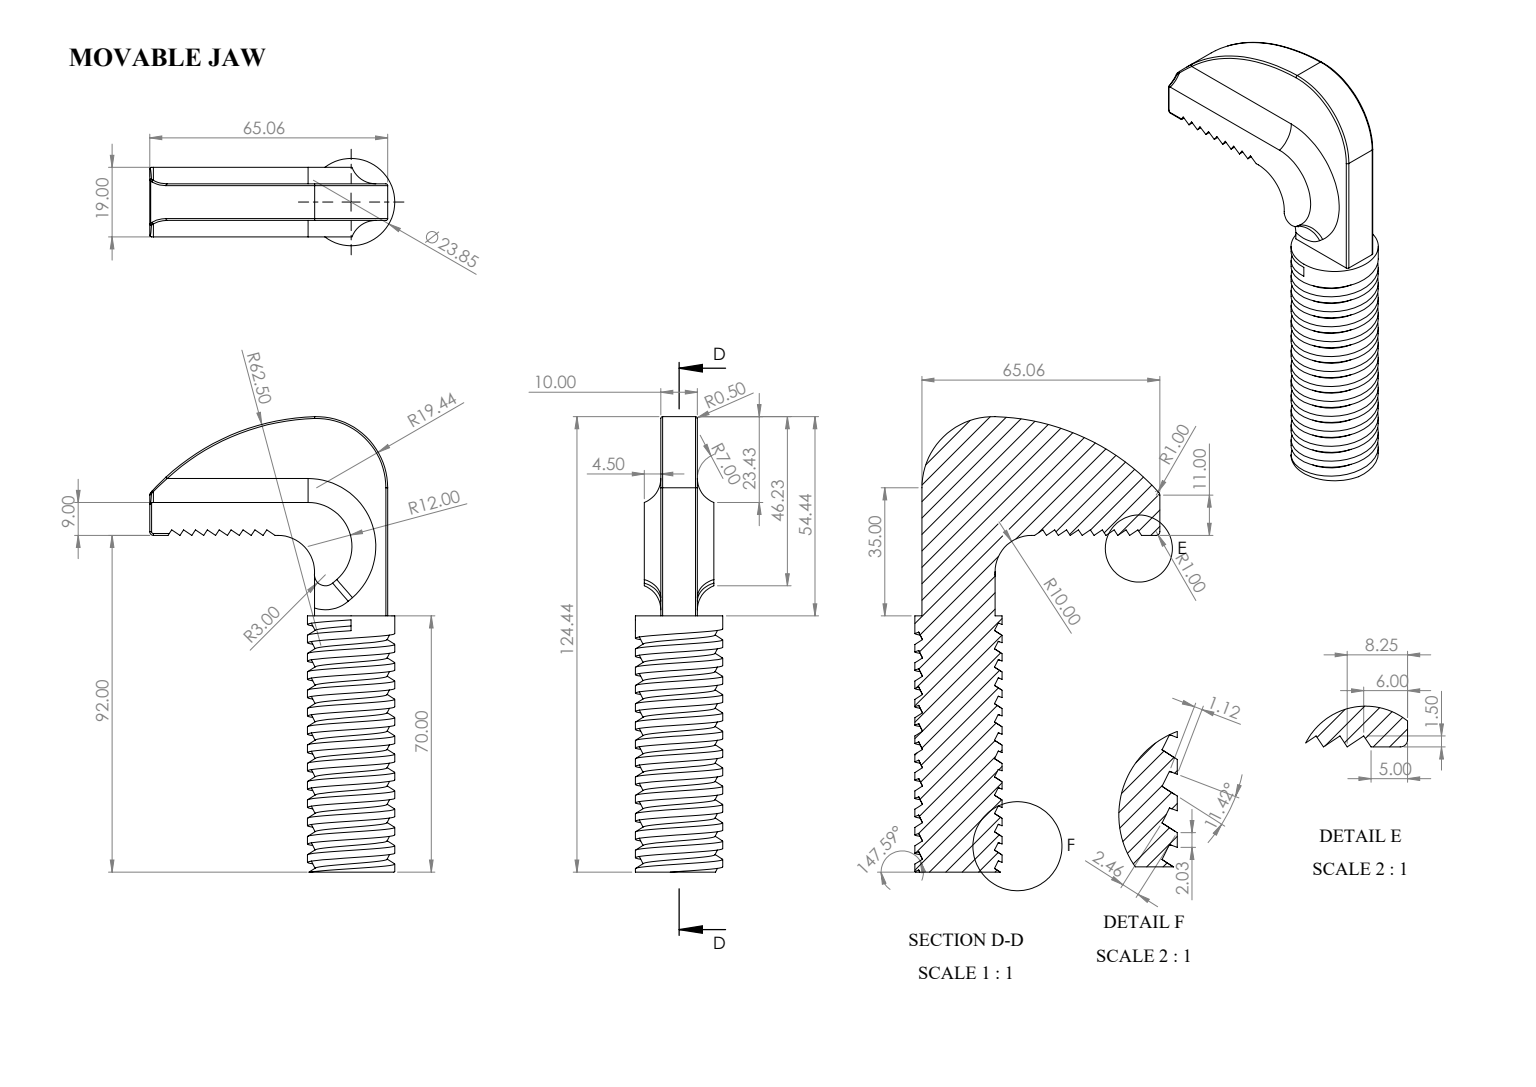
ISO-10303-21;
HEADER;
FILE_DESCRIPTION (('STEP AP214'),
    '1' );
FILE_NAME ('1.2 Movable Jaw.step',
    '2026-10-07T05:30:18',
    ( '' ),
    ( '' ),
    'SwSTEP 2.0',
    'SolidWorks 2021',
    '' );
FILE_SCHEMA (( 'AUTOMOTIVE_DESIGN' ));
ENDSEC;

DATA;
#1=CARTESIAN_POINT ( 'NONE',  ( 7.084665262690076126, 22.02201867748817321, -10.88017736071110164 ) ) ;
#3=CARTESIAN_POINT ( 'NONE',  ( 10.00000000000000000, 59.75893115100078745, -9.846743663894594434 ) ) ;
#5=CARTESIAN_POINT ( 'NONE',  ( 14.92337183194729988, 29.34226448433411960, -8.527530157486177487 ) ) ;
#6=CARTESIAN_POINT ( 'NONE',  ( -1.099225684535947600, 54.54030133659708923, 6.408140936763237150 ) ) ;
#9=CARTESIAN_POINT ( 'NONE',  ( 4.559911319644449179, 47.23035201082150536, -9.422509992056141925 ) ) ;
#10=CARTESIAN_POINT ( 'NONE',  ( 10.00000000000000000, 49.75893115100078745, -9.846743663894594434 ) ) ;
#11=CARTESIAN_POINT ( 'NONE',  ( 6.204703633549690345, 40.76208216824731778, -14.16423886937410259 ) ) ;
#13=CARTESIAN_POINT ( 'NONE',  ( 17.08211943468705840, 5.137082168247300906, -12.26659068614894466 ) ) ;
#14=CARTESIAN_POINT ( 'NONE',  ( 0.5774900079438590739, 67.64701867748817676, -5.440088680355550821 ) ) ;
#16=CARTESIAN_POINT ( 'NONE',  ( 24.16423886937410614, 59.51208216824728936, -3.795296366450302550 ) ) ;
#17=CARTESIAN_POINT ( 'NONE',  ( 13.43411237798106583, 7.665301336597086568, -12.81628187352647252 ) ) ;
#18=CARTESIAN_POINT ( 'NONE',  ( 18.95386800104995473, 43.23810908735726599, -6.499999999999990230 ) ) ;
#19=CARTESIAN_POINT ( 'NONE',  ( 0.5774900079438607392, 58.48035201082151247, 5.440088680355550821 ) ) ;
#21=CARTESIAN_POINT ( 'NONE',  ( -46.94000000000001194, 100.5254250115999923, -8.865097534344174690 ) ) ;
#22=CARTESIAN_POINT ( 'NONE',  ( 0.6178305044545818747, 33.49863466993042493, -9.382169495545419124 ) ) ;
#23=CARTESIAN_POINT ( 'NONE',  ( -2.266590686148945544, 67.22041550158063217, 7.082119434687048631 ) ) ;
#25=CARTESIAN_POINT ( 'NONE',  ( 20.88017736071110875, 15.77201867748817143, -2.915334737309920765 ) ) ;
#26=CARTESIAN_POINT ( 'NONE',  ( 19.42250999205614193, 30.14701867748817321, 5.440088680355555262 ) ) ;
#27=CARTESIAN_POINT ( 'NONE',  ( 7.361572987183169658, 49.96726448433410894, -9.846743663894592657 ) ) ;
#28=CARTESIAN_POINT ( 'NONE',  ( 19.84674366389459266, 58.71726448433411605, -2.638427012816827677 ) ) ;
#29=CARTESIAN_POINT ( 'NONE',  ( -2.816281873526473856, 49.12363466993042493, 9.499525473075851096E-16 ) ) ;
#34=CARTESIAN_POINT ( 'NONE',  ( 20.88017736071110875, 20.77201867748816611, -2.915334737309920765 ) ) ;
#35=CARTESIAN_POINT ( 'NONE',  ( 6.565887622018943937, 23.08196800326375708, -12.81628187352647608 ) ) ;
#37=CARTESIAN_POINT ( 'NONE',  ( 10.00000000000000000, 54.75893115100078745, -9.846743663894594434 ) ) ;
#38=CARTESIAN_POINT ( 'NONE',  ( 12.91533473730992121, 29.52201867748817321, 10.88017736071110164 ) ) ;
#39=CARTESIAN_POINT ( 'NONE',  ( 3.591859063236763294, 18.29030133659708568, -11.09922568453595026 ) ) ;
#40=CARTESIAN_POINT ( 'NONE',  ( -0.8801773607111008646, 43.27201867748817676, 2.915334737309923430 ) ) ;
#42=DIRECTION ( 'NONE',  ( -1.000000000000000000, 0.000000000000000000, 0.000000000000000000 ) ) ;
#43=CARTESIAN_POINT ( 'NONE',  ( 21.09922568453594849, 56.20696800326375353, 6.408140936763242479 ) ) ;
#45=CARTESIAN_POINT ( 'NONE',  ( 12.63842701281683034, 62.46726448433410894, 9.846743663894596210 ) ) ;
#46=CARTESIAN_POINT ( 'NONE',  ( -0.8801773607110991993, 42.85535201082150536, -2.915334737309923874 ) ) ;
#47=CARTESIAN_POINT ( 'NONE',  ( 13.43411237798106583, 32.66530133659708213, -12.81628187352647252 ) ) ;
#48=CARTESIAN_POINT ( 'NONE',  ( -4.164238869374099039, 6.803748834913967869, 8.674139862899312516E-16 ) ) ;
#49=CARTESIAN_POINT ( 'NONE',  ( 10.00000000000000000, 9.758931151000785675, -9.846743663894594434 ) ) ;
#50=CARTESIAN_POINT ( 'NONE',  ( 2.035157376598824452, 58.68868534415482685, 7.964842623401179544 ) ) ;
#51=CARTESIAN_POINT ( 'NONE',  ( -4.164238869374099039, 46.80374883491397497, 8.674139862899312516E-16 ) ) ;
#53=CARTESIAN_POINT ( 'NONE',  ( 0.1532563361054083140, 11.00893115100078568, 1.131784320476157264E-15 ) ) ;
#54=CARTESIAN_POINT ( 'NONE',  ( 0.1532563361054082862, 6.217264484334118713, 2.638427012816831674 ) ) ;
#56=CARTESIAN_POINT ( 'NONE',  ( 2.917880565312950480, 45.97041550158063927, -12.26659068614894821 ) ) ;
#58=CARTESIAN_POINT ( 'NONE',  ( 0.5774900079438590739, 12.64701867748817143, -5.440088680355550821 ) ) ;
#60=ORIENTED_EDGE ( 'NONE', *, *, #26638, .T. ) ;
#62=CARTESIAN_POINT ( 'NONE',  ( 15.44008868035555793, 11.39701867748817143, -9.422509992056140149 ) ) ;
#63=CARTESIAN_POINT ( 'NONE',  ( 22.26659068614895176, 59.72041550158063927, -7.082119434687042414 ) ) ;
#65=CARTESIAN_POINT ( 'NONE',  ( 17.20831665107776587, 42.88393115100077324, 7.208316651077764980 ) ) ;
#66=CARTESIAN_POINT ( 'NONE',  ( -2.816281873526473856, 34.33196800326376064, 3.434112377981055619 ) ) ;
#69=CARTESIAN_POINT ( 'NONE',  ( -2.266590686148945544, 11.38708216824730179, -7.082119434687050408 ) ) ;
#70=CARTESIAN_POINT ( 'NONE',  ( 12.91533473730992121, 29.52201867748817321, 10.88017736071110164 ) ) ;
#71=CARTESIAN_POINT ( 'NONE',  ( -0.8801773607111009756, 8.063685344154837509, 1.068504757029289695E-15 ) ) ;
#72=CARTESIAN_POINT ( 'NONE',  ( 19.84674366389459266, 48.71726448433413026, -2.638427012816827677 ) ) ;
#75=CARTESIAN_POINT ( 'NONE',  ( 17.20831665107776587, 17.88393115100078745, 7.208316651077764980 ) ) ;
#76=CARTESIAN_POINT ( 'NONE',  ( 1.274849032794231007, 33.57228050351031357, 6.499999999999895195 ) ) ;
#78=EDGE_LOOP ( 'NONE', ( #8782, #50817, #67592, #16515 ) ) ;
#81=CARTESIAN_POINT ( 'NONE',  ( 12.63842701281683922, 59.55059781766744464, -9.846743663894590881 ) ) ;
#82=CARTESIAN_POINT ( 'NONE',  ( 20.88017736071110519, 30.56368534415484106, 2.639326808657452039E-16 ) ) ;
#83=CARTESIAN_POINT ( 'NONE',  ( 2.035157376598824452, 33.68868534415484106, 7.964842623401179544 ) ) ;
#84=CARTESIAN_POINT ( 'NONE',  ( 2.791683348922240793, 56.63393115100078035, 7.208316651077764092 ) ) ;
#85=CARTESIAN_POINT ( 'NONE',  ( 16.40814093676323893, 25.79030133659708923, 11.09922568453595026 ) ) ;
#86=CARTESIAN_POINT ( 'NONE',  ( -2.266590686148945544, 21.38708216824730357, -7.082119434687050408 ) ) ;
#89=CARTESIAN_POINT ( 'NONE',  ( 19.38216949554541202, 40.99863466993042493, 9.382169495545424454 ) ) ;
#91=CARTESIAN_POINT ( 'NONE',  ( 0.1532563361054083140, 51.00893115100078745, 1.131784320476157264E-15 ) ) ;
#92=CARTESIAN_POINT ( 'NONE',  ( -0.8801773607110991993, 2.855352010821504471, -2.915334737309923874 ) ) ;
#94=CARTESIAN_POINT ( 'NONE',  ( 17.96484262340118221, 11.18868534415484106, -7.964842623401177768 ) ) ;
#95=ORIENTED_EDGE ( 'NONE', *, *, #4795, .T. ) ;
#96=CARTESIAN_POINT ( 'NONE',  ( 20.88017736071110164, 60.35535201082151957, 2.915334737309930979 ) ) ;
#97=CARTESIAN_POINT ( 'NONE',  ( 15.44008868035555793, 61.39701867748817676, -9.422509992056140149 ) ) ;
#98=CARTESIAN_POINT ( 'NONE',  ( 10.00000000000000178, 59.31368534415484106, 10.88017736071110342 ) ) ;
#100=CARTESIAN_POINT ( 'NONE',  ( 0.5774900079438590739, 52.64701867748817676, -5.440088680355550821 ) ) ;
#103=CARTESIAN_POINT ( 'NONE',  ( -46.78604402846880106, 100.7423487049318140, 9.213902555517821114 ) ) ;
#106=CARTESIAN_POINT ( 'NONE',  ( 7.361572987183170547, 42.05059781766745886, 9.846743663894590881 ) ) ;
#107=VERTEX_POINT ( 'NONE', #70238 ) ;
#108=CARTESIAN_POINT ( 'NONE',  ( 1.472469842513823179, 65.59226448433412315, -4.923371831947296329 ) ) ;
#110=CARTESIAN_POINT ( 'NONE',  ( -4.164238869374098151, 16.59541550158063927, -3.795296366450310543 ) ) ;
#113=CARTESIAN_POINT ( 'NONE',  ( 10.00000000000000178, 64.31368534415483396, 10.88017736071110342 ) ) ;
#114=CARTESIAN_POINT ( 'NONE',  ( 7.084665262690076126, 12.02201867748817321, -10.88017736071110164 ) ) ;
#115=CARTESIAN_POINT ( 'NONE',  ( 0.6081133539230425544, 48.33703382326399378, 6.499999999999948486 ) ) ;
#116=CARTESIAN_POINT ( 'NONE',  ( 6.565887622018943937, 45.16530133659708923, 12.81628187352647430 ) ) ;
#118=CARTESIAN_POINT ( 'NONE',  ( 5.076628168052703671, 46.84226448433412315, 8.527530157486179263 ) ) ;
#119=CARTESIAN_POINT ( 'NONE',  ( 12.63842701281683034, 2.467264484334118269, 9.846743663894596210 ) ) ;
#120=CARTESIAN_POINT ( 'NONE',  ( 16.40814093676324603, 17.45696800326375353, -11.09922568453594671 ) ) ;
#121=CARTESIAN_POINT ( 'NONE',  ( 14.92337183194729988, 19.34226448433411960, -8.527530157486177487 ) ) ;
#122=CARTESIAN_POINT ( 'NONE',  ( 0.6178305044545818747, 13.49863466993041783, -9.382169495545419124 ) ) ;
#125=CARTESIAN_POINT ( 'NONE',  ( 12.63842701281683034, 12.46726448433411782, 9.846743663894596210 ) ) ;
#126=EDGE_LOOP ( 'NONE', ( #78693, #55595, #4509, #60539 ) ) ;
#128=CARTESIAN_POINT ( 'NONE',  ( -0.8801773607110991993, 22.85535201082150181, -2.915334737309923874 ) ) ;
#129=CARTESIAN_POINT ( 'NONE',  ( 24.16423886937410614, 19.30374883491397142, 8.672049930838204340E-16 ) ) ;
#130=CARTESIAN_POINT ( 'NONE',  ( 0.1532563361054082862, 46.21726448433411605, 2.638427012816831674 ) ) ;
#131=CARTESIAN_POINT ( 'NONE',  ( 1.472469842513823179, 5.592264484334118713, -4.923371831947296329 ) ) ;
#132=CARTESIAN_POINT ( 'NONE',  ( -2.816281873526473856, 44.33196800326375353, 3.434112377981055619 ) ) ;
#134=CARTESIAN_POINT ( 'NONE',  ( -0.8801773607111008646, 18.27201867748817321, 2.915334737309923430 ) ) ;
#136=CARTESIAN_POINT ( 'NONE',  ( 6.565887622018943937, 13.08196800326374998, -12.81628187352647608 ) ) ;
#137=CARTESIAN_POINT ( 'NONE',  ( 3.591859063236761518, 4.956968003263753531, 11.09922568453594849 ) ) ;
#138=CARTESIAN_POINT ( 'NONE',  ( 19.84674366389459266, 33.30059781766744464, 2.638427012816836559 ) ) ;
#140=CARTESIAN_POINT ( 'NONE',  ( 19.38216949554541202, 30.99863466993042138, 9.382169495545424454 ) ) ;
#142=CARTESIAN_POINT ( 'NONE',  ( 2.035157376598822676, 42.43868534415483396, -7.964842623401177768 ) ) ;
#144=ADVANCED_FACE ( 'NONE', ( #16249 ), #24174, .T. ) ;
#146=CARTESIAN_POINT ( 'NONE',  ( 2.035157376598824452, 68.68868534415484817, 7.964842623401179544 ) ) ;
#147=CARTESIAN_POINT ( 'NONE',  ( 2.035157376598822676, 42.43868534415483396, -7.964842623401177768 ) ) ;
#149=CARTESIAN_POINT ( 'NONE',  ( 2.035157376598824452, 48.68868534415483396, 7.964842623401179544 ) ) ;
#150=CARTESIAN_POINT ( 'NONE',  ( 5.076628168052703671, 61.84226448433412315, 8.527530157486179263 ) ) ;
#151=CARTESIAN_POINT ( 'NONE',  ( 19.42250999205614548, 65.98035201082151957, -5.440088680355545492 ) ) ;
#152=CARTESIAN_POINT ( 'NONE',  ( 1.472469842513823179, 50.59226448433411605, -4.923371831947296329 ) ) ;
#153=CARTESIAN_POINT ( 'NONE',  ( 15.44008868035555793, 6.397018677488170546, -9.422509992056140149 ) ) ;
#155=CARTESIAN_POINT ( 'NONE',  ( 3.591859063236763294, 8.290301336597087456, -11.09922568453595026 ) ) ;
#156=VERTEX_POINT ( 'NONE', #67375 ) ;
#157=CARTESIAN_POINT ( 'NONE',  ( -0.8801773607111009756, 38.06368534415484106, 1.068504757029289695E-15 ) ) ;
#158=CARTESIAN_POINT ( 'NONE',  ( 19.84674366389459266, 63.71726448433412315, -2.638427012816827677 ) ) ;
#159=CARTESIAN_POINT ( 'NONE',  ( 0.9413316022086131163, 23.45508385108959004, 6.499999999999978684 ) ) ;
#160=CARTESIAN_POINT ( 'NONE',  ( 20.88017736071110164, 20.35535201082150891, 2.915334737309930979 ) ) ;
#161=CARTESIAN_POINT ( 'NONE',  ( 4.559911319644449179, 23.89701867748817321, 9.422509992056141925 ) ) ;
#162=CARTESIAN_POINT ( 'NONE',  ( 20.36894250292379738, 39.92874883491396787, -10.36894250292379027 ) ) ;
#163=CARTESIAN_POINT ( 'NONE',  ( 18.52753015748618282, 23.92559781766745530, -4.923371831947291888 ) ) ;
#164=CARTESIAN_POINT ( 'NONE',  ( 0.5774900079438590739, 42.64701867748816966, -5.440088680355550821 ) ) ;
#165=CARTESIAN_POINT ( 'NONE',  ( 24.16423886937410614, 4.512082168247300906, -3.795296366450302550 ) ) ;
#167=CARTESIAN_POINT ( 'NONE',  ( 7.361572987183170547, 57.05059781766744464, 9.846743663894590881 ) ) ;
#170=CARTESIAN_POINT ( 'NONE',  ( -2.266590686148945544, 32.22041550158063927, 7.082119434687048631 ) ) ;
#171=CARTESIAN_POINT ( 'NONE',  ( 13.79529636645030344, 23.26208216824730002, 14.16423886937410614 ) ) ;
#173=CARTESIAN_POINT ( 'NONE',  ( 0.1532563361054100626, 0.8005978176674514168, -2.638427012816831230 ) ) ;
#174=CARTESIAN_POINT ( 'NONE',  ( 17.20831665107776587, 47.88393115100078745, 7.208316651077764980 ) ) ;
#176=CARTESIAN_POINT ( 'NONE',  ( 4.559911319644449179, 52.23035201082151247, -9.422509992056141925 ) ) ;
#177=CARTESIAN_POINT ( 'NONE',  ( 16.40814093676324603, 22.45696800326375353, -11.09922568453594671 ) ) ;
#178=CARTESIAN_POINT ( 'NONE',  ( 6.204703633549690345, 30.76208216824730357, -14.16423886937410259 ) ) ;
#179=CARTESIAN_POINT ( 'NONE',  ( 0.5774900079438590739, 7.647018677488171434, -5.440088680355550821 ) ) ;
#180=CARTESIAN_POINT ( 'NONE',  ( 20.88017736071110519, 25.56368534415483751, 2.639326808657452039E-16 ) ) ;
#182=CARTESIAN_POINT ( 'NONE',  ( -0.8801773607110991993, 62.85535201082150536, -2.915334737309923874 ) ) ;
#183=CARTESIAN_POINT ( 'NONE',  ( -1.099225684535947600, 44.54030133659708923, 6.408140936763237150 ) ) ;
#191=CARTESIAN_POINT ( 'NONE',  ( -0.3689425029237881626, 62.42874883491396787, 10.36894250292379027 ) ) ;
#192=CARTESIAN_POINT ( 'NONE',  ( 17.08211943468705840, 60.13708216824729647, -12.26659068614894466 ) ) ;
#193=CARTESIAN_POINT ( 'NONE',  ( 19.84674366389459621, 18.50893115100078745, 7.409399052514197653E-17 ) ) ;
#194=CARTESIAN_POINT ( 'NONE',  ( 2.791683348922237240, 60.38393115100078745, -7.208316651077763204 ) ) ;
#197=CARTESIAN_POINT ( 'NONE',  ( 21.09922568453595559, 2.040301336597086568, -6.408140936763230044 ) ) ;
#200=CARTESIAN_POINT ( 'NONE',  ( 24.16423886937409904, 34.09541550158064638, 3.795296366450317205 ) ) ;
#202=CARTESIAN_POINT ( 'NONE',  ( 22.26659068614895176, 49.72041550158063927, -7.082119434687042414 ) ) ;
#204=CARTESIAN_POINT ( 'NONE',  ( 13.43411237798106583, 52.66530133659708213, -12.81628187352647252 ) ) ;
#206=CARTESIAN_POINT ( 'NONE',  ( -0.8801773607111008646, 28.27201867748817321, 2.915334737309923430 ) ) ;
#207=CARTESIAN_POINT ( 'NONE',  ( 1.472469842513823179, 50.59226448433411605, -4.923371831947296329 ) ) ;
#208=CARTESIAN_POINT ( 'NONE',  ( 19.42250999205614548, 25.98035201082150891, -5.440088680355545492 ) ) ;
#209=CARTESIAN_POINT ( 'NONE',  ( 22.81628187352647785, 61.41530133659709634, 3.434112377981063169 ) ) ;
#211=CARTESIAN_POINT ( 'NONE',  ( 0.1532563361054083140, 51.00893115100078745, 1.131784320476157264E-15 ) ) ;
#212=CARTESIAN_POINT ( 'NONE',  ( 7.361572987183169658, 54.96726448433413026, -9.846743663894592657 ) ) ;
#214=CARTESIAN_POINT ( 'NONE',  ( -46.30928139467842897, 104.0823827281712255, -5.529860068218142466 ) ) ;
#216=ORIENTED_EDGE ( 'NONE', *, *, #69949, .F. ) ;
#218=CARTESIAN_POINT ( 'NONE',  ( 18.52753015748617571, 3.092264484334118269, 4.923371831947298993 ) ) ;
#221=CARTESIAN_POINT ( 'NONE',  ( 0.9408516040111366552, 57.46693863883976405, -6.499999999999915623 ) ) ;
#222=CARTESIAN_POINT ( 'NONE',  ( 12.63842701281683034, 37.46726448433411605, 9.846743663894596210 ) ) ;
#224=CARTESIAN_POINT ( 'NONE',  ( 16.40814093676324603, 32.45696800326375353, -11.09922568453594671 ) ) ;
#229=CARTESIAN_POINT ( 'NONE',  ( 18.52753015748618282, 63.92559781766745886, -4.923371831947291888 ) ) ;
#231=CARTESIAN_POINT ( 'NONE',  ( 17.20831665107776587, 57.88393115100078745, 7.208316651077764980 ) ) ;
#232=CARTESIAN_POINT ( 'NONE',  ( 2.917880565312948704, 37.63708216824731068, 12.26659068614894643 ) ) ;
#233=CARTESIAN_POINT ( 'NONE',  ( 14.92337183194729633, 62.67559781766745886, 8.527530157486181039 ) ) ;
#235=CARTESIAN_POINT ( 'NONE',  ( 14.92337183194729988, 9.342264484334119601, -8.527530157486177487 ) ) ;
#236=CARTESIAN_POINT ( 'NONE',  ( 20.15039907845753220, 46.74884699246888431, 6.262539305110077947 ) ) ;
#237=CARTESIAN_POINT ( 'NONE',  ( 10.00000000000000000, 44.75893115100078745, -9.846743663894594434 ) ) ;
#238=CARTESIAN_POINT ( 'NONE',  ( 15.44008868035555260, 54.73035201082150536, 9.422509992056143702 ) ) ;
#239=CARTESIAN_POINT ( 'NONE',  ( 10.00000000000000178, 47.25893115100078745, 9.846743663894594434 ) ) ;
#242=CARTESIAN_POINT ( 'NONE',  ( 17.96484262340118221, 49.93868534415484106, 7.964842623401181321 ) ) ;
#245=CARTESIAN_POINT ( 'NONE',  ( 7.084665262690076126, 27.02201867748817676, -10.88017736071110164 ) ) ;
#246=CARTESIAN_POINT ( 'NONE',  ( -2.816281873526473856, -0.6680319967362464695, 3.434112377981055619 ) ) ;
#247=CARTESIAN_POINT ( 'NONE',  ( 19.42250999205614193, 60.14701867748817676, 5.440088680355555262 ) ) ;
#249=LINE ( 'NONE', #54676, #20391 ) ;
#251=CARTESIAN_POINT ( 'NONE',  ( 19.42250999205614193, 45.14701867748817676, 5.440088680355555262 ) ) ;
#252=CARTESIAN_POINT ( 'NONE',  ( -35.44000000000001194, 93.50000000000000000, 9.500000000000000000 ) ) ;
#253=CARTESIAN_POINT ( 'NONE',  ( 19.84674366389459266, 8.300597817667451750, 2.638427012816836559 ) ) ;
#254=CARTESIAN_POINT ( 'NONE',  ( 14.92337183194729633, 42.67559781766745886, 8.527530157486181039 ) ) ;
#256=CARTESIAN_POINT ( 'NONE',  ( 19.38216949554541202, 0.9986346699304200492, 9.382169495545424454 ) ) ;
#257=CARTESIAN_POINT ( 'NONE',  ( -4.164238869374098151, 61.59541550158063217, -3.795296366450310543 ) ) ;
#261=CARTESIAN_POINT ( 'NONE',  ( 24.16423886937410614, 24.30374883491396787, 8.672049930838204340E-16 ) ) ;
#262=EDGE_CURVE ( 'NONE', #31207, #19224, #78615, .T. ) ;
#263=CARTESIAN_POINT ( 'NONE',  ( -4.164238869374098151, 56.59541550158063927, -3.795296366450310543 ) ) ;
#265=( BOUNDED_CURVE ( )  B_SPLINE_CURVE ( 2, ( #5381, #12855, #20864, #27367, #66849, #65855, #27855, #66344, #19866 ),
 .UNSPECIFIED., .F., .F. ) 
 B_SPLINE_CURVE_WITH_KNOTS ( ( 3, 2, 2, 2, 3 ),
 ( 0.7962860886497512558, 0.7976190476190476719, 0.8035714285714286031, 0.8095238095238095344, 0.8108567684931060615 ),
 .UNSPECIFIED. ) 
 CURVE ( )  GEOMETRIC_REPRESENTATION_ITEM ( )  RATIONAL_B_SPLINE_CURVE ( ( 0.9881565478350734510, 0.9923695281211492025, 1.000000000000000000, 0.9659258262890683122, 1.000000000000000000, 0.9659258262890683122, 1.000000000000000000, 0.9923695281211484254, 0.9881565478350726739 ) ) 
 REPRESENTATION_ITEM ( '' )  );
#266=CARTESIAN_POINT ( 'NONE',  ( 17.20831665107776587, 14.13393115100078568, -7.208316651077762316 ) ) ;
#267=CARTESIAN_POINT ( 'NONE',  ( 19.88565890683626947, 32.71691075486303646, -6.480892540919838574 ) ) ;
#270=CARTESIAN_POINT ( 'NONE',  ( 14.92337183194729633, 22.67559781766745175, 8.527530157486181039 ) ) ;
#271=CARTESIAN_POINT ( 'NONE',  ( 7.084665262690076126, 24.10535201082150181, 10.88017736071109987 ) ) ;
#272=CARTESIAN_POINT ( 'NONE',  ( -1.099225684535947600, -1.293031996736246469, -6.408140936763238038 ) ) ;
#273=CARTESIAN_POINT ( 'NONE',  ( 6.204703633549690345, 12.84541550158063572, 14.16423886937410082 ) ) ;
#276=CARTESIAN_POINT ( 'NONE',  ( 14.92337183194729633, 12.67559781766745353, 8.527530157486181039 ) ) ;
#277=CARTESIAN_POINT ( 'NONE',  ( 13.43411237798105340, 40.58196800326375353, 12.81628187352647963 ) ) ;
#278=CARTESIAN_POINT ( 'NONE',  ( 0.1532563361054083140, 46.00893115100079456, 1.131784320476157264E-15 ) ) ;
#280=CARTESIAN_POINT ( 'NONE',  ( 1.472469842513823179, 16.42559781766745175, 4.923371831947296329 ) ) ;
#283=CARTESIAN_POINT ( 'NONE',  ( 24.16423886937410614, 59.30374883491397497, 8.672049930838204340E-16 ) ) ;
#284=CARTESIAN_POINT ( 'NONE',  ( 2.035157376598822676, 57.43868534415484106, -7.964842623401177768 ) ) ;
#287=CARTESIAN_POINT ( 'NONE',  ( 10.00000000000000000, 34.75893115100078745, -9.846743663894594434 ) ) ;
#288=CARTESIAN_POINT ( 'NONE',  ( -0.8801773607111008646, 3.272018677488171434, 2.915334737309923430 ) ) ;
#289=CARTESIAN_POINT ( 'NONE',  ( 10.00000000000000178, 42.25893115100078745, 9.846743663894594434 ) ) ;
#291=CARTESIAN_POINT ( 'NONE',  ( 17.20831665107776587, 52.88393115100078035, 7.208316651077764980 ) ) ;
#292=CARTESIAN_POINT ( 'NONE',  ( 7.084665262690076126, 49.10535201082149825, 10.88017736071109987 ) ) ;
#299=ADVANCED_FACE ( 'NONE', ( #45868 ), #51618, .T. ) ;
#300=CARTESIAN_POINT ( 'NONE',  ( 19.84674366389459621, 8.508931151000785675, 7.409399052514197653E-17 ) ) ;
#301=CARTESIAN_POINT ( 'NONE',  ( 22.81628187352647785, 56.41530133659708213, 3.434112377981063169 ) ) ;
#302=CARTESIAN_POINT ( 'NONE',  ( 7.084665262690076126, 2.022018677488171434, -10.88017736071110164 ) ) ;
#303=CARTESIAN_POINT ( 'NONE',  ( 2.791683348922237240, 55.38393115100078745, -7.208316651077763204 ) ) ;
#304=CARTESIAN_POINT ( 'NONE',  ( 20.00000000000000711, 81.00839193781131087, 4.500000000000000888 ) ) ;
#305=CARTESIAN_POINT ( 'NONE',  ( 6.204703633549690345, 30.76208216824730357, -14.16423886937410259 ) ) ;
#306=CARTESIAN_POINT ( 'NONE',  ( 2.917880565312948704, 52.63708216824730357, 12.26659068614894643 ) ) ;
#307=CARTESIAN_POINT ( 'NONE',  ( 18.52753015748617571, 58.09226448433411605, 4.923371831947298993 ) ) ;
#310=CARTESIAN_POINT ( 'NONE',  ( 17.96484262340118221, 56.18868534415484817, -7.964842623401177768 ) ) ;
#312=CARTESIAN_POINT ( 'NONE',  ( 1.472469842513823179, 0.5922644843341181575, -4.923371831947296329 ) ) ;
#314=CARTESIAN_POINT ( 'NONE',  ( 13.43411237798106583, 62.66530133659708923, -12.81628187352647252 ) ) ;
#317=CARTESIAN_POINT ( 'NONE',  ( 10.00000000000000178, 7.258931151000785675, 9.846743663894594434 ) ) ;
#319=CARTESIAN_POINT ( 'NONE',  ( 10.00000000000000178, 23.05374883491397142, 14.16423886937410082 ) ) ;
#320=CARTESIAN_POINT ( 'NONE',  ( 17.20831665107776587, 19.13393115100078035, -7.208316651077762316 ) ) ;
#321=CARTESIAN_POINT ( 'NONE',  ( 15.44008868035555260, 34.73035201082151247, 9.422509992056143702 ) ) ;
#322=CARTESIAN_POINT ( 'NONE',  ( 0.5600000000000076028, 107.5383484153110203, -5.000000000000000000 ) ) ;
#324=CARTESIAN_POINT ( 'NONE',  ( 12.91533473730993009, 21.60535201082150536, -10.88017736071109987 ) ) ;
#326=CARTESIAN_POINT ( 'NONE',  ( 17.96484262340118221, 34.93868534415482685, 7.964842623401181321 ) ) ;
#327=PRESENTATION_STYLE_ASSIGNMENT (( #76290 ) ) ;
#331=CARTESIAN_POINT ( 'NONE',  ( 16.40814093676324603, 22.45696800326375353, -11.09922568453594671 ) ) ;
#332=CARTESIAN_POINT ( 'NONE',  ( 2.603489959281199972, 21.58210964143324873, 6.499999999999559464 ) ) ;
#333=CARTESIAN_POINT ( 'NONE',  ( 0.1532563361054082862, 6.217264484334118713, 2.638427012816831674 ) ) ;
#335=CARTESIAN_POINT ( 'NONE',  ( -0.03932841506541424198, 58.12161441960502373, 6.397827110479012092 ) ) ;
#336=CARTESIAN_POINT ( 'NONE',  ( 2.791683348922240793, 21.63393115100078745, 7.208316651077764092 ) ) ;
#337=CARTESIAN_POINT ( 'NONE',  ( 7.084665262690076126, 29.10535201082150181, 10.88017736071109987 ) ) ;
#342=CARTESIAN_POINT ( 'NONE',  ( -0.1503990784575247319, 52.22266099184918176, -6.262539305110083276 ) ) ;
#343=CARTESIAN_POINT ( 'NONE',  ( 10.00000000000000000, 56.81368534415484106, -10.88017736071110342 ) ) ;
#345=CARTESIAN_POINT ( 'NONE',  ( 21.09922568453594849, 61.20696800326376064, 6.408140936763242479 ) ) ;
#346=CARTESIAN_POINT ( 'NONE',  ( 15.44008868035555260, 64.73035201082151957, 9.422509992056143702 ) ) ;
#347=CARTESIAN_POINT ( 'NONE',  ( 7.361572987183170547, 67.05059781766746596, 9.846743663894590881 ) ) ;
#349=CARTESIAN_POINT ( 'NONE',  ( 5.076628168052704559, 30.17559781766745175, -8.527530157486179263 ) ) ;
#350=CARTESIAN_POINT ( 'NONE',  ( 3.591859063236761518, 49.95696800326375353, 11.09922568453594849 ) ) ;
#352=CARTESIAN_POINT ( 'NONE',  ( 19.84674366389459266, 13.30059781766745353, 2.638427012816836559 ) ) ;
#353=CARTESIAN_POINT ( 'NONE',  ( 0.6178305044545838731, 14.74863466993041783, 9.382169495545420901 ) ) ;
#355=CARTESIAN_POINT ( 'NONE',  ( 19.42250999205614548, 30.98035201082150536, -5.440088680355545492 ) ) ;
#356=CARTESIAN_POINT ( 'NONE',  ( 10.00000000000000000, 64.75893115100078035, -9.846743663894594434 ) ) ;
#358=CARTESIAN_POINT ( 'NONE',  ( 5.076628168052704559, 20.17559781766745175, -8.527530157486179263 ) ) ;
#359=CARTESIAN_POINT ( 'NONE',  ( 5.076628168052703671, 1.842264484334118047, 8.527530157486179263 ) ) ;
#360=CARTESIAN_POINT ( 'NONE',  ( 0.5774900079438607392, 13.48035201082150358, 5.440088680355550821 ) ) ;
#361=CARTESIAN_POINT ( 'NONE',  ( 0.6178305044545838731, 19.74863466993042138, 9.382169495545420901 ) ) ;
#366=CARTESIAN_POINT ( 'NONE',  ( -2.266590686148945544, 67.22041550158063217, 7.082119434687048631 ) ) ;
#367=CARTESIAN_POINT ( 'NONE',  ( 7.361572987183169658, 49.96726448433410894, -9.846743663894592657 ) ) ;
#371=CARTESIAN_POINT ( 'NONE',  ( 2.035157376598824452, 23.68868534415484461, 7.964842623401179544 ) ) ;
#372=CARTESIAN_POINT ( 'NONE',  ( -0.8801773607111009756, 13.27201867748817321, 2.915334737309923874 ) ) ;
#374=CARTESIAN_POINT ( 'NONE',  ( 7.084665262690076126, 29.10535201082150181, 10.88017736071109987 ) ) ;
#375=CARTESIAN_POINT ( 'NONE',  ( 17.08211943468705840, 65.13708216824730357, -12.26659068614894466 ) ) ;
#377=( LENGTH_UNIT ( ) NAMED_UNIT ( * ) SI_UNIT ( .MILLI., .METRE. ) );
#378=CARTESIAN_POINT ( 'NONE',  ( 10.00000000000000000, 24.75893115100078745, -9.846743663894594434 ) ) ;
#379=CARTESIAN_POINT ( 'NONE',  ( 0.6178305044545818747, 8.498634669930421381, -9.382169495545419124 ) ) ;
#381=CARTESIAN_POINT ( 'NONE',  ( -2.816281873526473856, -0.8763653300695799508, 9.499525473075851096E-16 ) ) ;
#383=ADVANCED_FACE ( 'NONE', ( #38841 ), #20965, .T. ) ;
#385=CARTESIAN_POINT ( 'NONE',  ( -0.3689425029237898834, 11.17874883491396787, -10.36894250292378850 ) ) ;
#386=CARTESIAN_POINT ( 'NONE',  ( 5.076628168052703671, 31.84226448433412315, 8.527530157486179263 ) ) ;
#387=EDGE_LOOP ( 'NONE', ( #36571, #85483, #95211, #2832, #77271 ) ) ;
#388=CARTESIAN_POINT ( 'NONE',  ( 6.204703633549690345, 57.84541550158063927, 14.16423886937410082 ) ) ;
#390=CARTESIAN_POINT ( 'NONE',  ( 14.92337183194729633, 12.67559781766745353, 8.527530157486181039 ) ) ;
#393=CARTESIAN_POINT ( 'NONE',  ( 10.00000000000000178, 44.31368534415484106, 10.88017736071110342 ) ) ;
#394=CARTESIAN_POINT ( 'NONE',  ( 22.81628187352647785, 46.41530133659708213, 3.434112377981063169 ) ) ;
#395=CARTESIAN_POINT ( 'NONE',  ( 10.00000000000000000, 16.81368534415483751, -10.88017736071110342 ) ) ;
#396=CARTESIAN_POINT ( 'NONE',  ( 19.38216949554541557, 47.24863466993041783, -9.382169495545420901 ) ) ;
#397=CARTESIAN_POINT ( 'NONE',  ( 1.472469842513823179, 65.59226448433412315, -4.923371831947296329 ) ) ;
#401=CARTESIAN_POINT ( 'NONE',  ( -4.164238869374098151, 36.59541550158063217, -3.795296366450310543 ) ) ;
#402=CARTESIAN_POINT ( 'NONE',  ( 13.79529636645030344, 13.26208216824729824, 14.16423886937410614 ) ) ;
#403=CARTESIAN_POINT ( 'NONE',  ( 19.42250999205614193, 15.14701867748817143, 5.440088680355555262 ) ) ;
#404=CARTESIAN_POINT ( 'NONE',  ( 15.44008868035555260, 34.73035201082151247, 9.422509992056143702 ) ) ;
#407=CARTESIAN_POINT ( 'NONE',  ( 19.84674366389459621, 3.508931151000785231, 7.409399052514197653E-17 ) ) ;
#408=CARTESIAN_POINT ( 'NONE',  ( 0.5774900079438607392, 58.48035201082151247, 5.440088680355550821 ) ) ;
#409=CARTESIAN_POINT ( 'NONE',  ( -2.816281873526473856, 24.33196800326375353, 3.434112377981055619 ) ) ;
#410=DIRECTION ( 'NONE',  ( 1.000000000000000000, 0.000000000000000000, 0.000000000000000000 ) ) ;
#412=CARTESIAN_POINT ( 'NONE',  ( 7.361572987183170547, 37.05059781766744464, 9.846743663894590881 ) ) ;
#413=CARTESIAN_POINT ( 'NONE',  ( 19.42250999205614193, 20.14701867748817321, 5.440088680355555262 ) ) ;
#415=CARTESIAN_POINT ( 'NONE',  ( 6.565887622018943937, 18.08196800326375708, -12.81628187352647608 ) ) ;
#417=CARTESIAN_POINT ( 'NONE',  ( 10.00000000000000178, 12.25893115100078568, 9.846743663894594434 ) ) ;
#418=CARTESIAN_POINT ( 'NONE',  ( 15.44008868035555260, 14.73035201082150536, 9.422509992056143702 ) ) ;
#419=CARTESIAN_POINT ( 'NONE',  ( 5.076628168052704559, 35.17559781766745175, -8.527530157486179263 ) ) ;
#420=CARTESIAN_POINT ( 'NONE',  ( -2.816281873526473856, 59.33196800326374643, 3.434112377981055619 ) ) ;
#421=CARTESIAN_POINT ( 'NONE',  ( 17.20831665107776587, 37.88393115100078745, 7.208316651077764980 ) ) ;
#422=CARTESIAN_POINT ( 'NONE',  ( 17.08211943468705130, 3.470415501580634388, 12.26659068614894998 ) ) ;
#423=CARTESIAN_POINT ( 'NONE',  ( 22.26659068614894466, 13.88708216824730179, 7.082119434687054849 ) ) ;
#424=CARTESIAN_POINT ( 'NONE',  ( 0.5774900079438607392, 33.48035201082150536, 5.440088680355550821 ) ) ;
#425=CARTESIAN_POINT ( 'NONE',  ( -0.8801773607111008646, 13.27201867748817143, 2.915334737309923430 ) ) ;
#426=CARTESIAN_POINT ( 'NONE',  ( 20.36894250292379382, 43.67874883491397497, 10.36894250292379205 ) ) ;
#428=CARTESIAN_POINT ( 'NONE',  ( 2.035157376598822676, 37.43868534415484106, -7.964842623401177768 ) ) ;
#429=CARTESIAN_POINT ( 'NONE',  ( 15.44008868035555260, 14.73035201082150536, 9.422509992056143702 ) ) ;
#430=ORIENTED_EDGE ( 'NONE', *, *, #84794, .F. ) ;
#431=CARTESIAN_POINT ( 'NONE',  ( 10.00000000000000000, 36.81368534415484106, -10.88017736071110342 ) ) ;
#432=CARTESIAN_POINT ( 'NONE',  ( 16.40814093676324603, 57.45696800326375353, -11.09922568453594671 ) ) ;
#433=CARTESIAN_POINT ( 'NONE',  ( 7.084665262690076126, 44.10535201082151247, 10.88017736071109987 ) ) ;
#434=CARTESIAN_POINT ( 'NONE',  ( 15.44008868035555260, 44.73035201082151247, 9.422509992056143702 ) ) ;
#437=CARTESIAN_POINT ( 'NONE',  ( 12.91533473730993009, 46.60535201082150536, -10.88017736071109987 ) ) ;
#439=CARTESIAN_POINT ( 'NONE',  ( 20.36894250292379382, 48.67874883491396076, 10.36894250292379205 ) ) ;
#440=CARTESIAN_POINT ( 'NONE',  ( 20.88017736071110875, 65.77201867748817676, -2.915334737309920765 ) ) ;
#444=CARTESIAN_POINT ( 'NONE',  ( 19.84674366389459621, 38.50893115100078745, 7.409399052514197653E-17 ) ) ;
#447=CARTESIAN_POINT ( 'NONE',  ( 2.791683348922237240, 40.38393115100078035, -7.208316651077763204 ) ) ;
#448=CARTESIAN_POINT ( 'NONE',  ( 17.96484262340118221, 39.93868534415484106, 7.964842623401181321 ) ) ;
#449=CARTESIAN_POINT ( 'NONE',  ( 7.361572987183169658, 34.96726448433411605, -9.846743663894592657 ) ) ;
#450=CARTESIAN_POINT ( 'NONE',  ( 6.565887622018943937, 20.16530133659708213, 12.81628187352647430 ) ) ;
#452=CARTESIAN_POINT ( 'NONE',  ( 19.42250999205614548, 55.98035201082150536, -5.440088680355545492 ) ) ;
#453=CARTESIAN_POINT ( 'NONE',  ( 19.42250999205614193, 40.14701867748817676, 5.440088680355555262 ) ) ;
#454=CARTESIAN_POINT ( 'NONE',  ( 0.5774900079438607392, 3.480352010821504027, 5.440088680355550821 ) ) ;
#455=CARTESIAN_POINT ( 'NONE',  ( -4.164238869374099927, 52.01208216824729647, 3.795296366450308767 ) ) ;
#456=EDGE_CURVE ( 'NONE', #94075, #88696, #79322, .T. ) ;
#457=( GEOMETRIC_REPRESENTATION_CONTEXT ( 3 ) GLOBAL_UNCERTAINTY_ASSIGNED_CONTEXT ( ( #37162 ) ) GLOBAL_UNIT_ASSIGNED_CONTEXT ( ( #27747, #58230, #95771 ) ) REPRESENTATION_CONTEXT ( 'NONE', 'WORKASPACE' ) );
#458=CARTESIAN_POINT ( 'NONE',  ( 10.00000000000000000, 22.87363466993042138, -12.81628187352647608 ) ) ;
#459=CARTESIAN_POINT ( 'NONE',  ( 2.603489959281613420, 50.43575266056826933, -6.500000000000031086 ) ) ;
#461=CARTESIAN_POINT ( 'NONE',  ( 22.81628187352647785, 21.62363466993041783, 6.195893100308588602E-16 ) ) ;
#462=CARTESIAN_POINT ( 'NONE',  ( 4.559911319644449179, 22.23035201082150536, -9.422509992056141925 ) ) ;
#463=CARTESIAN_POINT ( 'NONE',  ( 17.96484262340118221, 59.93868534415484106, 7.964842623401181321 ) ) ;
#465=ORIENTED_EDGE ( 'NONE', *, *, #55676, .T. ) ;
#466=CARTESIAN_POINT ( 'NONE',  ( 7.361572987183170547, 2.050597817667451750, 9.846743663894590881 ) ) ;
#467=CARTESIAN_POINT ( 'NONE',  ( 18.52753015748618282, 48.92559781766745886, -4.923371831947291888 ) ) ;
#468=CARTESIAN_POINT ( 'NONE',  ( 1.472469842513823179, 40.59226448433411605, -4.923371831947296329 ) ) ;
#469=CARTESIAN_POINT ( 'NONE',  ( 7.361572987183170547, 32.05059781766745175, 9.846743663894590881 ) ) ;
#470=CARTESIAN_POINT ( 'NONE',  ( 0.2751277870542967463, 70.00000000000000000, 6.000000000000000000 ) ) ;
#472=CARTESIAN_POINT ( 'NONE',  ( -2.816281873526473856, 39.12363466993041783, 9.499525473075851096E-16 ) ) ;
#473=CARTESIAN_POINT ( 'NONE',  ( 19.84674366389459621, 13.50893115100078568, 7.409399052514197653E-17 ) ) ;
#474=CARTESIAN_POINT ( 'NONE',  ( 19.89103541497710737, 50.66234555792570404, -6.479102184480820981 ) ) ;
#476=CARTESIAN_POINT ( 'NONE',  ( 1.472469842513823179, 40.59226448433411605, -4.923371831947296329 ) ) ;
#479=CARTESIAN_POINT ( 'NONE',  ( 0.000000000000000000, 70.00000000000000000, 6.000000000000000000 ) ) ;
#480=CARTESIAN_POINT ( 'NONE',  ( 0.6178305044545838731, 9.748634669930416052, 9.382169495545420901 ) ) ;
#481=CARTESIAN_POINT ( 'NONE',  ( 4.559911319644449179, 48.89701867748817676, 9.422509992056141925 ) ) ;
#482=CARTESIAN_POINT ( 'NONE',  ( -2.266590686148945544, 37.22041550158063217, 7.082119434687048631 ) ) ;
#484=CARTESIAN_POINT ( 'NONE',  ( 20.00000000000000711, 93.00652443313256867, 4.825407043044950051 ) ) ;
#485=CARTESIAN_POINT ( 'NONE',  ( 24.16423886937409904, 29.09541550158063572, 3.795296366450317205 ) ) ;
#486=CARTESIAN_POINT ( 'NONE',  ( 17.08211943468705840, 65.13708216824730357, -12.26659068614894466 ) ) ;
#487=CARTESIAN_POINT ( 'NONE',  ( 24.16423886937410614, 14.30374883491396787, 8.672049930838204340E-16 ) ) ;
#488=CARTESIAN_POINT ( 'NONE',  ( -4.164238869374098151, 31.59541550158063927, -3.795296366450310543 ) ) ;
#490=CARTESIAN_POINT ( 'NONE',  ( 7.084665262690076126, 59.10535201082150536, 10.88017736071109987 ) ) ;
#491=CARTESIAN_POINT ( 'NONE',  ( 1.274849032794231007, 38.57228050351032067, 6.499999999999895195 ) ) ;
#494=CARTESIAN_POINT ( 'NONE',  ( 10.00000000000000000, 39.75893115100078745, -9.846743663894594434 ) ) ;
#495=CARTESIAN_POINT ( 'NONE',  ( 0.5774900079438607392, 23.48035201082150536, 5.440088680355550821 ) ) ;
#496=CARTESIAN_POINT ( 'NONE',  ( 20.24186590665278018, 55.59014588040356841, -6.114288769123040090 ) ) ;
#497=CARTESIAN_POINT ( 'NONE',  ( 1.472469842513823179, 66.42559781766745175, 4.923371831947296329 ) ) ;
#498=CARTESIAN_POINT ( 'NONE',  ( 20.00000000000000711, 85.79222437201093499, -4.885465336748874066 ) ) ;
#499=CARTESIAN_POINT ( 'NONE',  ( 7.361572987183169658, 34.96726448433411605, -9.846743663894592657 ) ) ;
#500=CARTESIAN_POINT ( 'NONE',  ( 22.81628187352647785, 51.62363466993042493, 6.195893100308588602E-16 ) ) ;
#503=CARTESIAN_POINT ( 'NONE',  ( 0.1532563361054083140, 36.00893115100078745, 1.131784320476157264E-15 ) ) ;
#504=CARTESIAN_POINT ( 'NONE',  ( 10.00000000000000000, 54.75893115100078745, -9.846743663894594434 ) ) ;
#506=CARTESIAN_POINT ( 'NONE',  ( -4.164238869374099927, 42.01208216824728936, 3.795296366450308767 ) ) ;
#507=VERTEX_POINT ( 'NONE', #94282 ) ;
#508=CARTESIAN_POINT ( 'NONE',  ( -2.266590686148945544, 7.220415501580634832, 7.082119434687048631 ) ) ;
#510=EDGE_CURVE ( 'NONE', #54365, #74552, #66998, .T. ) ;
#511=CARTESIAN_POINT ( 'NONE',  ( 19.42250999205614193, 60.14701867748817676, 5.440088680355555262 ) ) ;
#513=CARTESIAN_POINT ( 'NONE',  ( 22.26659068614894466, 53.88708216824731068, 7.082119434687054849 ) ) ;
#514=CARTESIAN_POINT ( 'NONE',  ( 16.40814093676323893, 10.79030133659708923, 11.09922568453595026 ) ) ;
#516=CARTESIAN_POINT ( 'NONE',  ( 19.84674366389459621, 3.508931151000785231, 7.409399052514197653E-17 ) ) ;
#517=AXIS2_PLACEMENT_3D ( 'NONE', #48549, #24101, #1611 ) ;
#519=CARTESIAN_POINT ( 'NONE',  ( 2.603489959281582777, 31.58210964143329136, 6.499999999999995559 ) ) ;
#520=CARTESIAN_POINT ( 'NONE',  ( 2.917880565312948704, 57.63708216824731068, 12.26659068614894643 ) ) ;
#521=LINE ( 'NONE', #78442, #17689 ) ;
#522=CARTESIAN_POINT ( 'NONE',  ( 4.559911319644449179, 28.89701867748817321, 9.422509992056141925 ) ) ;
#523=CARTESIAN_POINT ( 'NONE',  ( 20.88017736071110519, 30.56368534415484106, 2.639326808657452039E-16 ) ) ;
#524=VECTOR ( 'NONE', #59815, 1000.000000000000000 ) ;
#525=CARTESIAN_POINT ( 'NONE',  ( 10.00000000000000000, 54.75893115100078745, -9.846743663894594434 ) ) ;
#526=CARTESIAN_POINT ( 'NONE',  ( 22.81628187352647785, 51.62363466993042493, 6.195893100308588602E-16 ) ) ;
#529=CARTESIAN_POINT ( 'NONE',  ( 7.084665262690076126, 17.02201867748817676, -10.88017736071110164 ) ) ;
#530=CARTESIAN_POINT ( 'NONE',  ( -2.816281873526473856, 14.33196800326375531, 3.434112377981055619 ) ) ;
#531=CARTESIAN_POINT ( 'NONE',  ( -10.00000000000000000, 82.00000000000000000, 5.000000000000000000 ) ) ;
#532=CARTESIAN_POINT ( 'NONE',  ( 17.20831665107776587, 42.88393115100077324, 7.208316651077764980 ) ) ;
#533=CARTESIAN_POINT ( 'NONE',  ( -0.8801773607111009756, 48.06368534415484817, 1.068504757029289695E-15 ) ) ;
#534=CARTESIAN_POINT ( 'NONE',  ( 10.00000000000000000, 27.87363466993042138, -12.81628187352647608 ) ) ;
#535=CARTESIAN_POINT ( 'NONE',  ( 0.5774900079438590739, 52.64701867748817676, -5.440088680355550821 ) ) ;
#537=CARTESIAN_POINT ( 'NONE',  ( 19.50000000000000000, 3.304235192336776005E-17, -4.500000000000001776 ) ) ;
#541=CARTESIAN_POINT ( 'NONE',  ( 20.88017736071110164, 50.35535201082151247, 2.915334737309930979 ) ) ;
#542=CARTESIAN_POINT ( 'NONE',  ( 22.81628187352647785, 41.62363466993042493, 6.195893100308588602E-16 ) ) ;
#545=CARTESIAN_POINT ( 'NONE',  ( 18.52753015748618282, 63.92559781766745886, -4.923371831947291888 ) ) ;
#546=CARTESIAN_POINT ( 'NONE',  ( 14.92337183194729633, 32.67559781766745175, 8.527530157486181039 ) ) ;
#547=CARTESIAN_POINT ( 'NONE',  ( 1.472469842513823179, 10.59226448433411782, -4.923371831947296329 ) ) ;
#549=CARTESIAN_POINT ( 'NONE',  ( 10.00000000000000178, 48.05374883491396787, 14.16423886937410082 ) ) ;
#550=( BOUNDED_CURVE ( )  B_SPLINE_CURVE ( 2, ( #98605, #14593, #6092, #22091, #15581, #28586, #76549, #67588, #76059 ),
 .UNSPECIFIED., .F., .T. ) 
 B_SPLINE_CURVE_WITH_KNOTS ( ( 3, 2, 2, 2, 3 ),
 ( 0.5115695083688026612, 0.5119047619047618625, 0.5178571428571427937, 0.5238095238095238360, 0.5241447773454830372 ),
 .UNSPECIFIED. ) 
 CURVE ( )  GEOMETRIC_REPRESENTATION_ITEM ( )  RATIONAL_B_SPLINE_CURVE ( ( 0.9963778908391753841, 0.9980808541467917072, 1.000000000000000000, 0.9659258262890683122, 1.000000000000000000, 0.9659258262890683122, 1.000000000000000000, 0.9980808541467917072, 0.9963778908391753841 ) ) 
 REPRESENTATION_ITEM ( '' )  );
#551=CARTESIAN_POINT ( 'NONE',  ( 0.5774900079438607392, 3.480352010821504027, 5.440088680355550821 ) ) ;
#552=CARTESIAN_POINT ( 'NONE',  ( -0.8801773607111008646, 3.272018677488171434, 2.915334737309923430 ) ) ;
#555=ORIENTED_EDGE ( 'NONE', *, *, #26429, .F. ) ;
#557=VECTOR ( 'NONE', #45943, 1000.000000000000000 ) ;
#558=CARTESIAN_POINT ( 'NONE',  ( 2.035157376598824452, 3.688685344154837953, 7.964842623401179544 ) ) ;
#559=CARTESIAN_POINT ( 'NONE',  ( -0.8801773607110991993, 12.85535201082150358, -2.915334737309923874 ) ) ;
#560=CARTESIAN_POINT ( 'NONE',  ( 19.84674366389459266, 43.30059781766744464, 2.638427012816836559 ) ) ;
#561=CARTESIAN_POINT ( 'NONE',  ( 10.00000000000000178, 35.37363466993042493, 12.81628187352647608 ) ) ;
#562=CARTESIAN_POINT ( 'NONE',  ( -13.69000000000001549, 92.00000000000000000, -10.09898361729590199 ) ) ;
#564=CARTESIAN_POINT ( 'NONE',  ( 2.917880565312948704, 12.63708216824730179, 12.26659068614894643 ) ) ;
#565=CARTESIAN_POINT ( 'NONE',  ( 15.44008868035555793, 26.39701867748817321, -9.422509992056140149 ) ) ;
#566=CARTESIAN_POINT ( 'NONE',  ( 10.00000000000000178, 68.05374883491397497, 14.16423886937410082 ) ) ;
#567=CARTESIAN_POINT ( 'NONE',  ( 19.84674366389459266, 38.30059781766745175, 2.638427012816836559 ) ) ;
#569=CARTESIAN_POINT ( 'NONE',  ( 2.791683348922240793, 21.63393115100078745, 7.208316651077764092 ) ) ;
#570=SURFACE_SIDE_STYLE ('',( #91028 ) ) ;
#573=CARTESIAN_POINT ( 'NONE',  ( 2.035157376598822676, 2.438685344154837953, -7.964842623401177768 ) ) ;
#575=CARTESIAN_POINT ( 'NONE',  ( 0.1532563361054082862, 56.21726448433411605, 2.638427012816831674 ) ) ;
#576=CARTESIAN_POINT ( 'NONE',  ( 20.88017736071110875, 35.77201867748816966, -2.915334737309920765 ) ) ;
#577=CARTESIAN_POINT ( 'NONE',  ( 20.88017736071110875, 40.77201867748818387, -2.915334737309920765 ) ) ;
#578=CARTESIAN_POINT ( 'NONE',  ( 12.91533473730993009, 6.605352010821504471, -10.88017736071109987 ) ) ;
#579=CARTESIAN_POINT ( 'NONE',  ( 16.40814093676324603, 32.45696800326375353, -11.09922568453594671 ) ) ;
#580=CARTESIAN_POINT ( 'NONE',  ( 13.79529636645031943, 15.34541550158063750, -14.16423886937409904 ) ) ;
#582=CARTESIAN_POINT ( 'NONE',  ( 22.81628187352648496, 51.83196800326376064, -3.434112377981050290 ) ) ;
#583=ORIENTED_EDGE ( 'NONE', *, *, #80611, .T. ) ;
#585=CARTESIAN_POINT ( 'NONE',  ( 5.076628168052704559, 40.17559781766745175, -8.527530157486179263 ) ) ;
#586=CARTESIAN_POINT ( 'NONE',  ( 2.035157376598824452, 23.68868534415484461, 7.964842623401179544 ) ) ;
#588=AXIS2_PLACEMENT_3D ( 'NONE', #25960, #34918, #10951 ) ;
#589=CARTESIAN_POINT ( 'NONE',  ( 20.88017736071110875, 15.77201867748817143, -2.915334737309920765 ) ) ;
#591=CARTESIAN_POINT ( 'NONE',  ( 17.96484262340118221, 54.93868534415484106, 7.964842623401181321 ) ) ;
#592=CARTESIAN_POINT ( 'NONE',  ( -0.8801773607111008646, 68.27201867748817676, 2.915334737309923430 ) ) ;
#593=CARTESIAN_POINT ( 'NONE',  ( 20.88017736071110164, 60.35535201082151957, 2.915334737309930979 ) ) ;
#596=CARTESIAN_POINT ( 'NONE',  ( 2.791683348922237240, 15.38393115100078212, -7.208316651077763204 ) ) ;
#597=CARTESIAN_POINT ( 'NONE',  ( 7.084665262690076126, 49.10535201082149825, 10.88017736071109987 ) ) ;
#600=CARTESIAN_POINT ( 'NONE',  ( -46.94000000000001194, 100.9546402834806713, 8.718409068399685324 ) ) ;
#603=CARTESIAN_POINT ( 'NONE',  ( 5.076628168052704559, 40.17559781766745175, -8.527530157486179263 ) ) ;
#608=CARTESIAN_POINT ( 'NONE',  ( -0.3689425029237881626, 22.42874883491397142, 10.36894250292379027 ) ) ;
#609=CARTESIAN_POINT ( 'NONE',  ( 20.15039907845753220, 29.72266099184918531, 6.262539305110077947 ) ) ;
#610=CARTESIAN_POINT ( 'NONE',  ( 19.39188664607694079, 10.83703382326400266, -6.499999999999999112 ) ) ;
#611=CARTESIAN_POINT ( 'NONE',  ( 2.035157376598822676, 57.43868534415484106, -7.964842623401177768 ) ) ;
#612=CARTESIAN_POINT ( 'NONE',  ( -0.8801773607111008646, 3.272018677488171434, 2.915334737309923430 ) ) ;
#613=CARTESIAN_POINT ( 'NONE',  ( 1.472469842513823179, 65.59226448433412315, -4.923371831947296329 ) ) ;
#614=CARTESIAN_POINT ( 'NONE',  ( 5.076628168052703671, 1.842264484334118047, 8.527530157486179263 ) ) ;
#615=CARTESIAN_POINT ( 'NONE',  ( 7.361572987183169658, 4.967264484334119601, -9.846743663894592657 ) ) ;
#616=CARTESIAN_POINT ( 'NONE',  ( 10.00000000000000000, 37.87363466993041783, -12.81628187352647608 ) ) ;
#617=CARTESIAN_POINT ( 'NONE',  ( 5.076628168052704559, 25.17559781766745175, -8.527530157486179263 ) ) ;
#619=CARTESIAN_POINT ( 'NONE',  ( 22.81628187352647785, 21.41530133659708923, 3.434112377981063169 ) ) ;
#621=CARTESIAN_POINT ( 'NONE',  ( 7.361572987183169658, -0.03273551566588185635, -9.846743663894592657 ) ) ;
#625=CARTESIAN_POINT ( 'NONE',  ( 15.44008868035555260, 19.73035201082150536, 9.422509992056143702 ) ) ;
#626=CARTESIAN_POINT ( 'NONE',  ( 20.36894250292379382, 18.67874883491397142, 10.36894250292379205 ) ) ;
#627=CARTESIAN_POINT ( 'NONE',  ( 14.92337183194729633, 42.67559781766745886, 8.527530157486181039 ) ) ;
#628=CARTESIAN_POINT ( 'NONE',  ( 12.91533473730993009, 66.60535201082150536, -10.88017736071109987 ) ) ;
#629=CARTESIAN_POINT ( 'NONE',  ( 22.81628187352648496, 46.83196800326376064, -3.434112377981050290 ) ) ;
#631=CARTESIAN_POINT ( 'NONE',  ( 7.084665262690076126, 22.02201867748817321, -10.88017736071110164 ) ) ;
#633=CARTESIAN_POINT ( 'NONE',  ( 16.40814093676323893, 10.79030133659708923, 11.09922568453595026 ) ) ;
#634=CARTESIAN_POINT ( 'NONE',  ( 3.591859063236763294, 3.290301336597087012, -11.09922568453595026 ) ) ;
#635=CARTESIAN_POINT ( 'NONE',  ( 1.472469842513823179, 31.42559781766745530, 4.923371831947296329 ) ) ;
#637=CARTESIAN_POINT ( 'NONE',  ( 22.81628187352648496, 46.83196800326376064, -3.434112377981050290 ) ) ;
#638=CARTESIAN_POINT ( 'NONE',  ( 0.5774900079438607392, 48.48035201082150536, 5.440088680355550821 ) ) ;
#641=CARTESIAN_POINT ( 'NONE',  ( 20.10421743870887212, 20.60736173766201773, -6.337391062633416894 ) ) ;
#642=CARTESIAN_POINT ( 'NONE',  ( 19.42250999205614193, 45.14701867748817676, 5.440088680355555262 ) ) ;
#643=CARTESIAN_POINT ( 'NONE',  ( 19.42250999205614193, 50.14701867748817676, 5.440088680355555262 ) ) ;
#644=CARTESIAN_POINT ( 'NONE',  ( 18.52753015748618282, 63.92559781766745886, -4.923371831947291888 ) ) ;
#645=CARTESIAN_POINT ( 'NONE',  ( 7.084665262690076126, 62.02201867748816966, -10.88017736071110164 ) ) ;
#647=CARTESIAN_POINT ( 'NONE',  ( 10.00000000000000178, 52.25893115100078745, 9.846743663894594434 ) ) ;
#648=CARTESIAN_POINT ( 'NONE',  ( 4.559911319644449179, 13.89701867748817143, 9.422509992056141925 ) ) ;
#650=CARTESIAN_POINT ( 'NONE',  ( -2.816281873526471635, 13.91530133659708746, -3.434112377981056508 ) ) ;
#651=VERTEX_POINT ( 'NONE', #85315 ) ;
#652=CARTESIAN_POINT ( 'NONE',  ( -0.8801773607110991993, 37.85535201082151247, -2.915334737309923874 ) ) ;
#653=CARTESIAN_POINT ( 'NONE',  ( 3.591859063236763294, 3.290301336597087012, -11.09922568453595026 ) ) ;
#656=CARTESIAN_POINT ( 'NONE',  ( 17.96484262340118221, 16.18868534415483396, -7.964842623401177768 ) ) ;
#657=CARTESIAN_POINT ( 'NONE',  ( 0.5774900079438590739, 27.64701867748817676, -5.440088680355550821 ) ) ;
#658=CARTESIAN_POINT ( 'NONE',  ( 24.16423886937410614, 34.51208216824731068, -3.795296366450302550 ) ) ;
#659=CARTESIAN_POINT ( 'NONE',  ( 17.20831665107776587, 24.13393115100078035, -7.208316651077762316 ) ) ;
#660=CARTESIAN_POINT ( 'NONE',  ( 2.035157376598822676, 57.43868534415484106, -7.964842623401177768 ) ) ;
#662=CARTESIAN_POINT ( 'NONE',  ( 19.84674366389459621, 63.50893115100078745, 7.409399052514197653E-17 ) ) ;
#663=VERTEX_POINT ( 'NONE', #55810 ) ;
#665=CARTESIAN_POINT ( 'NONE',  ( 6.204703633549690345, 32.84541550158063927, 14.16423886937410082 ) ) ;
#666=CARTESIAN_POINT ( 'NONE',  ( 24.16423886937410614, 39.51208216824731068, -3.795296366450302550 ) ) ;
#667=CARTESIAN_POINT ( 'NONE',  ( 0.1532563361054082862, 1.217264484334117824, 2.638427012816831674 ) ) ;
#668=CARTESIAN_POINT ( 'NONE',  ( 19.84674366389459266, 58.30059781766745886, 2.638427012816836559 ) ) ;
#670=CARTESIAN_POINT ( 'NONE',  ( 19.42250999205614193, 60.14701867748817676, 5.440088680355555262 ) ) ;
#671=CARTESIAN_POINT ( 'NONE',  ( 22.81628187352648496, 21.83196800326374643, -3.434112377981050290 ) ) ;
#672=CARTESIAN_POINT ( 'NONE',  ( 17.08211943468705840, 25.13708216824730357, -12.26659068614894466 ) ) ;
#673=CARTESIAN_POINT ( 'NONE',  ( 10.00000000000000178, 19.31368534415484106, 10.88017736071110342 ) ) ;
#674=CARTESIAN_POINT ( 'NONE',  ( 12.91533473730993009, 26.60535201082150536, -10.88017736071109987 ) ) ;
#676=CARTESIAN_POINT ( 'NONE',  ( 2.035157376598822676, 57.43868534415484106, -7.964842623401177768 ) ) ;
#677=CARTESIAN_POINT ( 'NONE',  ( 10.00000000000000000, 52.87363466993041783, -12.81628187352647608 ) ) ;
#680=SURFACE_SIDE_STYLE ('',( #69155 ) ) ;
#681=ORIENTED_EDGE ( 'NONE', *, *, #51264, .T. ) ;
#682=CARTESIAN_POINT ( 'NONE',  ( -0.1503990784575277295, 54.24884699246889852, -6.262539305110077947 ) ) ;
#684=CARTESIAN_POINT ( 'NONE',  ( -4.164238869374099039, 56.80374883491397497, 8.674139862899312516E-16 ) ) ;
#685=CARTESIAN_POINT ( 'NONE',  ( -0.8801773607111008646, 3.272018677488171434, 2.915334737309923430 ) ) ;
#686=CARTESIAN_POINT ( 'NONE',  ( 12.63842701281683922, 34.55059781766745886, -9.846743663894590881 ) ) ;
#687=CARTESIAN_POINT ( 'NONE',  ( 1.472469842513823179, 56.42559781766745886, 4.923371831947296329 ) ) ;
#689=CARTESIAN_POINT ( 'NONE',  ( 0.1532563361054100626, 10.80059781766745175, -2.638427012816831230 ) ) ;
#690=CARTESIAN_POINT ( 'NONE',  ( 19.38216949554541557, 2.248634669930420049, -9.382169495545420901 ) ) ;
#693=CARTESIAN_POINT ( 'NONE',  ( 24.16423886937410614, 49.30374883491396787, 8.672049930838204340E-16 ) ) ;
#695=CARTESIAN_POINT ( 'NONE',  ( -0.3689425029237881626, 37.42874883491396787, 10.36894250292379027 ) ) ;
#697=CARTESIAN_POINT ( 'NONE',  ( 6.565887622018943937, 58.08196800326376064, -12.81628187352647608 ) ) ;
#698=CARTESIAN_POINT ( 'NONE',  ( 19.42250999205614193, 30.14701867748817321, 5.440088680355555262 ) ) ;
#699=CARTESIAN_POINT ( 'NONE',  ( 18.52753015748618282, 43.92559781766745175, -4.923371831947291888 ) ) ;
#700=CARTESIAN_POINT ( 'NONE',  ( 7.084665262690076126, 24.10535201082150181, 10.88017736071109987 ) ) ;
#701=CARTESIAN_POINT ( 'NONE',  ( -1.926860441876563801, 64.89664270246085209, 3.195792623639529761 ) ) ;
#702=CARTESIAN_POINT ( 'NONE',  ( 19.84674366389459266, 53.71726448433411605, -2.638427012816827677 ) ) ;
#703=CARTESIAN_POINT ( 'NONE',  ( 19.84674366389459266, 48.30059781766745175, 2.638427012816836559 ) ) ;
#708=CARTESIAN_POINT ( 'NONE',  ( 17.85158348494335812, 19.73726573380441351, -6.499999999999992895 ) ) ;
#709=EDGE_LOOP ( 'NONE', ( #92265, #29499, #42364, #81425, #71041, #49947 ) ) ;
#711=CARTESIAN_POINT ( 'NONE',  ( 2.791683348922237240, 35.38393115100079456, -7.208316651077763204 ) ) ;
#713=CARTESIAN_POINT ( 'NONE',  ( 13.43411237798106583, 32.66530133659708213, -12.81628187352647252 ) ) ;
#716=DIRECTION ( 'NONE',  ( 0.000000000000000000, 0.000000000000000000, 1.000000000000000000 ) ) ;
#718=CARTESIAN_POINT ( 'NONE',  ( 10.00000000000000000, 64.75893115100078035, -9.846743663894594434 ) ) ;
#720=CARTESIAN_POINT ( 'NONE',  ( 10.00000000000000178, 57.25893115100078745, 9.846743663894594434 ) ) ;
#721=CARTESIAN_POINT ( 'NONE',  ( 24.16423886937410614, 39.30374883491396787, 8.672049930838204340E-16 ) ) ;
#722=CARTESIAN_POINT ( 'NONE',  ( 2.791683348922237240, 60.38393115100078745, -7.208316651077763204 ) ) ;
#724=CARTESIAN_POINT ( 'NONE',  ( 2.791683348922237240, 15.38393115100078212, -7.208316651077763204 ) ) ;
#725=CARTESIAN_POINT ( 'NONE',  ( -2.816281873526471635, 53.91530133659709634, -3.434112377981056508 ) ) ;
#726=CARTESIAN_POINT ( 'NONE',  ( 5.076628168052703671, 61.84226448433412315, 8.527530157486179263 ) ) ;
#727=CARTESIAN_POINT ( 'NONE',  ( 7.084665262690076126, 49.10535201082149825, 10.88017736071109987 ) ) ;
#728=CARTESIAN_POINT ( 'NONE',  ( 7.361572987183170547, 47.05059781766745175, 9.846743663894590881 ) ) ;
#731=EDGE_CURVE ( 'NONE', #11978, #70278, #61820, .T. ) ;
#732=CARTESIAN_POINT ( 'NONE',  ( 0.5774900079438607392, 53.48035201082151247, 5.440088680355550821 ) ) ;
#733=ORIENTED_EDGE ( 'NONE', *, *, #34970, .T. ) ;
#736=CARTESIAN_POINT ( 'NONE',  ( 4.559911319644449179, 32.23035201082150536, -9.422509992056141925 ) ) ;
#737=CARTESIAN_POINT ( 'NONE',  ( 10.00000000000000000, 2.873634669930420049, -12.81628187352647608 ) ) ;
#738=CARTESIAN_POINT ( 'NONE',  ( 4.559911319644449179, 58.89701867748817676, 9.422509992056141925 ) ) ;
#740=CARTESIAN_POINT ( 'NONE',  ( 20.10421743870887568, 10.60736173766201773, -6.337391062633407124 ) ) ;
#742=CARTESIAN_POINT ( 'NONE',  ( 19.42250999205614548, 45.98035201082150536, -5.440088680355545492 ) ) ;
#744=CARTESIAN_POINT ( 'NONE',  ( 7.361572987183169658, 34.96726448433411605, -9.846743663894592657 ) ) ;
#745=DIRECTION ( 'NONE',  ( -0.8320502943378437211, 0.5547001962252290364, 0.000000000000000000 ) ) ;
#747=CARTESIAN_POINT ( 'NONE',  ( 7.361572987183170547, 62.05059781766745886, 9.846743663894590881 ) ) ;
#748=CARTESIAN_POINT ( 'NONE',  ( -0.8801773607110991993, 7.855352010821506248, -2.915334737309923874 ) ) ;
#751=CARTESIAN_POINT ( 'NONE',  ( 2.917880565312948704, 27.63708216824730357, 12.26659068614894643 ) ) ;
#752=CARTESIAN_POINT ( 'NONE',  ( 10.00000000000000178, 58.05374883491397497, 14.16423886937410082 ) ) ;
#753=CARTESIAN_POINT ( 'NONE',  ( 12.63842701281683922, 34.55059781766745886, -9.846743663894590881 ) ) ;
#754=CARTESIAN_POINT ( 'NONE',  ( 0.1532563361054082862, 21.21726448433412315, 2.638427012816831674 ) ) ;
#757=CARTESIAN_POINT ( 'NONE',  ( 18.52753015748618282, 28.92559781766745175, -4.923371831947291888 ) ) ;
#758=CARTESIAN_POINT ( 'NONE',  ( 0.5774900079438590739, 27.64701867748817676, -5.440088680355550821 ) ) ;
#759=CARTESIAN_POINT ( 'NONE',  ( 0.1532563361054100626, 55.80059781766745175, -2.638427012816831230 ) ) ;
#760=CARTESIAN_POINT ( 'NONE',  ( 22.26659068614894466, 3.887082168247300906, 7.082119434687054849 ) ) ;
#762=CARTESIAN_POINT ( 'NONE',  ( 0.1532563361054082862, 11.21726448433411605, 2.638427012816831674 ) ) ;
#763=CARTESIAN_POINT ( 'NONE',  ( 21.09922568453595559, 32.04030133659708923, -6.408140936763230044 ) ) ;
#764=CARTESIAN_POINT ( 'NONE',  ( 17.20831665107776587, 37.88393115100078745, 7.208316651077764980 ) ) ;
#766=CARTESIAN_POINT ( 'NONE',  ( 0.1532563361054082862, 21.21726448433412315, 2.638427012816831674 ) ) ;
#768=CARTESIAN_POINT ( 'NONE',  ( -46.58960623550384383, 101.6399765164375850, -8.033401704989589831 ) ) ;
#769=CARTESIAN_POINT ( 'NONE',  ( -4.164238869374099039, 51.80374883491396787, 8.674139862899312516E-16 ) ) ;
#770=CARTESIAN_POINT ( 'NONE',  ( 10.00000000000000178, 54.31368534415484106, 10.88017736071110342 ) ) ;
#771=CARTESIAN_POINT ( 'NONE',  ( 2.035157376598822676, 52.43868534415483396, -7.964842623401177768 ) ) ;
#772=CARTESIAN_POINT ( 'NONE',  ( 2.791683348922240793, 31.63393115100078745, 7.208316651077764092 ) ) ;
#773=CARTESIAN_POINT ( 'NONE',  ( 7.084665262690076126, 2.022018677488170990, -10.88017736071110164 ) ) ;
#775=CARTESIAN_POINT ( 'NONE',  ( 12.63842701281683922, 44.55059781766745175, -9.846743663894590881 ) ) ;
#777=CARTESIAN_POINT ( 'NONE',  ( 4.559911319644449179, 53.89701867748817676, 9.422509992056141925 ) ) ;
#778=CARTESIAN_POINT ( 'NONE',  ( 17.20831665107776587, 4.133931151000785675, -7.208316651077762316 ) ) ;
#783=CARTESIAN_POINT ( 'NONE',  ( 5.076628168052704559, 20.17559781766745175, -8.527530157486179263 ) ) ;
#784=CARTESIAN_POINT ( 'NONE',  ( 10.00000000000000178, 55.37363466993042493, 12.81628187352647608 ) ) ;
#785=CARTESIAN_POINT ( 'NONE',  ( 4.559911319644449179, 13.89701867748817321, 9.422509992056141925 ) ) ;
#786=CARTESIAN_POINT ( 'NONE',  ( 2.791683348922240793, 46.63393115100077324, 7.208316651077764092 ) ) ;
#788=CARTESIAN_POINT ( 'NONE',  ( 10.00000000000000178, 28.05374883491396787, 14.16423886937410082 ) ) ;
#789=CARTESIAN_POINT ( 'NONE',  ( 20.36894250292379738, 59.92874883491397497, -10.36894250292379027 ) ) ;
#790=CARTESIAN_POINT ( 'NONE',  ( 12.63842701281683922, 54.55059781766745175, -9.846743663894590881 ) ) ;
#791=CARTESIAN_POINT ( 'NONE',  ( 15.44008868035555260, 49.73035201082150536, 9.422509992056143702 ) ) ;
#793=CARTESIAN_POINT ( 'NONE',  ( 1.472469842513823179, 15.59226448433411960, -4.923371831947296329 ) ) ;
#795=EDGE_LOOP ( 'NONE', ( #13304, #46664, #87844, #53045 ) ) ;
#796=B_SPLINE_CURVE_WITH_KNOTS ( 'NONE', 3,
 ( #44696, #708, #68688, #75192 ),
 .UNSPECIFIED., .F., .F.,
 ( 4, 4 ),
 ( 0.000000000000000000, 0.002392975128318422604 ),
 .UNSPECIFIED. ) ;
#799=CARTESIAN_POINT ( 'NONE',  ( 19.84674366389459621, 8.508931151000785675, 7.409399052514197653E-17 ) ) ;
#800=VERTEX_POINT ( 'NONE', #21761 ) ;
#801=CARTESIAN_POINT ( 'NONE',  ( -4.164238869374098151, 21.59541550158063217, -3.795296366450310543 ) ) ;
#802=CARTESIAN_POINT ( 'NONE',  ( 19.84674366389459266, 18.71726448433411960, -2.638427012816827677 ) ) ;
#803=CARTESIAN_POINT ( 'NONE',  ( 15.44008868035555793, 41.39701867748817676, -9.422509992056140149 ) ) ;
#806=CARTESIAN_POINT ( 'NONE',  ( 2.035157376598824452, 23.68868534415484461, 7.964842623401179544 ) ) ;
#810=CARTESIAN_POINT ( 'NONE',  ( 2.035157376598822676, 32.43868534415483396, -7.964842623401177768 ) ) ;
#812=EDGE_LOOP ( 'NONE', ( #36804, #71222, #33329, #97808 ) ) ;
#813=CARTESIAN_POINT ( 'NONE',  ( 13.43411237798106583, 22.66530133659708923, -12.81628187352647252 ) ) ;
#815=CARTESIAN_POINT ( 'NONE',  ( 5.076628168052704559, 5.175597817667451750, -8.527530157486179263 ) ) ;
#816=CARTESIAN_POINT ( 'NONE',  ( 19.84674366389459621, 18.50893115100078745, 7.409399052514197653E-17 ) ) ;
#817=CARTESIAN_POINT ( 'NONE',  ( 2.035157376598824452, 33.68868534415484106, 7.964842623401179544 ) ) ;
#820=ORIENTED_EDGE ( 'NONE', *, *, #72852, .F. ) ;
#822=CARTESIAN_POINT ( 'NONE',  ( 0.5774900079438607392, 63.48035201082149825, 5.440088680355550821 ) ) ;
#824=CARTESIAN_POINT ( 'NONE',  ( 10.00000000000000000, 66.81368534415484817, -10.88017736071110342 ) ) ;
#825=CARTESIAN_POINT ( 'NONE',  ( 13.43411237798105340, 5.581968003263753531, 12.81628187352647963 ) ) ;
#827=CARTESIAN_POINT ( 'NONE',  ( 12.63842701281683034, 32.46726448433412315, 9.846743663894596210 ) ) ;
#828=CARTESIAN_POINT ( 'NONE',  ( -1.099225684535947600, 49.54030133659708923, 6.408140936763237150 ) ) ;
#829=CARTESIAN_POINT ( 'NONE',  ( 2.153642693323476909, 36.13791097397317742, -6.500000000000079936 ) ) ;
#830=CARTESIAN_POINT ( 'NONE',  ( 17.20831665107776587, 14.13393115100078568, -7.208316651077762316 ) ) ;
#831=CARTESIAN_POINT ( 'NONE',  ( -2.816281873526471635, 13.91530133659708746, -3.434112377981056508 ) ) ;
#833=CARTESIAN_POINT ( 'NONE',  ( 20.88017736071110164, 35.35535201082150536, 2.915334737309930979 ) ) ;
#834=CARTESIAN_POINT ( 'NONE',  ( 0.1532563361054083140, 61.00893115100078745, 1.131784320476157264E-15 ) ) ;
#836=CARTESIAN_POINT ( 'NONE',  ( 2.791683348922237240, 20.38393115100078745, -7.208316651077763204 ) ) ;
#837=CARTESIAN_POINT ( 'NONE',  ( 18.52753015748618282, 3.925597817667451306, -4.923371831947291888 ) ) ;
#838=CARTESIAN_POINT ( 'NONE',  ( 19.42250999205614548, 10.98035201082150358, -5.440088680355545492 ) ) ;
#839=CARTESIAN_POINT ( 'NONE',  ( 19.38216949554541557, 12.24863466993041961, -9.382169495545420901 ) ) ;
#840=CARTESIAN_POINT ( 'NONE',  ( 14.92337183194729988, 64.34226448433412315, -8.527530157486177487 ) ) ;
#841=EDGE_CURVE ( 'NONE', #25175, #32896, #62196, .T. ) ;
#844=CARTESIAN_POINT ( 'NONE',  ( 10.00000000000000178, 24.31368534415484106, 10.88017736071110342 ) ) ;
#845=CARTESIAN_POINT ( 'NONE',  ( 1.472469842513823179, 46.42559781766745175, 4.923371831947296329 ) ) ;
#848=ADVANCED_FACE ( 'NONE', ( #33166 ), #69709, .F. ) ;
#849=CARTESIAN_POINT ( 'NONE',  ( -0.8801773607111008646, 18.27201867748817321, 2.915334737309923430 ) ) ;
#851=CARTESIAN_POINT ( 'NONE',  ( -0.8801773607111009756, 28.06368534415484106, 1.068504757029289695E-15 ) ) ;
#852=CARTESIAN_POINT ( 'NONE',  ( -4.164238869374099039, 66.80374883491396076, 8.674139862899312516E-16 ) ) ;
#854=CARTESIAN_POINT ( 'NONE',  ( 1.472469842513823179, 0.5922644843341181575, -4.923371831947296329 ) ) ;
#855=CARTESIAN_POINT ( 'NONE',  ( 18.52753015748617571, 23.09226448433411960, 4.923371831947298993 ) ) ;
#856=CARTESIAN_POINT ( 'NONE',  ( 0.6178305044545838731, 9.748634669930416052, 9.382169495545420901 ) ) ;
#859=CARTESIAN_POINT ( 'NONE',  ( 14.92337183194729988, 64.34226448433412315, -8.527530157486177487 ) ) ;
#862=CARTESIAN_POINT ( 'NONE',  ( 2.917880565312950480, 10.97041550158063572, -12.26659068614894821 ) ) ;
#863=CARTESIAN_POINT ( 'NONE',  ( 1.472469842513823179, 35.59226448433412315, -4.923371831947296329 ) ) ;
#866=CARTESIAN_POINT ( 'NONE',  ( 22.26659068614894466, 53.88708216824731068, 7.082119434687054849 ) ) ;
#867=CARTESIAN_POINT ( 'NONE',  ( 2.791683348922240793, 16.63393115100078745, 7.208316651077764092 ) ) ;
#870=CARTESIAN_POINT ( 'NONE',  ( 4.559911319644449179, 43.89701867748816966, 9.422509992056141925 ) ) ;
#871=CARTESIAN_POINT ( 'NONE',  ( 21.09922568453594849, 56.20696800326375353, 6.408140936763242479 ) ) ;
#872=CARTESIAN_POINT ( 'NONE',  ( 4.559911319644449179, 23.89701867748817321, 9.422509992056141925 ) ) ;
#873=CARTESIAN_POINT ( 'NONE',  ( 21.09922568453594849, 46.20696800326376064, 6.408140936763242479 ) ) ;
#874=CARTESIAN_POINT ( 'NONE',  ( -1.099225684535947600, 3.706968003263753531, -6.408140936763238038 ) ) ;
#878=CARTESIAN_POINT ( 'NONE',  ( 20.36894250292379382, 53.67874883491397497, 10.36894250292379205 ) ) ;
#879=CARTESIAN_POINT ( 'NONE',  ( -0.3689425029237881626, 17.42874883491397142, 10.36894250292379027 ) ) ;
#880=CARTESIAN_POINT ( 'NONE',  ( 10.00000000000000178, 14.31368534415483751, 10.88017736071110342 ) ) ;
#881=CARTESIAN_POINT ( 'NONE',  ( 0.5774900079438607392, 33.48035201082150536, 5.440088680355550821 ) ) ;
#883=CARTESIAN_POINT ( 'NONE',  ( -46.76873188434316830, 100.6386073946591466, -9.384976975161267276 ) ) ;
#884=CARTESIAN_POINT ( 'NONE',  ( 7.084665262690076126, 64.10535201082150536, 10.88017736071109987 ) ) ;
#885=CARTESIAN_POINT ( 'NONE',  ( 17.96484262340118221, 66.18868534415483396, -7.964842623401177768 ) ) ;
#886=CARTESIAN_POINT ( 'NONE',  ( -2.816281873526473856, 29.33196800326376064, 3.434112377981055619 ) ) ;
#888=CARTESIAN_POINT ( 'NONE',  ( 17.20831665107776587, 14.13393115100078568, -7.208316651077762316 ) ) ;
#889=CARTESIAN_POINT ( 'NONE',  ( 18.52753015748617571, 43.09226448433412315, 4.923371831947298993 ) ) ;
#890=STYLED_ITEM ( 'NONE', ( #61535 ), #52669 ) ;
#891=EDGE_CURVE ( 'NONE', #46987, #90157, #82265, .T. ) ;
#892=CARTESIAN_POINT ( 'NONE',  ( 10.00000000000000178, 14.31368534415483751, 10.88017736071110342 ) ) ;
#893=CARTESIAN_POINT ( 'NONE',  ( 16.40814093676323893, 35.79030133659708923, 11.09922568453595026 ) ) ;
#895=CARTESIAN_POINT ( 'NONE',  ( 0.1532563361054100626, 10.80059781766745175, -2.638427012816831230 ) ) ;
#897=CARTESIAN_POINT ( 'NONE',  ( 19.84674366389459621, 53.50893115100078745, 7.409399052514197653E-17 ) ) ;
#898=CARTESIAN_POINT ( 'NONE',  ( 19.84674366389459266, 28.30059781766745886, 2.638427012816836559 ) ) ;
#899=CARTESIAN_POINT ( 'NONE',  ( 2.917880565312948704, 17.63708216824730357, 12.26659068614894643 ) ) ;
#900=CARTESIAN_POINT ( 'NONE',  ( 10.00000000000000000, 36.81368534415484106, -10.88017736071110342 ) ) ;
#901=CARTESIAN_POINT ( 'NONE',  ( 19.42250999205614193, 5.147018677488171434, 5.440088680355555262 ) ) ;
#902=EDGE_CURVE ( 'NONE', #80852, #61558, #58673, .T. ) ;
#903=CARTESIAN_POINT ( 'NONE',  ( 20.88017736071110519, 35.56368534415484106, 2.639326808657452039E-16 ) ) ;
#904=CARTESIAN_POINT ( 'NONE',  ( -0.8801773607111009756, 28.06368534415484106, 1.068504757029289695E-15 ) ) ;
#906=CARTESIAN_POINT ( 'NONE',  ( 20.88017736071110164, 35.35535201082150536, 2.915334737309930979 ) ) ;
#908=CARTESIAN_POINT ( 'NONE',  ( 0.6178305044545818747, 63.49863466993043204, -9.382169495545419124 ) ) ;
#909=CARTESIAN_POINT ( 'NONE',  ( 7.084665262690076126, 54.10535201082151247, 10.88017736071109987 ) ) ;
#911=ORIENTED_EDGE ( 'NONE', *, *, #98370, .F. ) ;
#912=CARTESIAN_POINT ( 'NONE',  ( 17.96484262340118221, 44.93868534415483396, 7.964842623401181321 ) ) ;
#914=CARTESIAN_POINT ( 'NONE',  ( -0.1503990784575247319, 37.22266099184918176, -6.262539305110083276 ) ) ;
#915=CARTESIAN_POINT ( 'NONE',  ( -0.3689425029237881626, 62.42874883491396787, 10.36894250292379027 ) ) ;
#916=CARTESIAN_POINT ( 'NONE',  ( 7.084665262690076126, 64.10535201082150536, 10.88017736071109987 ) ) ;
#919=CARTESIAN_POINT ( 'NONE',  ( 2.035157376598822676, 2.438685344154837953, -7.964842623401177768 ) ) ;
#920=CARTESIAN_POINT ( 'NONE',  ( 14.92337183194729988, 29.34226448433411960, -8.527530157486177487 ) ) ;
#922=CARTESIAN_POINT ( 'NONE',  ( 5.076628168052704559, 35.17559781766745175, -8.527530157486179263 ) ) ;
#923=CARTESIAN_POINT ( 'NONE',  ( 2.035157376598822676, 37.43868534415484106, -7.964842623401177768 ) ) ;
#924=CARTESIAN_POINT ( 'NONE',  ( 19.84674366389459266, 43.71726448433410894, -2.638427012816827677 ) ) ;
#925=CARTESIAN_POINT ( 'NONE',  ( 10.00000000000000000, 17.87363466993041783, -12.81628187352647608 ) ) ;
#926=CARTESIAN_POINT ( 'NONE',  ( -0.8801773607110991993, 67.85535201082151957, -2.915334737309923874 ) ) ;
#927=CARTESIAN_POINT ( 'NONE',  ( 0.5774900079438607392, 68.48035201082150536, 5.440088680355550821 ) ) ;
#928=CARTESIAN_POINT ( 'NONE',  ( 10.00000000000000000, 51.81368534415484106, -10.88017736071110342 ) ) ;
#929=CARTESIAN_POINT ( 'NONE',  ( -0.3689425029237898834, 56.17874883491396076, -10.36894250292378850 ) ) ;
#932=CARTESIAN_POINT ( 'NONE',  ( 3.591859063236761518, 19.95696800326375353, 11.09922568453594849 ) ) ;
#936=CARTESIAN_POINT ( 'NONE',  ( 22.81628187352648496, 21.83196800326374643, -3.434112377981050290 ) ) ;
#937=CARTESIAN_POINT ( 'NONE',  ( 2.035157376598824452, 23.68868534415484461, 7.964842623401179544 ) ) ;
#938=CARTESIAN_POINT ( 'NONE',  ( 4.559911319644449179, 62.23035201082150536, -9.422509992056141925 ) ) ;
#939=EDGE_LOOP ( 'NONE', ( #2928, #68689, #25232, #41405 ) ) ;
#940=CARTESIAN_POINT ( 'NONE',  ( 1.472469842513823179, 5.592264484334118713, -4.923371831947296329 ) ) ;
#941=CARTESIAN_POINT ( 'NONE',  ( 2.791683348922237240, 50.38393115100078035, -7.208316651077763204 ) ) ;
#943=CARTESIAN_POINT ( 'NONE',  ( 17.20831665107776587, 37.88393115100078745, 7.208316651077764980 ) ) ;
#945=CARTESIAN_POINT ( 'NONE',  ( 17.20831665107776587, 22.88393115100078745, 7.208316651077764980 ) ) ;
#948=CARTESIAN_POINT ( 'NONE',  ( 1.472469842513823179, 15.59226448433411960, -4.923371831947296329 ) ) ;
#951=CARTESIAN_POINT ( 'NONE',  ( 10.00000000000000178, 47.25893115100078745, 9.846743663894594434 ) ) ;
#954=CARTESIAN_POINT ( 'NONE',  ( 0.6178305044545838731, 14.74863466993041783, 9.382169495545420901 ) ) ;
#956=CARTESIAN_POINT ( 'NONE',  ( -0.8801773607110991993, 47.85535201082150536, -2.915334737309923874 ) ) ;
#957=CARTESIAN_POINT ( 'NONE',  ( 17.08211943468705130, 43.47041550158063927, 12.26659068614894998 ) ) ;
#958=CARTESIAN_POINT ( 'NONE',  ( 10.00000000000000178, 2.258931151000784787, 9.846743663894594434 ) ) ;
#959=CARTESIAN_POINT ( 'NONE',  ( -46.94000000000001194, 100.4376529975699981, 9.000000000001183054 ) ) ;
#961=CARTESIAN_POINT ( 'NONE',  ( 13.79529636645031943, 50.34541550158064638, -14.16423886937409904 ) ) ;
#962=CARTESIAN_POINT ( 'NONE',  ( 10.00000000000000000, 65.55374883491396076, -14.16423886937410082 ) ) ;
#963=CARTESIAN_POINT ( 'NONE',  ( 10.00000000000000000, 20.55374883491396787, -14.16423886937410082 ) ) ;
#964=CARTESIAN_POINT ( 'NONE',  ( 24.16423886937410614, 29.51208216824729647, -3.795296366450302550 ) ) ;
#968=CARTESIAN_POINT ( 'NONE',  ( 5.076628168052704559, 40.17559781766745175, -8.527530157486179263 ) ) ;
#969=CARTESIAN_POINT ( 'NONE',  ( 15.44008868035555793, 26.39701867748817321, -9.422509992056140149 ) ) ;
#971=CARTESIAN_POINT ( 'NONE',  ( 1.472469842513823179, 65.59226448433412315, -4.923371831947296329 ) ) ;
#972=CARTESIAN_POINT ( 'NONE',  ( 20.00000000000000711, 88.18949240714360371, -4.994480956907769276 ) ) ;
#973=CARTESIAN_POINT ( 'NONE',  ( 17.20831665107776587, 42.88393115100077324, 7.208316651077764980 ) ) ;
#974=CARTESIAN_POINT ( 'NONE',  ( 0.6178305044545838731, 59.74863466993041783, 9.382169495545420901 ) ) ;
#977=CARTESIAN_POINT ( 'NONE',  ( 1.472469842513823179, 36.42559781766745175, 4.923371831947296329 ) ) ;
#978=CARTESIAN_POINT ( 'NONE',  ( 17.20831665107776587, 57.88393115100078745, 7.208316651077764980 ) ) ;
#979=VECTOR ( 'NONE', #94838, 1000.000000000000000 ) ;
#980=CARTESIAN_POINT ( 'NONE',  ( 20.36894250292379382, 33.67874883491396076, 10.36894250292379205 ) ) ;
#982=CARTESIAN_POINT ( 'NONE',  ( 13.79529636645030344, 13.26208216824729824, 14.16423886937410614 ) ) ;
#987=CARTESIAN_POINT ( 'NONE',  ( 2.035157376598824452, 8.688685344154839285, 7.964842623401179544 ) ) ;
#988=CARTESIAN_POINT ( 'NONE',  ( 21.09922568453594849, 6.206968003263753531, 6.408140936763242479 ) ) ;
#990=CARTESIAN_POINT ( 'NONE',  ( 14.92337183194729988, 4.342264484334117824, -8.527530157486177487 ) ) ;
#992=CARTESIAN_POINT ( 'NONE',  ( -46.52365679472261206, 102.3054413859459828, -7.234551493516248932 ) ) ;
#993=CARTESIAN_POINT ( 'NONE',  ( 2.917880565312950480, 65.97041550158063217, -12.26659068614894821 ) ) ;
#995=CARTESIAN_POINT ( 'NONE',  ( 12.91533473730992121, 29.52201867748817321, 10.88017736071110164 ) ) ;
#996=CARTESIAN_POINT ( 'NONE',  ( -0.8801773607111009756, 18.06368534415484106, 1.068504757029289695E-15 ) ) ;
#997=CARTESIAN_POINT ( 'NONE',  ( 2.791683348922237240, 60.38393115100078745, -7.208316651077763204 ) ) ;
#998=CARTESIAN_POINT ( 'NONE',  ( 0.1532563361054082862, 51.21726448433412315, 2.638427012816831674 ) ) ;
#999=CARTESIAN_POINT ( 'NONE',  ( -44.79861740791880464, 105.6822567946284153, -4.824280223375575716 ) ) ;
#1001=ORIENTED_EDGE ( 'NONE', *, *, #82418, .F. ) ;
#1002=CARTESIAN_POINT ( 'NONE',  ( 4.559911319644449179, 33.89701867748817676, 9.422509992056141925 ) ) ;
#1004=CARTESIAN_POINT ( 'NONE',  ( 13.43411237798105340, 20.58196800326374643, 12.81628187352647963 ) ) ;
#1005=CARTESIAN_POINT ( 'NONE',  ( 19.39235739573469530, 34.87576471608600315, 6.499999999999993783 ) ) ;
#1006=CARTESIAN_POINT ( 'NONE',  ( 10.00000000000000178, 67.25893115100079456, 9.846743663894594434 ) ) ;
#1007=CARTESIAN_POINT ( 'NONE',  ( 0.5774900079438590739, 52.64701867748817676, -5.440088680355550821 ) ) ;
#1008=CARTESIAN_POINT ( 'NONE',  ( 0.6178305044545838731, 24.74863466993042493, 9.382169495545420901 ) ) ;
#1009=CARTESIAN_POINT ( 'NONE',  ( -0.8801773607110991993, 67.85535201082151957, -2.915334737309923874 ) ) ;
#1012=CARTESIAN_POINT ( 'NONE',  ( -1.099225684535947600, 64.54030133659709634, 6.408140936763237150 ) ) ;
#1014=CARTESIAN_POINT ( 'NONE',  ( -0.8801773607110990882, 47.85535201082150536, -2.915334737309924318 ) ) ;
#1015=CARTESIAN_POINT ( 'NONE',  ( -46.94000000000001194, 103.0000000000000000, 5.997726559847112782 ) ) ;
#1016=CARTESIAN_POINT ( 'NONE',  ( 12.91533473730992121, 49.52201867748817676, 10.88017736071110164 ) ) ;
#1017=CARTESIAN_POINT ( 'NONE',  ( 3.591859063236763294, 53.29030133659708923, -11.09922568453595026 ) ) ;
#1018=CARTESIAN_POINT ( 'NONE',  ( 10.00000000000000178, 13.05374883491396787, 14.16423886937410082 ) ) ;
#1020=CARTESIAN_POINT ( 'NONE',  ( 10.00000000000000000, 24.75893115100078745, -9.846743663894594434 ) ) ;
#1022=CARTESIAN_POINT ( 'NONE',  ( 13.79529636645031943, 55.34541550158062506, -14.16423886937409904 ) ) ;
#1025=CARTESIAN_POINT ( 'NONE',  ( 4.559911319644449179, 3.897018677488170990, 9.422509992056141925 ) ) ;
#1026=CARTESIAN_POINT ( 'NONE',  ( 0.5774900079438607392, 3.480352010821504027, 5.440088680355550821 ) ) ;
#1029=CARTESIAN_POINT ( 'NONE',  ( 20.88017736071110875, 5.772018677488170546, -2.915334737309920765 ) ) ;
#1030=CARTESIAN_POINT ( 'NONE',  ( 10.00000000000000000, 6.813685344154838397, -10.88017736071110342 ) ) ;
#1031=CARTESIAN_POINT ( 'NONE',  ( 1.472469842513823179, 45.59226448433412315, -4.923371831947296329 ) ) ;
#1032=CARTESIAN_POINT ( 'NONE',  ( 6.565887622018943937, 35.16530133659708923, 12.81628187352647430 ) ) ;
#1033=CARTESIAN_POINT ( 'NONE',  ( 19.80832241502127999, 64.75868815902069286, 6.499999999999992006 ) ) ;
#1034=CARTESIAN_POINT ( 'NONE',  ( 18.72515096720570327, 11.07228050351031712, -6.499999999999992006 ) ) ;
#1035=CARTESIAN_POINT ( 'NONE',  ( -4.164238869374099927, 22.01208216824730357, 3.795296366450308767 ) ) ;
#1036=CARTESIAN_POINT ( 'NONE',  ( 12.91533473730993009, 21.60535201082150536, -10.88017736071109987 ) ) ;
#1037=CARTESIAN_POINT ( 'NONE',  ( 24.16423886937410614, 64.30374883491396076, 8.672049930838204340E-16 ) ) ;
#1038=CARTESIAN_POINT ( 'NONE',  ( 5.076628168052704559, 45.17559781766745175, -8.527530157486179263 ) ) ;
#1039=CARTESIAN_POINT ( 'NONE',  ( -45.94000000000000483, 92.50000000000000000, -9.000000000000000000 ) ) ;
#1040=CARTESIAN_POINT ( 'NONE',  ( 10.00000000000000178, 22.25893115100078745, 9.846743663894594434 ) ) ;
#1041=DIRECTION ( 'NONE',  ( 0.000000000000000000, -1.000000000000000000, 0.000000000000000000 ) ) ;
#1045=CARTESIAN_POINT ( 'NONE',  ( 18.52753015748617571, 63.09226448433412315, 4.923371831947298993 ) ) ;
#1046=CARTESIAN_POINT ( 'NONE',  ( 10.00000000000000000, 36.81368534415484106, -10.88017736071110342 ) ) ;
#1047=CARTESIAN_POINT ( 'NONE',  ( 17.96484262340118221, 36.18868534415484106, -7.964842623401177768 ) ) ;
#1048=CARTESIAN_POINT ( 'NONE',  ( 21.09922568453594849, 31.20696800326375353, 6.408140936763242479 ) ) ;
#1049=CARTESIAN_POINT ( 'NONE',  ( -4.164238869374099927, 17.01208216824730357, 3.795296366450308767 ) ) ;
#1055=CARTESIAN_POINT ( 'NONE',  ( -1.099225684535947600, 38.70696800326375353, -6.408140936763238038 ) ) ;
#1058=CARTESIAN_POINT ( 'NONE',  ( 0.1532563361054082862, 46.21726448433411605, 2.638427012816831674 ) ) ;
#1059=CARTESIAN_POINT ( 'NONE',  ( -0.8801773607110991993, 17.85535201082150536, -2.915334737309923874 ) ) ;
#1061=CARTESIAN_POINT ( 'NONE',  ( 0.5774900079438590739, 12.64701867748817321, -5.440088680355550821 ) ) ;
#1063=ORIENTED_EDGE ( 'NONE', *, *, #45515, .F. ) ;
#1064=CARTESIAN_POINT ( 'NONE',  ( 15.44008868035555260, 59.73035201082151247, 9.422509992056143702 ) ) ;
#1065=CARTESIAN_POINT ( 'NONE',  ( 2.035157376598822676, 67.43868534415484817, -7.964842623401177768 ) ) ;
#1067=CARTESIAN_POINT ( 'NONE',  ( 5.076628168052704559, 5.175597817667451750, -8.527530157486179263 ) ) ;
#1068=CARTESIAN_POINT ( 'NONE',  ( 4.559911319644449179, 63.89701867748817676, 9.422509992056141925 ) ) ;
#1070=( GEOMETRIC_REPRESENTATION_CONTEXT ( 3 ) GLOBAL_UNCERTAINTY_ASSIGNED_CONTEXT ( ( #63324 ) ) GLOBAL_UNIT_ASSIGNED_CONTEXT ( ( #52443, #14458, #5965 ) ) REPRESENTATION_CONTEXT ( 'NONE', 'WORKASPACE' ) );
#1071=CARTESIAN_POINT ( 'NONE',  ( -46.67091953292581508, 101.1773697441846736, 8.660634561519810148 ) ) ;
#1072=CARTESIAN_POINT ( 'NONE',  ( 10.00000000000000000, 4.758931151000784787, -9.846743663894594434 ) ) ;
#1076=CARTESIAN_POINT ( 'NONE',  ( 7.361572987183170547, 47.05059781766745175, 9.846743663894590881 ) ) ;
#1078=VERTEX_POINT ( 'NONE', #64147 ) ;
#1079=CARTESIAN_POINT ( 'NONE',  ( 5.500000000000000000, 11.50000000000000000, -6.000000000000000000 ) ) ;
#1081=LINE ( 'NONE', #65482, #88658 ) ;
#1083=CARTESIAN_POINT ( 'NONE',  ( 13.79529636645030344, 8.262082168247300018, 14.16423886937410614 ) ) ;
#1084=CARTESIAN_POINT ( 'NONE',  ( -2.266590686148945544, 21.38708216824730357, -7.082119434687050408 ) ) ;
#1086=DIRECTION ( 'NONE',  ( 1.000000000000000000, 0.000000000000000000, 0.000000000000000000 ) ) ;
#1087=CARTESIAN_POINT ( 'NONE',  ( -0.8801773607110991993, 27.85535201082150181, -2.915334737309923874 ) ) ;
#1090=CARTESIAN_POINT ( 'NONE',  ( 1.472469842513823179, 6.425597817667451750, 4.923371831947296329 ) ) ;
#1091=STYLED_ITEM ( 'NONE', ( #64075 ), #55484 ) ;
#1092=CARTESIAN_POINT ( 'NONE',  ( 3.591859063236763294, 28.29030133659708568, -11.09922568453595026 ) ) ;
#1093=CARTESIAN_POINT ( 'NONE',  ( 19.84674366389459266, 23.71726448433412315, -2.638427012816827677 ) ) ;
#1095=CARTESIAN_POINT ( 'NONE',  ( 6.565887622018943937, 10.16530133659708746, 12.81628187352647430 ) ) ;
#1097=CARTESIAN_POINT ( 'NONE',  ( 14.92337183194729633, 2.675597817667451750, 8.527530157486181039 ) ) ;
#1098=ORIENTED_EDGE ( 'NONE', *, *, #58474, .T. ) ;
#1100=CARTESIAN_POINT ( 'NONE',  ( 7.084665262690076126, 17.02201867748817676, -10.88017736071110164 ) ) ;
#1101=CARTESIAN_POINT ( 'NONE',  ( -0.3689425029237898834, 36.17874883491396787, -10.36894250292378850 ) ) ;
#1102=CARTESIAN_POINT ( 'NONE',  ( 17.20831665107776587, 37.88393115100078745, 7.208316651077764980 ) ) ;
#1103=CARTESIAN_POINT ( 'NONE',  ( 0.1532563361054082862, 1.217264484334117824, 2.638427012816831674 ) ) ;
#1104=CARTESIAN_POINT ( 'NONE',  ( 10.00000000000000178, 50.37363466993042493, 12.81628187352647608 ) ) ;
#1106=CARTESIAN_POINT ( 'NONE',  ( -0.8801773607111008646, 23.27201867748817676, 2.915334737309923430 ) ) ;
#1108=CARTESIAN_POINT ( 'NONE',  ( -1.099225684535947600, 18.70696800326375353, -6.408140936763238038 ) ) ;
#1109=CARTESIAN_POINT ( 'NONE',  ( 22.81628187352648496, 6.831968003263753531, -3.434112377981050290 ) ) ;
#1110=CARTESIAN_POINT ( 'NONE',  ( 19.84674366389459266, 38.30059781766745175, 2.638427012816836559 ) ) ;
#1112=CARTESIAN_POINT ( 'NONE',  ( -1.099225684535947600, 44.54030133659708923, 6.408140936763237150 ) ) ;
#1115=CARTESIAN_POINT ( 'NONE',  ( 10.00000000000000178, 59.31368534415484106, 10.88017736071110342 ) ) ;
#1120=CARTESIAN_POINT ( 'NONE',  ( 19.42250999205614193, 60.14701867748817676, 5.440088680355555262 ) ) ;
#1121=CARTESIAN_POINT ( 'NONE',  ( 15.44008868035555260, 59.73035201082151247, 9.422509992056143702 ) ) ;
#1124=CARTESIAN_POINT ( 'NONE',  ( 20.88017736071110875, 5.772018677488170546, -2.915334737309920765 ) ) ;
#1125=CARTESIAN_POINT ( 'NONE',  ( 19.84674366389459266, 53.30059781766744464, 2.638427012816836559 ) ) ;
#1126=CARTESIAN_POINT ( 'NONE',  ( 10.00000000000000000, 21.81368534415484106, -10.88017736071110342 ) ) ;
#1128=CARTESIAN_POINT ( 'NONE',  ( 10.00000000000000178, 30.37363466993042138, 12.81628187352647608 ) ) ;
#1130=CARTESIAN_POINT ( 'NONE',  ( -0.8801773607111009756, 43.06368534415484106, 1.068504757029289695E-15 ) ) ;
#1131=CARTESIAN_POINT ( 'NONE',  ( 10.00000000000000178, 5.373634669930420493, 12.81628187352647608 ) ) ;
#1133=CARTESIAN_POINT ( 'NONE',  ( 10.00000000000000178, 9.313685344154839285, 10.88017736071110342 ) ) ;
#1134=CARTESIAN_POINT ( 'NONE',  ( -0.8801773607110991993, 42.85535201082150536, -2.915334737309923874 ) ) ;
#1135=CARTESIAN_POINT ( 'NONE',  ( -0.3689425029237898834, 41.17874883491397497, -10.36894250292378850 ) ) ;
#1136=CARTESIAN_POINT ( 'NONE',  ( 10.00000000000000178, 22.25893115100078745, 9.846743663894594434 ) ) ;
#1137=CARTESIAN_POINT ( 'NONE',  ( 10.00000000000000178, 64.31368534415483396, 10.88017736071110342 ) ) ;
#1139=CARTESIAN_POINT ( 'NONE',  ( 24.16423886937409904, 9.095415501580633943, 3.795296366450317205 ) ) ;
#1144=CARTESIAN_POINT ( 'NONE',  ( 1.472469842513823179, 55.59226448433412315, -4.923371831947296329 ) ) ;
#1147=CARTESIAN_POINT ( 'NONE',  ( -0.3689425029237898834, 36.17874883491396787, -10.36894250292378850 ) ) ;
#1148=CARTESIAN_POINT ( 'NONE',  ( 20.36894250292379738, 34.92874883491396076, -10.36894250292379027 ) ) ;
#1149=AXIS2_PLACEMENT_3D ( 'NONE', #2580, #34009, #40556 ) ;
#1150=CARTESIAN_POINT ( 'NONE',  ( 19.84674366389459266, 3.300597817667451750, 2.638427012816836559 ) ) ;
#1151=CARTESIAN_POINT ( 'NONE',  ( 19.38216949554541557, 7.248634669930421381, -9.382169495545420901 ) ) ;
#1152=CARTESIAN_POINT ( 'NONE',  ( 10.00000000000000178, 57.25893115100078745, 9.846743663894594434 ) ) ;
#1154=CARTESIAN_POINT ( 'NONE',  ( 19.42250999205614548, 65.98035201082151957, -5.440088680355545492 ) ) ;
#1155=CARTESIAN_POINT ( 'NONE',  ( 22.81628187352648496, 16.83196800326374998, -3.434112377981050290 ) ) ;
#1156=CARTESIAN_POINT ( 'NONE',  ( -4.164238869374099039, 31.80374883491396432, 8.674139862899312516E-16 ) ) ;
#1157=CARTESIAN_POINT ( 'NONE',  ( -0.8801773607110991993, 32.85535201082151247, -2.915334737309923874 ) ) ;
#1158=CARTESIAN_POINT ( 'NONE',  ( 15.44008868035555793, 26.39701867748817321, -9.422509992056140149 ) ) ;
#1160=CARTESIAN_POINT ( 'NONE',  ( 20.88017736071110519, 55.56368534415484817, 2.639326808657452039E-16 ) ) ;
#1169=CARTESIAN_POINT ( 'NONE',  ( 13.79529636645031943, 60.34541550158063927, -14.16423886937409904 ) ) ;
#1170=CARTESIAN_POINT ( 'NONE',  ( 2.035157376598824452, 3.688685344154837953, 7.964842623401179544 ) ) ;
#1171=CARTESIAN_POINT ( 'NONE',  ( 14.92337183194729988, 39.34226448433412315, -8.527530157486177487 ) ) ;
#1172=CARTESIAN_POINT ( 'NONE',  ( 1.472469842513823179, 66.42559781766745175, 4.923371831947296329 ) ) ;
#1174=CARTESIAN_POINT ( 'NONE',  ( 20.10493008474205823, 49.71697413083879269, 6.336235997365754713 ) ) ;
#1175=ADVANCED_FACE ( 'NONE', ( #75612 ), #52125, .F. ) ;
#1176=B_SPLINE_CURVE_WITH_KNOTS ( 'NONE', 3,
 ( #51662, #22649, #81158, #20665, #74645, #43162 ),
 .UNSPECIFIED., .F., .F.,
 ( 4, 2, 4 ),
 ( 7.822990134193277425E-18, 0.0002626113303185972870, 0.0005252226606371867678 ),
 .UNSPECIFIED. ) ;
#1177=CARTESIAN_POINT ( 'NONE',  ( 3.591859063236761518, 9.956968003263753531, 11.09922568453594849 ) ) ;
#1180=CARTESIAN_POINT ( 'NONE',  ( 2.917880565312948704, 42.63708216824729647, 12.26659068614894643 ) ) ;
#1181=CARTESIAN_POINT ( 'NONE',  ( 13.79529636645031943, 45.34541550158062506, -14.16423886937409904 ) ) ;
#1183=CARTESIAN_POINT ( 'NONE',  ( 7.084665262690076126, 22.02201867748817321, -10.88017736071110164 ) ) ;
#1184=CARTESIAN_POINT ( 'NONE',  ( 19.38216949554541202, 55.99863466993041072, 9.382169495545424454 ) ) ;
#1185=CARTESIAN_POINT ( 'NONE',  ( 15.44008868035555793, 26.39701867748817321, -9.422509992056140149 ) ) ;
#1186=CARTESIAN_POINT ( 'NONE',  ( 19.84674366389459621, 53.50893115100078745, 7.409399052514197653E-17 ) ) ;
#1187=CARTESIAN_POINT ( 'NONE',  ( 4.559911319644449179, 38.89701867748817676, 9.422509992056141925 ) ) ;
#1188=CARTESIAN_POINT ( 'NONE',  ( -0.3289641300568005855, 65.10497603579418069, 5.963430220938281678 ) ) ;
#1189=CARTESIAN_POINT ( 'NONE',  ( 19.84674366389459266, 58.71726448433411605, -2.638427012816827677 ) ) ;
#1191=CARTESIAN_POINT ( 'NONE',  ( 2.035157376598822676, 27.43868534415483396, -7.964842623401177768 ) ) ;
#1193=VECTOR ( 'NONE', #97289, 1000.000000000000000 ) ;
#1196=CARTESIAN_POINT ( 'NONE',  ( 5.076628168052704559, 0.1755978176674514724, -8.527530157486179263 ) ) ;
#1200=CIRCLE ( 'NONE', #26713, 0.5000000000000004441 ) ;
#1202=CARTESIAN_POINT ( 'NONE',  ( 0.1532563361054100626, 25.80059781766744820, -2.638427012816831230 ) ) ;
#1203=CARTESIAN_POINT ( 'NONE',  ( 20.15039907845753575, 47.62777174578613426, -6.262539305110073506 ) ) ;
#1204=CARTESIAN_POINT ( 'NONE',  ( -2.816281873526473856, 49.33196800326374643, 3.434112377981055619 ) ) ;
#1211=CARTESIAN_POINT ( 'NONE',  ( 7.361572987183170547, 57.05059781766744464, 9.846743663894590881 ) ) ;
#1212=CARTESIAN_POINT ( 'NONE',  ( -0.3689425029237881626, 52.42874883491396076, 10.36894250292379027 ) ) ;
#1213=CARTESIAN_POINT ( 'NONE',  ( 12.63842701281683922, 64.55059781766745175, -9.846743663894590881 ) ) ;
#1214=CARTESIAN_POINT ( 'NONE',  ( 19.80448550324509682, 41.82703681773342907, 6.500000000002703615 ) ) ;
#1215=CARTESIAN_POINT ( 'NONE',  ( 0.1532563361054082862, 16.21726448433411960, 2.638427012816831674 ) ) ;
#1216=CARTESIAN_POINT ( 'NONE',  ( -1.099225684535947600, 48.70696800326375353, -6.408140936763238038 ) ) ;
#1217=CARTESIAN_POINT ( 'NONE',  ( 1.472469842513823179, 55.59226448433412315, -4.923371831947296329 ) ) ;
#1218=CARTESIAN_POINT ( 'NONE',  ( 2.035157376598822676, 57.43868534415484106, -7.964842623401177768 ) ) ;
#1220=CARTESIAN_POINT ( 'NONE',  ( 10.00000000000000000, 49.75893115100078745, -9.846743663894594434 ) ) ;
#1223=CARTESIAN_POINT ( 'NONE',  ( 7.084665262690076126, 54.10535201082151247, 10.88017736071109987 ) ) ;
#1226=CARTESIAN_POINT ( 'NONE',  ( 20.88017736071110164, 35.35535201082150536, 2.915334737309930979 ) ) ;
#1227=CARTESIAN_POINT ( 'NONE',  ( 0.6178305044545838731, 9.748634669930416052, 9.382169495545420901 ) ) ;
#1228=CARTESIAN_POINT ( 'NONE',  ( 19.42250999205614548, 60.98035201082151247, -5.440088680355545492 ) ) ;
#1232=CARTESIAN_POINT ( 'NONE',  ( 2.035157376598822676, 42.43868534415483396, -7.964842623401177768 ) ) ;
#1233=CARTESIAN_POINT ( 'NONE',  ( -0.1503990784575277295, 54.24884699246889852, -6.262539305110077947 ) ) ;
#1234=CARTESIAN_POINT ( 'NONE',  ( 7.361572987183170547, 42.05059781766745886, 9.846743663894590881 ) ) ;
#1235=CARTESIAN_POINT ( 'NONE',  ( 7.361572987183169658, 4.967264484334119601, -9.846743663894592657 ) ) ;
#1237=CARTESIAN_POINT ( 'NONE',  ( 3.591859063236763294, 13.29030133659708746, -11.09922568453595026 ) ) ;
#1238=CARTESIAN_POINT ( 'NONE',  ( 0.5774900079438590739, 7.647018677488171434, -5.440088680355550821 ) ) ;
#1240=CARTESIAN_POINT ( 'NONE',  ( -4.164238869374098151, 26.59541550158063217, -3.795296366450310543 ) ) ;
#1241=CARTESIAN_POINT ( 'NONE',  ( -2.266590686148945544, 66.38708216824730357, -7.082119434687050408 ) ) ;
#1242=CARTESIAN_POINT ( 'NONE',  ( 2.791683348922237240, 35.38393115100079456, -7.208316651077763204 ) ) ;
#1243=CARTESIAN_POINT ( 'NONE',  ( 10.00000000000000000, 19.75893115100078390, -9.846743663894594434 ) ) ;
#1244=CARTESIAN_POINT ( 'NONE',  ( 0.5774900079438607392, 18.48035201082150536, 5.440088680355550821 ) ) ;
#1246=CARTESIAN_POINT ( 'NONE',  ( 14.92337183194729633, 42.67559781766745886, 8.527530157486181039 ) ) ;
#1247=CARTESIAN_POINT ( 'NONE',  ( 19.42250999205614548, 30.98035201082150536, -5.440088680355545492 ) ) ;
#1248=CARTESIAN_POINT ( 'NONE',  ( 5.076628168052703671, 66.84226448433412315, 8.527530157486179263 ) ) ;
#1249=CARTESIAN_POINT ( 'NONE',  ( 17.08211943468705130, 13.47041550158063572, 12.26659068614894998 ) ) ;
#1252=UNCERTAINTY_MEASURE_WITH_UNIT (LENGTH_MEASURE( 1.000000000000000082E-05 ), #79189, 'distance_accuracy_value', 'NONE');
#1253=CARTESIAN_POINT ( 'NONE',  ( 2.791683348922237240, 5.383931151000785675, -7.208316651077763204 ) ) ;
#1254=CARTESIAN_POINT ( 'NONE',  ( 3.591859063236763294, 38.29030133659708923, -11.09922568453595026 ) ) ;
#1255=CARTESIAN_POINT ( 'NONE',  ( 0.1532563361054100626, 60.80059781766744464, -2.638427012816831230 ) ) ;
#1257=CARTESIAN_POINT ( 'NONE',  ( 19.84674366389459266, 18.71726448433411960, -2.638427012816827677 ) ) ;
#1258=FACE_OUTER_BOUND ( 'NONE', #92860, .T. ) ;
#1259=CARTESIAN_POINT ( 'NONE',  ( 17.08211943468705840, 50.13708216824730357, -12.26659068614894466 ) ) ;
#1260=CARTESIAN_POINT ( 'NONE',  ( 12.91533473730992121, 49.52201867748817676, 10.88017736071110164 ) ) ;
#1261=CARTESIAN_POINT ( 'NONE',  ( 2.917880565312948704, 2.637082168247300906, 12.26659068614894643 ) ) ;
#1263=CARTESIAN_POINT ( 'NONE',  ( 19.42250999205614548, 60.98035201082151247, -5.440088680355545492 ) ) ;
#1264=CARTESIAN_POINT ( 'NONE',  ( 10.00000000000000000, 39.75893115100078745, -9.846743663894594434 ) ) ;
#1265=CARTESIAN_POINT ( 'NONE',  ( 10.00000000000000178, 19.31368534415484106, 10.88017736071110342 ) ) ;
#1266=CARTESIAN_POINT ( 'NONE',  ( 17.39651004071841101, 37.93575266056827644, 6.500000000000005329 ) ) ;
#1267=CARTESIAN_POINT ( 'NONE',  ( 1.472469842513823179, 45.59226448433412315, -4.923371831947296329 ) ) ;
#1269=CARTESIAN_POINT ( 'NONE',  ( 7.084665262690076126, 54.10535201082151247, 10.88017736071109987 ) ) ;
#1270=ORIENTED_EDGE ( 'NONE', *, *, #68403, .F. ) ;
#1277=CARTESIAN_POINT ( 'NONE',  ( 13.79529636645030344, 3.262082168247301350, 14.16423886937410614 ) ) ;
#1278=CARTESIAN_POINT ( 'NONE',  ( 12.63842701281683922, 44.55059781766745175, -9.846743663894590881 ) ) ;
#1279=CARTESIAN_POINT ( 'NONE',  ( 10.00000000000000178, 22.25893115100078745, 9.846743663894594434 ) ) ;
#1280=CARTESIAN_POINT ( 'NONE',  ( -1.099225684535947600, 53.70696800326376064, -6.408140936763238038 ) ) ;
#1281=CARTESIAN_POINT ( 'NONE',  ( 15.44008868035555793, 16.39701867748817321, -9.422509992056140149 ) ) ;
#1282=CARTESIAN_POINT ( 'NONE',  ( 10.00000000000000000, 54.75893115100078745, -9.846743663894594434 ) ) ;
#1284=CARTESIAN_POINT ( 'NONE',  ( 20.36894250292379738, 44.92874883491396787, -10.36894250292379027 ) ) ;
#1285=CARTESIAN_POINT ( 'NONE',  ( 17.08211943468705130, 53.47041550158063217, 12.26659068614894998 ) ) ;
#1286=CARTESIAN_POINT ( 'NONE',  ( 14.92337183194729633, 57.67559781766745886, 8.527530157486181039 ) ) ;
#1288=CARTESIAN_POINT ( 'NONE',  ( 0.5774900079438607392, 53.48035201082151247, 5.440088680355550821 ) ) ;
#1289=CARTESIAN_POINT ( 'NONE',  ( 7.361572987183169658, 19.96726448433411960, -9.846743663894592657 ) ) ;
#1296=CARTESIAN_POINT ( 'NONE',  ( 2.791683348922237240, 10.38393115100078390, -7.208316651077763204 ) ) ;
#1298=CARTESIAN_POINT ( 'NONE',  ( -0.3689425029237898834, 16.17874883491396076, -10.36894250292378850 ) ) ;
#1299=CARTESIAN_POINT ( 'NONE',  ( 2.791683348922237240, 15.38393115100078212, -7.208316651077763204 ) ) ;
#1300=CARTESIAN_POINT ( 'NONE',  ( 2.035157376598824452, 43.68868534415484106, 7.964842623401179544 ) ) ;
#1303=VECTOR ( 'NONE', #84637, 1000.000000000000114 ) ;
#1304=CARTESIAN_POINT ( 'NONE',  ( 17.96484262340118221, 39.93868534415484106, 7.964842623401181321 ) ) ;
#1306=CARTESIAN_POINT ( 'NONE',  ( -0.1042174387088607435, 43.10736173766202484, 6.337391062633419558 ) ) ;
#1308=ORIENTED_EDGE ( 'NONE', *, *, #88059, .T. ) ;
#1309=CARTESIAN_POINT ( 'NONE',  ( 10.00000000000000178, 3.053748834913967425, 14.16423886937410082 ) ) ;
#1312=CARTESIAN_POINT ( 'NONE',  ( 3.591859063236763294, 23.29030133659708568, -11.09922568453595026 ) ) ;
#1313=CARTESIAN_POINT ( 'NONE',  ( 2.791683348922240793, 16.63393115100078745, 7.208316651077764092 ) ) ;
#1315=CARTESIAN_POINT ( 'NONE',  ( 19.10478245763051319, 10.10160829253885950, 5.990408912944328534 ) ) ;
#1316=CARTESIAN_POINT ( 'NONE',  ( 18.52753015748618282, 13.92559781766745175, -4.923371831947291888 ) ) ;
#1317=CARTESIAN_POINT ( 'NONE',  ( 10.00000000000000000, 36.81368534415484106, -10.88017736071110342 ) ) ;
#1319=ORIENTED_EDGE ( 'NONE', *, *, #41541, .F. ) ;
#1321=CARTESIAN_POINT ( 'NONE',  ( -0.8801773607110991993, 57.85535201082149825, -2.915334737309923874 ) ) ;
#1323=CARTESIAN_POINT ( 'NONE',  ( 20.88017736071110519, 60.56368534415484106, 2.639326808657452039E-16 ) ) ;
#1325=CARTESIAN_POINT ( 'NONE',  ( 14.92337183194729633, 32.67559781766745175, 8.527530157486181039 ) ) ;
#1326=CARTESIAN_POINT ( 'NONE',  ( 10.00000000000000000, 57.87363466993042493, -12.81628187352647608 ) ) ;
#1328=CARTESIAN_POINT ( 'NONE',  ( 2.791683348922237240, 20.38393115100078745, -7.208316651077763204 ) ) ;
#1329=CARTESIAN_POINT ( 'NONE',  ( 0.6178305044545818747, 18.49863466993041428, -9.382169495545419124 ) ) ;
#1332=CARTESIAN_POINT ( 'NONE',  ( 17.96484262340118221, 46.18868534415484106, -7.964842623401177768 ) ) ;
#1333=CARTESIAN_POINT ( 'NONE',  ( 10.00000000000000178, 57.25893115100078745, 9.846743663894594434 ) ) ;
#1335=CARTESIAN_POINT ( 'NONE',  ( 19.84674366389459621, 33.50893115100078745, 7.409399052514197653E-17 ) ) ;
#1336=CARTESIAN_POINT ( 'NONE',  ( 0.1532563361054100626, 20.80059781766744464, -2.638427012816831230 ) ) ;
#1337=CARTESIAN_POINT ( 'NONE',  ( 17.96484262340118221, 14.93868534415483751, 7.964842623401181321 ) ) ;
#1338=CARTESIAN_POINT ( 'NONE',  ( 22.81628187352647785, 11.41530133659708390, 3.434112377981063169 ) ) ;
#1340=PRESENTATION_STYLE_ASSIGNMENT (( #34861 ) ) ;
#1342=CARTESIAN_POINT ( 'NONE',  ( 17.96484262340118221, 19.93868534415484106, 7.964842623401181321 ) ) ;
#1344=CARTESIAN_POINT ( 'NONE',  ( 18.52753015748617571, 33.09226448433411605, 4.923371831947298993 ) ) ;
#1345=CARTESIAN_POINT ( 'NONE',  ( 0.5774900079438607392, 13.48035201082150358, 5.440088680355550821 ) ) ;
#1347=CARTESIAN_POINT ( 'NONE',  ( 2.035157376598824452, 33.68868534415484106, 7.964842623401179544 ) ) ;
#1349=CARTESIAN_POINT ( 'NONE',  ( 22.26659068614894466, 63.88708216824730357, 7.082119434687054849 ) ) ;
#1351=CARTESIAN_POINT ( 'NONE',  ( 19.84674366389459266, 18.71726448433411960, -2.638427012816827677 ) ) ;
#1352=CARTESIAN_POINT ( 'NONE',  ( 0.1532563361054100626, 40.80059781766745886, -2.638427012816831230 ) ) ;
#1354=CARTESIAN_POINT ( 'NONE',  ( 19.84674366389459621, 63.50893115100078745, 7.409399052514197653E-17 ) ) ;
#1359=CARTESIAN_POINT ( 'NONE',  ( -4.164238869374098151, 21.59541550158063217, -3.795296366450310543 ) ) ;
#1360=CARTESIAN_POINT ( 'NONE',  ( 17.20831665107776587, 34.13393115100078745, -7.208316651077762316 ) ) ;
#1363=CARTESIAN_POINT ( 'NONE',  ( 2.917880565312950480, 50.97041550158064638, -12.26659068614894821 ) ) ;
#1364=CARTESIAN_POINT ( 'NONE',  ( 1.472469842513823179, 25.59226448433412315, -4.923371831947296329 ) ) ;
#1367=CARTESIAN_POINT ( 'NONE',  ( 12.91533473730993009, 51.60535201082149825, -10.88017736071109987 ) ) ;
#1368=CARTESIAN_POINT ( 'NONE',  ( 19.38216949554541557, 52.24863466993041072, -9.382169495545420901 ) ) ;
#1369=CARTESIAN_POINT ( 'NONE',  ( 20.88017736071110164, 20.35535201082150891, 2.915334737309930979 ) ) ;
#1370=CARTESIAN_POINT ( 'NONE',  ( 0.6178305044545818747, 43.49863466993042493, -9.382169495545419124 ) ) ;
#1371=CARTESIAN_POINT ( 'NONE',  ( 0.6178305044545838731, -0.2513653300695798953, 9.382169495545420901 ) ) ;
#1375=CARTESIAN_POINT ( 'NONE',  ( 24.16423886937410614, 59.51208216824728936, -3.795296366450302550 ) ) ;
#1376=CARTESIAN_POINT ( 'NONE',  ( 24.16423886937410614, 19.51208216824729647, -3.795296366450302550 ) ) ;
#1377=CARTESIAN_POINT ( 'NONE',  ( 7.084665262690076126, 19.10535201082150181, 10.88017736071109987 ) ) ;
#1378=CARTESIAN_POINT ( 'NONE',  ( 2.035157376598824452, 38.68868534415483396, 7.964842623401179544 ) ) ;
#1379=CARTESIAN_POINT ( 'NONE',  ( 20.15039907845753930, 70.00000000000000000, -6.262539305110068177 ) ) ;
#1380=CARTESIAN_POINT ( 'NONE',  ( 2.791683348922237240, 0.3839311510007847872, -7.208316651077763204 ) ) ;
#1382=CARTESIAN_POINT ( 'NONE',  ( 2.791683348922237240, 15.38393115100078212, -7.208316651077763204 ) ) ;
#1383=CARTESIAN_POINT ( 'NONE',  ( 2.603489959281614308, 61.58210964143329846, 6.500000000000031086 ) ) ;
#1385=CARTESIAN_POINT ( 'NONE',  ( 19.84674366389459266, 13.71726448433411782, -2.638427012816827677 ) ) ;
#1386=CARTESIAN_POINT ( 'NONE',  ( 1.472469842513823179, 35.59226448433412315, -4.923371831947296329 ) ) ;
#1388=CARTESIAN_POINT ( 'NONE',  ( 15.44008868035555793, 16.39701867748817321, -9.422509992056140149 ) ) ;
#1389=CARTESIAN_POINT ( 'NONE',  ( -1.099225684535947600, 34.54030133659708923, 6.408140936763237150 ) ) ;
#1390=CARTESIAN_POINT ( 'NONE',  ( 18.52753015748618282, 3.925597817667451306, -4.923371831947291888 ) ) ;
#1392=CARTESIAN_POINT ( 'NONE',  ( 1.472469842513823179, 46.42559781766745175, 4.923371831947296329 ) ) ;
#1393=CARTESIAN_POINT ( 'NONE',  ( 12.63842701281683922, 29.55059781766745175, -9.846743663894590881 ) ) ;
#1394=CARTESIAN_POINT ( 'NONE',  ( 22.26659068614894466, 3.887082168247300906, 7.082119434687054849 ) ) ;
#1395=CARTESIAN_POINT ( 'NONE',  ( -2.266590686148945544, 21.38708216824730357, -7.082119434687050408 ) ) ;
#1396=CARTESIAN_POINT ( 'NONE',  ( 2.035157376598822676, 52.43868534415483396, -7.964842623401177768 ) ) ;
#1397=CARTESIAN_POINT ( 'NONE',  ( 20.88017736071110164, 10.35535201082150714, 2.915334737309930979 ) ) ;
#1398=CARTESIAN_POINT ( 'NONE',  ( 17.96484262340118221, 44.93868534415483396, 7.964842623401181321 ) ) ;
#1399=CARTESIAN_POINT ( 'NONE',  ( 20.88017736071110519, 30.56368534415484106, 2.639326808657452039E-16 ) ) ;
#1401=CARTESIAN_POINT ( 'NONE',  ( 10.00000000000000178, 30.37363466993042138, 12.81628187352647608 ) ) ;
#1402=CARTESIAN_POINT ( 'NONE',  ( 7.084665262690076126, 42.02201867748816966, -10.88017736071110164 ) ) ;
#1403=ORIENTED_EDGE ( 'NONE', *, *, #70327, .T. ) ;
#1404=CARTESIAN_POINT ( 'NONE',  ( 21.09922568453594849, 56.20696800326375353, 6.408140936763242479 ) ) ;
#1405=CARTESIAN_POINT ( 'NONE',  ( 0.5774900079438607392, 53.48035201082151247, 5.440088680355550821 ) ) ;
#1408=CARTESIAN_POINT ( 'NONE',  ( 2.035157376598824452, 53.68868534415484817, 7.964842623401179544 ) ) ;
#1411=CARTESIAN_POINT ( 'NONE',  ( 10.00000000000000178, 70.00000000000000000, 0.000000000000000000 ) ) ;
#1412=CARTESIAN_POINT ( 'NONE',  ( 24.16423886937410614, 59.30374883491397497, 8.672049930838204340E-16 ) ) ;
#1413=CARTESIAN_POINT ( 'NONE',  ( 10.00000000000000178, 64.31368534415483396, 10.88017736071110342 ) ) ;
#1414=CARTESIAN_POINT ( 'NONE',  ( 2.917880565312950480, 10.97041550158063572, -12.26659068614894821 ) ) ;
#1415=SURFACE_STYLE_USAGE ( .BOTH. , #69895 ) ;
#1416=CARTESIAN_POINT ( 'NONE',  ( 4.559911319644449179, 12.23035201082150536, -9.422509992056141925 ) ) ;
#1417=CARTESIAN_POINT ( 'NONE',  ( 0.1532563361054083140, 41.00893115100078745, 1.131784320476157264E-15 ) ) ;
#1418=VERTEX_POINT ( 'NONE', #21138 ) ;
#1419=CARTESIAN_POINT ( 'NONE',  ( 12.63842701281683922, 34.55059781766745886, -9.846743663894590881 ) ) ;
#1421=CARTESIAN_POINT ( 'NONE',  ( 7.084665262690076126, 39.10535201082150536, 10.88017736071109987 ) ) ;
#1422=CARTESIAN_POINT ( 'NONE',  ( 17.20831665107776587, 44.13393115100078745, -7.208316651077762316 ) ) ;
#1423=CARTESIAN_POINT ( 'NONE',  ( 16.40814093676323893, 20.79030133659708923, 11.09922568453595026 ) ) ;
#1424=SURFACE_STYLE_USAGE ( .BOTH. , #10872 ) ;
#1426=CARTESIAN_POINT ( 'NONE',  ( 4.559911319644449179, 47.23035201082150536, -9.422509992056141925 ) ) ;
#1427=CARTESIAN_POINT ( 'NONE',  ( 10.00000000000000178, 53.05374883491396787, 14.16423886937410082 ) ) ;
#1430=CARTESIAN_POINT ( 'NONE',  ( -1.099225684535947600, 19.54030133659708568, 6.408140936763237150 ) ) ;
#1433=CARTESIAN_POINT ( 'NONE',  ( 0.6178305044545818747, 23.49863466993041783, -9.382169495545419124 ) ) ;
#1434=CARTESIAN_POINT ( 'NONE',  ( 20.88017736071110164, 15.35535201082150358, 2.915334737309930979 ) ) ;
#1438=CARTESIAN_POINT ( 'NONE',  ( 19.42250999205614193, 65.14701867748817676, 5.440088680355555262 ) ) ;
#1439=CARTESIAN_POINT ( 'NONE',  ( 19.84674366389459621, 48.50893115100078745, 7.409399052514197653E-17 ) ) ;
#1440=CARTESIAN_POINT ( 'NONE',  ( 19.84674366389459266, 33.71726448433410894, -2.638427012816827677 ) ) ;
#1442=CARTESIAN_POINT ( 'NONE',  ( -1.099225684535947600, 64.54030133659709634, 6.408140936763237150 ) ) ;
#1443=CARTESIAN_POINT ( 'NONE',  ( 0.1532563361054083140, 31.00893115100078390, 1.131784320476157264E-15 ) ) ;
#1447=CARTESIAN_POINT ( 'NONE',  ( 5.076628168052704559, 10.17559781766745175, -8.527530157486179263 ) ) ;
#1448=CARTESIAN_POINT ( 'NONE',  ( 10.00000000000000178, 2.258931151000784787, 9.846743663894594434 ) ) ;
#1449=CARTESIAN_POINT ( 'NONE',  ( 0.1532563361054082862, 46.21726448433411605, 2.638427012816831674 ) ) ;
#1451=CARTESIAN_POINT ( 'NONE',  ( 20.32896413005680003, 16.77164270246083788, 5.963430220938287007 ) ) ;
#1452=CARTESIAN_POINT ( 'NONE',  ( 13.43411237798106583, 27.66530133659708568, -12.81628187352647252 ) ) ;
#1453=CARTESIAN_POINT ( 'NONE',  ( 10.00000000000000000, 46.81368534415484106, -10.88017736071110342 ) ) ;
#1454=CARTESIAN_POINT ( 'NONE',  ( 22.26659068614895176, 39.72041550158063217, -7.082119434687042414 ) ) ;
#1455=CARTESIAN_POINT ( 'NONE',  ( 0.1532563361054100626, 0.8005978176674514168, -2.638427012816831230 ) ) ;
#1457=CARTESIAN_POINT ( 'NONE',  ( 24.16423886937410614, 39.30374883491396787, 8.672049930838204340E-16 ) ) ;
#1459=CARTESIAN_POINT ( 'NONE',  ( 20.36894250292379738, 54.92874883491396076, -10.36894250292379027 ) ) ;
#1460=CARTESIAN_POINT ( 'NONE',  ( 24.16423886937410614, 24.51208216824730002, -3.795296366450302550 ) ) ;
#1461=CARTESIAN_POINT ( 'NONE',  ( -4.164238869374099039, 31.80374883491396432, 8.674139862899312516E-16 ) ) ;
#1465=CARTESIAN_POINT ( 'NONE',  ( 5.076628168052703671, 46.84226448433412315, 8.527530157486179263 ) ) ;
#1466=CARTESIAN_POINT ( 'NONE',  ( -0.8801773607111008646, 43.27201867748817676, 2.915334737309923430 ) ) ;
#1467=CARTESIAN_POINT ( 'NONE',  ( 10.00000000000000178, 70.00000000000000000, 0.000000000000000000 ) ) ;
#1468=CARTESIAN_POINT ( 'NONE',  ( 20.00000000000000711, 92.21878522475820716, -5.248003389973252553 ) ) ;
#1469=CARTESIAN_POINT ( 'NONE',  ( 12.63842701281683922, 39.55059781766744464, -9.846743663894590881 ) ) ;
#1470=CARTESIAN_POINT ( 'NONE',  ( 10.00000000000000178, 50.37363466993042493, 12.81628187352647608 ) ) ;
#1472=CARTESIAN_POINT ( 'NONE',  ( 17.20831665107776587, 39.13393115100079456, -7.208316651077762316 ) ) ;
#1473=CARTESIAN_POINT ( 'NONE',  ( 1.472469842513823179, 66.42559781766745175, 4.923371831947296329 ) ) ;
#1474=CARTESIAN_POINT ( 'NONE',  ( 10.00000000000000178, 38.05374883491396787, 14.16423886937410082 ) ) ;
#1476=CARTESIAN_POINT ( 'NONE',  ( -2.266590686148945544, 16.38708216824730357, -7.082119434687050408 ) ) ;
#1480=CARTESIAN_POINT ( 'NONE',  ( 0.5774900079438590739, 2.647018677488171434, -5.440088680355550821 ) ) ;
#1481=CARTESIAN_POINT ( 'NONE',  ( 6.565887622018943937, 8.081968003263751754, -12.81628187352647608 ) ) ;
#1483=CARTESIAN_POINT ( 'NONE',  ( 10.00000000000000000, -0.2410688489992152128, -9.846743663894594434 ) ) ;
#1485=CARTESIAN_POINT ( 'NONE',  ( -0.03743638938523759230, 14.25197528031018557, -6.399506433553937335 ) ) ;
#1487=CARTESIAN_POINT ( 'NONE',  ( -2.266590686148945544, 62.22041550158063927, 7.082119434687048631 ) ) ;
#1489=CARTESIAN_POINT ( 'NONE',  ( 10.00000000000000178, 24.31368534415484106, 10.88017736071110342 ) ) ;
#1490=CARTESIAN_POINT ( 'NONE',  ( 15.44008868035555260, 19.73035201082150536, 9.422509992056143702 ) ) ;
#1491=CARTESIAN_POINT ( 'NONE',  ( 7.361572987183170547, 67.05059781766746596, 9.846743663894590881 ) ) ;
#1492=CARTESIAN_POINT ( 'NONE',  ( 12.63842701281683922, 54.55059781766745175, -9.846743663894590881 ) ) ;
#1493=CARTESIAN_POINT ( 'NONE',  ( 6.565887622018943937, 60.16530133659707502, 12.81628187352647430 ) ) ;
#1494=B_SPLINE_CURVE_WITH_KNOTS ( 'NONE', 3,
 ( #6532, #84018, #74530, #29510 ),
 .UNSPECIFIED., .F., .F.,
 ( 4, 4 ),
 ( 5.421010862427522170E-20, 0.002657014572711347174 ),
 .UNSPECIFIED. ) ;
#1498=CARTESIAN_POINT ( 'NONE',  ( 0.5774900079438590739, 32.64701867748816966, -5.440088680355550821 ) ) ;
#1500=CARTESIAN_POINT ( 'NONE',  ( 3.591859063236761518, 34.95696800326375353, 11.09922568453594849 ) ) ;
#1504=CARTESIAN_POINT ( 'NONE',  ( 1.472469842513823179, 55.59226448433412315, -4.923371831947296329 ) ) ;
#1506=CARTESIAN_POINT ( 'NONE',  ( 7.084665262690076126, 52.02201867748816255, -10.88017736071110164 ) ) ;
#1508=CARTESIAN_POINT ( 'NONE',  ( 2.791683348922240793, 11.63393115100078568, 7.208316651077764092 ) ) ;
#1509=CARTESIAN_POINT ( 'NONE',  ( 6.565887622018943937, 25.16530133659708213, 12.81628187352647430 ) ) ;
#1510=CARTESIAN_POINT ( 'NONE',  ( 10.00000000000000178, 64.31368534415483396, 10.88017736071110342 ) ) ;
#1511=CARTESIAN_POINT ( 'NONE',  ( 19.72487221294571569, 17.80223176428831522, -6.499999999999990230 ) ) ;
#1512=( BOUNDED_SURFACE ( )  B_SPLINE_SURFACE ( 3, 2, ( 
 ( #55462, #86934, #71457 ),
 ( #47941, #9463, #86457 ),
 ( #32453, #78447, #23989 ),
 ( #40469, #69481, #999 ),
 ( #17955, #31461, #48442 ),
 ( #78941, #10452, #2971 ),
 ( #33421, #94431, #18447 ),
 ( #54460, #16485, #57418 ) ),
 .UNSPECIFIED., .F., .F., .T. ) 
 B_SPLINE_SURFACE_WITH_KNOTS ( ( 4, 2, 2, 4 ),
 ( 3, 3 ),
 ( 8.673617379884035472E-19, 0.002726357873101972664, 0.004089536809652958779, 0.005452715746203944461 ),
 ( 0.000000000000000000, 1.000000000000000000 ),
 .UNSPECIFIED. ) 
 GEOMETRIC_REPRESENTATION_ITEM ( )  RATIONAL_B_SPLINE_SURFACE ( (
 ( 1.000000000000000000, 0.7071067811865475727, 1.000000000000000000),
 ( 1.000000000000000000, 0.7287458841150015187, 1.000000000000000000),
 ( 1.000000000000000000, 0.7487351283423555603, 1.000000000000000000),
 ( 1.000000000000000000, 0.7766004504404603326, 1.000000000000000000),
 ( 1.000000000000000000, 0.7855344611292480739, 1.000000000000000000),
 ( 1.000000000000000000, 0.8027290847944021923, 1.000000000000000000),
 ( 1.000000000000000000, 0.8110176777142721338, 1.000000000000000000),
 ( 1.000000000000000000, 0.8188293140827601624, 1.000000000000000000) ) ) 
 REPRESENTATION_ITEM ( '' )  SURFACE ( )  );
#1513=CARTESIAN_POINT ( 'NONE',  ( 18.28836319691949797, 54.34492782695772917, 6.499999999999920952 ) ) ;
#1514=CARTESIAN_POINT ( 'NONE',  ( 3.591859063236763294, 63.29030133659708923, -11.09922568453595026 ) ) ;
#1517=CARTESIAN_POINT ( 'NONE',  ( 19.05914839598885280, 24.96693863883976050, 6.499999999999962697 ) ) ;
#1518=CARTESIAN_POINT ( 'NONE',  ( 15.44008868035555260, 49.73035201082150536, 9.422509992056143702 ) ) ;
#1519=CARTESIAN_POINT ( 'NONE',  ( 22.81628187352648496, 41.83196800326375353, -3.434112377981050290 ) ) ;
#1520=CARTESIAN_POINT ( 'NONE',  ( 19.84674366389459266, 23.71726448433412315, -2.638427012816827677 ) ) ;
#1521=CARTESIAN_POINT ( 'NONE',  ( 0.5774900079438590739, 2.647018677488170990, -5.440088680355550821 ) ) ;
#1522=CARTESIAN_POINT ( 'NONE',  ( 0.1532563361054100626, 25.80059781766744820, -2.638427012816831230 ) ) ;
#1524=CARTESIAN_POINT ( 'NONE',  ( 20.36894250292379738, 59.92874883491397497, -10.36894250292379027 ) ) ;
#1527=CARTESIAN_POINT ( 'NONE',  ( 12.91533473730993009, 11.60535201082150536, -10.88017736071109987 ) ) ;
#1528=DIRECTION ( 'NONE',  ( 0.000000000000000000, -0.000000000000000000, 1.000000000000000000 ) ) ;
#1529=VERTEX_POINT ( 'NONE', #54573 ) ;
#1531=CARTESIAN_POINT ( 'NONE',  ( -0.8801773607110991993, 7.855352010821506248, -2.915334737309923874 ) ) ;
#1532=CARTESIAN_POINT ( 'NONE',  ( 20.88017736071110875, 15.77201867748817143, -2.915334737309920765 ) ) ;
#1533=CARTESIAN_POINT ( 'NONE',  ( 10.00000000000000000, 44.75893115100078745, -9.846743663894594434 ) ) ;
#1535=CARTESIAN_POINT ( 'NONE',  ( 22.81628187352648496, 51.83196800326376064, -3.434112377981050290 ) ) ;
#1537=CARTESIAN_POINT ( 'NONE',  ( 19.84674366389459266, 63.71726448433412315, -2.638427012816827677 ) ) ;
#1538=CARTESIAN_POINT ( 'NONE',  ( -4.164238869374099039, 26.80374883491397142, 8.674139862899312516E-16 ) ) ;
#1539=CARTESIAN_POINT ( 'NONE',  ( 20.88017736071110519, 25.56368534415483751, 2.639326808657452039E-16 ) ) ;
#1540=CARTESIAN_POINT ( 'NONE',  ( 4.559911319644449179, 2.230352010821504916, -9.422509992056141925 ) ) ;
#1541=CARTESIAN_POINT ( 'NONE',  ( 0.1532563361054082862, 36.21726448433410894, 2.638427012816831674 ) ) ;
#1543=CARTESIAN_POINT ( 'NONE',  ( 19.84674366389459266, 33.30059781766744464, 2.638427012816836559 ) ) ;
#1546=EDGE_LOOP ( 'NONE', ( #6604, #81096, #63230, #9148 ) ) ;
#1547=CARTESIAN_POINT ( 'NONE',  ( 20.88017736071110875, 5.772018677488170546, -2.915334737309920765 ) ) ;
#1548=CARTESIAN_POINT ( 'NONE',  ( 20.88017736071110519, 65.56368534415483396, 2.639326808657452039E-16 ) ) ;
#1549=CARTESIAN_POINT ( 'NONE',  ( 17.20831665107776587, 59.13393115100078745, -7.208316651077762316 ) ) ;
#1550=CARTESIAN_POINT ( 'NONE',  ( 17.96484262340118221, 41.18868534415484106, -7.964842623401177768 ) ) ;
#1551=CARTESIAN_POINT ( 'NONE',  ( 0.5774900079438590739, 7.647018677488171434, -5.440088680355550821 ) ) ;
#1552=CARTESIAN_POINT ( 'NONE',  ( 0.6178305044545838731, 34.74863466993042493, 9.382169495545420901 ) ) ;
#1553=CARTESIAN_POINT ( 'NONE',  ( 24.16423886937410614, 24.30374883491396787, 8.672049930838204340E-16 ) ) ;
#1555=CARTESIAN_POINT ( 'NONE',  ( 16.40814093676323893, 45.79030133659708923, 11.09922568453595026 ) ) ;
#1557=CARTESIAN_POINT ( 'NONE',  ( 18.52753015748617571, 53.09226448433412315, 4.923371831947298993 ) ) ;
#1558=CARTESIAN_POINT ( 'NONE',  ( 10.00000000000000000, 16.81368534415483751, -10.88017736071110342 ) ) ;
#1560=CARTESIAN_POINT ( 'NONE',  ( 4.559911319644449179, 23.89701867748817321, 9.422509992056141925 ) ) ;
#1562=CARTESIAN_POINT ( 'NONE',  ( 20.88017736071110164, 65.35535201082150536, 2.915334737309930979 ) ) ;
#1563=CARTESIAN_POINT ( 'NONE',  ( 20.15039907845753220, 31.74884699246888786, 6.262539305110077059 ) ) ;
#1564=CARTESIAN_POINT ( 'NONE',  ( 18.52753015748617571, 3.092264484334118269, 4.923371831947298993 ) ) ;
#1565=CARTESIAN_POINT ( 'NONE',  ( 10.00000000000000000, -0.2410688489992152128, -9.846743663894594434 ) ) ;
#1568=CARTESIAN_POINT ( 'NONE',  ( -46.58521628013341598, 101.6760492933278215, 7.987317478326372289 ) ) ;
#1569=CARTESIAN_POINT ( 'NONE',  ( 14.92337183194729633, 12.67559781766745353, 8.527530157486181039 ) ) ;
#1571=CARTESIAN_POINT ( 'NONE',  ( 14.92337183194729988, 44.34226448433412315, -8.527530157486177487 ) ) ;
#1572=VERTEX_POINT ( 'NONE', #23124 ) ;
#1575=CARTESIAN_POINT ( 'NONE',  ( -0.3689425029237881626, 12.42874883491396609, 10.36894250292379027 ) ) ;
#1576=CARTESIAN_POINT ( 'NONE',  ( 6.565887622018943937, 63.08196800326376064, -12.81628187352647608 ) ) ;
#1578=CARTESIAN_POINT ( 'NONE',  ( 24.16423886937410614, 14.51208216824730179, -3.795296366450302550 ) ) ;
#1581=CARTESIAN_POINT ( 'NONE',  ( -0.8801773607111008646, 63.27201867748817676, 2.915334737309923430 ) ) ;
#1582=CARTESIAN_POINT ( 'NONE',  ( 7.084665262690076126, 17.02201867748817676, -10.88017736071110164 ) ) ;
#1585=( LENGTH_UNIT ( ) NAMED_UNIT ( * ) SI_UNIT ( .MILLI., .METRE. ) );
#1586=CARTESIAN_POINT ( 'NONE',  ( 18.52753015748618282, 8.925597817667451750, -4.923371831947291888 ) ) ;
#1588=CARTESIAN_POINT ( 'NONE',  ( 22.81628187352648496, 36.83196800326376064, -3.434112377981050290 ) ) ;
#1589=CARTESIAN_POINT ( 'NONE',  ( 18.52753015748617571, 28.09226448433411960, 4.923371831947298993 ) ) ;
#1591=CARTESIAN_POINT ( 'NONE',  ( -2.816281873526473856, 19.12363466993042138, 9.499525473075851096E-16 ) ) ;
#1593=CARTESIAN_POINT ( 'NONE',  ( 1.472469842513823179, 11.42559781766745175, 4.923371831947296329 ) ) ;
#1595=ORIENTED_EDGE ( 'NONE', *, *, #22327, .T. ) ;
#1596=CARTESIAN_POINT ( 'NONE',  ( -0.8801773607111009756, 43.06368534415484106, 1.068504757029289695E-15 ) ) ;
#1597=CARTESIAN_POINT ( 'NONE',  ( 24.16423886937409904, 29.09541550158063572, 3.795296366450317205 ) ) ;
#1598=CARTESIAN_POINT ( 'NONE',  ( 19.84674366389459266, 43.30059781766744464, 2.638427012816836559 ) ) ;
#1600=CARTESIAN_POINT ( 'NONE',  ( 10.00000000000000178, 2.258931151000784787, 9.846743663894594434 ) ) ;
#1601=B_SPLINE_CURVE_WITH_KNOTS ( 'NONE', 3,
 ( #20973, #97472, #89943, #21460 ),
 .UNSPECIFIED., .F., .F.,
 ( 4, 4 ),
 ( 3.469446951953614189E-18, 0.002392975128318428242 ),
 .UNSPECIFIED. ) ;
#1602=CARTESIAN_POINT ( 'NONE',  ( 6.565887622018943937, 60.16530133659707502, 12.81628187352647430 ) ) ;
#1603=CARTESIAN_POINT ( 'NONE',  ( 13.99999999999999822, 61.50000000000000711, -6.000000000000000000 ) ) ;
#1604=CARTESIAN_POINT ( 'NONE',  ( 15.44008868035555260, 29.73035201082150891, 9.422509992056143702 ) ) ;
#1607=CARTESIAN_POINT ( 'NONE',  ( 19.38216949554541202, 25.99863466993042138, 9.382169495545424454 ) ) ;
#1608=CARTESIAN_POINT ( 'NONE',  ( 0.1532563361054083140, 36.00893115100078745, 1.131784320476157264E-15 ) ) ;
#1610=CARTESIAN_POINT ( 'NONE',  ( 0.6178305044545838731, 49.74863466993041072, 9.382169495545420901 ) ) ;
#1611=DIRECTION ( 'NONE',  ( -0.8320502943378437211, 0.5547001962252290364, 0.000000000000000000 ) ) ;
#1612=CARTESIAN_POINT ( 'NONE',  ( 4.559911319644449179, 47.23035201082150536, -9.422509992056141925 ) ) ;
#1616=CARTESIAN_POINT ( 'NONE',  ( 1.042145700049407653, 14.74216108172003104, -6.499999999999879208 ) ) ;
#1617=CARTESIAN_POINT ( 'NONE',  ( 0.5774900079438590739, 57.64701867748817676, -5.440088680355550821 ) ) ;
#1618=CARTESIAN_POINT ( 'NONE',  ( 19.42250999205614548, 55.98035201082150536, -5.440088680355545492 ) ) ;
#1621=EDGE_CURVE ( 'NONE', #64078, #31259, #50151, .T. ) ;
#1623=CARTESIAN_POINT ( 'NONE',  ( 17.96484262340118221, 11.18868534415484106, -7.964842623401177768 ) ) ;
#1624=CARTESIAN_POINT ( 'NONE',  ( 0.1532563361054083140, 51.00893115100078745, 1.131784320476157264E-15 ) ) ;
#1625=CARTESIAN_POINT ( 'NONE',  ( 2.035157376598822676, 17.43868534415483751, -7.964842623401177768 ) ) ;
#1627=CARTESIAN_POINT ( 'NONE',  ( 22.81628187352648496, 31.83196800326375353, -3.434112377981050290 ) ) ;
#1629=CARTESIAN_POINT ( 'NONE',  ( 2.035157376598824452, 43.68868534415484106, 7.964842623401179544 ) ) ;
#1630=CARTESIAN_POINT ( 'NONE',  ( 13.43411237798105340, 0.5819680032637533085, 12.81628187352647963 ) ) ;
#1632=CARTESIAN_POINT ( 'NONE',  ( -0.8801773607111008646, 18.27201867748817321, 2.915334737309923430 ) ) ;
#1633=CARTESIAN_POINT ( 'NONE',  ( 10.00000000000000178, 44.31368534415484106, 10.88017736071110342 ) ) ;
#1634=CARTESIAN_POINT ( 'NONE',  ( 2.917880565312948704, 57.63708216824731068, 12.26659068614894643 ) ) ;
#1635=CARTESIAN_POINT ( 'NONE',  ( 12.63842701281683922, 29.55059781766745175, -9.846743663894590881 ) ) ;
#1636=CARTESIAN_POINT ( 'NONE',  ( 19.42250999205614193, 65.14701867748817676, 5.440088680355555262 ) ) ;
#1638=CARTESIAN_POINT ( 'NONE',  ( 24.16423886937410614, 19.51208216824729647, -3.795296366450302550 ) ) ;
#1642=CARTESIAN_POINT ( 'NONE',  ( 2.917880565312950480, 40.97041550158063217, -12.26659068614894821 ) ) ;
#1643=CARTESIAN_POINT ( 'NONE',  ( 13.79529636645031943, 30.34541550158063927, -14.16423886937409904 ) ) ;
#1644=CARTESIAN_POINT ( 'NONE',  ( 19.84674366389459621, 3.508931151000785231, 7.409399052514197653E-17 ) ) ;
#1645=CARTESIAN_POINT ( 'NONE',  ( 12.63842701281683034, 62.46726448433410894, 9.846743663894596210 ) ) ;
#1646=CARTESIAN_POINT ( 'NONE',  ( 0.000000000000000000, 69.50000000000000000, -6.000000000000000000 ) ) ;
#1647=CARTESIAN_POINT ( 'NONE',  ( 17.96484262340118221, 61.18868534415482685, -7.964842623401177768 ) ) ;
#1648=CARTESIAN_POINT ( 'NONE',  ( 19.38216949554541557, 37.24863466993041783, -9.382169495545420901 ) ) ;
#1649=CARTESIAN_POINT ( 'NONE',  ( 13.79529636645031943, 30.34541550158063927, -14.16423886937409904 ) ) ;
#1651=CARTESIAN_POINT ( 'NONE',  ( 4.559911319644449179, 28.89701867748817321, 9.422509992056141925 ) ) ;
#1652=CARTESIAN_POINT ( 'NONE',  ( 10.00000000000000178, 29.31368534415483751, 10.88017736071110342 ) ) ;
#1654=CARTESIAN_POINT ( 'NONE',  ( 1.472469842513823179, 0.5922644843341181575, -4.923371831947296329 ) ) ;
#1663=CARTESIAN_POINT ( 'NONE',  ( 24.16423886937409904, 4.095415501580634832, 3.795296366450317205 ) ) ;
#1664=CARTESIAN_POINT ( 'NONE',  ( 17.08211943468705130, 63.47041550158063927, 12.26659068614894998 ) ) ;
#1665=CARTESIAN_POINT ( 'NONE',  ( 20.88017736071110519, 15.56368534415483751, 2.639326808657452039E-16 ) ) ;
#1666=CARTESIAN_POINT ( 'NONE',  ( 0.1532563361054100626, 30.80059781766744820, -2.638427012816831230 ) ) ;
#1667=CARTESIAN_POINT ( 'NONE',  ( 17.20831665107776587, 54.13393115100079456, -7.208316651077762316 ) ) ;
#1669=CARTESIAN_POINT ( 'NONE',  ( -1.099225684535947600, -0.4596986634029132657, 6.408140936763237150 ) ) ;
#1671=CARTESIAN_POINT ( 'NONE',  ( -0.3689425029237898834, 51.17874883491397497, -10.36894250292378850 ) ) ;
#1673=CARTESIAN_POINT ( 'NONE',  ( 13.79529636645030344, 43.26208216824730357, 14.16423886937410614 ) ) ;
#1674=ORIENTED_EDGE ( 'NONE', *, *, #63110, .F. ) ;
#1675=CARTESIAN_POINT ( 'NONE',  ( 20.88017736071110164, 25.35535201082150891, 2.915334737309930979 ) ) ;
#1677=CARTESIAN_POINT ( 'NONE',  ( 12.91533473730992121, 44.52201867748816966, 10.88017736071110164 ) ) ;
#1678=CARTESIAN_POINT ( 'NONE',  ( 2.791683348922237240, 45.38393115100079456, -7.208316651077763204 ) ) ;
#1679=CARTESIAN_POINT ( 'NONE',  ( 12.91533473730992121, 39.52201867748817676, 10.88017736071110164 ) ) ;
#1681=CARTESIAN_POINT ( 'NONE',  ( 17.96484262340118221, 61.18868534415482685, -7.964842623401177768 ) ) ;
#1682=CARTESIAN_POINT ( 'NONE',  ( 0.5774900079438607392, 33.48035201082150536, 5.440088680355550821 ) ) ;
#1685=CARTESIAN_POINT ( 'NONE',  ( 1.472469842513823179, 6.425597817667451750, 4.923371831947296329 ) ) ;
#1688=CARTESIAN_POINT ( 'NONE',  ( 18.52753015748617571, 43.09226448433412315, 4.923371831947298993 ) ) ;
#1689=CARTESIAN_POINT ( 'NONE',  ( 18.29284471827482150, 10.40189080397285437, -6.499999999999984901 ) ) ;
#1693=CARTESIAN_POINT ( 'NONE',  ( 0.8952175423695086787, 53.52576239577083328, 5.990408912944362285 ) ) ;
#1694=CARTESIAN_POINT ( 'NONE',  ( 19.84674366389459266, 53.30059781766744464, 2.638427012816836559 ) ) ;
#1695=CARTESIAN_POINT ( 'NONE',  ( 13.79529636645030344, 53.26208216824730357, 14.16423886937410614 ) ) ;
#1696=CARTESIAN_POINT ( 'NONE',  ( 1.472469842513823179, 61.42559781766745175, 4.923371831947296329 ) ) ;
#1699=CARTESIAN_POINT ( 'NONE',  ( 14.92337183194729633, 22.67559781766745175, 8.527530157486181039 ) ) ;
#1700=CARTESIAN_POINT ( 'NONE',  ( 13.43411237798105340, 55.58196800326374643, 12.81628187352647963 ) ) ;
#1701=EDGE_CURVE ( 'NONE', #97107, #26202, #14406, .T. ) ;
#1702=CARTESIAN_POINT ( 'NONE',  ( 14.92337183194729988, 64.34226448433412315, -8.527530157486177487 ) ) ;
#1703=CARTESIAN_POINT ( 'NONE',  ( 20.88017736071110164, 55.35535201082149825, 2.915334737309930979 ) ) ;
#1706=CARTESIAN_POINT ( 'NONE',  ( 10.00000000000000178, 63.05374883491396076, 14.16423886937410082 ) ) ;
#1708=CARTESIAN_POINT ( 'NONE',  ( 2.035157376598822676, 32.43868534415483396, -7.964842623401177768 ) ) ;
#1709=VECTOR ( 'NONE', #83376, 1000.000000000000114 ) ;
#1710=CARTESIAN_POINT ( 'NONE',  ( 6.565887622018943937, 10.16530133659708746, 12.81628187352647430 ) ) ;
#1711=CARTESIAN_POINT ( 'NONE',  ( 10.00000000000000000, 61.81368534415484106, -10.88017736071110342 ) ) ;
#1712=CARTESIAN_POINT ( 'NONE',  ( 18.72515096720583827, 65.05509018479936856, 6.499999999999810818 ) ) ;
#1716=CARTESIAN_POINT ( 'NONE',  ( 2.035157376598824452, 53.68868534415484817, 7.964842623401179544 ) ) ;
#1718=CARTESIAN_POINT ( 'NONE',  ( 2.791683348922240793, 41.63393115100078745, 7.208316651077764092 ) ) ;
#1719=CARTESIAN_POINT ( 'NONE',  ( 19.84674366389459266, 3.717264484334118713, -2.638427012816827677 ) ) ;
#1721=CARTESIAN_POINT ( 'NONE',  ( 0.6178305044545838731, 14.74863466993041783, 9.382169495545420901 ) ) ;
#1724=CARTESIAN_POINT ( 'NONE',  ( -0.8801773607111008646, 18.27201867748817321, 2.915334737309923430 ) ) ;
#1725=CARTESIAN_POINT ( 'NONE',  ( 1.274849032794292736, 67.55509018479936856, -6.499999999999977796 ) ) ;
#1726=CARTESIAN_POINT ( 'NONE',  ( 6.204703633549690345, 40.76208216824731778, -14.16423886937410259 ) ) ;
#1727=CARTESIAN_POINT ( 'NONE',  ( -2.266590686148945544, 26.38708216824730357, -7.082119434687050408 ) ) ;
#1728=CARTESIAN_POINT ( 'NONE',  ( -0.3689425029237881626, 62.42874883491396787, 10.36894250292379027 ) ) ;
#1729=CARTESIAN_POINT ( 'NONE',  ( 12.63842701281683922, 29.55059781766745175, -9.846743663894590881 ) ) ;
#1730=CARTESIAN_POINT ( 'NONE',  ( 12.63842701281683922, 24.55059781766745175, -9.846743663894590881 ) ) ;
#1731=CARTESIAN_POINT ( 'NONE',  ( 15.44008868035555793, 16.39701867748817321, -9.422509992056140149 ) ) ;
#1734=CARTESIAN_POINT ( 'NONE',  ( 10.00000000000000178, 42.25893115100078745, 9.846743663894594434 ) ) ;
#1735=CARTESIAN_POINT ( 'NONE',  ( 20.88017736071110519, 30.56368534415484106, 2.639326808657452039E-16 ) ) ;
#1736=CARTESIAN_POINT ( 'NONE',  ( 10.00000000000000000, 59.75893115100078745, -9.846743663894594434 ) ) ;
#1737=CARTESIAN_POINT ( 'NONE',  ( 13.79529636645030344, 18.26208216824730002, 14.16423886937410614 ) ) ;
#1738=CARTESIAN_POINT ( 'NONE',  ( 1.959929470562282283, 61.50257860105349295, 5.767676674365853629 ) ) ;
#1741=CARTESIAN_POINT ( 'NONE',  ( 12.63842701281683922, 9.550597817667449974, -9.846743663894590881 ) ) ;
#1742=CARTESIAN_POINT ( 'NONE',  ( 16.40814093676323893, 45.79030133659708923, 11.09922568453595026 ) ) ;
#1743=CARTESIAN_POINT ( 'NONE',  ( 5.076628168052704559, 55.17559781766745175, -8.527530157486179263 ) ) ;
#1747=CARTESIAN_POINT ( 'NONE',  ( 17.96484262340118221, 6.188685344154837509, -7.964842623401177768 ) ) ;
#1748=CARTESIAN_POINT ( 'NONE',  ( 7.084665262690076126, 52.02201867748816255, -10.88017736071110164 ) ) ;
#1749=CARTESIAN_POINT ( 'NONE',  ( 22.26659068614895176, 4.720415501580633943, -7.082119434687042414 ) ) ;
#1750=CARTESIAN_POINT ( 'NONE',  ( 4.559911319644449179, 53.89701867748817676, 9.422509992056141925 ) ) ;
#1751=CARTESIAN_POINT ( 'NONE',  ( 19.84674366389459266, 38.30059781766745175, 2.638427012816836559 ) ) ;
#1752=CARTESIAN_POINT ( 'NONE',  ( -0.8801773607111009756, 23.06368534415484106, 1.068504757029289695E-15 ) ) ;
#1754=CARTESIAN_POINT ( 'NONE',  ( 1.472469842513823179, 65.59226448433412315, -4.923371831947296329 ) ) ;
#1762=CARTESIAN_POINT ( 'NONE',  ( 0.1532563361054100626, 40.80059781766745886, -2.638427012816831230 ) ) ;
#1763=CARTESIAN_POINT ( 'NONE',  ( 1.472469842513823179, 16.42559781766745175, 4.923371831947296329 ) ) ;
#1764=CARTESIAN_POINT ( 'NONE',  ( 0.6178305044545818747, 63.49863466993043204, -9.382169495545419124 ) ) ;
#1765=CARTESIAN_POINT ( 'NONE',  ( 15.44008868035555260, 24.73035201082150891, 9.422509992056143702 ) ) ;
#1766=CARTESIAN_POINT ( 'NONE',  ( 5.076628168052703671, 46.84226448433412315, 8.527530157486179263 ) ) ;
#1768=CARTESIAN_POINT ( 'NONE',  ( 2.917880565312948704, 37.63708216824731068, 12.26659068614894643 ) ) ;
#1769=CARTESIAN_POINT ( 'NONE',  ( 22.26659068614894466, 53.88708216824731068, 7.082119434687054849 ) ) ;
#1772=CARTESIAN_POINT ( 'NONE',  ( 10.00000000000000000, 46.81368534415484106, -10.88017736071110342 ) ) ;
#1774=CARTESIAN_POINT ( 'NONE',  ( 1.472469842513823179, 20.59226448433411960, -4.923371831947296329 ) ) ;
#1779=CARTESIAN_POINT ( 'NONE',  ( 7.361572987183170547, 7.050597817667451750, 9.846743663894590881 ) ) ;
#1781=CARTESIAN_POINT ( 'NONE',  ( 13.79529636645030344, 23.26208216824730002, 14.16423886937410614 ) ) ;
#1782=CARTESIAN_POINT ( 'NONE',  ( 1.472469842513823179, 26.42559781766745175, 4.923371831947296329 ) ) ;
#1783=CARTESIAN_POINT ( 'NONE',  ( 19.42250999205614548, 45.98035201082150536, -5.440088680355545492 ) ) ;
#1786=STYLED_ITEM ( 'NONE', ( #71662 ), #61780 ) ;
#1787=CARTESIAN_POINT ( 'NONE',  ( -0.8801773607110991993, 42.85535201082150536, -2.915334737309923874 ) ) ;
#1791=CARTESIAN_POINT ( 'NONE',  ( 15.44008868035555793, 46.39701867748817676, -9.422509992056140149 ) ) ;
#1793=CARTESIAN_POINT ( 'NONE',  ( 10.00000000000000000, 10.55374883491396787, -14.16423886937410082 ) ) ;
#1794=MECHANICAL_DESIGN_GEOMETRIC_PRESENTATION_REPRESENTATION('',(#87976),#62411);
#1795=VERTEX_POINT ( 'NONE', #12892 ) ;
#1796=CARTESIAN_POINT ( 'NONE',  ( -1.099225684535947600, 28.70696800326375353, -6.408140936763238038 ) ) ;
#1797=CARTESIAN_POINT ( 'NONE',  ( 10.00000000000000000, 4.758931151000784787, -9.846743663894594434 ) ) ;
#1798=CARTESIAN_POINT ( 'NONE',  ( 19.42250999205614548, 5.980352010821504471, -5.440088680355545492 ) ) ;
#1800=CARTESIAN_POINT ( 'NONE',  ( 14.92337183194729988, 14.34226448433411782, -8.527530157486177487 ) ) ;
#1801=CARTESIAN_POINT ( 'NONE',  ( 20.88017736071110164, 50.35535201082151247, 2.915334737309930979 ) ) ;
#1803=CARTESIAN_POINT ( 'NONE',  ( 10.00000000000000000, 62.87363466993042493, -12.81628187352647608 ) ) ;
#1804=CARTESIAN_POINT ( 'NONE',  ( 19.42250999205614193, 55.14701867748817676, 5.440088680355555262 ) ) ;
#1807=CARTESIAN_POINT ( 'NONE',  ( 10.00000000000000178, 59.31368534415484106, 10.88017736071110342 ) ) ;
#1808=CARTESIAN_POINT ( 'NONE',  ( 0.6178305044545818747, 8.498634669930421381, -9.382169495545419124 ) ) ;
#1809=DIRECTION ( 'NONE',  ( 0.000000000000000000, -1.000000000000000000, 0.000000000000000000 ) ) ;
#1811=CARTESIAN_POINT ( 'NONE',  ( 5.076628168052704559, 25.17559781766745175, -8.527530157486179263 ) ) ;
#1812=CARTESIAN_POINT ( 'NONE',  ( 18.72515096720568906, 36.07228050351032778, -6.500000000000007105 ) ) ;
#1813=CARTESIAN_POINT ( 'NONE',  ( 6.204703633549690345, 5.762082168247301794, -14.16423886937410259 ) ) ;
#1814=CARTESIAN_POINT ( 'NONE',  ( 2.791683348922240793, 16.63393115100078745, 7.208316651077764092 ) ) ;
#1815=CARTESIAN_POINT ( 'NONE',  ( 19.38216949554541202, 20.99863466993042138, 9.382169495545424454 ) ) ;
#1816=CARTESIAN_POINT ( 'NONE',  ( 10.00000000000000178, 70.00000000000000000, 0.000000000000000000 ) ) ;
#1817=CARTESIAN_POINT ( 'NONE',  ( 20.88017736071110519, 55.56368534415484817, 2.639326808657452039E-16 ) ) ;
#1818=CARTESIAN_POINT ( 'NONE',  ( 5.076628168052704559, 65.17559781766745175, -8.527530157486179263 ) ) ;
#1823=CARTESIAN_POINT ( 'NONE',  ( 10.00000000000000000, 34.75893115100078745, -9.846743663894594434 ) ) ;
#1824=CARTESIAN_POINT ( 'NONE',  ( 19.84674366389459266, 28.30059781766745886, 2.638427012816836559 ) ) ;
#1825=CARTESIAN_POINT ( 'NONE',  ( 12.91533473730992121, 14.52201867748817143, 10.88017736071110164 ) ) ;
#1826=CARTESIAN_POINT ( 'NONE',  ( 16.40814093676323893, 15.79030133659708746, 11.09922568453595026 ) ) ;
#1827=CARTESIAN_POINT ( 'NONE',  ( 18.52753015748618282, 18.92559781766745175, -4.923371831947291888 ) ) ;
#1828=SHAPE_REPRESENTATION_RELATIONSHIP ( 'NONE' , 'NONE' ,  #19841, #54890 ) ;
#1831=CARTESIAN_POINT ( 'NONE',  ( 19.42250999205614548, 20.98035201082150891, -5.440088680355545492 ) ) ;
#1833=CARTESIAN_POINT ( 'NONE',  ( 0.1532563361054083140, 46.00893115100079456, 1.131784320476157264E-15 ) ) ;
#1834=CARTESIAN_POINT ( 'NONE',  ( 20.88017736071110875, 15.77201867748817143, -2.915334737309920765 ) ) ;
#1835=CARTESIAN_POINT ( 'NONE',  ( 20.88017736071110875, 40.77201867748818387, -2.915334737309920765 ) ) ;
#1836=CARTESIAN_POINT ( 'NONE',  ( 0.5774900079438607392, 13.48035201082150358, 5.440088680355550821 ) ) ;
#1837=CARTESIAN_POINT ( 'NONE',  ( -0.2418659066527494572, 19.26028685723174405, -6.114288769123083611 ) ) ;
#1838=CARTESIAN_POINT ( 'NONE',  ( 0.1532563361054100626, 20.80059781766744464, -2.638427012816831230 ) ) ;
#1839=CARTESIAN_POINT ( 'NONE',  ( 1.472469842513823179, 35.59226448433412315, -4.923371831947296329 ) ) ;
#1841=CARTESIAN_POINT ( 'NONE',  ( 19.72487221294571569, 30.71833443783938122, -6.499999999999989342 ) ) ;
#1842=CARTESIAN_POINT ( 'NONE',  ( 1.472469842513823179, 65.59226448433412315, -4.923371831947296329 ) ) ;
#1843=CARTESIAN_POINT ( 'NONE',  ( 10.00000000000000000, 0.5537488349139675359, -14.16423886937410082 ) ) ;
#1844=CARTESIAN_POINT ( 'NONE',  ( 13.79529636645031943, 30.34541550158063927, -14.16423886937409904 ) ) ;
#1846=CARTESIAN_POINT ( 'NONE',  ( 19.84674366389459266, 33.30059781766744464, 2.638427012816836559 ) ) ;
#1849=CARTESIAN_POINT ( 'NONE',  ( 10.00000000000000178, 58.05374883491397497, 14.16423886937410082 ) ) ;
#1850=CARTESIAN_POINT ( 'NONE',  ( 18.52753015748618282, 18.92559781766745175, -4.923371831947291888 ) ) ;
#1853=CARTESIAN_POINT ( 'NONE',  ( 20.88017736071110164, 45.35535201082149115, 2.915334737309930979 ) ) ;
#1856=CARTESIAN_POINT ( 'NONE',  ( 20.88017736071110519, 20.56368534415484106, 2.639326808657452039E-16 ) ) ;
#1857=VECTOR ( 'NONE', #90994, 1000.000000000000000 ) ;
#1858=CARTESIAN_POINT ( 'NONE',  ( 13.43411237798105340, 50.58196800326375353, 12.81628187352647963 ) ) ;
#1859=CARTESIAN_POINT ( 'NONE',  ( 19.38216949554541202, 15.99863466993042138, 9.382169495545424454 ) ) ;
#1860=CARTESIAN_POINT ( 'NONE',  ( 1.472469842513823179, 20.59226448433411960, -4.923371831947296329 ) ) ;
#1862=DIRECTION ( 'NONE',  ( -0.000000000000000000, -0.000000000000000000, -1.000000000000000000 ) ) ;
#1864=CARTESIAN_POINT ( 'NONE',  ( 13.79529636645031943, 50.34541550158064638, -14.16423886937409904 ) ) ;
#1865=CARTESIAN_POINT ( 'NONE',  ( -2.266590686148945544, 21.38708216824730357, -7.082119434687050408 ) ) ;
#1866=CARTESIAN_POINT ( 'NONE',  ( 19.42250999205614193, 20.14701867748817321, 5.440088680355555262 ) ) ;
#1867=CARTESIAN_POINT ( 'NONE',  ( 12.91533473730993009, 31.60535201082150891, -10.88017736071109987 ) ) ;
#1870=CARTESIAN_POINT ( 'NONE',  ( 2.791683348922240793, 1.633931151000784565, 7.208316651077764092 ) ) ;
#1871=CARTESIAN_POINT ( 'NONE',  ( 1.274849032794231007, 33.57228050351031357, 6.499999999999895195 ) ) ;
#1872=CARTESIAN_POINT ( 'NONE',  ( 14.92337183194729988, 19.34226448433411960, -8.527530157486177487 ) ) ;
#1875=CARTESIAN_POINT ( 'NONE',  ( 19.84674366389459621, 18.50893115100078745, 7.409399052514197653E-17 ) ) ;
#1876=CARTESIAN_POINT ( 'NONE',  ( 7.361572987183169658, 34.96726448433411605, -9.846743663894592657 ) ) ;
#1877=CARTESIAN_POINT ( 'NONE',  ( 2.035157376598824452, 8.688685344154839285, 7.964842623401179544 ) ) ;
#1878=B_SPLINE_CURVE_WITH_KNOTS ( 'NONE', 3,
 ( #8995, #40988, #86487, #77985, #32481, #31974 ),
 .UNSPECIFIED., .F., .F.,
 ( 4, 2, 4 ),
 ( 0.000000000000000000, 0.0002626113303184896258, 0.0005252226606369792515 ),
 .UNSPECIFIED. ) ;
#1879=CARTESIAN_POINT ( 'NONE',  ( 6.565887622018943937, 30.16530133659708568, 12.81628187352647430 ) ) ;
#1880=CARTESIAN_POINT ( 'NONE',  ( 10.00000000000000178, 59.31368534415484106, 10.88017736071110342 ) ) ;
#1881=CARTESIAN_POINT ( 'NONE',  ( -0.3689425029237881626, 52.42874883491396076, 10.36894250292379027 ) ) ;
#1882=CARTESIAN_POINT ( 'NONE',  ( 7.361572987183169658, 9.967264484334119601, -9.846743663894592657 ) ) ;
#1885=CARTESIAN_POINT ( 'NONE',  ( 5.076628168052704559, 50.17559781766745886, -8.527530157486179263 ) ) ;
#1886=CARTESIAN_POINT ( 'NONE',  ( 12.63842701281683034, 37.46726448433411605, 9.846743663894596210 ) ) ;
#1887=CARTESIAN_POINT ( 'NONE',  ( 24.16423886937410614, 14.51208216824730179, -3.795296366450302550 ) ) ;
#1888=CARTESIAN_POINT ( 'NONE',  ( 20.36894250292379382, 13.67874883491396965, 10.36894250292379205 ) ) ;
#1889=CARTESIAN_POINT ( 'NONE',  ( 7.084665262690076126, 44.10535201082151247, 10.88017736071109987 ) ) ;
#1890=CARTESIAN_POINT ( 'NONE',  ( 20.88017736071110519, 15.56368534415483751, 2.639326808657452039E-16 ) ) ;
#1892=CARTESIAN_POINT ( 'NONE',  ( 17.96484262340118221, 46.18868534415484106, -7.964842623401177768 ) ) ;
#1893=CARTESIAN_POINT ( 'NONE',  ( 12.91533473730993009, 26.60535201082150536, -10.88017736071109987 ) ) ;
#1895=CARTESIAN_POINT ( 'NONE',  ( 13.43411237798105340, 35.58196800326375353, 12.81628187352647963 ) ) ;
#1896=CARTESIAN_POINT ( 'NONE',  ( 20.88017736071110875, 40.77201867748818387, -2.915334737309920765 ) ) ;
#1898=VERTEX_POINT ( 'NONE', #63551 ) ;
#1899=CARTESIAN_POINT ( 'NONE',  ( -2.816281873526473856, 64.33196800326376774, 3.434112377981055619 ) ) ;
#1900=CARTESIAN_POINT ( 'NONE',  ( 12.91533473730992121, 54.52201867748816255, 10.88017736071110164 ) ) ;
#1902=CARTESIAN_POINT ( 'NONE',  ( 17.96484262340118221, 54.93868534415484106, 7.964842623401181321 ) ) ;
#1903=( NAMED_UNIT ( * ) SI_UNIT ( $, .STERADIAN. ) SOLID_ANGLE_UNIT ( ) );
#1904=CARTESIAN_POINT ( 'NONE',  ( 19.84674366389459266, 8.300597817667453526, 2.638427012816836559 ) ) ;
#1906=CARTESIAN_POINT ( 'NONE',  ( 20.36894250292379382, 58.67874883491396076, 10.36894250292379205 ) ) ;
#1907=CARTESIAN_POINT ( 'NONE',  ( 19.42250999205614193, 60.14701867748817676, 5.440088680355555262 ) ) ;
#1908=CARTESIAN_POINT ( 'NONE',  ( 0.1532563361054100626, 10.80059781766745175, -2.638427012816831230 ) ) ;
#1909=CARTESIAN_POINT ( 'NONE',  ( 15.44008868035555793, 16.39701867748817321, -9.422509992056140149 ) ) ;
#1910=CARTESIAN_POINT ( 'NONE',  ( 19.84674366389459621, 48.50893115100078745, 7.409399052514197653E-17 ) ) ;
#1911=VERTEX_POINT ( 'NONE', #18561 ) ;
#1912=CARTESIAN_POINT ( 'NONE',  ( 18.52753015748618282, 43.92559781766745175, -4.923371831947291888 ) ) ;
#1913=CARTESIAN_POINT ( 'NONE',  ( 17.96484262340118221, 41.18868534415484106, -7.964842623401177768 ) ) ;
#1914=CARTESIAN_POINT ( 'NONE',  ( 14.92337183194729633, 52.67559781766745175, 8.527530157486181039 ) ) ;
#1915=CARTESIAN_POINT ( 'NONE',  ( 13.43411237798106583, 27.66530133659708568, -12.81628187352647252 ) ) ;
#1916=SURFACE_SIDE_STYLE ('',( #70397 ) ) ;
#1917=CARTESIAN_POINT ( 'NONE',  ( 17.96484262340118221, 64.93868534415483396, 7.964842623401181321 ) ) ;
#1918=CARTESIAN_POINT ( 'NONE',  ( 20.88017736071110164, 50.35535201082151247, 2.915334737309930979 ) ) ;
#1919=CARTESIAN_POINT ( 'NONE',  ( 17.08211943468705840, 55.13708216824731068, -12.26659068614894466 ) ) ;
#1920=COLOUR_RGB ( '', 0.72549020, 0.75294118, 0.79215686) ;
#1921=MECHANICAL_DESIGN_GEOMETRIC_PRESENTATION_REPRESENTATION('',(#25810),#22686);
#1922=CARTESIAN_POINT ( 'NONE',  ( 10.00000000000000000, 27.87363466993042138, -12.81628187352647608 ) ) ;
#1925=CARTESIAN_POINT ( 'NONE',  ( 13.43411237798106583, 32.66530133659708213, -12.81628187352647252 ) ) ;
#1926=CARTESIAN_POINT ( 'NONE',  ( 2.035157376598822676, 27.43868534415483396, -7.964842623401177768 ) ) ;
#1928=ORIENTED_EDGE ( 'NONE', *, *, #82443, .T. ) ;
#1929=CARTESIAN_POINT ( 'NONE',  ( 12.91533473730993009, 66.60535201082150536, -10.88017736071109987 ) ) ;
#1930=COLOUR_RGB ( '', 0.31764706, 0.68627451, 0.89019608) ;
#1931=CARTESIAN_POINT ( 'NONE',  ( 10.00000000000000000, 44.75893115100078745, -9.846743663894594434 ) ) ;
#1932=CARTESIAN_POINT ( 'NONE',  ( 14.92337183194729988, 9.342264484334119601, -8.527530157486177487 ) ) ;
#1933=CARTESIAN_POINT ( 'NONE',  ( 0.1532563361054100626, 35.80059781766745175, -2.638427012816831230 ) ) ;
#1937=LINE ( 'NONE', #47399, #8515 ) ;
#1938=EDGE_CURVE ( 'NONE', #89108, #507, #93384, .T. ) ;
#1939=CARTESIAN_POINT ( 'NONE',  ( 14.92337183194729633, 27.67559781766745530, 8.527530157486181039 ) ) ;
#1941=CARTESIAN_POINT ( 'NONE',  ( 1.472469842513823179, 45.59226448433412315, -4.923371831947296329 ) ) ;
#1942=EDGE_LOOP ( 'NONE', ( #82166, #11641, #33187, #89350, #49488, #32510 ) ) ;
#1944=CARTESIAN_POINT ( 'NONE',  ( 22.81628187352648496, 26.83196800326374998, -3.434112377981050290 ) ) ;
#1946=CARTESIAN_POINT ( 'NONE',  ( 2.917880565312950480, 50.97041550158064638, -12.26659068614894821 ) ) ;
#1947=CARTESIAN_POINT ( 'NONE',  ( 7.361572987183169658, 24.96726448433412315, -9.846743663894592657 ) ) ;
#1949=CARTESIAN_POINT ( 'NONE',  ( 20.36894250292379382, 38.67874883491396076, 10.36894250292379205 ) ) ;
#1950=CARTESIAN_POINT ( 'NONE',  ( 2.791683348922237240, 65.38393115100078035, -7.208316651077763204 ) ) ;
#1951=CARTESIAN_POINT ( 'NONE',  ( 10.00000000000000000, 55.55374883491396787, -14.16423886937410082 ) ) ;
#1952=CARTESIAN_POINT ( 'NONE',  ( 2.917880565312948704, 27.63708216824730357, 12.26659068614894643 ) ) ;
#1953=CARTESIAN_POINT ( 'NONE',  ( -2.266590686148945544, 36.38708216824730357, -7.082119434687050408 ) ) ;
#1954=CARTESIAN_POINT ( 'NONE',  ( -45.72064753280899652, 104.7206091210568957, -5.189487810365704057 ) ) ;
#1957=CARTESIAN_POINT ( 'NONE',  ( 7.361572987183170547, 62.05059781766745886, 9.846743663894590881 ) ) ;
#1958=CARTESIAN_POINT ( 'NONE',  ( -0.8801773607110991993, 42.85535201082150536, -2.915334737309923874 ) ) ;
#1959=CARTESIAN_POINT ( 'NONE',  ( 0.2751277870542909176, 64.36607318730132477, -6.499999999999992006 ) ) ;
#1960=CARTESIAN_POINT ( 'NONE',  ( 10.00000000000000000, 34.75893115100078745, -9.846743663894594434 ) ) ;
#1961=CARTESIAN_POINT ( 'NONE',  ( 19.38216949554541557, 57.24863466993042493, -9.382169495545420901 ) ) ;
#1963=CARTESIAN_POINT ( 'NONE',  ( 19.84674366389459266, 48.71726448433413026, -2.638427012816827677 ) ) ;
#1968=CARTESIAN_POINT ( 'NONE',  ( -0.3689425029237881626, 17.42874883491397142, 10.36894250292379027 ) ) ;
#1972=CARTESIAN_POINT ( 'NONE',  ( 12.91533473730993009, 11.60535201082150714, -10.88017736071109987 ) ) ;
#1973=CARTESIAN_POINT ( 'NONE',  ( 22.81628187352647785, 11.41530133659708390, 3.434112377981063169 ) ) ;
#1975=CARTESIAN_POINT ( 'NONE',  ( 0.1957200283969096621, 55.25733960839544068, 6.499999999999992006 ) ) ;
#1976=CARTESIAN_POINT ( 'NONE',  ( 7.084665262690076126, 69.10535201082151957, 10.88017736071109987 ) ) ;
#1977=CARTESIAN_POINT ( 'NONE',  ( 20.15039907845753220, 26.74884699246889141, 6.262539305110078836 ) ) ;
#1980=CARTESIAN_POINT ( 'NONE',  ( 24.16423886937409904, 59.09541550158063217, 3.795296366450317205 ) ) ;
#1981=CARTESIAN_POINT ( 'NONE',  ( 17.39651004071838969, 44.08210964143329846, -6.500000000000027534 ) ) ;
#1983=CARTESIAN_POINT ( 'NONE',  ( 7.084665262690076126, 24.10535201082150181, 10.88017736071109987 ) ) ;
#1984=CARTESIAN_POINT ( 'NONE',  ( 7.084665262690076126, 39.10535201082150536, 10.88017736071109987 ) ) ;
#1985=CARTESIAN_POINT ( 'NONE',  ( -1.099225684535947600, 3.706968003263753531, -6.408140936763238038 ) ) ;
#1986=CARTESIAN_POINT ( 'NONE',  ( 10.00000000000000178, 52.25893115100078745, 9.846743663894594434 ) ) ;
#1987=CARTESIAN_POINT ( 'NONE',  ( 0.6178305044545838731, 59.74863466993041783, 9.382169495545420901 ) ) ;
#1988=ORIENTED_EDGE ( 'NONE', *, *, #46418, .F. ) ;
#1990=CARTESIAN_POINT ( 'NONE',  ( 20.88017736071110875, 25.77201867748816966, -2.915334737309920765 ) ) ;
#1991=CARTESIAN_POINT ( 'NONE',  ( 13.43411237798105340, 35.58196800326375353, 12.81628187352647963 ) ) ;
#1992=CARTESIAN_POINT ( 'NONE',  ( -1.319618665598680717E-31, 72.38931350946023713, 5.123507015312970481 ) ) ;
#1994=CARTESIAN_POINT ( 'NONE',  ( 1.472469842513823179, 66.42559781766745175, 4.923371831947296329 ) ) ;
#1995=CARTESIAN_POINT ( 'NONE',  ( 0.5774900079438607392, 48.48035201082150536, 5.440088680355550821 ) ) ;
#1996=CARTESIAN_POINT ( 'NONE',  ( 7.361572987183170547, 12.05059781766744997, 9.846743663894590881 ) ) ;
#1997=CARTESIAN_POINT ( 'NONE',  ( 0.6178305044545818747, 33.49863466993042493, -9.382169495545419124 ) ) ;
#1999=CARTESIAN_POINT ( 'NONE',  ( 4.559911319644449179, 57.23035201082150536, -9.422509992056141925 ) ) ;
#2001=PRESENTATION_STYLE_ASSIGNMENT (( #23520 ) ) ;
#2002=CARTESIAN_POINT ( 'NONE',  ( -2.816281873526473856, 59.33196800326374643, 3.434112377981055619 ) ) ;
#2005=CARTESIAN_POINT ( 'NONE',  ( 1.602071938427501063, 17.02224192338641373, -6.499999999999984901 ) ) ;
#2006=CARTESIAN_POINT ( 'NONE',  ( 7.084665262690076126, 7.022018677488169658, -10.88017736071110164 ) ) ;
#2007=CARTESIAN_POINT ( 'NONE',  ( 10.00000000000000000, 42.87363466993042493, -12.81628187352647608 ) ) ;
#2008=CARTESIAN_POINT ( 'NONE',  ( -4.164238869374099039, 16.80374883491396787, 8.674139862899312516E-16 ) ) ;
#2009=CARTESIAN_POINT ( 'NONE',  ( 0.1532563361054082862, 16.21726448433411960, 2.638427012816831674 ) ) ;
#2010=CARTESIAN_POINT ( 'NONE',  ( 12.91533473730992121, 4.522018677488169658, 10.88017736071110164 ) ) ;
#2011=CARTESIAN_POINT ( 'NONE',  ( 17.20831665107776587, 22.88393115100078745, 7.208316651077764980 ) ) ;
#2012=CARTESIAN_POINT ( 'NONE',  ( 10.00000000000000178, 53.05374883491396787, 14.16423886937410082 ) ) ;
#2017=CARTESIAN_POINT ( 'NONE',  ( 4.559911319644449179, 22.23035201082150536, -9.422509992056141925 ) ) ;
#2018=CARTESIAN_POINT ( 'NONE',  ( 1.492507162822237499, 32.19955587570479594, -6.499999999999986677 ) ) ;
#2022=CARTESIAN_POINT ( 'NONE',  ( 0.5774900079438590739, 17.64701867748817321, -5.440088680355550821 ) ) ;
#2023=CARTESIAN_POINT ( 'NONE',  ( 19.42250999205614193, 15.14701867748817143, 5.440088680355555262 ) ) ;
#2024=CARTESIAN_POINT ( 'NONE',  ( 1.472469842513823179, 51.42559781766745886, 4.923371831947296329 ) ) ;
#2025=CARTESIAN_POINT ( 'NONE',  ( -2.816281873526473856, 54.33196800326376064, 3.434112377981055619 ) ) ;
#2026=CARTESIAN_POINT ( 'NONE',  ( 20.10493008474205823, 64.71697413083879269, 6.336235997365761818 ) ) ;
#2028=CARTESIAN_POINT ( 'NONE',  ( 22.26659068614894466, 13.88708216824730179, 7.082119434687054849 ) ) ;
#2029=CARTESIAN_POINT ( 'NONE',  ( 4.559911319644449179, 22.23035201082150536, -9.422509992056141925 ) ) ;
#2030=CARTESIAN_POINT ( 'NONE',  ( 12.91533473730992121, 4.522018677488170546, 10.88017736071110164 ) ) ;
#2031=CARTESIAN_POINT ( 'NONE',  ( 5.076628168052703671, 56.84226448433412315, 8.527530157486179263 ) ) ;
#2033=CARTESIAN_POINT ( 'NONE',  ( 17.20831665107776587, 37.88393115100078745, 7.208316651077764980 ) ) ;
#2035=CARTESIAN_POINT ( 'NONE',  ( 19.84674366389459621, 3.508931151000785231, 7.409399052514197653E-17 ) ) ;
#2038=CARTESIAN_POINT ( 'NONE',  ( 17.96484262340118221, 6.188685344154836621, -7.964842623401177768 ) ) ;
#2039=CARTESIAN_POINT ( 'NONE',  ( 10.00000000000000178, 2.258931151000784787, 9.846743663894594434 ) ) ;
#2040=CARTESIAN_POINT ( 'NONE',  ( 3.591859063236763294, 3.290301336597087012, -11.09922568453595026 ) ) ;
#2041=CARTESIAN_POINT ( 'NONE',  ( 19.42250999205614193, 40.14701867748817676, 5.440088680355555262 ) ) ;
#2042=CARTESIAN_POINT ( 'NONE',  ( 7.084665262690076126, 47.02201867748818387, -10.88017736071110164 ) ) ;
#2043=CARTESIAN_POINT ( 'NONE',  ( -0.8801773607110991993, 12.85535201082150358, -2.915334737309923874 ) ) ;
#2044=CARTESIAN_POINT ( 'NONE',  ( 3.591859063236761518, 44.95696800326376064, 11.09922568453594849 ) ) ;
#2045=CARTESIAN_POINT ( 'NONE',  ( 24.16423886937409904, 19.09541550158063927, 3.795296366450317205 ) ) ;
#2047=CARTESIAN_POINT ( 'NONE',  ( 22.81628187352647785, 46.41530133659708213, 3.434112377981063169 ) ) ;
#2049=CARTESIAN_POINT ( 'NONE',  ( 0.1532563361054100626, 55.80059781766745175, -2.638427012816831230 ) ) ;
#2050=CARTESIAN_POINT ( 'NONE',  ( 19.42250999205614548, 20.98035201082150891, -5.440088680355545492 ) ) ;
#2051=CARTESIAN_POINT ( 'NONE',  ( 17.96484262340118221, 26.18868534415483396, -7.964842623401177768 ) ) ;
#2053=CARTESIAN_POINT ( 'NONE',  ( -0.8801773607111008646, 68.27201867748817676, 2.915334737309923430 ) ) ;
#2054=( NAMED_UNIT ( * ) PLANE_ANGLE_UNIT ( ) SI_UNIT ( $, .RADIAN. ) );
#2055=CARTESIAN_POINT ( 'NONE',  ( 20.15039907845753930, 70.00000000000000000, 6.262539305110068177 ) ) ;
#2056=CARTESIAN_POINT ( 'NONE',  ( 2.791683348922237240, 10.38393115100078390, -7.208316651077763204 ) ) ;
#2057=CARTESIAN_POINT ( 'NONE',  ( 2.791683348922237240, 0.3839311510007847872, -7.208316651077763204 ) ) ;
#2059=CARTESIAN_POINT ( 'NONE',  ( 10.00000000000000178, 54.31368534415484106, 10.88017736071110342 ) ) ;
#2061=CARTESIAN_POINT ( 'NONE',  ( 7.084665262690076126, 69.10535201082151957, 10.88017736071109987 ) ) ;
#2062=CARTESIAN_POINT ( 'NONE',  ( 7.361572987183170547, 7.050597817667451750, 9.846743663894590881 ) ) ;
#2064=ORIENTED_EDGE ( 'NONE', *, *, #89439, .F. ) ;
#2066=CARTESIAN_POINT ( 'NONE',  ( 2.791683348922240793, 61.63393115100079456, 7.208316651077764092 ) ) ;
#2070=CARTESIAN_POINT ( 'NONE',  ( 10.00000000000000000, 10.55374883491396787, -14.16423886937410082 ) ) ;
#2072=CARTESIAN_POINT ( 'NONE',  ( 13.43411237798106583, 57.66530133659708923, -12.81628187352647252 ) ) ;
#2073=( GEOMETRIC_REPRESENTATION_CONTEXT ( 3 ) GLOBAL_UNCERTAINTY_ASSIGNED_CONTEXT ( ( #64491 ) ) GLOBAL_UNIT_ASSIGNED_CONTEXT ( ( #85888, #78872, #74305 ) ) REPRESENTATION_CONTEXT ( 'NONE', 'WORKASPACE' ) );
#2074=CARTESIAN_POINT ( 'NONE',  ( 20.36894250292379382, 3.678748834913967869, 10.36894250292379205 ) ) ;
#2075=CARTESIAN_POINT ( 'NONE',  ( 17.08211943468705840, 20.13708216824730357, -12.26659068614894466 ) ) ;
#2076=CARTESIAN_POINT ( 'NONE',  ( 19.72487221294570858, 56.86607318730075633, 6.500000000000000888 ) ) ;
#2078=CARTESIAN_POINT ( 'NONE',  ( -0.8801773607111009756, 23.06368534415484106, 1.068504757029289695E-15 ) ) ;
#2080=CARTESIAN_POINT ( 'NONE',  ( 0.1532563361054083140, 1.008931151000784787, 1.131784320476157264E-15 ) ) ;
#2082=CARTESIAN_POINT ( 'NONE',  ( 22.81628187352647785, 26.62363466993042138, 6.195893100308588602E-16 ) ) ;
#2083=CARTESIAN_POINT ( 'NONE',  ( 10.00000000000000000, 34.75893115100078745, -9.846743663894594434 ) ) ;
#2085=CARTESIAN_POINT ( 'NONE',  ( 10.00000000000000000, 12.87363466993042138, -12.81628187352647608 ) ) ;
#2087=CARTESIAN_POINT ( 'NONE',  ( 19.84674366389459621, 23.50893115100078390, 7.409399052514197653E-17 ) ) ;
#2088=CARTESIAN_POINT ( 'NONE',  ( 10.00000000000000178, 12.25893115100078568, 9.846743663894594434 ) ) ;
#2092=CARTESIAN_POINT ( 'NONE',  ( 0.5774900079438607392, 38.48035201082150536, 5.440088680355550821 ) ) ;
#2093=CARTESIAN_POINT ( 'NONE',  ( -4.164238869374099039, 26.80374883491397142, 8.674139862899312516E-16 ) ) ;
#2094=CARTESIAN_POINT ( 'NONE',  ( 7.361572987183169658, 34.96726448433411605, -9.846743663894592657 ) ) ;
#2095=CARTESIAN_POINT ( 'NONE',  ( 1.472469842513823179, 15.59226448433411960, -4.923371831947296329 ) ) ;
#2096=CARTESIAN_POINT ( 'NONE',  ( -1.099225684535947600, 53.70696800326376064, -6.408140936763238038 ) ) ;
#2098=CARTESIAN_POINT ( 'NONE',  ( 2.035157376598824452, 33.68868534415484106, 7.964842623401179544 ) ) ;
#2100=CARTESIAN_POINT ( 'NONE',  ( -0.1503990784575328643, 70.00000000000000000, 6.262539305110068177 ) ) ;
#2101=CARTESIAN_POINT ( 'NONE',  ( 16.40814093676323893, 20.79030133659708923, 11.09922568453595026 ) ) ;
#2102=CARTESIAN_POINT ( 'NONE',  ( 22.81628187352647785, 16.41530133659708923, 3.434112377981063169 ) ) ;
#2103=CARTESIAN_POINT ( 'NONE',  ( 12.63842701281683922, 34.55059781766745886, -9.846743663894590881 ) ) ;
#2105=CARTESIAN_POINT ( 'NONE',  ( 10.00000000000000178, 45.37363466993041783, 12.81628187352647608 ) ) ;
#2106=FILL_AREA_STYLE ('',( #17588 ) ) ;
#2107=CARTESIAN_POINT ( 'NONE',  ( 10.00000000000000000, 56.81368534415484106, -10.88017736071110342 ) ) ;
#2111=CARTESIAN_POINT ( 'NONE',  ( 15.44008868035555793, 51.39701867748816966, -9.422509992056140149 ) ) ;
#2113=CARTESIAN_POINT ( 'NONE',  ( 20.88017736071110875, 55.77201867748816966, -2.915334737309920765 ) ) ;
#2116=CARTESIAN_POINT ( 'NONE',  ( 7.084665262690076126, 14.10535201082150358, 10.88017736071109987 ) ) ;
#2117=CARTESIAN_POINT ( 'NONE',  ( 5.076628168052704559, 60.17559781766745175, -8.527530157486179263 ) ) ;
#2118=CARTESIAN_POINT ( 'NONE',  ( 4.559911319644449179, 18.89701867748817321, 9.422509992056141925 ) ) ;
#2121=CARTESIAN_POINT ( 'NONE',  ( 22.81628187352648496, 21.83196800326374643, -3.434112377981050290 ) ) ;
#2123=CARTESIAN_POINT ( 'NONE',  ( 17.96484262340118221, 54.93868534415484106, 7.964842623401181321 ) ) ;
#2124=CARTESIAN_POINT ( 'NONE',  ( 5.076628168052704559, 40.17559781766745175, -8.527530157486179263 ) ) ;
#2125=CARTESIAN_POINT ( 'NONE',  ( 22.81628187352648496, 1.831968003263753753, -3.434112377981050290 ) ) ;
#2126=CARTESIAN_POINT ( 'NONE',  ( 19.80427997160309062, 47.75733960839543357, -6.499999999999980460 ) ) ;
#2127=CARTESIAN_POINT ( 'NONE',  ( 19.42250999205614548, 15.98035201082150714, -5.440088680355545492 ) ) ;
#2128=CARTESIAN_POINT ( 'NONE',  ( 19.42250999205614548, 40.98035201082150536, -5.440088680355545492 ) ) ;
#2129=CARTESIAN_POINT ( 'NONE',  ( 17.08211943468705840, 55.13708216824731068, -12.26659068614894466 ) ) ;
#2130=CARTESIAN_POINT ( 'NONE',  ( 10.00000000000000178, 37.25893115100078745, 9.846743663894594434 ) ) ;
#2131=CARTESIAN_POINT ( 'NONE',  ( 15.44008868035555793, 56.39701867748817676, -9.422509992056140149 ) ) ;
#2132=DIRECTION ( 'NONE',  ( 0.000000000000000000, -1.000000000000000000, 0.000000000000000000 ) ) ;
#2133=CARTESIAN_POINT ( 'NONE',  ( -4.164238869374098151, 11.59541550158063217, -3.795296366450310543 ) ) ;
#2139=CARTESIAN_POINT ( 'NONE',  ( -2.266590686148945544, 31.38708216824730002, -7.082119434687050408 ) ) ;
#2140=CARTESIAN_POINT ( 'NONE',  ( -0.3689425029237881626, 37.42874883491396787, 10.36894250292379027 ) ) ;
#2141=CARTESIAN_POINT ( 'NONE',  ( 1.472469842513823179, 5.592264484334118713, -4.923371831947296329 ) ) ;
#2142=CARTESIAN_POINT ( 'NONE',  ( 5.076628168052703671, 66.84226448433412315, 8.527530157486179263 ) ) ;
#2143=CARTESIAN_POINT ( 'NONE',  ( 19.72487221294570858, 70.00000000000000000, -6.000000000000000000 ) ) ;
#2144=CARTESIAN_POINT ( 'NONE',  ( 0.5774900079438590739, 62.64701867748817676, -5.440088680355550821 ) ) ;
#2145=CARTESIAN_POINT ( 'NONE',  ( -2.816281873526471635, 38.91530133659708213, -3.434112377981056508 ) ) ;
#2146=CARTESIAN_POINT ( 'NONE',  ( 20.36894250292379382, 28.67874883491396787, 10.36894250292379205 ) ) ;
#2147=CARTESIAN_POINT ( 'NONE',  ( -0.8801773607111009756, 28.06368534415484106, 1.068504757029289695E-15 ) ) ;
#2150=CARTESIAN_POINT ( 'NONE',  ( 10.00000000000000178, 2.258931151000784787, 9.846743663894594434 ) ) ;
#2152=EDGE_CURVE ( 'NONE', #46415, #92145, #11040, .T. ) ;
#2154=CARTESIAN_POINT ( 'NONE',  ( 19.84674366389459266, 8.300597817667451750, 2.638427012816836559 ) ) ;
#2161=CARTESIAN_POINT ( 'NONE',  ( 10.00000000000000178, 68.05374883491397497, 14.16423886937410082 ) ) ;
#2162=CARTESIAN_POINT ( 'NONE',  ( 7.084665262690076126, 17.02201867748817676, -10.88017736071110164 ) ) ;
#2163=CARTESIAN_POINT ( 'NONE',  ( 14.92337183194729633, 42.67559781766745886, 8.527530157486181039 ) ) ;
#2164=CARTESIAN_POINT ( 'NONE',  ( -1.099225684535947600, 9.540301336597087456, 6.408140936763237150 ) ) ;
#2167=CARTESIAN_POINT ( 'NONE',  ( 22.81628187352647785, 1.415301336597087012, 3.434112377981063169 ) ) ;
#2169=CARTESIAN_POINT ( 'NONE',  ( 10.00000000000000000, 45.55374883491397497, -14.16423886937410082 ) ) ;
#2171=CARTESIAN_POINT ( 'NONE',  ( 13.79529636645030344, 58.26208216824728936, 14.16423886937410614 ) ) ;
#2173=CARTESIAN_POINT ( 'NONE',  ( 19.42250999205614548, 30.98035201082150536, -5.440088680355545492 ) ) ;
#2174=CARTESIAN_POINT ( 'NONE',  ( 12.91533473730993009, 41.60535201082149825, -10.88017736071109987 ) ) ;
#2175=CARTESIAN_POINT ( 'NONE',  ( 10.00000000000000000, 64.75893115100078035, -9.846743663894594434 ) ) ;
#2176=CARTESIAN_POINT ( 'NONE',  ( 0.5774900079438607392, 38.48035201082150536, 5.440088680355550821 ) ) ;
#2177=CARTESIAN_POINT ( 'NONE',  ( 10.00000000000000000, 61.81368534415484106, -10.88017736071110342 ) ) ;
#2178=CARTESIAN_POINT ( 'NONE',  ( -0.8801773607111009756, 23.06368534415484106, 1.068504757029289695E-15 ) ) ;
#2179=EDGE_CURVE ( 'NONE', #80524, #56195, #29858, .T. ) ;
#2181=CARTESIAN_POINT ( 'NONE',  ( 0.1532563361054082862, 16.21726448433411960, 2.638427012816831674 ) ) ;
#2185=CARTESIAN_POINT ( 'NONE',  ( 5.076628168052704559, 40.17559781766745175, -8.527530157486179263 ) ) ;
#2186=ADVANCED_FACE ( 'NONE', ( #16355 ), #98403, .T. ) ;
#2187=FACE_OUTER_BOUND ( 'NONE', #9592, .T. ) ;
#2190=CARTESIAN_POINT ( 'NONE',  ( 0.2751277870542913062, 49.36607318730131055, -6.499999999999992006 ) ) ;
#2191=CARTESIAN_POINT ( 'NONE',  ( 18.52753015748618282, 48.92559781766745886, -4.923371831947291888 ) ) ;
#2192=CARTESIAN_POINT ( 'NONE',  ( 17.08211943468705840, 45.13708216824730357, -12.26659068614894466 ) ) ;
#2193=CARTESIAN_POINT ( 'NONE',  ( 2.791683348922240793, 61.63393115100079456, 7.208316651077764092 ) ) ;
#2194=ORIENTED_EDGE ( 'NONE', *, *, #27099, .F. ) ;
#2196=CARTESIAN_POINT ( 'NONE',  ( 19.84674366389459621, 23.50893115100078390, 7.409399052514197653E-17 ) ) ;
#2197=EDGE_CURVE ( 'NONE', #39981, #14329, #74238, .T. ) ;
#2198=CARTESIAN_POINT ( 'NONE',  ( 6.565887622018943937, 50.16530133659708213, 12.81628187352647430 ) ) ;
#2199=CARTESIAN_POINT ( 'NONE',  ( 7.361572987183170547, 67.05059781766746596, 9.846743663894590881 ) ) ;
#2200=CARTESIAN_POINT ( 'NONE',  ( 7.084665262690076126, 69.10535201082151957, 10.88017736071109987 ) ) ;
#2204=CARTESIAN_POINT ( 'NONE',  ( 13.79529636645031943, 60.34541550158063927, -14.16423886937409904 ) ) ;
#2205=CARTESIAN_POINT ( 'NONE',  ( 4.559911319644449179, 38.89701867748817676, 9.422509992056141925 ) ) ;
#2206=CARTESIAN_POINT ( 'NONE',  ( -2.816281873526473856, 9.331968003263753531, 3.434112377981055619 ) ) ;
#2207=CARTESIAN_POINT ( 'NONE',  ( 19.42250999205614548, 55.98035201082150536, -5.440088680355545492 ) ) ;
#2213=CARTESIAN_POINT ( 'NONE',  ( 18.52753015748618282, 53.92559781766745175, -4.923371831947291888 ) ) ;
#2214=CARTESIAN_POINT ( 'NONE',  ( 18.52753015748617571, 3.092264484334118269, 4.923371831947298993 ) ) ;
#2216=CARTESIAN_POINT ( 'NONE',  ( 10.00000000000000000, 2.873634669930420049, -12.81628187352647608 ) ) ;
#2218=CARTESIAN_POINT ( 'NONE',  ( 12.91533473730992121, 9.522018677488171434, 10.88017736071110164 ) ) ;
#2220=CARTESIAN_POINT ( 'NONE',  ( 10.00000000000000000, 30.55374883491397142, -14.16423886937410082 ) ) ;
#2221=CARTESIAN_POINT ( 'NONE',  ( 6.204703633549690345, 32.84541550158063927, 14.16423886937410082 ) ) ;
#2222=CARTESIAN_POINT ( 'NONE',  ( 13.79529636645031943, 65.34541550158063217, -14.16423886937409904 ) ) ;
#2223=CARTESIAN_POINT ( 'NONE',  ( 1.472469842513823179, 20.59226448433411960, -4.923371831947296329 ) ) ;
#2224=CARTESIAN_POINT ( 'NONE',  ( 12.91533473730992121, 9.522018677488171434, 10.88017736071110164 ) ) ;
#2225=B_SPLINE_CURVE_WITH_KNOTS ( 'NONE', 3,
 ( #42817, #4825, #20312, #72310 ),
 .UNSPECIFIED., .F., .F.,
 ( 4, 4 ),
 ( 5.421010862427522170E-20, 0.0003153491572467390460 ),
 .UNSPECIFIED. ) ;
#2226=ORIENTED_EDGE ( 'NONE', *, *, #49530, .F. ) ;
#2227=CARTESIAN_POINT ( 'NONE',  ( 14.92337183194729633, 32.67559781766745175, 8.527530157486181039 ) ) ;
#2228=CARTESIAN_POINT ( 'NONE',  ( 12.91533473730992121, 34.52201867748817676, 10.88017736071110164 ) ) ;
#2229=CARTESIAN_POINT ( 'NONE',  ( 10.00000000000000178, 62.25893115100078745, 9.846743663894594434 ) ) ;
#2230=CARTESIAN_POINT ( 'NONE',  ( -4.164238869374098151, 21.59541550158063217, -3.795296366450310543 ) ) ;
#2231=CARTESIAN_POINT ( 'NONE',  ( -0.1503990784575407469, 17.22266099184918531, -6.262539305110056631 ) ) ;
#2233=UNCERTAINTY_MEASURE_WITH_UNIT (LENGTH_MEASURE( 1.000000000000000082E-05 ), #61801, 'distance_accuracy_value', 'NONE');
#2234=CARTESIAN_POINT ( 'NONE',  ( 0.1532563361054083140, 31.00893115100078390, 1.131784320476157264E-15 ) ) ;
#2235=CARTESIAN_POINT ( 'NONE',  ( 19.38216949554541557, 47.24863466993041783, -9.382169495545420901 ) ) ;
#2236=CARTESIAN_POINT ( 'NONE',  ( 19.84674366389459266, 53.30059781766744464, 2.638427012816836559 ) ) ;
#2239=FACE_OUTER_BOUND ( 'NONE', #44031, .T. ) ;
#2240=CARTESIAN_POINT ( 'NONE',  ( 2.917880565312950480, 60.97041550158063927, -12.26659068614894821 ) ) ;
#2241=CARTESIAN_POINT ( 'NONE',  ( 4.559911319644449179, 57.23035201082150536, -9.422509992056141925 ) ) ;
#2242=CARTESIAN_POINT ( 'NONE',  ( 6.204703633549690345, 10.76208216824729824, -14.16423886937410259 ) ) ;
#2243=CARTESIAN_POINT ( 'NONE',  ( 18.52753015748617571, 3.092264484334118269, 4.923371831947298993 ) ) ;
#2244=CARTESIAN_POINT ( 'NONE',  ( 0.1532563361054100626, 55.80059781766745175, -2.638427012816831230 ) ) ;
#2245=CARTESIAN_POINT ( 'NONE',  ( 20.88017736071110875, 20.77201867748816611, -2.915334737309920765 ) ) ;
#2246=CARTESIAN_POINT ( 'NONE',  ( 18.28836319691944112, 39.34492782695771496, 6.500000000000040856 ) ) ;
#2247=CARTESIAN_POINT ( 'NONE',  ( 19.84674366389459266, 63.30059781766745886, 2.638427012816836559 ) ) ;
#2251=DIRECTION ( 'NONE',  ( -0.000000000000000000, -0.000000000000000000, 1.000000000000000000 ) ) ;
#2252=ORIENTED_EDGE ( 'NONE', *, *, #16102, .F. ) ;
#2253=ORIENTED_EDGE ( 'NONE', *, *, #72228, .F. ) ;
#2254=LINE ( 'NONE', #32711, #64468 ) ;
#2257=CARTESIAN_POINT ( 'NONE',  ( 13.79529636645031943, 45.34541550158062506, -14.16423886937409904 ) ) ;
#2258=CARTESIAN_POINT ( 'NONE',  ( 14.92337183194729633, 62.67559781766745886, 8.527530157486181039 ) ) ;
#2259=CARTESIAN_POINT ( 'NONE',  ( 17.20831665107776587, 24.13393115100078035, -7.208316651077762316 ) ) ;
#2260=CARTESIAN_POINT ( 'NONE',  ( 17.39651004071838614, 52.93575266056826933, 6.500000000000032863 ) ) ;
#2261=CARTESIAN_POINT ( 'NONE',  ( -0.8801773607111009756, 13.06368534415483929, 1.068504757029289695E-15 ) ) ;
#2262=CARTESIAN_POINT ( 'NONE',  ( 10.00000000000000000, -2.126365330069579951, -12.81628187352647608 ) ) ;
#2263=CARTESIAN_POINT ( 'NONE',  ( -0.1503990784575242878, 34.24884699246889141, -6.262539305110083276 ) ) ;
#2264=CARTESIAN_POINT ( 'NONE',  ( 17.08211943468705840, 40.13708216824731068, -12.26659068614894466 ) ) ;
#2265=CARTESIAN_POINT ( 'NONE',  ( -4.164238869374099039, 61.80374883491397497, 8.674139862899312516E-16 ) ) ;
#2266=CARTESIAN_POINT ( 'NONE',  ( 6.000000000000000000, 11.50000000000000000, 6.500000000000000888 ) ) ;
#2267=CARTESIAN_POINT ( 'NONE',  ( 2.603489959281590771, 66.58210964143327715, 6.500000000000003553 ) ) ;
#2268=CARTESIAN_POINT ( 'NONE',  ( 2.035157376598824452, 68.68868534415484817, 7.964842623401179544 ) ) ;
#2269=CARTESIAN_POINT ( 'NONE',  ( 18.52753015748618282, 13.92559781766745175, -4.923371831947291888 ) ) ;
#2272=CARTESIAN_POINT ( 'NONE',  ( 20.15039907845753220, 29.72266099184918531, 6.262539305110077947 ) ) ;
#2273=ORIENTED_EDGE ( 'NONE', *, *, #21380, .F. ) ;
#2274=CARTESIAN_POINT ( 'NONE',  ( 10.00000000000000000, 24.75893115100078745, -9.846743663894594434 ) ) ;
#2276=CARTESIAN_POINT ( 'NONE',  ( 24.16423886937409904, 34.09541550158064638, 3.795296366450317205 ) ) ;
#2277=CARTESIAN_POINT ( 'NONE',  ( 7.361572987183169658, 39.96726448433411605, -9.846743663894592657 ) ) ;
#2278=CARTESIAN_POINT ( 'NONE',  ( 2.035157376598824452, 48.68868534415483396, 7.964842623401179544 ) ) ;
#2281=CARTESIAN_POINT ( 'NONE',  ( 7.084665262690076126, 42.02201867748816966, -10.88017736071110164 ) ) ;
#2286=CARTESIAN_POINT ( 'NONE',  ( 20.36894250292379738, 9.928748834913966093, -10.36894250292379027 ) ) ;
#2289=( LENGTH_UNIT ( ) NAMED_UNIT ( * ) SI_UNIT ( .MILLI., .METRE. ) );
#2290=CARTESIAN_POINT ( 'NONE',  ( 3.591859063236763294, 28.29030133659708568, -11.09922568453595026 ) ) ;
#2292=CARTESIAN_POINT ( 'NONE',  ( 10.00000000000000000, 19.75893115100078390, -9.846743663894594434 ) ) ;
#2293=CARTESIAN_POINT ( 'NONE',  ( 7.084665262690076126, 2.022018677488170990, -10.88017736071110164 ) ) ;
#2295=CARTESIAN_POINT ( 'NONE',  ( 14.92337183194729633, 27.67559781766745530, 8.527530157486181039 ) ) ;
#2299=CARTESIAN_POINT ( 'NONE',  ( 10.00000000000000000, 51.81368534415484106, -10.88017736071110342 ) ) ;
#2302=CARTESIAN_POINT ( 'NONE',  ( 3.591859063236763294, 63.29030133659708923, -11.09922568453595026 ) ) ;
#2303=CARTESIAN_POINT ( 'NONE',  ( 5.076628168052704559, 10.17559781766745175, -8.527530157486179263 ) ) ;
#2305=CARTESIAN_POINT ( 'NONE',  ( 22.81628187352647785, 11.41530133659708390, 3.434112377981063169 ) ) ;
#2306=CARTESIAN_POINT ( 'NONE',  ( 4.999999999999999112, 60.50000000000000711, 6.000000000000000000 ) ) ;
#2307=B_SPLINE_CURVE_WITH_KNOTS ( 'NONE', 3,
 ( #22595, #53072, #115, #77058 ),
 .UNSPECIFIED., .F., .F.,
 ( 4, 4 ),
 ( 2.168404344971008868E-18, 0.001060528352561995475 ),
 .UNSPECIFIED. ) ;
#2308=CARTESIAN_POINT ( 'NONE',  ( 0.1532563361054100626, 25.80059781766744820, -2.638427012816831230 ) ) ;
#2309=DIRECTION ( 'NONE',  ( 1.000000000000000000, -0.000000000000000000, 0.000000000000000000 ) ) ;
#2310=CARTESIAN_POINT ( 'NONE',  ( 6.204703633549690345, 7.845415501580634832, 14.16423886937410082 ) ) ;
#2311=CARTESIAN_POINT ( 'NONE',  ( 14.92337183194729633, 22.67559781766745175, 8.527530157486181039 ) ) ;
#2312=CARTESIAN_POINT ( 'NONE',  ( 3.591859063236763294, 33.29030133659708213, -11.09922568453595026 ) ) ;
#2315=CARTESIAN_POINT ( 'NONE',  ( -0.8801773607110991993, 52.85535201082151247, -2.915334737309923874 ) ) ;
#2316=CARTESIAN_POINT ( 'NONE',  ( 19.38216949554541202, 5.998634669930420493, 9.382169495545424454 ) ) ;
#2319=CARTESIAN_POINT ( 'NONE',  ( 2.791683348922237240, 30.38393115100078390, -7.208316651077763204 ) ) ;
#2320=CARTESIAN_POINT ( 'NONE',  ( 14.92337183194729988, 24.34226448433411960, -8.527530157486177487 ) ) ;
#2321=CARTESIAN_POINT ( 'NONE',  ( 7.084665262690076126, 32.02201867748816966, -10.88017736071110164 ) ) ;
#2322=CARTESIAN_POINT ( 'NONE',  ( 6.565887622018943937, 23.08196800326375708, -12.81628187352647608 ) ) ;
#2323=CARTESIAN_POINT ( 'NONE',  ( 1.472469842513823179, 25.59226448433412315, -4.923371831947296329 ) ) ;
#2325=CARTESIAN_POINT ( 'NONE',  ( -0.8801773607111008646, 13.27201867748817321, 2.915334737309923430 ) ) ;
#2326=CARTESIAN_POINT ( 'NONE',  ( 0.5774900079438590739, 62.64701867748817676, -5.440088680355550821 ) ) ;
#2328=CARTESIAN_POINT ( 'NONE',  ( 19.84674366389459621, 48.50893115100078745, 7.409399052514197653E-17 ) ) ;
#2329=CARTESIAN_POINT ( 'NONE',  ( 7.084665262690076126, 22.02201867748817321, -10.88017736071110164 ) ) ;
#2331=ADVANCED_FACE ( 'NONE', ( #94301 ), #32810, .F. ) ;
#2332=CARTESIAN_POINT ( 'NONE',  ( 20.88017736071110519, 45.56368534415484106, 2.639326808657452039E-16 ) ) ;
#2333=CARTESIAN_POINT ( 'NONE',  ( 0.5774900079438590739, 7.647018677488171434, -5.440088680355550821 ) ) ;
#2334=CARTESIAN_POINT ( 'NONE',  ( 17.20831665107776587, 14.13393115100078568, -7.208316651077762316 ) ) ;
#2335=CARTESIAN_POINT ( 'NONE',  ( 18.52753015748618282, 33.92559781766745886, -4.923371831947291888 ) ) ;
#2338=CARTESIAN_POINT ( 'NONE',  ( -4.164238869374098151, 1.595415501580634388, -3.795296366450310543 ) ) ;
#2339=CARTESIAN_POINT ( 'NONE',  ( 17.08211943468705130, 23.47041550158063572, 12.26659068614894998 ) ) ;
#2340=CARTESIAN_POINT ( 'NONE',  ( 17.20831665107776587, 32.88393115100078745, 7.208316651077764980 ) ) ;
#2342=VERTEX_POINT ( 'NONE', #87294 ) ;
#2343=CARTESIAN_POINT ( 'NONE',  ( 12.91533473730993009, 6.605352010821504471, -10.88017736071109987 ) ) ;
#2344=CARTESIAN_POINT ( 'NONE',  ( 2.791683348922237240, 20.38393115100078745, -7.208316651077763204 ) ) ;
#2346=CARTESIAN_POINT ( 'NONE',  ( 4.559911319644449179, 47.23035201082150536, -9.422509992056141925 ) ) ;
#2349=CARTESIAN_POINT ( 'NONE',  ( 15.44008868035555793, 21.39701867748817321, -9.422509992056140149 ) ) ;
#2350=CARTESIAN_POINT ( 'NONE',  ( 10.00000000000000000, 47.87363466993042493, -12.81628187352647608 ) ) ;
#2351=CARTESIAN_POINT ( 'NONE',  ( -2.816281873526473856, 14.12363466993041961, 9.499525473075851096E-16 ) ) ;
#2352=CARTESIAN_POINT ( 'NONE',  ( 19.84674366389459266, 18.71726448433411960, -2.638427012816827677 ) ) ;
#2356=CARTESIAN_POINT ( 'NONE',  ( 22.26659068614895176, 54.72041550158063217, -7.082119434687042414 ) ) ;
#2357=CARTESIAN_POINT ( 'NONE',  ( 24.16423886937410614, 24.51208216824730002, -3.795296366450302550 ) ) ;
#2358=CARTESIAN_POINT ( 'NONE',  ( 17.96484262340118221, 19.93868534415484106, 7.964842623401181321 ) ) ;
#2359=CARTESIAN_POINT ( 'NONE',  ( -0.8801773607111009756, 53.06368534415484106, 1.068504757029289695E-15 ) ) ;
#2362=CARTESIAN_POINT ( 'NONE',  ( 7.084665262690076126, 67.02201867748817676, -10.88017736071110164 ) ) ;
#2363=DIRECTION ( 'NONE',  ( -0.8320502943378437211, 0.5547001962252290364, 0.000000000000000000 ) ) ;
#2364=CARTESIAN_POINT ( 'NONE',  ( 12.63842701281683922, 19.55059781766745175, -9.846743663894590881 ) ) ;
#2365=CARTESIAN_POINT ( 'NONE',  ( 17.20831665107776587, 17.88393115100078745, 7.208316651077764980 ) ) ;
#2366=CARTESIAN_POINT ( 'NONE',  ( 2.791683348922240793, 56.63393115100078035, 7.208316651077764092 ) ) ;
#2367=CARTESIAN_POINT ( 'NONE',  ( 4.559911319644449179, 8.897018677488171434, 9.422509992056141925 ) ) ;
#2368=UNCERTAINTY_MEASURE_WITH_UNIT (LENGTH_MEASURE( 1.000000000000000082E-05 ), #13505, 'distance_accuracy_value', 'NONE');
#2369=( BOUNDED_CURVE ( )  B_SPLINE_CURVE ( 2, ( #47773, #71759, #57235, #63747, #71279, #78271, #40779, #87733, #1812 ),
 .UNSPECIFIED., .F., .F. ) 
 B_SPLINE_CURVE_WITH_KNOTS ( ( 3, 2, 2, 2, 3 ),
 ( 0.4748575172211798034, 0.4761904761904761640, 0.4821428571428571508, 0.4880952380952380820, 0.4894281970645347202 ),
 .UNSPECIFIED. ) 
 CURVE ( )  GEOMETRIC_REPRESENTATION_ITEM ( )  RATIONAL_B_SPLINE_CURVE ( ( 0.9881565478350737841, 0.9923695281211494246, 1.000000000000000000, 0.9659258262890683122, 1.000000000000000000, 0.9659258262890683122, 1.000000000000000000, 0.9923695281211478703, 0.9881565478350720078 ) ) 
 REPRESENTATION_ITEM ( '' )  );
#2370=CARTESIAN_POINT ( 'NONE',  ( 13.43411237798105340, 25.58196800326374998, 12.81628187352647963 ) ) ;
#2372=CARTESIAN_POINT ( 'NONE',  ( -0.8801773607110991993, 52.85535201082151247, -2.915334737309923874 ) ) ;
#2373=CARTESIAN_POINT ( 'NONE',  ( 12.63842701281683922, 34.55059781766745886, -9.846743663894590881 ) ) ;
#2374=CARTESIAN_POINT ( 'NONE',  ( 24.16423886937410614, 44.51208216824730357, -3.795296366450302550 ) ) ;
#2375=CARTESIAN_POINT ( 'NONE',  ( 14.92337183194729633, 27.67559781766745530, 8.527530157486181039 ) ) ;
#2377=CARTESIAN_POINT ( 'NONE',  ( 0.1532563361054100626, 55.80059781766745175, -2.638427012816831230 ) ) ;
#2378=CARTESIAN_POINT ( 'NONE',  ( 1.472469842513823179, 35.59226448433412315, -4.923371831947296329 ) ) ;
#2379=CARTESIAN_POINT ( 'NONE',  ( 17.08211943468705840, 15.13708216824730179, -12.26659068614894466 ) ) ;
#2380=( BOUNDED_SURFACE ( )  B_SPLINE_SURFACE ( 1, 2, ( 
 ( #32034, #18046, #25556, #70552, #77060, #63039, #2080, #92066, #62538, #9550, #614, #56048, #16074, #31059, #8085, #71052, #48524, #38581, #78542, #61559, #23595, #16572, #85556, #10052, #62048, #2575, #86052, #17563, #40552, #54059, #78048, #77543, #8572, #84573, #46561, #33031, #9061, #39076, #69570, #17068, #92548, #24077, #54544, #85060, #47551, #39574, #70063, #32540, #93537, #57989, #42035, #57503, #65988, #49021, #20502, #87513, #71546, #79025, #49503, #11028, #19998, #33510, #56530, #72994, #42510, #96515, #18531, #64007, #64500, #35493, #94520, #64986, #72500, #4524, #4032, #87019, #27006, #27987, #34987, #11512, #34495, #95513, #50007, #65491, #41547, #72011, #73482, #87999, #42999, #3056, #80512, #19512, #95006, #12011, #27496, #79528, #96011, #80008, #26514, #88495, #26038, #50500, #57010, #3542, #58483, #80997, #34002, #12500, #5009, #19026, #88996, #10538, #41048, #44472, #31796, #8815, #14490, #20997, #6981, #44962, #35984, #74972, #52468, #12986, #39327, #58984, #43482, #50988, #14987, #81482, #28491, #21992, #59963, #67975, #89487, #13491, #43970, #6477, #52955, #69822, #36491, #21490, #36981, #67480, #75465, #62294, #98001, #29455, #51485, #13995, #92802, #73983, #81979, #74472, #5996, #66983, #83466, #82971, #97504, #90455, #1344, #98500, #5508, #29955, #37486, #51987, #66485, #97013, #28969, #77300, #59472, #60461, #90950, #22480, #46808, #89972, #82475, #9304, #33271, #79279, #11268, #79769, #72260, #24329, #25316, #39813, #10789, #55803, #86296, #32784, #56770, #47792, #63281, #70316, #94272, #3789, #18787, #85308, #25795, #93787, #16816, #78793, #41788, #34244, #24818, #85805, #56294, #17803, #87266, #71300, #55294, #86789, #18290, #41306, #64744, #10301, #62794, #33753, #40799, #93294, #48281, #54792, #1833, #78290, #2821, #63765, #48773, #71779, #3288, #64255, #94770, #32289, #9806, #77794, #2328, #47293, #17317, #26269, #49269, #40307, #70813, #27247, #74726, #36241, #21243, #27741, #28731, #95763, #19265, #66737, #89240, #35240, #36742, #81241, #35742, #13239, #57745, #4768, #58223, #50241, #97262, #51741, #65238, #11763, #88744, #87751, #26762, #50755, #65738, #28240, #12740, #88248, #19756, #59222, #43733, #74219, #89726, #57254, #66230, #96267, #80756, #49749, #13739, #5752, #20254, #4275, #42271, #43239, #95256, #12251, #42758, #82225, #73734, #44222, #73240, #80259, #6240, #72742, #5264, #96765, #34749, #58735, #20748, #51239, #81725, #67233, #37737, #98253, #8218, #21748, #44721, #61204, #30694, #84701, #6730, #52229, #52715, #23725, #82721, #53214, #60706, #91710, #30203, #75218, #15236 ),
 ( #37246, #22238, #91203, #22731, #38228, #23229, #68715, #246, #46211, #14240, #83222, #67735, #45219, #90215, #29711, #76698, #75716, #60219, #90713, #14745, #46689, #38712, #92201, #98753, #737, #7230, #68236, #69211, #53701, #83716, #8694, #45717, #7732, #84222, #76219, #15731, #31190, #61684, #54188, #16206, #77186, #97756, #29222, #59721, #69697, #93668, #78174, #71178, #25202, #9190, #33155, #18665, #55680, #32667, #39704, #2206, #49153, #1227, #70191, #1710, #62669, #16699, #71664, #40678, #47172, #63160, #10184, #63649, #2704, #94157, #18173, #54673, #93170, #92681, #17203, #62172, #77677, #48655, #47680, #24206, #85192, #32168, #79654, #79155, #64135, #70688, #3174, #24695, #55167, #10669, #25683, #9685, #39210, #86179, #78675, #56176, #85682, #40181, #17690, #48161, #41183, #94653, #86669, #33639, #26161, #31680, #56656, #87142, #50133, #43126, #65619, #80137, #5138, #89616, #96144, #4658, #11647, #73117, #21128, #72141, #42160, #72625, #34625, #87636, #43617, #12624, #19150, #27627, #59106, #58620, #51627, #89121, #58112, #12136, #41673, #3668, #34131, #36115, #49628, #88621, #50632, #73615, #81123, #35629, #57140, #95132, #20128, #66114, #97148, #66621, #11152, #64623, #42639, #26644, #96643, #35119, #28120, #19640, #74104, #65124, #80640, #4158, #20632, #95643, #5637, #27129, #51121, #81613, #57632, #13121, #28619, #88128, #82606, #44608, #83605, #52599, #46097, #30087, #14124, #15119, #76093, #38115, #92084, #37617, #21629, #91596, #68111, #52114, #14630, #13618, #59605, #37123, #45095, #75103, #97638, #75601, #74610, #44099, #98636, #22119, #45595, #60594, #6610, #7623, #61573, #91089, #7113, #67619, #22617, #23610, #6123, #98127, #29588, #60090, #90101, #15613, #68604, #90592, #53093, #31075, #30582, #82107, #61086, #132, #83102, #36629, #67113, #29103, #8101, #23112, #53584, #84098, #76581, #38597, #69095, #629, #39093, #63056, #10069, #41065, #10554, #3074, #54075, #55054, #69584, #40568, #85573, #17087, #62554, #86559, #77560, #93058, #1104, #25086, #33530, #48542, #16090, #55569, #24591, #46577, #9568, #71562, #64025, #54561, #16586, #86068, #47567, #18063, #2096, #85077, #17579, #48045, #71066, #94538, #40070, #92566, #63541, #70571, #24092, #78065, #84590, #31567, #9076, #32555, #93553, #78559, #2591, #33046, #94051, #25572, #62063, #39589, #8587, #32051, #77075, #47062, #56064, #79041, #70080, #1602, #57029, #5526, #66005, #51006, #57523, #58504, #26533, #49042, #96533, #20018, #65007, #66509, #12029, #65509, #43019, #87530, #34514, #88019, #80029, #28008, #81501, #19532, #26056, #19044, #49520 ) ),
 .UNSPECIFIED., .F., .F., .F. ) 
 B_SPLINE_SURFACE_WITH_KNOTS ( ( 2, 2 ),
 ( 3, 2, 2, 2, 2, 2, 2, 2, 2, 2, 2, 2, 2, 2, 2, 2, 2, 2, 2, 2, 2, 2, 2, 2, 2, 2, 2, 2, 2, 2, 2, 2, 2, 2, 2, 2, 2, 2, 2, 2, 2, 2, 2, 2, 2, 2, 2, 2, 2, 2, 2, 2, 2, 2, 2, 2, 2, 2, 2, 2, 2, 2, 2, 2, 2, 2, 2, 2, 2, 2, 2, 2, 2, 2, 2, 2, 2, 2, 2, 2, 2, 2, 2, 2, 2, 2, 2, 2, 2, 2, 2, 2, 2, 2, 2, 2, 2, 2, 2, 2, 2, 2, 2, 2, 2, 2, 2, 2, 2, 2, 2, 2, 2, 2, 2, 2, 2, 2, 2, 2, 2, 2, 2, 2, 2, 2, 2, 2, 2, 2, 2, 2, 2, 2, 2, 2, 2, 2, 2, 2, 2, 2, 2, 2, 2, 2, 2, 2, 2, 2, 2, 2, 2, 2, 2, 2, 2, 2, 2, 2, 2, 2, 3 ),
 ( 0.000000000000000000, 1.000000000000000000 ),
 ( 0.000000000000000000, 0.005952380952380952051, 0.01190476190476190410, 0.01785714285714285615, 0.02380952380952380820, 0.02976190476190476025, 0.03571428571428571230, 0.04166666666666666435, 0.04761904761904761640, 0.05357142857142856845, 0.05952380952380952051, 0.06547619047619047949, 0.07142857142857142461, 0.07738095238095238360, 0.08333333333333332871, 0.08928571428571428770, 0.09523809523809523281, 0.1011904761904761918, 0.1071428571428571369, 0.1130952380952380959, 0.1190476190476190410, 0.1250000000000000000, 0.1309523809523809590, 0.1369047619047619180, 0.1428571428571428492, 0.1488095238095238082, 0.1547619047619047672, 0.1607142857142857262, 0.1666666666666666574, 0.1726190476190476164, 0.1785714285714285754, 0.1845238095238095344, 0.1904761904761904656, 0.1964285714285714246, 0.2023809523809523836, 0.2083333333333333426, 0.2142857142857142738, 0.2202380952380952328, 0.2261904761904761918, 0.2321428571428571508, 0.2380952380952380820, 0.2440476190476190410, 0.2500000000000000000, 0.2559523809523809312, 0.2619047619047619180, 0.2678571428571428492, 0.2738095238095238360, 0.2797619047619047672, 0.2857142857142856984, 0.2916666666666666852, 0.2976190476190476164, 0.3035714285714285476, 0.3095238095238095344, 0.3154761904761904656, 0.3214285714285714524, 0.3273809523809523836, 0.3333333333333333148, 0.3392857142857143016, 0.3452380952380952328, 0.3511904761904761640, 0.3571428571428571508, 0.3630952380952380820, 0.3690476190476190688, 0.3750000000000000000, 0.3809523809523809312, 0.3869047619047619180, 0.3928571428571428492, 0.3988095238095238360, 0.4047619047619047672, 0.4107142857142856984, 0.4166666666666666852, 0.4226190476190476164, 0.4285714285714285476, 0.4345238095238095344, 0.4404761904761904656, 0.4464285714285714524, 0.4523809523809523836, 0.4583333333333333148, 0.4642857142857143016, 0.4702380952380952328, 0.4761904761904761640, 0.4821428571428571508, 0.4880952380952380820, 0.4940476190476190688, 0.5000000000000000000, 0.5059523809523809312, 0.5119047619047618625, 0.5178571428571429047, 0.5238095238095238360, 0.5297619047619047672, 0.5357142857142856984, 0.5416666666666666297, 0.5476190476190476719, 0.5535714285714286031, 0.5595238095238095344, 0.5654761904761904656, 0.5714285714285713969, 0.5773809523809523281, 0.5833333333333333703, 0.5892857142857143016, 0.5952380952380952328, 0.6011904761904761640, 0.6071428571428570953, 0.6130952380952381375, 0.6190476190476190688, 0.6250000000000000000, 0.6309523809523809312, 0.6369047619047618625, 0.6428571428571429047, 0.6488095238095238360, 0.6547619047619047672, 0.6607142857142856984, 0.6666666666666666297, 0.6726190476190476719, 0.6785714285714286031, 0.6845238095238095344, 0.6904761904761904656, 0.6964285714285713969, 0.7023809523809523281, 0.7083333333333333703, 0.7142857142857143016, 0.7202380952380952328, 0.7261904761904761640, 0.7321428571428570953, 0.7380952380952381375, 0.7440476190476190688, 0.7500000000000000000, 0.7559523809523809312, 0.7619047619047618625, 0.7678571428571429047, 0.7738095238095238360, 0.7797619047619047672, 0.7857142857142856984, 0.7916666666666666297, 0.7976190476190476719, 0.8035714285714286031, 0.8095238095238095344, 0.8154761904761904656, 0.8214285714285713969, 0.8273809523809523281, 0.8333333333333333703, 0.8392857142857143016, 0.8452380952380952328, 0.8511904761904761640, 0.8571428571428570953, 0.8630952380952381375, 0.8690476190476190688, 0.8750000000000000000, 0.8809523809523809312, 0.8869047619047618625, 0.8928571428571429047, 0.8988095238095238360, 0.9047619047619047672, 0.9107142857142856984, 0.9166666666666666297, 0.9226190476190476719, 0.9285714285714286031, 0.9345238095238095344, 0.9404761904761904656, 0.9464285714285713969, 0.9523809523809523281, 0.9583333333333333703, 0.9642857142857143016 ),
 .UNSPECIFIED. ) 
 GEOMETRIC_REPRESENTATION_ITEM ( )  RATIONAL_B_SPLINE_SURFACE ( (
 ( 1.000000000000000000, 0.9659258262890683122, 1.000000000000000000, 0.9659258262890683122, 1.000000000000000000, 0.9659258262890683122, 1.000000000000000000, 0.9659258262890683122, 1.000000000000000000, 0.9659258262890683122, 1.000000000000000000, 0.9659258262890683122, 1.000000000000000000, 0.9659258262890683122, 1.000000000000000000, 0.9659258262890683122, 1.000000000000000000, 0.9659258262890683122, 1.000000000000000000, 0.9659258262890683122, 1.000000000000000000, 0.9659258262890683122, 1.000000000000000000, 0.9659258262890683122, 1.000000000000000000, 0.9659258262890683122, 1.000000000000000000, 0.9659258262890683122, 1.000000000000000000, 0.9659258262890683122, 1.000000000000000000, 0.9659258262890683122, 1.000000000000000000, 0.9659258262890683122, 1.000000000000000000, 0.9659258262890683122, 1.000000000000000000, 0.9659258262890683122, 1.000000000000000000, 0.9659258262890683122, 1.000000000000000000, 0.9659258262890683122, 1.000000000000000000, 0.9659258262890683122, 1.000000000000000000, 0.9659258262890683122, 1.000000000000000000, 0.9659258262890683122, 1.000000000000000000, 0.9659258262890683122, 1.000000000000000000, 0.9659258262890683122, 1.000000000000000000, 0.9659258262890683122, 1.000000000000000000, 0.9659258262890683122, 1.000000000000000000, 0.9659258262890683122, 1.000000000000000000, 0.9659258262890683122, 1.000000000000000000, 0.9659258262890683122, 1.000000000000000000, 0.9659258262890683122, 1.000000000000000000, 0.9659258262890683122, 1.000000000000000000, 0.9659258262890683122, 1.000000000000000000, 0.9659258262890683122, 1.000000000000000000, 0.9659258262890683122, 1.000000000000000000, 0.9659258262890683122, 1.000000000000000000, 0.9659258262890683122, 1.000000000000000000, 0.9659258262890683122, 1.000000000000000000, 0.9659258262890683122, 1.000000000000000000, 0.9659258262890683122, 1.000000000000000000, 0.9659258262890683122, 1.000000000000000000, 0.9659258262890683122, 1.000000000000000000, 0.9659258262890683122, 1.000000000000000000, 0.9659258262890683122, 1.000000000000000000, 0.9659258262890683122, 1.000000000000000000, 0.9659258262890683122, 1.000000000000000000, 0.9659258262890683122, 1.000000000000000000, 0.9659258262890683122, 1.000000000000000000, 0.9659258262890683122, 1.000000000000000000, 0.9659258262890683122, 1.000000000000000000, 0.9659258262890683122, 1.000000000000000000, 0.9659258262890683122, 1.000000000000000000, 0.9659258262890683122, 1.000000000000000000, 0.9659258262890683122, 1.000000000000000000, 0.9659258262890683122, 1.000000000000000000, 0.9659258262890683122, 1.000000000000000000, 0.9659258262890683122, 1.000000000000000000, 0.9659258262890683122, 1.000000000000000000, 0.9659258262890683122, 1.000000000000000000, 0.9659258262890683122, 1.000000000000000000, 0.9659258262890683122, 1.000000000000000000, 0.9659258262890683122, 1.000000000000000000, 0.9659258262890683122, 1.000000000000000000, 0.9659258262890683122, 1.000000000000000000, 0.9659258262890683122, 1.000000000000000000, 0.9659258262890683122, 1.000000000000000000, 0.9659258262890683122, 1.000000000000000000, 0.9659258262890683122, 1.000000000000000000, 0.9659258262890683122, 1.000000000000000000, 0.9659258262890683122, 1.000000000000000000, 0.9659258262890683122, 1.000000000000000000, 0.9659258262890683122, 1.000000000000000000, 0.9659258262890683122, 1.000000000000000000, 0.9659258262890683122, 1.000000000000000000, 0.9659258262890683122, 1.000000000000000000, 0.9659258262890683122, 1.000000000000000000, 0.9659258262890683122, 1.000000000000000000, 0.9659258262890683122, 1.000000000000000000, 0.9659258262890683122, 1.000000000000000000, 0.9659258262890683122, 1.000000000000000000, 0.9659258262890683122, 1.000000000000000000, 0.9659258262890683122, 1.000000000000000000, 0.9659258262890683122, 1.000000000000000000, 0.9659258262890683122, 1.000000000000000000, 0.9659258262890683122, 1.000000000000000000, 0.9659258262890683122, 1.000000000000000000, 0.9659258262890683122, 1.000000000000000000, 0.9659258262890683122, 1.000000000000000000, 0.9659258262890683122, 1.000000000000000000, 0.9659258262890683122, 1.000000000000000000, 0.9659258262890683122, 1.000000000000000000, 0.9659258262890683122, 1.000000000000000000, 0.9659258262890683122, 1.000000000000000000, 0.9659258262890683122, 1.000000000000000000, 0.9659258262890683122, 1.000000000000000000, 0.9659258262890683122, 1.000000000000000000, 0.9659258262890683122, 1.000000000000000000, 0.9659258262890683122, 1.000000000000000000, 0.9659258262890683122, 1.000000000000000000, 0.9659258262890683122, 1.000000000000000000, 0.9659258262890683122, 1.000000000000000000, 0.9659258262890683122, 1.000000000000000000, 0.9659258262890683122, 1.000000000000000000, 0.9659258262890683122, 1.000000000000000000, 0.9659258262890683122, 1.000000000000000000, 0.9659258262890683122, 1.000000000000000000, 0.9659258262890683122, 1.000000000000000000, 0.9659258262890683122, 1.000000000000000000, 0.9659258262890683122, 1.000000000000000000, 0.9659258262890683122, 1.000000000000000000, 0.9659258262890683122, 1.000000000000000000, 0.9659258262890683122, 1.000000000000000000, 0.9659258262890683122, 1.000000000000000000, 0.9659258262890683122, 1.000000000000000000, 0.9659258262890683122, 1.000000000000000000, 0.9659258262890683122, 1.000000000000000000, 0.9659258262890683122, 1.000000000000000000, 0.9659258262890683122, 1.000000000000000000, 0.9659258262890683122, 1.000000000000000000, 0.9659258262890683122, 1.000000000000000000, 0.9659258262890683122, 1.000000000000000000, 0.9659258262890683122, 1.000000000000000000, 0.9659258262890683122, 1.000000000000000000, 0.9659258262890683122, 1.000000000000000000, 0.9659258262890683122, 1.000000000000000000, 0.9659258262890683122, 1.000000000000000000, 0.9659258262890683122, 1.000000000000000000, 0.9659258262890683122, 1.000000000000000000, 0.9659258262890683122, 1.000000000000000000, 0.9659258262890683122, 1.000000000000000000, 0.9659258262890683122, 1.000000000000000000, 0.9659258262890683122, 1.000000000000000000, 0.9659258262890683122, 1.000000000000000000, 0.9659258262890683122, 1.000000000000000000, 0.9659258262890683122, 1.000000000000000000, 0.9659258262890683122, 1.000000000000000000, 0.9659258262890683122, 1.000000000000000000, 0.9659258262890683122, 1.000000000000000000, 0.9659258262890683122, 1.000000000000000000, 0.9659258262890683122, 1.000000000000000000, 0.9659258262890683122, 1.000000000000000000, 0.9659258262890683122, 1.000000000000000000, 0.9659258262890683122, 1.000000000000000000, 0.9659258262890683122, 1.000000000000000000, 0.9659258262890683122, 1.000000000000000000, 0.9659258262890683122, 1.000000000000000000, 0.9659258262890683122, 1.000000000000000000, 0.9659258262890683122, 1.000000000000000000, 0.9659258262890683122, 1.000000000000000000, 0.9659258262890683122, 1.000000000000000000, 0.9659258262890683122, 1.000000000000000000, 0.9659258262890683122, 1.000000000000000000, 0.9659258262890683122, 1.000000000000000000, 0.9659258262890683122, 1.000000000000000000, 0.9659258262890683122, 1.000000000000000000, 0.9659258262890683122, 1.000000000000000000, 0.9659258262890683122, 1.000000000000000000, 0.9659258262890683122, 1.000000000000000000, 0.9659258262890683122, 1.000000000000000000, 0.9659258262890683122, 1.000000000000000000, 0.9659258262890683122, 1.000000000000000000),
 ( 1.000000000000000000, 0.9659258262890683122, 1.000000000000000000, 0.9659258262890683122, 1.000000000000000000, 0.9659258262890683122, 1.000000000000000000, 0.9659258262890683122, 1.000000000000000000, 0.9659258262890683122, 1.000000000000000000, 0.9659258262890683122, 1.000000000000000000, 0.9659258262890683122, 1.000000000000000000, 0.9659258262890683122, 1.000000000000000000, 0.9659258262890683122, 1.000000000000000000, 0.9659258262890683122, 1.000000000000000000, 0.9659258262890683122, 1.000000000000000000, 0.9659258262890683122, 1.000000000000000000, 0.9659258262890683122, 1.000000000000000000, 0.9659258262890683122, 1.000000000000000000, 0.9659258262890683122, 1.000000000000000000, 0.9659258262890683122, 1.000000000000000000, 0.9659258262890683122, 1.000000000000000000, 0.9659258262890683122, 1.000000000000000000, 0.9659258262890683122, 1.000000000000000000, 0.9659258262890683122, 1.000000000000000000, 0.9659258262890683122, 1.000000000000000000, 0.9659258262890683122, 1.000000000000000000, 0.9659258262890683122, 1.000000000000000000, 0.9659258262890683122, 1.000000000000000000, 0.9659258262890683122, 1.000000000000000000, 0.9659258262890683122, 1.000000000000000000, 0.9659258262890683122, 1.000000000000000000, 0.9659258262890683122, 1.000000000000000000, 0.9659258262890683122, 1.000000000000000000, 0.9659258262890683122, 1.000000000000000000, 0.9659258262890683122, 1.000000000000000000, 0.9659258262890683122, 1.000000000000000000, 0.9659258262890683122, 1.000000000000000000, 0.9659258262890683122, 1.000000000000000000, 0.9659258262890683122, 1.000000000000000000, 0.9659258262890683122, 1.000000000000000000, 0.9659258262890683122, 1.000000000000000000, 0.9659258262890683122, 1.000000000000000000, 0.9659258262890683122, 1.000000000000000000, 0.9659258262890683122, 1.000000000000000000, 0.9659258262890683122, 1.000000000000000000, 0.9659258262890683122, 1.000000000000000000, 0.9659258262890683122, 1.000000000000000000, 0.9659258262890683122, 1.000000000000000000, 0.9659258262890683122, 1.000000000000000000, 0.9659258262890683122, 1.000000000000000000, 0.9659258262890683122, 1.000000000000000000, 0.9659258262890683122, 1.000000000000000000, 0.9659258262890683122, 1.000000000000000000, 0.9659258262890683122, 1.000000000000000000, 0.9659258262890683122, 1.000000000000000000, 0.9659258262890683122, 1.000000000000000000, 0.9659258262890683122, 1.000000000000000000, 0.9659258262890683122, 1.000000000000000000, 0.9659258262890683122, 1.000000000000000000, 0.9659258262890683122, 1.000000000000000000, 0.9659258262890683122, 1.000000000000000000, 0.9659258262890683122, 1.000000000000000000, 0.9659258262890683122, 1.000000000000000000, 0.9659258262890683122, 1.000000000000000000, 0.9659258262890683122, 1.000000000000000000, 0.9659258262890683122, 1.000000000000000000, 0.9659258262890683122, 1.000000000000000000, 0.9659258262890683122, 1.000000000000000000, 0.9659258262890683122, 1.000000000000000000, 0.9659258262890683122, 1.000000000000000000, 0.9659258262890683122, 1.000000000000000000, 0.9659258262890683122, 1.000000000000000000, 0.9659258262890683122, 1.000000000000000000, 0.9659258262890683122, 1.000000000000000000, 0.9659258262890683122, 1.000000000000000000, 0.9659258262890683122, 1.000000000000000000, 0.9659258262890683122, 1.000000000000000000, 0.9659258262890683122, 1.000000000000000000, 0.9659258262890683122, 1.000000000000000000, 0.9659258262890683122, 1.000000000000000000, 0.9659258262890683122, 1.000000000000000000, 0.9659258262890683122, 1.000000000000000000, 0.9659258262890683122, 1.000000000000000000, 0.9659258262890683122, 1.000000000000000000, 0.9659258262890683122, 1.000000000000000000, 0.9659258262890683122, 1.000000000000000000, 0.9659258262890683122, 1.000000000000000000, 0.9659258262890683122, 1.000000000000000000, 0.9659258262890683122, 1.000000000000000000, 0.9659258262890683122, 1.000000000000000000, 0.9659258262890683122, 1.000000000000000000, 0.9659258262890683122, 1.000000000000000000, 0.9659258262890683122, 1.000000000000000000, 0.9659258262890683122, 1.000000000000000000, 0.9659258262890683122, 1.000000000000000000, 0.9659258262890683122, 1.000000000000000000, 0.9659258262890683122, 1.000000000000000000, 0.9659258262890683122, 1.000000000000000000, 0.9659258262890683122, 1.000000000000000000, 0.9659258262890683122, 1.000000000000000000, 0.9659258262890683122, 1.000000000000000000, 0.9659258262890683122, 1.000000000000000000, 0.9659258262890683122, 1.000000000000000000, 0.9659258262890683122, 1.000000000000000000, 0.9659258262890683122, 1.000000000000000000, 0.9659258262890683122, 1.000000000000000000, 0.9659258262890683122, 1.000000000000000000, 0.9659258262890683122, 1.000000000000000000, 0.9659258262890683122, 1.000000000000000000, 0.9659258262890683122, 1.000000000000000000, 0.9659258262890683122, 1.000000000000000000, 0.9659258262890683122, 1.000000000000000000, 0.9659258262890683122, 1.000000000000000000, 0.9659258262890683122, 1.000000000000000000, 0.9659258262890683122, 1.000000000000000000, 0.9659258262890683122, 1.000000000000000000, 0.9659258262890683122, 1.000000000000000000, 0.9659258262890683122, 1.000000000000000000, 0.9659258262890683122, 1.000000000000000000, 0.9659258262890683122, 1.000000000000000000, 0.9659258262890683122, 1.000000000000000000, 0.9659258262890683122, 1.000000000000000000, 0.9659258262890683122, 1.000000000000000000, 0.9659258262890683122, 1.000000000000000000, 0.9659258262890683122, 1.000000000000000000, 0.9659258262890683122, 1.000000000000000000, 0.9659258262890683122, 1.000000000000000000, 0.9659258262890683122, 1.000000000000000000, 0.9659258262890683122, 1.000000000000000000, 0.9659258262890683122, 1.000000000000000000, 0.9659258262890683122, 1.000000000000000000, 0.9659258262890683122, 1.000000000000000000, 0.9659258262890683122, 1.000000000000000000, 0.9659258262890683122, 1.000000000000000000, 0.9659258262890683122, 1.000000000000000000, 0.9659258262890683122, 1.000000000000000000, 0.9659258262890683122, 1.000000000000000000, 0.9659258262890683122, 1.000000000000000000, 0.9659258262890683122, 1.000000000000000000, 0.9659258262890683122, 1.000000000000000000, 0.9659258262890683122, 1.000000000000000000, 0.9659258262890683122, 1.000000000000000000, 0.9659258262890683122, 1.000000000000000000, 0.9659258262890683122, 1.000000000000000000, 0.9659258262890683122, 1.000000000000000000, 0.9659258262890683122, 1.000000000000000000, 0.9659258262890683122, 1.000000000000000000, 0.9659258262890683122, 1.000000000000000000, 0.9659258262890683122, 1.000000000000000000, 0.9659258262890683122, 1.000000000000000000, 0.9659258262890683122, 1.000000000000000000, 0.9659258262890683122, 1.000000000000000000, 0.9659258262890683122, 1.000000000000000000, 0.9659258262890683122, 1.000000000000000000, 0.9659258262890683122, 1.000000000000000000, 0.9659258262890683122, 1.000000000000000000, 0.9659258262890683122, 1.000000000000000000, 0.9659258262890683122, 1.000000000000000000, 0.9659258262890683122, 1.000000000000000000, 0.9659258262890683122, 1.000000000000000000, 0.9659258262890683122, 1.000000000000000000, 0.9659258262890683122, 1.000000000000000000, 0.9659258262890683122, 1.000000000000000000, 0.9659258262890683122, 1.000000000000000000, 0.9659258262890683122, 1.000000000000000000, 0.9659258262890683122, 1.000000000000000000) ) ) 
 REPRESENTATION_ITEM ( '' )  SURFACE ( )  );
#2381=CARTESIAN_POINT ( 'NONE',  ( 17.08211943468705840, 15.13708216824730179, -12.26659068614894466 ) ) ;
#2382=CARTESIAN_POINT ( 'NONE',  ( 5.076628168052703671, 26.84226448433411960, 8.527530157486179263 ) ) ;
#2383=CARTESIAN_POINT ( 'NONE',  ( 12.91533473730993009, 41.60535201082149825, -10.88017736071109987 ) ) ;
#2384=CARTESIAN_POINT ( 'NONE',  ( 2.035157376598824452, 18.68868534415484106, 7.964842623401179544 ) ) ;
#2385=CARTESIAN_POINT ( 'NONE',  ( 10.00000000000000178, 44.31368534415484106, 10.88017736071110342 ) ) ;
#2387=CARTESIAN_POINT ( 'NONE',  ( 17.96484262340118221, 29.93868534415484106, 7.964842623401181321 ) ) ;
#2388=VERTEX_POINT ( 'NONE', #48309 ) ;
#2389=CARTESIAN_POINT ( 'NONE',  ( 10.00000000000000000, 37.87363466993041783, -12.81628187352647608 ) ) ;
#2390=CARTESIAN_POINT ( 'NONE',  ( 7.084665262690076126, 44.10535201082151247, 10.88017736071109987 ) ) ;
#2393=CARTESIAN_POINT ( 'NONE',  ( -2.816281873526473856, 59.33196800326374643, 3.434112377981055619 ) ) ;
#2394=CARTESIAN_POINT ( 'NONE',  ( 2.035157376598824452, 63.68868534415484106, 7.964842623401179544 ) ) ;
#2396=CARTESIAN_POINT ( 'NONE',  ( 20.88017736071110164, 65.35535201082150536, 2.915334737309930979 ) ) ;
#2397=CARTESIAN_POINT ( 'NONE',  ( 2.603489959281614308, 61.58210964143329846, 6.500000000000031086 ) ) ;
#2399=CARTESIAN_POINT ( 'NONE',  ( -2.266590686148945544, 56.38708216824731068, -7.082119434687050408 ) ) ;
#2400=CARTESIAN_POINT ( 'NONE',  ( 7.361572987183169658, 9.967264484334119601, -9.846743663894592657 ) ) ;
#2402=( NAMED_UNIT ( * ) PLANE_ANGLE_UNIT ( ) SI_UNIT ( $, .RADIAN. ) );
#2403=CARTESIAN_POINT ( 'NONE',  ( 0.1532563361054083140, 6.008931151000784787, 1.131784320476157264E-15 ) ) ;
#2404=CARTESIAN_POINT ( 'NONE',  ( 12.91533473730992121, 4.522018677488169658, 10.88017736071110164 ) ) ;
#2405=CARTESIAN_POINT ( 'NONE',  ( 10.00000000000000000, 39.75893115100078745, -9.846743663894594434 ) ) ;
#2407=CARTESIAN_POINT ( 'NONE',  ( 17.20831665107776587, 49.13393115100078745, -7.208316651077762316 ) ) ;
#2408=CARTESIAN_POINT ( 'NONE',  ( 17.96484262340118221, 46.18868534415484106, -7.964842623401177768 ) ) ;
#2409=CARTESIAN_POINT ( 'NONE',  ( 18.52753015748617571, 48.09226448433412315, 4.923371831947298993 ) ) ;
#2412=CARTESIAN_POINT ( 'NONE',  ( 10.00000000000000178, 54.31368534415484106, 10.88017736071110342 ) ) ;
#2413=CARTESIAN_POINT ( 'NONE',  ( 19.42250999205614193, 10.14701867748816966, 5.440088680355555262 ) ) ;
#2414=EDGE_CURVE ( 'NONE', #37014, #48374, #2847, .T. ) ;
#2415=B_SPLINE_CURVE_WITH_KNOTS ( 'NONE', 3,
 ( #47096, #84620, #16124, #31600 ),
 .UNSPECIFIED., .F., .F.,
 ( 4, 4 ),
 ( 0.000000000000000000, 0.001036303429213394781 ),
 .UNSPECIFIED. ) ;
#2417=CARTESIAN_POINT ( 'NONE',  ( 13.43411237798105340, 40.58196800326375353, 12.81628187352647963 ) ) ;
#2420=CARTESIAN_POINT ( 'NONE',  ( -2.816281873526473856, 34.12363466993042493, 9.499525473075851096E-16 ) ) ;
#2421=CARTESIAN_POINT ( 'NONE',  ( -0.8801773607111009756, 28.06368534415484106, 1.068504757029289695E-15 ) ) ;
#2422=EDGE_CURVE ( 'NONE', #19080, #91846, #96963, .T. ) ;
#2425=CARTESIAN_POINT ( 'NONE',  ( 10.00000000000000000, -0.2410688489992152128, -9.846743663894594434 ) ) ;
#2426=CARTESIAN_POINT ( 'NONE',  ( 12.63842701281683922, 44.55059781766745175, -9.846743663894590881 ) ) ;
#2427=CARTESIAN_POINT ( 'NONE',  ( 18.52753015748618282, 13.92559781766745175, -4.923371831947291888 ) ) ;
#2428=CARTESIAN_POINT ( 'NONE',  ( 12.63842701281683034, 42.46726448433412315, 9.846743663894596210 ) ) ;
#2431=CARTESIAN_POINT ( 'NONE',  ( 7.361572987183169658, 29.96726448433411960, -9.846743663894592657 ) ) ;
#2433=CARTESIAN_POINT ( 'NONE',  ( 2.603489959281614308, 61.58210964143329846, 6.500000000000031086 ) ) ;
#2434=CARTESIAN_POINT ( 'NONE',  ( 14.92337183194729633, 32.67559781766745175, 8.527530157486181039 ) ) ;
#2435=CARTESIAN_POINT ( 'NONE',  ( 0.2751277870542967463, 70.00000000000000000, -6.000000000000000000 ) ) ;
#2437=CARTESIAN_POINT ( 'NONE',  ( 10.00000000000000000, 39.75893115100078745, -9.846743663894594434 ) ) ;
#2440=CARTESIAN_POINT ( 'NONE',  ( 6.565887622018943937, 23.08196800326375708, -12.81628187352647608 ) ) ;
#2444=CARTESIAN_POINT ( 'NONE',  ( -0.3689425029237881626, 42.42874883491396787, 10.36894250292379027 ) ) ;
#2445=CARTESIAN_POINT ( 'NONE',  ( 5.076628168052703671, 21.84226448433411960, 8.527530157486179263 ) ) ;
#2446=CARTESIAN_POINT ( 'NONE',  ( 14.92337183194729633, 2.675597817667451750, 8.527530157486181039 ) ) ;
#2448=CARTESIAN_POINT ( 'NONE',  ( -0.3689425029237898834, 46.17874883491397497, -10.36894250292378850 ) ) ;
#2449=CARTESIAN_POINT ( 'NONE',  ( 19.84674366389459266, 58.30059781766745886, 2.638427012816836559 ) ) ;
#2450=EDGE_CURVE ( 'NONE', #84403, #23604, #32460, .T. ) ;
#2451=CARTESIAN_POINT ( 'NONE',  ( 0.5774900079438607392, 8.480352010821505360, 5.440088680355550821 ) ) ;
#2452=CARTESIAN_POINT ( 'NONE',  ( 20.36894250292379382, 23.67874883491397142, 10.36894250292379205 ) ) ;
#2453=CARTESIAN_POINT ( 'NONE',  ( 10.00000000000000000, 35.55374883491396787, -14.16423886937410082 ) ) ;
#2456=CARTESIAN_POINT ( 'NONE',  ( 0.1532563361054100626, 50.80059781766745175, -2.638427012816831230 ) ) ;
#2458=CARTESIAN_POINT ( 'NONE',  ( 7.084665262690076126, 32.02201867748816966, -10.88017736071110164 ) ) ;
#2460=COLOUR_RGB ( '', 0.66274510, 0.83137255, 0.94901961) ;
#2462=CARTESIAN_POINT ( 'NONE',  ( 14.92337183194729988, 39.34226448433412315, -8.527530157486177487 ) ) ;
#2465=CARTESIAN_POINT ( 'NONE',  ( 0.1532563361054100626, 55.80059781766745175, -2.638427012816831230 ) ) ;
#2466=CARTESIAN_POINT ( 'NONE',  ( 12.63842701281683922, 64.55059781766745175, -9.846743663894590881 ) ) ;
#2469=CARTESIAN_POINT ( 'NONE',  ( 17.08211943468705130, 18.47041550158063572, 12.26659068614894998 ) ) ;
#2473=CARTESIAN_POINT ( 'NONE',  ( 0.5774900079438590739, 7.647018677488171434, -5.440088680355550821 ) ) ;
#2474=CARTESIAN_POINT ( 'NONE',  ( 13.43411237798106583, 22.66530133659708923, -12.81628187352647252 ) ) ;
#2475=CARTESIAN_POINT ( 'NONE',  ( -0.1503990784575328643, 55.12777174578612716, 6.262539305110068177 ) ) ;
#2476=CARTESIAN_POINT ( 'NONE',  ( 7.084665262690076126, 64.10535201082150536, 10.88017736071109987 ) ) ;
#2477=CARTESIAN_POINT ( 'NONE',  ( 21.92686044187656691, 42.18830936912751639, 4.562052436263911564E-16 ) ) ;
#2479=CARTESIAN_POINT ( 'NONE',  ( 7.084665262690076126, 14.10535201082150358, 10.88017736071109987 ) ) ;
#2481=CARTESIAN_POINT ( 'NONE',  ( 0.9413316022086114510, 3.455083851089586489, 6.499999999999963585 ) ) ;
#2482=CARTESIAN_POINT ( 'NONE',  ( 17.96484262340118221, 29.93868534415484106, 7.964842623401181321 ) ) ;
#2483=CARTESIAN_POINT ( 'NONE',  ( 20.88017736071110519, 40.56368534415484106, 2.639326808657452039E-16 ) ) ;
#2485=CARTESIAN_POINT ( 'NONE',  ( 3.591859063236763294, -1.709698663402913210, -11.09922568453595026 ) ) ;
#2486=DIRECTION ( 'NONE',  ( 0.000000000000000000, -1.000000000000000000, -0.000000000000000000 ) ) ;
#2487=CARTESIAN_POINT ( 'NONE',  ( 0.6178305044545838731, 64.74863466993043914, 9.382169495545420901 ) ) ;
#2488=CARTESIAN_POINT ( 'NONE',  ( 18.52753015748618282, 13.92559781766745175, -4.923371831947291888 ) ) ;
#2490=CARTESIAN_POINT ( 'NONE',  ( 12.91533473730992121, 24.52201867748816966, 10.88017736071110164 ) ) ;
#2491=CARTESIAN_POINT ( 'NONE',  ( 22.81628187352648496, 26.83196800326374998, -3.434112377981050290 ) ) ;
#2493=CARTESIAN_POINT ( 'NONE',  ( 19.84674366389459266, 63.71726448433412315, -2.638427012816827677 ) ) ;
#2494=CARTESIAN_POINT ( 'NONE',  ( 17.96484262340118221, 46.18868534415484106, -7.964842623401177768 ) ) ;
#2496=CARTESIAN_POINT ( 'NONE',  ( 2.791683348922237240, 15.38393115100078212, -7.208316651077763204 ) ) ;
#2497=CARTESIAN_POINT ( 'NONE',  ( 22.81628187352647785, 41.62363466993042493, 6.195893100308588602E-16 ) ) ;
#2498=CARTESIAN_POINT ( 'NONE',  ( -0.8801773607111008646, 68.27201867748817676, 2.915334737309923430 ) ) ;
#2501=CARTESIAN_POINT ( 'NONE',  ( -2.816281873526473856, 64.12363466993042493, 9.499525473075851096E-16 ) ) ;
#2505=( NAMED_UNIT ( * ) SI_UNIT ( $, .STERADIAN. ) SOLID_ANGLE_UNIT ( ) );
#2506=CARTESIAN_POINT ( 'NONE',  ( 13.43411237798106583, 52.66530133659708213, -12.81628187352647252 ) ) ;
#2507=CARTESIAN_POINT ( 'NONE',  ( -0.3689425029237881626, 17.42874883491397142, 10.36894250292379027 ) ) ;
#2508=CARTESIAN_POINT ( 'NONE',  ( 0.1532563361054100626, 10.80059781766745175, -2.638427012816831230 ) ) ;
#2509=CARTESIAN_POINT ( 'NONE',  ( 2.035157376598822676, 7.438685344154837509, -7.964842623401177768 ) ) ;
#2510=CARTESIAN_POINT ( 'NONE',  ( 19.84674366389459621, 13.50893115100078568, 7.409399052514197653E-17 ) ) ;
#2511=CARTESIAN_POINT ( 'NONE',  ( 13.79529636645031943, 60.34541550158063927, -14.16423886937409904 ) ) ;
#2513=CARTESIAN_POINT ( 'NONE',  ( 20.88017736071110875, 5.772018677488170546, -2.915334737309920765 ) ) ;
#2515=CARTESIAN_POINT ( 'NONE',  ( 7.084665262690076126, 24.10535201082150181, 10.88017736071109987 ) ) ;
#2517=ORIENTED_EDGE ( 'NONE', *, *, #4236, .T. ) ;
#2518=CARTESIAN_POINT ( 'NONE',  ( 4.559911319644449179, 13.89701867748817321, 9.422509992056141925 ) ) ;
#2519=CARTESIAN_POINT ( 'NONE',  ( 7.361572987183170547, 57.05059781766744464, 9.846743663894590881 ) ) ;
#2521=CARTESIAN_POINT ( 'NONE',  ( 21.09922568453594849, 56.20696800326375353, 6.408140936763242479 ) ) ;
#2524=CARTESIAN_POINT ( 'NONE',  ( -4.164238869374098151, 21.59541550158063217, -3.795296366450310543 ) ) ;
#2525=CARTESIAN_POINT ( 'NONE',  ( 2.035157376598822676, 42.43868534415483396, -7.964842623401177768 ) ) ;
#2526=CARTESIAN_POINT ( 'NONE',  ( -0.8801773607111009756, 23.06368534415484106, 1.068504757029289695E-15 ) ) ;
#2527=CARTESIAN_POINT ( 'NONE',  ( 1.472469842513823179, 56.42559781766745886, 4.923371831947296329 ) ) ;
#2529=CARTESIAN_POINT ( 'NONE',  ( 19.72487221294570858, 31.86607318730074567, 6.500000000000000888 ) ) ;
#2530=CARTESIAN_POINT ( 'NONE',  ( 14.92337183194729988, 34.34226448433411605, -8.527530157486177487 ) ) ;
#2531=CARTESIAN_POINT ( 'NONE',  ( 2.791683348922237240, 5.383931151000785675, -7.208316651077763204 ) ) ;
#2533=ORIENTED_EDGE ( 'NONE', *, *, #11199, .F. ) ;
#2534=CARTESIAN_POINT ( 'NONE',  ( 17.96484262340118221, 4.938685344154837509, 7.964842623401181321 ) ) ;
#2535=CARTESIAN_POINT ( 'NONE',  ( 14.92337183194729633, 17.67559781766745175, 8.527530157486181039 ) ) ;
#2536=CARTESIAN_POINT ( 'NONE',  ( 13.43411237798105340, 5.581968003263753531, 12.81628187352647963 ) ) ;
#2537=CARTESIAN_POINT ( 'NONE',  ( 2.035157376598824452, 43.68868534415484106, 7.964842623401179544 ) ) ;
#2538=CARTESIAN_POINT ( 'NONE',  ( 15.44008868035555793, 6.397018677488170546, -9.422509992056140149 ) ) ;
#2539=CARTESIAN_POINT ( 'NONE',  ( 6.565887622018943937, 43.08196800326374643, -12.81628187352647608 ) ) ;
#2540=CARTESIAN_POINT ( 'NONE',  ( 6.204703633549690345, 25.76208216824730712, -14.16423886937410259 ) ) ;
#2544=CARTESIAN_POINT ( 'NONE',  ( 3.591859063236763294, 63.29030133659708923, -11.09922568453595026 ) ) ;
#2545=ORIENTED_EDGE ( 'NONE', *, *, #97325, .F. ) ;
#2546=CARTESIAN_POINT ( 'NONE',  ( 19.84674366389459266, 58.71726448433411605, -2.638427012816827677 ) ) ;
#2548=CARTESIAN_POINT ( 'NONE',  ( 12.91533473730992121, 24.52201867748816966, 10.88017736071110164 ) ) ;
#2549=ORIENTED_EDGE ( 'NONE', *, *, #98491, .T. ) ;
#2550=CARTESIAN_POINT ( 'NONE',  ( 12.63842701281683034, 2.467264484334118269, 9.846743663894596210 ) ) ;
#2552=CARTESIAN_POINT ( 'NONE',  ( 5.076628168052703671, 11.84226448433411960, 8.527530157486179263 ) ) ;
#2553=CARTESIAN_POINT ( 'NONE',  ( 14.92337183194729633, 2.675597817667451750, 8.527530157486181039 ) ) ;
#2554=CARTESIAN_POINT ( 'NONE',  ( 20.88017736071110164, 60.35535201082151957, 2.915334737309930979 ) ) ;
#2556=CARTESIAN_POINT ( 'NONE',  ( -0.8801773607111008646, 68.27201867748817676, 2.915334737309923430 ) ) ;
#2558=CARTESIAN_POINT ( 'NONE',  ( 19.84674366389459266, 3.300597817667451750, 2.638427012816836559 ) ) ;
#2562=CARTESIAN_POINT ( 'NONE',  ( 0.1532563361054100626, 50.80059781766745175, -2.638427012816831230 ) ) ;
#2565=FACE_OUTER_BOUND ( 'NONE', #78621, .T. ) ;
#2567=CARTESIAN_POINT ( 'NONE',  ( -0.3689425029237898834, 6.178748834913968757, -10.36894250292378850 ) ) ;
#2568=CARTESIAN_POINT ( 'NONE',  ( -2.816281873526473856, 59.12363466993042493, 9.499525473075851096E-16 ) ) ;
#2569=CARTESIAN_POINT ( 'NONE',  ( -0.3689425029237898834, 6.178748834913968757, -10.36894250292378850 ) ) ;
#2570=CARTESIAN_POINT ( 'NONE',  ( 22.26659068614895176, 29.72041550158063572, -7.082119434687042414 ) ) ;
#2571=CARTESIAN_POINT ( 'NONE',  ( 0.1957200283969079413, 45.25733960839543357, 6.499999999999982236 ) ) ;
#2572=CARTESIAN_POINT ( 'NONE',  ( 19.42250999205614548, 25.98035201082150891, -5.440088680355545492 ) ) ;
#2574=ORIENTED_EDGE ( 'NONE', *, *, #72852, .T. ) ;
#2575=CARTESIAN_POINT ( 'NONE',  ( 7.361572987183169658, 4.967264484334119601, -9.846743663894592657 ) ) ;
#2576=CARTESIAN_POINT ( 'NONE',  ( 19.84674366389459266, 13.30059781766745353, 2.638427012816836559 ) ) ;
#2577=CARTESIAN_POINT ( 'NONE',  ( -1.099225684535947600, 28.70696800326375353, -6.408140936763238038 ) ) ;
#2578=CARTESIAN_POINT ( 'NONE',  ( 18.52753015748618282, 43.92559781766745175, -4.923371831947291888 ) ) ;
#2579=EDGE_CURVE ( 'NONE', #91901, #78236, #2756, .T. ) ;
#2580=CARTESIAN_POINT ( 'NONE',  ( 5.500000000000000000, 11.00000000000000000, -6.500000000000000888 ) ) ;
#2581=CARTESIAN_POINT ( 'NONE',  ( 16.40814093676324603, 32.45696800326375353, -11.09922568453594671 ) ) ;
#2582=CARTESIAN_POINT ( 'NONE',  ( 19.72487221294571569, 40.71833443783938122, -6.499999999999989342 ) ) ;
#2583=CARTESIAN_POINT ( 'NONE',  ( 12.63842701281683034, 32.46726448433412315, 9.846743663894596210 ) ) ;
#2584=AXIS2_PLACEMENT_3D ( 'NONE', #55942, #40945, #72394 ) ;
#2585=CARTESIAN_POINT ( 'NONE',  ( -2.266590686148945544, 12.22041550158063394, 7.082119434687048631 ) ) ;
#2586=ORIENTED_EDGE ( 'NONE', *, *, #2422, .T. ) ;
#2587=CARTESIAN_POINT ( 'NONE',  ( 20.88017736071110519, 30.56368534415484106, 2.639326808657452039E-16 ) ) ;
#2588=CARTESIAN_POINT ( 'NONE',  ( -4.164238869374098151, 31.59541550158063927, -3.795296366450310543 ) ) ;
#2589=CARTESIAN_POINT ( 'NONE',  ( 14.92337183194729988, 54.34226448433412315, -8.527530157486177487 ) ) ;
#2590=CARTESIAN_POINT ( 'NONE',  ( 0.1532563361054082862, 11.21726448433411605, 2.638427012816831674 ) ) ;
#2591=CARTESIAN_POINT ( 'NONE',  ( 16.40814093676324603, 57.45696800326375353, -11.09922568453594671 ) ) ;
#2593=CARTESIAN_POINT ( 'NONE',  ( 10.00000000000000178, 34.31368534415484106, 10.88017736071110342 ) ) ;
#2595=CARTESIAN_POINT ( 'NONE',  ( 16.40814093676324603, 17.45696800326375353, -11.09922568453594671 ) ) ;
#2596=CARTESIAN_POINT ( 'NONE',  ( 22.81628187352647785, 21.62363466993041783, 6.195893100308588602E-16 ) ) ;
#2597=CARTESIAN_POINT ( 'NONE',  ( 2.791683348922237240, 45.38393115100079456, -7.208316651077763204 ) ) ;
#2599=CARTESIAN_POINT ( 'NONE',  ( -2.816281873526471635, 43.91530133659708923, -3.434112377981056508 ) ) ;
#2600=CARTESIAN_POINT ( 'NONE',  ( 7.084665262690076126, 57.02201867748817676, -10.88017736071110164 ) ) ;
#2606=CARTESIAN_POINT ( 'NONE',  ( -0.8801773607111008646, 48.27201867748816966, 2.915334737309923430 ) ) ;
#2607=CARTESIAN_POINT ( 'NONE',  ( 10.00000000000000178, 54.31368534415484106, 10.88017736071110342 ) ) ;
#2608=LINE ( 'NONE', #24109, #48873 ) ;
#2610=CARTESIAN_POINT ( 'NONE',  ( -0.8801773607110991993, 2.855352010821504471, -2.915334737309923874 ) ) ;
#2611=CARTESIAN_POINT ( 'NONE',  ( 17.20831665107776587, 59.13393115100078745, -7.208316651077762316 ) ) ;
#2612=CARTESIAN_POINT ( 'NONE',  ( -0.8801773607110991993, 22.85535201082150181, -2.915334737309923874 ) ) ;
#2614=CARTESIAN_POINT ( 'NONE',  ( 20.32896413005680003, 51.77164270246084499, 5.963430220938287007 ) ) ;
#2615=CARTESIAN_POINT ( 'NONE',  ( -2.816281873526471635, 23.91530133659708568, -3.434112377981056508 ) ) ;
#2616=ORIENTED_EDGE ( 'NONE', *, *, #83073, .F. ) ;
#2617=CARTESIAN_POINT ( 'NONE',  ( 17.96484262340118221, 46.18868534415484106, -7.964842623401177768 ) ) ;
#2618=CARTESIAN_POINT ( 'NONE',  ( 17.20831665107776587, 39.13393115100079456, -7.208316651077762316 ) ) ;
#2619=CARTESIAN_POINT ( 'NONE',  ( -2.816281873526471635, 8.915301336597083903, -3.434112377981056508 ) ) ;
#2621=CARTESIAN_POINT ( 'NONE',  ( 12.91533473730993009, 31.60535201082150891, -10.88017736071109987 ) ) ;
#2622=CARTESIAN_POINT ( 'NONE',  ( 15.44008868035555260, 34.73035201082151247, 9.422509992056143702 ) ) ;
#2623=CARTESIAN_POINT ( 'NONE',  ( 13.79529636645030344, 48.26208216824728936, 14.16423886937410614 ) ) ;
#2624=CARTESIAN_POINT ( 'NONE',  ( 0.1532563361054083140, 41.00893115100078745, 1.131784320476157264E-15 ) ) ;
#2625=CARTESIAN_POINT ( 'NONE',  ( 15.44008868035555260, 59.73035201082151247, 9.422509992056143702 ) ) ;
#2627=CARTESIAN_POINT ( 'NONE',  ( 10.00000000000000178, 18.05374883491396787, 14.16423886937410082 ) ) ;
#2635=CARTESIAN_POINT ( 'NONE',  ( 20.36894250292379382, 43.67874883491397497, 10.36894250292379205 ) ) ;
#2636=CARTESIAN_POINT ( 'NONE',  ( -0.3689425029237881626, 42.42874883491396787, 10.36894250292379027 ) ) ;
#2637=CARTESIAN_POINT ( 'NONE',  ( 19.84674366389459621, 23.50893115100078390, 7.409399052514197653E-17 ) ) ;
#2638=CARTESIAN_POINT ( 'NONE',  ( 19.38216949554541202, 20.99863466993042138, 9.382169495545424454 ) ) ;
#2639=CARTESIAN_POINT ( 'NONE',  ( 5.076628168052703671, 61.84226448433412315, 8.527530157486179263 ) ) ;
#2640=CARTESIAN_POINT ( 'NONE',  ( 18.72515096720568906, 36.07228050351032778, -6.500000000000007105 ) ) ;
#2641=CARTESIAN_POINT ( 'NONE',  ( 4.559911319644449179, 53.89701867748817676, 9.422509992056141925 ) ) ;
#2642=CARTESIAN_POINT ( 'NONE',  ( 21.09922568453594849, 31.20696800326375353, 6.408140936763242479 ) ) ;
#2643=CARTESIAN_POINT ( 'NONE',  ( 17.08211943468705840, 40.13708216824731068, -12.26659068614894466 ) ) ;
#2644=VECTOR ( 'NONE', #2309, 1000.000000000000000 ) ;
#2646=CARTESIAN_POINT ( 'NONE',  ( 10.00000000000000000, 66.81368534415484817, -10.88017736071110342 ) ) ;
#2649=CARTESIAN_POINT ( 'NONE',  ( -0.1503990784575403861, 9.248846992468887862, -6.262539305110056631 ) ) ;
#2653=CARTESIAN_POINT ( 'NONE',  ( 10.00000000000000178, 3.053748834913967425, 14.16423886937410082 ) ) ;
#2654=CARTESIAN_POINT ( 'NONE',  ( 20.88017736071110519, 10.56368534415483929, 2.639326808657452039E-16 ) ) ;
#2655=CARTESIAN_POINT ( 'NONE',  ( 15.44008868035555793, 6.397018677488171434, -9.422509992056140149 ) ) ;
#2656=CARTESIAN_POINT ( 'NONE',  ( 14.92337183194729633, 32.67559781766745175, 8.527530157486181039 ) ) ;
#2657=CARTESIAN_POINT ( 'NONE',  ( -2.816281873526471635, 8.915301336597083903, -3.434112377981056508 ) ) ;
#2659=STYLED_ITEM ( 'NONE', ( #90423 ), #60882 ) ;
#2660=VECTOR ( 'NONE', #61914, 1000.000000000000000 ) ;
#2662=CARTESIAN_POINT ( 'NONE',  ( 21.09922568453595559, 17.04030133659708923, -6.408140936763230044 ) ) ;
#2663=ORIENTED_EDGE ( 'NONE', *, *, #69776, .T. ) ;
#2664=CARTESIAN_POINT ( 'NONE',  ( -2.266590686148945544, 47.22041550158063927, 7.082119434687048631 ) ) ;
#2665=ORIENTED_EDGE ( 'NONE', *, *, #18588, .T. ) ;
#2666=CARTESIAN_POINT ( 'NONE',  ( -4.164238869374099039, 56.80374883491397497, 8.674139862899312516E-16 ) ) ;
#2668=CARTESIAN_POINT ( 'NONE',  ( 12.91533473730993009, 36.60535201082151247, -10.88017736071109987 ) ) ;
#2669=CARTESIAN_POINT ( 'NONE',  ( 15.44008868035555260, 34.73035201082151247, 9.422509992056143702 ) ) ;
#2670=CARTESIAN_POINT ( 'NONE',  ( 19.42250999205614193, 40.14701867748817676, 5.440088680355555262 ) ) ;
#2671=CARTESIAN_POINT ( 'NONE',  ( 20.88017736071110164, 60.35535201082151957, 2.915334737309930979 ) ) ;
#2672=CARTESIAN_POINT ( 'NONE',  ( 19.42250999205614548, 30.98035201082150536, -5.440088680355545492 ) ) ;
#2676=CARTESIAN_POINT ( 'NONE',  ( 12.63842701281683922, 14.55059781766744997, -9.846743663894590881 ) ) ;
#2679=CARTESIAN_POINT ( 'NONE',  ( 14.92337183194729988, 39.34226448433412315, -8.527530157486177487 ) ) ;
#2680=CARTESIAN_POINT ( 'NONE',  ( 18.95386800104995828, 53.23810908735728020, -6.499999999999990230 ) ) ;
#2685=CARTESIAN_POINT ( 'NONE',  ( 1.472469842513823179, 61.42559781766745175, 4.923371831947296329 ) ) ;
#2686=CARTESIAN_POINT ( 'NONE',  ( 13.79529636645031943, 50.34541550158064638, -14.16423886937409904 ) ) ;
#2688=ORIENTED_EDGE ( 'NONE', *, *, #38184, .T. ) ;
#2690=CARTESIAN_POINT ( 'NONE',  ( 10.00000000000000000, 24.75893115100078745, -9.846743663894594434 ) ) ;
#2692=CARTESIAN_POINT ( 'NONE',  ( 14.92337183194729988, 59.34226448433412315, -8.527530157486177487 ) ) ;
#2693=CARTESIAN_POINT ( 'NONE',  ( 2.791683348922240793, 1.633931151000784565, 7.208316651077764092 ) ) ;
#2696=CARTESIAN_POINT ( 'NONE',  ( 7.361572987183170547, 57.05059781766744464, 9.846743663894590881 ) ) ;
#2699=ORIENTED_EDGE ( 'NONE', *, *, #38085, .F. ) ;
#2700=( BOUNDED_CURVE ( )  B_SPLINE_CURVE ( 2, ( #6769, #35777, #13774, #66266, #58264, #81279, #28277, #82759, #88780 ),
 .UNSPECIFIED., .F., .F. ) 
 B_SPLINE_CURVE_WITH_KNOTS ( ( 3, 2, 2, 2, 3 ),
 ( 0.4044266512259456214, 0.4047619047619047672, 0.4107142857142856984, 0.4166666666666666297, 0.4170019202026257754 ),
 .UNSPECIFIED. ) 
 CURVE ( )  GEOMETRIC_REPRESENTATION_ITEM ( )  RATIONAL_B_SPLINE_CURVE ( ( 0.9963778908391760503, 0.9980808541467920403, 1.000000000000000000, 0.9659258262890682012, 1.000000000000000000, 0.9659258262890682012, 1.000000000000000000, 0.9980808541467920403, 0.9963778908391760503 ) ) 
 REPRESENTATION_ITEM ( '' )  );
#2701=CARTESIAN_POINT ( 'NONE',  ( 22.26659068614894466, 63.88708216824730357, 7.082119434687054849 ) ) ;
#2703=CARTESIAN_POINT ( 'NONE',  ( -0.8801773607111008646, 38.27201867748816255, 2.915334737309923430 ) ) ;
#2704=CARTESIAN_POINT ( 'NONE',  ( 21.09922568453595559, 12.04030133659708746, -6.408140936763230044 ) ) ;
#2705=CARTESIAN_POINT ( 'NONE',  ( 19.42250999205614548, 65.98035201082151957, -5.440088680355545492 ) ) ;
#2707=CARTESIAN_POINT ( 'NONE',  ( 20.03932841506541962, 45.62161441960500241, -6.397827110479002322 ) ) ;
#2709=CARTESIAN_POINT ( 'NONE',  ( 17.20831665107776587, 47.88393115100078745, 7.208316651077764980 ) ) ;
#2710=CARTESIAN_POINT ( 'NONE',  ( 5.076628168052703671, 6.842264484334118713, 8.527530157486179263 ) ) ;
#2712=CARTESIAN_POINT ( 'NONE',  ( -2.816281873526471635, 3.915301336597087456, -3.434112377981056508 ) ) ;
#2713=CARTESIAN_POINT ( 'NONE',  ( -0.8801773607111008646, 13.27201867748817321, 2.915334737309923430 ) ) ;
#2714=CARTESIAN_POINT ( 'NONE',  ( 17.08211943468705130, 33.47041550158063927, 12.26659068614894998 ) ) ;
#2716=CARTESIAN_POINT ( 'NONE',  ( 17.08211943468705130, 33.47041550158063927, 12.26659068614894998 ) ) ;
#2717=CARTESIAN_POINT ( 'NONE',  ( -4.164238869374099927, 62.01208216824728936, 3.795296366450308767 ) ) ;
#2718=CARTESIAN_POINT ( 'NONE',  ( 0.1532563361054082862, 31.21726448433412315, 2.638427012816831674 ) ) ;
#2720=CARTESIAN_POINT ( 'NONE',  ( 22.81628187352647785, 36.41530133659707502, 3.434112377981063169 ) ) ;
#2721=CARTESIAN_POINT ( 'NONE',  ( 7.084665262690076126, 12.02201867748817143, -10.88017736071110164 ) ) ;
#2723=CARTESIAN_POINT ( 'NONE',  ( 7.361572987183170547, 32.05059781766745175, 9.846743663894590881 ) ) ;
#2724=CARTESIAN_POINT ( 'NONE',  ( 20.88017736071110875, 40.77201867748818387, -2.915334737309920765 ) ) ;
#2725=CARTESIAN_POINT ( 'NONE',  ( 0.6178305044545818747, 3.498634669930420049, -9.382169495545419124 ) ) ;
#2726=CARTESIAN_POINT ( 'NONE',  ( 6.204703633549690345, 27.84541550158063217, 14.16423886937410082 ) ) ;
#2727=CARTESIAN_POINT ( 'NONE',  ( 1.042145700049402990, 44.74216108172000617, -6.499999999999941380 ) ) ;
#2729=CARTESIAN_POINT ( 'NONE',  ( 12.63842701281683034, 22.46726448433411605, 9.846743663894596210 ) ) ;
#2730=CARTESIAN_POINT ( 'NONE',  ( 21.09922568453595559, 52.04030133659708923, -6.408140936763230044 ) ) ;
#2731=CARTESIAN_POINT ( 'NONE',  ( 7.361572987183170547, 52.05059781766745175, 9.846743663894590881 ) ) ;
#2734=CARTESIAN_POINT ( 'NONE',  ( 17.08211943468705130, 63.47041550158063927, 12.26659068614894998 ) ) ;
#2735=CARTESIAN_POINT ( 'NONE',  ( 24.16423886937409904, 9.095415501580633943, 3.795296366450317205 ) ) ;
#2736=CARTESIAN_POINT ( 'NONE',  ( 18.52753015748618282, 3.925597817667451306, -4.923371831947291888 ) ) ;
#2737=CARTESIAN_POINT ( 'NONE',  ( 10.00000000000000000, 54.75893115100078745, -9.846743663894594434 ) ) ;
#2738=CARTESIAN_POINT ( 'NONE',  ( 0.5774900079438590739, 17.64701867748817321, -5.440088680355550821 ) ) ;
#2743=B_SPLINE_CURVE_WITH_KNOTS ( 'NONE', 3,
 ( #67360, #29348, #73371, #12384 ),
 .UNSPECIFIED., .F., .F.,
 ( 4, 4 ),
 ( 4.336808689942017736E-19, 0.002562518741975335079 ),
 .UNSPECIFIED. ) ;
#2745=EDGE_LOOP ( 'NONE', ( #38210, #90387, #43418, #77232 ) ) ;
#2748=CARTESIAN_POINT ( 'NONE',  ( 22.26659068614895176, 14.72041550158063572, -7.082119434687042414 ) ) ;
#2749=CARTESIAN_POINT ( 'NONE',  ( 6.204703633549690345, 0.7620821682473009062, -14.16423886937410259 ) ) ;
#2750=CARTESIAN_POINT ( 'NONE',  ( 0.1532563361054082862, 51.21726448433412315, 2.638427012816831674 ) ) ;
#2751=CARTESIAN_POINT ( 'NONE',  ( 7.361572987183170547, 27.05059781766745175, 9.846743663894590881 ) ) ;
#2752=CARTESIAN_POINT ( 'NONE',  ( -2.816281873526471635, 63.91530133659708923, -3.434112377981056508 ) ) ;
#2753=CARTESIAN_POINT ( 'NONE',  ( 17.96484262340118221, 14.93868534415484106, 7.964842623401181321 ) ) ;
#2754=CARTESIAN_POINT ( 'NONE',  ( 10.00000000000000178, 62.25893115100078745, 9.846743663894594434 ) ) ;
#2756=B_SPLINE_CURVE_WITH_KNOTS ( 'NONE', 3,
 ( #65267, #72769, #81756, #43760, #19297, #4796, #88280, #59254, #49295, #87781 ),
 .UNSPECIFIED., .F., .F.,
 ( 4, 3, 3, 4 ),
 ( 1.474514954580286030E-17, 0.0006253016069560837905, 0.001250604074564929313, 0.002501455912506545670 ),
 .UNSPECIFIED. ) ;
#2758=CARTESIAN_POINT ( 'NONE',  ( 6.204703633549690345, 40.76208216824731778, -14.16423886937410259 ) ) ;
#2759=CARTESIAN_POINT ( 'NONE',  ( 12.91533473730992121, 9.522018677488171434, 10.88017736071110164 ) ) ;
#2761=CARTESIAN_POINT ( 'NONE',  ( 4.999999999999999112, 60.50000000000000000, -6.000000000000000000 ) ) ;
#2762=CARTESIAN_POINT ( 'NONE',  ( 17.96484262340118221, 61.18868534415482685, -7.964842623401177768 ) ) ;
#2763=CARTESIAN_POINT ( 'NONE',  ( 2.791683348922240793, 16.63393115100078745, 7.208316651077764092 ) ) ;
#2766=CYLINDRICAL_SURFACE ( 'NONE', #37890, 0.5000000000000004441 ) ;
#2768=CARTESIAN_POINT ( 'NONE',  ( 10.00000000000000178, 27.25893115100078390, 9.846743663894594434 ) ) ;
#2769=ORIENTED_EDGE ( 'NONE', *, *, #81676, .T. ) ;
#2770=CARTESIAN_POINT ( 'NONE',  ( 10.00000000000000000, 35.55374883491396787, -14.16423886937410082 ) ) ;
#2771=CARTESIAN_POINT ( 'NONE',  ( 19.84674366389459621, 28.50893115100078745, 7.409399052514197653E-17 ) ) ;
#2772=CARTESIAN_POINT ( 'NONE',  ( 2.035157376598822676, 47.43868534415484817, -7.964842623401177768 ) ) ;
#2775=CARTESIAN_POINT ( 'NONE',  ( 0.5774900079438590739, 42.64701867748816966, -5.440088680355550821 ) ) ;
#2777=AXIS2_PLACEMENT_3D ( 'NONE', #29083, #61553, #15591 ) ;
#2780=CARTESIAN_POINT ( 'NONE',  ( -4.164238869374098151, 1.595415501580634388, -3.795296366450310543 ) ) ;
#2783=ORIENTED_EDGE ( 'NONE', *, *, #80156, .F. ) ;
#2784=CARTESIAN_POINT ( 'NONE',  ( 13.43411237798106583, 27.66530133659708568, -12.81628187352647252 ) ) ;
#2786=CARTESIAN_POINT ( 'NONE',  ( 17.20831665107776587, 22.88393115100078745, 7.208316651077764980 ) ) ;
#2787=CARTESIAN_POINT ( 'NONE',  ( 0.5774900079438607392, 3.480352010821504027, 5.440088680355550821 ) ) ;
#2789=CARTESIAN_POINT ( 'NONE',  ( 12.63842701281683922, 34.55059781766745886, -9.846743663894590881 ) ) ;
#2790=STYLED_ITEM ( 'NONE', ( #32997 ), #31045 ) ;
#2791=VECTOR ( 'NONE', #20359, 1000.000000000000000 ) ;
#2793=CARTESIAN_POINT ( 'NONE',  ( 20.88017736071110164, 55.35535201082149825, 2.915334737309930979 ) ) ;
#2795=CARTESIAN_POINT ( 'NONE',  ( 19.42250999205614193, 65.14701867748817676, 5.440088680355555262 ) ) ;
#2797=CARTESIAN_POINT ( 'NONE',  ( 17.20831665107776587, 9.133931151000787452, -7.208316651077762316 ) ) ;
#2798=CARTESIAN_POINT ( 'NONE',  ( 6.565887622018943937, 13.08196800326374998, -12.81628187352647608 ) ) ;
#2800=CARTESIAN_POINT ( 'NONE',  ( 0.1532563361054082862, 41.21726448433411605, 2.638427012816831674 ) ) ;
#2801=CARTESIAN_POINT ( 'NONE',  ( -1.099225684535947600, 64.54030133659709634, 6.408140936763237150 ) ) ;
#2802=CARTESIAN_POINT ( 'NONE',  ( 2.917880565312950480, 10.97041550158063572, -12.26659068614894821 ) ) ;
#2803=CARTESIAN_POINT ( 'NONE',  ( 10.00000000000000178, 32.25893115100078745, 9.846743663894594434 ) ) ;
#2804=CARTESIAN_POINT ( 'NONE',  ( 0.6178305044545818747, 28.49863466993041783, -9.382169495545419124 ) ) ;
#2805=CARTESIAN_POINT ( 'NONE',  ( 2.603489959281115151, 16.58210964143323807, 6.499999999999462652 ) ) ;
#2807=CARTESIAN_POINT ( 'NONE',  ( 17.96484262340118221, 44.93868534415483396, 7.964842623401181321 ) ) ;
#2808=CARTESIAN_POINT ( 'NONE',  ( 10.00000000000000178, 5.373634669930420493, 12.81628187352647608 ) ) ;
#2811=CARTESIAN_POINT ( 'NONE',  ( 14.92337183194729633, 27.67559781766745530, 8.527530157486181039 ) ) ;
#2812=CARTESIAN_POINT ( 'NONE',  ( 4.559911319644449179, 23.89701867748817321, 9.422509992056141925 ) ) ;
#2813=EDGE_CURVE ( 'NONE', #50944, #76767, #55120, .T. ) ;
#2814=CARTESIAN_POINT ( 'NONE',  ( 3.591859063236761518, 29.95696800326375708, 11.09922568453594849 ) ) ;
#2816=CARTESIAN_POINT ( 'NONE',  ( 4.559911319644449179, 17.23035201082150536, -9.422509992056141925 ) ) ;
#2819=CARTESIAN_POINT ( 'NONE',  ( 20.88017736071110164, 55.35535201082149825, 2.915334737309930979 ) ) ;
#2820=CARTESIAN_POINT ( 'NONE',  ( 0.5774900079438590739, 2.647018677488170990, -5.440088680355550821 ) ) ;
#2821=CARTESIAN_POINT ( 'NONE',  ( 1.472469842513823179, 46.42559781766745175, 4.923371831947296329 ) ) ;
#2822=CARTESIAN_POINT ( 'NONE',  ( 20.88017736071110875, 30.77201867748816966, -2.915334737309920765 ) ) ;
#2823=CARTESIAN_POINT ( 'NONE',  ( 17.96484262340118221, 41.18868534415484106, -7.964842623401177768 ) ) ;
#2824=CARTESIAN_POINT ( 'NONE',  ( 2.035157376598824452, 13.68868534415483751, 7.964842623401179544 ) ) ;
#2826=CARTESIAN_POINT ( 'NONE',  ( 14.92337183194729988, 34.34226448433411605, -8.527530157486177487 ) ) ;
#2827=CARTESIAN_POINT ( 'NONE',  ( 1.274849032794280523, 48.57228050351032067, 6.499999999999960032 ) ) ;
#2828=CARTESIAN_POINT ( 'NONE',  ( 19.50000000000000711, 79.40087001978915282, -4.500000000000000888 ) ) ;
#2830=CARTESIAN_POINT ( 'NONE',  ( 13.79529636645030344, 23.26208216824730002, 14.16423886937410614 ) ) ;
#2832=ORIENTED_EDGE ( 'NONE', *, *, #61604, .F. ) ;
#2833=CARTESIAN_POINT ( 'NONE',  ( -4.164238869374098151, 61.59541550158063217, -3.795296366450310543 ) ) ;
#2834=CARTESIAN_POINT ( 'NONE',  ( 19.84674366389459621, 28.50893115100078745, 7.409399052514197653E-17 ) ) ;
#2837=CARTESIAN_POINT ( 'NONE',  ( 7.084665262690076126, 54.10535201082151247, 10.88017736071109987 ) ) ;
#2838=CARTESIAN_POINT ( 'NONE',  ( 19.38216949554541557, 62.24863466993041072, -9.382169495545420901 ) ) ;
#2840=CARTESIAN_POINT ( 'NONE',  ( 7.084665262690076126, 37.02201867748817676, -10.88017736071110164 ) ) ;
#2842=CARTESIAN_POINT ( 'NONE',  ( -1.099225684535947600, 8.706968003263753531, -6.408140936763238038 ) ) ;
#2844=CARTESIAN_POINT ( 'NONE',  ( 0.1532563361054083140, 11.00893115100078568, 1.131784320476157264E-15 ) ) ;
#2846=CARTESIAN_POINT ( 'NONE',  ( 5.076628168052704559, 0.1755978176674514724, -8.527530157486179263 ) ) ;
#2847=LINE ( 'NONE', #10328, #31688 ) ;
#2848=CARTESIAN_POINT ( 'NONE',  ( 10.00000000000000178, 53.05374883491396787, 14.16423886937410082 ) ) ;
#2849=CARTESIAN_POINT ( 'NONE',  ( -0.3689425029237881626, 22.42874883491397142, 10.36894250292379027 ) ) ;
#2850=AXIS2_PLACEMENT_3D ( 'NONE', #93611, #55110, #25148 ) ;
#2851=CARTESIAN_POINT ( 'NONE',  ( 19.42250999205614548, 45.98035201082150536, -5.440088680355545492 ) ) ;
#2854=CARTESIAN_POINT ( 'NONE',  ( 0.1532563361054083140, 6.008931151000784787, 1.131784320476157264E-15 ) ) ;
#2856=CARTESIAN_POINT ( 'NONE',  ( 0.1532563361054083140, 21.00893115100078745, 1.131784320476157264E-15 ) ) ;
#2857=CARTESIAN_POINT ( 'NONE',  ( 10.00000000000000178, 22.25893115100078745, 9.846743663894594434 ) ) ;
#2858=CARTESIAN_POINT ( 'NONE',  ( 0.1532563361054082862, 46.21726448433411605, 2.638427012816831674 ) ) ;
#2860=CARTESIAN_POINT ( 'NONE',  ( 2.035157376598824452, 28.68868534415484106, 7.964842623401179544 ) ) ;
#2862=VECTOR ( 'NONE', #79215, 1000.000000000000000 ) ;
#2863=CARTESIAN_POINT ( 'NONE',  ( 10.00000000000000178, 35.37363466993042493, 12.81628187352647608 ) ) ;
#2864=CARTESIAN_POINT ( 'NONE',  ( 4.559911319644449179, 53.89701867748817676, 9.422509992056141925 ) ) ;
#2865=CARTESIAN_POINT ( 'NONE',  ( 14.92337183194729633, 22.67559781766745175, 8.527530157486181039 ) ) ;
#2866=CARTESIAN_POINT ( 'NONE',  ( 24.16423886937409904, 44.09541550158063927, 3.795296366450317205 ) ) ;
#2867=CARTESIAN_POINT ( 'NONE',  ( 17.20831665107776587, 17.88393115100078745, 7.208316651077764980 ) ) ;
#2871=CARTESIAN_POINT ( 'NONE',  ( 17.20831665107776587, 52.88393115100078035, 7.208316651077764980 ) ) ;
#2872=CARTESIAN_POINT ( 'NONE',  ( 18.52753015748618282, 48.92559781766745886, -4.923371831947291888 ) ) ;
#2873=CARTESIAN_POINT ( 'NONE',  ( -4.164238869374099927, 7.012082168247302683, 3.795296366450308767 ) ) ;
#2874=CARTESIAN_POINT ( 'NONE',  ( 10.00000000000000178, 38.05374883491396787, 14.16423886937410082 ) ) ;
#2875=CARTESIAN_POINT ( 'NONE',  ( 0.1532563361054082862, 26.21726448433411605, 2.638427012816831674 ) ) ;
#2876=CARTESIAN_POINT ( 'NONE',  ( 20.88017736071110164, 25.35535201082150891, 2.915334737309930979 ) ) ;
#2877=CARTESIAN_POINT ( 'NONE',  ( 20.88017736071110164, 45.35535201082149115, 2.915334737309930979 ) ) ;
#2878=CARTESIAN_POINT ( 'NONE',  ( 12.91533473730993009, 31.60535201082150891, -10.88017736071109987 ) ) ;
#2880=CARTESIAN_POINT ( 'NONE',  ( 21.09922568453595559, 32.04030133659708923, -6.408140936763230044 ) ) ;
#2881=CARTESIAN_POINT ( 'NONE',  ( 20.88017736071110875, 55.77201867748816966, -2.915334737309920765 ) ) ;
#2882=ORIENTED_EDGE ( 'NONE', *, *, #91334, .T. ) ;
#2883=CARTESIAN_POINT ( 'NONE',  ( -0.8801773607110991993, 62.85535201082150536, -2.915334737309923874 ) ) ;
#2885=CARTESIAN_POINT ( 'NONE',  ( 15.44008868035555260, 59.73035201082151247, 9.422509992056143702 ) ) ;
#2886=CARTESIAN_POINT ( 'NONE',  ( 0.5774900079438590739, 2.647018677488170990, -5.440088680355550821 ) ) ;
#2889=CARTESIAN_POINT ( 'NONE',  ( 10.00000000000000000, 65.55374883491396076, -14.16423886937410082 ) ) ;
#2890=CARTESIAN_POINT ( 'NONE',  ( 1.472469842513823179, 15.59226448433411960, -4.923371831947296329 ) ) ;
#2892=CARTESIAN_POINT ( 'NONE',  ( 20.36894250292379382, 3.678748834913967869, 10.36894250292379205 ) ) ;
#2893=CARTESIAN_POINT ( 'NONE',  ( 1.472469842513823179, 0.5922644843341181575, -4.923371831947296329 ) ) ;
#2894=CARTESIAN_POINT ( 'NONE',  ( 10.00000000000000000, 6.813685344154838397, -10.88017736071110342 ) ) ;
#2895=CARTESIAN_POINT ( 'NONE',  ( 18.52753015748617571, 48.09226448433412315, 4.923371831947298993 ) ) ;
#2896=ORIENTED_EDGE ( 'NONE', *, *, #42226, .T. ) ;
#2897=ADVANCED_FACE ( 'NONE', ( #61715 ), #32200, .T. ) ;
#2898=CARTESIAN_POINT ( 'NONE',  ( 19.84674366389459266, 53.30059781766744464, 2.638427012816836559 ) ) ;
#2900=CARTESIAN_POINT ( 'NONE',  ( 12.91533473730992121, 59.52201867748816966, 10.88017736071110164 ) ) ;
#2901=CARTESIAN_POINT ( 'NONE',  ( 12.63842701281683034, 57.46726448433411605, 9.846743663894596210 ) ) ;
#2903=CARTESIAN_POINT ( 'NONE',  ( -0.8801773607111008646, 53.27201867748816966, 2.915334737309923430 ) ) ;
#2904=CARTESIAN_POINT ( 'NONE',  ( 17.96484262340118221, 9.938685344154839285, 7.964842623401181321 ) ) ;
#2906=CARTESIAN_POINT ( 'NONE',  ( 13.43411237798106583, 42.66530133659707502, -12.81628187352647252 ) ) ;
#2908=EDGE_LOOP ( 'NONE', ( #82923, #13926, #7024, #19525 ) ) ;
#2909=CARTESIAN_POINT ( 'NONE',  ( 3.591859063236761518, 34.95696800326375353, 11.09922568453594849 ) ) ;
#2910=CARTESIAN_POINT ( 'NONE',  ( -0.8801773607111008646, 33.27201867748817676, 2.915334737309923430 ) ) ;
#2914=CARTESIAN_POINT ( 'NONE',  ( 2.791683348922237240, 10.38393115100078390, -7.208316651077763204 ) ) ;
#2915=CARTESIAN_POINT ( 'NONE',  ( -1.099225684535947600, -0.4596986634029132657, 6.408140936763237150 ) ) ;
#2916=CARTESIAN_POINT ( 'NONE',  ( 10.00000000000000000, 9.758931151000785675, -9.846743663894594434 ) ) ;
#2917=CARTESIAN_POINT ( 'NONE',  ( 19.84674366389459266, 48.30059781766745175, 2.638427012816836559 ) ) ;
#2920=CARTESIAN_POINT ( 'NONE',  ( 19.84674366389459266, 43.30059781766744464, 2.638427012816836559 ) ) ;
#2923=CARTESIAN_POINT ( 'NONE',  ( 5.076628168052704559, 25.17559781766745175, -8.527530157486179263 ) ) ;
#2927=CARTESIAN_POINT ( 'NONE',  ( 10.00000000000000000, 64.75893115100078035, -9.846743663894594434 ) ) ;
#2928=ORIENTED_EDGE ( 'NONE', *, *, #29948, .T. ) ;
#2930=CARTESIAN_POINT ( 'NONE',  ( 0.8952175423694859191, 7.601608292538859502, -5.990408912944324094 ) ) ;
#2931=CARTESIAN_POINT ( 'NONE',  ( 13.43411237798106583, 22.66530133659708923, -12.81628187352647252 ) ) ;
#2932=CARTESIAN_POINT ( 'NONE',  ( 18.52753015748617571, 38.09226448433412315, 4.923371831947298993 ) ) ;
#2933=CARTESIAN_POINT ( 'NONE',  ( 13.99999999999999822, 61.50000000000000711, -6.500000000000000888 ) ) ;
#2934=CARTESIAN_POINT ( 'NONE',  ( -4.164238869374098151, 41.59541550158061796, -3.795296366450310543 ) ) ;
#2935=CARTESIAN_POINT ( 'NONE',  ( 19.84674366389459621, 18.50893115100078745, 7.409399052514197653E-17 ) ) ;
#2936=CARTESIAN_POINT ( 'NONE',  ( -0.1503990784575328643, 40.12777174578613426, 6.262539305110068177 ) ) ;
#2937=CARTESIAN_POINT ( 'NONE',  ( 6.204703633549690345, 45.76208216824729647, -14.16423886937410259 ) ) ;
#2938=CARTESIAN_POINT ( 'NONE',  ( 1.472469842513823179, 60.59226448433412315, -4.923371831947296329 ) ) ;
#2939=CARTESIAN_POINT ( 'NONE',  ( 10.00000000000000178, 68.05374883491397497, 14.16423886937410082 ) ) ;
#2940=CARTESIAN_POINT ( 'NONE',  ( 17.08211943468705840, 20.13708216824730357, -12.26659068614894466 ) ) ;
#2941=CARTESIAN_POINT ( 'NONE',  ( 13.79529636645031943, 40.34541550158063217, -14.16423886937409904 ) ) ;
#2942=FILL_AREA_STYLE ('',( #40929 ) ) ;
#2943=CARTESIAN_POINT ( 'NONE',  ( 1.274849032794317383, 27.55509018479935790, -6.500000000000010658 ) ) ;
#2944=CARTESIAN_POINT ( 'NONE',  ( 19.84674366389459266, 53.71726448433411605, -2.638427012816827677 ) ) ;
#2945=CARTESIAN_POINT ( 'NONE',  ( 20.88017736071110519, 30.56368534415484106, 2.639326808657452039E-16 ) ) ;
#2949=CARTESIAN_POINT ( 'NONE',  ( 16.40814093676324603, 62.45696800326376064, -11.09922568453594671 ) ) ;
#2951=CARTESIAN_POINT ( 'NONE',  ( 7.361572987183169658, 54.96726448433413026, -9.846743663894592657 ) ) ;
#2952=CARTESIAN_POINT ( 'NONE',  ( 5.076628168052703671, 61.84226448433412315, 8.527530157486179263 ) ) ;
#2953=VERTEX_POINT ( 'NONE', #77220 ) ;
#2954=CARTESIAN_POINT ( 'NONE',  ( -2.266590686148945544, 21.38708216824730357, -7.082119434687050408 ) ) ;
#2955=LINE ( 'NONE', #77940, #13527 ) ;
#2958=CARTESIAN_POINT ( 'NONE',  ( 12.91533473730992121, 9.522018677488171434, 10.88017736071110164 ) ) ;
#2959=CARTESIAN_POINT ( 'NONE',  ( 22.81628187352647785, 31.41530133659709279, 3.434112377981063169 ) ) ;
#2961=CARTESIAN_POINT ( 'NONE',  ( 10.00000000000000178, 17.25893115100078745, 9.846743663894594434 ) ) ;
#2963=CARTESIAN_POINT ( 'NONE',  ( -0.1503990784575403861, 9.248846992468887862, -6.262539305110056631 ) ) ;
#2965=CARTESIAN_POINT ( 'NONE',  ( 19.42250999205614548, 15.98035201082150714, -5.440088680355545492 ) ) ;
#2967=CARTESIAN_POINT ( 'NONE',  ( 2.035157376598822676, 42.43868534415483396, -7.964842623401177768 ) ) ;
#2968=CARTESIAN_POINT ( 'NONE',  ( 0.5774900079438590739, 32.64701867748816966, -5.440088680355550821 ) ) ;
#2969=CARTESIAN_POINT ( 'NONE',  ( 6.565887622018943937, 5.165301336597086568, 12.81628187352647430 ) ) ;
#2970=CARTESIAN_POINT ( 'NONE',  ( 18.52753015748618282, 63.92559781766745886, -4.923371831947291888 ) ) ;
#2971=CARTESIAN_POINT ( 'NONE',  ( -45.72097266785441150, 104.7202616008577678, -5.189651444387643586 ) ) ;
#2972=CARTESIAN_POINT ( 'NONE',  ( 7.361572987183169658, 9.967264484334119601, -9.846743663894592657 ) ) ;
#2973=EDGE_CURVE ( 'NONE', #97455, #75793, #44509, .T. ) ;
#2975=CARTESIAN_POINT ( 'NONE',  ( -0.8801773607111009756, 28.06368534415484106, 1.068504757029289695E-15 ) ) ;
#2976=CARTESIAN_POINT ( 'NONE',  ( 22.81628187352647785, 26.62363466993042138, 6.195893100308588602E-16 ) ) ;
#2977=CARTESIAN_POINT ( 'NONE',  ( 19.72487221294570858, 36.86607318730075633, 6.500000000000000888 ) ) ;
#2978=ADVANCED_FACE ( 'NONE', ( #1258 ), #62208, .T. ) ;
#2979=CARTESIAN_POINT ( 'NONE',  ( 14.92337183194729988, 64.34226448433412315, -8.527530157486177487 ) ) ;
#2980=CARTESIAN_POINT ( 'NONE',  ( -0.8801773607111009756, 68.06368534415484817, 1.068504757029289695E-15 ) ) ;
#2982=CARTESIAN_POINT ( 'NONE',  ( 12.63842701281683922, 9.550597817667449974, -9.846743663894590881 ) ) ;
#2983=CARTESIAN_POINT ( 'NONE',  ( 6.565887622018943937, 30.16530133659708568, 12.81628187352647430 ) ) ;
#2984=CARTESIAN_POINT ( 'NONE',  ( 12.91533473730993009, 56.60535201082151247, -10.88017736071109987 ) ) ;
#2988=CARTESIAN_POINT ( 'NONE',  ( 17.96484262340118221, 9.938685344154837509, 7.964842623401181321 ) ) ;
#2990=CARTESIAN_POINT ( 'NONE',  ( -1.099225684535947600, 58.70696800326375353, -6.408140936763238038 ) ) ;
#2991=CARTESIAN_POINT ( 'NONE',  ( 5.076628168052704559, 20.17559781766745175, -8.527530157486179263 ) ) ;
#2993=CARTESIAN_POINT ( 'NONE',  ( -0.8801773607110991993, 7.855352010821504471, -2.915334737309923874 ) ) ;
#2994=CARTESIAN_POINT ( 'NONE',  ( 14.92337183194729988, 24.34226448433411960, -8.527530157486177487 ) ) ;
#2995=CARTESIAN_POINT ( 'NONE',  ( -4.164238869374099039, 51.80374883491396787, 8.674139862899312516E-16 ) ) ;
#2996=ORIENTED_EDGE ( 'NONE', *, *, #76081, .F. ) ;
#2997=CARTESIAN_POINT ( 'NONE',  ( 7.084665262690076126, 12.02201867748817143, -10.88017736071110164 ) ) ;
#2999=CARTESIAN_POINT ( 'NONE',  ( 12.91533473730993009, 16.60535201082150891, -10.88017736071109987 ) ) ;
#3003=LINE ( 'NONE', #65925, #79619 ) ;
#3004=CARTESIAN_POINT ( 'NONE',  ( -0.8801773607111008646, 28.27201867748817321, 2.915334737309923430 ) ) ;
#3005=CARTESIAN_POINT ( 'NONE',  ( 0.1532563361054100626, 60.80059781766744464, -2.638427012816831230 ) ) ;
#3006=CARTESIAN_POINT ( 'NONE',  ( 6.565887622018943937, 48.08196800326375353, -12.81628187352647608 ) ) ;
#3008=CARTESIAN_POINT ( 'NONE',  ( -2.266590686148945544, 21.38708216824730357, -7.082119434687050408 ) ) ;
#3009=CARTESIAN_POINT ( 'NONE',  ( 15.44008868035555793, 36.39701867748816966, -9.422509992056140149 ) ) ;
#3010=CARTESIAN_POINT ( 'NONE',  ( 7.084665262690076126, 22.02201867748817321, -10.88017736071110164 ) ) ;
#3011=CARTESIAN_POINT ( 'NONE',  ( 12.63842701281683922, 49.55059781766744464, -9.846743663894590881 ) ) ;
#3013=CARTESIAN_POINT ( 'NONE',  ( 19.84674366389459266, 33.71726448433410894, -2.638427012816827677 ) ) ;
#3014=EDGE_CURVE ( 'NONE', #74488, #1418, #76428, .T. ) ;
#3015=CARTESIAN_POINT ( 'NONE',  ( 7.361572987183170547, 12.05059781766744997, 9.846743663894590881 ) ) ;
#3017=ORIENTED_EDGE ( 'NONE', *, *, #18470, .F. ) ;
#3019=CARTESIAN_POINT ( 'NONE',  ( 20.88017736071110519, 15.56368534415483751, 2.639326808657452039E-16 ) ) ;
#3020=CARTESIAN_POINT ( 'NONE',  ( 0.1532563361054100626, 5.800597817667452638, -2.638427012816831230 ) ) ;
#3021=CARTESIAN_POINT ( 'NONE',  ( 5.076628168052703671, 66.84226448433412315, 8.527530157486179263 ) ) ;
#3022=CARTESIAN_POINT ( 'NONE',  ( 10.00000000000000000, 41.81368534415484106, -10.88017736071110342 ) ) ;
#3023=CARTESIAN_POINT ( 'NONE',  ( 2.035157376598824452, 48.68868534415483396, 7.964842623401179544 ) ) ;
#3024=CARTESIAN_POINT ( 'NONE',  ( 2.035157376598824452, 23.68868534415484461, 7.964842623401179544 ) ) ;
#3025=CARTESIAN_POINT ( 'NONE',  ( 22.81628187352647785, 46.62363466993041783, 6.195893100308588602E-16 ) ) ;
#3026=CARTESIAN_POINT ( 'NONE',  ( 10.00000000000000178, 28.05374883491396787, 14.16423886937410082 ) ) ;
#3027=LINE ( 'NONE', #49469, #4344 ) ;
#3028=CARTESIAN_POINT ( 'NONE',  ( 13.43411237798106583, 57.66530133659708923, -12.81628187352647252 ) ) ;
#3029=ORIENTED_EDGE ( 'NONE', *, *, #67068, .F. ) ;
#3030=CARTESIAN_POINT ( 'NONE',  ( 10.00000000000000178, 52.25893115100078745, 9.846743663894594434 ) ) ;
#3031=CARTESIAN_POINT ( 'NONE',  ( 4.559911319644449179, 32.23035201082150536, -9.422509992056141925 ) ) ;
#3032=ORIENTED_EDGE ( 'NONE', *, *, #52405, .T. ) ;
#3033=CARTESIAN_POINT ( 'NONE',  ( 14.92337183194729633, 2.675597817667451750, 8.527530157486181039 ) ) ;
#3035=VECTOR ( 'NONE', #87176, 1000.000000000000000 ) ;
#3036=CARTESIAN_POINT ( 'NONE',  ( 12.63842701281683034, 22.46726448433411605, 9.846743663894596210 ) ) ;
#3037=CARTESIAN_POINT ( 'NONE',  ( 1.472469842513823179, 1.425597817667451528, 4.923371831947296329 ) ) ;
#3038=CARTESIAN_POINT ( 'NONE',  ( 18.52753015748618282, 3.925597817667451306, -4.923371831947291888 ) ) ;
#3039=CARTESIAN_POINT ( 'NONE',  ( 2.035157376598824452, 58.68868534415482685, 7.964842623401179544 ) ) ;
#3040=CARTESIAN_POINT ( 'NONE',  ( 15.44008868035555793, 66.39701867748817676, -9.422509992056140149 ) ) ;
#3041=ORIENTED_EDGE ( 'NONE', *, *, #39008, .T. ) ;
#3043=CARTESIAN_POINT ( 'NONE',  ( 17.20831665107776587, 52.88393115100078035, 7.208316651077764980 ) ) ;
#3044=VERTEX_POINT ( 'NONE', #33669 ) ;
#3046=CARTESIAN_POINT ( 'NONE',  ( -4.164238869374099927, 7.012082168247302683, 3.795296366450308767 ) ) ;
#3047=CARTESIAN_POINT ( 'NONE',  ( 3.059999999999993392, 76.92054879330447648, -9.500000000000000000 ) ) ;
#3048=CARTESIAN_POINT ( 'NONE',  ( 6.204703633549690345, 7.845415501580634832, 14.16423886937410082 ) ) ;
#3049=CARTESIAN_POINT ( 'NONE',  ( 6.204703633549690345, 32.84541550158063927, 14.16423886937410082 ) ) ;
#3051=DIRECTION ( 'NONE',  ( 0.000000000000000000, -1.000000000000000000, 0.000000000000000000 ) ) ;
#3052=CARTESIAN_POINT ( 'NONE',  ( 17.08211943468705840, 5.137082168247300906, -12.26659068614894466 ) ) ;
#3053=CARTESIAN_POINT ( 'NONE',  ( 10.00000000000000000, 26.81368534415484106, -10.88017736071110342 ) ) ;
#3054=FILL_AREA_STYLE_COLOUR ( '', #32366 ) ;
#3056=CARTESIAN_POINT ( 'NONE',  ( 19.84674366389459266, 18.30059781766745175, 2.638427012816836559 ) ) ;
#3057=CARTESIAN_POINT ( 'NONE',  ( 17.96484262340118221, 56.18868534415484817, -7.964842623401177768 ) ) ;
#3058=CARTESIAN_POINT ( 'NONE',  ( 5.076628168052704559, 20.17559781766745175, -8.527530157486179263 ) ) ;
#3059=CARTESIAN_POINT ( 'NONE',  ( 22.81628187352647785, 46.62363466993041783, 6.195893100308588602E-16 ) ) ;
#3060=CARTESIAN_POINT ( 'NONE',  ( 7.361572987183169658, 39.96726448433411605, -9.846743663894592657 ) ) ;
#3061=EDGE_CURVE ( 'NONE', #29028, #87186, #28152, .T. ) ;
#3062=MECHANICAL_DESIGN_GEOMETRIC_PRESENTATION_REPRESENTATION('',(#65331),#34994);
#3063=CARTESIAN_POINT ( 'NONE',  ( 0.1957200283969089960, 25.25733960839544423, 6.499999999999985789 ) ) ;
#3064=CARTESIAN_POINT ( 'NONE',  ( -0.8801773607111008646, 53.27201867748816966, 2.915334737309923430 ) ) ;
#3065=CARTESIAN_POINT ( 'NONE',  ( 3.591859063236761518, 29.95696800326375708, 11.09922568453594849 ) ) ;
#3066=COLOUR_RGB ( '', 0.31764706, 0.68627451, 0.89019608) ;
#3068=CARTESIAN_POINT ( 'NONE',  ( 17.20831665107776587, 27.88393115100078390, 7.208316651077764980 ) ) ;
#3069=CARTESIAN_POINT ( 'NONE',  ( 6.204703633549690345, 15.76208216824730179, -14.16423886937410259 ) ) ;
#3070=CARTESIAN_POINT ( 'NONE',  ( 15.44008868035555793, 36.39701867748816966, -9.422509992056140149 ) ) ;
#3071=CARTESIAN_POINT ( 'NONE',  ( 2.917880565312950480, 35.97041550158063217, -12.26659068614894821 ) ) ;
#3072=CARTESIAN_POINT ( 'NONE',  ( 5.076628168052703671, 51.84226448433412315, 8.527530157486179263 ) ) ;
#3073=CARTESIAN_POINT ( 'NONE',  ( 10.00000000000000178, 12.25893115100078568, 9.846743663894594434 ) ) ;
#3074=CARTESIAN_POINT ( 'NONE',  ( 6.565887622018943937, 48.08196800326375353, -12.81628187352647608 ) ) ;
#3076=CARTESIAN_POINT ( 'NONE',  ( 15.44008868035555793, 41.39701867748817676, -9.422509992056140149 ) ) ;
#3077=CARTESIAN_POINT ( 'NONE',  ( 3.591859063236763294, 18.29030133659708568, -11.09922568453595026 ) ) ;
#3078=CARTESIAN_POINT ( 'NONE',  ( 0.1532563361054082862, 46.21726448433411605, 2.638427012816831674 ) ) ;
#3081=CARTESIAN_POINT ( 'NONE',  ( 7.084665262690076126, 64.10535201082150536, 10.88017736071109987 ) ) ;
#3086=CARTESIAN_POINT ( 'NONE',  ( 10.00000000000000178, 59.31368534415484106, 10.88017736071110342 ) ) ;
#3087=CARTESIAN_POINT ( 'NONE',  ( 7.084665262690076126, 62.02201867748816966, -10.88017736071110164 ) ) ;
#3091=CARTESIAN_POINT ( 'NONE',  ( 17.20831665107776587, 22.88393115100078745, 7.208316651077764980 ) ) ;
#3092=CARTESIAN_POINT ( 'NONE',  ( 10.00000000000000000, 16.81368534415483751, -10.88017736071110342 ) ) ;
#3093=ADVANCED_FACE ( 'NONE', ( #27655 ), #42188, .T. ) ;
#3094=CARTESIAN_POINT ( 'NONE',  ( 22.81628187352647785, 1.415301336597087012, 3.434112377981063169 ) ) ;
#3095=CARTESIAN_POINT ( 'NONE',  ( -0.8801773607111008646, 23.27201867748817676, 2.915334737309923430 ) ) ;
#3098=CARTESIAN_POINT ( 'NONE',  ( 13.43411237798105340, 20.58196800326374643, 12.81628187352647963 ) ) ;
#3100=CARTESIAN_POINT ( 'NONE',  ( 4.559911319644449179, 52.23035201082151247, -9.422509992056141925 ) ) ;
#3101=CARTESIAN_POINT ( 'NONE',  ( 10.00000000000000178, 47.25893115100078745, 9.846743663894594434 ) ) ;
#3102=CARTESIAN_POINT ( 'NONE',  ( 13.43411237798105340, 25.58196800326374998, 12.81628187352647963 ) ) ;
#3103=CARTESIAN_POINT ( 'NONE',  ( 20.88017736071110164, 25.35535201082150891, 2.915334737309930979 ) ) ;
#3104=CARTESIAN_POINT ( 'NONE',  ( 2.035157376598824452, 38.68868534415483396, 7.964842623401179544 ) ) ;
#3105=CARTESIAN_POINT ( 'NONE',  ( 10.00000000000000178, 53.05374883491396787, 14.16423886937410082 ) ) ;
#3106=CARTESIAN_POINT ( 'NONE',  ( 0.1532563361054082862, 41.21726448433411605, 2.638427012816831674 ) ) ;
#3108=CARTESIAN_POINT ( 'NONE',  ( 10.00000000000000000, 9.758931151000785675, -9.846743663894594434 ) ) ;
#3109=CARTESIAN_POINT ( 'NONE',  ( 20.88017736071110519, 45.56368534415484106, 2.639326808657452039E-16 ) ) ;
#3111=CARTESIAN_POINT ( 'NONE',  ( -2.266590686148945544, 16.38708216824730357, -7.082119434687050408 ) ) ;
#3113=CARTESIAN_POINT ( 'NONE',  ( 1.472469842513823179, 66.42559781766745175, 4.923371831947296329 ) ) ;
#3115=CARTESIAN_POINT ( 'NONE',  ( 24.16423886937409904, 44.09541550158063927, 3.795296366450317205 ) ) ;
#3116=CARTESIAN_POINT ( 'NONE',  ( 20.36894250292379738, 44.92874883491396787, -10.36894250292379027 ) ) ;
#3117=CARTESIAN_POINT ( 'NONE',  ( 0.1532563361054100626, 15.80059781766745353, -2.638427012816831230 ) ) ;
#3120=CARTESIAN_POINT ( 'NONE',  ( -1.099225684535947600, 34.54030133659708923, 6.408140936763237150 ) ) ;
#3121=CARTESIAN_POINT ( 'NONE',  ( -4.164238869374099927, 42.01208216824728936, 3.795296366450308767 ) ) ;
#3122=EDGE_CURVE ( 'NONE', #26466, #76186, #72652, .T. ) ;
#3123=SURFACE_SIDE_STYLE ('',( #64567 ) ) ;
#3126=CARTESIAN_POINT ( 'NONE',  ( 14.92337183194729633, 17.67559781766745175, 8.527530157486181039 ) ) ;
#3127=LINE ( 'NONE', #32614, #20601 ) ;
#3129=CARTESIAN_POINT ( 'NONE',  ( 2.035157376598822676, 12.43868534415483751, -7.964842623401177768 ) ) ;
#3130=CARTESIAN_POINT ( 'NONE',  ( -0.8801773607110991993, 7.855352010821506248, -2.915334737309923874 ) ) ;
#3131=CARTESIAN_POINT ( 'NONE',  ( 0.1532563361054083140, 56.00893115100078745, 1.131784320476157264E-15 ) ) ;
#3132=CARTESIAN_POINT ( 'NONE',  ( 21.09922568453595559, 7.040301336597086568, -6.408140936763230044 ) ) ;
#3134=CARTESIAN_POINT ( 'NONE',  ( -2.816281873526473856, 14.12363466993041961, 9.499525473075851096E-16 ) ) ;
#3136=CARTESIAN_POINT ( 'NONE',  ( -2.266590686148945544, 57.22041550158063217, 7.082119434687048631 ) ) ;
#3138=CARTESIAN_POINT ( 'NONE',  ( -4.164238869374099039, 51.80374883491396787, 8.674139862899312516E-16 ) ) ;
#3139=ORIENTED_EDGE ( 'NONE', *, *, #48244, .T. ) ;
#3140=CARTESIAN_POINT ( 'NONE',  ( 2.035157376598824452, 33.68868534415484106, 7.964842623401179544 ) ) ;
#3142=CARTESIAN_POINT ( 'NONE',  ( 12.91533473730992121, 39.52201867748817676, 10.88017736071110164 ) ) ;
#3143=CARTESIAN_POINT ( 'NONE',  ( -0.8801773607111008646, 63.27201867748817676, 2.915334737309923430 ) ) ;
#3144=CARTESIAN_POINT ( 'NONE',  ( 7.084665262690076126, 32.02201867748816966, -10.88017736071110164 ) ) ;
#3146=CARTESIAN_POINT ( 'NONE',  ( 0.2751277870542911952, 33.21833443783938122, 6.499999999999992006 ) ) ;
#3147=CARTESIAN_POINT ( 'NONE',  ( 14.92337183194729633, 12.67559781766745353, 8.527530157486181039 ) ) ;
#3148=ORIENTED_EDGE ( 'NONE', *, *, #73132, .F. ) ;
#3150=CARTESIAN_POINT ( 'NONE',  ( 18.52753015748618282, 43.92559781766745175, -4.923371831947291888 ) ) ;
#3152=CARTESIAN_POINT ( 'NONE',  ( -1.099225684535947600, 48.70696800326375353, -6.408140936763238038 ) ) ;
#3153=( LENGTH_UNIT ( ) NAMED_UNIT ( * ) SI_UNIT ( .MILLI., .METRE. ) );
#3156=CARTESIAN_POINT ( 'NONE',  ( -44.76764016918902200, 105.1727941590568349, 5.383302543209945945 ) ) ;
#3158=CARTESIAN_POINT ( 'NONE',  ( -4.164238869374099039, 51.80374883491396787, 8.674139862899312516E-16 ) ) ;
#3159=CARTESIAN_POINT ( 'NONE',  ( 19.05866839779138999, 5.955083851089585600, -6.499999999999964473 ) ) ;
#3162=CARTESIAN_POINT ( 'NONE',  ( 14.92337183194729633, 27.67559781766745530, 8.527530157486181039 ) ) ;
#3164=CARTESIAN_POINT ( 'NONE',  ( 6.565887622018943937, 3.081968003263753531, -12.81628187352647608 ) ) ;
#3165=CARTESIAN_POINT ( 'NONE',  ( -0.8801773607111009756, 68.06368534415484817, 1.068504757029289695E-15 ) ) ;
#3166=EDGE_CURVE ( 'NONE', #66548, #85989, #98203, .T. ) ;
#3167=CARTESIAN_POINT ( 'NONE',  ( 0.1532563361054082862, 56.21726448433411605, 2.638427012816831674 ) ) ;
#3168=CARTESIAN_POINT ( 'NONE',  ( -0.1491070598754174470, 61.94583914210339515, 5.000000000000000000 ) ) ;
#3171=CARTESIAN_POINT ( 'NONE',  ( 10.00000000000000000, 1.813685344154838175, -10.88017736071110342 ) ) ;
#3173=CARTESIAN_POINT ( 'NONE',  ( 0.5774900079438590739, 42.64701867748816966, -5.440088680355550821 ) ) ;
#3174=CARTESIAN_POINT ( 'NONE',  ( 16.40814093676323893, 15.79030133659708746, 11.09922568453595026 ) ) ;
#3178=CARTESIAN_POINT ( 'NONE',  ( -0.1503990784575247319, 67.22266099184919597, -6.262539305110083276 ) ) ;
#3179=CARTESIAN_POINT ( 'NONE',  ( 2.791683348922237240, 45.38393115100079456, -7.208316651077763204 ) ) ;
#3180=CARTESIAN_POINT ( 'NONE',  ( 0.1532563361054100626, 0.8005978176674514168, -2.638427012816831230 ) ) ;
#3182=CARTESIAN_POINT ( 'NONE',  ( 19.38216949554541202, 10.99863466993042138, 9.382169495545424454 ) ) ;
#3184=CARTESIAN_POINT ( 'NONE',  ( 12.91533473730992121, 29.52201867748817321, 10.88017736071110164 ) ) ;
#3187=CARTESIAN_POINT ( 'NONE',  ( -4.164238869374098151, 36.59541550158063217, -3.795296366450310543 ) ) ;
#3188=CARTESIAN_POINT ( 'NONE',  ( 2.917880565312950480, 30.97041550158063572, -12.26659068614894821 ) ) ;
#3189=CARTESIAN_POINT ( 'NONE',  ( 10.00000000000000000, 6.813685344154838397, -10.88017736071110342 ) ) ;
#3190=CARTESIAN_POINT ( 'NONE',  ( 17.20831665107776587, 37.88393115100078745, 7.208316651077764980 ) ) ;
#3191=CARTESIAN_POINT ( 'NONE',  ( -1.099225684535947600, 39.54030133659708923, 6.408140936763237150 ) ) ;
#3192=CARTESIAN_POINT ( 'NONE',  ( 4.559911319644449179, 12.23035201082150536, -9.422509992056141925 ) ) ;
#3194=CARTESIAN_POINT ( 'NONE',  ( 10.00000000000000178, 32.25893115100078745, 9.846743663894594434 ) ) ;
#3196=CARTESIAN_POINT ( 'NONE',  ( 2.035157376598822676, 37.43868534415484106, -7.964842623401177768 ) ) ;
#3197=CARTESIAN_POINT ( 'NONE',  ( 10.00000000000000000, 2.873634669930420049, -12.81628187352647608 ) ) ;
#3198=CARTESIAN_POINT ( 'NONE',  ( 13.79529636645031943, 20.34541550158063572, -14.16423886937409904 ) ) ;
#3202=CARTESIAN_POINT ( 'NONE',  ( 12.63842701281683922, 24.55059781766745175, -9.846743663894590881 ) ) ;
#3203=CARTESIAN_POINT ( 'NONE',  ( 10.00000000000000178, 50.37363466993042493, 12.81628187352647608 ) ) ;
#3204=CARTESIAN_POINT ( 'NONE',  ( 5.076628168052704559, 60.17559781766745175, -8.527530157486179263 ) ) ;
#3209=CARTESIAN_POINT ( 'NONE',  ( 20.88017736071110875, 5.772018677488170546, -2.915334737309920765 ) ) ;
#3210=CARTESIAN_POINT ( 'NONE',  ( 24.16423886937410614, 9.512082168247301794, -3.795296366450302550 ) ) ;
#3211=CARTESIAN_POINT ( 'NONE',  ( 0.1532563361054082862, 1.217264484334117824, 2.638427012816831674 ) ) ;
#3212=CARTESIAN_POINT ( 'NONE',  ( 19.84674366389459266, 48.71726448433413026, -2.638427012816827677 ) ) ;
#3213=CARTESIAN_POINT ( 'NONE',  ( 10.00000000000000000, 26.81368534415484106, -10.88017736071110342 ) ) ;
#3215=CARTESIAN_POINT ( 'NONE',  ( 19.84674366389459266, 58.30059781766745886, 2.638427012816836559 ) ) ;
#3221=CARTESIAN_POINT ( 'NONE',  ( 2.917880565312950480, 5.970415501580634832, -12.26659068614894821 ) ) ;
#3222=CARTESIAN_POINT ( 'NONE',  ( 2.917880565312948704, 42.63708216824729647, 12.26659068614894643 ) ) ;
#3223=CARTESIAN_POINT ( 'NONE',  ( 17.20831665107776587, 54.13393115100079456, -7.208316651077762316 ) ) ;
#3224=CARTESIAN_POINT ( 'NONE',  ( 10.00000000000000000, 39.75893115100078745, -9.846743663894594434 ) ) ;
#3226=CARTESIAN_POINT ( 'NONE',  ( 12.91533473730993009, 26.60535201082150536, -10.88017736071109987 ) ) ;
#3227=CARTESIAN_POINT ( 'NONE',  ( 0.1532563361054082862, 66.21726448433413736, 2.638427012816831674 ) ) ;
#3228=CARTESIAN_POINT ( 'NONE',  ( 6.204703633549690345, 37.84541550158063927, 14.16423886937410082 ) ) ;
#3229=CARTESIAN_POINT ( 'NONE',  ( 19.42250999205614548, 10.98035201082150536, -5.440088680355545492 ) ) ;
#3230=CARTESIAN_POINT ( 'NONE',  ( 1.472469842513823179, 65.59226448433412315, -4.923371831947296329 ) ) ;
#3231=CARTESIAN_POINT ( 'NONE',  ( -0.8801773607111008646, 58.27201867748816966, 2.915334737309923430 ) ) ;
#3232=CARTESIAN_POINT ( 'NONE',  ( 12.63842701281683922, 24.55059781766745175, -9.846743663894590881 ) ) ;
#3234=EDGE_CURVE ( 'NONE', #1418, #39614, #35148, .T. ) ;
#3238=CARTESIAN_POINT ( 'NONE',  ( 1.472469842513823179, 21.42559781766745175, 4.923371831947296329 ) ) ;
#3240=CARTESIAN_POINT ( 'NONE',  ( 24.16423886937409904, 29.09541550158063572, 3.795296366450317205 ) ) ;
#3241=CARTESIAN_POINT ( 'NONE',  ( 12.63842701281683922, 29.55059781766745175, -9.846743663894590881 ) ) ;
#3242=CARTESIAN_POINT ( 'NONE',  ( 4.559911319644449179, 53.89701867748817676, 9.422509992056141925 ) ) ;
#3244=CARTESIAN_POINT ( 'NONE',  ( 15.44008868035555793, 41.39701867748817676, -9.422509992056140149 ) ) ;
#3245=CARTESIAN_POINT ( 'NONE',  ( 1.472469842513823179, 50.59226448433411605, -4.923371831947296329 ) ) ;
#3248=CARTESIAN_POINT ( 'NONE',  ( 7.084665262690076126, 42.02201867748816966, -10.88017736071110164 ) ) ;
#3249=CARTESIAN_POINT ( 'NONE',  ( -4.164238869374099927, 7.012082168247302683, 3.795296366450308767 ) ) ;
#3251=CARTESIAN_POINT ( 'NONE',  ( 22.81628187352647785, 31.62363466993042138, 6.195893100308588602E-16 ) ) ;
#3252=CARTESIAN_POINT ( 'NONE',  ( 1.472469842513823179, 26.42559781766745175, 4.923371831947296329 ) ) ;
#3254=CARTESIAN_POINT ( 'NONE',  ( 3.591859063236763294, 43.29030133659708923, -11.09922568453595026 ) ) ;
#3256=CARTESIAN_POINT ( 'NONE',  ( 19.84674366389459266, 28.71726448433411960, -2.638427012816827677 ) ) ;
#3257=CARTESIAN_POINT ( 'NONE',  ( 7.084665262690076126, 64.10535201082150536, 10.88017736071109987 ) ) ;
#3259=B_SPLINE_CURVE_WITH_KNOTS ( 'NONE', 3,
 ( #18118, #59547, #98575, #43068 ),
 .UNSPECIFIED., .F., .F.,
 ( 4, 4 ),
 ( 0.0004294207726287377542, 0.0005403323854458763099 ),
 .UNSPECIFIED. ) ;
#3263=CARTESIAN_POINT ( 'NONE',  ( 5.076628168052703671, 6.842264484334118713, 8.527530157486179263 ) ) ;
#3264=CARTESIAN_POINT ( 'NONE',  ( -2.816281873526473856, 14.33196800326375531, 3.434112377981055619 ) ) ;
#3268=CARTESIAN_POINT ( 'NONE',  ( 7.361572987183169658, 49.96726448433410894, -9.846743663894592657 ) ) ;
#3270=CARTESIAN_POINT ( 'NONE',  ( 24.16423886937409904, 9.095415501580633943, 3.795296366450317205 ) ) ;
#3271=CARTESIAN_POINT ( 'NONE',  ( 5.076628168052704559, 35.17559781766745175, -8.527530157486179263 ) ) ;
#3272=CARTESIAN_POINT ( 'NONE',  ( 10.00000000000000000, 32.87363466993042493, -12.81628187352647608 ) ) ;
#3275=CARTESIAN_POINT ( 'NONE',  ( 7.084665262690076126, 54.10535201082151247, 10.88017736071109987 ) ) ;
#3276=CARTESIAN_POINT ( 'NONE',  ( 21.09922568453595559, 7.040301336597086568, -6.408140936763230044 ) ) ;
#3278=CARTESIAN_POINT ( 'NONE',  ( 0.1532563361054082862, 21.21726448433412315, 2.638427012816831674 ) ) ;
#3279=CARTESIAN_POINT ( 'NONE',  ( -0.8801773607110991993, 22.85535201082150181, -2.915334737309923874 ) ) ;
#3281=CARTESIAN_POINT ( 'NONE',  ( 21.09922568453594849, 36.20696800326375353, 6.408140936763242479 ) ) ;
#3282=CARTESIAN_POINT ( 'NONE',  ( 19.84674366389459266, 23.30059781766745530, 2.638427012816836559 ) ) ;
#3285=CARTESIAN_POINT ( 'NONE',  ( 20.88017736071110164, 35.35535201082150536, 2.915334737309930979 ) ) ;
#3286=CARTESIAN_POINT ( 'NONE',  ( 2.035157376598822676, 62.43868534415483396, -7.964842623401177768 ) ) ;
#3287=CARTESIAN_POINT ( 'NONE',  ( -0.8801773607110991993, 2.855352010821504471, -2.915334737309923874 ) ) ;
#3288=CARTESIAN_POINT ( 'NONE',  ( 10.00000000000000178, 47.25893115100078745, 9.846743663894594434 ) ) ;
#3289=CARTESIAN_POINT ( 'NONE',  ( 17.96484262340118221, 24.93868534415484461, 7.964842623401181321 ) ) ;
#3290=PRESENTATION_STYLE_ASSIGNMENT (( #70815 ) ) ;
#3291=CARTESIAN_POINT ( 'NONE',  ( 2.035157376598824452, 43.68868534415484106, 7.964842623401179544 ) ) ;
#3292=CARTESIAN_POINT ( 'NONE',  ( 2.035157376598824452, 8.688685344154839285, 7.964842623401179544 ) ) ;
#3295=CARTESIAN_POINT ( 'NONE',  ( 12.63842701281683034, 42.46726448433412315, 9.846743663894596210 ) ) ;
#3296=CARTESIAN_POINT ( 'NONE',  ( 2.917880565312950480, 50.97041550158064638, -12.26659068614894821 ) ) ;
#3298=CARTESIAN_POINT ( 'NONE',  ( 24.16423886937410614, 19.51208216824729647, -3.795296366450302550 ) ) ;
#3303=CARTESIAN_POINT ( 'NONE',  ( 24.16423886937410614, 64.51208216824728936, -3.795296366450302550 ) ) ;
#3304=CARTESIAN_POINT ( 'NONE',  ( 17.20831665107776587, 34.13393115100078745, -7.208316651077762316 ) ) ;
#3306=CARTESIAN_POINT ( 'NONE',  ( 0.5774900079438590739, 57.64701867748817676, -5.440088680355550821 ) ) ;
#3307=CARTESIAN_POINT ( 'NONE',  ( -2.816281873526473856, 59.33196800326374643, 3.434112377981055619 ) ) ;
#3308=CARTESIAN_POINT ( 'NONE',  ( 15.44008868035555260, 24.73035201082150891, 9.422509992056143702 ) ) ;
#3309=CARTESIAN_POINT ( 'NONE',  ( 10.00000000000000178, 65.37363466993042493, 12.81628187352647608 ) ) ;
#3310=CARTESIAN_POINT ( 'NONE',  ( 13.43411237798105340, 15.58196800326374998, 12.81628187352647963 ) ) ;
#3311=CARTESIAN_POINT ( 'NONE',  ( 18.52753015748617571, 13.09226448433411960, 4.923371831947298993 ) ) ;
#3313=ORIENTED_EDGE ( 'NONE', *, *, #81525, .T. ) ;
#3315=CARTESIAN_POINT ( 'NONE',  ( 22.26659068614895176, 64.72041550158064638, -7.082119434687042414 ) ) ;
#3316=CARTESIAN_POINT ( 'NONE',  ( -4.164238869374098151, 21.59541550158063217, -3.795296366450310543 ) ) ;
#3317=CARTESIAN_POINT ( 'NONE',  ( 20.88017736071110164, 30.35535201082151247, 2.915334737309930979 ) ) ;
#3318=CARTESIAN_POINT ( 'NONE',  ( 17.96484262340118221, 44.93868534415483396, 7.964842623401181321 ) ) ;
#3321=CARTESIAN_POINT ( 'NONE',  ( 19.84674366389459621, 13.50893115100078568, 7.409399052514197653E-17 ) ) ;
#3322=FILL_AREA_STYLE ('',( #11307 ) ) ;
#3323=CARTESIAN_POINT ( 'NONE',  ( 5.076628168052703671, 21.84226448433411960, 8.527530157486179263 ) ) ;
#3326=CARTESIAN_POINT ( 'NONE',  ( 10.00000000000000000, 19.75893115100078390, -9.846743663894594434 ) ) ;
#3327=CARTESIAN_POINT ( 'NONE',  ( 19.84674366389459621, 53.50893115100078745, 7.409399052514197653E-17 ) ) ;
#3328=AXIS2_PLACEMENT_3D ( 'NONE', #4753, #95750, #57240 ) ;
#3329=CARTESIAN_POINT ( 'NONE',  ( 19.42250999205614548, 25.98035201082150891, -5.440088680355545492 ) ) ;
#3330=B_SPLINE_CURVE_WITH_KNOTS ( 'NONE', 3,
 ( #81763, #82258, #72294, #50278, #5302, #43767 ),
 .UNSPECIFIED., .F., .F.,
 ( 4, 2, 4 ),
 ( 0.000000000000000000, 0.0002626113303185885592, 0.0005252226606371771184 ),
 .UNSPECIFIED. ) ;
#3332=CARTESIAN_POINT ( 'NONE',  ( 10.00000000000000000, 47.87363466993042493, -12.81628187352647608 ) ) ;
#3333=CARTESIAN_POINT ( 'NONE',  ( -0.8801773607111008646, 48.27201867748816966, 2.915334737309923430 ) ) ;
#3334=CARTESIAN_POINT ( 'NONE',  ( 19.84674366389459266, 28.71726448433411960, -2.638427012816827677 ) ) ;
#3335=CARTESIAN_POINT ( 'NONE',  ( -4.164238869374098151, 41.59541550158061796, -3.795296366450310543 ) ) ;
#3336=CARTESIAN_POINT ( 'NONE',  ( 17.20831665107776587, 24.13393115100078035, -7.208316651077762316 ) ) ;
#3338=CARTESIAN_POINT ( 'NONE',  ( 12.63842701281683922, 64.55059781766745175, -9.846743663894590881 ) ) ;
#3339=CARTESIAN_POINT ( 'NONE',  ( 22.26659068614895176, 9.720415501580633943, -7.082119434687042414 ) ) ;
#3340=CARTESIAN_POINT ( 'NONE',  ( 13.79529636645031943, 25.34541550158063572, -14.16423886937409904 ) ) ;
#3341=CARTESIAN_POINT ( 'NONE',  ( 10.00000000000000178, 32.25893115100078745, 9.846743663894594434 ) ) ;
#3343=CARTESIAN_POINT ( 'NONE',  ( 20.88017736071110875, 20.77201867748816611, -2.915334737309920765 ) ) ;
#3344=CARTESIAN_POINT ( 'NONE',  ( 2.035157376598824452, 48.68868534415483396, 7.964842623401179544 ) ) ;
#3345=CARTESIAN_POINT ( 'NONE',  ( 7.084665262690076126, 44.10535201082151247, 10.88017736071109987 ) ) ;
#3347=CARTESIAN_POINT ( 'NONE',  ( 6.565887622018943937, 45.16530133659708923, 12.81628187352647430 ) ) ;
#3348=CARTESIAN_POINT ( 'NONE',  ( 20.88017736071110519, 50.56368534415484106, 2.639326808657452039E-16 ) ) ;
#3351=EDGE_CURVE ( 'NONE', #107, #61640, #69627, .T. ) ;
#3352=CARTESIAN_POINT ( 'NONE',  ( 20.88017736071110164, 65.35535201082150536, 2.915334737309930979 ) ) ;
#3353=ORIENTED_EDGE ( 'NONE', *, *, #39054, .T. ) ;
#3354=CARTESIAN_POINT ( 'NONE',  ( 2.035157376598824452, 63.68868534415484106, 7.964842623401179544 ) ) ;
#3355=CARTESIAN_POINT ( 'NONE',  ( 0.5774900079438607392, 3.480352010821504027, 5.440088680355550821 ) ) ;
#3356=CARTESIAN_POINT ( 'NONE',  ( 19.10478245763052740, 40.10160829253885595, 5.990408912944308994 ) ) ;
#3358=CARTESIAN_POINT ( 'NONE',  ( 19.42250999205614548, 5.980352010821504471, -5.440088680355545492 ) ) ;
#3359=CARTESIAN_POINT ( 'NONE',  ( 12.63842701281683034, 7.467264484334118713, 9.846743663894596210 ) ) ;
#3360=CARTESIAN_POINT ( 'NONE',  ( 13.79529636645031943, 10.34541550158063394, -14.16423886937409904 ) ) ;
#3361=CARTESIAN_POINT ( 'NONE',  ( 1.472469842513823179, 10.59226448433411782, -4.923371831947296329 ) ) ;
#3362=CARTESIAN_POINT ( 'NONE',  ( 7.084665262690076126, 12.02201867748817143, -10.88017736071110164 ) ) ;
#3363=CARTESIAN_POINT ( 'NONE',  ( 1.472469842513823179, 50.59226448433411605, -4.923371831947296329 ) ) ;
#3364=B_SPLINE_CURVE_WITH_KNOTS ( 'NONE', 3,
 ( #26424, #35900, #18945, #49421, #79924, #11432, #41952, #87914, #15801, #44427 ),
 .UNSPECIFIED., .F., .F.,
 ( 4, 3, 3, 4 ),
 ( 0.000000000000000000, 0.0006253016069560996199, 0.001250604074564917820, 0.002501455912506563017 ),
 .UNSPECIFIED. ) ;
#3367=CARTESIAN_POINT ( 'NONE',  ( 1.472469842513823179, 46.42559781766745175, 4.923371831947296329 ) ) ;
#3368=EDGE_LOOP ( 'NONE', ( #67416, #80626, #82600, #56636 ) ) ;
#3369=CARTESIAN_POINT ( 'NONE',  ( 18.29284471827483571, 30.40189080397291832, -6.500000000000035527 ) ) ;
#3370=CARTESIAN_POINT ( 'NONE',  ( 0.5774900079438607392, 53.48035201082151247, 5.440088680355550821 ) ) ;
#3371=CARTESIAN_POINT ( 'NONE',  ( 1.472469842513823179, 50.59226448433411605, -4.923371831947296329 ) ) ;
#3372=CARTESIAN_POINT ( 'NONE',  ( 22.81628187352647785, 31.62363466993042138, 6.195893100308588602E-16 ) ) ;
#3373=FILL_AREA_STYLE_COLOUR ( '', #62700 ) ;
#3374=CARTESIAN_POINT ( 'NONE',  ( 2.035157376598824452, 58.68868534415482685, 7.964842623401179544 ) ) ;
#3375=CARTESIAN_POINT ( 'NONE',  ( 4.559911319644449179, 2.230352010821504916, -9.422509992056141925 ) ) ;
#3376=CIRCLE ( 'NONE', #83233, 1.000000000000000888 ) ;
#3377=CARTESIAN_POINT ( 'NONE',  ( 22.81628187352647785, 41.62363466993042493, 6.195893100308588602E-16 ) ) ;
#3380=CARTESIAN_POINT ( 'NONE',  ( 16.40814093676324603, 22.45696800326375353, -11.09922568453594671 ) ) ;
#3381=CARTESIAN_POINT ( 'NONE',  ( 7.084665262690076126, 39.10535201082150536, 10.88017736071109987 ) ) ;
#3383=CARTESIAN_POINT ( 'NONE',  ( 12.63842701281683034, 7.467264484334118713, 9.846743663894596210 ) ) ;
#3384=CARTESIAN_POINT ( 'NONE',  ( -2.816281873526473856, -0.6680319967362464695, 3.434112377981055619 ) ) ;
#3385=CARTESIAN_POINT ( 'NONE',  ( 17.20831665107776587, 17.88393115100078745, 7.208316651077764980 ) ) ;
#3386=CARTESIAN_POINT ( 'NONE',  ( 14.92337183194729633, 52.67559781766745175, 8.527530157486181039 ) ) ;
#3388=SURFACE_SIDE_STYLE ('',( #25896 ) ) ;
#3390=CARTESIAN_POINT ( 'NONE',  ( 2.791683348922240793, 41.63393115100078745, 7.208316651077764092 ) ) ;
#3392=CARTESIAN_POINT ( 'NONE',  ( -29.94000000000000838, 92.00000000000000000, -10.09898361729590199 ) ) ;
#3393=CARTESIAN_POINT ( 'NONE',  ( 12.63842701281683922, 24.55059781766745175, -9.846743663894590881 ) ) ;
#3394=CARTESIAN_POINT ( 'NONE',  ( 7.361572987183169658, -0.03273551566588185635, -9.846743663894592657 ) ) ;
#3397=CARTESIAN_POINT ( 'NONE',  ( 19.84674366389459266, 63.71726448433412315, -2.638427012816827677 ) ) ;
#3400=CARTESIAN_POINT ( 'NONE',  ( 3.591859063236763294, 63.29030133659708923, -11.09922568453595026 ) ) ;
#3402=CARTESIAN_POINT ( 'NONE',  ( 22.81628187352648496, 21.83196800326374643, -3.434112377981050290 ) ) ;
#3403=CARTESIAN_POINT ( 'NONE',  ( 5.076628168052703671, 41.84226448433411605, 8.527530157486179263 ) ) ;
#3406=CARTESIAN_POINT ( 'NONE',  ( -4.164238869374098151, 61.59541550158063217, -3.795296366450310543 ) ) ;
#3408=CARTESIAN_POINT ( 'NONE',  ( 18.52753015748618282, 13.92559781766745175, -4.923371831947291888 ) ) ;
#3412=CARTESIAN_POINT ( 'NONE',  ( 13.79529636645030344, 63.26208216824730357, 14.16423886937410614 ) ) ;
#3413=CARTESIAN_POINT ( 'NONE',  ( 18.52753015748617571, 58.09226448433411605, 4.923371831947298993 ) ) ;
#3414=CARTESIAN_POINT ( 'NONE',  ( 17.96484262340118221, 9.938685344154839285, 7.964842623401181321 ) ) ;
#3415=CARTESIAN_POINT ( 'NONE',  ( -0.3689425029237881626, 37.42874883491396787, 10.36894250292379027 ) ) ;
#3416=CARTESIAN_POINT ( 'NONE',  ( 13.79529636645031943, 45.34541550158062506, -14.16423886937409904 ) ) ;
#3420=CARTESIAN_POINT ( 'NONE',  ( 19.84674366389459266, 53.30059781766744464, 2.638427012816836559 ) ) ;
#3421=B_SPLINE_CURVE_WITH_KNOTS ( 'NONE', 3,
 ( #98692, #60649, #91148, #22674, #13678, #53153 ),
 .UNSPECIFIED., .F., .F.,
 ( 4, 2, 4 ),
 ( 0.000000000000000000, 0.0002565770811490986373, 0.0005131541622981972747 ),
 .UNSPECIFIED. ) ;
#3423=CARTESIAN_POINT ( 'NONE',  ( 17.96484262340118221, 31.18868534415483751, -7.964842623401177768 ) ) ;
#3425=CARTESIAN_POINT ( 'NONE',  ( 19.84674366389459621, 48.50893115100078745, 7.409399052514197653E-17 ) ) ;
#3428=CARTESIAN_POINT ( 'NONE',  ( 0.1532563361054083140, 56.00893115100078745, 1.131784320476157264E-15 ) ) ;
#3429=CARTESIAN_POINT ( 'NONE',  ( 0.1532563361054082862, 66.21726448433413736, 2.638427012816831674 ) ) ;
#3432=CARTESIAN_POINT ( 'NONE',  ( 22.26659068614894466, 28.88708216824730357, 7.082119434687054849 ) ) ;
#3433=( NAMED_UNIT ( * ) PLANE_ANGLE_UNIT ( ) SI_UNIT ( $, .RADIAN. ) );
#3435=CARTESIAN_POINT ( 'NONE',  ( 18.72515096720571037, 45.05509018479935435, 6.499999999999982236 ) ) ;
#3436=CARTESIAN_POINT ( 'NONE',  ( -0.8801773607111009756, 23.06368534415484106, 1.068504757029289695E-15 ) ) ;
#3437=CARTESIAN_POINT ( 'NONE',  ( -1.099225684535947600, 29.54030133659708923, 6.408140936763237150 ) ) ;
#3438=DIRECTION ( 'NONE',  ( 0.000000000000000000, -1.000000000000000000, 0.000000000000000000 ) ) ;
#3439=CARTESIAN_POINT ( 'NONE',  ( 1.472469842513823179, 5.592264484334118713, -4.923371831947296329 ) ) ;
#3442=CARTESIAN_POINT ( 'NONE',  ( 22.26659068614894466, 28.88708216824730357, 7.082119434687054849 ) ) ;
#3445=CARTESIAN_POINT ( 'NONE',  ( 10.00000000000000000, 6.813685344154838397, -10.88017736071110342 ) ) ;
#3446=CYLINDRICAL_SURFACE ( 'NONE', #79772, 0.5000000000000004441 ) ;
#3448=CARTESIAN_POINT ( 'NONE',  ( 2.035157376598824452, 33.68868534415484106, 7.964842623401179544 ) ) ;
#3449=CARTESIAN_POINT ( 'NONE',  ( 4.559911319644449179, 42.23035201082151247, -9.422509992056141925 ) ) ;
#3450=CARTESIAN_POINT ( 'NONE',  ( -2.816281873526473856, -0.6680319967362464695, 3.434112377981055619 ) ) ;
#3451=CARTESIAN_POINT ( 'NONE',  ( 18.52753015748617571, 63.09226448433412315, 4.923371831947298993 ) ) ;
#3452=LINE ( 'NONE', #71931, #75477 ) ;
#3453=CARTESIAN_POINT ( 'NONE',  ( 19.84674366389459621, 3.508931151000785231, 7.409399052514197653E-17 ) ) ;
#3455=B_SPLINE_CURVE_WITH_KNOTS ( 'NONE', 3,
 ( #53189, #83196, #82201, #37705, #68690, #98728, #30670, #30178 ),
 .UNSPECIFIED., .F., .F.,
 ( 4, 2, 2, 4 ),
 ( 0.000000000000000000, 0.004806130321901048823, 0.007209195482851595352, 0.009612260643802141014 ),
 .UNSPECIFIED. ) ;
#3457=CARTESIAN_POINT ( 'NONE',  ( 0.5774900079438590739, 47.64701867748817676, -5.440088680355550821 ) ) ;
#3459=COLOUR_RGB ( '', 0.40784314, 0.44705882, 0.49803922) ;
#3460=CARTESIAN_POINT ( 'NONE',  ( 21.09922568453594849, 11.20696800326375531, 6.408140936763242479 ) ) ;
#3461=CARTESIAN_POINT ( 'NONE',  ( 12.91533473730992121, 59.52201867748816966, 10.88017736071110164 ) ) ;
#3462=CARTESIAN_POINT ( 'NONE',  ( 0.1532563361054082862, 26.21726448433411605, 2.638427012816831674 ) ) ;
#3463=CARTESIAN_POINT ( 'NONE',  ( 22.81628187352648496, 31.83196800326375353, -3.434112377981050290 ) ) ;
#3464=CARTESIAN_POINT ( 'NONE',  ( 14.92337183194729633, 7.675597817667451750, 8.527530157486181039 ) ) ;
#3467=CARTESIAN_POINT ( 'NONE',  ( 0.8952175423695025724, 48.52576239577081907, 5.990408912944351627 ) ) ;
#3469=CARTESIAN_POINT ( 'NONE',  ( 0.5774900079438607392, 8.480352010821505360, 5.440088680355550821 ) ) ;
#3470=CARTESIAN_POINT ( 'NONE',  ( -1.099225684535947600, 63.70696800326376774, -6.408140936763238038 ) ) ;
#3471=CARTESIAN_POINT ( 'NONE',  ( 18.52753015748617571, 13.09226448433411960, 4.923371831947298993 ) ) ;
#3472=PRESENTATION_STYLE_ASSIGNMENT (( #40980 ) ) ;
#3473=CARTESIAN_POINT ( 'NONE',  ( -0.8801773607110991993, 7.855352010821506248, -2.915334737309923874 ) ) ;
#3474=EDGE_LOOP ( 'NONE', ( #29821, #1595, #46121, #23054 ) ) ;
#3475=CARTESIAN_POINT ( 'NONE',  ( 7.084665262690076126, 17.02201867748817676, -10.88017736071110164 ) ) ;
#3477=CARTESIAN_POINT ( 'NONE',  ( -0.8801773607111008646, 18.27201867748817321, 2.915334737309923430 ) ) ;
#3478=CARTESIAN_POINT ( 'NONE',  ( 2.603489959281581889, 30.43575266056827999, -6.499999999999995559 ) ) ;
#3481=CARTESIAN_POINT ( 'NONE',  ( 10.00000000000000178, 62.25893115100078745, 9.846743663894594434 ) ) ;
#3482=CARTESIAN_POINT ( 'NONE',  ( 20.88017736071110519, 20.56368534415484106, 2.639326808657452039E-16 ) ) ;
#3483=CARTESIAN_POINT ( 'NONE',  ( 0.1532563361054100626, 50.80059781766745175, -2.638427012816831230 ) ) ;
#3484=STYLED_ITEM ( 'NONE', ( #72806 ), #32638 ) ;
#3486=CARTESIAN_POINT ( 'NONE',  ( -1.926860441876562025, 4.479976035794175360, -3.195792623639529761 ) ) ;
#3487=CARTESIAN_POINT ( 'NONE',  ( 24.16423886937410614, 29.30374883491396787, 8.672049930838204340E-16 ) ) ;
#3488=CARTESIAN_POINT ( 'NONE',  ( 2.035157376598824452, 38.68868534415483396, 7.964842623401179544 ) ) ;
#3489=CARTESIAN_POINT ( 'NONE',  ( 10.00000000000000000, 11.81368534415483751, -10.88017736071110342 ) ) ;
#3490=CARTESIAN_POINT ( 'NONE',  ( 2.791683348922237240, 60.38393115100078745, -7.208316651077763204 ) ) ;
#3492=CARTESIAN_POINT ( 'NONE',  ( 12.63842701281683034, 42.46726448433412315, 9.846743663894596210 ) ) ;
#3494=CARTESIAN_POINT ( 'NONE',  ( 17.20831665107776587, 12.88393115100078390, 7.208316651077764980 ) ) ;
#3498=CARTESIAN_POINT ( 'NONE',  ( 12.91533473730993009, 11.60535201082150536, -10.88017736071109987 ) ) ;
#3499=CARTESIAN_POINT ( 'NONE',  ( 12.63842701281683034, 12.46726448433411782, 9.846743663894596210 ) ) ;
#3500=CARTESIAN_POINT ( 'NONE',  ( 14.92337183194729988, 64.34226448433412315, -8.527530157486177487 ) ) ;
#3501=CARTESIAN_POINT ( 'NONE',  ( 19.42250999205614193, 45.14701867748817676, 5.440088680355555262 ) ) ;
#3502=CARTESIAN_POINT ( 'NONE',  ( 4.559911319644449179, 23.89701867748817321, 9.422509992056141925 ) ) ;
#3503=CARTESIAN_POINT ( 'NONE',  ( 10.00000000000000000, 42.87363466993042493, -12.81628187352647608 ) ) ;
#3504=CARTESIAN_POINT ( 'NONE',  ( 2.917880565312948704, 37.63708216824731068, 12.26659068614894643 ) ) ;
#3506=CARTESIAN_POINT ( 'NONE',  ( -1.099225684535947600, 64.54030133659709634, 6.408140936763237150 ) ) ;
#3508=CARTESIAN_POINT ( 'NONE',  ( 12.63842701281683034, 52.46726448433413026, 9.846743663894596210 ) ) ;
#3510=CARTESIAN_POINT ( 'NONE',  ( 2.035157376598824452, 33.68868534415484106, 7.964842623401179544 ) ) ;
#3512=CARTESIAN_POINT ( 'NONE',  ( 17.20831665107776587, 4.133931151000785675, -7.208316651077762316 ) ) ;
#3514=CARTESIAN_POINT ( 'NONE',  ( 18.52753015748617571, 8.092264484334117824, 4.923371831947298993 ) ) ;
#3515=CARTESIAN_POINT ( 'NONE',  ( 10.00000000000000000, 24.75893115100078745, -9.846743663894594434 ) ) ;
#3517=CARTESIAN_POINT ( 'NONE',  ( 7.361572987183169658, 4.967264484334119601, -9.846743663894592657 ) ) ;
#3518=CARTESIAN_POINT ( 'NONE',  ( 10.00000000000000000, -0.2410688489992152128, -9.846743663894594434 ) ) ;
#3519=CARTESIAN_POINT ( 'NONE',  ( 12.91533473730993009, 61.60535201082150536, -10.88017736071109987 ) ) ;
#3521=CARTESIAN_POINT ( 'NONE',  ( 20.88017736071110164, 60.35535201082151957, 2.915334737309930979 ) ) ;
#3522=CARTESIAN_POINT ( 'NONE',  ( 2.791683348922240793, 16.63393115100078745, 7.208316651077764092 ) ) ;
#3524=EDGE_CURVE ( 'NONE', #29181, #68203, #24300, .T. ) ;
#3527=CARTESIAN_POINT ( 'NONE',  ( 7.361572987183169658, 49.96726448433410894, -9.846743663894592657 ) ) ;
#3530=CARTESIAN_POINT ( 'NONE',  ( 13.79529636645030344, 3.262082168247301350, 14.16423886937410614 ) ) ;
#3531=EDGE_CURVE ( 'NONE', #34568, #83562, #70881, .T. ) ;
#3532=( BOUNDED_SURFACE ( )  B_SPLINE_SURFACE ( 1, 2, ( 
 ( #81264, #58756, #97280, #12763, #21263, #31705, #75737, #22263, #38250, #98276, #37270, #61227, #45743, #38735, #91732, #7256, #760, #85219, #23254, #31211, #47198, #46236, #8717, #67757, #37760, #68256, #30224, #83244, #39235, #8241, #14767, #53729, #54697, #54209, #16723, #84726, #84246, #7756, #29733, #60241, #90736, #62198, #45240, #69236, #91228, #98776, #69723, #61707, #52737, #60729, #15750, #92221, #92706, #24231, #6753, #22752, #68741, #53235, #23749, #273, #30718, #15262, #1249, #83740, #76239, #76722, #16231, #46711, #77211, #39725, #48677, #86201, #70218, #33180, #95157, #64646, #78195, #40206, #79180, #48185, #41694, #25708, #47703, #93193, #10207, #1737, #9212, #63673, #17713, #10695, #94177, #9708, #71687, #57160, #56200, #3198, #19171, #18197, #79677, #32191, #70712, #2230, #32689, #55193, #11174, #41207, #85710, #86692, #26666, #26185, #87658, #56677, #33662, #78697, #62693, #24720, #17224, #3691, #63184, #64158, #93691, #25225, #72164, #94676, #55705, #40700, #87166, #18692, #77701, #34152, #71203, #2726, #49175, #34650, #89141, #27646, #58132, #35140, #5659, #80662, #65640, #65146, #35646, #89634, #66644, #11669, #66133, #96164, #42182, #50654, #21146, #59125, #57653, #19662, #96664, #88642, #36137, #43143, #88150, #28144, #58642, #20651, #51646, #81142, #27151, #13138, #12645, #97168, #50152, #73634, #4179, #12157, #20149, #5160, #51142, #81631, #43636, #74122, #28636, #42662, #82126, #49651, #80159, #95666, #73138, #72646, #4678, #41357, #86343, #54840, #48331, #24864, #24375, #63328, #71348, #85854, #17366, #3335, #79328, #17846, #91510, #78835, #10346, #7537, #47835, #25362, #83518, #10838, #30498, #2866, #78338, #2374, #71826, #85353, #64304, #32340, #15037, #22533, #93342, #16867, #63812, #76009, #51, #40846, #33317, #33797, #61000, #38028, #9353, #53004, #68520, #9859, #40358, #94322, #70859, #47341, #32829, #45509, #25843, #55347, #93836, #55848, #56341, #86835, #18339, #48819, #77844, #39858, #70364, #1881, #62842, #57795, #80309, #73294, #43289, #57305, #34293, #81293, #35792, #19801, #87314, #96318, #42317, #3834, #13290, #58278, #26811, #20304, #95816, #95307, #35292, #73784, #88303, #50292, #74269, #51290, #88796, #64790, #50804, #12789, #79814, #80805, #27793, #56816, #81775, #87797, #18832, #94815, #58785, #26318, #72304, #65785, #4818, #5314, #19315, #49801, #11809, #12302, #96815, #72790, #4327, #34799, #66280, #42810, #43778, #49312, #28291, #5800, #36290, #65289, #89291, #20801, #27296, #11318, #41837, #45772, #68770, #28779, #37786, #75272, #67285, #21293, #84275, #37296, #8265 ),
 ( #59277, #302, #51786, #52276, #23281, #82272, #52764, #60267, #60756, #29759, #44274, #14796, #15774, #91256, #98305, #90766, #22291, #68283, #30746, #83272, #83767, #13787, #45269, #61253, #89776, #98804, #75764, #82775, #7285, #15290, #29274, #6288, #53261, #7782, #30252, #74779, #22782, #14295, #36791, #46263, #76265, #97813, #38277, #67783, #59770, #91758, #53757, #76748, #66788, #97307, #90263, #21796, #44767, #6782, #2261, #23776, #32221, #40237, #785, #94206, #46741, #31238, #38765, #2753, #69265, #16259, #9737, #47728, #55737, #77239, #1281, #31734, #93222, #40728, #92737, #62230, #24261, #78725, #55225, #25736, #61733, #10235, #56228, #79209, #47226, #24746, #71230, #54725, #33209, #86228, #17739, #63703, #92251, #70745, #77729, #39264, #54241, #86722, #9241, #84754, #8743, #69753, #62722, #85245, #16751, #39752, #48215, #17252, #18226, #70249, #1765, #48706, #85739, #78225, #32716, #63214, #93718, #25252, #19200, #3226, #10719, #80187, #41723, #50686, #64188, #87197, #4710, #73171, #28176, #49202, #43177, #34183, #49683, #56706, #80690, #58670, #5192, #71714, #12186, #11700, #33690, #65176, #89172, #96697, #11204, #72193, #42692, #42209, #73665, #57683, #3722, #35172, #65673, #96194, #20683, #95697, #79706, #20183, #27181, #35680, #64675, #88179, #94708, #95185, #72676, #4211, #27679, #58164, #88675, #81178, #12678, #26693, #51177, #41236, #66164, #26213, #57189, #18720, #34681, #87686, #19693, #50180, #61131, #22665, #7669, #14172, #15165, #82156, #5687, #53141, #75648, #21677, #23159, #67670, #22166, #98683, #44152, #90147, #44656, #36675, #83650, #38160, #51677, #97198, #75151, #74154, #13170, #37177, #52163, #14676, #98180, #13668, #7160, #91641, #29636, #37663, #81660, #52648, #45646, #43667, #74660, #6171, #67163, #59158, #76143, #83151, #89664, #60144, #30624, #30132, #36173, #60638, #90641, #82656, #66673, #28666, #21175, #68646, #97687, #45142, #29149, #59656, #176, #68163, #6661, #91139, #62598, #9617, #40615, #10117, #2641, #53634, #54606, #69142, #40118, #85122, #16633, #62105, #84633, #33095, #93602, #78608, #47108, #86114, #54120, #76629, #25139, #47616, #92615, #94097, #39636, #93103, #70619, #16135, #24139, #77608, #8631, #55617, #71114, #23658, #670, #9121, #46143, #84154, #70125, #1647, #85620, #32099, #46621, #78111, #63588, #24633, #2144, #15660, #55100, #17625, #8148, #77119, #39140, #69630, #31120, #48095, #17137, #61615, #32604, #38641, #63100, #92133, #1154, #31614, #26576, #56111, #86605, #48589, #50565, #64071, #57565, #11095, #94586, #27560, #19575, #71608, #10604, #34558, #80576 ) ),
 .UNSPECIFIED., .F., .F., .F. ) 
 B_SPLINE_SURFACE_WITH_KNOTS ( ( 2, 2 ),
 ( 3, 2, 2, 2, 2, 2, 2, 2, 2, 2, 2, 2, 2, 2, 2, 2, 2, 2, 2, 2, 2, 2, 2, 2, 2, 2, 2, 2, 2, 2, 2, 2, 2, 2, 2, 2, 2, 2, 2, 2, 2, 2, 2, 2, 2, 2, 2, 2, 2, 2, 2, 2, 2, 2, 2, 2, 2, 2, 2, 2, 2, 2, 2, 2, 2, 2, 2, 2, 2, 2, 2, 2, 2, 2, 2, 2, 2, 2, 2, 2, 2, 2, 2, 2, 2, 2, 2, 2, 2, 2, 2, 2, 2, 2, 2, 2, 2, 2, 2, 2, 2, 2, 2, 2, 2, 2, 2, 2, 2, 2, 2, 2, 2, 2, 2, 2, 2, 2, 2, 2, 2, 2, 2, 2, 2, 2, 2, 2, 2, 2, 2, 2, 2, 2, 2, 2, 2, 2, 2, 2, 2, 2, 2, 2, 2, 2, 2, 2, 2, 2, 2, 2, 2, 2, 2, 2, 2, 2, 2, 2, 2, 2, 3 ),
 ( 0.000000000000000000, 1.000000000000000000 ),
 ( 0.000000000000000000, 0.005952380952380952051, 0.01190476190476190410, 0.01785714285714285615, 0.02380952380952380820, 0.02976190476190476025, 0.03571428571428571230, 0.04166666666666666435, 0.04761904761904761640, 0.05357142857142856845, 0.05952380952380952051, 0.06547619047619047949, 0.07142857142857142461, 0.07738095238095238360, 0.08333333333333332871, 0.08928571428571428770, 0.09523809523809523281, 0.1011904761904761918, 0.1071428571428571369, 0.1130952380952380959, 0.1190476190476190410, 0.1250000000000000000, 0.1309523809523809590, 0.1369047619047619180, 0.1428571428571428492, 0.1488095238095238082, 0.1547619047619047672, 0.1607142857142857262, 0.1666666666666666574, 0.1726190476190476164, 0.1785714285714285754, 0.1845238095238095344, 0.1904761904761904656, 0.1964285714285714246, 0.2023809523809523836, 0.2083333333333333426, 0.2142857142857142738, 0.2202380952380952328, 0.2261904761904761918, 0.2321428571428571508, 0.2380952380952380820, 0.2440476190476190410, 0.2500000000000000000, 0.2559523809523809312, 0.2619047619047619180, 0.2678571428571428492, 0.2738095238095238360, 0.2797619047619047672, 0.2857142857142856984, 0.2916666666666666852, 0.2976190476190476164, 0.3035714285714285476, 0.3095238095238095344, 0.3154761904761904656, 0.3214285714285714524, 0.3273809523809523836, 0.3333333333333333148, 0.3392857142857143016, 0.3452380952380952328, 0.3511904761904761640, 0.3571428571428571508, 0.3630952380952380820, 0.3690476190476190688, 0.3750000000000000000, 0.3809523809523809312, 0.3869047619047619180, 0.3928571428571428492, 0.3988095238095238360, 0.4047619047619047672, 0.4107142857142856984, 0.4166666666666666852, 0.4226190476190476164, 0.4285714285714285476, 0.4345238095238095344, 0.4404761904761904656, 0.4464285714285714524, 0.4523809523809523836, 0.4583333333333333148, 0.4642857142857143016, 0.4702380952380952328, 0.4761904761904761640, 0.4821428571428571508, 0.4880952380952380820, 0.4940476190476190688, 0.5000000000000000000, 0.5059523809523809312, 0.5119047619047618625, 0.5178571428571429047, 0.5238095238095238360, 0.5297619047619047672, 0.5357142857142856984, 0.5416666666666666297, 0.5476190476190476719, 0.5535714285714286031, 0.5595238095238095344, 0.5654761904761904656, 0.5714285714285713969, 0.5773809523809523281, 0.5833333333333333703, 0.5892857142857143016, 0.5952380952380952328, 0.6011904761904761640, 0.6071428571428570953, 0.6130952380952381375, 0.6190476190476190688, 0.6250000000000000000, 0.6309523809523809312, 0.6369047619047618625, 0.6428571428571429047, 0.6488095238095238360, 0.6547619047619047672, 0.6607142857142856984, 0.6666666666666666297, 0.6726190476190476719, 0.6785714285714286031, 0.6845238095238095344, 0.6904761904761904656, 0.6964285714285713969, 0.7023809523809523281, 0.7083333333333333703, 0.7142857142857143016, 0.7202380952380952328, 0.7261904761904761640, 0.7321428571428570953, 0.7380952380952381375, 0.7440476190476190688, 0.7500000000000000000, 0.7559523809523809312, 0.7619047619047618625, 0.7678571428571429047, 0.7738095238095238360, 0.7797619047619047672, 0.7857142857142856984, 0.7916666666666666297, 0.7976190476190476719, 0.8035714285714286031, 0.8095238095238095344, 0.8154761904761904656, 0.8214285714285713969, 0.8273809523809523281, 0.8333333333333333703, 0.8392857142857143016, 0.8452380952380952328, 0.8511904761904761640, 0.8571428571428570953, 0.8630952380952381375, 0.8690476190476190688, 0.8750000000000000000, 0.8809523809523809312, 0.8869047619047618625, 0.8928571428571429047, 0.8988095238095238360, 0.9047619047619047672, 0.9107142857142856984, 0.9166666666666666297, 0.9226190476190476719, 0.9285714285714286031, 0.9345238095238095344, 0.9404761904761904656, 0.9464285714285713969, 0.9523809523809523281, 0.9583333333333333703, 0.9642857142857143016 ),
 .UNSPECIFIED. ) 
 GEOMETRIC_REPRESENTATION_ITEM ( )  RATIONAL_B_SPLINE_SURFACE ( (
 ( 1.000000000000000000, 0.9659258262890683122, 1.000000000000000000, 0.9659258262890683122, 1.000000000000000000, 0.9659258262890683122, 1.000000000000000000, 0.9659258262890683122, 1.000000000000000000, 0.9659258262890683122, 1.000000000000000000, 0.9659258262890683122, 1.000000000000000000, 0.9659258262890683122, 1.000000000000000000, 0.9659258262890683122, 1.000000000000000000, 0.9659258262890683122, 1.000000000000000000, 0.9659258262890683122, 1.000000000000000000, 0.9659258262890683122, 1.000000000000000000, 0.9659258262890683122, 1.000000000000000000, 0.9659258262890683122, 1.000000000000000000, 0.9659258262890683122, 1.000000000000000000, 0.9659258262890683122, 1.000000000000000000, 0.9659258262890683122, 1.000000000000000000, 0.9659258262890683122, 1.000000000000000000, 0.9659258262890683122, 1.000000000000000000, 0.9659258262890683122, 1.000000000000000000, 0.9659258262890683122, 1.000000000000000000, 0.9659258262890683122, 1.000000000000000000, 0.9659258262890683122, 1.000000000000000000, 0.9659258262890683122, 1.000000000000000000, 0.9659258262890683122, 1.000000000000000000, 0.9659258262890683122, 1.000000000000000000, 0.9659258262890683122, 1.000000000000000000, 0.9659258262890683122, 1.000000000000000000, 0.9659258262890683122, 1.000000000000000000, 0.9659258262890683122, 1.000000000000000000, 0.9659258262890683122, 1.000000000000000000, 0.9659258262890683122, 1.000000000000000000, 0.9659258262890683122, 1.000000000000000000, 0.9659258262890683122, 1.000000000000000000, 0.9659258262890683122, 1.000000000000000000, 0.9659258262890683122, 1.000000000000000000, 0.9659258262890683122, 1.000000000000000000, 0.9659258262890683122, 1.000000000000000000, 0.9659258262890683122, 1.000000000000000000, 0.9659258262890683122, 1.000000000000000000, 0.9659258262890683122, 1.000000000000000000, 0.9659258262890683122, 1.000000000000000000, 0.9659258262890683122, 1.000000000000000000, 0.9659258262890683122, 1.000000000000000000, 0.9659258262890683122, 1.000000000000000000, 0.9659258262890683122, 1.000000000000000000, 0.9659258262890683122, 1.000000000000000000, 0.9659258262890683122, 1.000000000000000000, 0.9659258262890683122, 1.000000000000000000, 0.9659258262890683122, 1.000000000000000000, 0.9659258262890683122, 1.000000000000000000, 0.9659258262890683122, 1.000000000000000000, 0.9659258262890683122, 1.000000000000000000, 0.9659258262890683122, 1.000000000000000000, 0.9659258262890683122, 1.000000000000000000, 0.9659258262890683122, 1.000000000000000000, 0.9659258262890683122, 1.000000000000000000, 0.9659258262890683122, 1.000000000000000000, 0.9659258262890683122, 1.000000000000000000, 0.9659258262890683122, 1.000000000000000000, 0.9659258262890683122, 1.000000000000000000, 0.9659258262890683122, 1.000000000000000000, 0.9659258262890683122, 1.000000000000000000, 0.9659258262890683122, 1.000000000000000000, 0.9659258262890683122, 1.000000000000000000, 0.9659258262890683122, 1.000000000000000000, 0.9659258262890683122, 1.000000000000000000, 0.9659258262890683122, 1.000000000000000000, 0.9659258262890683122, 1.000000000000000000, 0.9659258262890683122, 1.000000000000000000, 0.9659258262890683122, 1.000000000000000000, 0.9659258262890683122, 1.000000000000000000, 0.9659258262890683122, 1.000000000000000000, 0.9659258262890683122, 1.000000000000000000, 0.9659258262890683122, 1.000000000000000000, 0.9659258262890683122, 1.000000000000000000, 0.9659258262890683122, 1.000000000000000000, 0.9659258262890683122, 1.000000000000000000, 0.9659258262890683122, 1.000000000000000000, 0.9659258262890683122, 1.000000000000000000, 0.9659258262890683122, 1.000000000000000000, 0.9659258262890683122, 1.000000000000000000, 0.9659258262890683122, 1.000000000000000000, 0.9659258262890683122, 1.000000000000000000, 0.9659258262890683122, 1.000000000000000000, 0.9659258262890683122, 1.000000000000000000, 0.9659258262890683122, 1.000000000000000000, 0.9659258262890683122, 1.000000000000000000, 0.9659258262890683122, 1.000000000000000000, 0.9659258262890683122, 1.000000000000000000, 0.9659258262890683122, 1.000000000000000000, 0.9659258262890683122, 1.000000000000000000, 0.9659258262890683122, 1.000000000000000000, 0.9659258262890683122, 1.000000000000000000, 0.9659258262890683122, 1.000000000000000000, 0.9659258262890683122, 1.000000000000000000, 0.9659258262890683122, 1.000000000000000000, 0.9659258262890683122, 1.000000000000000000, 0.9659258262890683122, 1.000000000000000000, 0.9659258262890683122, 1.000000000000000000, 0.9659258262890683122, 1.000000000000000000, 0.9659258262890683122, 1.000000000000000000, 0.9659258262890683122, 1.000000000000000000, 0.9659258262890683122, 1.000000000000000000, 0.9659258262890683122, 1.000000000000000000, 0.9659258262890683122, 1.000000000000000000, 0.9659258262890683122, 1.000000000000000000, 0.9659258262890683122, 1.000000000000000000, 0.9659258262890683122, 1.000000000000000000, 0.9659258262890683122, 1.000000000000000000, 0.9659258262890683122, 1.000000000000000000, 0.9659258262890683122, 1.000000000000000000, 0.9659258262890683122, 1.000000000000000000, 0.9659258262890683122, 1.000000000000000000, 0.9659258262890683122, 1.000000000000000000, 0.9659258262890683122, 1.000000000000000000, 0.9659258262890683122, 1.000000000000000000, 0.9659258262890683122, 1.000000000000000000, 0.9659258262890683122, 1.000000000000000000, 0.9659258262890683122, 1.000000000000000000, 0.9659258262890683122, 1.000000000000000000, 0.9659258262890683122, 1.000000000000000000, 0.9659258262890683122, 1.000000000000000000, 0.9659258262890683122, 1.000000000000000000, 0.9659258262890683122, 1.000000000000000000, 0.9659258262890683122, 1.000000000000000000, 0.9659258262890683122, 1.000000000000000000, 0.9659258262890683122, 1.000000000000000000, 0.9659258262890683122, 1.000000000000000000, 0.9659258262890683122, 1.000000000000000000, 0.9659258262890683122, 1.000000000000000000, 0.9659258262890683122, 1.000000000000000000, 0.9659258262890683122, 1.000000000000000000, 0.9659258262890683122, 1.000000000000000000, 0.9659258262890683122, 1.000000000000000000, 0.9659258262890683122, 1.000000000000000000, 0.9659258262890683122, 1.000000000000000000, 0.9659258262890683122, 1.000000000000000000, 0.9659258262890683122, 1.000000000000000000, 0.9659258262890683122, 1.000000000000000000, 0.9659258262890683122, 1.000000000000000000, 0.9659258262890683122, 1.000000000000000000, 0.9659258262890683122, 1.000000000000000000, 0.9659258262890683122, 1.000000000000000000, 0.9659258262890683122, 1.000000000000000000, 0.9659258262890683122, 1.000000000000000000, 0.9659258262890683122, 1.000000000000000000, 0.9659258262890683122, 1.000000000000000000, 0.9659258262890683122, 1.000000000000000000, 0.9659258262890683122, 1.000000000000000000, 0.9659258262890683122, 1.000000000000000000, 0.9659258262890683122, 1.000000000000000000, 0.9659258262890683122, 1.000000000000000000, 0.9659258262890683122, 1.000000000000000000, 0.9659258262890683122, 1.000000000000000000, 0.9659258262890683122, 1.000000000000000000, 0.9659258262890683122, 1.000000000000000000, 0.9659258262890683122, 1.000000000000000000, 0.9659258262890683122, 1.000000000000000000, 0.9659258262890683122, 1.000000000000000000, 0.9659258262890683122, 1.000000000000000000, 0.9659258262890683122, 1.000000000000000000, 0.9659258262890683122, 1.000000000000000000),
 ( 1.000000000000000000, 0.9659258262890683122, 1.000000000000000000, 0.9659258262890683122, 1.000000000000000000, 0.9659258262890683122, 1.000000000000000000, 0.9659258262890683122, 1.000000000000000000, 0.9659258262890683122, 1.000000000000000000, 0.9659258262890683122, 1.000000000000000000, 0.9659258262890683122, 1.000000000000000000, 0.9659258262890683122, 1.000000000000000000, 0.9659258262890683122, 1.000000000000000000, 0.9659258262890683122, 1.000000000000000000, 0.9659258262890683122, 1.000000000000000000, 0.9659258262890683122, 1.000000000000000000, 0.9659258262890683122, 1.000000000000000000, 0.9659258262890683122, 1.000000000000000000, 0.9659258262890683122, 1.000000000000000000, 0.9659258262890683122, 1.000000000000000000, 0.9659258262890683122, 1.000000000000000000, 0.9659258262890683122, 1.000000000000000000, 0.9659258262890683122, 1.000000000000000000, 0.9659258262890683122, 1.000000000000000000, 0.9659258262890683122, 1.000000000000000000, 0.9659258262890683122, 1.000000000000000000, 0.9659258262890683122, 1.000000000000000000, 0.9659258262890683122, 1.000000000000000000, 0.9659258262890683122, 1.000000000000000000, 0.9659258262890683122, 1.000000000000000000, 0.9659258262890683122, 1.000000000000000000, 0.9659258262890683122, 1.000000000000000000, 0.9659258262890683122, 1.000000000000000000, 0.9659258262890683122, 1.000000000000000000, 0.9659258262890683122, 1.000000000000000000, 0.9659258262890683122, 1.000000000000000000, 0.9659258262890683122, 1.000000000000000000, 0.9659258262890683122, 1.000000000000000000, 0.9659258262890683122, 1.000000000000000000, 0.9659258262890683122, 1.000000000000000000, 0.9659258262890683122, 1.000000000000000000, 0.9659258262890683122, 1.000000000000000000, 0.9659258262890683122, 1.000000000000000000, 0.9659258262890683122, 1.000000000000000000, 0.9659258262890683122, 1.000000000000000000, 0.9659258262890683122, 1.000000000000000000, 0.9659258262890683122, 1.000000000000000000, 0.9659258262890683122, 1.000000000000000000, 0.9659258262890683122, 1.000000000000000000, 0.9659258262890683122, 1.000000000000000000, 0.9659258262890683122, 1.000000000000000000, 0.9659258262890683122, 1.000000000000000000, 0.9659258262890683122, 1.000000000000000000, 0.9659258262890683122, 1.000000000000000000, 0.9659258262890683122, 1.000000000000000000, 0.9659258262890683122, 1.000000000000000000, 0.9659258262890683122, 1.000000000000000000, 0.9659258262890683122, 1.000000000000000000, 0.9659258262890683122, 1.000000000000000000, 0.9659258262890683122, 1.000000000000000000, 0.9659258262890683122, 1.000000000000000000, 0.9659258262890683122, 1.000000000000000000, 0.9659258262890683122, 1.000000000000000000, 0.9659258262890683122, 1.000000000000000000, 0.9659258262890683122, 1.000000000000000000, 0.9659258262890683122, 1.000000000000000000, 0.9659258262890683122, 1.000000000000000000, 0.9659258262890683122, 1.000000000000000000, 0.9659258262890683122, 1.000000000000000000, 0.9659258262890683122, 1.000000000000000000, 0.9659258262890683122, 1.000000000000000000, 0.9659258262890683122, 1.000000000000000000, 0.9659258262890683122, 1.000000000000000000, 0.9659258262890683122, 1.000000000000000000, 0.9659258262890683122, 1.000000000000000000, 0.9659258262890683122, 1.000000000000000000, 0.9659258262890683122, 1.000000000000000000, 0.9659258262890683122, 1.000000000000000000, 0.9659258262890683122, 1.000000000000000000, 0.9659258262890683122, 1.000000000000000000, 0.9659258262890683122, 1.000000000000000000, 0.9659258262890683122, 1.000000000000000000, 0.9659258262890683122, 1.000000000000000000, 0.9659258262890683122, 1.000000000000000000, 0.9659258262890683122, 1.000000000000000000, 0.9659258262890683122, 1.000000000000000000, 0.9659258262890683122, 1.000000000000000000, 0.9659258262890683122, 1.000000000000000000, 0.9659258262890683122, 1.000000000000000000, 0.9659258262890683122, 1.000000000000000000, 0.9659258262890683122, 1.000000000000000000, 0.9659258262890683122, 1.000000000000000000, 0.9659258262890683122, 1.000000000000000000, 0.9659258262890683122, 1.000000000000000000, 0.9659258262890683122, 1.000000000000000000, 0.9659258262890683122, 1.000000000000000000, 0.9659258262890683122, 1.000000000000000000, 0.9659258262890683122, 1.000000000000000000, 0.9659258262890683122, 1.000000000000000000, 0.9659258262890683122, 1.000000000000000000, 0.9659258262890683122, 1.000000000000000000, 0.9659258262890683122, 1.000000000000000000, 0.9659258262890683122, 1.000000000000000000, 0.9659258262890683122, 1.000000000000000000, 0.9659258262890683122, 1.000000000000000000, 0.9659258262890683122, 1.000000000000000000, 0.9659258262890683122, 1.000000000000000000, 0.9659258262890683122, 1.000000000000000000, 0.9659258262890683122, 1.000000000000000000, 0.9659258262890683122, 1.000000000000000000, 0.9659258262890683122, 1.000000000000000000, 0.9659258262890683122, 1.000000000000000000, 0.9659258262890683122, 1.000000000000000000, 0.9659258262890683122, 1.000000000000000000, 0.9659258262890683122, 1.000000000000000000, 0.9659258262890683122, 1.000000000000000000, 0.9659258262890683122, 1.000000000000000000, 0.9659258262890683122, 1.000000000000000000, 0.9659258262890683122, 1.000000000000000000, 0.9659258262890683122, 1.000000000000000000, 0.9659258262890683122, 1.000000000000000000, 0.9659258262890683122, 1.000000000000000000, 0.9659258262890683122, 1.000000000000000000, 0.9659258262890683122, 1.000000000000000000, 0.9659258262890683122, 1.000000000000000000, 0.9659258262890683122, 1.000000000000000000, 0.9659258262890683122, 1.000000000000000000, 0.9659258262890683122, 1.000000000000000000, 0.9659258262890683122, 1.000000000000000000, 0.9659258262890683122, 1.000000000000000000, 0.9659258262890683122, 1.000000000000000000, 0.9659258262890683122, 1.000000000000000000, 0.9659258262890683122, 1.000000000000000000, 0.9659258262890683122, 1.000000000000000000, 0.9659258262890683122, 1.000000000000000000, 0.9659258262890683122, 1.000000000000000000, 0.9659258262890683122, 1.000000000000000000, 0.9659258262890683122, 1.000000000000000000, 0.9659258262890683122, 1.000000000000000000, 0.9659258262890683122, 1.000000000000000000, 0.9659258262890683122, 1.000000000000000000, 0.9659258262890683122, 1.000000000000000000, 0.9659258262890683122, 1.000000000000000000, 0.9659258262890683122, 1.000000000000000000, 0.9659258262890683122, 1.000000000000000000, 0.9659258262890683122, 1.000000000000000000, 0.9659258262890683122, 1.000000000000000000, 0.9659258262890683122, 1.000000000000000000, 0.9659258262890683122, 1.000000000000000000, 0.9659258262890683122, 1.000000000000000000, 0.9659258262890683122, 1.000000000000000000, 0.9659258262890683122, 1.000000000000000000, 0.9659258262890683122, 1.000000000000000000, 0.9659258262890683122, 1.000000000000000000, 0.9659258262890683122, 1.000000000000000000, 0.9659258262890683122, 1.000000000000000000, 0.9659258262890683122, 1.000000000000000000, 0.9659258262890683122, 1.000000000000000000, 0.9659258262890683122, 1.000000000000000000, 0.9659258262890683122, 1.000000000000000000, 0.9659258262890683122, 1.000000000000000000, 0.9659258262890683122, 1.000000000000000000, 0.9659258262890683122, 1.000000000000000000, 0.9659258262890683122, 1.000000000000000000, 0.9659258262890683122, 1.000000000000000000, 0.9659258262890683122, 1.000000000000000000) ) ) 
 REPRESENTATION_ITEM ( '' )  SURFACE ( )  );
#3533=UNCERTAINTY_MEASURE_WITH_UNIT (LENGTH_MEASURE( 1.000000000000000082E-05 ), #4520, 'distance_accuracy_value', 'NONE');
#3535=CARTESIAN_POINT ( 'NONE',  ( 13.79529636645030344, 23.26208216824730002, 14.16423886937410614 ) ) ;
#3536=CARTESIAN_POINT ( 'NONE',  ( 10.00000000000000178, 28.05374883491396787, 14.16423886937410082 ) ) ;
#3537=CARTESIAN_POINT ( 'NONE',  ( 2.917880565312948704, 2.637082168247300906, 12.26659068614894643 ) ) ;
#3538=CARTESIAN_POINT ( 'NONE',  ( 4.555630843329476320, 77.03495325336415078, 9.500000000000000000 ) ) ;
#3539=CARTESIAN_POINT ( 'NONE',  ( 0.5774900079438590739, 32.64701867748816966, -5.440088680355550821 ) ) ;
#3542=CARTESIAN_POINT ( 'NONE',  ( 0.1532563361054082862, 21.21726448433412315, 2.638427012816831674 ) ) ;
#3543=CARTESIAN_POINT ( 'NONE',  ( 7.084665262690076126, 52.02201867748816255, -10.88017736071110164 ) ) ;
#3544=CARTESIAN_POINT ( 'NONE',  ( 14.92337183194729988, 19.34226448433411960, -8.527530157486177487 ) ) ;
#3547=CARTESIAN_POINT ( 'NONE',  ( 19.38216949554541202, 45.99863466993041072, 9.382169495545424454 ) ) ;
#3548=CARTESIAN_POINT ( 'NONE',  ( 18.52753015748618282, 38.92559781766745175, -4.923371831947291888 ) ) ;
#3550=CARTESIAN_POINT ( 'NONE',  ( 19.38216949554541202, 30.99863466993042138, 9.382169495545424454 ) ) ;
#3552=COLOUR_RGB ( '', 0.40784314, 0.44705882, 0.49803922) ;
#3553=CARTESIAN_POINT ( 'NONE',  ( 5.076628168052704559, 25.17559781766745175, -8.527530157486179263 ) ) ;
#3554=CARTESIAN_POINT ( 'NONE',  ( 20.36894250292379382, 13.67874883491396965, 10.36894250292379205 ) ) ;
#3556=CARTESIAN_POINT ( 'NONE',  ( 19.42250999205614548, 40.98035201082150536, -5.440088680355545492 ) ) ;
#3557=CARTESIAN_POINT ( 'NONE',  ( 12.91533473730992121, 49.52201867748817676, 10.88017736071110164 ) ) ;
#3558=CARTESIAN_POINT ( 'NONE',  ( 13.79529636645031943, 40.34541550158063217, -14.16423886937409904 ) ) ;
#3559=CARTESIAN_POINT ( 'NONE',  ( 7.361572987183170547, 57.05059781766744464, 9.846743663894590881 ) ) ;
#3560=CARTESIAN_POINT ( 'NONE',  ( 17.20831665107776587, 14.13393115100078568, -7.208316651077762316 ) ) ;
#3564=CARTESIAN_POINT ( 'NONE',  ( -0.8801773607111008646, 43.27201867748817676, 2.915334737309923430 ) ) ;
#3565=EDGE_CURVE ( 'NONE', #78790, #60237, #48075, .T. ) ;
#3568=CARTESIAN_POINT ( 'NONE',  ( 21.09922568453594849, 16.20696800326375353, 6.408140936763242479 ) ) ;
#3569=CARTESIAN_POINT ( 'NONE',  ( 0.1532563361054083140, 51.00893115100078745, 1.131784320476157264E-15 ) ) ;
#3571=SURFACE_SIDE_STYLE ('',( #26063 ) ) ;
#3573=CARTESIAN_POINT ( 'NONE',  ( 12.91533473730992121, 64.52201867748817676, 10.88017736071110164 ) ) ;
#3577=CARTESIAN_POINT ( 'NONE',  ( 0.1532563361054083140, 1.008931151000784787, 1.131784320476157264E-15 ) ) ;
#3578=CARTESIAN_POINT ( 'NONE',  ( 7.361572987183169658, -0.03273551566588185635, -9.846743663894592657 ) ) ;
#3580=CARTESIAN_POINT ( 'NONE',  ( 0.1532563361054100626, 25.80059781766744820, -2.638427012816831230 ) ) ;
#3581=CARTESIAN_POINT ( 'NONE',  ( -0.8801773607110991993, 17.85535201082150536, -2.915334737309923874 ) ) ;
#3582=CARTESIAN_POINT ( 'NONE',  ( 7.361572987183170547, 62.05059781766745886, 9.846743663894590881 ) ) ;
#3583=CARTESIAN_POINT ( 'NONE',  ( 19.42250999205614548, 40.98035201082150536, -5.440088680355545492 ) ) ;
#3584=CARTESIAN_POINT ( 'NONE',  ( 19.39188664607695145, 55.83703382326400799, -6.499999999999960920 ) ) ;
#3585=CARTESIAN_POINT ( 'NONE',  ( -2.816281873526473856, 44.33196800326375353, 3.434112377981055619 ) ) ;
#3586=VERTEX_POINT ( 'NONE', #85602 ) ;
#3587=CARTESIAN_POINT ( 'NONE',  ( 20.88017736071110875, 50.77201867748817676, -2.915334737309920765 ) ) ;
#3588=CARTESIAN_POINT ( 'NONE',  ( -1.099225684535947600, 23.70696800326375708, -6.408140936763238038 ) ) ;
#3589=SURFACE_SIDE_STYLE ('',( #48571 ) ) ;
#3590=CARTESIAN_POINT ( 'NONE',  ( 17.08211943468705130, 48.47041550158063927, 12.26659068614894998 ) ) ;
#3591=CARTESIAN_POINT ( 'NONE',  ( 0.1532563361054082862, 46.21726448433411605, 2.638427012816831674 ) ) ;
#3592=CARTESIAN_POINT ( 'NONE',  ( 1.472469842513823179, 1.425597817667451528, 4.923371831947296329 ) ) ;
#3593=CARTESIAN_POINT ( 'NONE',  ( 7.084665262690076126, 69.10535201082151957, 10.88017736071109987 ) ) ;
#3595=CARTESIAN_POINT ( 'NONE',  ( 22.26659068614895176, 29.72041550158063572, -7.082119434687042414 ) ) ;
#3596=CARTESIAN_POINT ( 'NONE',  ( -45.94000000000001194, 107.5383484153110061, -12.00000000000000000 ) ) ;
#3601=CARTESIAN_POINT ( 'NONE',  ( 20.36894250292379382, 48.67874883491396076, 10.36894250292379205 ) ) ;
#3602=CARTESIAN_POINT ( 'NONE',  ( -4.164238869374099927, 52.01208216824729647, 3.795296366450308767 ) ) ;
#3603=CARTESIAN_POINT ( 'NONE',  ( 1.472469842513823179, 11.42559781766745175, 4.923371831947296329 ) ) ;
#3605=DIRECTION ( 'NONE',  ( 0.000000000000000000, 0.000000000000000000, -1.000000000000000000 ) ) ;
#3606=CARTESIAN_POINT ( 'NONE',  ( 19.42250999205614548, 5.980352010821504471, -5.440088680355545492 ) ) ;
#3607=CARTESIAN_POINT ( 'NONE',  ( 13.43411237798106583, 32.66530133659708213, -12.81628187352647252 ) ) ;
#3608=CARTESIAN_POINT ( 'NONE',  ( 20.36894250292379382, 48.67874883491396076, 10.36894250292379205 ) ) ;
#3611=VERTEX_POINT ( 'NONE', #54590 ) ;
#3612=CARTESIAN_POINT ( 'NONE',  ( 10.00000000000000000, 24.75893115100078745, -9.846743663894594434 ) ) ;
#3614=CARTESIAN_POINT ( 'NONE',  ( 10.00000000000000178, 9.313685344154839285, 10.88017736071110342 ) ) ;
#3615=CARTESIAN_POINT ( 'NONE',  ( 10.00000000000000178, 9.313685344154839285, 10.88017736071110342 ) ) ;
#3616=CARTESIAN_POINT ( 'NONE',  ( 7.361572987183169658, 44.96726448433412315, -9.846743663894592657 ) ) ;
#3617=CARTESIAN_POINT ( 'NONE',  ( -1.099225684535947600, 8.706968003263753531, -6.408140936763238038 ) ) ;
#3620=LINE ( 'NONE', #54624, #14493 ) ;
#3622=CARTESIAN_POINT ( 'NONE',  ( 19.38216949554541202, 20.99863466993042138, 9.382169495545424454 ) ) ;
#3624=VECTOR ( 'NONE', #76938, 1000.000000000000000 ) ;
#3625=CARTESIAN_POINT ( 'NONE',  ( 24.16423886937410614, 54.51208216824730357, -3.795296366450302550 ) ) ;
#3628=CARTESIAN_POINT ( 'NONE',  ( -4.164238869374098151, 56.59541550158063927, -3.795296366450310543 ) ) ;
#3630=CARTESIAN_POINT ( 'NONE',  ( 2.035157376598824452, 38.68868534415483396, 7.964842623401179544 ) ) ;
#3631=CARTESIAN_POINT ( 'NONE',  ( 4.559911319644449179, 47.23035201082150536, -9.422509992056141925 ) ) ;
#3632=CARTESIAN_POINT ( 'NONE',  ( 17.96484262340118221, 34.93868534415482685, 7.964842623401181321 ) ) ;
#3635=CARTESIAN_POINT ( 'NONE',  ( 10.00000000000000000, 46.81368534415484106, -10.88017736071110342 ) ) ;
#3637=EDGE_CURVE ( 'NONE', #55747, #22305, #17116, .T. ) ;
#3638=CARTESIAN_POINT ( 'NONE',  ( 1.472469842513823179, 15.59226448433411960, -4.923371831947296329 ) ) ;
#3641=CARTESIAN_POINT ( 'NONE',  ( 0.1532563361054100626, 40.80059781766745886, -2.638427012816831230 ) ) ;
#3642=DIRECTION ( 'NONE',  ( 0.000000000000000000, -1.000000000000000000, -0.000000000000000000 ) ) ;
#3643=EDGE_CURVE ( 'NONE', #45856, #25477, #79177, .T. ) ;
#3644=CARTESIAN_POINT ( 'NONE',  ( 13.43411237798105340, 60.58196800326376064, 12.81628187352647963 ) ) ;
#3647=LINE ( 'NONE', #34112, #18881 ) ;
#3648=CARTESIAN_POINT ( 'NONE',  ( -43.79988333157628233, 106.6859424350824668, 5.014248105693637214 ) ) ;
#3650=CARTESIAN_POINT ( 'NONE',  ( -0.3689425029237898834, 61.17874883491396076, -10.36894250292378850 ) ) ;
#3651=CARTESIAN_POINT ( 'NONE',  ( 1.274849032794278747, 57.55509018479938277, -6.499999999999960032 ) ) ;
#3652=ORIENTED_EDGE ( 'NONE', *, *, #46207, .T. ) ;
#3654=CARTESIAN_POINT ( 'NONE',  ( 10.00000000000000178, 32.25893115100078745, 9.846743663894594434 ) ) ;
#3656=CARTESIAN_POINT ( 'NONE',  ( 13.43411237798105340, 10.58196800326375353, 12.81628187352647963 ) ) ;
#3657=CARTESIAN_POINT ( 'NONE',  ( 20.88017736071110519, 60.56368534415484106, 2.639326808657452039E-16 ) ) ;
#3659=CARTESIAN_POINT ( 'NONE',  ( 5.076628168052704559, 15.17559781766745175, -8.527530157486179263 ) ) ;
#3660=CARTESIAN_POINT ( 'NONE',  ( 10.00000000000000000, 54.75893115100078745, -9.846743663894594434 ) ) ;
#3665=CARTESIAN_POINT ( 'NONE',  ( 24.16423886937410614, 64.51208216824728936, -3.795296366450302550 ) ) ;
#3667=CARTESIAN_POINT ( 'NONE',  ( 19.42250999205614193, 40.14701867748817676, 5.440088680355555262 ) ) ;
#3668=CARTESIAN_POINT ( 'NONE',  ( 19.38216949554541202, 25.99863466993042138, 9.382169495545424454 ) ) ;
#3674=CARTESIAN_POINT ( 'NONE',  ( 0.1532563361054100626, 50.80059781766745175, -2.638427012816831230 ) ) ;
#3675=CARTESIAN_POINT ( 'NONE',  ( 5.076628168052704559, 10.17559781766745175, -8.527530157486179263 ) ) ;
#3677=CARTESIAN_POINT ( 'NONE',  ( 0.6178305044545838731, 19.74863466993042138, 9.382169495545420901 ) ) ;
#3679=CARTESIAN_POINT ( 'NONE',  ( 7.084665262690076126, 24.10535201082150181, 10.88017736071109987 ) ) ;
#3682=CARTESIAN_POINT ( 'NONE',  ( 2.917880565312950480, 40.97041550158063217, -12.26659068614894821 ) ) ;
#3683=CARTESIAN_POINT ( 'NONE',  ( 13.79529636645031943, 35.34541550158063927, -14.16423886937409904 ) ) ;
#3685=CARTESIAN_POINT ( 'NONE',  ( 7.361572987183169658, 39.96726448433411605, -9.846743663894592657 ) ) ;
#3686=CARTESIAN_POINT ( 'NONE',  ( -2.816281873526473856, 34.12363466993042493, 9.499525473075851096E-16 ) ) ;
#3687=CARTESIAN_POINT ( 'NONE',  ( 7.084665262690076126, 27.02201867748817676, -10.88017736071110164 ) ) ;
#3688=CARTESIAN_POINT ( 'NONE',  ( 14.92337183194729988, 54.34226448433412315, -8.527530157486177487 ) ) ;
#3689=CARTESIAN_POINT ( 'NONE',  ( 4.559911319644449179, 42.23035201082151247, -9.422509992056141925 ) ) ;
#3690=CARTESIAN_POINT ( 'NONE',  ( 16.40814093676323893, 5.790301336597087456, 11.09922568453595026 ) ) ;
#3691=CARTESIAN_POINT ( 'NONE',  ( 20.36894250292379738, 24.92874883491396787, -10.36894250292379027 ) ) ;
#3692=CARTESIAN_POINT ( 'NONE',  ( -0.1503990784575359729, 13.10158574516642105, 6.262539305110062848 ) ) ;
#3693=VECTOR ( 'NONE', #41023, 1000.000000000000000 ) ;
#3695=CARTESIAN_POINT ( 'NONE',  ( 19.84674366389459266, 28.71726448433411960, -2.638427012816827677 ) ) ;
#3696=CARTESIAN_POINT ( 'NONE',  ( 21.09922568453594849, 51.20696800326375353, 6.408140936763242479 ) ) ;
#3697=CARTESIAN_POINT ( 'NONE',  ( -2.816281873526473856, 4.123634669930420493, 9.499525473075851096E-16 ) ) ;
#3700=CARTESIAN_POINT ( 'NONE',  ( 20.00000000000000355, 70.00000000000000000, 4.500000000000000888 ) ) ;
#3702=CARTESIAN_POINT ( 'NONE',  ( 10.00000000000000178, 68.05374883491397497, 14.16423886937410082 ) ) ;
#3703=CARTESIAN_POINT ( 'NONE',  ( 4.559911319644449179, 62.23035201082150536, -9.422509992056141925 ) ) ;
#3704=CARTESIAN_POINT ( 'NONE',  ( -4.164238869374099927, 17.01208216824730357, 3.795296366450308767 ) ) ;
#3705=CARTESIAN_POINT ( 'NONE',  ( 2.791683348922240793, 1.633931151000784565, 7.208316651077764092 ) ) ;
#3706=CARTESIAN_POINT ( 'NONE',  ( 19.84674366389459266, 48.30059781766745175, 2.638427012816836559 ) ) ;
#3707=CARTESIAN_POINT ( 'NONE',  ( 2.035157376598824452, 28.68868534415484106, 7.964842623401179544 ) ) ;
#3710=CARTESIAN_POINT ( 'NONE',  ( 7.361572987183169658, 64.96726448433412315, -9.846743663894592657 ) ) ;
#3716=CARTESIAN_POINT ( 'NONE',  ( -4.164238869374098151, 6.595415501580634832, -3.795296366450310543 ) ) ;
#3717=CARTESIAN_POINT ( 'NONE',  ( 20.36894250292379738, 4.928748834913967869, -10.36894250292379027 ) ) ;
#3718=CARTESIAN_POINT ( 'NONE',  ( -2.266590686148945544, 57.22041550158063217, 7.082119434687048631 ) ) ;
#3719=CARTESIAN_POINT ( 'NONE',  ( 18.52753015748617571, 63.09226448433412315, 4.923371831947298993 ) ) ;
#3720=CARTESIAN_POINT ( 'NONE',  ( 1.472469842513823179, 40.59226448433411605, -4.923371831947296329 ) ) ;
#3722=CARTESIAN_POINT ( 'NONE',  ( -0.8801773607111009756, 33.06368534415484106, 1.068504757029289695E-15 ) ) ;
#3723=CARTESIAN_POINT ( 'NONE',  ( 2.791683348922240793, 56.63393115100078035, 7.208316651077764092 ) ) ;
#3724=( NAMED_UNIT ( * ) PLANE_ANGLE_UNIT ( ) SI_UNIT ( $, .RADIAN. ) );
#3725=CARTESIAN_POINT ( 'NONE',  ( 22.26659068614894466, 53.88708216824731068, 7.082119434687054849 ) ) ;
#3726=CARTESIAN_POINT ( 'NONE',  ( 20.88017736071110519, 5.563685344154838397, 2.639326808657452039E-16 ) ) ;
#3729=CARTESIAN_POINT ( 'NONE',  ( 7.084665262690076126, 67.02201867748817676, -10.88017736071110164 ) ) ;
#3730=CARTESIAN_POINT ( 'NONE',  ( 17.20831665107776587, 34.13393115100078745, -7.208316651077762316 ) ) ;
#3733=CYLINDRICAL_SURFACE ( 'NONE', #61901, 0.5000000000000004441 ) ;
#3734=( BOUNDED_SURFACE ( )  B_SPLINE_SURFACE ( 1, 2, ( 
 ( #38910, #97953, #69397, #919, #92385, #21944, #82921, #6930, #37438, #60411, #67929, #22434, #33344, #2404, #40876, #39403, #86373, #24896, #87345, #79357, #71382, #62368, #70886, #78864, #2894, #55874, #56846, #48848, #18860, #94352, #70390, #10864, #63838, #17875, #56369, #16896, #41385, #40389, #32862, #86861, #69896, #77374, #47862, #18367, #63360, #62872, #64333, #93863, #71852, #3362, #1416, #26345, #32367, #9381, #33826, #94844, #25391, #8887, #55381, #93369, #31869, #92872, #77871, #24404, #78368, #54872, #85382, #47373, #39886, #85881, #1909, #17394, #9887, #57822, #80831, #73319, #66306, #27818, #34825, #19344, #49341, #19828, #74295, #4842, #88331, #81321, #35318, #43314, #96345, #28802, #41865, #50316, #89318, #95841, #12331, #42344, #5822, #20332, #42835, #3861, #49827, #80339, #36315, #34322, #65813, #66809, #96843, #57330, #26836, #58303, #88820, #28317, #87826, #50828, #12815, #73808, #65315, #11837, #51315, #5341, #81798, #97331, #59302, #35819, #58809, #89799, #20825, #72821, #13315, #4359, #64820, #95337, #27326, #43802, #79840, #11345, #72328, #60781, #91784, #75295, #60297, #37319, #46285, #52304, #90789, #21822, #52788, #810, #90284, #45295, #22316, #61275, #74801, #67811, #15314, #59792, #91283, #51809, #45798, #326, #15799, #82797, #98327, #76773, #23307, #6807, #22805, #75789, #29297, #29786, #38787, #31264, #37811, #53284, #84300, #8289, #83793, #30770, #13817, #44299, #76289, #69288, #7803, #61762, #21318, #38302, #82296, #6309, #36814, #67307, #97833, #24775, #9765, #3248, #70274, #71739, #55760, #40753, #24284, #18251, #55251, #17277, #33235, #46765, #39288, #62749, #63728, #85766, #77753, #79234, #48730, #10747, #41265, #69779, #1791, #32246, #93251, #81202, #12703, #80713, #81681, #11720, #19225, #72218, #64699, #80214, #73197, #65198, #4234, #96220, #50710, #73685, #5221, #85032, #84545, #87969, #95731, #20218, #44933, #74946, #44444, #30422, #75441, #43944, #59935, #22955, #66453, #83928, #6448, #14961, #90425, #67454, #15457, #7456, #96989, #6953, #81950, #52445, #21966, #36958, #97975, #74442, #60432, #22454, #5969, #82945, #28466, #52928, #53421, #37461, #90925, #58963, #67948, #13462, #29431, #82445, #14460, #36463, #59444, #37954, #66958, #97476, #45430, #83440, #13969, #98472, #28941, #45938, #29926, #75933, #5487, #68447, #89459, #98968, #51960, #60922, #35957, #91428, #89945, #20977, #21463, #51460, #8424, #32387, #1438, #39907, #38439, #85404, #23933, #17896, #78387, #1929, #61412, #31890, #77892, #62892, #54889, #55897, #47885, #76427, #93391, #69419, #9908, #47391, #9405 ),
 ( #2425, #24916, #15930, #62387, #93885, #68936, #7943, #77393, #85902, #92894, #39423, #466, #70905, #30914, #55401, #53923, #24426, #17416, #8907, #32882, #46421, #63381, #25413, #76913, #91921, #23446, #84433, #38931, #940, #31402, #61903, #92409, #54402, #84913, #16425, #46901, #41406, #3383, #73340, #64356, #94865, #88353, #50342, #56865, #41889, #4867, #27840, #35344, #58328, #88845, #48379, #2914, #78882, #10393, #33364, #68325, #97852, #89338, #29808, #43824, #20848, #51339, #75316, #44322, #82817, #81342, #29316, #66831, #30299, #22336, #14337, #5363, #13840, #21843, #44810, #59812, #98845, #90808, #60801, #37342, #13340, #52810, #90307, #52324, #67832, #58831, #83317, #82320, #74823, #6828, #12838, #20353, #89824, #98350, #6327, #5846, #7333, #36839, #60317, #14842, #43338, #50849, #74319, #81823, #45314, #75811, #67327, #37834, #97353, #36337, #73834, #35842, #28822, #66329, #21342, #96865, #28341, #59322, #51833, #53304, #70791, #92295, #1811, #46788, #54282, #2308, #93274, #83812, #62272, #68816, #39309, #77281, #23819, #84797, #61296, #47273, #9287, #30796, #8792, #15338, #39796, #40283, #24309, #77774, #45821, #54774, #349, #16306, #69305, #69802, #91805, #46307, #24797, #23327, #53808, #32266, #70296, #827, #1325, #84318, #32763, #31777, #85290, #91301, #92778, #76308, #16797, #38812, #47772, #22828, #62775, #15819, #55274, #76793, #8309, #31287, #85785, #17297, #78270, #7826, #9784, #61785, #38322, #65217, #26739, #48259, #56749, #64721, #57234, #41766, #42738, #34726, #4747, #80235, #56273, #95744, #34224, #72237, #11743, #2800, #27228, #26253, #87242, #87732, #25293, #73219, #33732, #3770, #18768, #48750, #50220, #49250, #42251, #57723, #55780, #12229, #18271, #94251, #72721, #4255, #79750, #80734, #10769, #79258, #88226, #19735, #63746, #11248, #64233, #63258, #93767, #33255, #86275, #78772, #86768, #25779, #41284, #17784, #95231, #19244, #94750, #3268, #10278, #49728, #71758, #40778, #71278, #89221, #35723, #66211, #90197, #59204, #97739, #96243, #44201, #81705, #45201, #37228, #29201, #20231, #28713, #36725, #59700, #13717, #14725, #6710, #75700, #52209, #28218, #67715, #6221, #74711, #82703, #73712, #98228, #97244, #89707, #21727, #27723, #35217, #5733, #67216, #21221, #20730, #22222, #51725, #44701, #29689, #58203, #83203, #51221, #13219, #75200, #60198, #82207, #52698, #43715, #74199, #90693, #88720, #36219, #81224, #66719, #12723, #43218, #5245, #85173, #91187, #229, #38212, #45696, #70176, #718, #46672, #76679, #46196, #32148, #77170, #76196, #61663, #24678, #68214, #85663, #8199, #16683 ) ),
 .UNSPECIFIED., .F., .F., .T. ) 
 B_SPLINE_SURFACE_WITH_KNOTS ( ( 2, 2 ),
 ( 3, 2, 2, 2, 2, 2, 2, 2, 2, 2, 2, 2, 2, 2, 2, 2, 2, 2, 2, 2, 2, 2, 2, 2, 2, 2, 2, 2, 2, 2, 2, 2, 2, 2, 2, 2, 2, 2, 2, 2, 2, 2, 2, 2, 2, 2, 2, 2, 2, 2, 2, 2, 2, 2, 2, 2, 2, 2, 2, 2, 2, 2, 2, 2, 2, 2, 2, 2, 2, 2, 2, 2, 2, 2, 2, 2, 2, 2, 2, 2, 2, 2, 2, 2, 2, 2, 2, 2, 2, 2, 2, 2, 2, 2, 2, 2, 2, 2, 2, 2, 2, 2, 2, 2, 2, 2, 2, 2, 2, 2, 2, 2, 2, 2, 2, 2, 2, 2, 2, 2, 2, 2, 2, 2, 2, 2, 2, 2, 2, 2, 2, 2, 2, 2, 2, 2, 2, 2, 2, 2, 2, 2, 2, 2, 2, 2, 2, 2, 2, 2, 2, 2, 2, 2, 2, 2, 2, 2, 2, 2, 2, 2, 3 ),
 ( 0.000000000000000000, 1.000000000000000000 ),
 ( 0.000000000000000000, 0.005952380952380952051, 0.01190476190476190410, 0.01785714285714285615, 0.02380952380952380820, 0.02976190476190476025, 0.03571428571428571230, 0.04166666666666666435, 0.04761904761904761640, 0.05357142857142856845, 0.05952380952380952051, 0.06547619047619047949, 0.07142857142857142461, 0.07738095238095238360, 0.08333333333333332871, 0.08928571428571428770, 0.09523809523809523281, 0.1011904761904761918, 0.1071428571428571369, 0.1130952380952380959, 0.1190476190476190410, 0.1250000000000000000, 0.1309523809523809590, 0.1369047619047619180, 0.1428571428571428492, 0.1488095238095238082, 0.1547619047619047672, 0.1607142857142857262, 0.1666666666666666574, 0.1726190476190476164, 0.1785714285714285754, 0.1845238095238095344, 0.1904761904761904656, 0.1964285714285714246, 0.2023809523809523836, 0.2083333333333333426, 0.2142857142857142738, 0.2202380952380952328, 0.2261904761904761918, 0.2321428571428571508, 0.2380952380952380820, 0.2440476190476190410, 0.2500000000000000000, 0.2559523809523809312, 0.2619047619047619180, 0.2678571428571428492, 0.2738095238095238360, 0.2797619047619047672, 0.2857142857142856984, 0.2916666666666666852, 0.2976190476190476164, 0.3035714285714285476, 0.3095238095238095344, 0.3154761904761904656, 0.3214285714285714524, 0.3273809523809523836, 0.3333333333333333148, 0.3392857142857143016, 0.3452380952380952328, 0.3511904761904761640, 0.3571428571428571508, 0.3630952380952380820, 0.3690476190476190688, 0.3750000000000000000, 0.3809523809523809312, 0.3869047619047619180, 0.3928571428571428492, 0.3988095238095238360, 0.4047619047619047672, 0.4107142857142856984, 0.4166666666666666852, 0.4226190476190476164, 0.4285714285714285476, 0.4345238095238095344, 0.4404761904761904656, 0.4464285714285714524, 0.4523809523809523836, 0.4583333333333333148, 0.4642857142857143016, 0.4702380952380952328, 0.4761904761904761640, 0.4821428571428571508, 0.4880952380952380820, 0.4940476190476190688, 0.5000000000000000000, 0.5059523809523809312, 0.5119047619047618625, 0.5178571428571429047, 0.5238095238095238360, 0.5297619047619047672, 0.5357142857142856984, 0.5416666666666666297, 0.5476190476190476719, 0.5535714285714286031, 0.5595238095238095344, 0.5654761904761904656, 0.5714285714285713969, 0.5773809523809523281, 0.5833333333333333703, 0.5892857142857143016, 0.5952380952380952328, 0.6011904761904761640, 0.6071428571428570953, 0.6130952380952381375, 0.6190476190476190688, 0.6250000000000000000, 0.6309523809523809312, 0.6369047619047618625, 0.6428571428571429047, 0.6488095238095238360, 0.6547619047619047672, 0.6607142857142856984, 0.6666666666666666297, 0.6726190476190476719, 0.6785714285714286031, 0.6845238095238095344, 0.6904761904761904656, 0.6964285714285713969, 0.7023809523809523281, 0.7083333333333333703, 0.7142857142857143016, 0.7202380952380952328, 0.7261904761904761640, 0.7321428571428570953, 0.7380952380952381375, 0.7440476190476190688, 0.7500000000000000000, 0.7559523809523809312, 0.7619047619047618625, 0.7678571428571429047, 0.7738095238095238360, 0.7797619047619047672, 0.7857142857142856984, 0.7916666666666666297, 0.7976190476190476719, 0.8035714285714286031, 0.8095238095238095344, 0.8154761904761904656, 0.8214285714285713969, 0.8273809523809523281, 0.8333333333333333703, 0.8392857142857143016, 0.8452380952380952328, 0.8511904761904761640, 0.8571428571428570953, 0.8630952380952381375, 0.8690476190476190688, 0.8750000000000000000, 0.8809523809523809312, 0.8869047619047618625, 0.8928571428571429047, 0.8988095238095238360, 0.9047619047619047672, 0.9107142857142856984, 0.9166666666666666297, 0.9226190476190476719, 0.9285714285714286031, 0.9345238095238095344, 0.9404761904761904656, 0.9464285714285713969, 0.9523809523809523281, 0.9583333333333333703, 0.9642857142857143016 ),
 .UNSPECIFIED. ) 
 GEOMETRIC_REPRESENTATION_ITEM ( )  RATIONAL_B_SPLINE_SURFACE ( (
 ( 1.000000000000000000, 0.9659258262890683122, 1.000000000000000000, 0.9659258262890683122, 1.000000000000000000, 0.9659258262890683122, 1.000000000000000000, 0.9659258262890683122, 1.000000000000000000, 0.9659258262890683122, 1.000000000000000000, 0.9659258262890683122, 1.000000000000000000, 0.9659258262890683122, 1.000000000000000000, 0.9659258262890683122, 1.000000000000000000, 0.9659258262890683122, 1.000000000000000000, 0.9659258262890683122, 1.000000000000000000, 0.9659258262890683122, 1.000000000000000000, 0.9659258262890683122, 1.000000000000000000, 0.9659258262890683122, 1.000000000000000000, 0.9659258262890683122, 1.000000000000000000, 0.9659258262890683122, 1.000000000000000000, 0.9659258262890683122, 1.000000000000000000, 0.9659258262890683122, 1.000000000000000000, 0.9659258262890683122, 1.000000000000000000, 0.9659258262890683122, 1.000000000000000000, 0.9659258262890683122, 1.000000000000000000, 0.9659258262890683122, 1.000000000000000000, 0.9659258262890683122, 1.000000000000000000, 0.9659258262890683122, 1.000000000000000000, 0.9659258262890683122, 1.000000000000000000, 0.9659258262890683122, 1.000000000000000000, 0.9659258262890683122, 1.000000000000000000, 0.9659258262890683122, 1.000000000000000000, 0.9659258262890683122, 1.000000000000000000, 0.9659258262890683122, 1.000000000000000000, 0.9659258262890683122, 1.000000000000000000, 0.9659258262890683122, 1.000000000000000000, 0.9659258262890683122, 1.000000000000000000, 0.9659258262890683122, 1.000000000000000000, 0.9659258262890683122, 1.000000000000000000, 0.9659258262890683122, 1.000000000000000000, 0.9659258262890683122, 1.000000000000000000, 0.9659258262890683122, 1.000000000000000000, 0.9659258262890683122, 1.000000000000000000, 0.9659258262890683122, 1.000000000000000000, 0.9659258262890683122, 1.000000000000000000, 0.9659258262890683122, 1.000000000000000000, 0.9659258262890683122, 1.000000000000000000, 0.9659258262890683122, 1.000000000000000000, 0.9659258262890683122, 1.000000000000000000, 0.9659258262890683122, 1.000000000000000000, 0.9659258262890683122, 1.000000000000000000, 0.9659258262890683122, 1.000000000000000000, 0.9659258262890683122, 1.000000000000000000, 0.9659258262890683122, 1.000000000000000000, 0.9659258262890683122, 1.000000000000000000, 0.9659258262890683122, 1.000000000000000000, 0.9659258262890683122, 1.000000000000000000, 0.9659258262890683122, 1.000000000000000000, 0.9659258262890683122, 1.000000000000000000, 0.9659258262890683122, 1.000000000000000000, 0.9659258262890683122, 1.000000000000000000, 0.9659258262890683122, 1.000000000000000000, 0.9659258262890683122, 1.000000000000000000, 0.9659258262890683122, 1.000000000000000000, 0.9659258262890683122, 1.000000000000000000, 0.9659258262890683122, 1.000000000000000000, 0.9659258262890683122, 1.000000000000000000, 0.9659258262890683122, 1.000000000000000000, 0.9659258262890683122, 1.000000000000000000, 0.9659258262890683122, 1.000000000000000000, 0.9659258262890683122, 1.000000000000000000, 0.9659258262890683122, 1.000000000000000000, 0.9659258262890683122, 1.000000000000000000, 0.9659258262890683122, 1.000000000000000000, 0.9659258262890683122, 1.000000000000000000, 0.9659258262890683122, 1.000000000000000000, 0.9659258262890683122, 1.000000000000000000, 0.9659258262890683122, 1.000000000000000000, 0.9659258262890683122, 1.000000000000000000, 0.9659258262890683122, 1.000000000000000000, 0.9659258262890683122, 1.000000000000000000, 0.9659258262890683122, 1.000000000000000000, 0.9659258262890683122, 1.000000000000000000, 0.9659258262890683122, 1.000000000000000000, 0.9659258262890683122, 1.000000000000000000, 0.9659258262890683122, 1.000000000000000000, 0.9659258262890683122, 1.000000000000000000, 0.9659258262890683122, 1.000000000000000000, 0.9659258262890683122, 1.000000000000000000, 0.9659258262890683122, 1.000000000000000000, 0.9659258262890683122, 1.000000000000000000, 0.9659258262890683122, 1.000000000000000000, 0.9659258262890683122, 1.000000000000000000, 0.9659258262890683122, 1.000000000000000000, 0.9659258262890683122, 1.000000000000000000, 0.9659258262890683122, 1.000000000000000000, 0.9659258262890683122, 1.000000000000000000, 0.9659258262890683122, 1.000000000000000000, 0.9659258262890683122, 1.000000000000000000, 0.9659258262890683122, 1.000000000000000000, 0.9659258262890683122, 1.000000000000000000, 0.9659258262890683122, 1.000000000000000000, 0.9659258262890683122, 1.000000000000000000, 0.9659258262890683122, 1.000000000000000000, 0.9659258262890683122, 1.000000000000000000, 0.9659258262890683122, 1.000000000000000000, 0.9659258262890683122, 1.000000000000000000, 0.9659258262890683122, 1.000000000000000000, 0.9659258262890683122, 1.000000000000000000, 0.9659258262890683122, 1.000000000000000000, 0.9659258262890683122, 1.000000000000000000, 0.9659258262890683122, 1.000000000000000000, 0.9659258262890683122, 1.000000000000000000, 0.9659258262890683122, 1.000000000000000000, 0.9659258262890683122, 1.000000000000000000, 0.9659258262890683122, 1.000000000000000000, 0.9659258262890683122, 1.000000000000000000, 0.9659258262890683122, 1.000000000000000000, 0.9659258262890683122, 1.000000000000000000, 0.9659258262890683122, 1.000000000000000000, 0.9659258262890683122, 1.000000000000000000, 0.9659258262890683122, 1.000000000000000000, 0.9659258262890683122, 1.000000000000000000, 0.9659258262890683122, 1.000000000000000000, 0.9659258262890683122, 1.000000000000000000, 0.9659258262890683122, 1.000000000000000000, 0.9659258262890683122, 1.000000000000000000, 0.9659258262890683122, 1.000000000000000000, 0.9659258262890683122, 1.000000000000000000, 0.9659258262890683122, 1.000000000000000000, 0.9659258262890683122, 1.000000000000000000, 0.9659258262890683122, 1.000000000000000000, 0.9659258262890683122, 1.000000000000000000, 0.9659258262890683122, 1.000000000000000000, 0.9659258262890683122, 1.000000000000000000, 0.9659258262890683122, 1.000000000000000000, 0.9659258262890683122, 1.000000000000000000, 0.9659258262890683122, 1.000000000000000000, 0.9659258262890683122, 1.000000000000000000, 0.9659258262890683122, 1.000000000000000000, 0.9659258262890683122, 1.000000000000000000, 0.9659258262890683122, 1.000000000000000000, 0.9659258262890683122, 1.000000000000000000, 0.9659258262890683122, 1.000000000000000000, 0.9659258262890683122, 1.000000000000000000, 0.9659258262890683122, 1.000000000000000000, 0.9659258262890683122, 1.000000000000000000, 0.9659258262890683122, 1.000000000000000000, 0.9659258262890683122, 1.000000000000000000, 0.9659258262890683122, 1.000000000000000000, 0.9659258262890683122, 1.000000000000000000, 0.9659258262890683122, 1.000000000000000000, 0.9659258262890683122, 1.000000000000000000, 0.9659258262890683122, 1.000000000000000000, 0.9659258262890683122, 1.000000000000000000, 0.9659258262890683122, 1.000000000000000000, 0.9659258262890683122, 1.000000000000000000, 0.9659258262890683122, 1.000000000000000000, 0.9659258262890683122, 1.000000000000000000, 0.9659258262890683122, 1.000000000000000000, 0.9659258262890683122, 1.000000000000000000, 0.9659258262890683122, 1.000000000000000000, 0.9659258262890683122, 1.000000000000000000, 0.9659258262890683122, 1.000000000000000000, 0.9659258262890683122, 1.000000000000000000, 0.9659258262890683122, 1.000000000000000000, 0.9659258262890683122, 1.000000000000000000),
 ( 1.000000000000000000, 0.9659258262890683122, 1.000000000000000000, 0.9659258262890683122, 1.000000000000000000, 0.9659258262890683122, 1.000000000000000000, 0.9659258262890683122, 1.000000000000000000, 0.9659258262890683122, 1.000000000000000000, 0.9659258262890683122, 1.000000000000000000, 0.9659258262890683122, 1.000000000000000000, 0.9659258262890683122, 1.000000000000000000, 0.9659258262890683122, 1.000000000000000000, 0.9659258262890683122, 1.000000000000000000, 0.9659258262890683122, 1.000000000000000000, 0.9659258262890683122, 1.000000000000000000, 0.9659258262890683122, 1.000000000000000000, 0.9659258262890683122, 1.000000000000000000, 0.9659258262890683122, 1.000000000000000000, 0.9659258262890683122, 1.000000000000000000, 0.9659258262890683122, 1.000000000000000000, 0.9659258262890683122, 1.000000000000000000, 0.9659258262890683122, 1.000000000000000000, 0.9659258262890683122, 1.000000000000000000, 0.9659258262890683122, 1.000000000000000000, 0.9659258262890683122, 1.000000000000000000, 0.9659258262890683122, 1.000000000000000000, 0.9659258262890683122, 1.000000000000000000, 0.9659258262890683122, 1.000000000000000000, 0.9659258262890683122, 1.000000000000000000, 0.9659258262890683122, 1.000000000000000000, 0.9659258262890683122, 1.000000000000000000, 0.9659258262890683122, 1.000000000000000000, 0.9659258262890683122, 1.000000000000000000, 0.9659258262890683122, 1.000000000000000000, 0.9659258262890683122, 1.000000000000000000, 0.9659258262890683122, 1.000000000000000000, 0.9659258262890683122, 1.000000000000000000, 0.9659258262890683122, 1.000000000000000000, 0.9659258262890683122, 1.000000000000000000, 0.9659258262890683122, 1.000000000000000000, 0.9659258262890683122, 1.000000000000000000, 0.9659258262890683122, 1.000000000000000000, 0.9659258262890683122, 1.000000000000000000, 0.9659258262890683122, 1.000000000000000000, 0.9659258262890683122, 1.000000000000000000, 0.9659258262890683122, 1.000000000000000000, 0.9659258262890683122, 1.000000000000000000, 0.9659258262890683122, 1.000000000000000000, 0.9659258262890683122, 1.000000000000000000, 0.9659258262890683122, 1.000000000000000000, 0.9659258262890683122, 1.000000000000000000, 0.9659258262890683122, 1.000000000000000000, 0.9659258262890683122, 1.000000000000000000, 0.9659258262890683122, 1.000000000000000000, 0.9659258262890683122, 1.000000000000000000, 0.9659258262890683122, 1.000000000000000000, 0.9659258262890683122, 1.000000000000000000, 0.9659258262890683122, 1.000000000000000000, 0.9659258262890683122, 1.000000000000000000, 0.9659258262890683122, 1.000000000000000000, 0.9659258262890683122, 1.000000000000000000, 0.9659258262890683122, 1.000000000000000000, 0.9659258262890683122, 1.000000000000000000, 0.9659258262890683122, 1.000000000000000000, 0.9659258262890683122, 1.000000000000000000, 0.9659258262890683122, 1.000000000000000000, 0.9659258262890683122, 1.000000000000000000, 0.9659258262890683122, 1.000000000000000000, 0.9659258262890683122, 1.000000000000000000, 0.9659258262890683122, 1.000000000000000000, 0.9659258262890683122, 1.000000000000000000, 0.9659258262890683122, 1.000000000000000000, 0.9659258262890683122, 1.000000000000000000, 0.9659258262890683122, 1.000000000000000000, 0.9659258262890683122, 1.000000000000000000, 0.9659258262890683122, 1.000000000000000000, 0.9659258262890683122, 1.000000000000000000, 0.9659258262890683122, 1.000000000000000000, 0.9659258262890683122, 1.000000000000000000, 0.9659258262890683122, 1.000000000000000000, 0.9659258262890683122, 1.000000000000000000, 0.9659258262890683122, 1.000000000000000000, 0.9659258262890683122, 1.000000000000000000, 0.9659258262890683122, 1.000000000000000000, 0.9659258262890683122, 1.000000000000000000, 0.9659258262890683122, 1.000000000000000000, 0.9659258262890683122, 1.000000000000000000, 0.9659258262890683122, 1.000000000000000000, 0.9659258262890683122, 1.000000000000000000, 0.9659258262890683122, 1.000000000000000000, 0.9659258262890683122, 1.000000000000000000, 0.9659258262890683122, 1.000000000000000000, 0.9659258262890683122, 1.000000000000000000, 0.9659258262890683122, 1.000000000000000000, 0.9659258262890683122, 1.000000000000000000, 0.9659258262890683122, 1.000000000000000000, 0.9659258262890683122, 1.000000000000000000, 0.9659258262890683122, 1.000000000000000000, 0.9659258262890683122, 1.000000000000000000, 0.9659258262890683122, 1.000000000000000000, 0.9659258262890683122, 1.000000000000000000, 0.9659258262890683122, 1.000000000000000000, 0.9659258262890683122, 1.000000000000000000, 0.9659258262890683122, 1.000000000000000000, 0.9659258262890683122, 1.000000000000000000, 0.9659258262890683122, 1.000000000000000000, 0.9659258262890683122, 1.000000000000000000, 0.9659258262890683122, 1.000000000000000000, 0.9659258262890683122, 1.000000000000000000, 0.9659258262890683122, 1.000000000000000000, 0.9659258262890683122, 1.000000000000000000, 0.9659258262890683122, 1.000000000000000000, 0.9659258262890683122, 1.000000000000000000, 0.9659258262890683122, 1.000000000000000000, 0.9659258262890683122, 1.000000000000000000, 0.9659258262890683122, 1.000000000000000000, 0.9659258262890683122, 1.000000000000000000, 0.9659258262890683122, 1.000000000000000000, 0.9659258262890683122, 1.000000000000000000, 0.9659258262890683122, 1.000000000000000000, 0.9659258262890683122, 1.000000000000000000, 0.9659258262890683122, 1.000000000000000000, 0.9659258262890683122, 1.000000000000000000, 0.9659258262890683122, 1.000000000000000000, 0.9659258262890683122, 1.000000000000000000, 0.9659258262890683122, 1.000000000000000000, 0.9659258262890683122, 1.000000000000000000, 0.9659258262890683122, 1.000000000000000000, 0.9659258262890683122, 1.000000000000000000, 0.9659258262890683122, 1.000000000000000000, 0.9659258262890683122, 1.000000000000000000, 0.9659258262890683122, 1.000000000000000000, 0.9659258262890683122, 1.000000000000000000, 0.9659258262890683122, 1.000000000000000000, 0.9659258262890683122, 1.000000000000000000, 0.9659258262890683122, 1.000000000000000000, 0.9659258262890683122, 1.000000000000000000, 0.9659258262890683122, 1.000000000000000000, 0.9659258262890683122, 1.000000000000000000, 0.9659258262890683122, 1.000000000000000000, 0.9659258262890683122, 1.000000000000000000, 0.9659258262890683122, 1.000000000000000000, 0.9659258262890683122, 1.000000000000000000, 0.9659258262890683122, 1.000000000000000000, 0.9659258262890683122, 1.000000000000000000, 0.9659258262890683122, 1.000000000000000000, 0.9659258262890683122, 1.000000000000000000, 0.9659258262890683122, 1.000000000000000000, 0.9659258262890683122, 1.000000000000000000, 0.9659258262890683122, 1.000000000000000000, 0.9659258262890683122, 1.000000000000000000, 0.9659258262890683122, 1.000000000000000000, 0.9659258262890683122, 1.000000000000000000, 0.9659258262890683122, 1.000000000000000000, 0.9659258262890683122, 1.000000000000000000, 0.9659258262890683122, 1.000000000000000000, 0.9659258262890683122, 1.000000000000000000, 0.9659258262890683122, 1.000000000000000000, 0.9659258262890683122, 1.000000000000000000, 0.9659258262890683122, 1.000000000000000000, 0.9659258262890683122, 1.000000000000000000, 0.9659258262890683122, 1.000000000000000000, 0.9659258262890683122, 1.000000000000000000, 0.9659258262890683122, 1.000000000000000000, 0.9659258262890683122, 1.000000000000000000) ) ) 
 REPRESENTATION_ITEM ( '' )  SURFACE ( )  );
#3736=CARTESIAN_POINT ( 'NONE',  ( 12.63842701281683034, 17.46726448433411250, 9.846743663894596210 ) ) ;
#3738=CARTESIAN_POINT ( 'NONE',  ( -2.266590686148945544, 37.22041550158063217, 7.082119434687048631 ) ) ;
#3739=CARTESIAN_POINT ( 'NONE',  ( 10.00000000000000178, 37.25893115100078745, 9.846743663894594434 ) ) ;
#3740=CARTESIAN_POINT ( 'NONE',  ( 10.00000000000000178, 54.31368534415484106, 10.88017736071110342 ) ) ;
#3742=FILL_AREA_STYLE ('',( #86247 ) ) ;
#3744=CARTESIAN_POINT ( 'NONE',  ( 10.00000000000000178, 54.31368534415484106, 10.88017736071110342 ) ) ;
#3746=CARTESIAN_POINT ( 'NONE',  ( 0.1532563361054082862, 46.21726448433411605, 2.638427012816831674 ) ) ;
#3749=CARTESIAN_POINT ( 'NONE',  ( -2.266590686148945544, 26.38708216824730357, -7.082119434687050408 ) ) ;
#3752=CARTESIAN_POINT ( 'NONE',  ( 0.6178305044545838731, 29.74863466993042138, 9.382169495545420901 ) ) ;
#3753=CARTESIAN_POINT ( 'NONE',  ( 19.84674366389459266, 18.71726448433411960, -2.638427012816827677 ) ) ;
#3754=SURFACE_SIDE_STYLE ('',( #78759 ) ) ;
#3755=CARTESIAN_POINT ( 'NONE',  ( -1.099225684535947600, 53.70696800326376064, -6.408140936763238038 ) ) ;
#3756=FACE_OUTER_BOUND ( 'NONE', #55982, .T. ) ;
#3757=CARTESIAN_POINT ( 'NONE',  ( 19.84674366389459266, 33.30059781766744464, 2.638427012816836559 ) ) ;
#3759=EDGE_CURVE ( 'NONE', #72785, #16271, #76612, .T. ) ;
#3761=CARTESIAN_POINT ( 'NONE',  ( -0.8801773607111009756, 68.06368534415484817, 1.068504757029289695E-15 ) ) ;
#3762=CARTESIAN_POINT ( 'NONE',  ( 17.39651004071838969, 39.08210964143329846, -6.500000000000027534 ) ) ;
#3764=CARTESIAN_POINT ( 'NONE',  ( 19.84674366389459621, 3.508931151000785231, 7.409399052514197653E-17 ) ) ;
#3767=CARTESIAN_POINT ( 'NONE',  ( 3.591859063236763294, 18.29030133659708568, -11.09922568453595026 ) ) ;
#3768=COLOUR_RGB ( '', 0.66274510, 0.83137255, 0.94901961) ;
#3770=CARTESIAN_POINT ( 'NONE',  ( 17.20831665107776587, 42.88393115100077324, 7.208316651077764980 ) ) ;
#3772=CARTESIAN_POINT ( 'NONE',  ( 24.16423886937410614, 9.512082168247301794, -3.795296366450302550 ) ) ;
#3773=CARTESIAN_POINT ( 'NONE',  ( 14.92337183194729988, 34.34226448433411605, -8.527530157486177487 ) ) ;
#3775=CARTESIAN_POINT ( 'NONE',  ( 3.591859063236761518, 29.95696800326375708, 11.09922568453594849 ) ) ;
#3776=CARTESIAN_POINT ( 'NONE',  ( 17.39651004071841456, 14.08210964143329669, -6.500000000000003553 ) ) ;
#3777=FACE_OUTER_BOUND ( 'NONE', #50735, .T. ) ;
#3778=CARTESIAN_POINT ( 'NONE',  ( 19.42250999205614548, 55.98035201082150536, -5.440088680355545492 ) ) ;
#3779=CARTESIAN_POINT ( 'NONE',  ( 0.6178305044545818747, 8.498634669930421381, -9.382169495545419124 ) ) ;
#3781=CARTESIAN_POINT ( 'NONE',  ( 0.1532563361054083140, 41.00893115100078745, 1.131784320476157264E-15 ) ) ;
#3782=CARTESIAN_POINT ( 'NONE',  ( 2.035157376598822676, 22.43868534415483396, -7.964842623401177768 ) ) ;
#3783=CARTESIAN_POINT ( 'NONE',  ( -1.099225684535947600, 28.70696800326375353, -6.408140936763238038 ) ) ;
#3784=CARTESIAN_POINT ( 'NONE',  ( 7.361572987183170547, 17.05059781766745530, 9.846743663894590881 ) ) ;
#3786=CARTESIAN_POINT ( 'NONE',  ( -0.8801773607111009756, 33.06368534415484106, 1.068504757029289695E-15 ) ) ;
#3787=CARTESIAN_POINT ( 'NONE',  ( 20.88017736071110875, 65.77201867748817676, -2.915334737309920765 ) ) ;
#3788=CARTESIAN_POINT ( 'NONE',  ( 12.91533473730993009, 6.605352010821504471, -10.88017736071109987 ) ) ;
#3789=CARTESIAN_POINT ( 'NONE',  ( 2.791683348922237240, 40.38393115100078035, -7.208316651077763204 ) ) ;
#3790=CARTESIAN_POINT ( 'NONE',  ( 0.5774900079438607392, 28.48035201082150891, 5.440088680355550821 ) ) ;
#3791=CARTESIAN_POINT ( 'NONE',  ( 5.500000000000000000, 11.00000000000000000, -6.500000000000000888 ) ) ;
#3792=CARTESIAN_POINT ( 'NONE',  ( 19.42250999205614548, 40.98035201082150536, -5.440088680355545492 ) ) ;
#3793=CARTESIAN_POINT ( 'NONE',  ( 10.00000000000000000, 6.813685344154838397, -10.88017736071110342 ) ) ;
#3794=FACE_OUTER_BOUND ( 'NONE', #19494, .T. ) ;
#3796=CARTESIAN_POINT ( 'NONE',  ( 18.52753015748617571, 58.09226448433411605, 4.923371831947298993 ) ) ;
#3797=CARTESIAN_POINT ( 'NONE',  ( 20.36894250292379382, 48.67874883491396076, 10.36894250292379205 ) ) ;
#3801=CARTESIAN_POINT ( 'NONE',  ( 20.36894250292379738, 39.92874883491396787, -10.36894250292379027 ) ) ;
#3804=CARTESIAN_POINT ( 'NONE',  ( 24.16423886937409904, 64.09541550158064638, 3.795296366450317205 ) ) ;
#3805=CARTESIAN_POINT ( 'NONE',  ( 0.1532563361054083140, 36.00893115100078745, 1.131784320476157264E-15 ) ) ;
#3808=CARTESIAN_POINT ( 'NONE',  ( 2.035157376598824452, 63.68868534415484106, 7.964842623401179544 ) ) ;
#3809=CARTESIAN_POINT ( 'NONE',  ( 16.40814093676324603, 62.45696800326376064, -11.09922568453594671 ) ) ;
#3810=CARTESIAN_POINT ( 'NONE',  ( 15.44008868035555260, 34.73035201082151247, 9.422509992056143702 ) ) ;
#3811=CARTESIAN_POINT ( 'NONE',  ( 21.09922568453594849, 56.20696800326375353, 6.408140936763242479 ) ) ;
#3812=CARTESIAN_POINT ( 'NONE',  ( 21.09922568453595559, 17.04030133659708923, -6.408140936763230044 ) ) ;
#3813=CARTESIAN_POINT ( 'NONE',  ( 19.84674366389459266, 13.30059781766745353, 2.638427012816836559 ) ) ;
#3815=( NAMED_UNIT ( * ) SI_UNIT ( $, .STERADIAN. ) SOLID_ANGLE_UNIT ( ) );
#3817=CARTESIAN_POINT ( 'NONE',  ( -0.8801773607111008646, 3.272018677488171434, 2.915334737309923430 ) ) ;
#3818=CARTESIAN_POINT ( 'NONE',  ( -0.3689425029237881626, 32.42874883491395366, 10.36894250292379027 ) ) ;
#3819=CARTESIAN_POINT ( 'NONE',  ( 4.559911319644449179, 38.89701867748817676, 9.422509992056141925 ) ) ;
#3820=CARTESIAN_POINT ( 'NONE',  ( 12.91533473730993009, 46.60535201082150536, -10.88017736071109987 ) ) ;
#3823=CARTESIAN_POINT ( 'NONE',  ( 17.20831665107776587, 4.133931151000785675, -7.208316651077762316 ) ) ;
#3826=CARTESIAN_POINT ( 'NONE',  ( -46.52481518344757205, 102.2792363782860576, 7.261093659072778372 ) ) ;
#3827=CARTESIAN_POINT ( 'NONE',  ( 10.00000000000000000, 24.75893115100078745, -9.846743663894594434 ) ) ;
#3828=CARTESIAN_POINT ( 'NONE',  ( 0.1532563361054082862, 56.21726448433411605, 2.638427012816831674 ) ) ;
#3829=CARTESIAN_POINT ( 'NONE',  ( 0.5774900079438590739, 22.64701867748817321, -5.440088680355550821 ) ) ;
#3830=CARTESIAN_POINT ( 'NONE',  ( 22.81628187352648496, 41.83196800326375353, -3.434112377981050290 ) ) ;
#3832=CARTESIAN_POINT ( 'NONE',  ( 20.88017736071110875, 60.77201867748817676, -2.915334737309920765 ) ) ;
#3833=CARTESIAN_POINT ( 'NONE',  ( 5.076628168052703671, 26.84226448433411960, 8.527530157486179263 ) ) ;
#3834=CARTESIAN_POINT ( 'NONE',  ( 13.79529636645031943, 55.34541550158062506, -14.16423886937409904 ) ) ;
#3835=CARTESIAN_POINT ( 'NONE',  ( 12.63842701281683034, 27.46726448433411250, 9.846743663894596210 ) ) ;
#3836=CARTESIAN_POINT ( 'NONE',  ( 0.1129803114748860748, 44.29427333184091964, -6.480634945678686698 ) ) ;
#3837=CARTESIAN_POINT ( 'NONE',  ( -42.60666666666667624, 92.50000000000000000, -9.500000000000000000 ) ) ;
#3838=CARTESIAN_POINT ( 'NONE',  ( 2.917880565312950480, 5.970415501580634832, -12.26659068614894821 ) ) ;
#3839=CARTESIAN_POINT ( 'NONE',  ( 2.917880565312948704, 37.63708216824731068, 12.26659068614894643 ) ) ;
#3840=CARTESIAN_POINT ( 'NONE',  ( 2.791683348922240793, 31.63393115100078745, 7.208316651077764092 ) ) ;
#3842=CARTESIAN_POINT ( 'NONE',  ( 19.42250999205614193, 20.14701867748817321, 5.440088680355555262 ) ) ;
#3844=CARTESIAN_POINT ( 'NONE',  ( 0.5774900079438607392, 53.48035201082151247, 5.440088680355550821 ) ) ;
#3846=EDGE_LOOP ( 'NONE', ( #4746, #67108, #37781, #17654 ) ) ;
#3847=CARTESIAN_POINT ( 'NONE',  ( -1.099225684535947600, 38.70696800326375353, -6.408140936763238038 ) ) ;
#3848=CARTESIAN_POINT ( 'NONE',  ( 0.5774900079438607392, 48.48035201082150536, 5.440088680355550821 ) ) ;
#3850=FACE_OUTER_BOUND ( 'NONE', #26365, .T. ) ;
#3852=CARTESIAN_POINT ( 'NONE',  ( 12.91533473730993009, 61.60535201082150536, -10.88017736071109987 ) ) ;
#3854=CARTESIAN_POINT ( 'NONE',  ( 4.559911319644449179, 62.23035201082150536, -9.422509992056141925 ) ) ;
#3857=CARTESIAN_POINT ( 'NONE',  ( 2.035157376598822676, 7.438685344154837509, -7.964842623401177768 ) ) ;
#3858=CARTESIAN_POINT ( 'NONE',  ( 5.076628168052703671, 6.842264484334118713, 8.527530157486179263 ) ) ;
#3859=CARTESIAN_POINT ( 'NONE',  ( -0.3689425029237881626, 12.42874883491396609, 10.36894250292379027 ) ) ;
#3860=CARTESIAN_POINT ( 'NONE',  ( 18.52753015748618282, 8.925597817667451750, -4.923371831947291888 ) ) ;
#3861=CARTESIAN_POINT ( 'NONE',  ( 2.035157376598822676, 22.43868534415483396, -7.964842623401177768 ) ) ;
#3862=CARTESIAN_POINT ( 'NONE',  ( 10.00000000000000000, 59.75893115100078745, -9.846743663894594434 ) ) ;
#3863=VERTEX_POINT ( 'NONE', #72062 ) ;
#3864=CARTESIAN_POINT ( 'NONE',  ( 5.076628168052703671, 46.84226448433412315, 8.527530157486179263 ) ) ;
#3865=EDGE_LOOP ( 'NONE', ( #8215, #61037, #25643, #64355, #6806, #79339, #24164, #19615 ) ) ;
#3866=CARTESIAN_POINT ( 'NONE',  ( 19.72487221294570858, 70.00000000000000000, 6.000000000000000000 ) ) ;
#3867=CARTESIAN_POINT ( 'NONE',  ( 15.44008868035555793, 56.39701867748817676, -9.422509992056140149 ) ) ;
#3868=CARTESIAN_POINT ( 'NONE',  ( 17.20831665107776587, 52.88393115100078035, 7.208316651077764980 ) ) ;
#3869=CARTESIAN_POINT ( 'NONE',  ( 2.035157376598822676, 12.43868534415483751, -7.964842623401177768 ) ) ;
#3871=CARTESIAN_POINT ( 'NONE',  ( 7.084665262690076126, 64.10535201082150536, 10.88017736071109987 ) ) ;
#3872=CARTESIAN_POINT ( 'NONE',  ( 6.204703633549690345, 65.76208216824731778, -14.16423886937410259 ) ) ;
#3875=CARTESIAN_POINT ( 'NONE',  ( 0.6178305044545838731, 44.74863466993042493, 9.382169495545420901 ) ) ;
#3876=CARTESIAN_POINT ( 'NONE',  ( -0.8801773607111009756, 33.06368534415484106, 1.068504757029289695E-15 ) ) ;
#3879=CARTESIAN_POINT ( 'NONE',  ( 16.40814093676324603, 42.45696800326375353, -11.09922568453594671 ) ) ;
#3880=CARTESIAN_POINT ( 'NONE',  ( 10.00000000000000000, 36.81368534415484106, -10.88017736071110342 ) ) ;
#3881=EDGE_CURVE ( 'NONE', #85215, #57334, #12414, .T. ) ;
#3883=CARTESIAN_POINT ( 'NONE',  ( 0.1532563361054100626, 65.80059781766745175, -2.638427012816831230 ) ) ;
#3884=CARTESIAN_POINT ( 'NONE',  ( 12.63842701281683922, 14.55059781766744997, -9.846743663894590881 ) ) ;
#3885=CARTESIAN_POINT ( 'NONE',  ( 0.1532563361054100626, 45.80059781766745886, -2.638427012816831230 ) ) ;
#3886=CARTESIAN_POINT ( 'NONE',  ( 10.00000000000000000, 16.81368534415483751, -10.88017736071110342 ) ) ;
#3888=CARTESIAN_POINT ( 'NONE',  ( 2.791683348922237240, 40.38393115100078035, -7.208316651077763204 ) ) ;
#3891=CARTESIAN_POINT ( 'NONE',  ( 14.92337183194729988, 24.34226448433411960, -8.527530157486177487 ) ) ;
#3892=CARTESIAN_POINT ( 'NONE',  ( 17.20831665107776587, 14.13393115100078568, -7.208316651077762316 ) ) ;
#3894=CARTESIAN_POINT ( 'NONE',  ( 10.00000000000000178, 62.25893115100078745, 9.846743663894594434 ) ) ;
#3896=CARTESIAN_POINT ( 'NONE',  ( 20.10239578412225470, 7.633775574782964313, -6.340343622311918281 ) ) ;
#3897=CARTESIAN_POINT ( 'NONE',  ( -2.816281873526471635, 43.91530133659708923, -3.434112377981056508 ) ) ;
#3898=CARTESIAN_POINT ( 'NONE',  ( 2.791683348922240793, 46.63393115100077324, 7.208316651077764092 ) ) ;
#3900=CARTESIAN_POINT ( 'NONE',  ( 0.1916775849787255848, 12.25868815902069642, -6.500000000000001776 ) ) ;
#3901=CARTESIAN_POINT ( 'NONE',  ( 17.08211943468705130, 63.47041550158063927, 12.26659068614894998 ) ) ;
#3902=CARTESIAN_POINT ( 'NONE',  ( 12.63842701281683922, 24.55059781766745175, -9.846743663894590881 ) ) ;
#3905=CARTESIAN_POINT ( 'NONE',  ( 17.08211943468705130, 53.47041550158063217, 12.26659068614894998 ) ) ;
#3906=CARTESIAN_POINT ( 'NONE',  ( 19.84674366389459266, 63.71726448433412315, -2.638427012816827677 ) ) ;
#3907=CARTESIAN_POINT ( 'NONE',  ( 17.96484262340118221, 4.938685344154837509, 7.964842623401181321 ) ) ;
#3908=CARTESIAN_POINT ( 'NONE',  ( -2.266590686148945544, 31.38708216824730002, -7.082119434687050408 ) ) ;
#3909=CARTESIAN_POINT ( 'NONE',  ( 22.26659068614895176, 34.72041550158063927, -7.082119434687042414 ) ) ;
#3912=CARTESIAN_POINT ( 'NONE',  ( 0.1532563361054100626, 60.80059781766744464, -2.638427012816831230 ) ) ;
#3913=CARTESIAN_POINT ( 'NONE',  ( 19.42250999205614548, 45.98035201082150536, -5.440088680355545492 ) ) ;
#3917=CARTESIAN_POINT ( 'NONE',  ( 18.52753015748617571, 58.09226448433411605, 4.923371831947298993 ) ) ;
#3918=CARTESIAN_POINT ( 'NONE',  ( 2.917880565312950480, 0.9704155015806342766, -12.26659068614894821 ) ) ;
#3920=CARTESIAN_POINT ( 'NONE',  ( 24.16423886937410614, 24.30374883491396787, 8.672049930838204340E-16 ) ) ;
#3924=CARTESIAN_POINT ( 'NONE',  ( 2.035157376598822676, 17.43868534415483751, -7.964842623401177768 ) ) ;
#3925=CARTESIAN_POINT ( 'NONE',  ( 22.81628187352648496, 26.83196800326374998, -3.434112377981050290 ) ) ;
#3927=CARTESIAN_POINT ( 'NONE',  ( 7.361572987183170547, 12.05059781766744997, 9.846743663894590881 ) ) ;
#3933=CARTESIAN_POINT ( 'NONE',  ( 7.084665262690076126, 7.022018677488170546, -10.88017736071110164 ) ) ;
#3935=CARTESIAN_POINT ( 'NONE',  ( 20.88017736071110164, 35.35535201082150536, 2.915334737309930979 ) ) ;
#3936=CARTESIAN_POINT ( 'NONE',  ( -0.8801773607111008646, 43.27201867748817676, 2.915334737309923430 ) ) ;
#3937=CARTESIAN_POINT ( 'NONE',  ( 22.81628187352647785, 11.62363466993042138, 6.195893100308588602E-16 ) ) ;
#3938=CARTESIAN_POINT ( 'NONE',  ( 1.472469842513823179, 61.42559781766745175, 4.923371831947296329 ) ) ;
#3940=CARTESIAN_POINT ( 'NONE',  ( 19.84674366389459266, 13.71726448433411782, -2.638427012816827677 ) ) ;
#3943=CARTESIAN_POINT ( 'NONE',  ( 19.42250999205614548, 45.98035201082150536, -5.440088680355545492 ) ) ;
#3944=CARTESIAN_POINT ( 'NONE',  ( 13.43411237798105340, 0.5819680032637533085, 12.81628187352647963 ) ) ;
#3945=CARTESIAN_POINT ( 'NONE',  ( 19.42250999205614193, 60.14701867748817676, 5.440088680355555262 ) ) ;
#3946=CARTESIAN_POINT ( 'NONE',  ( 12.63842701281683922, 24.55059781766745175, -9.846743663894590881 ) ) ;
#3947=CARTESIAN_POINT ( 'NONE',  ( 13.43411237798105340, 45.58196800326374643, 12.81628187352647963 ) ) ;
#3948=CARTESIAN_POINT ( 'NONE',  ( 10.00000000000000000, -0.2410688489992152128, -9.846743663894594434 ) ) ;
#3949=CARTESIAN_POINT ( 'NONE',  ( 5.500000000000000000, 10.49999999999999822, 6.500000000000000888 ) ) ;
#3953=CARTESIAN_POINT ( 'NONE',  ( 19.42250999205614548, 5.980352010821504471, -5.440088680355545492 ) ) ;
#3954=CARTESIAN_POINT ( 'NONE',  ( 6.565887622018943937, 60.16530133659707502, 12.81628187352647430 ) ) ;
#3955=CARTESIAN_POINT ( 'NONE',  ( 17.08211943468705130, 23.47041550158063572, 12.26659068614894998 ) ) ;
#3956=CARTESIAN_POINT ( 'NONE',  ( 2.791683348922237240, 25.38393115100078390, -7.208316651077763204 ) ) ;
#3957=CARTESIAN_POINT ( 'NONE',  ( 20.88017736071110875, 20.77201867748816611, -2.915334737309920765 ) ) ;
#3958=CARTESIAN_POINT ( 'NONE',  ( 2.917880565312948704, 67.63708216824730357, 12.26659068614894643 ) ) ;
#3961=CARTESIAN_POINT ( 'NONE',  ( 20.88017736071110164, 15.35535201082150358, 2.915334737309930979 ) ) ;
#3962=EDGE_CURVE ( 'NONE', #97016, #51739, #66195, .T. ) ;
#3963=CARTESIAN_POINT ( 'NONE',  ( 4.559911319644449179, 27.23035201082150536, -9.422509992056141925 ) ) ;
#3965=CARTESIAN_POINT ( 'NONE',  ( 12.91533473730993009, 31.60535201082150891, -10.88017736071109987 ) ) ;
#3967=CARTESIAN_POINT ( 'NONE',  ( 18.52753015748617571, 63.09226448433412315, 4.923371831947298993 ) ) ;
#3968=CARTESIAN_POINT ( 'NONE',  ( 15.44008868035555260, 24.73035201082150891, 9.422509992056143702 ) ) ;
#3969=CARTESIAN_POINT ( 'NONE',  ( 18.52753015748617571, 63.09226448433412315, 4.923371831947298993 ) ) ;
#3971=CARTESIAN_POINT ( 'NONE',  ( 10.00000000000000000, 57.87363466993042493, -12.81628187352647608 ) ) ;
#3972=CARTESIAN_POINT ( 'NONE',  ( 0.8952175423694801459, 67.60160829253887016, -5.990408912944315212 ) ) ;
#3974=CARTESIAN_POINT ( 'NONE',  ( 20.36894250292379738, 34.92874883491396076, -10.36894250292379027 ) ) ;
#3975=CARTESIAN_POINT ( 'NONE',  ( 20.88017736071110875, 45.77201867748816966, -2.915334737309920765 ) ) ;
#3976=CARTESIAN_POINT ( 'NONE',  ( 4.559911319644449179, 12.23035201082150714, -9.422509992056141925 ) ) ;
#3977=ADVANCED_FACE ( 'NONE', ( #73527 ), #10732, .T. ) ;
#3978=CARTESIAN_POINT ( 'NONE',  ( 19.84674366389459266, 53.71726448433411605, -2.638427012816827677 ) ) ;
#3980=CARTESIAN_POINT ( 'NONE',  ( 0.1532563361054100626, 45.80059781766745886, -2.638427012816831230 ) ) ;
#3982=CARTESIAN_POINT ( 'NONE',  ( 20.15039907845753930, 70.00000000000000000, -6.262539305110068177 ) ) ;
#3983=CARTESIAN_POINT ( 'NONE',  ( 0.1532563361054083140, 11.00893115100078568, 1.131784320476157264E-15 ) ) ;
#3985=ORIENTED_EDGE ( 'NONE', *, *, #43233, .F. ) ;
#3987=CARTESIAN_POINT ( 'NONE',  ( 2.035157376598824452, 13.68868534415483751, 7.964842623401179544 ) ) ;
#3988=CARTESIAN_POINT ( 'NONE',  ( 12.63842701281683034, 7.467264484334118713, 9.846743663894596210 ) ) ;
#3990=CARTESIAN_POINT ( 'NONE',  ( 10.00000000000000000, 64.75893115100078035, -9.846743663894594434 ) ) ;
#3991=CARTESIAN_POINT ( 'NONE',  ( 20.88017736071110164, 65.35535201082150536, 2.915334737309930979 ) ) ;
#3992=CARTESIAN_POINT ( 'NONE',  ( 15.44008868035555260, 49.73035201082150536, 9.422509992056143702 ) ) ;
#3993=CARTESIAN_POINT ( 'NONE',  ( -0.8801773607110991993, 22.85535201082150181, -2.915334737309923874 ) ) ;
#3994=CARTESIAN_POINT ( 'NONE',  ( 10.00000000000000000, 62.87363466993042493, -12.81628187352647608 ) ) ;
#3995=CARTESIAN_POINT ( 'NONE',  ( 13.79529636645031943, 30.34541550158063927, -14.16423886937409904 ) ) ;
#3996=CARTESIAN_POINT ( 'NONE',  ( 2.791683348922240793, 11.63393115100078568, 7.208316651077764092 ) ) ;
#3999=CARTESIAN_POINT ( 'NONE',  ( 3.591859063236763294, 53.29030133659708923, -11.09922568453595026 ) ) ;
#4001=CARTESIAN_POINT ( 'NONE',  ( 10.00000000000000178, 5.373634669930420493, 12.81628187352647608 ) ) ;
#4003=CARTESIAN_POINT ( 'NONE',  ( 0.5774900079438607392, 28.48035201082150891, 5.440088680355550821 ) ) ;
#4007=CARTESIAN_POINT ( 'NONE',  ( 17.20831665107776587, 9.133931151000787452, -7.208316651077762316 ) ) ;
#4009=CARTESIAN_POINT ( 'NONE',  ( 19.84674366389459621, 8.508931151000785675, 7.409399052514197653E-17 ) ) ;
#4010=CARTESIAN_POINT ( 'NONE',  ( 1.472469842513823179, 25.59226448433412315, -4.923371831947296329 ) ) ;
#4011=CARTESIAN_POINT ( 'NONE',  ( 0.1532563361054082862, 11.21726448433411605, 2.638427012816831674 ) ) ;
#4012=CARTESIAN_POINT ( 'NONE',  ( 14.92337183194729633, 2.675597817667451750, 8.527530157486181039 ) ) ;
#4014=CARTESIAN_POINT ( 'NONE',  ( 0.5774900079438607392, 53.48035201082151247, 5.440088680355550821 ) ) ;
#4016=CARTESIAN_POINT ( 'NONE',  ( 19.42250999205614548, 60.98035201082151247, -5.440088680355545492 ) ) ;
#4017=CARTESIAN_POINT ( 'NONE',  ( 2.791683348922240793, 21.63393115100078745, 7.208316651077764092 ) ) ;
#4020=CARTESIAN_POINT ( 'NONE',  ( 12.63842701281683922, 54.55059781766745175, -9.846743663894590881 ) ) ;
#4022=CARTESIAN_POINT ( 'NONE',  ( 19.42250999205614193, 5.147018677488171434, 5.440088680355555262 ) ) ;
#4023=CARTESIAN_POINT ( 'NONE',  ( 22.26659068614895176, 24.72041550158063572, -7.082119434687042414 ) ) ;
#4026=CARTESIAN_POINT ( 'NONE',  ( 20.36894250292379738, 14.92874883491396432, -10.36894250292379027 ) ) ;
#4027=CARTESIAN_POINT ( 'NONE',  ( 13.79529636645031943, 30.34541550158063927, -14.16423886937409904 ) ) ;
#4029=( NAMED_UNIT ( * ) PLANE_ANGLE_UNIT ( ) SI_UNIT ( $, .RADIAN. ) );
#4030=CARTESIAN_POINT ( 'NONE',  ( 17.96484262340118221, 39.93868534415484106, 7.964842623401181321 ) ) ;
#4032=CARTESIAN_POINT ( 'NONE',  ( 5.076628168052704559, 15.17559781766745175, -8.527530157486179263 ) ) ;
#4033=CARTESIAN_POINT ( 'NONE',  ( 0.5774900079438607392, 58.48035201082151247, 5.440088680355550821 ) ) ;
#4034=CARTESIAN_POINT ( 'NONE',  ( 2.791683348922237240, 20.38393115100078745, -7.208316651077763204 ) ) ;
#4035=CARTESIAN_POINT ( 'NONE',  ( 17.96484262340118221, 9.938685344154839285, 7.964842623401181321 ) ) ;
#4036=CARTESIAN_POINT ( 'NONE',  ( 10.00000000000000000, 42.87363466993042493, -12.81628187352647608 ) ) ;
#4037=CARTESIAN_POINT ( 'NONE',  ( 7.361572987183169658, 44.96726448433412315, -9.846743663894592657 ) ) ;
#4038=CARTESIAN_POINT ( 'NONE',  ( 18.04007052943772749, 58.01528370094807485, 5.767676674365840306 ) ) ;
#4040=CARTESIAN_POINT ( 'NONE',  ( 13.43411237798106583, 32.66530133659708213, -12.81628187352647252 ) ) ;
#4042=CARTESIAN_POINT ( 'NONE',  ( 19.84674366389459621, 28.50893115100078745, 7.409399052514197653E-17 ) ) ;
#4043=CARTESIAN_POINT ( 'NONE',  ( 10.00000000000000000, 10.55374883491396787, -14.16423886937410082 ) ) ;
#4047=CARTESIAN_POINT ( 'NONE',  ( 19.42250999205614193, 45.14701867748817676, 5.440088680355555262 ) ) ;
#4048=CARTESIAN_POINT ( 'NONE',  ( 12.91533473730993009, 46.60535201082150536, -10.88017736071109987 ) ) ;
#4049=CARTESIAN_POINT ( 'NONE',  ( 20.36894250292379382, 48.67874883491396076, 10.36894250292379205 ) ) ;
#4050=CARTESIAN_POINT ( 'NONE',  ( 18.52753015748618282, 53.92559781766745175, -4.923371831947291888 ) ) ;
#4051=CARTESIAN_POINT ( 'NONE',  ( 19.84674366389459621, 8.508931151000785675, 7.409399052514197653E-17 ) ) ;
#4053=CARTESIAN_POINT ( 'NONE',  ( 2.035157376598822676, 47.43868534415484817, -7.964842623401177768 ) ) ;
#4054=FACE_OUTER_BOUND ( 'NONE', #51584, .T. ) ;
#4055=CARTESIAN_POINT ( 'NONE',  ( 16.40814093676324603, 27.45696800326375708, -11.09922568453594671 ) ) ;
#4056=CARTESIAN_POINT ( 'NONE',  ( 17.20831665107776587, 57.88393115100078745, 7.208316651077764980 ) ) ;
#4058=CARTESIAN_POINT ( 'NONE',  ( 10.00000000000000000, 66.81368534415484817, -10.88017736071110342 ) ) ;
#4059=( LENGTH_UNIT ( ) NAMED_UNIT ( * ) SI_UNIT ( .MILLI., .METRE. ) );
#4060=CARTESIAN_POINT ( 'NONE',  ( 10.00000000000000178, 2.258931151000784787, 9.846743663894594434 ) ) ;
#4061=CARTESIAN_POINT ( 'NONE',  ( 0.5774900079438607392, 68.48035201082150536, 5.440088680355550821 ) ) ;
#4063=AXIS2_PLACEMENT_3D ( 'NONE', #64970, #11991, #27478 ) ;
#4064=CARTESIAN_POINT ( 'NONE',  ( 18.52753015748617571, 33.09226448433411605, 4.923371831947298993 ) ) ;
#4065=CARTESIAN_POINT ( 'NONE',  ( 10.00000000000000000, 21.81368534415484106, -10.88017736071110342 ) ) ;
#4066=CARTESIAN_POINT ( 'NONE',  ( 0.1532563361054100626, 60.80059781766744464, -2.638427012816831230 ) ) ;
#4067=CARTESIAN_POINT ( 'NONE',  ( 2.035157376598824452, 33.68868534415484106, 7.964842623401179544 ) ) ;
#4070=CARTESIAN_POINT ( 'NONE',  ( 3.591859063236761518, 39.95696800326375353, 11.09922568453594849 ) ) ;
#4072=CARTESIAN_POINT ( 'NONE',  ( 19.42250999205614193, 55.14701867748817676, 5.440088680355555262 ) ) ;
#4073=CARTESIAN_POINT ( 'NONE',  ( 16.40814093676324603, 17.45696800326375353, -11.09922568453594671 ) ) ;
#4075=CARTESIAN_POINT ( 'NONE',  ( 12.63842701281683034, 2.467264484334118269, 9.846743663894596210 ) ) ;
#4076=CARTESIAN_POINT ( 'NONE',  ( 17.96484262340118221, 29.93868534415484106, 7.964842623401181321 ) ) ;
#4077=CARTESIAN_POINT ( 'NONE',  ( 22.26659068614895176, 59.72041550158063927, -7.082119434687042414 ) ) ;
#4078=CARTESIAN_POINT ( 'NONE',  ( 10.00000000000000000, 49.75893115100078745, -9.846743663894594434 ) ) ;
#4079=CARTESIAN_POINT ( 'NONE',  ( 17.20831665107776587, 7.883931151000784787, 7.208316651077764980 ) ) ;
#4080=CARTESIAN_POINT ( 'NONE',  ( 4.559911319644449179, 62.23035201082150536, -9.422509992056141925 ) ) ;
#4082=CARTESIAN_POINT ( 'NONE',  ( 24.16423886937409904, 29.09541550158063572, 3.795296366450317205 ) ) ;
#4088=CARTESIAN_POINT ( 'NONE',  ( 2.917880565312948704, 52.63708216824730357, 12.26659068614894643 ) ) ;
#4089=CARTESIAN_POINT ( 'NONE',  ( 2.917880565312948704, 47.63708216824730357, 12.26659068614894643 ) ) ;
#4090=CARTESIAN_POINT ( 'NONE',  ( 10.00000000000000178, 22.25893115100078745, 9.846743663894594434 ) ) ;
#4092=CARTESIAN_POINT ( 'NONE',  ( -1.099225684535947600, 14.54030133659708568, 6.408140936763237150 ) ) ;
#4095=SURFACE_SIDE_STYLE ('',( #12072 ) ) ;
#4096=CARTESIAN_POINT ( 'NONE',  ( 22.81628187352647785, 51.41530133659708923, 3.434112377981063169 ) ) ;
#4097=CARTESIAN_POINT ( 'NONE',  ( 22.26659068614894466, 48.88708216824730357, 7.082119434687054849 ) ) ;
#4101=CARTESIAN_POINT ( 'NONE',  ( 19.84674366389459266, 8.717264484334116048, -2.638427012816827677 ) ) ;
#4104=CARTESIAN_POINT ( 'NONE',  ( 18.52753015748618282, 13.92559781766745175, -4.923371831947291888 ) ) ;
#4106=CARTESIAN_POINT ( 'NONE',  ( 20.88017736071110164, 5.355352010821503583, 2.915334737309930979 ) ) ;
#4107=CARTESIAN_POINT ( 'NONE',  ( 19.42250999205614548, 30.98035201082150536, -5.440088680355545492 ) ) ;
#4108=CARTESIAN_POINT ( 'NONE',  ( 17.20831665107776587, 49.13393115100078745, -7.208316651077762316 ) ) ;
#4109=CARTESIAN_POINT ( 'NONE',  ( 21.09922568453594849, 6.206968003263753531, 6.408140936763242479 ) ) ;
#4113=CARTESIAN_POINT ( 'NONE',  ( 0.6178305044545818747, 18.49863466993041428, -9.382169495545419124 ) ) ;
#4114=ORIENTED_EDGE ( 'NONE', *, *, #3061, .T. ) ;
#4115=( BOUNDED_CURVE ( )  B_SPLINE_CURVE ( 2, ( #19207, #21682, #28182, #21182, #51682, #45149, #6666, #60643, #82161 ),
 .UNSPECIFIED., .F., .T. ) 
 B_SPLINE_CURVE_WITH_KNOTS ( ( 3, 2, 2, 2, 3 ),
 ( 0.9401409369402312644, 0.9404761904761904656, 0.9464285714285713969, 0.9523809523809524391, 0.9527162059169116404 ),
 .UNSPECIFIED. ) 
 CURVE ( )  GEOMETRIC_REPRESENTATION_ITEM ( )  RATIONAL_B_SPLINE_CURVE ( ( 0.9963778908391753841, 0.9980808541467917072, 1.000000000000000000, 0.9659258262890682012, 1.000000000000000000, 0.9659258262890682012, 1.000000000000000000, 0.9980808541467917072, 0.9963778908391753841 ) ) 
 REPRESENTATION_ITEM ( '' )  );
#4116=CARTESIAN_POINT ( 'NONE',  ( 1.472469842513823179, 35.59226448433412315, -4.923371831947296329 ) ) ;
#4117=CARTESIAN_POINT ( 'NONE',  ( -0.3689425029237881626, 57.42874883491397497, 10.36894250292379027 ) ) ;
#4120=CARTESIAN_POINT ( 'NONE',  ( 20.36894250292379382, 58.67874883491396076, 10.36894250292379205 ) ) ;
#4121=ORIENTED_EDGE ( 'NONE', *, *, #50935, .F. ) ;
#4122=CARTESIAN_POINT ( 'NONE',  ( 0.5774900079438607392, 28.48035201082150891, 5.440088680355550821 ) ) ;
#4123=CARTESIAN_POINT ( 'NONE',  ( 15.44008868035555793, 41.39701867748817676, -9.422509992056140149 ) ) ;
#4124=CARTESIAN_POINT ( 'NONE',  ( 2.035157376598822676, 52.43868534415483396, -7.964842623401177768 ) ) ;
#4126=CARTESIAN_POINT ( 'NONE',  ( 4.559911319644449179, 43.89701867748816966, 9.422509992056141925 ) ) ;
#4132=CARTESIAN_POINT ( 'NONE',  ( 19.84674366389459266, 18.30059781766745175, 2.638427012816836559 ) ) ;
#4135=CARTESIAN_POINT ( 'NONE',  ( 1.472469842513823179, 61.42559781766745175, 4.923371831947296329 ) ) ;
#4137=CARTESIAN_POINT ( 'NONE',  ( 22.81628187352647785, 61.41530133659709634, 3.434112377981063169 ) ) ;
#4142=CARTESIAN_POINT ( 'NONE',  ( 17.08211943468705130, 63.47041550158063927, 12.26659068614894998 ) ) ;
#4146=CARTESIAN_POINT ( 'NONE',  ( 19.84674366389459266, 33.30059781766744464, 2.638427012816836559 ) ) ;
#4147=CARTESIAN_POINT ( 'NONE',  ( 19.38216949554541557, 62.24863466993041072, -9.382169495545420901 ) ) ;
#4148=CARTESIAN_POINT ( 'NONE',  ( -1.099225684535947600, -0.4596986634029132657, 6.408140936763237150 ) ) ;
#4149=CARTESIAN_POINT ( 'NONE',  ( 17.96484262340118221, 61.18868534415482685, -7.964842623401177768 ) ) ;
#4151=CARTESIAN_POINT ( 'NONE',  ( 1.472469842513823179, 15.59226448433411960, -4.923371831947296329 ) ) ;
#4152=CARTESIAN_POINT ( 'NONE',  ( 0.1532563361054083140, 61.00893115100078745, 1.131784320476157264E-15 ) ) ;
#4155=CARTESIAN_POINT ( 'NONE',  ( 12.91533473730993009, 16.60535201082150891, -10.88017736071109987 ) ) ;
#4156=CARTESIAN_POINT ( 'NONE',  ( 0.1532563361054082862, 11.21726448433411605, 2.638427012816831674 ) ) ;
#4157=CARTESIAN_POINT ( 'NONE',  ( 10.00000000000000000, 36.81368534415484106, -10.88017736071110342 ) ) ;
#4158=CARTESIAN_POINT ( 'NONE',  ( 22.81628187352647785, 31.41530133659709279, 3.434112377981063169 ) ) ;
#4160=( NAMED_UNIT ( * ) PLANE_ANGLE_UNIT ( ) SI_UNIT ( $, .RADIAN. ) );
#4161=CARTESIAN_POINT ( 'NONE',  ( -0.2418659066527703572, 58.09014588040358262, 6.114288769123046308 ) ) ;
#4162=CARTESIAN_POINT ( 'NONE',  ( 1.472469842513823179, 50.59226448433411605, -4.923371831947296329 ) ) ;
#4163=CARTESIAN_POINT ( 'NONE',  ( 7.361572987183170547, 17.05059781766745530, 9.846743663894590881 ) ) ;
#4165=CARTESIAN_POINT ( 'NONE',  ( 6.565887622018943937, 20.16530133659708213, 12.81628187352647430 ) ) ;
#4166=FACE_OUTER_BOUND ( 'NONE', #50419, .T. ) ;
#4167=CARTESIAN_POINT ( 'NONE',  ( 17.96484262340118221, 26.18868534415483396, -7.964842623401177768 ) ) ;
#4171=CARTESIAN_POINT ( 'NONE',  ( 13.79529636645030344, 48.26208216824728936, 14.16423886937410614 ) ) ;
#4173=CARTESIAN_POINT ( 'NONE',  ( 12.63842701281683922, 39.55059781766744464, -9.846743663894590881 ) ) ;
#4174=CARTESIAN_POINT ( 'NONE',  ( 21.09922568453595559, 32.04030133659708923, -6.408140936763230044 ) ) ;
#4175=CARTESIAN_POINT ( 'NONE',  ( 17.96484262340118221, 31.18868534415483751, -7.964842623401177768 ) ) ;
#4176=CARTESIAN_POINT ( 'NONE',  ( 2.791683348922237240, 50.38393115100078035, -7.208316651077763204 ) ) ;
#4177=CARTESIAN_POINT ( 'NONE',  ( -0.8801773607111009756, 43.06368534415484106, 1.068504757029289695E-15 ) ) ;
#4178=CARTESIAN_POINT ( 'NONE',  ( 22.81628187352647785, 11.62363466993042138, 6.195893100308588602E-16 ) ) ;
#4179=CARTESIAN_POINT ( 'NONE',  ( 2.917880565312950480, 35.97041550158063217, -12.26659068614894821 ) ) ;
#4183=CARTESIAN_POINT ( 'NONE',  ( 5.076628168052704559, 25.17559781766745175, -8.527530157486179263 ) ) ;
#4184=CARTESIAN_POINT ( 'NONE',  ( 6.565887622018943937, 58.08196800326376064, -12.81628187352647608 ) ) ;
#4185=CARTESIAN_POINT ( 'NONE',  ( 5.076628168052703671, 61.84226448433412315, 8.527530157486179263 ) ) ;
#4186=ORIENTED_EDGE ( 'NONE', *, *, #89747, .T. ) ;
#4187=CARTESIAN_POINT ( 'NONE',  ( 20.15039907845753575, 7.627771745786129820, -6.262539305110077059 ) ) ;
#4189=CARTESIAN_POINT ( 'NONE',  ( -0.8801773607111008646, 8.272018677488171434, 2.915334737309923430 ) ) ;
#4190=CARTESIAN_POINT ( 'NONE',  ( 20.88017736071110519, 60.56368534415484106, 2.639326808657452039E-16 ) ) ;
#4191=CARTESIAN_POINT ( 'NONE',  ( 2.917880565312950480, 30.97041550158063572, -12.26659068614894821 ) ) ;
#4192=CARTESIAN_POINT ( 'NONE',  ( 0.1532563361054082862, 6.217264484334118713, 2.638427012816831674 ) ) ;
#4193=CARTESIAN_POINT ( 'NONE',  ( 18.52753015748618282, 53.92559781766745175, -4.923371831947291888 ) ) ;
#4194=CARTESIAN_POINT ( 'NONE',  ( 0.5774900079438607392, 38.48035201082150536, 5.440088680355550821 ) ) ;
#4196=CARTESIAN_POINT ( 'NONE',  ( -43.49126349454923712, 106.3716649516064479, -5.070890430955789618 ) ) ;
#4200=ADVANCED_FACE ( 'NONE', ( #30938 ), #97316, .T. ) ;
#4202=ORIENTED_EDGE ( 'NONE', *, *, #72345, .T. ) ;
#4204=CARTESIAN_POINT ( 'NONE',  ( 13.79529636645030344, 3.262082168247301350, 14.16423886937410614 ) ) ;
#4205=CARTESIAN_POINT ( 'NONE',  ( 13.79529636645031943, 15.34541550158063750, -14.16423886937409904 ) ) ;
#4206=CARTESIAN_POINT ( 'NONE',  ( 4.559911319644449179, 47.23035201082150536, -9.422509992056141925 ) ) ;
#4207=CARTESIAN_POINT ( 'NONE',  ( 6.204703633549690345, 60.76208216824730357, -14.16423886937410259 ) ) ;
#4208=CARTESIAN_POINT ( 'NONE',  ( 7.361572987183169658, 59.96726448433410894, -9.846743663894592657 ) ) ;
#4209=CARTESIAN_POINT ( 'NONE',  ( 18.52753015748618282, 33.92559781766745886, -4.923371831947291888 ) ) ;
#4211=CARTESIAN_POINT ( 'NONE',  ( 17.96484262340118221, 36.18868534415484106, -7.964842623401177768 ) ) ;
#4212=CARTESIAN_POINT ( 'NONE',  ( 5.076628168052703671, 56.84226448433412315, 8.527530157486179263 ) ) ;
#4213=( NAMED_UNIT ( * ) SI_UNIT ( $, .STERADIAN. ) SOLID_ANGLE_UNIT ( ) );
#4214=CARTESIAN_POINT ( 'NONE',  ( 2.917880565312948704, 47.63708216824730357, 12.26659068614894643 ) ) ;
#4215=EDGE_CURVE ( 'NONE', #90918, #14329, #66068, .T. ) ;
#4216=CARTESIAN_POINT ( 'NONE',  ( 10.00000000000000178, 4.313685344154837509, 10.88017736071110342 ) ) ;
#4217=CARTESIAN_POINT ( 'NONE',  ( 17.39651004071838969, 39.08210964143329846, -6.500000000000027534 ) ) ;
#4220=ORIENTED_EDGE ( 'NONE', *, *, #79658, .F. ) ;
#4223=CARTESIAN_POINT ( 'NONE',  ( 17.20831665107776587, 24.13393115100078035, -7.208316651077762316 ) ) ;
#4226=CARTESIAN_POINT ( 'NONE',  ( 24.16423886937410614, 39.51208216824731068, -3.795296366450302550 ) ) ;
#4227=CARTESIAN_POINT ( 'NONE',  ( 0.1532563361054082862, 31.21726448433412315, 2.638427012816831674 ) ) ;
#4228=CARTESIAN_POINT ( 'NONE',  ( 12.91533473730993009, 61.60535201082150536, -10.88017736071109987 ) ) ;
#4229=CARTESIAN_POINT ( 'NONE',  ( 19.88701968852527102, 36.79427333184084858, 6.480634945678612091 ) ) ;
#4230=CARTESIAN_POINT ( 'NONE',  ( 15.44008868035555793, 56.39701867748817676, -9.422509992056140149 ) ) ;
#4231=EDGE_CURVE ( 'NONE', #90354, #87694, #86076, .T. ) ;
#4233=ORIENTED_EDGE ( 'NONE', *, *, #87033, .T. ) ;
#4234=CARTESIAN_POINT ( 'NONE',  ( 10.00000000000000178, 49.31368534415484106, 10.88017736071110342 ) ) ;
#4235=CARTESIAN_POINT ( 'NONE',  ( -2.266590686148945544, 17.22041550158063572, 7.082119434687048631 ) ) ;
#4236=EDGE_CURVE ( 'NONE', #98371, #507, #24760, .T. ) ;
#4238=CARTESIAN_POINT ( 'NONE',  ( -2.816281873526471635, 48.91530133659708213, -3.434112377981056508 ) ) ;
#4239=CARTESIAN_POINT ( 'NONE',  ( 19.42250999205614193, 20.14701867748817321, 5.440088680355555262 ) ) ;
#4240=CARTESIAN_POINT ( 'NONE',  ( 7.361572987183170547, 22.05059781766745530, 9.846743663894590881 ) ) ;
#4241=CARTESIAN_POINT ( 'NONE',  ( 7.084665262690076126, 19.10535201082150181, 10.88017736071109987 ) ) ;
#4242=CARTESIAN_POINT ( 'NONE',  ( 0.6178305044545818747, 48.49863466993042493, -9.382169495545419124 ) ) ;
#4244=CARTESIAN_POINT ( 'NONE',  ( 0.1532563361054100626, 35.80059781766745175, -2.638427012816831230 ) ) ;
#4247=DIRECTION ( 'NONE',  ( 1.000000000000000000, 0.000000000000000000, 0.000000000000000000 ) ) ;
#4250=AXIS2_PLACEMENT_3D ( 'NONE', #22093, #75074, #61052 ) ;
#4251=CARTESIAN_POINT ( 'NONE',  ( -0.3289641300568005855, 44.27164270246084499, -5.963430220938281678 ) ) ;
#4252=CARTESIAN_POINT ( 'NONE',  ( 10.00000000000000000, -0.2410688489992152128, -9.846743663894594434 ) ) ;
#4253=CARTESIAN_POINT ( 'NONE',  ( 16.40814093676324603, 27.45696800326375708, -11.09922568453594671 ) ) ;
#4255=CARTESIAN_POINT ( 'NONE',  ( 2.791683348922237240, 45.38393115100079456, -7.208316651077763204 ) ) ;
#4257=CARTESIAN_POINT ( 'NONE',  ( 13.79529636645030344, 18.26208216824730002, 14.16423886937410614 ) ) ;
#4258=CARTESIAN_POINT ( 'NONE',  ( 2.791683348922240793, 26.63393115100078745, 7.208316651077764092 ) ) ;
#4259=CARTESIAN_POINT ( 'NONE',  ( -1.099225684535947600, 38.70696800326375353, -6.408140936763238038 ) ) ;
#4261=CARTESIAN_POINT ( 'NONE',  ( 19.72487221294570858, 70.00000000000000000, 6.000000000000000000 ) ) ;
#4262=CARTESIAN_POINT ( 'NONE',  ( 7.084665262690076126, 69.10535201082151957, 10.88017736071109987 ) ) ;
#4263=CARTESIAN_POINT ( 'NONE',  ( -2.816281873526471635, 3.915301336597087456, -3.434112377981056508 ) ) ;
#4264=CARTESIAN_POINT ( 'NONE',  ( 2.791683348922237240, 30.38393115100078390, -7.208316651077763204 ) ) ;
#4265=CARTESIAN_POINT ( 'NONE',  ( 12.91533473730993009, 21.60535201082150536, -10.88017736071109987 ) ) ;
#4266=CARTESIAN_POINT ( 'NONE',  ( 21.09922568453595559, 32.04030133659708923, -6.408140936763230044 ) ) ;
#4268=COLOUR_RGB ( '', 0.66274510, 0.83137255, 0.94901961) ;
#4271=CARTESIAN_POINT ( 'NONE',  ( 7.084665262690076126, 34.10535201082151247, 10.88017736071109987 ) ) ;
#4275=CARTESIAN_POINT ( 'NONE',  ( 17.20831665107776587, 59.13393115100078745, -7.208316651077762316 ) ) ;
#4276=CARTESIAN_POINT ( 'NONE',  ( 19.42250999205614193, 35.14701867748816966, 5.440088680355555262 ) ) ;
#4278=CARTESIAN_POINT ( 'NONE',  ( 0.5774900079438590739, 62.64701867748817676, -5.440088680355550821 ) ) ;
#4279=CARTESIAN_POINT ( 'NONE',  ( 7.084665262690076126, 27.02201867748817676, -10.88017736071110164 ) ) ;
#4281=CARTESIAN_POINT ( 'NONE',  ( 12.63842701281683034, 2.467264484334118269, 9.846743663894596210 ) ) ;
#4283=CARTESIAN_POINT ( 'NONE',  ( 19.84674366389459266, 53.30059781766744464, 2.638427012816836559 ) ) ;
#4284=CARTESIAN_POINT ( 'NONE',  ( 24.16423886937410614, 49.30374883491396787, 8.672049930838204340E-16 ) ) ;
#4287=EDGE_CURVE ( 'NONE', #94783, #87107, #77936, .T. ) ;
#4288=CARTESIAN_POINT ( 'NONE',  ( 24.16423886937410614, 14.51208216824730179, -3.795296366450302550 ) ) ;
#4289=CARTESIAN_POINT ( 'NONE',  ( 22.26659068614894466, 38.88708216824731068, 7.082119434687054849 ) ) ;
#4291=CARTESIAN_POINT ( 'NONE',  ( 19.38216949554541202, 10.99863466993042138, 9.382169495545424454 ) ) ;
#4294=CARTESIAN_POINT ( 'NONE',  ( -4.164238869374099927, 67.01208216824728936, 3.795296366450308767 ) ) ;
#4295=CARTESIAN_POINT ( 'NONE',  ( 12.63842701281683034, 37.46726448433411605, 9.846743663894596210 ) ) ;
#4298=CARTESIAN_POINT ( 'NONE',  ( 10.00000000000000178, 59.31368534415484106, 10.88017736071110342 ) ) ;
#4300=STYLED_ITEM ( 'NONE', ( #86456 ), #29558 ) ;
#4301=CARTESIAN_POINT ( 'NONE',  ( -2.816281873526471635, 63.91530133659708923, -3.434112377981056508 ) ) ;
#4302=CARTESIAN_POINT ( 'NONE',  ( 6.565887622018943937, 30.16530133659708568, 12.81628187352647430 ) ) ;
#4303=CARTESIAN_POINT ( 'NONE',  ( 0.1532563361054082862, 26.21726448433411605, 2.638427012816831674 ) ) ;
#4307=CARTESIAN_POINT ( 'NONE',  ( 10.00000000000000000, 1.813685344154838175, -10.88017736071110342 ) ) ;
#4308=CARTESIAN_POINT ( 'NONE',  ( 24.16423886937410614, 34.51208216824731068, -3.795296366450302550 ) ) ;
#4309=CARTESIAN_POINT ( 'NONE',  ( 0.5774900079438590739, 27.64701867748817676, -5.440088680355550821 ) ) ;
#4310=CARTESIAN_POINT ( 'NONE',  ( 10.00000000000000178, 49.31368534415484106, 10.88017736071110342 ) ) ;
#4313=CARTESIAN_POINT ( 'NONE',  ( 14.92337183194729988, 14.34226448433411782, -8.527530157486177487 ) ) ;
#4316=CARTESIAN_POINT ( 'NONE',  ( 2.791683348922237240, 40.38393115100078035, -7.208316651077763204 ) ) ;
#4317=CARTESIAN_POINT ( 'NONE',  ( 0.1532563361054100626, 50.80059781766745175, -2.638427012816831230 ) ) ;
#4318=CARTESIAN_POINT ( 'NONE',  ( 2.035157376598824452, 23.68868534415484461, 7.964842623401179544 ) ) ;
#4319=UNCERTAINTY_MEASURE_WITH_UNIT (LENGTH_MEASURE( 1.000000000000000082E-05 ), #64257, 'distance_accuracy_value', 'NONE');
#4320=( BOUNDED_CURVE ( )  B_SPLINE_CURVE ( 2, ( #86993, #57474, #27466, #49974, #42481, #26482, #34960, #18500, #65458 ),
 .UNSPECIFIED., .F., .T. ) 
 B_SPLINE_CURVE_WITH_KNOTS ( ( 3, 2, 2, 2, 3 ),
 ( 0.7258552226545170738, 0.7261904761904762751, 0.7321428571428572063, 0.7380952380952381375, 0.7384304916311973388 ),
 .UNSPECIFIED. ) 
 CURVE ( )  GEOMETRIC_REPRESENTATION_ITEM ( )  RATIONAL_B_SPLINE_CURVE ( ( 0.9963778908391753841, 0.9980808541467917072, 1.000000000000000000, 0.9659258262890683122, 1.000000000000000000, 0.9659258262890683122, 1.000000000000000000, 0.9980808541467917072, 0.9963778908391753841 ) ) 
 REPRESENTATION_ITEM ( '' )  );
#4321=ADVANCED_FACE ( 'NONE', ( #44348 ), #65368, .T. ) ;
#4323=CARTESIAN_POINT ( 'NONE',  ( 22.81628187352648496, 51.83196800326376064, -3.434112377981050290 ) ) ;
#4325=CARTESIAN_POINT ( 'NONE',  ( 4.559911319644449179, 68.89701867748817676, 9.422509992056141925 ) ) ;
#4326=CARTESIAN_POINT ( 'NONE',  ( 1.472469842513823179, 25.59226448433412315, -4.923371831947296329 ) ) ;
#4327=CARTESIAN_POINT ( 'NONE',  ( 10.00000000000000178, 63.05374883491396076, 14.16423886937410082 ) ) ;
#4328=CARTESIAN_POINT ( 'NONE',  ( 14.92337183194729633, 17.67559781766745175, 8.527530157486181039 ) ) ;
#4332=CARTESIAN_POINT ( 'NONE',  ( 20.36894250292379382, 23.67874883491397142, 10.36894250292379205 ) ) ;
#4334=CARTESIAN_POINT ( 'NONE',  ( 17.08211943468705130, 33.47041550158063927, 12.26659068614894998 ) ) ;
#4335=CARTESIAN_POINT ( 'NONE',  ( 19.84674366389459266, 43.71726448433410894, -2.638427012816827677 ) ) ;
#4337=CARTESIAN_POINT ( 'NONE',  ( 15.44008868035555260, 29.73035201082150891, 9.422509992056143702 ) ) ;
#4338=CARTESIAN_POINT ( 'NONE',  ( 12.91533473730993009, 56.60535201082151247, -10.88017736071109987 ) ) ;
#4341=CARTESIAN_POINT ( 'NONE',  ( 22.81628187352647785, 51.62363466993042493, 6.195893100308588602E-16 ) ) ;
#4344=VECTOR ( 'NONE', #48493, 1000.000000000000000 ) ;
#4345=CARTESIAN_POINT ( 'NONE',  ( 2.035157376598822676, 47.43868534415484817, -7.964842623401177768 ) ) ;
#4349=CARTESIAN_POINT ( 'NONE',  ( 2.347401019785370746, 0.3355287360789229734, -6.482960602445015041 ) ) ;
#4352=CARTESIAN_POINT ( 'NONE',  ( 4.559911319644449179, 67.23035201082150536, -9.422509992056141925 ) ) ;
#4353=CARTESIAN_POINT ( 'NONE',  ( 12.91533473730992121, 9.522018677488171434, 10.88017736071110164 ) ) ;
#4356=CARTESIAN_POINT ( 'NONE',  ( 20.88017736071110164, 5.355352010821503583, 2.915334737309930979 ) ) ;
#4357=CARTESIAN_POINT ( 'NONE',  ( 2.791683348922240793, 6.633931151000785675, 7.208316651077764092 ) ) ;
#4358=CARTESIAN_POINT ( 'NONE',  ( 17.08211943468705840, 15.13708216824730179, -12.26659068614894466 ) ) ;
#4359=CARTESIAN_POINT ( 'NONE',  ( 2.035157376598824452, 28.68868534415484106, 7.964842623401179544 ) ) ;
#4360=CARTESIAN_POINT ( 'NONE',  ( 2.791683348922237240, 60.38393115100078745, -7.208316651077763204 ) ) ;
#4361=ORIENTED_EDGE ( 'NONE', *, *, #26104, .T. ) ;
#4362=CARTESIAN_POINT ( 'NONE',  ( 12.63842701281683034, 62.46726448433410894, 9.846743663894596210 ) ) ;
#4365=CARTESIAN_POINT ( 'NONE',  ( -0.8801773607111008646, 53.27201867748816966, 2.915334737309923430 ) ) ;
#4366=CARTESIAN_POINT ( 'NONE',  ( 2.791683348922237240, 60.38393115100078745, -7.208316651077763204 ) ) ;
#4367=CARTESIAN_POINT ( 'NONE',  ( 19.38216949554541557, 42.24863466993041783, -9.382169495545420901 ) ) ;
#4368=CARTESIAN_POINT ( 'NONE',  ( 10.00000000000000000, 6.813685344154838397, -10.88017736071110342 ) ) ;
#4370=CARTESIAN_POINT ( 'NONE',  ( 12.91533473730993009, 56.60535201082151247, -10.88017736071109987 ) ) ;
#4371=CARTESIAN_POINT ( 'NONE',  ( 17.96484262340118221, 6.188685344154837509, -7.964842623401177768 ) ) ;
#4372=CARTESIAN_POINT ( 'NONE',  ( 21.09922568453595559, 47.04030133659708923, -6.408140936763230044 ) ) ;
#4373=CARTESIAN_POINT ( 'NONE',  ( 19.42250999205614193, 25.14701867748817321, 5.440088680355555262 ) ) ;
#4374=CARTESIAN_POINT ( 'NONE',  ( -46.94000000000002615, 100.7935499705929203, -8.437539667946047928 ) ) ;
#4376=CARTESIAN_POINT ( 'NONE',  ( 13.43411237798105340, 35.58196800326375353, 12.81628187352647963 ) ) ;
#4377=CARTESIAN_POINT ( 'NONE',  ( 19.42250999205614548, 40.98035201082150536, -5.440088680355545492 ) ) ;
#4378=CARTESIAN_POINT ( 'NONE',  ( 1.472469842513823179, 51.42559781766745886, 4.923371831947296329 ) ) ;
#4379=VERTEX_POINT ( 'NONE', #49878 ) ;
#4380=CARTESIAN_POINT ( 'NONE',  ( 10.00000000000000000, 59.75893115100078745, -9.846743663894594434 ) ) ;
#4382=CARTESIAN_POINT ( 'NONE',  ( 1.472469842513823179, 50.59226448433411605, -4.923371831947296329 ) ) ;
#4383=CARTESIAN_POINT ( 'NONE',  ( -0.8801773607111008646, 23.27201867748817676, 2.915334737309923430 ) ) ;
#4385=CARTESIAN_POINT ( 'NONE',  ( 19.84674366389459621, 33.50893115100078745, 7.409399052514197653E-17 ) ) ;
#4388=CARTESIAN_POINT ( 'NONE',  ( 7.361572987183170547, 47.05059781766745175, 9.846743663894590881 ) ) ;
#4389=( LENGTH_UNIT ( ) NAMED_UNIT ( * ) SI_UNIT ( .MILLI., .METRE. ) );
#4390=CARTESIAN_POINT ( 'NONE',  ( 17.20831665107776587, 52.88393115100078035, 7.208316651077764980 ) ) ;
#4392=( BOUNDED_SURFACE ( )  B_SPLINE_SURFACE ( 1, 2, ( 
 ( #71327, #56320, #2846, #63792, #42788, #94300, #25823, #65265, #27275, #88279, #58763, #51269, #44254, #66258, #29739, #21270, #5780, #68263, #89267, #43759, #20778, #50779, #36270, #6266, #60735, #66764, #21777, #90742, #13267, #83252, #37276, #75250, #59749, #12771, #81753, #74248, #14274, #35770, #98783, #60249, #90246, #28761, #97287, #37766, #59253, #97790, #30231, #67765, #29253, #52744, #89753, #43267, #22270, #98284, #82251, #14774, #51767, #13766, #74758, #36771, #73762, #20282, #67263, #7265, #52256, #6762, #82752, #44747, #45247, #75743, #81271, #5293, #96793, #28268, #85227, #77219, #84733, #16730, #54216, #16239, #280, #46719, #62207, #23756, #8724, #39242, #92713, #69730, #91740, #47207, #38744, #1257, #77708, #24239, #92230, #8247, #31712, #94556, #54706, #61234, #9220, #61714, #69245, #766, #41082, #31219, #26074, #72051, #15757, #71580, #30727, #3091, #33547, #23261, #64043, #56565, #87059, #18568, #49061, #46242, #79566, #53736, #11064, #84255, #41584, #3580, #34037, #91237, #22760, #53242, #76728, #83747, #15270, #45751, #76247, #7763, #38256, #68748, #65021, #58520, #12042, #50534, #89028, #66022, #65524, #80545, #43036, #66523, #73517, #34525, #81029, #35023, #42541, #73025, #5045, #4560, #97050, #44008, #88033, #96047, #4064, #20538, #27531, #95549, #35528, #13022, #58023, #88531, #74510, #20033, #96548, #28524, #51522, #28023, #49536, #12535, #51022, #26549, #21032, #72530, #57044, #64533, #59016, #95040, #42069, #81516, #43519, #74014, #27037, #57536, #5543, #11549, #36020, #89522, #50041, #13525, #19546, #82014, #6031, #87547, #19058, #80044, #76978, #52502, #38014, #8005, #29490, #532, #53485, #91496, #75996, #29002, #6513, #75008, #30485, #52021, #84493, #46002, #7524, #44998, #98036, #53985, #83010, #15023, #46482, #83996, #45494, #68999, #60000, #59513, #38503, #15520, #98540, #30979, #37021, #7015, #90493, #75503, #90007, #36531, #37522, #23513, #83506, #23017, #90988, #22029, #14528, #61477, #76492, #15994, #91983, #67020, #97541, #68013, #82512, #21527, #29992, #14030, #44508, #67518, #60499, #22519, #52991, #68507, #37, #60984, #24491, #69981, #1504, #77462, #48937, #54955, #86941, #32949, #54469, #10459, #77964, #71466, #55469, #8974, #55965, #62455, #63449, #32459, #62955, #46968, #17963, #93460, #17482, #47948, #38995, #40476, #92470, #85473, #93956, #48450, #78948, #86466, #85972, #25481, #23996, #92957, #61970, #16984, #84974, #31468, #40969, #2493, #39490, #47462, #2979, #25952, #33428, #63925, #39972, #94440, #31953, #16492, #56455, #18453, #1994, #9470, #8491, #69488, #1006 ),
 ( #70474, #78457, #9971, #24986, #70973, #11435, #4447, #26430, #88915, #80432, #64907, #28409, #18947, #3944, #79927, #10945, #95432, #65409, #20917, #26926, #80922, #50909, #72418, #43404, #96433, #35410, #19920, #71937, #49424, #41954, #73402, #94929, #58903, #20423, #50412, #87917, #34416, #96933, #57423, #95934, #19433, #4930, #49921, #27416, #65902, #12415, #11930, #42434, #57908, #81405, #88419, #72917, #42922, #34912, #27905, #58396, #12907, #73901, #5434, #89401, #35904, #66401, #79445, #41469, #3460, #33915, #64422, #56930, #87431, #44877, #30866, #90374, #60376, #83878, #38385, #14905, #36405, #75379, #52877, #13404, #7891, #59389, #43889, #51406, #15405, #81893, #28884, #22402, #90873, #68391, #89890, #82387, #6896, #97418, #60870, #52389, #36903, #415, #21408, #74889, #51903, #74387, #67395, #37408, #91873, #97921, #83387, #22897, #44391, #45888, #98912, #7404, #45377, #5913, #13911, #6388, #75883, #66899, #61364, #91371, #37902, #59883, #29381, #68886, #21913, #29874, #82889, #30365, #53369, #76376, #14405, #67896, #98419, #2370, #85351, #93833, #92360, #92847, #77347, #31844, #15886, #23395, #24374, #10342, #70362, #9856, #77842, #8858, #9351, #39374, #39856, #61856, #93340, #16373, #17363, #1879, #16863, #47832, #47339, #32338, #31355, #62839, #24861, #54838, #55345, #85852, #78335, #71345, #46852, #62340, #69372, #40355, #70855, #53880, #69869, #84864, #1389, #23886, #63809, #32825, #2863, #63325, #893, #25359, #55845, #86340, #17843, #54352, #48328, #78832, #40842, #33314, #84387, #46371, #76860, #8373, #38880, #34796, #25840, #27292, #79325, #72301, #50287, #35288, #65781, #42807, #42312, #19796, #10835, #49309, #48815, #3830, #41354, #18335, #80801, #88298, #94811, #79810, #12298, #12786, #96314, #20300, #26807, #27787, #26314, #71823, #58273, #73290, #87793, #34287, #81290, #73780, #4814, #56813, #64786, #57302, #11314, #88792, #50800, #64301, #3332, #19311, #86831, #56338, #49796, #95303, #57791, #80305, #87311, #43286, #33794, #18830, #95812, #5310, #35787, #94319, #41833, #11804, #72786, #4323, #65285, #98800, #30248, #14792, #52272, #15286, #45265, #45768, #51287, #36787, #22778, #51782, #60263, #58782, #36286, #97303, #6779, #22286, #29270, #67778, #75759, #7280, #89772, #91252, #52760, #53257, #83763, #76261, #66275, #67281, #81772, #83268, #44269, #13286, #28287, #37782, #28775, #74775, #97809, #21289, #68279, #7778, #66784, #43774, #59764, #89287, #96811, #21792, #6284, #98300, #82770, #59273, #20798, #74266, #82267, #29755, #60751, #5795, #90762, #13783, #90258, #44763, #14291, #75268, #37292 ) ),
 .UNSPECIFIED., .F., .F., .F. ) 
 B_SPLINE_SURFACE_WITH_KNOTS ( ( 2, 2 ),
 ( 3, 2, 2, 2, 2, 2, 2, 2, 2, 2, 2, 2, 2, 2, 2, 2, 2, 2, 2, 2, 2, 2, 2, 2, 2, 2, 2, 2, 2, 2, 2, 2, 2, 2, 2, 2, 2, 2, 2, 2, 2, 2, 2, 2, 2, 2, 2, 2, 2, 2, 2, 2, 2, 2, 2, 2, 2, 2, 2, 2, 2, 2, 2, 2, 2, 2, 2, 2, 2, 2, 2, 2, 2, 2, 2, 2, 2, 2, 2, 2, 2, 2, 2, 2, 2, 2, 2, 2, 2, 2, 2, 2, 2, 2, 2, 2, 2, 2, 2, 2, 2, 2, 2, 2, 2, 2, 2, 2, 2, 2, 2, 2, 2, 2, 2, 2, 2, 2, 2, 2, 2, 2, 2, 2, 2, 2, 2, 2, 2, 2, 2, 2, 2, 2, 2, 2, 2, 2, 2, 2, 2, 2, 2, 2, 2, 2, 2, 2, 2, 2, 2, 2, 2, 2, 2, 2, 2, 2, 2, 2, 2, 2, 3 ),
 ( 0.000000000000000000, 1.000000000000000000 ),
 ( 0.000000000000000000, 0.005952380952380952051, 0.01190476190476190410, 0.01785714285714285615, 0.02380952380952380820, 0.02976190476190476025, 0.03571428571428571230, 0.04166666666666666435, 0.04761904761904761640, 0.05357142857142856845, 0.05952380952380952051, 0.06547619047619047949, 0.07142857142857142461, 0.07738095238095238360, 0.08333333333333332871, 0.08928571428571428770, 0.09523809523809523281, 0.1011904761904761918, 0.1071428571428571369, 0.1130952380952380959, 0.1190476190476190410, 0.1250000000000000000, 0.1309523809523809590, 0.1369047619047619180, 0.1428571428571428492, 0.1488095238095238082, 0.1547619047619047672, 0.1607142857142857262, 0.1666666666666666574, 0.1726190476190476164, 0.1785714285714285754, 0.1845238095238095344, 0.1904761904761904656, 0.1964285714285714246, 0.2023809523809523836, 0.2083333333333333426, 0.2142857142857142738, 0.2202380952380952328, 0.2261904761904761918, 0.2321428571428571508, 0.2380952380952380820, 0.2440476190476190410, 0.2500000000000000000, 0.2559523809523809312, 0.2619047619047619180, 0.2678571428571428492, 0.2738095238095238360, 0.2797619047619047672, 0.2857142857142856984, 0.2916666666666666852, 0.2976190476190476164, 0.3035714285714285476, 0.3095238095238095344, 0.3154761904761904656, 0.3214285714285714524, 0.3273809523809523836, 0.3333333333333333148, 0.3392857142857143016, 0.3452380952380952328, 0.3511904761904761640, 0.3571428571428571508, 0.3630952380952380820, 0.3690476190476190688, 0.3750000000000000000, 0.3809523809523809312, 0.3869047619047619180, 0.3928571428571428492, 0.3988095238095238360, 0.4047619047619047672, 0.4107142857142856984, 0.4166666666666666852, 0.4226190476190476164, 0.4285714285714285476, 0.4345238095238095344, 0.4404761904761904656, 0.4464285714285714524, 0.4523809523809523836, 0.4583333333333333148, 0.4642857142857143016, 0.4702380952380952328, 0.4761904761904761640, 0.4821428571428571508, 0.4880952380952380820, 0.4940476190476190688, 0.5000000000000000000, 0.5059523809523809312, 0.5119047619047618625, 0.5178571428571429047, 0.5238095238095238360, 0.5297619047619047672, 0.5357142857142856984, 0.5416666666666666297, 0.5476190476190476719, 0.5535714285714286031, 0.5595238095238095344, 0.5654761904761904656, 0.5714285714285713969, 0.5773809523809523281, 0.5833333333333333703, 0.5892857142857143016, 0.5952380952380952328, 0.6011904761904761640, 0.6071428571428570953, 0.6130952380952381375, 0.6190476190476190688, 0.6250000000000000000, 0.6309523809523809312, 0.6369047619047618625, 0.6428571428571429047, 0.6488095238095238360, 0.6547619047619047672, 0.6607142857142856984, 0.6666666666666666297, 0.6726190476190476719, 0.6785714285714286031, 0.6845238095238095344, 0.6904761904761904656, 0.6964285714285713969, 0.7023809523809523281, 0.7083333333333333703, 0.7142857142857143016, 0.7202380952380952328, 0.7261904761904761640, 0.7321428571428570953, 0.7380952380952381375, 0.7440476190476190688, 0.7500000000000000000, 0.7559523809523809312, 0.7619047619047618625, 0.7678571428571429047, 0.7738095238095238360, 0.7797619047619047672, 0.7857142857142856984, 0.7916666666666666297, 0.7976190476190476719, 0.8035714285714286031, 0.8095238095238095344, 0.8154761904761904656, 0.8214285714285713969, 0.8273809523809523281, 0.8333333333333333703, 0.8392857142857143016, 0.8452380952380952328, 0.8511904761904761640, 0.8571428571428570953, 0.8630952380952381375, 0.8690476190476190688, 0.8750000000000000000, 0.8809523809523809312, 0.8869047619047618625, 0.8928571428571429047, 0.8988095238095238360, 0.9047619047619047672, 0.9107142857142856984, 0.9166666666666666297, 0.9226190476190476719, 0.9285714285714286031, 0.9345238095238095344, 0.9404761904761904656, 0.9464285714285713969, 0.9523809523809523281, 0.9583333333333333703, 0.9642857142857143016 ),
 .UNSPECIFIED. ) 
 GEOMETRIC_REPRESENTATION_ITEM ( )  RATIONAL_B_SPLINE_SURFACE ( (
 ( 1.000000000000000000, 0.9659258262890683122, 1.000000000000000000, 0.9659258262890683122, 1.000000000000000000, 0.9659258262890683122, 1.000000000000000000, 0.9659258262890683122, 1.000000000000000000, 0.9659258262890683122, 1.000000000000000000, 0.9659258262890683122, 1.000000000000000000, 0.9659258262890683122, 1.000000000000000000, 0.9659258262890683122, 1.000000000000000000, 0.9659258262890683122, 1.000000000000000000, 0.9659258262890683122, 1.000000000000000000, 0.9659258262890683122, 1.000000000000000000, 0.9659258262890683122, 1.000000000000000000, 0.9659258262890683122, 1.000000000000000000, 0.9659258262890683122, 1.000000000000000000, 0.9659258262890683122, 1.000000000000000000, 0.9659258262890683122, 1.000000000000000000, 0.9659258262890683122, 1.000000000000000000, 0.9659258262890683122, 1.000000000000000000, 0.9659258262890683122, 1.000000000000000000, 0.9659258262890683122, 1.000000000000000000, 0.9659258262890683122, 1.000000000000000000, 0.9659258262890683122, 1.000000000000000000, 0.9659258262890683122, 1.000000000000000000, 0.9659258262890683122, 1.000000000000000000, 0.9659258262890683122, 1.000000000000000000, 0.9659258262890683122, 1.000000000000000000, 0.9659258262890683122, 1.000000000000000000, 0.9659258262890683122, 1.000000000000000000, 0.9659258262890683122, 1.000000000000000000, 0.9659258262890683122, 1.000000000000000000, 0.9659258262890683122, 1.000000000000000000, 0.9659258262890683122, 1.000000000000000000, 0.9659258262890683122, 1.000000000000000000, 0.9659258262890683122, 1.000000000000000000, 0.9659258262890683122, 1.000000000000000000, 0.9659258262890683122, 1.000000000000000000, 0.9659258262890683122, 1.000000000000000000, 0.9659258262890683122, 1.000000000000000000, 0.9659258262890683122, 1.000000000000000000, 0.9659258262890683122, 1.000000000000000000, 0.9659258262890683122, 1.000000000000000000, 0.9659258262890683122, 1.000000000000000000, 0.9659258262890683122, 1.000000000000000000, 0.9659258262890683122, 1.000000000000000000, 0.9659258262890683122, 1.000000000000000000, 0.9659258262890683122, 1.000000000000000000, 0.9659258262890683122, 1.000000000000000000, 0.9659258262890683122, 1.000000000000000000, 0.9659258262890683122, 1.000000000000000000, 0.9659258262890683122, 1.000000000000000000, 0.9659258262890683122, 1.000000000000000000, 0.9659258262890683122, 1.000000000000000000, 0.9659258262890683122, 1.000000000000000000, 0.9659258262890683122, 1.000000000000000000, 0.9659258262890683122, 1.000000000000000000, 0.9659258262890683122, 1.000000000000000000, 0.9659258262890683122, 1.000000000000000000, 0.9659258262890683122, 1.000000000000000000, 0.9659258262890683122, 1.000000000000000000, 0.9659258262890683122, 1.000000000000000000, 0.9659258262890683122, 1.000000000000000000, 0.9659258262890683122, 1.000000000000000000, 0.9659258262890683122, 1.000000000000000000, 0.9659258262890683122, 1.000000000000000000, 0.9659258262890683122, 1.000000000000000000, 0.9659258262890683122, 1.000000000000000000, 0.9659258262890683122, 1.000000000000000000, 0.9659258262890683122, 1.000000000000000000, 0.9659258262890683122, 1.000000000000000000, 0.9659258262890683122, 1.000000000000000000, 0.9659258262890683122, 1.000000000000000000, 0.9659258262890683122, 1.000000000000000000, 0.9659258262890683122, 1.000000000000000000, 0.9659258262890683122, 1.000000000000000000, 0.9659258262890683122, 1.000000000000000000, 0.9659258262890683122, 1.000000000000000000, 0.9659258262890683122, 1.000000000000000000, 0.9659258262890683122, 1.000000000000000000, 0.9659258262890683122, 1.000000000000000000, 0.9659258262890683122, 1.000000000000000000, 0.9659258262890683122, 1.000000000000000000, 0.9659258262890683122, 1.000000000000000000, 0.9659258262890683122, 1.000000000000000000, 0.9659258262890683122, 1.000000000000000000, 0.9659258262890683122, 1.000000000000000000, 0.9659258262890683122, 1.000000000000000000, 0.9659258262890683122, 1.000000000000000000, 0.9659258262890683122, 1.000000000000000000, 0.9659258262890683122, 1.000000000000000000, 0.9659258262890683122, 1.000000000000000000, 0.9659258262890683122, 1.000000000000000000, 0.9659258262890683122, 1.000000000000000000, 0.9659258262890683122, 1.000000000000000000, 0.9659258262890683122, 1.000000000000000000, 0.9659258262890683122, 1.000000000000000000, 0.9659258262890683122, 1.000000000000000000, 0.9659258262890683122, 1.000000000000000000, 0.9659258262890683122, 1.000000000000000000, 0.9659258262890683122, 1.000000000000000000, 0.9659258262890683122, 1.000000000000000000, 0.9659258262890683122, 1.000000000000000000, 0.9659258262890683122, 1.000000000000000000, 0.9659258262890683122, 1.000000000000000000, 0.9659258262890683122, 1.000000000000000000, 0.9659258262890683122, 1.000000000000000000, 0.9659258262890683122, 1.000000000000000000, 0.9659258262890683122, 1.000000000000000000, 0.9659258262890683122, 1.000000000000000000, 0.9659258262890683122, 1.000000000000000000, 0.9659258262890683122, 1.000000000000000000, 0.9659258262890683122, 1.000000000000000000, 0.9659258262890683122, 1.000000000000000000, 0.9659258262890683122, 1.000000000000000000, 0.9659258262890683122, 1.000000000000000000, 0.9659258262890683122, 1.000000000000000000, 0.9659258262890683122, 1.000000000000000000, 0.9659258262890683122, 1.000000000000000000, 0.9659258262890683122, 1.000000000000000000, 0.9659258262890683122, 1.000000000000000000, 0.9659258262890683122, 1.000000000000000000, 0.9659258262890683122, 1.000000000000000000, 0.9659258262890683122, 1.000000000000000000, 0.9659258262890683122, 1.000000000000000000, 0.9659258262890683122, 1.000000000000000000, 0.9659258262890683122, 1.000000000000000000, 0.9659258262890683122, 1.000000000000000000, 0.9659258262890683122, 1.000000000000000000, 0.9659258262890683122, 1.000000000000000000, 0.9659258262890683122, 1.000000000000000000, 0.9659258262890683122, 1.000000000000000000, 0.9659258262890683122, 1.000000000000000000, 0.9659258262890683122, 1.000000000000000000, 0.9659258262890683122, 1.000000000000000000, 0.9659258262890683122, 1.000000000000000000, 0.9659258262890683122, 1.000000000000000000, 0.9659258262890683122, 1.000000000000000000, 0.9659258262890683122, 1.000000000000000000, 0.9659258262890683122, 1.000000000000000000, 0.9659258262890683122, 1.000000000000000000, 0.9659258262890683122, 1.000000000000000000, 0.9659258262890683122, 1.000000000000000000, 0.9659258262890683122, 1.000000000000000000, 0.9659258262890683122, 1.000000000000000000, 0.9659258262890683122, 1.000000000000000000, 0.9659258262890683122, 1.000000000000000000, 0.9659258262890683122, 1.000000000000000000, 0.9659258262890683122, 1.000000000000000000, 0.9659258262890683122, 1.000000000000000000, 0.9659258262890683122, 1.000000000000000000, 0.9659258262890683122, 1.000000000000000000, 0.9659258262890683122, 1.000000000000000000, 0.9659258262890683122, 1.000000000000000000, 0.9659258262890683122, 1.000000000000000000, 0.9659258262890683122, 1.000000000000000000, 0.9659258262890683122, 1.000000000000000000, 0.9659258262890683122, 1.000000000000000000, 0.9659258262890683122, 1.000000000000000000, 0.9659258262890683122, 1.000000000000000000, 0.9659258262890683122, 1.000000000000000000, 0.9659258262890683122, 1.000000000000000000, 0.9659258262890683122, 1.000000000000000000, 0.9659258262890683122, 1.000000000000000000),
 ( 1.000000000000000000, 0.9659258262890683122, 1.000000000000000000, 0.9659258262890683122, 1.000000000000000000, 0.9659258262890683122, 1.000000000000000000, 0.9659258262890683122, 1.000000000000000000, 0.9659258262890683122, 1.000000000000000000, 0.9659258262890683122, 1.000000000000000000, 0.9659258262890683122, 1.000000000000000000, 0.9659258262890683122, 1.000000000000000000, 0.9659258262890683122, 1.000000000000000000, 0.9659258262890683122, 1.000000000000000000, 0.9659258262890683122, 1.000000000000000000, 0.9659258262890683122, 1.000000000000000000, 0.9659258262890683122, 1.000000000000000000, 0.9659258262890683122, 1.000000000000000000, 0.9659258262890683122, 1.000000000000000000, 0.9659258262890683122, 1.000000000000000000, 0.9659258262890683122, 1.000000000000000000, 0.9659258262890683122, 1.000000000000000000, 0.9659258262890683122, 1.000000000000000000, 0.9659258262890683122, 1.000000000000000000, 0.9659258262890683122, 1.000000000000000000, 0.9659258262890683122, 1.000000000000000000, 0.9659258262890683122, 1.000000000000000000, 0.9659258262890683122, 1.000000000000000000, 0.9659258262890683122, 1.000000000000000000, 0.9659258262890683122, 1.000000000000000000, 0.9659258262890683122, 1.000000000000000000, 0.9659258262890683122, 1.000000000000000000, 0.9659258262890683122, 1.000000000000000000, 0.9659258262890683122, 1.000000000000000000, 0.9659258262890683122, 1.000000000000000000, 0.9659258262890683122, 1.000000000000000000, 0.9659258262890683122, 1.000000000000000000, 0.9659258262890683122, 1.000000000000000000, 0.9659258262890683122, 1.000000000000000000, 0.9659258262890683122, 1.000000000000000000, 0.9659258262890683122, 1.000000000000000000, 0.9659258262890683122, 1.000000000000000000, 0.9659258262890683122, 1.000000000000000000, 0.9659258262890683122, 1.000000000000000000, 0.9659258262890683122, 1.000000000000000000, 0.9659258262890683122, 1.000000000000000000, 0.9659258262890683122, 1.000000000000000000, 0.9659258262890683122, 1.000000000000000000, 0.9659258262890683122, 1.000000000000000000, 0.9659258262890683122, 1.000000000000000000, 0.9659258262890683122, 1.000000000000000000, 0.9659258262890683122, 1.000000000000000000, 0.9659258262890683122, 1.000000000000000000, 0.9659258262890683122, 1.000000000000000000, 0.9659258262890683122, 1.000000000000000000, 0.9659258262890683122, 1.000000000000000000, 0.9659258262890683122, 1.000000000000000000, 0.9659258262890683122, 1.000000000000000000, 0.9659258262890683122, 1.000000000000000000, 0.9659258262890683122, 1.000000000000000000, 0.9659258262890683122, 1.000000000000000000, 0.9659258262890683122, 1.000000000000000000, 0.9659258262890683122, 1.000000000000000000, 0.9659258262890683122, 1.000000000000000000, 0.9659258262890683122, 1.000000000000000000, 0.9659258262890683122, 1.000000000000000000, 0.9659258262890683122, 1.000000000000000000, 0.9659258262890683122, 1.000000000000000000, 0.9659258262890683122, 1.000000000000000000, 0.9659258262890683122, 1.000000000000000000, 0.9659258262890683122, 1.000000000000000000, 0.9659258262890683122, 1.000000000000000000, 0.9659258262890683122, 1.000000000000000000, 0.9659258262890683122, 1.000000000000000000, 0.9659258262890683122, 1.000000000000000000, 0.9659258262890683122, 1.000000000000000000, 0.9659258262890683122, 1.000000000000000000, 0.9659258262890683122, 1.000000000000000000, 0.9659258262890683122, 1.000000000000000000, 0.9659258262890683122, 1.000000000000000000, 0.9659258262890683122, 1.000000000000000000, 0.9659258262890683122, 1.000000000000000000, 0.9659258262890683122, 1.000000000000000000, 0.9659258262890683122, 1.000000000000000000, 0.9659258262890683122, 1.000000000000000000, 0.9659258262890683122, 1.000000000000000000, 0.9659258262890683122, 1.000000000000000000, 0.9659258262890683122, 1.000000000000000000, 0.9659258262890683122, 1.000000000000000000, 0.9659258262890683122, 1.000000000000000000, 0.9659258262890683122, 1.000000000000000000, 0.9659258262890683122, 1.000000000000000000, 0.9659258262890683122, 1.000000000000000000, 0.9659258262890683122, 1.000000000000000000, 0.9659258262890683122, 1.000000000000000000, 0.9659258262890683122, 1.000000000000000000, 0.9659258262890683122, 1.000000000000000000, 0.9659258262890683122, 1.000000000000000000, 0.9659258262890683122, 1.000000000000000000, 0.9659258262890683122, 1.000000000000000000, 0.9659258262890683122, 1.000000000000000000, 0.9659258262890683122, 1.000000000000000000, 0.9659258262890683122, 1.000000000000000000, 0.9659258262890683122, 1.000000000000000000, 0.9659258262890683122, 1.000000000000000000, 0.9659258262890683122, 1.000000000000000000, 0.9659258262890683122, 1.000000000000000000, 0.9659258262890683122, 1.000000000000000000, 0.9659258262890683122, 1.000000000000000000, 0.9659258262890683122, 1.000000000000000000, 0.9659258262890683122, 1.000000000000000000, 0.9659258262890683122, 1.000000000000000000, 0.9659258262890683122, 1.000000000000000000, 0.9659258262890683122, 1.000000000000000000, 0.9659258262890683122, 1.000000000000000000, 0.9659258262890683122, 1.000000000000000000, 0.9659258262890683122, 1.000000000000000000, 0.9659258262890683122, 1.000000000000000000, 0.9659258262890683122, 1.000000000000000000, 0.9659258262890683122, 1.000000000000000000, 0.9659258262890683122, 1.000000000000000000, 0.9659258262890683122, 1.000000000000000000, 0.9659258262890683122, 1.000000000000000000, 0.9659258262890683122, 1.000000000000000000, 0.9659258262890683122, 1.000000000000000000, 0.9659258262890683122, 1.000000000000000000, 0.9659258262890683122, 1.000000000000000000, 0.9659258262890683122, 1.000000000000000000, 0.9659258262890683122, 1.000000000000000000, 0.9659258262890683122, 1.000000000000000000, 0.9659258262890683122, 1.000000000000000000, 0.9659258262890683122, 1.000000000000000000, 0.9659258262890683122, 1.000000000000000000, 0.9659258262890683122, 1.000000000000000000, 0.9659258262890683122, 1.000000000000000000, 0.9659258262890683122, 1.000000000000000000, 0.9659258262890683122, 1.000000000000000000, 0.9659258262890683122, 1.000000000000000000, 0.9659258262890683122, 1.000000000000000000, 0.9659258262890683122, 1.000000000000000000, 0.9659258262890683122, 1.000000000000000000, 0.9659258262890683122, 1.000000000000000000, 0.9659258262890683122, 1.000000000000000000, 0.9659258262890683122, 1.000000000000000000, 0.9659258262890683122, 1.000000000000000000, 0.9659258262890683122, 1.000000000000000000, 0.9659258262890683122, 1.000000000000000000, 0.9659258262890683122, 1.000000000000000000, 0.9659258262890683122, 1.000000000000000000, 0.9659258262890683122, 1.000000000000000000, 0.9659258262890683122, 1.000000000000000000, 0.9659258262890683122, 1.000000000000000000, 0.9659258262890683122, 1.000000000000000000, 0.9659258262890683122, 1.000000000000000000, 0.9659258262890683122, 1.000000000000000000, 0.9659258262890683122, 1.000000000000000000, 0.9659258262890683122, 1.000000000000000000, 0.9659258262890683122, 1.000000000000000000, 0.9659258262890683122, 1.000000000000000000, 0.9659258262890683122, 1.000000000000000000, 0.9659258262890683122, 1.000000000000000000, 0.9659258262890683122, 1.000000000000000000, 0.9659258262890683122, 1.000000000000000000, 0.9659258262890683122, 1.000000000000000000, 0.9659258262890683122, 1.000000000000000000, 0.9659258262890683122, 1.000000000000000000) ) ) 
 REPRESENTATION_ITEM ( '' )  SURFACE ( )  );
#4394=CARTESIAN_POINT ( 'NONE',  ( 6.565887622018943937, 40.16530133659708923, 12.81628187352647430 ) ) ;
#4395=CARTESIAN_POINT ( 'NONE',  ( 5.076628168052704559, 45.17559781766745175, -8.527530157486179263 ) ) ;
#4397=CARTESIAN_POINT ( 'NONE',  ( -0.3689425029237881626, 57.42874883491397497, 10.36894250292379027 ) ) ;
#4398=CARTESIAN_POINT ( 'NONE',  ( 18.52753015748617571, 38.09226448433412315, 4.923371831947298993 ) ) ;
#4399=ORIENTED_EDGE ( 'NONE', *, *, #72108, .F. ) ;
#4401=CARTESIAN_POINT ( 'NONE',  ( 24.16423886937409904, 54.09541550158063217, 3.795296366450317205 ) ) ;
#4403=CARTESIAN_POINT ( 'NONE',  ( -0.3689425029237881626, 67.42874883491396076, 10.36894250292379027 ) ) ;
#4404=CARTESIAN_POINT ( 'NONE',  ( 24.16423886937409904, 39.09541550158062506, 3.795296366450317205 ) ) ;
#4406=CARTESIAN_POINT ( 'NONE',  ( 13.79529636645030344, 58.26208216824728936, 14.16423886937410614 ) ) ;
#4408=CARTESIAN_POINT ( 'NONE',  ( 19.42250999205614193, 5.147018677488171434, 5.440088680355555262 ) ) ;
#4409=CARTESIAN_POINT ( 'NONE',  ( 2.791683348922240793, 6.633931151000785675, 7.208316651077764092 ) ) ;
#4411=CARTESIAN_POINT ( 'NONE',  ( 21.09922568453594849, 1.206968003263753531, 6.408140936763242479 ) ) ;
#4413=CARTESIAN_POINT ( 'NONE',  ( 20.88017736071110519, 50.56368534415484106, 2.639326808657452039E-16 ) ) ;
#4414=CARTESIAN_POINT ( 'NONE',  ( -0.8801773607111009756, 18.06368534415484106, 1.068504757029289695E-15 ) ) ;
#4416=CARTESIAN_POINT ( 'NONE',  ( 18.52753015748617571, 48.09226448433412315, 4.923371831947298993 ) ) ;
#4419=CARTESIAN_POINT ( 'NONE',  ( 18.52753015748618282, 53.92559781766745175, -4.923371831947291888 ) ) ;
#4420=( NAMED_UNIT ( * ) SI_UNIT ( $, .STERADIAN. ) SOLID_ANGLE_UNIT ( ) );
#4421=CARTESIAN_POINT ( 'NONE',  ( 13.79529636645030344, 23.26208216824730002, 14.16423886937410614 ) ) ;
#4422=FILL_AREA_STYLE ('',( #88396 ) ) ;
#4424=FILL_AREA_STYLE ('',( #5889 ) ) ;
#4425=CARTESIAN_POINT ( 'NONE',  ( 20.88017736071110875, 25.77201867748816966, -2.915334737309920765 ) ) ;
#4426=CARTESIAN_POINT ( 'NONE',  ( -2.816281873526471635, 43.91530133659708923, -3.434112377981056508 ) ) ;
#4428=CARTESIAN_POINT ( 'NONE',  ( 18.52753015748617571, 8.092264484334117824, 4.923371831947298993 ) ) ;
#4429=CARTESIAN_POINT ( 'NONE',  ( 3.591859063236763294, 63.29030133659708923, -11.09922568453595026 ) ) ;
#4430=ORIENTED_EDGE ( 'NONE', *, *, #52943, .T. ) ;
#4432=CARTESIAN_POINT ( 'NONE',  ( 13.79529636645030344, 33.26208216824730357, 14.16423886937410614 ) ) ;
#4433=CARTESIAN_POINT ( 'NONE',  ( 0.1532563361054083140, 21.00893115100078745, 1.131784320476157264E-15 ) ) ;
#4434=CYLINDRICAL_SURFACE ( 'NONE', #75816, 11.92686044187656513 ) ;
#4435=CARTESIAN_POINT ( 'NONE',  ( 12.91533473730993009, 11.60535201082150714, -10.88017736071109987 ) ) ;
#4438=CARTESIAN_POINT ( 'NONE',  ( 2.035157376598824452, 43.68868534415484106, 7.964842623401179544 ) ) ;
#4439=CARTESIAN_POINT ( 'NONE',  ( -0.8801773607111009756, 48.06368534415484817, 1.068504757029289695E-15 ) ) ;
#4440=CARTESIAN_POINT ( 'NONE',  ( 13.43411237798105340, 15.58196800326374998, 12.81628187352647963 ) ) ;
#4441=CARTESIAN_POINT ( 'NONE',  ( 12.63842701281683034, 62.46726448433410894, 9.846743663894596210 ) ) ;
#4443=CARTESIAN_POINT ( 'NONE',  ( 18.52753015748618282, 3.925597817667451306, -4.923371831947291888 ) ) ;
#4445=CARTESIAN_POINT ( 'NONE',  ( 15.44008868035555793, 46.39701867748817676, -9.422509992056140149 ) ) ;
#4447=CARTESIAN_POINT ( 'NONE',  ( -2.816281873526473856, -0.8763653300695799508, 9.499525473075851096E-16 ) ) ;
#4448=CARTESIAN_POINT ( 'NONE',  ( 2.035157376598824452, 58.68868534415482685, 7.964842623401179544 ) ) ;
#4449=CARTESIAN_POINT ( 'NONE',  ( 0.1532563361054082862, 31.21726448433412315, 2.638427012816831674 ) ) ;
#4450=CARTESIAN_POINT ( 'NONE',  ( 0.6178305044545838731, 44.74863466993042493, 9.382169495545420901 ) ) ;
#4451=CARTESIAN_POINT ( 'NONE',  ( 18.52753015748617571, 8.092264484334117824, 4.923371831947298993 ) ) ;
#4455=CARTESIAN_POINT ( 'NONE',  ( 7.084665262690076126, 17.02201867748817676, -10.88017736071110164 ) ) ;
#4457=CARTESIAN_POINT ( 'NONE',  ( 5.076628168052703671, 26.84226448433411960, 8.527530157486179263 ) ) ;
#4458=CARTESIAN_POINT ( 'NONE',  ( 17.96484262340118221, 14.93868534415483751, 7.964842623401181321 ) ) ;
#4459=CARTESIAN_POINT ( 'NONE',  ( 15.44008868035555260, 4.730352010821505360, 9.422509992056143702 ) ) ;
#4461=CARTESIAN_POINT ( 'NONE',  ( 12.91533473730992121, 14.52201867748817143, 10.88017736071110164 ) ) ;
#4462=CARTESIAN_POINT ( 'NONE',  ( 12.91533473730992121, 29.52201867748817321, 10.88017736071110164 ) ) ;
#4464=CARTESIAN_POINT ( 'NONE',  ( 17.96484262340118221, 26.18868534415483396, -7.964842623401177768 ) ) ;
#4466=VERTEX_POINT ( 'NONE', #11893 ) ;
#4467=CARTESIAN_POINT ( 'NONE',  ( 20.24186590665277663, 26.76028685723174760, 6.114288769123037426 ) ) ;
#4468=CARTESIAN_POINT ( 'NONE',  ( -0.8801773607111008646, 18.27201867748817321, 2.915334737309923430 ) ) ;
#4471=CARTESIAN_POINT ( 'NONE',  ( 16.40814093676323893, 60.79030133659709634, 11.09922568453595026 ) ) ;
#4472=CARTESIAN_POINT ( 'NONE',  ( -0.8801773607110990882, 67.85535201082149115, -2.915334737309924318 ) ) ;
#4473=CARTESIAN_POINT ( 'NONE',  ( -4.164238869374098151, 36.59541550158063217, -3.795296366450310543 ) ) ;
#4474=CARTESIAN_POINT ( 'NONE',  ( 7.084665262690076126, 39.10535201082150536, 10.88017736071109987 ) ) ;
#4475=CARTESIAN_POINT ( 'NONE',  ( 10.00000000000000178, 14.31368534415483929, 10.88017736071110342 ) ) ;
#4476=CARTESIAN_POINT ( 'NONE',  ( 19.84674366389459266, 63.30059781766745886, 2.638427012816836559 ) ) ;
#4477=CARTESIAN_POINT ( 'NONE',  ( 10.00000000000000000, 54.75893115100078745, -9.846743663894594434 ) ) ;
#4478=CARTESIAN_POINT ( 'NONE',  ( 10.00000000000000000, 24.75893115100078745, -9.846743663894594434 ) ) ;
#4482=CARTESIAN_POINT ( 'NONE',  ( -0.8801773607110991993, 7.855352010821504471, -2.915334737309923874 ) ) ;
#4483=CARTESIAN_POINT ( 'NONE',  ( 10.00000000000000178, 7.258931151000785675, 9.846743663894594434 ) ) ;
#4484=CARTESIAN_POINT ( 'NONE',  ( 10.00000000000000000, 56.81368534415484106, -10.88017736071110342 ) ) ;
#4485=CARTESIAN_POINT ( 'NONE',  ( 12.91533473730992121, 24.52201867748816966, 10.88017736071110164 ) ) ;
#4486=CARTESIAN_POINT ( 'NONE',  ( 22.81628187352648496, 61.83196800326376774, -3.434112377981050290 ) ) ;
#4487=CARTESIAN_POINT ( 'NONE',  ( 17.08211943468705130, 33.47041550158063927, 12.26659068614894998 ) ) ;
#4490=CARTESIAN_POINT ( 'NONE',  ( 20.32896413005680714, 12.60497603579417536, -5.963430220938276349 ) ) ;
#4492=CARTESIAN_POINT ( 'NONE',  ( 13.43411237798106583, 52.66530133659708213, -12.81628187352647252 ) ) ;
#4493=ORIENTED_EDGE ( 'NONE', *, *, #93755, .F. ) ;
#4494=CARTESIAN_POINT ( 'NONE',  ( 2.791683348922237240, 65.38393115100078035, -7.208316651077763204 ) ) ;
#4496=CARTESIAN_POINT ( 'NONE',  ( 20.88017736071110875, 30.77201867748816966, -2.915334737309920765 ) ) ;
#4499=CARTESIAN_POINT ( 'NONE',  ( 2.791683348922240793, 11.63393115100078568, 7.208316651077764092 ) ) ;
#4501=B_SPLINE_CURVE_WITH_KNOTS ( 'NONE', 3,
 ( #26248, #33728, #64716, #40770 ),
 .UNSPECIFIED., .F., .F.,
 ( 4, 4 ),
 ( 0.000000000000000000, 0.001036303429213241041 ),
 .UNSPECIFIED. ) ;
#4502=CARTESIAN_POINT ( 'NONE',  ( 5.076628168052703671, 21.84226448433411960, 8.527530157486179263 ) ) ;
#4503=CARTESIAN_POINT ( 'NONE',  ( 10.00000000000000000, 9.758931151000785675, -9.846743663894594434 ) ) ;
#4504=CARTESIAN_POINT ( 'NONE',  ( 2.791683348922240793, 1.633931151000784565, 7.208316651077764092 ) ) ;
#4505=CARTESIAN_POINT ( 'NONE',  ( 10.00000000000000000, 66.81368534415484817, -10.88017736071110342 ) ) ;
#4507=CARTESIAN_POINT ( 'NONE',  ( 1.472469842513823179, 5.592264484334118713, -4.923371831947296329 ) ) ;
#4508=CARTESIAN_POINT ( 'NONE',  ( 5.076628168052704559, 15.17559781766745175, -8.527530157486179263 ) ) ;
#4509=ORIENTED_EDGE ( 'NONE', *, *, #3234, .F. ) ;
#4511=CARTESIAN_POINT ( 'NONE',  ( -1.099225684535947600, 4.540301336597087456, 6.408140936763237150 ) ) ;
#4512=ORIENTED_EDGE ( 'NONE', *, *, #83547, .F. ) ;
#4513=EDGE_LOOP ( 'NONE', ( #31366, #36200, #2533, #9399, #53295, #97738 ) ) ;
#4514=SURFACE_STYLE_FILL_AREA ( #72985 ) ;
#4515=CARTESIAN_POINT ( 'NONE',  ( 17.08211943468705130, 13.47041550158063572, 12.26659068614894998 ) ) ;
#4518=CARTESIAN_POINT ( 'NONE',  ( 24.16423886937410614, 14.30374883491396787, 8.672049930838204340E-16 ) ) ;
#4519=CARTESIAN_POINT ( 'NONE',  ( 17.08211943468705130, 33.47041550158063927, 12.26659068614894998 ) ) ;
#4520=( LENGTH_UNIT ( ) NAMED_UNIT ( * ) SI_UNIT ( .MILLI., .METRE. ) );
#4521=CARTESIAN_POINT ( 'NONE',  ( 17.08211943468705130, 3.470415501580634388, 12.26659068614894998 ) ) ;
#4522=CARTESIAN_POINT ( 'NONE',  ( 0.5774900079438607392, 38.48035201082150536, 5.440088680355550821 ) ) ;
#4524=CARTESIAN_POINT ( 'NONE',  ( 7.361572987183169658, 14.96726448433411960, -9.846743663894592657 ) ) ;
#4525=CARTESIAN_POINT ( 'NONE',  ( 15.44008868035555793, 51.39701867748816966, -9.422509992056140149 ) ) ;
#4526=CARTESIAN_POINT ( 'NONE',  ( 5.076628168052703671, 26.84226448433411960, 8.527530157486179263 ) ) ;
#4527=CARTESIAN_POINT ( 'NONE',  ( 19.42250999205614548, 10.98035201082150536, -5.440088680355545492 ) ) ;
#4528=CARTESIAN_POINT ( 'NONE',  ( 0.6178305044545818747, 48.49863466993042493, -9.382169495545419124 ) ) ;
#4529=CARTESIAN_POINT ( 'NONE',  ( 0.1532563361054083140, 46.00893115100079456, 1.131784320476157264E-15 ) ) ;
#4532=CARTESIAN_POINT ( 'NONE',  ( 19.38216949554541557, 27.24863466993041783, -9.382169495545420901 ) ) ;
#4535=CARTESIAN_POINT ( 'NONE',  ( 10.00000000000000000, 39.75893115100078745, -9.846743663894594434 ) ) ;
#4536=CARTESIAN_POINT ( 'NONE',  ( 6.204703633549690345, 7.845415501580634832, 14.16423886937410082 ) ) ;
#4537=EDGE_LOOP ( 'NONE', ( #85668, #68586, #87009, #52697 ) ) ;
#4540=CARTESIAN_POINT ( 'NONE',  ( 4.559911319644449179, 53.89701867748817676, 9.422509992056141925 ) ) ;
#4541=CARTESIAN_POINT ( 'NONE',  ( -0.8801773607110991993, 47.85535201082150536, -2.915334737309923874 ) ) ;
#4542=CARTESIAN_POINT ( 'NONE',  ( 2.917880565312950480, 45.97041550158063927, -12.26659068614894821 ) ) ;
#4543=CARTESIAN_POINT ( 'NONE',  ( 0.1532563361054082862, 51.21726448433412315, 2.638427012816831674 ) ) ;
#4545=CARTESIAN_POINT ( 'NONE',  ( 19.42250999205614193, 35.14701867748816966, 5.440088680355555262 ) ) ;
#4548=CARTESIAN_POINT ( 'NONE',  ( 14.92337183194729633, 57.67559781766745886, 8.527530157486181039 ) ) ;
#4550=CARTESIAN_POINT ( 'NONE',  ( 0.2751277870542983006, 13.21833443783938122, 6.500000000000002665 ) ) ;
#4552=CARTESIAN_POINT ( 'NONE',  ( 12.91533473730992121, 4.522018677488169658, 10.88017736071110164 ) ) ;
#4555=CARTESIAN_POINT ( 'NONE',  ( 15.44008868035555793, 61.39701867748817676, -9.422509992056140149 ) ) ;
#4556=B_SPLINE_CURVE_WITH_KNOTS ( 'NONE', 3,
 ( #9266, #39773, #40749, #25758, #93245, #18246 ),
 .UNSPECIFIED., .F., .F.,
 ( 4, 2, 4 ),
 ( 0.000000000000000000, 0.0002701661927229329508, 0.0005403323854458659016 ),
 .UNSPECIFIED. ) ;
#4557=CARTESIAN_POINT ( 'NONE',  ( 5.076628168052704559, 0.1755978176674514724, -8.527530157486179263 ) ) ;
#4560=CARTESIAN_POINT ( 'NONE',  ( 7.361572987183170547, 32.05059781766745175, 9.846743663894590881 ) ) ;
#4561=CARTESIAN_POINT ( 'NONE',  ( 17.96484262340118221, 16.18868534415483396, -7.964842623401177768 ) ) ;
#4562=CARTESIAN_POINT ( 'NONE',  ( 3.591859063236761518, 4.956968003263753531, 11.09922568453594849 ) ) ;
#4563=CARTESIAN_POINT ( 'NONE',  ( -0.8801773607110991993, 32.85535201082151247, -2.915334737309923874 ) ) ;
#4566=CARTESIAN_POINT ( 'NONE',  ( 13.43411237798106583, 37.66530133659708923, -12.81628187352647252 ) ) ;
#4568=CARTESIAN_POINT ( 'NONE',  ( -0.8801773607111008646, 63.27201867748817676, 2.915334737309923430 ) ) ;
#4570=CARTESIAN_POINT ( 'NONE',  ( 19.38216949554541557, 17.24863466993041783, -9.382169495545420901 ) ) ;
#4571=CARTESIAN_POINT ( 'NONE',  ( 19.84674366389459266, 18.30059781766745175, 2.638427012816836559 ) ) ;
#4572=( NAMED_UNIT ( * ) PLANE_ANGLE_UNIT ( ) SI_UNIT ( $, .RADIAN. ) );
#4573=CARTESIAN_POINT ( 'NONE',  ( 10.00000000000000178, 29.31368534415483751, 10.88017736071110342 ) ) ;
#4574=CARTESIAN_POINT ( 'NONE',  ( 10.00000000000000178, 63.05374883491396076, 14.16423886937410082 ) ) ;
#4575=CARTESIAN_POINT ( 'NONE',  ( 14.92337183194729988, 54.34226448433412315, -8.527530157486177487 ) ) ;
#4576=CARTESIAN_POINT ( 'NONE',  ( 2.791683348922240793, 1.633931151000784565, 7.208316651077764092 ) ) ;
#4577=CARTESIAN_POINT ( 'NONE',  ( 0.5774900079438607392, 58.48035201082151247, 5.440088680355550821 ) ) ;
#4578=CARTESIAN_POINT ( 'NONE',  ( 0.2751277870542914172, 43.21833443783938122, 6.499999999999992006 ) ) ;
#4579=CARTESIAN_POINT ( 'NONE',  ( 2.917880565312948704, 32.63708216824730357, 12.26659068614894643 ) ) ;
#4580=B_SPLINE_CURVE_WITH_KNOTS ( 'NONE', 3,
 ( #19206, #58677, #12190, #20689 ),
 .UNSPECIFIED., .F., .F.,
 ( 4, 4 ),
 ( 6.046421166978534523E-20, 0.0003153927346769890092 ),
 .UNSPECIFIED. ) ;
#4585=CARTESIAN_POINT ( 'NONE',  ( -4.164238869374098151, 46.59541550158063927, -3.795296366450310543 ) ) ;
#4586=CARTESIAN_POINT ( 'NONE',  ( 22.26659068614894466, 48.88708216824730357, 7.082119434687054849 ) ) ;
#4587=CARTESIAN_POINT ( 'NONE',  ( 18.52753015748617571, 23.09226448433411960, 4.923371831947298993 ) ) ;
#4588=CARTESIAN_POINT ( 'NONE',  ( 19.38216949554541557, 32.24863466993041783, -9.382169495545420901 ) ) ;
#4591=( LENGTH_UNIT ( ) NAMED_UNIT ( * ) SI_UNIT ( .MILLI., .METRE. ) );
#4592=CARTESIAN_POINT ( 'NONE',  ( 20.36894250292379738, 39.92874883491396787, -10.36894250292379027 ) ) ;
#4594=CARTESIAN_POINT ( 'NONE',  ( 5.076628168052704559, 10.17559781766745175, -8.527530157486179263 ) ) ;
#4597=ORIENTED_EDGE ( 'NONE', *, *, #73216, .F. ) ;
#4599=( BOUNDED_CURVE ( )  B_SPLINE_CURVE ( 2, ( #81791, #73801, #13308, #5331, #35812, #67301, #43794, #66804, #44294 ),
 .UNSPECIFIED., .F., .T. ) 
 B_SPLINE_CURVE_WITH_KNOTS ( ( 3, 2, 2, 2, 3 ),
 ( 0.08299807979737425234, 0.08333333333333337034, 0.08928571428571430157, 0.09523809523809523281, 0.09557334877405435081 ),
 .UNSPECIFIED. ) 
 CURVE ( )  GEOMETRIC_REPRESENTATION_ITEM ( )  RATIONAL_B_SPLINE_CURVE ( ( 0.9963778908391762723, 0.9980808541467921513, 1.000000000000000000, 0.9659258262890683122, 1.000000000000000000, 0.9659258262890683122, 1.000000000000000000, 0.9980808541467921513, 0.9963778908391762723 ) ) 
 REPRESENTATION_ITEM ( '' )  );
#4603=CARTESIAN_POINT ( 'NONE',  ( 6.204703633549690345, 12.84541550158063572, 14.16423886937410082 ) ) ;
#4604=CARTESIAN_POINT ( 'NONE',  ( 20.88017736071110519, 15.56368534415483751, 2.639326808657452039E-16 ) ) ;
#4605=CARTESIAN_POINT ( 'NONE',  ( 20.88017736071110519, 20.56368534415484106, 2.639326808657452039E-16 ) ) ;
#4606=CARTESIAN_POINT ( 'NONE',  ( 7.361572987183170547, 52.05059781766745175, 9.846743663894590881 ) ) ;
#4607=CARTESIAN_POINT ( 'NONE',  ( 13.43411237798106583, 17.66530133659708923, -12.81628187352647252 ) ) ;
#4610=CARTESIAN_POINT ( 'NONE',  ( 19.38216949554541557, 17.24863466993041783, -9.382169495545420901 ) ) ;
#4612=CARTESIAN_POINT ( 'NONE',  ( 19.84674366389459621, 33.50893115100078745, 7.409399052514197653E-17 ) ) ;
#4613=CARTESIAN_POINT ( 'NONE',  ( 10.00000000000000178, 63.05374883491396076, 14.16423886937410082 ) ) ;
#4615=CARTESIAN_POINT ( 'NONE',  ( 20.88017736071110519, 5.563685344154838397, 2.639326808657452039E-16 ) ) ;
#4617=CARTESIAN_POINT ( 'NONE',  ( 4.559911319644449179, 47.23035201082150536, -9.422509992056141925 ) ) ;
#4618=CARTESIAN_POINT ( 'NONE',  ( 17.96484262340118221, 49.93868534415484106, 7.964842623401181321 ) ) ;
#4620=CARTESIAN_POINT ( 'NONE',  ( 15.44008868035555260, 54.73035201082150536, 9.422509992056143702 ) ) ;
#4621=CARTESIAN_POINT ( 'NONE',  ( 0.5774900079438590739, 37.64701867748817676, -5.440088680355550821 ) ) ;
#4623=VECTOR ( 'NONE', #31133, 1000.000000000000000 ) ;
#4627=CARTESIAN_POINT ( 'NONE',  ( 1.472469842513823179, 26.42559781766745175, 4.923371831947296329 ) ) ;
#4628=ORIENTED_EDGE ( 'NONE', *, *, #66191, .F. ) ;
#4629=CARTESIAN_POINT ( 'NONE',  ( 14.92337183194729988, 54.34226448433412315, -8.527530157486177487 ) ) ;
#4635=CARTESIAN_POINT ( 'NONE',  ( 0.1532563361054083140, 66.00893115100079456, 1.131784320476157264E-15 ) ) ;
#4636=CARTESIAN_POINT ( 'NONE',  ( 1.472469842513823179, 30.59226448433411960, -4.923371831947296329 ) ) ;
#4637=CARTESIAN_POINT ( 'NONE',  ( 24.16423886937410614, 59.30374883491397497, 8.672049930838204340E-16 ) ) ;
#4641=CARTESIAN_POINT ( 'NONE',  ( 17.20831665107776587, 32.88393115100078745, 7.208316651077764980 ) ) ;
#4642=CARTESIAN_POINT ( 'NONE',  ( -2.816281873526473856, 59.33196800326374643, 3.434112377981055619 ) ) ;
#4643=CARTESIAN_POINT ( 'NONE',  ( 0.6178305044545838731, -0.2513653300695798953, 9.382169495545420901 ) ) ;
#4644=CARTESIAN_POINT ( 'NONE',  ( 17.20831665107776587, 14.13393115100078568, -7.208316651077762316 ) ) ;
#4648=CARTESIAN_POINT ( 'NONE',  ( 17.20831665107776587, 7.883931151000784787, 7.208316651077764980 ) ) ;
#4649=CARTESIAN_POINT ( 'NONE',  ( 5.076628168052704559, 65.17559781766745175, -8.527530157486179263 ) ) ;
#4651=ADVANCED_FACE ( 'NONE', ( #91330 ), #60829, .T. ) ;
#4653=EDGE_LOOP ( 'NONE', ( #16581, #78021, #48136, #88770 ) ) ;
#4654=CARTESIAN_POINT ( 'NONE',  ( -0.8801773607111009756, 8.063685344154837509, 1.068504757029289695E-15 ) ) ;
#4655=CARTESIAN_POINT ( 'NONE',  ( 10.00000000000000000, 10.55374883491396787, -14.16423886937410082 ) ) ;
#4656=CARTESIAN_POINT ( 'NONE',  ( 12.63842701281683922, 9.550597817667449974, -9.846743663894590881 ) ) ;
#4657=CARTESIAN_POINT ( 'NONE',  ( 4.559911319644449179, 53.89701867748817676, 9.422509992056141925 ) ) ;
#4658=CARTESIAN_POINT ( 'NONE',  ( 22.81628187352648496, 21.83196800326374643, -3.434112377981050290 ) ) ;
#4659=CARTESIAN_POINT ( 'NONE',  ( 15.44008868035555260, 64.73035201082151957, 9.422509992056143702 ) ) ;
#4663=CARTESIAN_POINT ( 'NONE',  ( 19.38216949554541557, 7.248634669930421381, -9.382169495545420901 ) ) ;
#4664=CARTESIAN_POINT ( 'NONE',  ( 6.565887622018943937, 0.1653013365970866511, 12.81628187352647430 ) ) ;
#4665=CARTESIAN_POINT ( 'NONE',  ( 12.63842701281683922, 9.550597817667449974, -9.846743663894590881 ) ) ;
#4667=CARTESIAN_POINT ( 'NONE',  ( 6.565887622018943937, 25.16530133659708213, 12.81628187352647430 ) ) ;
#4670=CARTESIAN_POINT ( 'NONE',  ( 0.5774900079438607392, 33.48035201082150536, 5.440088680355550821 ) ) ;
#4672=CARTESIAN_POINT ( 'NONE',  ( 20.36894250292379382, 48.67874883491396076, 10.36894250292379205 ) ) ;
#4674=CARTESIAN_POINT ( 'NONE',  ( 6.565887622018943937, 38.08196800326376064, -12.81628187352647608 ) ) ;
#4675=CARTESIAN_POINT ( 'NONE',  ( -0.8801773607111009756, 33.06368534415484106, 1.068504757029289695E-15 ) ) ;
#4676=CARTESIAN_POINT ( 'NONE',  ( 0.1532563361054082862, 46.21726448433411605, 2.638427012816831674 ) ) ;
#4677=CARTESIAN_POINT ( 'NONE',  ( 4.559911319644449179, 48.89701867748817676, 9.422509992056141925 ) ) ;
#4678=CARTESIAN_POINT ( 'NONE',  ( 24.16423886937410614, 39.30374883491396787, 8.672049930838204340E-16 ) ) ;
#4680=CARTESIAN_POINT ( 'NONE',  ( 10.00000000000000178, 32.25893115100078745, 9.846743663894594434 ) ) ;
#4681=CARTESIAN_POINT ( 'NONE',  ( 0.6178305044545838731, 64.74863466993043914, 9.382169495545420901 ) ) ;
#4682=CARTESIAN_POINT ( 'NONE',  ( 10.00000000000000000, 64.75893115100078035, -9.846743663894594434 ) ) ;
#4687=CARTESIAN_POINT ( 'NONE',  ( 19.42250999205614548, 15.98035201082150714, -5.440088680355545492 ) ) ;
#4688=CARTESIAN_POINT ( 'NONE',  ( 20.88017736071110164, 60.35535201082151957, 2.915334737309930979 ) ) ;
#4690=CARTESIAN_POINT ( 'NONE',  ( 20.36894250292379738, 24.92874883491396787, -10.36894250292379027 ) ) ;
#4691=CARTESIAN_POINT ( 'NONE',  ( 2.791683348922240793, 16.63393115100078745, 7.208316651077764092 ) ) ;
#4692=CARTESIAN_POINT ( 'NONE',  ( 7.361572987183170547, 67.05059781766746596, 9.846743663894590881 ) ) ;
#4693=CARTESIAN_POINT ( 'NONE',  ( 7.084665262690076126, 32.02201867748816966, -10.88017736071110164 ) ) ;
#4699=CARTESIAN_POINT ( 'NONE',  ( 0.1532563361054100626, 45.80059781766745886, -2.638427012816831230 ) ) ;
#4701=VERTEX_POINT ( 'NONE', #67859 ) ;
#4702=DIRECTION ( 'NONE',  ( -0.000000000000000000, 1.000000000000000000, 0.000000000000000000 ) ) ;
#4703=CARTESIAN_POINT ( 'NONE',  ( -4.164238869374099039, 11.80374883491396965, 8.674139862899312516E-16 ) ) ;
#4704=CARTESIAN_POINT ( 'NONE',  ( 24.16423886937409904, 9.095415501580633943, 3.795296366450317205 ) ) ;
#4705=CARTESIAN_POINT ( 'NONE',  ( 19.42250999205614548, 50.98035201082151247, -5.440088680355545492 ) ) ;
#4706=CARTESIAN_POINT ( 'NONE',  ( 22.26659068614894466, 48.88708216824730357, 7.082119434687054849 ) ) ;
#4707=CARTESIAN_POINT ( 'NONE',  ( 0.6178305044545838731, -0.2513653300695798953, 9.382169495545420901 ) ) ;
#4708=CARTESIAN_POINT ( 'NONE',  ( 17.20831665107776587, 34.13393115100078745, -7.208316651077762316 ) ) ;
#4710=CARTESIAN_POINT ( 'NONE',  ( -0.8801773607111009756, 28.06368534415484106, 1.068504757029289695E-15 ) ) ;
#4711=CARTESIAN_POINT ( 'NONE',  ( 0.6178305044545838731, 9.748634669930416052, 9.382169495545420901 ) ) ;
#4712=CARTESIAN_POINT ( 'NONE',  ( 24.16423886937409904, 4.095415501580634832, 3.795296366450317205 ) ) ;
#4713=CARTESIAN_POINT ( 'NONE',  ( -4.164238869374099039, 46.80374883491397497, 8.674139862899312516E-16 ) ) ;
#4714=CARTESIAN_POINT ( 'NONE',  ( -4.164238869374099039, 66.80374883491396076, 8.674139862899312516E-16 ) ) ;
#4715=CARTESIAN_POINT ( 'NONE',  ( -1.926860441876564023, 67.87045670184116375, 3.195792623639529761 ) ) ;
#4720=ORIENTED_EDGE ( 'NONE', *, *, #82743, .F. ) ;
#4721=CARTESIAN_POINT ( 'NONE',  ( -4.164238869374099039, 51.80374883491396787, 8.674139862899312516E-16 ) ) ;
#4722=CARTESIAN_POINT ( 'NONE',  ( 5.076628168052703671, 51.84226448433412315, 8.527530157486179263 ) ) ;
#4723=CARTESIAN_POINT ( 'NONE',  ( -0.8801773607111009756, 58.06368534415484106, 1.068504757029289695E-15 ) ) ;
#4726=CARTESIAN_POINT ( 'NONE',  ( 17.96484262340118221, 54.93868534415484106, 7.964842623401181321 ) ) ;
#4729=CARTESIAN_POINT ( 'NONE',  ( 10.00000000000000178, 23.05374883491397142, 14.16423886937410082 ) ) ;
#4730=CARTESIAN_POINT ( 'NONE',  ( 6.565887622018943937, 30.16530133659708568, 12.81628187352647430 ) ) ;
#4732=CARTESIAN_POINT ( 'NONE',  ( 13.43411237798105340, 50.58196800326375353, 12.81628187352647963 ) ) ;
#4734=CARTESIAN_POINT ( 'NONE',  ( 15.44008868035555260, 19.73035201082150536, 9.422509992056143702 ) ) ;
#4735=CARTESIAN_POINT ( 'NONE',  ( 5.076628168052703671, 41.84226448433411605, 8.527530157486179263 ) ) ;
#4736=CARTESIAN_POINT ( 'NONE',  ( 0.5774900079438607392, 13.48035201082150358, 5.440088680355550821 ) ) ;
#4737=CARTESIAN_POINT ( 'NONE',  ( 0.1532563361054082862, 41.21726448433411605, 2.638427012816831674 ) ) ;
#4741=CARTESIAN_POINT ( 'NONE',  ( 15.44008868035555793, 66.39701867748817676, -9.422509992056140149 ) ) ;
#4742=CARTESIAN_POINT ( 'NONE',  ( 19.72487221294570858, 69.50000000000000000, 6.500000000000000888 ) ) ;
#4744=CARTESIAN_POINT ( 'NONE',  ( 19.84674366389459266, 23.30059781766745530, 2.638427012816836559 ) ) ;
#4745=CARTESIAN_POINT ( 'NONE',  ( 3.591859063236763294, 23.29030133659708568, -11.09922568453595026 ) ) ;
#4746=ORIENTED_EDGE ( 'NONE', *, *, #35243, .T. ) ;
#4747=CARTESIAN_POINT ( 'NONE',  ( 10.00000000000000000, 39.75893115100078745, -9.846743663894594434 ) ) ;
#4749=CARTESIAN_POINT ( 'NONE',  ( 17.08211943468705840, 25.13708216824730357, -12.26659068614894466 ) ) ;
#4750=CARTESIAN_POINT ( 'NONE',  ( 19.84674366389459266, 33.71726448433410894, -2.638427012816827677 ) ) ;
#4751=CARTESIAN_POINT ( 'NONE',  ( 10.00000000000000178, 45.37363466993041783, 12.81628187352647608 ) ) ;
#4753=CARTESIAN_POINT ( 'NONE',  ( 19.50000000000000000, 3.304235192336776005E-17, -4.500000000000001776 ) ) ;
#4754=CARTESIAN_POINT ( 'NONE',  ( 17.96484262340118221, 61.18868534415482685, -7.964842623401177768 ) ) ;
#4756=CARTESIAN_POINT ( 'NONE',  ( -2.816281873526473856, 14.33196800326375531, 3.434112377981055619 ) ) ;
#4757=CARTESIAN_POINT ( 'NONE',  ( 4.999999999999999112, 60.50000000000000000, -6.500000000000000888 ) ) ;
#4758=CARTESIAN_POINT ( 'NONE',  ( 10.00000000000000000, 39.75893115100078745, -9.846743663894594434 ) ) ;
#4759=CARTESIAN_POINT ( 'NONE',  ( 4.559911319644449179, 37.23035201082150536, -9.422509992056141925 ) ) ;
#4760=CARTESIAN_POINT ( 'NONE',  ( 10.00000000000000178, 25.37363466993041783, 12.81628187352647608 ) ) ;
#4761=CARTESIAN_POINT ( 'NONE',  ( 5.076628168052703671, 31.84226448433412315, 8.527530157486179263 ) ) ;
#4765=CARTESIAN_POINT ( 'NONE',  ( 10.00000000000000000, 26.81368534415484106, -10.88017736071110342 ) ) ;
#4768=CARTESIAN_POINT ( 'NONE',  ( 19.84674366389459266, 53.30059781766744464, 2.638427012816836559 ) ) ;
#4769=CARTESIAN_POINT ( 'NONE',  ( 12.91533473730992121, 29.52201867748817321, 10.88017736071110164 ) ) ;
#4770=CARTESIAN_POINT ( 'NONE',  ( 2.035157376598822676, 62.43868534415483396, -7.964842623401177768 ) ) ;
#4772=CARTESIAN_POINT ( 'NONE',  ( 10.00000000000000178, 29.31368534415483751, 10.88017736071110342 ) ) ;
#4773=CARTESIAN_POINT ( 'NONE',  ( 3.640395162852212874, 107.5383484153110203, -12.00000000000000000 ) ) ;
#4774=PRESENTATION_STYLE_ASSIGNMENT (( #88750 ) ) ;
#4775=CARTESIAN_POINT ( 'NONE',  ( 2.791683348922237240, 30.38393115100078390, -7.208316651077763204 ) ) ;
#4776=CARTESIAN_POINT ( 'NONE',  ( 5.076628168052704559, 45.17559781766745175, -8.527530157486179263 ) ) ;
#4778=CARTESIAN_POINT ( 'NONE',  ( 22.26659068614895176, 54.72041550158063217, -7.082119434687042414 ) ) ;
#4781=CARTESIAN_POINT ( 'NONE',  ( -2.266590686148945544, 12.22041550158063394, 7.082119434687048631 ) ) ;
#4782=CARTESIAN_POINT ( 'NONE',  ( -0.3689425029237898834, 41.17874883491397497, -10.36894250292378850 ) ) ;
#4783=CARTESIAN_POINT ( 'NONE',  ( 21.09922568453594849, 11.20696800326375531, 6.408140936763242479 ) ) ;
#4784=LINE ( 'NONE', #12267, #31352 ) ;
#4785=CARTESIAN_POINT ( 'NONE',  ( -0.8801773607111009756, 18.06368534415484106, 1.068504757029289695E-15 ) ) ;
#4786=CARTESIAN_POINT ( 'NONE',  ( 17.20831665107776587, 37.88393115100078745, 7.208316651077764980 ) ) ;
#4788=CARTESIAN_POINT ( 'NONE',  ( 10.00000000000000178, 64.31368534415483396, 10.88017736071110342 ) ) ;
#4790=CARTESIAN_POINT ( 'NONE',  ( 13.43411237798105340, 60.58196800326376064, 12.81628187352647963 ) ) ;
#4791=CARTESIAN_POINT ( 'NONE',  ( -1.099225684535947600, 24.54030133659708923, 6.408140936763237150 ) ) ;
#4792=CARTESIAN_POINT ( 'NONE',  ( 14.92337183194729988, 34.34226448433411605, -8.527530157486177487 ) ) ;
#4795=EDGE_CURVE ( 'NONE', #96981, #27072, #60342, .T. ) ;
#4796=CARTESIAN_POINT ( 'NONE',  ( 18.17829156368507526, 4.167925641218962696, 6.500000000000000888 ) ) ;
#4797=CARTESIAN_POINT ( 'NONE',  ( 20.88017736071110164, 5.355352010821503583, 2.915334737309930979 ) ) ;
#4798=CARTESIAN_POINT ( 'NONE',  ( 4.559911319644449179, 12.23035201082150536, -9.422509992056141925 ) ) ;
#4799=CARTESIAN_POINT ( 'NONE',  ( 17.08211943468705840, 45.13708216824730357, -12.26659068614894466 ) ) ;
#4800=CARTESIAN_POINT ( 'NONE',  ( 12.91533473730992121, 34.52201867748817676, 10.88017736071110164 ) ) ;
#4801=CARTESIAN_POINT ( 'NONE',  ( -0.8801773607111009756, 63.06368534415484106, 1.068504757029289695E-15 ) ) ;
#4805=CARTESIAN_POINT ( 'NONE',  ( 10.00000000000000000, 14.75893115100078568, -9.846743663894594434 ) ) ;
#4806=( LENGTH_UNIT ( ) NAMED_UNIT ( * ) SI_UNIT ( .MILLI., .METRE. ) );
#4807=CARTESIAN_POINT ( 'NONE',  ( 12.63842701281683034, 7.467264484334118713, 9.846743663894596210 ) ) ;
#4808=DIRECTION ( 'NONE',  ( -0.000000000000000000, -1.000000000000000000, 0.000000000000000000 ) ) ;
#4809=CARTESIAN_POINT ( 'NONE',  ( 14.92337183194729988, 34.34226448433411605, -8.527530157486177487 ) ) ;
#4810=CARTESIAN_POINT ( 'NONE',  ( -2.816281873526473856, -0.8763653300695799508, 9.499525473075851096E-16 ) ) ;
#4811=CARTESIAN_POINT ( 'NONE',  ( 10.00000000000000178, 24.31368534415484106, 10.88017736071110342 ) ) ;
#4814=CARTESIAN_POINT ( 'NONE',  ( 21.09922568453594849, 46.20696800326376064, 6.408140936763242479 ) ) ;
#4815=CARTESIAN_POINT ( 'NONE',  ( -46.70923076923077133, 98.84615384615385381, -9.500000000000000000 ) ) ;
#4816=CARTESIAN_POINT ( 'NONE',  ( 10.00000000000000000, -0.2410688489992152128, -9.846743663894594434 ) ) ;
#4817=CARTESIAN_POINT ( 'NONE',  ( 22.81628187352647785, 41.62363466993042493, 6.195893100308588602E-16 ) ) ;
#4818=CARTESIAN_POINT ( 'NONE',  ( -2.266590686148945544, 61.38708216824730357, -7.082119434687050408 ) ) ;
#4819=CARTESIAN_POINT ( 'NONE',  ( 10.00000000000000000, 29.75893115100078745, -9.846743663894594434 ) ) ;
#4821=CARTESIAN_POINT ( 'NONE',  ( 19.84674366389459266, 58.71726448433411605, -2.638427012816827677 ) ) ;
#4822=CARTESIAN_POINT ( 'NONE',  ( -0.3689425029237881626, 17.42874883491397142, 10.36894250292379027 ) ) ;
#4823=CARTESIAN_POINT ( 'NONE',  ( 24.16423886937409904, 34.09541550158064638, 3.795296366450317205 ) ) ;
#4824=CARTESIAN_POINT ( 'NONE',  ( 10.00000000000000000, 49.75893115100078745, -9.846743663894594434 ) ) ;
#4825=CARTESIAN_POINT ( 'NONE',  ( -0.2002492713866858565, 69.97537705844109723, 6.181741512438951425 ) ) ;
#4826=CARTESIAN_POINT ( 'NONE',  ( 7.084665262690076126, 42.02201867748816966, -10.88017736071110164 ) ) ;
#4827=CARTESIAN_POINT ( 'NONE',  ( 4.559911319644449179, 52.23035201082151247, -9.422509992056141925 ) ) ;
#4830=CARTESIAN_POINT ( 'NONE',  ( 22.81628187352647785, 41.41530133659708923, 3.434112377981063169 ) ) ;
#4831=CARTESIAN_POINT ( 'NONE',  ( 12.63842701281683034, 2.467264484334118269, 9.846743663894596210 ) ) ;
#4835=DIRECTION ( 'NONE',  ( -0.000000000000000000, -1.000000000000000000, -0.000000000000000000 ) ) ;
#4839=CARTESIAN_POINT ( 'NONE',  ( 19.42250999205614548, 15.98035201082150714, -5.440088680355545492 ) ) ;
#4841=CARTESIAN_POINT ( 'NONE',  ( -0.3689425029237898834, 21.17874883491396432, -10.36894250292378850 ) ) ;
#4842=CARTESIAN_POINT ( 'NONE',  ( 7.084665262690076126, 19.10535201082150181, 10.88017736071109987 ) ) ;
#4843=CARTESIAN_POINT ( 'NONE',  ( 14.92337183194729633, 57.67559781766745886, 8.527530157486181039 ) ) ;
#4844=ORIENTED_EDGE ( 'NONE', *, *, #25859, .F. ) ;
#4845=AXIS2_PLACEMENT_3D ( 'NONE', #76117, #69606, #55077 ) ;
#4846=CARTESIAN_POINT ( 'NONE',  ( 17.20831665107776587, 62.88393115100078745, 7.208316651077764980 ) ) ;
#4849=CARTESIAN_POINT ( 'NONE',  ( -0.8801773607110991993, 52.85535201082151247, -2.915334737309923874 ) ) ;
#4850=CARTESIAN_POINT ( 'NONE',  ( 0.1532563361054082862, 61.21726448433412315, 2.638427012816831674 ) ) ;
#4851=CARTESIAN_POINT ( 'NONE',  ( -2.816281873526473856, 34.12363466993042493, 9.499525473075851096E-16 ) ) ;
#4852=CARTESIAN_POINT ( 'NONE',  ( 12.91533473730992121, 9.522018677488171434, 10.88017736071110164 ) ) ;
#4854=CARTESIAN_POINT ( 'NONE',  ( 2.791683348922237240, 5.383931151000785675, -7.208316651077763204 ) ) ;
#4855=VECTOR ( 'NONE', #70283, 1000.000000000000000 ) ;
#4856=CARTESIAN_POINT ( 'NONE',  ( -0.8801773607111009756, 23.06368534415484106, 1.068504757029289695E-15 ) ) ;
#4859=CARTESIAN_POINT ( 'NONE',  ( -2.816281873526473856, 59.12363466993042493, 9.499525473075851096E-16 ) ) ;
#4860=CARTESIAN_POINT ( 'NONE',  ( 12.91533473730992121, 29.52201867748817321, 10.88017736071110164 ) ) ;
#4861=CARTESIAN_POINT ( 'NONE',  ( 19.65595853167378948, 92.20263838533996648, 5.361990343729008401 ) ) ;
#4862=CARTESIAN_POINT ( 'NONE',  ( 10.00000000000000178, 40.37363466993042493, 12.81628187352647608 ) ) ;
#4863=CARTESIAN_POINT ( 'NONE',  ( 7.084665262690076126, 52.02201867748816255, -10.88017736071110164 ) ) ;
#4864=CARTESIAN_POINT ( 'NONE',  ( 19.84674366389459621, 53.50893115100078745, 7.409399052514197653E-17 ) ) ;
#4866=CARTESIAN_POINT ( 'NONE',  ( -0.03743638938522138304, 49.25197528031019090, -6.399506433553975526 ) ) ;
#4867=CARTESIAN_POINT ( 'NONE',  ( 17.20831665107776587, 9.133931151000787452, -7.208316651077762316 ) ) ;
#4868=CARTESIAN_POINT ( 'NONE',  ( 7.361572987183170547, 67.05059781766746596, 9.846743663894590881 ) ) ;
#4869=CARTESIAN_POINT ( 'NONE',  ( 17.39651004071841811, 4.082109641433293135, -6.499999999999999112 ) ) ;
#4870=CARTESIAN_POINT ( 'NONE',  ( 14.92337183194729988, 49.34226448433411605, -8.527530157486177487 ) ) ;
#4871=CARTESIAN_POINT ( 'NONE',  ( 19.42250999205614548, 15.98035201082150714, -5.440088680355545492 ) ) ;
#4872=CARTESIAN_POINT ( 'NONE',  ( 5.076628168052703671, 36.84226448433412315, 8.527530157486179263 ) ) ;
#4874=SURFACE_STYLE_FILL_AREA ( #50350 ) ;
#4875=CARTESIAN_POINT ( 'NONE',  ( 0.1532563361054082862, 41.21726448433411605, 2.638427012816831674 ) ) ;
#4876=CARTESIAN_POINT ( 'NONE',  ( 18.52753015748617571, 8.092264484334117824, 4.923371831947298993 ) ) ;
#4877=CARTESIAN_POINT ( 'NONE',  ( 19.84674366389459266, 53.30059781766744464, 2.638427012816836559 ) ) ;
#4881=VECTOR ( 'NONE', #65106, 1000.000000000000000 ) ;
#4882=CARTESIAN_POINT ( 'NONE',  ( -1.099225684535947600, 38.70696800326375353, -6.408140936763238038 ) ) ;
#4883=CARTESIAN_POINT ( 'NONE',  ( 1.472469842513823179, 46.42559781766745175, 4.923371831947296329 ) ) ;
#4885=CARTESIAN_POINT ( 'NONE',  ( 22.26659068614895176, 59.72041550158063927, -7.082119434687042414 ) ) ;
#4886=CARTESIAN_POINT ( 'NONE',  ( 5.076628168052703671, 31.84226448433412315, 8.527530157486179263 ) ) ;
#4887=EDGE_CURVE ( 'NONE', #4978, #24202, #32405, .T. ) ;
#4888=CARTESIAN_POINT ( 'NONE',  ( 20.00000000000000000, 88.20477317201525125, 5.338983947147861286 ) ) ;
#4889=CARTESIAN_POINT ( 'NONE',  ( 2.917880565312948704, 52.63708216824730357, 12.26659068614894643 ) ) ;
#4891=CARTESIAN_POINT ( 'NONE',  ( 20.88017736071110519, 20.56368534415484106, 2.639326808657452039E-16 ) ) ;
#4892=CARTESIAN_POINT ( 'NONE',  ( -4.164238869374099927, 42.01208216824728936, 3.795296366450308767 ) ) ;
#4893=CARTESIAN_POINT ( 'NONE',  ( 13.79529636645030344, 53.26208216824730357, 14.16423886937410614 ) ) ;
#4894=CARTESIAN_POINT ( 'NONE',  ( 20.88017736071110519, 5.563685344154838397, 2.639326808657452039E-16 ) ) ;
#4895=CARTESIAN_POINT ( 'NONE',  ( 19.84674366389459266, 18.30059781766745175, 2.638427012816836559 ) ) ;
#4896=CARTESIAN_POINT ( 'NONE',  ( 6.565887622018943937, 0.1653013365970866511, 12.81628187352647430 ) ) ;
#4897=CARTESIAN_POINT ( 'NONE',  ( 4.559911319644449179, 43.89701867748816966, 9.422509992056141925 ) ) ;
#4898=CARTESIAN_POINT ( 'NONE',  ( 1.274849032794305170, 17.55509018479936145, -6.499999999999995559 ) ) ;
#4900=( BOUNDED_SURFACE ( )  B_SPLINE_SURFACE ( 1, 2, ( 
 ( #35972, #66472, #88485, #28478, #20988, #51473, #81964, #87988, #5986, #36478, #66972, #42024, #19500, #97491, #19987, #72489, #4022, #34979, #50487, #64979, #80987, #4999, #11999, #35480, #42501, #65976, #84811, #69316, #70804, #16317, #69814, #47284, #91818, #38825, #61798, #54296, #77786, #8805, #15831, #45833, #92306, #21477, #59460, #46800, #838, #62287, #77293, #24320, #39318, #9797, #51976, #76804, #16809, #23833, #82462, #89961, #360, #61307, #23339, #32278, #31298, #1825, #85302, #1337, #15349, #31788, #92791, #85795, #54786, #9298, #39808, #38336, #17308, #53819, #70309, #76319, #62786, #47785, #28957, #84331, #24809, #7837, #30809, #93285, #68829, #46318, #8321, #55286, #78282, #40296, #49740, #95755, #33265, #79269, #57734, #4265, #63757, #72248, #34738, #3782, #41778, #3279, #26751, #34236, #64732, #80247, #2812, #50231, #80745, #72732, #25305, #40789, #11754, #10779, #19746, #27239, #41295, #71769, #55792, #18283, #64244, #17795, #49261, #42263, #79761, #56760, #33743, #42750, #87254, #95244, #19255, #94263, #94762, #26262, #18779, #65229, #11260, #86780, #48270, #57246, #93778, #32774, #87743, #88238, #12240, #2321, #63269, #86287, #78784, #10291, #48762, #71288, #25789, #56284, #35230, #43230, #5255, #96752, #50746, #6721, #74720, #81234, #98241, #82714, #43725, #44212, #97253, #74211, #83214, #28227, #4759, #96254, #29700, #12733, #6232, #58726, #73724, #75210, #89230, #35733, #14232, #51735, #29213, #60209, #90704, #22232, #5741, #97749, #36735, #67226, #52220, #66222, #52707, #14735, #44711, #27733, #20739, #37237, #81716, #73231, #65728, #51232, #36230, #58215, #13228, #66729, #88731, #21232, #67727, #82217, #28723, #59213, #20243, #89718, #13727, #90208, #59712, #21738, #76688, #69203, #62165, #23719, #30686, #60696, #8209, #37722, #75709, #727, #84214, #77179, #31183, #39200, #92193, #24688, #68226, #91702, #31673, #38704, #98746, #7223, #15227, #76207, #68706, #22721, #77667, #46682, #53204, #70186, #54665, #15720, #16200, #61673, #46205, #55160, #238, #30195, #91195, #1703, #83709, #8686, #61194, #45706, #47162, #23220, #7724, #85181, #54178, #1218, #32159, #62661, #93163, #38221, #9181, #53693, #16692, #92670, #84690, #69687, #24198, #39698, #85674, #45211, #3657, #10659, #25192, #4149, #10173, #25674, #78168, #71656, #34614, #17193, #48154, #11633, #47673, #86171, #56647, #9677, #70679, #55671, #94643, #40175, #11143, #64614, #42149, #78667, #94147, #72614, #19139, #40671, #87132, #49616, #18655, #49143, #57128, #65109, #57619, #56168, #3165, #79644, #33627, #86660, #41662, #2200, #87625 ),
 ( #80126, #71169, #17680, #95632, #26153, #72130, #27120, #32661, #63154, #2693, #93657, #18165, #33145, #34122, #48643, #63639, #64126, #95123, #79147, #26630, #41173, #81598, #96134, #75092, #81112, #96631, #50120, #43606, #6598, #88118, #20118, #82595, #19628, #58101, #28607, #80630, #42627, #27615, #66609, #12126, #82097, #36617, #14110, #50621, #66102, #44594, #90090, #12613, #59096, #21617, #89605, #21114, #89110, #13608, #51614, #44089, #67104, #88608, #37111, #67608, #59592, #73105, #43114, #97628, #28108, #98114, #29576, #58608, #20621, #4644, #5128, #51111, #35108, #36103, #29092, #97137, #74092, #13110, #65607, #5626, #74598, #6112, #73603, #52103, #35617, #84084, #77064, #38584, #45584, #75590, #91584, #52587, #90581, #15599, #121, #92070, #46082, #54062, #8088, #39577, #83090, #7608, #46563, #23100, #14619, #22107, #30075, #91076, #53080, #76079, #61562, #83592, #69082, #77546, #22603, #1093, #62050, #15107, #53571, #76570, #16077, #98626, #617, #45085, #60584, #84576, #23598, #9065, #38103, #8575, #68591, #30568, #70066, #31063, #16575, #39079, #1589, #69573, #60080, #31554, #92552, #7102, #24080, #37604, #54547, #61072, #85064, #68099, #47050, #32038, #34008, #33034, #87023, #94038, #17567, #10541, #79532, #93540, #70555, #18535, #72018, #56052, #24580, #33515, #78545, #87517, #80014, #41051, #2083, #19030, #86055, #63530, #32543, #25559, #18050, #64012, #86543, #49507, #94524, #63043, #49026, #26043, #17071, #48527, #56534, #11032, #71550, #11517, #3548, #62541, #95010, #93047, #9554, #3060, #41552, #64504, #25071, #26518, #79029, #57015, #42041, #48032, #71055, #72505, #55554, #55041, #85559, #47554, #78051, #40056, #10056, #40555, #2578, #5513, #20507, #12505, #73988, #4037, #43975, #35990, #96018, #43004, #4529, #57509, #21495, #73488, #44478, #34500, #42515, #89001, #5015, #74477, #27011, #21002, #81488, #36496, #72999, #43487, #95518, #88006, #34993, #12991, #64991, #97019, #51490, #97510, #65498, #81003, #59477, #6002, #27501, #66492, #66988, #28496, #58989, #35498, #89493, #81985, #13496, #28974, #57996, #51992, #82481, #89978, #19517, #88502, #14000, #65993, #50014, #80518, #96520, #27993, #12016, #20005, #58489, #50505, #50993, #84461, #53451, #30451, #14992, #16454, #60951, #15486, #91950, #37491, #83471, #7490, #3, #23482, #83960, #60466, #90461, #37986, #67485, #6483, #91460, #45463, #7974, #22986, #68965, #45969, #54434, #98007, #22487, #61444, #68477, #29460, #36988, #44968, #6987, #98506, #52472, #8453, #76459, #82977, #971, #15959, #75962, #38473, #497, #30946, #84943, #29960, #59968 ) ),
 .UNSPECIFIED., .F., .F., .F. ) 
 B_SPLINE_SURFACE_WITH_KNOTS ( ( 2, 2 ),
 ( 3, 2, 2, 2, 2, 2, 2, 2, 2, 2, 2, 2, 2, 2, 2, 2, 2, 2, 2, 2, 2, 2, 2, 2, 2, 2, 2, 2, 2, 2, 2, 2, 2, 2, 2, 2, 2, 2, 2, 2, 2, 2, 2, 2, 2, 2, 2, 2, 2, 2, 2, 2, 2, 2, 2, 2, 2, 2, 2, 2, 2, 2, 2, 2, 2, 2, 2, 2, 2, 2, 2, 2, 2, 2, 2, 2, 2, 2, 2, 2, 2, 2, 2, 2, 2, 2, 2, 2, 2, 2, 2, 2, 2, 2, 2, 2, 2, 2, 2, 2, 2, 2, 2, 2, 2, 2, 2, 2, 2, 2, 2, 2, 2, 2, 2, 2, 2, 2, 2, 2, 2, 2, 2, 2, 2, 2, 2, 2, 2, 2, 2, 2, 2, 2, 2, 2, 2, 2, 2, 2, 2, 2, 2, 2, 2, 2, 2, 2, 2, 2, 2, 2, 2, 2, 2, 2, 2, 2, 2, 2, 2, 2, 3 ),
 ( 0.000000000000000000, 1.000000000000000000 ),
 ( 0.000000000000000000, 0.005952380952380952051, 0.01190476190476190410, 0.01785714285714285615, 0.02380952380952380820, 0.02976190476190476025, 0.03571428571428571230, 0.04166666666666666435, 0.04761904761904761640, 0.05357142857142856845, 0.05952380952380952051, 0.06547619047619047949, 0.07142857142857142461, 0.07738095238095238360, 0.08333333333333332871, 0.08928571428571428770, 0.09523809523809523281, 0.1011904761904761918, 0.1071428571428571369, 0.1130952380952380959, 0.1190476190476190410, 0.1250000000000000000, 0.1309523809523809590, 0.1369047619047619180, 0.1428571428571428492, 0.1488095238095238082, 0.1547619047619047672, 0.1607142857142857262, 0.1666666666666666574, 0.1726190476190476164, 0.1785714285714285754, 0.1845238095238095344, 0.1904761904761904656, 0.1964285714285714246, 0.2023809523809523836, 0.2083333333333333426, 0.2142857142857142738, 0.2202380952380952328, 0.2261904761904761918, 0.2321428571428571508, 0.2380952380952380820, 0.2440476190476190410, 0.2500000000000000000, 0.2559523809523809312, 0.2619047619047619180, 0.2678571428571428492, 0.2738095238095238360, 0.2797619047619047672, 0.2857142857142856984, 0.2916666666666666852, 0.2976190476190476164, 0.3035714285714285476, 0.3095238095238095344, 0.3154761904761904656, 0.3214285714285714524, 0.3273809523809523836, 0.3333333333333333148, 0.3392857142857143016, 0.3452380952380952328, 0.3511904761904761640, 0.3571428571428571508, 0.3630952380952380820, 0.3690476190476190688, 0.3750000000000000000, 0.3809523809523809312, 0.3869047619047619180, 0.3928571428571428492, 0.3988095238095238360, 0.4047619047619047672, 0.4107142857142856984, 0.4166666666666666852, 0.4226190476190476164, 0.4285714285714285476, 0.4345238095238095344, 0.4404761904761904656, 0.4464285714285714524, 0.4523809523809523836, 0.4583333333333333148, 0.4642857142857143016, 0.4702380952380952328, 0.4761904761904761640, 0.4821428571428571508, 0.4880952380952380820, 0.4940476190476190688, 0.5000000000000000000, 0.5059523809523809312, 0.5119047619047618625, 0.5178571428571429047, 0.5238095238095238360, 0.5297619047619047672, 0.5357142857142856984, 0.5416666666666666297, 0.5476190476190476719, 0.5535714285714286031, 0.5595238095238095344, 0.5654761904761904656, 0.5714285714285713969, 0.5773809523809523281, 0.5833333333333333703, 0.5892857142857143016, 0.5952380952380952328, 0.6011904761904761640, 0.6071428571428570953, 0.6130952380952381375, 0.6190476190476190688, 0.6250000000000000000, 0.6309523809523809312, 0.6369047619047618625, 0.6428571428571429047, 0.6488095238095238360, 0.6547619047619047672, 0.6607142857142856984, 0.6666666666666666297, 0.6726190476190476719, 0.6785714285714286031, 0.6845238095238095344, 0.6904761904761904656, 0.6964285714285713969, 0.7023809523809523281, 0.7083333333333333703, 0.7142857142857143016, 0.7202380952380952328, 0.7261904761904761640, 0.7321428571428570953, 0.7380952380952381375, 0.7440476190476190688, 0.7500000000000000000, 0.7559523809523809312, 0.7619047619047618625, 0.7678571428571429047, 0.7738095238095238360, 0.7797619047619047672, 0.7857142857142856984, 0.7916666666666666297, 0.7976190476190476719, 0.8035714285714286031, 0.8095238095238095344, 0.8154761904761904656, 0.8214285714285713969, 0.8273809523809523281, 0.8333333333333333703, 0.8392857142857143016, 0.8452380952380952328, 0.8511904761904761640, 0.8571428571428570953, 0.8630952380952381375, 0.8690476190476190688, 0.8750000000000000000, 0.8809523809523809312, 0.8869047619047618625, 0.8928571428571429047, 0.8988095238095238360, 0.9047619047619047672, 0.9107142857142856984, 0.9166666666666666297, 0.9226190476190476719, 0.9285714285714286031, 0.9345238095238095344, 0.9404761904761904656, 0.9464285714285713969, 0.9523809523809523281, 0.9583333333333333703, 0.9642857142857143016 ),
 .UNSPECIFIED. ) 
 GEOMETRIC_REPRESENTATION_ITEM ( )  RATIONAL_B_SPLINE_SURFACE ( (
 ( 1.000000000000000000, 0.9659258262890683122, 1.000000000000000000, 0.9659258262890683122, 1.000000000000000000, 0.9659258262890683122, 1.000000000000000000, 0.9659258262890683122, 1.000000000000000000, 0.9659258262890683122, 1.000000000000000000, 0.9659258262890683122, 1.000000000000000000, 0.9659258262890683122, 1.000000000000000000, 0.9659258262890683122, 1.000000000000000000, 0.9659258262890683122, 1.000000000000000000, 0.9659258262890683122, 1.000000000000000000, 0.9659258262890683122, 1.000000000000000000, 0.9659258262890683122, 1.000000000000000000, 0.9659258262890683122, 1.000000000000000000, 0.9659258262890683122, 1.000000000000000000, 0.9659258262890683122, 1.000000000000000000, 0.9659258262890683122, 1.000000000000000000, 0.9659258262890683122, 1.000000000000000000, 0.9659258262890683122, 1.000000000000000000, 0.9659258262890683122, 1.000000000000000000, 0.9659258262890683122, 1.000000000000000000, 0.9659258262890683122, 1.000000000000000000, 0.9659258262890683122, 1.000000000000000000, 0.9659258262890683122, 1.000000000000000000, 0.9659258262890683122, 1.000000000000000000, 0.9659258262890683122, 1.000000000000000000, 0.9659258262890683122, 1.000000000000000000, 0.9659258262890683122, 1.000000000000000000, 0.9659258262890683122, 1.000000000000000000, 0.9659258262890683122, 1.000000000000000000, 0.9659258262890683122, 1.000000000000000000, 0.9659258262890683122, 1.000000000000000000, 0.9659258262890683122, 1.000000000000000000, 0.9659258262890683122, 1.000000000000000000, 0.9659258262890683122, 1.000000000000000000, 0.9659258262890683122, 1.000000000000000000, 0.9659258262890683122, 1.000000000000000000, 0.9659258262890683122, 1.000000000000000000, 0.9659258262890683122, 1.000000000000000000, 0.9659258262890683122, 1.000000000000000000, 0.9659258262890683122, 1.000000000000000000, 0.9659258262890683122, 1.000000000000000000, 0.9659258262890683122, 1.000000000000000000, 0.9659258262890683122, 1.000000000000000000, 0.9659258262890683122, 1.000000000000000000, 0.9659258262890683122, 1.000000000000000000, 0.9659258262890683122, 1.000000000000000000, 0.9659258262890683122, 1.000000000000000000, 0.9659258262890683122, 1.000000000000000000, 0.9659258262890683122, 1.000000000000000000, 0.9659258262890683122, 1.000000000000000000, 0.9659258262890683122, 1.000000000000000000, 0.9659258262890683122, 1.000000000000000000, 0.9659258262890683122, 1.000000000000000000, 0.9659258262890683122, 1.000000000000000000, 0.9659258262890683122, 1.000000000000000000, 0.9659258262890683122, 1.000000000000000000, 0.9659258262890683122, 1.000000000000000000, 0.9659258262890683122, 1.000000000000000000, 0.9659258262890683122, 1.000000000000000000, 0.9659258262890683122, 1.000000000000000000, 0.9659258262890683122, 1.000000000000000000, 0.9659258262890683122, 1.000000000000000000, 0.9659258262890683122, 1.000000000000000000, 0.9659258262890683122, 1.000000000000000000, 0.9659258262890683122, 1.000000000000000000, 0.9659258262890683122, 1.000000000000000000, 0.9659258262890683122, 1.000000000000000000, 0.9659258262890683122, 1.000000000000000000, 0.9659258262890683122, 1.000000000000000000, 0.9659258262890683122, 1.000000000000000000, 0.9659258262890683122, 1.000000000000000000, 0.9659258262890683122, 1.000000000000000000, 0.9659258262890683122, 1.000000000000000000, 0.9659258262890683122, 1.000000000000000000, 0.9659258262890683122, 1.000000000000000000, 0.9659258262890683122, 1.000000000000000000, 0.9659258262890683122, 1.000000000000000000, 0.9659258262890683122, 1.000000000000000000, 0.9659258262890683122, 1.000000000000000000, 0.9659258262890683122, 1.000000000000000000, 0.9659258262890683122, 1.000000000000000000, 0.9659258262890683122, 1.000000000000000000, 0.9659258262890683122, 1.000000000000000000, 0.9659258262890683122, 1.000000000000000000, 0.9659258262890683122, 1.000000000000000000, 0.9659258262890683122, 1.000000000000000000, 0.9659258262890683122, 1.000000000000000000, 0.9659258262890683122, 1.000000000000000000, 0.9659258262890683122, 1.000000000000000000, 0.9659258262890683122, 1.000000000000000000, 0.9659258262890683122, 1.000000000000000000, 0.9659258262890683122, 1.000000000000000000, 0.9659258262890683122, 1.000000000000000000, 0.9659258262890683122, 1.000000000000000000, 0.9659258262890683122, 1.000000000000000000, 0.9659258262890683122, 1.000000000000000000, 0.9659258262890683122, 1.000000000000000000, 0.9659258262890683122, 1.000000000000000000, 0.9659258262890683122, 1.000000000000000000, 0.9659258262890683122, 1.000000000000000000, 0.9659258262890683122, 1.000000000000000000, 0.9659258262890683122, 1.000000000000000000, 0.9659258262890683122, 1.000000000000000000, 0.9659258262890683122, 1.000000000000000000, 0.9659258262890683122, 1.000000000000000000, 0.9659258262890683122, 1.000000000000000000, 0.9659258262890683122, 1.000000000000000000, 0.9659258262890683122, 1.000000000000000000, 0.9659258262890683122, 1.000000000000000000, 0.9659258262890683122, 1.000000000000000000, 0.9659258262890683122, 1.000000000000000000, 0.9659258262890683122, 1.000000000000000000, 0.9659258262890683122, 1.000000000000000000, 0.9659258262890683122, 1.000000000000000000, 0.9659258262890683122, 1.000000000000000000, 0.9659258262890683122, 1.000000000000000000, 0.9659258262890683122, 1.000000000000000000, 0.9659258262890683122, 1.000000000000000000, 0.9659258262890683122, 1.000000000000000000, 0.9659258262890683122, 1.000000000000000000, 0.9659258262890683122, 1.000000000000000000, 0.9659258262890683122, 1.000000000000000000, 0.9659258262890683122, 1.000000000000000000, 0.9659258262890683122, 1.000000000000000000, 0.9659258262890683122, 1.000000000000000000, 0.9659258262890683122, 1.000000000000000000, 0.9659258262890683122, 1.000000000000000000, 0.9659258262890683122, 1.000000000000000000, 0.9659258262890683122, 1.000000000000000000, 0.9659258262890683122, 1.000000000000000000, 0.9659258262890683122, 1.000000000000000000, 0.9659258262890683122, 1.000000000000000000, 0.9659258262890683122, 1.000000000000000000, 0.9659258262890683122, 1.000000000000000000, 0.9659258262890683122, 1.000000000000000000, 0.9659258262890683122, 1.000000000000000000, 0.9659258262890683122, 1.000000000000000000, 0.9659258262890683122, 1.000000000000000000, 0.9659258262890683122, 1.000000000000000000, 0.9659258262890683122, 1.000000000000000000, 0.9659258262890683122, 1.000000000000000000, 0.9659258262890683122, 1.000000000000000000, 0.9659258262890683122, 1.000000000000000000, 0.9659258262890683122, 1.000000000000000000, 0.9659258262890683122, 1.000000000000000000, 0.9659258262890683122, 1.000000000000000000, 0.9659258262890683122, 1.000000000000000000, 0.9659258262890683122, 1.000000000000000000, 0.9659258262890683122, 1.000000000000000000, 0.9659258262890683122, 1.000000000000000000, 0.9659258262890683122, 1.000000000000000000, 0.9659258262890683122, 1.000000000000000000, 0.9659258262890683122, 1.000000000000000000, 0.9659258262890683122, 1.000000000000000000, 0.9659258262890683122, 1.000000000000000000, 0.9659258262890683122, 1.000000000000000000, 0.9659258262890683122, 1.000000000000000000, 0.9659258262890683122, 1.000000000000000000, 0.9659258262890683122, 1.000000000000000000, 0.9659258262890683122, 1.000000000000000000, 0.9659258262890683122, 1.000000000000000000, 0.9659258262890683122, 1.000000000000000000),
 ( 1.000000000000000000, 0.9659258262890683122, 1.000000000000000000, 0.9659258262890683122, 1.000000000000000000, 0.9659258262890683122, 1.000000000000000000, 0.9659258262890683122, 1.000000000000000000, 0.9659258262890683122, 1.000000000000000000, 0.9659258262890683122, 1.000000000000000000, 0.9659258262890683122, 1.000000000000000000, 0.9659258262890683122, 1.000000000000000000, 0.9659258262890683122, 1.000000000000000000, 0.9659258262890683122, 1.000000000000000000, 0.9659258262890683122, 1.000000000000000000, 0.9659258262890683122, 1.000000000000000000, 0.9659258262890683122, 1.000000000000000000, 0.9659258262890683122, 1.000000000000000000, 0.9659258262890683122, 1.000000000000000000, 0.9659258262890683122, 1.000000000000000000, 0.9659258262890683122, 1.000000000000000000, 0.9659258262890683122, 1.000000000000000000, 0.9659258262890683122, 1.000000000000000000, 0.9659258262890683122, 1.000000000000000000, 0.9659258262890683122, 1.000000000000000000, 0.9659258262890683122, 1.000000000000000000, 0.9659258262890683122, 1.000000000000000000, 0.9659258262890683122, 1.000000000000000000, 0.9659258262890683122, 1.000000000000000000, 0.9659258262890683122, 1.000000000000000000, 0.9659258262890683122, 1.000000000000000000, 0.9659258262890683122, 1.000000000000000000, 0.9659258262890683122, 1.000000000000000000, 0.9659258262890683122, 1.000000000000000000, 0.9659258262890683122, 1.000000000000000000, 0.9659258262890683122, 1.000000000000000000, 0.9659258262890683122, 1.000000000000000000, 0.9659258262890683122, 1.000000000000000000, 0.9659258262890683122, 1.000000000000000000, 0.9659258262890683122, 1.000000000000000000, 0.9659258262890683122, 1.000000000000000000, 0.9659258262890683122, 1.000000000000000000, 0.9659258262890683122, 1.000000000000000000, 0.9659258262890683122, 1.000000000000000000, 0.9659258262890683122, 1.000000000000000000, 0.9659258262890683122, 1.000000000000000000, 0.9659258262890683122, 1.000000000000000000, 0.9659258262890683122, 1.000000000000000000, 0.9659258262890683122, 1.000000000000000000, 0.9659258262890683122, 1.000000000000000000, 0.9659258262890683122, 1.000000000000000000, 0.9659258262890683122, 1.000000000000000000, 0.9659258262890683122, 1.000000000000000000, 0.9659258262890683122, 1.000000000000000000, 0.9659258262890683122, 1.000000000000000000, 0.9659258262890683122, 1.000000000000000000, 0.9659258262890683122, 1.000000000000000000, 0.9659258262890683122, 1.000000000000000000, 0.9659258262890683122, 1.000000000000000000, 0.9659258262890683122, 1.000000000000000000, 0.9659258262890683122, 1.000000000000000000, 0.9659258262890683122, 1.000000000000000000, 0.9659258262890683122, 1.000000000000000000, 0.9659258262890683122, 1.000000000000000000, 0.9659258262890683122, 1.000000000000000000, 0.9659258262890683122, 1.000000000000000000, 0.9659258262890683122, 1.000000000000000000, 0.9659258262890683122, 1.000000000000000000, 0.9659258262890683122, 1.000000000000000000, 0.9659258262890683122, 1.000000000000000000, 0.9659258262890683122, 1.000000000000000000, 0.9659258262890683122, 1.000000000000000000, 0.9659258262890683122, 1.000000000000000000, 0.9659258262890683122, 1.000000000000000000, 0.9659258262890683122, 1.000000000000000000, 0.9659258262890683122, 1.000000000000000000, 0.9659258262890683122, 1.000000000000000000, 0.9659258262890683122, 1.000000000000000000, 0.9659258262890683122, 1.000000000000000000, 0.9659258262890683122, 1.000000000000000000, 0.9659258262890683122, 1.000000000000000000, 0.9659258262890683122, 1.000000000000000000, 0.9659258262890683122, 1.000000000000000000, 0.9659258262890683122, 1.000000000000000000, 0.9659258262890683122, 1.000000000000000000, 0.9659258262890683122, 1.000000000000000000, 0.9659258262890683122, 1.000000000000000000, 0.9659258262890683122, 1.000000000000000000, 0.9659258262890683122, 1.000000000000000000, 0.9659258262890683122, 1.000000000000000000, 0.9659258262890683122, 1.000000000000000000, 0.9659258262890683122, 1.000000000000000000, 0.9659258262890683122, 1.000000000000000000, 0.9659258262890683122, 1.000000000000000000, 0.9659258262890683122, 1.000000000000000000, 0.9659258262890683122, 1.000000000000000000, 0.9659258262890683122, 1.000000000000000000, 0.9659258262890683122, 1.000000000000000000, 0.9659258262890683122, 1.000000000000000000, 0.9659258262890683122, 1.000000000000000000, 0.9659258262890683122, 1.000000000000000000, 0.9659258262890683122, 1.000000000000000000, 0.9659258262890683122, 1.000000000000000000, 0.9659258262890683122, 1.000000000000000000, 0.9659258262890683122, 1.000000000000000000, 0.9659258262890683122, 1.000000000000000000, 0.9659258262890683122, 1.000000000000000000, 0.9659258262890683122, 1.000000000000000000, 0.9659258262890683122, 1.000000000000000000, 0.9659258262890683122, 1.000000000000000000, 0.9659258262890683122, 1.000000000000000000, 0.9659258262890683122, 1.000000000000000000, 0.9659258262890683122, 1.000000000000000000, 0.9659258262890683122, 1.000000000000000000, 0.9659258262890683122, 1.000000000000000000, 0.9659258262890683122, 1.000000000000000000, 0.9659258262890683122, 1.000000000000000000, 0.9659258262890683122, 1.000000000000000000, 0.9659258262890683122, 1.000000000000000000, 0.9659258262890683122, 1.000000000000000000, 0.9659258262890683122, 1.000000000000000000, 0.9659258262890683122, 1.000000000000000000, 0.9659258262890683122, 1.000000000000000000, 0.9659258262890683122, 1.000000000000000000, 0.9659258262890683122, 1.000000000000000000, 0.9659258262890683122, 1.000000000000000000, 0.9659258262890683122, 1.000000000000000000, 0.9659258262890683122, 1.000000000000000000, 0.9659258262890683122, 1.000000000000000000, 0.9659258262890683122, 1.000000000000000000, 0.9659258262890683122, 1.000000000000000000, 0.9659258262890683122, 1.000000000000000000, 0.9659258262890683122, 1.000000000000000000, 0.9659258262890683122, 1.000000000000000000, 0.9659258262890683122, 1.000000000000000000, 0.9659258262890683122, 1.000000000000000000, 0.9659258262890683122, 1.000000000000000000, 0.9659258262890683122, 1.000000000000000000, 0.9659258262890683122, 1.000000000000000000, 0.9659258262890683122, 1.000000000000000000, 0.9659258262890683122, 1.000000000000000000, 0.9659258262890683122, 1.000000000000000000, 0.9659258262890683122, 1.000000000000000000, 0.9659258262890683122, 1.000000000000000000, 0.9659258262890683122, 1.000000000000000000, 0.9659258262890683122, 1.000000000000000000, 0.9659258262890683122, 1.000000000000000000, 0.9659258262890683122, 1.000000000000000000, 0.9659258262890683122, 1.000000000000000000, 0.9659258262890683122, 1.000000000000000000, 0.9659258262890683122, 1.000000000000000000, 0.9659258262890683122, 1.000000000000000000, 0.9659258262890683122, 1.000000000000000000, 0.9659258262890683122, 1.000000000000000000, 0.9659258262890683122, 1.000000000000000000, 0.9659258262890683122, 1.000000000000000000, 0.9659258262890683122, 1.000000000000000000, 0.9659258262890683122, 1.000000000000000000, 0.9659258262890683122, 1.000000000000000000, 0.9659258262890683122, 1.000000000000000000, 0.9659258262890683122, 1.000000000000000000, 0.9659258262890683122, 1.000000000000000000, 0.9659258262890683122, 1.000000000000000000, 0.9659258262890683122, 1.000000000000000000, 0.9659258262890683122, 1.000000000000000000, 0.9659258262890683122, 1.000000000000000000) ) ) 
 REPRESENTATION_ITEM ( '' )  SURFACE ( )  );
#4902=CARTESIAN_POINT ( 'NONE',  ( -0.1503990784575328643, 60.12777174578613426, 6.262539305110068177 ) ) ;
#4905=CARTESIAN_POINT ( 'NONE',  ( -0.3689425029237898834, 41.17874883491397497, -10.36894250292378850 ) ) ;
#4906=( LENGTH_UNIT ( ) NAMED_UNIT ( * ) SI_UNIT ( .MILLI., .METRE. ) );
#4908=CARTESIAN_POINT ( 'NONE',  ( 17.96484262340118221, 19.93868534415484106, 7.964842623401181321 ) ) ;
#4909=CARTESIAN_POINT ( 'NONE',  ( -2.816281873526471635, 33.91530133659708213, -3.434112377981056508 ) ) ;
#4912=CARTESIAN_POINT ( 'NONE',  ( -2.816281873526473856, 59.12363466993042493, 9.499525473075851096E-16 ) ) ;
#4917=CARTESIAN_POINT ( 'NONE',  ( 17.08211943468705840, 25.13708216824730357, -12.26659068614894466 ) ) ;
#4918=CARTESIAN_POINT ( 'NONE',  ( 2.917880565312950480, 5.970415501580634832, -12.26659068614894821 ) ) ;
#4919=CARTESIAN_POINT ( 'NONE',  ( 20.03743638938529159, 61.75197528031018379, 6.399506433553906248 ) ) ;
#4920=CARTESIAN_POINT ( 'NONE',  ( 12.91533473730993009, 21.60535201082150536, -10.88017736071109987 ) ) ;
#4922=CARTESIAN_POINT ( 'NONE',  ( 20.88017736071110875, 40.77201867748818387, -2.915334737309920765 ) ) ;
#4923=CARTESIAN_POINT ( 'NONE',  ( 0.5774900079438590739, 57.64701867748817676, -5.440088680355550821 ) ) ;
#4924=CARTESIAN_POINT ( 'NONE',  ( 19.38216949554541557, 12.24863466993041961, -9.382169495545420901 ) ) ;
#4926=CYLINDRICAL_SURFACE ( 'NONE', #54689, 0.5000000000000004441 ) ;
#4927=CARTESIAN_POINT ( 'NONE',  ( 17.20831665107776587, 29.13393115100078390, -7.208316651077762316 ) ) ;
#4929=CARTESIAN_POINT ( 'NONE',  ( 10.00000000000000178, 39.31368534415484106, 10.88017736071110342 ) ) ;
#4930=CARTESIAN_POINT ( 'NONE',  ( 22.81628187352647785, 6.415301336597088344, 3.434112377981063169 ) ) ;
#4931=CARTESIAN_POINT ( 'NONE',  ( 12.91533473730993009, 56.60535201082151247, -10.88017736071109987 ) ) ;
#4932=CARTESIAN_POINT ( 'NONE',  ( 17.20831665107776587, 22.88393115100078745, 7.208316651077764980 ) ) ;
#4933=CARTESIAN_POINT ( 'NONE',  ( -1.099225684535947600, 53.70696800326376064, -6.408140936763238038 ) ) ;
#4934=CARTESIAN_POINT ( 'NONE',  ( 0.1532563361054083140, 11.00893115100078568, 1.131784320476157264E-15 ) ) ;
#4937=DIRECTION ( 'NONE',  ( 0.000000000000000000, -1.000000000000000000, 0.000000000000000000 ) ) ;
#4938=CARTESIAN_POINT ( 'NONE',  ( 20.88017736071110164, 15.35535201082150358, 2.915334737309930979 ) ) ;
#4939=CARTESIAN_POINT ( 'NONE',  ( 22.81628187352647785, 56.41530133659708213, 3.434112377981063169 ) ) ;
#4940=CARTESIAN_POINT ( 'NONE',  ( 6.204703633549690345, 22.84541550158062861, 14.16423886937410082 ) ) ;
#4941=CARTESIAN_POINT ( 'NONE',  ( 2.791683348922240793, 31.63393115100078745, 7.208316651077764092 ) ) ;
#4942=CARTESIAN_POINT ( 'NONE',  ( 10.00000000000000178, 19.31368534415484106, 10.88017736071110342 ) ) ;
#4943=CARTESIAN_POINT ( 'NONE',  ( -2.266590686148945544, 67.22041550158063217, 7.082119434687048631 ) ) ;
#4945=CARTESIAN_POINT ( 'NONE',  ( 4.559911319644449179, 17.23035201082150536, -9.422509992056141925 ) ) ;
#4946=CARTESIAN_POINT ( 'NONE',  ( 4.559911319644449179, 32.23035201082150536, -9.422509992056141925 ) ) ;
#4948=CARTESIAN_POINT ( 'NONE',  ( 4.559911319644449179, 43.89701867748816966, 9.422509992056141925 ) ) ;
#4949=ORIENTED_EDGE ( 'NONE', *, *, #43822, .T. ) ;
#4950=CARTESIAN_POINT ( 'NONE',  ( 0.1532563361054082862, 66.21726448433413736, 2.638427012816831674 ) ) ;
#4951=CARTESIAN_POINT ( 'NONE',  ( 4.559911319644449179, 18.89701867748817321, 9.422509992056141925 ) ) ;
#4953=COLOUR_RGB ( '', 0.08235294, 0.09019608, 0.10196078) ;
#4955=CARTESIAN_POINT ( 'NONE',  ( -2.816281873526473856, 64.12363466993042493, 9.499525473075851096E-16 ) ) ;
#4956=CARTESIAN_POINT ( 'NONE',  ( 20.15039907845753220, 30.60158574516642815, -6.262539305110077947 ) ) ;
#4957=CARTESIAN_POINT ( 'NONE',  ( -2.266590686148945544, 27.22041550158063572, 7.082119434687048631 ) ) ;
#4958=CARTESIAN_POINT ( 'NONE',  ( -0.8801773607111008646, 53.27201867748816966, 2.915334737309923430 ) ) ;
#4959=CARTESIAN_POINT ( 'NONE',  ( 19.42250999205614193, 35.14701867748816966, 5.440088680355555262 ) ) ;
#4962=CARTESIAN_POINT ( 'NONE',  ( 17.20831665107776587, 52.88393115100078035, 7.208316651077764980 ) ) ;
#4963=ORIENTED_EDGE ( 'NONE', *, *, #8053, .F. ) ;
#4964=CARTESIAN_POINT ( 'NONE',  ( 0.1077916266722469679, 22.24062864464239553, -6.478736007405950126 ) ) ;
#4965=CARTESIAN_POINT ( 'NONE',  ( 7.361572987183170547, 22.05059781766745530, 9.846743663894590881 ) ) ;
#4967=CARTESIAN_POINT ( 'NONE',  ( 4.559911319644449179, 17.23035201082150536, -9.422509992056141925 ) ) ;
#4968=CARTESIAN_POINT ( 'NONE',  ( 2.791683348922237240, 30.38393115100078390, -7.208316651077763204 ) ) ;
#4970=CARTESIAN_POINT ( 'NONE',  ( 3.591859063236761518, 14.95696800326375531, 11.09922568453594849 ) ) ;
#4971=CARTESIAN_POINT ( 'NONE',  ( 2.035157376598824452, 58.68868534415482685, 7.964842623401179544 ) ) ;
#4972=CARTESIAN_POINT ( 'NONE',  ( 12.91533473730993009, 16.60535201082150891, -10.88017736071109987 ) ) ;
#4973=CARTESIAN_POINT ( 'NONE',  ( 6.565887622018943937, 55.16530133659709634, 12.81628187352647430 ) ) ;
#4974=CARTESIAN_POINT ( 'NONE',  ( 24.16423886937410614, 49.30374883491396787, 8.672049930838204340E-16 ) ) ;
#4975=EDGE_CURVE ( 'NONE', #65472, #96338, #92100, .T. ) ;
#4977=CARTESIAN_POINT ( 'NONE',  ( -42.83369174045569849, 106.9566484930309684, 5.017862233661315230 ) ) ;
#4978=VERTEX_POINT ( 'NONE', #79774 ) ;
#4979=CARTESIAN_POINT ( 'NONE',  ( -2.816281873526473856, -0.8763653300695799508, 9.499525473075851096E-16 ) ) ;
#4980=CARTESIAN_POINT ( 'NONE',  ( 19.05866839779139355, 20.95508385108958649, -6.499999999999974243 ) ) ;
#4981=CARTESIAN_POINT ( 'NONE',  ( 10.00000000000000178, 29.31368534415483751, 10.88017736071110342 ) ) ;
#4982=CARTESIAN_POINT ( 'NONE',  ( 19.84674366389459266, 63.30059781766745886, 2.638427012816836559 ) ) ;
#4984=CARTESIAN_POINT ( 'NONE',  ( 19.84674366389459621, 13.50893115100078568, 7.409399052514197653E-17 ) ) ;
#4985=CARTESIAN_POINT ( 'NONE',  ( 10.00000000000000000, 14.75893115100078568, -9.846743663894594434 ) ) ;
#4986=CARTESIAN_POINT ( 'NONE',  ( 19.84674366389459266, 28.30059781766745886, 2.638427012816836559 ) ) ;
#4987=CARTESIAN_POINT ( 'NONE',  ( 5.076628168052704559, 5.175597817667451750, -8.527530157486179263 ) ) ;
#4988=CARTESIAN_POINT ( 'NONE',  ( 19.84674366389459266, 3.717264484334118713, -2.638427012816827677 ) ) ;
#4990=CARTESIAN_POINT ( 'NONE',  ( 17.20831665107776587, 4.133931151000785675, -7.208316651077762316 ) ) ;
#4992=CARTESIAN_POINT ( 'NONE',  ( 18.52753015748617571, 8.092264484334117824, 4.923371831947298993 ) ) ;
#4993=CARTESIAN_POINT ( 'NONE',  ( 19.84674366389459266, 23.71726448433412315, -2.638427012816827677 ) ) ;
#4996=EDGE_CURVE ( 'NONE', #91846, #36347, #58603, .T. ) ;
#4997=CARTESIAN_POINT ( 'NONE',  ( 10.00000000000000178, 62.25893115100078745, 9.846743663894594434 ) ) ;
#4999=CARTESIAN_POINT ( 'NONE',  ( 17.96484262340118221, 6.188685344154836621, -7.964842623401177768 ) ) ;
#5000=CARTESIAN_POINT ( 'NONE',  ( 2.917880565312948704, 22.63708216824730002, 12.26659068614894643 ) ) ;
#5003=CARTESIAN_POINT ( 'NONE',  ( 13.79529636645031943, 15.34541550158063750, -14.16423886937409904 ) ) ;
#5004=CARTESIAN_POINT ( 'NONE',  ( 2.917880565312950480, 45.97041550158063927, -12.26659068614894821 ) ) ;
#5005=FILL_AREA_STYLE_COLOUR ( '', #71005 ) ;
#5006=CARTESIAN_POINT ( 'NONE',  ( 22.26659068614894466, 18.88708216824730002, 7.082119434687054849 ) ) ;
#5007=CARTESIAN_POINT ( 'NONE',  ( -0.8801773607111009756, 33.06368534415484106, 1.068504757029289695E-15 ) ) ;
#5009=CARTESIAN_POINT ( 'NONE',  ( 10.00000000000000178, 22.25893115100078745, 9.846743663894594434 ) ) ;
#5010=CARTESIAN_POINT ( 'NONE',  ( 0.5774900079438590739, 52.64701867748817676, -5.440088680355550821 ) ) ;
#5011=CARTESIAN_POINT ( 'NONE',  ( 18.52753015748617571, 23.09226448433411960, 4.923371831947298993 ) ) ;
#5013=CARTESIAN_POINT ( 'NONE',  ( -0.8801773607110991993, 12.85535201082150358, -2.915334737309923874 ) ) ;
#5014=CARTESIAN_POINT ( 'NONE',  ( 3.591859063236763294, 48.29030133659708923, -11.09922568453595026 ) ) ;
#5015=CARTESIAN_POINT ( 'NONE',  ( 14.92337183194729633, 47.67559781766745175, 8.527530157486181039 ) ) ;
#5017=CARTESIAN_POINT ( 'NONE',  ( -2.816281873526471635, 48.91530133659708213, -3.434112377981056508 ) ) ;
#5019=CARTESIAN_POINT ( 'NONE',  ( 10.00000000000000000, 34.75893115100078745, -9.846743663894594434 ) ) ;
#5020=CARTESIAN_POINT ( 'NONE',  ( 24.16423886937410614, 24.30374883491396787, 8.672049930838204340E-16 ) ) ;
#5023=CARTESIAN_POINT ( 'NONE',  ( 20.88017736071110875, 55.77201867748816966, -2.915334737309920765 ) ) ;
#5024=CARTESIAN_POINT ( 'NONE',  ( 0.5774900079438590739, 62.64701867748817676, -5.440088680355550821 ) ) ;
#5025=CARTESIAN_POINT ( 'NONE',  ( -4.164238869374099039, 41.80374883491397497, 8.674139862899312516E-16 ) ) ;
#5026=CARTESIAN_POINT ( 'NONE',  ( 2.791683348922240793, 66.63393115100079456, 7.208316651077764092 ) ) ;
#5027=CARTESIAN_POINT ( 'NONE',  ( -0.04068437667222699061, 57.21974360917722180, -6.396802510829763477 ) ) ;
#5028=CARTESIAN_POINT ( 'NONE',  ( 20.88017736071110519, 35.56368534415484106, 2.639326808657452039E-16 ) ) ;
#5030=CARTESIAN_POINT ( 'NONE',  ( 13.43411237798106583, 27.66530133659708568, -12.81628187352647252 ) ) ;
#5031=CARTESIAN_POINT ( 'NONE',  ( 2.791683348922237240, 55.38393115100078745, -7.208316651077763204 ) ) ;
#5034=CARTESIAN_POINT ( 'NONE',  ( 4.559911319644449179, 13.89701867748817321, 9.422509992056141925 ) ) ;
#5039=CARTESIAN_POINT ( 'NONE',  ( 10.00000000000000000, 6.813685344154838397, -10.88017736071110342 ) ) ;
#5040=PLANE ( 'NONE',  #44846 ) ;
#5041=CARTESIAN_POINT ( 'NONE',  ( 12.91533473730993009, 66.60535201082150536, -10.88017736071109987 ) ) ;
#5043=CARTESIAN_POINT ( 'NONE',  ( 20.88017736071110519, 65.56368534415483396, 2.639326808657452039E-16 ) ) ;
#5045=CARTESIAN_POINT ( 'NONE',  ( 5.076628168052703671, 31.84226448433412315, 8.527530157486179263 ) ) ;
#5046=CARTESIAN_POINT ( 'NONE',  ( 20.88017736071110519, 25.56368534415483751, 2.639326808657452039E-16 ) ) ;
#5047=CARTESIAN_POINT ( 'NONE',  ( 13.43411237798106583, 12.66530133659708746, -12.81628187352647252 ) ) ;
#5048=CARTESIAN_POINT ( 'NONE',  ( 12.91533473730992121, 29.52201867748817321, 10.88017736071110164 ) ) ;
#5051=CARTESIAN_POINT ( 'NONE',  ( -2.816281873526471635, 33.91530133659708213, -3.434112377981056508 ) ) ;
#5053=CARTESIAN_POINT ( 'NONE',  ( 2.035157376598824452, 63.68868534415484106, 7.964842623401179544 ) ) ;
#5054=CARTESIAN_POINT ( 'NONE',  ( -1.099225684535947600, 24.54030133659708923, 6.408140936763237150 ) ) ;
#5055=FILL_AREA_STYLE ('',( #42553 ) ) ;
#5056=CARTESIAN_POINT ( 'NONE',  ( 7.084665262690076126, 44.10535201082151247, 10.88017736071109987 ) ) ;
#5057=CARTESIAN_POINT ( 'NONE',  ( 0.1957200283969144639, 15.25733960839543890, 6.500000000000003553 ) ) ;
#5058=CARTESIAN_POINT ( 'NONE',  ( -4.164238869374098151, 66.59541550158060375, -3.795296366450310543 ) ) ;
#5059=CARTESIAN_POINT ( 'NONE',  ( 17.20831665107776587, 54.13393115100079456, -7.208316651077762316 ) ) ;
#5060=CARTESIAN_POINT ( 'NONE',  ( 7.084665262690076126, 67.02201867748817676, -10.88017736071110164 ) ) ;
#5061=CARTESIAN_POINT ( 'NONE',  ( 2.035157376598822676, 67.43868534415484817, -7.964842623401177768 ) ) ;
#5063=CARTESIAN_POINT ( 'NONE',  ( 20.36894250292379738, 24.92874883491396787, -10.36894250292379027 ) ) ;
#5068=CARTESIAN_POINT ( 'NONE',  ( 22.26659068614894466, 63.88708216824730357, 7.082119434687054849 ) ) ;
#5069=CARTESIAN_POINT ( 'NONE',  ( 10.00000000000000000, 55.55374883491396787, -14.16423886937410082 ) ) ;
#5070=CARTESIAN_POINT ( 'NONE',  ( 7.361572987183169658, 24.96726448433412315, -9.846743663894592657 ) ) ;
#5071=CARTESIAN_POINT ( 'NONE',  ( 10.00000000000000000, 22.87363466993042138, -12.81628187352647608 ) ) ;
#5074=CARTESIAN_POINT ( 'NONE',  ( 0.5774900079438607392, 3.480352010821504027, 5.440088680355550821 ) ) ;
#5075=CARTESIAN_POINT ( 'NONE',  ( -4.164238869374099039, 61.80374883491397497, 8.674139862899312516E-16 ) ) ;
#5077=CARTESIAN_POINT ( 'NONE',  ( 0.1532563361054083140, 6.008931151000784787, 1.131784320476157264E-15 ) ) ;
#5084=CARTESIAN_POINT ( 'NONE',  ( 22.26659068614894466, 13.88708216824730179, 7.082119434687054849 ) ) ;
#5085=CARTESIAN_POINT ( 'NONE',  ( -0.8801773607111009756, 23.06368534415484106, 1.068504757029289695E-15 ) ) ;
#5086=CARTESIAN_POINT ( 'NONE',  ( 0.5774900079438590739, 22.64701867748817321, -5.440088680355550821 ) ) ;
#5087=CARTESIAN_POINT ( 'NONE',  ( 7.361572987183169658, 49.96726448433410894, -9.846743663894592657 ) ) ;
#5088=CARTESIAN_POINT ( 'NONE',  ( -1.099225684535947600, 19.54030133659708568, 6.408140936763237150 ) ) ;
#5090=MECHANICAL_DESIGN_GEOMETRIC_PRESENTATION_REPRESENTATION('',(#9945),#64154);
#5091=CARTESIAN_POINT ( 'NONE',  ( -2.816281873526473856, 34.12363466993042493, 9.499525473075851096E-16 ) ) ;
#5093=CARTESIAN_POINT ( 'NONE',  ( 19.84674366389459266, 33.30059781766744464, 2.638427012816836559 ) ) ;
#5094=CARTESIAN_POINT ( 'NONE',  ( 20.36894250292379382, 58.67874883491396076, 10.36894250292379205 ) ) ;
#5096=CARTESIAN_POINT ( 'NONE',  ( 7.084665262690076126, 7.022018677488170546, -10.88017736071110164 ) ) ;
#5097=ORIENTED_EDGE ( 'NONE', *, *, #26477, .F. ) ;
#5098=CARTESIAN_POINT ( 'NONE',  ( -0.8801773607110991993, 42.85535201082150536, -2.915334737309923874 ) ) ;
#5099=CARTESIAN_POINT ( 'NONE',  ( 19.42250999205614193, 45.14701867748817676, 5.440088680355555262 ) ) ;
#5100=CARTESIAN_POINT ( 'NONE',  ( 0.5774900079438590739, 52.64701867748817676, -5.440088680355550821 ) ) ;
#5101=CARTESIAN_POINT ( 'NONE',  ( 20.88017736071110164, 40.35535201082150536, 2.915334737309930979 ) ) ;
#5102=CARTESIAN_POINT ( 'NONE',  ( 20.15039907845753220, 64.72266099184918176, 6.262539305110077947 ) ) ;
#5104=AXIS2_PLACEMENT_3D ( 'NONE', #58198, #88713, #20223 ) ;
#5105=VERTEX_POINT ( 'NONE', #73740 ) ;
#5107=EDGE_CURVE ( 'NONE', #27101, #17129, #42763, .T. ) ;
#5108=CARTESIAN_POINT ( 'NONE',  ( 1.472469842513823179, 25.59226448433412315, -4.923371831947296329 ) ) ;
#5110=CARTESIAN_POINT ( 'NONE',  ( 7.361572987183170547, 62.05059781766745886, 9.846743663894590881 ) ) ;
#5111=FACE_OUTER_BOUND ( 'NONE', #56104, .T. ) ;
#5112=AXIS2_PLACEMENT_3D ( 'NONE', #92284, #31765, #46290 ) ;
#5113=EDGE_CURVE ( 'NONE', #46963, #88123, #79864, .T. ) ;
#5118=DIRECTION ( 'NONE',  ( -0.000000000000000000, -0.000000000000000000, 1.000000000000000000 ) ) ;
#5119=CARTESIAN_POINT ( 'NONE',  ( 18.72515096720571037, 45.05509018479935435, 6.499999999999982236 ) ) ;
#5121=CARTESIAN_POINT ( 'NONE',  ( 22.26659068614895176, 54.72041550158063217, -7.082119434687042414 ) ) ;
#5122=CARTESIAN_POINT ( 'NONE',  ( 18.61655166652077398, 64.87718327197430312, 6.499999999999981348 ) ) ;
#5125=CARTESIAN_POINT ( 'NONE',  ( 0.1532563361054100626, 35.80059781766745175, -2.638427012816831230 ) ) ;
#5126=DIRECTION ( 'NONE',  ( 0.000000000000000000, 0.000000000000000000, -1.000000000000000000 ) ) ;
#5127=CARTESIAN_POINT ( 'NONE',  ( 6.565887622018943937, 8.081968003263751754, -12.81628187352647608 ) ) ;
#5128=CARTESIAN_POINT ( 'NONE',  ( 14.92337183194729988, 14.34226448433411782, -8.527530157486177487 ) ) ;
#5130=CARTESIAN_POINT ( 'NONE',  ( 5.076628168052704559, 5.175597817667451750, -8.527530157486179263 ) ) ;
#5131=CARTESIAN_POINT ( 'NONE',  ( -2.816281873526471635, -1.084698663402913210, -3.434112377981056508 ) ) ;
#5132=DIRECTION ( 'NONE',  ( -1.000000000000000000, 0.000000000000000000, 0.000000000000000000 ) ) ;
#5134=CARTESIAN_POINT ( 'NONE',  ( 2.035157376598824452, 3.688685344154837953, 7.964842623401179544 ) ) ;
#5135=CARTESIAN_POINT ( 'NONE',  ( 24.16423886937409904, 4.095415501580634832, 3.795296366450317205 ) ) ;
#5136=CARTESIAN_POINT ( 'NONE',  ( 5.076628168052704559, 25.17559781766745175, -8.527530157486179263 ) ) ;
#5137=CARTESIAN_POINT ( 'NONE',  ( 7.084665262690076126, 49.10535201082149825, 10.88017736071109987 ) ) ;
#5138=CARTESIAN_POINT ( 'NONE',  ( 21.09922568453594849, 21.20696800326375353, 6.408140936763242479 ) ) ;
#5140=CARTESIAN_POINT ( 'NONE',  ( 0.5774900079438590739, 2.647018677488170990, -5.440088680355550821 ) ) ;
#5143=CARTESIAN_POINT ( 'NONE',  ( 3.591859063236763294, 3.290301336597087012, -11.09922568453595026 ) ) ;
#5144=CARTESIAN_POINT ( 'NONE',  ( 16.40814093676323893, 0.7903013365970867898, 11.09922568453595026 ) ) ;
#5145=CARTESIAN_POINT ( 'NONE',  ( 19.84674366389459266, 13.71726448433411782, -2.638427012816827677 ) ) ;
#5147=CARTESIAN_POINT ( 'NONE',  ( 22.81628187352648496, 21.83196800326374643, -3.434112377981050290 ) ) ;
#5149=CARTESIAN_POINT ( 'NONE',  ( 4.559911319644449179, 23.89701867748817321, 9.422509992056141925 ) ) ;
#5153=CARTESIAN_POINT ( 'NONE',  ( 20.36894250292379738, 49.92874883491396787, -10.36894250292379027 ) ) ;
#5155=DIRECTION ( 'NONE',  ( 0.000000000000000000, -1.000000000000000000, 0.000000000000000000 ) ) ;
#5156=CARTESIAN_POINT ( 'NONE',  ( 19.42250999205614548, 30.98035201082150536, -5.440088680355545492 ) ) ;
#5157=AXIS2_PLACEMENT_3D ( 'NONE', #29918, #67941, #91914 ) ;
#5158=CARTESIAN_POINT ( 'NONE',  ( 2.791683348922240793, 46.63393115100077324, 7.208316651077764092 ) ) ;
#5159=CARTESIAN_POINT ( 'NONE',  ( 20.88017736071110875, 50.77201867748817676, -2.915334737309920765 ) ) ;
#5160=CARTESIAN_POINT ( 'NONE',  ( -4.164238869374098151, 36.59541550158063217, -3.795296366450310543 ) ) ;
#5162=UNCERTAINTY_MEASURE_WITH_UNIT (LENGTH_MEASURE( 1.000000000000000082E-05 ), #13393, 'distance_accuracy_value', 'NONE');
#5163=CARTESIAN_POINT ( 'NONE',  ( 1.472469842513823179, 41.42559781766745886, 4.923371831947296329 ) ) ;
#5164=CARTESIAN_POINT ( 'NONE',  ( 3.591859063236763294, 63.29030133659708923, -11.09922568453595026 ) ) ;
#5165=CARTESIAN_POINT ( 'NONE',  ( -1.099225684535947600, -0.4596986634029132657, 6.408140936763237150 ) ) ;
#5167=CARTESIAN_POINT ( 'NONE',  ( 7.084665262690076126, 19.10535201082150181, 10.88017736071109987 ) ) ;
#5169=CARTESIAN_POINT ( 'NONE',  ( 20.15039907845753930, 70.00000000000000000, 6.262539305110068177 ) ) ;
#5170=CARTESIAN_POINT ( 'NONE',  ( -0.8801773607111009756, 3.063685344154837509, 1.068504757029289695E-15 ) ) ;
#5171=CARTESIAN_POINT ( 'NONE',  ( -0.8801773607111009756, 13.06368534415483929, 1.068504757029289695E-15 ) ) ;
#5172=CARTESIAN_POINT ( 'NONE',  ( 0.1532563361054100626, 5.800597817667452638, -2.638427012816831230 ) ) ;
#5173=CARTESIAN_POINT ( 'NONE',  ( 10.00000000000000178, 18.05374883491396787, 14.16423886937410082 ) ) ;
#5174=CARTESIAN_POINT ( 'NONE',  ( 14.92337183194729988, 19.34226448433411960, -8.527530157486177487 ) ) ;
#5175=CARTESIAN_POINT ( 'NONE',  ( 14.92337183194729633, 62.67559781766745886, 8.527530157486181039 ) ) ;
#5176=CARTESIAN_POINT ( 'NONE',  ( 19.42250999205614548, 35.98035201082151247, -5.440088680355545492 ) ) ;
#5177=( BOUNDED_SURFACE ( )  B_SPLINE_SURFACE ( 1, 2, ( 
 ( #33333, #63827, #94341, #56833, #75781, #37803, #5814, #66803, #29776, #60286, #51308, #67802, #50819, #81312, #96832, #37313, #97324, #7304, #83290, #36307, #28794, #51804, #88811, #52295, #6799, #52781, #89309, #59296, #14815, #90783, #20817, #29289, #82288, #66298, #89793, #68300, #98819, #21311, #13808, #22309, #45286, #81790, #98322, #12807, #43307, #28309, #58295, #44292, #20323, #73800, #74796, #6304, #36806, #67300, #5330, #82791, #97827, #14313, #35811, #75289, #58801, #59786, #90279, #21811, #13307, #43793, #44783, #74287, #54258, #47245, #8764, #15791, #32240, #55243, #22798, #1299, #84769, #69280, #62247, #16278, #24278, #77255, #9754, #53276, #76764, #16770, #61751, #83783, #23298, #85757, #31752, #802, #15306, #320, #30762, #17268, #45791, #91276, #62739, #47743, #38293, #7797, #92269, #46760, #77746, #68788, #39281, #23793, #92753, #46279, #61268, #93239, #54742, #24765, #78240, #40256, #69769, #9259, #70763, #70266, #91776, #85263, #53776, #76282, #84292, #8284, #39766, #38781, #1782, #30272, #60774, #31255, #71731, #33225, #32733, #93736, #63720, #41256, #2771, #33707, #80704, #71248, #26229, #3241, #65190, #94223, #56722, #34697, #40744, #79721, #95203, #4227, #19706, #50193, #64207, #87700, #12199, #42224, #25753, #11221, #56247, #55753, #48234, #86740, #19216, #86244, #94722, #41740, #72211, #72690, #87214, #18242, #63233, #25270, #48723, #18737, #79227, #49217, #42708, #10737, #3739, #34199, #95712, #64692, #26708, #27195, #57203, #49697, #17757, #80206, #11712, #57697, #88197, #2277, #78743, #10251, #35694, #44170, #97212, #81193, #81673, #90660, #52667, #20699, #13188, #44674, #75168, #66178, #82674, #65687, #96211, #12694, #52180, #43680, #22186, #98198, #51191, #74167, #66687, #51692, #21694, #97705, #5701, #29171, #60164, #90164, #83169, #82171, #36187, #89679, #14190, #96712, #28680, #59174, #21192, #6678, #13684, #58685, #37198, #29655, #27693, #74678, #6190, #36694, #67182, #59672, #67689, #14694, #73186, #58177, #4722, #35185, #88689, #20197, #28190, #50699, #43190, #73678, #5210, #89186, #45665, #1667, #98700, #7179, #47123, #32116, #53162, #22681, #8167, #69163, #62123, #83667, #687, #38658, #77139, #30641, #15185, #77623, #62614, #31138, #24154, #39654, #37682, #93121, #9138, #53654, #61631, #46163, #92150, #24648, #91659, #194, #70146, #55117, #76162, #23675, #15678, #85635, #45164, #7684, #54622, #30149, #38177, #68667, #61150, #75668, #54137, #84650, #76646, #84173, #68181, #16153, #23177, #46637, #60658, #91157, #8648, #39158, #85143, #69648, #1172, #31632, #92631, #16651, #87100 ),
 ( #41133, #49580, #55631, #94602, #47632, #11109, #64577, #11595, #48112, #94109, #72576, #19099, #78626, #18614, #71621, #25154, #25637, #34573, #95595, #63604, #56127, #87587, #80090, #10137, #26591, #9638, #40136, #86131, #95086, #86622, #65069, #42114, #18133, #48605, #10621, #26119, #57093, #41628, #79109, #72093, #4109, #34086, #27080, #56611, #3132, #33592, #57581, #40632, #64087, #49103, #79606, #17153, #3617, #2657, #78128, #70636, #2164, #32619, #63117, #93619, #17644, #71130, #33109, #36069, #67570, #80591, #35575, #74560, #20585, #42591, #81077, #13069, #6076, #27575, #43561, #51070, #21076, #73564, #58070, #90055, #82060, #21578, #6562, #37072, #81562, #36577, #98082, #29051, #20077, #66570, #50582, #73071, #35068, #12580, #67065, #4607, #74059, #97099, #28570, #59558, #58566, #43078, #19589, #12086, #5088, #28069, #88573, #5592, #29541, #66066, #59063, #89071, #52066, #96594, #89567, #82561, #51574, #13568, #50087, #44055, #97591, #14077, #44557, #75053, #88077, #65567, #96093, #31024, #84044, #68059, #68553, #77505, #39536, #7575, #85, #31516, #62015, #53037, #69535, #52551, #83055, #98589, #39041, #30532, #9019, #85025, #38061, #61033, #53531, #38550, #8540, #84540, #91545, #16037, #47015, #77026, #70028, #69045, #23062, #76535, #1048, #22568, #15565, #46049, #8050, #92515, #579, #45545, #24040, #16538, #14576, #61520, #92030, #23560, #54028, #46526, #54512, #1552, #60046, #45043, #90544, #22076, #75552, #7068, #83553, #37568, #30038, #60546, #91039, #15076, #76042, #87475, #85520, #93007, #33960, #18990, #40017, #9517, #93999, #49467, #79973, #63497, #18494, #11479, #71978, #63003, #10498, #93505, #17030, #78010, #25030, #48982, #47509, #25523, #41011, #71511, #3503, #2539, #55517, #62504, #24541, #86016, #71017, #32505, #56009, #41996, #2044, #86513, #32994, #94972, #17529, #18010, #64465, #70521, #3025, #55002, #26000, #79491, #26474, #47996, #10019, #72460, #56972, #78506, #33473, #48490, #40520, #78993, #31998, #63970, #94482, #56495, #86985, #10991, #41512, #13446, #95478, #26966, #42473, #81936, #12461, #21451, #28928, #80961, #73447, #96476, #81448, #51450, #28450, #42966, #58947, #89934, #20962, #82433, #12949, #4973, #20464, #43933, #65451, #35453, #65949, #27949, #74430, #43444, #88459, #5958, #59432, #57467, #73945, #58441, #88955, #35946, #50953, #96976, #5474, #13958, #87960, #50455, #89449, #66442, #19476, #95976, #51948, #36451, #66943, #49966, #72957, #4486, #44432, #80472, #64950, #97463, #3994, #11970, #34953, #34459, #27459, #57952, #19960, #75921, #83429, #22942, #67939, #82932, #30904 ) ),
 .UNSPECIFIED., .F., .F., .F. ) 
 B_SPLINE_SURFACE_WITH_KNOTS ( ( 2, 2 ),
 ( 3, 2, 2, 2, 2, 2, 2, 2, 2, 2, 2, 2, 2, 2, 2, 2, 2, 2, 2, 2, 2, 2, 2, 2, 2, 2, 2, 2, 2, 2, 2, 2, 2, 2, 2, 2, 2, 2, 2, 2, 2, 2, 2, 2, 2, 2, 2, 2, 2, 2, 2, 2, 2, 2, 2, 2, 2, 2, 2, 2, 2, 2, 2, 2, 2, 2, 2, 2, 2, 2, 2, 2, 2, 2, 2, 2, 2, 2, 2, 2, 2, 2, 2, 2, 2, 2, 2, 2, 2, 2, 2, 2, 2, 2, 2, 2, 2, 2, 2, 2, 2, 2, 2, 2, 2, 2, 2, 2, 2, 2, 2, 2, 2, 2, 2, 2, 2, 2, 2, 2, 2, 2, 2, 2, 2, 2, 2, 2, 2, 2, 2, 2, 2, 2, 2, 2, 2, 2, 2, 2, 2, 2, 2, 2, 2, 2, 2, 2, 2, 2, 2, 2, 2, 2, 2, 2, 2, 2, 2, 2, 2, 2, 3 ),
 ( 0.000000000000000000, 1.000000000000000000 ),
 ( 0.000000000000000000, 0.005952380952380952051, 0.01190476190476190410, 0.01785714285714285615, 0.02380952380952380820, 0.02976190476190476025, 0.03571428571428571230, 0.04166666666666666435, 0.04761904761904761640, 0.05357142857142856845, 0.05952380952380952051, 0.06547619047619047949, 0.07142857142857142461, 0.07738095238095238360, 0.08333333333333332871, 0.08928571428571428770, 0.09523809523809523281, 0.1011904761904761918, 0.1071428571428571369, 0.1130952380952380959, 0.1190476190476190410, 0.1250000000000000000, 0.1309523809523809590, 0.1369047619047619180, 0.1428571428571428492, 0.1488095238095238082, 0.1547619047619047672, 0.1607142857142857262, 0.1666666666666666574, 0.1726190476190476164, 0.1785714285714285754, 0.1845238095238095344, 0.1904761904761904656, 0.1964285714285714246, 0.2023809523809523836, 0.2083333333333333426, 0.2142857142857142738, 0.2202380952380952328, 0.2261904761904761918, 0.2321428571428571508, 0.2380952380952380820, 0.2440476190476190410, 0.2500000000000000000, 0.2559523809523809312, 0.2619047619047619180, 0.2678571428571428492, 0.2738095238095238360, 0.2797619047619047672, 0.2857142857142856984, 0.2916666666666666852, 0.2976190476190476164, 0.3035714285714285476, 0.3095238095238095344, 0.3154761904761904656, 0.3214285714285714524, 0.3273809523809523836, 0.3333333333333333148, 0.3392857142857143016, 0.3452380952380952328, 0.3511904761904761640, 0.3571428571428571508, 0.3630952380952380820, 0.3690476190476190688, 0.3750000000000000000, 0.3809523809523809312, 0.3869047619047619180, 0.3928571428571428492, 0.3988095238095238360, 0.4047619047619047672, 0.4107142857142856984, 0.4166666666666666852, 0.4226190476190476164, 0.4285714285714285476, 0.4345238095238095344, 0.4404761904761904656, 0.4464285714285714524, 0.4523809523809523836, 0.4583333333333333148, 0.4642857142857143016, 0.4702380952380952328, 0.4761904761904761640, 0.4821428571428571508, 0.4880952380952380820, 0.4940476190476190688, 0.5000000000000000000, 0.5059523809523809312, 0.5119047619047618625, 0.5178571428571429047, 0.5238095238095238360, 0.5297619047619047672, 0.5357142857142856984, 0.5416666666666666297, 0.5476190476190476719, 0.5535714285714286031, 0.5595238095238095344, 0.5654761904761904656, 0.5714285714285713969, 0.5773809523809523281, 0.5833333333333333703, 0.5892857142857143016, 0.5952380952380952328, 0.6011904761904761640, 0.6071428571428570953, 0.6130952380952381375, 0.6190476190476190688, 0.6250000000000000000, 0.6309523809523809312, 0.6369047619047618625, 0.6428571428571429047, 0.6488095238095238360, 0.6547619047619047672, 0.6607142857142856984, 0.6666666666666666297, 0.6726190476190476719, 0.6785714285714286031, 0.6845238095238095344, 0.6904761904761904656, 0.6964285714285713969, 0.7023809523809523281, 0.7083333333333333703, 0.7142857142857143016, 0.7202380952380952328, 0.7261904761904761640, 0.7321428571428570953, 0.7380952380952381375, 0.7440476190476190688, 0.7500000000000000000, 0.7559523809523809312, 0.7619047619047618625, 0.7678571428571429047, 0.7738095238095238360, 0.7797619047619047672, 0.7857142857142856984, 0.7916666666666666297, 0.7976190476190476719, 0.8035714285714286031, 0.8095238095238095344, 0.8154761904761904656, 0.8214285714285713969, 0.8273809523809523281, 0.8333333333333333703, 0.8392857142857143016, 0.8452380952380952328, 0.8511904761904761640, 0.8571428571428570953, 0.8630952380952381375, 0.8690476190476190688, 0.8750000000000000000, 0.8809523809523809312, 0.8869047619047618625, 0.8928571428571429047, 0.8988095238095238360, 0.9047619047619047672, 0.9107142857142856984, 0.9166666666666666297, 0.9226190476190476719, 0.9285714285714286031, 0.9345238095238095344, 0.9404761904761904656, 0.9464285714285713969, 0.9523809523809523281, 0.9583333333333333703, 0.9642857142857143016 ),
 .UNSPECIFIED. ) 
 GEOMETRIC_REPRESENTATION_ITEM ( )  RATIONAL_B_SPLINE_SURFACE ( (
 ( 1.000000000000000000, 0.9659258262890683122, 1.000000000000000000, 0.9659258262890683122, 1.000000000000000000, 0.9659258262890683122, 1.000000000000000000, 0.9659258262890683122, 1.000000000000000000, 0.9659258262890683122, 1.000000000000000000, 0.9659258262890683122, 1.000000000000000000, 0.9659258262890683122, 1.000000000000000000, 0.9659258262890683122, 1.000000000000000000, 0.9659258262890683122, 1.000000000000000000, 0.9659258262890683122, 1.000000000000000000, 0.9659258262890683122, 1.000000000000000000, 0.9659258262890683122, 1.000000000000000000, 0.9659258262890683122, 1.000000000000000000, 0.9659258262890683122, 1.000000000000000000, 0.9659258262890683122, 1.000000000000000000, 0.9659258262890683122, 1.000000000000000000, 0.9659258262890683122, 1.000000000000000000, 0.9659258262890683122, 1.000000000000000000, 0.9659258262890683122, 1.000000000000000000, 0.9659258262890683122, 1.000000000000000000, 0.9659258262890683122, 1.000000000000000000, 0.9659258262890683122, 1.000000000000000000, 0.9659258262890683122, 1.000000000000000000, 0.9659258262890683122, 1.000000000000000000, 0.9659258262890683122, 1.000000000000000000, 0.9659258262890683122, 1.000000000000000000, 0.9659258262890683122, 1.000000000000000000, 0.9659258262890683122, 1.000000000000000000, 0.9659258262890683122, 1.000000000000000000, 0.9659258262890683122, 1.000000000000000000, 0.9659258262890683122, 1.000000000000000000, 0.9659258262890683122, 1.000000000000000000, 0.9659258262890683122, 1.000000000000000000, 0.9659258262890683122, 1.000000000000000000, 0.9659258262890683122, 1.000000000000000000, 0.9659258262890683122, 1.000000000000000000, 0.9659258262890683122, 1.000000000000000000, 0.9659258262890683122, 1.000000000000000000, 0.9659258262890683122, 1.000000000000000000, 0.9659258262890683122, 1.000000000000000000, 0.9659258262890683122, 1.000000000000000000, 0.9659258262890683122, 1.000000000000000000, 0.9659258262890683122, 1.000000000000000000, 0.9659258262890683122, 1.000000000000000000, 0.9659258262890683122, 1.000000000000000000, 0.9659258262890683122, 1.000000000000000000, 0.9659258262890683122, 1.000000000000000000, 0.9659258262890683122, 1.000000000000000000, 0.9659258262890683122, 1.000000000000000000, 0.9659258262890683122, 1.000000000000000000, 0.9659258262890683122, 1.000000000000000000, 0.9659258262890683122, 1.000000000000000000, 0.9659258262890683122, 1.000000000000000000, 0.9659258262890683122, 1.000000000000000000, 0.9659258262890683122, 1.000000000000000000, 0.9659258262890683122, 1.000000000000000000, 0.9659258262890683122, 1.000000000000000000, 0.9659258262890683122, 1.000000000000000000, 0.9659258262890683122, 1.000000000000000000, 0.9659258262890683122, 1.000000000000000000, 0.9659258262890683122, 1.000000000000000000, 0.9659258262890683122, 1.000000000000000000, 0.9659258262890683122, 1.000000000000000000, 0.9659258262890683122, 1.000000000000000000, 0.9659258262890683122, 1.000000000000000000, 0.9659258262890683122, 1.000000000000000000, 0.9659258262890683122, 1.000000000000000000, 0.9659258262890683122, 1.000000000000000000, 0.9659258262890683122, 1.000000000000000000, 0.9659258262890683122, 1.000000000000000000, 0.9659258262890683122, 1.000000000000000000, 0.9659258262890683122, 1.000000000000000000, 0.9659258262890683122, 1.000000000000000000, 0.9659258262890683122, 1.000000000000000000, 0.9659258262890683122, 1.000000000000000000, 0.9659258262890683122, 1.000000000000000000, 0.9659258262890683122, 1.000000000000000000, 0.9659258262890683122, 1.000000000000000000, 0.9659258262890683122, 1.000000000000000000, 0.9659258262890683122, 1.000000000000000000, 0.9659258262890683122, 1.000000000000000000, 0.9659258262890683122, 1.000000000000000000, 0.9659258262890683122, 1.000000000000000000, 0.9659258262890683122, 1.000000000000000000, 0.9659258262890683122, 1.000000000000000000, 0.9659258262890683122, 1.000000000000000000, 0.9659258262890683122, 1.000000000000000000, 0.9659258262890683122, 1.000000000000000000, 0.9659258262890683122, 1.000000000000000000, 0.9659258262890683122, 1.000000000000000000, 0.9659258262890683122, 1.000000000000000000, 0.9659258262890683122, 1.000000000000000000, 0.9659258262890683122, 1.000000000000000000, 0.9659258262890683122, 1.000000000000000000, 0.9659258262890683122, 1.000000000000000000, 0.9659258262890683122, 1.000000000000000000, 0.9659258262890683122, 1.000000000000000000, 0.9659258262890683122, 1.000000000000000000, 0.9659258262890683122, 1.000000000000000000, 0.9659258262890683122, 1.000000000000000000, 0.9659258262890683122, 1.000000000000000000, 0.9659258262890683122, 1.000000000000000000, 0.9659258262890683122, 1.000000000000000000, 0.9659258262890683122, 1.000000000000000000, 0.9659258262890683122, 1.000000000000000000, 0.9659258262890683122, 1.000000000000000000, 0.9659258262890683122, 1.000000000000000000, 0.9659258262890683122, 1.000000000000000000, 0.9659258262890683122, 1.000000000000000000, 0.9659258262890683122, 1.000000000000000000, 0.9659258262890683122, 1.000000000000000000, 0.9659258262890683122, 1.000000000000000000, 0.9659258262890683122, 1.000000000000000000, 0.9659258262890683122, 1.000000000000000000, 0.9659258262890683122, 1.000000000000000000, 0.9659258262890683122, 1.000000000000000000, 0.9659258262890683122, 1.000000000000000000, 0.9659258262890683122, 1.000000000000000000, 0.9659258262890683122, 1.000000000000000000, 0.9659258262890683122, 1.000000000000000000, 0.9659258262890683122, 1.000000000000000000, 0.9659258262890683122, 1.000000000000000000, 0.9659258262890683122, 1.000000000000000000, 0.9659258262890683122, 1.000000000000000000, 0.9659258262890683122, 1.000000000000000000, 0.9659258262890683122, 1.000000000000000000, 0.9659258262890683122, 1.000000000000000000, 0.9659258262890683122, 1.000000000000000000, 0.9659258262890683122, 1.000000000000000000, 0.9659258262890683122, 1.000000000000000000, 0.9659258262890683122, 1.000000000000000000, 0.9659258262890683122, 1.000000000000000000, 0.9659258262890683122, 1.000000000000000000, 0.9659258262890683122, 1.000000000000000000, 0.9659258262890683122, 1.000000000000000000, 0.9659258262890683122, 1.000000000000000000, 0.9659258262890683122, 1.000000000000000000, 0.9659258262890683122, 1.000000000000000000, 0.9659258262890683122, 1.000000000000000000, 0.9659258262890683122, 1.000000000000000000, 0.9659258262890683122, 1.000000000000000000, 0.9659258262890683122, 1.000000000000000000, 0.9659258262890683122, 1.000000000000000000, 0.9659258262890683122, 1.000000000000000000, 0.9659258262890683122, 1.000000000000000000, 0.9659258262890683122, 1.000000000000000000, 0.9659258262890683122, 1.000000000000000000, 0.9659258262890683122, 1.000000000000000000, 0.9659258262890683122, 1.000000000000000000, 0.9659258262890683122, 1.000000000000000000, 0.9659258262890683122, 1.000000000000000000, 0.9659258262890683122, 1.000000000000000000, 0.9659258262890683122, 1.000000000000000000, 0.9659258262890683122, 1.000000000000000000, 0.9659258262890683122, 1.000000000000000000, 0.9659258262890683122, 1.000000000000000000, 0.9659258262890683122, 1.000000000000000000, 0.9659258262890683122, 1.000000000000000000, 0.9659258262890683122, 1.000000000000000000, 0.9659258262890683122, 1.000000000000000000, 0.9659258262890683122, 1.000000000000000000, 0.9659258262890683122, 1.000000000000000000),
 ( 1.000000000000000000, 0.9659258262890683122, 1.000000000000000000, 0.9659258262890683122, 1.000000000000000000, 0.9659258262890683122, 1.000000000000000000, 0.9659258262890683122, 1.000000000000000000, 0.9659258262890683122, 1.000000000000000000, 0.9659258262890683122, 1.000000000000000000, 0.9659258262890683122, 1.000000000000000000, 0.9659258262890683122, 1.000000000000000000, 0.9659258262890683122, 1.000000000000000000, 0.9659258262890683122, 1.000000000000000000, 0.9659258262890683122, 1.000000000000000000, 0.9659258262890683122, 1.000000000000000000, 0.9659258262890683122, 1.000000000000000000, 0.9659258262890683122, 1.000000000000000000, 0.9659258262890683122, 1.000000000000000000, 0.9659258262890683122, 1.000000000000000000, 0.9659258262890683122, 1.000000000000000000, 0.9659258262890683122, 1.000000000000000000, 0.9659258262890683122, 1.000000000000000000, 0.9659258262890683122, 1.000000000000000000, 0.9659258262890683122, 1.000000000000000000, 0.9659258262890683122, 1.000000000000000000, 0.9659258262890683122, 1.000000000000000000, 0.9659258262890683122, 1.000000000000000000, 0.9659258262890683122, 1.000000000000000000, 0.9659258262890683122, 1.000000000000000000, 0.9659258262890683122, 1.000000000000000000, 0.9659258262890683122, 1.000000000000000000, 0.9659258262890683122, 1.000000000000000000, 0.9659258262890683122, 1.000000000000000000, 0.9659258262890683122, 1.000000000000000000, 0.9659258262890683122, 1.000000000000000000, 0.9659258262890683122, 1.000000000000000000, 0.9659258262890683122, 1.000000000000000000, 0.9659258262890683122, 1.000000000000000000, 0.9659258262890683122, 1.000000000000000000, 0.9659258262890683122, 1.000000000000000000, 0.9659258262890683122, 1.000000000000000000, 0.9659258262890683122, 1.000000000000000000, 0.9659258262890683122, 1.000000000000000000, 0.9659258262890683122, 1.000000000000000000, 0.9659258262890683122, 1.000000000000000000, 0.9659258262890683122, 1.000000000000000000, 0.9659258262890683122, 1.000000000000000000, 0.9659258262890683122, 1.000000000000000000, 0.9659258262890683122, 1.000000000000000000, 0.9659258262890683122, 1.000000000000000000, 0.9659258262890683122, 1.000000000000000000, 0.9659258262890683122, 1.000000000000000000, 0.9659258262890683122, 1.000000000000000000, 0.9659258262890683122, 1.000000000000000000, 0.9659258262890683122, 1.000000000000000000, 0.9659258262890683122, 1.000000000000000000, 0.9659258262890683122, 1.000000000000000000, 0.9659258262890683122, 1.000000000000000000, 0.9659258262890683122, 1.000000000000000000, 0.9659258262890683122, 1.000000000000000000, 0.9659258262890683122, 1.000000000000000000, 0.9659258262890683122, 1.000000000000000000, 0.9659258262890683122, 1.000000000000000000, 0.9659258262890683122, 1.000000000000000000, 0.9659258262890683122, 1.000000000000000000, 0.9659258262890683122, 1.000000000000000000, 0.9659258262890683122, 1.000000000000000000, 0.9659258262890683122, 1.000000000000000000, 0.9659258262890683122, 1.000000000000000000, 0.9659258262890683122, 1.000000000000000000, 0.9659258262890683122, 1.000000000000000000, 0.9659258262890683122, 1.000000000000000000, 0.9659258262890683122, 1.000000000000000000, 0.9659258262890683122, 1.000000000000000000, 0.9659258262890683122, 1.000000000000000000, 0.9659258262890683122, 1.000000000000000000, 0.9659258262890683122, 1.000000000000000000, 0.9659258262890683122, 1.000000000000000000, 0.9659258262890683122, 1.000000000000000000, 0.9659258262890683122, 1.000000000000000000, 0.9659258262890683122, 1.000000000000000000, 0.9659258262890683122, 1.000000000000000000, 0.9659258262890683122, 1.000000000000000000, 0.9659258262890683122, 1.000000000000000000, 0.9659258262890683122, 1.000000000000000000, 0.9659258262890683122, 1.000000000000000000, 0.9659258262890683122, 1.000000000000000000, 0.9659258262890683122, 1.000000000000000000, 0.9659258262890683122, 1.000000000000000000, 0.9659258262890683122, 1.000000000000000000, 0.9659258262890683122, 1.000000000000000000, 0.9659258262890683122, 1.000000000000000000, 0.9659258262890683122, 1.000000000000000000, 0.9659258262890683122, 1.000000000000000000, 0.9659258262890683122, 1.000000000000000000, 0.9659258262890683122, 1.000000000000000000, 0.9659258262890683122, 1.000000000000000000, 0.9659258262890683122, 1.000000000000000000, 0.9659258262890683122, 1.000000000000000000, 0.9659258262890683122, 1.000000000000000000, 0.9659258262890683122, 1.000000000000000000, 0.9659258262890683122, 1.000000000000000000, 0.9659258262890683122, 1.000000000000000000, 0.9659258262890683122, 1.000000000000000000, 0.9659258262890683122, 1.000000000000000000, 0.9659258262890683122, 1.000000000000000000, 0.9659258262890683122, 1.000000000000000000, 0.9659258262890683122, 1.000000000000000000, 0.9659258262890683122, 1.000000000000000000, 0.9659258262890683122, 1.000000000000000000, 0.9659258262890683122, 1.000000000000000000, 0.9659258262890683122, 1.000000000000000000, 0.9659258262890683122, 1.000000000000000000, 0.9659258262890683122, 1.000000000000000000, 0.9659258262890683122, 1.000000000000000000, 0.9659258262890683122, 1.000000000000000000, 0.9659258262890683122, 1.000000000000000000, 0.9659258262890683122, 1.000000000000000000, 0.9659258262890683122, 1.000000000000000000, 0.9659258262890683122, 1.000000000000000000, 0.9659258262890683122, 1.000000000000000000, 0.9659258262890683122, 1.000000000000000000, 0.9659258262890683122, 1.000000000000000000, 0.9659258262890683122, 1.000000000000000000, 0.9659258262890683122, 1.000000000000000000, 0.9659258262890683122, 1.000000000000000000, 0.9659258262890683122, 1.000000000000000000, 0.9659258262890683122, 1.000000000000000000, 0.9659258262890683122, 1.000000000000000000, 0.9659258262890683122, 1.000000000000000000, 0.9659258262890683122, 1.000000000000000000, 0.9659258262890683122, 1.000000000000000000, 0.9659258262890683122, 1.000000000000000000, 0.9659258262890683122, 1.000000000000000000, 0.9659258262890683122, 1.000000000000000000, 0.9659258262890683122, 1.000000000000000000, 0.9659258262890683122, 1.000000000000000000, 0.9659258262890683122, 1.000000000000000000, 0.9659258262890683122, 1.000000000000000000, 0.9659258262890683122, 1.000000000000000000, 0.9659258262890683122, 1.000000000000000000, 0.9659258262890683122, 1.000000000000000000, 0.9659258262890683122, 1.000000000000000000, 0.9659258262890683122, 1.000000000000000000, 0.9659258262890683122, 1.000000000000000000, 0.9659258262890683122, 1.000000000000000000, 0.9659258262890683122, 1.000000000000000000, 0.9659258262890683122, 1.000000000000000000, 0.9659258262890683122, 1.000000000000000000, 0.9659258262890683122, 1.000000000000000000, 0.9659258262890683122, 1.000000000000000000, 0.9659258262890683122, 1.000000000000000000, 0.9659258262890683122, 1.000000000000000000, 0.9659258262890683122, 1.000000000000000000, 0.9659258262890683122, 1.000000000000000000, 0.9659258262890683122, 1.000000000000000000, 0.9659258262890683122, 1.000000000000000000, 0.9659258262890683122, 1.000000000000000000, 0.9659258262890683122, 1.000000000000000000, 0.9659258262890683122, 1.000000000000000000, 0.9659258262890683122, 1.000000000000000000, 0.9659258262890683122, 1.000000000000000000, 0.9659258262890683122, 1.000000000000000000, 0.9659258262890683122, 1.000000000000000000, 0.9659258262890683122, 1.000000000000000000) ) ) 
 REPRESENTATION_ITEM ( '' )  SURFACE ( )  );
#5179=ORIENTED_EDGE ( 'NONE', *, *, #70842, .T. ) ;
#5182=CARTESIAN_POINT ( 'NONE',  ( 18.52753015748617571, 43.09226448433412315, 4.923371831947298993 ) ) ;
#5183=ORIENTED_EDGE ( 'NONE', *, *, #2414, .T. ) ;
#5186=CARTESIAN_POINT ( 'NONE',  ( 6.204703633549690345, 15.76208216824730179, -14.16423886937410259 ) ) ;
#5187=CARTESIAN_POINT ( 'NONE',  ( 6.204703633549690345, 12.84541550158063572, 14.16423886937410082 ) ) ;
#5188=CARTESIAN_POINT ( 'NONE',  ( 19.42250999205614193, 55.14701867748817676, 5.440088680355555262 ) ) ;
#5189=CARTESIAN_POINT ( 'NONE',  ( 20.36894250292379382, 53.67874883491397497, 10.36894250292379205 ) ) ;
#5190=CARTESIAN_POINT ( 'NONE',  ( 19.84674366389459621, 38.50893115100078745, 7.409399052514197653E-17 ) ) ;
#5192=CARTESIAN_POINT ( 'NONE',  ( 19.42250999205614193, 30.14701867748817321, 5.440088680355555262 ) ) ;
#5193=CARTESIAN_POINT ( 'NONE',  ( 22.81628187352647785, 1.623634669930420271, 6.195893100308588602E-16 ) ) ;
#5194=CARTESIAN_POINT ( 'NONE',  ( 24.16423886937409904, 9.095415501580633943, 3.795296366450317205 ) ) ;
#5195=CARTESIAN_POINT ( 'NONE',  ( 6.204703633549690345, 55.76208216824730357, -14.16423886937410259 ) ) ;
#5197=CARTESIAN_POINT ( 'NONE',  ( 12.91533473730993009, 21.60535201082150536, -10.88017736071109987 ) ) ;
#5198=CARTESIAN_POINT ( 'NONE',  ( 18.52753015748617571, 38.09226448433412315, 4.923371831947298993 ) ) ;
#5201=CARTESIAN_POINT ( 'NONE',  ( 19.42250999205614193, 50.14701867748817676, 5.440088680355555262 ) ) ;
#5204=ORIENTED_EDGE ( 'NONE', *, *, #10522, .T. ) ;
#5208=ORIENTED_EDGE ( 'NONE', *, *, #82294, .F. ) ;
#5209=CARTESIAN_POINT ( 'NONE',  ( 24.16423886937409904, 44.09541550158063927, 3.795296366450317205 ) ) ;
#5210=CARTESIAN_POINT ( 'NONE',  ( 19.84674366389459621, 53.50893115100078745, 7.409399052514197653E-17 ) ) ;
#5211=CARTESIAN_POINT ( 'NONE',  ( 0.5774900079438590739, 62.64701867748817676, -5.440088680355550821 ) ) ;
#5213=EDGE_CURVE ( 'NONE', #72980, #65756, #51552, .T. ) ;
#5215=CARTESIAN_POINT ( 'NONE',  ( 2.035157376598822676, 52.43868534415483396, -7.964842623401177768 ) ) ;
#5217=EDGE_CURVE ( 'NONE', #34081, #74857, #90844, .T. ) ;
#5218=CARTESIAN_POINT ( 'NONE',  ( 10.00000000000000178, 60.37363466993041783, 12.81628187352647608 ) ) ;
#5221=CARTESIAN_POINT ( 'NONE',  ( 19.42250999205614193, 50.14701867748817676, 5.440088680355555262 ) ) ;
#5222=CARTESIAN_POINT ( 'NONE',  ( 6.204703633549690345, 15.76208216824730179, -14.16423886937410259 ) ) ;
#5223=CARTESIAN_POINT ( 'NONE',  ( 22.81628187352647785, 21.41530133659708923, 3.434112377981063169 ) ) ;
#5226=CARTESIAN_POINT ( 'NONE',  ( 19.38216949554541202, 40.99863466993042493, 9.382169495545424454 ) ) ;
#5227=CARTESIAN_POINT ( 'NONE',  ( 2.035157376598824452, 18.68868534415484106, 7.964842623401179544 ) ) ;
#5228=CARTESIAN_POINT ( 'NONE',  ( 10.00000000000000000, 39.75893115100078745, -9.846743663894594434 ) ) ;
#5229=CARTESIAN_POINT ( 'NONE',  ( 10.00000000000000000, 6.813685344154838397, -10.88017736071110342 ) ) ;
#5231=DIRECTION ( 'NONE',  ( 0.000000000000000000, 0.000000000000000000, -1.000000000000000000 ) ) ;
#5232=CARTESIAN_POINT ( 'NONE',  ( 18.52753015748618282, 48.92559781766745886, -4.923371831947291888 ) ) ;
#5233=CARTESIAN_POINT ( 'NONE',  ( 20.15039907845753220, 21.74884699246888786, 6.262539305110078836 ) ) ;
#5235=VECTOR ( 'NONE', #31884, 1000.000000000000000 ) ;
#5236=CARTESIAN_POINT ( 'NONE',  ( -0.1503990784575328088, 3.101585745166421493, 6.262539305110068177 ) ) ;
#5239=CARTESIAN_POINT ( 'NONE',  ( -0.1503990784575242878, 44.24884699246889852, -6.262539305110083276 ) ) ;
#5240=CARTESIAN_POINT ( 'NONE',  ( 12.63842701281683922, 24.55059781766745175, -9.846743663894590881 ) ) ;
#5241=CARTESIAN_POINT ( 'NONE',  ( 13.43411237798105340, 20.58196800326374643, 12.81628187352647963 ) ) ;
#5245=CARTESIAN_POINT ( 'NONE',  ( 19.84674366389459266, 63.30059781766745886, 2.638427012816836559 ) ) ;
#5247=CARTESIAN_POINT ( 'NONE',  ( -4.164238869374098151, 26.59541550158063217, -3.795296366450310543 ) ) ;
#5248=CARTESIAN_POINT ( 'NONE',  ( 2.791683348922237240, 45.38393115100079456, -7.208316651077763204 ) ) ;
#5249=CARTESIAN_POINT ( 'NONE',  ( 19.38216949554541202, 40.99863466993042493, 9.382169495545424454 ) ) ;
#5252=CARTESIAN_POINT ( 'NONE',  ( 19.42250999205614193, 60.14701867748817676, 5.440088680355555262 ) ) ;
#5254=CARTESIAN_POINT ( 'NONE',  ( 5.076628168052704559, 30.17559781766745175, -8.527530157486179263 ) ) ;
#5255=CARTESIAN_POINT ( 'NONE',  ( 10.00000000000000178, 34.31368534415484106, 10.88017736071110342 ) ) ;
#5256=CARTESIAN_POINT ( 'NONE',  ( 19.38216949554541202, 40.99863466993042493, 9.382169495545424454 ) ) ;
#5257=( GEOMETRIC_REPRESENTATION_CONTEXT ( 3 ) GLOBAL_UNCERTAINTY_ASSIGNED_CONTEXT ( ( #75265 ) ) GLOBAL_UNIT_ASSIGNED_CONTEXT ( ( #40154, #55139, #53674 ) ) REPRESENTATION_CONTEXT ( 'NONE', 'WORKASPACE' ) );
#5258=CARTESIAN_POINT ( 'NONE',  ( -45.94000000000000483, 92.00000000000000000, 9.500000000000000000 ) ) ;
#5259=CARTESIAN_POINT ( 'NONE',  ( 4.559911319644449179, 28.89701867748817321, 9.422509992056141925 ) ) ;
#5262=CARTESIAN_POINT ( 'NONE',  ( -45.94000000000001194, 107.5383484153110061, 12.00000000000000000 ) ) ;
#5263=CARTESIAN_POINT ( 'NONE',  ( 15.44008868035555793, 21.39701867748817321, -9.422509992056140149 ) ) ;
#5264=CARTESIAN_POINT ( 'NONE',  ( 5.076628168052703671, 61.84226448433412315, 8.527530157486179263 ) ) ;
#5265=CARTESIAN_POINT ( 'NONE',  ( 10.00000000000000178, 39.31368534415484106, 10.88017736071110342 ) ) ;
#5267=STYLED_ITEM ( 'NONE', ( #27313 ), #91888 ) ;
#5268=CARTESIAN_POINT ( 'NONE',  ( 19.42250999205614193, 55.14701867748817676, 5.440088680355555262 ) ) ;
#5269=CARTESIAN_POINT ( 'NONE',  ( 10.00000000000000000, 31.81368534415483751, -10.88017736071110342 ) ) ;
#5270=DIRECTION ( 'NONE',  ( -1.000000000000000000, -2.653152395358074805E-16, 0.000000000000000000 ) ) ;
#5271=CARTESIAN_POINT ( 'NONE',  ( 17.20831665107776587, 2.883931151000785231, 7.208316651077764980 ) ) ;
#5272=CARTESIAN_POINT ( 'NONE',  ( 19.84674366389459621, 28.50893115100078745, 7.409399052514197653E-17 ) ) ;
#5275=CARTESIAN_POINT ( 'NONE',  ( 5.076628168052704559, 55.17559781766745175, -8.527530157486179263 ) ) ;
#5276=CARTESIAN_POINT ( 'NONE',  ( 24.16423886937409904, 49.09541550158063217, 3.795296366450317205 ) ) ;
#5278=CARTESIAN_POINT ( 'NONE',  ( 6.000000000000000000, 11.50000000000000000, -6.500000000000000888 ) ) ;
#5279=CARTESIAN_POINT ( 'NONE',  ( -0.3689425029237898834, 11.17874883491396787, -10.36894250292378850 ) ) ;
#5281=CARTESIAN_POINT ( 'NONE',  ( 24.16423886937410614, 34.51208216824731068, -3.795296366450302550 ) ) ;
#5282=CARTESIAN_POINT ( 'NONE',  ( 21.09922568453595559, 7.040301336597086568, -6.408140936763230044 ) ) ;
#5284=CARTESIAN_POINT ( 'NONE',  ( 4.559911319644449179, 12.23035201082150714, -9.422509992056141925 ) ) ;
#5285=CARTESIAN_POINT ( 'NONE',  ( 2.791683348922237240, 30.38393115100078390, -7.208316651077763204 ) ) ;
#5289=CARTESIAN_POINT ( 'NONE',  ( 18.52753015748617571, 3.092264484334118269, 4.923371831947298993 ) ) ;
#5290=CARTESIAN_POINT ( 'NONE',  ( 0.6178305044545818747, 23.49863466993041783, -9.382169495545419124 ) ) ;
#5291=CARTESIAN_POINT ( 'NONE',  ( 19.84674366389459266, 23.30059781766745530, 2.638427012816836559 ) ) ;
#5293=CARTESIAN_POINT ( 'NONE',  ( 12.63842701281683922, 14.55059781766744997, -9.846743663894590881 ) ) ;
#5294=CARTESIAN_POINT ( 'NONE',  ( 0.5774900079438590739, 2.647018677488171434, -5.440088680355550821 ) ) ;
#5295=CARTESIAN_POINT ( 'NONE',  ( 20.88017736071110875, 10.77201867748817143, -2.915334737309920765 ) ) ;
#5297=CARTESIAN_POINT ( 'NONE',  ( -2.266590686148945544, 36.38708216824730357, -7.082119434687050408 ) ) ;
#5298=CARTESIAN_POINT ( 'NONE',  ( 20.88017736071110875, 60.77201867748817676, -2.915334737309920765 ) ) ;
#5299=DIRECTION ( 'NONE',  ( 0.000000000000000000, -1.000000000000000000, 0.000000000000000000 ) ) ;
#5300=CARTESIAN_POINT ( 'NONE',  ( 17.39651004071843232, 17.93575266056828355, 6.499999999999984013 ) ) ;
#5301=CARTESIAN_POINT ( 'NONE',  ( 2.791683348922240793, 21.63393115100078745, 7.208316651077764092 ) ) ;
#5302=CARTESIAN_POINT ( 'NONE',  ( 19.80448550324510038, 21.82703681773340421, 6.500000000002801315 ) ) ;
#5303=CARTESIAN_POINT ( 'NONE',  ( 1.472469842513823179, 1.425597817667451528, 4.923371831947296329 ) ) ;
#5304=LINE ( 'NONE', #19791, #19655 ) ;
#5305=CARTESIAN_POINT ( 'NONE',  ( 14.92337183194729633, 32.67559781766745175, 8.527530157486181039 ) ) ;
#5306=CARTESIAN_POINT ( 'NONE',  ( 2.791683348922237240, 60.38393115100078745, -7.208316651077763204 ) ) ;
#5308=CARTESIAN_POINT ( 'NONE',  ( 10.00000000000000178, 34.31368534415484106, 10.88017736071110342 ) ) ;
#5310=CARTESIAN_POINT ( 'NONE',  ( 13.43411237798105340, 50.58196800326375353, 12.81628187352647963 ) ) ;
#5312=CARTESIAN_POINT ( 'NONE',  ( 12.91533473730992121, 64.52201867748817676, 10.88017736071110164 ) ) ;
#5313=CARTESIAN_POINT ( 'NONE',  ( -2.816281873526473856, 44.12363466993042493, 9.499525473075851096E-16 ) ) ;
#5314=CARTESIAN_POINT ( 'NONE',  ( -4.164238869374098151, 61.59541550158063217, -3.795296366450310543 ) ) ;
#5315=CARTESIAN_POINT ( 'NONE',  ( 14.92337183194729633, 32.67559781766745175, 8.527530157486181039 ) ) ;
#5318=CARTESIAN_POINT ( 'NONE',  ( 17.08211943468705840, 20.13708216824730357, -12.26659068614894466 ) ) ;
#5319=CARTESIAN_POINT ( 'NONE',  ( 10.00000000000000000, 45.55374883491397497, -14.16423886937410082 ) ) ;
#5320=CARTESIAN_POINT ( 'NONE',  ( 7.361572987183169658, 49.96726448433410894, -9.846743663894592657 ) ) ;
#5321=CARTESIAN_POINT ( 'NONE',  ( 20.10239578412225825, 12.63377557478296609, -6.340343622311917393 ) ) ;
#5322=CARTESIAN_POINT ( 'NONE',  ( -0.8801773607111009756, 38.06368534415484106, 1.068504757029289695E-15 ) ) ;
#5323=CARTESIAN_POINT ( 'NONE',  ( 17.96484262340118221, 56.18868534415484817, -7.964842623401177768 ) ) ;
#5324=ORIENTED_EDGE ( 'NONE', *, *, #51919, .T. ) ;
#5325=CARTESIAN_POINT ( 'NONE',  ( 13.43411237798105340, 40.58196800326375353, 12.81628187352647963 ) ) ;
#5327=CARTESIAN_POINT ( 'NONE',  ( 20.88017736071110519, 65.56368534415483396, 2.639326808657452039E-16 ) ) ;
#5329=CARTESIAN_POINT ( 'NONE',  ( -4.164238869374099039, 1.803748834913967647, 8.674139862899312516E-16 ) ) ;
#5330=CARTESIAN_POINT ( 'NONE',  ( 0.1532563361054083140, 11.00893115100078568, 1.131784320476157264E-15 ) ) ;
#5331=CARTESIAN_POINT ( 'NONE',  ( -1.926860441876563801, 59.89664270246083788, 3.195792623639529761 ) ) ;
#5335=CARTESIAN_POINT ( 'NONE',  ( 2.035157376598824452, 13.68868534415483751, 7.964842623401179544 ) ) ;
#5337=CARTESIAN_POINT ( 'NONE',  ( -4.164238869374099039, 21.80374883491396787, 8.674139862899312516E-16 ) ) ;
#5339=EDGE_CURVE ( 'NONE', #41390, #43512, #29659, .T. ) ;
#5341=CARTESIAN_POINT ( 'NONE',  ( 12.91533473730993009, 26.60535201082150536, -10.88017736071109987 ) ) ;
#5342=CARTESIAN_POINT ( 'NONE',  ( 0.1532563361054082862, 66.21726448433413736, 2.638427012816831674 ) ) ;
#5343=ORIENTED_EDGE ( 'NONE', *, *, #15317, .T. ) ;
#5345=CARTESIAN_POINT ( 'NONE',  ( 10.00000000000000000, 59.75893115100078745, -9.846743663894594434 ) ) ;
#5347=CARTESIAN_POINT ( 'NONE',  ( 14.92337183194729633, 2.675597817667451750, 8.527530157486181039 ) ) ;
#5348=CARTESIAN_POINT ( 'NONE',  ( 2.791683348922240793, 66.63393115100079456, 7.208316651077764092 ) ) ;
#5349=CARTESIAN_POINT ( 'NONE',  ( 6.565887622018943937, 38.08196800326376064, -12.81628187352647608 ) ) ;
#5350=CARTESIAN_POINT ( 'NONE',  ( 10.00000000000000000, 11.81368534415483751, -10.88017736071110342 ) ) ;
#5352=CARTESIAN_POINT ( 'NONE',  ( 2.035157376598824452, 68.68868534415484817, 7.964842623401179544 ) ) ;
#5353=CARTESIAN_POINT ( 'NONE',  ( -0.8801773607111009756, 13.06368534415483929, 1.068504757029289695E-15 ) ) ;
#5355=CARTESIAN_POINT ( 'NONE',  ( 13.43411237798105340, 55.58196800326374643, 12.81628187352647963 ) ) ;
#5356=CARTESIAN_POINT ( 'NONE',  ( 17.96484262340118221, 41.18868534415484106, -7.964842623401177768 ) ) ;
#5357=CARTESIAN_POINT ( 'NONE',  ( 19.67858290521088449, 89.80181819993967451, 5.461713021790604472 ) ) ;
#5358=CARTESIAN_POINT ( 'NONE',  ( 21.09922568453595559, 42.04030133659708213, -6.408140936763230044 ) ) ;
#5359=CARTESIAN_POINT ( 'NONE',  ( 17.96484262340118221, 49.93868534415484106, 7.964842623401181321 ) ) ;
#5360=CARTESIAN_POINT ( 'NONE',  ( 18.52753015748617571, 53.09226448433412315, 4.923371831947298993 ) ) ;
#5362=VERTEX_POINT ( 'NONE', #98759 ) ;
#5363=CARTESIAN_POINT ( 'NONE',  ( 12.63842701281683922, 14.55059781766744997, -9.846743663894590881 ) ) ;
#5364=CARTESIAN_POINT ( 'NONE',  ( 10.00000000000000000, 2.873634669930420049, -12.81628187352647608 ) ) ;
#5366=CARTESIAN_POINT ( 'NONE',  ( 19.84674366389459266, 58.30059781766745886, 2.638427012816836559 ) ) ;
#5367=CARTESIAN_POINT ( 'NONE',  ( 2.035157376598822676, 17.43868534415483751, -7.964842623401177768 ) ) ;
#5368=CARTESIAN_POINT ( 'NONE',  ( 2.791683348922237240, 55.38393115100078745, -7.208316651077763204 ) ) ;
#5369=CARTESIAN_POINT ( 'NONE',  ( 5.500000000000000000, 11.00000000000000000, -6.000000000000000000 ) ) ;
#5370=( NAMED_UNIT ( * ) PLANE_ANGLE_UNIT ( ) SI_UNIT ( $, .RADIAN. ) );
#5372=CARTESIAN_POINT ( 'NONE',  ( 1.472469842513823179, 11.42559781766745175, 4.923371831947296329 ) ) ;
#5373=FILL_AREA_STYLE_COLOUR ( '', #4268 ) ;
#5374=CARTESIAN_POINT ( 'NONE',  ( -2.816281873526473856, -0.8763653300695799508, 9.499525473075851096E-16 ) ) ;
#5377=CARTESIAN_POINT ( 'NONE',  ( 1.274849032794294290, 63.57228050351031357, 6.499999999999979572 ) ) ;
#5379=CARTESIAN_POINT ( 'NONE',  ( 6.565887622018943937, 43.08196800326374643, -12.81628187352647608 ) ) ;
#5380=CARTESIAN_POINT ( 'NONE',  ( 7.361572987183169658, 29.96726448433411960, -9.846743663894592657 ) ) ;
#5381=CARTESIAN_POINT ( 'NONE',  ( 1.274849032794278747, 57.55509018479938277, -6.499999999999960032 ) ) ;
#5382=CARTESIAN_POINT ( 'NONE',  ( 17.08211943468705130, 58.47041550158063927, 12.26659068614894998 ) ) ;
#5383=CARTESIAN_POINT ( 'NONE',  ( 1.472469842513823179, 31.42559781766745530, 4.923371831947296329 ) ) ;
#5386=CARTESIAN_POINT ( 'NONE',  ( 10.00000000000000000, 50.55374883491396787, -14.16423886937410082 ) ) ;
#5388=CARTESIAN_POINT ( 'NONE',  ( 12.91533473730992121, 14.52201867748817143, 10.88017736071110164 ) ) ;
#5389=CARTESIAN_POINT ( 'NONE',  ( 6.204703633549690345, 35.76208216824729647, -14.16423886937410259 ) ) ;
#5390=CARTESIAN_POINT ( 'NONE',  ( 24.16423886937410614, 59.51208216824728936, -3.795296366450302550 ) ) ;
#5391=CARTESIAN_POINT ( 'NONE',  ( 0.2751277870542967463, 70.00000000000000000, -6.000000000000000000 ) ) ;
#5393=CARTESIAN_POINT ( 'NONE',  ( 2.791683348922240793, 11.63393115100078568, 7.208316651077764092 ) ) ;
#5394=CARTESIAN_POINT ( 'NONE',  ( 13.43411237798105340, 5.581968003263753531, 12.81628187352647963 ) ) ;
#5395=CARTESIAN_POINT ( 'NONE',  ( 18.28836319691945889, 14.34492782695770785, 6.500000000000000888 ) ) ;
#5396=ORIENTED_EDGE ( 'NONE', *, *, #9194, .T. ) ;
#5397=CARTESIAN_POINT ( 'NONE',  ( 10.00000000000000000, 51.81368534415484106, -10.88017736071110342 ) ) ;
#5398=FACE_OUTER_BOUND ( 'NONE', #18255, .T. ) ;
#5401=CARTESIAN_POINT ( 'NONE',  ( 20.00000000000000711, 79.40087001978915282, -4.500000000000000000 ) ) ;
#5404=CARTESIAN_POINT ( 'NONE',  ( -0.3689425029237881626, 37.42874883491396787, 10.36894250292379027 ) ) ;
#5405=EDGE_LOOP ( 'NONE', ( #34767, #10259, #30265, #6912, #72865, #6651 ) ) ;
#5406=CARTESIAN_POINT ( 'NONE',  ( 5.076628168052704559, 0.1755978176674514724, -8.527530157486179263 ) ) ;
#5409=CARTESIAN_POINT ( 'NONE',  ( 20.88017736071110519, 20.56368534415484106, 2.639326808657452039E-16 ) ) ;
#5410=CARTESIAN_POINT ( 'NONE',  ( 13.43411237798106583, 42.66530133659707502, -12.81628187352647252 ) ) ;
#5411=CARTESIAN_POINT ( 'NONE',  ( 10.00000000000000000, 6.813685344154838397, -10.88017736071110342 ) ) ;
#5412=CARTESIAN_POINT ( 'NONE',  ( -1.099225684535947600, 28.70696800326375353, -6.408140936763238038 ) ) ;
#5413=CARTESIAN_POINT ( 'NONE',  ( 16.40814093676324603, 57.45696800326375353, -11.09922568453594671 ) ) ;
#5415=AXIS2_PLACEMENT_3D ( 'NONE', #52469, #75958, #14491 ) ;
#5418=CARTESIAN_POINT ( 'NONE',  ( 24.16423886937410614, 24.30374883491396787, 8.672049930838204340E-16 ) ) ;
#5419=CARTESIAN_POINT ( 'NONE',  ( -2.266590686148945544, 6.387082168247300906, -7.082119434687050408 ) ) ;
#5421=CARTESIAN_POINT ( 'NONE',  ( 0.5774900079438607392, 28.48035201082150891, 5.440088680355550821 ) ) ;
#5424=CARTESIAN_POINT ( 'NONE',  ( -0.8801773607111009756, 58.06368534415484106, 1.068504757029289695E-15 ) ) ;
#5425=CARTESIAN_POINT ( 'NONE',  ( 17.96484262340118221, 49.93868534415484106, 7.964842623401181321 ) ) ;
#5426=CARTESIAN_POINT ( 'NONE',  ( 19.38216949554541202, 15.99863466993042138, 9.382169495545424454 ) ) ;
#5427=CARTESIAN_POINT ( 'NONE',  ( 0.1089645850228985746, 48.16234555792571115, 6.479102184480827198 ) ) ;
#5429=CARTESIAN_POINT ( 'NONE',  ( 7.361572987183169658, 24.96726448433412315, -9.846743663894592657 ) ) ;
#5432=CARTESIAN_POINT ( 'NONE',  ( -0.8801773607111008646, 38.27201867748816255, 2.915334737309923430 ) ) ;
#5434=CARTESIAN_POINT ( 'NONE',  ( 3.591859063236761518, 9.956968003263753531, 11.09922568453594849 ) ) ;
#5435=CARTESIAN_POINT ( 'NONE',  ( 1.472469842513823179, 26.42559781766745175, 4.923371831947296329 ) ) ;
#5436=CARTESIAN_POINT ( 'NONE',  ( 0.6178305044545838731, 54.74863466993042493, 9.382169495545420901 ) ) ;
#5437=CARTESIAN_POINT ( 'NONE',  ( 0.1532563361054100626, 10.80059781766745175, -2.638427012816831230 ) ) ;
#5438=ORIENTED_EDGE ( 'NONE', *, *, #12359, .T. ) ;
#5439=CARTESIAN_POINT ( 'NONE',  ( 20.15039907845753220, 41.74884699246887720, 6.262539305110078836 ) ) ;
#5440=CARTESIAN_POINT ( 'NONE',  ( 18.95785429995060767, 27.24216108172003104, 6.499999999999853451 ) ) ;
#5441=CARTESIAN_POINT ( 'NONE',  ( 0.5774900079438607392, 13.48035201082150358, 5.440088680355550821 ) ) ;
#5442=( NAMED_UNIT ( * ) PLANE_ANGLE_UNIT ( ) SI_UNIT ( $, .RADIAN. ) );
#5443=CARTESIAN_POINT ( 'NONE',  ( 17.08211943468705840, 30.13708216824730357, -12.26659068614894466 ) ) ;
#5444=CARTESIAN_POINT ( 'NONE',  ( 1.472469842513823179, 30.59226448433411960, -4.923371831947296329 ) ) ;
#5445=CARTESIAN_POINT ( 'NONE',  ( 19.42250999205614548, 15.98035201082150714, -5.440088680355545492 ) ) ;
#5446=CARTESIAN_POINT ( 'NONE',  ( 0.5774900079438607392, 3.480352010821504916, 5.440088680355550821 ) ) ;
#5448=CARTESIAN_POINT ( 'NONE',  ( 19.42250999205614548, 30.98035201082150536, -5.440088680355545492 ) ) ;
#5449=CARTESIAN_POINT ( 'NONE',  ( -0.8801773607111009756, 38.06368534415484106, 1.068504757029289695E-15 ) ) ;
#5451=ORIENTED_EDGE ( 'NONE', *, *, #51194, .F. ) ;
#5452=CARTESIAN_POINT ( 'NONE',  ( 0.1532563361054082862, 51.21726448433412315, 2.638427012816831674 ) ) ;
#5453=CARTESIAN_POINT ( 'NONE',  ( -0.8801773607110991993, 37.85535201082151247, -2.915334737309923874 ) ) ;
#5457=CARTESIAN_POINT ( 'NONE',  ( 10.00000000000000178, 65.37363466993042493, 12.81628187352647608 ) ) ;
#5459=CARTESIAN_POINT ( 'NONE',  ( 6.204703633549690345, 37.84541550158063927, 14.16423886937410082 ) ) ;
#5460=CARTESIAN_POINT ( 'NONE',  ( 19.42250999205614193, 55.14701867748817676, 5.440088680355555262 ) ) ;
#5464=CARTESIAN_POINT ( 'NONE',  ( 12.63842701281683922, 44.55059781766745175, -9.846743663894590881 ) ) ;
#5467=CARTESIAN_POINT ( 'NONE',  ( 0.1532563361054083140, 16.00893115100078390, 1.131784320476157264E-15 ) ) ;
#5469=CARTESIAN_POINT ( 'NONE',  ( 2.035157376598822676, 27.43868534415483396, -7.964842623401177768 ) ) ;
#5470=CARTESIAN_POINT ( 'NONE',  ( 12.63842701281683034, 27.46726448433411250, 9.846743663894596210 ) ) ;
#5471=CARTESIAN_POINT ( 'NONE',  ( 21.09922568453594849, 6.206968003263753531, 6.408140936763242479 ) ) ;
#5472=CARTESIAN_POINT ( 'NONE',  ( 0.5774900079438607392, 53.48035201082151247, 5.440088680355550821 ) ) ;
#5473=CARTESIAN_POINT ( 'NONE',  ( 4.559911319644449179, 32.23035201082150536, -9.422509992056141925 ) ) ;
#5474=CARTESIAN_POINT ( 'NONE',  ( -2.816281873526473856, 59.12363466993042493, 9.499525473075851096E-16 ) ) ;
#5475=CARTESIAN_POINT ( 'NONE',  ( 20.36894250292379382, 43.67874883491397497, 10.36894250292379205 ) ) ;
#5476=CARTESIAN_POINT ( 'NONE',  ( 21.92686044187657046, 35.16212336850780673, 4.562052436263912550E-16 ) ) ;
#5477=ORIENTED_EDGE ( 'NONE', *, *, #33964, .F. ) ;
#5478=CARTESIAN_POINT ( 'NONE',  ( 1.472469842513823179, 66.42559781766745175, 4.923371831947296329 ) ) ;
#5479=CARTESIAN_POINT ( 'NONE',  ( 0.5774900079438590739, 12.64701867748817143, -5.440088680355550821 ) ) ;
#5480=CARTESIAN_POINT ( 'NONE',  ( 19.42250999205614548, 50.98035201082151247, -5.440088680355545492 ) ) ;
#5481=CARTESIAN_POINT ( 'NONE',  ( 1.472469842513823179, 61.42559781766745175, 4.923371831947296329 ) ) ;
#5483=EDGE_CURVE ( 'NONE', #35669, #12094, #7472, .T. ) ;
#5485=CARTESIAN_POINT ( 'NONE',  ( 19.84674366389459621, 18.50893115100078745, 7.409399052514197653E-17 ) ) ;
#5487=CARTESIAN_POINT ( 'NONE',  ( 4.559911319644449179, 62.23035201082150536, -9.422509992056141925 ) ) ;
#5488=CARTESIAN_POINT ( 'NONE',  ( 14.92337183194729633, 42.67559781766745886, 8.527530157486181039 ) ) ;
#5489=CARTESIAN_POINT ( 'NONE',  ( 5.076628168052704559, 15.17559781766745175, -8.527530157486179263 ) ) ;
#5490=CARTESIAN_POINT ( 'NONE',  ( 5.076628168052704559, 15.17559781766745175, -8.527530157486179263 ) ) ;
#5491=CARTESIAN_POINT ( 'NONE',  ( 19.50000000000000711, 79.40087001978915282, 4.500000000000000888 ) ) ;
#5492=CARTESIAN_POINT ( 'NONE',  ( 4.559911319644449179, 67.23035201082150536, -9.422509992056141925 ) ) ;
#5494=CARTESIAN_POINT ( 'NONE',  ( 10.00000000000000178, 7.258931151000785675, 9.846743663894594434 ) ) ;
#5495=CARTESIAN_POINT ( 'NONE',  ( 0.1532563361054100626, 30.80059781766744820, -2.638427012816831230 ) ) ;
#5496=VERTEX_POINT ( 'NONE', #252 ) ;
#5498=CARTESIAN_POINT ( 'NONE',  ( 3.591859063236763294, 3.290301336597087012, -11.09922568453595026 ) ) ;
#5499=CARTESIAN_POINT ( 'NONE',  ( -4.164238869374099039, 21.80374883491396787, 8.674139862899312516E-16 ) ) ;
#5502=CARTESIAN_POINT ( 'NONE',  ( 20.36894250292379738, 19.92874883491396787, -10.36894250292379027 ) ) ;
#5503=CARTESIAN_POINT ( 'NONE',  ( -0.3689425029237898834, 41.17874883491397497, -10.36894250292378850 ) ) ;
#5504=CARTESIAN_POINT ( 'NONE',  ( 24.16423886937410614, 19.51208216824729647, -3.795296366450302550 ) ) ;
#5505=CARTESIAN_POINT ( 'NONE',  ( -0.8801773607111008646, 68.27201867748817676, 2.915334737309923430 ) ) ;
#5506=CARTESIAN_POINT ( 'NONE',  ( 15.44008868035555793, 36.39701867748816966, -9.422509992056140149 ) ) ;
#5508=CARTESIAN_POINT ( 'NONE',  ( 19.84674366389459621, 33.50893115100078745, 7.409399052514197653E-17 ) ) ;
#5509=CARTESIAN_POINT ( 'NONE',  ( 0.2751277870542967463, 70.00000000000000000, -6.500000000000000888 ) ) ;
#5510=CARTESIAN_POINT ( 'NONE',  ( 17.20831665107776587, 22.88393115100078745, 7.208316651077764980 ) ) ;
#5511=CARTESIAN_POINT ( 'NONE',  ( 15.44008868035555793, 11.39701867748817143, -9.422509992056140149 ) ) ;
#5512=CARTESIAN_POINT ( 'NONE',  ( 19.38216949554541557, 57.24863466993042493, -9.382169495545420901 ) ) ;
#5513=CARTESIAN_POINT ( 'NONE',  ( 17.20831665107776587, 44.13393115100078745, -7.208316651077762316 ) ) ;
#5516=CARTESIAN_POINT ( 'NONE',  ( -1.099225684535947600, 44.54030133659708923, 6.408140936763237150 ) ) ;
#5518=CARTESIAN_POINT ( 'NONE',  ( 10.00000000000000178, 49.31368534415484106, 10.88017736071110342 ) ) ;
#5519=CARTESIAN_POINT ( 'NONE',  ( 0.1532563361054100626, 45.80059781766745886, -2.638427012816831230 ) ) ;
#5520=CARTESIAN_POINT ( 'NONE',  ( 17.08211943468705840, 20.13708216824730357, -12.26659068614894466 ) ) ;
#5521=ORIENTED_EDGE ( 'NONE', *, *, #52221, .F. ) ;
#5522=CARTESIAN_POINT ( 'NONE',  ( 17.96484262340118221, 54.93868534415484106, 7.964842623401181321 ) ) ;
#5524=CARTESIAN_POINT ( 'NONE',  ( -2.266590686148945544, 52.22041550158064638, 7.082119434687048631 ) ) ;
#5525=CARTESIAN_POINT ( 'NONE',  ( 16.40814093676324603, 2.456968003263753531, -11.09922568453594671 ) ) ;
#5526=CARTESIAN_POINT ( 'NONE',  ( 13.43411237798105340, 60.58196800326376064, 12.81628187352647963 ) ) ;
#5527=CARTESIAN_POINT ( 'NONE',  ( 20.88017736071110164, 60.35535201082151957, 2.915334737309930979 ) ) ;
#5529=CARTESIAN_POINT ( 'NONE',  ( 10.00000000000000000, 27.87363466993042138, -12.81628187352647608 ) ) ;
#5530=CARTESIAN_POINT ( 'NONE',  ( 22.81628187352647785, 1.623634669930420271, 6.195893100308588602E-16 ) ) ;
#5532=CARTESIAN_POINT ( 'NONE',  ( -0.8801773607110991993, 17.85535201082150536, -2.915334737309923874 ) ) ;
#5533=CARTESIAN_POINT ( 'NONE',  ( 10.00000000000000178, 9.313685344154839285, 10.88017736071110342 ) ) ;
#5537=EDGE_CURVE ( 'NONE', #26466, #93630, #20565, .T. ) ;
#5538=CARTESIAN_POINT ( 'NONE',  ( 19.42250999205614193, 10.14701867748816966, 5.440088680355555262 ) ) ;
#5540=CARTESIAN_POINT ( 'NONE',  ( 10.00000000000000178, 69.31368534415484817, 10.88017736071110342 ) ) ;
#5541=CARTESIAN_POINT ( 'NONE',  ( 2.791683348922240793, 1.633931151000784565, 7.208316651077764092 ) ) ;
#5542=STYLED_ITEM ( 'NONE', ( #14352 ), #54890 ) ;
#5543=CARTESIAN_POINT ( 'NONE',  ( 14.92337183194729988, 39.34226448433412315, -8.527530157486177487 ) ) ;
#5544=CARTESIAN_POINT ( 'NONE',  ( 15.44008868035555793, 31.39701867748817676, -9.422509992056140149 ) ) ;
#5546=CARTESIAN_POINT ( 'NONE',  ( 22.81628187352647785, 6.415301336597088344, 3.434112377981063169 ) ) ;
#5547=CARTESIAN_POINT ( 'NONE',  ( 12.91533473730993009, 41.60535201082149825, -10.88017736071109987 ) ) ;
#5549=CARTESIAN_POINT ( 'NONE',  ( 0.6178305044545818747, 38.49863466993042493, -9.382169495545419124 ) ) ;
#5550=ORIENTED_EDGE ( 'NONE', *, *, #43101, .T. ) ;
#5551=CARTESIAN_POINT ( 'NONE',  ( 17.96484262340118221, 61.18868534415482685, -7.964842623401177768 ) ) ;
#5553=CARTESIAN_POINT ( 'NONE',  ( 0.6178305044545838731, 34.74863466993042493, 9.382169495545420901 ) ) ;
#5554=CARTESIAN_POINT ( 'NONE',  ( -2.266590686148945544, 7.220415501580634832, 7.082119434687048631 ) ) ;
#5555=CARTESIAN_POINT ( 'NONE',  ( 1.472469842513823179, 0.5922644843341181575, -4.923371831947296329 ) ) ;
#5556=CARTESIAN_POINT ( 'NONE',  ( 10.00000000000000000, 41.81368534415484106, -10.88017736071110342 ) ) ;
#5558=CARTESIAN_POINT ( 'NONE',  ( 17.08211943468705840, 60.13708216824729647, -12.26659068614894466 ) ) ;
#5559=CARTESIAN_POINT ( 'NONE',  ( 14.92337183194729633, 47.67559781766745175, 8.527530157486181039 ) ) ;
#5560=CARTESIAN_POINT ( 'NONE',  ( 19.84674366389459266, 13.71726448433411782, -2.638427012816827677 ) ) ;
#5561=CARTESIAN_POINT ( 'NONE',  ( 4.559911319644449179, 67.23035201082150536, -9.422509992056141925 ) ) ;
#5563=CARTESIAN_POINT ( 'NONE',  ( 2.917880565312948704, 27.63708216824730357, 12.26659068614894643 ) ) ;
#5566=( BOUNDED_SURFACE ( )  B_SPLINE_SURFACE ( 1, 2, ( 
 ( #7722, #83707, #53691, #38219, #90702, #68704, #84688, #84211, #30684, #61192, #15718, #46203, #8207, #44709, #38702, #37235, #69201, #46680, #92191, #6719, #23716, #60694, #67724, #60207, #83212, #14733, #7219, #37720, #68224, #30193, #11524, #80021, #86552, #71556, #42046, #4536, #27016, #12021, #18542, #19524, #18056, #10062, #57515, #72510, #26050, #27506, #72026, #26524, #4043, #48534, #94531, #49034, #41058, #88012, #42521, #56058, #2585, #79539, #78551, #17572, #41560, #56540, #19037, #3554, #79034, #34505, #65502, #34014, #11038, #10548, #64511, #96025, #48039, #3069, #33523, #64019, #63536, #50020, #87522, #94044, #95015, #34999, #64997, #86061, #87030, #57020, #80523, #49513, #95524, #40560, #73004, #71060, #33039, #25566, #5520, #29468, #58997, #12998, #90469, #35998, #14006, #44975, #14504, #6994, #58001, #89499, #73493, #44485, #21010, #51497, #66501, #22004, #81494, #97026, #5020, #28981, #37498, #52479, #20010, #59485, #28503, #50512, #13503, #75480, #43494, #67988, #74486, #81992, #81009, #89985, #43984, #12510, #6009, #98514, #73994, #88508, #36503, #66995, #97518, #82985, #21502, #58497, #51999, #82489, #74986, #43011, #6489, #96526, #67493, #36997, #89007, #98014, #35504, #65998, #59976, #27999, #50999, #20514, #54441, #980, #31442, #8948, #45470, #83969, #83479, #7981, #75972, #52967, #84951, #23967, #30459, #15494, #16461, #48781, #69955, #56304, #61452, #63771, #60959, #15000, #1474, #46941, #68974, #71787, #15966, #69460, #77435, #91468, #38480, #91960, #45976, #31928, #86797, #11, #7499, #23489, #22495, #60473, #84468, #506, #61943, #46458, #22993, #39465, #10797, #76952, #53961, #53459, #8462, #41315, #90962, #76466, #30953, #38968, #37992, #94281, #92444, #68484, #25802, #79288, #18298, #29967, #80271, #11771, #73745, #12260, #96277, #94776, #72269, #34252, #56778, #3797, #49759, #5276, #4284, #57265, #35753, #42280, #58235, #89250, #58746, #51250, #3296, #34758, #18794, #88755, #65248, #95775, #72751, #66240, #26770, #27255, #49277, #73251, #81736, #96775, #20265, #65747, #87273, #57755, #4778, #64264, #20760, #11276, #26276, #33760, #28252, #79777, #41796, #35251, #42769, #50764, #64753, #95265, #87760, #88258, #13252, #43743, #19275, #19764, #50249, #80765, #27751, #81253, #43250, #12752, #15741, #82734, #29724, #45730, #67245, #38239, #91215, #257, #68730, #5763, #76231, #13751, #68247, #89736, #23242, #59733, #44235, #14252, #59234, #91721, #44734, #7745, #21254, #22743, #52727, #30706, #97770, #66748, #61218, #53226, #37260, #83232, #53714, #74738, #74230, #75230, #97272, #36252, #6743 ),
 ( #84234, #90725, #67748, #98267, #28744, #22250, #6251, #7244, #98765, #30215, #51752, #60230, #36755, #83729, #14757, #29235, #15252, #82236, #90229, #37749, #21760, #52241, #45230, #60719, #75728, #47690, #25212, #61694, #1238, #748, #24218, #92210, #69223, #70698, #40191, #46701, #31693, #2218, #63659, #86190, #71188, #77687, #78684, #77200, #31201, #17701, #32676, #85206, #86678, #17213, #63170, #46224, #55692, #76710, #55178, #2713, #32178, #33165, #9202, #62184, #24707, #93677, #16216, #62681, #16710, #92694, #54684, #85693, #47183, #48171, #25695, #69708, #39714, #84715, #10194, #70203, #8705, #78183, #40687, #1724, #93181, #56185, #94165, #9696, #39223, #8229, #38723, #23737, #54199, #19651, #79165, #73626, #26172, #10678, #18184, #81133, #48663, #94663, #88138, #27139, #35131, #56664, #79666, #11162, #72635, #20140, #5149, #3679, #87646, #42172, #34636, #35639, #41194, #58123, #66125, #58633, #26653, #4167, #88631, #41682, #12636, #65630, #43134, #96654, #71674, #50644, #87152, #12146, #33650, #28133, #34141, #18677, #57149, #3184, #64146, #19160, #49163, #72151, #96155, #95655, #64633, #95143, #49639, #80147, #27638, #11658, #57643, #65134, #50143, #80652, #42651, #73128, #4670, #59616, #21137, #30097, #43628, #66633, #83112, #52611, #7634, #28629, #60604, #6622, #44109, #51132, #75115, #82618, #14642, #52124, #97161, #37135, #38125, #45104, #21638, #14134, #44619, #51638, #91099, #74114, #59116, #75611, #7122, #68613, #89626, #22627, #67630, #74621, #81623, #98140, #29601, #37626, #60102, #82118, #90603, #142, #68122, #22129, #98648, #53105, #83615, #15130, #30591, #45606, #20643, #76104, #89133, #13131, #5648, #36124, #6135, #13628, #36640, #67123, #97650, #90113, #29113, #39104, #1612, #8596, #63063, #40579, #84601, #77085, #638, #85582, #62071, #61582, #32061, #9579, #24102, #54572, #71075, #17589, #24599, #31087, #17096, #55064, #46109, #85087, #62565, #23123, #48054, #69105, #53594, #61096, #25096, #91606, #38606, #93068, #70088, #78074, #92093, #23621, #54086, #16595, #93562, #78569, #46588, #31577, #47073, #77570, #10078, #84108, #2107, #2600, #15624, #69594, #9086, #32565, #16100, #55579, #40079, #86077, #76593, #8111, #1115, #92579, #47578, #39600, #70581, #18560, #71569, #72043, #18070, #50526, #41575, #65516, #48550, #50034, #11542, #96038, #26064, #25581, #35015, #12035, #95032, #42061, #20025, #3081, #73510, #3573, #56073, #33054, #34030, #63550, #72524, #88523, #19051, #58013, #26541, #49052, #4058, #80537, #33539, #49529, #64526, #79555, #11055, #34519, #57037, #27522, #12525, #56555, #87539 ) ),
 .UNSPECIFIED., .F., .F., .F. ) 
 B_SPLINE_SURFACE_WITH_KNOTS ( ( 2, 2 ),
 ( 3, 2, 2, 2, 2, 2, 2, 2, 2, 2, 2, 2, 2, 2, 2, 2, 2, 2, 2, 2, 2, 2, 2, 2, 2, 2, 2, 2, 2, 2, 2, 2, 2, 2, 2, 2, 2, 2, 2, 2, 2, 2, 2, 2, 2, 2, 2, 2, 2, 2, 2, 2, 2, 2, 2, 2, 2, 2, 2, 2, 2, 2, 2, 2, 2, 2, 2, 2, 2, 2, 2, 2, 2, 2, 2, 2, 2, 2, 2, 2, 2, 2, 2, 2, 2, 2, 2, 2, 2, 2, 2, 2, 2, 2, 2, 2, 2, 2, 2, 2, 2, 2, 2, 2, 2, 2, 2, 2, 2, 2, 2, 2, 2, 2, 2, 2, 2, 2, 2, 2, 2, 2, 2, 2, 2, 2, 2, 2, 2, 2, 2, 2, 2, 2, 2, 2, 2, 2, 2, 2, 2, 2, 2, 2, 2, 2, 2, 2, 2, 2, 2, 2, 2, 2, 2, 2, 2, 2, 2, 2, 2, 2, 3 ),
 ( 0.000000000000000000, 1.000000000000000000 ),
 ( 0.000000000000000000, 0.005952380952380952051, 0.01190476190476190410, 0.01785714285714285615, 0.02380952380952380820, 0.02976190476190476025, 0.03571428571428571230, 0.04166666666666666435, 0.04761904761904761640, 0.05357142857142856845, 0.05952380952380952051, 0.06547619047619047949, 0.07142857142857142461, 0.07738095238095238360, 0.08333333333333332871, 0.08928571428571428770, 0.09523809523809523281, 0.1011904761904761918, 0.1071428571428571369, 0.1130952380952380959, 0.1190476190476190410, 0.1250000000000000000, 0.1309523809523809590, 0.1369047619047619180, 0.1428571428571428492, 0.1488095238095238082, 0.1547619047619047672, 0.1607142857142857262, 0.1666666666666666574, 0.1726190476190476164, 0.1785714285714285754, 0.1845238095238095344, 0.1904761904761904656, 0.1964285714285714246, 0.2023809523809523836, 0.2083333333333333426, 0.2142857142857142738, 0.2202380952380952328, 0.2261904761904761918, 0.2321428571428571508, 0.2380952380952380820, 0.2440476190476190410, 0.2500000000000000000, 0.2559523809523809312, 0.2619047619047619180, 0.2678571428571428492, 0.2738095238095238360, 0.2797619047619047672, 0.2857142857142856984, 0.2916666666666666852, 0.2976190476190476164, 0.3035714285714285476, 0.3095238095238095344, 0.3154761904761904656, 0.3214285714285714524, 0.3273809523809523836, 0.3333333333333333148, 0.3392857142857143016, 0.3452380952380952328, 0.3511904761904761640, 0.3571428571428571508, 0.3630952380952380820, 0.3690476190476190688, 0.3750000000000000000, 0.3809523809523809312, 0.3869047619047619180, 0.3928571428571428492, 0.3988095238095238360, 0.4047619047619047672, 0.4107142857142856984, 0.4166666666666666852, 0.4226190476190476164, 0.4285714285714285476, 0.4345238095238095344, 0.4404761904761904656, 0.4464285714285714524, 0.4523809523809523836, 0.4583333333333333148, 0.4642857142857143016, 0.4702380952380952328, 0.4761904761904761640, 0.4821428571428571508, 0.4880952380952380820, 0.4940476190476190688, 0.5000000000000000000, 0.5059523809523809312, 0.5119047619047618625, 0.5178571428571429047, 0.5238095238095238360, 0.5297619047619047672, 0.5357142857142856984, 0.5416666666666666297, 0.5476190476190476719, 0.5535714285714286031, 0.5595238095238095344, 0.5654761904761904656, 0.5714285714285713969, 0.5773809523809523281, 0.5833333333333333703, 0.5892857142857143016, 0.5952380952380952328, 0.6011904761904761640, 0.6071428571428570953, 0.6130952380952381375, 0.6190476190476190688, 0.6250000000000000000, 0.6309523809523809312, 0.6369047619047618625, 0.6428571428571429047, 0.6488095238095238360, 0.6547619047619047672, 0.6607142857142856984, 0.6666666666666666297, 0.6726190476190476719, 0.6785714285714286031, 0.6845238095238095344, 0.6904761904761904656, 0.6964285714285713969, 0.7023809523809523281, 0.7083333333333333703, 0.7142857142857143016, 0.7202380952380952328, 0.7261904761904761640, 0.7321428571428570953, 0.7380952380952381375, 0.7440476190476190688, 0.7500000000000000000, 0.7559523809523809312, 0.7619047619047618625, 0.7678571428571429047, 0.7738095238095238360, 0.7797619047619047672, 0.7857142857142856984, 0.7916666666666666297, 0.7976190476190476719, 0.8035714285714286031, 0.8095238095238095344, 0.8154761904761904656, 0.8214285714285713969, 0.8273809523809523281, 0.8333333333333333703, 0.8392857142857143016, 0.8452380952380952328, 0.8511904761904761640, 0.8571428571428570953, 0.8630952380952381375, 0.8690476190476190688, 0.8750000000000000000, 0.8809523809523809312, 0.8869047619047618625, 0.8928571428571429047, 0.8988095238095238360, 0.9047619047619047672, 0.9107142857142856984, 0.9166666666666666297, 0.9226190476190476719, 0.9285714285714286031, 0.9345238095238095344, 0.9404761904761904656, 0.9464285714285713969, 0.9523809523809523281, 0.9583333333333333703, 0.9642857142857143016 ),
 .UNSPECIFIED. ) 
 GEOMETRIC_REPRESENTATION_ITEM ( )  RATIONAL_B_SPLINE_SURFACE ( (
 ( 1.000000000000000000, 0.9659258262890683122, 1.000000000000000000, 0.9659258262890683122, 1.000000000000000000, 0.9659258262890683122, 1.000000000000000000, 0.9659258262890683122, 1.000000000000000000, 0.9659258262890683122, 1.000000000000000000, 0.9659258262890683122, 1.000000000000000000, 0.9659258262890683122, 1.000000000000000000, 0.9659258262890683122, 1.000000000000000000, 0.9659258262890683122, 1.000000000000000000, 0.9659258262890683122, 1.000000000000000000, 0.9659258262890683122, 1.000000000000000000, 0.9659258262890683122, 1.000000000000000000, 0.9659258262890683122, 1.000000000000000000, 0.9659258262890683122, 1.000000000000000000, 0.9659258262890683122, 1.000000000000000000, 0.9659258262890683122, 1.000000000000000000, 0.9659258262890683122, 1.000000000000000000, 0.9659258262890683122, 1.000000000000000000, 0.9659258262890683122, 1.000000000000000000, 0.9659258262890683122, 1.000000000000000000, 0.9659258262890683122, 1.000000000000000000, 0.9659258262890683122, 1.000000000000000000, 0.9659258262890683122, 1.000000000000000000, 0.9659258262890683122, 1.000000000000000000, 0.9659258262890683122, 1.000000000000000000, 0.9659258262890683122, 1.000000000000000000, 0.9659258262890683122, 1.000000000000000000, 0.9659258262890683122, 1.000000000000000000, 0.9659258262890683122, 1.000000000000000000, 0.9659258262890683122, 1.000000000000000000, 0.9659258262890683122, 1.000000000000000000, 0.9659258262890683122, 1.000000000000000000, 0.9659258262890683122, 1.000000000000000000, 0.9659258262890683122, 1.000000000000000000, 0.9659258262890683122, 1.000000000000000000, 0.9659258262890683122, 1.000000000000000000, 0.9659258262890683122, 1.000000000000000000, 0.9659258262890683122, 1.000000000000000000, 0.9659258262890683122, 1.000000000000000000, 0.9659258262890683122, 1.000000000000000000, 0.9659258262890683122, 1.000000000000000000, 0.9659258262890683122, 1.000000000000000000, 0.9659258262890683122, 1.000000000000000000, 0.9659258262890683122, 1.000000000000000000, 0.9659258262890683122, 1.000000000000000000, 0.9659258262890683122, 1.000000000000000000, 0.9659258262890683122, 1.000000000000000000, 0.9659258262890683122, 1.000000000000000000, 0.9659258262890683122, 1.000000000000000000, 0.9659258262890683122, 1.000000000000000000, 0.9659258262890683122, 1.000000000000000000, 0.9659258262890683122, 1.000000000000000000, 0.9659258262890683122, 1.000000000000000000, 0.9659258262890683122, 1.000000000000000000, 0.9659258262890683122, 1.000000000000000000, 0.9659258262890683122, 1.000000000000000000, 0.9659258262890683122, 1.000000000000000000, 0.9659258262890683122, 1.000000000000000000, 0.9659258262890683122, 1.000000000000000000, 0.9659258262890683122, 1.000000000000000000, 0.9659258262890683122, 1.000000000000000000, 0.9659258262890683122, 1.000000000000000000, 0.9659258262890683122, 1.000000000000000000, 0.9659258262890683122, 1.000000000000000000, 0.9659258262890683122, 1.000000000000000000, 0.9659258262890683122, 1.000000000000000000, 0.9659258262890683122, 1.000000000000000000, 0.9659258262890683122, 1.000000000000000000, 0.9659258262890683122, 1.000000000000000000, 0.9659258262890683122, 1.000000000000000000, 0.9659258262890683122, 1.000000000000000000, 0.9659258262890683122, 1.000000000000000000, 0.9659258262890683122, 1.000000000000000000, 0.9659258262890683122, 1.000000000000000000, 0.9659258262890683122, 1.000000000000000000, 0.9659258262890683122, 1.000000000000000000, 0.9659258262890683122, 1.000000000000000000, 0.9659258262890683122, 1.000000000000000000, 0.9659258262890683122, 1.000000000000000000, 0.9659258262890683122, 1.000000000000000000, 0.9659258262890683122, 1.000000000000000000, 0.9659258262890683122, 1.000000000000000000, 0.9659258262890683122, 1.000000000000000000, 0.9659258262890683122, 1.000000000000000000, 0.9659258262890683122, 1.000000000000000000, 0.9659258262890683122, 1.000000000000000000, 0.9659258262890683122, 1.000000000000000000, 0.9659258262890683122, 1.000000000000000000, 0.9659258262890683122, 1.000000000000000000, 0.9659258262890683122, 1.000000000000000000, 0.9659258262890683122, 1.000000000000000000, 0.9659258262890683122, 1.000000000000000000, 0.9659258262890683122, 1.000000000000000000, 0.9659258262890683122, 1.000000000000000000, 0.9659258262890683122, 1.000000000000000000, 0.9659258262890683122, 1.000000000000000000, 0.9659258262890683122, 1.000000000000000000, 0.9659258262890683122, 1.000000000000000000, 0.9659258262890683122, 1.000000000000000000, 0.9659258262890683122, 1.000000000000000000, 0.9659258262890683122, 1.000000000000000000, 0.9659258262890683122, 1.000000000000000000, 0.9659258262890683122, 1.000000000000000000, 0.9659258262890683122, 1.000000000000000000, 0.9659258262890683122, 1.000000000000000000, 0.9659258262890683122, 1.000000000000000000, 0.9659258262890683122, 1.000000000000000000, 0.9659258262890683122, 1.000000000000000000, 0.9659258262890683122, 1.000000000000000000, 0.9659258262890683122, 1.000000000000000000, 0.9659258262890683122, 1.000000000000000000, 0.9659258262890683122, 1.000000000000000000, 0.9659258262890683122, 1.000000000000000000, 0.9659258262890683122, 1.000000000000000000, 0.9659258262890683122, 1.000000000000000000, 0.9659258262890683122, 1.000000000000000000, 0.9659258262890683122, 1.000000000000000000, 0.9659258262890683122, 1.000000000000000000, 0.9659258262890683122, 1.000000000000000000, 0.9659258262890683122, 1.000000000000000000, 0.9659258262890683122, 1.000000000000000000, 0.9659258262890683122, 1.000000000000000000, 0.9659258262890683122, 1.000000000000000000, 0.9659258262890683122, 1.000000000000000000, 0.9659258262890683122, 1.000000000000000000, 0.9659258262890683122, 1.000000000000000000, 0.9659258262890683122, 1.000000000000000000, 0.9659258262890683122, 1.000000000000000000, 0.9659258262890683122, 1.000000000000000000, 0.9659258262890683122, 1.000000000000000000, 0.9659258262890683122, 1.000000000000000000, 0.9659258262890683122, 1.000000000000000000, 0.9659258262890683122, 1.000000000000000000, 0.9659258262890683122, 1.000000000000000000, 0.9659258262890683122, 1.000000000000000000, 0.9659258262890683122, 1.000000000000000000, 0.9659258262890683122, 1.000000000000000000, 0.9659258262890683122, 1.000000000000000000, 0.9659258262890683122, 1.000000000000000000, 0.9659258262890683122, 1.000000000000000000, 0.9659258262890683122, 1.000000000000000000, 0.9659258262890683122, 1.000000000000000000, 0.9659258262890683122, 1.000000000000000000, 0.9659258262890683122, 1.000000000000000000, 0.9659258262890683122, 1.000000000000000000, 0.9659258262890683122, 1.000000000000000000, 0.9659258262890683122, 1.000000000000000000, 0.9659258262890683122, 1.000000000000000000, 0.9659258262890683122, 1.000000000000000000, 0.9659258262890683122, 1.000000000000000000, 0.9659258262890683122, 1.000000000000000000, 0.9659258262890683122, 1.000000000000000000, 0.9659258262890683122, 1.000000000000000000, 0.9659258262890683122, 1.000000000000000000, 0.9659258262890683122, 1.000000000000000000, 0.9659258262890683122, 1.000000000000000000, 0.9659258262890683122, 1.000000000000000000, 0.9659258262890683122, 1.000000000000000000, 0.9659258262890683122, 1.000000000000000000, 0.9659258262890683122, 1.000000000000000000, 0.9659258262890683122, 1.000000000000000000, 0.9659258262890683122, 1.000000000000000000),
 ( 1.000000000000000000, 0.9659258262890683122, 1.000000000000000000, 0.9659258262890683122, 1.000000000000000000, 0.9659258262890683122, 1.000000000000000000, 0.9659258262890683122, 1.000000000000000000, 0.9659258262890683122, 1.000000000000000000, 0.9659258262890683122, 1.000000000000000000, 0.9659258262890683122, 1.000000000000000000, 0.9659258262890683122, 1.000000000000000000, 0.9659258262890683122, 1.000000000000000000, 0.9659258262890683122, 1.000000000000000000, 0.9659258262890683122, 1.000000000000000000, 0.9659258262890683122, 1.000000000000000000, 0.9659258262890683122, 1.000000000000000000, 0.9659258262890683122, 1.000000000000000000, 0.9659258262890683122, 1.000000000000000000, 0.9659258262890683122, 1.000000000000000000, 0.9659258262890683122, 1.000000000000000000, 0.9659258262890683122, 1.000000000000000000, 0.9659258262890683122, 1.000000000000000000, 0.9659258262890683122, 1.000000000000000000, 0.9659258262890683122, 1.000000000000000000, 0.9659258262890683122, 1.000000000000000000, 0.9659258262890683122, 1.000000000000000000, 0.9659258262890683122, 1.000000000000000000, 0.9659258262890683122, 1.000000000000000000, 0.9659258262890683122, 1.000000000000000000, 0.9659258262890683122, 1.000000000000000000, 0.9659258262890683122, 1.000000000000000000, 0.9659258262890683122, 1.000000000000000000, 0.9659258262890683122, 1.000000000000000000, 0.9659258262890683122, 1.000000000000000000, 0.9659258262890683122, 1.000000000000000000, 0.9659258262890683122, 1.000000000000000000, 0.9659258262890683122, 1.000000000000000000, 0.9659258262890683122, 1.000000000000000000, 0.9659258262890683122, 1.000000000000000000, 0.9659258262890683122, 1.000000000000000000, 0.9659258262890683122, 1.000000000000000000, 0.9659258262890683122, 1.000000000000000000, 0.9659258262890683122, 1.000000000000000000, 0.9659258262890683122, 1.000000000000000000, 0.9659258262890683122, 1.000000000000000000, 0.9659258262890683122, 1.000000000000000000, 0.9659258262890683122, 1.000000000000000000, 0.9659258262890683122, 1.000000000000000000, 0.9659258262890683122, 1.000000000000000000, 0.9659258262890683122, 1.000000000000000000, 0.9659258262890683122, 1.000000000000000000, 0.9659258262890683122, 1.000000000000000000, 0.9659258262890683122, 1.000000000000000000, 0.9659258262890683122, 1.000000000000000000, 0.9659258262890683122, 1.000000000000000000, 0.9659258262890683122, 1.000000000000000000, 0.9659258262890683122, 1.000000000000000000, 0.9659258262890683122, 1.000000000000000000, 0.9659258262890683122, 1.000000000000000000, 0.9659258262890683122, 1.000000000000000000, 0.9659258262890683122, 1.000000000000000000, 0.9659258262890683122, 1.000000000000000000, 0.9659258262890683122, 1.000000000000000000, 0.9659258262890683122, 1.000000000000000000, 0.9659258262890683122, 1.000000000000000000, 0.9659258262890683122, 1.000000000000000000, 0.9659258262890683122, 1.000000000000000000, 0.9659258262890683122, 1.000000000000000000, 0.9659258262890683122, 1.000000000000000000, 0.9659258262890683122, 1.000000000000000000, 0.9659258262890683122, 1.000000000000000000, 0.9659258262890683122, 1.000000000000000000, 0.9659258262890683122, 1.000000000000000000, 0.9659258262890683122, 1.000000000000000000, 0.9659258262890683122, 1.000000000000000000, 0.9659258262890683122, 1.000000000000000000, 0.9659258262890683122, 1.000000000000000000, 0.9659258262890683122, 1.000000000000000000, 0.9659258262890683122, 1.000000000000000000, 0.9659258262890683122, 1.000000000000000000, 0.9659258262890683122, 1.000000000000000000, 0.9659258262890683122, 1.000000000000000000, 0.9659258262890683122, 1.000000000000000000, 0.9659258262890683122, 1.000000000000000000, 0.9659258262890683122, 1.000000000000000000, 0.9659258262890683122, 1.000000000000000000, 0.9659258262890683122, 1.000000000000000000, 0.9659258262890683122, 1.000000000000000000, 0.9659258262890683122, 1.000000000000000000, 0.9659258262890683122, 1.000000000000000000, 0.9659258262890683122, 1.000000000000000000, 0.9659258262890683122, 1.000000000000000000, 0.9659258262890683122, 1.000000000000000000, 0.9659258262890683122, 1.000000000000000000, 0.9659258262890683122, 1.000000000000000000, 0.9659258262890683122, 1.000000000000000000, 0.9659258262890683122, 1.000000000000000000, 0.9659258262890683122, 1.000000000000000000, 0.9659258262890683122, 1.000000000000000000, 0.9659258262890683122, 1.000000000000000000, 0.9659258262890683122, 1.000000000000000000, 0.9659258262890683122, 1.000000000000000000, 0.9659258262890683122, 1.000000000000000000, 0.9659258262890683122, 1.000000000000000000, 0.9659258262890683122, 1.000000000000000000, 0.9659258262890683122, 1.000000000000000000, 0.9659258262890683122, 1.000000000000000000, 0.9659258262890683122, 1.000000000000000000, 0.9659258262890683122, 1.000000000000000000, 0.9659258262890683122, 1.000000000000000000, 0.9659258262890683122, 1.000000000000000000, 0.9659258262890683122, 1.000000000000000000, 0.9659258262890683122, 1.000000000000000000, 0.9659258262890683122, 1.000000000000000000, 0.9659258262890683122, 1.000000000000000000, 0.9659258262890683122, 1.000000000000000000, 0.9659258262890683122, 1.000000000000000000, 0.9659258262890683122, 1.000000000000000000, 0.9659258262890683122, 1.000000000000000000, 0.9659258262890683122, 1.000000000000000000, 0.9659258262890683122, 1.000000000000000000, 0.9659258262890683122, 1.000000000000000000, 0.9659258262890683122, 1.000000000000000000, 0.9659258262890683122, 1.000000000000000000, 0.9659258262890683122, 1.000000000000000000, 0.9659258262890683122, 1.000000000000000000, 0.9659258262890683122, 1.000000000000000000, 0.9659258262890683122, 1.000000000000000000, 0.9659258262890683122, 1.000000000000000000, 0.9659258262890683122, 1.000000000000000000, 0.9659258262890683122, 1.000000000000000000, 0.9659258262890683122, 1.000000000000000000, 0.9659258262890683122, 1.000000000000000000, 0.9659258262890683122, 1.000000000000000000, 0.9659258262890683122, 1.000000000000000000, 0.9659258262890683122, 1.000000000000000000, 0.9659258262890683122, 1.000000000000000000, 0.9659258262890683122, 1.000000000000000000, 0.9659258262890683122, 1.000000000000000000, 0.9659258262890683122, 1.000000000000000000, 0.9659258262890683122, 1.000000000000000000, 0.9659258262890683122, 1.000000000000000000, 0.9659258262890683122, 1.000000000000000000, 0.9659258262890683122, 1.000000000000000000, 0.9659258262890683122, 1.000000000000000000, 0.9659258262890683122, 1.000000000000000000, 0.9659258262890683122, 1.000000000000000000, 0.9659258262890683122, 1.000000000000000000, 0.9659258262890683122, 1.000000000000000000, 0.9659258262890683122, 1.000000000000000000, 0.9659258262890683122, 1.000000000000000000, 0.9659258262890683122, 1.000000000000000000, 0.9659258262890683122, 1.000000000000000000, 0.9659258262890683122, 1.000000000000000000, 0.9659258262890683122, 1.000000000000000000, 0.9659258262890683122, 1.000000000000000000, 0.9659258262890683122, 1.000000000000000000, 0.9659258262890683122, 1.000000000000000000, 0.9659258262890683122, 1.000000000000000000, 0.9659258262890683122, 1.000000000000000000, 0.9659258262890683122, 1.000000000000000000, 0.9659258262890683122, 1.000000000000000000, 0.9659258262890683122, 1.000000000000000000, 0.9659258262890683122, 1.000000000000000000, 0.9659258262890683122, 1.000000000000000000) ) ) 
 REPRESENTATION_ITEM ( '' )  SURFACE ( )  );
#5568=ORIENTED_EDGE ( 'NONE', *, *, #25107, .T. ) ;
#5569=CARTESIAN_POINT ( 'NONE',  ( -4.164238869374099039, 56.80374883491397497, 8.674139862899312516E-16 ) ) ;
#5570=CARTESIAN_POINT ( 'NONE',  ( -0.8801773607111009756, 3.063685344154838397, 1.068504757029289695E-15 ) ) ;
#5572=CARTESIAN_POINT ( 'NONE',  ( 14.92337183194729988, 29.34226448433411960, -8.527530157486177487 ) ) ;
#5574=CARTESIAN_POINT ( 'NONE',  ( -2.816281873526473856, 29.12363466993041783, 9.499525473075851096E-16 ) ) ;
#5577=CARTESIAN_POINT ( 'NONE',  ( 20.88017736071110519, 15.56368534415483751, 2.639326808657452039E-16 ) ) ;
#5578=CARTESIAN_POINT ( 'NONE',  ( -4.164238869374099927, 62.01208216824728936, 3.795296366450308767 ) ) ;
#5579=CARTESIAN_POINT ( 'NONE',  ( 17.20831665107776587, 22.88393115100078745, 7.208316651077764980 ) ) ;
#5582=CARTESIAN_POINT ( 'NONE',  ( 0.1532563361054083140, 11.00893115100078568, 1.131784320476157264E-15 ) ) ;
#5583=CARTESIAN_POINT ( 'NONE',  ( 18.61655166652078108, 59.87718327197428181, 6.499999999999962697 ) ) ;
#5589=CARTESIAN_POINT ( 'NONE',  ( 10.00000000000000178, 14.31368534415483929, 10.88017736071110342 ) ) ;
#5590=CARTESIAN_POINT ( 'NONE',  ( 4.559911319644449179, 18.89701867748817321, 9.422509992056141925 ) ) ;
#5591=CARTESIAN_POINT ( 'NONE',  ( 19.84674366389459266, 58.30059781766745886, 2.638427012816836559 ) ) ;
#5592=CARTESIAN_POINT ( 'NONE',  ( 6.565887622018943937, 20.16530133659708213, 12.81628187352647430 ) ) ;
#5593=CARTESIAN_POINT ( 'NONE',  ( -2.266590686148945544, 11.38708216824730179, -7.082119434687050408 ) ) ;
#5594=CARTESIAN_POINT ( 'NONE',  ( 22.81628187352647785, 36.41530133659707502, 3.434112377981063169 ) ) ;
#5596=CARTESIAN_POINT ( 'NONE',  ( 12.63842701281683922, 29.55059781766745175, -9.846743663894590881 ) ) ;
#5597=CARTESIAN_POINT ( 'NONE',  ( 12.91533473730992121, 4.522018677488170546, 10.88017736071110164 ) ) ;
#5599=CARTESIAN_POINT ( 'NONE',  ( 2.035157376598822676, 7.438685344154837509, -7.964842623401177768 ) ) ;
#5600=VERTEX_POINT ( 'NONE', #3178 ) ;
#5601=CARTESIAN_POINT ( 'NONE',  ( 15.44008868035555260, 49.73035201082150536, 9.422509992056143702 ) ) ;
#5602=CARTESIAN_POINT ( 'NONE',  ( 17.96484262340118221, 61.18868534415482685, -7.964842623401177768 ) ) ;
#5603=CARTESIAN_POINT ( 'NONE',  ( 2.035157376598822676, 47.43868534415484817, -7.964842623401177768 ) ) ;
#5606=CARTESIAN_POINT ( 'NONE',  ( 19.42250999205614548, 40.98035201082150536, -5.440088680355545492 ) ) ;
#5607=CARTESIAN_POINT ( 'NONE',  ( 1.492507162822263256, 47.19955587570481725, -6.500000000000077272 ) ) ;
#5609=CARTESIAN_POINT ( 'NONE',  ( 10.00000000000000000, 34.75893115100078745, -9.846743663894594434 ) ) ;
#5610=ORIENTED_EDGE ( 'NONE', *, *, #17730, .F. ) ;
#5611=CARTESIAN_POINT ( 'NONE',  ( 0.1532563361054100626, 55.80059781766745175, -2.638427012816831230 ) ) ;
#5614=CARTESIAN_POINT ( 'NONE',  ( 24.16423886937410614, 4.512082168247300906, -3.795296366450302550 ) ) ;
#5615=ORIENTED_EDGE ( 'NONE', *, *, #37205, .F. ) ;
#5619=CARTESIAN_POINT ( 'NONE',  ( 17.08211943468705840, 55.13708216824731068, -12.26659068614894466 ) ) ;
#5621=ORIENTED_EDGE ( 'NONE', *, *, #24086, .F. ) ;
#5623=CARTESIAN_POINT ( 'NONE',  ( 0.1532563361054100626, 45.80059781766745886, -2.638427012816831230 ) ) ;
#5624=DIRECTION ( 'NONE',  ( -0.000000000000000000, -1.000000000000000000, 0.000000000000000000 ) ) ;
#5625=CARTESIAN_POINT ( 'NONE',  ( 6.565887622018943937, 23.08196800326375708, -12.81628187352647608 ) ) ;
#5626=CARTESIAN_POINT ( 'NONE',  ( 0.1532563361054082862, 16.21726448433411960, 2.638427012816831674 ) ) ;
#5628=CARTESIAN_POINT ( 'NONE',  ( 18.52753015748618282, 3.925597817667451306, -4.923371831947291888 ) ) ;
#5629=CARTESIAN_POINT ( 'NONE',  ( 0.6178305044545838731, -0.2513653300695798953, 9.382169495545420901 ) ) ;
#5633=CARTESIAN_POINT ( 'NONE',  ( 17.96484262340118221, 16.18868534415483396, -7.964842623401177768 ) ) ;
#5634=CARTESIAN_POINT ( 'NONE',  ( 6.204703633549690345, 7.845415501580634832, 14.16423886937410082 ) ) ;
#5635=CARTESIAN_POINT ( 'NONE',  ( 10.00000000000000178, 22.25893115100078745, 9.846743663894594434 ) ) ;
#5636=CARTESIAN_POINT ( 'NONE',  ( 20.88017736071110875, 50.77201867748817676, -2.915334737309920765 ) ) ;
#5637=CARTESIAN_POINT ( 'NONE',  ( 21.09922568453595559, 32.04030133659708923, -6.408140936763230044 ) ) ;
#5639=CARTESIAN_POINT ( 'NONE',  ( 7.084665262690076126, 7.022018677488169658, -10.88017736071110164 ) ) ;
#5642=CARTESIAN_POINT ( 'NONE',  ( -2.816281873526473856, 4.123634669930420493, 9.499525473075851096E-16 ) ) ;
#5643=CARTESIAN_POINT ( 'NONE',  ( 19.84674366389459266, 63.30059781766745886, 2.638427012816836559 ) ) ;
#5644=CARTESIAN_POINT ( 'NONE',  ( 18.52753015748618282, 18.92559781766745175, -4.923371831947291888 ) ) ;
#5646=CARTESIAN_POINT ( 'NONE',  ( 13.43411237798106583, 22.66530133659708923, -12.81628187352647252 ) ) ;
#5647=CARTESIAN_POINT ( 'NONE',  ( 2.603489959281613420, 50.43575266056826933, -6.500000000000031086 ) ) ;
#5648=CARTESIAN_POINT ( 'NONE',  ( 19.42250999205614193, 45.14701867748817676, 5.440088680355555262 ) ) ;
#5652=EDGE_CURVE ( 'NONE', #97107, #57318, #38453, .T. ) ;
#5654=CARTESIAN_POINT ( 'NONE',  ( 0.5774900079438607392, 33.48035201082150536, 5.440088680355550821 ) ) ;
#5655=CARTESIAN_POINT ( 'NONE',  ( 12.91533473730993009, 26.60535201082150536, -10.88017736071109987 ) ) ;
#5656=CARTESIAN_POINT ( 'NONE',  ( 0.1532563361054100626, 50.80059781766745175, -2.638427012816831230 ) ) ;
#5657=CARTESIAN_POINT ( 'NONE',  ( 19.42250999205614548, 50.98035201082151247, -5.440088680355545492 ) ) ;
#5659=CARTESIAN_POINT ( 'NONE',  ( 24.16423886937410614, 29.30374883491396787, 8.672049930838204340E-16 ) ) ;
#5660=CARTESIAN_POINT ( 'NONE',  ( 0.1532563361054083140, 36.00893115100078745, 1.131784320476157264E-15 ) ) ;
#5661=CARTESIAN_POINT ( 'NONE',  ( 19.38216949554541202, 60.99863466993042493, 9.382169495545424454 ) ) ;
#5662=CARTESIAN_POINT ( 'NONE',  ( 22.81628187352648496, 1.831968003263753753, -3.434112377981050290 ) ) ;
#5664=CARTESIAN_POINT ( 'NONE',  ( 17.96484262340118221, 19.93868534415484106, 7.964842623401181321 ) ) ;
#5665=CARTESIAN_POINT ( 'NONE',  ( 10.00000000000000000, 6.813685344154838397, -10.88017736071110342 ) ) ;
#5666=CARTESIAN_POINT ( 'NONE',  ( 19.42250999205614193, 10.14701867748816966, 5.440088680355555262 ) ) ;
#5667=CARTESIAN_POINT ( 'NONE',  ( 12.91533473730993009, 66.60535201082150536, -10.88017736071109987 ) ) ;
#5668=CARTESIAN_POINT ( 'NONE',  ( -2.266590686148945544, 27.22041550158063572, 7.082119434687048631 ) ) ;
#5669=CARTESIAN_POINT ( 'NONE',  ( 1.472469842513823179, 20.59226448433411960, -4.923371831947296329 ) ) ;
#5670=CARTESIAN_POINT ( 'NONE',  ( 19.84674366389459266, 63.30059781766745886, 2.638427012816836559 ) ) ;
#5671=CARTESIAN_POINT ( 'NONE',  ( 7.084665262690076126, 29.10535201082150181, 10.88017736071109987 ) ) ;
#5675=CARTESIAN_POINT ( 'NONE',  ( 3.558677480090427281, 70.40124509038875544, 5.000000000000000000 ) ) ;
#5676=CARTESIAN_POINT ( 'NONE',  ( 19.84674366389459621, 43.50893115100078745, 7.409399052514197653E-17 ) ) ;
#5680=CARTESIAN_POINT ( 'NONE',  ( -4.164238869374099927, 27.01208216824730357, 3.795296366450308767 ) ) ;
#5681=CARTESIAN_POINT ( 'NONE',  ( 13.79529636645030344, 13.26208216824729824, 14.16423886937410614 ) ) ;
#5682=EDGE_CURVE ( 'NONE', #507, #90918, #33633, .T. ) ;
#5683=CARTESIAN_POINT ( 'NONE',  ( 20.88017736071110519, 60.56368534415484106, 2.639326808657452039E-16 ) ) ;
#5684=CARTESIAN_POINT ( 'NONE',  ( 6.204703633549690345, 57.84541550158063927, 14.16423886937410082 ) ) ;
#5685=CARTESIAN_POINT ( 'NONE',  ( 0.6178305044545818747, -1.501365330069579951, -9.382169495545419124 ) ) ;
#5686=CARTESIAN_POINT ( 'NONE',  ( 19.84674366389459621, 48.50893115100078745, 7.409399052514197653E-17 ) ) ;
#5687=CARTESIAN_POINT ( 'NONE',  ( 19.42250999205614548, 40.98035201082150536, -5.440088680355545492 ) ) ;
#5688=CARTESIAN_POINT ( 'NONE',  ( 0.6178305044545838731, -0.2513653300695798953, 9.382169495545420901 ) ) ;
#5689=CARTESIAN_POINT ( 'NONE',  ( 10.00000000000000000, 15.55374883491396787, -14.16423886937410082 ) ) ;
#5691=CARTESIAN_POINT ( 'NONE',  ( 20.88017736071110519, 15.56368534415483751, 2.639326808657452039E-16 ) ) ;
#5692=CARTESIAN_POINT ( 'NONE',  ( 20.04068437667225666, 14.71974360917720226, 6.396802510829714628 ) ) ;
#5694=CARTESIAN_POINT ( 'NONE',  ( -0.8801773607110991993, 47.85535201082150536, -2.915334737309923874 ) ) ;
#5696=EDGE_LOOP ( 'NONE', ( #72256, #44786, #30246, #34006 ) ) ;
#5699=ORIENTED_EDGE ( 'NONE', *, *, #5339, .T. ) ;
#5700=CARTESIAN_POINT ( 'NONE',  ( 17.08211943468705130, 43.47041550158063927, 12.26659068614894998 ) ) ;
#5701=CARTESIAN_POINT ( 'NONE',  ( 0.1532563361054083140, 46.00893115100079456, 1.131784320476157264E-15 ) ) ;
#5702=CARTESIAN_POINT ( 'NONE',  ( 12.91533473730992121, 64.52201867748817676, 10.88017736071110164 ) ) ;
#5704=CARTESIAN_POINT ( 'NONE',  ( 19.42250999205614193, 60.14701867748817676, 5.440088680355555262 ) ) ;
#5706=CARTESIAN_POINT ( 'NONE',  ( -1.099225684535947600, 54.54030133659708923, 6.408140936763237150 ) ) ;
#5709=CARTESIAN_POINT ( 'NONE',  ( 2.917880565312948704, 22.63708216824730002, 12.26659068614894643 ) ) ;
#5710=CARTESIAN_POINT ( 'NONE',  ( 3.591859063236763294, 18.29030133659708568, -11.09922568453595026 ) ) ;
#5712=CARTESIAN_POINT ( 'NONE',  ( 6.565887622018943937, 45.16530133659708923, 12.81628187352647430 ) ) ;
#5714=CARTESIAN_POINT ( 'NONE',  ( 2.791683348922240793, 31.63393115100078745, 7.208316651077764092 ) ) ;
#5715=CARTESIAN_POINT ( 'NONE',  ( 7.084665262690076126, 9.105352010821503583, 10.88017736071109987 ) ) ;
#5716=CARTESIAN_POINT ( 'NONE',  ( 0.6178305044545818747, 53.49863466993041072, -9.382169495545419124 ) ) ;
#5718=CARTESIAN_POINT ( 'NONE',  ( 18.52753015748617571, 48.09226448433412315, 4.923371831947298993 ) ) ;
#5720=EDGE_CURVE ( 'NONE', #4379, #97455, #15796, .T. ) ;
#5721=CARTESIAN_POINT ( 'NONE',  ( 18.72515096720568550, 20.05509018479935790, 6.500000000000015099 ) ) ;
#5725=CARTESIAN_POINT ( 'NONE',  ( 14.49999999999999822, 60.50000000000000000, 6.000000000000000000 ) ) ;
#5728=CARTESIAN_POINT ( 'NONE',  ( 19.84674366389459266, 13.71726448433411782, -2.638427012816827677 ) ) ;
#5729=CARTESIAN_POINT ( 'NONE',  ( -2.816281873526473856, 19.33196800326375708, 3.434112377981055619 ) ) ;
#5732=ORIENTED_EDGE ( 'NONE', *, *, #57354, .F. ) ;
#5733=CARTESIAN_POINT ( 'NONE',  ( 18.52753015748617571, 58.09226448433411605, 4.923371831947298993 ) ) ;
#5734=CARTESIAN_POINT ( 'NONE',  ( 18.72515096720570327, 6.072280503510315341, -6.499999999999985789 ) ) ;
#5735=CARTESIAN_POINT ( 'NONE',  ( 20.36894250292379738, 24.92874883491396787, -10.36894250292379027 ) ) ;
#5736=CARTESIAN_POINT ( 'NONE',  ( 17.20831665107776587, 47.88393115100078745, 7.208316651077764980 ) ) ;
#5737=CARTESIAN_POINT ( 'NONE',  ( 16.40814093676324603, 42.45696800326375353, -11.09922568453594671 ) ) ;
#5739=CARTESIAN_POINT ( 'NONE',  ( 7.361572987183169658, 9.967264484334119601, -9.846743663894592657 ) ) ;
#5740=CARTESIAN_POINT ( 'NONE',  ( 14.92337183194729633, 37.67559781766745175, 8.527530157486181039 ) ) ;
#5741=CARTESIAN_POINT ( 'NONE',  ( 20.88017736071110519, 40.56368534415484106, 2.639326808657452039E-16 ) ) ;
#5743=CARTESIAN_POINT ( 'NONE',  ( 14.92337183194729988, 34.34226448433411605, -8.527530157486177487 ) ) ;
#5747=CARTESIAN_POINT ( 'NONE',  ( 7.084665262690076126, 52.02201867748816255, -10.88017736071110164 ) ) ;
#5748=STYLED_ITEM ( 'NONE', ( #82397 ), #86608 ) ;
#5751=CARTESIAN_POINT ( 'NONE',  ( 19.42250999205614548, 10.98035201082150358, -5.440088680355545492 ) ) ;
#5752=CARTESIAN_POINT ( 'NONE',  ( 19.84674366389459266, 58.71726448433411605, -2.638427012816827677 ) ) ;
#5753=CARTESIAN_POINT ( 'NONE',  ( 17.96484262340118221, 44.93868534415483396, 7.964842623401181321 ) ) ;
#5755=CARTESIAN_POINT ( 'NONE',  ( 15.44008868035555793, 56.39701867748817676, -9.422509992056140149 ) ) ;
#5756=CARTESIAN_POINT ( 'NONE',  ( 20.88017736071110519, 20.56368534415484106, 2.639326808657452039E-16 ) ) ;
#5758=CARTESIAN_POINT ( 'NONE',  ( 18.72515096720571037, 50.05509018479936856, 6.499999999999982236 ) ) ;
#5759=CARTESIAN_POINT ( 'NONE',  ( 18.52753015748618282, 18.92559781766745175, -4.923371831947291888 ) ) ;
#5760=CARTESIAN_POINT ( 'NONE',  ( -46.68456736488007408, 103.6675473310227034, 5.000000000000000000 ) ) ;
#5762=CARTESIAN_POINT ( 'NONE',  ( 17.20831665107776587, 49.13393115100078745, -7.208316651077762316 ) ) ;
#5763=CARTESIAN_POINT ( 'NONE',  ( -4.164238869374099927, 62.01208216824728936, 3.795296366450308767 ) ) ;
#5764=CARTESIAN_POINT ( 'NONE',  ( 2.153642693323417845, 61.13791097397316321, -6.499999999999922728 ) ) ;
#5765=CARTESIAN_POINT ( 'NONE',  ( 20.36894250292379382, 13.67874883491396965, 10.36894250292379205 ) ) ;
#5767=CARTESIAN_POINT ( 'NONE',  ( 22.26659068614894466, 33.88708216824730357, 7.082119434687054849 ) ) ;
#5768=CARTESIAN_POINT ( 'NONE',  ( 0.6178305044545838731, 9.748634669930416052, 9.382169495545420901 ) ) ;
#5770=CARTESIAN_POINT ( 'NONE',  ( 20.88017736071110875, 15.77201867748817143, -2.915334737309920765 ) ) ;
#5771=EDGE_CURVE ( 'NONE', #59748, #53014, #17034, .T. ) ;
#5772=CARTESIAN_POINT ( 'NONE',  ( 10.00000000000000178, 52.25893115100078745, 9.846743663894594434 ) ) ;
#5776=CARTESIAN_POINT ( 'NONE',  ( 14.92337183194729988, 4.342264484334117824, -8.527530157486177487 ) ) ;
#5777=CARTESIAN_POINT ( 'NONE',  ( 0.6178305044545838731, 29.74863466993042138, 9.382169495545420901 ) ) ;
#5778=CARTESIAN_POINT ( 'NONE',  ( 5.076628168052703671, 26.84226448433411960, 8.527530157486179263 ) ) ;
#5779=EDGE_LOOP ( 'NONE', ( #78866, #86254, #22881, #76246 ) ) ;
#5780=CARTESIAN_POINT ( 'NONE',  ( 18.52753015748617571, 3.092264484334118269, 4.923371831947298993 ) ) ;
#5783=CARTESIAN_POINT ( 'NONE',  ( 7.084665262690076126, 17.02201867748817676, -10.88017736071110164 ) ) ;
#5784=CARTESIAN_POINT ( 'NONE',  ( -2.266590686148945544, 42.22041550158063217, 7.082119434687048631 ) ) ;
#5785=CARTESIAN_POINT ( 'NONE',  ( 10.00000000000000178, 59.31368534415484106, 10.88017736071110342 ) ) ;
#5786=CARTESIAN_POINT ( 'NONE',  ( 14.92337183194729988, 19.34226448433411960, -8.527530157486177487 ) ) ;
#5787=CARTESIAN_POINT ( 'NONE',  ( 17.20831665107776587, 9.133931151000787452, -7.208316651077762316 ) ) ;
#5788=CARTESIAN_POINT ( 'NONE',  ( -1.468748247964608566, 5.397528278722328812E-15, 2.247705202101426103 ) ) ;
#5789=CARTESIAN_POINT ( 'NONE',  ( 7.361572987183169658, 34.96726448433411605, -9.846743663894592657 ) ) ;
#5790=CARTESIAN_POINT ( 'NONE',  ( 12.63842701281683034, 57.46726448433411605, 9.846743663894596210 ) ) ;
#5793=CARTESIAN_POINT ( 'NONE',  ( 12.91533473730993009, 36.60535201082151247, -10.88017736071109987 ) ) ;
#5794=ORIENTED_EDGE ( 'NONE', *, *, #82294, .T. ) ;
#5795=CARTESIAN_POINT ( 'NONE',  ( -2.816281873526471635, 63.91530133659708923, -3.434112377981056508 ) ) ;
#5798=CARTESIAN_POINT ( 'NONE',  ( 17.96484262340118221, 66.18868534415483396, -7.964842623401177768 ) ) ;
#5799=CARTESIAN_POINT ( 'NONE',  ( 21.09922568453594849, 46.20696800326376064, 6.408140936763242479 ) ) ;
#5800=CARTESIAN_POINT ( 'NONE',  ( 24.16423886937410614, 64.51208216824728936, -3.795296366450302550 ) ) ;
#5801=CARTESIAN_POINT ( 'NONE',  ( 2.791683348922240793, 36.63393115100078035, 7.208316651077764092 ) ) ;
#5802=CARTESIAN_POINT ( 'NONE',  ( 2.917880565312948704, 42.63708216824729647, 12.26659068614894643 ) ) ;
#5803=CARTESIAN_POINT ( 'NONE',  ( 18.52753015748617571, 48.09226448433412315, 4.923371831947298993 ) ) ;
#5805=CARTESIAN_POINT ( 'NONE',  ( -0.8801773607111008646, 43.27201867748817676, 2.915334737309923430 ) ) ;
#5807=CARTESIAN_POINT ( 'NONE',  ( 2.791683348922237240, 0.3839311510007847872, -7.208316651077763204 ) ) ;
#5808=CARTESIAN_POINT ( 'NONE',  ( 1.959929470562272291, 55.51528370094808906, -5.767676674365837641 ) ) ;
#5810=CARTESIAN_POINT ( 'NONE',  ( 19.38216949554541202, 60.99863466993042493, 9.382169495545424454 ) ) ;
#5812=CARTESIAN_POINT ( 'NONE',  ( 19.84674366389459621, 3.508931151000785231, 7.409399052514197653E-17 ) ) ;
#5814=CARTESIAN_POINT ( 'NONE',  ( 0.1532563361054083140, 1.008931151000784787, 1.131784320476157264E-15 ) ) ;
#5815=CARTESIAN_POINT ( 'NONE',  ( 1.361758211743682168, 0.02824709245459683729, -6.170260303628292142 ) ) ;
#5816=COLOUR_RGB ( '', 0.08235294, 0.09019608, 0.10196078) ;
#5819=CARTESIAN_POINT ( 'NONE',  ( 7.084665262690076126, 14.10535201082150358, 10.88017736071109987 ) ) ;
#5822=CARTESIAN_POINT ( 'NONE',  ( 10.00000000000000000, 21.81368534415484106, -10.88017736071110342 ) ) ;
#5823=CARTESIAN_POINT ( 'NONE',  ( 7.361572987183170547, 62.05059781766745886, 9.846743663894590881 ) ) ;
#5825=CARTESIAN_POINT ( 'NONE',  ( 1.472469842513823179, 65.59226448433412315, -4.923371831947296329 ) ) ;
#5827=CARTESIAN_POINT ( 'NONE',  ( 20.88017736071110519, 60.56368534415484106, 2.639326808657452039E-16 ) ) ;
#5828=CARTESIAN_POINT ( 'NONE',  ( 5.076628168052704559, 65.17559781766745175, -8.527530157486179263 ) ) ;
#5829=CARTESIAN_POINT ( 'NONE',  ( 3.591859063236761518, 39.95696800326375353, 11.09922568453594849 ) ) ;
#5830=CARTESIAN_POINT ( 'NONE',  ( 20.88017736071110164, 5.355352010821502695, 2.915334737309930979 ) ) ;
#5832=CARTESIAN_POINT ( 'NONE',  ( 0.1532563361054083140, 1.008931151000784787, 1.131784320476157264E-15 ) ) ;
#5833=CARTESIAN_POINT ( 'NONE',  ( 15.44008868035555260, 24.73035201082150891, 9.422509992056143702 ) ) ;
#5836=ORIENTED_EDGE ( 'NONE', *, *, #96583, .F. ) ;
#5838=CARTESIAN_POINT ( 'NONE',  ( -2.816281873526471635, 53.91530133659709634, -3.434112377981056508 ) ) ;
#5839=CARTESIAN_POINT ( 'NONE',  ( -0.8801773607111008646, 43.27201867748817676, 2.915334737309923430 ) ) ;
#5841=CARTESIAN_POINT ( 'NONE',  ( 10.00000000000000178, 60.37363466993041783, 12.81628187352647608 ) ) ;
#5842=CARTESIAN_POINT ( 'NONE',  ( 19.42250999205614193, 50.14701867748817676, 5.440088680355555262 ) ) ;
#5843=CARTESIAN_POINT ( 'NONE',  ( 1.472469842513823179, 60.59226448433412315, -4.923371831947296329 ) ) ;
#5844=CARTESIAN_POINT ( 'NONE',  ( 0.1129803114748853671, 49.29427333184091964, -6.480634945678684922 ) ) ;
#5845=B_SPLINE_CURVE_WITH_KNOTS ( 'NONE', 3,
 ( #87370, #63385, #86398, #63862, #9409, #55405 ),
 .UNSPECIFIED., .F., .F.,
 ( 4, 2, 4 ),
 ( 0.000000000000000000, 0.0002605067024380848333, 0.0005210134048761696666 ),
 .UNSPECIFIED. ) ;
#5846=CARTESIAN_POINT ( 'NONE',  ( 12.63842701281683922, 19.55059781766745175, -9.846743663894590881 ) ) ;
#5847=CARTESIAN_POINT ( 'NONE',  ( 6.565887622018943937, 3.081968003263753531, -12.81628187352647608 ) ) ;
#5848=FACE_OUTER_BOUND ( 'NONE', #62243, .T. ) ;
#5849=CARTESIAN_POINT ( 'NONE',  ( 19.50000000000000711, 105.0000000000000000, 4.500000000000000888 ) ) ;
#5850=CARTESIAN_POINT ( 'NONE',  ( 20.88017736071110519, 25.56368534415483751, 2.639326808657452039E-16 ) ) ;
#5851=CARTESIAN_POINT ( 'NONE',  ( 0.1532563361054083140, 56.00893115100078745, 1.131784320476157264E-15 ) ) ;
#5852=CARTESIAN_POINT ( 'NONE',  ( 17.20831665107776587, 4.133931151000785675, -7.208316651077762316 ) ) ;
#5854=CARTESIAN_POINT ( 'NONE',  ( 3.591859063236763294, 3.290301336597087012, -11.09922568453595026 ) ) ;
#5855=ORIENTED_EDGE ( 'NONE', *, *, #56361, .T. ) ;
#5858=CARTESIAN_POINT ( 'NONE',  ( -2.816281873526473856, 44.33196800326375353, 3.434112377981055619 ) ) ;
#5859=CARTESIAN_POINT ( 'NONE',  ( 7.361572987183170547, 32.05059781766745175, 9.846743663894590881 ) ) ;
#5861=CARTESIAN_POINT ( 'NONE',  ( 4.559911319644449179, 12.23035201082150714, -9.422509992056141925 ) ) ;
#5862=CARTESIAN_POINT ( 'NONE',  ( 5.076628168052703671, 36.84226448433412315, 8.527530157486179263 ) ) ;
#5863=VECTOR ( 'NONE', #21053, 1000.000000000000000 ) ;
#5867=CARTESIAN_POINT ( 'NONE',  ( 22.26659068614894466, 63.88708216824730357, 7.082119434687054849 ) ) ;
#5869=CARTESIAN_POINT ( 'NONE',  ( 4.559911319644449179, 13.89701867748817321, 9.422509992056141925 ) ) ;
#5870=CARTESIAN_POINT ( 'NONE',  ( 13.79529636645030344, 43.26208216824730357, 14.16423886937410614 ) ) ;
#5871=CARTESIAN_POINT ( 'NONE',  ( 6.204703633549690345, 50.76208216824730357, -14.16423886937410259 ) ) ;
#5873=CARTESIAN_POINT ( 'NONE',  ( 18.52753015748618282, 13.92559781766745175, -4.923371831947291888 ) ) ;
#5874=CARTESIAN_POINT ( 'NONE',  ( 6.565887622018943937, -1.918031996736246692, -12.81628187352647608 ) ) ;
#5875=CARTESIAN_POINT ( 'NONE',  ( 19.42250999205614193, 45.14701867748817676, 5.440088680355555262 ) ) ;
#5878=CARTESIAN_POINT ( 'NONE',  ( 1.472469842513823179, 66.42559781766745175, 4.923371831947296329 ) ) ;
#5879=CARTESIAN_POINT ( 'NONE',  ( -4.164238869374099039, 1.803748834913967647, 8.674139862899312516E-16 ) ) ;
#5881=CARTESIAN_POINT ( 'NONE',  ( 10.00000000000000000, 29.75893115100078745, -9.846743663894594434 ) ) ;
#5884=CARTESIAN_POINT ( 'NONE',  ( 22.26659068614894466, 43.88708216824729647, 7.082119434687054849 ) ) ;
#5887=EDGE_CURVE ( 'NONE', #31069, #43200, #20133, .T. ) ;
#5888=CARTESIAN_POINT ( 'NONE',  ( 7.361572987183169658, 14.96726448433411960, -9.846743663894592657 ) ) ;
#5889=FILL_AREA_STYLE_COLOUR ( '', #83789 ) ;
#5890=CARTESIAN_POINT ( 'NONE',  ( 10.00000000000000178, 34.31368534415484106, 10.88017736071110342 ) ) ;
#5891=CARTESIAN_POINT ( 'NONE',  ( 16.40814093676323893, 35.79030133659708923, 11.09922568453595026 ) ) ;
#5892=( BOUNDED_CURVE ( )  B_SPLINE_CURVE ( 2, ( #7354, #20868, #54304, #15842, #46807, #91828, #54791, #93293, #45842 ),
 .UNSPECIFIED., .F., .F. ) 
 B_SPLINE_CURVE_WITH_KNOTS ( ( 3, 2, 2, 2, 3 ),
 ( 0.2258552226545170460, 0.2261904761904761640, 0.2321428571428572063, 0.2380952380952381375, 0.2384304916311972555 ),
 .UNSPECIFIED. ) 
 CURVE ( )  GEOMETRIC_REPRESENTATION_ITEM ( )  RATIONAL_B_SPLINE_CURVE ( ( 0.9963778908391762723, 0.9980808541467921513, 1.000000000000000000, 0.9659258262890683122, 1.000000000000000000, 0.9659258262890683122, 1.000000000000000000, 0.9980808541467921513, 0.9963778908391762723 ) ) 
 REPRESENTATION_ITEM ( '' )  );
#5893=CARTESIAN_POINT ( 'NONE',  ( -0.8801773607111009756, 3.063685344154837509, 1.068504757029289695E-15 ) ) ;
#5894=CARTESIAN_POINT ( 'NONE',  ( 6.565887622018943937, 35.16530133659708923, 12.81628187352647430 ) ) ;
#5895=CARTESIAN_POINT ( 'NONE',  ( 10.00000000000000000, 57.87363466993042493, -12.81628187352647608 ) ) ;
#5897=CARTESIAN_POINT ( 'NONE',  ( -4.164238869374099039, 46.80374883491397497, 8.674139862899312516E-16 ) ) ;
#5899=CARTESIAN_POINT ( 'NONE',  ( 17.96484262340118221, 9.938685344154837509, 7.964842623401181321 ) ) ;
#5900=CARTESIAN_POINT ( 'NONE',  ( -0.8801773607111008646, 18.27201867748817321, 2.915334737309923430 ) ) ;
#5903=CARTESIAN_POINT ( 'NONE',  ( 12.91533473730992121, 54.52201867748816255, 10.88017736071110164 ) ) ;
#5904=CARTESIAN_POINT ( 'NONE',  ( 15.44008868035555260, 49.73035201082150536, 9.422509992056143702 ) ) ;
#5905=CARTESIAN_POINT ( 'NONE',  ( 16.40814093676324603, 17.45696800326375353, -11.09922568453594671 ) ) ;
#5906=FACE_OUTER_BOUND ( 'NONE', #48931, .T. ) ;
#5908=CARTESIAN_POINT ( 'NONE',  ( 1.472469842513823179, 25.59226448433412315, -4.923371831947296329 ) ) ;
#5909=CARTESIAN_POINT ( 'NONE',  ( -0.8801773607111009756, 58.06368534415484106, 1.068504757029289695E-15 ) ) ;
#5910=STYLED_ITEM ( 'NONE', ( #81472 ), #56452 ) ;
#5911=AXIS2_PLACEMENT_3D ( 'NONE', #24622, #2132, #91629 ) ;
#5913=CARTESIAN_POINT ( 'NONE',  ( 22.81628187352647785, 21.41530133659708923, 3.434112377981063169 ) ) ;
#5914=CARTESIAN_POINT ( 'NONE',  ( 0.1532563361054083140, 1.008931151000784787, 1.131784320476157264E-15 ) ) ;
#5915=CARTESIAN_POINT ( 'NONE',  ( 14.92337183194729988, 44.34226448433412315, -8.527530157486177487 ) ) ;
#5916=CARTESIAN_POINT ( 'NONE',  ( -2.816281873526471635, 43.91530133659708923, -3.434112377981056508 ) ) ;
#5917=CARTESIAN_POINT ( 'NONE',  ( 10.00000000000000000, 24.75893115100078745, -9.846743663894594434 ) ) ;
#5918=CARTESIAN_POINT ( 'NONE',  ( 6.204703633549690345, 0.7620821682473009062, -14.16423886937410259 ) ) ;
#5920=CARTESIAN_POINT ( 'NONE',  ( 12.91533473730993009, 16.60535201082150891, -10.88017736071109987 ) ) ;
#5922=CARTESIAN_POINT ( 'NONE',  ( 22.26659068614895176, 29.72041550158063572, -7.082119434687042414 ) ) ;
#5924=CARTESIAN_POINT ( 'NONE',  ( 7.361572987183170547, 32.05059781766745175, 9.846743663894590881 ) ) ;
#5925=CARTESIAN_POINT ( 'NONE',  ( 15.44008868035555260, 19.73035201082150536, 9.422509992056143702 ) ) ;
#5927=CARTESIAN_POINT ( 'NONE',  ( -0.8801773607111008646, 23.27201867748817676, 2.915334737309923430 ) ) ;
#5930=CARTESIAN_POINT ( 'NONE',  ( 17.96484262340118221, 26.18868534415483396, -7.964842623401177768 ) ) ;
#5931=CARTESIAN_POINT ( 'NONE',  ( -1.099225684535947600, 43.70696800326375353, -6.408140936763238038 ) ) ;
#5932=CARTESIAN_POINT ( 'NONE',  ( 4.559911319644449179, 38.89701867748817676, 9.422509992056141925 ) ) ;
#5934=CARTESIAN_POINT ( 'NONE',  ( 0.5774900079438607392, 38.48035201082150536, 5.440088680355550821 ) ) ;
#5937=CARTESIAN_POINT ( 'NONE',  ( 18.52753015748618282, 58.92559781766745886, -4.923371831947291888 ) ) ;
#5938=CARTESIAN_POINT ( 'NONE',  ( 20.88017736071110519, 35.56368534415484106, 2.639326808657452039E-16 ) ) ;
#5941=CARTESIAN_POINT ( 'NONE',  ( -2.816281873526473856, 59.33196800326374643, 3.434112377981055619 ) ) ;
#5943=CARTESIAN_POINT ( 'NONE',  ( -2.266590686148945544, 52.22041550158064638, 7.082119434687048631 ) ) ;
#5944=CARTESIAN_POINT ( 'NONE',  ( 4.559911319644449179, 53.89701867748817676, 9.422509992056141925 ) ) ;
#5945=CARTESIAN_POINT ( 'NONE',  ( 1.472469842513823179, 66.42559781766745175, 4.923371831947296329 ) ) ;
#5948=CARTESIAN_POINT ( 'NONE',  ( 18.52753015748618282, 53.92559781766745175, -4.923371831947291888 ) ) ;
#5949=CARTESIAN_POINT ( 'NONE',  ( 7.361572987183169658, 14.96726448433411960, -9.846743663894592657 ) ) ;
#5951=CARTESIAN_POINT ( 'NONE',  ( 0.1532563361054082862, 26.21726448433411605, 2.638427012816831674 ) ) ;
#5953=CARTESIAN_POINT ( 'NONE',  ( 2.035157376598824452, 28.68868534415484106, 7.964842623401179544 ) ) ;
#5954=CARTESIAN_POINT ( 'NONE',  ( 5.076628168052703671, 26.84226448433411960, 8.527530157486179263 ) ) ;
#5955=CARTESIAN_POINT ( 'NONE',  ( 12.91533473730992121, 64.52201867748817676, 10.88017736071110164 ) ) ;
#5956=CARTESIAN_POINT ( 'NONE',  ( 2.035157376598822676, 52.43868534415483396, -7.964842623401177768 ) ) ;
#5957=CARTESIAN_POINT ( 'NONE',  ( -0.8801773607110991993, 37.85535201082151247, -2.915334737309923874 ) ) ;
#5958=CARTESIAN_POINT ( 'NONE',  ( 19.38216949554541557, 57.24863466993042493, -9.382169495545420901 ) ) ;
#5959=CARTESIAN_POINT ( 'NONE',  ( 13.79529636645031943, 50.34541550158064638, -14.16423886937409904 ) ) ;
#5962=CARTESIAN_POINT ( 'NONE',  ( 3.591859063236761518, 4.956968003263753531, 11.09922568453594849 ) ) ;
#5963=CARTESIAN_POINT ( 'NONE',  ( 0.5774900079438590739, 2.647018677488170990, -5.440088680355550821 ) ) ;
#5964=CARTESIAN_POINT ( 'NONE',  ( 7.084665262690076126, 52.02201867748816255, -10.88017736071110164 ) ) ;
#5965=( NAMED_UNIT ( * ) SI_UNIT ( $, .STERADIAN. ) SOLID_ANGLE_UNIT ( ) );
#5966=ORIENTED_EDGE ( 'NONE', *, *, #11212, .T. ) ;
#5967=CARTESIAN_POINT ( 'NONE',  ( 1.472469842513823179, 16.42559781766745175, 4.923371831947296329 ) ) ;
#5969=CARTESIAN_POINT ( 'NONE',  ( 10.00000000000000000, 56.81368534415484106, -10.88017736071110342 ) ) ;
#5970=CARTESIAN_POINT ( 'NONE',  ( 19.84674366389459266, 33.30059781766744464, 2.638427012816836559 ) ) ;
#5971=CARTESIAN_POINT ( 'NONE',  ( 17.20831665107776587, 27.88393115100078390, 7.208316651077764980 ) ) ;
#5972=CARTESIAN_POINT ( 'NONE',  ( 1.472469842513823179, 16.42559781766745175, 4.923371831947296329 ) ) ;
#5975=CARTESIAN_POINT ( 'NONE',  ( 22.81628187352647785, 36.62363466993041783, 6.195893100308588602E-16 ) ) ;
#5976=CARTESIAN_POINT ( 'NONE',  ( 12.91533473730992121, 64.52201867748817676, 10.88017736071110164 ) ) ;
#5980=CARTESIAN_POINT ( 'NONE',  ( 17.20831665107776587, 37.88393115100078745, 7.208316651077764980 ) ) ;
#5981=ORIENTED_EDGE ( 'NONE', *, *, #47684, .F. ) ;
#5983=CARTESIAN_POINT ( 'NONE',  ( 16.40814093676323893, 55.79030133659708923, 11.09922568453595026 ) ) ;
#5984=CARTESIAN_POINT ( 'NONE',  ( 17.39651004071838969, 54.08210964143329846, -6.500000000000027534 ) ) ;
#5985=CARTESIAN_POINT ( 'NONE',  ( 17.20831665107776587, 64.13393115100079456, -7.208316651077762316 ) ) ;
#5986=CARTESIAN_POINT ( 'NONE',  ( 0.5774900079438607392, 3.480352010821504027, 5.440088680355550821 ) ) ;
#5987=CARTESIAN_POINT ( 'NONE',  ( 22.26659068614894466, 13.88708216824730179, 7.082119434687054849 ) ) ;
#5989=CARTESIAN_POINT ( 'NONE',  ( 2.917880565312950480, 30.97041550158063572, -12.26659068614894821 ) ) ;
#5990=CARTESIAN_POINT ( 'NONE',  ( 6.204703633549690345, 42.84541550158063217, 14.16423886937410082 ) ) ;
#5991=CARTESIAN_POINT ( 'NONE',  ( 6.204703633549690345, 15.76208216824730179, -14.16423886937410259 ) ) ;
#5992=CARTESIAN_POINT ( 'NONE',  ( -2.266590686148945544, 16.38708216824730357, -7.082119434687050408 ) ) ;
#5993=CARTESIAN_POINT ( 'NONE',  ( 19.42250999205614548, 65.98035201082151957, -5.440088680355545492 ) ) ;
#5994=CARTESIAN_POINT ( 'NONE',  ( 20.88017736071110519, 50.56368534415484106, 2.639326808657452039E-16 ) ) ;
#5996=CARTESIAN_POINT ( 'NONE',  ( 5.076628168052703671, 31.84226448433412315, 8.527530157486179263 ) ) ;
#5998=CARTESIAN_POINT ( 'NONE',  ( 17.96484262340118221, 64.93868534415483396, 7.964842623401181321 ) ) ;
#5999=CARTESIAN_POINT ( 'NONE',  ( 0.1532563361054100626, 25.80059781766744820, -2.638427012816831230 ) ) ;
#6000=CARTESIAN_POINT ( 'NONE',  ( -0.8801773607110991993, 7.855352010821506248, -2.915334737309923874 ) ) ;
#6001=CARTESIAN_POINT ( 'NONE',  ( -2.816281873526473856, 64.33196800326376774, 3.434112377981055619 ) ) ;
#6002=CARTESIAN_POINT ( 'NONE',  ( 2.791683348922240793, 51.63393115100078745, 7.208316651077764092 ) ) ;
#6003=CARTESIAN_POINT ( 'NONE',  ( 0.1532563361054082862, 26.21726448433411605, 2.638427012816831674 ) ) ;
#6004=CARTESIAN_POINT ( 'NONE',  ( -2.816281873526473856, 44.12363466993042493, 9.499525473075851096E-16 ) ) ;
#6006=CARTESIAN_POINT ( 'NONE',  ( 15.44008868035555260, 39.73035201082150536, 9.422509992056143702 ) ) ;
#6007=CARTESIAN_POINT ( 'NONE',  ( 12.63842701281683034, 42.46726448433412315, 9.846743663894596210 ) ) ;
#6008=EDGE_CURVE ( 'NONE', #65472, #14954, #19310, .T. ) ;
#6009=CARTESIAN_POINT ( 'NONE',  ( 10.00000000000000178, 28.05374883491396787, 14.16423886937410082 ) ) ;
#6011=CARTESIAN_POINT ( 'NONE',  ( 22.26659068614894466, 3.887082168247300906, 7.082119434687054849 ) ) ;
#6012=EDGE_CURVE ( 'NONE', #55863, #70171, #56003, .T. ) ;
#6014=CARTESIAN_POINT ( 'NONE',  ( 20.88017736071110519, 50.56368534415484106, 2.639326808657452039E-16 ) ) ;
#6015=CARTESIAN_POINT ( 'NONE',  ( 19.42250999205614193, 60.14701867748817676, 5.440088680355555262 ) ) ;
#6016=CARTESIAN_POINT ( 'NONE',  ( 6.204703633549690345, 60.76208216824730357, -14.16423886937410259 ) ) ;
#6017=CARTESIAN_POINT ( 'NONE',  ( 6.565887622018943937, 3.081968003263753531, -12.81628187352647608 ) ) ;
#6018=CARTESIAN_POINT ( 'NONE',  ( -0.1042174387088606741, 53.10736173766203905, 6.337391062633418670 ) ) ;
#6019=CARTESIAN_POINT ( 'NONE',  ( 19.42250999205614548, 60.98035201082151247, -5.440088680355545492 ) ) ;
#6020=CARTESIAN_POINT ( 'NONE',  ( 21.09922568453594849, 1.206968003263753531, 6.408140936763242479 ) ) ;
#6022=CARTESIAN_POINT ( 'NONE',  ( 17.96484262340118221, 9.938685344154837509, 7.964842623401181321 ) ) ;
#6023=CARTESIAN_POINT ( 'NONE',  ( 19.42250999205614193, 10.14701867748816966, 5.440088680355555262 ) ) ;
#6024=CARTESIAN_POINT ( 'NONE',  ( 12.63842701281683034, 47.46726448433412315, 9.846743663894596210 ) ) ;
#6025=LINE ( 'NONE', #59992, #61549 ) ;
#6027=SURFACE_SIDE_STYLE ('',( #49531 ) ) ;
#6028=CARTESIAN_POINT ( 'NONE',  ( 21.09922568453595559, 7.040301336597086568, -6.408140936763230044 ) ) ;
#6029=CARTESIAN_POINT ( 'NONE',  ( 0.5600000000000083800, 105.0000000000000000, 5.000000000000000000 ) ) ;
#6030=CARTESIAN_POINT ( 'NONE',  ( 5.076628168052704559, 5.175597817667451750, -8.527530157486179263 ) ) ;
#6031=CARTESIAN_POINT ( 'NONE',  ( 0.1532563361054083140, 41.00893115100078745, 1.131784320476157264E-15 ) ) ;
#6032=CARTESIAN_POINT ( 'NONE',  ( 20.88017736071110519, 40.56368534415484106, 2.639326808657452039E-16 ) ) ;
#6033=B_SPLINE_CURVE_WITH_KNOTS ( 'NONE', 3,
 ( #39635, #18113, #34066, #71607 ),
 .UNSPECIFIED., .F., .F.,
 ( 4, 4 ),
 ( 2.168404344971008868E-18, 0.001060528352562004149 ),
 .UNSPECIFIED. ) ;
#6034=CARTESIAN_POINT ( 'NONE',  ( 3.591859063236763294, 3.290301336597087012, -11.09922568453595026 ) ) ;
#6035=CARTESIAN_POINT ( 'NONE',  ( 19.42250999205614193, 50.14701867748817676, 5.440088680355555262 ) ) ;
#6037=CARTESIAN_POINT ( 'NONE',  ( 19.38216949554541557, 47.24863466993041783, -9.382169495545420901 ) ) ;
#6039=CARTESIAN_POINT ( 'NONE',  ( 7.084665262690076126, 69.10535201082151957, 10.88017736071109987 ) ) ;
#6040=CARTESIAN_POINT ( 'NONE',  ( 16.40814093676324603, 37.45696800326376064, -11.09922568453594671 ) ) ;
#6042=CARTESIAN_POINT ( 'NONE',  ( 7.361572987183170547, 2.050597817667451750, 9.846743663894590881 ) ) ;
#6043=CARTESIAN_POINT ( 'NONE',  ( 7.084665262690076126, 39.10535201082150536, 10.88017736071109987 ) ) ;
#6044=CARTESIAN_POINT ( 'NONE',  ( 7.361572987183169658, 64.96726448433412315, -9.846743663894592657 ) ) ;
#6046=CARTESIAN_POINT ( 'NONE',  ( 18.52753015748618282, 58.92559781766745886, -4.923371831947291888 ) ) ;
#6047=CARTESIAN_POINT ( 'NONE',  ( 1.472469842513823179, 21.42559781766745175, 4.923371831947296329 ) ) ;
#6048=CARTESIAN_POINT ( 'NONE',  ( 1.472469842513823179, 1.425597817667451528, 4.923371831947296329 ) ) ;
#6050=CARTESIAN_POINT ( 'NONE',  ( 13.79529636645030344, 48.26208216824728936, 14.16423886937410614 ) ) ;
#6054=ORIENTED_EDGE ( 'NONE', *, *, #17895, .T. ) ;
#6055=CARTESIAN_POINT ( 'NONE',  ( 6.204703633549690345, 55.76208216824730357, -14.16423886937410259 ) ) ;
#6056=CARTESIAN_POINT ( 'NONE',  ( 2.917880565312950480, 65.97041550158063217, -12.26659068614894821 ) ) ;
#6057=CARTESIAN_POINT ( 'NONE',  ( 7.361572987183170547, 32.05059781766745175, 9.846743663894590881 ) ) ;
#6059=( NAMED_UNIT ( * ) PLANE_ANGLE_UNIT ( ) SI_UNIT ( $, .RADIAN. ) );
#6060=CARTESIAN_POINT ( 'NONE',  ( -4.164238869374098151, 11.59541550158063217, -3.795296366450310543 ) ) ;
#6061=CARTESIAN_POINT ( 'NONE',  ( 12.91533473730992121, 9.522018677488171434, 10.88017736071110164 ) ) ;
#6062=CARTESIAN_POINT ( 'NONE',  ( 22.26659068614895176, 54.72041550158063217, -7.082119434687042414 ) ) ;
#6063=CARTESIAN_POINT ( 'NONE',  ( 1.472469842513823179, 30.59226448433411960, -4.923371831947296329 ) ) ;
#6065=CARTESIAN_POINT ( 'NONE',  ( 18.52753015748618282, 8.925597817667451750, -4.923371831947291888 ) ) ;
#6066=CARTESIAN_POINT ( 'NONE',  ( 18.72515096720571037, 55.05509018479936145, 6.499999999999982236 ) ) ;
#6068=VERTEX_POINT ( 'NONE', #72145 ) ;
#6069=EDGE_LOOP ( 'NONE', ( #37105, #93758, #9070, #87712 ) ) ;
#6071=EDGE_LOOP ( 'NONE', ( #98466, #96969, #7617, #47754 ) ) ;
#6072=CARTESIAN_POINT ( 'NONE',  ( 17.20831665107776587, 42.88393115100077324, 7.208316651077764980 ) ) ;
#6073=CARTESIAN_POINT ( 'NONE',  ( 4.559911319644449179, 23.89701867748817321, 9.422509992056141925 ) ) ;
#6074=CARTESIAN_POINT ( 'NONE',  ( 17.96484262340118221, 24.93868534415484461, 7.964842623401181321 ) ) ;
#6075=CARTESIAN_POINT ( 'NONE',  ( 0.1532563361054100626, 60.80059781766744464, -2.638427012816831230 ) ) ;
#6076=CARTESIAN_POINT ( 'NONE',  ( 10.00000000000000000, 12.87363466993042138, -12.81628187352647608 ) ) ;
#6077=CARTESIAN_POINT ( 'NONE',  ( -2.266590686148945544, 6.387082168247300906, -7.082119434687050408 ) ) ;
#6079=CARTESIAN_POINT ( 'NONE',  ( 3.591859063236761518, 29.95696800326375708, 11.09922568453594849 ) ) ;
#6081=CARTESIAN_POINT ( 'NONE',  ( 17.20831665107776587, 34.13393115100078745, -7.208316651077762316 ) ) ;
#6082=CARTESIAN_POINT ( 'NONE',  ( 20.88017736071110519, 10.56368534415483929, 2.639326808657452039E-16 ) ) ;
#6083=ORIENTED_EDGE ( 'NONE', *, *, #26901, .T. ) ;
#6084=CARTESIAN_POINT ( 'NONE',  ( 20.88017736071110164, 5.355352010821503583, 2.915334737309930979 ) ) ;
#6086=CARTESIAN_POINT ( 'NONE',  ( -0.8801773607110991993, 47.85535201082150536, -2.915334737309923874 ) ) ;
#6087=CARTESIAN_POINT ( 'NONE',  ( 4.559911319644449179, 62.23035201082150536, -9.422509992056141925 ) ) ;
#6088=CARTESIAN_POINT ( 'NONE',  ( -0.8801773607111009756, 48.06368534415484817, 1.068504757029289695E-15 ) ) ;
#6091=CARTESIAN_POINT ( 'NONE',  ( 4.559911319644449179, 58.89701867748817676, 9.422509992056141925 ) ) ;
#6092=CARTESIAN_POINT ( 'NONE',  ( -0.3289641300568005855, 30.10497603579417714, 5.963430220938281678 ) ) ;
#6095=CARTESIAN_POINT ( 'NONE',  ( 1.472469842513823179, 31.42559781766745530, 4.923371831947296329 ) ) ;
#6097=CARTESIAN_POINT ( 'NONE',  ( 10.00000000000000000, 59.75893115100078745, -9.846743663894594434 ) ) ;
#6099=CARTESIAN_POINT ( 'NONE',  ( 2.917880565312948704, 12.63708216824730179, 12.26659068614894643 ) ) ;
#6101=VERTEX_POINT ( 'NONE', #23973 ) ;
#6105=CARTESIAN_POINT ( 'NONE',  ( 4.559911319644449179, 2.230352010821504916, -9.422509992056141925 ) ) ;
#6109=CARTESIAN_POINT ( 'NONE',  ( 7.361572987183169658, 39.96726448433411605, -9.846743663894592657 ) ) ;
#6111=CARTESIAN_POINT ( 'NONE',  ( 21.09922568453594849, 16.20696800326375353, 6.408140936763242479 ) ) ;
#6112=CARTESIAN_POINT ( 'NONE',  ( 2.791683348922240793, 16.63393115100078745, 7.208316651077764092 ) ) ;
#6114=DIRECTION ( 'NONE',  ( 0.000000000000000000, 0.000000000000000000, -1.000000000000000000 ) ) ;
#6115=CARTESIAN_POINT ( 'NONE',  ( -2.816281873526473856, 4.123634669930420493, 9.499525473075851096E-16 ) ) ;
#6117=ORIENTED_EDGE ( 'NONE', *, *, #3759, .F. ) ;
#6119=CARTESIAN_POINT ( 'NONE',  ( 0.5774900079438590739, 12.64701867748817321, -5.440088680355550821 ) ) ;
#6120=CARTESIAN_POINT ( 'NONE',  ( -0.3689425029237898834, 6.178748834913968757, -10.36894250292378850 ) ) ;
#6121=CARTESIAN_POINT ( 'NONE',  ( 1.472469842513823179, 21.42559781766745175, 4.923371831947296329 ) ) ;
#6122=CARTESIAN_POINT ( 'NONE',  ( 19.42250999205614193, 55.14701867748817676, 5.440088680355555262 ) ) ;
#6123=CARTESIAN_POINT ( 'NONE',  ( 22.81628187352647785, 41.62363466993042493, 6.195893100308588602E-16 ) ) ;
#6125=CARTESIAN_POINT ( 'NONE',  ( 7.084665262690076126, 9.105352010821503583, 10.88017736071109987 ) ) ;
#6129=CARTESIAN_POINT ( 'NONE',  ( 0.6178305044545818747, 3.498634669930420049, -9.382169495545419124 ) ) ;
#6130=CARTESIAN_POINT ( 'NONE',  ( 5.076628168052704559, 65.17559781766745175, -8.527530157486179263 ) ) ;
#6131=CARTESIAN_POINT ( 'NONE',  ( 12.63842701281683034, 27.46726448433411250, 9.846743663894596210 ) ) ;
#6133=CARTESIAN_POINT ( 'NONE',  ( 16.40814093676323893, 30.79030133659708923, 11.09922568453595026 ) ) ;
#6135=CARTESIAN_POINT ( 'NONE',  ( 20.88017736071110519, 45.56368534415484106, 2.639326808657452039E-16 ) ) ;
#6138=( BOUNDED_CURVE ( )  B_SPLINE_CURVE ( 2, ( #34182, #57188, #80186, #42208, #89171 ),
 .UNSPECIFIED., .F., .F. ) 
 B_SPLINE_CURVE_WITH_KNOTS ( ( 3, 2, 3 ),
 ( 0.9401409369402312644, 0.9404761904761904656, 0.9419949716883659896 ),
 .UNSPECIFIED. ) 
 CURVE ( )  GEOMETRIC_REPRESENTATION_ITEM ( )  RATIONAL_B_SPLINE_CURVE ( ( 0.9963778908391753841, 0.9980808541467917072, 1.000000000000000000, 0.9913057959047685275, 0.9870483353379817526 ) ) 
 REPRESENTATION_ITEM ( '' )  );
#6139=CARTESIAN_POINT ( 'NONE',  ( 20.88017736071110519, 45.56368534415484106, 2.639326808657452039E-16 ) ) ;
#6140=CARTESIAN_POINT ( 'NONE',  ( 2.035157376598822676, 32.43868534415483396, -7.964842623401177768 ) ) ;
#6141=CARTESIAN_POINT ( 'NONE',  ( 1.472469842513823179, 61.42559781766745175, 4.923371831947296329 ) ) ;
#6142=CARTESIAN_POINT ( 'NONE',  ( 17.96484262340118221, 59.93868534415484106, 7.964842623401181321 ) ) ;
#6144=CARTESIAN_POINT ( 'NONE',  ( 19.84674366389459266, 33.30059781766744464, 2.638427012816836559 ) ) ;
#6145=CARTESIAN_POINT ( 'NONE',  ( -40.17076923076924544, 96.15384615384614619, -9.500000000000000000 ) ) ;
#6146=CARTESIAN_POINT ( 'NONE',  ( 22.81628187352647785, 16.41530133659708923, 3.434112377981063169 ) ) ;
#6148=CARTESIAN_POINT ( 'NONE',  ( 20.88017736071110519, 20.56368534415484106, 2.639326808657452039E-16 ) ) ;
#6149=CARTESIAN_POINT ( 'NONE',  ( 4.559911319644449179, 12.23035201082150714, -9.422509992056141925 ) ) ;
#6150=CARTESIAN_POINT ( 'NONE',  ( 14.92337183194729988, 4.342264484334117824, -8.527530157486177487 ) ) ;
#6151=CARTESIAN_POINT ( 'NONE',  ( -4.164238869374098151, 26.59541550158063217, -3.795296366450310543 ) ) ;
#6152=CARTESIAN_POINT ( 'NONE',  ( 7.361572987183170547, 12.05059781766744997, 9.846743663894590881 ) ) ;
#6153=CARTESIAN_POINT ( 'NONE',  ( 17.20831665107776587, 62.88393115100078745, 7.208316651077764980 ) ) ;
#6154=CARTESIAN_POINT ( 'NONE',  ( 2.035157376598822676, 47.43868534415484817, -7.964842623401177768 ) ) ;
#6156=FACE_OUTER_BOUND ( 'NONE', #93578, .T. ) ;
#6160=CARTESIAN_POINT ( 'NONE',  ( 19.84674366389459266, 48.30059781766745175, 2.638427012816836559 ) ) ;
#6164=CARTESIAN_POINT ( 'NONE',  ( 6.204703633549690345, 20.76208216824730357, -14.16423886937410259 ) ) ;
#6165=CARTESIAN_POINT ( 'NONE',  ( -4.164238869374099039, 21.80374883491396787, 8.674139862899312516E-16 ) ) ;
#6166=CARTESIAN_POINT ( 'NONE',  ( 7.084665262690076126, 59.10535201082150536, 10.88017736071109987 ) ) ;
#6167=CARTESIAN_POINT ( 'NONE',  ( -0.8801773607111009756, 3.063685344154838397, 1.068504757029289695E-15 ) ) ;
#6168=CARTESIAN_POINT ( 'NONE',  ( -2.816281873526473856, 4.331968003263754419, 3.434112377981055619 ) ) ;
#6169=CARTESIAN_POINT ( 'NONE',  ( 7.361572987183169658, 49.96726448433410894, -9.846743663894592657 ) ) ;
#6171=CARTESIAN_POINT ( 'NONE',  ( -0.8801773607110991993, 47.85535201082150536, -2.915334737309923874 ) ) ;
#6172=CARTESIAN_POINT ( 'NONE',  ( 21.09922568453595559, 2.040301336597086568, -6.408140936763230044 ) ) ;
#6173=CARTESIAN_POINT ( 'NONE',  ( -4.164238869374099039, 16.80374883491396787, 8.674139862899312516E-16 ) ) ;
#6174=CARTESIAN_POINT ( 'NONE',  ( 17.96484262340118221, 19.93868534415484106, 7.964842623401181321 ) ) ;
#6175=CARTESIAN_POINT ( 'NONE',  ( 2.035157376598822676, 12.43868534415483751, -7.964842623401177768 ) ) ;
#6177=CARTESIAN_POINT ( 'NONE',  ( 2.035157376598824452, 43.68868534415484106, 7.964842623401179544 ) ) ;
#6178=( GEOMETRIC_REPRESENTATION_CONTEXT ( 3 ) GLOBAL_UNCERTAINTY_ASSIGNED_CONTEXT ( ( #39237 ) ) GLOBAL_UNIT_ASSIGNED_CONTEXT ( ( #47414, #69936, #55418 ) ) REPRESENTATION_CONTEXT ( 'NONE', 'WORKASPACE' ) );
#6179=CARTESIAN_POINT ( 'NONE',  ( 13.43411237798105340, 45.58196800326374643, 12.81628187352647963 ) ) ;
#6182=CARTESIAN_POINT ( 'NONE',  ( 20.10493008474208665, 4.716974130838791801, 6.336235997365754713 ) ) ;
#6184=CARTESIAN_POINT ( 'NONE',  ( 1.472469842513823179, 30.59226448433411960, -4.923371831947296329 ) ) ;
#6186=DIRECTION ( 'NONE',  ( 0.000000000000000000, 0.000000000000000000, 1.000000000000000000 ) ) ;
#6187=CARTESIAN_POINT ( 'NONE',  ( -2.266590686148945544, 47.22041550158063927, 7.082119434687048631 ) ) ;
#6188=CARTESIAN_POINT ( 'NONE',  ( 10.00000000000000178, 4.313685344154837509, 10.88017736071110342 ) ) ;
#6189=CARTESIAN_POINT ( 'NONE',  ( 17.20831665107776587, 27.88393115100078390, 7.208316651077764980 ) ) ;
#6190=CARTESIAN_POINT ( 'NONE',  ( 5.076628168052704559, 50.17559781766745886, -8.527530157486179263 ) ) ;
#6195=CARTESIAN_POINT ( 'NONE',  ( 1.472469842513823179, 0.5922644843341181575, -4.923371831947296329 ) ) ;
#6198=CARTESIAN_POINT ( 'NONE',  ( -0.3689425029237881626, 32.42874883491395366, 10.36894250292379027 ) ) ;
#6199=CARTESIAN_POINT ( 'NONE',  ( 6.565887622018943937, 28.08196800326375353, -12.81628187352647608 ) ) ;
#6201=CARTESIAN_POINT ( 'NONE',  ( 10.00000000000000000, 47.87363466993042493, -12.81628187352647608 ) ) ;
#6202=CARTESIAN_POINT ( 'NONE',  ( 17.96484262340118221, 14.93868534415484106, 7.964842623401181321 ) ) ;
#6203=CARTESIAN_POINT ( 'NONE',  ( 7.361572987183170547, 32.05059781766745175, 9.846743663894590881 ) ) ;
#6204=CARTESIAN_POINT ( 'NONE',  ( -0.8801773607110991993, 17.85535201082150536, -2.915334737309923874 ) ) ;
#6207=CARTESIAN_POINT ( 'NONE',  ( 5.076628168052703671, 46.84226448433412315, 8.527530157486179263 ) ) ;
#6208=CARTESIAN_POINT ( 'NONE',  ( 1.472469842513823179, 50.59226448433411605, -4.923371831947296329 ) ) ;
#6216=CARTESIAN_POINT ( 'NONE',  ( 14.92337183194729988, 19.34226448433411960, -8.527530157486177487 ) ) ;
#6217=CARTESIAN_POINT ( 'NONE',  ( 13.43411237798105340, 40.58196800326375353, 12.81628187352647963 ) ) ;
#6221=CARTESIAN_POINT ( 'NONE',  ( 0.1532563361054083140, 56.00893115100078745, 1.131784320476157264E-15 ) ) ;
#6222=CARTESIAN_POINT ( 'NONE',  ( 17.39651004071841811, 4.082109641433293135, -6.499999999999999112 ) ) ;
#6223=CARTESIAN_POINT ( 'NONE',  ( 22.26659068614895176, 29.72041550158063572, -7.082119434687042414 ) ) ;
#6224=CARTESIAN_POINT ( 'NONE',  ( 2.791683348922240793, 41.63393115100078745, 7.208316651077764092 ) ) ;
#6225=CARTESIAN_POINT ( 'NONE',  ( 22.81628187352647785, 46.41530133659708213, 3.434112377981063169 ) ) ;
#6229=CARTESIAN_POINT ( 'NONE',  ( 17.20831665107776587, 2.883931151000785231, 7.208316651077764980 ) ) ;
#6231=CARTESIAN_POINT ( 'NONE',  ( 12.63842701281683034, 47.46726448433412315, 9.846743663894596210 ) ) ;
#6232=CARTESIAN_POINT ( 'NONE',  ( -0.8801773607111009756, 38.06368534415484106, 1.068504757029289695E-15 ) ) ;
#6233=CARTESIAN_POINT ( 'NONE',  ( 19.50000000000000711, 105.0000000000000000, 5.000000000000000000 ) ) ;
#6235=CARTESIAN_POINT ( 'NONE',  ( 2.035157376598824452, 43.68868534415484106, 7.964842623401179544 ) ) ;
#6238=DIRECTION ( 'NONE',  ( -1.000000000000000000, -2.799047438454523236E-16, 0.000000000000000000 ) ) ;
#6239=CARTESIAN_POINT ( 'NONE',  ( 20.88017736071110164, 10.35535201082150714, 2.915334737309930979 ) ) ;
#6240=CARTESIAN_POINT ( 'NONE',  ( 1.472469842513823179, 61.42559781766745175, 4.923371831947296329 ) ) ;
#6241=CARTESIAN_POINT ( 'NONE',  ( 10.00000000000000178, 44.31368534415484106, 10.88017736071110342 ) ) ;
#6242=CARTESIAN_POINT ( 'NONE',  ( 4.559911319644449179, 63.89701867748817676, 9.422509992056141925 ) ) ;
#6244=CARTESIAN_POINT ( 'NONE',  ( 4.559911319644449179, 22.23035201082150536, -9.422509992056141925 ) ) ;
#6246=CARTESIAN_POINT ( 'NONE',  ( 19.84674366389459621, 13.50893115100078568, 7.409399052514197653E-17 ) ) ;
#6247=CARTESIAN_POINT ( 'NONE',  ( 17.20831665107776587, 19.13393115100078035, -7.208316651077762316 ) ) ;
#6250=CARTESIAN_POINT ( 'NONE',  ( 2.791683348922237240, 65.38393115100078035, -7.208316651077763204 ) ) ;
#6251=CARTESIAN_POINT ( 'NONE',  ( -0.8801773607111009756, 3.063685344154838397, 1.068504757029289695E-15 ) ) ;
#6253=CARTESIAN_POINT ( 'NONE',  ( 24.16423886937410614, 9.512082168247301794, -3.795296366450302550 ) ) ;
#6255=CARTESIAN_POINT ( 'NONE',  ( -2.266590686148945544, 51.38708216824730357, -7.082119434687050408 ) ) ;
#6256=CARTESIAN_POINT ( 'NONE',  ( 13.43411237798106583, 7.665301336597086568, -12.81628187352647252 ) ) ;
#6257=ORIENTED_EDGE ( 'NONE', *, *, #4996, .T. ) ;
#6258=CARTESIAN_POINT ( 'NONE',  ( 19.84674366389459266, 8.717264484334116048, -2.638427012816827677 ) ) ;
#6259=CARTESIAN_POINT ( 'NONE',  ( 10.00000000000000000, 11.81368534415483751, -10.88017736071110342 ) ) ;
#6260=CARTESIAN_POINT ( 'NONE',  ( 14.92337183194729633, 42.67559781766745886, 8.527530157486181039 ) ) ;
#6261=DIRECTION ( 'NONE',  ( -0.000000000000000000, -0.000000000000000000, 1.000000000000000000 ) ) ;
#6263=CARTESIAN_POINT ( 'NONE',  ( 22.81628187352647785, 21.62363466993041783, 6.195893100308588602E-16 ) ) ;
#6264=CARTESIAN_POINT ( 'NONE',  ( 19.84674366389459621, 23.50893115100078390, 7.409399052514197653E-17 ) ) ;
#6265=VERTEX_POINT ( 'NONE', #16962 ) ;
#6266=CARTESIAN_POINT ( 'NONE',  ( 12.63842701281683922, 4.550597817667451750, -9.846743663894590881 ) ) ;
#6268=CARTESIAN_POINT ( 'NONE',  ( -46.70132286185116044, 101.0484326958216599, -8.835676566301254198 ) ) ;
#6269=CARTESIAN_POINT ( 'NONE',  ( 7.084665262690076126, 14.10535201082150358, 10.88017736071109987 ) ) ;
#6270=CARTESIAN_POINT ( 'NONE',  ( -2.266590686148945544, 46.38708216824730357, -7.082119434687050408 ) ) ;
#6271=CARTESIAN_POINT ( 'NONE',  ( 7.084665262690076126, 57.02201867748817676, -10.88017736071110164 ) ) ;
#6274=CARTESIAN_POINT ( 'NONE',  ( 10.00000000000000000, 24.75893115100078745, -9.846743663894594434 ) ) ;
#6275=CARTESIAN_POINT ( 'NONE',  ( 17.96484262340118221, 6.188685344154836621, -7.964842623401177768 ) ) ;
#6276=CARTESIAN_POINT ( 'NONE',  ( 2.791683348922240793, 11.63393115100078568, 7.208316651077764092 ) ) ;
#6278=CARTESIAN_POINT ( 'NONE',  ( 18.52753015748617571, 38.09226448433412315, 4.923371831947298993 ) ) ;
#6280=STYLED_ITEM ( 'NONE', ( #76066 ), #26594 ) ;
#6281=CARTESIAN_POINT ( 'NONE',  ( 2.035157376598822676, 37.43868534415484106, -7.964842623401177768 ) ) ;
#6282=UNCERTAINTY_MEASURE_WITH_UNIT (LENGTH_MEASURE( 1.000000000000000082E-05 ), #74854, 'distance_accuracy_value', 'NONE');
#6284=CARTESIAN_POINT ( 'NONE',  ( 21.09922568453595559, 62.04030133659709634, -6.408140936763230044 ) ) ;
#6286=CARTESIAN_POINT ( 'NONE',  ( 19.84674366389459266, 8.300597817667451750, 2.638427012816836559 ) ) ;
#6287=CARTESIAN_POINT ( 'NONE',  ( -2.816281873526473856, 39.33196800326374643, 3.434112377981055619 ) ) ;
#6288=CARTESIAN_POINT ( 'NONE',  ( -0.8801773607111008646, 8.272018677488171434, 2.915334737309923430 ) ) ;
#6289=CARTESIAN_POINT ( 'NONE',  ( 0.1532563361054083140, 31.00893115100078390, 1.131784320476157264E-15 ) ) ;
#6291=SURFACE_SIDE_STYLE ('',( #59773 ) ) ;
#6292=CARTESIAN_POINT ( 'NONE',  ( 6.204703633549690345, 22.84541550158062861, 14.16423886937410082 ) ) ;
#6293=CARTESIAN_POINT ( 'NONE',  ( -2.266590686148945544, 47.22041550158063927, 7.082119434687048631 ) ) ;
#6294=CARTESIAN_POINT ( 'NONE',  ( 10.00000000000000178, 47.25893115100078745, 9.846743663894594434 ) ) ;
#6296=CARTESIAN_POINT ( 'NONE',  ( 0.5774900079438590739, 32.64701867748816966, -5.440088680355550821 ) ) ;
#6297=CARTESIAN_POINT ( 'NONE',  ( 20.88017736071110519, 65.56368534415483396, 2.639326808657452039E-16 ) ) ;
#6299=VERTEX_POINT ( 'NONE', #21632 ) ;
#6300=CARTESIAN_POINT ( 'NONE',  ( 19.38216949554541557, 57.24863466993042493, -9.382169495545420901 ) ) ;
#6301=CARTESIAN_POINT ( 'NONE',  ( 4.559911319644449179, 68.89701867748817676, 9.422509992056141925 ) ) ;
#6303=CARTESIAN_POINT ( 'NONE',  ( -4.164238869374099927, 7.012082168247302683, 3.795296366450308767 ) ) ;
#6304=CARTESIAN_POINT ( 'NONE',  ( 2.791683348922237240, 10.38393115100078390, -7.208316651077763204 ) ) ;
#6307=CARTESIAN_POINT ( 'NONE',  ( 17.96484262340118221, 16.18868534415483396, -7.964842623401177768 ) ) ;
#6309=CARTESIAN_POINT ( 'NONE',  ( 20.88017736071110875, 40.77201867748818387, -2.915334737309920765 ) ) ;
#6311=CARTESIAN_POINT ( 'NONE',  ( 22.81628187352647785, 11.62363466993042138, 6.195893100308588602E-16 ) ) ;
#6312=ORIENTED_EDGE ( 'NONE', *, *, #62855, .F. ) ;
#6313=CARTESIAN_POINT ( 'NONE',  ( 2.791683348922237240, 0.3839311510007847872, -7.208316651077763204 ) ) ;
#6314=CARTESIAN_POINT ( 'NONE',  ( 19.84674366389459266, 58.30059781766745886, 2.638427012816836559 ) ) ;
#6315=CARTESIAN_POINT ( 'NONE',  ( 2.035157376598824452, 18.68868534415484106, 7.964842623401179544 ) ) ;
#6317=CARTESIAN_POINT ( 'NONE',  ( 0.1532563361054083140, 6.008931151000784787, 1.131784320476157264E-15 ) ) ;
#6318=CARTESIAN_POINT ( 'NONE',  ( 15.44008868035555260, 14.73035201082150536, 9.422509992056143702 ) ) ;
#6320=CARTESIAN_POINT ( 'NONE',  ( -2.816281873526471635, 58.91530133659707502, -3.434112377981056508 ) ) ;
#6321=CARTESIAN_POINT ( 'NONE',  ( 0.5774900079438590739, 42.64701867748816966, -5.440088680355550821 ) ) ;
#6322=CARTESIAN_POINT ( 'NONE',  ( 0.2751277870542909731, 47.28217586085238366, -6.499999999999992006 ) ) ;
#6323=CARTESIAN_POINT ( 'NONE',  ( 22.81628187352647785, 51.62363466993042493, 6.195893100308588602E-16 ) ) ;
#6324=CARTESIAN_POINT ( 'NONE',  ( 17.96484262340118221, 41.18868534415484106, -7.964842623401177768 ) ) ;
#6326=VECTOR ( 'NONE', #51893, 1000.000000000000000 ) ;
#6327=CARTESIAN_POINT ( 'NONE',  ( 14.92337183194729988, 19.34226448433411960, -8.527530157486177487 ) ) ;
#6328=CARTESIAN_POINT ( 'NONE',  ( 21.09922568453595559, 7.040301336597086568, -6.408140936763230044 ) ) ;
#6330=CARTESIAN_POINT ( 'NONE',  ( 5.076628168052704559, 65.17559781766745175, -8.527530157486179263 ) ) ;
#6331=CARTESIAN_POINT ( 'NONE',  ( 20.88017736071110875, 40.77201867748818387, -2.915334737309920765 ) ) ;
#6333=CARTESIAN_POINT ( 'NONE',  ( 14.92337183194729988, 44.34226448433412315, -8.527530157486177487 ) ) ;
#6335=CARTESIAN_POINT ( 'NONE',  ( 0.1532563361054083140, 21.00893115100078745, 1.131784320476157264E-15 ) ) ;
#6336=CARTESIAN_POINT ( 'NONE',  ( 7.361572987183170547, 12.05059781766744997, 9.846743663894590881 ) ) ;
#6337=CARTESIAN_POINT ( 'NONE',  ( 10.00000000000000178, 5.373634669930420493, 12.81628187352647608 ) ) ;
#6339=CARTESIAN_POINT ( 'NONE',  ( 0.1532563361054082862, 66.21726448433413736, 2.638427012816831674 ) ) ;
#6340=CARTESIAN_POINT ( 'NONE',  ( 10.00000000000000178, 50.37363466993042493, 12.81628187352647608 ) ) ;
#6342=CARTESIAN_POINT ( 'NONE',  ( 14.92337183194729988, 29.34226448433411960, -8.527530157486177487 ) ) ;
#6344=CARTESIAN_POINT ( 'NONE',  ( 2.035157376598822676, 2.438685344154838397, -7.964842623401177768 ) ) ;
#6345=CARTESIAN_POINT ( 'NONE',  ( 2.791683348922237240, 30.38393115100078390, -7.208316651077763204 ) ) ;
#6349=CARTESIAN_POINT ( 'NONE',  ( 12.91533473730993009, 6.605352010821504471, -10.88017736071109987 ) ) ;
#6351=CARTESIAN_POINT ( 'NONE',  ( 7.084665262690076126, 24.10535201082150181, 10.88017736071109987 ) ) ;
#6352=CARTESIAN_POINT ( 'NONE',  ( 10.00000000000000000, 50.55374883491396787, -14.16423886937410082 ) ) ;
#6353=CARTESIAN_POINT ( 'NONE',  ( 17.08211943468705840, 55.13708216824731068, -12.26659068614894466 ) ) ;
#6354=DIRECTION ( 'NONE',  ( 0.000000000000000000, 0.000000000000000000, -1.000000000000000000 ) ) ;
#6356=CARTESIAN_POINT ( 'NONE',  ( 2.791683348922237240, 15.38393115100078212, -7.208316651077763204 ) ) ;
#6357=CARTESIAN_POINT ( 'NONE',  ( -1.099225684535947600, -0.4596986634029132657, 6.408140936763237150 ) ) ;
#6360=CARTESIAN_POINT ( 'NONE',  ( 0.5600000000000083800, 105.0000000000000000, -4.500000000000001776 ) ) ;
#6361=CARTESIAN_POINT ( 'NONE',  ( -0.3689425029237881626, 12.42874883491396609, 10.36894250292379027 ) ) ;
#6362=CARTESIAN_POINT ( 'NONE',  ( 1.472469842513823179, 26.42559781766745175, 4.923371831947296329 ) ) ;
#6363=DIRECTION ( 'NONE',  ( -0.000000000000000000, -0.000000000000000000, 1.000000000000000000 ) ) ;
#6364=CARTESIAN_POINT ( 'NONE',  ( -2.266590686148945544, 46.38708216824730357, -7.082119434687050408 ) ) ;
#6365=CARTESIAN_POINT ( 'NONE',  ( 19.84674366389459266, 3.300597817667451750, 2.638427012816836559 ) ) ;
#6366=CARTESIAN_POINT ( 'NONE',  ( 1.274849032794131976, 13.57228050351029403, 6.499999999999760192 ) ) ;
#6368=CARTESIAN_POINT ( 'NONE',  ( -0.8801773607111008646, 28.27201867748817321, 2.915334737309923430 ) ) ;
#6369=CARTESIAN_POINT ( 'NONE',  ( 16.40814093676324603, 32.45696800326375353, -11.09922568453594671 ) ) ;
#6370=( NAMED_UNIT ( * ) SI_UNIT ( $, .STERADIAN. ) SOLID_ANGLE_UNIT ( ) );
#6371=CARTESIAN_POINT ( 'NONE',  ( 10.00000000000000178, 30.37363466993042138, 12.81628187352647608 ) ) ;
#6372=CARTESIAN_POINT ( 'NONE',  ( 6.565887622018943937, 63.08196800326376064, -12.81628187352647608 ) ) ;
#6374=CARTESIAN_POINT ( 'NONE',  ( 2.603489959281591659, 10.43575266056827644, -6.500000000000006217 ) ) ;
#6375=DIRECTION ( 'NONE',  ( 0.000000000000000000, 0.000000000000000000, -1.000000000000000000 ) ) ;
#6376=CARTESIAN_POINT ( 'NONE',  ( 17.08211943468705840, 35.13708216824730357, -12.26659068614894466 ) ) ;
#6377=CARTESIAN_POINT ( 'NONE',  ( 10.00000000000000000, 0.5537488349139675359, -14.16423886937410082 ) ) ;
#6378=CARTESIAN_POINT ( 'NONE',  ( 12.91533473730992121, 9.522018677488171434, 10.88017736071110164 ) ) ;
#6379=CARTESIAN_POINT ( 'NONE',  ( 0.5774900079438590739, 27.64701867748817676, -5.440088680355550821 ) ) ;
#6381=CARTESIAN_POINT ( 'NONE',  ( 20.88017736071110875, 50.77201867748817676, -2.915334737309920765 ) ) ;
#6382=CARTESIAN_POINT ( 'NONE',  ( 19.42250999205614548, 45.98035201082150536, -5.440088680355545492 ) ) ;
#6383=CARTESIAN_POINT ( 'NONE',  ( 10.00000000000000000, 22.87363466993042138, -12.81628187352647608 ) ) ;
#6384=CARTESIAN_POINT ( 'NONE',  ( 20.15039907845753220, 26.74884699246889141, 6.262539305110078836 ) ) ;
#6385=CARTESIAN_POINT ( 'NONE',  ( 1.472469842513823179, 21.42559781766745175, 4.923371831947296329 ) ) ;
#6386=CARTESIAN_POINT ( 'NONE',  ( 7.084665262690076126, 52.02201867748816255, -10.88017736071110164 ) ) ;
#6388=CARTESIAN_POINT ( 'NONE',  ( 22.81628187352648496, 21.83196800326374643, -3.434112377981050290 ) ) ;
#6389=FILL_AREA_STYLE ('',( #97419 ) ) ;
#6390=CARTESIAN_POINT ( 'NONE',  ( 10.00000000000000000, 6.813685344154838397, -10.88017736071110342 ) ) ;
#6391=CARTESIAN_POINT ( 'NONE',  ( 19.84674366389459621, 33.50893115100078745, 7.409399052514197653E-17 ) ) ;
#6392=CARTESIAN_POINT ( 'NONE',  ( -2.816281873526471635, 63.91530133659708923, -3.434112377981056508 ) ) ;
#6393=CARTESIAN_POINT ( 'NONE',  ( 12.63842701281683922, 14.55059781766744997, -9.846743663894590881 ) ) ;
#6394=CARTESIAN_POINT ( 'NONE',  ( 10.00000000000000178, 8.053748834913967869, 14.16423886937410082 ) ) ;
#6396=CARTESIAN_POINT ( 'NONE',  ( -0.8801773607111008646, 38.27201867748816255, 2.915334737309923430 ) ) ;
#6397=CARTESIAN_POINT ( 'NONE',  ( 0.5774900079438590739, 2.647018677488170990, -5.440088680355550821 ) ) ;
#6398=CARTESIAN_POINT ( 'NONE',  ( 24.16423886937410614, 29.51208216824729647, -3.795296366450302550 ) ) ;
#6399=CARTESIAN_POINT ( 'NONE',  ( 10.00000000000000178, 42.25893115100078745, 9.846743663894594434 ) ) ;
#6402=B_SPLINE_CURVE_WITH_KNOTS ( 'NONE', 3,
 ( #57336, #17880, #3369, #64338 ),
 .UNSPECIFIED., .F., .F.,
 ( 4, 4 ),
 ( 2.146014906638809613E-16, 0.002392975128318425206 ),
 .UNSPECIFIED. ) ;
#6403=CARTESIAN_POINT ( 'NONE',  ( -0.8801773607111009756, 38.06368534415484106, 1.068504757029289695E-15 ) ) ;
#6404=CARTESIAN_POINT ( 'NONE',  ( 10.00000000000000178, 14.31368534415483929, 10.88017736071110342 ) ) ;
#6407=CARTESIAN_POINT ( 'NONE',  ( 12.91533473730992121, 29.52201867748817321, 10.88017736071110164 ) ) ;
#6409=CARTESIAN_POINT ( 'NONE',  ( -1.099225684535947600, 39.54030133659708923, 6.408140936763237150 ) ) ;
#6410=CARTESIAN_POINT ( 'NONE',  ( 7.084665262690076126, 37.02201867748817676, -10.88017736071110164 ) ) ;
#6411=CARTESIAN_POINT ( 'NONE',  ( 0.1532563361054082862, 46.21726448433411605, 2.638427012816831674 ) ) ;
#6412=CARTESIAN_POINT ( 'NONE',  ( 15.44008868035555260, 34.73035201082151247, 9.422509992056143702 ) ) ;
#6413=ORIENTED_EDGE ( 'NONE', *, *, #44925, .F. ) ;
#6414=CARTESIAN_POINT ( 'NONE',  ( 17.20831665107776587, 59.13393115100078745, -7.208316651077762316 ) ) ;
#6415=CARTESIAN_POINT ( 'NONE',  ( 7.084665262690076126, 34.10535201082151247, 10.88017736071109987 ) ) ;
#6418=CARTESIAN_POINT ( 'NONE',  ( -2.266590686148945544, 46.38708216824730357, -7.082119434687050408 ) ) ;
#6419=CARTESIAN_POINT ( 'NONE',  ( -0.8801773607111009756, 48.06368534415484817, 1.068504757029289695E-15 ) ) ;
#6420=CARTESIAN_POINT ( 'NONE',  ( 17.20831665107776587, 62.88393115100078745, 7.208316651077764980 ) ) ;
#6422=CARTESIAN_POINT ( 'NONE',  ( 14.92337183194729633, 62.67559781766745886, 8.527530157486181039 ) ) ;
#6423=SURFACE_STYLE_USAGE ( .BOTH. , #45916 ) ;
#6424=CARTESIAN_POINT ( 'NONE',  ( 14.92337183194729633, 2.675597817667451750, 8.527530157486181039 ) ) ;
#6425=CARTESIAN_POINT ( 'NONE',  ( 5.076628168052704559, 20.17559781766745175, -8.527530157486179263 ) ) ;
#6426=ORIENTED_EDGE ( 'NONE', *, *, #39741, .T. ) ;
#6427=CARTESIAN_POINT ( 'NONE',  ( 12.63842701281683034, 27.46726448433411250, 9.846743663894596210 ) ) ;
#6429=CARTESIAN_POINT ( 'NONE',  ( 4.559911319644449179, 23.89701867748817321, 9.422509992056141925 ) ) ;
#6430=CARTESIAN_POINT ( 'NONE',  ( 12.63842701281683034, 22.46726448433411605, 9.846743663894596210 ) ) ;
#6432=CARTESIAN_POINT ( 'NONE',  ( 0.6178305044545818747, 13.49863466993041783, -9.382169495545419124 ) ) ;
#6433=CARTESIAN_POINT ( 'NONE',  ( 18.72515096720568195, 26.07228050351032778, -6.500000000000018652 ) ) ;
#6434=CARTESIAN_POINT ( 'NONE',  ( 10.00000000000000000, 56.81368534415484106, -10.88017736071110342 ) ) ;
#6435=CARTESIAN_POINT ( 'NONE',  ( 12.91533473730992121, 34.52201867748817676, 10.88017736071110164 ) ) ;
#6436=CARTESIAN_POINT ( 'NONE',  ( 7.084665262690076126, 4.105352010821503583, 10.88017736071109987 ) ) ;
#6437=CARTESIAN_POINT ( 'NONE',  ( 22.26659068614894466, 48.88708216824730357, 7.082119434687054849 ) ) ;
#6439=B_SPLINE_CURVE_WITH_KNOTS ( 'NONE', 3,
 ( #36105, #36619, #75591, #20119, #60081, #98115 ),
 .UNSPECIFIED., .F., .F.,
 ( 4, 2, 4 ),
 ( 0.000000000000000000, 0.0004042018129159926330, 0.0008084036258319852661 ),
 .UNSPECIFIED. ) ;
#6442=EDGE_CURVE ( 'NONE', #89305, #57072, #69420, .T. ) ;
#6444=CARTESIAN_POINT ( 'NONE',  ( -1.099225684535947600, 18.70696800326375353, -6.408140936763238038 ) ) ;
#6445=CARTESIAN_POINT ( 'NONE',  ( 12.91533473730992121, 49.52201867748817676, 10.88017736071110164 ) ) ;
#6446=FILL_AREA_STYLE ('',( #67946 ) ) ;
#6447=ORIENTED_EDGE ( 'NONE', *, *, #70155, .F. ) ;
#6448=CARTESIAN_POINT ( 'NONE',  ( 0.5774900079438607392, 53.48035201082151247, 5.440088680355550821 ) ) ;
#6449=CARTESIAN_POINT ( 'NONE',  ( 19.84674366389459621, 38.50893115100078745, 7.409399052514197653E-17 ) ) ;
#6451=CARTESIAN_POINT ( 'NONE',  ( 7.361572987183169658, 19.96726448433411960, -9.846743663894592657 ) ) ;
#6452=CARTESIAN_POINT ( 'NONE',  ( 17.20831665107776587, 12.88393115100078390, 7.208316651077764980 ) ) ;
#6453=DIRECTION ( 'NONE',  ( 0.000000000000000000, -1.000000000000000000, 0.000000000000000000 ) ) ;
#6454=CARTESIAN_POINT ( 'NONE',  ( -1.099225684535947600, 39.54030133659708923, 6.408140936763237150 ) ) ;
#6455=CARTESIAN_POINT ( 'NONE',  ( -0.8801773607111009756, 68.06368534415484817, 1.068504757029289695E-15 ) ) ;
#6458=CARTESIAN_POINT ( 'NONE',  ( 0.1532563361054083140, 31.00893115100078390, 1.131784320476157264E-15 ) ) ;
#6459=VERTEX_POINT ( 'NONE', #94908 ) ;
#6461=CARTESIAN_POINT ( 'NONE',  ( 10.00000000000000178, 55.37363466993042493, 12.81628187352647608 ) ) ;
#6463=CARTESIAN_POINT ( 'NONE',  ( 14.92337183194729633, 62.67559781766745886, 8.527530157486181039 ) ) ;
#6464=EDGE_CURVE ( 'NONE', #73005, #90157, #41933, .T. ) ;
#6465=CARTESIAN_POINT ( 'NONE',  ( 13.79529636645031943, 30.34541550158063927, -14.16423886937409904 ) ) ;
#6469=ADVANCED_FACE ( 'NONE', ( #87890 ), #11412, .T. ) ;
#6470=CARTESIAN_POINT ( 'NONE',  ( 13.79529636645031943, 30.34541550158063927, -14.16423886937409904 ) ) ;
#6471=CARTESIAN_POINT ( 'NONE',  ( 17.08211943468705130, 48.47041550158063927, 12.26659068614894998 ) ) ;
#6472=CARTESIAN_POINT ( 'NONE',  ( 2.917880565312948704, 12.63708216824730179, 12.26659068614894643 ) ) ;
#6473=CARTESIAN_POINT ( 'NONE',  ( 17.08211943468705130, 18.47041550158063572, 12.26659068614894998 ) ) ;
#6475=CARTESIAN_POINT ( 'NONE',  ( 15.44008868035555260, 44.73035201082151247, 9.422509992056143702 ) ) ;
#6477=CARTESIAN_POINT ( 'NONE',  ( 19.84674366389459266, 28.30059781766745886, 2.638427012816836559 ) ) ;
#6478=CARTESIAN_POINT ( 'NONE',  ( 12.91533473730993009, 66.60535201082150536, -10.88017736071109987 ) ) ;
#6479=CARTESIAN_POINT ( 'NONE',  ( 17.20831665107776587, 29.13393115100078390, -7.208316651077762316 ) ) ;
#6481=CARTESIAN_POINT ( 'NONE',  ( 12.91533473730992121, 19.52201867748816611, 10.88017736071110164 ) ) ;
#6482=CARTESIAN_POINT ( 'NONE',  ( 0.6178305044545818747, 53.49863466993041072, -9.382169495545419124 ) ) ;
#6483=CARTESIAN_POINT ( 'NONE',  ( 0.1532563361054082862, 61.21726448433412315, 2.638427012816831674 ) ) ;
#6484=CARTESIAN_POINT ( 'NONE',  ( 2.791683348922237240, 30.38393115100078390, -7.208316651077763204 ) ) ;
#6485=CARTESIAN_POINT ( 'NONE',  ( 22.81628187352648496, 36.83196800326376064, -3.434112377981050290 ) ) ;
#6487=CARTESIAN_POINT ( 'NONE',  ( 2.035157376598824452, 38.68868534415483396, 7.964842623401179544 ) ) ;
#6488=CARTESIAN_POINT ( 'NONE',  ( 1.472469842513823179, 45.59226448433412315, -4.923371831947296329 ) ) ;
#6489=CARTESIAN_POINT ( 'NONE',  ( 2.917880565312950480, 30.97041550158063572, -12.26659068614894821 ) ) ;
#6490=EDGE_LOOP ( 'NONE', ( #733, #24227, #78705, #12836, #93610, #35062, #85868, #41735 ) ) ;
#6491=SURFACE_STYLE_USAGE ( .BOTH. , #98016 ) ;
#6492=CARTESIAN_POINT ( 'NONE',  ( 10.00000000000000178, 69.31368534415484817, 10.88017736071110342 ) ) ;
#6493=CARTESIAN_POINT ( 'NONE',  ( 12.91533473730993009, 61.60535201082150536, -10.88017736071109987 ) ) ;
#6494=CARTESIAN_POINT ( 'NONE',  ( 6.204703633549690345, 57.84541550158063927, 14.16423886937410082 ) ) ;
#6495=CARTESIAN_POINT ( 'NONE',  ( 19.84674366389459266, 63.30059781766745886, 2.638427012816836559 ) ) ;
#6497=CARTESIAN_POINT ( 'NONE',  ( 12.91533473730992121, 54.52201867748816255, 10.88017736071110164 ) ) ;
#6501=CARTESIAN_POINT ( 'NONE',  ( 17.96484262340118221, 11.18868534415483929, -7.964842623401177768 ) ) ;
#6502=CARTESIAN_POINT ( 'NONE',  ( 4.559911319644449179, 17.23035201082150536, -9.422509992056141925 ) ) ;
#6503=CARTESIAN_POINT ( 'NONE',  ( 12.63842701281683034, 37.46726448433411605, 9.846743663894596210 ) ) ;
#6504=CARTESIAN_POINT ( 'NONE',  ( 13.43411237798105340, 45.58196800326374643, 12.81628187352647963 ) ) ;
#6508=CARTESIAN_POINT ( 'NONE',  ( -0.8801773607111008646, 23.27201867748817676, 2.915334737309923430 ) ) ;
#6510=CARTESIAN_POINT ( 'NONE',  ( 13.43411237798105340, 25.58196800326374998, 12.81628187352647963 ) ) ;
#6511=CARTESIAN_POINT ( 'NONE',  ( 19.89220837332773684, 39.74062864464239908, 6.478736007406005193 ) ) ;
#6512=CARTESIAN_POINT ( 'NONE',  ( 1.472469842513823179, 5.592264484334118713, -4.923371831947296329 ) ) ;
#6513=CARTESIAN_POINT ( 'NONE',  ( 18.52753015748618282, 43.92559781766745175, -4.923371831947291888 ) ) ;
#6514=CARTESIAN_POINT ( 'NONE',  ( 17.96484262340118221, 36.18868534415484106, -7.964842623401177768 ) ) ;
#6515=CARTESIAN_POINT ( 'NONE',  ( -1.099225684535947600, 14.54030133659708568, 6.408140936763237150 ) ) ;
#6516=CARTESIAN_POINT ( 'NONE',  ( 17.96484262340118221, 54.93868534415484106, 7.964842623401181321 ) ) ;
#6518=DIRECTION ( 'NONE',  ( 0.000000000000000000, 0.000000000000000000, 1.000000000000000000 ) ) ;
#6519=CARTESIAN_POINT ( 'NONE',  ( 21.09922568453594849, 51.20696800326375353, 6.408140936763242479 ) ) ;
#6521=CARTESIAN_POINT ( 'NONE',  ( 20.88017736071110875, 65.77201867748817676, -2.915334737309920765 ) ) ;
#6522=CARTESIAN_POINT ( 'NONE',  ( 13.43411237798105340, 30.58196800326374998, 12.81628187352647963 ) ) ;
#6523=CARTESIAN_POINT ( 'NONE',  ( 24.16423886937410614, 4.512082168247300906, -3.795296366450302550 ) ) ;
#6524=CARTESIAN_POINT ( 'NONE',  ( 18.52753015748618282, 3.925597817667451306, -4.923371831947291888 ) ) ;
#6525=CARTESIAN_POINT ( 'NONE',  ( 20.88017736071110164, 35.35535201082150536, 2.915334737309930979 ) ) ;
#6527=CARTESIAN_POINT ( 'NONE',  ( 0.1532563361054100626, 65.80059781766745175, -2.638427012816831230 ) ) ;
#6528=CARTESIAN_POINT ( 'NONE',  ( 18.52753015748617571, 18.09226448433411960, 4.923371831947298993 ) ) ;
#6529=CARTESIAN_POINT ( 'NONE',  ( 12.63842701281683034, 7.467264484334118713, 9.846743663894596210 ) ) ;
#6531=CARTESIAN_POINT ( 'NONE',  ( 22.26659068614895176, 44.72041550158063927, -7.082119434687042414 ) ) ;
#6532=CARTESIAN_POINT ( 'NONE',  ( 0.2751277870542911397, 55.30223176428831522, 6.499999999999992006 ) ) ;
#6534=CARTESIAN_POINT ( 'NONE',  ( 0.1077916266722467875, 7.240628644642391087, -6.478736007405949238 ) ) ;
#6538=CARTESIAN_POINT ( 'NONE',  ( 22.26659068614895176, 64.72041550158064638, -7.082119434687042414 ) ) ;
#6539=CARTESIAN_POINT ( 'NONE',  ( 20.36894250292379382, 63.67874883491396787, 10.36894250292379205 ) ) ;
#6540=CARTESIAN_POINT ( 'NONE',  ( 1.472469842513823179, 26.42559781766745175, 4.923371831947296329 ) ) ;
#6541=CARTESIAN_POINT ( 'NONE',  ( 0.6178305044545838731, 24.74863466993042493, 9.382169495545420901 ) ) ;
#6543=CARTESIAN_POINT ( 'NONE',  ( 10.00000000000000000, 5.553748834913967869, -14.16423886937410082 ) ) ;
#6544=CARTESIAN_POINT ( 'NONE',  ( 10.00000000000000000, 16.81368534415483751, -10.88017736071110342 ) ) ;
#6545=CARTESIAN_POINT ( 'NONE',  ( 24.16423886937410614, 59.30374883491397497, 8.672049930838204340E-16 ) ) ;
#6546=CARTESIAN_POINT ( 'NONE',  ( 17.20831665107776587, 27.88393115100078390, 7.208316651077764980 ) ) ;
#6548=CARTESIAN_POINT ( 'NONE',  ( 14.92337183194729988, 24.34226448433411960, -8.527530157486177487 ) ) ;
#6550=CARTESIAN_POINT ( 'NONE',  ( 19.84674366389459266, 3.300597817667451750, 2.638427012816836559 ) ) ;
#6557=CARTESIAN_POINT ( 'NONE',  ( 17.20831665107776587, 49.13393115100078745, -7.208316651077762316 ) ) ;
#6558=CARTESIAN_POINT ( 'NONE',  ( 13.79529636645031943, 20.34541550158063572, -14.16423886937409904 ) ) ;
#6559=CARTESIAN_POINT ( 'NONE',  ( 7.084665262690076126, 24.10535201082150181, 10.88017736071109987 ) ) ;
#6560=CARTESIAN_POINT ( 'NONE',  ( 12.91533473730992121, 44.52201867748816966, 10.88017736071110164 ) ) ;
#6561=CARTESIAN_POINT ( 'NONE',  ( 5.076628168052703671, 66.84226448433412315, 8.527530157486179263 ) ) ;
#6562=CARTESIAN_POINT ( 'NONE',  ( 3.591859063236761518, 14.95696800326375531, 11.09922568453594849 ) ) ;
#6563=ADVANCED_FACE ( 'NONE', ( #24963 ), #55448, .T. ) ;
#6564=CARTESIAN_POINT ( 'NONE',  ( 19.38216949554541202, 25.99863466993042138, 9.382169495545424454 ) ) ;
#6567=CARTESIAN_POINT ( 'NONE',  ( 0.1532563361054083140, 46.00893115100079456, 1.131784320476157264E-15 ) ) ;
#6568=CARTESIAN_POINT ( 'NONE',  ( 4.559911319644449179, 2.230352010821504916, -9.422509992056141925 ) ) ;
#6570=CARTESIAN_POINT ( 'NONE',  ( -0.8801773607110991993, 2.855352010821504471, -2.915334737309923874 ) ) ;
#6572=CARTESIAN_POINT ( 'NONE',  ( 15.44008868035555793, 46.39701867748817676, -9.422509992056140149 ) ) ;
#6573=CARTESIAN_POINT ( 'NONE',  ( -0.8801773607110991993, 62.85535201082150536, -2.915334737309923874 ) ) ;
#6574=FILL_AREA_STYLE ('',( #44068 ) ) ;
#6575=CARTESIAN_POINT ( 'NONE',  ( -0.8801773607110991993, 57.85535201082149825, -2.915334737309923874 ) ) ;
#6576=AXIS2_PLACEMENT_3D ( 'NONE', #39343, #77314, #8828 ) ;
#6582=CARTESIAN_POINT ( 'NONE',  ( 19.84674366389459266, 33.30059781766744464, 2.638427012816836559 ) ) ;
#6585=CARTESIAN_POINT ( 'NONE',  ( 20.30776406404415724, 70.00000000000000000, -6.000000000000001776 ) ) ;
#6587=CARTESIAN_POINT ( 'NONE',  ( 13.79529636645030344, 3.262082168247301350, 14.16423886937410614 ) ) ;
#6591=CARTESIAN_POINT ( 'NONE',  ( 0.5774900079438590739, 12.64701867748817321, -5.440088680355550821 ) ) ;
#6592=CARTESIAN_POINT ( 'NONE',  ( 18.39792806157253224, 64.52224192338641728, 6.499999999999917399 ) ) ;
#6594=SURFACE_STYLE_FILL_AREA ( #14106 ) ;
#6595=CARTESIAN_POINT ( 'NONE',  ( 17.20831665107776587, 44.13393115100078745, -7.208316651077762316 ) ) ;
#6597=CARTESIAN_POINT ( 'NONE',  ( 21.09922568453595559, 22.04030133659708923, -6.408140936763230044 ) ) ;
#6598=CARTESIAN_POINT ( 'NONE',  ( 1.472469842513823179, 5.592264484334118713, -4.923371831947296329 ) ) ;
#6600=CARTESIAN_POINT ( 'NONE',  ( 7.361572987183169658, 19.96726448433411960, -9.846743663894592657 ) ) ;
#6601=CARTESIAN_POINT ( 'NONE',  ( 6.565887622018943937, 8.081968003263751754, -12.81628187352647608 ) ) ;
#6602=CARTESIAN_POINT ( 'NONE',  ( 0.1532563361054100626, 25.80059781766744820, -2.638427012816831230 ) ) ;
#6604=ORIENTED_EDGE ( 'NONE', *, *, #19988, .F. ) ;
#6605=ORIENTED_EDGE ( 'NONE', *, *, #39008, .F. ) ;
#6606=CARTESIAN_POINT ( 'NONE',  ( -0.8801773607111008646, 18.27201867748817321, 2.915334737309923430 ) ) ;
#6607=CARTESIAN_POINT ( 'NONE',  ( -2.266590686148945544, 17.22041550158063572, 7.082119434687048631 ) ) ;
#6608=CARTESIAN_POINT ( 'NONE',  ( 19.84674366389459621, 33.50893115100078745, 7.409399052514197653E-17 ) ) ;
#6609=CARTESIAN_POINT ( 'NONE',  ( 4.559911319644449179, 58.89701867748817676, 9.422509992056141925 ) ) ;
#6610=CARTESIAN_POINT ( 'NONE',  ( 3.591859063236761518, 39.95696800326375353, 11.09922568453594849 ) ) ;
#6612=CARTESIAN_POINT ( 'NONE',  ( 4.559911319644449179, 12.23035201082150536, -9.422509992056141925 ) ) ;
#6615=CARTESIAN_POINT ( 'NONE',  ( 0.6178305044545838731, 9.748634669930416052, 9.382169495545420901 ) ) ;
#6616=CARTESIAN_POINT ( 'NONE',  ( 0.1532563361054100626, 65.80059781766745175, -2.638427012816831230 ) ) ;
#6617=CARTESIAN_POINT ( 'NONE',  ( 5.076628168052704559, 30.17559781766745175, -8.527530157486179263 ) ) ;
#6619=CARTESIAN_POINT ( 'NONE',  ( 21.09922568453595559, 42.04030133659708213, -6.408140936763230044 ) ) ;
#6621=( GEOMETRIC_REPRESENTATION_CONTEXT ( 3 ) GLOBAL_UNCERTAINTY_ASSIGNED_CONTEXT ( ( #69131 ) ) GLOBAL_UNIT_ASSIGNED_CONTEXT ( ( #47099, #83640, #40107 ) ) REPRESENTATION_CONTEXT ( 'NONE', 'WORKASPACE' ) );
#6622=CARTESIAN_POINT ( 'NONE',  ( 20.88017736071110875, 35.77201867748816966, -2.915334737309920765 ) ) ;
#6625=CARTESIAN_POINT ( 'NONE',  ( 0.5774900079438590739, 67.64701867748817676, -5.440088680355550821 ) ) ;
#6626=CARTESIAN_POINT ( 'NONE',  ( 12.91533473730993009, 46.60535201082150536, -10.88017736071109987 ) ) ;
#6628=CARTESIAN_POINT ( 'NONE',  ( -0.8801773607111009756, 43.06368534415484106, 1.068504757029289695E-15 ) ) ;
#6629=CARTESIAN_POINT ( 'NONE',  ( 19.84674366389459266, 63.71726448433412315, -2.638427012816827677 ) ) ;
#6630=CARTESIAN_POINT ( 'NONE',  ( 7.084665262690076126, 67.02201867748817676, -10.88017736071110164 ) ) ;
#6631=CARTESIAN_POINT ( 'NONE',  ( 10.00000000000000178, 37.25893115100078745, 9.846743663894594434 ) ) ;
#6632=CARTESIAN_POINT ( 'NONE',  ( 4.559911319644449179, 2.230352010821504471, -9.422509992056141925 ) ) ;
#6633=CARTESIAN_POINT ( 'NONE',  ( 21.09922568453594849, 6.206968003263753531, 6.408140936763242479 ) ) ;
#6635=CARTESIAN_POINT ( 'NONE',  ( 7.084665262690076126, 29.10535201082150181, 10.88017736071109987 ) ) ;
#6636=CARTESIAN_POINT ( 'NONE',  ( 2.035157376598824452, 33.68868534415484106, 7.964842623401179544 ) ) ;
#6637=CARTESIAN_POINT ( 'NONE',  ( 7.084665262690076126, 69.10535201082151957, 10.88017736071109987 ) ) ;
#6638=CARTESIAN_POINT ( 'NONE',  ( 13.79529636645030344, 43.26208216824730357, 14.16423886937410614 ) ) ;
#6640=CARTESIAN_POINT ( 'NONE',  ( 2.791683348922240793, 11.63393115100078568, 7.208316651077764092 ) ) ;
#6641=CARTESIAN_POINT ( 'NONE',  ( -0.8801773607111008646, 53.27201867748816966, 2.915334737309923430 ) ) ;
#6643=CARTESIAN_POINT ( 'NONE',  ( 22.26659068614895176, 4.720415501580633943, -7.082119434687042414 ) ) ;
#6645=ADVANCED_FACE ( 'NONE', ( #28862 ), #65385, .F. ) ;
#6648=CARTESIAN_POINT ( 'NONE',  ( 5.076628168052704559, 65.17559781766745175, -8.527530157486179263 ) ) ;
#6649=( BOUNDED_SURFACE ( )  B_SPLINE_SURFACE ( 1, 2, ( 
 ( #97964, #59925, #75428, #76416, #29420, #52917, #68433, #30411, #454, #14948, #44920, #6436, #67445, #6942, #37943, #98460, #91416, #8413, #83917, #15446, #45927, #23434, #68925, #84422, #15919, #52434, #74935, #90413, #59256, #13770, #59753, #96297, #43271, #21780, #67266, #27774, #36272, #89270, #73276, #73766, #82754, #44750, #12774, #5295, #36774, #97794, #58259, #74761, #57776, #88282, #4798, #44257, #35773, #14277, #90248, #66261, #96796, #58766, #43762, #6269, #89757, #28271, #21274, #52259, #82254, #75253, #74251, #20781, #81758, #29256, #88774, #51272, #13270, #5783, #6766, #66767, #50783, #65269, #95797, #19782, #97290, #28764, #51770, #27278, #50270, #80787, #12284, #42791, #35274, #65769, #20285, #81274, #93636, #33606, #77154, #18147, #56143, #71633, #69665, #26133, #41148, #85649, #2178, #78144, #70656, #94620, #63134, #48130, #54643, #25170, #55646, #9654, #40151, #47142, #33123, #32636, #87113, #86146, #39175, #25650, #56624, #10151, #63617, #1191, #40646, #85160, #17659, #55135, #78645, #16668, #32134, #10636, #77639, #9156, #48619, #94124, #17169, #71144, #39674, #18628, #2672, #86638, #8663, #79123, #31650, #3144, #24665, #64102, #62140, #92648, #70165, #24172, #1682, #62634, #93138, #47649, #87601, #11610, #58584, #58083, #95606, #59075, #51087, #12592, #34101, #42607, #50599, #43091, #27594, #28585, #20600, #49120, #4621, #42126, #81091, #20095, #88587, #66081, #19112, #81578, #12104, #73085, #73577, #65084, #88093, #5101, #49592, #65582, #5606, #79622, #89086, #28086, #43582, #41642, #97114, #13084, #57596, #35083, #50101, #96109, #66587, #27093, #4126, #74073, #36084, #80104, #35594, #19606, #89580, #11123, #72592, #72106, #64592, #34590, #80607, #96609, #3635, #95100, #26607, #57105, #60061, #46062, #91054, #59576, #75569, #38563, #82075, #597, #22090, #30546, #7081, #90562, #22581, #37583, #31039, #67587, #29556, #91562, #23079, #14090, #61048, #13586, #44069, #90069, #100, #52566, #69059, #76548, #98096, #83071, #14590, #98604, #68569, #45562, #45059, #76058, #8067, #38080, #61539, #30054, #68076, #60563, #53548, #82576, #53054, #83571, #15090, #84061, #7588, #6575, #15580, #21091, #74575, #51591, #6091, #36594, #67080, #97607, #29068, #21593, #52083, #44573, #75071, #37088, #24558, #46542, #54044, #62028, #24056, #16554, #77043, #92528, #54525, #48503, #8556, #84554, #94011, #79006, #1068, #69552, #55017, #17047, #10031, #31532, #47527, #85534, #25045, #77520, #85041, #25534, #86028, #56025, #10509, #41025, #78029, #78517, #71527, #33010, #47028, #70535, #9037, #39057, #39554, #70043, #40532 ),
 ( #1565, #40033, #9531, #2057, #32519, #32014, #48009, #63017, #3037, #93518, #16054, #71030, #33487, #55531, #2553, #62517, #17542, #93022, #63509, #86523, #18021, #92047, #23575, #96491, #33975, #3517, #4987, #49482, #64478, #65964, #57967, #27962, #81460, #12963, #95492, #50471, #43458, #35468, #94985, #42490, #26491, #18507, #11008, #56985, #80976, #48997, #26985, #72972, #4503, #58456, #34473, #87492, #94496, #56510, #19006, #4011, #79990, #57483, #73960, #11492, #87978, #64966, #88971, #42013, #19489, #20480, #72478, #34968, #26015, #88471, #12475, #50966, #49982, #80490, #5489, #63986, #11987, #65465, #95992, #71992, #27474, #87001, #79506, #19974, #42979, #41524, #73459, #28944, #45433, #28468, #58965, #74444, #14963, #44446, #53423, #60925, #13971, #6451, #29433, #14462, #83442, #60434, #74948, #90927, #22958, #52931, #15459, #44937, #36961, #52447, #75935, #97478, #67456, #97977, #59937, #7458, #75443, #21465, #37956, #91430, #89461, #6955, #90427, #21968, #67950, #82947, #29928, #37463, #45940, #20979, #82447, #22456, #98474, #51462, #96991, #5971, #66960, #59446, #81952, #36465, #89947, #83930, #13465, #43946, #68449, #76430, #51963, #98970, #30424, #35960, #66455, #46423, #62390, #69919, #39910, #8426, #63384, #61416, #68938, #9911, #93888, #15932, #84435, #1440, #31892, #24919, #76916, #92898, #24429, #70413, #92411, #38933, #40413, #1933, #70908, #25416, #55900, #39426, #93394, #86397, #47888, #69422, #85408, #943, #91923, #53925, #31404, #55404, #23448, #54893, #16918, #47394, #78390, #77396, #61905, #38441, #468, #23935, #46903, #54404, #77896, #17900, #84916, #9408, #8909, #2428, #16427, #32390, #32885, #62895, #85905, #30916, #17419, #48383, #7945, #10886, #56868, #35347, #80856, #41410, #49856, #3885, #86880, #87369, #96370, #58331, #26369, #18884, #50345, #12353, #71874, #88356, #71401, #2917, #18390, #57846, #49365, #27843, #4870, #79867, #11371, #72353, #57359, #27353, #4382, #41893, #34847, #65841, #95871, #88848, #87853, #34352, #95362, #19852, #3386, #64843, #26862, #19371, #42860, #80365, #64359, #73343, #20356, #33367, #11865, #42372, #72846, #65343, #78885, #10396, #40900, #63861, #94375, #25894, #56393, #48869, #79381, #33851, #94868, #81827, #74323, #5366, #20851, #97356, #59325, #22342, #52815, #43827, #60323, #43341, #73838, #89341, #29814, #89828, #68331, #75818, #28825, #21345, #44325, #29319, #98356, #75320, #51836, #6833, #37840, #67838, #30305, #59816, #82323, #67330, #90813, #13343, #13843, #74826, #6330, #83323, #90311, #36340, #14849, #7339, #35845, #21847, #36842, #97856, #82821 ) ),
 .UNSPECIFIED., .F., .F., .T. ) 
 B_SPLINE_SURFACE_WITH_KNOTS ( ( 2, 2 ),
 ( 3, 2, 2, 2, 2, 2, 2, 2, 2, 2, 2, 2, 2, 2, 2, 2, 2, 2, 2, 2, 2, 2, 2, 2, 2, 2, 2, 2, 2, 2, 2, 2, 2, 2, 2, 2, 2, 2, 2, 2, 2, 2, 2, 2, 2, 2, 2, 2, 2, 2, 2, 2, 2, 2, 2, 2, 2, 2, 2, 2, 2, 2, 2, 2, 2, 2, 2, 2, 2, 2, 2, 2, 2, 2, 2, 2, 2, 2, 2, 2, 2, 2, 2, 2, 2, 2, 2, 2, 2, 2, 2, 2, 2, 2, 2, 2, 2, 2, 2, 2, 2, 2, 2, 2, 2, 2, 2, 2, 2, 2, 2, 2, 2, 2, 2, 2, 2, 2, 2, 2, 2, 2, 2, 2, 2, 2, 2, 2, 2, 2, 2, 2, 2, 2, 2, 2, 2, 2, 2, 2, 2, 2, 2, 2, 2, 2, 2, 2, 2, 2, 2, 2, 2, 2, 2, 2, 2, 2, 2, 2, 2, 2, 3 ),
 ( 0.000000000000000000, 1.000000000000000000 ),
 ( 0.000000000000000000, 0.005952380952380952051, 0.01190476190476190410, 0.01785714285714285615, 0.02380952380952380820, 0.02976190476190476025, 0.03571428571428571230, 0.04166666666666666435, 0.04761904761904761640, 0.05357142857142856845, 0.05952380952380952051, 0.06547619047619047949, 0.07142857142857142461, 0.07738095238095238360, 0.08333333333333332871, 0.08928571428571428770, 0.09523809523809523281, 0.1011904761904761918, 0.1071428571428571369, 0.1130952380952380959, 0.1190476190476190410, 0.1250000000000000000, 0.1309523809523809590, 0.1369047619047619180, 0.1428571428571428492, 0.1488095238095238082, 0.1547619047619047672, 0.1607142857142857262, 0.1666666666666666574, 0.1726190476190476164, 0.1785714285714285754, 0.1845238095238095344, 0.1904761904761904656, 0.1964285714285714246, 0.2023809523809523836, 0.2083333333333333426, 0.2142857142857142738, 0.2202380952380952328, 0.2261904761904761918, 0.2321428571428571508, 0.2380952380952380820, 0.2440476190476190410, 0.2500000000000000000, 0.2559523809523809312, 0.2619047619047619180, 0.2678571428571428492, 0.2738095238095238360, 0.2797619047619047672, 0.2857142857142856984, 0.2916666666666666852, 0.2976190476190476164, 0.3035714285714285476, 0.3095238095238095344, 0.3154761904761904656, 0.3214285714285714524, 0.3273809523809523836, 0.3333333333333333148, 0.3392857142857143016, 0.3452380952380952328, 0.3511904761904761640, 0.3571428571428571508, 0.3630952380952380820, 0.3690476190476190688, 0.3750000000000000000, 0.3809523809523809312, 0.3869047619047619180, 0.3928571428571428492, 0.3988095238095238360, 0.4047619047619047672, 0.4107142857142856984, 0.4166666666666666852, 0.4226190476190476164, 0.4285714285714285476, 0.4345238095238095344, 0.4404761904761904656, 0.4464285714285714524, 0.4523809523809523836, 0.4583333333333333148, 0.4642857142857143016, 0.4702380952380952328, 0.4761904761904761640, 0.4821428571428571508, 0.4880952380952380820, 0.4940476190476190688, 0.5000000000000000000, 0.5059523809523809312, 0.5119047619047618625, 0.5178571428571429047, 0.5238095238095238360, 0.5297619047619047672, 0.5357142857142856984, 0.5416666666666666297, 0.5476190476190476719, 0.5535714285714286031, 0.5595238095238095344, 0.5654761904761904656, 0.5714285714285713969, 0.5773809523809523281, 0.5833333333333333703, 0.5892857142857143016, 0.5952380952380952328, 0.6011904761904761640, 0.6071428571428570953, 0.6130952380952381375, 0.6190476190476190688, 0.6250000000000000000, 0.6309523809523809312, 0.6369047619047618625, 0.6428571428571429047, 0.6488095238095238360, 0.6547619047619047672, 0.6607142857142856984, 0.6666666666666666297, 0.6726190476190476719, 0.6785714285714286031, 0.6845238095238095344, 0.6904761904761904656, 0.6964285714285713969, 0.7023809523809523281, 0.7083333333333333703, 0.7142857142857143016, 0.7202380952380952328, 0.7261904761904761640, 0.7321428571428570953, 0.7380952380952381375, 0.7440476190476190688, 0.7500000000000000000, 0.7559523809523809312, 0.7619047619047618625, 0.7678571428571429047, 0.7738095238095238360, 0.7797619047619047672, 0.7857142857142856984, 0.7916666666666666297, 0.7976190476190476719, 0.8035714285714286031, 0.8095238095238095344, 0.8154761904761904656, 0.8214285714285713969, 0.8273809523809523281, 0.8333333333333333703, 0.8392857142857143016, 0.8452380952380952328, 0.8511904761904761640, 0.8571428571428570953, 0.8630952380952381375, 0.8690476190476190688, 0.8750000000000000000, 0.8809523809523809312, 0.8869047619047618625, 0.8928571428571429047, 0.8988095238095238360, 0.9047619047619047672, 0.9107142857142856984, 0.9166666666666666297, 0.9226190476190476719, 0.9285714285714286031, 0.9345238095238095344, 0.9404761904761904656, 0.9464285714285713969, 0.9523809523809523281, 0.9583333333333333703, 0.9642857142857143016 ),
 .UNSPECIFIED. ) 
 GEOMETRIC_REPRESENTATION_ITEM ( )  RATIONAL_B_SPLINE_SURFACE ( (
 ( 1.000000000000000000, 0.9659258262890683122, 1.000000000000000000, 0.9659258262890683122, 1.000000000000000000, 0.9659258262890683122, 1.000000000000000000, 0.9659258262890683122, 1.000000000000000000, 0.9659258262890683122, 1.000000000000000000, 0.9659258262890683122, 1.000000000000000000, 0.9659258262890683122, 1.000000000000000000, 0.9659258262890683122, 1.000000000000000000, 0.9659258262890683122, 1.000000000000000000, 0.9659258262890683122, 1.000000000000000000, 0.9659258262890683122, 1.000000000000000000, 0.9659258262890683122, 1.000000000000000000, 0.9659258262890683122, 1.000000000000000000, 0.9659258262890683122, 1.000000000000000000, 0.9659258262890683122, 1.000000000000000000, 0.9659258262890683122, 1.000000000000000000, 0.9659258262890683122, 1.000000000000000000, 0.9659258262890683122, 1.000000000000000000, 0.9659258262890683122, 1.000000000000000000, 0.9659258262890683122, 1.000000000000000000, 0.9659258262890683122, 1.000000000000000000, 0.9659258262890683122, 1.000000000000000000, 0.9659258262890683122, 1.000000000000000000, 0.9659258262890683122, 1.000000000000000000, 0.9659258262890683122, 1.000000000000000000, 0.9659258262890683122, 1.000000000000000000, 0.9659258262890683122, 1.000000000000000000, 0.9659258262890683122, 1.000000000000000000, 0.9659258262890683122, 1.000000000000000000, 0.9659258262890683122, 1.000000000000000000, 0.9659258262890683122, 1.000000000000000000, 0.9659258262890683122, 1.000000000000000000, 0.9659258262890683122, 1.000000000000000000, 0.9659258262890683122, 1.000000000000000000, 0.9659258262890683122, 1.000000000000000000, 0.9659258262890683122, 1.000000000000000000, 0.9659258262890683122, 1.000000000000000000, 0.9659258262890683122, 1.000000000000000000, 0.9659258262890683122, 1.000000000000000000, 0.9659258262890683122, 1.000000000000000000, 0.9659258262890683122, 1.000000000000000000, 0.9659258262890683122, 1.000000000000000000, 0.9659258262890683122, 1.000000000000000000, 0.9659258262890683122, 1.000000000000000000, 0.9659258262890683122, 1.000000000000000000, 0.9659258262890683122, 1.000000000000000000, 0.9659258262890683122, 1.000000000000000000, 0.9659258262890683122, 1.000000000000000000, 0.9659258262890683122, 1.000000000000000000, 0.9659258262890683122, 1.000000000000000000, 0.9659258262890683122, 1.000000000000000000, 0.9659258262890683122, 1.000000000000000000, 0.9659258262890683122, 1.000000000000000000, 0.9659258262890683122, 1.000000000000000000, 0.9659258262890683122, 1.000000000000000000, 0.9659258262890683122, 1.000000000000000000, 0.9659258262890683122, 1.000000000000000000, 0.9659258262890683122, 1.000000000000000000, 0.9659258262890683122, 1.000000000000000000, 0.9659258262890683122, 1.000000000000000000, 0.9659258262890683122, 1.000000000000000000, 0.9659258262890683122, 1.000000000000000000, 0.9659258262890683122, 1.000000000000000000, 0.9659258262890683122, 1.000000000000000000, 0.9659258262890683122, 1.000000000000000000, 0.9659258262890683122, 1.000000000000000000, 0.9659258262890683122, 1.000000000000000000, 0.9659258262890683122, 1.000000000000000000, 0.9659258262890683122, 1.000000000000000000, 0.9659258262890683122, 1.000000000000000000, 0.9659258262890683122, 1.000000000000000000, 0.9659258262890683122, 1.000000000000000000, 0.9659258262890683122, 1.000000000000000000, 0.9659258262890683122, 1.000000000000000000, 0.9659258262890683122, 1.000000000000000000, 0.9659258262890683122, 1.000000000000000000, 0.9659258262890683122, 1.000000000000000000, 0.9659258262890683122, 1.000000000000000000, 0.9659258262890683122, 1.000000000000000000, 0.9659258262890683122, 1.000000000000000000, 0.9659258262890683122, 1.000000000000000000, 0.9659258262890683122, 1.000000000000000000, 0.9659258262890683122, 1.000000000000000000, 0.9659258262890683122, 1.000000000000000000, 0.9659258262890683122, 1.000000000000000000, 0.9659258262890683122, 1.000000000000000000, 0.9659258262890683122, 1.000000000000000000, 0.9659258262890683122, 1.000000000000000000, 0.9659258262890683122, 1.000000000000000000, 0.9659258262890683122, 1.000000000000000000, 0.9659258262890683122, 1.000000000000000000, 0.9659258262890683122, 1.000000000000000000, 0.9659258262890683122, 1.000000000000000000, 0.9659258262890683122, 1.000000000000000000, 0.9659258262890683122, 1.000000000000000000, 0.9659258262890683122, 1.000000000000000000, 0.9659258262890683122, 1.000000000000000000, 0.9659258262890683122, 1.000000000000000000, 0.9659258262890683122, 1.000000000000000000, 0.9659258262890683122, 1.000000000000000000, 0.9659258262890683122, 1.000000000000000000, 0.9659258262890683122, 1.000000000000000000, 0.9659258262890683122, 1.000000000000000000, 0.9659258262890683122, 1.000000000000000000, 0.9659258262890683122, 1.000000000000000000, 0.9659258262890683122, 1.000000000000000000, 0.9659258262890683122, 1.000000000000000000, 0.9659258262890683122, 1.000000000000000000, 0.9659258262890683122, 1.000000000000000000, 0.9659258262890683122, 1.000000000000000000, 0.9659258262890683122, 1.000000000000000000, 0.9659258262890683122, 1.000000000000000000, 0.9659258262890683122, 1.000000000000000000, 0.9659258262890683122, 1.000000000000000000, 0.9659258262890683122, 1.000000000000000000, 0.9659258262890683122, 1.000000000000000000, 0.9659258262890683122, 1.000000000000000000, 0.9659258262890683122, 1.000000000000000000, 0.9659258262890683122, 1.000000000000000000, 0.9659258262890683122, 1.000000000000000000, 0.9659258262890683122, 1.000000000000000000, 0.9659258262890683122, 1.000000000000000000, 0.9659258262890683122, 1.000000000000000000, 0.9659258262890683122, 1.000000000000000000, 0.9659258262890683122, 1.000000000000000000, 0.9659258262890683122, 1.000000000000000000, 0.9659258262890683122, 1.000000000000000000, 0.9659258262890683122, 1.000000000000000000, 0.9659258262890683122, 1.000000000000000000, 0.9659258262890683122, 1.000000000000000000, 0.9659258262890683122, 1.000000000000000000, 0.9659258262890683122, 1.000000000000000000, 0.9659258262890683122, 1.000000000000000000, 0.9659258262890683122, 1.000000000000000000, 0.9659258262890683122, 1.000000000000000000, 0.9659258262890683122, 1.000000000000000000, 0.9659258262890683122, 1.000000000000000000, 0.9659258262890683122, 1.000000000000000000, 0.9659258262890683122, 1.000000000000000000, 0.9659258262890683122, 1.000000000000000000, 0.9659258262890683122, 1.000000000000000000, 0.9659258262890683122, 1.000000000000000000, 0.9659258262890683122, 1.000000000000000000, 0.9659258262890683122, 1.000000000000000000, 0.9659258262890683122, 1.000000000000000000, 0.9659258262890683122, 1.000000000000000000, 0.9659258262890683122, 1.000000000000000000, 0.9659258262890683122, 1.000000000000000000, 0.9659258262890683122, 1.000000000000000000, 0.9659258262890683122, 1.000000000000000000, 0.9659258262890683122, 1.000000000000000000, 0.9659258262890683122, 1.000000000000000000, 0.9659258262890683122, 1.000000000000000000, 0.9659258262890683122, 1.000000000000000000, 0.9659258262890683122, 1.000000000000000000, 0.9659258262890683122, 1.000000000000000000, 0.9659258262890683122, 1.000000000000000000, 0.9659258262890683122, 1.000000000000000000, 0.9659258262890683122, 1.000000000000000000, 0.9659258262890683122, 1.000000000000000000, 0.9659258262890683122, 1.000000000000000000, 0.9659258262890683122, 1.000000000000000000),
 ( 1.000000000000000000, 0.9659258262890683122, 1.000000000000000000, 0.9659258262890683122, 1.000000000000000000, 0.9659258262890683122, 1.000000000000000000, 0.9659258262890683122, 1.000000000000000000, 0.9659258262890683122, 1.000000000000000000, 0.9659258262890683122, 1.000000000000000000, 0.9659258262890683122, 1.000000000000000000, 0.9659258262890683122, 1.000000000000000000, 0.9659258262890683122, 1.000000000000000000, 0.9659258262890683122, 1.000000000000000000, 0.9659258262890683122, 1.000000000000000000, 0.9659258262890683122, 1.000000000000000000, 0.9659258262890683122, 1.000000000000000000, 0.9659258262890683122, 1.000000000000000000, 0.9659258262890683122, 1.000000000000000000, 0.9659258262890683122, 1.000000000000000000, 0.9659258262890683122, 1.000000000000000000, 0.9659258262890683122, 1.000000000000000000, 0.9659258262890683122, 1.000000000000000000, 0.9659258262890683122, 1.000000000000000000, 0.9659258262890683122, 1.000000000000000000, 0.9659258262890683122, 1.000000000000000000, 0.9659258262890683122, 1.000000000000000000, 0.9659258262890683122, 1.000000000000000000, 0.9659258262890683122, 1.000000000000000000, 0.9659258262890683122, 1.000000000000000000, 0.9659258262890683122, 1.000000000000000000, 0.9659258262890683122, 1.000000000000000000, 0.9659258262890683122, 1.000000000000000000, 0.9659258262890683122, 1.000000000000000000, 0.9659258262890683122, 1.000000000000000000, 0.9659258262890683122, 1.000000000000000000, 0.9659258262890683122, 1.000000000000000000, 0.9659258262890683122, 1.000000000000000000, 0.9659258262890683122, 1.000000000000000000, 0.9659258262890683122, 1.000000000000000000, 0.9659258262890683122, 1.000000000000000000, 0.9659258262890683122, 1.000000000000000000, 0.9659258262890683122, 1.000000000000000000, 0.9659258262890683122, 1.000000000000000000, 0.9659258262890683122, 1.000000000000000000, 0.9659258262890683122, 1.000000000000000000, 0.9659258262890683122, 1.000000000000000000, 0.9659258262890683122, 1.000000000000000000, 0.9659258262890683122, 1.000000000000000000, 0.9659258262890683122, 1.000000000000000000, 0.9659258262890683122, 1.000000000000000000, 0.9659258262890683122, 1.000000000000000000, 0.9659258262890683122, 1.000000000000000000, 0.9659258262890683122, 1.000000000000000000, 0.9659258262890683122, 1.000000000000000000, 0.9659258262890683122, 1.000000000000000000, 0.9659258262890683122, 1.000000000000000000, 0.9659258262890683122, 1.000000000000000000, 0.9659258262890683122, 1.000000000000000000, 0.9659258262890683122, 1.000000000000000000, 0.9659258262890683122, 1.000000000000000000, 0.9659258262890683122, 1.000000000000000000, 0.9659258262890683122, 1.000000000000000000, 0.9659258262890683122, 1.000000000000000000, 0.9659258262890683122, 1.000000000000000000, 0.9659258262890683122, 1.000000000000000000, 0.9659258262890683122, 1.000000000000000000, 0.9659258262890683122, 1.000000000000000000, 0.9659258262890683122, 1.000000000000000000, 0.9659258262890683122, 1.000000000000000000, 0.9659258262890683122, 1.000000000000000000, 0.9659258262890683122, 1.000000000000000000, 0.9659258262890683122, 1.000000000000000000, 0.9659258262890683122, 1.000000000000000000, 0.9659258262890683122, 1.000000000000000000, 0.9659258262890683122, 1.000000000000000000, 0.9659258262890683122, 1.000000000000000000, 0.9659258262890683122, 1.000000000000000000, 0.9659258262890683122, 1.000000000000000000, 0.9659258262890683122, 1.000000000000000000, 0.9659258262890683122, 1.000000000000000000, 0.9659258262890683122, 1.000000000000000000, 0.9659258262890683122, 1.000000000000000000, 0.9659258262890683122, 1.000000000000000000, 0.9659258262890683122, 1.000000000000000000, 0.9659258262890683122, 1.000000000000000000, 0.9659258262890683122, 1.000000000000000000, 0.9659258262890683122, 1.000000000000000000, 0.9659258262890683122, 1.000000000000000000, 0.9659258262890683122, 1.000000000000000000, 0.9659258262890683122, 1.000000000000000000, 0.9659258262890683122, 1.000000000000000000, 0.9659258262890683122, 1.000000000000000000, 0.9659258262890683122, 1.000000000000000000, 0.9659258262890683122, 1.000000000000000000, 0.9659258262890683122, 1.000000000000000000, 0.9659258262890683122, 1.000000000000000000, 0.9659258262890683122, 1.000000000000000000, 0.9659258262890683122, 1.000000000000000000, 0.9659258262890683122, 1.000000000000000000, 0.9659258262890683122, 1.000000000000000000, 0.9659258262890683122, 1.000000000000000000, 0.9659258262890683122, 1.000000000000000000, 0.9659258262890683122, 1.000000000000000000, 0.9659258262890683122, 1.000000000000000000, 0.9659258262890683122, 1.000000000000000000, 0.9659258262890683122, 1.000000000000000000, 0.9659258262890683122, 1.000000000000000000, 0.9659258262890683122, 1.000000000000000000, 0.9659258262890683122, 1.000000000000000000, 0.9659258262890683122, 1.000000000000000000, 0.9659258262890683122, 1.000000000000000000, 0.9659258262890683122, 1.000000000000000000, 0.9659258262890683122, 1.000000000000000000, 0.9659258262890683122, 1.000000000000000000, 0.9659258262890683122, 1.000000000000000000, 0.9659258262890683122, 1.000000000000000000, 0.9659258262890683122, 1.000000000000000000, 0.9659258262890683122, 1.000000000000000000, 0.9659258262890683122, 1.000000000000000000, 0.9659258262890683122, 1.000000000000000000, 0.9659258262890683122, 1.000000000000000000, 0.9659258262890683122, 1.000000000000000000, 0.9659258262890683122, 1.000000000000000000, 0.9659258262890683122, 1.000000000000000000, 0.9659258262890683122, 1.000000000000000000, 0.9659258262890683122, 1.000000000000000000, 0.9659258262890683122, 1.000000000000000000, 0.9659258262890683122, 1.000000000000000000, 0.9659258262890683122, 1.000000000000000000, 0.9659258262890683122, 1.000000000000000000, 0.9659258262890683122, 1.000000000000000000, 0.9659258262890683122, 1.000000000000000000, 0.9659258262890683122, 1.000000000000000000, 0.9659258262890683122, 1.000000000000000000, 0.9659258262890683122, 1.000000000000000000, 0.9659258262890683122, 1.000000000000000000, 0.9659258262890683122, 1.000000000000000000, 0.9659258262890683122, 1.000000000000000000, 0.9659258262890683122, 1.000000000000000000, 0.9659258262890683122, 1.000000000000000000, 0.9659258262890683122, 1.000000000000000000, 0.9659258262890683122, 1.000000000000000000, 0.9659258262890683122, 1.000000000000000000, 0.9659258262890683122, 1.000000000000000000, 0.9659258262890683122, 1.000000000000000000, 0.9659258262890683122, 1.000000000000000000, 0.9659258262890683122, 1.000000000000000000, 0.9659258262890683122, 1.000000000000000000, 0.9659258262890683122, 1.000000000000000000, 0.9659258262890683122, 1.000000000000000000, 0.9659258262890683122, 1.000000000000000000, 0.9659258262890683122, 1.000000000000000000, 0.9659258262890683122, 1.000000000000000000, 0.9659258262890683122, 1.000000000000000000, 0.9659258262890683122, 1.000000000000000000, 0.9659258262890683122, 1.000000000000000000, 0.9659258262890683122, 1.000000000000000000, 0.9659258262890683122, 1.000000000000000000, 0.9659258262890683122, 1.000000000000000000, 0.9659258262890683122, 1.000000000000000000, 0.9659258262890683122, 1.000000000000000000, 0.9659258262890683122, 1.000000000000000000, 0.9659258262890683122, 1.000000000000000000, 0.9659258262890683122, 1.000000000000000000, 0.9659258262890683122, 1.000000000000000000) ) ) 
 REPRESENTATION_ITEM ( '' )  SURFACE ( )  );
#6650=EDGE_LOOP ( 'NONE', ( #51499, #60296, #62086, #64666 ) ) ;
#6651=ORIENTED_EDGE ( 'NONE', *, *, #48371, .F. ) ;
#6654=CARTESIAN_POINT ( 'NONE',  ( 10.00000000000000178, 18.05374883491396787, 14.16423886937410082 ) ) ;
#6655=CARTESIAN_POINT ( 'NONE',  ( 24.16423886937409904, 19.09541550158063927, 3.795296366450317205 ) ) ;
#6656=CARTESIAN_POINT ( 'NONE',  ( 17.96484262340118221, 59.93868534415484106, 7.964842623401181321 ) ) ;
#6657=CARTESIAN_POINT ( 'NONE',  ( 10.00000000000000000, 1.813685344154838175, -10.88017736071110342 ) ) ;
#6658=CARTESIAN_POINT ( 'NONE',  ( -1.099225684535947600, -0.4596986634029132657, 6.408140936763237150 ) ) ;
#6659=CARTESIAN_POINT ( 'NONE',  ( 17.20831665107776587, 42.88393115100077324, 7.208316651077764980 ) ) ;
#6661=CARTESIAN_POINT ( 'NONE',  ( 0.5774900079438590739, 52.64701867748817676, -5.440088680355550821 ) ) ;
#6662=CARTESIAN_POINT ( 'NONE',  ( 21.09922568453594849, 1.206968003263753531, 6.408140936763242479 ) ) ;
#6663=CARTESIAN_POINT ( 'NONE',  ( 24.16423886937409904, 14.09541550158063217, 3.795296366450317205 ) ) ;
#6664=CARTESIAN_POINT ( 'NONE',  ( -0.8801773607110991993, 12.85535201082150358, -2.915334737309923874 ) ) ;
#6665=CARTESIAN_POINT ( 'NONE',  ( 7.084665262690076126, 12.02201867748817321, -10.88017736071110164 ) ) ;
#6666=CARTESIAN_POINT ( 'NONE',  ( -0.3289641300568009741, 2.245456701841137548, -5.963430220938281678 ) ) ;
#6667=CARTESIAN_POINT ( 'NONE',  ( 10.00000000000000178, 54.31368534415484106, 10.88017736071110342 ) ) ;
#6668=CARTESIAN_POINT ( 'NONE',  ( 19.38216949554541557, 47.24863466993041783, -9.382169495545420901 ) ) ;
#6670=ORIENTED_EDGE ( 'NONE', *, *, #86362, .F. ) ;
#6671=CARTESIAN_POINT ( 'NONE',  ( -46.20903833114419967, 103.7402771300235855, -6.114030023718171059 ) ) ;
#6672=ORIENTED_EDGE ( 'NONE', *, *, #25922, .T. ) ;
#6674=CARTESIAN_POINT ( 'NONE',  ( -0.1503990784575242878, 19.24884699246888786, -6.262539305110083276 ) ) ;
#6675=CARTESIAN_POINT ( 'NONE',  ( 20.36894250292379738, 49.92874883491396787, -10.36894250292379027 ) ) ;
#6676=CARTESIAN_POINT ( 'NONE',  ( 24.16423886937410614, 64.51208216824728936, -3.795296366450302550 ) ) ;
#6677=CARTESIAN_POINT ( 'NONE',  ( 14.92337183194729988, 29.34226448433411960, -8.527530157486177487 ) ) ;
#6678=CARTESIAN_POINT ( 'NONE',  ( 19.84674366389459266, 48.71726448433413026, -2.638427012816827677 ) ) ;
#6681=CARTESIAN_POINT ( 'NONE',  ( 19.84674366389459266, 3.300597817667451750, 2.638427012816836559 ) ) ;
#6682=EDGE_CURVE ( 'NONE', #66913, #69767, #42313, .T. ) ;
#6687=CARTESIAN_POINT ( 'NONE',  ( 6.204703633549690345, 32.84541550158063927, 14.16423886937410082 ) ) ;
#6688=CARTESIAN_POINT ( 'NONE',  ( -1.099225684535947600, 29.54030133659708923, 6.408140936763237150 ) ) ;
#6690=CARTESIAN_POINT ( 'NONE',  ( -2.816281873526473856, 64.12363466993042493, 9.499525473075851096E-16 ) ) ;
#6691=CARTESIAN_POINT ( 'NONE',  ( 7.084665262690076126, 29.10535201082150181, 10.88017736071109987 ) ) ;
#6692=CARTESIAN_POINT ( 'NONE',  ( 19.84674366389459266, 33.71726448433410894, -2.638427012816827677 ) ) ;
#6693=CARTESIAN_POINT ( 'NONE',  ( -0.8801773607111009756, 33.06368534415484106, 1.068504757029289695E-15 ) ) ;
#6695=CARTESIAN_POINT ( 'NONE',  ( 19.38216949554541557, 62.24863466993041072, -9.382169495545420901 ) ) ;
#6697=CARTESIAN_POINT ( 'NONE',  ( 10.00000000000000000, 44.75893115100078745, -9.846743663894594434 ) ) ;
#6698=CARTESIAN_POINT ( 'NONE',  ( 0.1532563361054082862, 56.21726448433411605, 2.638427012816831674 ) ) ;
#6705=CARTESIAN_POINT ( 'NONE',  ( 18.52753015748618282, 13.92559781766745175, -4.923371831947291888 ) ) ;
#6706=CARTESIAN_POINT ( 'NONE',  ( 0.6178305044545838731, 34.74863466993042493, 9.382169495545420901 ) ) ;
#6708=EDGE_CURVE ( 'NONE', #22423, #28167, #51881, .T. ) ;
#6710=CARTESIAN_POINT ( 'NONE',  ( 7.361572987183169658, 54.96726448433413026, -9.846743663894592657 ) ) ;
#6712=CARTESIAN_POINT ( 'NONE',  ( 19.84674366389459266, 43.71726448433410894, -2.638427012816827677 ) ) ;
#6713=CARTESIAN_POINT ( 'NONE',  ( 24.16423886937409904, 29.09541550158063572, 3.795296366450317205 ) ) ;
#6714=CARTESIAN_POINT ( 'NONE',  ( 14.92337183194729988, 49.34226448433411605, -8.527530157486177487 ) ) ;
#6715=CARTESIAN_POINT ( 'NONE',  ( 22.81628187352648496, 46.83196800326376064, -3.434112377981050290 ) ) ;
#6717=CARTESIAN_POINT ( 'NONE',  ( 1.816707512666851709, 10.10290668512023338, -6.499999999999988454 ) ) ;
#6718=CARTESIAN_POINT ( 'NONE',  ( 18.52753015748617571, 3.092264484334118269, 4.923371831947298993 ) ) ;
#6719=CARTESIAN_POINT ( 'NONE',  ( 24.16423886937410614, 4.512082168247300906, -3.795296366450302550 ) ) ;
#6720=CARTESIAN_POINT ( 'NONE',  ( 10.00000000000000000, 54.75893115100078745, -9.846743663894594434 ) ) ;
#6721=CARTESIAN_POINT ( 'NONE',  ( 17.96484262340118221, 34.93868534415482685, 7.964842623401181321 ) ) ;
#6722=CARTESIAN_POINT ( 'NONE',  ( 1.472469842513823179, 45.59226448433412315, -4.923371831947296329 ) ) ;
#6726=CARTESIAN_POINT ( 'NONE',  ( 20.88017736071110519, 50.56368534415484106, 2.639326808657452039E-16 ) ) ;
#6727=ORIENTED_EDGE ( 'NONE', *, *, #91334, .F. ) ;
#6729=CARTESIAN_POINT ( 'NONE',  ( 12.91533473730993009, 21.60535201082150536, -10.88017736071109987 ) ) ;
#6730=CARTESIAN_POINT ( 'NONE',  ( 5.076628168052704559, 65.17559781766745175, -8.527530157486179263 ) ) ;
#6731=CARTESIAN_POINT ( 'NONE',  ( 2.035157376598824452, 38.68868534415483396, 7.964842623401179544 ) ) ;
#6735=CARTESIAN_POINT ( 'NONE',  ( 20.88017736071110875, 35.77201867748816966, -2.915334737309920765 ) ) ;
#6736=CARTESIAN_POINT ( 'NONE',  ( 20.00000000000000711, 92.18909449965150316, -4.886738312308601451 ) ) ;
#6737=CARTESIAN_POINT ( 'NONE',  ( 17.20831665107776587, 14.13393115100078568, -7.208316651077762316 ) ) ;
#6739=CARTESIAN_POINT ( 'NONE',  ( 7.361572987183170547, 27.05059781766745175, 9.846743663894590881 ) ) ;
#6740=FACE_OUTER_BOUND ( 'NONE', #43969, .T. ) ;
#6742=CARTESIAN_POINT ( 'NONE',  ( 6.565887622018943937, 0.1653013365970866511, 12.81628187352647430 ) ) ;
#6743=CARTESIAN_POINT ( 'NONE',  ( 10.00000000000000178, 68.05374883491397497, 14.16423886937410082 ) ) ;
#6745=CARTESIAN_POINT ( 'NONE',  ( 10.00000000000000178, 23.05374883491397142, 14.16423886937410082 ) ) ;
#6746=CARTESIAN_POINT ( 'NONE',  ( -4.164238869374099927, 57.01208216824731068, 3.795296366450308767 ) ) ;
#6748=DIRECTION ( 'NONE',  ( 0.000000000000000000, 0.000000000000000000, 1.000000000000000000 ) ) ;
#6749=VERTEX_POINT ( 'NONE', #57884 ) ;
#6750=CARTESIAN_POINT ( 'NONE',  ( 19.84674366389459266, 28.30059781766745886, 2.638427012816836559 ) ) ;
#6751=CARTESIAN_POINT ( 'NONE',  ( 12.91533473730992121, 14.52201867748817143, 10.88017736071110164 ) ) ;
#6752=CARTESIAN_POINT ( 'NONE',  ( 19.84674366389459621, 53.50893115100078745, 7.409399052514197653E-17 ) ) ;
#6753=CARTESIAN_POINT ( 'NONE',  ( -4.164238869374099039, 11.80374883491396965, 8.674139862899312516E-16 ) ) ;
#6755=CARTESIAN_POINT ( 'NONE',  ( 14.49999999999999822, 60.50000000000000000, 5.000000000000000000 ) ) ;
#6758=CARTESIAN_POINT ( 'NONE',  ( 2.791683348922237240, 0.3839311510007847872, -7.208316651077763204 ) ) ;
#6759=CARTESIAN_POINT ( 'NONE',  ( 22.81628187352647785, 36.41530133659707502, 3.434112377981063169 ) ) ;
#6760=CARTESIAN_POINT ( 'NONE',  ( 19.84674366389459266, 38.71726448433412315, -2.638427012816827677 ) ) ;
#6762=CARTESIAN_POINT ( 'NONE',  ( 19.84674366389459266, 13.30059781766745353, 2.638427012816836559 ) ) ;
#6765=CARTESIAN_POINT ( 'NONE',  ( 20.15039907845753575, 16.74884699246888431, 6.262539305110077059 ) ) ;
#6766=CARTESIAN_POINT ( 'NONE',  ( 4.559911319644449179, 17.23035201082150536, -9.422509992056141925 ) ) ;
#6767=CARTESIAN_POINT ( 'NONE',  ( 10.00000000000000000, 60.55374883491397497, -14.16423886937410082 ) ) ;
#6768=CARTESIAN_POINT ( 'NONE',  ( 4.559911319644449179, 68.89701867748817676, 9.422509992056141925 ) ) ;
#6769=CARTESIAN_POINT ( 'NONE',  ( 20.15039907845753220, 40.60158574516643171, -6.262539305110077947 ) ) ;
#6770=CARTESIAN_POINT ( 'NONE',  ( 18.52753015748617571, 18.09226448433411960, 4.923371831947298993 ) ) ;
#6771=CARTESIAN_POINT ( 'NONE',  ( 19.42250999205614193, 10.14701867748816966, 5.440088680355555262 ) ) ;
#6772=CARTESIAN_POINT ( 'NONE',  ( 2.791683348922237240, 0.3839311510007847872, -7.208316651077763204 ) ) ;
#6775=CARTESIAN_POINT ( 'NONE',  ( 7.361572987183169658, 44.96726448433412315, -9.846743663894592657 ) ) ;
#6777=CARTESIAN_POINT ( 'NONE',  ( 15.44008868035555260, 39.73035201082150536, 9.422509992056143702 ) ) ;
#6779=CARTESIAN_POINT ( 'NONE',  ( 10.00000000000000178, 55.37363466993042493, 12.81628187352647608 ) ) ;
#6780=CARTESIAN_POINT ( 'NONE',  ( 2.791683348922240793, 6.633931151000785675, 7.208316651077764092 ) ) ;
#6781=CARTESIAN_POINT ( 'NONE',  ( 16.40814093676323893, 40.79030133659708923, 11.09922568453595026 ) ) ;
#6782=CARTESIAN_POINT ( 'NONE',  ( -0.8801773607110991993, 12.85535201082150358, -2.915334737309923874 ) ) ;
#6783=CARTESIAN_POINT ( 'NONE',  ( 17.20831665107776587, 37.88393115100078745, 7.208316651077764980 ) ) ;
#6784=( LENGTH_UNIT ( ) NAMED_UNIT ( * ) SI_UNIT ( .MILLI., .METRE. ) );
#6785=FILL_AREA_STYLE ('',( #98807 ) ) ;
#6786=CARTESIAN_POINT ( 'NONE',  ( 24.16423886937410614, 34.51208216824731068, -3.795296366450302550 ) ) ;
#6787=CARTESIAN_POINT ( 'NONE',  ( 13.79529636645031943, 45.34541550158062506, -14.16423886937409904 ) ) ;
#6788=CARTESIAN_POINT ( 'NONE',  ( 5.076628168052704559, 55.17559781766745175, -8.527530157486179263 ) ) ;
#6790=CARTESIAN_POINT ( 'NONE',  ( 2.035157376598822676, 42.43868534415483396, -7.964842623401177768 ) ) ;
#6791=CARTESIAN_POINT ( 'NONE',  ( 7.361572987183169658, 4.967264484334119601, -9.846743663894592657 ) ) ;
#6795=CARTESIAN_POINT ( 'NONE',  ( 3.591859063236761518, 64.95696800326376774, 11.09922568453594849 ) ) ;
#6796=CARTESIAN_POINT ( 'NONE',  ( 20.88017736071110519, 60.56368534415484106, 2.639326808657452039E-16 ) ) ;
#6797=ORIENTED_EDGE ( 'NONE', *, *, #50588, .T. ) ;
#6798=CARTESIAN_POINT ( 'NONE',  ( -4.164238869374099927, 12.01208216824730357, 3.795296366450308767 ) ) ;
#6799=CARTESIAN_POINT ( 'NONE',  ( 10.00000000000000000, 4.758931151000784787, -9.846743663894594434 ) ) ;
#6800=CARTESIAN_POINT ( 'NONE',  ( 20.88017736071110164, 25.35535201082150891, 2.915334737309930979 ) ) ;
#6802=CARTESIAN_POINT ( 'NONE',  ( 7.084665262690076126, 24.10535201082150181, 10.88017736071109987 ) ) ;
#6806=ORIENTED_EDGE ( 'NONE', *, *, #49225, .F. ) ;
#6807=CARTESIAN_POINT ( 'NONE',  ( 17.96484262340118221, 36.18868534415484106, -7.964842623401177768 ) ) ;
#6810=ORIENTED_EDGE ( 'NONE', *, *, #86183, .T. ) ;
#6811=CARTESIAN_POINT ( 'NONE',  ( 2.035157376598822676, 62.43868534415483396, -7.964842623401177768 ) ) ;
#6813=CARTESIAN_POINT ( 'NONE',  ( 0.5774900079438607392, 18.48035201082150536, 5.440088680355550821 ) ) ;
#6815=CARTESIAN_POINT ( 'NONE',  ( 0.1532563361054082862, 1.217264484334117824, 2.638427012816831674 ) ) ;
#6816=CARTESIAN_POINT ( 'NONE',  ( 12.91533473730992121, 14.52201867748817143, 10.88017736071110164 ) ) ;
#6817=COLOUR_RGB ( '', 0.40784314, 0.44705882, 0.49803922) ;
#6819=CARTESIAN_POINT ( 'NONE',  ( 19.38216949554541557, 57.24863466993042493, -9.382169495545420901 ) ) ;
#6820=CARTESIAN_POINT ( 'NONE',  ( 0.5774900079438607392, 38.48035201082150536, 5.440088680355550821 ) ) ;
#6821=CARTESIAN_POINT ( 'NONE',  ( -0.3289641300568009741, 22.24545670184114243, -5.963430220938281678 ) ) ;
#6822=CARTESIAN_POINT ( 'NONE',  ( 22.81628187352647785, 56.41530133659708213, 3.434112377981063169 ) ) ;
#6823=CARTESIAN_POINT ( 'NONE',  ( 12.91533473730993009, 41.60535201082149825, -10.88017736071109987 ) ) ;
#6826=CARTESIAN_POINT ( 'NONE',  ( 1.472469842513823179, 65.59226448433412315, -4.923371831947296329 ) ) ;
#6828=CARTESIAN_POINT ( 'NONE',  ( 19.84674366389459266, 18.30059781766745175, 2.638427012816836559 ) ) ;
#6829=CARTESIAN_POINT ( 'NONE',  ( -2.816281873526473856, 59.12363466993042493, 9.499525473075851096E-16 ) ) ;
#6830=CARTESIAN_POINT ( 'NONE',  ( 1.383448333479235348, 37.37718327197428181, -6.499999999999977796 ) ) ;
#6831=CARTESIAN_POINT ( 'NONE',  ( 13.43411237798105340, 5.581968003263753531, 12.81628187352647963 ) ) ;
#6833=CARTESIAN_POINT ( 'NONE',  ( 17.20831665107776587, 62.88393115100078745, 7.208316651077764980 ) ) ;
#6834=CARTESIAN_POINT ( 'NONE',  ( -0.8801773607111009756, 33.06368534415484106, 1.068504757029289695E-15 ) ) ;
#6835=CARTESIAN_POINT ( 'NONE',  ( 0.1532563361054083140, 51.00893115100078745, 1.131784320476157264E-15 ) ) ;
#6838=CARTESIAN_POINT ( 'NONE',  ( 1.472469842513823179, 10.59226448433411782, -4.923371831947296329 ) ) ;
#6839=CARTESIAN_POINT ( 'NONE',  ( -2.816281873526471635, -1.084698663402913210, -3.434112377981056508 ) ) ;
#6841=CARTESIAN_POINT ( 'NONE',  ( 20.88017736071110519, 5.563685344154837509, 2.639326808657452039E-16 ) ) ;
#6843=CARTESIAN_POINT ( 'NONE',  ( 19.84674366389459266, 63.30059781766745886, 2.638427012816836559 ) ) ;
#6845=CARTESIAN_POINT ( 'NONE',  ( 7.084665262690076126, 7.022018677488170546, -10.88017736071110164 ) ) ;
#6846=CARTESIAN_POINT ( 'NONE',  ( 12.63842701281683922, 39.55059781766744464, -9.846743663894590881 ) ) ;
#6848=LINE ( 'NONE', #66348, #15402 ) ;
#6849=CARTESIAN_POINT ( 'NONE',  ( 0.5774900079438607392, 3.480352010821504916, 5.440088680355550821 ) ) ;
#6850=CARTESIAN_POINT ( 'NONE',  ( 0.1532563361054082862, 6.217264484334118713, 2.638427012816831674 ) ) ;
#6851=CARTESIAN_POINT ( 'NONE',  ( 12.91533473730993009, 21.60535201082150536, -10.88017736071109987 ) ) ;
#6853=CARTESIAN_POINT ( 'NONE',  ( -0.3689425029237898834, 51.17874883491397497, -10.36894250292378850 ) ) ;
#6854=CARTESIAN_POINT ( 'NONE',  ( 2.917880565312948704, 67.63708216824730357, 12.26659068614894643 ) ) ;
#6856=CARTESIAN_POINT ( 'NONE',  ( 0.1532563361054100626, 5.800597817667452638, -2.638427012816831230 ) ) ;
#6857=CARTESIAN_POINT ( 'NONE',  ( 2.791683348922240793, 21.63393115100078745, 7.208316651077764092 ) ) ;
#6858=CARTESIAN_POINT ( 'NONE',  ( 3.591859063236763294, 13.29030133659708746, -11.09922568453595026 ) ) ;
#6861=TOROIDAL_SURFACE ( 'NONE', #91518, 1.000000000000000000, 0.5000000000000000000 ) ;
#6864=CARTESIAN_POINT ( 'NONE',  ( 5.076628168052704559, 65.17559781766745175, -8.527530157486179263 ) ) ;
#6865=CARTESIAN_POINT ( 'NONE',  ( 20.36894250292379738, 4.928748834913967869, -10.36894250292379027 ) ) ;
#6867=CARTESIAN_POINT ( 'NONE',  ( 12.63842701281683922, 29.55059781766745175, -9.846743663894590881 ) ) ;
#6870=CARTESIAN_POINT ( 'NONE',  ( 20.36894250292379738, 34.92874883491396076, -10.36894250292379027 ) ) ;
#6871=CARTESIAN_POINT ( 'NONE',  ( 19.84674366389459621, 13.50893115100078568, 7.409399052514197653E-17 ) ) ;
#6874=CARTESIAN_POINT ( 'NONE',  ( 20.88017736071110164, 35.35535201082150536, 2.915334737309930979 ) ) ;
#6875=CARTESIAN_POINT ( 'NONE',  ( -2.816281873526471635, 53.91530133659709634, -3.434112377981056508 ) ) ;
#6876=CARTESIAN_POINT ( 'NONE',  ( 2.035157376598824452, 3.688685344154837953, 7.964842623401179544 ) ) ;
#6877=CARTESIAN_POINT ( 'NONE',  ( 0.6178305044545838731, 39.74863466993041072, 9.382169495545420901 ) ) ;
#6878=CARTESIAN_POINT ( 'NONE',  ( 5.076628168052703671, 1.842264484334118047, 8.527530157486179263 ) ) ;
#6881=CARTESIAN_POINT ( 'NONE',  ( 1.274849032793998305, 2.555090184799397424, -6.499999999999581668 ) ) ;
#6882=CARTESIAN_POINT ( 'NONE',  ( 13.79529636645031943, 40.34541550158063217, -14.16423886937409904 ) ) ;
#6883=CARTESIAN_POINT ( 'NONE',  ( 2.035157376598824452, 8.688685344154839285, 7.964842623401179544 ) ) ;
#6884=CARTESIAN_POINT ( 'NONE',  ( 19.42250999205614548, 20.98035201082150891, -5.440088680355545492 ) ) ;
#6887=CARTESIAN_POINT ( 'NONE',  ( 4.559911319644449179, 58.89701867748817676, 9.422509992056141925 ) ) ;
#6888=CARTESIAN_POINT ( 'NONE',  ( 4.559911319644449179, 67.23035201082150536, -9.422509992056141925 ) ) ;
#6889=CARTESIAN_POINT ( 'NONE',  ( 6.565887622018943937, 20.16530133659708213, 12.81628187352647430 ) ) ;
#6890=CARTESIAN_POINT ( 'NONE',  ( 0.2751277870542876980, 48.21833443783936701, 6.499999999999984901 ) ) ;
#6892=CARTESIAN_POINT ( 'NONE',  ( 5.076628168052704559, 20.17559781766745175, -8.527530157486179263 ) ) ;
#6893=CARTESIAN_POINT ( 'NONE',  ( 10.00000000000000000, 56.81368534415484106, -10.88017736071110342 ) ) ;
#6896=CARTESIAN_POINT ( 'NONE',  ( 21.09922568453595559, 17.04030133659708923, -6.408140936763230044 ) ) ;
#6897=CARTESIAN_POINT ( 'NONE',  ( 2.035157376598824452, 8.688685344154839285, 7.964842623401179544 ) ) ;
#6898=CARTESIAN_POINT ( 'NONE',  ( 12.63842701281683034, 42.46726448433412315, 9.846743663894596210 ) ) ;
#6899=CARTESIAN_POINT ( 'NONE',  ( 22.81628187352647785, 61.41530133659709634, 3.434112377981063169 ) ) ;
#6901=CARTESIAN_POINT ( 'NONE',  ( 12.63842701281683034, 17.46726448433411250, 9.846743663894596210 ) ) ;
#6902=VECTOR ( 'NONE', #42884, 1000.000000000000000 ) ;
#6903=CARTESIAN_POINT ( 'NONE',  ( -4.164238869374098151, 1.595415501580634388, -3.795296366450310543 ) ) ;
#6905=CARTESIAN_POINT ( 'NONE',  ( 20.88017736071110875, 30.77201867748816966, -2.915334737309920765 ) ) ;
#6906=CARTESIAN_POINT ( 'NONE',  ( 4.559911319644449179, 3.897018677488170990, 9.422509992056141925 ) ) ;
#6907=CARTESIAN_POINT ( 'NONE',  ( 10.00000000000000000, 35.55374883491396787, -14.16423886937410082 ) ) ;
#6908=CARTESIAN_POINT ( 'NONE',  ( 19.84674366389459266, 48.71726448433413026, -2.638427012816827677 ) ) ;
#6910=CARTESIAN_POINT ( 'NONE',  ( 4.559911319644449179, 27.23035201082150536, -9.422509992056141925 ) ) ;
#6911=CARTESIAN_POINT ( 'NONE',  ( -0.8801773607111008646, 13.27201867748817321, 2.915334737309923430 ) ) ;
#6912=ORIENTED_EDGE ( 'NONE', *, *, #88945, .F. ) ;
#6914=CARTESIAN_POINT ( 'NONE',  ( 2.035157376598822676, 22.43868534415483396, -7.964842623401177768 ) ) ;
#6915=CARTESIAN_POINT ( 'NONE',  ( 21.09922568453594849, 51.20696800326375353, 6.408140936763242479 ) ) ;
#6916=CARTESIAN_POINT ( 'NONE',  ( 2.035157376598824452, 48.68868534415483396, 7.964842623401179544 ) ) ;
#6918=CARTESIAN_POINT ( 'NONE',  ( 20.88017736071110519, 40.56368534415484106, 2.639326808657452039E-16 ) ) ;
#6920=CARTESIAN_POINT ( 'NONE',  ( 12.63842701281683034, 57.46726448433411605, 9.846743663894596210 ) ) ;
#6921=CARTESIAN_POINT ( 'NONE',  ( -0.8801773607111008646, 43.27201867748817676, 2.915334737309923430 ) ) ;
#6924=ADVANCED_FACE ( 'NONE', ( #8348 ), #7128, .T. ) ;
#6925=CYLINDRICAL_SURFACE ( 'NONE', #61969, 0.5000000000000004441 ) ;
#6926=CARTESIAN_POINT ( 'NONE',  ( 2.917880565312948704, 42.63708216824729647, 12.26659068614894643 ) ) ;
#6927=CARTESIAN_POINT ( 'NONE',  ( 2.035157376598822676, 52.43868534415483396, -7.964842623401177768 ) ) ;
#6929=CARTESIAN_POINT ( 'NONE',  ( 10.00000000000000000, 64.75893115100078035, -9.846743663894594434 ) ) ;
#6930=CARTESIAN_POINT ( 'NONE',  ( -0.8801773607111008646, 3.272018677488171434, 2.915334737309923430 ) ) ;
#6931=CARTESIAN_POINT ( 'NONE',  ( 0.1532563361054083140, 36.00893115100078745, 1.131784320476157264E-15 ) ) ;
#6934=CARTESIAN_POINT ( 'NONE',  ( 19.84674366389459621, 28.50893115100078745, 7.409399052514197653E-17 ) ) ;
#6936=CARTESIAN_POINT ( 'NONE',  ( 15.44008868035555260, 24.73035201082150891, 9.422509992056143702 ) ) ;
#6937=CARTESIAN_POINT ( 'NONE',  ( 19.84674366389459621, 28.50893115100078745, 7.409399052514197653E-17 ) ) ;
#6938=CARTESIAN_POINT ( 'NONE',  ( -2.816281873526471635, 18.91530133659708213, -3.434112377981056508 ) ) ;
#6939=CARTESIAN_POINT ( 'NONE',  ( 2.148416515056620124, 37.23726573380441351, 6.499999999999959144 ) ) ;
#6940=CARTESIAN_POINT ( 'NONE',  ( -0.8801773607111008646, 58.27201867748816966, 2.915334737309923430 ) ) ;
#6941=CARTESIAN_POINT ( 'NONE',  ( 0.5774900079438590739, 37.64701867748817676, -5.440088680355550821 ) ) ;
#6942=CARTESIAN_POINT ( 'NONE',  ( 12.91533473730992121, 4.522018677488169658, 10.88017736071110164 ) ) ;
#6943=CARTESIAN_POINT ( 'NONE',  ( 24.16423886937409904, 44.09541550158063927, 3.795296366450317205 ) ) ;
#6948=CARTESIAN_POINT ( 'NONE',  ( 0.6178305044545818747, 13.49863466993041783, -9.382169495545419124 ) ) ;
#6949=CARTESIAN_POINT ( 'NONE',  ( 15.44008868035555260, 4.730352010821504471, 9.422509992056143702 ) ) ;
#6950=CARTESIAN_POINT ( 'NONE',  ( 12.91533473730993009, 46.60535201082150536, -10.88017736071109987 ) ) ;
#6951=VERTEX_POINT ( 'NONE', #92336 ) ;
#6953=CARTESIAN_POINT ( 'NONE',  ( 17.96484262340118221, 54.93868534415484106, 7.964842623401181321 ) ) ;
#6954=CARTESIAN_POINT ( 'NONE',  ( 12.63842701281683922, 39.55059781766744464, -9.846743663894590881 ) ) ;
#6955=CARTESIAN_POINT ( 'NONE',  ( 7.361572987183169658, 24.96726448433412315, -9.846743663894592657 ) ) ;
#6956=CARTESIAN_POINT ( 'NONE',  ( 12.63842701281683922, 9.550597817667449974, -9.846743663894590881 ) ) ;
#6959=CARTESIAN_POINT ( 'NONE',  ( 7.361572987183170547, 17.05059781766745530, 9.846743663894590881 ) ) ;
#6962=CARTESIAN_POINT ( 'NONE',  ( 2.791683348922240793, 36.63393115100078035, 7.208316651077764092 ) ) ;
#6963=VERTEX_POINT ( 'NONE', #83362 ) ;
#6964=CARTESIAN_POINT ( 'NONE',  ( 19.38216949554541202, 55.99863466993041072, 9.382169495545424454 ) ) ;
#6965=CARTESIAN_POINT ( 'NONE',  ( 19.72487221294570858, 5.718334437839381224, -6.500000000000000888 ) ) ;
#6966=CARTESIAN_POINT ( 'NONE',  ( 3.591859063236763294, 8.290301336597087456, -11.09922568453595026 ) ) ;
#6968=CARTESIAN_POINT ( 'NONE',  ( 2.035157376598824452, 58.68868534415482685, 7.964842623401179544 ) ) ;
#6969=CARTESIAN_POINT ( 'NONE',  ( 24.16423886937410614, 34.30374883491396787, 8.672049930838204340E-16 ) ) ;
#6972=VECTOR ( 'NONE', #59473, 1000.000000000000000 ) ;
#6973=CARTESIAN_POINT ( 'NONE',  ( 22.26659068614895176, 24.72041550158063572, -7.082119434687042414 ) ) ;
#6975=CARTESIAN_POINT ( 'NONE',  ( 2.917880565312950480, 50.97041550158064638, -12.26659068614894821 ) ) ;
#6976=CARTESIAN_POINT ( 'NONE',  ( 24.16423886937410614, 9.512082168247301794, -3.795296366450302550 ) ) ;
#6977=CARTESIAN_POINT ( 'NONE',  ( 22.26659068614895176, 9.720415501580633943, -7.082119434687042414 ) ) ;
#6978=CARTESIAN_POINT ( 'NONE',  ( -1.926860441876562247, 37.45379003517448524, -3.195792623639530650 ) ) ;
#6979=CARTESIAN_POINT ( 'NONE',  ( 2.035157376598824452, 43.68868534415484106, 7.964842623401179544 ) ) ;
#6981=CARTESIAN_POINT ( 'NONE',  ( 14.92337183194729988, 24.34226448433411960, -8.527530157486177487 ) ) ;
#6982=LINE ( 'NONE', #29956, #62853 ) ;
#6983=CARTESIAN_POINT ( 'NONE',  ( 1.472469842513823179, 41.42559781766745886, 4.923371831947296329 ) ) ;
#6985=CARTESIAN_POINT ( 'NONE',  ( 20.88017736071110519, 25.56368534415483751, 2.639326808657452039E-16 ) ) ;
#6986=CARTESIAN_POINT ( 'NONE',  ( 21.09922568453595559, 62.04030133659709634, -6.408140936763230044 ) ) ;
#6987=CARTESIAN_POINT ( 'NONE',  ( 14.92337183194729988, 64.34226448433412315, -8.527530157486177487 ) ) ;
#6989=CARTESIAN_POINT ( 'NONE',  ( 1.472469842513823179, 30.59226448433411960, -4.923371831947296329 ) ) ;
#6990=CARTESIAN_POINT ( 'NONE',  ( -2.816281873526471635, 38.91530133659708213, -3.434112377981056508 ) ) ;
#6992=CARTESIAN_POINT ( 'NONE',  ( 2.035157376598824452, 43.68868534415484106, 7.964842623401179544 ) ) ;
#6993=CARTESIAN_POINT ( 'NONE',  ( 14.92337183194729988, 49.34226448433411605, -8.527530157486177487 ) ) ;
#6994=CARTESIAN_POINT ( 'NONE',  ( -4.164238869374099927, 22.01208216824730357, 3.795296366450308767 ) ) ;
#6995=ORIENTED_EDGE ( 'NONE', *, *, #64077, .F. ) ;
#6996=CARTESIAN_POINT ( 'NONE',  ( -0.8801773607111008646, 58.27201867748816966, 2.915334737309923430 ) ) ;
#6997=CARTESIAN_POINT ( 'NONE',  ( 17.96484262340118221, 64.93868534415483396, 7.964842623401181321 ) ) ;
#6998=CARTESIAN_POINT ( 'NONE',  ( 20.36894250292379738, 64.92874883491397497, -10.36894250292379027 ) ) ;
#6999=CARTESIAN_POINT ( 'NONE',  ( 2.791683348922240793, 61.63393115100079456, 7.208316651077764092 ) ) ;
#7001=CARTESIAN_POINT ( 'NONE',  ( 2.035157376598824452, 53.68868534415484817, 7.964842623401179544 ) ) ;
#7003=CARTESIAN_POINT ( 'NONE',  ( -0.3689425029237898834, 46.17874883491397497, -10.36894250292378850 ) ) ;
#7005=CARTESIAN_POINT ( 'NONE',  ( 12.91533473730992121, 9.522018677488171434, 10.88017736071110164 ) ) ;
#7006=CARTESIAN_POINT ( 'NONE',  ( 10.00000000000000178, 24.31368534415484106, 10.88017736071110342 ) ) ;
#7007=CARTESIAN_POINT ( 'NONE',  ( 7.361572987183170547, 52.05059781766745175, 9.846743663894590881 ) ) ;
#7008=CARTESIAN_POINT ( 'NONE',  ( 16.40814093676324603, 57.45696800326375353, -11.09922568453594671 ) ) ;
#7011=CARTESIAN_POINT ( 'NONE',  ( 12.91533473730993009, 11.60535201082150536, -10.88017736071109987 ) ) ;
#7013=CARTESIAN_POINT ( 'NONE',  ( -2.816281873526471635, 18.91530133659708213, -3.434112377981056508 ) ) ;
#7015=CARTESIAN_POINT ( 'NONE',  ( 19.84674366389459266, 48.71726448433413026, -2.638427012816827677 ) ) ;
#7016=B_SPLINE_CURVE_WITH_KNOTS ( 'NONE', 3,
 ( #85392, #38918, #56380, #93873, #23919, #25399 ),
 .UNSPECIFIED., .F., .F.,
 ( 4, 2, 4 ),
 ( 0.000000000000000000, 0.0002626113303184793800, 0.0005252226606369587601 ),
 .UNSPECIFIED. ) ;
#7018=CARTESIAN_POINT ( 'NONE',  ( 2.035157376598824452, 33.68868534415484106, 7.964842623401179544 ) ) ;
#7019=CARTESIAN_POINT ( 'NONE',  ( 16.40814093676324603, 27.45696800326375708, -11.09922568453594671 ) ) ;
#7020=CARTESIAN_POINT ( 'NONE',  ( -0.8801773607110991993, 47.85535201082150536, -2.915334737309923874 ) ) ;
#7023=CARTESIAN_POINT ( 'NONE',  ( -2.816281873526473856, 49.12363466993042493, 9.499525473075851096E-16 ) ) ;
#7024=ORIENTED_EDGE ( 'NONE', *, *, #64473, .F. ) ;
#7026=CARTESIAN_POINT ( 'NONE',  ( 4.559911319644449179, 53.89701867748817676, 9.422509992056141925 ) ) ;
#7027=CARTESIAN_POINT ( 'NONE',  ( 6.565887622018943937, 40.16530133659708923, 12.81628187352647430 ) ) ;
#7028=CARTESIAN_POINT ( 'NONE',  ( 5.076628168052703671, 6.842264484334118713, 8.527530157486179263 ) ) ;
#7029=CARTESIAN_POINT ( 'NONE',  ( 19.42250999205614548, 45.98035201082150536, -5.440088680355545492 ) ) ;
#7030=CARTESIAN_POINT ( 'NONE',  ( -0.03447792253739143109, 15.15514106990689847, 6.401564815979740253 ) ) ;
#7031=SURFACE_STYLE_FILL_AREA ( #69503 ) ;
#7032=CARTESIAN_POINT ( 'NONE',  ( 0.1532563361054083140, 21.00893115100078745, 1.131784320476157264E-15 ) ) ;
#7033=CARTESIAN_POINT ( 'NONE',  ( 1.472469842513823179, 0.5922644843341181575, -4.923371831947296329 ) ) ;
#7034=CARTESIAN_POINT ( 'NONE',  ( -0.03447792253739536544, 5.155141069906901130, 6.401564815979722489 ) ) ;
#7035=CARTESIAN_POINT ( 'NONE',  ( 6.204703633549690345, 37.84541550158063927, 14.16423886937410082 ) ) ;
#7036=ADVANCED_FACE ( 'NONE', ( #30341 ), #38856, .T. ) ;
#7038=CARTESIAN_POINT ( 'NONE',  ( 2.035157376598822676, 12.43868534415483751, -7.964842623401177768 ) ) ;
#7041=CARTESIAN_POINT ( 'NONE',  ( 17.08211943468705840, 60.13708216824729647, -12.26659068614894466 ) ) ;
#7042=CARTESIAN_POINT ( 'NONE',  ( 6.204703633549690345, 62.84541550158063927, 14.16423886937410082 ) ) ;
#7043=CARTESIAN_POINT ( 'NONE',  ( 2.791683348922240793, 36.63393115100078035, 7.208316651077764092 ) ) ;
#7045=CARTESIAN_POINT ( 'NONE',  ( -1.099225684535947600, 39.54030133659708923, 6.408140936763237150 ) ) ;
#7049=CARTESIAN_POINT ( 'NONE',  ( -0.3689425029237898834, 1.178748834913967869, -10.36894250292378850 ) ) ;
#7050=CARTESIAN_POINT ( 'NONE',  ( 12.91533473730992121, 19.52201867748816611, 10.88017736071110164 ) ) ;
#7051=CARTESIAN_POINT ( 'NONE',  ( 10.00000000000000178, 63.05374883491396076, 14.16423886937410082 ) ) ;
#7052=CARTESIAN_POINT ( 'NONE',  ( 12.63842701281683034, 37.46726448433411605, 9.846743663894596210 ) ) ;
#7054=CARTESIAN_POINT ( 'NONE',  ( 19.84674366389459266, 28.30059781766745886, 2.638427012816836559 ) ) ;
#7063=CARTESIAN_POINT ( 'NONE',  ( 17.20831665107776587, 57.88393115100078745, 7.208316651077764980 ) ) ;
#7064=CARTESIAN_POINT ( 'NONE',  ( -4.164238869374098151, 21.59541550158063217, -3.795296366450310543 ) ) ;
#7065=CARTESIAN_POINT ( 'NONE',  ( 17.96484262340118221, 31.18868534415483751, -7.964842623401177768 ) ) ;
#7066=CARTESIAN_POINT ( 'NONE',  ( 4.559911319644449179, 33.89701867748817676, 9.422509992056141925 ) ) ;
#7067=CARTESIAN_POINT ( 'NONE',  ( 5.076628168052703671, 56.84226448433412315, 8.527530157486179263 ) ) ;
#7068=CARTESIAN_POINT ( 'NONE',  ( 19.38216949554541202, 35.99863466993041072, 9.382169495545424454 ) ) ;
#7069=CARTESIAN_POINT ( 'NONE',  ( 10.00000000000000000, 5.553748834913967869, -14.16423886937410082 ) ) ;
#7070=CARTESIAN_POINT ( 'NONE',  ( 4.559911319644449179, 68.89701867748817676, 9.422509992056141925 ) ) ;
#7071=CARTESIAN_POINT ( 'NONE',  ( 10.00000000000000178, 25.37363466993041783, 12.81628187352647608 ) ) ;
#7073=CARTESIAN_POINT ( 'NONE',  ( 18.52753015748617571, 43.09226448433412315, 4.923371831947298993 ) ) ;
#7074=CARTESIAN_POINT ( 'NONE',  ( -0.8801773607111009756, 3.063685344154838397, 1.068504757029289695E-15 ) ) ;
#7075=ORIENTED_EDGE ( 'NONE', *, *, #77438, .T. ) ;
#7076=CARTESIAN_POINT ( 'NONE',  ( 20.88017736071110519, 15.56368534415483751, 2.639326808657452039E-16 ) ) ;
#7078=CARTESIAN_POINT ( 'NONE',  ( 17.96484262340118221, 66.18868534415483396, -7.964842623401177768 ) ) ;
#7079=CARTESIAN_POINT ( 'NONE',  ( 2.035157376598822676, 52.43868534415483396, -7.964842623401177768 ) ) ;
#7080=CARTESIAN_POINT ( 'NONE',  ( 12.91533473730992121, 64.52201867748817676, 10.88017736071110164 ) ) ;
#7081=CARTESIAN_POINT ( 'NONE',  ( 15.44008868035555260, 49.73035201082150536, 9.422509992056143702 ) ) ;
#7084=CARTESIAN_POINT ( 'NONE',  ( 20.15039907845753930, 70.00000000000000000, -6.262539305110068177 ) ) ;
#7087=CARTESIAN_POINT ( 'NONE',  ( 12.63842701281683034, 47.46726448433412315, 9.846743663894596210 ) ) ;
#7089=DIRECTION ( 'NONE',  ( 0.000000000000000000, -1.000000000000000000, 0.000000000000000000 ) ) ;
#7090=CARTESIAN_POINT ( 'NONE',  ( 20.36894250292379382, 8.678748834913967869, 10.36894250292379205 ) ) ;
#7093=CARTESIAN_POINT ( 'NONE',  ( 17.39651004071838614, 42.93575266056826933, 6.500000000000032863 ) ) ;
#7094=CARTESIAN_POINT ( 'NONE',  ( 0.5774900079438607392, 8.480352010821505360, 5.440088680355550821 ) ) ;
#7096=CARTESIAN_POINT ( 'NONE',  ( 16.40814093676324603, 37.45696800326376064, -11.09922568453594671 ) ) ;
#7099=CARTESIAN_POINT ( 'NONE',  ( 0.1532563361054083140, 41.00893115100078745, 1.131784320476157264E-15 ) ) ;
#7101=CARTESIAN_POINT ( 'NONE',  ( -2.816281873526471635, 13.91530133659708746, -3.434112377981056508 ) ) ;
#7102=CARTESIAN_POINT ( 'NONE',  ( 17.20831665107776587, 29.13393115100078390, -7.208316651077762316 ) ) ;
#7103=CARTESIAN_POINT ( 'NONE',  ( 17.20831665107776587, 17.88393115100078745, 7.208316651077764980 ) ) ;
#7104=CARTESIAN_POINT ( 'NONE',  ( 13.43411237798106583, 2.665301336597086568, -12.81628187352647252 ) ) ;
#7107=ORIENTED_EDGE ( 'NONE', *, *, #16746, .F. ) ;
#7109=CARTESIAN_POINT ( 'NONE',  ( 17.96484262340118221, 24.93868534415484461, 7.964842623401181321 ) ) ;
#7110=CARTESIAN_POINT ( 'NONE',  ( 24.16423886937410614, 14.51208216824730179, -3.795296366450302550 ) ) ;
#7111=CARTESIAN_POINT ( 'NONE',  ( 7.361572987183170547, 32.05059781766745175, 9.846743663894590881 ) ) ;
#7112=CARTESIAN_POINT ( 'NONE',  ( 7.084665262690076126, 69.10535201082151957, 10.88017736071109987 ) ) ;
#7113=CARTESIAN_POINT ( 'NONE',  ( 16.40814093676323893, 40.79030133659708923, 11.09922568453595026 ) ) ;
#7114=CARTESIAN_POINT ( 'NONE',  ( -0.8801773607110991993, 12.85535201082150358, -2.915334737309923874 ) ) ;
#7116=CARTESIAN_POINT ( 'NONE',  ( -0.1503990784575328643, 70.00000000000000000, 6.262539305110068177 ) ) ;
#7117=CARTESIAN_POINT ( 'NONE',  ( 0.6178305044545818747, 3.498634669930420049, -9.382169495545419124 ) ) ;
#7118=CARTESIAN_POINT ( 'NONE',  ( 18.52753015748618282, 28.92559781766745175, -4.923371831947291888 ) ) ;
#7120=CARTESIAN_POINT ( 'NONE',  ( 3.591859063236763294, 38.29030133659708923, -11.09922568453595026 ) ) ;
#7122=CARTESIAN_POINT ( 'NONE',  ( 15.44008868035555260, 39.73035201082150536, 9.422509992056143702 ) ) ;
#7125=CARTESIAN_POINT ( 'NONE',  ( 15.44008868035555793, 41.39701867748817676, -9.422509992056140149 ) ) ;
#7126=CARTESIAN_POINT ( 'NONE',  ( -0.8801773607110991993, 47.85535201082150536, -2.915334737309923874 ) ) ;
#7127=DIRECTION ( 'NONE',  ( 1.000000000000000000, 1.790682297782510536E-15, 0.000000000000000000 ) ) ;
#7128=TOROIDAL_SURFACE ( 'NONE', #96574, 62.00000000000000000, 0.5000000000000000000 ) ;
#7129=CARTESIAN_POINT ( 'NONE',  ( 0.5774900079438590739, 62.64701867748817676, -5.440088680355550821 ) ) ;
#7130=ADVANCED_FACE ( 'NONE', ( #90849 ), #72277, .F. ) ;
#7133=CARTESIAN_POINT ( 'NONE',  ( 10.00000000000000000, 54.75893115100078745, -9.846743663894594434 ) ) ;
#7134=CARTESIAN_POINT ( 'NONE',  ( 2.035157376598822676, 7.438685344154837509, -7.964842623401177768 ) ) ;
#7136=CARTESIAN_POINT ( 'NONE',  ( 13.43411237798105340, 10.58196800326375353, 12.81628187352647963 ) ) ;
#7138=CARTESIAN_POINT ( 'NONE',  ( 17.96484262340118221, 36.18868534415484106, -7.964842623401177768 ) ) ;
#7140=CARTESIAN_POINT ( 'NONE',  ( 10.00000000000000178, 24.31368534415484106, 10.88017736071110342 ) ) ;
#7141=CARTESIAN_POINT ( 'NONE',  ( 14.92337183194729633, 2.675597817667451750, 8.527530157486181039 ) ) ;
#7142=CARTESIAN_POINT ( 'NONE',  ( 13.79529636645031943, 40.34541550158063217, -14.16423886937409904 ) ) ;
#7143=CARTESIAN_POINT ( 'NONE',  ( 1.472469842513823179, 31.42559781766745530, 4.923371831947296329 ) ) ;
#7144=CARTESIAN_POINT ( 'NONE',  ( -0.8801773607111008646, 48.27201867748816966, 2.915334737309923430 ) ) ;
#7146=SURFACE_STYLE_FILL_AREA ( #75634 ) ;
#7150=CARTESIAN_POINT ( 'NONE',  ( 12.63842701281683034, 57.46726448433411605, 9.846743663894596210 ) ) ;
#7151=ORIENTED_EDGE ( 'NONE', *, *, #42484, .T. ) ;
#7153=CARTESIAN_POINT ( 'NONE',  ( -4.164238869374099039, 16.80374883491396787, 8.674139862899312516E-16 ) ) ;
#7154=CARTESIAN_POINT ( 'NONE',  ( 6.204703633549690345, 25.76208216824730712, -14.16423886937410259 ) ) ;
#7155=CARTESIAN_POINT ( 'NONE',  ( -0.8801773607111008646, 63.27201867748817676, 2.915334737309923430 ) ) ;
#7156=CARTESIAN_POINT ( 'NONE',  ( -4.164238869374099927, 67.01208216824728936, 3.795296366450308767 ) ) ;
#7157=CARTESIAN_POINT ( 'NONE',  ( 13.43411237798106583, 7.665301336597086568, -12.81628187352647252 ) ) ;
#7158=CARTESIAN_POINT ( 'NONE',  ( 2.791683348922240793, 46.63393115100077324, 7.208316651077764092 ) ) ;
#7160=CARTESIAN_POINT ( 'NONE',  ( 19.42250999205614548, 45.98035201082150536, -5.440088680355545492 ) ) ;
#7161=CARTESIAN_POINT ( 'NONE',  ( 22.81628187352647785, 16.62363466993042138, 6.195893100308588602E-16 ) ) ;
#7162=CARTESIAN_POINT ( 'NONE',  ( 10.00000000000000178, 18.05374883491396787, 14.16423886937410082 ) ) ;
#7163=CARTESIAN_POINT ( 'NONE',  ( 2.035157376598824452, 8.688685344154839285, 7.964842623401179544 ) ) ;
#7164=CARTESIAN_POINT ( 'NONE',  ( 7.084665262690076126, 24.10535201082150181, 10.88017736071109987 ) ) ;
#7166=CARTESIAN_POINT ( 'NONE',  ( 2.035157376598824452, 53.68868534415484817, 7.964842623401179544 ) ) ;
#7171=STYLED_ITEM ( 'NONE', ( #11421 ), #10384 ) ;
#7172=ORIENTED_EDGE ( 'NONE', *, *, #91952, .T. ) ;
#7173=PLANE ( 'NONE',  #27096 ) ;
#7175=CARTESIAN_POINT ( 'NONE',  ( -0.1491070598754174470, 61.94583914210339515, 5.000000000000000000 ) ) ;
#7176=CARTESIAN_POINT ( 'NONE',  ( 10.00000000000000000, 65.55374883491396076, -14.16423886937410082 ) ) ;
#7177=CARTESIAN_POINT ( 'NONE',  ( -4.164238869374098151, 66.59541550158060375, -3.795296366450310543 ) ) ;
#7178=CARTESIAN_POINT ( 'NONE',  ( 12.63842701281683922, 29.55059781766745175, -9.846743663894590881 ) ) ;
#7179=CARTESIAN_POINT ( 'NONE',  ( 12.63842701281683922, 54.55059781766745175, -9.846743663894590881 ) ) ;
#7180=CARTESIAN_POINT ( 'NONE',  ( 7.084665262690076126, 67.02201867748817676, -10.88017736071110164 ) ) ;
#7181=CARTESIAN_POINT ( 'NONE',  ( 17.96484262340118221, 64.93868534415483396, 7.964842623401181321 ) ) ;
#7186=CARTESIAN_POINT ( 'NONE',  ( 20.36894250292379738, 39.92874883491396787, -10.36894250292379027 ) ) ;
#7188=CARTESIAN_POINT ( 'NONE',  ( -4.164238869374098151, 41.59541550158061796, -3.795296366450310543 ) ) ;
#7190=CARTESIAN_POINT ( 'NONE',  ( -2.816281873526471635, 53.91530133659709634, -3.434112377981056508 ) ) ;
#7191=CARTESIAN_POINT ( 'NONE',  ( 0.5774900079438590739, 22.64701867748817321, -5.440088680355550821 ) ) ;
#7192=CARTESIAN_POINT ( 'NONE',  ( 10.00000000000000000, 49.75893115100078745, -9.846743663894594434 ) ) ;
#7193=CARTESIAN_POINT ( 'NONE',  ( 7.084665262690076126, 22.02201867748817321, -10.88017736071110164 ) ) ;
#7196=CARTESIAN_POINT ( 'NONE',  ( 2.791683348922237240, 55.38393115100078745, -7.208316651077763204 ) ) ;
#7197=CARTESIAN_POINT ( 'NONE',  ( 19.84674366389459621, 53.50893115100078745, 7.409399052514197653E-17 ) ) ;
#7202=FACE_OUTER_BOUND ( 'NONE', #83288, .T. ) ;
#7204=CARTESIAN_POINT ( 'NONE',  ( 0.6076426042653103599, 67.37576471608602446, -6.499999999999992006 ) ) ;
#7205=CARTESIAN_POINT ( 'NONE',  ( 7.361572987183169658, 24.96726448433412315, -9.846743663894592657 ) ) ;
#7206=CYLINDRICAL_SURFACE ( 'NONE', #61199, 0.5000000000000004441 ) ;
#7207=CARTESIAN_POINT ( 'NONE',  ( 21.09922568453595559, 32.04030133659708923, -6.408140936763230044 ) ) ;
#7212=CARTESIAN_POINT ( 'NONE',  ( 0.1143410931637171279, 65.21691075486303646, 6.480892540919849232 ) ) ;
#7213=CARTESIAN_POINT ( 'NONE',  ( 18.52753015748618282, 38.92559781766745175, -4.923371831947291888 ) ) ;
#7214=CARTESIAN_POINT ( 'NONE',  ( 2.917880565312948704, 32.63708216824730357, 12.26659068614894643 ) ) ;
#7215=CARTESIAN_POINT ( 'NONE',  ( 0.1532563361054100626, 50.80059781766745175, -2.638427012816831230 ) ) ;
#7218=CARTESIAN_POINT ( 'NONE',  ( 0.1532563361054083140, 1.008931151000784787, 1.131784320476157264E-15 ) ) ;
#7219=CARTESIAN_POINT ( 'NONE',  ( 2.917880565312950480, 5.970415501580634832, -12.26659068614894821 ) ) ;
#7222=CARTESIAN_POINT ( 'NONE',  ( 5.076628168052703671, 46.84226448433412315, 8.527530157486179263 ) ) ;
#7223=CARTESIAN_POINT ( 'NONE',  ( 12.91533473730993009, 51.60535201082149825, -10.88017736071109987 ) ) ;
#7224=CARTESIAN_POINT ( 'NONE',  ( 0.1532563361054100626, 45.80059781766745886, -2.638427012816831230 ) ) ;
#7226=CARTESIAN_POINT ( 'NONE',  ( 17.96484262340118221, 44.93868534415483396, 7.964842623401181321 ) ) ;
#7229=CARTESIAN_POINT ( 'NONE',  ( 4.559911319644449179, 18.89701867748817321, 9.422509992056141925 ) ) ;
#7230=CARTESIAN_POINT ( 'NONE',  ( 6.565887622018943937, 3.081968003263753531, -12.81628187352647608 ) ) ;
#7231=CARTESIAN_POINT ( 'NONE',  ( 10.00000000000000178, 49.31368534415484106, 10.88017736071110342 ) ) ;
#7232=CARTESIAN_POINT ( 'NONE',  ( -1.926860441876563801, 47.66212336850780673, 1.004413902775740978E-15 ) ) ;
#7233=CARTESIAN_POINT ( 'NONE',  ( 20.15039907845753575, 10.60158574516642460, -6.262539305110077059 ) ) ;
#7235=CARTESIAN_POINT ( 'NONE',  ( 20.88017736071110519, 45.56368534415484106, 2.639326808657452039E-16 ) ) ;
#7237=CARTESIAN_POINT ( 'NONE',  ( 18.52753015748618282, 13.92559781766745175, -4.923371831947291888 ) ) ;
#7239=CARTESIAN_POINT ( 'NONE',  ( 5.076628168052703671, 36.84226448433412315, 8.527530157486179263 ) ) ;
#7242=CARTESIAN_POINT ( 'NONE',  ( 7.361572987183170547, 67.05059781766746596, 9.846743663894590881 ) ) ;
#7244=CARTESIAN_POINT ( 'NONE',  ( -0.8801773607111008646, 3.272018677488171434, 2.915334737309923430 ) ) ;
#7246=CARTESIAN_POINT ( 'NONE',  ( 13.79529636645031943, 25.34541550158063572, -14.16423886937409904 ) ) ;
#7247=B_SPLINE_CURVE_WITH_KNOTS ( 'NONE', 3,
 ( #80036, #64033, #73018, #65014, #94547, #4550 ),
 .UNSPECIFIED., .F., .F.,
 ( 4, 2, 4 ),
 ( 0.000000000000000000, 0.0002605067024380935069, 0.0005210134048761870139 ),
 .UNSPECIFIED. ) ;
#7248=CARTESIAN_POINT ( 'NONE',  ( 13.79529636645030344, 48.26208216824728936, 14.16423886937410614 ) ) ;
#7249=FILL_AREA_STYLE ('',( #45234 ) ) ;
#7252=CARTESIAN_POINT ( 'NONE',  ( 18.52753015748617571, 23.09226448433411960, 4.923371831947298993 ) ) ;
#7254=CARTESIAN_POINT ( 'NONE',  ( -0.8801773607111008646, 33.27201867748817676, 2.915334737309923430 ) ) ;
#7255=CARTESIAN_POINT ( 'NONE',  ( 0.1532563361054100626, 50.80059781766745175, -2.638427012816831230 ) ) ;
#7256=CARTESIAN_POINT ( 'NONE',  ( 20.36894250292379382, 3.678748834913967869, 10.36894250292379205 ) ) ;
#7261=CARTESIAN_POINT ( 'NONE',  ( 19.38216949554541202, 40.99863466993042493, 9.382169495545424454 ) ) ;
#7263=CARTESIAN_POINT ( 'NONE',  ( 18.52753015748618282, 38.92559781766745175, -4.923371831947291888 ) ) ;
#7264=ORIENTED_EDGE ( 'NONE', *, *, #86712, .T. ) ;
#7265=CARTESIAN_POINT ( 'NONE',  ( 17.20831665107776587, 12.88393115100078390, 7.208316651077764980 ) ) ;
#7267=CARTESIAN_POINT ( 'NONE',  ( 20.10384461210892226, 16.74302437010793199, 6.337995344473751125 ) ) ;
#7268=CARTESIAN_POINT ( 'NONE',  ( 4.559911319644449179, 8.897018677488173211, 9.422509992056141925 ) ) ;
#7269=CARTESIAN_POINT ( 'NONE',  ( 22.26659068614894466, 48.88708216824730357, 7.082119434687054849 ) ) ;
#7270=CARTESIAN_POINT ( 'NONE',  ( 4.559911319644449179, 43.89701867748816966, 9.422509992056141925 ) ) ;
#7271=CARTESIAN_POINT ( 'NONE',  ( 0.2751277870542908621, 32.28217586085237656, -6.499999999999992006 ) ) ;
#7272=LINE ( 'NONE', #47593, #83200 ) ;
#7273=CARTESIAN_POINT ( 'NONE',  ( 17.20831665107776587, 32.88393115100078745, 7.208316651077764980 ) ) ;
#7274=CARTESIAN_POINT ( 'NONE',  ( 19.42250999205614548, 5.980352010821504471, -5.440088680355545492 ) ) ;
#7275=CARTESIAN_POINT ( 'NONE',  ( 5.076628168052704559, 45.17559781766745175, -8.527530157486179263 ) ) ;
#7276=CARTESIAN_POINT ( 'NONE',  ( 17.20831665107776587, 54.13393115100079456, -7.208316651077762316 ) ) ;
#7277=CARTESIAN_POINT ( 'NONE',  ( 17.96484262340118221, 29.93868534415484106, 7.964842623401181321 ) ) ;
#7280=CARTESIAN_POINT ( 'NONE',  ( 22.81628187352647785, 56.41530133659708213, 3.434112377981063169 ) ) ;
#7281=VECTOR ( 'NONE', #85220, 1000.000000000000000 ) ;
#7282=CARTESIAN_POINT ( 'NONE',  ( 6.000000000000000000, 61.00000000000000711, -6.500000000000000888 ) ) ;
#7283=CARTESIAN_POINT ( 'NONE',  ( 10.00000000000000000, 9.758931151000785675, -9.846743663894594434 ) ) ;
#7284=CARTESIAN_POINT ( 'NONE',  ( 21.09922568453595559, 52.04030133659708923, -6.408140936763230044 ) ) ;
#7285=CARTESIAN_POINT ( 'NONE',  ( 0.5774900079438590739, 7.647018677488171434, -5.440088680355550821 ) ) ;
#7286=CARTESIAN_POINT ( 'NONE',  ( 10.00000000000000178, 52.25893115100078745, 9.846743663894594434 ) ) ;
#7287=FILL_AREA_STYLE_COLOUR ( '', #48816 ) ;
#7288=B_SPLINE_CURVE_WITH_KNOTS ( 'NONE', 3,
 ( #67598, #8078, #97620, #69073, #29566, #609 ),
 .UNSPECIFIED., .F., .F.,
 ( 4, 2, 4 ),
 ( 0.000000000000000000, 0.0002565770811490998300, 0.0005131541622981996599 ),
 .UNSPECIFIED. ) ;
#7289=CARTESIAN_POINT ( 'NONE',  ( 17.08211943468705840, 25.13708216824730357, -12.26659068614894466 ) ) ;
#7290=CARTESIAN_POINT ( 'NONE',  ( -4.164238869374098151, 51.59541550158063217, -3.795296366450310543 ) ) ;
#7291=CARTESIAN_POINT ( 'NONE',  ( 7.361572987183169658, 59.96726448433410894, -9.846743663894592657 ) ) ;
#7293=CARTESIAN_POINT ( 'NONE',  ( 15.44008868035555260, 54.73035201082150536, 9.422509992056143702 ) ) ;
#7295=CARTESIAN_POINT ( 'NONE',  ( 2.791683348922237240, 5.383931151000785675, -7.208316651077763204 ) ) ;
#7298=CARTESIAN_POINT ( 'NONE',  ( 0.6178305044545838731, 54.74863466993042493, 9.382169495545420901 ) ) ;
#7300=CARTESIAN_POINT ( 'NONE',  ( 5.076628168052704559, 10.17559781766745175, -8.527530157486179263 ) ) ;
#7303=CARTESIAN_POINT ( 'NONE',  ( 6.204703633549690345, 25.76208216824730712, -14.16423886937410259 ) ) ;
#7304=CARTESIAN_POINT ( 'NONE',  ( 19.84674366389459266, 3.300597817667451750, 2.638427012816836559 ) ) ;
#7305=CARTESIAN_POINT ( 'NONE',  ( 0.5774900079438607392, 28.48035201082150891, 5.440088680355550821 ) ) ;
#7306=DIRECTION ( 'NONE',  ( 0.7353630527936689809, 0.6776733583268385042, 0.000000000000000000 ) ) ;
#7307=ORIENTED_EDGE ( 'NONE', *, *, #48449, .T. ) ;
#7308=CARTESIAN_POINT ( 'NONE',  ( 7.084665262690076126, 32.02201867748816966, -10.88017736071110164 ) ) ;
#7313=CARTESIAN_POINT ( 'NONE',  ( 13.43411237798106583, 12.66530133659708746, -12.81628187352647252 ) ) ;
#7314=CARTESIAN_POINT ( 'NONE',  ( 19.42250999205614548, 60.98035201082151247, -5.440088680355545492 ) ) ;
#7317=CARTESIAN_POINT ( 'NONE',  ( 1.472469842513823179, 11.42559781766745175, 4.923371831947296329 ) ) ;
#7318=CARTESIAN_POINT ( 'NONE',  ( -0.8801773607111008646, 38.27201867748816255, 2.915334737309923430 ) ) ;
#7319=COLOUR_RGB ( '', 0.08235294, 0.09019608, 0.10196078) ;
#7323=ORIENTED_EDGE ( 'NONE', *, *, #9855, .F. ) ;
#7325=CARTESIAN_POINT ( 'NONE',  ( 15.44008868035555260, 44.73035201082151247, 9.422509992056143702 ) ) ;
#7326=CARTESIAN_POINT ( 'NONE',  ( -1.926860441876563801, 22.66212336850780673, 1.004413902775740978E-15 ) ) ;
#7329=CARTESIAN_POINT ( 'NONE',  ( 13.43411237798106583, 52.66530133659708213, -12.81628187352647252 ) ) ;
#7330=CARTESIAN_POINT ( 'NONE',  ( 12.91533473730993009, 56.60535201082151247, -10.88017736071109987 ) ) ;
#7331=CARTESIAN_POINT ( 'NONE',  ( -2.816281873526471635, -1.084698663402913210, -3.434112377981056508 ) ) ;
#7333=CARTESIAN_POINT ( 'NONE',  ( 10.00000000000000000, 19.75893115100078390, -9.846743663894594434 ) ) ;
#7334=CARTESIAN_POINT ( 'NONE',  ( 21.09922568453595559, 57.04030133659708923, -6.408140936763230044 ) ) ;
#7336=CARTESIAN_POINT ( 'NONE',  ( 10.00000000000000178, 2.258931151000784787, 9.846743663894594434 ) ) ;
#7337=CARTESIAN_POINT ( 'NONE',  ( 6.565887622018943937, 8.081968003263751754, -12.81628187352647608 ) ) ;
#7339=CARTESIAN_POINT ( 'NONE',  ( 0.1532563361054082862, 66.21726448433413736, 2.638427012816831674 ) ) ;
#7340=CARTESIAN_POINT ( 'NONE',  ( 4.559911319644449179, 33.89701867748817676, 9.422509992056141925 ) ) ;
#7341=CARTESIAN_POINT ( 'NONE',  ( 10.00000000000000000, 44.75893115100078745, -9.846743663894594434 ) ) ;
#7342=CARTESIAN_POINT ( 'NONE',  ( -1.926860441876563801, 32.66212336850780673, 1.004413902775740978E-15 ) ) ;
#7344=CARTESIAN_POINT ( 'NONE',  ( 2.791683348922237240, 15.38393115100078212, -7.208316651077763204 ) ) ;
#7345=CARTESIAN_POINT ( 'NONE',  ( 12.63842701281683034, 7.467264484334118713, 9.846743663894596210 ) ) ;
#7346=CARTESIAN_POINT ( 'NONE',  ( 3.591859063236761518, -0.04303199673624671928, 11.09922568453594849 ) ) ;
#7348=CARTESIAN_POINT ( 'NONE',  ( 2.035157376598824452, 3.688685344154837953, 7.964842623401179544 ) ) ;
#7349=CARTESIAN_POINT ( 'NONE',  ( 19.84674366389459266, 63.71726448433412315, -2.638427012816827677 ) ) ;
#7352=CARTESIAN_POINT ( 'NONE',  ( 0.5774900079438590739, 7.647018677488171434, -5.440088680355550821 ) ) ;
#7353=CARTESIAN_POINT ( 'NONE',  ( 7.361572987183169658, 39.96726448433411605, -9.846743663894592657 ) ) ;
#7354=CARTESIAN_POINT ( 'NONE',  ( -0.1503990784575328643, 50.12777174578613426, 6.262539305110068177 ) ) ;
#7355=CARTESIAN_POINT ( 'NONE',  ( -0.8801773607111008646, 8.272018677488171434, 2.915334737309923430 ) ) ;
#7357=CARTESIAN_POINT ( 'NONE',  ( 10.00000000000000178, 39.31368534415484106, 10.88017736071110342 ) ) ;
#7358=CARTESIAN_POINT ( 'NONE',  ( 13.79529636645031943, 45.34541550158062506, -14.16423886937409904 ) ) ;
#7359=CARTESIAN_POINT ( 'NONE',  ( 6.204703633549690345, 62.84541550158063927, 14.16423886937410082 ) ) ;
#7361=CARTESIAN_POINT ( 'NONE',  ( 5.076628168052703671, 6.842264484334118713, 8.527530157486179263 ) ) ;
#7362=CARTESIAN_POINT ( 'NONE',  ( 1.472469842513823179, 31.42559781766745530, 4.923371831947296329 ) ) ;
#7363=CARTESIAN_POINT ( 'NONE',  ( 19.38216949554541202, 15.99863466993042138, 9.382169495545424454 ) ) ;
#7368=CARTESIAN_POINT ( 'NONE',  ( 12.63842701281683034, 57.46726448433411605, 9.846743663894596210 ) ) ;
#7371=CARTESIAN_POINT ( 'NONE',  ( -4.164238869374098151, 6.595415501580634832, -3.795296366450310543 ) ) ;
#7372=CARTESIAN_POINT ( 'NONE',  ( 14.92337183194729633, 22.67559781766745175, 8.527530157486181039 ) ) ;
#7376=CARTESIAN_POINT ( 'NONE',  ( -2.266590686148945544, 52.22041550158064638, 7.082119434687048631 ) ) ;
#7377=CARTESIAN_POINT ( 'NONE',  ( 1.472469842513823179, 11.42559781766745175, 4.923371831947296329 ) ) ;
#7380=CARTESIAN_POINT ( 'NONE',  ( 15.44008868035555260, 34.73035201082151247, 9.422509992056143702 ) ) ;
#7381=CARTESIAN_POINT ( 'NONE',  ( 10.00000000000000000, 47.87363466993042493, -12.81628187352647608 ) ) ;
#7383=CARTESIAN_POINT ( 'NONE',  ( 19.42250999205614193, 10.14701867748816966, 5.440088680355555262 ) ) ;
#7384=CARTESIAN_POINT ( 'NONE',  ( 3.591859063236761518, 34.95696800326375353, 11.09922568453594849 ) ) ;
#7386=CARTESIAN_POINT ( 'NONE',  ( 2.791683348922237240, 5.383931151000785675, -7.208316651077763204 ) ) ;
#7389=CARTESIAN_POINT ( 'NONE',  ( -0.3689425029237881626, 42.42874883491396787, 10.36894250292379027 ) ) ;
#7390=CARTESIAN_POINT ( 'NONE',  ( 6.204703633549690345, 12.84541550158063572, 14.16423886937410082 ) ) ;
#7391=CARTESIAN_POINT ( 'NONE',  ( 15.44008868035555260, 4.730352010821504471, 9.422509992056143702 ) ) ;
#7392=CARTESIAN_POINT ( 'NONE',  ( 19.42250999205614548, 40.98035201082150536, -5.440088680355545492 ) ) ;
#7395=CARTESIAN_POINT ( 'NONE',  ( 12.91533473730992121, 59.52201867748816966, 10.88017736071110164 ) ) ;
#7396=CARTESIAN_POINT ( 'NONE',  ( 19.42250999205614193, 65.14701867748817676, 5.440088680355555262 ) ) ;
#7397=CARTESIAN_POINT ( 'NONE',  ( 19.38216949554541202, 25.99863466993042138, 9.382169495545424454 ) ) ;
#7400=CARTESIAN_POINT ( 'NONE',  ( 0.1532563361054100626, 30.80059781766744820, -2.638427012816831230 ) ) ;
#7404=CARTESIAN_POINT ( 'NONE',  ( 19.38216949554541202, 20.99863466993042138, 9.382169495545424454 ) ) ;
#7405=EDGE_CURVE ( 'NONE', #53047, #62035, #19287, .T. ) ;
#7406=CARTESIAN_POINT ( 'NONE',  ( 7.361572987183169658, -0.03273551566588185635, -9.846743663894592657 ) ) ;
#7407=CARTESIAN_POINT ( 'NONE',  ( 4.559911319644449179, 8.897018677488171434, 9.422509992056141925 ) ) ;
#7409=CARTESIAN_POINT ( 'NONE',  ( 19.84674366389459266, 38.71726448433412315, -2.638427012816827677 ) ) ;
#7410=CARTESIAN_POINT ( 'NONE',  ( -23.44000000000000838, 92.00000000000000000, -10.09898361729590199 ) ) ;
#7411=CARTESIAN_POINT ( 'NONE',  ( 10.00000000000000178, 17.25893115100078745, 9.846743663894594434 ) ) ;
#7412=CARTESIAN_POINT ( 'NONE',  ( 6.204703633549690345, 2.845415501580634388, 14.16423886937410082 ) ) ;
#7413=CARTESIAN_POINT ( 'NONE',  ( 2.917880565312950480, 0.9704155015806342766, -12.26659068614894821 ) ) ;
#7415=CARTESIAN_POINT ( 'NONE',  ( 4.559911319644449179, 38.89701867748817676, 9.422509992056141925 ) ) ;
#7417=CARTESIAN_POINT ( 'NONE',  ( 20.36894250292379738, 44.92874883491396787, -10.36894250292379027 ) ) ;
#7418=CARTESIAN_POINT ( 'NONE',  ( 20.88017736071110519, 25.56368534415483751, 2.639326808657452039E-16 ) ) ;
#7419=CARTESIAN_POINT ( 'NONE',  ( 4.559911319644449179, 13.89701867748817321, 9.422509992056141925 ) ) ;
#7420=ORIENTED_EDGE ( 'NONE', *, *, #36870, .F. ) ;
#7421=CARTESIAN_POINT ( 'NONE',  ( 12.91533473730992121, 24.52201867748816966, 10.88017736071110164 ) ) ;
#7422=CARTESIAN_POINT ( 'NONE',  ( 22.81628187352647785, 46.41530133659708213, 3.434112377981063169 ) ) ;
#7423=CARTESIAN_POINT ( 'NONE',  ( 20.88017736071110875, 45.77201867748816966, -2.915334737309920765 ) ) ;
#7425=CARTESIAN_POINT ( 'NONE',  ( 0.5774900079438590739, 57.64701867748817676, -5.440088680355550821 ) ) ;
#7427=MECHANICAL_DESIGN_GEOMETRIC_PRESENTATION_REPRESENTATION('',(#95248),#79273);
#7428=CARTESIAN_POINT ( 'NONE',  ( -0.8801773607111009756, 38.06368534415484106, 1.068504757029289695E-15 ) ) ;
#7431=CARTESIAN_POINT ( 'NONE',  ( -4.164238869374099039, 41.80374883491397497, 8.674139862899312516E-16 ) ) ;
#7432=CARTESIAN_POINT ( 'NONE',  ( 2.035157376598822676, 67.43868534415484817, -7.964842623401177768 ) ) ;
#7433=CARTESIAN_POINT ( 'NONE',  ( 19.80777595082616216, 25.68878173731741299, -6.499999999999960920 ) ) ;
#7434=CARTESIAN_POINT ( 'NONE',  ( 10.00000000000000000, -0.2410688489992152128, -9.846743663894594434 ) ) ;
#7435=CARTESIAN_POINT ( 'NONE',  ( 0.1532563361054100626, 60.80059781766744464, -2.638427012816831230 ) ) ;
#7437=CARTESIAN_POINT ( 'NONE',  ( 12.63842701281683034, 27.46726448433411250, 9.846743663894596210 ) ) ;
#7438=CARTESIAN_POINT ( 'NONE',  ( 17.20831665107776587, 39.13393115100079456, -7.208316651077762316 ) ) ;
#7440=CARTESIAN_POINT ( 'NONE',  ( 4.559911319644449179, 27.23035201082150536, -9.422509992056141925 ) ) ;
#7441=CARTESIAN_POINT ( 'NONE',  ( 17.20831665107776587, 42.88393115100077324, 7.208316651077764980 ) ) ;
#7442=CARTESIAN_POINT ( 'NONE',  ( 19.39188664607695500, 25.83703382326400089, -6.499999999999964473 ) ) ;
#7443=CARTESIAN_POINT ( 'NONE',  ( 17.96484262340118221, 56.18868534415484817, -7.964842623401177768 ) ) ;
#7444=CARTESIAN_POINT ( 'NONE',  ( 2.035157376598822676, 37.43868534415484106, -7.964842623401177768 ) ) ;
#7445=PRESENTATION_STYLE_ASSIGNMENT (( #98955 ) ) ;
#7446=CARTESIAN_POINT ( 'NONE',  ( 20.36894250292379382, 53.67874883491397497, 10.36894250292379205 ) ) ;
#7447=MECHANICAL_DESIGN_GEOMETRIC_PRESENTATION_REPRESENTATION('',(#1091),#26608);
#7449=CARTESIAN_POINT ( 'NONE',  ( -1.099225684535947600, 23.70696800326375708, -6.408140936763238038 ) ) ;
#7450=DIRECTION ( 'NONE',  ( -0.000000000000000000, -1.000000000000000000, 0.000000000000000000 ) ) ;
#7452=CARTESIAN_POINT ( 'NONE',  ( -2.816281873526473856, 14.33196800326375531, 3.434112377981055619 ) ) ;
#7453=CARTESIAN_POINT ( 'NONE',  ( 0.5774900079438607392, 13.48035201082150358, 5.440088680355550821 ) ) ;
#7454=CARTESIAN_POINT ( 'NONE',  ( 7.084665262690076126, 47.02201867748818387, -10.88017736071110164 ) ) ;
#7456=CARTESIAN_POINT ( 'NONE',  ( 12.91533473730992121, 54.52201867748816255, 10.88017736071110164 ) ) ;
#7457=CARTESIAN_POINT ( 'NONE',  ( 14.92337183194729988, 39.34226448433412315, -8.527530157486177487 ) ) ;
#7458=CARTESIAN_POINT ( 'NONE',  ( 19.84674366389459266, 23.71726448433412315, -2.638427012816827677 ) ) ;
#7460=CARTESIAN_POINT ( 'NONE',  ( 19.84674366389459266, 18.71726448433411960, -2.638427012816827677 ) ) ;
#7463=CARTESIAN_POINT ( 'NONE',  ( 19.38216949554541202, 35.99863466993041072, 9.382169495545424454 ) ) ;
#7465=CARTESIAN_POINT ( 'NONE',  ( 0.1532563361054082862, 16.21726448433411960, 2.638427012816831674 ) ) ;
#7469=CARTESIAN_POINT ( 'NONE',  ( 18.52753015748618282, 28.92559781766745175, -4.923371831947291888 ) ) ;
#7472=B_SPLINE_CURVE_WITH_KNOTS ( 'NONE', 3,
 ( #54194, #97762, #91715, #29718, #29227, #68723 ),
 .UNSPECIFIED., .F., .F.,
 ( 4, 2, 4 ),
 ( 2.221529986854170345E-17, 0.0002504968758227833921, 0.0005009937516455445581 ),
 .UNSPECIFIED. ) ;
#7473=CARTESIAN_POINT ( 'NONE',  ( 10.00000000000000178, 15.37363466993042138, 12.81628187352647608 ) ) ;
#7474=CARTESIAN_POINT ( 'NONE',  ( 4.559911319644449179, 58.89701867748817676, 9.422509992056141925 ) ) ;
#7475=CIRCLE ( 'NONE', #44120, 0.5000000000000004441 ) ;
#7476=CARTESIAN_POINT ( 'NONE',  ( 24.16423886937410614, 34.51208216824731068, -3.795296366450302550 ) ) ;
#7479=CARTESIAN_POINT ( 'NONE',  ( 13.79529636645030344, 33.26208216824730357, 14.16423886937410614 ) ) ;
#7480=CARTESIAN_POINT ( 'NONE',  ( -0.3689425029237898834, 56.17874883491396076, -10.36894250292378850 ) ) ;
#7481=CARTESIAN_POINT ( 'NONE',  ( 22.26659068614894466, 8.887082168247300018, 7.082119434687054849 ) ) ;
#7482=CARTESIAN_POINT ( 'NONE',  ( 13.79529636645031943, 20.34541550158063572, -14.16423886937409904 ) ) ;
#7483=CARTESIAN_POINT ( 'NONE',  ( -0.3289641300567998083, 38.07879003517447103, 5.963430220938281678 ) ) ;
#7484=CARTESIAN_POINT ( 'NONE',  ( 10.00000000000000178, 49.31368534415484106, 10.88017736071110342 ) ) ;
#7486=DIRECTION ( 'NONE',  ( -1.000000000000000000, 0.000000000000000000, -0.000000000000000000 ) ) ;
#7487=CARTESIAN_POINT ( 'NONE',  ( 17.20831665107776587, 47.88393115100078745, 7.208316651077764980 ) ) ;
#7488=CARTESIAN_POINT ( 'NONE',  ( 2.035157376598824452, 18.68868534415484106, 7.964842623401179544 ) ) ;
#7489=CARTESIAN_POINT ( 'NONE',  ( 13.43411237798106583, 57.66530133659708923, -12.81628187352647252 ) ) ;
#7490=CARTESIAN_POINT ( 'NONE',  ( 12.63842701281683922, 59.55059781766744464, -9.846743663894590881 ) ) ;
#7491=CARTESIAN_POINT ( 'NONE',  ( 20.00000000000000711, 79.40087001978915282, -4.500000000000000888 ) ) ;
#7492=CARTESIAN_POINT ( 'NONE',  ( 7.361572987183169658, 29.96726448433411960, -9.846743663894592657 ) ) ;
#7494=CARTESIAN_POINT ( 'NONE',  ( 0.6178305044545818747, 58.49863466993042493, -9.382169495545419124 ) ) ;
#7497=CARTESIAN_POINT ( 'NONE',  ( 7.084665262690076126, 47.02201867748818387, -10.88017736071110164 ) ) ;
#7498=CARTESIAN_POINT ( 'NONE',  ( 1.472469842513823179, 50.59226448433411605, -4.923371831947296329 ) ) ;
#7499=CARTESIAN_POINT ( 'NONE',  ( 2.917880565312950480, 40.97041550158063217, -12.26659068614894821 ) ) ;
#7503=CARTESIAN_POINT ( 'NONE',  ( 24.16423886937410614, 4.512082168247300906, -3.795296366450302550 ) ) ;
#7504=CARTESIAN_POINT ( 'NONE',  ( 12.91533473730992121, 64.52201867748817676, 10.88017736071110164 ) ) ;
#7506=CARTESIAN_POINT ( 'NONE',  ( 24.16423886937409904, 59.09541550158063217, 3.795296366450317205 ) ) ;
#7507=CARTESIAN_POINT ( 'NONE',  ( 19.38216949554541202, 15.99863466993042138, 9.382169495545424454 ) ) ;
#7509=CARTESIAN_POINT ( 'NONE',  ( 4.559911319644449179, 57.23035201082150536, -9.422509992056141925 ) ) ;
#7511=CARTESIAN_POINT ( 'NONE',  ( -46.69421152571126044, 101.0768001808267229, -8.798454068542781670 ) ) ;
#7512=CARTESIAN_POINT ( 'NONE',  ( 7.084665262690076126, 2.022018677488171434, -10.88017736071110164 ) ) ;
#7514=CARTESIAN_POINT ( 'NONE',  ( 10.00000000000000000, 11.81368534415483751, -10.88017736071110342 ) ) ;
#7515=CARTESIAN_POINT ( 'NONE',  ( 15.44008868035555793, 21.39701867748817321, -9.422509992056140149 ) ) ;
#7516=CARTESIAN_POINT ( 'NONE',  ( 14.92337183194729988, 59.34226448433412315, -8.527530157486177487 ) ) ;
#7517=CARTESIAN_POINT ( 'NONE',  ( 19.38216949554541557, 52.24863466993041072, -9.382169495545420901 ) ) ;
#7518=FACE_OUTER_BOUND ( 'NONE', #65659, .T. ) ;
#7520=CARTESIAN_POINT ( 'NONE',  ( 2.035157376598824452, 13.68868534415483751, 7.964842623401179544 ) ) ;
#7521=CARTESIAN_POINT ( 'NONE',  ( 21.09922568453594849, 21.20696800326375353, 6.408140936763242479 ) ) ;
#7524=CARTESIAN_POINT ( 'NONE',  ( 5.076628168052704559, 45.17559781766745175, -8.527530157486179263 ) ) ;
#7525=CARTESIAN_POINT ( 'NONE',  ( 2.035157376598822676, 32.43868534415483396, -7.964842623401177768 ) ) ;
#7526=CARTESIAN_POINT ( 'NONE',  ( 0.6178305044545818747, 28.49863466993041783, -9.382169495545419124 ) ) ;
#7527=CARTESIAN_POINT ( 'NONE',  ( 4.559911319644449179, 43.89701867748816966, 9.422509992056141925 ) ) ;
#7528=CARTESIAN_POINT ( 'NONE',  ( 19.10478245763048477, 16.02576239577082262, -5.990408912944377384 ) ) ;
#7530=CARTESIAN_POINT ( 'NONE',  ( 10.00000000000000000, 52.87363466993041783, -12.81628187352647608 ) ) ;
#7532=CARTESIAN_POINT ( 'NONE',  ( 20.88017736071110519, 55.56368534415484817, 2.639326808657452039E-16 ) ) ;
#7533=CARTESIAN_POINT ( 'NONE',  ( 10.00000000000000000, 27.87363466993042138, -12.81628187352647608 ) ) ;
#7534=CARTESIAN_POINT ( 'NONE',  ( 2.917880565312948704, 7.637082168247301794, 12.26659068614894643 ) ) ;
#7535=CARTESIAN_POINT ( 'NONE',  ( 2.791683348922237240, 5.383931151000785675, -7.208316651077763204 ) ) ;
#7536=CARTESIAN_POINT ( 'NONE',  ( -0.8801773607111008646, 58.27201867748816966, 2.915334737309923430 ) ) ;
#7537=CARTESIAN_POINT ( 'NONE',  ( 6.204703633549690345, 42.84541550158063217, 14.16423886937410082 ) ) ;
#7538=CARTESIAN_POINT ( 'NONE',  ( 12.63842701281683034, 62.46726448433410894, 9.846743663894596210 ) ) ;
#7539=CARTESIAN_POINT ( 'NONE',  ( 17.20831665107776587, 12.88393115100078390, 7.208316651077764980 ) ) ;
#7541=CARTESIAN_POINT ( 'NONE',  ( 2.791683348922237240, 5.383931151000785675, -7.208316651077763204 ) ) ;
#7543=CARTESIAN_POINT ( 'NONE',  ( -2.266590686148945544, 42.22041550158063217, 7.082119434687048631 ) ) ;
#7544=( BOUNDED_CURVE ( )  B_SPLINE_CURVE ( 2, ( #57325, #87819, #13311, #11339, #95836, #74291, #73806, #64813, #34315 ),
 .UNSPECIFIED., .F., .T. ) 
 B_SPLINE_CURVE_WITH_KNOTS ( ( 3, 2, 2, 2, 3 ),
 ( 0.009663273234349279567, 0.01190476190476190410, 0.01785714285714285615, 0.02380952380952380820, 0.02605726409658919510 ),
 .UNSPECIFIED. ) 
 CURVE ( )  GEOMETRIC_REPRESENTATION_ITEM ( )  RATIONAL_B_SPLINE_CURVE ( ( 0.9840011491998950088, 0.9871686851131101781, 1.000000000000000000, 0.9659258262890683122, 1.000000000000000000, 0.9659258262890683122, 1.000000000000000000, 0.9871328979762477029, 0.9839835555609426354 ) ) 
 REPRESENTATION_ITEM ( '' )  );
#7547=CARTESIAN_POINT ( 'NONE',  ( 20.88017736071110164, 10.35535201082150714, 2.915334737309930979 ) ) ;
#7549=COLOUR_RGB ( '', 0.40784314, 0.44705882, 0.49803922) ;
#7550=VERTEX_POINT ( 'NONE', #14266 ) ;
#7551=CARTESIAN_POINT ( 'NONE',  ( 15.44008868035555260, 4.730352010821505360, 9.422509992056143702 ) ) ;
#7552=CARTESIAN_POINT ( 'NONE',  ( 0.5774900079438590739, 2.647018677488171434, -5.440088680355550821 ) ) ;
#7553=CARTESIAN_POINT ( 'NONE',  ( 12.63842701281683922, 49.55059781766744464, -9.846743663894590881 ) ) ;
#7554=CARTESIAN_POINT ( 'NONE',  ( 22.81628187352648496, 41.83196800326375353, -3.434112377981050290 ) ) ;
#7557=CARTESIAN_POINT ( 'NONE',  ( 13.79529636645030344, 3.262082168247301350, 14.16423886937410614 ) ) ;
#7558=CARTESIAN_POINT ( 'NONE',  ( -0.8801773607110991993, 12.85535201082150358, -2.915334737309923874 ) ) ;
#7559=CARTESIAN_POINT ( 'NONE',  ( 2.917880565312948704, 67.63708216824730357, 12.26659068614894643 ) ) ;
#7562=CARTESIAN_POINT ( 'NONE',  ( 14.92337183194729633, 47.67559781766745175, 8.527530157486181039 ) ) ;
#7563=CARTESIAN_POINT ( 'NONE',  ( 18.06765999051787119, 43.99127512925446126, 6.499999999999926281 ) ) ;
#7564=CARTESIAN_POINT ( 'NONE',  ( 1.472469842513823179, 26.42559781766745175, 4.923371831947296329 ) ) ;
#7565=CARTESIAN_POINT ( 'NONE',  ( 0.8952175423694952450, 33.52576239577081907, 5.990408912944338304 ) ) ;
#7567=ORIENTED_EDGE ( 'NONE', *, *, #23183, .F. ) ;
#7568=ORIENTED_EDGE ( 'NONE', *, *, #83927, .F. ) ;
#7569=CARTESIAN_POINT ( 'NONE',  ( -22.44000000000001194, 93.50000000000000000, -10.09898361729590199 ) ) ;
#7570=EDGE_LOOP ( 'NONE', ( #82632, #60248, #32625, #25427, #36388, #54669 ) ) ;
#7571=CARTESIAN_POINT ( 'NONE',  ( 14.92337183194729633, 52.67559781766745175, 8.527530157486181039 ) ) ;
#7572=CARTESIAN_POINT ( 'NONE',  ( 4.559911319644449179, 28.89701867748817321, 9.422509992056141925 ) ) ;
#7573=CARTESIAN_POINT ( 'NONE',  ( 20.88017736071110519, 35.56368534415484106, 2.639326808657452039E-16 ) ) ;
#7574=CARTESIAN_POINT ( 'NONE',  ( 14.92337183194729988, 59.34226448433412315, -8.527530157486177487 ) ) ;
#7575=CARTESIAN_POINT ( 'NONE',  ( 13.43411237798105340, 25.58196800326374998, 12.81628187352647963 ) ) ;
#7578=CARTESIAN_POINT ( 'NONE',  ( 21.09922568453595559, 42.04030133659708213, -6.408140936763230044 ) ) ;
#7580=CARTESIAN_POINT ( 'NONE',  ( 17.20831665107776587, 49.13393115100078745, -7.208316651077762316 ) ) ;
#7581=CARTESIAN_POINT ( 'NONE',  ( 20.88017736071110519, 5.563685344154838397, 2.639326808657452039E-16 ) ) ;
#7583=CARTESIAN_POINT ( 'NONE',  ( 12.91533473730993009, 21.60535201082150536, -10.88017736071109987 ) ) ;
#7585=CARTESIAN_POINT ( 'NONE',  ( 2.035157376598824452, 63.68868534415484106, 7.964842623401179544 ) ) ;
#7586=CARTESIAN_POINT ( 'NONE',  ( 20.88017736071110164, 60.35535201082151957, 2.915334737309930979 ) ) ;
#7588=CARTESIAN_POINT ( 'NONE',  ( 0.5774900079438590739, 57.64701867748817676, -5.440088680355550821 ) ) ;
#7589=EDGE_CURVE ( 'NONE', #35045, #55728, #38736, .T. ) ;
#7590=CARTESIAN_POINT ( 'NONE',  ( -46.94000000000240647, 102.7387969410439723, 6.737038697110675045 ) ) ;
#7591=ORIENTED_EDGE ( 'NONE', *, *, #42129, .T. ) ;
#7592=CARTESIAN_POINT ( 'NONE',  ( 12.63842701281683034, 42.46726448433412315, 9.846743663894596210 ) ) ;
#7599=CARTESIAN_POINT ( 'NONE',  ( 2.035157376598824452, 58.68868534415482685, 7.964842623401179544 ) ) ;
#7600=CARTESIAN_POINT ( 'NONE',  ( 10.00000000000000178, 9.313685344154839285, 10.88017736071110342 ) ) ;
#7601=CARTESIAN_POINT ( 'NONE',  ( -0.03743638938522109161, 59.25197528031019090, -6.399506433553975526 ) ) ;
#7602=CARTESIAN_POINT ( 'NONE',  ( 21.09922568453594849, 41.20696800326375353, 6.408140936763242479 ) ) ;
#7605=CARTESIAN_POINT ( 'NONE',  ( 18.52753015748617571, 43.09226448433412315, 4.923371831947298993 ) ) ;
#7606=CARTESIAN_POINT ( 'NONE',  ( 12.63842701281683922, 4.550597817667451750, -9.846743663894590881 ) ) ;
#7607=CARTESIAN_POINT ( 'NONE',  ( 0.6178305044545838731, 24.74863466993042493, 9.382169495545420901 ) ) ;
#7608=CARTESIAN_POINT ( 'NONE',  ( 0.1532563361054100626, 20.80059781766744464, -2.638427012816831230 ) ) ;
#7610=CARTESIAN_POINT ( 'NONE',  ( 0.1532563361054100626, 20.80059781766744464, -2.638427012816831230 ) ) ;
#7611=CARTESIAN_POINT ( 'NONE',  ( -1.099225684535947600, 14.54030133659708568, 6.408140936763237150 ) ) ;
#7612=( BOUNDED_CURVE ( )  B_SPLINE_CURVE ( 2, ( #90633, #22157, #73658, #96689, #58662, #48510, #33495, #63994, #56517 ),
 .UNSPECIFIED., .F., .F. ) 
 B_SPLINE_CURVE_WITH_KNOTS ( ( 3, 2, 2, 2, 3 ),
 ( 0.8677146600783226527, 0.8690476190476190688, 0.8750000000000000000, 0.8809523809523809312, 0.8822853399216774584 ),
 .UNSPECIFIED. ) 
 CURVE ( )  GEOMETRIC_REPRESENTATION_ITEM ( )  RATIONAL_B_SPLINE_CURVE ( ( 0.9881565478350733400, 0.9923695281211490915, 1.000000000000000000, 0.9659258262890683122, 1.000000000000000000, 0.9659258262890683122, 1.000000000000000000, 0.9923695281211484254, 0.9881565478350726739 ) ) 
 REPRESENTATION_ITEM ( '' )  );
#7615=CARTESIAN_POINT ( 'NONE',  ( 5.076628168052704559, 5.175597817667451750, -8.527530157486179263 ) ) ;
#7616=EDGE_CURVE ( 'NONE', #45856, #9878, #63951, .T. ) ;
#7617=ORIENTED_EDGE ( 'NONE', *, *, #48609, .T. ) ;
#7619=CARTESIAN_POINT ( 'NONE',  ( 4.559911319644449179, 23.89701867748817321, 9.422509992056141925 ) ) ;
#7620=CARTESIAN_POINT ( 'NONE',  ( -4.164238869374099039, 21.80374883491396787, 8.674139862899312516E-16 ) ) ;
#7621=CARTESIAN_POINT ( 'NONE',  ( 0.1532563361054100626, 45.80059781766745886, -2.638427012816831230 ) ) ;
#7622=CARTESIAN_POINT ( 'NONE',  ( 10.00000000000000178, 64.31368534415483396, 10.88017736071110342 ) ) ;
#7623=CARTESIAN_POINT ( 'NONE',  ( 6.565887622018943937, 40.16530133659708923, 12.81628187352647430 ) ) ;
#7625=CARTESIAN_POINT ( 'NONE',  ( 20.88017736071110519, 15.56368534415483751, 2.639326808657452039E-16 ) ) ;
#7629=CARTESIAN_POINT ( 'NONE',  ( -2.816281873526473856, 9.123634669930421381, 9.499525473075851096E-16 ) ) ;
#7630=CARTESIAN_POINT ( 'NONE',  ( 5.076628168052703671, 21.84226448433411960, 8.527530157486179263 ) ) ;
#7632=CARTESIAN_POINT ( 'NONE',  ( 3.591859063236761518, 34.95696800326375353, 11.09922568453594849 ) ) ;
#7634=CARTESIAN_POINT ( 'NONE',  ( 19.42250999205614193, 35.14701867748816966, 5.440088680355555262 ) ) ;
#7638=CARTESIAN_POINT ( 'NONE',  ( 20.03932841506543383, 20.62161441960503083, -6.397827110478934820 ) ) ;
#7640=CARTESIAN_POINT ( 'NONE',  ( 10.00000000000000000, 41.81368534415484106, -10.88017736071110342 ) ) ;
#7641=CARTESIAN_POINT ( 'NONE',  ( 10.00000000000000178, 39.31368534415484106, 10.88017736071110342 ) ) ;
#7642=CARTESIAN_POINT ( 'NONE',  ( 0.1532563361054100626, 60.80059781766744464, -2.638427012816831230 ) ) ;
#7643=CARTESIAN_POINT ( 'NONE',  ( 2.035157376598822676, 67.43868534415484817, -7.964842623401177768 ) ) ;
#7644=CARTESIAN_POINT ( 'NONE',  ( 7.361572987183169658, 49.96726448433410894, -9.846743663894592657 ) ) ;
#7645=CARTESIAN_POINT ( 'NONE',  ( -0.8801773607110991993, 12.85535201082150358, -2.915334737309923874 ) ) ;
#7647=CARTESIAN_POINT ( 'NONE',  ( -1.099225684535947600, 14.54030133659708568, 6.408140936763237150 ) ) ;
#7649=CARTESIAN_POINT ( 'NONE',  ( -0.8801773607110991993, 32.85535201082151247, -2.915334737309923874 ) ) ;
#7650=CARTESIAN_POINT ( 'NONE',  ( 3.591859063236761518, -0.04303199673624671928, 11.09922568453594849 ) ) ;
#7651=CARTESIAN_POINT ( 'NONE',  ( 7.084665262690076126, 19.10535201082150181, 10.88017736071109987 ) ) ;
#7652=CARTESIAN_POINT ( 'NONE',  ( 17.96484262340118221, 31.18868534415483751, -7.964842623401177768 ) ) ;
#7653=CARTESIAN_POINT ( 'NONE',  ( 24.16423886937410614, 39.51208216824731068, -3.795296366450302550 ) ) ;
#7654=CARTESIAN_POINT ( 'NONE',  ( 1.472469842513823179, 25.59226448433412315, -4.923371831947296329 ) ) ;
#7655=CARTESIAN_POINT ( 'NONE',  ( 7.084665262690076126, 49.10535201082149825, 10.88017736071109987 ) ) ;
#7657=CARTESIAN_POINT ( 'NONE',  ( 6.204703633549690345, 0.7620821682473009062, -14.16423886937410259 ) ) ;
#7659=FILL_AREA_STYLE ('',( #70116 ) ) ;
#7660=CARTESIAN_POINT ( 'NONE',  ( 14.92337183194729988, 59.34226448433412315, -8.527530157486177487 ) ) ;
#7663=CARTESIAN_POINT ( 'NONE',  ( 13.79529636645030344, 38.26208216824729647, 14.16423886937410614 ) ) ;
#7664=CARTESIAN_POINT ( 'NONE',  ( 2.917880565312948704, 17.63708216824730357, 12.26659068614894643 ) ) ;
#7665=CARTESIAN_POINT ( 'NONE',  ( 18.52753015748618282, 8.925597817667451750, -4.923371831947291888 ) ) ;
#7666=CARTESIAN_POINT ( 'NONE',  ( 3.591859063236761518, 9.956968003263753531, 11.09922568453594849 ) ) ;
#7667=CARTESIAN_POINT ( 'NONE',  ( 19.84674366389459621, 53.50893115100078745, 7.409399052514197653E-17 ) ) ;
#7669=CARTESIAN_POINT ( 'NONE',  ( 19.42250999205614193, 40.14701867748817676, 5.440088680355555262 ) ) ;
#7670=CARTESIAN_POINT ( 'NONE',  ( 22.81628187352647785, 16.41530133659708923, 3.434112377981063169 ) ) ;
#7671=CARTESIAN_POINT ( 'NONE',  ( 13.79529636645031943, 20.34541550158063572, -14.16423886937409904 ) ) ;
#7672=CARTESIAN_POINT ( 'NONE',  ( -0.8801773607111008646, 18.27201867748817321, 2.915334737309923430 ) ) ;
#7673=CARTESIAN_POINT ( 'NONE',  ( 7.084665262690076126, 29.10535201082150181, 10.88017736071109987 ) ) ;
#7674=CARTESIAN_POINT ( 'NONE',  ( 17.96484262340118221, 59.93868534415484106, 7.964842623401181321 ) ) ;
#7676=ORIENTED_EDGE ( 'NONE', *, *, #49106, .T. ) ;
#7681=CARTESIAN_POINT ( 'NONE',  ( 17.08211943468705840, 55.13708216824731068, -12.26659068614894466 ) ) ;
#7682=CARTESIAN_POINT ( 'NONE',  ( -2.266590686148945544, 62.22041550158063927, 7.082119434687048631 ) ) ;
#7683=CARTESIAN_POINT ( 'NONE',  ( 14.92337183194729633, 17.67559781766745175, 8.527530157486181039 ) ) ;
#7684=CARTESIAN_POINT ( 'NONE',  ( 7.361572987183170547, 62.05059781766745886, 9.846743663894590881 ) ) ;
#7685=CARTESIAN_POINT ( 'NONE',  ( 2.035157376598822676, 67.43868534415484817, -7.964842623401177768 ) ) ;
#7686=CARTESIAN_POINT ( 'NONE',  ( 0.1532563361054082862, 11.21726448433411605, 2.638427012816831674 ) ) ;
#7688=ORIENTED_EDGE ( 'NONE', *, *, #14714, .F. ) ;
#7690=CARTESIAN_POINT ( 'NONE',  ( -4.164238869374099927, 32.01208216824730357, 3.795296366450308767 ) ) ;
#7691=CARTESIAN_POINT ( 'NONE',  ( 20.36894250292379382, 48.67874883491396076, 10.36894250292379205 ) ) ;
#7693=CARTESIAN_POINT ( 'NONE',  ( 3.591859063236761518, 54.95696800326376064, 11.09922568453594849 ) ) ;
#7695=CARTESIAN_POINT ( 'NONE',  ( 15.44008868035555260, 24.73035201082150891, 9.422509992056143702 ) ) ;
#7696=CARTESIAN_POINT ( 'NONE',  ( 19.84674366389459621, 43.50893115100078745, 7.409399052514197653E-17 ) ) ;
#7697=CARTESIAN_POINT ( 'NONE',  ( 19.42250999205614193, 20.14701867748817321, 5.440088680355555262 ) ) ;
#7699=CARTESIAN_POINT ( 'NONE',  ( 1.472469842513823179, 60.59226448433412315, -4.923371831947296329 ) ) ;
#7700=CARTESIAN_POINT ( 'NONE',  ( 18.52753015748618282, 53.92559781766745175, -4.923371831947291888 ) ) ;
#7702=EDGE_CURVE ( 'NONE', #42198, #39274, #22192, .T. ) ;
#7704=CARTESIAN_POINT ( 'NONE',  ( 19.50000000000000355, 98.59912998021083297, -5.000000000000000000 ) ) ;
#7708=CARTESIAN_POINT ( 'NONE',  ( 0.9408516040111539747, 7.466938638839759612, -6.499999999999972466 ) ) ;
#7709=CARTESIAN_POINT ( 'NONE',  ( 5.076628168052704559, 35.17559781766745175, -8.527530157486179263 ) ) ;
#7712=CARTESIAN_POINT ( 'NONE',  ( 22.81628187352647785, 31.41530133659709279, 3.434112377981063169 ) ) ;
#7713=CARTESIAN_POINT ( 'NONE',  ( 1.274849032794231007, 38.57228050351032067, 6.499999999999895195 ) ) ;
#7717=CARTESIAN_POINT ( 'NONE',  ( 12.63842701281683922, 39.55059781766744464, -9.846743663894590881 ) ) ;
#7718=CARTESIAN_POINT ( 'NONE',  ( 2.917880565312950480, 30.97041550158063572, -12.26659068614894821 ) ) ;
#7719=CARTESIAN_POINT ( 'NONE',  ( 18.52753015748618282, 58.92559781766745886, -4.923371831947291888 ) ) ;
#7721=CARTESIAN_POINT ( 'NONE',  ( 10.00000000000000178, 69.31368534415484817, 10.88017736071110342 ) ) ;
#7722=CARTESIAN_POINT ( 'NONE',  ( 10.00000000000000000, 0.5537488349139675359, -14.16423886937410082 ) ) ;
#7723=CARTESIAN_POINT ( 'NONE',  ( 17.20831665107776587, 47.88393115100078745, 7.208316651077764980 ) ) ;
#7724=CARTESIAN_POINT ( 'NONE',  ( 10.00000000000000000, 56.81368534415484106, -10.88017736071110342 ) ) ;
#7725=CARTESIAN_POINT ( 'NONE',  ( 5.076628168052703671, 46.84226448433412315, 8.527530157486179263 ) ) ;
#7728=CARTESIAN_POINT ( 'NONE',  ( 12.91533473730992121, 49.52201867748817676, 10.88017736071110164 ) ) ;
#7730=CARTESIAN_POINT ( 'NONE',  ( 0.8719017118913385822, 123.9374316453451144, -4.500000000000000888 ) ) ;
#7731=CARTESIAN_POINT ( 'NONE',  ( 20.88017736071110519, 25.56368534415483751, 2.639326808657452039E-16 ) ) ;
#7732=CARTESIAN_POINT ( 'NONE',  ( -1.099225684535947600, 4.540301336597087456, 6.408140936763237150 ) ) ;
#7733=CARTESIAN_POINT ( 'NONE',  ( -0.8801773607110991993, 57.85535201082149825, -2.915334737309923874 ) ) ;
#7736=CARTESIAN_POINT ( 'NONE',  ( 2.035157376598824452, 68.68868534415484817, 7.964842623401179544 ) ) ;
#7737=CARTESIAN_POINT ( 'NONE',  ( -46.48928645636213730, 103.2957187381727238, -6.397878122524045530 ) ) ;
#7738=CARTESIAN_POINT ( 'NONE',  ( 0.5774900079438590739, 42.64701867748816966, -5.440088680355550821 ) ) ;
#7739=CARTESIAN_POINT ( 'NONE',  ( 10.00000000000000000, 14.75893115100078568, -9.846743663894594434 ) ) ;
#7740=AXIS2_PLACEMENT_3D ( 'NONE', #9337, #56798, #55830 ) ;
#7741=CARTESIAN_POINT ( 'NONE',  ( 18.52753015748618282, 33.92559781766745886, -4.923371831947291888 ) ) ;
#7744=CARTESIAN_POINT ( 'NONE',  ( 1.472469842513823179, 61.42559781766745175, 4.923371831947296329 ) ) ;
#7745=CARTESIAN_POINT ( 'NONE',  ( 24.16423886937410614, 64.51208216824728936, -3.795296366450302550 ) ) ;
#7747=CARTESIAN_POINT ( 'NONE',  ( -2.266590686148945544, 26.38708216824730357, -7.082119434687050408 ) ) ;
#7748=CARTESIAN_POINT ( 'NONE',  ( 17.08211943468705840, 55.13708216824731068, -12.26659068614894466 ) ) ;
#7750=CARTESIAN_POINT ( 'NONE',  ( 12.63842701281683922, 19.55059781766745175, -9.846743663894590881 ) ) ;
#7751=CARTESIAN_POINT ( 'NONE',  ( -0.8801773607110991993, 2.855352010821504471, -2.915334737309923874 ) ) ;
#7753=CARTESIAN_POINT ( 'NONE',  ( 17.20831665107776587, 27.88393115100078390, 7.208316651077764980 ) ) ;
#7754=CARTESIAN_POINT ( 'NONE',  ( 7.084665262690076126, 22.02201867748817321, -10.88017736071110164 ) ) ;
#7755=CARTESIAN_POINT ( 'NONE',  ( 7.361572987183169658, 49.96726448433410894, -9.846743663894592657 ) ) ;
#7756=CARTESIAN_POINT ( 'NONE',  ( 13.79529636645030344, 8.262082168247300018, 14.16423886937410614 ) ) ;
#7759=CARTESIAN_POINT ( 'NONE',  ( 5.076628168052704559, 5.175597817667451750, -8.527530157486179263 ) ) ;
#7760=CARTESIAN_POINT ( 'NONE',  ( 16.40814093676324603, 37.45696800326376064, -11.09922568453594671 ) ) ;
#7761=CARTESIAN_POINT ( 'NONE',  ( 12.63842701281683922, 44.55059781766745175, -9.846743663894590881 ) ) ;
#7762=EDGE_LOOP ( 'NONE', ( #4949, #82036, #54167, #23373, #61872, #75045 ) ) ;
#7763=CARTESIAN_POINT ( 'NONE',  ( 17.20831665107776587, 27.88393115100078390, 7.208316651077764980 ) ) ;
#7765=CARTESIAN_POINT ( 'NONE',  ( -0.3689425029237898834, 56.17874883491396076, -10.36894250292378850 ) ) ;
#7766=CARTESIAN_POINT ( 'NONE',  ( 17.96484262340118221, 51.18868534415483396, -7.964842623401177768 ) ) ;
#7769=CARTESIAN_POINT ( 'NONE',  ( 0.1532563361054083140, 36.00893115100078745, 1.131784320476157264E-15 ) ) ;
#7770=CARTESIAN_POINT ( 'NONE',  ( 2.035157376598822676, 7.438685344154837509, -7.964842623401177768 ) ) ;
#7771=CARTESIAN_POINT ( 'NONE',  ( 7.361572987183170547, 37.05059781766744464, 9.846743663894590881 ) ) ;
#7773=CARTESIAN_POINT ( 'NONE',  ( 5.076628168052703671, 51.84226448433412315, 8.527530157486179263 ) ) ;
#7774=CARTESIAN_POINT ( 'NONE',  ( 20.88017736071110164, 45.35535201082149115, 2.915334737309930979 ) ) ;
#7777=ORIENTED_EDGE ( 'NONE', *, *, #25585, .F. ) ;
#7778=CARTESIAN_POINT ( 'NONE',  ( 13.43411237798105340, 60.58196800326376064, 12.81628187352647963 ) ) ;
#7779=DIRECTION ( 'NONE',  ( 0.000000000000000000, -0.000000000000000000, -1.000000000000000000 ) ) ;
#7780=CARTESIAN_POINT ( 'NONE',  ( 18.52753015748618282, 13.92559781766745175, -4.923371831947291888 ) ) ;
#7781=CARTESIAN_POINT ( 'NONE',  ( 13.43411237798105340, 55.58196800326374643, 12.81628187352647963 ) ) ;
#7782=CARTESIAN_POINT ( 'NONE',  ( 2.035157376598824452, 8.688685344154839285, 7.964842623401179544 ) ) ;
#7783=CARTESIAN_POINT ( 'NONE',  ( 19.84674366389459266, 53.71726448433411605, -2.638427012816827677 ) ) ;
#7785=CARTESIAN_POINT ( 'NONE',  ( 6.204703633549690345, 25.76208216824730712, -14.16423886937410259 ) ) ;
#7786=CARTESIAN_POINT ( 'NONE',  ( 17.08211943468705130, 58.47041550158063927, 12.26659068614894998 ) ) ;
#7787=CARTESIAN_POINT ( 'NONE',  ( 1.472469842513823179, 61.42559781766745175, 4.923371831947296329 ) ) ;
#7789=CARTESIAN_POINT ( 'NONE',  ( 12.91533473730992121, 54.52201867748816255, 10.88017736071110164 ) ) ;
#7790=CARTESIAN_POINT ( 'NONE',  ( 10.00000000000000178, 69.31368534415484817, 10.88017736071110342 ) ) ;
#7791=ORIENTED_EDGE ( 'NONE', *, *, #81606, .F. ) ;
#7792=CARTESIAN_POINT ( 'NONE',  ( 13.43411237798106583, 52.66530133659708213, -12.81628187352647252 ) ) ;
#7794=CARTESIAN_POINT ( 'NONE',  ( 18.52753015748618282, 3.925597817667451306, -4.923371831947291888 ) ) ;
#7796=CARTESIAN_POINT ( 'NONE',  ( -2.266590686148945544, 16.38708216824730357, -7.082119434687050408 ) ) ;
#7797=CARTESIAN_POINT ( 'NONE',  ( 0.1532563361054100626, 20.80059781766744464, -2.638427012816831230 ) ) ;
#7798=CARTESIAN_POINT ( 'NONE',  ( 7.084665262690076126, 27.02201867748817676, -10.88017736071110164 ) ) ;
#7801=CARTESIAN_POINT ( 'NONE',  ( 12.91533473730992121, 29.52201867748817321, 10.88017736071110164 ) ) ;
#7803=CARTESIAN_POINT ( 'NONE',  ( 15.44008868035555260, 39.73035201082150536, 9.422509992056143702 ) ) ;
#7807=CARTESIAN_POINT ( 'NONE',  ( 13.43411237798105340, 20.58196800326374643, 12.81628187352647963 ) ) ;
#7809=( BOUNDED_SURFACE ( )  B_SPLINE_SURFACE ( 3, 2, ( 
 ( #35201, #49714, #57221 ),
 ( #58194, #56262, #65208 ),
 ( #42241, #80224, #26726 ),
 ( #56737, #50210, #42725 ) ),
 .UNSPECIFIED., .F., .F., .F. ) 
 B_SPLINE_SURFACE_WITH_KNOTS ( ( 4, 4 ),
 ( 3, 3 ),
 ( 2.168404344971008868E-19, 0.0006068291151710755033 ),
 ( 0.000000000000000000, 1.000000000000000000 ),
 .UNSPECIFIED. ) 
 GEOMETRIC_REPRESENTATION_ITEM ( )  RATIONAL_B_SPLINE_SURFACE ( (
 ( 1.000000000000000000, 0.8188293140827536121, 1.000000000000000000),
 ( 1.000000000000000000, 0.8260591074388915489, 1.000000000000000000),
 ( 1.000000000000000000, 0.8336435218269933056, 1.000000000000000000),
 ( 1.000000000000000000, 0.8414823709351006986, 1.000000000000000000) ) ) 
 REPRESENTATION_ITEM ( '' )  SURFACE ( )  );
#7810=CARTESIAN_POINT ( 'NONE',  ( 5.076628168052704559, 10.17559781766745175, -8.527530157486179263 ) ) ;
#7812=EDGE_CURVE ( 'NONE', #25175, #10365, #82848, .T. ) ;
#7814=CARTESIAN_POINT ( 'NONE',  ( 14.92337183194729988, 19.34226448433411960, -8.527530157486177487 ) ) ;
#7815=CARTESIAN_POINT ( 'NONE',  ( 20.88017736071110875, 35.77201867748816966, -2.915334737309920765 ) ) ;
#7819=CARTESIAN_POINT ( 'NONE',  ( 19.42250999205614548, 50.98035201082151247, -5.440088680355545492 ) ) ;
#7821=CARTESIAN_POINT ( 'NONE',  ( -2.816281873526473856, 59.33196800326374643, 3.434112377981055619 ) ) ;
#7822=CARTESIAN_POINT ( 'NONE',  ( 17.96484262340118221, 56.18868534415484817, -7.964842623401177768 ) ) ;
#7824=CARTESIAN_POINT ( 'NONE',  ( 19.38216949554541557, 2.248634669930420049, -9.382169495545420901 ) ) ;
#7826=CARTESIAN_POINT ( 'NONE',  ( 7.361572987183170547, 37.05059781766744464, 9.846743663894590881 ) ) ;
#7827=CARTESIAN_POINT ( 'NONE',  ( -1.099225684535947600, 53.70696800326376064, -6.408140936763238038 ) ) ;
#7828=CARTESIAN_POINT ( 'NONE',  ( 20.15039907845753220, 37.62777174578614847, -6.262539305110077947 ) ) ;
#7829=CARTESIAN_POINT ( 'NONE',  ( 19.84674366389459266, 3.300597817667451750, 2.638427012816836559 ) ) ;
#7830=CARTESIAN_POINT ( 'NONE',  ( 3.591859063236763294, 18.29030133659708568, -11.09922568453595026 ) ) ;
#7833=CARTESIAN_POINT ( 'NONE',  ( 10.00000000000000000, 31.81368534415483751, -10.88017736071110342 ) ) ;
#7834=CARTESIAN_POINT ( 'NONE',  ( 14.92337183194729633, 57.67559781766745886, 8.527530157486181039 ) ) ;
#7836=CARTESIAN_POINT ( 'NONE',  ( 5.076628168052703671, 6.842264484334118713, 8.527530157486179263 ) ) ;
#7837=CARTESIAN_POINT ( 'NONE',  ( 2.035157376598824452, 18.68868534415484106, 7.964842623401179544 ) ) ;
#7838=CARTESIAN_POINT ( 'NONE',  ( 0.6178305044545838731, 14.74863466993041783, 9.382169495545420901 ) ) ;
#7839=STYLED_ITEM ( 'NONE', ( #31868 ), #71516 ) ;
#7840=( NAMED_UNIT ( * ) SI_UNIT ( $, .STERADIAN. ) SOLID_ANGLE_UNIT ( ) );
#7843=CARTESIAN_POINT ( 'NONE',  ( 20.88017736071110519, 10.56368534415483929, 2.639326808657452039E-16 ) ) ;
#7844=CARTESIAN_POINT ( 'NONE',  ( 12.63842701281683922, 44.55059781766745175, -9.846743663894590881 ) ) ;
#7846=CARTESIAN_POINT ( 'NONE',  ( 15.44008868035555260, 4.730352010821505360, 9.422509992056143702 ) ) ;
#7848=CARTESIAN_POINT ( 'NONE',  ( 7.084665262690076126, 34.10535201082151247, 10.88017736071109987 ) ) ;
#7849=CARTESIAN_POINT ( 'NONE',  ( 13.79529636645030344, 63.26208216824730357, 14.16423886937410614 ) ) ;
#7851=CARTESIAN_POINT ( 'NONE',  ( 5.076628168052703671, 21.84226448433411960, 8.527530157486179263 ) ) ;
#7852=CARTESIAN_POINT ( 'NONE',  ( 13.43411237798105340, 10.58196800326375353, 12.81628187352647963 ) ) ;
#7855=CARTESIAN_POINT ( 'NONE',  ( 17.20831665107776587, 64.13393115100079456, -7.208316651077762316 ) ) ;
#7858=EDGE_CURVE ( 'NONE', #16435, #9403, #52194, .T. ) ;
#7860=CARTESIAN_POINT ( 'NONE',  ( -2.266590686148945544, 16.38708216824730357, -7.082119434687050408 ) ) ;
#7861=CARTESIAN_POINT ( 'NONE',  ( 0.1532563361054083140, 21.00893115100078745, 1.131784320476157264E-15 ) ) ;
#7862=LINE ( 'NONE', #44848, #80011 ) ;
#7864=CARTESIAN_POINT ( 'NONE',  ( 22.26659068614895176, 49.72041550158063927, -7.082119434687042414 ) ) ;
#7865=CARTESIAN_POINT ( 'NONE',  ( 17.20831665107776587, 7.883931151000784787, 7.208316651077764980 ) ) ;
#7868=CARTESIAN_POINT ( 'NONE',  ( 7.084665262690076126, 39.10535201082150536, 10.88017736071109987 ) ) ;
#7869=CARTESIAN_POINT ( 'NONE',  ( 21.09922568453594849, 46.20696800326376064, 6.408140936763242479 ) ) ;
#7870=CARTESIAN_POINT ( 'NONE',  ( -0.8801773607111008646, 13.27201867748817143, 2.915334737309923430 ) ) ;
#7871=CARTESIAN_POINT ( 'NONE',  ( 6.565887622018943937, 45.16530133659708923, 12.81628187352647430 ) ) ;
#7872=CARTESIAN_POINT ( 'NONE',  ( 2.791683348922237240, 65.38393115100078035, -7.208316651077763204 ) ) ;
#7873=CARTESIAN_POINT ( 'NONE',  ( 0.1532563361054082862, 1.217264484334117824, 2.638427012816831674 ) ) ;
#7877=CARTESIAN_POINT ( 'NONE',  ( 24.16423886937410614, 44.51208216824730357, -3.795296366450302550 ) ) ;
#7878=CARTESIAN_POINT ( 'NONE',  ( -2.266590686148945544, 11.38708216824730179, -7.082119434687050408 ) ) ;
#7879=CARTESIAN_POINT ( 'NONE',  ( 0.5774900079438590739, 7.647018677488171434, -5.440088680355550821 ) ) ;
#7880=CARTESIAN_POINT ( 'NONE',  ( 0.5774900079438607392, 38.48035201082150536, 5.440088680355550821 ) ) ;
#7884=CARTESIAN_POINT ( 'NONE',  ( -0.8801773607111008646, 63.27201867748817676, 2.915334737309923430 ) ) ;
#7886=CARTESIAN_POINT ( 'NONE',  ( 16.40814093676323893, 30.79030133659708923, 11.09922568453595026 ) ) ;
#7889=CARTESIAN_POINT ( 'NONE',  ( 19.84674366389459266, 38.71726448433412315, -2.638427012816827677 ) ) ;
#7890=CARTESIAN_POINT ( 'NONE',  ( 10.00000000000000000, 16.81368534415483751, -10.88017736071110342 ) ) ;
#7891=CARTESIAN_POINT ( 'NONE',  ( -1.099225684535947600, 14.54030133659708568, 6.408140936763237150 ) ) ;
#7892=CARTESIAN_POINT ( 'NONE',  ( 10.00000000000000000, 4.758931151000784787, -9.846743663894594434 ) ) ;
#7893=CARTESIAN_POINT ( 'NONE',  ( -0.8801773607110991993, 12.85535201082150358, -2.915334737309923874 ) ) ;
#7894=CARTESIAN_POINT ( 'NONE',  ( 7.361572987183169658, 34.96726448433411605, -9.846743663894592657 ) ) ;
#7895=CARTESIAN_POINT ( 'NONE',  ( 16.40814093676324603, 62.45696800326376064, -11.09922568453594671 ) ) ;
#7896=CARTESIAN_POINT ( 'NONE',  ( 19.84674366389459621, 23.50893115100078390, 7.409399052514197653E-17 ) ) ;
#7897=CARTESIAN_POINT ( 'NONE',  ( 13.79529636645030344, 8.262082168247300018, 14.16423886937410614 ) ) ;
#7899=CARTESIAN_POINT ( 'NONE',  ( 0.5774900079438607392, 28.48035201082150891, 5.440088680355550821 ) ) ;
#7900=CARTESIAN_POINT ( 'NONE',  ( 19.42250999205614548, 5.980352010821504471, -5.440088680355545492 ) ) ;
#7901=CARTESIAN_POINT ( 'NONE',  ( 24.16423886937410614, 39.51208216824731068, -3.795296366450302550 ) ) ;
#7902=CARTESIAN_POINT ( 'NONE',  ( 4.559911319644449179, 33.89701867748817676, 9.422509992056141925 ) ) ;
#7904=CARTESIAN_POINT ( 'NONE',  ( 20.88017736071110875, 10.77201867748817143, -2.915334737309920765 ) ) ;
#7905=ORIENTED_EDGE ( 'NONE', *, *, #68674, .T. ) ;
#7906=CARTESIAN_POINT ( 'NONE',  ( 20.88017736071110875, 45.77201867748816966, -2.915334737309920765 ) ) ;
#7907=EDGE_CURVE ( 'NONE', #13653, #26237, #78196, .T. ) ;
#7908=CARTESIAN_POINT ( 'NONE',  ( 0.6178305044545818747, 53.49863466993041072, -9.382169495545419124 ) ) ;
#7909=CARTESIAN_POINT ( 'NONE',  ( 12.91533473730993009, 46.60535201082150536, -10.88017736071109987 ) ) ;
#7910=CARTESIAN_POINT ( 'NONE',  ( 19.42250999205614548, 55.98035201082150536, -5.440088680355545492 ) ) ;
#7912=CARTESIAN_POINT ( 'NONE',  ( 19.42250999205614193, 50.14701867748817676, 5.440088680355555262 ) ) ;
#7914=CARTESIAN_POINT ( 'NONE',  ( -0.1503990784575260087, 24.24884699246888786, -6.262539305110081500 ) ) ;
#7915=CARTESIAN_POINT ( 'NONE',  ( 17.08211943468705840, 50.13708216824730357, -12.26659068614894466 ) ) ;
#7916=CARTESIAN_POINT ( 'NONE',  ( 0.1532563361054082862, 1.217264484334117824, 2.638427012816831674 ) ) ;
#7919=CARTESIAN_POINT ( 'NONE',  ( 12.63842701281683922, 59.55059781766744464, -9.846743663894590881 ) ) ;
#7920=( LENGTH_UNIT ( ) NAMED_UNIT ( * ) SI_UNIT ( .MILLI., .METRE. ) );
#7921=CARTESIAN_POINT ( 'NONE',  ( 19.84674366389459266, 33.71726448433410894, -2.638427012816827677 ) ) ;
#7922=ORIENTED_EDGE ( 'NONE', *, *, #2450, .T. ) ;
#7923=CARTESIAN_POINT ( 'NONE',  ( 2.791683348922237240, 35.38393115100079456, -7.208316651077763204 ) ) ;
#7925=CARTESIAN_POINT ( 'NONE',  ( -0.8801773607111009756, 43.06368534415484106, 1.068504757029289695E-15 ) ) ;
#7926=CARTESIAN_POINT ( 'NONE',  ( 2.791683348922240793, 31.63393115100078745, 7.208316651077764092 ) ) ;
#7927=CARTESIAN_POINT ( 'NONE',  ( 3.591859063236761518, 24.95696800326375353, 11.09922568453594849 ) ) ;
#7928=CARTESIAN_POINT ( 'NONE',  ( 10.00000000000000178, 70.00000000000000000, 0.000000000000000000 ) ) ;
#7929=CARTESIAN_POINT ( 'NONE',  ( 19.42250999205614193, 55.14701867748817676, 5.440088680355555262 ) ) ;
#7930=CARTESIAN_POINT ( 'NONE',  ( 17.96484262340118221, 44.93868534415483396, 7.964842623401181321 ) ) ;
#7931=( LENGTH_UNIT ( ) NAMED_UNIT ( * ) SI_UNIT ( .MILLI., .METRE. ) );
#7932=CARTESIAN_POINT ( 'NONE',  ( 20.36894250292379382, 58.67874883491396076, 10.36894250292379205 ) ) ;
#7933=EDGE_CURVE ( 'NONE', #87224, #2388, #51928, .T. ) ;
#7934=CARTESIAN_POINT ( 'NONE',  ( 16.40814093676324603, 17.45696800326375353, -11.09922568453594671 ) ) ;
#7935=LINE ( 'NONE', #8417, #91441 ) ;
#7937=CARTESIAN_POINT ( 'NONE',  ( 19.38216949554541557, 12.24863466993041961, -9.382169495545420901 ) ) ;
#7938=CARTESIAN_POINT ( 'NONE',  ( 19.42250999205614193, 15.14701867748817143, 5.440088680355555262 ) ) ;
#7940=CARTESIAN_POINT ( 'NONE',  ( 7.084665262690076126, 54.10535201082151247, 10.88017736071109987 ) ) ;
#7941=ORIENTED_EDGE ( 'NONE', *, *, #92769, .T. ) ;
#7943=CARTESIAN_POINT ( 'NONE',  ( 0.1532563361054083140, 1.008931151000784787, 1.131784320476157264E-15 ) ) ;
#7944=CARTESIAN_POINT ( 'NONE',  ( 1.472469842513823179, 55.59226448433412315, -4.923371831947296329 ) ) ;
#7945=CARTESIAN_POINT ( 'NONE',  ( 14.92337183194729988, 44.34226448433412315, -8.527530157486177487 ) ) ;
#7946=CARTESIAN_POINT ( 'NONE',  ( 0.1532563361054082862, 31.21726448433412315, 2.638427012816831674 ) ) ;
#7950=CARTESIAN_POINT ( 'NONE',  ( -1.099225684535947600, 34.54030133659708923, 6.408140936763237150 ) ) ;
#7951=CARTESIAN_POINT ( 'NONE',  ( 2.791683348922237240, 20.38393115100078745, -7.208316651077763204 ) ) ;
#7953=CARTESIAN_POINT ( 'NONE',  ( 21.92686044187657046, 45.16212336850780673, 4.562052436263912550E-16 ) ) ;
#7954=CARTESIAN_POINT ( 'NONE',  ( 14.92337183194729988, 44.34226448433412315, -8.527530157486177487 ) ) ;
#7955=ORIENTED_EDGE ( 'NONE', *, *, #51347, .F. ) ;
#7957=CARTESIAN_POINT ( 'NONE',  ( 16.40814093676323893, 15.79030133659708746, 11.09922568453595026 ) ) ;
#7959=CARTESIAN_POINT ( 'NONE',  ( 10.00000000000000000, 51.81368534415484106, -10.88017736071110342 ) ) ;
#7960=CARTESIAN_POINT ( 'NONE',  ( -4.164238869374099927, 27.01208216824730357, 3.795296366450308767 ) ) ;
#7961=CARTESIAN_POINT ( 'NONE',  ( 1.602071938427519049, 42.02224192338641018, -6.500000000000035527 ) ) ;
#7962=CARTESIAN_POINT ( 'NONE',  ( 17.08211943468705840, 30.13708216824730357, -12.26659068614894466 ) ) ;
#7963=ADVANCED_FACE ( 'NONE', ( #16556 ), #86656, .T. ) ;
#7964=CARTESIAN_POINT ( 'NONE',  ( 6.204703633549690345, 55.76208216824730357, -14.16423886937410259 ) ) ;
#7965=CARTESIAN_POINT ( 'NONE',  ( 13.79529636645030344, 8.262082168247300018, 14.16423886937410614 ) ) ;
#7966=CARTESIAN_POINT ( 'NONE',  ( 10.00000000000000000, 30.55374883491397142, -14.16423886937410082 ) ) ;
#7968=CARTESIAN_POINT ( 'NONE',  ( 15.44008868035555793, 56.39701867748817676, -9.422509992056140149 ) ) ;
#7969=CARTESIAN_POINT ( 'NONE',  ( 19.89220837332776526, 24.74062864464239553, 6.478736007405958119 ) ) ;
#7971=CARTESIAN_POINT ( 'NONE',  ( 17.20831665107776587, 49.13393115100078745, -7.208316651077762316 ) ) ;
#7972=CARTESIAN_POINT ( 'NONE',  ( 15.44008868035555793, 21.39701867748817321, -9.422509992056140149 ) ) ;
#7974=CARTESIAN_POINT ( 'NONE',  ( 5.076628168052703671, 61.84226448433412315, 8.527530157486179263 ) ) ;
#7976=CARTESIAN_POINT ( 'NONE',  ( 0.1532563361054083140, 31.00893115100078390, 1.131784320476157264E-15 ) ) ;
#7977=CARTESIAN_POINT ( 'NONE',  ( 13.43411237798105340, 50.58196800326375353, 12.81628187352647963 ) ) ;
#7979=CARTESIAN_POINT ( 'NONE',  ( 14.92337183194729988, 44.34226448433412315, -8.527530157486177487 ) ) ;
#7980=CARTESIAN_POINT ( 'NONE',  ( 0.1532563361054083140, 56.00893115100078745, 1.131784320476157264E-15 ) ) ;
#7981=CARTESIAN_POINT ( 'NONE',  ( 20.36894250292379738, 34.92874883491396076, -10.36894250292379027 ) ) ;
#7983=CARTESIAN_POINT ( 'NONE',  ( 17.08211943468705130, 8.470415501580635720, 12.26659068614894998 ) ) ;
#7984=CARTESIAN_POINT ( 'NONE',  ( 7.084665262690076126, 64.10535201082150536, 10.88017736071109987 ) ) ;
#7986=CARTESIAN_POINT ( 'NONE',  ( -4.164238869374099039, 56.80374883491397497, 8.674139862899312516E-16 ) ) ;
#7987=CARTESIAN_POINT ( 'NONE',  ( 16.40814093676324603, 17.45696800326375353, -11.09922568453594671 ) ) ;
#7989=CARTESIAN_POINT ( 'NONE',  ( 17.20831665107776587, 2.883931151000785231, 7.208316651077764980 ) ) ;
#7992=CARTESIAN_POINT ( 'NONE',  ( 13.79529636645031943, 60.34541550158063927, -14.16423886937409904 ) ) ;
#7994=CARTESIAN_POINT ( 'NONE',  ( 20.88017736071110875, 25.77201867748816966, -2.915334737309920765 ) ) ;
#7995=CARTESIAN_POINT ( 'NONE',  ( -0.8801773607111008646, 28.27201867748817321, 2.915334737309923430 ) ) ;
#7996=CARTESIAN_POINT ( 'NONE',  ( 10.00000000000000178, 57.25893115100078745, 9.846743663894594434 ) ) ;
#7997=CARTESIAN_POINT ( 'NONE',  ( 10.00000000000000000, 59.75893115100078745, -9.846743663894594434 ) ) ;
#7998=CARTESIAN_POINT ( 'NONE',  ( 21.09922568453594849, 51.20696800326375353, 6.408140936763242479 ) ) ;
#7999=VECTOR ( 'NONE', #78259, 1000.000000000000000 ) ;
#8002=CARTESIAN_POINT ( 'NONE',  ( -0.8801773607111008646, 18.27201867748817321, 2.915334737309923430 ) ) ;
#8003=CARTESIAN_POINT ( 'NONE',  ( 16.40814093676323893, 25.79030133659708923, 11.09922568453595026 ) ) ;
#8005=CARTESIAN_POINT ( 'NONE',  ( 12.63842701281683034, 42.46726448433412315, 9.846743663894596210 ) ) ;
#8006=CARTESIAN_POINT ( 'NONE',  ( -0.8801773607110991993, 47.85535201082150536, -2.915334737309923874 ) ) ;
#8007=CARTESIAN_POINT ( 'NONE',  ( 10.00000000000000178, 20.37363466993042138, 12.81628187352647608 ) ) ;
#8008=CARTESIAN_POINT ( 'NONE',  ( 10.00000000000000000, 51.81368534415484106, -10.88017736071110342 ) ) ;
#8010=DIRECTION ( 'NONE',  ( 0.000000000000000000, -1.000000000000000000, 0.000000000000000000 ) ) ;
#8011=CARTESIAN_POINT ( 'NONE',  ( 10.00000000000000178, 45.37363466993041783, 12.81628187352647608 ) ) ;
#8013=CARTESIAN_POINT ( 'NONE',  ( 7.361572987183170547, 57.05059781766744464, 9.846743663894590881 ) ) ;
#8015=CARTESIAN_POINT ( 'NONE',  ( 10.00000000000000178, 54.31368534415484106, 10.88017736071110342 ) ) ;
#8016=CARTESIAN_POINT ( 'NONE',  ( 10.00000000000000178, 45.37363466993041783, 12.81628187352647608 ) ) ;
#8017=CARTESIAN_POINT ( 'NONE',  ( 24.16423886937410614, 19.51208216824729647, -3.795296366450302550 ) ) ;
#8018=CARTESIAN_POINT ( 'NONE',  ( 1.472469842513823179, 10.59226448433411782, -4.923371831947296329 ) ) ;
#8019=DIRECTION ( 'NONE',  ( 0.000000000000000000, -1.000000000000000000, 0.000000000000000000 ) ) ;
#8020=CARTESIAN_POINT ( 'NONE',  ( 19.84674366389459621, 28.50893115100078745, 7.409399052514197653E-17 ) ) ;
#8021=CARTESIAN_POINT ( 'NONE',  ( 14.92337183194729988, 9.342264484334119601, -8.527530157486177487 ) ) ;
#8022=CARTESIAN_POINT ( 'NONE',  ( -42.16485527613927076, 107.5383484153110061, 5.000000000000000000 ) ) ;
#8023=CARTESIAN_POINT ( 'NONE',  ( -2.266590686148945544, 46.38708216824730357, -7.082119434687050408 ) ) ;
#8026=CARTESIAN_POINT ( 'NONE',  ( 20.88017736071110875, 10.77201867748817143, -2.915334737309920765 ) ) ;
#8029=CARTESIAN_POINT ( 'NONE',  ( 19.42250999205614193, 15.14701867748817143, 5.440088680355555262 ) ) ;
#8030=CARTESIAN_POINT ( 'NONE',  ( 2.035157376598822676, 7.438685344154837509, -7.964842623401177768 ) ) ;
#8031=CARTESIAN_POINT ( 'NONE',  ( 7.361572987183169658, 39.96726448433411605, -9.846743663894592657 ) ) ;
#8032=CARTESIAN_POINT ( 'NONE',  ( 10.00000000000000000, 37.87363466993041783, -12.81628187352647608 ) ) ;
#8034=CARTESIAN_POINT ( 'NONE',  ( 1.274849032794199255, 23.57228050351030646, 6.499999999999850786 ) ) ;
#8035=CARTESIAN_POINT ( 'NONE',  ( 13.79529636645031943, 5.345415501580634832, -14.16423886937409904 ) ) ;
#8036=CARTESIAN_POINT ( 'NONE',  ( 17.96484262340118221, 29.93868534415484106, 7.964842623401181321 ) ) ;
#8037=CARTESIAN_POINT ( 'NONE',  ( -0.3689425029237898834, 66.17874883491396076, -10.36894250292378850 ) ) ;
#8038=CARTESIAN_POINT ( 'NONE',  ( 19.84674366389459266, 43.71726448433410894, -2.638427012816827677 ) ) ;
#8039=DIRECTION ( 'NONE',  ( 1.000000000000000000, -0.000000000000000000, -0.000000000000000000 ) ) ;
#8040=CARTESIAN_POINT ( 'NONE',  ( 2.791683348922240793, 26.63393115100078745, 7.208316651077764092 ) ) ;
#8041=FILL_AREA_STYLE_COLOUR ( '', #84950 ) ;
#8047=CARTESIAN_POINT ( 'NONE',  ( 10.00000000000000178, 34.31368534415484106, 10.88017736071110342 ) ) ;
#8048=CARTESIAN_POINT ( 'NONE',  ( 20.88017736071110519, 40.56368534415484106, 2.639326808657452039E-16 ) ) ;
#8049=CARTESIAN_POINT ( 'NONE',  ( 7.084665262690076126, 2.022018677488170990, -10.88017736071110164 ) ) ;
#8050=CARTESIAN_POINT ( 'NONE',  ( 21.09922568453595559, 32.04030133659708923, -6.408140936763230044 ) ) ;
#8051=CARTESIAN_POINT ( 'NONE',  ( 24.16423886937410614, 19.51208216824729647, -3.795296366450302550 ) ) ;
#8053=EDGE_CURVE ( 'NONE', #68797, #97455, #34947, .T. ) ;
#8054=CARTESIAN_POINT ( 'NONE',  ( 19.38216949554541557, 42.24863466993041783, -9.382169495545420901 ) ) ;
#8056=CARTESIAN_POINT ( 'NONE',  ( 0.1532563361054100626, 50.80059781766745175, -2.638427012816831230 ) ) ;
#8057=EDGE_CURVE ( 'NONE', #25434, #98109, #45062, .T. ) ;
#8058=CARTESIAN_POINT ( 'NONE',  ( 17.96484262340118221, 24.93868534415484461, 7.964842623401181321 ) ) ;
#8061=CARTESIAN_POINT ( 'NONE',  ( 2.035157376598822676, 22.43868534415483396, -7.964842623401177768 ) ) ;
#8063=CARTESIAN_POINT ( 'NONE',  ( 10.00000000000000000, 56.81368534415484106, -10.88017736071110342 ) ) ;
#8065=CARTESIAN_POINT ( 'NONE',  ( 12.91533473730993009, 61.60535201082150536, -10.88017736071109987 ) ) ;
#8066=CARTESIAN_POINT ( 'NONE',  ( 1.472469842513823179, 0.5922644843341181575, -4.923371831947296329 ) ) ;
#8067=CARTESIAN_POINT ( 'NONE',  ( 19.42250999205614193, 55.14701867748817676, 5.440088680355555262 ) ) ;
#8068=CARTESIAN_POINT ( 'NONE',  ( -46.94000000000000483, 101.1610691152320953, 7.882642855612810528 ) ) ;
#8069=CARTESIAN_POINT ( 'NONE',  ( 1.472469842513823179, 10.59226448433411782, -4.923371831947296329 ) ) ;
#8070=FACE_OUTER_BOUND ( 'NONE', #91251, .T. ) ;
#8071=ORIENTED_EDGE ( 'NONE', *, *, #891, .T. ) ;
#8072=CARTESIAN_POINT ( 'NONE',  ( 19.84674366389459621, 43.50893115100078745, 7.409399052514197653E-17 ) ) ;
#8074=CARTESIAN_POINT ( 'NONE',  ( 5.076628168052703671, 66.84226448433412315, 8.527530157486179263 ) ) ;
#8075=CARTESIAN_POINT ( 'NONE',  ( 17.08211943468705840, 15.13708216824730179, -12.26659068614894466 ) ) ;
#8076=VERTEX_POINT ( 'NONE', #63989 ) ;
#8078=CARTESIAN_POINT ( 'NONE',  ( 19.80832241502127289, 29.75868815902069997, 6.499999999999991118 ) ) ;
#8079=CARTESIAN_POINT ( 'NONE',  ( 19.72487221294570858, 9.782175860852373006, 6.500000000000000000 ) ) ;
#8080=CARTESIAN_POINT ( 'NONE',  ( 7.084665262690076126, 59.10535201082150536, 10.88017736071109987 ) ) ;
#8081=CARTESIAN_POINT ( 'NONE',  ( -0.8801773607110991993, 7.855352010821506248, -2.915334737309923874 ) ) ;
#8083=CARTESIAN_POINT ( 'NONE',  ( 6.565887622018943937, 40.16530133659708923, 12.81628187352647430 ) ) ;
#8085=CARTESIAN_POINT ( 'NONE',  ( 14.92337183194729633, 2.675597817667451750, 8.527530157486181039 ) ) ;
#8086=( NAMED_UNIT ( * ) PLANE_ANGLE_UNIT ( ) SI_UNIT ( $, .RADIAN. ) );
#8087=CARTESIAN_POINT ( 'NONE',  ( 3.591859063236763294, 33.29030133659708213, -11.09922568453595026 ) ) ;
#8088=CARTESIAN_POINT ( 'NONE',  ( 5.076628168052704559, 20.17559781766745175, -8.527530157486179263 ) ) ;
#8091=CARTESIAN_POINT ( 'NONE',  ( -2.816281873526473856, 19.33196800326375708, 3.434112377981055619 ) ) ;
#8094=CARTESIAN_POINT ( 'NONE',  ( 1.472469842513823179, 6.425597817667451750, 4.923371831947296329 ) ) ;
#8097=CARTESIAN_POINT ( 'NONE',  ( 10.00000000000000000, 16.81368534415483751, -10.88017736071110342 ) ) ;
#8098=CARTESIAN_POINT ( 'NONE',  ( 10.00000000000000178, 13.05374883491396787, 14.16423886937410082 ) ) ;
#8099=CARTESIAN_POINT ( 'NONE',  ( 2.791683348922237240, 35.38393115100079456, -7.208316651077763204 ) ) ;
#8100=CARTESIAN_POINT ( 'NONE',  ( 2.035157376598824452, 68.68868534415484817, 7.964842623401179544 ) ) ;
#8101=CARTESIAN_POINT ( 'NONE',  ( 10.00000000000000178, 45.37363466993041783, 12.81628187352647608 ) ) ;
#8103=CARTESIAN_POINT ( 'NONE',  ( 2.035157376598822676, 12.43868534415483751, -7.964842623401177768 ) ) ;
#8105=CARTESIAN_POINT ( 'NONE',  ( -2.816281873526473856, 14.33196800326375531, 3.434112377981055619 ) ) ;
#8106=CARTESIAN_POINT ( 'NONE',  ( 13.43411237798106583, 7.665301336597086568, -12.81628187352647252 ) ) ;
#8107=CARTESIAN_POINT ( 'NONE',  ( 14.92337183194729633, 22.67559781766745175, 8.527530157486181039 ) ) ;
#8109=CARTESIAN_POINT ( 'NONE',  ( -2.816281873526473856, 29.33196800326376064, 3.434112377981055619 ) ) ;
#8111=CARTESIAN_POINT ( 'NONE',  ( 7.084665262690076126, 59.10535201082150536, 10.88017736071109987 ) ) ;
#8114=CARTESIAN_POINT ( 'NONE',  ( 7.084665262690076126, 69.10535201082151957, 10.88017736071109987 ) ) ;
#8115=CARTESIAN_POINT ( 'NONE',  ( 4.559911319644449179, 43.89701867748816966, 9.422509992056141925 ) ) ;
#8117=CARTESIAN_POINT ( 'NONE',  ( 20.88017736071110164, 40.35535201082150536, 2.915334737309930979 ) ) ;
#8118=CARTESIAN_POINT ( 'NONE',  ( 20.15039907845753220, 56.74884699246889141, 6.262539305110074395 ) ) ;
#8120=CARTESIAN_POINT ( 'NONE',  ( 2.791683348922237240, 50.38393115100078035, -7.208316651077763204 ) ) ;
#8121=CARTESIAN_POINT ( 'NONE',  ( 7.084665262690076126, 7.022018677488169658, -10.88017736071110164 ) ) ;
#8124=CARTESIAN_POINT ( 'NONE',  ( 16.40814093676324603, 7.456968003263754419, -11.09922568453594671 ) ) ;
#8126=CARTESIAN_POINT ( 'NONE',  ( 20.88017736071110164, 35.35535201082150536, 2.915334737309930979 ) ) ;
#8127=CARTESIAN_POINT ( 'NONE',  ( 0.6178305044545818747, 3.498634669930420049, -9.382169495545419124 ) ) ;
#8128=CARTESIAN_POINT ( 'NONE',  ( -20.19000000000001194, 92.00000000000000000, -10.09898361729590199 ) ) ;
#8129=CARTESIAN_POINT ( 'NONE',  ( -0.8801773607110991993, 12.85535201082150358, -2.915334737309923874 ) ) ;
#8131=CARTESIAN_POINT ( 'NONE',  ( 19.42250999205614548, 30.98035201082150536, -5.440088680355545492 ) ) ;
#8132=CARTESIAN_POINT ( 'NONE',  ( 17.08211943468705840, 35.13708216824730357, -12.26659068614894466 ) ) ;
#8133=CARTESIAN_POINT ( 'NONE',  ( 19.84674366389459621, 33.50893115100078745, 7.409399052514197653E-17 ) ) ;
#8134=CARTESIAN_POINT ( 'NONE',  ( 20.88017736071110164, 45.35535201082149115, 2.915334737309930979 ) ) ;
#8136=CARTESIAN_POINT ( 'NONE',  ( 2.917880565312950480, 5.970415501580634832, -12.26659068614894821 ) ) ;
#8140=CARTESIAN_POINT ( 'NONE',  ( 19.84674366389459266, 63.71726448433412315, -2.638427012816827677 ) ) ;
#8142=ORIENTED_EDGE ( 'NONE', *, *, #52894, .T. ) ;
#8143=CARTESIAN_POINT ( 'NONE',  ( 10.00000000000000178, 33.05374883491396787, 14.16423886937410082 ) ) ;
#8144=CARTESIAN_POINT ( 'NONE',  ( 10.00000000000000178, 18.05374883491396787, 14.16423886937410082 ) ) ;
#8145=CARTESIAN_POINT ( 'NONE',  ( 18.52753015748617571, 3.092264484334118269, 4.923371831947298993 ) ) ;
#8146=CARTESIAN_POINT ( 'NONE',  ( 17.20831665107776587, 62.88393115100078745, 7.208316651077764980 ) ) ;
#8148=CARTESIAN_POINT ( 'NONE',  ( 0.5774900079438607392, 63.48035201082149825, 5.440088680355550821 ) ) ;
#8149=CARTESIAN_POINT ( 'NONE',  ( 13.43411237798105340, 15.58196800326374998, 12.81628187352647963 ) ) ;
#8150=CARTESIAN_POINT ( 'NONE',  ( -2.266590686148945544, 27.22041550158063572, 7.082119434687048631 ) ) ;
#8151=CARTESIAN_POINT ( 'NONE',  ( 2.035157376598822676, 17.43868534415483751, -7.964842623401177768 ) ) ;
#8152=CARTESIAN_POINT ( 'NONE',  ( 20.88017736071110164, 35.35535201082150536, 2.915334737309930979 ) ) ;
#8153=LINE ( 'NONE', #15665, #1303 ) ;
#8154=CARTESIAN_POINT ( 'NONE',  ( 17.96484262340118221, 56.18868534415484817, -7.964842623401177768 ) ) ;
#8155=CARTESIAN_POINT ( 'NONE',  ( 13.43411237798106583, 52.66530133659708213, -12.81628187352647252 ) ) ;
#8157=EDGE_LOOP ( 'NONE', ( #43861, #13677, #27585, #4220, #97678, #42682 ) ) ;
#8158=FILL_AREA_STYLE_COLOUR ( '', #93820 ) ;
#8164=CARTESIAN_POINT ( 'NONE',  ( 13.79529636645031943, 55.34541550158062506, -14.16423886937409904 ) ) ;
#8165=CARTESIAN_POINT ( 'NONE',  ( 10.00000000000000000, 65.55374883491396076, -14.16423886937410082 ) ) ;
#8166=CARTESIAN_POINT ( 'NONE',  ( 19.84674366389459266, 18.30059781766745175, 2.638427012816836559 ) ) ;
#8167=CARTESIAN_POINT ( 'NONE',  ( 1.472469842513823179, 55.59226448433412315, -4.923371831947296329 ) ) ;
#8169=STYLED_ITEM ( 'NONE', ( #35882 ), #80046 ) ;
#8171=CARTESIAN_POINT ( 'NONE',  ( -2.816281873526473856, -0.8763653300695799508, 9.499525473075851096E-16 ) ) ;
#8173=ORIENTED_EDGE ( 'NONE', *, *, #29529, .F. ) ;
#8174=CARTESIAN_POINT ( 'NONE',  ( 17.08211943468705130, 28.47041550158063572, 12.26659068614894998 ) ) ;
#8176=CARTESIAN_POINT ( 'NONE',  ( 22.26659068614895176, 39.72041550158063217, -7.082119434687042414 ) ) ;
#8177=ORIENTED_EDGE ( 'NONE', *, *, #62796, .F. ) ;
#8178=CARTESIAN_POINT ( 'NONE',  ( -1.099225684535947600, 54.54030133659708923, 6.408140936763237150 ) ) ;
#8179=CARTESIAN_POINT ( 'NONE',  ( 19.84674366389459266, 48.30059781766745175, 2.638427012816836559 ) ) ;
#8180=CARTESIAN_POINT ( 'NONE',  ( 2.035157376598822676, 22.43868534415483396, -7.964842623401177768 ) ) ;
#8182=CARTESIAN_POINT ( 'NONE',  ( 12.63842701281683034, 52.46726448433413026, 9.846743663894596210 ) ) ;
#8183=CARTESIAN_POINT ( 'NONE',  ( 7.361572987183170547, 47.05059781766745175, 9.846743663894590881 ) ) ;
#8184=STYLED_ITEM ( 'NONE', ( #77535 ), #33405 ) ;
#8188=CARTESIAN_POINT ( 'NONE',  ( 12.63842701281683922, 4.550597817667451750, -9.846743663894590881 ) ) ;
#8189=DIRECTION ( 'NONE',  ( -0.000000000000000000, -0.000000000000000000, 1.000000000000000000 ) ) ;
#8192=CARTESIAN_POINT ( 'NONE',  ( 19.84674366389459621, 33.50893115100078745, 7.409399052514197653E-17 ) ) ;
#8194=CARTESIAN_POINT ( 'NONE',  ( 3.591859063236763294, 38.29030133659708923, -11.09922568453595026 ) ) ;
#8197=DIRECTION ( 'NONE',  ( -0.8320502943378436100, 0.5547001962252291474, -0.000000000000000000 ) ) ;
#8199=CARTESIAN_POINT ( 'NONE',  ( 7.361572987183170547, 67.05059781766746596, 9.846743663894590881 ) ) ;
#8201=CARTESIAN_POINT ( 'NONE',  ( 17.20831665107776587, 59.13393115100078745, -7.208316651077762316 ) ) ;
#8202=CARTESIAN_POINT ( 'NONE',  ( 13.79529636645030344, 28.26208216824729647, 14.16423886937410614 ) ) ;
#8203=CARTESIAN_POINT ( 'NONE',  ( 0.1532563361054083140, 56.00893115100078745, 1.131784320476157264E-15 ) ) ;
#8205=CARTESIAN_POINT ( 'NONE',  ( 14.92337183194729988, 24.34226448433411960, -8.527530157486177487 ) ) ;
#8206=CARTESIAN_POINT ( 'NONE',  ( 3.591859063236763294, 48.29030133659708923, -11.09922568453595026 ) ) ;
#8207=CARTESIAN_POINT ( 'NONE',  ( 10.00000000000000178, 3.053748834913967425, 14.16423886937410082 ) ) ;
#8208=CARTESIAN_POINT ( 'NONE',  ( 7.361572987183170547, 52.05059781766745175, 9.846743663894590881 ) ) ;
#8209=CARTESIAN_POINT ( 'NONE',  ( 0.5774900079438607392, 48.48035201082150536, 5.440088680355550821 ) ) ;
#8211=CARTESIAN_POINT ( 'NONE',  ( 10.00000000000000000, 39.75893115100078745, -9.846743663894594434 ) ) ;
#8213=ORIENTED_EDGE ( 'NONE', *, *, #11124, .F. ) ;
#8214=CARTESIAN_POINT ( 'NONE',  ( 19.42250999205614548, 60.98035201082151247, -5.440088680355545492 ) ) ;
#8215=ORIENTED_EDGE ( 'NONE', *, *, #47389, .F. ) ;
#8217=CARTESIAN_POINT ( 'NONE',  ( 19.42250999205614548, 25.98035201082150891, -5.440088680355545492 ) ) ;
#8218=CARTESIAN_POINT ( 'NONE',  ( 18.52753015748618282, 63.92559781766745886, -4.923371831947291888 ) ) ;
#8219=CARTESIAN_POINT ( 'NONE',  ( 4.559911319644449179, 57.23035201082150536, -9.422509992056141925 ) ) ;
#8220=CARTESIAN_POINT ( 'NONE',  ( 7.084665262690076126, 69.10535201082151957, 10.88017736071109987 ) ) ;
#8222=CARTESIAN_POINT ( 'NONE',  ( -0.8801773607111008646, 43.27201867748817676, 2.915334737309923430 ) ) ;
#8225=CARTESIAN_POINT ( 'NONE',  ( 19.84674366389459621, 43.50893115100078745, 7.409399052514197653E-17 ) ) ;
#8228=CARTESIAN_POINT ( 'NONE',  ( 0.1532563361054082862, 61.21726448433412315, 2.638427012816831674 ) ) ;
#8229=CARTESIAN_POINT ( 'NONE',  ( 12.91533473730992121, 19.52201867748816611, 10.88017736071110164 ) ) ;
#8232=CARTESIAN_POINT ( 'NONE',  ( 24.16423886937409904, 19.09541550158063927, 3.795296366450317205 ) ) ;
#8233=CARTESIAN_POINT ( 'NONE',  ( 2.917880565312950480, 55.97041550158063217, -12.26659068614894821 ) ) ;
#8234=CARTESIAN_POINT ( 'NONE',  ( 19.84674366389459621, 18.50893115100078745, 7.409399052514197653E-17 ) ) ;
#8235=CARTESIAN_POINT ( 'NONE',  ( 20.15039907845753575, 32.62777174578613426, -6.262539305110076171 ) ) ;
#8238=CARTESIAN_POINT ( 'NONE',  ( 5.076628168052704559, 20.17559781766745175, -8.527530157486179263 ) ) ;
#8239=CARTESIAN_POINT ( 'NONE',  ( -0.8801773607110991993, 22.85535201082150181, -2.915334737309923874 ) ) ;
#8240=CARTESIAN_POINT ( 'NONE',  ( 19.84674366389459266, 63.71726448433412315, -2.638427012816827677 ) ) ;
#8241=CARTESIAN_POINT ( 'NONE',  ( -4.164238869374098151, 6.595415501580634832, -3.795296366450310543 ) ) ;
#8243=CARTESIAN_POINT ( 'NONE',  ( 0.1532563361054100626, 15.80059781766745353, -2.638427012816831230 ) ) ;
#8244=CARTESIAN_POINT ( 'NONE',  ( -2.816281873526473856, 44.12363466993042493, 9.499525473075851096E-16 ) ) ;
#8245=CARTESIAN_POINT ( 'NONE',  ( 1.472469842513823179, 40.59226448433411605, -4.923371831947296329 ) ) ;
#8247=CARTESIAN_POINT ( 'NONE',  ( 12.63842701281683922, 19.55059781766745175, -9.846743663894590881 ) ) ;
#8249=CARTESIAN_POINT ( 'NONE',  ( -4.164238869374099927, 57.01208216824731068, 3.795296366450308767 ) ) ;
#8251=CARTESIAN_POINT ( 'NONE',  ( 2.791683348922237240, 35.38393115100079456, -7.208316651077763204 ) ) ;
#8252=CARTESIAN_POINT ( 'NONE',  ( 20.88017736071110164, 5.355352010821502695, 2.915334737309930979 ) ) ;
#8253=CARTESIAN_POINT ( 'NONE',  ( 14.92337183194729633, 52.67559781766745175, 8.527530157486181039 ) ) ;
#8254=CARTESIAN_POINT ( 'NONE',  ( 20.88017736071110164, 55.35535201082149825, 2.915334737309930979 ) ) ;
#8256=CARTESIAN_POINT ( 'NONE',  ( 10.00000000000000178, 2.258931151000784787, 9.846743663894594434 ) ) ;
#8260=ORIENTED_EDGE ( 'NONE', *, *, #60753, .F. ) ;
#8263=CARTESIAN_POINT ( 'NONE',  ( 2.791683348922237240, 25.38393115100078390, -7.208316651077763204 ) ) ;
#8264=CARTESIAN_POINT ( 'NONE',  ( 6.565887622018943937, 63.08196800326376064, -12.81628187352647608 ) ) ;
#8265=CARTESIAN_POINT ( 'NONE',  ( 10.00000000000000178, 68.05374883491397497, 14.16423886937410082 ) ) ;
#8266=CARTESIAN_POINT ( 'NONE',  ( 17.20831665107776587, 42.88393115100077324, 7.208316651077764980 ) ) ;
#8268=EDGE_CURVE ( 'NONE', #50375, #49115, #21547, .T. ) ;
#8269=CARTESIAN_POINT ( 'NONE',  ( 24.16423886937410614, 24.30374883491396787, 8.672049930838204340E-16 ) ) ;
#8270=CARTESIAN_POINT ( 'NONE',  ( 24.16423886937409904, 54.09541550158063217, 3.795296366450317205 ) ) ;
#8271=CARTESIAN_POINT ( 'NONE',  ( 14.92337183194729633, 62.67559781766745886, 8.527530157486181039 ) ) ;
#8272=CARTESIAN_POINT ( 'NONE',  ( 1.707155281725165397, 67.90189080397283306, 6.499999999999919176 ) ) ;
#8273=CARTESIAN_POINT ( 'NONE',  ( 19.42250999205614548, 50.98035201082151247, -5.440088680355545492 ) ) ;
#8274=CARTESIAN_POINT ( 'NONE',  ( 12.63842701281683922, 9.550597817667449974, -9.846743663894590881 ) ) ;
#8278=CIRCLE ( 'NONE', #35448, 9.538348415311009632 ) ;
#8281=CARTESIAN_POINT ( 'NONE',  ( 1.472469842513823179, 5.592264484334118713, -4.923371831947296329 ) ) ;
#8283=CARTESIAN_POINT ( 'NONE',  ( -0.3689425029237881626, 22.42874883491397142, 10.36894250292379027 ) ) ;
#8284=CARTESIAN_POINT ( 'NONE',  ( 0.1532563361054100626, 25.80059781766744820, -2.638427012816831230 ) ) ;
#8285=CARTESIAN_POINT ( 'NONE',  ( -0.8801773607110991993, 32.85535201082151247, -2.915334737309923874 ) ) ;
#8287=CARTESIAN_POINT ( 'NONE',  ( 10.00000000000000178, 24.31368534415484106, 10.88017736071110342 ) ) ;
#8289=CARTESIAN_POINT ( 'NONE',  ( -0.8801773607111008646, 38.27201867748816255, 2.915334737309923430 ) ) ;
#8290=( LENGTH_UNIT ( ) NAMED_UNIT ( * ) SI_UNIT ( .MILLI., .METRE. ) );
#8293=ORIENTED_EDGE ( 'NONE', *, *, #60962, .T. ) ;
#8294=CARTESIAN_POINT ( 'NONE',  ( 16.40814093676323893, 20.79030133659708923, 11.09922568453595026 ) ) ;
#8295=CARTESIAN_POINT ( 'NONE',  ( 1.472469842513823179, 10.59226448433411782, -4.923371831947296329 ) ) ;
#8297=CARTESIAN_POINT ( 'NONE',  ( 1.472469842513823179, 15.59226448433411960, -4.923371831947296329 ) ) ;
#8298=CARTESIAN_POINT ( 'NONE',  ( 0.5774900079438590739, 27.64701867748817676, -5.440088680355550821 ) ) ;
#8299=VERTEX_POINT ( 'NONE', #95995 ) ;
#8302=CARTESIAN_POINT ( 'NONE',  ( 19.38216949554541557, 62.24863466993041072, -9.382169495545420901 ) ) ;
#8303=CARTESIAN_POINT ( 'NONE',  ( 20.88017736071110519, 60.56368534415484106, 2.639326808657452039E-16 ) ) ;
#8306=CARTESIAN_POINT ( 'NONE',  ( 20.88017736071110519, 55.56368534415484817, 2.639326808657452039E-16 ) ) ;
#8307=CARTESIAN_POINT ( 'NONE',  ( 3.591859063236761518, 4.956968003263753531, 11.09922568453594849 ) ) ;
#8309=CARTESIAN_POINT ( 'NONE',  ( 0.1532563361054083140, 36.00893115100078745, 1.131784320476157264E-15 ) ) ;
#8310=CARTESIAN_POINT ( 'NONE',  ( 21.09922568453595559, 52.04030133659708923, -6.408140936763230044 ) ) ;
#8312=CARTESIAN_POINT ( 'NONE',  ( 18.52753015748617571, 18.09226448433411960, 4.923371831947298993 ) ) ;
#8313=CARTESIAN_POINT ( 'NONE',  ( 21.09922568453594849, 21.20696800326375353, 6.408140936763242479 ) ) ;
#8315=CARTESIAN_POINT ( 'NONE',  ( 14.49999999999999822, 11.00000000000000000, 5.000000000000000000 ) ) ;
#8316=CARTESIAN_POINT ( 'NONE',  ( 20.88017736071110875, 30.77201867748816966, -2.915334737309920765 ) ) ;
#8317=CARTESIAN_POINT ( 'NONE',  ( 10.00000000000000178, 67.25893115100079456, 9.846743663894594434 ) ) ;
#8319=CARTESIAN_POINT ( 'NONE',  ( 0.1532563361054100626, 25.80059781766744820, -2.638427012816831230 ) ) ;
#8320=CARTESIAN_POINT ( 'NONE',  ( 19.84674366389459266, 3.717264484334118713, -2.638427012816827677 ) ) ;
#8321=CARTESIAN_POINT ( 'NONE',  ( 15.44008868035555260, 19.73035201082150536, 9.422509992056143702 ) ) ;
#8322=EDGE_CURVE ( 'NONE', #8299, #93646, #58274, .T. ) ;
#8323=CARTESIAN_POINT ( 'NONE',  ( 6.565887622018943937, 20.16530133659708213, 12.81628187352647430 ) ) ;
#8324=CARTESIAN_POINT ( 'NONE',  ( 10.00000000000000178, 67.25893115100079456, 9.846743663894594434 ) ) ;
#8326=CARTESIAN_POINT ( 'NONE',  ( 20.88017736071110519, 20.56368534415484106, 2.639326808657452039E-16 ) ) ;
#8327=CARTESIAN_POINT ( 'NONE',  ( 10.00000000000000000, 49.75893115100078745, -9.846743663894594434 ) ) ;
#8328=MECHANICAL_DESIGN_GEOMETRIC_PRESENTATION_REPRESENTATION('',(#19531),#29079);
#8329=CARTESIAN_POINT ( 'NONE',  ( 15.44008868035555793, 21.39701867748817321, -9.422509992056140149 ) ) ;
#8330=CARTESIAN_POINT ( 'NONE',  ( 0.1532563361054100626, 5.800597817667451750, -2.638427012816831230 ) ) ;
#8332=CARTESIAN_POINT ( 'NONE',  ( 10.00000000000000000, 31.81368534415483751, -10.88017736071110342 ) ) ;
#8333=CARTESIAN_POINT ( 'NONE',  ( 19.42250999205614193, 5.147018677488171434, 5.440088680355555262 ) ) ;
#8335=( NAMED_UNIT ( * ) SI_UNIT ( $, .STERADIAN. ) SOLID_ANGLE_UNIT ( ) );
#8336=CARTESIAN_POINT ( 'NONE',  ( 19.84674366389459266, 28.71726448433411960, -2.638427012816827677 ) ) ;
#8337=CARTESIAN_POINT ( 'NONE',  ( 16.40814093676323893, 10.79030133659708923, 11.09922568453595026 ) ) ;
#8341=CARTESIAN_POINT ( 'NONE',  ( 6.204703633549690345, 12.84541550158063572, 14.16423886937410082 ) ) ;
#8342=CARTESIAN_POINT ( 'NONE',  ( 18.52753015748618282, 33.92559781766745886, -4.923371831947291888 ) ) ;
#8345=CARTESIAN_POINT ( 'NONE',  ( 10.00000000000000178, 48.05374883491396787, 14.16423886937410082 ) ) ;
#8346=CARTESIAN_POINT ( 'NONE',  ( 12.63842701281683034, 22.46726448433411605, 9.846743663894596210 ) ) ;
#8348=FACE_OUTER_BOUND ( 'NONE', #30508, .T. ) ;
#8349=CARTESIAN_POINT ( 'NONE',  ( -0.8801773607110991993, 47.85535201082150536, -2.915334737309923874 ) ) ;
#8350=CARTESIAN_POINT ( 'NONE',  ( 0.6178305044545818747, 48.49863466993042493, -9.382169495545419124 ) ) ;
#8351=CARTESIAN_POINT ( 'NONE',  ( -0.8801773607111009756, 18.06368534415484106, 1.068504757029289695E-15 ) ) ;
#8352=CARTESIAN_POINT ( 'NONE',  ( 10.00000000000000178, 50.37363466993042493, 12.81628187352647608 ) ) ;
#8353=CARTESIAN_POINT ( 'NONE',  ( -2.816281873526471635, -1.084698663402913210, -3.434112377981056508 ) ) ;
#8354=CARTESIAN_POINT ( 'NONE',  ( 0.1532563361054100626, 5.800597817667452638, -2.638427012816831230 ) ) ;
#8355=ORIENTED_EDGE ( 'NONE', *, *, #29891, .T. ) ;
#8357=CARTESIAN_POINT ( 'NONE',  ( 0.000000000000000000, 10.49999999999999822, -6.500000000000000888 ) ) ;
#8358=CARTESIAN_POINT ( 'NONE',  ( 20.36894250292379738, 59.92874883491397497, -10.36894250292379027 ) ) ;
#8359=CARTESIAN_POINT ( 'NONE',  ( 24.16423886937410614, 14.51208216824730179, -3.795296366450302550 ) ) ;
#8360=CARTESIAN_POINT ( 'NONE',  ( 10.00000000000000178, 24.31368534415484106, 10.88017736071110342 ) ) ;
#8361=CARTESIAN_POINT ( 'NONE',  ( 4.559911319644449179, 38.89701867748817676, 9.422509992056141925 ) ) ;
#8364=CARTESIAN_POINT ( 'NONE',  ( 20.88017736071110875, 65.77201867748817676, -2.915334737309920765 ) ) ;
#8365=CARTESIAN_POINT ( 'NONE',  ( 20.88017736071110875, 60.77201867748817676, -2.915334737309920765 ) ) ;
#8366=CARTESIAN_POINT ( 'NONE',  ( 6.565887622018943937, 25.16530133659708213, 12.81628187352647430 ) ) ;
#8367=CYLINDRICAL_SURFACE ( 'NONE', #74584, 0.5000000000000004441 ) ;
#8369=CARTESIAN_POINT ( 'NONE',  ( 14.92337183194729633, 7.675597817667451750, 8.527530157486181039 ) ) ;
#8370=CARTESIAN_POINT ( 'NONE',  ( 14.92337183194729633, 42.67559781766745886, 8.527530157486181039 ) ) ;
#8371=CARTESIAN_POINT ( 'NONE',  ( 19.42250999205614548, 10.98035201082150358, -5.440088680355545492 ) ) ;
#8373=CARTESIAN_POINT ( 'NONE',  ( 0.6178305044545818747, 38.49863466993042493, -9.382169495545419124 ) ) ;
#8374=CARTESIAN_POINT ( 'NONE',  ( 19.84674366389459621, 13.50893115100078568, 7.409399052514197653E-17 ) ) ;
#8378=CARTESIAN_POINT ( 'NONE',  ( 17.20831665107776587, 57.88393115100078745, 7.208316651077764980 ) ) ;
#8379=CARTESIAN_POINT ( 'NONE',  ( 0.1532563361054100626, 25.80059781766744820, -2.638427012816831230 ) ) ;
#8380=CARTESIAN_POINT ( 'NONE',  ( 20.36894250292379382, 3.678748834913967869, 10.36894250292379205 ) ) ;
#8381=CARTESIAN_POINT ( 'NONE',  ( -2.266590686148945544, 12.22041550158063394, 7.082119434687048631 ) ) ;
#8382=CARTESIAN_POINT ( 'NONE',  ( 0.5774900079438590739, 32.64701867748816966, -5.440088680355550821 ) ) ;
#8383=CARTESIAN_POINT ( 'NONE',  ( 15.44008868035555793, 6.397018677488170546, -9.422509992056140149 ) ) ;
#8384=CARTESIAN_POINT ( 'NONE',  ( -0.8801773607111008646, 28.27201867748817321, 2.915334737309923430 ) ) ;
#8385=CARTESIAN_POINT ( 'NONE',  ( 19.42250999205614193, 35.14701867748816966, 5.440088680355555262 ) ) ;
#8387=( BOUNDED_SURFACE ( )  B_SPLINE_SURFACE ( 1, 2, ( 
 ( #38391, #54846, #22904, #15412, #46860, #69874, #14912, #68894, #45895, #14412, #67902, #7412, #54357, #37908, #422, #8380, #1394, #49316, #78840, #25848, #55853, #25368, #11322, #56345, #24871, #71354, #3838, #47346, #64794, #86348, #94819, #2873, #48336, #95313, #87319, #77849, #86839, #62848, #33322, #63817, #17851, #10351, #55353, #41363, #3339, #47840, #94327, #9358, #33801, #34297, #18344, #71830, #79333, #18836, #26815, #85360, #10842, #64308, #16872, #26322, #78343, #79820, #9864, #39863, #32345, #40363, #41841, #1887, #72307, #70864, #2379, #32834, #63336, #93841, #73298, #82276, #88307, #96323, #19805, #20309, #36794, #4822, #12793, #43293, #97310, #11813, #35296, #81779, #65789, #35797, #19321, #13294, #28783, #51789, #5318, #66284, #13793, #59280, #96819, #89295, #20805, #74273, #89780, #74783, #67288, #21297, #44279, #6292, #49805, #80313, #72794, #4332, #34803, #67787, #8269, #37789, #46745, #54244, #7289, #98808, #22786, #7785, #69268, #53760, #68287, #15777, #16262, #46266, #8747, #38280, #60760, #45775, #788, #52768, #91260, #53264, #83770, #31241, #68775, #14801, #98309, #90266, #15293, #84756, #76268, #305, #61256, #30749, #23284, #91761, #39267, #21799, #61736, #92254, #69755, #52281, #83276, #82779, #14299, #44770, #75275, #29763, #60271, #6786, #37299, #45273, #71233, #10238, #9244, #77732, #63218, #25255, #18228, #70252, #55740, #93721, #63706, #85742, #1768, #3228, #70750, #56709, #86231, #40240, #94209, #17742, #25739, #78728, #11207, #92740, #2264, #41240, #40730, #2758, #93225, #87200, #56231, #86725, #54728, #32224, #62725, #18723, #48709, #79212, #10722, #71717, #24750, #55228, #33693, #64191, #94710, #17255, #41726, #1284, #31737, #62233, #24264, #85249, #16754, #47229, #89667, #21178, #4713, #58674, #51680, #13173, #4214, #81180, #34684, #26696, #19204, #65178, #20686, #57191, #35175, #12681, #43180, #43670, #27184, #12188, #88182, #97201, #95701, #42695, #72678, #65676, #82159, #42212, #96198, #73174, #36176, #87689, #19696, #66167, #57687, #73668, #3725, #96700, #51180, #66676, #50183, #80693, #28669, #59161, #27682, #5195, #58167, #80190, #88678, #13671, #72196, #20186, #35683, #34186, #64678, #28179, #95188, #49686, #29653, #45162, #84648, #15183, #24152, #31630, #83665, #76160, #192, #84171, #54135, #31136, #45663, #61629, #92629, #23673, #85141, #15676, #7682, #23175, #16151, #68179, #38175, #68665, #30639, #46635, #46161, #91155, #75666, #6676, #38656, #47121, #61148, #98196, #8165, #53160, #62121, #54620, #76644, #7177, #77137, #30147, #37680, #98698, #16649, #60656, #22679 ),
 ( #69161, #37196, #8646, #67687, #39156, #91657, #69646, #685, #92148, #1170, #53652, #60162, #90658, #22184, #52665, #83167, #14692, #48110, #56125, #71128, #63115, #64575, #2655, #56609, #72091, #70144, #26589, #17642, #63602, #3130, #33107, #94107, #95084, #25152, #32617, #11107, #3615, #78126, #25635, #78624, #19097, #77621, #17151, #87098, #62612, #70634, #9636, #47630, #41626, #86620, #18131, #10135, #40630, #34084, #48603, #40134, #79107, #57091, #39652, #87585, #10619, #18612, #41131, #71619, #9136, #79604, #1665, #33590, #55115, #64085, #94600, #26117, #49101, #2162, #32114, #93119, #93617, #24646, #85633, #55629, #86129, #81560, #5590, #11593, #13067, #27078, #43076, #27573, #12578, #57579, #4605, #82058, #19587, #88075, #89566, #66568, #58068, #73562, #12084, #29049, #5086, #96091, #43559, #50085, #28067, #80088, #74057, #97097, #44053, #80589, #88571, #6074, #51572, #42589, #20583, #35573, #73069, #20075, #67063, #90053, #50580, #81075, #21074, #13566, #35066, #59061, #42112, #72574, #65565, #28568, #66064, #97589, #74558, #96592, #58564, #89069, #51068, #36575, #36067, #49578, #4107, #34571, #65067, #95593, #30530, #98587, #38059, #38548, #83054, #30036, #53035, #45543, #69043, #83, #7066, #90542, #21576, #91037, #46524, #76040, #60544, #53529, #7573, #15563, #68552, #1047, #14075, #22566, #61518, #68057, #83551, #14574, #77024, #91543, #15074, #75051, #22074, #52549, #8538, #61031, #76533, #23060, #84042, #29539, #98080, #46048, #8048, #577, #60044, #31022, #92028, #23558, #37566, #45041, #54027, #84538, #16035, #39039, #69533, #31514, #62013, #52064, #82559, #75550, #44555, #6560, #37070, #67568, #55000, #41009, #9017, #25029, #32992, #25521, #63968, #70519, #32503, #2042, #41510, #85518, #63001, #47994, #18008, #92513, #78991, #3023, #86983, #31996, #18988, #19958, #3992, #27947, #50453, #51448, #13444, #58439, #34457, #89447, #80470, #64948, #12459, #43931, #20462, #5956, #94970, #26472, #82930, #46408, #38426, #98953, #21449, #29914, #37941, #30409, #14946, #15917, #7929, #76896, #53408, #29418, #452, #7443, #45415, #45925, #6434, #30902, #98458, #60419, #91414, #97461, #36449, #6940, #75919, #22443, #21953, #23432, #52915, #76414, #91907, #28926, #84420, #75426, #83427, #22940, #68431, #53911, #66941, #14448, #90411, #59430, #51946, #67443, #82431, #37447, #13956, #44430, #97962, #59923, #52432, #44918, #39410, #46890, #71389, #1917, #47870, #77879, #47380, #33352, #78375, #77381, #62881, #25879, #69406, #86869, #9391, #17884, #93378, #70398, #18378, #10381, #927, #9896, #84900, #55388, #24905 ) ),
 .UNSPECIFIED., .F., .F., .F. ) 
 B_SPLINE_SURFACE_WITH_KNOTS ( ( 2, 2 ),
 ( 3, 2, 2, 2, 2, 2, 2, 2, 2, 2, 2, 2, 2, 2, 2, 2, 2, 2, 2, 2, 2, 2, 2, 2, 2, 2, 2, 2, 2, 2, 2, 2, 2, 2, 2, 2, 2, 2, 2, 2, 2, 2, 2, 2, 2, 2, 2, 2, 2, 2, 2, 2, 2, 2, 2, 2, 2, 2, 2, 2, 2, 2, 2, 2, 2, 2, 2, 2, 2, 2, 2, 2, 2, 2, 2, 2, 2, 2, 2, 2, 2, 2, 2, 2, 2, 2, 2, 2, 2, 2, 2, 2, 2, 2, 2, 2, 2, 2, 2, 2, 2, 2, 2, 2, 2, 2, 2, 2, 2, 2, 2, 2, 2, 2, 2, 2, 2, 2, 2, 2, 2, 2, 2, 2, 2, 2, 2, 2, 2, 2, 2, 2, 2, 2, 2, 2, 2, 2, 2, 2, 2, 2, 2, 2, 2, 2, 2, 2, 2, 2, 2, 2, 2, 2, 2, 2, 2, 2, 2, 2, 2, 2, 3 ),
 ( 0.000000000000000000, 1.000000000000000000 ),
 ( 0.000000000000000000, 0.005952380952380952051, 0.01190476190476190410, 0.01785714285714285615, 0.02380952380952380820, 0.02976190476190476025, 0.03571428571428571230, 0.04166666666666666435, 0.04761904761904761640, 0.05357142857142856845, 0.05952380952380952051, 0.06547619047619047949, 0.07142857142857142461, 0.07738095238095238360, 0.08333333333333332871, 0.08928571428571428770, 0.09523809523809523281, 0.1011904761904761918, 0.1071428571428571369, 0.1130952380952380959, 0.1190476190476190410, 0.1250000000000000000, 0.1309523809523809590, 0.1369047619047619180, 0.1428571428571428492, 0.1488095238095238082, 0.1547619047619047672, 0.1607142857142857262, 0.1666666666666666574, 0.1726190476190476164, 0.1785714285714285754, 0.1845238095238095344, 0.1904761904761904656, 0.1964285714285714246, 0.2023809523809523836, 0.2083333333333333426, 0.2142857142857142738, 0.2202380952380952328, 0.2261904761904761918, 0.2321428571428571508, 0.2380952380952380820, 0.2440476190476190410, 0.2500000000000000000, 0.2559523809523809312, 0.2619047619047619180, 0.2678571428571428492, 0.2738095238095238360, 0.2797619047619047672, 0.2857142857142856984, 0.2916666666666666852, 0.2976190476190476164, 0.3035714285714285476, 0.3095238095238095344, 0.3154761904761904656, 0.3214285714285714524, 0.3273809523809523836, 0.3333333333333333148, 0.3392857142857143016, 0.3452380952380952328, 0.3511904761904761640, 0.3571428571428571508, 0.3630952380952380820, 0.3690476190476190688, 0.3750000000000000000, 0.3809523809523809312, 0.3869047619047619180, 0.3928571428571428492, 0.3988095238095238360, 0.4047619047619047672, 0.4107142857142856984, 0.4166666666666666852, 0.4226190476190476164, 0.4285714285714285476, 0.4345238095238095344, 0.4404761904761904656, 0.4464285714285714524, 0.4523809523809523836, 0.4583333333333333148, 0.4642857142857143016, 0.4702380952380952328, 0.4761904761904761640, 0.4821428571428571508, 0.4880952380952380820, 0.4940476190476190688, 0.5000000000000000000, 0.5059523809523809312, 0.5119047619047618625, 0.5178571428571429047, 0.5238095238095238360, 0.5297619047619047672, 0.5357142857142856984, 0.5416666666666666297, 0.5476190476190476719, 0.5535714285714286031, 0.5595238095238095344, 0.5654761904761904656, 0.5714285714285713969, 0.5773809523809523281, 0.5833333333333333703, 0.5892857142857143016, 0.5952380952380952328, 0.6011904761904761640, 0.6071428571428570953, 0.6130952380952381375, 0.6190476190476190688, 0.6250000000000000000, 0.6309523809523809312, 0.6369047619047618625, 0.6428571428571429047, 0.6488095238095238360, 0.6547619047619047672, 0.6607142857142856984, 0.6666666666666666297, 0.6726190476190476719, 0.6785714285714286031, 0.6845238095238095344, 0.6904761904761904656, 0.6964285714285713969, 0.7023809523809523281, 0.7083333333333333703, 0.7142857142857143016, 0.7202380952380952328, 0.7261904761904761640, 0.7321428571428570953, 0.7380952380952381375, 0.7440476190476190688, 0.7500000000000000000, 0.7559523809523809312, 0.7619047619047618625, 0.7678571428571429047, 0.7738095238095238360, 0.7797619047619047672, 0.7857142857142856984, 0.7916666666666666297, 0.7976190476190476719, 0.8035714285714286031, 0.8095238095238095344, 0.8154761904761904656, 0.8214285714285713969, 0.8273809523809523281, 0.8333333333333333703, 0.8392857142857143016, 0.8452380952380952328, 0.8511904761904761640, 0.8571428571428570953, 0.8630952380952381375, 0.8690476190476190688, 0.8750000000000000000, 0.8809523809523809312, 0.8869047619047618625, 0.8928571428571429047, 0.8988095238095238360, 0.9047619047619047672, 0.9107142857142856984, 0.9166666666666666297, 0.9226190476190476719, 0.9285714285714286031, 0.9345238095238095344, 0.9404761904761904656, 0.9464285714285713969, 0.9523809523809523281, 0.9583333333333333703, 0.9642857142857143016 ),
 .UNSPECIFIED. ) 
 GEOMETRIC_REPRESENTATION_ITEM ( )  RATIONAL_B_SPLINE_SURFACE ( (
 ( 1.000000000000000000, 0.9659258262890683122, 1.000000000000000000, 0.9659258262890683122, 1.000000000000000000, 0.9659258262890683122, 1.000000000000000000, 0.9659258262890683122, 1.000000000000000000, 0.9659258262890683122, 1.000000000000000000, 0.9659258262890683122, 1.000000000000000000, 0.9659258262890683122, 1.000000000000000000, 0.9659258262890683122, 1.000000000000000000, 0.9659258262890683122, 1.000000000000000000, 0.9659258262890683122, 1.000000000000000000, 0.9659258262890683122, 1.000000000000000000, 0.9659258262890683122, 1.000000000000000000, 0.9659258262890683122, 1.000000000000000000, 0.9659258262890683122, 1.000000000000000000, 0.9659258262890683122, 1.000000000000000000, 0.9659258262890683122, 1.000000000000000000, 0.9659258262890683122, 1.000000000000000000, 0.9659258262890683122, 1.000000000000000000, 0.9659258262890683122, 1.000000000000000000, 0.9659258262890683122, 1.000000000000000000, 0.9659258262890683122, 1.000000000000000000, 0.9659258262890683122, 1.000000000000000000, 0.9659258262890683122, 1.000000000000000000, 0.9659258262890683122, 1.000000000000000000, 0.9659258262890683122, 1.000000000000000000, 0.9659258262890683122, 1.000000000000000000, 0.9659258262890683122, 1.000000000000000000, 0.9659258262890683122, 1.000000000000000000, 0.9659258262890683122, 1.000000000000000000, 0.9659258262890683122, 1.000000000000000000, 0.9659258262890683122, 1.000000000000000000, 0.9659258262890683122, 1.000000000000000000, 0.9659258262890683122, 1.000000000000000000, 0.9659258262890683122, 1.000000000000000000, 0.9659258262890683122, 1.000000000000000000, 0.9659258262890683122, 1.000000000000000000, 0.9659258262890683122, 1.000000000000000000, 0.9659258262890683122, 1.000000000000000000, 0.9659258262890683122, 1.000000000000000000, 0.9659258262890683122, 1.000000000000000000, 0.9659258262890683122, 1.000000000000000000, 0.9659258262890683122, 1.000000000000000000, 0.9659258262890683122, 1.000000000000000000, 0.9659258262890683122, 1.000000000000000000, 0.9659258262890683122, 1.000000000000000000, 0.9659258262890683122, 1.000000000000000000, 0.9659258262890683122, 1.000000000000000000, 0.9659258262890683122, 1.000000000000000000, 0.9659258262890683122, 1.000000000000000000, 0.9659258262890683122, 1.000000000000000000, 0.9659258262890683122, 1.000000000000000000, 0.9659258262890683122, 1.000000000000000000, 0.9659258262890683122, 1.000000000000000000, 0.9659258262890683122, 1.000000000000000000, 0.9659258262890683122, 1.000000000000000000, 0.9659258262890683122, 1.000000000000000000, 0.9659258262890683122, 1.000000000000000000, 0.9659258262890683122, 1.000000000000000000, 0.9659258262890683122, 1.000000000000000000, 0.9659258262890683122, 1.000000000000000000, 0.9659258262890683122, 1.000000000000000000, 0.9659258262890683122, 1.000000000000000000, 0.9659258262890683122, 1.000000000000000000, 0.9659258262890683122, 1.000000000000000000, 0.9659258262890683122, 1.000000000000000000, 0.9659258262890683122, 1.000000000000000000, 0.9659258262890683122, 1.000000000000000000, 0.9659258262890683122, 1.000000000000000000, 0.9659258262890683122, 1.000000000000000000, 0.9659258262890683122, 1.000000000000000000, 0.9659258262890683122, 1.000000000000000000, 0.9659258262890683122, 1.000000000000000000, 0.9659258262890683122, 1.000000000000000000, 0.9659258262890683122, 1.000000000000000000, 0.9659258262890683122, 1.000000000000000000, 0.9659258262890683122, 1.000000000000000000, 0.9659258262890683122, 1.000000000000000000, 0.9659258262890683122, 1.000000000000000000, 0.9659258262890683122, 1.000000000000000000, 0.9659258262890683122, 1.000000000000000000, 0.9659258262890683122, 1.000000000000000000, 0.9659258262890683122, 1.000000000000000000, 0.9659258262890683122, 1.000000000000000000, 0.9659258262890683122, 1.000000000000000000, 0.9659258262890683122, 1.000000000000000000, 0.9659258262890683122, 1.000000000000000000, 0.9659258262890683122, 1.000000000000000000, 0.9659258262890683122, 1.000000000000000000, 0.9659258262890683122, 1.000000000000000000, 0.9659258262890683122, 1.000000000000000000, 0.9659258262890683122, 1.000000000000000000, 0.9659258262890683122, 1.000000000000000000, 0.9659258262890683122, 1.000000000000000000, 0.9659258262890683122, 1.000000000000000000, 0.9659258262890683122, 1.000000000000000000, 0.9659258262890683122, 1.000000000000000000, 0.9659258262890683122, 1.000000000000000000, 0.9659258262890683122, 1.000000000000000000, 0.9659258262890683122, 1.000000000000000000, 0.9659258262890683122, 1.000000000000000000, 0.9659258262890683122, 1.000000000000000000, 0.9659258262890683122, 1.000000000000000000, 0.9659258262890683122, 1.000000000000000000, 0.9659258262890683122, 1.000000000000000000, 0.9659258262890683122, 1.000000000000000000, 0.9659258262890683122, 1.000000000000000000, 0.9659258262890683122, 1.000000000000000000, 0.9659258262890683122, 1.000000000000000000, 0.9659258262890683122, 1.000000000000000000, 0.9659258262890683122, 1.000000000000000000, 0.9659258262890683122, 1.000000000000000000, 0.9659258262890683122, 1.000000000000000000, 0.9659258262890683122, 1.000000000000000000, 0.9659258262890683122, 1.000000000000000000, 0.9659258262890683122, 1.000000000000000000, 0.9659258262890683122, 1.000000000000000000, 0.9659258262890683122, 1.000000000000000000, 0.9659258262890683122, 1.000000000000000000, 0.9659258262890683122, 1.000000000000000000, 0.9659258262890683122, 1.000000000000000000, 0.9659258262890683122, 1.000000000000000000, 0.9659258262890683122, 1.000000000000000000, 0.9659258262890683122, 1.000000000000000000, 0.9659258262890683122, 1.000000000000000000, 0.9659258262890683122, 1.000000000000000000, 0.9659258262890683122, 1.000000000000000000, 0.9659258262890683122, 1.000000000000000000, 0.9659258262890683122, 1.000000000000000000, 0.9659258262890683122, 1.000000000000000000, 0.9659258262890683122, 1.000000000000000000, 0.9659258262890683122, 1.000000000000000000, 0.9659258262890683122, 1.000000000000000000, 0.9659258262890683122, 1.000000000000000000, 0.9659258262890683122, 1.000000000000000000, 0.9659258262890683122, 1.000000000000000000, 0.9659258262890683122, 1.000000000000000000, 0.9659258262890683122, 1.000000000000000000, 0.9659258262890683122, 1.000000000000000000, 0.9659258262890683122, 1.000000000000000000, 0.9659258262890683122, 1.000000000000000000, 0.9659258262890683122, 1.000000000000000000, 0.9659258262890683122, 1.000000000000000000, 0.9659258262890683122, 1.000000000000000000, 0.9659258262890683122, 1.000000000000000000, 0.9659258262890683122, 1.000000000000000000, 0.9659258262890683122, 1.000000000000000000, 0.9659258262890683122, 1.000000000000000000, 0.9659258262890683122, 1.000000000000000000, 0.9659258262890683122, 1.000000000000000000, 0.9659258262890683122, 1.000000000000000000, 0.9659258262890683122, 1.000000000000000000, 0.9659258262890683122, 1.000000000000000000, 0.9659258262890683122, 1.000000000000000000, 0.9659258262890683122, 1.000000000000000000, 0.9659258262890683122, 1.000000000000000000, 0.9659258262890683122, 1.000000000000000000, 0.9659258262890683122, 1.000000000000000000, 0.9659258262890683122, 1.000000000000000000, 0.9659258262890683122, 1.000000000000000000, 0.9659258262890683122, 1.000000000000000000, 0.9659258262890683122, 1.000000000000000000, 0.9659258262890683122, 1.000000000000000000),
 ( 1.000000000000000000, 0.9659258262890683122, 1.000000000000000000, 0.9659258262890683122, 1.000000000000000000, 0.9659258262890683122, 1.000000000000000000, 0.9659258262890683122, 1.000000000000000000, 0.9659258262890683122, 1.000000000000000000, 0.9659258262890683122, 1.000000000000000000, 0.9659258262890683122, 1.000000000000000000, 0.9659258262890683122, 1.000000000000000000, 0.9659258262890683122, 1.000000000000000000, 0.9659258262890683122, 1.000000000000000000, 0.9659258262890683122, 1.000000000000000000, 0.9659258262890683122, 1.000000000000000000, 0.9659258262890683122, 1.000000000000000000, 0.9659258262890683122, 1.000000000000000000, 0.9659258262890683122, 1.000000000000000000, 0.9659258262890683122, 1.000000000000000000, 0.9659258262890683122, 1.000000000000000000, 0.9659258262890683122, 1.000000000000000000, 0.9659258262890683122, 1.000000000000000000, 0.9659258262890683122, 1.000000000000000000, 0.9659258262890683122, 1.000000000000000000, 0.9659258262890683122, 1.000000000000000000, 0.9659258262890683122, 1.000000000000000000, 0.9659258262890683122, 1.000000000000000000, 0.9659258262890683122, 1.000000000000000000, 0.9659258262890683122, 1.000000000000000000, 0.9659258262890683122, 1.000000000000000000, 0.9659258262890683122, 1.000000000000000000, 0.9659258262890683122, 1.000000000000000000, 0.9659258262890683122, 1.000000000000000000, 0.9659258262890683122, 1.000000000000000000, 0.9659258262890683122, 1.000000000000000000, 0.9659258262890683122, 1.000000000000000000, 0.9659258262890683122, 1.000000000000000000, 0.9659258262890683122, 1.000000000000000000, 0.9659258262890683122, 1.000000000000000000, 0.9659258262890683122, 1.000000000000000000, 0.9659258262890683122, 1.000000000000000000, 0.9659258262890683122, 1.000000000000000000, 0.9659258262890683122, 1.000000000000000000, 0.9659258262890683122, 1.000000000000000000, 0.9659258262890683122, 1.000000000000000000, 0.9659258262890683122, 1.000000000000000000, 0.9659258262890683122, 1.000000000000000000, 0.9659258262890683122, 1.000000000000000000, 0.9659258262890683122, 1.000000000000000000, 0.9659258262890683122, 1.000000000000000000, 0.9659258262890683122, 1.000000000000000000, 0.9659258262890683122, 1.000000000000000000, 0.9659258262890683122, 1.000000000000000000, 0.9659258262890683122, 1.000000000000000000, 0.9659258262890683122, 1.000000000000000000, 0.9659258262890683122, 1.000000000000000000, 0.9659258262890683122, 1.000000000000000000, 0.9659258262890683122, 1.000000000000000000, 0.9659258262890683122, 1.000000000000000000, 0.9659258262890683122, 1.000000000000000000, 0.9659258262890683122, 1.000000000000000000, 0.9659258262890683122, 1.000000000000000000, 0.9659258262890683122, 1.000000000000000000, 0.9659258262890683122, 1.000000000000000000, 0.9659258262890683122, 1.000000000000000000, 0.9659258262890683122, 1.000000000000000000, 0.9659258262890683122, 1.000000000000000000, 0.9659258262890683122, 1.000000000000000000, 0.9659258262890683122, 1.000000000000000000, 0.9659258262890683122, 1.000000000000000000, 0.9659258262890683122, 1.000000000000000000, 0.9659258262890683122, 1.000000000000000000, 0.9659258262890683122, 1.000000000000000000, 0.9659258262890683122, 1.000000000000000000, 0.9659258262890683122, 1.000000000000000000, 0.9659258262890683122, 1.000000000000000000, 0.9659258262890683122, 1.000000000000000000, 0.9659258262890683122, 1.000000000000000000, 0.9659258262890683122, 1.000000000000000000, 0.9659258262890683122, 1.000000000000000000, 0.9659258262890683122, 1.000000000000000000, 0.9659258262890683122, 1.000000000000000000, 0.9659258262890683122, 1.000000000000000000, 0.9659258262890683122, 1.000000000000000000, 0.9659258262890683122, 1.000000000000000000, 0.9659258262890683122, 1.000000000000000000, 0.9659258262890683122, 1.000000000000000000, 0.9659258262890683122, 1.000000000000000000, 0.9659258262890683122, 1.000000000000000000, 0.9659258262890683122, 1.000000000000000000, 0.9659258262890683122, 1.000000000000000000, 0.9659258262890683122, 1.000000000000000000, 0.9659258262890683122, 1.000000000000000000, 0.9659258262890683122, 1.000000000000000000, 0.9659258262890683122, 1.000000000000000000, 0.9659258262890683122, 1.000000000000000000, 0.9659258262890683122, 1.000000000000000000, 0.9659258262890683122, 1.000000000000000000, 0.9659258262890683122, 1.000000000000000000, 0.9659258262890683122, 1.000000000000000000, 0.9659258262890683122, 1.000000000000000000, 0.9659258262890683122, 1.000000000000000000, 0.9659258262890683122, 1.000000000000000000, 0.9659258262890683122, 1.000000000000000000, 0.9659258262890683122, 1.000000000000000000, 0.9659258262890683122, 1.000000000000000000, 0.9659258262890683122, 1.000000000000000000, 0.9659258262890683122, 1.000000000000000000, 0.9659258262890683122, 1.000000000000000000, 0.9659258262890683122, 1.000000000000000000, 0.9659258262890683122, 1.000000000000000000, 0.9659258262890683122, 1.000000000000000000, 0.9659258262890683122, 1.000000000000000000, 0.9659258262890683122, 1.000000000000000000, 0.9659258262890683122, 1.000000000000000000, 0.9659258262890683122, 1.000000000000000000, 0.9659258262890683122, 1.000000000000000000, 0.9659258262890683122, 1.000000000000000000, 0.9659258262890683122, 1.000000000000000000, 0.9659258262890683122, 1.000000000000000000, 0.9659258262890683122, 1.000000000000000000, 0.9659258262890683122, 1.000000000000000000, 0.9659258262890683122, 1.000000000000000000, 0.9659258262890683122, 1.000000000000000000, 0.9659258262890683122, 1.000000000000000000, 0.9659258262890683122, 1.000000000000000000, 0.9659258262890683122, 1.000000000000000000, 0.9659258262890683122, 1.000000000000000000, 0.9659258262890683122, 1.000000000000000000, 0.9659258262890683122, 1.000000000000000000, 0.9659258262890683122, 1.000000000000000000, 0.9659258262890683122, 1.000000000000000000, 0.9659258262890683122, 1.000000000000000000, 0.9659258262890683122, 1.000000000000000000, 0.9659258262890683122, 1.000000000000000000, 0.9659258262890683122, 1.000000000000000000, 0.9659258262890683122, 1.000000000000000000, 0.9659258262890683122, 1.000000000000000000, 0.9659258262890683122, 1.000000000000000000, 0.9659258262890683122, 1.000000000000000000, 0.9659258262890683122, 1.000000000000000000, 0.9659258262890683122, 1.000000000000000000, 0.9659258262890683122, 1.000000000000000000, 0.9659258262890683122, 1.000000000000000000, 0.9659258262890683122, 1.000000000000000000, 0.9659258262890683122, 1.000000000000000000, 0.9659258262890683122, 1.000000000000000000, 0.9659258262890683122, 1.000000000000000000, 0.9659258262890683122, 1.000000000000000000, 0.9659258262890683122, 1.000000000000000000, 0.9659258262890683122, 1.000000000000000000, 0.9659258262890683122, 1.000000000000000000, 0.9659258262890683122, 1.000000000000000000, 0.9659258262890683122, 1.000000000000000000, 0.9659258262890683122, 1.000000000000000000, 0.9659258262890683122, 1.000000000000000000, 0.9659258262890683122, 1.000000000000000000, 0.9659258262890683122, 1.000000000000000000, 0.9659258262890683122, 1.000000000000000000, 0.9659258262890683122, 1.000000000000000000, 0.9659258262890683122, 1.000000000000000000, 0.9659258262890683122, 1.000000000000000000, 0.9659258262890683122, 1.000000000000000000, 0.9659258262890683122, 1.000000000000000000, 0.9659258262890683122, 1.000000000000000000) ) ) 
 REPRESENTATION_ITEM ( '' )  SURFACE ( )  );
#8388=CARTESIAN_POINT ( 'NONE',  ( 19.42250999205614193, 35.14701867748816966, 5.440088680355555262 ) ) ;
#8389=EDGE_LOOP ( 'NONE', ( #87511, #90186, #92006, #53340 ) ) ;
#8390=CARTESIAN_POINT ( 'NONE',  ( 13.43411237798106583, 57.66530133659708923, -12.81628187352647252 ) ) ;
#8391=CARTESIAN_POINT ( 'NONE',  ( -0.8801773607111008646, 48.27201867748816966, 2.915334737309923430 ) ) ;
#8392=AXIS2_PLACEMENT_3D ( 'NONE', #51612, #73601, #5126 ) ;
#8394=CARTESIAN_POINT ( 'NONE',  ( 15.44008868035555793, 51.39701867748816966, -9.422509992056140149 ) ) ;
#8397=CARTESIAN_POINT ( 'NONE',  ( -0.3689425029237881626, 57.42874883491397497, 10.36894250292379027 ) ) ;
#8398=CARTESIAN_POINT ( 'NONE',  ( -0.8801773607111008646, 63.27201867748817676, 2.915334737309923430 ) ) ;
#8402=CARTESIAN_POINT ( 'NONE',  ( 19.84674366389459266, 33.30059781766744464, 2.638427012816836559 ) ) ;
#8403=ORIENTED_EDGE ( 'NONE', *, *, #62283, .T. ) ;
#8406=CARTESIAN_POINT ( 'NONE',  ( 10.00000000000000178, 37.25893115100078745, 9.846743663894594434 ) ) ;
#8407=CARTESIAN_POINT ( 'NONE',  ( 20.88017736071110875, 35.77201867748816966, -2.915334737309920765 ) ) ;
#8408=CARTESIAN_POINT ( 'NONE',  ( 14.92337183194729633, 42.67559781766745886, 8.527530157486181039 ) ) ;
#8409=CARTESIAN_POINT ( 'NONE',  ( -2.816281873526473856, 19.33196800326375708, 3.434112377981055619 ) ) ;
#8410=CARTESIAN_POINT ( 'NONE',  ( 19.88565890683628723, 2.716910754863021804, -6.480892540919843903 ) ) ;
#8412=CARTESIAN_POINT ( 'NONE',  ( 12.91533473730993009, 51.60535201082149825, -10.88017736071109987 ) ) ;
#8413=CARTESIAN_POINT ( 'NONE',  ( 20.88017736071110164, 5.355352010821502695, 2.915334737309930979 ) ) ;
#8414=CARTESIAN_POINT ( 'NONE',  ( 10.00000000000000178, 58.05374883491397497, 14.16423886937410082 ) ) ;
#8415=MECHANICAL_DESIGN_GEOMETRIC_PRESENTATION_REPRESENTATION('',(#54644),#457);
#8416=CARTESIAN_POINT ( 'NONE',  ( 3.591859063236761518, 24.95696800326375353, 11.09922568453594849 ) ) ;
#8417=CARTESIAN_POINT ( 'NONE',  ( 19.72487221294570858, 70.00000000000000000, 6.500000000000000888 ) ) ;
#8418=ORIENTED_EDGE ( 'NONE', *, *, #70327, .F. ) ;
#8419=CARTESIAN_POINT ( 'NONE',  ( 6.565887622018943937, 15.16530133659708568, 12.81628187352647430 ) ) ;
#8420=CARTESIAN_POINT ( 'NONE',  ( 20.88017736071110875, 25.77201867748816966, -2.915334737309920765 ) ) ;
#8421=CARTESIAN_POINT ( 'NONE',  ( 12.91533473730993009, 66.60535201082150536, -10.88017736071109987 ) ) ;
#8424=CARTESIAN_POINT ( 'NONE',  ( 15.44008868035555260, 64.73035201082151957, 9.422509992056143702 ) ) ;
#8425=CARTESIAN_POINT ( 'NONE',  ( 7.361572987183170547, 47.05059781766745175, 9.846743663894590881 ) ) ;
#8426=CARTESIAN_POINT ( 'NONE',  ( 7.361572987183170547, 32.05059781766745175, 9.846743663894590881 ) ) ;
#8428=CARTESIAN_POINT ( 'NONE',  ( 5.076628168052704559, 30.17559781766745175, -8.527530157486179263 ) ) ;
#8429=CYLINDRICAL_SURFACE ( 'NONE', #60422, 0.5000000000000004441 ) ;
#8431=CARTESIAN_POINT ( 'NONE',  ( 2.791683348922237240, 15.38393115100078212, -7.208316651077763204 ) ) ;
#8434=CARTESIAN_POINT ( 'NONE',  ( 2.791683348922237240, 45.38393115100079456, -7.208316651077763204 ) ) ;
#8438=CARTESIAN_POINT ( 'NONE',  ( 0.6178305044545818747, 18.49863466993041428, -9.382169495545419124 ) ) ;
#8439=CARTESIAN_POINT ( 'NONE',  ( 17.96484262340118221, 54.93868534415484106, 7.964842623401181321 ) ) ;
#8440=CARTESIAN_POINT ( 'NONE',  ( -4.164238869374099039, 36.80374883491396787, 8.674139862899312516E-16 ) ) ;
#8442=CARTESIAN_POINT ( 'NONE',  ( 20.36894250292379738, 39.92874883491396787, -10.36894250292379027 ) ) ;
#8443=CARTESIAN_POINT ( 'NONE',  ( 17.08211943468705840, 55.13708216824731068, -12.26659068614894466 ) ) ;
#8444=CARTESIAN_POINT ( 'NONE',  ( 24.16423886937410614, 24.30374883491396787, 8.672049930838204340E-16 ) ) ;
#8445=CARTESIAN_POINT ( 'NONE',  ( 24.16423886937409904, 24.09541550158063927, 3.795296366450317205 ) ) ;
#8446=CARTESIAN_POINT ( 'NONE',  ( -0.1503990784575280903, 38.10158574516643171, 6.262539305110076171 ) ) ;
#8449=CARTESIAN_POINT ( 'NONE',  ( 7.361572987183169658, 39.96726448433411605, -9.846743663894592657 ) ) ;
#8451=CARTESIAN_POINT ( 'NONE',  ( -0.8801773607111008646, 23.27201867748817676, 2.915334737309923430 ) ) ;
#8453=CARTESIAN_POINT ( 'NONE',  ( 7.361572987183169658, 64.96726448433412315, -9.846743663894592657 ) ) ;
#8455=CARTESIAN_POINT ( 'NONE',  ( 19.67853978997394293, 88.18036594423148244, -5.461515559775651063 ) ) ;
#8456=CARTESIAN_POINT ( 'NONE',  ( 0.1532563361054100626, 45.80059781766745886, -2.638427012816831230 ) ) ;
#8457=CARTESIAN_POINT ( 'NONE',  ( -1.099225684535947600, 49.54030133659708923, 6.408140936763237150 ) ) ;
#8460=CARTESIAN_POINT ( 'NONE',  ( 5.076628168052703671, 36.84226448433412315, 8.527530157486179263 ) ) ;
#8461=CARTESIAN_POINT ( 'NONE',  ( 18.52753015748618282, 48.92559781766745886, -4.923371831947291888 ) ) ;
#8462=CARTESIAN_POINT ( 'NONE',  ( 22.26659068614894466, 43.88708216824729647, 7.082119434687054849 ) ) ;
#8463=ORIENTED_EDGE ( 'NONE', *, *, #88174, .T. ) ;
#8464=CARTESIAN_POINT ( 'NONE',  ( -4.164238869374099927, 17.01208216824730357, 3.795296366450308767 ) ) ;
#8465=CARTESIAN_POINT ( 'NONE',  ( 15.44008868035555260, 64.73035201082151957, 9.422509992056143702 ) ) ;
#8467=CARTESIAN_POINT ( 'NONE',  ( -0.8801773607111008646, 3.272018677488171434, 2.915334737309923430 ) ) ;
#8468=CARTESIAN_POINT ( 'NONE',  ( -1.099225684535947600, 14.54030133659708568, 6.408140936763237150 ) ) ;
#8469=AXIS2_PLACEMENT_3D ( 'NONE', #97882, #44349, #6354 ) ;
#8470=CARTESIAN_POINT ( 'NONE',  ( 20.24186590665274821, 1.760286857231739610, 6.114288769123088052 ) ) ;
#8471=CARTESIAN_POINT ( 'NONE',  ( 18.52753015748618282, 3.925597817667451306, -4.923371831947291888 ) ) ;
#8472=( GEOMETRIC_REPRESENTATION_CONTEXT ( 3 ) GLOBAL_UNCERTAINTY_ASSIGNED_CONTEXT ( ( #95505 ) ) GLOBAL_UNIT_ASSIGNED_CONTEXT ( ( #47072, #92092, #9085 ) ) REPRESENTATION_CONTEXT ( 'NONE', 'WORKASPACE' ) );
#8476=CARTESIAN_POINT ( 'NONE',  ( 13.79529636645031943, 65.34541550158063217, -14.16423886937409904 ) ) ;
#8478=CARTESIAN_POINT ( 'NONE',  ( 15.44008868035555260, 24.73035201082150891, 9.422509992056143702 ) ) ;
#8479=CARTESIAN_POINT ( 'NONE',  ( 17.96484262340118221, 26.18868534415483396, -7.964842623401177768 ) ) ;
#8481=CARTESIAN_POINT ( 'NONE',  ( 0.1532563361054082862, 56.21726448433411605, 2.638427012816831674 ) ) ;
#8482=CARTESIAN_POINT ( 'NONE',  ( 14.92337183194729633, 52.67559781766745175, 8.527530157486181039 ) ) ;
#8483=CARTESIAN_POINT ( 'NONE',  ( -2.816281873526473856, 59.33196800326374643, 3.434112377981055619 ) ) ;
#8484=CARTESIAN_POINT ( 'NONE',  ( 17.20831665107776587, 2.883931151000785231, 7.208316651077764980 ) ) ;
#8486=ORIENTED_EDGE ( 'NONE', *, *, #70639, .F. ) ;
#8487=CARTESIAN_POINT ( 'NONE',  ( 7.084665262690076126, 22.02201867748817321, -10.88017736071110164 ) ) ;
#8488=CARTESIAN_POINT ( 'NONE',  ( -2.816281873526473856, 19.33196800326375708, 3.434112377981055619 ) ) ;
#8491=CARTESIAN_POINT ( 'NONE',  ( 5.076628168052703671, 66.84226448433412315, 8.527530157486179263 ) ) ;
#8492=CARTESIAN_POINT ( 'NONE',  ( 17.96484262340118221, 51.18868534415483396, -7.964842623401177768 ) ) ;
#8494=CARTESIAN_POINT ( 'NONE',  ( -2.816281873526473856, 24.33196800326375353, 3.434112377981055619 ) ) ;
#8495=CARTESIAN_POINT ( 'NONE',  ( 0.5774900079438607392, 58.48035201082151247, 5.440088680355550821 ) ) ;
#8502=CARTESIAN_POINT ( 'NONE',  ( 10.00000000000000178, 49.31368534415484106, 10.88017736071110342 ) ) ;
#8503=CARTESIAN_POINT ( 'NONE',  ( 22.81628187352648496, 51.83196800326376064, -3.434112377981050290 ) ) ;
#8504=CARTESIAN_POINT ( 'NONE',  ( 6.204703633549690345, 17.84541550158063217, 14.16423886937410082 ) ) ;
#8505=CARTESIAN_POINT ( 'NONE',  ( 19.84674366389459266, 3.717264484334118713, -2.638427012816827677 ) ) ;
#8507=CARTESIAN_POINT ( 'NONE',  ( 19.84674366389459621, 23.50893115100078390, 7.409399052514197653E-17 ) ) ;
#8509=CARTESIAN_POINT ( 'NONE',  ( 2.917880565312950480, 55.97041550158063217, -12.26659068614894821 ) ) ;
#8510=FILL_AREA_STYLE_COLOUR ( '', #9071 ) ;
#8511=CARTESIAN_POINT ( 'NONE',  ( 7.084665262690076126, 7.022018677488169658, -10.88017736071110164 ) ) ;
#8514=ORIENTED_EDGE ( 'NONE', *, *, #46418, .T. ) ;
#8515=VECTOR ( 'NONE', #32395, 1000.000000000000000 ) ;
#8516=CARTESIAN_POINT ( 'NONE',  ( 19.42250999205614548, 10.98035201082150536, -5.440088680355545492 ) ) ;
#8517=CARTESIAN_POINT ( 'NONE',  ( 10.00000000000000178, 14.31368534415483929, 10.88017736071110342 ) ) ;
#8518=CARTESIAN_POINT ( 'NONE',  ( 7.361572987183170547, 37.05059781766744464, 9.846743663894590881 ) ) ;
#8519=CARTESIAN_POINT ( 'NONE',  ( -1.099225684535947600, 34.54030133659708923, 6.408140936763237150 ) ) ;
#8522=CARTESIAN_POINT ( 'NONE',  ( -0.3689425029237898834, 16.17874883491396076, -10.36894250292378850 ) ) ;
#8523=CARTESIAN_POINT ( 'NONE',  ( 0.5774900079438590739, 22.64701867748817321, -5.440088680355550821 ) ) ;
#8524=EDGE_CURVE ( 'NONE', #38545, #83562, #30665, .T. ) ;
#8525=CARTESIAN_POINT ( 'NONE',  ( -4.164238869374098151, 66.59541550158060375, -3.795296366450310543 ) ) ;
#8527=CARTESIAN_POINT ( 'NONE',  ( 5.076628168052703671, 41.84226448433411605, 8.527530157486179263 ) ) ;
#8529=CARTESIAN_POINT ( 'NONE',  ( 19.84674366389459266, 23.71726448433412315, -2.638427012816827677 ) ) ;
#8531=CARTESIAN_POINT ( 'NONE',  ( 0.1532563361054083140, 1.008931151000784787, 1.131784320476157264E-15 ) ) ;
#8534=SURFACE_STYLE_USAGE ( .BOTH. , #47503 ) ;
#8536=CARTESIAN_POINT ( 'NONE',  ( 17.20831665107776587, 62.88393115100078745, 7.208316651077764980 ) ) ;
#8537=CARTESIAN_POINT ( 'NONE',  ( 0.5774900079438590739, 27.64701867748817676, -5.440088680355550821 ) ) ;
#8538=CARTESIAN_POINT ( 'NONE',  ( 4.559911319644449179, 38.89701867748817676, 9.422509992056141925 ) ) ;
#8539=( LENGTH_UNIT ( ) NAMED_UNIT ( * ) SI_UNIT ( .MILLI., .METRE. ) );
#8540=CARTESIAN_POINT ( 'NONE',  ( -2.816281873526473856, 29.12363466993041783, 9.499525473075851096E-16 ) ) ;
#8541=CARTESIAN_POINT ( 'NONE',  ( 22.26659068614894466, 23.88708216824730357, 7.082119434687054849 ) ) ;
#8542=EDGE_CURVE ( 'NONE', #76182, #68558, #89953, .T. ) ;
#8544=CARTESIAN_POINT ( 'NONE',  ( 10.00000000000000000, 42.87363466993042493, -12.81628187352647608 ) ) ;
#8545=ORIENTED_EDGE ( 'NONE', *, *, #58920, .T. ) ;
#8547=CARTESIAN_POINT ( 'NONE',  ( 19.84674366389459266, 48.30059781766745175, 2.638427012816836559 ) ) ;
#8548=CARTESIAN_POINT ( 'NONE',  ( 12.91533473730993009, 26.60535201082150536, -10.88017736071109987 ) ) ;
#8550=CARTESIAN_POINT ( 'NONE',  ( 0.5774900079438607392, 23.48035201082150536, 5.440088680355550821 ) ) ;
#8551=ORIENTED_EDGE ( 'NONE', *, *, #76610, .T. ) ;
#8552=CARTESIAN_POINT ( 'NONE',  ( 15.44008868035555793, 56.39701867748817676, -9.422509992056140149 ) ) ;
#8553=CARTESIAN_POINT ( 'NONE',  ( 10.00000000000000178, 70.00000000000000000, 0.000000000000000000 ) ) ;
#8554=CARTESIAN_POINT ( 'NONE',  ( 2.035157376598824452, 68.68868534415484817, 7.964842623401179544 ) ) ;
#8555=CARTESIAN_POINT ( 'NONE',  ( 18.52753015748618282, 3.925597817667451306, -4.923371831947291888 ) ) ;
#8556=CARTESIAN_POINT ( 'NONE',  ( -0.8801773607111009756, 63.06368534415484106, 1.068504757029289695E-15 ) ) ;
#8558=CARTESIAN_POINT ( 'NONE',  ( -46.94000000000001194, 101.5930487410390270, 7.918115197747519929 ) ) ;
#8559=CARTESIAN_POINT ( 'NONE',  ( 10.00000000000000178, 12.25893115100078568, 9.846743663894594434 ) ) ;
#8561=CARTESIAN_POINT ( 'NONE',  ( 12.63842701281683922, 39.55059781766744464, -9.846743663894590881 ) ) ;
#8562=VERTEX_POINT ( 'NONE', #74953 ) ;
#8563=CARTESIAN_POINT ( 'NONE',  ( 19.72487221294571569, 19.78217586085237301, 6.499999999999990230 ) ) ;
#8564=CARTESIAN_POINT ( 'NONE',  ( 20.25387647958519821, 70.00000000000000000, -6.092576751097364074 ) ) ;
#8566=CARTESIAN_POINT ( 'NONE',  ( 6.204703633549690345, 15.76208216824730179, -14.16423886937410259 ) ) ;
#8569=CARTESIAN_POINT ( 'NONE',  ( 4.559911319644449179, 27.23035201082150536, -9.422509992056141925 ) ) ;
#8572=CARTESIAN_POINT ( 'NONE',  ( 1.472469842513823179, 6.425597817667451750, 4.923371831947296329 ) ) ;
#8573=CARTESIAN_POINT ( 'NONE',  ( 7.361572987183169658, -0.03273551566588185635, -9.846743663894592657 ) ) ;
#8574=CARTESIAN_POINT ( 'NONE',  ( 10.00000000000000178, 35.37363466993042493, 12.81628187352647608 ) ) ;
#8575=CARTESIAN_POINT ( 'NONE',  ( 2.791683348922240793, 26.63393115100078745, 7.208316651077764092 ) ) ;
#8578=CARTESIAN_POINT ( 'NONE',  ( 13.43411237798105340, 15.58196800326374998, 12.81628187352647963 ) ) ;
#8580=CARTESIAN_POINT ( 'NONE',  ( 7.361572987183169658, 4.967264484334119601, -9.846743663894592657 ) ) ;
#8583=CARTESIAN_POINT ( 'NONE',  ( 2.035157376598822676, 17.43868534415483751, -7.964842623401177768 ) ) ;
#8584=CARTESIAN_POINT ( 'NONE',  ( 17.08211943468705130, 13.47041550158063572, 12.26659068614894998 ) ) ;
#8585=CARTESIAN_POINT ( 'NONE',  ( 17.20831665107776587, 42.88393115100077324, 7.208316651077764980 ) ) ;
#8586=CARTESIAN_POINT ( 'NONE',  ( 20.88017736071110875, 65.77201867748817676, -2.915334737309920765 ) ) ;
#8587=CARTESIAN_POINT ( 'NONE',  ( -1.099225684535947600, 58.70696800326375353, -6.408140936763238038 ) ) ;
#8589=CARTESIAN_POINT ( 'NONE',  ( 4.559911319644449179, 22.23035201082150536, -9.422509992056141925 ) ) ;
#8591=CARTESIAN_POINT ( 'NONE',  ( 0.6178305044545838731, 14.74863466993041783, 9.382169495545420901 ) ) ;
#8592=CARTESIAN_POINT ( 'NONE',  ( 10.00000000000000178, 47.25893115100078745, 9.846743663894594434 ) ) ;
#8594=CARTESIAN_POINT ( 'NONE',  ( 16.40814093676324603, 42.45696800326375353, -11.09922568453594671 ) ) ;
#8596=CARTESIAN_POINT ( 'NONE',  ( 2.035157376598822676, 47.43868534415484817, -7.964842623401177768 ) ) ;
#8599=CARTESIAN_POINT ( 'NONE',  ( 10.00000000000000000, 56.81368534415484106, -10.88017736071110342 ) ) ;
#8600=CARTESIAN_POINT ( 'NONE',  ( 10.00000000000000000, 46.81368534415484106, -10.88017736071110342 ) ) ;
#8603=CARTESIAN_POINT ( 'NONE',  ( 4.559911319644449179, 67.23035201082150536, -9.422509992056141925 ) ) ;
#8606=CARTESIAN_POINT ( 'NONE',  ( 0.1532563361054083140, 56.00893115100078745, 1.131784320476157264E-15 ) ) ;
#8607=CARTESIAN_POINT ( 'NONE',  ( 0.5774900079438607392, 28.48035201082150891, 5.440088680355550821 ) ) ;
#8609=CARTESIAN_POINT ( 'NONE',  ( 0.6178305044545838731, 19.74863466993042138, 9.382169495545420901 ) ) ;
#8611=CARTESIAN_POINT ( 'NONE',  ( -0.8801773607110991993, 42.85535201082150536, -2.915334737309923874 ) ) ;
#8613=CARTESIAN_POINT ( 'NONE',  ( 6.565887622018943937, 10.16530133659708746, 12.81628187352647430 ) ) ;
#8614=CARTESIAN_POINT ( 'NONE',  ( 0.2751277870542914172, 23.21833443783937767, 6.499999999999992006 ) ) ;
#8615=CARTESIAN_POINT ( 'NONE',  ( 7.084665262690076126, 12.02201867748817143, -10.88017736071110164 ) ) ;
#8616=CARTESIAN_POINT ( 'NONE',  ( 20.88017736071110519, 30.56368534415484106, 2.639326808657452039E-16 ) ) ;
#8617=CARTESIAN_POINT ( 'NONE',  ( 17.08211943468705130, 38.47041550158063217, 12.26659068614894998 ) ) ;
#8618=CARTESIAN_POINT ( 'NONE',  ( 19.84674366389459621, 28.50893115100078745, 7.409399052514197653E-17 ) ) ;
#8619=CARTESIAN_POINT ( 'NONE',  ( 7.084665262690076126, 57.02201867748817676, -10.88017736071110164 ) ) ;
#8621=CARTESIAN_POINT ( 'NONE',  ( -4.164238869374099039, 6.803748834913967869, 8.674139862899312516E-16 ) ) ;
#8623=CARTESIAN_POINT ( 'NONE',  ( 10.00000000000000000, 54.75893115100078745, -9.846743663894594434 ) ) ;
#8626=CARTESIAN_POINT ( 'NONE',  ( 10.00000000000000000, 30.55374883491397142, -14.16423886937410082 ) ) ;
#8627=CARTESIAN_POINT ( 'NONE',  ( -2.266590686148945544, 36.38708216824730357, -7.082119434687050408 ) ) ;
#8628=CARTESIAN_POINT ( 'NONE',  ( 18.52753015748618282, 3.925597817667451306, -4.923371831947291888 ) ) ;
#8629=CARTESIAN_POINT ( 'NONE',  ( 7.361572987183169658, 59.96726448433410894, -9.846743663894592657 ) ) ;
#8631=CARTESIAN_POINT ( 'NONE',  ( 10.00000000000000178, 59.31368534415484106, 10.88017736071110342 ) ) ;
#8632=CARTESIAN_POINT ( 'NONE',  ( -2.816281873526473856, 24.12363466993042138, 9.499525473075851096E-16 ) ) ;
#8633=CARTESIAN_POINT ( 'NONE',  ( -0.3689425029237898834, 36.17874883491396787, -10.36894250292378850 ) ) ;
#8634=CARTESIAN_POINT ( 'NONE',  ( -0.8801773607111009756, 23.06368534415484106, 1.068504757029289695E-15 ) ) ;
#8635=CARTESIAN_POINT ( 'NONE',  ( 19.42250999205614193, 35.14701867748816966, 5.440088680355555262 ) ) ;
#8637=CARTESIAN_POINT ( 'NONE',  ( 4.559911319644449179, 52.23035201082151247, -9.422509992056141925 ) ) ;
#8641=ORIENTED_EDGE ( 'NONE', *, *, #95637, .T. ) ;
#8644=CARTESIAN_POINT ( 'NONE',  ( -0.3689425029237898834, 1.178748834913967869, -10.36894250292378850 ) ) ;
#8645=CARTESIAN_POINT ( 'NONE',  ( 22.26659068614895176, 54.72041550158063217, -7.082119434687042414 ) ) ;
#8646=CARTESIAN_POINT ( 'NONE',  ( 4.559911319644449179, 2.230352010821504916, -9.422509992056141925 ) ) ;
#8647=CARTESIAN_POINT ( 'NONE',  ( 10.00000000000000000, 39.75893115100078745, -9.846743663894594434 ) ) ;
#8648=CARTESIAN_POINT ( 'NONE',  ( 1.472469842513823179, 65.59226448433412315, -4.923371831947296329 ) ) ;
#8650=CARTESIAN_POINT ( 'NONE',  ( -2.816281873526473856, 9.331968003263753531, 3.434112377981055619 ) ) ;
#8652=CARTESIAN_POINT ( 'NONE',  ( 6.204703633549690345, 45.76208216824729647, -14.16423886937410259 ) ) ;
#8653=CARTESIAN_POINT ( 'NONE',  ( -2.266590686148945544, 42.22041550158063217, 7.082119434687048631 ) ) ;
#8654=ORIENTED_EDGE ( 'NONE', *, *, #42653, .T. ) ;
#8655=CARTESIAN_POINT ( 'NONE',  ( 2.035157376598822676, 17.43868534415483751, -7.964842623401177768 ) ) ;
#8656=CARTESIAN_POINT ( 'NONE',  ( 16.40814093676324603, 57.45696800326375353, -11.09922568453594671 ) ) ;
#8657=CARTESIAN_POINT ( 'NONE',  ( 17.96484262340118221, 26.18868534415483396, -7.964842623401177768 ) ) ;
#8658=CARTESIAN_POINT ( 'NONE',  ( 18.52753015748617571, 48.09226448433412315, 4.923371831947298993 ) ) ;
#8659=CARTESIAN_POINT ( 'NONE',  ( 12.91533473730993009, 21.60535201082150536, -10.88017736071109987 ) ) ;
#8661=CARTESIAN_POINT ( 'NONE',  ( 7.361572987183170547, 57.05059781766744464, 9.846743663894590881 ) ) ;
#8663=CARTESIAN_POINT ( 'NONE',  ( 15.44008868035555793, 31.39701867748817676, -9.422509992056140149 ) ) ;
#8668=SURFACE_STYLE_USAGE ( .BOTH. , #16179 ) ;
#8672=CARTESIAN_POINT ( 'NONE',  ( 19.84674366389459266, 33.30059781766744464, 2.638427012816836559 ) ) ;
#8674=CARTESIAN_POINT ( 'NONE',  ( -2.816281873526471635, 48.91530133659708213, -3.434112377981056508 ) ) ;
#8675=DIRECTION ( 'NONE',  ( 0.000000000000000000, 0.000000000000000000, -1.000000000000000000 ) ) ;
#8680=CARTESIAN_POINT ( 'NONE',  ( 2.791683348922237240, 60.38393115100078745, -7.208316651077763204 ) ) ;
#8681=CARTESIAN_POINT ( 'NONE',  ( -2.266590686148945544, 52.22041550158064638, 7.082119434687048631 ) ) ;
#8682=CARTESIAN_POINT ( 'NONE',  ( 17.20831665107776587, 57.88393115100078745, 7.208316651077764980 ) ) ;
#8683=CARTESIAN_POINT ( 'NONE',  ( 12.63842701281683922, 19.55059781766745175, -9.846743663894590881 ) ) ;
#8684=CARTESIAN_POINT ( 'NONE',  ( 16.40814093676323893, 55.79030133659708923, 11.09922568453595026 ) ) ;
#8685=CARTESIAN_POINT ( 'NONE',  ( 7.361572987183170547, 62.05059781766745886, 9.846743663894590881 ) ) ;
#8686=CARTESIAN_POINT ( 'NONE',  ( 20.88017736071110875, 55.77201867748816966, -2.915334737309920765 ) ) ;
#8688=CARTESIAN_POINT ( 'NONE',  ( 12.63842701281683922, 44.55059781766745175, -9.846743663894590881 ) ) ;
#8690=CARTESIAN_POINT ( 'NONE',  ( 2.035157376598824452, 53.68868534415484817, 7.964842623401179544 ) ) ;
#8693=CARTESIAN_POINT ( 'NONE',  ( 20.88017736071110519, 30.56368534415484106, 2.639326808657452039E-16 ) ) ;
#8694=CARTESIAN_POINT ( 'NONE',  ( -2.816281873526473856, 4.123634669930420493, 9.499525473075851096E-16 ) ) ;
#8695=CARTESIAN_POINT ( 'NONE',  ( 12.91533473730993009, 51.60535201082149825, -10.88017736071109987 ) ) ;
#8697=CARTESIAN_POINT ( 'NONE',  ( 7.084665262690076126, 67.02201867748817676, -10.88017736071110164 ) ) ;
#8699=CARTESIAN_POINT ( 'NONE',  ( 7.084665262690076126, 37.02201867748817676, -10.88017736071110164 ) ) ;
#8700=CARTESIAN_POINT ( 'NONE',  ( -0.1503990784575247319, 62.22266099184918176, -6.262539305110083276 ) ) ;
#8701=CARTESIAN_POINT ( 'NONE',  ( 19.84674366389459266, 38.30059781766745175, 2.638427012816836559 ) ) ;
#8702=CARTESIAN_POINT ( 'NONE',  ( 19.84674366389459266, 3.300597817667451750, 2.638427012816836559 ) ) ;
#8704=CARTESIAN_POINT ( 'NONE',  ( -2.816281873526471635, 13.91530133659708746, -3.434112377981056508 ) ) ;
#8705=CARTESIAN_POINT ( 'NONE',  ( 0.5774900079438590739, 17.64701867748817321, -5.440088680355550821 ) ) ;
#8706=( NAMED_UNIT ( * ) SI_UNIT ( $, .STERADIAN. ) SOLID_ANGLE_UNIT ( ) );
#8708=CARTESIAN_POINT ( 'NONE',  ( -0.3689425029237898834, 21.17874883491396432, -10.36894250292378850 ) ) ;
#8709=CARTESIAN_POINT ( 'NONE',  ( 10.00000000000000178, 63.05374883491396076, 14.16423886937410082 ) ) ;
#8710=CARTESIAN_POINT ( 'NONE',  ( 14.92337183194729988, 14.34226448433411782, -8.527530157486177487 ) ) ;
#8711=SURFACE_STYLE_USAGE ( .BOTH. , #77206 ) ;
#8713=CARTESIAN_POINT ( 'NONE',  ( 0.1532563361054082862, 21.21726448433412315, 2.638427012816831674 ) ) ;
#8714=EDGE_CURVE ( 'NONE', #93646, #32106, #89848, .T. ) ;
#8715=CARTESIAN_POINT ( 'NONE',  ( 20.88017736071110875, 20.77201867748816611, -2.915334737309920765 ) ) ;
#8716=CARTESIAN_POINT ( 'NONE',  ( 0.1532563361054100626, 60.80059781766744464, -2.638427012816831230 ) ) ;
#8717=CARTESIAN_POINT ( 'NONE',  ( 17.08211943468705840, 5.137082168247300906, -12.26659068614894466 ) ) ;
#8720=CARTESIAN_POINT ( 'NONE',  ( 18.52753015748618282, 13.92559781766745175, -4.923371831947291888 ) ) ;
#8721=CARTESIAN_POINT ( 'NONE',  ( 19.38216949554541557, 37.24863466993041783, -9.382169495545420901 ) ) ;
#8722=CARTESIAN_POINT ( 'NONE',  ( 19.84674366389459266, 43.30059781766744464, 2.638427012816836559 ) ) ;
#8724=CARTESIAN_POINT ( 'NONE',  ( 10.00000000000000178, 17.25893115100078745, 9.846743663894594434 ) ) ;
#8725=CARTESIAN_POINT ( 'NONE',  ( 2.603489959281592991, 11.58210964143329313, 6.500000000000006217 ) ) ;
#8726=CARTESIAN_POINT ( 'NONE',  ( 2.917880565312948704, 47.63708216824730357, 12.26659068614894643 ) ) ;
#8727=CARTESIAN_POINT ( 'NONE',  ( 15.44008868035555260, 49.73035201082150536, 9.422509992056143702 ) ) ;
#8728=CARTESIAN_POINT ( 'NONE',  ( -0.04068437667224335946, 32.21974360917720759, -6.396802510829702193 ) ) ;
#8729=CARTESIAN_POINT ( 'NONE',  ( 12.91533473730993009, 56.60535201082151247, -10.88017736071109987 ) ) ;
#8730=CARTESIAN_POINT ( 'NONE',  ( 5.076628168052703671, 31.84226448433412315, 8.527530157486179263 ) ) ;
#8731=CARTESIAN_POINT ( 'NONE',  ( 12.91533473730992121, 14.52201867748817143, 10.88017736071110164 ) ) ;
#8733=CARTESIAN_POINT ( 'NONE',  ( 1.472469842513823179, 55.59226448433412315, -4.923371831947296329 ) ) ;
#8734=CARTESIAN_POINT ( 'NONE',  ( 7.084665262690076126, 47.02201867748818387, -10.88017736071110164 ) ) ;
#8735=CARTESIAN_POINT ( 'NONE',  ( 5.076628168052704559, 0.1755978176674514724, -8.527530157486179263 ) ) ;
#8740=CARTESIAN_POINT ( 'NONE',  ( 18.52753015748618282, 43.92559781766745175, -4.923371831947291888 ) ) ;
#8741=CARTESIAN_POINT ( 'NONE',  ( 1.472469842513823179, 21.42559781766745175, 4.923371831947296329 ) ) ;
#8742=CARTESIAN_POINT ( 'NONE',  ( 13.43411237798106583, 57.66530133659708923, -12.81628187352647252 ) ) ;
#8743=CARTESIAN_POINT ( 'NONE',  ( 0.5774900079438590739, 22.64701867748817321, -5.440088680355550821 ) ) ;
#8744=CARTESIAN_POINT ( 'NONE',  ( 18.52753015748617571, 53.09226448433412315, 4.923371831947298993 ) ) ;
#8747=CARTESIAN_POINT ( 'NONE',  ( -2.266590686148945544, 27.22041550158063572, 7.082119434687048631 ) ) ;
#8749=CARTESIAN_POINT ( 'NONE',  ( 22.26659068614895176, 54.72041550158063217, -7.082119434687042414 ) ) ;
#8750=CARTESIAN_POINT ( 'NONE',  ( 19.84674366389459266, 63.30059781766745886, 2.638427012816836559 ) ) ;
#8752=CARTESIAN_POINT ( 'NONE',  ( 20.88017736071110519, 50.56368534415484106, 2.639326808657452039E-16 ) ) ;
#8754=CARTESIAN_POINT ( 'NONE',  ( 17.20831665107776587, 9.133931151000787452, -7.208316651077762316 ) ) ;
#8756=EDGE_CURVE ( 'NONE', #80446, #51688, #61650, .T. ) ;
#8758=DIRECTION ( 'NONE',  ( 0.000000000000000000, 0.000000000000000000, -1.000000000000000000 ) ) ;
#8761=CARTESIAN_POINT ( 'NONE',  ( 7.361572987183169658, 14.96726448433411960, -9.846743663894592657 ) ) ;
#8763=CARTESIAN_POINT ( 'NONE',  ( 24.16423886937410614, 14.30374883491396787, 8.672049930838204340E-16 ) ) ;
#8764=CARTESIAN_POINT ( 'NONE',  ( 14.92337183194729988, 14.34226448433411782, -8.527530157486177487 ) ) ;
#8765=CARTESIAN_POINT ( 'NONE',  ( 2.035157376598822676, 42.43868534415483396, -7.964842623401177768 ) ) ;
#8769=CARTESIAN_POINT ( 'NONE',  ( 20.88017736071110519, 25.56368534415483751, 2.639326808657452039E-16 ) ) ;
#8773=CARTESIAN_POINT ( 'NONE',  ( 6.204703633549690345, 7.845415501580634832, 14.16423886937410082 ) ) ;
#8775=CARTESIAN_POINT ( 'NONE',  ( -2.816281873526473856, 24.33196800326375353, 3.434112377981055619 ) ) ;
#8776=CARTESIAN_POINT ( 'NONE',  ( 14.92337183194729633, 12.67559781766745353, 8.527530157486181039 ) ) ;
#8779=CARTESIAN_POINT ( 'NONE',  ( 12.63842701281683922, 19.55059781766745175, -9.846743663894590881 ) ) ;
#8780=CARTESIAN_POINT ( 'NONE',  ( -0.8801773607111009756, 28.06368534415484106, 1.068504757029289695E-15 ) ) ;
#8782=ORIENTED_EDGE ( 'NONE', *, *, #22584, .F. ) ;
#8784=CARTESIAN_POINT ( 'NONE',  ( 19.42250999205614548, 55.98035201082150536, -5.440088680355545492 ) ) ;
#8787=CARTESIAN_POINT ( 'NONE',  ( 7.084665262690076126, 67.02201867748817676, -10.88017736071110164 ) ) ;
#8788=CARTESIAN_POINT ( 'NONE',  ( 21.09922568453595559, 17.04030133659708923, -6.408140936763230044 ) ) ;
#8789=B_SPLINE_CURVE_WITH_KNOTS ( 'NONE', 3,
 ( #9844, #69362, #32326, #46842, #883, #85341 ),
 .UNSPECIFIED., .F., .F.,
 ( 4, 2, 4 ),
 ( 0.000000000000000000, 0.0002496607219482335272, 0.0004993214438964670545 ),
 .UNSPECIFIED. ) ;
#8791=DIRECTION ( 'NONE',  ( -0.000000000000000000, -1.000000000000000000, -0.000000000000000000 ) ) ;
#8792=CARTESIAN_POINT ( 'NONE',  ( 19.84674366389459621, 28.50893115100078745, 7.409399052514197653E-17 ) ) ;
#8793=CARTESIAN_POINT ( 'NONE',  ( 21.09922568453594849, 56.20696800326375353, 6.408140936763242479 ) ) ;
#8794=CARTESIAN_POINT ( 'NONE',  ( 1.821708436314968482, 36.66792564121895026, -6.500000000000079936 ) ) ;
#8795=CARTESIAN_POINT ( 'NONE',  ( 19.84674366389459621, 18.50893115100078745, 7.409399052514197653E-17 ) ) ;
#8796=CARTESIAN_POINT ( 'NONE',  ( 0.6178305044545818747, 23.49863466993041783, -9.382169495545419124 ) ) ;
#8800=CARTESIAN_POINT ( 'NONE',  ( 20.88017736071110164, 55.35535201082149825, 2.915334737309930979 ) ) ;
#8801=CARTESIAN_POINT ( 'NONE',  ( 2.791683348922240793, 56.63393115100078035, 7.208316651077764092 ) ) ;
#8803=CARTESIAN_POINT ( 'NONE',  ( 12.63842701281683922, 29.55059781766745175, -9.846743663894590881 ) ) ;
#8804=CARTESIAN_POINT ( 'NONE',  ( 14.92337183194729633, 17.67559781766745175, 8.527530157486181039 ) ) ;
#8805=CARTESIAN_POINT ( 'NONE',  ( 12.91533473730992121, 9.522018677488171434, 10.88017736071110164 ) ) ;
#8806=EDGE_CURVE ( 'NONE', #31975, #10378, #36715, .T. ) ;
#8807=CARTESIAN_POINT ( 'NONE',  ( -1.099225684535947600, 14.54030133659708568, 6.408140936763237150 ) ) ;
#8808=CARTESIAN_POINT ( 'NONE',  ( -0.8801773607111008646, 3.272018677488171434, 2.915334737309923430 ) ) ;
#8809=CARTESIAN_POINT ( 'NONE',  ( 0.000000000000000000, 81.99999999999992895, 5.000000000000000000 ) ) ;
#8811=CARTESIAN_POINT ( 'NONE',  ( 2.035157376598824452, 18.68868534415484106, 7.964842623401179544 ) ) ;
#8815=CARTESIAN_POINT ( 'NONE',  ( 19.84674366389459266, 23.71726448433412315, -2.638427012816827677 ) ) ;
#8816=CARTESIAN_POINT ( 'NONE',  ( 17.96484262340118221, 11.18868534415484106, -7.964842623401177768 ) ) ;
#8817=CARTESIAN_POINT ( 'NONE',  ( 7.084665262690076126, 37.02201867748817676, -10.88017736071110164 ) ) ;
#8818=CARTESIAN_POINT ( 'NONE',  ( -0.3689425029237881626, 67.42874883491396076, 10.36894250292379027 ) ) ;
#8819=CARTESIAN_POINT ( 'NONE',  ( 1.046131998950050601, 40.73810908735726599, 6.499999999999992006 ) ) ;
#8820=CARTESIAN_POINT ( 'NONE',  ( 1.472469842513823179, 1.425597817667451528, 4.923371831947296329 ) ) ;
#8821=CARTESIAN_POINT ( 'NONE',  ( 0.1532563361054100626, 35.80059781766745175, -2.638427012816831230 ) ) ;
#8822=DIRECTION ( 'NONE',  ( 2.478176394252579169E-16, -1.000000000000000000, 0.000000000000000000 ) ) ;
#8826=CARTESIAN_POINT ( 'NONE',  ( 24.16423886937410614, 24.30374883491396787, 8.672049930838204340E-16 ) ) ;
#8827=CARTESIAN_POINT ( 'NONE',  ( 7.361572987183169658, 39.96726448433411605, -9.846743663894592657 ) ) ;
#8828=DIRECTION ( 'NONE',  ( 0.000000000000000000, 0.000000000000000000, -1.000000000000000000 ) ) ;
#8831=CARTESIAN_POINT ( 'NONE',  ( 22.26659068614894466, 48.88708216824730357, 7.082119434687054849 ) ) ;
#8832=CARTESIAN_POINT ( 'NONE',  ( 10.00000000000000000, 24.75893115100078745, -9.846743663894594434 ) ) ;
#8835=CARTESIAN_POINT ( 'NONE',  ( -0.8801773607110991993, 42.85535201082150536, -2.915334737309923874 ) ) ;
#8836=CARTESIAN_POINT ( 'NONE',  ( 13.43411237798106583, 57.66530133659708923, -12.81628187352647252 ) ) ;
#8837=CARTESIAN_POINT ( 'NONE',  ( 17.96484262340118221, 19.93868534415484106, 7.964842623401181321 ) ) ;
#8838=CARTESIAN_POINT ( 'NONE',  ( 6.565887622018943937, 53.08196800326374643, -12.81628187352647608 ) ) ;
#8839=CARTESIAN_POINT ( 'NONE',  ( 18.52753015748617571, 63.09226448433412315, 4.923371831947298993 ) ) ;
#8843=CARTESIAN_POINT ( 'NONE',  ( -0.1503990784575328643, 20.12777174578613071, 6.262539305110068177 ) ) ;
#8844=CARTESIAN_POINT ( 'NONE',  ( 10.00000000000000178, 48.05374883491396787, 14.16423886937410082 ) ) ;
#8845=CARTESIAN_POINT ( 'NONE',  ( 20.36894250292379382, 8.678748834913967869, 10.36894250292379205 ) ) ;
#8846=CARTESIAN_POINT ( 'NONE',  ( 15.44008868035555260, 24.73035201082150891, 9.422509992056143702 ) ) ;
#8847=CARTESIAN_POINT ( 'NONE',  ( 0.5774900079438590739, 42.64701867748816966, -5.440088680355550821 ) ) ;
#8850=CARTESIAN_POINT ( 'NONE',  ( 10.00000000000000178, 69.31368534415484817, 10.88017736071110342 ) ) ;
#8851=CARTESIAN_POINT ( 'NONE',  ( 19.42250999205614193, 60.14701867748817676, 5.440088680355555262 ) ) ;
#8852=CARTESIAN_POINT ( 'NONE',  ( 1.472469842513823179, 26.42559781766745175, 4.923371831947296329 ) ) ;
#8854=CARTESIAN_POINT ( 'NONE',  ( 17.20831665107776587, 12.88393115100078390, 7.208316651077764980 ) ) ;
#8855=CARTESIAN_POINT ( 'NONE',  ( 10.00000000000000000, 34.75893115100078745, -9.846743663894594434 ) ) ;
#8857=CARTESIAN_POINT ( 'NONE',  ( -0.8801773607111008646, 8.272018677488171434, 2.915334737309923430 ) ) ;
#8858=CARTESIAN_POINT ( 'NONE',  ( 0.6178305044545818747, 28.49863466993041783, -9.382169495545419124 ) ) ;
#8860=CARTESIAN_POINT ( 'NONE',  ( 1.472469842513823179, 6.425597817667451750, 4.923371831947296329 ) ) ;
#8862=CARTESIAN_POINT ( 'NONE',  ( 17.20831665107776587, 47.88393115100078745, 7.208316651077764980 ) ) ;
#8863=CARTESIAN_POINT ( 'NONE',  ( 14.92337183194729633, 32.67559781766745175, 8.527530157486181039 ) ) ;
#8864=CARTESIAN_POINT ( 'NONE',  ( -4.164238869374098151, 16.59541550158063927, -3.795296366450310543 ) ) ;
#8865=CARTESIAN_POINT ( 'NONE',  ( 7.084665262690076126, 52.02201867748816255, -10.88017736071110164 ) ) ;
#8866=CARTESIAN_POINT ( 'NONE',  ( 7.084665262690076126, 9.105352010821503583, 10.88017736071109987 ) ) ;
#8867=CARTESIAN_POINT ( 'NONE',  ( 12.91533473730993009, 51.60535201082149825, -10.88017736071109987 ) ) ;
#8868=CARTESIAN_POINT ( 'NONE',  ( 15.44008868035555793, 36.39701867748816966, -9.422509992056140149 ) ) ;
#8870=CARTESIAN_POINT ( 'NONE',  ( 12.91533473730993009, 41.60535201082149825, -10.88017736071109987 ) ) ;
#8872=CARTESIAN_POINT ( 'NONE',  ( 0.6178305044545838731, 54.74863466993042493, 9.382169495545420901 ) ) ;
#8874=CARTESIAN_POINT ( 'NONE',  ( 20.88017736071110164, 50.35535201082151247, 2.915334737309930979 ) ) ;
#8876=ORIENTED_EDGE ( 'NONE', *, *, #68114, .T. ) ;
#8877=CARTESIAN_POINT ( 'NONE',  ( 15.44008868035555260, 49.73035201082150536, 9.422509992056143702 ) ) ;
#8878=FILL_AREA_STYLE ('',( #91394 ) ) ;
#8879=CARTESIAN_POINT ( 'NONE',  ( 1.383448333479224024, 27.37718327197428891, -6.499999999999968026 ) ) ;
#8881=CARTESIAN_POINT ( 'NONE',  ( 2.917880565312950480, 60.97041550158063927, -12.26659068614894821 ) ) ;
#8882=CARTESIAN_POINT ( 'NONE',  ( 10.00000000000000000, 61.81368534415484106, -10.88017736071110342 ) ) ;
#8884=CARTESIAN_POINT ( 'NONE',  ( 13.79529636645031943, 5.345415501580634832, -14.16423886937409904 ) ) ;
#8886=FILL_AREA_STYLE_COLOUR ( '', #3066 ) ;
#8887=CARTESIAN_POINT ( 'NONE',  ( 2.035157376598824452, 13.68868534415483751, 7.964842623401179544 ) ) ;
#8888=CARTESIAN_POINT ( 'NONE',  ( 18.52753015748618282, 33.92559781766745886, -4.923371831947291888 ) ) ;
#8889=ORIENTED_EDGE ( 'NONE', *, *, #86910, .F. ) ;
#8890=CARTESIAN_POINT ( 'NONE',  ( 7.361572987183170547, 32.05059781766745175, 9.846743663894590881 ) ) ;
#8891=CARTESIAN_POINT ( 'NONE',  ( 20.88017736071110164, 35.35535201082150536, 2.915334737309930979 ) ) ;
#8892=CARTESIAN_POINT ( 'NONE',  ( 1.472469842513823179, 41.42559781766745886, 4.923371831947296329 ) ) ;
#8893=CARTESIAN_POINT ( 'NONE',  ( 21.09922568453595559, 17.04030133659708923, -6.408140936763230044 ) ) ;
#8895=CARTESIAN_POINT ( 'NONE',  ( -0.8801773607110991993, 52.85535201082151247, -2.915334737309923874 ) ) ;
#8896=CARTESIAN_POINT ( 'NONE',  ( 2.917880565312948704, 57.63708216824731068, 12.26659068614894643 ) ) ;
#8898=CARTESIAN_POINT ( 'NONE',  ( 16.40814093676323893, 15.79030133659708746, 11.09922568453595026 ) ) ;
#8901=CARTESIAN_POINT ( 'NONE',  ( 3.591859063236761518, 29.95696800326375708, 11.09922568453594849 ) ) ;
#8902=CARTESIAN_POINT ( 'NONE',  ( -0.8801773607111009756, 23.06368534415484106, 1.068504757029289695E-15 ) ) ;
#8904=ORIENTED_EDGE ( 'NONE', *, *, #91447, .T. ) ;
#8907=CARTESIAN_POINT ( 'NONE',  ( 19.84674366389459621, 3.508931151000785231, 7.409399052514197653E-17 ) ) ;
#8908=CARTESIAN_POINT ( 'NONE',  ( 19.84674366389459266, 43.71726448433410894, -2.638427012816827677 ) ) ;
#8909=CARTESIAN_POINT ( 'NONE',  ( 10.00000000000000178, 42.25893115100078745, 9.846743663894594434 ) ) ;
#8911=CARTESIAN_POINT ( 'NONE',  ( 19.39235739573469530, 14.87576471608601203, 6.499999999999995559 ) ) ;
#8912=CARTESIAN_POINT ( 'NONE',  ( 10.00000000000000178, 27.25893115100078390, 9.846743663894594434 ) ) ;
#8916=CARTESIAN_POINT ( 'NONE',  ( 19.84674366389459621, 8.508931151000785675, 7.409399052514197653E-17 ) ) ;
#8920=CARTESIAN_POINT ( 'NONE',  ( 7.361572987183169658, 39.96726448433411605, -9.846743663894592657 ) ) ;
#8922=DIRECTION ( 'NONE',  ( 1.000000000000000000, -0.000000000000000000, -0.000000000000000000 ) ) ;
#8923=CARTESIAN_POINT ( 'NONE',  ( 21.09922568453594849, 6.206968003263753531, 6.408140936763242479 ) ) ;
#8925=CARTESIAN_POINT ( 'NONE',  ( 20.88017736071110164, 50.35535201082151247, 2.915334737309930979 ) ) ;
#8926=CARTESIAN_POINT ( 'NONE',  ( 2.917880565312948704, 52.63708216824730357, 12.26659068614894643 ) ) ;
#8930=CARTESIAN_POINT ( 'NONE',  ( -4.164238869374098151, 46.59541550158063927, -3.795296366450310543 ) ) ;
#8931=CARTESIAN_POINT ( 'NONE',  ( 24.16423886937409904, 59.09541550158063217, 3.795296366450317205 ) ) ;
#8932=CARTESIAN_POINT ( 'NONE',  ( -0.3689425029237898834, 26.17874883491396432, -10.36894250292378850 ) ) ;
#8933=CARTESIAN_POINT ( 'NONE',  ( -4.164238869374099927, 22.01208216824730357, 3.795296366450308767 ) ) ;
#8936=CARTESIAN_POINT ( 'NONE',  ( 1.472469842513823179, 36.42559781766745175, 4.923371831947296329 ) ) ;
#8938=CARTESIAN_POINT ( 'NONE',  ( -0.8801773607111009756, 43.06368534415484106, 1.068504757029289695E-15 ) ) ;
#8939=CARTESIAN_POINT ( 'NONE',  ( 20.10239578412225470, 22.63377557478296964, -6.340343622311920058 ) ) ;
#8941=CARTESIAN_POINT ( 'NONE',  ( 1.472469842513823179, 40.59226448433411605, -4.923371831947296329 ) ) ;
#8942=CARTESIAN_POINT ( 'NONE',  ( -2.816281873526471635, 58.91530133659707502, -3.434112377981056508 ) ) ;
#8945=CARTESIAN_POINT ( 'NONE',  ( 0.1532563361054100626, 35.80059781766745175, -2.638427012816831230 ) ) ;
#8946=CARTESIAN_POINT ( 'NONE',  ( 19.84674366389459621, 63.50893115100078745, 7.409399052514197653E-17 ) ) ;
#8947=COLOUR_RGB ( '', 0.66274510, 0.83137255, 0.94901961) ;
#8948=CARTESIAN_POINT ( 'NONE',  ( 24.16423886937409904, 34.09541550158064638, 3.795296366450317205 ) ) ;
#8950=CARTESIAN_POINT ( 'NONE',  ( -2.266590686148945544, 11.38708216824730179, -7.082119434687050408 ) ) ;
#8951=VECTOR ( 'NONE', #28893, 1000.000000000000000 ) ;
#8952=CARTESIAN_POINT ( 'NONE',  ( 0.1922240491738397838, 68.18878173731741299, 6.499999999999944933 ) ) ;
#8954=CARTESIAN_POINT ( 'NONE',  ( 19.42250999205614193, 10.14701867748816966, 5.440088680355555262 ) ) ;
#8955=CARTESIAN_POINT ( 'NONE',  ( 3.591859063236763294, 13.29030133659708746, -11.09922568453595026 ) ) ;
#8957=CARTESIAN_POINT ( 'NONE',  ( 0.1532563361054100626, 0.8005978176674514168, -2.638427012816831230 ) ) ;
#8958=ADVANCED_FACE ( 'NONE', ( #86405 ), #92905, .T. ) ;
#8959=CARTESIAN_POINT ( 'NONE',  ( 0.2751277870542980231, 14.36607318730130878, -6.500000000000002665 ) ) ;
#8960=DIRECTION ( 'NONE',  ( 0.000000000000000000, 0.000000000000000000, 1.000000000000000000 ) ) ;
#8961=CARTESIAN_POINT ( 'NONE',  ( 22.26659068614895176, 64.72041550158064638, -7.082119434687042414 ) ) ;
#8963=( BOUNDED_SURFACE ( )  B_SPLINE_SURFACE ( 1, 2, ( 
 ( #23671, #9134, #93615, #8644, #47628, #92146, #86127, #17640, #63600, #31628, #70142, #25633, #2653, #62119, #40132, #24644, #77135, #1663, #86618, #48601, #32112, #62610, #33105, #94105, #92627, #78622, #54133, #84646, #39154, #10133, #55113, #18129, #56123, #85631, #78124, #9634, #70632, #79105, #10617, #69159, #16149, #46633, #69644, #24150, #54618, #85139, #80587, #58066, #34082, #42110, #72572, #65065, #50578, #12082, #87583, #11105, #41129, #73067, #28065, #4603, #65563, #96089, #81073, #12576, #5084, #20581, #64083, #35571, #58562, #89067, #51066, #64573, #91035, #98078, #29047, #97095, #21072, #51570, #15072, #97587, #83052, #29537, #37068, #82056, #28566, #52062, #82557, #14572, #90051, #21574, #74556, #45541, #75049, #90540, #13065, #6558, #36573, #45039, #67566, #74055, #75548, #7064, #68055, #30034, #26912, #34400, #64888, #51392, #41941, #57408, #43390, #12400, #49907, #13391, #5418, #96417, #87415, #95920, #4917, #58380, #80906, #81879, #73887, #43874, #20409, #87900, #35888, #73389, #42906, #50895, #72404, #66384, #65394, #27400, #88900, #64408, #3442, #72898, #81390, #57892, #19415, #89389, #88407, #96918, #28394, #94914, #33900, #42418, #19905, #58888, #50396, #20903, #26413, #80418, #11916, #56914, #18932, #4432, #49410, #34898, #79911, #11419, #13894, #53356, #59374, #67379, #6376, #44378, #38370, #67882, #14894, #44864, #14393, #401, #45364, #74877, #29859, #91859, #36392, #53861, #75367, #83863, #60362, #37394, #84372, #76363, #66886, #75868, #51889, #22389, #90858, #6882, #98404, #36891, #30351, #91358, #97908, #52865, #97404, #22884, #23377, #7389, #60858, #28872, #37887, #82371, #83371, #52372, #68380, #29368, #59870, #7877, #90357, #21895, #15387, #45872, #98899, #68871, #30853, #61350, #15871, #74370, #5897, #89879, #21395, #82878, #62825, #63307, #8844, #54824, #77823, #70346, #93817, #24846, #31829, #16356, #46356, #16849, #71329, #1864, #85336, #78319, #32322, #40340, #93325, #25825, #38866, #47324, #86325, #92833, #9338, #39358, #2848, #17349, #39840, #878, #46837, #77332, #33302, #24361, #2356, #47819, #55328, #54335, #23871, #85835, #9839, #25348, #84849, #70843, #32811, #55831, #62325, #69852, #48310, #17829, #78819, #63794, #94302, #10329, #40828, #56322, #86818, #1375, #76844, #8358, #31338, #92345, #69357, #61838, #71809, #49784, #95796, #57775, #88773, #72285, #57288, #34272, #43270, #49296, #87782, #18814, #80291, #96795, #87295, #42298, #19298, #58258, #3315, #64773, #12283, #56799, #27277, #48802, #42790, #65768, #12773, #79798, #95289, #73765, #20284, #11300, #88281, #72770, #26299 ),
 ( #4307, #10818, #19781, #26791, #5294, #66260, #50269, #3817, #27773, #11790, #34781, #73275, #65268, #28270, #41338, #80786, #50782, #4797, #35273, #96296, #35772, #81273, #58765, #33778, #18321, #79311, #64284, #94797, #179, #15168, #53144, #52166, #82659, #7163, #68166, #61134, #14175, #98686, #37666, #76147, #29639, #44659, #46146, #38163, #76632, #61618, #92136, #75651, #30627, #23661, #84157, #75154, #22668, #6664, #97690, #90150, #37180, #91644, #29152, #30135, #83653, #45649, #15663, #98183, #83154, #60147, #69145, #67673, #14679, #90644, #60641, #54123, #22169, #91142, #45145, #8151, #59659, #52651, #68649, #7672, #23162, #74663, #53637, #38644, #673, #31123, #44155, #6174, #36678, #67166, #86117, #40121, #54609, #24636, #34932, #95953, #62601, #55103, #87936, #19452, #9124, #26945, #8634, #39143, #85125, #95454, #85623, #65429, #42453, #93106, #17140, #9621, #93605, #64926, #40618, #47619, #71117, #4464, #34433, #27434, #25143, #78114, #32607, #57446, #77611, #70622, #2147, #63103, #49946, #55620, #1651, #16636, #16138, #17628, #72935, #48099, #78611, #10120, #39639, #47111, #70130, #57929, #32102, #3965, #80451, #11949, #46624, #77122, #69633, #1157, #31617, #62108, #92618, #51923, #66919, #67916, #59901, #29894, #6412, #81424, #52409, #89912, #97440, #36924, #27924, #82910, #51424, #13424, #82407, #50431, #98438, #58923, #28904, #81914, #73924, #75399, #5934, #67414, #14428, #80940, #88438, #28425, #36426, #13933, #21426, #44409, #6918, #35923, #43422, #44897, #19938, #88931, #74912, #89423, #12433, #42941, #58416, #97942, #73424, #12927, #20441, #50929, #4948, #29400, #96452, #20936, #434, #85372, #31373, #98933, #15900, #77861, #22422, #39874, #61381, #69886, #46391, #23412, #70381, #62358, #52896, #61871, #37922, #8391, #76877, #91890, #53895, #30388, #16389, #77364, #60891, #38901, #83406, #8874, #9372, #92376, #46874, #14928, #23902, #68411, #84401, #38405, #69388, #91390, #15428, #92862, #22919, #53388, #1405, #39392, #68906, #909, #83896, #1900, #54371, #84882, #60397, #31859, #45394, #24392, #7910, #16883, #90894, #54860, #45907, #47361, #76394, #75900, #7425, #30885, #49818, #80327, #63829, #18849, #11827, #72318, #63348, #10854, #93853, #85871, #78357, #25381, #49329, #17383, #94342, #41375, #71842, #3852, #86363, #71369, #48347, #57321, #55865, #2883, #32847, #25860, #42335, #2394, #56356, #33334, #34310, #47852, #78853, #26336, #70877, #3352, #62863, #56834, #79831, #26827, #17862, #10364, #87814, #64807, #40863, #33814, #86852, #40376, #18358, #72807, #32356, #48834, #79346, #95327, #19335 ) ),
 .UNSPECIFIED., .F., .F., .F. ) 
 B_SPLINE_SURFACE_WITH_KNOTS ( ( 2, 2 ),
 ( 3, 2, 2, 2, 2, 2, 2, 2, 2, 2, 2, 2, 2, 2, 2, 2, 2, 2, 2, 2, 2, 2, 2, 2, 2, 2, 2, 2, 2, 2, 2, 2, 2, 2, 2, 2, 2, 2, 2, 2, 2, 2, 2, 2, 2, 2, 2, 2, 2, 2, 2, 2, 2, 2, 2, 2, 2, 2, 2, 2, 2, 2, 2, 2, 2, 2, 2, 2, 2, 2, 2, 2, 2, 2, 2, 2, 2, 2, 2, 2, 2, 2, 2, 2, 2, 2, 2, 2, 2, 2, 2, 2, 2, 2, 2, 2, 2, 2, 2, 2, 2, 2, 2, 2, 2, 2, 2, 2, 2, 2, 2, 2, 2, 2, 2, 2, 2, 2, 2, 2, 2, 2, 2, 2, 2, 2, 2, 2, 2, 2, 2, 2, 2, 2, 2, 2, 2, 2, 2, 2, 2, 2, 2, 2, 2, 2, 2, 2, 2, 2, 2, 2, 2, 2, 2, 2, 2, 2, 2, 2, 2, 2, 3 ),
 ( 0.000000000000000000, 1.000000000000000000 ),
 ( 0.000000000000000000, 0.005952380952380952051, 0.01190476190476190410, 0.01785714285714285615, 0.02380952380952380820, 0.02976190476190476025, 0.03571428571428571230, 0.04166666666666666435, 0.04761904761904761640, 0.05357142857142856845, 0.05952380952380952051, 0.06547619047619047949, 0.07142857142857142461, 0.07738095238095238360, 0.08333333333333332871, 0.08928571428571428770, 0.09523809523809523281, 0.1011904761904761918, 0.1071428571428571369, 0.1130952380952380959, 0.1190476190476190410, 0.1250000000000000000, 0.1309523809523809590, 0.1369047619047619180, 0.1428571428571428492, 0.1488095238095238082, 0.1547619047619047672, 0.1607142857142857262, 0.1666666666666666574, 0.1726190476190476164, 0.1785714285714285754, 0.1845238095238095344, 0.1904761904761904656, 0.1964285714285714246, 0.2023809523809523836, 0.2083333333333333426, 0.2142857142857142738, 0.2202380952380952328, 0.2261904761904761918, 0.2321428571428571508, 0.2380952380952380820, 0.2440476190476190410, 0.2500000000000000000, 0.2559523809523809312, 0.2619047619047619180, 0.2678571428571428492, 0.2738095238095238360, 0.2797619047619047672, 0.2857142857142856984, 0.2916666666666666852, 0.2976190476190476164, 0.3035714285714285476, 0.3095238095238095344, 0.3154761904761904656, 0.3214285714285714524, 0.3273809523809523836, 0.3333333333333333148, 0.3392857142857143016, 0.3452380952380952328, 0.3511904761904761640, 0.3571428571428571508, 0.3630952380952380820, 0.3690476190476190688, 0.3750000000000000000, 0.3809523809523809312, 0.3869047619047619180, 0.3928571428571428492, 0.3988095238095238360, 0.4047619047619047672, 0.4107142857142856984, 0.4166666666666666852, 0.4226190476190476164, 0.4285714285714285476, 0.4345238095238095344, 0.4404761904761904656, 0.4464285714285714524, 0.4523809523809523836, 0.4583333333333333148, 0.4642857142857143016, 0.4702380952380952328, 0.4761904761904761640, 0.4821428571428571508, 0.4880952380952380820, 0.4940476190476190688, 0.5000000000000000000, 0.5059523809523809312, 0.5119047619047618625, 0.5178571428571429047, 0.5238095238095238360, 0.5297619047619047672, 0.5357142857142856984, 0.5416666666666666297, 0.5476190476190476719, 0.5535714285714286031, 0.5595238095238095344, 0.5654761904761904656, 0.5714285714285713969, 0.5773809523809523281, 0.5833333333333333703, 0.5892857142857143016, 0.5952380952380952328, 0.6011904761904761640, 0.6071428571428570953, 0.6130952380952381375, 0.6190476190476190688, 0.6250000000000000000, 0.6309523809523809312, 0.6369047619047618625, 0.6428571428571429047, 0.6488095238095238360, 0.6547619047619047672, 0.6607142857142856984, 0.6666666666666666297, 0.6726190476190476719, 0.6785714285714286031, 0.6845238095238095344, 0.6904761904761904656, 0.6964285714285713969, 0.7023809523809523281, 0.7083333333333333703, 0.7142857142857143016, 0.7202380952380952328, 0.7261904761904761640, 0.7321428571428570953, 0.7380952380952381375, 0.7440476190476190688, 0.7500000000000000000, 0.7559523809523809312, 0.7619047619047618625, 0.7678571428571429047, 0.7738095238095238360, 0.7797619047619047672, 0.7857142857142856984, 0.7916666666666666297, 0.7976190476190476719, 0.8035714285714286031, 0.8095238095238095344, 0.8154761904761904656, 0.8214285714285713969, 0.8273809523809523281, 0.8333333333333333703, 0.8392857142857143016, 0.8452380952380952328, 0.8511904761904761640, 0.8571428571428570953, 0.8630952380952381375, 0.8690476190476190688, 0.8750000000000000000, 0.8809523809523809312, 0.8869047619047618625, 0.8928571428571429047, 0.8988095238095238360, 0.9047619047619047672, 0.9107142857142856984, 0.9166666666666666297, 0.9226190476190476719, 0.9285714285714286031, 0.9345238095238095344, 0.9404761904761904656, 0.9464285714285713969, 0.9523809523809523281, 0.9583333333333333703, 0.9642857142857143016 ),
 .UNSPECIFIED. ) 
 GEOMETRIC_REPRESENTATION_ITEM ( )  RATIONAL_B_SPLINE_SURFACE ( (
 ( 1.000000000000000000, 0.9659258262890683122, 1.000000000000000000, 0.9659258262890683122, 1.000000000000000000, 0.9659258262890683122, 1.000000000000000000, 0.9659258262890683122, 1.000000000000000000, 0.9659258262890683122, 1.000000000000000000, 0.9659258262890683122, 1.000000000000000000, 0.9659258262890683122, 1.000000000000000000, 0.9659258262890683122, 1.000000000000000000, 0.9659258262890683122, 1.000000000000000000, 0.9659258262890683122, 1.000000000000000000, 0.9659258262890683122, 1.000000000000000000, 0.9659258262890683122, 1.000000000000000000, 0.9659258262890683122, 1.000000000000000000, 0.9659258262890683122, 1.000000000000000000, 0.9659258262890683122, 1.000000000000000000, 0.9659258262890683122, 1.000000000000000000, 0.9659258262890683122, 1.000000000000000000, 0.9659258262890683122, 1.000000000000000000, 0.9659258262890683122, 1.000000000000000000, 0.9659258262890683122, 1.000000000000000000, 0.9659258262890683122, 1.000000000000000000, 0.9659258262890683122, 1.000000000000000000, 0.9659258262890683122, 1.000000000000000000, 0.9659258262890683122, 1.000000000000000000, 0.9659258262890683122, 1.000000000000000000, 0.9659258262890683122, 1.000000000000000000, 0.9659258262890683122, 1.000000000000000000, 0.9659258262890683122, 1.000000000000000000, 0.9659258262890683122, 1.000000000000000000, 0.9659258262890683122, 1.000000000000000000, 0.9659258262890683122, 1.000000000000000000, 0.9659258262890683122, 1.000000000000000000, 0.9659258262890683122, 1.000000000000000000, 0.9659258262890683122, 1.000000000000000000, 0.9659258262890683122, 1.000000000000000000, 0.9659258262890683122, 1.000000000000000000, 0.9659258262890683122, 1.000000000000000000, 0.9659258262890683122, 1.000000000000000000, 0.9659258262890683122, 1.000000000000000000, 0.9659258262890683122, 1.000000000000000000, 0.9659258262890683122, 1.000000000000000000, 0.9659258262890683122, 1.000000000000000000, 0.9659258262890683122, 1.000000000000000000, 0.9659258262890683122, 1.000000000000000000, 0.9659258262890683122, 1.000000000000000000, 0.9659258262890683122, 1.000000000000000000, 0.9659258262890683122, 1.000000000000000000, 0.9659258262890683122, 1.000000000000000000, 0.9659258262890683122, 1.000000000000000000, 0.9659258262890683122, 1.000000000000000000, 0.9659258262890683122, 1.000000000000000000, 0.9659258262890683122, 1.000000000000000000, 0.9659258262890683122, 1.000000000000000000, 0.9659258262890683122, 1.000000000000000000, 0.9659258262890683122, 1.000000000000000000, 0.9659258262890683122, 1.000000000000000000, 0.9659258262890683122, 1.000000000000000000, 0.9659258262890683122, 1.000000000000000000, 0.9659258262890683122, 1.000000000000000000, 0.9659258262890683122, 1.000000000000000000, 0.9659258262890683122, 1.000000000000000000, 0.9659258262890683122, 1.000000000000000000, 0.9659258262890683122, 1.000000000000000000, 0.9659258262890683122, 1.000000000000000000, 0.9659258262890683122, 1.000000000000000000, 0.9659258262890683122, 1.000000000000000000, 0.9659258262890683122, 1.000000000000000000, 0.9659258262890683122, 1.000000000000000000, 0.9659258262890683122, 1.000000000000000000, 0.9659258262890683122, 1.000000000000000000, 0.9659258262890683122, 1.000000000000000000, 0.9659258262890683122, 1.000000000000000000, 0.9659258262890683122, 1.000000000000000000, 0.9659258262890683122, 1.000000000000000000, 0.9659258262890683122, 1.000000000000000000, 0.9659258262890683122, 1.000000000000000000, 0.9659258262890683122, 1.000000000000000000, 0.9659258262890683122, 1.000000000000000000, 0.9659258262890683122, 1.000000000000000000, 0.9659258262890683122, 1.000000000000000000, 0.9659258262890683122, 1.000000000000000000, 0.9659258262890683122, 1.000000000000000000, 0.9659258262890683122, 1.000000000000000000, 0.9659258262890683122, 1.000000000000000000, 0.9659258262890683122, 1.000000000000000000, 0.9659258262890683122, 1.000000000000000000, 0.9659258262890683122, 1.000000000000000000, 0.9659258262890683122, 1.000000000000000000, 0.9659258262890683122, 1.000000000000000000, 0.9659258262890683122, 1.000000000000000000, 0.9659258262890683122, 1.000000000000000000, 0.9659258262890683122, 1.000000000000000000, 0.9659258262890683122, 1.000000000000000000, 0.9659258262890683122, 1.000000000000000000, 0.9659258262890683122, 1.000000000000000000, 0.9659258262890683122, 1.000000000000000000, 0.9659258262890683122, 1.000000000000000000, 0.9659258262890683122, 1.000000000000000000, 0.9659258262890683122, 1.000000000000000000, 0.9659258262890683122, 1.000000000000000000, 0.9659258262890683122, 1.000000000000000000, 0.9659258262890683122, 1.000000000000000000, 0.9659258262890683122, 1.000000000000000000, 0.9659258262890683122, 1.000000000000000000, 0.9659258262890683122, 1.000000000000000000, 0.9659258262890683122, 1.000000000000000000, 0.9659258262890683122, 1.000000000000000000, 0.9659258262890683122, 1.000000000000000000, 0.9659258262890683122, 1.000000000000000000, 0.9659258262890683122, 1.000000000000000000, 0.9659258262890683122, 1.000000000000000000, 0.9659258262890683122, 1.000000000000000000, 0.9659258262890683122, 1.000000000000000000, 0.9659258262890683122, 1.000000000000000000, 0.9659258262890683122, 1.000000000000000000, 0.9659258262890683122, 1.000000000000000000, 0.9659258262890683122, 1.000000000000000000, 0.9659258262890683122, 1.000000000000000000, 0.9659258262890683122, 1.000000000000000000, 0.9659258262890683122, 1.000000000000000000, 0.9659258262890683122, 1.000000000000000000, 0.9659258262890683122, 1.000000000000000000, 0.9659258262890683122, 1.000000000000000000, 0.9659258262890683122, 1.000000000000000000, 0.9659258262890683122, 1.000000000000000000, 0.9659258262890683122, 1.000000000000000000, 0.9659258262890683122, 1.000000000000000000, 0.9659258262890683122, 1.000000000000000000, 0.9659258262890683122, 1.000000000000000000, 0.9659258262890683122, 1.000000000000000000, 0.9659258262890683122, 1.000000000000000000, 0.9659258262890683122, 1.000000000000000000, 0.9659258262890683122, 1.000000000000000000, 0.9659258262890683122, 1.000000000000000000, 0.9659258262890683122, 1.000000000000000000, 0.9659258262890683122, 1.000000000000000000, 0.9659258262890683122, 1.000000000000000000, 0.9659258262890683122, 1.000000000000000000, 0.9659258262890683122, 1.000000000000000000, 0.9659258262890683122, 1.000000000000000000, 0.9659258262890683122, 1.000000000000000000, 0.9659258262890683122, 1.000000000000000000, 0.9659258262890683122, 1.000000000000000000, 0.9659258262890683122, 1.000000000000000000, 0.9659258262890683122, 1.000000000000000000, 0.9659258262890683122, 1.000000000000000000, 0.9659258262890683122, 1.000000000000000000, 0.9659258262890683122, 1.000000000000000000, 0.9659258262890683122, 1.000000000000000000, 0.9659258262890683122, 1.000000000000000000, 0.9659258262890683122, 1.000000000000000000, 0.9659258262890683122, 1.000000000000000000, 0.9659258262890683122, 1.000000000000000000, 0.9659258262890683122, 1.000000000000000000, 0.9659258262890683122, 1.000000000000000000, 0.9659258262890683122, 1.000000000000000000, 0.9659258262890683122, 1.000000000000000000, 0.9659258262890683122, 1.000000000000000000, 0.9659258262890683122, 1.000000000000000000, 0.9659258262890683122, 1.000000000000000000, 0.9659258262890683122, 1.000000000000000000, 0.9659258262890683122, 1.000000000000000000),
 ( 1.000000000000000000, 0.9659258262890683122, 1.000000000000000000, 0.9659258262890683122, 1.000000000000000000, 0.9659258262890683122, 1.000000000000000000, 0.9659258262890683122, 1.000000000000000000, 0.9659258262890683122, 1.000000000000000000, 0.9659258262890683122, 1.000000000000000000, 0.9659258262890683122, 1.000000000000000000, 0.9659258262890683122, 1.000000000000000000, 0.9659258262890683122, 1.000000000000000000, 0.9659258262890683122, 1.000000000000000000, 0.9659258262890683122, 1.000000000000000000, 0.9659258262890683122, 1.000000000000000000, 0.9659258262890683122, 1.000000000000000000, 0.9659258262890683122, 1.000000000000000000, 0.9659258262890683122, 1.000000000000000000, 0.9659258262890683122, 1.000000000000000000, 0.9659258262890683122, 1.000000000000000000, 0.9659258262890683122, 1.000000000000000000, 0.9659258262890683122, 1.000000000000000000, 0.9659258262890683122, 1.000000000000000000, 0.9659258262890683122, 1.000000000000000000, 0.9659258262890683122, 1.000000000000000000, 0.9659258262890683122, 1.000000000000000000, 0.9659258262890683122, 1.000000000000000000, 0.9659258262890683122, 1.000000000000000000, 0.9659258262890683122, 1.000000000000000000, 0.9659258262890683122, 1.000000000000000000, 0.9659258262890683122, 1.000000000000000000, 0.9659258262890683122, 1.000000000000000000, 0.9659258262890683122, 1.000000000000000000, 0.9659258262890683122, 1.000000000000000000, 0.9659258262890683122, 1.000000000000000000, 0.9659258262890683122, 1.000000000000000000, 0.9659258262890683122, 1.000000000000000000, 0.9659258262890683122, 1.000000000000000000, 0.9659258262890683122, 1.000000000000000000, 0.9659258262890683122, 1.000000000000000000, 0.9659258262890683122, 1.000000000000000000, 0.9659258262890683122, 1.000000000000000000, 0.9659258262890683122, 1.000000000000000000, 0.9659258262890683122, 1.000000000000000000, 0.9659258262890683122, 1.000000000000000000, 0.9659258262890683122, 1.000000000000000000, 0.9659258262890683122, 1.000000000000000000, 0.9659258262890683122, 1.000000000000000000, 0.9659258262890683122, 1.000000000000000000, 0.9659258262890683122, 1.000000000000000000, 0.9659258262890683122, 1.000000000000000000, 0.9659258262890683122, 1.000000000000000000, 0.9659258262890683122, 1.000000000000000000, 0.9659258262890683122, 1.000000000000000000, 0.9659258262890683122, 1.000000000000000000, 0.9659258262890683122, 1.000000000000000000, 0.9659258262890683122, 1.000000000000000000, 0.9659258262890683122, 1.000000000000000000, 0.9659258262890683122, 1.000000000000000000, 0.9659258262890683122, 1.000000000000000000, 0.9659258262890683122, 1.000000000000000000, 0.9659258262890683122, 1.000000000000000000, 0.9659258262890683122, 1.000000000000000000, 0.9659258262890683122, 1.000000000000000000, 0.9659258262890683122, 1.000000000000000000, 0.9659258262890683122, 1.000000000000000000, 0.9659258262890683122, 1.000000000000000000, 0.9659258262890683122, 1.000000000000000000, 0.9659258262890683122, 1.000000000000000000, 0.9659258262890683122, 1.000000000000000000, 0.9659258262890683122, 1.000000000000000000, 0.9659258262890683122, 1.000000000000000000, 0.9659258262890683122, 1.000000000000000000, 0.9659258262890683122, 1.000000000000000000, 0.9659258262890683122, 1.000000000000000000, 0.9659258262890683122, 1.000000000000000000, 0.9659258262890683122, 1.000000000000000000, 0.9659258262890683122, 1.000000000000000000, 0.9659258262890683122, 1.000000000000000000, 0.9659258262890683122, 1.000000000000000000, 0.9659258262890683122, 1.000000000000000000, 0.9659258262890683122, 1.000000000000000000, 0.9659258262890683122, 1.000000000000000000, 0.9659258262890683122, 1.000000000000000000, 0.9659258262890683122, 1.000000000000000000, 0.9659258262890683122, 1.000000000000000000, 0.9659258262890683122, 1.000000000000000000, 0.9659258262890683122, 1.000000000000000000, 0.9659258262890683122, 1.000000000000000000, 0.9659258262890683122, 1.000000000000000000, 0.9659258262890683122, 1.000000000000000000, 0.9659258262890683122, 1.000000000000000000, 0.9659258262890683122, 1.000000000000000000, 0.9659258262890683122, 1.000000000000000000, 0.9659258262890683122, 1.000000000000000000, 0.9659258262890683122, 1.000000000000000000, 0.9659258262890683122, 1.000000000000000000, 0.9659258262890683122, 1.000000000000000000, 0.9659258262890683122, 1.000000000000000000, 0.9659258262890683122, 1.000000000000000000, 0.9659258262890683122, 1.000000000000000000, 0.9659258262890683122, 1.000000000000000000, 0.9659258262890683122, 1.000000000000000000, 0.9659258262890683122, 1.000000000000000000, 0.9659258262890683122, 1.000000000000000000, 0.9659258262890683122, 1.000000000000000000, 0.9659258262890683122, 1.000000000000000000, 0.9659258262890683122, 1.000000000000000000, 0.9659258262890683122, 1.000000000000000000, 0.9659258262890683122, 1.000000000000000000, 0.9659258262890683122, 1.000000000000000000, 0.9659258262890683122, 1.000000000000000000, 0.9659258262890683122, 1.000000000000000000, 0.9659258262890683122, 1.000000000000000000, 0.9659258262890683122, 1.000000000000000000, 0.9659258262890683122, 1.000000000000000000, 0.9659258262890683122, 1.000000000000000000, 0.9659258262890683122, 1.000000000000000000, 0.9659258262890683122, 1.000000000000000000, 0.9659258262890683122, 1.000000000000000000, 0.9659258262890683122, 1.000000000000000000, 0.9659258262890683122, 1.000000000000000000, 0.9659258262890683122, 1.000000000000000000, 0.9659258262890683122, 1.000000000000000000, 0.9659258262890683122, 1.000000000000000000, 0.9659258262890683122, 1.000000000000000000, 0.9659258262890683122, 1.000000000000000000, 0.9659258262890683122, 1.000000000000000000, 0.9659258262890683122, 1.000000000000000000, 0.9659258262890683122, 1.000000000000000000, 0.9659258262890683122, 1.000000000000000000, 0.9659258262890683122, 1.000000000000000000, 0.9659258262890683122, 1.000000000000000000, 0.9659258262890683122, 1.000000000000000000, 0.9659258262890683122, 1.000000000000000000, 0.9659258262890683122, 1.000000000000000000, 0.9659258262890683122, 1.000000000000000000, 0.9659258262890683122, 1.000000000000000000, 0.9659258262890683122, 1.000000000000000000, 0.9659258262890683122, 1.000000000000000000, 0.9659258262890683122, 1.000000000000000000, 0.9659258262890683122, 1.000000000000000000, 0.9659258262890683122, 1.000000000000000000, 0.9659258262890683122, 1.000000000000000000, 0.9659258262890683122, 1.000000000000000000, 0.9659258262890683122, 1.000000000000000000, 0.9659258262890683122, 1.000000000000000000, 0.9659258262890683122, 1.000000000000000000, 0.9659258262890683122, 1.000000000000000000, 0.9659258262890683122, 1.000000000000000000, 0.9659258262890683122, 1.000000000000000000, 0.9659258262890683122, 1.000000000000000000, 0.9659258262890683122, 1.000000000000000000, 0.9659258262890683122, 1.000000000000000000, 0.9659258262890683122, 1.000000000000000000, 0.9659258262890683122, 1.000000000000000000, 0.9659258262890683122, 1.000000000000000000, 0.9659258262890683122, 1.000000000000000000, 0.9659258262890683122, 1.000000000000000000, 0.9659258262890683122, 1.000000000000000000, 0.9659258262890683122, 1.000000000000000000, 0.9659258262890683122, 1.000000000000000000, 0.9659258262890683122, 1.000000000000000000, 0.9659258262890683122, 1.000000000000000000, 0.9659258262890683122, 1.000000000000000000) ) ) 
 REPRESENTATION_ITEM ( '' )  SURFACE ( )  );
#8964=CARTESIAN_POINT ( 'NONE',  ( 20.88017736071110875, 30.77201867748816966, -2.915334737309920765 ) ) ;
#8965=CARTESIAN_POINT ( 'NONE',  ( 2.035157376598824452, 28.68868534415484106, 7.964842623401179544 ) ) ;
#8966=CARTESIAN_POINT ( 'NONE',  ( 13.43411237798106583, 2.665301336597086568, -12.81628187352647252 ) ) ;
#8967=CARTESIAN_POINT ( 'NONE',  ( 2.791683348922237240, 55.38393115100078745, -7.208316651077763204 ) ) ;
#8968=CARTESIAN_POINT ( 'NONE',  ( 3.591859063236763294, 58.29030133659708923, -11.09922568453595026 ) ) ;
#8971=CARTESIAN_POINT ( 'NONE',  ( 15.44008868035555260, 24.73035201082150891, 9.422509992056143702 ) ) ;
#8972=CARTESIAN_POINT ( 'NONE',  ( 19.38216949554541202, 30.99863466993042138, 9.382169495545424454 ) ) ;
#8973=CARTESIAN_POINT ( 'NONE',  ( 19.05914839598885635, 34.96693863883976405, 6.499999999999962697 ) ) ;
#8974=CARTESIAN_POINT ( 'NONE',  ( 17.20831665107776587, 57.88393115100078745, 7.208316651077764980 ) ) ;
#8975=CARTESIAN_POINT ( 'NONE',  ( 10.00000000000000178, 44.31368534415484106, 10.88017736071110342 ) ) ;
#8976=CARTESIAN_POINT ( 'NONE',  ( 17.20831665107776587, 17.88393115100078745, 7.208316651077764980 ) ) ;
#8977=CARTESIAN_POINT ( 'NONE',  ( 16.40814093676324603, 17.45696800326375353, -11.09922568453594671 ) ) ;
#8978=CARTESIAN_POINT ( 'NONE',  ( 7.084665262690076126, 62.02201867748816966, -10.88017736071110164 ) ) ;
#8979=CARTESIAN_POINT ( 'NONE',  ( 19.42250999205614548, 15.98035201082150714, -5.440088680355545492 ) ) ;
#8980=FILL_AREA_STYLE_COLOUR ( '', #13029 ) ;
#8982=CARTESIAN_POINT ( 'NONE',  ( 0.5774900079438607392, 48.48035201082150536, 5.440088680355550821 ) ) ;
#8983=CARTESIAN_POINT ( 'NONE',  ( 19.39235739573469175, 24.87576471608601381, 6.499999999999993783 ) ) ;
#8984=CARTESIAN_POINT ( 'NONE',  ( -0.8801773607111009756, 43.06368534415484106, 1.068504757029289695E-15 ) ) ;
#8985=CARTESIAN_POINT ( 'NONE',  ( 16.40814093676324603, 47.45696800326375353, -11.09922568453594671 ) ) ;
#8986=CARTESIAN_POINT ( 'NONE',  ( 24.16423886937410614, 9.512082168247301794, -3.795296366450302550 ) ) ;
#8987=CARTESIAN_POINT ( 'NONE',  ( 18.52753015748617571, 23.09226448433411960, 4.923371831947298993 ) ) ;
#8988=CARTESIAN_POINT ( 'NONE',  ( 20.88017736071110164, 10.35535201082150714, 2.915334737309930979 ) ) ;
#8989=CARTESIAN_POINT ( 'NONE',  ( 7.361572987183170547, 17.05059781766745530, 9.846743663894590881 ) ) ;
#8991=CARTESIAN_POINT ( 'NONE',  ( 24.16423886937410614, 59.30374883491397497, 8.672049930838204340E-16 ) ) ;
#8995=CARTESIAN_POINT ( 'NONE',  ( 20.15039907845753220, 46.74884699246888431, 6.262539305110077947 ) ) ;
#8998=CARTESIAN_POINT ( 'NONE',  ( 17.96484262340118221, 11.18868534415484106, -7.964842623401177768 ) ) ;
#8999=CARTESIAN_POINT ( 'NONE',  ( 19.42250999205614193, 5.147018677488171434, 5.440088680355555262 ) ) ;
#9000=CARTESIAN_POINT ( 'NONE',  ( 14.92337183194729633, 42.67559781766745886, 8.527530157486181039 ) ) ;
#9001=CARTESIAN_POINT ( 'NONE',  ( 16.40814093676324603, 42.45696800326375353, -11.09922568453594671 ) ) ;
#9002=CARTESIAN_POINT ( 'NONE',  ( 20.04068437667222469, 64.71974360917720048, 6.396802510829778576 ) ) ;
#9004=CARTESIAN_POINT ( 'NONE',  ( 24.16423886937409904, 14.09541550158063217, 3.795296366450317205 ) ) ;
#9005=CARTESIAN_POINT ( 'NONE',  ( 19.42250999205614548, 30.98035201082150536, -5.440088680355545492 ) ) ;
#9006=CARTESIAN_POINT ( 'NONE',  ( 6.204703633549690345, 65.76208216824731778, -14.16423886937410259 ) ) ;
#9007=CARTESIAN_POINT ( 'NONE',  ( 12.63842701281683034, 42.46726448433412315, 9.846743663894596210 ) ) ;
#9008=LINE ( 'NONE', #91534, #34860 ) ;
#9009=CARTESIAN_POINT ( 'NONE',  ( 0.1532563361054082862, 41.21726448433411605, 2.638427012816831674 ) ) ;
#9010=CARTESIAN_POINT ( 'NONE',  ( 2.791683348922237240, 0.3839311510007847872, -7.208316651077763204 ) ) ;
#9012=VERTEX_POINT ( 'NONE', #10893 ) ;
#9013=CARTESIAN_POINT ( 'NONE',  ( 20.88017736071110164, 5.355352010821502695, 2.915334737309930979 ) ) ;
#9014=CARTESIAN_POINT ( 'NONE',  ( 15.44008868035555260, 64.73035201082151957, 9.422509992056143702 ) ) ;
#9015=CARTESIAN_POINT ( 'NONE',  ( 2.791683348922240793, 56.63393115100078035, 7.208316651077764092 ) ) ;
#9016=CARTESIAN_POINT ( 'NONE',  ( 7.084665262690076126, 47.02201867748818387, -10.88017736071110164 ) ) ;
#9017=CARTESIAN_POINT ( 'NONE',  ( 20.88017736071110519, 45.56368534415484106, 2.639326808657452039E-16 ) ) ;
#9018=CARTESIAN_POINT ( 'NONE',  ( 19.42250999205614548, 10.98035201082150358, -5.440088680355545492 ) ) ;
#9019=CARTESIAN_POINT ( 'NONE',  ( 10.00000000000000000, 27.87363466993042138, -12.81628187352647608 ) ) ;
#9020=CARTESIAN_POINT ( 'NONE',  ( -0.3689425029237881626, 22.42874883491397142, 10.36894250292379027 ) ) ;
#9021=EDGE_CURVE ( 'NONE', #97143, #17007, #48391, .T. ) ;
#9023=CIRCLE ( 'NONE', #80892, 0.5000000000000004441 ) ;
#9026=CARTESIAN_POINT ( 'NONE',  ( -2.816281873526473856, 49.33196800326374643, 3.434112377981055619 ) ) ;
#9028=CARTESIAN_POINT ( 'NONE',  ( 12.63842701281683034, 57.46726448433411605, 9.846743663894596210 ) ) ;
#9029=CARTESIAN_POINT ( 'NONE',  ( 20.88017736071110164, 15.35535201082150358, 2.915334737309930979 ) ) ;
#9031=CARTESIAN_POINT ( 'NONE',  ( 19.42250999205614193, 20.14701867748817321, 5.440088680355555262 ) ) ;
#9032=ORIENTED_EDGE ( 'NONE', *, *, #77438, .F. ) ;
#9033=CARTESIAN_POINT ( 'NONE',  ( 17.96484262340118221, 64.93868534415483396, 7.964842623401181321 ) ) ;
#9034=FILL_AREA_STYLE ('',( #69547 ) ) ;
#9035=CARTESIAN_POINT ( 'NONE',  ( 10.00000000000000000, 9.758931151000785675, -9.846743663894594434 ) ) ;
#9037=CARTESIAN_POINT ( 'NONE',  ( 0.5774900079438607392, 68.48035201082150536, 5.440088680355550821 ) ) ;
#9038=COLOUR_RGB ( '', 0.66274510, 0.83137255, 0.94901961) ;
#9041=CARTESIAN_POINT ( 'NONE',  ( -46.94000000000001194, 100.3306229069515325, 9.153711987617667134 ) ) ;
#9042=CARTESIAN_POINT ( 'NONE',  ( 1.472469842513823179, 11.42559781766745175, 4.923371831947296329 ) ) ;
#9043=VERTEX_POINT ( 'NONE', #63391 ) ;
#9047=CARTESIAN_POINT ( 'NONE',  ( 10.00000000000000000, 44.75893115100078745, -9.846743663894594434 ) ) ;
#9050=CARTESIAN_POINT ( 'NONE',  ( 2.917880565312948704, 7.637082168247301794, 12.26659068614894643 ) ) ;
#9051=ADVANCED_FACE ( 'NONE', ( #39433 ), #31747, .T. ) ;
#9052=CARTESIAN_POINT ( 'NONE',  ( 13.43411237798106583, 62.66530133659708923, -12.81628187352647252 ) ) ;
#9053=CARTESIAN_POINT ( 'NONE',  ( -2.266590686148945544, 1.387082168247301128, -7.082119434687050408 ) ) ;
#9054=CARTESIAN_POINT ( 'NONE',  ( 24.16423886937409904, 14.09541550158063217, 3.795296366450317205 ) ) ;
#9057=CARTESIAN_POINT ( 'NONE',  ( 2.035157376598822676, 62.43868534415483396, -7.964842623401177768 ) ) ;
#9058=CARTESIAN_POINT ( 'NONE',  ( 17.96484262340118221, 14.93868534415484106, 7.964842623401181321 ) ) ;
#9059=CARTESIAN_POINT ( 'NONE',  ( 1.472469842513823179, 66.42559781766745175, 4.923371831947296329 ) ) ;
#9060=ORIENTED_EDGE ( 'NONE', *, *, #95734, .T. ) ;
#9061=CARTESIAN_POINT ( 'NONE',  ( 10.00000000000000178, 7.258931151000785675, 9.846743663894594434 ) ) ;
#9062=CARTESIAN_POINT ( 'NONE',  ( 18.52753015748617571, 8.092264484334117824, 4.923371831947298993 ) ) ;
#9063=COLOUR_RGB ( '', 0.09019608, 0.27058824, 0.51372549) ;
#9064=CARTESIAN_POINT ( 'NONE',  ( 13.43411237798105340, 30.58196800326374998, 12.81628187352647963 ) ) ;
#9065=CARTESIAN_POINT ( 'NONE',  ( 0.1532563361054082862, 26.21726448433411605, 2.638427012816831674 ) ) ;
#9067=CARTESIAN_POINT ( 'NONE',  ( 22.81628187352648496, 16.83196800326374998, -3.434112377981050290 ) ) ;
#9069=CARTESIAN_POINT ( 'NONE',  ( 7.361572987183170547, 2.050597817667451750, 9.846743663894590881 ) ) ;
#9070=ORIENTED_EDGE ( 'NONE', *, *, #41733, .T. ) ;
#9071=COLOUR_RGB ( '', 0.66274510, 0.83137255, 0.94901961) ;
#9072=CARTESIAN_POINT ( 'NONE',  ( 4.559911319644449179, 42.23035201082151247, -9.422509992056141925 ) ) ;
#9073=CARTESIAN_POINT ( 'NONE',  ( -2.266590686148945544, 31.38708216824730002, -7.082119434687050408 ) ) ;
#9074=CARTESIAN_POINT ( 'NONE',  ( 14.92337183194729633, 37.67559781766745175, 8.527530157486181039 ) ) ;
#9075=CARTESIAN_POINT ( 'NONE',  ( 19.84674366389459621, 3.508931151000785231, 7.409399052514197653E-17 ) ) ;
#9076=CARTESIAN_POINT ( 'NONE',  ( 22.81628187352647785, 56.62363466993042493, 6.195893100308588602E-16 ) ) ;
#9078=CARTESIAN_POINT ( 'NONE',  ( 7.084665262690076126, 24.10535201082150181, 10.88017736071109987 ) ) ;
#9081=CARTESIAN_POINT ( 'NONE',  ( 0.6178305044545818747, 8.498634669930421381, -9.382169495545419124 ) ) ;
#9082=CARTESIAN_POINT ( 'NONE',  ( 5.076628168052703671, 41.84226448433411605, 8.527530157486179263 ) ) ;
#9084=CARTESIAN_POINT ( 'NONE',  ( 3.591859063236761518, 54.95696800326376064, 11.09922568453594849 ) ) ;
#9085=( NAMED_UNIT ( * ) SI_UNIT ( $, .STERADIAN. ) SOLID_ANGLE_UNIT ( ) );
#9086=CARTESIAN_POINT ( 'NONE',  ( 0.5774900079438590739, 57.64701867748817676, -5.440088680355550821 ) ) ;
#9090=CARTESIAN_POINT ( 'NONE',  ( 4.559911319644449179, 53.89701867748817676, 9.422509992056141925 ) ) ;
#9091=CARTESIAN_POINT ( 'NONE',  ( 15.44008868035555260, 54.73035201082150536, 9.422509992056143702 ) ) ;
#9095=CARTESIAN_POINT ( 'NONE',  ( 10.00000000000000178, 9.313685344154839285, 10.88017736071110342 ) ) ;
#9096=CARTESIAN_POINT ( 'NONE',  ( 0.1532563361054100626, 50.80059781766745175, -2.638427012816831230 ) ) ;
#9097=CARTESIAN_POINT ( 'NONE',  ( 19.42250999205614193, 20.14701867748817321, 5.440088680355555262 ) ) ;
#9099=CARTESIAN_POINT ( 'NONE',  ( -2.816281873526471635, 28.91530133659708213, -3.434112377981056508 ) ) ;
#9101=CARTESIAN_POINT ( 'NONE',  ( 15.44008868035555793, 36.39701867748816966, -9.422509992056140149 ) ) ;
#9102=CARTESIAN_POINT ( 'NONE',  ( 21.09922568453595559, 12.04030133659708746, -6.408140936763230044 ) ) ;
#9104=CARTESIAN_POINT ( 'NONE',  ( 20.88017736071110164, 10.35535201082150714, 2.915334737309930979 ) ) ;
#9105=CARTESIAN_POINT ( 'NONE',  ( 4.559911319644449179, 42.23035201082151247, -9.422509992056141925 ) ) ;
#9106=CARTESIAN_POINT ( 'NONE',  ( -0.3689425029237881626, 47.42874883491396787, 10.36894250292379027 ) ) ;
#9107=CARTESIAN_POINT ( 'NONE',  ( 17.20831665107776587, 29.13393115100078390, -7.208316651077762316 ) ) ;
#9108=CARTESIAN_POINT ( 'NONE',  ( 7.084665262690076126, 62.02201867748816966, -10.88017736071110164 ) ) ;
#9109=LINE ( 'NONE', #39623, #87335 ) ;
#9110=CARTESIAN_POINT ( 'NONE',  ( 13.79529636645030344, 23.26208216824730002, 14.16423886937410614 ) ) ;
#9112=SURFACE_SIDE_STYLE ('',( #54110 ) ) ;
#9113=CARTESIAN_POINT ( 'NONE',  ( 1.932340009482153231, 21.49127512925448613, -6.500000000000008882 ) ) ;
#9116=CARTESIAN_POINT ( 'NONE',  ( 13.79529636645031943, 40.34541550158063217, -14.16423886937409904 ) ) ;
#9117=CARTESIAN_POINT ( 'NONE',  ( -2.266590686148945544, 31.38708216824730002, -7.082119434687050408 ) ) ;
#9118=CARTESIAN_POINT ( 'NONE',  ( 5.076628168052704559, 0.1755978176674514724, -8.527530157486179263 ) ) ;
#9119=CARTESIAN_POINT ( 'NONE',  ( 18.52753015748618282, 63.92559781766745886, -4.923371831947291888 ) ) ;
#9121=CARTESIAN_POINT ( 'NONE',  ( 20.88017736071110164, 60.35535201082151957, 2.915334737309930979 ) ) ;
#9122=CARTESIAN_POINT ( 'NONE',  ( 10.00000000000000000, 22.87363466993042138, -12.81628187352647608 ) ) ;
#9123=CARTESIAN_POINT ( 'NONE',  ( -2.266590686148945544, 36.38708216824730357, -7.082119434687050408 ) ) ;
#9124=CARTESIAN_POINT ( 'NONE',  ( 0.5774900079438590739, 22.64701867748817321, -5.440088680355550821 ) ) ;
#9125=CARTESIAN_POINT ( 'NONE',  ( 10.00000000000000000, 26.81368534415484106, -10.88017736071110342 ) ) ;
#9126=DIRECTION ( 'NONE',  ( 0.000000000000000000, -1.000000000000000000, 0.000000000000000000 ) ) ;
#9130=CARTESIAN_POINT ( 'NONE',  ( 19.72487221294570858, 0.5000000000000000000, 6.500000000000000888 ) ) ;
#9131=VERTEX_POINT ( 'NONE', #23193 ) ;
#9133=ORIENTED_EDGE ( 'NONE', *, *, #86940, .F. ) ;
#9134=CARTESIAN_POINT ( 'NONE',  ( 6.204703633549690345, 0.7620821682473009062, -14.16423886937410259 ) ) ;
#9135=CARTESIAN_POINT ( 'NONE',  ( 24.16423886937410614, 54.30374883491396787, 8.672049930838204340E-16 ) ) ;
#9136=CARTESIAN_POINT ( 'NONE',  ( 19.42250999205614193, 15.14701867748817143, 5.440088680355555262 ) ) ;
#9137=CARTESIAN_POINT ( 'NONE',  ( 7.361572987183170547, 37.05059781766744464, 9.846743663894590881 ) ) ;
#9138=CARTESIAN_POINT ( 'NONE',  ( 18.52753015748618282, 58.92559781766745886, -4.923371831947291888 ) ) ;
#9142=CARTESIAN_POINT ( 'NONE',  ( 6.565887622018943937, 3.081968003263753531, -12.81628187352647608 ) ) ;
#9143=AXIS2_PLACEMENT_3D ( 'NONE', #60867, #91367, #22893 ) ;
#9144=ORIENTED_EDGE ( 'NONE', *, *, #98768, .T. ) ;
#9145=CARTESIAN_POINT ( 'NONE',  ( -4.164238869374099927, 47.01208216824729647, 3.795296366450308767 ) ) ;
#9147=CARTESIAN_POINT ( 'NONE',  ( 6.204703633549690345, 37.84541550158063927, 14.16423886937410082 ) ) ;
#9148=ORIENTED_EDGE ( 'NONE', *, *, #12731, .T. ) ;
#9149=CARTESIAN_POINT ( 'NONE',  ( 10.00000000000000178, 24.31368534415484106, 10.88017736071110342 ) ) ;
#9151=CARTESIAN_POINT ( 'NONE',  ( 4.559911319644449179, 33.89701867748817676, 9.422509992056141925 ) ) ;
#9152=CARTESIAN_POINT ( 'NONE',  ( 19.84674366389459266, 53.30059781766744464, 2.638427012816836559 ) ) ;
#9153=CARTESIAN_POINT ( 'NONE',  ( 12.91533473730992121, 34.52201867748817676, 10.88017736071110164 ) ) ;
#9155=CARTESIAN_POINT ( 'NONE',  ( -0.8801773607111008646, 68.27201867748817676, 2.915334737309923430 ) ) ;
#9156=CARTESIAN_POINT ( 'NONE',  ( 12.91533473730992121, 29.52201867748817321, 10.88017736071110164 ) ) ;
#9160=CARTESIAN_POINT ( 'NONE',  ( 17.20831665107776587, 4.133931151000785675, -7.208316651077762316 ) ) ;
#9164=CARTESIAN_POINT ( 'NONE',  ( 17.20831665107776587, 29.13393115100078390, -7.208316651077762316 ) ) ;
#9172=CARTESIAN_POINT ( 'NONE',  ( 14.92337183194729633, 52.67559781766745175, 8.527530157486181039 ) ) ;
#9173=CARTESIAN_POINT ( 'NONE',  ( 22.26659068614894466, 48.88708216824730357, 7.082119434687054849 ) ) ;
#9174=CARTESIAN_POINT ( 'NONE',  ( 2.791683348922237240, 65.38393115100078035, -7.208316651077763204 ) ) ;
#9177=CARTESIAN_POINT ( 'NONE',  ( 19.84674366389459266, 18.30059781766745175, 2.638427012816836559 ) ) ;
#9179=CARTESIAN_POINT ( 'NONE',  ( 16.40814093676323893, 45.79030133659708923, 11.09922568453595026 ) ) ;
#9180=CARTESIAN_POINT ( 'NONE',  ( 1.472469842513823179, 60.59226448433412315, -4.923371831947296329 ) ) ;
#9181=CARTESIAN_POINT ( 'NONE',  ( 0.5774900079438607392, 58.48035201082151247, 5.440088680355550821 ) ) ;
#9183=CARTESIAN_POINT ( 'NONE',  ( 17.20831665107776587, 49.13393115100078745, -7.208316651077762316 ) ) ;
#9187=CARTESIAN_POINT ( 'NONE',  ( 6.204703633549690345, 50.76208216824730357, -14.16423886937410259 ) ) ;
#9188=SURFACE_STYLE_FILL_AREA ( #17201 ) ;
#9189=CARTESIAN_POINT ( 'NONE',  ( 4.559911319644449179, 23.89701867748817321, 9.422509992056141925 ) ) ;
#9190=CARTESIAN_POINT ( 'NONE',  ( 6.565887622018943937, 8.081968003263751754, -12.81628187352647608 ) ) ;
#9191=CARTESIAN_POINT ( 'NONE',  ( -0.8801773607110991993, 62.85535201082150536, -2.915334737309923874 ) ) ;
#9194=EDGE_CURVE ( 'NONE', #36460, #52625, #45181, .T. ) ;
#9195=CARTESIAN_POINT ( 'NONE',  ( 20.10421743870887568, 45.60736173766201063, -6.337391062633419558 ) ) ;
#9196=CARTESIAN_POINT ( 'NONE',  ( -0.8801773607111009756, 58.06368534415484106, 1.068504757029289695E-15 ) ) ;
#9197=CARTESIAN_POINT ( 'NONE',  ( 0.1955144967549070634, 54.32703681773340065, -6.500000000002873257 ) ) ;
#9198=CARTESIAN_POINT ( 'NONE',  ( 7.361572987183170547, 37.05059781766744464, 9.846743663894590881 ) ) ;
#9199=FILL_AREA_STYLE_COLOUR ( '', #12218 ) ;
#9201=CARTESIAN_POINT ( 'NONE',  ( 3.591859063236763294, 3.290301336597087012, -11.09922568453595026 ) ) ;
#9202=CARTESIAN_POINT ( 'NONE',  ( 4.559911319644449179, 13.89701867748817321, 9.422509992056141925 ) ) ;
#9204=CARTESIAN_POINT ( 'NONE',  ( -2.266590686148945544, 42.22041550158063217, 7.082119434687048631 ) ) ;
#9205=CARTESIAN_POINT ( 'NONE',  ( 24.16423886937410614, 59.51208216824728936, -3.795296366450302550 ) ) ;
#9206=CARTESIAN_POINT ( 'NONE',  ( 1.472469842513823179, 15.59226448433411960, -4.923371831947296329 ) ) ;
#9207=CARTESIAN_POINT ( 'NONE',  ( 19.42250999205614193, 10.14701867748816966, 5.440088680355555262 ) ) ;
#9209=CARTESIAN_POINT ( 'NONE',  ( 17.20831665107776587, 37.88393115100078745, 7.208316651077764980 ) ) ;
#9210=CARTESIAN_POINT ( 'NONE',  ( -0.8801773607111009756, 28.06368534415484106, 1.068504757029289695E-15 ) ) ;
#9211=CARTESIAN_POINT ( 'NONE',  ( 6.565887622018943937, -1.918031996736246692, -12.81628187352647608 ) ) ;
#9212=CARTESIAN_POINT ( 'NONE',  ( 17.08211943468705130, 18.47041550158063572, 12.26659068614894998 ) ) ;
#9213=CARTESIAN_POINT ( 'NONE',  ( 0.1532563361054100626, 60.80059781766744464, -2.638427012816831230 ) ) ;
#9216=CARTESIAN_POINT ( 'NONE',  ( 2.791683348922237240, 10.38393115100078390, -7.208316651077763204 ) ) ;
#9217=CARTESIAN_POINT ( 'NONE',  ( 13.43411237798106583, 57.66530133659708923, -12.81628187352647252 ) ) ;
#9218=CARTESIAN_POINT ( 'NONE',  ( 14.92337183194729633, 57.67559781766745886, 8.527530157486181039 ) ) ;
#9220=CARTESIAN_POINT ( 'NONE',  ( 1.472469842513823179, 20.59226448433411960, -4.923371831947296329 ) ) ;
#9223=CARTESIAN_POINT ( 'NONE',  ( 10.00000000000000000, 1.813685344154838175, -10.88017736071110342 ) ) ;
#9224=CARTESIAN_POINT ( 'NONE',  ( 19.42250999205614548, 55.98035201082150536, -5.440088680355545492 ) ) ;
#9225=CARTESIAN_POINT ( 'NONE',  ( 13.79529636645031943, 10.34541550158063394, -14.16423886937409904 ) ) ;
#9227=CARTESIAN_POINT ( 'NONE',  ( 20.88017736071110519, 50.56368534415484106, 2.639326808657452039E-16 ) ) ;
#9228=CARTESIAN_POINT ( 'NONE',  ( 5.076628168052704559, 35.17559781766745175, -8.527530157486179263 ) ) ;
#9229=CARTESIAN_POINT ( 'NONE',  ( 7.084665262690076126, 22.02201867748817321, -10.88017736071110164 ) ) ;
#9231=CARTESIAN_POINT ( 'NONE',  ( 17.20831665107776587, 57.88393115100078745, 7.208316651077764980 ) ) ;
#9237=CARTESIAN_POINT ( 'NONE',  ( 0.2751277870542908621, 32.28217586085237656, -6.499999999999992006 ) ) ;
#9238=CARTESIAN_POINT ( 'NONE',  ( 0.1532563361054082862, 46.21726448433411605, 2.638427012816831674 ) ) ;
#9239=CARTESIAN_POINT ( 'NONE',  ( 0.1532563361054082862, 26.21726448433411605, 2.638427012816831674 ) ) ;
#9240=CARTESIAN_POINT ( 'NONE',  ( 3.591859063236763294, 63.29030133659708923, -11.09922568453595026 ) ) ;
#9241=CARTESIAN_POINT ( 'NONE',  ( 4.559911319644449179, 22.23035201082150536, -9.422509992056141925 ) ) ;
#9242=CARTESIAN_POINT ( 'NONE',  ( 14.92337183194729633, 47.67559781766745175, 8.527530157486181039 ) ) ;
#9243=CARTESIAN_POINT ( 'NONE',  ( -0.2418659066527639179, 34.26028685723174050, -6.114288769123057854 ) ) ;
#9244=CARTESIAN_POINT ( 'NONE',  ( 10.00000000000000000, 35.55374883491396787, -14.16423886937410082 ) ) ;
#9245=CARTESIAN_POINT ( 'NONE',  ( 24.16423886937410614, 54.30374883491396787, 8.672049930838204340E-16 ) ) ;
#9248=CARTESIAN_POINT ( 'NONE',  ( 7.084665262690076126, 54.10535201082151247, 10.88017736071109987 ) ) ;
#9249=CARTESIAN_POINT ( 'NONE',  ( 14.92337183194729633, 17.67559781766745175, 8.527530157486181039 ) ) ;
#9253=CARTESIAN_POINT ( 'NONE',  ( 0.8719017118913385822, 123.9374316453451144, 4.500000000000000888 ) ) ;
#9256=CARTESIAN_POINT ( 'NONE',  ( 2.791683348922240793, 11.63393115100078568, 7.208316651077764092 ) ) ;
#9258=CARTESIAN_POINT ( 'NONE',  ( 17.08211943468705130, 18.47041550158063572, 12.26659068614894998 ) ) ;
#9259=CARTESIAN_POINT ( 'NONE',  ( 17.20831665107776587, 24.13393115100078035, -7.208316651077762316 ) ) ;
#9260=CARTESIAN_POINT ( 'NONE',  ( -0.8801773607111008646, 38.27201867748816255, 2.915334737309923430 ) ) ;
#9262=MECHANICAL_DESIGN_GEOMETRIC_PRESENTATION_REPRESENTATION('',(#47580),#14047);
#9265=CARTESIAN_POINT ( 'NONE',  ( 17.96484262340118221, 41.18868534415484106, -7.964842623401177768 ) ) ;
#9266=CARTESIAN_POINT ( 'NONE',  ( 19.72487221294571214, 37.80223176428831522, -6.499999999999988454 ) ) ;
#9267=ORIENTED_EDGE ( 'NONE', *, *, #38200, .T. ) ;
#9268=CARTESIAN_POINT ( 'NONE',  ( 6.204703633549690345, 5.762082168247301794, -14.16423886937410259 ) ) ;
#9270=ORIENTED_EDGE ( 'NONE', *, *, #65480, .T. ) ;
#9271=CARTESIAN_POINT ( 'NONE',  ( -2.816281873526473856, 29.33196800326376064, 3.434112377981055619 ) ) ;
#9272=CARTESIAN_POINT ( 'NONE',  ( 19.84674366389459621, 8.508931151000785675, 7.409399052514197653E-17 ) ) ;
#9275=CARTESIAN_POINT ( 'NONE',  ( 7.361572987183169658, 19.96726448433411960, -9.846743663894592657 ) ) ;
#9276=CARTESIAN_POINT ( 'NONE',  ( 19.42250999205614193, 30.14701867748817321, 5.440088680355555262 ) ) ;
#9281=CARTESIAN_POINT ( 'NONE',  ( 2.035157376598824452, 58.68868534415482685, 7.964842623401179544 ) ) ;
#9283=CARTESIAN_POINT ( 'NONE',  ( 15.44008868035555260, 54.73035201082150536, 9.422509992056143702 ) ) ;
#9284=EDGE_CURVE ( 'NONE', #18606, #78790, #58035, .T. ) ;
#9287=CARTESIAN_POINT ( 'NONE',  ( 18.52753015748617571, 28.09226448433411960, 4.923371831947298993 ) ) ;
#9288=CARTESIAN_POINT ( 'NONE',  ( 22.81628187352648496, 61.83196800326376774, -3.434112377981050290 ) ) ;
#9289=CARTESIAN_POINT ( 'NONE',  ( 24.16423886937410614, 14.30374883491396787, 8.672049930838204340E-16 ) ) ;
#9290=CARTESIAN_POINT ( 'NONE',  ( 1.472469842513823179, 21.42559781766745175, 4.923371831947296329 ) ) ;
#9291=CARTESIAN_POINT ( 'NONE',  ( 0.6178305044545838731, 19.74863466993042138, 9.382169495545420901 ) ) ;
#9293=CYLINDRICAL_SURFACE ( 'NONE', #54552, 11.92686044187656513 ) ;
#9294=CARTESIAN_POINT ( 'NONE',  ( -0.8801773607110991993, 47.85535201082150536, -2.915334737309923874 ) ) ;
#9295=CARTESIAN_POINT ( 'NONE',  ( 2.791683348922237240, 65.38393115100078035, -7.208316651077763204 ) ) ;
#9297=CARTESIAN_POINT ( 'NONE',  ( 2.791683348922240793, 16.63393115100078745, 7.208316651077764092 ) ) ;
#9298=CARTESIAN_POINT ( 'NONE',  ( 17.96484262340118221, 16.18868534415483396, -7.964842623401177768 ) ) ;
#9299=CARTESIAN_POINT ( 'NONE',  ( 22.81628187352648496, 16.83196800326374998, -3.434112377981050290 ) ) ;
#9300=CARTESIAN_POINT ( 'NONE',  ( 19.84674366389459266, 18.71726448433411960, -2.638427012816827677 ) ) ;
#9302=CARTESIAN_POINT ( 'NONE',  ( 19.42250999205614548, 15.98035201082150714, -5.440088680355545492 ) ) ;
#9304=CARTESIAN_POINT ( 'NONE',  ( 2.791683348922240793, 36.63393115100078035, 7.208316651077764092 ) ) ;
#9305=CARTESIAN_POINT ( 'NONE',  ( 19.42250999205614548, 20.98035201082150891, -5.440088680355545492 ) ) ;
#9306=LINE ( 'NONE', #24331, #51965 ) ;
#9307=CARTESIAN_POINT ( 'NONE',  ( 17.96484262340118221, 36.18868534415484106, -7.964842623401177768 ) ) ;
#9308=CARTESIAN_POINT ( 'NONE',  ( 10.00000000000000178, 9.313685344154839285, 10.88017736071110342 ) ) ;
#9310=CARTESIAN_POINT ( 'NONE',  ( 2.791683348922237240, 10.38393115100078390, -7.208316651077763204 ) ) ;
#9312=CARTESIAN_POINT ( 'NONE',  ( 18.52753015748617571, 43.09226448433412315, 4.923371831947298993 ) ) ;
#9315=ADVANCED_FACE ( 'NONE', ( #74024 ), #75260, .T. ) ;
#9320=CARTESIAN_POINT ( 'NONE',  ( 24.16423886937409904, 29.09541550158063572, 3.795296366450317205 ) ) ;
#9321=CARTESIAN_POINT ( 'NONE',  ( 18.52753015748617571, 33.09226448433411605, 4.923371831947298993 ) ) ;
#9324=CARTESIAN_POINT ( 'NONE',  ( -0.3689425029237881626, 57.42874883491397497, 10.36894250292379027 ) ) ;
#9325=CARTESIAN_POINT ( 'NONE',  ( 0.1532563361054083140, 21.00893115100078745, 1.131784320476157264E-15 ) ) ;
#9328=CARTESIAN_POINT ( 'NONE',  ( 15.44008868035555260, 44.73035201082151247, 9.422509992056143702 ) ) ;
#9329=CARTESIAN_POINT ( 'NONE',  ( 0.6178305044545818747, 58.49863466993042493, -9.382169495545419124 ) ) ;
#9331=CARTESIAN_POINT ( 'NONE',  ( 15.44008868035555260, 19.73035201082150536, 9.422509992056143702 ) ) ;
#9332=CARTESIAN_POINT ( 'NONE',  ( 22.81628187352648496, 46.83196800326376064, -3.434112377981050290 ) ) ;
#9333=CARTESIAN_POINT ( 'NONE',  ( 0.6178305044545838731, 14.74863466993041783, 9.382169495545420901 ) ) ;
#9334=CARTESIAN_POINT ( 'NONE',  ( 18.52753015748618282, 13.92559781766745175, -4.923371831947291888 ) ) ;
#9337=CARTESIAN_POINT ( 'NONE',  ( 14.49999999999999822, 11.00000000000000000, -6.500000000000000888 ) ) ;
#9338=CARTESIAN_POINT ( 'NONE',  ( 2.917880565312948704, 52.63708216824730357, 12.26659068614894643 ) ) ;
#9339=CARTESIAN_POINT ( 'NONE',  ( -0.3689425029237881626, 12.42874883491396609, 10.36894250292379027 ) ) ;
#9340=CARTESIAN_POINT ( 'NONE',  ( 17.96484262340118221, 21.18868534415483396, -7.964842623401177768 ) ) ;
#9341=CARTESIAN_POINT ( 'NONE',  ( 2.035157376598822676, 37.43868534415484106, -7.964842623401177768 ) ) ;
#9342=CARTESIAN_POINT ( 'NONE',  ( 20.15039907845753220, 21.74884699246888786, 6.262539305110078836 ) ) ;
#9343=CARTESIAN_POINT ( 'NONE',  ( 19.42250999205614548, 60.98035201082151247, -5.440088680355545492 ) ) ;
#9344=CARTESIAN_POINT ( 'NONE',  ( 12.63842701281683922, 24.55059781766745175, -9.846743663894590881 ) ) ;
#9347=CARTESIAN_POINT ( 'NONE',  ( 14.92337183194729988, 14.34226448433411782, -8.527530157486177487 ) ) ;
#9348=CARTESIAN_POINT ( 'NONE',  ( 18.52753015748617571, 33.09226448433411605, 4.923371831947298993 ) ) ;
#9349=CARTESIAN_POINT ( 'NONE',  ( 0.5774900079438590739, 7.647018677488171434, -5.440088680355550821 ) ) ;
#9351=CARTESIAN_POINT ( 'NONE',  ( -1.099225684535947600, 28.70696800326375353, -6.408140936763238038 ) ) ;
#9352=CARTESIAN_POINT ( 'NONE',  ( 15.44008868035555793, 56.39701867748817676, -9.422509992056140149 ) ) ;
#9353=CARTESIAN_POINT ( 'NONE',  ( 10.00000000000000178, 48.05374883491396787, 14.16423886937410082 ) ) ;
#9354=CARTESIAN_POINT ( 'NONE',  ( 14.92337183194729988, 14.34226448433411782, -8.527530157486177487 ) ) ;
#9356=CARTESIAN_POINT ( 'NONE',  ( 0.1532563361054083140, 46.00893115100079456, 1.131784320476157264E-15 ) ) ;
#9357=CARTESIAN_POINT ( 'NONE',  ( 18.52753015748617571, 33.09226448433411605, 4.923371831947298993 ) ) ;
#9358=CARTESIAN_POINT ( 'NONE',  ( 13.79529636645031943, 10.34541550158063394, -14.16423886937409904 ) ) ;
#9360=CARTESIAN_POINT ( 'NONE',  ( 24.16423886937410614, 24.30374883491396787, 8.672049930838204340E-16 ) ) ;
#9361=CARTESIAN_POINT ( 'NONE',  ( 12.91533473730992121, 44.52201867748816966, 10.88017736071110164 ) ) ;
#9362=CARTESIAN_POINT ( 'NONE',  ( 20.88017736071110164, 15.35535201082150358, 2.915334737309930979 ) ) ;
#9363=CARTESIAN_POINT ( 'NONE',  ( 10.00000000000000000, 41.81368534415484106, -10.88017736071110342 ) ) ;
#9365=CARTESIAN_POINT ( 'NONE',  ( 4.559911319644449179, 32.23035201082150536, -9.422509992056141925 ) ) ;
#9367=CARTESIAN_POINT ( 'NONE',  ( 3.591859063236763294, 33.29030133659708213, -11.09922568453595026 ) ) ;
#9368=CARTESIAN_POINT ( 'NONE',  ( 2.035157376598824452, 38.68868534415483396, 7.964842623401179544 ) ) ;
#9370=CARTESIAN_POINT ( 'NONE',  ( 3.591859063236763294, 63.29030133659708923, -11.09922568453595026 ) ) ;
#9372=CARTESIAN_POINT ( 'NONE',  ( 20.88017736071110519, 50.56368534415484106, 2.639326808657452039E-16 ) ) ;
#9374=CARTESIAN_POINT ( 'NONE',  ( 0.5774900079438590739, 52.64701867748817676, -5.440088680355550821 ) ) ;
#9375=CARTESIAN_POINT ( 'NONE',  ( 12.91533473730992121, 4.522018677488169658, 10.88017736071110164 ) ) ;
#9376=FACE_OUTER_BOUND ( 'NONE', #92952, .T. ) ;
#9378=CARTESIAN_POINT ( 'NONE',  ( 24.16423886937410614, 64.51208216824728936, -3.795296366450302550 ) ) ;
#9379=CARTESIAN_POINT ( 'NONE',  ( 0.1532563361054100626, 0.8005978176674514168, -2.638427012816831230 ) ) ;
#9380=CARTESIAN_POINT ( 'NONE',  ( -4.164238869374098151, 1.595415501580634388, -3.795296366450310543 ) ) ;
#9381=CARTESIAN_POINT ( 'NONE',  ( -0.8801773607110991993, 12.85535201082150358, -2.915334737309923874 ) ) ;
#9382=CARTESIAN_POINT ( 'NONE',  ( 5.076628168052704559, 45.17559781766745175, -8.527530157486179263 ) ) ;
#9384=B_SPLINE_CURVE_WITH_KNOTS ( 'NONE', 3,
 ( #58656, #74138, #21161, #12172, #80176, #4196, #51663, #34666 ),
 .UNSPECIFIED., .F., .F.,
 ( 4, 2, 2, 4 ),
 ( 1.734723475976807094E-18, 0.001337541016207008859, 0.002675082032414015983, 0.005350164064828043242 ),
 .UNSPECIFIED. ) ;
#9385=CARTESIAN_POINT ( 'NONE',  ( 0.1532563361054083140, 51.00893115100078745, 1.131784320476157264E-15 ) ) ;
#9386=STYLED_ITEM ( 'NONE', ( #1340 ), #13909 ) ;
#9387=CARTESIAN_POINT ( 'NONE',  ( -0.8801773607111009756, 68.06368534415484817, 1.068504757029289695E-15 ) ) ;
#9388=CARTESIAN_POINT ( 'NONE',  ( 20.88017736071110164, 40.35535201082150536, 2.915334737309930979 ) ) ;
#9389=CARTESIAN_POINT ( 'NONE',  ( 0.1532563361054083140, 41.00893115100078745, 1.131784320476157264E-15 ) ) ;
#9391=CARTESIAN_POINT ( 'NONE',  ( 4.559911319644449179, 67.23035201082150536, -9.422509992056141925 ) ) ;
#9392=CARTESIAN_POINT ( 'NONE',  ( 7.084665262690076126, 52.02201867748816255, -10.88017736071110164 ) ) ;
#9393=CARTESIAN_POINT ( 'NONE',  ( 24.16423886937410614, 64.30374883491396076, 8.672049930838204340E-16 ) ) ;
#9395=MECHANICAL_DESIGN_GEOMETRIC_PRESENTATION_REPRESENTATION('',(#7839),#14195);
#9397=CARTESIAN_POINT ( 'NONE',  ( -2.816281873526473856, 19.33196800326375708, 3.434112377981055619 ) ) ;
#9398=CYLINDRICAL_SURFACE ( 'NONE', #32337, 0.5000000000000004441 ) ;
#9399=ORIENTED_EDGE ( 'NONE', *, *, #65693, .F. ) ;
#9400=CARTESIAN_POINT ( 'NONE',  ( 22.81628187352647785, 31.41530133659709279, 3.434112377981063169 ) ) ;
#9401=CARTESIAN_POINT ( 'NONE',  ( 12.91533473730993009, 16.60535201082150891, -10.88017736071109987 ) ) ;
#9402=EDGE_CURVE ( 'NONE', #30783, #74488, #79351, .T. ) ;
#9403=VERTEX_POINT ( 'NONE', #2397 ) ;
#9405=CARTESIAN_POINT ( 'NONE',  ( 10.00000000000000178, 69.31368534415484817, 10.88017736071110342 ) ) ;
#9406=CARTESIAN_POINT ( 'NONE',  ( 2.791683348922237240, 45.38393115100079456, -7.208316651077763204 ) ) ;
#9407=CARTESIAN_POINT ( 'NONE',  ( 1.472469842513823179, 10.59226448433411782, -4.923371831947296329 ) ) ;
#9408=CARTESIAN_POINT ( 'NONE',  ( 7.361572987183170547, 42.05059781766745886, 9.846743663894590881 ) ) ;
#9409=CARTESIAN_POINT ( 'NONE',  ( 0.1922240491738394785, 28.18878173731741299, 6.499999999999960920 ) ) ;
#9411=CARTESIAN_POINT ( 'NONE',  ( 5.076628168052703671, 21.84226448433411960, 8.527530157486179263 ) ) ;
#9415=CARTESIAN_POINT ( 'NONE',  ( 2.791683348922240793, 31.63393115100078745, 7.208316651077764092 ) ) ;
#9417=CARTESIAN_POINT ( 'NONE',  ( 7.361572987183169658, 44.96726448433412315, -9.846743663894592657 ) ) ;
#9420=CARTESIAN_POINT ( 'NONE',  ( 21.09922568453595559, 32.04030133659708923, -6.408140936763230044 ) ) ;
#9422=CARTESIAN_POINT ( 'NONE',  ( -4.164238869374098151, 51.59541550158063217, -3.795296366450310543 ) ) ;
#9423=CARTESIAN_POINT ( 'NONE',  ( 7.361572987183169658, 19.96726448433411960, -9.846743663894592657 ) ) ;
#9425=CARTESIAN_POINT ( 'NONE',  ( 2.917880565312948704, 37.63708216824731068, 12.26659068614894643 ) ) ;
#9426=CARTESIAN_POINT ( 'NONE',  ( 7.361572987183169658, 59.96726448433410894, -9.846743663894592657 ) ) ;
#9427=CARTESIAN_POINT ( 'NONE',  ( -2.266590686148945544, 57.22041550158063217, 7.082119434687048631 ) ) ;
#9428=CARTESIAN_POINT ( 'NONE',  ( 13.79529636645030344, 23.26208216824730002, 14.16423886937410614 ) ) ;
#9429=CARTESIAN_POINT ( 'NONE',  ( -4.164238869374099039, 21.80374883491396787, 8.674139862899312516E-16 ) ) ;
#9433=CARTESIAN_POINT ( 'NONE',  ( 1.472469842513823179, 61.42559781766745175, 4.923371831947296329 ) ) ;
#9435=CARTESIAN_POINT ( 'NONE',  ( 15.44008868035555260, 39.73035201082150536, 9.422509992056143702 ) ) ;
#9439=CARTESIAN_POINT ( 'NONE',  ( 19.84674366389459621, 38.50893115100078745, 7.409399052514197653E-17 ) ) ;
#9440=CARTESIAN_POINT ( 'NONE',  ( 22.81628187352647785, 56.41530133659708213, 3.434112377981063169 ) ) ;
#9442=CARTESIAN_POINT ( 'NONE',  ( 19.84674366389459266, 48.30059781766745175, 2.638427012816836559 ) ) ;
#9445=CARTESIAN_POINT ( 'NONE',  ( 6.204703633549690345, 15.76208216824730179, -14.16423886937410259 ) ) ;
#9446=LINE ( 'NONE', #23971, #48628 ) ;
#9447=CARTESIAN_POINT ( 'NONE',  ( 18.72515096720571037, 45.05509018479935435, 6.499999999999982236 ) ) ;
#9449=CARTESIAN_POINT ( 'NONE',  ( 17.96484262340118221, 11.18868534415484106, -7.964842623401177768 ) ) ;
#9450=CARTESIAN_POINT ( 'NONE',  ( 22.81628187352648496, 6.831968003263753531, -3.434112377981050290 ) ) ;
#9452=CARTESIAN_POINT ( 'NONE',  ( 12.91533473730993009, 61.60535201082150536, -10.88017736071109987 ) ) ;
#9455=CARTESIAN_POINT ( 'NONE',  ( -46.94000000000001194, 101.0890360526157252, -7.984865333617746863 ) ) ;
#9457=CARTESIAN_POINT ( 'NONE',  ( 22.26659068614895176, 59.72041550158063927, -7.082119434687042414 ) ) ;
#9459=CARTESIAN_POINT ( 'NONE',  ( 19.42250999205614548, 25.98035201082150891, -5.440088680355545492 ) ) ;
#9460=CARTESIAN_POINT ( 'NONE',  ( 0.5774900079438590739, 37.64701867748817676, -5.440088680355550821 ) ) ;
#9461=CARTESIAN_POINT ( 'NONE',  ( 21.09922568453595559, 2.040301336597086568, -6.408140936763230044 ) ) ;
#9462=CARTESIAN_POINT ( 'NONE',  ( 1.472469842513823179, 51.42559781766745886, 4.923371831947296329 ) ) ;
#9463=CARTESIAN_POINT ( 'NONE',  ( -43.14624366973443870, 107.3138868136391864, -4.970300893257880048 ) ) ;
#9464=CARTESIAN_POINT ( 'NONE',  ( 19.84674366389459266, 3.300597817667451750, 2.638427012816836559 ) ) ;
#9467=CARTESIAN_POINT ( 'NONE',  ( 20.88017736071110164, 30.35535201082151247, 2.915334737309930979 ) ) ;
#9468=CARTESIAN_POINT ( 'NONE',  ( 10.00000000000000178, 35.37363466993042493, 12.81628187352647608 ) ) ;
#9469=CARTESIAN_POINT ( 'NONE',  ( -1.926860441876563801, 54.89664270246084499, 3.195792623639529761 ) ) ;
#9470=CARTESIAN_POINT ( 'NONE',  ( 2.791683348922240793, 66.63393115100079456, 7.208316651077764092 ) ) ;
#9471=CARTESIAN_POINT ( 'NONE',  ( 15.44008868035555260, 54.73035201082150536, 9.422509992056143702 ) ) ;
#9472=CARTESIAN_POINT ( 'NONE',  ( 14.92337183194729633, 12.67559781766745353, 8.527530157486181039 ) ) ;
#9473=CARTESIAN_POINT ( 'NONE',  ( 0.6178305044545818747, 38.49863466993042493, -9.382169495545419124 ) ) ;
#9474=CARTESIAN_POINT ( 'NONE',  ( 20.88017736071110164, 65.35535201082150536, 2.915334737309930979 ) ) ;
#9475=DIRECTION ( 'NONE',  ( -0.000000000000000000, 1.000000000000000000, -0.000000000000000000 ) ) ;
#9476=CARTESIAN_POINT ( 'NONE',  ( 19.42250999205614548, 55.98035201082150536, -5.440088680355545492 ) ) ;
#9477=CARTESIAN_POINT ( 'NONE',  ( 6.565887622018943937, 65.16530133659709634, 12.81628187352647430 ) ) ;
#9481=CARTESIAN_POINT ( 'NONE',  ( 20.88017736071110519, 10.56368534415483751, 2.639326808657452039E-16 ) ) ;
#9482=CARTESIAN_POINT ( 'NONE',  ( 19.38216949554541202, 50.99863466993042493, 9.382169495545424454 ) ) ;
#9483=CARTESIAN_POINT ( 'NONE',  ( 10.00000000000000000, 10.55374883491396787, -14.16423886937410082 ) ) ;
#9484=CARTESIAN_POINT ( 'NONE',  ( 14.92337183194729633, 22.67559781766745175, 8.527530157486181039 ) ) ;
#9485=CARTESIAN_POINT ( 'NONE',  ( 5.076628168052704559, 15.17559781766745175, -8.527530157486179263 ) ) ;
#9486=CARTESIAN_POINT ( 'NONE',  ( 17.08211943468705840, 50.13708216824730357, -12.26659068614894466 ) ) ;
#9488=VECTOR ( 'NONE', #28891, 1000.000000000000000 ) ;
#9489=EDGE_CURVE ( 'NONE', #19583, #72554, #75842, .T. ) ;
#9490=CARTESIAN_POINT ( 'NONE',  ( -0.8801773607110991993, 22.85535201082150181, -2.915334737309923874 ) ) ;
#9491=CARTESIAN_POINT ( 'NONE',  ( 1.602071938427508391, 32.02224192338639597, -6.499999999999986677 ) ) ;
#9494=CARTESIAN_POINT ( 'NONE',  ( 0.5774900079438590739, 12.64701867748817321, -5.440088680355550821 ) ) ;
#9495=CARTESIAN_POINT ( 'NONE',  ( 0.5774900079438607392, 13.48035201082150358, 5.440088680355550821 ) ) ;
#9496=CARTESIAN_POINT ( 'NONE',  ( 19.84674366389459621, 63.50893115100078745, 7.409399052514197653E-17 ) ) ;
#9497=CARTESIAN_POINT ( 'NONE',  ( 13.43411237798105340, 50.58196800326375353, 12.81628187352647963 ) ) ;
#9498=DIRECTION ( 'NONE',  ( 0.000000000000000000, -1.000000000000000000, 0.000000000000000000 ) ) ;
#9499=CARTESIAN_POINT ( 'NONE',  ( 17.39651004071838614, 62.93575266056827644, 6.500000000000032863 ) ) ;
#9500=CARTESIAN_POINT ( 'NONE',  ( 10.00000000000000000, 15.55374883491396787, -14.16423886937410082 ) ) ;
#9501=CARTESIAN_POINT ( 'NONE',  ( 19.42250999205614193, 30.14701867748817321, 5.440088680355555262 ) ) ;
#9502=CARTESIAN_POINT ( 'NONE',  ( -0.8801773607111009756, 3.063685344154838397, 1.068504757029289695E-15 ) ) ;
#9504=CARTESIAN_POINT ( 'NONE',  ( 7.361572987183170547, 62.05059781766745886, 9.846743663894590881 ) ) ;
#9505=CARTESIAN_POINT ( 'NONE',  ( 18.17829156368508592, 44.16792564121893605, 6.499999999999926281 ) ) ;
#9506=CARTESIAN_POINT ( 'NONE',  ( 0.1532563361054100626, 35.80059781766745175, -2.638427012816831230 ) ) ;
#9507=CARTESIAN_POINT ( 'NONE',  ( 14.92337183194729633, 2.675597817667451750, 8.527530157486181039 ) ) ;
#9511=CARTESIAN_POINT ( 'NONE',  ( 7.084665262690076126, 2.022018677488170990, -10.88017736071110164 ) ) ;
#9512=CARTESIAN_POINT ( 'NONE',  ( 0.1532563361054083140, 1.008931151000784787, 1.131784320476157264E-15 ) ) ;
#9514=CARTESIAN_POINT ( 'NONE',  ( 21.09922568453595559, 2.040301336597086568, -6.408140936763230044 ) ) ;
#9515=CARTESIAN_POINT ( 'NONE',  ( 17.96484262340118221, 46.18868534415484106, -7.964842623401177768 ) ) ;
#9516=CARTESIAN_POINT ( 'NONE',  ( 4.559911319644449179, 12.23035201082150536, -9.422509992056141925 ) ) ;
#9517=CARTESIAN_POINT ( 'NONE',  ( -2.816281873526471635, 38.91530133659708213, -3.434112377981056508 ) ) ;
#9518=CARTESIAN_POINT ( 'NONE',  ( -0.3689425029237898834, 16.17874883491396076, -10.36894250292378850 ) ) ;
#9519=EDGE_CURVE ( 'NONE', #91046, #6749, #21198, .T. ) ;
#9520=CARTESIAN_POINT ( 'NONE',  ( -2.816281873526471635, 38.91530133659708213, -3.434112377981056508 ) ) ;
#9521=VERTEX_POINT ( 'NONE', #56362 ) ;
#9522=CARTESIAN_POINT ( 'NONE',  ( 17.20831665107776587, 57.88393115100078745, 7.208316651077764980 ) ) ;
#9523=CARTESIAN_POINT ( 'NONE',  ( 4.559911319644449179, 13.89701867748817321, 9.422509992056141925 ) ) ;
#9525=CARTESIAN_POINT ( 'NONE',  ( 2.035157376598824452, 33.68868534415484106, 7.964842623401179544 ) ) ;
#9526=ORIENTED_EDGE ( 'NONE', *, *, #3962, .T. ) ;
#9527=CARTESIAN_POINT ( 'NONE',  ( 1.472469842513823179, 10.59226448433411782, -4.923371831947296329 ) ) ;
#9528=SURFACE_SIDE_STYLE ('',( #54523 ) ) ;
#9530=CARTESIAN_POINT ( 'NONE',  ( 19.84674366389459621, 13.50893115100078568, 7.409399052514197653E-17 ) ) ;
#9531=CARTESIAN_POINT ( 'NONE',  ( 5.076628168052704559, 0.1755978176674514724, -8.527530157486179263 ) ) ;
#9532=CARTESIAN_POINT ( 'NONE',  ( 19.72487221294571569, 49.78217586085237656, 6.499999999999993783 ) ) ;
#9533=CARTESIAN_POINT ( 'NONE',  ( 1.274849032794231007, 38.57228050351032067, 6.499999999999895195 ) ) ;
#9534=CARTESIAN_POINT ( 'NONE',  ( 2.035157376598822676, 67.43868534415484817, -7.964842623401177768 ) ) ;
#9535=CARTESIAN_POINT ( 'NONE',  ( 1.472469842513823179, 5.592264484334118713, -4.923371831947296329 ) ) ;
#9537=CARTESIAN_POINT ( 'NONE',  ( 0.1532563361054082862, 61.21726448433412315, 2.638427012816831674 ) ) ;
#9539=VERTEX_POINT ( 'NONE', #69890 ) ;
#9540=DIRECTION ( 'NONE',  ( -0.8320502943378437211, 0.5547001962252290364, 0.000000000000000000 ) ) ;
#9541=CARTESIAN_POINT ( 'NONE',  ( -2.266590686148945544, 7.220415501580634832, 7.082119434687048631 ) ) ;
#9542=CARTESIAN_POINT ( 'NONE',  ( -1.099225684535947600, 54.54030133659708923, 6.408140936763237150 ) ) ;
#9543=CARTESIAN_POINT ( 'NONE',  ( 2.917880565312948704, 2.637082168247300906, 12.26659068614894643 ) ) ;
#9545=CARTESIAN_POINT ( 'NONE',  ( -4.164238869374099927, 22.01208216824730357, 3.795296366450308767 ) ) ;
#9547=CARTESIAN_POINT ( 'NONE',  ( 19.42250999205614193, 60.14701867748817676, 5.440088680355555262 ) ) ;
#9548=CARTESIAN_POINT ( 'NONE',  ( 20.88017736071110875, 15.77201867748817143, -2.915334737309920765 ) ) ;
#9549=ORIENTED_EDGE ( 'NONE', *, *, #75097, .F. ) ;
#9550=CARTESIAN_POINT ( 'NONE',  ( 2.791683348922240793, 1.633931151000784565, 7.208316651077764092 ) ) ;
#9551=CARTESIAN_POINT ( 'NONE',  ( 12.63842701281683034, 7.467264484334118713, 9.846743663894596210 ) ) ;
#9553=CARTESIAN_POINT ( 'NONE',  ( 22.81628187352647785, 31.62363466993042138, 6.195893100308588602E-16 ) ) ;
#9554=CARTESIAN_POINT ( 'NONE',  ( 10.00000000000000000, 39.75893115100078745, -9.846743663894594434 ) ) ;
#9556=ADVANCED_FACE ( 'NONE', ( #9376 ), #70385, .T. ) ;
#9557=CARTESIAN_POINT ( 'NONE',  ( 16.40814093676324603, 17.45696800326375353, -11.09922568453594671 ) ) ;
#9559=CARTESIAN_POINT ( 'NONE',  ( 12.63842701281683922, 29.55059781766745175, -9.846743663894590881 ) ) ;
#9560=CARTESIAN_POINT ( 'NONE',  ( 0.1532563361054083140, 11.00893115100078568, 1.131784320476157264E-15 ) ) ;
#9562=B_SPLINE_CURVE_WITH_KNOTS ( 'NONE', 3,
 ( #17251, #25735, #33689, #93221, #49682, #40236 ),
 .UNSPECIFIED., .F., .F.,
 ( 4, 2, 4 ),
 ( 0.000000000000000000, 0.0002605067024380875980, 0.0005210134048761751960 ),
 .UNSPECIFIED. ) ;
#9564=CARTESIAN_POINT ( 'NONE',  ( 12.91533473730993009, 31.60535201082150891, -10.88017736071109987 ) ) ;
#9565=CARTESIAN_POINT ( 'NONE',  ( 17.08211943468705130, 38.47041550158063217, 12.26659068614894998 ) ) ;
#9566=CARTESIAN_POINT ( 'NONE',  ( 12.63842701281683922, 44.55059781766745175, -9.846743663894590881 ) ) ;
#9567=CARTESIAN_POINT ( 'NONE',  ( 19.84674366389459266, 13.71726448433411782, -2.638427012816827677 ) ) ;
#9568=CARTESIAN_POINT ( 'NONE',  ( 21.09922568453595559, 52.04030133659708923, -6.408140936763230044 ) ) ;
#9570=CARTESIAN_POINT ( 'NONE',  ( 10.00000000000000178, 24.31368534415484106, 10.88017736071110342 ) ) ;
#9571=DIRECTION ( 'NONE',  ( -0.000000000000000000, 1.000000000000000000, -0.000000000000000000 ) ) ;
#9573=CARTESIAN_POINT ( 'NONE',  ( 21.09922568453594849, 16.20696800326375353, 6.408140936763242479 ) ) ;
#9574=CARTESIAN_POINT ( 'NONE',  ( 13.43411237798105340, 15.58196800326374998, 12.81628187352647963 ) ) ;
#9575=CARTESIAN_POINT ( 'NONE',  ( 10.00000000000000000, 44.75893115100078745, -9.846743663894594434 ) ) ;
#9577=CARTESIAN_POINT ( 'NONE',  ( 13.43411237798106583, 42.66530133659707502, -12.81628187352647252 ) ) ;
#9579=CARTESIAN_POINT ( 'NONE',  ( 12.91533473730992121, 49.52201867748817676, 10.88017736071110164 ) ) ;
#9583=CARTESIAN_POINT ( 'NONE',  ( 7.084665262690076126, 49.10535201082149825, 10.88017736071109987 ) ) ;
#9584=CARTESIAN_POINT ( 'NONE',  ( 7.084665262690076126, 64.10535201082150536, 10.88017736071109987 ) ) ;
#9587=CARTESIAN_POINT ( 'NONE',  ( 19.42250999205614548, 5.980352010821504471, -5.440088680355545492 ) ) ;
#9588=CARTESIAN_POINT ( 'NONE',  ( 7.361572987183169658, 64.96726448433412315, -9.846743663894592657 ) ) ;
#9589=CARTESIAN_POINT ( 'NONE',  ( 19.42250999205614193, 25.14701867748817321, 5.440088680355555262 ) ) ;
#9591=CARTESIAN_POINT ( 'NONE',  ( 0.6178305044545838731, 24.74863466993042493, 9.382169495545420901 ) ) ;
#9592=EDGE_LOOP ( 'NONE', ( #77530, #49576, #88467, #68377 ) ) ;
#9593=CARTESIAN_POINT ( 'NONE',  ( -0.8801773607110991993, 52.85535201082151247, -2.915334737309923874 ) ) ;
#9594=CARTESIAN_POINT ( 'NONE',  ( 10.00000000000000000, 34.75893115100078745, -9.846743663894594434 ) ) ;
#9595=CARTESIAN_POINT ( 'NONE',  ( 16.40814093676324603, 2.456968003263753531, -11.09922568453594671 ) ) ;
#9597=CARTESIAN_POINT ( 'NONE',  ( 15.44008868035555793, 11.39701867748817143, -9.422509992056140149 ) ) ;
#9598=CARTESIAN_POINT ( 'NONE',  ( 17.96484262340118221, 36.18868534415484106, -7.964842623401177768 ) ) ;
#9599=CARTESIAN_POINT ( 'NONE',  ( -0.3689425029237881626, 52.42874883491396076, 10.36894250292379027 ) ) ;
#9600=CARTESIAN_POINT ( 'NONE',  ( 10.00000000000000000, 39.75893115100078745, -9.846743663894594434 ) ) ;
#9601=CARTESIAN_POINT ( 'NONE',  ( 0.5774900079438607392, 58.48035201082151247, 5.440088680355550821 ) ) ;
#9603=CARTESIAN_POINT ( 'NONE',  ( -2.266590686148945544, 11.38708216824730179, -7.082119434687050408 ) ) ;
#9604=EDGE_CURVE ( 'NONE', #107, #91043, #35549, .T. ) ;
#9606=CARTESIAN_POINT ( 'NONE',  ( 1.602071938427508169, 22.02224192338640307, -6.499999999999988454 ) ) ;
#9611=CARTESIAN_POINT ( 'NONE',  ( 17.08211943468705130, 33.47041550158063927, 12.26659068614894998 ) ) ;
#9612=CARTESIAN_POINT ( 'NONE',  ( -4.164238869374099927, 42.01208216824728936, 3.795296366450308767 ) ) ;
#9613=CARTESIAN_POINT ( 'NONE',  ( 0.5774900079438607392, 68.48035201082150536, 5.440088680355550821 ) ) ;
#9614=CARTESIAN_POINT ( 'NONE',  ( 21.09922568453595559, 17.04030133659708923, -6.408140936763230044 ) ) ;
#9615=CARTESIAN_POINT ( 'NONE',  ( 2.791683348922240793, 61.63393115100079456, 7.208316651077764092 ) ) ;
#9616=CARTESIAN_POINT ( 'NONE',  ( 17.39651004071838614, 52.93575266056826933, 6.500000000000032863 ) ) ;
#9617=CARTESIAN_POINT ( 'NONE',  ( -0.8801773607111008646, 53.27201867748816966, 2.915334737309923430 ) ) ;
#9618=CARTESIAN_POINT ( 'NONE',  ( 13.43411237798106583, 27.66530133659708568, -12.81628187352647252 ) ) ;
#9619=CARTESIAN_POINT ( 'NONE',  ( 13.79529636645030344, 33.26208216824730357, 14.16423886937410614 ) ) ;
#9620=EDGE_CURVE ( 'NONE', #21055, #93709, #7544, .T. ) ;
#9621=CARTESIAN_POINT ( 'NONE',  ( 17.96484262340118221, 24.93868534415484461, 7.964842623401181321 ) ) ;
#9623=DIRECTION ( 'NONE',  ( 0.000000000000000000, 0.000000000000000000, 1.000000000000000000 ) ) ;
#9624=CARTESIAN_POINT ( 'NONE',  ( -0.8801773607111008646, 68.27201867748817676, 2.915334737309923430 ) ) ;
#9627=CARTESIAN_POINT ( 'NONE',  ( 5.076628168052703671, 6.842264484334118713, 8.527530157486179263 ) ) ;
#9628=EDGE_LOOP ( 'NONE', ( #42076, #20815, #49514, #74021, #76422 ) ) ;
#9630=ORIENTED_EDGE ( 'NONE', *, *, #67068, .T. ) ;
#9633=ORIENTED_EDGE ( 'NONE', *, *, #75189, .F. ) ;
#9634=CARTESIAN_POINT ( 'NONE',  ( 6.204703633549690345, 7.845415501580634832, 14.16423886937410082 ) ) ;
#9635=CARTESIAN_POINT ( 'NONE',  ( 19.42250999205614548, 5.980352010821504471, -5.440088680355545492 ) ) ;
#9636=CARTESIAN_POINT ( 'NONE',  ( 15.44008868035555793, 11.39701867748817143, -9.422509992056140149 ) ) ;
#9637=CARTESIAN_POINT ( 'NONE',  ( 19.84674366389459621, 33.50893115100078745, 7.409399052514197653E-17 ) ) ;
#9638=CARTESIAN_POINT ( 'NONE',  ( 6.565887622018943937, 3.081968003263753531, -12.81628187352647608 ) ) ;
#9641=CARTESIAN_POINT ( 'NONE',  ( 19.38216949554541202, 5.998634669930420493, 9.382169495545424454 ) ) ;
#9644=CARTESIAN_POINT ( 'NONE',  ( -0.3689425029237881626, 47.42874883491396787, 10.36894250292379027 ) ) ;
#9647=CARTESIAN_POINT ( 'NONE',  ( 13.79529636645031943, 55.34541550158062506, -14.16423886937409904 ) ) ;
#9649=CARTESIAN_POINT ( 'NONE',  ( 12.91533473730993009, 26.60535201082150536, -10.88017736071109987 ) ) ;
#9650=CARTESIAN_POINT ( 'NONE',  ( 4.559911319644449179, 38.89701867748817676, 9.422509992056141925 ) ) ;
#9651=CARTESIAN_POINT ( 'NONE',  ( 14.92337183194729988, 59.34226448433412315, -8.527530157486177487 ) ) ;
#9652=CARTESIAN_POINT ( 'NONE',  ( 12.91533473730993009, 41.60535201082149825, -10.88017736071109987 ) ) ;
#9653=CARTESIAN_POINT ( 'NONE',  ( 7.084665262690076126, 59.10535201082150536, 10.88017736071109987 ) ) ;
#9654=CARTESIAN_POINT ( 'NONE',  ( 17.96484262340118221, 24.93868534415484461, 7.964842623401181321 ) ) ;
#9655=B_SPLINE_CURVE_WITH_KNOTS ( 'NONE', 3,
 ( #2805, #47777, #87247, #25298 ),
 .UNSPECIFIED., .F., .F.,
 ( 4, 4 ),
 ( 2.138679957953595447E-16, 0.002392975128318489825 ),
 .UNSPECIFIED. ) ;
#9658=ORIENTED_EDGE ( 'NONE', *, *, #66371, .T. ) ;
#9660=FILL_AREA_STYLE_COLOUR ( '', #51425 ) ;
#9663=CARTESIAN_POINT ( 'NONE',  ( 19.84674366389459266, 43.71726448433410894, -2.638427012816827677 ) ) ;
#9667=CARTESIAN_POINT ( 'NONE',  ( -46.68456736488007408, 103.6675473310227034, 5.775421524742653467 ) ) ;
#9669=CARTESIAN_POINT ( 'NONE',  ( 5.076628168052704559, 55.17559781766745175, -8.527530157486179263 ) ) ;
#9670=CARTESIAN_POINT ( 'NONE',  ( 24.16423886937410614, 54.30374883491396787, 8.672049930838204340E-16 ) ) ;
#9671=CARTESIAN_POINT ( 'NONE',  ( 7.361572987183170547, 57.05059781766744464, 9.846743663894590881 ) ) ;
#9674=CARTESIAN_POINT ( 'NONE',  ( 18.52753015748618282, 23.92559781766745530, -4.923371831947291888 ) ) ;
#9675=CARTESIAN_POINT ( 'NONE',  ( 22.81628187352648496, 46.83196800326376064, -3.434112377981050290 ) ) ;
#9676=CARTESIAN_POINT ( 'NONE',  ( 7.361572987183169658, 64.96726448433412315, -9.846743663894592657 ) ) ;
#9677=CARTESIAN_POINT ( 'NONE',  ( 2.035157376598824452, 63.68868534415484106, 7.964842623401179544 ) ) ;
#9681=( BOUNDED_CURVE ( )  B_SPLINE_CURVE ( 3, ( #66859, #97378, #21368, #50372 ),
 .UNSPECIFIED., .F., .F. ) 
 B_SPLINE_CURVE_WITH_KNOTS ( ( 4, 4 ),
 ( 3.694400132159521011, 4.712388980384689674 ),
 .UNSPECIFIED. ) 
 CURVE ( )  GEOMETRIC_REPRESENTATION_ITEM ( )  RATIONAL_B_SPLINE_CURVE ( ( 1.000000000000000000, 0.9154899770527742398, 0.9154899770527742398, 1.000000000000000000 ) ) 
 REPRESENTATION_ITEM ( '' )  );
#9682=CARTESIAN_POINT ( 'NONE',  ( -4.164238869374098151, 56.59541550158063927, -3.795296366450310543 ) ) ;
#9683=CARTESIAN_POINT ( 'NONE',  ( 12.91533473730992121, 24.52201867748816966, 10.88017736071110164 ) ) ;
#9685=CARTESIAN_POINT ( 'NONE',  ( 22.81628187352648496, 16.83196800326374998, -3.434112377981050290 ) ) ;
#9686=CARTESIAN_POINT ( 'NONE',  ( 7.084665262690076126, 57.02201867748817676, -10.88017736071110164 ) ) ;
#9691=EDGE_CURVE ( 'NONE', #14954, #31369, #45786, .T. ) ;
#9692=CARTESIAN_POINT ( 'NONE',  ( 19.84674366389459621, 48.50893115100078745, 7.409399052514197653E-17 ) ) ;
#9695=CARTESIAN_POINT ( 'NONE',  ( 21.09922568453595559, 7.040301336597086568, -6.408140936763230044 ) ) ;
#9696=CARTESIAN_POINT ( 'NONE',  ( 7.084665262690076126, 19.10535201082150181, 10.88017736071109987 ) ) ;
#9698=CARTESIAN_POINT ( 'NONE',  ( -4.164238869374099039, 36.80374883491396787, 8.674139862899312516E-16 ) ) ;
#9699=CARTESIAN_POINT ( 'NONE',  ( -0.3689425029237881626, 27.42874883491397142, 10.36894250292379027 ) ) ;
#9700=CARTESIAN_POINT ( 'NONE',  ( 13.79529636645030344, 58.26208216824728936, 14.16423886937410614 ) ) ;
#9701=CARTESIAN_POINT ( 'NONE',  ( 10.00000000000000000, 29.75893115100078745, -9.846743663894594434 ) ) ;
#9702=CARTESIAN_POINT ( 'NONE',  ( 2.791683348922237240, 20.38393115100078745, -7.208316651077763204 ) ) ;
#9703=CARTESIAN_POINT ( 'NONE',  ( 10.00000000000000000, 16.81368534415483751, -10.88017736071110342 ) ) ;
#9705=CARTESIAN_POINT ( 'NONE',  ( 12.63842701281683922, 44.55059781766745175, -9.846743663894590881 ) ) ;
#9706=CARTESIAN_POINT ( 'NONE',  ( 20.88017736071110164, 45.35535201082149115, 2.915334737309930979 ) ) ;
#9707=CARTESIAN_POINT ( 'NONE',  ( 10.00000000000000178, 57.25893115100078745, 9.846743663894594434 ) ) ;
#9708=CARTESIAN_POINT ( 'NONE',  ( 24.16423886937410614, 19.51208216824729647, -3.795296366450302550 ) ) ;
#9711=CARTESIAN_POINT ( 'NONE',  ( 1.472469842513823179, 15.59226448433411960, -4.923371831947296329 ) ) ;
#9712=CARTESIAN_POINT ( 'NONE',  ( 22.81628187352647785, 51.62363466993042493, 6.195893100308588602E-16 ) ) ;
#9713=CARTESIAN_POINT ( 'NONE',  ( 0.1532563361054100626, 50.80059781766745175, -2.638427012816831230 ) ) ;
#9716=CYLINDRICAL_SURFACE ( 'NONE', #50768, 0.5000000000000004441 ) ;
#9717=CARTESIAN_POINT ( 'NONE',  ( 4.559911319644449179, 7.230352010821505360, -9.422509992056141925 ) ) ;
#9718=CARTESIAN_POINT ( 'NONE',  ( 15.44008868035555793, 56.39701867748817676, -9.422509992056140149 ) ) ;
#9719=CARTESIAN_POINT ( 'NONE',  ( -4.164238869374098151, 6.595415501580634832, -3.795296366450310543 ) ) ;
#9720=CARTESIAN_POINT ( 'NONE',  ( 5.076628168052704559, 0.1755978176674514724, -8.527530157486179263 ) ) ;
#9721=CARTESIAN_POINT ( 'NONE',  ( 2.791683348922237240, 55.38393115100078745, -7.208316651077763204 ) ) ;
#9722=CARTESIAN_POINT ( 'NONE',  ( 10.00000000000000000, 21.81368534415484106, -10.88017736071110342 ) ) ;
#9725=CARTESIAN_POINT ( 'NONE',  ( 19.84674366389459266, 3.717264484334118713, -2.638427012816827677 ) ) ;
#9726=CARTESIAN_POINT ( 'NONE',  ( 10.00000000000000178, 55.37363466993042493, 12.81628187352647608 ) ) ;
#9729=ORIENTED_EDGE ( 'NONE', *, *, #85921, .F. ) ;
#9733=CARTESIAN_POINT ( 'NONE',  ( 17.08211943468705840, 45.13708216824730357, -12.26659068614894466 ) ) ;
#9734=CARTESIAN_POINT ( 'NONE',  ( 5.076628168052703671, 41.84226448433411605, 8.527530157486179263 ) ) ;
#9735=CARTESIAN_POINT ( 'NONE',  ( 2.791683348922237240, 20.38393115100078745, -7.208316651077763204 ) ) ;
#9737=CARTESIAN_POINT ( 'NONE',  ( 20.88017736071110519, 15.56368534415483751, 2.639326808657452039E-16 ) ) ;
#9738=CARTESIAN_POINT ( 'NONE',  ( 2.791683348922237240, 65.38393115100078035, -7.208316651077763204 ) ) ;
#9741=CARTESIAN_POINT ( 'NONE',  ( 6.204703633549690345, 60.76208216824730357, -14.16423886937410259 ) ) ;
#9744=CARTESIAN_POINT ( 'NONE',  ( 19.42250999205614548, 60.98035201082151247, -5.440088680355545492 ) ) ;
#9745=CARTESIAN_POINT ( 'NONE',  ( 1.472469842513823179, 10.59226448433411782, -4.923371831947296329 ) ) ;
#9747=ORIENTED_EDGE ( 'NONE', *, *, #42576, .T. ) ;
#9749=EDGE_LOOP ( 'NONE', ( #80712, #87828, #97382, #65064 ) ) ;
#9751=CARTESIAN_POINT ( 'NONE',  ( 19.84674366389459266, 28.30059781766745886, 2.638427012816836559 ) ) ;
#9753=CARTESIAN_POINT ( 'NONE',  ( 6.204703633549690345, 30.76208216824730357, -14.16423886937410259 ) ) ;
#9754=CARTESIAN_POINT ( 'NONE',  ( 5.076628168052703671, 16.84226448433411960, 8.527530157486179263 ) ) ;
#9755=CARTESIAN_POINT ( 'NONE',  ( 19.42250999205614548, 40.98035201082150536, -5.440088680355545492 ) ) ;
#9758=AXIS2_PLACEMENT_3D ( 'NONE', #41077, #93566, #25099 ) ;
#9759=CARTESIAN_POINT ( 'NONE',  ( 2.035157376598824452, 38.68868534415483396, 7.964842623401179544 ) ) ;
#9761=EDGE_CURVE ( 'NONE', #53936, #51000, #85652, .T. ) ;
#9765=CARTESIAN_POINT ( 'NONE',  ( 10.00000000000000000, 41.81368534415484106, -10.88017736071110342 ) ) ;
#9767=CARTESIAN_POINT ( 'NONE',  ( -0.3689425029237898834, 11.17874883491396787, -10.36894250292378850 ) ) ;
#9768=EDGE_LOOP ( 'NONE', ( #56220, #97938, #49430, #27017, #64205, #41047 ) ) ;
#9771=CARTESIAN_POINT ( 'NONE',  ( 6.565887622018943937, 35.16530133659708923, 12.81628187352647430 ) ) ;
#9772=CARTESIAN_POINT ( 'NONE',  ( 19.84674366389459266, 8.300597817667451750, 2.638427012816836559 ) ) ;
#9773=DIRECTION ( 'NONE',  ( 0.000000000000000000, -1.000000000000000000, 0.000000000000000000 ) ) ;
#9775=CARTESIAN_POINT ( 'NONE',  ( 0.1532563361054082862, 31.21726448433412315, 2.638427012816831674 ) ) ;
#9776=ORIENTED_EDGE ( 'NONE', *, *, #81843, .T. ) ;
#9778=CARTESIAN_POINT ( 'NONE',  ( 7.084665262690076126, 52.02201867748816255, -10.88017736071110164 ) ) ;
#9781=CARTESIAN_POINT ( 'NONE',  ( 12.63842701281683922, 9.550597817667449974, -9.846743663894590881 ) ) ;
#9782=CARTESIAN_POINT ( 'NONE',  ( 6.565887622018943937, 10.16530133659708746, 12.81628187352647430 ) ) ;
#9784=CARTESIAN_POINT ( 'NONE',  ( 10.00000000000000178, 37.25893115100078745, 9.846743663894594434 ) ) ;
#9786=CARTESIAN_POINT ( 'NONE',  ( 2.917880565312948704, 7.637082168247301794, 12.26659068614894643 ) ) ;
#9787=CARTESIAN_POINT ( 'NONE',  ( 7.361572987183169658, 19.96726448433411960, -9.846743663894592657 ) ) ;
#9788=CARTESIAN_POINT ( 'NONE',  ( -2.816281873526471635, 23.91530133659708568, -3.434112377981056508 ) ) ;
#9791=CARTESIAN_POINT ( 'NONE',  ( 7.084665262690076126, 44.10535201082151247, 10.88017736071109987 ) ) ;
#9792=CARTESIAN_POINT ( 'NONE',  ( 0.6178305044545818747, -1.501365330069579951, -9.382169495545419124 ) ) ;
#9796=CARTESIAN_POINT ( 'NONE',  ( 1.472469842513823179, 25.59226448433412315, -4.923371831947296329 ) ) ;
#9797=CARTESIAN_POINT ( 'NONE',  ( 7.084665262690076126, 12.02201867748817143, -10.88017736071110164 ) ) ;
#9798=CARTESIAN_POINT ( 'NONE',  ( -1.099225684535947600, 18.70696800326375353, -6.408140936763238038 ) ) ;
#9799=CARTESIAN_POINT ( 'NONE',  ( 1.472469842513823179, 20.59226448433411960, -4.923371831947296329 ) ) ;
#9802=CARTESIAN_POINT ( 'NONE',  ( 10.00000000000000000, 21.81368534415484106, -10.88017736071110342 ) ) ;
#9803=EDGE_LOOP ( 'NONE', ( #85046, #23767, #55361, #74914 ) ) ;
#9804=CARTESIAN_POINT ( 'NONE',  ( 20.88017736071110875, 60.77201867748817676, -2.915334737309920765 ) ) ;
#9806=CARTESIAN_POINT ( 'NONE',  ( 18.52753015748617571, 48.09226448433412315, 4.923371831947298993 ) ) ;
#9807=CARTESIAN_POINT ( 'NONE',  ( 17.96484262340118221, 21.18868534415483396, -7.964842623401177768 ) ) ;
#9809=CARTESIAN_POINT ( 'NONE',  ( 20.88017736071110164, 40.35535201082150536, 2.915334737309930979 ) ) ;
#9810=CARTESIAN_POINT ( 'NONE',  ( -0.8801773607110991993, 12.85535201082150358, -2.915334737309923874 ) ) ;
#9811=CARTESIAN_POINT ( 'NONE',  ( -1.926860441876562025, 19.47997603579417358, -3.195792623639529761 ) ) ;
#9812=CARTESIAN_POINT ( 'NONE',  ( 1.472469842513823179, 10.59226448433411782, -4.923371831947296329 ) ) ;
#9813=CARTESIAN_POINT ( 'NONE',  ( 0.1532563361054082862, 41.21726448433411605, 2.638427012816831674 ) ) ;
#9818=CARTESIAN_POINT ( 'NONE',  ( 1.472469842513823179, 66.42559781766745175, 4.923371831947296329 ) ) ;
#9820=CARTESIAN_POINT ( 'NONE',  ( 22.26659068614894466, 18.88708216824730002, 7.082119434687054849 ) ) ;
#9822=CARTESIAN_POINT ( 'NONE',  ( 14.92337183194729633, 42.67559781766745886, 8.527530157486181039 ) ) ;
#9825=CARTESIAN_POINT ( 'NONE',  ( 19.42250999205614548, 5.980352010821504471, -5.440088680355545492 ) ) ;
#9826=CARTESIAN_POINT ( 'NONE',  ( 14.92337183194729988, 19.34226448433411960, -8.527530157486177487 ) ) ;
#9829=CARTESIAN_POINT ( 'NONE',  ( 7.084665262690076126, 52.02201867748816255, -10.88017736071110164 ) ) ;
#9831=CARTESIAN_POINT ( 'NONE',  ( 0.5774900079438607392, 13.48035201082150358, 5.440088680355550821 ) ) ;
#9833=CARTESIAN_POINT ( 'NONE',  ( 3.591859063236761518, 49.95696800326375353, 11.09922568453594849 ) ) ;
#9834=CARTESIAN_POINT ( 'NONE',  ( 6.565887622018943937, 10.16530133659708746, 12.81628187352647430 ) ) ;
#9835=CARTESIAN_POINT ( 'NONE',  ( 2.791683348922237240, 15.38393115100078212, -7.208316651077763204 ) ) ;
#9839=CARTESIAN_POINT ( 'NONE',  ( 2.917880565312950480, 55.97041550158063217, -12.26659068614894821 ) ) ;
#9840=CARTESIAN_POINT ( 'NONE',  ( 13.79529636645030344, 23.26208216824730002, 14.16423886937410614 ) ) ;
#9841=CARTESIAN_POINT ( 'NONE',  ( 10.00000000000000178, 19.31368534415484106, 10.88017736071110342 ) ) ;
#9842=CARTESIAN_POINT ( 'NONE',  ( 20.88017736071110519, 55.56368534415484817, 2.639326808657452039E-16 ) ) ;
#9843=FILL_AREA_STYLE_COLOUR ( '', #65485 ) ;
#9844=CARTESIAN_POINT ( 'NONE',  ( -46.44000000000001194, 100.8660254037844339, -9.500000000000000000 ) ) ;
#9845=CARTESIAN_POINT ( 'NONE',  ( 12.63842701281683034, 2.467264484334118269, 9.846743663894596210 ) ) ;
#9846=PRESENTATION_STYLE_ASSIGNMENT (( #92839 ) ) ;
#9847=CARTESIAN_POINT ( 'NONE',  ( 0.1532563361054100626, 15.80059781766745353, -2.638427012816831230 ) ) ;
#9848=CARTESIAN_POINT ( 'NONE',  ( 7.361572987183169658, -0.03273551566588185635, -9.846743663894592657 ) ) ;
#9849=STYLED_ITEM ( 'NONE', ( #84623 ), #74133 ) ;
#9851=CARTESIAN_POINT ( 'NONE',  ( 2.791683348922237240, 30.38393115100078390, -7.208316651077763204 ) ) ;
#9852=CARTESIAN_POINT ( 'NONE',  ( 1.472469842513823179, 55.59226448433412315, -4.923371831947296329 ) ) ;
#9853=CARTESIAN_POINT ( 'NONE',  ( 12.91533473730992121, 14.52201867748817143, 10.88017736071110164 ) ) ;
#9855=EDGE_CURVE ( 'NONE', #86126, #63027, #4556, .T. ) ;
#9856=CARTESIAN_POINT ( 'NONE',  ( 6.565887622018943937, 28.08196800326375353, -12.81628187352647608 ) ) ;
#9857=CARTESIAN_POINT ( 'NONE',  ( 17.96484262340118221, 51.18868534415483396, -7.964842623401177768 ) ) ;
#9858=CARTESIAN_POINT ( 'NONE',  ( 18.52753015748617571, 23.09226448433411960, 4.923371831947298993 ) ) ;
#9859=CARTESIAN_POINT ( 'NONE',  ( 20.36894250292379382, 48.67874883491396076, 10.36894250292379205 ) ) ;
#9860=CARTESIAN_POINT ( 'NONE',  ( 0.1532563361054083140, 11.00893115100078568, 1.131784320476157264E-15 ) ) ;
#9862=CARTESIAN_POINT ( 'NONE',  ( 2.791683348922237240, 55.38393115100078745, -7.208316651077763204 ) ) ;
#9863=CARTESIAN_POINT ( 'NONE',  ( 5.076628168052704559, 30.17559781766745175, -8.527530157486179263 ) ) ;
#9864=CARTESIAN_POINT ( 'NONE',  ( 17.08211943468705130, 13.47041550158063572, 12.26659068614894998 ) ) ;
#9866=CARTESIAN_POINT ( 'NONE',  ( 24.16423886937410614, 24.51208216824730002, -3.795296366450302550 ) ) ;
#9867=CARTESIAN_POINT ( 'NONE',  ( 0.1532563361054083140, 36.00893115100078745, 1.131784320476157264E-15 ) ) ;
#9868=CARTESIAN_POINT ( 'NONE',  ( -0.8801773607111008646, 48.27201867748816966, 2.915334737309923430 ) ) ;
#9869=CARTESIAN_POINT ( 'NONE',  ( 19.42250999205614548, 25.98035201082150891, -5.440088680355545492 ) ) ;
#9870=CARTESIAN_POINT ( 'NONE',  ( 20.88017736071110875, 40.77201867748818387, -2.915334737309920765 ) ) ;
#9871=CARTESIAN_POINT ( 'NONE',  ( 12.91533473730992121, 29.52201867748817321, 10.88017736071110164 ) ) ;
#9873=CARTESIAN_POINT ( 'NONE',  ( 10.00000000000000178, 35.37363466993042493, 12.81628187352647608 ) ) ;
#9874=CARTESIAN_POINT ( 'NONE',  ( 2.035157376598822676, 37.43868534415484106, -7.964842623401177768 ) ) ;
#9876=CARTESIAN_POINT ( 'NONE',  ( 3.591859063236763294, 53.29030133659708923, -11.09922568453595026 ) ) ;
#9878=VERTEX_POINT ( 'NONE', #54262 ) ;
#9879=CARTESIAN_POINT ( 'NONE',  ( -0.8801773607110991993, 52.85535201082151247, -2.915334737309923874 ) ) ;
#9880=MECHANICAL_DESIGN_GEOMETRIC_PRESENTATION_REPRESENTATION('',(#22587),#81652);
#9883=CARTESIAN_POINT ( 'NONE',  ( 13.79529636645030344, 63.26208216824730357, 14.16423886937410614 ) ) ;
#9884=CARTESIAN_POINT ( 'NONE',  ( 0.1532563361054100626, 10.80059781766745175, -2.638427012816831230 ) ) ;
#9885=CARTESIAN_POINT ( 'NONE',  ( -2.266590686148945544, 1.387082168247301128, -7.082119434687050408 ) ) ;
#9886=CARTESIAN_POINT ( 'NONE',  ( 17.20831665107776587, 9.133931151000787452, -7.208316651077762316 ) ) ;
#9887=CARTESIAN_POINT ( 'NONE',  ( 10.00000000000000000, 16.81368534415483751, -10.88017736071110342 ) ) ;
#9888=CARTESIAN_POINT ( 'NONE',  ( 1.472469842513823179, 45.59226448433412315, -4.923371831947296329 ) ) ;
#9890=CARTESIAN_POINT ( 'NONE',  ( 10.00000000000000178, 52.25893115100078745, 9.846743663894594434 ) ) ;
#9891=CARTESIAN_POINT ( 'NONE',  ( 2.831191079880678085, 79.91181047996344944, 9.500000000000000000 ) ) ;
#9892=CARTESIAN_POINT ( 'NONE',  ( 20.88017736071110875, 45.77201867748816966, -2.915334737309920765 ) ) ;
#9893=CARTESIAN_POINT ( 'NONE',  ( 19.84674366389459621, 48.50893115100078745, 7.409399052514197653E-17 ) ) ;
#9894=CARTESIAN_POINT ( 'NONE',  ( 19.38216949554541557, 27.24863466993041783, -9.382169495545420901 ) ) ;
#9895=FACE_OUTER_BOUND ( 'NONE', #17618, .T. ) ;
#9896=CARTESIAN_POINT ( 'NONE',  ( 2.035157376598824452, 68.68868534415484817, 7.964842623401179544 ) ) ;
#9897=CARTESIAN_POINT ( 'NONE',  ( 20.88017736071110875, 45.77201867748816966, -2.915334737309920765 ) ) ;
#9898=CARTESIAN_POINT ( 'NONE',  ( 10.00000000000000000, 6.813685344154838397, -10.88017736071110342 ) ) ;
#9900=CARTESIAN_POINT ( 'NONE',  ( 16.40814093676324603, 47.45696800326375353, -11.09922568453594671 ) ) ;
#9902=ORIENTED_EDGE ( 'NONE', *, *, #6008, .F. ) ;
#9903=CARTESIAN_POINT ( 'NONE',  ( 10.00000000000000000, 27.87363466993042138, -12.81628187352647608 ) ) ;
#9904=CARTESIAN_POINT ( 'NONE',  ( 10.00000000000000000, 21.81368534415484106, -10.88017736071110342 ) ) ;
#9905=CIRCLE ( 'NONE', #5112, 1.000000000000000888 ) ;
#9907=B_SPLINE_CURVE_WITH_KNOTS ( 'NONE', 3,
 ( #21904, #27900, #96925, #5427, #81399, #6890 ),
 .UNSPECIFIED., .F., .F.,
 ( 4, 2, 4 ),
 ( 0.000000000000000000, 0.0002605067024380873270, 0.0005210134048761746539 ),
 .UNSPECIFIED. ) ;
#9908=CARTESIAN_POINT ( 'NONE',  ( 4.559911319644449179, 68.89701867748817676, 9.422509992056141925 ) ) ;
#9909=CARTESIAN_POINT ( 'NONE',  ( 17.20831665107776587, 44.13393115100078745, -7.208316651077762316 ) ) ;
#9910=CARTESIAN_POINT ( 'NONE',  ( 18.52753015748618282, 18.92559781766745175, -4.923371831947291888 ) ) ;
#9911=CARTESIAN_POINT ( 'NONE',  ( 17.20831665107776587, 32.88393115100078745, 7.208316651077764980 ) ) ;
#9914=CARTESIAN_POINT ( 'NONE',  ( 12.63842701281683922, 29.55059781766745175, -9.846743663894590881 ) ) ;
#9915=CARTESIAN_POINT ( 'NONE',  ( 0.1077916266722770133, 52.24062864464239198, -6.478736007406002528 ) ) ;
#9916=CARTESIAN_POINT ( 'NONE',  ( -15.94000000000001371, 93.50000000000000000, 9.500000000000000000 ) ) ;
#9917=CARTESIAN_POINT ( 'NONE',  ( 7.361572987183170547, 22.05059781766745530, 9.846743663894590881 ) ) ;
#9918=CARTESIAN_POINT ( 'NONE',  ( 5.076628168052703671, 1.842264484334118047, 8.527530157486179263 ) ) ;
#9919=CARTESIAN_POINT ( 'NONE',  ( 5.076628168052704559, 40.17559781766745175, -8.527530157486179263 ) ) ;
#9922=CARTESIAN_POINT ( 'NONE',  ( -1.099225684535947600, 24.54030133659708923, 6.408140936763237150 ) ) ;
#9924=CARTESIAN_POINT ( 'NONE',  ( 2.917880565312950480, 40.97041550158063217, -12.26659068614894821 ) ) ;
#9925=CARTESIAN_POINT ( 'NONE',  ( 0.1532563361054082862, 21.21726448433412315, 2.638427012816831674 ) ) ;
#9926=CARTESIAN_POINT ( 'NONE',  ( 1.472469842513823179, 5.592264484334118713, -4.923371831947296329 ) ) ;
#9928=CARTESIAN_POINT ( 'NONE',  ( 6.204703633549690345, 47.84541550158064638, 14.16423886937410082 ) ) ;
#9929=CARTESIAN_POINT ( 'NONE',  ( 12.63842701281683922, 59.55059781766744464, -9.846743663894590881 ) ) ;
#9930=CARTESIAN_POINT ( 'NONE',  ( 17.96484262340118221, 6.188685344154837509, -7.964842623401177768 ) ) ;
#9931=CARTESIAN_POINT ( 'NONE',  ( -4.164238869374098151, 16.59541550158063927, -3.795296366450310543 ) ) ;
#9932=CARTESIAN_POINT ( 'NONE',  ( -4.164238869374099039, 41.80374883491397497, 8.674139862899312516E-16 ) ) ;
#9935=CARTESIAN_POINT ( 'NONE',  ( 1.472469842513823179, 55.59226448433412315, -4.923371831947296329 ) ) ;
#9936=CARTESIAN_POINT ( 'NONE',  ( 10.00000000000000178, 34.31368534415484106, 10.88017736071110342 ) ) ;
#9938=CARTESIAN_POINT ( 'NONE',  ( 19.59274024544229675, 95.43182565554037922, -5.128398454507786752 ) ) ;
#9939=EDGE_CURVE ( 'NONE', #15989, #67813, #18898, .T. ) ;
#9940=CARTESIAN_POINT ( 'NONE',  ( 12.63842701281683034, 37.46726448433411605, 9.846743663894596210 ) ) ;
#9943=CARTESIAN_POINT ( 'NONE',  ( 14.92337183194729633, 37.67559781766745175, 8.527530157486181039 ) ) ;
#9944=CARTESIAN_POINT ( 'NONE',  ( 10.00000000000000000, 59.75893115100078745, -9.846743663894594434 ) ) ;
#9945=STYLED_ITEM ( 'NONE', ( #28279 ), #80618 ) ;
#9947=CARTESIAN_POINT ( 'NONE',  ( 22.26659068614895176, 9.720415501580633943, -7.082119434687042414 ) ) ;
#9950=CARTESIAN_POINT ( 'NONE',  ( -4.164238869374098151, 66.59541550158060375, -3.795296366450310543 ) ) ;
#9951=CARTESIAN_POINT ( 'NONE',  ( 21.09922568453594849, 21.20696800326375353, 6.408140936763242479 ) ) ;
#9952=CARTESIAN_POINT ( 'NONE',  ( 7.084665262690076126, 67.02201867748817676, -10.88017736071110164 ) ) ;
#9956=CARTESIAN_POINT ( 'NONE',  ( 4.559911319644449179, 13.89701867748817321, 9.422509992056141925 ) ) ;
#9958=CARTESIAN_POINT ( 'NONE',  ( 0.5774900079438590739, 22.64701867748817321, -5.440088680355550821 ) ) ;
#9959=CARTESIAN_POINT ( 'NONE',  ( 2.035157376598822676, 37.43868534415484106, -7.964842623401177768 ) ) ;
#9960=CARTESIAN_POINT ( 'NONE',  ( 10.00000000000000178, 0.3736346699304200492, 12.81628187352647608 ) ) ;
#9962=CARTESIAN_POINT ( 'NONE',  ( 7.361572987183170547, 52.05059781766745175, 9.846743663894590881 ) ) ;
#9963=CARTESIAN_POINT ( 'NONE',  ( 22.81628187352647785, 61.62363466993041783, 6.195893100308588602E-16 ) ) ;
#9964=CARTESIAN_POINT ( 'NONE',  ( 1.472469842513823179, 11.42559781766745175, 4.923371831947296329 ) ) ;
#9966=CARTESIAN_POINT ( 'NONE',  ( 4.559911319644449179, 28.89701867748817321, 9.422509992056141925 ) ) ;
#9967=CARTESIAN_POINT ( 'NONE',  ( -2.816281873526473856, 34.33196800326376064, 3.434112377981055619 ) ) ;
#9970=EDGE_CURVE ( 'NONE', #85332, #79199, #56389, .T. ) ;
#9971=CARTESIAN_POINT ( 'NONE',  ( 3.591859063236763294, -1.709698663402913210, -11.09922568453595026 ) ) ;
#9972=CARTESIAN_POINT ( 'NONE',  ( -0.8801773607110991993, 42.85535201082150536, -2.915334737309923874 ) ) ;
#9973=CARTESIAN_POINT ( 'NONE',  ( 17.20831665107776587, 9.133931151000787452, -7.208316651077762316 ) ) ;
#9974=CARTESIAN_POINT ( 'NONE',  ( 19.38216949554541202, 40.99863466993042493, 9.382169495545424454 ) ) ;
#9975=CARTESIAN_POINT ( 'NONE',  ( 15.44008868035555793, 56.39701867748817676, -9.422509992056140149 ) ) ;
#9976=CARTESIAN_POINT ( 'NONE',  ( -0.1503990784575328643, 69.92552686551195507, -6.262539305110068177 ) ) ;
#9978=CARTESIAN_POINT ( 'NONE',  ( 0.6178305044545818747, 63.49863466993043204, -9.382169495545419124 ) ) ;
#9979=ORIENTED_EDGE ( 'NONE', *, *, #11731, .T. ) ;
#9983=CARTESIAN_POINT ( 'NONE',  ( 0.6178305044545818747, 43.49863466993042493, -9.382169495545419124 ) ) ;
#9984=CARTESIAN_POINT ( 'NONE',  ( 22.26659068614894466, 18.88708216824730002, 7.082119434687054849 ) ) ;
#9985=CARTESIAN_POINT ( 'NONE',  ( 0.1532563361054083140, 21.00893115100078745, 1.131784320476157264E-15 ) ) ;
#9987=CARTESIAN_POINT ( 'NONE',  ( 7.084665262690076126, 2.022018677488170990, -10.88017736071110164 ) ) ;
#9988=CARTESIAN_POINT ( 'NONE',  ( 7.361572987183169658, 19.96726448433411960, -9.846743663894592657 ) ) ;
#9990=CARTESIAN_POINT ( 'NONE',  ( 10.00000000000000000, 50.55374883491396787, -14.16423886937410082 ) ) ;
#9993=CARTESIAN_POINT ( 'NONE',  ( 12.91533473730992121, 4.522018677488169658, 10.88017736071110164 ) ) ;
#9994=CARTESIAN_POINT ( 'NONE',  ( 20.88017736071110164, 20.35535201082150891, 2.915334737309930979 ) ) ;
#9997=EDGE_LOOP ( 'NONE', ( #37064, #42220, #32695, #55711 ) ) ;
#9998=CARTESIAN_POINT ( 'NONE',  ( 20.88017736071110875, 10.77201867748817143, -2.915334737309920765 ) ) ;
#9999=CARTESIAN_POINT ( 'NONE',  ( 19.84674366389459621, 53.50893115100078745, 7.409399052514197653E-17 ) ) ;
#10000=CARTESIAN_POINT ( 'NONE',  ( 13.43411237798105340, 55.58196800326374643, 12.81628187352647963 ) ) ;
#10002=SURFACE_STYLE_USAGE ( .BOTH. , #78488 ) ;
#10003=CARTESIAN_POINT ( 'NONE',  ( 2.917880565312950480, 15.97041550158063217, -12.26659068614894821 ) ) ;
#10004=CARTESIAN_POINT ( 'NONE',  ( 4.559911319644449179, 27.23035201082150536, -9.422509992056141925 ) ) ;
#10005=CARTESIAN_POINT ( 'NONE',  ( 15.44008868035555793, 16.39701867748817321, -9.422509992056140149 ) ) ;
#10006=CARTESIAN_POINT ( 'NONE',  ( 19.84674366389459266, 53.30059781766744464, 2.638427012816836559 ) ) ;
#10008=CARTESIAN_POINT ( 'NONE',  ( 2.791683348922240793, 36.63393115100078035, 7.208316651077764092 ) ) ;
#10009=CARTESIAN_POINT ( 'NONE',  ( -19.19000000000001194, 93.50000000000000000, -10.09898361729590199 ) ) ;
#10011=CARTESIAN_POINT ( 'NONE',  ( 0.1532563361054082862, 11.21726448433411605, 2.638427012816831674 ) ) ;
#10015=CARTESIAN_POINT ( 'NONE',  ( 2.791683348922237240, 5.383931151000785675, -7.208316651077763204 ) ) ;
#10016=CARTESIAN_POINT ( 'NONE',  ( 22.81628187352647785, 1.623634669930420271, 6.195893100308588602E-16 ) ) ;
#10017=CARTESIAN_POINT ( 'NONE',  ( 4.559911319644449179, 47.23035201082150536, -9.422509992056141925 ) ) ;
#10018=CARTESIAN_POINT ( 'NONE',  ( -0.8801773607110991993, 7.855352010821504471, -2.915334737309923874 ) ) ;
#10019=CARTESIAN_POINT ( 'NONE',  ( 10.00000000000000000, 47.87363466993042493, -12.81628187352647608 ) ) ;
#10020=CARTESIAN_POINT ( 'NONE',  ( -2.266590686148945544, 17.22041550158063572, 7.082119434687048631 ) ) ;
#10023=CARTESIAN_POINT ( 'NONE',  ( 21.09922568453594849, 56.20696800326375353, 6.408140936763242479 ) ) ;
#10025=CARTESIAN_POINT ( 'NONE',  ( 2.791683348922240793, 61.63393115100079456, 7.208316651077764092 ) ) ;
#10026=CARTESIAN_POINT ( 'NONE',  ( 4.559911319644449179, 23.89701867748817321, 9.422509992056141925 ) ) ;
#10028=CARTESIAN_POINT ( 'NONE',  ( 0.1532563361054082862, 6.217264484334118713, 2.638427012816831674 ) ) ;
#10030=CARTESIAN_POINT ( 'NONE',  ( 14.92337183194729988, 9.342264484334119601, -8.527530157486177487 ) ) ;
#10031=CARTESIAN_POINT ( 'NONE',  ( 15.44008868035555260, 64.73035201082151957, 9.422509992056143702 ) ) ;
#10033=CARTESIAN_POINT ( 'NONE',  ( 10.00000000000000178, 59.31368534415484106, 10.88017736071110342 ) ) ;
#10034=CARTESIAN_POINT ( 'NONE',  ( 0.5774900079438607392, 68.48035201082150536, 5.440088680355550821 ) ) ;
#10035=CARTESIAN_POINT ( 'NONE',  ( 19.84674366389459621, 8.508931151000785675, 7.409399052514197653E-17 ) ) ;
#10039=CARTESIAN_POINT ( 'NONE',  ( 10.00000000000000000, 49.75893115100078745, -9.846743663894594434 ) ) ;
#10043=CARTESIAN_POINT ( 'NONE',  ( -4.164238869374099039, 1.803748834913967647, 8.674139862899312516E-16 ) ) ;
#10045=AXIS2_PLACEMENT_3D ( 'NONE', #49388, #85933, #24943 ) ;
#10046=CARTESIAN_POINT ( 'NONE',  ( 21.09922568453595559, 62.04030133659709634, -6.408140936763230044 ) ) ;
#10047=AXIS2_PLACEMENT_3D ( 'NONE', #6360, #67865, #22370 ) ;
#10048=CARTESIAN_POINT ( 'NONE',  ( 6.204703633549690345, 22.84541550158062861, 14.16423886937410082 ) ) ;
#10049=CARTESIAN_POINT ( 'NONE',  ( -0.3689425029237881626, 2.428748834913967869, 10.36894250292379027 ) ) ;
#10050=CARTESIAN_POINT ( 'NONE',  ( 12.91533473730993009, 21.60535201082150536, -10.88017736071109987 ) ) ;
#10051=ORIENTED_EDGE ( 'NONE', *, *, #59021, .F. ) ;
#10052=CARTESIAN_POINT ( 'NONE',  ( 12.63842701281683922, 4.550597817667451750, -9.846743663894590881 ) ) ;
#10054=CARTESIAN_POINT ( 'NONE',  ( 0.1532563361054083140, 16.00893115100078390, 1.131784320476157264E-15 ) ) ;
#10055=CARTESIAN_POINT ( 'NONE',  ( 0.6178305044545818747, 28.49863466993041783, -9.382169495545419124 ) ) ;
#10056=CARTESIAN_POINT ( 'NONE',  ( 19.84674366389459621, 43.50893115100078745, 7.409399052514197653E-17 ) ) ;
#10059=CARTESIAN_POINT ( 'NONE',  ( -2.816281873526473856, 24.12363466993042138, 9.499525473075851096E-16 ) ) ;
#10061=CARTESIAN_POINT ( 'NONE',  ( 12.63842701281683034, 22.46726448433411605, 9.846743663894596210 ) ) ;
#10062=CARTESIAN_POINT ( 'NONE',  ( 24.16423886937409904, 9.095415501580633943, 3.795296366450317205 ) ) ;
#10063=VERTEX_POINT ( 'NONE', #55950 ) ;
#10065=CARTESIAN_POINT ( 'NONE',  ( 19.42250999205614548, 30.98035201082150536, -5.440088680355545492 ) ) ;
#10066=CARTESIAN_POINT ( 'NONE',  ( 6.204703633549690345, 37.84541550158063927, 14.16423886937410082 ) ) ;
#10067=CARTESIAN_POINT ( 'NONE',  ( 19.84674366389459621, 53.50893115100078745, 7.409399052514197653E-17 ) ) ;
#10068=CARTESIAN_POINT ( 'NONE',  ( 0.1532563361054083140, 16.00893115100078390, 1.131784320476157264E-15 ) ) ;
#10069=CARTESIAN_POINT ( 'NONE',  ( 16.40814093676324603, 47.45696800326375353, -11.09922568453594671 ) ) ;
#10071=CARTESIAN_POINT ( 'NONE',  ( -0.8801773607111008646, 33.27201867748817676, 2.915334737309923430 ) ) ;
#10073=CARTESIAN_POINT ( 'NONE',  ( 10.00000000000000000, 22.87363466993042138, -12.81628187352647608 ) ) ;
#10074=CARTESIAN_POINT ( 'NONE',  ( 17.20831665107776587, 39.13393115100079456, -7.208316651077762316 ) ) ;
#10076=CARTESIAN_POINT ( 'NONE',  ( 19.38216949554541557, 52.24863466993041072, -9.382169495545420901 ) ) ;
#10078=CARTESIAN_POINT ( 'NONE',  ( 15.44008868035555793, 56.39701867748817676, -9.422509992056140149 ) ) ;
#10083=CARTESIAN_POINT ( 'NONE',  ( 0.5774900079438607392, 58.48035201082151247, 5.440088680355550821 ) ) ;
#10085=CARTESIAN_POINT ( 'NONE',  ( 20.88017736071110875, 60.77201867748817676, -2.915334737309920765 ) ) ;
#10086=CARTESIAN_POINT ( 'NONE',  ( -10.00000000000007105, 92.00000000000000000, -9.500000000000000000 ) ) ;
#10089=CARTESIAN_POINT ( 'NONE',  ( 0.5774900079438590739, 7.647018677488171434, -5.440088680355550821 ) ) ;
#10090=CARTESIAN_POINT ( 'NONE',  ( 0.6178305044545818747, -1.501365330069579951, -9.382169495545419124 ) ) ;
#10091=CARTESIAN_POINT ( 'NONE',  ( 2.035157376598822676, 22.43868534415483396, -7.964842623401177768 ) ) ;
#10094=CARTESIAN_POINT ( 'NONE',  ( -1.099225684535947600, 28.70696800326375353, -6.408140936763238038 ) ) ;
#10095=VERTEX_POINT ( 'NONE', #31453 ) ;
#10096=CARTESIAN_POINT ( 'NONE',  ( 12.91533473730993009, 46.60535201082150536, -10.88017736071109987 ) ) ;
#10098=CARTESIAN_POINT ( 'NONE',  ( 12.63842701281683034, 42.46726448433412315, 9.846743663894596210 ) ) ;
#10099=CARTESIAN_POINT ( 'NONE',  ( 16.40814093676323893, 5.790301336597087456, 11.09922568453595026 ) ) ;
#10101=CARTESIAN_POINT ( 'NONE',  ( 15.44008868035555793, 21.39701867748817321, -9.422509992056140149 ) ) ;
#10102=CARTESIAN_POINT ( 'NONE',  ( 20.88017736071110164, 35.35535201082150536, 2.915334737309930979 ) ) ;
#10103=CARTESIAN_POINT ( 'NONE',  ( -2.266590686148945544, 52.22041550158064638, 7.082119434687048631 ) ) ;
#10104=CARTESIAN_POINT ( 'NONE',  ( 1.472469842513823179, 45.59226448433412315, -4.923371831947296329 ) ) ;
#10105=CARTESIAN_POINT ( 'NONE',  ( -0.8801773607111008646, 63.27201867748817676, 2.915334737309923430 ) ) ;
#10107=CARTESIAN_POINT ( 'NONE',  ( 10.00000000000000178, 13.05374883491396787, 14.16423886937410082 ) ) ;
#10111=CARTESIAN_POINT ( 'NONE',  ( -2.266590686148945544, 52.22041550158064638, 7.082119434687048631 ) ) ;
#10112=CARTESIAN_POINT ( 'NONE',  ( 2.917880565312948704, 42.63708216824729647, 12.26659068614894643 ) ) ;
#10113=CARTESIAN_POINT ( 'NONE',  ( 0.1532563361054083140, 21.00893115100078745, 1.131784320476157264E-15 ) ) ;
#10114=CARTESIAN_POINT ( 'NONE',  ( 3.591859063236761518, 19.95696800326375353, 11.09922568453594849 ) ) ;
#10115=CARTESIAN_POINT ( 'NONE',  ( 7.361572987183170547, 57.05059781766744464, 9.846743663894590881 ) ) ;
#10116=DIRECTION ( 'NONE',  ( 0.000000000000000000, -1.000000000000000000, 0.000000000000000000 ) ) ;
#10117=CARTESIAN_POINT ( 'NONE',  ( 2.035157376598824452, 53.68868534415484817, 7.964842623401179544 ) ) ;
#10118=CARTESIAN_POINT ( 'NONE',  ( 6.565887622018943937, 28.08196800326375353, -12.81628187352647608 ) ) ;
#10119=CARTESIAN_POINT ( 'NONE',  ( 24.16423886937410614, 39.30374883491396787, 8.672049930838204340E-16 ) ) ;
#10120=CARTESIAN_POINT ( 'NONE',  ( 20.88017736071110164, 30.35535201082151247, 2.915334737309930979 ) ) ;
#10123=CARTESIAN_POINT ( 'NONE',  ( 12.91533473730993009, 66.60535201082150536, -10.88017736071109987 ) ) ;
#10126=CARTESIAN_POINT ( 'NONE',  ( 1.472469842513823179, 6.425597817667451750, 4.923371831947296329 ) ) ;
#10133=CARTESIAN_POINT ( 'NONE',  ( -4.164238869374098151, 6.595415501580634832, -3.795296366450310543 ) ) ;
#10134=CARTESIAN_POINT ( 'NONE',  ( 0.5774900079438590739, 7.647018677488171434, -5.440088680355550821 ) ) ;
#10135=CARTESIAN_POINT ( 'NONE',  ( 2.035157376598822676, 12.43868534415483751, -7.964842623401177768 ) ) ;
#10136=CARTESIAN_POINT ( 'NONE',  ( 19.84674366389459266, 38.30059781766745175, 2.638427012816836559 ) ) ;
#10137=CARTESIAN_POINT ( 'NONE',  ( 13.43411237798106583, 2.665301336597086568, -12.81628187352647252 ) ) ;
#10140=ADVANCED_FACE ( 'NONE', ( #46953 ), #85957, .T. ) ;
#10141=CARTESIAN_POINT ( 'NONE',  ( 22.81628187352647785, 16.62363466993042138, 6.195893100308588602E-16 ) ) ;
#10143=CARTESIAN_POINT ( 'NONE',  ( -2.266590686148945544, 52.22041550158064638, 7.082119434687048631 ) ) ;
#10145=CARTESIAN_POINT ( 'NONE',  ( 6.204703633549690345, 52.84541550158062506, 14.16423886937410082 ) ) ;
#10147=CARTESIAN_POINT ( 'NONE',  ( 12.91533473730992121, 29.52201867748817321, 10.88017736071110164 ) ) ;
#10148=CARTESIAN_POINT ( 'NONE',  ( 2.035157376598824452, 38.68868534415483396, 7.964842623401179544 ) ) ;
#10149=CARTESIAN_POINT ( 'NONE',  ( 19.42250999205614548, 35.98035201082151247, -5.440088680355545492 ) ) ;
#10150=DIRECTION ( 'NONE',  ( 0.8320502943378436100, -0.5547001962252291474, 0.000000000000000000 ) ) ;
#10151=CARTESIAN_POINT ( 'NONE',  ( 7.084665262690076126, 27.02201867748817676, -10.88017736071110164 ) ) ;
#10155=CARTESIAN_POINT ( 'NONE',  ( 5.076628168052704559, 10.17559781766745175, -8.527530157486179263 ) ) ;
#10157=ORIENTED_EDGE ( 'NONE', *, *, #43796, .T. ) ;
#10158=CARTESIAN_POINT ( 'NONE',  ( 10.00000000000000000, 49.75893115100078745, -9.846743663894594434 ) ) ;
#10160=CARTESIAN_POINT ( 'NONE',  ( 13.43411237798105340, 45.58196800326374643, 12.81628187352647963 ) ) ;
#10161=LINE ( 'NONE', #92658, #10758 ) ;
#10163=DIRECTION ( 'NONE',  ( 0.000000000000000000, 1.000000000000000000, -0.000000000000000000 ) ) ;
#10164=CARTESIAN_POINT ( 'NONE',  ( 14.92337183194729633, 57.67559781766745886, 8.527530157486181039 ) ) ;
#10165=CARTESIAN_POINT ( 'NONE',  ( -2.266590686148945544, 42.22041550158063217, 7.082119434687048631 ) ) ;
#10167=B_SPLINE_CURVE_WITH_KNOTS ( 'NONE', 3,
 ( #76310, #6830, #29810, #38814, #69307, #8794, #60319, #829, #37836, #14844 ),
 .UNSPECIFIED., .F., .F.,
 ( 4, 3, 3, 4 ),
 ( 0.000000000000000000, 0.0006253016069561017883, 0.001250604074564958586, 0.002501455912506553476 ),
 .UNSPECIFIED. ) ;
#10170=CARTESIAN_POINT ( 'NONE',  ( 0.1532563361054083140, 16.00893115100078390, 1.131784320476157264E-15 ) ) ;
#10171=CARTESIAN_POINT ( 'NONE',  ( 19.38216949554541202, 60.99863466993042493, 9.382169495545424454 ) ) ;
#10172=CARTESIAN_POINT ( 'NONE',  ( 18.52753015748618282, 58.92559781766745886, -4.923371831947291888 ) ) ;
#10173=CARTESIAN_POINT ( 'NONE',  ( 15.44008868035555793, 61.39701867748817676, -9.422509992056140149 ) ) ;
#10174=CARTESIAN_POINT ( 'NONE',  ( 12.63842701281683034, 42.46726448433412315, 9.846743663894596210 ) ) ;
#10181=CARTESIAN_POINT ( 'NONE',  ( 20.36894250292379738, 64.92874883491397497, -10.36894250292379027 ) ) ;
#10182=CARTESIAN_POINT ( 'NONE',  ( -45.94000000000001194, 100.9999999999999858, 9.500000000000000000 ) ) ;
#10183=CARTESIAN_POINT ( 'NONE',  ( 0.5774900079438590739, 47.64701867748817676, -5.440088680355550821 ) ) ;
#10184=CARTESIAN_POINT ( 'NONE',  ( 22.81628187352647785, 11.62363466993042138, 6.195893100308588602E-16 ) ) ;
#10185=CARTESIAN_POINT ( 'NONE',  ( 20.88017736071110875, 65.77201867748817676, -2.915334737309920765 ) ) ;
#10186=CARTESIAN_POINT ( 'NONE',  ( -0.1503990784575277573, 63.10158574516643171, 6.262539305110076171 ) ) ;
#10191=CARTESIAN_POINT ( 'NONE',  ( 19.84674366389459266, 53.30059781766744464, 2.638427012816836559 ) ) ;
#10193=CARTESIAN_POINT ( 'NONE',  ( 0.6178305044545838731, 9.748634669930416052, 9.382169495545420901 ) ) ;
#10194=CARTESIAN_POINT ( 'NONE',  ( 4.559911319644449179, 17.23035201082150536, -9.422509992056141925 ) ) ;
#10197=CARTESIAN_POINT ( 'NONE',  ( 6.204703633549690345, 35.76208216824729647, -14.16423886937410259 ) ) ;
#10198=CARTESIAN_POINT ( 'NONE',  ( 20.36894250292379382, 28.67874883491396787, 10.36894250292379205 ) ) ;
#10199=CARTESIAN_POINT ( 'NONE',  ( -4.164238869374099927, 67.01208216824728936, 3.795296366450308767 ) ) ;
#10200=CARTESIAN_POINT ( 'NONE',  ( 10.00000000000000178, 32.25893115100078745, 9.846743663894594434 ) ) ;
#10201=CARTESIAN_POINT ( 'NONE',  ( 16.40814093676324603, 32.45696800326375353, -11.09922568453594671 ) ) ;
#10202=CARTESIAN_POINT ( 'NONE',  ( 12.91533473730993009, 16.60535201082150891, -10.88017736071109987 ) ) ;
#10204=CARTESIAN_POINT ( 'NONE',  ( 2.791683348922240793, 41.63393115100078745, 7.208316651077764092 ) ) ;
#10205=CARTESIAN_POINT ( 'NONE',  ( 4.559911319644449179, 47.23035201082150536, -9.422509992056141925 ) ) ;
#10206=CARTESIAN_POINT ( 'NONE',  ( 1.472469842513823179, 66.42559781766745175, 4.923371831947296329 ) ) ;
#10207=CARTESIAN_POINT ( 'NONE',  ( 10.00000000000000178, 18.05374883491396787, 14.16423886937410082 ) ) ;
#10208=CARTESIAN_POINT ( 'NONE',  ( 2.603489959281613420, 45.43575266056827644, -6.500000000000031086 ) ) ;
#10209=CARTESIAN_POINT ( 'NONE',  ( 18.28836319691945889, 34.34492782695770785, 6.500000000000000888 ) ) ;
#10211=CARTESIAN_POINT ( 'NONE',  ( 7.361572987183169658, 29.96726448433411960, -9.846743663894592657 ) ) ;
#10212=CARTESIAN_POINT ( 'NONE',  ( 3.591859063236763294, 53.29030133659708923, -11.09922568453595026 ) ) ;
#10213=CARTESIAN_POINT ( 'NONE',  ( 17.20831665107776587, 57.88393115100078745, 7.208316651077764980 ) ) ;
#10217=CARTESIAN_POINT ( 'NONE',  ( -46.50634649544846866, 102.7699257839083486, -6.812960513223167425 ) ) ;
#10218=CARTESIAN_POINT ( 'NONE',  ( 10.00000000000000178, 4.313685344154837509, 10.88017736071110342 ) ) ;
#10219=CARTESIAN_POINT ( 'NONE',  ( 12.91533473730992121, 59.52201867748816966, 10.88017736071110164 ) ) ;
#10220=CARTESIAN_POINT ( 'NONE',  ( 24.16423886937409904, 14.09541550158063217, 3.795296366450317205 ) ) ;
#10221=CARTESIAN_POINT ( 'NONE',  ( 19.84674366389459621, 3.508931151000785231, 7.409399052514197653E-17 ) ) ;
#10222=CARTESIAN_POINT ( 'NONE',  ( 17.20831665107776587, 52.88393115100078035, 7.208316651077764980 ) ) ;
#10223=CARTESIAN_POINT ( 'NONE',  ( 17.96484262340118221, 21.18868534415483396, -7.964842623401177768 ) ) ;
#10230=CARTESIAN_POINT ( 'NONE',  ( 24.16423886937409904, 14.09541550158063217, 3.795296366450317205 ) ) ;
#10231=CARTESIAN_POINT ( 'NONE',  ( -4.164238869374099039, 41.80374883491397497, 8.674139862899312516E-16 ) ) ;
#10232=CARTESIAN_POINT ( 'NONE',  ( 12.63842701281683922, 54.55059781766745175, -9.846743663894590881 ) ) ;
#10233=CARTESIAN_POINT ( 'NONE',  ( 18.52753015748618282, 23.92559781766745530, -4.923371831947291888 ) ) ;
#10235=CARTESIAN_POINT ( 'NONE',  ( 2.035157376598824452, 18.68868534415484106, 7.964842623401179544 ) ) ;
#10236=CARTESIAN_POINT ( 'NONE',  ( 18.52753015748618282, 58.92559781766745886, -4.923371831947291888 ) ) ;
#10238=CARTESIAN_POINT ( 'NONE',  ( 13.79529636645031943, 35.34541550158063927, -14.16423886937409904 ) ) ;
#10239=CARTESIAN_POINT ( 'NONE',  ( 17.96484262340118221, 6.188685344154837509, -7.964842623401177768 ) ) ;
#10242=CARTESIAN_POINT ( 'NONE',  ( 15.44008868035555260, 59.73035201082151247, 9.422509992056143702 ) ) ;
#10243=CARTESIAN_POINT ( 'NONE',  ( 18.52753015748617571, 13.09226448433411960, 4.923371831947298993 ) ) ;
#10248=CARTESIAN_POINT ( 'NONE',  ( 17.20831665107776587, 19.13393115100078035, -7.208316651077762316 ) ) ;
#10250=CARTESIAN_POINT ( 'NONE',  ( 17.08211943468705130, 33.47041550158063927, 12.26659068614894998 ) ) ;
#10251=CARTESIAN_POINT ( 'NONE',  ( 2.791683348922237240, 40.38393115100078035, -7.208316651077763204 ) ) ;
#10252=CARTESIAN_POINT ( 'NONE',  ( 19.42250999205614193, 45.14701867748817676, 5.440088680355555262 ) ) ;
#10254=ORIENTED_EDGE ( 'NONE', *, *, #85921, .T. ) ;
#10255=CARTESIAN_POINT ( 'NONE',  ( 0.5774900079438590739, 37.64701867748817676, -5.440088680355550821 ) ) ;
#10257=VECTOR ( 'NONE', #72982, 1000.000000000000114 ) ;
#10259=ORIENTED_EDGE ( 'NONE', *, *, #38991, .F. ) ;
#10260=CARTESIAN_POINT ( 'NONE',  ( 6.204703633549690345, 2.845415501580634388, 14.16423886937410082 ) ) ;
#10264=CARTESIAN_POINT ( 'NONE',  ( -2.816281873526473856, 34.12363466993042493, 9.499525473075851096E-16 ) ) ;
#10265=CARTESIAN_POINT ( 'NONE',  ( 7.361572987183169658, 29.96726448433411960, -9.846743663894592657 ) ) ;
#10267=CARTESIAN_POINT ( 'NONE',  ( 13.43411237798105340, 45.58196800326374643, 12.81628187352647963 ) ) ;
#10268=CARTESIAN_POINT ( 'NONE',  ( 12.63842701281683034, 32.46726448433412315, 9.846743663894596210 ) ) ;
#10269=ADVANCED_FACE ( 'NONE', ( #64890 ), #4434, .T. ) ;
#10270=CARTESIAN_POINT ( 'NONE',  ( 7.084665262690076126, 57.02201867748817676, -10.88017736071110164 ) ) ;
#10275=CARTESIAN_POINT ( 'NONE',  ( 1.472469842513823179, 0.5922644843341181575, -4.923371831947296329 ) ) ;
#10276=CARTESIAN_POINT ( 'NONE',  ( 0.6178305044545838731, 14.74863466993041783, 9.382169495545420901 ) ) ;
#10278=CARTESIAN_POINT ( 'NONE',  ( 5.076628168052704559, 50.17559781766745886, -8.527530157486179263 ) ) ;
#10280=CARTESIAN_POINT ( 'NONE',  ( 13.79529636645031943, 10.34541550158063394, -14.16423886937409904 ) ) ;
#10281=CARTESIAN_POINT ( 'NONE',  ( 18.52753015748617571, 23.09226448433411960, 4.923371831947298993 ) ) ;
#10282=CARTESIAN_POINT ( 'NONE',  ( 0.6178305044545818747, 33.49863466993042493, -9.382169495545419124 ) ) ;
#10284=CARTESIAN_POINT ( 'NONE',  ( 0.5774900079438607392, 23.48035201082150536, 5.440088680355550821 ) ) ;
#10285=CARTESIAN_POINT ( 'NONE',  ( 0.5774900079438590739, 47.64701867748817676, -5.440088680355550821 ) ) ;
#10286=EDGE_CURVE ( 'NONE', #49769, #36460, #10932, .T. ) ;
#10287=CARTESIAN_POINT ( 'NONE',  ( -1.099225684535947600, 3.706968003263753531, -6.408140936763238038 ) ) ;
#10290=CARTESIAN_POINT ( 'NONE',  ( 0.1532563361054083140, 21.00893115100078745, 1.131784320476157264E-15 ) ) ;
#10291=CARTESIAN_POINT ( 'NONE',  ( -0.8801773607110991993, 32.85535201082151247, -2.915334737309923874 ) ) ;
#10292=CARTESIAN_POINT ( 'NONE',  ( 22.81628187352647785, 36.41530133659707502, 3.434112377981063169 ) ) ;
#10293=CARTESIAN_POINT ( 'NONE',  ( 17.20831665107776587, 22.88393115100078745, 7.208316651077764980 ) ) ;
#10296=CARTESIAN_POINT ( 'NONE',  ( -0.8801773607111008646, 23.27201867748817676, 2.915334737309923430 ) ) ;
#10297=EDGE_CURVE ( 'NONE', #14567, #83178, #49864, .T. ) ;
#10299=CARTESIAN_POINT ( 'NONE',  ( 10.00000000000000000, 56.81368534415484106, -10.88017736071110342 ) ) ;
#10300=PRESENTATION_STYLE_ASSIGNMENT (( #86788 ) ) ;
#10301=CARTESIAN_POINT ( 'NONE',  ( 12.63842701281683922, 44.55059781766745175, -9.846743663894590881 ) ) ;
#10302=CARTESIAN_POINT ( 'NONE',  ( -0.8801773607111008646, 23.27201867748817676, 2.915334737309923430 ) ) ;
#10304=CARTESIAN_POINT ( 'NONE',  ( 10.00000000000000000, 51.81368534415484106, -10.88017736071110342 ) ) ;
#10305=CARTESIAN_POINT ( 'NONE',  ( 10.00000000000000000, 11.81368534415483751, -10.88017736071110342 ) ) ;
#10306=CARTESIAN_POINT ( 'NONE',  ( -0.1503990784575242878, 19.24884699246888786, -6.262539305110083276 ) ) ;
#10308=CARTESIAN_POINT ( 'NONE',  ( 17.20831665107776587, 34.13393115100078745, -7.208316651077762316 ) ) ;
#10310=DIRECTION ( 'NONE',  ( 0.000000000000000000, 0.000000000000000000, -1.000000000000000000 ) ) ;
#10311=CARTESIAN_POINT ( 'NONE',  ( -4.164238869374098151, 26.59541550158063217, -3.795296366450310543 ) ) ;
#10315=CARTESIAN_POINT ( 'NONE',  ( 6.204703633549690345, 62.84541550158063927, 14.16423886937410082 ) ) ;
#10316=CARTESIAN_POINT ( 'NONE',  ( 0.1532563361054082862, 16.21726448433411960, 2.638427012816831674 ) ) ;
#10318=CARTESIAN_POINT ( 'NONE',  ( 19.42250999205614193, 50.14701867748817676, 5.440088680355555262 ) ) ;
#10320=CARTESIAN_POINT ( 'NONE',  ( 10.00000000000000178, 34.31368534415484106, 10.88017736071110342 ) ) ;
#10321=CARTESIAN_POINT ( 'NONE',  ( 0.6178305044545838731, 59.74863466993041783, 9.382169495545420901 ) ) ;
#10322=CARTESIAN_POINT ( 'NONE',  ( 13.43411237798105340, 5.581968003263753531, 12.81628187352647963 ) ) ;
#10323=CARTESIAN_POINT ( 'NONE',  ( 19.84674366389459266, 8.300597817667451750, 2.638427012816836559 ) ) ;
#10326=SURFACE_STYLE_USAGE ( .BOTH. , #57286 ) ;
#10328=CARTESIAN_POINT ( 'NONE',  ( 0.000000000000000000, 61.50000000000000711, -6.500000000000000888 ) ) ;
#10329=CARTESIAN_POINT ( 'NONE',  ( 20.36894250292379382, 58.67874883491396076, 10.36894250292379205 ) ) ;
#10330=CARTESIAN_POINT ( 'NONE',  ( 22.26659068614895176, 29.72041550158063572, -7.082119434687042414 ) ) ;
#10331=CARTESIAN_POINT ( 'NONE',  ( -0.8801773607111008646, 23.27201867748817676, 2.915334737309923430 ) ) ;
#10332=CARTESIAN_POINT ( 'NONE',  ( 17.96484262340118221, 54.93868534415484106, 7.964842623401181321 ) ) ;
#10333=DIRECTION ( 'NONE',  ( 0.5547001962252290364, 0.8320502943378437211, 0.000000000000000000 ) ) ;
#10335=CARTESIAN_POINT ( 'NONE',  ( 5.076628168052703671, 16.84226448433411960, 8.527530157486179263 ) ) ;
#10337=CARTESIAN_POINT ( 'NONE',  ( 19.84674366389459266, 18.30059781766745175, 2.638427012816836559 ) ) ;
#10339=FACE_OUTER_BOUND ( 'NONE', #85895, .T. ) ;
#10340=CARTESIAN_POINT ( 'NONE',  ( 14.92337183194729988, 19.34226448433411960, -8.527530157486177487 ) ) ;
#10341=CARTESIAN_POINT ( 'NONE',  ( 12.63842701281683034, 52.46726448433413026, 9.846743663894596210 ) ) ;
#10342=CARTESIAN_POINT ( 'NONE',  ( 13.43411237798106583, 27.66530133659708568, -12.81628187352647252 ) ) ;
#10344=CARTESIAN_POINT ( 'NONE',  ( 10.00000000000000000, 46.81368534415484106, -10.88017736071110342 ) ) ;
#10345=CARTESIAN_POINT ( 'NONE',  ( 12.63842701281683922, 29.55059781766745175, -9.846743663894590881 ) ) ;
#10346=CARTESIAN_POINT ( 'NONE',  ( 2.917880565312948704, 42.63708216824729647, 12.26659068614894643 ) ) ;
#10347=CARTESIAN_POINT ( 'NONE',  ( 7.361572987183170547, 17.05059781766745530, 9.846743663894590881 ) ) ;
#10349=CARTESIAN_POINT ( 'NONE',  ( 2.791683348922240793, 56.63393115100078035, 7.208316651077764092 ) ) ;
#10350=CARTESIAN_POINT ( 'NONE',  ( 10.00000000000000000, 44.75893115100078745, -9.846743663894594434 ) ) ;
#10351=CARTESIAN_POINT ( 'NONE',  ( 24.16423886937409904, 9.095415501580633943, 3.795296366450317205 ) ) ;
#10352=CARTESIAN_POINT ( 'NONE',  ( -2.266590686148945544, 36.38708216824730357, -7.082119434687050408 ) ) ;
#10353=CARTESIAN_POINT ( 'NONE',  ( 2.791683348922240793, 26.63393115100078745, 7.208316651077764092 ) ) ;
#10354=CARTESIAN_POINT ( 'NONE',  ( 0.5774900079438590739, 42.64701867748816966, -5.440088680355550821 ) ) ;
#10355=CARTESIAN_POINT ( 'NONE',  ( 19.42250999205614548, 20.98035201082150891, -5.440088680355545492 ) ) ;
#10356=CARTESIAN_POINT ( 'NONE',  ( 12.91533473730992121, 44.52201867748816966, 10.88017736071110164 ) ) ;
#10357=CARTESIAN_POINT ( 'NONE',  ( 4.559911319644449179, 27.23035201082150536, -9.422509992056141925 ) ) ;
#10359=CARTESIAN_POINT ( 'NONE',  ( 13.43411237798105340, 30.58196800326374998, 12.81628187352647963 ) ) ;
#10360=CARTESIAN_POINT ( 'NONE',  ( 7.084665262690076126, 59.10535201082150536, 10.88017736071109987 ) ) ;
#10364=CARTESIAN_POINT ( 'NONE',  ( 12.91533473730993009, 66.60535201082150536, -10.88017736071109987 ) ) ;
#10365=VERTEX_POINT ( 'NONE', #26415 ) ;
#10367=CARTESIAN_POINT ( 'NONE',  ( 10.00000000000000000, 61.81368534415484106, -10.88017736071110342 ) ) ;
#10368=( LENGTH_UNIT ( ) NAMED_UNIT ( * ) SI_UNIT ( .MILLI., .METRE. ) );
#10369=DIRECTION ( 'NONE',  ( 0.000000000000000000, -1.000000000000000000, 0.000000000000000000 ) ) ;
#10371=CARTESIAN_POINT ( 'NONE',  ( 10.00000000000000000, 55.55374883491396787, -14.16423886937410082 ) ) ;
#10372=CARTESIAN_POINT ( 'NONE',  ( 12.63842701281683922, 9.550597817667449974, -9.846743663894590881 ) ) ;
#10373=CARTESIAN_POINT ( 'NONE',  ( 24.16423886937410614, 4.303748834913967869, 8.672049930838204340E-16 ) ) ;
#10374=CARTESIAN_POINT ( 'NONE',  ( 0.1532563361054082862, 1.217264484334117824, 2.638427012816831674 ) ) ;
#10375=CARTESIAN_POINT ( 'NONE',  ( 18.52753015748618282, 43.92559781766745175, -4.923371831947291888 ) ) ;
#10377=CARTESIAN_POINT ( 'NONE',  ( 19.84674366389459621, 53.50893115100078745, 7.409399052514197653E-17 ) ) ;
#10378=VERTEX_POINT ( 'NONE', #33902 ) ;
#10379=CARTESIAN_POINT ( 'NONE',  ( 7.084665262690076126, 59.10535201082150536, 10.88017736071109987 ) ) ;
#10380=CARTESIAN_POINT ( 'NONE',  ( 14.92337183194729988, 54.34226448433412315, -8.527530157486177487 ) ) ;
#10381=CARTESIAN_POINT ( 'NONE',  ( -0.8801773607111008646, 68.27201867748817676, 2.915334737309923430 ) ) ;
#10382=CARTESIAN_POINT ( 'NONE',  ( 17.96484262340118221, 61.18868534415482685, -7.964842623401177768 ) ) ;
#10383=CARTESIAN_POINT ( 'NONE',  ( 20.88017736071110875, 5.772018677488170546, -2.915334737309920765 ) ) ;
#10384=ADVANCED_FACE ( 'NONE', ( #19417 ), #72041, .T. ) ;
#10386=CARTESIAN_POINT ( 'NONE',  ( 22.81628187352648496, 41.83196800326375353, -3.434112377981050290 ) ) ;
#10390=CARTESIAN_POINT ( 'NONE',  ( 22.81628187352648496, 26.83196800326374998, -3.434112377981050290 ) ) ;
#10391=CARTESIAN_POINT ( 'NONE',  ( -0.8801773607111008646, 28.27201867748817321, 2.915334737309923430 ) ) ;
#10393=CARTESIAN_POINT ( 'NONE',  ( 0.1532563361054100626, 10.80059781766745175, -2.638427012816831230 ) ) ;
#10394=CARTESIAN_POINT ( 'NONE',  ( 10.00000000000000178, 67.25893115100079456, 9.846743663894594434 ) ) ;
#10395=CARTESIAN_POINT ( 'NONE',  ( 18.52753015748617571, 8.092264484334117824, 4.923371831947298993 ) ) ;
#10396=CARTESIAN_POINT ( 'NONE',  ( 0.1532563361054100626, 55.80059781766745175, -2.638427012816831230 ) ) ;
#10398=CARTESIAN_POINT ( 'NONE',  ( 19.84674366389459266, 33.71726448433410894, -2.638427012816827677 ) ) ;
#10401=CARTESIAN_POINT ( 'NONE',  ( 17.20831665107776587, 32.88393115100078745, 7.208316651077764980 ) ) ;
#10402=DIRECTION ( 'NONE',  ( 0.000000000000000000, -1.000000000000000000, 0.000000000000000000 ) ) ;
#10404=CARTESIAN_POINT ( 'NONE',  ( 2.791683348922240793, 56.63393115100078035, 7.208316651077764092 ) ) ;
#10408=CARTESIAN_POINT ( 'NONE',  ( -2.816281873526473856, 29.33196800326376064, 3.434112377981055619 ) ) ;
#10409=CARTESIAN_POINT ( 'NONE',  ( 2.791683348922237240, 50.38393115100078035, -7.208316651077763204 ) ) ;
#10411=CARTESIAN_POINT ( 'NONE',  ( 6.204703633549690345, 40.76208216824731778, -14.16423886937410259 ) ) ;
#10412=CARTESIAN_POINT ( 'NONE',  ( 2.791683348922240793, 16.63393115100078745, 7.208316651077764092 ) ) ;
#10414=CARTESIAN_POINT ( 'NONE',  ( 19.84674366389459266, 3.300597817667451750, 2.638427012816836559 ) ) ;
#10415=CARTESIAN_POINT ( 'NONE',  ( -46.90021668353733730, 100.5602553471094183, 9.231058622660704316 ) ) ;
#10416=CARTESIAN_POINT ( 'NONE',  ( -4.164238869374098151, 41.59541550158061796, -3.795296366450310543 ) ) ;
#10417=CARTESIAN_POINT ( 'NONE',  ( 14.92337183194729633, 62.67559781766745886, 8.527530157486181039 ) ) ;
#10418=CARTESIAN_POINT ( 'NONE',  ( 20.88017736071110519, 10.56368534415483929, 2.639326808657452039E-16 ) ) ;
#10419=CARTESIAN_POINT ( 'NONE',  ( 10.00000000000000178, 28.05374883491396787, 14.16423886937410082 ) ) ;
#10420=CARTESIAN_POINT ( 'NONE',  ( 13.79529636645030344, 33.26208216824730357, 14.16423886937410614 ) ) ;
#10421=CARTESIAN_POINT ( 'NONE',  ( 19.84674366389459621, 33.50893115100078745, 7.409399052514197653E-17 ) ) ;
#10423=CARTESIAN_POINT ( 'NONE',  ( -0.8801773607111009756, 28.27201867748817321, 2.915334737309923874 ) ) ;
#10424=CARTESIAN_POINT ( 'NONE',  ( 19.84674366389459266, 58.71726448433411605, -2.638427012816827677 ) ) ;
#10425=VERTEX_POINT ( 'NONE', #96322 ) ;
#10426=CARTESIAN_POINT ( 'NONE',  ( 7.084665262690076126, 39.10535201082150536, 10.88017736071109987 ) ) ;
#10429=CARTESIAN_POINT ( 'NONE',  ( 3.591859063236761518, 64.95696800326376774, 11.09922568453594849 ) ) ;
#10431=CARTESIAN_POINT ( 'NONE',  ( 10.00000000000000000, 59.75893115100078745, -9.846743663894594434 ) ) ;
#10432=CARTESIAN_POINT ( 'NONE',  ( 0.1532563361054100626, 65.80059781766745175, -2.638427012816831230 ) ) ;
#10435=CARTESIAN_POINT ( 'NONE',  ( 24.16423886937409904, 24.09541550158063927, 3.795296366450317205 ) ) ;
#10438=DIRECTION ( 'NONE',  ( 0.000000000000000000, 1.000000000000000000, -0.000000000000000000 ) ) ;
#10439=CARTESIAN_POINT ( 'NONE',  ( 2.917880565312950480, 65.97041550158063217, -12.26659068614894821 ) ) ;
#10440=CARTESIAN_POINT ( 'NONE',  ( 22.81628187352647785, 21.62363466993041783, 6.195893100308588602E-16 ) ) ;
#10442=CARTESIAN_POINT ( 'NONE',  ( 5.076628168052703671, 16.84226448433411960, 8.527530157486179263 ) ) ;
#10443=CARTESIAN_POINT ( 'NONE',  ( -0.1503990784575328643, 5.127771745786130708, 6.262539305110068177 ) ) ;
#10446=CARTESIAN_POINT ( 'NONE',  ( 20.88017736071110519, 15.56368534415483751, 2.639326808657452039E-16 ) ) ;
#10448=CARTESIAN_POINT ( 'NONE',  ( -0.8801773607110991993, 37.85535201082151247, -2.915334737309923874 ) ) ;
#10449=CARTESIAN_POINT ( 'NONE',  ( 4.559911319644449179, 33.89701867748817676, 9.422509992056141925 ) ) ;
#10450=CARTESIAN_POINT ( 'NONE',  ( -1.099225684535947600, 4.540301336597087456, 6.408140936763237150 ) ) ;
#10451=CARTESIAN_POINT ( 'NONE',  ( 0.1532563361054100626, 60.80059781766744464, -2.638427012816831230 ) ) ;
#10452=CARTESIAN_POINT ( 'NONE',  ( -45.63603160005279591, 104.8105884637807890, -5.540438805289570112 ) ) ;
#10453=CARTESIAN_POINT ( 'NONE',  ( 14.92337183194729988, 9.342264484334119601, -8.527530157486177487 ) ) ;
#10455=CARTESIAN_POINT ( 'NONE',  ( 19.42250999205614193, 25.14701867748817321, 5.440088680355555262 ) ) ;
#10456=CARTESIAN_POINT ( 'NONE',  ( 16.40814093676324603, 32.45696800326375353, -11.09922568453594671 ) ) ;
#10457=CARTESIAN_POINT ( 'NONE',  ( -1.926860441876562025, 54.47997603579417358, -3.195792623639529761 ) ) ;
#10458=( BOUNDED_SURFACE ( )  B_SPLINE_SURFACE ( 3, 2, ( 
 ( #93443, #39476, #16475 ),
 ( #31938, #23003, #47449 ),
 ( #992, #46952, #68984 ),
 ( #62439, #53470, #24477 ),
 ( #52978, #77948, #9455 ),
 ( #75982, #62942, #15010 ),
 ( #7511, #15979, #38002 ),
 ( #68495, #38490, #21 ),
 ( #30469, #30965, #94422 ),
 ( #24969, #63433, #10930 ) ),
 .UNSPECIFIED., .F., .F., .F. ) 
 B_SPLINE_SURFACE_WITH_KNOTS ( ( 4, 2, 2, 2, 4 ),
 ( 3, 3 ),
 ( 0.000000000000000000, 0.002067014858588510882, 0.003100522287882766324, 0.003617276002529893827, 0.004134029717177021765 ),
 ( 0.000000000000000000, 1.000000000000000000 ),
 .UNSPECIFIED. ) 
 GEOMETRIC_REPRESENTATION_ITEM ( )  RATIONAL_B_SPLINE_SURFACE ( (
 ( 1.000000000000000000, 0.7411386215561424073, 1.000000000000000000),
 ( 1.000000000000000000, 0.7517628147009809414, 1.000000000000000000),
 ( 1.000000000000000000, 0.7644153482607498606, 1.000000000000000000),
 ( 1.000000000000000000, 0.8033584422216667464, 1.000000000000000000),
 ( 1.000000000000000000, 0.8197614970480194829, 1.000000000000000000),
 ( 1.000000000000000000, 0.8550190949536496943, 1.000000000000000000),
 ( 1.000000000000000000, 0.8686037895732486858, 1.000000000000000000),
 ( 1.000000000000000000, 0.9009153382757982831, 1.000000000000000000),
 ( 1.000000000000000000, 0.9197777054298900135, 1.000000000000000000),
 ( 1.000000000000000000, 0.9412039349194007976, 1.000000000000000000) ) ) 
 REPRESENTATION_ITEM ( '' )  SURFACE ( )  );
#10459=CARTESIAN_POINT ( 'NONE',  ( 7.361572987183170547, 57.05059781766744464, 9.846743663894590881 ) ) ;
#10460=CARTESIAN_POINT ( 'NONE',  ( 15.44008868035555793, 66.39701867748817676, -9.422509992056140149 ) ) ;
#10461=CARTESIAN_POINT ( 'NONE',  ( 19.84674366389459621, 18.50893115100078745, 7.409399052514197653E-17 ) ) ;
#10462=CARTESIAN_POINT ( 'NONE',  ( 16.40814093676323893, 30.79030133659708923, 11.09922568453595026 ) ) ;
#10463=CARTESIAN_POINT ( 'NONE',  ( 17.96484262340118221, 59.93868534415484106, 7.964842623401181321 ) ) ;
#10464=CARTESIAN_POINT ( 'NONE',  ( 18.72515096720579209, 51.07228050351030646, -6.499999999999869438 ) ) ;
#10465=CARTESIAN_POINT ( 'NONE',  ( 6.565887622018943937, 63.08196800326376064, -12.81628187352647608 ) ) ;
#10468=CARTESIAN_POINT ( 'NONE',  ( 15.44008868035555793, 11.39701867748817143, -9.422509992056140149 ) ) ;
#10469=CARTESIAN_POINT ( 'NONE',  ( 6.565887622018943937, 65.16530133659709634, 12.81628187352647430 ) ) ;
#10470=CARTESIAN_POINT ( 'NONE',  ( 10.00000000000000178, 22.25893115100078745, 9.846743663894594434 ) ) ;
#10471=CARTESIAN_POINT ( 'NONE',  ( 10.00000000000000000, 1.813685344154837731, -10.88017736071110342 ) ) ;
#10472=CARTESIAN_POINT ( 'NONE',  ( 19.84674366389459266, 23.30059781766745530, 2.638427012816836559 ) ) ;
#10473=CARTESIAN_POINT ( 'NONE',  ( 24.16423886937410614, 59.51208216824728936, -3.795296366450302550 ) ) ;
#10474=ORIENTED_EDGE ( 'NONE', *, *, #77960, .T. ) ;
#10475=CARTESIAN_POINT ( 'NONE',  ( -0.8801773607110991993, 7.855352010821504471, -2.915334737309923874 ) ) ;
#10476=CARTESIAN_POINT ( 'NONE',  ( -0.8801773607110991993, 27.85535201082150181, -2.915334737309923874 ) ) ;
#10477=CARTESIAN_POINT ( 'NONE',  ( -0.1503990784575327533, 7.222660991849186196, -6.262539305110070842 ) ) ;
#10480=CARTESIAN_POINT ( 'NONE',  ( 7.084665262690076126, 22.02201867748817321, -10.88017736071110164 ) ) ;
#10481=CARTESIAN_POINT ( 'NONE',  ( 5.076628168052704559, 55.17559781766745175, -8.527530157486179263 ) ) ;
#10483=CARTESIAN_POINT ( 'NONE',  ( 6.565887622018943937, 50.16530133659708213, 12.81628187352647430 ) ) ;
#10485=CARTESIAN_POINT ( 'NONE',  ( 24.16423886937410614, 24.51208216824730002, -3.795296366450302550 ) ) ;
#10486=CARTESIAN_POINT ( 'NONE',  ( 12.91533473730992121, 39.52201867748817676, 10.88017736071110164 ) ) ;
#10487=CARTESIAN_POINT ( 'NONE',  ( 7.084665262690076126, 12.02201867748817321, -10.88017736071110164 ) ) ;
#10488=CARTESIAN_POINT ( 'NONE',  ( 10.00000000000000000, 59.75893115100078745, -9.846743663894594434 ) ) ;
#10490=CARTESIAN_POINT ( 'NONE',  ( 12.63842701281683922, 34.55059781766745886, -9.846743663894590881 ) ) ;
#10491=CARTESIAN_POINT ( 'NONE',  ( 7.361572987183170547, 7.050597817667451750, 9.846743663894590881 ) ) ;
#10494=CARTESIAN_POINT ( 'NONE',  ( 10.00000000000000000, 9.758931151000785675, -9.846743663894594434 ) ) ;
#10495=CARTESIAN_POINT ( 'NONE',  ( 10.00000000000000178, 67.25893115100079456, 9.846743663894594434 ) ) ;
#10496=CARTESIAN_POINT ( 'NONE',  ( 10.00000000000000178, 49.31368534415484106, 10.88017736071110342 ) ) ;
#10497=CARTESIAN_POINT ( 'NONE',  ( 7.084665262690076126, 19.10535201082150181, 10.88017736071109987 ) ) ;
#10498=CARTESIAN_POINT ( 'NONE',  ( 16.40814093676323893, 40.79030133659708923, 11.09922568453595026 ) ) ;
#10499=CARTESIAN_POINT ( 'NONE',  ( -4.164238869374099039, 26.80374883491397142, 8.674139862899312516E-16 ) ) ;
#10500=EDGE_CURVE ( 'NONE', #23770, #60007, #65292, .T. ) ;
#10501=CARTESIAN_POINT ( 'NONE',  ( 20.15039907845753930, 11.74884699246888964, 6.262539305110064625 ) ) ;
#10502=CARTESIAN_POINT ( 'NONE',  ( 22.81628187352647785, 61.41530133659709634, 3.434112377981063169 ) ) ;
#10504=CARTESIAN_POINT ( 'NONE',  ( 12.63842701281683922, 59.55059781766744464, -9.846743663894590881 ) ) ;
#10505=CARTESIAN_POINT ( 'NONE',  ( 10.00000000000000178, 39.31368534415484106, 10.88017736071110342 ) ) ;
#10507=CARTESIAN_POINT ( 'NONE',  ( 0.1532563361054082862, 1.217264484334117824, 2.638427012816831674 ) ) ;
#10508=CARTESIAN_POINT ( 'NONE',  ( 19.84674366389459621, 28.50893115100078745, 7.409399052514197653E-17 ) ) ;
#10509=CARTESIAN_POINT ( 'NONE',  ( 10.00000000000000000, 66.81368534415484817, -10.88017736071110342 ) ) ;
#10511=( NAMED_UNIT ( * ) SI_UNIT ( $, .STERADIAN. ) SOLID_ANGLE_UNIT ( ) );
#10512=CARTESIAN_POINT ( 'NONE',  ( 20.88017736071110519, 55.56368534415484817, 2.639326808657452039E-16 ) ) ;
#10514=CARTESIAN_POINT ( 'NONE',  ( 12.91533473730992121, 64.52201867748817676, 10.88017736071110164 ) ) ;
#10516=CARTESIAN_POINT ( 'NONE',  ( 0.1532563361054100626, 10.80059781766745175, -2.638427012816831230 ) ) ;
#10520=B_SPLINE_CURVE_WITH_KNOTS ( 'NONE', 3,
 ( #35098, #97127, #28597, #89594 ),
 .UNSPECIFIED., .F., .F.,
 ( 4, 4 ),
 ( 6.254634441385501671E-17, 0.001060528352561988753 ),
 .UNSPECIFIED. ) ;
#10522=EDGE_CURVE ( 'NONE', #15284, #18635, #44589, .T. ) ;
#10523=CARTESIAN_POINT ( 'NONE',  ( 19.84674366389459621, 58.50893115100078745, 7.409399052514197653E-17 ) ) ;
#10524=ORIENTED_EDGE ( 'NONE', *, *, #45654, .T. ) ;
#10526=CARTESIAN_POINT ( 'NONE',  ( 13.99999999999999822, 10.49999999999999822, -6.500000000000000888 ) ) ;
#10528=CARTESIAN_POINT ( 'NONE',  ( 22.26659068614895176, 9.720415501580633943, -7.082119434687042414 ) ) ;
#10529=( BOUNDED_SURFACE ( )  B_SPLINE_SURFACE ( 1, 2, ( 
 ( #64496, #94516, #19508, #10534, #56527, #33028, #34492, #34984, #72991, #10049, #64984, #95003, #40548, #95509, #4521, #27492, #48520, #41044, #57500, #87995, #86048, #17559, #3052, #94031, #25552, #56044, #33506, #64004, #96510, #67477, #43964, #90451, #88992, #13486, #42995, #12981, #20993, #51480, #28964, #82470, #59467, #89969, #36977, #58479, #6977, #37482, #29452, #80992, #27982, #97997, #66480, #75461, #82967, #35979, #28486, #59959, #14486, #89483, #21989, #20496, #12495, #52465, #51983, #97008, #98496, #74468, #97500, #74968, #50984, #58980, #81974, #43478, #44958, #67971, #81479, #73477, #5992, #50495, #88491, #36487, #66979, #21485, #13991, #73979, #44466, #57986, #6473, #19993, #5006, #35488, #65984, #5504, #91824, #60942, #53443, #7482, #62414, #31424, #37979, #15952, #77923, #77417, #9429, #8933, #76936, #30937, #69941, #53946, #22476, #61928, #76450, #85430, #39933, #8445, #30443, #54427, #61436, #91453, #69444, #39450, #91942, #23473, #70436, #16939, #92429, #22978, #84936, #23954, #14983, #84453, #16447, #90946, #47421, #68469, #52951, #29951, #92919, #60456, #83952, #964, #38952, #46925, #15478, #45961, #7966, #46445, #31912, #38464, #68956, #488, #1461, #24449, #83462, #45454, #54916, #75955, #42392, #10420, #56416, #72380, #93913, #64865, #18911, #79888, #3909, #62919, #71893, #40928, #2453, #55424, #19391, #71426, #1953, #32417, #40436, #94399, #93419, #25441, #55924, #49387, #79409, #34376, #86423, #24942, #95386, #11395, #63887, #10910, #87875, #70935, #85932, #2941, #17442, #47909, #33389, #32909, #41917, #78414, #9932, #94892, #64382, #49877, #63409, #17924, #48408, #57381, #78911, #86902, #25914, #26390, #18412, #48895, #41432, #80389, #56890, #3416, #33877, #87394, #26888, #11892, #96892, #89850, #88380, #89362, #36862, #65367, #43849, #35865, #58351, #51364, #21366, #35373, #12377, #59347, #96392, #81365, #19877, #74343, #21870, #67354, #34873, #5871, #12864, #95897, #28369, #90331, #59841, #73365, #65864, #36363, #43362, #97880, #20873, #4893, #66858, #97376, #28844, #82845, #58856, #42882, #82346, #81851, #6353, #27866, #13364, #57869, #88873, #66354, #51861, #13867, #44347, #74852, #29340, #52348, #20380, #14365, #72871, #4406, #27376, #50873, #50370, #73862, #80878, #5390, #22855, #15361, #84822, #69826, #76333, #77304, #45339, #67858, #16329, #38836, #83836, #85312, #30823, #84344, #61811, #7359, #53327, #7849, #98871, #46812, #1349, #14867, #60341, #38347, #37365, #75339, #375, #45846, #76816, #61321, #75839, #69330, #24335, #91832, #852, #44835, #15846, #8818, #6854, #37861, #68353 ),
 ( #39332, #98377, #46330, #68842, #30326, #29833, #62298, #23350, #90835, #22362, #83345, #53832, #52836, #60828, #91329, #92317, #8333, #31801, #31309, #23842, #92806, #54309, #54795, #94276, #3793, #85809, #57260, #78797, #2333, #25799, #64260, #78294, #55298, #3292, #56774, #40804, #9308, #18294, #63285, #72265, #64748, #56299, #17322, #41311, #17806, #47795, #86793, #94773, #10305, #71304, #95260, #34248, #79284, #9810, #71783, #10793, #1836, #2824, #48777, #77798, #26766, #24822, #39816, #16820, #79773, #47296, #93298, #33756, #26272, #87269, #40312, #70817, #32788, #33276, #18791, #93791, #25321, #55807, #49274, #63768, #70321, #32293, #11272, #62798, #86300, #48286, #41792, #59226, #80760, #51746, #5756, #66741, #89730, #49753, #58739, #96272, #88252, #42276, #6244, #58228, #29226, #87755, #27251, #81246, #19269, #12255, #42762, #36245, #66234, #21247, #73245, #80264, #82229, #97266, #50759, #96769, #74731, #57750, #11767, #27745, #72746, #4279, #88748, #19760, #28736, #34753, #65243, #81729, #51242, #36748, #50244, #95769, #4772, #44227, #35245, #73739, #12745, #13244, #43243, #65742, #35746, #67238, #43736, #20258, #5269, #28244, #89244, #13744, #20753, #97761, #74223, #76224, #23730, #52234, #30699, #82726, #84708, #98259, #91714, #45223, #29717, #61688, #53706, #6735, #44726, #68722, #15734, #46695, #16211, #8699, #59726, #60711, #75223, #46217, #91208, #22736, #68241, #92205, #83225, #98758, #37251, #61210, #39215, #54193, #21753, #23234, #30208, #14245, #15243, #77193, #69702, #60224, #22243, #84226, #53219, #1232, #7738, #90718, #76703, #8222, #38717, #90221, #45722, #52720, #69216, #38232, #67740, #14750, #251, #75720, #7235, #83721, #742, #31195, #37742, #4048, #34510, #12026, #32172, #81013, #12514, #4541, #54678, #70196, #42525, #41563, #50516, #58004, #11042, #3557, #73009, #88513, #64514, #65506, #62675, #85199, #35003, #27020, #72030, #73498, #19040, #72514, #50025, #93175, #34017, #95020, #87036, #96028, #20015, #1716, #47177, #26528, #24212, #62177, #87526, #57025, #65003, #49516, #24701, #57520, #43016, #80025, #88016, #31685, #95530, #27510, #92687, #55172, #18546, #49038, #9196, #16704, #19528, #39709, #11529, #77682, #80527, #79542, #42050, #52004, #6015, #35508, #66002, #59980, #67497, #89011, #97522, #6493, #96530, #60477, #13003, #28005, #5024, #67994, #58501, #81498, #74990, #14009, #22008, #43498, #66506, #97031, #59490, #6997, #59001, #28507, #89503, #44978, #21506, #90966, #20518, #75484, #22500, #45474, #13507, #89990, #37502, #21014, #98519, #52482, #82990, #29972, #51003, #37001, #43989 ) ),
 .UNSPECIFIED., .F., .F., .T. ) 
 B_SPLINE_SURFACE_WITH_KNOTS ( ( 2, 2 ),
 ( 3, 2, 2, 2, 2, 2, 2, 2, 2, 2, 2, 2, 2, 2, 2, 2, 2, 2, 2, 2, 2, 2, 2, 2, 2, 2, 2, 2, 2, 2, 2, 2, 2, 2, 2, 2, 2, 2, 2, 2, 2, 2, 2, 2, 2, 2, 2, 2, 2, 2, 2, 2, 2, 2, 2, 2, 2, 2, 2, 2, 2, 2, 2, 2, 2, 2, 2, 2, 2, 2, 2, 2, 2, 2, 2, 2, 2, 2, 2, 2, 2, 2, 2, 2, 2, 2, 2, 2, 2, 2, 2, 2, 2, 2, 2, 2, 2, 2, 2, 2, 2, 2, 2, 2, 2, 2, 2, 2, 2, 2, 2, 2, 2, 2, 2, 2, 2, 2, 2, 2, 2, 2, 2, 2, 2, 2, 2, 2, 2, 2, 2, 2, 2, 2, 2, 2, 2, 2, 2, 2, 2, 2, 2, 2, 2, 2, 2, 2, 2, 2, 2, 2, 2, 2, 2, 2, 2, 2, 2, 2, 2, 2, 3 ),
 ( 0.000000000000000000, 1.000000000000000000 ),
 ( 0.000000000000000000, 0.005952380952380952051, 0.01190476190476190410, 0.01785714285714285615, 0.02380952380952380820, 0.02976190476190476025, 0.03571428571428571230, 0.04166666666666666435, 0.04761904761904761640, 0.05357142857142856845, 0.05952380952380952051, 0.06547619047619047949, 0.07142857142857142461, 0.07738095238095238360, 0.08333333333333332871, 0.08928571428571428770, 0.09523809523809523281, 0.1011904761904761918, 0.1071428571428571369, 0.1130952380952380959, 0.1190476190476190410, 0.1250000000000000000, 0.1309523809523809590, 0.1369047619047619180, 0.1428571428571428492, 0.1488095238095238082, 0.1547619047619047672, 0.1607142857142857262, 0.1666666666666666574, 0.1726190476190476164, 0.1785714285714285754, 0.1845238095238095344, 0.1904761904761904656, 0.1964285714285714246, 0.2023809523809523836, 0.2083333333333333426, 0.2142857142857142738, 0.2202380952380952328, 0.2261904761904761918, 0.2321428571428571508, 0.2380952380952380820, 0.2440476190476190410, 0.2500000000000000000, 0.2559523809523809312, 0.2619047619047619180, 0.2678571428571428492, 0.2738095238095238360, 0.2797619047619047672, 0.2857142857142856984, 0.2916666666666666852, 0.2976190476190476164, 0.3035714285714285476, 0.3095238095238095344, 0.3154761904761904656, 0.3214285714285714524, 0.3273809523809523836, 0.3333333333333333148, 0.3392857142857143016, 0.3452380952380952328, 0.3511904761904761640, 0.3571428571428571508, 0.3630952380952380820, 0.3690476190476190688, 0.3750000000000000000, 0.3809523809523809312, 0.3869047619047619180, 0.3928571428571428492, 0.3988095238095238360, 0.4047619047619047672, 0.4107142857142856984, 0.4166666666666666852, 0.4226190476190476164, 0.4285714285714285476, 0.4345238095238095344, 0.4404761904761904656, 0.4464285714285714524, 0.4523809523809523836, 0.4583333333333333148, 0.4642857142857143016, 0.4702380952380952328, 0.4761904761904761640, 0.4821428571428571508, 0.4880952380952380820, 0.4940476190476190688, 0.5000000000000000000, 0.5059523809523809312, 0.5119047619047618625, 0.5178571428571429047, 0.5238095238095238360, 0.5297619047619047672, 0.5357142857142856984, 0.5416666666666666297, 0.5476190476190476719, 0.5535714285714286031, 0.5595238095238095344, 0.5654761904761904656, 0.5714285714285713969, 0.5773809523809523281, 0.5833333333333333703, 0.5892857142857143016, 0.5952380952380952328, 0.6011904761904761640, 0.6071428571428570953, 0.6130952380952381375, 0.6190476190476190688, 0.6250000000000000000, 0.6309523809523809312, 0.6369047619047618625, 0.6428571428571429047, 0.6488095238095238360, 0.6547619047619047672, 0.6607142857142856984, 0.6666666666666666297, 0.6726190476190476719, 0.6785714285714286031, 0.6845238095238095344, 0.6904761904761904656, 0.6964285714285713969, 0.7023809523809523281, 0.7083333333333333703, 0.7142857142857143016, 0.7202380952380952328, 0.7261904761904761640, 0.7321428571428570953, 0.7380952380952381375, 0.7440476190476190688, 0.7500000000000000000, 0.7559523809523809312, 0.7619047619047618625, 0.7678571428571429047, 0.7738095238095238360, 0.7797619047619047672, 0.7857142857142856984, 0.7916666666666666297, 0.7976190476190476719, 0.8035714285714286031, 0.8095238095238095344, 0.8154761904761904656, 0.8214285714285713969, 0.8273809523809523281, 0.8333333333333333703, 0.8392857142857143016, 0.8452380952380952328, 0.8511904761904761640, 0.8571428571428570953, 0.8630952380952381375, 0.8690476190476190688, 0.8750000000000000000, 0.8809523809523809312, 0.8869047619047618625, 0.8928571428571429047, 0.8988095238095238360, 0.9047619047619047672, 0.9107142857142856984, 0.9166666666666666297, 0.9226190476190476719, 0.9285714285714286031, 0.9345238095238095344, 0.9404761904761904656, 0.9464285714285713969, 0.9523809523809523281, 0.9583333333333333703, 0.9642857142857143016 ),
 .UNSPECIFIED. ) 
 GEOMETRIC_REPRESENTATION_ITEM ( )  RATIONAL_B_SPLINE_SURFACE ( (
 ( 1.000000000000000000, 0.9659258262890683122, 1.000000000000000000, 0.9659258262890683122, 1.000000000000000000, 0.9659258262890683122, 1.000000000000000000, 0.9659258262890683122, 1.000000000000000000, 0.9659258262890683122, 1.000000000000000000, 0.9659258262890683122, 1.000000000000000000, 0.9659258262890683122, 1.000000000000000000, 0.9659258262890683122, 1.000000000000000000, 0.9659258262890683122, 1.000000000000000000, 0.9659258262890683122, 1.000000000000000000, 0.9659258262890683122, 1.000000000000000000, 0.9659258262890683122, 1.000000000000000000, 0.9659258262890683122, 1.000000000000000000, 0.9659258262890683122, 1.000000000000000000, 0.9659258262890683122, 1.000000000000000000, 0.9659258262890683122, 1.000000000000000000, 0.9659258262890683122, 1.000000000000000000, 0.9659258262890683122, 1.000000000000000000, 0.9659258262890683122, 1.000000000000000000, 0.9659258262890683122, 1.000000000000000000, 0.9659258262890683122, 1.000000000000000000, 0.9659258262890683122, 1.000000000000000000, 0.9659258262890683122, 1.000000000000000000, 0.9659258262890683122, 1.000000000000000000, 0.9659258262890683122, 1.000000000000000000, 0.9659258262890683122, 1.000000000000000000, 0.9659258262890683122, 1.000000000000000000, 0.9659258262890683122, 1.000000000000000000, 0.9659258262890683122, 1.000000000000000000, 0.9659258262890683122, 1.000000000000000000, 0.9659258262890683122, 1.000000000000000000, 0.9659258262890683122, 1.000000000000000000, 0.9659258262890683122, 1.000000000000000000, 0.9659258262890683122, 1.000000000000000000, 0.9659258262890683122, 1.000000000000000000, 0.9659258262890683122, 1.000000000000000000, 0.9659258262890683122, 1.000000000000000000, 0.9659258262890683122, 1.000000000000000000, 0.9659258262890683122, 1.000000000000000000, 0.9659258262890683122, 1.000000000000000000, 0.9659258262890683122, 1.000000000000000000, 0.9659258262890683122, 1.000000000000000000, 0.9659258262890683122, 1.000000000000000000, 0.9659258262890683122, 1.000000000000000000, 0.9659258262890683122, 1.000000000000000000, 0.9659258262890683122, 1.000000000000000000, 0.9659258262890683122, 1.000000000000000000, 0.9659258262890683122, 1.000000000000000000, 0.9659258262890683122, 1.000000000000000000, 0.9659258262890683122, 1.000000000000000000, 0.9659258262890683122, 1.000000000000000000, 0.9659258262890683122, 1.000000000000000000, 0.9659258262890683122, 1.000000000000000000, 0.9659258262890683122, 1.000000000000000000, 0.9659258262890683122, 1.000000000000000000, 0.9659258262890683122, 1.000000000000000000, 0.9659258262890683122, 1.000000000000000000, 0.9659258262890683122, 1.000000000000000000, 0.9659258262890683122, 1.000000000000000000, 0.9659258262890683122, 1.000000000000000000, 0.9659258262890683122, 1.000000000000000000, 0.9659258262890683122, 1.000000000000000000, 0.9659258262890683122, 1.000000000000000000, 0.9659258262890683122, 1.000000000000000000, 0.9659258262890683122, 1.000000000000000000, 0.9659258262890683122, 1.000000000000000000, 0.9659258262890683122, 1.000000000000000000, 0.9659258262890683122, 1.000000000000000000, 0.9659258262890683122, 1.000000000000000000, 0.9659258262890683122, 1.000000000000000000, 0.9659258262890683122, 1.000000000000000000, 0.9659258262890683122, 1.000000000000000000, 0.9659258262890683122, 1.000000000000000000, 0.9659258262890683122, 1.000000000000000000, 0.9659258262890683122, 1.000000000000000000, 0.9659258262890683122, 1.000000000000000000, 0.9659258262890683122, 1.000000000000000000, 0.9659258262890683122, 1.000000000000000000, 0.9659258262890683122, 1.000000000000000000, 0.9659258262890683122, 1.000000000000000000, 0.9659258262890683122, 1.000000000000000000, 0.9659258262890683122, 1.000000000000000000, 0.9659258262890683122, 1.000000000000000000, 0.9659258262890683122, 1.000000000000000000, 0.9659258262890683122, 1.000000000000000000, 0.9659258262890683122, 1.000000000000000000, 0.9659258262890683122, 1.000000000000000000, 0.9659258262890683122, 1.000000000000000000, 0.9659258262890683122, 1.000000000000000000, 0.9659258262890683122, 1.000000000000000000, 0.9659258262890683122, 1.000000000000000000, 0.9659258262890683122, 1.000000000000000000, 0.9659258262890683122, 1.000000000000000000, 0.9659258262890683122, 1.000000000000000000, 0.9659258262890683122, 1.000000000000000000, 0.9659258262890683122, 1.000000000000000000, 0.9659258262890683122, 1.000000000000000000, 0.9659258262890683122, 1.000000000000000000, 0.9659258262890683122, 1.000000000000000000, 0.9659258262890683122, 1.000000000000000000, 0.9659258262890683122, 1.000000000000000000, 0.9659258262890683122, 1.000000000000000000, 0.9659258262890683122, 1.000000000000000000, 0.9659258262890683122, 1.000000000000000000, 0.9659258262890683122, 1.000000000000000000, 0.9659258262890683122, 1.000000000000000000, 0.9659258262890683122, 1.000000000000000000, 0.9659258262890683122, 1.000000000000000000, 0.9659258262890683122, 1.000000000000000000, 0.9659258262890683122, 1.000000000000000000, 0.9659258262890683122, 1.000000000000000000, 0.9659258262890683122, 1.000000000000000000, 0.9659258262890683122, 1.000000000000000000, 0.9659258262890683122, 1.000000000000000000, 0.9659258262890683122, 1.000000000000000000, 0.9659258262890683122, 1.000000000000000000, 0.9659258262890683122, 1.000000000000000000, 0.9659258262890683122, 1.000000000000000000, 0.9659258262890683122, 1.000000000000000000, 0.9659258262890683122, 1.000000000000000000, 0.9659258262890683122, 1.000000000000000000, 0.9659258262890683122, 1.000000000000000000, 0.9659258262890683122, 1.000000000000000000, 0.9659258262890683122, 1.000000000000000000, 0.9659258262890683122, 1.000000000000000000, 0.9659258262890683122, 1.000000000000000000, 0.9659258262890683122, 1.000000000000000000, 0.9659258262890683122, 1.000000000000000000, 0.9659258262890683122, 1.000000000000000000, 0.9659258262890683122, 1.000000000000000000, 0.9659258262890683122, 1.000000000000000000, 0.9659258262890683122, 1.000000000000000000, 0.9659258262890683122, 1.000000000000000000, 0.9659258262890683122, 1.000000000000000000, 0.9659258262890683122, 1.000000000000000000, 0.9659258262890683122, 1.000000000000000000, 0.9659258262890683122, 1.000000000000000000, 0.9659258262890683122, 1.000000000000000000, 0.9659258262890683122, 1.000000000000000000, 0.9659258262890683122, 1.000000000000000000, 0.9659258262890683122, 1.000000000000000000, 0.9659258262890683122, 1.000000000000000000, 0.9659258262890683122, 1.000000000000000000, 0.9659258262890683122, 1.000000000000000000, 0.9659258262890683122, 1.000000000000000000, 0.9659258262890683122, 1.000000000000000000, 0.9659258262890683122, 1.000000000000000000, 0.9659258262890683122, 1.000000000000000000, 0.9659258262890683122, 1.000000000000000000, 0.9659258262890683122, 1.000000000000000000, 0.9659258262890683122, 1.000000000000000000, 0.9659258262890683122, 1.000000000000000000, 0.9659258262890683122, 1.000000000000000000, 0.9659258262890683122, 1.000000000000000000, 0.9659258262890683122, 1.000000000000000000, 0.9659258262890683122, 1.000000000000000000, 0.9659258262890683122, 1.000000000000000000, 0.9659258262890683122, 1.000000000000000000, 0.9659258262890683122, 1.000000000000000000, 0.9659258262890683122, 1.000000000000000000, 0.9659258262890683122, 1.000000000000000000, 0.9659258262890683122, 1.000000000000000000),
 ( 1.000000000000000000, 0.9659258262890683122, 1.000000000000000000, 0.9659258262890683122, 1.000000000000000000, 0.9659258262890683122, 1.000000000000000000, 0.9659258262890683122, 1.000000000000000000, 0.9659258262890683122, 1.000000000000000000, 0.9659258262890683122, 1.000000000000000000, 0.9659258262890683122, 1.000000000000000000, 0.9659258262890683122, 1.000000000000000000, 0.9659258262890683122, 1.000000000000000000, 0.9659258262890683122, 1.000000000000000000, 0.9659258262890683122, 1.000000000000000000, 0.9659258262890683122, 1.000000000000000000, 0.9659258262890683122, 1.000000000000000000, 0.9659258262890683122, 1.000000000000000000, 0.9659258262890683122, 1.000000000000000000, 0.9659258262890683122, 1.000000000000000000, 0.9659258262890683122, 1.000000000000000000, 0.9659258262890683122, 1.000000000000000000, 0.9659258262890683122, 1.000000000000000000, 0.9659258262890683122, 1.000000000000000000, 0.9659258262890683122, 1.000000000000000000, 0.9659258262890683122, 1.000000000000000000, 0.9659258262890683122, 1.000000000000000000, 0.9659258262890683122, 1.000000000000000000, 0.9659258262890683122, 1.000000000000000000, 0.9659258262890683122, 1.000000000000000000, 0.9659258262890683122, 1.000000000000000000, 0.9659258262890683122, 1.000000000000000000, 0.9659258262890683122, 1.000000000000000000, 0.9659258262890683122, 1.000000000000000000, 0.9659258262890683122, 1.000000000000000000, 0.9659258262890683122, 1.000000000000000000, 0.9659258262890683122, 1.000000000000000000, 0.9659258262890683122, 1.000000000000000000, 0.9659258262890683122, 1.000000000000000000, 0.9659258262890683122, 1.000000000000000000, 0.9659258262890683122, 1.000000000000000000, 0.9659258262890683122, 1.000000000000000000, 0.9659258262890683122, 1.000000000000000000, 0.9659258262890683122, 1.000000000000000000, 0.9659258262890683122, 1.000000000000000000, 0.9659258262890683122, 1.000000000000000000, 0.9659258262890683122, 1.000000000000000000, 0.9659258262890683122, 1.000000000000000000, 0.9659258262890683122, 1.000000000000000000, 0.9659258262890683122, 1.000000000000000000, 0.9659258262890683122, 1.000000000000000000, 0.9659258262890683122, 1.000000000000000000, 0.9659258262890683122, 1.000000000000000000, 0.9659258262890683122, 1.000000000000000000, 0.9659258262890683122, 1.000000000000000000, 0.9659258262890683122, 1.000000000000000000, 0.9659258262890683122, 1.000000000000000000, 0.9659258262890683122, 1.000000000000000000, 0.9659258262890683122, 1.000000000000000000, 0.9659258262890683122, 1.000000000000000000, 0.9659258262890683122, 1.000000000000000000, 0.9659258262890683122, 1.000000000000000000, 0.9659258262890683122, 1.000000000000000000, 0.9659258262890683122, 1.000000000000000000, 0.9659258262890683122, 1.000000000000000000, 0.9659258262890683122, 1.000000000000000000, 0.9659258262890683122, 1.000000000000000000, 0.9659258262890683122, 1.000000000000000000, 0.9659258262890683122, 1.000000000000000000, 0.9659258262890683122, 1.000000000000000000, 0.9659258262890683122, 1.000000000000000000, 0.9659258262890683122, 1.000000000000000000, 0.9659258262890683122, 1.000000000000000000, 0.9659258262890683122, 1.000000000000000000, 0.9659258262890683122, 1.000000000000000000, 0.9659258262890683122, 1.000000000000000000, 0.9659258262890683122, 1.000000000000000000, 0.9659258262890683122, 1.000000000000000000, 0.9659258262890683122, 1.000000000000000000, 0.9659258262890683122, 1.000000000000000000, 0.9659258262890683122, 1.000000000000000000, 0.9659258262890683122, 1.000000000000000000, 0.9659258262890683122, 1.000000000000000000, 0.9659258262890683122, 1.000000000000000000, 0.9659258262890683122, 1.000000000000000000, 0.9659258262890683122, 1.000000000000000000, 0.9659258262890683122, 1.000000000000000000, 0.9659258262890683122, 1.000000000000000000, 0.9659258262890683122, 1.000000000000000000, 0.9659258262890683122, 1.000000000000000000, 0.9659258262890683122, 1.000000000000000000, 0.9659258262890683122, 1.000000000000000000, 0.9659258262890683122, 1.000000000000000000, 0.9659258262890683122, 1.000000000000000000, 0.9659258262890683122, 1.000000000000000000, 0.9659258262890683122, 1.000000000000000000, 0.9659258262890683122, 1.000000000000000000, 0.9659258262890683122, 1.000000000000000000, 0.9659258262890683122, 1.000000000000000000, 0.9659258262890683122, 1.000000000000000000, 0.9659258262890683122, 1.000000000000000000, 0.9659258262890683122, 1.000000000000000000, 0.9659258262890683122, 1.000000000000000000, 0.9659258262890683122, 1.000000000000000000, 0.9659258262890683122, 1.000000000000000000, 0.9659258262890683122, 1.000000000000000000, 0.9659258262890683122, 1.000000000000000000, 0.9659258262890683122, 1.000000000000000000, 0.9659258262890683122, 1.000000000000000000, 0.9659258262890683122, 1.000000000000000000, 0.9659258262890683122, 1.000000000000000000, 0.9659258262890683122, 1.000000000000000000, 0.9659258262890683122, 1.000000000000000000, 0.9659258262890683122, 1.000000000000000000, 0.9659258262890683122, 1.000000000000000000, 0.9659258262890683122, 1.000000000000000000, 0.9659258262890683122, 1.000000000000000000, 0.9659258262890683122, 1.000000000000000000, 0.9659258262890683122, 1.000000000000000000, 0.9659258262890683122, 1.000000000000000000, 0.9659258262890683122, 1.000000000000000000, 0.9659258262890683122, 1.000000000000000000, 0.9659258262890683122, 1.000000000000000000, 0.9659258262890683122, 1.000000000000000000, 0.9659258262890683122, 1.000000000000000000, 0.9659258262890683122, 1.000000000000000000, 0.9659258262890683122, 1.000000000000000000, 0.9659258262890683122, 1.000000000000000000, 0.9659258262890683122, 1.000000000000000000, 0.9659258262890683122, 1.000000000000000000, 0.9659258262890683122, 1.000000000000000000, 0.9659258262890683122, 1.000000000000000000, 0.9659258262890683122, 1.000000000000000000, 0.9659258262890683122, 1.000000000000000000, 0.9659258262890683122, 1.000000000000000000, 0.9659258262890683122, 1.000000000000000000, 0.9659258262890683122, 1.000000000000000000, 0.9659258262890683122, 1.000000000000000000, 0.9659258262890683122, 1.000000000000000000, 0.9659258262890683122, 1.000000000000000000, 0.9659258262890683122, 1.000000000000000000, 0.9659258262890683122, 1.000000000000000000, 0.9659258262890683122, 1.000000000000000000, 0.9659258262890683122, 1.000000000000000000, 0.9659258262890683122, 1.000000000000000000, 0.9659258262890683122, 1.000000000000000000, 0.9659258262890683122, 1.000000000000000000, 0.9659258262890683122, 1.000000000000000000, 0.9659258262890683122, 1.000000000000000000, 0.9659258262890683122, 1.000000000000000000, 0.9659258262890683122, 1.000000000000000000, 0.9659258262890683122, 1.000000000000000000, 0.9659258262890683122, 1.000000000000000000, 0.9659258262890683122, 1.000000000000000000, 0.9659258262890683122, 1.000000000000000000, 0.9659258262890683122, 1.000000000000000000, 0.9659258262890683122, 1.000000000000000000, 0.9659258262890683122, 1.000000000000000000, 0.9659258262890683122, 1.000000000000000000, 0.9659258262890683122, 1.000000000000000000, 0.9659258262890683122, 1.000000000000000000, 0.9659258262890683122, 1.000000000000000000, 0.9659258262890683122, 1.000000000000000000, 0.9659258262890683122, 1.000000000000000000, 0.9659258262890683122, 1.000000000000000000, 0.9659258262890683122, 1.000000000000000000) ) ) 
 REPRESENTATION_ITEM ( '' )  SURFACE ( )  );
#10530=CARTESIAN_POINT ( 'NONE',  ( 10.00000000000000178, 65.37363466993042493, 12.81628187352647608 ) ) ;
#10531=CARTESIAN_POINT ( 'NONE',  ( -2.266590686148945544, 6.387082168247300906, -7.082119434687050408 ) ) ;
#10532=CARTESIAN_POINT ( 'NONE',  ( -2.266590686148945544, 36.38708216824730357, -7.082119434687050408 ) ) ;
#10534=CARTESIAN_POINT ( 'NONE',  ( -0.3689425029237898834, 1.178748834913967869, -10.36894250292378850 ) ) ;
#10535=CARTESIAN_POINT ( 'NONE',  ( 15.44008868035555260, 19.73035201082150536, 9.422509992056143702 ) ) ;
#10536=FACE_OUTER_BOUND ( 'NONE', #14421, .T. ) ;
#10538=CARTESIAN_POINT ( 'NONE',  ( 17.20831665107776587, 22.88393115100078745, 7.208316651077764980 ) ) ;
#10539=CARTESIAN_POINT ( 'NONE',  ( 7.361572987183170547, 17.05059781766745530, 9.846743663894590881 ) ) ;
#10540=CARTESIAN_POINT ( 'NONE',  ( 22.81628187352647785, 46.41530133659708213, 3.434112377981063169 ) ) ;
#10541=CARTESIAN_POINT ( 'NONE',  ( 7.361572987183170547, 32.05059781766745175, 9.846743663894590881 ) ) ;
#10543=CARTESIAN_POINT ( 'NONE',  ( 17.96484262340118221, 56.18868534415484817, -7.964842623401177768 ) ) ;
#10544=CARTESIAN_POINT ( 'NONE',  ( -1.099225684535947600, 23.70696800326375708, -6.408140936763238038 ) ) ;
#10546=CARTESIAN_POINT ( 'NONE',  ( 5.076628168052704559, 20.17559781766745175, -8.527530157486179263 ) ) ;
#10548=CARTESIAN_POINT ( 'NONE',  ( 20.36894250292379738, 14.92874883491396432, -10.36894250292379027 ) ) ;
#10550=CARTESIAN_POINT ( 'NONE',  ( 17.96484262340118221, 36.18868534415484106, -7.964842623401177768 ) ) ;
#10551=CARTESIAN_POINT ( 'NONE',  ( 20.36894250292379738, 34.92874883491396076, -10.36894250292379027 ) ) ;
#10552=CARTESIAN_POINT ( 'NONE',  ( 10.00000000000000000, 54.75893115100078745, -9.846743663894594434 ) ) ;
#10553=CARTESIAN_POINT ( 'NONE',  ( 10.00000000000000178, 7.258931151000785675, 9.846743663894594434 ) ) ;
#10554=CARTESIAN_POINT ( 'NONE',  ( 10.00000000000000000, 47.87363466993042493, -12.81628187352647608 ) ) ;
#10556=CARTESIAN_POINT ( 'NONE',  ( 20.88017736071110519, 40.56368534415484106, 2.639326808657452039E-16 ) ) ;
#10559=CARTESIAN_POINT ( 'NONE',  ( 0.6178305044545818747, 23.49863466993041783, -9.382169495545419124 ) ) ;
#10560=CARTESIAN_POINT ( 'NONE',  ( 17.20831665107776587, 44.13393115100078745, -7.208316651077762316 ) ) ;
#10563=DIRECTION ( 'NONE',  ( -0.000000000000000000, -0.000000000000000000, -1.000000000000000000 ) ) ;
#10570=CARTESIAN_POINT ( 'NONE',  ( 17.96484262340118221, 54.93868534415484106, 7.964842623401181321 ) ) ;
#10571=CARTESIAN_POINT ( 'NONE',  ( 19.42250999205614548, 60.98035201082151247, -5.440088680355545492 ) ) ;
#10574=CARTESIAN_POINT ( 'NONE',  ( -0.8801773607111009756, 28.06368534415484106, 1.068504757029289695E-15 ) ) ;
#10575=CARTESIAN_POINT ( 'NONE',  ( -2.816281873526471635, -1.084698663402913210, -3.434112377981056508 ) ) ;
#10576=CARTESIAN_POINT ( 'NONE',  ( 7.084665262690076126, 24.10535201082150181, 10.88017736071109987 ) ) ;
#10577=CARTESIAN_POINT ( 'NONE',  ( 18.95785429995050464, 37.24216108172004880, 6.499999999999924505 ) ) ;
#10579=CARTESIAN_POINT ( 'NONE',  ( 16.40814093676323893, 20.79030133659708923, 11.09922568453595026 ) ) ;
#10581=CARTESIAN_POINT ( 'NONE',  ( 0.5774900079438590739, 57.64701867748817676, -5.440088680355550821 ) ) ;
#10582=CARTESIAN_POINT ( 'NONE',  ( 0.1532563361054083140, 36.00893115100078745, 1.131784320476157264E-15 ) ) ;
#10583=CARTESIAN_POINT ( 'NONE',  ( 3.591859063236761518, 19.95696800326375353, 11.09922568453594849 ) ) ;
#10584=CARTESIAN_POINT ( 'NONE',  ( 20.03743638938529159, 51.75197528031018379, 6.399506433553905360 ) ) ;
#10585=CARTESIAN_POINT ( 'NONE',  ( 12.91533473730992121, 34.52201867748817676, 10.88017736071110164 ) ) ;
#10586=CARTESIAN_POINT ( 'NONE',  ( 22.26659068614895176, 54.72041550158063217, -7.082119434687042414 ) ) ;
#10587=CARTESIAN_POINT ( 'NONE',  ( 5.076628168052704559, 35.17559781766745175, -8.527530157486179263 ) ) ;
#10588=CARTESIAN_POINT ( 'NONE',  ( 12.91533473730993009, 61.60535201082150536, -10.88017736071109987 ) ) ;
#10589=CARTESIAN_POINT ( 'NONE',  ( 12.91533473730992121, 49.52201867748817676, 10.88017736071110164 ) ) ;
#10591=CARTESIAN_POINT ( 'NONE',  ( 10.00000000000000000, 10.55374883491396787, -14.16423886937410082 ) ) ;
#10594=CARTESIAN_POINT ( 'NONE',  ( 7.361572987183170547, 67.05059781766746596, 9.846743663894590881 ) ) ;
#10596=CIRCLE ( 'NONE', #69689, 0.5000000000000041078 ) ;
#10598=CARTESIAN_POINT ( 'NONE',  ( 20.36894250292379738, 49.92874883491396787, -10.36894250292379027 ) ) ;
#10599=CARTESIAN_POINT ( 'NONE',  ( 10.00000000000000000, 50.55374883491396787, -14.16423886937410082 ) ) ;
#10600=CARTESIAN_POINT ( 'NONE',  ( 17.20831665107776587, 12.88393115100078390, 7.208316651077764980 ) ) ;
#10601=CARTESIAN_POINT ( 'NONE',  ( 13.43411237798106583, 12.66530133659708746, -12.81628187352647252 ) ) ;
#10603=CARTESIAN_POINT ( 'NONE',  ( 19.88565890683627657, 52.71691075486304356, -6.480892540919849232 ) ) ;
#10604=CARTESIAN_POINT ( 'NONE',  ( 4.559911319644449179, 68.89701867748817676, 9.422509992056141925 ) ) ;
#10605=CARTESIAN_POINT ( 'NONE',  ( 10.00000000000000000, 32.87363466993042493, -12.81628187352647608 ) ) ;
#10606=CARTESIAN_POINT ( 'NONE',  ( 20.36894250292379382, 38.67874883491396076, 10.36894250292379205 ) ) ;
#10609=CARTESIAN_POINT ( 'NONE',  ( 4.559911319644449179, 68.89701867748817676, 9.422509992056141925 ) ) ;
#10610=B_SPLINE_CURVE_WITH_KNOTS ( 'NONE', 3,
 ( #48147, #3159, #42144, #87126 ),
 .UNSPECIFIED., .F., .F.,
 ( 4, 4 ),
 ( 1.453963218420191702E-17, 0.001060528352561989837 ),
 .UNSPECIFIED. ) ;
#10614=CARTESIAN_POINT ( 'NONE',  ( 1.472469842513823179, 21.42559781766745175, 4.923371831947296329 ) ) ;
#10617=CARTESIAN_POINT ( 'NONE',  ( 17.08211943468705130, 8.470415501580635720, 12.26659068614894998 ) ) ;
#10618=CARTESIAN_POINT ( 'NONE',  ( 19.42250999205614193, 5.147018677488171434, 5.440088680355555262 ) ) ;
#10619=CARTESIAN_POINT ( 'NONE',  ( 10.00000000000000178, 14.31368534415483929, 10.88017736071110342 ) ) ;
#10620=CARTESIAN_POINT ( 'NONE',  ( 2.791683348922240793, 36.63393115100078035, 7.208316651077764092 ) ) ;
#10621=CARTESIAN_POINT ( 'NONE',  ( 3.591859063236761518, 4.956968003263753531, 11.09922568453594849 ) ) ;
#10622=DIRECTION ( 'NONE',  ( 1.000000000000000000, 0.000000000000000000, 0.000000000000000000 ) ) ;
#10627=CARTESIAN_POINT ( 'NONE',  ( -2.816281873526471635, 13.91530133659708746, -3.434112377981056508 ) ) ;
#10629=CARTESIAN_POINT ( 'NONE',  ( 24.16423886937409904, 44.09541550158063927, 3.795296366450317205 ) ) ;
#10631=CARTESIAN_POINT ( 'NONE',  ( 13.79529636645030344, 53.26208216824730357, 14.16423886937410614 ) ) ;
#10633=CARTESIAN_POINT ( 'NONE',  ( 7.084665262690076126, 32.02201867748816966, -10.88017736071110164 ) ) ;
#10634=CARTESIAN_POINT ( 'NONE',  ( 20.88017736071110875, 40.77201867748818387, -2.915334737309920765 ) ) ;
#10635=CARTESIAN_POINT ( 'NONE',  ( -0.8801773607110991993, 62.85535201082150536, -2.915334737309923874 ) ) ;
#10636=CARTESIAN_POINT ( 'NONE',  ( 7.084665262690076126, 29.10535201082150181, 10.88017736071109987 ) ) ;
#10637=CARTESIAN_POINT ( 'NONE',  ( 0.1922240491738455848, 33.18878173731742010, 6.499999999999968914 ) ) ;
#10638=ADVANCED_FACE ( 'NONE', ( #67786 ), #31131, .T. ) ;
#10639=CARTESIAN_POINT ( 'NONE',  ( 2.791683348922240793, 16.63393115100078745, 7.208316651077764092 ) ) ;
#10641=ORIENTED_EDGE ( 'NONE', *, *, #4975, .F. ) ;
#10643=CARTESIAN_POINT ( 'NONE',  ( 18.52753015748617571, 48.09226448433412315, 4.923371831947298993 ) ) ;
#10645=CARTESIAN_POINT ( 'NONE',  ( 21.09922568453595559, 47.04030133659708923, -6.408140936763230044 ) ) ;
#10648=CARTESIAN_POINT ( 'NONE',  ( 18.95785429995060767, 22.24216108172003459, 6.499999999999853451 ) ) ;
#10650=CARTESIAN_POINT ( 'NONE',  ( 12.63842701281683034, 62.46726448433410894, 9.846743663894596210 ) ) ;
#10651=CARTESIAN_POINT ( 'NONE',  ( 6.204703633549690345, 50.76208216824730357, -14.16423886937410259 ) ) ;
#10653=ORIENTED_EDGE ( 'NONE', *, *, #61201, .T. ) ;
#10655=CARTESIAN_POINT ( 'NONE',  ( 10.00000000000000178, 37.25893115100078745, 9.846743663894594434 ) ) ;
#10656=CARTESIAN_POINT ( 'NONE',  ( 6.565887622018943937, 63.08196800326376064, -12.81628187352647608 ) ) ;
#10658=CARTESIAN_POINT ( 'NONE',  ( -2.816281873526473856, 9.331968003263753531, 3.434112377981055619 ) ) ;
#10659=CARTESIAN_POINT ( 'NONE',  ( 20.88017736071110875, 60.77201867748817676, -2.915334737309920765 ) ) ;
#10661=CIRCLE ( 'NONE', #23392, 2.999999999999999112 ) ;
#10662=CARTESIAN_POINT ( 'NONE',  ( 2.791683348922240793, 61.63393115100079456, 7.208316651077764092 ) ) ;
#10666=CARTESIAN_POINT ( 'NONE',  ( 13.79529636645031943, 65.34541550158063217, -14.16423886937409904 ) ) ;
#10668=CARTESIAN_POINT ( 'NONE',  ( 20.88017736071110519, 40.56368534415484106, 2.639326808657452039E-16 ) ) ;
#10669=CARTESIAN_POINT ( 'NONE',  ( 22.81628187352647785, 16.41530133659708923, 3.434112377981063169 ) ) ;
#10670=CARTESIAN_POINT ( 'NONE',  ( 0.5774900079438607392, 68.48035201082150536, 5.440088680355550821 ) ) ;
#10674=CARTESIAN_POINT ( 'NONE',  ( 2.791683348922240793, 46.63393115100077324, 7.208316651077764092 ) ) ;
#10675=CARTESIAN_POINT ( 'NONE',  ( 10.00000000000000178, 2.258931151000784787, 9.846743663894594434 ) ) ;
#10677=CARTESIAN_POINT ( 'NONE',  ( 0.6178305044545818747, 3.498634669930420049, -9.382169495545419124 ) ) ;
#10678=CARTESIAN_POINT ( 'NONE',  ( 17.96484262340118221, 21.18868534415483396, -7.964842623401177768 ) ) ;
#10681=CARTESIAN_POINT ( 'NONE',  ( 17.08211943468705840, 30.13708216824730357, -12.26659068614894466 ) ) ;
#10682=ADVANCED_FACE ( 'NONE', ( #52767 ), #54798, .T. ) ;
#10683=CIRCLE ( 'NONE', #73047, 0.5000000000000004441 ) ;
#10684=CARTESIAN_POINT ( 'NONE',  ( -4.164238869374099039, 31.80374883491396432, 8.674139862899312516E-16 ) ) ;
#10685=CARTESIAN_POINT ( 'NONE',  ( 2.035157376598822676, 12.43868534415483751, -7.964842623401177768 ) ) ;
#10686=CARTESIAN_POINT ( 'NONE',  ( 12.63842701281683922, 49.55059781766744464, -9.846743663894590881 ) ) ;
#10688=CARTESIAN_POINT ( 'NONE',  ( -2.816281873526473856, 44.12363466993042493, 9.499525473075851096E-16 ) ) ;
#10689=CARTESIAN_POINT ( 'NONE',  ( 4.559911319644449179, 8.897018677488171434, 9.422509992056141925 ) ) ;
#10691=CARTESIAN_POINT ( 'NONE',  ( 18.52753015748617571, 38.09226448433412315, 4.923371831947298993 ) ) ;
#10693=CARTESIAN_POINT ( 'NONE',  ( 7.084665262690076126, 42.02201867748816966, -10.88017736071110164 ) ) ;
#10694=CARTESIAN_POINT ( 'NONE',  ( 16.40814093676324603, 12.45696800326375353, -11.09922568453594671 ) ) ;
#10695=CARTESIAN_POINT ( 'NONE',  ( 24.16423886937409904, 19.09541550158063927, 3.795296366450317205 ) ) ;
#10698=CARTESIAN_POINT ( 'NONE',  ( 1.472469842513823179, 20.59226448433411960, -4.923371831947296329 ) ) ;
#10699=CARTESIAN_POINT ( 'NONE',  ( 21.09922568453595559, 47.04030133659708923, -6.408140936763230044 ) ) ;
#10700=CARTESIAN_POINT ( 'NONE',  ( 12.63842701281683922, 49.55059781766744464, -9.846743663894590881 ) ) ;
#10703=CARTESIAN_POINT ( 'NONE',  ( -0.3689425029237898834, 66.17874883491396076, -10.36894250292378850 ) ) ;
#10704=CARTESIAN_POINT ( 'NONE',  ( 20.36894250292379738, 4.928748834913967869, -10.36894250292379027 ) ) ;
#10705=CARTESIAN_POINT ( 'NONE',  ( 7.361572987183169658, -0.03273551566588185635, -9.846743663894592657 ) ) ;
#10706=CARTESIAN_POINT ( 'NONE',  ( 12.63842701281683922, 49.55059781766744464, -9.846743663894590881 ) ) ;
#10707=CARTESIAN_POINT ( 'NONE',  ( 20.88017736071110164, 15.35535201082150358, 2.915334737309930979 ) ) ;
#10708=DIRECTION ( 'NONE',  ( -0.000000000000000000, -0.000000000000000000, 1.000000000000000000 ) ) ;
#10709=CARTESIAN_POINT ( 'NONE',  ( 18.72515096720609051, 25.05509018479941119, 6.499999999999470646 ) ) ;
#10711=ORIENTED_EDGE ( 'NONE', *, *, #731, .F. ) ;
#10714=CARTESIAN_POINT ( 'NONE',  ( 20.36894250292379382, 8.678748834913967869, 10.36894250292379205 ) ) ;
#10716=CARTESIAN_POINT ( 'NONE',  ( 6.204703633549690345, 40.76208216824731778, -14.16423886937410259 ) ) ;
#10717=CARTESIAN_POINT ( 'NONE',  ( 7.361572987183169658, 54.96726448433413026, -9.846743663894592657 ) ) ;
#10718=CARTESIAN_POINT ( 'NONE',  ( 12.63842701281683922, 39.55059781766744464, -9.846743663894590881 ) ) ;
#10719=CARTESIAN_POINT ( 'NONE',  ( 10.00000000000000000, 26.81368534415484106, -10.88017736071110342 ) ) ;
#10720=CARTESIAN_POINT ( 'NONE',  ( 2.791683348922237240, 60.38393115100078745, -7.208316651077763204 ) ) ;
#10721=CARTESIAN_POINT ( 'NONE',  ( 20.36894250292379738, 9.928748834913966093, -10.36894250292379027 ) ) ;
#10722=CARTESIAN_POINT ( 'NONE',  ( 10.00000000000000178, 43.05374883491397497, 14.16423886937410082 ) ) ;
#10724=CARTESIAN_POINT ( 'NONE',  ( 20.88017736071110519, 10.56368534415483929, 2.639326808657452039E-16 ) ) ;
#10728=CARTESIAN_POINT ( 'NONE',  ( 7.084665262690076126, 64.10535201082150536, 10.88017736071109987 ) ) ;
#10729=CARTESIAN_POINT ( 'NONE',  ( 10.00000000000000000, 24.75893115100078745, -9.846743663894594434 ) ) ;
#10732=( BOUNDED_SURFACE ( )  B_SPLINE_SURFACE ( 1, 2, ( 
 ( #74521, #51532, #98550, #90999, #44519, #38025, #67030, #36541, #53002, #45507, #21043, #75018, #21538, #60996, #20548, #59027, #51033, #22039, #37033, #6523, #89533, #15034, #67529, #90505, #22530, #45008, #52514, #14538, #82024, #75514, #48, #43528, #5554, #76007, #7534, #36031, #44018, #97060, #28533, #97552, #29014, #30990, #39503, #8986, #24006, #54478, #61489, #47476, #9483, #91994, #46981, #84009, #39986, #40487, #24504, #77976, #15533, #54966, #23525, #84988, #1018, #16504, #53997, #46492, #55483, #84504, #16004, #32473, #70488, #31478, #69992, #76991, #70985, #62467, #85488, #91508, #92972, #46014, #2008, #39007, #47960, #2507, #62968, #8504, #93473, #85984, #17495, #78470, #9984, #23027, #76503, #8017, #38514, #61981, #92481, #65419, #94940, #12425, #50424, #56940, #87442, #42931, #49934, #79939, #73412, #49435, #72429, #4940, #10955, #63464, #3955, #95444, #57435, #80442, #25963, #72927, #57920, #93965, #25491, #55976, #48948, #33439, #86477, #48460, #40978, #63936, #56464, #86950, #18463, #79456, #13922, #14917, #27914, #36416, #75389, #81904, #74399, #28417, #90884, #6398, #5922, #20432, #5443, #66412, #83397, #50919, #97428, #35420, #82898, #43414, #12917, #28894, #59399, #14417, #73914, #89902, #21418, #29390, #51415, #96944, #37419, #44399, #29884, #59892, #58912, #90382, #21920, #65914, #6907, #96444, #98429, #60386, #58407, #81415, #89411, #13413, #60881, #40233, #86225, #78721, #79206, #48702, #26210, #40724, #25249, #38396, #47724, #7901, #70741, #87193, #76386, #32712, #78222, #10716, #91381, #55221, #33205, #45900, #10231, #37913, #63699, #56224, #3222, #68898, #85735, #56703, #41233, #426, #71226, #63210, #15418, #17248, #18716, #7417, #9733, #2257, #33686, #68401, #32217, #18222, #30378, #22909, #62718, #86718, #25732, #93714, #55733, #93218, #83889, #94202, #24742, #21171, #4706, #72189, #81174, #27177, #36169, #28662, #58160, #49679, #42688, #43664, #12674, #89168, #35676, #35169, #43174, #41720, #88671, #57680, #89661, #81657, #73662, #64671, #73167, #5189, #66160, #20179, #59154, #51173, #79702, #96693, #72672, #13166, #50682, #28173, #58666, #19196, #74150, #65669, #96191, #20679, #3718, #11200, #50176, #5684, #27675, #65173, #66669, #97194, #34179, #95181, #26689, #57185, #34677, #11696, #87682, #80183, #42205, #4207, #88176, #95693, #19689, #80686, #12182, #37173, #75147, #45643, #51674, #97684, #82152, #14673, #90637, #60140, #29146, #22661, #98176, #83148, #37660, #75645, #45139, #22162, #59652, #52644, #15162, #44148, #13664, #29632, #60635, #7156, #82652, #53138, #68159, #21673, #98680 ),
 ( #6657, #30129, #90143, #91136, #74656, #83647, #6167, #36671, #44652, #67159, #52159, #14168, #67666, #12989, #65991, #50012, #50503, #66986, #42513, #35496, #12503, #82479, #42039, #80516, #72503, #43485, #58487, #27991, #12014, #6000, #96518, #81486, #28494, #66490, #73986, #88999, #72997, #20505, #59475, #4035, #21493, #43002, #51488, #50991, #4527, #43973, #5511, #34991, #35988, #19515, #97017, #58987, #73486, #5013, #65496, #89491, #21000, #96016, #81983, #34498, #13494, #89976, #74475, #36494, #64989, #97508, #27499, #28972, #20003, #51990, #57994, #88500, #95516, #81001, #27009, #57507, #88004, #22485, #75960, #75469, #92434, #7488, #45967, #54432, #37984, #6481, #76457, #60464, #69450, #61933, #91458, #82975, #68475, #76942, #7972, #23480, #68963, #1, #38471, #74976, #22984, #90952, #23958, #8451, #495, #98005, #30449, #30944, #61442, #53449, #13998, #84459, #44476, #91948, #6985, #38958, #83958, #53951, #969, #14495, #31430, #60949, #36986, #67483, #29458, #59966, #83469, #90459, #21995, #98504, #44966, #37489, #67978, #29958, #52958, #14990, #45461, #16944, #2945, #33394, #78420, #3423, #32423, #39937, #18417, #2458, #94897, #62924, #64386, #93920, #93425, #32915, #63892, #47428, #24947, #17448, #9936, #94406, #63415, #70439, #54921, #84941, #55431, #10915, #40440, #85937, #17929, #70941, #78915, #25446, #26394, #77424, #47914, #25919, #55929, #86428, #77928, #41438, #48412, #10426, #39456, #85435, #9435, #71899, #69946, #40933, #33882, #56422, #92924, #62420, #71431, #86907, #48902, #24455, #79416, #16452, #46931, #1958, #8938, #1466, #31920, #51371, #4897, #26895, #88386, #43368, #74348, #96896, #5875, #19885, #81858, #56895, #3913, #19397, #73867, #11401, #50376, #35378, #96397, #28375, #58864, #36370, #88879, #73370, #87880, #95903, #57389, #80885, #66864, #49884, #12383, #27384, #89368, #41923, #4413, #50879, #95394, #65870, #87400, #81372, #5397, #13369, #80396, #34880, #43854, #20879, #11898, #27873, #42888, #64870, #65374, #97383, #18916, #57874, #58359, #49392, #79893, #42400, #66360, #72385, #34382, #72878, #35871, #20388, #12869, #24574, #76564, #611, #55034, #24073, #84569, #17065, #31055, #7599, #77539, #8080, #47547, #78045, #61555, #92063, #9547, #16569, #16070, #91067, #23591, #39073, #53070, #69566, #38095, #62044, #92544, #9057, #39570, #30559, #70059, #1581, #32030, #62534, #68582, #53562, #113, #84076, #48026, #36978, #66481, #50985, #43965, #97009, #5993, #20994, #90452, #27493, #12982, #82471, #20497, #73980, #35489, #97998, #81975, #5505, #19994, #80993, #12496, #59960, #50496 ) ),
 .UNSPECIFIED., .F., .F., .F. ) 
 B_SPLINE_SURFACE_WITH_KNOTS ( ( 2, 2 ),
 ( 3, 2, 2, 2, 2, 2, 2, 2, 2, 2, 2, 2, 2, 2, 2, 2, 2, 2, 2, 2, 2, 2, 2, 2, 2, 2, 2, 2, 2, 2, 2, 2, 2, 2, 2, 2, 2, 2, 2, 2, 2, 2, 2, 2, 2, 2, 2, 2, 2, 2, 2, 2, 2, 2, 2, 2, 2, 2, 2, 2, 2, 2, 2, 2, 2, 2, 2, 2, 2, 2, 2, 2, 2, 2, 2, 2, 2, 2, 2, 2, 2, 2, 2, 2, 2, 2, 2, 2, 2, 2, 2, 2, 2, 2, 2, 2, 2, 2, 2, 2, 2, 2, 2, 2, 2, 2, 2, 2, 2, 2, 2, 2, 2, 2, 2, 2, 2, 2, 2, 2, 2, 2, 2, 2, 2, 2, 2, 2, 2, 2, 2, 2, 2, 2, 2, 2, 2, 2, 2, 2, 2, 2, 2, 2, 2, 2, 2, 2, 2, 2, 2, 2, 2, 2, 2, 2, 2, 2, 2, 2, 2, 2, 3 ),
 ( 0.000000000000000000, 1.000000000000000000 ),
 ( 0.000000000000000000, 0.005952380952380952051, 0.01190476190476190410, 0.01785714285714285615, 0.02380952380952380820, 0.02976190476190476025, 0.03571428571428571230, 0.04166666666666666435, 0.04761904761904761640, 0.05357142857142856845, 0.05952380952380952051, 0.06547619047619047949, 0.07142857142857142461, 0.07738095238095238360, 0.08333333333333332871, 0.08928571428571428770, 0.09523809523809523281, 0.1011904761904761918, 0.1071428571428571369, 0.1130952380952380959, 0.1190476190476190410, 0.1250000000000000000, 0.1309523809523809590, 0.1369047619047619180, 0.1428571428571428492, 0.1488095238095238082, 0.1547619047619047672, 0.1607142857142857262, 0.1666666666666666574, 0.1726190476190476164, 0.1785714285714285754, 0.1845238095238095344, 0.1904761904761904656, 0.1964285714285714246, 0.2023809523809523836, 0.2083333333333333426, 0.2142857142857142738, 0.2202380952380952328, 0.2261904761904761918, 0.2321428571428571508, 0.2380952380952380820, 0.2440476190476190410, 0.2500000000000000000, 0.2559523809523809312, 0.2619047619047619180, 0.2678571428571428492, 0.2738095238095238360, 0.2797619047619047672, 0.2857142857142856984, 0.2916666666666666852, 0.2976190476190476164, 0.3035714285714285476, 0.3095238095238095344, 0.3154761904761904656, 0.3214285714285714524, 0.3273809523809523836, 0.3333333333333333148, 0.3392857142857143016, 0.3452380952380952328, 0.3511904761904761640, 0.3571428571428571508, 0.3630952380952380820, 0.3690476190476190688, 0.3750000000000000000, 0.3809523809523809312, 0.3869047619047619180, 0.3928571428571428492, 0.3988095238095238360, 0.4047619047619047672, 0.4107142857142856984, 0.4166666666666666852, 0.4226190476190476164, 0.4285714285714285476, 0.4345238095238095344, 0.4404761904761904656, 0.4464285714285714524, 0.4523809523809523836, 0.4583333333333333148, 0.4642857142857143016, 0.4702380952380952328, 0.4761904761904761640, 0.4821428571428571508, 0.4880952380952380820, 0.4940476190476190688, 0.5000000000000000000, 0.5059523809523809312, 0.5119047619047618625, 0.5178571428571429047, 0.5238095238095238360, 0.5297619047619047672, 0.5357142857142856984, 0.5416666666666666297, 0.5476190476190476719, 0.5535714285714286031, 0.5595238095238095344, 0.5654761904761904656, 0.5714285714285713969, 0.5773809523809523281, 0.5833333333333333703, 0.5892857142857143016, 0.5952380952380952328, 0.6011904761904761640, 0.6071428571428570953, 0.6130952380952381375, 0.6190476190476190688, 0.6250000000000000000, 0.6309523809523809312, 0.6369047619047618625, 0.6428571428571429047, 0.6488095238095238360, 0.6547619047619047672, 0.6607142857142856984, 0.6666666666666666297, 0.6726190476190476719, 0.6785714285714286031, 0.6845238095238095344, 0.6904761904761904656, 0.6964285714285713969, 0.7023809523809523281, 0.7083333333333333703, 0.7142857142857143016, 0.7202380952380952328, 0.7261904761904761640, 0.7321428571428570953, 0.7380952380952381375, 0.7440476190476190688, 0.7500000000000000000, 0.7559523809523809312, 0.7619047619047618625, 0.7678571428571429047, 0.7738095238095238360, 0.7797619047619047672, 0.7857142857142856984, 0.7916666666666666297, 0.7976190476190476719, 0.8035714285714286031, 0.8095238095238095344, 0.8154761904761904656, 0.8214285714285713969, 0.8273809523809523281, 0.8333333333333333703, 0.8392857142857143016, 0.8452380952380952328, 0.8511904761904761640, 0.8571428571428570953, 0.8630952380952381375, 0.8690476190476190688, 0.8750000000000000000, 0.8809523809523809312, 0.8869047619047618625, 0.8928571428571429047, 0.8988095238095238360, 0.9047619047619047672, 0.9107142857142856984, 0.9166666666666666297, 0.9226190476190476719, 0.9285714285714286031, 0.9345238095238095344, 0.9404761904761904656, 0.9464285714285713969, 0.9523809523809523281, 0.9583333333333333703, 0.9642857142857143016 ),
 .UNSPECIFIED. ) 
 GEOMETRIC_REPRESENTATION_ITEM ( )  RATIONAL_B_SPLINE_SURFACE ( (
 ( 1.000000000000000000, 0.9659258262890683122, 1.000000000000000000, 0.9659258262890683122, 1.000000000000000000, 0.9659258262890683122, 1.000000000000000000, 0.9659258262890683122, 1.000000000000000000, 0.9659258262890683122, 1.000000000000000000, 0.9659258262890683122, 1.000000000000000000, 0.9659258262890683122, 1.000000000000000000, 0.9659258262890683122, 1.000000000000000000, 0.9659258262890683122, 1.000000000000000000, 0.9659258262890683122, 1.000000000000000000, 0.9659258262890683122, 1.000000000000000000, 0.9659258262890683122, 1.000000000000000000, 0.9659258262890683122, 1.000000000000000000, 0.9659258262890683122, 1.000000000000000000, 0.9659258262890683122, 1.000000000000000000, 0.9659258262890683122, 1.000000000000000000, 0.9659258262890683122, 1.000000000000000000, 0.9659258262890683122, 1.000000000000000000, 0.9659258262890683122, 1.000000000000000000, 0.9659258262890683122, 1.000000000000000000, 0.9659258262890683122, 1.000000000000000000, 0.9659258262890683122, 1.000000000000000000, 0.9659258262890683122, 1.000000000000000000, 0.9659258262890683122, 1.000000000000000000, 0.9659258262890683122, 1.000000000000000000, 0.9659258262890683122, 1.000000000000000000, 0.9659258262890683122, 1.000000000000000000, 0.9659258262890683122, 1.000000000000000000, 0.9659258262890683122, 1.000000000000000000, 0.9659258262890683122, 1.000000000000000000, 0.9659258262890683122, 1.000000000000000000, 0.9659258262890683122, 1.000000000000000000, 0.9659258262890683122, 1.000000000000000000, 0.9659258262890683122, 1.000000000000000000, 0.9659258262890683122, 1.000000000000000000, 0.9659258262890683122, 1.000000000000000000, 0.9659258262890683122, 1.000000000000000000, 0.9659258262890683122, 1.000000000000000000, 0.9659258262890683122, 1.000000000000000000, 0.9659258262890683122, 1.000000000000000000, 0.9659258262890683122, 1.000000000000000000, 0.9659258262890683122, 1.000000000000000000, 0.9659258262890683122, 1.000000000000000000, 0.9659258262890683122, 1.000000000000000000, 0.9659258262890683122, 1.000000000000000000, 0.9659258262890683122, 1.000000000000000000, 0.9659258262890683122, 1.000000000000000000, 0.9659258262890683122, 1.000000000000000000, 0.9659258262890683122, 1.000000000000000000, 0.9659258262890683122, 1.000000000000000000, 0.9659258262890683122, 1.000000000000000000, 0.9659258262890683122, 1.000000000000000000, 0.9659258262890683122, 1.000000000000000000, 0.9659258262890683122, 1.000000000000000000, 0.9659258262890683122, 1.000000000000000000, 0.9659258262890683122, 1.000000000000000000, 0.9659258262890683122, 1.000000000000000000, 0.9659258262890683122, 1.000000000000000000, 0.9659258262890683122, 1.000000000000000000, 0.9659258262890683122, 1.000000000000000000, 0.9659258262890683122, 1.000000000000000000, 0.9659258262890683122, 1.000000000000000000, 0.9659258262890683122, 1.000000000000000000, 0.9659258262890683122, 1.000000000000000000, 0.9659258262890683122, 1.000000000000000000, 0.9659258262890683122, 1.000000000000000000, 0.9659258262890683122, 1.000000000000000000, 0.9659258262890683122, 1.000000000000000000, 0.9659258262890683122, 1.000000000000000000, 0.9659258262890683122, 1.000000000000000000, 0.9659258262890683122, 1.000000000000000000, 0.9659258262890683122, 1.000000000000000000, 0.9659258262890683122, 1.000000000000000000, 0.9659258262890683122, 1.000000000000000000, 0.9659258262890683122, 1.000000000000000000, 0.9659258262890683122, 1.000000000000000000, 0.9659258262890683122, 1.000000000000000000, 0.9659258262890683122, 1.000000000000000000, 0.9659258262890683122, 1.000000000000000000, 0.9659258262890683122, 1.000000000000000000, 0.9659258262890683122, 1.000000000000000000, 0.9659258262890683122, 1.000000000000000000, 0.9659258262890683122, 1.000000000000000000, 0.9659258262890683122, 1.000000000000000000, 0.9659258262890683122, 1.000000000000000000, 0.9659258262890683122, 1.000000000000000000, 0.9659258262890683122, 1.000000000000000000, 0.9659258262890683122, 1.000000000000000000, 0.9659258262890683122, 1.000000000000000000, 0.9659258262890683122, 1.000000000000000000, 0.9659258262890683122, 1.000000000000000000, 0.9659258262890683122, 1.000000000000000000, 0.9659258262890683122, 1.000000000000000000, 0.9659258262890683122, 1.000000000000000000, 0.9659258262890683122, 1.000000000000000000, 0.9659258262890683122, 1.000000000000000000, 0.9659258262890683122, 1.000000000000000000, 0.9659258262890683122, 1.000000000000000000, 0.9659258262890683122, 1.000000000000000000, 0.9659258262890683122, 1.000000000000000000, 0.9659258262890683122, 1.000000000000000000, 0.9659258262890683122, 1.000000000000000000, 0.9659258262890683122, 1.000000000000000000, 0.9659258262890683122, 1.000000000000000000, 0.9659258262890683122, 1.000000000000000000, 0.9659258262890683122, 1.000000000000000000, 0.9659258262890683122, 1.000000000000000000, 0.9659258262890683122, 1.000000000000000000, 0.9659258262890683122, 1.000000000000000000, 0.9659258262890683122, 1.000000000000000000, 0.9659258262890683122, 1.000000000000000000, 0.9659258262890683122, 1.000000000000000000, 0.9659258262890683122, 1.000000000000000000, 0.9659258262890683122, 1.000000000000000000, 0.9659258262890683122, 1.000000000000000000, 0.9659258262890683122, 1.000000000000000000, 0.9659258262890683122, 1.000000000000000000, 0.9659258262890683122, 1.000000000000000000, 0.9659258262890683122, 1.000000000000000000, 0.9659258262890683122, 1.000000000000000000, 0.9659258262890683122, 1.000000000000000000, 0.9659258262890683122, 1.000000000000000000, 0.9659258262890683122, 1.000000000000000000, 0.9659258262890683122, 1.000000000000000000, 0.9659258262890683122, 1.000000000000000000, 0.9659258262890683122, 1.000000000000000000, 0.9659258262890683122, 1.000000000000000000, 0.9659258262890683122, 1.000000000000000000, 0.9659258262890683122, 1.000000000000000000, 0.9659258262890683122, 1.000000000000000000, 0.9659258262890683122, 1.000000000000000000, 0.9659258262890683122, 1.000000000000000000, 0.9659258262890683122, 1.000000000000000000, 0.9659258262890683122, 1.000000000000000000, 0.9659258262890683122, 1.000000000000000000, 0.9659258262890683122, 1.000000000000000000, 0.9659258262890683122, 1.000000000000000000, 0.9659258262890683122, 1.000000000000000000, 0.9659258262890683122, 1.000000000000000000, 0.9659258262890683122, 1.000000000000000000, 0.9659258262890683122, 1.000000000000000000, 0.9659258262890683122, 1.000000000000000000, 0.9659258262890683122, 1.000000000000000000, 0.9659258262890683122, 1.000000000000000000, 0.9659258262890683122, 1.000000000000000000, 0.9659258262890683122, 1.000000000000000000, 0.9659258262890683122, 1.000000000000000000, 0.9659258262890683122, 1.000000000000000000, 0.9659258262890683122, 1.000000000000000000, 0.9659258262890683122, 1.000000000000000000, 0.9659258262890683122, 1.000000000000000000, 0.9659258262890683122, 1.000000000000000000, 0.9659258262890683122, 1.000000000000000000, 0.9659258262890683122, 1.000000000000000000, 0.9659258262890683122, 1.000000000000000000, 0.9659258262890683122, 1.000000000000000000, 0.9659258262890683122, 1.000000000000000000, 0.9659258262890683122, 1.000000000000000000, 0.9659258262890683122, 1.000000000000000000, 0.9659258262890683122, 1.000000000000000000, 0.9659258262890683122, 1.000000000000000000, 0.9659258262890683122, 1.000000000000000000),
 ( 1.000000000000000000, 0.9659258262890683122, 1.000000000000000000, 0.9659258262890683122, 1.000000000000000000, 0.9659258262890683122, 1.000000000000000000, 0.9659258262890683122, 1.000000000000000000, 0.9659258262890683122, 1.000000000000000000, 0.9659258262890683122, 1.000000000000000000, 0.9659258262890683122, 1.000000000000000000, 0.9659258262890683122, 1.000000000000000000, 0.9659258262890683122, 1.000000000000000000, 0.9659258262890683122, 1.000000000000000000, 0.9659258262890683122, 1.000000000000000000, 0.9659258262890683122, 1.000000000000000000, 0.9659258262890683122, 1.000000000000000000, 0.9659258262890683122, 1.000000000000000000, 0.9659258262890683122, 1.000000000000000000, 0.9659258262890683122, 1.000000000000000000, 0.9659258262890683122, 1.000000000000000000, 0.9659258262890683122, 1.000000000000000000, 0.9659258262890683122, 1.000000000000000000, 0.9659258262890683122, 1.000000000000000000, 0.9659258262890683122, 1.000000000000000000, 0.9659258262890683122, 1.000000000000000000, 0.9659258262890683122, 1.000000000000000000, 0.9659258262890683122, 1.000000000000000000, 0.9659258262890683122, 1.000000000000000000, 0.9659258262890683122, 1.000000000000000000, 0.9659258262890683122, 1.000000000000000000, 0.9659258262890683122, 1.000000000000000000, 0.9659258262890683122, 1.000000000000000000, 0.9659258262890683122, 1.000000000000000000, 0.9659258262890683122, 1.000000000000000000, 0.9659258262890683122, 1.000000000000000000, 0.9659258262890683122, 1.000000000000000000, 0.9659258262890683122, 1.000000000000000000, 0.9659258262890683122, 1.000000000000000000, 0.9659258262890683122, 1.000000000000000000, 0.9659258262890683122, 1.000000000000000000, 0.9659258262890683122, 1.000000000000000000, 0.9659258262890683122, 1.000000000000000000, 0.9659258262890683122, 1.000000000000000000, 0.9659258262890683122, 1.000000000000000000, 0.9659258262890683122, 1.000000000000000000, 0.9659258262890683122, 1.000000000000000000, 0.9659258262890683122, 1.000000000000000000, 0.9659258262890683122, 1.000000000000000000, 0.9659258262890683122, 1.000000000000000000, 0.9659258262890683122, 1.000000000000000000, 0.9659258262890683122, 1.000000000000000000, 0.9659258262890683122, 1.000000000000000000, 0.9659258262890683122, 1.000000000000000000, 0.9659258262890683122, 1.000000000000000000, 0.9659258262890683122, 1.000000000000000000, 0.9659258262890683122, 1.000000000000000000, 0.9659258262890683122, 1.000000000000000000, 0.9659258262890683122, 1.000000000000000000, 0.9659258262890683122, 1.000000000000000000, 0.9659258262890683122, 1.000000000000000000, 0.9659258262890683122, 1.000000000000000000, 0.9659258262890683122, 1.000000000000000000, 0.9659258262890683122, 1.000000000000000000, 0.9659258262890683122, 1.000000000000000000, 0.9659258262890683122, 1.000000000000000000, 0.9659258262890683122, 1.000000000000000000, 0.9659258262890683122, 1.000000000000000000, 0.9659258262890683122, 1.000000000000000000, 0.9659258262890683122, 1.000000000000000000, 0.9659258262890683122, 1.000000000000000000, 0.9659258262890683122, 1.000000000000000000, 0.9659258262890683122, 1.000000000000000000, 0.9659258262890683122, 1.000000000000000000, 0.9659258262890683122, 1.000000000000000000, 0.9659258262890683122, 1.000000000000000000, 0.9659258262890683122, 1.000000000000000000, 0.9659258262890683122, 1.000000000000000000, 0.9659258262890683122, 1.000000000000000000, 0.9659258262890683122, 1.000000000000000000, 0.9659258262890683122, 1.000000000000000000, 0.9659258262890683122, 1.000000000000000000, 0.9659258262890683122, 1.000000000000000000, 0.9659258262890683122, 1.000000000000000000, 0.9659258262890683122, 1.000000000000000000, 0.9659258262890683122, 1.000000000000000000, 0.9659258262890683122, 1.000000000000000000, 0.9659258262890683122, 1.000000000000000000, 0.9659258262890683122, 1.000000000000000000, 0.9659258262890683122, 1.000000000000000000, 0.9659258262890683122, 1.000000000000000000, 0.9659258262890683122, 1.000000000000000000, 0.9659258262890683122, 1.000000000000000000, 0.9659258262890683122, 1.000000000000000000, 0.9659258262890683122, 1.000000000000000000, 0.9659258262890683122, 1.000000000000000000, 0.9659258262890683122, 1.000000000000000000, 0.9659258262890683122, 1.000000000000000000, 0.9659258262890683122, 1.000000000000000000, 0.9659258262890683122, 1.000000000000000000, 0.9659258262890683122, 1.000000000000000000, 0.9659258262890683122, 1.000000000000000000, 0.9659258262890683122, 1.000000000000000000, 0.9659258262890683122, 1.000000000000000000, 0.9659258262890683122, 1.000000000000000000, 0.9659258262890683122, 1.000000000000000000, 0.9659258262890683122, 1.000000000000000000, 0.9659258262890683122, 1.000000000000000000, 0.9659258262890683122, 1.000000000000000000, 0.9659258262890683122, 1.000000000000000000, 0.9659258262890683122, 1.000000000000000000, 0.9659258262890683122, 1.000000000000000000, 0.9659258262890683122, 1.000000000000000000, 0.9659258262890683122, 1.000000000000000000, 0.9659258262890683122, 1.000000000000000000, 0.9659258262890683122, 1.000000000000000000, 0.9659258262890683122, 1.000000000000000000, 0.9659258262890683122, 1.000000000000000000, 0.9659258262890683122, 1.000000000000000000, 0.9659258262890683122, 1.000000000000000000, 0.9659258262890683122, 1.000000000000000000, 0.9659258262890683122, 1.000000000000000000, 0.9659258262890683122, 1.000000000000000000, 0.9659258262890683122, 1.000000000000000000, 0.9659258262890683122, 1.000000000000000000, 0.9659258262890683122, 1.000000000000000000, 0.9659258262890683122, 1.000000000000000000, 0.9659258262890683122, 1.000000000000000000, 0.9659258262890683122, 1.000000000000000000, 0.9659258262890683122, 1.000000000000000000, 0.9659258262890683122, 1.000000000000000000, 0.9659258262890683122, 1.000000000000000000, 0.9659258262890683122, 1.000000000000000000, 0.9659258262890683122, 1.000000000000000000, 0.9659258262890683122, 1.000000000000000000, 0.9659258262890683122, 1.000000000000000000, 0.9659258262890683122, 1.000000000000000000, 0.9659258262890683122, 1.000000000000000000, 0.9659258262890683122, 1.000000000000000000, 0.9659258262890683122, 1.000000000000000000, 0.9659258262890683122, 1.000000000000000000, 0.9659258262890683122, 1.000000000000000000, 0.9659258262890683122, 1.000000000000000000, 0.9659258262890683122, 1.000000000000000000, 0.9659258262890683122, 1.000000000000000000, 0.9659258262890683122, 1.000000000000000000, 0.9659258262890683122, 1.000000000000000000, 0.9659258262890683122, 1.000000000000000000, 0.9659258262890683122, 1.000000000000000000, 0.9659258262890683122, 1.000000000000000000, 0.9659258262890683122, 1.000000000000000000, 0.9659258262890683122, 1.000000000000000000, 0.9659258262890683122, 1.000000000000000000, 0.9659258262890683122, 1.000000000000000000, 0.9659258262890683122, 1.000000000000000000, 0.9659258262890683122, 1.000000000000000000, 0.9659258262890683122, 1.000000000000000000, 0.9659258262890683122, 1.000000000000000000, 0.9659258262890683122, 1.000000000000000000, 0.9659258262890683122, 1.000000000000000000, 0.9659258262890683122, 1.000000000000000000, 0.9659258262890683122, 1.000000000000000000, 0.9659258262890683122, 1.000000000000000000, 0.9659258262890683122, 1.000000000000000000, 0.9659258262890683122, 1.000000000000000000, 0.9659258262890683122, 1.000000000000000000) ) ) 
 REPRESENTATION_ITEM ( '' )  SURFACE ( )  );
#10733=VERTEX_POINT ( 'NONE', #92772 ) ;
#10734=CARTESIAN_POINT ( 'NONE',  ( 19.84674366389459266, 23.71726448433412315, -2.638427012816827677 ) ) ;
#10735=VERTEX_POINT ( 'NONE', #342 ) ;
#10736=CARTESIAN_POINT ( 'NONE',  ( 6.204703633549690345, 32.84541550158063927, 14.16423886937410082 ) ) ;
#10737=CARTESIAN_POINT ( 'NONE',  ( 7.361572987183170547, 37.05059781766744464, 9.846743663894590881 ) ) ;
#10738=CARTESIAN_POINT ( 'NONE',  ( -0.8801773607111008646, 48.27201867748816966, 2.915334737309923430 ) ) ;
#10739=FACE_BOUND ( 'NONE', #63716, .T. ) ;
#10741=CARTESIAN_POINT ( 'NONE',  ( -0.8801773607111009756, 38.06368534415484106, 1.068504757029289695E-15 ) ) ;
#10747=CARTESIAN_POINT ( 'NONE',  ( 20.88017736071110875, 45.77201867748816966, -2.915334737309920765 ) ) ;
#10748=CARTESIAN_POINT ( 'NONE',  ( -4.164238869374099039, 1.803748834913967647, 8.674139862899312516E-16 ) ) ;
#10749=ORIENTED_EDGE ( 'NONE', *, *, #28284, .T. ) ;
#10750=CARTESIAN_POINT ( 'NONE',  ( 19.38216949554541557, 27.24863466993041783, -9.382169495545420901 ) ) ;
#10751=AXIS2_PLACEMENT_3D ( 'NONE', #9253, #70261, #63226 ) ;
#10752=( NAMED_UNIT ( * ) PLANE_ANGLE_UNIT ( ) SI_UNIT ( $, .RADIAN. ) );
#10753=CARTESIAN_POINT ( 'NONE',  ( 14.92337183194729988, 24.34226448433411960, -8.527530157486177487 ) ) ;
#10755=CARTESIAN_POINT ( 'NONE',  ( 21.09922568453595559, 47.04030133659708923, -6.408140936763230044 ) ) ;
#10757=CARTESIAN_POINT ( 'NONE',  ( 19.84674366389459621, 23.50893115100078390, 7.409399052514197653E-17 ) ) ;
#10758=VECTOR ( 'NONE', #8197, 1000.000000000000000 ) ;
#10759=CIRCLE ( 'NONE', #45887, 0.5000000000000004441 ) ;
#10760=CARTESIAN_POINT ( 'NONE',  ( 4.559911319644449179, 58.89701867748817676, 9.422509992056141925 ) ) ;
#10765=CARTESIAN_POINT ( 'NONE',  ( 5.076628168052703671, 1.842264484334118047, 8.527530157486179263 ) ) ;
#10766=CARTESIAN_POINT ( 'NONE',  ( 16.40814093676324603, 12.45696800326375353, -11.09922568453594671 ) ) ;
#10769=CARTESIAN_POINT ( 'NONE',  ( 0.1532563361054083140, 46.00893115100079456, 1.131784320476157264E-15 ) ) ;
#10770=CARTESIAN_POINT ( 'NONE',  ( -42.94000000000001194, 92.00000000000000000, -8.999999999999998224 ) ) ;
#10771=CARTESIAN_POINT ( 'NONE',  ( -4.164238869374099039, 1.803748834913967647, 8.674139862899312516E-16 ) ) ;
#10772=CARTESIAN_POINT ( 'NONE',  ( 19.84674366389459621, 33.50893115100078745, 7.409399052514197653E-17 ) ) ;
#10773=CARTESIAN_POINT ( 'NONE',  ( 10.00000000000000178, 30.37363466993042138, 12.81628187352647608 ) ) ;
#10775=CARTESIAN_POINT ( 'NONE',  ( 10.00000000000000178, 49.31368534415484106, 10.88017736071110342 ) ) ;
#10776=CARTESIAN_POINT ( 'NONE',  ( 21.09922568453595559, 2.040301336597086568, -6.408140936763230044 ) ) ;
#10778=CARTESIAN_POINT ( 'NONE',  ( 19.84674366389459266, 18.30059781766745175, 2.638427012816836559 ) ) ;
#10779=CARTESIAN_POINT ( 'NONE',  ( 20.88017736071110164, 25.35535201082150891, 2.915334737309930979 ) ) ;
#10780=CARTESIAN_POINT ( 'NONE',  ( -2.816281873526471635, 28.91530133659708213, -3.434112377981056508 ) ) ;
#10783=CARTESIAN_POINT ( 'NONE',  ( 10.00000000000000178, 39.31368534415484106, 10.88017736071110342 ) ) ;
#10786=CARTESIAN_POINT ( 'NONE',  ( 10.00000000000000178, 59.31368534415484106, 10.88017736071110342 ) ) ;
#10787=B_SPLINE_CURVE_WITH_KNOTS ( 'NONE', 3,
 ( #6384, #67389, #83381, #36900, #90869, #14903 ),
 .UNSPECIFIED., .F., .F.,
 ( 4, 2, 4 ),
 ( 0.000000000000000000, 0.0002626113303185870955, 0.0005252226606371741911 ),
 .UNSPECIFIED. ) ;
#10788=FILL_AREA_STYLE ('',( #79278 ) ) ;
#10789=CARTESIAN_POINT ( 'NONE',  ( 19.84674366389459621, 38.50893115100078745, 7.409399052514197653E-17 ) ) ;
#10790=CARTESIAN_POINT ( 'NONE',  ( 4.559911319644449179, 28.89701867748817321, 9.422509992056141925 ) ) ;
#10791=PLANE ( 'NONE',  #66361 ) ;
#10792=CARTESIAN_POINT ( 'NONE',  ( 12.91533473730992121, 44.52201867748816966, 10.88017736071110164 ) ) ;
#10793=CARTESIAN_POINT ( 'NONE',  ( -0.8801773607111008646, 13.27201867748817321, 2.915334737309923430 ) ) ;
#10795=CARTESIAN_POINT ( 'NONE',  ( 21.92686044187657401, 55.37045670184114954, -3.195792623639525765 ) ) ;
#10796=CARTESIAN_POINT ( 'NONE',  ( 19.84674366389459266, 33.30059781766744464, 2.638427012816836559 ) ) ;
#10797=CARTESIAN_POINT ( 'NONE',  ( 10.00000000000000178, 43.05374883491397497, 14.16423886937410082 ) ) ;
#10802=( BOUNDED_CURVE ( )  B_SPLINE_CURVE ( 2, ( #67005, #93939, #61953, #84478, #2477, #55453, #54938, #69965, #48432 ),
 .UNSPECIFIED., .F., .F. ) 
 B_SPLINE_CURVE_WITH_KNOTS ( ( 3, 2, 2, 2, 3 ),
 ( 0.3329980797973742246, 0.3333333333333333703, 0.3392857142857143016, 0.3452380952380952328, 0.3455733487740543786 ),
 .UNSPECIFIED. ) 
 CURVE ( )  GEOMETRIC_REPRESENTATION_ITEM ( )  RATIONAL_B_SPLINE_CURVE ( ( 0.9963778908391760503, 0.9980808541467920403, 1.000000000000000000, 0.9659258262890683122, 1.000000000000000000, 0.9659258262890683122, 1.000000000000000000, 0.9980808541467920403, 0.9963778908391759392 ) ) 
 REPRESENTATION_ITEM ( '' )  );
#10803=CARTESIAN_POINT ( 'NONE',  ( -4.164238869374099039, 26.80374883491397142, 8.674139862899312516E-16 ) ) ;
#10804=AXIS2_PLACEMENT_3D ( 'NONE', #46508, #9498, #40000 ) ;
#10806=CARTESIAN_POINT ( 'NONE',  ( -4.164238869374099039, 66.80374883491396076, 8.674139862899312516E-16 ) ) ;
#10807=CARTESIAN_POINT ( 'NONE',  ( 5.076628168052703671, 41.84226448433411605, 8.527530157486179263 ) ) ;
#10810=CARTESIAN_POINT ( 'NONE',  ( 20.88017736071110519, 55.56368534415484817, 2.639326808657452039E-16 ) ) ;
#10811=CARTESIAN_POINT ( 'NONE',  ( 13.43411237798106583, 62.66530133659708923, -12.81628187352647252 ) ) ;
#10812=CARTESIAN_POINT ( 'NONE',  ( 19.42250999205614193, 35.14701867748816966, 5.440088680355555262 ) ) ;
#10813=CARTESIAN_POINT ( 'NONE',  ( -2.816281873526473856, 64.12363466993042493, 9.499525473075851096E-16 ) ) ;
#10814=CARTESIAN_POINT ( 'NONE',  ( 13.43411237798106583, 7.665301336597086568, -12.81628187352647252 ) ) ;
#10815=CARTESIAN_POINT ( 'NONE',  ( 19.84674366389459266, 13.71726448433411782, -2.638427012816827677 ) ) ;
#10817=CARTESIAN_POINT ( 'NONE',  ( -0.1023957841222418036, 20.13377557478296609, 6.340343622311920946 ) ) ;
#10818=CARTESIAN_POINT ( 'NONE',  ( 7.084665262690076126, 2.022018677488171434, -10.88017736071110164 ) ) ;
#10819=CARTESIAN_POINT ( 'NONE',  ( 24.16423886937409904, 29.09541550158063572, 3.795296366450317205 ) ) ;
#10820=CARTESIAN_POINT ( 'NONE',  ( 20.88017736071110164, 35.35535201082150536, 2.915334737309930979 ) ) ;
#10822=CARTESIAN_POINT ( 'NONE',  ( 20.88017736071110164, 45.35535201082149115, 2.915334737309930979 ) ) ;
#10823=DIRECTION ( 'NONE',  ( 0.000000000000000000, 0.000000000000000000, -1.000000000000000000 ) ) ;
#10824=CARTESIAN_POINT ( 'NONE',  ( 18.52753015748618282, 48.92559781766745886, -4.923371831947291888 ) ) ;
#10825=CARTESIAN_POINT ( 'NONE',  ( 7.361572987183169658, 4.967264484334119601, -9.846743663894592657 ) ) ;
#10827=CARTESIAN_POINT ( 'NONE',  ( 0.1532563361054083140, 26.00893115100078745, 1.131784320476157264E-15 ) ) ;
#10830=CARTESIAN_POINT ( 'NONE',  ( 7.361572987183169658, 29.96726448433411960, -9.846743663894592657 ) ) ;
#10831=CARTESIAN_POINT ( 'NONE',  ( 5.076628168052704559, 50.17559781766745886, -8.527530157486179263 ) ) ;
#10835=CARTESIAN_POINT ( 'NONE',  ( 21.09922568453594849, 41.20696800326375353, 6.408140936763242479 ) ) ;
#10836=CARTESIAN_POINT ( 'NONE',  ( 12.91533473730993009, 51.60535201082149825, -10.88017736071109987 ) ) ;
#10837=CARTESIAN_POINT ( 'NONE',  ( 5.076628168052704559, 25.17559781766745175, -8.527530157486179263 ) ) ;
#10838=CARTESIAN_POINT ( 'NONE',  ( 20.36894250292379382, 43.67874883491397497, 10.36894250292379205 ) ) ;
#10839=CARTESIAN_POINT ( 'NONE',  ( 12.63842701281683034, 17.46726448433411250, 9.846743663894596210 ) ) ;
#10840=CARTESIAN_POINT ( 'NONE',  ( -0.1049300847420624183, 47.21697413083880690, -6.336235997365760930 ) ) ;
#10841=DIRECTION ( 'NONE',  ( 0.000000000000000000, -1.000000000000000000, 0.000000000000000000 ) ) ;
#10842=CARTESIAN_POINT ( 'NONE',  ( -2.266590686148945544, 12.22041550158063394, 7.082119434687048631 ) ) ;
#10843=CARTESIAN_POINT ( 'NONE',  ( 2.917880565312948704, 27.63708216824730357, 12.26659068614894643 ) ) ;
#10844=CARTESIAN_POINT ( 'NONE',  ( 18.52753015748618282, 23.92559781766745530, -4.923371831947291888 ) ) ;
#10846=CARTESIAN_POINT ( 'NONE',  ( 12.91533473730993009, 26.60535201082150536, -10.88017736071109987 ) ) ;
#10847=CARTESIAN_POINT ( 'NONE',  ( 19.42250999205614548, 40.98035201082150536, -5.440088680355545492 ) ) ;
#10848=CARTESIAN_POINT ( 'NONE',  ( 19.42250999205614548, 40.98035201082150536, -5.440088680355545492 ) ) ;
#10851=CARTESIAN_POINT ( 'NONE',  ( 15.44008868035555260, 59.73035201082151247, 9.422509992056143702 ) ) ;
#10854=CARTESIAN_POINT ( 'NONE',  ( 12.91533473730992121, 59.52201867748816966, 10.88017736071110164 ) ) ;
#10856=CARTESIAN_POINT ( 'NONE',  ( 10.00000000000000000, 66.81368534415484817, -10.88017736071110342 ) ) ;
#10858=CARTESIAN_POINT ( 'NONE',  ( -12.69000000000001371, 93.50000000000000000, -10.09898361729590199 ) ) ;
#10860=CARTESIAN_POINT ( 'NONE',  ( -0.8801773607110991993, 12.85535201082150358, -2.915334737309923874 ) ) ;
#10861=CARTESIAN_POINT ( 'NONE',  ( 2.791683348922240793, 11.63393115100078568, 7.208316651077764092 ) ) ;
#10863=CARTESIAN_POINT ( 'NONE',  ( 5.076628168052703671, 1.842264484334118047, 8.527530157486179263 ) ) ;
#10864=CARTESIAN_POINT ( 'NONE',  ( -0.8801773607111008646, 8.272018677488171434, 2.915334737309923430 ) ) ;
#10865=CARTESIAN_POINT ( 'NONE',  ( 10.00000000000000000, 49.75893115100078745, -9.846743663894594434 ) ) ;
#10866=VERTEX_POINT ( 'NONE', #16790 ) ;
#10867=CARTESIAN_POINT ( 'NONE',  ( 18.52753015748617571, 48.09226448433412315, 4.923371831947298993 ) ) ;
#10868=ORIENTED_EDGE ( 'NONE', *, *, #68033, .T. ) ;
#10870=CARTESIAN_POINT ( 'NONE',  ( -0.8801773607111009756, 53.06368534415484106, 1.068504757029289695E-15 ) ) ;
#10871=CARTESIAN_POINT ( 'NONE',  ( 0.1532563361054083140, 51.00893115100078745, 1.131784320476157264E-15 ) ) ;
#10872=SURFACE_SIDE_STYLE ('',( #47379 ) ) ;
#10874=CARTESIAN_POINT ( 'NONE',  ( -0.8801773607111009756, 53.06368534415484106, 1.068504757029289695E-15 ) ) ;
#10875=CARTESIAN_POINT ( 'NONE',  ( -4.164238869374098151, 66.59541550158060375, -3.795296366450310543 ) ) ;
#10876=CARTESIAN_POINT ( 'NONE',  ( 6.565887622018943937, 38.08196800326376064, -12.81628187352647608 ) ) ;
#10879=CARTESIAN_POINT ( 'NONE',  ( 22.81628187352647785, 26.62363466993042138, 6.195893100308588602E-16 ) ) ;
#10880=CARTESIAN_POINT ( 'NONE',  ( 19.42250999205614193, 30.14701867748817321, 5.440088680355555262 ) ) ;
#10883=MECHANICAL_DESIGN_GEOMETRIC_PRESENTATION_REPRESENTATION('',(#55642),#73179);
#10884=CARTESIAN_POINT ( 'NONE',  ( 0.6178305044545818747, -1.501365330069579951, -9.382169495545419124 ) ) ;
#10885=CARTESIAN_POINT ( 'NONE',  ( 12.63842701281683034, 7.467264484334118713, 9.846743663894596210 ) ) ;
#10886=CARTESIAN_POINT ( 'NONE',  ( 12.63842701281683922, 44.55059781766745175, -9.846743663894590881 ) ) ;
#10888=( NAMED_UNIT ( * ) PLANE_ANGLE_UNIT ( ) SI_UNIT ( $, .RADIAN. ) );
#10889=CARTESIAN_POINT ( 'NONE',  ( 7.361572987183169658, 39.96726448433411605, -9.846743663894592657 ) ) ;
#10891=CARTESIAN_POINT ( 'NONE',  ( 19.84674366389459266, 28.30059781766745886, 2.638427012816836559 ) ) ;
#10893=CARTESIAN_POINT ( 'NONE',  ( 15.00000000000000000, 60.50000000000000711, -6.500000000000000888 ) ) ;
#10895=CARTESIAN_POINT ( 'NONE',  ( 18.52753015748617571, 63.09226448433412315, 4.923371831947298993 ) ) ;
#10900=CARTESIAN_POINT ( 'NONE',  ( -1.099225684535947600, 19.54030133659708568, 6.408140936763237150 ) ) ;
#10901=CARTESIAN_POINT ( 'NONE',  ( 2.791683348922240793, 41.63393115100078745, 7.208316651077764092 ) ) ;
#10903=CARTESIAN_POINT ( 'NONE',  ( -2.266590686148945544, 41.38708216824729647, -7.082119434687050408 ) ) ;
#10904=CARTESIAN_POINT ( 'NONE',  ( 18.52753015748617571, 23.09226448433411960, 4.923371831947298993 ) ) ;
#10905=CARTESIAN_POINT ( 'NONE',  ( 19.54746220608152285, 80.97929546852273575, 5.000000000000000000 ) ) ;
#10906=CARTESIAN_POINT ( 'NONE',  ( -0.3689425029237898834, 61.17874883491396076, -10.36894250292378850 ) ) ;
#10907=CARTESIAN_POINT ( 'NONE',  ( 5.076628168052703671, 61.84226448433412315, 8.527530157486179263 ) ) ;
#10908=CARTESIAN_POINT ( 'NONE',  ( 19.42250999205614548, 10.98035201082150536, -5.440088680355545492 ) ) ;
#10909=CARTESIAN_POINT ( 'NONE',  ( 2.917880565312948704, 32.63708216824730357, 12.26659068614894643 ) ) ;
#10910=CARTESIAN_POINT ( 'NONE',  ( 24.16423886937410614, 39.51208216824731068, -3.795296366450302550 ) ) ;
#10913=CARTESIAN_POINT ( 'NONE',  ( 12.63842701281683922, 54.55059781766745175, -9.846743663894590881 ) ) ;
#10915=CARTESIAN_POINT ( 'NONE',  ( 20.88017736071110875, 35.77201867748816966, -2.915334737309920765 ) ) ;
#10917=CARTESIAN_POINT ( 'NONE',  ( -1.099225684535947600, 63.70696800326376774, -6.408140936763238038 ) ) ;
#10919=CARTESIAN_POINT ( 'NONE',  ( 2.791683348922237240, 55.38393115100078745, -7.208316651077763204 ) ) ;
#10922=CARTESIAN_POINT ( 'NONE',  ( 20.36894250292379382, 33.67874883491396076, 10.36894250292379205 ) ) ;
#10925=CARTESIAN_POINT ( 'NONE',  ( 4.559911319644449179, 22.23035201082150536, -9.422509992056141925 ) ) ;
#10926=CARTESIAN_POINT ( 'NONE',  ( -1.099225684535947600, 23.70696800326375708, -6.408140936763238038 ) ) ;
#10928=CARTESIAN_POINT ( 'NONE',  ( 10.00000000000000000, 14.75893115100078568, -9.846743663894594434 ) ) ;
#10929=CARTESIAN_POINT ( 'NONE',  ( -45.94000000000000483, 93.00000000000000000, 9.000000000000000000 ) ) ;
#10930=CARTESIAN_POINT ( 'NONE',  ( -46.94000000000001194, 100.3306229069515325, -9.153711987617667134 ) ) ;
#10932=LINE ( 'NONE', #87417, #48695 ) ;
#10933=CARTESIAN_POINT ( 'NONE',  ( -0.8801773607111009756, 13.06368534415483929, 1.068504757029289695E-15 ) ) ;
#10935=CARTESIAN_POINT ( 'NONE',  ( -0.8801773607111008646, 38.27201867748816255, 2.915334737309923430 ) ) ;
#10936=CARTESIAN_POINT ( 'NONE',  ( 0.5774900079438607392, 33.48035201082150536, 5.440088680355550821 ) ) ;
#10937=CARTESIAN_POINT ( 'NONE',  ( 2.791683348922240793, 66.63393115100079456, 7.208316651077764092 ) ) ;
#10938=CARTESIAN_POINT ( 'NONE',  ( 2.791683348922240793, 66.63393115100079456, 7.208316651077764092 ) ) ;
#10940=CARTESIAN_POINT ( 'NONE',  ( 10.00000000000000000, 9.758931151000785675, -9.846743663894594434 ) ) ;
#10941=ORIENTED_EDGE ( 'NONE', *, *, #11090, .T. ) ;
#10943=CARTESIAN_POINT ( 'NONE',  ( 10.00000000000000000, 31.81368534415483751, -10.88017736071110342 ) ) ;
#10945=CARTESIAN_POINT ( 'NONE',  ( 19.38216949554541202, 0.9986346699304200492, 9.382169495545424454 ) ) ;
#10946=CARTESIAN_POINT ( 'NONE',  ( 4.559911319644449179, 63.89701867748817676, 9.422509992056141925 ) ) ;
#10947=CARTESIAN_POINT ( 'NONE',  ( 5.076628168052703671, 6.842264484334118713, 8.527530157486179263 ) ) ;
#10948=CARTESIAN_POINT ( 'NONE',  ( -1.099225684535947600, 34.54030133659708923, 6.408140936763237150 ) ) ;
#10949=CARTESIAN_POINT ( 'NONE',  ( 5.076628168052703671, 6.842264484334118713, 8.527530157486179263 ) ) ;
#10951=DIRECTION ( 'NONE',  ( 0.000000000000000000, 0.000000000000000000, -1.000000000000000000 ) ) ;
#10952=CARTESIAN_POINT ( 'NONE',  ( 2.603489959281591659, 15.43575266056827999, -6.500000000000006217 ) ) ;
#10953=CARTESIAN_POINT ( 'NONE',  ( 19.42250999205614548, 10.98035201082150358, -5.440088680355545492 ) ) ;
#10954=CARTESIAN_POINT ( 'NONE',  ( -1.099225684535947600, 54.54030133659708923, 6.408140936763237150 ) ) ;
#10955=CARTESIAN_POINT ( 'NONE',  ( 10.00000000000000178, 23.05374883491397142, 14.16423886937410082 ) ) ;
#10956=CARTESIAN_POINT ( 'NONE',  ( 0.1532563361054100626, 20.80059781766744464, -2.638427012816831230 ) ) ;
#10957=( GEOMETRIC_REPRESENTATION_CONTEXT ( 3 ) GLOBAL_UNCERTAINTY_ASSIGNED_CONTEXT ( ( #2233 ) ) GLOBAL_UNIT_ASSIGNED_CONTEXT ( ( #61801, #46320, #23835 ) ) REPRESENTATION_CONTEXT ( 'NONE', 'WORKASPACE' ) );
#10958=CARTESIAN_POINT ( 'NONE',  ( 7.361572987183170547, 27.05059781766745175, 9.846743663894590881 ) ) ;
#10959=CARTESIAN_POINT ( 'NONE',  ( 20.88017736071110875, 5.772018677488170546, -2.915334737309920765 ) ) ;
#10961=CARTESIAN_POINT ( 'NONE',  ( 4.559911319644449179, 13.89701867748817143, 9.422509992056141925 ) ) ;
#10962=CARTESIAN_POINT ( 'NONE',  ( 15.44008868035555793, 21.39701867748817321, -9.422509992056140149 ) ) ;
#10968=CARTESIAN_POINT ( 'NONE',  ( 17.96484262340118221, 24.93868534415484461, 7.964842623401181321 ) ) ;
#10970=CARTESIAN_POINT ( 'NONE',  ( 12.63842701281683034, 62.46726448433410894, 9.846743663894596210 ) ) ;
#10972=CARTESIAN_POINT ( 'NONE',  ( 10.00000000000000178, 50.37363466993042493, 12.81628187352647608 ) ) ;
#10974=CARTESIAN_POINT ( 'NONE',  ( 17.08211943468705130, 38.47041550158063217, 12.26659068614894998 ) ) ;
#10975=CARTESIAN_POINT ( 'NONE',  ( 0.5774900079438607392, 38.48035201082150536, 5.440088680355550821 ) ) ;
#10976=CARTESIAN_POINT ( 'NONE',  ( 2.035157376598824452, 13.68868534415483751, 7.964842623401179544 ) ) ;
#10977=CARTESIAN_POINT ( 'NONE',  ( 17.20831665107776587, 57.88393115100078745, 7.208316651077764980 ) ) ;
#10979=CARTESIAN_POINT ( 'NONE',  ( 18.18329248733322245, 32.60290668512019607, 6.499999999999997335 ) ) ;
#10980=CARTESIAN_POINT ( 'NONE',  ( 1.472469842513823179, 40.59226448433411605, -4.923371831947296329 ) ) ;
#10982=CARTESIAN_POINT ( 'NONE',  ( 7.361572987183169658, 9.967264484334119601, -9.846743663894592657 ) ) ;
#10984=VERTEX_POINT ( 'NONE', #55266 ) ;
#10986=CARTESIAN_POINT ( 'NONE',  ( 10.00000000000000178, 9.313685344154839285, 10.88017736071110342 ) ) ;
#10987=CARTESIAN_POINT ( 'NONE',  ( 2.791683348922240793, 11.63393115100078568, 7.208316651077764092 ) ) ;
#10988=CARTESIAN_POINT ( 'NONE',  ( 10.00000000000000000, -2.126365330069579951, -12.81628187352647608 ) ) ;
#10989=CARTESIAN_POINT ( 'NONE',  ( 0.5774900079438590739, 42.64701867748816966, -5.440088680355550821 ) ) ;
#10990=CARTESIAN_POINT ( 'NONE',  ( 4.559911319644449179, 17.23035201082150536, -9.422509992056141925 ) ) ;
#10991=CARTESIAN_POINT ( 'NONE',  ( 13.43411237798105340, 50.58196800326375353, 12.81628187352647963 ) ) ;
#10992=CARTESIAN_POINT ( 'NONE',  ( 13.79529636645031943, 35.34541550158063927, -14.16423886937409904 ) ) ;
#10995=CARTESIAN_POINT ( 'NONE',  ( 16.40814093676323893, 60.79030133659709634, 11.09922568453595026 ) ) ;
#10996=EDGE_LOOP ( 'NONE', ( #88322, #32306, #13258, #77937 ) ) ;
#10997=CARTESIAN_POINT ( 'NONE',  ( 19.84674366389459621, 63.50893115100078745, 7.409399052514197653E-17 ) ) ;
#10999=CARTESIAN_POINT ( 'NONE',  ( 17.96484262340118221, 36.18868534415484106, -7.964842623401177768 ) ) ;
#11001=ORIENTED_EDGE ( 'NONE', *, *, #46255, .T. ) ;
#11002=CARTESIAN_POINT ( 'NONE',  ( 17.20831665107776587, 2.883931151000785231, 7.208316651077764980 ) ) ;
#11006=CARTESIAN_POINT ( 'NONE',  ( 10.00000000000000178, 12.25893115100078568, 9.846743663894594434 ) ) ;
#11007=CARTESIAN_POINT ( 'NONE',  ( 12.63842701281683922, 24.55059781766745175, -9.846743663894590881 ) ) ;
#11008=CARTESIAN_POINT ( 'NONE',  ( 19.84674366389459621, 8.508931151000785675, 7.409399052514197653E-17 ) ) ;
#11009=CARTESIAN_POINT ( 'NONE',  ( 12.91533473730992121, 54.52201867748816255, 10.88017736071110164 ) ) ;
#11011=CARTESIAN_POINT ( 'NONE',  ( 10.00000000000000000, 66.81368534415484817, -10.88017736071110342 ) ) ;
#11012=CARTESIAN_POINT ( 'NONE',  ( 14.92337183194729988, 19.34226448433411960, -8.527530157486177487 ) ) ;
#11015=CARTESIAN_POINT ( 'NONE',  ( 10.00000000000000178, 57.25893115100078745, 9.846743663894594434 ) ) ;
#11016=ORIENTED_EDGE ( 'NONE', *, *, #47770, .F. ) ;
#11019=CARTESIAN_POINT ( 'NONE',  ( -4.164238869374098151, 11.59541550158063217, -3.795296366450310543 ) ) ;
#11021=CARTESIAN_POINT ( 'NONE',  ( 17.08211943468705130, 23.47041550158063572, 12.26659068614894998 ) ) ;
#11022=CARTESIAN_POINT ( 'NONE',  ( -4.164238869374098151, 26.59541550158063217, -3.795296366450310543 ) ) ;
#11024=CARTESIAN_POINT ( 'NONE',  ( -4.164238869374099039, 1.803748834913967647, 8.674139862899312516E-16 ) ) ;
#11026=CARTESIAN_POINT ( 'NONE',  ( 17.96484262340118221, 41.18868534415484106, -7.964842623401177768 ) ) ;
#11028=CARTESIAN_POINT ( 'NONE',  ( 7.361572987183170547, 12.05059781766744997, 9.846743663894590881 ) ) ;
#11029=CARTESIAN_POINT ( 'NONE',  ( 20.88017736071110519, 60.56368534415484106, 2.639326808657452039E-16 ) ) ;
#11030=CARTESIAN_POINT ( 'NONE',  ( 0.1532563361054082862, 16.21726448433411960, 2.638427012816831674 ) ) ;
#11031=CARTESIAN_POINT ( 'NONE',  ( -2.816281873526471635, 43.91530133659708923, -3.434112377981056508 ) ) ;
#11032=CARTESIAN_POINT ( 'NONE',  ( 19.84674366389459266, 38.30059781766745175, 2.638427012816836559 ) ) ;
#11034=CARTESIAN_POINT ( 'NONE',  ( 0.5774900079438607392, 58.48035201082151247, 5.440088680355550821 ) ) ;
#11035=CARTESIAN_POINT ( 'NONE',  ( 19.38216949554541202, 25.99863466993042138, 9.382169495545424454 ) ) ;
#11037=CARTESIAN_POINT ( 'NONE',  ( 18.52753015748618282, 28.92559781766745175, -4.923371831947291888 ) ) ;
#11038=CARTESIAN_POINT ( 'NONE',  ( 22.26659068614895176, 14.72041550158063572, -7.082119434687042414 ) ) ;
#11040=B_SPLINE_CURVE_WITH_KNOTS ( 'NONE', 3,
 ( #6881, #68870, #84848, #67881, #53860, #15870, #76843 ),
 .UNSPECIFIED., .F., .F.,
 ( 4, 3, 4 ),
 ( 1.788497222143715241E-16, 0.001212392164850256563, 0.002424962242136481996 ),
 .UNSPECIFIED. ) ;
#11041=CARTESIAN_POINT ( 'NONE',  ( 20.88017736071110164, 40.35535201082150536, 2.915334737309930979 ) ) ;
#11042=CARTESIAN_POINT ( 'NONE',  ( 10.00000000000000178, 49.31368534415484106, 10.88017736071110342 ) ) ;
#11043=CARTESIAN_POINT ( 'NONE',  ( -0.3689425029237881626, 52.42874883491396076, 10.36894250292379027 ) ) ;
#11044=CARTESIAN_POINT ( 'NONE',  ( 2.791683348922240793, 56.63393115100078035, 7.208316651077764092 ) ) ;
#11045=CARTESIAN_POINT ( 'NONE',  ( 18.52753015748617571, 13.09226448433411960, 4.923371831947298993 ) ) ;
#11046=DIRECTION ( 'NONE',  ( 1.000000000000000000, 0.000000000000000000, 0.000000000000000000 ) ) ;
#11048=CARTESIAN_POINT ( 'NONE',  ( 2.035157376598824452, 38.68868534415483396, 7.964842623401179544 ) ) ;
#11049=DIRECTION ( 'NONE',  ( 0.000000000000000000, 0.000000000000000000, -1.000000000000000000 ) ) ;
#11050=CARTESIAN_POINT ( 'NONE',  ( 0.6178305044545818747, 18.49863466993041428, -9.382169495545419124 ) ) ;
#11051=CARTESIAN_POINT ( 'NONE',  ( 3.591859063236761518, 19.95696800326375353, 11.09922568453594849 ) ) ;
#11052=CARTESIAN_POINT ( 'NONE',  ( 17.20831665107776587, 49.13393115100078745, -7.208316651077762316 ) ) ;
#11054=CARTESIAN_POINT ( 'NONE',  ( 7.084665262690076126, 4.105352010821503583, 10.88017736071109987 ) ) ;
#11055=CARTESIAN_POINT ( 'NONE',  ( -0.8801773607111009756, 68.06368534415484817, 1.068504757029289695E-15 ) ) ;
#11060=CARTESIAN_POINT ( 'NONE',  ( 20.88017736071110164, 65.35535201082150536, 2.915334737309930979 ) ) ;
#11061=CARTESIAN_POINT ( 'NONE',  ( -0.8801773607111008646, 63.27201867748817676, 2.915334737309923430 ) ) ;
#11064=CARTESIAN_POINT ( 'NONE',  ( 5.076628168052704559, 25.17559781766745175, -8.527530157486179263 ) ) ;
#11065=CARTESIAN_POINT ( 'NONE',  ( 7.084665262690076126, 19.10535201082150181, 10.88017736071109987 ) ) ;
#11066=CARTESIAN_POINT ( 'NONE',  ( 10.00000000000000000, 59.75893115100078745, -9.846743663894594434 ) ) ;
#11067=CARTESIAN_POINT ( 'NONE',  ( 12.91533473730993009, 36.60535201082151247, -10.88017736071109987 ) ) ;
#11070=CARTESIAN_POINT ( 'NONE',  ( -1.099225684535947600, 43.70696800326375353, -6.408140936763238038 ) ) ;
#11071=ORIENTED_EDGE ( 'NONE', *, *, #35481, .T. ) ;
#11072=CARTESIAN_POINT ( 'NONE',  ( 7.084665262690076126, 49.10535201082149825, 10.88017736071109987 ) ) ;
#11073=CARTESIAN_POINT ( 'NONE',  ( -2.816281873526473856, 24.12363466993042138, 9.499525473075851096E-16 ) ) ;
#11075=CARTESIAN_POINT ( 'NONE',  ( 20.88017736071110875, 20.77201867748816611, -2.915334737309920765 ) ) ;
#11076=CARTESIAN_POINT ( 'NONE',  ( 2.917880565312948704, 52.63708216824730357, 12.26659068614894643 ) ) ;
#11077=CARTESIAN_POINT ( 'NONE',  ( 1.472469842513823179, 46.42559781766745175, 4.923371831947296329 ) ) ;
#11079=CARTESIAN_POINT ( 'NONE',  ( 14.92337183194729633, 2.675597817667451750, 8.527530157486181039 ) ) ;
#11080=CARTESIAN_POINT ( 'NONE',  ( 4.559911319644449179, 43.89701867748816966, 9.422509992056141925 ) ) ;
#11082=CARTESIAN_POINT ( 'NONE',  ( -4.164238869374099039, 21.80374883491396787, 8.674139862899312516E-16 ) ) ;
#11088=CARTESIAN_POINT ( 'NONE',  ( -4.164238869374099039, 46.80374883491397497, 8.674139862899312516E-16 ) ) ;
#11089=CARTESIAN_POINT ( 'NONE',  ( -4.164238869374099927, 47.01208216824729647, 3.795296366450308767 ) ) ;
#11090=EDGE_CURVE ( 'NONE', #73676, #30064, #79049, .T. ) ;
#11091=CARTESIAN_POINT ( 'NONE',  ( 19.84674366389459266, 13.71726448433411782, -2.638427012816827677 ) ) ;
#11092=CARTESIAN_POINT ( 'NONE',  ( 0.6178305044545818747, 18.49863466993041428, -9.382169495545419124 ) ) ;
#11095=CARTESIAN_POINT ( 'NONE',  ( -0.8801773607110991993, 67.85535201082151957, -2.915334737309923874 ) ) ;
#11096=CARTESIAN_POINT ( 'NONE',  ( 22.81628187352647785, 31.62363466993042138, 6.195893100308588602E-16 ) ) ;
#11097=CARTESIAN_POINT ( 'NONE',  ( 10.00000000000000178, 43.05374883491397497, 14.16423886937410082 ) ) ;
#11103=CARTESIAN_POINT ( 'NONE',  ( 17.20831665107776587, 17.88393115100078745, 7.208316651077764980 ) ) ;
#11105=CARTESIAN_POINT ( 'NONE',  ( -4.164238869374099927, 12.01208216824730357, 3.795296366450308767 ) ) ;
#11106=CARTESIAN_POINT ( 'NONE',  ( 10.00000000000000000, 6.813685344154838397, -10.88017736071110342 ) ) ;
#11107=CARTESIAN_POINT ( 'NONE',  ( 7.084665262690076126, 9.105352010821503583, 10.88017736071109987 ) ) ;
#11108=CARTESIAN_POINT ( 'NONE',  ( 1.472469842513823179, 46.42559781766745175, 4.923371831947296329 ) ) ;
#11109=CARTESIAN_POINT ( 'NONE',  ( -2.816281873526471635, -1.084698663402913210, -3.434112377981056508 ) ) ;
#11110=CARTESIAN_POINT ( 'NONE',  ( -29.94000000000001549, 92.00000000000000000, 9.500000000000000000 ) ) ;
#11112=CARTESIAN_POINT ( 'NONE',  ( 10.00000000000000178, 20.37363466993042138, 12.81628187352647608 ) ) ;
#11114=CARTESIAN_POINT ( 'NONE',  ( 24.16423886937409904, 64.09541550158064638, 3.795296366450317205 ) ) ;
#11115=ORIENTED_EDGE ( 'NONE', *, *, #64113, .T. ) ;
#11116=CARTESIAN_POINT ( 'NONE',  ( 17.08211943468705130, 53.47041550158063217, 12.26659068614894998 ) ) ;
#11118=CARTESIAN_POINT ( 'NONE',  ( 20.88017736071110164, 35.35535201082150536, 2.915334737309930979 ) ) ;
#11120=CARTESIAN_POINT ( 'NONE',  ( 20.88017736071110875, 40.77201867748818387, -2.915334737309920765 ) ) ;
#11121=CARTESIAN_POINT ( 'NONE',  ( 7.084665262690076126, 39.10535201082150536, 10.88017736071109987 ) ) ;
#11123=CARTESIAN_POINT ( 'NONE',  ( 20.88017736071110164, 45.35535201082149115, 2.915334737309930979 ) ) ;
#11124=EDGE_CURVE ( 'NONE', #26718, #87224, #82033, .T. ) ;
#11127=CARTESIAN_POINT ( 'NONE',  ( 18.52753015748617571, 13.09226448433411960, 4.923371831947298993 ) ) ;
#11130=CARTESIAN_POINT ( 'NONE',  ( 5.076628168052704559, 45.17559781766745175, -8.527530157486179263 ) ) ;
#11133=CARTESIAN_POINT ( 'NONE',  ( -46.43544119129182945, 103.9441758960464455, 5.610234333949799534 ) ) ;
#11134=CARTESIAN_POINT ( 'NONE',  ( -45.12746704901013572, 105.3510678274659540, 4.910681296974491516 ) ) ;
#11136=CARTESIAN_POINT ( 'NONE',  ( -4.164238869374099039, 56.80374883491397497, 8.674139862899312516E-16 ) ) ;
#11140=CARTESIAN_POINT ( 'NONE',  ( 2.791683348922240793, 31.63393115100078745, 7.208316651077764092 ) ) ;
#11141=CARTESIAN_POINT ( 'NONE',  ( 16.40814093676324603, 62.45696800326376064, -11.09922568453594671 ) ) ;
#11142=CARTESIAN_POINT ( 'NONE',  ( 19.38216949554541557, 7.248634669930421381, -9.382169495545420901 ) ) ;
#11143=CARTESIAN_POINT ( 'NONE',  ( 15.44008868035555260, 64.73035201082151957, 9.422509992056143702 ) ) ;
#11145=CARTESIAN_POINT ( 'NONE',  ( 17.20831665107776587, 14.13393115100078568, -7.208316651077762316 ) ) ;
#11146=CARTESIAN_POINT ( 'NONE',  ( 14.92337183194729988, 54.34226448433412315, -8.527530157486177487 ) ) ;
#11149=CARTESIAN_POINT ( 'NONE',  ( 24.16423886937410614, 59.30374883491397497, 8.672049930838204340E-16 ) ) ;
#11150=FACE_OUTER_BOUND ( 'NONE', #58326, .T. ) ;
#11151=CARTESIAN_POINT ( 'NONE',  ( 17.96484262340118221, 36.18868534415484106, -7.964842623401177768 ) ) ;
#11152=CARTESIAN_POINT ( 'NONE',  ( -2.816281873526473856, 29.12363466993041783, 9.499525473075851096E-16 ) ) ;
#11154=SURFACE_SIDE_STYLE ('',( #95134 ) ) ;
#11157=CARTESIAN_POINT ( 'NONE',  ( 0.1532563361054082862, 46.21726448433411605, 2.638427012816831674 ) ) ;
#11158=CARTESIAN_POINT ( 'NONE',  ( 18.52753015748618282, 13.92559781766745175, -4.923371831947291888 ) ) ;
#11160=CARTESIAN_POINT ( 'NONE',  ( 13.43411237798106583, 27.66530133659708568, -12.81628187352647252 ) ) ;
#11162=CARTESIAN_POINT ( 'NONE',  ( -0.8801773607111008646, 23.27201867748817676, 2.915334737309923430 ) ) ;
#11164=CARTESIAN_POINT ( 'NONE',  ( 24.16423886937410614, 39.51208216824731068, -3.795296366450302550 ) ) ;
#11165=EDGE_CURVE ( 'NONE', #76576, #10735, #89279, .T. ) ;
#11166=CARTESIAN_POINT ( 'NONE',  ( 20.36894250292379738, 29.92874883491396432, -10.36894250292379027 ) ) ;
#11167=CARTESIAN_POINT ( 'NONE',  ( 2.035157376598824452, 8.688685344154839285, 7.964842623401179544 ) ) ;
#11168=CARTESIAN_POINT ( 'NONE',  ( 19.84674366389459266, 48.30059781766745175, 2.638427012816836559 ) ) ;
#11169=CARTESIAN_POINT ( 'NONE',  ( 6.565887622018943937, 43.08196800326374643, -12.81628187352647608 ) ) ;
#11170=CARTESIAN_POINT ( 'NONE',  ( 2.035157376598822676, 17.43868534415483751, -7.964842623401177768 ) ) ;
#11171=CARTESIAN_POINT ( 'NONE',  ( 5.076628168052703671, 41.84226448433411605, 8.527530157486179263 ) ) ;
#11172=CARTESIAN_POINT ( 'NONE',  ( 20.88017736071110164, 35.35535201082150536, 2.915334737309930979 ) ) ;
#11173=CARTESIAN_POINT ( 'NONE',  ( 22.81628187352647785, 1.623634669930420271, 6.195893100308588602E-16 ) ) ;
#11174=CARTESIAN_POINT ( 'NONE',  ( -2.266590686148945544, 22.22041550158063572, 7.082119434687048631 ) ) ;
#11177=CARTESIAN_POINT ( 'NONE',  ( 10.00000000000000178, 27.25893115100078390, 9.846743663894594434 ) ) ;
#11178=CARTESIAN_POINT ( 'NONE',  ( 22.81628187352648496, 56.83196800326374643, -3.434112377981050290 ) ) ;
#11179=CARTESIAN_POINT ( 'NONE',  ( 0.1532563361054082862, 56.21726448433411605, 2.638427012816831674 ) ) ;
#11182=FILL_AREA_STYLE_COLOUR ( '', #49122 ) ;
#11183=MECHANICAL_DESIGN_GEOMETRIC_PRESENTATION_REPRESENTATION('',(#43155),#86274);
#11184=CARTESIAN_POINT ( 'NONE',  ( -4.164238869374099039, 66.80374883491396076, 8.674139862899312516E-16 ) ) ;
#11185=CARTESIAN_POINT ( 'NONE',  ( 17.08211943468705130, 8.470415501580635720, 12.26659068614894998 ) ) ;
#11186=CARTESIAN_POINT ( 'NONE',  ( 10.00000000000000000, 66.81368534415484817, -10.88017736071110342 ) ) ;
#11187=CARTESIAN_POINT ( 'NONE',  ( 10.00000000000000000, 49.75893115100078745, -9.846743663894594434 ) ) ;
#11188=CARTESIAN_POINT ( 'NONE',  ( 7.084665262690076126, 37.02201867748817676, -10.88017736071110164 ) ) ;
#11190=CARTESIAN_POINT ( 'NONE',  ( 20.88017736071110164, 25.35535201082150891, 2.915334737309930979 ) ) ;
#11197=CARTESIAN_POINT ( 'NONE',  ( 22.26659068614895176, 9.720415501580633943, -7.082119434687042414 ) ) ;
#11198=CARTESIAN_POINT ( 'NONE',  ( -4.164238869374098151, 16.59541550158063927, -3.795296366450310543 ) ) ;
#11199=EDGE_CURVE ( 'NONE', #27072, #85384, #550, .T. ) ;
#11200=CARTESIAN_POINT ( 'NONE',  ( -0.3689425029237881626, 57.42874883491397497, 10.36894250292379027 ) ) ;
#11201=CARTESIAN_POINT ( 'NONE',  ( 19.84674366389459266, 58.30059781766745886, 2.638427012816836559 ) ) ;
#11202=CARTESIAN_POINT ( 'NONE',  ( 7.361572987183169658, 39.96726448433411605, -9.846743663894592657 ) ) ;
#11204=CARTESIAN_POINT ( 'NONE',  ( 10.00000000000000000, 31.81368534415483751, -10.88017736071110342 ) ) ;
#11205=CARTESIAN_POINT ( 'NONE',  ( 10.00000000000000178, 57.25893115100078745, 9.846743663894594434 ) ) ;
#11206=CARTESIAN_POINT ( 'NONE',  ( -4.164238869374099039, 6.803748834913967869, 8.674139862899312516E-16 ) ) ;
#11207=CARTESIAN_POINT ( 'NONE',  ( 22.26659068614895176, 39.72041550158063217, -7.082119434687042414 ) ) ;
#11208=CARTESIAN_POINT ( 'NONE',  ( -0.3689425029237898834, 66.17874883491396076, -10.36894250292378850 ) ) ;
#11209=CARTESIAN_POINT ( 'NONE',  ( 17.20831665107776587, 64.13393115100079456, -7.208316651077762316 ) ) ;
#11211=CARTESIAN_POINT ( 'NONE',  ( 12.91533473730993009, 66.60535201082150536, -10.88017736071109987 ) ) ;
#11212=EDGE_CURVE ( 'NONE', #32729, #27101, #24858, .T. ) ;
#11213=CARTESIAN_POINT ( 'NONE',  ( 14.92337183194729988, 29.34226448433411960, -8.527530157486177487 ) ) ;
#11215=ORIENTED_EDGE ( 'NONE', *, *, #5107, .T. ) ;
#11218=CARTESIAN_POINT ( 'NONE',  ( 0.1532563361054083140, 26.00893115100078745, 1.131784320476157264E-15 ) ) ;
#11220=CARTESIAN_POINT ( 'NONE',  ( -2.266590686148945544, 36.38708216824730357, -7.082119434687050408 ) ) ;
#11221=CARTESIAN_POINT ( 'NONE',  ( 17.20831665107776587, 32.88393115100078745, 7.208316651077764980 ) ) ;
#11222=CARTESIAN_POINT ( 'NONE',  ( 7.084665262690076126, 54.10535201082151247, 10.88017736071109987 ) ) ;
#11224=B_SPLINE_CURVE_WITH_KNOTS ( 'NONE', 3,
 ( #95378, #3900, #97368, #96383, #58342, #88862 ),
 .UNSPECIFIED., .F., .F.,
 ( 4, 2, 4 ),
 ( 0.000000000000000000, 0.0002565770811491102925, 0.0005131541622982205850 ),
 .UNSPECIFIED. ) ;
#11225=CARTESIAN_POINT ( 'NONE',  ( 12.91533473730992121, 59.52201867748816966, 10.88017736071110164 ) ) ;
#11226=CARTESIAN_POINT ( 'NONE',  ( 19.84674366389459621, 48.50893115100078745, 7.409399052514197653E-17 ) ) ;
#11229=CARTESIAN_POINT ( 'NONE',  ( 24.16423886937410614, 24.30374883491396787, 8.672049930838204340E-16 ) ) ;
#11232=CARTESIAN_POINT ( 'NONE',  ( 10.00000000000000000, 32.87363466993042493, -12.81628187352647608 ) ) ;
#11233=CARTESIAN_POINT ( 'NONE',  ( 0.1532563361054100626, 20.80059781766744464, -2.638427012816831230 ) ) ;
#11234=CARTESIAN_POINT ( 'NONE',  ( 4.559911319644449179, 3.897018677488170990, 9.422509992056141925 ) ) ;
#11235=CARTESIAN_POINT ( 'NONE',  ( 19.38216949554541202, 50.99863466993042493, 9.382169495545424454 ) ) ;
#11237=CARTESIAN_POINT ( 'NONE',  ( 18.52753015748617571, 28.09226448433411960, 4.923371831947298993 ) ) ;
#11239=CARTESIAN_POINT ( 'NONE',  ( 19.42250999205614193, 65.14701867748817676, 5.440088680355555262 ) ) ;
#11242=CARTESIAN_POINT ( 'NONE',  ( -0.1503990784575407469, 17.22266099184918531, -6.262539305110056631 ) ) ;
#11243=CARTESIAN_POINT ( 'NONE',  ( 10.00000000000000178, 2.258931151000784787, 9.846743663894594434 ) ) ;
#11244=CARTESIAN_POINT ( 'NONE',  ( -1.099225684535947600, 29.54030133659708923, 6.408140936763237150 ) ) ;
#11247=VECTOR ( 'NONE', #95437, 1000.000000000000000 ) ;
#11248=CARTESIAN_POINT ( 'NONE',  ( 7.361572987183170547, 47.05059781766745175, 9.846743663894590881 ) ) ;
#11250=CARTESIAN_POINT ( 'NONE',  ( -0.3689425029237881626, 12.42874883491396609, 10.36894250292379027 ) ) ;
#11251=CARTESIAN_POINT ( 'NONE',  ( 0.1532563361054083140, 31.00893115100078390, 1.131784320476157264E-15 ) ) ;
#11252=CARTESIAN_POINT ( 'NONE',  ( 13.43411237798105340, 35.58196800326375353, 12.81628187352647963 ) ) ;
#11255=CARTESIAN_POINT ( 'NONE',  ( 20.88017736071110875, 65.77201867748817676, -2.915334737309920765 ) ) ;
#11257=CARTESIAN_POINT ( 'NONE',  ( -2.816281873526473856, 4.331968003263754419, 3.434112377981055619 ) ) ;
#11259=CARTESIAN_POINT ( 'NONE',  ( 1.472469842513823179, 35.59226448433412315, -4.923371831947296329 ) ) ;
#11260=CARTESIAN_POINT ( 'NONE',  ( 19.42250999205614193, 30.14701867748817321, 5.440088680355555262 ) ) ;
#11261=CARTESIAN_POINT ( 'NONE',  ( -1.099225684535947600, 23.70696800326375708, -6.408140936763238038 ) ) ;
#11262=CARTESIAN_POINT ( 'NONE',  ( 10.00000000000000178, 27.25893115100078390, 9.846743663894594434 ) ) ;
#11264=CARTESIAN_POINT ( 'NONE',  ( 0.5774900079438607392, 33.48035201082150536, 5.440088680355550821 ) ) ;
#11266=CARTESIAN_POINT ( 'NONE',  ( 12.91533473730993009, 56.60535201082151247, -10.88017736071109987 ) ) ;
#11267=CARTESIAN_POINT ( 'NONE',  ( 10.00000000000000178, 4.313685344154837509, 10.88017736071110342 ) ) ;
#11268=CARTESIAN_POINT ( 'NONE',  ( 10.00000000000000178, 37.25893115100078745, 9.846743663894594434 ) ) ;
#11269=CARTESIAN_POINT ( 'NONE',  ( 7.084665262690076126, 27.02201867748817676, -10.88017736071110164 ) ) ;
#11271=CARTESIAN_POINT ( 'NONE',  ( 17.96484262340118221, 49.93868534415484106, 7.964842623401181321 ) ) ;
#11272=CARTESIAN_POINT ( 'NONE',  ( 4.559911319644449179, 18.89701867748817321, 9.422509992056141925 ) ) ;
#11275=CARTESIAN_POINT ( 'NONE',  ( 7.361572987183169658, 54.96726448433413026, -9.846743663894592657 ) ) ;
#11276=CARTESIAN_POINT ( 'NONE',  ( 13.79529636645031943, 55.34541550158062506, -14.16423886937409904 ) ) ;
#11280=CARTESIAN_POINT ( 'NONE',  ( 6.204703633549690345, 0.7620821682473009062, -14.16423886937410259 ) ) ;
#11282=CARTESIAN_POINT ( 'NONE',  ( -0.3689425029237881626, 37.42874883491396787, 10.36894250292379027 ) ) ;
#11286=CARTESIAN_POINT ( 'NONE',  ( 13.79529636645031943, 65.34541550158063217, -14.16423886937409904 ) ) ;
#11288=CARTESIAN_POINT ( 'NONE',  ( 1.472469842513823179, 35.59226448433412315, -4.923371831947296329 ) ) ;
#11291=CARTESIAN_POINT ( 'NONE',  ( 0.5774900079438590739, 62.64701867748817676, -5.440088680355550821 ) ) ;
#11293=CARTESIAN_POINT ( 'NONE',  ( 7.084665262690076126, 32.02201867748816966, -10.88017736071110164 ) ) ;
#11294=CARTESIAN_POINT ( 'NONE',  ( -1.099225684535947600, 64.54030133659709634, 6.408140936763237150 ) ) ;
#11295=CARTESIAN_POINT ( 'NONE',  ( 0.6178305044545838731, 9.748634669930416052, 9.382169495545420901 ) ) ;
#11296=CARTESIAN_POINT ( 'NONE',  ( 18.52753015748618282, 18.92559781766745175, -4.923371831947291888 ) ) ;
#11297=ORIENTED_EDGE ( 'NONE', *, *, #24384, .F. ) ;
#11300=CARTESIAN_POINT ( 'NONE',  ( -0.3689425029237881626, 67.42874883491396076, 10.36894250292379027 ) ) ;
#11301=CARTESIAN_POINT ( 'NONE',  ( -0.3689425029237898834, 26.17874883491396432, -10.36894250292378850 ) ) ;
#11302=CARTESIAN_POINT ( 'NONE',  ( 0.5774900079438607392, 38.48035201082150536, 5.440088680355550821 ) ) ;
#11303=CARTESIAN_POINT ( 'NONE',  ( 12.91533473730992121, 44.52201867748816966, 10.88017736071110164 ) ) ;
#11305=CARTESIAN_POINT ( 'NONE',  ( 17.39651004071838614, 47.93575266056826933, 6.500000000000032863 ) ) ;
#11306=CARTESIAN_POINT ( 'NONE',  ( 12.63842701281683922, 14.55059781766744997, -9.846743663894590881 ) ) ;
#11307=FILL_AREA_STYLE_COLOUR ( '', #3459 ) ;
#11310=CARTESIAN_POINT ( 'NONE',  ( 5.076628168052703671, 26.84226448433411960, 8.527530157486179263 ) ) ;
#11311=CARTESIAN_POINT ( 'NONE',  ( 1.472469842513823179, 50.59226448433411605, -4.923371831947296329 ) ) ;
#11314=CARTESIAN_POINT ( 'NONE',  ( 21.09922568453595559, 47.04030133659708923, -6.408140936763230044 ) ) ;
#11316=CARTESIAN_POINT ( 'NONE',  ( 7.361572987183170547, 2.050597817667451750, 9.846743663894590881 ) ) ;
#11317=CARTESIAN_POINT ( 'NONE',  ( 17.20831665107776587, 22.88393115100078745, 7.208316651077764980 ) ) ;
#11318=CARTESIAN_POINT ( 'NONE',  ( 6.204703633549690345, 65.76208216824731778, -14.16423886937410259 ) ) ;
#11319=CARTESIAN_POINT ( 'NONE',  ( 0.1532563361054100626, 20.80059781766744464, -2.638427012816831230 ) ) ;
#11320=CARTESIAN_POINT ( 'NONE',  ( -0.03743638938522149406, 44.25197528031021221, -6.399506433553973750 ) ) ;
#11321=CARTESIAN_POINT ( 'NONE',  ( 1.472469842513823179, 66.42559781766745175, 4.923371831947296329 ) ) ;
#11322=CARTESIAN_POINT ( 'NONE',  ( 17.08211943468705840, 5.137082168247300906, -12.26659068614894466 ) ) ;
#11323=CARTESIAN_POINT ( 'NONE',  ( -2.266590686148945544, 37.22041550158063217, 7.082119434687048631 ) ) ;
#11324=CARTESIAN_POINT ( 'NONE',  ( 5.076628168052704559, 35.17559781766745175, -8.527530157486179263 ) ) ;
#11326=CARTESIAN_POINT ( 'NONE',  ( -0.8801773607110991993, 22.85535201082150181, -2.915334737309923874 ) ) ;
#11327=ADVANCED_FACE ( 'NONE', ( #61049 ), #15091, .T. ) ;
#11329=CARTESIAN_POINT ( 'NONE',  ( 0.5774900079438590739, 62.64701867748817676, -5.440088680355550821 ) ) ;
#11332=CARTESIAN_POINT ( 'NONE',  ( 10.00000000000000178, 50.37363466993042493, 12.81628187352647608 ) ) ;
#11333=CARTESIAN_POINT ( 'NONE',  ( 7.084665262690076126, 47.02201867748818387, -10.88017736071110164 ) ) ;
#11337=CARTESIAN_POINT ( 'NONE',  ( 7.084665262690076126, 69.10535201082151957, 10.88017736071109987 ) ) ;
#11338=CARTESIAN_POINT ( 'NONE',  ( 10.00000000000000000, 6.813685344154838397, -10.88017736071110342 ) ) ;
#11339=CARTESIAN_POINT ( 'NONE',  ( 0.1532563361054100626, 0.8005978176674514168, -2.638427012816831230 ) ) ;
#11341=CARTESIAN_POINT ( 'NONE',  ( 20.88017736071110875, 10.77201867748817143, -2.915334737309920765 ) ) ;
#11342=CARTESIAN_POINT ( 'NONE',  ( 19.84674366389459266, 13.71726448433411782, -2.638427012816827677 ) ) ;
#11343=CARTESIAN_POINT ( 'NONE',  ( 22.26659068614894466, 13.88708216824730179, 7.082119434687054849 ) ) ;
#11344=CARTESIAN_POINT ( 'NONE',  ( 14.92337183194729988, 4.342264484334117824, -8.527530157486177487 ) ) ;
#11345=CARTESIAN_POINT ( 'NONE',  ( 17.96484262340118221, 29.93868534415484106, 7.964842623401181321 ) ) ;
#11346=CARTESIAN_POINT ( 'NONE',  ( 1.472469842513823179, 40.59226448433411605, -4.923371831947296329 ) ) ;
#11348=CARTESIAN_POINT ( 'NONE',  ( 2.791683348922240793, 46.63393115100077324, 7.208316651077764092 ) ) ;
#11351=CARTESIAN_POINT ( 'NONE',  ( -0.8801773607110991993, 47.85535201082150536, -2.915334737309923874 ) ) ;
#11352=CARTESIAN_POINT ( 'NONE',  ( 18.52753015748618282, 48.92559781766745886, -4.923371831947291888 ) ) ;
#11353=CARTESIAN_POINT ( 'NONE',  ( 19.42250999205614548, 5.980352010821504471, -5.440088680355545492 ) ) ;
#11355=CARTESIAN_POINT ( 'NONE',  ( 4.559911319644449179, 57.23035201082150536, -9.422509992056141925 ) ) ;
#11356=CARTESIAN_POINT ( 'NONE',  ( 10.00000000000000000, 1.813685344154838175, -10.88017736071110342 ) ) ;
#11360=CARTESIAN_POINT ( 'NONE',  ( 6.565887622018943937, 40.16530133659708923, 12.81628187352647430 ) ) ;
#11361=CARTESIAN_POINT ( 'NONE',  ( 20.88017736071110519, 30.56368534415484106, 2.639326808657452039E-16 ) ) ;
#11362=CARTESIAN_POINT ( 'NONE',  ( -45.94000000000001194, 99.99999999999998579, 12.00000000000000000 ) ) ;
#11364=CARTESIAN_POINT ( 'NONE',  ( 6.565887622018943937, 48.08196800326375353, -12.81628187352647608 ) ) ;
#11365=CARTESIAN_POINT ( 'NONE',  ( 20.88017736071110164, 30.35535201082151247, 2.915334737309930979 ) ) ;
#11369=CARTESIAN_POINT ( 'NONE',  ( 18.52753015748618282, 63.92559781766745886, -4.923371831947291888 ) ) ;
#11370=CARTESIAN_POINT ( 'NONE',  ( 10.00000000000000178, 7.258931151000785675, 9.846743663894594434 ) ) ;
#11371=CARTESIAN_POINT ( 'NONE',  ( 10.00000000000000000, 49.75893115100078745, -9.846743663894594434 ) ) ;
#11372=CARTESIAN_POINT ( 'NONE',  ( 17.96484262340118221, 24.93868534415484461, 7.964842623401181321 ) ) ;
#11374=CARTESIAN_POINT ( 'NONE',  ( 12.63842701281683034, 37.46726448433411605, 9.846743663894596210 ) ) ;
#11376=DIRECTION ( 'NONE',  ( -0.000000000000000000, -0.000000000000000000, 1.000000000000000000 ) ) ;
#11377=CARTESIAN_POINT ( 'NONE',  ( 0.1532563361054082862, 26.21726448433411605, 2.638427012816831674 ) ) ;
#11378=CARTESIAN_POINT ( 'NONE',  ( 0.1532563361054083140, 11.00893115100078568, 1.131784320476157264E-15 ) ) ;
#11379=CARTESIAN_POINT ( 'NONE',  ( 18.04007052943773104, 28.01528370094808551, 5.767676674365834977 ) ) ;
#11380=CARTESIAN_POINT ( 'NONE',  ( 10.00000000000000000, 54.75893115100078745, -9.846743663894594434 ) ) ;
#11382=VECTOR ( 'NONE', #82121, 1000.000000000000000 ) ;
#11383=CARTESIAN_POINT ( 'NONE',  ( 0.8952175423694405110, 8.525762395770811963, 5.990408912944244157 ) ) ;
#11384=CARTESIAN_POINT ( 'NONE',  ( 13.43411237798105340, 20.58196800326374643, 12.81628187352647963 ) ) ;
#11385=CARTESIAN_POINT ( 'NONE',  ( 7.361572987183170547, 47.05059781766745175, 9.846743663894590881 ) ) ;
#11386=CARTESIAN_POINT ( 'NONE',  ( -0.1503990784575321704, 8.101585745166424601, 6.262539305110068177 ) ) ;
#11387=CARTESIAN_POINT ( 'NONE',  ( 24.16423886937410614, 54.30374883491396787, 8.672049930838204340E-16 ) ) ;
#11388=CARTESIAN_POINT ( 'NONE',  ( 18.52753015748618282, 23.92559781766745530, -4.923371831947291888 ) ) ;
#11390=CARTESIAN_POINT ( 'NONE',  ( 20.00000000000000711, 79.40087001978916703, 4.999999999999999112 ) ) ;
#11391=CARTESIAN_POINT ( 'NONE',  ( 6.204703633549690345, 57.84541550158063927, 14.16423886937410082 ) ) ;
#11392=CARTESIAN_POINT ( 'NONE',  ( 19.84674366389459621, 58.50893115100078745, 7.409399052514197653E-17 ) ) ;
#11393=CARTESIAN_POINT ( 'NONE',  ( 10.00000000000000000, 1.813685344154838175, -10.88017736071110342 ) ) ;
#11394=CARTESIAN_POINT ( 'NONE',  ( 22.26659068614895176, 39.72041550158063217, -7.082119434687042414 ) ) ;
#11395=CARTESIAN_POINT ( 'NONE',  ( 24.16423886937409904, 39.09541550158062506, 3.795296366450317205 ) ) ;
#11399=CARTESIAN_POINT ( 'NONE',  ( 0.1532563361054083140, 56.00893115100078745, 1.131784320476157264E-15 ) ) ;
#11401=CARTESIAN_POINT ( 'NONE',  ( 12.91533473730993009, 46.60535201082150536, -10.88017736071109987 ) ) ;
#11404=CARTESIAN_POINT ( 'NONE',  ( 12.63842701281683922, 54.55059781766745175, -9.846743663894590881 ) ) ;
#11407=CARTESIAN_POINT ( 'NONE',  ( 6.204703633549690345, 22.84541550158062861, 14.16423886937410082 ) ) ;
#11412=CYLINDRICAL_SURFACE ( 'NONE', #2584, 11.92686044187656513 ) ;
#11413=CARTESIAN_POINT ( 'NONE',  ( 0.5774900079438607392, 23.48035201082150536, 5.440088680355550821 ) ) ;
#11414=CARTESIAN_POINT ( 'NONE',  ( -1.099225684535947600, 19.54030133659708568, 6.408140936763237150 ) ) ;
#11415=CARTESIAN_POINT ( 'NONE',  ( 20.24186590665277308, 61.76028685723174050, 6.114288769123050749 ) ) ;
#11416=CARTESIAN_POINT ( 'NONE',  ( 17.20831665107776587, 12.88393115100078390, 7.208316651077764980 ) ) ;
#11419=CARTESIAN_POINT ( 'NONE',  ( 24.16423886937409904, 34.09541550158064638, 3.795296366450317205 ) ) ;
#11420=CARTESIAN_POINT ( 'NONE',  ( -0.3289641300568005855, 10.10497603579417536, 5.963430220938281678 ) ) ;
#11421=PRESENTATION_STYLE_ASSIGNMENT (( #42420 ) ) ;
#11422=CARTESIAN_POINT ( 'NONE',  ( 20.88017736071110164, 5.355352010821503583, 2.915334737309930979 ) ) ;
#11423=CARTESIAN_POINT ( 'NONE',  ( 0.2751277870542967463, 70.00000000000000000, 6.000000000000000000 ) ) ;
#11425=CARTESIAN_POINT ( 'NONE',  ( 15.44008868035555260, 34.73035201082151247, 9.422509992056143702 ) ) ;
#11426=CARTESIAN_POINT ( 'NONE',  ( 19.42250999205614548, 40.98035201082150536, -5.440088680355545492 ) ) ;
#11427=CARTESIAN_POINT ( 'NONE',  ( -2.816281873526473856, 19.33196800326375708, 3.434112377981055619 ) ) ;
#11428=CARTESIAN_POINT ( 'NONE',  ( 0.1532563361054083140, 66.00893115100079456, 1.131784320476157264E-15 ) ) ;
#11429=CARTESIAN_POINT ( 'NONE',  ( 0.2751277870542979120, 15.30223176428831344, 6.500000000000003553 ) ) ;
#11430=CARTESIAN_POINT ( 'NONE',  ( 19.84674366389459266, 13.30059781766745353, 2.638427012816836559 ) ) ;
#11431=VERTEX_POINT ( 'NONE', #47528 ) ;
#11432=CARTESIAN_POINT ( 'NONE',  ( 18.17829156368509302, 49.16792564121895026, 6.499999999999931610 ) ) ;
#11433=CARTESIAN_POINT ( 'NONE',  ( 19.42250999205614548, 40.98035201082150536, -5.440088680355545492 ) ) ;
#11434=UNCERTAINTY_MEASURE_WITH_UNIT (LENGTH_MEASURE( 1.000000000000000082E-05 ), #57163, 'distance_accuracy_value', 'NONE');
#11435=CARTESIAN_POINT ( 'NONE',  ( -2.816281873526471635, -1.084698663402913210, -3.434112377981056508 ) ) ;
#11436=CARTESIAN_POINT ( 'NONE',  ( -0.8801773607111008646, 63.27201867748817676, 2.915334737309923430 ) ) ;
#11437=CARTESIAN_POINT ( 'NONE',  ( 0.1532563361054083140, 31.00893115100078390, 1.131784320476157264E-15 ) ) ;
#11438=CARTESIAN_POINT ( 'NONE',  ( 6.565887622018943937, 35.16530133659708923, 12.81628187352647430 ) ) ;
#11439=CARTESIAN_POINT ( 'NONE',  ( 12.63842701281683922, 9.550597817667449974, -9.846743663894590881 ) ) ;
#11441=ORIENTED_EDGE ( 'NONE', *, *, #69115, .T. ) ;
#11444=CARTESIAN_POINT ( 'NONE',  ( 0.5774900079438590739, 12.64701867748817143, -5.440088680355550821 ) ) ;
#11445=CARTESIAN_POINT ( 'NONE',  ( 16.40814093676324603, 62.45696800326376064, -11.09922568453594671 ) ) ;
#11447=CARTESIAN_POINT ( 'NONE',  ( 0.1532563361054100626, 35.80059781766745175, -2.638427012816831230 ) ) ;
#11448=CARTESIAN_POINT ( 'NONE',  ( 12.91533473730993009, 16.60535201082150891, -10.88017736071109987 ) ) ;
#11449=CARTESIAN_POINT ( 'NONE',  ( 15.44008868035555793, 6.397018677488171434, -9.422509992056140149 ) ) ;
#11451=CARTESIAN_POINT ( 'NONE',  ( 4.559911319644449179, 12.23035201082150536, -9.422509992056141925 ) ) ;
#11452=CARTESIAN_POINT ( 'NONE',  ( 20.88017736071110164, 25.35535201082150891, 2.915334737309930979 ) ) ;
#11457=CARTESIAN_POINT ( 'NONE',  ( 2.791683348922240793, 61.63393115100079456, 7.208316651077764092 ) ) ;
#11458=CARTESIAN_POINT ( 'NONE',  ( -0.8801773607111009756, 23.06368534415484106, 1.068504757029289695E-15 ) ) ;
#11459=CARTESIAN_POINT ( 'NONE',  ( 10.00000000000000178, 57.25893115100078745, 9.846743663894594434 ) ) ;
#11460=CARTESIAN_POINT ( 'NONE',  ( -1.099225684535947600, 48.70696800326375353, -6.408140936763238038 ) ) ;
#11462=CARTESIAN_POINT ( 'NONE',  ( 22.26659068614894466, 28.88708216824730357, 7.082119434687054849 ) ) ;
#11463=CARTESIAN_POINT ( 'NONE',  ( 0.5774900079438590739, 42.64701867748816966, -5.440088680355550821 ) ) ;
#11464=CARTESIAN_POINT ( 'NONE',  ( 17.96484262340118221, 14.93868534415484106, 7.964842623401181321 ) ) ;
#11465=CARTESIAN_POINT ( 'NONE',  ( 10.00000000000000000, 49.75893115100078745, -9.846743663894594434 ) ) ;
#11467=CARTESIAN_POINT ( 'NONE',  ( 0.1532563361054082862, 56.21726448433411605, 2.638427012816831674 ) ) ;
#11468=STYLED_ITEM ( 'NONE', ( #91894 ), #47247 ) ;
#11469=CARTESIAN_POINT ( 'NONE',  ( 20.15039907845753930, 70.00000000000000000, -6.262539305110068177 ) ) ;
#11470=CARTESIAN_POINT ( 'NONE',  ( 5.076628168052703671, 1.842264484334118047, 8.527530157486179263 ) ) ;
#11474=CARTESIAN_POINT ( 'NONE',  ( 2.035157376598822676, 12.43868534415483751, -7.964842623401177768 ) ) ;
#11475=CARTESIAN_POINT ( 'NONE',  ( 5.076628168052704559, 5.175597817667451750, -8.527530157486179263 ) ) ;
#11476=CARTESIAN_POINT ( 'NONE',  ( 3.591859063236763294, -1.709698663402913210, -11.09922568453595026 ) ) ;
#11477=CARTESIAN_POINT ( 'NONE',  ( 7.084665262690076126, 62.02201867748816966, -10.88017736071110164 ) ) ;
#11478=CARTESIAN_POINT ( 'NONE',  ( 10.00000000000000178, 24.31368534415484106, 10.88017736071110342 ) ) ;
#11479=CARTESIAN_POINT ( 'NONE',  ( 6.565887622018943937, 40.16530133659708923, 12.81628187352647430 ) ) ;
#11480=CARTESIAN_POINT ( 'NONE',  ( 13.79529636645031943, 25.34541550158063572, -14.16423886937409904 ) ) ;
#11481=CARTESIAN_POINT ( 'NONE',  ( 6.565887622018943937, 60.16530133659707502, 12.81628187352647430 ) ) ;
#11483=CARTESIAN_POINT ( 'NONE',  ( 7.361572987183170547, 67.05059781766746596, 9.846743663894590881 ) ) ;
#11485=CARTESIAN_POINT ( 'NONE',  ( -0.8801773607111008646, 28.27201867748817321, 2.915334737309923430 ) ) ;
#11486=CARTESIAN_POINT ( 'NONE',  ( 7.361572987183169658, 64.96726448433412315, -9.846743663894592657 ) ) ;
#11488=CARTESIAN_POINT ( 'NONE',  ( 18.52753015748617571, 8.092264484334117824, 4.923371831947298993 ) ) ;
#11490=CARTESIAN_POINT ( 'NONE',  ( 17.20831665107776587, 14.13393115100078568, -7.208316651077762316 ) ) ;
#11491=CARTESIAN_POINT ( 'NONE',  ( 0.1532563361054082862, 21.21726448433412315, 2.638427012816831674 ) ) ;
#11492=CARTESIAN_POINT ( 'NONE',  ( 7.361572987183170547, 12.05059781766744997, 9.846743663894590881 ) ) ;
#11494=CARTESIAN_POINT ( 'NONE',  ( 7.084665262690076126, 52.02201867748816255, -10.88017736071110164 ) ) ;
#11496=CARTESIAN_POINT ( 'NONE',  ( -0.8801773607111009756, 68.06368534415484817, 1.068504757029289695E-15 ) ) ;
#11497=CARTESIAN_POINT ( 'NONE',  ( 17.20831665107776587, 12.88393115100078390, 7.208316651077764980 ) ) ;
#11501=CARTESIAN_POINT ( 'NONE',  ( 12.63842701281683034, 57.46726448433411605, 9.846743663894596210 ) ) ;
#11503=CARTESIAN_POINT ( 'NONE',  ( 17.08211943468705130, 23.47041550158063572, 12.26659068614894998 ) ) ;
#11504=UNCERTAINTY_MEASURE_WITH_UNIT (LENGTH_MEASURE( 1.000000000000000082E-05 ), #29322, 'distance_accuracy_value', 'NONE');
#11505=DIRECTION ( 'NONE',  ( -0.000000000000000000, -0.000000000000000000, 1.000000000000000000 ) ) ;
#11506=CARTESIAN_POINT ( 'NONE',  ( -2.266590686148945544, 11.38708216824730179, -7.082119434687050408 ) ) ;
#11507=CARTESIAN_POINT ( 'NONE',  ( -2.266590686148945544, 27.22041550158063572, 7.082119434687048631 ) ) ;
#11509=FILL_AREA_STYLE_COLOUR ( '', #41828 ) ;
#11510=CARTESIAN_POINT ( 'NONE',  ( 4.559911319644449179, 33.89701867748817676, 9.422509992056141925 ) ) ;
#11511=VERTEX_POINT ( 'NONE', #39058 ) ;
#11512=CARTESIAN_POINT ( 'NONE',  ( 0.1532563361054082862, 16.21726448433411960, 2.638427012816831674 ) ) ;
#11514=CARTESIAN_POINT ( 'NONE',  ( 19.42250999205614193, 60.14701867748817676, 5.440088680355555262 ) ) ;
#11515=CARTESIAN_POINT ( 'NONE',  ( 14.92337183194729988, 14.34226448433411782, -8.527530157486177487 ) ) ;
#11516=CARTESIAN_POINT ( 'NONE',  ( 0.6178305044545838731, 49.74863466993041072, 9.382169495545420901 ) ) ;
#11517=CARTESIAN_POINT ( 'NONE',  ( 19.84674366389459266, 38.71726448433412315, -2.638427012816827677 ) ) ;
#11519=CARTESIAN_POINT ( 'NONE',  ( 22.81628187352648496, 31.83196800326375353, -3.434112377981050290 ) ) ;
#11522=CARTESIAN_POINT ( 'NONE',  ( 19.84674366389459266, 23.71726448433412315, -2.638427012816827677 ) ) ;
#11524=CARTESIAN_POINT ( 'NONE',  ( -4.164238869374099039, 6.803748834913967869, 8.674139862899312516E-16 ) ) ;
#11528=CARTESIAN_POINT ( 'NONE',  ( 4.559911319644449179, 52.23035201082151247, -9.422509992056141925 ) ) ;
#11529=CARTESIAN_POINT ( 'NONE',  ( 4.559911319644449179, 58.89701867748817676, 9.422509992056141925 ) ) ;
#11530=CARTESIAN_POINT ( 'NONE',  ( 17.08211943468705130, 43.47041550158063927, 12.26659068614894998 ) ) ;
#11531=CARTESIAN_POINT ( 'NONE',  ( 17.20831665107776587, 52.88393115100078035, 7.208316651077764980 ) ) ;
#11532=CARTESIAN_POINT ( 'NONE',  ( 7.361572987183170547, 17.05059781766745530, 9.846743663894590881 ) ) ;
#11535=CARTESIAN_POINT ( 'NONE',  ( 0.5774900079438590739, 37.64701867748817676, -5.440088680355550821 ) ) ;
#11536=( GEOMETRIC_REPRESENTATION_CONTEXT ( 3 ) GLOBAL_UNCERTAINTY_ASSIGNED_CONTEXT ( ( #41536 ) ) GLOBAL_UNIT_ASSIGNED_CONTEXT ( ( #51555, #6059, #42573 ) ) REPRESENTATION_CONTEXT ( 'NONE', 'WORKASPACE' ) );
#11538=CARTESIAN_POINT ( 'NONE',  ( 12.63842701281683034, 57.46726448433411605, 9.846743663894596210 ) ) ;
#11541=AXIS2_PLACEMENT_3D ( 'NONE', #36507, #82493, #98018 ) ;
#11542=CARTESIAN_POINT ( 'NONE',  ( 4.559911319644449179, 62.23035201082150536, -9.422509992056141925 ) ) ;
#11543=SURFACE_STYLE_USAGE ( .BOTH. , #6027 ) ;
#11545=STYLED_ITEM ( 'NONE', ( #14269 ), #73503 ) ;
#11546=CARTESIAN_POINT ( 'NONE',  ( 10.00000000000000000, -0.2410688489992152128, -9.846743663894594434 ) ) ;
#11547=CARTESIAN_POINT ( 'NONE',  ( 0.1532563361054100626, 0.8005978176674514168, -2.638427012816831230 ) ) ;
#11549=CARTESIAN_POINT ( 'NONE',  ( 12.63842701281683922, 39.55059781766744464, -9.846743663894590881 ) ) ;
#11550=CARTESIAN_POINT ( 'NONE',  ( 7.084665262690076126, 17.02201867748817676, -10.88017736071110164 ) ) ;
#11551=CARTESIAN_POINT ( 'NONE',  ( 17.20831665107776587, 64.13393115100079456, -7.208316651077762316 ) ) ;
#11552=CARTESIAN_POINT ( 'NONE',  ( 20.88017736071110875, 30.77201867748816966, -2.915334737309920765 ) ) ;
#11554=CARTESIAN_POINT ( 'NONE',  ( 18.29284471827482506, 65.40189080397281884, -6.499999999999912070 ) ) ;
#11555=CARTESIAN_POINT ( 'NONE',  ( -1.099225684535947600, 38.70696800326375353, -6.408140936763238038 ) ) ;
#11556=VERTEX_POINT ( 'NONE', #9532 ) ;
#11557=CARTESIAN_POINT ( 'NONE',  ( 10.00000000000000000, 51.81368534415484106, -10.88017736071110342 ) ) ;
#11558=CARTESIAN_POINT ( 'NONE',  ( 0.6178305044545818747, 18.49863466993041428, -9.382169495545419124 ) ) ;
#11559=CARTESIAN_POINT ( 'NONE',  ( 18.04007052943773459, 18.01528370094808196, 5.767676674365826983 ) ) ;
#11561=CARTESIAN_POINT ( 'NONE',  ( 17.96484262340118221, 21.18868534415483396, -7.964842623401177768 ) ) ;
#11562=CARTESIAN_POINT ( 'NONE',  ( -4.164238869374099927, 67.01208216824728936, 3.795296366450308767 ) ) ;
#11563=MECHANICAL_DESIGN_GEOMETRIC_PRESENTATION_REPRESENTATION('',(#29182),#80218);
#11564=CARTESIAN_POINT ( 'NONE',  ( 14.92337183194729633, 37.67559781766745175, 8.527530157486181039 ) ) ;
#11565=CARTESIAN_POINT ( 'NONE',  ( 10.00000000000000178, 7.258931151000785675, 9.846743663894594434 ) ) ;
#11566=CARTESIAN_POINT ( 'NONE',  ( 12.91533473730993009, 56.60535201082151247, -10.88017736071109987 ) ) ;
#11567=B_SPLINE_CURVE_WITH_KNOTS ( 'NONE', 3,
 ( #72851, #94380, #19376, #70913 ),
 .UNSPECIFIED., .F., .F.,
 ( 4, 4 ),
 ( 0.000000000000000000, 0.002657014572711341102 ),
 .UNSPECIFIED. ) ;
#11569=CARTESIAN_POINT ( 'NONE',  ( 10.00000000000000000, 35.55374883491396787, -14.16423886937410082 ) ) ;
#11572=ORIENTED_EDGE ( 'NONE', *, *, #35734, .F. ) ;
#11574=TOROIDAL_SURFACE ( 'NONE', #48252, 7.538348415311010520, 7.000000000000000000 ) ;
#11575=CARTESIAN_POINT ( 'NONE',  ( 24.16423886937410614, 54.51208216824730357, -3.795296366450302550 ) ) ;
#11576=CARTESIAN_POINT ( 'NONE',  ( -2.266590686148945544, 56.38708216824731068, -7.082119434687050408 ) ) ;
#11577=CARTESIAN_POINT ( 'NONE',  ( 2.791683348922240793, 11.63393115100078568, 7.208316651077764092 ) ) ;
#11578=CARTESIAN_POINT ( 'NONE',  ( -1.099225684535947600, 18.70696800326375353, -6.408140936763238038 ) ) ;
#11580=FACE_OUTER_BOUND ( 'NONE', #795, .T. ) ;
#11582=CARTESIAN_POINT ( 'NONE',  ( 22.81628187352648496, 36.83196800326376064, -3.434112377981050290 ) ) ;
#11583=CARTESIAN_POINT ( 'NONE',  ( 10.00000000000000000, 40.55374883491397497, -14.16423886937410082 ) ) ;
#11585=CARTESIAN_POINT ( 'NONE',  ( 18.52753015748617571, 13.09226448433411960, 4.923371831947298993 ) ) ;
#11589=CARTESIAN_POINT ( 'NONE',  ( 18.52753015748617571, 18.09226448433411960, 4.923371831947298993 ) ) ;
#11591=ORIENTED_EDGE ( 'NONE', *, *, #72949, .F. ) ;
#11592=CARTESIAN_POINT ( 'NONE',  ( 12.91533473730992121, 9.522018677488171434, 10.88017736071110164 ) ) ;
#11593=CARTESIAN_POINT ( 'NONE',  ( 7.084665262690076126, 19.10535201082150181, 10.88017736071109987 ) ) ;
#11594=CARTESIAN_POINT ( 'NONE',  ( 1.472469842513823179, 56.42559781766745886, 4.923371831947296329 ) ) ;
#11595=CARTESIAN_POINT ( 'NONE',  ( -2.816281873526473856, -0.6680319967362464695, 3.434112377981055619 ) ) ;
#11596=CIRCLE ( 'NONE', #40377, 9.999999999999994671 ) ;
#11597=CARTESIAN_POINT ( 'NONE',  ( 6.565887622018943937, 18.08196800326375708, -12.81628187352647608 ) ) ;
#11600=CARTESIAN_POINT ( 'NONE',  ( 24.16423886937409904, 59.09541550158063217, 3.795296366450317205 ) ) ;
#11602=AXIS2_PLACEMENT_3D ( 'NONE', #77878, #32375, #69904 ) ;
#11603=CARTESIAN_POINT ( 'NONE',  ( -2.266590686148945544, 62.22041550158063927, 7.082119434687048631 ) ) ;
#11605=CARTESIAN_POINT ( 'NONE',  ( -0.8801773607111009756, 28.06368534415484106, 1.068504757029289695E-15 ) ) ;
#11606=CARTESIAN_POINT ( 'NONE',  ( 15.44008868035555793, 51.39701867748816966, -9.422509992056140149 ) ) ;
#11607=CARTESIAN_POINT ( 'NONE',  ( 4.559911319644449179, 57.23035201082150536, -9.422509992056141925 ) ) ;
#11610=CARTESIAN_POINT ( 'NONE',  ( 12.91533473730992121, 34.52201867748817676, 10.88017736071110164 ) ) ;
#11614=CARTESIAN_POINT ( 'NONE',  ( 1.472469842513823179, 10.59226448433411782, -4.923371831947296329 ) ) ;
#11617=CARTESIAN_POINT ( 'NONE',  ( 5.076628168052703671, 46.84226448433412315, 8.527530157486179263 ) ) ;
#11619=CARTESIAN_POINT ( 'NONE',  ( 16.40814093676323893, 60.79030133659709634, 11.09922568453595026 ) ) ;
#11626=CARTESIAN_POINT ( 'NONE',  ( 7.361572987183169658, 29.96726448433411960, -9.846743663894592657 ) ) ;
#11627=CARTESIAN_POINT ( 'NONE',  ( 10.00000000000000000, 55.55374883491396787, -14.16423886937410082 ) ) ;
#11631=CARTESIAN_POINT ( 'NONE',  ( 1.472469842513823179, 35.59226448433412315, -4.923371831947296329 ) ) ;
#11632=CARTESIAN_POINT ( 'NONE',  ( 21.09922568453595559, 7.040301336597086568, -6.408140936763230044 ) ) ;
#11633=CARTESIAN_POINT ( 'NONE',  ( -0.8801773607110991993, 62.85535201082150536, -2.915334737309923874 ) ) ;
#11635=B_SPLINE_CURVE_WITH_KNOTS ( 'NONE', 3,
 ( #75432, #20967, #4977, #74938, #51452, #96480, #44436, #59929 ),
 .UNSPECIFIED., .F., .F.,
 ( 4, 2, 2, 4 ),
 ( 0.000000000000000000, 0.001329205578904317682, 0.002658411157808635364, 0.005316822315617270728 ),
 .UNSPECIFIED. ) ;
#11636=CARTESIAN_POINT ( 'NONE',  ( 19.84674366389459266, 13.30059781766745353, 2.638427012816836559 ) ) ;
#11637=CARTESIAN_POINT ( 'NONE',  ( 5.076628168052704559, 60.17559781766745175, -8.527530157486179263 ) ) ;
#11638=CARTESIAN_POINT ( 'NONE',  ( 1.042145700049395884, 19.74216108172003104, -6.499999999999846345 ) ) ;
#11640=ADVANCED_FACE ( 'NONE', ( #71993 ), #20956, .T. ) ;
#11641=ORIENTED_EDGE ( 'NONE', *, *, #86749, .F. ) ;
#11643=CARTESIAN_POINT ( 'NONE',  ( 15.44008868035555260, 4.730352010821505360, 9.422509992056143702 ) ) ;
#11644=CARTESIAN_POINT ( 'NONE',  ( -2.266590686148945544, 7.220415501580634832, 7.082119434687048631 ) ) ;
#11645=CARTESIAN_POINT ( 'NONE',  ( 5.076628168052704559, 15.17559781766745175, -8.527530157486179263 ) ) ;
#11646=CARTESIAN_POINT ( 'NONE',  ( 0.5774900079438607392, 48.48035201082150536, 5.440088680355550821 ) ) ;
#11647=CARTESIAN_POINT ( 'NONE',  ( 21.09922568453595559, 22.04030133659708923, -6.408140936763230044 ) ) ;
#11649=CARTESIAN_POINT ( 'NONE',  ( 0.5774900079438590739, 7.647018677488171434, -5.440088680355550821 ) ) ;
#11652=CARTESIAN_POINT ( 'NONE',  ( 7.361572987183169658, 54.96726448433413026, -9.846743663894592657 ) ) ;
#11653=CARTESIAN_POINT ( 'NONE',  ( 0.1532563361054100626, 15.80059781766745353, -2.638427012816831230 ) ) ;
#11655=CARTESIAN_POINT ( 'NONE',  ( 3.591859063236763294, 28.29030133659708568, -11.09922568453595026 ) ) ;
#11656=DIRECTION ( 'NONE',  ( 0.000000000000000000, 0.000000000000000000, -1.000000000000000000 ) ) ;
#11658=CARTESIAN_POINT ( 'NONE',  ( 7.084665262690076126, 32.02201867748816966, -10.88017736071110164 ) ) ;
#11660=CARTESIAN_POINT ( 'NONE',  ( 10.00000000000000000, 55.55374883491396787, -14.16423886937410082 ) ) ;
#11661=CARTESIAN_POINT ( 'NONE',  ( 13.79529636645031943, 30.34541550158063927, -14.16423886937409904 ) ) ;
#11662=CIRCLE ( 'NONE', #59561, 0.5000000000000004441 ) ;
#11663=CARTESIAN_POINT ( 'NONE',  ( 19.84674366389459621, 43.50893115100078745, 7.409399052514197653E-17 ) ) ;
#11664=CARTESIAN_POINT ( 'NONE',  ( -2.816281873526473856, 39.33196800326374643, 3.434112377981055619 ) ) ;
#11665=CARTESIAN_POINT ( 'NONE',  ( 2.035157376598824452, 23.68868534415484461, 7.964842623401179544 ) ) ;
#11666=CARTESIAN_POINT ( 'NONE',  ( 19.84674366389459621, 53.50893115100078745, 7.409399052514197653E-17 ) ) ;
#11667=CARTESIAN_POINT ( 'NONE',  ( 4.559911319644449179, 38.89701867748817676, 9.422509992056141925 ) ) ;
#11668=CARTESIAN_POINT ( 'NONE',  ( 19.38216949554541202, 10.99863466993042138, 9.382169495545424454 ) ) ;
#11669=CARTESIAN_POINT ( 'NONE',  ( 6.204703633549690345, 30.76208216824730357, -14.16423886937410259 ) ) ;
#11671=CARTESIAN_POINT ( 'NONE',  ( 17.62281668512003208, 33.28593319516822646, 6.499999999999993783 ) ) ;
#11674=CARTESIAN_POINT ( 'NONE',  ( 0.1532563361054082862, 31.21726448433412315, 2.638427012816831674 ) ) ;
#11675=CARTESIAN_POINT ( 'NONE',  ( 21.09922568453595559, 62.04030133659709634, -6.408140936763230044 ) ) ;
#11676=CARTESIAN_POINT ( 'NONE',  ( 2.791683348922240793, 66.63393115100079456, 7.208316651077764092 ) ) ;
#11679=DIRECTION ( 'NONE',  ( 0.000000000000000000, 0.000000000000000000, -1.000000000000000000 ) ) ;
#11681=CARTESIAN_POINT ( 'NONE',  ( 2.035157376598822676, 17.43868534415483751, -7.964842623401177768 ) ) ;
#11682=CARTESIAN_POINT ( 'NONE',  ( 6.204703633549690345, 27.84541550158063217, 14.16423886937410082 ) ) ;
#11683=CARTESIAN_POINT ( 'NONE',  ( 10.00000000000000178, 7.258931151000785675, 9.846743663894594434 ) ) ;
#11684=CARTESIAN_POINT ( 'NONE',  ( 14.92337183194729633, 52.67559781766745175, 8.527530157486181039 ) ) ;
#11685=CARTESIAN_POINT ( 'NONE',  ( 20.88017736071110164, 35.35535201082150536, 2.915334737309930979 ) ) ;
#11690=CARTESIAN_POINT ( 'NONE',  ( 20.15039907845753575, 65.60158574516643171, -6.262539305110073506 ) ) ;
#11693=CARTESIAN_POINT ( 'NONE',  ( -41.70923076923077844, 106.3461538461538396, -9.500000000000000000 ) ) ;
#11694=CARTESIAN_POINT ( 'NONE',  ( 10.00000000000000178, 13.05374883491396787, 14.16423886937410082 ) ) ;
#11695=CARTESIAN_POINT ( 'NONE',  ( 22.26659068614895176, 9.720415501580633943, -7.082119434687042414 ) ) ;
#11696=CARTESIAN_POINT ( 'NONE',  ( 20.36894250292379738, 59.92874883491397497, -10.36894250292379027 ) ) ;
#11697=CARTESIAN_POINT ( 'NONE',  ( 12.63842701281683034, 52.46726448433413026, 9.846743663894596210 ) ) ;
#11698=CARTESIAN_POINT ( 'NONE',  ( 5.076628168052703671, 41.84226448433411605, 8.527530157486179263 ) ) ;
#11699=CARTESIAN_POINT ( 'NONE',  ( 19.72487221294570858, 51.86607318730076344, 6.500000000000000888 ) ) ;
#11700=CARTESIAN_POINT ( 'NONE',  ( 20.88017736071110875, 30.77201867748816966, -2.915334737309920765 ) ) ;
#11701=CARTESIAN_POINT ( 'NONE',  ( 12.63842701281683034, 62.46726448433410894, 9.846743663894596210 ) ) ;
#11702=CARTESIAN_POINT ( 'NONE',  ( -4.164238869374098151, 1.595415501580634388, -3.795296366450310543 ) ) ;
#11703=CARTESIAN_POINT ( 'NONE',  ( 10.00000000000000178, 9.313685344154839285, 10.88017736071110342 ) ) ;
#11704=CARTESIAN_POINT ( 'NONE',  ( -0.2418659066527706625, 67.23410085661205926, -6.114288769123047196 ) ) ;
#11709=CARTESIAN_POINT ( 'NONE',  ( 14.92337183194729633, 27.67559781766745530, 8.527530157486181039 ) ) ;
#11711=CARTESIAN_POINT ( 'NONE',  ( 10.00000000000000178, 38.05374883491396787, 14.16423886937410082 ) ) ;
#11712=CARTESIAN_POINT ( 'NONE',  ( 14.92337183194729988, 39.34226448433412315, -8.527530157486177487 ) ) ;
#11713=CARTESIAN_POINT ( 'NONE',  ( 19.42250999205614548, 55.98035201082150536, -5.440088680355545492 ) ) ;
#11714=AXIS2_PLACEMENT_3D ( 'NONE', #98525, #50144, #22506 ) ;
#11716=CARTESIAN_POINT ( 'NONE',  ( 20.88017736071110875, 50.77201867748817676, -2.915334737309920765 ) ) ;
#11717=CARTESIAN_POINT ( 'NONE',  ( 16.40814093676324603, 62.45696800326376064, -11.09922568453594671 ) ) ;
#11720=CARTESIAN_POINT ( 'NONE',  ( -0.8801773607110991993, 47.85535201082150536, -2.915334737309923874 ) ) ;
#11721=CARTESIAN_POINT ( 'NONE',  ( -4.164238869374099039, 21.80374883491396787, 8.674139862899312516E-16 ) ) ;
#11723=CARTESIAN_POINT ( 'NONE',  ( 22.81628187352647785, 46.62363466993041783, 6.195893100308588602E-16 ) ) ;
#11724=CARTESIAN_POINT ( 'NONE',  ( 17.96484262340118221, 19.93868534415484106, 7.964842623401181321 ) ) ;
#11725=CARTESIAN_POINT ( 'NONE',  ( 18.52753015748617571, 28.09226448433411960, 4.923371831947298993 ) ) ;
#11726=CARTESIAN_POINT ( 'NONE',  ( 19.42250999205614548, 15.98035201082150714, -5.440088680355545492 ) ) ;
#11727=CARTESIAN_POINT ( 'NONE',  ( 21.09922568453595559, 52.04030133659708923, -6.408140936763230044 ) ) ;
#11729=CARTESIAN_POINT ( 'NONE',  ( 5.076628168052704559, 35.17559781766745175, -8.527530157486179263 ) ) ;
#11731=EDGE_CURVE ( 'NONE', #14724, #39677, #80974, .T. ) ;
#11735=CARTESIAN_POINT ( 'NONE',  ( 20.88017736071110875, 65.77201867748817676, -2.915334737309920765 ) ) ;
#11736=CARTESIAN_POINT ( 'NONE',  ( 0.6076426042653181314, 27.37576471608601025, -6.500000000000012434 ) ) ;
#11738=CARTESIAN_POINT ( 'NONE',  ( 7.361572987183170547, 2.050597817667451750, 9.846743663894590881 ) ) ;
#11739=AXIS2_PLACEMENT_3D ( 'NONE', #28094, #82583, #34599 ) ;
#11740=CARTESIAN_POINT ( 'NONE',  ( -1.099225684535947600, 28.70696800326375353, -6.408140936763238038 ) ) ;
#11743=CARTESIAN_POINT ( 'NONE',  ( 0.1532563361054083140, 41.00893115100078745, 1.131784320476157264E-15 ) ) ;
#11744=CARTESIAN_POINT ( 'NONE',  ( 20.15039907845754286, 14.72266099184918531, 6.262539305110064625 ) ) ;
#11745=CARTESIAN_POINT ( 'NONE',  ( -2.266590686148945544, 22.22041550158063572, 7.082119434687048631 ) ) ;
#11746=CARTESIAN_POINT ( 'NONE',  ( 7.361572987183169658, 29.96726448433411960, -9.846743663894592657 ) ) ;
#11747=CARTESIAN_POINT ( 'NONE',  ( 13.43411237798105340, 30.58196800326374998, 12.81628187352647963 ) ) ;
#11750=CARTESIAN_POINT ( 'NONE',  ( 2.035157376598824452, 68.68868534415484817, 7.964842623401179544 ) ) ;
#11751=CARTESIAN_POINT ( 'NONE',  ( 16.40814093676323893, 10.79030133659708923, 11.09922568453595026 ) ) ;
#11752=CARTESIAN_POINT ( 'NONE',  ( -26.69000000000001194, 92.00000000000000000, -10.09898361729590199 ) ) ;
#11753=CARTESIAN_POINT ( 'NONE',  ( 12.63842701281683922, 39.55059781766744464, -9.846743663894590881 ) ) ;
#11754=CARTESIAN_POINT ( 'NONE',  ( 19.42250999205614193, 25.14701867748817321, 5.440088680355555262 ) ) ;
#11755=CARTESIAN_POINT ( 'NONE',  ( 16.40814093676324603, 27.45696800326375708, -11.09922568453594671 ) ) ;
#11759=CARTESIAN_POINT ( 'NONE',  ( 12.91533473730993009, 26.60535201082150536, -10.88017736071109987 ) ) ;
#11760=VERTEX_POINT ( 'NONE', #24759 ) ;
#11761=DIRECTION ( 'NONE',  ( 0.000000000000000000, -1.000000000000000000, 0.000000000000000000 ) ) ;
#11763=CARTESIAN_POINT ( 'NONE',  ( 12.63842701281683922, 54.55059781766745175, -9.846743663894590881 ) ) ;
#11764=CARTESIAN_POINT ( 'NONE',  ( 20.88017736071110519, 30.56368534415484106, 2.639326808657452039E-16 ) ) ;
#11766=CARTESIAN_POINT ( 'NONE',  ( 19.42250999205614548, 50.98035201082151247, -5.440088680355545492 ) ) ;
#11767=CARTESIAN_POINT ( 'NONE',  ( 15.44008868035555793, 26.39701867748817321, -9.422509992056140149 ) ) ;
#11770=CARTESIAN_POINT ( 'NONE',  ( 7.361572987183170547, 52.05059781766745175, 9.846743663894590881 ) ) ;
#11771=CARTESIAN_POINT ( 'NONE',  ( -4.164238869374099927, 47.01208216824729647, 3.795296366450308767 ) ) ;
#11773=CARTESIAN_POINT ( 'NONE',  ( -29.94000000000001549, 92.00000000000000000, -9.500000000000000000 ) ) ;
#11774=CARTESIAN_POINT ( 'NONE',  ( -2.266590686148945544, 6.387082168247300906, -7.082119434687050408 ) ) ;
#11775=CARTESIAN_POINT ( 'NONE',  ( 24.16423886937410614, 39.51208216824731068, -3.795296366450302550 ) ) ;
#11776=CARTESIAN_POINT ( 'NONE',  ( 3.591859063236761518, 9.956968003263753531, 11.09922568453594849 ) ) ;
#11778=VERTEX_POINT ( 'NONE', #39761 ) ;
#11779=B_SPLINE_CURVE_WITH_KNOTS ( 'NONE', 3,
 ( #19551, #79063, #10577, #80549 ),
 .UNSPECIFIED., .F., .F.,
 ( 4, 4 ),
 ( 0.000000000000000000, 0.002562518741975561461 ),
 .UNSPECIFIED. ) ;
#11780=CARTESIAN_POINT ( 'NONE',  ( 2.035157376598822676, 2.438685344154838397, -7.964842623401177768 ) ) ;
#11781=CARTESIAN_POINT ( 'NONE',  ( 18.52753015748617571, 33.09226448433411605, 4.923371831947298993 ) ) ;
#11782=CARTESIAN_POINT ( 'NONE',  ( 2.035157376598824452, 58.68868534415482685, 7.964842623401179544 ) ) ;
#11783=CARTESIAN_POINT ( 'NONE',  ( 0.2751277870542967463, 70.00000000000000000, -6.500000000000000888 ) ) ;
#11784=CARTESIAN_POINT ( 'NONE',  ( -0.8801773607111009756, 28.06368534415484106, 1.068504757029289695E-15 ) ) ;
#11785=CARTESIAN_POINT ( 'NONE',  ( 6.565887622018943937, 58.08196800326376064, -12.81628187352647608 ) ) ;
#11786=CARTESIAN_POINT ( 'NONE',  ( 19.38216949554541202, 25.99863466993042138, 9.382169495545424454 ) ) ;
#11787=CARTESIAN_POINT ( 'NONE',  ( 12.63842701281683034, 22.46726448433411605, 9.846743663894596210 ) ) ;
#11790=CARTESIAN_POINT ( 'NONE',  ( 2.035157376598824452, 3.688685344154837953, 7.964842623401179544 ) ) ;
#11791=CARTESIAN_POINT ( 'NONE',  ( -4.164238869374098151, 46.59541550158063927, -3.795296366450310543 ) ) ;
#11792=CARTESIAN_POINT ( 'NONE',  ( -0.8801773607111008646, 33.27201867748817676, 2.915334737309923430 ) ) ;
#11793=CARTESIAN_POINT ( 'NONE',  ( 7.084665262690076126, 52.02201867748816255, -10.88017736071110164 ) ) ;
#11797=CARTESIAN_POINT ( 'NONE',  ( 7.361572987183170547, 7.050597817667451750, 9.846743663894590881 ) ) ;
#11800=CARTESIAN_POINT ( 'NONE',  ( 12.63842701281683034, 27.46726448433411250, 9.846743663894596210 ) ) ;
#11801=CARTESIAN_POINT ( 'NONE',  ( 2.791683348922237240, 50.38393115100078035, -7.208316651077763204 ) ) ;
#11803=ORIENTED_EDGE ( 'NONE', *, *, #40200, .F. ) ;
#11804=CARTESIAN_POINT ( 'NONE',  ( 22.81628187352647785, 51.41530133659708923, 3.434112377981063169 ) ) ;
#11807=CARTESIAN_POINT ( 'NONE',  ( 7.084665262690076126, 67.02201867748817676, -10.88017736071110164 ) ) ;
#11808=CARTESIAN_POINT ( 'NONE',  ( 5.076628168052704559, 35.17559781766745175, -8.527530157486179263 ) ) ;
#11809=CARTESIAN_POINT ( 'NONE',  ( -2.266590686148945544, 62.22041550158063927, 7.082119434687048631 ) ) ;
#11810=CARTESIAN_POINT ( 'NONE',  ( 12.63842701281683034, 22.46726448433411605, 9.846743663894596210 ) ) ;
#11812=CARTESIAN_POINT ( 'NONE',  ( 19.84674366389459266, 63.30059781766745886, 2.638427012816836559 ) ) ;
#11813=CARTESIAN_POINT ( 'NONE',  ( 13.79529636645030344, 18.26208216824730002, 14.16423886937410614 ) ) ;
#11814=CARTESIAN_POINT ( 'NONE',  ( 6.204703633549690345, 37.84541550158063927, 14.16423886937410082 ) ) ;
#11815=CARTESIAN_POINT ( 'NONE',  ( 5.076628168052704559, 40.17559781766745175, -8.527530157486179263 ) ) ;
#11817=CARTESIAN_POINT ( 'NONE',  ( 17.96484262340118221, 31.18868534415483751, -7.964842623401177768 ) ) ;
#11819=CARTESIAN_POINT ( 'NONE',  ( 10.00000000000000178, 64.31368534415483396, 10.88017736071110342 ) ) ;
#11820=CARTESIAN_POINT ( 'NONE',  ( -0.1310148450194394409, 0.09385736792626404867, 6.293957503965299516 ) ) ;
#11822=CARTESIAN_POINT ( 'NONE',  ( 21.09922568453594849, 51.20696800326375353, 6.408140936763242479 ) ) ;
#11823=CARTESIAN_POINT ( 'NONE',  ( 10.00000000000000000, 51.81368534415484106, -10.88017736071110342 ) ) ;
#11827=CARTESIAN_POINT ( 'NONE',  ( 4.559911319644449179, 58.89701867748817676, 9.422509992056141925 ) ) ;
#11829=CARTESIAN_POINT ( 'NONE',  ( 0.5774900079438590739, 67.64701867748817676, -5.440088680355550821 ) ) ;
#11830=CARTESIAN_POINT ( 'NONE',  ( -0.8801773607111008646, 18.27201867748817321, 2.915334737309923430 ) ) ;
#11832=CARTESIAN_POINT ( 'NONE',  ( 20.30776406404399026, 0.000000000000000000, 6.000000000000280664 ) ) ;
#11833=CARTESIAN_POINT ( 'NONE',  ( 4.559911319644449179, 3.897018677488171434, 9.422509992056141925 ) ) ;
#11834=CARTESIAN_POINT ( 'NONE',  ( 18.52753015748617571, 13.09226448433411960, 4.923371831947298993 ) ) ;
#11835=CARTESIAN_POINT ( 'NONE',  ( 24.16423886937410614, 19.30374883491397142, 8.672049930838204340E-16 ) ) ;
#11836=B_SPLINE_CURVE_WITH_KNOTS ( 'NONE', 3,
 ( #54482, #39507, #30008, #69505 ),
 .UNSPECIFIED., .F., .F.,
 ( 4, 4 ),
 ( 0.000000000000000000, 0.001036303429213355533 ),
 .UNSPECIFIED. ) ;
#11837=CARTESIAN_POINT ( 'NONE',  ( 17.96484262340118221, 26.18868534415483396, -7.964842623401177768 ) ) ;
#11838=CARTESIAN_POINT ( 'NONE',  ( 18.52753015748618282, 53.92559781766745175, -4.923371831947291888 ) ) ;
#11840=CARTESIAN_POINT ( 'NONE',  ( 1.472469842513823179, 55.59226448433412315, -4.923371831947296329 ) ) ;
#11843=CARTESIAN_POINT ( 'NONE',  ( 19.42250999205614548, 55.98035201082150536, -5.440088680355545492 ) ) ;
#11844=CARTESIAN_POINT ( 'NONE',  ( 5.076628168052704559, 45.17559781766745175, -8.527530157486179263 ) ) ;
#11845=CARTESIAN_POINT ( 'NONE',  ( 21.09922568453595559, 42.04030133659708213, -6.408140936763230044 ) ) ;
#11846=CARTESIAN_POINT ( 'NONE',  ( 15.44008868035555260, 9.730352010821505360, 9.422509992056143702 ) ) ;
#11847=FACE_OUTER_BOUND ( 'NONE', #45035, .T. ) ;
#11848=CARTESIAN_POINT ( 'NONE',  ( 20.88017736071110519, 65.56368534415483396, 2.639326808657452039E-16 ) ) ;
#11849=CARTESIAN_POINT ( 'NONE',  ( 0.5774900079438607392, 8.480352010821505360, 5.440088680355550821 ) ) ;
#11851=CARTESIAN_POINT ( 'NONE',  ( 19.38216949554541557, 42.24863466993041783, -9.382169495545420901 ) ) ;
#11852=CARTESIAN_POINT ( 'NONE',  ( 15.44008868035555793, 26.39701867748817321, -9.422509992056140149 ) ) ;
#11853=CARTESIAN_POINT ( 'NONE',  ( 19.67388390623025529, 90.60261632297043377, 5.439653449514034733 ) ) ;
#11854=ADVANCED_FACE ( 'NONE', ( #63715 ), #2766, .T. ) ;
#11856=B_SPLINE_CURVE_WITH_KNOTS ( 'NONE', 3,
 ( #34888, #80405, #88889, #19893 ),
 .UNSPECIFIED., .F., .F.,
 ( 4, 4 ),
 ( 0.000000000000000000, 0.001036303429213364423 ),
 .UNSPECIFIED. ) ;
#11857=CARTESIAN_POINT ( 'NONE',  ( 0.6178305044545818747, 43.49863466993042493, -9.382169495545419124 ) ) ;
#11858=CARTESIAN_POINT ( 'NONE',  ( 20.88017736071110875, 40.77201867748818387, -2.915334737309920765 ) ) ;
#11859=CARTESIAN_POINT ( 'NONE',  ( 17.20831665107776587, 62.88393115100078745, 7.208316651077764980 ) ) ;
#11861=B_SPLINE_CURVE_WITH_KNOTS ( 'NONE', 3,
 ( #33852, #31206, #267, #75237, #23743, #8235 ),
 .UNSPECIFIED., .F., .F.,
 ( 4, 2, 4 ),
 ( 0.000000000000000000, 0.0002701661927229507859, 0.0005403323854459015719 ),
 .UNSPECIFIED. ) ;
#11862=CARTESIAN_POINT ( 'NONE',  ( 0.1532563361054082862, 56.21726448433411605, 2.638427012816831674 ) ) ;
#11865=CARTESIAN_POINT ( 'NONE',  ( 10.00000000000000000, 54.75893115100078745, -9.846743663894594434 ) ) ;
#11866=CARTESIAN_POINT ( 'NONE',  ( 7.084665262690076126, 27.02201867748817676, -10.88017736071110164 ) ) ;
#11867=( LENGTH_UNIT ( ) NAMED_UNIT ( * ) SI_UNIT ( .MILLI., .METRE. ) );
#11868=CARTESIAN_POINT ( 'NONE',  ( 5.076628168052704559, 35.17559781766745175, -8.527530157486179263 ) ) ;
#11871=CARTESIAN_POINT ( 'NONE',  ( 10.00000000000000178, 37.25893115100078745, 9.846743663894594434 ) ) ;
#11872=CARTESIAN_POINT ( 'NONE',  ( 18.52753015748618282, 8.925597817667451750, -4.923371831947291888 ) ) ;
#11873=PRESENTATION_STYLE_ASSIGNMENT (( #73352 ) ) ;
#11874=CARTESIAN_POINT ( 'NONE',  ( 7.361572987183169658, 64.96726448433412315, -9.846743663894592657 ) ) ;
#11875=ORIENTED_EDGE ( 'NONE', *, *, #9604, .T. ) ;
#11876=CARTESIAN_POINT ( 'NONE',  ( 0.6178305044545838731, 64.74863466993043914, 9.382169495545420901 ) ) ;
#11877=CARTESIAN_POINT ( 'NONE',  ( 16.40814093676324603, 32.45696800326375353, -11.09922568453594671 ) ) ;
#11878=EDGE_CURVE ( 'NONE', #49769, #48349, #96893, .T. ) ;
#11879=CARTESIAN_POINT ( 'NONE',  ( 18.52753015748618282, 38.92559781766745175, -4.923371831947291888 ) ) ;
#11882=CARTESIAN_POINT ( 'NONE',  ( 20.36894250292379382, 53.67874883491397497, 10.36894250292379205 ) ) ;
#11883=CARTESIAN_POINT ( 'NONE',  ( 14.92337183194729633, 37.67559781766745175, 8.527530157486181039 ) ) ;
#11888=CARTESIAN_POINT ( 'NONE',  ( 17.08211943468705130, 58.47041550158063927, 12.26659068614894998 ) ) ;
#11890=CARTESIAN_POINT ( 'NONE',  ( 4.559911319644449179, 7.230352010821505360, -9.422509992056141925 ) ) ;
#11891=CARTESIAN_POINT ( 'NONE',  ( 24.16423886937409904, 34.09541550158064638, 3.795296366450317205 ) ) ;
#11892=CARTESIAN_POINT ( 'NONE',  ( -0.3689425029237898834, 46.17874883491397497, -10.36894250292378850 ) ) ;
#11893=CARTESIAN_POINT ( 'NONE',  ( 1.274849032794116210, 8.572280503510292249, 6.499999999999738876 ) ) ;
#11894=CARTESIAN_POINT ( 'NONE',  ( 18.72515096720569971, 5.055090184799359676, 6.500000000000000000 ) ) ;
#11895=CARTESIAN_POINT ( 'NONE',  ( 18.52753015748617571, 18.09226448433411960, 4.923371831947298993 ) ) ;
#11897=CARTESIAN_POINT ( 'NONE',  ( 3.591859063236763294, 3.290301336597087012, -11.09922568453595026 ) ) ;
#11898=CARTESIAN_POINT ( 'NONE',  ( -0.8801773607111009756, 53.06368534415484106, 1.068504757029289695E-15 ) ) ;
#11900=CARTESIAN_POINT ( 'NONE',  ( 14.92337183194729633, 52.67559781766745175, 8.527530157486181039 ) ) ;
#11902=( BOUNDED_CURVE ( )  B_SPLINE_CURVE ( 2, ( #1712, #85685, #31682, #77679, #23727, #25685, #24697, #78677, #17205 ),
 .UNSPECIFIED., .F., .T. ) 
 B_SPLINE_CURVE_WITH_KNOTS ( ( 3, 2, 2, 2, 3 ),
 ( 0.9034289457926085731, 0.9047619047619047672, 0.9107142857142856984, 0.9166666666666666297, 0.9179996256359628237 ),
 .UNSPECIFIED. ) 
 CURVE ( )  GEOMETRIC_REPRESENTATION_ITEM ( )  RATIONAL_B_SPLINE_CURVE ( ( 0.9881565478350746723, 0.9923695281211503127, 1.000000000000000000, 0.9659258262890683122, 1.000000000000000000, 0.9659258262890683122, 1.000000000000000000, 0.9923695281211504238, 0.9881565478350746723 ) ) 
 REPRESENTATION_ITEM ( '' )  );
#11903=CARTESIAN_POINT ( 'NONE',  ( 17.20831665107776587, 54.13393115100079456, -7.208316651077762316 ) ) ;
#11906=CARTESIAN_POINT ( 'NONE',  ( 17.08211943468705130, 28.47041550158063572, 12.26659068614894998 ) ) ;
#11907=CARTESIAN_POINT ( 'NONE',  ( -0.1503990784575280903, 38.10158574516643171, 6.262539305110076171 ) ) ;
#11909=CARTESIAN_POINT ( 'NONE',  ( 19.42250999205614193, 25.14701867748817321, 5.440088680355555262 ) ) ;
#11910=CARTESIAN_POINT ( 'NONE',  ( 6.565887622018943937, 20.16530133659708213, 12.81628187352647430 ) ) ;
#11912=CARTESIAN_POINT ( 'NONE',  ( 0.1532563361054083140, 16.00893115100078390, 1.131784320476157264E-15 ) ) ;
#11913=CARTESIAN_POINT ( 'NONE',  ( 22.81628187352647785, 61.41530133659709634, 3.434112377981063169 ) ) ;
#11916=CARTESIAN_POINT ( 'NONE',  ( 2.917880565312948704, 32.63708216824730357, 12.26659068614894643 ) ) ;
#11917=CARTESIAN_POINT ( 'NONE',  ( 15.44008868035555793, 11.39701867748817143, -9.422509992056140149 ) ) ;
#11920=CARTESIAN_POINT ( 'NONE',  ( 0.5774900079438590739, 37.64701867748817676, -5.440088680355550821 ) ) ;
#11921=CARTESIAN_POINT ( 'NONE',  ( 2.035157376598822676, 52.43868534415483396, -7.964842623401177768 ) ) ;
#11922=CARTESIAN_POINT ( 'NONE',  ( 0.6178305044545818747, 13.49863466993041783, -9.382169495545419124 ) ) ;
#11923=CARTESIAN_POINT ( 'NONE',  ( 19.84674366389459266, 63.71726448433412315, -2.638427012816827677 ) ) ;
#11925=CARTESIAN_POINT ( 'NONE',  ( 10.00000000000000178, 7.258931151000785675, 9.846743663894594434 ) ) ;
#11928=CARTESIAN_POINT ( 'NONE',  ( 17.96484262340118221, 49.93868534415484106, 7.964842623401181321 ) ) ;
#11930=CARTESIAN_POINT ( 'NONE',  ( 16.40814093676324603, 7.456968003263754419, -11.09922568453594671 ) ) ;
#11931=CARTESIAN_POINT ( 'NONE',  ( 19.42250999205614548, 65.98035201082151957, -5.440088680355545492 ) ) ;
#11932=CARTESIAN_POINT ( 'NONE',  ( 19.84674366389459266, 18.71726448433411960, -2.638427012816827677 ) ) ;
#11933=CARTESIAN_POINT ( 'NONE',  ( 13.43411237798106583, 52.66530133659708213, -12.81628187352647252 ) ) ;
#11934=CARTESIAN_POINT ( 'NONE',  ( 7.361572987183169658, -0.03273551566588185635, -9.846743663894592657 ) ) ;
#11935=ORIENTED_EDGE ( 'NONE', *, *, #70927, .T. ) ;
#11936=CARTESIAN_POINT ( 'NONE',  ( 1.821708436314942503, 56.66792564121897158, -6.500000000000043521 ) ) ;
#11937=CARTESIAN_POINT ( 'NONE',  ( 0.2751277870542889192, 28.21833443783938122, 6.499999999999990230 ) ) ;
#11938=CARTESIAN_POINT ( 'NONE',  ( 17.96484262340118221, 24.93868534415484461, 7.964842623401181321 ) ) ;
#11939=CARTESIAN_POINT ( 'NONE',  ( 10.00000000000000178, 60.37363466993041783, 12.81628187352647608 ) ) ;
#11940=CARTESIAN_POINT ( 'NONE',  ( 2.791683348922240793, 36.63393115100078035, 7.208316651077764092 ) ) ;
#11941=CARTESIAN_POINT ( 'NONE',  ( 2.035157376598824452, 23.68868534415484461, 7.964842623401179544 ) ) ;
#11942=CARTESIAN_POINT ( 'NONE',  ( 10.00000000000000000, 65.55374883491396076, -14.16423886937410082 ) ) ;
#11945=B_SPLINE_CURVE_WITH_KNOTS ( 'NONE', 3,
 ( #16688, #69683, #18161, #55667, #1214, #40170 ),
 .UNSPECIFIED., .F., .F.,
 ( 4, 2, 4 ),
 ( 0.000000000000000000, 0.0002626113303184855600, 0.0005252226606369711200 ),
 .UNSPECIFIED. ) ;
#11946=CARTESIAN_POINT ( 'NONE',  ( 2.035157376598822676, 12.43868534415483751, -7.964842623401177768 ) ) ;
#11947=CARTESIAN_POINT ( 'NONE',  ( 2.035157376598824452, 28.68868534415484106, 7.964842623401179544 ) ) ;
#11949=CARTESIAN_POINT ( 'NONE',  ( 7.084665262690076126, 32.02201867748816966, -10.88017736071110164 ) ) ;
#11951=CARTESIAN_POINT ( 'NONE',  ( 0.1532563361054083140, 61.00893115100078745, 1.131784320476157264E-15 ) ) ;
#11952=CARTESIAN_POINT ( 'NONE',  ( 2.035157376598822676, 27.43868534415483396, -7.964842623401177768 ) ) ;
#11953=CARTESIAN_POINT ( 'NONE',  ( 18.52753015748618282, 63.92559781766745886, -4.923371831947291888 ) ) ;
#11954=CARTESIAN_POINT ( 'NONE',  ( 19.72487221294570858, 70.00000000000000000, -6.000000000000000000 ) ) ;
#11955=CARTESIAN_POINT ( 'NONE',  ( 6.565887622018943937, 58.08196800326376064, -12.81628187352647608 ) ) ;
#11956=CARTESIAN_POINT ( 'NONE',  ( -4.164238869374099039, 31.80374883491396432, 8.674139862899312516E-16 ) ) ;
#11957=CARTESIAN_POINT ( 'NONE',  ( 2.035157376598824452, 33.68868534415484106, 7.964842623401179544 ) ) ;
#11958=CARTESIAN_POINT ( 'NONE',  ( 7.084665262690076126, 17.02201867748817676, -10.88017736071110164 ) ) ;
#11959=CARTESIAN_POINT ( 'NONE',  ( 3.208591742434494964, 70.37446617634741131, -5.000000000000000000 ) ) ;
#11960=CARTESIAN_POINT ( 'NONE',  ( 14.92337183194729633, 52.67559781766745175, 8.527530157486181039 ) ) ;
#11962=CARTESIAN_POINT ( 'NONE',  ( -0.1503990784575247319, 22.22266099184918886, -6.262539305110083276 ) ) ;
#11963=CARTESIAN_POINT ( 'NONE',  ( 19.84674366389459621, 18.50893115100078745, 7.409399052514197653E-17 ) ) ;
#11965=CARTESIAN_POINT ( 'NONE',  ( 7.084665262690076126, 7.022018677488169658, -10.88017736071110164 ) ) ;
#11966=CARTESIAN_POINT ( 'NONE',  ( 5.076628168052703671, 6.842264484334118713, 8.527530157486179263 ) ) ;
#11967=CARTESIAN_POINT ( 'NONE',  ( 10.00000000000000178, 15.37363466993042138, 12.81628187352647608 ) ) ;
#11968=CARTESIAN_POINT ( 'NONE',  ( 12.91533473730992121, 59.52201867748816966, 10.88017736071110164 ) ) ;
#11969=CARTESIAN_POINT ( 'NONE',  ( 15.44008868035555793, 21.39701867748817321, -9.422509992056140149 ) ) ;
#11970=CARTESIAN_POINT ( 'NONE',  ( 6.565887622018943937, 63.08196800326376064, -12.81628187352647608 ) ) ;
#11971=CARTESIAN_POINT ( 'NONE',  ( 10.00000000000000178, 33.05374883491396787, 14.16423886937410082 ) ) ;
#11972=SURFACE_STYLE_FILL_AREA ( #80474 ) ;
#11976=CARTESIAN_POINT ( 'NONE',  ( 0.6178305044545818747, 58.49863466993042493, -9.382169495545419124 ) ) ;
#11978=VERTEX_POINT ( 'NONE', #27689 ) ;
#11979=CARTESIAN_POINT ( 'NONE',  ( -2.816281873526473856, 4.331968003263754419, 3.434112377981055619 ) ) ;
#11980=CARTESIAN_POINT ( 'NONE',  ( 19.39188664607694790, 20.83703382326399733, -6.499999999999962697 ) ) ;
#11981=CARTESIAN_POINT ( 'NONE',  ( -0.8801773607110991993, 32.85535201082151247, -2.915334737309923874 ) ) ;
#11984=CARTESIAN_POINT ( 'NONE',  ( 17.20831665107776587, 19.13393115100078035, -7.208316651077762316 ) ) ;
#11985=CARTESIAN_POINT ( 'NONE',  ( 14.92337183194729633, 7.675597817667451750, 8.527530157486181039 ) ) ;
#11986=CARTESIAN_POINT ( 'NONE',  ( 0.1532563361054083140, 26.00893115100078745, 1.131784320476157264E-15 ) ) ;
#11987=CARTESIAN_POINT ( 'NONE',  ( 1.472469842513823179, 15.59226448433411960, -4.923371831947296329 ) ) ;
#11988=FILL_AREA_STYLE_COLOUR ( '', #12312 ) ;
#11989=CIRCLE ( 'NONE', #34383, 0.5000000000000004441 ) ;
#11990=CARTESIAN_POINT ( 'NONE',  ( -0.8801773607110991993, 67.85535201082151957, -2.915334737309923874 ) ) ;
#11991=DIRECTION ( 'NONE',  ( 0.000000000000000000, 0.000000000000000000, -1.000000000000000000 ) ) ;
#11992=CARTESIAN_POINT ( 'NONE',  ( 14.92337183194729633, 7.675597817667451750, 8.527530157486181039 ) ) ;
#11993=CARTESIAN_POINT ( 'NONE',  ( 0.1532563361054100626, 25.80059781766744820, -2.638427012816831230 ) ) ;
#11996=CARTESIAN_POINT ( 'NONE',  ( 19.38216949554541202, 0.9986346699304200492, 9.382169495545424454 ) ) ;
#11999=CARTESIAN_POINT ( 'NONE',  ( 15.44008868035555793, 6.397018677488170546, -9.422509992056140149 ) ) ;
#12000=CARTESIAN_POINT ( 'NONE',  ( 17.08211943468705840, 20.13708216824730357, -12.26659068614894466 ) ) ;
#12003=CARTESIAN_POINT ( 'NONE',  ( 10.00000000000000000, 20.55374883491396787, -14.16423886937410082 ) ) ;
#12004=CARTESIAN_POINT ( 'NONE',  ( -4.164238869374098151, 36.59541550158063217, -3.795296366450310543 ) ) ;
#12005=SURFACE_SIDE_STYLE ('',( #87016 ) ) ;
#12007=CARTESIAN_POINT ( 'NONE',  ( -0.8801773607110991993, 37.85535201082151247, -2.915334737309923874 ) ) ;
#12009=CIRCLE ( 'NONE', #95079, 1.000000000000000888 ) ;
#12010=ORIENTED_EDGE ( 'NONE', *, *, #27413, .F. ) ;
#12011=CARTESIAN_POINT ( 'NONE',  ( 17.20831665107776587, 19.13393115100078035, -7.208316651077762316 ) ) ;
#12012=CARTESIAN_POINT ( 'NONE',  ( 0.5774900079438590739, 62.64701867748817676, -5.440088680355550821 ) ) ;
#12013=CARTESIAN_POINT ( 'NONE',  ( 1.472469842513823179, 16.42559781766745175, 4.923371831947296329 ) ) ;
#12014=CARTESIAN_POINT ( 'NONE',  ( 0.5774900079438590739, 7.647018677488171434, -5.440088680355550821 ) ) ;
#12015=CARTESIAN_POINT ( 'NONE',  ( -2.816281873526473856, 49.12363466993042493, 9.499525473075851096E-16 ) ) ;
#12016=CARTESIAN_POINT ( 'NONE',  ( 1.472469842513823179, 56.42559781766745886, 4.923371831947296329 ) ) ;
#12017=CARTESIAN_POINT ( 'NONE',  ( 19.84674366389459266, 58.71726448433412315, -2.638427012816827677 ) ) ;
#12018=CARTESIAN_POINT ( 'NONE',  ( 10.00000000000000000, 32.87363466993042493, -12.81628187352647608 ) ) ;
#12020=CARTESIAN_POINT ( 'NONE',  ( 7.361572987183169658, 34.96726448433411605, -9.846743663894592657 ) ) ;
#12021=CARTESIAN_POINT ( 'NONE',  ( 13.79529636645030344, 8.262082168247300018, 14.16423886937410614 ) ) ;
#12025=CARTESIAN_POINT ( 'NONE',  ( 4.559911319644449179, 47.23035201082150536, -9.422509992056141925 ) ) ;
#12026=CARTESIAN_POINT ( 'NONE',  ( 7.084665262690076126, 47.02201867748818387, -10.88017736071110164 ) ) ;
#12027=CARTESIAN_POINT ( 'NONE',  ( 6.204703633549690345, 45.76208216824729647, -14.16423886937410259 ) ) ;
#12028=CARTESIAN_POINT ( 'NONE',  ( 0.1532563361054083140, 61.00893115100078745, 1.131784320476157264E-15 ) ) ;
#12029=CARTESIAN_POINT ( 'NONE',  ( 10.00000000000000000, 62.87363466993042493, -12.81628187352647608 ) ) ;
#12030=CARTESIAN_POINT ( 'NONE',  ( 4.559911319644449179, 37.23035201082150536, -9.422509992056141925 ) ) ;
#12032=CARTESIAN_POINT ( 'NONE',  ( 22.81628187352647785, 21.41530133659708923, 3.434112377981063169 ) ) ;
#12033=CARTESIAN_POINT ( 'NONE',  ( 19.84674366389459266, 53.30059781766744464, 2.638427012816836559 ) ) ;
#12035=CARTESIAN_POINT ( 'NONE',  ( -0.8801773607111008646, 63.27201867748817676, 2.915334737309923430 ) ) ;
#12036=CARTESIAN_POINT ( 'NONE',  ( -0.8801773607111009756, 3.063685344154837509, 1.068504757029289695E-15 ) ) ;
#12037=CARTESIAN_POINT ( 'NONE',  ( 1.816707512666844604, 60.10290668512023871, -6.499999999999958256 ) ) ;
#12038=CARTESIAN_POINT ( 'NONE',  ( 0.1532563361054100626, 0.8005978176674514168, -2.638427012816831230 ) ) ;
#12039=CARTESIAN_POINT ( 'NONE',  ( -0.8801773607111009756, 68.06368534415484817, 1.068504757029289695E-15 ) ) ;
#12042=CARTESIAN_POINT ( 'NONE',  ( 18.52753015748618282, 28.92559781766745175, -4.923371831947291888 ) ) ;
#12043=CARTESIAN_POINT ( 'NONE',  ( 0.5774900079438590739, 27.64701867748817676, -5.440088680355550821 ) ) ;
#12044=CARTESIAN_POINT ( 'NONE',  ( 22.81628187352647785, 11.41530133659708390, 3.434112377981063169 ) ) ;
#12045=CARTESIAN_POINT ( 'NONE',  ( 7.084665262690076126, 32.02201867748816966, -10.88017736071110164 ) ) ;
#12047=CARTESIAN_POINT ( 'NONE',  ( 13.43411237798106583, 32.66530133659708213, -12.81628187352647252 ) ) ;
#12049=FACE_OUTER_BOUND ( 'NONE', #23072, .T. ) ;
#12050=CARTESIAN_POINT ( 'NONE',  ( 19.38216949554541202, 20.99863466993042138, 9.382169495545424454 ) ) ;
#12053=CARTESIAN_POINT ( 'NONE',  ( -0.8801773607111008646, 28.27201867748817321, 2.915334737309923430 ) ) ;
#12054=CARTESIAN_POINT ( 'NONE',  ( 24.16423886937409904, 59.09541550158063217, 3.795296366450317205 ) ) ;
#12055=CARTESIAN_POINT ( 'NONE',  ( 19.84674366389459266, 48.30059781766745175, 2.638427012816836559 ) ) ;
#12056=CARTESIAN_POINT ( 'NONE',  ( 12.63842701281683922, 9.550597817667449974, -9.846743663894590881 ) ) ;
#12057=CARTESIAN_POINT ( 'NONE',  ( 17.96484262340118221, 64.93868534415483396, 7.964842623401181321 ) ) ;
#12059=CARTESIAN_POINT ( 'NONE',  ( 10.00000000000000000, 30.55374883491397142, -14.16423886937410082 ) ) ;
#12060=( GEOMETRIC_REPRESENTATION_CONTEXT ( 3 ) GLOBAL_UNCERTAINTY_ASSIGNED_CONTEXT ( ( #4319 ) ) GLOBAL_UNIT_ASSIGNED_CONTEXT ( ( #64257, #56772, #49271 ) ) REPRESENTATION_CONTEXT ( 'NONE', 'WORKASPACE' ) );
#12065=CARTESIAN_POINT ( 'NONE',  ( 22.26659068614895176, 54.72041550158063217, -7.082119434687042414 ) ) ;
#12066=CARTESIAN_POINT ( 'NONE',  ( 17.08211943468705840, 45.13708216824730357, -12.26659068614894466 ) ) ;
#12067=CARTESIAN_POINT ( 'NONE',  ( 14.92337183194729633, 17.67559781766745175, 8.527530157486181039 ) ) ;
#12069=CARTESIAN_POINT ( 'NONE',  ( 16.40814093676323893, 30.79030133659708923, 11.09922568453595026 ) ) ;
#12072=SURFACE_STYLE_FILL_AREA ( #42574 ) ;
#12073=CARTESIAN_POINT ( 'NONE',  ( -2.266590686148945544, 37.22041550158063217, 7.082119434687048631 ) ) ;
#12074=CARTESIAN_POINT ( 'NONE',  ( 10.00000000000000178, 7.258931151000785675, 9.846743663894594434 ) ) ;
#12080=ADVANCED_FACE ( 'NONE', ( #34692 ), #3733, .T. ) ;
#12082=CARTESIAN_POINT ( 'NONE',  ( -4.164238869374098151, 11.59541550158063217, -3.795296366450310543 ) ) ;
#12083=CARTESIAN_POINT ( 'NONE',  ( 15.44008868035555793, 26.39701867748817321, -9.422509992056140149 ) ) ;
#12084=CARTESIAN_POINT ( 'NONE',  ( 4.559911319644449179, 22.23035201082150536, -9.422509992056141925 ) ) ;
#12085=CARTESIAN_POINT ( 'NONE',  ( 2.791683348922240793, 51.63393115100078745, 7.208316651077764092 ) ) ;
#12086=CARTESIAN_POINT ( 'NONE',  ( -2.816281873526473856, 19.33196800326375708, 3.434112377981055619 ) ) ;
#12092=CARTESIAN_POINT ( 'NONE',  ( -1.099225684535947600, 14.54030133659708568, 6.408140936763237150 ) ) ;
#12094=VERTEX_POINT ( 'NONE', #42703 ) ;
#12095=CARTESIAN_POINT ( 'NONE',  ( 1.472469842513823179, 26.42559781766745175, 4.923371831947296329 ) ) ;
#12096=CARTESIAN_POINT ( 'NONE',  ( -4.164238869374099039, 66.80374883491396076, 8.674139862899312516E-16 ) ) ;
#12097=EDGE_LOOP ( 'NONE', ( #4844, #67880, #1063, #67306 ) ) ;
#12098=CARTESIAN_POINT ( 'NONE',  ( -0.8801773607111008646, 8.272018677488171434, 2.915334737309923430 ) ) ;
#12100=CARTESIAN_POINT ( 'NONE',  ( 19.42250999205614548, 40.98035201082150536, -5.440088680355545492 ) ) ;
#12101=CARTESIAN_POINT ( 'NONE',  ( 20.88017736071110875, 50.77201867748817676, -2.915334737309920765 ) ) ;
#12102=CARTESIAN_POINT ( 'NONE',  ( -0.8801773607110991993, 57.85535201082149825, -2.915334737309923874 ) ) ;
#12103=CARTESIAN_POINT ( 'NONE',  ( 20.03932841506543738, 5.621614419605015733, -6.397827110478957024 ) ) ;
#12104=CARTESIAN_POINT ( 'NONE',  ( 10.00000000000000178, 39.31368534415484106, 10.88017736071110342 ) ) ;
#12108=CARTESIAN_POINT ( 'NONE',  ( 0.1532563361054100626, 20.80059781766744464, -2.638427012816831230 ) ) ;
#12109=ORIENTED_EDGE ( 'NONE', *, *, #85272, .T. ) ;
#12110=CARTESIAN_POINT ( 'NONE',  ( 1.472469842513823179, 51.42559781766745886, 4.923371831947296329 ) ) ;
#12111=CARTESIAN_POINT ( 'NONE',  ( 1.274849032794292736, 62.55509018479936145, -6.499999999999977796 ) ) ;
#12116=CARTESIAN_POINT ( 'NONE',  ( 17.20831665107776587, 64.13393115100079456, -7.208316651077762316 ) ) ;
#12117=CARTESIAN_POINT ( 'NONE',  ( 10.00000000000000178, 32.25893115100078745, 9.846743663894594434 ) ) ;
#12118=CARTESIAN_POINT ( 'NONE',  ( -4.164238869374099927, 67.01208216824728936, 3.795296366450308767 ) ) ;
#12120=ORIENTED_EDGE ( 'NONE', *, *, #13330, .F. ) ;
#12122=CARTESIAN_POINT ( 'NONE',  ( 5.076628168052703671, 36.84226448433412315, 8.527530157486179263 ) ) ;
#12123=CARTESIAN_POINT ( 'NONE',  ( -1.099225684535947600, 64.54030133659709634, 6.408140936763237150 ) ) ;
#12125=CARTESIAN_POINT ( 'NONE',  ( 3.591859063236763294, 3.290301336597087012, -11.09922568453595026 ) ) ;
#12126=CARTESIAN_POINT ( 'NONE',  ( 17.20831665107776587, 7.883931151000784787, 7.208316651077764980 ) ) ;
#12128=CARTESIAN_POINT ( 'NONE',  ( 2.791683348922237240, 5.383931151000785675, -7.208316651077763204 ) ) ;
#12129=CARTESIAN_POINT ( 'NONE',  ( 12.63842701281683034, 57.46726448433411605, 9.846743663894596210 ) ) ;
#12133=CARTESIAN_POINT ( 'NONE',  ( 20.88017736071110164, 10.35535201082150714, 2.915334737309930979 ) ) ;
#12134=CARTESIAN_POINT ( 'NONE',  ( 18.52753015748617571, 13.09226448433411960, 4.923371831947298993 ) ) ;
#12135=CARTESIAN_POINT ( 'NONE',  ( 20.88017736071110164, 45.35535201082149115, 2.915334737309930979 ) ) ;
#12136=CARTESIAN_POINT ( 'NONE',  ( 13.43411237798105340, 25.58196800326374998, 12.81628187352647963 ) ) ;
#12140=CARTESIAN_POINT ( 'NONE',  ( 22.81628187352648496, 6.831968003263753531, -3.434112377981050290 ) ) ;
#12141=CARTESIAN_POINT ( 'NONE',  ( 19.84674366389459621, 63.50893115100078745, 7.409399052514197653E-17 ) ) ;
#12142=CARTESIAN_POINT ( 'NONE',  ( 10.00000000000000178, 12.25893115100078568, 9.846743663894594434 ) ) ;
#12144=CARTESIAN_POINT ( 'NONE',  ( 10.00000000000000000, 22.87363466993042138, -12.81628187352647608 ) ) ;
#12145=CARTESIAN_POINT ( 'NONE',  ( 1.711636803080569313, 51.84492782695771496, -6.500000000000077272 ) ) ;
#12146=CARTESIAN_POINT ( 'NONE',  ( -0.8801773607111008646, 28.27201867748817321, 2.915334737309923430 ) ) ;
#12149=CARTESIAN_POINT ( 'NONE',  ( -0.3689425029237898834, 51.17874883491397497, -10.36894250292378850 ) ) ;
#12151=CARTESIAN_POINT ( 'NONE',  ( 13.43411237798105340, 35.58196800326375353, 12.81628187352647963 ) ) ;
#12152=CARTESIAN_POINT ( 'NONE',  ( 17.96484262340118221, 21.18868534415483396, -7.964842623401177768 ) ) ;
#12155=CARTESIAN_POINT ( 'NONE',  ( 12.63842701281683922, 54.55059781766745175, -9.846743663894590881 ) ) ;
#12156=CARTESIAN_POINT ( 'NONE',  ( 12.91533473730992121, 49.52201867748817676, 10.88017736071110164 ) ) ;
#12157=CARTESIAN_POINT ( 'NONE',  ( -0.3689425029237898834, 36.17874883491396787, -10.36894250292378850 ) ) ;
#12159=CARTESIAN_POINT ( 'NONE',  ( 17.20831665107776587, 27.88393115100078390, 7.208316651077764980 ) ) ;
#12160=SURFACE_STYLE_FILL_AREA ( #73144 ) ;
#12161=CARTESIAN_POINT ( 'NONE',  ( 0.6178305044545818747, 3.498634669930420049, -9.382169495545419124 ) ) ;
#12163=CARTESIAN_POINT ( 'NONE',  ( 20.15039907845753930, 11.74884699246888964, 6.262539305110064625 ) ) ;
#12164=CARTESIAN_POINT ( 'NONE',  ( 20.88017736071110164, 15.35535201082150358, 2.915334737309930979 ) ) ;
#12165=CARTESIAN_POINT ( 'NONE',  ( -4.164238869374098151, 21.59541550158063217, -3.795296366450310543 ) ) ;
#12167=CARTESIAN_POINT ( 'NONE',  ( 5.076628168052704559, 15.17559781766745175, -8.527530157486179263 ) ) ;
#12168=CARTESIAN_POINT ( 'NONE',  ( 12.63842701281683922, 64.55059781766745175, -9.846743663894590881 ) ) ;
#12169=CARTESIAN_POINT ( 'NONE',  ( 20.88017736071110164, 30.35535201082151247, 2.915334737309930979 ) ) ;
#12170=( BOUNDED_CURVE ( )  B_SPLINE_CURVE ( 2, ( #46006, #52995, #24000, #54959, #84980, #15027, #8979, #7528, #85480 ),
 .UNSPECIFIED., .F., .F. ) 
 B_SPLINE_CURVE_WITH_KNOTS ( ( 3, 2, 2, 2, 3 ),
 ( 0.1891432315068940218, 0.1904761904761904656, 0.1964285714285714246, 0.2023809523809523836, 0.2037139113502489662 ),
 .UNSPECIFIED. ) 
 CURVE ( )  GEOMETRIC_REPRESENTATION_ITEM ( )  RATIONAL_B_SPLINE_CURVE ( ( 0.9881565478350731180, 0.9923695281211488695, 1.000000000000000000, 0.9659258262890683122, 1.000000000000000000, 0.9659258262890683122, 1.000000000000000000, 0.9923695281211482033, 0.9881565478350723408 ) ) 
 REPRESENTATION_ITEM ( '' )  );
#12172=CARTESIAN_POINT ( 'NONE',  ( -44.74606106857038412, 105.1870489192399845, -5.398875195867286259 ) ) ;
#12173=EDGE_CURVE ( 'NONE', #31069, #97822, #30004, .T. ) ;
#12175=CARTESIAN_POINT ( 'NONE',  ( 1.472469842513823179, 40.59226448433411605, -4.923371831947296329 ) ) ;
#12179=CARTESIAN_POINT ( 'NONE',  ( 10.00000000000000178, 3.053748834913967425, 14.16423886937410082 ) ) ;
#12180=CARTESIAN_POINT ( 'NONE',  ( 6.204703633549690345, 10.76208216824729824, -14.16423886937410259 ) ) ;
#12181=CARTESIAN_POINT ( 'NONE',  ( -0.8801773607110991993, 47.85535201082150536, -2.915334737309923874 ) ) ;
#12182=CARTESIAN_POINT ( 'NONE',  ( -4.164238869374099039, 61.80374883491397497, 8.674139862899312516E-16 ) ) ;
#12183=CARTESIAN_POINT ( 'NONE',  ( 7.361572987183170547, 67.05059781766746596, 9.846743663894590881 ) ) ;
#12184=CARTESIAN_POINT ( 'NONE',  ( 7.361572987183169658, 34.96726448433411605, -9.846743663894592657 ) ) ;
#12186=CARTESIAN_POINT ( 'NONE',  ( 20.88017736071110519, 30.56368534415484106, 2.639326808657452039E-16 ) ) ;
#12187=CARTESIAN_POINT ( 'NONE',  ( -1.099225684535947600, 8.706968003263753531, -6.408140936763238038 ) ) ;
#12188=CARTESIAN_POINT ( 'NONE',  ( 13.79529636645031943, 50.34541550158064638, -14.16423886937409904 ) ) ;
#12189=CARTESIAN_POINT ( 'NONE',  ( 4.559911319644449179, 7.230352010821505360, -9.422509992056141925 ) ) ;
#12190=CARTESIAN_POINT ( 'NONE',  ( -0.2002127540270661199, 0.02465945891864366329, 6.181800700214927780 ) ) ;
#12196=ORIENTED_EDGE ( 'NONE', *, *, #39446, .F. ) ;
#12198=CARTESIAN_POINT ( 'NONE',  ( -4.164238869374098151, 51.59541550158063217, -3.795296366450310543 ) ) ;
#12199=CARTESIAN_POINT ( 'NONE',  ( 10.00000000000000178, 32.25893115100078745, 9.846743663894594434 ) ) ;
#12200=CARTESIAN_POINT ( 'NONE',  ( 17.96484262340118221, 56.18868534415484817, -7.964842623401177768 ) ) ;
#12201=CARTESIAN_POINT ( 'NONE',  ( 19.72487221294570858, 36.86607318730075633, 6.500000000000000888 ) ) ;
#12202=CARTESIAN_POINT ( 'NONE',  ( 20.88017736071110519, 60.56368534415484106, 2.639326808657452039E-16 ) ) ;
#12204=EDGE_CURVE ( 'NONE', #651, #3863, #90651, .T. ) ;
#12205=CARTESIAN_POINT ( 'NONE',  ( 22.81628187352648496, 56.83196800326374643, -3.434112377981050290 ) ) ;
#12209=CARTESIAN_POINT ( 'NONE',  ( 6.204703633549690345, 22.84541550158062861, 14.16423886937410082 ) ) ;
#12211=CARTESIAN_POINT ( 'NONE',  ( 3.591859063236763294, 23.29030133659708568, -11.09922568453595026 ) ) ;
#12213=CARTESIAN_POINT ( 'NONE',  ( -2.816281873526473856, 49.12363466993042493, 9.499525473075851096E-16 ) ) ;
#12214=CARTESIAN_POINT ( 'NONE',  ( 14.92337183194729988, 19.34226448433411960, -8.527530157486177487 ) ) ;
#12215=CARTESIAN_POINT ( 'NONE',  ( 0.5774900079438607392, 18.48035201082150536, 5.440088680355550821 ) ) ;
#12216=CARTESIAN_POINT ( 'NONE',  ( 3.591859063236761518, 54.95696800326376064, 11.09922568453594849 ) ) ;
#12217=CARTESIAN_POINT ( 'NONE',  ( 14.92337183194729633, 37.67559781766745175, 8.527530157486181039 ) ) ;
#12218=COLOUR_RGB ( '', 0.66274510, 0.83137255, 0.94901961) ;
#12220=EDGE_LOOP ( 'NONE', ( #19228, #69543, #61895, #7567 ) ) ;
#12221=CARTESIAN_POINT ( 'NONE',  ( 17.96484262340118221, 66.18868534415483396, -7.964842623401177768 ) ) ;
#12223=STYLED_ITEM ( 'NONE', ( #44071 ), #88026 ) ;
#12225=CARTESIAN_POINT ( 'NONE',  ( 17.20831665107776587, 12.88393115100078390, 7.208316651077764980 ) ) ;
#12226=CARTESIAN_POINT ( 'NONE',  ( 16.40814093676323893, 20.79030133659708923, 11.09922568453595026 ) ) ;
#12229=CARTESIAN_POINT ( 'NONE',  ( 12.63842701281683922, 44.55059781766745175, -9.846743663894590881 ) ) ;
#12231=CARTESIAN_POINT ( 'NONE',  ( 2.917880565312948704, 22.63708216824730002, 12.26659068614894643 ) ) ;
#12232=CARTESIAN_POINT ( 'NONE',  ( 2.791683348922237240, 30.38393115100078390, -7.208316651077763204 ) ) ;
#12233=CARTESIAN_POINT ( 'NONE',  ( 10.00000000000000000, 47.87363466993042493, -12.81628187352647608 ) ) ;
#12235=CARTESIAN_POINT ( 'NONE',  ( 1.274849032794199255, 23.57228050351030646, 6.499999999999850786 ) ) ;
#12236=CARTESIAN_POINT ( 'NONE',  ( 15.44008868035555260, 59.73035201082151247, 9.422509992056143702 ) ) ;
#12237=CARTESIAN_POINT ( 'NONE',  ( 6.565887622018943937, 15.16530133659708568, 12.81628187352647430 ) ) ;
#12239=CARTESIAN_POINT ( 'NONE',  ( 7.361572987183170547, 37.05059781766744464, 9.846743663894590881 ) ) ;
#12240=CARTESIAN_POINT ( 'NONE',  ( 10.00000000000000000, 31.81368534415483751, -10.88017736071110342 ) ) ;
#12241=CARTESIAN_POINT ( 'NONE',  ( 6.565887622018943937, 35.16530133659708923, 12.81628187352647430 ) ) ;
#12242=VECTOR ( 'NONE', #66735, 1000.000000000000000 ) ;
#12243=CARTESIAN_POINT ( 'NONE',  ( 2.791683348922240793, 36.63393115100078035, 7.208316651077764092 ) ) ;
#12247=CARTESIAN_POINT ( 'NONE',  ( 20.88017736071110875, 35.77201867748816966, -2.915334737309920765 ) ) ;
#12250=CARTESIAN_POINT ( 'NONE',  ( 2.035157376598824452, 3.688685344154837953, 7.964842623401179544 ) ) ;
#12251=CARTESIAN_POINT ( 'NONE',  ( 7.361572987183169658, 59.96726448433410894, -9.846743663894592657 ) ) ;
#12252=CARTESIAN_POINT ( 'NONE',  ( 10.00000000000000000, 26.81368534415484106, -10.88017736071110342 ) ) ;
#12254=CARTESIAN_POINT ( 'NONE',  ( -0.8801773607111008646, 53.27201867748816966, 2.915334737309923430 ) ) ;
#12255=CARTESIAN_POINT ( 'NONE',  ( 2.035157376598824452, 23.68868534415484461, 7.964842623401179544 ) ) ;
#12256=CARTESIAN_POINT ( 'NONE',  ( 19.05914839598885635, 49.96693863883977116, 6.499999999999962697 ) ) ;
#12257=CARTESIAN_POINT ( 'NONE',  ( 14.92337183194729988, 29.34226448433411960, -8.527530157486177487 ) ) ;
#12259=CARTESIAN_POINT ( 'NONE',  ( 17.20831665107776587, 47.88393115100078745, 7.208316651077764980 ) ) ;
#12260=CARTESIAN_POINT ( 'NONE',  ( -0.3689425029237881626, 47.42874883491396787, 10.36894250292379027 ) ) ;
#12263=CARTESIAN_POINT ( 'NONE',  ( 2.917880565312950480, 5.970415501580634832, -12.26659068614894821 ) ) ;
#12264=CARTESIAN_POINT ( 'NONE',  ( 22.26659068614895176, 34.72041550158063927, -7.082119434687042414 ) ) ;
#12265=STYLED_ITEM ( 'NONE', ( #95921 ), #40986 ) ;
#12266=CARTESIAN_POINT ( 'NONE',  ( 6.565887622018943937, 10.16530133659708746, 12.81628187352647430 ) ) ;
#12267=CARTESIAN_POINT ( 'NONE',  ( -10.00000000000007105, 92.00000000000000000, 5.000000000000000000 ) ) ;
#12268=CARTESIAN_POINT ( 'NONE',  ( 4.559911319644449179, 13.89701867748817321, 9.422509992056141925 ) ) ;
#12269=CARTESIAN_POINT ( 'NONE',  ( 0.1532563361054082862, 31.21726448433412315, 2.638427012816831674 ) ) ;
#12271=CARTESIAN_POINT ( 'NONE',  ( 17.96484262340118221, 61.18868534415482685, -7.964842623401177768 ) ) ;
#12276=( BOUNDED_SURFACE ( )  B_SPLINE_SURFACE ( 1, 2, ( 
 ( #31508, #9511, #41005, #573, #62009, #56004, #92509, #24037, #40012, #54507, #16534, #47010, #70516, #77501, #93501, #2534, #86507, #9013, #39530, #1547, #63491, #2038, #25026, #73442, #42469, #11965, #72455, #95970, #72952, #4482, #50449, #71974, #20458, #50948, #42961, #94478, #10986, #80956, #79968, #88950, #96471, #49462, #41991, #25995, #87470, #34453, #86979, #3498, #56490, #12455, #65447, #11474, #12944, #57462, #34948, #88454, #33955, #3987, #64945, #95472, #19955, #49962, #56967, #18489, #26962, #63964, #3019, #87955, #19472, #27455, #80466, #41506, #57947, #81443, #4967, #18984, #35449, #65944, #48977, #33468, #64459, #94966, #26468, #79486, #27943, #58435, #71506, #68427, #52910, #13952, #14444, #44425, #74930, #67438, #98949, #73941, #66437, #30405, #81932, #75421, #28923, #13440, #45411, #37443, #89443, #90911, #6429, #36941, #22936, #60907, #6936, #43927, #98454, #67934, #28445, #97959, #44914, #29910, #21949, #53404, #14942, #43440, #7440, #5469, #20957, #60416, #52428, #22439, #74425, #5953, #36445, #29414, #75916, #59427, #82426, #83424, #66937, #59919, #91410, #35941, #37937, #83913, #96972, #51942, #90407, #58942, #82926, #51444, #97458, #89929, #21444, #77876, #77378, #23915, #15913, #68920, #32867, #84897, #55881, #15441, #53907, #8891, #45921, #8407, #38914, #32372, #92877, #47868, #69402, #31385, #16901, #923, #24411, #63367, #76893, #55385, #17400, #61885, #46887, #1421, #70395, #84416, #69901, #448, #46404, #9388, #39892, #93869, #92390, #1913, #54384, #16409, #25396, #39407, #70891, #93375, #76410, #62877, #7925, #47377, #24902, #38422, #85886, #91903, #31873, #62373, #54877, #23428, #85388, #30899, #78373, #9892, #40396, #2408, #61393, #64826, #34831, #48853, #25876, #72827, #27331, #11351, #78870, #87832, #33831, #42840, #35323, #95343, #56377, #73324, #41391, #18865, #86866, #57828, #88337, #71859, #49347, #72335, #42351, #18374, #41871, #71387, #79362, #80346, #49834, #4849, #10870, #4365, #3370, #64339, #96353, #79848, #65818, #65323, #27823, #95846, #86379, #19350, #19834, #48365, #11843, #63844, #3867, #94850, #34330, #94357, #26350, #17881, #50323, #87351, #80836, #26842, #56852, #57337, #12336, #10379, #40882, #2900, #33350, #82301, #50833, #59797, #5827, #14825, #7314, #36820, #28323, #45301, #13322, #89804, #58814, #6811, #21326, #51814, #37817, #75796, #21825, #89323, #14323, #52309, #43320, #13823, #90288, #82801, #67312, #68309, #29790, #58309, #22321, #88825, #35826, #29302, #97837, #75299, #96848, #20831, #51320, #44304, #60302, #74302, #97336, #44794, #81804, #74807, #98831 ),
 ( #37327, #59307, #28809, #6313, #83300, #20337, #81326, #12821, #43807, #67817, #36321, #66814, #90795, #98333, #5347, #73813, #52795, #66312, #17282, #85771, #78256, #91790, #32252, #38793, #1797, #85276, #815, #16781, #68802, #84782, #15321, #333, #24290, #92764, #47758, #30777, #47257, #46289, #23311, #40268, #61767, #9772, #9272, #70776, #77758, #30285, #62258, #39782, #91287, #54756, #7810, #23805, #8295, #92283, #38307, #84305, #60787, #62753, #31267, #70280, #54266, #15804, #8776, #93257, #53790, #61281, #24781, #55257, #16291, #22810, #31764, #76778, #53290, #83799, #39293, #69293, #45803, #46771, #77265, #69784, #76294, #1313, #94736, #80718, #57710, #64706, #71262, #57218, #95216, #86258, #26242, #3753, #26723, #79736, #12214, #72704, #2292, #65205, #32748, #78758, #72223, #11233, #19230, #40759, #63735, #94235, #56735, #4240, #18257, #41271, #87715, #2786, #18750, #88210, #63245, #42238, #19718, #42722, #10753, #87227, #34213, #49234, #71746, #49710, #41752, #25766, #80221, #64219, #3252, #33240, #55766, #50207, #33720, #93750, #25283, #56259, #11725, #17771, #86752, #48734, #34709, #95725, #27209, #79240, #48247, #10265, #66192, #82188, #90675, #35706, #14204, #75180, #28202, #5714, #59187, #6203, #50716, #66700, #51206, #36202, #81209, #58698, #73203, #6692, #74183, #29185, #97228, #89202, #51705, #21707, #96726, #12709, #59683, #44685, #28695, #65701, #74693, #20715, #29669, #22201, #13698, #43203, #60178, #81689, #89692, #73693, #52192, #21207, #44183, #52680, #83181, #36706, #5228, #90177, #67196, #58190, #97721, #82687, #37211, #67699, #14705, #98211, #4735, #35198, #96228, #13203, #27707, #88702, #20212, #43696, #7696, #38192, #699, #47138, #61164, #84182, #69660, #45677, #61642, #1678, #45179, #85156, #32131, #85646, #53666, #31152, #46653, #92163, #15691, #16169, #23688, #68679, #8658, #8179, #46176, #76175, #98714, #62630, #76660, #75678, #7192, #83680, #38675, #37695, #207, #30657, #62135, #54151, #77635, #91672, #23191, #77149, #69176, #84661, #93135, #39171, #16664, #9152, #1186, #31645, #92643, #24168, #15195, #54638, #30165, #39670, #70161, #24662, #55132, #68193, #60669, #91167, #22695, #53174, #49976, #73955, #96485, #66450, #65958, #96985, #50466, #73454, #78141, #47646, #87485, #57962, #9651, #70652, #56980, #95988, #40148, #12470, #27957, #12958, #49475, #95487, #5481, #20473, #79984, #88466, #50960, #19968, #80970, #19484, #42974, #4982, #35462, #58450, #19000, #28462, #58956, #88965, #2175, #11486, #81456, #26978, #35954, #43453, #57477, #87972, #32633, #34468, #80482, #63131, #42006 ) ),
 .UNSPECIFIED., .F., .F., .F. ) 
 B_SPLINE_SURFACE_WITH_KNOTS ( ( 2, 2 ),
 ( 3, 2, 2, 2, 2, 2, 2, 2, 2, 2, 2, 2, 2, 2, 2, 2, 2, 2, 2, 2, 2, 2, 2, 2, 2, 2, 2, 2, 2, 2, 2, 2, 2, 2, 2, 2, 2, 2, 2, 2, 2, 2, 2, 2, 2, 2, 2, 2, 2, 2, 2, 2, 2, 2, 2, 2, 2, 2, 2, 2, 2, 2, 2, 2, 2, 2, 2, 2, 2, 2, 2, 2, 2, 2, 2, 2, 2, 2, 2, 2, 2, 2, 2, 2, 2, 2, 2, 2, 2, 2, 2, 2, 2, 2, 2, 2, 2, 2, 2, 2, 2, 2, 2, 2, 2, 2, 2, 2, 2, 2, 2, 2, 2, 2, 2, 2, 2, 2, 2, 2, 2, 2, 2, 2, 2, 2, 2, 2, 2, 2, 2, 2, 2, 2, 2, 2, 2, 2, 2, 2, 2, 2, 2, 2, 2, 2, 2, 2, 2, 2, 2, 2, 2, 2, 2, 2, 2, 2, 2, 2, 2, 2, 3 ),
 ( 0.000000000000000000, 1.000000000000000000 ),
 ( 0.000000000000000000, 0.005952380952380952051, 0.01190476190476190410, 0.01785714285714285615, 0.02380952380952380820, 0.02976190476190476025, 0.03571428571428571230, 0.04166666666666666435, 0.04761904761904761640, 0.05357142857142856845, 0.05952380952380952051, 0.06547619047619047949, 0.07142857142857142461, 0.07738095238095238360, 0.08333333333333332871, 0.08928571428571428770, 0.09523809523809523281, 0.1011904761904761918, 0.1071428571428571369, 0.1130952380952380959, 0.1190476190476190410, 0.1250000000000000000, 0.1309523809523809590, 0.1369047619047619180, 0.1428571428571428492, 0.1488095238095238082, 0.1547619047619047672, 0.1607142857142857262, 0.1666666666666666574, 0.1726190476190476164, 0.1785714285714285754, 0.1845238095238095344, 0.1904761904761904656, 0.1964285714285714246, 0.2023809523809523836, 0.2083333333333333426, 0.2142857142857142738, 0.2202380952380952328, 0.2261904761904761918, 0.2321428571428571508, 0.2380952380952380820, 0.2440476190476190410, 0.2500000000000000000, 0.2559523809523809312, 0.2619047619047619180, 0.2678571428571428492, 0.2738095238095238360, 0.2797619047619047672, 0.2857142857142856984, 0.2916666666666666852, 0.2976190476190476164, 0.3035714285714285476, 0.3095238095238095344, 0.3154761904761904656, 0.3214285714285714524, 0.3273809523809523836, 0.3333333333333333148, 0.3392857142857143016, 0.3452380952380952328, 0.3511904761904761640, 0.3571428571428571508, 0.3630952380952380820, 0.3690476190476190688, 0.3750000000000000000, 0.3809523809523809312, 0.3869047619047619180, 0.3928571428571428492, 0.3988095238095238360, 0.4047619047619047672, 0.4107142857142856984, 0.4166666666666666852, 0.4226190476190476164, 0.4285714285714285476, 0.4345238095238095344, 0.4404761904761904656, 0.4464285714285714524, 0.4523809523809523836, 0.4583333333333333148, 0.4642857142857143016, 0.4702380952380952328, 0.4761904761904761640, 0.4821428571428571508, 0.4880952380952380820, 0.4940476190476190688, 0.5000000000000000000, 0.5059523809523809312, 0.5119047619047618625, 0.5178571428571429047, 0.5238095238095238360, 0.5297619047619047672, 0.5357142857142856984, 0.5416666666666666297, 0.5476190476190476719, 0.5535714285714286031, 0.5595238095238095344, 0.5654761904761904656, 0.5714285714285713969, 0.5773809523809523281, 0.5833333333333333703, 0.5892857142857143016, 0.5952380952380952328, 0.6011904761904761640, 0.6071428571428570953, 0.6130952380952381375, 0.6190476190476190688, 0.6250000000000000000, 0.6309523809523809312, 0.6369047619047618625, 0.6428571428571429047, 0.6488095238095238360, 0.6547619047619047672, 0.6607142857142856984, 0.6666666666666666297, 0.6726190476190476719, 0.6785714285714286031, 0.6845238095238095344, 0.6904761904761904656, 0.6964285714285713969, 0.7023809523809523281, 0.7083333333333333703, 0.7142857142857143016, 0.7202380952380952328, 0.7261904761904761640, 0.7321428571428570953, 0.7380952380952381375, 0.7440476190476190688, 0.7500000000000000000, 0.7559523809523809312, 0.7619047619047618625, 0.7678571428571429047, 0.7738095238095238360, 0.7797619047619047672, 0.7857142857142856984, 0.7916666666666666297, 0.7976190476190476719, 0.8035714285714286031, 0.8095238095238095344, 0.8154761904761904656, 0.8214285714285713969, 0.8273809523809523281, 0.8333333333333333703, 0.8392857142857143016, 0.8452380952380952328, 0.8511904761904761640, 0.8571428571428570953, 0.8630952380952381375, 0.8690476190476190688, 0.8750000000000000000, 0.8809523809523809312, 0.8869047619047618625, 0.8928571428571429047, 0.8988095238095238360, 0.9047619047619047672, 0.9107142857142856984, 0.9166666666666666297, 0.9226190476190476719, 0.9285714285714286031, 0.9345238095238095344, 0.9404761904761904656, 0.9464285714285713969, 0.9523809523809523281, 0.9583333333333333703, 0.9642857142857143016 ),
 .UNSPECIFIED. ) 
 GEOMETRIC_REPRESENTATION_ITEM ( )  RATIONAL_B_SPLINE_SURFACE ( (
 ( 1.000000000000000000, 0.9659258262890683122, 1.000000000000000000, 0.9659258262890683122, 1.000000000000000000, 0.9659258262890683122, 1.000000000000000000, 0.9659258262890683122, 1.000000000000000000, 0.9659258262890683122, 1.000000000000000000, 0.9659258262890683122, 1.000000000000000000, 0.9659258262890683122, 1.000000000000000000, 0.9659258262890683122, 1.000000000000000000, 0.9659258262890683122, 1.000000000000000000, 0.9659258262890683122, 1.000000000000000000, 0.9659258262890683122, 1.000000000000000000, 0.9659258262890683122, 1.000000000000000000, 0.9659258262890683122, 1.000000000000000000, 0.9659258262890683122, 1.000000000000000000, 0.9659258262890683122, 1.000000000000000000, 0.9659258262890683122, 1.000000000000000000, 0.9659258262890683122, 1.000000000000000000, 0.9659258262890683122, 1.000000000000000000, 0.9659258262890683122, 1.000000000000000000, 0.9659258262890683122, 1.000000000000000000, 0.9659258262890683122, 1.000000000000000000, 0.9659258262890683122, 1.000000000000000000, 0.9659258262890683122, 1.000000000000000000, 0.9659258262890683122, 1.000000000000000000, 0.9659258262890683122, 1.000000000000000000, 0.9659258262890683122, 1.000000000000000000, 0.9659258262890683122, 1.000000000000000000, 0.9659258262890683122, 1.000000000000000000, 0.9659258262890683122, 1.000000000000000000, 0.9659258262890683122, 1.000000000000000000, 0.9659258262890683122, 1.000000000000000000, 0.9659258262890683122, 1.000000000000000000, 0.9659258262890683122, 1.000000000000000000, 0.9659258262890683122, 1.000000000000000000, 0.9659258262890683122, 1.000000000000000000, 0.9659258262890683122, 1.000000000000000000, 0.9659258262890683122, 1.000000000000000000, 0.9659258262890683122, 1.000000000000000000, 0.9659258262890683122, 1.000000000000000000, 0.9659258262890683122, 1.000000000000000000, 0.9659258262890683122, 1.000000000000000000, 0.9659258262890683122, 1.000000000000000000, 0.9659258262890683122, 1.000000000000000000, 0.9659258262890683122, 1.000000000000000000, 0.9659258262890683122, 1.000000000000000000, 0.9659258262890683122, 1.000000000000000000, 0.9659258262890683122, 1.000000000000000000, 0.9659258262890683122, 1.000000000000000000, 0.9659258262890683122, 1.000000000000000000, 0.9659258262890683122, 1.000000000000000000, 0.9659258262890683122, 1.000000000000000000, 0.9659258262890683122, 1.000000000000000000, 0.9659258262890683122, 1.000000000000000000, 0.9659258262890683122, 1.000000000000000000, 0.9659258262890683122, 1.000000000000000000, 0.9659258262890683122, 1.000000000000000000, 0.9659258262890683122, 1.000000000000000000, 0.9659258262890683122, 1.000000000000000000, 0.9659258262890683122, 1.000000000000000000, 0.9659258262890683122, 1.000000000000000000, 0.9659258262890683122, 1.000000000000000000, 0.9659258262890683122, 1.000000000000000000, 0.9659258262890683122, 1.000000000000000000, 0.9659258262890683122, 1.000000000000000000, 0.9659258262890683122, 1.000000000000000000, 0.9659258262890683122, 1.000000000000000000, 0.9659258262890683122, 1.000000000000000000, 0.9659258262890683122, 1.000000000000000000, 0.9659258262890683122, 1.000000000000000000, 0.9659258262890683122, 1.000000000000000000, 0.9659258262890683122, 1.000000000000000000, 0.9659258262890683122, 1.000000000000000000, 0.9659258262890683122, 1.000000000000000000, 0.9659258262890683122, 1.000000000000000000, 0.9659258262890683122, 1.000000000000000000, 0.9659258262890683122, 1.000000000000000000, 0.9659258262890683122, 1.000000000000000000, 0.9659258262890683122, 1.000000000000000000, 0.9659258262890683122, 1.000000000000000000, 0.9659258262890683122, 1.000000000000000000, 0.9659258262890683122, 1.000000000000000000, 0.9659258262890683122, 1.000000000000000000, 0.9659258262890683122, 1.000000000000000000, 0.9659258262890683122, 1.000000000000000000, 0.9659258262890683122, 1.000000000000000000, 0.9659258262890683122, 1.000000000000000000, 0.9659258262890683122, 1.000000000000000000, 0.9659258262890683122, 1.000000000000000000, 0.9659258262890683122, 1.000000000000000000, 0.9659258262890683122, 1.000000000000000000, 0.9659258262890683122, 1.000000000000000000, 0.9659258262890683122, 1.000000000000000000, 0.9659258262890683122, 1.000000000000000000, 0.9659258262890683122, 1.000000000000000000, 0.9659258262890683122, 1.000000000000000000, 0.9659258262890683122, 1.000000000000000000, 0.9659258262890683122, 1.000000000000000000, 0.9659258262890683122, 1.000000000000000000, 0.9659258262890683122, 1.000000000000000000, 0.9659258262890683122, 1.000000000000000000, 0.9659258262890683122, 1.000000000000000000, 0.9659258262890683122, 1.000000000000000000, 0.9659258262890683122, 1.000000000000000000, 0.9659258262890683122, 1.000000000000000000, 0.9659258262890683122, 1.000000000000000000, 0.9659258262890683122, 1.000000000000000000, 0.9659258262890683122, 1.000000000000000000, 0.9659258262890683122, 1.000000000000000000, 0.9659258262890683122, 1.000000000000000000, 0.9659258262890683122, 1.000000000000000000, 0.9659258262890683122, 1.000000000000000000, 0.9659258262890683122, 1.000000000000000000, 0.9659258262890683122, 1.000000000000000000, 0.9659258262890683122, 1.000000000000000000, 0.9659258262890683122, 1.000000000000000000, 0.9659258262890683122, 1.000000000000000000, 0.9659258262890683122, 1.000000000000000000, 0.9659258262890683122, 1.000000000000000000, 0.9659258262890683122, 1.000000000000000000, 0.9659258262890683122, 1.000000000000000000, 0.9659258262890683122, 1.000000000000000000, 0.9659258262890683122, 1.000000000000000000, 0.9659258262890683122, 1.000000000000000000, 0.9659258262890683122, 1.000000000000000000, 0.9659258262890683122, 1.000000000000000000, 0.9659258262890683122, 1.000000000000000000, 0.9659258262890683122, 1.000000000000000000, 0.9659258262890683122, 1.000000000000000000, 0.9659258262890683122, 1.000000000000000000, 0.9659258262890683122, 1.000000000000000000, 0.9659258262890683122, 1.000000000000000000, 0.9659258262890683122, 1.000000000000000000, 0.9659258262890683122, 1.000000000000000000, 0.9659258262890683122, 1.000000000000000000, 0.9659258262890683122, 1.000000000000000000, 0.9659258262890683122, 1.000000000000000000, 0.9659258262890683122, 1.000000000000000000, 0.9659258262890683122, 1.000000000000000000, 0.9659258262890683122, 1.000000000000000000, 0.9659258262890683122, 1.000000000000000000, 0.9659258262890683122, 1.000000000000000000, 0.9659258262890683122, 1.000000000000000000, 0.9659258262890683122, 1.000000000000000000, 0.9659258262890683122, 1.000000000000000000, 0.9659258262890683122, 1.000000000000000000, 0.9659258262890683122, 1.000000000000000000, 0.9659258262890683122, 1.000000000000000000, 0.9659258262890683122, 1.000000000000000000, 0.9659258262890683122, 1.000000000000000000, 0.9659258262890683122, 1.000000000000000000, 0.9659258262890683122, 1.000000000000000000, 0.9659258262890683122, 1.000000000000000000, 0.9659258262890683122, 1.000000000000000000, 0.9659258262890683122, 1.000000000000000000, 0.9659258262890683122, 1.000000000000000000, 0.9659258262890683122, 1.000000000000000000, 0.9659258262890683122, 1.000000000000000000, 0.9659258262890683122, 1.000000000000000000, 0.9659258262890683122, 1.000000000000000000, 0.9659258262890683122, 1.000000000000000000, 0.9659258262890683122, 1.000000000000000000, 0.9659258262890683122, 1.000000000000000000),
 ( 1.000000000000000000, 0.9659258262890683122, 1.000000000000000000, 0.9659258262890683122, 1.000000000000000000, 0.9659258262890683122, 1.000000000000000000, 0.9659258262890683122, 1.000000000000000000, 0.9659258262890683122, 1.000000000000000000, 0.9659258262890683122, 1.000000000000000000, 0.9659258262890683122, 1.000000000000000000, 0.9659258262890683122, 1.000000000000000000, 0.9659258262890683122, 1.000000000000000000, 0.9659258262890683122, 1.000000000000000000, 0.9659258262890683122, 1.000000000000000000, 0.9659258262890683122, 1.000000000000000000, 0.9659258262890683122, 1.000000000000000000, 0.9659258262890683122, 1.000000000000000000, 0.9659258262890683122, 1.000000000000000000, 0.9659258262890683122, 1.000000000000000000, 0.9659258262890683122, 1.000000000000000000, 0.9659258262890683122, 1.000000000000000000, 0.9659258262890683122, 1.000000000000000000, 0.9659258262890683122, 1.000000000000000000, 0.9659258262890683122, 1.000000000000000000, 0.9659258262890683122, 1.000000000000000000, 0.9659258262890683122, 1.000000000000000000, 0.9659258262890683122, 1.000000000000000000, 0.9659258262890683122, 1.000000000000000000, 0.9659258262890683122, 1.000000000000000000, 0.9659258262890683122, 1.000000000000000000, 0.9659258262890683122, 1.000000000000000000, 0.9659258262890683122, 1.000000000000000000, 0.9659258262890683122, 1.000000000000000000, 0.9659258262890683122, 1.000000000000000000, 0.9659258262890683122, 1.000000000000000000, 0.9659258262890683122, 1.000000000000000000, 0.9659258262890683122, 1.000000000000000000, 0.9659258262890683122, 1.000000000000000000, 0.9659258262890683122, 1.000000000000000000, 0.9659258262890683122, 1.000000000000000000, 0.9659258262890683122, 1.000000000000000000, 0.9659258262890683122, 1.000000000000000000, 0.9659258262890683122, 1.000000000000000000, 0.9659258262890683122, 1.000000000000000000, 0.9659258262890683122, 1.000000000000000000, 0.9659258262890683122, 1.000000000000000000, 0.9659258262890683122, 1.000000000000000000, 0.9659258262890683122, 1.000000000000000000, 0.9659258262890683122, 1.000000000000000000, 0.9659258262890683122, 1.000000000000000000, 0.9659258262890683122, 1.000000000000000000, 0.9659258262890683122, 1.000000000000000000, 0.9659258262890683122, 1.000000000000000000, 0.9659258262890683122, 1.000000000000000000, 0.9659258262890683122, 1.000000000000000000, 0.9659258262890683122, 1.000000000000000000, 0.9659258262890683122, 1.000000000000000000, 0.9659258262890683122, 1.000000000000000000, 0.9659258262890683122, 1.000000000000000000, 0.9659258262890683122, 1.000000000000000000, 0.9659258262890683122, 1.000000000000000000, 0.9659258262890683122, 1.000000000000000000, 0.9659258262890683122, 1.000000000000000000, 0.9659258262890683122, 1.000000000000000000, 0.9659258262890683122, 1.000000000000000000, 0.9659258262890683122, 1.000000000000000000, 0.9659258262890683122, 1.000000000000000000, 0.9659258262890683122, 1.000000000000000000, 0.9659258262890683122, 1.000000000000000000, 0.9659258262890683122, 1.000000000000000000, 0.9659258262890683122, 1.000000000000000000, 0.9659258262890683122, 1.000000000000000000, 0.9659258262890683122, 1.000000000000000000, 0.9659258262890683122, 1.000000000000000000, 0.9659258262890683122, 1.000000000000000000, 0.9659258262890683122, 1.000000000000000000, 0.9659258262890683122, 1.000000000000000000, 0.9659258262890683122, 1.000000000000000000, 0.9659258262890683122, 1.000000000000000000, 0.9659258262890683122, 1.000000000000000000, 0.9659258262890683122, 1.000000000000000000, 0.9659258262890683122, 1.000000000000000000, 0.9659258262890683122, 1.000000000000000000, 0.9659258262890683122, 1.000000000000000000, 0.9659258262890683122, 1.000000000000000000, 0.9659258262890683122, 1.000000000000000000, 0.9659258262890683122, 1.000000000000000000, 0.9659258262890683122, 1.000000000000000000, 0.9659258262890683122, 1.000000000000000000, 0.9659258262890683122, 1.000000000000000000, 0.9659258262890683122, 1.000000000000000000, 0.9659258262890683122, 1.000000000000000000, 0.9659258262890683122, 1.000000000000000000, 0.9659258262890683122, 1.000000000000000000, 0.9659258262890683122, 1.000000000000000000, 0.9659258262890683122, 1.000000000000000000, 0.9659258262890683122, 1.000000000000000000, 0.9659258262890683122, 1.000000000000000000, 0.9659258262890683122, 1.000000000000000000, 0.9659258262890683122, 1.000000000000000000, 0.9659258262890683122, 1.000000000000000000, 0.9659258262890683122, 1.000000000000000000, 0.9659258262890683122, 1.000000000000000000, 0.9659258262890683122, 1.000000000000000000, 0.9659258262890683122, 1.000000000000000000, 0.9659258262890683122, 1.000000000000000000, 0.9659258262890683122, 1.000000000000000000, 0.9659258262890683122, 1.000000000000000000, 0.9659258262890683122, 1.000000000000000000, 0.9659258262890683122, 1.000000000000000000, 0.9659258262890683122, 1.000000000000000000, 0.9659258262890683122, 1.000000000000000000, 0.9659258262890683122, 1.000000000000000000, 0.9659258262890683122, 1.000000000000000000, 0.9659258262890683122, 1.000000000000000000, 0.9659258262890683122, 1.000000000000000000, 0.9659258262890683122, 1.000000000000000000, 0.9659258262890683122, 1.000000000000000000, 0.9659258262890683122, 1.000000000000000000, 0.9659258262890683122, 1.000000000000000000, 0.9659258262890683122, 1.000000000000000000, 0.9659258262890683122, 1.000000000000000000, 0.9659258262890683122, 1.000000000000000000, 0.9659258262890683122, 1.000000000000000000, 0.9659258262890683122, 1.000000000000000000, 0.9659258262890683122, 1.000000000000000000, 0.9659258262890683122, 1.000000000000000000, 0.9659258262890683122, 1.000000000000000000, 0.9659258262890683122, 1.000000000000000000, 0.9659258262890683122, 1.000000000000000000, 0.9659258262890683122, 1.000000000000000000, 0.9659258262890683122, 1.000000000000000000, 0.9659258262890683122, 1.000000000000000000, 0.9659258262890683122, 1.000000000000000000, 0.9659258262890683122, 1.000000000000000000, 0.9659258262890683122, 1.000000000000000000, 0.9659258262890683122, 1.000000000000000000, 0.9659258262890683122, 1.000000000000000000, 0.9659258262890683122, 1.000000000000000000, 0.9659258262890683122, 1.000000000000000000, 0.9659258262890683122, 1.000000000000000000, 0.9659258262890683122, 1.000000000000000000, 0.9659258262890683122, 1.000000000000000000, 0.9659258262890683122, 1.000000000000000000, 0.9659258262890683122, 1.000000000000000000, 0.9659258262890683122, 1.000000000000000000, 0.9659258262890683122, 1.000000000000000000, 0.9659258262890683122, 1.000000000000000000, 0.9659258262890683122, 1.000000000000000000, 0.9659258262890683122, 1.000000000000000000, 0.9659258262890683122, 1.000000000000000000, 0.9659258262890683122, 1.000000000000000000, 0.9659258262890683122, 1.000000000000000000, 0.9659258262890683122, 1.000000000000000000, 0.9659258262890683122, 1.000000000000000000, 0.9659258262890683122, 1.000000000000000000, 0.9659258262890683122, 1.000000000000000000, 0.9659258262890683122, 1.000000000000000000, 0.9659258262890683122, 1.000000000000000000, 0.9659258262890683122, 1.000000000000000000, 0.9659258262890683122, 1.000000000000000000, 0.9659258262890683122, 1.000000000000000000, 0.9659258262890683122, 1.000000000000000000, 0.9659258262890683122, 1.000000000000000000, 0.9659258262890683122, 1.000000000000000000) ) ) 
 REPRESENTATION_ITEM ( '' )  SURFACE ( )  );
#12277=CARTESIAN_POINT ( 'NONE',  ( 16.40814093676323893, 60.79030133659709634, 11.09922568453595026 ) ) ;
#12278=CARTESIAN_POINT ( 'NONE',  ( 21.09922568453595559, 27.04030133659708568, -6.408140936763230044 ) ) ;
#12279=CARTESIAN_POINT ( 'NONE',  ( 17.20831665107776587, 27.88393115100078390, 7.208316651077764980 ) ) ;
#12281=CARTESIAN_POINT ( 'NONE',  ( 8.673617379884035472E-16, 78.91966277462714174, 5.000000000000000000 ) ) ;
#12283=CARTESIAN_POINT ( 'NONE',  ( 17.08211943468705840, 65.13708216824730357, -12.26659068614894466 ) ) ;
#12284=CARTESIAN_POINT ( 'NONE',  ( 15.44008868035555260, 19.73035201082150536, 9.422509992056143702 ) ) ;
#12285=CARTESIAN_POINT ( 'NONE',  ( 20.36894250292379738, 44.92874883491396787, -10.36894250292379027 ) ) ;
#12286=CARTESIAN_POINT ( 'NONE',  ( 19.42250999205614193, 35.14701867748816966, 5.440088680355555262 ) ) ;
#12287=CARTESIAN_POINT ( 'NONE',  ( -0.8801773607111009756, 58.06368534415484106, 1.068504757029289695E-15 ) ) ;
#12289=CARTESIAN_POINT ( 'NONE',  ( 19.84674366389459266, 13.30059781766745353, 2.638427012816836559 ) ) ;
#12291=CARTESIAN_POINT ( 'NONE',  ( 18.52753015748617571, 13.09226448433411960, 4.923371831947298993 ) ) ;
#12293=CARTESIAN_POINT ( 'NONE',  ( 0.1532563361054083140, 41.00893115100078745, 1.131784320476157264E-15 ) ) ;
#12294=CARTESIAN_POINT ( 'NONE',  ( 1.472469842513823179, 60.59226448433412315, -4.923371831947296329 ) ) ;
#12297=ORIENTED_EDGE ( 'NONE', *, *, #61201, .F. ) ;
#12298=CARTESIAN_POINT ( 'NONE',  ( 3.591859063236763294, 43.29030133659708923, -11.09922568453595026 ) ) ;
#12300=CARTESIAN_POINT ( 'NONE',  ( 20.88017736071110875, 65.77201867748817676, -2.915334737309920765 ) ) ;
#12301=CARTESIAN_POINT ( 'NONE',  ( 3.591859063236761518, 44.95696800326376064, 11.09922568453594849 ) ) ;
#12302=CARTESIAN_POINT ( 'NONE',  ( -0.3689425029237881626, 62.42874883491396787, 10.36894250292379027 ) ) ;
#12303=CARTESIAN_POINT ( 'NONE',  ( 2.791683348922240793, 41.63393115100078745, 7.208316651077764092 ) ) ;
#12306=CARTESIAN_POINT ( 'NONE',  ( 7.361572987183169658, 64.96726448433412315, -9.846743663894592657 ) ) ;
#12307=CARTESIAN_POINT ( 'NONE',  ( -4.164238869374099039, 26.80374883491397142, 8.674139862899312516E-16 ) ) ;
#12308=CARTESIAN_POINT ( 'NONE',  ( 10.00000000000000178, 37.25893115100078745, 9.846743663894594434 ) ) ;
#12310=CARTESIAN_POINT ( 'NONE',  ( 17.96484262340118221, 39.93868534415484106, 7.964842623401181321 ) ) ;
#12311=CARTESIAN_POINT ( 'NONE',  ( 4.559911319644449179, 57.23035201082150536, -9.422509992056141925 ) ) ;
#12312=COLOUR_RGB ( '', 0.31764706, 0.68627451, 0.89019608) ;
#12315=CARTESIAN_POINT ( 'NONE',  ( 3.591859063236761518, 39.95696800326375353, 11.09922568453594849 ) ) ;
#12316=VECTOR ( 'NONE', #71434, 1000.000000000000000 ) ;
#12317=CARTESIAN_POINT ( 'NONE',  ( 4.559911319644449179, 47.23035201082150536, -9.422509992056141925 ) ) ;
#12322=ORIENTED_EDGE ( 'NONE', *, *, #2179, .T. ) ;
#12325=CARTESIAN_POINT ( 'NONE',  ( 20.88017736071110164, 15.35535201082150358, 2.915334737309930979 ) ) ;
#12328=CARTESIAN_POINT ( 'NONE',  ( 6.204703633549690345, 67.84541550158060375, 14.16423886937410082 ) ) ;
#12329=CARTESIAN_POINT ( 'NONE',  ( 6.204703633549690345, 20.76208216824730357, -14.16423886937410259 ) ) ;
#12331=CARTESIAN_POINT ( 'NONE',  ( 15.44008868035555793, 21.39701867748817321, -9.422509992056140149 ) ) ;
#12332=CARTESIAN_POINT ( 'NONE',  ( 5.076628168052703671, 61.84226448433412315, 8.527530157486179263 ) ) ;
#12333=ORIENTED_EDGE ( 'NONE', *, *, #69416, .F. ) ;
#12334=CARTESIAN_POINT ( 'NONE',  ( 18.52753015748618282, 63.92559781766745886, -4.923371831947291888 ) ) ;
#12336=CARTESIAN_POINT ( 'NONE',  ( 4.559911319644449179, 58.89701867748817676, 9.422509992056141925 ) ) ;
#12337=CARTESIAN_POINT ( 'NONE',  ( 1.472469842513823179, 61.42559781766745175, 4.923371831947296329 ) ) ;
#12338=CARTESIAN_POINT ( 'NONE',  ( 12.91533473730993009, 6.605352010821504471, -10.88017736071109987 ) ) ;
#12340=CARTESIAN_POINT ( 'NONE',  ( 17.96484262340118221, 66.18868534415483396, -7.964842623401177768 ) ) ;
#12341=CARTESIAN_POINT ( 'NONE',  ( 0.5774900079438590739, 12.64701867748817321, -5.440088680355550821 ) ) ;
#12342=CARTESIAN_POINT ( 'NONE',  ( 6.565887622018943937, 53.08196800326374643, -12.81628187352647608 ) ) ;
#12343=CARTESIAN_POINT ( 'NONE',  ( 4.559911319644449179, 28.89701867748817321, 9.422509992056141925 ) ) ;
#12345=CARTESIAN_POINT ( 'NONE',  ( 19.38216949554541202, 45.99863466993041072, 9.382169495545424454 ) ) ;
#12346=CARTESIAN_POINT ( 'NONE',  ( 2.035157376598822676, 52.43868534415483396, -7.964842623401177768 ) ) ;
#12348=CARTESIAN_POINT ( 'NONE',  ( 5.076628168052703671, 61.84226448433412315, 8.527530157486179263 ) ) ;
#12351=CARTESIAN_POINT ( 'NONE',  ( 10.00000000000000000, -2.126365330069579951, -12.81628187352647608 ) ) ;
#12352=DIRECTION ( 'NONE',  ( 0.000000000000000000, -1.000000000000000000, 0.000000000000000000 ) ) ;
#12353=CARTESIAN_POINT ( 'NONE',  ( 12.63842701281683034, 47.46726448433412315, 9.846743663894596210 ) ) ;
#12354=CARTESIAN_POINT ( 'NONE',  ( 17.96484262340118221, 21.18868534415483396, -7.964842623401177768 ) ) ;
#12356=CARTESIAN_POINT ( 'NONE',  ( 14.92337183194729633, 42.67559781766745886, 8.527530157486181039 ) ) ;
#12358=PRESENTATION_STYLE_ASSIGNMENT (( #67333 ) ) ;
#12359=EDGE_CURVE ( 'NONE', #28561, #80817, #66634, .T. ) ;
#12360=CARTESIAN_POINT ( 'NONE',  ( 7.361572987183169658, 44.96726448433412315, -9.846743663894592657 ) ) ;
#12361=CARTESIAN_POINT ( 'NONE',  ( 1.472469842513823179, 5.592264484334118713, -4.923371831947296329 ) ) ;
#12363=CARTESIAN_POINT ( 'NONE',  ( 18.52753015748618282, 58.92559781766745886, -4.923371831947291888 ) ) ;
#12366=CARTESIAN_POINT ( 'NONE',  ( 22.81628187352647785, 41.41530133659708923, 3.434112377981063169 ) ) ;
#12367=CARTESIAN_POINT ( 'NONE',  ( 18.52753015748618282, 43.92559781766745175, -4.923371831947291888 ) ) ;
#12369=CARTESIAN_POINT ( 'NONE',  ( 13.79529636645030344, 53.26208216824730357, 14.16423886937410614 ) ) ;
#12370=CARTESIAN_POINT ( 'NONE',  ( 7.361572987183170547, 32.05059781766745175, 9.846743663894590881 ) ) ;
#12371=CARTESIAN_POINT ( 'NONE',  ( 20.00000000000000711, 87.41133749856676616, 4.971011742375448073 ) ) ;
#12372=CARTESIAN_POINT ( 'NONE',  ( 20.36894250292379738, 59.92874883491397497, -10.36894250292379027 ) ) ;
#12374=CARTESIAN_POINT ( 'NONE',  ( 19.42250999205614193, 15.14701867748817143, 5.440088680355555262 ) ) ;
#12375=CARTESIAN_POINT ( 'NONE',  ( 2.917880565312950480, 30.97041550158063572, -12.26659068614894821 ) ) ;
#12377=CARTESIAN_POINT ( 'NONE',  ( 22.26659068614894466, 48.88708216824730357, 7.082119434687054849 ) ) ;
#12380=CARTESIAN_POINT ( 'NONE',  ( 10.00000000000000000, 14.75893115100078568, -9.846743663894594434 ) ) ;
#12381=CARTESIAN_POINT ( 'NONE',  ( 0.1532563361054100626, 65.80059781766745175, -2.638427012816831230 ) ) ;
#12383=CARTESIAN_POINT ( 'NONE',  ( 15.44008868035555260, 49.73035201082150536, 9.422509992056143702 ) ) ;
#12384=CARTESIAN_POINT ( 'NONE',  ( 0.2751277870542874204, 39.36607318730131055, -6.499999999999984901 ) ) ;
#12388=CARTESIAN_POINT ( 'NONE',  ( 0.1532563361054100626, 60.80059781766744464, -2.638427012816831230 ) ) ;
#12389=SURFACE_SIDE_STYLE ('',( #34884 ) ) ;
#12391=CARTESIAN_POINT ( 'NONE',  ( 10.00000000000000178, 23.05374883491397142, 14.16423886937410082 ) ) ;
#12394=CARTESIAN_POINT ( 'NONE',  ( 12.91533473730992121, 19.52201867748816611, 10.88017736071110164 ) ) ;
#12395=CARTESIAN_POINT ( 'NONE',  ( -2.816281873526473856, 39.12363466993041783, 9.499525473075851096E-16 ) ) ;
#12400=CARTESIAN_POINT ( 'NONE',  ( 20.36894250292379382, 23.67874883491397142, 10.36894250292379205 ) ) ;
#12401=CARTESIAN_POINT ( 'NONE',  ( 24.16423886937410614, 4.303748834913967869, 8.672049930838204340E-16 ) ) ;
#12403=CARTESIAN_POINT ( 'NONE',  ( 0.5774900079438590739, 22.64701867748817321, -5.440088680355550821 ) ) ;
#12404=CYLINDRICAL_SURFACE ( 'NONE', #84565, 6.999999999999995559 ) ;
#12406=CARTESIAN_POINT ( 'NONE',  ( 7.084665262690076126, 39.10535201082150536, 10.88017736071109987 ) ) ;
#12407=CARTESIAN_POINT ( 'NONE',  ( 17.96484262340118221, 56.18868534415484817, -7.964842623401177768 ) ) ;
#12408=CARTESIAN_POINT ( 'NONE',  ( -2.816281873526473856, 9.123634669930421381, 9.499525473075851096E-16 ) ) ;
#12409=LINE ( 'NONE', #48928, #17082 ) ;
#12410=CARTESIAN_POINT ( 'NONE',  ( 0.8952175423693563561, 2.601608292538878597, -5.990408912944101161 ) ) ;
#12411=CARTESIAN_POINT ( 'NONE',  ( 14.92337183194729633, 17.67559781766745175, 8.527530157486181039 ) ) ;
#12412=CARTESIAN_POINT ( 'NONE',  ( 2.035157376598824452, 38.68868534415483396, 7.964842623401179544 ) ) ;
#12414=B_SPLINE_CURVE_WITH_KNOTS ( 'NONE', 3,
 ( #87070, #34537, #10584, #96057, #28034, #80557 ),
 .UNSPECIFIED., .F., .F.,
 ( 4, 2, 4 ),
 ( 0.000000000000000000, 0.0002626113303184835542, 0.0005252226606369671084 ),
 .UNSPECIFIED. ) ;
#12415=CARTESIAN_POINT ( 'NONE',  ( 19.38216949554541557, 7.248634669930421381, -9.382169495545420901 ) ) ;
#12416=CARTESIAN_POINT ( 'NONE',  ( 17.96484262340118221, 61.18868534415482685, -7.964842623401177768 ) ) ;
#12417=CARTESIAN_POINT ( 'NONE',  ( 19.84674366389459266, 23.71726448433412315, -2.638427012816827677 ) ) ;
#12418=CARTESIAN_POINT ( 'NONE',  ( 16.40814093676324603, 42.45696800326375353, -11.09922568453594671 ) ) ;
#12419=CARTESIAN_POINT ( 'NONE',  ( 5.076628168052704559, 0.1755978176674514724, -8.527530157486179263 ) ) ;
#12422=DIRECTION ( 'NONE',  ( 0.000000000000000000, 0.000000000000000000, -1.000000000000000000 ) ) ;
#12423=CARTESIAN_POINT ( 'NONE',  ( 17.96484262340118221, 19.93868534415484106, 7.964842623401181321 ) ) ;
#12424=CARTESIAN_POINT ( 'NONE',  ( 22.81628187352647785, 61.62363466993041783, 6.195893100308588602E-16 ) ) ;
#12425=CARTESIAN_POINT ( 'NONE',  ( 6.204703633549690345, 20.76208216824730357, -14.16423886937410259 ) ) ;
#12426=CARTESIAN_POINT ( 'NONE',  ( 7.361572987183169658, 29.96726448433411960, -9.846743663894592657 ) ) ;
#12427=CARTESIAN_POINT ( 'NONE',  ( 15.44008868035555260, 14.73035201082150536, 9.422509992056143702 ) ) ;
#12428=CARTESIAN_POINT ( 'NONE',  ( 4.559911319644449179, 2.230352010821504916, -9.422509992056141925 ) ) ;
#12429=ORIENTED_EDGE ( 'NONE', *, *, #12204, .F. ) ;
#12430=CARTESIAN_POINT ( 'NONE',  ( 0.5774900079438590739, 17.64701867748817321, -5.440088680355550821 ) ) ;
#12431=CARTESIAN_POINT ( 'NONE',  ( 15.44008868035555260, 34.73035201082151247, 9.422509992056143702 ) ) ;
#12433=CARTESIAN_POINT ( 'NONE',  ( 4.559911319644449179, 42.23035201082151247, -9.422509992056141925 ) ) ;
#12434=( GEOMETRIC_REPRESENTATION_CONTEXT ( 3 ) GLOBAL_UNCERTAINTY_ASSIGNED_CONTEXT ( ( #1252 ) ) GLOBAL_UNIT_ASSIGNED_CONTEXT ( ( #79189, #56685, #42669 ) ) REPRESENTATION_CONTEXT ( 'NONE', 'WORKASPACE' ) );
#12436=CARTESIAN_POINT ( 'NONE',  ( 19.84674366389459266, 63.71726448433412315, -2.638427012816827677 ) ) ;
#12437=CARTESIAN_POINT ( 'NONE',  ( 19.42250999205614193, 30.14701867748817321, 5.440088680355555262 ) ) ;
#12438=CARTESIAN_POINT ( 'NONE',  ( 0.1532563361054082862, 66.21726448433413736, 2.638427012816831674 ) ) ;
#12441=CARTESIAN_POINT ( 'NONE',  ( 22.81628187352647785, 56.62363466993042493, 6.195893100308588602E-16 ) ) ;
#12442=CARTESIAN_POINT ( 'NONE',  ( 20.10421743870886147, 30.60736173766201773, -6.337391062633416006 ) ) ;
#12443=CARTESIAN_POINT ( 'NONE',  ( 17.08211943468705130, 33.47041550158063927, 12.26659068614894998 ) ) ;
#12444=CARTESIAN_POINT ( 'NONE',  ( 15.44008868035555260, 49.73035201082150536, 9.422509992056143702 ) ) ;
#12445=CARTESIAN_POINT ( 'NONE',  ( 15.44008868035555793, 36.39701867748816966, -9.422509992056140149 ) ) ;
#12446=CARTESIAN_POINT ( 'NONE',  ( 5.076628168052703671, 66.84226448433412315, 8.527530157486179263 ) ) ;
#12447=DIRECTION ( 'NONE',  ( 1.000000000000000000, 0.000000000000000000, -0.000000000000000000 ) ) ;
#12448=CARTESIAN_POINT ( 'NONE',  ( 19.84674366389459266, 43.71726448433410894, -2.638427012816827677 ) ) ;
#12449=EDGE_CURVE ( 'NONE', #61453, #8076, #14685, .T. ) ;
#12452=CARTESIAN_POINT ( 'NONE',  ( 2.791683348922240793, 21.63393115100078745, 7.208316651077764092 ) ) ;
#12455=CARTESIAN_POINT ( 'NONE',  ( 7.084665262690076126, 12.02201867748817143, -10.88017736071110164 ) ) ;
#12456=CARTESIAN_POINT ( 'NONE',  ( 10.00000000000000000, 29.75893115100078745, -9.846743663894594434 ) ) ;
#12457=CARTESIAN_POINT ( 'NONE',  ( 13.43411237798106583, 12.66530133659708746, -12.81628187352647252 ) ) ;
#12458=CARTESIAN_POINT ( 'NONE',  ( 0.5774900079438590739, 57.64701867748817676, -5.440088680355550821 ) ) ;
#12459=CARTESIAN_POINT ( 'NONE',  ( 10.00000000000000000, 51.81368534415484106, -10.88017736071110342 ) ) ;
#12460=CARTESIAN_POINT ( 'NONE',  ( 19.42250999205614193, 25.14701867748817321, 5.440088680355555262 ) ) ;
#12461=CARTESIAN_POINT ( 'NONE',  ( 21.09922568453595559, 52.04030133659708923, -6.408140936763230044 ) ) ;
#12462=CARTESIAN_POINT ( 'NONE',  ( 6.204703633549690345, 32.84541550158063927, 14.16423886937410082 ) ) ;
#12465=CARTESIAN_POINT ( 'NONE',  ( 20.24186590665276597, 34.73410085661203084, 6.114288769123062295 ) ) ;
#12466=ORIENTED_EDGE ( 'NONE', *, *, #54625, .F. ) ;
#12467=CARTESIAN_POINT ( 'NONE',  ( -1.099225684535947600, -0.4596986634029132657, 6.408140936763237150 ) ) ;
#12468=CARTESIAN_POINT ( 'NONE',  ( 0.6178305044545838731, 64.74863466993043914, 9.382169495545420901 ) ) ;
#12469=CARTESIAN_POINT ( 'NONE',  ( 19.42250999205614548, 30.98035201082150536, -5.440088680355545492 ) ) ;
#12470=CARTESIAN_POINT ( 'NONE',  ( 2.791683348922237240, 60.38393115100078745, -7.208316651077763204 ) ) ;
#12472=CARTESIAN_POINT ( 'NONE',  ( 7.361572987183169658, 19.96726448433411960, -9.846743663894592657 ) ) ;
#12473=CARTESIAN_POINT ( 'NONE',  ( 12.63842701281683034, 7.467264484334118713, 9.846743663894596210 ) ) ;
#12474=CARTESIAN_POINT ( 'NONE',  ( 0.1532563361054082862, 26.21726448433411605, 2.638427012816831674 ) ) ;
#12475=CARTESIAN_POINT ( 'NONE',  ( 14.92337183194729988, 14.34226448433411782, -8.527530157486177487 ) ) ;
#12476=CARTESIAN_POINT ( 'NONE',  ( 7.361572987183169658, -0.03273551566588185635, -9.846743663894592657 ) ) ;
#12478=EDGE_CURVE ( 'NONE', #72922, #45554, #3421, .T. ) ;
#12479=CARTESIAN_POINT ( 'NONE',  ( 0.1532563361054083140, 1.008931151000784787, 1.131784320476157264E-15 ) ) ;
#12481=CARTESIAN_POINT ( 'NONE',  ( 2.791683348922237240, 5.383931151000785675, -7.208316651077763204 ) ) ;
#12482=CARTESIAN_POINT ( 'NONE',  ( 14.92337183194729988, 24.34226448433411960, -8.527530157486177487 ) ) ;
#12483=ORIENTED_EDGE ( 'NONE', *, *, #76081, .T. ) ;
#12485=CARTESIAN_POINT ( 'NONE',  ( 10.00000000000000178, 5.373634669930420493, 12.81628187352647608 ) ) ;
#12487=FACE_OUTER_BOUND ( 'NONE', #91149, .T. ) ;
#12488=CARTESIAN_POINT ( 'NONE',  ( 22.26659068614894466, 18.88708216824730002, 7.082119434687054849 ) ) ;
#12490=DIRECTION ( 'NONE',  ( 1.000000000000000000, 0.000000000000000000, 0.000000000000000000 ) ) ;
#12491=CARTESIAN_POINT ( 'NONE',  ( -0.3689425029237898834, 21.17874883491396432, -10.36894250292378850 ) ) ;
#12493=CARTESIAN_POINT ( 'NONE',  ( -4.164238869374099039, 26.80374883491397142, 8.674139862899312516E-16 ) ) ;
#12494=CARTESIAN_POINT ( 'NONE',  ( 10.00000000000000000, 0.5537488349139675359, -14.16423886937410082 ) ) ;
#12495=CARTESIAN_POINT ( 'NONE',  ( 10.00000000000000178, 13.05374883491396787, 14.16423886937410082 ) ) ;
#12496=CARTESIAN_POINT ( 'NONE',  ( 4.559911319644449179, 68.89701867748817676, 9.422509992056141925 ) ) ;
#12497=CARTESIAN_POINT ( 'NONE',  ( -0.8801773607111008646, 28.27201867748817321, 2.915334737309923430 ) ) ;
#12500=CARTESIAN_POINT ( 'NONE',  ( 7.361572987183170547, 22.05059781766745530, 9.846743663894590881 ) ) ;
#12501=CARTESIAN_POINT ( 'NONE',  ( 19.42250999205614548, 50.98035201082151247, -5.440088680355545492 ) ) ;
#12502=CARTESIAN_POINT ( 'NONE',  ( 2.791683348922237240, 35.38393115100079456, -7.208316651077763204 ) ) ;
#12503=CARTESIAN_POINT ( 'NONE',  ( 19.42250999205614548, 5.980352010821504471, -5.440088680355545492 ) ) ;
#12504=CARTESIAN_POINT ( 'NONE',  ( -1.099225684535947600, 44.54030133659708923, 6.408140936763237150 ) ) ;
#12505=CARTESIAN_POINT ( 'NONE',  ( 12.63842701281683922, 44.55059781766745175, -9.846743663894590881 ) ) ;
#12507=CARTESIAN_POINT ( 'NONE',  ( -1.099225684535947600, 48.70696800326375353, -6.408140936763238038 ) ) ;
#12509=CARTESIAN_POINT ( 'NONE',  ( 7.361572987183169658, 44.96726448433412315, -9.846743663894592657 ) ) ;
#12510=CARTESIAN_POINT ( 'NONE',  ( 6.204703633549690345, 27.84541550158063217, 14.16423886937410082 ) ) ;
#12513=CARTESIAN_POINT ( 'NONE',  ( 10.00000000000000178, 49.31368534415484106, 10.88017736071110342 ) ) ;
#12514=CARTESIAN_POINT ( 'NONE',  ( 0.5774900079438590739, 47.64701867748817676, -5.440088680355550821 ) ) ;
#12515=CARTESIAN_POINT ( 'NONE',  ( 24.16423886937410614, 44.51208216824730357, -3.795296366450302550 ) ) ;
#12516=CARTESIAN_POINT ( 'NONE',  ( 0.1532563361054082862, 61.21726448433412315, 2.638427012816831674 ) ) ;
#12517=CARTESIAN_POINT ( 'NONE',  ( 0.1077916266722667299, 57.24062864464239908, -6.478736007405996311 ) ) ;
#12518=CARTESIAN_POINT ( 'NONE',  ( 15.44008868035555793, 36.39701867748816966, -9.422509992056140149 ) ) ;
#12521=CARTESIAN_POINT ( 'NONE',  ( 16.40814093676323893, 25.79030133659708923, 11.09922568453595026 ) ) ;
#12522=CARTESIAN_POINT ( 'NONE',  ( 10.00000000000000000, 59.75893115100078745, -9.846743663894594434 ) ) ;
#12524=CARTESIAN_POINT ( 'NONE',  ( 0.5774900079438590739, 2.647018677488170990, -5.440088680355550821 ) ) ;
#12525=CARTESIAN_POINT ( 'NONE',  ( 4.559911319644449179, 68.89701867748817676, 9.422509992056141925 ) ) ;
#12528=FACE_OUTER_BOUND ( 'NONE', #32685, .T. ) ;
#12529=EDGE_CURVE ( 'NONE', #58088, #39614, #36522, .T. ) ;
#12532=CARTESIAN_POINT ( 'NONE',  ( 20.88017736071110875, 60.77201867748817676, -2.915334737309920765 ) ) ;
#12533=CARTESIAN_POINT ( 'NONE',  ( 2.791683348922237240, 5.383931151000785675, -7.208316651077763204 ) ) ;
#12535=CARTESIAN_POINT ( 'NONE',  ( 0.1532563361054082862, 36.21726448433410894, 2.638427012816831674 ) ) ;
#12537=CARTESIAN_POINT ( 'NONE',  ( 17.96484262340118221, 19.93868534415484106, 7.964842623401181321 ) ) ;
#12538=CARTESIAN_POINT ( 'NONE',  ( -1.099225684535947600, 8.706968003263753531, -6.408140936763238038 ) ) ;
#12539=CARTESIAN_POINT ( 'NONE',  ( 0.5774900079438607392, 38.48035201082150536, 5.440088680355550821 ) ) ;
#12542=CARTESIAN_POINT ( 'NONE',  ( 13.43411237798106583, 42.66530133659707502, -12.81628187352647252 ) ) ;
#12544=CARTESIAN_POINT ( 'NONE',  ( 0.5774900079438590739, 62.64701867748817676, -5.440088680355550821 ) ) ;
#12545=CARTESIAN_POINT ( 'NONE',  ( 10.00000000000000000, 22.87363466993042138, -12.81628187352647608 ) ) ;
#12546=CARTESIAN_POINT ( 'NONE',  ( 18.52753015748617571, 18.09226448433411960, 4.923371831947298993 ) ) ;
#12548=CARTESIAN_POINT ( 'NONE',  ( 20.88017736071110519, 35.56368534415484106, 2.639326808657452039E-16 ) ) ;
#12549=CARTESIAN_POINT ( 'NONE',  ( 17.20831665107776587, 64.13393115100079456, -7.208316651077762316 ) ) ;
#12550=CARTESIAN_POINT ( 'NONE',  ( -2.266590686148945544, 62.22041550158063927, 7.082119434687048631 ) ) ;
#12551=CARTESIAN_POINT ( 'NONE',  ( 18.52753015748618282, 48.92559781766745886, -4.923371831947291888 ) ) ;
#12552=CARTESIAN_POINT ( 'NONE',  ( 19.84674366389459621, 3.508931151000785231, 7.409399052514197653E-17 ) ) ;
#12553=CARTESIAN_POINT ( 'NONE',  ( 10.00000000000000000, 66.81368534415484817, -10.88017736071110342 ) ) ;
#12554=CARTESIAN_POINT ( 'NONE',  ( 0.2751277870542980231, 5.302231764288316107, 6.500000000000002665 ) ) ;
#12555=CARTESIAN_POINT ( 'NONE',  ( -4.164238869374099927, 27.01208216824730357, 3.795296366450308767 ) ) ;
#12559=CARTESIAN_POINT ( 'NONE',  ( 10.00000000000000000, 1.813685344154838175, -10.88017736071110342 ) ) ;
#12560=CARTESIAN_POINT ( 'NONE',  ( 6.204703633549690345, 52.84541550158062506, 14.16423886937410082 ) ) ;
#12561=CARTESIAN_POINT ( 'NONE',  ( 19.84674366389459621, 28.50893115100078745, 7.409399052514197653E-17 ) ) ;
#12562=CARTESIAN_POINT ( 'NONE',  ( 22.81628187352647785, 31.41530133659709279, 3.434112377981063169 ) ) ;
#12564=SURFACE_SIDE_STYLE ('',( #43066 ) ) ;
#12565=SURFACE_STYLE_USAGE ( .BOTH. , #4095 ) ;
#12566=CARTESIAN_POINT ( 'NONE',  ( -4.164238869374098151, 61.59541550158063217, -3.795296366450310543 ) ) ;
#12568=CARTESIAN_POINT ( 'NONE',  ( 7.361572987183169658, 4.967264484334119601, -9.846743663894592657 ) ) ;
#12572=VECTOR ( 'NONE', #64166, 1000.000000000000000 ) ;
#12573=VERTEX_POINT ( 'NONE', #85135 ) ;
#12576=CARTESIAN_POINT ( 'NONE',  ( 20.36894250292379382, 13.67874883491396965, 10.36894250292379205 ) ) ;
#12577=CARTESIAN_POINT ( 'NONE',  ( 12.91533473730992121, 14.52201867748817143, 10.88017736071110164 ) ) ;
#12578=CARTESIAN_POINT ( 'NONE',  ( 19.42250999205614193, 20.14701867748817321, 5.440088680355555262 ) ) ;
#12579=CARTESIAN_POINT ( 'NONE',  ( 5.076628168052704559, 45.17559781766745175, -8.527530157486179263 ) ) ;
#12580=CARTESIAN_POINT ( 'NONE',  ( 19.38216949554541557, 17.24863466993041783, -9.382169495545420901 ) ) ;
#12581=DIRECTION ( 'NONE',  ( 0.000000000000000000, 0.000000000000000000, -1.000000000000000000 ) ) ;
#12582=CARTESIAN_POINT ( 'NONE',  ( 21.09922568453595559, 27.04030133659708568, -6.408140936763230044 ) ) ;
#12584=CARTESIAN_POINT ( 'NONE',  ( 14.92337183194729633, 37.67559781766745175, 8.527530157486181039 ) ) ;
#12585=CARTESIAN_POINT ( 'NONE',  ( 20.36894250292379738, 64.92874883491397497, -10.36894250292379027 ) ) ;
#12586=CARTESIAN_POINT ( 'NONE',  ( -0.8801773607111009756, 8.063685344154837509, 1.068504757029289695E-15 ) ) ;
#12587=ORIENTED_EDGE ( 'NONE', *, *, #77642, .T. ) ;
#12588=CARTESIAN_POINT ( 'NONE',  ( 2.035157376598822676, 47.43868534415484817, -7.964842623401177768 ) ) ;
#12589=CARTESIAN_POINT ( 'NONE',  ( 7.084665262690076126, 44.10535201082151247, 10.88017736071109987 ) ) ;
#12590=CARTESIAN_POINT ( 'NONE',  ( 10.00000000000000178, 49.31368534415484106, 10.88017736071110342 ) ) ;
#12592=CARTESIAN_POINT ( 'NONE',  ( 20.88017736071110875, 35.77201867748816966, -2.915334737309920765 ) ) ;
#12595=ADVANCED_FACE ( 'NONE', ( #17635 ), #61625, .T. ) ;
#12597=CARTESIAN_POINT ( 'NONE',  ( 19.84674366389459621, 23.50893115100078390, 7.409399052514197653E-17 ) ) ;
#12599=CARTESIAN_POINT ( 'NONE',  ( 5.076628168052704559, 60.17559781766745175, -8.527530157486179263 ) ) ;
#12602=ORIENTED_EDGE ( 'NONE', *, *, #3122, .F. ) ;
#12605=CARTESIAN_POINT ( 'NONE',  ( 2.791683348922237240, 65.38393115100078035, -7.208316651077763204 ) ) ;
#12606=CARTESIAN_POINT ( 'NONE',  ( 24.16423886937409904, 64.09541550158064638, 3.795296366450317205 ) ) ;
#12607=CARTESIAN_POINT ( 'NONE',  ( 18.72515096720583827, 65.05509018479936856, 6.499999999999810818 ) ) ;
#12610=CARTESIAN_POINT ( 'NONE',  ( 7.361572987183170547, 32.05059781766745175, 9.846743663894590881 ) ) ;
#12612=CARTESIAN_POINT ( 'NONE',  ( 10.00000000000000000, 7.873634669930421381, -12.81628187352647608 ) ) ;
#12613=CARTESIAN_POINT ( 'NONE',  ( 12.63842701281683922, 9.550597817667449974, -9.846743663894590881 ) ) ;
#12616=CARTESIAN_POINT ( 'NONE',  ( 7.361572987183169658, 9.967264484334119601, -9.846743663894592657 ) ) ;
#12617=CARTESIAN_POINT ( 'NONE',  ( 2.791683348922237240, 60.38393115100078745, -7.208316651077763204 ) ) ;
#12620=CARTESIAN_POINT ( 'NONE',  ( 0.5774900079438607392, 3.480352010821504916, 5.440088680355550821 ) ) ;
#12621=CARTESIAN_POINT ( 'NONE',  ( -0.3689425029237898834, 11.17874883491396787, -10.36894250292378850 ) ) ;
#12622=CARTESIAN_POINT ( 'NONE',  ( 19.84674366389459621, 18.50893115100078745, 7.409399052514197653E-17 ) ) ;
#12623=CARTESIAN_POINT ( 'NONE',  ( 17.96484262340118221, 54.93868534415484106, 7.964842623401181321 ) ) ;
#12624=CARTESIAN_POINT ( 'NONE',  ( -2.816281873526471635, 23.91530133659708568, -3.434112377981056508 ) ) ;
#12627=CARTESIAN_POINT ( 'NONE',  ( -0.1503990784575282014, 57.22266099184919597, -6.262539305110077947 ) ) ;
#12630=CARTESIAN_POINT ( 'NONE',  ( 3.591859063236763294, -1.709698663402913210, -11.09922568453595026 ) ) ;
#12631=CARTESIAN_POINT ( 'NONE',  ( 12.63842701281683034, 17.46726448433411250, 9.846743663894596210 ) ) ;
#12633=CARTESIAN_POINT ( 'NONE',  ( 13.43411237798106583, 17.66530133659708923, -12.81628187352647252 ) ) ;
#12636=CARTESIAN_POINT ( 'NONE',  ( 10.00000000000000000, 26.81368534415484106, -10.88017736071110342 ) ) ;
#12639=CARTESIAN_POINT ( 'NONE',  ( 24.16423886937409904, 44.09541550158063927, 3.795296366450317205 ) ) ;
#12641=CARTESIAN_POINT ( 'NONE',  ( 15.44008868035555793, 21.39701867748817321, -9.422509992056140149 ) ) ;
#12643=CARTESIAN_POINT ( 'NONE',  ( 5.076628168052704559, 45.17559781766745175, -8.527530157486179263 ) ) ;
#12644=CARTESIAN_POINT ( 'NONE',  ( 2.035157376598824452, 58.68868534415482685, 7.964842623401179544 ) ) ;
#12645=CARTESIAN_POINT ( 'NONE',  ( 17.08211943468705840, 35.13708216824730357, -12.26659068614894466 ) ) ;
#12646=DIRECTION ( 'NONE',  ( 1.000000000000000000, 0.000000000000000000, 0.000000000000000000 ) ) ;
#12649=CARTESIAN_POINT ( 'NONE',  ( 18.52753015748617571, 33.09226448433411605, 4.923371831947298993 ) ) ;
#12650=LINE ( 'NONE', #6145, #53550 ) ;
#12651=CARTESIAN_POINT ( 'NONE',  ( 21.09922568453594849, 1.206968003263753531, 6.408140936763242479 ) ) ;
#12653=CARTESIAN_POINT ( 'NONE',  ( 0.5774900079438607392, 23.48035201082150536, 5.440088680355550821 ) ) ;
#12655=FACE_OUTER_BOUND ( 'NONE', #939, .T. ) ;
#12656=CARTESIAN_POINT ( 'NONE',  ( 2.035157376598824452, 8.688685344154839285, 7.964842623401179544 ) ) ;
#12657=CARTESIAN_POINT ( 'NONE',  ( 1.472469842513823179, 1.425597817667451528, 4.923371831947296329 ) ) ;
#12659=CARTESIAN_POINT ( 'NONE',  ( 6.204703633549690345, 20.76208216824730357, -14.16423886937410259 ) ) ;
#12660=CARTESIAN_POINT ( 'NONE',  ( 5.076628168052703671, 16.84226448433411960, 8.527530157486179263 ) ) ;
#12661=CARTESIAN_POINT ( 'NONE',  ( 10.00000000000000000, 59.75893115100078745, -9.846743663894594434 ) ) ;
#12662=CARTESIAN_POINT ( 'NONE',  ( -0.8801773607110991993, 32.85535201082151247, -2.915334737309923874 ) ) ;
#12667=CARTESIAN_POINT ( 'NONE',  ( 7.361572987183169658, 49.96726448433410894, -9.846743663894592657 ) ) ;
#12669=VERTEX_POINT ( 'NONE', #2649 ) ;
#12671=CARTESIAN_POINT ( 'NONE',  ( -2.266590686148945544, 26.38708216824730357, -7.082119434687050408 ) ) ;
#12672=CARTESIAN_POINT ( 'NONE',  ( -4.164238869374099039, 11.80374883491396965, 8.674139862899312516E-16 ) ) ;
#12673=CARTESIAN_POINT ( 'NONE',  ( 12.91533473730992121, 59.52201867748816966, 10.88017736071110164 ) ) ;
#12674=CARTESIAN_POINT ( 'NONE',  ( 2.917880565312950480, 50.97041550158064638, -12.26659068614894821 ) ) ;
#12675=CARTESIAN_POINT ( 'NONE',  ( 19.38216949554541557, 2.248634669930420049, -9.382169495545420901 ) ) ;
#12676=CARTESIAN_POINT ( 'NONE',  ( 12.63842701281683034, 32.46726448433412315, 9.846743663894596210 ) ) ;
#12678=CARTESIAN_POINT ( 'NONE',  ( 4.559911319644449179, 37.23035201082150536, -9.422509992056141925 ) ) ;
#12679=CARTESIAN_POINT ( 'NONE',  ( 0.6178305044545818747, 3.498634669930420049, -9.382169495545419124 ) ) ;
#12680=CARTESIAN_POINT ( 'NONE',  ( 20.36894250292379382, 8.678748834913967869, 10.36894250292379205 ) ) ;
#12681=CARTESIAN_POINT ( 'NONE',  ( 24.16423886937410614, 49.51208216824730357, -3.795296366450302550 ) ) ;
#12682=CARTESIAN_POINT ( 'NONE',  ( 17.96484262340118221, 14.93868534415484106, 7.964842623401181321 ) ) ;
#12683=CARTESIAN_POINT ( 'NONE',  ( 19.39235739573468820, 4.875764716086009365, 6.500000000000002665 ) ) ;
#12685=CARTESIAN_POINT ( 'NONE',  ( 15.44008868035555793, 41.39701867748817676, -9.422509992056140149 ) ) ;
#12689=ORIENTED_EDGE ( 'NONE', *, *, #78395, .F. ) ;
#12691=ORIENTED_EDGE ( 'NONE', *, *, #18470, .T. ) ;
#12692=VERTEX_POINT ( 'NONE', #77131 ) ;
#12693=CARTESIAN_POINT ( 'NONE',  ( 2.917880565312948704, 52.63708216824730357, 12.26659068614894643 ) ) ;
#12694=CARTESIAN_POINT ( 'NONE',  ( 19.84674366389459266, 43.71726448433410894, -2.638427012816827677 ) ) ;
#12695=CARTESIAN_POINT ( 'NONE',  ( 15.44008868035555793, 61.39701867748817676, -9.422509992056140149 ) ) ;
#12697=PLANE ( 'NONE',  #43227 ) ;
#12699=CARTESIAN_POINT ( 'NONE',  ( 4.559911319644449179, 58.89701867748817676, 9.422509992056141925 ) ) ;
#12700=CARTESIAN_POINT ( 'NONE',  ( 16.40814093676324603, 57.45696800326375353, -11.09922568453594671 ) ) ;
#12703=CARTESIAN_POINT ( 'NONE',  ( 4.559911319644449179, 47.23035201082150536, -9.422509992056141925 ) ) ;
#12704=CARTESIAN_POINT ( 'NONE',  ( 17.08211943468705130, 18.47041550158063572, 12.26659068614894998 ) ) ;
#12705=CARTESIAN_POINT ( 'NONE',  ( 22.81628187352647785, 26.62363466993042138, 6.195893100308588602E-16 ) ) ;
#12707=CARTESIAN_POINT ( 'NONE',  ( 16.40814093676323893, 40.79030133659708923, 11.09922568453595026 ) ) ;
#12708=CARTESIAN_POINT ( 'NONE',  ( 15.44008868035555793, 16.39701867748817321, -9.422509992056140149 ) ) ;
#12709=CARTESIAN_POINT ( 'NONE',  ( 2.791683348922237240, 35.38393115100079456, -7.208316651077763204 ) ) ;
#12710=CARTESIAN_POINT ( 'NONE',  ( 12.91533473730993009, 6.605352010821504471, -10.88017736071109987 ) ) ;
#12711=CARTESIAN_POINT ( 'NONE',  ( 10.00000000000000178, 50.37363466993042493, 12.81628187352647608 ) ) ;
#12712=DIRECTION ( 'NONE',  ( 0.000000000000000000, -1.000000000000000000, 0.000000000000000000 ) ) ;
#12713=CARTESIAN_POINT ( 'NONE',  ( 12.63842701281683034, 42.46726448433412315, 9.846743663894596210 ) ) ;
#12716=EDGE_LOOP ( 'NONE', ( #86106, #51577, #17910, #72488, #59666 ) ) ;
#12720=CARTESIAN_POINT ( 'NONE',  ( 17.20831665107776587, 24.13393115100078035, -7.208316651077762316 ) ) ;
#12721=CARTESIAN_POINT ( 'NONE',  ( 10.00000000000000178, 25.37363466993041783, 12.81628187352647608 ) ) ;
#12723=CARTESIAN_POINT ( 'NONE',  ( 17.20831665107776587, 62.88393115100078745, 7.208316651077764980 ) ) ;
#12725=CARTESIAN_POINT ( 'NONE',  ( 24.16423886937410614, 14.51208216824730179, -3.795296366450302550 ) ) ;
#12726=CARTESIAN_POINT ( 'NONE',  ( 14.92337183194729633, 47.67559781766745175, 8.527530157486181039 ) ) ;
#12727=CARTESIAN_POINT ( 'NONE',  ( -1.099225684535947600, 43.70696800326375353, -6.408140936763238038 ) ) ;
#12729=CARTESIAN_POINT ( 'NONE',  ( 12.91533473730992121, 64.52201867748817676, 10.88017736071110164 ) ) ;
#12731=EDGE_CURVE ( 'NONE', #55238, #44298, #41407, .T. ) ;
#12732=CARTESIAN_POINT ( 'NONE',  ( 18.52753015748618282, 33.92559781766745886, -4.923371831947291888 ) ) ;
#12733=CARTESIAN_POINT ( 'NONE',  ( -0.8801773607110991993, 37.85535201082151247, -2.915334737309923874 ) ) ;
#12734=CARTESIAN_POINT ( 'NONE',  ( -1.099225684535947600, 44.54030133659708923, 6.408140936763237150 ) ) ;
#12735=CARTESIAN_POINT ( 'NONE',  ( 19.72487221294570858, 70.00000000000000000, -6.000000000000000000 ) ) ;
#12736=CARTESIAN_POINT ( 'NONE',  ( -0.8801773607111008646, 33.27201867748817676, 2.915334737309923430 ) ) ;
#12738=FACE_OUTER_BOUND ( 'NONE', #387, .T. ) ;
#12739=CARTESIAN_POINT ( 'NONE',  ( 12.91533473730993009, 11.60535201082150536, -10.88017736071109987 ) ) ;
#12740=CARTESIAN_POINT ( 'NONE',  ( 0.1532563361054083140, 56.00893115100078745, 1.131784320476157264E-15 ) ) ;
#12741=CARTESIAN_POINT ( 'NONE',  ( 20.88017736071110519, 50.56368534415484106, 2.639326808657452039E-16 ) ) ;
#12742=DIRECTION ( 'NONE',  ( -1.000000000000000000, 0.000000000000000000, 0.000000000000000000 ) ) ;
#12743=CARTESIAN_POINT ( 'NONE',  ( 15.44008868035555260, 64.73035201082151957, 9.422509992056143702 ) ) ;
#12744=VECTOR ( 'NONE', #89391, 1000.000000000000000 ) ;
#12745=CARTESIAN_POINT ( 'NONE',  ( 19.42250999205614193, 30.14701867748817321, 5.440088680355555262 ) ) ;
#12746=CARTESIAN_POINT ( 'NONE',  ( 0.000000000000000000, 73.93174988520466684, -5.598587842719937591 ) ) ;
#12747=CARTESIAN_POINT ( 'NONE',  ( 19.84674366389459266, 23.30059781766745530, 2.638427012816836559 ) ) ;
#12750=CARTESIAN_POINT ( 'NONE',  ( 0.1532563361054082862, 46.21726448433411605, 2.638427012816831674 ) ) ;
#12752=CARTESIAN_POINT ( 'NONE',  ( 20.36894250292379738, 59.92874883491397497, -10.36894250292379027 ) ) ;
#12756=CARTESIAN_POINT ( 'NONE',  ( 13.79529636645030344, 8.262082168247300018, 14.16423886937410614 ) ) ;
#12757=CARTESIAN_POINT ( 'NONE',  ( 10.00000000000000000, 40.55374883491397497, -14.16423886937410082 ) ) ;
#12758=CARTESIAN_POINT ( 'NONE',  ( 19.38216949554541202, 5.998634669930420493, 9.382169495545424454 ) ) ;
#12759=ADVANCED_FACE ( 'NONE', ( #91651 ), #92625, .T. ) ;
#12761=CARTESIAN_POINT ( 'NONE',  ( -0.8801773607110991993, 12.85535201082150358, -2.915334737309923874 ) ) ;
#12762=CARTESIAN_POINT ( 'NONE',  ( 2.791683348922240793, 31.63393115100078745, 7.208316651077764092 ) ) ;
#12763=CARTESIAN_POINT ( 'NONE',  ( -0.3689425029237898834, 1.178748834913967869, -10.36894250292378850 ) ) ;
#12766=ADVANCED_FACE ( 'NONE', ( #54129, #46155 ), #76639, .F. ) ;
#12768=CARTESIAN_POINT ( 'NONE',  ( 3.591859063236761518, 19.95696800326375353, 11.09922568453594849 ) ) ;
#12769=CARTESIAN_POINT ( 'NONE',  ( 12.63842701281683034, 27.46726448433411250, 9.846743663894596210 ) ) ;
#12771=CARTESIAN_POINT ( 'NONE',  ( 2.791683348922240793, 6.633931151000785675, 7.208316651077764092 ) ) ;
#12773=CARTESIAN_POINT ( 'NONE',  ( -2.266590686148945544, 66.38708216824730357, -7.082119434687050408 ) ) ;
#12774=CARTESIAN_POINT ( 'NONE',  ( 20.88017736071110519, 10.56368534415483751, 2.639326808657452039E-16 ) ) ;
#12775=CARTESIAN_POINT ( 'NONE',  ( 17.08211943468705130, 38.47041550158063217, 12.26659068614894998 ) ) ;
#12776=CARTESIAN_POINT ( 'NONE',  ( -0.8801773607110991993, 27.85535201082150181, -2.915334737309923874 ) ) ;
#12777=CARTESIAN_POINT ( 'NONE',  ( 0.5774900079438590739, 62.64701867748817676, -5.440088680355550821 ) ) ;
#12778=CYLINDRICAL_SURFACE ( 'NONE', #83066, 0.5000000000000004441 ) ;
#12779=CARTESIAN_POINT ( 'NONE',  ( 7.361572987183169658, 29.96726448433411960, -9.846743663894592657 ) ) ;
#12781=CARTESIAN_POINT ( 'NONE',  ( 19.84674366389459266, 8.300597817667451750, 2.638427012816836559 ) ) ;
#12782=CARTESIAN_POINT ( 'NONE',  ( 0.1532563361054082862, 31.21726448433412315, 2.638427012816831674 ) ) ;
#12783=CARTESIAN_POINT ( 'NONE',  ( 7.361572987183170547, 67.05059781766746596, 9.846743663894590881 ) ) ;
#12784=CARTESIAN_POINT ( 'NONE',  ( 2.035157376598822676, 42.43868534415483396, -7.964842623401177768 ) ) ;
#12786=CARTESIAN_POINT ( 'NONE',  ( 0.6178305044545818747, 43.49863466993042493, -9.382169495545419124 ) ) ;
#12787=CARTESIAN_POINT ( 'NONE',  ( 15.44008868035555793, 61.39701867748817676, -9.422509992056140149 ) ) ;
#12788=CARTESIAN_POINT ( 'NONE',  ( 10.00000000000000000, 42.87363466993042493, -12.81628187352647608 ) ) ;
#12789=CARTESIAN_POINT ( 'NONE',  ( 20.36894250292379382, 58.67874883491396076, 10.36894250292379205 ) ) ;
#12790=CARTESIAN_POINT ( 'NONE',  ( 18.52753015748618282, 33.92559781766745886, -4.923371831947291888 ) ) ;
#12792=CARTESIAN_POINT ( 'NONE',  ( 10.00000000000000000, 59.75893115100078745, -9.846743663894594434 ) ) ;
#12793=CARTESIAN_POINT ( 'NONE',  ( 2.917880565312948704, 17.63708216824730357, 12.26659068614894643 ) ) ;
#12794=CARTESIAN_POINT ( 'NONE',  ( 24.16423886937410614, 39.30374883491396787, 8.672049930838204340E-16 ) ) ;
#12795=CARTESIAN_POINT ( 'NONE',  ( 19.84674366389459266, 48.30059781766745175, 2.638427012816836559 ) ) ;
#12797=CARTESIAN_POINT ( 'NONE',  ( 20.88017736071110875, 35.77201867748816966, -2.915334737309920765 ) ) ;
#12799=CARTESIAN_POINT ( 'NONE',  ( 10.00000000000000000, 61.81368534415484106, -10.88017736071110342 ) ) ;
#12802=CARTESIAN_POINT ( 'NONE',  ( 13.43411237798106583, 47.66530133659709634, -12.81628187352647252 ) ) ;
#12803=EDGE_LOOP ( 'NONE', ( #20578, #3029, #84427, #39509, #67087, #68786 ) ) ;
#12804=CARTESIAN_POINT ( 'NONE',  ( 15.44008868035555260, 64.73035201082151957, 9.422509992056143702 ) ) ;
#12806=CARTESIAN_POINT ( 'NONE',  ( 24.16423886937410614, 9.303748834913967869, 8.672049930838204340E-16 ) ) ;
#12807=CARTESIAN_POINT ( 'NONE',  ( 19.84674366389459266, 8.717264484334116048, -2.638427012816827677 ) ) ;
#12808=CARTESIAN_POINT ( 'NONE',  ( 1.720799100035159679, 0.1239429031973928452, -6.333916461130630005 ) ) ;
#12812=CARTESIAN_POINT ( 'NONE',  ( 2.035157376598822676, 12.43868534415483751, -7.964842623401177768 ) ) ;
#12813=CARTESIAN_POINT ( 'NONE',  ( 20.88017736071110519, 60.56368534415484106, 2.639326808657452039E-16 ) ) ;
#12814=CARTESIAN_POINT ( 'NONE',  ( 24.16423886937410614, 19.51208216824729647, -3.795296366450302550 ) ) ;
#12815=CARTESIAN_POINT ( 'NONE',  ( 20.88017736071110519, 25.56368534415483751, 2.639326808657452039E-16 ) ) ;
#12817=CARTESIAN_POINT ( 'NONE',  ( 17.20831665107776587, 59.13393115100078745, -7.208316651077762316 ) ) ;
#12819=CARTESIAN_POINT ( 'NONE',  ( 2.791683348922240793, 61.63393115100079456, 7.208316651077764092 ) ) ;
#12821=CARTESIAN_POINT ( 'NONE',  ( 0.1532563361054082862, 1.217264484334117824, 2.638427012816831674 ) ) ;
#12822=CARTESIAN_POINT ( 'NONE',  ( 18.52753015748618282, 58.92559781766745886, -4.923371831947291888 ) ) ;
#12823=CARTESIAN_POINT ( 'NONE',  ( 21.09922568453594849, 36.20696800326375353, 6.408140936763242479 ) ) ;
#12824=CARTESIAN_POINT ( 'NONE',  ( 2.035157376598824452, 3.688685344154837953, 7.964842623401179544 ) ) ;
#12826=CARTESIAN_POINT ( 'NONE',  ( 5.076628168052704559, 5.175597817667451750, -8.527530157486179263 ) ) ;
#12828=CARTESIAN_POINT ( 'NONE',  ( -0.8801773607111008646, 23.27201867748817676, 2.915334737309923430 ) ) ;
#12830=CARTESIAN_POINT ( 'NONE',  ( -2.816281873526473856, 59.33196800326374643, 3.434112377981055619 ) ) ;
#12831=CARTESIAN_POINT ( 'NONE',  ( 10.00000000000000178, 44.31368534415484106, 10.88017736071110342 ) ) ;
#12832=CARTESIAN_POINT ( 'NONE',  ( 1.274849032794292736, 47.55509018479936856, -6.499999999999977796 ) ) ;
#12833=CARTESIAN_POINT ( 'NONE',  ( 21.09922568453594849, 41.20696800326375353, 6.408140936763242479 ) ) ;
#12834=CARTESIAN_POINT ( 'NONE',  ( 15.44008868035555260, 44.73035201082151247, 9.422509992056143702 ) ) ;
#12835=CARTESIAN_POINT ( 'NONE',  ( 7.361572987183170547, 57.05059781766744464, 9.846743663894590881 ) ) ;
#12836=ORIENTED_EDGE ( 'NONE', *, *, #12173, .F. ) ;
#12838=CARTESIAN_POINT ( 'NONE',  ( 19.84674366389459621, 18.50893115100078745, 7.409399052514197653E-17 ) ) ;
#12839=CARTESIAN_POINT ( 'NONE',  ( 21.09922568453595559, 12.04030133659708746, -6.408140936763230044 ) ) ;
#12842=CARTESIAN_POINT ( 'NONE',  ( 2.035157376598824452, 18.68868534415484106, 7.964842623401179544 ) ) ;
#12843=CARTESIAN_POINT ( 'NONE',  ( 12.63842701281683922, 54.55059781766745175, -9.846743663894590881 ) ) ;
#12846=CARTESIAN_POINT ( 'NONE',  ( 5.076628168052704559, 10.17559781766745175, -8.527530157486179263 ) ) ;
#12847=( NAMED_UNIT ( * ) PLANE_ANGLE_UNIT ( ) SI_UNIT ( $, .RADIAN. ) );
#12848=CARTESIAN_POINT ( 'NONE',  ( 10.00000000000000178, 0.3736346699304200492, 12.81628187352647608 ) ) ;
#12851=CARTESIAN_POINT ( 'NONE',  ( -36.44000000000000483, 92.00000000000000000, -10.09898361729590199 ) ) ;
#12853=CARTESIAN_POINT ( 'NONE',  ( -1.099225684535947600, 39.54030133659708923, 6.408140936763237150 ) ) ;
#12854=CARTESIAN_POINT ( 'NONE',  ( 17.20831665107776587, 29.13393115100078390, -7.208316651077762316 ) ) ;
#12855=CARTESIAN_POINT ( 'NONE',  ( 0.8952175423694743728, 57.60160829253887016, -5.990408912944304554 ) ) ;
#12856=CARTESIAN_POINT ( 'NONE',  ( 2.917880565312948704, 57.63708216824731068, 12.26659068614894643 ) ) ;
#12857=CARTESIAN_POINT ( 'NONE',  ( 0.1532563361054100626, 25.80059781766744820, -2.638427012816831230 ) ) ;
#12858=ORIENTED_EDGE ( 'NONE', *, *, #58474, .F. ) ;
#12859=CARTESIAN_POINT ( 'NONE',  ( 20.00000000000000711, 85.01043265489317946, 4.826711382686302620 ) ) ;
#12860=CARTESIAN_POINT ( 'NONE',  ( 17.08211943468705840, 55.13708216824731068, -12.26659068614894466 ) ) ;
#12862=CARTESIAN_POINT ( 'NONE',  ( 20.88017736071110519, 25.56368534415483751, 2.639326808657452039E-16 ) ) ;
#12863=CARTESIAN_POINT ( 'NONE',  ( 6.204703633549690345, 42.84541550158063217, 14.16423886937410082 ) ) ;
#12864=CARTESIAN_POINT ( 'NONE',  ( 2.917880565312950480, 50.97041550158064638, -12.26659068614894821 ) ) ;
#12866=CARTESIAN_POINT ( 'NONE',  ( 19.84674366389459621, 8.508931151000785675, 7.409399052514197653E-17 ) ) ;
#12867=CARTESIAN_POINT ( 'NONE',  ( 3.591859063236761518, 4.956968003263753531, 11.09922568453594849 ) ) ;
#12869=CARTESIAN_POINT ( 'NONE',  ( 10.00000000000000000, 56.81368534415484106, -10.88017736071110342 ) ) ;
#12871=CARTESIAN_POINT ( 'NONE',  ( 18.52753015748618282, 58.92559781766745886, -4.923371831947291888 ) ) ;
#12873=CARTESIAN_POINT ( 'NONE',  ( 0.1532563361054083140, 66.00893115100079456, 1.131784320476157264E-15 ) ) ;
#12875=( GEOMETRIC_REPRESENTATION_CONTEXT ( 3 ) GLOBAL_UNCERTAINTY_ASSIGNED_CONTEXT ( ( #32335 ) ) GLOBAL_UNIT_ASSIGNED_CONTEXT ( ( #55165, #63158, #82104 ) ) REPRESENTATION_CONTEXT ( 'NONE', 'WORKASPACE' ) );
#12877=FACE_OUTER_BOUND ( 'NONE', #8389, .T. ) ;
#12879=CARTESIAN_POINT ( 'NONE',  ( -2.266590686148945544, 42.22041550158063217, 7.082119434687048631 ) ) ;
#12881=CARTESIAN_POINT ( 'NONE',  ( -0.8801773607111009756, 13.06368534415483929, 1.068504757029289695E-15 ) ) ;
#12882=CARTESIAN_POINT ( 'NONE',  ( -2.816281873526473856, 39.33196800326374643, 3.434112377981055619 ) ) ;
#12883=( BOUNDED_CURVE ( )  B_SPLINE_CURVE ( 2, ( #21278, #13274, #64048, #68755, #17110, #37773, #2614, #68270, #53247 ),
 .UNSPECIFIED., .F., .T. ) 
 B_SPLINE_CURVE_WITH_KNOTS ( ( 3, 2, 2, 2, 3 ),
 ( 0.1901409369402313476, 0.1904761904761904656, 0.1964285714285713969, 0.2023809523809524391, 0.2027162059169115571 ),
 .UNSPECIFIED. ) 
 CURVE ( )  GEOMETRIC_REPRESENTATION_ITEM ( )  RATIONAL_B_SPLINE_CURVE ( ( 0.9963778908391762723, 0.9980808541467921513, 1.000000000000000000, 0.9659258262890683122, 1.000000000000000000, 0.9659258262890683122, 1.000000000000000000, 0.9980808541467921513, 0.9963778908391762723 ) ) 
 REPRESENTATION_ITEM ( '' )  );
#12884=ADVANCED_FACE ( 'NONE', ( #95080 ), #64079, .F. ) ;
#12885=CARTESIAN_POINT ( 'NONE',  ( 12.91533473730992121, 9.522018677488171434, 10.88017736071110164 ) ) ;
#12887=CARTESIAN_POINT ( 'NONE',  ( 6.565887622018943937, 23.08196800326375708, -12.81628187352647608 ) ) ;
#12892=CARTESIAN_POINT ( 'NONE',  ( -45.94000000000000483, 92.50000000000000000, 9.500000000000000000 ) ) ;
#12893=CARTESIAN_POINT ( 'NONE',  ( -0.3689425029237898834, 6.178748834913968757, -10.36894250292378850 ) ) ;
#12895=CARTESIAN_POINT ( 'NONE',  ( 2.035157376598822676, 27.43868534415483396, -7.964842623401177768 ) ) ;
#12896=CARTESIAN_POINT ( 'NONE',  ( 5.500000000000000000, 61.00000000000000711, 5.000000000000000000 ) ) ;
#12898=CARTESIAN_POINT ( 'NONE',  ( -0.8801773607111008646, 53.27201867748816966, 2.915334737309923430 ) ) ;
#12899=CARTESIAN_POINT ( 'NONE',  ( 20.88017736071110164, 45.35535201082149115, 2.915334737309930979 ) ) ;
#12900=CARTESIAN_POINT ( 'NONE',  ( 21.09922568453594849, 11.20696800326375531, 6.408140936763242479 ) ) ;
#12903=CARTESIAN_POINT ( 'NONE',  ( 19.84674366389459266, 28.30059781766745886, 2.638427012816836559 ) ) ;
#12906=CARTESIAN_POINT ( 'NONE',  ( 2.035157376598822676, 42.43868534415483396, -7.964842623401177768 ) ) ;
#12907=CARTESIAN_POINT ( 'NONE',  ( -1.099225684535947600, 9.540301336597087456, 6.408140936763237150 ) ) ;
#12908=CARTESIAN_POINT ( 'NONE',  ( 5.076628168052703671, 1.842264484334118047, 8.527530157486179263 ) ) ;
#12909=CARTESIAN_POINT ( 'NONE',  ( 17.20831665107776587, 24.13393115100078035, -7.208316651077762316 ) ) ;
#12910=CARTESIAN_POINT ( 'NONE',  ( -1.099225684535947600, 48.70696800326375353, -6.408140936763238038 ) ) ;
#12911=CARTESIAN_POINT ( 'NONE',  ( 7.361572987183170547, 2.050597817667451750, 9.846743663894590881 ) ) ;
#12915=CARTESIAN_POINT ( 'NONE',  ( 20.88017736071110164, 25.35535201082150891, 2.915334737309930979 ) ) ;
#12916=CARTESIAN_POINT ( 'NONE',  ( 19.50000000000000711, 98.59912998021083297, -4.500000000000000888 ) ) ;
#12917=CARTESIAN_POINT ( 'NONE',  ( -4.164238869374099039, 31.80374883491396432, 8.674139862899312516E-16 ) ) ;
#12918=CARTESIAN_POINT ( 'NONE',  ( 2.791683348922240793, 26.63393115100078745, 7.208316651077764092 ) ) ;
#12919=CARTESIAN_POINT ( 'NONE',  ( 20.88017736071110519, 20.56368534415484106, 2.639326808657452039E-16 ) ) ;
#12920=CARTESIAN_POINT ( 'NONE',  ( 7.084665262690076126, 9.105352010821503583, 10.88017736071109987 ) ) ;
#12923=CARTESIAN_POINT ( 'NONE',  ( -0.8801773607111008646, 33.27201867748817676, 2.915334737309923430 ) ) ;
#12925=CARTESIAN_POINT ( 'NONE',  ( -0.8801773607111009756, 33.06368534415484106, 1.068504757029289695E-15 ) ) ;
#12927=CARTESIAN_POINT ( 'NONE',  ( -0.8801773607111008646, 43.27201867748817676, 2.915334737309923430 ) ) ;
#12929=CARTESIAN_POINT ( 'NONE',  ( 21.92686044187657046, 10.16212336850780673, 4.562052436263912550E-16 ) ) ;
#12930=CARTESIAN_POINT ( 'NONE',  ( 20.88017736071110519, 40.56368534415484106, 2.639326808657452039E-16 ) ) ;
#12934=CARTESIAN_POINT ( 'NONE',  ( 3.591859063236763294, 63.29030133659708923, -11.09922568453595026 ) ) ;
#12936=CARTESIAN_POINT ( 'NONE',  ( 22.26659068614895176, 34.72041550158063927, -7.082119434687042414 ) ) ;
#12937=CARTESIAN_POINT ( 'NONE',  ( 12.91533473730992121, 54.52201867748816255, 10.88017736071110164 ) ) ;
#12940=CARTESIAN_POINT ( 'NONE',  ( 12.63842701281683034, 47.46726448433412315, 9.846743663894596210 ) ) ;
#12942=CARTESIAN_POINT ( 'NONE',  ( 1.472469842513823179, 20.59226448433411960, -4.923371831947296329 ) ) ;
#12944=CARTESIAN_POINT ( 'NONE',  ( 0.5774900079438590739, 12.64701867748817143, -5.440088680355550821 ) ) ;
#12945=CARTESIAN_POINT ( 'NONE',  ( 1.472469842513823179, 31.42559781766745530, 4.923371831947296329 ) ) ;
#12946=CARTESIAN_POINT ( 'NONE',  ( 19.38216949554541557, 7.248634669930421381, -9.382169495545420901 ) ) ;
#12947=CARTESIAN_POINT ( 'NONE',  ( 20.88017736071110519, 60.56368534415484106, 2.639326808657452039E-16 ) ) ;
#12948=CARTESIAN_POINT ( 'NONE',  ( 4.559911319644449179, 27.23035201082150536, -9.422509992056141925 ) ) ;
#12949=CARTESIAN_POINT ( 'NONE',  ( 3.591859063236761518, 54.95696800326376064, 11.09922568453594849 ) ) ;
#12950=CARTESIAN_POINT ( 'NONE',  ( 17.08211943468705840, 45.13708216824730357, -12.26659068614894466 ) ) ;
#12954=CARTESIAN_POINT ( 'NONE',  ( 0.6178305044545818747, -1.501365330069579951, -9.382169495545419124 ) ) ;
#12955=CARTESIAN_POINT ( 'NONE',  ( 10.00000000000000178, 4.313685344154837509, 10.88017736071110342 ) ) ;
#12956=CARTESIAN_POINT ( 'NONE',  ( 4.559911319644449179, 48.89701867748817676, 9.422509992056141925 ) ) ;
#12958=CARTESIAN_POINT ( 'NONE',  ( 0.1532563361054100626, 60.80059781766744464, -2.638427012816831230 ) ) ;
#12959=ORIENTED_EDGE ( 'NONE', *, *, #84150, .F. ) ;
#12960=CARTESIAN_POINT ( 'NONE',  ( 7.361572987183170547, 17.05059781766745530, 9.846743663894590881 ) ) ;
#12961=CARTESIAN_POINT ( 'NONE',  ( 5.076628168052704559, 10.17559781766745175, -8.527530157486179263 ) ) ;
#12962=CARTESIAN_POINT ( 'NONE',  ( 1.472469842513823179, 36.42559781766745175, 4.923371831947296329 ) ) ;
#12963=CARTESIAN_POINT ( 'NONE',  ( 2.791683348922240793, 6.633931151000785675, 7.208316651077764092 ) ) ;
#12965=CARTESIAN_POINT ( 'NONE',  ( 5.076628168052704559, 20.17559781766745175, -8.527530157486179263 ) ) ;
#12967=EDGE_CURVE ( 'NONE', #64078, #85989, #57573, .T. ) ;
#12968=CARTESIAN_POINT ( 'NONE',  ( 12.63842701281683034, 2.467264484334118269, 9.846743663894596210 ) ) ;
#12970=CARTESIAN_POINT ( 'NONE',  ( 2.791683348922237240, 10.38393115100078390, -7.208316651077763204 ) ) ;
#12971=CARTESIAN_POINT ( 'NONE',  ( 19.84674366389459266, 13.71726448433411782, -2.638427012816827677 ) ) ;
#12974=CARTESIAN_POINT ( 'NONE',  ( 10.00000000000000000, 2.873634669930420049, -12.81628187352647608 ) ) ;
#12975=( NAMED_UNIT ( * ) SI_UNIT ( $, .STERADIAN. ) SOLID_ANGLE_UNIT ( ) );
#12976=CARTESIAN_POINT ( 'NONE',  ( 22.26659068614895176, 19.72041550158063572, -7.082119434687042414 ) ) ;
#12978=CARTESIAN_POINT ( 'NONE',  ( -0.3689425029237881626, 12.42874883491396609, 10.36894250292379027 ) ) ;
#12979=CARTESIAN_POINT ( 'NONE',  ( -0.3689425029237898834, 46.17874883491397497, -10.36894250292378850 ) ) ;
#12980=SURFACE_STYLE_USAGE ( .BOTH. , #27981 ) ;
#12981=CARTESIAN_POINT ( 'NONE',  ( 6.204703633549690345, 7.845415501580634832, 14.16423886937410082 ) ) ;
#12982=CARTESIAN_POINT ( 'NONE',  ( 10.00000000000000000, 66.81368534415484817, -10.88017736071110342 ) ) ;
#12983=CARTESIAN_POINT ( 'NONE',  ( -0.8801773607111009756, 28.06368534415484106, 1.068504757029289695E-15 ) ) ;
#12986=CARTESIAN_POINT ( 'NONE',  ( 2.791683348922237240, 25.38393115100078390, -7.208316651077763204 ) ) ;
#12987=CARTESIAN_POINT ( 'NONE',  ( 4.559911319644449179, 53.89701867748817676, 9.422509992056141925 ) ) ;
#12988=CARTESIAN_POINT ( 'NONE',  ( 1.472469842513823179, 31.42559781766745530, 4.923371831947296329 ) ) ;
#12989=CARTESIAN_POINT ( 'NONE',  ( 12.91533473730992121, 4.522018677488170546, 10.88017736071110164 ) ) ;
#12990=CARTESIAN_POINT ( 'NONE',  ( 16.40814093676324603, 57.45696800326375353, -11.09922568453594671 ) ) ;
#12991=CARTESIAN_POINT ( 'NONE',  ( 7.361572987183169658, 49.96726448433410894, -9.846743663894592657 ) ) ;
#12993=CARTESIAN_POINT ( 'NONE',  ( 0.6178305044545818747, 43.49863466993042493, -9.382169495545419124 ) ) ;
#12995=CARTESIAN_POINT ( 'NONE',  ( 2.035157376598824452, 48.68868534415483396, 7.964842623401179544 ) ) ;
#12996=CARTESIAN_POINT ( 'NONE',  ( 19.84674366389459266, 38.30059781766745175, 2.638427012816836559 ) ) ;
#12998=CARTESIAN_POINT ( 'NONE',  ( 6.204703633549690345, 20.76208216824730357, -14.16423886937410259 ) ) ;
#13001=CARTESIAN_POINT ( 'NONE',  ( 13.79529636645030344, 3.262082168247301350, 14.16423886937410614 ) ) ;
#13002=CARTESIAN_POINT ( 'NONE',  ( 15.44008868035555793, 56.39701867748817676, -9.422509992056140149 ) ) ;
#13003=CARTESIAN_POINT ( 'NONE',  ( 4.559911319644449179, 62.23035201082150536, -9.422509992056141925 ) ) ;
#13004=CARTESIAN_POINT ( 'NONE',  ( 10.00000000000000178, 48.05374883491396787, 14.16423886937410082 ) ) ;
#13005=CARTESIAN_POINT ( 'NONE',  ( 22.81628187352648496, 1.831968003263753753, -3.434112377981050290 ) ) ;
#13007=CARTESIAN_POINT ( 'NONE',  ( 19.42250999205614193, 60.14701867748817676, 5.440088680355555262 ) ) ;
#13008=DIRECTION ( 'NONE',  ( 1.000000000000000000, 0.000000000000000000, 0.000000000000000000 ) ) ;
#13009=CARTESIAN_POINT ( 'NONE',  ( -2.816281873526473856, 24.12363466993042138, 9.499525473075851096E-16 ) ) ;
#13010=CARTESIAN_POINT ( 'NONE',  ( 14.92337183194729633, 52.67559781766745175, 8.527530157486181039 ) ) ;
#13012=( NAMED_UNIT ( * ) PLANE_ANGLE_UNIT ( ) SI_UNIT ( $, .RADIAN. ) );
#13013=CARTESIAN_POINT ( 'NONE',  ( 0.5774900079438607392, 8.480352010821505360, 5.440088680355550821 ) ) ;
#13016=CARTESIAN_POINT ( 'NONE',  ( 15.44008868035555793, 6.397018677488170546, -9.422509992056140149 ) ) ;
#13018=CARTESIAN_POINT ( 'NONE',  ( 10.00000000000000000, 61.81368534415484106, -10.88017736071110342 ) ) ;
#13020=CARTESIAN_POINT ( 'NONE',  ( 1.472469842513823179, 1.425597817667451528, 4.923371831947296329 ) ) ;
#13021=CIRCLE ( 'NONE', #16252, 0.4999999999999993894 ) ;
#13022=CARTESIAN_POINT ( 'NONE',  ( 17.20831665107776587, 34.13393115100078745, -7.208316651077762316 ) ) ;
#13023=B_SPLINE_CURVE_WITH_KNOTS ( 'NONE', 3,
 ( #18573, #72055, #34531, #17598 ),
 .UNSPECIFIED., .F., .F.,
 ( 4, 4 ),
 ( 1.571840398521015072E-16, 0.001060528352561993307 ),
 .UNSPECIFIED. ) ;
#13024=CARTESIAN_POINT ( 'NONE',  ( 20.88017736071110164, 40.35535201082150536, 2.915334737309930979 ) ) ;
#13025=CARTESIAN_POINT ( 'NONE',  ( 0.6178305044545818747, 13.49863466993041783, -9.382169495545419124 ) ) ;
#13026=CARTESIAN_POINT ( 'NONE',  ( 19.42250999205614193, 40.14701867748817676, 5.440088680355555262 ) ) ;
#13029=COLOUR_RGB ( '', 0.40784314, 0.44705882, 0.49803922) ;
#13030=CARTESIAN_POINT ( 'NONE',  ( 6.565887622018943937, 43.08196800326374643, -12.81628187352647608 ) ) ;
#13032=CARTESIAN_POINT ( 'NONE',  ( 10.00000000000000178, 64.31368534415483396, 10.88017736071110342 ) ) ;
#13033=CARTESIAN_POINT ( 'NONE',  ( 13.43411237798106583, 27.66530133659708568, -12.81628187352647252 ) ) ;
#13034=CARTESIAN_POINT ( 'NONE',  ( 17.96484262340118221, 41.18868534415484106, -7.964842623401177768 ) ) ;
#13035=CARTESIAN_POINT ( 'NONE',  ( 0.1532563361054100626, 65.80059781766745175, -2.638427012816831230 ) ) ;
#13036=CARTESIAN_POINT ( 'NONE',  ( -4.164238869374099927, 62.01208216824728936, 3.795296366450308767 ) ) ;
#13037=CARTESIAN_POINT ( 'NONE',  ( 5.076628168052703671, 56.84226448433412315, 8.527530157486179263 ) ) ;
#13038=CARTESIAN_POINT ( 'NONE',  ( 4.559911319644449179, 68.89701867748817676, 9.422509992056141925 ) ) ;
#13040=CARTESIAN_POINT ( 'NONE',  ( 12.91533473730992121, 64.52201867748817676, 10.88017736071110164 ) ) ;
#13042=CARTESIAN_POINT ( 'NONE',  ( -2.266590686148945544, 26.38708216824730357, -7.082119434687050408 ) ) ;
#13045=( NAMED_UNIT ( * ) SI_UNIT ( $, .STERADIAN. ) SOLID_ANGLE_UNIT ( ) );
#13047=VERTEX_POINT ( 'NONE', #14439 ) ;
#13048=CARTESIAN_POINT ( 'NONE',  ( 6.204703633549690345, 65.76208216824731778, -14.16423886937410259 ) ) ;
#13049=CARTESIAN_POINT ( 'NONE',  ( 7.084665262690076126, 2.022018677488171434, -10.88017736071110164 ) ) ;
#13050=CARTESIAN_POINT ( 'NONE',  ( 14.92337183194729633, 32.67559781766745175, 8.527530157486181039 ) ) ;
#13051=CARTESIAN_POINT ( 'NONE',  ( -1.099225684535947600, 29.54030133659708923, 6.408140936763237150 ) ) ;
#13054=CARTESIAN_POINT ( 'NONE',  ( 20.88017736071110875, 10.77201867748817143, -2.915334737309920765 ) ) ;
#13055=CARTESIAN_POINT ( 'NONE',  ( 20.36894250292379382, 58.67874883491396076, 10.36894250292379205 ) ) ;
#13056=CARTESIAN_POINT ( 'NONE',  ( 12.63842701281683034, 27.46726448433411250, 9.846743663894596210 ) ) ;
#13057=CARTESIAN_POINT ( 'NONE',  ( 20.15039907845753220, 19.72266099184918886, 6.262539305110075283 ) ) ;
#13058=CARTESIAN_POINT ( 'NONE',  ( 19.84674366389459621, 13.50893115100078568, 7.409399052514197653E-17 ) ) ;
#13060=CARTESIAN_POINT ( 'NONE',  ( 18.06765999051783567, 58.99127512925446837, 6.500000000000043521 ) ) ;
#13063=ORIENTED_EDGE ( 'NONE', *, *, #27562, .F. ) ;
#13065=CARTESIAN_POINT ( 'NONE',  ( 17.08211943468705840, 20.13708216824730357, -12.26659068614894466 ) ) ;
#13066=CARTESIAN_POINT ( 'NONE',  ( 12.91533473730992121, 24.52201867748816966, 10.88017736071110164 ) ) ;
#13067=CARTESIAN_POINT ( 'NONE',  ( 10.00000000000000178, 19.31368534415484106, 10.88017736071110342 ) ) ;
#13068=CARTESIAN_POINT ( 'NONE',  ( 18.52753015748618282, 43.92559781766745175, -4.923371831947291888 ) ) ;
#13069=CARTESIAN_POINT ( 'NONE',  ( 13.43411237798106583, 12.66530133659708746, -12.81628187352647252 ) ) ;
#13070=CARTESIAN_POINT ( 'NONE',  ( 2.917880565312950480, 10.97041550158063572, -12.26659068614894821 ) ) ;
#13071=CARTESIAN_POINT ( 'NONE',  ( 18.52753015748618282, 43.92559781766745175, -4.923371831947291888 ) ) ;
#13072=AXIS2_PLACEMENT_3D ( 'NONE', #2266, #94712, #55230 ) ;
#13073=CARTESIAN_POINT ( 'NONE',  ( -1.099225684535947600, 29.54030133659708923, 6.408140936763237150 ) ) ;
#13074=CARTESIAN_POINT ( 'NONE',  ( 0.1532563361054082862, 1.217264484334117824, 2.638427012816831674 ) ) ;
#13076=CARTESIAN_POINT ( 'NONE',  ( 10.00000000000000000, 29.75893115100078745, -9.846743663894594434 ) ) ;
#13077=CARTESIAN_POINT ( 'NONE',  ( 20.36894250292379738, 54.92874883491396076, -10.36894250292379027 ) ) ;
#13079=CARTESIAN_POINT ( 'NONE',  ( 17.96484262340118221, 6.188685344154837509, -7.964842623401177768 ) ) ;
#13081=CARTESIAN_POINT ( 'NONE',  ( 0.5774900079438607392, 43.48035201082151247, 5.440088680355550821 ) ) ;
#13082=CARTESIAN_POINT ( 'NONE',  ( 7.084665262690076126, 49.10535201082149825, 10.88017736071109987 ) ) ;
#13083=CARTESIAN_POINT ( 'NONE',  ( 20.88017736071110164, 50.35535201082151247, 2.915334737309930979 ) ) ;
#13084=CARTESIAN_POINT ( 'NONE',  ( 2.035157376598822676, 42.43868534415483396, -7.964842623401177768 ) ) ;
#13090=VECTOR ( 'NONE', #77288, 1000.000000000000000 ) ;
#13091=CARTESIAN_POINT ( 'NONE',  ( 18.52753015748618282, 33.92559781766745886, -4.923371831947291888 ) ) ;
#13093=CARTESIAN_POINT ( 'NONE',  ( 12.63842701281683922, 54.55059781766745175, -9.846743663894590881 ) ) ;
#13098=CARTESIAN_POINT ( 'NONE',  ( -0.3689425029237881626, 2.428748834913967869, 10.36894250292379027 ) ) ;
#13100=CARTESIAN_POINT ( 'NONE',  ( -42.50369195530267774, 107.9060299417078426, 4.500000000000000888 ) ) ;
#13102=CARTESIAN_POINT ( 'NONE',  ( 22.26659068614894466, 63.88708216824730357, 7.082119434687054849 ) ) ;
#13107=CARTESIAN_POINT ( 'NONE',  ( 2.791683348922240793, 41.63393115100078745, 7.208316651077764092 ) ) ;
#13109=CARTESIAN_POINT ( 'NONE',  ( -1.099225684535947600, 18.70696800326375353, -6.408140936763238038 ) ) ;
#13110=CARTESIAN_POINT ( 'NONE',  ( 0.1532563361054100626, 15.80059781766745353, -2.638427012816831230 ) ) ;
#13112=CARTESIAN_POINT ( 'NONE',  ( 14.92337183194729633, 12.67559781766745353, 8.527530157486181039 ) ) ;
#13113=CARTESIAN_POINT ( 'NONE',  ( 0.6178305044545818747, -1.501365330069579951, -9.382169495545419124 ) ) ;
#13115=ADVANCED_FACE ( 'NONE', ( #29905 ), #3734, .T. ) ;
#13117=CARTESIAN_POINT ( 'NONE',  ( 7.084665262690076126, 14.10535201082150358, 10.88017736071109987 ) ) ;
#13118=CARTESIAN_POINT ( 'NONE',  ( -4.164238869374099039, 6.803748834913967869, 8.674139862899312516E-16 ) ) ;
#13119=CARTESIAN_POINT ( 'NONE',  ( 0.1532563361054100626, 25.80059781766744820, -2.638427012816831230 ) ) ;
#13120=CARTESIAN_POINT ( 'NONE',  ( 0.5774900079438590739, 52.64701867748817676, -5.440088680355550821 ) ) ;
#13121=CARTESIAN_POINT ( 'NONE',  ( 6.565887622018943937, 33.08196800326374643, -12.81628187352647608 ) ) ;
#13125=CARTESIAN_POINT ( 'NONE',  ( 13.43411237798105340, 0.5819680032637533085, 12.81628187352647963 ) ) ;
#13126=CARTESIAN_POINT ( 'NONE',  ( 7.361572987183170547, 62.05059781766745886, 9.846743663894590881 ) ) ;
#13127=CARTESIAN_POINT ( 'NONE',  ( 10.00000000000000000, 19.75893115100078390, -9.846743663894594434 ) ) ;
#13129=CARTESIAN_POINT ( 'NONE',  ( 16.40814093676324603, 27.45696800326375708, -11.09922568453594671 ) ) ;
#13131=CARTESIAN_POINT ( 'NONE',  ( 17.96484262340118221, 44.93868534415483396, 7.964842623401181321 ) ) ;
#13133=( BOUNDED_CURVE ( )  B_SPLINE_CURVE ( 2, ( #97082, #28553, #13553, #57564, #44039, #97570, #29033, #27065, #50071 ),
 .UNSPECIFIED., .F., .T. ) 
 B_SPLINE_CURVE_WITH_KNOTS ( ( 3, 2, 2, 2, 3 ),
 ( 0.3687123655116599230, 0.3690476190476190688, 0.3750000000000000000, 0.3809523809523809312, 0.3812876344883400770 ),
 .UNSPECIFIED. ) 
 CURVE ( )  GEOMETRIC_REPRESENTATION_ITEM ( )  RATIONAL_B_SPLINE_CURVE ( ( 0.9963778908391760503, 0.9980808541467920403, 1.000000000000000000, 0.9659258262890682012, 1.000000000000000000, 0.9659258262890682012, 1.000000000000000000, 0.9980808541467920403, 0.9963778908391760503 ) ) 
 REPRESENTATION_ITEM ( '' )  );
#13134=CARTESIAN_POINT ( 'NONE',  ( 4.559911319644449179, 32.23035201082150536, -9.422509992056141925 ) ) ;
#13136=CARTESIAN_POINT ( 'NONE',  ( 10.00000000000000178, 52.25893115100078745, 9.846743663894594434 ) ) ;
#13137=CARTESIAN_POINT ( 'NONE',  ( 17.96484262340118221, 56.18868534415484817, -7.964842623401177768 ) ) ;
#13138=CARTESIAN_POINT ( 'NONE',  ( 20.36894250292379738, 34.92874883491396076, -10.36894250292379027 ) ) ;
#13141=( BOUNDED_CURVE ( )  B_SPLINE_CURVE ( 2, ( #24966, #62939, #53967, #77945, #70455, #30961, #86444, #8470, #61459 ),
 .UNSPECIFIED., .F., .F. ) 
 B_SPLINE_CURVE_WITH_KNOTS ( ( 3, 2, 2, 2, 3 ),
 ( 0.9044266512259456769, 0.9047619047619047672, 0.9107142857142856984, 0.9166666666666667407, 0.9170019202026259419 ),
 .UNSPECIFIED. ) 
 CURVE ( )  GEOMETRIC_REPRESENTATION_ITEM ( )  RATIONAL_B_SPLINE_CURVE ( ( 0.9963778908391764944, 0.9980808541467923733, 1.000000000000000000, 0.9659258262890683122, 1.000000000000000000, 0.9659258262890683122, 1.000000000000000000, 0.9980808541467917072, 0.9963778908391753841 ) ) 
 REPRESENTATION_ITEM ( '' )  );
#13142=CARTESIAN_POINT ( 'NONE',  ( 17.20831665107776587, 39.13393115100079456, -7.208316651077762316 ) ) ;
#13143=CARTESIAN_POINT ( 'NONE',  ( 18.52753015748617571, 63.09226448433412315, 4.923371831947298993 ) ) ;
#13145=CARTESIAN_POINT ( 'NONE',  ( 2.035157376598822676, 27.43868534415483396, -7.964842623401177768 ) ) ;
#13146=CARTESIAN_POINT ( 'NONE',  ( 15.44008868035555793, 6.397018677488170546, -9.422509992056140149 ) ) ;
#13147=CARTESIAN_POINT ( 'NONE',  ( 7.084665262690076126, 9.105352010821503583, 10.88017736071109987 ) ) ;
#13148=CARTESIAN_POINT ( 'NONE',  ( 1.472469842513823179, 0.5922644843341181575, -4.923371831947296329 ) ) ;
#13149=CARTESIAN_POINT ( 'NONE',  ( 24.16423886937409904, 19.09541550158063927, 3.795296366450317205 ) ) ;
#13150=CARTESIAN_POINT ( 'NONE',  ( 5.076628168052704559, 20.17559781766745175, -8.527530157486179263 ) ) ;
#13151=CARTESIAN_POINT ( 'NONE',  ( 14.92337183194729633, 57.67559781766745886, 8.527530157486181039 ) ) ;
#13152=CARTESIAN_POINT ( 'NONE',  ( 7.084665262690076126, 39.10535201082150536, 10.88017736071109987 ) ) ;
#13156=ORIENTED_EDGE ( 'NONE', *, *, #43233, .T. ) ;
#13159=CARTESIAN_POINT ( 'NONE',  ( 19.84674366389459266, 43.30059781766744464, 2.638427012816836559 ) ) ;
#13163=CARTESIAN_POINT ( 'NONE',  ( 10.00000000000000178, 28.05374883491396787, 14.16423886937410082 ) ) ;
#13164=CARTESIAN_POINT ( 'NONE',  ( -0.3689425029237898834, 11.17874883491396787, -10.36894250292378850 ) ) ;
#13165=CARTESIAN_POINT ( 'NONE',  ( 20.88017736071110164, 60.35535201082151957, 2.915334737309930979 ) ) ;
#13166=CARTESIAN_POINT ( 'NONE',  ( 13.79529636645031943, 55.34541550158062506, -14.16423886937409904 ) ) ;
#13167=CARTESIAN_POINT ( 'NONE',  ( 6.565887622018943937, -1.918031996736246692, -12.81628187352647608 ) ) ;
#13168=CARTESIAN_POINT ( 'NONE',  ( 19.84674366389459266, 43.30059781766744464, 2.638427012816836559 ) ) ;
#13170=CARTESIAN_POINT ( 'NONE',  ( 15.44008868035555260, 44.73035201082151247, 9.422509992056143702 ) ) ;
#13171=CARTESIAN_POINT ( 'NONE',  ( 6.565887622018943937, 5.165301336597086568, 12.81628187352647430 ) ) ;
#13172=CARTESIAN_POINT ( 'NONE',  ( -4.164238869374099927, 22.01208216824730357, 3.795296366450308767 ) ) ;
#13173=CARTESIAN_POINT ( 'NONE',  ( -0.3689425029237881626, 47.42874883491396787, 10.36894250292379027 ) ) ;
#13175=CARTESIAN_POINT ( 'NONE',  ( 20.88017736071110875, 20.77201867748816611, -2.915334737309920765 ) ) ;
#13177=CIRCLE ( 'NONE', #59419, 0.5000000000000004441 ) ;
#13179=CARTESIAN_POINT ( 'NONE',  ( 0.5774900079438607392, 43.48035201082151247, 5.440088680355550821 ) ) ;
#13183=CARTESIAN_POINT ( 'NONE',  ( 19.72487221294570858, 4.782175860852374782, 6.500000000000002665 ) ) ;
#13187=CARTESIAN_POINT ( 'NONE',  ( 2.917880565312950480, 40.97041550158063217, -12.26659068614894821 ) ) ;
#13188=CARTESIAN_POINT ( 'NONE',  ( 10.00000000000000178, 42.25893115100078745, 9.846743663894594434 ) ) ;
#13189=CARTESIAN_POINT ( 'NONE',  ( 20.32896413005680358, 49.74545670184114954, 5.963430220938287007 ) ) ;
#13192=CARTESIAN_POINT ( 'NONE',  ( 15.44008868035555260, 59.73035201082151247, 9.422509992056143702 ) ) ;
#13193=CARTESIAN_POINT ( 'NONE',  ( 19.38216949554541202, 55.99863466993041072, 9.382169495545424454 ) ) ;
#13196=ADVANCED_FACE ( 'NONE', ( #38694 ), #23210, .T. ) ;
#13197=CARTESIAN_POINT ( 'NONE',  ( 17.08211943468705840, 20.13708216824730357, -12.26659068614894466 ) ) ;
#13199=CARTESIAN_POINT ( 'NONE',  ( 6.565887622018943937, 18.08196800326375708, -12.81628187352647608 ) ) ;
#13202=CARTESIAN_POINT ( 'NONE',  ( 13.43411237798105340, 45.58196800326374643, 12.81628187352647963 ) ) ;
#13203=CARTESIAN_POINT ( 'NONE',  ( 12.63842701281683034, 42.46726448433412315, 9.846743663894596210 ) ) ;
#13204=CARTESIAN_POINT ( 'NONE',  ( 15.44008868035555260, 9.730352010821505360, 9.422509992056143702 ) ) ;
#13205=CARTESIAN_POINT ( 'NONE',  ( -2.816281873526473856, 59.12363466993042493, 9.499525473075851096E-16 ) ) ;
#13206=CARTESIAN_POINT ( 'NONE',  ( 0.1532563361054100626, 45.80059781766745886, -2.638427012816831230 ) ) ;
#13210=DIRECTION ( 'NONE',  ( -0.000000000000000000, -0.000000000000000000, 1.000000000000000000 ) ) ;
#13211=CARTESIAN_POINT ( 'NONE',  ( 18.17884179759848706, 8.666888798595232757, -6.499999999999968914 ) ) ;
#13214=CARTESIAN_POINT ( 'NONE',  ( 17.20831665107776587, 19.13393115100078035, -7.208316651077762316 ) ) ;
#13215=EDGE_CURVE ( 'NONE', #75354, #79733, #30677, .T. ) ;
#13216=CARTESIAN_POINT ( 'NONE',  ( 10.00000000000000000, 27.87363466993042138, -12.81628187352647608 ) ) ;
#13217=CARTESIAN_POINT ( 'NONE',  ( 0.9413316022086131163, 38.45508385108959004, 6.499999999999978684 ) ) ;
#13219=CARTESIAN_POINT ( 'NONE',  ( 2.791683348922237240, 60.38393115100078745, -7.208316651077763204 ) ) ;
#13220=CARTESIAN_POINT ( 'NONE',  ( 17.85158348494336167, 4.737265733804413514, -6.499999999999994671 ) ) ;
#13221=CARTESIAN_POINT ( 'NONE',  ( 10.00000000000000000, 20.55374883491396787, -14.16423886937410082 ) ) ;
#13222=CARTESIAN_POINT ( 'NONE',  ( 2.791683348922240793, 46.63393115100077324, 7.208316651077764092 ) ) ;
#13223=CARTESIAN_POINT ( 'NONE',  ( -2.816281873526473856, 49.12363466993042493, 9.499525473075851096E-16 ) ) ;
#13224=CARTESIAN_POINT ( 'NONE',  ( 20.32896413005680714, 37.60497603579418069, -5.963430220938276349 ) ) ;
#13225=CARTESIAN_POINT ( 'NONE',  ( 17.96484262340118221, 59.93868534415484106, 7.964842623401181321 ) ) ;
#13226=CARTESIAN_POINT ( 'NONE',  ( 20.32896413005680714, 47.60497603579417358, -5.963430220938276349 ) ) ;
#13227=CARTESIAN_POINT ( 'NONE',  ( 1.472469842513823179, 30.59226448433411960, -4.923371831947296329 ) ) ;
#13228=CARTESIAN_POINT ( 'NONE',  ( 10.00000000000000178, 44.31368534415484106, 10.88017736071110342 ) ) ;
#13230=CARTESIAN_POINT ( 'NONE',  ( 0.1532563361054100626, 30.80059781766744820, -2.638427012816831230 ) ) ;
#13233=CARTESIAN_POINT ( 'NONE',  ( 0.5774900079438607392, 43.48035201082151247, 5.440088680355550821 ) ) ;
#13234=( GEOMETRIC_REPRESENTATION_CONTEXT ( 3 ) GLOBAL_UNCERTAINTY_ASSIGNED_CONTEXT ( ( #86204 ) ) GLOBAL_UNIT_ASSIGNED_CONTEXT ( ( #63143, #55659, #69191 ) ) REPRESENTATION_CONTEXT ( 'NONE', 'WORKASPACE' ) );
#13238=CARTESIAN_POINT ( 'NONE',  ( 17.96484262340118221, 14.93868534415483751, 7.964842623401181321 ) ) ;
#13239=CARTESIAN_POINT ( 'NONE',  ( 17.20831665107776587, 52.88393115100078035, 7.208316651077764980 ) ) ;
#13240=CARTESIAN_POINT ( 'NONE',  ( 15.44008868035555793, 41.39701867748817676, -9.422509992056140149 ) ) ;
#13243=CARTESIAN_POINT ( 'NONE',  ( 7.084665262690076126, 64.10535201082150536, 10.88017736071109987 ) ) ;
#13244=CARTESIAN_POINT ( 'NONE',  ( 20.88017736071110164, 30.35535201082151247, 2.915334737309930979 ) ) ;
#13245=CARTESIAN_POINT ( 'NONE',  ( 0.000000000000000000, 70.80332830338373640, -5.000000000000000000 ) ) ;
#13246=CARTESIAN_POINT ( 'NONE',  ( 0.1532563361054083140, 1.008931151000784787, 1.131784320476157264E-15 ) ) ;
#13247=CARTESIAN_POINT ( 'NONE',  ( 19.84674366389459266, 28.71726448433411960, -2.638427012816827677 ) ) ;
#13251=CARTESIAN_POINT ( 'NONE',  ( 0.1532563361054082862, 51.21726448433412315, 2.638427012816831674 ) ) ;
#13252=CARTESIAN_POINT ( 'NONE',  ( 10.00000000000000178, 58.05374883491397497, 14.16423886937410082 ) ) ;
#13254=CARTESIAN_POINT ( 'NONE',  ( 17.08211943468705130, 13.47041550158063572, 12.26659068614894998 ) ) ;
#13255=B_SPLINE_CURVE_WITH_KNOTS ( 'NONE', 3,
 ( #80333, #33339, #49823, #11832 ),
 .UNSPECIFIED., .F., .F.,
 ( 4, 4 ),
 ( 0.000000000000000000, 0.0003153491572464160622 ),
 .UNSPECIFIED. ) ;
#13256=CARTESIAN_POINT ( 'NONE',  ( -2.266590686148945544, 31.38708216824730002, -7.082119434687050408 ) ) ;
#13257=CARTESIAN_POINT ( 'NONE',  ( -1.099225684535947600, 9.540301336597087456, 6.408140936763237150 ) ) ;
#13258=ORIENTED_EDGE ( 'NONE', *, *, #28207, .F. ) ;
#13259=CARTESIAN_POINT ( 'NONE',  ( 19.42250999205614193, 10.14701867748816966, 5.440088680355555262 ) ) ;
#13260=CARTESIAN_POINT ( 'NONE',  ( 1.472469842513823179, 45.59226448433412315, -4.923371831947296329 ) ) ;
#13263=CARTESIAN_POINT ( 'NONE',  ( 17.20831665107776587, 4.133931151000785675, -7.208316651077762316 ) ) ;
#13264=CARTESIAN_POINT ( 'NONE',  ( 10.00000000000000178, 20.37363466993042138, 12.81628187352647608 ) ) ;
#13265=CARTESIAN_POINT ( 'NONE',  ( 12.63842701281683922, 29.55059781766745175, -9.846743663894590881 ) ) ;
#13267=CARTESIAN_POINT ( 'NONE',  ( 1.472469842513823179, 5.592264484334118713, -4.923371831947296329 ) ) ;
#13270=CARTESIAN_POINT ( 'NONE',  ( 10.00000000000000000, 16.81368534415483751, -10.88017736071110342 ) ) ;
#13271=CARTESIAN_POINT ( 'NONE',  ( -0.3689425029237881626, 42.42874883491396787, 10.36894250292379027 ) ) ;
#13272=CARTESIAN_POINT ( 'NONE',  ( -0.8801773607111009756, 68.06368534415484817, 1.068504757029289695E-15 ) ) ;
#13274=CARTESIAN_POINT ( 'NONE',  ( 20.24186590665278018, 52.61633188102327807, -6.114288769123040090 ) ) ;
#13275=CARTESIAN_POINT ( 'NONE',  ( 5.076628168052704559, 30.17559781766745175, -8.527530157486179263 ) ) ;
#13277=CARTESIAN_POINT ( 'NONE',  ( 18.52753015748618282, 3.925597817667451306, -4.923371831947291888 ) ) ;
#13278=CARTESIAN_POINT ( 'NONE',  ( -1.066947046745619687, -5.787280142670764339E-16, -1.918137652920613778 ) ) ;
#13279=CARTESIAN_POINT ( 'NONE',  ( 5.076628168052703671, 31.84226448433412315, 8.527530157486179263 ) ) ;
#13280=CARTESIAN_POINT ( 'NONE',  ( 18.52753015748618282, 63.92559781766745886, -4.923371831947291888 ) ) ;
#13282=CARTESIAN_POINT ( 'NONE',  ( 19.42250999205614193, 40.14701867748817676, 5.440088680355555262 ) ) ;
#13286=CARTESIAN_POINT ( 'NONE',  ( -2.816281873526471635, 58.91530133659707502, -3.434112377981056508 ) ) ;
#13288=CARTESIAN_POINT ( 'NONE',  ( 12.91533473730993009, 61.60535201082150536, -10.88017736071109987 ) ) ;
#13289=CARTESIAN_POINT ( 'NONE',  ( 0.6178305044545838731, 39.74863466993041072, 9.382169495545420901 ) ) ;
#13290=CARTESIAN_POINT ( 'NONE',  ( 10.00000000000000000, 55.55374883491396787, -14.16423886937410082 ) ) ;
#13291=CARTESIAN_POINT ( 'NONE',  ( 5.076628168052703671, 31.84226448433412315, 8.527530157486179263 ) ) ;
#13292=SURFACE_STYLE_USAGE ( .BOTH. , #91258 ) ;
#13293=PRESENTATION_STYLE_ASSIGNMENT (( #83275 ) ) ;
#13294=CARTESIAN_POINT ( 'NONE',  ( 24.16423886937410614, 19.51208216824729647, -3.795296366450302550 ) ) ;
#13295=CARTESIAN_POINT ( 'NONE',  ( -2.266590686148945544, 42.22041550158063217, 7.082119434687048631 ) ) ;
#13296=CARTESIAN_POINT ( 'NONE',  ( 1.472469842513823179, 46.42559781766745175, 4.923371831947296329 ) ) ;
#13297=CARTESIAN_POINT ( 'NONE',  ( 10.00000000000000000, 41.81368534415484106, -10.88017736071110342 ) ) ;
#13298=CARTESIAN_POINT ( 'NONE',  ( 0.5774900079438607392, 58.48035201082151247, 5.440088680355550821 ) ) ;
#13300=VERTEX_POINT ( 'NONE', #53684 ) ;
#13301=CARTESIAN_POINT ( 'NONE',  ( 10.00000000000000178, 40.37363466993042493, 12.81628187352647608 ) ) ;
#13302=B_SPLINE_CURVE_WITH_KNOTS ( 'NONE', 3,
 ( #5984, #82460, #51973, #96499 ),
 .UNSPECIFIED., .F., .F.,
 ( 4, 4 ),
 ( 0.000000000000000000, 0.002392975128318497631 ),
 .UNSPECIFIED. ) ;
#13303=CARTESIAN_POINT ( 'NONE',  ( 7.084665262690076126, 67.02201867748817676, -10.88017736071110164 ) ) ;
#13304=ORIENTED_EDGE ( 'NONE', *, *, #36865, .T. ) ;
#13306=CARTESIAN_POINT ( 'NONE',  ( 13.79529636645031943, 10.34541550158063394, -14.16423886937409904 ) ) ;
#13307=CARTESIAN_POINT ( 'NONE',  ( 18.52753015748617571, 13.09226448433411960, 4.923371831947298993 ) ) ;
#13308=CARTESIAN_POINT ( 'NONE',  ( -0.3289641300568005855, 60.10497603579418069, 5.963430220938281678 ) ) ;
#13309=ORIENTED_EDGE ( 'NONE', *, *, #91952, .F. ) ;
#13310=CARTESIAN_POINT ( 'NONE',  ( 4.559911319644449179, 18.89701867748817321, 9.422509992056141925 ) ) ;
#13311=CARTESIAN_POINT ( 'NONE',  ( 1.472469842513823179, 0.5922644843341181575, -4.923371831947296329 ) ) ;
#13313=CARTESIAN_POINT ( 'NONE',  ( 10.00000000000000178, 13.05374883491396787, 14.16423886937410082 ) ) ;
#13314=VERTEX_POINT ( 'NONE', #79633 ) ;
#13315=CARTESIAN_POINT ( 'NONE',  ( 0.5774900079438607392, 28.48035201082150891, 5.440088680355550821 ) ) ;
#13316=CARTESIAN_POINT ( 'NONE',  ( 18.52753015748617571, 53.09226448433412315, 4.923371831947298993 ) ) ;
#13318=VECTOR ( 'NONE', #78913, 1000.000000000000000 ) ;
#13319=CARTESIAN_POINT ( 'NONE',  ( 2.791683348922237240, 60.38393115100078745, -7.208316651077763204 ) ) ;
#13320=ORIENTED_EDGE ( 'NONE', *, *, #63943, .T. ) ;
#13322=CARTESIAN_POINT ( 'NONE',  ( 10.00000000000000000, 61.81368534415484106, -10.88017736071110342 ) ) ;
#13323=CARTESIAN_POINT ( 'NONE',  ( 12.63842701281683922, 59.55059781766744464, -9.846743663894590881 ) ) ;
#13325=CARTESIAN_POINT ( 'NONE',  ( -2.816281873526473856, 39.33196800326374643, 3.434112377981055619 ) ) ;
#13326=CARTESIAN_POINT ( 'NONE',  ( 19.42250999205614193, 5.147018677488171434, 5.440088680355555262 ) ) ;
#13328=CARTESIAN_POINT ( 'NONE',  ( 10.00000000000000178, 2.258931151000784787, 9.846743663894594434 ) ) ;
#13329=CARTESIAN_POINT ( 'NONE',  ( 12.91533473730992121, 24.52201867748816966, 10.88017736071110164 ) ) ;
#13330=EDGE_CURVE ( 'NONE', #97093, #76767, #3647, .T. ) ;
#13332=CARTESIAN_POINT ( 'NONE',  ( 16.40814093676324603, 52.45696800326375353, -11.09922568453594671 ) ) ;
#13333=CARTESIAN_POINT ( 'NONE',  ( 2.035157376598822676, 47.43868534415484817, -7.964842623401177768 ) ) ;
#13335=CARTESIAN_POINT ( 'NONE',  ( 22.81628187352648496, 41.83196800326375353, -3.434112377981050290 ) ) ;
#13336=CARTESIAN_POINT ( 'NONE',  ( 2.035157376598824452, 43.68868534415484106, 7.964842623401179544 ) ) ;
#13338=CARTESIAN_POINT ( 'NONE',  ( 17.20831665107776587, 59.13393115100078745, -7.208316651077762316 ) ) ;
#13340=CARTESIAN_POINT ( 'NONE',  ( 1.472469842513823179, 16.42559781766745175, 4.923371831947296329 ) ) ;
#13341=CARTESIAN_POINT ( 'NONE',  ( 6.565887622018943937, 13.08196800326374998, -12.81628187352647608 ) ) ;
#13343=CARTESIAN_POINT ( 'NONE',  ( 12.63842701281683922, 64.55059781766745175, -9.846743663894590881 ) ) ;
#13344=CARTESIAN_POINT ( 'NONE',  ( 12.91533473730992121, 24.52201867748816966, 10.88017736071110164 ) ) ;
#13345=CARTESIAN_POINT ( 'NONE',  ( 19.84674366389459266, 53.30059781766744464, 2.638427012816836559 ) ) ;
#13347=CARTESIAN_POINT ( 'NONE',  ( 17.20831665107776587, 12.88393115100078390, 7.208316651077764980 ) ) ;
#13348=CARTESIAN_POINT ( 'NONE',  ( 0.1532563361054082862, 1.217264484334117824, 2.638427012816831674 ) ) ;
#13349=CARTESIAN_POINT ( 'NONE',  ( 16.40814093676324603, 2.456968003263753531, -11.09922568453594671 ) ) ;
#13350=ORIENTED_EDGE ( 'NONE', *, *, #24010, .F. ) ;
#13351=CARTESIAN_POINT ( 'NONE',  ( -40.70923076923077844, 107.8461538461538396, -9.500000000000000000 ) ) ;
#13352=CARTESIAN_POINT ( 'NONE',  ( 13.43411237798105340, 40.58196800326375353, 12.81628187352647963 ) ) ;
#13353=CARTESIAN_POINT ( 'NONE',  ( 19.84674366389459266, 28.30059781766745886, 2.638427012816836559 ) ) ;
#13355=CARTESIAN_POINT ( 'NONE',  ( -2.266590686148945544, 57.22041550158063217, 7.082119434687048631 ) ) ;
#13356=CARTESIAN_POINT ( 'NONE',  ( 0.1532563361054082862, 36.21726448433410894, 2.638427012816831674 ) ) ;
#13358=DIRECTION ( 'NONE',  ( 0.000000000000000000, -1.000000000000000000, 0.000000000000000000 ) ) ;
#13359=CARTESIAN_POINT ( 'NONE',  ( 20.88017736071110164, 10.35535201082150714, 2.915334737309930979 ) ) ;
#13360=CARTESIAN_POINT ( 'NONE',  ( -42.80192881254231452, 92.20710678118653902, 9.500000000000000000 ) ) ;
#13362=CARTESIAN_POINT ( 'NONE',  ( 0.5774900079438607392, 13.48035201082150358, 5.440088680355550821 ) ) ;
#13363=CARTESIAN_POINT ( 'NONE',  ( -2.266590686148945544, 47.22041550158063927, 7.082119434687048631 ) ) ;
#13364=CARTESIAN_POINT ( 'NONE',  ( 10.00000000000000000, 55.55374883491396787, -14.16423886937410082 ) ) ;
#13366=CARTESIAN_POINT ( 'NONE',  ( 1.472469842513823179, 6.425597817667451750, 4.923371831947296329 ) ) ;
#13367=CARTESIAN_POINT ( 'NONE',  ( 16.40814093676323893, 0.7903013365970867898, 11.09922568453595026 ) ) ;
#13369=CARTESIAN_POINT ( 'NONE',  ( 7.084665262690076126, 52.02201867748816255, -10.88017736071110164 ) ) ;
#13371=ADVANCED_FACE ( 'NONE', ( #26621 ), #48633, .T. ) ;
#13372=CARTESIAN_POINT ( 'NONE',  ( 0.1532563361054100626, 65.80059781766745175, -2.638427012816831230 ) ) ;
#13373=VERTEX_POINT ( 'NONE', #32651 ) ;
#13374=CARTESIAN_POINT ( 'NONE',  ( 12.63842701281683034, 32.46726448433412315, 9.846743663894596210 ) ) ;
#13375=DIRECTION ( 'NONE',  ( 0.000000000000000000, 0.000000000000000000, -1.000000000000000000 ) ) ;
#13377=VECTOR ( 'NONE', #69261, 1000.000000000000000 ) ;
#13378=CARTESIAN_POINT ( 'NONE',  ( 2.917880565312948704, 42.63708216824729647, 12.26659068614894643 ) ) ;
#13380=CARTESIAN_POINT ( 'NONE',  ( 18.52753015748618282, 13.92559781766745175, -4.923371831947291888 ) ) ;
#13383=CARTESIAN_POINT ( 'NONE',  ( 12.91533473730992121, 29.52201867748817321, 10.88017736071110164 ) ) ;
#13384=CARTESIAN_POINT ( 'NONE',  ( 22.81628187352648496, 31.83196800326375353, -3.434112377981050290 ) ) ;
#13385=CARTESIAN_POINT ( 'NONE',  ( 3.591859063236763294, 38.29030133659708923, -11.09922568453595026 ) ) ;
#13386=CARTESIAN_POINT ( 'NONE',  ( 13.43411237798106583, 57.66530133659708923, -12.81628187352647252 ) ) ;
#13387=EDGE_LOOP ( 'NONE', ( #24565, #42596, #63901, #80699, #98621, #42716 ) ) ;
#13391=CARTESIAN_POINT ( 'NONE',  ( 24.16423886937409904, 24.09541550158063927, 3.795296366450317205 ) ) ;
#13392=FILL_AREA_STYLE ('',( #50397 ) ) ;
#13393=( LENGTH_UNIT ( ) NAMED_UNIT ( * ) SI_UNIT ( .MILLI., .METRE. ) );
#13394=CARTESIAN_POINT ( 'NONE',  ( 2.035157376598824452, 23.68868534415484461, 7.964842623401179544 ) ) ;
#13396=DIRECTION ( 'NONE',  ( 0.000000000000000000, 0.000000000000000000, -1.000000000000000000 ) ) ;
#13397=CARTESIAN_POINT ( 'NONE',  ( -0.8801773607110991993, 47.85535201082150536, -2.915334737309923874 ) ) ;
#13398=CARTESIAN_POINT ( 'NONE',  ( -0.8801773607110991993, 52.85535201082151247, -2.915334737309923874 ) ) ;
#13399=CARTESIAN_POINT ( 'NONE',  ( 3.591859063236763294, 13.29030133659708746, -11.09922568453595026 ) ) ;
#13402=CARTESIAN_POINT ( 'NONE',  ( 5.076628168052703671, 21.84226448433411960, 8.527530157486179263 ) ) ;
#13403=CARTESIAN_POINT ( 'NONE',  ( 10.00000000000000000, 46.81368534415484106, -10.88017736071110342 ) ) ;
#13404=CARTESIAN_POINT ( 'NONE',  ( -2.816281873526473856, 14.33196800326375531, 3.434112377981055619 ) ) ;
#13405=CARTESIAN_POINT ( 'NONE',  ( 2.791683348922237240, 0.3839311510007847872, -7.208316651077763204 ) ) ;
#13406=CARTESIAN_POINT ( 'NONE',  ( 0.1532563361054083140, 21.00893115100078745, 1.131784320476157264E-15 ) ) ;
#13407=CARTESIAN_POINT ( 'NONE',  ( 3.591859063236763294, 48.29030133659708923, -11.09922568453595026 ) ) ;
#13408=CARTESIAN_POINT ( 'NONE',  ( 5.076628168052704559, 25.17559781766745175, -8.527530157486179263 ) ) ;
#13410=CARTESIAN_POINT ( 'NONE',  ( 22.26659068614894466, 3.887082168247300906, 7.082119434687054849 ) ) ;
#13411=DIRECTION ( 'NONE',  ( 0.000000000000000000, 0.000000000000000000, 1.000000000000000000 ) ) ;
#13412=CARTESIAN_POINT ( 'NONE',  ( -0.8801773607111008646, 23.27201867748817676, 2.915334737309923430 ) ) ;
#13413=CARTESIAN_POINT ( 'NONE',  ( -4.164238869374099927, 37.01208216824731068, 3.795296366450308767 ) ) ;
#13414=CARTESIAN_POINT ( 'NONE',  ( 5.076628168052704559, 35.17559781766745175, -8.527530157486179263 ) ) ;
#13415=CARTESIAN_POINT ( 'NONE',  ( -0.8801773607111008646, 23.27201867748817676, 2.915334737309923430 ) ) ;
#13416=EDGE_CURVE ( 'NONE', #42599, #63730, #29422, .T. ) ;
#13417=CARTESIAN_POINT ( 'NONE',  ( 2.035157376598822676, 22.43868534415483396, -7.964842623401177768 ) ) ;
#13419=CARTESIAN_POINT ( 'NONE',  ( 2.035157376598824452, 23.68868534415484461, 7.964842623401179544 ) ) ;
#13421=CARTESIAN_POINT ( 'NONE',  ( 21.09922568453594849, 41.20696800326375353, 6.408140936763242479 ) ) ;
#13422=CARTESIAN_POINT ( 'NONE',  ( 19.42250999205614548, 35.98035201082151247, -5.440088680355545492 ) ) ;
#13424=CARTESIAN_POINT ( 'NONE',  ( 12.91533473730993009, 36.60535201082151247, -10.88017736071109987 ) ) ;
#13426=CARTESIAN_POINT ( 'NONE',  ( 10.00000000000000178, 52.25893115100078745, 9.846743663894594434 ) ) ;
#13427=CARTESIAN_POINT ( 'NONE',  ( 15.44008868035555793, 41.39701867748817676, -9.422509992056140149 ) ) ;
#13429=CARTESIAN_POINT ( 'NONE',  ( -0.03743638938523772414, 9.251975280310178462, -6.399506433553937335 ) ) ;
#13430=CARTESIAN_POINT ( 'NONE',  ( -4.164238869374099927, 47.01208216824729647, 3.795296366450308767 ) ) ;
#13431=CARTESIAN_POINT ( 'NONE',  ( 17.96484262340118221, 49.93868534415484106, 7.964842623401181321 ) ) ;
#13432=CARTESIAN_POINT ( 'NONE',  ( 0.2751277870542911397, 50.30223176428831522, 6.499999999999992006 ) ) ;
#13433=CARTESIAN_POINT ( 'NONE',  ( 0.000000000000000000, 0.5000000000000000000, -5.999999999999999112 ) ) ;
#13434=CARTESIAN_POINT ( 'NONE',  ( 18.52753015748618282, 48.92559781766745886, -4.923371831947291888 ) ) ;
#13435=CARTESIAN_POINT ( 'NONE',  ( 5.076628168052704559, 5.175597817667451750, -8.527530157486179263 ) ) ;
#13436=CARTESIAN_POINT ( 'NONE',  ( 7.361572987183169658, 24.96726448433412315, -9.846743663894592657 ) ) ;
#13437=ORIENTED_EDGE ( 'NONE', *, *, #20763, .T. ) ;
#13438=CARTESIAN_POINT ( 'NONE',  ( 2.791683348922237240, 15.38393115100078212, -7.208316651077763204 ) ) ;
#13440=CARTESIAN_POINT ( 'NONE',  ( -0.8801773607110991993, 22.85535201082150181, -2.915334737309923874 ) ) ;
#13441=CARTESIAN_POINT ( 'NONE',  ( 1.472469842513823179, 25.59226448433412315, -4.923371831947296329 ) ) ;
#13442=CARTESIAN_POINT ( 'NONE',  ( 0.6178305044545838731, 9.748634669930416052, 9.382169495545420901 ) ) ;
#13443=CARTESIAN_POINT ( 'NONE',  ( 4.559911319644449179, 63.89701867748817676, 9.422509992056141925 ) ) ;
#13444=CARTESIAN_POINT ( 'NONE',  ( 20.88017736071110519, 50.56368534415484106, 2.639326808657452039E-16 ) ) ;
#13445=CARTESIAN_POINT ( 'NONE',  ( 15.44008868035555793, 31.39701867748817676, -9.422509992056140149 ) ) ;
#13446=CARTESIAN_POINT ( 'NONE',  ( 19.38216949554541202, 50.99863466993042493, 9.382169495545424454 ) ) ;
#13447=CARTESIAN_POINT ( 'NONE',  ( 17.08211943468705840, 40.13708216824731068, -12.26659068614894466 ) ) ;
#13448=ADVANCED_FACE ( 'NONE', ( #34604 ), #55573, .T. ) ;
#13452=CARTESIAN_POINT ( 'NONE',  ( -2.816281873526471635, 3.915301336597087456, -3.434112377981056508 ) ) ;
#13453=CARTESIAN_POINT ( 'NONE',  ( 4.559911319644449179, 3.897018677488170990, 9.422509992056141925 ) ) ;
#13455=CARTESIAN_POINT ( 'NONE',  ( 20.88017736071110875, 50.77201867748817676, -2.915334737309920765 ) ) ;
#13456=SURFACE_SIDE_STYLE ('',( #37458 ) ) ;
#13458=EDGE_LOOP ( 'NONE', ( #51419, #49191, #84612, #40562, #30478, #1403, #37948, #27953 ) ) ;
#13459=CARTESIAN_POINT ( 'NONE',  ( 0.1532563361054082862, 11.21726448433411605, 2.638427012816831674 ) ) ;
#13462=CARTESIAN_POINT ( 'NONE',  ( 2.035157376598824452, 58.68868534415482685, 7.964842623401179544 ) ) ;
#13463=CARTESIAN_POINT ( 'NONE',  ( 5.076628168052704559, 30.17559781766745175, -8.527530157486179263 ) ) ;
#13465=CARTESIAN_POINT ( 'NONE',  ( 14.92337183194729988, 29.34226448433411960, -8.527530157486177487 ) ) ;
#13466=CARTESIAN_POINT ( 'NONE',  ( 19.84674366389459266, 8.300597817667451750, 2.638427012816836559 ) ) ;
#13468=CARTESIAN_POINT ( 'NONE',  ( -1.099225684535947600, 43.70696800326375353, -6.408140936763238038 ) ) ;
#13469=CARTESIAN_POINT ( 'NONE',  ( 7.084665262690076126, 67.02201867748817676, -10.88017736071110164 ) ) ;
#13472=CARTESIAN_POINT ( 'NONE',  ( 5.076628168052704559, 35.17559781766745175, -8.527530157486179263 ) ) ;
#13474=CARTESIAN_POINT ( 'NONE',  ( 6.565887622018943937, 55.16530133659709634, 12.81628187352647430 ) ) ;
#13476=CARTESIAN_POINT ( 'NONE',  ( 1.472469842513823179, 65.59226448433412315, -4.923371831947296329 ) ) ;
#13479=CARTESIAN_POINT ( 'NONE',  ( 20.36894250292379382, 13.67874883491396965, 10.36894250292379205 ) ) ;
#13481=UNCERTAINTY_MEASURE_WITH_UNIT (LENGTH_MEASURE( 1.000000000000000082E-05 ), #48766, 'distance_accuracy_value', 'NONE');
#13482=CARTESIAN_POINT ( 'NONE',  ( 2.603489959281588995, 40.43575266056827644, -6.500000000000003553 ) ) ;
#13483=CARTESIAN_POINT ( 'NONE',  ( -2.266590686148945544, 26.38708216824730357, -7.082119434687050408 ) ) ;
#13484=CARTESIAN_POINT ( 'NONE',  ( -2.266590686148945544, 41.38708216824729647, -7.082119434687050408 ) ) ;
#13485=CARTESIAN_POINT ( 'NONE',  ( 20.36894250292379738, 9.928748834913966093, -10.36894250292379027 ) ) ;
#13486=CARTESIAN_POINT ( 'NONE',  ( -0.3689425029237881626, 7.428748834913967869, 10.36894250292379027 ) ) ;
#13488=CARTESIAN_POINT ( 'NONE',  ( 10.00000000000000178, 54.31368534415484106, 10.88017736071110342 ) ) ;
#13491=CARTESIAN_POINT ( 'NONE',  ( 17.20831665107776587, 27.88393115100078390, 7.208316651077764980 ) ) ;
#13492=CARTESIAN_POINT ( 'NONE',  ( 17.96484262340118221, 66.18868534415483396, -7.964842623401177768 ) ) ;
#13493=CARTESIAN_POINT ( 'NONE',  ( 17.20831665107776587, 27.88393115100078390, 7.208316651077764980 ) ) ;
#13494=CARTESIAN_POINT ( 'NONE',  ( 10.00000000000000178, 14.31368534415483929, 10.88017736071110342 ) ) ;
#13495=CARTESIAN_POINT ( 'NONE',  ( 10.00000000000000000, 52.87363466993041783, -12.81628187352647608 ) ) ;
#13496=CARTESIAN_POINT ( 'NONE',  ( 19.84674366389459621, 53.50893115100078745, 7.409399052514197653E-17 ) ) ;
#13498=CARTESIAN_POINT ( 'NONE',  ( 19.84674366389459621, 33.50893115100078745, 7.409399052514197653E-17 ) ) ;
#13499=CARTESIAN_POINT ( 'NONE',  ( 22.81628187352647785, 36.62363466993041783, 6.195893100308588602E-16 ) ) ;
#13501=CARTESIAN_POINT ( 'NONE',  ( 12.91533473730992121, 49.52201867748817676, 10.88017736071110164 ) ) ;
#13502=CARTESIAN_POINT ( 'NONE',  ( 10.00000000000000178, 42.25893115100078745, 9.846743663894594434 ) ) ;
#13503=CARTESIAN_POINT ( 'NONE',  ( 2.917880565312950480, 25.97041550158063572, -12.26659068614894821 ) ) ;
#13504=ORIENTED_EDGE ( 'NONE', *, *, #62767, .F. ) ;
#13505=( LENGTH_UNIT ( ) NAMED_UNIT ( * ) SI_UNIT ( .MILLI., .METRE. ) );
#13506=CARTESIAN_POINT ( 'NONE',  ( 7.084665262690076126, 47.02201867748818387, -10.88017736071110164 ) ) ;
#13507=CARTESIAN_POINT ( 'NONE',  ( 4.559911319644449179, 67.23035201082150536, -9.422509992056141925 ) ) ;
#13508=CARTESIAN_POINT ( 'NONE',  ( 22.26659068614895176, 54.72041550158063217, -7.082119434687042414 ) ) ;
#13509=CARTESIAN_POINT ( 'NONE',  ( -1.099225684535947600, -0.4596986634029132657, 6.408140936763237150 ) ) ;
#13511=CARTESIAN_POINT ( 'NONE',  ( 7.084665262690076126, 59.10535201082150536, 10.88017736071109987 ) ) ;
#13512=CARTESIAN_POINT ( 'NONE',  ( -1.926860441876563801, 27.66212336850780673, 1.004413902775740978E-15 ) ) ;
#13513=CARTESIAN_POINT ( 'NONE',  ( 22.81628187352648496, 31.83196800326375353, -3.434112377981050290 ) ) ;
#13514=CARTESIAN_POINT ( 'NONE',  ( 2.791683348922240793, 61.63393115100079456, 7.208316651077764092 ) ) ;
#13516=CARTESIAN_POINT ( 'NONE',  ( -0.8801773607111008646, 8.272018677488171434, 2.915334737309923430 ) ) ;
#13517=CARTESIAN_POINT ( 'NONE',  ( 7.084665262690076126, 7.022018677488170546, -10.88017736071110164 ) ) ;
#13518=CARTESIAN_POINT ( 'NONE',  ( 1.472469842513823179, 45.59226448433412315, -4.923371831947296329 ) ) ;
#13519=CARTESIAN_POINT ( 'NONE',  ( 17.39651004071838614, 62.93575266056827644, 6.500000000000032863 ) ) ;
#13521=CARTESIAN_POINT ( 'NONE',  ( 10.00000000000000178, 9.313685344154839285, 10.88017736071110342 ) ) ;
#13522=CARTESIAN_POINT ( 'NONE',  ( 22.81628187352648496, 11.83196800326375531, -3.434112377981050290 ) ) ;
#13524=CARTESIAN_POINT ( 'NONE',  ( 19.84674366389459266, 13.30059781766745353, 2.638427012816836559 ) ) ;
#13525=CARTESIAN_POINT ( 'NONE',  ( 2.791683348922237240, 40.38393115100078035, -7.208316651077763204 ) ) ;
#13526=CARTESIAN_POINT ( 'NONE',  ( 4.559911319644449179, 42.23035201082151247, -9.422509992056141925 ) ) ;
#13527=VECTOR ( 'NONE', #77439, 1000.000000000000000 ) ;
#13528=CARTESIAN_POINT ( 'NONE',  ( 22.81628187352648496, 6.831968003263753531, -3.434112377981050290 ) ) ;
#13529=CARTESIAN_POINT ( 'NONE',  ( 20.88017736071110164, 50.35535201082151247, 2.915334737309930979 ) ) ;
#13531=CARTESIAN_POINT ( 'NONE',  ( 19.38216949554541557, 57.24863466993042493, -9.382169495545420901 ) ) ;
#13533=CARTESIAN_POINT ( 'NONE',  ( 0.5774900079438607392, 68.48035201082150536, 5.440088680355550821 ) ) ;
#13534=CARTESIAN_POINT ( 'NONE',  ( 6.565887622018943937, 30.16530133659708568, 12.81628187352647430 ) ) ;
#13535=CARTESIAN_POINT ( 'NONE',  ( 20.24186590665276597, 31.76028685723174405, 6.114288769123062295 ) ) ;
#13536=CARTESIAN_POINT ( 'NONE',  ( 17.96484262340118221, 36.18868534415484106, -7.964842623401177768 ) ) ;
#13537=CARTESIAN_POINT ( 'NONE',  ( 10.00000000000000178, 62.25893115100078745, 9.846743663894594434 ) ) ;
#13538=CARTESIAN_POINT ( 'NONE',  ( 7.361572987183169658, 59.96726448433410894, -9.846743663894592657 ) ) ;
#13539=CARTESIAN_POINT ( 'NONE',  ( 19.84674366389459266, 18.71726448433411960, -2.638427012816827677 ) ) ;
#13540=CARTESIAN_POINT ( 'NONE',  ( 2.791683348922240793, 6.633931151000785675, 7.208316651077764092 ) ) ;
#13541=CARTESIAN_POINT ( 'NONE',  ( -0.1023957841222509352, 5.133775574782962536, 6.340343622311908511 ) ) ;
#13542=CARTESIAN_POINT ( 'NONE',  ( 17.08211943468705840, 30.13708216824730357, -12.26659068614894466 ) ) ;
#13547=ORIENTED_EDGE ( 'NONE', *, *, #54303, .F. ) ;
#13548=CARTESIAN_POINT ( 'NONE',  ( -0.3689425029237898834, 56.17874883491396076, -10.36894250292378850 ) ) ;
#13549=CARTESIAN_POINT ( 'NONE',  ( -0.3689425029237898834, 66.17874883491396076, -10.36894250292378850 ) ) ;
#13550=CARTESIAN_POINT ( 'NONE',  ( 0.1532563361054083140, 36.00893115100078745, 1.131784320476157264E-15 ) ) ;
#13551=CARTESIAN_POINT ( 'NONE',  ( 21.09922568453595559, 32.04030133659708923, -6.408140936763230044 ) ) ;
#13553=CARTESIAN_POINT ( 'NONE',  ( -0.3289641300567998083, 43.07879003517447813, 5.963430220938281678 ) ) ;
#13554=CARTESIAN_POINT ( 'NONE',  ( -0.8801773607111009756, 18.06368534415484106, 1.068504757029289695E-15 ) ) ;
#13555=CARTESIAN_POINT ( 'NONE',  ( 10.00000000000000000, 50.55374883491396787, -14.16423886937410082 ) ) ;
#13556=CARTESIAN_POINT ( 'NONE',  ( 18.52753015748618282, 28.92559781766745175, -4.923371831947291888 ) ) ;
#13558=CARTESIAN_POINT ( 'NONE',  ( 0.1532563361054083140, 16.00893115100078390, 1.131784320476157264E-15 ) ) ;
#13559=CARTESIAN_POINT ( 'NONE',  ( 18.72515096720578853, 60.05509018479938277, 6.499999999999877431 ) ) ;
#13564=CARTESIAN_POINT ( 'NONE',  ( 10.00000000000000000, 44.75893115100078745, -9.846743663894594434 ) ) ;
#13565=CARTESIAN_POINT ( 'NONE',  ( 12.91533473730993009, 16.60535201082150891, -10.88017736071109987 ) ) ;
#13566=CARTESIAN_POINT ( 'NONE',  ( 2.035157376598822676, 27.43868534415483396, -7.964842623401177768 ) ) ;
#13567=CARTESIAN_POINT ( 'NONE',  ( 7.361572987183170547, 57.05059781766744464, 9.846743663894590881 ) ) ;
#13568=CARTESIAN_POINT ( 'NONE',  ( 19.38216949554541557, 22.24863466993041428, -9.382169495545420901 ) ) ;
#13569=CARTESIAN_POINT ( 'NONE',  ( -2.266590686148945544, 1.387082168247301128, -7.082119434687050408 ) ) ;
#13572=ADVANCED_FACE ( 'NONE', ( #88107 ), #51609, .T. ) ;
#13573=CARTESIAN_POINT ( 'NONE',  ( 10.00000000000000000, 37.87363466993041783, -12.81628187352647608 ) ) ;
#13575=CARTESIAN_POINT ( 'NONE',  ( 19.84674366389459266, 33.71726448433410894, -2.638427012816827677 ) ) ;
#13577=CARTESIAN_POINT ( 'NONE',  ( -0.8801773607111008646, 3.272018677488171434, 2.915334737309923430 ) ) ;
#13579=CARTESIAN_POINT ( 'NONE',  ( 0.5774900079438590739, 2.647018677488171434, -5.440088680355550821 ) ) ;
#13581=CARTESIAN_POINT ( 'NONE',  ( 10.00000000000000000, 51.81368534415484106, -10.88017736071110342 ) ) ;
#13582=CARTESIAN_POINT ( 'NONE',  ( 10.00000000000000000, 56.81368534415484106, -10.88017736071110342 ) ) ;
#13583=CARTESIAN_POINT ( 'NONE',  ( 12.91533473730993009, 46.60535201082150536, -10.88017736071109987 ) ) ;
#13585=CARTESIAN_POINT ( 'NONE',  ( 5.076628168052703671, 1.842264484334118047, 8.527530157486179263 ) ) ;
#13586=CARTESIAN_POINT ( 'NONE',  ( 7.084665262690076126, 52.02201867748816255, -10.88017736071110164 ) ) ;
#13588=SURFACE_STYLE_USAGE ( .BOTH. , #21093 ) ;
#13590=CARTESIAN_POINT ( 'NONE',  ( 19.84674366389459266, 33.71726448433410894, -2.638427012816827677 ) ) ;
#13591=ORIENTED_EDGE ( 'NONE', *, *, #9489, .F. ) ;
#13592=CARTESIAN_POINT ( 'NONE',  ( 7.361572987183170547, 57.05059781766744464, 9.846743663894590881 ) ) ;
#13595=CARTESIAN_POINT ( 'NONE',  ( -0.3689425029237881626, 12.42874883491396609, 10.36894250292379027 ) ) ;
#13601=CARTESIAN_POINT ( 'NONE',  ( 2.035157376598822676, 7.438685344154837509, -7.964842623401177768 ) ) ;
#13605=CARTESIAN_POINT ( 'NONE',  ( 7.361572987183169658, 49.96726448433410894, -9.846743663894592657 ) ) ;
#13606=CARTESIAN_POINT ( 'NONE',  ( 10.00000000000000178, 70.00000000000000000, 0.000000000000000000 ) ) ;
#13607=CARTESIAN_POINT ( 'NONE',  ( 22.81628187352648496, 16.83196800326374998, -3.434112377981050290 ) ) ;
#13608=CARTESIAN_POINT ( 'NONE',  ( 0.1532563361054100626, 10.80059781766745175, -2.638427012816831230 ) ) ;
#13610=LINE ( 'NONE', #97138, #98515 ) ;
#13611=CARTESIAN_POINT ( 'NONE',  ( 19.84674366389459266, 18.30059781766745175, 2.638427012816836559 ) ) ;
#13612=CARTESIAN_POINT ( 'NONE',  ( 21.09922568453595559, 2.040301336597086568, -6.408140936763230044 ) ) ;
#13615=CARTESIAN_POINT ( 'NONE',  ( 12.91533473730992121, 9.522018677488171434, 10.88017736071110164 ) ) ;
#13616=CARTESIAN_POINT ( 'NONE',  ( 17.20831665107776587, 29.13393115100078390, -7.208316651077762316 ) ) ;
#13617=CARTESIAN_POINT ( 'NONE',  ( 17.96484262340118221, 51.18868534415483396, -7.964842623401177768 ) ) ;
#13618=CARTESIAN_POINT ( 'NONE',  ( 19.38216949554541557, 37.24863466993041783, -9.382169495545420901 ) ) ;
#13620=CARTESIAN_POINT ( 'NONE',  ( 19.42250999205614193, 15.14701867748817143, 5.440088680355555262 ) ) ;
#13623=CARTESIAN_POINT ( 'NONE',  ( 10.00000000000000000, 64.75893115100078035, -9.846743663894594434 ) ) ;
#13624=CARTESIAN_POINT ( 'NONE',  ( 14.92337183194729633, 27.67559781766745530, 8.527530157486181039 ) ) ;
#13626=CARTESIAN_POINT ( 'NONE',  ( 16.40814093676323893, 40.79030133659708923, 11.09922568453595026 ) ) ;
#13628=CARTESIAN_POINT ( 'NONE',  ( 20.88017736071110875, 45.77201867748816966, -2.915334737309920765 ) ) ;
#13632=CARTESIAN_POINT ( 'NONE',  ( 2.035157376598824452, 43.68868534415484106, 7.964842623401179544 ) ) ;
#13633=CARTESIAN_POINT ( 'NONE',  ( 2.035157376598822676, 27.43868534415483396, -7.964842623401177768 ) ) ;
#13634=CARTESIAN_POINT ( 'NONE',  ( 2.603489959281590771, 46.58210964143328425, 6.500000000000003553 ) ) ;
#13635=CARTESIAN_POINT ( 'NONE',  ( 20.88017736071110164, 60.35535201082151957, 2.915334737309930979 ) ) ;
#13637=CARTESIAN_POINT ( 'NONE',  ( 19.84674366389459266, 43.71726448433410894, -2.638427012816827677 ) ) ;
#13638=CARTESIAN_POINT ( 'NONE',  ( 6.565887622018943937, 60.16530133659707502, 12.81628187352647430 ) ) ;
#13639=CARTESIAN_POINT ( 'NONE',  ( -1.099225684535947600, 9.540301336597087456, 6.408140936763237150 ) ) ;
#13640=VERTEX_POINT ( 'NONE', #90080 ) ;
#13641=CARTESIAN_POINT ( 'NONE',  ( 20.88017736071110164, 25.35535201082150891, 2.915334737309930979 ) ) ;
#13643=CARTESIAN_POINT ( 'NONE',  ( 4.559911319644449179, 13.89701867748817321, 9.422509992056141925 ) ) ;
#13644=CARTESIAN_POINT ( 'NONE',  ( 0.5774900079438590739, 67.64701867748817676, -5.440088680355550821 ) ) ;
#13645=CARTESIAN_POINT ( 'NONE',  ( 17.08211943468705840, 20.13708216824730357, -12.26659068614894466 ) ) ;
#13646=CARTESIAN_POINT ( 'NONE',  ( 0.1532563361054100626, 15.80059781766745353, -2.638427012816831230 ) ) ;
#13647=CARTESIAN_POINT ( 'NONE',  ( 10.00000000000000178, 57.25893115100078745, 9.846743663894594434 ) ) ;
#13648=CARTESIAN_POINT ( 'NONE',  ( 19.42250999205614193, 50.14701867748817676, 5.440088680355555262 ) ) ;
#13653=VERTEX_POINT ( 'NONE', #61430 ) ;
#13656=CARTESIAN_POINT ( 'NONE',  ( 12.63842701281683034, 42.46726448433412315, 9.846743663894596210 ) ) ;
#13657=( BOUNDED_CURVE ( )  B_SPLINE_CURVE ( 2, ( #93661, #24690, #16202, #25197, #16694, #25677, #48647, #55673, #86173 ),
 .UNSPECIFIED., .F., .T. ) 
 B_SPLINE_CURVE_WITH_KNOTS ( ( 3, 2, 2, 2, 3 ),
 ( 0.7615695083688026612, 0.7619047619047618625, 0.7678571428571429047, 0.7738095238095238360, 0.7741447773454829262 ),
 .UNSPECIFIED. ) 
 CURVE ( )  GEOMETRIC_REPRESENTATION_ITEM ( )  RATIONAL_B_SPLINE_CURVE ( ( 0.9963778908391753841, 0.9980808541467917072, 1.000000000000000000, 0.9659258262890682012, 1.000000000000000000, 0.9659258262890682012, 1.000000000000000000, 0.9980808541467922623, 0.9963778908391764944 ) ) 
 REPRESENTATION_ITEM ( '' )  );
#13661=CARTESIAN_POINT ( 'NONE',  ( 13.79529636645031943, 20.34541550158063572, -14.16423886937409904 ) ) ;
#13662=CARTESIAN_POINT ( 'NONE',  ( 22.26659068614895176, 29.72041550158063572, -7.082119434687042414 ) ) ;
#13663=CARTESIAN_POINT ( 'NONE',  ( -0.8801773607111008646, 58.27201867748816966, 2.915334737309923430 ) ) ;
#13664=CARTESIAN_POINT ( 'NONE',  ( -2.266590686148945544, 66.38708216824730357, -7.082119434687050408 ) ) ;
#13665=CARTESIAN_POINT ( 'NONE',  ( 13.43411237798106583, 2.665301336597086568, -12.81628187352647252 ) ) ;
#13666=CARTESIAN_POINT ( 'NONE',  ( 2.791683348922237240, 50.38393115100078035, -7.208316651077763204 ) ) ;
#13668=CARTESIAN_POINT ( 'NONE',  ( 20.88017736071110875, 45.77201867748816966, -2.915334737309920765 ) ) ;
#13669=CARTESIAN_POINT ( 'NONE',  ( 3.591859063236761518, 9.956968003263753531, 11.09922568453594849 ) ) ;
#13670=CARTESIAN_POINT ( 'NONE',  ( 13.79529636645030344, 23.26208216824730002, 14.16423886937410614 ) ) ;
#13671=CARTESIAN_POINT ( 'NONE',  ( -4.164238869374098151, 56.59541550158063927, -3.795296366450310543 ) ) ;
#13673=CARTESIAN_POINT ( 'NONE',  ( 12.91533473730992121, 19.52201867748816611, 10.88017736071110164 ) ) ;
#13674=CARTESIAN_POINT ( 'NONE',  ( 17.39651004071838969, 54.08210964143329846, -6.500000000000027534 ) ) ;
#13675=CARTESIAN_POINT ( 'NONE',  ( 10.00000000000000178, 39.31368534415484106, 10.88017736071110342 ) ) ;
#13677=ORIENTED_EDGE ( 'NONE', *, *, #88960, .T. ) ;
#13678=CARTESIAN_POINT ( 'NONE',  ( 20.10493008474206178, 34.71697413083879269, 6.336235997365760930 ) ) ;
#13681=PRESENTATION_STYLE_ASSIGNMENT (( #80827 ) ) ;
#13682=CARTESIAN_POINT ( 'NONE',  ( -4.164238869374099039, 46.80374883491397497, 8.674139862899312516E-16 ) ) ;
#13683=CARTESIAN_POINT ( 'NONE',  ( 10.00000000000000000, 19.75893115100078390, -9.846743663894594434 ) ) ;
#13684=CARTESIAN_POINT ( 'NONE',  ( 18.52753015748618282, 48.92559781766745886, -4.923371831947291888 ) ) ;
#13687=CARTESIAN_POINT ( 'NONE',  ( 17.20831665107776587, 2.883931151000785231, 7.208316651077764980 ) ) ;
#13690=CARTESIAN_POINT ( 'NONE',  ( -2.816281873526471635, 53.91530133659709634, -3.434112377981056508 ) ) ;
#13693=CARTESIAN_POINT ( 'NONE',  ( 2.917880565312948704, 32.63708216824730357, 12.26659068614894643 ) ) ;
#13694=EDGE_CURVE ( 'NONE', #21520, #10378, #10520, .T. ) ;
#13695=CARTESIAN_POINT ( 'NONE',  ( 19.38216949554541557, 27.24863466993041783, -9.382169495545420901 ) ) ;
#13696=ORIENTED_EDGE ( 'NONE', *, *, #23853, .F. ) ;
#13697=CARTESIAN_POINT ( 'NONE',  ( -2.816281873526471635, 43.91530133659708923, -3.434112377981056508 ) ) ;
#13698=CARTESIAN_POINT ( 'NONE',  ( 10.00000000000000178, 37.25893115100078745, 9.846743663894594434 ) ) ;
#13699=CARTESIAN_POINT ( 'NONE',  ( 0.5774900079438590739, 17.64701867748817321, -5.440088680355550821 ) ) ;
#13700=CARTESIAN_POINT ( 'NONE',  ( 6.565887622018943937, 60.16530133659707502, 12.81628187352647430 ) ) ;
#13702=CARTESIAN_POINT ( 'NONE',  ( 2.791683348922240793, 46.63393115100077324, 7.208316651077764092 ) ) ;
#13703=CARTESIAN_POINT ( 'NONE',  ( 0.1532563361054082862, 51.21726448433412315, 2.638427012816831674 ) ) ;
#13707=EDGE_LOOP ( 'NONE', ( #12858, #35700, #64064, #38559 ) ) ;
#13708=MECHANICAL_DESIGN_GEOMETRIC_PRESENTATION_REPRESENTATION('',(#66149),#74356);
#13711=CARTESIAN_POINT ( 'NONE',  ( 17.39651004071841456, 9.082109641433294911, -6.500000000000003553 ) ) ;
#13713=CARTESIAN_POINT ( 'NONE',  ( 2.791683348922240793, 16.63393115100078745, 7.208316651077764092 ) ) ;
#13714=CARTESIAN_POINT ( 'NONE',  ( 19.38216949554541557, 32.24863466993041783, -9.382169495545420901 ) ) ;
#13717=CARTESIAN_POINT ( 'NONE',  ( 12.63842701281683922, 54.55059781766745175, -9.846743663894590881 ) ) ;
#13718=CARTESIAN_POINT ( 'NONE',  ( 20.15039907845753220, 52.62777174578612716, -6.262539305110077947 ) ) ;
#13719=CARTESIAN_POINT ( 'NONE',  ( 6.204703633549690345, 20.76208216824730357, -14.16423886937410259 ) ) ;
#13720=CARTESIAN_POINT ( 'NONE',  ( 14.92337183194729633, 52.67559781766745175, 8.527530157486181039 ) ) ;
#13721=CARTESIAN_POINT ( 'NONE',  ( 19.38216949554541202, 45.99863466993041072, 9.382169495545424454 ) ) ;
#13724=CARTESIAN_POINT ( 'NONE',  ( 7.361572987183170547, 12.05059781766744997, 9.846743663894590881 ) ) ;
#13726=CARTESIAN_POINT ( 'NONE',  ( 2.791683348922237240, 45.38393115100079456, -7.208316651077763204 ) ) ;
#13727=CARTESIAN_POINT ( 'NONE',  ( 15.44008868035555793, 46.39701867748817676, -9.422509992056140149 ) ) ;
#13729=AXIS2_PLACEMENT_3D ( 'NONE', #71416, #48885, #85421 ) ;
#13730=CARTESIAN_POINT ( 'NONE',  ( 7.361572987183169658, 34.96726448433411605, -9.846743663894592657 ) ) ;
#13734=CARTESIAN_POINT ( 'NONE',  ( 17.96484262340118221, 46.18868534415484106, -7.964842623401177768 ) ) ;
#13736=EDGE_LOOP ( 'NONE', ( #81771, #25165, #44601, #52316, #16114, #93082 ) ) ;
#13738=CARTESIAN_POINT ( 'NONE',  ( 10.00000000000000178, 9.313685344154839285, 10.88017736071110342 ) ) ;
#13739=CARTESIAN_POINT ( 'NONE',  ( 19.84674366389459621, 58.50893115100078745, 7.409399052514197653E-17 ) ) ;
#13740=CARTESIAN_POINT ( 'NONE',  ( 0.5774900079438607392, 48.48035201082150536, 5.440088680355550821 ) ) ;
#13742=CARTESIAN_POINT ( 'NONE',  ( 20.88017736071110519, 60.56368534415484106, 2.639326808657452039E-16 ) ) ;
#13744=CARTESIAN_POINT ( 'NONE',  ( 2.035157376598822676, 32.43868534415483396, -7.964842623401177768 ) ) ;
#13746=CARTESIAN_POINT ( 'NONE',  ( 2.791683348922237240, 10.38393115100078390, -7.208316651077763204 ) ) ;
#13747=CARTESIAN_POINT ( 'NONE',  ( 14.92337183194729633, 22.67559781766745175, 8.527530157486181039 ) ) ;
#13750=CARTESIAN_POINT ( 'NONE',  ( 10.00000000000000178, 67.25893115100079456, 9.846743663894594434 ) ) ;
#13751=CARTESIAN_POINT ( 'NONE',  ( -0.3689425029237881626, 62.42874883491396787, 10.36894250292379027 ) ) ;
#13752=CARTESIAN_POINT ( 'NONE',  ( -0.3689425029237881626, 12.42874883491396609, 10.36894250292379027 ) ) ;
#13753=CARTESIAN_POINT ( 'NONE',  ( -0.3689425029237881626, 57.42874883491397497, 10.36894250292379027 ) ) ;
#13754=CARTESIAN_POINT ( 'NONE',  ( 22.81628187352648496, 1.831968003263753753, -3.434112377981050290 ) ) ;
#13756=CARTESIAN_POINT ( 'NONE',  ( 7.361572987183169658, 14.96726448433411960, -9.846743663894592657 ) ) ;
#13757=CARTESIAN_POINT ( 'NONE',  ( 12.91533473730993009, 16.60535201082150891, -10.88017736071109987 ) ) ;
#13758=CARTESIAN_POINT ( 'NONE',  ( 18.52753015748618282, 43.92559781766745175, -4.923371831947291888 ) ) ;
#13762=CARTESIAN_POINT ( 'NONE',  ( 2.791683348922240793, 1.633931151000784565, 7.208316651077764092 ) ) ;
#13763=CARTESIAN_POINT ( 'NONE',  ( 6.565887622018943937, 23.08196800326375708, -12.81628187352647608 ) ) ;
#13764=CARTESIAN_POINT ( 'NONE',  ( 12.63842701281683034, 32.46726448433412315, 9.846743663894596210 ) ) ;
#13766=CARTESIAN_POINT ( 'NONE',  ( 2.791683348922240793, 11.63393115100078568, 7.208316651077764092 ) ) ;
#13767=B_SPLINE_CURVE_WITH_KNOTS ( 'NONE', 3,
 ( #34618, #80634, #11638, #42153 ),
 .UNSPECIFIED., .F., .F.,
 ( 4, 4 ),
 ( 0.000000000000000000, 0.002562518741975322069 ),
 .UNSPECIFIED. ) ;
#13770=CARTESIAN_POINT ( 'NONE',  ( -0.8801773607110991993, 7.855352010821504471, -2.915334737309923874 ) ) ;
#13771=CARTESIAN_POINT ( 'NONE',  ( -0.3689425029237898834, 41.17874883491397497, -10.36894250292378850 ) ) ;
#13772=CARTESIAN_POINT ( 'NONE',  ( -0.8801773607111009756, 43.06368534415484106, 1.068504757029289695E-15 ) ) ;
#13773=CARTESIAN_POINT ( 'NONE',  ( 4.559911319644449179, 63.89701867748817676, 9.422509992056141925 ) ) ;
#13774=CARTESIAN_POINT ( 'NONE',  ( 20.32896413005680714, 40.57879003517447103, -5.963430220938276349 ) ) ;
#13775=CARTESIAN_POINT ( 'NONE',  ( 10.00000000000000000, 19.75893115100078390, -9.846743663894594434 ) ) ;
#13776=CARTESIAN_POINT ( 'NONE',  ( 5.076628168052703671, 6.842264484334118713, 8.527530157486179263 ) ) ;
#13777=CARTESIAN_POINT ( 'NONE',  ( -1.372027372252927480, 1.950157826164670856E-16, -0.5557468924052827441 ) ) ;
#13778=CARTESIAN_POINT ( 'NONE',  ( 18.52753015748618282, 38.92559781766745175, -4.923371831947291888 ) ) ;
#13780=CARTESIAN_POINT ( 'NONE',  ( 17.96484262340118221, 34.93868534415482685, 7.964842623401181321 ) ) ;
#13781=EDGE_CURVE ( 'NONE', #15284, #16048, #73591, .T. ) ;
#13783=CARTESIAN_POINT ( 'NONE',  ( -2.816281873526473856, 64.33196800326376774, 3.434112377981055619 ) ) ;
#13785=CARTESIAN_POINT ( 'NONE',  ( 14.92337183194729633, 12.67559781766745353, 8.527530157486181039 ) ) ;
#13786=CARTESIAN_POINT ( 'NONE',  ( 13.43411237798105340, 45.58196800326374643, 12.81628187352647963 ) ) ;
#13787=CARTESIAN_POINT ( 'NONE',  ( 17.96484262340118221, 6.188685344154837509, -7.964842623401177768 ) ) ;
#13788=CARTESIAN_POINT ( 'NONE',  ( 18.52753015748617571, 33.09226448433411605, 4.923371831947298993 ) ) ;
#13789=FILL_AREA_STYLE ('',( #7287 ) ) ;
#13793=CARTESIAN_POINT ( 'NONE',  ( 10.00000000000000000, 20.55374883491396787, -14.16423886937410082 ) ) ;
#13794=CARTESIAN_POINT ( 'NONE',  ( 22.26659068614894466, 38.88708216824731068, 7.082119434687054849 ) ) ;
#13795=CARTESIAN_POINT ( 'NONE',  ( 2.791683348922237240, 40.38393115100078035, -7.208316651077763204 ) ) ;
#13797=CARTESIAN_POINT ( 'NONE',  ( 7.084665262690076126, 34.10535201082151247, 10.88017736071109987 ) ) ;
#13798=CARTESIAN_POINT ( 'NONE',  ( 14.92337183194729633, 7.675597817667451750, 8.527530157486181039 ) ) ;
#13800=VERTEX_POINT ( 'NONE', #77916 ) ;
#13801=CARTESIAN_POINT ( 'NONE',  ( 6.565887622018943937, 53.08196800326374643, -12.81628187352647608 ) ) ;
#13803=ADVANCED_FACE ( 'NONE', ( #15947 ), #61814, .T. ) ;
#13804=CARTESIAN_POINT ( 'NONE',  ( -0.8801773607110991993, 67.85535201082151957, -2.915334737309923874 ) ) ;
#13805=COLOUR_RGB ( '', 0.08235294, 0.09019608, 0.10196078) ;
#13807=CARTESIAN_POINT ( 'NONE',  ( -2.266590686148945544, 7.220415501580634832, 7.082119434687048631 ) ) ;
#13808=CARTESIAN_POINT ( 'NONE',  ( 14.92337183194729633, 7.675597817667451750, 8.527530157486181039 ) ) ;
#13813=CARTESIAN_POINT ( 'NONE',  ( 4.559911319644449179, 12.23035201082150536, -9.422509992056141925 ) ) ;
#13815=VECTOR ( 'NONE', #72593, 1000.000000000000000 ) ;
#13816=ORIENTED_EDGE ( 'NONE', *, *, #55674, .F. ) ;
#13817=CARTESIAN_POINT ( 'NONE',  ( 4.559911319644449179, 38.89701867748817676, 9.422509992056141925 ) ) ;
#13818=LINE ( 'NONE', #15800, #55269 ) ;
#13820=EDGE_CURVE ( 'NONE', #37993, #58317, #28408, .T. ) ;
#13821=CARTESIAN_POINT ( 'NONE',  ( 17.20831665107776587, 64.13393115100079456, -7.208316651077762316 ) ) ;
#13822=ORIENTED_EDGE ( 'NONE', *, *, #80963, .T. ) ;
#13823=CARTESIAN_POINT ( 'NONE',  ( 12.91533473730992121, 64.52201867748817676, 10.88017736071110164 ) ) ;
#13825=CARTESIAN_POINT ( 'NONE',  ( 13.43411237798105340, 35.58196800326375353, 12.81628187352647963 ) ) ;
#13826=CARTESIAN_POINT ( 'NONE',  ( 2.035157376598822676, 27.43868534415483396, -7.964842623401177768 ) ) ;
#13827=CARTESIAN_POINT ( 'NONE',  ( -0.1503990784575275907, 58.10158574516644592, 6.262539305110076171 ) ) ;
#13828=CARTESIAN_POINT ( 'NONE',  ( 17.20831665107776587, 2.883931151000785231, 7.208316651077764980 ) ) ;
#13829=CARTESIAN_POINT ( 'NONE',  ( 2.035157376598822676, 12.43868534415483751, -7.964842623401177768 ) ) ;
#13833=CARTESIAN_POINT ( 'NONE',  ( -2.816281873526471635, 48.91530133659708213, -3.434112377981056508 ) ) ;
#13834=CARTESIAN_POINT ( 'NONE',  ( 7.084665262690076126, 49.10535201082149825, 10.88017736071109987 ) ) ;
#13835=CARTESIAN_POINT ( 'NONE',  ( 19.50000000000000355, 98.59912998021083297, 5.000000000000000000 ) ) ;
#13836=CARTESIAN_POINT ( 'NONE',  ( 3.591859063236761518, 59.95696800326375353, 11.09922568453594849 ) ) ;
#13837=CARTESIAN_POINT ( 'NONE',  ( -0.8801773607111008646, 43.27201867748817676, 2.915334737309923430 ) ) ;
#13838=CARTESIAN_POINT ( 'NONE',  ( 14.92337183194729988, 59.34226448433412315, -8.527530157486177487 ) ) ;
#13840=CARTESIAN_POINT ( 'NONE',  ( 10.00000000000000000, 14.75893115100078568, -9.846743663894594434 ) ) ;
#13841=CARTESIAN_POINT ( 'NONE',  ( -2.816281873526473856, 9.123634669930421381, 9.499525473075851096E-16 ) ) ;
#13843=CARTESIAN_POINT ( 'NONE',  ( 10.00000000000000000, 64.75893115100078035, -9.846743663894594434 ) ) ;
#13844=CARTESIAN_POINT ( 'NONE',  ( 0.5774900079438607392, 38.48035201082150536, 5.440088680355550821 ) ) ;
#13845=CARTESIAN_POINT ( 'NONE',  ( 0.1532563361054100626, 50.80059781766745175, -2.638427012816831230 ) ) ;
#13848=CARTESIAN_POINT ( 'NONE',  ( 0.1532563361054100626, 15.80059781766745353, -2.638427012816831230 ) ) ;
#13849=CARTESIAN_POINT ( 'NONE',  ( 17.20831665107776587, 7.883931151000784787, 7.208316651077764980 ) ) ;
#13851=CARTESIAN_POINT ( 'NONE',  ( -2.816281873526473856, -0.6680319967362464695, 3.434112377981055619 ) ) ;
#13854=CARTESIAN_POINT ( 'NONE',  ( 5.076628168052704559, 60.17559781766745175, -8.527530157486179263 ) ) ;
#13855=CARTESIAN_POINT ( 'NONE',  ( 22.81628187352648496, 41.83196800326375353, -3.434112377981050290 ) ) ;
#13856=CARTESIAN_POINT ( 'NONE',  ( 0.1532563361054100626, 35.80059781766745175, -2.638427012816831230 ) ) ;
#13857=CARTESIAN_POINT ( 'NONE',  ( -45.94000000000000483, 103.7452903794826824, -5.529860068218139801 ) ) ;
#13858=CARTESIAN_POINT ( 'NONE',  ( 6.204703633549690345, 67.84541550158060375, 14.16423886937410082 ) ) ;
#13859=CARTESIAN_POINT ( 'NONE',  ( 7.361572987183169658, 34.96726448433411605, -9.846743663894592657 ) ) ;
#13862=LINE ( 'NONE', #29827, #83968 ) ;
#13863=CARTESIAN_POINT ( 'NONE',  ( -0.8801773607111009756, 8.063685344154837509, 1.068504757029289695E-15 ) ) ;
#13865=CARTESIAN_POINT ( 'NONE',  ( 17.96484262340118221, 21.18868534415483396, -7.964842623401177768 ) ) ;
#13866=CARTESIAN_POINT ( 'NONE',  ( 22.26659068614895176, 54.72041550158063217, -7.082119434687042414 ) ) ;
#13867=CARTESIAN_POINT ( 'NONE',  ( -4.164238869374098151, 56.59541550158063927, -3.795296366450310543 ) ) ;
#13869=FACE_OUTER_BOUND ( 'NONE', #97836, .T. ) ;
#13870=CARTESIAN_POINT ( 'NONE',  ( 19.84674366389459266, 13.30059781766745353, 2.638427012816836559 ) ) ;
#13871=CARTESIAN_POINT ( 'NONE',  ( 21.09922568453594849, 6.206968003263753531, 6.408140936763242479 ) ) ;
#13874=CARTESIAN_POINT ( 'NONE',  ( 18.52753015748617571, 58.09226448433411605, 4.923371831947298993 ) ) ;
#13876=CARTESIAN_POINT ( 'NONE',  ( 10.00000000000000000, 64.75893115100078035, -9.846743663894594434 ) ) ;
#13877=CARTESIAN_POINT ( 'NONE',  ( 24.16423886937409904, 9.095415501580633943, 3.795296366450317205 ) ) ;
#13878=CARTESIAN_POINT ( 'NONE',  ( 10.00000000000000000, 19.75893115100078390, -9.846743663894594434 ) ) ;
#13880=ORIENTED_EDGE ( 'NONE', *, *, #42450, .T. ) ;
#13881=CARTESIAN_POINT ( 'NONE',  ( 24.16423886937409904, 34.09541550158064638, 3.795296366450317205 ) ) ;
#13883=CARTESIAN_POINT ( 'NONE',  ( 1.472469842513823179, 5.592264484334118713, -4.923371831947296329 ) ) ;
#13886=CARTESIAN_POINT ( 'NONE',  ( 4.559911319644449179, 37.23035201082150536, -9.422509992056141925 ) ) ;
#13887=CARTESIAN_POINT ( 'NONE',  ( 6.565887622018943937, 40.16530133659708923, 12.81628187352647430 ) ) ;
#13888=CARTESIAN_POINT ( 'NONE',  ( 2.035157376598822676, 7.438685344154837509, -7.964842623401177768 ) ) ;
#13889=CARTESIAN_POINT ( 'NONE',  ( -2.816281873526473856, 34.12363466993042493, 9.499525473075851096E-16 ) ) ;
#13890=CARTESIAN_POINT ( 'NONE',  ( 22.81628187352648496, 56.83196800326374643, -3.434112377981050290 ) ) ;
#13891=ORIENTED_EDGE ( 'NONE', *, *, #92635, .F. ) ;
#13894=CARTESIAN_POINT ( 'NONE',  ( 24.16423886937410614, 34.30374883491396787, 8.672049930838204340E-16 ) ) ;
#13895=CARTESIAN_POINT ( 'NONE',  ( 4.559911319644449179, 7.230352010821504471, -9.422509992056141925 ) ) ;
#13896=CARTESIAN_POINT ( 'NONE',  ( 17.96484262340118221, 24.93868534415484461, 7.964842623401181321 ) ) ;
#13899=CARTESIAN_POINT ( 'NONE',  ( 12.91533473730993009, 56.60535201082151247, -10.88017736071109987 ) ) ;
#13900=CARTESIAN_POINT ( 'NONE',  ( -0.8801773607111009756, 53.06368534415484106, 1.068504757029289695E-15 ) ) ;
#13901=CARTESIAN_POINT ( 'NONE',  ( 16.40814093676324603, 32.45696800326375353, -11.09922568453594671 ) ) ;
#13904=CARTESIAN_POINT ( 'NONE',  ( 12.63842701281683034, 17.46726448433411250, 9.846743663894596210 ) ) ;
#13906=( GEOMETRIC_REPRESENTATION_CONTEXT ( 3 ) GLOBAL_UNCERTAINTY_ASSIGNED_CONTEXT ( ( #83121 ) ) GLOBAL_UNIT_ASSIGNED_CONTEXT ( ( #64268, #86802, #77803 ) ) REPRESENTATION_CONTEXT ( 'NONE', 'WORKASPACE' ) );
#13907=CARTESIAN_POINT ( 'NONE',  ( 0.5774900079438607392, 58.48035201082151247, 5.440088680355550821 ) ) ;
#13909=ADVANCED_FACE ( 'NONE', ( #82332 ), #82260, .T. ) ;
#13911=CARTESIAN_POINT ( 'NONE',  ( 22.81628187352647785, 21.62363466993041783, 6.195893100308588602E-16 ) ) ;
#13912=SURFACE_STYLE_USAGE ( .BOTH. , #67396 ) ;
#13913=CARTESIAN_POINT ( 'NONE',  ( 12.91533473730992121, 14.52201867748817143, 10.88017736071110164 ) ) ;
#13915=CARTESIAN_POINT ( 'NONE',  ( 1.472469842513823179, 36.42559781766745175, 4.923371831947296329 ) ) ;
#13916=CARTESIAN_POINT ( 'NONE',  ( -2.816281873526473856, 54.12363466993041783, 9.499525473075851096E-16 ) ) ;
#13917=CARTESIAN_POINT ( 'NONE',  ( 2.791683348922237240, 20.38393115100078745, -7.208316651077763204 ) ) ;
#13918=CARTESIAN_POINT ( 'NONE',  ( -2.266590686148945544, 11.38708216824730179, -7.082119434687050408 ) ) ;
#13919=CARTESIAN_POINT ( 'NONE',  ( 18.18329248733315140, 27.60290668512023515, 6.499999999999997335 ) ) ;
#13920=CARTESIAN_POINT ( 'NONE',  ( 0.5774900079438607392, 23.48035201082150536, 5.440088680355550821 ) ) ;
#13921=( NAMED_UNIT ( * ) SI_UNIT ( $, .STERADIAN. ) SOLID_ANGLE_UNIT ( ) );
#13922=CARTESIAN_POINT ( 'NONE',  ( 2.917880565312948704, 27.63708216824730357, 12.26659068614894643 ) ) ;
#13923=CARTESIAN_POINT ( 'NONE',  ( 2.791683348922237240, 50.38393115100078035, -7.208316651077763204 ) ) ;
#13924=CARTESIAN_POINT ( 'NONE',  ( -0.8801773607111008646, 33.27201867748817676, 2.915334737309923430 ) ) ;
#13925=CARTESIAN_POINT ( 'NONE',  ( 17.96484262340118221, 19.93868534415484106, 7.964842623401181321 ) ) ;
#13926=ORIENTED_EDGE ( 'NONE', *, *, #85924, .T. ) ;
#13927=COLOUR_RGB ( '', 0.72549020, 0.75294118, 0.79215686) ;
#13928=CARTESIAN_POINT ( 'NONE',  ( 4.559911319644449179, 22.23035201082150536, -9.422509992056141925 ) ) ;
#13929=EDGE_CURVE ( 'NONE', #71042, #96104, #92487, .T. ) ;
#13930=CARTESIAN_POINT ( 'NONE',  ( 6.565887622018943937, 48.08196800326375353, -12.81628187352647608 ) ) ;
#13931=CARTESIAN_POINT ( 'NONE',  ( 0.5774900079438590739, 32.64701867748816966, -5.440088680355550821 ) ) ;
#13932=CARTESIAN_POINT ( 'NONE',  ( 0.1532563361054083140, 46.00893115100079456, 1.131784320476157264E-15 ) ) ;
#13933=CARTESIAN_POINT ( 'NONE',  ( 17.96484262340118221, 39.93868534415484106, 7.964842623401181321 ) ) ;
#13935=CARTESIAN_POINT ( 'NONE',  ( 18.52753015748617571, 58.09226448433411605, 4.923371831947298993 ) ) ;
#13936=CARTESIAN_POINT ( 'NONE',  ( 0.5774900079438607392, 43.48035201082151247, 5.440088680355550821 ) ) ;
#13939=CARTESIAN_POINT ( 'NONE',  ( 20.36894250292379738, 49.92874883491396787, -10.36894250292379027 ) ) ;
#13940=CARTESIAN_POINT ( 'NONE',  ( -0.8801773607110991993, 52.85535201082151247, -2.915334737309923874 ) ) ;
#13941=CARTESIAN_POINT ( 'NONE',  ( 0.1532563361054083140, 66.00893115100079456, 1.131784320476157264E-15 ) ) ;
#13944=CARTESIAN_POINT ( 'NONE',  ( 5.076628168052704559, 65.17559781766745175, -8.527530157486179263 ) ) ;
#13945=( NAMED_UNIT ( * ) SI_UNIT ( $, .STERADIAN. ) SOLID_ANGLE_UNIT ( ) );
#13946=CARTESIAN_POINT ( 'NONE',  ( 1.472469842513823179, 15.59226448433411960, -4.923371831947296329 ) ) ;
#13948=EDGE_CURVE ( 'NONE', #25434, #31259, #13951, .T. ) ;
#13949=CARTESIAN_POINT ( 'NONE',  ( 18.52753015748617571, 28.09226448433411960, 4.923371831947298993 ) ) ;
#13951=( BOUNDED_CURVE ( )  B_SPLINE_CURVE ( 2, ( #19455, #65431, #95955, #33452, #12929, #27436, #19940, #80942, #35431 ),
 .UNSPECIFIED., .F., .T. ) 
 B_SPLINE_CURVE_WITH_KNOTS ( ( 3, 2, 2, 2, 3 ),
 ( 0.8329980797973741691, 0.8333333333333333703, 0.8392857142857143016, 0.8452380952380952328, 0.8455733487740543231 ),
 .UNSPECIFIED. ) 
 CURVE ( )  GEOMETRIC_REPRESENTATION_ITEM ( )  RATIONAL_B_SPLINE_CURVE ( ( 0.9963778908391753841, 0.9980808541467917072, 1.000000000000000000, 0.9659258262890682012, 1.000000000000000000, 0.9659258262890682012, 1.000000000000000000, 0.9980808541467922623, 0.9963778908391764944 ) ) 
 REPRESENTATION_ITEM ( '' )  );
#13952=CARTESIAN_POINT ( 'NONE',  ( 20.88017736071110164, 20.35535201082150891, 2.915334737309930979 ) ) ;
#13953=CARTESIAN_POINT ( 'NONE',  ( 2.791683348922237240, 25.38393115100078390, -7.208316651077763204 ) ) ;
#13954=CARTESIAN_POINT ( 'NONE',  ( -1.099225684535947600, 8.706968003263753531, -6.408140936763238038 ) ) ;
#13955=CARTESIAN_POINT ( 'NONE',  ( -0.8801773607111008646, 68.27201867748817676, 2.915334737309923430 ) ) ;
#13956=CARTESIAN_POINT ( 'NONE',  ( -0.8801773607111009756, 63.06368534415484106, 1.068504757029289695E-15 ) ) ;
#13957=CARTESIAN_POINT ( 'NONE',  ( -0.8801773607111009756, 33.06368534415484106, 1.068504757029289695E-15 ) ) ;
#13958=CARTESIAN_POINT ( 'NONE',  ( -2.816281873526473856, 59.33196800326374643, 3.434112377981055619 ) ) ;
#13959=CARTESIAN_POINT ( 'NONE',  ( -2.266590686148945544, 51.38708216824730357, -7.082119434687050408 ) ) ;
#13960=EDGE_CURVE ( 'NONE', #13640, #1529, #3003, .T. ) ;
#13961=CARTESIAN_POINT ( 'NONE',  ( 20.15039907845753220, 34.72266099184918176, 6.262539305110077059 ) ) ;
#13962=ORIENTED_EDGE ( 'NONE', *, *, #91312, .F. ) ;
#13963=CARTESIAN_POINT ( 'NONE',  ( 0.6178305044545838731, 14.74863466993041783, 9.382169495545420901 ) ) ;
#13964=CARTESIAN_POINT ( 'NONE',  ( 2.035157376598824452, 8.688685344154839285, 7.964842623401179544 ) ) ;
#13965=CARTESIAN_POINT ( 'NONE',  ( -0.8801773607111009756, 43.06368534415484106, 1.068504757029289695E-15 ) ) ;
#13967=LINE ( 'NONE', #68445, #77690 ) ;
#13969=CARTESIAN_POINT ( 'NONE',  ( 19.42250999205614548, 60.98035201082151247, -5.440088680355545492 ) ) ;
#13970=CARTESIAN_POINT ( 'NONE',  ( 5.076628168052703671, 31.84226448433412315, 8.527530157486179263 ) ) ;
#13971=CARTESIAN_POINT ( 'NONE',  ( 10.00000000000000000, 19.75893115100078390, -9.846743663894594434 ) ) ;
#13972=CARTESIAN_POINT ( 'NONE',  ( 14.92337183194729633, 12.67559781766745353, 8.527530157486181039 ) ) ;
#13974=CARTESIAN_POINT ( 'NONE',  ( -2.816281873526471635, 38.91530133659708213, -3.434112377981056508 ) ) ;
#13975=CARTESIAN_POINT ( 'NONE',  ( 14.92337183194729988, 4.342264484334117824, -8.527530157486177487 ) ) ;
#13977=CARTESIAN_POINT ( 'NONE',  ( 0.1089645850228807833, 23.16234555792570760, 6.479102184480781013 ) ) ;
#13979=CARTESIAN_POINT ( 'NONE',  ( 2.791683348922237240, 30.38393115100078390, -7.208316651077763204 ) ) ;
#13982=CARTESIAN_POINT ( 'NONE',  ( 6.565887622018943937, 58.08196800326376064, -12.81628187352647608 ) ) ;
#13984=CARTESIAN_POINT ( 'NONE',  ( 12.63842701281683034, 62.46726448433410894, 9.846743663894596210 ) ) ;
#13985=CARTESIAN_POINT ( 'NONE',  ( -2.266590686148945544, 27.22041550158063572, 7.082119434687048631 ) ) ;
#13987=CARTESIAN_POINT ( 'NONE',  ( 13.79529636645031943, 25.34541550158063572, -14.16423886937409904 ) ) ;
#13988=CARTESIAN_POINT ( 'NONE',  ( 13.79529636645030344, 48.26208216824728936, 14.16423886937410614 ) ) ;
#13990=CARTESIAN_POINT ( 'NONE',  ( -2.266590686148945544, 12.22041550158063394, 7.082119434687048631 ) ) ;
#13991=CARTESIAN_POINT ( 'NONE',  ( 2.917880565312948704, 17.63708216824730357, 12.26659068614894643 ) ) ;
#13993=CARTESIAN_POINT ( 'NONE',  ( 15.44008868035555260, 49.73035201082150536, 9.422509992056143702 ) ) ;
#13995=CARTESIAN_POINT ( 'NONE',  ( 0.1532563361054100626, 30.80059781766744820, -2.638427012816831230 ) ) ;
#13996=CARTESIAN_POINT ( 'NONE',  ( 2.035157376598822676, 67.43868534415484817, -7.964842623401177768 ) ) ;
#13997=CARTESIAN_POINT ( 'NONE',  ( 18.52753015748617571, 33.09226448433411605, 4.923371831947298993 ) ) ;
#13998=CARTESIAN_POINT ( 'NONE',  ( 15.44008868035555260, 24.73035201082150891, 9.422509992056143702 ) ) ;
#13999=CARTESIAN_POINT ( 'NONE',  ( 3.591859063236761518, 59.95696800326375353, 11.09922568453594849 ) ) ;
#14000=CARTESIAN_POINT ( 'NONE',  ( 5.076628168052704559, 55.17559781766745175, -8.527530157486179263 ) ) ;
#14002=CARTESIAN_POINT ( 'NONE',  ( 22.81628187352648496, 46.83196800326376064, -3.434112377981050290 ) ) ;
#14004=CARTESIAN_POINT ( 'NONE',  ( -0.8801773607110991993, 37.85535201082151247, -2.915334737309923874 ) ) ;
#14005=CARTESIAN_POINT ( 'NONE',  ( 2.791683348922237240, 35.38393115100079456, -7.208316651077763204 ) ) ;
#14006=CARTESIAN_POINT ( 'NONE',  ( -2.266590686148945544, 21.38708216824730357, -7.082119434687050408 ) ) ;
#14007=ORIENTED_EDGE ( 'NONE', *, *, #85898, .T. ) ;
#14008=CARTESIAN_POINT ( 'NONE',  ( 20.88017736071110875, 60.77201867748817676, -2.915334737309920765 ) ) ;
#14009=CARTESIAN_POINT ( 'NONE',  ( 2.035157376598824452, 63.68868534415484106, 7.964842623401179544 ) ) ;
#14010=CARTESIAN_POINT ( 'NONE',  ( 24.16423886937410614, 54.30374883491396787, 8.672049930838204340E-16 ) ) ;
#14011=CARTESIAN_POINT ( 'NONE',  ( 7.361572987183169658, 64.96726448433412315, -9.846743663894592657 ) ) ;
#14013=CARTESIAN_POINT ( 'NONE',  ( 2.035157376598824452, 48.68868534415483396, 7.964842623401179544 ) ) ;
#14016=CARTESIAN_POINT ( 'NONE',  ( 22.81628187352647785, 31.62363466993042138, 6.195893100308588602E-16 ) ) ;
#14018=CARTESIAN_POINT ( 'NONE',  ( -0.8801773607111009756, 13.06368534415483929, 1.068504757029289695E-15 ) ) ;
#14019=CARTESIAN_POINT ( 'NONE',  ( 15.44008868035555260, 14.73035201082150536, 9.422509992056143702 ) ) ;
#14020=CARTESIAN_POINT ( 'NONE',  ( 0.1532563361054100626, 45.80059781766745886, -2.638427012816831230 ) ) ;
#14021=CARTESIAN_POINT ( 'NONE',  ( 21.09922568453595559, 52.04030133659708923, -6.408140936763230044 ) ) ;
#14024=CARTESIAN_POINT ( 'NONE',  ( -0.8801773607111009756, 23.06368534415484106, 1.068504757029289695E-15 ) ) ;
#14025=CARTESIAN_POINT ( 'NONE',  ( -1.099225684535947600, -0.4596986634029132657, 6.408140936763237150 ) ) ;
#14027=CARTESIAN_POINT ( 'NONE',  ( 12.63842701281683034, 7.467264484334118713, 9.846743663894596210 ) ) ;
#14030=CARTESIAN_POINT ( 'NONE',  ( 19.84674366389459266, 53.30059781766744464, 2.638427012816836559 ) ) ;
#14031=CARTESIAN_POINT ( 'NONE',  ( 19.42250999205614193, 35.14701867748816966, 5.440088680355555262 ) ) ;
#14033=CARTESIAN_POINT ( 'NONE',  ( -1.099225684535947600, 4.540301336597087456, 6.408140936763237150 ) ) ;
#14034=CARTESIAN_POINT ( 'NONE',  ( 20.88017736071110519, 45.56368534415484106, 2.639326808657452039E-16 ) ) ;
#14036=CARTESIAN_POINT ( 'NONE',  ( 19.38216949554541202, 55.99863466993041072, 9.382169495545424454 ) ) ;
#14038=CARTESIAN_POINT ( 'NONE',  ( 12.91533473730992121, 59.52201867748816966, 10.88017736071110164 ) ) ;
#14039=CARTESIAN_POINT ( 'NONE',  ( -1.099225684535947600, 38.70696800326375353, -6.408140936763238038 ) ) ;
#14040=CARTESIAN_POINT ( 'NONE',  ( 10.00000000000000178, 39.31368534415484106, 10.88017736071110342 ) ) ;
#14041=CARTESIAN_POINT ( 'NONE',  ( 7.361572987183170547, 67.05059781766746596, 9.846743663894590881 ) ) ;
#14042=CARTESIAN_POINT ( 'NONE',  ( 10.00000000000000000, 54.75893115100078745, -9.846743663894594434 ) ) ;
#14043=CARTESIAN_POINT ( 'NONE',  ( 5.076628168052704559, 15.17559781766745175, -8.527530157486179263 ) ) ;
#14044=CARTESIAN_POINT ( 'NONE',  ( 19.84674366389459266, 3.300597817667451750, 2.638427012816836559 ) ) ;
#14045=CARTESIAN_POINT ( 'NONE',  ( 17.08211943468705130, 38.47041550158063217, 12.26659068614894998 ) ) ;
#14047=( GEOMETRIC_REPRESENTATION_CONTEXT ( 3 ) GLOBAL_UNCERTAINTY_ASSIGNED_CONTEXT ( ( #57301 ) ) GLOBAL_UNIT_ASSIGNED_CONTEXT ( ( #3153, #49131, #67091 ) ) REPRESENTATION_CONTEXT ( 'NONE', 'WORKASPACE' ) );
#14051=ORIENTED_EDGE ( 'NONE', *, *, #17478, .F. ) ;
#14053=CARTESIAN_POINT ( 'NONE',  ( 13.79529636645031943, 55.34541550158062506, -14.16423886937409904 ) ) ;
#14054=CARTESIAN_POINT ( 'NONE',  ( 6.204703633549690345, 57.84541550158063927, 14.16423886937410082 ) ) ;
#14055=CARTESIAN_POINT ( 'NONE',  ( 7.361572987183169658, 29.96726448433411960, -9.846743663894592657 ) ) ;
#14056=CARTESIAN_POINT ( 'NONE',  ( 6.565887622018943937, 28.08196800326375353, -12.81628187352647608 ) ) ;
#14057=CARTESIAN_POINT ( 'NONE',  ( 2.148416515056672971, 22.23726573380438509, 6.499999999999995559 ) ) ;
#14058=CARTESIAN_POINT ( 'NONE',  ( -2.266590686148945544, 2.220415501580634388, 7.082119434687048631 ) ) ;
#14059=CARTESIAN_POINT ( 'NONE',  ( 4.559911319644449179, 12.23035201082150536, -9.422509992056141925 ) ) ;
#14060=CARTESIAN_POINT ( 'NONE',  ( -4.164238869374099039, 51.80374883491396787, 8.674139862899312516E-16 ) ) ;
#14062=CARTESIAN_POINT ( 'NONE',  ( 2.791683348922240793, 31.63393115100078745, 7.208316651077764092 ) ) ;
#14064=CARTESIAN_POINT ( 'NONE',  ( 10.00000000000000178, 17.25893115100078745, 9.846743663894594434 ) ) ;
#14069=B_SPLINE_CURVE_WITH_KNOTS ( 'NONE', 3,
 ( #48744, #41761, #64228, #49243, #55773, #56743, #24792, #47267 ),
 .UNSPECIFIED., .F., .F.,
 ( 4, 2, 2, 4 ),
 ( 0.000000000000000000, 0.002750327629744753200, 0.004125491444617137606, 0.005500655259489521144 ),
 .UNSPECIFIED. ) ;
#14071=SURFACE_STYLE_USAGE ( .BOTH. , #75545 ) ;
#14072=ORIENTED_EDGE ( 'NONE', *, *, #86749, .T. ) ;
#14073=CARTESIAN_POINT ( 'NONE',  ( 14.92337183194729988, 44.34226448433412315, -8.527530157486177487 ) ) ;
#14074=CARTESIAN_POINT ( 'NONE',  ( -0.8801773607110991993, 22.85535201082150181, -2.915334737309923874 ) ) ;
#14075=CARTESIAN_POINT ( 'NONE',  ( 15.44008868035555793, 36.39701867748816966, -9.422509992056140149 ) ) ;
#14076=CARTESIAN_POINT ( 'NONE',  ( 19.84674366389459266, 63.30059781766745886, 2.638427012816836559 ) ) ;
#14077=CARTESIAN_POINT ( 'NONE',  ( 6.565887622018943937, 23.08196800326375708, -12.81628187352647608 ) ) ;
#14078=CARTESIAN_POINT ( 'NONE',  ( 17.08211943468705130, 8.470415501580635720, 12.26659068614894998 ) ) ;
#14079=CARTESIAN_POINT ( 'NONE',  ( 20.88017736071110164, 65.35535201082150536, 2.915334737309930979 ) ) ;
#14080=CARTESIAN_POINT ( 'NONE',  ( 13.43411237798105340, 25.58196800326374998, 12.81628187352647963 ) ) ;
#14082=CARTESIAN_POINT ( 'NONE',  ( 2.791683348922237240, 25.38393115100078390, -7.208316651077763204 ) ) ;
#14083=CARTESIAN_POINT ( 'NONE',  ( 2.035157376598822676, 7.438685344154837509, -7.964842623401177768 ) ) ;
#14085=CARTESIAN_POINT ( 'NONE',  ( 7.084665262690076126, 9.105352010821503583, 10.88017736071109987 ) ) ;
#14086=VERTEX_POINT ( 'NONE', #58392 ) ;
#14087=CARTESIAN_POINT ( 'NONE',  ( -0.8801773607111008646, 43.27201867748817676, 2.915334737309923430 ) ) ;
#14088=CARTESIAN_POINT ( 'NONE',  ( -0.8801773607111009756, 58.06368534415484106, 1.068504757029289695E-15 ) ) ;
#14089=CARTESIAN_POINT ( 'NONE',  ( 7.361572987183170547, 2.050597817667451750, 9.846743663894590881 ) ) ;
#14090=CARTESIAN_POINT ( 'NONE',  ( 12.91533473730993009, 51.60535201082149825, -10.88017736071109987 ) ) ;
#14093=CARTESIAN_POINT ( 'NONE',  ( 0.1532563361054082862, 26.21726448433411605, 2.638427012816831674 ) ) ;
#14095=CARTESIAN_POINT ( 'NONE',  ( 20.15039907845753220, 19.72266099184918886, 6.262539305110075283 ) ) ;
#14097=CARTESIAN_POINT ( 'NONE',  ( 6.204703633549690345, 0.7620821682473009062, -14.16423886937410259 ) ) ;
#14103=CARTESIAN_POINT ( 'NONE',  ( 20.88017736071110519, 5.563685344154838397, 2.639326808657452039E-16 ) ) ;
#14104=DIRECTION ( 'NONE',  ( 1.000000000000000000, 0.000000000000000000, -0.000000000000000000 ) ) ;
#14105=VERTEX_POINT ( 'NONE', #57420 ) ;
#14106=FILL_AREA_STYLE ('',( #90086 ) ) ;
#14107=CARTESIAN_POINT ( 'NONE',  ( 0.1532563361054083140, 46.00893115100079456, 1.131784320476157264E-15 ) ) ;
#14109=CARTESIAN_POINT ( 'NONE',  ( 0.6178305044545818747, 23.49863466993041783, -9.382169495545419124 ) ) ;
#14110=CARTESIAN_POINT ( 'NONE',  ( 19.84674366389459621, 8.508931151000785675, 7.409399052514197653E-17 ) ) ;
#14111=EDGE_CURVE ( 'NONE', #43572, #39677, #17398, .T. ) ;
#14114=CARTESIAN_POINT ( 'NONE',  ( 21.09922568453595559, 7.040301336597086568, -6.408140936763230044 ) ) ;
#14120=CARTESIAN_POINT ( 'NONE',  ( 7.084665262690076126, 22.02201867748817321, -10.88017736071110164 ) ) ;
#14121=CARTESIAN_POINT ( 'NONE',  ( 13.79529636645031943, 25.34541550158063572, -14.16423886937409904 ) ) ;
#14122=CARTESIAN_POINT ( 'NONE',  ( 5.076628168052703671, 31.84226448433412315, 8.527530157486179263 ) ) ;
#14123=CARTESIAN_POINT ( 'NONE',  ( 20.88017736071110164, 60.35535201082151957, 2.915334737309930979 ) ) ;
#14124=CARTESIAN_POINT ( 'NONE',  ( 3.591859063236761518, 34.95696800326375353, 11.09922568453594849 ) ) ;
#14125=CARTESIAN_POINT ( 'NONE',  ( 15.44008868035555260, 14.73035201082150536, 9.422509992056143702 ) ) ;
#14126=CARTESIAN_POINT ( 'NONE',  ( 0.9413316022086124502, 43.45508385108959004, 6.499999999999978684 ) ) ;
#14128=CARTESIAN_POINT ( 'NONE',  ( 16.40814093676323893, 15.79030133659708746, 11.09922568453595026 ) ) ;
#14129=CARTESIAN_POINT ( 'NONE',  ( 12.63842701281683922, 59.55059781766744464, -9.846743663894590881 ) ) ;
#14130=CARTESIAN_POINT ( 'NONE',  ( 1.472469842513823179, 26.42559781766745175, 4.923371831947296329 ) ) ;
#14132=CARTESIAN_POINT ( 'NONE',  ( 13.43411237798105340, 35.58196800326375353, 12.81628187352647963 ) ) ;
#14133=CARTESIAN_POINT ( 'NONE',  ( 18.61655166652077042, 24.87718327197429602, 6.499999999999981348 ) ) ;
#14134=CARTESIAN_POINT ( 'NONE',  ( -0.8801773607111008646, 38.27201867748816255, 2.915334737309923430 ) ) ;
#14139=CARTESIAN_POINT ( 'NONE',  ( 20.88017736071110875, 35.77201867748816966, -2.915334737309920765 ) ) ;
#14140=CARTESIAN_POINT ( 'NONE',  ( 7.084665262690076126, 44.10535201082151247, 10.88017736071109987 ) ) ;
#14141=CARTESIAN_POINT ( 'NONE',  ( 19.84674366389459621, 63.50893115100078745, 7.409399052514197653E-17 ) ) ;
#14143=CARTESIAN_POINT ( 'NONE',  ( 2.035157376598822676, 47.43868534415484817, -7.964842623401177768 ) ) ;
#14144=EDGE_CURVE ( 'NONE', #6265, #33986, #3364, .T. ) ;
#14145=CARTESIAN_POINT ( 'NONE',  ( 12.63842701281683922, 44.55059781766745175, -9.846743663894590881 ) ) ;
#14146=CARTESIAN_POINT ( 'NONE',  ( 2.035157376598822676, 12.43868534415483751, -7.964842623401177768 ) ) ;
#14147=CARTESIAN_POINT ( 'NONE',  ( 13.43411237798106583, 12.66530133659708746, -12.81628187352647252 ) ) ;
#14149=CARTESIAN_POINT ( 'NONE',  ( -0.8801773607111008646, 18.27201867748817321, 2.915334737309923430 ) ) ;
#14152=CARTESIAN_POINT ( 'NONE',  ( 2.035157376598824452, 3.688685344154837953, 7.964842623401179544 ) ) ;
#14153=CARTESIAN_POINT ( 'NONE',  ( 10.00000000000000000, 31.81368534415483751, -10.88017736071110342 ) ) ;
#14154=CARTESIAN_POINT ( 'NONE',  ( 0.1532563361054083140, 1.008931151000784787, 1.131784320476157264E-15 ) ) ;
#14155=CARTESIAN_POINT ( 'NONE',  ( 22.26659068614894466, 38.88708216824731068, 7.082119434687054849 ) ) ;
#14156=CARTESIAN_POINT ( 'NONE',  ( 12.63842701281683034, 17.46726448433411250, 9.846743663894596210 ) ) ;
#14158=CARTESIAN_POINT ( 'NONE',  ( 4.559911319644449179, 47.23035201082150536, -9.422509992056141925 ) ) ;
#14159=CARTESIAN_POINT ( 'NONE',  ( 19.05866839779139355, 45.95508385108959715, -6.499999999999974243 ) ) ;
#14160=ORIENTED_EDGE ( 'NONE', *, *, #6682, .F. ) ;
#14162=CARTESIAN_POINT ( 'NONE',  ( 7.361572987183169658, 64.96726448433412315, -9.846743663894592657 ) ) ;
#14163=ORIENTED_EDGE ( 'NONE', *, *, #6008, .T. ) ;
#14165=CARTESIAN_POINT ( 'NONE',  ( 6.204703633549690345, 22.84541550158062861, 14.16423886937410082 ) ) ;
#14166=CARTESIAN_POINT ( 'NONE',  ( 24.16423886937409904, 24.09541550158063927, 3.795296366450317205 ) ) ;
#14167=CARTESIAN_POINT ( 'NONE',  ( 2.035157376598822676, 62.43868534415483396, -7.964842623401177768 ) ) ;
#14168=CARTESIAN_POINT ( 'NONE',  ( 7.084665262690076126, 4.105352010821503583, 10.88017736071109987 ) ) ;
#14169=CARTESIAN_POINT ( 'NONE',  ( 3.591859063236761518, 4.956968003263753531, 11.09922568453594849 ) ) ;
#14170=CARTESIAN_POINT ( 'NONE',  ( 14.92337183194729988, 44.34226448433412315, -8.527530157486177487 ) ) ;
#14172=CARTESIAN_POINT ( 'NONE',  ( 20.88017736071110164, 40.35535201082150536, 2.915334737309930979 ) ) ;
#14173=CARTESIAN_POINT ( 'NONE',  ( 16.40814093676323893, 0.7903013365970867898, 11.09922568453595026 ) ) ;
#14174=CARTESIAN_POINT ( 'NONE',  ( 24.16423886937410614, 19.30374883491397142, 8.672049930838204340E-16 ) ) ;
#14175=CARTESIAN_POINT ( 'NONE',  ( 10.00000000000000178, 9.313685344154839285, 10.88017736071110342 ) ) ;
#14176=CARTESIAN_POINT ( 'NONE',  ( 7.084665262690076126, 17.02201867748817676, -10.88017736071110164 ) ) ;
#14177=CARTESIAN_POINT ( 'NONE',  ( 18.52753015748617571, 53.09226448433412315, 4.923371831947298993 ) ) ;
#14178=CARTESIAN_POINT ( 'NONE',  ( 17.96484262340118221, 39.93868534415484106, 7.964842623401181321 ) ) ;
#14181=ORIENTED_EDGE ( 'NONE', *, *, #3643, .F. ) ;
#14184=CARTESIAN_POINT ( 'NONE',  ( 2.791683348922240793, 31.63393115100078745, 7.208316651077764092 ) ) ;
#14186=CARTESIAN_POINT ( 'NONE',  ( -46.94000000000001194, 103.0000000000000000, -5.997726559847240679 ) ) ;
#14187=CARTESIAN_POINT ( 'NONE',  ( 22.26659068614894466, 48.88708216824730357, 7.082119434687054849 ) ) ;
#14188=CARTESIAN_POINT ( 'NONE',  ( 7.084665262690076126, 4.105352010821503583, 10.88017736071109987 ) ) ;
#14189=CARTESIAN_POINT ( 'NONE',  ( 18.52753015748617571, 28.09226448433411960, 4.923371831947298993 ) ) ;
#14190=CARTESIAN_POINT ( 'NONE',  ( 14.92337183194729633, 47.67559781766745175, 8.527530157486181039 ) ) ;
#14191=CARTESIAN_POINT ( 'NONE',  ( 21.92686044187657046, 50.16212336850781384, 4.562052436263912550E-16 ) ) ;
#14195=( GEOMETRIC_REPRESENTATION_CONTEXT ( 3 ) GLOBAL_UNCERTAINTY_ASSIGNED_CONTEXT ( ( #32211 ) ) GLOBAL_UNIT_ASSIGNED_CONTEXT ( ( #85381, #60409, #22432 ) ) REPRESENTATION_CONTEXT ( 'NONE', 'WORKASPACE' ) );
#14196=CARTESIAN_POINT ( 'NONE',  ( 0.1532563361054100626, 0.8005978176674514168, -2.638427012816831230 ) ) ;
#14199=CARTESIAN_POINT ( 'NONE',  ( -0.3689425029237898834, 36.17874883491396787, -10.36894250292378850 ) ) ;
#14200=CARTESIAN_POINT ( 'NONE',  ( 16.40814093676323893, 20.79030133659708923, 11.09922568453595026 ) ) ;
#14201=ORIENTED_EDGE ( 'NONE', *, *, #52504, .T. ) ;
#14202=CARTESIAN_POINT ( 'NONE',  ( -2.816281873526471635, 58.91530133659707502, -3.434112377981056508 ) ) ;
#14203=CARTESIAN_POINT ( 'NONE',  ( -0.8801773607110991993, 27.85535201082150181, -2.915334737309923874 ) ) ;
#14204=CARTESIAN_POINT ( 'NONE',  ( 0.1532563361054083140, 31.00893115100078390, 1.131784320476157264E-15 ) ) ;
#14205=CARTESIAN_POINT ( 'NONE',  ( -0.8801773607111008646, 28.27201867748817321, 2.915334737309923430 ) ) ;
#14206=CARTESIAN_POINT ( 'NONE',  ( 20.15039907845753575, 32.62777174578613426, -6.262539305110076171 ) ) ;
#14208=CARTESIAN_POINT ( 'NONE',  ( 17.20831665107776587, 37.88393115100078745, 7.208316651077764980 ) ) ;
#14209=CARTESIAN_POINT ( 'NONE',  ( 14.92337183194729633, 52.67559781766745175, 8.527530157486181039 ) ) ;
#14211=CARTESIAN_POINT ( 'NONE',  ( 0.6178305044545838731, 29.74863466993042138, 9.382169495545420901 ) ) ;
#14212=CARTESIAN_POINT ( 'NONE',  ( 17.39651004071842166, 27.93575266056828355, 6.499999999999998224 ) ) ;
#14216=CARTESIAN_POINT ( 'NONE',  ( 18.72515096720590577, 61.07228050351029935, -6.499999999999718447 ) ) ;
#14218=CARTESIAN_POINT ( 'NONE',  ( 17.20831665107776587, 17.88393115100078745, 7.208316651077764980 ) ) ;
#14219=CARTESIAN_POINT ( 'NONE',  ( 10.00000000000000178, 35.37363466993042493, 12.81628187352647608 ) ) ;
#14223=CARTESIAN_POINT ( 'NONE',  ( 1.472469842513823179, 36.42559781766745175, 4.923371831947296329 ) ) ;
#14224=CARTESIAN_POINT ( 'NONE',  ( 2.917880565312950480, 40.97041550158063217, -12.26659068614894821 ) ) ;
#14225=CARTESIAN_POINT ( 'NONE',  ( 1.472469842513823179, 45.59226448433412315, -4.923371831947296329 ) ) ;
#14226=CARTESIAN_POINT ( 'NONE',  ( 16.40814093676324603, 52.45696800326375353, -11.09922568453594671 ) ) ;
#14227=CYLINDRICAL_SURFACE ( 'NONE', #14527, 11.92686044187656513 ) ;
#14229=CARTESIAN_POINT ( 'NONE',  ( 5.076628168052703671, 11.84226448433411960, 8.527530157486179263 ) ) ;
#14230=SURFACE_STYLE_FILL_AREA ( #22230 ) ;
#14231=CARTESIAN_POINT ( 'NONE',  ( 19.84674366389459266, 48.71726448433413026, -2.638427012816827677 ) ) ;
#14232=CARTESIAN_POINT ( 'NONE',  ( 10.00000000000000178, 39.31368534415484106, 10.88017736071110342 ) ) ;
#14234=CARTESIAN_POINT ( 'NONE',  ( 19.84674366389459266, 38.71726448433412315, -2.638427012816827677 ) ) ;
#14236=CARTESIAN_POINT ( 'NONE',  ( 12.91533473730993009, 46.60535201082150536, -10.88017736071109987 ) ) ;
#14239=CARTESIAN_POINT ( 'NONE',  ( 17.96484262340118221, 21.18868534415483396, -7.964842623401177768 ) ) ;
#14240=CARTESIAN_POINT ( 'NONE',  ( 0.6178305044545838731, -0.2513653300695798953, 9.382169495545420901 ) ) ;
#14241=CARTESIAN_POINT ( 'NONE',  ( 7.084665262690076126, 49.10535201082149825, 10.88017736071109987 ) ) ;
#14242=CARTESIAN_POINT ( 'NONE',  ( 7.084665262690076126, 62.02201867748816966, -10.88017736071110164 ) ) ;
#14245=CARTESIAN_POINT ( 'NONE',  ( 20.88017736071110875, 40.77201867748818387, -2.915334737309920765 ) ) ;
#14247=CARTESIAN_POINT ( 'NONE',  ( 0.1532563361054082862, 11.21726448433411605, 2.638427012816831674 ) ) ;
#14248=CARTESIAN_POINT ( 'NONE',  ( 0.1532563361054100626, 25.80059781766744820, -2.638427012816831230 ) ) ;
#14251=CARTESIAN_POINT ( 'NONE',  ( 14.92337183194729633, 62.67559781766745886, 8.527530157486181039 ) ) ;
#14252=CARTESIAN_POINT ( 'NONE',  ( 20.36894250292379382, 63.67874883491396787, 10.36894250292379205 ) ) ;
#14255=CARTESIAN_POINT ( 'NONE',  ( 10.00000000000000178, 28.05374883491396787, 14.16423886937410082 ) ) ;
#14256=VECTOR ( 'NONE', #77649, 1000.000000000000000 ) ;
#14257=CARTESIAN_POINT ( 'NONE',  ( -4.164238869374098151, 46.59541550158063927, -3.795296366450310543 ) ) ;
#14258=( LENGTH_UNIT ( ) NAMED_UNIT ( * ) SI_UNIT ( .MILLI., .METRE. ) );
#14260=EDGE_LOOP ( 'NONE', ( #81308, #17652, #76152, #48684, #18193, #48717 ) ) ;
#14261=CARTESIAN_POINT ( 'NONE',  ( 1.472469842513823179, 25.59226448433412315, -4.923371831947296329 ) ) ;
#14263=CARTESIAN_POINT ( 'NONE',  ( 2.035157376598824452, 18.68868534415484106, 7.964842623401179544 ) ) ;
#14264=CARTESIAN_POINT ( 'NONE',  ( 0.1532563361054082862, 51.21726448433412315, 2.638427012816831674 ) ) ;
#14265=FACE_OUTER_BOUND ( 'NONE', #65559, .T. ) ;
#14266=CARTESIAN_POINT ( 'NONE',  ( 20.15039907845753575, 16.74884699246888431, 6.262539305110077059 ) ) ;
#14269=PRESENTATION_STYLE_ASSIGNMENT (( #89749 ) ) ;
#14270=CARTESIAN_POINT ( 'NONE',  ( 16.40814093676324603, 32.45696800326375353, -11.09922568453594671 ) ) ;
#14271=CARTESIAN_POINT ( 'NONE',  ( 7.361572987183170547, 47.05059781766745175, 9.846743663894590881 ) ) ;
#14274=CARTESIAN_POINT ( 'NONE',  ( 10.00000000000000178, 7.258931151000785675, 9.846743663894594434 ) ) ;
#14277=CARTESIAN_POINT ( 'NONE',  ( -0.8801773607110991993, 12.85535201082150358, -2.915334737309923874 ) ) ;
#14278=CARTESIAN_POINT ( 'NONE',  ( 20.36894250292379738, 59.92874883491397497, -10.36894250292379027 ) ) ;
#14279=CARTESIAN_POINT ( 'NONE',  ( 15.44008868035555793, 46.39701867748817676, -9.422509992056140149 ) ) ;
#14280=CARTESIAN_POINT ( 'NONE',  ( 15.44008868035555793, 66.39701867748817676, -9.422509992056140149 ) ) ;
#14282=CARTESIAN_POINT ( 'NONE',  ( 19.84674366389459621, 18.50893115100078745, 7.409399052514197653E-17 ) ) ;
#14283=CARTESIAN_POINT ( 'NONE',  ( 7.084665262690076126, 7.022018677488169658, -10.88017736071110164 ) ) ;
#14284=CARTESIAN_POINT ( 'NONE',  ( 10.00000000000000178, 12.25893115100078568, 9.846743663894594434 ) ) ;
#14286=CARTESIAN_POINT ( 'NONE',  ( 1.472469842513823179, 31.42559781766745530, 4.923371831947296329 ) ) ;
#14288=CARTESIAN_POINT ( 'NONE',  ( 4.559911319644449179, 32.23035201082150536, -9.422509992056141925 ) ) ;
#14289=UNCERTAINTY_MEASURE_WITH_UNIT (LENGTH_MEASURE( 1.000000000000000082E-05 ), #40489, 'distance_accuracy_value', 'NONE');
#14291=CARTESIAN_POINT ( 'NONE',  ( 3.591859063236761518, 64.95696800326376774, 11.09922568453594849 ) ) ;
#14293=CARTESIAN_POINT ( 'NONE',  ( 5.076628168052704559, 15.17559781766745175, -8.527530157486179263 ) ) ;
#14294=CARTESIAN_POINT ( 'NONE',  ( 6.565887622018943937, 50.16530133659708213, 12.81628187352647430 ) ) ;
#14295=CARTESIAN_POINT ( 'NONE',  ( 12.91533473730992121, 9.522018677488171434, 10.88017736071110164 ) ) ;
#14296=CARTESIAN_POINT ( 'NONE',  ( 14.92337183194729988, 29.34226448433411960, -8.527530157486177487 ) ) ;
#14297=DIRECTION ( 'NONE',  ( -0.8320502943378437211, 0.5547001962252290364, 0.000000000000000000 ) ) ;
#14299=CARTESIAN_POINT ( 'NONE',  ( 17.08211943468705130, 33.47041550158063927, 12.26659068614894998 ) ) ;
#14300=CARTESIAN_POINT ( 'NONE',  ( 20.36894250292379738, 39.92874883491396787, -10.36894250292379027 ) ) ;
#14301=CARTESIAN_POINT ( 'NONE',  ( 19.84674366389459266, 53.71726448433411605, -2.638427012816827677 ) ) ;
#14303=CARTESIAN_POINT ( 'NONE',  ( 2.035157376598824452, 38.68868534415483396, 7.964842623401179544 ) ) ;
#14304=CARTESIAN_POINT ( 'NONE',  ( 7.084665262690076126, 67.02201867748817676, -10.88017736071110164 ) ) ;
#14307=ORIENTED_EDGE ( 'NONE', *, *, #84150, .T. ) ;
#14308=CARTESIAN_POINT ( 'NONE',  ( -1.099225684535947600, 58.70696800326375353, -6.408140936763238038 ) ) ;
#14310=CARTESIAN_POINT ( 'NONE',  ( 2.791683348922237240, 0.3839311510007847872, -7.208316651077763204 ) ) ;
#14311=ORIENTED_EDGE ( 'NONE', *, *, #39425, .F. ) ;
#14312=CARTESIAN_POINT ( 'NONE',  ( 2.917880565312950480, 10.97041550158063572, -12.26659068614894821 ) ) ;
#14313=CARTESIAN_POINT ( 'NONE',  ( 2.791683348922240793, 11.63393115100078568, 7.208316651077764092 ) ) ;
#14314=CARTESIAN_POINT ( 'NONE',  ( -0.8801773607111009756, 33.06368534415484106, 1.068504757029289695E-15 ) ) ;
#14315=EDGE_CURVE ( 'NONE', #96219, #19780, #16473, .T. ) ;
#14316=CARTESIAN_POINT ( 'NONE',  ( 1.152268111383477178, 1.024801820426059406E-17, -6.000000000000281553 ) ) ;
#14318=CARTESIAN_POINT ( 'NONE',  ( 10.00000000000000178, 34.31368534415484106, 10.88017736071110342 ) ) ;
#14319=ORIENTED_EDGE ( 'NONE', *, *, #93755, .T. ) ;
#14321=ORIENTED_EDGE ( 'NONE', *, *, #94726, .T. ) ;
#14322=ORIENTED_EDGE ( 'NONE', *, *, #16304, .F. ) ;
#14323=CARTESIAN_POINT ( 'NONE',  ( 4.559911319644449179, 63.89701867748817676, 9.422509992056141925 ) ) ;
#14325=CARTESIAN_POINT ( 'NONE',  ( 12.91533473730992121, 14.52201867748817143, 10.88017736071110164 ) ) ;
#14327=CARTESIAN_POINT ( 'NONE',  ( 1.472469842513823179, 0.5922644843341181575, -4.923371831947296329 ) ) ;
#14328=CARTESIAN_POINT ( 'NONE',  ( 7.084665262690076126, 14.10535201082150358, 10.88017736071109987 ) ) ;
#14329=VERTEX_POINT ( 'NONE', #24841 ) ;
#14330=CARTESIAN_POINT ( 'NONE',  ( 21.09922568453594849, 51.20696800326375353, 6.408140936763242479 ) ) ;
#14331=CARTESIAN_POINT ( 'NONE',  ( 4.559911319644449179, 42.23035201082151247, -9.422509992056141925 ) ) ;
#14333=CARTESIAN_POINT ( 'NONE',  ( 19.38216949554541202, 60.99863466993042493, 9.382169495545424454 ) ) ;
#14334=CARTESIAN_POINT ( 'NONE',  ( 2.035157376598822676, 42.43868534415483396, -7.964842623401177768 ) ) ;
#14335=CARTESIAN_POINT ( 'NONE',  ( 22.81628187352647785, 6.415301336597088344, 3.434112377981063169 ) ) ;
#14336=PLANE ( 'NONE',  #29078 ) ;
#14337=CARTESIAN_POINT ( 'NONE',  ( 14.92337183194729988, 14.34226448433411782, -8.527530157486177487 ) ) ;
#14339=CARTESIAN_POINT ( 'NONE',  ( 3.591859063236763294, 8.290301336597087456, -11.09922568453595026 ) ) ;
#14342=CARTESIAN_POINT ( 'NONE',  ( 19.42250999205614193, 40.14701867748817676, 5.440088680355555262 ) ) ;
#14344=CARTESIAN_POINT ( 'NONE',  ( 7.361572987183170547, 47.05059781766745175, 9.846743663894590881 ) ) ;
#14346=CARTESIAN_POINT ( 'NONE',  ( 5.076628168052703671, 16.84226448433411960, 8.527530157486179263 ) ) ;
#14347=CARTESIAN_POINT ( 'NONE',  ( 7.361572987183170547, 2.050597817667451750, 9.846743663894590881 ) ) ;
#14349=CARTESIAN_POINT ( 'NONE',  ( 7.361572987183170547, 67.05059781766746596, 9.846743663894590881 ) ) ;
#14351=CARTESIAN_POINT ( 'NONE',  ( 20.88017736071110164, 5.355352010821502695, 2.915334737309930979 ) ) ;
#14352=PRESENTATION_STYLE_ASSIGNMENT (( #69320 ) ) ;
#14353=CARTESIAN_POINT ( 'NONE',  ( 19.84674366389459266, 58.71726448433411605, -2.638427012816827677 ) ) ;
#14354=CARTESIAN_POINT ( 'NONE',  ( 19.84674366389459266, 28.71726448433411960, -2.638427012816827677 ) ) ;
#14356=CARTESIAN_POINT ( 'NONE',  ( 10.00000000000000000, 6.813685344154838397, -10.88017736071110342 ) ) ;
#14357=EDGE_CURVE ( 'NONE', #61681, #31263, #24170, .T. ) ;
#14358=CARTESIAN_POINT ( 'NONE',  ( 14.92337183194729633, 47.67559781766745175, 8.527530157486181039 ) ) ;
#14361=CARTESIAN_POINT ( 'NONE',  ( 2.035157376598822676, 2.438685344154838397, -7.964842623401177768 ) ) ;
#14362=CARTESIAN_POINT ( 'NONE',  ( 0.5774900079438607392, 13.48035201082150358, 5.440088680355550821 ) ) ;
#14363=CARTESIAN_POINT ( 'NONE',  ( 0.5774900079438607392, 18.48035201082150536, 5.440088680355550821 ) ) ;
#14364=CARTESIAN_POINT ( 'NONE',  ( 24.16423886937410614, 54.51208216824730357, -3.795296366450302550 ) ) ;
#14365=CARTESIAN_POINT ( 'NONE',  ( 6.204703633549690345, 57.84541550158063927, 14.16423886937410082 ) ) ;
#14367=CARTESIAN_POINT ( 'NONE',  ( 7.361572987183170547, 2.050597817667451750, 9.846743663894590881 ) ) ;
#14368=B_SPLINE_CURVE_WITH_KNOTS ( 'NONE', 3,
 ( #41904, #16929, #72365, #26875, #3896, #93407 ),
 .UNSPECIFIED., .F., .F.,
 ( 4, 2, 4 ),
 ( 0.000000000000000000, 0.0002701661927229378839, 0.0005403323854458757678 ),
 .UNSPECIFIED. ) ;
#14369=CARTESIAN_POINT ( 'NONE',  ( 7.361572987183170547, 22.05059781766745530, 9.846743663894590881 ) ) ;
#14371=CARTESIAN_POINT ( 'NONE',  ( -1.099225684535947600, 13.70696800326375353, -6.408140936763238038 ) ) ;
#14374=CARTESIAN_POINT ( 'NONE',  ( 1.472469842513823179, 56.42559781766745886, 4.923371831947296329 ) ) ;
#14377=CARTESIAN_POINT ( 'NONE',  ( 24.16423886937410614, 4.303748834913967869, 8.672049930838204340E-16 ) ) ;
#14378=CARTESIAN_POINT ( 'NONE',  ( 2.791683348922237240, 25.38393115100078390, -7.208316651077763204 ) ) ;
#14381=CARTESIAN_POINT ( 'NONE',  ( -2.266590686148945544, 41.38708216824729647, -7.082119434687050408 ) ) ;
#14382=CARTESIAN_POINT ( 'NONE',  ( 12.63842701281683034, 2.467264484334118269, 9.846743663894596210 ) ) ;
#14384=CARTESIAN_POINT ( 'NONE',  ( 19.42250999205614548, 30.98035201082150536, -5.440088680355545492 ) ) ;
#14385=CARTESIAN_POINT ( 'NONE',  ( 6.565887622018943937, 43.08196800326374643, -12.81628187352647608 ) ) ;
#14386=CARTESIAN_POINT ( 'NONE',  ( 2.035157376598824452, 8.688685344154839285, 7.964842623401179544 ) ) ;
#14387=CARTESIAN_POINT ( 'NONE',  ( 16.40814093676323893, 30.79030133659708923, 11.09922568453595026 ) ) ;
#14388=CARTESIAN_POINT ( 'NONE',  ( 5.076628168052704559, 5.175597817667451750, -8.527530157486179263 ) ) ;
#14390=ORIENTED_EDGE ( 'NONE', *, *, #87839, .T. ) ;
#14393=CARTESIAN_POINT ( 'NONE',  ( -2.266590686148945544, 36.38708216824730357, -7.082119434687050408 ) ) ;
#14394=CARTESIAN_POINT ( 'NONE',  ( 19.42250999205614548, 5.980352010821504471, -5.440088680355545492 ) ) ;
#14395=CARTESIAN_POINT ( 'NONE',  ( 20.88017736071110519, 25.56368534415483751, 2.639326808657452039E-16 ) ) ;
#14397=DIRECTION ( 'NONE',  ( 0.000000000000000000, 0.000000000000000000, -1.000000000000000000 ) ) ;
#14398=CARTESIAN_POINT ( 'NONE',  ( 19.42250999205614193, 50.14701867748817676, 5.440088680355555262 ) ) ;
#14399=CARTESIAN_POINT ( 'NONE',  ( 2.035157376598824452, 63.68868534415484106, 7.964842623401179544 ) ) ;
#14400=CARTESIAN_POINT ( 'NONE',  ( 0.6178305044545838731, 24.74863466993042493, 9.382169495545420901 ) ) ;
#14401=CARTESIAN_POINT ( 'NONE',  ( -36.44000000000001194, 92.00000000000000000, -10.09898361729590199 ) ) ;
#14402=CARTESIAN_POINT ( 'NONE',  ( -0.1503990784575328643, 30.12777174578613781, 6.262539305110068177 ) ) ;
#14403=CARTESIAN_POINT ( 'NONE',  ( 19.84674366389459621, 23.50893115100078390, 7.409399052514197653E-17 ) ) ;
#14404=CARTESIAN_POINT ( 'NONE',  ( 20.88017736071110875, 55.77201867748816966, -2.915334737309920765 ) ) ;
#14405=CARTESIAN_POINT ( 'NONE',  ( 3.591859063236761518, 24.95696800326375353, 11.09922568453594849 ) ) ;
#14406=B_SPLINE_CURVE_WITH_KNOTS ( 'NONE', 3,
 ( #54087, #69595, #84109, #46110 ),
 .UNSPECIFIED., .F., .F.,
 ( 4, 4 ),
 ( 0.000000000000000000, 0.001036303429213365941 ),
 .UNSPECIFIED. ) ;
#14407=CARTESIAN_POINT ( 'NONE',  ( 0.1532563361054100626, 0.8005978176674514168, -2.638427012816831230 ) ) ;
#14408=CARTESIAN_POINT ( 'NONE',  ( 17.96484262340118221, 11.18868534415483929, -7.964842623401177768 ) ) ;
#14409=CARTESIAN_POINT ( 'NONE',  ( 19.84674366389459621, 43.50893115100078745, 7.409399052514197653E-17 ) ) ;
#14410=CARTESIAN_POINT ( 'NONE',  ( 21.09922568453595559, 57.04030133659708923, -6.408140936763230044 ) ) ;
#14411=CARTESIAN_POINT ( 'NONE',  ( 18.52753015748618282, 18.92559781766745175, -4.923371831947291888 ) ) ;
#14412=CARTESIAN_POINT ( 'NONE',  ( -0.3689425029237881626, 2.428748834913967869, 10.36894250292379027 ) ) ;
#14413=CARTESIAN_POINT ( 'NONE',  ( 10.00000000000000000, 0.5537488349139675359, -14.16423886937410082 ) ) ;
#14415=CARTESIAN_POINT ( 'NONE',  ( 10.00000000000000178, 39.31368534415484106, 10.88017736071110342 ) ) ;
#14416=FILL_AREA_STYLE ('',( #67404 ) ) ;
#14417=CARTESIAN_POINT ( 'NONE',  ( -0.3689425029237881626, 32.42874883491395366, 10.36894250292379027 ) ) ;
#14418=CARTESIAN_POINT ( 'NONE',  ( 2.791683348922237240, 40.38393115100078035, -7.208316651077763204 ) ) ;
#14419=CARTESIAN_POINT ( 'NONE',  ( 20.88017736071110875, 30.77201867748816966, -2.915334737309920765 ) ) ;
#14420=CARTESIAN_POINT ( 'NONE',  ( 0.5774900079438590739, 17.64701867748817321, -5.440088680355550821 ) ) ;
#14421=EDGE_LOOP ( 'NONE', ( #82401, #48232, #61079, #36600, #31018, #86483, #54097, #97718, #95483, #13962, #98341, #41268, #96085, #36314, #7777, #26625, #78238, #46671, #53088, #430, #12429, #5732, #95324, #17056, #24789, #92005, #73090, #29411, #18057, #81583, #52999, #8641, #72437 ) ) ;
#14423=CARTESIAN_POINT ( 'NONE',  ( 17.96484262340118221, 31.18868534415483751, -7.964842623401177768 ) ) ;
#14424=CARTESIAN_POINT ( 'NONE',  ( -1.099225684535947600, 48.70696800326375353, -6.408140936763238038 ) ) ;
#14425=EDGE_CURVE ( 'NONE', #11778, #93697, #34349, .T. ) ;
#14426=CARTESIAN_POINT ( 'NONE',  ( 19.42250999205614193, 45.14701867748817676, 5.440088680355555262 ) ) ;
#14428=CARTESIAN_POINT ( 'NONE',  ( 4.559911319644449179, 38.89701867748817676, 9.422509992056141925 ) ) ;
#14430=CARTESIAN_POINT ( 'NONE',  ( 2.791683348922240793, 51.63393115100078745, 7.208316651077764092 ) ) ;
#14431=CARTESIAN_POINT ( 'NONE',  ( 2.035157376598822676, 37.43868534415484106, -7.964842623401177768 ) ) ;
#14434=CARTESIAN_POINT ( 'NONE',  ( 20.36894250292379382, 43.67874883491397497, 10.36894250292379205 ) ) ;
#14435=CARTESIAN_POINT ( 'NONE',  ( -0.8801773607110991993, 47.85535201082150536, -2.915334737309923874 ) ) ;
#14436=FACE_OUTER_BOUND ( 'NONE', #709, .T. ) ;
#14438=CARTESIAN_POINT ( 'NONE',  ( 2.791683348922240793, 61.63393115100079456, 7.208316651077764092 ) ) ;
#14439=CARTESIAN_POINT ( 'NONE',  ( -25.69000000000001194, 93.50000000000000000, 9.500000000000000000 ) ) ;
#14440=CARTESIAN_POINT ( 'NONE',  ( 7.361572987183169658, 29.96726448433411960, -9.846743663894592657 ) ) ;
#14442=CARTESIAN_POINT ( 'NONE',  ( 2.791683348922240793, 36.63393115100078035, 7.208316651077764092 ) ) ;
#14444=CARTESIAN_POINT ( 'NONE',  ( 20.88017736071110519, 20.56368534415484106, 2.639326808657452039E-16 ) ) ;
#14445=CARTESIAN_POINT ( 'NONE',  ( 17.20831665107776587, 27.88393115100078390, 7.208316651077764980 ) ) ;
#14446=CARTESIAN_POINT ( 'NONE',  ( -1.099225684535947600, 19.54030133659708568, 6.408140936763237150 ) ) ;
#14447=CARTESIAN_POINT ( 'NONE',  ( 18.72515096720569971, 5.055090184799359676, 6.500000000000000000 ) ) ;
#14448=CARTESIAN_POINT ( 'NONE',  ( 12.91533473730993009, 61.60535201082150536, -10.88017736071109987 ) ) ;
#14449=CARTESIAN_POINT ( 'NONE',  ( 15.44008868035555260, 34.73035201082151247, 9.422509992056143702 ) ) ;
#14450=SURFACE_SIDE_STYLE ('',( #76898 ) ) ;
#14451=CARTESIAN_POINT ( 'NONE',  ( -2.266590686148945544, 41.38708216824729647, -7.082119434687050408 ) ) ;
#14455=CARTESIAN_POINT ( 'NONE',  ( 21.09922568453594849, 16.20696800326375353, 6.408140936763242479 ) ) ;
#14456=CARTESIAN_POINT ( 'NONE',  ( 17.96484262340118221, 6.188685344154836621, -7.964842623401177768 ) ) ;
#14457=CARTESIAN_POINT ( 'NONE',  ( 0.5774900079438607392, 53.48035201082151247, 5.440088680355550821 ) ) ;
#14458=( NAMED_UNIT ( * ) PLANE_ANGLE_UNIT ( ) SI_UNIT ( $, .RADIAN. ) );
#14460=CARTESIAN_POINT ( 'NONE',  ( 10.00000000000000178, 59.31368534415484106, 10.88017736071110342 ) ) ;
#14461=CARTESIAN_POINT ( 'NONE',  ( 19.84674366389459266, 38.30059781766745175, 2.638427012816836559 ) ) ;
#14462=CARTESIAN_POINT ( 'NONE',  ( 2.791683348922237240, 20.38393115100078745, -7.208316651077763204 ) ) ;
#14463=CARTESIAN_POINT ( 'NONE',  ( 10.00000000000000000, 9.758931151000785675, -9.846743663894594434 ) ) ;
#14465=CARTESIAN_POINT ( 'NONE',  ( 3.591859063236763294, 38.29030133659708923, -11.09922568453595026 ) ) ;
#14466=CARTESIAN_POINT ( 'NONE',  ( 17.20831665107776587, 17.88393115100078745, 7.208316651077764980 ) ) ;
#14469=CARTESIAN_POINT ( 'NONE',  ( 12.63842701281683922, 29.55059781766745175, -9.846743663894590881 ) ) ;
#14472=EDGE_CURVE ( 'NONE', #6265, #21520, #18331, .T. ) ;
#14473=CARTESIAN_POINT ( 'NONE',  ( -1.099225684535947600, 54.54030133659708923, 6.408140936763237150 ) ) ;
#14475=CARTESIAN_POINT ( 'NONE',  ( 10.00000000000000000, 12.87363466993042138, -12.81628187352647608 ) ) ;
#14477=CARTESIAN_POINT ( 'NONE',  ( 17.96484262340118221, 46.18868534415484106, -7.964842623401177768 ) ) ;
#14478=CARTESIAN_POINT ( 'NONE',  ( 20.36894250292379738, 34.92874883491396076, -10.36894250292379027 ) ) ;
#14480=AXIS2_PLACEMENT_3D ( 'NONE', #22394, #13396, #43879 ) ;
#14482=CARTESIAN_POINT ( 'NONE',  ( 1.932340009482166776, 41.49127512925448258, -6.500000000000040856 ) ) ;
#14483=CARTESIAN_POINT ( 'NONE',  ( 24.16423886937409904, 24.09541550158063927, 3.795296366450317205 ) ) ;
#14484=CARTESIAN_POINT ( 'NONE',  ( 22.26659068614895176, 39.72041550158063217, -7.082119434687042414 ) ) ;
#14485=CARTESIAN_POINT ( 'NONE',  ( 13.79529636645030344, 3.262082168247301350, 14.16423886937410614 ) ) ;
#14486=CARTESIAN_POINT ( 'NONE',  ( -2.266590686148945544, 12.22041550158063394, 7.082119434687048631 ) ) ;
#14487=CARTESIAN_POINT ( 'NONE',  ( -1.926860441876564023, 37.87045670184114954, 3.195792623639529761 ) ) ;
#14488=CARTESIAN_POINT ( 'NONE',  ( 2.035157376598822676, 47.43868534415484817, -7.964842623401177768 ) ) ;
#14490=CARTESIAN_POINT ( 'NONE',  ( 18.52753015748618282, 23.92559781766745530, -4.923371831947291888 ) ) ;
#14491=DIRECTION ( 'NONE',  ( 1.000000000000000000, 0.000000000000000000, 0.000000000000000000 ) ) ;
#14492=CARTESIAN_POINT ( 'NONE',  ( 1.472469842513823179, 26.42559781766745175, 4.923371831947296329 ) ) ;
#14493=VECTOR ( 'NONE', #85145, 1000.000000000000000 ) ;
#14495=CARTESIAN_POINT ( 'NONE',  ( 12.91533473730993009, 26.60535201082150536, -10.88017736071109987 ) ) ;
#14496=CARTESIAN_POINT ( 'NONE',  ( 16.40814093676323893, 60.79030133659709634, 11.09922568453595026 ) ) ;
#14499=CARTESIAN_POINT ( 'NONE',  ( 10.00000000000000000, 24.75893115100078745, -9.846743663894594434 ) ) ;
#14500=CARTESIAN_POINT ( 'NONE',  ( 16.40814093676324603, 47.45696800326375353, -11.09922568453594671 ) ) ;
#14502=CARTESIAN_POINT ( 'NONE',  ( 19.42250999205614193, 40.14701867748817676, 5.440088680355555262 ) ) ;
#14503=CARTESIAN_POINT ( 'NONE',  ( 19.84674366389459266, 53.71726448433411605, -2.638427012816827677 ) ) ;
#14504=CARTESIAN_POINT ( 'NONE',  ( -4.164238869374099039, 21.80374883491396787, 8.674139862899312516E-16 ) ) ;
#14507=CARTESIAN_POINT ( 'NONE',  ( -0.8801773607111008646, 68.27201867748817676, 2.915334737309923430 ) ) ;
#14509=CARTESIAN_POINT ( 'NONE',  ( -2.266590686148945544, 62.22041550158063927, 7.082119434687048631 ) ) ;
#14510=CARTESIAN_POINT ( 'NONE',  ( -1.099225684535947600, 4.540301336597087456, 6.408140936763237150 ) ) ;
#14512=CARTESIAN_POINT ( 'NONE',  ( 17.96484262340118221, 51.18868534415483396, -7.964842623401177768 ) ) ;
#14514=CARTESIAN_POINT ( 'NONE',  ( 6.000000000000000000, 10.49999999999999822, 6.500000000000000888 ) ) ;
#14515=CARTESIAN_POINT ( 'NONE',  ( 6.204703633549690345, 55.76208216824730357, -14.16423886937410259 ) ) ;
#14517=CARTESIAN_POINT ( 'NONE',  ( 20.88017736071110519, 10.56368534415483751, 2.639326808657452039E-16 ) ) ;
#14518=CARTESIAN_POINT ( 'NONE',  ( 4.559911319644449179, 27.23035201082150536, -9.422509992056141925 ) ) ;
#14519=CARTESIAN_POINT ( 'NONE',  ( 12.63842701281683034, 62.46726448433410894, 9.846743663894596210 ) ) ;
#14520=CARTESIAN_POINT ( 'NONE',  ( 21.09922568453594849, 46.20696800326376064, 6.408140936763242479 ) ) ;
#14524=CARTESIAN_POINT ( 'NONE',  ( 0.5774900079438607392, 13.48035201082150358, 5.440088680355550821 ) ) ;
#14525=CARTESIAN_POINT ( 'NONE',  ( 21.09922568453595559, 22.04030133659708923, -6.408140936763230044 ) ) ;
#14527=AXIS2_PLACEMENT_3D ( 'NONE', #44706, #75206, #37233 ) ;
#14528=CARTESIAN_POINT ( 'NONE',  ( 0.1532563361054083140, 51.00893115100078745, 1.131784320476157264E-15 ) ) ;
#14529=CARTESIAN_POINT ( 'NONE',  ( 0.5774900079438607392, 38.48035201082150536, 5.440088680355550821 ) ) ;
#14530=CARTESIAN_POINT ( 'NONE',  ( 22.81628187352648496, 26.83196800326374998, -3.434112377981050290 ) ) ;
#14531=CARTESIAN_POINT ( 'NONE',  ( 2.035157376598822676, 47.43868534415484817, -7.964842623401177768 ) ) ;
#14533=CARTESIAN_POINT ( 'NONE',  ( 13.43411237798106583, 47.66530133659709634, -12.81628187352647252 ) ) ;
#14534=VERTEX_POINT ( 'NONE', #71240 ) ;
#14535=CARTESIAN_POINT ( 'NONE',  ( 1.274849032794305170, 17.55509018479936145, -6.499999999999995559 ) ) ;
#14536=CARTESIAN_POINT ( 'NONE',  ( 20.88017736071110519, 50.56368534415484106, 2.639326808657452039E-16 ) ) ;
#14537=CARTESIAN_POINT ( 'NONE',  ( 0.6178305044545838731, 39.74863466993041072, 9.382169495545420901 ) ) ;
#14538=CARTESIAN_POINT ( 'NONE',  ( -0.3689425029237898834, 6.178748834913968757, -10.36894250292378850 ) ) ;
#14539=CARTESIAN_POINT ( 'NONE',  ( 20.88017736071110164, 45.35535201082149115, 2.915334737309930979 ) ) ;
#14540=CARTESIAN_POINT ( 'NONE',  ( 1.472469842513823179, 66.42559781766745175, 4.923371831947296329 ) ) ;
#14541=CARTESIAN_POINT ( 'NONE',  ( 1.472469842513823179, 61.42559781766745175, 4.923371831947296329 ) ) ;
#14542=CARTESIAN_POINT ( 'NONE',  ( 18.52753015748618282, 13.92559781766745175, -4.923371831947291888 ) ) ;
#14543=CARTESIAN_POINT ( 'NONE',  ( 17.20831665107776587, 12.88393115100078390, 7.208316651077764980 ) ) ;
#14545=CARTESIAN_POINT ( 'NONE',  ( 22.26659068614895176, 49.72041550158063927, -7.082119434687042414 ) ) ;
#14549=( BOUNDED_SURFACE ( )  B_SPLINE_SURFACE ( 1, 2, ( 
 ( #67944, #20471, #66448, #75435, #5963, #14956, #22450, #74438, #66952, #50958, #13453, #59439, #12955, #44439, #6949, #74941, #51955, #97470, #37950, #82440, #36953, #14456, #58954, #28934, #89941, #21458, #44928, #67450, #81944, #37456, #52923, #98468, #28460, #13964, #97971, #29427, #59932, #90420, #21960, #75928, #88963, #43939, #82939, #52441, #81454, #58448, #96983, #89454, #20970, #73952, #29921, #60427, #5479, #83436, #90920, #45423, #7453, #96483, #27955, #43451, #51455, #98962, #91423, #93388, #7938, #1434, #53920, #38434, #70408, #91917, #76424, #9401, #46898, #24422, #55397, #24913, #17414, #22951, #53417, #85897, #54886, #85402, #38927, #30418, #16421, #77389, #47880, #69914, #16914, #61897, #68932, #78384, #61408, #76907, #60918, #23927, #9904, #68442, #462, #62889, #83924, #30910, #8902, #15454, #45933, #937, #92404, #47387, #39419, #84429, #77889, #23441, #39902, #15926, #54398, #8420, #31887, #84909, #62385, #92890, #46417, #69414, #31397, #1926, #32384, #93881, #2421, #10391, #71396, #63856, #17892, #72839, #41884, #48376, #65337, #49849, #10880, #11365, #64353, #41404, #50338, #94370, #70901, #63376, #95863, #78880, #72348, #25888, #40895, #42366, #56387, #2910, #80358, #18878, #95357, #27346, #57839, #88348, #25408, #55895, #19846, #26856, #57353, #71870, #32878, #87364, #49360, #80849, #3880, #87846, #33844, #33361, #40407, #86876, #48865, #86391, #94861, #18386, #79375, #3381, #34842, #26364, #56863, #79862, #34344, #64838, #19366, #11858, #4377, #6324, #59809, #6823, #43334, #89334, #67829, #14334, #73826, #82317, #44807, #13837, #51829, #13336, #36834, #44318, #74819, #90303, #12834, #60313, #90805, #82814, #35339, #50845, #21838, #20844, #29804, #37339, #51336, #81818, #65832, #28336, #74316, #27837, #59319, #52321, #89818, #66827, #43820, #52807, #97349, #67325, #29313, #5359, #5842, #35838, #28820, #36332, #97848, #21339, #75313, #98347, #22333, #4863, #58826, #12346, #42853, #96364, #73336, #81337, #66326, #96861, #88841, #58324, #20349, #60798, #9283, #92776, #53805, #54276, #8306, #84316, #93270, #7822, #14838, #7330, #39792, #22822, #16302, #68813, #53301, #85286, #38317, #91298, #24305, #61782, #39306, #70292, #1807, #32264, #37831, #68321, #62769, #69798, #1323, #15816, #45312, #31282, #92292, #24794, #84793, #31774, #76789, #83809, #83314, #76305, #91802, #75808, #38806, #98840, #30295, #15335, #77771, #45817, #346, #23815, #30788, #61293, #23324, #46783, #46302, #77277, #62267, #69302, #824, #8787, #54767, #16794, #47270, #26250, #57230, #56745, #94745, #56270, #79747, #87239, #18764 ),
 ( #4252, #33730, #25291, #42247, #10275, #86762, #55775, #18267, #41280, #49245, #10765, #11738, #11243, #86269, #41763, #72234, #40279, #48746, #3764, #34221, #64230, #34722, #26736, #64718, #72717, #95227, #33250, #79254, #63255, #40773, #55270, #87728, #71754, #19241, #3263, #71275, #49723, #80232, #17781, #93763, #65215, #95740, #85782, #47769, #17293, #2797, #78267, #9781, #70786, #48256, #2303, #63743, #32759, #78766, #94246, #25775, #59199, #81702, #82699, #89703, #96239, #82202, #21217, #12225, #20727, #28708, #51719, #5728, #6705, #97735, #66715, #44698, #36720, #75194, #97239, #36215, #44196, #65713, #29197, #89214, #51216, #13713, #43212, #66207, #74706, #27719, #43708, #14218, #27222, #67210, #37225, #67710, #35718, #13214, #6216, #74195, #96739, #59695, #57720, #90192, #21722, #20226, #28214, #58200, #80730, #88221, #58712, #19731, #50217, #88716, #52205, #42735, #73213, #4744, #35210, #50731, #81219, #12720, #73707, #5240, #46189, #7205, #16677, #60683, #39184, #1202, #53190, #30671, #84195, #54163, #37706, #53678, #83197, #68207, #92177, #61655, #47149, #98729, #84675, #15211, #91182, #9164, #61179, #54650, #77164, #77650, #46666, #39682, #31165, #16183, #60193, #23703, #75693, #91684, #76189, #68691, #22216, #45690, #23203, #14721, #76673, #8672, #8192, #15704, #38204, #98223, #38689, #69188, #69673, #22708, #7709, #711, #31660, #62147, #92655, #83693, #24181, #85168, #29684, #30179, #90688, #222, #52693, #45195, #64111, #18153, #49601, #62643, #17665, #56631, #2679, #24672, #32142, #40158, #2185, #93643, #47658, #3641, #71642, #78152, #95107, #79629, #40655, #41157, #94131, #71153, #80110, #25176, #1688, #93148, #26614, #9663, #3150, #55657, #70664, #72115, #86154, #32644, #11130, #48627, #26138, #57111, #87609, #19120, #55143, #85657, #11617, #87119, #18637, #33130, #17176, #79131, #10643, #70172, #33615, #49127, #63625, #63140, #48138, #78653, #10158, #25658, #56151, #86645, #94627, #41648, #64597, #34106, #12110, #81584, #34598, #95616, #80615, #20607, #72599, #36089, #89589, #36601, #73091, #20102, #97616, #44074, #4629, #13093, #74582, #43589, #74078, #43099, #66594, #5611, #97121, #21098, #42612, #90074, #21600, #13592, #65092, #35092, #51598, #50605, #59581, #67088, #28592, #58591, #81097, #59082, #42133, #82082, #6097, #65591, #12599, #96117, #27103, #52089, #73586, #82582, #4135, #27601, #28093, #5110, #29076, #57603, #88103, #51096, #19612, #58089, #50107, #88593, #89093, #35599, #66087, #96616, #54051, #16064, #68083, #45569, #108, #69068, #52574, #68576, #98101, #83078, #8074, #76556, #31540 ) ),
 .UNSPECIFIED., .F., .F., .F. ) 
 B_SPLINE_SURFACE_WITH_KNOTS ( ( 2, 2 ),
 ( 3, 2, 2, 2, 2, 2, 2, 2, 2, 2, 2, 2, 2, 2, 2, 2, 2, 2, 2, 2, 2, 2, 2, 2, 2, 2, 2, 2, 2, 2, 2, 2, 2, 2, 2, 2, 2, 2, 2, 2, 2, 2, 2, 2, 2, 2, 2, 2, 2, 2, 2, 2, 2, 2, 2, 2, 2, 2, 2, 2, 2, 2, 2, 2, 2, 2, 2, 2, 2, 2, 2, 2, 2, 2, 2, 2, 2, 2, 2, 2, 2, 2, 2, 2, 2, 2, 2, 2, 2, 2, 2, 2, 2, 2, 2, 2, 2, 2, 2, 2, 2, 2, 2, 2, 2, 2, 2, 2, 2, 2, 2, 2, 2, 2, 2, 2, 2, 2, 2, 2, 2, 2, 2, 2, 2, 2, 2, 2, 2, 2, 2, 2, 2, 2, 2, 2, 2, 2, 2, 2, 2, 2, 2, 2, 2, 2, 2, 2, 2, 2, 2, 2, 2, 2, 2, 2, 2, 2, 2, 2, 2, 2, 3 ),
 ( 0.000000000000000000, 1.000000000000000000 ),
 ( 0.000000000000000000, 0.005952380952380952051, 0.01190476190476190410, 0.01785714285714285615, 0.02380952380952380820, 0.02976190476190476025, 0.03571428571428571230, 0.04166666666666666435, 0.04761904761904761640, 0.05357142857142856845, 0.05952380952380952051, 0.06547619047619047949, 0.07142857142857142461, 0.07738095238095238360, 0.08333333333333332871, 0.08928571428571428770, 0.09523809523809523281, 0.1011904761904761918, 0.1071428571428571369, 0.1130952380952380959, 0.1190476190476190410, 0.1250000000000000000, 0.1309523809523809590, 0.1369047619047619180, 0.1428571428571428492, 0.1488095238095238082, 0.1547619047619047672, 0.1607142857142857262, 0.1666666666666666574, 0.1726190476190476164, 0.1785714285714285754, 0.1845238095238095344, 0.1904761904761904656, 0.1964285714285714246, 0.2023809523809523836, 0.2083333333333333426, 0.2142857142857142738, 0.2202380952380952328, 0.2261904761904761918, 0.2321428571428571508, 0.2380952380952380820, 0.2440476190476190410, 0.2500000000000000000, 0.2559523809523809312, 0.2619047619047619180, 0.2678571428571428492, 0.2738095238095238360, 0.2797619047619047672, 0.2857142857142856984, 0.2916666666666666852, 0.2976190476190476164, 0.3035714285714285476, 0.3095238095238095344, 0.3154761904761904656, 0.3214285714285714524, 0.3273809523809523836, 0.3333333333333333148, 0.3392857142857143016, 0.3452380952380952328, 0.3511904761904761640, 0.3571428571428571508, 0.3630952380952380820, 0.3690476190476190688, 0.3750000000000000000, 0.3809523809523809312, 0.3869047619047619180, 0.3928571428571428492, 0.3988095238095238360, 0.4047619047619047672, 0.4107142857142856984, 0.4166666666666666852, 0.4226190476190476164, 0.4285714285714285476, 0.4345238095238095344, 0.4404761904761904656, 0.4464285714285714524, 0.4523809523809523836, 0.4583333333333333148, 0.4642857142857143016, 0.4702380952380952328, 0.4761904761904761640, 0.4821428571428571508, 0.4880952380952380820, 0.4940476190476190688, 0.5000000000000000000, 0.5059523809523809312, 0.5119047619047618625, 0.5178571428571429047, 0.5238095238095238360, 0.5297619047619047672, 0.5357142857142856984, 0.5416666666666666297, 0.5476190476190476719, 0.5535714285714286031, 0.5595238095238095344, 0.5654761904761904656, 0.5714285714285713969, 0.5773809523809523281, 0.5833333333333333703, 0.5892857142857143016, 0.5952380952380952328, 0.6011904761904761640, 0.6071428571428570953, 0.6130952380952381375, 0.6190476190476190688, 0.6250000000000000000, 0.6309523809523809312, 0.6369047619047618625, 0.6428571428571429047, 0.6488095238095238360, 0.6547619047619047672, 0.6607142857142856984, 0.6666666666666666297, 0.6726190476190476719, 0.6785714285714286031, 0.6845238095238095344, 0.6904761904761904656, 0.6964285714285713969, 0.7023809523809523281, 0.7083333333333333703, 0.7142857142857143016, 0.7202380952380952328, 0.7261904761904761640, 0.7321428571428570953, 0.7380952380952381375, 0.7440476190476190688, 0.7500000000000000000, 0.7559523809523809312, 0.7619047619047618625, 0.7678571428571429047, 0.7738095238095238360, 0.7797619047619047672, 0.7857142857142856984, 0.7916666666666666297, 0.7976190476190476719, 0.8035714285714286031, 0.8095238095238095344, 0.8154761904761904656, 0.8214285714285713969, 0.8273809523809523281, 0.8333333333333333703, 0.8392857142857143016, 0.8452380952380952328, 0.8511904761904761640, 0.8571428571428570953, 0.8630952380952381375, 0.8690476190476190688, 0.8750000000000000000, 0.8809523809523809312, 0.8869047619047618625, 0.8928571428571429047, 0.8988095238095238360, 0.9047619047619047672, 0.9107142857142856984, 0.9166666666666666297, 0.9226190476190476719, 0.9285714285714286031, 0.9345238095238095344, 0.9404761904761904656, 0.9464285714285713969, 0.9523809523809523281, 0.9583333333333333703, 0.9642857142857143016 ),
 .UNSPECIFIED. ) 
 GEOMETRIC_REPRESENTATION_ITEM ( )  RATIONAL_B_SPLINE_SURFACE ( (
 ( 1.000000000000000000, 0.9659258262890683122, 1.000000000000000000, 0.9659258262890683122, 1.000000000000000000, 0.9659258262890683122, 1.000000000000000000, 0.9659258262890683122, 1.000000000000000000, 0.9659258262890683122, 1.000000000000000000, 0.9659258262890683122, 1.000000000000000000, 0.9659258262890683122, 1.000000000000000000, 0.9659258262890683122, 1.000000000000000000, 0.9659258262890683122, 1.000000000000000000, 0.9659258262890683122, 1.000000000000000000, 0.9659258262890683122, 1.000000000000000000, 0.9659258262890683122, 1.000000000000000000, 0.9659258262890683122, 1.000000000000000000, 0.9659258262890683122, 1.000000000000000000, 0.9659258262890683122, 1.000000000000000000, 0.9659258262890683122, 1.000000000000000000, 0.9659258262890683122, 1.000000000000000000, 0.9659258262890683122, 1.000000000000000000, 0.9659258262890683122, 1.000000000000000000, 0.9659258262890683122, 1.000000000000000000, 0.9659258262890683122, 1.000000000000000000, 0.9659258262890683122, 1.000000000000000000, 0.9659258262890683122, 1.000000000000000000, 0.9659258262890683122, 1.000000000000000000, 0.9659258262890683122, 1.000000000000000000, 0.9659258262890683122, 1.000000000000000000, 0.9659258262890683122, 1.000000000000000000, 0.9659258262890683122, 1.000000000000000000, 0.9659258262890683122, 1.000000000000000000, 0.9659258262890683122, 1.000000000000000000, 0.9659258262890683122, 1.000000000000000000, 0.9659258262890683122, 1.000000000000000000, 0.9659258262890683122, 1.000000000000000000, 0.9659258262890683122, 1.000000000000000000, 0.9659258262890683122, 1.000000000000000000, 0.9659258262890683122, 1.000000000000000000, 0.9659258262890683122, 1.000000000000000000, 0.9659258262890683122, 1.000000000000000000, 0.9659258262890683122, 1.000000000000000000, 0.9659258262890683122, 1.000000000000000000, 0.9659258262890683122, 1.000000000000000000, 0.9659258262890683122, 1.000000000000000000, 0.9659258262890683122, 1.000000000000000000, 0.9659258262890683122, 1.000000000000000000, 0.9659258262890683122, 1.000000000000000000, 0.9659258262890683122, 1.000000000000000000, 0.9659258262890683122, 1.000000000000000000, 0.9659258262890683122, 1.000000000000000000, 0.9659258262890683122, 1.000000000000000000, 0.9659258262890683122, 1.000000000000000000, 0.9659258262890683122, 1.000000000000000000, 0.9659258262890683122, 1.000000000000000000, 0.9659258262890683122, 1.000000000000000000, 0.9659258262890683122, 1.000000000000000000, 0.9659258262890683122, 1.000000000000000000, 0.9659258262890683122, 1.000000000000000000, 0.9659258262890683122, 1.000000000000000000, 0.9659258262890683122, 1.000000000000000000, 0.9659258262890683122, 1.000000000000000000, 0.9659258262890683122, 1.000000000000000000, 0.9659258262890683122, 1.000000000000000000, 0.9659258262890683122, 1.000000000000000000, 0.9659258262890683122, 1.000000000000000000, 0.9659258262890683122, 1.000000000000000000, 0.9659258262890683122, 1.000000000000000000, 0.9659258262890683122, 1.000000000000000000, 0.9659258262890683122, 1.000000000000000000, 0.9659258262890683122, 1.000000000000000000, 0.9659258262890683122, 1.000000000000000000, 0.9659258262890683122, 1.000000000000000000, 0.9659258262890683122, 1.000000000000000000, 0.9659258262890683122, 1.000000000000000000, 0.9659258262890683122, 1.000000000000000000, 0.9659258262890683122, 1.000000000000000000, 0.9659258262890683122, 1.000000000000000000, 0.9659258262890683122, 1.000000000000000000, 0.9659258262890683122, 1.000000000000000000, 0.9659258262890683122, 1.000000000000000000, 0.9659258262890683122, 1.000000000000000000, 0.9659258262890683122, 1.000000000000000000, 0.9659258262890683122, 1.000000000000000000, 0.9659258262890683122, 1.000000000000000000, 0.9659258262890683122, 1.000000000000000000, 0.9659258262890683122, 1.000000000000000000, 0.9659258262890683122, 1.000000000000000000, 0.9659258262890683122, 1.000000000000000000, 0.9659258262890683122, 1.000000000000000000, 0.9659258262890683122, 1.000000000000000000, 0.9659258262890683122, 1.000000000000000000, 0.9659258262890683122, 1.000000000000000000, 0.9659258262890683122, 1.000000000000000000, 0.9659258262890683122, 1.000000000000000000, 0.9659258262890683122, 1.000000000000000000, 0.9659258262890683122, 1.000000000000000000, 0.9659258262890683122, 1.000000000000000000, 0.9659258262890683122, 1.000000000000000000, 0.9659258262890683122, 1.000000000000000000, 0.9659258262890683122, 1.000000000000000000, 0.9659258262890683122, 1.000000000000000000, 0.9659258262890683122, 1.000000000000000000, 0.9659258262890683122, 1.000000000000000000, 0.9659258262890683122, 1.000000000000000000, 0.9659258262890683122, 1.000000000000000000, 0.9659258262890683122, 1.000000000000000000, 0.9659258262890683122, 1.000000000000000000, 0.9659258262890683122, 1.000000000000000000, 0.9659258262890683122, 1.000000000000000000, 0.9659258262890683122, 1.000000000000000000, 0.9659258262890683122, 1.000000000000000000, 0.9659258262890683122, 1.000000000000000000, 0.9659258262890683122, 1.000000000000000000, 0.9659258262890683122, 1.000000000000000000, 0.9659258262890683122, 1.000000000000000000, 0.9659258262890683122, 1.000000000000000000, 0.9659258262890683122, 1.000000000000000000, 0.9659258262890683122, 1.000000000000000000, 0.9659258262890683122, 1.000000000000000000, 0.9659258262890683122, 1.000000000000000000, 0.9659258262890683122, 1.000000000000000000, 0.9659258262890683122, 1.000000000000000000, 0.9659258262890683122, 1.000000000000000000, 0.9659258262890683122, 1.000000000000000000, 0.9659258262890683122, 1.000000000000000000, 0.9659258262890683122, 1.000000000000000000, 0.9659258262890683122, 1.000000000000000000, 0.9659258262890683122, 1.000000000000000000, 0.9659258262890683122, 1.000000000000000000, 0.9659258262890683122, 1.000000000000000000, 0.9659258262890683122, 1.000000000000000000, 0.9659258262890683122, 1.000000000000000000, 0.9659258262890683122, 1.000000000000000000, 0.9659258262890683122, 1.000000000000000000, 0.9659258262890683122, 1.000000000000000000, 0.9659258262890683122, 1.000000000000000000, 0.9659258262890683122, 1.000000000000000000, 0.9659258262890683122, 1.000000000000000000, 0.9659258262890683122, 1.000000000000000000, 0.9659258262890683122, 1.000000000000000000, 0.9659258262890683122, 1.000000000000000000, 0.9659258262890683122, 1.000000000000000000, 0.9659258262890683122, 1.000000000000000000, 0.9659258262890683122, 1.000000000000000000, 0.9659258262890683122, 1.000000000000000000, 0.9659258262890683122, 1.000000000000000000, 0.9659258262890683122, 1.000000000000000000, 0.9659258262890683122, 1.000000000000000000, 0.9659258262890683122, 1.000000000000000000, 0.9659258262890683122, 1.000000000000000000, 0.9659258262890683122, 1.000000000000000000, 0.9659258262890683122, 1.000000000000000000, 0.9659258262890683122, 1.000000000000000000, 0.9659258262890683122, 1.000000000000000000, 0.9659258262890683122, 1.000000000000000000, 0.9659258262890683122, 1.000000000000000000, 0.9659258262890683122, 1.000000000000000000, 0.9659258262890683122, 1.000000000000000000, 0.9659258262890683122, 1.000000000000000000, 0.9659258262890683122, 1.000000000000000000, 0.9659258262890683122, 1.000000000000000000, 0.9659258262890683122, 1.000000000000000000, 0.9659258262890683122, 1.000000000000000000, 0.9659258262890683122, 1.000000000000000000),
 ( 1.000000000000000000, 0.9659258262890683122, 1.000000000000000000, 0.9659258262890683122, 1.000000000000000000, 0.9659258262890683122, 1.000000000000000000, 0.9659258262890683122, 1.000000000000000000, 0.9659258262890683122, 1.000000000000000000, 0.9659258262890683122, 1.000000000000000000, 0.9659258262890683122, 1.000000000000000000, 0.9659258262890683122, 1.000000000000000000, 0.9659258262890683122, 1.000000000000000000, 0.9659258262890683122, 1.000000000000000000, 0.9659258262890683122, 1.000000000000000000, 0.9659258262890683122, 1.000000000000000000, 0.9659258262890683122, 1.000000000000000000, 0.9659258262890683122, 1.000000000000000000, 0.9659258262890683122, 1.000000000000000000, 0.9659258262890683122, 1.000000000000000000, 0.9659258262890683122, 1.000000000000000000, 0.9659258262890683122, 1.000000000000000000, 0.9659258262890683122, 1.000000000000000000, 0.9659258262890683122, 1.000000000000000000, 0.9659258262890683122, 1.000000000000000000, 0.9659258262890683122, 1.000000000000000000, 0.9659258262890683122, 1.000000000000000000, 0.9659258262890683122, 1.000000000000000000, 0.9659258262890683122, 1.000000000000000000, 0.9659258262890683122, 1.000000000000000000, 0.9659258262890683122, 1.000000000000000000, 0.9659258262890683122, 1.000000000000000000, 0.9659258262890683122, 1.000000000000000000, 0.9659258262890683122, 1.000000000000000000, 0.9659258262890683122, 1.000000000000000000, 0.9659258262890683122, 1.000000000000000000, 0.9659258262890683122, 1.000000000000000000, 0.9659258262890683122, 1.000000000000000000, 0.9659258262890683122, 1.000000000000000000, 0.9659258262890683122, 1.000000000000000000, 0.9659258262890683122, 1.000000000000000000, 0.9659258262890683122, 1.000000000000000000, 0.9659258262890683122, 1.000000000000000000, 0.9659258262890683122, 1.000000000000000000, 0.9659258262890683122, 1.000000000000000000, 0.9659258262890683122, 1.000000000000000000, 0.9659258262890683122, 1.000000000000000000, 0.9659258262890683122, 1.000000000000000000, 0.9659258262890683122, 1.000000000000000000, 0.9659258262890683122, 1.000000000000000000, 0.9659258262890683122, 1.000000000000000000, 0.9659258262890683122, 1.000000000000000000, 0.9659258262890683122, 1.000000000000000000, 0.9659258262890683122, 1.000000000000000000, 0.9659258262890683122, 1.000000000000000000, 0.9659258262890683122, 1.000000000000000000, 0.9659258262890683122, 1.000000000000000000, 0.9659258262890683122, 1.000000000000000000, 0.9659258262890683122, 1.000000000000000000, 0.9659258262890683122, 1.000000000000000000, 0.9659258262890683122, 1.000000000000000000, 0.9659258262890683122, 1.000000000000000000, 0.9659258262890683122, 1.000000000000000000, 0.9659258262890683122, 1.000000000000000000, 0.9659258262890683122, 1.000000000000000000, 0.9659258262890683122, 1.000000000000000000, 0.9659258262890683122, 1.000000000000000000, 0.9659258262890683122, 1.000000000000000000, 0.9659258262890683122, 1.000000000000000000, 0.9659258262890683122, 1.000000000000000000, 0.9659258262890683122, 1.000000000000000000, 0.9659258262890683122, 1.000000000000000000, 0.9659258262890683122, 1.000000000000000000, 0.9659258262890683122, 1.000000000000000000, 0.9659258262890683122, 1.000000000000000000, 0.9659258262890683122, 1.000000000000000000, 0.9659258262890683122, 1.000000000000000000, 0.9659258262890683122, 1.000000000000000000, 0.9659258262890683122, 1.000000000000000000, 0.9659258262890683122, 1.000000000000000000, 0.9659258262890683122, 1.000000000000000000, 0.9659258262890683122, 1.000000000000000000, 0.9659258262890683122, 1.000000000000000000, 0.9659258262890683122, 1.000000000000000000, 0.9659258262890683122, 1.000000000000000000, 0.9659258262890683122, 1.000000000000000000, 0.9659258262890683122, 1.000000000000000000, 0.9659258262890683122, 1.000000000000000000, 0.9659258262890683122, 1.000000000000000000, 0.9659258262890683122, 1.000000000000000000, 0.9659258262890683122, 1.000000000000000000, 0.9659258262890683122, 1.000000000000000000, 0.9659258262890683122, 1.000000000000000000, 0.9659258262890683122, 1.000000000000000000, 0.9659258262890683122, 1.000000000000000000, 0.9659258262890683122, 1.000000000000000000, 0.9659258262890683122, 1.000000000000000000, 0.9659258262890683122, 1.000000000000000000, 0.9659258262890683122, 1.000000000000000000, 0.9659258262890683122, 1.000000000000000000, 0.9659258262890683122, 1.000000000000000000, 0.9659258262890683122, 1.000000000000000000, 0.9659258262890683122, 1.000000000000000000, 0.9659258262890683122, 1.000000000000000000, 0.9659258262890683122, 1.000000000000000000, 0.9659258262890683122, 1.000000000000000000, 0.9659258262890683122, 1.000000000000000000, 0.9659258262890683122, 1.000000000000000000, 0.9659258262890683122, 1.000000000000000000, 0.9659258262890683122, 1.000000000000000000, 0.9659258262890683122, 1.000000000000000000, 0.9659258262890683122, 1.000000000000000000, 0.9659258262890683122, 1.000000000000000000, 0.9659258262890683122, 1.000000000000000000, 0.9659258262890683122, 1.000000000000000000, 0.9659258262890683122, 1.000000000000000000, 0.9659258262890683122, 1.000000000000000000, 0.9659258262890683122, 1.000000000000000000, 0.9659258262890683122, 1.000000000000000000, 0.9659258262890683122, 1.000000000000000000, 0.9659258262890683122, 1.000000000000000000, 0.9659258262890683122, 1.000000000000000000, 0.9659258262890683122, 1.000000000000000000, 0.9659258262890683122, 1.000000000000000000, 0.9659258262890683122, 1.000000000000000000, 0.9659258262890683122, 1.000000000000000000, 0.9659258262890683122, 1.000000000000000000, 0.9659258262890683122, 1.000000000000000000, 0.9659258262890683122, 1.000000000000000000, 0.9659258262890683122, 1.000000000000000000, 0.9659258262890683122, 1.000000000000000000, 0.9659258262890683122, 1.000000000000000000, 0.9659258262890683122, 1.000000000000000000, 0.9659258262890683122, 1.000000000000000000, 0.9659258262890683122, 1.000000000000000000, 0.9659258262890683122, 1.000000000000000000, 0.9659258262890683122, 1.000000000000000000, 0.9659258262890683122, 1.000000000000000000, 0.9659258262890683122, 1.000000000000000000, 0.9659258262890683122, 1.000000000000000000, 0.9659258262890683122, 1.000000000000000000, 0.9659258262890683122, 1.000000000000000000, 0.9659258262890683122, 1.000000000000000000, 0.9659258262890683122, 1.000000000000000000, 0.9659258262890683122, 1.000000000000000000, 0.9659258262890683122, 1.000000000000000000, 0.9659258262890683122, 1.000000000000000000, 0.9659258262890683122, 1.000000000000000000, 0.9659258262890683122, 1.000000000000000000, 0.9659258262890683122, 1.000000000000000000, 0.9659258262890683122, 1.000000000000000000, 0.9659258262890683122, 1.000000000000000000, 0.9659258262890683122, 1.000000000000000000, 0.9659258262890683122, 1.000000000000000000, 0.9659258262890683122, 1.000000000000000000, 0.9659258262890683122, 1.000000000000000000, 0.9659258262890683122, 1.000000000000000000, 0.9659258262890683122, 1.000000000000000000, 0.9659258262890683122, 1.000000000000000000, 0.9659258262890683122, 1.000000000000000000, 0.9659258262890683122, 1.000000000000000000, 0.9659258262890683122, 1.000000000000000000, 0.9659258262890683122, 1.000000000000000000, 0.9659258262890683122, 1.000000000000000000, 0.9659258262890683122, 1.000000000000000000, 0.9659258262890683122, 1.000000000000000000) ) ) 
 REPRESENTATION_ITEM ( '' )  SURFACE ( )  );
#14552=CARTESIAN_POINT ( 'NONE',  ( -4.164238869374099039, 66.80374883491396076, 8.674139862899312516E-16 ) ) ;
#14553=CARTESIAN_POINT ( 'NONE',  ( -2.266590686148945544, 62.22041550158063927, 7.082119434687048631 ) ) ;
#14554=CARTESIAN_POINT ( 'NONE',  ( 0.1532563361054082862, 36.21726448433410894, 2.638427012816831674 ) ) ;
#14555=CARTESIAN_POINT ( 'NONE',  ( 6.565887622018943937, 45.16530133659708923, 12.81628187352647430 ) ) ;
#14557=CARTESIAN_POINT ( 'NONE',  ( 17.08211943468705840, 10.13708216824730179, -12.26659068614894466 ) ) ;
#14558=CARTESIAN_POINT ( 'NONE',  ( 7.084665262690076126, 9.105352010821503583, 10.88017736071109987 ) ) ;
#14559=CARTESIAN_POINT ( 'NONE',  ( 22.26659068614894466, 53.88708216824731068, 7.082119434687054849 ) ) ;
#14560=CARTESIAN_POINT ( 'NONE',  ( 2.791683348922240793, 46.63393115100077324, 7.208316651077764092 ) ) ;
#14562=CARTESIAN_POINT ( 'NONE',  ( 17.20831665107776587, 22.88393115100078745, 7.208316651077764980 ) ) ;
#14565=FACE_OUTER_BOUND ( 'NONE', #74792, .T. ) ;
#14567=VERTEX_POINT ( 'NONE', #17748 ) ;
#14570=EDGE_LOOP ( 'NONE', ( #73425, #27850, #11071, #70629 ) ) ;
#14571=CARTESIAN_POINT ( 'NONE',  ( 2.791683348922237240, 50.38393115100078035, -7.208316651077763204 ) ) ;
#14572=CARTESIAN_POINT ( 'NONE',  ( 20.36894250292379382, 18.67874883491397142, 10.36894250292379205 ) ) ;
#14573=CARTESIAN_POINT ( 'NONE',  ( 10.00000000000000178, 39.31368534415484106, 10.88017736071110342 ) ) ;
#14574=CARTESIAN_POINT ( 'NONE',  ( 2.035157376598822676, 37.43868534415484106, -7.964842623401177768 ) ) ;
#14575=CARTESIAN_POINT ( 'NONE',  ( 7.361572987183169658, 59.96726448433410894, -9.846743663894592657 ) ) ;
#14576=CARTESIAN_POINT ( 'NONE',  ( 3.591859063236763294, 33.29030133659708213, -11.09922568453595026 ) ) ;
#14577=CARTESIAN_POINT ( 'NONE',  ( -0.3689425029237881626, 2.428748834913967869, 10.36894250292379027 ) ) ;
#14579=CARTESIAN_POINT ( 'NONE',  ( 6.565887622018943937, 28.08196800326375353, -12.81628187352647608 ) ) ;
#14581=CARTESIAN_POINT ( 'NONE',  ( 19.84674366389459266, 38.71726448433412315, -2.638427012816827677 ) ) ;
#14582=CARTESIAN_POINT ( 'NONE',  ( 2.035157376598822676, 12.43868534415483751, -7.964842623401177768 ) ) ;
#14584=CARTESIAN_POINT ( 'NONE',  ( 10.00000000000000000, 16.81368534415483751, -10.88017736071110342 ) ) ;
#14586=CARTESIAN_POINT ( 'NONE',  ( 20.88017736071110875, 65.77201867748817676, -2.915334737309920765 ) ) ;
#14587=CARTESIAN_POINT ( 'NONE',  ( 20.88017736071110164, 55.35535201082149825, 2.915334737309930979 ) ) ;
#14588=CARTESIAN_POINT ( 'NONE',  ( 20.88017736071110519, 65.56368534415483396, 2.639326808657452039E-16 ) ) ;
#14589=EDGE_CURVE ( 'NONE', #88856, #5496, #77248, .T. ) ;
#14590=CARTESIAN_POINT ( 'NONE',  ( 4.559911319644449179, 53.89701867748817676, 9.422509992056141925 ) ) ;
#14593=CARTESIAN_POINT ( 'NONE',  ( -0.2418659066527493184, 30.11633188102328162, 6.114288769123083611 ) ) ;
#14596=( NAMED_UNIT ( * ) SI_UNIT ( $, .STERADIAN. ) SOLID_ANGLE_UNIT ( ) );
#14597=EDGE_LOOP ( 'NONE', ( #56864, #26283, #47747, #47972 ) ) ;
#14600=CARTESIAN_POINT ( 'NONE',  ( 12.63842701281683922, 44.55059781766745175, -9.846743663894590881 ) ) ;
#14604=LINE ( 'NONE', #38573, #62141 ) ;
#14606=CARTESIAN_POINT ( 'NONE',  ( -0.3689425029237898834, 6.178748834913968757, -10.36894250292378850 ) ) ;
#14608=CARTESIAN_POINT ( 'NONE',  ( -1.926860441876564023, 7.870456701841140656, 3.195792623639529761 ) ) ;
#14609=CARTESIAN_POINT ( 'NONE',  ( -46.94000000000003325, 103.1207406662227157, -5.953111867825573000 ) ) ;
#14610=CARTESIAN_POINT ( 'NONE',  ( 2.035157376598822676, 2.438685344154838397, -7.964842623401177768 ) ) ;
#14611=DIRECTION ( 'NONE',  ( -0.000000000000000000, 0.000000000000000000, -1.000000000000000000 ) ) ;
#14612=CARTESIAN_POINT ( 'NONE',  ( -2.816281873526471635, 38.91530133659708213, -3.434112377981056508 ) ) ;
#14615=CARTESIAN_POINT ( 'NONE',  ( 1.472469842513823179, 45.59226448433412315, -4.923371831947296329 ) ) ;
#14617=CARTESIAN_POINT ( 'NONE',  ( 17.39651004071890128, 29.08210964143323096, -6.499999999999448441 ) ) ;
#14618=CARTESIAN_POINT ( 'NONE',  ( 6.565887622018943937, 25.16530133659708213, 12.81628187352647430 ) ) ;
#14619=CARTESIAN_POINT ( 'NONE',  ( 1.472469842513823179, 21.42559781766745175, 4.923371831947296329 ) ) ;
#14621=CARTESIAN_POINT ( 'NONE',  ( 6.565887622018943937, 3.081968003263753531, -12.81628187352647608 ) ) ;
#14626=CARTESIAN_POINT ( 'NONE',  ( -0.8801773607111009756, 23.06368534415484106, 1.068504757029289695E-15 ) ) ;
#14627=CARTESIAN_POINT ( 'NONE',  ( 24.16423886937410614, 19.51208216824729647, -3.795296366450302550 ) ) ;
#14628=CARTESIAN_POINT ( 'NONE',  ( 0.1532563361054082862, 26.21726448433411605, 2.638427012816831674 ) ) ;
#14629=CARTESIAN_POINT ( 'NONE',  ( 7.084665262690076126, 62.02201867748816966, -10.88017736071110164 ) ) ;
#14630=CARTESIAN_POINT ( 'NONE',  ( 21.09922568453595559, 37.04030133659708923, -6.408140936763230044 ) ) ;
#14632=CARTESIAN_POINT ( 'NONE',  ( 15.44008868035555793, 11.39701867748817143, -9.422509992056140149 ) ) ;
#14634=CARTESIAN_POINT ( 'NONE',  ( 0.2751277870542914172, 43.21833443783938122, 6.499999999999992006 ) ) ;
#14635=CARTESIAN_POINT ( 'NONE',  ( -1.099225684535947600, 14.54030133659708568, 6.408140936763237150 ) ) ;
#14636=CARTESIAN_POINT ( 'NONE',  ( 19.38216949554541557, 12.24863466993041961, -9.382169495545420901 ) ) ;
#14637=CARTESIAN_POINT ( 'NONE',  ( 2.791683348922240793, 21.63393115100078745, 7.208316651077764092 ) ) ;
#14639=CARTESIAN_POINT ( 'NONE',  ( 6.565887622018943937, 38.08196800326376064, -12.81628187352647608 ) ) ;
#14642=CARTESIAN_POINT ( 'NONE',  ( 10.00000000000000000, 36.81368534415484106, -10.88017736071110342 ) ) ;
#14646=CARTESIAN_POINT ( 'NONE',  ( 15.44008868035555260, 34.73035201082151247, 9.422509992056143702 ) ) ;
#14647=CARTESIAN_POINT ( 'NONE',  ( 10.00000000000000178, 44.31368534415484106, 10.88017736071110342 ) ) ;
#14648=CARTESIAN_POINT ( 'NONE',  ( 5.076628168052704559, 65.17559781766745175, -8.527530157486179263 ) ) ;
#14649=CARTESIAN_POINT ( 'NONE',  ( 12.91533473730993009, 66.60535201082150536, -10.88017736071109987 ) ) ;
#14650=CARTESIAN_POINT ( 'NONE',  ( 10.00000000000000000, 39.75893115100078745, -9.846743663894594434 ) ) ;
#14651=CARTESIAN_POINT ( 'NONE',  ( 10.00000000000000178, 4.313685344154837509, 10.88017736071110342 ) ) ;
#14652=CARTESIAN_POINT ( 'NONE',  ( 3.591859063236763294, 18.29030133659708568, -11.09922568453595026 ) ) ;
#14653=EDGE_LOOP ( 'NONE', ( #75162, #40145, #96122, #13591 ) ) ;
#14654=CARTESIAN_POINT ( 'NONE',  ( 12.91533473730993009, 21.60535201082150536, -10.88017736071109987 ) ) ;
#14656=CARTESIAN_POINT ( 'NONE',  ( 15.44008868035555793, 21.39701867748817321, -9.422509992056140149 ) ) ;
#14657=CARTESIAN_POINT ( 'NONE',  ( 0.1532563361054100626, 0.8005978176674514168, -2.638427012816831230 ) ) ;
#14658=CARTESIAN_POINT ( 'NONE',  ( -4.164238869374099039, 36.80374883491396787, 8.674139862899312516E-16 ) ) ;
#14659=CARTESIAN_POINT ( 'NONE',  ( 12.63842701281683922, 24.55059781766745175, -9.846743663894590881 ) ) ;
#14660=CARTESIAN_POINT ( 'NONE',  ( 17.96484262340118221, 41.18868534415484106, -7.964842623401177768 ) ) ;
#14662=CARTESIAN_POINT ( 'NONE',  ( -2.266590686148945544, 6.387082168247300906, -7.082119434687050408 ) ) ;
#14666=CARTESIAN_POINT ( 'NONE',  ( 19.84674366389459266, 53.30059781766744464, 2.638427012816836559 ) ) ;
#14670=CARTESIAN_POINT ( 'NONE',  ( 22.26659068614894466, 23.88708216824730357, 7.082119434687054849 ) ) ;
#14671=CARTESIAN_POINT ( 'NONE',  ( 22.26659068614894466, 18.88708216824730002, 7.082119434687054849 ) ) ;
#14672=CARTESIAN_POINT ( 'NONE',  ( 2.035157376598822676, 57.43868534415484106, -7.964842623401177768 ) ) ;
#14673=CARTESIAN_POINT ( 'NONE',  ( 13.79529636645030344, 63.26208216824730357, 14.16423886937410614 ) ) ;
#14674=CARTESIAN_POINT ( 'NONE',  ( 19.84674366389459266, 48.71726448433413026, -2.638427012816827677 ) ) ;
#14676=CARTESIAN_POINT ( 'NONE',  ( 20.88017736071110164, 45.35535201082149115, 2.915334737309930979 ) ) ;
#14677=CARTESIAN_POINT ( 'NONE',  ( 16.40814093676323893, 25.79030133659708923, 11.09922568453595026 ) ) ;
#14678=CARTESIAN_POINT ( 'NONE',  ( -4.164238869374099927, 17.01208216824730357, 3.795296366450308767 ) ) ;
#14679=CARTESIAN_POINT ( 'NONE',  ( 19.42250999205614548, 15.98035201082150714, -5.440088680355545492 ) ) ;
#14680=CARTESIAN_POINT ( 'NONE',  ( 4.559911319644449179, 17.23035201082150536, -9.422509992056141925 ) ) ;
#14681=CARTESIAN_POINT ( 'NONE',  ( 10.00000000000000000, 61.81368534415484106, -10.88017736071110342 ) ) ;
#14682=CARTESIAN_POINT ( 'NONE',  ( -2.816281873526473856, 49.12363466993042493, 9.499525473075851096E-16 ) ) ;
#14685=LINE ( 'NONE', #82165, #41161 ) ;
#14687=CARTESIAN_POINT ( 'NONE',  ( -1.926860441876562247, 12.45379003517447458, -3.195792623639530650 ) ) ;
#14691=CARTESIAN_POINT ( 'NONE',  ( 20.36894250292379382, 53.67874883491397497, 10.36894250292379205 ) ) ;
#14692=CARTESIAN_POINT ( 'NONE',  ( 19.42250999205614193, 5.147018677488171434, 5.440088680355555262 ) ) ;
#14693=CARTESIAN_POINT ( 'NONE',  ( 12.63842701281683034, 22.46726448433411605, 9.846743663894596210 ) ) ;
#14694=CARTESIAN_POINT ( 'NONE',  ( 0.1532563361054082862, 51.21726448433412315, 2.638427012816831674 ) ) ;
#14695=CARTESIAN_POINT ( 'NONE',  ( 2.035157376598824452, 68.68868534415484817, 7.964842623401179544 ) ) ;
#14697=MECHANICAL_DESIGN_GEOMETRIC_PRESENTATION_REPRESENTATION('',(#59333),#21030);
#14698=CARTESIAN_POINT ( 'NONE',  ( 12.91533473730992121, 64.52201867748817676, 10.88017736071110164 ) ) ;
#14700=EDGE_LOOP ( 'NONE', ( #54950, #27703, #14201, #20436 ) ) ;
#14701=CARTESIAN_POINT ( 'NONE',  ( -4.164238869374098151, 31.59541550158063927, -3.795296366450310543 ) ) ;
#14702=CARTESIAN_POINT ( 'NONE',  ( 24.16423886937410614, 39.51208216824731068, -3.795296366450302550 ) ) ;
#14704=CARTESIAN_POINT ( 'NONE',  ( 3.591859063236763294, 53.29030133659708923, -11.09922568453595026 ) ) ;
#14705=CARTESIAN_POINT ( 'NONE',  ( 1.472469842513823179, 41.42559781766745886, 4.923371831947296329 ) ) ;
#14706=CARTESIAN_POINT ( 'NONE',  ( 4.559911319644449179, 23.89701867748817321, 9.422509992056141925 ) ) ;
#14708=CARTESIAN_POINT ( 'NONE',  ( 0.6178305044545838731, 64.74863466993043914, 9.382169495545420901 ) ) ;
#14710=CARTESIAN_POINT ( 'NONE',  ( 0.1532563361054082862, 51.21726448433412315, 2.638427012816831674 ) ) ;
#14711=CARTESIAN_POINT ( 'NONE',  ( 2.791683348922237240, 45.38393115100079456, -7.208316651077763204 ) ) ;
#14714=EDGE_CURVE ( 'NONE', #31231, #43572, #80197, .T. ) ;
#14717=CARTESIAN_POINT ( 'NONE',  ( 3.640395162852214650, 89.00000000000000000, -5.000000000000000000 ) ) ;
#14720=CARTESIAN_POINT ( 'NONE',  ( 0.6076426042653030324, 57.37576471608601025, -6.499999999999985789 ) ) ;
#14721=CARTESIAN_POINT ( 'NONE',  ( 17.20831665107776587, 32.88393115100078745, 7.208316651077764980 ) ) ;
#14724=VERTEX_POINT ( 'NONE', #15272 ) ;
#14725=CARTESIAN_POINT ( 'NONE',  ( 10.00000000000000000, 54.75893115100078745, -9.846743663894594434 ) ) ;
#14727=CARTESIAN_POINT ( 'NONE',  ( 18.52753015748617571, 43.09226448433412315, 4.923371831947298993 ) ) ;
#14728=CARTESIAN_POINT ( 'NONE',  ( 10.00000000000000000, 30.55374883491397142, -14.16423886937410082 ) ) ;
#14729=CARTESIAN_POINT ( 'NONE',  ( 19.84674366389459266, 48.30059781766745175, 2.638427012816836559 ) ) ;
#14732=CARTESIAN_POINT ( 'NONE',  ( 0.1532563361054100626, 5.800597817667452638, -2.638427012816831230 ) ) ;
#14733=CARTESIAN_POINT ( 'NONE',  ( 6.204703633549690345, 5.762082168247301794, -14.16423886937410259 ) ) ;
#14734=CARTESIAN_POINT ( 'NONE',  ( 19.84674366389459266, 43.30059781766744464, 2.638427012816836559 ) ) ;
#14735=CARTESIAN_POINT ( 'NONE',  ( 7.084665262690076126, 42.02201867748816966, -10.88017736071110164 ) ) ;
#14736=CARTESIAN_POINT ( 'NONE',  ( 1.472469842513823179, 40.59226448433411605, -4.923371831947296329 ) ) ;
#14738=AXIS2_PLACEMENT_3D ( 'NONE', #38052, #1041, #76525 ) ;
#14740=CARTESIAN_POINT ( 'NONE',  ( 15.44008868035555793, 51.39701867748816966, -9.422509992056140149 ) ) ;
#14744=CARTESIAN_POINT ( 'NONE',  ( -0.8801773607111008646, 13.27201867748817143, 2.915334737309923430 ) ) ;
#14745=CARTESIAN_POINT ( 'NONE',  ( 22.81628187352648496, 1.831968003263753753, -3.434112377981050290 ) ) ;
#14746=CARTESIAN_POINT ( 'NONE',  ( 2.035157376598822676, 42.43868534415483396, -7.964842623401177768 ) ) ;
#14748=CARTESIAN_POINT ( 'NONE',  ( 18.04007052943773104, 13.01528370094808196, 5.767676674365834977 ) ) ;
#14750=CARTESIAN_POINT ( 'NONE',  ( 17.96484262340118221, 44.93868534415483396, 7.964842623401181321 ) ) ;
#14752=CARTESIAN_POINT ( 'NONE',  ( 2.791683348922240793, 16.63393115100078745, 7.208316651077764092 ) ) ;
#14753=CARTESIAN_POINT ( 'NONE',  ( 1.472469842513823179, 36.42559781766745175, 4.923371831947296329 ) ) ;
#14755=CARTESIAN_POINT ( 'NONE',  ( 0.1532563361054082862, 66.21726448433413736, 2.638427012816831674 ) ) ;
#14757=CARTESIAN_POINT ( 'NONE',  ( 15.44008868035555260, 4.730352010821505360, 9.422509992056143702 ) ) ;
#14759=CARTESIAN_POINT ( 'NONE',  ( 17.08211943468705130, 23.47041550158063572, 12.26659068614894998 ) ) ;
#14760=CARTESIAN_POINT ( 'NONE',  ( 22.26659068614894466, 53.88708216824731068, 7.082119434687054849 ) ) ;
#14762=CARTESIAN_POINT ( 'NONE',  ( 7.084665262690076126, 7.022018677488169658, -10.88017736071110164 ) ) ;
#14763=VERTEX_POINT ( 'NONE', #97793 ) ;
#14764=CARTESIAN_POINT ( 'NONE',  ( 12.63842701281683034, 27.46726448433411250, 9.846743663894596210 ) ) ;
#14765=CARTESIAN_POINT ( 'NONE',  ( 0.5774900079438590739, 32.64701867748816966, -5.440088680355550821 ) ) ;
#14766=CARTESIAN_POINT ( 'NONE',  ( 5.076628168052703671, 46.84226448433412315, 8.527530157486179263 ) ) ;
#14767=CARTESIAN_POINT ( 'NONE',  ( -4.164238869374099039, 6.803748834913967869, 8.674139862899312516E-16 ) ) ;
#14769=VECTOR ( 'NONE', #40776, 1000.000000000000000 ) ;
#14770=FILL_AREA_STYLE_COLOUR ( '', #19541 ) ;
#14771=CARTESIAN_POINT ( 'NONE',  ( 22.81628187352647785, 36.62363466993041783, 6.195893100308588602E-16 ) ) ;
#14772=CARTESIAN_POINT ( 'NONE',  ( 18.52753015748617571, 48.09226448433412315, 4.923371831947298993 ) ) ;
#14774=CARTESIAN_POINT ( 'NONE',  ( 0.1532563361054082862, 11.21726448433411605, 2.638427012816831674 ) ) ;
#14778=CARTESIAN_POINT ( 'NONE',  ( 20.88017736071110519, 15.56368534415483751, 2.639326808657452039E-16 ) ) ;
#14779=CARTESIAN_POINT ( 'NONE',  ( 10.00000000000000000, 50.55374883491396787, -14.16423886937410082 ) ) ;
#14780=CARTESIAN_POINT ( 'NONE',  ( 17.96484262340118221, 41.18868534415484106, -7.964842623401177768 ) ) ;
#14781=CARTESIAN_POINT ( 'NONE',  ( 6.204703633549690345, 0.7620821682473009062, -14.16423886937410259 ) ) ;
#14784=CARTESIAN_POINT ( 'NONE',  ( 19.84674366389459266, 28.30059781766745886, 2.638427012816836559 ) ) ;
#14785=CARTESIAN_POINT ( 'NONE',  ( -0.8801773607110991993, 2.855352010821504471, -2.915334737309923874 ) ) ;
#14786=CARTESIAN_POINT ( 'NONE',  ( 17.20831665107776587, 37.88393115100078745, 7.208316651077764980 ) ) ;
#14788=CARTESIAN_POINT ( 'NONE',  ( 19.84674366389459266, 48.71726448433413026, -2.638427012816827677 ) ) ;
#14789=CARTESIAN_POINT ( 'NONE',  ( 4.559911319644449179, 42.23035201082151247, -9.422509992056141925 ) ) ;
#14791=ORIENTED_EDGE ( 'NONE', *, *, #94068, .F. ) ;
#14792=CARTESIAN_POINT ( 'NONE',  ( 13.43411237798106583, 52.66530133659708213, -12.81628187352647252 ) ) ;
#14794=CARTESIAN_POINT ( 'NONE',  ( 10.00000000000000178, 2.258931151000784787, 9.846743663894594434 ) ) ;
#14795=CARTESIAN_POINT ( 'NONE',  ( 22.81628187352647785, 51.62363466993042493, 6.195893100308588602E-16 ) ) ;
#14796=CARTESIAN_POINT ( 'NONE',  ( 7.084665262690076126, 4.105352010821503583, 10.88017736071109987 ) ) ;
#14797=CARTESIAN_POINT ( 'NONE',  ( 7.361572987183170547, 52.05059781766745175, 9.846743663894590881 ) ) ;
#14801=CARTESIAN_POINT ( 'NONE',  ( 24.16423886937410614, 29.51208216824729647, -3.795296366450302550 ) ) ;
#14802=CARTESIAN_POINT ( 'NONE',  ( 10.00000000000000178, 43.05374883491397497, 14.16423886937410082 ) ) ;
#14803=CARTESIAN_POINT ( 'NONE',  ( 19.84674366389459621, 53.50893115100078745, 7.409399052514197653E-17 ) ) ;
#14805=CARTESIAN_POINT ( 'NONE',  ( 4.559911319644449179, 47.23035201082150536, -9.422509992056141925 ) ) ;
#14806=CARTESIAN_POINT ( 'NONE',  ( 1.472469842513823179, 1.425597817667451528, 4.923371831947296329 ) ) ;
#14807=AXIS2_PLACEMENT_3D ( 'NONE', #2435, #10402, #71408 ) ;
#14810=CARTESIAN_POINT ( 'NONE',  ( 10.00000000000000178, 60.37363466993041783, 12.81628187352647608 ) ) ;
#14812=CARTESIAN_POINT ( 'NONE',  ( 20.88017736071110164, 60.35535201082151957, 2.915334737309930979 ) ) ;
#14814=CARTESIAN_POINT ( 'NONE',  ( 24.16423886937410614, 4.512082168247300906, -3.795296366450302550 ) ) ;
#14815=CARTESIAN_POINT ( 'NONE',  ( 1.472469842513823179, 5.592264484334118713, -4.923371831947296329 ) ) ;
#14816=CARTESIAN_POINT ( 'NONE',  ( 2.035157376598822676, 27.43868534415483396, -7.964842623401177768 ) ) ;
#14818=ORIENTED_EDGE ( 'NONE', *, *, #81525, .F. ) ;
#14819=CARTESIAN_POINT ( 'NONE',  ( 10.00000000000000000, 26.81368534415484106, -10.88017736071110342 ) ) ;
#14822=CARTESIAN_POINT ( 'NONE',  ( 1.046131998950039499, 45.73810908735726599, 6.499999999999985789 ) ) ;
#14824=CARTESIAN_POINT ( 'NONE',  ( -2.816281873526473856, 19.33196800326375708, 3.434112377981055619 ) ) ;
#14825=CARTESIAN_POINT ( 'NONE',  ( 20.88017736071110875, 60.77201867748817676, -2.915334737309920765 ) ) ;
#14828=CARTESIAN_POINT ( 'NONE',  ( 12.63842701281683034, 2.467264484334118269, 9.846743663894596210 ) ) ;
#14829=CARTESIAN_POINT ( 'NONE',  ( 4.559911319644449179, 32.23035201082150536, -9.422509992056141925 ) ) ;
#14833=CARTESIAN_POINT ( 'NONE',  ( 6.565887622018943937, 63.08196800326376064, -12.81628187352647608 ) ) ;
#14834=CARTESIAN_POINT ( 'NONE',  ( -0.8801773607111008646, 38.27201867748816255, 2.915334737309923430 ) ) ;
#14835=CARTESIAN_POINT ( 'NONE',  ( -46.77276111675546844, 103.6220771345834919, -6.142410991622097249 ) ) ;
#14837=CARTESIAN_POINT ( 'NONE',  ( 16.40814093676323893, 55.79030133659708923, 11.09922568453595026 ) ) ;
#14838=CARTESIAN_POINT ( 'NONE',  ( 15.44008868035555793, 56.39701867748817676, -9.422509992056140149 ) ) ;
#14840=CARTESIAN_POINT ( 'NONE',  ( 22.81628187352647785, 1.415301336597087012, 3.434112377981063169 ) ) ;
#14841=TOROIDAL_SURFACE ( 'NONE', #10047, 18.93999999999999773, 0.5000000000000000000 ) ;
#14842=CARTESIAN_POINT ( 'NONE',  ( 2.791683348922237240, 20.38393115100078745, -7.208316651077763204 ) ) ;
#14843=CARTESIAN_POINT ( 'NONE',  ( 19.38216949554541202, 60.99863466993042493, 9.382169495545424454 ) ) ;
#14844=CARTESIAN_POINT ( 'NONE',  ( 2.603489959281613420, 35.43575266056827644, -6.500000000000031086 ) ) ;
#14845=CARTESIAN_POINT ( 'NONE',  ( 1.472469842513823179, 6.425597817667451750, 4.923371831947296329 ) ) ;
#14847=CARTESIAN_POINT ( 'NONE',  ( 3.591859063236763294, 3.290301336597087012, -11.09922568453595026 ) ) ;
#14849=CARTESIAN_POINT ( 'NONE',  ( 0.1532563361054083140, 66.00893115100079456, 1.131784320476157264E-15 ) ) ;
#14850=CARTESIAN_POINT ( 'NONE',  ( 0.5774900079438590739, 32.64701867748816966, -5.440088680355550821 ) ) ;
#14851=CARTESIAN_POINT ( 'NONE',  ( 17.20831665107776587, 52.88393115100078035, 7.208316651077764980 ) ) ;
#14852=CARTESIAN_POINT ( 'NONE',  ( -1.926860441876564023, 32.87045670184114954, 3.195792623639529761 ) ) ;
#14853=CARTESIAN_POINT ( 'NONE',  ( 19.84674366389459266, 18.71726448433411960, -2.638427012816827677 ) ) ;
#14854=CARTESIAN_POINT ( 'NONE',  ( 1.472469842513823179, 5.592264484334118713, -4.923371831947296329 ) ) ;
#14855=CARTESIAN_POINT ( 'NONE',  ( 19.38216949554541202, 5.998634669930420493, 9.382169495545424454 ) ) ;
#14858=CARTESIAN_POINT ( 'NONE',  ( 14.92337183194729988, 59.34226448433412315, -8.527530157486177487 ) ) ;
#14859=CARTESIAN_POINT ( 'NONE',  ( 12.91533473730992121, 4.522018677488170546, 10.88017736071110164 ) ) ;
#14860=CARTESIAN_POINT ( 'NONE',  ( 0.1532563361054083140, 46.00893115100079456, 1.131784320476157264E-15 ) ) ;
#14861=ORIENTED_EDGE ( 'NONE', *, *, #76418, .T. ) ;
#14863=CARTESIAN_POINT ( 'NONE',  ( 22.26659068614895176, 64.72041550158064638, -7.082119434687042414 ) ) ;
#14864=CARTESIAN_POINT ( 'NONE',  ( 1.274849032794131976, 13.57228050351029403, 6.499999999999760192 ) ) ;
#14865=CARTESIAN_POINT ( 'NONE',  ( 20.88017736071110164, 35.35535201082150536, 2.915334737309930979 ) ) ;
#14866=CARTESIAN_POINT ( 'NONE',  ( 13.79529636645031943, 50.34541550158064638, -14.16423886937409904 ) ) ;
#14867=CARTESIAN_POINT ( 'NONE',  ( 24.16423886937409904, 64.09541550158064638, 3.795296366450317205 ) ) ;
#14869=CARTESIAN_POINT ( 'NONE',  ( 1.472469842513823179, 6.425597817667451750, 4.923371831947296329 ) ) ;
#14871=CARTESIAN_POINT ( 'NONE',  ( 0.1532563361054083140, 26.00893115100078745, 1.131784320476157264E-15 ) ) ;
#14872=CARTESIAN_POINT ( 'NONE',  ( 21.09922568453594849, 16.20696800326375353, 6.408140936763242479 ) ) ;
#14878=CARTESIAN_POINT ( 'NONE',  ( 2.917880565312950480, 5.970415501580634832, -12.26659068614894821 ) ) ;
#14880=CARTESIAN_POINT ( 'NONE',  ( 1.472469842513823179, 30.59226448433411960, -4.923371831947296329 ) ) ;
#14882=CARTESIAN_POINT ( 'NONE',  ( 13.79529636645030344, 38.26208216824729647, 14.16423886937410614 ) ) ;
#14883=CARTESIAN_POINT ( 'NONE',  ( 14.92337183194729988, 9.342264484334119601, -8.527530157486177487 ) ) ;
#14886=CARTESIAN_POINT ( 'NONE',  ( -0.8801773607110991993, 27.85535201082150181, -2.915334737309923874 ) ) ;
#14887=CARTESIAN_POINT ( 'NONE',  ( -1.099225684535947600, 54.54030133659708923, 6.408140936763237150 ) ) ;
#14888=CARTESIAN_POINT ( 'NONE',  ( 20.88017736071110875, 5.772018677488170546, -2.915334737309920765 ) ) ;
#14889=CARTESIAN_POINT ( 'NONE',  ( 16.40814093676324603, 32.45696800326375353, -11.09922568453594671 ) ) ;
#14890=CARTESIAN_POINT ( 'NONE',  ( 12.63842701281683034, 2.467264484334118269, 9.846743663894596210 ) ) ;
#14894=CARTESIAN_POINT ( 'NONE',  ( 2.917880565312950480, 35.97041550158063217, -12.26659068614894821 ) ) ;
#14895=CARTESIAN_POINT ( 'NONE',  ( 22.26659068614895176, 19.72041550158063572, -7.082119434687042414 ) ) ;
#14896=CARTESIAN_POINT ( 'NONE',  ( -0.8801773607111009756, 38.06368534415484106, 1.068504757029289695E-15 ) ) ;
#14899=CARTESIAN_POINT ( 'NONE',  ( 2.035157376598822676, 57.43868534415484106, -7.964842623401177768 ) ) ;
#14900=CARTESIAN_POINT ( 'NONE',  ( 20.88017736071110875, 65.77201867748817676, -2.915334737309920765 ) ) ;
#14901=CARTESIAN_POINT ( 'NONE',  ( 21.09922568453595559, 27.04030133659708568, -6.408140936763230044 ) ) ;
#14903=CARTESIAN_POINT ( 'NONE',  ( 19.72487221294570858, 26.86607318730131055, 6.500000000000000888 ) ) ;
#14904=CARTESIAN_POINT ( 'NONE',  ( 5.076628168052703671, 31.84226448433412315, 8.527530157486179263 ) ) ;
#14905=CARTESIAN_POINT ( 'NONE',  ( 0.6178305044545818747, 13.49863466993041783, -9.382169495545419124 ) ) ;
#14906=CARTESIAN_POINT ( 'NONE',  ( 1.472469842513823179, 0.5922644843341181575, -4.923371831947296329 ) ) ;
#14907=CARTESIAN_POINT ( 'NONE',  ( -0.8801773607110991993, 2.855352010821504471, -2.915334737309923874 ) ) ;
#14908=CARTESIAN_POINT ( 'NONE',  ( 18.52753015748617571, 38.09226448433412315, 4.923371831947298993 ) ) ;
#14911=CARTESIAN_POINT ( 'NONE',  ( 17.20831665107776587, 14.13393115100078568, -7.208316651077762316 ) ) ;
#14912=CARTESIAN_POINT ( 'NONE',  ( -4.164238869374099039, 1.803748834913967647, 8.674139862899312516E-16 ) ) ;
#14913=CARTESIAN_POINT ( 'NONE',  ( 13.79529636645030344, 3.262082168247301350, 14.16423886937410614 ) ) ;
#14915=CARTESIAN_POINT ( 'NONE',  ( 12.91533473730992121, 34.52201867748817676, 10.88017736071110164 ) ) ;
#14916=CARTESIAN_POINT ( 'NONE',  ( 10.00000000000000178, 4.313685344154837509, 10.88017736071110342 ) ) ;
#14917=CARTESIAN_POINT ( 'NONE',  ( 6.204703633549690345, 27.84541550158063217, 14.16423886937410082 ) ) ;
#14918=VECTOR ( 'NONE', #97648, 1000.000000000000000 ) ;
#14919=CARTESIAN_POINT ( 'NONE',  ( 19.42250999205614193, 35.14701867748816966, 5.440088680355555262 ) ) ;
#14920=CARTESIAN_POINT ( 'NONE',  ( -0.8801773607111009756, 23.06368534415484106, 1.068504757029289695E-15 ) ) ;
#14923=CARTESIAN_POINT ( 'NONE',  ( 4.559911319644449179, 28.89701867748817321, 9.422509992056141925 ) ) ;
#14924=CARTESIAN_POINT ( 'NONE',  ( 13.43411237798105340, 45.58196800326374643, 12.81628187352647963 ) ) ;
#14926=CARTESIAN_POINT ( 'NONE',  ( -0.8801773607111009756, 43.06368534415484106, 1.068504757029289695E-15 ) ) ;
#14928=CARTESIAN_POINT ( 'NONE',  ( 17.96484262340118221, 51.18868534415483396, -7.964842623401177768 ) ) ;
#14930=CARTESIAN_POINT ( 'NONE',  ( 15.44008868035555260, 34.73035201082151247, 9.422509992056143702 ) ) ;
#14932=CARTESIAN_POINT ( 'NONE',  ( 0.2751277870542906956, 37.28217586085238366, -6.499999999999992006 ) ) ;
#14933=CARTESIAN_POINT ( 'NONE',  ( 2.917880565312950480, 40.97041550158063217, -12.26659068614894821 ) ) ;
#14934=CARTESIAN_POINT ( 'NONE',  ( 7.361572987183170547, 2.050597817667451750, 9.846743663894590881 ) ) ;
#14935=EDGE_CURVE ( 'NONE', #7550, #91796, #76558, .T. ) ;
#14936=CARTESIAN_POINT ( 'NONE',  ( 19.84674366389459266, 58.30059781766745886, 2.638427012816836559 ) ) ;
#14938=CARTESIAN_POINT ( 'NONE',  ( 12.63842701281683034, 37.46726448433411605, 9.846743663894596210 ) ) ;
#14940=CARTESIAN_POINT ( 'NONE',  ( 10.00000000000000000, 29.75893115100078745, -9.846743663894594434 ) ) ;
#14942=CARTESIAN_POINT ( 'NONE',  ( 10.00000000000000000, 26.81368534415484106, -10.88017736071110342 ) ) ;
#14943=CARTESIAN_POINT ( 'NONE',  ( 19.84674366389459266, 38.71726448433412315, -2.638427012816827677 ) ) ;
#14944=CARTESIAN_POINT ( 'NONE',  ( 10.00000000000000000, 22.87363466993042138, -12.81628187352647608 ) ) ;
#14946=CARTESIAN_POINT ( 'NONE',  ( 15.44008868035555260, 54.73035201082150536, 9.422509992056143702 ) ) ;
#14947=CARTESIAN_POINT ( 'NONE',  ( 10.00000000000000000, 31.81368534415483751, -10.88017736071110342 ) ) ;
#14948=CARTESIAN_POINT ( 'NONE',  ( 2.035157376598824452, 3.688685344154837953, 7.964842623401179544 ) ) ;
#14949=CARTESIAN_POINT ( 'NONE',  ( -0.3689425029237898834, 61.17874883491396076, -10.36894250292378850 ) ) ;
#14954=VERTEX_POINT ( 'NONE', #68265 ) ;
#14955=CARTESIAN_POINT ( 'NONE',  ( -2.816281873526473856, 19.33196800326375708, 3.434112377981055619 ) ) ;
#14956=CARTESIAN_POINT ( 'NONE',  ( -0.8801773607110991993, 2.855352010821504471, -2.915334737309923874 ) ) ;
#14957=CARTESIAN_POINT ( 'NONE',  ( 0.5774900079438607392, 43.48035201082151247, 5.440088680355550821 ) ) ;
#14960=B_SPLINE_CURVE_WITH_KNOTS ( 'NONE', 3,
 ( #44005, #12037, #65520, #49532 ),
 .UNSPECIFIED., .F., .F.,
 ( 4, 4 ),
 ( 5.444379262168902198E-17, 0.002562518741975295181 ),
 .UNSPECIFIED. ) ;
#14961=CARTESIAN_POINT ( 'NONE',  ( 2.035157376598824452, 53.68868534415484817, 7.964842623401179544 ) ) ;
#14962=CARTESIAN_POINT ( 'NONE',  ( 2.791683348922240793, 41.63393115100078745, 7.208316651077764092 ) ) ;
#14963=CARTESIAN_POINT ( 'NONE',  ( 18.52753015748618282, 18.92559781766745175, -4.923371831947291888 ) ) ;
#14964=CARTESIAN_POINT ( 'NONE',  ( 5.076628168052703671, 16.84226448433411960, 8.527530157486179263 ) ) ;
#14967=CARTESIAN_POINT ( 'NONE',  ( 13.43411237798105340, 35.58196800326375353, 12.81628187352647963 ) ) ;
#14968=CARTESIAN_POINT ( 'NONE',  ( 5.076628168052703671, 11.84226448433411960, 8.527530157486179263 ) ) ;
#14971=CARTESIAN_POINT ( 'NONE',  ( 17.20831665107776587, 29.13393115100078390, -7.208316651077762316 ) ) ;
#14974=CARTESIAN_POINT ( 'NONE',  ( 22.81628187352648496, 11.83196800326375531, -3.434112377981050290 ) ) ;
#14976=CARTESIAN_POINT ( 'NONE',  ( 4.559911319644449179, 57.23035201082150536, -9.422509992056141925 ) ) ;
#14977=CARTESIAN_POINT ( 'NONE',  ( 6.204703633549690345, 30.76208216824730357, -14.16423886937410259 ) ) ;
#14980=CARTESIAN_POINT ( 'NONE',  ( 20.36894250292379738, 34.92874883491396076, -10.36894250292379027 ) ) ;
#14981=CARTESIAN_POINT ( 'NONE',  ( -4.164238869374099039, 56.80374883491397497, 8.674139862899312516E-16 ) ) ;
#14982=CARTESIAN_POINT ( 'NONE',  ( 17.08211943468705130, 8.470415501580635720, 12.26659068614894998 ) ) ;
#14983=CARTESIAN_POINT ( 'NONE',  ( -2.266590686148945544, 27.22041550158063572, 7.082119434687048631 ) ) ;
#14985=CARTESIAN_POINT ( 'NONE',  ( 2.035157376598822676, 52.43868534415483396, -7.964842623401177768 ) ) ;
#14987=CARTESIAN_POINT ( 'NONE',  ( 1.472469842513823179, 26.42559781766745175, 4.923371831947296329 ) ) ;
#14988=CARTESIAN_POINT ( 'NONE',  ( 20.88017736071110875, 65.77201867748817676, -2.915334737309920765 ) ) ;
#14989=CARTESIAN_POINT ( 'NONE',  ( 12.63842701281683034, 42.46726448433412315, 9.846743663894596210 ) ) ;
#14990=CARTESIAN_POINT ( 'NONE',  ( 17.96484262340118221, 29.93868534415484106, 7.964842623401181321 ) ) ;
#14991=CARTESIAN_POINT ( 'NONE',  ( 22.81628187352647785, 56.62363466993042493, 6.195893100308588602E-16 ) ) ;
#14992=CARTESIAN_POINT ( 'NONE',  ( 18.52753015748617571, 58.09226448433411605, 4.923371831947298993 ) ) ;
#14994=EDGE_CURVE ( 'NONE', #55728, #45005, #83749, .T. ) ;
#14995=CARTESIAN_POINT ( 'NONE',  ( 5.076628168052703671, 26.84226448433411960, 8.527530157486179263 ) ) ;
#14996=CARTESIAN_POINT ( 'NONE',  ( 22.81628187352648496, 51.83196800326376064, -3.434112377981050290 ) ) ;
#14998=CARTESIAN_POINT ( 'NONE',  ( 20.88017736071110875, 45.77201867748816966, -2.915334737309920765 ) ) ;
#14999=CARTESIAN_POINT ( 'NONE',  ( 0.1532563361054082862, 56.21726448433411605, 2.638427012816831674 ) ) ;
#15000=CARTESIAN_POINT ( 'NONE',  ( 6.204703633549690345, 37.84541550158063927, 14.16423886937410082 ) ) ;
#15002=CARTESIAN_POINT ( 'NONE',  ( 24.16423886937410614, 4.303748834913967869, 8.672049930838204340E-16 ) ) ;
#15003=CARTESIAN_POINT ( 'NONE',  ( 7.084665262690076126, 57.02201867748817676, -10.88017736071110164 ) ) ;
#15005=CARTESIAN_POINT ( 'NONE',  ( 6.204703633549690345, 55.76208216824730357, -14.16423886937410259 ) ) ;
#15006=CARTESIAN_POINT ( 'NONE',  ( 21.09922568453594849, 11.20696800326375531, 6.408140936763242479 ) ) ;
#15008=CARTESIAN_POINT ( 'NONE',  ( 15.44008868035555793, 51.39701867748816966, -9.422509992056140149 ) ) ;
#15010=CARTESIAN_POINT ( 'NONE',  ( -46.94000000000001194, 100.8028158894829289, -8.422108456579607605 ) ) ;
#15011=CARTESIAN_POINT ( 'NONE',  ( 22.81628187352647785, 31.41530133659709279, 3.434112377981063169 ) ) ;
#15012=CARTESIAN_POINT ( 'NONE',  ( 10.00000000000000178, 48.05374883491396787, 14.16423886937410082 ) ) ;
#15014=CARTESIAN_POINT ( 'NONE',  ( 15.44008868035555260, 14.73035201082150536, 9.422509992056143702 ) ) ;
#15015=CARTESIAN_POINT ( 'NONE',  ( 10.00000000000000178, 29.31368534415483751, 10.88017736071110342 ) ) ;
#15016=CARTESIAN_POINT ( 'NONE',  ( 17.20831665107776587, 54.13393115100079456, -7.208316651077762316 ) ) ;
#15017=CARTESIAN_POINT ( 'NONE',  ( 22.81628187352648496, 46.83196800326376064, -3.434112377981050290 ) ) ;
#15020=CARTESIAN_POINT ( 'NONE',  ( -0.8801773607110991993, 17.85535201082150536, -2.915334737309923874 ) ) ;
#15021=CARTESIAN_POINT ( 'NONE',  ( 19.38216949554541202, 20.99863466993042138, 9.382169495545424454 ) ) ;
#15023=CARTESIAN_POINT ( 'NONE',  ( 0.1532563361054082862, 46.21726448433411605, 2.638427012816831674 ) ) ;
#15024=CARTESIAN_POINT ( 'NONE',  ( 12.91533473730993009, 36.60535201082151247, -10.88017736071109987 ) ) ;
#15025=CARTESIAN_POINT ( 'NONE',  ( 3.591859063236763294, 23.29030133659708568, -11.09922568453595026 ) ) ;
#15026=CARTESIAN_POINT ( 'NONE',  ( 7.084665262690076126, 47.02201867748818387, -10.88017736071110164 ) ) ;
#15027=CARTESIAN_POINT ( 'NONE',  ( 20.88017736071110875, 15.77201867748817143, -2.915334737309920321 ) ) ;
#15028=EDGE_CURVE ( 'NONE', #57285, #58602, #26432, .T. ) ;
#15030=CARTESIAN_POINT ( 'NONE',  ( 16.40814093676323893, 55.79030133659708923, 11.09922568453595026 ) ) ;
#15032=CARTESIAN_POINT ( 'NONE',  ( 17.96484262340118221, 54.93868534415484106, 7.964842623401181321 ) ) ;
#15033=CARTESIAN_POINT ( 'NONE',  ( -1.099225684535947600, 28.70696800326375353, -6.408140936763238038 ) ) ;
#15034=CARTESIAN_POINT ( 'NONE',  ( 20.36894250292379738, 4.928748834913967869, -10.36894250292379027 ) ) ;
#15035=CARTESIAN_POINT ( 'NONE',  ( 5.076628168052704559, 5.175597817667451750, -8.527530157486179263 ) ) ;
#15036=CARTESIAN_POINT ( 'NONE',  ( 7.084665262690076126, 57.02201867748817676, -10.88017736071110164 ) ) ;
#15037=CARTESIAN_POINT ( 'NONE',  ( 10.00000000000000000, 45.55374883491397497, -14.16423886937410082 ) ) ;
#15039=CARTESIAN_POINT ( 'NONE',  ( 12.63842701281683034, 12.46726448433411782, 9.846743663894596210 ) ) ;
#15040=CARTESIAN_POINT ( 'NONE',  ( 2.791683348922240793, 1.633931151000784565, 7.208316651077764092 ) ) ;
#15042=CARTESIAN_POINT ( 'NONE',  ( -4.164238869374099927, 47.01208216824729647, 3.795296366450308767 ) ) ;
#15043=CARTESIAN_POINT ( 'NONE',  ( 20.24186590665277663, 24.73410085661204150, 6.114288769123037426 ) ) ;
#15045=CARTESIAN_POINT ( 'NONE',  ( -0.8801773607111008646, 13.27201867748817143, 2.915334737309923430 ) ) ;
#15048=CARTESIAN_POINT ( 'NONE',  ( 4.559911319644449179, 13.89701867748817321, 9.422509992056141925 ) ) ;
#15049=CARTESIAN_POINT ( 'NONE',  ( 24.16423886937410614, 64.51208216824728936, -3.795296366450302550 ) ) ;
#15050=CARTESIAN_POINT ( 'NONE',  ( 17.20831665107776587, 49.13393115100078745, -7.208316651077762316 ) ) ;
#15051=CARTESIAN_POINT ( 'NONE',  ( 19.38216949554541557, 42.24863466993041783, -9.382169495545420901 ) ) ;
#15055=CARTESIAN_POINT ( 'NONE',  ( 24.16423886937409904, 9.095415501580633943, 3.795296366450317205 ) ) ;
#15056=CARTESIAN_POINT ( 'NONE',  ( 4.559911319644449179, 18.89701867748817321, 9.422509992056141925 ) ) ;
#15057=CARTESIAN_POINT ( 'NONE',  ( 19.42250999205614193, 10.14701867748816966, 5.440088680355555262 ) ) ;
#15058=EDGE_CURVE ( 'NONE', #72922, #62857, #32201, .T. ) ;
#15060=CARTESIAN_POINT ( 'NONE',  ( 0.1532563361054100626, 40.80059781766745886, -2.638427012816831230 ) ) ;
#15062=CARTESIAN_POINT ( 'NONE',  ( 10.00000000000000178, 27.25893115100078390, 9.846743663894594434 ) ) ;
#15067=ORIENTED_EDGE ( 'NONE', *, *, #64680, .T. ) ;
#15069=FILL_AREA_STYLE ('',( #22562 ) ) ;
#15071=CARTESIAN_POINT ( 'NONE',  ( 0.1532563361054083140, 56.00893115100078745, 1.131784320476157264E-15 ) ) ;
#15072=CARTESIAN_POINT ( 'NONE',  ( -4.164238869374099039, 16.80374883491396787, 8.674139862899312516E-16 ) ) ;
#15073=CARTESIAN_POINT ( 'NONE',  ( 15.44008868035555260, 39.73035201082150536, 9.422509992056143702 ) ) ;
#15074=CARTESIAN_POINT ( 'NONE',  ( -0.8801773607111009756, 38.06368534415484106, 1.068504757029289695E-15 ) ) ;
#15075=FACE_OUTER_BOUND ( 'NONE', #78243, .T. ) ;
#15076=CARTESIAN_POINT ( 'NONE',  ( 19.38216949554541557, 37.24863466993041783, -9.382169495545420901 ) ) ;
#15077=CARTESIAN_POINT ( 'NONE',  ( 24.16423886937410614, 4.512082168247300906, -3.795296366450302550 ) ) ;
#15079=CARTESIAN_POINT ( 'NONE',  ( 0.6178305044545838731, 39.74863466993041072, 9.382169495545420901 ) ) ;
#15081=CARTESIAN_POINT ( 'NONE',  ( 7.361572987183169658, 39.96726448433411605, -9.846743663894592657 ) ) ;
#15082=CARTESIAN_POINT ( 'NONE',  ( 17.96484262340118221, 6.188685344154837509, -7.964842623401177768 ) ) ;
#15085=CARTESIAN_POINT ( 'NONE',  ( 20.88017736071110875, 10.77201867748817143, -2.915334737309920765 ) ) ;
#15086=ORIENTED_EDGE ( 'NONE', *, *, #52894, .F. ) ;
#15087=CARTESIAN_POINT ( 'NONE',  ( -0.8801773607111008646, 63.27201867748817676, 2.915334737309923430 ) ) ;
#15088=CARTESIAN_POINT ( 'NONE',  ( 10.00000000000000178, 59.31368534415484106, 10.88017736071110342 ) ) ;
#15089=CARTESIAN_POINT ( 'NONE',  ( 15.44008868035555793, 66.39701867748817676, -9.422509992056140149 ) ) ;
#15090=CARTESIAN_POINT ( 'NONE',  ( 4.559911319644449179, 57.23035201082150536, -9.422509992056141925 ) ) ;
#15091=CYLINDRICAL_SURFACE ( 'NONE', #69855, 0.5000000000000004441 ) ;
#15094=CARTESIAN_POINT ( 'NONE',  ( 1.472469842513823179, 35.59226448433412315, -4.923371831947296329 ) ) ;
#15097=CARTESIAN_POINT ( 'NONE',  ( -0.3689425029237881626, 7.428748834913967869, 10.36894250292379027 ) ) ;
#15100=CARTESIAN_POINT ( 'NONE',  ( -0.8801773607110991993, 2.855352010821504471, -2.915334737309923874 ) ) ;
#15102=CARTESIAN_POINT ( 'NONE',  ( 19.38216949554541557, 47.24863466993041783, -9.382169495545420901 ) ) ;
#15105=CARTESIAN_POINT ( 'NONE',  ( 17.20831665107776587, 49.13393115100078745, -7.208316651077762316 ) ) ;
#15106=CARTESIAN_POINT ( 'NONE',  ( -2.816281873526473856, 24.33196800326375353, 3.434112377981055619 ) ) ;
#15107=CARTESIAN_POINT ( 'NONE',  ( 17.20831665107776587, 24.13393115100078035, -7.208316651077762316 ) ) ;
#15108=CARTESIAN_POINT ( 'NONE',  ( 18.72515096720568195, 26.07228050351032778, -6.500000000000018652 ) ) ;
#15109=CARTESIAN_POINT ( 'NONE',  ( 5.076628168052703671, 66.84226448433412315, 8.527530157486179263 ) ) ;
#15111=CARTESIAN_POINT ( 'NONE',  ( 2.791683348922237240, 10.38393115100078390, -7.208316651077763204 ) ) ;
#15115=CARTESIAN_POINT ( 'NONE',  ( 0.5774900079438590739, 17.64701867748817321, -5.440088680355550821 ) ) ;
#15116=CARTESIAN_POINT ( 'NONE',  ( -0.3689425029237898834, 21.17874883491396432, -10.36894250292378850 ) ) ;
#15117=CARTESIAN_POINT ( 'NONE',  ( 17.20831665107776587, 27.88393115100078390, 7.208316651077764980 ) ) ;
#15118=CARTESIAN_POINT ( 'NONE',  ( 10.00000000000000178, 69.31368534415484817, 10.88017736071110342 ) ) ;
#15119=CARTESIAN_POINT ( 'NONE',  ( 6.565887622018943937, 35.16530133659708923, 12.81628187352647430 ) ) ;
#15121=CARTESIAN_POINT ( 'NONE',  ( 7.084665262690076126, 17.02201867748817676, -10.88017736071110164 ) ) ;
#15124=CARTESIAN_POINT ( 'NONE',  ( 13.43411237798106583, 12.66530133659708746, -12.81628187352647252 ) ) ;
#15125=CARTESIAN_POINT ( 'NONE',  ( 13.43411237798105340, 10.58196800326375353, 12.81628187352647963 ) ) ;
#15126=CARTESIAN_POINT ( 'NONE',  ( 7.361572987183169658, 29.96726448433411960, -9.846743663894592657 ) ) ;
#15128=CARTESIAN_POINT ( 'NONE',  ( 13.43411237798105340, 30.58196800326374998, 12.81628187352647963 ) ) ;
#15129=DIRECTION ( 'NONE',  ( 0.000000000000000000, -0.000000000000000000, -1.000000000000000000 ) ) ;
#15130=CARTESIAN_POINT ( 'NONE',  ( 2.035157376598824452, 43.68868534415484106, 7.964842623401179544 ) ) ;
#15134=( BOUNDED_SURFACE ( )  B_SPLINE_SURFACE ( 1, 2, ( 
 ( #29081, #14097, #60069, #82584, #83579, #90570, #97124, #83080, #22097, #13098, #21604, #29565, #52576, #6587, #38091, #98615, #28095, #91064, #58596, #5614, #98103, #67595, #45074, #66597, #30062, #90078, #44581, #14606, #74585, #97618, #75578, #28595, #75081, #15097, #89096, #68086, #45573, #68579, #36604, #7090, #37592, #60574, #59583, #22592, #53067, #51601, #76067, #20610, #51098, #59084, #81587, #43593, #74080, #36091, #89592, #21102, #82085, #13595, #6099, #92060, #17062, #77536, #69563, #61062, #47040, #9054, #55546, #1578, #85550, #92541, #8075, #86045, #23587, #8566, #91573, #54538, #17558, #110, #31052, #93530, #30556, #69072, #39566, #23090, #53558, #38574, #70055, #84073, #93038, #47544, #25061, #61552, #77054, #48023, #2075, #54053, #32027, #32535, #62531, #24571, #1084, #55031, #78042, #9545, #40047, #608, #78536, #10048, #70547, #15590, #84566, #63033, #39070, #40547, #46073, #31545, #62040, #76560, #16066, #24070, #46555, #85054, #16566, #49499, #26509, #11022, #12493, #57005, #11507, #87993, #33504, #79522, #3536, #95001, #19505, #80002, #56526, #86536, #33996, #63523, #2570, #87508, #41540, #4027, #19020, #64983, #42031, #50494, #94028, #18525, #57498, #64494, #25550, #33026, #41042, #3049, #94514, #48518, #4519, #72495, #79021, #96007, #80508, #72007, #34490, #95508, #27000, #50002, #27490, #56042, #18041, #57983, #10532, #12004, #87015, #71542, #72989, #42507, #64002, #26033, #34983, #65486, #88490, #19992, #80991, #49015, #71047, #51478, #14484, #97995, #81972, #83460, #28962, #82468, #59957, #5503, #13484, #74464, #66977, #90449, #21483, #28484, #58478, #5990, #35486, #73475, #97498, #43962, #74966, #59465, #36975, #89967, #22474, #65982, #89481, #29450, #36485, #96507, #5004, #12979, #73977, #66478, #20494, #75459, #44464, #50982, #67969, #52462, #51981, #13988, #6471, #67475, #21987, #98494, #27980, #88990, #29949, #81477, #82965, #58978, #43476, #44956, #6975, #35976, #97006, #37480, #60454, #90943, #52949, #42992, #20992, #16937, #23471, #85428, #69939, #84451, #75953, #61926, #92427, #70434, #16445, #1459, #8443, #22976, #1951, #7964, #53944, #7480, #69442, #32415, #14981, #45959, #9427, #45452, #83950, #54425, #37977, #68467, #53441, #23952, #98987, #8931, #62412, #39931, #76448, #91940, #62917, #47419, #38462, #84934, #77921, #46923, #77415, #15950, #39448, #31910, #92917, #24447, #15476, #93417, #24940, #55422, #30441, #68954, #54914, #46443, #60940, #91451, #76934, #38950, #486, #30935, #962, #61434, #31422, #95384, #64380, #41430, #25439, #79886, #49385, #4403, #55922, #41915, #2939 ),
 ( #11393, #34374, #80387, #17922, #63885, #42390, #87873, #48406, #56888, #19389, #87391, #26388, #86900, #72378, #18909, #3907, #64863, #86421, #34871, #65365, #57379, #9930, #78909, #26886, #94397, #95895, #11890, #25912, #56414, #40434, #33387, #48893, #2451, #33875, #49874, #94890, #71891, #18410, #27374, #3414, #72869, #85930, #10418, #79406, #10908, #17440, #47907, #78412, #71423, #32907, #70933, #63406, #93911, #40926, #96890, #89847, #13362, #51859, #5869, #37363, #50368, #5388, #44344, #89360, #12374, #19875, #27864, #88871, #81363, #35371, #90329, #59345, #65861, #82843, #67352, #28366, #28842, #58854, #20871, #81848, #14363, #88378, #80876, #44832, #96390, #21364, #43360, #58349, #59839, #82344, #4891, #42880, #66856, #13865, #75337, #6851, #67856, #20377, #21868, #66352, #29338, #74850, #51362, #73363, #36360, #97374, #98375, #6351, #36860, #43847, #50871, #73859, #74341, #97878, #12862, #52346, #57866, #35863, #69825, #16819, #70320, #38346, #84342, #31308, #46329, #68841, #851, #15845, #53326, #92315, #91831, #374, #30324, #83343, #47295, #30821, #29831, #60339, #68351, #23349, #90833, #22853, #83835, #46811, #8332, #62297, #15360, #45845, #61810, #76331, #38835, #77797, #91327, #1347, #31799, #7848, #61320, #76815, #84821, #98869, #69329, #14865, #60826, #23841, #54308, #9307, #53831, #16328, #77303, #8817, #39815, #39331, #85311, #92805, #22360, #24334, #52834, #54794, #45337, #75837, #7357, #37859, #94275, #78796, #63767, #9809, #55805, #1835, #3792, #2823, #56773, #25798, #86299, #79283, #49272, #63284, #40311, #87268, #41791, #56298, #93297, #3291, #48285, #57258, #49752, #10792, #70816, #87754, #17805, #33274, #2332, #86792, #18293, #33755, #48776, #19268, #64259, #32787, #18790, #94772, #85808, #41309, #26271, #79771, #71782, #80263, #72264, #32292, #64747, #62797, #78293, #11271, #34247, #95259, #93790, #26765, #11766, #42275, #24821, #55297, #10304, #17320, #47794, #25319, #40803, #71303, #57748, #12254, #66740, #36244, #90219, #42761, #28734, #88747, #35244, #82724, #5268, #29224, #51745, #21751, #21246, #52232, #5755, #59225, #34752, #97264, #50243, #66233, #50758, #35745, #80759, #27744, #72745, #74729, #73738, #89729, #96768, #58227, #51241, #82228, #65741, #73243, #13742, #44225, #28243, #65241, #74222, #20257, #59724, #14242, #81728, #4770, #4278, #81244, #58738, #96271, #89243, #20751, #6242, #13243, #95767, #36745, #12743, #67236, #97759, #88251, #43735, #27250, #19759, #43242, #24210, #16209, #44724, #8697, #75221, #22240, #15733, #53704, #61687, #83224, #46693, #7736, #68719, #8220, #60709 ) ),
 .UNSPECIFIED., .F., .F., .T. ) 
 B_SPLINE_SURFACE_WITH_KNOTS ( ( 2, 2 ),
 ( 3, 2, 2, 2, 2, 2, 2, 2, 2, 2, 2, 2, 2, 2, 2, 2, 2, 2, 2, 2, 2, 2, 2, 2, 2, 2, 2, 2, 2, 2, 2, 2, 2, 2, 2, 2, 2, 2, 2, 2, 2, 2, 2, 2, 2, 2, 2, 2, 2, 2, 2, 2, 2, 2, 2, 2, 2, 2, 2, 2, 2, 2, 2, 2, 2, 2, 2, 2, 2, 2, 2, 2, 2, 2, 2, 2, 2, 2, 2, 2, 2, 2, 2, 2, 2, 2, 2, 2, 2, 2, 2, 2, 2, 2, 2, 2, 2, 2, 2, 2, 2, 2, 2, 2, 2, 2, 2, 2, 2, 2, 2, 2, 2, 2, 2, 2, 2, 2, 2, 2, 2, 2, 2, 2, 2, 2, 2, 2, 2, 2, 2, 2, 2, 2, 2, 2, 2, 2, 2, 2, 2, 2, 2, 2, 2, 2, 2, 2, 2, 2, 2, 2, 2, 2, 2, 2, 2, 2, 2, 2, 2, 2, 3 ),
 ( 0.000000000000000000, 1.000000000000000000 ),
 ( 0.000000000000000000, 0.005952380952380952051, 0.01190476190476190410, 0.01785714285714285615, 0.02380952380952380820, 0.02976190476190476025, 0.03571428571428571230, 0.04166666666666666435, 0.04761904761904761640, 0.05357142857142856845, 0.05952380952380952051, 0.06547619047619047949, 0.07142857142857142461, 0.07738095238095238360, 0.08333333333333332871, 0.08928571428571428770, 0.09523809523809523281, 0.1011904761904761918, 0.1071428571428571369, 0.1130952380952380959, 0.1190476190476190410, 0.1250000000000000000, 0.1309523809523809590, 0.1369047619047619180, 0.1428571428571428492, 0.1488095238095238082, 0.1547619047619047672, 0.1607142857142857262, 0.1666666666666666574, 0.1726190476190476164, 0.1785714285714285754, 0.1845238095238095344, 0.1904761904761904656, 0.1964285714285714246, 0.2023809523809523836, 0.2083333333333333426, 0.2142857142857142738, 0.2202380952380952328, 0.2261904761904761918, 0.2321428571428571508, 0.2380952380952380820, 0.2440476190476190410, 0.2500000000000000000, 0.2559523809523809312, 0.2619047619047619180, 0.2678571428571428492, 0.2738095238095238360, 0.2797619047619047672, 0.2857142857142856984, 0.2916666666666666852, 0.2976190476190476164, 0.3035714285714285476, 0.3095238095238095344, 0.3154761904761904656, 0.3214285714285714524, 0.3273809523809523836, 0.3333333333333333148, 0.3392857142857143016, 0.3452380952380952328, 0.3511904761904761640, 0.3571428571428571508, 0.3630952380952380820, 0.3690476190476190688, 0.3750000000000000000, 0.3809523809523809312, 0.3869047619047619180, 0.3928571428571428492, 0.3988095238095238360, 0.4047619047619047672, 0.4107142857142856984, 0.4166666666666666852, 0.4226190476190476164, 0.4285714285714285476, 0.4345238095238095344, 0.4404761904761904656, 0.4464285714285714524, 0.4523809523809523836, 0.4583333333333333148, 0.4642857142857143016, 0.4702380952380952328, 0.4761904761904761640, 0.4821428571428571508, 0.4880952380952380820, 0.4940476190476190688, 0.5000000000000000000, 0.5059523809523809312, 0.5119047619047618625, 0.5178571428571429047, 0.5238095238095238360, 0.5297619047619047672, 0.5357142857142856984, 0.5416666666666666297, 0.5476190476190476719, 0.5535714285714286031, 0.5595238095238095344, 0.5654761904761904656, 0.5714285714285713969, 0.5773809523809523281, 0.5833333333333333703, 0.5892857142857143016, 0.5952380952380952328, 0.6011904761904761640, 0.6071428571428570953, 0.6130952380952381375, 0.6190476190476190688, 0.6250000000000000000, 0.6309523809523809312, 0.6369047619047618625, 0.6428571428571429047, 0.6488095238095238360, 0.6547619047619047672, 0.6607142857142856984, 0.6666666666666666297, 0.6726190476190476719, 0.6785714285714286031, 0.6845238095238095344, 0.6904761904761904656, 0.6964285714285713969, 0.7023809523809523281, 0.7083333333333333703, 0.7142857142857143016, 0.7202380952380952328, 0.7261904761904761640, 0.7321428571428570953, 0.7380952380952381375, 0.7440476190476190688, 0.7500000000000000000, 0.7559523809523809312, 0.7619047619047618625, 0.7678571428571429047, 0.7738095238095238360, 0.7797619047619047672, 0.7857142857142856984, 0.7916666666666666297, 0.7976190476190476719, 0.8035714285714286031, 0.8095238095238095344, 0.8154761904761904656, 0.8214285714285713969, 0.8273809523809523281, 0.8333333333333333703, 0.8392857142857143016, 0.8452380952380952328, 0.8511904761904761640, 0.8571428571428570953, 0.8630952380952381375, 0.8690476190476190688, 0.8750000000000000000, 0.8809523809523809312, 0.8869047619047618625, 0.8928571428571429047, 0.8988095238095238360, 0.9047619047619047672, 0.9107142857142856984, 0.9166666666666666297, 0.9226190476190476719, 0.9285714285714286031, 0.9345238095238095344, 0.9404761904761904656, 0.9464285714285713969, 0.9523809523809523281, 0.9583333333333333703, 0.9642857142857143016 ),
 .UNSPECIFIED. ) 
 GEOMETRIC_REPRESENTATION_ITEM ( )  RATIONAL_B_SPLINE_SURFACE ( (
 ( 1.000000000000000000, 0.9659258262890683122, 1.000000000000000000, 0.9659258262890683122, 1.000000000000000000, 0.9659258262890683122, 1.000000000000000000, 0.9659258262890683122, 1.000000000000000000, 0.9659258262890683122, 1.000000000000000000, 0.9659258262890683122, 1.000000000000000000, 0.9659258262890683122, 1.000000000000000000, 0.9659258262890683122, 1.000000000000000000, 0.9659258262890683122, 1.000000000000000000, 0.9659258262890683122, 1.000000000000000000, 0.9659258262890683122, 1.000000000000000000, 0.9659258262890683122, 1.000000000000000000, 0.9659258262890683122, 1.000000000000000000, 0.9659258262890683122, 1.000000000000000000, 0.9659258262890683122, 1.000000000000000000, 0.9659258262890683122, 1.000000000000000000, 0.9659258262890683122, 1.000000000000000000, 0.9659258262890683122, 1.000000000000000000, 0.9659258262890683122, 1.000000000000000000, 0.9659258262890683122, 1.000000000000000000, 0.9659258262890683122, 1.000000000000000000, 0.9659258262890683122, 1.000000000000000000, 0.9659258262890683122, 1.000000000000000000, 0.9659258262890683122, 1.000000000000000000, 0.9659258262890683122, 1.000000000000000000, 0.9659258262890683122, 1.000000000000000000, 0.9659258262890683122, 1.000000000000000000, 0.9659258262890683122, 1.000000000000000000, 0.9659258262890683122, 1.000000000000000000, 0.9659258262890683122, 1.000000000000000000, 0.9659258262890683122, 1.000000000000000000, 0.9659258262890683122, 1.000000000000000000, 0.9659258262890683122, 1.000000000000000000, 0.9659258262890683122, 1.000000000000000000, 0.9659258262890683122, 1.000000000000000000, 0.9659258262890683122, 1.000000000000000000, 0.9659258262890683122, 1.000000000000000000, 0.9659258262890683122, 1.000000000000000000, 0.9659258262890683122, 1.000000000000000000, 0.9659258262890683122, 1.000000000000000000, 0.9659258262890683122, 1.000000000000000000, 0.9659258262890683122, 1.000000000000000000, 0.9659258262890683122, 1.000000000000000000, 0.9659258262890683122, 1.000000000000000000, 0.9659258262890683122, 1.000000000000000000, 0.9659258262890683122, 1.000000000000000000, 0.9659258262890683122, 1.000000000000000000, 0.9659258262890683122, 1.000000000000000000, 0.9659258262890683122, 1.000000000000000000, 0.9659258262890683122, 1.000000000000000000, 0.9659258262890683122, 1.000000000000000000, 0.9659258262890683122, 1.000000000000000000, 0.9659258262890683122, 1.000000000000000000, 0.9659258262890683122, 1.000000000000000000, 0.9659258262890683122, 1.000000000000000000, 0.9659258262890683122, 1.000000000000000000, 0.9659258262890683122, 1.000000000000000000, 0.9659258262890683122, 1.000000000000000000, 0.9659258262890683122, 1.000000000000000000, 0.9659258262890683122, 1.000000000000000000, 0.9659258262890683122, 1.000000000000000000, 0.9659258262890683122, 1.000000000000000000, 0.9659258262890683122, 1.000000000000000000, 0.9659258262890683122, 1.000000000000000000, 0.9659258262890683122, 1.000000000000000000, 0.9659258262890683122, 1.000000000000000000, 0.9659258262890683122, 1.000000000000000000, 0.9659258262890683122, 1.000000000000000000, 0.9659258262890683122, 1.000000000000000000, 0.9659258262890683122, 1.000000000000000000, 0.9659258262890683122, 1.000000000000000000, 0.9659258262890683122, 1.000000000000000000, 0.9659258262890683122, 1.000000000000000000, 0.9659258262890683122, 1.000000000000000000, 0.9659258262890683122, 1.000000000000000000, 0.9659258262890683122, 1.000000000000000000, 0.9659258262890683122, 1.000000000000000000, 0.9659258262890683122, 1.000000000000000000, 0.9659258262890683122, 1.000000000000000000, 0.9659258262890683122, 1.000000000000000000, 0.9659258262890683122, 1.000000000000000000, 0.9659258262890683122, 1.000000000000000000, 0.9659258262890683122, 1.000000000000000000, 0.9659258262890683122, 1.000000000000000000, 0.9659258262890683122, 1.000000000000000000, 0.9659258262890683122, 1.000000000000000000, 0.9659258262890683122, 1.000000000000000000, 0.9659258262890683122, 1.000000000000000000, 0.9659258262890683122, 1.000000000000000000, 0.9659258262890683122, 1.000000000000000000, 0.9659258262890683122, 1.000000000000000000, 0.9659258262890683122, 1.000000000000000000, 0.9659258262890683122, 1.000000000000000000, 0.9659258262890683122, 1.000000000000000000, 0.9659258262890683122, 1.000000000000000000, 0.9659258262890683122, 1.000000000000000000, 0.9659258262890683122, 1.000000000000000000, 0.9659258262890683122, 1.000000000000000000, 0.9659258262890683122, 1.000000000000000000, 0.9659258262890683122, 1.000000000000000000, 0.9659258262890683122, 1.000000000000000000, 0.9659258262890683122, 1.000000000000000000, 0.9659258262890683122, 1.000000000000000000, 0.9659258262890683122, 1.000000000000000000, 0.9659258262890683122, 1.000000000000000000, 0.9659258262890683122, 1.000000000000000000, 0.9659258262890683122, 1.000000000000000000, 0.9659258262890683122, 1.000000000000000000, 0.9659258262890683122, 1.000000000000000000, 0.9659258262890683122, 1.000000000000000000, 0.9659258262890683122, 1.000000000000000000, 0.9659258262890683122, 1.000000000000000000, 0.9659258262890683122, 1.000000000000000000, 0.9659258262890683122, 1.000000000000000000, 0.9659258262890683122, 1.000000000000000000, 0.9659258262890683122, 1.000000000000000000, 0.9659258262890683122, 1.000000000000000000, 0.9659258262890683122, 1.000000000000000000, 0.9659258262890683122, 1.000000000000000000, 0.9659258262890683122, 1.000000000000000000, 0.9659258262890683122, 1.000000000000000000, 0.9659258262890683122, 1.000000000000000000, 0.9659258262890683122, 1.000000000000000000, 0.9659258262890683122, 1.000000000000000000, 0.9659258262890683122, 1.000000000000000000, 0.9659258262890683122, 1.000000000000000000, 0.9659258262890683122, 1.000000000000000000, 0.9659258262890683122, 1.000000000000000000, 0.9659258262890683122, 1.000000000000000000, 0.9659258262890683122, 1.000000000000000000, 0.9659258262890683122, 1.000000000000000000, 0.9659258262890683122, 1.000000000000000000, 0.9659258262890683122, 1.000000000000000000, 0.9659258262890683122, 1.000000000000000000, 0.9659258262890683122, 1.000000000000000000, 0.9659258262890683122, 1.000000000000000000, 0.9659258262890683122, 1.000000000000000000, 0.9659258262890683122, 1.000000000000000000, 0.9659258262890683122, 1.000000000000000000, 0.9659258262890683122, 1.000000000000000000, 0.9659258262890683122, 1.000000000000000000, 0.9659258262890683122, 1.000000000000000000, 0.9659258262890683122, 1.000000000000000000, 0.9659258262890683122, 1.000000000000000000, 0.9659258262890683122, 1.000000000000000000, 0.9659258262890683122, 1.000000000000000000, 0.9659258262890683122, 1.000000000000000000, 0.9659258262890683122, 1.000000000000000000, 0.9659258262890683122, 1.000000000000000000, 0.9659258262890683122, 1.000000000000000000, 0.9659258262890683122, 1.000000000000000000, 0.9659258262890683122, 1.000000000000000000, 0.9659258262890683122, 1.000000000000000000, 0.9659258262890683122, 1.000000000000000000, 0.9659258262890683122, 1.000000000000000000, 0.9659258262890683122, 1.000000000000000000, 0.9659258262890683122, 1.000000000000000000, 0.9659258262890683122, 1.000000000000000000, 0.9659258262890683122, 1.000000000000000000, 0.9659258262890683122, 1.000000000000000000, 0.9659258262890683122, 1.000000000000000000, 0.9659258262890683122, 1.000000000000000000),
 ( 1.000000000000000000, 0.9659258262890683122, 1.000000000000000000, 0.9659258262890683122, 1.000000000000000000, 0.9659258262890683122, 1.000000000000000000, 0.9659258262890683122, 1.000000000000000000, 0.9659258262890683122, 1.000000000000000000, 0.9659258262890683122, 1.000000000000000000, 0.9659258262890683122, 1.000000000000000000, 0.9659258262890683122, 1.000000000000000000, 0.9659258262890683122, 1.000000000000000000, 0.9659258262890683122, 1.000000000000000000, 0.9659258262890683122, 1.000000000000000000, 0.9659258262890683122, 1.000000000000000000, 0.9659258262890683122, 1.000000000000000000, 0.9659258262890683122, 1.000000000000000000, 0.9659258262890683122, 1.000000000000000000, 0.9659258262890683122, 1.000000000000000000, 0.9659258262890683122, 1.000000000000000000, 0.9659258262890683122, 1.000000000000000000, 0.9659258262890683122, 1.000000000000000000, 0.9659258262890683122, 1.000000000000000000, 0.9659258262890683122, 1.000000000000000000, 0.9659258262890683122, 1.000000000000000000, 0.9659258262890683122, 1.000000000000000000, 0.9659258262890683122, 1.000000000000000000, 0.9659258262890683122, 1.000000000000000000, 0.9659258262890683122, 1.000000000000000000, 0.9659258262890683122, 1.000000000000000000, 0.9659258262890683122, 1.000000000000000000, 0.9659258262890683122, 1.000000000000000000, 0.9659258262890683122, 1.000000000000000000, 0.9659258262890683122, 1.000000000000000000, 0.9659258262890683122, 1.000000000000000000, 0.9659258262890683122, 1.000000000000000000, 0.9659258262890683122, 1.000000000000000000, 0.9659258262890683122, 1.000000000000000000, 0.9659258262890683122, 1.000000000000000000, 0.9659258262890683122, 1.000000000000000000, 0.9659258262890683122, 1.000000000000000000, 0.9659258262890683122, 1.000000000000000000, 0.9659258262890683122, 1.000000000000000000, 0.9659258262890683122, 1.000000000000000000, 0.9659258262890683122, 1.000000000000000000, 0.9659258262890683122, 1.000000000000000000, 0.9659258262890683122, 1.000000000000000000, 0.9659258262890683122, 1.000000000000000000, 0.9659258262890683122, 1.000000000000000000, 0.9659258262890683122, 1.000000000000000000, 0.9659258262890683122, 1.000000000000000000, 0.9659258262890683122, 1.000000000000000000, 0.9659258262890683122, 1.000000000000000000, 0.9659258262890683122, 1.000000000000000000, 0.9659258262890683122, 1.000000000000000000, 0.9659258262890683122, 1.000000000000000000, 0.9659258262890683122, 1.000000000000000000, 0.9659258262890683122, 1.000000000000000000, 0.9659258262890683122, 1.000000000000000000, 0.9659258262890683122, 1.000000000000000000, 0.9659258262890683122, 1.000000000000000000, 0.9659258262890683122, 1.000000000000000000, 0.9659258262890683122, 1.000000000000000000, 0.9659258262890683122, 1.000000000000000000, 0.9659258262890683122, 1.000000000000000000, 0.9659258262890683122, 1.000000000000000000, 0.9659258262890683122, 1.000000000000000000, 0.9659258262890683122, 1.000000000000000000, 0.9659258262890683122, 1.000000000000000000, 0.9659258262890683122, 1.000000000000000000, 0.9659258262890683122, 1.000000000000000000, 0.9659258262890683122, 1.000000000000000000, 0.9659258262890683122, 1.000000000000000000, 0.9659258262890683122, 1.000000000000000000, 0.9659258262890683122, 1.000000000000000000, 0.9659258262890683122, 1.000000000000000000, 0.9659258262890683122, 1.000000000000000000, 0.9659258262890683122, 1.000000000000000000, 0.9659258262890683122, 1.000000000000000000, 0.9659258262890683122, 1.000000000000000000, 0.9659258262890683122, 1.000000000000000000, 0.9659258262890683122, 1.000000000000000000, 0.9659258262890683122, 1.000000000000000000, 0.9659258262890683122, 1.000000000000000000, 0.9659258262890683122, 1.000000000000000000, 0.9659258262890683122, 1.000000000000000000, 0.9659258262890683122, 1.000000000000000000, 0.9659258262890683122, 1.000000000000000000, 0.9659258262890683122, 1.000000000000000000, 0.9659258262890683122, 1.000000000000000000, 0.9659258262890683122, 1.000000000000000000, 0.9659258262890683122, 1.000000000000000000, 0.9659258262890683122, 1.000000000000000000, 0.9659258262890683122, 1.000000000000000000, 0.9659258262890683122, 1.000000000000000000, 0.9659258262890683122, 1.000000000000000000, 0.9659258262890683122, 1.000000000000000000, 0.9659258262890683122, 1.000000000000000000, 0.9659258262890683122, 1.000000000000000000, 0.9659258262890683122, 1.000000000000000000, 0.9659258262890683122, 1.000000000000000000, 0.9659258262890683122, 1.000000000000000000, 0.9659258262890683122, 1.000000000000000000, 0.9659258262890683122, 1.000000000000000000, 0.9659258262890683122, 1.000000000000000000, 0.9659258262890683122, 1.000000000000000000, 0.9659258262890683122, 1.000000000000000000, 0.9659258262890683122, 1.000000000000000000, 0.9659258262890683122, 1.000000000000000000, 0.9659258262890683122, 1.000000000000000000, 0.9659258262890683122, 1.000000000000000000, 0.9659258262890683122, 1.000000000000000000, 0.9659258262890683122, 1.000000000000000000, 0.9659258262890683122, 1.000000000000000000, 0.9659258262890683122, 1.000000000000000000, 0.9659258262890683122, 1.000000000000000000, 0.9659258262890683122, 1.000000000000000000, 0.9659258262890683122, 1.000000000000000000, 0.9659258262890683122, 1.000000000000000000, 0.9659258262890683122, 1.000000000000000000, 0.9659258262890683122, 1.000000000000000000, 0.9659258262890683122, 1.000000000000000000, 0.9659258262890683122, 1.000000000000000000, 0.9659258262890683122, 1.000000000000000000, 0.9659258262890683122, 1.000000000000000000, 0.9659258262890683122, 1.000000000000000000, 0.9659258262890683122, 1.000000000000000000, 0.9659258262890683122, 1.000000000000000000, 0.9659258262890683122, 1.000000000000000000, 0.9659258262890683122, 1.000000000000000000, 0.9659258262890683122, 1.000000000000000000, 0.9659258262890683122, 1.000000000000000000, 0.9659258262890683122, 1.000000000000000000, 0.9659258262890683122, 1.000000000000000000, 0.9659258262890683122, 1.000000000000000000, 0.9659258262890683122, 1.000000000000000000, 0.9659258262890683122, 1.000000000000000000, 0.9659258262890683122, 1.000000000000000000, 0.9659258262890683122, 1.000000000000000000, 0.9659258262890683122, 1.000000000000000000, 0.9659258262890683122, 1.000000000000000000, 0.9659258262890683122, 1.000000000000000000, 0.9659258262890683122, 1.000000000000000000, 0.9659258262890683122, 1.000000000000000000, 0.9659258262890683122, 1.000000000000000000, 0.9659258262890683122, 1.000000000000000000, 0.9659258262890683122, 1.000000000000000000, 0.9659258262890683122, 1.000000000000000000, 0.9659258262890683122, 1.000000000000000000, 0.9659258262890683122, 1.000000000000000000, 0.9659258262890683122, 1.000000000000000000, 0.9659258262890683122, 1.000000000000000000, 0.9659258262890683122, 1.000000000000000000, 0.9659258262890683122, 1.000000000000000000, 0.9659258262890683122, 1.000000000000000000, 0.9659258262890683122, 1.000000000000000000, 0.9659258262890683122, 1.000000000000000000, 0.9659258262890683122, 1.000000000000000000, 0.9659258262890683122, 1.000000000000000000, 0.9659258262890683122, 1.000000000000000000, 0.9659258262890683122, 1.000000000000000000, 0.9659258262890683122, 1.000000000000000000, 0.9659258262890683122, 1.000000000000000000, 0.9659258262890683122, 1.000000000000000000, 0.9659258262890683122, 1.000000000000000000) ) ) 
 REPRESENTATION_ITEM ( '' )  SURFACE ( )  );
#15135=CARTESIAN_POINT ( 'NONE',  ( 19.42250999205614193, 35.14701867748816966, 5.440088680355555262 ) ) ;
#15136=CARTESIAN_POINT ( 'NONE',  ( 17.96484262340118221, 44.93868534415483396, 7.964842623401181321 ) ) ;
#15137=CARTESIAN_POINT ( 'NONE',  ( -0.1491070598754174470, 61.94583914210339515, -5.000000000000000000 ) ) ;
#15138=DIRECTION ( 'NONE',  ( -0.000000000000000000, 1.000000000000000000, -0.000000000000000000 ) ) ;
#15140=CARTESIAN_POINT ( 'NONE',  ( 0.1532563361054082862, 51.21726448433412315, 2.638427012816831674 ) ) ;
#15141=CARTESIAN_POINT ( 'NONE',  ( 19.42250999205614548, 5.980352010821504471, -5.440088680355545492 ) ) ;
#15143=CARTESIAN_POINT ( 'NONE',  ( 3.591859063236761518, 14.95696800326375531, 11.09922568453594849 ) ) ;
#15144=ORIENTED_EDGE ( 'NONE', *, *, #77356, .F. ) ;
#15145=CARTESIAN_POINT ( 'NONE',  ( 20.88017736071110519, 40.56368534415484106, 2.639326808657452039E-16 ) ) ;
#15146=CARTESIAN_POINT ( 'NONE',  ( 0.1532563361054082862, 66.21726448433413736, 2.638427012816831674 ) ) ;
#15148=CARTESIAN_POINT ( 'NONE',  ( 4.559911319644449179, 22.23035201082150536, -9.422509992056141925 ) ) ;
#15149=CARTESIAN_POINT ( 'NONE',  ( -2.266590686148945544, 37.22041550158063217, 7.082119434687048631 ) ) ;
#15150=CARTESIAN_POINT ( 'NONE',  ( 12.63842701281683034, 32.46726448433412315, 9.846743663894596210 ) ) ;
#15151=CARTESIAN_POINT ( 'NONE',  ( 15.44008868035555793, 51.39701867748816966, -9.422509992056140149 ) ) ;
#15153=ADVANCED_FACE ( 'NONE', ( #2239 ), #9716, .T. ) ;
#15155=CARTESIAN_POINT ( 'NONE',  ( 19.84674366389459621, 58.50893115100078745, 7.409399052514197653E-17 ) ) ;
#15158=ORIENTED_EDGE ( 'NONE', *, *, #9970, .T. ) ;
#15159=CARTESIAN_POINT ( 'NONE',  ( 24.16423886937409904, 29.09541550158063572, 3.795296366450317205 ) ) ;
#15160=CARTESIAN_POINT ( 'NONE',  ( 6.204703633549690345, 27.84541550158063217, 14.16423886937410082 ) ) ;
#15161=CARTESIAN_POINT ( 'NONE',  ( 2.791683348922237240, 0.3839311510007847872, -7.208316651077763204 ) ) ;
#15162=CARTESIAN_POINT ( 'NONE',  ( 2.917880565312950480, 65.97041550158063217, -12.26659068614894821 ) ) ;
#15163=CARTESIAN_POINT ( 'NONE',  ( 18.52753015748617571, 53.09226448433412315, 4.923371831947298993 ) ) ;
#15165=CARTESIAN_POINT ( 'NONE',  ( 20.88017736071110519, 40.56368534415484106, 2.639326808657452039E-16 ) ) ;
#15166=CARTESIAN_POINT ( 'NONE',  ( 22.81628187352647785, 21.62363466993041783, 6.195893100308588602E-16 ) ) ;
#15167=CARTESIAN_POINT ( 'NONE',  ( 22.26659068614895176, 14.72041550158063572, -7.082119434687042414 ) ) ;
#15168=CARTESIAN_POINT ( 'NONE',  ( -0.8801773607110991993, 7.855352010821506248, -2.915334737309923874 ) ) ;
#15170=CARTESIAN_POINT ( 'NONE',  ( 7.084665262690076126, 34.10535201082151247, 10.88017736071109987 ) ) ;
#15172=CARTESIAN_POINT ( 'NONE',  ( 19.42250999205614193, 55.14701867748817676, 5.440088680355555262 ) ) ;
#15173=CARTESIAN_POINT ( 'NONE',  ( 21.09922568453594849, 51.20696800326375353, 6.408140936763242479 ) ) ;
#15177=VECTOR ( 'NONE', #10841, 1000.000000000000000 ) ;
#15182=CARTESIAN_POINT ( 'NONE',  ( -2.266590686148945544, 56.38708216824731068, -7.082119434687050408 ) ) ;
#15183=CARTESIAN_POINT ( 'NONE',  ( 24.16423886937409904, 59.09541550158063217, 3.795296366450317205 ) ) ;
#15184=CARTESIAN_POINT ( 'NONE',  ( 7.361572987183170547, 27.05059781766745175, 9.846743663894590881 ) ) ;
#15185=CARTESIAN_POINT ( 'NONE',  ( 10.00000000000000178, 57.25893115100078745, 9.846743663894594434 ) ) ;
#15186=CARTESIAN_POINT ( 'NONE',  ( -0.8801773607111008646, 68.27201867748817676, 2.915334737309923430 ) ) ;
#15188=ORIENTED_EDGE ( 'NONE', *, *, #25103, .T. ) ;
#15189=CARTESIAN_POINT ( 'NONE',  ( 10.00000000000000178, 33.05374883491396787, 14.16423886937410082 ) ) ;
#15190=EDGE_CURVE ( 'NONE', #49358, #10984, #49658, .T. ) ;
#15191=CARTESIAN_POINT ( 'NONE',  ( 22.26659068614894466, 43.88708216824729647, 7.082119434687054849 ) ) ;
#15192=ORIENTED_EDGE ( 'NONE', *, *, #80003, .T. ) ;
#15193=CARTESIAN_POINT ( 'NONE',  ( 19.38216949554541557, 57.24863466993042493, -9.382169495545420901 ) ) ;
#15194=CARTESIAN_POINT ( 'NONE',  ( 4.559911319644449179, 22.23035201082150536, -9.422509992056141925 ) ) ;
#15195=CARTESIAN_POINT ( 'NONE',  ( 14.92337183194729988, 54.34226448433412315, -8.527530157486177487 ) ) ;
#15196=CARTESIAN_POINT ( 'NONE',  ( 20.88017736071110519, 25.56368534415483751, 2.639326808657452039E-16 ) ) ;
#15197=CARTESIAN_POINT ( 'NONE',  ( 19.38216949554541202, 60.99863466993042493, 9.382169495545424454 ) ) ;
#15199=CARTESIAN_POINT ( 'NONE',  ( 12.63842701281683922, 59.55059781766744464, -9.846743663894590881 ) ) ;
#15200=CARTESIAN_POINT ( 'NONE',  ( 0.1532563361054100626, 45.80059781766745886, -2.638427012816831230 ) ) ;
#15201=ADVANCED_FACE ( 'NONE', ( #12655 ), #35221, .T. ) ;
#15202=( BOUNDED_CURVE ( )  B_SPLINE_CURVE ( 2, ( #40185, #4161, #43127, #51124, #65622, #96148, #82111, #42642, #12627 ),
 .UNSPECIFIED., .F., .F. ) 
 B_SPLINE_CURVE_WITH_KNOTS ( ( 3, 2, 2, 2, 3 ),
 ( 0.1544266512259456492, 0.1547619047619047672, 0.1607142857142856984, 0.1666666666666666297, 0.1670019202026257477 ),
 .UNSPECIFIED. ) 
 CURVE ( )  GEOMETRIC_REPRESENTATION_ITEM ( )  RATIONAL_B_SPLINE_CURVE ( ( 0.9963778908391762723, 0.9980808541467921513, 1.000000000000000000, 0.9659258262890682012, 1.000000000000000000, 0.9659258262890682012, 1.000000000000000000, 0.9980808541467922623, 0.9963778908391763833 ) ) 
 REPRESENTATION_ITEM ( '' )  );
#15204=ORIENTED_EDGE ( 'NONE', *, *, #55912, .F. ) ;
#15207=CARTESIAN_POINT ( 'NONE',  ( 19.84674366389459621, 8.508931151000785675, 7.409399052514197653E-17 ) ) ;
#15211=CARTESIAN_POINT ( 'NONE',  ( 19.84674366389459266, 28.71726448433411960, -2.638427012816827677 ) ) ;
#15213=CARTESIAN_POINT ( 'NONE',  ( 0.6178305044545818747, 33.49863466993042493, -9.382169495545419124 ) ) ;
#15214=DIRECTION ( 'NONE',  ( 0.000000000000000000, -1.000000000000000000, 0.000000000000000000 ) ) ;
#15218=CARTESIAN_POINT ( 'NONE',  ( -33.19000000000001194, 92.00000000000000000, 9.500000000000000000 ) ) ;
#15219=CARTESIAN_POINT ( 'NONE',  ( 17.20831665107776587, 42.88393115100077324, 7.208316651077764980 ) ) ;
#15220=CARTESIAN_POINT ( 'NONE',  ( 13.79529636645031943, 35.34541550158063927, -14.16423886937409904 ) ) ;
#15221=CARTESIAN_POINT ( 'NONE',  ( 19.84674366389459266, 58.71726448433411605, -2.638427012816827677 ) ) ;
#15223=CARTESIAN_POINT ( 'NONE',  ( 5.076628168052703671, 6.842264484334118713, 8.527530157486179263 ) ) ;
#15224=( NAMED_UNIT ( * ) SI_UNIT ( $, .STERADIAN. ) SOLID_ANGLE_UNIT ( ) );
#15226=CARTESIAN_POINT ( 'NONE',  ( 7.361572987183170547, 47.05059781766745175, 9.846743663894590881 ) ) ;
#15227=CARTESIAN_POINT ( 'NONE',  ( 10.00000000000000000, 51.81368534415484106, -10.88017736071110342 ) ) ;
#15228=CARTESIAN_POINT ( 'NONE',  ( 5.076628168052704559, 45.17559781766745175, -8.527530157486179263 ) ) ;
#15232=CARTESIAN_POINT ( 'NONE',  ( 20.88017736071110875, 45.77201867748816966, -2.915334737309920765 ) ) ;
#15235=CARTESIAN_POINT ( 'NONE',  ( 2.035157376598824452, 33.68868534415484106, 7.964842623401179544 ) ) ;
#15236=CARTESIAN_POINT ( 'NONE',  ( 10.00000000000000178, 67.25893115100079456, 9.846743663894594434 ) ) ;
#15237=CARTESIAN_POINT ( 'NONE',  ( -0.8801773607111008646, 53.27201867748816966, 2.915334737309923430 ) ) ;
#15241=CARTESIAN_POINT ( 'NONE',  ( -46.43608953664445949, 103.5215118185570589, -6.243227838361740112 ) ) ;
#15243=CARTESIAN_POINT ( 'NONE',  ( 19.42250999205614548, 40.98035201082150536, -5.440088680355545492 ) ) ;
#15245=CARTESIAN_POINT ( 'NONE',  ( 14.92337183194729988, 9.342264484334119601, -8.527530157486177487 ) ) ;
#15248=CARTESIAN_POINT ( 'NONE',  ( 19.84674366389459266, 33.71726448433410894, -2.638427012816827677 ) ) ;
#15251=CARTESIAN_POINT ( 'NONE',  ( 6.565887622018943937, -1.918031996736246692, -12.81628187352647608 ) ) ;
#15252=CARTESIAN_POINT ( 'NONE',  ( 19.42250999205614193, 5.147018677488171434, 5.440088680355555262 ) ) ;
#15255=CARTESIAN_POINT ( 'NONE',  ( 22.26659068614894466, 18.88708216824730002, 7.082119434687054849 ) ) ;
#15256=CARTESIAN_POINT ( 'NONE',  ( 20.36894250292379738, 44.92874883491396787, -10.36894250292379027 ) ) ;
#15257=CARTESIAN_POINT ( 'NONE',  ( 2.791683348922237240, 15.38393115100078212, -7.208316651077763204 ) ) ;
#15258=ORIENTED_EDGE ( 'NONE', *, *, #95193, .T. ) ;
#15259=CARTESIAN_POINT ( 'NONE',  ( 17.20831665107776587, 22.88393115100078745, 7.208316651077764980 ) ) ;
#15260=CARTESIAN_POINT ( 'NONE',  ( 20.88017736071110519, 25.56368534415483751, 2.639326808657452039E-16 ) ) ;
#15261=CARTESIAN_POINT ( 'NONE',  ( 12.63842701281683922, 49.55059781766744464, -9.846743663894590881 ) ) ;
#15262=CARTESIAN_POINT ( 'NONE',  ( 13.79529636645030344, 13.26208216824729824, 14.16423886937410614 ) ) ;
#15266=CARTESIAN_POINT ( 'NONE',  ( 18.52753015748617571, 13.09226448433411960, 4.923371831947298993 ) ) ;
#15267=CARTESIAN_POINT ( 'NONE',  ( -1.099225684535947600, 33.70696800326375353, -6.408140936763238038 ) ) ;
#15268=CARTESIAN_POINT ( 'NONE',  ( 18.52753015748617571, 43.09226448433412315, 4.923371831947298993 ) ) ;
#15270=CARTESIAN_POINT ( 'NONE',  ( 10.00000000000000178, 27.25893115100078390, 9.846743663894594434 ) ) ;
#15272=CARTESIAN_POINT ( 'NONE',  ( 0.8801356535991349261, 124.4373638429518962, 4.500000000000000888 ) ) ;
#15273=CARTESIAN_POINT ( 'NONE',  ( 22.26659068614895176, 49.72041550158063927, -7.082119434687042414 ) ) ;
#15274=CARTESIAN_POINT ( 'NONE',  ( 17.96484262340118221, 56.18868534415484817, -7.964842623401177768 ) ) ;
#15277=CARTESIAN_POINT ( 'NONE',  ( 12.63842701281683034, 32.46726448433412315, 9.846743663894596210 ) ) ;
#15278=CARTESIAN_POINT ( 'NONE',  ( 17.96484262340118221, 4.938685344154837509, 7.964842623401181321 ) ) ;
#15279=CARTESIAN_POINT ( 'NONE',  ( 17.20831665107776587, 42.88393115100077324, 7.208316651077764980 ) ) ;
#15281=CARTESIAN_POINT ( 'NONE',  ( 10.00000000000000000, 44.75893115100078745, -9.846743663894594434 ) ) ;
#15282=CARTESIAN_POINT ( 'NONE',  ( 17.96484262340118221, 54.93868534415484106, 7.964842623401181321 ) ) ;
#15284=VERTEX_POINT ( 'NONE', #19085 ) ;
#15286=CARTESIAN_POINT ( 'NONE',  ( 6.565887622018943937, 53.08196800326374643, -12.81628187352647608 ) ) ;
#15288=CARTESIAN_POINT ( 'NONE',  ( 19.84674366389459266, 3.300597817667451750, 2.638427012816836559 ) ) ;
#15289=CARTESIAN_POINT ( 'NONE',  ( 22.81628187352647785, 51.41530133659708923, 3.434112377981063169 ) ) ;
#15290=CARTESIAN_POINT ( 'NONE',  ( -0.8801773607110991993, 7.855352010821506248, -2.915334737309923874 ) ) ;
#15291=CARTESIAN_POINT ( 'NONE',  ( 10.00000000000000000, 49.75893115100078745, -9.846743663894594434 ) ) ;
#15293=CARTESIAN_POINT ( 'NONE',  ( 17.08211943468705840, 30.13708216824730357, -12.26659068614894466 ) ) ;
#15295=CARTESIAN_POINT ( 'NONE',  ( 10.00000000000000178, 63.05374883491396076, 14.16423886937410082 ) ) ;
#15296=CARTESIAN_POINT ( 'NONE',  ( 0.1532563361054100626, 60.80059781766744464, -2.638427012816831230 ) ) ;
#15297=CARTESIAN_POINT ( 'NONE',  ( 19.42250999205614193, 55.14701867748817676, 5.440088680355555262 ) ) ;
#15298=CARTESIAN_POINT ( 'NONE',  ( 18.52753015748618282, 8.925597817667451750, -4.923371831947291888 ) ) ;
#15300=ORIENTED_EDGE ( 'NONE', *, *, #61757, .T. ) ;
#15301=CARTESIAN_POINT ( 'NONE',  ( 3.591859063236763294, 53.29030133659708923, -11.09922568453595026 ) ) ;
#15303=CARTESIAN_POINT ( 'NONE',  ( 10.00000000000000000, 9.758931151000785675, -9.846743663894594434 ) ) ;
#15305=CARTESIAN_POINT ( 'NONE',  ( -2.266590686148945544, 21.38708216824730357, -7.082119434687050408 ) ) ;
#15306=CARTESIAN_POINT ( 'NONE',  ( 18.52753015748618282, 18.92559781766745175, -4.923371831947291888 ) ) ;
#15307=CARTESIAN_POINT ( 'NONE',  ( 17.96484262340118221, 24.93868534415484461, 7.964842623401181321 ) ) ;
#15310=CARTESIAN_POINT ( 'NONE',  ( 20.88017736071110875, 30.77201867748816966, -2.915334737309920765 ) ) ;
#15314=CARTESIAN_POINT ( 'NONE',  ( 4.559911319644449179, 33.89701867748817676, 9.422509992056141925 ) ) ;
#15315=CARTESIAN_POINT ( 'NONE',  ( 1.472469842513823179, 66.42559781766745175, 4.923371831947296329 ) ) ;
#15317=EDGE_CURVE ( 'NONE', #27101, #32140, #29991, .T. ) ;
#15319=CARTESIAN_POINT ( 'NONE',  ( 3.591859063236761518, 14.95696800326375531, 11.09922568453594849 ) ) ;
#15321=CARTESIAN_POINT ( 'NONE',  ( 0.1532563361054083140, 6.008931151000784787, 1.131784320476157264E-15 ) ) ;
#15323=CARTESIAN_POINT ( 'NONE',  ( 20.03743638938530225, 6.751975280310174021, 6.399506433553884932 ) ) ;
#15324=CARTESIAN_POINT ( 'NONE',  ( 14.92337183194729633, 12.67559781766745353, 8.527530157486181039 ) ) ;
#15325=CARTESIAN_POINT ( 'NONE',  ( -0.8801773607110991993, 27.85535201082150181, -2.915334737309923874 ) ) ;
#15330=CARTESIAN_POINT ( 'NONE',  ( -2.816281873526473856, 64.12363466993042493, 9.499525473075851096E-16 ) ) ;
#15331=CARTESIAN_POINT ( 'NONE',  ( 2.035157376598822676, 57.43868534415484106, -7.964842623401177768 ) ) ;
#15334=CARTESIAN_POINT ( 'NONE',  ( 0.6178305044545818747, 58.49863466993042493, -9.382169495545419124 ) ) ;
#15335=CARTESIAN_POINT ( 'NONE',  ( 7.084665262690076126, 64.10535201082150536, 10.88017736071109987 ) ) ;
#15336=CARTESIAN_POINT ( 'NONE',  ( 2.791683348922237240, 65.38393115100078035, -7.208316651077763204 ) ) ;
#15338=CARTESIAN_POINT ( 'NONE',  ( 19.84674366389459266, 28.71726448433411960, -2.638427012816827677 ) ) ;
#15339=CARTESIAN_POINT ( 'NONE',  ( 19.38216949554541202, 55.99863466993041072, 9.382169495545424454 ) ) ;
#15340=LINE ( 'NONE', #68327, #96044 ) ;
#15341=CARTESIAN_POINT ( 'NONE',  ( 2.791683348922240793, 6.633931151000785675, 7.208316651077764092 ) ) ;
#15342=CARTESIAN_POINT ( 'NONE',  ( 6.565887622018943937, 25.16530133659708213, 12.81628187352647430 ) ) ;
#15343=CARTESIAN_POINT ( 'NONE',  ( -46.56032276184168950, 103.8061269828102837, 5.692785089662784515 ) ) ;
#15344=CARTESIAN_POINT ( 'NONE',  ( -42.16485527613927076, 107.5383484153110061, 4.500000000000000888 ) ) ;
#15345=CARTESIAN_POINT ( 'NONE',  ( 0.5774900079438607392, 33.48035201082150536, 5.440088680355550821 ) ) ;
#15346=CARTESIAN_POINT ( 'NONE',  ( -2.816281873526473856, -0.6680319967362464695, 3.434112377981055619 ) ) ;
#15347=CARTESIAN_POINT ( 'NONE',  ( 1.472469842513823179, 20.59226448433411960, -4.923371831947296329 ) ) ;
#15348=CARTESIAN_POINT ( 'NONE',  ( 1.472469842513823179, 6.425597817667451750, 4.923371831947296329 ) ) ;
#15349=CARTESIAN_POINT ( 'NONE',  ( 19.42250999205614193, 15.14701867748817143, 5.440088680355555262 ) ) ;
#15350=CARTESIAN_POINT ( 'NONE',  ( 16.40814093676324603, 12.45696800326375353, -11.09922568453594671 ) ) ;
#15351=ORIENTED_EDGE ( 'NONE', *, *, #54980, .F. ) ;
#15355=CARTESIAN_POINT ( 'NONE',  ( 19.42250999205614193, 10.14701867748816966, 5.440088680355555262 ) ) ;
#15356=CARTESIAN_POINT ( 'NONE',  ( 19.84674366389459266, 43.30059781766744464, 2.638427012816836559 ) ) ;
#15359=CARTESIAN_POINT ( 'NONE',  ( -4.164238869374099039, 66.80374883491396076, 8.674139862899312516E-16 ) ) ;
#15360=CARTESIAN_POINT ( 'NONE',  ( 4.559911319644449179, 32.23035201082150536, -9.422509992056141925 ) ) ;
#15361=CARTESIAN_POINT ( 'NONE',  ( 20.36894250292379738, 59.92874883491397497, -10.36894250292379027 ) ) ;
#15363=CARTESIAN_POINT ( 'NONE',  ( 12.63842701281683034, 7.467264484334118713, 9.846743663894596210 ) ) ;
#15364=CARTESIAN_POINT ( 'NONE',  ( 10.00000000000000178, 22.25893115100078745, 9.846743663894594434 ) ) ;
#15365=CARTESIAN_POINT ( 'NONE',  ( 13.43411237798106583, 7.665301336597086568, -12.81628187352647252 ) ) ;
#15366=CARTESIAN_POINT ( 'NONE',  ( -46.48622585131851537, 103.4028339409962172, 6.319095158313501770 ) ) ;
#15372=CARTESIAN_POINT ( 'NONE',  ( -0.3689425029237898834, 16.17874883491396076, -10.36894250292378850 ) ) ;
#15373=CARTESIAN_POINT ( 'NONE',  ( 10.00000000000000178, 27.25893115100078390, 9.846743663894594434 ) ) ;
#15376=CARTESIAN_POINT ( 'NONE',  ( 13.79529636645030344, 53.26208216824730357, 14.16423886937410614 ) ) ;
#15377=CARTESIAN_POINT ( 'NONE',  ( 10.00000000000000000, 4.758931151000784787, -9.846743663894594434 ) ) ;
#15378=CARTESIAN_POINT ( 'NONE',  ( 2.035157376598824452, 38.68868534415483396, 7.964842623401179544 ) ) ;
#15379=CARTESIAN_POINT ( 'NONE',  ( 3.591859063236763294, 48.29030133659708923, -11.09922568453595026 ) ) ;
#15380=CARTESIAN_POINT ( 'NONE',  ( -0.8801773607110991993, 12.85535201082150358, -2.915334737309923874 ) ) ;
#15381=CARTESIAN_POINT ( 'NONE',  ( 19.38216949554541202, 50.99863466993042493, 9.382169495545424454 ) ) ;
#15382=CARTESIAN_POINT ( 'NONE',  ( 5.076628168052703671, 61.84226448433412315, 8.527530157486179263 ) ) ;
#15383=SURFACE_STYLE_USAGE ( .BOTH. , #22385 ) ;
#15385=CARTESIAN_POINT ( 'NONE',  ( 1.383448333479229797, 12.37718327197428536, -6.499999999999972466 ) ) ;
#15387=CARTESIAN_POINT ( 'NONE',  ( 17.08211943468705840, 45.13708216824730357, -12.26659068614894466 ) ) ;
#15388=CARTESIAN_POINT ( 'NONE',  ( 10.00000000000000000, 20.55374883491396787, -14.16423886937410082 ) ) ;
#15389=CARTESIAN_POINT ( 'NONE',  ( 10.00000000000000000, 11.81368534415483751, -10.88017736071110342 ) ) ;
#15390=CARTESIAN_POINT ( 'NONE',  ( 20.88017736071110164, 35.35535201082150536, 2.915334737309930979 ) ) ;
#15393=CARTESIAN_POINT ( 'NONE',  ( 14.92337183194729633, 2.675597817667451750, 8.527530157486181039 ) ) ;
#15394=CARTESIAN_POINT ( 'NONE',  ( -0.8801773607111008646, 68.27201867748817676, 2.915334737309923430 ) ) ;
#15395=CARTESIAN_POINT ( 'NONE',  ( 19.38216949554541557, 32.24863466993041783, -9.382169495545420901 ) ) ;
#15396=DIRECTION ( 'NONE',  ( -0.000000000000000000, 1.000000000000000000, 0.000000000000000000 ) ) ;
#15397=CARTESIAN_POINT ( 'NONE',  ( 0.1143410931637246636, 30.21691075486303291, 6.480892540919863443 ) ) ;
#15398=CARTESIAN_POINT ( 'NONE',  ( 12.63842701281683922, 39.55059781766744464, -9.846743663894590881 ) ) ;
#15399=CARTESIAN_POINT ( 'NONE',  ( 0.5774900079438607392, 8.480352010821505360, 5.440088680355550821 ) ) ;
#15402=VECTOR ( 'NONE', #44828, 1000.000000000000000 ) ;
#15405=CARTESIAN_POINT ( 'NONE',  ( 10.00000000000000178, 15.37363466993042138, 12.81628187352647608 ) ) ;
#15406=CARTESIAN_POINT ( 'NONE',  ( 7.361572987183169658, 14.96726448433411960, -9.846743663894592657 ) ) ;
#15407=CARTESIAN_POINT ( 'NONE',  ( 2.035157376598824452, 3.688685344154837953, 7.964842623401179544 ) ) ;
#15409=CARTESIAN_POINT ( 'NONE',  ( 2.791683348922237240, 40.38393115100078035, -7.208316651077763204 ) ) ;
#15410=CARTESIAN_POINT ( 'NONE',  ( 3.591859063236761518, 59.95696800326375353, 11.09922568453594849 ) ) ;
#15411=CARTESIAN_POINT ( 'NONE',  ( 18.52753015748617571, 18.09226448433411960, 4.923371831947298993 ) ) ;
#15412=CARTESIAN_POINT ( 'NONE',  ( -0.3689425029237898834, 1.178748834913967869, -10.36894250292378850 ) ) ;
#15414=CARTESIAN_POINT ( 'NONE',  ( 20.36894250292379382, 8.678748834913967869, 10.36894250292379205 ) ) ;
#15416=CARTESIAN_POINT ( 'NONE',  ( 17.96484262340118221, 29.93868534415484106, 7.964842623401181321 ) ) ;
#15417=CARTESIAN_POINT ( 'NONE',  ( -0.8801773607110991993, 17.85535201082150536, -2.915334737309923874 ) ) ;
#15418=CARTESIAN_POINT ( 'NONE',  ( 24.16423886937410614, 44.30374883491397497, 8.672049930838204340E-16 ) ) ;
#15419=CARTESIAN_POINT ( 'NONE',  ( 0.5774900079438590739, 27.64701867748817676, -5.440088680355550821 ) ) ;
#15420=CARTESIAN_POINT ( 'NONE',  ( 20.88017736071110164, 20.35535201082150891, 2.915334737309930979 ) ) ;
#15421=ORIENTED_EDGE ( 'NONE', *, *, #46150, .T. ) ;
#15422=( BOUNDED_CURVE ( )  B_SPLINE_CURVE ( 2, ( #40503, #3972, #87945, #4472, #40995, #86964, #65436, #42460, #71492 ),
 .UNSPECIFIED., .F., .F. ) 
 B_SPLINE_CURVE_WITH_KNOTS ( ( 3, 2, 2, 2, 3 ),
 ( 0.9391432315068940495, 0.9404761904761904656, 0.9464285714285713969, 0.9523809523809523281, 0.9537139113502488552 ),
 .UNSPECIFIED. ) 
 CURVE ( )  GEOMETRIC_REPRESENTATION_ITEM ( )  RATIONAL_B_SPLINE_CURVE ( ( 0.9881565478350733400, 0.9923695281211490915, 1.000000000000000000, 0.9659258262890683122, 1.000000000000000000, 0.9659258262890683122, 1.000000000000000000, 0.9923695281211485364, 0.9881565478350726739 ) ) 
 REPRESENTATION_ITEM ( '' )  );
#15423=CARTESIAN_POINT ( 'NONE',  ( -0.8801773607110991993, 42.85535201082150536, -2.915334737309923874 ) ) ;
#15424=CARTESIAN_POINT ( 'NONE',  ( 22.81628187352648496, 56.83196800326374643, -3.434112377981050290 ) ) ;
#15425=CARTESIAN_POINT ( 'NONE',  ( 20.88017736071110519, 45.56368534415484106, 2.639326808657452039E-16 ) ) ;
#15426=AXIS2_PLACEMENT_3D ( 'NONE', #7730, #61202, #31678 ) ;
#15428=CARTESIAN_POINT ( 'NONE',  ( 0.5774900079438590739, 52.64701867748817676, -5.440088680355550821 ) ) ;
#15431=CARTESIAN_POINT ( 'NONE',  ( 12.91533473730993009, 56.60535201082151247, -10.88017736071109987 ) ) ;
#15432=CARTESIAN_POINT ( 'NONE',  ( -1.926860441876562025, 24.47997603579417358, -3.195792623639529761 ) ) ;
#15433=CARTESIAN_POINT ( 'NONE',  ( 22.26659068614895176, 44.72041550158063927, -7.082119434687042414 ) ) ;
#15434=CARTESIAN_POINT ( 'NONE',  ( 2.035157376598824452, 68.68868534415484817, 7.964842623401179544 ) ) ;
#15436=CARTESIAN_POINT ( 'NONE',  ( 12.63842701281683034, 57.46726448433411605, 9.846743663894596210 ) ) ;
#15437=FILL_AREA_STYLE_COLOUR ( '', #98788 ) ;
#15438=CARTESIAN_POINT ( 'NONE',  ( 5.076628168052703671, 36.84226448433412315, 8.527530157486179263 ) ) ;
#15439=CARTESIAN_POINT ( 'NONE',  ( 12.63842701281683922, 39.55059781766744464, -9.846743663894590881 ) ) ;
#15441=CARTESIAN_POINT ( 'NONE',  ( 17.96484262340118221, 34.93868534415482685, 7.964842623401181321 ) ) ;
#15442=CARTESIAN_POINT ( 'NONE',  ( 19.84674366389459621, 43.50893115100078745, 7.409399052514197653E-17 ) ) ;
#15443=CARTESIAN_POINT ( 'NONE',  ( 21.09922568453595559, 22.04030133659708923, -6.408140936763230044 ) ) ;
#15445=CARTESIAN_POINT ( 'NONE',  ( 19.42250999205614548, 40.98035201082150536, -5.440088680355545492 ) ) ;
#15446=CARTESIAN_POINT ( 'NONE',  ( 20.88017736071110875, 5.772018677488170546, -2.915334737309920765 ) ) ;
#15447=CARTESIAN_POINT ( 'NONE',  ( 6.204703633549690345, 55.76208216824730357, -14.16423886937410259 ) ) ;
#15448=STYLED_ITEM ( 'NONE', ( #79981 ), #55723 ) ;
#15450=CARTESIAN_POINT ( 'NONE',  ( -2.816281873526471635, 28.91530133659708213, -3.434112377981056508 ) ) ;
#15453=CARTESIAN_POINT ( 'NONE',  ( -2.816281873526471635, 13.91530133659708746, -3.434112377981056508 ) ) ;
#15454=CARTESIAN_POINT ( 'NONE',  ( -0.8801773607111008646, 23.27201867748817676, 2.915334737309923430 ) ) ;
#15455=CARTESIAN_POINT ( 'NONE',  ( 20.88017736071110875, 65.77201867748817676, -2.915334737309920765 ) ) ;
#15457=CARTESIAN_POINT ( 'NONE',  ( 10.00000000000000178, 54.31368534415484106, 10.88017736071110342 ) ) ;
#15458=CARTESIAN_POINT ( 'NONE',  ( 1.472469842513823179, 45.59226448433412315, -4.923371831947296329 ) ) ;
#15459=CARTESIAN_POINT ( 'NONE',  ( 5.076628168052703671, 21.84226448433411960, 8.527530157486179263 ) ) ;
#15460=CARTESIAN_POINT ( 'NONE',  ( 12.63842701281683034, 22.46726448433411605, 9.846743663894596210 ) ) ;
#15461=CARTESIAN_POINT ( 'NONE',  ( 6.000000000000000000, 11.50000000000000000, 5.000000000000000000 ) ) ;
#15463=CARTESIAN_POINT ( 'NONE',  ( 16.40814093676324603, 42.45696800326375353, -11.09922568453594671 ) ) ;
#15464=CARTESIAN_POINT ( 'NONE',  ( 17.20831665107776587, 19.13393115100078035, -7.208316651077762316 ) ) ;
#15468=CARTESIAN_POINT ( 'NONE',  ( 19.84674366389459621, 33.50893115100078745, 7.409399052514197653E-17 ) ) ;
#15470=LINE ( 'NONE', #479, #94882 ) ;
#15471=CARTESIAN_POINT ( 'NONE',  ( 22.81628187352647785, 6.415301336597088344, 3.434112377981063169 ) ) ;
#15472=CARTESIAN_POINT ( 'NONE',  ( 19.42250999205614193, 50.14701867748817676, 5.440088680355555262 ) ) ;
#15473=CARTESIAN_POINT ( 'NONE',  ( 13.79529636645030344, 33.26208216824730357, 14.16423886937410614 ) ) ;
#15475=CARTESIAN_POINT ( 'NONE',  ( 6.204703633549690345, 25.76208216824730712, -14.16423886937410259 ) ) ;
#15476=CARTESIAN_POINT ( 'NONE',  ( 2.917880565312948704, 62.63708216824730357, 12.26659068614894643 ) ) ;
#15477=CARTESIAN_POINT ( 'NONE',  ( 2.917880565312950480, 10.97041550158063572, -12.26659068614894821 ) ) ;
#15478=CARTESIAN_POINT ( 'NONE',  ( 17.08211943468705840, 30.13708216824730357, -12.26659068614894466 ) ) ;
#15479=CARTESIAN_POINT ( 'NONE',  ( -0.2418659066527643342, 37.23410085661203794, -6.114288769123057854 ) ) ;
#15480=CARTESIAN_POINT ( 'NONE',  ( 10.00000000000000000, 51.81368534415484106, -10.88017736071110342 ) ) ;
#15483=CARTESIAN_POINT ( 'NONE',  ( 19.84674366389459266, 43.71726448433410894, -2.638427012816827677 ) ) ;
#15486=CARTESIAN_POINT ( 'NONE',  ( 19.84674366389459266, 58.71726448433411605, -2.638427012816827677 ) ) ;
#15489=CARTESIAN_POINT ( 'NONE',  ( -1.099225684535947600, 58.70696800326375353, -6.408140936763238038 ) ) ;
#15492=CARTESIAN_POINT ( 'NONE',  ( 0.1532563361054082862, 41.21726448433411605, 2.638427012816831674 ) ) ;
#15493=CARTESIAN_POINT ( 'NONE',  ( 7.361572987183169658, 54.96726448433413026, -9.846743663894592657 ) ) ;
#15494=CARTESIAN_POINT ( 'NONE',  ( -0.3689425029237898834, 36.17874883491396787, -10.36894250292378850 ) ) ;
#15496=ORIENTED_EDGE ( 'NONE', *, *, #26882, .F. ) ;
#15497=CARTESIAN_POINT ( 'NONE',  ( 20.36894250292379382, 18.67874883491397142, 10.36894250292379205 ) ) ;
#15498=CARTESIAN_POINT ( 'NONE',  ( 10.00000000000000178, 59.31368534415484106, 10.88017736071110342 ) ) ;
#15500=CARTESIAN_POINT ( 'NONE',  ( 13.79529636645030344, 58.26208216824728936, 14.16423886937410614 ) ) ;
#15501=CARTESIAN_POINT ( 'NONE',  ( 16.40814093676323893, 15.79030133659708746, 11.09922568453595026 ) ) ;
#15503=CARTESIAN_POINT ( 'NONE',  ( 5.076628168052703671, 1.842264484334118047, 8.527530157486179263 ) ) ;
#15504=CARTESIAN_POINT ( 'NONE',  ( -0.1503990784575287842, 28.10158574516642815, 6.262539305110075283 ) ) ;
#15505=CARTESIAN_POINT ( 'NONE',  ( 1.959929470562269183, 30.51528370094808196, -5.767676674365832312 ) ) ;
#15506=CARTESIAN_POINT ( 'NONE',  ( 21.09922568453594849, 31.20696800326375353, 6.408140936763242479 ) ) ;
#15507=CARTESIAN_POINT ( 'NONE',  ( 24.16423886937410614, 59.51208216824728936, -3.795296366450302550 ) ) ;
#15509=CARTESIAN_POINT ( 'NONE',  ( 17.96484262340118221, 16.18868534415483396, -7.964842623401177768 ) ) ;
#15510=CARTESIAN_POINT ( 'NONE',  ( -0.8801773607111009756, 28.06368534415484106, 1.068504757029289695E-15 ) ) ;
#15511=CARTESIAN_POINT ( 'NONE',  ( 5.076628168052703671, 51.84226448433412315, 8.527530157486179263 ) ) ;
#15512=CARTESIAN_POINT ( 'NONE',  ( 18.52753015748617571, 58.09226448433411605, 4.923371831947298993 ) ) ;
#15513=CARTESIAN_POINT ( 'NONE',  ( 16.40814093676324603, 52.45696800326375353, -11.09922568453594671 ) ) ;
#15516=CARTESIAN_POINT ( 'NONE',  ( 12.91533473730992121, 14.52201867748817143, 10.88017736071110164 ) ) ;
#15517=CARTESIAN_POINT ( 'NONE',  ( 3.591859063236761518, 14.95696800326375531, 11.09922568453594849 ) ) ;
#15520=CARTESIAN_POINT ( 'NONE',  ( 17.20831665107776587, 47.88393115100078745, 7.208316651077764980 ) ) ;
#15521=CARTESIAN_POINT ( 'NONE',  ( 19.42250999205614193, 55.14701867748817676, 5.440088680355555262 ) ) ;
#15523=CARTESIAN_POINT ( 'NONE',  ( -1.099225684535947600, 18.70696800326375353, -6.408140936763238038 ) ) ;
#15524=CARTESIAN_POINT ( 'NONE',  ( 2.035157376598824452, 53.68868534415484817, 7.964842623401179544 ) ) ;
#15526=( BOUNDED_SURFACE ( )  B_SPLINE_SURFACE ( 1, 2, ( 
 ( #89456, #36459, #66954, #39798, #70298, #78272, #10771, #25295, #55782, #41768, #18770, #25781, #32268, #18273, #56275, #47275, #86277, #63748, #86770, #40780, #72239, #33734, #62274, #26254, #92780, #1813, #33257, #71280, #79260, #62777, #24799, #55276, #17786, #64235, #9786, #2310, #48752, #93276, #78774, #49252, #24311, #3270, #79752, #3772, #70793, #48261, #94253, #10280, #32765, #41286, #2802, #85786, #71760, #94752, #63260, #17299, #16799, #11250, #93769, #54776, #85292, #47774, #56751, #77776, #40285, #87244, #9289, #12725, #66722, #27230, #50222, #35725, #57725, #43220, #51727, #95746, #74201, #36221, #88228, #65719, #20233, #89223, #72723, #88722, #19246, #4257, #28220, #96744, #82209, #34728, #20732, #80736, #19737, #44203, #96245, #89709, #13221, #13719, #81707, #74713, #66213, #51223, #95233, #58718, #11745, #27725, #12231, #58205, #42253, #42740, #34226, #97246, #35219, #43717, #50737, #73221, #73714, #5735, #4749, #65219, #28715, #59206, #81226, #26741, #21223, #5247, #64723, #57236, #87734, #49730, #80237, #98231, #60690, #8202, #22225, #45204, #30680, #6713, #22715, #61666, #6223, #46198, #92185, #46675, #14728, #91190, #7718, #53199, #75703, #76199, #83703, #29692, #68700, #68217, #7214, #37230, #59703, #23711, #37715, #36727, #67218, #44703, #98738, #97741, #60201, #90696, #23213, #15220, #38697, #52701, #83206, #38215, #30189, #45699, #54172, #67718, #76682, #69196, #232, #61188, #91694, #53686, #75203, #84204, #90200, #15712, #721, #31175, #84683, #16193, #29204, #21730, #52212, #82706, #14224, #33620, #56160, #26146, #25667, #56640, #10165, #33137, #39193, #40663, #54660, #70672, #55152, #40167, #85176, #32151, #77173, #79140, #78160, #63632, #2192, #62653, #55664, #86653, #39691, #16686, #94139, #18158, #32654, #69681, #78660, #24681, #64119, #87125, #86163, #47156, #71161, #77659, #9173, #93157, #48636, #63148, #93650, #18646, #94636, #2686, #70179, #10651, #41166, #62157, #25184, #71650, #3158, #17673, #8681, #1212, #31667, #92663, #24191, #1695, #48146, #85666, #17186, #47666, #9670, #58095, #5121, #36095, #5619, #97130, #11627, #51104, #57612, #20615, #35609, #19620, #11136, #96127, #27608, #66602, #50614, #66095, #42620, #57120, #28600, #42143, #88111, #41655, #4637, #59089, #49135, #80119, #43598, #79637, #19131, #88600, #72122, #3650, #87618, #20110, #34115, #43107, #96624, #74086, #72607, #27113, #89598, #81591, #4142, #81105, #13102, #12606, #73594, #50114, #28099, #58600, #89102, #64607, #49609, #95115, #26623, #34607, #65103, #95624, #80624, #12118, #73099, #35101, #65599, #90574, #51606 ),
 ( #76070, #83583, #6105, #14610, #22594, #15100, #98619, #612, #91576, #21107, #84077, #82090, #97622, #91068, #30067, #38096, #59587, #82589, #14103, #75582, #23093, #37103, #60073, #45576, #21610, #37596, #76565, #13601, #61066, #8081, #61556, #29569, #7094, #53071, #68090, #22100, #7600, #60577, #44586, #68583, #83083, #52580, #52095, #74591, #38577, #45077, #44081, #36610, #90083, #114, #67097, #75085, #6591, #29085, #67600, #30560, #53563, #15592, #98107, #46076, #69075, #31056, #94032, #9058, #32031, #17560, #92545, #9548, #48521, #92064, #33029, #79023, #33507, #1582, #47548, #93534, #40050, #62535, #63036, #78046, #16570, #55549, #55035, #93041, #24074, #46558, #10535, #24575, #23592, #54056, #31549, #85553, #84570, #85057, #47043, #10050, #70550, #25553, #77540, #39571, #25064, #70060, #2078, #41045, #54541, #63525, #56045, #17066, #32538, #86049, #48027, #62045, #78539, #77057, #40549, #71049, #2572, #71544, #86538, #18043, #3053, #16071, #8569, #39074, #69567, #1087, #12983, #12497, #43479, #96009, #19995, #26036, #27494, #41544, #57501, #42033, #27004, #72008, #19023, #64005, #65985, #64985, #50497, #87996, #49500, #42508, #42996, #26512, #3539, #80994, #5007, #19509, #56528, #65489, #11510, #20498, #73981, #72992, #33999, #57987, #64497, #95004, #80005, #73478, #50004, #80510, #5506, #50986, #88492, #57007, #35490, #96512, #49018, #12007, #27983, #58480, #4522, #94517, #88993, #87017, #81480, #87509, #72497, #4030, #34985, #18528, #34493, #95510, #79525, #11026, #52466, #91454, #35980, #75956, #22980, #76452, #44468, #90453, #37484, #82969, #74970, #6979, #21990, #59469, #98498, #97999, #6475, #36489, #89484, #53445, #36979, #66482, #97010, #74470, #29453, #28488, #28966, #89971, #52953, #14488, #68471, #21487, #51984, #67973, #82472, #44960, #83954, #97502, #7484, #37981, #13993, #67478, #75463, #90948, #5994, #29953, #20995, #66980, #60458, #22478, #15480, #59961, #83464, #14985, #45456, #45963, #34337, #58981, #30444, #51482, #60944, #81976, #13488, #43966, #68958, #41304, #85804, #2819, #86294, #71299, #17314, #63279, #7968, #11266, #10299, #64253, #33269, #93785, #86787, #56768, #70811, #47790, #94768, #49268, #63763, #490, #10786, #55800, #64742, #57252, #18289, #78288, #71777, #9804, #40305, #25314, #87264, #94270, #25794, #87749, #95254, #3286, #2326, #26267, #33751, #93292, #56293, #18785, #79768, #48772, #19263, #41786, #38466, #72258, #30939, #32782, #79277, #3787, #34242, #62792, #26760, #17801, #49747, #48279, #24816, #78791, #40798, #55292, #82223, #81239, #36239, #43237, #65736, #58733, #28729 ) ),
 .UNSPECIFIED., .F., .F., .F. ) 
 B_SPLINE_SURFACE_WITH_KNOTS ( ( 2, 2 ),
 ( 3, 2, 2, 2, 2, 2, 2, 2, 2, 2, 2, 2, 2, 2, 2, 2, 2, 2, 2, 2, 2, 2, 2, 2, 2, 2, 2, 2, 2, 2, 2, 2, 2, 2, 2, 2, 2, 2, 2, 2, 2, 2, 2, 2, 2, 2, 2, 2, 2, 2, 2, 2, 2, 2, 2, 2, 2, 2, 2, 2, 2, 2, 2, 2, 2, 2, 2, 2, 2, 2, 2, 2, 2, 2, 2, 2, 2, 2, 2, 2, 2, 2, 2, 2, 2, 2, 2, 2, 2, 2, 2, 2, 2, 2, 2, 2, 2, 2, 2, 2, 2, 2, 2, 2, 2, 2, 2, 2, 2, 2, 2, 2, 2, 2, 2, 2, 2, 2, 2, 2, 2, 2, 2, 2, 2, 2, 2, 2, 2, 2, 2, 2, 2, 2, 2, 2, 2, 2, 2, 2, 2, 2, 2, 2, 2, 2, 2, 2, 2, 2, 2, 2, 2, 2, 2, 2, 2, 2, 2, 2, 2, 2, 3 ),
 ( 0.000000000000000000, 1.000000000000000000 ),
 ( 0.000000000000000000, 0.005952380952380952051, 0.01190476190476190410, 0.01785714285714285615, 0.02380952380952380820, 0.02976190476190476025, 0.03571428571428571230, 0.04166666666666666435, 0.04761904761904761640, 0.05357142857142856845, 0.05952380952380952051, 0.06547619047619047949, 0.07142857142857142461, 0.07738095238095238360, 0.08333333333333332871, 0.08928571428571428770, 0.09523809523809523281, 0.1011904761904761918, 0.1071428571428571369, 0.1130952380952380959, 0.1190476190476190410, 0.1250000000000000000, 0.1309523809523809590, 0.1369047619047619180, 0.1428571428571428492, 0.1488095238095238082, 0.1547619047619047672, 0.1607142857142857262, 0.1666666666666666574, 0.1726190476190476164, 0.1785714285714285754, 0.1845238095238095344, 0.1904761904761904656, 0.1964285714285714246, 0.2023809523809523836, 0.2083333333333333426, 0.2142857142857142738, 0.2202380952380952328, 0.2261904761904761918, 0.2321428571428571508, 0.2380952380952380820, 0.2440476190476190410, 0.2500000000000000000, 0.2559523809523809312, 0.2619047619047619180, 0.2678571428571428492, 0.2738095238095238360, 0.2797619047619047672, 0.2857142857142856984, 0.2916666666666666852, 0.2976190476190476164, 0.3035714285714285476, 0.3095238095238095344, 0.3154761904761904656, 0.3214285714285714524, 0.3273809523809523836, 0.3333333333333333148, 0.3392857142857143016, 0.3452380952380952328, 0.3511904761904761640, 0.3571428571428571508, 0.3630952380952380820, 0.3690476190476190688, 0.3750000000000000000, 0.3809523809523809312, 0.3869047619047619180, 0.3928571428571428492, 0.3988095238095238360, 0.4047619047619047672, 0.4107142857142856984, 0.4166666666666666852, 0.4226190476190476164, 0.4285714285714285476, 0.4345238095238095344, 0.4404761904761904656, 0.4464285714285714524, 0.4523809523809523836, 0.4583333333333333148, 0.4642857142857143016, 0.4702380952380952328, 0.4761904761904761640, 0.4821428571428571508, 0.4880952380952380820, 0.4940476190476190688, 0.5000000000000000000, 0.5059523809523809312, 0.5119047619047618625, 0.5178571428571429047, 0.5238095238095238360, 0.5297619047619047672, 0.5357142857142856984, 0.5416666666666666297, 0.5476190476190476719, 0.5535714285714286031, 0.5595238095238095344, 0.5654761904761904656, 0.5714285714285713969, 0.5773809523809523281, 0.5833333333333333703, 0.5892857142857143016, 0.5952380952380952328, 0.6011904761904761640, 0.6071428571428570953, 0.6130952380952381375, 0.6190476190476190688, 0.6250000000000000000, 0.6309523809523809312, 0.6369047619047618625, 0.6428571428571429047, 0.6488095238095238360, 0.6547619047619047672, 0.6607142857142856984, 0.6666666666666666297, 0.6726190476190476719, 0.6785714285714286031, 0.6845238095238095344, 0.6904761904761904656, 0.6964285714285713969, 0.7023809523809523281, 0.7083333333333333703, 0.7142857142857143016, 0.7202380952380952328, 0.7261904761904761640, 0.7321428571428570953, 0.7380952380952381375, 0.7440476190476190688, 0.7500000000000000000, 0.7559523809523809312, 0.7619047619047618625, 0.7678571428571429047, 0.7738095238095238360, 0.7797619047619047672, 0.7857142857142856984, 0.7916666666666666297, 0.7976190476190476719, 0.8035714285714286031, 0.8095238095238095344, 0.8154761904761904656, 0.8214285714285713969, 0.8273809523809523281, 0.8333333333333333703, 0.8392857142857143016, 0.8452380952380952328, 0.8511904761904761640, 0.8571428571428570953, 0.8630952380952381375, 0.8690476190476190688, 0.8750000000000000000, 0.8809523809523809312, 0.8869047619047618625, 0.8928571428571429047, 0.8988095238095238360, 0.9047619047619047672, 0.9107142857142856984, 0.9166666666666666297, 0.9226190476190476719, 0.9285714285714286031, 0.9345238095238095344, 0.9404761904761904656, 0.9464285714285713969, 0.9523809523809523281, 0.9583333333333333703, 0.9642857142857143016 ),
 .UNSPECIFIED. ) 
 GEOMETRIC_REPRESENTATION_ITEM ( )  RATIONAL_B_SPLINE_SURFACE ( (
 ( 1.000000000000000000, 0.9659258262890683122, 1.000000000000000000, 0.9659258262890683122, 1.000000000000000000, 0.9659258262890683122, 1.000000000000000000, 0.9659258262890683122, 1.000000000000000000, 0.9659258262890683122, 1.000000000000000000, 0.9659258262890683122, 1.000000000000000000, 0.9659258262890683122, 1.000000000000000000, 0.9659258262890683122, 1.000000000000000000, 0.9659258262890683122, 1.000000000000000000, 0.9659258262890683122, 1.000000000000000000, 0.9659258262890683122, 1.000000000000000000, 0.9659258262890683122, 1.000000000000000000, 0.9659258262890683122, 1.000000000000000000, 0.9659258262890683122, 1.000000000000000000, 0.9659258262890683122, 1.000000000000000000, 0.9659258262890683122, 1.000000000000000000, 0.9659258262890683122, 1.000000000000000000, 0.9659258262890683122, 1.000000000000000000, 0.9659258262890683122, 1.000000000000000000, 0.9659258262890683122, 1.000000000000000000, 0.9659258262890683122, 1.000000000000000000, 0.9659258262890683122, 1.000000000000000000, 0.9659258262890683122, 1.000000000000000000, 0.9659258262890683122, 1.000000000000000000, 0.9659258262890683122, 1.000000000000000000, 0.9659258262890683122, 1.000000000000000000, 0.9659258262890683122, 1.000000000000000000, 0.9659258262890683122, 1.000000000000000000, 0.9659258262890683122, 1.000000000000000000, 0.9659258262890683122, 1.000000000000000000, 0.9659258262890683122, 1.000000000000000000, 0.9659258262890683122, 1.000000000000000000, 0.9659258262890683122, 1.000000000000000000, 0.9659258262890683122, 1.000000000000000000, 0.9659258262890683122, 1.000000000000000000, 0.9659258262890683122, 1.000000000000000000, 0.9659258262890683122, 1.000000000000000000, 0.9659258262890683122, 1.000000000000000000, 0.9659258262890683122, 1.000000000000000000, 0.9659258262890683122, 1.000000000000000000, 0.9659258262890683122, 1.000000000000000000, 0.9659258262890683122, 1.000000000000000000, 0.9659258262890683122, 1.000000000000000000, 0.9659258262890683122, 1.000000000000000000, 0.9659258262890683122, 1.000000000000000000, 0.9659258262890683122, 1.000000000000000000, 0.9659258262890683122, 1.000000000000000000, 0.9659258262890683122, 1.000000000000000000, 0.9659258262890683122, 1.000000000000000000, 0.9659258262890683122, 1.000000000000000000, 0.9659258262890683122, 1.000000000000000000, 0.9659258262890683122, 1.000000000000000000, 0.9659258262890683122, 1.000000000000000000, 0.9659258262890683122, 1.000000000000000000, 0.9659258262890683122, 1.000000000000000000, 0.9659258262890683122, 1.000000000000000000, 0.9659258262890683122, 1.000000000000000000, 0.9659258262890683122, 1.000000000000000000, 0.9659258262890683122, 1.000000000000000000, 0.9659258262890683122, 1.000000000000000000, 0.9659258262890683122, 1.000000000000000000, 0.9659258262890683122, 1.000000000000000000, 0.9659258262890683122, 1.000000000000000000, 0.9659258262890683122, 1.000000000000000000, 0.9659258262890683122, 1.000000000000000000, 0.9659258262890683122, 1.000000000000000000, 0.9659258262890683122, 1.000000000000000000, 0.9659258262890683122, 1.000000000000000000, 0.9659258262890683122, 1.000000000000000000, 0.9659258262890683122, 1.000000000000000000, 0.9659258262890683122, 1.000000000000000000, 0.9659258262890683122, 1.000000000000000000, 0.9659258262890683122, 1.000000000000000000, 0.9659258262890683122, 1.000000000000000000, 0.9659258262890683122, 1.000000000000000000, 0.9659258262890683122, 1.000000000000000000, 0.9659258262890683122, 1.000000000000000000, 0.9659258262890683122, 1.000000000000000000, 0.9659258262890683122, 1.000000000000000000, 0.9659258262890683122, 1.000000000000000000, 0.9659258262890683122, 1.000000000000000000, 0.9659258262890683122, 1.000000000000000000, 0.9659258262890683122, 1.000000000000000000, 0.9659258262890683122, 1.000000000000000000, 0.9659258262890683122, 1.000000000000000000, 0.9659258262890683122, 1.000000000000000000, 0.9659258262890683122, 1.000000000000000000, 0.9659258262890683122, 1.000000000000000000, 0.9659258262890683122, 1.000000000000000000, 0.9659258262890683122, 1.000000000000000000, 0.9659258262890683122, 1.000000000000000000, 0.9659258262890683122, 1.000000000000000000, 0.9659258262890683122, 1.000000000000000000, 0.9659258262890683122, 1.000000000000000000, 0.9659258262890683122, 1.000000000000000000, 0.9659258262890683122, 1.000000000000000000, 0.9659258262890683122, 1.000000000000000000, 0.9659258262890683122, 1.000000000000000000, 0.9659258262890683122, 1.000000000000000000, 0.9659258262890683122, 1.000000000000000000, 0.9659258262890683122, 1.000000000000000000, 0.9659258262890683122, 1.000000000000000000, 0.9659258262890683122, 1.000000000000000000, 0.9659258262890683122, 1.000000000000000000, 0.9659258262890683122, 1.000000000000000000, 0.9659258262890683122, 1.000000000000000000, 0.9659258262890683122, 1.000000000000000000, 0.9659258262890683122, 1.000000000000000000, 0.9659258262890683122, 1.000000000000000000, 0.9659258262890683122, 1.000000000000000000, 0.9659258262890683122, 1.000000000000000000, 0.9659258262890683122, 1.000000000000000000, 0.9659258262890683122, 1.000000000000000000, 0.9659258262890683122, 1.000000000000000000, 0.9659258262890683122, 1.000000000000000000, 0.9659258262890683122, 1.000000000000000000, 0.9659258262890683122, 1.000000000000000000, 0.9659258262890683122, 1.000000000000000000, 0.9659258262890683122, 1.000000000000000000, 0.9659258262890683122, 1.000000000000000000, 0.9659258262890683122, 1.000000000000000000, 0.9659258262890683122, 1.000000000000000000, 0.9659258262890683122, 1.000000000000000000, 0.9659258262890683122, 1.000000000000000000, 0.9659258262890683122, 1.000000000000000000, 0.9659258262890683122, 1.000000000000000000, 0.9659258262890683122, 1.000000000000000000, 0.9659258262890683122, 1.000000000000000000, 0.9659258262890683122, 1.000000000000000000, 0.9659258262890683122, 1.000000000000000000, 0.9659258262890683122, 1.000000000000000000, 0.9659258262890683122, 1.000000000000000000, 0.9659258262890683122, 1.000000000000000000, 0.9659258262890683122, 1.000000000000000000, 0.9659258262890683122, 1.000000000000000000, 0.9659258262890683122, 1.000000000000000000, 0.9659258262890683122, 1.000000000000000000, 0.9659258262890683122, 1.000000000000000000, 0.9659258262890683122, 1.000000000000000000, 0.9659258262890683122, 1.000000000000000000, 0.9659258262890683122, 1.000000000000000000, 0.9659258262890683122, 1.000000000000000000, 0.9659258262890683122, 1.000000000000000000, 0.9659258262890683122, 1.000000000000000000, 0.9659258262890683122, 1.000000000000000000, 0.9659258262890683122, 1.000000000000000000, 0.9659258262890683122, 1.000000000000000000, 0.9659258262890683122, 1.000000000000000000, 0.9659258262890683122, 1.000000000000000000, 0.9659258262890683122, 1.000000000000000000, 0.9659258262890683122, 1.000000000000000000, 0.9659258262890683122, 1.000000000000000000, 0.9659258262890683122, 1.000000000000000000, 0.9659258262890683122, 1.000000000000000000, 0.9659258262890683122, 1.000000000000000000, 0.9659258262890683122, 1.000000000000000000, 0.9659258262890683122, 1.000000000000000000, 0.9659258262890683122, 1.000000000000000000, 0.9659258262890683122, 1.000000000000000000, 0.9659258262890683122, 1.000000000000000000, 0.9659258262890683122, 1.000000000000000000, 0.9659258262890683122, 1.000000000000000000),
 ( 1.000000000000000000, 0.9659258262890683122, 1.000000000000000000, 0.9659258262890683122, 1.000000000000000000, 0.9659258262890683122, 1.000000000000000000, 0.9659258262890683122, 1.000000000000000000, 0.9659258262890683122, 1.000000000000000000, 0.9659258262890683122, 1.000000000000000000, 0.9659258262890683122, 1.000000000000000000, 0.9659258262890683122, 1.000000000000000000, 0.9659258262890683122, 1.000000000000000000, 0.9659258262890683122, 1.000000000000000000, 0.9659258262890683122, 1.000000000000000000, 0.9659258262890683122, 1.000000000000000000, 0.9659258262890683122, 1.000000000000000000, 0.9659258262890683122, 1.000000000000000000, 0.9659258262890683122, 1.000000000000000000, 0.9659258262890683122, 1.000000000000000000, 0.9659258262890683122, 1.000000000000000000, 0.9659258262890683122, 1.000000000000000000, 0.9659258262890683122, 1.000000000000000000, 0.9659258262890683122, 1.000000000000000000, 0.9659258262890683122, 1.000000000000000000, 0.9659258262890683122, 1.000000000000000000, 0.9659258262890683122, 1.000000000000000000, 0.9659258262890683122, 1.000000000000000000, 0.9659258262890683122, 1.000000000000000000, 0.9659258262890683122, 1.000000000000000000, 0.9659258262890683122, 1.000000000000000000, 0.9659258262890683122, 1.000000000000000000, 0.9659258262890683122, 1.000000000000000000, 0.9659258262890683122, 1.000000000000000000, 0.9659258262890683122, 1.000000000000000000, 0.9659258262890683122, 1.000000000000000000, 0.9659258262890683122, 1.000000000000000000, 0.9659258262890683122, 1.000000000000000000, 0.9659258262890683122, 1.000000000000000000, 0.9659258262890683122, 1.000000000000000000, 0.9659258262890683122, 1.000000000000000000, 0.9659258262890683122, 1.000000000000000000, 0.9659258262890683122, 1.000000000000000000, 0.9659258262890683122, 1.000000000000000000, 0.9659258262890683122, 1.000000000000000000, 0.9659258262890683122, 1.000000000000000000, 0.9659258262890683122, 1.000000000000000000, 0.9659258262890683122, 1.000000000000000000, 0.9659258262890683122, 1.000000000000000000, 0.9659258262890683122, 1.000000000000000000, 0.9659258262890683122, 1.000000000000000000, 0.9659258262890683122, 1.000000000000000000, 0.9659258262890683122, 1.000000000000000000, 0.9659258262890683122, 1.000000000000000000, 0.9659258262890683122, 1.000000000000000000, 0.9659258262890683122, 1.000000000000000000, 0.9659258262890683122, 1.000000000000000000, 0.9659258262890683122, 1.000000000000000000, 0.9659258262890683122, 1.000000000000000000, 0.9659258262890683122, 1.000000000000000000, 0.9659258262890683122, 1.000000000000000000, 0.9659258262890683122, 1.000000000000000000, 0.9659258262890683122, 1.000000000000000000, 0.9659258262890683122, 1.000000000000000000, 0.9659258262890683122, 1.000000000000000000, 0.9659258262890683122, 1.000000000000000000, 0.9659258262890683122, 1.000000000000000000, 0.9659258262890683122, 1.000000000000000000, 0.9659258262890683122, 1.000000000000000000, 0.9659258262890683122, 1.000000000000000000, 0.9659258262890683122, 1.000000000000000000, 0.9659258262890683122, 1.000000000000000000, 0.9659258262890683122, 1.000000000000000000, 0.9659258262890683122, 1.000000000000000000, 0.9659258262890683122, 1.000000000000000000, 0.9659258262890683122, 1.000000000000000000, 0.9659258262890683122, 1.000000000000000000, 0.9659258262890683122, 1.000000000000000000, 0.9659258262890683122, 1.000000000000000000, 0.9659258262890683122, 1.000000000000000000, 0.9659258262890683122, 1.000000000000000000, 0.9659258262890683122, 1.000000000000000000, 0.9659258262890683122, 1.000000000000000000, 0.9659258262890683122, 1.000000000000000000, 0.9659258262890683122, 1.000000000000000000, 0.9659258262890683122, 1.000000000000000000, 0.9659258262890683122, 1.000000000000000000, 0.9659258262890683122, 1.000000000000000000, 0.9659258262890683122, 1.000000000000000000, 0.9659258262890683122, 1.000000000000000000, 0.9659258262890683122, 1.000000000000000000, 0.9659258262890683122, 1.000000000000000000, 0.9659258262890683122, 1.000000000000000000, 0.9659258262890683122, 1.000000000000000000, 0.9659258262890683122, 1.000000000000000000, 0.9659258262890683122, 1.000000000000000000, 0.9659258262890683122, 1.000000000000000000, 0.9659258262890683122, 1.000000000000000000, 0.9659258262890683122, 1.000000000000000000, 0.9659258262890683122, 1.000000000000000000, 0.9659258262890683122, 1.000000000000000000, 0.9659258262890683122, 1.000000000000000000, 0.9659258262890683122, 1.000000000000000000, 0.9659258262890683122, 1.000000000000000000, 0.9659258262890683122, 1.000000000000000000, 0.9659258262890683122, 1.000000000000000000, 0.9659258262890683122, 1.000000000000000000, 0.9659258262890683122, 1.000000000000000000, 0.9659258262890683122, 1.000000000000000000, 0.9659258262890683122, 1.000000000000000000, 0.9659258262890683122, 1.000000000000000000, 0.9659258262890683122, 1.000000000000000000, 0.9659258262890683122, 1.000000000000000000, 0.9659258262890683122, 1.000000000000000000, 0.9659258262890683122, 1.000000000000000000, 0.9659258262890683122, 1.000000000000000000, 0.9659258262890683122, 1.000000000000000000, 0.9659258262890683122, 1.000000000000000000, 0.9659258262890683122, 1.000000000000000000, 0.9659258262890683122, 1.000000000000000000, 0.9659258262890683122, 1.000000000000000000, 0.9659258262890683122, 1.000000000000000000, 0.9659258262890683122, 1.000000000000000000, 0.9659258262890683122, 1.000000000000000000, 0.9659258262890683122, 1.000000000000000000, 0.9659258262890683122, 1.000000000000000000, 0.9659258262890683122, 1.000000000000000000, 0.9659258262890683122, 1.000000000000000000, 0.9659258262890683122, 1.000000000000000000, 0.9659258262890683122, 1.000000000000000000, 0.9659258262890683122, 1.000000000000000000, 0.9659258262890683122, 1.000000000000000000, 0.9659258262890683122, 1.000000000000000000, 0.9659258262890683122, 1.000000000000000000, 0.9659258262890683122, 1.000000000000000000, 0.9659258262890683122, 1.000000000000000000, 0.9659258262890683122, 1.000000000000000000, 0.9659258262890683122, 1.000000000000000000, 0.9659258262890683122, 1.000000000000000000, 0.9659258262890683122, 1.000000000000000000, 0.9659258262890683122, 1.000000000000000000, 0.9659258262890683122, 1.000000000000000000, 0.9659258262890683122, 1.000000000000000000, 0.9659258262890683122, 1.000000000000000000, 0.9659258262890683122, 1.000000000000000000, 0.9659258262890683122, 1.000000000000000000, 0.9659258262890683122, 1.000000000000000000, 0.9659258262890683122, 1.000000000000000000, 0.9659258262890683122, 1.000000000000000000, 0.9659258262890683122, 1.000000000000000000, 0.9659258262890683122, 1.000000000000000000, 0.9659258262890683122, 1.000000000000000000, 0.9659258262890683122, 1.000000000000000000, 0.9659258262890683122, 1.000000000000000000, 0.9659258262890683122, 1.000000000000000000, 0.9659258262890683122, 1.000000000000000000, 0.9659258262890683122, 1.000000000000000000, 0.9659258262890683122, 1.000000000000000000, 0.9659258262890683122, 1.000000000000000000, 0.9659258262890683122, 1.000000000000000000, 0.9659258262890683122, 1.000000000000000000, 0.9659258262890683122, 1.000000000000000000, 0.9659258262890683122, 1.000000000000000000, 0.9659258262890683122, 1.000000000000000000, 0.9659258262890683122, 1.000000000000000000, 0.9659258262890683122, 1.000000000000000000) ) ) 
 REPRESENTATION_ITEM ( '' )  SURFACE ( )  );
#15527=CARTESIAN_POINT ( 'NONE',  ( 22.81628187352647785, 56.62363466993042493, 6.195893100308588602E-16 ) ) ;
#15528=ORIENTED_EDGE ( 'NONE', *, *, #52791, .F. ) ;
#15529=CARTESIAN_POINT ( 'NONE',  ( 5.076628168052703671, 61.84226448433412315, 8.527530157486179263 ) ) ;
#15531=CARTESIAN_POINT ( 'NONE',  ( -0.8801773607111009756, 48.06368534415484817, 1.068504757029289695E-15 ) ) ;
#15532=CARTESIAN_POINT ( 'NONE',  ( 16.40814093676324603, 42.45696800326375353, -11.09922568453594671 ) ) ;
#15533=CARTESIAN_POINT ( 'NONE',  ( -2.266590686148945544, 12.22041550158063394, 7.082119434687048631 ) ) ;
#15535=CARTESIAN_POINT ( 'NONE',  ( 17.20831665107776587, 34.13393115100078745, -7.208316651077762316 ) ) ;
#15536=CARTESIAN_POINT ( 'NONE',  ( 5.076628168052704559, 5.175597817667451750, -8.527530157486179263 ) ) ;
#15538=CARTESIAN_POINT ( 'NONE',  ( -2.266590686148945544, 37.22041550158063217, 7.082119434687048631 ) ) ;
#15540=CARTESIAN_POINT ( 'NONE',  ( 7.084665262690076126, 14.10535201082150358, 10.88017736071109987 ) ) ;
#15544=CARTESIAN_POINT ( 'NONE',  ( 15.44008868035555260, 14.73035201082150536, 9.422509992056143702 ) ) ;
#15545=CARTESIAN_POINT ( 'NONE',  ( 0.5774900079438590739, 7.647018677488171434, -5.440088680355550821 ) ) ;
#15546=CARTESIAN_POINT ( 'NONE',  ( 10.00000000000000000, 39.75893115100078745, -9.846743663894594434 ) ) ;
#15547=CARTESIAN_POINT ( 'NONE',  ( 22.81628187352647785, 36.41530133659707502, 3.434112377981063169 ) ) ;
#15549=CARTESIAN_POINT ( 'NONE',  ( 2.917880565312950480, 5.970415501580634832, -12.26659068614894821 ) ) ;
#15550=CARTESIAN_POINT ( 'NONE',  ( -0.8801773607110991993, 22.85535201082150181, -2.915334737309923874 ) ) ;
#15551=CARTESIAN_POINT ( 'NONE',  ( 20.36894250292379738, 64.92874883491397497, -10.36894250292379027 ) ) ;
#15553=CARTESIAN_POINT ( 'NONE',  ( 0.1532563361054083140, 36.00893115100078745, 1.131784320476157264E-15 ) ) ;
#15554=LINE ( 'NONE', #84528, #25329 ) ;
#15555=CARTESIAN_POINT ( 'NONE',  ( 19.84674366389459266, 18.30059781766745175, 2.638427012816836559 ) ) ;
#15559=FACE_OUTER_BOUND ( 'NONE', #14570, .T. ) ;
#15561=CARTESIAN_POINT ( 'NONE',  ( 1.472469842513823179, 56.42559781766745886, 4.923371831947296329 ) ) ;
#15562=CARTESIAN_POINT ( 'NONE',  ( 10.00000000000000178, 29.31368534415483751, 10.88017736071110342 ) ) ;
#15563=CARTESIAN_POINT ( 'NONE',  ( 20.88017736071110875, 35.77201867748816966, -2.915334737309920765 ) ) ;
#15564=CARTESIAN_POINT ( 'NONE',  ( -0.8801773607110991993, 2.855352010821504471, -2.915334737309923874 ) ) ;
#15565=CARTESIAN_POINT ( 'NONE',  ( 22.81628187352647785, 31.62363466993042138, 6.195893100308588602E-16 ) ) ;
#15566=CARTESIAN_POINT ( 'NONE',  ( 2.917880565312950480, 20.97041550158063217, -12.26659068614894821 ) ) ;
#15570=CARTESIAN_POINT ( 'NONE',  ( 10.00000000000000178, 50.37363466993042493, 12.81628187352647608 ) ) ;
#15572=CARTESIAN_POINT ( 'NONE',  ( 7.361572987183170547, 47.05059781766745175, 9.846743663894590881 ) ) ;
#15573=CARTESIAN_POINT ( 'NONE',  ( 19.42250999205614193, 25.14701867748817321, 5.440088680355555262 ) ) ;
#15575=CARTESIAN_POINT ( 'NONE',  ( 15.44008868035555260, 19.73035201082150536, 9.422509992056143702 ) ) ;
#15578=CARTESIAN_POINT ( 'NONE',  ( 0.5774900079438590739, 57.64701867748817676, -5.440088680355550821 ) ) ;
#15579=CARTESIAN_POINT ( 'NONE',  ( 12.91533473730993009, 61.60535201082150536, -10.88017736071109987 ) ) ;
#15580=CARTESIAN_POINT ( 'NONE',  ( -0.8801773607111009756, 58.06368534415484106, 1.068504757029289695E-15 ) ) ;
#15581=CARTESIAN_POINT ( 'NONE',  ( -1.926860441876564023, 29.68830936912750573, 1.004413902775740781E-15 ) ) ;
#15582=CARTESIAN_POINT ( 'NONE',  ( -46.94000000000126960, 101.3832071409885884, 8.175121524388728744 ) ) ;
#15583=CARTESIAN_POINT ( 'NONE',  ( 20.15039907845753220, 54.72266099184918886, 6.262539305110078836 ) ) ;
#15585=CARTESIAN_POINT ( 'NONE',  ( 0.1532563361054083140, 41.00893115100078745, 1.131784320476157264E-15 ) ) ;
#15587=CARTESIAN_POINT ( 'NONE',  ( 0.2751277870542967463, 70.00000000000000000, 6.000000000000000000 ) ) ;
#15588=( LENGTH_UNIT ( ) NAMED_UNIT ( * ) SI_UNIT ( .MILLI., .METRE. ) );
#15589=VECTOR ( 'NONE', #15396, 1000.000000000000000 ) ;
#15590=CARTESIAN_POINT ( 'NONE',  ( 13.79529636645030344, 23.26208216824730002, 14.16423886937410614 ) ) ;
#15591=DIRECTION ( 'NONE',  ( 0.000000000000000000, 0.000000000000000000, 1.000000000000000000 ) ) ;
#15592=CARTESIAN_POINT ( 'NONE',  ( 2.035157376598824452, 13.68868534415483751, 7.964842623401179544 ) ) ;
#15593=CARTESIAN_POINT ( 'NONE',  ( 0.2751277870542871984, 68.21833443783938833, 6.499999999999984901 ) ) ;
#15594=CARTESIAN_POINT ( 'NONE',  ( 22.81628187352648496, 36.83196800326376064, -3.434112377981050290 ) ) ;
#15595=ORIENTED_EDGE ( 'NONE', *, *, #13820, .T. ) ;
#15596=CARTESIAN_POINT ( 'NONE',  ( 19.80427997160309417, 62.75733960839542647, -6.499999999999983125 ) ) ;
#15597=CARTESIAN_POINT ( 'NONE',  ( 14.92337183194729633, 2.675597817667451750, 8.527530157486181039 ) ) ;
#15598=CARTESIAN_POINT ( 'NONE',  ( 13.43411237798106583, 32.66530133659708213, -12.81628187352647252 ) ) ;
#15599=CARTESIAN_POINT ( 'NONE',  ( 17.20831665107776587, 19.13393115100078035, -7.208316651077762316 ) ) ;
#15601=CARTESIAN_POINT ( 'NONE',  ( -1.099225684535947600, 13.70696800326375353, -6.408140936763238038 ) ) ;
#15604=CARTESIAN_POINT ( 'NONE',  ( 10.00000000000000000, -0.2410688489992152128, -9.846743663894594434 ) ) ;
#15605=ORIENTED_EDGE ( 'NONE', *, *, #39446, .T. ) ;
#15608=EDGE_LOOP ( 'NONE', ( #8355, #9526, #16776, #67796 ) ) ;
#15609=CARTESIAN_POINT ( 'NONE',  ( 0.5774900079438590739, 22.64701867748817321, -5.440088680355550821 ) ) ;
#15610=CARTESIAN_POINT ( 'NONE',  ( 17.08211943468705130, 23.47041550158063572, 12.26659068614894998 ) ) ;
#15611=CARTESIAN_POINT ( 'NONE',  ( 12.63842701281683034, 47.46726448433412315, 9.846743663894596210 ) ) ;
#15612=CARTESIAN_POINT ( 'NONE',  ( 17.96484262340118221, 66.18868534415483396, -7.964842623401177768 ) ) ;
#15613=CARTESIAN_POINT ( 'NONE',  ( 13.43411237798106583, 42.66530133659707502, -12.81628187352647252 ) ) ;
#15615=CARTESIAN_POINT ( 'NONE',  ( -0.8801773607111008646, 8.272018677488171434, 2.915334737309923430 ) ) ;
#15616=DIRECTION ( 'NONE',  ( -0.000000000000000000, 1.000000000000000000, -0.000000000000000000 ) ) ;
#15618=CARTESIAN_POINT ( 'NONE',  ( -1.099225684535947600, 8.706968003263753531, -6.408140936763238038 ) ) ;
#15619=CARTESIAN_POINT ( 'NONE',  ( -1.099225684535947600, 13.70696800326375353, -6.408140936763238038 ) ) ;
#15620=CARTESIAN_POINT ( 'NONE',  ( 19.84674366389459266, 33.71726448433410894, -2.638427012816827677 ) ) ;
#15622=CARTESIAN_POINT ( 'NONE',  ( -2.816281873526473856, 34.12363466993042493, 9.499525473075851096E-16 ) ) ;
#15624=CARTESIAN_POINT ( 'NONE',  ( 4.559911319644449179, 57.23035201082150536, -9.422509992056141925 ) ) ;
#15625=CARTESIAN_POINT ( 'NONE',  ( 20.15039907845753930, 9.722660991849181755, 6.262539305110064625 ) ) ;
#15626=AXIS2_PLACEMENT_3D ( 'NONE', #97889, #88389, #19888 ) ;
#15629=VECTOR ( 'NONE', #49207, 1000.000000000000000 ) ;
#15630=CARTESIAN_POINT ( 'NONE',  ( 7.084665262690076126, 34.10535201082151247, 10.88017736071109987 ) ) ;
#15631=CARTESIAN_POINT ( 'NONE',  ( 12.91533473730993009, 46.60535201082150536, -10.88017736071109987 ) ) ;
#15632=CARTESIAN_POINT ( 'NONE',  ( 10.00000000000000178, 67.25893115100079456, 9.846743663894594434 ) ) ;
#15634=CARTESIAN_POINT ( 'NONE',  ( 12.63842701281683034, 52.46726448433413026, 9.846743663894596210 ) ) ;
#15635=CARTESIAN_POINT ( 'NONE',  ( -0.8801773607111009756, 3.063685344154837509, 1.068504757029289695E-15 ) ) ;
#15637=CARTESIAN_POINT ( 'NONE',  ( 22.81628187352647785, 6.415301336597088344, 3.434112377981063169 ) ) ;
#15639=CARTESIAN_POINT ( 'NONE',  ( 19.42250999205614548, 40.98035201082150536, -5.440088680355545492 ) ) ;
#15640=ADVANCED_FACE ( 'NONE', ( #36557 ), #83534, .F. ) ;
#15641=CARTESIAN_POINT ( 'NONE',  ( 0.1532563361054083140, 61.00893115100078745, 1.131784320476157264E-15 ) ) ;
#15643=CARTESIAN_POINT ( 'NONE',  ( 15.44008868035555260, 9.730352010821505360, 9.422509992056143702 ) ) ;
#15644=CARTESIAN_POINT ( 'NONE',  ( 0.5774900079438590739, 32.64701867748816966, -5.440088680355550821 ) ) ;
#15645=CARTESIAN_POINT ( 'NONE',  ( -0.3689425029237881626, 42.42874883491396787, 10.36894250292379027 ) ) ;
#15646=CARTESIAN_POINT ( 'NONE',  ( 5.076628168052703671, 31.84226448433412315, 8.527530157486179263 ) ) ;
#15647=CARTESIAN_POINT ( 'NONE',  ( 0.5774900079438590739, 52.64701867748817676, -5.440088680355550821 ) ) ;
#15649=CARTESIAN_POINT ( 'NONE',  ( 10.00000000000000178, 3.053748834913967425, 14.16423886937410082 ) ) ;
#15651=CARTESIAN_POINT ( 'NONE',  ( 1.472469842513823179, 60.59226448433412315, -4.923371831947296329 ) ) ;
#15654=CARTESIAN_POINT ( 'NONE',  ( -0.3689425029237881626, 37.42874883491396787, 10.36894250292379027 ) ) ;
#15655=CARTESIAN_POINT ( 'NONE',  ( 24.16423886937410614, 24.51208216824730002, -3.795296366450302550 ) ) ;
#15656=CARTESIAN_POINT ( 'NONE',  ( 2.035157376598824452, 68.68868534415484817, 7.964842623401179544 ) ) ;
#15657=CARTESIAN_POINT ( 'NONE',  ( 10.00000000000000178, 10.37363466993041961, 12.81628187352647608 ) ) ;
#15660=CARTESIAN_POINT ( 'NONE',  ( -0.8801773607110991993, 62.85535201082150536, -2.915334737309923874 ) ) ;
#15661=CARTESIAN_POINT ( 'NONE',  ( 6.565887622018943937, 23.08196800326375708, -12.81628187352647608 ) ) ;
#15662=CARTESIAN_POINT ( 'NONE',  ( -0.3689425029237898834, 31.17874883491396787, -10.36894250292378850 ) ) ;
#15663=CARTESIAN_POINT ( 'NONE',  ( 15.44008868035555260, 14.73035201082150536, 9.422509992056143702 ) ) ;
#15664=CARTESIAN_POINT ( 'NONE',  ( 0.5774900079438590739, 27.64701867748817676, -5.440088680355550821 ) ) ;
#15665=CARTESIAN_POINT ( 'NONE',  ( -31.17076923076924544, 90.15384615384616041, -9.500000000000000000 ) ) ;
#15666=CARTESIAN_POINT ( 'NONE',  ( 12.91533473730993009, 51.60535201082149825, -10.88017736071109987 ) ) ;
#15667=CARTESIAN_POINT ( 'NONE',  ( 21.09922568453595559, 52.04030133659708923, -6.408140936763230044 ) ) ;
#15670=DIRECTION ( 'NONE',  ( 0.000000000000000000, 0.000000000000000000, -1.000000000000000000 ) ) ;
#15671=EDGE_LOOP ( 'NONE', ( #75714, #70152, #61547, #22318 ) ) ;
#15675=CARTESIAN_POINT ( 'NONE',  ( -4.164238869374099927, 57.01208216824731068, 3.795296366450308767 ) ) ;
#15676=CARTESIAN_POINT ( 'NONE',  ( -4.164238869374099927, 62.01208216824728936, 3.795296366450308767 ) ) ;
#15677=CARTESIAN_POINT ( 'NONE',  ( 18.52753015748618282, 28.92559781766745175, -4.923371831947291888 ) ) ;
#15678=CARTESIAN_POINT ( 'NONE',  ( 1.472469842513823179, 61.42559781766745175, 4.923371831947296329 ) ) ;
#15679=CARTESIAN_POINT ( 'NONE',  ( 19.80832241502127644, 49.75868815902069997, 6.499999999999990230 ) ) ;
#15682=CARTESIAN_POINT ( 'NONE',  ( 13.43411237798105340, 10.58196800326375353, 12.81628187352647963 ) ) ;
#15684=ORIENTED_EDGE ( 'NONE', *, *, #72107, .T. ) ;
#15685=CARTESIAN_POINT ( 'NONE',  ( -4.164238869374099039, 36.80374883491396787, 8.674139862899312516E-16 ) ) ;
#15686=CARTESIAN_POINT ( 'NONE',  ( 22.26659068614894466, 48.88708216824730357, 7.082119434687054849 ) ) ;
#15688=CARTESIAN_POINT ( 'NONE',  ( 16.40814093676323893, 55.79030133659708923, 11.09922568453595026 ) ) ;
#15690=CARTESIAN_POINT ( 'NONE',  ( 17.96484262340118221, 24.93868534415484461, 7.964842623401181321 ) ) ;
#15691=CARTESIAN_POINT ( 'NONE',  ( 10.00000000000000178, 47.25893115100078745, 9.846743663894594434 ) ) ;
#15692=CARTESIAN_POINT ( 'NONE',  ( 10.00000000000000000, 26.81368534415484106, -10.88017736071110342 ) ) ;
#15693=DIRECTION ( 'NONE',  ( 0.6186827199538796895, 0.6777609120374844531, -0.3973308925122567281 ) ) ;
#15694=CARTESIAN_POINT ( 'NONE',  ( 10.00000000000000000, 59.75893115100078745, -9.846743663894594434 ) ) ;
#15695=CARTESIAN_POINT ( 'NONE',  ( 17.20831665107776587, 52.88393115100078035, 7.208316651077764980 ) ) ;
#15698=CARTESIAN_POINT ( 'NONE',  ( 20.00000000000000355, 70.00000000000000000, 4.500000000000000888 ) ) ;
#15700=CARTESIAN_POINT ( 'NONE',  ( 7.361572987183169658, -0.03273551566588185635, -9.846743663894592657 ) ) ;
#15704=CARTESIAN_POINT ( 'NONE',  ( 19.84674366389459266, 33.71726448433410894, -2.638427012816827677 ) ) ;
#15706=CARTESIAN_POINT ( 'NONE',  ( 22.81628187352647785, 41.41530133659708923, 3.434112377981063169 ) ) ;
#15711=CARTESIAN_POINT ( 'NONE',  ( 12.63842701281683034, 52.46726448433413026, 9.846743663894596210 ) ) ;
#15712=CARTESIAN_POINT ( 'NONE',  ( 24.16423886937409904, 39.09541550158062506, 3.795296366450317205 ) ) ;
#15713=CARTESIAN_POINT ( 'NONE',  ( 0.1532563361054100626, 55.80059781766745175, -2.638427012816831230 ) ) ;
#15715=CARTESIAN_POINT ( 'NONE',  ( 2.791683348922240793, 6.633931151000785675, 7.208316651077764092 ) ) ;
#15717=CARTESIAN_POINT ( 'NONE',  ( 22.81628187352647785, 51.62363466993042493, 6.195893100308588602E-16 ) ) ;
#15718=CARTESIAN_POINT ( 'NONE',  ( 2.917880565312948704, 2.637082168247300906, 12.26659068614894643 ) ) ;
#15719=CARTESIAN_POINT ( 'NONE',  ( 17.20831665107776587, 49.13393115100078745, -7.208316651077762316 ) ) ;
#15720=CARTESIAN_POINT ( 'NONE',  ( 2.035157376598824452, 53.68868534415484817, 7.964842623401179544 ) ) ;
#15721=CARTESIAN_POINT ( 'NONE',  ( 12.63842701281683922, 39.55059781766744464, -9.846743663894590881 ) ) ;
#15723=CARTESIAN_POINT ( 'NONE',  ( 19.72487221294570858, 31.86607318730074567, 6.500000000000000888 ) ) ;
#15725=CARTESIAN_POINT ( 'NONE',  ( 4.559911319644449179, 62.23035201082150536, -9.422509992056141925 ) ) ;
#15730=CARTESIAN_POINT ( 'NONE',  ( 12.91533473730993009, 31.60535201082150891, -10.88017736071109987 ) ) ;
#15731=CARTESIAN_POINT ( 'NONE',  ( 6.565887622018943937, 5.165301336597086568, 12.81628187352647430 ) ) ;
#15732=CARTESIAN_POINT ( 'NONE',  ( 4.559911319644449179, 52.23035201082151247, -9.422509992056141925 ) ) ;
#15733=CARTESIAN_POINT ( 'NONE',  ( 0.5774900079438590739, 67.64701867748817676, -5.440088680355550821 ) ) ;
#15734=CARTESIAN_POINT ( 'NONE',  ( 15.44008868035555793, 36.39701867748816966, -9.422509992056140149 ) ) ;
#15735=CARTESIAN_POINT ( 'NONE',  ( 20.00000000000000711, 92.98956734509515343, -4.826711383682784628 ) ) ;
#15736=CARTESIAN_POINT ( 'NONE',  ( 0.1532563361054083140, 11.00893115100078568, 1.131784320476157264E-15 ) ) ;
#15737=CARTESIAN_POINT ( 'NONE',  ( 17.20831665107776587, 32.88393115100078745, 7.208316651077764980 ) ) ;
#15740=CARTESIAN_POINT ( 'NONE',  ( 12.63842701281683922, 64.55059781766745175, -9.846743663894590881 ) ) ;
#15741=CARTESIAN_POINT ( 'NONE',  ( 17.08211943468705840, 60.13708216824729647, -12.26659068614894466 ) ) ;
#15743=CARTESIAN_POINT ( 'NONE',  ( 13.79529636645030344, 28.26208216824729647, 14.16423886937410614 ) ) ;
#15744=CARTESIAN_POINT ( 'NONE',  ( 24.16423886937410614, 54.30374883491396787, 8.672049930838204340E-16 ) ) ;
#15745=CARTESIAN_POINT ( 'NONE',  ( 19.84674366389459266, 13.30059781766745353, 2.638427012816836559 ) ) ;
#15747=CARTESIAN_POINT ( 'NONE',  ( 5.076628168052703671, 26.84226448433411960, 8.527530157486179263 ) ) ;
#15748=CARTESIAN_POINT ( 'NONE',  ( 12.91533473730993009, 21.60535201082150536, -10.88017736071109987 ) ) ;
#15749=CARTESIAN_POINT ( 'NONE',  ( 5.076628168052704559, 60.17559781766745175, -8.527530157486179263 ) ) ;
#15750=CARTESIAN_POINT ( 'NONE',  ( 2.917880565312950480, 10.97041550158063572, -12.26659068614894821 ) ) ;
#15751=CARTESIAN_POINT ( 'NONE',  ( 0.2751277870542980231, 5.302231764288316107, 6.500000000000002665 ) ) ;
#15753=CARTESIAN_POINT ( 'NONE',  ( 19.84674366389459621, 13.50893115100078568, 7.409399052514197653E-17 ) ) ;
#15754=CARTESIAN_POINT ( 'NONE',  ( 19.38216949554541557, 42.24863466993041783, -9.382169495545420901 ) ) ;
#15755=CARTESIAN_POINT ( 'NONE',  ( 5.076628168052704559, 45.17559781766745175, -8.527530157486179263 ) ) ;
#15756=ORIENTED_EDGE ( 'NONE', *, *, #98332, .T. ) ;
#15757=CARTESIAN_POINT ( 'NONE',  ( 10.00000000000000178, 22.25893115100078745, 9.846743663894594434 ) ) ;
#15760=CARTESIAN_POINT ( 'NONE',  ( 10.00000000000000178, 48.05374883491396787, 14.16423886937410082 ) ) ;
#15761=CARTESIAN_POINT ( 'NONE',  ( 19.42250999205614193, 50.14701867748817676, 5.440088680355555262 ) ) ;
#15763=CARTESIAN_POINT ( 'NONE',  ( 17.20831665107776587, 42.88393115100077324, 7.208316651077764980 ) ) ;
#15764=CARTESIAN_POINT ( 'NONE',  ( 7.084665262690076126, 12.02201867748817143, -10.88017736071110164 ) ) ;
#15765=CARTESIAN_POINT ( 'NONE',  ( 18.52753015748618282, 48.92559781766745886, -4.923371831947291888 ) ) ;
#15766=CARTESIAN_POINT ( 'NONE',  ( 19.42250999205614193, 50.14701867748817676, 5.440088680355555262 ) ) ;
#15767=B_SPLINE_CURVE_WITH_KNOTS ( 'NONE', 3,
 ( #4956, #12442, #75406, #37432, #67922, #66427 ),
 .UNSPECIFIED., .F., .F.,
 ( 4, 2, 4 ),
 ( 5.553824967135427403E-18, 0.0002605067024380902543, 0.0005210134048761749792 ),
 .UNSPECIFIED. ) ;
#15770=CARTESIAN_POINT ( 'NONE',  ( -0.1503990784575328643, 70.00000000000000000, -6.262539305110068177 ) ) ;
#15772=CARTESIAN_POINT ( 'NONE',  ( 2.791683348922237240, 10.38393115100078390, -7.208316651077763204 ) ) ;
#15773=CARTESIAN_POINT ( 'NONE',  ( 13.43411237798106583, 62.66530133659708923, -12.81628187352647252 ) ) ;
#15774=CARTESIAN_POINT ( 'NONE',  ( 10.00000000000000178, 4.313685344154837509, 10.88017736071110342 ) ) ;
#15775=CARTESIAN_POINT ( 'NONE',  ( 19.84674366389459266, 48.30059781766745175, 2.638427012816836559 ) ) ;
#15777=CARTESIAN_POINT ( 'NONE',  ( -4.164238869374098151, 26.59541550158063217, -3.795296366450310543 ) ) ;
#15778=CARTESIAN_POINT ( 'NONE',  ( -2.266590686148945544, 61.38708216824730357, -7.082119434687050408 ) ) ;
#15779=CARTESIAN_POINT ( 'NONE',  ( 5.076628168052703671, 61.84226448433412315, 8.527530157486179263 ) ) ;
#15781=CARTESIAN_POINT ( 'NONE',  ( 20.88017736071110164, 45.35535201082149115, 2.915334737309930979 ) ) ;
#15782=CARTESIAN_POINT ( 'NONE',  ( 7.361572987183169658, -0.03273551566588185635, -9.846743663894592657 ) ) ;
#15786=CARTESIAN_POINT ( 'NONE',  ( 3.591859063236761518, 54.95696800326376064, 11.09922568453594849 ) ) ;
#15788=CARTESIAN_POINT ( 'NONE',  ( 2.791683348922240793, 6.633931151000785675, 7.208316651077764092 ) ) ;
#15790=CARTESIAN_POINT ( 'NONE',  ( 13.79529636645031943, 15.34541550158063750, -14.16423886937409904 ) ) ;
#15791=CARTESIAN_POINT ( 'NONE',  ( 12.63842701281683922, 14.55059781766744997, -9.846743663894590881 ) ) ;
#15792=CARTESIAN_POINT ( 'NONE',  ( 2.035157376598824452, 33.68868534415484106, 7.964842623401179544 ) ) ;
#15795=CARTESIAN_POINT ( 'NONE',  ( 19.42250999205614193, 25.14701867748817321, 5.440088680355555262 ) ) ;
#15796=B_SPLINE_CURVE_WITH_KNOTS ( 'NONE', 3,
 ( #32671, #16705, #55173, #85200 ),
 .UNSPECIFIED., .F., .F.,
 ( 4, 4 ),
 ( 0.000000000000000000, 0.002657014572711318551 ),
 .UNSPECIFIED. ) ;
#15797=( BOUNDED_SURFACE ( )  B_SPLINE_SURFACE ( 3, 2, ( 
 ( #22331, #46300, #67827 ),
 ( #37829, #14835, #91296 ),
 ( #45815, #52319, #45310 ),
 ( #69300, #30786, #84791 ) ),
 .UNSPECIFIED., .F., .F., .F. ) 
 B_SPLINE_SURFACE_WITH_KNOTS ( ( 4, 4 ),
 ( 3, 3 ),
 ( 0.000000000000000000, 0.0004264778881141670364 ),
 ( 0.000000000000000000, 1.000000000000000000 ),
 .UNSPECIFIED. ) 
 GEOMETRIC_REPRESENTATION_ITEM ( )  RATIONAL_B_SPLINE_SURFACE ( (
 ( 1.000000000000000000, 0.8414823709351039183, 1.000000000000000000),
 ( 1.000000000000000000, 0.8184116177158143879, 1.000000000000000000),
 ( 1.000000000000000000, 0.7848884419355106612, 1.000000000000000000),
 ( 1.000000000000000000, 0.7411386215560255009, 1.000000000000000000) ) ) 
 REPRESENTATION_ITEM ( '' )  SURFACE ( )  );
#15798=ORIENTED_EDGE ( 'NONE', *, *, #84556, .T. ) ;
#15799=CARTESIAN_POINT ( 'NONE',  ( 19.42250999205614193, 35.14701867748816966, 5.440088680355555262 ) ) ;
#15800=CARTESIAN_POINT ( 'NONE',  ( -39.69000000000001194, 92.00000000000000000, 9.500000000000000000 ) ) ;
#15801=CARTESIAN_POINT ( 'NONE',  ( 17.62281668512000365, 48.28593319516822646, 6.500000000000063061 ) ) ;
#15803=CARTESIAN_POINT ( 'NONE',  ( -1.099225684535947600, 13.70696800326375353, -6.408140936763238038 ) ) ;
#15804=CARTESIAN_POINT ( 'NONE',  ( 12.63842701281683034, 12.46726448433411782, 9.846743663894596210 ) ) ;
#15808=CARTESIAN_POINT ( 'NONE',  ( 18.52753015748617571, 18.09226448433411960, 4.923371831947298993 ) ) ;
#15809=CARTESIAN_POINT ( 'NONE',  ( 19.42250999205614548, 25.98035201082150891, -5.440088680355545492 ) ) ;
#15811=ORIENTED_EDGE ( 'NONE', *, *, #81515, .T. ) ;
#15813=CARTESIAN_POINT ( 'NONE',  ( 19.42250999205614193, 60.14701867748817676, 5.440088680355555262 ) ) ;
#15815=CARTESIAN_POINT ( 'NONE',  ( 13.43411237798106583, 57.66530133659708923, -12.81628187352647252 ) ) ;
#15816=CARTESIAN_POINT ( 'NONE',  ( 20.88017736071110875, 60.77201867748817676, -2.915334737309920765 ) ) ;
#15817=CARTESIAN_POINT ( 'NONE',  ( 0.6178305044545838731, 4.748634669930420493, 9.382169495545420901 ) ) ;
#15819=CARTESIAN_POINT ( 'NONE',  ( 2.791683348922237240, 35.38393115100079456, -7.208316651077763204 ) ) ;
#15820=CARTESIAN_POINT ( 'NONE',  ( 22.81628187352648496, 51.83196800326376064, -3.434112377981050290 ) ) ;
#15821=CARTESIAN_POINT ( 'NONE',  ( 2.602085213965210642E-15, 78.91966277462714174, 9.500000000000000000 ) ) ;
#15822=CARTESIAN_POINT ( 'NONE',  ( 7.361572987183169658, 24.96726448433412315, -9.846743663894592657 ) ) ;
#15823=CARTESIAN_POINT ( 'NONE',  ( 0.6178305044545818747, 13.49863466993041783, -9.382169495545419124 ) ) ;
#15824=CARTESIAN_POINT ( 'NONE',  ( 19.50000000000000711, 105.0000000000000000, -5.000000000000000000 ) ) ;
#15825=CARTESIAN_POINT ( 'NONE',  ( 17.96484262340118221, 39.93868534415484106, 7.964842623401181321 ) ) ;
#15826=CARTESIAN_POINT ( 'NONE',  ( -1.099225684535947600, -0.4596986634029132657, 6.408140936763237150 ) ) ;
#15829=CARTESIAN_POINT ( 'NONE',  ( 5.076628168052704559, 25.17559781766745175, -8.527530157486179263 ) ) ;
#15830=CARTESIAN_POINT ( 'NONE',  ( 18.52753015748618282, 8.925597817667451750, -4.923371831947291888 ) ) ;
#15831=CARTESIAN_POINT ( 'NONE',  ( 15.44008868035555260, 9.730352010821505360, 9.422509992056143702 ) ) ;
#15832=CARTESIAN_POINT ( 'NONE',  ( 16.40814093676324603, 17.45696800326375353, -11.09922568453594671 ) ) ;
#15834=B_SPLINE_CURVE_WITH_KNOTS ( 'NONE', 3,
 ( #79030, #3063, #87518, #86544, #79533, #50015 ),
 .UNSPECIFIED., .F., .F.,
 ( 4, 2, 4 ),
 ( 0.000000000000000000, 0.0002701661927229300235, 0.0005403323854458600469 ),
 .UNSPECIFIED. ) ;
#15836=CARTESIAN_POINT ( 'NONE',  ( 5.076628168052704559, 65.17559781766745175, -8.527530157486179263 ) ) ;
#15839=CARTESIAN_POINT ( 'NONE',  ( 4.559911319644449179, 23.89701867748817321, 9.422509992056141925 ) ) ;
#15840=CARTESIAN_POINT ( 'NONE',  ( 18.52753015748617571, 48.09226448433412315, 4.923371831947298993 ) ) ;
#15841=ADVANCED_FACE ( 'NONE', ( #68536 ), #84522, .T. ) ;
#15842=CARTESIAN_POINT ( 'NONE',  ( -1.926860441876563801, 49.89664270246083078, 3.195792623639529761 ) ) ;
#15843=CARTESIAN_POINT ( 'NONE',  ( 4.559911319644449179, 23.89701867748817321, 9.422509992056141925 ) ) ;
#15844=CARTESIAN_POINT ( 'NONE',  ( 1.472469842513823179, 6.425597817667451750, 4.923371831947296329 ) ) ;
#15845=CARTESIAN_POINT ( 'NONE',  ( -0.8801773607111008646, 28.27201867748817321, 2.915334737309923430 ) ) ;
#15846=CARTESIAN_POINT ( 'NONE',  ( -2.266590686148945544, 67.22041550158063217, 7.082119434687048631 ) ) ;
#15848=CARTESIAN_POINT ( 'NONE',  ( 14.92337183194729633, 27.67559781766745530, 8.527530157486181039 ) ) ;
#15849=CARTESIAN_POINT ( 'NONE',  ( -2.816281873526473856, 9.123634669930421381, 9.499525473075851096E-16 ) ) ;
#15852=CARTESIAN_POINT ( 'NONE',  ( 0.2751277870542893633, 25.30223176428832232, 6.499999999999988454 ) ) ;
#15854=CARTESIAN_POINT ( 'NONE',  ( 22.26659068614894466, 13.88708216824730179, 7.082119434687054849 ) ) ;
#15855=CARTESIAN_POINT ( 'NONE',  ( 7.361572987183170547, 42.05059781766745886, 9.846743663894590881 ) ) ;
#15858=CARTESIAN_POINT ( 'NONE',  ( 24.16423886937410614, 54.51208216824730357, -3.795296366450302550 ) ) ;
#15859=CARTESIAN_POINT ( 'NONE',  ( 10.00000000000000178, 17.25893115100078745, 9.846743663894594434 ) ) ;
#15862=CARTESIAN_POINT ( 'NONE',  ( 7.084665262690076126, 49.10535201082149825, 10.88017736071109987 ) ) ;
#15863=CARTESIAN_POINT ( 'NONE',  ( 10.00000000000000178, 45.37363466993041783, 12.81628187352647608 ) ) ;
#15864=CARTESIAN_POINT ( 'NONE',  ( -0.8801773607111008646, 23.27201867748817676, 2.915334737309923430 ) ) ;
#15865=CARTESIAN_POINT ( 'NONE',  ( 22.81628187352647785, 46.41530133659708213, 3.434112377981063169 ) ) ;
#15866=CARTESIAN_POINT ( 'NONE',  ( -2.816281873526473856, -0.8763653300695799508, 9.499525473075851096E-16 ) ) ;
#15867=ORIENTED_EDGE ( 'NONE', *, *, #75684, .F. ) ;
#15868=CARTESIAN_POINT ( 'NONE',  ( -0.1503990784575321704, 8.101585745166424601, 6.262539305110068177 ) ) ;
#15870=CARTESIAN_POINT ( 'NONE',  ( 2.342957944459074682, 0.8396798841124157864, -6.500000000000004441 ) ) ;
#15871=CARTESIAN_POINT ( 'NONE',  ( -2.266590686148945544, 46.38708216824730357, -7.082119434687050408 ) ) ;
#15872=CARTESIAN_POINT ( 'NONE',  ( 6.204703633549690345, 15.76208216824730179, -14.16423886937410259 ) ) ;
#15873=CARTESIAN_POINT ( 'NONE',  ( 19.42250999205614548, 25.98035201082150891, -5.440088680355545492 ) ) ;
#15874=CARTESIAN_POINT ( 'NONE',  ( 7.084665262690076126, 37.02201867748817676, -10.88017736071110164 ) ) ;
#15878=CARTESIAN_POINT ( 'NONE',  ( 12.91533473730992121, 64.52201867748817676, 10.88017736071110164 ) ) ;
#15879=CARTESIAN_POINT ( 'NONE',  ( 0.5774900079438590739, 67.64701867748817676, -5.440088680355550821 ) ) ;
#15880=CARTESIAN_POINT ( 'NONE',  ( 13.43411237798105340, 30.58196800326374998, 12.81628187352647963 ) ) ;
#15883=CARTESIAN_POINT ( 'NONE',  ( 1.472469842513823179, 11.42559781766745175, 4.923371831947296329 ) ) ;
#15884=CARTESIAN_POINT ( 'NONE',  ( 7.361572987183170547, 42.05059781766745886, 9.846743663894590881 ) ) ;
#15885=CARTESIAN_POINT ( 'NONE',  ( 0.5774900079438590739, 12.64701867748817143, -5.440088680355550821 ) ) ;
#15886=CARTESIAN_POINT ( 'NONE',  ( 21.09922568453595559, 27.04030133659708568, -6.408140936763230044 ) ) ;
#15887=CARTESIAN_POINT ( 'NONE',  ( 12.63842701281683922, 9.550597817667449974, -9.846743663894590881 ) ) ;
#15888=CARTESIAN_POINT ( 'NONE',  ( 20.88017736071110164, 5.355352010821502695, 2.915334737309930979 ) ) ;
#15889=CARTESIAN_POINT ( 'NONE',  ( 0.1532563361054083140, 36.00893115100078745, 1.131784320476157264E-15 ) ) ;
#15890=CARTESIAN_POINT ( 'NONE',  ( 19.84674366389459266, 38.71726448433412315, -2.638427012816827677 ) ) ;
#15891=CARTESIAN_POINT ( 'NONE',  ( -0.3689425029237881626, 22.42874883491397142, 10.36894250292379027 ) ) ;
#15892=CARTESIAN_POINT ( 'NONE',  ( 20.88017736071110164, 30.35535201082151247, 2.915334737309930979 ) ) ;
#15893=CARTESIAN_POINT ( 'NONE',  ( 10.00000000000000000, 6.813685344154838397, -10.88017736071110342 ) ) ;
#15894=CARTESIAN_POINT ( 'NONE',  ( -0.8801773607110991993, 37.85535201082151247, -2.915334737309923874 ) ) ;
#15895=CARTESIAN_POINT ( 'NONE',  ( 19.42250999205614548, 30.98035201082150536, -5.440088680355545492 ) ) ;
#15897=CARTESIAN_POINT ( 'NONE',  ( 15.44008868035555260, 44.73035201082151247, 9.422509992056143702 ) ) ;
#15898=CARTESIAN_POINT ( 'NONE',  ( 19.38216949554541202, 55.99863466993041072, 9.382169495545424454 ) ) ;
#15899=CARTESIAN_POINT ( 'NONE',  ( 10.00000000000000000, 41.81368534415484106, -10.88017736071110342 ) ) ;
#15900=CARTESIAN_POINT ( 'NONE',  ( 20.88017736071110519, 45.56368534415484106, 2.639326808657452039E-16 ) ) ;
#15901=ORIENTED_EDGE ( 'NONE', *, *, #77882, .F. ) ;
#15902=CARTESIAN_POINT ( 'NONE',  ( 20.88017736071110519, 55.56368534415484817, 2.639326808657452039E-16 ) ) ;
#15906=CARTESIAN_POINT ( 'NONE',  ( -2.266590686148945544, 57.22041550158063217, 7.082119434687048631 ) ) ;
#15907=CARTESIAN_POINT ( 'NONE',  ( -0.8801773607111009756, 63.06368534415484106, 1.068504757029289695E-15 ) ) ;
#15910=CARTESIAN_POINT ( 'NONE',  ( 19.84674366389459621, 28.50893115100078745, 7.409399052514197653E-17 ) ) ;
#15911=ORIENTED_EDGE ( 'NONE', *, *, #44603, .F. ) ;
#15912=CARTESIAN_POINT ( 'NONE',  ( 1.472469842513823179, 36.42559781766745175, 4.923371831947296329 ) ) ;
#15913=CARTESIAN_POINT ( 'NONE',  ( 4.559911319644449179, 33.89701867748817676, 9.422509992056141925 ) ) ;
#15914=CARTESIAN_POINT ( 'NONE',  ( 14.92337183194729633, 37.67559781766745175, 8.527530157486181039 ) ) ;
#15915=CARTESIAN_POINT ( 'NONE',  ( 16.40814093676323893, 25.79030133659708923, 11.09922568453595026 ) ) ;
#15917=CARTESIAN_POINT ( 'NONE',  ( 17.96484262340118221, 54.93868534415484106, 7.964842623401181321 ) ) ;
#15918=CARTESIAN_POINT ( 'NONE',  ( 17.96484262340118221, 39.93868534415484106, 7.964842623401181321 ) ) ;
#15919=CARTESIAN_POINT ( 'NONE',  ( 10.00000000000000000, 6.813685344154838397, -10.88017736071110342 ) ) ;
#15920=CARTESIAN_POINT ( 'NONE',  ( 2.917880565312950480, 55.97041550158063217, -12.26659068614894821 ) ) ;
#15922=CARTESIAN_POINT ( 'NONE',  ( 21.09922568453595559, 22.04030133659708923, -6.408140936763230044 ) ) ;
#15925=CARTESIAN_POINT ( 'NONE',  ( 21.09922568453595559, 17.04030133659708923, -6.408140936763230044 ) ) ;
#15926=CARTESIAN_POINT ( 'NONE',  ( 20.88017736071110164, 25.35535201082150891, 2.915334737309930979 ) ) ;
#15927=CARTESIAN_POINT ( 'NONE',  ( 10.00000000000000178, 54.31368534415484106, 10.88017736071110342 ) ) ;
#15930=CARTESIAN_POINT ( 'NONE',  ( 5.076628168052704559, 0.1755978176674514724, -8.527530157486179263 ) ) ;
#15931=CARTESIAN_POINT ( 'NONE',  ( 19.84674366389459266, 48.71726448433413026, -2.638427012816827677 ) ) ;
#15932=CARTESIAN_POINT ( 'NONE',  ( 19.84674366389459266, 33.30059781766744464, 2.638427012816836559 ) ) ;
#15934=CARTESIAN_POINT ( 'NONE',  ( 2.791683348922240793, 21.63393115100078745, 7.208316651077764092 ) ) ;
#15935=CARTESIAN_POINT ( 'NONE',  ( 19.89220837332778302, 54.74062864464239908, 6.478736007405906605 ) ) ;
#15937=CARTESIAN_POINT ( 'NONE',  ( 7.361572987183170547, 12.05059781766744997, 9.846743663894590881 ) ) ;
#15940=CARTESIAN_POINT ( 'NONE',  ( 7.361572987183170547, 52.05059781766745175, 9.846743663894590881 ) ) ;
#15942=EDGE_CURVE ( 'NONE', #53047, #30064, #78966, .T. ) ;
#15943=CARTESIAN_POINT ( 'NONE',  ( 22.81628187352648496, 6.831968003263753531, -3.434112377981050290 ) ) ;
#15944=CARTESIAN_POINT ( 'NONE',  ( 20.88017736071110519, 55.56368534415484817, 2.639326808657452039E-16 ) ) ;
#15945=CARTESIAN_POINT ( 'NONE',  ( 17.08211943468705130, 38.47041550158063217, 12.26659068614894998 ) ) ;
#15947=FACE_OUTER_BOUND ( 'NONE', #88835, .T. ) ;
#15948=CARTESIAN_POINT ( 'NONE',  ( 19.67853978997394293, 89.81963405576850334, 5.461515559775651063 ) ) ;
#15949=CARTESIAN_POINT ( 'NONE',  ( 17.08211943468705840, 40.13708216824731068, -12.26659068614894466 ) ) ;
#15950=CARTESIAN_POINT ( 'NONE',  ( -4.164238869374098151, 61.59541550158063217, -3.795296366450310543 ) ) ;
#15951=CARTESIAN_POINT ( 'NONE',  ( 22.26659068614895176, 29.72041550158063572, -7.082119434687042414 ) ) ;
#15952=CARTESIAN_POINT ( 'NONE',  ( -0.3689425029237898834, 21.17874883491396432, -10.36894250292378850 ) ) ;
#15954=CARTESIAN_POINT ( 'NONE',  ( 0.1129803114748920007, 29.29427333184091609, -6.480634945678687586 ) ) ;
#15956=CARTESIAN_POINT ( 'NONE',  ( 2.791683348922237240, 40.38393115100078035, -7.208316651077763204 ) ) ;
#15957=EDGE_LOOP ( 'NONE', ( #31871, #39002, #7905, #72984, #44582, #86746 ) ) ;
#15959=CARTESIAN_POINT ( 'NONE',  ( 0.1532563361054100626, 65.80059781766745175, -2.638427012816831230 ) ) ;
#15960=CARTESIAN_POINT ( 'NONE',  ( -0.1503990784575328643, 45.12777174578613426, 6.262539305110068177 ) ) ;
#15961=CARTESIAN_POINT ( 'NONE',  ( 1.472469842513823179, 45.59226448433412315, -4.923371831947296329 ) ) ;
#15962=CARTESIAN_POINT ( 'NONE',  ( -2.816281873526473856, 49.12363466993042493, 9.499525473075851096E-16 ) ) ;
#15964=CARTESIAN_POINT ( 'NONE',  ( 1.472469842513823179, 45.59226448433412315, -4.923371831947296329 ) ) ;
#15965=CARTESIAN_POINT ( 'NONE',  ( 10.00000000000000178, 57.25893115100078745, 9.846743663894594434 ) ) ;
#15966=CARTESIAN_POINT ( 'NONE',  ( 22.26659068614894466, 38.88708216824731068, 7.082119434687054849 ) ) ;
#15968=B_SPLINE_CURVE_WITH_KNOTS ( 'NONE', 3,
 ( #1383, #93334, #76372, #47332 ),
 .UNSPECIFIED., .F., .F.,
 ( 4, 4 ),
 ( 3.418109631315660599E-17, 0.002392975128318410027 ),
 .UNSPECIFIED. ) ;
#15969=CARTESIAN_POINT ( 'NONE',  ( 20.36894250292379738, 14.92874883491396432, -10.36894250292379027 ) ) ;
#15971=CARTESIAN_POINT ( 'NONE',  ( -0.8801773607111008646, 63.27201867748817676, 2.915334737309923430 ) ) ;
#15974=CARTESIAN_POINT ( 'NONE',  ( 0.5774900079438607392, 3.480352010821504916, 5.440088680355550821 ) ) ;
#15975=CARTESIAN_POINT ( 'NONE',  ( 22.81628187352648496, 16.83196800326374998, -3.434112377981050290 ) ) ;
#15977=CARTESIAN_POINT ( 'NONE',  ( 19.84674366389459266, 3.300597817667451750, 2.638427012816836559 ) ) ;
#15978=VECTOR ( 'NONE', #5299, 1000.000000000000000 ) ;
#15979=CARTESIAN_POINT ( 'NONE',  ( -46.94000000000001194, 100.9546402834806713, -8.718409068399685324 ) ) ;
#15981=CARTESIAN_POINT ( 'NONE',  ( 24.16423886937410614, 59.30374883491397497, 8.672049930838204340E-16 ) ) ;
#15983=CARTESIAN_POINT ( 'NONE',  ( 20.88017736071110164, 20.35535201082150891, 2.915334737309930979 ) ) ;
#15984=CARTESIAN_POINT ( 'NONE',  ( 19.42250999205614193, 25.14701867748817321, 5.440088680355555262 ) ) ;
#15985=CARTESIAN_POINT ( 'NONE',  ( 12.63842701281683922, 59.55059781766744464, -9.846743663894590881 ) ) ;
#15986=CARTESIAN_POINT ( 'NONE',  ( 18.52753015748618282, 58.92559781766745886, -4.923371831947291888 ) ) ;
#15987=CARTESIAN_POINT ( 'NONE',  ( -1.099225684535947600, 48.70696800326375353, -6.408140936763238038 ) ) ;
#15989=VERTEX_POINT ( 'NONE', #39022 ) ;
#15990=VECTOR ( 'NONE', #80953, 1000.000000000000000 ) ;
#15991=CARTESIAN_POINT ( 'NONE',  ( 2.035157376598822676, 22.43868534415483396, -7.964842623401177768 ) ) ;
#15992=CARTESIAN_POINT ( 'NONE',  ( 10.00000000000000178, 15.37363466993042138, 12.81628187352647608 ) ) ;
#15994=CARTESIAN_POINT ( 'NONE',  ( 2.791683348922240793, 51.63393115100078745, 7.208316651077764092 ) ) ;
#15995=CARTESIAN_POINT ( 'NONE',  ( 0.5774900079438590739, 47.64701867748817676, -5.440088680355550821 ) ) ;
#15996=CARTESIAN_POINT ( 'NONE',  ( 21.09922568453595559, 17.04030133659708923, -6.408140936763230044 ) ) ;
#15997=CARTESIAN_POINT ( 'NONE',  ( 2.035157376598822676, 62.43868534415483396, -7.964842623401177768 ) ) ;
#15998=CARTESIAN_POINT ( 'NONE',  ( -0.1503990784575328643, 70.00000000000000000, 6.262539305110068177 ) ) ;
#15999=CARTESIAN_POINT ( 'NONE',  ( -0.03447792253739274948, 50.15514106990690379, 6.401564815979743805 ) ) ;
#16002=CARTESIAN_POINT ( 'NONE',  ( -0.8801773607111008646, 43.27201867748817676, 2.915334737309923430 ) ) ;
#16003=CARTESIAN_POINT ( 'NONE',  ( 19.38216949554541557, 42.24863466993041783, -9.382169495545420901 ) ) ;
#16004=CARTESIAN_POINT ( 'NONE',  ( 24.16423886937410614, 14.30374883491396787, 8.672049930838204340E-16 ) ) ;
#16006=CARTESIAN_POINT ( 'NONE',  ( 0.1532563361054083140, 21.00893115100078745, 1.131784320476157264E-15 ) ) ;
#16008=CARTESIAN_POINT ( 'NONE',  ( 6.204703633549690345, 45.76208216824729647, -14.16423886937410259 ) ) ;
#16009=FACE_OUTER_BOUND ( 'NONE', #60979, .T. ) ;
#16010=CARTESIAN_POINT ( 'NONE',  ( 4.559911319644449179, 7.230352010821504471, -9.422509992056141925 ) ) ;
#16014=CARTESIAN_POINT ( 'NONE',  ( -0.8801773607111008646, 3.272018677488171434, 2.915334737309923430 ) ) ;
#16015=CARTESIAN_POINT ( 'NONE',  ( 4.559911319644449179, 12.23035201082150714, -9.422509992056141925 ) ) ;
#16016=CARTESIAN_POINT ( 'NONE',  ( 2.791683348922237240, 40.38393115100078035, -7.208316651077763204 ) ) ;
#16018=CARTESIAN_POINT ( 'NONE',  ( 16.40814093676324603, 37.45696800326376064, -11.09922568453594671 ) ) ;
#16020=CARTESIAN_POINT ( 'NONE',  ( 0.9408516040111536416, 2.466938638839759168, -6.499999999999972466 ) ) ;
#16021=CARTESIAN_POINT ( 'NONE',  ( 2.917880565312948704, 7.637082168247301794, 12.26659068614894643 ) ) ;
#16022=CARTESIAN_POINT ( 'NONE',  ( 15.44008868035555793, 31.39701867748817676, -9.422509992056140149 ) ) ;
#16023=CARTESIAN_POINT ( 'NONE',  ( 19.42250999205614548, 5.980352010821504471, -5.440088680355545492 ) ) ;
#16024=CARTESIAN_POINT ( 'NONE',  ( 10.00000000000000178, 37.25893115100078745, 9.846743663894594434 ) ) ;
#16026=DIRECTION ( 'NONE',  ( -0.000000000000000000, -0.000000000000000000, 1.000000000000000000 ) ) ;
#16027=CARTESIAN_POINT ( 'NONE',  ( 1.472469842513823179, 16.42559781766745175, 4.923371831947296329 ) ) ;
#16032=ORIENTED_EDGE ( 'NONE', *, *, #3014, .F. ) ;
#16033=CARTESIAN_POINT ( 'NONE',  ( 10.00000000000000000, 59.75893115100078745, -9.846743663894594434 ) ) ;
#16034=CARTESIAN_POINT ( 'NONE',  ( -0.8801773607111009756, 28.06368534415484106, 1.068504757029289695E-15 ) ) ;
#16035=CARTESIAN_POINT ( 'NONE',  ( 0.5774900079438590739, 42.64701867748816966, -5.440088680355550821 ) ) ;
#16036=CARTESIAN_POINT ( 'NONE',  ( 15.44008868035555260, 9.730352010821505360, 9.422509992056143702 ) ) ;
#16037=CARTESIAN_POINT ( 'NONE',  ( 0.6178305044545838731, 29.74863466993042138, 9.382169495545420901 ) ) ;
#16038=CARTESIAN_POINT ( 'NONE',  ( 24.16423886937410614, 19.30374883491397142, 8.672049930838204340E-16 ) ) ;
#16041=CARTESIAN_POINT ( 'NONE',  ( 6.565887622018943937, 43.08196800326374643, -12.81628187352647608 ) ) ;
#16042=ORIENTED_EDGE ( 'NONE', *, *, #5771, .F. ) ;
#16043=CARTESIAN_POINT ( 'NONE',  ( 0.1532563361054082862, 41.21726448433411605, 2.638427012816831674 ) ) ;
#16044=CARTESIAN_POINT ( 'NONE',  ( 15.44008868035555793, 21.39701867748817321, -9.422509992056140149 ) ) ;
#16047=CARTESIAN_POINT ( 'NONE',  ( -0.8801773607111009756, 23.06368534415484106, 1.068504757029289695E-15 ) ) ;
#16048=VERTEX_POINT ( 'NONE', #70011 ) ;
#16049=CARTESIAN_POINT ( 'NONE',  ( -0.8801773607111008646, 58.27201867748816966, 2.915334737309923430 ) ) ;
#16051=CARTESIAN_POINT ( 'NONE',  ( 0.5774900079438590739, 67.64701867748817676, -5.440088680355550821 ) ) ;
#16052=CARTESIAN_POINT ( 'NONE',  ( 20.88017736071110875, 60.77201867748817676, -2.915334737309920765 ) ) ;
#16053=CARTESIAN_POINT ( 'NONE',  ( 0.1532563361054083140, 16.00893115100078390, 1.131784320476157264E-15 ) ) ;
#16054=CARTESIAN_POINT ( 'NONE',  ( 5.076628168052703671, 1.842264484334118047, 8.527530157486179263 ) ) ;
#16058=CARTESIAN_POINT ( 'NONE',  ( 19.84674366389459621, 3.508931151000785231, 7.409399052514197653E-17 ) ) ;
#16060=ADVANCED_FACE ( 'NONE', ( #31980 ), #32488, .F. ) ;
#16061=CARTESIAN_POINT ( 'NONE',  ( 0.1532563361054100626, 45.80059781766745886, -2.638427012816831230 ) ) ;
#16064=CARTESIAN_POINT ( 'NONE',  ( 7.361572987183169658, 64.96726448433412315, -9.846743663894592657 ) ) ;
#16066=CARTESIAN_POINT ( 'NONE',  ( 17.08211943468705840, 25.13708216824730357, -12.26659068614894466 ) ) ;
#16068=CARTESIAN_POINT ( 'NONE',  ( -0.2418659066527787949, 7.234100856612040609, -6.114288769123032985 ) ) ;
#16069=DIRECTION ( 'NONE',  ( 0.000000000000000000, 0.000000000000000000, 1.000000000000000000 ) ) ;
#16070=CARTESIAN_POINT ( 'NONE',  ( 20.88017736071110519, 60.56368534415484106, 2.639326808657452039E-16 ) ) ;
#16071=CARTESIAN_POINT ( 'NONE',  ( 7.084665262690076126, 27.02201867748817676, -10.88017736071110164 ) ) ;
#16072=CARTESIAN_POINT ( 'NONE',  ( 13.99999999999999822, 11.50000000000000000, -6.500000000000000888 ) ) ;
#16074=CARTESIAN_POINT ( 'NONE',  ( 10.00000000000000178, 2.258931151000784787, 9.846743663894594434 ) ) ;
#16076=CARTESIAN_POINT ( 'NONE',  ( 22.81628187352648496, 26.83196800326374998, -3.434112377981050290 ) ) ;
#16077=CARTESIAN_POINT ( 'NONE',  ( 10.00000000000000000, 24.75893115100078745, -9.846743663894594434 ) ) ;
#16078=DIRECTION ( 'NONE',  ( -0.000000000000000000, -1.000000000000000000, 0.000000000000000000 ) ) ;
#16079=CARTESIAN_POINT ( 'NONE',  ( 3.591859063236763294, 13.29030133659708746, -11.09922568453595026 ) ) ;
#16080=CARTESIAN_POINT ( 'NONE',  ( 20.15039907845753220, 40.60158574516643171, -6.262539305110077947 ) ) ;
#16082=CARTESIAN_POINT ( 'NONE',  ( 1.472469842513823179, 10.59226448433411782, -4.923371831947296329 ) ) ;
#16084=ORIENTED_EDGE ( 'NONE', *, *, #69416, .T. ) ;
#16085=CARTESIAN_POINT ( 'NONE',  ( -0.8801773607110991993, 17.85535201082150536, -2.915334737309923874 ) ) ;
#16086=CARTESIAN_POINT ( 'NONE',  ( 20.36894250292379738, 19.92874883491396787, -10.36894250292379027 ) ) ;
#16087=CARTESIAN_POINT ( 'NONE',  ( 12.63842701281683922, 39.55059781766744464, -9.846743663894590881 ) ) ;
#16088=( BOUNDED_CURVE ( )  B_SPLINE_CURVE ( 2, ( #73314, #68659, #91653, #38652, #73803, #14687, #61626, #23669, #35814 ),
 .UNSPECIFIED., .F., .F. ) 
 B_SPLINE_CURVE_WITH_KNOTS ( ( 3, 2, 2, 2, 3 ),
 ( 0.7972837940830885817, 0.7976190476190476719, 0.8035714285714286031, 0.8095238095238095344, 0.8098590630597686246 ),
 .UNSPECIFIED. ) 
 CURVE ( )  GEOMETRIC_REPRESENTATION_ITEM ( )  RATIONAL_B_SPLINE_CURVE ( ( 0.9963778908391764944, 0.9980808541467923733, 1.000000000000000000, 0.9659258262890682012, 1.000000000000000000, 0.9659258262890682012, 1.000000000000000000, 0.9980808541467922623, 0.9963778908391764944 ) ) 
 REPRESENTATION_ITEM ( '' )  );
#16089=CARTESIAN_POINT ( 'NONE',  ( 17.20831665107776587, 2.883931151000785231, 7.208316651077764980 ) ) ;
#16090=CARTESIAN_POINT ( 'NONE',  ( 21.09922568453594849, 51.20696800326375353, 6.408140936763242479 ) ) ;
#16092=CARTESIAN_POINT ( 'NONE',  ( 12.91533473730993009, 31.60535201082150891, -10.88017736071109987 ) ) ;
#16094=EDGE_CURVE ( 'NONE', #96185, #85865, #45458, .T. ) ;
#16095=CARTESIAN_POINT ( 'NONE',  ( -1.099225684535947600, 14.54030133659708568, 6.408140936763237150 ) ) ;
#16096=CARTESIAN_POINT ( 'NONE',  ( 18.52753015748617571, 38.09226448433412315, 4.923371831947298993 ) ) ;
#16098=CARTESIAN_POINT ( 'NONE',  ( 10.00000000000000000, 42.87363466993042493, -12.81628187352647608 ) ) ;
#16100=CARTESIAN_POINT ( 'NONE',  ( -0.8801773607111009756, 58.06368534415484106, 1.068504757029289695E-15 ) ) ;
#16102=EDGE_CURVE ( 'NONE', #80852, #6068, #15422, .T. ) ;
#16104=CARTESIAN_POINT ( 'NONE',  ( 17.39651004071842166, 27.93575266056828355, 6.499999999999998224 ) ) ;
#16105=CARTESIAN_POINT ( 'NONE',  ( 12.91533473730993009, 56.60535201082151247, -10.88017736071109987 ) ) ;
#16106=CARTESIAN_POINT ( 'NONE',  ( 19.42250999205614548, 40.98035201082150536, -5.440088680355545492 ) ) ;
#16108=CARTESIAN_POINT ( 'NONE',  ( 0.5774900079438590739, 67.64701867748817676, -5.440088680355550821 ) ) ;
#16109=CARTESIAN_POINT ( 'NONE',  ( 5.076628168052704559, 45.17559781766745175, -8.527530157486179263 ) ) ;
#16110=CARTESIAN_POINT ( 'NONE',  ( 2.035157376598824452, 3.688685344154837953, 7.964842623401179544 ) ) ;
#16113=CARTESIAN_POINT ( 'NONE',  ( 16.40814093676323893, 25.79030133659708923, 11.09922568453595026 ) ) ;
#16114=ORIENTED_EDGE ( 'NONE', *, *, #4231, .T. ) ;
#16115=CARTESIAN_POINT ( 'NONE',  ( 7.084665262690076126, 34.10535201082151247, 10.88017736071109987 ) ) ;
#16117=CARTESIAN_POINT ( 'NONE',  ( 6.565887622018943937, 3.081968003263753531, -12.81628187352647608 ) ) ;
#16119=CARTESIAN_POINT ( 'NONE',  ( 20.88017736071110519, 15.56368534415483751, 2.639326808657452039E-16 ) ) ;
#16120=CARTESIAN_POINT ( 'NONE',  ( 17.96484262340118221, 26.18868534415483396, -7.964842623401177768 ) ) ;
#16121=CARTESIAN_POINT ( 'NONE',  ( 13.79529636645030344, 38.26208216824729647, 14.16423886937410614 ) ) ;
#16122=CARTESIAN_POINT ( 'NONE',  ( 5.076628168052704559, 25.17559781766745175, -8.527530157486179263 ) ) ;
#16123=CARTESIAN_POINT ( 'NONE',  ( 2.035157376598824452, 53.68868534415484817, 7.964842623401179544 ) ) ;
#16124=CARTESIAN_POINT ( 'NONE',  ( 0.9408516040111475354, 32.46693863883975695, -6.499999999999953815 ) ) ;
#16125=CARTESIAN_POINT ( 'NONE',  ( -0.3689425029237898834, 1.178748834913967869, -10.36894250292378850 ) ) ;
#16126=UNCERTAINTY_MEASURE_WITH_UNIT (LENGTH_MEASURE( 1.000000000000000082E-05 ), #21549, 'distance_accuracy_value', 'NONE');
#16127=CARTESIAN_POINT ( 'NONE',  ( 14.92337183194729633, 62.67559781766745886, 8.527530157486181039 ) ) ;
#16130=CARTESIAN_POINT ( 'NONE',  ( -4.164238869374098151, 36.59541550158063217, -3.795296366450310543 ) ) ;
#16131=CARTESIAN_POINT ( 'NONE',  ( 2.917880565312950480, 40.97041550158063217, -12.26659068614894821 ) ) ;
#16132=CARTESIAN_POINT ( 'NONE',  ( -0.8801773607111009756, 68.06368534415484817, 1.068504757029289695E-15 ) ) ;
#16133=CARTESIAN_POINT ( 'NONE',  ( 1.472469842513823179, 55.59226448433412315, -4.923371831947296329 ) ) ;
#16135=CARTESIAN_POINT ( 'NONE',  ( 2.035157376598824452, 58.68868534415482685, 7.964842623401179544 ) ) ;
#16136=CARTESIAN_POINT ( 'NONE',  ( 3.591859063236761518, 14.95696800326375531, 11.09922568453594849 ) ) ;
#16137=CARTESIAN_POINT ( 'NONE',  ( -0.3689425029237898834, 26.17874883491396432, -10.36894250292378850 ) ) ;
#16138=CARTESIAN_POINT ( 'NONE',  ( 10.00000000000000178, 29.31368534415483751, 10.88017736071110342 ) ) ;
#16139=CARTESIAN_POINT ( 'NONE',  ( 17.96484262340118221, 36.18868534415484106, -7.964842623401177768 ) ) ;
#16140=CARTESIAN_POINT ( 'NONE',  ( 20.30776406404399737, 70.00000000000000000, 6.000000000000270894 ) ) ;
#16141=CARTESIAN_POINT ( 'NONE',  ( 19.42250999205614548, 50.98035201082151247, -5.440088680355545492 ) ) ;
#16145=VERTEX_POINT ( 'NONE', #25982 ) ;
#16149=CARTESIAN_POINT ( 'NONE',  ( 22.26659068614894466, 8.887082168247300018, 7.082119434687054849 ) ) ;
#16150=CARTESIAN_POINT ( 'NONE',  ( -4.164238869374098151, 56.59541550158063927, -3.795296366450310543 ) ) ;
#16151=CARTESIAN_POINT ( 'NONE',  ( 2.917880565312948704, 62.63708216824730357, 12.26659068614894643 ) ) ;
#16152=CARTESIAN_POINT ( 'NONE',  ( 7.361572987183169658, 34.96726448433411605, -9.846743663894592657 ) ) ;
#16153=CARTESIAN_POINT ( 'NONE',  ( 12.63842701281683922, 64.55059781766745175, -9.846743663894590881 ) ) ;
#16156=CARTESIAN_POINT ( 'NONE',  ( 20.04068437667227087, 44.71974360917720759, 6.396802510829643573 ) ) ;
#16160=CARTESIAN_POINT ( 'NONE',  ( 3.591859063236761518, 4.956968003263753531, 11.09922568453594849 ) ) ;
#16162=ORIENTED_EDGE ( 'NONE', *, *, #71749, .T. ) ;
#16163=CARTESIAN_POINT ( 'NONE',  ( 2.917880565312950480, 40.97041550158063217, -12.26659068614894821 ) ) ;
#16164=CARTESIAN_POINT ( 'NONE',  ( 6.204703633549690345, 42.84541550158063217, 14.16423886937410082 ) ) ;
#16165=ORIENTED_EDGE ( 'NONE', *, *, #4287, .F. ) ;
#16166=CARTESIAN_POINT ( 'NONE',  ( 19.42250999205614193, 25.14701867748817321, 5.440088680355555262 ) ) ;
#16167=CARTESIAN_POINT ( 'NONE',  ( 16.40814093676323893, 60.79030133659709634, 11.09922568453595026 ) ) ;
#16168=CARTESIAN_POINT ( 'NONE',  ( 0.5774900079438607392, 28.48035201082150891, 5.440088680355550821 ) ) ;
#16169=CARTESIAN_POINT ( 'NONE',  ( 12.63842701281683034, 47.46726448433412315, 9.846743663894596210 ) ) ;
#16170=CARTESIAN_POINT ( 'NONE',  ( 17.96484262340118221, 21.18868534415483396, -7.964842623401177768 ) ) ;
#16172=CARTESIAN_POINT ( 'NONE',  ( 14.92337183194729988, 54.34226448433412315, -8.527530157486177487 ) ) ;
#16173=CARTESIAN_POINT ( 'NONE',  ( 12.91533473730993009, 66.60535201082150536, -10.88017736071109987 ) ) ;
#16177=EDGE_CURVE ( 'NONE', #97822, #43200, #90730, .T. ) ;
#16179=SURFACE_SIDE_STYLE ('',( #62638 ) ) ;
#16180=DIRECTION ( 'NONE',  ( -1.000000000000000000, 0.000000000000000000, 0.000000000000000000 ) ) ;
#16181=ORIENTED_EDGE ( 'NONE', *, *, #5217, .F. ) ;
#16183=CARTESIAN_POINT ( 'NONE',  ( 0.1532563361054100626, 30.80059781766744820, -2.638427012816831230 ) ) ;
#16184=DIRECTION ( 'NONE',  ( 0.000000000000000000, -1.000000000000000000, 0.000000000000000000 ) ) ;
#16185=CARTESIAN_POINT ( 'NONE',  ( 16.40814093676323893, 45.79030133659708923, 11.09922568453595026 ) ) ;
#16192=CARTESIAN_POINT ( 'NONE',  ( 7.361572987183169658, 59.96726448433410894, -9.846743663894592657 ) ) ;
#16193=CARTESIAN_POINT ( 'NONE',  ( 20.36894250292379738, 39.92874883491396787, -10.36894250292379027 ) ) ;
#16194=CARTESIAN_POINT ( 'NONE',  ( 7.361572987183169658, 54.96726448433413026, -9.846743663894592657 ) ) ;
#16197=CARTESIAN_POINT ( 'NONE',  ( 12.63842701281683922, 14.55059781766744997, -9.846743663894590881 ) ) ;
#16198=CARTESIAN_POINT ( 'NONE',  ( 19.38216949554541202, 50.99863466993042493, 9.382169495545424454 ) ) ;
#16199=CARTESIAN_POINT ( 'NONE',  ( 0.6178305044545818747, -1.501365330069579951, -9.382169495545419124 ) ) ;
#16200=CARTESIAN_POINT ( 'NONE',  ( 4.559911319644449179, 53.89701867748817676, 9.422509992056141925 ) ) ;
#16201=CARTESIAN_POINT ( 'NONE',  ( 5.076628168052704559, 40.17559781766745175, -8.527530157486179263 ) ) ;
#16202=CARTESIAN_POINT ( 'NONE',  ( 20.32896413005680714, 15.57879003517447281, -5.963430220938276349 ) ) ;
#16203=VERTEX_POINT ( 'NONE', #88444 ) ;
#16205=CARTESIAN_POINT ( 'NONE',  ( 2.035157376598822676, 22.43868534415483396, -7.964842623401177768 ) ) ;
#16206=CARTESIAN_POINT ( 'NONE',  ( 19.38216949554541202, 5.998634669930420493, 9.382169495545424454 ) ) ;
#16207=CARTESIAN_POINT ( 'NONE',  ( 19.42250999205614548, 50.98035201082151247, -5.440088680355545492 ) ) ;
#16209=CARTESIAN_POINT ( 'NONE',  ( 12.91533473730993009, 66.60535201082150536, -10.88017736071109987 ) ) ;
#16211=CARTESIAN_POINT ( 'NONE',  ( 10.00000000000000000, 36.81368534415484106, -10.88017736071110342 ) ) ;
#16213=CARTESIAN_POINT ( 'NONE',  ( 12.63842701281683034, 37.46726448433411605, 9.846743663894596210 ) ) ;
#16215=CARTESIAN_POINT ( 'NONE',  ( -2.816281873526473856, 4.331968003263754419, 3.434112377981055619 ) ) ;
#16216=CARTESIAN_POINT ( 'NONE',  ( 15.44008868035555260, 14.73035201082150536, 9.422509992056143702 ) ) ;
#16217=PRESENTATION_STYLE_ASSIGNMENT (( #46225 ) ) ;
#16219=AXIS2_PLACEMENT_3D ( 'NONE', #5278, #88260, #50251 ) ;
#16220=CARTESIAN_POINT ( 'NONE',  ( 10.00000000000000000, 25.55374883491396787, -14.16423886937410082 ) ) ;
#16222=CARTESIAN_POINT ( 'NONE',  ( 20.36894250292379738, 64.92874883491397497, -10.36894250292379027 ) ) ;
#16223=CARTESIAN_POINT ( 'NONE',  ( 10.00000000000000000, 34.75893115100078745, -9.846743663894594434 ) ) ;
#16224=CARTESIAN_POINT ( 'NONE',  ( 5.076628168052703671, 21.84226448433411960, 8.527530157486179263 ) ) ;
#16225=DIRECTION ( 'NONE',  ( 1.000000000000000000, 0.000000000000000000, 0.000000000000000000 ) ) ;
#16227=ORIENTED_EDGE ( 'NONE', *, *, #65518, .T. ) ;
#16228=CARTESIAN_POINT ( 'NONE',  ( 7.361572987183169658, 24.96726448433412315, -9.846743663894592657 ) ) ;
#16229=CARTESIAN_POINT ( 'NONE',  ( 2.035157376598822676, 22.43868534415483396, -7.964842623401177768 ) ) ;
#16230=CARTESIAN_POINT ( 'NONE',  ( 7.361572987183170547, 62.05059781766745886, 9.846743663894590881 ) ) ;
#16231=CARTESIAN_POINT ( 'NONE',  ( 24.16423886937410614, 14.30374883491396787, 8.672049930838204340E-16 ) ) ;
#16235=CARTESIAN_POINT ( 'NONE',  ( 14.92337183194729988, 9.342264484334119601, -8.527530157486177487 ) ) ;
#16236=CARTESIAN_POINT ( 'NONE',  ( 19.38216949554541557, 32.24863466993041783, -9.382169495545420901 ) ) ;
#16237=CARTESIAN_POINT ( 'NONE',  ( 17.20831665107776587, 39.13393115100079456, -7.208316651077762316 ) ) ;
#16238=ORIENTED_EDGE ( 'NONE', *, *, #30268, .T. ) ;
#16239=CARTESIAN_POINT ( 'NONE',  ( 0.1532563361054082862, 16.21726448433411960, 2.638427012816831674 ) ) ;
#16240=CARTESIAN_POINT ( 'NONE',  ( 1.042145700049403434, 34.74216108172000617, -6.499999999999937828 ) ) ;
#16241=CARTESIAN_POINT ( 'NONE',  ( 20.36894250292379738, 54.92874883491396076, -10.36894250292379027 ) ) ;
#16242=CARTESIAN_POINT ( 'NONE',  ( 6.204703633549690345, 2.845415501580634388, 14.16423886937410082 ) ) ;
#16243=CARTESIAN_POINT ( 'NONE',  ( 17.96484262340118221, 51.18868534415483396, -7.964842623401177768 ) ) ;
#16244=CARTESIAN_POINT ( 'NONE',  ( 18.52753015748618282, 33.92559781766745886, -4.923371831947291888 ) ) ;
#16245=CARTESIAN_POINT ( 'NONE',  ( 17.96484262340118221, 19.93868534415484106, 7.964842623401181321 ) ) ;
#16247=CARTESIAN_POINT ( 'NONE',  ( 10.00000000000000000, 54.75893115100078745, -9.846743663894594434 ) ) ;
#16248=CARTESIAN_POINT ( 'NONE',  ( 0.5774900079438607392, 53.48035201082151247, 5.440088680355550821 ) ) ;
#16249=FACE_OUTER_BOUND ( 'NONE', #5405, .T. ) ;
#16250=COLOUR_RGB ( '', 0.09019608, 0.27058824, 0.51372549) ;
#16251=EDGE_LOOP ( 'NONE', ( #27169, #70544, #76718, #85544 ) ) ;
#16252=AXIS2_PLACEMENT_3D ( 'NONE', #15344, #70797, #85789 ) ;
#16255=CARTESIAN_POINT ( 'NONE',  ( 2.917880565312948704, 2.637082168247300906, 12.26659068614894643 ) ) ;
#16256=CARTESIAN_POINT ( 'NONE',  ( 10.00000000000000000, 44.75893115100078745, -9.846743663894594434 ) ) ;
#16257=CARTESIAN_POINT ( 'NONE',  ( 7.361572987183170547, 17.05059781766745530, 9.846743663894590881 ) ) ;
#16258=CARTESIAN_POINT ( 'NONE',  ( 3.591859063236763294, 53.29030133659708923, -11.09922568453595026 ) ) ;
#16259=CARTESIAN_POINT ( 'NONE',  ( 20.88017736071110164, 15.35535201082150358, 2.915334737309930979 ) ) ;
#16260=CARTESIAN_POINT ( 'NONE',  ( 5.076628168052703671, 51.84226448433412315, 8.527530157486179263 ) ) ;
#16261=FILL_AREA_STYLE_COLOUR ( '', #71032 ) ;
#16262=CARTESIAN_POINT ( 'NONE',  ( -4.164238869374099039, 26.80374883491397142, 8.674139862899312516E-16 ) ) ;
#16263=CARTESIAN_POINT ( 'NONE',  ( 20.36894250292379382, 63.67874883491396787, 10.36894250292379205 ) ) ;
#16264=CARTESIAN_POINT ( 'NONE',  ( 12.63842701281683922, 59.55059781766744464, -9.846743663894590881 ) ) ;
#16268=CARTESIAN_POINT ( 'NONE',  ( 2.035157376598824452, 53.68868534415484817, 7.964842623401179544 ) ) ;
#16269=CARTESIAN_POINT ( 'NONE',  ( 0.1532563361054100626, 15.80059781766745353, -2.638427012816831230 ) ) ;
#16271=VERTEX_POINT ( 'NONE', #95461 ) ;
#16275=CARTESIAN_POINT ( 'NONE',  ( 0.1532563361054083140, 6.008931151000784787, 1.131784320476157264E-15 ) ) ;
#16277=CARTESIAN_POINT ( 'NONE',  ( -0.3689425029237898834, 26.17874883491396432, -10.36894250292378850 ) ) ;
#16278=CARTESIAN_POINT ( 'NONE',  ( 0.1532563361054082862, 16.21726448433411960, 2.638427012816831674 ) ) ;
#16279=CARTESIAN_POINT ( 'NONE',  ( 15.44008868035555260, 44.73035201082151247, 9.422509992056143702 ) ) ;
#16280=DIRECTION ( 'NONE',  ( 0.000000000000000000, 0.000000000000000000, 1.000000000000000000 ) ) ;
#16282=CARTESIAN_POINT ( 'NONE',  ( 15.44008868035555793, 21.39701867748817321, -9.422509992056140149 ) ) ;
#16286=CARTESIAN_POINT ( 'NONE',  ( -2.266590686148945544, 2.220415501580634388, 7.082119434687048631 ) ) ;
#16288=B_SPLINE_CURVE_WITH_KNOTS ( 'NONE', 3,
 ( #50294, #58787, #71828, #26813 ),
 .UNSPECIFIED., .F., .F.,
 ( 4, 4 ),
 ( 5.421010862427522170E-20, 0.002657014572711347174 ),
 .UNSPECIFIED. ) ;
#16290=CARTESIAN_POINT ( 'NONE',  ( -2.816281873526473856, 24.12363466993042138, 9.499525473075851096E-16 ) ) ;
#16291=CARTESIAN_POINT ( 'NONE',  ( 18.52753015748618282, 13.92559781766745175, -4.923371831947291888 ) ) ;
#16292=CARTESIAN_POINT ( 'NONE',  ( -0.3077640640439943676, 70.00000000000000000, -6.000000000000270894 ) ) ;
#16294=CARTESIAN_POINT ( 'NONE',  ( 7.361572987183170547, 17.05059781766745530, 9.846743663894590881 ) ) ;
#16295=CARTESIAN_POINT ( 'NONE',  ( 20.88017736071110875, 30.77201867748816966, -2.915334737309920765 ) ) ;
#16298=CARTESIAN_POINT ( 'NONE',  ( 16.40814093676324603, 62.45696800326376064, -11.09922568453594671 ) ) ;
#16299=CARTESIAN_POINT ( 'NONE',  ( -0.8801773607111009756, 53.06368534415484106, 1.068504757029289695E-15 ) ) ;
#16302=CARTESIAN_POINT ( 'NONE',  ( 4.559911319644449179, 57.23035201082150536, -9.422509992056141925 ) ) ;
#16303=CARTESIAN_POINT ( 'NONE',  ( 19.84674366389459266, 63.30059781766745886, 2.638427012816836559 ) ) ;
#16304=EDGE_CURVE ( 'NONE', #11556, #57334, #73930, .T. ) ;
#16306=CARTESIAN_POINT ( 'NONE',  ( 2.791683348922237240, 30.38393115100078390, -7.208316651077763204 ) ) ;
#16307=CARTESIAN_POINT ( 'NONE',  ( -1.099225684535947600, 54.54030133659708923, 6.408140936763237150 ) ) ;
#16308=LINE ( 'NONE', #68818, #64039 ) ;
#16309=CARTESIAN_POINT ( 'NONE',  ( 0.1532563361054082862, 26.21726448433411605, 2.638427012816831674 ) ) ;
#16310=CARTESIAN_POINT ( 'NONE',  ( 10.00000000000000000, 22.87363466993042138, -12.81628187352647608 ) ) ;
#16311=FACE_OUTER_BOUND ( 'NONE', #22068, .T. ) ;
#16312=CARTESIAN_POINT ( 'NONE',  ( 2.035157376598822676, 47.43868534415484817, -7.964842623401177768 ) ) ;
#16313=CARTESIAN_POINT ( 'NONE',  ( 12.63842701281683034, 57.46726448433411605, 9.846743663894596210 ) ) ;
#16315=CARTESIAN_POINT ( 'NONE',  ( 18.52753015748617571, 33.09226448433411605, 4.923371831947298993 ) ) ;
#16316=CARTESIAN_POINT ( 'NONE',  ( 12.63842701281683034, 22.46726448433411605, 9.846743663894596210 ) ) ;
#16317=CARTESIAN_POINT ( 'NONE',  ( -0.8801773607110991993, 7.855352010821504471, -2.915334737309923874 ) ) ;
#16318=CARTESIAN_POINT ( 'NONE',  ( 3.591859063236763294, 18.29030133659708568, -11.09922568453595026 ) ) ;
#16322=CARTESIAN_POINT ( 'NONE',  ( 15.44008868035555260, 24.73035201082150891, 9.422509992056143702 ) ) ;
#16326=CARTESIAN_POINT ( 'NONE',  ( 7.084665262690076126, 17.02201867748817676, -10.88017736071110164 ) ) ;
#16327=CARTESIAN_POINT ( 'NONE',  ( 1.959929470562270959, 5.515283700948081957, -5.767676674365834977 ) ) ;
#16328=CARTESIAN_POINT ( 'NONE',  ( 12.91533473730993009, 36.60535201082151247, -10.88017736071109987 ) ) ;
#16329=CARTESIAN_POINT ( 'NONE',  ( -2.266590686148945544, 61.38708216824730357, -7.082119434687050408 ) ) ;
#16332=CARTESIAN_POINT ( 'NONE',  ( 5.076628168052704559, 20.17559781766745175, -8.527530157486179263 ) ) ;
#16335=CARTESIAN_POINT ( 'NONE',  ( 0.1532563361054082862, 66.21726448433413736, 2.638427012816831674 ) ) ;
#16336=CARTESIAN_POINT ( 'NONE',  ( 19.72487221294571569, 54.78217586085238366, 6.499999999999995559 ) ) ;
#16338=CARTESIAN_POINT ( 'NONE',  ( 6.204703633549690345, 17.84541550158063217, 14.16423886937410082 ) ) ;
#16340=CARTESIAN_POINT ( 'NONE',  ( 14.92337183194729988, 34.34226448433411605, -8.527530157486177487 ) ) ;
#16342=ORIENTED_EDGE ( 'NONE', *, *, #16597, .F. ) ;
#16343=CARTESIAN_POINT ( 'NONE',  ( 6.204703633549690345, 52.84541550158062506, 14.16423886937410082 ) ) ;
#16344=CARTESIAN_POINT ( 'NONE',  ( 5.076628168052703671, 21.84226448433411960, 8.527530157486179263 ) ) ;
#16347=CARTESIAN_POINT ( 'NONE',  ( 17.96484262340118221, 51.18868534415483396, -7.964842623401177768 ) ) ;
#16348=CARTESIAN_POINT ( 'NONE',  ( 16.40814093676324603, 52.45696800326375353, -11.09922568453594671 ) ) ;
#16349=CARTESIAN_POINT ( 'NONE',  ( 12.91533473730993009, 16.60535201082150891, -10.88017736071109987 ) ) ;
#16350=CARTESIAN_POINT ( 'NONE',  ( 0.6178305044545838731, 44.74863466993042493, 9.382169495545420901 ) ) ;
#16351=CARTESIAN_POINT ( 'NONE',  ( 19.84674366389459621, 63.50893115100078745, 7.409399052514197653E-17 ) ) ;
#16352=CARTESIAN_POINT ( 'NONE',  ( 18.52753015748618282, 3.925597817667451306, -4.923371831947291888 ) ) ;
#16355=FACE_OUTER_BOUND ( 'NONE', #96836, .T. ) ;
#16356=CARTESIAN_POINT ( 'NONE',  ( 24.16423886937410614, 49.51208216824730357, -3.795296366450302550 ) ) ;
#16357=CARTESIAN_POINT ( 'NONE',  ( 24.16423886937410614, 19.30374883491397142, 8.672049930838204340E-16 ) ) ;
#16358=CARTESIAN_POINT ( 'NONE',  ( 10.00000000000000000, 21.81368534415484106, -10.88017736071110342 ) ) ;
#16359=CARTESIAN_POINT ( 'NONE',  ( -0.8801773607111009756, 33.06368534415484106, 1.068504757029289695E-15 ) ) ;
#16362=CARTESIAN_POINT ( 'NONE',  ( 15.44008868035555793, 61.39701867748817676, -9.422509992056140149 ) ) ;
#16363=CARTESIAN_POINT ( 'NONE',  ( 20.15039907845753930, 70.00000000000000000, 6.262539305110068177 ) ) ;
#16364=CARTESIAN_POINT ( 'NONE',  ( 12.63842701281683034, 17.46726448433411250, 9.846743663894596210 ) ) ;
#16366=DIRECTION ( 'NONE',  ( 0.000000000000000000, 0.000000000000000000, -1.000000000000000000 ) ) ;
#16367=CARTESIAN_POINT ( 'NONE',  ( 7.361572987183170547, 7.050597817667451750, 9.846743663894590881 ) ) ;
#16368=CARTESIAN_POINT ( 'NONE',  ( 7.361572987183170547, 32.05059781766745175, 9.846743663894590881 ) ) ;
#16370=CARTESIAN_POINT ( 'NONE',  ( 20.88017736071110519, 10.56368534415483751, 2.639326808657452039E-16 ) ) ;
#16371=( BOUNDED_SURFACE ( )  B_SPLINE_SURFACE ( 1, 2, ( 
 ( #20322, #36306, #90782, #20816, #29288, #27810, #5329, #66297, #35810, #75780, #35309, #52294, #83289, #59295, #66802, #89792, #90278, #22308, #52780, #14814, #65801, #97323, #50818, #21810, #21310, #51803, #43792, #67801, #58800, #74286, #81311, #6303, #13807, #96335, #51307, #96831, #28308, #89308, #58294, #81789, #45285, #59785, #12806, #37312, #44291, #98321, #74795, #13306, #82790, #36805, #14312, #67299, #97826, #44782, #75288, #6798, #29775, #60285, #88810, #43306, #91275, #84291, #62246, #47244, #31751, #77254, #8763, #85262, #22797, #61267, #60773, #15790, #53275, #30271, #92752, #1298, #7796, #91775, #24277, #24764, #77745, #32239, #38780, #39765, #38292, #83782, #9258, #54741, #46278, #47742, #92268, #46759, #16769, #68787, #76763, #69279, #23297, #70265, #62738, #76281, #15305, #801, #98818, #37802, #61750, #8283, #39280, #23792, #319, #1781, #85756, #54257, #69768, #93238, #55242, #17267, #68299, #30761, #53775, #31254, #45790, #7303, #84768, #16277, #79225, #78742, #18736, #26707, #41255, #71730, #57696, #34696, #41739, #48233, #34198, #72210, #63232, #3240, #79720, #40255, #65189, #86243, #70762, #78239, #42223, #9753, #55752, #49216, #87213, #95202, #17756, #40743, #71247, #33706, #80205, #10736, #63719, #27194, #10250, #94721, #95711, #2276, #19215, #88196, #19705, #86739, #64206, #49696, #2770, #72689, #57202, #64691, #11220, #32732, #33224, #94222, #3738, #93735, #25269, #25752, #11711, #56246, #87699, #18241, #26228, #56721, #48722, #4226, #28679, #82671, #43189, #42707, #52177, #29168, #13187, #59173, #37195, #20196, #90657, #58684, #73185, #50192, #20698, #67686, #97211, #36691, #5700, #35693, #36186, #5209, #66686, #88688, #21191, #73677, #44168, #89678, #43679, #74676, #74166, #51690, #58176, #82169, #13682, #81672, #6187, #67179, #97702, #59669, #50698, #90161, #96711, #21691, #14187, #44671, #51190, #75165, #66177, #6675, #98195, #81192, #29652, #60161, #28189, #89185, #80703, #12198, #4721, #35184, #65686, #96210, #12693, #27692, #91154, #62611, #30638, #14691, #22183, #91656, #9135, #69160, #8645, #76643, #7681, #8164, #76159, #38655, #60655, #92147, #15182, #16150, #684, #15675, #46634, #84170, #46160, #30146, #31135, #23672, #53651, #61628, #54134, #84647, #77136, #22678, #39155, #68664, #69645, #1169, #31629, #23174, #62120, #38174, #92628, #24151, #53159, #54619, #85140, #191, #61147, #16648, #47120, #77620, #1664, #45662, #39651, #83664, #70143, #32113, #52664, #83166, #45161, #75665, #7176, #37679, #68178, #98697, #63114, #49100, #56608, #78125, #86619, #94599, #55114, #49577, #2161 ),
 ( #93616, #87097, #72573, #79106, #26116, #34083, #42111, #18611, #85632, #25151, #55628, #17641, #70633, #26588, #79603, #32616, #10618, #4106, #41625, #34570, #9635, #63601, #80087, #78623, #11106, #17150, #86128, #48109, #10134, #93118, #24645, #72090, #47629, #18130, #94106, #48602, #3614, #11592, #40133, #40629, #71127, #25634, #2654, #64574, #56124, #95083, #33106, #41130, #57090, #87584, #71618, #3129, #33589, #64084, #19096, #35065, #51067, #35572, #81074, #43075, #5589, #12577, #67062, #44554, #88570, #73561, #4604, #89565, #66063, #65564, #36066, #13565, #28066, #58563, #75050, #21575, #28567, #96090, #21073, #59060, #50084, #89068, #66567, #27077, #52063, #73068, #57578, #65066, #29048, #95592, #42588, #97096, #74056, #82057, #27572, #58067, #20074, #20582, #97588, #96591, #50579, #14074, #5085, #81559, #82558, #88074, #6073, #6559, #19586, #13066, #43558, #36574, #51571, #59556, #44052, #74557, #90052, #80588, #12083, #75549, #31021, #52548, #85023, #68056, #8537, #98079, #16034, #76039, #84041, #30529, #7572, #54026, #15562, #69532, #30035, #29538, #39038, #46523, #82, #46047, #24039, #7065, #77503, #45542, #60043, #37069, #38058, #54510, #76532, #23557, #91542, #22565, #23059, #91036, #53528, #37565, #8047, #60543, #61517, #38547, #61030, #92027, #69042, #576, #45040, #84537, #77023, #68551, #1046, #31513, #62012, #92512, #98586, #16536, #53034, #47013, #67567, #90541, #22073, #83053, #14573, #83550, #15073, #79489, #2041, #71976, #25998, #63967, #48488, #1550, #78008, #47507, #3022, #24539, #56970, #40015, #10989, #70026, #86982, #47993, #56008, #2537, #78504, #56493, #86511, #41509, #32502, #31995, #3501, #18492, #71015, #18007, #94969, #9515, #49465, #17527, #62502, #9016, #10017, #26471, #78990, #94480, #63495, #93504, #93997, #63000, #25520, #70518, #10496, #25028, #33471, #41008, #32991, #48980, #71509, #33958, #17028, #64463, #87473, #40518, #18987, #39534, #93005, #54999, #55515, #85517, #86014, #65947, #5472, #81446, #80959, #42964, #65449, #58438, #28448, #49964, #96474, #50452, #95974, #57950, #20461, #27457, #81934, #59429, #4484, #88457, #19474, #35944, #12458, #80469, #50951, #58945, #73445, #4971, #89932, #36448, #43442, #11968, #66440, #73943, #64947, #35451, #12947, #41994, #66940, #87958, #72458, #79971, #43930, #11477, #57465, #96974, #88953, #89446, #42471, #72955, #34951, #27946, #13443, #20960, #19957, #5955, #51447, #95476, #74428, #3991, #34456, #97460, #28925, #21448, #26964, #21952, #45924, #31388, #37940, #53407, #91906, #926, #83915, #13955, #52431, #82929, #75425, #29417, #84419 ) ),
 .UNSPECIFIED., .F., .F., .F. ) 
 B_SPLINE_SURFACE_WITH_KNOTS ( ( 2, 2 ),
 ( 3, 2, 2, 2, 2, 2, 2, 2, 2, 2, 2, 2, 2, 2, 2, 2, 2, 2, 2, 2, 2, 2, 2, 2, 2, 2, 2, 2, 2, 2, 2, 2, 2, 2, 2, 2, 2, 2, 2, 2, 2, 2, 2, 2, 2, 2, 2, 2, 2, 2, 2, 2, 2, 2, 2, 2, 2, 2, 2, 2, 2, 2, 2, 2, 2, 2, 2, 2, 2, 2, 2, 2, 2, 2, 2, 2, 2, 2, 2, 2, 2, 2, 2, 2, 2, 2, 2, 2, 2, 2, 2, 2, 2, 2, 2, 2, 2, 2, 2, 2, 2, 2, 2, 2, 2, 2, 2, 2, 2, 2, 2, 2, 2, 2, 2, 2, 2, 2, 2, 2, 2, 2, 2, 2, 2, 2, 2, 2, 2, 2, 2, 2, 2, 2, 2, 2, 2, 2, 2, 2, 2, 2, 2, 2, 2, 2, 2, 2, 2, 2, 2, 2, 2, 2, 2, 2, 2, 2, 2, 2, 2, 2, 3 ),
 ( 0.000000000000000000, 1.000000000000000000 ),
 ( 0.000000000000000000, 0.005952380952380952051, 0.01190476190476190410, 0.01785714285714285615, 0.02380952380952380820, 0.02976190476190476025, 0.03571428571428571230, 0.04166666666666666435, 0.04761904761904761640, 0.05357142857142856845, 0.05952380952380952051, 0.06547619047619047949, 0.07142857142857142461, 0.07738095238095238360, 0.08333333333333332871, 0.08928571428571428770, 0.09523809523809523281, 0.1011904761904761918, 0.1071428571428571369, 0.1130952380952380959, 0.1190476190476190410, 0.1250000000000000000, 0.1309523809523809590, 0.1369047619047619180, 0.1428571428571428492, 0.1488095238095238082, 0.1547619047619047672, 0.1607142857142857262, 0.1666666666666666574, 0.1726190476190476164, 0.1785714285714285754, 0.1845238095238095344, 0.1904761904761904656, 0.1964285714285714246, 0.2023809523809523836, 0.2083333333333333426, 0.2142857142857142738, 0.2202380952380952328, 0.2261904761904761918, 0.2321428571428571508, 0.2380952380952380820, 0.2440476190476190410, 0.2500000000000000000, 0.2559523809523809312, 0.2619047619047619180, 0.2678571428571428492, 0.2738095238095238360, 0.2797619047619047672, 0.2857142857142856984, 0.2916666666666666852, 0.2976190476190476164, 0.3035714285714285476, 0.3095238095238095344, 0.3154761904761904656, 0.3214285714285714524, 0.3273809523809523836, 0.3333333333333333148, 0.3392857142857143016, 0.3452380952380952328, 0.3511904761904761640, 0.3571428571428571508, 0.3630952380952380820, 0.3690476190476190688, 0.3750000000000000000, 0.3809523809523809312, 0.3869047619047619180, 0.3928571428571428492, 0.3988095238095238360, 0.4047619047619047672, 0.4107142857142856984, 0.4166666666666666852, 0.4226190476190476164, 0.4285714285714285476, 0.4345238095238095344, 0.4404761904761904656, 0.4464285714285714524, 0.4523809523809523836, 0.4583333333333333148, 0.4642857142857143016, 0.4702380952380952328, 0.4761904761904761640, 0.4821428571428571508, 0.4880952380952380820, 0.4940476190476190688, 0.5000000000000000000, 0.5059523809523809312, 0.5119047619047618625, 0.5178571428571429047, 0.5238095238095238360, 0.5297619047619047672, 0.5357142857142856984, 0.5416666666666666297, 0.5476190476190476719, 0.5535714285714286031, 0.5595238095238095344, 0.5654761904761904656, 0.5714285714285713969, 0.5773809523809523281, 0.5833333333333333703, 0.5892857142857143016, 0.5952380952380952328, 0.6011904761904761640, 0.6071428571428570953, 0.6130952380952381375, 0.6190476190476190688, 0.6250000000000000000, 0.6309523809523809312, 0.6369047619047618625, 0.6428571428571429047, 0.6488095238095238360, 0.6547619047619047672, 0.6607142857142856984, 0.6666666666666666297, 0.6726190476190476719, 0.6785714285714286031, 0.6845238095238095344, 0.6904761904761904656, 0.6964285714285713969, 0.7023809523809523281, 0.7083333333333333703, 0.7142857142857143016, 0.7202380952380952328, 0.7261904761904761640, 0.7321428571428570953, 0.7380952380952381375, 0.7440476190476190688, 0.7500000000000000000, 0.7559523809523809312, 0.7619047619047618625, 0.7678571428571429047, 0.7738095238095238360, 0.7797619047619047672, 0.7857142857142856984, 0.7916666666666666297, 0.7976190476190476719, 0.8035714285714286031, 0.8095238095238095344, 0.8154761904761904656, 0.8214285714285713969, 0.8273809523809523281, 0.8333333333333333703, 0.8392857142857143016, 0.8452380952380952328, 0.8511904761904761640, 0.8571428571428570953, 0.8630952380952381375, 0.8690476190476190688, 0.8750000000000000000, 0.8809523809523809312, 0.8869047619047618625, 0.8928571428571429047, 0.8988095238095238360, 0.9047619047619047672, 0.9107142857142856984, 0.9166666666666666297, 0.9226190476190476719, 0.9285714285714286031, 0.9345238095238095344, 0.9404761904761904656, 0.9464285714285713969, 0.9523809523809523281, 0.9583333333333333703, 0.9642857142857143016 ),
 .UNSPECIFIED. ) 
 GEOMETRIC_REPRESENTATION_ITEM ( )  RATIONAL_B_SPLINE_SURFACE ( (
 ( 1.000000000000000000, 0.9659258262890683122, 1.000000000000000000, 0.9659258262890683122, 1.000000000000000000, 0.9659258262890683122, 1.000000000000000000, 0.9659258262890683122, 1.000000000000000000, 0.9659258262890683122, 1.000000000000000000, 0.9659258262890683122, 1.000000000000000000, 0.9659258262890683122, 1.000000000000000000, 0.9659258262890683122, 1.000000000000000000, 0.9659258262890683122, 1.000000000000000000, 0.9659258262890683122, 1.000000000000000000, 0.9659258262890683122, 1.000000000000000000, 0.9659258262890683122, 1.000000000000000000, 0.9659258262890683122, 1.000000000000000000, 0.9659258262890683122, 1.000000000000000000, 0.9659258262890683122, 1.000000000000000000, 0.9659258262890683122, 1.000000000000000000, 0.9659258262890683122, 1.000000000000000000, 0.9659258262890683122, 1.000000000000000000, 0.9659258262890683122, 1.000000000000000000, 0.9659258262890683122, 1.000000000000000000, 0.9659258262890683122, 1.000000000000000000, 0.9659258262890683122, 1.000000000000000000, 0.9659258262890683122, 1.000000000000000000, 0.9659258262890683122, 1.000000000000000000, 0.9659258262890683122, 1.000000000000000000, 0.9659258262890683122, 1.000000000000000000, 0.9659258262890683122, 1.000000000000000000, 0.9659258262890683122, 1.000000000000000000, 0.9659258262890683122, 1.000000000000000000, 0.9659258262890683122, 1.000000000000000000, 0.9659258262890683122, 1.000000000000000000, 0.9659258262890683122, 1.000000000000000000, 0.9659258262890683122, 1.000000000000000000, 0.9659258262890683122, 1.000000000000000000, 0.9659258262890683122, 1.000000000000000000, 0.9659258262890683122, 1.000000000000000000, 0.9659258262890683122, 1.000000000000000000, 0.9659258262890683122, 1.000000000000000000, 0.9659258262890683122, 1.000000000000000000, 0.9659258262890683122, 1.000000000000000000, 0.9659258262890683122, 1.000000000000000000, 0.9659258262890683122, 1.000000000000000000, 0.9659258262890683122, 1.000000000000000000, 0.9659258262890683122, 1.000000000000000000, 0.9659258262890683122, 1.000000000000000000, 0.9659258262890683122, 1.000000000000000000, 0.9659258262890683122, 1.000000000000000000, 0.9659258262890683122, 1.000000000000000000, 0.9659258262890683122, 1.000000000000000000, 0.9659258262890683122, 1.000000000000000000, 0.9659258262890683122, 1.000000000000000000, 0.9659258262890683122, 1.000000000000000000, 0.9659258262890683122, 1.000000000000000000, 0.9659258262890683122, 1.000000000000000000, 0.9659258262890683122, 1.000000000000000000, 0.9659258262890683122, 1.000000000000000000, 0.9659258262890683122, 1.000000000000000000, 0.9659258262890683122, 1.000000000000000000, 0.9659258262890683122, 1.000000000000000000, 0.9659258262890683122, 1.000000000000000000, 0.9659258262890683122, 1.000000000000000000, 0.9659258262890683122, 1.000000000000000000, 0.9659258262890683122, 1.000000000000000000, 0.9659258262890683122, 1.000000000000000000, 0.9659258262890683122, 1.000000000000000000, 0.9659258262890683122, 1.000000000000000000, 0.9659258262890683122, 1.000000000000000000, 0.9659258262890683122, 1.000000000000000000, 0.9659258262890683122, 1.000000000000000000, 0.9659258262890683122, 1.000000000000000000, 0.9659258262890683122, 1.000000000000000000, 0.9659258262890683122, 1.000000000000000000, 0.9659258262890683122, 1.000000000000000000, 0.9659258262890683122, 1.000000000000000000, 0.9659258262890683122, 1.000000000000000000, 0.9659258262890683122, 1.000000000000000000, 0.9659258262890683122, 1.000000000000000000, 0.9659258262890683122, 1.000000000000000000, 0.9659258262890683122, 1.000000000000000000, 0.9659258262890683122, 1.000000000000000000, 0.9659258262890683122, 1.000000000000000000, 0.9659258262890683122, 1.000000000000000000, 0.9659258262890683122, 1.000000000000000000, 0.9659258262890683122, 1.000000000000000000, 0.9659258262890683122, 1.000000000000000000, 0.9659258262890683122, 1.000000000000000000, 0.9659258262890683122, 1.000000000000000000, 0.9659258262890683122, 1.000000000000000000, 0.9659258262890683122, 1.000000000000000000, 0.9659258262890683122, 1.000000000000000000, 0.9659258262890683122, 1.000000000000000000, 0.9659258262890683122, 1.000000000000000000, 0.9659258262890683122, 1.000000000000000000, 0.9659258262890683122, 1.000000000000000000, 0.9659258262890683122, 1.000000000000000000, 0.9659258262890683122, 1.000000000000000000, 0.9659258262890683122, 1.000000000000000000, 0.9659258262890683122, 1.000000000000000000, 0.9659258262890683122, 1.000000000000000000, 0.9659258262890683122, 1.000000000000000000, 0.9659258262890683122, 1.000000000000000000, 0.9659258262890683122, 1.000000000000000000, 0.9659258262890683122, 1.000000000000000000, 0.9659258262890683122, 1.000000000000000000, 0.9659258262890683122, 1.000000000000000000, 0.9659258262890683122, 1.000000000000000000, 0.9659258262890683122, 1.000000000000000000, 0.9659258262890683122, 1.000000000000000000, 0.9659258262890683122, 1.000000000000000000, 0.9659258262890683122, 1.000000000000000000, 0.9659258262890683122, 1.000000000000000000, 0.9659258262890683122, 1.000000000000000000, 0.9659258262890683122, 1.000000000000000000, 0.9659258262890683122, 1.000000000000000000, 0.9659258262890683122, 1.000000000000000000, 0.9659258262890683122, 1.000000000000000000, 0.9659258262890683122, 1.000000000000000000, 0.9659258262890683122, 1.000000000000000000, 0.9659258262890683122, 1.000000000000000000, 0.9659258262890683122, 1.000000000000000000, 0.9659258262890683122, 1.000000000000000000, 0.9659258262890683122, 1.000000000000000000, 0.9659258262890683122, 1.000000000000000000, 0.9659258262890683122, 1.000000000000000000, 0.9659258262890683122, 1.000000000000000000, 0.9659258262890683122, 1.000000000000000000, 0.9659258262890683122, 1.000000000000000000, 0.9659258262890683122, 1.000000000000000000, 0.9659258262890683122, 1.000000000000000000, 0.9659258262890683122, 1.000000000000000000, 0.9659258262890683122, 1.000000000000000000, 0.9659258262890683122, 1.000000000000000000, 0.9659258262890683122, 1.000000000000000000, 0.9659258262890683122, 1.000000000000000000, 0.9659258262890683122, 1.000000000000000000, 0.9659258262890683122, 1.000000000000000000, 0.9659258262890683122, 1.000000000000000000, 0.9659258262890683122, 1.000000000000000000, 0.9659258262890683122, 1.000000000000000000, 0.9659258262890683122, 1.000000000000000000, 0.9659258262890683122, 1.000000000000000000, 0.9659258262890683122, 1.000000000000000000, 0.9659258262890683122, 1.000000000000000000, 0.9659258262890683122, 1.000000000000000000, 0.9659258262890683122, 1.000000000000000000, 0.9659258262890683122, 1.000000000000000000, 0.9659258262890683122, 1.000000000000000000, 0.9659258262890683122, 1.000000000000000000, 0.9659258262890683122, 1.000000000000000000, 0.9659258262890683122, 1.000000000000000000, 0.9659258262890683122, 1.000000000000000000, 0.9659258262890683122, 1.000000000000000000, 0.9659258262890683122, 1.000000000000000000, 0.9659258262890683122, 1.000000000000000000, 0.9659258262890683122, 1.000000000000000000, 0.9659258262890683122, 1.000000000000000000, 0.9659258262890683122, 1.000000000000000000, 0.9659258262890683122, 1.000000000000000000, 0.9659258262890683122, 1.000000000000000000, 0.9659258262890683122, 1.000000000000000000, 0.9659258262890683122, 1.000000000000000000, 0.9659258262890683122, 1.000000000000000000),
 ( 1.000000000000000000, 0.9659258262890683122, 1.000000000000000000, 0.9659258262890683122, 1.000000000000000000, 0.9659258262890683122, 1.000000000000000000, 0.9659258262890683122, 1.000000000000000000, 0.9659258262890683122, 1.000000000000000000, 0.9659258262890683122, 1.000000000000000000, 0.9659258262890683122, 1.000000000000000000, 0.9659258262890683122, 1.000000000000000000, 0.9659258262890683122, 1.000000000000000000, 0.9659258262890683122, 1.000000000000000000, 0.9659258262890683122, 1.000000000000000000, 0.9659258262890683122, 1.000000000000000000, 0.9659258262890683122, 1.000000000000000000, 0.9659258262890683122, 1.000000000000000000, 0.9659258262890683122, 1.000000000000000000, 0.9659258262890683122, 1.000000000000000000, 0.9659258262890683122, 1.000000000000000000, 0.9659258262890683122, 1.000000000000000000, 0.9659258262890683122, 1.000000000000000000, 0.9659258262890683122, 1.000000000000000000, 0.9659258262890683122, 1.000000000000000000, 0.9659258262890683122, 1.000000000000000000, 0.9659258262890683122, 1.000000000000000000, 0.9659258262890683122, 1.000000000000000000, 0.9659258262890683122, 1.000000000000000000, 0.9659258262890683122, 1.000000000000000000, 0.9659258262890683122, 1.000000000000000000, 0.9659258262890683122, 1.000000000000000000, 0.9659258262890683122, 1.000000000000000000, 0.9659258262890683122, 1.000000000000000000, 0.9659258262890683122, 1.000000000000000000, 0.9659258262890683122, 1.000000000000000000, 0.9659258262890683122, 1.000000000000000000, 0.9659258262890683122, 1.000000000000000000, 0.9659258262890683122, 1.000000000000000000, 0.9659258262890683122, 1.000000000000000000, 0.9659258262890683122, 1.000000000000000000, 0.9659258262890683122, 1.000000000000000000, 0.9659258262890683122, 1.000000000000000000, 0.9659258262890683122, 1.000000000000000000, 0.9659258262890683122, 1.000000000000000000, 0.9659258262890683122, 1.000000000000000000, 0.9659258262890683122, 1.000000000000000000, 0.9659258262890683122, 1.000000000000000000, 0.9659258262890683122, 1.000000000000000000, 0.9659258262890683122, 1.000000000000000000, 0.9659258262890683122, 1.000000000000000000, 0.9659258262890683122, 1.000000000000000000, 0.9659258262890683122, 1.000000000000000000, 0.9659258262890683122, 1.000000000000000000, 0.9659258262890683122, 1.000000000000000000, 0.9659258262890683122, 1.000000000000000000, 0.9659258262890683122, 1.000000000000000000, 0.9659258262890683122, 1.000000000000000000, 0.9659258262890683122, 1.000000000000000000, 0.9659258262890683122, 1.000000000000000000, 0.9659258262890683122, 1.000000000000000000, 0.9659258262890683122, 1.000000000000000000, 0.9659258262890683122, 1.000000000000000000, 0.9659258262890683122, 1.000000000000000000, 0.9659258262890683122, 1.000000000000000000, 0.9659258262890683122, 1.000000000000000000, 0.9659258262890683122, 1.000000000000000000, 0.9659258262890683122, 1.000000000000000000, 0.9659258262890683122, 1.000000000000000000, 0.9659258262890683122, 1.000000000000000000, 0.9659258262890683122, 1.000000000000000000, 0.9659258262890683122, 1.000000000000000000, 0.9659258262890683122, 1.000000000000000000, 0.9659258262890683122, 1.000000000000000000, 0.9659258262890683122, 1.000000000000000000, 0.9659258262890683122, 1.000000000000000000, 0.9659258262890683122, 1.000000000000000000, 0.9659258262890683122, 1.000000000000000000, 0.9659258262890683122, 1.000000000000000000, 0.9659258262890683122, 1.000000000000000000, 0.9659258262890683122, 1.000000000000000000, 0.9659258262890683122, 1.000000000000000000, 0.9659258262890683122, 1.000000000000000000, 0.9659258262890683122, 1.000000000000000000, 0.9659258262890683122, 1.000000000000000000, 0.9659258262890683122, 1.000000000000000000, 0.9659258262890683122, 1.000000000000000000, 0.9659258262890683122, 1.000000000000000000, 0.9659258262890683122, 1.000000000000000000, 0.9659258262890683122, 1.000000000000000000, 0.9659258262890683122, 1.000000000000000000, 0.9659258262890683122, 1.000000000000000000, 0.9659258262890683122, 1.000000000000000000, 0.9659258262890683122, 1.000000000000000000, 0.9659258262890683122, 1.000000000000000000, 0.9659258262890683122, 1.000000000000000000, 0.9659258262890683122, 1.000000000000000000, 0.9659258262890683122, 1.000000000000000000, 0.9659258262890683122, 1.000000000000000000, 0.9659258262890683122, 1.000000000000000000, 0.9659258262890683122, 1.000000000000000000, 0.9659258262890683122, 1.000000000000000000, 0.9659258262890683122, 1.000000000000000000, 0.9659258262890683122, 1.000000000000000000, 0.9659258262890683122, 1.000000000000000000, 0.9659258262890683122, 1.000000000000000000, 0.9659258262890683122, 1.000000000000000000, 0.9659258262890683122, 1.000000000000000000, 0.9659258262890683122, 1.000000000000000000, 0.9659258262890683122, 1.000000000000000000, 0.9659258262890683122, 1.000000000000000000, 0.9659258262890683122, 1.000000000000000000, 0.9659258262890683122, 1.000000000000000000, 0.9659258262890683122, 1.000000000000000000, 0.9659258262890683122, 1.000000000000000000, 0.9659258262890683122, 1.000000000000000000, 0.9659258262890683122, 1.000000000000000000, 0.9659258262890683122, 1.000000000000000000, 0.9659258262890683122, 1.000000000000000000, 0.9659258262890683122, 1.000000000000000000, 0.9659258262890683122, 1.000000000000000000, 0.9659258262890683122, 1.000000000000000000, 0.9659258262890683122, 1.000000000000000000, 0.9659258262890683122, 1.000000000000000000, 0.9659258262890683122, 1.000000000000000000, 0.9659258262890683122, 1.000000000000000000, 0.9659258262890683122, 1.000000000000000000, 0.9659258262890683122, 1.000000000000000000, 0.9659258262890683122, 1.000000000000000000, 0.9659258262890683122, 1.000000000000000000, 0.9659258262890683122, 1.000000000000000000, 0.9659258262890683122, 1.000000000000000000, 0.9659258262890683122, 1.000000000000000000, 0.9659258262890683122, 1.000000000000000000, 0.9659258262890683122, 1.000000000000000000, 0.9659258262890683122, 1.000000000000000000, 0.9659258262890683122, 1.000000000000000000, 0.9659258262890683122, 1.000000000000000000, 0.9659258262890683122, 1.000000000000000000, 0.9659258262890683122, 1.000000000000000000, 0.9659258262890683122, 1.000000000000000000, 0.9659258262890683122, 1.000000000000000000, 0.9659258262890683122, 1.000000000000000000, 0.9659258262890683122, 1.000000000000000000, 0.9659258262890683122, 1.000000000000000000, 0.9659258262890683122, 1.000000000000000000, 0.9659258262890683122, 1.000000000000000000, 0.9659258262890683122, 1.000000000000000000, 0.9659258262890683122, 1.000000000000000000, 0.9659258262890683122, 1.000000000000000000, 0.9659258262890683122, 1.000000000000000000, 0.9659258262890683122, 1.000000000000000000, 0.9659258262890683122, 1.000000000000000000, 0.9659258262890683122, 1.000000000000000000, 0.9659258262890683122, 1.000000000000000000, 0.9659258262890683122, 1.000000000000000000, 0.9659258262890683122, 1.000000000000000000, 0.9659258262890683122, 1.000000000000000000, 0.9659258262890683122, 1.000000000000000000, 0.9659258262890683122, 1.000000000000000000, 0.9659258262890683122, 1.000000000000000000, 0.9659258262890683122, 1.000000000000000000, 0.9659258262890683122, 1.000000000000000000, 0.9659258262890683122, 1.000000000000000000, 0.9659258262890683122, 1.000000000000000000, 0.9659258262890683122, 1.000000000000000000) ) ) 
 REPRESENTATION_ITEM ( '' )  SURFACE ( )  );
#16373=CARTESIAN_POINT ( 'NONE',  ( 0.6178305044545838731, 29.74863466993042138, 9.382169495545420901 ) ) ;
#16374=CARTESIAN_POINT ( 'NONE',  ( 17.20831665107776587, 9.133931151000787452, -7.208316651077762316 ) ) ;
#16376=CARTESIAN_POINT ( 'NONE',  ( 5.076628168052703671, 46.84226448433412315, 8.527530157486179263 ) ) ;
#16377=CARTESIAN_POINT ( 'NONE',  ( 5.076628168052704559, 35.17559781766745175, -8.527530157486179263 ) ) ;
#16378=CARTESIAN_POINT ( 'NONE',  ( 22.26659068614895176, 14.72041550158063572, -7.082119434687042414 ) ) ;
#16379=CARTESIAN_POINT ( 'NONE',  ( 2.035157376598822676, 32.43868534415483396, -7.964842623401177768 ) ) ;
#16380=CARTESIAN_POINT ( 'NONE',  ( 20.88017736071110519, 5.563685344154837509, 2.639326808657452039E-16 ) ) ;
#16381=CARTESIAN_POINT ( 'NONE',  ( 17.96484262340118221, 51.18868534415483396, -7.964842623401177768 ) ) ;
#16382=CARTESIAN_POINT ( 'NONE',  ( 20.88017736071110519, 35.56368534415484106, 2.639326808657452039E-16 ) ) ;
#16384=CARTESIAN_POINT ( 'NONE',  ( 6.565887622018943937, 38.08196800326376064, -12.81628187352647608 ) ) ;
#16386=CARTESIAN_POINT ( 'NONE',  ( 17.96484262340118221, 41.18868534415484106, -7.964842623401177768 ) ) ;
#16388=CARTESIAN_POINT ( 'NONE',  ( -1.099225684535947600, 54.54030133659708923, 6.408140936763237150 ) ) ;
#16389=CARTESIAN_POINT ( 'NONE',  ( 10.00000000000000178, 49.31368534415484106, 10.88017736071110342 ) ) ;
#16391=EDGE_LOOP ( 'NONE', ( #77260, #27669, #95687 ) ) ;
#16392=CARTESIAN_POINT ( 'NONE',  ( 4.559911319644449179, 53.89701867748817676, 9.422509992056141925 ) ) ;
#16393=ADVANCED_FACE ( 'NONE', ( #60404 ), #97446, .T. ) ;
#16396=CARTESIAN_POINT ( 'NONE',  ( 24.16423886937409904, 59.09541550158063217, 3.795296366450317205 ) ) ;
#16397=CARTESIAN_POINT ( 'NONE',  ( 4.559911319644449179, 67.23035201082150536, -9.422509992056141925 ) ) ;
#16398=CARTESIAN_POINT ( 'NONE',  ( 19.10478245763055227, 56.02576239577081196, -5.990408912944265474 ) ) ;
#16399=EDGE_CURVE ( 'NONE', #12669, #27569, #65734, .T. ) ;
#16400=VECTOR ( 'NONE', #56272, 1000.000000000000000 ) ;
#16401=FACE_OUTER_BOUND ( 'NONE', #7762, .T. ) ;
#16404=CARTESIAN_POINT ( 'NONE',  ( 12.63842701281683034, 32.46726448433412315, 9.846743663894596210 ) ) ;
#16407=CARTESIAN_POINT ( 'NONE',  ( 0.1532563361054083140, 36.00893115100078745, 1.131784320476157264E-15 ) ) ;
#16408=COLOUR_RGB ( '', 0.09019608, 0.27058824, 0.51372549) ;
#16409=CARTESIAN_POINT ( 'NONE',  ( 12.91533473730993009, 41.60535201082149825, -10.88017736071109987 ) ) ;
#16410=CARTESIAN_POINT ( 'NONE',  ( 18.52753015748618282, 38.92559781766745175, -4.923371831947291888 ) ) ;
#16411=CARTESIAN_POINT ( 'NONE',  ( 22.81628187352647785, 21.62363466993041783, 6.195893100308588602E-16 ) ) ;
#16414=CARTESIAN_POINT ( 'NONE',  ( 17.96484262340118221, 51.18868534415483396, -7.964842623401177768 ) ) ;
#16415=CARTESIAN_POINT ( 'NONE',  ( 22.26659068614894466, 53.88708216824731068, 7.082119434687054849 ) ) ;
#16417=CARTESIAN_POINT ( 'NONE',  ( -1.099225684535947600, 18.70696800326375353, -6.408140936763238038 ) ) ;
#16418=CARTESIAN_POINT ( 'NONE',  ( 0.1532563361054082862, 51.21726448433412315, 2.638427012816831674 ) ) ;
#16420=CARTESIAN_POINT ( 'NONE',  ( 3.591859063236763294, 28.29030133659708568, -11.09922568453595026 ) ) ;
#16421=CARTESIAN_POINT ( 'NONE',  ( 10.00000000000000178, 19.31368534415484106, 10.88017736071110342 ) ) ;
#16422=ADVANCED_FACE ( 'NONE', ( #43915 ), #6925, .T. ) ;
#16424=VECTOR ( 'NONE', #88045, 1000.000000000000000 ) ;
#16425=CARTESIAN_POINT ( 'NONE',  ( 5.076628168052703671, 6.842264484334118713, 8.527530157486179263 ) ) ;
#16426=CARTESIAN_POINT ( 'NONE',  ( 18.52753015748617571, 43.09226448433412315, 4.923371831947298993 ) ) ;
#16427=CARTESIAN_POINT ( 'NONE',  ( 14.92337183194729633, 42.67559781766745886, 8.527530157486181039 ) ) ;
#16429=CARTESIAN_POINT ( 'NONE',  ( 7.361572987183170547, 27.05059781766745175, 9.846743663894590881 ) ) ;
#16431=CARTESIAN_POINT ( 'NONE',  ( 14.92337183194729633, 7.675597817667451750, 8.527530157486181039 ) ) ;
#16433=CARTESIAN_POINT ( 'NONE',  ( 18.72515096720571393, 41.07228050351032778, -6.499999999999974243 ) ) ;
#16434=CARTESIAN_POINT ( 'NONE',  ( 0.1532563361054082862, 41.21726448433411605, 2.638427012816831674 ) ) ;
#16435=VERTEX_POINT ( 'NONE', #89919 ) ;
#16437=CARTESIAN_POINT ( 'NONE',  ( 19.38216949554541557, 62.24863466993041072, -9.382169495545420901 ) ) ;
#16439=CARTESIAN_POINT ( 'NONE',  ( 21.92686044187656336, 16.97997603579417358, 3.195792623639536423 ) ) ;
#16440=CARTESIAN_POINT ( 'NONE',  ( 21.09922568453594849, 11.20696800326375531, 6.408140936763242479 ) ) ;
#16441=CARTESIAN_POINT ( 'NONE',  ( 10.00000000000000178, 54.31368534415484106, 10.88017736071110342 ) ) ;
#16442=CARTESIAN_POINT ( 'NONE',  ( -4.164238869374099039, 51.80374883491396787, 8.674139862899312516E-16 ) ) ;
#16443=CARTESIAN_POINT ( 'NONE',  ( 20.00000000000000711, 96.99991098592576577, 4.500000004388789776 ) ) ;
#16444=CARTESIAN_POINT ( 'NONE',  ( -2.266590686148945544, 41.38708216824729647, -7.082119434687050408 ) ) ;
#16445=CARTESIAN_POINT ( 'NONE',  ( 22.26659068614895176, 54.72041550158063217, -7.082119434687042414 ) ) ;
#16446=CARTESIAN_POINT ( 'NONE',  ( 24.16423886937410614, 19.30374883491397142, 8.672049930838204340E-16 ) ) ;
#16447=CARTESIAN_POINT ( 'NONE',  ( 2.917880565312948704, 27.63708216824730357, 12.26659068614894643 ) ) ;
#16451=CARTESIAN_POINT ( 'NONE',  ( 7.361572987183169658, 44.96726448433412315, -9.846743663894592657 ) ) ;
#16452=CARTESIAN_POINT ( 'NONE',  ( 2.035157376598822676, 42.43868534415483396, -7.964842623401177768 ) ) ;
#16454=CARTESIAN_POINT ( 'NONE',  ( 19.84674366389459266, 58.30059781766745886, 2.638427012816836559 ) ) ;
#16455=FACE_OUTER_BOUND ( 'NONE', #68338, .T. ) ;
#16456=CARTESIAN_POINT ( 'NONE',  ( 18.52753015748618282, 43.92559781766745175, -4.923371831947291888 ) ) ;
#16457=CARTESIAN_POINT ( 'NONE',  ( 22.81628187352647785, 61.41530133659709634, 3.434112377981063169 ) ) ;
#16459=CARTESIAN_POINT ( 'NONE',  ( 0.1532563361054082862, 36.21726448433410894, 2.638427012816831674 ) ) ;
#16460=CARTESIAN_POINT ( 'NONE',  ( 2.791683348922240793, 51.63393115100078745, 7.208316651077764092 ) ) ;
#16461=CARTESIAN_POINT ( 'NONE',  ( -2.266590686148945544, 36.38708216824730357, -7.082119434687050408 ) ) ;
#16463=CARTESIAN_POINT ( 'NONE',  ( 20.36894250292379382, 13.67874883491396965, 10.36894250292379205 ) ) ;
#16465=CARTESIAN_POINT ( 'NONE',  ( -0.1503990784575294781, 68.10158574516643171, 6.262539305110072618 ) ) ;
#16467=CARTESIAN_POINT ( 'NONE',  ( 4.559911319644449179, 3.897018677488171434, 9.422509992056141925 ) ) ;
#16469=CARTESIAN_POINT ( 'NONE',  ( 0.6178305044545818747, 13.49863466993041783, -9.382169495545419124 ) ) ;
#16471=CARTESIAN_POINT ( 'NONE',  ( 0.1143410931637271200, 55.21691075486304356, 6.480892540919860778 ) ) ;
#16472=CARTESIAN_POINT ( 'NONE',  ( 20.88017736071110164, 65.35535201082150536, 2.915334737309930979 ) ) ;
#16473=B_SPLINE_CURVE_WITH_KNOTS ( 'NONE', 3,
 ( #54339, #81370, #27872, #20386, #5395, #35870, #58357, #50877, #88878, #32316 ),
 .UNSPECIFIED., .F., .F.,
 ( 4, 3, 3, 4 ),
 ( 2.173602285337623399E-17, 0.0006253016069560831400, 0.001250604074564932782, 0.002501455912506543068 ),
 .UNSPECIFIED. ) ;
#16474=MECHANICAL_DESIGN_GEOMETRIC_PRESENTATION_REPRESENTATION('',(#27654),#8472);
#16475=CARTESIAN_POINT ( 'NONE',  ( -46.94000000000001194, 103.0000000000000000, -5.997726559847112782 ) ) ;
#16477=CARTESIAN_POINT ( 'NONE',  ( 0.1089645850229078172, 43.16234555792571825, 6.479102184480833415 ) ) ;
#16478=CARTESIAN_POINT ( 'NONE',  ( 17.08211943468705130, 58.47041550158063927, 12.26659068614894998 ) ) ;
#16479=DIRECTION ( 'NONE',  ( 0.000000000000000000, 0.000000000000000000, 1.000000000000000000 ) ) ;
#16480=CARTESIAN_POINT ( 'NONE',  ( 17.96484262340118221, 31.18868534415483751, -7.964842623401177768 ) ) ;
#16481=CARTESIAN_POINT ( 'NONE',  ( 7.084665262690076126, 22.02201867748817321, -10.88017736071110164 ) ) ;
#16483=CARTESIAN_POINT ( 'NONE',  ( 10.00000000000000000, 49.75893115100078745, -9.846743663894594434 ) ) ;
#16484=CARTESIAN_POINT ( 'NONE',  ( 10.00000000000000000, 54.75893115100078745, -9.846743663894594434 ) ) ;
#16485=CARTESIAN_POINT ( 'NONE',  ( -46.21538524526005176, 104.1852450480875802, -5.851526435683381600 ) ) ;
#16486=CARTESIAN_POINT ( 'NONE',  ( 12.63842701281683034, 2.467264484334118269, 9.846743663894596210 ) ) ;
#16489=CARTESIAN_POINT ( 'NONE',  ( 15.44008868035555260, 34.73035201082151247, 9.422509992056143702 ) ) ;
#16490=CARTESIAN_POINT ( 'NONE',  ( 21.09922568453594849, 31.20696800326375353, 6.408140936763242479 ) ) ;
#16492=CARTESIAN_POINT ( 'NONE',  ( 0.1532563361054100626, 65.80059781766745175, -2.638427012816831230 ) ) ;
#16493=CARTESIAN_POINT ( 'NONE',  ( 0.5774900079438607392, 43.48035201082151247, 5.440088680355550821 ) ) ;
#16494=CARTESIAN_POINT ( 'NONE',  ( 12.63842701281683034, 12.46726448433411782, 9.846743663894596210 ) ) ;
#16495=CARTESIAN_POINT ( 'NONE',  ( 16.40814093676324603, 22.45696800326375353, -11.09922568453594671 ) ) ;
#16496=CARTESIAN_POINT ( 'NONE',  ( -0.8801773607111009756, 58.06368534415484106, 1.068504757029289695E-15 ) ) ;
#16500=CARTESIAN_POINT ( 'NONE',  ( 1.274849032794292736, 47.55509018479936856, -6.499999999999977796 ) ) ;
#16502=CARTESIAN_POINT ( 'NONE',  ( 12.91533473730993009, 51.60535201082149825, -10.88017736071109987 ) ) ;
#16503=CARTESIAN_POINT ( 'NONE',  ( 13.43411237798106583, 47.66530133659709634, -12.81628187352647252 ) ) ;
#16504=CARTESIAN_POINT ( 'NONE',  ( 13.79529636645030344, 13.26208216824729824, 14.16423886937410614 ) ) ;
#16505=CARTESIAN_POINT ( 'NONE',  ( 12.63842701281683922, 19.55059781766745175, -9.846743663894590881 ) ) ;
#16506=CARTESIAN_POINT ( 'NONE',  ( 17.20831665107776587, 64.13393115100079456, -7.208316651077762316 ) ) ;
#16507=CARTESIAN_POINT ( 'NONE',  ( 12.63842701281683034, 17.46726448433411250, 9.846743663894596210 ) ) ;
#16508=DIRECTION ( 'NONE',  ( 1.000000000000000000, 0.000000000000000000, 0.000000000000000000 ) ) ;
#16509=CARTESIAN_POINT ( 'NONE',  ( 6.204703633549690345, 60.76208216824730357, -14.16423886937410259 ) ) ;
#16511=( LENGTH_UNIT ( ) NAMED_UNIT ( * ) SI_UNIT ( .MILLI., .METRE. ) );
#16513=CARTESIAN_POINT ( 'NONE',  ( 17.96484262340118221, 11.18868534415483929, -7.964842623401177768 ) ) ;
#16514=CARTESIAN_POINT ( 'NONE',  ( -0.1503990784575242878, 19.24884699246888786, -6.262539305110083276 ) ) ;
#16515=ORIENTED_EDGE ( 'NONE', *, *, #79817, .T. ) ;
#16517=CARTESIAN_POINT ( 'NONE',  ( 20.88017736071110164, 5.355352010821503583, 2.915334737309930979 ) ) ;
#16518=CARTESIAN_POINT ( 'NONE',  ( 4.559911319644449179, 7.230352010821505360, -9.422509992056141925 ) ) ;
#16520=CARTESIAN_POINT ( 'NONE',  ( 12.63842701281683034, 37.46726448433411605, 9.846743663894596210 ) ) ;
#16521=CARTESIAN_POINT ( 'NONE',  ( -1.099225684535947600, 33.70696800326375353, -6.408140936763238038 ) ) ;
#16522=CARTESIAN_POINT ( 'NONE',  ( 19.89220837332772263, 64.74062864464239908, 6.478736007406007857 ) ) ;
#16524=CARTESIAN_POINT ( 'NONE',  ( -2.266590686148945544, 22.22041550158063572, 7.082119434687048631 ) ) ;
#16525=CARTESIAN_POINT ( 'NONE',  ( 17.96484262340118221, 26.18868534415483396, -7.964842623401177768 ) ) ;
#16526=CARTESIAN_POINT ( 'NONE',  ( 4.559911319644449179, 8.897018677488173211, 9.422509992056141925 ) ) ;
#16527=CARTESIAN_POINT ( 'NONE',  ( 18.52753015748617571, 48.09226448433412315, 4.923371831947298993 ) ) ;
#16530=CARTESIAN_POINT ( 'NONE',  ( 0.1532563361054083140, 41.00893115100078745, 1.131784320476157264E-15 ) ) ;
#16531=FILL_AREA_STYLE ('',( #8041 ) ) ;
#16533=ORIENTED_EDGE ( 'NONE', *, *, #65807, .F. ) ;
#16534=CARTESIAN_POINT ( 'NONE',  ( 4.559911319644449179, 3.897018677488170990, 9.422509992056141925 ) ) ;
#16535=CARTESIAN_POINT ( 'NONE',  ( 10.00000000000000178, 69.31368534415484817, 10.88017736071110342 ) ) ;
#16536=CARTESIAN_POINT ( 'NONE',  ( -0.8801773607110991993, 37.85535201082151247, -2.915334737309923874 ) ) ;
#16537=CARTESIAN_POINT ( 'NONE',  ( 20.88017736071110164, 10.35535201082150714, 2.915334737309930979 ) ) ;
#16538=CARTESIAN_POINT ( 'NONE',  ( 6.565887622018943937, 33.08196800326374643, -12.81628187352647608 ) ) ;
#16539=CARTESIAN_POINT ( 'NONE',  ( 17.08211943468705130, 23.47041550158063572, 12.26659068614894998 ) ) ;
#16543=CARTESIAN_POINT ( 'NONE',  ( 21.09922568453594849, 41.20696800326375353, 6.408140936763242479 ) ) ;
#16545=CARTESIAN_POINT ( 'NONE',  ( 2.791683348922240793, 41.63393115100078745, 7.208316651077764092 ) ) ;
#16546=CARTESIAN_POINT ( 'NONE',  ( 2.035157376598822676, 17.43868534415483751, -7.964842623401177768 ) ) ;
#16547=CIRCLE ( 'NONE', #5415, 0.5000000000000004441 ) ;
#16548=CARTESIAN_POINT ( 'NONE',  ( -0.8801773607110991993, 17.85535201082150536, -2.915334737309923874 ) ) ;
#16550=CARTESIAN_POINT ( 'NONE',  ( -0.8801773607110991993, 62.85535201082150536, -2.915334737309923874 ) ) ;
#16551=( LENGTH_UNIT ( ) NAMED_UNIT ( * ) SI_UNIT ( .MILLI., .METRE. ) );
#16553=CARTESIAN_POINT ( 'NONE',  ( 17.20831665107776587, 2.883931151000785231, 7.208316651077764980 ) ) ;
#16554=CARTESIAN_POINT ( 'NONE',  ( 7.084665262690076126, 62.02201867748816966, -10.88017736071110164 ) ) ;
#16556=FACE_OUTER_BOUND ( 'NONE', #45420, .T. ) ;
#16557=CARTESIAN_POINT ( 'NONE',  ( 14.92337183194729988, 4.342264484334117824, -8.527530157486177487 ) ) ;
#16558=EDGE_LOOP ( 'NONE', ( #6810, #96099, #51201, #77028 ) ) ;
#16559=CARTESIAN_POINT ( 'NONE',  ( 14.92337183194729988, 39.34226448433412315, -8.527530157486177487 ) ) ;
#16562=DIRECTION ( 'NONE',  ( -0.5547001962252290364, -0.8320502943378437211, 0.000000000000000000 ) ) ;
#16563=CARTESIAN_POINT ( 'NONE',  ( -2.266590686148945544, 12.22041550158063394, 7.082119434687048631 ) ) ;
#16564=CARTESIAN_POINT ( 'NONE',  ( 19.38216949554541557, 62.24863466993041072, -9.382169495545420901 ) ) ;
#16565=CARTESIAN_POINT ( 'NONE',  ( 24.16423886937410614, 9.303748834913967869, 8.672049930838204340E-16 ) ) ;
#16566=CARTESIAN_POINT ( 'NONE',  ( 2.917880565312950480, 25.97041550158063572, -12.26659068614894821 ) ) ;
#16568=DIRECTION ( 'NONE',  ( 1.000000000000000000, 1.454946622157118376E-15, 0.000000000000000000 ) ) ;
#16569=CARTESIAN_POINT ( 'NONE',  ( 20.88017736071110164, 60.35535201082151957, 2.915334737309930979 ) ) ;
#16570=CARTESIAN_POINT ( 'NONE',  ( 0.5774900079438607392, 18.48035201082150536, 5.440088680355550821 ) ) ;
#16572=CARTESIAN_POINT ( 'NONE',  ( 17.20831665107776587, 4.133931151000785675, -7.208316651077762316 ) ) ;
#16573=CARTESIAN_POINT ( 'NONE',  ( 5.076628168052703671, 6.842264484334118713, 8.527530157486179263 ) ) ;
#16574=CARTESIAN_POINT ( 'NONE',  ( 19.38216949554541202, 25.99863466993042138, 9.382169495545424454 ) ) ;
#16575=CARTESIAN_POINT ( 'NONE',  ( 14.92337183194729633, 27.67559781766745530, 8.527530157486181039 ) ) ;
#16577=CARTESIAN_POINT ( 'NONE',  ( 3.591859063236761518, 9.956968003263753531, 11.09922568453594849 ) ) ;
#16579=CARTESIAN_POINT ( 'NONE',  ( 14.92337183194729988, 9.342264484334119601, -8.527530157486177487 ) ) ;
#16581=ORIENTED_EDGE ( 'NONE', *, *, #45704, .T. ) ;
#16582=CARTESIAN_POINT ( 'NONE',  ( 12.91533473730993009, 41.60535201082149825, -10.88017736071109987 ) ) ;
#16583=CARTESIAN_POINT ( 'NONE',  ( -0.3689425029237898834, 26.17874883491396432, -10.36894250292378850 ) ) ;
#16584=CARTESIAN_POINT ( 'NONE',  ( 1.472469842513823179, 35.59226448433412315, -4.923371831947296329 ) ) ;
#16585=CARTESIAN_POINT ( 'NONE',  ( 15.44008868035555793, 66.39701867748817676, -9.422509992056140149 ) ) ;
#16586=CARTESIAN_POINT ( 'NONE',  ( 10.00000000000000000, 52.87363466993041783, -12.81628187352647608 ) ) ;
#16588=CARTESIAN_POINT ( 'NONE',  ( 10.00000000000000000, 31.81368534415483751, -10.88017736071110342 ) ) ;
#16590=CARTESIAN_POINT ( 'NONE',  ( 10.00000000000000178, 10.37363466993041961, 12.81628187352647608 ) ) ;
#16591=CARTESIAN_POINT ( 'NONE',  ( 2.791683348922237240, 40.38393115100078035, -7.208316651077763204 ) ) ;
#16593=CARTESIAN_POINT ( 'NONE',  ( -1.099225684535947600, 49.54030133659708923, 6.408140936763237150 ) ) ;
#16595=CARTESIAN_POINT ( 'NONE',  ( 17.96484262340118221, 54.93868534415484106, 7.964842623401181321 ) ) ;
#16597=EDGE_CURVE ( 'NONE', #49769, #39417, #15767, .T. ) ;
#16598=DIRECTION ( 'NONE',  ( 1.000000000000000000, 0.000000000000000000, 0.000000000000000000 ) ) ;
#16600=CARTESIAN_POINT ( 'NONE',  ( 20.88017736071110519, 50.56368534415484106, 2.639326808657452039E-16 ) ) ;
#16602=CARTESIAN_POINT ( 'NONE',  ( 0.5774900079438607392, 63.48035201082149825, 5.440088680355550821 ) ) ;
#16603=LINE ( 'NONE', #78576, #31316 ) ;
#16604=CARTESIAN_POINT ( 'NONE',  ( 0.5774900079438607392, 63.48035201082149825, 5.440088680355550821 ) ) ;
#16605=CARTESIAN_POINT ( 'NONE',  ( 19.42250999205614193, 5.147018677488171434, 5.440088680355555262 ) ) ;
#16606=CARTESIAN_POINT ( 'NONE',  ( 1.472469842513823179, 46.42559781766745175, 4.923371831947296329 ) ) ;
#16607=CARTESIAN_POINT ( 'NONE',  ( 7.084665262690076126, 19.10535201082150181, 10.88017736071109987 ) ) ;
#16608=FACE_OUTER_BOUND ( 'NONE', #75401, .T. ) ;
#16609=CARTESIAN_POINT ( 'NONE',  ( 6.565887622018943937, 30.16530133659708568, 12.81628187352647430 ) ) ;
#16611=CARTESIAN_POINT ( 'NONE',  ( 2.035157376598822676, 32.43868534415483396, -7.964842623401177768 ) ) ;
#16613=CARTESIAN_POINT ( 'NONE',  ( 6.565887622018943937, 8.081968003263751754, -12.81628187352647608 ) ) ;
#16615=CARTESIAN_POINT ( 'NONE',  ( 15.44008868035555260, 14.73035201082150536, 9.422509992056143702 ) ) ;
#16616=CARTESIAN_POINT ( 'NONE',  ( 19.42250999205614548, 35.98035201082151247, -5.440088680355545492 ) ) ;
#16617=CARTESIAN_POINT ( 'NONE',  ( 17.08211943468705130, 53.47041550158063217, 12.26659068614894998 ) ) ;
#16618=CARTESIAN_POINT ( 'NONE',  ( 12.63842701281683034, 22.46726448433411605, 9.846743663894596210 ) ) ;
#16619=CARTESIAN_POINT ( 'NONE',  ( 20.88017736071110519, 65.56368534415483396, 2.639326808657452039E-16 ) ) ;
#16621=CARTESIAN_POINT ( 'NONE',  ( 6.204703633549690345, 22.84541550158062861, 14.16423886937410082 ) ) ;
#16626=CARTESIAN_POINT ( 'NONE',  ( 22.26659068614894466, 28.88708216824730357, 7.082119434687054849 ) ) ;
#16627=CARTESIAN_POINT ( 'NONE',  ( 6.204703633549690345, 37.84541550158063927, 14.16423886937410082 ) ) ;
#16629=CARTESIAN_POINT ( 'NONE',  ( 7.361572987183169658, 4.967264484334119601, -9.846743663894592657 ) ) ;
#16630=CARTESIAN_POINT ( 'NONE',  ( 3.591859063236763294, 8.290301336597087456, -11.09922568453595026 ) ) ;
#16631=CARTESIAN_POINT ( 'NONE',  ( 12.63842701281683922, 59.55059781766744464, -9.846743663894590881 ) ) ;
#16633=CARTESIAN_POINT ( 'NONE',  ( 19.42250999205614193, 55.14701867748817676, 5.440088680355555262 ) ) ;
#16634=CARTESIAN_POINT ( 'NONE',  ( 3.591859063236763294, 13.29030133659708746, -11.09922568453595026 ) ) ;
#16635=CARTESIAN_POINT ( 'NONE',  ( 24.16423886937410614, 24.30374883491396787, 8.672049930838204340E-16 ) ) ;
#16636=CARTESIAN_POINT ( 'NONE',  ( 7.084665262690076126, 29.10535201082150181, 10.88017736071109987 ) ) ;
#16637=CARTESIAN_POINT ( 'NONE',  ( 12.91533473730992121, 34.52201867748817676, 10.88017736071110164 ) ) ;
#16639=B_SPLINE_CURVE_WITH_KNOTS ( 'NONE', 3,
 ( #41829, #72295, #3826, #34281, #64781, #97803, #21787, #52755, #29264, #20791 ),
 .UNSPECIFIED., .F., .F.,
 ( 4, 2, 2, 2, 4 ),
 ( 8.673617379884034509E-19, 0.001992649090385492476, 0.002988973635578252158, 0.003487135908174629831, 0.003985298180771007504 ),
 .UNSPECIFIED. ) ;
#16641=CARTESIAN_POINT ( 'NONE',  ( 20.88017736071110164, 60.35535201082151957, 2.915334737309930979 ) ) ;
#16646=LINE ( 'NONE', #94596, #81257 ) ;
#16648=CARTESIAN_POINT ( 'NONE',  ( 6.204703633549690345, 62.84541550158063927, 14.16423886937410082 ) ) ;
#16649=CARTESIAN_POINT ( 'NONE',  ( 2.917880565312948704, 67.63708216824730357, 12.26659068614894643 ) ) ;
#16650=CARTESIAN_POINT ( 'NONE',  ( 0.1532563361054082862, 41.21726448433411605, 2.638427012816831674 ) ) ;
#16651=CARTESIAN_POINT ( 'NONE',  ( 7.361572987183170547, 67.05059781766746596, 9.846743663894590881 ) ) ;
#16654=CARTESIAN_POINT ( 'NONE',  ( 21.09922568453594849, 11.20696800326375531, 6.408140936763242479 ) ) ;
#16657=CARTESIAN_POINT ( 'NONE',  ( 6.204703633549690345, 50.76208216824730357, -14.16423886937410259 ) ) ;
#16658=CARTESIAN_POINT ( 'NONE',  ( -4.164238869374098151, 46.59541550158063927, -3.795296366450310543 ) ) ;
#16660=CARTESIAN_POINT ( 'NONE',  ( 17.96484262340118221, 16.18868534415483396, -7.964842623401177768 ) ) ;
#16663=CARTESIAN_POINT ( 'NONE',  ( 17.96484262340118221, 39.93868534415484106, 7.964842623401181321 ) ) ;
#16664=CARTESIAN_POINT ( 'NONE',  ( 18.52753015748617571, 53.09226448433412315, 4.923371831947298993 ) ) ;
#16665=CARTESIAN_POINT ( 'NONE',  ( 10.00000000000000000, 36.81368534415484106, -10.88017736071110342 ) ) ;
#16667=CARTESIAN_POINT ( 'NONE',  ( 10.00000000000000178, 59.31368534415484106, 10.88017736071110342 ) ) ;
#16668=CARTESIAN_POINT ( 'NONE',  ( 2.035157376598824452, 28.68868534415484106, 7.964842623401179544 ) ) ;
#16670=CARTESIAN_POINT ( 'NONE',  ( 5.500000000000000000, 61.00000000000000711, 6.500000000000000888 ) ) ;
#16671=ORIENTED_EDGE ( 'NONE', *, *, #97240, .F. ) ;
#16673=CARTESIAN_POINT ( 'NONE',  ( 10.00000000000000178, 2.258931151000784787, 9.846743663894594434 ) ) ;
#16675=ORIENTED_EDGE ( 'NONE', *, *, #37822, .T. ) ;
#16677=CARTESIAN_POINT ( 'NONE',  ( 5.076628168052704559, 25.17559781766745175, -8.527530157486179263 ) ) ;
#16683=CARTESIAN_POINT ( 'NONE',  ( 10.00000000000000178, 67.25893115100079456, 9.846743663894594434 ) ) ;
#16684=CARTESIAN_POINT ( 'NONE',  ( -43.18361233615330974, 107.2794497428041041, 4.499999999210813506 ) ) ;
#16685=CARTESIAN_POINT ( 'NONE',  ( 14.92337183194729988, 49.34226448433411605, -8.527530157486177487 ) ) ;
#16686=CARTESIAN_POINT ( 'NONE',  ( -0.3689425029237898834, 46.17874883491397497, -10.36894250292378850 ) ) ;
#16687=CARTESIAN_POINT ( 'NONE',  ( 19.84674366389459266, 53.30059781766744464, 2.638427012816836559 ) ) ;
#16688=CARTESIAN_POINT ( 'NONE',  ( 20.15039907845753220, 41.74884699246887720, 6.262539305110078836 ) ) ;
#16689=CARTESIAN_POINT ( 'NONE',  ( 7.361572987183169658, 14.96726448433411960, -9.846743663894592657 ) ) ;
#16690=CARTESIAN_POINT ( 'NONE',  ( 16.40814093676324603, 47.45696800326375353, -11.09922568453594671 ) ) ;
#16691=CARTESIAN_POINT ( 'NONE',  ( 19.84674366389459266, 63.71726448433412315, -2.638427012816827677 ) ) ;
#16692=CARTESIAN_POINT ( 'NONE',  ( 4.559911319644449179, 58.89701867748817676, 9.422509992056141925 ) ) ;
#16693=CARTESIAN_POINT ( 'NONE',  ( 12.63842701281683922, 49.55059781766744464, -9.846743663894590881 ) ) ;
#16694=CARTESIAN_POINT ( 'NONE',  ( 21.92686044187657046, 15.16212336850780318, 4.562052436263912550E-16 ) ) ;
#16696=CARTESIAN_POINT ( 'NONE',  ( 2.917880565312948704, 52.63708216824730357, 12.26659068614894643 ) ) ;
#16698=CARTESIAN_POINT ( 'NONE',  ( 15.44008868035555260, 29.73035201082150891, 9.422509992056143702 ) ) ;
#16699=CARTESIAN_POINT ( 'NONE',  ( 13.43411237798105340, 10.58196800326375353, 12.81628187352647963 ) ) ;
#16700=CARTESIAN_POINT ( 'NONE',  ( 2.035157376598822676, 62.43868534415483396, -7.964842623401177768 ) ) ;
#16704=CARTESIAN_POINT ( 'NONE',  ( -0.8801773607111008646, 58.27201867748816966, 2.915334737309923430 ) ) ;
#16705=CARTESIAN_POINT ( 'NONE',  ( 1.046131998950049047, 10.73810908735726777, 6.500000000000002665 ) ) ;
#16706=CARTESIAN_POINT ( 'NONE',  ( 14.92337183194729988, 34.34226448433411605, -8.527530157486177487 ) ) ;
#16707=FACE_OUTER_BOUND ( 'NONE', #97302, .T. ) ;
#16709=CARTESIAN_POINT ( 'NONE',  ( 19.38216949554541557, 12.24863466993041961, -9.382169495545420901 ) ) ;
#16710=CARTESIAN_POINT ( 'NONE',  ( 19.42250999205614193, 15.14701867748817143, 5.440088680355555262 ) ) ;
#16711=DIRECTION ( 'NONE',  ( 0.000000000000000000, 0.000000000000000000, -1.000000000000000000 ) ) ;
#16713=CARTESIAN_POINT ( 'NONE',  ( 10.00000000000000178, 38.05374883491396787, 14.16423886937410082 ) ) ;
#16714=EDGE_CURVE ( 'NONE', #25641, #87694, #95610, .T. ) ;
#16715=CARTESIAN_POINT ( 'NONE',  ( -0.3689425029237881626, 67.42874883491396076, 10.36894250292379027 ) ) ;
#16716=CARTESIAN_POINT ( 'NONE',  ( 1.472469842513823179, 30.59226448433411960, -4.923371831947296329 ) ) ;
#16717=CARTESIAN_POINT ( 'NONE',  ( 17.20831665107776587, 19.13393115100078035, -7.208316651077762316 ) ) ;
#16718=CARTESIAN_POINT ( 'NONE',  ( 19.42250999205614193, 20.14701867748817321, 5.440088680355555262 ) ) ;
#16720=CARTESIAN_POINT ( 'NONE',  ( 18.52753015748618282, 43.92559781766745175, -4.923371831947291888 ) ) ;
#16721=CARTESIAN_POINT ( 'NONE',  ( 2.035157376598822676, 32.43868534415483396, -7.964842623401177768 ) ) ;
#16722=CARTESIAN_POINT ( 'NONE',  ( 10.00000000000000000, 64.75893115100078035, -9.846743663894594434 ) ) ;
#16723=CARTESIAN_POINT ( 'NONE',  ( 2.917880565312948704, 7.637082168247301794, 12.26659068614894643 ) ) ;
#16724=CARTESIAN_POINT ( 'NONE',  ( 0.2751277870542909731, 44.36607318730131055, -6.499999999999992006 ) ) ;
#16726=CARTESIAN_POINT ( 'NONE',  ( 18.52753015748617571, 18.09226448433411960, 4.923371831947298993 ) ) ;
#16727=CARTESIAN_POINT ( 'NONE',  ( 22.81628187352647785, 56.41530133659708213, 3.434112377981063169 ) ) ;
#16728=CARTESIAN_POINT ( 'NONE',  ( 1.472469842513823179, 61.42559781766745175, 4.923371831947296329 ) ) ;
#16730=CARTESIAN_POINT ( 'NONE',  ( 0.1532563361054100626, 15.80059781766745353, -2.638427012816831230 ) ) ;
#16733=CARTESIAN_POINT ( 'NONE',  ( 0.5774900079438590739, 2.647018677488171434, -5.440088680355550821 ) ) ;
#16734=CARTESIAN_POINT ( 'NONE',  ( 0.5774900079438607392, 48.48035201082150536, 5.440088680355550821 ) ) ;
#16736=CARTESIAN_POINT ( 'NONE',  ( 12.91533473730993009, 61.60535201082150536, -10.88017736071109987 ) ) ;
#16737=CARTESIAN_POINT ( 'NONE',  ( 7.361572987183170547, 42.05059781766745886, 9.846743663894590881 ) ) ;
#16738=CARTESIAN_POINT ( 'NONE',  ( 15.44008868035555260, 14.73035201082150536, 9.422509992056143702 ) ) ;
#16741=B_SPLINE_CURVE_WITH_KNOTS ( 'NONE', 3,
 ( #46677, #70182, #48639, #92187 ),
 .UNSPECIFIED., .F., .F.,
 ( 4, 4 ),
 ( 7.410741937918042371E-18, 0.002562518741975316431 ),
 .UNSPECIFIED. ) ;
#16742=( LENGTH_UNIT ( ) NAMED_UNIT ( * ) SI_UNIT ( .MILLI., .METRE. ) );
#16746=EDGE_CURVE ( 'NONE', #6951, #31758, #83136, .T. ) ;
#16748=CARTESIAN_POINT ( 'NONE',  ( 10.00000000000000000, 39.75893115100078745, -9.846743663894594434 ) ) ;
#16749=CARTESIAN_POINT ( 'NONE',  ( 19.84674366389459621, 18.50893115100078745, 7.409399052514197653E-17 ) ) ;
#16750=CARTESIAN_POINT ( 'NONE',  ( 0.6178305044545818747, 58.49863466993042493, -9.382169495545419124 ) ) ;
#16751=CARTESIAN_POINT ( 'NONE',  ( 0.5774900079438607392, 23.48035201082150536, 5.440088680355550821 ) ) ;
#16752=CARTESIAN_POINT ( 'NONE',  ( 12.63842701281683034, 47.46726448433412315, 9.846743663894596210 ) ) ;
#16753=CARTESIAN_POINT ( 'NONE',  ( -1.926860441876563801, 34.89664270246083788, 3.195792623639529761 ) ) ;
#16754=CARTESIAN_POINT ( 'NONE',  ( 2.917880565312950480, 45.97041550158063927, -12.26659068614894821 ) ) ;
#16756=CARTESIAN_POINT ( 'NONE',  ( 20.36894250292379738, 64.92874883491397497, -10.36894250292379027 ) ) ;
#16758=DIRECTION ( 'NONE',  ( 0.000000000000000000, 0.000000000000000000, 1.000000000000000000 ) ) ;
#16759=CARTESIAN_POINT ( 'NONE',  ( 12.91533473730992121, 49.52201867748817676, 10.88017736071110164 ) ) ;
#16762=CARTESIAN_POINT ( 'NONE',  ( 18.52753015748618282, 18.92559781766745175, -4.923371831947291888 ) ) ;
#16766=ORIENTED_EDGE ( 'NONE', *, *, #40716, .F. ) ;
#16767=CARTESIAN_POINT ( 'NONE',  ( 19.84674366389459266, 3.717264484334118713, -2.638427012816827677 ) ) ;
#16769=CARTESIAN_POINT ( 'NONE',  ( 22.26659068614895176, 19.72041550158063572, -7.082119434687042414 ) ) ;
#16770=CARTESIAN_POINT ( 'NONE',  ( 12.63842701281683034, 17.46726448433411250, 9.846743663894596210 ) ) ;
#16771=CARTESIAN_POINT ( 'NONE',  ( 20.88017736071110164, 50.35535201082151247, 2.915334737309930979 ) ) ;
#16774=CARTESIAN_POINT ( 'NONE',  ( 20.88017736071110519, 45.56368534415484106, 2.639326808657452039E-16 ) ) ;
#16776=ORIENTED_EDGE ( 'NONE', *, *, #83698, .T. ) ;
#16777=CARTESIAN_POINT ( 'NONE',  ( 17.08211943468705130, 3.470415501580634388, 12.26659068614894998 ) ) ;
#16780=CARTESIAN_POINT ( 'NONE',  ( 19.38216949554541557, 17.24863466993041783, -9.382169495545420901 ) ) ;
#16781=CARTESIAN_POINT ( 'NONE',  ( 2.791683348922237240, 5.383931151000785675, -7.208316651077763204 ) ) ;
#16782=CARTESIAN_POINT ( 'NONE',  ( 2.035157376598822676, 2.438685344154837953, -7.964842623401177768 ) ) ;
#16785=CARTESIAN_POINT ( 'NONE',  ( 18.52753015748617571, 23.09226448433411960, 4.923371831947298993 ) ) ;
#16786=CARTESIAN_POINT ( 'NONE',  ( -0.8801773607110991993, 32.85535201082151247, -2.915334737309923874 ) ) ;
#16787=AXIS2_PLACEMENT_3D ( 'NONE', #88574, #49104, #43079 ) ;
#16790=CARTESIAN_POINT ( 'NONE',  ( -10.44000000000001194, 92.00000000000000000, -9.500000000000000000 ) ) ;
#16791=CARTESIAN_POINT ( 'NONE',  ( -0.8801773607111009756, 58.06368534415484106, 1.068504757029289695E-15 ) ) ;
#16793=CARTESIAN_POINT ( 'NONE',  ( 6.565887622018943937, 63.08196800326376064, -12.81628187352647608 ) ) ;
#16794=CARTESIAN_POINT ( 'NONE',  ( 2.035157376598822676, 67.43868534415484817, -7.964842623401177768 ) ) ;
#16795=CARTESIAN_POINT ( 'NONE',  ( -2.816281873526471635, 8.915301336597083903, -3.434112377981056508 ) ) ;
#16797=CARTESIAN_POINT ( 'NONE',  ( 14.92337183194729988, 34.34226448433411605, -8.527530157486177487 ) ) ;
#16798=CARTESIAN_POINT ( 'NONE',  ( -1.099225684535947600, 58.70696800326375353, -6.408140936763238038 ) ) ;
#16799=CARTESIAN_POINT ( 'NONE',  ( -2.266590686148945544, 12.22041550158063394, 7.082119434687048631 ) ) ;
#16800=CARTESIAN_POINT ( 'NONE',  ( 14.92337183194729633, 17.67559781766745175, 8.527530157486181039 ) ) ;
#16801=CARTESIAN_POINT ( 'NONE',  ( -1.099225684535947600, 23.70696800326375708, -6.408140936763238038 ) ) ;
#16805=CARTESIAN_POINT ( 'NONE',  ( 20.88017736071110164, 45.35535201082149115, 2.915334737309930979 ) ) ;
#16806=CARTESIAN_POINT ( 'NONE',  ( 14.92337183194729633, 62.67559781766745886, 8.527530157486181039 ) ) ;
#16808=CARTESIAN_POINT ( 'NONE',  ( 2.791683348922240793, 26.63393115100078745, 7.208316651077764092 ) ) ;
#16809=CARTESIAN_POINT ( 'NONE',  ( 0.5774900079438590739, 12.64701867748817143, -5.440088680355550821 ) ) ;
#16810=CARTESIAN_POINT ( 'NONE',  ( 21.09922568453595559, 22.04030133659708923, -6.408140936763230044 ) ) ;
#16811=CARTESIAN_POINT ( 'NONE',  ( 18.52753015748617571, 23.09226448433411960, 4.923371831947298993 ) ) ;
#16813=CARTESIAN_POINT ( 'NONE',  ( -0.8801773607111009756, 18.06368534415484106, 1.068504757029289695E-15 ) ) ;
#16814=B_SPLINE_CURVE_WITH_KNOTS ( 'NONE', 3,
 ( #96736, #52201, #89210, #36211 ),
 .UNSPECIFIED., .F., .F.,
 ( 4, 4 ),
 ( 0.000000000000000000, 0.002392975128318465105 ),
 .UNSPECIFIED. ) ;
#16816=CARTESIAN_POINT ( 'NONE',  ( 1.472469842513823179, 41.42559781766745886, 4.923371831947296329 ) ) ;
#16817=CARTESIAN_POINT ( 'NONE',  ( 15.44008868035555793, 16.39701867748817321, -9.422509992056140149 ) ) ;
#16819=CARTESIAN_POINT ( 'NONE',  ( 12.91533473730993009, 26.60535201082150536, -10.88017736071109987 ) ) ;
#16820=CARTESIAN_POINT ( 'NONE',  ( 17.96484262340118221, 14.93868534415484106, 7.964842623401181321 ) ) ;
#16821=CARTESIAN_POINT ( 'NONE',  ( -1.926860441876564023, 19.68830936912750573, 1.004413902775740781E-15 ) ) ;
#16822=CARTESIAN_POINT ( 'NONE',  ( 7.361572987183169658, 19.96726448433411960, -9.846743663894592657 ) ) ;
#16823=CARTESIAN_POINT ( 'NONE',  ( 12.63842701281683922, 44.55059781766745175, -9.846743663894590881 ) ) ;
#16825=CARTESIAN_POINT ( 'NONE',  ( 20.15039907845753930, 4.722660991849187972, 6.262539305110067289 ) ) ;
#16826=CARTESIAN_POINT ( 'NONE',  ( 7.361572987183170547, 67.05059781766746596, 9.846743663894590881 ) ) ;
#16830=CARTESIAN_POINT ( 'NONE',  ( -0.3689425029237881626, 27.42874883491397142, 10.36894250292379027 ) ) ;
#16831=CARTESIAN_POINT ( 'NONE',  ( 0.1532563361054082862, 41.21726448433411605, 2.638427012816831674 ) ) ;
#16832=FACE_OUTER_BOUND ( 'NONE', #26940, .T. ) ;
#16833=ORIENTED_EDGE ( 'NONE', *, *, #23445, .T. ) ;
#16835=CARTESIAN_POINT ( 'NONE',  ( 6.204703633549690345, 55.76208216824730357, -14.16423886937410259 ) ) ;
#16838=CARTESIAN_POINT ( 'NONE',  ( 1.472469842513823179, 15.59226448433411960, -4.923371831947296329 ) ) ;
#16840=CARTESIAN_POINT ( 'NONE',  ( 19.42250999205614548, 40.98035201082150536, -5.440088680355545492 ) ) ;
#16841=CARTESIAN_POINT ( 'NONE',  ( 3.591859063236761518, 44.95696800326376064, 11.09922568453594849 ) ) ;
#16842=CARTESIAN_POINT ( 'NONE',  ( 10.00000000000000178, 14.31368534415483751, 10.88017736071110342 ) ) ;
#16843=CARTESIAN_POINT ( 'NONE',  ( 6.565887622018943937, 43.08196800326374643, -12.81628187352647608 ) ) ;
#16844=CARTESIAN_POINT ( 'NONE',  ( 10.00000000000000178, 67.25893115100079456, 9.846743663894594434 ) ) ;
#16845=CARTESIAN_POINT ( 'NONE',  ( 19.84674366389459266, 8.717264484334116048, -2.638427012816827677 ) ) ;
#16849=CARTESIAN_POINT ( 'NONE',  ( 20.36894250292379738, 49.92874883491396787, -10.36894250292379027 ) ) ;
#16850=CARTESIAN_POINT ( 'NONE',  ( 24.16423886937410614, 9.512082168247301794, -3.795296366450302550 ) ) ;
#16851=CARTESIAN_POINT ( 'NONE',  ( 12.91533473730992121, 19.52201867748816611, 10.88017736071110164 ) ) ;
#16852=CARTESIAN_POINT ( 'NONE',  ( 17.96484262340118221, 29.93868534415484106, 7.964842623401181321 ) ) ;
#16853=FACE_OUTER_BOUND ( 'NONE', #45784, .T. ) ;
#16854=CARTESIAN_POINT ( 'NONE',  ( 4.559911319644449179, 67.23035201082150536, -9.422509992056141925 ) ) ;
#16855=CARTESIAN_POINT ( 'NONE',  ( -19.19000000000001194, 93.50000000000000000, -10.09898361729590199 ) ) ;
#16856=CARTESIAN_POINT ( 'NONE',  ( 2.791683348922240793, 21.63393115100078745, 7.208316651077764092 ) ) ;
#16858=CYLINDRICAL_SURFACE ( 'NONE', #85043, 0.5000000000000004441 ) ;
#16859=CARTESIAN_POINT ( 'NONE',  ( 1.472469842513823179, 10.59226448433411782, -4.923371831947296329 ) ) ;
#16860=CARTESIAN_POINT ( 'NONE',  ( 19.84674366389459266, 38.30059781766745175, 2.638427012816836559 ) ) ;
#16862=CARTESIAN_POINT ( 'NONE',  ( 15.44008868035555260, 9.730352010821505360, 9.422509992056143702 ) ) ;
#16863=CARTESIAN_POINT ( 'NONE',  ( 10.00000000000000178, 30.37363466993042138, 12.81628187352647608 ) ) ;
#16864=ADVANCED_FACE ( 'NONE', ( #18362 ), #56841, .T. ) ;
#16866=CARTESIAN_POINT ( 'NONE',  ( 15.44008868035555260, 54.73035201082150536, 9.422509992056143702 ) ) ;
#16867=CARTESIAN_POINT ( 'NONE',  ( -0.3689425029237898834, 46.17874883491397497, -10.36894250292378850 ) ) ;
#16868=CARTESIAN_POINT ( 'NONE',  ( 18.52753015748618282, 13.92559781766745175, -4.923371831947291888 ) ) ;
#16870=CARTESIAN_POINT ( 'NONE',  ( 10.00000000000000000, 49.75893115100078745, -9.846743663894594434 ) ) ;
#16871=CARTESIAN_POINT ( 'NONE',  ( 18.52753015748617571, 28.09226448433411960, 4.923371831947298993 ) ) ;
#16872=CARTESIAN_POINT ( 'NONE',  ( 2.917880565312948704, 12.63708216824730179, 12.26659068614894643 ) ) ;
#16873=CARTESIAN_POINT ( 'NONE',  ( 6.204703633549690345, 22.84541550158062861, 14.16423886937410082 ) ) ;
#16874=CARTESIAN_POINT ( 'NONE',  ( 19.42250999205614193, 40.14701867748817676, 5.440088680355555262 ) ) ;
#16875=CARTESIAN_POINT ( 'NONE',  ( 10.00000000000000178, 9.313685344154839285, 10.88017736071110342 ) ) ;
#16877=CARTESIAN_POINT ( 'NONE',  ( -0.8801773607110991993, 42.85535201082150536, -2.915334737309923874 ) ) ;
#16878=CARTESIAN_POINT ( 'NONE',  ( 4.559911319644449179, 23.89701867748817321, 9.422509992056141925 ) ) ;
#16879=ORIENTED_EDGE ( 'NONE', *, *, #53879, .T. ) ;
#16880=CARTESIAN_POINT ( 'NONE',  ( 10.00000000000000178, 39.31368534415484106, 10.88017736071110342 ) ) ;
#16882=CARTESIAN_POINT ( 'NONE',  ( 19.38216949554541557, 62.24863466993041072, -9.382169495545420901 ) ) ;
#16883=CARTESIAN_POINT ( 'NONE',  ( 17.96484262340118221, 56.18868534415484817, -7.964842623401177768 ) ) ;
#16885=VERTEX_POINT ( 'NONE', #72815 ) ;
#16886=( BOUNDED_SURFACE ( )  B_SPLINE_SURFACE ( 1, 2, ( 
 ( #64649, #42185, #6632, #91616, #68133, #92104, #15635, #84609, #84123, #16110, #68623, #45619, #14651, #53117, #53606, #98153, #45114, #98660, #60614, #46118, #15141, #22139, #153, #54094, #75622, #8121, #91112, #7134, #30602, #22636, #61107, #83625, #46596, #29126, #83123, #23133, #30108, #90122, #97659, #37148, #67644, #60116, #21650, #29611, #90615, #23635, #52135, #59627, #38616, #77095, #44630, #14146, #76116, #7645, #76605, #75125, #38136, #69117, #648, #52623, #37636, #31097, #61591, #36647, #67134, #82630, #40092, #94071, #26077, #48562, #39611, #86087, #70100, #62083, #54583, #1625, #25592, #92590, #70592, #17597, #48066, #79062, #2118, #16607, #94559, #32073, #62575, #47591, #9097, #32577, #87062, #77581, #63073, #78085, #93079, #78581, #1126, #24113, #47086, #10091, #39115, #2612, #56084, #3095, #24609, #85595, #64046, #10576, #55076, #40590, #93574, #17108, #9589, #56571, #18572, #25109, #55592, #41086, #71583, #71087, #18086, #31588, #85098, #33067, #86578, #63563, #49065, #33550, #8607, #69605, #73030, #58027, #28027, #5048, #19550, #35531, #66526, #96552, #59019, #11552, #34040, #26552, #42072, #58523, #64536, #12045, #88535, #20036, #51026, #4563, #87550, #97053, #72533, #4067, #50045, #80048, #42545, #89526, #49539, #35026, #80548, #34530, #50538, #72054, #95044, #19061, #81032, #11067, #73520, #89031, #74017, #65024, #57539, #36024, #81519, #95552, #12539, #65527, #27040, #88036, #28527, #21035, #96050, #27534, #13026, #43522, #43040, #20541, #3583, #57048, #66025, #5547, #79569, #41588, #76495, #29494, #22032, #45001, #29995, #40, #75999, #90497, #7527, #38506, #68510, #30982, #60502, #60003, #68016, #30489, #14034, #52506, #83013, #75506, #60987, #90992, #37025, #15026, #69003, #14531, #23020, #7020, #37526, #83509, #98543, #45499, #22522, #61481, #44011, #98039, #38017, #52994, #6035, #13529, #21531, #82516, #75011, #36534, #52024, #44512, #8008, #67023, #74515, #53489, #535, #59516, #29006, #91499, #84000, #15524, #90010, #46005, #91986, #51525, #67522, #6516, #82017, #97544, #25485, #40973, #71471, #54958, #9975, #2984, #63456, #54472, #1999, #84979, #76981, #69493, #16496, #40480, #8495, #85479, #32464, #62959, #93960, #16988, #31471, #10463, #46973, #77467, #62459, #23999, #47467, #33432, #92473, #77967, #92962, #8978, #93465, #15997, #38998, #61974, #24991, #53988, #17486, #70977, #17968, #39495, #1510, #78952, #55970, #69985, #55474, #9474, #31957, #24495, #63929, #23518, #39977, #70478, #86470, #48454, #85976, #32952, #46485, #1009, #47952, #2498, #78462, #84496, #20426, #72422, #64911 ),
 ( #3948, #11934, #12419, #56934, #34421, #26930, #19438, #42926, #72921, #79932, #57914, #12911, #95436, #65907, #49926, #57428, #27420, #80436, #88424, #42439, #73907, #86945, #41959, #80926, #87921, #48941, #56459, #64426, #26436, #18951, #79450, #94933, #87436, #50913, #10949, #18458, #96438, #81409, #3464, #71941, #4451, #34916, #73406, #33920, #65413, #95938, #19924, #11439, #49428, #27908, #50417, #58401, #43408, #5437, #4934, #35414, #35909, #88919, #94444, #25956, #41474, #45382, #74894, #83884, #91376, #44395, #36908, #59887, #44882, #14911, #90879, #6393, #22407, #53374, #83392, #45894, #75384, #67400, #82895, #75888, #28889, #97927, #29386, #90378, #7411, #6901, #51908, #29879, #15411, #21917, #37907, #52395, #14411, #98425, #37414, #60381, #67901, #76381, #58907, #13917, #52882, #68396, #20921, #28412, #36410, #97423, #89896, #51410, #66904, #59393, #22903, #81898, #89405, #98917, #7896, #74393, #43893, #30372, #60876, #66406, #5917, #96937, #13408, #21413, #82393, #8379, #40362, #32344, #70863, #55852, #86347, #69873, #24870, #17850, #78342, #69376, #16871, #898, #91879, #84391, #31360, #55352, #23400, #1393, #47345, #77848, #9863, #31848, #46375, #25367, #61860, #92364, #77352, #38888, #62346, #48335, #23891, #92851, #8863, #54356, #9357, #30873, #53884, #76864, #39862, #68893, #62847, #85858, #32833, #84868, #16377, #93840, #2378, #46859, #70368, #24379, #39379, #54845, #78839, #38390, #85359, #1886, #63335, #421, #93346, #47839, #61369, #15890, #17370, #58153, #67152, #59646, #89161, #80679, #21165, #35162, #12175, #42680, #90136, #50169, #73160, #51667, #20670, #88663, #21666, #13656, #74143, #94326, #5182, #13159, #5676, #51166, #52151, #82145, #44139, #58659, #10350, #97187, #81649, #43657, #28655, #4699, #74649, #73654, #35668, #36160, #27667, #50675, #66662, #65661, #28164, #97676, #40850, #6160, #89654, #36664, #2872, #71353, #29140, #20170, #66152, #12667, #96686, #33321, #81166, #96184, #63816, #25847, #43167, #59146, #57673, #88168, #19682, #22154, #61606, #67659, #75638, #14666, #52638, #46612, #76132, #23150, #53132, #22654, #8623, #53622, #83141, #38151, #1144, #44646, #62098, #83641, #92122, #68638, #45133, #167, #98169, #7150, #84142, #60132, #30615, #61123, #15155, #45634, #37653, #38631, #7660, #39133, #23650, #31604, #31112, #92606, #15651, #69134, #75140, #46134, #90630, #91632, #60628, #76620, #68151, #98674, #16127, #30123, #91130, #54111, #662, #8140, #84624, #77110, #24131, #69620, #82645, #14162, #6648, #37165, #29626, #25129, #48085, #33085, #3113, #79082, #93590, #10594, #41604 ) ),
 .UNSPECIFIED., .F., .F., .F. ) 
 B_SPLINE_SURFACE_WITH_KNOTS ( ( 2, 2 ),
 ( 3, 2, 2, 2, 2, 2, 2, 2, 2, 2, 2, 2, 2, 2, 2, 2, 2, 2, 2, 2, 2, 2, 2, 2, 2, 2, 2, 2, 2, 2, 2, 2, 2, 2, 2, 2, 2, 2, 2, 2, 2, 2, 2, 2, 2, 2, 2, 2, 2, 2, 2, 2, 2, 2, 2, 2, 2, 2, 2, 2, 2, 2, 2, 2, 2, 2, 2, 2, 2, 2, 2, 2, 2, 2, 2, 2, 2, 2, 2, 2, 2, 2, 2, 2, 2, 2, 2, 2, 2, 2, 2, 2, 2, 2, 2, 2, 2, 2, 2, 2, 2, 2, 2, 2, 2, 2, 2, 2, 2, 2, 2, 2, 2, 2, 2, 2, 2, 2, 2, 2, 2, 2, 2, 2, 2, 2, 2, 2, 2, 2, 2, 2, 2, 2, 2, 2, 2, 2, 2, 2, 2, 2, 2, 2, 2, 2, 2, 2, 2, 2, 2, 2, 2, 2, 2, 2, 2, 2, 2, 2, 2, 2, 3 ),
 ( 0.000000000000000000, 1.000000000000000000 ),
 ( 0.000000000000000000, 0.005952380952380952051, 0.01190476190476190410, 0.01785714285714285615, 0.02380952380952380820, 0.02976190476190476025, 0.03571428571428571230, 0.04166666666666666435, 0.04761904761904761640, 0.05357142857142856845, 0.05952380952380952051, 0.06547619047619047949, 0.07142857142857142461, 0.07738095238095238360, 0.08333333333333332871, 0.08928571428571428770, 0.09523809523809523281, 0.1011904761904761918, 0.1071428571428571369, 0.1130952380952380959, 0.1190476190476190410, 0.1250000000000000000, 0.1309523809523809590, 0.1369047619047619180, 0.1428571428571428492, 0.1488095238095238082, 0.1547619047619047672, 0.1607142857142857262, 0.1666666666666666574, 0.1726190476190476164, 0.1785714285714285754, 0.1845238095238095344, 0.1904761904761904656, 0.1964285714285714246, 0.2023809523809523836, 0.2083333333333333426, 0.2142857142857142738, 0.2202380952380952328, 0.2261904761904761918, 0.2321428571428571508, 0.2380952380952380820, 0.2440476190476190410, 0.2500000000000000000, 0.2559523809523809312, 0.2619047619047619180, 0.2678571428571428492, 0.2738095238095238360, 0.2797619047619047672, 0.2857142857142856984, 0.2916666666666666852, 0.2976190476190476164, 0.3035714285714285476, 0.3095238095238095344, 0.3154761904761904656, 0.3214285714285714524, 0.3273809523809523836, 0.3333333333333333148, 0.3392857142857143016, 0.3452380952380952328, 0.3511904761904761640, 0.3571428571428571508, 0.3630952380952380820, 0.3690476190476190688, 0.3750000000000000000, 0.3809523809523809312, 0.3869047619047619180, 0.3928571428571428492, 0.3988095238095238360, 0.4047619047619047672, 0.4107142857142856984, 0.4166666666666666852, 0.4226190476190476164, 0.4285714285714285476, 0.4345238095238095344, 0.4404761904761904656, 0.4464285714285714524, 0.4523809523809523836, 0.4583333333333333148, 0.4642857142857143016, 0.4702380952380952328, 0.4761904761904761640, 0.4821428571428571508, 0.4880952380952380820, 0.4940476190476190688, 0.5000000000000000000, 0.5059523809523809312, 0.5119047619047618625, 0.5178571428571429047, 0.5238095238095238360, 0.5297619047619047672, 0.5357142857142856984, 0.5416666666666666297, 0.5476190476190476719, 0.5535714285714286031, 0.5595238095238095344, 0.5654761904761904656, 0.5714285714285713969, 0.5773809523809523281, 0.5833333333333333703, 0.5892857142857143016, 0.5952380952380952328, 0.6011904761904761640, 0.6071428571428570953, 0.6130952380952381375, 0.6190476190476190688, 0.6250000000000000000, 0.6309523809523809312, 0.6369047619047618625, 0.6428571428571429047, 0.6488095238095238360, 0.6547619047619047672, 0.6607142857142856984, 0.6666666666666666297, 0.6726190476190476719, 0.6785714285714286031, 0.6845238095238095344, 0.6904761904761904656, 0.6964285714285713969, 0.7023809523809523281, 0.7083333333333333703, 0.7142857142857143016, 0.7202380952380952328, 0.7261904761904761640, 0.7321428571428570953, 0.7380952380952381375, 0.7440476190476190688, 0.7500000000000000000, 0.7559523809523809312, 0.7619047619047618625, 0.7678571428571429047, 0.7738095238095238360, 0.7797619047619047672, 0.7857142857142856984, 0.7916666666666666297, 0.7976190476190476719, 0.8035714285714286031, 0.8095238095238095344, 0.8154761904761904656, 0.8214285714285713969, 0.8273809523809523281, 0.8333333333333333703, 0.8392857142857143016, 0.8452380952380952328, 0.8511904761904761640, 0.8571428571428570953, 0.8630952380952381375, 0.8690476190476190688, 0.8750000000000000000, 0.8809523809523809312, 0.8869047619047618625, 0.8928571428571429047, 0.8988095238095238360, 0.9047619047619047672, 0.9107142857142856984, 0.9166666666666666297, 0.9226190476190476719, 0.9285714285714286031, 0.9345238095238095344, 0.9404761904761904656, 0.9464285714285713969, 0.9523809523809523281, 0.9583333333333333703, 0.9642857142857143016 ),
 .UNSPECIFIED. ) 
 GEOMETRIC_REPRESENTATION_ITEM ( )  RATIONAL_B_SPLINE_SURFACE ( (
 ( 1.000000000000000000, 0.9659258262890683122, 1.000000000000000000, 0.9659258262890683122, 1.000000000000000000, 0.9659258262890683122, 1.000000000000000000, 0.9659258262890683122, 1.000000000000000000, 0.9659258262890683122, 1.000000000000000000, 0.9659258262890683122, 1.000000000000000000, 0.9659258262890683122, 1.000000000000000000, 0.9659258262890683122, 1.000000000000000000, 0.9659258262890683122, 1.000000000000000000, 0.9659258262890683122, 1.000000000000000000, 0.9659258262890683122, 1.000000000000000000, 0.9659258262890683122, 1.000000000000000000, 0.9659258262890683122, 1.000000000000000000, 0.9659258262890683122, 1.000000000000000000, 0.9659258262890683122, 1.000000000000000000, 0.9659258262890683122, 1.000000000000000000, 0.9659258262890683122, 1.000000000000000000, 0.9659258262890683122, 1.000000000000000000, 0.9659258262890683122, 1.000000000000000000, 0.9659258262890683122, 1.000000000000000000, 0.9659258262890683122, 1.000000000000000000, 0.9659258262890683122, 1.000000000000000000, 0.9659258262890683122, 1.000000000000000000, 0.9659258262890683122, 1.000000000000000000, 0.9659258262890683122, 1.000000000000000000, 0.9659258262890683122, 1.000000000000000000, 0.9659258262890683122, 1.000000000000000000, 0.9659258262890683122, 1.000000000000000000, 0.9659258262890683122, 1.000000000000000000, 0.9659258262890683122, 1.000000000000000000, 0.9659258262890683122, 1.000000000000000000, 0.9659258262890683122, 1.000000000000000000, 0.9659258262890683122, 1.000000000000000000, 0.9659258262890683122, 1.000000000000000000, 0.9659258262890683122, 1.000000000000000000, 0.9659258262890683122, 1.000000000000000000, 0.9659258262890683122, 1.000000000000000000, 0.9659258262890683122, 1.000000000000000000, 0.9659258262890683122, 1.000000000000000000, 0.9659258262890683122, 1.000000000000000000, 0.9659258262890683122, 1.000000000000000000, 0.9659258262890683122, 1.000000000000000000, 0.9659258262890683122, 1.000000000000000000, 0.9659258262890683122, 1.000000000000000000, 0.9659258262890683122, 1.000000000000000000, 0.9659258262890683122, 1.000000000000000000, 0.9659258262890683122, 1.000000000000000000, 0.9659258262890683122, 1.000000000000000000, 0.9659258262890683122, 1.000000000000000000, 0.9659258262890683122, 1.000000000000000000, 0.9659258262890683122, 1.000000000000000000, 0.9659258262890683122, 1.000000000000000000, 0.9659258262890683122, 1.000000000000000000, 0.9659258262890683122, 1.000000000000000000, 0.9659258262890683122, 1.000000000000000000, 0.9659258262890683122, 1.000000000000000000, 0.9659258262890683122, 1.000000000000000000, 0.9659258262890683122, 1.000000000000000000, 0.9659258262890683122, 1.000000000000000000, 0.9659258262890683122, 1.000000000000000000, 0.9659258262890683122, 1.000000000000000000, 0.9659258262890683122, 1.000000000000000000, 0.9659258262890683122, 1.000000000000000000, 0.9659258262890683122, 1.000000000000000000, 0.9659258262890683122, 1.000000000000000000, 0.9659258262890683122, 1.000000000000000000, 0.9659258262890683122, 1.000000000000000000, 0.9659258262890683122, 1.000000000000000000, 0.9659258262890683122, 1.000000000000000000, 0.9659258262890683122, 1.000000000000000000, 0.9659258262890683122, 1.000000000000000000, 0.9659258262890683122, 1.000000000000000000, 0.9659258262890683122, 1.000000000000000000, 0.9659258262890683122, 1.000000000000000000, 0.9659258262890683122, 1.000000000000000000, 0.9659258262890683122, 1.000000000000000000, 0.9659258262890683122, 1.000000000000000000, 0.9659258262890683122, 1.000000000000000000, 0.9659258262890683122, 1.000000000000000000, 0.9659258262890683122, 1.000000000000000000, 0.9659258262890683122, 1.000000000000000000, 0.9659258262890683122, 1.000000000000000000, 0.9659258262890683122, 1.000000000000000000, 0.9659258262890683122, 1.000000000000000000, 0.9659258262890683122, 1.000000000000000000, 0.9659258262890683122, 1.000000000000000000, 0.9659258262890683122, 1.000000000000000000, 0.9659258262890683122, 1.000000000000000000, 0.9659258262890683122, 1.000000000000000000, 0.9659258262890683122, 1.000000000000000000, 0.9659258262890683122, 1.000000000000000000, 0.9659258262890683122, 1.000000000000000000, 0.9659258262890683122, 1.000000000000000000, 0.9659258262890683122, 1.000000000000000000, 0.9659258262890683122, 1.000000000000000000, 0.9659258262890683122, 1.000000000000000000, 0.9659258262890683122, 1.000000000000000000, 0.9659258262890683122, 1.000000000000000000, 0.9659258262890683122, 1.000000000000000000, 0.9659258262890683122, 1.000000000000000000, 0.9659258262890683122, 1.000000000000000000, 0.9659258262890683122, 1.000000000000000000, 0.9659258262890683122, 1.000000000000000000, 0.9659258262890683122, 1.000000000000000000, 0.9659258262890683122, 1.000000000000000000, 0.9659258262890683122, 1.000000000000000000, 0.9659258262890683122, 1.000000000000000000, 0.9659258262890683122, 1.000000000000000000, 0.9659258262890683122, 1.000000000000000000, 0.9659258262890683122, 1.000000000000000000, 0.9659258262890683122, 1.000000000000000000, 0.9659258262890683122, 1.000000000000000000, 0.9659258262890683122, 1.000000000000000000, 0.9659258262890683122, 1.000000000000000000, 0.9659258262890683122, 1.000000000000000000, 0.9659258262890683122, 1.000000000000000000, 0.9659258262890683122, 1.000000000000000000, 0.9659258262890683122, 1.000000000000000000, 0.9659258262890683122, 1.000000000000000000, 0.9659258262890683122, 1.000000000000000000, 0.9659258262890683122, 1.000000000000000000, 0.9659258262890683122, 1.000000000000000000, 0.9659258262890683122, 1.000000000000000000, 0.9659258262890683122, 1.000000000000000000, 0.9659258262890683122, 1.000000000000000000, 0.9659258262890683122, 1.000000000000000000, 0.9659258262890683122, 1.000000000000000000, 0.9659258262890683122, 1.000000000000000000, 0.9659258262890683122, 1.000000000000000000, 0.9659258262890683122, 1.000000000000000000, 0.9659258262890683122, 1.000000000000000000, 0.9659258262890683122, 1.000000000000000000, 0.9659258262890683122, 1.000000000000000000, 0.9659258262890683122, 1.000000000000000000, 0.9659258262890683122, 1.000000000000000000, 0.9659258262890683122, 1.000000000000000000, 0.9659258262890683122, 1.000000000000000000, 0.9659258262890683122, 1.000000000000000000, 0.9659258262890683122, 1.000000000000000000, 0.9659258262890683122, 1.000000000000000000, 0.9659258262890683122, 1.000000000000000000, 0.9659258262890683122, 1.000000000000000000, 0.9659258262890683122, 1.000000000000000000, 0.9659258262890683122, 1.000000000000000000, 0.9659258262890683122, 1.000000000000000000, 0.9659258262890683122, 1.000000000000000000, 0.9659258262890683122, 1.000000000000000000, 0.9659258262890683122, 1.000000000000000000, 0.9659258262890683122, 1.000000000000000000, 0.9659258262890683122, 1.000000000000000000, 0.9659258262890683122, 1.000000000000000000, 0.9659258262890683122, 1.000000000000000000, 0.9659258262890683122, 1.000000000000000000, 0.9659258262890683122, 1.000000000000000000, 0.9659258262890683122, 1.000000000000000000, 0.9659258262890683122, 1.000000000000000000, 0.9659258262890683122, 1.000000000000000000, 0.9659258262890683122, 1.000000000000000000, 0.9659258262890683122, 1.000000000000000000, 0.9659258262890683122, 1.000000000000000000, 0.9659258262890683122, 1.000000000000000000, 0.9659258262890683122, 1.000000000000000000),
 ( 1.000000000000000000, 0.9659258262890683122, 1.000000000000000000, 0.9659258262890683122, 1.000000000000000000, 0.9659258262890683122, 1.000000000000000000, 0.9659258262890683122, 1.000000000000000000, 0.9659258262890683122, 1.000000000000000000, 0.9659258262890683122, 1.000000000000000000, 0.9659258262890683122, 1.000000000000000000, 0.9659258262890683122, 1.000000000000000000, 0.9659258262890683122, 1.000000000000000000, 0.9659258262890683122, 1.000000000000000000, 0.9659258262890683122, 1.000000000000000000, 0.9659258262890683122, 1.000000000000000000, 0.9659258262890683122, 1.000000000000000000, 0.9659258262890683122, 1.000000000000000000, 0.9659258262890683122, 1.000000000000000000, 0.9659258262890683122, 1.000000000000000000, 0.9659258262890683122, 1.000000000000000000, 0.9659258262890683122, 1.000000000000000000, 0.9659258262890683122, 1.000000000000000000, 0.9659258262890683122, 1.000000000000000000, 0.9659258262890683122, 1.000000000000000000, 0.9659258262890683122, 1.000000000000000000, 0.9659258262890683122, 1.000000000000000000, 0.9659258262890683122, 1.000000000000000000, 0.9659258262890683122, 1.000000000000000000, 0.9659258262890683122, 1.000000000000000000, 0.9659258262890683122, 1.000000000000000000, 0.9659258262890683122, 1.000000000000000000, 0.9659258262890683122, 1.000000000000000000, 0.9659258262890683122, 1.000000000000000000, 0.9659258262890683122, 1.000000000000000000, 0.9659258262890683122, 1.000000000000000000, 0.9659258262890683122, 1.000000000000000000, 0.9659258262890683122, 1.000000000000000000, 0.9659258262890683122, 1.000000000000000000, 0.9659258262890683122, 1.000000000000000000, 0.9659258262890683122, 1.000000000000000000, 0.9659258262890683122, 1.000000000000000000, 0.9659258262890683122, 1.000000000000000000, 0.9659258262890683122, 1.000000000000000000, 0.9659258262890683122, 1.000000000000000000, 0.9659258262890683122, 1.000000000000000000, 0.9659258262890683122, 1.000000000000000000, 0.9659258262890683122, 1.000000000000000000, 0.9659258262890683122, 1.000000000000000000, 0.9659258262890683122, 1.000000000000000000, 0.9659258262890683122, 1.000000000000000000, 0.9659258262890683122, 1.000000000000000000, 0.9659258262890683122, 1.000000000000000000, 0.9659258262890683122, 1.000000000000000000, 0.9659258262890683122, 1.000000000000000000, 0.9659258262890683122, 1.000000000000000000, 0.9659258262890683122, 1.000000000000000000, 0.9659258262890683122, 1.000000000000000000, 0.9659258262890683122, 1.000000000000000000, 0.9659258262890683122, 1.000000000000000000, 0.9659258262890683122, 1.000000000000000000, 0.9659258262890683122, 1.000000000000000000, 0.9659258262890683122, 1.000000000000000000, 0.9659258262890683122, 1.000000000000000000, 0.9659258262890683122, 1.000000000000000000, 0.9659258262890683122, 1.000000000000000000, 0.9659258262890683122, 1.000000000000000000, 0.9659258262890683122, 1.000000000000000000, 0.9659258262890683122, 1.000000000000000000, 0.9659258262890683122, 1.000000000000000000, 0.9659258262890683122, 1.000000000000000000, 0.9659258262890683122, 1.000000000000000000, 0.9659258262890683122, 1.000000000000000000, 0.9659258262890683122, 1.000000000000000000, 0.9659258262890683122, 1.000000000000000000, 0.9659258262890683122, 1.000000000000000000, 0.9659258262890683122, 1.000000000000000000, 0.9659258262890683122, 1.000000000000000000, 0.9659258262890683122, 1.000000000000000000, 0.9659258262890683122, 1.000000000000000000, 0.9659258262890683122, 1.000000000000000000, 0.9659258262890683122, 1.000000000000000000, 0.9659258262890683122, 1.000000000000000000, 0.9659258262890683122, 1.000000000000000000, 0.9659258262890683122, 1.000000000000000000, 0.9659258262890683122, 1.000000000000000000, 0.9659258262890683122, 1.000000000000000000, 0.9659258262890683122, 1.000000000000000000, 0.9659258262890683122, 1.000000000000000000, 0.9659258262890683122, 1.000000000000000000, 0.9659258262890683122, 1.000000000000000000, 0.9659258262890683122, 1.000000000000000000, 0.9659258262890683122, 1.000000000000000000, 0.9659258262890683122, 1.000000000000000000, 0.9659258262890683122, 1.000000000000000000, 0.9659258262890683122, 1.000000000000000000, 0.9659258262890683122, 1.000000000000000000, 0.9659258262890683122, 1.000000000000000000, 0.9659258262890683122, 1.000000000000000000, 0.9659258262890683122, 1.000000000000000000, 0.9659258262890683122, 1.000000000000000000, 0.9659258262890683122, 1.000000000000000000, 0.9659258262890683122, 1.000000000000000000, 0.9659258262890683122, 1.000000000000000000, 0.9659258262890683122, 1.000000000000000000, 0.9659258262890683122, 1.000000000000000000, 0.9659258262890683122, 1.000000000000000000, 0.9659258262890683122, 1.000000000000000000, 0.9659258262890683122, 1.000000000000000000, 0.9659258262890683122, 1.000000000000000000, 0.9659258262890683122, 1.000000000000000000, 0.9659258262890683122, 1.000000000000000000, 0.9659258262890683122, 1.000000000000000000, 0.9659258262890683122, 1.000000000000000000, 0.9659258262890683122, 1.000000000000000000, 0.9659258262890683122, 1.000000000000000000, 0.9659258262890683122, 1.000000000000000000, 0.9659258262890683122, 1.000000000000000000, 0.9659258262890683122, 1.000000000000000000, 0.9659258262890683122, 1.000000000000000000, 0.9659258262890683122, 1.000000000000000000, 0.9659258262890683122, 1.000000000000000000, 0.9659258262890683122, 1.000000000000000000, 0.9659258262890683122, 1.000000000000000000, 0.9659258262890683122, 1.000000000000000000, 0.9659258262890683122, 1.000000000000000000, 0.9659258262890683122, 1.000000000000000000, 0.9659258262890683122, 1.000000000000000000, 0.9659258262890683122, 1.000000000000000000, 0.9659258262890683122, 1.000000000000000000, 0.9659258262890683122, 1.000000000000000000, 0.9659258262890683122, 1.000000000000000000, 0.9659258262890683122, 1.000000000000000000, 0.9659258262890683122, 1.000000000000000000, 0.9659258262890683122, 1.000000000000000000, 0.9659258262890683122, 1.000000000000000000, 0.9659258262890683122, 1.000000000000000000, 0.9659258262890683122, 1.000000000000000000, 0.9659258262890683122, 1.000000000000000000, 0.9659258262890683122, 1.000000000000000000, 0.9659258262890683122, 1.000000000000000000, 0.9659258262890683122, 1.000000000000000000, 0.9659258262890683122, 1.000000000000000000, 0.9659258262890683122, 1.000000000000000000, 0.9659258262890683122, 1.000000000000000000, 0.9659258262890683122, 1.000000000000000000, 0.9659258262890683122, 1.000000000000000000, 0.9659258262890683122, 1.000000000000000000, 0.9659258262890683122, 1.000000000000000000, 0.9659258262890683122, 1.000000000000000000, 0.9659258262890683122, 1.000000000000000000, 0.9659258262890683122, 1.000000000000000000, 0.9659258262890683122, 1.000000000000000000, 0.9659258262890683122, 1.000000000000000000, 0.9659258262890683122, 1.000000000000000000, 0.9659258262890683122, 1.000000000000000000, 0.9659258262890683122, 1.000000000000000000, 0.9659258262890683122, 1.000000000000000000, 0.9659258262890683122, 1.000000000000000000, 0.9659258262890683122, 1.000000000000000000, 0.9659258262890683122, 1.000000000000000000, 0.9659258262890683122, 1.000000000000000000, 0.9659258262890683122, 1.000000000000000000, 0.9659258262890683122, 1.000000000000000000, 0.9659258262890683122, 1.000000000000000000, 0.9659258262890683122, 1.000000000000000000) ) ) 
 REPRESENTATION_ITEM ( '' )  SURFACE ( )  );
#16887=CARTESIAN_POINT ( 'NONE',  ( 20.88017736071110164, 45.35535201082149115, 2.915334737309930979 ) ) ;
#16889=CARTESIAN_POINT ( 'NONE',  ( -0.2418659066527510948, 24.26028685723174050, -6.114288769123079170 ) ) ;
#16890=CARTESIAN_POINT ( 'NONE',  ( 20.36894250292379382, 53.67874883491397497, 10.36894250292379205 ) ) ;
#16891=CARTESIAN_POINT ( 'NONE',  ( 4.559911319644449179, 63.89701867748817676, 9.422509992056141925 ) ) ;
#16893=CARTESIAN_POINT ( 'NONE',  ( -4.164238869374099927, 12.01208216824730357, 3.795296366450308767 ) ) ;
#16896=CARTESIAN_POINT ( 'NONE',  ( 7.084665262690076126, 9.105352010821503583, 10.88017736071109987 ) ) ;
#16897=CARTESIAN_POINT ( 'NONE',  ( 17.20831665107776587, 52.88393115100078035, 7.208316651077764980 ) ) ;
#16899=CARTESIAN_POINT ( 'NONE',  ( 19.84674366389459266, 48.71726448433413026, -2.638427012816827677 ) ) ;
#16900=CARTESIAN_POINT ( 'NONE',  ( 0.5774900079438607392, 63.48035201082149825, 5.440088680355550821 ) ) ;
#16901=CARTESIAN_POINT ( 'NONE',  ( 4.559911319644449179, 37.23035201082150536, -9.422509992056141925 ) ) ;
#16902=CARTESIAN_POINT ( 'NONE',  ( 10.00000000000000178, 32.25893115100078745, 9.846743663894594434 ) ) ;
#16903=CARTESIAN_POINT ( 'NONE',  ( 22.81628187352648496, 31.83196800326375353, -3.434112377981050290 ) ) ;
#16906=CARTESIAN_POINT ( 'NONE',  ( -0.8801773607110991993, 42.85535201082150536, -2.915334737309923874 ) ) ;
#16907=CARTESIAN_POINT ( 'NONE',  ( 17.08211943468705130, 58.47041550158063927, 12.26659068614894998 ) ) ;
#16910=CARTESIAN_POINT ( 'NONE',  ( 21.09922568453595559, 17.04030133659708923, -6.408140936763230044 ) ) ;
#16911=LINE ( 'NONE', #53917, #22803 ) ;
#16912=ORIENTED_EDGE ( 'NONE', *, *, #68349, .T. ) ;
#16913=CARTESIAN_POINT ( 'NONE',  ( -2.816281873526473856, 29.33196800326376064, 3.434112377981055619 ) ) ;
#16914=CARTESIAN_POINT ( 'NONE',  ( 19.42250999205614193, 20.14701867748817321, 5.440088680355555262 ) ) ;
#16916=CARTESIAN_POINT ( 'NONE',  ( 0.1532563361054100626, 45.80059781766745886, -2.638427012816831230 ) ) ;
#16917=CARTESIAN_POINT ( 'NONE',  ( 1.472469842513823179, 15.59226448433411960, -4.923371831947296329 ) ) ;
#16918=CARTESIAN_POINT ( 'NONE',  ( 14.92337183194729988, 39.34226448433412315, -8.527530157486177487 ) ) ;
#16921=CARTESIAN_POINT ( 'NONE',  ( 10.00000000000000178, 22.25893115100078745, 9.846743663894594434 ) ) ;
#16922=LINE ( 'NONE', #77900, #87541 ) ;
#16925=CARTESIAN_POINT ( 'NONE',  ( 0.1532563361054100626, 25.80059781766744820, -2.638427012816831230 ) ) ;
#16926=CARTESIAN_POINT ( 'NONE',  ( 0.1532563361054100626, 0.8005978176674514168, -2.638427012816831230 ) ) ;
#16927=CARTESIAN_POINT ( 'NONE',  ( 5.076628168052703671, 41.84226448433411605, 8.527530157486179263 ) ) ;
#16928=ORIENTED_EDGE ( 'NONE', *, *, #7933, .F. ) ;
#16929=CARTESIAN_POINT ( 'NONE',  ( 19.80427997160309417, 7.757339608395445119, -6.499999999999999112 ) ) ;
#16930=CARTESIAN_POINT ( 'NONE',  ( 19.38216949554541202, 30.99863466993042138, 9.382169495545424454 ) ) ;
#16932=CARTESIAN_POINT ( 'NONE',  ( 10.00000000000000000, 50.55374883491396787, -14.16423886937410082 ) ) ;
#16933=CARTESIAN_POINT ( 'NONE',  ( 19.84674366389459621, 23.50893115100078390, 7.409399052514197653E-17 ) ) ;
#16935=CARTESIAN_POINT ( 'NONE',  ( 10.00000000000000178, 43.05374883491397497, 14.16423886937410082 ) ) ;
#16936=CARTESIAN_POINT ( 'NONE',  ( 14.92337183194729633, 57.67559781766745886, 8.527530157486181039 ) ) ;
#16937=CARTESIAN_POINT ( 'NONE',  ( 6.204703633549690345, 52.84541550158062506, 14.16423886937410082 ) ) ;
#16938=CARTESIAN_POINT ( 'NONE',  ( -4.164238869374098151, 26.59541550158063217, -3.795296366450310543 ) ) ;
#16939=CARTESIAN_POINT ( 'NONE',  ( -0.3689425029237898834, 26.17874883491396432, -10.36894250292378850 ) ) ;
#16943=CARTESIAN_POINT ( 'NONE',  ( 2.791683348922237240, 45.38393115100079456, -7.208316651077763204 ) ) ;
#16944=CARTESIAN_POINT ( 'NONE',  ( 20.88017736071110164, 30.35535201082151247, 2.915334737309930979 ) ) ;
#16947=CARTESIAN_POINT ( 'NONE',  ( 7.361572987183170547, 37.05059781766744464, 9.846743663894590881 ) ) ;
#16948=CARTESIAN_POINT ( 'NONE',  ( 21.09922568453594849, 51.20696800326375353, 6.408140936763242479 ) ) ;
#16950=CIRCLE ( 'NONE', #45707, 0.4999999999999967248 ) ;
#16951=CARTESIAN_POINT ( 'NONE',  ( 18.52753015748617571, 48.09226448433412315, 4.923371831947298993 ) ) ;
#16956=CARTESIAN_POINT ( 'NONE',  ( 24.16423886937409904, 9.095415501580633943, 3.795296366450317205 ) ) ;
#16957=EDGE_CURVE ( 'NONE', #87897, #98547, #79835, .T. ) ;
#16958=CIRCLE ( 'NONE', #91963, 0.5000000000000004441 ) ;
#16962=CARTESIAN_POINT ( 'NONE',  ( 18.72515096720571037, 50.05509018479936856, 6.499999999999982236 ) ) ;
#16963=CARTESIAN_POINT ( 'NONE',  ( 17.96484262340118221, 6.188685344154837509, -7.964842623401177768 ) ) ;
#16964=CARTESIAN_POINT ( 'NONE',  ( 13.43411237798105340, 15.58196800326374998, 12.81628187352647963 ) ) ;
#16965=( BOUNDED_CURVE ( )  B_SPLINE_CURVE ( 2, ( #65388, #79906, #81384, #57403, #80411, #88401, #49406, #11415, #64883 ),
 .UNSPECIFIED., .F., .T. ) 
 B_SPLINE_CURVE_WITH_KNOTS ( ( 3, 2, 2, 2, 3 ),
 ( 0.04728379408308854698, 0.04761904761904767192, 0.05357142857142860315, 0.05952380952380953438, 0.05985906305976865238 ),
 .UNSPECIFIED. ) 
 CURVE ( )  GEOMETRIC_REPRESENTATION_ITEM ( )  RATIONAL_B_SPLINE_CURVE ( ( 0.9963778908391762723, 0.9980808541467921513, 1.000000000000000000, 0.9659258262890683122, 1.000000000000000000, 0.9659258262890683122, 1.000000000000000000, 0.9980808541467921513, 0.9963778908391762723 ) ) 
 REPRESENTATION_ITEM ( '' )  );
#16967=CARTESIAN_POINT ( 'NONE',  ( 10.00000000000000000, 61.81368534415484106, -10.88017736071110342 ) ) ;
#16971=CARTESIAN_POINT ( 'NONE',  ( -4.164238869374099927, 67.01208216824728936, 3.795296366450308767 ) ) ;
#16973=CARTESIAN_POINT ( 'NONE',  ( 20.88017736071110519, 25.56368534415483751, 2.639326808657452039E-16 ) ) ;
#16974=CARTESIAN_POINT ( 'NONE',  ( 10.00000000000000178, 44.31368534415484106, 10.88017736071110342 ) ) ;
#16975=CARTESIAN_POINT ( 'NONE',  ( 22.81628187352647785, 6.623634669930420493, 6.195893100308588602E-16 ) ) ;
#16976=CARTESIAN_POINT ( 'NONE',  ( 19.84674366389459266, 53.30059781766744464, 2.638427012816836559 ) ) ;
#16977=CARTESIAN_POINT ( 'NONE',  ( 6.565887622018943937, 58.08196800326376064, -12.81628187352647608 ) ) ;
#16978=( LENGTH_UNIT ( ) NAMED_UNIT ( * ) SI_UNIT ( .MILLI., .METRE. ) );
#16979=ORIENTED_EDGE ( 'NONE', *, *, #63943, .F. ) ;
#16981=CARTESIAN_POINT ( 'NONE',  ( 20.88017736071110164, 35.35535201082150536, 2.915334737309930979 ) ) ;
#16982=CARTESIAN_POINT ( 'NONE',  ( 22.81628187352648496, 31.83196800326375353, -3.434112377981050290 ) ) ;
#16984=CARTESIAN_POINT ( 'NONE',  ( 17.20831665107776587, 62.88393115100078745, 7.208316651077764980 ) ) ;
#16985=CARTESIAN_POINT ( 'NONE',  ( 12.91533473730992121, 54.52201867748816255, 10.88017736071110164 ) ) ;
#16986=CARTESIAN_POINT ( 'NONE',  ( 12.63842701281683034, 17.46726448433411250, 9.846743663894596210 ) ) ;
#16987=CARTESIAN_POINT ( 'NONE',  ( 22.81628187352647785, 36.41530133659707502, 3.434112377981063169 ) ) ;
#16988=CARTESIAN_POINT ( 'NONE',  ( 12.91533473730992121, 59.52201867748816966, 10.88017736071110164 ) ) ;
#16991=CARTESIAN_POINT ( 'NONE',  ( -1.099225684535947600, 63.70696800326376774, -6.408140936763238038 ) ) ;
#16992=ORIENTED_EDGE ( 'NONE', *, *, #57910, .T. ) ;
#16995=CARTESIAN_POINT ( 'NONE',  ( -0.8801773607110991993, 2.855352010821504471, -2.915334737309923874 ) ) ;
#16996=CARTESIAN_POINT ( 'NONE',  ( 16.40814093676323893, 45.79030133659708923, 11.09922568453595026 ) ) ;
#16998=CARTESIAN_POINT ( 'NONE',  ( 5.076628168052703671, 16.84226448433411960, 8.527530157486179263 ) ) ;
#16999=CARTESIAN_POINT ( 'NONE',  ( -0.8801773607111009756, 8.063685344154837509, 1.068504757029289695E-15 ) ) ;
#17000=CARTESIAN_POINT ( 'NONE',  ( 1.472469842513823179, 26.42559781766745175, 4.923371831947296329 ) ) ;
#17001=CARTESIAN_POINT ( 'NONE',  ( 20.36894250292379382, 53.67874883491397497, 10.36894250292379205 ) ) ;
#17003=AXIS2_PLACEMENT_3D ( 'NONE', #15137, #84116, #7127 ) ;
#17004=CARTESIAN_POINT ( 'NONE',  ( 7.084665262690076126, 12.02201867748817143, -10.88017736071110164 ) ) ;
#17005=EDGE_CURVE ( 'NONE', #44298, #76727, #13255, .T. ) ;
#17007=VERTEX_POINT ( 'NONE', #40382 ) ;
#17008=CARTESIAN_POINT ( 'NONE',  ( 20.88017736071110519, 5.563685344154838397, 2.639326808657452039E-16 ) ) ;
#17009=CARTESIAN_POINT ( 'NONE',  ( 10.00000000000000000, 11.81368534415483751, -10.88017736071110342 ) ) ;
#17010=CARTESIAN_POINT ( 'NONE',  ( 5.076628168052703671, 41.84226448433411605, 8.527530157486179263 ) ) ;
#17011=CARTESIAN_POINT ( 'NONE',  ( 0.6178305044545838731, 54.74863466993042493, 9.382169495545420901 ) ) ;
#17014=CARTESIAN_POINT ( 'NONE',  ( -4.164238869374098151, 16.59541550158063927, -3.795296366450310543 ) ) ;
#17015=CARTESIAN_POINT ( 'NONE',  ( 4.559911319644449179, 28.89701867748817321, 9.422509992056141925 ) ) ;
#17016=CARTESIAN_POINT ( 'NONE',  ( 10.00000000000000178, 9.313685344154839285, 10.88017736071110342 ) ) ;
#17017=CARTESIAN_POINT ( 'NONE',  ( 2.791683348922240793, 61.63393115100079456, 7.208316651077764092 ) ) ;
#17020=CARTESIAN_POINT ( 'NONE',  ( 12.63842701281683034, 32.46726448433412315, 9.846743663894596210 ) ) ;
#17021=DIRECTION ( 'NONE',  ( 0.000000000000000000, 0.000000000000000000, -1.000000000000000000 ) ) ;
#17022=CARTESIAN_POINT ( 'NONE',  ( 7.361572987183169658, -0.03273551566588185635, -9.846743663894592657 ) ) ;
#17024=ORIENTED_EDGE ( 'NONE', *, *, #84469, .T. ) ;
#17026=CARTESIAN_POINT ( 'NONE',  ( 19.42250999205614548, 65.98035201082151957, -5.440088680355545492 ) ) ;
#17027=CARTESIAN_POINT ( 'NONE',  ( 10.00000000000000178, 0.3736346699304200492, 12.81628187352647608 ) ) ;
#17028=CARTESIAN_POINT ( 'NONE',  ( 19.42250999205614548, 50.98035201082151247, -5.440088680355545492 ) ) ;
#17029=CARTESIAN_POINT ( 'NONE',  ( 10.00000000000000000, 1.813685344154837731, -10.88017736071110342 ) ) ;
#17030=CARTESIAN_POINT ( 'NONE',  ( 21.09922568453594849, 41.20696800326375353, 6.408140936763242479 ) ) ;
#17032=CARTESIAN_POINT ( 'NONE',  ( -4.164238869374098151, 21.59541550158063217, -3.795296366450310543 ) ) ;
#17034=B_SPLINE_CURVE_WITH_KNOTS ( 'NONE', 3,
 ( #1233, #56180, #31686, #25689, #9197, #18178 ),
 .UNSPECIFIED., .F., .F.,
 ( 4, 2, 4 ),
 ( 5.780498387344536870E-18, 0.0002626113303185893724, 0.0005252226606371728900 ),
 .UNSPECIFIED. ) ;
#17036=CARTESIAN_POINT ( 'NONE',  ( -2.816281873526471635, 48.91530133659708213, -3.434112377981056508 ) ) ;
#17037=ORIENTED_EDGE ( 'NONE', *, *, #3351, .T. ) ;
#17038=CARTESIAN_POINT ( 'NONE',  ( 10.00000000000000178, 57.25893115100078745, 9.846743663894594434 ) ) ;
#17039=CARTESIAN_POINT ( 'NONE',  ( 4.559911319644449179, 17.23035201082150536, -9.422509992056141925 ) ) ;
#17040=CARTESIAN_POINT ( 'NONE',  ( 0.5774900079438607392, 33.48035201082150536, 5.440088680355550821 ) ) ;
#17042=CARTESIAN_POINT ( 'NONE',  ( 7.361572987183169658, 9.967264484334119601, -9.846743663894592657 ) ) ;
#17043=CARTESIAN_POINT ( 'NONE',  ( 4.559911319644449179, 68.89701867748817676, 9.422509992056141925 ) ) ;
#17044=CARTESIAN_POINT ( 'NONE',  ( -46.34323875807881166, 103.6109741468810483, 6.190393423093146552 ) ) ;
#17046=CARTESIAN_POINT ( 'NONE',  ( 12.63842701281683034, 7.467264484334118713, 9.846743663894596210 ) ) ;
#17047=CARTESIAN_POINT ( 'NONE',  ( 12.91533473730992121, 64.52201867748817676, 10.88017736071110164 ) ) ;
#17050=CARTESIAN_POINT ( 'NONE',  ( 20.88017736071110875, 60.77201867748817676, -2.915334737309920765 ) ) ;
#17051=CARTESIAN_POINT ( 'NONE',  ( 14.92337183194729633, 7.675597817667451750, 8.527530157486181039 ) ) ;
#17055=CARTESIAN_POINT ( 'NONE',  ( 14.92337183194729988, 49.34226448433411605, -8.527530157486177487 ) ) ;
#17056=ORIENTED_EDGE ( 'NONE', *, *, #65475, .T. ) ;
#17057=EDGE_LOOP ( 'NONE', ( #80966, #98877, #39779, #1270, #91553 ) ) ;
#17059=CARTESIAN_POINT ( 'NONE',  ( 10.00000000000000000, 0.5537488349139675359, -14.16423886937410082 ) ) ;
#17060=CARTESIAN_POINT ( 'NONE',  ( 3.591859063236761518, 54.95696800326376064, 11.09922568453594849 ) ) ;
#17061=CARTESIAN_POINT ( 'NONE',  ( -0.3689425029237881626, 2.428748834913967869, 10.36894250292379027 ) ) ;
#17062=CARTESIAN_POINT ( 'NONE',  ( 10.00000000000000178, 13.05374883491396787, 14.16423886937410082 ) ) ;
#17064=CARTESIAN_POINT ( 'NONE',  ( 20.20021275402702443, 69.97534054108130874, 6.181800700215005939 ) ) ;
#17065=CARTESIAN_POINT ( 'NONE',  ( -0.8801773607111008646, 58.27201867748816966, 2.915334737309923430 ) ) ;
#17066=CARTESIAN_POINT ( 'NONE',  ( 7.084665262690076126, 24.10535201082150181, 10.88017736071109987 ) ) ;
#17068=CARTESIAN_POINT ( 'NONE',  ( 17.20831665107776587, 7.883931151000784787, 7.208316651077764980 ) ) ;
#17069=CARTESIAN_POINT ( 'NONE',  ( 10.00000000000000000, 4.758931151000784787, -9.846743663894594434 ) ) ;
#17070=CARTESIAN_POINT ( 'NONE',  ( 21.09922568453594849, 31.20696800326375353, 6.408140936763242479 ) ) ;
#17071=CARTESIAN_POINT ( 'NONE',  ( 14.92337183194729633, 37.67559781766745175, 8.527530157486181039 ) ) ;
#17073=CARTESIAN_POINT ( 'NONE',  ( 0.6178305044545818747, 18.49863466993041428, -9.382169495545419124 ) ) ;
#17076=CARTESIAN_POINT ( 'NONE',  ( 17.20831665107776587, 22.88393115100078745, 7.208316651077764980 ) ) ;
#17077=EDGE_CURVE ( 'NONE', #92463, #28728, #94347, .T. ) ;
#17078=CARTESIAN_POINT ( 'NONE',  ( 17.20831665107776587, 4.133931151000785675, -7.208316651077762316 ) ) ;
#17081=EDGE_CURVE ( 'NONE', #46987, #5600, #71376, .T. ) ;
#17082=VECTOR ( 'NONE', #34407, 1000.000000000000000 ) ;
#17083=CARTESIAN_POINT ( 'NONE',  ( 2.035157376598822676, 42.43868534415483396, -7.964842623401177768 ) ) ;
#17084=CARTESIAN_POINT ( 'NONE',  ( -4.164238869374098151, 26.59541550158063217, -3.795296366450310543 ) ) ;
#17085=CARTESIAN_POINT ( 'NONE',  ( 17.20831665107776587, 44.13393115100078745, -7.208316651077762316 ) ) ;
#17086=CARTESIAN_POINT ( 'NONE',  ( 10.00000000000000178, 17.25893115100078745, 9.846743663894594434 ) ) ;
#17087=CARTESIAN_POINT ( 'NONE',  ( -2.816281873526473856, 49.33196800326374643, 3.434112377981055619 ) ) ;
#17089=CARTESIAN_POINT ( 'NONE',  ( 0.5774900079438590739, 27.64701867748817676, -5.440088680355550821 ) ) ;
#17091=CARTESIAN_POINT ( 'NONE',  ( 13.43411237798106583, 27.66530133659708568, -12.81628187352647252 ) ) ;
#17092=CARTESIAN_POINT ( 'NONE',  ( 0.1532563361054100626, 40.80059781766745886, -2.638427012816831230 ) ) ;
#17094=CARTESIAN_POINT ( 'NONE',  ( 16.40814093676323893, 45.79030133659708923, 11.09922568453595026 ) ) ;
#17096=CARTESIAN_POINT ( 'NONE',  ( 19.42250999205614548, 50.98035201082151247, -5.440088680355545492 ) ) ;
#17100=CARTESIAN_POINT ( 'NONE',  ( 4.559911319644449179, 48.89701867748817676, 9.422509992056141925 ) ) ;
#17101=CARTESIAN_POINT ( 'NONE',  ( 2.035157376598824452, 53.68868534415484817, 7.964842623401179544 ) ) ;
#17104=EDGE_CURVE ( 'NONE', #39677, #68278, #52069, .T. ) ;
#17106=CARTESIAN_POINT ( 'NONE',  ( 4.559911319644449179, 3.897018677488171434, 9.422509992056141925 ) ) ;
#17107=CARTESIAN_POINT ( 'NONE',  ( 1.472469842513823179, 61.42559781766745175, 4.923371831947296329 ) ) ;
#17108=CARTESIAN_POINT ( 'NONE',  ( 17.96484262340118221, 24.93868534415484461, 7.964842623401181321 ) ) ;
#17109=CARTESIAN_POINT ( 'NONE',  ( 18.04007052943773459, 24.00257860105348939, -5.767676674365828760 ) ) ;
#17110=CARTESIAN_POINT ( 'NONE',  ( 21.92686044187656691, 52.18830936912750929, 4.562052436263911564E-16 ) ) ;
#17111=CARTESIAN_POINT ( 'NONE',  ( -2.816281873526473856, 24.33196800326375353, 3.434112377981055619 ) ) ;
#17112=ORIENTED_EDGE ( 'NONE', *, *, #81084, .F. ) ;
#17113=CARTESIAN_POINT ( 'NONE',  ( 12.91533473730992121, 34.52201867748817676, 10.88017736071110164 ) ) ;
#17114=CARTESIAN_POINT ( 'NONE',  ( 1.472469842513823179, 41.42559781766745886, 4.923371831947296329 ) ) ;
#17115=CARTESIAN_POINT ( 'NONE',  ( -1.099225684535947600, 4.540301336597087456, 6.408140936763237150 ) ) ;
#17116=LINE ( 'NONE', #86585, #70175 ) ;
#17117=EDGE_CURVE ( 'NONE', #35522, #46963, #29704, .T. ) ;
#17118=CARTESIAN_POINT ( 'NONE',  ( 0.5774900079438590739, 12.64701867748817143, -5.440088680355550821 ) ) ;
#17119=CARTESIAN_POINT ( 'NONE',  ( 10.00000000000000000, 41.81368534415484106, -10.88017736071110342 ) ) ;
#17120=CARTESIAN_POINT ( 'NONE',  ( 24.16423886937410614, 49.30374883491396787, 8.672049930838204340E-16 ) ) ;
#17121=CARTESIAN_POINT ( 'NONE',  ( 12.63842701281683034, 42.46726448433412315, 9.846743663894596210 ) ) ;
#17122=CARTESIAN_POINT ( 'NONE',  ( 20.88017736071110875, 60.77201867748817676, -2.915334737309920765 ) ) ;
#17123=CARTESIAN_POINT ( 'NONE',  ( 19.50000000000000355, 70.00000000000000000, -4.500000000000001776 ) ) ;
#17124=CARTESIAN_POINT ( 'NONE',  ( 6.204703633549690345, 15.76208216824730179, -14.16423886937410259 ) ) ;
#17129=VERTEX_POINT ( 'NONE', #14186 ) ;
#17131=CARTESIAN_POINT ( 'NONE',  ( 2.917880565312950480, 35.97041550158063217, -12.26659068614894821 ) ) ;
#17132=CARTESIAN_POINT ( 'NONE',  ( 13.79529636645030344, 33.26208216824730357, 14.16423886937410614 ) ) ;
#17133=CARTESIAN_POINT ( 'NONE',  ( 19.84674366389459266, 8.717264484334116048, -2.638427012816827677 ) ) ;
#17134=CARTESIAN_POINT ( 'NONE',  ( 0.6178305044545838731, 19.74863466993042138, 9.382169495545420901 ) ) ;
#17135=CARTESIAN_POINT ( 'NONE',  ( 1.472469842513823179, 60.59226448433412315, -4.923371831947296329 ) ) ;
#17137=CARTESIAN_POINT ( 'NONE',  ( 15.44008868035555260, 64.73035201082151957, 9.422509992056143702 ) ) ;
#17138=CARTESIAN_POINT ( 'NONE',  ( 3.591859063236763294, 38.29030133659708923, -11.09922568453595026 ) ) ;
#17139=CARTESIAN_POINT ( 'NONE',  ( 24.16423886937410614, 29.51208216824729647, -3.795296366450302550 ) ) ;
#17140=CARTESIAN_POINT ( 'NONE',  ( 15.44008868035555260, 24.73035201082150891, 9.422509992056143702 ) ) ;
#17142=CARTESIAN_POINT ( 'NONE',  ( 2.791683348922240793, 1.633931151000784565, 7.208316651077764092 ) ) ;
#17147=CARTESIAN_POINT ( 'NONE',  ( -0.1503990784575282014, 42.22266099184918886, -6.262539305110077947 ) ) ;
#17150=CARTESIAN_POINT ( 'NONE',  ( 7.084665262690076126, 7.022018677488170546, -10.88017736071110164 ) ) ;
#17151=CARTESIAN_POINT ( 'NONE',  ( 20.88017736071110519, 10.56368534415483929, 2.639326808657452039E-16 ) ) ;
#17152=CARTESIAN_POINT ( 'NONE',  ( 0.1532563361054100626, 35.80059781766745175, -2.638427012816831230 ) ) ;
#17153=CARTESIAN_POINT ( 'NONE',  ( 0.6178305044545818747, 8.498634669930421381, -9.382169495545419124 ) ) ;
#17155=CARTESIAN_POINT ( 'NONE',  ( 20.15039907845753930, 1.748846992468885198, 6.262539305110068177 ) ) ;
#17156=CARTESIAN_POINT ( 'NONE',  ( 13.43411237798105340, 0.5819680032637533085, 12.81628187352647963 ) ) ;
#17157=AXIS2_PLACEMENT_3D ( 'NONE', #60371, #82885, #58898 ) ;
#17159=CARTESIAN_POINT ( 'NONE',  ( 13.79529636645030344, 43.26208216824730357, 14.16423886937410614 ) ) ;
#17161=CARTESIAN_POINT ( 'NONE',  ( -0.3689425029237881626, 62.42874883491396787, 10.36894250292379027 ) ) ;
#17163=CARTESIAN_POINT ( 'NONE',  ( 19.42250999205614548, 25.98035201082150891, -5.440088680355545492 ) ) ;
#17164=CARTESIAN_POINT ( 'NONE',  ( 20.88017736071110875, 35.77201867748816966, -2.915334737309920765 ) ) ;
#17166=CARTESIAN_POINT ( 'NONE',  ( 12.91533473730993009, 36.60535201082151247, -10.88017736071109987 ) ) ;
#17168=CARTESIAN_POINT ( 'NONE',  ( 12.91533473730993009, 61.60535201082150536, -10.88017736071109987 ) ) ;
#17169=CARTESIAN_POINT ( 'NONE',  ( 19.42250999205614193, 30.14701867748817321, 5.440088680355555262 ) ) ;
#17172=CARTESIAN_POINT ( 'NONE',  ( 19.84674366389459266, 3.717264484334118713, -2.638427012816827677 ) ) ;
#17176=CARTESIAN_POINT ( 'NONE',  ( 14.92337183194729633, 47.67559781766745175, 8.527530157486181039 ) ) ;
#17178=CARTESIAN_POINT ( 'NONE',  ( 22.81628187352647785, 46.62363466993041783, 6.195893100308588602E-16 ) ) ;
#17184=CARTESIAN_POINT ( 'NONE',  ( -0.8801773607110990882, 52.85535201082151247, -2.915334737309924318 ) ) ;
#17185=CARTESIAN_POINT ( 'NONE',  ( 10.00000000000000178, 52.25893115100078745, 9.846743663894594434 ) ) ;
#17186=CARTESIAN_POINT ( 'NONE',  ( 22.26659068614894466, 53.88708216824731068, 7.082119434687054849 ) ) ;
#17187=CARTESIAN_POINT ( 'NONE',  ( 18.52753015748618282, 63.92559781766745886, -4.923371831947291888 ) ) ;
#17189=CARTESIAN_POINT ( 'NONE',  ( 10.00000000000000000, 19.75893115100078390, -9.846743663894594434 ) ) ;
#17191=CARTESIAN_POINT ( 'NONE',  ( 22.81628187352647785, 46.41530133659708213, 3.434112377981063169 ) ) ;
#17192=CARTESIAN_POINT ( 'NONE',  ( 19.84674366389459266, 63.30059781766745886, 2.638427012816836559 ) ) ;
#17193=CARTESIAN_POINT ( 'NONE',  ( 2.035157376598822676, 62.43868534415483396, -7.964842623401177768 ) ) ;
#17198=ORIENTED_EDGE ( 'NONE', *, *, #80382, .F. ) ;
#17200=CARTESIAN_POINT ( 'NONE',  ( -2.266590686148945544, 57.22041550158063217, 7.082119434687048631 ) ) ;
#17201=FILL_AREA_STYLE ('',( #54671 ) ) ;
#17202=CARTESIAN_POINT ( 'NONE',  ( 19.42250999205614193, 30.14701867748817321, 5.440088680355555262 ) ) ;
#17203=CARTESIAN_POINT ( 'NONE',  ( 3.591859063236763294, 13.29030133659708746, -11.09922568453595026 ) ) ;
#17204=CARTESIAN_POINT ( 'NONE',  ( 0.5774900079438590739, 52.64701867748817676, -5.440088680355550821 ) ) ;
#17205=CARTESIAN_POINT ( 'NONE',  ( 18.72515096720591643, 66.07228050351029935, -6.499999999999699796 ) ) ;
#17209=CARTESIAN_POINT ( 'NONE',  ( 19.84674366389459266, 48.71726448433413026, -2.638427012816827677 ) ) ;
#17210=CARTESIAN_POINT ( 'NONE',  ( 12.63842701281683034, 2.467264484334118269, 9.846743663894596210 ) ) ;
#17212=CARTESIAN_POINT ( 'NONE',  ( 6.565887622018943937, 3.081968003263753531, -12.81628187352647608 ) ) ;
#17213=CARTESIAN_POINT ( 'NONE',  ( 7.084665262690076126, 12.02201867748817321, -10.88017736071110164 ) ) ;
#17215=CARTESIAN_POINT ( 'NONE',  ( 2.917880565312948704, 42.63708216824729647, 12.26659068614894643 ) ) ;
#17216=CARTESIAN_POINT ( 'NONE',  ( -2.266590686148945544, 36.38708216824730357, -7.082119434687050408 ) ) ;
#17217=CARTESIAN_POINT ( 'NONE',  ( -0.3689425029237898834, 61.17874883491396076, -10.36894250292378850 ) ) ;
#17218=CARTESIAN_POINT ( 'NONE',  ( 1.472469842513823179, 16.42559781766745175, 4.923371831947296329 ) ) ;
#17219=CARTESIAN_POINT ( 'NONE',  ( 10.00000000000000000, 11.81368534415483751, -10.88017736071110342 ) ) ;
#17220=ORIENTED_EDGE ( 'NONE', *, *, #2973, .T. ) ;
#17221=CARTESIAN_POINT ( 'NONE',  ( 5.076628168052703671, 31.84226448433412315, 8.527530157486179263 ) ) ;
#17222=CARTESIAN_POINT ( 'NONE',  ( 10.00000000000000178, 34.31368534415484106, 10.88017736071110342 ) ) ;
#17223=CARTESIAN_POINT ( 'NONE',  ( 1.472469842513823179, 61.42559781766745175, 4.923371831947296329 ) ) ;
#17224=CARTESIAN_POINT ( 'NONE',  ( 22.26659068614895176, 24.72041550158063572, -7.082119434687042414 ) ) ;
#17225=CARTESIAN_POINT ( 'NONE',  ( -0.3289641300567998083, 18.07879003517447103, 5.963430220938281678 ) ) ;
#17227=UNCERTAINTY_MEASURE_WITH_UNIT (LENGTH_MEASURE( 1.000000000000000082E-05 ), #48315, 'distance_accuracy_value', 'NONE');
#17228=CARTESIAN_POINT ( 'NONE',  ( 19.84674366389459266, 8.717264484334116048, -2.638427012816827677 ) ) ;
#17229=CARTESIAN_POINT ( 'NONE',  ( 13.43411237798105340, 50.58196800326375353, 12.81628187352647963 ) ) ;
#17230=CARTESIAN_POINT ( 'NONE',  ( 10.00000000000000000, 49.75893115100078745, -9.846743663894594434 ) ) ;
#17233=CARTESIAN_POINT ( 'NONE',  ( 20.88017736071110519, 5.563685344154838397, 2.639326808657452039E-16 ) ) ;
#17234=CARTESIAN_POINT ( 'NONE',  ( -0.3689425029237881626, 17.42874883491397142, 10.36894250292379027 ) ) ;
#17235=CARTESIAN_POINT ( 'NONE',  ( 4.559911319644449179, 67.23035201082150536, -9.422509992056141925 ) ) ;
#17236=CARTESIAN_POINT ( 'NONE',  ( 19.84674366389459266, 43.30059781766744464, 2.638427012816836559 ) ) ;
#17237=CARTESIAN_POINT ( 'NONE',  ( 20.88017736071110519, 15.56368534415483751, 2.639326808657452039E-16 ) ) ;
#17239=CARTESIAN_POINT ( 'NONE',  ( 19.84674366389459621, 63.50893115100078745, 7.409399052514197653E-17 ) ) ;
#17241=CARTESIAN_POINT ( 'NONE',  ( 7.361572987183170547, 2.050597817667451750, 9.846743663894590881 ) ) ;
#17243=CARTESIAN_POINT ( 'NONE',  ( 16.40814093676324603, 57.45696800326375353, -11.09922568453594671 ) ) ;
#17245=VERTEX_POINT ( 'NONE', #88326 ) ;
#17248=CARTESIAN_POINT ( 'NONE',  ( 24.16423886937410614, 44.51208216824730357, -3.795296366450302550 ) ) ;
#17249=CARTESIAN_POINT ( 'NONE',  ( 18.52753015748618282, 38.92559781766745175, -4.923371831947291888 ) ) ;
#17250=CARTESIAN_POINT ( 'NONE',  ( 19.84674366389459266, 23.30059781766745530, 2.638427012816836559 ) ) ;
#17251=CARTESIAN_POINT ( 'NONE',  ( -0.1503990784575280903, 38.10158574516643171, 6.262539305110076171 ) ) ;
#17252=CARTESIAN_POINT ( 'NONE',  ( 7.084665262690076126, 24.10535201082150181, 10.88017736071109987 ) ) ;
#17253=CARTESIAN_POINT ( 'NONE',  ( 1.472469842513823179, 56.42559781766745886, 4.923371831947296329 ) ) ;
#17255=CARTESIAN_POINT ( 'NONE',  ( 24.16423886937410614, 44.51208216824730357, -3.795296366450302550 ) ) ;
#17256=CARTESIAN_POINT ( 'NONE',  ( 13.79529636645030344, 53.26208216824730357, 14.16423886937410614 ) ) ;
#17259=CARTESIAN_POINT ( 'NONE',  ( -0.8801773607111009756, 68.06368534415484817, 1.068504757029289695E-15 ) ) ;
#17260=CARTESIAN_POINT ( 'NONE',  ( 19.84674366389459621, 13.50893115100078568, 7.409399052514197653E-17 ) ) ;
#17262=VERTEX_POINT ( 'NONE', #75164 ) ;
#17263=CARTESIAN_POINT ( 'NONE',  ( 20.24186590665277663, 29.73410085661204150, 6.114288769123037426 ) ) ;
#17265=CARTESIAN_POINT ( 'NONE',  ( 0.1532563361054100626, 15.80059781766745353, -2.638427012816831230 ) ) ;
#17267=CARTESIAN_POINT ( 'NONE',  ( 24.16423886937410614, 24.51208216824730002, -3.795296366450302550 ) ) ;
#17268=CARTESIAN_POINT ( 'NONE',  ( 12.63842701281683922, 19.55059781766745175, -9.846743663894590881 ) ) ;
#17269=CARTESIAN_POINT ( 'NONE',  ( -0.8801773607111009756, 38.06368534415484106, 1.068504757029289695E-15 ) ) ;
#17274=CARTESIAN_POINT ( 'NONE',  ( -0.8801773607110991993, 47.85535201082150536, -2.915334737309923874 ) ) ;
#17277=CARTESIAN_POINT ( 'NONE',  ( 2.035157376598824452, 43.68868534415484106, 7.964842623401179544 ) ) ;
#17278=CARTESIAN_POINT ( 'NONE',  ( 13.79529636645030344, 8.262082168247300018, 14.16423886937410614 ) ) ;
#17281=CARTESIAN_POINT ( 'NONE',  ( 10.00000000000000000, 27.87363466993042138, -12.81628187352647608 ) ) ;
#17282=CARTESIAN_POINT ( 'NONE',  ( 19.84674366389459621, 3.508931151000785231, 7.409399052514197653E-17 ) ) ;
#17283=CARTESIAN_POINT ( 'NONE',  ( 10.00000000000000178, 45.37363466993041783, 12.81628187352647608 ) ) ;
#17285=CARTESIAN_POINT ( 'NONE',  ( 19.84674366389459621, 28.50893115100078745, 7.409399052514197653E-17 ) ) ;
#17286=CARTESIAN_POINT ( 'NONE',  ( 20.88017736071110519, 50.56368534415484106, 2.639326808657452039E-16 ) ) ;
#17290=CARTESIAN_POINT ( 'NONE',  ( -0.8801773607111008646, 53.27201867748816966, 2.915334737309923430 ) ) ;
#17293=CARTESIAN_POINT ( 'NONE',  ( 18.52753015748618282, 8.925597817667451750, -4.923371831947291888 ) ) ;
#17294=CARTESIAN_POINT ( 'NONE',  ( 3.591859063236763294, 13.29030133659708746, -11.09922568453595026 ) ) ;
#17295=LINE ( 'NONE', #18269, #38738 ) ;
#17297=CARTESIAN_POINT ( 'NONE',  ( 2.791683348922240793, 36.63393115100078035, 7.208316651077764092 ) ) ;
#17298=CARTESIAN_POINT ( 'NONE',  ( 10.00000000000000000, 62.87363466993042493, -12.81628187352647608 ) ) ;
#17299=CARTESIAN_POINT ( 'NONE',  ( -4.164238869374099927, 12.01208216824730357, 3.795296366450308767 ) ) ;
#17300=CARTESIAN_POINT ( 'NONE',  ( 19.84674366389459266, 13.71726448433411782, -2.638427012816827677 ) ) ;
#17301=CARTESIAN_POINT ( 'NONE',  ( 19.38216949554541557, 22.24863466993041428, -9.382169495545420901 ) ) ;
#17304=CARTESIAN_POINT ( 'NONE',  ( 15.44008868035555793, 46.39701867748817676, -9.422509992056140149 ) ) ;
#17305=CARTESIAN_POINT ( 'NONE',  ( 17.20831665107776587, 62.88393115100078745, 7.208316651077764980 ) ) ;
#17306=DIRECTION ( 'NONE',  ( 1.000000000000000000, -0.000000000000000000, 0.000000000000000000 ) ) ;
#17307=CARTESIAN_POINT ( 'NONE',  ( 18.52753015748618282, 23.92559781766745530, -4.923371831947291888 ) ) ;
#17308=CARTESIAN_POINT ( 'NONE',  ( 10.00000000000000000, 16.81368534415483751, -10.88017736071110342 ) ) ;
#17309=CARTESIAN_POINT ( 'NONE',  ( 6.565887622018943937, 18.08196800326375708, -12.81628187352647608 ) ) ;
#17310=CARTESIAN_POINT ( 'NONE',  ( 19.84674366389459621, 18.50893115100078745, 7.409399052514197653E-17 ) ) ;
#17313=CARTESIAN_POINT ( 'NONE',  ( 20.88017736071110875, 20.77201867748816611, -2.915334737309920765 ) ) ;
#17314=CARTESIAN_POINT ( 'NONE',  ( 19.42250999205614548, 55.98035201082150536, -5.440088680355545492 ) ) ;
#17317=CARTESIAN_POINT ( 'NONE',  ( 18.52753015748618282, 48.92559781766745886, -4.923371831947291888 ) ) ;
#17318=CARTESIAN_POINT ( 'NONE',  ( 20.88017736071110875, 10.77201867748817143, -2.915334737309920765 ) ) ;
#17320=CARTESIAN_POINT ( 'NONE',  ( 7.084665262690076126, 52.02201867748816255, -10.88017736071110164 ) ) ;
#17322=CARTESIAN_POINT ( 'NONE',  ( 20.88017736071110519, 10.56368534415483929, 2.639326808657452039E-16 ) ) ;
#17324=CARTESIAN_POINT ( 'NONE',  ( 17.20831665107776587, 19.13393115100078035, -7.208316651077762316 ) ) ;
#17325=CARTESIAN_POINT ( 'NONE',  ( 12.63842701281683034, 37.46726448433411605, 9.846743663894596210 ) ) ;
#17328=CARTESIAN_POINT ( 'NONE',  ( -1.099225684535947600, -1.293031996736246469, -6.408140936763238038 ) ) ;
#17332=CARTESIAN_POINT ( 'NONE',  ( 20.36894250292379738, 19.92874883491396787, -10.36894250292379027 ) ) ;
#17333=CARTESIAN_POINT ( 'NONE',  ( 2.791683348922240793, 41.63393115100078745, 7.208316651077764092 ) ) ;
#17336=CARTESIAN_POINT ( 'NONE',  ( -0.3689425029237898834, 56.17874883491396076, -10.36894250292378850 ) ) ;
#17337=CARTESIAN_POINT ( 'NONE',  ( 17.20831665107776587, 17.88393115100078745, 7.208316651077764980 ) ) ;
#17338=CARTESIAN_POINT ( 'NONE',  ( -0.1503990784575328643, 70.00000000000000000, 6.262539305110068177 ) ) ;
#17340=CARTESIAN_POINT ( 'NONE',  ( 17.96484262340118221, 46.18868534415484106, -7.964842623401177768 ) ) ;
#17341=CARTESIAN_POINT ( 'NONE',  ( 10.00000000000000000, 62.87363466993042493, -12.81628187352647608 ) ) ;
#17342=CARTESIAN_POINT ( 'NONE',  ( -0.8801773607110991993, 17.85535201082150536, -2.915334737309923874 ) ) ;
#17343=CARTESIAN_POINT ( 'NONE',  ( 22.81628187352647785, 46.62363466993041783, 6.195893100308588602E-16 ) ) ;
#17344=CARTESIAN_POINT ( 'NONE',  ( -2.816281873526473856, 9.331968003263753531, 3.434112377981055619 ) ) ;
#17345=CARTESIAN_POINT ( 'NONE',  ( 10.00000000000000000, 9.758931151000785675, -9.846743663894594434 ) ) ;
#17349=CARTESIAN_POINT ( 'NONE',  ( 13.79529636645030344, 53.26208216824730357, 14.16423886937410614 ) ) ;
#17350=CARTESIAN_POINT ( 'NONE',  ( -4.164238869374099039, 21.80374883491396787, 8.674139862899312516E-16 ) ) ;
#17351=CARTESIAN_POINT ( 'NONE',  ( 4.559911319644449179, 22.23035201082150536, -9.422509992056141925 ) ) ;
#17352=CARTESIAN_POINT ( 'NONE',  ( 12.91533473730992121, 49.52201867748817676, 10.88017736071110164 ) ) ;
#17355=CARTESIAN_POINT ( 'NONE',  ( 6.000000000000000000, 11.00000000000000000, -5.000000000000000000 ) ) ;
#17356=CARTESIAN_POINT ( 'NONE',  ( 10.00000000000000178, 2.258931151000784787, 9.846743663894594434 ) ) ;
#17358=CARTESIAN_POINT ( 'NONE',  ( 0.1532563361054082862, 16.21726448433411960, 2.638427012816831674 ) ) ;
#17359=CARTESIAN_POINT ( 'NONE',  ( 18.52753015748618282, 28.92559781766745175, -4.923371831947291888 ) ) ;
#17360=CARTESIAN_POINT ( 'NONE',  ( 14.92337183194729633, 52.67559781766745175, 8.527530157486181039 ) ) ;
#17361=EDGE_CURVE ( 'NONE', #36347, #67137, #60084, .T. ) ;
#17362=CARTESIAN_POINT ( 'NONE',  ( -0.8801773607110991993, 17.85535201082150536, -2.915334737309923874 ) ) ;
#17363=CARTESIAN_POINT ( 'NONE',  ( 3.591859063236761518, 29.95696800326375708, 11.09922568453594849 ) ) ;
#17364=CARTESIAN_POINT ( 'NONE',  ( 0.5774900079438590739, 47.64701867748817676, -5.440088680355550821 ) ) ;
#17365=CARTESIAN_POINT ( 'NONE',  ( 17.20831665107776587, 24.13393115100078035, -7.208316651077762316 ) ) ;
#17366=CARTESIAN_POINT ( 'NONE',  ( -2.266590686148945544, 41.38708216824729647, -7.082119434687050408 ) ) ;
#17367=CARTESIAN_POINT ( 'NONE',  ( 18.52753015748617571, 8.092264484334117824, 4.923371831947298993 ) ) ;
#17369=CARTESIAN_POINT ( 'NONE',  ( 18.52753015748617571, 53.09226448433412315, 4.923371831947298993 ) ) ;
#17370=CARTESIAN_POINT ( 'NONE',  ( 18.52753015748618282, 38.92559781766745175, -4.923371831947291888 ) ) ;
#17371=CARTESIAN_POINT ( 'NONE',  ( 2.917880565312950480, 15.97041550158063217, -12.26659068614894821 ) ) ;
#17372=CARTESIAN_POINT ( 'NONE',  ( 2.791683348922237240, 30.38393115100078390, -7.208316651077763204 ) ) ;
#17373=CARTESIAN_POINT ( 'NONE',  ( 20.88017736071110519, 50.56368534415484106, 2.639326808657452039E-16 ) ) ;
#17374=CARTESIAN_POINT ( 'NONE',  ( 0.5774900079438590739, 7.647018677488171434, -5.440088680355550821 ) ) ;
#17376=CARTESIAN_POINT ( 'NONE',  ( 2.035157376598822676, 47.43868534415484817, -7.964842623401177768 ) ) ;
#17377=CARTESIAN_POINT ( 'NONE',  ( 15.44008868035555260, 24.73035201082150891, 9.422509992056143702 ) ) ;
#17379=CARTESIAN_POINT ( 'NONE',  ( 6.565887622018943937, 33.08196800326374643, -12.81628187352647608 ) ) ;
#17380=CARTESIAN_POINT ( 'NONE',  ( 0.5774900079438590739, 42.64701867748816966, -5.440088680355550821 ) ) ;
#17383=CARTESIAN_POINT ( 'NONE',  ( 20.88017736071110875, 60.77201867748817676, -2.915334737309920765 ) ) ;
#17384=ORIENTED_EDGE ( 'NONE', *, *, #5213, .T. ) ;
#17385=CARTESIAN_POINT ( 'NONE',  ( 4.559911319644449179, 43.89701867748816966, 9.422509992056141925 ) ) ;
#17386=CARTESIAN_POINT ( 'NONE',  ( 4.559911319644449179, 3.897018677488170990, 9.422509992056141925 ) ) ;
#17387=CARTESIAN_POINT ( 'NONE',  ( 20.88017736071110519, 40.56368534415484106, 2.639326808657452039E-16 ) ) ;
#17388=DIRECTION ( 'NONE',  ( 0.000000000000000000, 0.000000000000000000, -1.000000000000000000 ) ) ;
#17389=CARTESIAN_POINT ( 'NONE',  ( 10.00000000000000178, 63.05374883491396076, 14.16423886937410082 ) ) ;
#17390=CARTESIAN_POINT ( 'NONE',  ( 10.00000000000000000, 4.758931151000784787, -9.846743663894594434 ) ) ;
#17391=CARTESIAN_POINT ( 'NONE',  ( 20.36894250292379738, 9.928748834913966093, -10.36894250292379027 ) ) ;
#17392=CARTESIAN_POINT ( 'NONE',  ( 0.1532563361054082862, 11.21726448433411605, 2.638427012816831674 ) ) ;
#17394=CARTESIAN_POINT ( 'NONE',  ( 12.91533473730993009, 16.60535201082150891, -10.88017736071109987 ) ) ;
#17395=CARTESIAN_POINT ( 'NONE',  ( 17.20831665107776587, 44.13393115100078745, -7.208316651077762316 ) ) ;
#17397=CARTESIAN_POINT ( 'NONE',  ( 0.1532563361054082862, 51.21726448433412315, 2.638427012816831674 ) ) ;
#17398=CIRCLE ( 'NONE', #86046, 18.93999999999999773 ) ;
#17400=CARTESIAN_POINT ( 'NONE',  ( 0.5774900079438607392, 38.48035201082150536, 5.440088680355550821 ) ) ;
#17401=CARTESIAN_POINT ( 'NONE',  ( 0.1532563361054082862, 56.21726448433411605, 2.638427012816831674 ) ) ;
#17402=CARTESIAN_POINT ( 'NONE',  ( 19.38216949554541557, 32.24863466993041783, -9.382169495545420901 ) ) ;
#17404=CARTESIAN_POINT ( 'NONE',  ( 12.91533473730993009, 41.60535201082149825, -10.88017736071109987 ) ) ;
#17405=CARTESIAN_POINT ( 'NONE',  ( 15.44008868035555260, 4.730352010821505360, 9.422509992056143702 ) ) ;
#17407=ADVANCED_FACE ( 'NONE', ( #27320 ), #8963, .T. ) ;
#17409=CARTESIAN_POINT ( 'NONE',  ( -2.816281873526473856, 19.12363466993042138, 9.499525473075851096E-16 ) ) ;
#17412=ORIENTED_EDGE ( 'NONE', *, *, #69776, .F. ) ;
#17413=CARTESIAN_POINT ( 'NONE',  ( -1.099225684535947600, 23.70696800326375708, -6.408140936763238038 ) ) ;
#17414=CARTESIAN_POINT ( 'NONE',  ( 0.5774900079438590739, 17.64701867748817321, -5.440088680355550821 ) ) ;
#17416=CARTESIAN_POINT ( 'NONE',  ( 19.84674366389459266, 3.300597817667451750, 2.638427012816836559 ) ) ;
#17417=CARTESIAN_POINT ( 'NONE',  ( 14.92337183194729988, 54.34226448433412315, -8.527530157486177487 ) ) ;
#17418=CARTESIAN_POINT ( 'NONE',  ( 19.84674366389459266, 13.71726448433411782, -2.638427012816827677 ) ) ;
#17419=CARTESIAN_POINT ( 'NONE',  ( 18.52753015748618282, 43.92559781766745175, -4.923371831947291888 ) ) ;
#17422=CARTESIAN_POINT ( 'NONE',  ( 0.1532563361054100626, 25.80059781766744820, -2.638427012816831230 ) ) ;
#17423=CARTESIAN_POINT ( 'NONE',  ( -0.1503990784575328088, 3.101585745166421493, 6.262539305110068177 ) ) ;
#17425=CARTESIAN_POINT ( 'NONE',  ( 1.472469842513823179, 21.42559781766745175, 4.923371831947296329 ) ) ;
#17426=CARTESIAN_POINT ( 'NONE',  ( -0.1503990784575328643, 70.00000000000000000, 6.262539305110068177 ) ) ;
#17427=CARTESIAN_POINT ( 'NONE',  ( 12.63842701281683922, 39.55059781766744464, -9.846743663894590881 ) ) ;
#17430=CARTESIAN_POINT ( 'NONE',  ( 3.591859063236761518, 29.95696800326375708, 11.09922568453594849 ) ) ;
#17433=CARTESIAN_POINT ( 'NONE',  ( -0.3689425029237881626, 47.42874883491396787, 10.36894250292379027 ) ) ;
#17434=CARTESIAN_POINT ( 'NONE',  ( 12.63842701281683034, 17.46726448433411250, 9.846743663894596210 ) ) ;
#17435=CARTESIAN_POINT ( 'NONE',  ( 5.076628168052704559, 5.175597817667451750, -8.527530157486179263 ) ) ;
#17438=CARTESIAN_POINT ( 'NONE',  ( 24.16423886937410614, 44.30374883491397497, 8.672049930838204340E-16 ) ) ;
#17439=CARTESIAN_POINT ( 'NONE',  ( 17.20831665107776587, 64.13393115100079456, -7.208316651077762316 ) ) ;
#17440=CARTESIAN_POINT ( 'NONE',  ( 17.96484262340118221, 11.18868534415484106, -7.964842623401177768 ) ) ;
#17441=CARTESIAN_POINT ( 'NONE',  ( -0.3689425029237881626, 27.42874883491397142, 10.36894250292379027 ) ) ;
#17442=CARTESIAN_POINT ( 'NONE',  ( 10.00000000000000000, 40.55374883491397497, -14.16423886937410082 ) ) ;
#17443=CARTESIAN_POINT ( 'NONE',  ( -42.94000000000001194, 92.00000000000000000, 9.500000000000000000 ) ) ;
#17446=CARTESIAN_POINT ( 'NONE',  ( 17.20831665107776587, 54.13393115100079456, -7.208316651077762316 ) ) ;
#17448=CARTESIAN_POINT ( 'NONE',  ( 7.084665262690076126, 34.10535201082151247, 10.88017736071109987 ) ) ;
#17449=CARTESIAN_POINT ( 'NONE',  ( 20.03447792253739124, 22.65514106990690379, -6.401564815979733147 ) ) ;
#17450=CARTESIAN_POINT ( 'NONE',  ( 19.64232630867097384, 93.02620456798111093, -5.304930624720125998 ) ) ;
#17451=CARTESIAN_POINT ( 'NONE',  ( 5.076628168052703671, 41.84226448433411605, 8.527530157486179263 ) ) ;
#17452=CARTESIAN_POINT ( 'NONE',  ( 0.2751277870542911397, 35.30223176428830811, 6.499999999999992006 ) ) ;
#17454=CARTESIAN_POINT ( 'NONE',  ( 7.361572987183170547, 42.05059781766745886, 9.846743663894590881 ) ) ;
#17455=CARTESIAN_POINT ( 'NONE',  ( 10.00000000000000000, 64.75893115100078035, -9.846743663894594434 ) ) ;
#17457=CARTESIAN_POINT ( 'NONE',  ( 24.16423886937410614, 9.512082168247301794, -3.795296366450302550 ) ) ;
#17460=DIRECTION ( 'NONE',  ( 1.000000000000000000, 0.000000000000000000, 0.000000000000000000 ) ) ;
#17461=CARTESIAN_POINT ( 'NONE',  ( -0.3689425029237898834, 66.17874883491396076, -10.36894250292378850 ) ) ;
#17462=CARTESIAN_POINT ( 'NONE',  ( -2.816281873526473856, 29.33196800326376064, 3.434112377981055619 ) ) ;
#17463=CARTESIAN_POINT ( 'NONE',  ( 1.472469842513823179, 0.5922644843341181575, -4.923371831947296329 ) ) ;
#17465=VECTOR ( 'NONE', #94715, 1000.000000000000000 ) ;
#17466=CARTESIAN_POINT ( 'NONE',  ( -0.1503990784575328643, 10.12777174578612716, 6.262539305110068177 ) ) ;
#17467=CARTESIAN_POINT ( 'NONE',  ( -46.44000000000001194, 103.0000000000000000, -8.999999999999998224 ) ) ;
#17468=CARTESIAN_POINT ( 'NONE',  ( 6.204703633549690345, 65.76208216824731778, -14.16423886937410259 ) ) ;
#17469=CARTESIAN_POINT ( 'NONE',  ( -0.1503990784575282014, 42.22266099184918886, -6.262539305110077947 ) ) ;
#17470=CARTESIAN_POINT ( 'NONE',  ( 10.00000000000000000, 26.81368534415484106, -10.88017736071110342 ) ) ;
#17471=CARTESIAN_POINT ( 'NONE',  ( 10.00000000000000000, 31.81368534415483751, -10.88017736071110342 ) ) ;
#17472=CARTESIAN_POINT ( 'NONE',  ( 2.791683348922237240, 65.38393115100078035, -7.208316651077763204 ) ) ;
#17473=CARTESIAN_POINT ( 'NONE',  ( 21.09922568453595559, 62.04030133659709634, -6.408140936763230044 ) ) ;
#17474=SURFACE_SIDE_STYLE ('',( #23990 ) ) ;
#17477=CARTESIAN_POINT ( 'NONE',  ( 10.00000000000000000, 36.81368534415484106, -10.88017736071110342 ) ) ;
#17478=EDGE_CURVE ( 'NONE', #52153, #49358, #57812, .T. ) ;
#17479=CARTESIAN_POINT ( 'NONE',  ( 3.591859063236761518, 29.95696800326375708, 11.09922568453594849 ) ) ;
#17480=CARTESIAN_POINT ( 'NONE',  ( 18.72515096720573879, 35.05509018479936145, 6.499999999999937828 ) ) ;
#17481=UNCERTAINTY_MEASURE_WITH_UNIT (LENGTH_MEASURE( 1.000000000000000082E-05 ), #34309, 'distance_accuracy_value', 'NONE');
#17482=CARTESIAN_POINT ( 'NONE',  ( 10.00000000000000000, 59.75893115100078745, -9.846743663894594434 ) ) ;
#17483=CARTESIAN_POINT ( 'NONE',  ( 20.88017736071110519, 50.56368534415484106, 2.639326808657452039E-16 ) ) ;
#17484=CARTESIAN_POINT ( 'NONE',  ( 1.472469842513823179, 15.59226448433411960, -4.923371831947296329 ) ) ;
#17485=CARTESIAN_POINT ( 'NONE',  ( 13.43411237798105340, 30.58196800326374998, 12.81628187352647963 ) ) ;
#17486=CARTESIAN_POINT ( 'NONE',  ( 0.5774900079438607392, 63.48035201082149825, 5.440088680355550821 ) ) ;
#17487=FILL_AREA_STYLE_COLOUR ( '', #32083 ) ;
#17489=CARTESIAN_POINT ( 'NONE',  ( 10.00000000000000178, 65.37363466993042493, 12.81628187352647608 ) ) ;
#17493=CARTESIAN_POINT ( 'NONE',  ( 17.96484262340118221, 6.188685344154836621, -7.964842623401177768 ) ) ;
#17494=CARTESIAN_POINT ( 'NONE',  ( 22.81628187352647785, 51.62363466993042493, 6.195893100308588602E-16 ) ) ;
#17495=CARTESIAN_POINT ( 'NONE',  ( 17.08211943468705130, 18.47041550158063572, 12.26659068614894998 ) ) ;
#17496=CARTESIAN_POINT ( 'NONE',  ( 2.791683348922237240, 20.38393115100078745, -7.208316651077763204 ) ) ;
#17497=AXIS2_PLACEMENT_3D ( 'NONE', #92634, #56130, #10622 ) ;
#17498=CARTESIAN_POINT ( 'NONE',  ( -0.8801773607111009756, 3.063685344154837509, 1.068504757029289695E-15 ) ) ;
#17499=CARTESIAN_POINT ( 'NONE',  ( 10.00000000000000000, 14.75893115100078568, -9.846743663894594434 ) ) ;
#17500=CARTESIAN_POINT ( 'NONE',  ( 22.26659068614894466, 53.88708216824731068, 7.082119434687054849 ) ) ;
#17502=CARTESIAN_POINT ( 'NONE',  ( 0.5774900079438590739, 2.647018677488170990, -5.440088680355550821 ) ) ;
#17504=CARTESIAN_POINT ( 'NONE',  ( 19.42250999205614548, 15.98035201082150714, -5.440088680355545492 ) ) ;
#17505=DIRECTION ( 'NONE',  ( 0.000000000000000000, -1.000000000000000000, 0.000000000000000000 ) ) ;
#17507=ORIENTED_EDGE ( 'NONE', *, *, #40802, .T. ) ;
#17508=CARTESIAN_POINT ( 'NONE',  ( -0.8801773607110991993, 17.85535201082150536, -2.915334737309923874 ) ) ;
#17509=CARTESIAN_POINT ( 'NONE',  ( 12.91533473730992121, 14.52201867748817143, 10.88017736071110164 ) ) ;
#17510=CARTESIAN_POINT ( 'NONE',  ( 14.92337183194729633, 57.67559781766745886, 8.527530157486181039 ) ) ;
#17511=CARTESIAN_POINT ( 'NONE',  ( 22.81628187352648496, 46.83196800326376064, -3.434112377981050290 ) ) ;
#17513=CARTESIAN_POINT ( 'NONE',  ( 24.16423886937410614, 14.51208216824730179, -3.795296366450302550 ) ) ;
#17514=CARTESIAN_POINT ( 'NONE',  ( 20.88017736071110519, 20.56368534415484106, 2.639326808657452039E-16 ) ) ;
#17515=CARTESIAN_POINT ( 'NONE',  ( 12.91533473730992121, 14.52201867748817143, 10.88017736071110164 ) ) ;
#17516=CARTESIAN_POINT ( 'NONE',  ( 19.84674366389459621, 53.50893115100078745, 7.409399052514197653E-17 ) ) ;
#17518=CARTESIAN_POINT ( 'NONE',  ( 2.791683348922237240, 35.38393115100079456, -7.208316651077763204 ) ) ;
#17520=CARTESIAN_POINT ( 'NONE',  ( 14.92337183194729633, 7.675597817667451750, 8.527530157486181039 ) ) ;
#17522=ORIENTED_EDGE ( 'NONE', *, *, #68890, .T. ) ;
#17524=FILL_AREA_STYLE_COLOUR ( '', #71702 ) ;
#17525=CARTESIAN_POINT ( 'NONE',  ( 19.84674366389459266, 8.300597817667451750, 2.638427012816836559 ) ) ;
#17526=CARTESIAN_POINT ( 'NONE',  ( 3.591859063236761518, 4.956968003263753531, 11.09922568453594849 ) ) ;
#17527=CARTESIAN_POINT ( 'NONE',  ( 12.91533473730993009, 46.60535201082150536, -10.88017736071109987 ) ) ;
#17528=( NAMED_UNIT ( * ) PLANE_ANGLE_UNIT ( ) SI_UNIT ( $, .RADIAN. ) );
#17529=CARTESIAN_POINT ( 'NONE',  ( 16.40814093676323893, 45.79030133659708923, 11.09922568453595026 ) ) ;
#17530=CARTESIAN_POINT ( 'NONE',  ( 13.79529636645031943, 20.34541550158063572, -14.16423886937409904 ) ) ;
#17532=CARTESIAN_POINT ( 'NONE',  ( 21.09922568453595559, 57.04030133659708923, -6.408140936763230044 ) ) ;
#17534=ORIENTED_EDGE ( 'NONE', *, *, #72028, .F. ) ;
#17535=CARTESIAN_POINT ( 'NONE',  ( 19.84674366389459621, 53.50893115100078745, 7.409399052514197653E-17 ) ) ;
#17536=CARTESIAN_POINT ( 'NONE',  ( 17.96484262340118221, 19.93868534415484106, 7.964842623401181321 ) ) ;
#17538=CARTESIAN_POINT ( 'NONE',  ( 10.00000000000000178, 69.31368534415484817, 10.88017736071110342 ) ) ;
#17539=CARTESIAN_POINT ( 'NONE',  ( 15.00000000000000000, 60.50000000000000711, -6.000000000000000000 ) ) ;
#17541=CARTESIAN_POINT ( 'NONE',  ( 10.00000000000000000, 14.75893115100078568, -9.846743663894594434 ) ) ;
#17542=CARTESIAN_POINT ( 'NONE',  ( 18.52753015748617571, 3.092264484334118269, 4.923371831947298993 ) ) ;
#17544=CARTESIAN_POINT ( 'NONE',  ( 17.96484262340118221, 61.18868534415482685, -7.964842623401177768 ) ) ;
#17545=CARTESIAN_POINT ( 'NONE',  ( 0.5774900079438590739, 62.64701867748817676, -5.440088680355550821 ) ) ;
#17546=CARTESIAN_POINT ( 'NONE',  ( 5.076628168052703671, 6.842264484334118713, 8.527530157486179263 ) ) ;
#17549=CARTESIAN_POINT ( 'NONE',  ( 7.361572987183170547, 52.05059781766745175, 9.846743663894590881 ) ) ;
#17554=CARTESIAN_POINT ( 'NONE',  ( -0.3689425029237898834, 1.178748834913967869, -10.36894250292378850 ) ) ;
#17555=CARTESIAN_POINT ( 'NONE',  ( 21.09922568453594849, 56.20696800326375353, 6.408140936763242479 ) ) ;
#17558=CARTESIAN_POINT ( 'NONE',  ( -2.266590686148945544, 16.38708216824730357, -7.082119434687050408 ) ) ;
#17559=CARTESIAN_POINT ( 'NONE',  ( 20.36894250292379738, 4.928748834913967869, -10.36894250292379027 ) ) ;
#17560=CARTESIAN_POINT ( 'NONE',  ( 20.88017736071110164, 15.35535201082150358, 2.915334737309930979 ) ) ;
#17561=CARTESIAN_POINT ( 'NONE',  ( -28.94000000000001549, 93.50000000000000000, 9.500000000000000000 ) ) ;
#17563=CARTESIAN_POINT ( 'NONE',  ( 2.791683348922237240, 5.383931151000785675, -7.208316651077763204 ) ) ;
#17564=CARTESIAN_POINT ( 'NONE',  ( 18.52753015748617571, 13.09226448433411960, 4.923371831947298993 ) ) ;
#17565=VECTOR ( 'NONE', #82804, 1000.000000000000000 ) ;
#17566=CARTESIAN_POINT ( 'NONE',  ( -1.099225684535947600, 33.70696800326375353, -6.408140936763238038 ) ) ;
#17567=CARTESIAN_POINT ( 'NONE',  ( 5.076628168052703671, 31.84226448433412315, 8.527530157486179263 ) ) ;
#17569=CARTESIAN_POINT ( 'NONE',  ( 6.565887622018943937, 33.08196800326374643, -12.81628187352647608 ) ) ;
#17571=CARTESIAN_POINT ( 'NONE',  ( 5.076628168052703671, 31.84226448433412315, 8.527530157486179263 ) ) ;
#17572=CARTESIAN_POINT ( 'NONE',  ( 6.204703633549690345, 12.84541550158063572, 14.16423886937410082 ) ) ;
#17575=CARTESIAN_POINT ( 'NONE',  ( 0.5774900079438607392, 33.48035201082150536, 5.440088680355550821 ) ) ;
#17576=CARTESIAN_POINT ( 'NONE',  ( 20.36894250292379382, 28.67874883491396787, 10.36894250292379205 ) ) ;
#17577=CARTESIAN_POINT ( 'NONE',  ( 19.84674366389459266, 58.30059781766745886, 2.638427012816836559 ) ) ;
#17578=CARTESIAN_POINT ( 'NONE',  ( 0.1532563361054100626, 15.80059781766745353, -2.638427012816831230 ) ) ;
#17579=CARTESIAN_POINT ( 'NONE',  ( -2.816281873526473856, 54.12363466993041783, 9.499525473075851096E-16 ) ) ;
#17580=DIRECTION ( 'NONE',  ( -0.000000000000000000, -1.000000000000000000, 0.000000000000000000 ) ) ;
#17581=CARTESIAN_POINT ( 'NONE',  ( 19.42250999205614548, 30.98035201082150536, -5.440088680355545492 ) ) ;
#17583=CARTESIAN_POINT ( 'NONE',  ( 13.43411237798105340, 20.58196800326374643, 12.81628187352647963 ) ) ;
#17584=CARTESIAN_POINT ( 'NONE',  ( 10.00000000000000000, 27.87363466993042138, -12.81628187352647608 ) ) ;
#17585=CARTESIAN_POINT ( 'NONE',  ( 0.1532563361054100626, 45.80059781766745886, -2.638427012816831230 ) ) ;
#17587=CARTESIAN_POINT ( 'NONE',  ( 21.09922568453594849, 51.20696800326375353, 6.408140936763242479 ) ) ;
#17588=FILL_AREA_STYLE_COLOUR ( '', #18121 ) ;
#17589=CARTESIAN_POINT ( 'NONE',  ( 20.88017736071110164, 50.35535201082151247, 2.915334737309930979 ) ) ;
#17590=CARTESIAN_POINT ( 'NONE',  ( 20.10493008474207244, 9.716974130838785584, 6.336235997365739614 ) ) ;
#17591=CARTESIAN_POINT ( 'NONE',  ( -45.94000000000000483, 93.00000000000000000, 9.500000000000000000 ) ) ;
#17592=CARTESIAN_POINT ( 'NONE',  ( 17.96484262340118221, 51.18868534415483396, -7.964842623401177768 ) ) ;
#17593=CARTESIAN_POINT ( 'NONE',  ( 15.44008868035555793, 51.39701867748816966, -9.422509992056140149 ) ) ;
#17595=CARTESIAN_POINT ( 'NONE',  ( 7.084665262690076126, 9.105352010821503583, 10.88017736071109987 ) ) ;
#17596=CARTESIAN_POINT ( 'NONE',  ( 0.1532563361054100626, 65.80059781766745175, -2.638427012816831230 ) ) ;
#17597=CARTESIAN_POINT ( 'NONE',  ( -0.8801773607111008646, 18.27201867748817321, 2.915334737309923430 ) ) ;
#17598=CARTESIAN_POINT ( 'NONE',  ( 0.2751277870542983006, 13.21833443783938122, 6.500000000000002665 ) ) ;
#17600=CARTESIAN_POINT ( 'NONE',  ( 22.81628187352648496, 26.83196800326374998, -3.434112377981050290 ) ) ;
#17602=CARTESIAN_POINT ( 'NONE',  ( 7.084665262690076126, 47.02201867748818387, -10.88017736071110164 ) ) ;
#17603=CARTESIAN_POINT ( 'NONE',  ( 2.791683348922237240, 40.38393115100078035, -7.208316651077763204 ) ) ;
#17604=CARTESIAN_POINT ( 'NONE',  ( -1.099225684535947600, 13.70696800326375353, -6.408140936763238038 ) ) ;
#17606=CARTESIAN_POINT ( 'NONE',  ( 12.91533473730992121, 19.52201867748816611, 10.88017736071110164 ) ) ;
#17607=CARTESIAN_POINT ( 'NONE',  ( 19.42250999205614193, 35.14701867748816966, 5.440088680355555262 ) ) ;
#17608=CARTESIAN_POINT ( 'NONE',  ( 2.917880565312948704, 47.63708216824730357, 12.26659068614894643 ) ) ;
#17609=CARTESIAN_POINT ( 'NONE',  ( 2.791683348922237240, 35.38393115100079456, -7.208316651077763204 ) ) ;
#17610=CARTESIAN_POINT ( 'NONE',  ( 2.035157376598824452, 58.68868534415482685, 7.964842623401179544 ) ) ;
#17612=CARTESIAN_POINT ( 'NONE',  ( 22.26659068614894466, 13.88708216824730179, 7.082119434687054849 ) ) ;
#17615=LINE ( 'NONE', #86596, #55184 ) ;
#17618=EDGE_LOOP ( 'NONE', ( #91652, #60083, #59534, #49137 ) ) ;
#17619=CARTESIAN_POINT ( 'NONE',  ( 13.79529636645030344, 43.26208216824730357, 14.16423886937410614 ) ) ;
#17620=CARTESIAN_POINT ( 'NONE',  ( 24.16423886937410614, 39.30374883491396787, 8.672049930838204340E-16 ) ) ;
#17621=CARTESIAN_POINT ( 'NONE',  ( 14.92337183194729988, 19.34226448433411960, -8.527530157486177487 ) ) ;
#17622=CARTESIAN_POINT ( 'NONE',  ( 22.81628187352647785, 16.62363466993042138, 6.195893100308588602E-16 ) ) ;
#17625=CARTESIAN_POINT ( 'NONE',  ( -0.8801773607111008646, 63.27201867748817676, 2.915334737309923430 ) ) ;
#17626=CARTESIAN_POINT ( 'NONE',  ( 21.09922568453594849, 36.20696800326375353, 6.408140936763242479 ) ) ;
#17627=CARTESIAN_POINT ( 'NONE',  ( 17.08211943468705840, 30.13708216824730357, -12.26659068614894466 ) ) ;
#17628=CARTESIAN_POINT ( 'NONE',  ( 12.91533473730992121, 29.52201867748817321, 10.88017736071110164 ) ) ;
#17630=CARTESIAN_POINT ( 'NONE',  ( 19.42250999205614193, 65.14701867748817676, 5.440088680355555262 ) ) ;
#17633=CARTESIAN_POINT ( 'NONE',  ( 1.472469842513823179, 5.592264484334118713, -4.923371831947296329 ) ) ;
#17635=FACE_OUTER_BOUND ( 'NONE', #41878, .T. ) ;
#17640=CARTESIAN_POINT ( 'NONE',  ( -4.164238869374099927, 2.012082168247300906, 3.795296366450308767 ) ) ;
#17641=CARTESIAN_POINT ( 'NONE',  ( 7.084665262690076126, 4.105352010821503583, 10.88017736071109987 ) ) ;
#17642=CARTESIAN_POINT ( 'NONE',  ( 2.035157376598822676, 7.438685344154837509, -7.964842623401177768 ) ) ;
#17643=CARTESIAN_POINT ( 'NONE',  ( 18.52753015748617571, 38.09226448433412315, 4.923371831947298993 ) ) ;
#17644=CARTESIAN_POINT ( 'NONE',  ( 10.00000000000000178, 10.37363466993041961, 12.81628187352647608 ) ) ;
#17646=CARTESIAN_POINT ( 'NONE',  ( 1.472469842513823179, 6.425597817667451750, 4.923371831947296329 ) ) ;
#17648=CARTESIAN_POINT ( 'NONE',  ( 3.591859063236761518, -0.04303199673624671928, 11.09922568453594849 ) ) ;
#17651=CARTESIAN_POINT ( 'NONE',  ( -4.164238869374099039, 51.80374883491396787, 8.674139862899312516E-16 ) ) ;
#17652=ORIENTED_EDGE ( 'NONE', *, *, #23633, .F. ) ;
#17653=CARTESIAN_POINT ( 'NONE',  ( -0.3689425029237898834, 51.17874883491397497, -10.36894250292378850 ) ) ;
#17654=ORIENTED_EDGE ( 'NONE', *, *, #62796, .T. ) ;
#17655=CARTESIAN_POINT ( 'NONE',  ( 20.88017736071110875, 40.77201867748818387, -2.915334737309920765 ) ) ;
#17656=CARTESIAN_POINT ( 'NONE',  ( 7.084665262690076126, 34.10535201082151247, 10.88017736071109987 ) ) ;
#17657=CARTESIAN_POINT ( 'NONE',  ( 15.44008868035555793, 36.39701867748816966, -9.422509992056140149 ) ) ;
#17658=CARTESIAN_POINT ( 'NONE',  ( -44.70923076923077133, 101.8461538461538396, -9.500000000000000000 ) ) ;
#17659=CARTESIAN_POINT ( 'NONE',  ( -0.8801773607111009756, 28.06368534415484106, 1.068504757029289695E-15 ) ) ;
#17662=CARTESIAN_POINT ( 'NONE',  ( 2.791683348922240793, 21.63393115100078745, 7.208316651077764092 ) ) ;
#17665=CARTESIAN_POINT ( 'NONE',  ( 18.52753015748618282, 38.92559781766745175, -4.923371831947291888 ) ) ;
#17667=SURFACE_STYLE_FILL_AREA ( #55146 ) ;
#17668=EDGE_CURVE ( 'NONE', #75865, #21055, #76931, .T. ) ;
#17671=CARTESIAN_POINT ( 'NONE',  ( -46.21538524526005887, 104.1852450480875660, 5.851526435683383376 ) ) ;
#17672=CARTESIAN_POINT ( 'NONE',  ( 1.472469842513823179, 50.59226448433411605, -4.923371831947296329 ) ) ;
#17673=CARTESIAN_POINT ( 'NONE',  ( -4.164238869374099927, 52.01208216824729647, 3.795296366450308767 ) ) ;
#17677=CARTESIAN_POINT ( 'NONE',  ( 5.076628168052704559, 15.17559781766745175, -8.527530157486179263 ) ) ;
#17678=CARTESIAN_POINT ( 'NONE',  ( -2.816281873526473856, 64.12363466993042493, 9.499525473075851096E-16 ) ) ;
#17679=CARTESIAN_POINT ( 'NONE',  ( 18.52753015748617571, 63.09226448433412315, 4.923371831947298993 ) ) ;
#17680=CARTESIAN_POINT ( 'NONE',  ( 5.076628168052704559, 0.1755978176674514724, -8.527530157486179263 ) ) ;
#17681=CARTESIAN_POINT ( 'NONE',  ( 0.1532563361054100626, 50.80059781766745175, -2.638427012816831230 ) ) ;
#17682=EDGE_CURVE ( 'NONE', #80255, #75354, #4599, .T. ) ;
#17683=DIRECTION ( 'NONE',  ( 0.000000000000000000, -0.000000000000000000, 1.000000000000000000 ) ) ;
#17686=CARTESIAN_POINT ( 'NONE',  ( 22.26659068614894466, 58.88708216824729647, 7.082119434687054849 ) ) ;
#17688=CARTESIAN_POINT ( 'NONE',  ( 19.42250999205614548, 45.98035201082150536, -5.440088680355545492 ) ) ;
#17689=VECTOR ( 'NONE', #77951, 1000.000000000000000 ) ;
#17690=CARTESIAN_POINT ( 'NONE',  ( 3.591859063236763294, 18.29030133659708568, -11.09922568453595026 ) ) ;
#17695=CARTESIAN_POINT ( 'NONE',  ( -0.04068437667222131460, 62.21974360917720048, -6.396802510829771471 ) ) ;
#17696=CARTESIAN_POINT ( 'NONE',  ( 17.20831665107776587, 49.13393115100078745, -7.208316651077762316 ) ) ;
#17697=LINE ( 'NONE', #79162, #55343 ) ;
#17699=CARTESIAN_POINT ( 'NONE',  ( 21.09922568453595559, 12.04030133659708746, -6.408140936763230044 ) ) ;
#17701=CARTESIAN_POINT ( 'NONE',  ( 17.96484262340118221, 11.18868534415484106, -7.964842623401177768 ) ) ;
#17702=CARTESIAN_POINT ( 'NONE',  ( 1.383448333479232906, 67.37718327197430312, -6.499999999999977796 ) ) ;
#17704=CARTESIAN_POINT ( 'NONE',  ( 22.26659068614895176, 34.72041550158063927, -7.082119434687042414 ) ) ;
#17705=CARTESIAN_POINT ( 'NONE',  ( 20.36894250292379738, 34.92874883491396076, -10.36894250292379027 ) ) ;
#17706=CARTESIAN_POINT ( 'NONE',  ( 2.917880565312948704, 57.63708216824731068, 12.26659068614894643 ) ) ;
#17707=CARTESIAN_POINT ( 'NONE',  ( -2.816281873526471635, 38.91530133659708213, -3.434112377981056508 ) ) ;
#17708=CARTESIAN_POINT ( 'NONE',  ( -0.8801773607111009756, 8.063685344154837509, 1.068504757029289695E-15 ) ) ;
#17710=CARTESIAN_POINT ( 'NONE',  ( 0.1532563361054082862, 41.21726448433411605, 2.638427012816831674 ) ) ;
#17711=CARTESIAN_POINT ( 'NONE',  ( 7.084665262690076126, 47.02201867748818387, -10.88017736071110164 ) ) ;
#17712=CARTESIAN_POINT ( 'NONE',  ( 12.63842701281683034, 62.46726448433410894, 9.846743663894596210 ) ) ;
#17713=CARTESIAN_POINT ( 'NONE',  ( 22.26659068614894466, 18.88708216824730002, 7.082119434687054849 ) ) ;
#17714=CARTESIAN_POINT ( 'NONE',  ( -39.69000000000001194, 92.00000000000000000, -10.09898361729590199 ) ) ;
#17715=CARTESIAN_POINT ( 'NONE',  ( 18.39792806157249672, 34.52224192338640307, 6.500000000000000888 ) ) ;
#17716=CARTESIAN_POINT ( 'NONE',  ( 0.1532563361054100626, 25.80059781766744820, -2.638427012816831230 ) ) ;
#17717=CARTESIAN_POINT ( 'NONE',  ( 16.40814093676324603, 47.45696800326375353, -11.09922568453594671 ) ) ;
#17718=CARTESIAN_POINT ( 'NONE',  ( 19.84674366389459266, 48.71726448433413026, -2.638427012816827677 ) ) ;
#17721=CARTESIAN_POINT ( 'NONE',  ( 17.08211943468705840, 65.13708216824730357, -12.26659068614894466 ) ) ;
#17722=CARTESIAN_POINT ( 'NONE',  ( 19.42250999205614193, 60.14701867748817676, 5.440088680355555262 ) ) ;
#17723=CARTESIAN_POINT ( 'NONE',  ( 24.16423886937410614, 14.51208216824730179, -3.795296366450302550 ) ) ;
#17724=CARTESIAN_POINT ( 'NONE',  ( 1.472469842513823179, 1.425597817667451528, 4.923371831947296329 ) ) ;
#17725=CARTESIAN_POINT ( 'NONE',  ( 7.361572987183170547, 47.05059781766745175, 9.846743663894590881 ) ) ;
#17726=CARTESIAN_POINT ( 'NONE',  ( 20.88017736071110519, 20.56368534415484106, 2.639326808657452039E-16 ) ) ;
#17728=CARTESIAN_POINT ( 'NONE',  ( 2.791683348922240793, 61.63393115100079456, 7.208316651077764092 ) ) ;
#17730=EDGE_CURVE ( 'NONE', #28561, #56172, #25035, .T. ) ;
#17736=( NAMED_UNIT ( * ) PLANE_ANGLE_UNIT ( ) SI_UNIT ( $, .RADIAN. ) );
#17737=CARTESIAN_POINT ( 'NONE',  ( 19.84674366389459266, 63.71726448433412315, -2.638427012816827677 ) ) ;
#17738=CARTESIAN_POINT ( 'NONE',  ( 2.791683348922240793, 21.63393115100078745, 7.208316651077764092 ) ) ;
#17739=CARTESIAN_POINT ( 'NONE',  ( 20.88017736071110519, 20.56368534415484106, 2.639326808657452039E-16 ) ) ;
#17740=CARTESIAN_POINT ( 'NONE',  ( 1.472469842513823179, 60.59226448433412315, -4.923371831947296329 ) ) ;
#17742=CARTESIAN_POINT ( 'NONE',  ( 24.16423886937409904, 39.09541550158062506, 3.795296366450317205 ) ) ;
#17743=CARTESIAN_POINT ( 'NONE',  ( 17.08211943468705840, 65.13708216824730357, -12.26659068614894466 ) ) ;
#17744=CARTESIAN_POINT ( 'NONE',  ( 1.472469842513823179, 66.42559781766745175, 4.923371831947296329 ) ) ;
#17746=CARTESIAN_POINT ( 'NONE',  ( 4.559911319644449179, 68.89701867748817676, 9.422509992056141925 ) ) ;
#17747=CARTESIAN_POINT ( 'NONE',  ( 1.472469842513823179, 11.42559781766745175, 4.923371831947296329 ) ) ;
#17748=CARTESIAN_POINT ( 'NONE',  ( 20.15039907845753220, 61.74884699246888431, 6.262539305110078836 ) ) ;
#17753=COLOUR_RGB ( '', 0.09019608, 0.27058824, 0.51372549) ;
#17754=CARTESIAN_POINT ( 'NONE',  ( 7.361572987183169658, 24.96726448433412315, -9.846743663894592657 ) ) ;
#17756=CARTESIAN_POINT ( 'NONE',  ( -4.164238869374099039, 31.80374883491396432, 8.674139862899312516E-16 ) ) ;
#17757=CARTESIAN_POINT ( 'NONE',  ( 18.52753015748618282, 38.92559781766745175, -4.923371831947291888 ) ) ;
#17758=CARTESIAN_POINT ( 'NONE',  ( 4.559911319644449179, 38.89701867748817676, 9.422509992056141925 ) ) ;
#17760=( BOUNDED_CURVE ( )  B_SPLINE_CURVE ( 2, ( #10186, #40680, #93172, #84703, #70690, #32669, #79157, #25204, #71180 ),
 .UNSPECIFIED., .F., .T. ) 
 B_SPLINE_CURVE_WITH_KNOTS ( ( 3, 2, 2, 2, 3 ),
 ( 0.08299807979737425234, 0.08333333333333337034, 0.08928571428571430157, 0.09523809523809523281, 0.09557334877405435081 ),
 .UNSPECIFIED. ) 
 CURVE ( )  GEOMETRIC_REPRESENTATION_ITEM ( )  RATIONAL_B_SPLINE_CURVE ( ( 0.9963778908391762723, 0.9980808541467921513, 1.000000000000000000, 0.9659258262890682012, 1.000000000000000000, 0.9659258262890682012, 1.000000000000000000, 0.9980808541467921513, 0.9963778908391762723 ) ) 
 REPRESENTATION_ITEM ( '' )  );
#17761=CARTESIAN_POINT ( 'NONE',  ( 10.00000000000000178, 44.31368534415484106, 10.88017736071110342 ) ) ;
#17767=CARTESIAN_POINT ( 'NONE',  ( -4.164238869374099927, 12.01208216824730357, 3.795296366450308767 ) ) ;
#17769=ORIENTED_EDGE ( 'NONE', *, *, #57907, .F. ) ;
#17770=CARTESIAN_POINT ( 'NONE',  ( 0.6178305044545818747, 28.49863466993041783, -9.382169495545419124 ) ) ;
#17771=CARTESIAN_POINT ( 'NONE',  ( 19.84674366389459266, 28.30059781766745886, 2.638427012816836559 ) ) ;
#17774=CARTESIAN_POINT ( 'NONE',  ( 12.63842701281683034, 27.46726448433411250, 9.846743663894596210 ) ) ;
#17775=CARTESIAN_POINT ( 'NONE',  ( 12.91533473730992121, 54.52201867748816255, 10.88017736071110164 ) ) ;
#17776=CARTESIAN_POINT ( 'NONE',  ( 2.377183314879994125, 45.78593319516822646, -6.500000000000057732 ) ) ;
#17777=LINE ( 'NONE', #33247, #37091 ) ;
#17779=EDGE_CURVE ( 'NONE', #62008, #94783, #10596, .T. ) ;
#17780=CARTESIAN_POINT ( 'NONE',  ( -2.816281873526473856, 64.33196800326376774, 3.434112377981055619 ) ) ;
#17781=CARTESIAN_POINT ( 'NONE',  ( 14.92337183194729633, 7.675597817667451750, 8.527530157486181039 ) ) ;
#17782=CARTESIAN_POINT ( 'NONE',  ( -2.816281873526473856, 9.331968003263753531, 3.434112377981055619 ) ) ;
#17783=CARTESIAN_POINT ( 'NONE',  ( -26.69000000000001194, 92.00000000000000000, 9.500000000000000000 ) ) ;
#17784=CARTESIAN_POINT ( 'NONE',  ( 17.20831665107776587, 49.13393115100078745, -7.208316651077762316 ) ) ;
#17786=CARTESIAN_POINT ( 'NONE',  ( -2.266590686148945544, 7.220415501580634832, 7.082119434687048631 ) ) ;
#17787=CARTESIAN_POINT ( 'NONE',  ( 7.361572987183170547, 17.05059781766745530, 9.846743663894590881 ) ) ;
#17788=CARTESIAN_POINT ( 'NONE',  ( 0.6178305044545838731, 39.74863466993041072, 9.382169495545420901 ) ) ;
#17791=CARTESIAN_POINT ( 'NONE',  ( 19.42250999205614548, 45.98035201082150536, -5.440088680355545492 ) ) ;
#17792=CARTESIAN_POINT ( 'NONE',  ( 6.565887622018943937, 8.081968003263751754, -12.81628187352647608 ) ) ;
#17794=CARTESIAN_POINT ( 'NONE',  ( 10.00000000000000178, 17.25893115100078745, 9.846743663894594434 ) ) ;
#17795=CARTESIAN_POINT ( 'NONE',  ( 7.084665262690076126, 27.02201867748817676, -10.88017736071110164 ) ) ;
#17796=CARTESIAN_POINT ( 'NONE',  ( 10.00000000000000178, 35.37363466993042493, 12.81628187352647608 ) ) ;
#17797=CARTESIAN_POINT ( 'NONE',  ( 10.00000000000000000, 19.75893115100078390, -9.846743663894594434 ) ) ;
#17800=CARTESIAN_POINT ( 'NONE',  ( 19.42250999205614193, 20.14701867748817321, 5.440088680355555262 ) ) ;
#17801=CARTESIAN_POINT ( 'NONE',  ( 12.91533473730993009, 66.60535201082150536, -10.88017736071109987 ) ) ;
#17802=SURFACE_SIDE_STYLE ('',( #94769 ) ) ;
#17803=CARTESIAN_POINT ( 'NONE',  ( 17.20831665107776587, 42.88393115100077324, 7.208316651077764980 ) ) ;
#17804=CARTESIAN_POINT ( 'NONE',  ( 19.42250999205614193, 20.14701867748817321, 5.440088680355555262 ) ) ;
#17805=CARTESIAN_POINT ( 'NONE',  ( 19.42250999205614193, 45.14701867748817676, 5.440088680355555262 ) ) ;
#17806=CARTESIAN_POINT ( 'NONE',  ( 19.42250999205614548, 10.98035201082150536, -5.440088680355545492 ) ) ;
#17807=CARTESIAN_POINT ( 'NONE',  ( 14.92337183194729633, 32.67559781766745175, 8.527530157486181039 ) ) ;
#17808=DIRECTION ( 'NONE',  ( -1.000000000000000000, -2.653152395358074805E-16, -0.000000000000000000 ) ) ;
#17810=CARTESIAN_POINT ( 'NONE',  ( 21.09922568453594849, 6.206968003263753531, 6.408140936763242479 ) ) ;
#17813=CARTESIAN_POINT ( 'NONE',  ( 24.16423886937410614, 19.30374883491397142, 8.672049930838204340E-16 ) ) ;
#17816=CARTESIAN_POINT ( 'NONE',  ( 20.36894250292379738, 64.92874883491397497, -10.36894250292379027 ) ) ;
#17817=CARTESIAN_POINT ( 'NONE',  ( 1.472469842513823179, 26.42559781766745175, 4.923371831947296329 ) ) ;
#17820=CARTESIAN_POINT ( 'NONE',  ( 7.084665262690076126, 47.02201867748818387, -10.88017736071110164 ) ) ;
#17821=CARTESIAN_POINT ( 'NONE',  ( 3.591859063236763294, 58.29030133659708923, -11.09922568453595026 ) ) ;
#17822=CARTESIAN_POINT ( 'NONE',  ( 7.084665262690076126, 29.10535201082150181, 10.88017736071109987 ) ) ;
#17824=CARTESIAN_POINT ( 'NONE',  ( 10.00000000000000178, 70.00000000000000000, 0.000000000000000000 ) ) ;
#17825=CARTESIAN_POINT ( 'NONE',  ( 3.591859063236761518, 14.95696800326375531, 11.09922568453594849 ) ) ;
#17826=CARTESIAN_POINT ( 'NONE',  ( 7.361572987183169658, 14.96726448433411960, -9.846743663894592657 ) ) ;
#17827=ORIENTED_EDGE ( 'NONE', *, *, #28143, .T. ) ;
#17829=CARTESIAN_POINT ( 'NONE',  ( 6.204703633549690345, 57.84541550158063927, 14.16423886937410082 ) ) ;
#17830=CARTESIAN_POINT ( 'NONE',  ( -2.266590686148945544, 22.22041550158063572, 7.082119434687048631 ) ) ;
#17831=CARTESIAN_POINT ( 'NONE',  ( -0.8801773607111008646, 13.27201867748817143, 2.915334737309923430 ) ) ;
#17832=CARTESIAN_POINT ( 'NONE',  ( 19.42250999205614548, 55.98035201082150536, -5.440088680355545492 ) ) ;
#17833=SURFACE_STYLE_USAGE ( .BOTH. , #62829 ) ;
#17835=CARTESIAN_POINT ( 'NONE',  ( 1.472469842513823179, 16.42559781766745175, 4.923371831947296329 ) ) ;
#17837=CARTESIAN_POINT ( 'NONE',  ( 10.00000000000000178, 22.25893115100078745, 9.846743663894594434 ) ) ;
#17839=CARTESIAN_POINT ( 'NONE',  ( 10.00000000000000000, 29.75893115100078745, -9.846743663894594434 ) ) ;
#17840=CARTESIAN_POINT ( 'NONE',  ( 14.92337183194729988, 44.34226448433412315, -8.527530157486177487 ) ) ;
#17842=CARTESIAN_POINT ( 'NONE',  ( 7.084665262690076126, 24.10535201082150181, 10.88017736071109987 ) ) ;
#17843=CARTESIAN_POINT ( 'NONE',  ( 22.81628187352647785, 36.62363466993041783, 6.195893100308588602E-16 ) ) ;
#17844=CARTESIAN_POINT ( 'NONE',  ( 19.42250999205614548, 50.98035201082151247, -5.440088680355545492 ) ) ;
#17845=CARTESIAN_POINT ( 'NONE',  ( 19.84674366389459266, 23.71726448433412315, -2.638427012816827677 ) ) ;
#17846=CARTESIAN_POINT ( 'NONE',  ( -4.164238869374099927, 42.01208216824728936, 3.795296366450308767 ) ) ;
#17847=CARTESIAN_POINT ( 'NONE',  ( 18.52753015748618282, 28.92559781766745175, -4.923371831947291888 ) ) ;
#17849=CARTESIAN_POINT ( 'NONE',  ( 7.361572987183170547, 52.05059781766745175, 9.846743663894590881 ) ) ;
#17850=CARTESIAN_POINT ( 'NONE',  ( 12.63842701281683034, 27.46726448433411250, 9.846743663894596210 ) ) ;
#17851=CARTESIAN_POINT ( 'NONE',  ( 22.26659068614894466, 8.887082168247300018, 7.082119434687054849 ) ) ;
#17852=CARTESIAN_POINT ( 'NONE',  ( 2.917880565312948704, 12.63708216824730179, 12.26659068614894643 ) ) ;
#17853=CARTESIAN_POINT ( 'NONE',  ( 5.076628168052704559, 30.17559781766745175, -8.527530157486179263 ) ) ;
#17854=CARTESIAN_POINT ( 'NONE',  ( 20.88017736071110519, 45.56368534415484106, 2.639326808657452039E-16 ) ) ;
#17855=CARTESIAN_POINT ( 'NONE',  ( -0.8801773607111009756, 23.06368534415484106, 1.068504757029289695E-15 ) ) ;
#17856=CARTESIAN_POINT ( 'NONE',  ( 4.559911319644449179, 38.89701867748817676, 9.422509992056141925 ) ) ;
#17857=CARTESIAN_POINT ( 'NONE',  ( 7.084665262690076126, 24.10535201082150181, 10.88017736071109987 ) ) ;
#17859=CARTESIAN_POINT ( 'NONE',  ( 17.96484262340118221, 56.18868534415484817, -7.964842623401177768 ) ) ;
#17861=SURFACE_STYLE_FILL_AREA ( #42333 ) ;
#17862=CARTESIAN_POINT ( 'NONE',  ( 15.44008868035555793, 66.39701867748817676, -9.422509992056140149 ) ) ;
#17865=CARTESIAN_POINT ( 'NONE',  ( 20.88017736071110875, 65.77201867748817676, -2.915334737309920765 ) ) ;
#17867=EDGE_CURVE ( 'NONE', #75287, #49705, #9023, .T. ) ;
#17870=CARTESIAN_POINT ( 'NONE',  ( 24.16423886937409904, 64.09541550158064638, 3.795296366450317205 ) ) ;
#17871=CARTESIAN_POINT ( 'NONE',  ( 12.63842701281683034, 12.46726448433411782, 9.846743663894596210 ) ) ;
#17872=( NAMED_UNIT ( * ) SI_UNIT ( $, .STERADIAN. ) SOLID_ANGLE_UNIT ( ) );
#17874=CARTESIAN_POINT ( 'NONE',  ( 5.076628168052703671, 6.842264484334118713, 8.527530157486179263 ) ) ;
#17875=CARTESIAN_POINT ( 'NONE',  ( 2.035157376598824452, 8.688685344154839285, 7.964842623401179544 ) ) ;
#17876=CARTESIAN_POINT ( 'NONE',  ( 14.92337183194729633, 47.67559781766745175, 8.527530157486181039 ) ) ;
#17878=CARTESIAN_POINT ( 'NONE',  ( 12.63842701281683922, 44.55059781766745175, -9.846743663894590881 ) ) ;
#17880=CARTESIAN_POINT ( 'NONE',  ( 17.85158348494331904, 29.73726573380435667, -6.499999999999992895 ) ) ;
#17881=CARTESIAN_POINT ( 'NONE',  ( 2.035157376598822676, 57.43868534415484106, -7.964842623401177768 ) ) ;
#17882=CARTESIAN_POINT ( 'NONE',  ( 1.472469842513823179, 46.42559781766745175, 4.923371831947296329 ) ) ;
#17884=CARTESIAN_POINT ( 'NONE',  ( 2.035157376598822676, 67.43868534415484817, -7.964842623401177768 ) ) ;
#17885=CARTESIAN_POINT ( 'NONE',  ( 10.00000000000000178, 59.31368534415484106, 10.88017736071110342 ) ) ;
#17886=CARTESIAN_POINT ( 'NONE',  ( 10.00000000000000178, 68.05374883491397497, 14.16423886937410082 ) ) ;
#17889=CARTESIAN_POINT ( 'NONE',  ( -2.816281873526473856, 39.12363466993041783, 9.499525473075851096E-16 ) ) ;
#17891=CARTESIAN_POINT ( 'NONE',  ( 6.565887622018943937, 25.16530133659708213, 12.81628187352647430 ) ) ;
#17892=CARTESIAN_POINT ( 'NONE',  ( 4.559911319644449179, 28.89701867748817321, 9.422509992056141925 ) ) ;
#17895=EDGE_CURVE ( 'NONE', #88123, #62008, #39283, .T. ) ;
#17896=CARTESIAN_POINT ( 'NONE',  ( 17.96484262340118221, 66.18868534415483396, -7.964842623401177768 ) ) ;
#17898=CARTESIAN_POINT ( 'NONE',  ( 5.076628168052704559, 60.17559781766745175, -8.527530157486179263 ) ) ;
#17899=CARTESIAN_POINT ( 'NONE',  ( 0.1532563361054100626, 15.80059781766745353, -2.638427012816831230 ) ) ;
#17900=CARTESIAN_POINT ( 'NONE',  ( 2.791683348922240793, 41.63393115100078745, 7.208316651077764092 ) ) ;
#17902=CARTESIAN_POINT ( 'NONE',  ( 19.05914839598885635, 14.96693863883975872, 6.499999999999962697 ) ) ;
#17903=CARTESIAN_POINT ( 'NONE',  ( 19.84674366389459266, 38.30059781766745175, 2.638427012816836559 ) ) ;
#17907=CARTESIAN_POINT ( 'NONE',  ( 14.92337183194729988, 29.34226448433411960, -8.527530157486177487 ) ) ;
#17909=CARTESIAN_POINT ( 'NONE',  ( 1.472469842513823179, 41.42559781766745886, 4.923371831947296329 ) ) ;
#17910=ORIENTED_EDGE ( 'NONE', *, *, #14111, .T. ) ;
#17912=CARTESIAN_POINT ( 'NONE',  ( -2.816281873526473856, 19.12363466993042138, 9.499525473075851096E-16 ) ) ;
#17913=CARTESIAN_POINT ( 'NONE',  ( 10.00000000000000000, 49.75893115100078745, -9.846743663894594434 ) ) ;
#17915=CARTESIAN_POINT ( 'NONE',  ( 22.26659068614895176, 44.72041550158063927, -7.082119434687042414 ) ) ;
#17916=CARTESIAN_POINT ( 'NONE',  ( 18.52753015748617571, 13.09226448433411960, 4.923371831947298993 ) ) ;
#17918=CARTESIAN_POINT ( 'NONE',  ( 0.1532563361054083140, 6.008931151000784787, 1.131784320476157264E-15 ) ) ;
#17920=CARTESIAN_POINT ( 'NONE',  ( 13.79529636645031943, 45.34541550158062506, -14.16423886937409904 ) ) ;
#17921=CARTESIAN_POINT ( 'NONE',  ( 12.63842701281683034, 62.46726448433410894, 9.846743663894596210 ) ) ;
#17922=CARTESIAN_POINT ( 'NONE',  ( 2.035157376598822676, 2.438685344154838397, -7.964842623401177768 ) ) ;
#17923=CARTESIAN_POINT ( 'NONE',  ( 22.26659068614894466, 23.88708216824730357, 7.082119434687054849 ) ) ;
#17924=CARTESIAN_POINT ( 'NONE',  ( 6.204703633549690345, 42.84541550158063217, 14.16423886937410082 ) ) ;
#17925=FACE_OUTER_BOUND ( 'NONE', #57915, .T. ) ;
#17926=LINE ( 'NONE', #19882, #13318 ) ;
#17927=CARTESIAN_POINT ( 'NONE',  ( 19.84674366389459621, 58.50893115100078745, 7.409399052514197653E-17 ) ) ;
#17928=ORIENTED_EDGE ( 'NONE', *, *, #5887, .T. ) ;
#17929=CARTESIAN_POINT ( 'NONE',  ( 15.44008868035555793, 36.39701867748816966, -9.422509992056140149 ) ) ;
#17931=CARTESIAN_POINT ( 'NONE',  ( 20.00000000000000355, 95.46878211396317226, -5.047406989011700595 ) ) ;
#17932=DIRECTION ( 'NONE',  ( 0.000000000000000000, -1.000000000000000000, 0.000000000000000000 ) ) ;
#17934=CARTESIAN_POINT ( 'NONE',  ( 0.1532563361054100626, 50.80059781766745175, -2.638427012816831230 ) ) ;
#17935=CARTESIAN_POINT ( 'NONE',  ( 12.63842701281683034, 62.46726448433410894, 9.846743663894596210 ) ) ;
#17938=CARTESIAN_POINT ( 'NONE',  ( -4.164238869374099927, 22.01208216824730357, 3.795296366450308767 ) ) ;
#17941=CARTESIAN_POINT ( 'NONE',  ( 20.88017736071110164, 10.35535201082150714, 2.915334737309930979 ) ) ;
#17942=CARTESIAN_POINT ( 'NONE',  ( 0.6178305044545818747, 23.49863466993041783, -9.382169495545419124 ) ) ;
#17944=CARTESIAN_POINT ( 'NONE',  ( 2.791683348922240793, 16.63393115100078745, 7.208316651077764092 ) ) ;
#17946=CARTESIAN_POINT ( 'NONE',  ( 0.1532563361054100626, 20.80059781766744820, -2.638427012816831230 ) ) ;
#17948=CARTESIAN_POINT ( 'NONE',  ( 17.96484262340118221, 6.188685344154837509, -7.964842623401177768 ) ) ;
#17949=FACE_OUTER_BOUND ( 'NONE', #62263, .T. ) ;
#17951=CARTESIAN_POINT ( 'NONE',  ( 12.91533473730993009, 31.60535201082150891, -10.88017736071109987 ) ) ;
#17952=CARTESIAN_POINT ( 'NONE',  ( 0.5774900079438590739, 42.64701867748816966, -5.440088680355550821 ) ) ;
#17953=CARTESIAN_POINT ( 'NONE',  ( 14.92337183194729988, 64.34226448433412315, -8.527530157486177487 ) ) ;
#17954=CARTESIAN_POINT ( 'NONE',  ( 10.00000000000000000, 64.75893115100078035, -9.846743663894594434 ) ) ;
#17955=CARTESIAN_POINT ( 'NONE',  ( -44.75051794150706286, 105.1827308279087703, -5.400450157393513528 ) ) ;
#17956=CARTESIAN_POINT ( 'NONE',  ( 1.472469842513823179, 10.59226448433411782, -4.923371831947296329 ) ) ;
#17958=CARTESIAN_POINT ( 'NONE',  ( 4.559911319644449179, 32.23035201082150536, -9.422509992056141925 ) ) ;
#17960=CARTESIAN_POINT ( 'NONE',  ( 10.00000000000000000, 27.87363466993042138, -12.81628187352647608 ) ) ;
#17963=CARTESIAN_POINT ( 'NONE',  ( 14.92337183194729988, 59.34226448433412315, -8.527530157486177487 ) ) ;
#17964=CARTESIAN_POINT ( 'NONE',  ( -0.8801773607111009756, 58.06368534415484106, 1.068504757029289695E-15 ) ) ;
#17965=CARTESIAN_POINT ( 'NONE',  ( 2.791683348922240793, 6.633931151000785675, 7.208316651077764092 ) ) ;
#17966=CARTESIAN_POINT ( 'NONE',  ( 3.591859063236761518, 34.95696800326375353, 11.09922568453594849 ) ) ;
#17967=VECTOR ( 'NONE', #1809, 1000.000000000000000 ) ;
#17968=CARTESIAN_POINT ( 'NONE',  ( 4.559911319644449179, 63.89701867748817676, 9.422509992056141925 ) ) ;
#17971=CARTESIAN_POINT ( 'NONE',  ( 13.43411237798106583, 62.66530133659708923, -12.81628187352647252 ) ) ;
#17975=CARTESIAN_POINT ( 'NONE',  ( 10.00000000000000000, 62.87363466993042493, -12.81628187352647608 ) ) ;
#17976=CARTESIAN_POINT ( 'NONE',  ( 12.63842701281683922, 14.55059781766744997, -9.846743663894590881 ) ) ;
#17978=CARTESIAN_POINT ( 'NONE',  ( 19.42250999205614193, 10.14701867748816966, 5.440088680355555262 ) ) ;
#17979=CARTESIAN_POINT ( 'NONE',  ( 2.791683348922240793, 21.63393115100078745, 7.208316651077764092 ) ) ;
#17980=CARTESIAN_POINT ( 'NONE',  ( 24.16423886937410614, 54.30374883491396787, 8.672049930838204340E-16 ) ) ;
#17981=EDGE_LOOP ( 'NONE', ( #46384, #84413, #44549, #5794 ) ) ;
#17983=CARTESIAN_POINT ( 'NONE',  ( 15.44008868035555793, 11.39701867748817143, -9.422509992056140149 ) ) ;
#17984=CARTESIAN_POINT ( 'NONE',  ( 19.42250999205614193, 25.14701867748817321, 5.440088680355555262 ) ) ;
#17989=CARTESIAN_POINT ( 'NONE',  ( 20.88017736071110519, 25.56368534415483751, 2.639326808657452039E-16 ) ) ;
#17990=CARTESIAN_POINT ( 'NONE',  ( 12.63842701281683922, 59.55059781766744464, -9.846743663894590881 ) ) ;
#17992=CARTESIAN_POINT ( 'NONE',  ( 6.565887622018943937, 53.08196800326374643, -12.81628187352647608 ) ) ;
#17994=CARTESIAN_POINT ( 'NONE',  ( 24.16423886937409904, 24.09541550158063927, 3.795296366450317205 ) ) ;
#17995=CARTESIAN_POINT ( 'NONE',  ( -0.8801773607111009756, 43.06368534415484106, 1.068504757029289695E-15 ) ) ;
#17996=CARTESIAN_POINT ( 'NONE',  ( 19.42250999205614548, 15.98035201082150714, -5.440088680355545492 ) ) ;
#17997=CARTESIAN_POINT ( 'NONE',  ( 18.52753015748617571, 58.09226448433411605, 4.923371831947298993 ) ) ;
#17999=CARTESIAN_POINT ( 'NONE',  ( 0.1532563361054082862, 36.21726448433410894, 2.638427012816831674 ) ) ;
#18002=CARTESIAN_POINT ( 'NONE',  ( 17.20831665107776587, 4.133931151000785675, -7.208316651077762316 ) ) ;
#18005=CARTESIAN_POINT ( 'NONE',  ( 10.00000000000000000, 14.75893115100078568, -9.846743663894594434 ) ) ;
#18006=CARTESIAN_POINT ( 'NONE',  ( 6.565887622018943937, 0.1653013365970866511, 12.81628187352647430 ) ) ;
#18007=CARTESIAN_POINT ( 'NONE',  ( 20.88017736071110875, 45.77201867748816966, -2.915334737309920765 ) ) ;
#18008=CARTESIAN_POINT ( 'NONE',  ( -0.8801773607111009756, 48.06368534415484817, 1.068504757029289695E-15 ) ) ;
#18009=CARTESIAN_POINT ( 'NONE',  ( 7.084665262690076126, 22.02201867748817321, -10.88017736071110164 ) ) ;
#18010=CARTESIAN_POINT ( 'NONE',  ( 19.38216949554541202, 45.99863466993041072, 9.382169495545424454 ) ) ;
#18011=CARTESIAN_POINT ( 'NONE',  ( -2.266590686148945544, 36.38708216824730357, -7.082119434687050408 ) ) ;
#18013=CARTESIAN_POINT ( 'NONE',  ( -1.099225684535947600, 59.54030133659708923, 6.408140936763237150 ) ) ;
#18015=CARTESIAN_POINT ( 'NONE',  ( 17.20831665107776587, 62.88393115100078745, 7.208316651077764980 ) ) ;
#18016=CARTESIAN_POINT ( 'NONE',  ( 15.44008868035555793, 31.39701867748817676, -9.422509992056140149 ) ) ;
#18018=CARTESIAN_POINT ( 'NONE',  ( 7.361572987183169658, -0.03273551566588185635, -9.846743663894592657 ) ) ;
#18020=CARTESIAN_POINT ( 'NONE',  ( 19.84674366389459266, 8.717264484334116048, -2.638427012816827677 ) ) ;
#18021=CARTESIAN_POINT ( 'NONE',  ( 18.52753015748618282, 3.925597817667451306, -4.923371831947291888 ) ) ;
#18024=CARTESIAN_POINT ( 'NONE',  ( 20.88017736071110519, 60.56368534415484106, 2.639326808657452039E-16 ) ) ;
#18026=CARTESIAN_POINT ( 'NONE',  ( 20.88017736071110875, 65.77201867748817676, -2.915334737309920765 ) ) ;
#18027=CARTESIAN_POINT ( 'NONE',  ( 1.472469842513823179, 10.59226448433411782, -4.923371831947296329 ) ) ;
#18031=CARTESIAN_POINT ( 'NONE',  ( 14.92337183194729633, 52.67559781766745175, 8.527530157486181039 ) ) ;
#18034=CARTESIAN_POINT ( 'NONE',  ( 6.000000000000000000, 11.50000000000000000, -6.500000000000000888 ) ) ;
#18036=CARTESIAN_POINT ( 'NONE',  ( 13.79529636645030344, 8.262082168247300018, 14.16423886937410614 ) ) ;
#18037=MECHANICAL_DESIGN_GEOMETRIC_PRESENTATION_REPRESENTATION('',(#43568),#13234);
#18039=CARTESIAN_POINT ( 'NONE',  ( 3.591859063236763294, 58.29030133659708923, -11.09922568453595026 ) ) ;
#18040=CARTESIAN_POINT ( 'NONE',  ( -4.164238869374098151, 1.595415501580634388, -3.795296366450310543 ) ) ;
#18041=CARTESIAN_POINT ( 'NONE',  ( 2.917880565312950480, 35.97041550158063217, -12.26659068614894821 ) ) ;
#18042=SURFACE_STYLE_USAGE ( .BOTH. , #12005 ) ;
#18043=CARTESIAN_POINT ( 'NONE',  ( 12.91533473730993009, 26.60535201082150536, -10.88017736071109987 ) ) ;
#18045=VERTEX_POINT ( 'NONE', #77748 ) ;
#18046=CARTESIAN_POINT ( 'NONE',  ( 7.361572987183169658, -0.03273551566588185635, -9.846743663894592657 ) ) ;
#18047=STYLED_ITEM ( 'NONE', ( #58053 ), #76824 ) ;
#18048=CARTESIAN_POINT ( 'NONE',  ( 19.84674366389459266, 18.30059781766745175, 2.638427012816836559 ) ) ;
#18049=CARTESIAN_POINT ( 'NONE',  ( 19.38216949554541557, 47.24863466993041783, -9.382169495545420901 ) ) ;
#18050=CARTESIAN_POINT ( 'NONE',  ( 0.1532563361054083140, 36.00893115100078745, 1.131784320476157264E-15 ) ) ;
#18052=CARTESIAN_POINT ( 'NONE',  ( 20.88017736071110519, 55.56368534415484817, 2.639326808657452039E-16 ) ) ;
#18053=CARTESIAN_POINT ( 'NONE',  ( 5.076628168052703671, 21.84226448433411960, 8.527530157486179263 ) ) ;
#18054=CARTESIAN_POINT ( 'NONE',  ( 0.6178305044545838731, 34.74863466993042493, 9.382169495545420901 ) ) ;
#18055=CARTESIAN_POINT ( 'NONE',  ( 14.92337183194729633, 22.67559781766745175, 8.527530157486181039 ) ) ;
#18056=CARTESIAN_POINT ( 'NONE',  ( 22.26659068614894466, 8.887082168247300018, 7.082119434687054849 ) ) ;
#18057=ORIENTED_EDGE ( 'NONE', *, *, #55358, .T. ) ;
#18058=CARTESIAN_POINT ( 'NONE',  ( 19.42250999205614193, 35.14701867748816966, 5.440088680355555262 ) ) ;
#18059=CARTESIAN_POINT ( 'NONE',  ( -0.3689425029237881626, 32.42874883491395366, 10.36894250292379027 ) ) ;
#18060=CARTESIAN_POINT ( 'NONE',  ( 19.84674366389459266, 48.71726448433413026, -2.638427012816827677 ) ) ;
#18062=CARTESIAN_POINT ( 'NONE',  ( 14.92337183194729988, 9.342264484334119601, -8.527530157486177487 ) ) ;
#18063=CARTESIAN_POINT ( 'NONE',  ( 0.6178305044545818747, 53.49863466993041072, -9.382169495545419124 ) ) ;
#18065=CARTESIAN_POINT ( 'NONE',  ( 0.5774900079438607392, 28.48035201082150891, 5.440088680355550821 ) ) ;
#18067=CARTESIAN_POINT ( 'NONE',  ( 3.591859063236763294, 23.29030133659708568, -11.09922568453595026 ) ) ;
#18068=CARTESIAN_POINT ( 'NONE',  ( 7.361572987183169658, 39.96726448433411605, -9.846743663894592657 ) ) ;
#18070=CARTESIAN_POINT ( 'NONE',  ( 19.42250999205614548, 60.98035201082151247, -5.440088680355545492 ) ) ;
#18071=CARTESIAN_POINT ( 'NONE',  ( 19.72487221294569792, 32.80223176428832232, -6.500000000000008882 ) ) ;
#18075=DIRECTION ( 'NONE',  ( 0.000000000000000000, 0.000000000000000000, 1.000000000000000000 ) ) ;
#18076=CARTESIAN_POINT ( 'NONE',  ( 10.00000000000000178, 54.31368534415484106, 10.88017736071110342 ) ) ;
#18078=CARTESIAN_POINT ( 'NONE',  ( 20.88017736071110519, 60.56368534415484106, 2.639326808657452039E-16 ) ) ;
#18079=CARTESIAN_POINT ( 'NONE',  ( 19.80448550324510038, 56.82703681773343618, 6.500000000002678746 ) ) ;
#18084=CARTESIAN_POINT ( 'NONE',  ( 7.084665262690076126, 7.022018677488170546, -10.88017736071110164 ) ) ;
#18085=CARTESIAN_POINT ( 'NONE',  ( 2.791683348922240793, 61.63393115100079456, 7.208316651077764092 ) ) ;
#18086=CARTESIAN_POINT ( 'NONE',  ( 10.00000000000000000, 26.81368534415484106, -10.88017736071110342 ) ) ;
#18089=CARTESIAN_POINT ( 'NONE',  ( -1.099225684535947600, 29.54030133659708923, 6.408140936763237150 ) ) ;
#18091=CARTESIAN_POINT ( 'NONE',  ( 4.559911319644449179, 57.23035201082150536, -9.422509992056141925 ) ) ;
#18092=CARTESIAN_POINT ( 'NONE',  ( 18.52753015748617571, 43.09226448433412315, 4.923371831947298993 ) ) ;
#18093=CARTESIAN_POINT ( 'NONE',  ( 13.43411237798106583, 7.665301336597086568, -12.81628187352647252 ) ) ;
#18095=CARTESIAN_POINT ( 'NONE',  ( -0.8801773607111009756, 28.06368534415484106, 1.068504757029289695E-15 ) ) ;
#18096=CARTESIAN_POINT ( 'NONE',  ( 7.084665262690076126, 42.02201867748816966, -10.88017736071110164 ) ) ;
#18097=CARTESIAN_POINT ( 'NONE',  ( 10.00000000000000178, 48.05374883491396787, 14.16423886937410082 ) ) ;
#18098=CARTESIAN_POINT ( 'NONE',  ( 7.361572987183170547, 37.05059781766744464, 9.846743663894590881 ) ) ;
#18099=CARTESIAN_POINT ( 'NONE',  ( 17.96484262340118221, 59.93868534415484106, 7.964842623401181321 ) ) ;
#18100=CARTESIAN_POINT ( 'NONE',  ( 19.42250999205614193, 45.14701867748817676, 5.440088680355555262 ) ) ;
#18101=DIRECTION ( 'NONE',  ( 0.000000000000000000, 0.000000000000000000, -1.000000000000000000 ) ) ;
#18102=CARTESIAN_POINT ( 'NONE',  ( 22.26659068614895176, 19.72041550158063572, -7.082119434687042414 ) ) ;
#18105=ORIENTED_EDGE ( 'NONE', *, *, #70206, .F. ) ;
#18107=CARTESIAN_POINT ( 'NONE',  ( 22.26659068614895176, 49.72041550158063927, -7.082119434687042414 ) ) ;
#18108=CARTESIAN_POINT ( 'NONE',  ( 2.917880565312948704, 37.63708216824731068, 12.26659068614894643 ) ) ;
#18109=CARTESIAN_POINT ( 'NONE',  ( 0.1532563361054082862, 21.21726448433412315, 2.638427012816831674 ) ) ;
#18110=ADVANCED_FACE ( 'NONE', ( #10739, #93738 ), #25274, .F. ) ;
#18111=CARTESIAN_POINT ( 'NONE',  ( 22.81628187352648496, 11.83196800326375531, -3.434112377981050290 ) ) ;
#18113=CARTESIAN_POINT ( 'NONE',  ( 0.9413316022086140045, 58.45508385108959004, 6.499999999999978684 ) ) ;
#18114=CARTESIAN_POINT ( 'NONE',  ( 10.00000000000000178, 4.313685344154837509, 10.88017736071110342 ) ) ;
#18115=CARTESIAN_POINT ( 'NONE',  ( -2.816281873526473856, 34.33196800326376064, 3.434112377981055619 ) ) ;
#18116=CARTESIAN_POINT ( 'NONE',  ( -0.3689425029237898834, 46.17874883491397497, -10.36894250292378850 ) ) ;
#18118=CARTESIAN_POINT ( 'NONE',  ( -0.08248232600719085372, 0.1423898869303599768, 6.349449577244200782 ) ) ;
#18119=CARTESIAN_POINT ( 'NONE',  ( 20.88017736071110875, 65.77201867748817676, -2.915334737309920765 ) ) ;
#18121=COLOUR_RGB ( '', 0.40784314, 0.44705882, 0.49803922) ;
#18123=CARTESIAN_POINT ( 'NONE',  ( 12.63842701281683034, 7.467264484334118713, 9.846743663894596210 ) ) ;
#18125=CARTESIAN_POINT ( 'NONE',  ( 12.63842701281683922, 14.55059781766744997, -9.846743663894590881 ) ) ;
#18126=AXIS2_PLACEMENT_3D ( 'NONE', #95870, #27352, #57845 ) ;
#18128=ORIENTED_EDGE ( 'NONE', *, *, #14111, .F. ) ;
#18129=CARTESIAN_POINT ( 'NONE',  ( -4.164238869374099927, 7.012082168247302683, 3.795296366450308767 ) ) ;
#18130=CARTESIAN_POINT ( 'NONE',  ( 2.035157376598824452, 8.688685344154839285, 7.964842623401179544 ) ) ;
#18131=CARTESIAN_POINT ( 'NONE',  ( 4.559911319644449179, 12.23035201082150714, -9.422509992056141925 ) ) ;
#18132=CARTESIAN_POINT ( 'NONE',  ( 0.1532563361054083140, 36.00893115100078745, 1.131784320476157264E-15 ) ) ;
#18133=CARTESIAN_POINT ( 'NONE',  ( -1.099225684535947600, 4.540301336597087456, 6.408140936763237150 ) ) ;
#18136=B_SPLINE_CURVE_WITH_KNOTS ( 'NONE', 3,
 ( #56305, #70326, #94283, #93796, #86799, #48783, #79291, #26278, #41317, #71789 ),
 .UNSPECIFIED., .F., .F.,
 ( 4, 3, 3, 4 ),
 ( 1.528532816688728551E-17, 0.0006253016069560878021, 0.001250604074564932566, 0.002501455912506543068 ),
 .UNSPECIFIED. ) ;
#18137=CARTESIAN_POINT ( 'NONE',  ( 16.40814093676324603, 17.45696800326375353, -11.09922568453594671 ) ) ;
#18138=ORIENTED_EDGE ( 'NONE', *, *, #75431, .F. ) ;
#18139=( BOUNDED_SURFACE ( )  B_SPLINE_SURFACE ( 1, 2, ( 
 ( #58251, #36767, #20774, #6758, #51763, #51265, #97786, #37272, #82247, #13762, #88767, #20278, #67761, #81749, #98280, #29735, #5289, #67259, #22266, #81267, #96788, #13263, #5776, #36265, #52739, #60731, #7759, #1253, #39238, #47203, #68744, #91736, #23257, #84729, #32195, #46238, #69240, #54702, #30723, #46715, #85713, #30227, #70222, #17228, #70718, #38740, #16235, #1741, #53732, #93197, #77704, #9216, #62696, #91232, #31708, #762, #61230, #83742, #47705, #31215, #22756, #53238, #276, #23752, #15266, #84251, #15753, #39728, #8720, #24723, #76724, #45747, #55199, #78199, #92226, #69726, #9711, #8243, #76243, #40211, #61710, #54212, #77215, #62203, #38252, #92709, #24235, #85223, #16726, #19666, #40703, #55708, #86696, #57655, #86205, #87171, #94680, #95161, #64162, #78702, #10698, #50155, #27154, #79184, #71690, #42184, #88152, #33665, #34654, #2729, #25229, #72648, #26668, #41212, #42664, #18694, #41697, #19173, #63676, #3202, #26188, #56203, #4183, #80664, #71207, #17716, #56680, #93694, #32692, #49178, #79679, #34156, #11177, #33184, #57162, #12159, #72168, #48681, #87660, #3695, #48189, #63189, #94181, #25710, #18202, #10211, #65149, #64648, #49653, #80163, #2234, #11674, #95668, #52134, #21148, #74124, #4680, #35143, #96166, #98152, #12649, #6144, #58644, #43146, #75124, #67133, #20153, #58136, #82128, #29125, #60115, #29610, #22138, #73143, #5660, #88645, #59626, #36142, #66646, #81633, #6631, #90614, #50656, #90121, #52622, #83122, #67643, #65642, #44122, #13142, #27649, #28637, #14650, #81145, #73635, #35649, #74632, #43639, #37147, #51648, #5163, #36646, #97658, #21649, #66135, #59127, #96667, #82629, #89637, #28148, #89143, #13637, #20653, #51147, #97170, #14145, #44629, #69604, #16109, #46595, #24112, #45618, #93078, #24608, #16606, #68132, #83624, #54582, #85097, #70099, #76604, #77580, #76115, #98659, #47085, #39114, #84122, #85594, #31096, #84608, #62082, #7644, #53605, #8120, #152, #9096, #1624, #15140, #60613, #38615, #37635, #75621, #647, #15634, #77094, #61590, #38135, #1125, #55075, #92103, #91615, #31587, #69116, #30107, #7133, #68622, #30601, #61106, #22635, #39610, #8606, #53116, #23634, #45113, #92589, #91111, #32072, #54093, #46117, #23132, #62574, #40091, #42071, #55591, #49064, #2611, #86086, #19060, #11066, #63072, #2117, #26076, #72053, #4066, #72532, #65023, #17107, #18085, #32576, #3582, #48561, #79061, #25591, #49538, #34529, #93573, #34039, #95551, #27039, #11551, #78084, #87061, #56083, #9588, #71582, #57538, #47590, #17596, #78580, #18571, #86577, #80047, #64045, #48065, #79568 ),
 ( #25108, #33549, #70591, #10090, #41587, #10575, #33066, #94558, #64535, #40589, #71086, #95043, #57047, #41085, #63562, #26551, #94070, #3094, #56570, #87549, #58026, #82016, #28026, #29493, #74016, #28526, #6034, #50537, #96551, #20540, #43039, #59515, #14033, #88534, #4562, #51025, #80547, #19549, #43521, #58522, #21034, #5546, #20035, #13528, #67521, #36023, #35530, #74514, #81518, #42544, #50044, #81031, #12538, #73519, #65526, #21530, #89525, #96049, #66525, #37024, #36533, #98038, #67022, #97052, #89030, #12044, #73029, #35025, #44511, #27533, #51524, #5047, #66024, #90009, #44010, #13025, #59018, #97543, #29005, #75010, #6515, #88035, #52023, #82515, #75505, #46484, #91498, #23019, #68509, #92472, #46972, #37525, #15996, #84977, #8977, #54471, #22031, #30981, #39, #52505, #15523, #77466, #39494, #60501, #22521, #61480, #30488, #23998, #8007, #90991, #91985, #53987, #76980, #69984, #46004, #98542, #69492, #76494, #16495, #52993, #38505, #45000, #15025, #53488, #83999, #23517, #84495, #8494, #38997, #1008, #83508, #1509, #60002, #31470, #83012, #29994, #61973, #60986, #90496, #14530, #38016, #69002, #7019, #68015, #534, #45498, #75998, #7526, #71940, #55969, #48940, #47466, #48453, #94932, #24494, #2983, #93959, #17485, #10462, #79449, #93464, #70477, #18457, #3463, #86469, #54957, #33431, #78461, #87435, #79931, #40972, #1997, #56458, #32951, #32463, #71470, #10948, #25484, #17966, #11438, #18950, #94443, #62958, #86944, #25955, #16987, #78951, #63928, #92960, #49427, #39976, #85478, #31956, #26435, #62458, #9473, #41473, #33918, #64425, #24990, #55473, #85975, #56933, #41957, #47951, #70976, #72421, #9974, #77966, #40479, #2497, #63455, #89894, #44394, #12418, #58400, #74392, #95937, #66903, #20920, #81896, #5916, #64910, #73905, #42925, #4450, #57427, #21412, #73405, #3947, #34420, #42438, #96437, #95435, #27419, #57912, #51409, #81408, #36409, #88423, #26929, #97422, #13407, #65905, #12910, #51907, #72920, #87920, #28888, #34915, #35413, #65412, #19923, #43892, #19437, #80435, #96936, #66405, #82392, #50416, #49924, #80925, #59392, #11933, #88918, #27907, #28411, #20425, #4933, #50912, #13916, #58906, #43407, #5436, #35908, #89404, #9726, #67399, #45893, #37906, #60380, #53373, #24736, #37413, #14410, #61368, #17243, #98916, #97925, #76380, #22406, #32708, #25243, #83883, #44881, #420, #75887, #75383, #15410, #55213, #68395, #30371, #55727, #63205, #38389, #6899, #30871, #68892, #59886, #60875, #7895, #36907, #93708, #82894, #29385, #74893, #40226, #6392, #52394, #91878, #85729, #47719, #67900, #98424, #29878 ) ),
 .UNSPECIFIED., .F., .F., .F. ) 
 B_SPLINE_SURFACE_WITH_KNOTS ( ( 2, 2 ),
 ( 3, 2, 2, 2, 2, 2, 2, 2, 2, 2, 2, 2, 2, 2, 2, 2, 2, 2, 2, 2, 2, 2, 2, 2, 2, 2, 2, 2, 2, 2, 2, 2, 2, 2, 2, 2, 2, 2, 2, 2, 2, 2, 2, 2, 2, 2, 2, 2, 2, 2, 2, 2, 2, 2, 2, 2, 2, 2, 2, 2, 2, 2, 2, 2, 2, 2, 2, 2, 2, 2, 2, 2, 2, 2, 2, 2, 2, 2, 2, 2, 2, 2, 2, 2, 2, 2, 2, 2, 2, 2, 2, 2, 2, 2, 2, 2, 2, 2, 2, 2, 2, 2, 2, 2, 2, 2, 2, 2, 2, 2, 2, 2, 2, 2, 2, 2, 2, 2, 2, 2, 2, 2, 2, 2, 2, 2, 2, 2, 2, 2, 2, 2, 2, 2, 2, 2, 2, 2, 2, 2, 2, 2, 2, 2, 2, 2, 2, 2, 2, 2, 2, 2, 2, 2, 2, 2, 2, 2, 2, 2, 2, 2, 3 ),
 ( 0.000000000000000000, 1.000000000000000000 ),
 ( 0.000000000000000000, 0.005952380952380952051, 0.01190476190476190410, 0.01785714285714285615, 0.02380952380952380820, 0.02976190476190476025, 0.03571428571428571230, 0.04166666666666666435, 0.04761904761904761640, 0.05357142857142856845, 0.05952380952380952051, 0.06547619047619047949, 0.07142857142857142461, 0.07738095238095238360, 0.08333333333333332871, 0.08928571428571428770, 0.09523809523809523281, 0.1011904761904761918, 0.1071428571428571369, 0.1130952380952380959, 0.1190476190476190410, 0.1250000000000000000, 0.1309523809523809590, 0.1369047619047619180, 0.1428571428571428492, 0.1488095238095238082, 0.1547619047619047672, 0.1607142857142857262, 0.1666666666666666574, 0.1726190476190476164, 0.1785714285714285754, 0.1845238095238095344, 0.1904761904761904656, 0.1964285714285714246, 0.2023809523809523836, 0.2083333333333333426, 0.2142857142857142738, 0.2202380952380952328, 0.2261904761904761918, 0.2321428571428571508, 0.2380952380952380820, 0.2440476190476190410, 0.2500000000000000000, 0.2559523809523809312, 0.2619047619047619180, 0.2678571428571428492, 0.2738095238095238360, 0.2797619047619047672, 0.2857142857142856984, 0.2916666666666666852, 0.2976190476190476164, 0.3035714285714285476, 0.3095238095238095344, 0.3154761904761904656, 0.3214285714285714524, 0.3273809523809523836, 0.3333333333333333148, 0.3392857142857143016, 0.3452380952380952328, 0.3511904761904761640, 0.3571428571428571508, 0.3630952380952380820, 0.3690476190476190688, 0.3750000000000000000, 0.3809523809523809312, 0.3869047619047619180, 0.3928571428571428492, 0.3988095238095238360, 0.4047619047619047672, 0.4107142857142856984, 0.4166666666666666852, 0.4226190476190476164, 0.4285714285714285476, 0.4345238095238095344, 0.4404761904761904656, 0.4464285714285714524, 0.4523809523809523836, 0.4583333333333333148, 0.4642857142857143016, 0.4702380952380952328, 0.4761904761904761640, 0.4821428571428571508, 0.4880952380952380820, 0.4940476190476190688, 0.5000000000000000000, 0.5059523809523809312, 0.5119047619047618625, 0.5178571428571429047, 0.5238095238095238360, 0.5297619047619047672, 0.5357142857142856984, 0.5416666666666666297, 0.5476190476190476719, 0.5535714285714286031, 0.5595238095238095344, 0.5654761904761904656, 0.5714285714285713969, 0.5773809523809523281, 0.5833333333333333703, 0.5892857142857143016, 0.5952380952380952328, 0.6011904761904761640, 0.6071428571428570953, 0.6130952380952381375, 0.6190476190476190688, 0.6250000000000000000, 0.6309523809523809312, 0.6369047619047618625, 0.6428571428571429047, 0.6488095238095238360, 0.6547619047619047672, 0.6607142857142856984, 0.6666666666666666297, 0.6726190476190476719, 0.6785714285714286031, 0.6845238095238095344, 0.6904761904761904656, 0.6964285714285713969, 0.7023809523809523281, 0.7083333333333333703, 0.7142857142857143016, 0.7202380952380952328, 0.7261904761904761640, 0.7321428571428570953, 0.7380952380952381375, 0.7440476190476190688, 0.7500000000000000000, 0.7559523809523809312, 0.7619047619047618625, 0.7678571428571429047, 0.7738095238095238360, 0.7797619047619047672, 0.7857142857142856984, 0.7916666666666666297, 0.7976190476190476719, 0.8035714285714286031, 0.8095238095238095344, 0.8154761904761904656, 0.8214285714285713969, 0.8273809523809523281, 0.8333333333333333703, 0.8392857142857143016, 0.8452380952380952328, 0.8511904761904761640, 0.8571428571428570953, 0.8630952380952381375, 0.8690476190476190688, 0.8750000000000000000, 0.8809523809523809312, 0.8869047619047618625, 0.8928571428571429047, 0.8988095238095238360, 0.9047619047619047672, 0.9107142857142856984, 0.9166666666666666297, 0.9226190476190476719, 0.9285714285714286031, 0.9345238095238095344, 0.9404761904761904656, 0.9464285714285713969, 0.9523809523809523281, 0.9583333333333333703, 0.9642857142857143016 ),
 .UNSPECIFIED. ) 
 GEOMETRIC_REPRESENTATION_ITEM ( )  RATIONAL_B_SPLINE_SURFACE ( (
 ( 1.000000000000000000, 0.9659258262890683122, 1.000000000000000000, 0.9659258262890683122, 1.000000000000000000, 0.9659258262890683122, 1.000000000000000000, 0.9659258262890683122, 1.000000000000000000, 0.9659258262890683122, 1.000000000000000000, 0.9659258262890683122, 1.000000000000000000, 0.9659258262890683122, 1.000000000000000000, 0.9659258262890683122, 1.000000000000000000, 0.9659258262890683122, 1.000000000000000000, 0.9659258262890683122, 1.000000000000000000, 0.9659258262890683122, 1.000000000000000000, 0.9659258262890683122, 1.000000000000000000, 0.9659258262890683122, 1.000000000000000000, 0.9659258262890683122, 1.000000000000000000, 0.9659258262890683122, 1.000000000000000000, 0.9659258262890683122, 1.000000000000000000, 0.9659258262890683122, 1.000000000000000000, 0.9659258262890683122, 1.000000000000000000, 0.9659258262890683122, 1.000000000000000000, 0.9659258262890683122, 1.000000000000000000, 0.9659258262890683122, 1.000000000000000000, 0.9659258262890683122, 1.000000000000000000, 0.9659258262890683122, 1.000000000000000000, 0.9659258262890683122, 1.000000000000000000, 0.9659258262890683122, 1.000000000000000000, 0.9659258262890683122, 1.000000000000000000, 0.9659258262890683122, 1.000000000000000000, 0.9659258262890683122, 1.000000000000000000, 0.9659258262890683122, 1.000000000000000000, 0.9659258262890683122, 1.000000000000000000, 0.9659258262890683122, 1.000000000000000000, 0.9659258262890683122, 1.000000000000000000, 0.9659258262890683122, 1.000000000000000000, 0.9659258262890683122, 1.000000000000000000, 0.9659258262890683122, 1.000000000000000000, 0.9659258262890683122, 1.000000000000000000, 0.9659258262890683122, 1.000000000000000000, 0.9659258262890683122, 1.000000000000000000, 0.9659258262890683122, 1.000000000000000000, 0.9659258262890683122, 1.000000000000000000, 0.9659258262890683122, 1.000000000000000000, 0.9659258262890683122, 1.000000000000000000, 0.9659258262890683122, 1.000000000000000000, 0.9659258262890683122, 1.000000000000000000, 0.9659258262890683122, 1.000000000000000000, 0.9659258262890683122, 1.000000000000000000, 0.9659258262890683122, 1.000000000000000000, 0.9659258262890683122, 1.000000000000000000, 0.9659258262890683122, 1.000000000000000000, 0.9659258262890683122, 1.000000000000000000, 0.9659258262890683122, 1.000000000000000000, 0.9659258262890683122, 1.000000000000000000, 0.9659258262890683122, 1.000000000000000000, 0.9659258262890683122, 1.000000000000000000, 0.9659258262890683122, 1.000000000000000000, 0.9659258262890683122, 1.000000000000000000, 0.9659258262890683122, 1.000000000000000000, 0.9659258262890683122, 1.000000000000000000, 0.9659258262890683122, 1.000000000000000000, 0.9659258262890683122, 1.000000000000000000, 0.9659258262890683122, 1.000000000000000000, 0.9659258262890683122, 1.000000000000000000, 0.9659258262890683122, 1.000000000000000000, 0.9659258262890683122, 1.000000000000000000, 0.9659258262890683122, 1.000000000000000000, 0.9659258262890683122, 1.000000000000000000, 0.9659258262890683122, 1.000000000000000000, 0.9659258262890683122, 1.000000000000000000, 0.9659258262890683122, 1.000000000000000000, 0.9659258262890683122, 1.000000000000000000, 0.9659258262890683122, 1.000000000000000000, 0.9659258262890683122, 1.000000000000000000, 0.9659258262890683122, 1.000000000000000000, 0.9659258262890683122, 1.000000000000000000, 0.9659258262890683122, 1.000000000000000000, 0.9659258262890683122, 1.000000000000000000, 0.9659258262890683122, 1.000000000000000000, 0.9659258262890683122, 1.000000000000000000, 0.9659258262890683122, 1.000000000000000000, 0.9659258262890683122, 1.000000000000000000, 0.9659258262890683122, 1.000000000000000000, 0.9659258262890683122, 1.000000000000000000, 0.9659258262890683122, 1.000000000000000000, 0.9659258262890683122, 1.000000000000000000, 0.9659258262890683122, 1.000000000000000000, 0.9659258262890683122, 1.000000000000000000, 0.9659258262890683122, 1.000000000000000000, 0.9659258262890683122, 1.000000000000000000, 0.9659258262890683122, 1.000000000000000000, 0.9659258262890683122, 1.000000000000000000, 0.9659258262890683122, 1.000000000000000000, 0.9659258262890683122, 1.000000000000000000, 0.9659258262890683122, 1.000000000000000000, 0.9659258262890683122, 1.000000000000000000, 0.9659258262890683122, 1.000000000000000000, 0.9659258262890683122, 1.000000000000000000, 0.9659258262890683122, 1.000000000000000000, 0.9659258262890683122, 1.000000000000000000, 0.9659258262890683122, 1.000000000000000000, 0.9659258262890683122, 1.000000000000000000, 0.9659258262890683122, 1.000000000000000000, 0.9659258262890683122, 1.000000000000000000, 0.9659258262890683122, 1.000000000000000000, 0.9659258262890683122, 1.000000000000000000, 0.9659258262890683122, 1.000000000000000000, 0.9659258262890683122, 1.000000000000000000, 0.9659258262890683122, 1.000000000000000000, 0.9659258262890683122, 1.000000000000000000, 0.9659258262890683122, 1.000000000000000000, 0.9659258262890683122, 1.000000000000000000, 0.9659258262890683122, 1.000000000000000000, 0.9659258262890683122, 1.000000000000000000, 0.9659258262890683122, 1.000000000000000000, 0.9659258262890683122, 1.000000000000000000, 0.9659258262890683122, 1.000000000000000000, 0.9659258262890683122, 1.000000000000000000, 0.9659258262890683122, 1.000000000000000000, 0.9659258262890683122, 1.000000000000000000, 0.9659258262890683122, 1.000000000000000000, 0.9659258262890683122, 1.000000000000000000, 0.9659258262890683122, 1.000000000000000000, 0.9659258262890683122, 1.000000000000000000, 0.9659258262890683122, 1.000000000000000000, 0.9659258262890683122, 1.000000000000000000, 0.9659258262890683122, 1.000000000000000000, 0.9659258262890683122, 1.000000000000000000, 0.9659258262890683122, 1.000000000000000000, 0.9659258262890683122, 1.000000000000000000, 0.9659258262890683122, 1.000000000000000000, 0.9659258262890683122, 1.000000000000000000, 0.9659258262890683122, 1.000000000000000000, 0.9659258262890683122, 1.000000000000000000, 0.9659258262890683122, 1.000000000000000000, 0.9659258262890683122, 1.000000000000000000, 0.9659258262890683122, 1.000000000000000000, 0.9659258262890683122, 1.000000000000000000, 0.9659258262890683122, 1.000000000000000000, 0.9659258262890683122, 1.000000000000000000, 0.9659258262890683122, 1.000000000000000000, 0.9659258262890683122, 1.000000000000000000, 0.9659258262890683122, 1.000000000000000000, 0.9659258262890683122, 1.000000000000000000, 0.9659258262890683122, 1.000000000000000000, 0.9659258262890683122, 1.000000000000000000, 0.9659258262890683122, 1.000000000000000000, 0.9659258262890683122, 1.000000000000000000, 0.9659258262890683122, 1.000000000000000000, 0.9659258262890683122, 1.000000000000000000, 0.9659258262890683122, 1.000000000000000000, 0.9659258262890683122, 1.000000000000000000, 0.9659258262890683122, 1.000000000000000000, 0.9659258262890683122, 1.000000000000000000, 0.9659258262890683122, 1.000000000000000000, 0.9659258262890683122, 1.000000000000000000, 0.9659258262890683122, 1.000000000000000000, 0.9659258262890683122, 1.000000000000000000, 0.9659258262890683122, 1.000000000000000000, 0.9659258262890683122, 1.000000000000000000, 0.9659258262890683122, 1.000000000000000000, 0.9659258262890683122, 1.000000000000000000, 0.9659258262890683122, 1.000000000000000000, 0.9659258262890683122, 1.000000000000000000),
 ( 1.000000000000000000, 0.9659258262890683122, 1.000000000000000000, 0.9659258262890683122, 1.000000000000000000, 0.9659258262890683122, 1.000000000000000000, 0.9659258262890683122, 1.000000000000000000, 0.9659258262890683122, 1.000000000000000000, 0.9659258262890683122, 1.000000000000000000, 0.9659258262890683122, 1.000000000000000000, 0.9659258262890683122, 1.000000000000000000, 0.9659258262890683122, 1.000000000000000000, 0.9659258262890683122, 1.000000000000000000, 0.9659258262890683122, 1.000000000000000000, 0.9659258262890683122, 1.000000000000000000, 0.9659258262890683122, 1.000000000000000000, 0.9659258262890683122, 1.000000000000000000, 0.9659258262890683122, 1.000000000000000000, 0.9659258262890683122, 1.000000000000000000, 0.9659258262890683122, 1.000000000000000000, 0.9659258262890683122, 1.000000000000000000, 0.9659258262890683122, 1.000000000000000000, 0.9659258262890683122, 1.000000000000000000, 0.9659258262890683122, 1.000000000000000000, 0.9659258262890683122, 1.000000000000000000, 0.9659258262890683122, 1.000000000000000000, 0.9659258262890683122, 1.000000000000000000, 0.9659258262890683122, 1.000000000000000000, 0.9659258262890683122, 1.000000000000000000, 0.9659258262890683122, 1.000000000000000000, 0.9659258262890683122, 1.000000000000000000, 0.9659258262890683122, 1.000000000000000000, 0.9659258262890683122, 1.000000000000000000, 0.9659258262890683122, 1.000000000000000000, 0.9659258262890683122, 1.000000000000000000, 0.9659258262890683122, 1.000000000000000000, 0.9659258262890683122, 1.000000000000000000, 0.9659258262890683122, 1.000000000000000000, 0.9659258262890683122, 1.000000000000000000, 0.9659258262890683122, 1.000000000000000000, 0.9659258262890683122, 1.000000000000000000, 0.9659258262890683122, 1.000000000000000000, 0.9659258262890683122, 1.000000000000000000, 0.9659258262890683122, 1.000000000000000000, 0.9659258262890683122, 1.000000000000000000, 0.9659258262890683122, 1.000000000000000000, 0.9659258262890683122, 1.000000000000000000, 0.9659258262890683122, 1.000000000000000000, 0.9659258262890683122, 1.000000000000000000, 0.9659258262890683122, 1.000000000000000000, 0.9659258262890683122, 1.000000000000000000, 0.9659258262890683122, 1.000000000000000000, 0.9659258262890683122, 1.000000000000000000, 0.9659258262890683122, 1.000000000000000000, 0.9659258262890683122, 1.000000000000000000, 0.9659258262890683122, 1.000000000000000000, 0.9659258262890683122, 1.000000000000000000, 0.9659258262890683122, 1.000000000000000000, 0.9659258262890683122, 1.000000000000000000, 0.9659258262890683122, 1.000000000000000000, 0.9659258262890683122, 1.000000000000000000, 0.9659258262890683122, 1.000000000000000000, 0.9659258262890683122, 1.000000000000000000, 0.9659258262890683122, 1.000000000000000000, 0.9659258262890683122, 1.000000000000000000, 0.9659258262890683122, 1.000000000000000000, 0.9659258262890683122, 1.000000000000000000, 0.9659258262890683122, 1.000000000000000000, 0.9659258262890683122, 1.000000000000000000, 0.9659258262890683122, 1.000000000000000000, 0.9659258262890683122, 1.000000000000000000, 0.9659258262890683122, 1.000000000000000000, 0.9659258262890683122, 1.000000000000000000, 0.9659258262890683122, 1.000000000000000000, 0.9659258262890683122, 1.000000000000000000, 0.9659258262890683122, 1.000000000000000000, 0.9659258262890683122, 1.000000000000000000, 0.9659258262890683122, 1.000000000000000000, 0.9659258262890683122, 1.000000000000000000, 0.9659258262890683122, 1.000000000000000000, 0.9659258262890683122, 1.000000000000000000, 0.9659258262890683122, 1.000000000000000000, 0.9659258262890683122, 1.000000000000000000, 0.9659258262890683122, 1.000000000000000000, 0.9659258262890683122, 1.000000000000000000, 0.9659258262890683122, 1.000000000000000000, 0.9659258262890683122, 1.000000000000000000, 0.9659258262890683122, 1.000000000000000000, 0.9659258262890683122, 1.000000000000000000, 0.9659258262890683122, 1.000000000000000000, 0.9659258262890683122, 1.000000000000000000, 0.9659258262890683122, 1.000000000000000000, 0.9659258262890683122, 1.000000000000000000, 0.9659258262890683122, 1.000000000000000000, 0.9659258262890683122, 1.000000000000000000, 0.9659258262890683122, 1.000000000000000000, 0.9659258262890683122, 1.000000000000000000, 0.9659258262890683122, 1.000000000000000000, 0.9659258262890683122, 1.000000000000000000, 0.9659258262890683122, 1.000000000000000000, 0.9659258262890683122, 1.000000000000000000, 0.9659258262890683122, 1.000000000000000000, 0.9659258262890683122, 1.000000000000000000, 0.9659258262890683122, 1.000000000000000000, 0.9659258262890683122, 1.000000000000000000, 0.9659258262890683122, 1.000000000000000000, 0.9659258262890683122, 1.000000000000000000, 0.9659258262890683122, 1.000000000000000000, 0.9659258262890683122, 1.000000000000000000, 0.9659258262890683122, 1.000000000000000000, 0.9659258262890683122, 1.000000000000000000, 0.9659258262890683122, 1.000000000000000000, 0.9659258262890683122, 1.000000000000000000, 0.9659258262890683122, 1.000000000000000000, 0.9659258262890683122, 1.000000000000000000, 0.9659258262890683122, 1.000000000000000000, 0.9659258262890683122, 1.000000000000000000, 0.9659258262890683122, 1.000000000000000000, 0.9659258262890683122, 1.000000000000000000, 0.9659258262890683122, 1.000000000000000000, 0.9659258262890683122, 1.000000000000000000, 0.9659258262890683122, 1.000000000000000000, 0.9659258262890683122, 1.000000000000000000, 0.9659258262890683122, 1.000000000000000000, 0.9659258262890683122, 1.000000000000000000, 0.9659258262890683122, 1.000000000000000000, 0.9659258262890683122, 1.000000000000000000, 0.9659258262890683122, 1.000000000000000000, 0.9659258262890683122, 1.000000000000000000, 0.9659258262890683122, 1.000000000000000000, 0.9659258262890683122, 1.000000000000000000, 0.9659258262890683122, 1.000000000000000000, 0.9659258262890683122, 1.000000000000000000, 0.9659258262890683122, 1.000000000000000000, 0.9659258262890683122, 1.000000000000000000, 0.9659258262890683122, 1.000000000000000000, 0.9659258262890683122, 1.000000000000000000, 0.9659258262890683122, 1.000000000000000000, 0.9659258262890683122, 1.000000000000000000, 0.9659258262890683122, 1.000000000000000000, 0.9659258262890683122, 1.000000000000000000, 0.9659258262890683122, 1.000000000000000000, 0.9659258262890683122, 1.000000000000000000, 0.9659258262890683122, 1.000000000000000000, 0.9659258262890683122, 1.000000000000000000, 0.9659258262890683122, 1.000000000000000000, 0.9659258262890683122, 1.000000000000000000, 0.9659258262890683122, 1.000000000000000000, 0.9659258262890683122, 1.000000000000000000, 0.9659258262890683122, 1.000000000000000000, 0.9659258262890683122, 1.000000000000000000, 0.9659258262890683122, 1.000000000000000000, 0.9659258262890683122, 1.000000000000000000, 0.9659258262890683122, 1.000000000000000000, 0.9659258262890683122, 1.000000000000000000, 0.9659258262890683122, 1.000000000000000000, 0.9659258262890683122, 1.000000000000000000, 0.9659258262890683122, 1.000000000000000000, 0.9659258262890683122, 1.000000000000000000, 0.9659258262890683122, 1.000000000000000000, 0.9659258262890683122, 1.000000000000000000, 0.9659258262890683122, 1.000000000000000000, 0.9659258262890683122, 1.000000000000000000, 0.9659258262890683122, 1.000000000000000000, 0.9659258262890683122, 1.000000000000000000) ) ) 
 REPRESENTATION_ITEM ( '' )  SURFACE ( )  );
#18140=CARTESIAN_POINT ( 'NONE',  ( 17.08211943468705130, 53.47041550158063217, 12.26659068614894998 ) ) ;
#18142=CARTESIAN_POINT ( 'NONE',  ( 6.204703633549690345, 50.76208216824730357, -14.16423886937410259 ) ) ;
#18144=CARTESIAN_POINT ( 'NONE',  ( 19.42250999205614193, 35.14701867748816966, 5.440088680355555262 ) ) ;
#18145=CARTESIAN_POINT ( 'NONE',  ( 12.91533473730992121, 34.52201867748817676, 10.88017736071110164 ) ) ;
#18147=CARTESIAN_POINT ( 'NONE',  ( 12.91533473730993009, 21.60535201082150536, -10.88017736071109987 ) ) ;
#18149=CARTESIAN_POINT ( 'NONE',  ( 1.472469842513823179, 11.42559781766745175, 4.923371831947296329 ) ) ;
#18153=CARTESIAN_POINT ( 'NONE',  ( 19.84674366389459266, 38.30059781766745175, 2.638427012816836559 ) ) ;
#18155=ORIENTED_EDGE ( 'NONE', *, *, #37205, .T. ) ;
#18158=CARTESIAN_POINT ( 'NONE',  ( -4.164238869374098151, 46.59541550158063927, -3.795296366450310543 ) ) ;
#18161=CARTESIAN_POINT ( 'NONE',  ( 20.03743638938529870, 41.75197528031017669, 6.399506433553907137 ) ) ;
#18162=CARTESIAN_POINT ( 'NONE',  ( 17.20831665107776587, 14.13393115100078568, -7.208316651077762316 ) ) ;
#18164=CARTESIAN_POINT ( 'NONE',  ( 2.791683348922237240, 65.38393115100078035, -7.208316651077763204 ) ) ;
#18165=CARTESIAN_POINT ( 'NONE',  ( 7.361572987183170547, 2.050597817667451750, 9.846743663894590881 ) ) ;
#18166=CARTESIAN_POINT ( 'NONE',  ( 19.84674366389459621, 63.50893115100078745, 7.409399052514197653E-17 ) ) ;
#18170=CARTESIAN_POINT ( 'NONE',  ( -4.164238869374099927, 67.01208216824728936, 3.795296366450308767 ) ) ;
#18171=CARTESIAN_POINT ( 'NONE',  ( 19.72487221294570858, 6.866073187300758107, 6.500000000000000888 ) ) ;
#18172=CARTESIAN_POINT ( 'NONE',  ( 0.5774900079438590739, 37.64701867748817676, -5.440088680355550821 ) ) ;
#18173=CARTESIAN_POINT ( 'NONE',  ( 16.40814093676324603, 12.45696800326375353, -11.09922568453594671 ) ) ;
#18174=CARTESIAN_POINT ( 'NONE',  ( 20.88017736071110519, 65.56368534415483396, 2.639326808657452039E-16 ) ) ;
#18178=CARTESIAN_POINT ( 'NONE',  ( 0.2751277870542870319, 54.36607318730131055, -6.499999999999985789 ) ) ;
#18179=CARTESIAN_POINT ( 'NONE',  ( 0.1532563361054082862, 56.21726448433411605, 2.638427012816831674 ) ) ;
#18180=CARTESIAN_POINT ( 'NONE',  ( 1.472469842513823179, 5.592264484334118713, -4.923371831947296329 ) ) ;
#18182=CARTESIAN_POINT ( 'NONE',  ( -2.816281873526473856, 4.123634669930420493, 9.499525473075851096E-16 ) ) ;
#18183=ADVANCED_FACE ( 'NONE', ( #67183 ), #12697, .F. ) ;
#18184=CARTESIAN_POINT ( 'NONE',  ( 15.44008868035555793, 21.39701867748817321, -9.422509992056140149 ) ) ;
#18185=CYLINDRICAL_SURFACE ( 'NONE', #19627, 0.5000000000000004441 ) ;
#18186=CARTESIAN_POINT ( 'NONE',  ( 6.204703633549690345, 30.76208216824730357, -14.16423886937410259 ) ) ;
#18187=CARTESIAN_POINT ( 'NONE',  ( -0.3689425029237898834, 31.17874883491396787, -10.36894250292378850 ) ) ;
#18188=CARTESIAN_POINT ( 'NONE',  ( 10.00000000000000178, 68.05374883491397497, 14.16423886937410082 ) ) ;
#18189=CARTESIAN_POINT ( 'NONE',  ( 1.472469842513823179, 46.42559781766745175, 4.923371831947296329 ) ) ;
#18190=CARTESIAN_POINT ( 'NONE',  ( -2.816281873526471635, 43.91530133659708923, -3.434112377981056508 ) ) ;
#18191=CARTESIAN_POINT ( 'NONE',  ( 0.5774900079438607392, 13.48035201082150358, 5.440088680355550821 ) ) ;
#18193=ORIENTED_EDGE ( 'NONE', *, *, #51498, .T. ) ;
#18194=CARTESIAN_POINT ( 'NONE',  ( 19.84674366389459621, 33.50893115100078745, 7.409399052514197653E-17 ) ) ;
#18195=CARTESIAN_POINT ( 'NONE',  ( 0.5774900079438590739, 42.64701867748816966, -5.440088680355550821 ) ) ;
#18196=CARTESIAN_POINT ( 'NONE',  ( 13.43411237798106583, 7.665301336597086568, -12.81628187352647252 ) ) ;
#18197=CARTESIAN_POINT ( 'NONE',  ( 6.204703633549690345, 20.76208216824730357, -14.16423886937410259 ) ) ;
#18201=UNCERTAINTY_MEASURE_WITH_UNIT (LENGTH_MEASURE( 1.000000000000000082E-05 ), #30257, 'distance_accuracy_value', 'NONE');
#18202=CARTESIAN_POINT ( 'NONE',  ( 10.00000000000000000, 29.75893115100078745, -9.846743663894594434 ) ) ;
#18203=CARTESIAN_POINT ( 'NONE',  ( 0.6178305044545818747, 53.49863466993041072, -9.382169495545419124 ) ) ;
#18204=CARTESIAN_POINT ( 'NONE',  ( 12.63842701281683034, 57.46726448433411605, 9.846743663894596210 ) ) ;
#18208=CARTESIAN_POINT ( 'NONE',  ( -4.164238869374098151, 61.59541550158063217, -3.795296366450310543 ) ) ;
#18209=CARTESIAN_POINT ( 'NONE',  ( 2.035157376598824452, 58.68868534415482685, 7.964842623401179544 ) ) ;
#18210=CARTESIAN_POINT ( 'NONE',  ( 6.204703633549690345, 7.845415501580634832, 14.16423886937410082 ) ) ;
#18211=CARTESIAN_POINT ( 'NONE',  ( 7.084665262690076126, 69.10535201082151957, 10.88017736071109987 ) ) ;
#18212=CARTESIAN_POINT ( 'NONE',  ( 19.84674366389459266, 53.71726448433411605, -2.638427012816827677 ) ) ;
#18213=CARTESIAN_POINT ( 'NONE',  ( 20.88017736071110875, 15.77201867748817143, -2.915334737309920765 ) ) ;
#18214=CARTESIAN_POINT ( 'NONE',  ( 18.72515096720583827, 65.05509018479936856, 6.499999999999810818 ) ) ;
#18215=CARTESIAN_POINT ( 'NONE',  ( 5.076628168052704559, 60.17559781766745175, -8.527530157486179263 ) ) ;
#18220=CARTESIAN_POINT ( 'NONE',  ( 17.08211943468705130, 13.47041550158063572, 12.26659068614894998 ) ) ;
#18221=CARTESIAN_POINT ( 'NONE',  ( -2.266590686148945544, 2.220415501580634388, 7.082119434687048631 ) ) ;
#18222=CARTESIAN_POINT ( 'NONE',  ( -0.3689425029237898834, 46.17874883491397497, -10.36894250292378850 ) ) ;
#18223=CARTESIAN_POINT ( 'NONE',  ( 12.63842701281683034, 57.46726448433411605, 9.846743663894596210 ) ) ;
#18224=CARTESIAN_POINT ( 'NONE',  ( 19.84674366389459266, 23.71726448433412315, -2.638427012816827677 ) ) ;
#18226=CARTESIAN_POINT ( 'NONE',  ( 10.00000000000000178, 24.31368534415484106, 10.88017736071110342 ) ) ;
#18227=CARTESIAN_POINT ( 'NONE',  ( 19.84674366389459621, 58.50893115100078745, 7.409399052514197653E-17 ) ) ;
#18228=CARTESIAN_POINT ( 'NONE',  ( -2.266590686148945544, 36.38708216824730357, -7.082119434687050408 ) ) ;
#18229=CARTESIAN_POINT ( 'NONE',  ( 19.42250999205614548, 5.980352010821504471, -5.440088680355545492 ) ) ;
#18232=CARTESIAN_POINT ( 'NONE',  ( -0.8801773607111008646, 63.27201867748817676, 2.915334737309923430 ) ) ;
#18234=CARTESIAN_POINT ( 'NONE',  ( 10.00000000000000178, 17.25893115100078745, 9.846743663894594434 ) ) ;
#18239=CARTESIAN_POINT ( 'NONE',  ( 2.791683348922240793, 21.63393115100078745, 7.208316651077764092 ) ) ;
#18241=CARTESIAN_POINT ( 'NONE',  ( 20.36894250292379382, 38.67874883491396076, 10.36894250292379205 ) ) ;
#18242=CARTESIAN_POINT ( 'NONE',  ( 2.791683348922237240, 35.38393115100079456, -7.208316651077763204 ) ) ;
#18243=CARTESIAN_POINT ( 'NONE',  ( 12.91533473730992121, 49.52201867748817676, 10.88017736071110164 ) ) ;
#18244=( NAMED_UNIT ( * ) SI_UNIT ( $, .STERADIAN. ) SOLID_ANGLE_UNIT ( ) );
#18245=CARTESIAN_POINT ( 'NONE',  ( 17.96484262340118221, 36.18868534415484106, -7.964842623401177768 ) ) ;
#18246=CARTESIAN_POINT ( 'NONE',  ( 20.15039907845753220, 37.62777174578614847, -6.262539305110077947 ) ) ;
#18251=CARTESIAN_POINT ( 'NONE',  ( -0.8801773607111008646, 43.27201867748817676, 2.915334737309923430 ) ) ;
#18252=CARTESIAN_POINT ( 'NONE',  ( 20.36894250292379382, 3.678748834913967869, 10.36894250292379205 ) ) ;
#18255=EDGE_LOOP ( 'NONE', ( #2783, #41226, #1001, #29889 ) ) ;
#18256=CARTESIAN_POINT ( 'NONE',  ( 21.09922568453594849, 31.20696800326375353, 6.408140936763242479 ) ) ;
#18257=CARTESIAN_POINT ( 'NONE',  ( 10.00000000000000178, 22.25893115100078745, 9.846743663894594434 ) ) ;
#18259=CARTESIAN_POINT ( 'NONE',  ( 19.38216949554541202, 45.99863466993041072, 9.382169495545424454 ) ) ;
#18261=CARTESIAN_POINT ( 'NONE',  ( 5.076628168052703671, 31.84226448433412315, 8.527530157486179263 ) ) ;
#18262=CARTESIAN_POINT ( 'NONE',  ( 2.035157376598822676, 62.43868534415483396, -7.964842623401177768 ) ) ;
#18264=CARTESIAN_POINT ( 'NONE',  ( 12.91533473730993009, 66.60535201082150536, -10.88017736071109987 ) ) ;
#18266=CARTESIAN_POINT ( 'NONE',  ( 0.6178305044545838731, 64.74863466993043914, 9.382169495545420901 ) ) ;
#18267=CARTESIAN_POINT ( 'NONE',  ( 0.1532563361054082862, 1.217264484334117824, 2.638427012816831674 ) ) ;
#18268=CARTESIAN_POINT ( 'NONE',  ( 19.38216949554541202, 15.99863466993042138, 9.382169495545424454 ) ) ;
#18269=CARTESIAN_POINT ( 'NONE',  ( -45.70923076923077133, 100.3461538461538538, -9.500000000000000000 ) ) ;
#18270=EDGE_CURVE ( 'NONE', #49843, #30282, #20692, .T. ) ;
#18271=CARTESIAN_POINT ( 'NONE',  ( 10.00000000000000000, 44.75893115100078745, -9.846743663894594434 ) ) ;
#18273=CARTESIAN_POINT ( 'NONE',  ( 13.79529636645030344, 3.262082168247301350, 14.16423886937410614 ) ) ;
#18274=CARTESIAN_POINT ( 'NONE',  ( 14.92337183194729988, 39.34226448433412315, -8.527530157486177487 ) ) ;
#18275=CARTESIAN_POINT ( 'NONE',  ( 10.00000000000000000, 27.87363466993042138, -12.81628187352647608 ) ) ;
#18276=CARTESIAN_POINT ( 'NONE',  ( 1.274849032794324932, 22.55509018479936145, -6.500000000000021316 ) ) ;
#18277=CARTESIAN_POINT ( 'NONE',  ( 4.559911319644449179, 48.89701867748817676, 9.422509992056141925 ) ) ;
#18278=CARTESIAN_POINT ( 'NONE',  ( 21.09922568453595559, 12.04030133659708746, -6.408140936763230044 ) ) ;
#18282=CARTESIAN_POINT ( 'NONE',  ( 2.791683348922240793, 21.63393115100078745, 7.208316651077764092 ) ) ;
#18283=CARTESIAN_POINT ( 'NONE',  ( 12.91533473730993009, 26.60535201082150536, -10.88017736071109987 ) ) ;
#18284=CARTESIAN_POINT ( 'NONE',  ( 19.38216949554541202, 35.99863466993041072, 9.382169495545424454 ) ) ;
#18285=CARTESIAN_POINT ( 'NONE',  ( 14.92337183194729988, 24.34226448433411960, -8.527530157486177487 ) ) ;
#18287=CARTESIAN_POINT ( 'NONE',  ( 15.44008868035555793, 36.39701867748816966, -9.422509992056140149 ) ) ;
#18289=CARTESIAN_POINT ( 'NONE',  ( 19.42250999205614193, 60.14701867748817676, 5.440088680355555262 ) ) ;
#18290=CARTESIAN_POINT ( 'NONE',  ( 18.52753015748618282, 43.92559781766745175, -4.923371831947291888 ) ) ;
#18291=CARTESIAN_POINT ( 'NONE',  ( 7.084665262690076126, 37.02201867748817676, -10.88017736071110164 ) ) ;
#18292=LINE ( 'NONE', #25797, #23218 ) ;
#18293=CARTESIAN_POINT ( 'NONE',  ( 19.42250999205614548, 45.98035201082150536, -5.440088680355545492 ) ) ;
#18294=CARTESIAN_POINT ( 'NONE',  ( 12.91533473730992121, 9.522018677488171434, 10.88017736071110164 ) ) ;
#18297=CARTESIAN_POINT ( 'NONE',  ( 7.361572987183169658, 39.96726448433411605, -9.846743663894592657 ) ) ;
#18298=CARTESIAN_POINT ( 'NONE',  ( -2.266590686148945544, 46.38708216824730357, -7.082119434687050408 ) ) ;
#18299=CARTESIAN_POINT ( 'NONE',  ( 3.640395162852212874, 107.5383484153110203, 12.00000000000000000 ) ) ;
#18302=CARTESIAN_POINT ( 'NONE',  ( 17.08211943468705840, 30.13708216824730357, -12.26659068614894466 ) ) ;
#18307=CARTESIAN_POINT ( 'NONE',  ( 10.00000000000000000, 1.813685344154838175, -10.88017736071110342 ) ) ;
#18308=CARTESIAN_POINT ( 'NONE',  ( 10.00000000000000000, 34.75893115100078745, -9.846743663894594434 ) ) ;
#18311=CARTESIAN_POINT ( 'NONE',  ( 7.084665262690076126, 64.10535201082150536, 10.88017736071109987 ) ) ;
#18313=AXIS2_PLACEMENT_3D ( 'NONE', #48423, #32434, #47925 ) ;
#18315=CARTESIAN_POINT ( 'NONE',  ( 15.44008868035555793, 31.39701867748817676, -9.422509992056140149 ) ) ;
#18316=CARTESIAN_POINT ( 'NONE',  ( 22.81628187352647785, 56.62363466993042493, 6.195893100308588602E-16 ) ) ;
#18317=CARTESIAN_POINT ( 'NONE',  ( 0.6178305044545818747, 13.49863466993041783, -9.382169495545419124 ) ) ;
#18318=CARTESIAN_POINT ( 'NONE',  ( 17.20831665107776587, 14.13393115100078568, -7.208316651077762316 ) ) ;
#18321=CARTESIAN_POINT ( 'NONE',  ( 10.00000000000000000, 6.813685344154838397, -10.88017736071110342 ) ) ;
#18322=CARTESIAN_POINT ( 'NONE',  ( 6.204703633549690345, 25.76208216824730712, -14.16423886937410259 ) ) ;
#18323=CARTESIAN_POINT ( 'NONE',  ( 15.44008868035555793, 36.39701867748816966, -9.422509992056140149 ) ) ;
#18324=CARTESIAN_POINT ( 'NONE',  ( 15.44008868035555793, 46.39701867748817676, -9.422509992056140149 ) ) ;
#18325=DIRECTION ( 'NONE',  ( 0.000000000000000000, -1.000000000000000000, 0.000000000000000000 ) ) ;
#18327=CARTESIAN_POINT ( 'NONE',  ( 10.00000000000000178, 12.25893115100078568, 9.846743663894594434 ) ) ;
#18329=CARTESIAN_POINT ( 'NONE',  ( 1.472469842513823179, 25.59226448433412315, -4.923371831947296329 ) ) ;
#18330=CARTESIAN_POINT ( 'NONE',  ( 10.00000000000000000, -0.2410688489992152128, -9.846743663894594434 ) ) ;
#18331=( BOUNDED_CURVE ( )  B_SPLINE_CURVE ( 2, ( #65795, #64801, #95320, #26821, #43300, #66291, #57314, #87807, #80319 ),
 .UNSPECIFIED., .F., .T. ) 
 B_SPLINE_CURVE_WITH_KNOTS ( ( 3, 2, 2, 2, 3 ),
 ( 0.6891432315068940495, 0.6904761904761904656, 0.6964285714285713969, 0.7023809523809523281, 0.7037139113502487442 ),
 .UNSPECIFIED. ) 
 CURVE ( )  GEOMETRIC_REPRESENTATION_ITEM ( )  RATIONAL_B_SPLINE_CURVE ( ( 0.9881565478350733400, 0.9923695281211490915, 1.000000000000000000, 0.9659258262890683122, 1.000000000000000000, 0.9659258262890683122, 1.000000000000000000, 0.9923695281211492025, 0.9881565478350733400 ) ) 
 REPRESENTATION_ITEM ( '' )  );
#18332=LINE ( 'NONE', #48812, #43139 ) ;
#18333=CARTESIAN_POINT ( 'NONE',  ( 18.52753015748617571, 18.09226448433411960, 4.923371831947298993 ) ) ;
#18334=CARTESIAN_POINT ( 'NONE',  ( 0.1532563361054083140, 46.00893115100079456, 1.131784320476157264E-15 ) ) ;
#18335=CARTESIAN_POINT ( 'NONE',  ( 19.38216949554541557, 42.24863466993041783, -9.382169495545420901 ) ) ;
#18337=CARTESIAN_POINT ( 'NONE',  ( 2.035157376598822676, 52.43868534415483396, -7.964842623401177768 ) ) ;
#18338=CARTESIAN_POINT ( 'NONE',  ( 7.361572987183169658, 24.96726448433412315, -9.846743663894592657 ) ) ;
#18339=CARTESIAN_POINT ( 'NONE',  ( -2.266590686148945544, 51.38708216824730357, -7.082119434687050408 ) ) ;
#18340=CARTESIAN_POINT ( 'NONE',  ( 7.361572987183169658, 19.96726448433411960, -9.846743663894592657 ) ) ;
#18343=CARTESIAN_POINT ( 'NONE',  ( 7.361572987183169658, 59.96726448433410894, -9.846743663894592657 ) ) ;
#18344=CARTESIAN_POINT ( 'NONE',  ( 2.917880565312950480, 10.97041550158063572, -12.26659068614894821 ) ) ;
#18345=CARTESIAN_POINT ( 'NONE',  ( 10.00000000000000000, 35.55374883491396787, -14.16423886937410082 ) ) ;
#18346=CARTESIAN_POINT ( 'NONE',  ( 19.84674366389459266, 28.71726448433411960, -2.638427012816827677 ) ) ;
#18348=CARTESIAN_POINT ( 'NONE',  ( 10.00000000000000178, 24.31368534415484106, 10.88017736071110342 ) ) ;
#18350=CARTESIAN_POINT ( 'NONE',  ( 15.44008868035555793, 46.39701867748817676, -9.422509992056140149 ) ) ;
#18351=CARTESIAN_POINT ( 'NONE',  ( 7.084665262690076126, 49.10535201082149825, 10.88017736071109987 ) ) ;
#18353=CARTESIAN_POINT ( 'NONE',  ( 21.09922568453594849, 36.20696800326375353, 6.408140936763242479 ) ) ;
#18354=CARTESIAN_POINT ( 'NONE',  ( 17.96484262340118221, 51.18868534415483396, -7.964842623401177768 ) ) ;
#18357=CARTESIAN_POINT ( 'NONE',  ( -36.44000000000001194, 92.00000000000000000, 9.500000000000000000 ) ) ;
#18358=CARTESIAN_POINT ( 'NONE',  ( -0.8801773607111009756, 68.06368534415484817, 1.068504757029289695E-15 ) ) ;
#18360=CARTESIAN_POINT ( 'NONE',  ( -0.8801773607111009756, 63.06368534415484106, 1.068504757029289695E-15 ) ) ;
#18361=CARTESIAN_POINT ( 'NONE',  ( 10.00000000000000178, 4.313685344154837509, 10.88017736071110342 ) ) ;
#18362=FACE_OUTER_BOUND ( 'NONE', #90298, .T. ) ;
#18363=CARTESIAN_POINT ( 'NONE',  ( -0.8801773607111008646, 3.272018677488171434, 2.915334737309923430 ) ) ;
#18364=CARTESIAN_POINT ( 'NONE',  ( 18.52753015748618282, 8.925597817667451750, -4.923371831947291888 ) ) ;
#18365=CARTESIAN_POINT ( 'NONE',  ( 13.79529636645030344, 8.262082168247300018, 14.16423886937410614 ) ) ;
#18366=CARTESIAN_POINT ( 'NONE',  ( 7.361572987183170547, 2.050597817667451750, 9.846743663894590881 ) ) ;
#18367=CARTESIAN_POINT ( 'NONE',  ( 20.88017736071110875, 10.77201867748817143, -2.915334737309920765 ) ) ;
#18368=CARTESIAN_POINT ( 'NONE',  ( 14.92337183194729633, 42.67559781766745886, 8.527530157486181039 ) ) ;
#18370=CARTESIAN_POINT ( 'NONE',  ( 12.63842701281683922, 54.55059781766745175, -9.846743663894590881 ) ) ;
#18374=CARTESIAN_POINT ( 'NONE',  ( 12.91533473730993009, 51.60535201082149825, -10.88017736071109987 ) ) ;
#18375=CARTESIAN_POINT ( 'NONE',  ( 17.20831665107776587, 54.13393115100079456, -7.208316651077762316 ) ) ;
#18376=CARTESIAN_POINT ( 'NONE',  ( 3.591859063236763294, 28.29030133659708568, -11.09922568453595026 ) ) ;
#18378=CARTESIAN_POINT ( 'NONE',  ( -0.8801773607111009756, 68.06368534415484817, 1.068504757029289695E-15 ) ) ;
#18379=CARTESIAN_POINT ( 'NONE',  ( 4.559911319644449179, 62.23035201082150536, -9.422509992056141925 ) ) ;
#18380=CARTESIAN_POINT ( 'NONE',  ( -2.266590686148945544, 66.38708216824730357, -7.082119434687050408 ) ) ;
#18382=CARTESIAN_POINT ( 'NONE',  ( 22.81628187352647785, 46.62363466993041783, 6.195893100308588602E-16 ) ) ;
#18385=CARTESIAN_POINT ( 'NONE',  ( 0.6178305044545818747, 28.49863466993041783, -9.382169495545419124 ) ) ;
#18386=CARTESIAN_POINT ( 'NONE',  ( 2.035157376598824452, 38.68868534415483396, 7.964842623401179544 ) ) ;
#18388=CARTESIAN_POINT ( 'NONE',  ( 7.361572987183170547, 62.05059781766745886, 9.846743663894590881 ) ) ;
#18389=CARTESIAN_POINT ( 'NONE',  ( 0.1532563361054082862, 11.21726448433411605, 2.638427012816831674 ) ) ;
#18390=CARTESIAN_POINT ( 'NONE',  ( 19.84674366389459621, 48.50893115100078745, 7.409399052514197653E-17 ) ) ;
#18395=CARTESIAN_POINT ( 'NONE',  ( 19.84674366389459266, 33.71726448433410894, -2.638427012816827677 ) ) ;
#18396=CARTESIAN_POINT ( 'NONE',  ( 1.472469842513823179, 0.5922644843341181575, -4.923371831947296329 ) ) ;
#18397=CARTESIAN_POINT ( 'NONE',  ( 10.00000000000000178, 57.25893115100078745, 9.846743663894594434 ) ) ;
#18400=CARTESIAN_POINT ( 'NONE',  ( -1.099225684535947600, 23.70696800326375708, -6.408140936763238038 ) ) ;
#18402=CARTESIAN_POINT ( 'NONE',  ( 0.1532563361054100626, 50.80059781766745175, -2.638427012816831230 ) ) ;
#18403=DIRECTION ( 'NONE',  ( 0.000000000000000000, 0.000000000000000000, 1.000000000000000000 ) ) ;
#18404=CARTESIAN_POINT ( 'NONE',  ( 24.16423886937410614, 49.51208216824730357, -3.795296366450302550 ) ) ;
#18405=CARTESIAN_POINT ( 'NONE',  ( 5.076628168052704559, 15.17559781766745175, -8.527530157486179263 ) ) ;
#18408=CARTESIAN_POINT ( 'NONE',  ( -4.164238869374099927, 52.01208216824729647, 3.795296366450308767 ) ) ;
#18409=CARTESIAN_POINT ( 'NONE',  ( 0.1532563361054083140, 56.00893115100078745, 1.131784320476157264E-15 ) ) ;
#18410=CARTESIAN_POINT ( 'NONE',  ( 12.91533473730992121, 9.522018677488171434, 10.88017736071110164 ) ) ;
#18411=CARTESIAN_POINT ( 'NONE',  ( 24.16423886937410614, 39.51208216824731068, -3.795296366450302550 ) ) ;
#18412=CARTESIAN_POINT ( 'NONE',  ( 24.16423886937410614, 44.30374883491397497, 8.672049930838204340E-16 ) ) ;
#18415=CARTESIAN_POINT ( 'NONE',  ( 19.84674366389459266, 58.30059781766745886, 2.638427012816836559 ) ) ;
#18416=VERTEX_POINT ( 'NONE', #51694 ) ;
#18417=CARTESIAN_POINT ( 'NONE',  ( 10.00000000000000000, 31.81368534415483751, -10.88017736071110342 ) ) ;
#18418=DIRECTION ( 'NONE',  ( 0.000000000000000000, -1.000000000000000000, 0.000000000000000000 ) ) ;
#18419=VECTOR ( 'NONE', #96595, 1000.000000000000000 ) ;
#18420=CARTESIAN_POINT ( 'NONE',  ( 20.00000000000000711, 98.59912998021083297, -4.999999999999999112 ) ) ;
#18421=CARTESIAN_POINT ( 'NONE',  ( 18.52753015748618282, 53.92559781766745175, -4.923371831947291888 ) ) ;
#18422=CYLINDRICAL_SURFACE ( 'NONE', #77762, 0.5000000000000004441 ) ;
#18424=CARTESIAN_POINT ( 'NONE',  ( 1.472469842513823179, 61.42559781766745175, 4.923371831947296329 ) ) ;
#18429=CARTESIAN_POINT ( 'NONE',  ( 13.79529636645030344, 33.26208216824730357, 14.16423886937410614 ) ) ;
#18430=FACE_OUTER_BOUND ( 'NONE', #34094, .T. ) ;
#18432=CARTESIAN_POINT ( 'NONE',  ( 19.10478245763052030, 45.10160829253886305, 5.990408912944319653 ) ) ;
#18433=CARTESIAN_POINT ( 'NONE',  ( 20.88017736071110519, 15.56368534415483751, 2.639326808657452039E-16 ) ) ;
#18434=CARTESIAN_POINT ( 'NONE',  ( -1.099225684535947600, 24.54030133659708923, 6.408140936763237150 ) ) ;
#18437=CARTESIAN_POINT ( 'NONE',  ( 19.84674366389459621, 13.50893115100078568, 7.409399052514197653E-17 ) ) ;
#18438=CARTESIAN_POINT ( 'NONE',  ( 0.1532563361054082862, 21.21726448433411605, 2.638427012816831674 ) ) ;
#18440=CARTESIAN_POINT ( 'NONE',  ( 4.559911319644449179, 12.23035201082150714, -9.422509992056141925 ) ) ;
#18443=CARTESIAN_POINT ( 'NONE',  ( 10.00000000000000178, 34.31368534415484106, 10.88017736071110342 ) ) ;
#18444=CARTESIAN_POINT ( 'NONE',  ( 20.88017736071110519, 35.56368534415484106, 2.639326808657452039E-16 ) ) ;
#18445=CARTESIAN_POINT ( 'NONE',  ( -2.816281873526473856, -0.8763653300695799508, 9.499525473075851096E-16 ) ) ;
#18447=CARTESIAN_POINT ( 'NONE',  ( -46.02116055762927971, 104.3980163073828606, -5.346303181598003995 ) ) ;
#18448=CARTESIAN_POINT ( 'NONE',  ( 14.92337183194729988, 4.342264484334117824, -8.527530157486177487 ) ) ;
#18449=ORIENTED_EDGE ( 'NONE', *, *, #9604, .F. ) ;
#18450=CARTESIAN_POINT ( 'NONE',  ( 10.00000000000000178, 29.31368534415483751, 10.88017736071110342 ) ) ;
#18451=CARTESIAN_POINT ( 'NONE',  ( 0.6178305044545818747, 33.49863466993042493, -9.382169495545419124 ) ) ;
#18453=CARTESIAN_POINT ( 'NONE',  ( 0.1532563361054082862, 66.21726448433413736, 2.638427012816831674 ) ) ;
#18454=CARTESIAN_POINT ( 'NONE',  ( 0.5774900079438590739, 57.64701867748817676, -5.440088680355550821 ) ) ;
#18455=VECTOR ( 'NONE', #94059, 1000.000000000000000 ) ;
#18456=CARTESIAN_POINT ( 'NONE',  ( 7.361572987183170547, 17.05059781766745530, 9.846743663894590881 ) ) ;
#18457=CARTESIAN_POINT ( 'NONE',  ( 22.81628187352647785, 31.62363466993042138, 6.195893100308588602E-16 ) ) ;
#18458=CARTESIAN_POINT ( 'NONE',  ( 7.361572987183170547, 7.050597817667451750, 9.846743663894590881 ) ) ;
#18461=CARTESIAN_POINT ( 'NONE',  ( 10.00000000000000000, 11.81368534415483751, -10.88017736071110342 ) ) ;
#18462=CARTESIAN_POINT ( 'NONE',  ( -2.816281873526473856, 54.33196800326376064, 3.434112377981055619 ) ) ;
#18463=CARTESIAN_POINT ( 'NONE',  ( -2.266590686148945544, 27.22041550158063572, 7.082119434687048631 ) ) ;
#18464=CARTESIAN_POINT ( 'NONE',  ( 0.1532563361054100626, 15.80059781766745353, -2.638427012816831230 ) ) ;
#18465=CARTESIAN_POINT ( 'NONE',  ( 20.88017736071110875, 10.77201867748817143, -2.915334737309920765 ) ) ;
#18466=CARTESIAN_POINT ( 'NONE',  ( 5.076628168052703671, 26.84226448433411960, 8.527530157486179263 ) ) ;
#18467=CARTESIAN_POINT ( 'NONE',  ( -4.164238869374098151, 66.59541550158060375, -3.795296366450310543 ) ) ;
#18468=ORIENTED_EDGE ( 'NONE', *, *, #90664, .F. ) ;
#18469=CARTESIAN_POINT ( 'NONE',  ( 15.44008868035555260, 9.730352010821505360, 9.422509992056143702 ) ) ;
#18470=EDGE_CURVE ( 'NONE', #54853, #62857, #43449, .T. ) ;
#18471=CARTESIAN_POINT ( 'NONE',  ( 4.559911319644449179, 18.89701867748817321, 9.422509992056141925 ) ) ;
#18472=CARTESIAN_POINT ( 'NONE',  ( 2.603489959281115151, 16.58210964143323807, 6.499999999999462652 ) ) ;
#18473=ORIENTED_EDGE ( 'NONE', *, *, #54980, .T. ) ;
#18474=CARTESIAN_POINT ( 'NONE',  ( 10.00000000000000000, 64.75893115100078035, -9.846743663894594434 ) ) ;
#18475=CARTESIAN_POINT ( 'NONE',  ( 2.035157376598824452, 28.68868534415484106, 7.964842623401179544 ) ) ;
#18476=CARTESIAN_POINT ( 'NONE',  ( 14.92337183194729988, 59.34226448433412315, -8.527530157486177487 ) ) ;
#18480=CARTESIAN_POINT ( 'NONE',  ( 22.26659068614895176, 39.72041550158063217, -7.082119434687042414 ) ) ;
#18481=CARTESIAN_POINT ( 'NONE',  ( 12.91533473730992121, 44.52201867748816966, 10.88017736071110164 ) ) ;
#18482=CARTESIAN_POINT ( 'NONE',  ( 20.88017736071110164, 20.35535201082150891, 2.915334737309930979 ) ) ;
#18483=CARTESIAN_POINT ( 'NONE',  ( 2.791683348922237240, 55.38393115100078745, -7.208316651077763204 ) ) ;
#18485=CARTESIAN_POINT ( 'NONE',  ( 19.84674366389459621, 33.50893115100078745, 7.409399052514197653E-17 ) ) ;
#18486=CARTESIAN_POINT ( 'NONE',  ( 17.20831665107776587, 2.883931151000785231, 7.208316651077764980 ) ) ;
#18489=CARTESIAN_POINT ( 'NONE',  ( 17.96484262340118221, 14.93868534415483751, 7.964842623401181321 ) ) ;
#18490=CARTESIAN_POINT ( 'NONE',  ( 14.92337183194729988, 9.342264484334119601, -8.527530157486177487 ) ) ;
#18491=CARTESIAN_POINT ( 'NONE',  ( -1.099225684535947600, -0.4596986634029132657, 6.408140936763237150 ) ) ;
#18492=CARTESIAN_POINT ( 'NONE',  ( 20.88017736071110164, 45.35535201082149115, 2.915334737309930979 ) ) ;
#18493=CARTESIAN_POINT ( 'NONE',  ( 20.88017736071110164, 15.35535201082150358, 2.915334737309930979 ) ) ;
#18494=CARTESIAN_POINT ( 'NONE',  ( 3.591859063236761518, 39.95696800326375353, 11.09922568453594849 ) ) ;
#18495=CARTESIAN_POINT ( 'NONE',  ( -4.164238869374099927, 37.01208216824731068, 3.795296366450308767 ) ) ;
#18497=CARTESIAN_POINT ( 'NONE',  ( -2.816281873526471635, 63.91530133659708923, -3.434112377981056508 ) ) ;
#18499=CARTESIAN_POINT ( 'NONE',  ( 18.52753015748618282, 63.92559781766745886, -4.923371831947291888 ) ) ;
#18500=CARTESIAN_POINT ( 'NONE',  ( -0.2418659066527494572, 14.26028685723174050, -6.114288769123083611 ) ) ;
#18501=CARTESIAN_POINT ( 'NONE',  ( 0.5774900079438590739, 32.64701867748816966, -5.440088680355550821 ) ) ;
#18503=CARTESIAN_POINT ( 'NONE',  ( 18.52753015748617571, 3.092264484334118269, 4.923371831947298993 ) ) ;
#18506=CARTESIAN_POINT ( 'NONE',  ( 19.84674366389459266, 28.71726448433411960, -2.638427012816827677 ) ) ;
#18507=CARTESIAN_POINT ( 'NONE',  ( 19.84674366389459266, 8.300597817667451750, 2.638427012816836559 ) ) ;
#18508=CARTESIAN_POINT ( 'NONE',  ( 10.00000000000000178, 7.258931151000785675, 9.846743663894594434 ) ) ;
#18510=CARTESIAN_POINT ( 'NONE',  ( 2.035157376598822676, 57.43868534415484106, -7.964842623401177768 ) ) ;
#18512=CARTESIAN_POINT ( 'NONE',  ( 2.035157376598822676, 62.43868534415483396, -7.964842623401177768 ) ) ;
#18513=TOROIDAL_SURFACE ( 'NONE', #47262, 1.000000000000000000, 0.5000000000000000000 ) ;
#18514=CARTESIAN_POINT ( 'NONE',  ( 10.00000000000000178, 17.25893115100078745, 9.846743663894594434 ) ) ;
#18515=ORIENTED_EDGE ( 'NONE', *, *, #43101, .F. ) ;
#18516=VECTOR ( 'NONE', #78858, 1000.000000000000000 ) ;
#18518=CARTESIAN_POINT ( 'NONE',  ( 18.52753015748618282, 58.92559781766745886, -4.923371831947291888 ) ) ;
#18521=CARTESIAN_POINT ( 'NONE',  ( 13.79529636645031943, 10.34541550158063394, -14.16423886937409904 ) ) ;
#18523=DIRECTION ( 'NONE',  ( 0.000000000000000000, -1.000000000000000000, 0.000000000000000000 ) ) ;
#18524=( NAMED_UNIT ( * ) PLANE_ANGLE_UNIT ( ) SI_UNIT ( $, .RADIAN. ) );
#18525=CARTESIAN_POINT ( 'NONE',  ( -4.164238869374098151, 31.59541550158063927, -3.795296366450310543 ) ) ;
#18527=PRESENTATION_STYLE_ASSIGNMENT (( #18042 ) ) ;
#18528=CARTESIAN_POINT ( 'NONE',  ( 20.88017736071110164, 40.35535201082150536, 2.915334737309930979 ) ) ;
#18531=CARTESIAN_POINT ( 'NONE',  ( 19.84674366389459621, 13.50893115100078568, 7.409399052514197653E-17 ) ) ;
#18532=CARTESIAN_POINT ( 'NONE',  ( -0.8801773607111008646, 58.27201867748816966, 2.915334737309923430 ) ) ;
#18533=CARTESIAN_POINT ( 'NONE',  ( 0.1532563361054083140, 11.00893115100078568, 1.131784320476157264E-15 ) ) ;
#18534=CARTESIAN_POINT ( 'NONE',  ( 19.38216949554541557, 42.24863466993041783, -9.382169495545420901 ) ) ;
#18535=CARTESIAN_POINT ( 'NONE',  ( 17.20831665107776587, 32.88393115100078745, 7.208316651077764980 ) ) ;
#18537=CARTESIAN_POINT ( 'NONE',  ( 20.88017736071110164, 60.35535201082151957, 2.915334737309930979 ) ) ;
#18538=CARTESIAN_POINT ( 'NONE',  ( 10.00000000000000178, 22.25893115100078745, 9.846743663894594434 ) ) ;
#18539=CARTESIAN_POINT ( 'NONE',  ( 22.81628187352648496, 26.83196800326374998, -3.434112377981050290 ) ) ;
#18541=CARTESIAN_POINT ( 'NONE',  ( 14.92337183194729988, 24.34226448433411960, -8.527530157486177487 ) ) ;
#18542=CARTESIAN_POINT ( 'NONE',  ( 17.08211943468705130, 8.470415501580635720, 12.26659068614894998 ) ) ;
#18545=CARTESIAN_POINT ( 'NONE',  ( -0.8801773607111008646, 38.27201867748816255, 2.915334737309923430 ) ) ;
#18546=CARTESIAN_POINT ( 'NONE',  ( 0.5774900079438590739, 57.64701867748817676, -5.440088680355550821 ) ) ;
#18547=CARTESIAN_POINT ( 'NONE',  ( 10.00000000000000178, 33.05374883491396787, 14.16423886937410082 ) ) ;
#18548=CARTESIAN_POINT ( 'NONE',  ( 5.076628168052704559, 50.17559781766745886, -8.527530157486179263 ) ) ;
#18549=CARTESIAN_POINT ( 'NONE',  ( 19.84674366389459266, 13.30059781766745353, 2.638427012816836559 ) ) ;
#18552=CARTESIAN_POINT ( 'NONE',  ( 19.42250999205614548, 45.98035201082150536, -5.440088680355545492 ) ) ;
#18554=FACE_OUTER_BOUND ( 'NONE', #73711, .T. ) ;
#18555=CARTESIAN_POINT ( 'NONE',  ( 22.81628187352647785, 16.62363466993042138, 6.195893100308588602E-16 ) ) ;
#18556=CARTESIAN_POINT ( 'NONE',  ( 19.38216949554541557, 27.24863466993041783, -9.382169495545420901 ) ) ;
#18557=CARTESIAN_POINT ( 'NONE',  ( 19.84674366389459266, 53.71726448433411605, -2.638427012816827677 ) ) ;
#18559=CARTESIAN_POINT ( 'NONE',  ( 2.035157376598824452, 3.688685344154837953, 7.964842623401179544 ) ) ;
#18560=CARTESIAN_POINT ( 'NONE',  ( 20.88017736071110164, 60.35535201082151957, 2.915334737309930979 ) ) ;
#18561=CARTESIAN_POINT ( 'NONE',  ( -22.44000000000001194, 93.50000000000000000, -9.500000000000000000 ) ) ;
#18564=CARTESIAN_POINT ( 'NONE',  ( 0.5600000000000083800, 105.0000000000000000, -5.000000000000000000 ) ) ;
#18565=CARTESIAN_POINT ( 'NONE',  ( 17.96484262340118221, 61.18868534415482685, -7.964842623401177768 ) ) ;
#18566=CARTESIAN_POINT ( 'NONE',  ( 17.96484262340118221, 54.93868534415484106, 7.964842623401181321 ) ) ;
#18568=CARTESIAN_POINT ( 'NONE',  ( 17.20831665107776587, 24.13393115100078035, -7.208316651077762316 ) ) ;
#18569=CARTESIAN_POINT ( 'NONE',  ( 20.88017736071110164, 20.35535201082150891, 2.915334737309930979 ) ) ;
#18571=CARTESIAN_POINT ( 'NONE',  ( 0.1532563361054082862, 66.21726448433413736, 2.638427012816831674 ) ) ;
#18572=CARTESIAN_POINT ( 'NONE',  ( 20.88017736071110519, 25.56368534415483751, 2.639326808657452039E-16 ) ) ;
#18573=CARTESIAN_POINT ( 'NONE',  ( 1.274849032794131976, 13.57228050351029403, 6.499999999999760192 ) ) ;
#18575=CARTESIAN_POINT ( 'NONE',  ( 21.09922568453594849, 36.20696800326375353, 6.408140936763242479 ) ) ;
#18577=CARTESIAN_POINT ( 'NONE',  ( 12.91533473730992121, 49.52201867748817676, 10.88017736071110164 ) ) ;
#18578=CARTESIAN_POINT ( 'NONE',  ( 16.40814093676323893, 15.79030133659708746, 11.09922568453595026 ) ) ;
#18579=CARTESIAN_POINT ( 'NONE',  ( 17.39651004071843232, 17.93575266056828355, 6.499999999999984013 ) ) ;
#18580=CARTESIAN_POINT ( 'NONE',  ( 10.00000000000000000, 21.81368534415484106, -10.88017736071110342 ) ) ;
#18581=CARTESIAN_POINT ( 'NONE',  ( 13.79529636645030344, 53.26208216824730357, 14.16423886937410614 ) ) ;
#18582=CARTESIAN_POINT ( 'NONE',  ( 19.84674366389459266, 38.30059781766745175, 2.638427012816836559 ) ) ;
#18583=CARTESIAN_POINT ( 'NONE',  ( 2.791683348922240793, 6.633931151000785675, 7.208316651077764092 ) ) ;
#18584=CARTESIAN_POINT ( 'NONE',  ( 2.035157376598824452, 48.68868534415483396, 7.964842623401179544 ) ) ;
#18586=CARTESIAN_POINT ( 'NONE',  ( 2.917880565312950480, 20.97041550158063217, -12.26659068614894821 ) ) ;
#18588=EDGE_CURVE ( 'NONE', #13640, #20501, #56569, .T. ) ;
#18591=ORIENTED_EDGE ( 'NONE', *, *, #83822, .F. ) ;
#18592=CARTESIAN_POINT ( 'NONE',  ( 22.26659068614894466, 43.88708216824729647, 7.082119434687054849 ) ) ;
#18593=CARTESIAN_POINT ( 'NONE',  ( -4.164238869374099039, 56.80374883491397497, 8.674139862899312516E-16 ) ) ;
#18594=CARTESIAN_POINT ( 'NONE',  ( 0.1532563361054083140, 11.00893115100078568, 1.131784320476157264E-15 ) ) ;
#18595=CARTESIAN_POINT ( 'NONE',  ( 16.40814093676324603, 17.45696800326375353, -11.09922568453594671 ) ) ;
#18597=DIRECTION ( 'NONE',  ( 0.000000000000000000, -0.000000000000000000, 1.000000000000000000 ) ) ;
#18598=CARTESIAN_POINT ( 'NONE',  ( 17.96484262340118221, 4.938685344154837509, 7.964842623401181321 ) ) ;
#18599=CARTESIAN_POINT ( 'NONE',  ( -1.099225684535947600, 29.54030133659708923, 6.408140936763237150 ) ) ;
#18600=CARTESIAN_POINT ( 'NONE',  ( 2.917880565312950480, 40.97041550158063217, -12.26659068614894821 ) ) ;
#18603=CARTESIAN_POINT ( 'NONE',  ( -0.8801773607111009756, 68.06368534415484817, 1.068504757029289695E-15 ) ) ;
#18606=VERTEX_POINT ( 'NONE', #52670 ) ;
#18607=PRESENTATION_STYLE_ASSIGNMENT (( #35061 ) ) ;
#18608=CARTESIAN_POINT ( 'NONE',  ( 14.92337183194729988, 14.34226448433411782, -8.527530157486177487 ) ) ;
#18609=B_SPLINE_CURVE_WITH_KNOTS ( 'NONE', 3,
 ( #74388, #51407, #29875, #22403 ),
 .UNSPECIFIED., .F., .F.,
 ( 4, 4 ),
 ( 2.388857365163340366E-16, 0.002392975128318463370 ),
 .UNSPECIFIED. ) ;
#18611=CARTESIAN_POINT ( 'NONE',  ( -0.8801773607111008646, 3.272018677488171434, 2.915334737309923430 ) ) ;
#18612=CARTESIAN_POINT ( 'NONE',  ( 12.91533473730992121, 14.52201867748817143, 10.88017736071110164 ) ) ;
#18613=CARTESIAN_POINT ( 'NONE',  ( 1.472469842513823179, 50.59226448433411605, -4.923371831947296329 ) ) ;
#18614=CARTESIAN_POINT ( 'NONE',  ( 13.43411237798105340, 0.5819680032637533085, 12.81628187352647963 ) ) ;
#18615=LINE ( 'NONE', #11110, #18419 ) ;
#18619=CARTESIAN_POINT ( 'NONE',  ( -2.816281873526473856, 24.12363466993042138, 9.499525473075851096E-16 ) ) ;
#18621=CARTESIAN_POINT ( 'NONE',  ( 24.16423886937410614, 59.30374883491397497, 8.672049930838204340E-16 ) ) ;
#18623=CARTESIAN_POINT ( 'NONE',  ( 6.204703633549690345, 55.76208216824730357, -14.16423886937410259 ) ) ;
#18624=VERTEX_POINT ( 'NONE', #53165 ) ;
#18625=CARTESIAN_POINT ( 'NONE',  ( 2.035157376598822676, 32.43868534415483396, -7.964842623401177768 ) ) ;
#18626=CARTESIAN_POINT ( 'NONE',  ( 15.44008868035555260, 39.73035201082150536, 9.422509992056143702 ) ) ;
#18628=CARTESIAN_POINT ( 'NONE',  ( 20.88017736071110875, 30.77201867748816966, -2.915334737309920765 ) ) ;
#18630=( GEOMETRIC_REPRESENTATION_CONTEXT ( 3 ) GLOBAL_UNCERTAINTY_ASSIGNED_CONTEXT ( ( #97301 ) ) GLOBAL_UNIT_ASSIGNED_CONTEXT ( ( #32129, #41518, #18997 ) ) REPRESENTATION_CONTEXT ( 'NONE', 'WORKASPACE' ) );
#18633=ORIENTED_EDGE ( 'NONE', *, *, #59927, .T. ) ;
#18634=CARTESIAN_POINT ( 'NONE',  ( 1.472469842513823179, 16.42559781766745175, 4.923371831947296329 ) ) ;
#18635=VERTEX_POINT ( 'NONE', #60166 ) ;
#18637=CARTESIAN_POINT ( 'NONE',  ( 10.00000000000000178, 47.25893115100078745, 9.846743663894594434 ) ) ;
#18638=EDGE_CURVE ( 'NONE', #11556, #30617, #70749, .T. ) ;
#18640=CARTESIAN_POINT ( 'NONE',  ( -2.816281873526473856, 59.33196800326374643, 3.434112377981055619 ) ) ;
#18643=CARTESIAN_POINT ( 'NONE',  ( -46.34161155552018840, 104.0475784593821658, 5.921604558742994406 ) ) ;
#18645=DIRECTION ( 'NONE',  ( 0.000000000000000000, 0.000000000000000000, -1.000000000000000000 ) ) ;
#18646=CARTESIAN_POINT ( 'NONE',  ( 20.36894250292379738, 49.92874883491396787, -10.36894250292379027 ) ) ;
#18650=CARTESIAN_POINT ( 'NONE',  ( 18.52753015748617571, 33.09226448433411605, 4.923371831947298993 ) ) ;
#18654=CARTESIAN_POINT ( 'NONE',  ( 10.00000000000000178, 10.37363466993041961, 12.81628187352647608 ) ) ;
#18655=CARTESIAN_POINT ( 'NONE',  ( 10.00000000000000000, 66.81368534415484817, -10.88017736071110342 ) ) ;
#18656=CARTESIAN_POINT ( 'NONE',  ( 0.2751277870542949144, 4.366073187301309666, -6.499999999999997335 ) ) ;
#18657=STYLED_ITEM ( 'NONE', ( #26168 ), #35550 ) ;
#18658=CARTESIAN_POINT ( 'NONE',  ( 19.84674366389459266, 63.30059781766745886, 2.638427012816836559 ) ) ;
#18660=CIRCLE ( 'NONE', #2777, 0.5000000000000004441 ) ;
#18662=CARTESIAN_POINT ( 'NONE',  ( 4.559911319644449179, 2.230352010821504916, -9.422509992056141925 ) ) ;
#18664=CARTESIAN_POINT ( 'NONE',  ( 0.5774900079438607392, 38.48035201082150536, 5.440088680355550821 ) ) ;
#18665=CARTESIAN_POINT ( 'NONE',  ( 0.6178305044545818747, 8.498634669930421381, -9.382169495545419124 ) ) ;
#18666=CARTESIAN_POINT ( 'NONE',  ( 10.00000000000000000, 66.81368534415484817, -10.88017736071110342 ) ) ;
#18668=CARTESIAN_POINT ( 'NONE',  ( 0.5774900079438607392, 3.480352010821504027, 5.440088680355550821 ) ) ;
#18672=CARTESIAN_POINT ( 'NONE',  ( 7.361572987183169658, 49.96726448433410894, -9.846743663894592657 ) ) ;
#18673=CARTESIAN_POINT ( 'NONE',  ( 17.20831665107776587, 17.88393115100078745, 7.208316651077764980 ) ) ;
#18675=CARTESIAN_POINT ( 'NONE',  ( 3.591859063236763294, 18.29030133659708568, -11.09922568453595026 ) ) ;
#18677=CARTESIAN_POINT ( 'NONE',  ( 7.084665262690076126, 29.10535201082150181, 10.88017736071109987 ) ) ;
#18680=CARTESIAN_POINT ( 'NONE',  ( -0.3689425029237881626, 37.42874883491396787, 10.36894250292379027 ) ) ;
#18681=CARTESIAN_POINT ( 'NONE',  ( -4.164238869374098151, 31.59541550158063927, -3.795296366450310543 ) ) ;
#18682=CARTESIAN_POINT ( 'NONE',  ( 2.035157376598822676, 7.438685344154837509, -7.964842623401177768 ) ) ;
#18683=CARTESIAN_POINT ( 'NONE',  ( 7.361572987183169658, 44.96726448433412315, -9.846743663894592657 ) ) ;
#18685=CARTESIAN_POINT ( 'NONE',  ( 19.38216949554541557, 42.24863466993041783, -9.382169495545420901 ) ) ;
#18686=CARTESIAN_POINT ( 'NONE',  ( -0.8801773607111008646, 13.27201867748817143, 2.915334737309923430 ) ) ;
#18688=CARTESIAN_POINT ( 'NONE',  ( 19.84674366389459266, 33.30059781766744464, 2.638427012816836559 ) ) ;
#18689=AXIS2_PLACEMENT_3D ( 'NONE', #34995, #89002, #82978 ) ;
#18690=CARTESIAN_POINT ( 'NONE',  ( 0.5774900079438607392, 43.48035201082151247, 5.440088680355550821 ) ) ;
#18691=CARTESIAN_POINT ( 'NONE',  ( -1.099225684535947600, 9.540301336597087456, 6.408140936763237150 ) ) ;
#18692=CARTESIAN_POINT ( 'NONE',  ( -4.164238869374099927, 27.01208216824730357, 3.795296366450308767 ) ) ;
#18694=CARTESIAN_POINT ( 'NONE',  ( 19.84674366389459266, 23.71726448433412315, -2.638427012816827677 ) ) ;
#18695=CARTESIAN_POINT ( 'NONE',  ( 22.81628187352647785, 56.62363466993042493, 6.195893100308588602E-16 ) ) ;
#18696=CARTESIAN_POINT ( 'NONE',  ( 1.472469842513823179, 55.59226448433412315, -4.923371831947296329 ) ) ;
#18700=CARTESIAN_POINT ( 'NONE',  ( 0.5774900079438607392, 3.480352010821504916, 5.440088680355550821 ) ) ;
#18701=CARTESIAN_POINT ( 'NONE',  ( -0.3689425029237898834, 6.178748834913968757, -10.36894250292378850 ) ) ;
#18702=CARTESIAN_POINT ( 'NONE',  ( 14.92337183194729988, 4.342264484334117824, -8.527530157486177487 ) ) ;
#18703=CARTESIAN_POINT ( 'NONE',  ( 17.20831665107776587, 49.13393115100078745, -7.208316651077762316 ) ) ;
#18704=CARTESIAN_POINT ( 'NONE',  ( 12.91533473730992121, 29.52201867748817321, 10.88017736071110164 ) ) ;
#18706=CARTESIAN_POINT ( 'NONE',  ( 19.84674366389459266, 63.71726448433412315, -2.638427012816827677 ) ) ;
#18707=( GEOMETRIC_REPRESENTATION_CONTEXT ( 3 ) GLOBAL_UNCERTAINTY_ASSIGNED_CONTEXT ( ( #58134 ) ) GLOBAL_UNIT_ASSIGNED_CONTEXT ( ( #61346, #44859, #23372 ) ) REPRESENTATION_CONTEXT ( 'NONE', 'WORKASPACE' ) );
#18709=ORIENTED_EDGE ( 'NONE', *, *, #79080, .F. ) ;
#18712=VERTEX_POINT ( 'NONE', #17155 ) ;
#18714=CARTESIAN_POINT ( 'NONE',  ( -4.164238869374099927, 12.01208216824730357, 3.795296366450308767 ) ) ;
#18715=CARTESIAN_POINT ( 'NONE',  ( 24.16423886937409904, 14.09541550158063217, 3.795296366450317205 ) ) ;
#18716=CARTESIAN_POINT ( 'NONE',  ( 22.26659068614895176, 44.72041550158063927, -7.082119434687042414 ) ) ;
#18717=CARTESIAN_POINT ( 'NONE',  ( 7.361572987183170547, 52.05059781766745175, 9.846743663894590881 ) ) ;
#18718=CARTESIAN_POINT ( 'NONE',  ( 19.84674366389459266, 33.30059781766744464, 2.638427012816836559 ) ) ;
#18720=CARTESIAN_POINT ( 'NONE',  ( 2.035157376598824452, 38.68868534415483396, 7.964842623401179544 ) ) ;
#18721=CARTESIAN_POINT ( 'NONE',  ( 14.92337183194729633, 57.67559781766745886, 8.527530157486181039 ) ) ;
#18722=CARTESIAN_POINT ( 'NONE',  ( -0.3689425029237898834, 6.178748834913968757, -10.36894250292378850 ) ) ;
#18723=CARTESIAN_POINT ( 'NONE',  ( -0.3689425029237881626, 42.42874883491396787, 10.36894250292379027 ) ) ;
#18725=CARTESIAN_POINT ( 'NONE',  ( 17.96484262340118221, 4.938685344154837509, 7.964842623401181321 ) ) ;
#18728=CARTESIAN_POINT ( 'NONE',  ( 17.96484262340118221, 66.18868534415483396, -7.964842623401177768 ) ) ;
#18729=CARTESIAN_POINT ( 'NONE',  ( 18.52753015748617571, 23.09226448433411960, 4.923371831947298993 ) ) ;
#18734=CARTESIAN_POINT ( 'NONE',  ( 0.1532563361054082862, 21.21726448433412315, 2.638427012816831674 ) ) ;
#18736=CARTESIAN_POINT ( 'NONE',  ( -4.164238869374099039, 26.80374883491397142, 8.674139862899312516E-16 ) ) ;
#18737=CARTESIAN_POINT ( 'NONE',  ( 0.1532563361054082862, 36.21726448433410894, 2.638427012816831674 ) ) ;
#18738=CARTESIAN_POINT ( 'NONE',  ( 19.42250999205614548, 60.98035201082151247, -5.440088680355545492 ) ) ;
#18740=CARTESIAN_POINT ( 'NONE',  ( -0.8801773607111008646, 43.27201867748817676, 2.915334737309923430 ) ) ;
#18741=CARTESIAN_POINT ( 'NONE',  ( 0.1532563361054082862, 51.21726448433412315, 2.638427012816831674 ) ) ;
#18745=CARTESIAN_POINT ( 'NONE',  ( -2.266590686148945544, 22.22041550158063572, 7.082119434687048631 ) ) ;
#18748=CARTESIAN_POINT ( 'NONE',  ( 0.6178305044545838731, 34.74863466993042493, 9.382169495545420901 ) ) ;
#18750=CARTESIAN_POINT ( 'NONE',  ( 18.52753015748617571, 23.09226448433411960, 4.923371831947298993 ) ) ;
#18751=FACE_OUTER_BOUND ( 'NONE', #17057, .T. ) ;
#18752=CARTESIAN_POINT ( 'NONE',  ( -2.816281873526471635, 48.91530133659708213, -3.434112377981056508 ) ) ;
#18754=CARTESIAN_POINT ( 'NONE',  ( 17.20831665107776587, 24.13393115100078035, -7.208316651077762316 ) ) ;
#18757=CARTESIAN_POINT ( 'NONE',  ( -0.8801773607110991993, 62.85535201082150536, -2.915334737309923874 ) ) ;
#18758=EDGE_CURVE ( 'NONE', #85730, #48374, #51229, .T. ) ;
#18762=EDGE_CURVE ( 'NONE', #61441, #13300, #3620, .T. ) ;
#18764=CARTESIAN_POINT ( 'NONE',  ( 10.00000000000000178, 69.31368534415484817, 10.88017736071110342 ) ) ;
#18766=CARTESIAN_POINT ( 'NONE',  ( 22.81628187352647785, 16.62363466993042138, 6.195893100308588602E-16 ) ) ;
#18768=CARTESIAN_POINT ( 'NONE',  ( 18.52753015748617571, 43.09226448433412315, 4.923371831947298993 ) ) ;
#18769=CARTESIAN_POINT ( 'NONE',  ( 10.00000000000000178, 65.37363466993042493, 12.81628187352647608 ) ) ;
#18770=CARTESIAN_POINT ( 'NONE',  ( 2.917880565312948704, 2.637082168247300906, 12.26659068614894643 ) ) ;
#18771=CARTESIAN_POINT ( 'NONE',  ( 1.472469842513823179, 36.42559781766745175, 4.923371831947296329 ) ) ;
#18772=CARTESIAN_POINT ( 'NONE',  ( -1.099225684535947600, 29.54030133659708923, 6.408140936763237150 ) ) ;
#18775=CARTESIAN_POINT ( 'NONE',  ( 4.559911319644449179, 58.89701867748817676, 9.422509992056141925 ) ) ;
#18776=CARTESIAN_POINT ( 'NONE',  ( 22.81628187352648496, 6.831968003263753531, -3.434112377981050290 ) ) ;
#18777=CARTESIAN_POINT ( 'NONE',  ( 1.959929470562282283, 41.50257860105349295, 5.767676674365853629 ) ) ;
#18778=CARTESIAN_POINT ( 'NONE',  ( 10.00000000000000000, 29.75893115100078745, -9.846743663894594434 ) ) ;
#18779=CARTESIAN_POINT ( 'NONE',  ( 15.44008868035555260, 29.73035201082150891, 9.422509992056143702 ) ) ;
#18780=CARTESIAN_POINT ( 'NONE',  ( 0.6178305044545838731, 24.74863466993042493, 9.382169495545420901 ) ) ;
#18781=CARTESIAN_POINT ( 'NONE',  ( 0.1532563361054100626, 25.80059781766744820, -2.638427012816831230 ) ) ;
#18783=CARTESIAN_POINT ( 'NONE',  ( 19.42250999205614193, 30.14701867748817321, 5.440088680355555262 ) ) ;
#18784=ORIENTED_EDGE ( 'NONE', *, *, #70799, .F. ) ;
#18785=CARTESIAN_POINT ( 'NONE',  ( 2.035157376598824452, 63.68868534415484106, 7.964842623401179544 ) ) ;
#18786=CARTESIAN_POINT ( 'NONE',  ( 19.42250999205614193, 5.147018677488171434, 5.440088680355555262 ) ) ;
#18787=CARTESIAN_POINT ( 'NONE',  ( 1.472469842513823179, 40.59226448433411605, -4.923371831947296329 ) ) ;
#18788=CARTESIAN_POINT ( 'NONE',  ( 2.035157376598822676, 32.43868534415483396, -7.964842623401177768 ) ) ;
#18790=CARTESIAN_POINT ( 'NONE',  ( 4.559911319644449179, 47.23035201082150536, -9.422509992056141925 ) ) ;
#18791=CARTESIAN_POINT ( 'NONE',  ( 4.559911319644449179, 17.23035201082150536, -9.422509992056141925 ) ) ;
#18793=CARTESIAN_POINT ( 'NONE',  ( 18.52753015748617571, 33.09226448433411605, 4.923371831947298993 ) ) ;
#18794=CARTESIAN_POINT ( 'NONE',  ( -2.266590686148945544, 51.38708216824730357, -7.082119434687050408 ) ) ;
#18797=CARTESIAN_POINT ( 'NONE',  ( 13.79529636645030344, 38.26208216824729647, 14.16423886937410614 ) ) ;
#18801=CARTESIAN_POINT ( 'NONE',  ( 0.5774900079438607392, 3.480352010821504916, 5.440088680355550821 ) ) ;
#18802=CARTESIAN_POINT ( 'NONE',  ( 5.076628168052704559, 35.17559781766745175, -8.527530157486179263 ) ) ;
#18804=CARTESIAN_POINT ( 'NONE',  ( -45.94000000000001194, 99.99999999999998579, 5.000000000000000000 ) ) ;
#18805=CARTESIAN_POINT ( 'NONE',  ( -0.8801773607110991993, 57.85535201082149825, -2.915334737309923874 ) ) ;
#18806=CARTESIAN_POINT ( 'NONE',  ( -2.816281873526473856, 59.12363466993042493, 9.499525473075851096E-16 ) ) ;
#18807=CARTESIAN_POINT ( 'NONE',  ( 10.00000000000000000, 26.81368534415484106, -10.88017736071110342 ) ) ;
#18808=CARTESIAN_POINT ( 'NONE',  ( 22.81628187352648496, 61.83196800326376774, -3.434112377981050290 ) ) ;
#18809=CARTESIAN_POINT ( 'NONE',  ( 10.00000000000000178, 10.37363466993041961, 12.81628187352647608 ) ) ;
#18810=CARTESIAN_POINT ( 'NONE',  ( 5.076628168052703671, 11.84226448433411960, 8.527530157486179263 ) ) ;
#18811=ORIENTED_EDGE ( 'NONE', *, *, #94726, .F. ) ;
#18812=FACE_OUTER_BOUND ( 'NONE', #63093, .T. ) ;
#18814=CARTESIAN_POINT ( 'NONE',  ( 13.79529636645030344, 63.26208216824730357, 14.16423886937410614 ) ) ;
#18815=CARTESIAN_POINT ( 'NONE',  ( 10.00000000000000000, 30.55374883491397142, -14.16423886937410082 ) ) ;
#18816=CARTESIAN_POINT ( 'NONE',  ( 2.035157376598824452, 28.68868534415484106, 7.964842623401179544 ) ) ;
#18818=CARTESIAN_POINT ( 'NONE',  ( 2.035157376598824452, 43.68868534415484106, 7.964842623401179544 ) ) ;
#18819=FACE_OUTER_BOUND ( 'NONE', #56257, .T. ) ;
#18821=CARTESIAN_POINT ( 'NONE',  ( 12.63842701281683034, 12.46726448433411782, 9.846743663894596210 ) ) ;
#18823=CARTESIAN_POINT ( 'NONE',  ( 12.63842701281683034, 27.46726448433411250, 9.846743663894596210 ) ) ;
#18825=CARTESIAN_POINT ( 'NONE',  ( 1.472469842513823179, 26.42559781766745175, 4.923371831947296329 ) ) ;
#18826=CARTESIAN_POINT ( 'NONE',  ( 14.92337183194729988, 54.34226448433412315, -8.527530157486177487 ) ) ;
#18827=CARTESIAN_POINT ( 'NONE',  ( -0.8801773607110991993, 22.85535201082150181, -2.915334737309923874 ) ) ;
#18830=CARTESIAN_POINT ( 'NONE',  ( 6.565887622018943937, 50.16530133659708213, 12.81628187352647430 ) ) ;
#18831=CARTESIAN_POINT ( 'NONE',  ( 19.84674366389459266, 33.71726448433410894, -2.638427012816827677 ) ) ;
#18832=CARTESIAN_POINT ( 'NONE',  ( 17.08211943468705840, 60.13708216824729647, -12.26659068614894466 ) ) ;
#18833=CARTESIAN_POINT ( 'NONE',  ( 19.84674366389459266, 18.71726448433411960, -2.638427012816827677 ) ) ;
#18835=CARTESIAN_POINT ( 'NONE',  ( 18.52753015748617571, 63.09226448433412315, 4.923371831947298993 ) ) ;
#18836=CARTESIAN_POINT ( 'NONE',  ( -4.164238869374098151, 11.59541550158063217, -3.795296366450310543 ) ) ;
#18837=CARTESIAN_POINT ( 'NONE',  ( 2.917880565312948704, 32.63708216824730357, 12.26659068614894643 ) ) ;
#18838=CARTESIAN_POINT ( 'NONE',  ( 18.52753015748617571, 33.09226448433411605, 4.923371831947298993 ) ) ;
#18840=CARTESIAN_POINT ( 'NONE',  ( 15.44008868035555260, 24.73035201082150891, 9.422509992056143702 ) ) ;
#18841=CARTESIAN_POINT ( 'NONE',  ( 10.00000000000000178, 54.31368534415484106, 10.88017736071110342 ) ) ;
#18842=CARTESIAN_POINT ( 'NONE',  ( -0.8801773607111008646, 43.27201867748817676, 2.915334737309923430 ) ) ;
#18844=CARTESIAN_POINT ( 'NONE',  ( 3.591859063236761518, 49.95696800326375353, 11.09922568453594849 ) ) ;
#18845=CARTESIAN_POINT ( 'NONE',  ( 12.91533473730993009, 51.60535201082149825, -10.88017736071109987 ) ) ;
#18846=ORIENTED_EDGE ( 'NONE', *, *, #1621, .F. ) ;
#18848=SURFACE_SIDE_STYLE ('',( #17861 ) ) ;
#18849=CARTESIAN_POINT ( 'NONE',  ( 2.035157376598824452, 58.68868534415482685, 7.964842623401179544 ) ) ;
#18850=ORIENTED_EDGE ( 'NONE', *, *, #16102, .T. ) ;
#18851=CARTESIAN_POINT ( 'NONE',  ( -0.8801773607111009756, 58.06368534415484106, 1.068504757029289695E-15 ) ) ;
#18852=CARTESIAN_POINT ( 'NONE',  ( 12.91533473730993009, 6.605352010821504471, -10.88017736071109987 ) ) ;
#18853=B_SPLINE_CURVE_WITH_KNOTS ( 'NONE', 3,
 ( #19465, #10979, #95466, #2529 ),
 .UNSPECIFIED., .F., .F.,
 ( 4, 4 ),
 ( 3.469446951953614189E-18, 0.002562518741975564063 ),
 .UNSPECIFIED. ) ;
#18856=CARTESIAN_POINT ( 'NONE',  ( -0.8801773607111009756, 8.063685344154837509, 1.068504757029289695E-15 ) ) ;
#18857=CARTESIAN_POINT ( 'NONE',  ( 14.92337183194729633, 12.67559781766745353, 8.527530157486181039 ) ) ;
#18858=CARTESIAN_POINT ( 'NONE',  ( 20.36894250292379738, 4.928748834913967869, -10.36894250292379027 ) ) ;
#18859=CARTESIAN_POINT ( 'NONE',  ( 19.84674366389459266, 8.717264484334116048, -2.638427012816827677 ) ) ;
#18860=CARTESIAN_POINT ( 'NONE',  ( 0.5774900079438590739, 7.647018677488171434, -5.440088680355550821 ) ) ;
#18861=CARTESIAN_POINT ( 'NONE',  ( 7.361572987183170547, 52.05059781766745175, 9.846743663894590881 ) ) ;
#18863=CARTESIAN_POINT ( 'NONE',  ( 5.076628168052703671, 41.84226448433411605, 8.527530157486179263 ) ) ;
#18865=CARTESIAN_POINT ( 'NONE',  ( 17.96484262340118221, 49.93868534415484106, 7.964842623401181321 ) ) ;
#18866=CARTESIAN_POINT ( 'NONE',  ( 18.52753015748617571, 58.09226448433411605, 4.923371831947298993 ) ) ;
#18868=CARTESIAN_POINT ( 'NONE',  ( -0.8801773607111008646, 8.272018677488171434, 2.915334737309923430 ) ) ;
#18870=CARTESIAN_POINT ( 'NONE',  ( -0.8801773607111008646, 63.27201867748817676, 2.915334737309923430 ) ) ;
#18871=CARTESIAN_POINT ( 'NONE',  ( 19.42250999205614193, 5.147018677488171434, 5.440088680355555262 ) ) ;
#18873=CARTESIAN_POINT ( 'NONE',  ( -2.816281873526473856, 44.12363466993042493, 9.499525473075851096E-16 ) ) ;
#18874=CARTESIAN_POINT ( 'NONE',  ( 20.88017736071110164, 30.35535201082151247, 2.915334737309930979 ) ) ;
#18875=CARTESIAN_POINT ( 'NONE',  ( -0.03447792253739070251, 10.15514106990689669, 6.401564815979740253 ) ) ;
#18877=CARTESIAN_POINT ( 'NONE',  ( -1.099225684535947600, 39.54030133659708923, 6.408140936763237150 ) ) ;
#18878=CARTESIAN_POINT ( 'NONE',  ( 2.035157376598824452, 33.68868534415484106, 7.964842623401179544 ) ) ;
#18881=VECTOR ( 'NONE', #94633, 1000.000000000000000 ) ;
#18882=CARTESIAN_POINT ( 'NONE',  ( 5.076628168052704559, 65.17559781766745175, -8.527530157486179263 ) ) ;
#18883=CARTESIAN_POINT ( 'NONE',  ( 2.791683348922240793, 11.63393115100078568, 7.208316651077764092 ) ) ;
#18884=CARTESIAN_POINT ( 'NONE',  ( 7.361572987183170547, 47.05059781766745175, 9.846743663894590881 ) ) ;
#18885=CARTESIAN_POINT ( 'NONE',  ( 4.559911319644449179, 22.23035201082150536, -9.422509992056141925 ) ) ;
#18887=CARTESIAN_POINT ( 'NONE',  ( 10.00000000000000000, 34.75893115100078745, -9.846743663894594434 ) ) ;
#18890=CARTESIAN_POINT ( 'NONE',  ( 1.472469842513823179, 30.59226448433411960, -4.923371831947296329 ) ) ;
#18894=CARTESIAN_POINT ( 'NONE',  ( 19.84674366389459266, 58.71726448433411605, -2.638427012816827677 ) ) ;
#18897=CARTESIAN_POINT ( 'NONE',  ( -2.816281873526471635, 63.91530133659708923, -3.434112377981056508 ) ) ;
#18898=B_SPLINE_CURVE_WITH_KNOTS ( 'NONE', 3,
 ( #69775, #1306, #78935, #16477, #62440, #71450 ),
 .UNSPECIFIED., .F., .F.,
 ( 4, 2, 4 ),
 ( 0.000000000000000000, 0.0002605067024380874896, 0.0005210134048761749792 ),
 .UNSPECIFIED. ) ;
#18899=CARTESIAN_POINT ( 'NONE',  ( 1.274849032794306947, 7.555090184799359676, -6.499999999999997335 ) ) ;
#18900=CARTESIAN_POINT ( 'NONE',  ( -2.816281873526473856, 24.12363466993042138, 9.499525473075851096E-16 ) ) ;
#18901=CARTESIAN_POINT ( 'NONE',  ( 0.1532563361054082862, 46.21726448433411605, 2.638427012816831674 ) ) ;
#18903=CARTESIAN_POINT ( 'NONE',  ( 17.08211943468705840, 65.13708216824730357, -12.26659068614894466 ) ) ;
#18904=CARTESIAN_POINT ( 'NONE',  ( 10.00000000000000178, 17.25893115100078745, 9.846743663894594434 ) ) ;
#18906=CARTESIAN_POINT ( 'NONE',  ( -4.164238869374098151, 51.59541550158063217, -3.795296366450310543 ) ) ;
#18907=CARTESIAN_POINT ( 'NONE',  ( 19.84674366389459266, 58.71726448433411605, -2.638427012816827677 ) ) ;
#18909=CARTESIAN_POINT ( 'NONE',  ( 15.44008868035555260, 4.730352010821505360, 9.422509992056143702 ) ) ;
#18910=CARTESIAN_POINT ( 'NONE',  ( -2.266590686148945544, 36.38708216824730357, -7.082119434687050408 ) ) ;
#18911=CARTESIAN_POINT ( 'NONE',  ( 24.16423886937410614, 34.30374883491396787, 8.672049930838204340E-16 ) ) ;
#18914=CARTESIAN_POINT ( 'NONE',  ( 2.791683348922237240, 60.38393115100078745, -7.208316651077763204 ) ) ;
#18916=CARTESIAN_POINT ( 'NONE',  ( 10.00000000000000178, 54.31368534415484106, 10.88017736071110342 ) ) ;
#18917=CARTESIAN_POINT ( 'NONE',  ( 19.64275089555621179, 93.00209110515163502, -5.306638067702549755 ) ) ;
#18918=CARTESIAN_POINT ( 'NONE',  ( 7.361572987183170547, 52.05059781766745175, 9.846743663894590881 ) ) ;
#18921=CARTESIAN_POINT ( 'NONE',  ( 14.92337183194729633, 57.67559781766745886, 8.527530157486181039 ) ) ;
#18924=CARTESIAN_POINT ( 'NONE',  ( 13.79529636645030344, 28.26208216824729647, 14.16423886937410614 ) ) ;
#18925=CARTESIAN_POINT ( 'NONE',  ( 2.791683348922237240, 0.3839311510007847872, -7.208316651077763204 ) ) ;
#18927=CARTESIAN_POINT ( 'NONE',  ( -0.8801773607111008646, 13.27201867748817321, 2.915334737309923430 ) ) ;
#18928=CARTESIAN_POINT ( 'NONE',  ( 10.00000000000000000, 27.87363466993042138, -12.81628187352647608 ) ) ;
#18930=CARTESIAN_POINT ( 'NONE',  ( 19.84674366389459266, 13.71726448433411782, -2.638427012816827677 ) ) ;
#18932=CARTESIAN_POINT ( 'NONE',  ( 10.00000000000000178, 33.05374883491396787, 14.16423886937410082 ) ) ;
#18934=CARTESIAN_POINT ( 'NONE',  ( 19.88701968852526747, 61.79427333184084148, 6.480634945678621861 ) ) ;
#18935=CARTESIAN_POINT ( 'NONE',  ( -0.8801773607110991993, 7.855352010821506248, -2.915334737309923874 ) ) ;
#18938=CARTESIAN_POINT ( 'NONE',  ( 20.88017736071110519, 40.56368534415484106, 2.639326808657452039E-16 ) ) ;
#18939=CARTESIAN_POINT ( 'NONE',  ( 2.035157376598822676, 32.43868534415483396, -7.964842623401177768 ) ) ;
#18940=CARTESIAN_POINT ( 'NONE',  ( 19.38216949554541202, 0.9986346699304200492, 9.382169495545424454 ) ) ;
#18941=SURFACE_STYLE_USAGE ( .BOTH. , #57900 ) ;
#18943=CARTESIAN_POINT ( 'NONE',  ( 10.00000000000000178, 12.25893115100078568, 9.846743663894594434 ) ) ;
#18944=EDGE_LOOP ( 'NONE', ( #39276, #54888, #58813, #95527 ) ) ;
#18945=CARTESIAN_POINT ( 'NONE',  ( 18.50749283717773963, 49.69955587570481015, 6.500000000000079936 ) ) ;
#18946=CARTESIAN_POINT ( 'NONE',  ( 4.559911319644449179, 48.89701867748817676, 9.422509992056141925 ) ) ;
#18947=CARTESIAN_POINT ( 'NONE',  ( 10.00000000000000178, 0.3736346699304200492, 12.81628187352647608 ) ) ;
#18948=CARTESIAN_POINT ( 'NONE',  ( 17.96484262340118221, 59.93868534415484106, 7.964842623401181321 ) ) ;
#18949=CARTESIAN_POINT ( 'NONE',  ( 2.791683348922237240, 30.38393115100078390, -7.208316651077763204 ) ) ;
#18950=CARTESIAN_POINT ( 'NONE',  ( 10.00000000000000178, 35.37363466993042493, 12.81628187352647608 ) ) ;
#18951=CARTESIAN_POINT ( 'NONE',  ( 0.1532563361054100626, 5.800597817667452638, -2.638427012816831230 ) ) ;
#18956=CARTESIAN_POINT ( 'NONE',  ( 12.91533473730992121, 4.522018677488169658, 10.88017736071110164 ) ) ;
#18957=CARTESIAN_POINT ( 'NONE',  ( 10.00000000000000000, 57.87363466993042493, -12.81628187352647608 ) ) ;
#18958=CARTESIAN_POINT ( 'NONE',  ( 1.472469842513823179, 31.42559781766745530, 4.923371831947296329 ) ) ;
#18959=CARTESIAN_POINT ( 'NONE',  ( 4.559911319644449179, 13.89701867748817143, 9.422509992056141925 ) ) ;
#18960=CARTESIAN_POINT ( 'NONE',  ( -0.8801773607111009756, 3.063685344154838397, 1.068504757029289695E-15 ) ) ;
#18962=CARTESIAN_POINT ( 'NONE',  ( -0.8801773607111008646, 18.27201867748817321, 2.915334737309923430 ) ) ;
#18964=AXIS2_PLACEMENT_3D ( 'NONE', #54616, #71616, #39647 ) ;
#18965=CARTESIAN_POINT ( 'NONE',  ( 15.44008868035555793, 16.39701867748817321, -9.422509992056140149 ) ) ;
#18966=DIRECTION ( 'NONE',  ( 0.000000000000000000, 0.000000000000000000, -1.000000000000000000 ) ) ;
#18968=CARTESIAN_POINT ( 'NONE',  ( 5.076628168052703671, 66.84226448433412315, 8.527530157486179263 ) ) ;
#18969=CARTESIAN_POINT ( 'NONE',  ( 7.084665262690076126, 24.10535201082150181, 10.88017736071109987 ) ) ;
#18970=CARTESIAN_POINT ( 'NONE',  ( 14.92337183194729988, 54.34226448433412315, -8.527530157486177487 ) ) ;
#18972=CARTESIAN_POINT ( 'NONE',  ( 0.6178305044545818747, 53.49863466993041072, -9.382169495545419124 ) ) ;
#18974=CARTESIAN_POINT ( 'NONE',  ( -4.164238869374098151, 31.59541550158063927, -3.795296366450310543 ) ) ;
#18975=CARTESIAN_POINT ( 'NONE',  ( 15.44008868035555260, 44.73035201082151247, 9.422509992056143702 ) ) ;
#18976=CARTESIAN_POINT ( 'NONE',  ( 4.559911319644449179, 13.89701867748817321, 9.422509992056141925 ) ) ;
#18977=CARTESIAN_POINT ( 'NONE',  ( 1.472469842513823179, 55.59226448433412315, -4.923371831947296329 ) ) ;
#18979=CARTESIAN_POINT ( 'NONE',  ( 7.361572987183170547, 47.05059781766745175, 9.846743663894590881 ) ) ;
#18980=CARTESIAN_POINT ( 'NONE',  ( 15.00000000000000000, 11.50000000000000000, -6.500000000000000888 ) ) ;
#18981=CARTESIAN_POINT ( 'NONE',  ( 17.20831665107776587, 9.133931151000787452, -7.208316651077762316 ) ) ;
#18984=CARTESIAN_POINT ( 'NONE',  ( 2.035157376598822676, 17.43868534415483751, -7.964842623401177768 ) ) ;
#18985=CARTESIAN_POINT ( 'NONE',  ( 17.20831665107776587, 7.883931151000784787, 7.208316651077764980 ) ) ;
#18986=CARTESIAN_POINT ( 'NONE',  ( -2.816281873526473856, -0.8763653300695799508, 9.499525473075851096E-16 ) ) ;
#18987=CARTESIAN_POINT ( 'NONE',  ( 10.00000000000000000, 51.81368534415484106, -10.88017736071110342 ) ) ;
#18988=CARTESIAN_POINT ( 'NONE',  ( 10.00000000000000178, 49.31368534415484106, 10.88017736071110342 ) ) ;
#18989=CARTESIAN_POINT ( 'NONE',  ( 20.88017736071110519, 20.56368534415484106, 2.639326808657452039E-16 ) ) ;
#18990=CARTESIAN_POINT ( 'NONE',  ( 0.6178305044545818747, 38.49863466993042493, -9.382169495545419124 ) ) ;
#18991=CARTESIAN_POINT ( 'NONE',  ( 6.204703633549690345, 37.84541550158063927, 14.16423886937410082 ) ) ;
#18992=CARTESIAN_POINT ( 'NONE',  ( 21.92686044187656336, 11.97997603579417536, 3.195792623639536423 ) ) ;
#18994=CARTESIAN_POINT ( 'NONE',  ( 10.00000000000000178, 55.37363466993042493, 12.81628187352647608 ) ) ;
#18996=CARTESIAN_POINT ( 'NONE',  ( 21.09922568453594849, 6.206968003263753531, 6.408140936763242479 ) ) ;
#18997=( NAMED_UNIT ( * ) SI_UNIT ( $, .STERADIAN. ) SOLID_ANGLE_UNIT ( ) );
#18999=CARTESIAN_POINT ( 'NONE',  ( 15.44008868035555260, 34.73035201082151247, 9.422509992056143702 ) ) ;
#19000=CARTESIAN_POINT ( 'NONE',  ( 18.52753015748618282, 63.92559781766745886, -4.923371831947291888 ) ) ;
#19001=ORIENTED_EDGE ( 'NONE', *, *, #36308, .F. ) ;
#19002=CARTESIAN_POINT ( 'NONE',  ( 12.63842701281683034, 7.467264484334118713, 9.846743663894596210 ) ) ;
#19003=CARTESIAN_POINT ( 'NONE',  ( -1.926860441876564023, 64.68830936912750929, 1.004413902775740781E-15 ) ) ;
#19004=EDGE_CURVE ( 'NONE', #74710, #72967, #73481, .T. ) ;
#19005=CARTESIAN_POINT ( 'NONE',  ( 18.52753015748618282, 18.92559781766745175, -4.923371831947291888 ) ) ;
#19006=CARTESIAN_POINT ( 'NONE',  ( 0.1532563361054083140, 11.00893115100078568, 1.131784320476157264E-15 ) ) ;
#19008=CARTESIAN_POINT ( 'NONE',  ( 4.559911319644449179, 53.89701867748817676, 9.422509992056141925 ) ) ;
#19009=CARTESIAN_POINT ( 'NONE',  ( 0.5774900079438590739, 37.64701867748817676, -5.440088680355550821 ) ) ;
#19010=CARTESIAN_POINT ( 'NONE',  ( 20.88017736071110519, 60.56368534415484106, 2.639326808657452039E-16 ) ) ;
#19011=CARTESIAN_POINT ( 'NONE',  ( 1.472469842513823179, 21.42559781766745175, 4.923371831947296329 ) ) ;
#19014=CARTESIAN_POINT ( 'NONE',  ( 2.791683348922237240, 50.38393115100078035, -7.208316651077763204 ) ) ;
#19017=CARTESIAN_POINT ( 'NONE',  ( -0.3689425029237898834, 21.17874883491396432, -10.36894250292378850 ) ) ;
#19019=CARTESIAN_POINT ( 'NONE',  ( 6.204703633549690345, 12.84541550158063572, 14.16423886937410082 ) ) ;
#19020=CARTESIAN_POINT ( 'NONE',  ( 10.00000000000000000, 30.55374883491397142, -14.16423886937410082 ) ) ;
#19023=CARTESIAN_POINT ( 'NONE',  ( 20.88017736071110519, 30.56368534415484106, 2.639326808657452039E-16 ) ) ;
#19025=ORIENTED_EDGE ( 'NONE', *, *, #59229, .F. ) ;
#19026=CARTESIAN_POINT ( 'NONE',  ( 12.63842701281683034, 22.46726448433411605, 9.846743663894596210 ) ) ;
#19027=CARTESIAN_POINT ( 'NONE',  ( 17.96484262340118221, 59.93868534415484106, 7.964842623401181321 ) ) ;
#19028=CARTESIAN_POINT ( 'NONE',  ( 7.361572987183169658, 9.967264484334119601, -9.846743663894592657 ) ) ;
#19029=CARTESIAN_POINT ( 'NONE',  ( 22.81628187352648496, 41.83196800326375353, -3.434112377981050290 ) ) ;
#19030=CARTESIAN_POINT ( 'NONE',  ( 7.361572987183169658, 34.96726448433411605, -9.846743663894592657 ) ) ;
#19033=CARTESIAN_POINT ( 'NONE',  ( 22.81628187352647785, 31.62363466993042138, 6.195893100308588602E-16 ) ) ;
#19036=CARTESIAN_POINT ( 'NONE',  ( 7.361572987183169658, 29.96726448433411960, -9.846743663894592657 ) ) ;
#19037=CARTESIAN_POINT ( 'NONE',  ( 17.08211943468705130, 13.47041550158063572, 12.26659068614894998 ) ) ;
#19039=CARTESIAN_POINT ( 'NONE',  ( 10.00000000000000178, 44.31368534415484106, 10.88017736071110342 ) ) ;
#19040=CARTESIAN_POINT ( 'NONE',  ( 10.00000000000000000, 51.81368534415484106, -10.88017736071110342 ) ) ;
#19041=CARTESIAN_POINT ( 'NONE',  ( 22.26659068614895176, 44.72041550158063927, -7.082119434687042414 ) ) ;
#19042=CARTESIAN_POINT ( 'NONE',  ( 5.076628168052703671, 56.84226448433412315, 8.527530157486179263 ) ) ;
#19043=CARTESIAN_POINT ( 'NONE',  ( 14.92337183194729988, 14.34226448433411782, -8.527530157486177487 ) ) ;
#19044=CARTESIAN_POINT ( 'NONE',  ( 6.565887622018943937, 65.16530133659709634, 12.81628187352647430 ) ) ;
#19046=CARTESIAN_POINT ( 'NONE',  ( 19.42250999205614193, 40.14701867748817676, 5.440088680355555262 ) ) ;
#19048=CARTESIAN_POINT ( 'NONE',  ( -2.816281873526473856, 29.12363466993041783, 9.499525473075851096E-16 ) ) ;
#19049=CARTESIAN_POINT ( 'NONE',  ( 0.1532563361054100626, 50.80059781766745175, -2.638427012816831230 ) ) ;
#19051=CARTESIAN_POINT ( 'NONE',  ( 19.42250999205614548, 65.98035201082151957, -5.440088680355545492 ) ) ;
#19053=CARTESIAN_POINT ( 'NONE',  ( 4.559911319644449179, 8.897018677488171434, 9.422509992056141925 ) ) ;
#19054=DIRECTION ( 'NONE',  ( 1.000000000000000000, 0.000000000000000000, -0.000000000000000000 ) ) ;
#19055=CARTESIAN_POINT ( 'NONE',  ( -0.8801773607110991993, 67.85535201082151957, -2.915334737309923874 ) ) ;
#19056=CARTESIAN_POINT ( 'NONE',  ( 0.5774900079438590739, 67.64701867748817676, -5.440088680355550821 ) ) ;
#19058=CARTESIAN_POINT ( 'NONE',  ( 1.472469842513823179, 41.42559781766745886, 4.923371831947296329 ) ) ;
#19059=CARTESIAN_POINT ( 'NONE',  ( 0.5774900079438590739, 17.64701867748817321, -5.440088680355550821 ) ) ;
#19060=CARTESIAN_POINT ( 'NONE',  ( 12.63842701281683922, 59.55059781766744464, -9.846743663894590881 ) ) ;
#19061=CARTESIAN_POINT ( 'NONE',  ( 17.96484262340118221, 36.18868534415484106, -7.964842623401177768 ) ) ;
#19063=CARTESIAN_POINT ( 'NONE',  ( 16.40814093676323893, 40.79030133659708923, 11.09922568453595026 ) ) ;
#19065=CARTESIAN_POINT ( 'NONE',  ( 2.035157376598822676, 47.43868534415484817, -7.964842623401177768 ) ) ;
#19066=CARTESIAN_POINT ( 'NONE',  ( 21.09922568453595559, 27.04030133659708568, -6.408140936763230044 ) ) ;
#19067=CARTESIAN_POINT ( 'NONE',  ( 0.5774900079438607392, 28.48035201082150891, 5.440088680355550821 ) ) ;
#19068=CARTESIAN_POINT ( 'NONE',  ( 4.559911319644449179, 2.230352010821504916, -9.422509992056141925 ) ) ;
#19069=CARTESIAN_POINT ( 'NONE',  ( 14.92337183194729633, 42.67559781766745886, 8.527530157486181039 ) ) ;
#19071=CARTESIAN_POINT ( 'NONE',  ( 5.076628168052703671, 6.842264484334118713, 8.527530157486179263 ) ) ;
#19072=CARTESIAN_POINT ( 'NONE',  ( -0.8801773607111008646, 58.27201867748816966, 2.915334737309923430 ) ) ;
#19074=CARTESIAN_POINT ( 'NONE',  ( 20.36894250292379738, 34.92874883491396076, -10.36894250292379027 ) ) ;
#19080=VERTEX_POINT ( 'NONE', #71925 ) ;
#19081=CARTESIAN_POINT ( 'NONE',  ( -4.164238869374099927, 47.01208216824729647, 3.795296366450308767 ) ) ;
#19082=CARTESIAN_POINT ( 'NONE',  ( 17.08211943468705840, 55.13708216824731068, -12.26659068614894466 ) ) ;
#19083=CARTESIAN_POINT ( 'NONE',  ( 0.1532563361054100626, 10.80059781766745175, -2.638427012816831230 ) ) ;
#19084=CARTESIAN_POINT ( 'NONE',  ( 10.00000000000000000, 17.87363466993041783, -12.81628187352647608 ) ) ;
#19085=CARTESIAN_POINT ( 'NONE',  ( -42.94000000000001194, 92.00000000000000000, -8.999999999999998224 ) ) ;
#19086=CARTESIAN_POINT ( 'NONE',  ( 0.5774900079438590739, 2.647018677488170990, -5.440088680355550821 ) ) ;
#19087=CARTESIAN_POINT ( 'NONE',  ( 22.81628187352647785, 36.41530133659707502, 3.434112377981063169 ) ) ;
#19088=CARTESIAN_POINT ( 'NONE',  ( 6.204703633549690345, 45.76208216824729647, -14.16423886937410259 ) ) ;
#19090=CARTESIAN_POINT ( 'NONE',  ( 20.88017736071110164, 65.35535201082150536, 2.915334737309930979 ) ) ;
#19093=CARTESIAN_POINT ( 'NONE',  ( -33.19000000000001194, 92.00000000000000000, -10.09898361729590199 ) ) ;
#19094=CARTESIAN_POINT ( 'NONE',  ( 19.84674366389459266, 13.30059781766745353, 2.638427012816836559 ) ) ;
#19095=EDGE_LOOP ( 'NONE', ( #42235, #54972, #63922, #6426 ) ) ;
#19096=CARTESIAN_POINT ( 'NONE',  ( -0.8801773607111009756, 13.06368534415483929, 1.068504757029289695E-15 ) ) ;
#19097=CARTESIAN_POINT ( 'NONE',  ( 19.42250999205614193, 10.14701867748816966, 5.440088680355555262 ) ) ;
#19098=CARTESIAN_POINT ( 'NONE',  ( 18.52753015748618282, 53.92559781766745175, -4.923371831947291888 ) ) ;
#19099=CARTESIAN_POINT ( 'NONE',  ( 6.565887622018943937, 0.1653013365970866511, 12.81628187352647430 ) ) ;
#19100=ADVANCED_FACE ( 'NONE', ( #17949 ), #3446, .T. ) ;
#19101=CARTESIAN_POINT ( 'NONE',  ( 10.00000000000000000, 17.87363466993041783, -12.81628187352647608 ) ) ;
#19103=CARTESIAN_POINT ( 'NONE',  ( 10.00000000000000000, 65.55374883491396076, -14.16423886937410082 ) ) ;
#19105=CARTESIAN_POINT ( 'NONE',  ( -4.164238869374099039, 61.80374883491397497, 8.674139862899312516E-16 ) ) ;
#19107=CARTESIAN_POINT ( 'NONE',  ( 17.96484262340118221, 31.18868534415483751, -7.964842623401177768 ) ) ;
#19109=CARTESIAN_POINT ( 'NONE',  ( 19.42250999205614548, 50.98035201082151247, -5.440088680355545492 ) ) ;
#19110=CARTESIAN_POINT ( 'NONE',  ( 19.42250999205614548, 50.98035201082151247, -5.440088680355545492 ) ) ;
#19112=CARTESIAN_POINT ( 'NONE',  ( 4.559911319644449179, 38.89701867748817676, 9.422509992056141925 ) ) ;
#19117=CARTESIAN_POINT ( 'NONE',  ( 10.00000000000000000, 9.758931151000785675, -9.846743663894594434 ) ) ;
#19120=CARTESIAN_POINT ( 'NONE',  ( 0.1532563361054082862, 46.21726448433411605, 2.638427012816831674 ) ) ;
#19121=CARTESIAN_POINT ( 'NONE',  ( 19.72487221294571569, 52.80223176428831522, -6.499999999999990230 ) ) ;
#19122=CARTESIAN_POINT ( 'NONE',  ( 3.591859063236763294, 58.29030133659708923, -11.09922568453595026 ) ) ;
#19128=CARTESIAN_POINT ( 'NONE',  ( 18.72515096720568195, 31.07228050351032422, -6.500000000000018652 ) ) ;
#19129=FACE_OUTER_BOUND ( 'NONE', #41124, .T. ) ;
#19130=CARTESIAN_POINT ( 'NONE',  ( 14.92337183194729988, 29.34226448433411960, -8.527530157486177487 ) ) ;
#19131=CARTESIAN_POINT ( 'NONE',  ( 10.00000000000000000, 60.55374883491397497, -14.16423886937410082 ) ) ;
#19136=CARTESIAN_POINT ( 'NONE',  ( 18.52753015748617571, 28.09226448433411960, 4.923371831947298993 ) ) ;
#19137=CARTESIAN_POINT ( 'NONE',  ( 21.09922568453595559, 62.04030133659709634, -6.408140936763230044 ) ) ;
#19138=CARTESIAN_POINT ( 'NONE',  ( 22.81628187352647785, 11.62363466993042138, 6.195893100308588602E-16 ) ) ;
#19139=CARTESIAN_POINT ( 'NONE',  ( 19.42250999205614548, 65.98035201082151957, -5.440088680355545492 ) ) ;
#19142=CARTESIAN_POINT ( 'NONE',  ( 18.52753015748617571, 3.092264484334118269, 4.923371831947298993 ) ) ;
#19143=CARTESIAN_POINT ( 'NONE',  ( 1.472469842513823179, 56.42559781766745886, 4.923371831947296329 ) ) ;
#19146=CARTESIAN_POINT ( 'NONE',  ( 20.36894250292379382, 58.67874883491396076, 10.36894250292379205 ) ) ;
#19147=CARTESIAN_POINT ( 'NONE',  ( -4.164238869374099927, 12.01208216824730357, 3.795296366450308767 ) ) ;
#19148=CARTESIAN_POINT ( 'NONE',  ( 1.472469842513823179, 16.42559781766745175, 4.923371831947296329 ) ) ;
#19149=CARTESIAN_POINT ( 'NONE',  ( 15.44008868035555793, 36.39701867748816966, -9.422509992056140149 ) ) ;
#19150=CARTESIAN_POINT ( 'NONE',  ( -2.816281873526473856, 24.12363466993042138, 9.499525473075851096E-16 ) ) ;
#19152=CARTESIAN_POINT ( 'NONE',  ( 4.559911319644449179, 3.897018677488170990, 9.422509992056141925 ) ) ;
#19153=EDGE_CURVE ( 'NONE', #13047, #24064, #28398, .T. ) ;
#19155=CARTESIAN_POINT ( 'NONE',  ( 5.076628168052704559, 45.17559781766745175, -8.527530157486179263 ) ) ;
#19156=CARTESIAN_POINT ( 'NONE',  ( 2.791683348922237240, 10.38393115100078390, -7.208316651077763204 ) ) ;
#19158=CARTESIAN_POINT ( 'NONE',  ( 6.565887622018943937, 28.08196800326375353, -12.81628187352647608 ) ) ;
#19160=CARTESIAN_POINT ( 'NONE',  ( 17.96484262340118221, 29.93868534415484106, 7.964842623401181321 ) ) ;
#19163=CARTESIAN_POINT ( 'NONE',  ( 13.79529636645031943, 45.34541550158062506, -14.16423886937409904 ) ) ;
#19164=CARTESIAN_POINT ( 'NONE',  ( 13.79529636645030344, 33.26208216824730357, 14.16423886937410614 ) ) ;
#19165=CARTESIAN_POINT ( 'NONE',  ( 0.1532563361054100626, 40.80059781766745886, -2.638427012816831230 ) ) ;
#19166=CARTESIAN_POINT ( 'NONE',  ( 22.81628187352647785, 31.62363466993042138, 6.195893100308588602E-16 ) ) ;
#19167=CARTESIAN_POINT ( 'NONE',  ( 17.96484262340118221, 29.93868534415484106, 7.964842623401181321 ) ) ;
#19168=CARTESIAN_POINT ( 'NONE',  ( 10.00000000000000178, 57.25893115100078745, 9.846743663894594434 ) ) ;
#19169=CARTESIAN_POINT ( 'NONE',  ( 17.96484262340118221, 36.18868534415484106, -7.964842623401177768 ) ) ;
#19170=CARTESIAN_POINT ( 'NONE',  ( 6.565887622018943937, 8.081968003263751754, -12.81628187352647608 ) ) ;
#19171=CARTESIAN_POINT ( 'NONE',  ( 10.00000000000000000, 20.55374883491396787, -14.16423886937410082 ) ) ;
#19173=CARTESIAN_POINT ( 'NONE',  ( 17.20831665107776587, 24.13393115100078035, -7.208316651077762316 ) ) ;
#19174=CARTESIAN_POINT ( 'NONE',  ( 22.81628187352648496, 61.83196800326376774, -3.434112377981050290 ) ) ;
#19175=CARTESIAN_POINT ( 'NONE',  ( 7.361572987183169658, 64.96726448433412315, -9.846743663894592657 ) ) ;
#19176=ORIENTED_EDGE ( 'NONE', *, *, #70639, .T. ) ;
#19179=CARTESIAN_POINT ( 'NONE',  ( -0.8801773607111008646, 13.27201867748817321, 2.915334737309923430 ) ) ;
#19180=CARTESIAN_POINT ( 'NONE',  ( 13.79529636645030344, 8.262082168247300018, 14.16423886937410614 ) ) ;
#19181=CARTESIAN_POINT ( 'NONE',  ( 4.559911319644449179, 68.89701867748817676, 9.422509992056141925 ) ) ;
#19182=CARTESIAN_POINT ( 'NONE',  ( 2.791683348922240793, 51.63393115100078745, 7.208316651077764092 ) ) ;
#19183=CARTESIAN_POINT ( 'NONE',  ( 17.96484262340118221, 31.18868534415483751, -7.964842623401177768 ) ) ;
#19194=CARTESIAN_POINT ( 'NONE',  ( -4.164238869374099039, 6.803748834913967869, 8.674139862899312516E-16 ) ) ;
#19195=CARTESIAN_POINT ( 'NONE',  ( 17.08211943468705840, 15.13708216824730179, -12.26659068614894466 ) ) ;
#19196=CARTESIAN_POINT ( 'NONE',  ( -0.3689425029237898834, 56.17874883491396076, -10.36894250292378850 ) ) ;
#19197=CARTESIAN_POINT ( 'NONE',  ( 1.472469842513823179, 61.42559781766745175, 4.923371831947296329 ) ) ;
#19198=CARTESIAN_POINT ( 'NONE',  ( 5.076628168052703671, 36.84226448433412315, 8.527530157486179263 ) ) ;
#19199=CARTESIAN_POINT ( 'NONE',  ( 6.565887622018943937, 65.16530133659709634, 12.81628187352647430 ) ) ;
#19200=CARTESIAN_POINT ( 'NONE',  ( 15.44008868035555793, 26.39701867748817321, -9.422509992056140149 ) ) ;
#19201=CARTESIAN_POINT ( 'NONE',  ( 10.00000000000000178, 67.25893115100079456, 9.846743663894594434 ) ) ;
#19202=CARTESIAN_POINT ( 'NONE',  ( 2.917880565312950480, 5.970415501580634832, -12.26659068614894821 ) ) ;
#19204=CARTESIAN_POINT ( 'NONE',  ( 17.08211943468705130, 48.47041550158063927, 12.26659068614894998 ) ) ;
#19205=CARTESIAN_POINT ( 'NONE',  ( -4.164238869374098151, 66.59541550158060375, -3.795296366450310543 ) ) ;
#19206=CARTESIAN_POINT ( 'NONE',  ( -0.3077640640441539621, 0.000000000000000000, 5.999999999999999112 ) ) ;
#19207=CARTESIAN_POINT ( 'NONE',  ( -0.1503990784575328088, 3.101585745166421493, 6.262539305110068177 ) ) ;
#19208=CARTESIAN_POINT ( 'NONE',  ( -2.816281873526473856, 44.33196800326375353, 3.434112377981055619 ) ) ;
#19213=CARTESIAN_POINT ( 'NONE',  ( 7.361572987183170547, 27.05059781766745175, 9.846743663894590881 ) ) ;
#19215=CARTESIAN_POINT ( 'NONE',  ( 24.16423886937410614, 34.30374883491396787, 8.672049930838204340E-16 ) ) ;
#19216=CARTESIAN_POINT ( 'NONE',  ( 18.52753015748618282, 33.92559781766745886, -4.923371831947291888 ) ) ;
#19217=CARTESIAN_POINT ( 'NONE',  ( 4.559911319644449179, 58.89701867748817676, 9.422509992056141925 ) ) ;
#19218=DIRECTION ( 'NONE',  ( -0.8320502943378437211, 0.5547001962252290364, 0.000000000000000000 ) ) ;
#19219=CARTESIAN_POINT ( 'NONE',  ( 20.88017736071110519, 55.56368534415484817, 2.639326808657452039E-16 ) ) ;
#19220=CARTESIAN_POINT ( 'NONE',  ( 12.63842701281683922, 44.55059781766745175, -9.846743663894590881 ) ) ;
#19222=CARTESIAN_POINT ( 'NONE',  ( 22.81628187352648496, 61.83196800326376774, -3.434112377981050290 ) ) ;
#19224=VERTEX_POINT ( 'NONE', #58892 ) ;
#19225=CARTESIAN_POINT ( 'NONE',  ( -0.8801773607111009756, 48.06368534415484817, 1.068504757029289695E-15 ) ) ;
#19226=CARTESIAN_POINT ( 'NONE',  ( -2.266590686148945544, 21.38708216824730357, -7.082119434687050408 ) ) ;
#19228=ORIENTED_EDGE ( 'NONE', *, *, #46768, .T. ) ;
#19229=CARTESIAN_POINT ( 'NONE',  ( -2.816281873526473856, 29.12363466993041783, 9.499525473075851096E-16 ) ) ;
#19230=CARTESIAN_POINT ( 'NONE',  ( 0.1532563361054083140, 21.00893115100078745, 1.131784320476157264E-15 ) ) ;
#19231=CARTESIAN_POINT ( 'NONE',  ( 17.96484262340118221, 16.18868534415483396, -7.964842623401177768 ) ) ;
#19232=CARTESIAN_POINT ( 'NONE',  ( 6.565887622018943937, 53.08196800326374643, -12.81628187352647608 ) ) ;
#19233=FACE_OUTER_BOUND ( 'NONE', #2908, .T. ) ;
#19234=CARTESIAN_POINT ( 'NONE',  ( 5.076628168052704559, 30.17559781766745175, -8.527530157486179263 ) ) ;
#19235=CARTESIAN_POINT ( 'NONE',  ( 19.72487221294571569, 19.78217586085237301, 6.499999999999990230 ) ) ;
#19239=CARTESIAN_POINT ( 'NONE',  ( 0.2751277870542914172, 23.21833443783937767, 6.499999999999992006 ) ) ;
#19241=CARTESIAN_POINT ( 'NONE',  ( 2.791683348922240793, 6.633931151000785675, 7.208316651077764092 ) ) ;
#19242=CARTESIAN_POINT ( 'NONE',  ( 0.6178305044545818747, 18.49863466993041428, -9.382169495545419124 ) ) ;
#19244=CARTESIAN_POINT ( 'NONE',  ( 12.63842701281683922, 49.55059781766744464, -9.846743663894590881 ) ) ;
#19246=CARTESIAN_POINT ( 'NONE',  ( 10.00000000000000178, 18.05374883491396787, 14.16423886937410082 ) ) ;
#19247=CARTESIAN_POINT ( 'NONE',  ( 2.791683348922237240, 35.38393115100079456, -7.208316651077763204 ) ) ;
#19248=CARTESIAN_POINT ( 'NONE',  ( -2.816281873526473856, 29.33196800326376064, 3.434112377981055619 ) ) ;
#19251=CARTESIAN_POINT ( 'NONE',  ( -0.8801773607111008646, 68.27201867748817676, 2.915334737309923430 ) ) ;
#19252=CARTESIAN_POINT ( 'NONE',  ( 10.00000000000000000, 2.873634669930420049, -12.81628187352647608 ) ) ;
#19254=CARTESIAN_POINT ( 'NONE',  ( 19.84674366389459621, 38.50893115100078745, 7.409399052514197653E-17 ) ) ;
#19255=CARTESIAN_POINT ( 'NONE',  ( 4.559911319644449179, 28.89701867748817321, 9.422509992056141925 ) ) ;
#19257=CARTESIAN_POINT ( 'NONE',  ( 6.565887622018943937, 30.16530133659708568, 12.81628187352647430 ) ) ;
#19258=CARTESIAN_POINT ( 'NONE',  ( 19.84674366389459621, 28.50893115100078745, 7.409399052514197653E-17 ) ) ;
#19261=CARTESIAN_POINT ( 'NONE',  ( 10.00000000000000178, 29.31368534415483751, 10.88017736071110342 ) ) ;
#19263=CARTESIAN_POINT ( 'NONE',  ( 10.00000000000000178, 64.31368534415483396, 10.88017736071110342 ) ) ;
#19265=CARTESIAN_POINT ( 'NONE',  ( 1.472469842513823179, 51.42559781766745886, 4.923371831947296329 ) ) ;
#19266=CARTESIAN_POINT ( 'NONE',  ( 15.44008868035555260, 24.73035201082150891, 9.422509992056143702 ) ) ;
#19267=CARTESIAN_POINT ( 'NONE',  ( 19.72487221294571569, 52.80223176428831522, -6.499999999999990230 ) ) ;
#19268=CARTESIAN_POINT ( 'NONE',  ( 12.91533473730993009, 46.60535201082150536, -10.88017736071109987 ) ) ;
#19269=CARTESIAN_POINT ( 'NONE',  ( 0.5774900079438607392, 23.48035201082150536, 5.440088680355550821 ) ) ;
#19270=CARTESIAN_POINT ( 'NONE',  ( 20.00000000000000355, 89.78870847431082325, -4.994901225422943902 ) ) ;
#19272=CARTESIAN_POINT ( 'NONE',  ( 0.1532563361054083140, 6.008931151000784787, 1.131784320476157264E-15 ) ) ;
#19274=CARTESIAN_POINT ( 'NONE',  ( 1.472469842513823179, 45.59226448433412315, -4.923371831947296329 ) ) ;
#19275=CARTESIAN_POINT ( 'NONE',  ( 17.08211943468705130, 58.47041550158063927, 12.26659068614894998 ) ) ;
#19278=CARTESIAN_POINT ( 'NONE',  ( 22.26659068614894466, 13.88708216824730179, 7.082119434687054849 ) ) ;
#19279=CARTESIAN_POINT ( 'NONE',  ( -0.3689425029237898834, 36.17874883491396787, -10.36894250292378850 ) ) ;
#19280=CARTESIAN_POINT ( 'NONE',  ( 13.43411237798105340, 5.581968003263753531, 12.81628187352647963 ) ) ;
#19283=EDGE_LOOP ( 'NONE', ( #96687, #51458, #52016, #78385 ) ) ;
#19284=CARTESIAN_POINT ( 'NONE',  ( 7.084665262690076126, 4.105352010821503583, 10.88017736071109987 ) ) ;
#19285=CARTESIAN_POINT ( 'NONE',  ( 17.20831665107776587, 32.88393115100078745, 7.208316651077764980 ) ) ;
#19287=LINE ( 'NONE', #42289, #29518 ) ;
#19288=CARTESIAN_POINT ( 'NONE',  ( 20.88017736071110875, 65.77201867748817676, -2.915334737309920765 ) ) ;
#19289=CARTESIAN_POINT ( 'NONE',  ( 20.15039907845753930, 70.00000000000000000, 6.262539305110068177 ) ) ;
#19290=CARTESIAN_POINT ( 'NONE',  ( 20.88017736071110164, 25.35535201082150891, 2.915334737309930979 ) ) ;
#19291=EDGE_CURVE ( 'NONE', #66685, #63139, #65891, .T. ) ;
#19292=CARTESIAN_POINT ( 'NONE',  ( 0.6178305044545818747, 58.49863466993042493, -9.382169495545419124 ) ) ;
#19293=CARTESIAN_POINT ( 'NONE',  ( 21.09922568453595559, 12.04030133659708746, -6.408140936763230044 ) ) ;
#19294=CARTESIAN_POINT ( 'NONE',  ( 17.20831665107776587, 32.88393115100078745, 7.208316651077764980 ) ) ;
#19296=FILL_AREA_STYLE_COLOUR ( '', #83623 ) ;
#19297=CARTESIAN_POINT ( 'NONE',  ( 18.28836319691945889, 4.344927826957708739, 6.500000000000004441 ) ) ;
#19298=CARTESIAN_POINT ( 'NONE',  ( 24.16423886937410614, 64.30374883491396076, 8.672049930838204340E-16 ) ) ;
#19299=CARTESIAN_POINT ( 'NONE',  ( 22.26659068614895176, 24.72041550158063572, -7.082119434687042414 ) ) ;
#19300=CARTESIAN_POINT ( 'NONE',  ( 19.42250999205614548, 35.98035201082151247, -5.440088680355545492 ) ) ;
#19301=CARTESIAN_POINT ( 'NONE',  ( 2.035157376598822676, 47.43868534415484817, -7.964842623401177768 ) ) ;
#19302=DIRECTION ( 'NONE',  ( 0.000000000000000000, -1.000000000000000000, 0.000000000000000000 ) ) ;
#19304=CARTESIAN_POINT ( 'NONE',  ( 19.84674366389459621, 8.508931151000785675, 7.409399052514197653E-17 ) ) ;
#19306=CARTESIAN_POINT ( 'NONE',  ( 7.361572987183170547, 22.05059781766745530, 9.846743663894590881 ) ) ;
#19307=CARTESIAN_POINT ( 'NONE',  ( 10.00000000000000000, 54.75893115100078745, -9.846743663894594434 ) ) ;
#19309=EDGE_CURVE ( 'NONE', #47024, #58376, #81394, .T. ) ;
#19310=B_SPLINE_CURVE_WITH_KNOTS ( 'NONE', 3,
 ( #34629, #87146, #79660, #96149 ),
 .UNSPECIFIED., .F., .F.,
 ( 4, 4 ),
 ( 0.000000000000000000, 0.001036303429213300022 ),
 .UNSPECIFIED. ) ;
#19311=CARTESIAN_POINT ( 'NONE',  ( 6.565887622018943937, 48.08196800326375353, -12.81628187352647608 ) ) ;
#19313=CARTESIAN_POINT ( 'NONE',  ( 2.035157376598824452, 63.68868534415484106, 7.964842623401179544 ) ) ;
#19314=CARTESIAN_POINT ( 'NONE',  ( 0.1532563361054083140, 31.00893115100078390, 1.131784320476157264E-15 ) ) ;
#19315=CARTESIAN_POINT ( 'NONE',  ( -4.164238869374099039, 61.80374883491397497, 8.674139862899312516E-16 ) ) ;
#19316=CARTESIAN_POINT ( 'NONE',  ( 18.52753015748618282, 23.92559781766745530, -4.923371831947291888 ) ) ;
#19317=CARTESIAN_POINT ( 'NONE',  ( 0.2751277870542909176, 60.30223176428830101, 6.499999999999992006 ) ) ;
#19321=CARTESIAN_POINT ( 'NONE',  ( 24.16423886937410614, 19.30374883491397142, 8.672049930838204340E-16 ) ) ;
#19322=CARTESIAN_POINT ( 'NONE',  ( 24.16423886937410614, 29.51208216824729647, -3.795296366450302550 ) ) ;
#19323=CARTESIAN_POINT ( 'NONE',  ( 10.00000000000000000, 39.75893115100078745, -9.846743663894594434 ) ) ;
#19325=CARTESIAN_POINT ( 'NONE',  ( 19.80427997160309417, 12.75733960839543890, -6.500000000000000888 ) ) ;
#19326=CARTESIAN_POINT ( 'NONE',  ( 20.88017736071110519, 30.56368534415484106, 2.639326808657452039E-16 ) ) ;
#19327=CARTESIAN_POINT ( 'NONE',  ( -0.8801773607111008646, 53.27201867748816966, 2.915334737309923430 ) ) ;
#19330=CARTESIAN_POINT ( 'NONE',  ( 16.40814093676323893, 50.79030133659708923, 11.09922568453595026 ) ) ;
#19331=CARTESIAN_POINT ( 'NONE',  ( -0.8801773607111008646, 58.27201867748816966, 2.915334737309923430 ) ) ;
#19335=CARTESIAN_POINT ( 'NONE',  ( 10.00000000000000178, 69.31368534415484817, 10.88017736071110342 ) ) ;
#19337=CARTESIAN_POINT ( 'NONE',  ( 7.084665262690076126, 64.10535201082150536, 10.88017736071109987 ) ) ;
#19338=CARTESIAN_POINT ( 'NONE',  ( 19.42250999205614548, 20.98035201082150891, -5.440088680355545492 ) ) ;
#19341=CARTESIAN_POINT ( 'NONE',  ( 0.5774900079438607392, 8.480352010821505360, 5.440088680355550821 ) ) ;
#19342=CARTESIAN_POINT ( 'NONE',  ( 14.92337183194729988, 9.342264484334119601, -8.527530157486177487 ) ) ;
#19343=CARTESIAN_POINT ( 'NONE',  ( 17.08211943468705130, 13.47041550158063572, 12.26659068614894998 ) ) ;
#19344=CARTESIAN_POINT ( 'NONE',  ( -0.8801773607111008646, 18.27201867748817321, 2.915334737309923430 ) ) ;
#19345=CARTESIAN_POINT ( 'NONE',  ( 1.472469842513823179, 61.42559781766745175, 4.923371831947296329 ) ) ;
#19348=CARTESIAN_POINT ( 'NONE',  ( 2.791683348922240793, 56.63393115100078035, 7.208316651077764092 ) ) ;
#19350=CARTESIAN_POINT ( 'NONE',  ( 20.88017736071110164, 55.35535201082149825, 2.915334737309930979 ) ) ;
#19351=CARTESIAN_POINT ( 'NONE',  ( 5.076628168052703671, 46.84226448433412315, 8.527530157486179263 ) ) ;
#19352=CARTESIAN_POINT ( 'NONE',  ( 21.09922568453594849, 41.20696800326375353, 6.408140936763242479 ) ) ;
#19353=CARTESIAN_POINT ( 'NONE',  ( 4.559911319644449179, 7.230352010821504471, -9.422509992056141925 ) ) ;
#19355=CARTESIAN_POINT ( 'NONE',  ( 20.88017736071110519, 55.56368534415484817, 2.639326808657452039E-16 ) ) ;
#19356=CARTESIAN_POINT ( 'NONE',  ( 0.5774900079438590739, 7.647018677488171434, -5.440088680355550821 ) ) ;
#19360=CARTESIAN_POINT ( 'NONE',  ( 10.00000000000000000, 42.87363466993042493, -12.81628187352647608 ) ) ;
#19361=CARTESIAN_POINT ( 'NONE',  ( 12.91533473730993009, 36.60535201082151247, -10.88017736071109987 ) ) ;
#19362=CARTESIAN_POINT ( 'NONE',  ( 0.2751277870542980231, 10.30223176428831522, 6.500000000000002665 ) ) ;
#19365=CARTESIAN_POINT ( 'NONE',  ( 19.38216949554541557, 47.24863466993041783, -9.382169495545420901 ) ) ;
#19366=CARTESIAN_POINT ( 'NONE',  ( 20.88017736071110519, 40.56368534415484106, 2.639326808657452039E-16 ) ) ;
#19367=CARTESIAN_POINT ( 'NONE',  ( 7.361572987183169658, 59.96726448433410894, -9.846743663894592657 ) ) ;
#19369=CARTESIAN_POINT ( 'NONE',  ( 5.076628168052703671, 61.84226448433412315, 8.527530157486179263 ) ) ;
#19371=CARTESIAN_POINT ( 'NONE',  ( 19.84674366389459266, 53.30059781766744464, 2.638427012816836559 ) ) ;
#19372=CARTESIAN_POINT ( 'NONE',  ( 7.084665262690076126, 24.10535201082150181, 10.88017736071109987 ) ) ;
#19373=DIRECTION ( 'NONE',  ( -0.8320502943378437211, 0.5547001962252290364, 0.000000000000000000 ) ) ;
#19374=CARTESIAN_POINT ( 'NONE',  ( 1.472469842513823179, 40.59226448433411605, -4.923371831947296329 ) ) ;
#19376=CARTESIAN_POINT ( 'NONE',  ( 18.17884179759845509, 58.66688879859523098, -6.500000000000054179 ) ) ;
#19377=CARTESIAN_POINT ( 'NONE',  ( 0.1532563361054082862, 46.21726448433411605, 2.638427012816831674 ) ) ;
#19378=FILL_AREA_STYLE ('',( #5373 ) ) ;
#19379=CARTESIAN_POINT ( 'NONE',  ( 0.1532563361054083140, 56.00893115100078745, 1.131784320476157264E-15 ) ) ;
#19382=CARTESIAN_POINT ( 'NONE',  ( 13.43411237798105340, 45.58196800326374643, 12.81628187352647963 ) ) ;
#19383=CARTESIAN_POINT ( 'NONE',  ( 2.791683348922237240, 45.38393115100079456, -7.208316651077763204 ) ) ;
#19384=CARTESIAN_POINT ( 'NONE',  ( 2.917880565312950480, 65.97041550158063217, -12.26659068614894821 ) ) ;
#19385=CARTESIAN_POINT ( 'NONE',  ( 18.52753015748617571, 28.09226448433411960, 4.923371831947298993 ) ) ;
#19387=CARTESIAN_POINT ( 'NONE',  ( 22.26659068614894466, 53.88708216824731068, 7.082119434687054849 ) ) ;
#19388=CARTESIAN_POINT ( 'NONE',  ( 2.791683348922240793, 66.63393115100079456, 7.208316651077764092 ) ) ;
#19389=CARTESIAN_POINT ( 'NONE',  ( 2.035157376598824452, 3.688685344154837953, 7.964842623401179544 ) ) ;
#19390=CARTESIAN_POINT ( 'NONE',  ( 10.00000000000000000, 35.55374883491396787, -14.16423886937410082 ) ) ;
#19391=CARTESIAN_POINT ( 'NONE',  ( 2.917880565312950480, 35.97041550158063217, -12.26659068614894821 ) ) ;
#19394=CARTESIAN_POINT ( 'NONE',  ( 10.00000000000000178, 17.25893115100078745, 9.846743663894594434 ) ) ;
#19396=CARTESIAN_POINT ( 'NONE',  ( 10.00000000000000178, 5.373634669930420493, 12.81628187352647608 ) ) ;
#19397=CARTESIAN_POINT ( 'NONE',  ( 17.96484262340118221, 46.18868534415484106, -7.964842623401177768 ) ) ;
#19400=CARTESIAN_POINT ( 'NONE',  ( 0.1532563361054100626, 50.80059781766745175, -2.638427012816831230 ) ) ;
#19402=CARTESIAN_POINT ( 'NONE',  ( 14.92337183194729988, 49.34226448433411605, -8.527530157486177487 ) ) ;
#19403=CARTESIAN_POINT ( 'NONE',  ( 6.204703633549690345, 0.7620821682473009062, -14.16423886937410259 ) ) ;
#19405=CARTESIAN_POINT ( 'NONE',  ( 6.204703633549690345, 25.76208216824730712, -14.16423886937410259 ) ) ;
#19407=CARTESIAN_POINT ( 'NONE',  ( 0.2751277870542967463, 70.00000000000000000, -6.500000000000000888 ) ) ;
#19408=CARTESIAN_POINT ( 'NONE',  ( 15.44008868035555260, 24.73035201082150891, 9.422509992056143702 ) ) ;
#19409=CARTESIAN_POINT ( 'NONE',  ( 16.40814093676323893, 25.79030133659708923, 11.09922568453595026 ) ) ;
#19411=CARTESIAN_POINT ( 'NONE',  ( 18.52753015748617571, 13.09226448433411960, 4.923371831947298993 ) ) ;
#19412=CARTESIAN_POINT ( 'NONE',  ( 21.09922568453595559, 52.04030133659708923, -6.408140936763230044 ) ) ;
#19415=CARTESIAN_POINT ( 'NONE',  ( 22.26659068614895176, 29.72041550158063572, -7.082119434687042414 ) ) ;
#19417=FACE_OUTER_BOUND ( 'NONE', #80323, .T. ) ;
#19418=CARTESIAN_POINT ( 'NONE',  ( 2.035157376598824452, 13.68868534415483751, 7.964842623401179544 ) ) ;
#19421=CARTESIAN_POINT ( 'NONE',  ( 17.96484262340118221, 46.18868534415484106, -7.964842623401177768 ) ) ;
#19422=CARTESIAN_POINT ( 'NONE',  ( 20.88017736071110164, 50.35535201082151247, 2.915334737309930979 ) ) ;
#19423=CARTESIAN_POINT ( 'NONE',  ( 6.565887622018943937, 10.16530133659708746, 12.81628187352647430 ) ) ;
#19424=CARTESIAN_POINT ( 'NONE',  ( 5.076628168052704559, 65.17559781766745175, -8.527530157486179263 ) ) ;
#19425=CARTESIAN_POINT ( 'NONE',  ( 19.72487221294571569, 59.78217586085237656, 6.499999999999986677 ) ) ;
#19426=CARTESIAN_POINT ( 'NONE',  ( 1.472469842513823179, 6.425597817667451750, 4.923371831947296329 ) ) ;
#19427=EDGE_CURVE ( 'NONE', #74440, #39993, #36396, .T. ) ;
#19429=CARTESIAN_POINT ( 'NONE',  ( 19.42250999205614193, 45.14701867748817676, 5.440088680355555262 ) ) ;
#19431=ADVANCED_FACE ( 'NONE', ( #97408 ), #12404, .F. ) ;
#19433=CARTESIAN_POINT ( 'NONE',  ( 21.09922568453594849, 6.206968003263753531, 6.408140936763242479 ) ) ;
#19434=CARTESIAN_POINT ( 'NONE',  ( 20.88017736071110875, 65.77201867748817676, -2.915334737309920765 ) ) ;
#19436=CARTESIAN_POINT ( 'NONE',  ( 5.076628168052703671, 31.84226448433412315, 8.527530157486179263 ) ) ;
#19437=CARTESIAN_POINT ( 'NONE',  ( 16.40814093676323893, 50.79030133659708923, 11.09922568453595026 ) ) ;
#19438=CARTESIAN_POINT ( 'NONE',  ( 0.1532563361054083140, 1.008931151000784787, 1.131784320476157264E-15 ) ) ;
#19441=CARTESIAN_POINT ( 'NONE',  ( 1.492507162822247491, 57.19955587570483146, -6.500000000000039080 ) ) ;
#19443=CARTESIAN_POINT ( 'NONE',  ( 20.88017736071110875, 20.77201867748816611, -2.915334737309920765 ) ) ;
#19444=CARTESIAN_POINT ( 'NONE',  ( 3.591859063236761518, 54.95696800326376064, 11.09922568453594849 ) ) ;
#19445=CARTESIAN_POINT ( 'NONE',  ( 0.1532563361054082862, 36.21726448433410894, 2.638427012816831674 ) ) ;
#19446=CARTESIAN_POINT ( 'NONE',  ( 0.5774900079438607392, 18.48035201082150536, 5.440088680355550821 ) ) ;
#19447=CARTESIAN_POINT ( 'NONE',  ( -4.164238869374099927, 67.01208216824728936, 3.795296366450308767 ) ) ;
#19449=CARTESIAN_POINT ( 'NONE',  ( -0.8801773607111009756, 8.063685344154837509, 1.068504757029289695E-15 ) ) ;
#19450=CARTESIAN_POINT ( 'NONE',  ( 12.91533473730993009, 26.60535201082150536, -10.88017736071109987 ) ) ;
#19452=CARTESIAN_POINT ( 'NONE',  ( 2.035157376598822676, 22.43868534415483396, -7.964842623401177768 ) ) ;
#19455=CARTESIAN_POINT ( 'NONE',  ( 20.15039907845753575, 10.60158574516642460, -6.262539305110077059 ) ) ;
#19456=CARTESIAN_POINT ( 'NONE',  ( 2.035157376598822676, 22.43868534415483396, -7.964842623401177768 ) ) ;
#19457=CARTESIAN_POINT ( 'NONE',  ( 2.791683348922237240, 55.38393115100078745, -7.208316651077763204 ) ) ;
#19458=CYLINDRICAL_SURFACE ( 'NONE', #88865, 0.5000000000000004441 ) ;
#19459=CARTESIAN_POINT ( 'NONE',  ( 0.6178305044545818747, 63.49863466993043204, -9.382169495545419124 ) ) ;
#19461=CARTESIAN_POINT ( 'NONE',  ( 2.917880565312948704, 32.63708216824730357, 12.26659068614894643 ) ) ;
#19462=CARTESIAN_POINT ( 'NONE',  ( 10.00000000000000178, 34.31368534415484106, 10.88017736071110342 ) ) ;
#19463=CARTESIAN_POINT ( 'NONE',  ( -0.8801773607110991993, 22.85535201082150181, -2.915334737309923874 ) ) ;
#19464=CARTESIAN_POINT ( 'NONE',  ( 20.15039907845753220, 42.62777174578613426, -6.262539305110077947 ) ) ;
#19465=CARTESIAN_POINT ( 'NONE',  ( 17.39651004071842166, 32.93575266056827644, 6.499999999999998224 ) ) ;
#19466=CARTESIAN_POINT ( 'NONE',  ( 7.361572987183169658, 44.96726448433412315, -9.846743663894592657 ) ) ;
#19469=CARTESIAN_POINT ( 'NONE',  ( 19.84674366389459266, 23.71726448433412315, -2.638427012816827677 ) ) ;
#19472=CARTESIAN_POINT ( 'NONE',  ( 19.42250999205614548, 15.98035201082150714, -5.440088680355545492 ) ) ;
#19473=CARTESIAN_POINT ( 'NONE',  ( 7.361572987183169658, 9.967264484334119601, -9.846743663894592657 ) ) ;
#19474=CARTESIAN_POINT ( 'NONE',  ( 4.559911319644449179, 57.23035201082150536, -9.422509992056141925 ) ) ;
#19475=CARTESIAN_POINT ( 'NONE',  ( 20.88017736071110164, 20.35535201082150891, 2.915334737309930979 ) ) ;
#19476=CARTESIAN_POINT ( 'NONE',  ( 10.00000000000000178, 60.37363466993041783, 12.81628187352647608 ) ) ;
#19477=CARTESIAN_POINT ( 'NONE',  ( 2.917880565312948704, 27.63708216824730357, 12.26659068614894643 ) ) ;
#19479=CARTESIAN_POINT ( 'NONE',  ( -2.816281873526471635, 58.91530133659707502, -3.434112377981056508 ) ) ;
#19481=CARTESIAN_POINT ( 'NONE',  ( 10.00000000000000000, -2.126365330069579951, -12.81628187352647608 ) ) ;
#19482=CARTESIAN_POINT ( 'NONE',  ( 1.274849032794324932, 32.55509018479936145, -6.500000000000021316 ) ) ;
#19483=CARTESIAN_POINT ( 'NONE',  ( -0.8801773607110991993, 37.85535201082151247, -2.915334737309923874 ) ) ;
#19484=CARTESIAN_POINT ( 'NONE',  ( 17.20831665107776587, 62.88393115100078745, 7.208316651077764980 ) ) ;
#19486=CARTESIAN_POINT ( 'NONE',  ( 19.84674366389459266, 18.30059781766745175, 2.638427012816836559 ) ) ;
#19487=CARTESIAN_POINT ( 'NONE',  ( 18.52753015748618282, 8.925597817667451750, -4.923371831947291888 ) ) ;
#19488=CARTESIAN_POINT ( 'NONE',  ( 17.20831665107776587, 17.88393115100078745, 7.208316651077764980 ) ) ;
#19489=CARTESIAN_POINT ( 'NONE',  ( 18.52753015748617571, 13.09226448433411960, 4.923371831947298993 ) ) ;
#19490=CARTESIAN_POINT ( 'NONE',  ( 15.44008868035555260, 59.73035201082151247, 9.422509992056143702 ) ) ;
#19492=CARTESIAN_POINT ( 'NONE',  ( 18.52753015748618282, 3.925597817667451306, -4.923371831947291888 ) ) ;
#19493=CARTESIAN_POINT ( 'NONE',  ( 5.076628168052703671, 21.84226448433411960, 8.527530157486179263 ) ) ;
#19494=EDGE_LOOP ( 'NONE', ( #25079, #555, #7107, #62245, #68213, #22526 ) ) ;
#19497=CARTESIAN_POINT ( 'NONE',  ( -1.099225684535947600, 3.706968003263753531, -6.408140936763238038 ) ) ;
#19500=CARTESIAN_POINT ( 'NONE',  ( 10.00000000000000178, 4.313685344154837509, 10.88017736071110342 ) ) ;
#19501=CARTESIAN_POINT ( 'NONE',  ( 6.204703633549690345, 15.76208216824730179, -14.16423886937410259 ) ) ;
#19504=CARTESIAN_POINT ( 'NONE',  ( 22.26659068614895176, 19.72041550158063572, -7.082119434687042414 ) ) ;
#19505=CARTESIAN_POINT ( 'NONE',  ( 17.08211943468705130, 28.47041550158063572, 12.26659068614894998 ) ) ;
#19508=CARTESIAN_POINT ( 'NONE',  ( 2.917880565312950480, 0.9704155015806342766, -12.26659068614894821 ) ) ;
#19509=CARTESIAN_POINT ( 'NONE',  ( -0.8801773607111008646, 33.27201867748817676, 2.915334737309923430 ) ) ;
#19512=CARTESIAN_POINT ( 'NONE',  ( 19.84674366389459266, 18.71726448433411960, -2.638427012816827677 ) ) ;
#19513=CARTESIAN_POINT ( 'NONE',  ( 15.44008868035555793, 61.39701867748817676, -9.422509992056140149 ) ) ;
#19514=CARTESIAN_POINT ( 'NONE',  ( 1.472469842513823179, 10.59226448433411782, -4.923371831947296329 ) ) ;
#19515=CARTESIAN_POINT ( 'NONE',  ( 7.084665262690076126, 12.02201867748817321, -10.88017736071110164 ) ) ;
#19516=CARTESIAN_POINT ( 'NONE',  ( 22.81628187352647785, 51.62363466993042493, 6.195893100308588602E-16 ) ) ;
#19517=CARTESIAN_POINT ( 'NONE',  ( 10.00000000000000000, 54.75893115100078745, -9.846743663894594434 ) ) ;
#19520=CARTESIAN_POINT ( 'NONE',  ( 0.6178305044545818747, 23.49863466993041783, -9.382169495545419124 ) ) ;
#19523=CARTESIAN_POINT ( 'NONE',  ( 19.84674366389459266, 43.30059781766744464, 2.638427012816836559 ) ) ;
#19524=CARTESIAN_POINT ( 'NONE',  ( 20.36894250292379382, 8.678748834913967869, 10.36894250292379205 ) ) ;
#19525=ORIENTED_EDGE ( 'NONE', *, *, #76871, .T. ) ;
#19527=CARTESIAN_POINT ( 'NONE',  ( 15.44008868035555793, 46.39701867748817676, -9.422509992056140149 ) ) ;
#19528=CARTESIAN_POINT ( 'NONE',  ( 0.5774900079438607392, 58.48035201082151247, 5.440088680355550821 ) ) ;
#19529=CARTESIAN_POINT ( 'NONE',  ( 13.79529636645031943, 50.34541550158064638, -14.16423886937409904 ) ) ;
#19530=CARTESIAN_POINT ( 'NONE',  ( 10.00000000000000178, 52.25893115100078745, 9.846743663894594434 ) ) ;
#19531=STYLED_ITEM ( 'NONE', ( #48735 ), #47653 ) ;
#19532=CARTESIAN_POINT ( 'NONE',  ( 0.6178305044545838731, 64.74863466993043914, 9.382169495545420901 ) ) ;
#19533=CARTESIAN_POINT ( 'NONE',  ( 17.96484262340118221, 46.18868534415484106, -7.964842623401177768 ) ) ;
#19535=CARTESIAN_POINT ( 'NONE',  ( 10.00000000000000000, 54.75893115100078745, -9.846743663894594434 ) ) ;
#19538=CARTESIAN_POINT ( 'NONE',  ( 19.72487221294570858, 11.86607318730075633, 6.500000000000000888 ) ) ;
#19539=DIRECTION ( 'NONE',  ( -0.000000000000000000, -0.000000000000000000, -1.000000000000000000 ) ) ;
#19541=COLOUR_RGB ( '', 0.72549020, 0.75294118, 0.79215686) ;
#19542=CARTESIAN_POINT ( 'NONE',  ( 18.52753015748617571, 3.092264484334118269, 4.923371831947298993 ) ) ;
#19543=CARTESIAN_POINT ( 'NONE',  ( 2.035157376598822676, 67.43868534415484817, -7.964842623401177768 ) ) ;
#19546=CARTESIAN_POINT ( 'NONE',  ( 1.472469842513823179, 40.59226448433411605, -4.923371831947296329 ) ) ;
#19547=CARTESIAN_POINT ( 'NONE',  ( 15.44008868035555793, 26.39701867748817321, -9.422509992056140149 ) ) ;
#19549=CARTESIAN_POINT ( 'NONE',  ( 13.43411237798105340, 5.581968003263753531, 12.81628187352647963 ) ) ;
#19550=CARTESIAN_POINT ( 'NONE',  ( 15.44008868035555260, 29.73035201082150891, 9.422509992056143702 ) ) ;
#19551=CARTESIAN_POINT ( 'NONE',  ( 17.39651004071841101, 37.93575266056827644, 6.500000000000005329 ) ) ;
#19552=CARTESIAN_POINT ( 'NONE',  ( 10.00000000000000000, 32.87363466993042493, -12.81628187352647608 ) ) ;
#19554=CARTESIAN_POINT ( 'NONE',  ( 15.44008868035555260, 49.73035201082150536, 9.422509992056143702 ) ) ;
#19555=CARTESIAN_POINT ( 'NONE',  ( 6.565887622018943937, 20.16530133659708213, 12.81628187352647430 ) ) ;
#19557=CARTESIAN_POINT ( 'NONE',  ( 20.32896413005680003, 31.77164270246084143, 5.963430220938287007 ) ) ;
#19558=CARTESIAN_POINT ( 'NONE',  ( 4.559911319644449179, 32.23035201082150536, -9.422509992056141925 ) ) ;
#19559=CARTESIAN_POINT ( 'NONE',  ( -2.266590686148945544, 67.22041550158063217, 7.082119434687048631 ) ) ;
#19561=CARTESIAN_POINT ( 'NONE',  ( 0.1532563361054083140, 56.00893115100078745, 1.131784320476157264E-15 ) ) ;
#19562=CARTESIAN_POINT ( 'NONE',  ( 0.1532563361054082862, 1.217264484334117824, 2.638427012816831674 ) ) ;
#19563=CARTESIAN_POINT ( 'NONE',  ( 20.88017736071110519, 65.56368534415483396, 2.639326808657452039E-16 ) ) ;
#19565=CARTESIAN_POINT ( 'NONE',  ( 17.08211943468705130, 28.47041550158063572, 12.26659068614894998 ) ) ;
#19568=EDGE_LOOP ( 'NONE', ( #29354, #8551, #5699, #66300 ) ) ;
#19569=CARTESIAN_POINT ( 'NONE',  ( 24.16423886937410614, 54.30374883491396787, 8.672049930838204340E-16 ) ) ;
#19570=CARTESIAN_POINT ( 'NONE',  ( 20.36894250292379738, 49.92874883491396787, -10.36894250292379027 ) ) ;
#19571=CARTESIAN_POINT ( 'NONE',  ( 14.92337183194729633, 22.67559781766745175, 8.527530157486181039 ) ) ;
#19572=CARTESIAN_POINT ( 'NONE',  ( 21.09922568453594849, 26.20696800326375353, 6.408140936763242479 ) ) ;
#19575=CARTESIAN_POINT ( 'NONE',  ( 0.5774900079438607392, 68.48035201082150536, 5.440088680355550821 ) ) ;
#19576=CARTESIAN_POINT ( 'NONE',  ( 22.26659068614895176, 49.72041550158063927, -7.082119434687042414 ) ) ;
#19579=CARTESIAN_POINT ( 'NONE',  ( 17.20831665107776587, 9.133931151000787452, -7.208316651077762316 ) ) ;
#19583=VERTEX_POINT ( 'NONE', #38374 ) ;
#19586=CARTESIAN_POINT ( 'NONE',  ( 10.00000000000000178, 24.31368534415484106, 10.88017736071110342 ) ) ;
#19587=CARTESIAN_POINT ( 'NONE',  ( 19.42250999205614548, 20.98035201082150891, -5.440088680355545492 ) ) ;
#19588=CARTESIAN_POINT ( 'NONE',  ( 19.84674366389459621, 48.50893115100078745, 7.409399052514197653E-17 ) ) ;
#19589=CARTESIAN_POINT ( 'NONE',  ( -2.816281873526473856, 19.12363466993042138, 9.499525473075851096E-16 ) ) ;
#19590=FACE_OUTER_BOUND ( 'NONE', #84488, .T. ) ;
#19592=CARTESIAN_POINT ( 'NONE',  ( -2.816281873526471635, 23.91530133659708568, -3.434112377981056508 ) ) ;
#19593=ORIENTED_EDGE ( 'NONE', *, *, #62664, .T. ) ;
#19595=CARTESIAN_POINT ( 'NONE',  ( 5.076628168052704559, 25.17559781766745175, -8.527530157486179263 ) ) ;
#19596=STYLED_ITEM ( 'NONE', ( #58858 ), #49361 ) ;
#19597=CARTESIAN_POINT ( 'NONE',  ( 2.917880565312948704, 62.63708216824730357, 12.26659068614894643 ) ) ;
#19600=CARTESIAN_POINT ( 'NONE',  ( 2.035157376598824452, 8.688685344154839285, 7.964842623401179544 ) ) ;
#19601=ORIENTED_EDGE ( 'NONE', *, *, #6682, .T. ) ;
#19602=CARTESIAN_POINT ( 'NONE',  ( 19.42250999205614548, 35.98035201082151247, -5.440088680355545492 ) ) ;
#19603=CARTESIAN_POINT ( 'NONE',  ( 12.91533473730993009, 51.60535201082149825, -10.88017736071109987 ) ) ;
#19604=CARTESIAN_POINT ( 'NONE',  ( 19.42250999205614193, 55.14701867748817676, 5.440088680355555262 ) ) ;
#19606=CARTESIAN_POINT ( 'NONE',  ( 17.96484262340118221, 44.93868534415483396, 7.964842623401181321 ) ) ;
#19609=CARTESIAN_POINT ( 'NONE',  ( 5.076628168052703671, 11.84226448433411960, 8.527530157486179263 ) ) ;
#19612=CARTESIAN_POINT ( 'NONE',  ( 18.52753015748617571, 63.09226448433412315, 4.923371831947298993 ) ) ;
#19613=CARTESIAN_POINT ( 'NONE',  ( 0.1129803114748865051, 24.29427333184091964, -6.480634945678684922 ) ) ;
#19615=ORIENTED_EDGE ( 'NONE', *, *, #70722, .T. ) ;
#19618=CARTESIAN_POINT ( 'NONE',  ( 2.791683348922240793, 66.63393115100079456, 7.208316651077764092 ) ) ;
#19619=CARTESIAN_POINT ( 'NONE',  ( 2.791683348922240793, 31.63393115100078745, 7.208316651077764092 ) ) ;
#19620=CARTESIAN_POINT ( 'NONE',  ( -4.164238869374098151, 56.59541550158063927, -3.795296366450310543 ) ) ;
#19624=CARTESIAN_POINT ( 'NONE',  ( 0.1532563361054082862, 26.21726448433411605, 2.638427012816831674 ) ) ;
#19625=CARTESIAN_POINT ( 'NONE',  ( 6.565887622018943937, 60.16530133659707502, 12.81628187352647430 ) ) ;
#19626=CARTESIAN_POINT ( 'NONE',  ( 0.6178305044545818747, 3.498634669930420049, -9.382169495545419124 ) ) ;
#19627=AXIS2_PLACEMENT_3D ( 'NONE', #24220, #85208, #16711 ) ;
#19628=CARTESIAN_POINT ( 'NONE',  ( 1.472469842513823179, 6.425597817667451750, 4.923371831947296329 ) ) ;
#19631=CARTESIAN_POINT ( 'NONE',  ( 2.791683348922240793, 6.633931151000785675, 7.208316651077764092 ) ) ;
#19632=CARTESIAN_POINT ( 'NONE',  ( 17.20831665107776587, 64.13393115100079456, -7.208316651077762316 ) ) ;
#19633=CARTESIAN_POINT ( 'NONE',  ( 19.42250999205614193, 20.14701867748817321, 5.440088680355555262 ) ) ;
#19636=CARTESIAN_POINT ( 'NONE',  ( -0.8801773607110991993, 12.85535201082150358, -2.915334737309923874 ) ) ;
#19637=CARTESIAN_POINT ( 'NONE',  ( 24.16423886937410614, 9.303748834913967869, 8.672049930838204340E-16 ) ) ;
#19638=CARTESIAN_POINT ( 'NONE',  ( 5.076628168052703671, 16.84226448433411960, 8.527530157486179263 ) ) ;
#19639=CARTESIAN_POINT ( 'NONE',  ( 2.035157376598822676, 42.43868534415483396, -7.964842623401177768 ) ) ;
#19640=CARTESIAN_POINT ( 'NONE',  ( 13.43411237798105340, 30.58196800326374998, 12.81628187352647963 ) ) ;
#19642=FILL_AREA_STYLE ('',( #27131 ) ) ;
#19643=CARTESIAN_POINT ( 'NONE',  ( 20.15039907845753220, 17.62777174578612716, -6.262539305110077947 ) ) ;
#19645=CARTESIAN_POINT ( 'NONE',  ( 10.00000000000000178, 0.3736346699304200492, 12.81628187352647608 ) ) ;
#19646=CARTESIAN_POINT ( 'NONE',  ( 18.52753015748618282, 58.92559781766745886, -4.923371831947291888 ) ) ;
#19647=CARTESIAN_POINT ( 'NONE',  ( 17.20831665107776587, 9.133931151000787452, -7.208316651077762316 ) ) ;
#19649=CARTESIAN_POINT ( 'NONE',  ( 3.591859063236761518, 19.95696800326375353, 11.09922568453594849 ) ) ;
#19651=CARTESIAN_POINT ( 'NONE',  ( 20.88017736071110164, 20.35535201082150891, 2.915334737309930979 ) ) ;
#19653=CARTESIAN_POINT ( 'NONE',  ( -4.164238869374099039, 51.80374883491396787, 8.674139862899312516E-16 ) ) ;
#19655=VECTOR ( 'NONE', #4808, 1000.000000000000000 ) ;
#19656=CARTESIAN_POINT ( 'NONE',  ( 13.43411237798106583, 32.66530133659708213, -12.81628187352647252 ) ) ;
#19657=CARTESIAN_POINT ( 'NONE',  ( 7.084665262690076126, 32.02201867748816966, -10.88017736071110164 ) ) ;
#19658=CARTESIAN_POINT ( 'NONE',  ( 10.00000000000000000, 49.75893115100078745, -9.846743663894594434 ) ) ;
#19660=CARTESIAN_POINT ( 'NONE',  ( 20.88017736071110875, 55.77201867748816966, -2.915334737309920765 ) ) ;
#19661=CARTESIAN_POINT ( 'NONE',  ( 19.38216949554541202, 0.9986346699304200492, 9.382169495545424454 ) ) ;
#19662=CARTESIAN_POINT ( 'NONE',  ( -0.3689425029237881626, 32.42874883491395366, 10.36894250292379027 ) ) ;
#19666=CARTESIAN_POINT ( 'NONE',  ( 19.84674366389459266, 18.30059781766745175, 2.638427012816836559 ) ) ;
#19667=CARTESIAN_POINT ( 'NONE',  ( -1.099225684535947600, 64.54030133659709634, 6.408140936763237150 ) ) ;
#19668=CARTESIAN_POINT ( 'NONE',  ( 13.43411237798105340, 0.5819680032637533085, 12.81628187352647963 ) ) ;
#19670=VECTOR ( 'NONE', #15129, 1000.000000000000000 ) ;
#19671=CARTESIAN_POINT ( 'NONE',  ( 20.10384461210893647, 11.74302437010793554, 6.337995344473741355 ) ) ;
#19672=CARTESIAN_POINT ( 'NONE',  ( 19.42250999205614193, 15.14701867748817143, 5.440088680355555262 ) ) ;
#19673=CARTESIAN_POINT ( 'NONE',  ( 17.08211943468705130, 18.47041550158063572, 12.26659068614894998 ) ) ;
#19674=CARTESIAN_POINT ( 'NONE',  ( 12.63842701281683922, 14.55059781766744997, -9.846743663894590881 ) ) ;
#19675=CARTESIAN_POINT ( 'NONE',  ( 14.92337183194729988, 44.34226448433412315, -8.527530157486177487 ) ) ;
#19676=CARTESIAN_POINT ( 'NONE',  ( 0.5774900079438590739, 27.64701867748817676, -5.440088680355550821 ) ) ;
#19678=CARTESIAN_POINT ( 'NONE',  ( 19.72487221294570858, 12.80223176428831167, -6.500000000000000888 ) ) ;
#19679=DIRECTION ( 'NONE',  ( 0.000000000000000000, 0.000000000000000000, 1.000000000000000000 ) ) ;
#19682=CARTESIAN_POINT ( 'NONE',  ( 10.00000000000000178, 52.25893115100078745, 9.846743663894594434 ) ) ;
#19684=VERTEX_POINT ( 'NONE', #37892 ) ;
#19686=CARTESIAN_POINT ( 'NONE',  ( 24.16423886937410614, 14.30374883491396787, 8.672049930838204340E-16 ) ) ;
#19687=CARTESIAN_POINT ( 'NONE',  ( -0.3689425029237898834, 6.178748834913968757, -10.36894250292378850 ) ) ;
#19688=CARTESIAN_POINT ( 'NONE',  ( 20.88017736071110164, 40.35535201082150536, 2.915334737309930979 ) ) ;
#19689=CARTESIAN_POINT ( 'NONE',  ( -2.266590686148945544, 61.38708216824730357, -7.082119434687050408 ) ) ;
#19690=CARTESIAN_POINT ( 'NONE',  ( 14.92337183194729988, 54.34226448433412315, -8.527530157486177487 ) ) ;
#19691=CARTESIAN_POINT ( 'NONE',  ( 17.20831665107776587, 32.88393115100078745, 7.208316651077764980 ) ) ;
#19693=CARTESIAN_POINT ( 'NONE',  ( 10.00000000000000178, 39.31368534415484106, 10.88017736071110342 ) ) ;
#19694=CARTESIAN_POINT ( 'NONE',  ( -2.816281873526473856, 4.123634669930420493, 9.499525473075851096E-16 ) ) ;
#19695=CARTESIAN_POINT ( 'NONE',  ( 17.08211943468705840, 5.137082168247300906, -12.26659068614894466 ) ) ;
#19696=CARTESIAN_POINT ( 'NONE',  ( 10.00000000000000178, 53.05374883491396787, 14.16423886937410082 ) ) ;
#19697=CARTESIAN_POINT ( 'NONE',  ( 19.42250999205614193, 10.14701867748816966, 5.440088680355555262 ) ) ;
#19698=CARTESIAN_POINT ( 'NONE',  ( -1.926860441876563801, 67.66212336850780673, 1.004413902775740978E-15 ) ) ;
#19704=ORIENTED_EDGE ( 'NONE', *, *, #93727, .T. ) ;
#19705=CARTESIAN_POINT ( 'NONE',  ( 22.26659068614895176, 34.72041550158063927, -7.082119434687042414 ) ) ;
#19706=CARTESIAN_POINT ( 'NONE',  ( 1.472469842513823179, 31.42559781766745530, 4.923371831947296329 ) ) ;
#19707=CARTESIAN_POINT ( 'NONE',  ( 12.91533473730992121, 59.52201867748816966, 10.88017736071110164 ) ) ;
#19710=CARTESIAN_POINT ( 'NONE',  ( 19.42250999205614193, 55.14701867748817676, 5.440088680355555262 ) ) ;
#19712=CARTESIAN_POINT ( 'NONE',  ( 21.09922568453594849, 61.20696800326376064, 6.408140936763242479 ) ) ;
#19715=CARTESIAN_POINT ( 'NONE',  ( 17.08211943468705840, 15.13708216824730179, -12.26659068614894466 ) ) ;
#19717=CARTESIAN_POINT ( 'NONE',  ( -1.099225684535947600, 43.70696800326375353, -6.408140936763238038 ) ) ;
#19718=CARTESIAN_POINT ( 'NONE',  ( 18.52753015748618282, 23.92559781766745530, -4.923371831947291888 ) ) ;
#19719=CARTESIAN_POINT ( 'NONE',  ( 15.44008868035555793, 11.39701867748817143, -9.422509992056140149 ) ) ;
#19720=CARTESIAN_POINT ( 'NONE',  ( 21.09922568453594849, 51.20696800326375353, 6.408140936763242479 ) ) ;
#19722=CARTESIAN_POINT ( 'NONE',  ( 10.00000000000000178, 37.25893115100078745, 9.846743663894594434 ) ) ;
#19725=ORIENTED_EDGE ( 'NONE', *, *, #74833, .T. ) ;
#19730=CARTESIAN_POINT ( 'NONE',  ( -0.2418659066527639179, 44.26028685723174050, -6.114288769123057854 ) ) ;
#19731=CARTESIAN_POINT ( 'NONE',  ( 7.361572987183170547, 22.05059781766745530, 9.846743663894590881 ) ) ;
#19732=CARTESIAN_POINT ( 'NONE',  ( 21.09922568453595559, 22.04030133659708923, -6.408140936763230044 ) ) ;
#19735=CARTESIAN_POINT ( 'NONE',  ( 2.791683348922240793, 46.63393115100077324, 7.208316651077764092 ) ) ;
#19736=CARTESIAN_POINT ( 'NONE',  ( 18.29284471827481084, 5.401890803972852595, -6.499999999999990230 ) ) ;
#19737=CARTESIAN_POINT ( 'NONE',  ( 22.26659068614895176, 19.72041550158063572, -7.082119434687042414 ) ) ;
#19738=CARTESIAN_POINT ( 'NONE',  ( 19.84674366389459621, 28.50893115100078745, 7.409399052514197653E-17 ) ) ;
#19739=CARTESIAN_POINT ( 'NONE',  ( 16.40814093676324603, 27.45696800326375708, -11.09922568453594671 ) ) ;
#19742=CARTESIAN_POINT ( 'NONE',  ( 4.559911319644449179, 57.23035201082150536, -9.422509992056141925 ) ) ;
#19743=CARTESIAN_POINT ( 'NONE',  ( 21.09922568453594849, 6.206968003263753531, 6.408140936763242479 ) ) ;
#19745=CARTESIAN_POINT ( 'NONE',  ( 2.791683348922240793, 36.63393115100078035, 7.208316651077764092 ) ) ;
#19746=CARTESIAN_POINT ( 'NONE',  ( 20.88017736071110519, 25.56368534415483751, 2.639326808657452039E-16 ) ) ;
#19747=EDGE_CURVE ( 'NONE', #83096, #25751, #47933, .T. ) ;
#19748=CARTESIAN_POINT ( 'NONE',  ( 22.81628187352648496, 31.83196800326375353, -3.434112377981050290 ) ) ;
#19749=CARTESIAN_POINT ( 'NONE',  ( 12.63842701281683922, 34.55059781766745886, -9.846743663894590881 ) ) ;
#19752=CARTESIAN_POINT ( 'NONE',  ( 0.5774900079438590739, 27.64701867748817676, -5.440088680355550821 ) ) ;
#19755=( LENGTH_UNIT ( ) NAMED_UNIT ( * ) SI_UNIT ( .MILLI., .METRE. ) );
#19756=CARTESIAN_POINT ( 'NONE',  ( 1.472469842513823179, 56.42559781766745886, 4.923371831947296329 ) ) ;
#19757=CARTESIAN_POINT ( 'NONE',  ( 12.91533473730993009, 31.60535201082150891, -10.88017736071109987 ) ) ;
#19759=CARTESIAN_POINT ( 'NONE',  ( 19.42250999205614548, 65.98035201082151957, -5.440088680355545492 ) ) ;
#19760=CARTESIAN_POINT ( 'NONE',  ( 2.035157376598822676, 27.43868534415483396, -7.964842623401177768 ) ) ;
#19762=CARTESIAN_POINT ( 'NONE',  ( 2.791683348922240793, 6.633931151000785675, 7.208316651077764092 ) ) ;
#19763=CARTESIAN_POINT ( 'NONE',  ( 10.00000000000000178, 52.25893115100078745, 9.846743663894594434 ) ) ;
#19764=CARTESIAN_POINT ( 'NONE',  ( 20.36894250292379382, 58.67874883491396076, 10.36894250292379205 ) ) ;
#19766=CARTESIAN_POINT ( 'NONE',  ( 10.00000000000000000, 15.55374883491396787, -14.16423886937410082 ) ) ;
#19767=CARTESIAN_POINT ( 'NONE',  ( -4.164238869374099927, 42.01208216824728936, 3.795296366450308767 ) ) ;
#19768=CARTESIAN_POINT ( 'NONE',  ( -2.816281873526473856, 4.123634669930420493, 9.499525473075851096E-16 ) ) ;
#19771=CARTESIAN_POINT ( 'NONE',  ( 17.96484262340118221, 11.18868534415484106, -7.964842623401177768 ) ) ;
#19772=CARTESIAN_POINT ( 'NONE',  ( 2.791683348922240793, 41.63393115100078745, 7.208316651077764092 ) ) ;
#19774=CARTESIAN_POINT ( 'NONE',  ( 19.42250999205614193, 60.14701867748817676, 5.440088680355555262 ) ) ;
#19776=CARTESIAN_POINT ( 'NONE',  ( 22.81628187352647785, 56.41530133659708213, 3.434112377981063169 ) ) ;
#19777=CARTESIAN_POINT ( 'NONE',  ( 21.09922568453594849, 26.20696800326375353, 6.408140936763242479 ) ) ;
#19778=CARTESIAN_POINT ( 'NONE',  ( 14.92337183194729988, 24.34226448433411960, -8.527530157486177487 ) ) ;
#19780=VERTEX_POINT ( 'NONE', #56327 ) ;
#19781=CARTESIAN_POINT ( 'NONE',  ( 4.559911319644449179, 2.230352010821504916, -9.422509992056141925 ) ) ;
#19782=CARTESIAN_POINT ( 'NONE',  ( -0.8801773607111008646, 18.27201867748817321, 2.915334737309923430 ) ) ;
#19783=CARTESIAN_POINT ( 'NONE',  ( -2.266590686148945544, 47.22041550158063927, 7.082119434687048631 ) ) ;
#19784=CARTESIAN_POINT ( 'NONE',  ( 7.084665262690076126, 34.10535201082151247, 10.88017736071109987 ) ) ;
#19785=CARTESIAN_POINT ( 'NONE',  ( -0.8801773607110991993, 57.85535201082149825, -2.915334737309923874 ) ) ;
#19788=CARTESIAN_POINT ( 'NONE',  ( 17.20831665107776587, 7.883931151000784787, 7.208316651077764980 ) ) ;
#19789=FACE_OUTER_BOUND ( 'NONE', #49113, .T. ) ;
#19790=CARTESIAN_POINT ( 'NONE',  ( 0.1532563361054082862, 6.217264484334118713, 2.638427012816831674 ) ) ;
#19791=CARTESIAN_POINT ( 'NONE',  ( 19.72487221294570858, 0.000000000000000000, -6.500000000000000888 ) ) ;
#19792=CARTESIAN_POINT ( 'NONE',  ( 17.20831665107776587, 44.13393115100078745, -7.208316651077762316 ) ) ;
#19793=CARTESIAN_POINT ( 'NONE',  ( 5.076628168052703671, 66.84226448433412315, 8.527530157486179263 ) ) ;
#19794=CARTESIAN_POINT ( 'NONE',  ( 4.559911319644449179, 23.89701867748817321, 9.422509992056141925 ) ) ;
#19795=ORIENTED_EDGE ( 'NONE', *, *, #35308, .T. ) ;
#19796=CARTESIAN_POINT ( 'NONE',  ( 19.38216949554541202, 40.99863466993042493, 9.382169495545424454 ) ) ;
#19797=LINE ( 'NONE', #4815, #41258 ) ;
#19799=CARTESIAN_POINT ( 'NONE',  ( 19.42250999205614548, 60.98035201082151247, -5.440088680355545492 ) ) ;
#19800=CARTESIAN_POINT ( 'NONE',  ( 21.09922568453594849, 41.20696800326375353, 6.408140936763242479 ) ) ;
#19801=CARTESIAN_POINT ( 'NONE',  ( 24.16423886937410614, 54.51208216824730357, -3.795296366450302550 ) ) ;
#19802=CARTESIAN_POINT ( 'NONE',  ( 5.076628168052703671, 16.84226448433411960, 8.527530157486179263 ) ) ;
#19805=CARTESIAN_POINT ( 'NONE',  ( -4.164238869374099039, 16.80374883491396787, 8.674139862899312516E-16 ) ) ;
#19806=CARTESIAN_POINT ( 'NONE',  ( 24.16423886937409904, 29.09541550158063572, 3.795296366450317205 ) ) ;
#19807=CARTESIAN_POINT ( 'NONE',  ( 14.92337183194729633, 47.67559781766745175, 8.527530157486181039 ) ) ;
#19808=CARTESIAN_POINT ( 'NONE',  ( 18.06765999051786054, 8.991275129254484355, 6.499999999999990230 ) ) ;
#19809=CARTESIAN_POINT ( 'NONE',  ( 15.44008868035555793, 21.39701867748817321, -9.422509992056140149 ) ) ;
#19811=CARTESIAN_POINT ( 'NONE',  ( 20.88017736071110164, 65.35535201082150536, 2.915334737309930979 ) ) ;
#19812=CARTESIAN_POINT ( 'NONE',  ( 0.1532563361054083140, 56.00893115100078745, 1.131784320476157264E-15 ) ) ;
#19814=CARTESIAN_POINT ( 'NONE',  ( 22.81628187352647785, 46.41530133659708213, 3.434112377981063169 ) ) ;
#19815=CARTESIAN_POINT ( 'NONE',  ( 15.44008868035555793, 51.39701867748816966, -9.422509992056140149 ) ) ;
#19821=CARTESIAN_POINT ( 'NONE',  ( 10.00000000000000178, 64.31368534415483396, 10.88017736071110342 ) ) ;
#19822=CARTESIAN_POINT ( 'NONE',  ( 10.00000000000000178, 14.31368534415483751, 10.88017736071110342 ) ) ;
#19825=CARTESIAN_POINT ( 'NONE',  ( 17.96484262340118221, 9.938685344154839285, 7.964842623401181321 ) ) ;
#19826=CARTESIAN_POINT ( 'NONE',  ( 7.361572987183169658, 24.96726448433412315, -9.846743663894592657 ) ) ;
#19827=CARTESIAN_POINT ( 'NONE',  ( 20.36894250292379738, 19.92874883491396787, -10.36894250292379027 ) ) ;
#19828=CARTESIAN_POINT ( 'NONE',  ( 2.035157376598824452, 18.68868534415484106, 7.964842623401179544 ) ) ;
#19829=CARTESIAN_POINT ( 'NONE',  ( 2.791683348922237240, 65.38393115100078035, -7.208316651077763204 ) ) ;
#19831=ADVANCED_FACE ( 'NONE', ( #63312 ), #93329, .F. ) ;
#19832=CARTESIAN_POINT ( 'NONE',  ( 5.076628168052703671, 56.84226448433412315, 8.527530157486179263 ) ) ;
#19833=ORIENTED_EDGE ( 'NONE', *, *, #92478, .T. ) ;
#19834=CARTESIAN_POINT ( 'NONE',  ( 20.88017736071110519, 55.56368534415484817, 2.639326808657452039E-16 ) ) ;
#19835=CARTESIAN_POINT ( 'NONE',  ( 0.1532563361054083140, 66.00893115100079456, 1.131784320476157264E-15 ) ) ;
#19836=CARTESIAN_POINT ( 'NONE',  ( 10.00000000000000000, 42.87363466993042493, -12.81628187352647608 ) ) ;
#19837=CARTESIAN_POINT ( 'NONE',  ( 7.084665262690076126, 4.105352010821503583, 10.88017736071109987 ) ) ;
#19839=CARTESIAN_POINT ( 'NONE',  ( 2.035157376598824452, 53.68868534415484817, 7.964842623401179544 ) ) ;
#19840=CARTESIAN_POINT ( 'NONE',  ( 20.88017736071110519, 15.56368534415483751, 2.639326808657452039E-16 ) ) ;
#19841=SHAPE_REPRESENTATION ( '1.2 Movable Jaw', ( #27931 ), #40723 ) ;
#19842=CARTESIAN_POINT ( 'NONE',  ( -1.099225684535947600, 44.54030133659708923, 6.408140936763237150 ) ) ;
#19843=CARTESIAN_POINT ( 'NONE',  ( -0.8801773607111009756, 28.06368534415484106, 1.068504757029289695E-15 ) ) ;
#19845=CARTESIAN_POINT ( 'NONE',  ( -1.099225684535947600, 38.70696800326375353, -6.408140936763238038 ) ) ;
#19846=CARTESIAN_POINT ( 'NONE',  ( 19.42250999205614193, 35.14701867748816966, 5.440088680355555262 ) ) ;
#19847=CARTESIAN_POINT ( 'NONE',  ( 19.84674366389459621, 58.50893115100078745, 7.409399052514197653E-17 ) ) ;
#19850=CARTESIAN_POINT ( 'NONE',  ( 7.361572987183169658, 59.96726448433410894, -9.846743663894592657 ) ) ;
#19852=CARTESIAN_POINT ( 'NONE',  ( 12.63842701281683034, 52.46726448433413026, 9.846743663894596210 ) ) ;
#19853=CARTESIAN_POINT ( 'NONE',  ( 0.5774900079438590739, 22.64701867748817321, -5.440088680355550821 ) ) ;
#19855=CARTESIAN_POINT ( 'NONE',  ( 0.1955144967549090895, 39.32703681773340776, -6.500000000002870593 ) ) ;
#19857=CARTESIAN_POINT ( 'NONE',  ( 12.63842701281683034, 42.46726448433412315, 9.846743663894596210 ) ) ;
#19858=CARTESIAN_POINT ( 'NONE',  ( 14.92337183194729988, 4.342264484334117824, -8.527530157486177487 ) ) ;
#19859=CARTESIAN_POINT ( 'NONE',  ( 18.52753015748617571, 28.09226448433411960, 4.923371831947298993 ) ) ;
#19861=CARTESIAN_POINT ( 'NONE',  ( 12.63842701281683922, 64.55059781766745175, -9.846743663894590881 ) ) ;
#19862=VERTEX_POINT ( 'NONE', #71332 ) ;
#19863=CARTESIAN_POINT ( 'NONE',  ( 21.09922568453595559, 37.04030133659708923, -6.408140936763230044 ) ) ;
#19864=CARTESIAN_POINT ( 'NONE',  ( 10.00000000000000000, 39.75893115100078745, -9.846743663894594434 ) ) ;
#19866=CARTESIAN_POINT ( 'NONE',  ( 1.274849032794294290, 58.57228050351032778, 6.499999999999979572 ) ) ;
#19867=CARTESIAN_POINT ( 'NONE',  ( 6.204703633549690345, 57.84541550158063927, 14.16423886937410082 ) ) ;
#19868=ADVANCED_FACE ( 'NONE', ( #18819 ), #94305, .T. ) ;
#19869=CARTESIAN_POINT ( 'NONE',  ( 0.1532563361054083140, 26.00893115100078745, 1.131784320476157264E-15 ) ) ;
#19873=CARTESIAN_POINT ( 'NONE',  ( 22.26659068614895176, 59.72041550158063927, -7.082119434687042414 ) ) ;
#19875=CARTESIAN_POINT ( 'NONE',  ( 20.88017736071110164, 15.35535201082150358, 2.915334737309930979 ) ) ;
#19876=CARTESIAN_POINT ( 'NONE',  ( 24.16423886937410614, 34.51208216824731068, -3.795296366450302550 ) ) ;
#19877=CARTESIAN_POINT ( 'NONE',  ( 22.26659068614895176, 49.72041550158063927, -7.082119434687042414 ) ) ;
#19880=CARTESIAN_POINT ( 'NONE',  ( 19.84674366389459621, 13.50893115100078568, 7.409399052514197653E-17 ) ) ;
#19881=ADVANCED_FACE ( 'NONE', ( #33782, #16853 ), #64289, .F. ) ;
#19882=CARTESIAN_POINT ( 'NONE',  ( 15.00000000000000000, 11.00000000000000000, 6.500000000000000888 ) ) ;
#19883=CARTESIAN_POINT ( 'NONE',  ( 18.52753015748618282, 63.92559781766745886, -4.923371831947291888 ) ) ;
#19885=CARTESIAN_POINT ( 'NONE',  ( 20.88017736071110164, 45.35535201082149115, 2.915334737309930979 ) ) ;
#19886=CARTESIAN_POINT ( 'NONE',  ( 0.8952175423694853640, 17.60160829253886305, -5.990408912944323205 ) ) ;
#19887=CARTESIAN_POINT ( 'NONE',  ( 10.00000000000000000, 49.75893115100078745, -9.846743663894594434 ) ) ;
#19888=DIRECTION ( 'NONE',  ( -0.7445673648800779088, 0.6675473310227050261, 0.000000000000000000 ) ) ;
#19889=CARTESIAN_POINT ( 'NONE',  ( 0.1532563361054082862, 56.21726448433411605, 2.638427012816831674 ) ) ;
#19890=CARTESIAN_POINT ( 'NONE',  ( 13.79529636645030344, 3.262082168247301350, 14.16423886937410614 ) ) ;
#19892=CARTESIAN_POINT ( 'NONE',  ( -4.164238869374099927, 27.01208216824730357, 3.795296366450308767 ) ) ;
#19893=CARTESIAN_POINT ( 'NONE',  ( 1.274849032794292736, 37.55509018479936145, -6.499999999999977796 ) ) ;
#19896=CARTESIAN_POINT ( 'NONE',  ( 17.96484262340118221, 16.18868534415483396, -7.964842623401177768 ) ) ;
#19897=CARTESIAN_POINT ( 'NONE',  ( -2.816281873526473856, 44.12363466993042493, 9.499525473075851096E-16 ) ) ;
#19898=( BOUNDED_CURVE ( )  B_SPLINE_CURVE ( 2, ( #11894, #72873, #4408, #73367, #4894, #88875, #30825, #75841, #84824 ),
 .UNSPECIFIED., .F., .F. ) 
 B_SPLINE_CURVE_WITH_KNOTS ( ( 3, 2, 2, 2, 3 ),
 ( 0.04628608864975117254, 0.04761904761904761640, 0.05357142857142856845, 0.05952380952380952051, 0.06085676849310609621 ),
 .UNSPECIFIED. ) 
 CURVE ( )  GEOMETRIC_REPRESENTATION_ITEM ( )  RATIONAL_B_SPLINE_CURVE ( ( 0.9881565478350731180, 0.9923695281211489805, 1.000000000000000000, 0.9659258262890683122, 1.000000000000000000, 0.9659258262890683122, 1.000000000000000000, 0.9923695281211482033, 0.9881565478350724518 ) ) 
 REPRESENTATION_ITEM ( '' )  );
#19900=CARTESIAN_POINT ( 'NONE',  ( 5.076628168052704559, 5.175597817667451750, -8.527530157486179263 ) ) ;
#19903=EDGE_CURVE ( 'NONE', #75285, #59946, #69857, .T. ) ;
#19905=CARTESIAN_POINT ( 'NONE',  ( -2.266590686148945544, 31.38708216824730002, -7.082119434687050408 ) ) ;
#19906=CARTESIAN_POINT ( 'NONE',  ( 2.917880565312948704, 2.637082168247300906, 12.26659068614894643 ) ) ;
#19908=CARTESIAN_POINT ( 'NONE',  ( 2.035157376598822676, 12.43868534415483751, -7.964842623401177768 ) ) ;
#19911=CARTESIAN_POINT ( 'NONE',  ( 4.559911319644449179, 33.89701867748817676, 9.422509992056141925 ) ) ;
#19912=CARTESIAN_POINT ( 'NONE',  ( 20.88017736071110875, 55.77201867748816966, -2.915334737309920765 ) ) ;
#19913=CARTESIAN_POINT ( 'NONE',  ( 0.6178305044545838731, 19.74863466993042138, 9.382169495545420901 ) ) ;
#19914=CARTESIAN_POINT ( 'NONE',  ( 17.20831665107776587, 62.88393115100078745, 7.208316651077764980 ) ) ;
#19916=CARTESIAN_POINT ( 'NONE',  ( 0.1532563361054100626, 20.80059781766744464, -2.638427012816831230 ) ) ;
#19919=CARTESIAN_POINT ( 'NONE',  ( 20.88017736071110164, 50.35535201082151247, 2.915334737309930979 ) ) ;
#19920=CARTESIAN_POINT ( 'NONE',  ( 3.591859063236763294, 3.290301336597087012, -11.09922568453595026 ) ) ;
#19921=CARTESIAN_POINT ( 'NONE',  ( 12.91533473730993009, 66.60535201082150536, -10.88017736071109987 ) ) ;
#19922=CARTESIAN_POINT ( 'NONE',  ( 0.1532563361054100626, 20.80059781766744464, -2.638427012816831230 ) ) ;
#19923=CARTESIAN_POINT ( 'NONE',  ( 10.00000000000000178, 50.37363466993042493, 12.81628187352647608 ) ) ;
#19924=CARTESIAN_POINT ( 'NONE',  ( 14.92337183194729988, 9.342264484334119601, -8.527530157486177487 ) ) ;
#19925=ORIENTED_EDGE ( 'NONE', *, *, #63790, .T. ) ;
#19927=CARTESIAN_POINT ( 'NONE',  ( 19.72487221294570858, 70.00000000000000000, -6.000000000000000000 ) ) ;
#19928=CARTESIAN_POINT ( 'NONE',  ( 19.42250999205614548, 20.98035201082150891, -5.440088680355545492 ) ) ;
#19929=CARTESIAN_POINT ( 'NONE',  ( 3.591859063236761518, 64.95696800326376774, 11.09922568453594849 ) ) ;
#19930=CARTESIAN_POINT ( 'NONE',  ( 7.361572987183170547, 27.05059781766745175, 9.846743663894590881 ) ) ;
#19931=CARTESIAN_POINT ( 'NONE',  ( 10.00000000000000178, 14.31368534415483751, 10.88017736071110342 ) ) ;
#19932=CARTESIAN_POINT ( 'NONE',  ( 17.96484262340118221, 4.938685344154837509, 7.964842623401181321 ) ) ;
#19934=CARTESIAN_POINT ( 'NONE',  ( 12.91533473730993009, 11.60535201082150536, -10.88017736071109987 ) ) ;
#19936=CARTESIAN_POINT ( 'NONE',  ( 2.035157376598824452, 33.68868534415484106, 7.964842623401179544 ) ) ;
#19938=CARTESIAN_POINT ( 'NONE',  ( 15.44008868035555793, 41.39701867748817676, -9.422509992056140149 ) ) ;
#19940=CARTESIAN_POINT ( 'NONE',  ( 20.32896413005680358, 9.745456701841137104, 5.963430220938287007 ) ) ;
#19941=CARTESIAN_POINT ( 'NONE',  ( 15.44008868035555260, 29.73035201082150891, 9.422509992056143702 ) ) ;
#19942=CARTESIAN_POINT ( 'NONE',  ( 7.361572987183169658, 64.96726448433412315, -9.846743663894592657 ) ) ;
#19944=CARTESIAN_POINT ( 'NONE',  ( -0.3289641300568005855, 5.104976035794174472, 5.963430220938281678 ) ) ;
#19945=CARTESIAN_POINT ( 'NONE',  ( 2.917880565312950480, 35.97041550158063217, -12.26659068614894821 ) ) ;
#19946=CARTESIAN_POINT ( 'NONE',  ( 0.5774900079438607392, 33.48035201082150536, 5.440088680355550821 ) ) ;
#19947=CARTESIAN_POINT ( 'NONE',  ( 0.5774900079438607392, 33.48035201082150536, 5.440088680355550821 ) ) ;
#19948=CARTESIAN_POINT ( 'NONE',  ( 7.361572987183169658, 64.96726448433412315, -9.846743663894592657 ) ) ;
#19951=CARTESIAN_POINT ( 'NONE',  ( 0.1532563361054083140, 46.00893115100079456, 1.131784320476157264E-15 ) ) ;
#19953=CARTESIAN_POINT ( 'NONE',  ( 10.00000000000000000, 19.75893115100078390, -9.846743663894594434 ) ) ;
#19955=CARTESIAN_POINT ( 'NONE',  ( 10.00000000000000178, 14.31368534415483751, 10.88017736071110342 ) ) ;
#19956=CARTESIAN_POINT ( 'NONE',  ( 17.20831665107776587, 22.88393115100078745, 7.208316651077764980 ) ) ;
#19957=CARTESIAN_POINT ( 'NONE',  ( 10.00000000000000178, 64.31368534415483396, 10.88017736071110342 ) ) ;
#19958=CARTESIAN_POINT ( 'NONE',  ( 12.91533473730992121, 49.52201867748817676, 10.88017736071110164 ) ) ;
#19959=CARTESIAN_POINT ( 'NONE',  ( -0.8801773607111009756, 23.06368534415484106, 1.068504757029289695E-15 ) ) ;
#19960=CARTESIAN_POINT ( 'NONE',  ( -2.816281873526473856, 64.12363466993042493, 9.499525473075851096E-16 ) ) ;
#19961=CARTESIAN_POINT ( 'NONE',  ( -0.3689425029237898834, 31.17874883491396787, -10.36894250292378850 ) ) ;
#19965=CARTESIAN_POINT ( 'NONE',  ( 21.09922568453595559, 7.040301336597086568, -6.408140936763230044 ) ) ;
#19966=SURFACE_STYLE_FILL_AREA ( #88464 ) ;
#19967=CARTESIAN_POINT ( 'NONE',  ( 12.91533473730993009, 31.60535201082150891, -10.88017736071109987 ) ) ;
#19968=CARTESIAN_POINT ( 'NONE',  ( 12.63842701281683034, 62.46726448433410894, 9.846743663894596210 ) ) ;
#19970=CARTESIAN_POINT ( 'NONE',  ( 0.1532563361054082862, 16.21726448433411960, 2.638427012816831674 ) ) ;
#19971=CARTESIAN_POINT ( 'NONE',  ( 5.076628168052704559, 15.17559781766745175, -8.527530157486179263 ) ) ;
#19972=CARTESIAN_POINT ( 'NONE',  ( 12.63842701281683922, 19.55059781766745175, -9.846743663894590881 ) ) ;
#19974=CARTESIAN_POINT ( 'NONE',  ( 7.361572987183170547, 17.05059781766745530, 9.846743663894590881 ) ) ;
#19975=( LENGTH_UNIT ( ) NAMED_UNIT ( * ) SI_UNIT ( .MILLI., .METRE. ) );
#19978=CARTESIAN_POINT ( 'NONE',  ( 2.791683348922237240, 0.3839311510007847872, -7.208316651077763204 ) ) ;
#19980=CARTESIAN_POINT ( 'NONE',  ( 0.1532563361054083140, 1.008931151000784787, 1.131784320476157264E-15 ) ) ;
#19981=CARTESIAN_POINT ( 'NONE',  ( 1.472469842513823179, 25.59226448433412315, -4.923371831947296329 ) ) ;
#19982=EDGE_LOOP ( 'NONE', ( #11441, #2252, #73810, #27571 ) ) ;
#19985=CARTESIAN_POINT ( 'NONE',  ( 16.40814093676323893, 0.7903013365970867898, 11.09922568453595026 ) ) ;
#19987=CARTESIAN_POINT ( 'NONE',  ( 15.44008868035555260, 4.730352010821504471, 9.422509992056143702 ) ) ;
#19988=EDGE_CURVE ( 'NONE', #18712, #44298, #64777, .T. ) ;
#19989=CARTESIAN_POINT ( 'NONE',  ( 10.00000000000000000, 20.55374883491396787, -14.16423886937410082 ) ) ;
#19991=CARTESIAN_POINT ( 'NONE',  ( 22.26659068614894466, 18.88708216824730002, 7.082119434687054849 ) ) ;
#19992=CARTESIAN_POINT ( 'NONE',  ( 20.36894250292379382, 38.67874883491396076, 10.36894250292379205 ) ) ;
#19993=CARTESIAN_POINT ( 'NONE',  ( 20.36894250292379382, 18.67874883491397142, 10.36894250292379205 ) ) ;
#19994=CARTESIAN_POINT ( 'NONE',  ( 0.5774900079438607392, 68.48035201082150536, 5.440088680355550821 ) ) ;
#19995=CARTESIAN_POINT ( 'NONE',  ( 4.559911319644449179, 28.89701867748817321, 9.422509992056141925 ) ) ;
#19998=CARTESIAN_POINT ( 'NONE',  ( 10.00000000000000178, 12.25893115100078568, 9.846743663894594434 ) ) ;
#20000=CARTESIAN_POINT ( 'NONE',  ( -0.8801773607111009756, 53.06368534415484106, 1.068504757029289695E-15 ) ) ;
#20001=CARTESIAN_POINT ( 'NONE',  ( 12.63842701281683922, 34.55059781766745886, -9.846743663894590881 ) ) ;
#20003=CARTESIAN_POINT ( 'NONE',  ( 19.42250999205614548, 15.98035201082150714, -5.440088680355545492 ) ) ;
#20004=CARTESIAN_POINT ( 'NONE',  ( -1.099225684535947600, 39.54030133659708923, 6.408140936763237150 ) ) ;
#20005=CARTESIAN_POINT ( 'NONE',  ( 2.791683348922240793, 56.63393115100078035, 7.208316651077764092 ) ) ;
#20007=CARTESIAN_POINT ( 'NONE',  ( 3.591859063236763294, 48.29030133659708923, -11.09922568453595026 ) ) ;
#20009=CARTESIAN_POINT ( 'NONE',  ( 0.1532563361054082862, 41.21726448433411605, 2.638427012816831674 ) ) ;
#20010=CARTESIAN_POINT ( 'NONE',  ( 17.08211943468705840, 25.13708216824730357, -12.26659068614894466 ) ) ;
#20013=COLOUR_RGB ( '', 0.09019608, 0.27058824, 0.51372549) ;
#20014=CARTESIAN_POINT ( 'NONE',  ( 2.035157376598822676, 52.43868534415483396, -7.964842623401177768 ) ) ;
#20015=CARTESIAN_POINT ( 'NONE',  ( 0.5774900079438607392, 53.48035201082151247, 5.440088680355550821 ) ) ;
#20016=CARTESIAN_POINT ( 'NONE',  ( 22.26659068614894466, 48.88708216824730357, 7.082119434687054849 ) ) ;
#20017=CARTESIAN_POINT ( 'NONE',  ( 0.1532563361054083140, 66.00893115100079456, 1.131784320476157264E-15 ) ) ;
#20018=CARTESIAN_POINT ( 'NONE',  ( 19.38216949554541557, 62.24863466993041072, -9.382169495545420901 ) ) ;
#20019=CARTESIAN_POINT ( 'NONE',  ( 17.96484262340118221, 39.93868534415484106, 7.964842623401181321 ) ) ;
#20022=CARTESIAN_POINT ( 'NONE',  ( 22.81628187352647785, 21.62363466993041783, 6.195893100308588602E-16 ) ) ;
#20023=CARTESIAN_POINT ( 'NONE',  ( 12.63842701281683034, 52.46726448433413026, 9.846743663894596210 ) ) ;
#20025=CARTESIAN_POINT ( 'NONE',  ( 4.559911319644449179, 63.89701867748817676, 9.422509992056141925 ) ) ;
#20029=CARTESIAN_POINT ( 'NONE',  ( 4.559911319644449179, 68.89701867748817676, 9.422509992056141925 ) ) ;
#20030=CARTESIAN_POINT ( 'NONE',  ( 19.84674366389459621, 3.508931151000785231, 7.409399052514197653E-17 ) ) ;
#20033=CARTESIAN_POINT ( 'NONE',  ( 7.361572987183169658, 34.96726448433411605, -9.846743663894592657 ) ) ;
#20034=CARTESIAN_POINT ( 'NONE',  ( 4.559911319644449179, 28.89701867748817321, 9.422509992056141925 ) ) ;
#20035=CARTESIAN_POINT ( 'NONE',  ( 22.81628187352647785, 6.623634669930420493, 6.195893100308588602E-16 ) ) ;
#20036=CARTESIAN_POINT ( 'NONE',  ( 2.035157376598822676, 32.43868534415483396, -7.964842623401177768 ) ) ;
#20037=CARTESIAN_POINT ( 'NONE',  ( 13.99999999999999822, 11.00000000000000000, 6.000000000000000000 ) ) ;
#20039=CARTESIAN_POINT ( 'NONE',  ( 19.38216949554541202, 35.99863466993041072, 9.382169495545424454 ) ) ;
#20041=CARTESIAN_POINT ( 'NONE',  ( 10.00000000000000178, 59.31368534415484106, 10.88017736071110342 ) ) ;
#20042=CARTESIAN_POINT ( 'NONE',  ( 22.81628187352647785, 21.62363466993041783, 6.195893100308588602E-16 ) ) ;
#20043=CARTESIAN_POINT ( 'NONE',  ( 19.84674366389459621, 18.50893115100078745, 7.409399052514197653E-17 ) ) ;
#20044=SURFACE_SIDE_STYLE ('',( #88543 ) ) ;
#20045=CARTESIAN_POINT ( 'NONE',  ( 0.5774900079438607392, 43.48035201082151247, 5.440088680355550821 ) ) ;
#20046=CARTESIAN_POINT ( 'NONE',  ( 24.16423886937410614, 64.30374883491396076, 8.672049930838204340E-16 ) ) ;
#20047=CARTESIAN_POINT ( 'NONE',  ( 10.00000000000000178, 57.25893115100078745, 9.846743663894594434 ) ) ;
#20048=CARTESIAN_POINT ( 'NONE',  ( 2.791683348922237240, 10.38393115100078390, -7.208316651077763204 ) ) ;
#20049=CARTESIAN_POINT ( 'NONE',  ( 2.035157376598822676, 62.43868534415483396, -7.964842623401177768 ) ) ;
#20051=CARTESIAN_POINT ( 'NONE',  ( 24.16423886937410614, 29.30374883491396787, 8.672049930838204340E-16 ) ) ;
#20052=COLOUR_RGB ( '', 0.66274510, 0.83137255, 0.94901961) ;
#20053=FACE_OUTER_BOUND ( 'NONE', #94862, .T. ) ;
#20054=CARTESIAN_POINT ( 'NONE',  ( 19.59355871817327710, 82.60099334974556484, -5.130928526377548593 ) ) ;
#20055=ORIENTED_EDGE ( 'NONE', *, *, #82443, .F. ) ;
#20057=CARTESIAN_POINT ( 'NONE',  ( 13.79529636645031943, 60.34541550158063927, -14.16423886937409904 ) ) ;
#20058=CARTESIAN_POINT ( 'NONE',  ( 17.08211943468705130, 53.47041550158063217, 12.26659068614894998 ) ) ;
#20059=CARTESIAN_POINT ( 'NONE',  ( 19.84674366389459266, 28.30059781766745886, 2.638427012816836559 ) ) ;
#20061=CARTESIAN_POINT ( 'NONE',  ( 0.6178305044545818747, 23.49863466993041783, -9.382169495545419124 ) ) ;
#20063=SURFACE_STYLE_USAGE ( .BOTH. , #12564 ) ;
#20064=CARTESIAN_POINT ( 'NONE',  ( -4.164238869374099927, 47.01208216824729647, 3.795296366450308767 ) ) ;
#20066=CARTESIAN_POINT ( 'NONE',  ( 14.92337183194729988, 4.342264484334117824, -8.527530157486177487 ) ) ;
#20071=ORIENTED_EDGE ( 'NONE', *, *, #35702, .T. ) ;
#20074=CARTESIAN_POINT ( 'NONE',  ( 10.00000000000000000, 21.81368534415484106, -10.88017736071110342 ) ) ;
#20075=CARTESIAN_POINT ( 'NONE',  ( 17.96484262340118221, 26.18868534415483396, -7.964842623401177768 ) ) ;
#20076=CARTESIAN_POINT ( 'NONE',  ( 10.00000000000000178, 52.25893115100078745, 9.846743663894594434 ) ) ;
#20077=CARTESIAN_POINT ( 'NONE',  ( 21.09922568453594849, 16.20696800326375353, 6.408140936763242479 ) ) ;
#20079=ADVANCED_FACE ( 'NONE', ( #22637 ), #12778, .T. ) ;
#20080=STYLED_ITEM ( 'NONE', ( #65643 ), #35604 ) ;
#20081=MECHANICAL_DESIGN_GEOMETRIC_PRESENTATION_REPRESENTATION('',(#77599),#53623);
#20082=B_SPLINE_CURVE_WITH_KNOTS ( 'NONE', 3,
 ( #79823, #34806, #33804, #34300, #64798, #58284, #19808, #73790, #26818, #57311 ),
 .UNSPECIFIED., .F., .F.,
 ( 4, 3, 3, 4 ),
 ( 1.398578778534940505E-17, 0.0006253016069560823811, 0.001250604074564926060, 0.002501455912506542201 ),
 .UNSPECIFIED. ) ;
#20085=CARTESIAN_POINT ( 'NONE',  ( 16.40814093676323893, 15.79030133659708746, 11.09922568453595026 ) ) ;
#20087=CARTESIAN_POINT ( 'NONE',  ( 10.00000000000000178, 37.25893115100078745, 9.846743663894594434 ) ) ;
#20088=CARTESIAN_POINT ( 'NONE',  ( 13.79529636645030344, 63.26208216824730357, 14.16423886937410614 ) ) ;
#20089=CARTESIAN_POINT ( 'NONE',  ( 12.91533473730992121, 4.522018677488170546, 10.88017736071110164 ) ) ;
#20091=CARTESIAN_POINT ( 'NONE',  ( -0.8801773607110991993, 52.85535201082151247, -2.915334737309923874 ) ) ;
#20092=CARTESIAN_POINT ( 'NONE',  ( 19.42250999205614193, 40.14701867748817676, 5.440088680355555262 ) ) ;
#20093=CARTESIAN_POINT ( 'NONE',  ( 15.44008868035555260, 49.73035201082150536, 9.422509992056143702 ) ) ;
#20095=CARTESIAN_POINT ( 'NONE',  ( -0.8801773607111008646, 38.27201867748816255, 2.915334737309923430 ) ) ;
#20096=CARTESIAN_POINT ( 'NONE',  ( 21.92686044187657401, 65.37045670184114954, -3.195792623639525765 ) ) ;
#20099=CARTESIAN_POINT ( 'NONE',  ( 0.1532563361054082862, 31.21726448433412315, 2.638427012816831674 ) ) ;
#20101=ORIENTED_EDGE ( 'NONE', *, *, #90664, .T. ) ;
#20102=CARTESIAN_POINT ( 'NONE',  ( 19.84674366389459266, 53.71726448433411605, -2.638427012816827677 ) ) ;
#20110=CARTESIAN_POINT ( 'NONE',  ( -4.164238869374098151, 61.59541550158063217, -3.795296366450310543 ) ) ;
#20114=CARTESIAN_POINT ( 'NONE',  ( 14.92337183194729988, 29.34226448433411960, -8.527530157486177487 ) ) ;
#20117=CARTESIAN_POINT ( 'NONE',  ( 16.40814093676324603, 7.456968003263754419, -11.09922568453594671 ) ) ;
#20118=CARTESIAN_POINT ( 'NONE',  ( 0.1532563361054083140, 6.008931151000784787, 1.131784320476157264E-15 ) ) ;
#20119=CARTESIAN_POINT ( 'NONE',  ( 0.1516233060550335465, 0.2505839662184247141, 6.438133714914693329 ) ) ;
#20120=CARTESIAN_POINT ( 'NONE',  ( 19.84674366389459266, 8.300597817667451750, 2.638427012816836559 ) ) ;
#20121=CARTESIAN_POINT ( 'NONE',  ( 5.076628168052704559, 55.17559781766745175, -8.527530157486179263 ) ) ;
#20123=ORIENTED_EDGE ( 'NONE', *, *, #6464, .T. ) ;
#20124=CARTESIAN_POINT ( 'NONE',  ( 19.42250999205614548, 5.980352010821504471, -5.440088680355545492 ) ) ;
#20125=CARTESIAN_POINT ( 'NONE',  ( 6.204703633549690345, 2.845415501580634388, 14.16423886937410082 ) ) ;
#20126=CARTESIAN_POINT ( 'NONE',  ( 0.1532563361054100626, 10.80059781766745175, -2.638427012816831230 ) ) ;
#20127=CARTESIAN_POINT ( 'NONE',  ( 17.96484262340118221, 49.93868534415484106, 7.964842623401181321 ) ) ;
#20128=CARTESIAN_POINT ( 'NONE',  ( 3.591859063236763294, 28.29030133659708568, -11.09922568453595026 ) ) ;
#20130=CARTESIAN_POINT ( 'NONE',  ( 10.00000000000000000, 1.813685344154837731, -10.88017736071110342 ) ) ;
#20133=LINE ( 'NONE', #66118, #36019 ) ;
#20134=CARTESIAN_POINT ( 'NONE',  ( 13.43411237798106583, 2.665301336597086568, -12.81628187352647252 ) ) ;
#20135=CARTESIAN_POINT ( 'NONE',  ( 18.52753015748617571, 63.09226448433412315, 4.923371831947298993 ) ) ;
#20136=CARTESIAN_POINT ( 'NONE',  ( 1.472469842513823179, 10.59226448433411782, -4.923371831947296329 ) ) ;
#20138=CARTESIAN_POINT ( 'NONE',  ( -1.099225684535947600, 19.54030133659708568, 6.408140936763237150 ) ) ;
#20139=CARTESIAN_POINT ( 'NONE',  ( 1.383448333479234904, 52.37718327197428891, -6.499999999999977796 ) ) ;
#20140=CARTESIAN_POINT ( 'NONE',  ( 2.035157376598824452, 23.68868534415484461, 7.964842623401179544 ) ) ;
#20142=CARTESIAN_POINT ( 'NONE',  ( 13.79529636645030344, 53.26208216824730357, 14.16423886937410614 ) ) ;
#20145=CARTESIAN_POINT ( 'NONE',  ( 15.44008868035555260, 24.73035201082150891, 9.422509992056143702 ) ) ;
#20147=CARTESIAN_POINT ( 'NONE',  ( 0.1532563361054082862, 56.21726448433411605, 2.638427012816831674 ) ) ;
#20148=CARTESIAN_POINT ( 'NONE',  ( 0.5774900079438590739, 57.64701867748817676, -5.440088680355550821 ) ) ;
#20149=CARTESIAN_POINT ( 'NONE',  ( -2.266590686148945544, 36.38708216824730357, -7.082119434687050408 ) ) ;
#20151=( GEOMETRIC_REPRESENTATION_CONTEXT ( 3 ) GLOBAL_UNCERTAINTY_ASSIGNED_CONTEXT ( ( #80505 ) ) GLOBAL_UNIT_ASSIGNED_CONTEXT ( ( #8290, #23801, #74802 ) ) REPRESENTATION_CONTEXT ( 'NONE', 'WORKASPACE' ) );
#20153=CARTESIAN_POINT ( 'NONE',  ( 14.92337183194729988, 34.34226448433411605, -8.527530157486177487 ) ) ;
#20154=CARTESIAN_POINT ( 'NONE',  ( 3.591859063236763294, 58.29030133659708923, -11.09922568453595026 ) ) ;
#20155=CARTESIAN_POINT ( 'NONE',  ( 14.92337183194729633, 62.67559781766745886, 8.527530157486181039 ) ) ;
#20157=CARTESIAN_POINT ( 'NONE',  ( 0.5774900079438607392, 18.48035201082150536, 5.440088680355550821 ) ) ;
#20160=CARTESIAN_POINT ( 'NONE',  ( 10.00000000000000000, 11.81368534415483751, -10.88017736071110342 ) ) ;
#20161=CARTESIAN_POINT ( 'NONE',  ( 15.44008868035555260, 64.73035201082151957, 9.422509992056143702 ) ) ;
#20162=CARTESIAN_POINT ( 'NONE',  ( 17.08211943468705840, 25.13708216824730357, -12.26659068614894466 ) ) ;
#20163=CARTESIAN_POINT ( 'NONE',  ( 17.20831665107776587, 14.13393115100078568, -7.208316651077762316 ) ) ;
#20164=CARTESIAN_POINT ( 'NONE',  ( 12.63842701281683034, 57.46726448433411605, 9.846743663894596210 ) ) ;
#20165=CARTESIAN_POINT ( 'NONE',  ( 15.44008868035555793, 31.39701867748817676, -9.422509992056140149 ) ) ;
#20168=VERTEX_POINT ( 'NONE', #81761 ) ;
#20170=CARTESIAN_POINT ( 'NONE',  ( 12.63842701281683922, 49.55059781766744464, -9.846743663894590881 ) ) ;
#20175=CARTESIAN_POINT ( 'NONE',  ( 24.16423886937409904, 9.095415501580633943, 3.795296366450317205 ) ) ;
#20176=CARTESIAN_POINT ( 'NONE',  ( 2.917880565312948704, 12.63708216824730179, 12.26659068614894643 ) ) ;
#20178=CARTESIAN_POINT ( 'NONE',  ( 0.5774900079438590739, 47.64701867748817676, -5.440088680355550821 ) ) ;
#20179=CARTESIAN_POINT ( 'NONE',  ( 24.16423886937409904, 54.09541550158063217, 3.795296366450317205 ) ) ;
#20180=CARTESIAN_POINT ( 'NONE',  ( 22.81628187352647785, 6.623634669930420493, 6.195893100308588602E-16 ) ) ;
#20181=CARTESIAN_POINT ( 'NONE',  ( 17.20831665107776587, 39.13393115100079456, -7.208316651077762316 ) ) ;
#20183=CARTESIAN_POINT ( 'NONE',  ( 12.91533473730992121, 34.52201867748817676, 10.88017736071110164 ) ) ;
#20184=CARTESIAN_POINT ( 'NONE',  ( 21.09922568453595559, 7.040301336597086568, -6.408140936763230044 ) ) ;
#20185=CARTESIAN_POINT ( 'NONE',  ( 10.00000000000000178, 8.053748834913967869, 14.16423886937410082 ) ) ;
#20186=CARTESIAN_POINT ( 'NONE',  ( -4.164238869374099927, 57.01208216824731068, 3.795296366450308767 ) ) ;
#20187=CARTESIAN_POINT ( 'NONE',  ( 19.42250999205614548, 15.98035201082150714, -5.440088680355545492 ) ) ;
#20188=CARTESIAN_POINT ( 'NONE',  ( 17.39651004071841101, 37.93575266056827644, 6.500000000000005329 ) ) ;
#20196=CARTESIAN_POINT ( 'NONE',  ( -4.164238869374098151, 41.59541550158061796, -3.795296366450310543 ) ) ;
#20197=CARTESIAN_POINT ( 'NONE',  ( 12.63842701281683034, 52.46726448433413026, 9.846743663894596210 ) ) ;
#20198=CARTESIAN_POINT ( 'NONE',  ( 19.42250999205614548, 50.98035201082151247, -5.440088680355545492 ) ) ;
#20201=CARTESIAN_POINT ( 'NONE',  ( -0.8801773607111009756, 58.06368534415484106, 1.068504757029289695E-15 ) ) ;
#20202=CARTESIAN_POINT ( 'NONE',  ( 6.565887622018943937, 58.08196800326376064, -12.81628187352647608 ) ) ;
#20206=CARTESIAN_POINT ( 'NONE',  ( 13.79529636645031943, 20.34541550158063572, -14.16423886937409904 ) ) ;
#20207=CARTESIAN_POINT ( 'NONE',  ( 0.6178305044545818747, 23.49863466993041783, -9.382169495545419124 ) ) ;
#20208=B_SPLINE_CURVE_WITH_KNOTS ( 'NONE', 3,
 ( #90067, #93020, #71525, #63982 ),
 .UNSPECIFIED., .F., .F.,
 ( 4, 4 ),
 ( 0.000000000000000000, 0.001036303429213355966 ),
 .UNSPECIFIED. ) ;
#20209=ORIENTED_EDGE ( 'NONE', *, *, #97449, .F. ) ;
#20210=CARTESIAN_POINT ( 'NONE',  ( -2.816281873526473856, 39.33196800326374643, 3.434112377981055619 ) ) ;
#20211=CARTESIAN_POINT ( 'NONE',  ( 15.44008868035555260, 14.73035201082150536, 9.422509992056143702 ) ) ;
#20212=CARTESIAN_POINT ( 'NONE',  ( 18.52753015748617571, 43.09226448433412315, 4.923371831947298993 ) ) ;
#20213=CARTESIAN_POINT ( 'NONE',  ( 10.00000000000000000, 11.81368534415483751, -10.88017736071110342 ) ) ;
#20214=CARTESIAN_POINT ( 'NONE',  ( 19.38216949554541202, 55.99863466993041072, 9.382169495545424454 ) ) ;
#20215=CARTESIAN_POINT ( 'NONE',  ( 0.2751277870542967463, 70.00000000000000000, 6.000000000000000000 ) ) ;
#20216=CARTESIAN_POINT ( 'NONE',  ( 1.472469842513823179, 46.42559781766745175, 4.923371831947296329 ) ) ;
#20218=CARTESIAN_POINT ( 'NONE',  ( 17.96484262340118221, 51.18868534415483396, -7.964842623401177768 ) ) ;
#20220=ORIENTED_EDGE ( 'NONE', *, *, #24086, .T. ) ;
#20223=DIRECTION ( 'NONE',  ( -1.000000000000000000, 0.000000000000000000, 0.000000000000000000 ) ) ;
#20225=CARTESIAN_POINT ( 'NONE',  ( 2.603489959281588106, 1.582109641433292690, 6.500000000000000888 ) ) ;
#20226=CARTESIAN_POINT ( 'NONE',  ( 0.1532563361054100626, 20.80059781766744464, -2.638427012816831230 ) ) ;
#20228=CARTESIAN_POINT ( 'NONE',  ( -1.099225684535947600, 23.70696800326375708, -6.408140936763238038 ) ) ;
#20231=CARTESIAN_POINT ( 'NONE',  ( 19.84674366389459266, 53.71726448433411605, -2.638427012816827677 ) ) ;
#20233=CARTESIAN_POINT ( 'NONE',  ( -2.266590686148945544, 17.22041550158063572, 7.082119434687048631 ) ) ;
#20234=CARTESIAN_POINT ( 'NONE',  ( 1.472469842513823179, 35.59226448433412315, -4.923371831947296329 ) ) ;
#20235=CARTESIAN_POINT ( 'NONE',  ( 13.43411237798106583, 42.66530133659707502, -12.81628187352647252 ) ) ;
#20238=CARTESIAN_POINT ( 'NONE',  ( 0.5774900079438590739, 62.64701867748817676, -5.440088680355550821 ) ) ;
#20239=CARTESIAN_POINT ( 'NONE',  ( 10.00000000000000178, 15.37363466993042138, 12.81628187352647608 ) ) ;
#20242=CARTESIAN_POINT ( 'NONE',  ( 12.63842701281683034, 37.46726448433411605, 9.846743663894596210 ) ) ;
#20243=CARTESIAN_POINT ( 'NONE',  ( 19.42250999205614548, 45.98035201082150536, -5.440088680355545492 ) ) ;
#20244=CARTESIAN_POINT ( 'NONE',  ( 3.591859063236763294, 43.29030133659708923, -11.09922568453595026 ) ) ;
#20245=CIRCLE ( 'NONE', #29873, 6.999999999999995559 ) ;
#20246=CARTESIAN_POINT ( 'NONE',  ( 17.20831665107776587, 32.88393115100078745, 7.208316651077764980 ) ) ;
#20250=CARTESIAN_POINT ( 'NONE',  ( 2.035157376598824452, 28.68868534415484106, 7.964842623401179544 ) ) ;
#20253=CARTESIAN_POINT ( 'NONE',  ( 10.00000000000000000, 11.81368534415483751, -10.88017736071110342 ) ) ;
#20254=CARTESIAN_POINT ( 'NONE',  ( 18.52753015748618282, 58.92559781766745886, -4.923371831947291888 ) ) ;
#20255=CARTESIAN_POINT ( 'NONE',  ( 2.035157376598824452, 28.68868534415484106, 7.964842623401179544 ) ) ;
#20256=CARTESIAN_POINT ( 'NONE',  ( 15.00000000000000000, 11.50000000000000000, -6.000000000000000000 ) ) ;
#20257=CARTESIAN_POINT ( 'NONE',  ( 12.91533473730993009, 61.60535201082150536, -10.88017736071109987 ) ) ;
#20258=CARTESIAN_POINT ( 'NONE',  ( 12.91533473730993009, 31.60535201082150891, -10.88017736071109987 ) ) ;
#20259=CARTESIAN_POINT ( 'NONE',  ( 0.000000000000000000, 77.50050546096726123, -8.104077677183505912 ) ) ;
#20261=CARTESIAN_POINT ( 'NONE',  ( 0.1532563361054100626, 30.80059781766744820, -2.638427012816831230 ) ) ;
#20264=CARTESIAN_POINT ( 'NONE',  ( 0.1532563361054100626, 50.80059781766745175, -2.638427012816831230 ) ) ;
#20265=CARTESIAN_POINT ( 'NONE',  ( 22.26659068614894466, 53.88708216824731068, 7.082119434687054849 ) ) ;
#20269=CARTESIAN_POINT ( 'NONE',  ( 6.204703633549690345, 7.845415501580634832, 14.16423886937410082 ) ) ;
#20270=CARTESIAN_POINT ( 'NONE',  ( -4.164238869374098151, 36.59541550158063217, -3.795296366450310543 ) ) ;
#20271=CARTESIAN_POINT ( 'NONE',  ( 21.09922568453594849, 6.206968003263753531, 6.408140936763242479 ) ) ;
#20273=ORIENTED_EDGE ( 'NONE', *, *, #80611, .F. ) ;
#20274=CARTESIAN_POINT ( 'NONE',  ( 19.42250999205614548, 15.98035201082150714, -5.440088680355545492 ) ) ;
#20275=CARTESIAN_POINT ( 'NONE',  ( 10.00000000000000178, 37.25893115100078745, 9.846743663894594434 ) ) ;
#20278=CARTESIAN_POINT ( 'NONE',  ( 7.361572987183170547, 2.050597817667451750, 9.846743663894590881 ) ) ;
#20279=CARTESIAN_POINT ( 'NONE',  ( 13.43411237798105340, 25.58196800326374998, 12.81628187352647963 ) ) ;
#20280=CARTESIAN_POINT ( 'NONE',  ( 14.92337183194729633, 22.67559781766745175, 8.527530157486181039 ) ) ;
#20282=CARTESIAN_POINT ( 'NONE',  ( 12.63842701281683034, 12.46726448433411782, 9.846743663894596210 ) ) ;
#20284=CARTESIAN_POINT ( 'NONE',  ( -2.266590686148945544, 67.22041550158063217, 7.082119434687048631 ) ) ;
#20285=CARTESIAN_POINT ( 'NONE',  ( 20.88017736071110519, 20.56368534415484106, 2.639326808657452039E-16 ) ) ;
#20286=CARTESIAN_POINT ( 'NONE',  ( 13.79529636645031943, 35.34541550158063927, -14.16423886937409904 ) ) ;
#20287=CARTESIAN_POINT ( 'NONE',  ( 7.084665262690076126, 29.10535201082150181, 10.88017736071109987 ) ) ;
#20288=CARTESIAN_POINT ( 'NONE',  ( 10.00000000000000178, 64.31368534415483396, 10.88017736071110342 ) ) ;
#20289=CARTESIAN_POINT ( 'NONE',  ( 0.2751277870542967463, 70.00000000000000000, 6.000000000000000000 ) ) ;
#20291=CARTESIAN_POINT ( 'NONE',  ( 14.92337183194729988, 29.34226448433411960, -8.527530157486177487 ) ) ;
#20293=CARTESIAN_POINT ( 'NONE',  ( 0.1532563361054100626, 0.8005978176674514168, -2.638427012816831230 ) ) ;
#20295=CARTESIAN_POINT ( 'NONE',  ( 0.1532563361054082862, 36.21726448433410894, 2.638427012816831674 ) ) ;
#20296=CARTESIAN_POINT ( 'NONE',  ( 5.076628168052704559, 60.17559781766745175, -8.527530157486179263 ) ) ;
#20297=CARTESIAN_POINT ( 'NONE',  ( 4.559911319644449179, 33.89701867748817676, 9.422509992056141925 ) ) ;
#20298=UNCERTAINTY_MEASURE_WITH_UNIT (LENGTH_MEASURE( 1.000000000000000082E-05 ), #64498, 'distance_accuracy_value', 'NONE');
#20300=CARTESIAN_POINT ( 'NONE',  ( -2.816281873526471635, 43.91530133659708923, -3.434112377981056508 ) ) ;
#20302=CARTESIAN_POINT ( 'NONE',  ( 20.88017736071110164, 60.35535201082151957, 2.915334737309930979 ) ) ;
#20303=CARTESIAN_POINT ( 'NONE',  ( 0.6178305044545818747, 38.49863466993042493, -9.382169495545419124 ) ) ;
#20304=CARTESIAN_POINT ( 'NONE',  ( -0.3689425029237898834, 56.17874883491396076, -10.36894250292378850 ) ) ;
#20305=CARTESIAN_POINT ( 'NONE',  ( 5.076628168052704559, 35.17559781766745175, -8.527530157486179263 ) ) ;
#20307=AXIS2_PLACEMENT_3D ( 'NONE', #77055, #67094, #90081 ) ;
#20308=CARTESIAN_POINT ( 'NONE',  ( 5.076628168052703671, 61.84226448433412315, 8.527530157486179263 ) ) ;
#20309=CARTESIAN_POINT ( 'NONE',  ( -4.164238869374099927, 17.01208216824730357, 3.795296366450308767 ) ) ;
#20310=CARTESIAN_POINT ( 'NONE',  ( 2.917880565312950480, 35.97041550158063217, -12.26659068614894821 ) ) ;
#20311=CARTESIAN_POINT ( 'NONE',  ( 19.84674366389459621, 43.50893115100078745, 7.409399052514197653E-17 ) ) ;
#20312=CARTESIAN_POINT ( 'NONE',  ( -0.2538764795851958800, 70.00000000000000000, 6.092576751097361409 ) ) ;
#20313=CARTESIAN_POINT ( 'NONE',  ( 19.42250999205614193, 35.14701867748816966, 5.440088680355555262 ) ) ;
#20314=CARTESIAN_POINT ( 'NONE',  ( 15.44008868035555793, 56.39701867748817676, -9.422509992056140149 ) ) ;
#20318=CARTESIAN_POINT ( 'NONE',  ( 13.43411237798106583, 42.66530133659707502, -12.81628187352647252 ) ) ;
#20320=CARTESIAN_POINT ( 'NONE',  ( 18.52753015748617571, 3.092264484334118269, 4.923371831947298993 ) ) ;
#20322=CARTESIAN_POINT ( 'NONE',  ( 10.00000000000000000, 0.5537488349139675359, -14.16423886937410082 ) ) ;
#20323=CARTESIAN_POINT ( 'NONE',  ( 10.00000000000000000, 9.758931151000785675, -9.846743663894594434 ) ) ;
#20326=CARTESIAN_POINT ( 'NONE',  ( 1.598469098248223030, 0.08731616080489693066, -6.289747708190945197 ) ) ;
#20327=ORIENTED_EDGE ( 'NONE', *, *, #92769, .F. ) ;
#20329=CARTESIAN_POINT ( 'NONE',  ( 20.88017736071110875, 10.77201867748817143, -2.915334737309920765 ) ) ;
#20331=CARTESIAN_POINT ( 'NONE',  ( 20.36894250292379382, 18.67874883491397142, 10.36894250292379205 ) ) ;
#20332=CARTESIAN_POINT ( 'NONE',  ( 7.084665262690076126, 22.02201867748817321, -10.88017736071110164 ) ) ;
#20333=CARTESIAN_POINT ( 'NONE',  ( 0.1532563361054100626, 65.80059781766745175, -2.638427012816831230 ) ) ;
#20335=CARTESIAN_POINT ( 'NONE',  ( 12.63842701281683034, 57.46726448433411605, 9.846743663894596210 ) ) ;
#20336=EDGE_LOOP ( 'NONE', ( #1928, #60541, #50574, #30774, #63581, #34978 ) ) ;
#20337=CARTESIAN_POINT ( 'NONE',  ( 0.1532563361054100626, 0.8005978176674514168, -2.638427012816831230 ) ) ;
#20338=CARTESIAN_POINT ( 'NONE',  ( 0.1532563361054083140, 61.00893115100078745, 1.131784320476157264E-15 ) ) ;
#20339=CARTESIAN_POINT ( 'NONE',  ( 17.96484262340118221, 11.18868534415483929, -7.964842623401177768 ) ) ;
#20341=CARTESIAN_POINT ( 'NONE',  ( 12.91533473730993009, 66.60535201082150536, -10.88017736071109987 ) ) ;
#20342=CARTESIAN_POINT ( 'NONE',  ( 10.00000000000000178, 19.31368534415484106, 10.88017736071110342 ) ) ;
#20343=ORIENTED_EDGE ( 'NONE', *, *, #86509, .T. ) ;
#20345=CARTESIAN_POINT ( 'NONE',  ( 13.43411237798105340, 60.58196800326376064, 12.81628187352647963 ) ) ;
#20346=CARTESIAN_POINT ( 'NONE',  ( 2.035157376598824452, 28.68868534415484106, 7.964842623401179544 ) ) ;
#20347=CARTESIAN_POINT ( 'NONE',  ( -46.94000000000001194, 100.5295635078804253, -8.861295791668675648 ) ) ;
#20348=CARTESIAN_POINT ( 'NONE',  ( 10.00000000000000178, 45.37363466993041783, 12.81628187352647608 ) ) ;
#20349=CARTESIAN_POINT ( 'NONE',  ( 10.00000000000000178, 54.31368534415484106, 10.88017736071110342 ) ) ;
#20351=CARTESIAN_POINT ( 'NONE',  ( 14.92337183194729988, 54.34226448433412315, -8.527530157486177487 ) ) ;
#20353=CARTESIAN_POINT ( 'NONE',  ( 19.84674366389459266, 18.71726448433411960, -2.638427012816827677 ) ) ;
#20354=CARTESIAN_POINT ( 'NONE',  ( 6.565887622018943937, 5.165301336597086568, 12.81628187352647430 ) ) ;
#20355=CARTESIAN_POINT ( 'NONE',  ( 18.17884179759847996, 3.666888798595233645, -6.499999999999976019 ) ) ;
#20356=CARTESIAN_POINT ( 'NONE',  ( 14.92337183194729988, 54.34226448433412315, -8.527530157486177487 ) ) ;
#20357=CARTESIAN_POINT ( 'NONE',  ( 19.42250999205614193, 25.14701867748817321, 5.440088680355555262 ) ) ;
#20358=CARTESIAN_POINT ( 'NONE',  ( 1.472469842513823179, 51.42559781766745886, 4.923371831947296329 ) ) ;
#20359=DIRECTION ( 'NONE',  ( -1.000000000000000000, -0.000000000000000000, -0.000000000000000000 ) ) ;
#20362=CARTESIAN_POINT ( 'NONE',  ( 19.84674366389459621, 8.508931151000785675, 7.409399052514197653E-17 ) ) ;
#20364=CARTESIAN_POINT ( 'NONE',  ( 13.43411237798105340, 0.5819680032637533085, 12.81628187352647963 ) ) ;
#20365=ORIENTED_EDGE ( 'NONE', *, *, #51664, .T. ) ;
#20367=CARTESIAN_POINT ( 'NONE',  ( 3.591859063236761518, 64.95696800326376774, 11.09922568453594849 ) ) ;
#20369=CARTESIAN_POINT ( 'NONE',  ( 19.38216949554541202, 35.99863466993041072, 9.382169495545424454 ) ) ;
#20370=CARTESIAN_POINT ( 'NONE',  ( 17.20831665107776587, 34.13393115100078745, -7.208316651077762316 ) ) ;
#20372=CARTESIAN_POINT ( 'NONE',  ( -2.266590686148945544, 61.38708216824730357, -7.082119434687050408 ) ) ;
#20373=CARTESIAN_POINT ( 'NONE',  ( 12.63842701281683034, 27.46726448433411250, 9.846743663894596210 ) ) ;
#20374=CARTESIAN_POINT ( 'NONE',  ( -0.3289641300568005855, 39.27164270246084499, -5.963430220938281678 ) ) ;
#20375=CARTESIAN_POINT ( 'NONE',  ( 10.00000000000000000, 60.55374883491397497, -14.16423886937410082 ) ) ;
#20376=CARTESIAN_POINT ( 'NONE',  ( 13.99999999999999822, 60.50000000000000711, -6.500000000000000888 ) ) ;
#20377=CARTESIAN_POINT ( 'NONE',  ( 7.084665262690076126, 22.02201867748817321, -10.88017736071110164 ) ) ;
#20378=CARTESIAN_POINT ( 'NONE',  ( -2.266590686148945544, 32.22041550158063927, 7.082119434687048631 ) ) ;
#20380=CARTESIAN_POINT ( 'NONE',  ( 2.917880565312948704, 57.63708216824731068, 12.26659068614894643 ) ) ;
#20384=CARTESIAN_POINT ( 'NONE',  ( 5.076628168052703671, 6.842264484334118713, 8.527530157486179263 ) ) ;
#20385=CARTESIAN_POINT ( 'NONE',  ( 19.84674366389459266, 63.71726448433412315, -2.638427012816827677 ) ) ;
#20386=CARTESIAN_POINT ( 'NONE',  ( 18.39792806157249672, 14.52224192338640663, 6.500000000000000888 ) ) ;
#20388=CARTESIAN_POINT ( 'NONE',  ( 12.91533473730993009, 56.60535201082151247, -10.88017736071109987 ) ) ;
#20391=VECTOR ( 'NONE', #91206, 1000.000000000000000 ) ;
#20397=CARTESIAN_POINT ( 'NONE',  ( -4.164238869374099039, 46.80374883491397497, 8.674139862899312516E-16 ) ) ;
#20398=SURFACE_STYLE_USAGE ( .BOTH. , #65383 ) ;
#20401=CARTESIAN_POINT ( 'NONE',  ( 15.44008868035555260, 14.73035201082150536, 9.422509992056143702 ) ) ;
#20402=CARTESIAN_POINT ( 'NONE',  ( 3.591859063236763294, 33.29030133659708213, -11.09922568453595026 ) ) ;
#20404=CARTESIAN_POINT ( 'NONE',  ( -2.816281873526471635, 18.91530133659708213, -3.434112377981056508 ) ) ;
#20405=CARTESIAN_POINT ( 'NONE',  ( 6.565887622018943937, 65.16530133659709634, 12.81628187352647430 ) ) ;
#20409=CARTESIAN_POINT ( 'NONE',  ( -2.266590686148945544, 26.38708216824730357, -7.082119434687050408 ) ) ;
#20410=( NAMED_UNIT ( * ) SI_UNIT ( $, .STERADIAN. ) SOLID_ANGLE_UNIT ( ) );
#20412=CARTESIAN_POINT ( 'NONE',  ( 10.00000000000000000, 21.81368534415484106, -10.88017736071110342 ) ) ;
#20413=DIRECTION ( 'NONE',  ( 0.000000000000000000, 0.000000000000000000, -1.000000000000000000 ) ) ;
#20415=CARTESIAN_POINT ( 'NONE',  ( 20.88017736071110519, 50.56368534415484106, 2.639326808657452039E-16 ) ) ;
#20416=CARTESIAN_POINT ( 'NONE',  ( 15.44008868035555793, 46.39701867748817676, -9.422509992056140149 ) ) ;
#20417=CARTESIAN_POINT ( 'NONE',  ( 6.565887622018943937, 15.16530133659708568, 12.81628187352647430 ) ) ;
#20419=CARTESIAN_POINT ( 'NONE',  ( -0.8801773607111009756, 3.272018677488171434, 2.915334737309923874 ) ) ;
#20420=CARTESIAN_POINT ( 'NONE',  ( 19.84674366389459621, 18.50893115100078745, 7.409399052514197653E-17 ) ) ;
#20422=CARTESIAN_POINT ( 'NONE',  ( 0.5774900079438607392, 43.48035201082151247, 5.440088680355550821 ) ) ;
#20423=CARTESIAN_POINT ( 'NONE',  ( 0.6178305044545838731, 4.748634669930420493, 9.382169495545420901 ) ) ;
#20424=CARTESIAN_POINT ( 'NONE',  ( 12.63842701281683034, 27.46726448433411250, 9.846743663894596210 ) ) ;
#20425=CARTESIAN_POINT ( 'NONE',  ( 0.6178305044545818747, 53.49863466993041072, -9.382169495545419124 ) ) ;
#20426=CARTESIAN_POINT ( 'NONE',  ( 4.559911319644449179, 68.89701867748817676, 9.422509992056141925 ) ) ;
#20429=CARTESIAN_POINT ( 'NONE',  ( 1.472469842513823179, 36.42559781766745175, 4.923371831947296329 ) ) ;
#20430=CARTESIAN_POINT ( 'NONE',  ( 17.96484262340118221, 16.18868534415483396, -7.964842623401177768 ) ) ;
#20432=CARTESIAN_POINT ( 'NONE',  ( 20.36894250292379738, 29.92874883491396432, -10.36894250292379027 ) ) ;
#20433=CARTESIAN_POINT ( 'NONE',  ( 0.1532563361054082862, 31.21726448433412315, 2.638427012816831674 ) ) ;
#20434=CARTESIAN_POINT ( 'NONE',  ( 10.00000000000000000, 16.81368534415483751, -10.88017736071110342 ) ) ;
#20435=CARTESIAN_POINT ( 'NONE',  ( -4.164238869374099039, 66.80374883491396076, 8.674139862899312516E-16 ) ) ;
#20436=ORIENTED_EDGE ( 'NONE', *, *, #84695, .F. ) ;
#20437=CARTESIAN_POINT ( 'NONE',  ( 7.084665262690076126, 32.02201867748816966, -10.88017736071110164 ) ) ;
#20439=CARTESIAN_POINT ( 'NONE',  ( 17.96484262340118221, 29.93868534415484106, 7.964842623401181321 ) ) ;
#20441=CARTESIAN_POINT ( 'NONE',  ( 0.5774900079438607392, 43.48035201082151247, 5.440088680355550821 ) ) ;
#20443=CARTESIAN_POINT ( 'NONE',  ( 17.20831665107776587, 62.88393115100078745, 7.208316651077764980 ) ) ;
#20444=CARTESIAN_POINT ( 'NONE',  ( 7.084665262690076126, 32.02201867748816966, -10.88017736071110164 ) ) ;
#20446=CARTESIAN_POINT ( 'NONE',  ( -1.099225684535947600, 63.70696800326376774, -6.408140936763238038 ) ) ;
#20447=DIRECTION ( 'NONE',  ( -0.000000000000000000, 1.000000000000000000, 0.000000000000000000 ) ) ;
#20448=CARTESIAN_POINT ( 'NONE',  ( 6.204703633549690345, 32.84541550158063927, 14.16423886937410082 ) ) ;
#20449=CARTESIAN_POINT ( 'NONE',  ( 17.96484262340118221, 54.93868534415484106, 7.964842623401181321 ) ) ;
#20450=ADVANCED_FACE ( 'NONE', ( #16608 ), #63074, .F. ) ;
#20451=CARTESIAN_POINT ( 'NONE',  ( 19.80427997160309417, 42.75733960839543357, -6.499999999999988454 ) ) ;
#20452=DIRECTION ( 'NONE',  ( 0.000000000000000000, 0.000000000000000000, 1.000000000000000000 ) ) ;
#20453=CARTESIAN_POINT ( 'NONE',  ( 1.472469842513823179, 45.59226448433412315, -4.923371831947296329 ) ) ;
#20455=CARTESIAN_POINT ( 'NONE',  ( 14.92337183194729988, 24.34226448433411960, -8.527530157486177487 ) ) ;
#20458=CARTESIAN_POINT ( 'NONE',  ( 0.5774900079438607392, 8.480352010821505360, 5.440088680355550821 ) ) ;
#20459=CARTESIAN_POINT ( 'NONE',  ( 10.00000000000000000, 24.75893115100078745, -9.846743663894594434 ) ) ;
#20460=CARTESIAN_POINT ( 'NONE',  ( 21.09922568453595559, 7.040301336597086568, -6.408140936763230044 ) ) ;
#20461=CARTESIAN_POINT ( 'NONE',  ( 19.42250999205614548, 55.98035201082150536, -5.440088680355545492 ) ) ;
#20462=CARTESIAN_POINT ( 'NONE',  ( 4.559911319644449179, 52.23035201082151247, -9.422509992056141925 ) ) ;
#20463=CARTESIAN_POINT ( 'NONE',  ( 20.88017736071110519, 35.56368534415484106, 2.639326808657452039E-16 ) ) ;
#20464=CARTESIAN_POINT ( 'NONE',  ( 10.00000000000000178, 55.37363466993042493, 12.81628187352647608 ) ) ;
#20465=CARTESIAN_POINT ( 'NONE',  ( 22.26659068614895176, 49.72041550158063927, -7.082119434687042414 ) ) ;
#20470=CARTESIAN_POINT ( 'NONE',  ( 10.00000000000000178, 67.25893115100079456, 9.846743663894594434 ) ) ;
#20471=CARTESIAN_POINT ( 'NONE',  ( 7.084665262690076126, 2.022018677488170990, -10.88017736071110164 ) ) ;
#20472=CARTESIAN_POINT ( 'NONE',  ( 15.44008868035555260, 44.73035201082151247, 9.422509992056143702 ) ) ;
#20473=CARTESIAN_POINT ( 'NONE',  ( 2.791683348922240793, 61.63393115100079456, 7.208316651077764092 ) ) ;
#20474=EDGE_CURVE ( 'NONE', #42599, #40639, #32012, .T. ) ;
#20476=CARTESIAN_POINT ( 'NONE',  ( 14.92337183194729988, 14.34226448433411782, -8.527530157486177487 ) ) ;
#20478=CARTESIAN_POINT ( 'NONE',  ( 17.20831665107776587, 12.88393115100078390, 7.208316651077764980 ) ) ;
#20479=CARTESIAN_POINT ( 'NONE',  ( 10.00000000000000178, 22.25893115100078745, 9.846743663894594434 ) ) ;
#20480=CARTESIAN_POINT ( 'NONE',  ( 19.84674366389459266, 13.30059781766745353, 2.638427012816836559 ) ) ;
#20482=CARTESIAN_POINT ( 'NONE',  ( 7.361572987183170547, 7.050597817667451750, 9.846743663894590881 ) ) ;
#20484=CARTESIAN_POINT ( 'NONE',  ( 17.20831665107776587, 2.883931151000785231, 7.208316651077764980 ) ) ;
#20485=CARTESIAN_POINT ( 'NONE',  ( 18.52753015748617571, 18.09226448433411960, 4.923371831947298993 ) ) ;
#20488=CARTESIAN_POINT ( 'NONE',  ( 14.92337183194729988, 64.34226448433412315, -8.527530157486177487 ) ) ;
#20491=CARTESIAN_POINT ( 'NONE',  ( -4.164238869374099927, 17.01208216824730357, 3.795296366450308767 ) ) ;
#20493=CARTESIAN_POINT ( 'NONE',  ( -2.266590686148945544, 22.22041550158063572, 7.082119434687048631 ) ) ;
#20494=CARTESIAN_POINT ( 'NONE',  ( -4.164238869374099039, 46.80374883491397497, 8.674139862899312516E-16 ) ) ;
#20495=( NAMED_UNIT ( * ) SI_UNIT ( $, .STERADIAN. ) SOLID_ANGLE_UNIT ( ) );
#20496=CARTESIAN_POINT ( 'NONE',  ( 6.204703633549690345, 12.84541550158063572, 14.16423886937410082 ) ) ;
#20497=CARTESIAN_POINT ( 'NONE',  ( 4.559911319644449179, 67.23035201082150536, -9.422509992056141925 ) ) ;
#20498=CARTESIAN_POINT ( 'NONE',  ( 7.084665262690076126, 34.10535201082151247, 10.88017736071109987 ) ) ;
#20501=VERTEX_POINT ( 'NONE', #40093 ) ;
#20502=CARTESIAN_POINT ( 'NONE',  ( 0.1532563361054083140, 11.00893115100078568, 1.131784320476157264E-15 ) ) ;
#20503=CARTESIAN_POINT ( 'NONE',  ( 19.42250999205614193, 50.14701867748817676, 5.440088680355555262 ) ) ;
#20504=CARTESIAN_POINT ( 'NONE',  ( 14.92337183194729988, 29.34226448433411960, -8.527530157486177487 ) ) ;
#20505=CARTESIAN_POINT ( 'NONE',  ( 12.91533473730992121, 9.522018677488171434, 10.88017736071110164 ) ) ;
#20506=CARTESIAN_POINT ( 'NONE',  ( -2.816281873526471635, 63.91530133659708923, -3.434112377981056508 ) ) ;
#20507=CARTESIAN_POINT ( 'NONE',  ( 14.92337183194729988, 44.34226448433412315, -8.527530157486177487 ) ) ;
#20510=CARTESIAN_POINT ( 'NONE',  ( 6.565887622018943937, 40.16530133659708923, 12.81628187352647430 ) ) ;
#20512=CARTESIAN_POINT ( 'NONE',  ( 2.035157376598822676, 47.43868534415484817, -7.964842623401177768 ) ) ;
#20513=CARTESIAN_POINT ( 'NONE',  ( 2.791683348922240793, 36.63393115100078035, 7.208316651077764092 ) ) ;
#20514=CARTESIAN_POINT ( 'NONE',  ( 13.79529636645030344, 33.26208216824730357, 14.16423886937410614 ) ) ;
#20517=CARTESIAN_POINT ( 'NONE',  ( 15.44008868035555793, 51.39701867748816966, -9.422509992056140149 ) ) ;
#20518=CARTESIAN_POINT ( 'NONE',  ( 15.44008868035555793, 66.39701867748817676, -9.422509992056140149 ) ) ;
#20519=CARTESIAN_POINT ( 'NONE',  ( 17.08211943468705840, 45.13708216824730357, -12.26659068614894466 ) ) ;
#20520=CARTESIAN_POINT ( 'NONE',  ( 3.591859063236763294, -1.709698663402913210, -11.09922568453595026 ) ) ;
#20522=CARTESIAN_POINT ( 'NONE',  ( 12.91533473730993009, 41.60535201082149825, -10.88017736071109987 ) ) ;
#20524=STYLED_ITEM ( 'NONE', ( #54422 ), #13803 ) ;
#20525=CARTESIAN_POINT ( 'NONE',  ( 13.43411237798106583, 22.66530133659708923, -12.81628187352647252 ) ) ;
#20526=CARTESIAN_POINT ( 'NONE',  ( 19.84674366389459266, 48.71726448433413026, -2.638427012816827677 ) ) ;
#20529=CARTESIAN_POINT ( 'NONE',  ( 7.084665262690076126, 17.02201867748817676, -10.88017736071110164 ) ) ;
#20532=VECTOR ( 'NONE', #7779, 1000.000000000000000 ) ;
#20533=CARTESIAN_POINT ( 'NONE',  ( 15.44008868035555260, 4.730352010821504471, 9.422509992056143702 ) ) ;
#20536=CARTESIAN_POINT ( 'NONE',  ( 7.361572987183170547, 2.050597817667451750, 9.846743663894590881 ) ) ;
#20537=CARTESIAN_POINT ( 'NONE',  ( 19.84674366389459266, 3.300597817667451750, 2.638427012816836559 ) ) ;
#20538=CARTESIAN_POINT ( 'NONE',  ( 19.84674366389459266, 33.30059781766744464, 2.638427012816836559 ) ) ;
#20539=CARTESIAN_POINT ( 'NONE',  ( 15.44008868035555260, 24.73035201082150891, 9.422509992056143702 ) ) ;
#20540=CARTESIAN_POINT ( 'NONE',  ( -2.816281873526471635, 3.915301336597087456, -3.434112377981056508 ) ) ;
#20541=CARTESIAN_POINT ( 'NONE',  ( 20.88017736071110875, 40.77201867748818387, -2.915334737309920765 ) ) ;
#20544=CARTESIAN_POINT ( 'NONE',  ( 10.00000000000000178, 40.37363466993042493, 12.81628187352647608 ) ) ;
#20546=CARTESIAN_POINT ( 'NONE',  ( 19.42250999205614193, 60.14701867748817676, 5.440088680355555262 ) ) ;
#20547=CARTESIAN_POINT ( 'NONE',  ( 3.591859063236761518, 14.95696800326375531, 11.09922568453594849 ) ) ;
#20548=CARTESIAN_POINT ( 'NONE',  ( 17.08211943468705130, 3.470415501580634388, 12.26659068614894998 ) ) ;
#20549=CARTESIAN_POINT ( 'NONE',  ( 7.361572987183169658, -0.03273551566588185635, -9.846743663894592657 ) ) ;
#20550=CARTESIAN_POINT ( 'NONE',  ( 2.035157376598822676, 37.43868534415484106, -7.964842623401177768 ) ) ;
#20552=CARTESIAN_POINT ( 'NONE',  ( 10.00000000000000178, 68.05374883491397497, 14.16423886937410082 ) ) ;
#20553=CARTESIAN_POINT ( 'NONE',  ( 0.1532563361054100626, 50.80059781766745175, -2.638427012816831230 ) ) ;
#20554=CARTESIAN_POINT ( 'NONE',  ( 7.361572987183169658, -0.03273551566588185635, -9.846743663894592657 ) ) ;
#20555=CARTESIAN_POINT ( 'NONE',  ( 0.5774900079438607392, 63.48035201082149825, 5.440088680355550821 ) ) ;
#20557=CARTESIAN_POINT ( 'NONE',  ( -2.266590686148945544, 27.22041550158063572, 7.082119434687048631 ) ) ;
#20559=CARTESIAN_POINT ( 'NONE',  ( 19.50000000000000355, 79.40087001978915282, -5.000000000000000000 ) ) ;
#20562=CARTESIAN_POINT ( 'NONE',  ( 13.79529636645030344, 63.26208216824730357, 14.16423886937410614 ) ) ;
#20563=CARTESIAN_POINT ( 'NONE',  ( 17.08211943468705840, 50.13708216824730357, -12.26659068614894466 ) ) ;
#20564=CARTESIAN_POINT ( 'NONE',  ( 0.1532563361054083140, 26.00893115100078745, 1.131784320476157264E-15 ) ) ;
#20565=B_SPLINE_CURVE_WITH_KNOTS ( 'NONE', 3,
 ( #78679, #33159, #86673, #47178 ),
 .UNSPECIFIED., .F., .F.,
 ( 4, 4 ),
 ( 1.084202172485504434E-19, 0.002657014572711316382 ),
 .UNSPECIFIED. ) ;
#20566=CARTESIAN_POINT ( 'NONE',  ( 10.00000000000000000, 27.87363466993042138, -12.81628187352647608 ) ) ;
#20569=CARTESIAN_POINT ( 'NONE',  ( 0.5774900079438590739, 7.647018677488171434, -5.440088680355550821 ) ) ;
#20570=CARTESIAN_POINT ( 'NONE',  ( 24.16423886937410614, 54.30374883491396787, 8.672049930838204340E-16 ) ) ;
#20572=ADVANCED_FACE ( 'NONE', ( #30603 ), #65528, .T. ) ;
#20573=CARTESIAN_POINT ( 'NONE',  ( 5.076628168052703671, 26.84226448433411960, 8.527530157486179263 ) ) ;
#20575=CARTESIAN_POINT ( 'NONE',  ( 12.63842701281683034, 7.467264484334118713, 9.846743663894596210 ) ) ;
#20576=CARTESIAN_POINT ( 'NONE',  ( 20.15039907845754286, 14.72266099184918531, 6.262539305110064625 ) ) ;
#20578=ORIENTED_EDGE ( 'NONE', *, *, #2813, .T. ) ;
#20579=ORIENTED_EDGE ( 'NONE', *, *, #55220, .T. ) ;
#20581=CARTESIAN_POINT ( 'NONE',  ( 24.16423886937409904, 14.09541550158063217, 3.795296366450317205 ) ) ;
#20582=CARTESIAN_POINT ( 'NONE',  ( 7.084665262690076126, 22.02201867748817321, -10.88017736071110164 ) ) ;
#20583=CARTESIAN_POINT ( 'NONE',  ( 20.88017736071110519, 25.56368534415483751, 2.639326808657452039E-16 ) ) ;
#20584=CARTESIAN_POINT ( 'NONE',  ( 19.84674366389459266, 48.71726448433413026, -2.638427012816827677 ) ) ;
#20585=CARTESIAN_POINT ( 'NONE',  ( 21.09922568453595559, 12.04030133659708746, -6.408140936763230044 ) ) ;
#20586=CARTESIAN_POINT ( 'NONE',  ( 10.00000000000000178, 3.053748834913967425, 14.16423886937410082 ) ) ;
#20587=CARTESIAN_POINT ( 'NONE',  ( 16.40814093676323893, 25.79030133659708923, 11.09922568453595026 ) ) ;
#20588=( NAMED_UNIT ( * ) SI_UNIT ( $, .STERADIAN. ) SOLID_ANGLE_UNIT ( ) );
#20590=CARTESIAN_POINT ( 'NONE',  ( 19.84674366389459266, 28.30059781766745886, 2.638427012816836559 ) ) ;
#20591=CARTESIAN_POINT ( 'NONE',  ( 10.00000000000000000, 55.55374883491396787, -14.16423886937410082 ) ) ;
#20592=ORIENTED_EDGE ( 'NONE', *, *, #17668, .F. ) ;
#20593=EDGE_CURVE ( 'NONE', #91503, #21162, #97711, .T. ) ;
#20594=CARTESIAN_POINT ( 'NONE',  ( 6.204703633549690345, 67.84541550158060375, 14.16423886937410082 ) ) ;
#20595=ORIENTED_EDGE ( 'NONE', *, *, #98732, .F. ) ;
#20596=CARTESIAN_POINT ( 'NONE',  ( 20.88017736071110519, 45.56368534415484106, 2.639326808657452039E-16 ) ) ;
#20597=CARTESIAN_POINT ( 'NONE',  ( 0.5774900079438607392, 48.48035201082150536, 5.440088680355550821 ) ) ;
#20599=CARTESIAN_POINT ( 'NONE',  ( 17.96484262340118221, 54.93868534415484106, 7.964842623401181321 ) ) ;
#20600=CARTESIAN_POINT ( 'NONE',  ( 4.559911319644449179, 37.23035201082150536, -9.422509992056141925 ) ) ;
#20601=VECTOR ( 'NONE', #71125, 1000.000000000000114 ) ;
#20605=CARTESIAN_POINT ( 'NONE',  ( 5.076628168052703671, 26.84226448433411960, 8.527530157486179263 ) ) ;
#20606=VERTEX_POINT ( 'NONE', #33551 ) ;
#20607=CARTESIAN_POINT ( 'NONE',  ( 12.63842701281683034, 52.46726448433413026, 9.846743663894596210 ) ) ;
#20609=CARTESIAN_POINT ( 'NONE',  ( -0.03743638938522729498, 24.25197528031018734, -6.399506433553966644 ) ) ;
#20610=CARTESIAN_POINT ( 'NONE',  ( 13.79529636645031943, 10.34541550158063394, -14.16423886937409904 ) ) ;
#20611=ORIENTED_EDGE ( 'NONE', *, *, #71835, .F. ) ;
#20612=CARTESIAN_POINT ( 'NONE',  ( -42.94000000000001194, 92.00000000000000000, -10.09898361729590199 ) ) ;
#20614=CARTESIAN_POINT ( 'NONE',  ( -46.94000000000001194, 103.0000000000000000, -5.997726559847240679 ) ) ;
#20615=CARTESIAN_POINT ( 'NONE',  ( -0.3689425029237898834, 56.17874883491396076, -10.36894250292378850 ) ) ;
#20617=DIRECTION ( 'NONE',  ( 0.000000000000000000, 1.000000000000000000, -0.000000000000000000 ) ) ;
#20618=CARTESIAN_POINT ( 'NONE',  ( 0.1532563361054082862, 51.21726448433412315, 2.638427012816831674 ) ) ;
#20619=FACE_OUTER_BOUND ( 'NONE', #40624, .T. ) ;
#20620=CARTESIAN_POINT ( 'NONE',  ( -2.816281873526473856, -0.8763653300695799508, 9.499525473075851096E-16 ) ) ;
#20621=CARTESIAN_POINT ( 'NONE',  ( 18.52753015748618282, 13.92559781766745175, -4.923371831947291888 ) ) ;
#20622=VECTOR ( 'NONE', #40881, 1000.000000000000000 ) ;
#20624=CARTESIAN_POINT ( 'NONE',  ( 1.472469842513823179, 11.42559781766745175, 4.923371831947296329 ) ) ;
#20625=CARTESIAN_POINT ( 'NONE',  ( 13.43411237798106583, 7.665301336597086568, -12.81628187352647252 ) ) ;
#20627=EDGE_LOOP ( 'NONE', ( #6672, #58045, #44001, #65827, #51565, #71090 ) ) ;
#20628=CARTESIAN_POINT ( 'NONE',  ( 17.96484262340118221, 14.93868534415484106, 7.964842623401181321 ) ) ;
#20629=CARTESIAN_POINT ( 'NONE',  ( -4.164238869374099927, 7.012082168247302683, 3.795296366450308767 ) ) ;
#20630=CARTESIAN_POINT ( 'NONE',  ( 14.92337183194729633, 27.67559781766745530, 8.527530157486181039 ) ) ;
#20631=CARTESIAN_POINT ( 'NONE',  ( 0.5774900079438590739, 57.64701867748817676, -5.440088680355550821 ) ) ;
#20632=CARTESIAN_POINT ( 'NONE',  ( 22.81628187352647785, 31.62363466993042138, 6.195893100308588602E-16 ) ) ;
#20634=CARTESIAN_POINT ( 'NONE',  ( 12.91533473730993009, 6.605352010821504471, -10.88017736071109987 ) ) ;
#20637=CARTESIAN_POINT ( 'NONE',  ( 19.38216949554541202, 0.9986346699304200492, 9.382169495545424454 ) ) ;
#20638=CARTESIAN_POINT ( 'NONE',  ( 17.20831665107776587, 64.13393115100079456, -7.208316651077762316 ) ) ;
#20639=CARTESIAN_POINT ( 'NONE',  ( 19.84674366389459621, 18.50893115100078745, 7.409399052514197653E-17 ) ) ;
#20641=CARTESIAN_POINT ( 'NONE',  ( 22.81628187352647785, 26.62363466993042138, 6.195893100308588602E-16 ) ) ;
#20643=CARTESIAN_POINT ( 'NONE',  ( 10.00000000000000178, 44.31368534415484106, 10.88017736071110342 ) ) ;
#20648=CARTESIAN_POINT ( 'NONE',  ( 20.88017736071110164, 30.35535201082151247, 2.915334737309930979 ) ) ;
#20649=CARTESIAN_POINT ( 'NONE',  ( 19.84674366389459621, 48.50893115100078745, 7.409399052514197653E-17 ) ) ;
#20650=CARTESIAN_POINT ( 'NONE',  ( 12.91533473730992121, 54.52201867748816255, 10.88017736071110164 ) ) ;
#20651=CARTESIAN_POINT ( 'NONE',  ( 24.16423886937409904, 34.09541550158064638, 3.795296366450317205 ) ) ;
#20652=CARTESIAN_POINT ( 'NONE',  ( 18.06765999051784988, 33.99127512925449679, 6.500000000000019540 ) ) ;
#20653=CARTESIAN_POINT ( 'NONE',  ( 18.52753015748618282, 43.92559781766745175, -4.923371831947291888 ) ) ;
#20654=( NAMED_UNIT ( * ) SI_UNIT ( $, .STERADIAN. ) SOLID_ANGLE_UNIT ( ) );
#20655=CARTESIAN_POINT ( 'NONE',  ( 1.472469842513823179, 65.59226448433412315, -4.923371831947296329 ) ) ;
#20657=CARTESIAN_POINT ( 'NONE',  ( -0.8801773607111009756, 28.06368534415484106, 1.068504757029289695E-15 ) ) ;
#20658=CARTESIAN_POINT ( 'NONE',  ( 20.88017736071110875, 5.772018677488170546, -2.915334737309920765 ) ) ;
#20659=CARTESIAN_POINT ( 'NONE',  ( 0.5774900079438590739, 17.64701867748817321, -5.440088680355550821 ) ) ;
#20660=CARTESIAN_POINT ( 'NONE',  ( 5.076628168052704559, 5.175597817667451750, -8.527530157486179263 ) ) ;
#20661=CARTESIAN_POINT ( 'NONE',  ( 20.36894250292379382, 23.67874883491397142, 10.36894250292379205 ) ) ;
#20662=CARTESIAN_POINT ( 'NONE',  ( 10.00000000000000000, 19.75893115100078390, -9.846743663894594434 ) ) ;
#20663=CARTESIAN_POINT ( 'NONE',  ( 2.791683348922240793, 61.63393115100079456, 7.208316651077764092 ) ) ;
#20664=CARTESIAN_POINT ( 'NONE',  ( 10.00000000000000000, 31.81368534415483751, -10.88017736071110342 ) ) ;
#20665=CARTESIAN_POINT ( 'NONE',  ( 0.1129803114748866161, 34.29427333184091964, -6.480634945678686698 ) ) ;
#20666=CARTESIAN_POINT ( 'NONE',  ( 19.42250999205614548, 25.98035201082150891, -5.440088680355545492 ) ) ;
#20668=ORIENTED_EDGE ( 'NONE', *, *, #10297, .T. ) ;
#20670=CARTESIAN_POINT ( 'NONE',  ( 5.076628168052703671, 41.84226448433411605, 8.527530157486179263 ) ) ;
#20671=( BOUNDED_CURVE ( )  B_SPLINE_CURVE ( 2, ( #41942, #63913, #86926, #17946, #4433, #18438, #56915, #65395, #48921 ),
 .UNSPECIFIED., .F., .T. ) 
 B_SPLINE_CURVE_WITH_KNOTS ( ( 3, 2, 2, 2, 3 ),
 ( 0.2953713073319822469, 0.2976190476190476164, 0.3035714285714285476, 0.3095238095238095344, 0.3117715498108742378 ),
 .UNSPECIFIED. ) 
 CURVE ( )  GEOMETRIC_REPRESENTATION_ITEM ( )  RATIONAL_B_SPLINE_CURVE ( ( 0.9839835555609424134, 0.9871328979762477029, 1.000000000000000000, 0.9659258262890683122, 1.000000000000000000, 0.9659258262890683122, 1.000000000000000000, 0.9871328979762515887, 0.9839835555609444118 ) ) 
 REPRESENTATION_ITEM ( '' )  );
#20672=EDGE_CURVE ( 'NONE', #75793, #27193, #13023, .T. ) ;
#20676=CARTESIAN_POINT ( 'NONE',  ( 2.917880565312950480, 15.97041550158063217, -12.26659068614894821 ) ) ;
#20677=CARTESIAN_POINT ( 'NONE',  ( 6.204703633549690345, 15.76208216824730179, -14.16423886937410259 ) ) ;
#20678=CARTESIAN_POINT ( 'NONE',  ( 4.559911319644449179, 57.23035201082150536, -9.422509992056141925 ) ) ;
#20679=CARTESIAN_POINT ( 'NONE',  ( -4.164238869374099927, 57.01208216824731068, 3.795296366450308767 ) ) ;
#20680=CARTESIAN_POINT ( 'NONE',  ( 1.472469842513823179, 65.59226448433412315, -4.923371831947296329 ) ) ;
#20681=CARTESIAN_POINT ( 'NONE',  ( 5.076628168052703671, 31.84226448433412315, 8.527530157486179263 ) ) ;
#20683=CARTESIAN_POINT ( 'NONE',  ( 4.559911319644449179, 33.89701867748817676, 9.422509992056141925 ) ) ;
#20684=CARTESIAN_POINT ( 'NONE',  ( -1.099225684535947600, -0.4596986634029132657, 6.408140936763237150 ) ) ;
#20685=CARTESIAN_POINT ( 'NONE',  ( -0.3689425029237898834, 21.17874883491396432, -10.36894250292378850 ) ) ;
#20686=CARTESIAN_POINT ( 'NONE',  ( 22.26659068614894466, 48.88708216824730357, 7.082119434687054849 ) ) ;
#20688=CARTESIAN_POINT ( 'NONE',  ( 15.44008868035555260, 24.73035201082150891, 9.422509992056143702 ) ) ;
#20689=CARTESIAN_POINT ( 'NONE',  ( -0.1503990784575328643, 0.07447313448805115144, 6.262539305110068177 ) ) ;
#20691=CARTESIAN_POINT ( 'NONE',  ( 4.559911319644449179, 37.23035201082150536, -9.422509992056141925 ) ) ;
#20692=CIRCLE ( 'NONE', #38470, 9.999999999999994671 ) ;
#20694=VERTEX_POINT ( 'NONE', #65025 ) ;
#20698=CARTESIAN_POINT ( 'NONE',  ( 2.917880565312948704, 42.63708216824729647, 12.26659068614894643 ) ) ;
#20699=CARTESIAN_POINT ( 'NONE',  ( 7.361572987183170547, 42.05059781766745886, 9.846743663894590881 ) ) ;
#20700=CARTESIAN_POINT ( 'NONE',  ( 0.5774900079438590739, 52.64701867748817676, -5.440088680355550821 ) ) ;
#20703=CARTESIAN_POINT ( 'NONE',  ( 7.084665262690076126, 54.10535201082151247, 10.88017736071109987 ) ) ;
#20704=CARTESIAN_POINT ( 'NONE',  ( 3.591859063236763294, 58.29030133659708923, -11.09922568453595026 ) ) ;
#20707=CARTESIAN_POINT ( 'NONE',  ( 13.79529636645031943, 25.34541550158063572, -14.16423886937409904 ) ) ;
#20710=CARTESIAN_POINT ( 'NONE',  ( 3.591859063236761518, 19.95696800326375353, 11.09922568453594849 ) ) ;
#20711=ORIENTED_EDGE ( 'NONE', *, *, #67409, .T. ) ;
#20712=CARTESIAN_POINT ( 'NONE',  ( 3.591859063236761518, 39.95696800326375353, 11.09922568453594849 ) ) ;
#20714=CARTESIAN_POINT ( 'NONE',  ( 10.00000000000000178, 14.31368534415483929, 10.88017736071110342 ) ) ;
#20715=CARTESIAN_POINT ( 'NONE',  ( 2.791683348922240793, 36.63393115100078035, 7.208316651077764092 ) ) ;
#20716=CARTESIAN_POINT ( 'NONE',  ( 10.00000000000000178, 14.31368534415483751, 10.88017736071110342 ) ) ;
#20717=CARTESIAN_POINT ( 'NONE',  ( 22.81628187352648496, 56.83196800326374643, -3.434112377981050290 ) ) ;
#20718=FACE_OUTER_BOUND ( 'NONE', #18944, .T. ) ;
#20719=CARTESIAN_POINT ( 'NONE',  ( 0.1532563361054083140, 41.00893115100078745, 1.131784320476157264E-15 ) ) ;
#20720=CARTESIAN_POINT ( 'NONE',  ( 0.5774900079438607392, 68.48035201082150536, 5.440088680355550821 ) ) ;
#20727=CARTESIAN_POINT ( 'NONE',  ( 18.52753015748617571, 13.09226448433411960, 4.923371831947298993 ) ) ;
#20728=CARTESIAN_POINT ( 'NONE',  ( 0.6178305044545818747, 23.49863466993041783, -9.382169495545419124 ) ) ;
#20730=CARTESIAN_POINT ( 'NONE',  ( 19.84674366389459266, 58.71726448433411605, -2.638427012816827677 ) ) ;
#20732=CARTESIAN_POINT ( 'NONE',  ( 24.16423886937410614, 19.30374883491397142, 8.672049930838204340E-16 ) ) ;
#20733=CARTESIAN_POINT ( 'NONE',  ( 10.00000000000000178, 42.25893115100078745, 9.846743663894594434 ) ) ;
#20734=CARTESIAN_POINT ( 'NONE',  ( 0.6178305044545818747, 48.49863466993042493, -9.382169495545419124 ) ) ;
#20735=CARTESIAN_POINT ( 'NONE',  ( 20.24186590665277308, 37.61633188102327807, -6.114288769123051637 ) ) ;
#20736=CARTESIAN_POINT ( 'NONE',  ( 17.96484262340118221, 56.18868534415484817, -7.964842623401177768 ) ) ;
#20738=CARTESIAN_POINT ( 'NONE',  ( 0.1532563361054100626, 30.80059781766744820, -2.638427012816831230 ) ) ;
#20739=CARTESIAN_POINT ( 'NONE',  ( 0.5774900079438590739, 42.64701867748816966, -5.440088680355550821 ) ) ;
#20740=CARTESIAN_POINT ( 'NONE',  ( 19.38216949554541202, 45.99863466993041072, 9.382169495545424454 ) ) ;
#20741=CARTESIAN_POINT ( 'NONE',  ( 12.63842701281683034, 32.46726448433412315, 9.846743663894596210 ) ) ;
#20744=CARTESIAN_POINT ( 'NONE',  ( 17.96484262340118221, 51.18868534415483396, -7.964842623401177768 ) ) ;
#20747=CARTESIAN_POINT ( 'NONE',  ( -0.8801773607111009756, 13.06368534415483929, 1.068504757029289695E-15 ) ) ;
#20748=CARTESIAN_POINT ( 'NONE',  ( 14.92337183194729633, 62.67559781766745886, 8.527530157486181039 ) ) ;
#20749=CARTESIAN_POINT ( 'NONE',  ( -0.8801773607110991993, 42.85535201082150536, -2.915334737309923874 ) ) ;
#20751=CARTESIAN_POINT ( 'NONE',  ( 2.035157376598824452, 63.68868534415484106, 7.964842623401179544 ) ) ;
#20753=CARTESIAN_POINT ( 'NONE',  ( 0.5774900079438590739, 32.64701867748816966, -5.440088680355550821 ) ) ;
#20754=CARTESIAN_POINT ( 'NONE',  ( 9.629649721936188023E-32, 78.62578230273079782, -9.232066091999506341 ) ) ;
#20755=CARTESIAN_POINT ( 'NONE',  ( 7.361572987183169658, 4.967264484334119601, -9.846743663894592657 ) ) ;
#20756=CARTESIAN_POINT ( 'NONE',  ( 10.00000000000000000, 24.75893115100078745, -9.846743663894594434 ) ) ;
#20759=CARTESIAN_POINT ( 'NONE',  ( 19.84674366389459621, 48.50893115100078745, 7.409399052514197653E-17 ) ) ;
#20760=CARTESIAN_POINT ( 'NONE',  ( 17.08211943468705840, 55.13708216824731068, -12.26659068614894466 ) ) ;
#20762=CARTESIAN_POINT ( 'NONE',  ( 1.711636803080574420, 61.84492782695771496, -6.500000000000073719 ) ) ;
#20763=EDGE_CURVE ( 'NONE', #16885, #62857, #11779, .T. ) ;
#20765=CARTESIAN_POINT ( 'NONE',  ( -4.164238869374099927, 12.01208216824730357, 3.795296366450308767 ) ) ;
#20766=CARTESIAN_POINT ( 'NONE',  ( 10.00000000000000178, 43.05374883491397497, 14.16423886937410082 ) ) ;
#20767=CARTESIAN_POINT ( 'NONE',  ( -2.816281873526471635, 3.915301336597087456, -3.434112377981056508 ) ) ;
#20769=CARTESIAN_POINT ( 'NONE',  ( 12.91533473730993009, 11.60535201082150714, -10.88017736071109987 ) ) ;
#20770=CARTESIAN_POINT ( 'NONE',  ( 7.361572987183170547, 47.05059781766745175, 9.846743663894590881 ) ) ;
#20774=CARTESIAN_POINT ( 'NONE',  ( 5.076628168052704559, 0.1755978176674514724, -8.527530157486179263 ) ) ;
#20775=CARTESIAN_POINT ( 'NONE',  ( -2.816281873526471635, 18.91530133659708213, -3.434112377981056508 ) ) ;
#20776=CARTESIAN_POINT ( 'NONE',  ( 18.52753015748617571, 23.09226448433411960, 4.923371831947298993 ) ) ;
#20777=EDGE_LOOP ( 'NONE', ( #75543, #64569, #49543, #17412 ) ) ;
#20778=CARTESIAN_POINT ( 'NONE',  ( 18.52753015748618282, 3.925597817667451306, -4.923371831947291888 ) ) ;
#20781=CARTESIAN_POINT ( 'NONE',  ( 20.88017736071110875, 15.77201867748817143, -2.915334737309920765 ) ) ;
#20782=CARTESIAN_POINT ( 'NONE',  ( 13.79529636645030344, 38.26208216824729647, 14.16423886937410614 ) ) ;
#20783=CARTESIAN_POINT ( 'NONE',  ( 0.5774900079438590739, 47.64701867748817676, -5.440088680355550821 ) ) ;
#20784=CARTESIAN_POINT ( 'NONE',  ( 7.084665262690076126, 67.02201867748817676, -10.88017736071110164 ) ) ;
#20788=CARTESIAN_POINT ( 'NONE',  ( 19.84674366389459266, 23.71726448433412315, -2.638427012816827677 ) ) ;
#20790=CARTESIAN_POINT ( 'NONE',  ( 1.472469842513823179, 5.592264484334118713, -4.923371831947296329 ) ) ;
#20791=CARTESIAN_POINT ( 'NONE',  ( -46.82017113615791004, 100.6079546444643427, 9.324761308090124601 ) ) ;
#20792=CARTESIAN_POINT ( 'NONE',  ( 5.076628168052704559, 35.17559781766745175, -8.527530157486179263 ) ) ;
#20793=CARTESIAN_POINT ( 'NONE',  ( 10.00000000000000178, 62.25893115100078745, 9.846743663894594434 ) ) ;
#20794=CARTESIAN_POINT ( 'NONE',  ( 12.91533473730992121, 39.52201867748817676, 10.88017736071110164 ) ) ;
#20795=B_SPLINE_CURVE_WITH_KNOTS ( 'NONE', 3,
 ( #58103, #49617, #48644, #88119, #26154, #18656 ),
 .UNSPECIFIED., .F., .F.,
 ( 4, 2, 4 ),
 ( 1.170549273921106170E-18, 0.0002626113303185924623, 0.0005252226606371837320 ),
 .UNSPECIFIED. ) ;
#20797=ORIENTED_EDGE ( 'NONE', *, *, #98370, .T. ) ;
#20798=CARTESIAN_POINT ( 'NONE',  ( 10.00000000000000000, 62.87363466993042493, -12.81628187352647608 ) ) ;
#20800=CARTESIAN_POINT ( 'NONE',  ( 22.81628187352647785, 41.41530133659708923, 3.434112377981063169 ) ) ;
#20801=CARTESIAN_POINT ( 'NONE',  ( 13.79529636645031943, 65.34541550158063217, -14.16423886937409904 ) ) ;
#20802=CARTESIAN_POINT ( 'NONE',  ( 12.63842701281683034, 32.46726448433412315, 9.846743663894596210 ) ) ;
#20803=CARTESIAN_POINT ( 'NONE',  ( -0.1503990784575328643, 60.12777174578613426, 6.262539305110068177 ) ) ;
#20804=CARTESIAN_POINT ( 'NONE',  ( 2.791683348922240793, 1.633931151000784565, 7.208316651077764092 ) ) ;
#20805=CARTESIAN_POINT ( 'NONE',  ( -2.266590686148945544, 21.38708216824730357, -7.082119434687050408 ) ) ;
#20807=CARTESIAN_POINT ( 'NONE',  ( 17.08211943468705840, 50.13708216824730357, -12.26659068614894466 ) ) ;
#20808=CARTESIAN_POINT ( 'NONE',  ( 0.1532563361054082862, 41.21726448433411605, 2.638427012816831674 ) ) ;
#20810=CARTESIAN_POINT ( 'NONE',  ( 20.88017736071110164, 40.35535201082150536, 2.915334737309930979 ) ) ;
#20811=CARTESIAN_POINT ( 'NONE',  ( 17.96484262340118221, 54.93868534415484106, 7.964842623401181321 ) ) ;
#20813=CARTESIAN_POINT ( 'NONE',  ( -2.816281873526473856, 49.12363466993042493, 9.499525473075851096E-16 ) ) ;
#20814=CARTESIAN_POINT ( 'NONE',  ( 0.1532563361054100626, 0.8005978176674514168, -2.638427012816831230 ) ) ;
#20815=ORIENTED_EDGE ( 'NONE', *, *, #79843, .F. ) ;
#20816=CARTESIAN_POINT ( 'NONE',  ( -0.3689425029237898834, 1.178748834913967869, -10.36894250292378850 ) ) ;
#20817=CARTESIAN_POINT ( 'NONE',  ( 0.1532563361054083140, 6.008931151000784787, 1.131784320476157264E-15 ) ) ;
#20821=CARTESIAN_POINT ( 'NONE',  ( 12.91533473730992121, 19.52201867748816611, 10.88017736071110164 ) ) ;
#20823=CARTESIAN_POINT ( 'NONE',  ( 13.79529636645031943, 20.34541550158063572, -14.16423886937409904 ) ) ;
#20825=CARTESIAN_POINT ( 'NONE',  ( -0.8801773607111009756, 28.06368534415484106, 1.068504757029289695E-15 ) ) ;
#20827=CARTESIAN_POINT ( 'NONE',  ( 18.52753015748617571, 63.09226448433412315, 4.923371831947298993 ) ) ;
#20829=CARTESIAN_POINT ( 'NONE',  ( 19.84674366389459266, 63.71726448433412315, -2.638427012816827677 ) ) ;
#20831=CARTESIAN_POINT ( 'NONE',  ( 2.035157376598822676, 67.43868534415484817, -7.964842623401177768 ) ) ;
#20833=CARTESIAN_POINT ( 'NONE',  ( 22.81628187352648496, 36.83196800326376064, -3.434112377981050290 ) ) ;
#20834=CARTESIAN_POINT ( 'NONE',  ( -0.8801773607111009756, 13.06368534415483929, 1.068504757029289695E-15 ) ) ;
#20836=CARTESIAN_POINT ( 'NONE',  ( -0.8801773607110991993, 67.85535201082151957, -2.915334737309923874 ) ) ;
#20838=CARTESIAN_POINT ( 'NONE',  ( 10.00000000000000178, 24.31368534415484106, 10.88017736071110342 ) ) ;
#20840=CARTESIAN_POINT ( 'NONE',  ( 0.6178305044545818747, 53.49863466993041072, -9.382169495545419124 ) ) ;
#20841=CARTESIAN_POINT ( 'NONE',  ( -0.8801773607110991993, 42.85535201082150536, -2.915334737309923874 ) ) ;
#20843=CARTESIAN_POINT ( 'NONE',  ( -2.816281873526473856, 44.12363466993042493, 9.499525473075851096E-16 ) ) ;
#20844=CARTESIAN_POINT ( 'NONE',  ( 17.96484262340118221, 46.18868534415484106, -7.964842623401177768 ) ) ;
#20845=CARTESIAN_POINT ( 'NONE',  ( 18.52753015748617571, 58.09226448433411605, 4.923371831947298993 ) ) ;
#20848=CARTESIAN_POINT ( 'NONE',  ( 10.00000000000000178, 12.25893115100078568, 9.846743663894594434 ) ) ;
#20849=CARTESIAN_POINT ( 'NONE',  ( -1.099225684535947600, 9.540301336597087456, 6.408140936763237150 ) ) ;
#20850=DIRECTION ( 'NONE',  ( 0.000000000000000000, 0.000000000000000000, -1.000000000000000000 ) ) ;
#20851=CARTESIAN_POINT ( 'NONE',  ( 19.84674366389459621, 58.50893115100078745, 7.409399052514197653E-17 ) ) ;
#20852=CARTESIAN_POINT ( 'NONE',  ( 2.035157376598822676, 22.43868534415483396, -7.964842623401177768 ) ) ;
#20853=CARTESIAN_POINT ( 'NONE',  ( 1.472469842513823179, 55.59226448433412315, -4.923371831947296329 ) ) ;
#20857=CARTESIAN_POINT ( 'NONE',  ( 2.791683348922240793, 11.63393115100078568, 7.208316651077764092 ) ) ;
#20858=CARTESIAN_POINT ( 'NONE',  ( 0.1532563361054083140, 1.008931151000784787, 1.131784320476157264E-15 ) ) ;
#20859=CARTESIAN_POINT ( 'NONE',  ( 10.00000000000000178, 67.25893115100079456, 9.846743663894594434 ) ) ;
#20862=CARTESIAN_POINT ( 'NONE',  ( 0.6178305044545838731, 39.74863466993041072, 9.382169495545420901 ) ) ;
#20863=CARTESIAN_POINT ( 'NONE',  ( 19.84674366389459621, 28.50893115100078745, 7.409399052514197653E-17 ) ) ;
#20864=CARTESIAN_POINT ( 'NONE',  ( 0.5774900079438590739, 57.64701867748817676, -5.440088680355550821 ) ) ;
#20865=CARTESIAN_POINT ( 'NONE',  ( -4.164238869374099039, 56.80374883491397497, 8.674139862899312516E-16 ) ) ;
#20866=CARTESIAN_POINT ( 'NONE',  ( 17.20831665107776587, 27.88393115100078390, 7.208316651077764980 ) ) ;
#20868=CARTESIAN_POINT ( 'NONE',  ( -0.2418659066527710233, 50.11633188102328518, 6.114288769123046308 ) ) ;
#20869=CARTESIAN_POINT ( 'NONE',  ( 2.035157376598824452, 8.688685344154839285, 7.964842623401179544 ) ) ;
#20871=CARTESIAN_POINT ( 'NONE',  ( -0.8801773607111009756, 18.06368534415484106, 1.068504757029289695E-15 ) ) ;
#20872=CARTESIAN_POINT ( 'NONE',  ( -4.164238869374099039, 46.80374883491397497, 8.674139862899312516E-16 ) ) ;
#20873=CARTESIAN_POINT ( 'NONE',  ( 10.00000000000000178, 53.05374883491396787, 14.16423886937410082 ) ) ;
#20874=DIRECTION ( 'NONE',  ( 0.000000000000000000, 0.000000000000000000, -1.000000000000000000 ) ) ;
#20875=LINE ( 'NONE', #42394, #6902 ) ;
#20876=CARTESIAN_POINT ( 'NONE',  ( 0.1532563361054100626, 15.80059781766745353, -2.638427012816831230 ) ) ;
#20877=CARTESIAN_POINT ( 'NONE',  ( 22.81628187352647785, 1.415301336597087012, 3.434112377981063169 ) ) ;
#20878=VERTEX_POINT ( 'NONE', #20037 ) ;
#20879=CARTESIAN_POINT ( 'NONE',  ( -0.8801773607110991993, 52.85535201082151247, -2.915334737309923874 ) ) ;
#20882=CARTESIAN_POINT ( 'NONE',  ( 0.1532563361054100626, 55.80059781766745175, -2.638427012816831230 ) ) ;
#20884=CARTESIAN_POINT ( 'NONE',  ( 14.92337183194729988, 64.34226448433412315, -8.527530157486177487 ) ) ;
#20888=CARTESIAN_POINT ( 'NONE',  ( 0.1532563361054082862, 26.21726448433411605, 2.638427012816831674 ) ) ;
#20890=CARTESIAN_POINT ( 'NONE',  ( 6.204703633549690345, 37.84541550158063927, 14.16423886937410082 ) ) ;
#20891=DIRECTION ( 'NONE',  ( 1.000000000000000000, 0.000000000000000000, 0.000000000000000000 ) ) ;
#20893=DIRECTION ( 'NONE',  ( 0.000000000000000000, 0.000000000000000000, 1.000000000000000000 ) ) ;
#20894=CARTESIAN_POINT ( 'NONE',  ( 15.44008868035555793, 26.39701867748817321, -9.422509992056140149 ) ) ;
#20895=CARTESIAN_POINT ( 'NONE',  ( -2.816281873526473856, 34.12363466993042493, 9.499525473075851096E-16 ) ) ;
#20896=CARTESIAN_POINT ( 'NONE',  ( 20.88017736071110519, 10.56368534415483751, 2.639326808657452039E-16 ) ) ;
#20898=CARTESIAN_POINT ( 'NONE',  ( 21.09922568453594849, 41.20696800326375353, 6.408140936763242479 ) ) ;
#20899=CARTESIAN_POINT ( 'NONE',  ( 21.09922568453594849, 56.20696800326375353, 6.408140936763242479 ) ) ;
#20903=CARTESIAN_POINT ( 'NONE',  ( -4.164238869374099927, 32.01208216824730357, 3.795296366450308767 ) ) ;
#20904=CARTESIAN_POINT ( 'NONE',  ( 17.08211943468705130, 3.470415501580634388, 12.26659068614894998 ) ) ;
#20905=CARTESIAN_POINT ( 'NONE',  ( -0.8801773607110991993, 7.855352010821504471, -2.915334737309923874 ) ) ;
#20906=CARTESIAN_POINT ( 'NONE',  ( 15.44008868035555793, 21.39701867748817321, -9.422509992056140149 ) ) ;
#20908=FACE_OUTER_BOUND ( 'NONE', #1546, .T. ) ;
#20909=CARTESIAN_POINT ( 'NONE',  ( 12.91533473730992121, 49.52201867748817676, 10.88017736071110164 ) ) ;
#20910=CARTESIAN_POINT ( 'NONE',  ( 20.88017736071110875, 45.77201867748816966, -2.915334737309920765 ) ) ;
#20911=CARTESIAN_POINT ( 'NONE',  ( -2.816281873526471635, 13.91530133659708746, -3.434112377981056508 ) ) ;
#20914=CARTESIAN_POINT ( 'NONE',  ( 17.20831665107776587, 19.13393115100078035, -7.208316651077762316 ) ) ;
#20915=CARTESIAN_POINT ( 'NONE',  ( 19.42250999205614193, 40.14701867748817676, 5.440088680355555262 ) ) ;
#20917=CARTESIAN_POINT ( 'NONE',  ( 22.81628187352647785, 1.623634669930420271, 6.195893100308588602E-16 ) ) ;
#20918=CARTESIAN_POINT ( 'NONE',  ( 1.274849032794231007, 43.57228050351031357, 6.499999999999895195 ) ) ;
#20919=CARTESIAN_POINT ( 'NONE',  ( 18.52753015748618282, 18.92559781766745175, -4.923371831947291888 ) ) ;
#20920=CARTESIAN_POINT ( 'NONE',  ( 0.6178305044545818747, 43.49863466993042493, -9.382169495545419124 ) ) ;
#20921=CARTESIAN_POINT ( 'NONE',  ( 0.1532563361054083140, 21.00893115100078745, 1.131784320476157264E-15 ) ) ;
#20923=CARTESIAN_POINT ( 'NONE',  ( 24.16423886937410614, 4.303748834913967869, 8.672049930838204340E-16 ) ) ;
#20925=CARTESIAN_POINT ( 'NONE',  ( 15.44008868035555793, 21.39701867748817321, -9.422509992056140149 ) ) ;
#20926=CARTESIAN_POINT ( 'NONE',  ( 2.035157376598824452, 3.688685344154837953, 7.964842623401179544 ) ) ;
#20927=CARTESIAN_POINT ( 'NONE',  ( 10.00000000000000000, 34.75893115100078745, -9.846743663894594434 ) ) ;
#20928=CARTESIAN_POINT ( 'NONE',  ( 7.084665262690076126, 14.10535201082150358, 10.88017736071109987 ) ) ;
#20929=CARTESIAN_POINT ( 'NONE',  ( 10.00000000000000000, 21.81368534415484106, -10.88017736071110342 ) ) ;
#20930=ORIENTED_EDGE ( 'NONE', *, *, #75923, .T. ) ;
#20932=CARTESIAN_POINT ( 'NONE',  ( 20.88017736071110875, 20.77201867748816611, -2.915334737309920765 ) ) ;
#20933=CARTESIAN_POINT ( 'NONE',  ( 13.43411237798106583, 52.66530133659708213, -12.81628187352647252 ) ) ;
#20934=CARTESIAN_POINT ( 'NONE',  ( 4.559911319644449179, 28.89701867748817321, 9.422509992056141925 ) ) ;
#20936=CARTESIAN_POINT ( 'NONE',  ( 12.91533473730992121, 44.52201867748816966, 10.88017736071110164 ) ) ;
#20938=CARTESIAN_POINT ( 'NONE',  ( 19.84674366389459266, 53.30059781766744464, 2.638427012816836559 ) ) ;
#20939=CARTESIAN_POINT ( 'NONE',  ( 19.42250999205614548, 40.98035201082150536, -5.440088680355545492 ) ) ;
#20940=CARTESIAN_POINT ( 'NONE',  ( 14.92337183194729988, 64.34226448433412315, -8.527530157486177487 ) ) ;
#20941=MECHANICAL_DESIGN_GEOMETRIC_PRESENTATION_REPRESENTATION('',(#8169),#38569);
#20943=CARTESIAN_POINT ( 'NONE',  ( 3.591859063236763294, 58.29030133659708923, -11.09922568453595026 ) ) ;
#20945=CARTESIAN_POINT ( 'NONE',  ( -4.164238869374099039, 51.80374883491396787, 8.674139862899312516E-16 ) ) ;
#20946=CARTESIAN_POINT ( 'NONE',  ( 19.42250999205614548, 50.98035201082151247, -5.440088680355545492 ) ) ;
#20949=CARTESIAN_POINT ( 'NONE',  ( 19.84674366389459621, 48.50893115100078745, 7.409399052514197653E-17 ) ) ;
#20950=CARTESIAN_POINT ( 'NONE',  ( 12.63842701281683922, 4.550597817667451750, -9.846743663894590881 ) ) ;
#20951=CARTESIAN_POINT ( 'NONE',  ( 0.1532563361054082862, 21.21726448433412315, 2.638427012816831674 ) ) ;
#20952=ORIENTED_EDGE ( 'NONE', *, *, #43747, .F. ) ;
#20953=CARTESIAN_POINT ( 'NONE',  ( 14.92337183194729633, 22.67559781766745175, 8.527530157486181039 ) ) ;
#20956=( BOUNDED_SURFACE ( )  B_SPLINE_SURFACE ( 1, 2, ( 
 ( #3518, #12476, #80491, #49983, #27475, #48998, #42980, #72479, #64967, #4504, #71528, #41026, #42014, #34969, #4012, #94986, #96492, #95493, #50473, #4988, #3038, #88972, #64479, #41525, #73460, #35469, #57484, #33488, #65466, #26492, #63987, #94497, #33976, #95993, #26016, #56511, #18508, #79507, #60435, #66458, #74446, #13466, #20980, #45434, #74949, #21969, #67951, #6956, #14463, #29434, #51463, #36962, #98971, #43459, #60926, #82449, #90928, #67457, #44447, #58966, #59938, #97978, #13972, #6452, #81953, #37464, #98475, #43947, #90429, #73961, #29930, #30425, #44938, #22457, #5490, #75444, #89462, #52448, #59447, #82948, #5972, #36466, #14964, #66961, #97479, #52932, #83443, #89948, #75936, #28945, #91432, #7460, #37959, #22959, #68450, #35961, #81461, #21466, #12965, #96992, #28469, #51964, #93397, #76918, #53928, #15934, #9411, #77399, #16921, #15460, #62393, #945, #63387, #85908, #47397, #38442, #46906, #54896, #77899, #31895, #32888, #24922, #93891, #70416, #46424, #17422, #24432, #92901, #32393, #91925, #47890, #16429, #8912, #39913, #45941, #53424, #23937, #85411, #39429, #38935, #40415, #69922, #78392, #9914, #76431, #2431, #8428, #69424, #70911, #83931, #1443, #7946, #31406, #61907, #68939, #469, #92413, #30917, #54406, #61417, #23451, #84918, #4385, #10398, #48871, #86882, #63864, #50348, #18887, #64846, #11868, #42374, #87856, #72355, #94378, #79870, #42863, #86401, #4872, #26372, #34850, #11374, #87372, #35350, #27355, #17903, #95365, #25897, #79383, #65345, #95874, #94870, #49368, #10889, #55903, #3888, #19374, #48386, #34355, #78888, #26864, #3390, #80859, #73345, #57849, #41413, #12356, #40903, #71404, #2920, #52330, #21347, #59818, #58333, #6333, #43829, #7341, #98358, #90313, #81347, #89830, #97858, #21849, #74828, #75820, #67840, #37842, #14344, #89343, #29816, #67332, #29321, #44815, #35847, #60325, #59327, #51838, #82823, #88850, #96372, #66836, #75322, #82325, #81829, #83325, #13845, #6835, #90815, #20358, #45322, #51344, #28346, #37349, #22344, #44327, #14851, #74325, #13345, #52817, #27845, #96870, #50854, #97358, #12843, #43343, #66334, #73840, #5368, #20853, #58836, #5851, #36342, #28827, #8801, #54782, #92787, #1333, #16313, #7834, #23828, #85791, #30307, #47780, #69313, #77783, #54291, #31294, #78279, #70305, #60809, #39316, #45828, #46797, #84804, #834, #61794, #38331, #24317, #85298, #68824, #77290, #91309, #16806, #17305, #31785, #47281, #22837, #62281, #76316, #92302, #46315, #69811, #356, #23335, #1818, #9295, #39803, #32275, #53815, #30805, #68333, #38821, #93281, #62782, #8317 ),
 ( #24805, #84326, #55282, #9792, #98853, #53312, #83820, #15346, #15826, #61303, #91814, #76801, #33739, #57731, #86777, #94260, #72729, #65226, #40786, #64241, #10776, #80742, #40291, #78780, #19252, #25301, #33263, #71285, #10287, #4263, #94759, #11257, #26748, #64729, #72245, #87251, #2808, #56756, #88234, #2316, #19743, #41292, #49736, #18776, #3276, #50227, #42259, #32770, #41774, #17792, #49259, #3779, #71766, #34232, #63754, #95239, #57242, #25786, #87740, #63266, #80244, #70800, #11751, #34734, #93775, #95752, #48267, #27236, #18278, #55788, #56281, #48759, #86284, #79266, #73227, #88728, #58211, #35227, #65725, #4756, #50743, #96251, #27730, #12237, #20239, #42746, #8898, #53916, #62885, #55393, #84905, #76420, #16910, #30906, #7934, #38430, #62380, #31393, #69910, #68438, #16417, #84425, #17409, #9397, #1430, #91419, #932, #39415, #31883, #85893, #61402, #68928, #24418, #54883, #61893, #24909, #15922, #91913, #39898, #32380, #458, #92400, #76903, #47876, #7449, #45929, #85397, #22945, #23437, #46413, #8416, #70404, #23923, #46894, #92886, #47383, #77884, #54394, #38923, #77385, #37946, #98958, #30414, #69409, #1922, #93382, #60914, #53412, #83920, #15450, #84186, #21715, #61648, #14211, #96111, #55362, #1401, #10359, #40858, #69881, #85866, #92372, #71363, #41371, #2880, #33330, #23898, #63824, #39387, #17379, #9367, #78352, #24387, #85367, #94338, #54854, #77857, #25855, #56352, #39870, #9873, #1895, #31367, #40372, #18353, #61867, #70873, #54366, #32842, #62858, #48830, #84876, #2389, #16384, #46869, #26823, #3847, #34305, #58289, #27308, #65797, #64316, #12315, #49814, #13301, #5325, #96331, #87327, #95827, #4830, #27806, #80815, #81786, #73795, #43788, #20318, #95322, #35806, #73307, #42822, #50814, #41849, #66293, #65301, #57807, #88807, #94828, #3347, #72802, #35305, #88315, #87809, #89304, #19814, #81307, #96827, #26331, #28304, #56830, #12802, #79827, #50303, #43302, #34812, #58796, #72315, #20813, #51303, #64803, #33810, #18844, #49324, #11332, #57316, #19330, #80321, #11822, #42328, #4341, #52289, #37308, #82283, #29285, #7792, #44287, #13801, #15301, #91270, #82787, #67797, #36802, #53770, #98316, #7298, #15786, #29770, #66798, #75777, #21807, #30757, #23293, #52777, #74791, #83778, #97823, #6300, #67296, #30266, #60280, #37798, #36302, #83284, #14308, #84286, #76277, #68295, #59291, #90777, #98815, #60769, #14810, #74281, #45785, #5810, #22794, #59782, #38288, #45281, #53271, #68782, #90273, #314, #22304, #61263, #91771, #97318, #28791, #44778, #89789, #21306, #75283, #51798, #6795, #25265, #40739 ) ),
 .UNSPECIFIED., .F., .F., .T. ) 
 B_SPLINE_SURFACE_WITH_KNOTS ( ( 2, 2 ),
 ( 3, 2, 2, 2, 2, 2, 2, 2, 2, 2, 2, 2, 2, 2, 2, 2, 2, 2, 2, 2, 2, 2, 2, 2, 2, 2, 2, 2, 2, 2, 2, 2, 2, 2, 2, 2, 2, 2, 2, 2, 2, 2, 2, 2, 2, 2, 2, 2, 2, 2, 2, 2, 2, 2, 2, 2, 2, 2, 2, 2, 2, 2, 2, 2, 2, 2, 2, 2, 2, 2, 2, 2, 2, 2, 2, 2, 2, 2, 2, 2, 2, 2, 2, 2, 2, 2, 2, 2, 2, 2, 2, 2, 2, 2, 2, 2, 2, 2, 2, 2, 2, 2, 2, 2, 2, 2, 2, 2, 2, 2, 2, 2, 2, 2, 2, 2, 2, 2, 2, 2, 2, 2, 2, 2, 2, 2, 2, 2, 2, 2, 2, 2, 2, 2, 2, 2, 2, 2, 2, 2, 2, 2, 2, 2, 2, 2, 2, 2, 2, 2, 2, 2, 2, 2, 2, 2, 2, 2, 2, 2, 2, 2, 3 ),
 ( 0.000000000000000000, 1.000000000000000000 ),
 ( 0.000000000000000000, 0.005952380952380952051, 0.01190476190476190410, 0.01785714285714285615, 0.02380952380952380820, 0.02976190476190476025, 0.03571428571428571230, 0.04166666666666666435, 0.04761904761904761640, 0.05357142857142856845, 0.05952380952380952051, 0.06547619047619047949, 0.07142857142857142461, 0.07738095238095238360, 0.08333333333333332871, 0.08928571428571428770, 0.09523809523809523281, 0.1011904761904761918, 0.1071428571428571369, 0.1130952380952380959, 0.1190476190476190410, 0.1250000000000000000, 0.1309523809523809590, 0.1369047619047619180, 0.1428571428571428492, 0.1488095238095238082, 0.1547619047619047672, 0.1607142857142857262, 0.1666666666666666574, 0.1726190476190476164, 0.1785714285714285754, 0.1845238095238095344, 0.1904761904761904656, 0.1964285714285714246, 0.2023809523809523836, 0.2083333333333333426, 0.2142857142857142738, 0.2202380952380952328, 0.2261904761904761918, 0.2321428571428571508, 0.2380952380952380820, 0.2440476190476190410, 0.2500000000000000000, 0.2559523809523809312, 0.2619047619047619180, 0.2678571428571428492, 0.2738095238095238360, 0.2797619047619047672, 0.2857142857142856984, 0.2916666666666666852, 0.2976190476190476164, 0.3035714285714285476, 0.3095238095238095344, 0.3154761904761904656, 0.3214285714285714524, 0.3273809523809523836, 0.3333333333333333148, 0.3392857142857143016, 0.3452380952380952328, 0.3511904761904761640, 0.3571428571428571508, 0.3630952380952380820, 0.3690476190476190688, 0.3750000000000000000, 0.3809523809523809312, 0.3869047619047619180, 0.3928571428571428492, 0.3988095238095238360, 0.4047619047619047672, 0.4107142857142856984, 0.4166666666666666852, 0.4226190476190476164, 0.4285714285714285476, 0.4345238095238095344, 0.4404761904761904656, 0.4464285714285714524, 0.4523809523809523836, 0.4583333333333333148, 0.4642857142857143016, 0.4702380952380952328, 0.4761904761904761640, 0.4821428571428571508, 0.4880952380952380820, 0.4940476190476190688, 0.5000000000000000000, 0.5059523809523809312, 0.5119047619047618625, 0.5178571428571429047, 0.5238095238095238360, 0.5297619047619047672, 0.5357142857142856984, 0.5416666666666666297, 0.5476190476190476719, 0.5535714285714286031, 0.5595238095238095344, 0.5654761904761904656, 0.5714285714285713969, 0.5773809523809523281, 0.5833333333333333703, 0.5892857142857143016, 0.5952380952380952328, 0.6011904761904761640, 0.6071428571428570953, 0.6130952380952381375, 0.6190476190476190688, 0.6250000000000000000, 0.6309523809523809312, 0.6369047619047618625, 0.6428571428571429047, 0.6488095238095238360, 0.6547619047619047672, 0.6607142857142856984, 0.6666666666666666297, 0.6726190476190476719, 0.6785714285714286031, 0.6845238095238095344, 0.6904761904761904656, 0.6964285714285713969, 0.7023809523809523281, 0.7083333333333333703, 0.7142857142857143016, 0.7202380952380952328, 0.7261904761904761640, 0.7321428571428570953, 0.7380952380952381375, 0.7440476190476190688, 0.7500000000000000000, 0.7559523809523809312, 0.7619047619047618625, 0.7678571428571429047, 0.7738095238095238360, 0.7797619047619047672, 0.7857142857142856984, 0.7916666666666666297, 0.7976190476190476719, 0.8035714285714286031, 0.8095238095238095344, 0.8154761904761904656, 0.8214285714285713969, 0.8273809523809523281, 0.8333333333333333703, 0.8392857142857143016, 0.8452380952380952328, 0.8511904761904761640, 0.8571428571428570953, 0.8630952380952381375, 0.8690476190476190688, 0.8750000000000000000, 0.8809523809523809312, 0.8869047619047618625, 0.8928571428571429047, 0.8988095238095238360, 0.9047619047619047672, 0.9107142857142856984, 0.9166666666666666297, 0.9226190476190476719, 0.9285714285714286031, 0.9345238095238095344, 0.9404761904761904656, 0.9464285714285713969, 0.9523809523809523281, 0.9583333333333333703, 0.9642857142857143016 ),
 .UNSPECIFIED. ) 
 GEOMETRIC_REPRESENTATION_ITEM ( )  RATIONAL_B_SPLINE_SURFACE ( (
 ( 1.000000000000000000, 0.9659258262890683122, 1.000000000000000000, 0.9659258262890683122, 1.000000000000000000, 0.9659258262890683122, 1.000000000000000000, 0.9659258262890683122, 1.000000000000000000, 0.9659258262890683122, 1.000000000000000000, 0.9659258262890683122, 1.000000000000000000, 0.9659258262890683122, 1.000000000000000000, 0.9659258262890683122, 1.000000000000000000, 0.9659258262890683122, 1.000000000000000000, 0.9659258262890683122, 1.000000000000000000, 0.9659258262890683122, 1.000000000000000000, 0.9659258262890683122, 1.000000000000000000, 0.9659258262890683122, 1.000000000000000000, 0.9659258262890683122, 1.000000000000000000, 0.9659258262890683122, 1.000000000000000000, 0.9659258262890683122, 1.000000000000000000, 0.9659258262890683122, 1.000000000000000000, 0.9659258262890683122, 1.000000000000000000, 0.9659258262890683122, 1.000000000000000000, 0.9659258262890683122, 1.000000000000000000, 0.9659258262890683122, 1.000000000000000000, 0.9659258262890683122, 1.000000000000000000, 0.9659258262890683122, 1.000000000000000000, 0.9659258262890683122, 1.000000000000000000, 0.9659258262890683122, 1.000000000000000000, 0.9659258262890683122, 1.000000000000000000, 0.9659258262890683122, 1.000000000000000000, 0.9659258262890683122, 1.000000000000000000, 0.9659258262890683122, 1.000000000000000000, 0.9659258262890683122, 1.000000000000000000, 0.9659258262890683122, 1.000000000000000000, 0.9659258262890683122, 1.000000000000000000, 0.9659258262890683122, 1.000000000000000000, 0.9659258262890683122, 1.000000000000000000, 0.9659258262890683122, 1.000000000000000000, 0.9659258262890683122, 1.000000000000000000, 0.9659258262890683122, 1.000000000000000000, 0.9659258262890683122, 1.000000000000000000, 0.9659258262890683122, 1.000000000000000000, 0.9659258262890683122, 1.000000000000000000, 0.9659258262890683122, 1.000000000000000000, 0.9659258262890683122, 1.000000000000000000, 0.9659258262890683122, 1.000000000000000000, 0.9659258262890683122, 1.000000000000000000, 0.9659258262890683122, 1.000000000000000000, 0.9659258262890683122, 1.000000000000000000, 0.9659258262890683122, 1.000000000000000000, 0.9659258262890683122, 1.000000000000000000, 0.9659258262890683122, 1.000000000000000000, 0.9659258262890683122, 1.000000000000000000, 0.9659258262890683122, 1.000000000000000000, 0.9659258262890683122, 1.000000000000000000, 0.9659258262890683122, 1.000000000000000000, 0.9659258262890683122, 1.000000000000000000, 0.9659258262890683122, 1.000000000000000000, 0.9659258262890683122, 1.000000000000000000, 0.9659258262890683122, 1.000000000000000000, 0.9659258262890683122, 1.000000000000000000, 0.9659258262890683122, 1.000000000000000000, 0.9659258262890683122, 1.000000000000000000, 0.9659258262890683122, 1.000000000000000000, 0.9659258262890683122, 1.000000000000000000, 0.9659258262890683122, 1.000000000000000000, 0.9659258262890683122, 1.000000000000000000, 0.9659258262890683122, 1.000000000000000000, 0.9659258262890683122, 1.000000000000000000, 0.9659258262890683122, 1.000000000000000000, 0.9659258262890683122, 1.000000000000000000, 0.9659258262890683122, 1.000000000000000000, 0.9659258262890683122, 1.000000000000000000, 0.9659258262890683122, 1.000000000000000000, 0.9659258262890683122, 1.000000000000000000, 0.9659258262890683122, 1.000000000000000000, 0.9659258262890683122, 1.000000000000000000, 0.9659258262890683122, 1.000000000000000000, 0.9659258262890683122, 1.000000000000000000, 0.9659258262890683122, 1.000000000000000000, 0.9659258262890683122, 1.000000000000000000, 0.9659258262890683122, 1.000000000000000000, 0.9659258262890683122, 1.000000000000000000, 0.9659258262890683122, 1.000000000000000000, 0.9659258262890683122, 1.000000000000000000, 0.9659258262890683122, 1.000000000000000000, 0.9659258262890683122, 1.000000000000000000, 0.9659258262890683122, 1.000000000000000000, 0.9659258262890683122, 1.000000000000000000, 0.9659258262890683122, 1.000000000000000000, 0.9659258262890683122, 1.000000000000000000, 0.9659258262890683122, 1.000000000000000000, 0.9659258262890683122, 1.000000000000000000, 0.9659258262890683122, 1.000000000000000000, 0.9659258262890683122, 1.000000000000000000, 0.9659258262890683122, 1.000000000000000000, 0.9659258262890683122, 1.000000000000000000, 0.9659258262890683122, 1.000000000000000000, 0.9659258262890683122, 1.000000000000000000, 0.9659258262890683122, 1.000000000000000000, 0.9659258262890683122, 1.000000000000000000, 0.9659258262890683122, 1.000000000000000000, 0.9659258262890683122, 1.000000000000000000, 0.9659258262890683122, 1.000000000000000000, 0.9659258262890683122, 1.000000000000000000, 0.9659258262890683122, 1.000000000000000000, 0.9659258262890683122, 1.000000000000000000, 0.9659258262890683122, 1.000000000000000000, 0.9659258262890683122, 1.000000000000000000, 0.9659258262890683122, 1.000000000000000000, 0.9659258262890683122, 1.000000000000000000, 0.9659258262890683122, 1.000000000000000000, 0.9659258262890683122, 1.000000000000000000, 0.9659258262890683122, 1.000000000000000000, 0.9659258262890683122, 1.000000000000000000, 0.9659258262890683122, 1.000000000000000000, 0.9659258262890683122, 1.000000000000000000, 0.9659258262890683122, 1.000000000000000000, 0.9659258262890683122, 1.000000000000000000, 0.9659258262890683122, 1.000000000000000000, 0.9659258262890683122, 1.000000000000000000, 0.9659258262890683122, 1.000000000000000000, 0.9659258262890683122, 1.000000000000000000, 0.9659258262890683122, 1.000000000000000000, 0.9659258262890683122, 1.000000000000000000, 0.9659258262890683122, 1.000000000000000000, 0.9659258262890683122, 1.000000000000000000, 0.9659258262890683122, 1.000000000000000000, 0.9659258262890683122, 1.000000000000000000, 0.9659258262890683122, 1.000000000000000000, 0.9659258262890683122, 1.000000000000000000, 0.9659258262890683122, 1.000000000000000000, 0.9659258262890683122, 1.000000000000000000, 0.9659258262890683122, 1.000000000000000000, 0.9659258262890683122, 1.000000000000000000, 0.9659258262890683122, 1.000000000000000000, 0.9659258262890683122, 1.000000000000000000, 0.9659258262890683122, 1.000000000000000000, 0.9659258262890683122, 1.000000000000000000, 0.9659258262890683122, 1.000000000000000000, 0.9659258262890683122, 1.000000000000000000, 0.9659258262890683122, 1.000000000000000000, 0.9659258262890683122, 1.000000000000000000, 0.9659258262890683122, 1.000000000000000000, 0.9659258262890683122, 1.000000000000000000, 0.9659258262890683122, 1.000000000000000000, 0.9659258262890683122, 1.000000000000000000, 0.9659258262890683122, 1.000000000000000000, 0.9659258262890683122, 1.000000000000000000, 0.9659258262890683122, 1.000000000000000000, 0.9659258262890683122, 1.000000000000000000, 0.9659258262890683122, 1.000000000000000000, 0.9659258262890683122, 1.000000000000000000, 0.9659258262890683122, 1.000000000000000000, 0.9659258262890683122, 1.000000000000000000, 0.9659258262890683122, 1.000000000000000000, 0.9659258262890683122, 1.000000000000000000, 0.9659258262890683122, 1.000000000000000000, 0.9659258262890683122, 1.000000000000000000, 0.9659258262890683122, 1.000000000000000000, 0.9659258262890683122, 1.000000000000000000, 0.9659258262890683122, 1.000000000000000000, 0.9659258262890683122, 1.000000000000000000, 0.9659258262890683122, 1.000000000000000000, 0.9659258262890683122, 1.000000000000000000),
 ( 1.000000000000000000, 0.9659258262890683122, 1.000000000000000000, 0.9659258262890683122, 1.000000000000000000, 0.9659258262890683122, 1.000000000000000000, 0.9659258262890683122, 1.000000000000000000, 0.9659258262890683122, 1.000000000000000000, 0.9659258262890683122, 1.000000000000000000, 0.9659258262890683122, 1.000000000000000000, 0.9659258262890683122, 1.000000000000000000, 0.9659258262890683122, 1.000000000000000000, 0.9659258262890683122, 1.000000000000000000, 0.9659258262890683122, 1.000000000000000000, 0.9659258262890683122, 1.000000000000000000, 0.9659258262890683122, 1.000000000000000000, 0.9659258262890683122, 1.000000000000000000, 0.9659258262890683122, 1.000000000000000000, 0.9659258262890683122, 1.000000000000000000, 0.9659258262890683122, 1.000000000000000000, 0.9659258262890683122, 1.000000000000000000, 0.9659258262890683122, 1.000000000000000000, 0.9659258262890683122, 1.000000000000000000, 0.9659258262890683122, 1.000000000000000000, 0.9659258262890683122, 1.000000000000000000, 0.9659258262890683122, 1.000000000000000000, 0.9659258262890683122, 1.000000000000000000, 0.9659258262890683122, 1.000000000000000000, 0.9659258262890683122, 1.000000000000000000, 0.9659258262890683122, 1.000000000000000000, 0.9659258262890683122, 1.000000000000000000, 0.9659258262890683122, 1.000000000000000000, 0.9659258262890683122, 1.000000000000000000, 0.9659258262890683122, 1.000000000000000000, 0.9659258262890683122, 1.000000000000000000, 0.9659258262890683122, 1.000000000000000000, 0.9659258262890683122, 1.000000000000000000, 0.9659258262890683122, 1.000000000000000000, 0.9659258262890683122, 1.000000000000000000, 0.9659258262890683122, 1.000000000000000000, 0.9659258262890683122, 1.000000000000000000, 0.9659258262890683122, 1.000000000000000000, 0.9659258262890683122, 1.000000000000000000, 0.9659258262890683122, 1.000000000000000000, 0.9659258262890683122, 1.000000000000000000, 0.9659258262890683122, 1.000000000000000000, 0.9659258262890683122, 1.000000000000000000, 0.9659258262890683122, 1.000000000000000000, 0.9659258262890683122, 1.000000000000000000, 0.9659258262890683122, 1.000000000000000000, 0.9659258262890683122, 1.000000000000000000, 0.9659258262890683122, 1.000000000000000000, 0.9659258262890683122, 1.000000000000000000, 0.9659258262890683122, 1.000000000000000000, 0.9659258262890683122, 1.000000000000000000, 0.9659258262890683122, 1.000000000000000000, 0.9659258262890683122, 1.000000000000000000, 0.9659258262890683122, 1.000000000000000000, 0.9659258262890683122, 1.000000000000000000, 0.9659258262890683122, 1.000000000000000000, 0.9659258262890683122, 1.000000000000000000, 0.9659258262890683122, 1.000000000000000000, 0.9659258262890683122, 1.000000000000000000, 0.9659258262890683122, 1.000000000000000000, 0.9659258262890683122, 1.000000000000000000, 0.9659258262890683122, 1.000000000000000000, 0.9659258262890683122, 1.000000000000000000, 0.9659258262890683122, 1.000000000000000000, 0.9659258262890683122, 1.000000000000000000, 0.9659258262890683122, 1.000000000000000000, 0.9659258262890683122, 1.000000000000000000, 0.9659258262890683122, 1.000000000000000000, 0.9659258262890683122, 1.000000000000000000, 0.9659258262890683122, 1.000000000000000000, 0.9659258262890683122, 1.000000000000000000, 0.9659258262890683122, 1.000000000000000000, 0.9659258262890683122, 1.000000000000000000, 0.9659258262890683122, 1.000000000000000000, 0.9659258262890683122, 1.000000000000000000, 0.9659258262890683122, 1.000000000000000000, 0.9659258262890683122, 1.000000000000000000, 0.9659258262890683122, 1.000000000000000000, 0.9659258262890683122, 1.000000000000000000, 0.9659258262890683122, 1.000000000000000000, 0.9659258262890683122, 1.000000000000000000, 0.9659258262890683122, 1.000000000000000000, 0.9659258262890683122, 1.000000000000000000, 0.9659258262890683122, 1.000000000000000000, 0.9659258262890683122, 1.000000000000000000, 0.9659258262890683122, 1.000000000000000000, 0.9659258262890683122, 1.000000000000000000, 0.9659258262890683122, 1.000000000000000000, 0.9659258262890683122, 1.000000000000000000, 0.9659258262890683122, 1.000000000000000000, 0.9659258262890683122, 1.000000000000000000, 0.9659258262890683122, 1.000000000000000000, 0.9659258262890683122, 1.000000000000000000, 0.9659258262890683122, 1.000000000000000000, 0.9659258262890683122, 1.000000000000000000, 0.9659258262890683122, 1.000000000000000000, 0.9659258262890683122, 1.000000000000000000, 0.9659258262890683122, 1.000000000000000000, 0.9659258262890683122, 1.000000000000000000, 0.9659258262890683122, 1.000000000000000000, 0.9659258262890683122, 1.000000000000000000, 0.9659258262890683122, 1.000000000000000000, 0.9659258262890683122, 1.000000000000000000, 0.9659258262890683122, 1.000000000000000000, 0.9659258262890683122, 1.000000000000000000, 0.9659258262890683122, 1.000000000000000000, 0.9659258262890683122, 1.000000000000000000, 0.9659258262890683122, 1.000000000000000000, 0.9659258262890683122, 1.000000000000000000, 0.9659258262890683122, 1.000000000000000000, 0.9659258262890683122, 1.000000000000000000, 0.9659258262890683122, 1.000000000000000000, 0.9659258262890683122, 1.000000000000000000, 0.9659258262890683122, 1.000000000000000000, 0.9659258262890683122, 1.000000000000000000, 0.9659258262890683122, 1.000000000000000000, 0.9659258262890683122, 1.000000000000000000, 0.9659258262890683122, 1.000000000000000000, 0.9659258262890683122, 1.000000000000000000, 0.9659258262890683122, 1.000000000000000000, 0.9659258262890683122, 1.000000000000000000, 0.9659258262890683122, 1.000000000000000000, 0.9659258262890683122, 1.000000000000000000, 0.9659258262890683122, 1.000000000000000000, 0.9659258262890683122, 1.000000000000000000, 0.9659258262890683122, 1.000000000000000000, 0.9659258262890683122, 1.000000000000000000, 0.9659258262890683122, 1.000000000000000000, 0.9659258262890683122, 1.000000000000000000, 0.9659258262890683122, 1.000000000000000000, 0.9659258262890683122, 1.000000000000000000, 0.9659258262890683122, 1.000000000000000000, 0.9659258262890683122, 1.000000000000000000, 0.9659258262890683122, 1.000000000000000000, 0.9659258262890683122, 1.000000000000000000, 0.9659258262890683122, 1.000000000000000000, 0.9659258262890683122, 1.000000000000000000, 0.9659258262890683122, 1.000000000000000000, 0.9659258262890683122, 1.000000000000000000, 0.9659258262890683122, 1.000000000000000000, 0.9659258262890683122, 1.000000000000000000, 0.9659258262890683122, 1.000000000000000000, 0.9659258262890683122, 1.000000000000000000, 0.9659258262890683122, 1.000000000000000000, 0.9659258262890683122, 1.000000000000000000, 0.9659258262890683122, 1.000000000000000000, 0.9659258262890683122, 1.000000000000000000, 0.9659258262890683122, 1.000000000000000000, 0.9659258262890683122, 1.000000000000000000, 0.9659258262890683122, 1.000000000000000000, 0.9659258262890683122, 1.000000000000000000, 0.9659258262890683122, 1.000000000000000000, 0.9659258262890683122, 1.000000000000000000, 0.9659258262890683122, 1.000000000000000000, 0.9659258262890683122, 1.000000000000000000, 0.9659258262890683122, 1.000000000000000000, 0.9659258262890683122, 1.000000000000000000, 0.9659258262890683122, 1.000000000000000000, 0.9659258262890683122, 1.000000000000000000, 0.9659258262890683122, 1.000000000000000000, 0.9659258262890683122, 1.000000000000000000) ) ) 
 REPRESENTATION_ITEM ( '' )  SURFACE ( )  );
#20957=CARTESIAN_POINT ( 'NONE',  ( 0.5774900079438590739, 27.64701867748817676, -5.440088680355550821 ) ) ;
#20958=CARTESIAN_POINT ( 'NONE',  ( 5.076628168052704559, 25.17559781766745175, -8.527530157486179263 ) ) ;
#20959=CARTESIAN_POINT ( 'NONE',  ( -2.816281873526473856, 9.331968003263753531, 3.434112377981055619 ) ) ;
#20960=CARTESIAN_POINT ( 'NONE',  ( 7.084665262690076126, 64.10535201082150536, 10.88017736071109987 ) ) ;
#20961=CARTESIAN_POINT ( 'NONE',  ( 20.88017736071110875, 30.77201867748816966, -2.915334737309920765 ) ) ;
#20962=CARTESIAN_POINT ( 'NONE',  ( -1.099225684535947600, 54.54030133659708923, 6.408140936763237150 ) ) ;
#20963=CARTESIAN_POINT ( 'NONE',  ( 22.26659068614895176, 44.72041550158063927, -7.082119434687042414 ) ) ;
#20965=( BOUNDED_SURFACE ( )  B_SPLINE_SURFACE ( 3, 2, ( 
 ( #60834, #83841, #38353 ),
 ( #15366, #30828, #61327 ),
 ( #91838, #53837, #69333 ),
 ( #28850, #54800, #33280 ) ),
 .UNSPECIFIED., .F., .F., .F. ) 
 B_SPLINE_SURFACE_WITH_KNOTS ( ( 4, 4 ),
 ( 3, 3 ),
 ( 0.000000000000000000, 0.0004252381714231216660 ),
 ( 0.000000000000000000, 1.000000000000000000 ),
 .UNSPECIFIED. ) 
 GEOMETRIC_REPRESENTATION_ITEM ( )  RATIONAL_B_SPLINE_SURFACE ( (
 ( 1.000000000000000000, 0.7411386215561424073, 1.000000000000000000),
 ( 1.000000000000000000, 0.7847835171315882263, 1.000000000000000000),
 ( 1.000000000000000000, 0.8182188757360080444, 1.000000000000000000),
 ( 1.000000000000000000, 0.8414823709351041403, 1.000000000000000000) ) ) 
 REPRESENTATION_ITEM ( '' )  SURFACE ( )  );
#20967=CARTESIAN_POINT ( 'NONE',  ( -42.50123216575902063, 107.2490263651838802, 4.999999999999999112 ) ) ;
#20969=CARTESIAN_POINT ( 'NONE',  ( 0.6178305044545818747, 3.498634669930420049, -9.382169495545419124 ) ) ;
#20970=CARTESIAN_POINT ( 'NONE',  ( 10.00000000000000000, 11.81368534415483751, -10.88017736071110342 ) ) ;
#20971=CARTESIAN_POINT ( 'NONE',  ( 0.5774900079438590739, 42.64701867748816966, -5.440088680355550821 ) ) ;
#20972=MECHANICAL_DESIGN_GEOMETRIC_PRESENTATION_REPRESENTATION('',(#56087),#81682);
#20973=CARTESIAN_POINT ( 'NONE',  ( 17.39651004071842522, 24.08210964143329491, -6.499999999999992895 ) ) ;
#20975=CARTESIAN_POINT ( 'NONE',  ( 0.1532563361054100626, 20.80059781766744464, -2.638427012816831230 ) ) ;
#20976=CARTESIAN_POINT ( 'NONE',  ( 1.274849032794305170, 17.55509018479936145, -6.499999999999995559 ) ) ;
#20977=CARTESIAN_POINT ( 'NONE',  ( 7.084665262690076126, 64.10535201082150536, 10.88017736071109987 ) ) ;
#20978=CARTESIAN_POINT ( 'NONE',  ( 0.1532563361054083140, 36.00893115100078745, 1.131784320476157264E-15 ) ) ;
#20979=CARTESIAN_POINT ( 'NONE',  ( 2.791683348922240793, 26.63393115100078745, 7.208316651077764092 ) ) ;
#20980=CARTESIAN_POINT ( 'NONE',  ( 19.84674366389459621, 8.508931151000785675, 7.409399052514197653E-17 ) ) ;
#20982=CARTESIAN_POINT ( 'NONE',  ( 4.559911319644449179, 68.89701867748817676, 9.422509992056141925 ) ) ;
#20983=CARTESIAN_POINT ( 'NONE',  ( 7.361572987183170547, 37.05059781766744464, 9.846743663894590881 ) ) ;
#20985=CARTESIAN_POINT ( 'NONE',  ( 10.00000000000000000, 52.87363466993041783, -12.81628187352647608 ) ) ;
#20987=CARTESIAN_POINT ( 'NONE',  ( 5.076628168052704559, 65.17559781766745175, -8.527530157486179263 ) ) ;
#20988=CARTESIAN_POINT ( 'NONE',  ( 0.5774900079438590739, 2.647018677488170990, -5.440088680355550821 ) ) ;
#20989=CARTESIAN_POINT ( 'NONE',  ( 22.26659068614894466, 23.88708216824730357, 7.082119434687054849 ) ) ;
#20991=CARTESIAN_POINT ( 'NONE',  ( 2.917880565312948704, 22.63708216824730002, 12.26659068614894643 ) ) ;
#20992=CARTESIAN_POINT ( 'NONE',  ( 2.917880565312948704, 52.63708216824730357, 12.26659068614894643 ) ) ;
#20993=CARTESIAN_POINT ( 'NONE',  ( 10.00000000000000178, 8.053748834913967869, 14.16423886937410082 ) ) ;
#20994=CARTESIAN_POINT ( 'NONE',  ( 17.96484262340118221, 66.18868534415483396, -7.964842623401177768 ) ) ;
#20995=CARTESIAN_POINT ( 'NONE',  ( 19.42250999205614548, 50.98035201082151247, -5.440088680355545492 ) ) ;
#20997=CARTESIAN_POINT ( 'NONE',  ( 17.20831665107776587, 24.13393115100078035, -7.208316651077762316 ) ) ;
#20999=CARTESIAN_POINT ( 'NONE',  ( 5.076628168052704559, 30.17559781766745175, -8.527530157486179263 ) ) ;
#21000=CARTESIAN_POINT ( 'NONE',  ( 0.5774900079438607392, 13.48035201082150358, 5.440088680355550821 ) ) ;
#21001=CARTESIAN_POINT ( 'NONE',  ( 3.591859063236763294, 53.29030133659708923, -11.09922568453595026 ) ) ;
#21002=CARTESIAN_POINT ( 'NONE',  ( 19.84674366389459266, 48.30059781766745175, 2.638427012816836559 ) ) ;
#21005=CARTESIAN_POINT ( 'NONE',  ( 7.361572987183170547, 32.05059781766745175, 9.846743663894590881 ) ) ;
#21006=CARTESIAN_POINT ( 'NONE',  ( -2.816281873526473856, 39.33196800326374643, 3.434112377981055619 ) ) ;
#21008=CARTESIAN_POINT ( 'NONE',  ( 17.96484262340118221, 46.18868534415484106, -7.964842623401177768 ) ) ;
#21009=CARTESIAN_POINT ( 'NONE',  ( 17.20831665107776587, 39.13393115100079456, -7.208316651077762316 ) ) ;
#21010=CARTESIAN_POINT ( 'NONE',  ( 10.00000000000000178, 23.05374883491397142, 14.16423886937410082 ) ) ;
#21013=CARTESIAN_POINT ( 'NONE',  ( 17.96484262340118221, 49.93868534415484106, 7.964842623401181321 ) ) ;
#21014=CARTESIAN_POINT ( 'NONE',  ( -0.8801773607110991993, 67.85535201082151957, -2.915334737309923874 ) ) ;
#21015=CARTESIAN_POINT ( 'NONE',  ( 22.26659068614895176, 49.72041550158063927, -7.082119434687042414 ) ) ;
#21016=CARTESIAN_POINT ( 'NONE',  ( 10.00000000000000000, 2.873634669930420049, -12.81628187352647608 ) ) ;
#21018=CARTESIAN_POINT ( 'NONE',  ( 10.00000000000000178, 49.31368534415484106, 10.88017736071110342 ) ) ;
#21020=CARTESIAN_POINT ( 'NONE',  ( -2.816281873526471635, 28.91530133659708213, -3.434112377981056508 ) ) ;
#21021=CARTESIAN_POINT ( 'NONE',  ( 6.565887622018943937, 3.081968003263753531, -12.81628187352647608 ) ) ;
#21023=CARTESIAN_POINT ( 'NONE',  ( 10.00000000000000178, 19.31368534415484106, 10.88017736071110342 ) ) ;
#21024=CARTESIAN_POINT ( 'NONE',  ( 0.5774900079438607392, 13.48035201082150358, 5.440088680355550821 ) ) ;
#21025=CARTESIAN_POINT ( 'NONE',  ( 12.63842701281683922, 44.55059781766745175, -9.846743663894590881 ) ) ;
#21029=CARTESIAN_POINT ( 'NONE',  ( 17.20831665107776587, 9.133931151000787452, -7.208316651077762316 ) ) ;
#21030=( GEOMETRIC_REPRESENTATION_CONTEXT ( 3 ) GLOBAL_UNCERTAINTY_ASSIGNED_CONTEXT ( ( #14289 ) ) GLOBAL_UNIT_ASSIGNED_CONTEXT ( ( #40489, #26443, #78472 ) ) REPRESENTATION_CONTEXT ( 'NONE', 'WORKASPACE' ) );
#21032=CARTESIAN_POINT ( 'NONE',  ( 5.076628168052703671, 36.84226448433412315, 8.527530157486179263 ) ) ;
#21033=CARTESIAN_POINT ( 'NONE',  ( 12.91533473730993009, 31.60535201082150891, -10.88017736071109987 ) ) ;
#21034=CARTESIAN_POINT ( 'NONE',  ( 21.09922568453594849, 6.206968003263753531, 6.408140936763242479 ) ) ;
#21035=CARTESIAN_POINT ( 'NONE',  ( 12.91533473730992121, 39.52201867748817676, 10.88017736071110164 ) ) ;
#21038=CARTESIAN_POINT ( 'NONE',  ( -2.816281873526473856, 49.33196800326374643, 3.434112377981055619 ) ) ;
#21040=CARTESIAN_POINT ( 'NONE',  ( 20.88017736071110875, 60.77201867748817676, -2.915334737309920765 ) ) ;
#21042=CARTESIAN_POINT ( 'NONE',  ( 6.565887622018943937, 35.16530133659708923, 12.81628187352647430 ) ) ;
#21043=CARTESIAN_POINT ( 'NONE',  ( 2.917880565312948704, 2.637082168247300906, 12.26659068614894643 ) ) ;
#21044=( LENGTH_UNIT ( ) NAMED_UNIT ( * ) SI_UNIT ( .MILLI., .METRE. ) );
#21045=CARTESIAN_POINT ( 'NONE',  ( 0.5774900079438590739, 42.64701867748816966, -5.440088680355550821 ) ) ;
#21046=CARTESIAN_POINT ( 'NONE',  ( 12.63842701281683922, 64.55059781766745175, -9.846743663894590881 ) ) ;
#21047=CARTESIAN_POINT ( 'NONE',  ( 2.791683348922240793, 56.63393115100078035, 7.208316651077764092 ) ) ;
#21048=CARTESIAN_POINT ( 'NONE',  ( 2.791683348922237240, 20.38393115100078745, -7.208316651077763204 ) ) ;
#21049=CARTESIAN_POINT ( 'NONE',  ( 17.96484262340118221, 61.18868534415482685, -7.964842623401177768 ) ) ;
#21050=CARTESIAN_POINT ( 'NONE',  ( -0.1503990784575328643, 5.127771745786130708, 6.262539305110068177 ) ) ;
#21051=CARTESIAN_POINT ( 'NONE',  ( -0.3689425029237898834, 26.17874883491396432, -10.36894250292378850 ) ) ;
#21053=DIRECTION ( 'NONE',  ( 0.000000000000000000, -1.000000000000000000, 0.000000000000000000 ) ) ;
#21055=VERTEX_POINT ( 'NONE', #27535 ) ;
#21056=CARTESIAN_POINT ( 'NONE',  ( -2.266590686148945544, 57.22041550158063217, 7.082119434687048631 ) ) ;
#21057=CARTESIAN_POINT ( 'NONE',  ( 17.08211943468705130, 58.47041550158063927, 12.26659068614894998 ) ) ;
#21058=CARTESIAN_POINT ( 'NONE',  ( 10.00000000000000000, 34.75893115100078745, -9.846743663894594434 ) ) ;
#21059=CARTESIAN_POINT ( 'NONE',  ( 21.09922568453595559, 22.04030133659708923, -6.408140936763230044 ) ) ;
#21061=CARTESIAN_POINT ( 'NONE',  ( 12.91533473730992121, 14.52201867748817143, 10.88017736071110164 ) ) ;
#21062=CARTESIAN_POINT ( 'NONE',  ( 10.00000000000000000, 55.55374883491396787, -14.16423886937410082 ) ) ;
#21063=CARTESIAN_POINT ( 'NONE',  ( 7.361572987183170547, 27.05059781766745175, 9.846743663894590881 ) ) ;
#21065=CARTESIAN_POINT ( 'NONE',  ( 17.20831665107776587, 14.13393115100078568, -7.208316651077762316 ) ) ;
#21066=CARTESIAN_POINT ( 'NONE',  ( 17.39651004071841811, 4.082109641433293135, -6.499999999999999112 ) ) ;
#21068=EDGE_LOOP ( 'NONE', ( #5179, #13547, #39389, #10641, #14163, #93641 ) ) ;
#21070=DIRECTION ( 'NONE',  ( 0.5547001962252290364, 0.8320502943378437211, 0.000000000000000000 ) ) ;
#21071=ORIENTED_EDGE ( 'NONE', *, *, #27915, .T. ) ;
#21072=CARTESIAN_POINT ( 'NONE',  ( -2.266590686148945544, 16.38708216824730357, -7.082119434687050408 ) ) ;
#21073=CARTESIAN_POINT ( 'NONE',  ( -0.8801773607111009756, 18.06368534415484106, 1.068504757029289695E-15 ) ) ;
#21074=CARTESIAN_POINT ( 'NONE',  ( 4.559911319644449179, 27.23035201082150536, -9.422509992056141925 ) ) ;
#21075=CARTESIAN_POINT ( 'NONE',  ( 10.00000000000000000, 59.75893115100078745, -9.846743663894594434 ) ) ;
#21076=CARTESIAN_POINT ( 'NONE',  ( -1.099225684535947600, 13.70696800326375353, -6.408140936763238038 ) ) ;
#21077=CARTESIAN_POINT ( 'NONE',  ( 24.16423886937410614, 4.303748834913967869, 8.672049930838204340E-16 ) ) ;
#21080=CARTESIAN_POINT ( 'NONE',  ( 16.40814093676323893, 30.79030133659708923, 11.09922568453595026 ) ) ;
#21082=CARTESIAN_POINT ( 'NONE',  ( 19.84674366389459621, 28.50893115100078745, 7.409399052514197653E-17 ) ) ;
#21083=CARTESIAN_POINT ( 'NONE',  ( 19.42250999205614548, 5.980352010821504471, -5.440088680355545492 ) ) ;
#21085=CARTESIAN_POINT ( 'NONE',  ( 20.36894250292379738, 64.92874883491397497, -10.36894250292379027 ) ) ;
#21087=CARTESIAN_POINT ( 'NONE',  ( 7.084665262690076126, 42.02201867748816966, -10.88017736071110164 ) ) ;
#21088=CARTESIAN_POINT ( 'NONE',  ( 2.035157376598824452, 63.68868534415484106, 7.964842623401179544 ) ) ;
#21089=CARTESIAN_POINT ( 'NONE',  ( 20.88017736071110875, 45.77201867748816966, -2.915334737309920765 ) ) ;
#21091=CARTESIAN_POINT ( 'NONE',  ( -0.8801773607111008646, 58.27201867748816966, 2.915334737309923430 ) ) ;
#21093=SURFACE_SIDE_STYLE ('',( #91565 ) ) ;
#21096=CARTESIAN_POINT ( 'NONE',  ( 10.00000000000000178, 27.25893115100078390, 9.846743663894594434 ) ) ;
#21097=VERTEX_POINT ( 'NONE', #97545 ) ;
#21098=CARTESIAN_POINT ( 'NONE',  ( 0.1532563361054082862, 56.21726448433411605, 2.638427012816831674 ) ) ;
#21100=CIRCLE ( 'NONE', #76984, 1.000000000000000888 ) ;
#21102=CARTESIAN_POINT ( 'NONE',  ( -4.164238869374099927, 12.01208216824730357, 3.795296366450308767 ) ) ;
#21107=CARTESIAN_POINT ( 'NONE',  ( 2.035157376598824452, 3.688685344154837953, 7.964842623401179544 ) ) ;
#21108=FACE_OUTER_BOUND ( 'NONE', #22315, .T. ) ;
#21111=VECTOR ( 'NONE', #84837, 1000.000000000000000 ) ;
#21112=CARTESIAN_POINT ( 'NONE',  ( 19.84674366389459266, 43.71726448433410894, -2.638427012816827677 ) ) ;
#21113=CARTESIAN_POINT ( 'NONE',  ( 16.40814093676324603, 12.45696800326375353, -11.09922568453594671 ) ) ;
#21114=CARTESIAN_POINT ( 'NONE',  ( 2.791683348922237240, 10.38393115100078390, -7.208316651077763204 ) ) ;
#21117=CARTESIAN_POINT ( 'NONE',  ( 0.1532563361054100626, 10.80059781766745175, -2.638427012816831230 ) ) ;
#21118=CARTESIAN_POINT ( 'NONE',  ( 6.565887622018943937, -1.918031996736246692, -12.81628187352647608 ) ) ;
#21119=VECTOR ( 'NONE', #43755, 1000.000000000000000 ) ;
#21120=CARTESIAN_POINT ( 'NONE',  ( 1.472469842513823179, 26.42559781766745175, 4.923371831947296329 ) ) ;
#21124=CARTESIAN_POINT ( 'NONE',  ( 10.00000000000000000, 11.81368534415483751, -10.88017736071110342 ) ) ;
#21125=CARTESIAN_POINT ( 'NONE',  ( 13.79529636645031943, 10.34541550158063394, -14.16423886937409904 ) ) ;
#21126=CARTESIAN_POINT ( 'NONE',  ( 2.791683348922240793, 31.63393115100078745, 7.208316651077764092 ) ) ;
#21127=CARTESIAN_POINT ( 'NONE',  ( 20.88017736071110519, 60.56368534415484106, 2.639326808657452039E-16 ) ) ;
#21128=CARTESIAN_POINT ( 'NONE',  ( 16.40814093676324603, 22.45696800326375353, -11.09922568453594671 ) ) ;
#21130=CARTESIAN_POINT ( 'NONE',  ( 20.88017736071110519, 10.56368534415483751, 2.639326808657452039E-16 ) ) ;
#21131=DIRECTION ( 'NONE',  ( 0.5547001962252290364, 0.8320502943378437211, 0.000000000000000000 ) ) ;
#21133=CARTESIAN_POINT ( 'NONE',  ( 1.472469842513823179, 61.42559781766745175, 4.923371831947296329 ) ) ;
#21134=CARTESIAN_POINT ( 'NONE',  ( 17.20831665107776587, 34.13393115100078745, -7.208316651077762316 ) ) ;
#21136=CARTESIAN_POINT ( 'NONE',  ( 3.591859063236761518, 39.95696800326375353, 11.09922568453594849 ) ) ;
#21137=CARTESIAN_POINT ( 'NONE',  ( 4.559911319644449179, 33.89701867748817676, 9.422509992056141925 ) ) ;
#21138=CARTESIAN_POINT ( 'NONE',  ( 20.15039907845753575, 6.748846992468889638, 6.262539305110063736 ) ) ;
#21139=FACE_OUTER_BOUND ( 'NONE', #59243, .T. ) ;
#21140=CARTESIAN_POINT ( 'NONE',  ( 17.96484262340118221, 26.18868534415483396, -7.964842623401177768 ) ) ;
#21142=CARTESIAN_POINT ( 'NONE',  ( 19.42250999205614193, 30.14701867748817321, 5.440088680355555262 ) ) ;
#21143=CARTESIAN_POINT ( 'NONE',  ( 17.20831665107776587, 52.88393115100078035, 7.208316651077764980 ) ) ;
#21145=CARTESIAN_POINT ( 'NONE',  ( -0.8801773607111009756, 48.06368534415484817, 1.068504757029289695E-15 ) ) ;
#21146=CARTESIAN_POINT ( 'NONE',  ( -4.164238869374099039, 31.80374883491396432, 8.674139862899312516E-16 ) ) ;
#21148=CARTESIAN_POINT ( 'NONE',  ( 5.076628168052703671, 31.84226448433412315, 8.527530157486179263 ) ) ;
#21149=CARTESIAN_POINT ( 'NONE',  ( -2.816281873526473856, -0.8763653300695799508, 9.499525473075851096E-16 ) ) ;
#21150=ORIENTED_EDGE ( 'NONE', *, *, #29943, .F. ) ;
#21151=CARTESIAN_POINT ( 'NONE',  ( 4.559911319644449179, 22.23035201082150536, -9.422509992056141925 ) ) ;
#21154=CARTESIAN_POINT ( 'NONE',  ( 4.559911319644449179, 18.89701867748817321, 9.422509992056141925 ) ) ;
#21155=CARTESIAN_POINT ( 'NONE',  ( 7.084665262690076126, 64.10535201082150536, 10.88017736071109987 ) ) ;
#21156=CARTESIAN_POINT ( 'NONE',  ( -2.266590686148945544, 21.38708216824730357, -7.082119434687050408 ) ) ;
#21157=CARTESIAN_POINT ( 'NONE',  ( 1.472469842513823179, 15.59226448433411960, -4.923371831947296329 ) ) ;
#21158=CARTESIAN_POINT ( 'NONE',  ( 18.52753015748618282, 58.92559781766745886, -4.923371831947291888 ) ) ;
#21159=CARTESIAN_POINT ( 'NONE',  ( 2.035157376598824452, 43.68868534415484106, 7.964842623401179544 ) ) ;
#21161=CARTESIAN_POINT ( 'NONE',  ( -45.35355022568786154, 104.5915939144275342, -5.642319926932224838 ) ) ;
#21162=VERTEX_POINT ( 'NONE', #91987 ) ;
#21165=CARTESIAN_POINT ( 'NONE',  ( 5.076628168052704559, 40.17559781766745175, -8.527530157486179263 ) ) ;
#21166=VERTEX_POINT ( 'NONE', #1511 ) ;
#21168=CARTESIAN_POINT ( 'NONE',  ( 13.79529636645030344, 18.26208216824730002, 14.16423886937410614 ) ) ;
#21169=CARTESIAN_POINT ( 'NONE',  ( 6.204703633549690345, 20.76208216824730357, -14.16423886937410259 ) ) ;
#21170=CARTESIAN_POINT ( 'NONE',  ( 20.88017736071110519, 55.56368534415484817, 2.639326808657452039E-16 ) ) ;
#21171=CARTESIAN_POINT ( 'NONE',  ( 20.36894250292379382, 48.67874883491396076, 10.36894250292379205 ) ) ;
#21172=CARTESIAN_POINT ( 'NONE',  ( 12.63842701281683922, 64.55059781766745175, -9.846743663894590881 ) ) ;
#21173=CARTESIAN_POINT ( 'NONE',  ( 1.472469842513823179, 46.42559781766745175, 4.923371831947296329 ) ) ;
#21175=CARTESIAN_POINT ( 'NONE',  ( 19.42250999205614548, 50.98035201082151247, -5.440088680355545492 ) ) ;
#21176=CARTESIAN_POINT ( 'NONE',  ( 10.00000000000000178, 5.373634669930420493, 12.81628187352647608 ) ) ;
#21177=CARTESIAN_POINT ( 'NONE',  ( 6.204703633549690345, 22.84541550158062861, 14.16423886937410082 ) ) ;
#21178=CARTESIAN_POINT ( 'NONE',  ( -4.164238869374098151, 46.59541550158063927, -3.795296366450310543 ) ) ;
#21180=CARTESIAN_POINT ( 'NONE',  ( 19.42250999205614193, 25.14701867748817321, 5.440088680355555262 ) ) ;
#21181=AXIS2_PLACEMENT_3D ( 'NONE', #67356, #80879, #87876 ) ;
#21182=CARTESIAN_POINT ( 'NONE',  ( -1.926860441876564023, 2.870456701841137992, 3.195792623639529761 ) ) ;
#21183=CARTESIAN_POINT ( 'NONE',  ( -0.8801773607111009756, 38.06368534415484106, 1.068504757029289695E-15 ) ) ;
#21188=STYLED_ITEM ( 'NONE', ( #96284 ), #76770 ) ;
#21189=ORIENTED_EDGE ( 'NONE', *, *, #8524, .F. ) ;
#21191=CARTESIAN_POINT ( 'NONE',  ( 22.26659068614895176, 44.72041550158063927, -7.082119434687042414 ) ) ;
#21192=CARTESIAN_POINT ( 'NONE',  ( 19.84674366389459621, 48.50893115100078745, 7.409399052514197653E-17 ) ) ;
#21193=CARTESIAN_POINT ( 'NONE',  ( 7.084665262690076126, 69.10535201082151957, 10.88017736071109987 ) ) ;
#21194=CARTESIAN_POINT ( 'NONE',  ( -10.00000000000000000, 82.00000000000000000, 5.000000000000000000 ) ) ;
#21196=COLOUR_RGB ( '', 0.09019608, 0.27058824, 0.51372549) ;
#21197=CARTESIAN_POINT ( 'NONE',  ( -0.8801773607111008646, 58.27201867748816966, 2.915334737309923430 ) ) ;
#21198=B_SPLINE_CURVE_WITH_KNOTS ( 'NONE', 3,
 ( #46877, #8879, #25385, #85376, #47856, #48840, #86367, #94346, #40870, #48351 ),
 .UNSPECIFIED., .F., .F.,
 ( 4, 3, 3, 4 ),
 ( 2.388396739587122319E-17, 0.0006253016069560766348, 0.001250604074564918254, 0.002501455912506555211 ),
 .UNSPECIFIED. ) ;
#21199=CARTESIAN_POINT ( 'NONE',  ( 0.6178305044545818747, 58.49863466993042493, -9.382169495545419124 ) ) ;
#21202=CARTESIAN_POINT ( 'NONE',  ( 13.79529636645030344, 38.26208216824729647, 14.16423886937410614 ) ) ;
#21203=CARTESIAN_POINT ( 'NONE',  ( 19.38216949554541202, 25.99863466993042138, 9.382169495545424454 ) ) ;
#21206=CARTESIAN_POINT ( 'NONE',  ( 19.38216949554541557, 42.24863466993041783, -9.382169495545420901 ) ) ;
#21207=CARTESIAN_POINT ( 'NONE',  ( 19.84674366389459266, 38.71726448433412315, -2.638427012816827677 ) ) ;
#21208=CARTESIAN_POINT ( 'NONE',  ( 20.88017736071110519, 15.56368534415483751, 2.639326808657452039E-16 ) ) ;
#21210=CARTESIAN_POINT ( 'NONE',  ( 19.84674366389459266, 38.30059781766745175, 2.638427012816836559 ) ) ;
#21216=DIRECTION ( 'NONE',  ( 0.9970872288863216193, 0.07626964003977222684, -0.000000000000000000 ) ) ;
#21217=CARTESIAN_POINT ( 'NONE',  ( 14.92337183194729633, 12.67559781766745353, 8.527530157486181039 ) ) ;
#21218=CARTESIAN_POINT ( 'NONE',  ( 21.09922568453594849, 26.20696800326375353, 6.408140936763242479 ) ) ;
#21221=CARTESIAN_POINT ( 'NONE',  ( 19.84674366389459621, 58.50893115100078745, 7.409399052514197653E-17 ) ) ;
#21223=CARTESIAN_POINT ( 'NONE',  ( -2.266590686148945544, 26.38708216824730357, -7.082119434687050408 ) ) ;
#21224=CARTESIAN_POINT ( 'NONE',  ( 19.84674366389459266, 48.71726448433413026, -2.638427012816827677 ) ) ;
#21225=CARTESIAN_POINT ( 'NONE',  ( 22.81628187352648496, 41.83196800326375353, -3.434112377981050290 ) ) ;
#21228=CARTESIAN_POINT ( 'NONE',  ( 0.1532563361054082862, 11.21726448433411605, 2.638427012816831674 ) ) ;
#21230=CARTESIAN_POINT ( 'NONE',  ( -0.1049300847420626126, 67.21697413083880690, -6.336235997365760042 ) ) ;
#21231=CARTESIAN_POINT ( 'NONE',  ( 18.52753015748617571, 53.09226448433412315, 4.923371831947298993 ) ) ;
#21232=CARTESIAN_POINT ( 'NONE',  ( 17.96484262340118221, 44.93868534415483396, 7.964842623401181321 ) ) ;
#21237=CARTESIAN_POINT ( 'NONE',  ( 7.084665262690076126, 44.10535201082151247, 10.88017736071109987 ) ) ;
#21241=MECHANICAL_DESIGN_GEOMETRIC_PRESENTATION_REPRESENTATION('',(#89897),#46785);
#21242=CARTESIAN_POINT ( 'NONE',  ( 0.5774900079438590739, 17.64701867748817321, -5.440088680355550821 ) ) ;
#21243=CARTESIAN_POINT ( 'NONE',  ( 1.472469842513823179, 50.59226448433411605, -4.923371831947296329 ) ) ;
#21244=CARTESIAN_POINT ( 'NONE',  ( 2.035157376598822676, 37.43868534415484106, -7.964842623401177768 ) ) ;
#21246=CARTESIAN_POINT ( 'NONE',  ( 19.42250999205614548, 55.98035201082150536, -5.440088680355545492 ) ) ;
#21247=CARTESIAN_POINT ( 'NONE',  ( 12.91533473730992121, 24.52201867748816966, 10.88017736071110164 ) ) ;
#21248=CARTESIAN_POINT ( 'NONE',  ( 20.00000000000000355, 81.00009212066629516, -4.499999999999997335 ) ) ;
#21249=CARTESIAN_POINT ( 'NONE',  ( 5.076628168052704559, 5.175597817667451750, -8.527530157486179263 ) ) ;
#21250=CARTESIAN_POINT ( 'NONE',  ( 17.20831665107776587, 27.88393115100078390, 7.208316651077764980 ) ) ;
#21253=CARTESIAN_POINT ( 'NONE',  ( 7.361572987183170547, 57.05059781766744464, 9.846743663894590881 ) ) ;
#21254=CARTESIAN_POINT ( 'NONE',  ( 22.26659068614895176, 64.72041550158064638, -7.082119434687042414 ) ) ;
#21256=CARTESIAN_POINT ( 'NONE',  ( 2.377183314879995013, 60.78593319516821936, -6.500000000000057732 ) ) ;
#21257=CARTESIAN_POINT ( 'NONE',  ( 17.08211943468705130, 3.470415501580634388, 12.26659068614894998 ) ) ;
#21258=CARTESIAN_POINT ( 'NONE',  ( 10.00000000000000000, 55.55374883491396787, -14.16423886937410082 ) ) ;
#21259=CARTESIAN_POINT ( 'NONE',  ( -2.816281873526471635, 8.915301336597083903, -3.434112377981056508 ) ) ;
#21261=CARTESIAN_POINT ( 'NONE',  ( 7.084665262690076126, 14.10535201082150358, 10.88017736071109987 ) ) ;
#21262=CARTESIAN_POINT ( 'NONE',  ( 14.92337183194729633, 47.67559781766745175, 8.527530157486181039 ) ) ;
#21263=CARTESIAN_POINT ( 'NONE',  ( -2.266590686148945544, 1.387082168247301128, -7.082119434687050408 ) ) ;
#21266=( LENGTH_UNIT ( ) NAMED_UNIT ( * ) SI_UNIT ( .MILLI., .METRE. ) );
#21267=CARTESIAN_POINT ( 'NONE',  ( 22.81628187352647785, 26.41530133659708923, 3.434112377981063169 ) ) ;
#21268=CARTESIAN_POINT ( 'NONE',  ( 19.84674366389459266, 28.71726448433411960, -2.638427012816827677 ) ) ;
#21270=CARTESIAN_POINT ( 'NONE',  ( 17.20831665107776587, 2.883931151000785231, 7.208316651077764980 ) ) ;
#21274=CARTESIAN_POINT ( 'NONE',  ( 15.44008868035555260, 14.73035201082150536, 9.422509992056143702 ) ) ;
#21275=CARTESIAN_POINT ( 'NONE',  ( 24.16423886937410614, 34.30374883491396787, 8.672049930838204340E-16 ) ) ;
#21276=CARTESIAN_POINT ( 'NONE',  ( 2.035157376598824452, 43.68868534415484106, 7.964842623401179544 ) ) ;
#21277=CARTESIAN_POINT ( 'NONE',  ( 2.035157376598822676, 67.43868534415484817, -7.964842623401177768 ) ) ;
#21278=CARTESIAN_POINT ( 'NONE',  ( 20.15039907845753220, 52.62777174578612716, -6.262539305110077947 ) ) ;
#21279=CARTESIAN_POINT ( 'NONE',  ( 18.52753015748618282, 23.92559781766745530, -4.923371831947291888 ) ) ;
#21281=CARTESIAN_POINT ( 'NONE',  ( 7.361572987183170547, 2.050597817667451750, 9.846743663894590881 ) ) ;
#21283=CARTESIAN_POINT ( 'NONE',  ( 18.52753015748617571, 33.09226448433411605, 4.923371831947298993 ) ) ;
#21285=CARTESIAN_POINT ( 'NONE',  ( 12.91533473730992121, 34.52201867748817676, 10.88017736071110164 ) ) ;
#21288=ORIENTED_EDGE ( 'NONE', *, *, #75730, .F. ) ;
#21289=CARTESIAN_POINT ( 'NONE',  ( 6.565887622018943937, 60.16530133659707502, 12.81628187352647430 ) ) ;
#21291=CARTESIAN_POINT ( 'NONE',  ( 14.92337183194729633, 7.675597817667451750, 8.527530157486181039 ) ) ;
#21292=CARTESIAN_POINT ( 'NONE',  ( -1.099225684535947600, 48.70696800326375353, -6.408140936763238038 ) ) ;
#21293=CARTESIAN_POINT ( 'NONE',  ( -0.3689425029237881626, 67.42874883491396076, 10.36894250292379027 ) ) ;
#21294=CARTESIAN_POINT ( 'NONE',  ( 0.1532563361054083140, 41.00893115100078745, 1.131784320476157264E-15 ) ) ;
#21296=CARTESIAN_POINT ( 'NONE',  ( 12.63842701281683034, 2.467264484334118269, 9.846743663894596210 ) ) ;
#21297=CARTESIAN_POINT ( 'NONE',  ( -0.3689425029237881626, 22.42874883491397142, 10.36894250292379027 ) ) ;
#21298=CARTESIAN_POINT ( 'NONE',  ( 22.26659068614895176, 39.72041550158063217, -7.082119434687042414 ) ) ;
#21299=CARTESIAN_POINT ( 'NONE',  ( 14.92337183194729633, 37.67559781766745175, 8.527530157486181039 ) ) ;
#21301=CARTESIAN_POINT ( 'NONE',  ( 10.00000000000000178, 44.31368534415484106, 10.88017736071110342 ) ) ;
#21302=CARTESIAN_POINT ( 'NONE',  ( 10.00000000000000000, 4.758931151000784787, -9.846743663894594434 ) ) ;
#21304=PRODUCT_DEFINITION_SHAPE ( 'NONE', 'NONE',  #70937 ) ;
#21306=CARTESIAN_POINT ( 'NONE',  ( -2.816281873526473856, 64.33196800326376774, 3.434112377981055619 ) ) ;
#21308=CARTESIAN_POINT ( 'NONE',  ( 20.88017736071110164, 65.35535201082150536, 2.915334737309930979 ) ) ;
#21309=ORIENTED_EDGE ( 'NONE', *, *, #29943, .T. ) ;
#21310=CARTESIAN_POINT ( 'NONE',  ( 10.00000000000000000, 5.553748834913967869, -14.16423886937410082 ) ) ;
#21311=CARTESIAN_POINT ( 'NONE',  ( 12.63842701281683034, 7.467264484334118713, 9.846743663894596210 ) ) ;
#21314=CARTESIAN_POINT ( 'NONE',  ( 19.42250999205614193, 20.14701867748817321, 5.440088680355555262 ) ) ;
#21316=VECTOR ( 'NONE', #61180, 1000.000000000000000 ) ;
#21318=CARTESIAN_POINT ( 'NONE',  ( 19.42250999205614193, 40.14701867748817676, 5.440088680355555262 ) ) ;
#21319=CARTESIAN_POINT ( 'NONE',  ( 2.791683348922240793, 56.63393115100078035, 7.208316651077764092 ) ) ;
#21322=CARTESIAN_POINT ( 'NONE',  ( 0.1532563361054083140, 61.00893115100078745, 1.131784320476157264E-15 ) ) ;
#21324=EDGE_CURVE ( 'NONE', #90354, #79846, #92474, .T. ) ;
#21326=CARTESIAN_POINT ( 'NONE',  ( 0.5774900079438590739, 62.64701867748817676, -5.440088680355550821 ) ) ;
#21327=CARTESIAN_POINT ( 'NONE',  ( 14.92337183194729988, 64.34226448433412315, -8.527530157486177487 ) ) ;
#21328=CARTESIAN_POINT ( 'NONE',  ( 0.6178305044545818747, 33.49863466993042493, -9.382169495545419124 ) ) ;
#21329=CARTESIAN_POINT ( 'NONE',  ( 7.084665262690076126, 27.02201867748817676, -10.88017736071110164 ) ) ;
#21330=CARTESIAN_POINT ( 'NONE',  ( 0.1089645850229091079, 58.16234555792573246, 6.479102184480836080 ) ) ;
#21331=CARTESIAN_POINT ( 'NONE',  ( 7.361572987183170547, 7.050597817667451750, 9.846743663894590881 ) ) ;
#21332=CARTESIAN_POINT ( 'NONE',  ( 19.42250999205614193, 15.14701867748817143, 5.440088680355555262 ) ) ;
#21335=CARTESIAN_POINT ( 'NONE',  ( 22.81628187352647785, 51.41530133659708923, 3.434112377981063169 ) ) ;
#21336=CARTESIAN_POINT ( 'NONE',  ( 20.88017736071110519, 40.56368534415484106, 2.639326808657452039E-16 ) ) ;
#21337=CARTESIAN_POINT ( 'NONE',  ( -46.94000000000001194, 103.0000000000000000, -5.997726559847240679 ) ) ;
#21338=CARTESIAN_POINT ( 'NONE',  ( 6.565887622018943937, 60.16530133659707502, 12.81628187352647430 ) ) ;
#21339=CARTESIAN_POINT ( 'NONE',  ( 17.96484262340118221, 51.18868534415483396, -7.964842623401177768 ) ) ;
#21340=CARTESIAN_POINT ( 'NONE',  ( 19.84674366389459266, 53.71726448433411605, -2.638427012816827677 ) ) ;
#21342=CARTESIAN_POINT ( 'NONE',  ( 19.84674366389459621, 23.50893115100078390, 7.409399052514197653E-17 ) ) ;
#21343=CARTESIAN_POINT ( 'NONE',  ( 13.43411237798106583, 2.665301336597086568, -12.81628187352647252 ) ) ;
#21344=CYLINDRICAL_SURFACE ( 'NONE', #42036, 11.92686044187656513 ) ;
#21345=CARTESIAN_POINT ( 'NONE',  ( 2.791683348922240793, 61.63393115100079456, 7.208316651077764092 ) ) ;
#21346=CARTESIAN_POINT ( 'NONE',  ( 15.44008868035555793, 36.39701867748816966, -9.422509992056140149 ) ) ;
#21347=CARTESIAN_POINT ( 'NONE',  ( 19.84674366389459266, 43.71726448433410894, -2.638427012816827677 ) ) ;
#21350=CARTESIAN_POINT ( 'NONE',  ( 3.591859063236763294, 8.290301336597087456, -11.09922568453595026 ) ) ;
#21351=VERTEX_POINT ( 'NONE', #61975 ) ;
#21352=CARTESIAN_POINT ( 'NONE',  ( 0.6081133539230525464, 63.33703382326400089, 6.499999999999970690 ) ) ;
#21355=CARTESIAN_POINT ( 'NONE',  ( 13.43411237798105340, 35.58196800326375353, 12.81628187352647963 ) ) ;
#21356=CARTESIAN_POINT ( 'NONE',  ( 5.076628168052704559, 35.17559781766745175, -8.527530157486179263 ) ) ;
#21357=CARTESIAN_POINT ( 'NONE',  ( 17.96484262340118221, 9.938685344154839285, 7.964842623401181321 ) ) ;
#21358=CARTESIAN_POINT ( 'NONE',  ( 1.472469842513823179, 30.59226448433411960, -4.923371831947296329 ) ) ;
#21362=CARTESIAN_POINT ( 'NONE',  ( 20.88017736071110875, 5.772018677488170546, -2.915334737309920765 ) ) ;
#21364=CARTESIAN_POINT ( 'NONE',  ( 12.91533473730992121, 19.52201867748816611, 10.88017736071110164 ) ) ;
#21365=CARTESIAN_POINT ( 'NONE',  ( -4.164238869374098151, 46.59541550158063927, -3.795296366450310543 ) ) ;
#21366=CARTESIAN_POINT ( 'NONE',  ( 17.08211943468705130, 48.47041550158063927, 12.26659068614894998 ) ) ;
#21368=CARTESIAN_POINT ( 'NONE',  ( 0.09770025222076675342, 69.67742753483354079, 6.500000000000000000 ) ) ;
#21369=CARTESIAN_POINT ( 'NONE',  ( 5.076628168052704559, 15.17559781766745175, -8.527530157486179263 ) ) ;
#21370=CARTESIAN_POINT ( 'NONE',  ( 0.1532563361054082862, 66.21726448433413736, 2.638427012816831674 ) ) ;
#21373=CARTESIAN_POINT ( 'NONE',  ( 7.361572987183169658, 59.96726448433410894, -9.846743663894592657 ) ) ;
#21376=CARTESIAN_POINT ( 'NONE',  ( 1.472469842513823179, 21.42559781766745175, 4.923371831947296329 ) ) ;
#21380=EDGE_CURVE ( 'NONE', #96219, #29181, #12170, .T. ) ;
#21381=CARTESIAN_POINT ( 'NONE',  ( 6.204703633549690345, 42.84541550158063217, 14.16423886937410082 ) ) ;
#21382=CARTESIAN_POINT ( 'NONE',  ( 0.1532563361054100626, 10.80059781766745175, -2.638427012816831230 ) ) ;
#21383=CARTESIAN_POINT ( 'NONE',  ( 0.1089645850229080254, 63.16234555792569694, 6.479102184480831639 ) ) ;
#21384=PRESENTATION_STYLE_ASSIGNMENT (( #34889 ) ) ;
#21385=CARTESIAN_POINT ( 'NONE',  ( 0.5774900079438607392, 33.48035201082150536, 5.440088680355550821 ) ) ;
#21386=CARTESIAN_POINT ( 'NONE',  ( 21.09922568453595559, 32.04030133659708923, -6.408140936763230044 ) ) ;
#21387=CARTESIAN_POINT ( 'NONE',  ( 19.42250999205614193, 5.147018677488171434, 5.440088680355555262 ) ) ;
#21388=CARTESIAN_POINT ( 'NONE',  ( -2.816281873526471635, 33.91530133659708213, -3.434112377981056508 ) ) ;
#21389=CARTESIAN_POINT ( 'NONE',  ( -2.816281873526473856, 64.12363466993042493, 9.499525473075851096E-16 ) ) ;
#21395=CARTESIAN_POINT ( 'NONE',  ( -2.266590686148945544, 47.22041550158063927, 7.082119434687048631 ) ) ;
#21397=CARTESIAN_POINT ( 'NONE',  ( 19.42250999205614193, 5.147018677488171434, 5.440088680355555262 ) ) ;
#21398=CARTESIAN_POINT ( 'NONE',  ( -0.8801773607111009756, 18.06368534415484106, 1.068504757029289695E-15 ) ) ;
#21401=CARTESIAN_POINT ( 'NONE',  ( 7.084665262690076126, 47.02201867748818387, -10.88017736071110164 ) ) ;
#21402=CARTESIAN_POINT ( 'NONE',  ( 15.44008868035555793, 56.39701867748817676, -9.422509992056140149 ) ) ;
#21403=CARTESIAN_POINT ( 'NONE',  ( 22.81628187352647785, 16.62363466993042138, 6.195893100308588602E-16 ) ) ;
#21405=CARTESIAN_POINT ( 'NONE',  ( 18.52753015748618282, 23.92559781766745530, -4.923371831947291888 ) ) ;
#21406=CARTESIAN_POINT ( 'NONE',  ( 19.42250999205614548, 50.98035201082151247, -5.440088680355545492 ) ) ;
#21408=CARTESIAN_POINT ( 'NONE',  ( 3.591859063236763294, 18.29030133659708568, -11.09922568453595026 ) ) ;
#21410=CARTESIAN_POINT ( 'NONE',  ( 2.035157376598822676, 7.438685344154837509, -7.964842623401177768 ) ) ;
#21411=CARTESIAN_POINT ( 'NONE',  ( 7.361572987183169658, 44.96726448433412315, -9.846743663894592657 ) ) ;
#21412=CARTESIAN_POINT ( 'NONE',  ( 6.565887622018943937, 45.16530133659708923, 12.81628187352647430 ) ) ;
#21413=CARTESIAN_POINT ( 'NONE',  ( 2.791683348922237240, 25.38393115100078390, -7.208316651077763204 ) ) ;
#21414=CARTESIAN_POINT ( 'NONE',  ( 24.16423886937409904, 4.095415501580634832, 3.795296366450317205 ) ) ;
#21415=CARTESIAN_POINT ( 'NONE',  ( 17.39651004071842166, 27.93575266056828355, 6.499999999999998224 ) ) ;
#21416=CARTESIAN_POINT ( 'NONE',  ( 15.44008868035555793, 26.39701867748817321, -9.422509992056140149 ) ) ;
#21417=CARTESIAN_POINT ( 'NONE',  ( 0.2751277870542967463, 0.000000000000000000, 6.500000000000000888 ) ) ;
#21418=CARTESIAN_POINT ( 'NONE',  ( 10.00000000000000178, 33.05374883491396787, 14.16423886937410082 ) ) ;
#21419=CARTESIAN_POINT ( 'NONE',  ( 10.00000000000000000, 49.75893115100078745, -9.846743663894594434 ) ) ;
#21420=CARTESIAN_POINT ( 'NONE',  ( 0.5774900079438607392, 28.48035201082150891, 5.440088680355550821 ) ) ;
#21421=CARTESIAN_POINT ( 'NONE',  ( 19.42250999205614193, 20.14701867748817321, 5.440088680355555262 ) ) ;
#21423=CARTESIAN_POINT ( 'NONE',  ( 17.96484262340118221, 24.93868534415484461, 7.964842623401181321 ) ) ;
#21424=CARTESIAN_POINT ( 'NONE',  ( 10.00000000000000178, 50.37363466993042493, 12.81628187352647608 ) ) ;
#21425=CARTESIAN_POINT ( 'NONE',  ( 20.88017736071110164, 40.35535201082150536, 2.915334737309930979 ) ) ;
#21426=CARTESIAN_POINT ( 'NONE',  ( 19.42250999205614193, 40.14701867748817676, 5.440088680355555262 ) ) ;
#21428=CARTESIAN_POINT ( 'NONE',  ( 0.1532563361054082862, 56.21726448433411605, 2.638427012816831674 ) ) ;
#21429=CARTESIAN_POINT ( 'NONE',  ( 15.44008868035555793, 31.39701867748817676, -9.422509992056140149 ) ) ;
#21432=CARTESIAN_POINT ( 'NONE',  ( 22.81628187352647785, 61.62363466993041783, 6.195893100308588602E-16 ) ) ;
#21434=CARTESIAN_POINT ( 'NONE',  ( 13.79529636645030344, 53.26208216824730357, 14.16423886937410614 ) ) ;
#21435=CARTESIAN_POINT ( 'NONE',  ( 2.035157376598824452, 48.68868534415483396, 7.964842623401179544 ) ) ;
#21438=CARTESIAN_POINT ( 'NONE',  ( 1.472469842513823179, 65.59226448433412315, -4.923371831947296329 ) ) ;
#21439=CARTESIAN_POINT ( 'NONE',  ( 19.84674366389459266, 3.300597817667451750, 2.638427012816836559 ) ) ;
#21440=CARTESIAN_POINT ( 'NONE',  ( 5.076628168052704559, 25.17559781766745175, -8.527530157486179263 ) ) ;
#21442=CARTESIAN_POINT ( 'NONE',  ( 7.361572987183170547, 27.05059781766745175, 9.846743663894590881 ) ) ;
#21444=CARTESIAN_POINT ( 'NONE',  ( -0.8801773607111009756, 33.06368534415484106, 1.068504757029289695E-15 ) ) ;
#21445=CARTESIAN_POINT ( 'NONE',  ( 12.63842701281683922, 24.55059781766745175, -9.846743663894590881 ) ) ;
#21447=CARTESIAN_POINT ( 'NONE',  ( -1.099225684535947600, 13.70696800326375353, -6.408140936763238038 ) ) ;
#21448=CARTESIAN_POINT ( 'NONE',  ( 17.96484262340118221, 66.18868534415483396, -7.964842623401177768 ) ) ;
#21449=CARTESIAN_POINT ( 'NONE',  ( 4.559911319644449179, 53.89701867748817676, 9.422509992056141925 ) ) ;
#21450=CARTESIAN_POINT ( 'NONE',  ( 17.96484262340118221, 31.18868534415483751, -7.964842623401177768 ) ) ;
#21451=CARTESIAN_POINT ( 'NONE',  ( 19.38216949554541557, 52.24863466993041072, -9.382169495545420901 ) ) ;
#21452=CARTESIAN_POINT ( 'NONE',  ( -4.164238869374099927, 42.01208216824728936, 3.795296366450308767 ) ) ;
#21457=CARTESIAN_POINT ( 'NONE',  ( 22.81628187352647785, 11.41530133659708390, 3.434112377981063169 ) ) ;
#21458=CARTESIAN_POINT ( 'NONE',  ( 7.084665262690076126, 7.022018677488169658, -10.88017736071110164 ) ) ;
#21459=CARTESIAN_POINT ( 'NONE',  ( 12.91533473730993009, 51.60535201082149825, -10.88017736071109987 ) ) ;
#21460=CARTESIAN_POINT ( 'NONE',  ( 18.72515096720568195, 26.07228050351032778, -6.500000000000018652 ) ) ;
#21461=AXIS2_PLACEMENT_3D ( 'NONE', #38979, #32443, #70457 ) ;
#21463=CARTESIAN_POINT ( 'NONE',  ( 10.00000000000000178, 64.31368534415483396, 10.88017736071110342 ) ) ;
#21464=CARTESIAN_POINT ( 'NONE',  ( 19.84674366389459266, 33.71726448433410894, -2.638427012816827677 ) ) ;
#21465=CARTESIAN_POINT ( 'NONE',  ( 17.20831665107776587, 24.13393115100078035, -7.208316651077762316 ) ) ;
#21466=CARTESIAN_POINT ( 'NONE',  ( 7.361572987183169658, 19.96726448433411960, -9.846743663894592657 ) ) ;
#21468=CARTESIAN_POINT ( 'NONE',  ( 7.361572987183170547, 2.050597817667451750, 9.846743663894590881 ) ) ;
#21469=CARTESIAN_POINT ( 'NONE',  ( -0.03932841506543475335, 23.12161441960502373, 6.397827110478943702 ) ) ;
#21471=CARTESIAN_POINT ( 'NONE',  ( 10.00000000000000178, 37.25893115100078745, 9.846743663894594434 ) ) ;
#21473=CARTESIAN_POINT ( 'NONE',  ( 13.43411237798106583, 57.66530133659708923, -12.81628187352647252 ) ) ;
#21476=CARTESIAN_POINT ( 'NONE',  ( 21.09922568453594849, 1.206968003263753531, 6.408140936763242479 ) ) ;
#21477=CARTESIAN_POINT ( 'NONE',  ( 20.88017736071110164, 10.35535201082150714, 2.915334737309930979 ) ) ;
#21478=CARTESIAN_POINT ( 'NONE',  ( -0.3689425029237881626, 32.42874883491395366, 10.36894250292379027 ) ) ;
#21482=CARTESIAN_POINT ( 'NONE',  ( 2.917880565312950480, 25.97041550158063572, -12.26659068614894821 ) ) ;
#21483=CARTESIAN_POINT ( 'NONE',  ( -2.266590686148945544, 42.22041550158063217, 7.082119434687048631 ) ) ;
#21484=CARTESIAN_POINT ( 'NONE',  ( 24.16423886937409904, 4.095415501580634832, 3.795296366450317205 ) ) ;
#21485=CARTESIAN_POINT ( 'NONE',  ( -0.3689425029237881626, 17.42874883491397142, 10.36894250292379027 ) ) ;
#21487=CARTESIAN_POINT ( 'NONE',  ( -0.8801773607110991993, 47.85535201082150536, -2.915334737309923874 ) ) ;
#21490=CARTESIAN_POINT ( 'NONE',  ( 17.20831665107776587, 29.13393115100078390, -7.208316651077762316 ) ) ;
#21491=DIRECTION ( 'NONE',  ( -1.000000000000000000, 0.000000000000000000, 0.000000000000000000 ) ) ;
#21492=CARTESIAN_POINT ( 'NONE',  ( 18.52753015748617571, 28.09226448433411960, 4.923371831947298993 ) ) ;
#21493=CARTESIAN_POINT ( 'NONE',  ( 19.42250999205614193, 10.14701867748816966, 5.440088680355555262 ) ) ;
#21494=CARTESIAN_POINT ( 'NONE',  ( -1.099225684535947600, 59.54030133659708923, 6.408140936763237150 ) ) ;
#21495=CARTESIAN_POINT ( 'NONE',  ( 1.472469842513823179, 46.42559781766745175, 4.923371831947296329 ) ) ;
#21496=VECTOR ( 'NONE', #57797, 1000.000000000000114 ) ;
#21498=CARTESIAN_POINT ( 'NONE',  ( 13.43411237798106583, 37.66530133659708923, -12.81628187352647252 ) ) ;
#21500=CARTESIAN_POINT ( 'NONE',  ( 4.559911319644449179, 37.23035201082150536, -9.422509992056141925 ) ) ;
#21501=CARTESIAN_POINT ( 'NONE',  ( 2.791683348922237240, 45.38393115100079456, -7.208316651077763204 ) ) ;
#21502=CARTESIAN_POINT ( 'NONE',  ( 22.26659068614895176, 29.72041550158063572, -7.082119434687042414 ) ) ;
#21504=CARTESIAN_POINT ( 'NONE',  ( 6.204703633549690345, 2.845415501580634388, 14.16423886937410082 ) ) ;
#21505=CARTESIAN_POINT ( 'NONE',  ( 19.42250999205614193, 65.14701867748817676, 5.440088680355555262 ) ) ;
#21506=CARTESIAN_POINT ( 'NONE',  ( 19.42250999205614548, 65.98035201082151957, -5.440088680355545492 ) ) ;
#21507=CARTESIAN_POINT ( 'NONE',  ( 2.917880565312950480, 60.97041550158063927, -12.26659068614894821 ) ) ;
#21508=CARTESIAN_POINT ( 'NONE',  ( 22.81628187352647785, 1.623634669930420271, 6.195893100308588602E-16 ) ) ;
#21510=CARTESIAN_POINT ( 'NONE',  ( 12.91533473730992121, 59.52201867748816966, 10.88017736071110164 ) ) ;
#21512=CARTESIAN_POINT ( 'NONE',  ( 0.6178305044545838731, 34.74863466993042493, 9.382169495545420901 ) ) ;
#21514=CARTESIAN_POINT ( 'NONE',  ( 15.44008868035555793, 11.39701867748817143, -9.422509992056140149 ) ) ;
#21515=CARTESIAN_POINT ( 'NONE',  ( 12.91533473730992121, 14.52201867748817143, 10.88017736071110164 ) ) ;
#21517=CARTESIAN_POINT ( 'NONE',  ( 5.076628168052704559, 40.17559781766745175, -8.527530157486179263 ) ) ;
#21518=CARTESIAN_POINT ( 'NONE',  ( 3.591859063236761518, 49.95696800326375353, 11.09922568453594849 ) ) ;
#21519=CARTESIAN_POINT ( 'NONE',  ( 20.00000000000000711, 105.0000000000000000, 4.500000000000000888 ) ) ;
#21520=VERTEX_POINT ( 'NONE', #10464 ) ;
#21521=B_SPLINE_CURVE_WITH_KNOTS ( 'NONE', 3,
 ( #53309, #15343, #76313, #38818 ),
 .UNSPECIFIED., .F., .F.,
 ( 4, 4 ),
 ( 0.000000000000000000, 0.0006109242138661632711 ),
 .UNSPECIFIED. ) ;
#21523=CARTESIAN_POINT ( 'NONE',  ( 19.42250999205614193, 15.14701867748817143, 5.440088680355555262 ) ) ;
#21524=CARTESIAN_POINT ( 'NONE',  ( 21.09922568453594849, 1.206968003263753531, 6.408140936763242479 ) ) ;
#21526=CARTESIAN_POINT ( 'NONE',  ( 0.1532563361054082862, 16.21726448433411960, 2.638427012816831674 ) ) ;
#21527=CARTESIAN_POINT ( 'NONE',  ( 17.20831665107776587, 52.88393115100078035, 7.208316651077764980 ) ) ;
#21528=CARTESIAN_POINT ( 'NONE',  ( 7.084665262690076126, 32.02201867748816966, -10.88017736071110164 ) ) ;
#21529=COLOUR_RGB ( '', 0.40784314, 0.44705882, 0.49803922) ;
#21530=CARTESIAN_POINT ( 'NONE',  ( -2.816281873526473856, 9.331968003263753531, 3.434112377981055619 ) ) ;
#21531=CARTESIAN_POINT ( 'NONE',  ( 20.88017736071110519, 50.56368534415484106, 2.639326808657452039E-16 ) ) ;
#21533=CARTESIAN_POINT ( 'NONE',  ( 16.40814093676324603, 52.45696800326375353, -11.09922568453594671 ) ) ;
#21535=CARTESIAN_POINT ( 'NONE',  ( 17.96484262340118221, 64.93868534415483396, 7.964842623401181321 ) ) ;
#21537=CARTESIAN_POINT ( 'NONE',  ( 22.81628187352647785, 31.41530133659709279, 3.434112377981063169 ) ) ;
#21538=CARTESIAN_POINT ( 'NONE',  ( 10.00000000000000178, 3.053748834913967425, 14.16423886937410082 ) ) ;
#21540=CARTESIAN_POINT ( 'NONE',  ( 19.42250999205614193, 40.14701867748817676, 5.440088680355555262 ) ) ;
#21541=CARTESIAN_POINT ( 'NONE',  ( 19.84674366389459621, 63.50893115100078745, 7.409399052514197653E-17 ) ) ;
#21542=CARTESIAN_POINT ( 'NONE',  ( 12.63842701281683922, 49.55059781766744464, -9.846743663894590881 ) ) ;
#21543=CARTESIAN_POINT ( 'NONE',  ( 7.361572987183170547, 22.05059781766745530, 9.846743663894590881 ) ) ;
#21544=CARTESIAN_POINT ( 'NONE',  ( 2.791683348922240793, 11.63393115100078568, 7.208316651077764092 ) ) ;
#21546=CARTESIAN_POINT ( 'NONE',  ( 22.26659068614894466, 48.88708216824730357, 7.082119434687054849 ) ) ;
#21547=( BOUNDED_CURVE ( )  B_SPLINE_CURVE ( 2, ( #56991, #87494, #19009, #49485, #79992, #42016, #47529, #78031, #9533 ),
 .UNSPECIFIED., .F., .T. ) 
 B_SPLINE_CURVE_WITH_KNOTS ( ( 3, 2, 2, 2, 3 ),
 ( 0.5105718029354654464, 0.5119047619047618625, 0.5178571428571429047, 0.5238095238095238360, 0.5251424827788202521 ),
 .UNSPECIFIED. ) 
 CURVE ( )  GEOMETRIC_REPRESENTATION_ITEM ( )  RATIONAL_B_SPLINE_CURVE ( ( 0.9881565478350733400, 0.9923695281211490915, 1.000000000000000000, 0.9659258262890683122, 1.000000000000000000, 0.9659258262890683122, 1.000000000000000000, 0.9923695281211490915, 0.9881565478350733400 ) ) 
 REPRESENTATION_ITEM ( '' )  );
#21548=CARTESIAN_POINT ( 'NONE',  ( 20.32896413005680714, 25.57879003517447458, -5.963430220938276349 ) ) ;
#21549=( LENGTH_UNIT ( ) NAMED_UNIT ( * ) SI_UNIT ( .MILLI., .METRE. ) );
#21550=CARTESIAN_POINT ( 'NONE',  ( 0.1916775849787289987, 7.258688159020694641, -6.500000000000003553 ) ) ;
#21551=( BOUNDED_CURVE ( )  B_SPLINE_CURVE ( 2, ( #40239, #61735, #55739, #16753, #47228, #70747, #39266, #9243, #2263 ),
 .UNSPECIFIED., .F., .F. ) 
 B_SPLINE_CURVE_WITH_KNOTS ( ( 3, 2, 2, 2, 3 ),
 ( 0.4401409369402313199, 0.4404761904761904656, 0.4464285714285713969, 0.4523809523809524391, 0.4527162059169115849 ),
 .UNSPECIFIED. ) 
 CURVE ( )  GEOMETRIC_REPRESENTATION_ITEM ( )  RATIONAL_B_SPLINE_CURVE ( ( 0.9963778908391760503, 0.9980808541467920403, 1.000000000000000000, 0.9659258262890683122, 1.000000000000000000, 0.9659258262890683122, 1.000000000000000000, 0.9980808541467920403, 0.9963778908391759392 ) ) 
 REPRESENTATION_ITEM ( '' )  );
#21552=ORIENTED_EDGE ( 'NONE', *, *, #37731, .F. ) ;
#21554=CARTESIAN_POINT ( 'NONE',  ( 13.79529636645031943, 65.34541550158063217, -14.16423886937409904 ) ) ;
#21555=CARTESIAN_POINT ( 'NONE',  ( 10.00000000000000000, 1.813685344154838175, -10.88017736071110342 ) ) ;
#21556=CARTESIAN_POINT ( 'NONE',  ( 10.00000000000000000, 29.75893115100078745, -9.846743663894594434 ) ) ;
#21558=CARTESIAN_POINT ( 'NONE',  ( 16.40814093676324603, 22.45696800326375353, -11.09922568453594671 ) ) ;
#21561=CARTESIAN_POINT ( 'NONE',  ( 17.08211943468705130, 13.47041550158063572, 12.26659068614894998 ) ) ;
#21562=CARTESIAN_POINT ( 'NONE',  ( 10.00000000000000178, 19.31368534415484106, 10.88017736071110342 ) ) ;
#21563=CARTESIAN_POINT ( 'NONE',  ( -2.266590686148945544, 61.38708216824730357, -7.082119434687050408 ) ) ;
#21564=CARTESIAN_POINT ( 'NONE',  ( 7.361572987183170547, 32.05059781766745175, 9.846743663894590881 ) ) ;
#21566=CARTESIAN_POINT ( 'NONE',  ( 19.84674366389459621, 28.50893115100078745, 7.409399052514197653E-17 ) ) ;
#21569=ORIENTED_EDGE ( 'NONE', *, *, #18758, .T. ) ;
#21573=CARTESIAN_POINT ( 'NONE',  ( 10.00000000000000178, 47.25893115100078745, 9.846743663894594434 ) ) ;
#21574=CARTESIAN_POINT ( 'NONE',  ( 24.16423886937409904, 19.09541550158063927, 3.795296366450317205 ) ) ;
#21575=CARTESIAN_POINT ( 'NONE',  ( 2.035157376598822676, 17.43868534415483751, -7.964842623401177768 ) ) ;
#21576=CARTESIAN_POINT ( 'NONE',  ( 10.00000000000000178, 34.31368534415484106, 10.88017736071110342 ) ) ;
#21577=CARTESIAN_POINT ( 'NONE',  ( 0.1532563361054083140, 66.00893115100079456, 1.131784320476157264E-15 ) ) ;
#21578=CARTESIAN_POINT ( 'NONE',  ( 0.6178305044545838731, 14.74863466993041783, 9.382169495545420901 ) ) ;
#21579=CARTESIAN_POINT ( 'NONE',  ( -2.266590686148945544, 7.220415501580634832, 7.082119434687048631 ) ) ;
#21580=CARTESIAN_POINT ( 'NONE',  ( 2.035157376598824452, 68.68868534415484817, 7.964842623401179544 ) ) ;
#21581=EDGE_CURVE ( 'NONE', #60237, #16271, #57429, .T. ) ;
#21582=CARTESIAN_POINT ( 'NONE',  ( -1.099225684535947600, 28.70696800326375353, -6.408140936763238038 ) ) ;
#21583=VERTEX_POINT ( 'NONE', #55971 ) ;
#21584=CARTESIAN_POINT ( 'NONE',  ( 5.076628168052703671, 26.84226448433411960, 8.527530157486179263 ) ) ;
#21585=CARTESIAN_POINT ( 'NONE',  ( 6.204703633549690345, 67.84541550158060375, 14.16423886937410082 ) ) ;
#21586=EDGE_LOOP ( 'NONE', ( #80199, #75059, #38152, #46431, #66467, #48696 ) ) ;
#21587=CARTESIAN_POINT ( 'NONE',  ( 20.88017736071110875, 5.772018677488170546, -2.915334737309920765 ) ) ;
#21589=CARTESIAN_POINT ( 'NONE',  ( 19.42250999205614193, 50.14701867748817676, 5.440088680355555262 ) ) ;
#21590=CARTESIAN_POINT ( 'NONE',  ( 17.96484262340118221, 64.93868534415483396, 7.964842623401181321 ) ) ;
#21591=CARTESIAN_POINT ( 'NONE',  ( 2.035157376598822676, 62.43868534415483396, -7.964842623401177768 ) ) ;
#21593=CARTESIAN_POINT ( 'NONE',  ( 17.96484262340118221, 59.93868534415484106, 7.964842623401181321 ) ) ;
#21598=CARTESIAN_POINT ( 'NONE',  ( 17.20831665107776587, 34.13393115100078745, -7.208316651077762316 ) ) ;
#21600=CARTESIAN_POINT ( 'NONE',  ( 5.076628168052703671, 56.84226448433412315, 8.527530157486179263 ) ) ;
#21603=EDGE_CURVE ( 'NONE', #16203, #95857, #48942, .T. ) ;
#21604=CARTESIAN_POINT ( 'NONE',  ( 2.917880565312948704, 2.637082168247300906, 12.26659068614894643 ) ) ;
#21609=CARTESIAN_POINT ( 'NONE',  ( 7.361572987183169658, 39.96726448433411605, -9.846743663894592657 ) ) ;
#21610=CARTESIAN_POINT ( 'NONE',  ( 10.00000000000000000, 6.813685344154838397, -10.88017736071110342 ) ) ;
#21612=ORIENTED_EDGE ( 'NONE', *, *, #83216, .F. ) ;
#21614=CARTESIAN_POINT ( 'NONE',  ( 18.52753015748618282, 43.92559781766745175, -4.923371831947291888 ) ) ;
#21616=CARTESIAN_POINT ( 'NONE',  ( -1.099225684535947600, 13.70696800326375353, -6.408140936763238038 ) ) ;
#21617=CARTESIAN_POINT ( 'NONE',  ( 7.361572987183169658, 9.967264484334119601, -9.846743663894592657 ) ) ;
#21619=CARTESIAN_POINT ( 'NONE',  ( 19.38216949554541557, 7.248634669930421381, -9.382169495545420901 ) ) ;
#21623=B_SPLINE_CURVE_WITH_KNOTS ( 'NONE', 3,
 ( #45202, #75701, #7212, #30187, #68215, #64117 ),
 .UNSPECIFIED., .F., .F.,
 ( 4, 2, 4 ),
 ( 0.000000000000000000, 0.0002701661927229328424, 0.0005403323854458656848 ),
 .UNSPECIFIED. ) ;
#21625=CARTESIAN_POINT ( 'NONE',  ( 19.42250999205614548, 15.98035201082150714, -5.440088680355545492 ) ) ;
#21626=CARTESIAN_POINT ( 'NONE',  ( -0.3689425029237898834, 16.17874883491396076, -10.36894250292378850 ) ) ;
#21627=CARTESIAN_POINT ( 'NONE',  ( 18.52753015748618282, 28.92559781766745175, -4.923371831947291888 ) ) ;
#21628=CARTESIAN_POINT ( 'NONE',  ( 20.88017736071110875, 55.77201867748816966, -2.915334737309920765 ) ) ;
#21629=CARTESIAN_POINT ( 'NONE',  ( 21.09922568453594849, 36.20696800326375353, 6.408140936763242479 ) ) ;
#21630=CARTESIAN_POINT ( 'NONE',  ( 17.96484262340118221, 21.18868534415483396, -7.964842623401177768 ) ) ;
#21632=CARTESIAN_POINT ( 'NONE',  ( 13.99999999999999822, 61.00000000000000711, 6.000000000000000000 ) ) ;
#21633=CARTESIAN_POINT ( 'NONE',  ( 18.52753015748617571, 58.09226448433411605, 4.923371831947298993 ) ) ;
#21634=CARTESIAN_POINT ( 'NONE',  ( 0.1532563361054082862, 26.21726448433411605, 2.638427012816831674 ) ) ;
#21636=CARTESIAN_POINT ( 'NONE',  ( -2.816281873526473856, 34.33196800326376064, 3.434112377981055619 ) ) ;
#21637=CARTESIAN_POINT ( 'NONE',  ( 0.2751277870542967463, 70.00000000000000000, -6.500000000000000888 ) ) ;
#21638=CARTESIAN_POINT ( 'NONE',  ( -0.8801773607111009756, 38.06368534415484106, 1.068504757029289695E-15 ) ) ;
#21643=CARTESIAN_POINT ( 'NONE',  ( 19.42250999205614548, 60.98035201082151247, -5.440088680355545492 ) ) ;
#21644=CARTESIAN_POINT ( 'NONE',  ( 15.44008868035555793, 46.39701867748817676, -9.422509992056140149 ) ) ;
#21645=CARTESIAN_POINT ( 'NONE',  ( 17.96484262340118221, 39.93868534415484106, 7.964842623401181321 ) ) ;
#21647=CARTESIAN_POINT ( 'NONE',  ( 2.035157376598822676, 52.43868534415483396, -7.964842623401177768 ) ) ;
#21649=CARTESIAN_POINT ( 'NONE',  ( 7.361572987183170547, 42.05059781766745886, 9.846743663894590881 ) ) ;
#21650=CARTESIAN_POINT ( 'NONE',  ( 20.88017736071110519, 10.56368534415483751, 2.639326808657452039E-16 ) ) ;
#21651=CARTESIAN_POINT ( 'NONE',  ( 16.40814093676324603, 17.45696800326375353, -11.09922568453594671 ) ) ;
#21653=CARTESIAN_POINT ( 'NONE',  ( 15.44008868035555793, 26.39701867748817321, -9.422509992056140149 ) ) ;
#21655=CARTESIAN_POINT ( 'NONE',  ( 0.6081133539230539897, 23.33703382326399733, 6.499999999999968914 ) ) ;
#21656=CARTESIAN_POINT ( 'NONE',  ( -0.8801773607110991993, 27.85535201082150181, -2.915334737309923874 ) ) ;
#21657=CARTESIAN_POINT ( 'NONE',  ( 12.91533473730992121, 64.52201867748817676, 10.88017736071110164 ) ) ;
#21658=CARTESIAN_POINT ( 'NONE',  ( 24.16423886937410614, 29.30374883491396787, 8.672049930838204340E-16 ) ) ;
#21659=CARTESIAN_POINT ( 'NONE',  ( 7.361572987183169658, 9.967264484334119601, -9.846743663894592657 ) ) ;
#21660=CARTESIAN_POINT ( 'NONE',  ( 10.00000000000000000, 46.81368534415484106, -10.88017736071110342 ) ) ;
#21662=CARTESIAN_POINT ( 'NONE',  ( 10.00000000000000000, 0.5537488349139675359, -14.16423886937410082 ) ) ;
#21666=CARTESIAN_POINT ( 'NONE',  ( 10.00000000000000178, 42.25893115100078745, 9.846743663894594434 ) ) ;
#21670=CARTESIAN_POINT ( 'NONE',  ( -0.3689425029237898834, 21.17874883491396432, -10.36894250292378850 ) ) ;
#21671=CARTESIAN_POINT ( 'NONE',  ( 2.917880565312948704, 22.63708216824730002, 12.26659068614894643 ) ) ;
#21672=CARTESIAN_POINT ( 'NONE',  ( 2.035157376598824452, 53.68868534415484817, 7.964842623401179544 ) ) ;
#21673=CARTESIAN_POINT ( 'NONE',  ( 6.204703633549690345, 67.84541550158060375, 14.16423886937410082 ) ) ;
#21674=CARTESIAN_POINT ( 'NONE',  ( 13.43411237798105340, 0.5819680032637533085, 12.81628187352647963 ) ) ;
#21675=CARTESIAN_POINT ( 'NONE',  ( 7.361572987183169658, 54.96726448433413026, -9.846743663894592657 ) ) ;
#21677=CARTESIAN_POINT ( 'NONE',  ( 12.91533473730993009, 41.60535201082149825, -10.88017736071109987 ) ) ;
#21678=CARTESIAN_POINT ( 'NONE',  ( 16.40814093676323893, 10.79030133659708923, 11.09922568453595026 ) ) ;
#21679=CARTESIAN_POINT ( 'NONE',  ( -2.266590686148945544, 11.38708216824730179, -7.082119434687050408 ) ) ;
#21681=CARTESIAN_POINT ( 'NONE',  ( 15.44008868035555260, 14.73035201082150536, 9.422509992056143702 ) ) ;
#21682=CARTESIAN_POINT ( 'NONE',  ( -0.2418659066527486246, 3.090145880403572409, 6.114288769123083611 ) ) ;
#21683=CARTESIAN_POINT ( 'NONE',  ( 20.88017736071110519, 45.56368534415484106, 2.639326808657452039E-16 ) ) ;
#21684=CARTESIAN_POINT ( 'NONE',  ( 0.6178305044545838731, 44.74863466993042493, 9.382169495545420901 ) ) ;
#21687=CARTESIAN_POINT ( 'NONE',  ( -13.69000000000001549, 92.00000000000000000, 9.500000000000000000 ) ) ;
#21691=CARTESIAN_POINT ( 'NONE',  ( 20.36894250292379382, 48.67874883491396076, 10.36894250292379205 ) ) ;
#21692=CARTESIAN_POINT ( 'NONE',  ( -0.8801773607111008646, 8.272018677488171434, 2.915334737309923430 ) ) ;
#21693=CARTESIAN_POINT ( 'NONE',  ( 18.52753015748617571, 23.09226448433411960, 4.923371831947298993 ) ) ;
#21694=CARTESIAN_POINT ( 'NONE',  ( 1.472469842513823179, 45.59226448433412315, -4.923371831947296329 ) ) ;
#21695=CARTESIAN_POINT ( 'NONE',  ( 10.00000000000000178, 69.31368534415484817, 10.88017736071110342 ) ) ;
#21696=ADVANCED_FACE ( 'NONE', ( #55475 ), #8387, .T. ) ;
#21697=CARTESIAN_POINT ( 'NONE',  ( 20.88017736071110875, 65.77201867748817676, -2.915334737309920765 ) ) ;
#21702=CARTESIAN_POINT ( 'NONE',  ( 2.917880565312948704, 27.63708216824730357, 12.26659068614894643 ) ) ;
#21703=CARTESIAN_POINT ( 'NONE',  ( -2.816281873526473856, 19.33196800326375708, 3.434112377981055619 ) ) ;
#21705=CARTESIAN_POINT ( 'NONE',  ( -1.099225684535947600, 39.54030133659708923, 6.408140936763237150 ) ) ;
#21706=CARTESIAN_POINT ( 'NONE',  ( 4.559911319644449179, 17.23035201082150536, -9.422509992056141925 ) ) ;
#21707=CARTESIAN_POINT ( 'NONE',  ( 7.361572987183169658, 34.96726448433411605, -9.846743663894592657 ) ) ;
#21708=CARTESIAN_POINT ( 'NONE',  ( 15.44008868035555793, 26.39701867748817321, -9.422509992056140149 ) ) ;
#21712=CARTESIAN_POINT ( 'NONE',  ( 10.00000000000000178, 42.25893115100078745, 9.846743663894594434 ) ) ;
#21713=CARTESIAN_POINT ( 'NONE',  ( 2.791683348922240793, 51.63393115100078745, 7.208316651077764092 ) ) ;
#21715=CARTESIAN_POINT ( 'NONE',  ( -2.816281873526473856, 29.33196800326376064, 3.434112377981055619 ) ) ;
#21719=CARTESIAN_POINT ( 'NONE',  ( -0.1503990784575328643, 10.12777174578612716, 6.262539305110068177 ) ) ;
#21722=CARTESIAN_POINT ( 'NONE',  ( 1.472469842513823179, 20.59226448433411960, -4.923371831947296329 ) ) ;
#21723=CARTESIAN_POINT ( 'NONE',  ( 21.09922568453594849, 31.20696800326375353, 6.408140936763242479 ) ) ;
#21725=DIRECTION ( 'NONE',  ( -1.000000000000000000, 0.000000000000000000, 0.000000000000000000 ) ) ;
#21727=CARTESIAN_POINT ( 'NONE',  ( 12.63842701281683034, 57.46726448433411605, 9.846743663894596210 ) ) ;
#21729=CARTESIAN_POINT ( 'NONE',  ( 17.20831665107776587, 37.88393115100078745, 7.208316651077764980 ) ) ;
#21730=CARTESIAN_POINT ( 'NONE',  ( 13.79529636645031943, 40.34541550158063217, -14.16423886937409904 ) ) ;
#21731=CARTESIAN_POINT ( 'NONE',  ( 1.472469842513823179, 46.42559781766745175, 4.923371831947296329 ) ) ;
#21732=CARTESIAN_POINT ( 'NONE',  ( 21.09922568453595559, 52.04030133659708923, -6.408140936763230044 ) ) ;
#21734=FACE_OUTER_BOUND ( 'NONE', #32198, .T. ) ;
#21735=CARTESIAN_POINT ( 'NONE',  ( 18.52753015748618282, 8.925597817667451750, -4.923371831947291888 ) ) ;
#21737=CARTESIAN_POINT ( 'NONE',  ( 18.52753015748618282, 53.92559781766745175, -4.923371831947291888 ) ) ;
#21738=CARTESIAN_POINT ( 'NONE',  ( 7.084665262690076126, 47.02201867748818387, -10.88017736071110164 ) ) ;
#21743=CARTESIAN_POINT ( 'NONE',  ( 0.5774900079438590739, 47.64701867748817676, -5.440088680355550821 ) ) ;
#21747=CARTESIAN_POINT ( 'NONE',  ( 19.42250999205614548, 15.98035201082150714, -5.440088680355545492 ) ) ;
#21748=CARTESIAN_POINT ( 'NONE',  ( 17.20831665107776587, 64.13393115100079456, -7.208316651077762316 ) ) ;
#21749=CARTESIAN_POINT ( 'NONE',  ( 4.559911319644449179, 47.23035201082150536, -9.422509992056141925 ) ) ;
#21751=CARTESIAN_POINT ( 'NONE',  ( 20.88017736071110875, 55.77201867748816966, -2.915334737309920765 ) ) ;
#21753=CARTESIAN_POINT ( 'NONE',  ( 19.42250999205614193, 40.14701867748817676, 5.440088680355555262 ) ) ;
#21755=CARTESIAN_POINT ( 'NONE',  ( 12.63842701281683034, 7.467264484334118713, 9.846743663894596210 ) ) ;
#21756=CARTESIAN_POINT ( 'NONE',  ( 2.791683348922237240, 20.38393115100078745, -7.208316651077763204 ) ) ;
#21759=CARTESIAN_POINT ( 'NONE',  ( 0.1532563361054100626, 65.80059781766745175, -2.638427012816831230 ) ) ;
#21760=CARTESIAN_POINT ( 'NONE',  ( 19.42250999205614548, 5.980352010821504471, -5.440088680355545492 ) ) ;
#21761=CARTESIAN_POINT ( 'NONE',  ( 2.603489959281115151, 16.58210964143323807, 6.499999999999462652 ) ) ;
#21763=CARTESIAN_POINT ( 'NONE',  ( 24.16423886937410614, 29.30374883491396787, 8.672049930838204340E-16 ) ) ;
#21765=CARTESIAN_POINT ( 'NONE',  ( 20.36894250292379382, 53.67874883491397497, 10.36894250292379205 ) ) ;
#21766=CARTESIAN_POINT ( 'NONE',  ( 17.96484262340118221, 4.938685344154837509, 7.964842623401181321 ) ) ;
#21768=CARTESIAN_POINT ( 'NONE',  ( 5.076628168052703671, 21.84226448433411960, 8.527530157486179263 ) ) ;
#21769=CARTESIAN_POINT ( 'NONE',  ( 15.44008868035555793, 11.39701867748817143, -9.422509992056140149 ) ) ;
#21770=CARTESIAN_POINT ( 'NONE',  ( 17.20831665107776587, 49.13393115100078745, -7.208316651077762316 ) ) ;
#21774=CARTESIAN_POINT ( 'NONE',  ( 22.81628187352647785, 31.62363466993042138, 6.195893100308588602E-16 ) ) ;
#21775=CARTESIAN_POINT ( 'NONE',  ( 0.1532563361054083140, 41.00893115100078745, 1.131784320476157264E-15 ) ) ;
#21777=CARTESIAN_POINT ( 'NONE',  ( 5.076628168052704559, 5.175597817667451750, -8.527530157486179263 ) ) ;
#21780=CARTESIAN_POINT ( 'NONE',  ( 2.035157376598824452, 8.688685344154839285, 7.964842623401179544 ) ) ;
#21781=CARTESIAN_POINT ( 'NONE',  ( 2.917880565312948704, 42.63708216824729647, 12.26659068614894643 ) ) ;
#21782=CARTESIAN_POINT ( 'NONE',  ( 19.42250999205614193, 45.14701867748817676, 5.440088680355555262 ) ) ;
#21783=CARTESIAN_POINT ( 'NONE',  ( 15.44008868035555260, 64.73035201082151957, 9.422509992056143702 ) ) ;
#21784=CARTESIAN_POINT ( 'NONE',  ( 19.84674366389459266, 23.30059781766745530, 2.638427012816836559 ) ) ;
#21785=CARTESIAN_POINT ( 'NONE',  ( 15.44008868035555260, 4.730352010821504471, 9.422509992056143702 ) ) ;
#21786=CARTESIAN_POINT ( 'NONE',  ( 19.84674366389459621, 8.508931151000785675, 7.409399052514197653E-17 ) ) ;
#21787=CARTESIAN_POINT ( 'NONE',  ( -46.70105855243338766, 101.0494761711182718, 8.834315900847478531 ) ) ;
#21788=CARTESIAN_POINT ( 'NONE',  ( 19.84674366389459266, 43.30059781766744464, 2.638427012816836559 ) ) ;
#21790=CARTESIAN_POINT ( 'NONE',  ( 10.00000000000000178, 39.31368534415484106, 10.88017736071110342 ) ) ;
#21792=CARTESIAN_POINT ( 'NONE',  ( 22.81628187352648496, 61.83196800326376774, -3.434112377981050290 ) ) ;
#21794=CARTESIAN_POINT ( 'NONE',  ( 14.92337183194729633, 2.675597817667451750, 8.527530157486181039 ) ) ;
#21795=CARTESIAN_POINT ( 'NONE',  ( 13.43411237798106583, 42.66530133659707502, -12.81628187352647252 ) ) ;
#21796=CARTESIAN_POINT ( 'NONE',  ( 2.035157376598822676, 12.43868534415483751, -7.964842623401177768 ) ) ;
#21797=CARTESIAN_POINT ( 'NONE',  ( 10.00000000000000178, 42.25893115100078745, 9.846743663894594434 ) ) ;
#21798=SURFACE_STYLE_FILL_AREA ( #13789 ) ;
#21799=CARTESIAN_POINT ( 'NONE',  ( -4.164238869374099927, 32.01208216824730357, 3.795296366450308767 ) ) ;
#21801=CARTESIAN_POINT ( 'NONE',  ( 10.00000000000000000, 50.55374883491396787, -14.16423886937410082 ) ) ;
#21802=CARTESIAN_POINT ( 'NONE',  ( 19.84674366389459266, 63.71726448433412315, -2.638427012816827677 ) ) ;
#21804=CARTESIAN_POINT ( 'NONE',  ( 4.559911319644449179, 37.23035201082150536, -9.422509992056141925 ) ) ;
#21805=CARTESIAN_POINT ( 'NONE',  ( 17.20831665107776587, 2.883931151000785231, 7.208316651077764980 ) ) ;
#21807=CARTESIAN_POINT ( 'NONE',  ( 16.40814093676323893, 55.79030133659708923, 11.09922568453595026 ) ) ;
#21808=CARTESIAN_POINT ( 'NONE',  ( 0.5774900079438590739, 62.64701867748817676, -5.440088680355550821 ) ) ;
#21810=CARTESIAN_POINT ( 'NONE',  ( 13.79529636645031943, 5.345415501580634832, -14.16423886937409904 ) ) ;
#21811=CARTESIAN_POINT ( 'NONE',  ( 17.20831665107776587, 12.88393115100078390, 7.208316651077764980 ) ) ;
#21812=CARTESIAN_POINT ( 'NONE',  ( 20.88017736071110519, 30.56368534415484106, 2.639326808657452039E-16 ) ) ;
#21817=CARTESIAN_POINT ( 'NONE',  ( 4.559911319644449179, 33.89701867748817676, 9.422509992056141925 ) ) ;
#21818=EDGE_CURVE ( 'NONE', #18712, #33937, #7016, .T. ) ;
#21822=CARTESIAN_POINT ( 'NONE',  ( 7.084665262690076126, 32.02201867748816966, -10.88017736071110164 ) ) ;
#21825=CARTESIAN_POINT ( 'NONE',  ( 0.5774900079438607392, 63.48035201082149825, 5.440088680355550821 ) ) ;
#21827=CARTESIAN_POINT ( 'NONE',  ( 7.361572987183169658, 64.96726448433412315, -9.846743663894592657 ) ) ;
#21828=CARTESIAN_POINT ( 'NONE',  ( 17.96484262340118221, 24.93868534415484461, 7.964842623401181321 ) ) ;
#21829=CARTESIAN_POINT ( 'NONE',  ( 19.72487221294570858, 6.866073187300758107, 6.500000000000000888 ) ) ;
#21830=CARTESIAN_POINT ( 'NONE',  ( 18.52753015748617571, 3.092264484334118269, 4.923371831947298993 ) ) ;
#21831=CARTESIAN_POINT ( 'NONE',  ( 19.42250999205614548, 20.98035201082150891, -5.440088680355545492 ) ) ;
#21835=CARTESIAN_POINT ( 'NONE',  ( 7.084665262690076126, 39.10535201082150536, 10.88017736071109987 ) ) ;
#21837=CARTESIAN_POINT ( 'NONE',  ( 3.591859063236763294, 58.29030133659708923, -11.09922568453595026 ) ) ;
#21838=CARTESIAN_POINT ( 'NONE',  ( 19.42250999205614548, 45.98035201082150536, -5.440088680355545492 ) ) ;
#21839=CARTESIAN_POINT ( 'NONE',  ( 0.6178305044545818747, 3.498634669930420049, -9.382169495545419124 ) ) ;
#21841=DIRECTION ( 'NONE',  ( -0.8320502943378437211, 0.5547001962252290364, 0.000000000000000000 ) ) ;
#21843=CARTESIAN_POINT ( 'NONE',  ( 7.361572987183169658, 14.96726448433411960, -9.846743663894592657 ) ) ;
#21845=CARTESIAN_POINT ( 'NONE',  ( 16.40814093676324603, 7.456968003263754419, -11.09922568453594671 ) ) ;
#21847=CARTESIAN_POINT ( 'NONE',  ( 2.791683348922240793, 66.63393115100079456, 7.208316651077764092 ) ) ;
#21848=CARTESIAN_POINT ( 'NONE',  ( 2.035157376598822676, 37.43868534415484106, -7.964842623401177768 ) ) ;
#21849=CARTESIAN_POINT ( 'NONE',  ( 0.1532563361054083140, 46.00893115100079456, 1.131784320476157264E-15 ) ) ;
#21851=CARTESIAN_POINT ( 'NONE',  ( 0.2751277870542967463, 70.00000000000000000, 6.000000000000000000 ) ) ;
#21852=CARTESIAN_POINT ( 'NONE',  ( 12.63842701281683034, 17.46726448433411250, 9.846743663894596210 ) ) ;
#21853=CARTESIAN_POINT ( 'NONE',  ( 14.92337183194729988, 4.342264484334117824, -8.527530157486177487 ) ) ;
#21854=CARTESIAN_POINT ( 'NONE',  ( -1.099225684535947600, -0.4596986634029132657, 6.408140936763237150 ) ) ;
#21855=ORIENTED_EDGE ( 'NONE', *, *, #15190, .F. ) ;
#21858=CARTESIAN_POINT ( 'NONE',  ( 0.1532563361054082862, 61.21726448433412315, 2.638427012816831674 ) ) ;
#21859=CARTESIAN_POINT ( 'NONE',  ( 18.52753015748618282, 33.92559781766745886, -4.923371831947291888 ) ) ;
#21861=CARTESIAN_POINT ( 'NONE',  ( 10.00000000000000000, 1.813685344154838175, -10.88017736071110342 ) ) ;
#21863=CARTESIAN_POINT ( 'NONE',  ( 19.84674366389459621, 43.50893115100078745, 7.409399052514197653E-17 ) ) ;
#21865=CARTESIAN_POINT ( 'NONE',  ( 17.39651004071841456, 64.08210964143329136, -6.500000000000001776 ) ) ;
#21866=CARTESIAN_POINT ( 'NONE',  ( 24.16423886937410614, 64.51208216824728936, -3.795296366450302550 ) ) ;
#21868=CARTESIAN_POINT ( 'NONE',  ( 4.559911319644449179, 22.23035201082150536, -9.422509992056141925 ) ) ;
#21869=CARTESIAN_POINT ( 'NONE',  ( 22.26659068614894466, 53.88708216824731068, 7.082119434687054849 ) ) ;
#21870=CARTESIAN_POINT ( 'NONE',  ( 17.08211943468705840, 50.13708216824730357, -12.26659068614894466 ) ) ;
#21872=CARTESIAN_POINT ( 'NONE',  ( 18.52753015748617571, 3.092264484334118269, 4.923371831947298993 ) ) ;
#21873=CARTESIAN_POINT ( 'NONE',  ( 12.63842701281683922, 29.55059781766745175, -9.846743663894590881 ) ) ;
#21874=CARTESIAN_POINT ( 'NONE',  ( 10.00000000000000000, 12.87363466993042138, -12.81628187352647608 ) ) ;
#21878=CARTESIAN_POINT ( 'NONE',  ( 7.361572987183170547, 67.05059781766746596, 9.846743663894590881 ) ) ;
#21879=CARTESIAN_POINT ( 'NONE',  ( 10.00000000000000000, 5.553748834913967869, -14.16423886937410082 ) ) ;
#21880=CARTESIAN_POINT ( 'NONE',  ( 1.472469842513823179, 20.59226448433411960, -4.923371831947296329 ) ) ;
#21882=CARTESIAN_POINT ( 'NONE',  ( 20.36894250292379738, 39.92874883491396787, -10.36894250292379027 ) ) ;
#21884=CARTESIAN_POINT ( 'NONE',  ( 1.472469842513823179, 10.59226448433411782, -4.923371831947296329 ) ) ;
#21887=CARTESIAN_POINT ( 'NONE',  ( 2.035157376598824452, 28.68868534415484106, 7.964842623401179544 ) ) ;
#21888=CARTESIAN_POINT ( 'NONE',  ( -1.099225684535947600, 39.54030133659708923, 6.408140936763237150 ) ) ;
#21889=CARTESIAN_POINT ( 'NONE',  ( 4.559911319644449179, 7.230352010821504471, -9.422509992056141925 ) ) ;
#21890=CARTESIAN_POINT ( 'NONE',  ( -2.816281873526473856, 39.33196800326374643, 3.434112377981055619 ) ) ;
#21891=CARTESIAN_POINT ( 'NONE',  ( 22.81628187352647785, 56.62363466993042493, 6.195893100308588602E-16 ) ) ;
#21893=CARTESIAN_POINT ( 'NONE',  ( 1.821708436314931179, 11.66792564121895381, -6.499999999999995559 ) ) ;
#21895=CARTESIAN_POINT ( 'NONE',  ( 20.36894250292379738, 44.92874883491396787, -10.36894250292379027 ) ) ;
#21896=CARTESIAN_POINT ( 'NONE',  ( 13.79529636645031943, 5.345415501580634832, -14.16423886937409904 ) ) ;
#21897=CARTESIAN_POINT ( 'NONE',  ( 4.559911319644449179, 2.230352010821504471, -9.422509992056141925 ) ) ;
#21898=CARTESIAN_POINT ( 'NONE',  ( 4.559911319644449179, 27.23035201082150536, -9.422509992056141925 ) ) ;
#21901=CARTESIAN_POINT ( 'NONE',  ( 20.88017736071110164, 55.35535201082149825, 2.915334737309930979 ) ) ;
#21902=CARTESIAN_POINT ( 'NONE',  ( 12.91533473730992121, 64.52201867748817676, 10.88017736071110164 ) ) ;
#21903=CARTESIAN_POINT ( 'NONE',  ( 21.09922568453595559, 22.04030133659708923, -6.408140936763230044 ) ) ;
#21904=CARTESIAN_POINT ( 'NONE',  ( -0.1503990784575294781, 48.10158574516642460, 6.262539305110072618 ) ) ;
#21905=APPLICATION_CONTEXT ( 'automotive_design' ) ;
#21907=CARTESIAN_POINT ( 'NONE',  ( 18.52753015748618282, 18.92559781766745175, -4.923371831947291888 ) ) ;
#21909=ADVANCED_FACE ( 'NONE', ( #11847 ), #41395, .T. ) ;
#21910=CARTESIAN_POINT ( 'NONE',  ( 20.88017736071110164, 60.35535201082151957, 2.915334737309930979 ) ) ;
#21913=CARTESIAN_POINT ( 'NONE',  ( -1.099225684535947600, 23.70696800326375708, -6.408140936763238038 ) ) ;
#21914=CARTESIAN_POINT ( 'NONE',  ( -0.8801773607111009756, 3.063685344154837509, 1.068504757029289695E-15 ) ) ;
#21915=CARTESIAN_POINT ( 'NONE',  ( 12.63842701281683922, 34.55059781766745886, -9.846743663894590881 ) ) ;
#21917=CARTESIAN_POINT ( 'NONE',  ( 19.84674366389459266, 18.30059781766745175, 2.638427012816836559 ) ) ;
#21918=CARTESIAN_POINT ( 'NONE',  ( 20.88017736071110875, 30.77201867748816966, -2.915334737309920321 ) ) ;
#21919=CARTESIAN_POINT ( 'NONE',  ( 15.44008868035555260, 39.73035201082150536, 9.422509992056143702 ) ) ;
#21920=CARTESIAN_POINT ( 'NONE',  ( 17.08211943468705840, 35.13708216824730357, -12.26659068614894466 ) ) ;
#21921=CARTESIAN_POINT ( 'NONE',  ( 17.20831665107776587, 39.13393115100079456, -7.208316651077762316 ) ) ;
#21922=CARTESIAN_POINT ( 'NONE',  ( 12.91533473730993009, 31.60535201082150891, -10.88017736071109987 ) ) ;
#21923=CARTESIAN_POINT ( 'NONE',  ( 10.00000000000000000, 11.81368534415483751, -10.88017736071110342 ) ) ;
#21926=CARTESIAN_POINT ( 'NONE',  ( -0.8801773607111008646, 23.27201867748817676, 2.915334737309923430 ) ) ;
#21927=CARTESIAN_POINT ( 'NONE',  ( 0.6178305044545818747, 43.49863466993042493, -9.382169495545419124 ) ) ;
#21928=CARTESIAN_POINT ( 'NONE',  ( 0.5774900079438590739, 47.64701867748817676, -5.440088680355550821 ) ) ;
#21931=CARTESIAN_POINT ( 'NONE',  ( 12.63842701281683922, 54.55059781766745175, -9.846743663894590881 ) ) ;
#21932=CARTESIAN_POINT ( 'NONE',  ( 12.91533473730993009, 41.60535201082149825, -10.88017736071109987 ) ) ;
#21936=CARTESIAN_POINT ( 'NONE',  ( 0.1129803114748714477, 9.294273331840907204, -6.480634945678661829 ) ) ;
#21937=CARTESIAN_POINT ( 'NONE',  ( 17.08211943468705130, 43.47041550158063927, 12.26659068614894998 ) ) ;
#21938=CARTESIAN_POINT ( 'NONE',  ( 10.00000000000000178, 59.31368534415484106, 10.88017736071110342 ) ) ;
#21939=SURFACE_STYLE_USAGE ( .BOTH. , #90904 ) ;
#21941=STYLED_ITEM ( 'NONE', ( #85845 ), #30196 ) ;
#21943=CARTESIAN_POINT ( 'NONE',  ( 10.00000000000000178, 67.25893115100079456, 9.846743663894594434 ) ) ;
#21944=CARTESIAN_POINT ( 'NONE',  ( -0.8801773607110991993, 2.855352010821504471, -2.915334737309923874 ) ) ;
#21945=CARTESIAN_POINT ( 'NONE',  ( 14.92337183194729988, 34.34226448433411605, -8.527530157486177487 ) ) ;
#21947=CARTESIAN_POINT ( 'NONE',  ( 1.472469842513823179, 41.42559781766745886, 4.923371831947296329 ) ) ;
#21949=CARTESIAN_POINT ( 'NONE',  ( 15.44008868035555793, 26.39701867748817321, -9.422509992056140149 ) ) ;
#21950=CARTESIAN_POINT ( 'NONE',  ( 14.92337183194729633, 22.67559781766745175, 8.527530157486181039 ) ) ;
#21951=CARTESIAN_POINT ( 'NONE',  ( 16.40814093676324603, 22.45696800326375353, -11.09922568453594671 ) ) ;
#21952=CARTESIAN_POINT ( 'NONE',  ( 12.91533473730993009, 66.60535201082150536, -10.88017736071109987 ) ) ;
#21953=CARTESIAN_POINT ( 'NONE',  ( 4.559911319644449179, 58.89701867748817676, 9.422509992056141925 ) ) ;
#21954=CARTESIAN_POINT ( 'NONE',  ( 4.559911319644449179, 38.89701867748817676, 9.422509992056141925 ) ) ;
#21955=FACE_OUTER_BOUND ( 'NONE', #85115, .T. ) ;
#21956=CARTESIAN_POINT ( 'NONE',  ( 10.00000000000000178, 48.05374883491396787, 14.16423886937410082 ) ) ;
#21958=EDGE_LOOP ( 'NONE', ( #84269, #20930, #71362, #71221 ) ) ;
#21959=CARTESIAN_POINT ( 'NONE',  ( 22.81628187352648496, 16.83196800326374998, -3.434112377981050290 ) ) ;
#21960=CARTESIAN_POINT ( 'NONE',  ( 15.44008868035555260, 9.730352010821505360, 9.422509992056143702 ) ) ;
#21961=CARTESIAN_POINT ( 'NONE',  ( -0.8801773607111009756, 53.06368534415484106, 1.068504757029289695E-15 ) ) ;
#21962=CARTESIAN_POINT ( 'NONE',  ( 10.00000000000000178, 70.00000000000000000, 0.000000000000000000 ) ) ;
#21966=CARTESIAN_POINT ( 'NONE',  ( 20.88017736071110519, 55.56368534415484817, 2.639326808657452039E-16 ) ) ;
#21967=CARTESIAN_POINT ( 'NONE',  ( 10.00000000000000178, 32.25893115100078745, 9.846743663894594434 ) ) ;
#21968=CARTESIAN_POINT ( 'NONE',  ( 2.791683348922237240, 25.38393115100078390, -7.208316651077763204 ) ) ;
#21969=CARTESIAN_POINT ( 'NONE',  ( 17.20831665107776587, 9.133931151000787452, -7.208316651077762316 ) ) ;
#21970=CARTESIAN_POINT ( 'NONE',  ( 1.042145700049404766, 49.74216108172002038, -6.499999999999937828 ) ) ;
#21971=CARTESIAN_POINT ( 'NONE',  ( 10.00000000000000178, 35.37363466993042493, 12.81628187352647608 ) ) ;
#21972=CARTESIAN_POINT ( 'NONE',  ( 0.1532563361054100626, 5.800597817667452638, -2.638427012816831230 ) ) ;
#21976=CARTESIAN_POINT ( 'NONE',  ( 14.92337183194729633, 32.67559781766745175, 8.527530157486181039 ) ) ;
#21980=CARTESIAN_POINT ( 'NONE',  ( 6.565887622018943937, 50.16530133659708213, 12.81628187352647430 ) ) ;
#21982=CARTESIAN_POINT ( 'NONE',  ( 3.591859063236761518, 14.95696800326375531, 11.09922568453594849 ) ) ;
#21983=CARTESIAN_POINT ( 'NONE',  ( 20.88017736071110519, 50.56368534415484106, 2.639326808657452039E-16 ) ) ;
#21984=CARTESIAN_POINT ( 'NONE',  ( -0.3689425029237881626, 27.42874883491397142, 10.36894250292379027 ) ) ;
#21986=CARTESIAN_POINT ( 'NONE',  ( 22.26659068614895176, 29.72041550158063572, -7.082119434687042414 ) ) ;
#21987=CARTESIAN_POINT ( 'NONE',  ( 22.26659068614894466, 48.88708216824730357, 7.082119434687054849 ) ) ;
#21988=CARTESIAN_POINT ( 'NONE',  ( 24.16423886937410614, 4.512082168247300906, -3.795296366450302550 ) ) ;
#21989=CARTESIAN_POINT ( 'NONE',  ( 2.917880565312948704, 12.63708216824730179, 12.26659068614894643 ) ) ;
#21990=CARTESIAN_POINT ( 'NONE',  ( 4.559911319644449179, 43.89701867748816966, 9.422509992056141925 ) ) ;
#21992=CARTESIAN_POINT ( 'NONE',  ( 7.361572987183170547, 27.05059781766745175, 9.846743663894590881 ) ) ;
#21993=CARTESIAN_POINT ( 'NONE',  ( -45.94000000000000483, 92.00000000000000000, -8.999999999999998224 ) ) ;
#21994=CARTESIAN_POINT ( 'NONE',  ( 0.1532563361054083140, 31.00893115100078390, 1.131784320476157264E-15 ) ) ;
#21995=CARTESIAN_POINT ( 'NONE',  ( 0.5774900079438607392, 28.48035201082150891, 5.440088680355550821 ) ) ;
#21996=CARTESIAN_POINT ( 'NONE',  ( 3.591859063236763294, 58.29030133659708923, -11.09922568453595026 ) ) ;
#21997=LINE ( 'NONE', #61935, #63347 ) ;
#21998=FACE_OUTER_BOUND ( 'NONE', #53286, .T. ) ;
#21999=CARTESIAN_POINT ( 'NONE',  ( 19.84674366389459266, 23.30059781766745530, 2.638427012816836559 ) ) ;
#22000=CARTESIAN_POINT ( 'NONE',  ( -1.099225684535947600, 38.70696800326375353, -6.408140936763238038 ) ) ;
#22002=CARTESIAN_POINT ( 'NONE',  ( 15.44008868035555793, 41.39701867748817676, -9.422509992056140149 ) ) ;
#22003=CARTESIAN_POINT ( 'NONE',  ( 5.076628168052703671, 56.84226448433412315, 8.527530157486179263 ) ) ;
#22004=CARTESIAN_POINT ( 'NONE',  ( 20.36894250292379382, 23.67874883491397142, 10.36894250292379205 ) ) ;
#22006=SURFACE_STYLE_FILL_AREA ( #98517 ) ;
#22007=CARTESIAN_POINT ( 'NONE',  ( 0.5774900079438607392, 63.48035201082149825, 5.440088680355550821 ) ) ;
#22008=CARTESIAN_POINT ( 'NONE',  ( 4.559911319644449179, 63.89701867748817676, 9.422509992056141925 ) ) ;
#22009=CARTESIAN_POINT ( 'NONE',  ( -2.266590686148945544, 61.38708216824730357, -7.082119434687050408 ) ) ;
#22010=CARTESIAN_POINT ( 'NONE',  ( 10.00000000000000000, -2.126365330069579951, -12.81628187352647608 ) ) ;
#22012=CARTESIAN_POINT ( 'NONE',  ( 4.559911319644449179, 58.89701867748817676, 9.422509992056141925 ) ) ;
#22013=CARTESIAN_POINT ( 'NONE',  ( -0.2418659066527792945, 28.09014588040356841, 6.114288769123030320 ) ) ;
#22015=CARTESIAN_POINT ( 'NONE',  ( 10.00000000000000000, 32.87363466993042493, -12.81628187352647608 ) ) ;
#22016=CARTESIAN_POINT ( 'NONE',  ( 13.79529636645030344, 43.26208216824730357, 14.16423886937410614 ) ) ;
#22018=CARTESIAN_POINT ( 'NONE',  ( 7.084665262690076126, 9.105352010821503583, 10.88017736071109987 ) ) ;
#22019=CARTESIAN_POINT ( 'NONE',  ( 19.42250999205614548, 15.98035201082150714, -5.440088680355545492 ) ) ;
#22020=CARTESIAN_POINT ( 'NONE',  ( 7.361572987183169658, 54.96726448433413026, -9.846743663894592657 ) ) ;
#22021=CARTESIAN_POINT ( 'NONE',  ( -1.099225684535947600, 54.54030133659708923, 6.408140936763237150 ) ) ;
#22025=CARTESIAN_POINT ( 'NONE',  ( 0.5774900079438607392, 18.48035201082150536, 5.440088680355550821 ) ) ;
#22026=CARTESIAN_POINT ( 'NONE',  ( -1.099225684535947600, 13.70696800326375353, -6.408140936763238038 ) ) ;
#22029=CARTESIAN_POINT ( 'NONE',  ( 0.1532563361054100626, 50.80059781766745175, -2.638427012816831230 ) ) ;
#22030=CARTESIAN_POINT ( 'NONE',  ( 10.00000000000000000, 36.81368534415484106, -10.88017736071110342 ) ) ;
#22031=CARTESIAN_POINT ( 'NONE',  ( 10.00000000000000000, 17.87363466993041783, -12.81628187352647608 ) ) ;
#22032=CARTESIAN_POINT ( 'NONE',  ( 0.5774900079438590739, 42.64701867748816966, -5.440088680355550821 ) ) ;
#22034=CARTESIAN_POINT ( 'NONE',  ( 14.49999999999999822, 61.00000000000000000, 6.000000000000000000 ) ) ;
#22035=CARTESIAN_POINT ( 'NONE',  ( 19.38216949554541202, 50.99863466993042493, 9.382169495545424454 ) ) ;
#22037=CARTESIAN_POINT ( 'NONE',  ( 19.42250999205614548, 45.98035201082150536, -5.440088680355545492 ) ) ;
#22038=CARTESIAN_POINT ( 'NONE',  ( -2.816281873526473856, 29.33196800326376064, 3.434112377981055619 ) ) ;
#22039=CARTESIAN_POINT ( 'NONE',  ( 24.16423886937409904, 4.095415501580634832, 3.795296366450317205 ) ) ;
#22040=CARTESIAN_POINT ( 'NONE',  ( 2.035157376598824452, 43.68868534415484106, 7.964842623401179544 ) ) ;
#22042=AXIS2_PLACEMENT_3D ( 'NONE', #52172, #22177, #30634 ) ;
#22043=CARTESIAN_POINT ( 'NONE',  ( 12.63842701281683922, 64.55059781766745175, -9.846743663894590881 ) ) ;
#22044=CARTESIAN_POINT ( 'NONE',  ( 5.076628168052703671, 16.84226448433411960, 8.527530157486179263 ) ) ;
#22045=CARTESIAN_POINT ( 'NONE',  ( 5.076628168052703671, 11.84226448433411960, 8.527530157486179263 ) ) ;
#22047=CARTESIAN_POINT ( 'NONE',  ( 24.16423886937410614, 49.30374883491396787, 8.672049930838204340E-16 ) ) ;
#22053=CARTESIAN_POINT ( 'NONE',  ( 13.79529636645030344, 58.26208216824728936, 14.16423886937410614 ) ) ;
#22054=CARTESIAN_POINT ( 'NONE',  ( 4.559911319644449179, 2.230352010821504916, -9.422509992056141925 ) ) ;
#22056=CARTESIAN_POINT ( 'NONE',  ( 5.076628168052704559, 35.17559781766745175, -8.527530157486179263 ) ) ;
#22057=CARTESIAN_POINT ( 'NONE',  ( -2.816281873526473856, 39.12363466993041783, 9.499525473075851096E-16 ) ) ;
#22059=CARTESIAN_POINT ( 'NONE',  ( 17.08211943468705130, 8.470415501580635720, 12.26659068614894998 ) ) ;
#22060=CARTESIAN_POINT ( 'NONE',  ( 0.5774900079438590739, 12.64701867748817143, -5.440088680355550821 ) ) ;
#22061=CARTESIAN_POINT ( 'NONE',  ( 24.16423886937410614, 54.51208216824730357, -3.795296366450302550 ) ) ;
#22062=CARTESIAN_POINT ( 'NONE',  ( 18.52753015748618282, 38.92559781766745175, -4.923371831947291888 ) ) ;
#22064=CARTESIAN_POINT ( 'NONE',  ( 19.39188664607695500, 40.83703382326399378, -6.499999999999968026 ) ) ;
#22065=CARTESIAN_POINT ( 'NONE',  ( 5.076628168052703671, 21.84226448433411960, 8.527530157486179263 ) ) ;
#22068=EDGE_LOOP ( 'NONE', ( #56616, #26569, #8486, #80635 ) ) ;
#22072=CARTESIAN_POINT ( 'NONE',  ( 5.076628168052704559, 50.17559781766745886, -8.527530157486179263 ) ) ;
#22073=CARTESIAN_POINT ( 'NONE',  ( 4.559911319644449179, 38.89701867748817676, 9.422509992056141925 ) ) ;
#22074=CARTESIAN_POINT ( 'NONE',  ( 0.5774900079438607392, 38.48035201082150536, 5.440088680355550821 ) ) ;
#22075=CARTESIAN_POINT ( 'NONE',  ( 0.1532563361054082862, 66.21726448433413736, 2.638427012816831674 ) ) ;
#22076=CARTESIAN_POINT ( 'NONE',  ( 13.43411237798105340, 35.58196800326375353, 12.81628187352647963 ) ) ;
#22077=CARTESIAN_POINT ( 'NONE',  ( 10.00000000000000178, 8.053748834913967869, 14.16423886937410082 ) ) ;
#22078=CARTESIAN_POINT ( 'NONE',  ( 0.5774900079438590739, 67.64701867748817676, -5.440088680355550821 ) ) ;
#22079=CARTESIAN_POINT ( 'NONE',  ( 10.00000000000000000, 32.87363466993042493, -12.81628187352647608 ) ) ;
#22081=CARTESIAN_POINT ( 'NONE',  ( 2.791683348922237240, 50.38393115100078035, -7.208316651077763204 ) ) ;
#22082=CARTESIAN_POINT ( 'NONE',  ( -0.8801773607110991993, 7.855352010821506248, -2.915334737309923874 ) ) ;
#22084=CARTESIAN_POINT ( 'NONE',  ( 15.44008868035555793, 11.39701867748817143, -9.422509992056140149 ) ) ;
#22086=CARTESIAN_POINT ( 'NONE',  ( 15.44008868035555793, 51.39701867748816966, -9.422509992056140149 ) ) ;
#22087=CARTESIAN_POINT ( 'NONE',  ( 20.88017736071110519, 60.56368534415484106, 2.639326808657452039E-16 ) ) ;
#22088=CARTESIAN_POINT ( 'NONE',  ( 10.00000000000000178, 64.31368534415483396, 10.88017736071110342 ) ) ;
#22090=CARTESIAN_POINT ( 'NONE',  ( 10.00000000000000178, 49.31368534415484106, 10.88017736071110342 ) ) ;
#22091=CARTESIAN_POINT ( 'NONE',  ( -1.926860441876563801, 29.89664270246084499, 3.195792623639529761 ) ) ;
#22092=CARTESIAN_POINT ( 'NONE',  ( 0.1532563361054083140, 11.00893115100078568, 1.131784320476157264E-15 ) ) ;
#22093=CARTESIAN_POINT ( 'NONE',  ( 19.72487221294570858, 70.00000000000000000, 6.000000000000000000 ) ) ;
#22094=CARTESIAN_POINT ( 'NONE',  ( 12.63842701281683034, 27.46726448433411250, 9.846743663894596210 ) ) ;
#22097=CARTESIAN_POINT ( 'NONE',  ( -2.266590686148945544, 2.220415501580634388, 7.082119434687048631 ) ) ;
#22100=CARTESIAN_POINT ( 'NONE',  ( 7.084665262690076126, 9.105352010821503583, 10.88017736071109987 ) ) ;
#22101=CARTESIAN_POINT ( 'NONE',  ( -0.1503990784575242878, 59.24884699246888431, -6.262539305110083276 ) ) ;
#22104=CARTESIAN_POINT ( 'NONE',  ( 5.076628168052703671, 41.84226448433411605, 8.527530157486179263 ) ) ;
#22106=CARTESIAN_POINT ( 'NONE',  ( -2.816281873526471635, 23.91530133659708568, -3.434112377981056508 ) ) ;
#22107=CARTESIAN_POINT ( 'NONE',  ( 2.791683348922240793, 21.63393115100078745, 7.208316651077764092 ) ) ;
#22109=CARTESIAN_POINT ( 'NONE',  ( 0.1532563361054082862, 21.21726448433412315, 2.638427012816831674 ) ) ;
#22110=CARTESIAN_POINT ( 'NONE',  ( -2.816281873526473856, -0.6680319967362464695, 3.434112377981055619 ) ) ;
#22115=CARTESIAN_POINT ( 'NONE',  ( 17.96484262340118221, 29.93868534415484106, 7.964842623401181321 ) ) ;
#22116=CARTESIAN_POINT ( 'NONE',  ( 10.00000000000000178, 18.05374883491396787, 14.16423886937410082 ) ) ;
#22117=CARTESIAN_POINT ( 'NONE',  ( 19.84674366389459266, 28.30059781766745886, 2.638427012816836559 ) ) ;
#22118=CARTESIAN_POINT ( 'NONE',  ( 15.44008868035555260, 59.73035201082151247, 9.422509992056143702 ) ) ;
#22119=CARTESIAN_POINT ( 'NONE',  ( -2.816281873526473856, 39.33196800326374643, 3.434112377981055619 ) ) ;
#22121=CARTESIAN_POINT ( 'NONE',  ( 7.084665262690076126, 12.02201867748817143, -10.88017736071110164 ) ) ;
#22125=CARTESIAN_POINT ( 'NONE',  ( 13.43411237798105340, 5.581968003263753531, 12.81628187352647963 ) ) ;
#22126=CARTESIAN_POINT ( 'NONE',  ( 1.472469842513823179, 21.42559781766745175, 4.923371831947296329 ) ) ;
#22128=CARTESIAN_POINT ( 'NONE',  ( 3.591859063236763294, 33.29030133659708213, -11.09922568453595026 ) ) ;
#22129=CARTESIAN_POINT ( 'NONE',  ( -0.8801773607110991993, 42.85535201082150536, -2.915334737309923874 ) ) ;
#22134=CARTESIAN_POINT ( 'NONE',  ( 4.559911319644449179, 37.23035201082150536, -9.422509992056141925 ) ) ;
#22135=CARTESIAN_POINT ( 'NONE',  ( 2.035157376598824452, 38.68868534415483396, 7.964842623401179544 ) ) ;
#22138=CARTESIAN_POINT ( 'NONE',  ( 1.472469842513823179, 35.59226448433412315, -4.923371831947296329 ) ) ;
#22139=CARTESIAN_POINT ( 'NONE',  ( 17.96484262340118221, 6.188685344154836621, -7.964842623401177768 ) ) ;
#22140=CARTESIAN_POINT ( 'NONE',  ( 13.43411237798106583, 17.66530133659708923, -12.81628187352647252 ) ) ;
#22142=CARTESIAN_POINT ( 'NONE',  ( 20.88017736071110164, 30.35535201082151247, 2.915334737309930979 ) ) ;
#22144=CARTESIAN_POINT ( 'NONE',  ( 15.44008868035555793, 31.39701867748817676, -9.422509992056140149 ) ) ;
#22145=CARTESIAN_POINT ( 'NONE',  ( 7.084665262690076126, 67.02201867748817676, -10.88017736071110164 ) ) ;
#22146=CARTESIAN_POINT ( 'NONE',  ( 6.204703633549690345, 40.76208216824731778, -14.16423886937410259 ) ) ;
#22147=CARTESIAN_POINT ( 'NONE',  ( 0.1532563361054100626, 30.80059781766744820, -2.638427012816831230 ) ) ;
#22149=CARTESIAN_POINT ( 'NONE',  ( 20.88017736071110875, 45.77201867748816966, -2.915334737309920765 ) ) ;
#22151=CARTESIAN_POINT ( 'NONE',  ( 10.00000000000000000, 5.553748834913967869, -14.16423886937410082 ) ) ;
#22152=VERTEX_POINT ( 'NONE', #35829 ) ;
#22154=CARTESIAN_POINT ( 'NONE',  ( 12.63842701281683034, 52.46726448433413026, 9.846743663894596210 ) ) ;
#22157=CARTESIAN_POINT ( 'NONE',  ( 0.8952175423694801459, 62.60160829253887016, -5.990408912944315212 ) ) ;
#22158=CARTESIAN_POINT ( 'NONE',  ( 20.36894250292379738, 19.92874883491396787, -10.36894250292379027 ) ) ;
#22159=CARTESIAN_POINT ( 'NONE',  ( 17.08211943468705130, 18.47041550158063572, 12.26659068614894998 ) ) ;
#22161=CARTESIAN_POINT ( 'NONE',  ( 10.00000000000000000, 56.81368534415484106, -10.88017736071110342 ) ) ;
#22162=CARTESIAN_POINT ( 'NONE',  ( 13.79529636645031943, 65.34541550158063217, -14.16423886937409904 ) ) ;
#22163=CARTESIAN_POINT ( 'NONE',  ( 10.00000000000000000, -2.126365330069579951, -12.81628187352647608 ) ) ;
#22164=CARTESIAN_POINT ( 'NONE',  ( 12.63842701281683034, 42.46726448433412315, 9.846743663894596210 ) ) ;
#22166=CARTESIAN_POINT ( 'NONE',  ( 4.559911319644449179, 42.23035201082151247, -9.422509992056141925 ) ) ;
#22167=CARTESIAN_POINT ( 'NONE',  ( 13.43411237798105340, 25.58196800326374998, 12.81628187352647963 ) ) ;
#22168=CARTESIAN_POINT ( 'NONE',  ( -2.266590686148945544, 12.22041550158063394, 7.082119434687048631 ) ) ;
#22169=CARTESIAN_POINT ( 'NONE',  ( 10.00000000000000000, 16.81368534415483751, -10.88017736071110342 ) ) ;
#22170=CARTESIAN_POINT ( 'NONE',  ( 0.5774900079438590739, 17.64701867748817321, -5.440088680355550821 ) ) ;
#22172=CARTESIAN_POINT ( 'NONE',  ( 17.96484262340118221, 61.18868534415482685, -7.964842623401177768 ) ) ;
#22174=CARTESIAN_POINT ( 'NONE',  ( 3.591859063236763294, 48.29030133659708923, -11.09922568453595026 ) ) ;
#22177=DIRECTION ( 'NONE',  ( 0.000000000000000000, 0.000000000000000000, -1.000000000000000000 ) ) ;
#22182=CARTESIAN_POINT ( 'NONE',  ( -0.03743638938522463044, 19.25197528031019090, -6.399506433553971974 ) ) ;
#22183=CARTESIAN_POINT ( 'NONE',  ( 22.26659068614894466, 53.88708216824731068, 7.082119434687054849 ) ) ;
#22184=CARTESIAN_POINT ( 'NONE',  ( 12.91533473730992121, 4.522018677488170546, 10.88017736071110164 ) ) ;
#22185=CARTESIAN_POINT ( 'NONE',  ( 2.791683348922240793, 16.63393115100078745, 7.208316651077764092 ) ) ;
#22186=CARTESIAN_POINT ( 'NONE',  ( 14.92337183194729988, 44.34226448433412315, -8.527530157486177487 ) ) ;
#22188=STYLED_ITEM ( 'NONE', ( #85734 ), #59599 ) ;
#22189=CARTESIAN_POINT ( 'NONE',  ( 20.10493008474206178, 44.71697413083879979, 6.336235997365762707 ) ) ;
#22190=AXIS2_PLACEMENT_3D ( 'NONE', #51434, #20452, #12447 ) ;
#22191=CARTESIAN_POINT ( 'NONE',  ( 7.084665262690076126, 67.02201867748817676, -10.88017736071110164 ) ) ;
#22192=B_SPLINE_CURVE_WITH_KNOTS ( 'NONE', 3,
 ( #15751, #22264, #30719, #83245 ),
 .UNSPECIFIED., .F., .F.,
 ( 4, 4 ),
 ( 1.388456241783856658E-18, 0.002657014572711311178 ),
 .UNSPECIFIED. ) ;
#22195=CARTESIAN_POINT ( 'NONE',  ( 24.16423886937410614, 39.51208216824731068, -3.795296366450302550 ) ) ;
#22196=CARTESIAN_POINT ( 'NONE',  ( 0.6178305044545838731, 19.74863466993042138, 9.382169495545420901 ) ) ;
#22198=CARTESIAN_POINT ( 'NONE',  ( 10.00000000000000178, 55.37363466993042493, 12.81628187352647608 ) ) ;
#22200=CARTESIAN_POINT ( 'NONE',  ( -0.8801773607111009756, 23.06368534415484106, 1.068504757029289695E-15 ) ) ;
#22201=CARTESIAN_POINT ( 'NONE',  ( 7.361572987183170547, 37.05059781766744464, 9.846743663894590881 ) ) ;
#22202=CARTESIAN_POINT ( 'NONE',  ( 2.035157376598824452, 28.68868534415484106, 7.964842623401179544 ) ) ;
#22203=CARTESIAN_POINT ( 'NONE',  ( 22.81628187352648496, 61.83196800326376774, -3.434112377981050290 ) ) ;
#22204=CARTESIAN_POINT ( 'NONE',  ( 19.72487221294570858, 70.00000000000000000, 6.000000000000000000 ) ) ;
#22205=CARTESIAN_POINT ( 'NONE',  ( 12.63842701281683922, 54.55059781766745175, -9.846743663894590881 ) ) ;
#22206=CARTESIAN_POINT ( 'NONE',  ( 5.076628168052704559, 50.17559781766745886, -8.527530157486179263 ) ) ;
#22216=CARTESIAN_POINT ( 'NONE',  ( 10.00000000000000178, 32.25893115100078745, 9.846743663894594434 ) ) ;
#22218=CARTESIAN_POINT ( 'NONE',  ( -2.816281873526473856, 39.33196800326374643, 3.434112377981055619 ) ) ;
#22222=CARTESIAN_POINT ( 'NONE',  ( 18.52753015748618282, 58.92559781766745886, -4.923371831947291888 ) ) ;
#22224=CARTESIAN_POINT ( 'NONE',  ( 5.076628168052704559, 35.17559781766745175, -8.527530157486179263 ) ) ;
#22225=CARTESIAN_POINT ( 'NONE',  ( 17.08211943468705130, 28.47041550158063572, 12.26659068614894998 ) ) ;
#22226=CARTESIAN_POINT ( 'NONE',  ( 17.20831665107776587, 44.13393115100078745, -7.208316651077762316 ) ) ;
#22227=CARTESIAN_POINT ( 'NONE',  ( 6.565887622018943937, 53.08196800326374643, -12.81628187352647608 ) ) ;
#22229=CARTESIAN_POINT ( 'NONE',  ( 19.84674366389459621, 8.508931151000785675, 7.409399052514197653E-17 ) ) ;
#22230=FILL_AREA_STYLE ('',( #75208 ) ) ;
#22231=CARTESIAN_POINT ( 'NONE',  ( 14.92337183194729988, 44.34226448433412315, -8.527530157486177487 ) ) ;
#22232=CARTESIAN_POINT ( 'NONE',  ( 20.88017736071110164, 40.35535201082150536, 2.915334737309930979 ) ) ;
#22234=CARTESIAN_POINT ( 'NONE',  ( -0.8801773607110991993, 52.85535201082151247, -2.915334737309923874 ) ) ;
#22237=CARTESIAN_POINT ( 'NONE',  ( 20.88017736071110519, 20.56368534415484106, 2.639326808657452039E-16 ) ) ;
#22238=CARTESIAN_POINT ( 'NONE',  ( 6.565887622018943937, -1.918031996736246692, -12.81628187352647608 ) ) ;
#22239=CARTESIAN_POINT ( 'NONE',  ( 15.44008868035555260, 49.73035201082150536, 9.422509992056143702 ) ) ;
#22240=CARTESIAN_POINT ( 'NONE',  ( 2.035157376598822676, 67.43868534415484817, -7.964842623401177768 ) ) ;
#22243=CARTESIAN_POINT ( 'NONE',  ( 10.00000000000000000, 41.81368534415484106, -10.88017736071110342 ) ) ;
#22245=CARTESIAN_POINT ( 'NONE',  ( 5.076628168052703671, 6.842264484334118713, 8.527530157486179263 ) ) ;
#22246=CARTESIAN_POINT ( 'NONE',  ( 7.361572987183169658, 24.96726448433412315, -9.846743663894592657 ) ) ;
#22249=CARTESIAN_POINT ( 'NONE',  ( 0.1532563361054083140, 61.00893115100078745, 1.131784320476157264E-15 ) ) ;
#22250=CARTESIAN_POINT ( 'NONE',  ( -0.8801773607110991993, 2.855352010821504471, -2.915334737309923874 ) ) ;
#22251=CARTESIAN_POINT ( 'NONE',  ( 0.2751277870542981341, 18.21833443783937767, 6.500000000000002665 ) ) ;
#22254=CARTESIAN_POINT ( 'NONE',  ( 13.79529636645031943, 20.34541550158063572, -14.16423886937409904 ) ) ;
#22256=CARTESIAN_POINT ( 'NONE',  ( 22.26659068614894466, 48.88708216824730357, 7.082119434687054849 ) ) ;
#22257=CARTESIAN_POINT ( 'NONE',  ( 12.91533473730993009, 6.605352010821504471, -10.88017736071109987 ) ) ;
#22259=CARTESIAN_POINT ( 'NONE',  ( 18.52753015748618282, 18.92559781766745175, -4.923371831947291888 ) ) ;
#22260=CARTESIAN_POINT ( 'NONE',  ( 12.91533473730993009, 31.60535201082150891, -10.88017736071109987 ) ) ;
#22262=CARTESIAN_POINT ( 'NONE',  ( 19.84674366389459621, 43.50893115100078745, 7.409399052514197653E-17 ) ) ;
#22263=CARTESIAN_POINT ( 'NONE',  ( -4.164238869374099927, 2.012082168247300906, 3.795296366450308767 ) ) ;
#22264=CARTESIAN_POINT ( 'NONE',  ( 1.046131998950046382, 5.738109087357264215, 6.500000000000002665 ) ) ;
#22266=CARTESIAN_POINT ( 'NONE',  ( 19.84674366389459621, 3.508931151000785231, 7.409399052514197653E-17 ) ) ;
#22267=CARTESIAN_POINT ( 'NONE',  ( 3.591859063236761518, 34.95696800326375353, 11.09922568453594849 ) ) ;
#22268=CARTESIAN_POINT ( 'NONE',  ( 2.791683348922237240, 45.38393115100079456, -7.208316651077763204 ) ) ;
#22270=CARTESIAN_POINT ( 'NONE',  ( 1.472469842513823179, 10.59226448433411782, -4.923371831947296329 ) ) ;
#22273=CARTESIAN_POINT ( 'NONE',  ( 15.44008868035555260, 14.73035201082150536, 9.422509992056143702 ) ) ;
#22275=CARTESIAN_POINT ( 'NONE',  ( 6.204703633549690345, 47.84541550158064638, 14.16423886937410082 ) ) ;
#22276=CARTESIAN_POINT ( 'NONE',  ( 10.00000000000000178, 39.31368534415484106, 10.88017736071110342 ) ) ;
#22277=CARTESIAN_POINT ( 'NONE',  ( -0.1049300847420624322, 32.21697413083879269, -6.336235997365760042 ) ) ;
#22279=CARTESIAN_POINT ( 'NONE',  ( 1.472469842513823179, 21.42559781766745175, 4.923371831947296329 ) ) ;
#22280=CARTESIAN_POINT ( 'NONE',  ( 19.84674366389459266, 33.71726448433410894, -2.638427012816827677 ) ) ;
#22282=CARTESIAN_POINT ( 'NONE',  ( 17.20831665107776587, 47.88393115100078745, 7.208316651077764980 ) ) ;
#22284=CARTESIAN_POINT ( 'NONE',  ( 15.44008868035555793, 41.39701867748817676, -9.422509992056140149 ) ) ;
#22286=CARTESIAN_POINT ( 'NONE',  ( 13.43411237798105340, 55.58196800326374643, 12.81628187352647963 ) ) ;
#22288=EDGE_CURVE ( 'NONE', #31232, #51688, #60305, .T. ) ;
#22289=CARTESIAN_POINT ( 'NONE',  ( 14.92337183194729988, 4.342264484334117824, -8.527530157486177487 ) ) ;
#22290=CARTESIAN_POINT ( 'NONE',  ( 6.565887622018943937, 60.16530133659707502, 12.81628187352647430 ) ) ;
#22291=CARTESIAN_POINT ( 'NONE',  ( 19.42250999205614193, 5.147018677488171434, 5.440088680355555262 ) ) ;
#22292=CARTESIAN_POINT ( 'NONE',  ( 19.84674366389459266, 38.30059781766745175, 2.638427012816836559 ) ) ;
#22295=CARTESIAN_POINT ( 'NONE',  ( -2.266590686148945544, 41.38708216824729647, -7.082119434687050408 ) ) ;
#22296=CARTESIAN_POINT ( 'NONE',  ( 2.791683348922237240, 55.38393115100078745, -7.208316651077763204 ) ) ;
#22298=CARTESIAN_POINT ( 'NONE',  ( 7.084665262690076126, 32.02201867748816966, -10.88017736071110164 ) ) ;
#22299=EDGE_CURVE ( 'NONE', #1418, #61640, #28435, .T. ) ;
#22300=CARTESIAN_POINT ( 'NONE',  ( 19.84674366389459266, 3.717264484334118713, -2.638427012816827677 ) ) ;
#22304=CARTESIAN_POINT ( 'NONE',  ( 10.00000000000000000, 62.87363466993042493, -12.81628187352647608 ) ) ;
#22305=VERTEX_POINT ( 'NONE', #67315 ) ;
#22306=CARTESIAN_POINT ( 'NONE',  ( 10.00000000000000178, 2.258931151000784787, 9.846743663894594434 ) ) ;
#22308=CARTESIAN_POINT ( 'NONE',  ( 24.16423886937409904, 4.095415501580634832, 3.795296366450317205 ) ) ;
#22309=CARTESIAN_POINT ( 'NONE',  ( 17.20831665107776587, 7.883931151000784787, 7.208316651077764980 ) ) ;
#22310=CARTESIAN_POINT ( 'NONE',  ( 20.88017736071110875, 25.77201867748816966, -2.915334737309920765 ) ) ;
#22314=CARTESIAN_POINT ( 'NONE',  ( 0.5774900079438607392, 23.48035201082150536, 5.440088680355550821 ) ) ;
#22315=EDGE_LOOP ( 'NONE', ( #24287, #31511, #33362, #7941, #5966, #11215 ) ) ;
#22316=CARTESIAN_POINT ( 'NONE',  ( -0.8801773607111009756, 33.06368534415484106, 1.068504757029289695E-15 ) ) ;
#22318=ORIENTED_EDGE ( 'NONE', *, *, #9855, .T. ) ;
#22319=EDGE_LOOP ( 'NONE', ( #92932, #14861, #81947, #97585 ) ) ;
#22320=CARTESIAN_POINT ( 'NONE',  ( 3.591859063236763294, 18.29030133659708568, -11.09922568453595026 ) ) ;
#22321=CARTESIAN_POINT ( 'NONE',  ( 19.42250999205614548, 65.98035201082151957, -5.440088680355545492 ) ) ;
#22323=CARTESIAN_POINT ( 'NONE',  ( 10.00000000000000000, 21.81368534415484106, -10.88017736071110342 ) ) ;
#22325=CARTESIAN_POINT ( 'NONE',  ( 10.00000000000000000, 9.758931151000785675, -9.846743663894594434 ) ) ;
#22326=CARTESIAN_POINT ( 'NONE',  ( 20.88017736071110164, 30.35535201082151247, 2.915334737309930979 ) ) ;
#22327=EDGE_CURVE ( 'NONE', #48119, #58781, #53395, .T. ) ;
#22329=CARTESIAN_POINT ( 'NONE',  ( 19.38216949554541202, 60.99863466993042493, 9.382169495545424454 ) ) ;
#22330=CARTESIAN_POINT ( 'NONE',  ( 20.88017736071110519, 45.56368534415484106, 2.639326808657452039E-16 ) ) ;
#22331=CARTESIAN_POINT ( 'NONE',  ( -46.34323875807881166, 103.6109741468810483, -6.190393423093143888 ) ) ;
#22332=CARTESIAN_POINT ( 'NONE',  ( 10.00000000000000178, 50.37363466993042493, 12.81628187352647608 ) ) ;
#22333=CARTESIAN_POINT ( 'NONE',  ( 10.00000000000000000, 51.81368534415484106, -10.88017736071110342 ) ) ;
#22334=CARTESIAN_POINT ( 'NONE',  ( 3.591859063236763294, -1.709698663402913210, -11.09922568453595026 ) ) ;
#22335=PRESENTATION_STYLE_ASSIGNMENT (( #83811 ) ) ;
#22336=CARTESIAN_POINT ( 'NONE',  ( 17.20831665107776587, 14.13393115100078568, -7.208316651077762316 ) ) ;
#22337=CARTESIAN_POINT ( 'NONE',  ( 13.43411237798105340, 60.58196800326376064, 12.81628187352647963 ) ) ;
#22339=CARTESIAN_POINT ( 'NONE',  ( 0.1532563361054100626, 10.80059781766745175, -2.638427012816831230 ) ) ;
#22340=CARTESIAN_POINT ( 'NONE',  ( 21.09922568453594849, 6.206968003263753531, 6.408140936763242479 ) ) ;
#22342=CARTESIAN_POINT ( 'NONE',  ( 17.20831665107776587, 59.13393115100078745, -7.208316651077762316 ) ) ;
#22343=CARTESIAN_POINT ( 'NONE',  ( 7.084665262690076126, 39.10535201082150536, 10.88017736071109987 ) ) ;
#22344=CARTESIAN_POINT ( 'NONE',  ( 12.63842701281683034, 52.46726448433413026, 9.846743663894596210 ) ) ;
#22347=CARTESIAN_POINT ( 'NONE',  ( 17.20831665107776587, 24.13393115100078035, -7.208316651077762316 ) ) ;
#22348=CARTESIAN_POINT ( 'NONE',  ( 18.52753015748617571, 13.09226448433411960, 4.923371831947298993 ) ) ;
#22349=CARTESIAN_POINT ( 'NONE',  ( 10.00000000000000000, 2.873634669930420049, -12.81628187352647608 ) ) ;
#22351=CARTESIAN_POINT ( 'NONE',  ( 18.52753015748618282, 58.92559781766745886, -4.923371831947291888 ) ) ;
#22353=CARTESIAN_POINT ( 'NONE',  ( 2.917880565312948704, 67.63708216824730357, 12.26659068614894643 ) ) ;
#22354=CARTESIAN_POINT ( 'NONE',  ( 1.472469842513823179, 45.59226448433412315, -4.923371831947296329 ) ) ;
#22357=CARTESIAN_POINT ( 'NONE',  ( 18.72515096720591643, 66.07228050351029935, -6.499999999999699796 ) ) ;
#22358=CARTESIAN_POINT ( 'NONE',  ( 12.91533473730992121, 4.522018677488170546, 10.88017736071110164 ) ) ;
#22359=DIRECTION ( 'NONE',  ( -0.000000000000000000, -0.000000000000000000, -1.000000000000000000 ) ) ;
#22360=CARTESIAN_POINT ( 'NONE',  ( -0.8801773607111009756, 38.06368534415484106, 1.068504757029289695E-15 ) ) ;
#22361=CARTESIAN_POINT ( 'NONE',  ( 17.08211943468705840, 45.13708216824730357, -12.26659068614894466 ) ) ;
#22362=CARTESIAN_POINT ( 'NONE',  ( 2.035157376598824452, 3.688685344154837953, 7.964842623401179544 ) ) ;
#22364=CARTESIAN_POINT ( 'NONE',  ( 7.361572987183169658, 4.967264484334119601, -9.846743663894592657 ) ) ;
#22366=CARTESIAN_POINT ( 'NONE',  ( 19.84674366389459266, 28.30059781766745886, 2.638427012816836559 ) ) ;
#22367=CARTESIAN_POINT ( 'NONE',  ( 16.40814093676324603, 12.45696800326375353, -11.09922568453594671 ) ) ;
#22369=EDGE_CURVE ( 'NONE', #59748, #10735, #97840, .T. ) ;
#22370=DIRECTION ( 'NONE',  ( 1.000000000000000000, 0.000000000000000000, 0.000000000000000000 ) ) ;
#22371=CARTESIAN_POINT ( 'NONE',  ( 20.36894250292379738, 14.92874883491396432, -10.36894250292379027 ) ) ;
#22372=CARTESIAN_POINT ( 'NONE',  ( 2.791683348922240793, 26.63393115100078745, 7.208316651077764092 ) ) ;
#22375=CARTESIAN_POINT ( 'NONE',  ( 24.16423886937410614, 34.30374883491396787, 8.672049930838204340E-16 ) ) ;
#22378=CARTESIAN_POINT ( 'NONE',  ( 5.076628168052704559, 15.17559781766745175, -8.527530157486179263 ) ) ;
#22381=CARTESIAN_POINT ( 'NONE',  ( 15.44008868035555793, 31.39701867748817676, -9.422509992056140149 ) ) ;
#22382=CARTESIAN_POINT ( 'NONE',  ( 19.38216949554541557, 57.24863466993042493, -9.382169495545420901 ) ) ;
#22383=CARTESIAN_POINT ( 'NONE',  ( 10.00000000000000178, 9.313685344154839285, 10.88017736071110342 ) ) ;
#22384=CARTESIAN_POINT ( 'NONE',  ( 22.81628187352647785, 31.62363466993042138, 6.195893100308588602E-16 ) ) ;
#22385=SURFACE_SIDE_STYLE ('',( #52860 ) ) ;
#22389=CARTESIAN_POINT ( 'NONE',  ( 20.36894250292379738, 39.92874883491396787, -10.36894250292379027 ) ) ;
#22390=CARTESIAN_POINT ( 'NONE',  ( -4.164238869374099039, 11.80374883491396965, 8.674139862899312516E-16 ) ) ;
#22391=CARTESIAN_POINT ( 'NONE',  ( 20.88017736071110875, 10.77201867748817143, -2.915334737309920765 ) ) ;
#22392=CARTESIAN_POINT ( 'NONE',  ( 20.88017736071110164, 40.35535201082150536, 2.915334737309930979 ) ) ;
#22394=CARTESIAN_POINT ( 'NONE',  ( 13.99999999999999822, 11.50000000000000000, 6.000000000000000000 ) ) ;
#22395=CARTESIAN_POINT ( 'NONE',  ( 20.88017736071110519, 55.56368534415484817, 2.639326808657452039E-16 ) ) ;
#22396=CARTESIAN_POINT ( 'NONE',  ( 2.035157376598822676, 62.43868534415483396, -7.964842623401177768 ) ) ;
#22397=CARTESIAN_POINT ( 'NONE',  ( 21.09922568453594849, 21.20696800326375353, 6.408140936763242479 ) ) ;
#22398=CARTESIAN_POINT ( 'NONE',  ( -0.1023957841222421367, 30.13377557478298385, 6.340343622311920946 ) ) ;
#22399=CARTESIAN_POINT ( 'NONE',  ( 2.791683348922240793, 41.63393115100078745, 7.208316651077764092 ) ) ;
#22400=UNCERTAINTY_MEASURE_WITH_UNIT (LENGTH_MEASURE( 1.000000000000000082E-05 ), #69495, 'distance_accuracy_value', 'NONE');
#22402=CARTESIAN_POINT ( 'NONE',  ( 19.38216949554541202, 15.99863466993042138, 9.382169495545424454 ) ) ;
#22403=CARTESIAN_POINT ( 'NONE',  ( 1.274849032794223680, 28.57228050351031001, 6.499999999999884537 ) ) ;
#22404=CARTESIAN_POINT ( 'NONE',  ( 15.44008868035555260, 4.730352010821504471, 9.422509992056143702 ) ) ;
#22405=CARTESIAN_POINT ( 'NONE',  ( 18.52753015748618282, 38.92559781766745175, -4.923371831947291888 ) ) ;
#22406=CARTESIAN_POINT ( 'NONE',  ( 3.591859063236763294, 58.29030133659708923, -11.09922568453595026 ) ) ;
#22407=CARTESIAN_POINT ( 'NONE',  ( 10.00000000000000000, 14.75893115100078568, -9.846743663894594434 ) ) ;
#22408=CARTESIAN_POINT ( 'NONE',  ( 2.917880565312948704, 2.637082168247300906, 12.26659068614894643 ) ) ;
#22409=CARTESIAN_POINT ( 'NONE',  ( 18.72515096720568195, 31.07228050351032422, -6.500000000000018652 ) ) ;
#22410=CARTESIAN_POINT ( 'NONE',  ( 7.084665262690076126, 37.02201867748817676, -10.88017736071110164 ) ) ;
#22413=CARTESIAN_POINT ( 'NONE',  ( 4.559911319644449179, 32.23035201082150536, -9.422509992056141925 ) ) ;
#22414=CARTESIAN_POINT ( 'NONE',  ( 17.96484262340118221, 16.18868534415483396, -7.964842623401177768 ) ) ;
#22416=( BOUNDED_CURVE ( )  B_SPLINE_CURVE ( 2, ( #86223, #36910, #90881, #67402, #90380, #21918, #52397, #82896, #22409 ),
 .UNSPECIFIED., .F., .F. ) 
 B_SPLINE_CURVE_WITH_KNOTS ( ( 3, 2, 2, 2, 3 ),
 ( 0.4034289457926085731, 0.4047619047619047672, 0.4107142857142856984, 0.4166666666666666852, 0.4179996256359633233 ),
 .UNSPECIFIED. ) 
 CURVE ( )  GEOMETRIC_REPRESENTATION_ITEM ( )  RATIONAL_B_SPLINE_CURVE ( ( 0.9881565478350746723, 0.9923695281211503127, 1.000000000000000000, 0.9659258262890683122, 1.000000000000000000, 0.9659258262890683122, 1.000000000000000000, 0.9923695281211478703, 0.9881565478350720078 ) ) 
 REPRESENTATION_ITEM ( '' )  );
#22418=CARTESIAN_POINT ( 'NONE',  ( 10.00000000000000178, 24.31368534415484106, 10.88017736071110342 ) ) ;
#22419=CARTESIAN_POINT ( 'NONE',  ( 3.591859063236761518, 49.95696800326375353, 11.09922568453594849 ) ) ;
#22420=CARTESIAN_POINT ( 'NONE',  ( -0.8801773607111009756, 48.06368534415484817, 1.068504757029289695E-15 ) ) ;
#22422=CARTESIAN_POINT ( 'NONE',  ( 19.42250999205614548, 45.98035201082150536, -5.440088680355545492 ) ) ;
#22423=VERTEX_POINT ( 'NONE', #91792 ) ;
#22424=CARTESIAN_POINT ( 'NONE',  ( 17.20831665107776587, 57.88393115100078745, 7.208316651077764980 ) ) ;
#22425=CARTESIAN_POINT ( 'NONE',  ( 12.91533473730993009, 31.60535201082150891, -10.88017736071109987 ) ) ;
#22429=CARTESIAN_POINT ( 'NONE',  ( 6.204703633549690345, 47.84541550158064638, 14.16423886937410082 ) ) ;
#22430=CARTESIAN_POINT ( 'NONE',  ( 12.91533473730993009, 56.60535201082151247, -10.88017736071109987 ) ) ;
#22431=DIRECTION ( 'NONE',  ( 1.000000000000000000, 0.000000000000000000, 0.000000000000000000 ) ) ;
#22432=( NAMED_UNIT ( * ) SI_UNIT ( $, .STERADIAN. ) SOLID_ANGLE_UNIT ( ) );
#22433=CARTESIAN_POINT ( 'NONE',  ( 18.52753015748618282, 58.92559781766745886, -4.923371831947291888 ) ) ;
#22434=CARTESIAN_POINT ( 'NONE',  ( 7.084665262690076126, 4.105352010821503583, 10.88017736071109987 ) ) ;
#22435=CARTESIAN_POINT ( 'NONE',  ( 14.92337183194729633, 32.67559781766745175, 8.527530157486181039 ) ) ;
#22437=CARTESIAN_POINT ( 'NONE',  ( 19.84674366389459266, 33.71726448433410894, -2.638427012816827677 ) ) ;
#22439=CARTESIAN_POINT ( 'NONE',  ( -0.8801773607111008646, 28.27201867748817321, 2.915334737309923430 ) ) ;
#22440=CARTESIAN_POINT ( 'NONE',  ( 18.52753015748618282, 33.92559781766745886, -4.923371831947291888 ) ) ;
#22441=CARTESIAN_POINT ( 'NONE',  ( -2.816281873526473856, 19.12363466993042138, 9.499525473075851096E-16 ) ) ;
#22442=CARTESIAN_POINT ( 'NONE',  ( 13.99999999999999822, 11.50000000000000000, 6.500000000000000888 ) ) ;
#22443=CARTESIAN_POINT ( 'NONE',  ( 2.035157376598824452, 58.68868534415482685, 7.964842623401179544 ) ) ;
#22444=CARTESIAN_POINT ( 'NONE',  ( 20.88017736071110164, 35.35535201082150536, 2.915334737309930979 ) ) ;
#22445=CARTESIAN_POINT ( 'NONE',  ( 13.79529636645030344, 48.26208216824728936, 14.16423886937410614 ) ) ;
#22449=CARTESIAN_POINT ( 'NONE',  ( 3.591859063236761518, 19.95696800326375353, 11.09922568453594849 ) ) ;
#22450=CARTESIAN_POINT ( 'NONE',  ( -0.8801773607111009756, 3.063685344154837509, 1.068504757029289695E-15 ) ) ;
#22451=CARTESIAN_POINT ( 'NONE',  ( 17.96484262340118221, 41.18868534415484106, -7.964842623401177768 ) ) ;
#22452=FACE_OUTER_BOUND ( 'NONE', #5779, .T. ) ;
#22454=CARTESIAN_POINT ( 'NONE',  ( 12.91533473730993009, 56.60535201082151247, -10.88017736071109987 ) ) ;
#22455=CARTESIAN_POINT ( 'NONE',  ( 7.361572987183169658, 29.96726448433411960, -9.846743663894592657 ) ) ;
#22456=CARTESIAN_POINT ( 'NONE',  ( 7.361572987183170547, 27.05059781766745175, 9.846743663894590881 ) ) ;
#22457=CARTESIAN_POINT ( 'NONE',  ( 7.361572987183169658, 14.96726448433411960, -9.846743663894592657 ) ) ;
#22459=CARTESIAN_POINT ( 'NONE',  ( 22.81628187352647785, 41.62363466993042493, 6.195893100308588602E-16 ) ) ;
#22460=CARTESIAN_POINT ( 'NONE',  ( 18.52753015748617571, 13.09226448433411960, 4.923371831947298993 ) ) ;
#22463=CARTESIAN_POINT ( 'NONE',  ( 17.20831665107776587, 27.88393115100078390, 7.208316651077764980 ) ) ;
#22466=CARTESIAN_POINT ( 'NONE',  ( -2.816281873526473856, 14.12363466993041961, 9.499525473075851096E-16 ) ) ;
#22467=CARTESIAN_POINT ( 'NONE',  ( 12.91533473730993009, 51.60535201082149825, -10.88017736071109987 ) ) ;
#22468=CARTESIAN_POINT ( 'NONE',  ( 13.79529636645030344, 28.26208216824729647, 14.16423886937410614 ) ) ;
#22472=CARTESIAN_POINT ( 'NONE',  ( 24.16423886937410614, 34.51208216824731068, -3.795296366450302550 ) ) ;
#22474=CARTESIAN_POINT ( 'NONE',  ( 22.26659068614895176, 44.72041550158063927, -7.082119434687042414 ) ) ;
#22475=CARTESIAN_POINT ( 'NONE',  ( -2.266590686148945544, 7.220415501580634832, 7.082119434687048631 ) ) ;
#22476=CARTESIAN_POINT ( 'NONE',  ( 10.00000000000000178, 23.05374883491397142, 14.16423886937410082 ) ) ;
#22478=CARTESIAN_POINT ( 'NONE',  ( 12.91533473730993009, 51.60535201082149825, -10.88017736071109987 ) ) ;
#22480=CARTESIAN_POINT ( 'NONE',  ( 0.1532563361054100626, 35.80059781766745175, -2.638427012816831230 ) ) ;
#22483=CARTESIAN_POINT ( 'NONE',  ( 19.84674366389459266, 48.30059781766745175, 2.638427012816836559 ) ) ;
#22485=CARTESIAN_POINT ( 'NONE',  ( -0.8801773607110991993, 17.85535201082150536, -2.915334737309923874 ) ) ;
#22486=CARTESIAN_POINT ( 'NONE',  ( -1.099225684535947600, 54.54030133659708923, 6.408140936763237150 ) ) ;
#22487=CARTESIAN_POINT ( 'NONE',  ( 18.52753015748617571, 63.09226448433412315, 4.923371831947298993 ) ) ;
#22488=CARTESIAN_POINT ( 'NONE',  ( 20.00000000000000711, 81.00008901408247652, -4.500000004388789776 ) ) ;
#22489=CARTESIAN_POINT ( 'NONE',  ( 0.1532563361054100626, 25.80059781766744820, -2.638427012816831230 ) ) ;
#22490=CARTESIAN_POINT ( 'NONE',  ( 10.00000000000000000, 52.87363466993041783, -12.81628187352647608 ) ) ;
#22492=CARTESIAN_POINT ( 'NONE',  ( 19.42250999205614193, 45.14701867748817676, 5.440088680355555262 ) ) ;
#22493=CARTESIAN_POINT ( 'NONE',  ( 19.84674366389459266, 53.30059781766744464, 2.638427012816836559 ) ) ;
#22495=CARTESIAN_POINT ( 'NONE',  ( -2.266590686148945544, 41.38708216824729647, -7.082119434687050408 ) ) ;
#22497=CARTESIAN_POINT ( 'NONE',  ( 2.917880565312948704, 2.637082168247300906, 12.26659068614894643 ) ) ;
#22498=EDGE_CURVE ( 'NONE', #10866, #47816, #59800, .T. ) ;
#22499=CARTESIAN_POINT ( 'NONE',  ( 10.00000000000000000, 56.81368534415484106, -10.88017736071110342 ) ) ;
#22500=CARTESIAN_POINT ( 'NONE',  ( 10.00000000000000000, 66.81368534415484817, -10.88017736071110342 ) ) ;
#22501=CARTESIAN_POINT ( 'NONE',  ( 17.08211943468705840, 55.13708216824731068, -12.26659068614894466 ) ) ;
#22502=CARTESIAN_POINT ( 'NONE',  ( 22.81628187352648496, 11.83196800326375531, -3.434112377981050290 ) ) ;
#22504=CARTESIAN_POINT ( 'NONE',  ( -0.8801773607111009756, 48.06368534415484817, 1.068504757029289695E-15 ) ) ;
#22506=DIRECTION ( 'NONE',  ( -1.000000000000000000, 0.000000000000000000, 0.000000000000000000 ) ) ;
#22507=CARTESIAN_POINT ( 'NONE',  ( 20.36894250292379382, 53.67874883491397497, 10.36894250292379205 ) ) ;
#22509=CARTESIAN_POINT ( 'NONE',  ( 2.035157376598822676, 12.43868534415483751, -7.964842623401177768 ) ) ;
#22510=CARTESIAN_POINT ( 'NONE',  ( 12.91533473730992121, 24.52201867748816966, 10.88017736071110164 ) ) ;
#22511=CARTESIAN_POINT ( 'NONE',  ( 7.361572987183169658, 59.96726448433410894, -9.846743663894592657 ) ) ;
#22512=CARTESIAN_POINT ( 'NONE',  ( -2.816281873526473856, 44.33196800326375353, 3.434112377981055619 ) ) ;
#22513=CARTESIAN_POINT ( 'NONE',  ( 19.72487221294571214, 37.80223176428831522, -6.499999999999988454 ) ) ;
#22515=CARTESIAN_POINT ( 'NONE',  ( -0.8801773607111008646, 13.27201867748817143, 2.915334737309923430 ) ) ;
#22516=CARTESIAN_POINT ( 'NONE',  ( -2.816281873526473856, 14.12363466993041961, 9.499525473075851096E-16 ) ) ;
#22518=VECTOR ( 'NONE', #3438, 1000.000000000000000 ) ;
#22519=CARTESIAN_POINT ( 'NONE',  ( 17.20831665107776587, 54.13393115100079456, -7.208316651077762316 ) ) ;
#22520=CARTESIAN_POINT ( 'NONE',  ( 20.88017736071110519, 35.56368534415484106, 2.639326808657452039E-16 ) ) ;
#22521=CARTESIAN_POINT ( 'NONE',  ( -1.099225684535947600, 19.54030133659708568, 6.408140936763237150 ) ) ;
#22522=CARTESIAN_POINT ( 'NONE',  ( 4.559911319644449179, 48.89701867748817676, 9.422509992056141925 ) ) ;
#22524=CARTESIAN_POINT ( 'NONE',  ( 18.72515096720571037, 55.05509018479936145, 6.499999999999982236 ) ) ;
#22525=CARTESIAN_POINT ( 'NONE',  ( -2.816281873526473856, 54.12363466993041783, 9.499525473075851096E-16 ) ) ;
#22526=ORIENTED_EDGE ( 'NONE', *, *, #44244, .F. ) ;
#22528=CARTESIAN_POINT ( 'NONE',  ( 10.00000000000000000, 46.81368534415484106, -10.88017736071110342 ) ) ;
#22529=CARTESIAN_POINT ( 'NONE',  ( 0.6178305044545818747, 33.49863466993042493, -9.382169495545419124 ) ) ;
#22530=CARTESIAN_POINT ( 'NONE',  ( 10.00000000000000000, 5.553748834913967869, -14.16423886937410082 ) ) ;
#22532=CARTESIAN_POINT ( 'NONE',  ( 4.559911319644449179, 57.23035201082150536, -9.422509992056141925 ) ) ;
#22533=CARTESIAN_POINT ( 'NONE',  ( 6.204703633549690345, 45.76208216824729647, -14.16423886937410259 ) ) ;
#22535=CARTESIAN_POINT ( 'NONE',  ( 19.84674366389459266, 13.30059781766745353, 2.638427012816836559 ) ) ;
#22536=CARTESIAN_POINT ( 'NONE',  ( 12.63842701281683922, 4.550597817667451750, -9.846743663894590881 ) ) ;
#22537=CARTESIAN_POINT ( 'NONE',  ( 2.599899806584774264, 0.4361964623231012195, -6.495912400107028084 ) ) ;
#22538=CARTESIAN_POINT ( 'NONE',  ( 17.08211943468705840, 45.13708216824730357, -12.26659068614894466 ) ) ;
#22540=CARTESIAN_POINT ( 'NONE',  ( 20.24186590665278018, 25.59014588040357197, -6.114288769123027656 ) ) ;
#22542=AXIS2_PLACEMENT_3D ( 'NONE', #18564, #18075, #93072 ) ;
#22545=CARTESIAN_POINT ( 'NONE',  ( 2.035157376598822676, 12.43868534415483751, -7.964842623401177768 ) ) ;
#22546=CARTESIAN_POINT ( 'NONE',  ( -2.266590686148945544, 57.22041550158063217, 7.082119434687048631 ) ) ;
#22547=CARTESIAN_POINT ( 'NONE',  ( 19.84674366389459266, 48.30059781766745175, 2.638427012816836559 ) ) ;
#22548=CARTESIAN_POINT ( 'NONE',  ( 19.38216949554541202, 40.99863466993042493, 9.382169495545424454 ) ) ;
#22551=CARTESIAN_POINT ( 'NONE',  ( 6.204703633549690345, 0.7620821682473009062, -14.16423886937410259 ) ) ;
#22552=CARTESIAN_POINT ( 'NONE',  ( 10.00000000000000000, 6.813685344154838397, -10.88017736071110342 ) ) ;
#22553=CARTESIAN_POINT ( 'NONE',  ( -0.3689425029237898834, 61.17874883491396076, -10.36894250292378850 ) ) ;
#22554=CARTESIAN_POINT ( 'NONE',  ( 7.361572987183170547, 42.05059781766745886, 9.846743663894590881 ) ) ;
#22556=CARTESIAN_POINT ( 'NONE',  ( 0.1532563361054100626, 20.80059781766744464, -2.638427012816831230 ) ) ;
#22558=( LENGTH_UNIT ( ) NAMED_UNIT ( * ) SI_UNIT ( .MILLI., .METRE. ) );
#22562=FILL_AREA_STYLE_COLOUR ( '', #73331 ) ;
#22563=ORIENTED_EDGE ( 'NONE', *, *, #52791, .T. ) ;
#22564=CARTESIAN_POINT ( 'NONE',  ( 10.00000000000000178, 62.25893115100078745, 9.846743663894594434 ) ) ;
#22565=CARTESIAN_POINT ( 'NONE',  ( -0.8801773607111008646, 33.27201867748817676, 2.915334737309923430 ) ) ;
#22566=CARTESIAN_POINT ( 'NONE',  ( 12.91533473730993009, 36.60535201082151247, -10.88017736071109987 ) ) ;
#22567=CARTESIAN_POINT ( 'NONE',  ( 10.00000000000000178, 67.25893115100079456, 9.846743663894594434 ) ) ;
#22568=CARTESIAN_POINT ( 'NONE',  ( 22.81628187352647785, 31.41530133659709279, 3.434112377981063169 ) ) ;
#22569=CARTESIAN_POINT ( 'NONE',  ( 20.36894250292379738, 9.928748834913966093, -10.36894250292379027 ) ) ;
#22570=CARTESIAN_POINT ( 'NONE',  ( 3.591859063236761518, 39.95696800326375353, 11.09922568453594849 ) ) ;
#22571=ORIENTED_EDGE ( 'NONE', *, *, #63228, .T. ) ;
#22572=CARTESIAN_POINT ( 'NONE',  ( 17.20831665107776587, 47.88393115100078745, 7.208316651077764980 ) ) ;
#22573=CARTESIAN_POINT ( 'NONE',  ( -4.164238869374099927, 67.01208216824728936, 3.795296366450308767 ) ) ;
#22575=CARTESIAN_POINT ( 'NONE',  ( 15.44008868035555793, 21.39701867748817321, -9.422509992056140149 ) ) ;
#22577=CARTESIAN_POINT ( 'NONE',  ( 19.42250999205614193, 55.14701867748817676, 5.440088680355555262 ) ) ;
#22578=CARTESIAN_POINT ( 'NONE',  ( -0.8801773607111008646, 58.27201867748816966, 2.915334737309923430 ) ) ;
#22579=CARTESIAN_POINT ( 'NONE',  ( 4.559911319644449179, 58.89701867748817676, 9.422509992056141925 ) ) ;
#22581=CARTESIAN_POINT ( 'NONE',  ( 19.42250999205614193, 50.14701867748817676, 5.440088680355555262 ) ) ;
#22584=EDGE_CURVE ( 'NONE', #76576, #18416, #93260, .T. ) ;
#22587=STYLED_ITEM ( 'NONE', ( #9846 ), #80415 ) ;
#22588=CARTESIAN_POINT ( 'NONE',  ( 19.84674366389459266, 48.30059781766745175, 2.638427012816836559 ) ) ;
#22590=DIRECTION ( 'NONE',  ( 0.000000000000000000, 0.000000000000000000, -1.000000000000000000 ) ) ;
#22592=CARTESIAN_POINT ( 'NONE',  ( 24.16423886937410614, 9.512082168247301794, -3.795296366450302550 ) ) ;
#22593=CARTESIAN_POINT ( 'NONE',  ( -0.1503990784575321704, 8.101585745166424601, 6.262539305110068177 ) ) ;
#22594=CARTESIAN_POINT ( 'NONE',  ( 0.5774900079438590739, 2.647018677488171434, -5.440088680355550821 ) ) ;
#22595=CARTESIAN_POINT ( 'NONE',  ( 1.274849032794280523, 48.57228050351032067, 6.499999999999960032 ) ) ;
#22596=CARTESIAN_POINT ( 'NONE',  ( 0.6178305044545818747, 43.49863466993042493, -9.382169495545419124 ) ) ;
#22597=ORIENTED_EDGE ( 'NONE', *, *, #5887, .F. ) ;
#22598=CARTESIAN_POINT ( 'NONE',  ( 10.00000000000000178, 70.00000000000000000, 0.000000000000000000 ) ) ;
#22599=CARTESIAN_POINT ( 'NONE',  ( 14.92337183194729633, 47.67559781766745175, 8.527530157486181039 ) ) ;
#22601=CARTESIAN_POINT ( 'NONE',  ( 0.1532563361054083140, 1.008931151000784787, 1.131784320476157264E-15 ) ) ;
#22602=CARTESIAN_POINT ( 'NONE',  ( 3.591859063236761518, 14.95696800326375531, 11.09922568453594849 ) ) ;
#22603=CARTESIAN_POINT ( 'NONE',  ( 19.84674366389459621, 23.50893115100078390, 7.409399052514197653E-17 ) ) ;
#22604=CARTESIAN_POINT ( 'NONE',  ( 2.791683348922237240, 20.38393115100078745, -7.208316651077763204 ) ) ;
#22605=CARTESIAN_POINT ( 'NONE',  ( 22.81628187352647785, 1.623634669930420271, 6.195893100308588602E-16 ) ) ;
#22612=CARTESIAN_POINT ( 'NONE',  ( 4.559911319644449179, 18.89701867748817321, 9.422509992056141925 ) ) ;
#22613=CARTESIAN_POINT ( 'NONE',  ( 22.26659068614894466, 13.88708216824730179, 7.082119434687054849 ) ) ;
#22614=CARTESIAN_POINT ( 'NONE',  ( 7.361572987183170547, 27.05059781766745175, 9.846743663894590881 ) ) ;
#22615=CARTESIAN_POINT ( 'NONE',  ( 5.076628168052704559, 5.175597817667451750, -8.527530157486179263 ) ) ;
#22617=CARTESIAN_POINT ( 'NONE',  ( 21.09922568453594849, 41.20696800326375353, 6.408140936763242479 ) ) ;
#22619=CARTESIAN_POINT ( 'NONE',  ( 0.5774900079438590739, 17.64701867748817321, -5.440088680355550821 ) ) ;
#22620=LINE ( 'NONE', #53097, #77329 ) ;
#22621=CARTESIAN_POINT ( 'NONE',  ( 13.43411237798106583, 2.665301336597086568, -12.81628187352647252 ) ) ;
#22622=CARTESIAN_POINT ( 'NONE',  ( 19.84674366389459266, 23.71726448433412315, -2.638427012816827677 ) ) ;
#22624=CARTESIAN_POINT ( 'NONE',  ( 0.6178305044545838731, 39.74863466993041072, 9.382169495545420901 ) ) ;
#22627=CARTESIAN_POINT ( 'NONE',  ( 20.88017736071110164, 40.35535201082150536, 2.915334737309930979 ) ) ;
#22631=CARTESIAN_POINT ( 'NONE',  ( 15.44008868035555260, 44.73035201082151247, 9.422509992056143702 ) ) ;
#22632=CARTESIAN_POINT ( 'NONE',  ( -0.8801773607111008646, 38.27201867748816255, 2.915334737309923430 ) ) ;
#22633=CARTESIAN_POINT ( 'NONE',  ( 20.03932841506541607, 60.62161441960504504, -6.397827110479004986 ) ) ;
#22634=CARTESIAN_POINT ( 'NONE',  ( -0.8801773607111009756, 63.06368534415484106, 1.068504757029289695E-15 ) ) ;
#22635=CARTESIAN_POINT ( 'NONE',  ( 1.472469842513823179, 55.59226448433412315, -4.923371831947296329 ) ) ;
#22636=CARTESIAN_POINT ( 'NONE',  ( -0.8801773607110991993, 7.855352010821504471, -2.915334737309923874 ) ) ;
#22637=FACE_OUTER_BOUND ( 'NONE', #53774, .T. ) ;
#22638=CARTESIAN_POINT ( 'NONE',  ( 22.81628187352648496, 6.831968003263753531, -3.434112377981050290 ) ) ;
#22640=CARTESIAN_POINT ( 'NONE',  ( 7.084665262690076126, 44.10535201082151247, 10.88017736071109987 ) ) ;
#22641=CARTESIAN_POINT ( 'NONE',  ( 10.00000000000000178, 67.25893115100079456, 9.846743663894594434 ) ) ;
#22642=CARTESIAN_POINT ( 'NONE',  ( 18.95785429995052596, 7.242161081720063009, 6.499999999999870326 ) ) ;
#22644=CARTESIAN_POINT ( 'NONE',  ( 7.084665262690076126, 29.10535201082150181, 10.88017736071109987 ) ) ;
#22645=CARTESIAN_POINT ( 'NONE',  ( 0.1532563361054082862, 16.21726448433411960, 2.638427012816831674 ) ) ;
#22646=CARTESIAN_POINT ( 'NONE',  ( 22.26659068614894466, 33.88708216824730357, 7.082119434687054849 ) ) ;
#22647=CARTESIAN_POINT ( 'NONE',  ( 5.076628168052703671, 26.84226448433411960, 8.527530157486179263 ) ) ;
#22648=CARTESIAN_POINT ( 'NONE',  ( 20.88017736071110519, 40.56368534415484106, 2.639326808657452039E-16 ) ) ;
#22649=CARTESIAN_POINT ( 'NONE',  ( -0.1038446121089033197, 34.24302437010793909, -6.337995344473782211 ) ) ;
#22650=CARTESIAN_POINT ( 'NONE',  ( 24.16423886937410614, 9.303748834913967869, 8.672049930838204340E-16 ) ) ;
#22652=B_SPLINE_CURVE_WITH_KNOTS ( 'NONE', 3,
 ( #67013, #97534, #83500, #60491 ),
 .UNSPECIFIED., .F., .F.,
 ( 4, 4 ),
 ( 2.478060227011367563E-17, 0.002392975128318452962 ),
 .UNSPECIFIED. ) ;
#22654=CARTESIAN_POINT ( 'NONE',  ( 12.63842701281683922, 54.55059781766745175, -9.846743663894590881 ) ) ;
#22658=CARTESIAN_POINT ( 'NONE',  ( 2.917880565312950480, 25.97041550158063572, -12.26659068614894821 ) ) ;
#22659=CARTESIAN_POINT ( 'NONE',  ( 2.917880565312950480, 25.97041550158063572, -12.26659068614894821 ) ) ;
#22660=CARTESIAN_POINT ( 'NONE',  ( 10.00000000000000000, 9.758931151000785675, -9.846743663894594434 ) ) ;
#22661=CARTESIAN_POINT ( 'NONE',  ( 24.16423886937409904, 64.09541550158064638, 3.795296366450317205 ) ) ;
#22662=CARTESIAN_POINT ( 'NONE',  ( 0.6178305044545838731, 9.748634669930416052, 9.382169495545420901 ) ) ;
#22663=CARTESIAN_POINT ( 'NONE',  ( 14.92337183194729633, 52.67559781766745175, 8.527530157486181039 ) ) ;
#22665=CARTESIAN_POINT ( 'NONE',  ( 17.96484262340118221, 39.93868534415484106, 7.964842623401181321 ) ) ;
#22666=CARTESIAN_POINT ( 'NONE',  ( 21.09922568453595559, 17.04030133659708923, -6.408140936763230044 ) ) ;
#22667=CARTESIAN_POINT ( 'NONE',  ( -4.164238869374098151, 11.59541550158063217, -3.795296366450310543 ) ) ;
#22668=CARTESIAN_POINT ( 'NONE',  ( 0.5774900079438590739, 12.64701867748817321, -5.440088680355550821 ) ) ;
#22669=CARTESIAN_POINT ( 'NONE',  ( 2.035157376598822676, 27.43868534415483396, -7.964842623401177768 ) ) ;
#22670=CARTESIAN_POINT ( 'NONE',  ( -0.8801773607111009756, 53.06368534415484106, 1.068504757029289695E-15 ) ) ;
#22671=CARTESIAN_POINT ( 'NONE',  ( 16.40814093676323893, 50.79030133659708923, 11.09922568453595026 ) ) ;
#22674=CARTESIAN_POINT ( 'NONE',  ( 20.04068437667225311, 34.71974360917721469, 6.396802510829709298 ) ) ;
#22676=ORIENTED_EDGE ( 'NONE', *, *, #87309, .T. ) ;
#22677=CARTESIAN_POINT ( 'NONE',  ( 0.1955144967548954060, 19.32703681773340421, -6.500000000002791545 ) ) ;
#22678=CARTESIAN_POINT ( 'NONE',  ( 24.16423886937410614, 59.51208216824728936, -3.795296366450302550 ) ) ;
#22679=CARTESIAN_POINT ( 'NONE',  ( 10.00000000000000178, 68.05374883491397497, 14.16423886937410082 ) ) ;
#22680=CARTESIAN_POINT ( 'NONE',  ( 5.076628168052703671, 21.84226448433411960, 8.527530157486179263 ) ) ;
#22681=CARTESIAN_POINT ( 'NONE',  ( 2.791683348922237240, 55.38393115100078745, -7.208316651077763204 ) ) ;
#22682=CARTESIAN_POINT ( 'NONE',  ( 14.49999999999999822, 60.50000000000000711, -6.000000000000000000 ) ) ;
#22683=CARTESIAN_POINT ( 'NONE',  ( 20.15039907845753220, 44.72266099184918176, 6.262539305110078836 ) ) ;
#22684=CARTESIAN_POINT ( 'NONE',  ( 14.92337183194729988, 9.342264484334119601, -8.527530157486177487 ) ) ;
#22686=( GEOMETRIC_REPRESENTATION_CONTEXT ( 3 ) GLOBAL_UNCERTAINTY_ASSIGNED_CONTEXT ( ( #98150 ) ) GLOBAL_UNIT_ASSIGNED_CONTEXT ( ( #7931, #53913, #91909 ) ) REPRESENTATION_CONTEXT ( 'NONE', 'WORKASPACE' ) );
#22690=CARTESIAN_POINT ( 'NONE',  ( 13.79529636645031943, 30.34541550158063927, -14.16423886937409904 ) ) ;
#22691=CARTESIAN_POINT ( 'NONE',  ( 10.00000000000000178, 48.05374883491396787, 14.16423886937410082 ) ) ;
#22693=CARTESIAN_POINT ( 'NONE',  ( -1.099225684535947600, 63.70696800326376774, -6.408140936763238038 ) ) ;
#22694=CARTESIAN_POINT ( 'NONE',  ( 19.42250999205614548, 25.98035201082150891, -5.440088680355545492 ) ) ;
#22695=CARTESIAN_POINT ( 'NONE',  ( 1.472469842513823179, 56.42559781766745886, 4.923371831947296329 ) ) ;
#22696=CARTESIAN_POINT ( 'NONE',  ( 17.96484262340118221, 19.93868534415484106, 7.964842623401181321 ) ) ;
#22700=CARTESIAN_POINT ( 'NONE',  ( 5.076628168052704559, 55.17559781766745175, -8.527530157486179263 ) ) ;
#22701=CARTESIAN_POINT ( 'NONE',  ( 14.92337183194729988, 44.34226448433412315, -8.527530157486177487 ) ) ;
#22705=CARTESIAN_POINT ( 'NONE',  ( 18.52753015748617571, 8.092264484334117824, 4.923371831947298993 ) ) ;
#22708=CARTESIAN_POINT ( 'NONE',  ( 7.361572987183169658, 34.96726448433411605, -9.846743663894592657 ) ) ;
#22709=LINE ( 'NONE', #69674, #21316 ) ;
#22710=CARTESIAN_POINT ( 'NONE',  ( 16.40814093676323893, 40.79030133659708923, 11.09922568453595026 ) ) ;
#22714=CARTESIAN_POINT ( 'NONE',  ( 10.00000000000000178, 42.25893115100078745, 9.846743663894594434 ) ) ;
#22715=CARTESIAN_POINT ( 'NONE',  ( 24.16423886937410614, 29.30374883491396787, 8.672049930838204340E-16 ) ) ;
#22716=CARTESIAN_POINT ( 'NONE',  ( 0.1532563361054082862, 46.21726448433411605, 2.638427012816831674 ) ) ;
#22718=CARTESIAN_POINT ( 'NONE',  ( 1.472469842513823179, 5.592264484334118713, -4.923371831947296329 ) ) ;
#22719=PRESENTATION_STYLE_ASSIGNMENT (( #31180 ) ) ;
#22720=CARTESIAN_POINT ( 'NONE',  ( 14.92337183194729988, 49.34226448433411605, -8.527530157486177487 ) ) ;
#22721=CARTESIAN_POINT ( 'NONE',  ( 2.035157376598822676, 52.43868534415483396, -7.964842623401177768 ) ) ;
#22722=CARTESIAN_POINT ( 'NONE',  ( 18.52753015748617571, 38.09226448433412315, 4.923371831947298993 ) ) ;
#22725=EDGE_CURVE ( 'NONE', #13373, #91555, #55689, .T. ) ;
#22726=CARTESIAN_POINT ( 'NONE',  ( -0.8801773607111009756, 48.06368534415484817, 1.068504757029289695E-15 ) ) ;
#22727=EDGE_LOOP ( 'NONE', ( #48673, #52691, #63192, #5836, #58292 ) ) ;
#22730=CARTESIAN_POINT ( 'NONE',  ( 12.91533473730992121, 29.52201867748817321, 10.88017736071110164 ) ) ;
#22731=CARTESIAN_POINT ( 'NONE',  ( 0.6178305044545818747, -1.501365330069579951, -9.382169495545419124 ) ) ;
#22732=CARTESIAN_POINT ( 'NONE',  ( 12.91533473730993009, 46.60535201082150536, -10.88017736071109987 ) ) ;
#22734=CARTESIAN_POINT ( 'NONE',  ( 20.03932841506542673, 10.62161441960501307, -6.397827110478957913 ) ) ;
#22735=CARTESIAN_POINT ( 'NONE',  ( 18.72515096720568195, 21.07228050351032422, -6.500000000000018652 ) ) ;
#22736=CARTESIAN_POINT ( 'NONE',  ( -0.8801773607111008646, 38.27201867748816255, 2.915334737309923430 ) ) ;
#22737=CARTESIAN_POINT ( 'NONE',  ( 20.00000000000000711, 96.99160806218867492, -4.500000000000000888 ) ) ;
#22738=CARTESIAN_POINT ( 'NONE',  ( 14.92337183194729988, 14.34226448433411782, -8.527530157486177487 ) ) ;
#22739=CARTESIAN_POINT ( 'NONE',  ( 10.00000000000000178, 37.25893115100078745, 9.846743663894594434 ) ) ;
#22740=CARTESIAN_POINT ( 'NONE',  ( 20.10239578412224404, 57.63377557478296609, -6.340343622311915617 ) ) ;
#22742=CARTESIAN_POINT ( 'NONE',  ( 17.20831665107776587, 62.88393115100078745, 7.208316651077764980 ) ) ;
#22743=CARTESIAN_POINT ( 'NONE',  ( 20.36894250292379738, 64.92874883491397497, -10.36894250292379027 ) ) ;
#22745=CARTESIAN_POINT ( 'NONE',  ( -4.164238869374098151, 21.59541550158063217, -3.795296366450310543 ) ) ;
#22746=CARTESIAN_POINT ( 'NONE',  ( 20.36894250292379738, 49.92874883491396787, -10.36894250292379027 ) ) ;
#22747=CARTESIAN_POINT ( 'NONE',  ( 0.1532563361054083140, 16.00893115100078390, 1.131784320476157264E-15 ) ) ;
#22749=CARTESIAN_POINT ( 'NONE',  ( 0.1532563361054100626, 20.80059781766744464, -2.638427012816831230 ) ) ;
#22750=CARTESIAN_POINT ( 'NONE',  ( 12.91533473730993009, 26.60535201082150536, -10.88017736071109987 ) ) ;
#22751=CARTESIAN_POINT ( 'NONE',  ( 7.361572987183169658, 54.96726448433413026, -9.846743663894592657 ) ) ;
#22752=CARTESIAN_POINT ( 'NONE',  ( -4.164238869374099927, 12.01208216824730357, 3.795296366450308767 ) ) ;
#22756=CARTESIAN_POINT ( 'NONE',  ( 10.00000000000000178, 12.25893115100078568, 9.846743663894594434 ) ) ;
#22757=CARTESIAN_POINT ( 'NONE',  ( 0.6178305044545818747, 33.49863466993042493, -9.382169495545419124 ) ) ;
#22758=CARTESIAN_POINT ( 'NONE',  ( 19.84674366389459621, 38.50893115100078745, 7.409399052514197653E-17 ) ) ;
#22760=CARTESIAN_POINT ( 'NONE',  ( 1.472469842513823179, 26.42559781766745175, 4.923371831947296329 ) ) ;
#22761=VECTOR ( 'NONE', #93601, 1000.000000000000000 ) ;
#22764=CARTESIAN_POINT ( 'NONE',  ( -2.266590686148945544, 56.38708216824731068, -7.082119434687050408 ) ) ;
#22765=CARTESIAN_POINT ( 'NONE',  ( 19.42250999205614548, 45.98035201082150536, -5.440088680355545492 ) ) ;
#22767=CARTESIAN_POINT ( 'NONE',  ( 7.361572987183169658, 39.96726448433411605, -9.846743663894592657 ) ) ;
#22768=CARTESIAN_POINT ( 'NONE',  ( -0.8801773607111008646, 13.27201867748817143, 2.915334737309923430 ) ) ;
#22769=CARTESIAN_POINT ( 'NONE',  ( 10.00000000000000000, 39.75893115100078745, -9.846743663894594434 ) ) ;
#22772=CARTESIAN_POINT ( 'NONE',  ( 0.1532563361054083140, 51.00893115100078745, 1.131784320476157264E-15 ) ) ;
#22773=B_SPLINE_CURVE_WITH_KNOTS ( 'NONE', 3,
 ( #3776, #34731, #65222, #95749 ),
 .UNSPECIFIED., .F., .F.,
 ( 4, 4 ),
 ( 6.254634441385501517E-18, 0.002392975128318428676 ),
 .UNSPECIFIED. ) ;
#22775=CARTESIAN_POINT ( 'NONE',  ( 10.00000000000000178, 54.31368534415484106, 10.88017736071110342 ) ) ;
#22778=CARTESIAN_POINT ( 'NONE',  ( -2.816281873526473856, 54.12363466993041783, 9.499525473075851096E-16 ) ) ;
#22780=CARTESIAN_POINT ( 'NONE',  ( 18.52753015748617571, 13.09226448433411960, 4.923371831947298993 ) ) ;
#22781=CARTESIAN_POINT ( 'NONE',  ( -2.816281873526471635, 58.91530133659707502, -3.434112377981056508 ) ) ;
#22782=CARTESIAN_POINT ( 'NONE',  ( 10.00000000000000178, 9.313685344154839285, 10.88017736071110342 ) ) ;
#22783=CARTESIAN_POINT ( 'NONE',  ( 18.52753015748618282, 48.92559781766745886, -4.923371831947291888 ) ) ;
#22784=CARTESIAN_POINT ( 'NONE',  ( 20.00000000000000355, 95.40264689492315142, 4.636598376030806712 ) ) ;
#22785=CARTESIAN_POINT ( 'NONE',  ( 0.1532563361054082862, 1.217264484334117824, 2.638427012816831674 ) ) ;
#22786=CARTESIAN_POINT ( 'NONE',  ( 10.00000000000000000, 25.55374883491396787, -14.16423886937410082 ) ) ;
#22787=CARTESIAN_POINT ( 'NONE',  ( 24.16423886937410614, 44.30374883491397497, 8.672049930838204340E-16 ) ) ;
#22788=CARTESIAN_POINT ( 'NONE',  ( 18.52753015748618282, 58.92559781766745886, -4.923371831947291888 ) ) ;
#22790=CARTESIAN_POINT ( 'NONE',  ( -0.8801773607110991993, 47.85535201082150536, -2.915334737309923874 ) ) ;
#22791=CARTESIAN_POINT ( 'NONE',  ( 2.791683348922240793, 1.633931151000784565, 7.208316651077764092 ) ) ;
#22794=CARTESIAN_POINT ( 'NONE',  ( 21.09922568453594849, 61.20696800326376064, 6.408140936763242479 ) ) ;
#22795=CARTESIAN_POINT ( 'NONE',  ( 10.00000000000000000, 4.758931151000784787, -9.846743663894594434 ) ) ;
#22796=ORIENTED_EDGE ( 'NONE', *, *, #89716, .T. ) ;
#22797=CARTESIAN_POINT ( 'NONE',  ( 22.26659068614895176, 14.72041550158063572, -7.082119434687042414 ) ) ;
#22798=CARTESIAN_POINT ( 'NONE',  ( 5.076628168052704559, 15.17559781766745175, -8.527530157486179263 ) ) ;
#22799=CARTESIAN_POINT ( 'NONE',  ( 12.91533473730992121, 34.52201867748817676, 10.88017736071110164 ) ) ;
#22802=CARTESIAN_POINT ( 'NONE',  ( 20.88017736071110164, 25.35535201082150891, 2.915334737309930979 ) ) ;
#22803=VECTOR ( 'NONE', #7450, 1000.000000000000000 ) ;
#22805=CARTESIAN_POINT ( 'NONE',  ( 15.44008868035555793, 36.39701867748816966, -9.422509992056140149 ) ) ;
#22809=CARTESIAN_POINT ( 'NONE',  ( -2.816281873526473856, 19.12363466993042138, 9.499525473075851096E-16 ) ) ;
#22810=CARTESIAN_POINT ( 'NONE',  ( 17.20831665107776587, 14.13393115100078568, -7.208316651077762316 ) ) ;
#22812=CARTESIAN_POINT ( 'NONE',  ( 5.076628168052703671, 16.84226448433411960, 8.527530157486179263 ) ) ;
#22813=CARTESIAN_POINT ( 'NONE',  ( 10.00000000000000000, 31.81368534415483751, -10.88017736071110342 ) ) ;
#22817=CARTESIAN_POINT ( 'NONE',  ( 6.565887622018943937, 65.16530133659709634, 12.81628187352647430 ) ) ;
#22818=CARTESIAN_POINT ( 'NONE',  ( 7.084665262690076126, 44.10535201082151247, 10.88017736071109987 ) ) ;
#22819=CARTESIAN_POINT ( 'NONE',  ( -0.2418659066527499291, 22.23410085661203794, -6.114288769123083611 ) ) ;
#22821=CARTESIAN_POINT ( 'NONE',  ( -2.816281873526473856, 54.12363466993041783, 9.499525473075851096E-16 ) ) ;
#22822=CARTESIAN_POINT ( 'NONE',  ( 7.084665262690076126, 57.02201867748817676, -10.88017736071110164 ) ) ;
#22825=CARTESIAN_POINT ( 'NONE',  ( -2.816281873526473856, -0.6680319967362464695, 3.434112377981055619 ) ) ;
#22826=COLOUR_RGB ( '', 0.09019608, 0.27058824, 0.51372549) ;
#22827=FILL_AREA_STYLE ('',( #53303 ) ) ;
#22828=CARTESIAN_POINT ( 'NONE',  ( 7.361572987183169658, 34.96726448433411605, -9.846743663894592657 ) ) ;
#22829=CARTESIAN_POINT ( 'NONE',  ( -2.816281873526473856, 54.12363466993041783, 9.499525473075851096E-16 ) ) ;
#22831=CARTESIAN_POINT ( 'NONE',  ( 7.361572987183170547, 2.050597817667451750, 9.846743663894590881 ) ) ;
#22833=CARTESIAN_POINT ( 'NONE',  ( -2.816281873526473856, 14.12363466993041961, 9.499525473075851096E-16 ) ) ;
#22836=CARTESIAN_POINT ( 'NONE',  ( 20.88017736071110519, 35.56368534415484106, 2.639326808657452039E-16 ) ) ;
#22837=CARTESIAN_POINT ( 'NONE',  ( 19.84674366389459621, 63.50893115100078745, 7.409399052514197653E-17 ) ) ;
#22839=CARTESIAN_POINT ( 'NONE',  ( 14.92337183194729633, 17.67559781766745175, 8.527530157486181039 ) ) ;
#22840=CARTESIAN_POINT ( 'NONE',  ( 12.63842701281683922, 9.550597817667449974, -9.846743663894590881 ) ) ;
#22841=CARTESIAN_POINT ( 'NONE',  ( -2.816281873526473856, 19.12363466993042138, 9.499525473075851096E-16 ) ) ;
#22843=CARTESIAN_POINT ( 'NONE',  ( -0.8801773607111009756, 3.063685344154837509, 1.068504757029289695E-15 ) ) ;
#22844=CARTESIAN_POINT ( 'NONE',  ( 10.00000000000000000, 59.75893115100078745, -9.846743663894594434 ) ) ;
#22847=CARTESIAN_POINT ( 'NONE',  ( 12.91533473730992121, 9.522018677488171434, 10.88017736071110164 ) ) ;
#22848=CARTESIAN_POINT ( 'NONE',  ( 10.00000000000000000, 39.75893115100078745, -9.846743663894594434 ) ) ;
#22851=CARTESIAN_POINT ( 'NONE',  ( 7.084665262690076126, 9.105352010821503583, 10.88017736071109987 ) ) ;
#22852=CARTESIAN_POINT ( 'NONE',  ( 19.72487221294570858, 69.50000000000000000, -6.500000000000000888 ) ) ;
#22853=CARTESIAN_POINT ( 'NONE',  ( 17.96484262340118221, 31.18868534415483751, -7.964842623401177768 ) ) ;
#22855=CARTESIAN_POINT ( 'NONE',  ( 22.26659068614895176, 59.72041550158063927, -7.082119434687042414 ) ) ;
#22857=CARTESIAN_POINT ( 'NONE',  ( 14.92337183194729988, 4.342264484334117824, -8.527530157486177487 ) ) ;
#22858=CARTESIAN_POINT ( 'NONE',  ( 0.1532563361054100626, 20.80059781766744464, -2.638427012816831230 ) ) ;
#22859=CARTESIAN_POINT ( 'NONE',  ( -1.099225684535947600, 14.54030133659708568, 6.408140936763237150 ) ) ;
#22861=CARTESIAN_POINT ( 'NONE',  ( -0.3077640640441539621, 70.00000000000000000, 5.999999999999999112 ) ) ;
#22863=CARTESIAN_POINT ( 'NONE',  ( 19.84674366389459621, 58.50893115100078745, 7.409399052514197653E-17 ) ) ;
#22866=CARTESIAN_POINT ( 'NONE',  ( 10.00000000000000000, 15.55374883491396787, -14.16423886937410082 ) ) ;
#22868=CARTESIAN_POINT ( 'NONE',  ( 19.84674366389459266, 23.71726448433412315, -2.638427012816827677 ) ) ;
#22871=CARTESIAN_POINT ( 'NONE',  ( 24.16423886937410614, 59.51208216824728936, -3.795296366450302550 ) ) ;
#22872=CARTESIAN_POINT ( 'NONE',  ( 7.361572987183170547, 7.050597817667451750, 9.846743663894590881 ) ) ;
#22875=CARTESIAN_POINT ( 'NONE',  ( 12.91533473730992121, 34.52201867748817676, 10.88017736071110164 ) ) ;
#22876=CARTESIAN_POINT ( 'NONE',  ( 0.6178305044545838731, 49.74863466993041072, 9.382169495545420901 ) ) ;
#22877=CARTESIAN_POINT ( 'NONE',  ( 0.5774900079438607392, 8.480352010821505360, 5.440088680355550821 ) ) ;
#22878=CARTESIAN_POINT ( 'NONE',  ( 19.38216949554541557, 32.24863466993041783, -9.382169495545420901 ) ) ;
#22879=CARTESIAN_POINT ( 'NONE',  ( 13.43411237798105340, 0.5819680032637533085, 12.81628187352647963 ) ) ;
#22880=CARTESIAN_POINT ( 'NONE',  ( 18.52753015748617571, 8.092264484334117824, 4.923371831947298993 ) ) ;
#22881=ORIENTED_EDGE ( 'NONE', *, *, #23455, .T. ) ;
#22884=CARTESIAN_POINT ( 'NONE',  ( -4.164238869374099927, 42.01208216824728936, 3.795296366450308767 ) ) ;
#22885=CARTESIAN_POINT ( 'NONE',  ( 6.204703633549690345, 17.84541550158063217, 14.16423886937410082 ) ) ;
#22886=CARTESIAN_POINT ( 'NONE',  ( 20.88017736071110875, 5.772018677488170546, -2.915334737309920765 ) ) ;
#22887=CARTESIAN_POINT ( 'NONE',  ( 17.96484262340118221, 31.18868534415483751, -7.964842623401177768 ) ) ;
#22890=CARTESIAN_POINT ( 'NONE',  ( -0.8801773607110991993, 62.85535201082150536, -2.915334737309923874 ) ) ;
#22892=CARTESIAN_POINT ( 'NONE',  ( 16.40814093676323893, 25.79030133659708923, 11.09922568453595026 ) ) ;
#22893=DIRECTION ( 'NONE',  ( 1.000000000000000000, 0.000000000000000000, -0.000000000000000000 ) ) ;
#22895=CARTESIAN_POINT ( 'NONE',  ( 17.20831665107776587, 34.13393115100078745, -7.208316651077762316 ) ) ;
#22897=CARTESIAN_POINT ( 'NONE',  ( 6.565887622018943937, 20.16530133659708213, 12.81628187352647430 ) ) ;
#22898=CARTESIAN_POINT ( 'NONE',  ( 12.63842701281683922, 14.55059781766744997, -9.846743663894590881 ) ) ;
#22899=CARTESIAN_POINT ( 'NONE',  ( 19.42250999205614548, 5.980352010821504471, -5.440088680355545492 ) ) ;
#22900=CARTESIAN_POINT ( 'NONE',  ( 18.52753015748618282, 33.92559781766745886, -4.923371831947291888 ) ) ;
#22903=CARTESIAN_POINT ( 'NONE',  ( 14.92337183194729633, 22.67559781766745175, 8.527530157486181039 ) ) ;
#22904=CARTESIAN_POINT ( 'NONE',  ( 2.917880565312950480, 0.9704155015806342766, -12.26659068614894821 ) ) ;
#22905=CARTESIAN_POINT ( 'NONE',  ( 6.204703633549690345, 7.845415501580634832, 14.16423886937410082 ) ) ;
#22907=CARTESIAN_POINT ( 'NONE',  ( 15.44008868035555793, 36.39701867748816966, -9.422509992056140149 ) ) ;
#22908=CARTESIAN_POINT ( 'NONE',  ( 19.42250999205614193, 15.14701867748817143, 5.440088680355555262 ) ) ;
#22909=CARTESIAN_POINT ( 'NONE',  ( -4.164238869374098151, 46.59541550158063927, -3.795296366450310543 ) ) ;
#22912=CARTESIAN_POINT ( 'NONE',  ( 17.96484262340118221, 34.93868534415482685, 7.964842623401181321 ) ) ;
#22913=CARTESIAN_POINT ( 'NONE',  ( 0.5774900079438607392, 18.48035201082150536, 5.440088680355550821 ) ) ;
#22915=CARTESIAN_POINT ( 'NONE',  ( 19.42250999205614193, 45.14701867748817676, 5.440088680355555262 ) ) ;
#22916=CARTESIAN_POINT ( 'NONE',  ( 10.00000000000000000, 42.87363466993042493, -12.81628187352647608 ) ) ;
#22917=CARTESIAN_POINT ( 'NONE',  ( 15.44008868035555793, 46.39701867748817676, -9.422509992056140149 ) ) ;
#22918=CARTESIAN_POINT ( 'NONE',  ( 1.472469842513823179, 46.42559781766745175, 4.923371831947296329 ) ) ;
#22919=CARTESIAN_POINT ( 'NONE',  ( -0.8801773607111009756, 53.06368534415484106, 1.068504757029289695E-15 ) ) ;
#22921=CARTESIAN_POINT ( 'NONE',  ( 20.88017736071110875, 55.77201867748816966, -2.915334737309920765 ) ) ;
#22923=CARTESIAN_POINT ( 'NONE',  ( -0.1049300847420624738, 37.21697413083879979, -6.336235997365760930 ) ) ;
#22924=CARTESIAN_POINT ( 'NONE',  ( -4.164238869374098151, 46.59541550158063927, -3.795296366450310543 ) ) ;
#22925=CARTESIAN_POINT ( 'NONE',  ( 20.88017736071110164, 60.35535201082151957, 2.915334737309930979 ) ) ;
#22930=CARTESIAN_POINT ( 'NONE',  ( 7.361572987183170547, 62.05059781766745886, 9.846743663894590881 ) ) ;
#22931=PRESENTATION_STYLE_ASSIGNMENT (( #6423 ) ) ;
#22932=CARTESIAN_POINT ( 'NONE',  ( 18.52753015748617571, 38.09226448433412315, 4.923371831947298993 ) ) ;
#22934=CARTESIAN_POINT ( 'NONE',  ( 18.52753015748618282, 28.92559781766745175, -4.923371831947291888 ) ) ;
#22936=CARTESIAN_POINT ( 'NONE',  ( 10.00000000000000178, 24.31368534415484106, 10.88017736071110342 ) ) ;
#22937=CARTESIAN_POINT ( 'NONE',  ( 2.791683348922240793, 36.63393115100078035, 7.208316651077764092 ) ) ;
#22938=CARTESIAN_POINT ( 'NONE',  ( 3.591859063236763294, 18.29030133659708568, -11.09922568453595026 ) ) ;
#22939=FACE_OUTER_BOUND ( 'NONE', #12097, .T. ) ;
#22940=CARTESIAN_POINT ( 'NONE',  ( 20.88017736071110875, 60.77201867748817676, -2.915334737309920765 ) ) ;
#22941=CARTESIAN_POINT ( 'NONE',  ( 17.96484262340118221, 46.18868534415484106, -7.964842623401177768 ) ) ;
#22942=CARTESIAN_POINT ( 'NONE',  ( 0.6178305044545838731, 64.74863466993043914, 9.382169495545420901 ) ) ;
#22943=CARTESIAN_POINT ( 'NONE',  ( 24.16423886937410614, 59.30374883491397497, 8.672049930838204340E-16 ) ) ;
#22944=ADVANCED_FACE ( 'NONE', ( #3756 ), #7809, .T. ) ;
#22945=CARTESIAN_POINT ( 'NONE',  ( -2.816281873526473856, 24.33196800326375353, 3.434112377981055619 ) ) ;
#22947=DIRECTION ( 'NONE',  ( 0.000000000000000000, 0.000000000000000000, 1.000000000000000000 ) ) ;
#22950=CARTESIAN_POINT ( 'NONE',  ( 21.09922568453594849, 21.20696800326375353, 6.408140936763242479 ) ) ;
#22951=CARTESIAN_POINT ( 'NONE',  ( -0.8801773607110991993, 17.85535201082150536, -2.915334737309923874 ) ) ;
#22952=CARTESIAN_POINT ( 'NONE',  ( 2.035157376598824452, 63.68868534415484106, 7.964842623401179544 ) ) ;
#22953=CYLINDRICAL_SURFACE ( 'NONE', #45733, 11.92686044187656513 ) ;
#22954=EDGE_LOOP ( 'NONE', ( #45216, #16042, #6312, #85188, #90535, #73467 ) ) ;
#22955=CARTESIAN_POINT ( 'NONE',  ( -0.8801773607110991993, 52.85535201082151247, -2.915334737309923874 ) ) ;
#22956=CARTESIAN_POINT ( 'NONE',  ( 10.00000000000000178, 42.25893115100078745, 9.846743663894594434 ) ) ;
#22958=CARTESIAN_POINT ( 'NONE',  ( 1.472469842513823179, 21.42559781766745175, 4.923371831947296329 ) ) ;
#22959=CARTESIAN_POINT ( 'NONE',  ( 17.20831665107776587, 19.13393115100078035, -7.208316651077762316 ) ) ;
#22960=CARTESIAN_POINT ( 'NONE',  ( 21.92686044187656691, 57.18830936912751639, 4.562052436263911564E-16 ) ) ;
#22961=CARTESIAN_POINT ( 'NONE',  ( -1.028725271592155099, -1.208271517246092823E-15, 4.540618777627624780 ) ) ;
#22962=CARTESIAN_POINT ( 'NONE',  ( 21.09922568453595559, 37.04030133659708923, -6.408140936763230044 ) ) ;
#22963=CARTESIAN_POINT ( 'NONE',  ( 14.92337183194729633, 17.67559781766745175, 8.527530157486181039 ) ) ;
#22965=CARTESIAN_POINT ( 'NONE',  ( 5.076628168052703671, 36.84226448433412315, 8.527530157486179263 ) ) ;
#22967=LINE ( 'NONE', #30925, #96547 ) ;
#22968=CARTESIAN_POINT ( 'NONE',  ( 22.81628187352647785, 16.62363466993042138, 6.195893100308588602E-16 ) ) ;
#22970=CARTESIAN_POINT ( 'NONE',  ( 19.42250999205614548, 50.98035201082151247, -5.440088680355545492 ) ) ;
#22971=CARTESIAN_POINT ( 'NONE',  ( -4.164238869374098151, 36.59541550158063217, -3.795296366450310543 ) ) ;
#22975=CARTESIAN_POINT ( 'NONE',  ( 10.00000000000000178, 33.05374883491396787, 14.16423886937410082 ) ) ;
#22976=CARTESIAN_POINT ( 'NONE',  ( 13.79529636645031943, 55.34541550158062506, -14.16423886937409904 ) ) ;
#22977=CARTESIAN_POINT ( 'NONE',  ( 20.36894250292379738, 14.92874883491396432, -10.36894250292379027 ) ) ;
#22978=CARTESIAN_POINT ( 'NONE',  ( -4.164238869374098151, 26.59541550158063217, -3.795296366450310543 ) ) ;
#22979=CARTESIAN_POINT ( 'NONE',  ( 19.39188664607693013, 35.83703382326400089, -6.500000000000031974 ) ) ;
#22980=CARTESIAN_POINT ( 'NONE',  ( 4.559911319644449179, 42.23035201082151247, -9.422509992056141925 ) ) ;
#22982=CARTESIAN_POINT ( 'NONE',  ( 10.00000000000000178, 69.31368534415484817, 10.88017736071110342 ) ) ;
#22983=CARTESIAN_POINT ( 'NONE',  ( 19.84674366389459621, 43.50893115100078745, 7.409399052514197653E-17 ) ) ;
#22984=CARTESIAN_POINT ( 'NONE',  ( 0.5774900079438590739, 22.64701867748817321, -5.440088680355550821 ) ) ;
#22986=CARTESIAN_POINT ( 'NONE',  ( 7.361572987183170547, 62.05059781766745886, 9.846743663894590881 ) ) ;
#22987=CARTESIAN_POINT ( 'NONE',  ( 20.00000000000000711, 84.99347556687297356, -4.825407043045644606 ) ) ;
#22988=CARTESIAN_POINT ( 'NONE',  ( 14.92337183194729633, 32.67559781766745175, 8.527530157486181039 ) ) ;
#22989=CARTESIAN_POINT ( 'NONE',  ( 13.43411237798106583, 57.66530133659708923, -12.81628187352647252 ) ) ;
#22991=CARTESIAN_POINT ( 'NONE',  ( 12.63842701281683034, 42.46726448433412315, 9.846743663894596210 ) ) ;
#22992=CARTESIAN_POINT ( 'NONE',  ( 12.63842701281683034, 47.46726448433412315, 9.846743663894596210 ) ) ;
#22993=CARTESIAN_POINT ( 'NONE',  ( 2.917880565312948704, 42.63708216824729647, 12.26659068614894643 ) ) ;
#22995=CARTESIAN_POINT ( 'NONE',  ( -0.3689425029237898834, 11.17874883491396787, -10.36894250292378850 ) ) ;
#22996=CARTESIAN_POINT ( 'NONE',  ( 0.5774900079438607392, 68.48035201082150536, 5.440088680355550821 ) ) ;
#22998=CARTESIAN_POINT ( 'NONE',  ( 10.00000000000000178, 63.05374883491396076, 14.16423886937410082 ) ) ;
#22999=CARTESIAN_POINT ( 'NONE',  ( 6.565887622018943937, 15.16530133659708568, 12.81628187352647430 ) ) ;
#23000=CARTESIAN_POINT ( 'NONE',  ( -0.1503990784575279516, 53.10158574516643171, 6.262539305110076171 ) ) ;
#23001=CARTESIAN_POINT ( 'NONE',  ( 10.00000000000000178, 59.31368534415484106, 10.88017736071110342 ) ) ;
#23002=CARTESIAN_POINT ( 'NONE',  ( -0.3289641300567998083, 28.07879003517447458, 5.963430220938281678 ) ) ;
#23003=CARTESIAN_POINT ( 'NONE',  ( -46.94000000000240647, 102.7387969410441002, -6.737038697110588004 ) ) ;
#23004=CARTESIAN_POINT ( 'NONE',  ( -4.164238869374099039, 61.80374883491397497, 8.674139862899312516E-16 ) ) ;
#23006=CARTESIAN_POINT ( 'NONE',  ( 7.084665262690076126, 17.02201867748817676, -10.88017736071110164 ) ) ;
#23007=CARTESIAN_POINT ( 'NONE',  ( 7.084665262690076126, 24.10535201082150181, 10.88017736071109987 ) ) ;
#23008=CARTESIAN_POINT ( 'NONE',  ( 19.84674366389459266, 58.30059781766745886, 2.638427012816836559 ) ) ;
#23009=CARTESIAN_POINT ( 'NONE',  ( 14.92337183194729988, 54.34226448433412315, -8.527530157486177487 ) ) ;
#23010=CARTESIAN_POINT ( 'NONE',  ( 0.6178305044545838731, 44.74863466993042493, 9.382169495545420901 ) ) ;
#23011=CARTESIAN_POINT ( 'NONE',  ( 0.1532563361054082862, 1.217264484334117824, 2.638427012816831674 ) ) ;
#23013=CARTESIAN_POINT ( 'NONE',  ( 20.88017736071110519, 10.56368534415483751, 2.639326808657452039E-16 ) ) ;
#23014=ADVANCED_FACE ( 'NONE', ( #19233 ), #72226, .T. ) ;
#23015=CARTESIAN_POINT ( 'NONE',  ( -1.099225684535947600, 24.54030133659708923, 6.408140936763237150 ) ) ;
#23017=CARTESIAN_POINT ( 'NONE',  ( 2.791683348922237240, 50.38393115100078035, -7.208316651077763204 ) ) ;
#23018=CARTESIAN_POINT ( 'NONE',  ( 10.00000000000000178, 39.31368534415484106, 10.88017736071110342 ) ) ;
#23019=CARTESIAN_POINT ( 'NONE',  ( 19.38216949554541202, 15.99863466993042138, 9.382169495545424454 ) ) ;
#23020=CARTESIAN_POINT ( 'NONE',  ( 0.5774900079438590739, 47.64701867748817676, -5.440088680355550821 ) ) ;
#23022=CARTESIAN_POINT ( 'NONE',  ( 21.09922568453595559, 52.04030133659708923, -6.408140936763230044 ) ) ;
#23024=CARTESIAN_POINT ( 'NONE',  ( 0.1532563361054100626, 65.80059781766745175, -2.638427012816831230 ) ) ;
#23025=CARTESIAN_POINT ( 'NONE',  ( 7.084665262690076126, 52.02201867748816255, -10.88017736071110164 ) ) ;
#23026=CARTESIAN_POINT ( 'NONE',  ( 13.43411237798105340, 40.58196800326375353, 12.81628187352647963 ) ) ;
#23027=CARTESIAN_POINT ( 'NONE',  ( 24.16423886937409904, 19.09541550158063927, 3.795296366450317205 ) ) ;
#23028=CARTESIAN_POINT ( 'NONE',  ( 2.035157376598824452, 53.68868534415484817, 7.964842623401179544 ) ) ;
#23029=CARTESIAN_POINT ( 'NONE',  ( 19.84674366389459621, 63.50893115100078745, 7.409399052514197653E-17 ) ) ;
#23030=CARTESIAN_POINT ( 'NONE',  ( 5.076628168052704559, 20.17559781766745175, -8.527530157486179263 ) ) ;
#23031=CARTESIAN_POINT ( 'NONE',  ( 17.20831665107776587, 2.883931151000785231, 7.208316651077764980 ) ) ;
#23033=CARTESIAN_POINT ( 'NONE',  ( 17.08211943468705840, 40.13708216824731068, -12.26659068614894466 ) ) ;
#23034=CARTESIAN_POINT ( 'NONE',  ( 21.92686044187657046, 25.16212336850780673, 4.562052436263912550E-16 ) ) ;
#23035=CARTESIAN_POINT ( 'NONE',  ( 2.035157376598822676, 7.438685344154837509, -7.964842623401177768 ) ) ;
#23038=CARTESIAN_POINT ( 'NONE',  ( 0.5774900079438590739, 7.647018677488171434, -5.440088680355550821 ) ) ;
#23039=CARTESIAN_POINT ( 'NONE',  ( 6.204703633549690345, 67.84541550158060375, 14.16423886937410082 ) ) ;
#23040=CARTESIAN_POINT ( 'NONE',  ( 17.20831665107776587, 44.13393115100078745, -7.208316651077762316 ) ) ;
#23041=CARTESIAN_POINT ( 'NONE',  ( 6.565887622018943937, 40.16530133659708923, 12.81628187352647430 ) ) ;
#23042=( NAMED_UNIT ( * ) PLANE_ANGLE_UNIT ( ) SI_UNIT ( $, .RADIAN. ) );
#23044=CARTESIAN_POINT ( 'NONE',  ( 18.72515096720583827, 56.07228050351029225, -6.499999999999802824 ) ) ;
#23045=CARTESIAN_POINT ( 'NONE',  ( 6.204703633549690345, 2.845415501580634388, 14.16423886937410082 ) ) ;
#23046=CARTESIAN_POINT ( 'NONE',  ( 7.084665262690076126, 32.02201867748816966, -10.88017736071110164 ) ) ;
#23047=CARTESIAN_POINT ( 'NONE',  ( -4.164238869374099927, 67.01208216824728936, 3.795296366450308767 ) ) ;
#23048=CARTESIAN_POINT ( 'NONE',  ( 1.472469842513823179, 45.59226448433412315, -4.923371831947296329 ) ) ;
#23050=CARTESIAN_POINT ( 'NONE',  ( 2.791683348922237240, 20.38393115100078745, -7.208316651077763204 ) ) ;
#23052=( NAMED_UNIT ( * ) SI_UNIT ( $, .STERADIAN. ) SOLID_ANGLE_UNIT ( ) );
#23054=ORIENTED_EDGE ( 'NONE', *, *, #51347, .T. ) ;
#23058=CARTESIAN_POINT ( 'NONE',  ( 18.52753015748618282, 58.92559781766745886, -4.923371831947291888 ) ) ;
#23059=CARTESIAN_POINT ( 'NONE',  ( 0.5774900079438607392, 33.48035201082150536, 5.440088680355550821 ) ) ;
#23060=CARTESIAN_POINT ( 'NONE',  ( 12.91533473730992121, 39.52201867748817676, 10.88017736071110164 ) ) ;
#23061=FILL_AREA_STYLE ('',( #66569 ) ) ;
#23062=CARTESIAN_POINT ( 'NONE',  ( 16.40814093676323893, 30.79030133659708923, 11.09922568453595026 ) ) ;
#23063=CARTESIAN_POINT ( 'NONE',  ( 6.204703633549690345, 17.84541550158063217, 14.16423886937410082 ) ) ;
#23067=CARTESIAN_POINT ( 'NONE',  ( 10.00000000000000000, 47.87363466993042493, -12.81628187352647608 ) ) ;
#23070=CARTESIAN_POINT ( 'NONE',  ( 18.52753015748617571, 48.09226448433412315, 4.923371831947298993 ) ) ;
#23071=CARTESIAN_POINT ( 'NONE',  ( 0.5774900079438590739, 2.647018677488171434, -5.440088680355550821 ) ) ;
#23072=EDGE_LOOP ( 'NONE', ( #97333, #8514, #71398, #77742 ) ) ;
#23073=CARTESIAN_POINT ( 'NONE',  ( 7.084665262690076126, 22.02201867748817321, -10.88017736071110164 ) ) ;
#23075=CARTESIAN_POINT ( 'NONE',  ( 2.035157376598822676, 67.43868534415484817, -7.964842623401177768 ) ) ;
#23076=CARTESIAN_POINT ( 'NONE',  ( 19.42250999205614548, 55.98035201082150536, -5.440088680355545492 ) ) ;
#23077=CARTESIAN_POINT ( 'NONE',  ( 0.5774900079438590739, 67.64701867748817676, -5.440088680355550821 ) ) ;
#23079=CARTESIAN_POINT ( 'NONE',  ( 15.44008868035555793, 51.39701867748816966, -9.422509992056140149 ) ) ;
#23082=CARTESIAN_POINT ( 'NONE',  ( 1.959929470562273179, 10.51528370094808196, -5.767676674365838529 ) ) ;
#23083=( LENGTH_UNIT ( ) NAMED_UNIT ( * ) SI_UNIT ( .MILLI., .METRE. ) );
#23085=CARTESIAN_POINT ( 'NONE',  ( 7.361572987183170547, 37.05059781766744464, 9.846743663894590881 ) ) ;
#23086=ORIENTED_EDGE ( 'NONE', *, *, #13960, .T. ) ;
#23089=EDGE_CURVE ( 'NONE', #20606, #6963, #82689, .T. ) ;
#23090=CARTESIAN_POINT ( 'NONE',  ( 6.204703633549690345, 17.84541550158063217, 14.16423886937410082 ) ) ;
#23093=CARTESIAN_POINT ( 'NONE',  ( 19.42250999205614548, 5.980352010821504471, -5.440088680355545492 ) ) ;
#23094=CARTESIAN_POINT ( 'NONE',  ( 1.959929470562273179, 66.50257860105348584, 5.767676674365838529 ) ) ;
#23095=CARTESIAN_POINT ( 'NONE',  ( -2.816281873526473856, 39.33196800326374643, 3.434112377981055619 ) ) ;
#23098=CARTESIAN_POINT ( 'NONE',  ( 18.52753015748617571, 53.09226448433412315, 4.923371831947298993 ) ) ;
#23099=CARTESIAN_POINT ( 'NONE',  ( 10.00000000000000178, 15.37363466993042138, 12.81628187352647608 ) ) ;
#23100=CARTESIAN_POINT ( 'NONE',  ( 0.1532563361054082862, 21.21726448433412315, 2.638427012816831674 ) ) ;
#23102=CARTESIAN_POINT ( 'NONE',  ( 10.00000000000000178, 15.37363466993042138, 12.81628187352647608 ) ) ;
#23103=CARTESIAN_POINT ( 'NONE',  ( 12.63842701281683922, 9.550597817667449974, -9.846743663894590881 ) ) ;
#23107=CIRCLE ( 'NONE', #75767, 0.5000000000000005551 ) ;
#23108=CARTESIAN_POINT ( 'NONE',  ( 12.91533473730992121, 19.52201867748816611, 10.88017736071110164 ) ) ;
#23109=CARTESIAN_POINT ( 'NONE',  ( -2.266590686148945544, 21.38708216824730357, -7.082119434687050408 ) ) ;
#23110=CARTESIAN_POINT ( 'NONE',  ( 10.00000000000000178, 47.25893115100078745, 9.846743663894594434 ) ) ;
#23111=CARTESIAN_POINT ( 'NONE',  ( 2.035157376598824452, 63.68868534415484106, 7.964842623401179544 ) ) ;
#23112=CARTESIAN_POINT ( 'NONE',  ( 13.43411237798105340, 45.58196800326374643, 12.81628187352647963 ) ) ;
#23114=CARTESIAN_POINT ( 'NONE',  ( 4.559911319644449179, 13.89701867748817143, 9.422509992056141925 ) ) ;
#23117=CARTESIAN_POINT ( 'NONE',  ( 3.591859063236763294, 13.29030133659708746, -11.09922568453595026 ) ) ;
#23118=CARTESIAN_POINT ( 'NONE',  ( 1.472469842513823179, 30.59226448433411960, -4.923371831947296329 ) ) ;
#23120=CARTESIAN_POINT ( 'NONE',  ( -1.099225684535947600, 38.70696800326375353, -6.408140936763238038 ) ) ;
#23122=CARTESIAN_POINT ( 'NONE',  ( 18.72515096720609051, 25.05509018479941119, 6.499999999999470646 ) ) ;
#23123=CARTESIAN_POINT ( 'NONE',  ( 7.084665262690076126, 52.02201867748816255, -10.88017736071110164 ) ) ;
#23124=CARTESIAN_POINT ( 'NONE',  ( 2.603489959281060973, 26.58210964143323096, 6.499999999999401368 ) ) ;
#23125=CARTESIAN_POINT ( 'NONE',  ( 18.72515096720583827, 30.05509018479937566, 6.499999999999810818 ) ) ;
#23126=CARTESIAN_POINT ( 'NONE',  ( 7.084665262690076126, 37.02201867748817676, -10.88017736071110164 ) ) ;
#23127=CARTESIAN_POINT ( 'NONE',  ( -0.8801773607111008646, 43.27201867748817676, 2.915334737309923430 ) ) ;
#23128=CARTESIAN_POINT ( 'NONE',  ( 14.92337183194729988, 64.34226448433412315, -8.527530157486177487 ) ) ;
#23131=( BOUNDED_SURFACE ( )  B_SPLINE_SURFACE ( 1, 2, ( 
 ( #93856, #49333, #94345, #93362, #2886, #64812, #47365, #47855, #3355, #25384, #17386, #24887, #18361, #9375, #55372, #48839, #33817, #39877, #64324, #86366, #94835, #56839, #87337, #18852, #11338, #24396, #54864, #32359, #78360, #40380, #51311, #57324, #28314, #72812, #88816, #73315, #58300, #4353, #50311, #28798, #65309, #34819, #36312, #20329, #80826, #73804, #43797, #50823, #36812, #81316, #13813, #12812, #87818, #96838, #42830, #51807, #44297, #5335, #95835, #5819, #19822, #27318, #57815, #74799, #88324, #12325, #66806, #35815, #4839, #6307, #97328, #58805, #80331, #35314, #81793, #65808, #96340, #27815, #43311, #11830, #66301, #89312, #13310, #49821, #74290, #20821, #59299, #89796, #21314, #82291, #95331, #26830, #19338, #42338, #16282, #324, #23302, #29292, #30767, #44788, #60778, #45290, #30277, #75293, #22314, #806, #37316, #6802, #8287, #91281, #52786, #45795, #15795, #22802, #8769, #53281, #84774, #83787, #59790, #68793, #14819, #23798, #46763, #76287, #67808, #76769, #90787, #98325, #29782, #77258, #60293, #83294, #38784, #7801, #75785, #67303, #69285, #61272, #52301, #15310, #91781, #53780, #38298, #97830, #31260, #7308, #98823, #84298, #46283, #61756, #92274, #54261, #37809, #90282, #21817, #82795, #14318, #68304, #78244, #63725, #39771, #55757, #94724, #39285, #79230, #18245, #33711, #31756, #87217, #40748, #86249, #47748, #10255, #69774, #10741, #71253, #32243, #9759, #70270, #92757, #56726, #40261, #79725, #1304, #77750, #25277, #70767, #41260, #62252, #9265, #3244, #32738, #78749, #2281, #63237, #64210, #2775, #1787, #93740, #18740, #24282, #71734, #33231, #62744, #17761, #93244, #54747, #49223, #48238, #85267, #16774, #24769, #94225, #25757, #26232, #47250, #55247, #85762, #56249, #86743, #48725, #17274, #36191, #81197, #49701, #65692, #28683, #72214, #34700, #66181, #88201, #72693, #80211, #96215, #95206, #11716, #27697, #96716, #64694, #28193, #57700, #43193, #43685, #5215, #42711, #66691, #89191, #59177, #58690, #89682, #73681, #20703, #3744, #35697, #87704, #4726, #19710, #73193, #19219, #65195, #74170, #42228, #4230, #51195, #35188, #95716, #88692, #81677, #58181, #51696, #20201, #21197, #50704, #34202, #12699, #50196, #97218, #11225, #13192, #27199, #5704, #80708, #12202, #41745, #26711, #57208, #44677, #93003, #92510, #29658, #93502, #85515, #47011, #67185, #75670, #85021, #77502, #62010, #62998, #54997, #60168, #14698, #9014, #7181, #54508, #24038, #1548, #21697, #17026, #45167, #37686, #39531, #98202, #22191, #70023, #82677, #98704, #40013, #82175, #24537, #62500, #78006, #74683, #32500, #16535 ),
 ( #52182, #68184, #90663, #47504, #6195, #14196, #9512, #31509, #31993, #52671, #83172, #70517, #2039, #75171, #25027, #13687, #44173, #6681, #36699, #97709, #37200, #67691, #29176, #59676, #90166, #41507, #11475, #10015, #72456, #3020, #87471, #87956, #49463, #86980, #11966, #34454, #4483, #3988, #34949, #18985, #41992, #17525, #79969, #32989, #48978, #33469, #18490, #63492, #10494, #19473, #25518, #93995, #95473, #79487, #41006, #33956, #64946, #10987, #95971, #71975, #72953, #3499, #47991, #56968, #63965, #42470, #65448, #64460, #56005, #26963, #78988, #86508, #18005, #55513, #48486, #71507, #57463, #94967, #94479, #86012, #49963, #80467, #40516, #26469, #78502, #71013, #2535, #25996, #56491, #73942, #58943, #51943, #51445, #97459, #36446, #44426, #65945, #29415, #89444, #81933, #89930, #43441, #66438, #82427, #27944, #43928, #82927, #27456, #67439, #6430, #21950, #19956, #75422, #28924, #74426, #35942, #59428, #57948, #97960, #21445, #20459, #96973, #20958, #13953, #13441, #74931, #66938, #36942, #96472, #59920, #5954, #90408, #52429, #5470, #28446, #14445, #58436, #44915, #6937, #88455, #37444, #67935, #50450, #80957, #12456, #42962, #73443, #4968, #35450, #88951, #50949, #81444, #12945, #7926, #98950, #52911, #16902, #68921, #39893, #98455, #37938, #84417, #38423, #39408, #22440, #68428, #62374, #91904, #38915, #449, #30900, #24412, #69403, #30406, #53908, #47378, #60417, #22937, #54385, #76411, #60908, #91411, #15914, #83425, #53405, #46405, #84898, #14943, #16410, #45922, #31386, #31874, #92391, #61394, #54878, #77379, #77877, #46888, #9389, #61886, #8892, #90912, #23916, #75917, #23429, #76894, #8408, #7441, #83914, #92878, #15442, #924, #69902, #1422, #85389, #29911, #45412, #33351, #11844, #63845, #87833, #94358, #62878, #71860, #17882, #26843, #19351, #48854, #40397, #79849, #93870, #70892, #2409, #49835, #9893, #32868, #11352, #79363, #48366, #80347, #72336, #33832, #55386, #25877, #3371, #64340, #10871, #70396, #41872, #78871, #94851, #63368, #86867, #57338, #1914, #3868, #49348, #64827, #93376, #32373, #26351, #18375, #10380, #41392, #24903, #34331, #56853, #25397, #40883, #55882, #85887, #17401, #71388, #47869, #78374, #86380, #56378, #2901, #95344, #87352, #18866, #6314, #35827, #81805, #12822, #81327, #67313, #13323, #80837, #96849, #59798, #4366, #65819, #97337, #20338, #4850, #12337, #28324, #27332, #42841, #58815, #28810, #95848, #59308, #88826, #74303, #74808, #36322, #73814, #97838, #21327, #90289, #89806, #21827, #5828, #51815, #34832, #66815, #19835, #66313, #50834, #5348, #50324, #96354, #36821 ) ),
 .UNSPECIFIED., .F., .F., .F. ) 
 B_SPLINE_SURFACE_WITH_KNOTS ( ( 2, 2 ),
 ( 3, 2, 2, 2, 2, 2, 2, 2, 2, 2, 2, 2, 2, 2, 2, 2, 2, 2, 2, 2, 2, 2, 2, 2, 2, 2, 2, 2, 2, 2, 2, 2, 2, 2, 2, 2, 2, 2, 2, 2, 2, 2, 2, 2, 2, 2, 2, 2, 2, 2, 2, 2, 2, 2, 2, 2, 2, 2, 2, 2, 2, 2, 2, 2, 2, 2, 2, 2, 2, 2, 2, 2, 2, 2, 2, 2, 2, 2, 2, 2, 2, 2, 2, 2, 2, 2, 2, 2, 2, 2, 2, 2, 2, 2, 2, 2, 2, 2, 2, 2, 2, 2, 2, 2, 2, 2, 2, 2, 2, 2, 2, 2, 2, 2, 2, 2, 2, 2, 2, 2, 2, 2, 2, 2, 2, 2, 2, 2, 2, 2, 2, 2, 2, 2, 2, 2, 2, 2, 2, 2, 2, 2, 2, 2, 2, 2, 2, 2, 2, 2, 2, 2, 2, 2, 2, 2, 2, 2, 2, 2, 2, 2, 3 ),
 ( 0.000000000000000000, 1.000000000000000000 ),
 ( 0.000000000000000000, 0.005952380952380952051, 0.01190476190476190410, 0.01785714285714285615, 0.02380952380952380820, 0.02976190476190476025, 0.03571428571428571230, 0.04166666666666666435, 0.04761904761904761640, 0.05357142857142856845, 0.05952380952380952051, 0.06547619047619047949, 0.07142857142857142461, 0.07738095238095238360, 0.08333333333333332871, 0.08928571428571428770, 0.09523809523809523281, 0.1011904761904761918, 0.1071428571428571369, 0.1130952380952380959, 0.1190476190476190410, 0.1250000000000000000, 0.1309523809523809590, 0.1369047619047619180, 0.1428571428571428492, 0.1488095238095238082, 0.1547619047619047672, 0.1607142857142857262, 0.1666666666666666574, 0.1726190476190476164, 0.1785714285714285754, 0.1845238095238095344, 0.1904761904761904656, 0.1964285714285714246, 0.2023809523809523836, 0.2083333333333333426, 0.2142857142857142738, 0.2202380952380952328, 0.2261904761904761918, 0.2321428571428571508, 0.2380952380952380820, 0.2440476190476190410, 0.2500000000000000000, 0.2559523809523809312, 0.2619047619047619180, 0.2678571428571428492, 0.2738095238095238360, 0.2797619047619047672, 0.2857142857142856984, 0.2916666666666666852, 0.2976190476190476164, 0.3035714285714285476, 0.3095238095238095344, 0.3154761904761904656, 0.3214285714285714524, 0.3273809523809523836, 0.3333333333333333148, 0.3392857142857143016, 0.3452380952380952328, 0.3511904761904761640, 0.3571428571428571508, 0.3630952380952380820, 0.3690476190476190688, 0.3750000000000000000, 0.3809523809523809312, 0.3869047619047619180, 0.3928571428571428492, 0.3988095238095238360, 0.4047619047619047672, 0.4107142857142856984, 0.4166666666666666852, 0.4226190476190476164, 0.4285714285714285476, 0.4345238095238095344, 0.4404761904761904656, 0.4464285714285714524, 0.4523809523809523836, 0.4583333333333333148, 0.4642857142857143016, 0.4702380952380952328, 0.4761904761904761640, 0.4821428571428571508, 0.4880952380952380820, 0.4940476190476190688, 0.5000000000000000000, 0.5059523809523809312, 0.5119047619047618625, 0.5178571428571429047, 0.5238095238095238360, 0.5297619047619047672, 0.5357142857142856984, 0.5416666666666666297, 0.5476190476190476719, 0.5535714285714286031, 0.5595238095238095344, 0.5654761904761904656, 0.5714285714285713969, 0.5773809523809523281, 0.5833333333333333703, 0.5892857142857143016, 0.5952380952380952328, 0.6011904761904761640, 0.6071428571428570953, 0.6130952380952381375, 0.6190476190476190688, 0.6250000000000000000, 0.6309523809523809312, 0.6369047619047618625, 0.6428571428571429047, 0.6488095238095238360, 0.6547619047619047672, 0.6607142857142856984, 0.6666666666666666297, 0.6726190476190476719, 0.6785714285714286031, 0.6845238095238095344, 0.6904761904761904656, 0.6964285714285713969, 0.7023809523809523281, 0.7083333333333333703, 0.7142857142857143016, 0.7202380952380952328, 0.7261904761904761640, 0.7321428571428570953, 0.7380952380952381375, 0.7440476190476190688, 0.7500000000000000000, 0.7559523809523809312, 0.7619047619047618625, 0.7678571428571429047, 0.7738095238095238360, 0.7797619047619047672, 0.7857142857142856984, 0.7916666666666666297, 0.7976190476190476719, 0.8035714285714286031, 0.8095238095238095344, 0.8154761904761904656, 0.8214285714285713969, 0.8273809523809523281, 0.8333333333333333703, 0.8392857142857143016, 0.8452380952380952328, 0.8511904761904761640, 0.8571428571428570953, 0.8630952380952381375, 0.8690476190476190688, 0.8750000000000000000, 0.8809523809523809312, 0.8869047619047618625, 0.8928571428571429047, 0.8988095238095238360, 0.9047619047619047672, 0.9107142857142856984, 0.9166666666666666297, 0.9226190476190476719, 0.9285714285714286031, 0.9345238095238095344, 0.9404761904761904656, 0.9464285714285713969, 0.9523809523809523281, 0.9583333333333333703, 0.9642857142857143016 ),
 .UNSPECIFIED. ) 
 GEOMETRIC_REPRESENTATION_ITEM ( )  RATIONAL_B_SPLINE_SURFACE ( (
 ( 1.000000000000000000, 0.9659258262890683122, 1.000000000000000000, 0.9659258262890683122, 1.000000000000000000, 0.9659258262890683122, 1.000000000000000000, 0.9659258262890683122, 1.000000000000000000, 0.9659258262890683122, 1.000000000000000000, 0.9659258262890683122, 1.000000000000000000, 0.9659258262890683122, 1.000000000000000000, 0.9659258262890683122, 1.000000000000000000, 0.9659258262890683122, 1.000000000000000000, 0.9659258262890683122, 1.000000000000000000, 0.9659258262890683122, 1.000000000000000000, 0.9659258262890683122, 1.000000000000000000, 0.9659258262890683122, 1.000000000000000000, 0.9659258262890683122, 1.000000000000000000, 0.9659258262890683122, 1.000000000000000000, 0.9659258262890683122, 1.000000000000000000, 0.9659258262890683122, 1.000000000000000000, 0.9659258262890683122, 1.000000000000000000, 0.9659258262890683122, 1.000000000000000000, 0.9659258262890683122, 1.000000000000000000, 0.9659258262890683122, 1.000000000000000000, 0.9659258262890683122, 1.000000000000000000, 0.9659258262890683122, 1.000000000000000000, 0.9659258262890683122, 1.000000000000000000, 0.9659258262890683122, 1.000000000000000000, 0.9659258262890683122, 1.000000000000000000, 0.9659258262890683122, 1.000000000000000000, 0.9659258262890683122, 1.000000000000000000, 0.9659258262890683122, 1.000000000000000000, 0.9659258262890683122, 1.000000000000000000, 0.9659258262890683122, 1.000000000000000000, 0.9659258262890683122, 1.000000000000000000, 0.9659258262890683122, 1.000000000000000000, 0.9659258262890683122, 1.000000000000000000, 0.9659258262890683122, 1.000000000000000000, 0.9659258262890683122, 1.000000000000000000, 0.9659258262890683122, 1.000000000000000000, 0.9659258262890683122, 1.000000000000000000, 0.9659258262890683122, 1.000000000000000000, 0.9659258262890683122, 1.000000000000000000, 0.9659258262890683122, 1.000000000000000000, 0.9659258262890683122, 1.000000000000000000, 0.9659258262890683122, 1.000000000000000000, 0.9659258262890683122, 1.000000000000000000, 0.9659258262890683122, 1.000000000000000000, 0.9659258262890683122, 1.000000000000000000, 0.9659258262890683122, 1.000000000000000000, 0.9659258262890683122, 1.000000000000000000, 0.9659258262890683122, 1.000000000000000000, 0.9659258262890683122, 1.000000000000000000, 0.9659258262890683122, 1.000000000000000000, 0.9659258262890683122, 1.000000000000000000, 0.9659258262890683122, 1.000000000000000000, 0.9659258262890683122, 1.000000000000000000, 0.9659258262890683122, 1.000000000000000000, 0.9659258262890683122, 1.000000000000000000, 0.9659258262890683122, 1.000000000000000000, 0.9659258262890683122, 1.000000000000000000, 0.9659258262890683122, 1.000000000000000000, 0.9659258262890683122, 1.000000000000000000, 0.9659258262890683122, 1.000000000000000000, 0.9659258262890683122, 1.000000000000000000, 0.9659258262890683122, 1.000000000000000000, 0.9659258262890683122, 1.000000000000000000, 0.9659258262890683122, 1.000000000000000000, 0.9659258262890683122, 1.000000000000000000, 0.9659258262890683122, 1.000000000000000000, 0.9659258262890683122, 1.000000000000000000, 0.9659258262890683122, 1.000000000000000000, 0.9659258262890683122, 1.000000000000000000, 0.9659258262890683122, 1.000000000000000000, 0.9659258262890683122, 1.000000000000000000, 0.9659258262890683122, 1.000000000000000000, 0.9659258262890683122, 1.000000000000000000, 0.9659258262890683122, 1.000000000000000000, 0.9659258262890683122, 1.000000000000000000, 0.9659258262890683122, 1.000000000000000000, 0.9659258262890683122, 1.000000000000000000, 0.9659258262890683122, 1.000000000000000000, 0.9659258262890683122, 1.000000000000000000, 0.9659258262890683122, 1.000000000000000000, 0.9659258262890683122, 1.000000000000000000, 0.9659258262890683122, 1.000000000000000000, 0.9659258262890683122, 1.000000000000000000, 0.9659258262890683122, 1.000000000000000000, 0.9659258262890683122, 1.000000000000000000, 0.9659258262890683122, 1.000000000000000000, 0.9659258262890683122, 1.000000000000000000, 0.9659258262890683122, 1.000000000000000000, 0.9659258262890683122, 1.000000000000000000, 0.9659258262890683122, 1.000000000000000000, 0.9659258262890683122, 1.000000000000000000, 0.9659258262890683122, 1.000000000000000000, 0.9659258262890683122, 1.000000000000000000, 0.9659258262890683122, 1.000000000000000000, 0.9659258262890683122, 1.000000000000000000, 0.9659258262890683122, 1.000000000000000000, 0.9659258262890683122, 1.000000000000000000, 0.9659258262890683122, 1.000000000000000000, 0.9659258262890683122, 1.000000000000000000, 0.9659258262890683122, 1.000000000000000000, 0.9659258262890683122, 1.000000000000000000, 0.9659258262890683122, 1.000000000000000000, 0.9659258262890683122, 1.000000000000000000, 0.9659258262890683122, 1.000000000000000000, 0.9659258262890683122, 1.000000000000000000, 0.9659258262890683122, 1.000000000000000000, 0.9659258262890683122, 1.000000000000000000, 0.9659258262890683122, 1.000000000000000000, 0.9659258262890683122, 1.000000000000000000, 0.9659258262890683122, 1.000000000000000000, 0.9659258262890683122, 1.000000000000000000, 0.9659258262890683122, 1.000000000000000000, 0.9659258262890683122, 1.000000000000000000, 0.9659258262890683122, 1.000000000000000000, 0.9659258262890683122, 1.000000000000000000, 0.9659258262890683122, 1.000000000000000000, 0.9659258262890683122, 1.000000000000000000, 0.9659258262890683122, 1.000000000000000000, 0.9659258262890683122, 1.000000000000000000, 0.9659258262890683122, 1.000000000000000000, 0.9659258262890683122, 1.000000000000000000, 0.9659258262890683122, 1.000000000000000000, 0.9659258262890683122, 1.000000000000000000, 0.9659258262890683122, 1.000000000000000000, 0.9659258262890683122, 1.000000000000000000, 0.9659258262890683122, 1.000000000000000000, 0.9659258262890683122, 1.000000000000000000, 0.9659258262890683122, 1.000000000000000000, 0.9659258262890683122, 1.000000000000000000, 0.9659258262890683122, 1.000000000000000000, 0.9659258262890683122, 1.000000000000000000, 0.9659258262890683122, 1.000000000000000000, 0.9659258262890683122, 1.000000000000000000, 0.9659258262890683122, 1.000000000000000000, 0.9659258262890683122, 1.000000000000000000, 0.9659258262890683122, 1.000000000000000000, 0.9659258262890683122, 1.000000000000000000, 0.9659258262890683122, 1.000000000000000000, 0.9659258262890683122, 1.000000000000000000, 0.9659258262890683122, 1.000000000000000000, 0.9659258262890683122, 1.000000000000000000, 0.9659258262890683122, 1.000000000000000000, 0.9659258262890683122, 1.000000000000000000, 0.9659258262890683122, 1.000000000000000000, 0.9659258262890683122, 1.000000000000000000, 0.9659258262890683122, 1.000000000000000000, 0.9659258262890683122, 1.000000000000000000, 0.9659258262890683122, 1.000000000000000000, 0.9659258262890683122, 1.000000000000000000, 0.9659258262890683122, 1.000000000000000000, 0.9659258262890683122, 1.000000000000000000, 0.9659258262890683122, 1.000000000000000000, 0.9659258262890683122, 1.000000000000000000, 0.9659258262890683122, 1.000000000000000000, 0.9659258262890683122, 1.000000000000000000, 0.9659258262890683122, 1.000000000000000000, 0.9659258262890683122, 1.000000000000000000, 0.9659258262890683122, 1.000000000000000000, 0.9659258262890683122, 1.000000000000000000, 0.9659258262890683122, 1.000000000000000000, 0.9659258262890683122, 1.000000000000000000),
 ( 1.000000000000000000, 0.9659258262890683122, 1.000000000000000000, 0.9659258262890683122, 1.000000000000000000, 0.9659258262890683122, 1.000000000000000000, 0.9659258262890683122, 1.000000000000000000, 0.9659258262890683122, 1.000000000000000000, 0.9659258262890683122, 1.000000000000000000, 0.9659258262890683122, 1.000000000000000000, 0.9659258262890683122, 1.000000000000000000, 0.9659258262890683122, 1.000000000000000000, 0.9659258262890683122, 1.000000000000000000, 0.9659258262890683122, 1.000000000000000000, 0.9659258262890683122, 1.000000000000000000, 0.9659258262890683122, 1.000000000000000000, 0.9659258262890683122, 1.000000000000000000, 0.9659258262890683122, 1.000000000000000000, 0.9659258262890683122, 1.000000000000000000, 0.9659258262890683122, 1.000000000000000000, 0.9659258262890683122, 1.000000000000000000, 0.9659258262890683122, 1.000000000000000000, 0.9659258262890683122, 1.000000000000000000, 0.9659258262890683122, 1.000000000000000000, 0.9659258262890683122, 1.000000000000000000, 0.9659258262890683122, 1.000000000000000000, 0.9659258262890683122, 1.000000000000000000, 0.9659258262890683122, 1.000000000000000000, 0.9659258262890683122, 1.000000000000000000, 0.9659258262890683122, 1.000000000000000000, 0.9659258262890683122, 1.000000000000000000, 0.9659258262890683122, 1.000000000000000000, 0.9659258262890683122, 1.000000000000000000, 0.9659258262890683122, 1.000000000000000000, 0.9659258262890683122, 1.000000000000000000, 0.9659258262890683122, 1.000000000000000000, 0.9659258262890683122, 1.000000000000000000, 0.9659258262890683122, 1.000000000000000000, 0.9659258262890683122, 1.000000000000000000, 0.9659258262890683122, 1.000000000000000000, 0.9659258262890683122, 1.000000000000000000, 0.9659258262890683122, 1.000000000000000000, 0.9659258262890683122, 1.000000000000000000, 0.9659258262890683122, 1.000000000000000000, 0.9659258262890683122, 1.000000000000000000, 0.9659258262890683122, 1.000000000000000000, 0.9659258262890683122, 1.000000000000000000, 0.9659258262890683122, 1.000000000000000000, 0.9659258262890683122, 1.000000000000000000, 0.9659258262890683122, 1.000000000000000000, 0.9659258262890683122, 1.000000000000000000, 0.9659258262890683122, 1.000000000000000000, 0.9659258262890683122, 1.000000000000000000, 0.9659258262890683122, 1.000000000000000000, 0.9659258262890683122, 1.000000000000000000, 0.9659258262890683122, 1.000000000000000000, 0.9659258262890683122, 1.000000000000000000, 0.9659258262890683122, 1.000000000000000000, 0.9659258262890683122, 1.000000000000000000, 0.9659258262890683122, 1.000000000000000000, 0.9659258262890683122, 1.000000000000000000, 0.9659258262890683122, 1.000000000000000000, 0.9659258262890683122, 1.000000000000000000, 0.9659258262890683122, 1.000000000000000000, 0.9659258262890683122, 1.000000000000000000, 0.9659258262890683122, 1.000000000000000000, 0.9659258262890683122, 1.000000000000000000, 0.9659258262890683122, 1.000000000000000000, 0.9659258262890683122, 1.000000000000000000, 0.9659258262890683122, 1.000000000000000000, 0.9659258262890683122, 1.000000000000000000, 0.9659258262890683122, 1.000000000000000000, 0.9659258262890683122, 1.000000000000000000, 0.9659258262890683122, 1.000000000000000000, 0.9659258262890683122, 1.000000000000000000, 0.9659258262890683122, 1.000000000000000000, 0.9659258262890683122, 1.000000000000000000, 0.9659258262890683122, 1.000000000000000000, 0.9659258262890683122, 1.000000000000000000, 0.9659258262890683122, 1.000000000000000000, 0.9659258262890683122, 1.000000000000000000, 0.9659258262890683122, 1.000000000000000000, 0.9659258262890683122, 1.000000000000000000, 0.9659258262890683122, 1.000000000000000000, 0.9659258262890683122, 1.000000000000000000, 0.9659258262890683122, 1.000000000000000000, 0.9659258262890683122, 1.000000000000000000, 0.9659258262890683122, 1.000000000000000000, 0.9659258262890683122, 1.000000000000000000, 0.9659258262890683122, 1.000000000000000000, 0.9659258262890683122, 1.000000000000000000, 0.9659258262890683122, 1.000000000000000000, 0.9659258262890683122, 1.000000000000000000, 0.9659258262890683122, 1.000000000000000000, 0.9659258262890683122, 1.000000000000000000, 0.9659258262890683122, 1.000000000000000000, 0.9659258262890683122, 1.000000000000000000, 0.9659258262890683122, 1.000000000000000000, 0.9659258262890683122, 1.000000000000000000, 0.9659258262890683122, 1.000000000000000000, 0.9659258262890683122, 1.000000000000000000, 0.9659258262890683122, 1.000000000000000000, 0.9659258262890683122, 1.000000000000000000, 0.9659258262890683122, 1.000000000000000000, 0.9659258262890683122, 1.000000000000000000, 0.9659258262890683122, 1.000000000000000000, 0.9659258262890683122, 1.000000000000000000, 0.9659258262890683122, 1.000000000000000000, 0.9659258262890683122, 1.000000000000000000, 0.9659258262890683122, 1.000000000000000000, 0.9659258262890683122, 1.000000000000000000, 0.9659258262890683122, 1.000000000000000000, 0.9659258262890683122, 1.000000000000000000, 0.9659258262890683122, 1.000000000000000000, 0.9659258262890683122, 1.000000000000000000, 0.9659258262890683122, 1.000000000000000000, 0.9659258262890683122, 1.000000000000000000, 0.9659258262890683122, 1.000000000000000000, 0.9659258262890683122, 1.000000000000000000, 0.9659258262890683122, 1.000000000000000000, 0.9659258262890683122, 1.000000000000000000, 0.9659258262890683122, 1.000000000000000000, 0.9659258262890683122, 1.000000000000000000, 0.9659258262890683122, 1.000000000000000000, 0.9659258262890683122, 1.000000000000000000, 0.9659258262890683122, 1.000000000000000000, 0.9659258262890683122, 1.000000000000000000, 0.9659258262890683122, 1.000000000000000000, 0.9659258262890683122, 1.000000000000000000, 0.9659258262890683122, 1.000000000000000000, 0.9659258262890683122, 1.000000000000000000, 0.9659258262890683122, 1.000000000000000000, 0.9659258262890683122, 1.000000000000000000, 0.9659258262890683122, 1.000000000000000000, 0.9659258262890683122, 1.000000000000000000, 0.9659258262890683122, 1.000000000000000000, 0.9659258262890683122, 1.000000000000000000, 0.9659258262890683122, 1.000000000000000000, 0.9659258262890683122, 1.000000000000000000, 0.9659258262890683122, 1.000000000000000000, 0.9659258262890683122, 1.000000000000000000, 0.9659258262890683122, 1.000000000000000000, 0.9659258262890683122, 1.000000000000000000, 0.9659258262890683122, 1.000000000000000000, 0.9659258262890683122, 1.000000000000000000, 0.9659258262890683122, 1.000000000000000000, 0.9659258262890683122, 1.000000000000000000, 0.9659258262890683122, 1.000000000000000000, 0.9659258262890683122, 1.000000000000000000, 0.9659258262890683122, 1.000000000000000000, 0.9659258262890683122, 1.000000000000000000, 0.9659258262890683122, 1.000000000000000000, 0.9659258262890683122, 1.000000000000000000, 0.9659258262890683122, 1.000000000000000000, 0.9659258262890683122, 1.000000000000000000, 0.9659258262890683122, 1.000000000000000000, 0.9659258262890683122, 1.000000000000000000, 0.9659258262890683122, 1.000000000000000000, 0.9659258262890683122, 1.000000000000000000, 0.9659258262890683122, 1.000000000000000000, 0.9659258262890683122, 1.000000000000000000, 0.9659258262890683122, 1.000000000000000000, 0.9659258262890683122, 1.000000000000000000, 0.9659258262890683122, 1.000000000000000000, 0.9659258262890683122, 1.000000000000000000) ) ) 
 REPRESENTATION_ITEM ( '' )  SURFACE ( )  );
#23132=CARTESIAN_POINT ( 'NONE',  ( 17.20831665107776587, 57.88393115100078745, 7.208316651077764980 ) ) ;
#23133=CARTESIAN_POINT ( 'NONE',  ( 7.084665262690076126, 9.105352010821503583, 10.88017736071109987 ) ) ;
#23135=CARTESIAN_POINT ( 'NONE',  ( 13.43411237798105340, 15.58196800326374998, 12.81628187352647963 ) ) ;
#23137=CARTESIAN_POINT ( 'NONE',  ( 12.91533473730993009, 41.60535201082149825, -10.88017736071109987 ) ) ;
#23138=CARTESIAN_POINT ( 'NONE',  ( 17.20831665107776587, 62.88393115100078745, 7.208316651077764980 ) ) ;
#23140=CARTESIAN_POINT ( 'NONE',  ( 2.035157376598824452, 13.68868534415483751, 7.964842623401179544 ) ) ;
#23141=CARTESIAN_POINT ( 'NONE',  ( 10.00000000000000000, 21.81368534415484106, -10.88017736071110342 ) ) ;
#23142=CARTESIAN_POINT ( 'NONE',  ( -4.164238869374098151, 41.59541550158061796, -3.795296366450310543 ) ) ;
#23143=CARTESIAN_POINT ( 'NONE',  ( 2.791683348922237240, 30.38393115100078390, -7.208316651077763204 ) ) ;
#23144=CARTESIAN_POINT ( 'NONE',  ( 0.5774900079438607392, 53.48035201082151247, 5.440088680355550821 ) ) ;
#23146=CARTESIAN_POINT ( 'NONE',  ( -2.266590686148945544, 1.387082168247301128, -7.082119434687050408 ) ) ;
#23150=CARTESIAN_POINT ( 'NONE',  ( 17.20831665107776587, 54.13393115100079456, -7.208316651077762316 ) ) ;
#23152=VERTEX_POINT ( 'NONE', #59686 ) ;
#23153=CARTESIAN_POINT ( 'NONE',  ( 6.204703633549690345, 35.76208216824729647, -14.16423886937410259 ) ) ;
#23154=CARTESIAN_POINT ( 'NONE',  ( -2.266590686148945544, 17.22041550158063572, 7.082119434687048631 ) ) ;
#23155=CARTESIAN_POINT ( 'NONE',  ( 12.63842701281683034, 2.467264484334118269, 9.846743663894596210 ) ) ;
#23156=CARTESIAN_POINT ( 'NONE',  ( -1.099225684535947600, 8.706968003263753531, -6.408140936763238038 ) ) ;
#23159=CARTESIAN_POINT ( 'NONE',  ( 10.00000000000000000, 41.81368534415484106, -10.88017736071110342 ) ) ;
#23160=CARTESIAN_POINT ( 'NONE',  ( 3.591859063236763294, 18.29030133659708568, -11.09922568453595026 ) ) ;
#23161=CARTESIAN_POINT ( 'NONE',  ( -4.164238869374099927, 27.01208216824730357, 3.795296366450308767 ) ) ;
#23162=CARTESIAN_POINT ( 'NONE',  ( 0.5774900079438607392, 18.48035201082150536, 5.440088680355550821 ) ) ;
#23163=CARTESIAN_POINT ( 'NONE',  ( 20.88017736071110875, 25.77201867748816966, -2.915334737309920765 ) ) ;
#23165=CARTESIAN_POINT ( 'NONE',  ( 4.559911319644449179, 53.89701867748817676, 9.422509992056141925 ) ) ;
#23166=CARTESIAN_POINT ( 'NONE',  ( 22.81628187352648496, 51.83196800326376064, -3.434112377981050290 ) ) ;
#23169=CARTESIAN_POINT ( 'NONE',  ( 10.00000000000000178, 70.00000000000000000, 0.000000000000000000 ) ) ;
#23171=ORIENTED_EDGE ( 'NONE', *, *, #29581, .T. ) ;
#23173=VERTEX_POINT ( 'NONE', #67199 ) ;
#23174=CARTESIAN_POINT ( 'NONE',  ( 6.204703633549690345, 60.76208216824730357, -14.16423886937410259 ) ) ;
#23175=CARTESIAN_POINT ( 'NONE',  ( -0.3689425029237881626, 62.42874883491396787, 10.36894250292379027 ) ) ;
#23176=CARTESIAN_POINT ( 'NONE',  ( 14.92337183194729633, 27.67559781766745530, 8.527530157486181039 ) ) ;
#23177=CARTESIAN_POINT ( 'NONE',  ( 10.00000000000000000, 64.75893115100078035, -9.846743663894594434 ) ) ;
#23180=ADVANCED_FACE ( 'NONE', ( #20718 ), #44688, .T. ) ;
#23181=CARTESIAN_POINT ( 'NONE',  ( 0.6178305044545818747, 3.498634669930420049, -9.382169495545419124 ) ) ;
#23183=EDGE_CURVE ( 'NONE', #88041, #97822, #75183, .T. ) ;
#23185=CARTESIAN_POINT ( 'NONE',  ( -4.164238869374099927, 27.01208216824730357, 3.795296366450308767 ) ) ;
#23186=ORIENTED_EDGE ( 'NONE', *, *, #6708, .T. ) ;
#23187=CARTESIAN_POINT ( 'NONE',  ( 6.204703633549690345, 47.84541550158064638, 14.16423886937410082 ) ) ;
#23189=CARTESIAN_POINT ( 'NONE',  ( 6.565887622018943937, 63.08196800326376064, -12.81628187352647608 ) ) ;
#23190=CARTESIAN_POINT ( 'NONE',  ( 17.96484262340118221, 29.93868534415484106, 7.964842623401181321 ) ) ;
#23191=CARTESIAN_POINT ( 'NONE',  ( 5.076628168052703671, 51.84226448433412315, 8.527530157486179263 ) ) ;
#23192=CARTESIAN_POINT ( 'NONE',  ( 20.88017736071110875, 25.77201867748816966, -2.915334737309920765 ) ) ;
#23193=CARTESIAN_POINT ( 'NONE',  ( 13.99999999999999822, 61.50000000000000711, 6.500000000000000888 ) ) ;
#23195=CARTESIAN_POINT ( 'NONE',  ( 0.1532563361054082862, 56.21726448433411605, 2.638427012816831674 ) ) ;
#23196=CARTESIAN_POINT ( 'NONE',  ( 12.63842701281683922, 49.55059781766744464, -9.846743663894590881 ) ) ;
#23199=CARTESIAN_POINT ( 'NONE',  ( 10.00000000000000000, -0.2410688489992152128, -9.846743663894594434 ) ) ;
#23203=CARTESIAN_POINT ( 'NONE',  ( 14.92337183194729633, 32.67559781766745175, 8.527530157486181039 ) ) ;
#23205=CARTESIAN_POINT ( 'NONE',  ( 3.591859063236761518, 39.95696800326375353, 11.09922568453594849 ) ) ;
#23206=CARTESIAN_POINT ( 'NONE',  ( 10.00000000000000178, 0.000000000000000000, 0.000000000000000000 ) ) ;
#23209=ORIENTED_EDGE ( 'NONE', *, *, #8322, .F. ) ;
#23210=PLANE ( 'NONE',  #25260 ) ;
#23212=CARTESIAN_POINT ( 'NONE',  ( 2.791683348922237240, 55.38393115100078745, -7.208316651077763204 ) ) ;
#23213=CARTESIAN_POINT ( 'NONE',  ( 17.08211943468705840, 35.13708216824730357, -12.26659068614894466 ) ) ;
#23214=CARTESIAN_POINT ( 'NONE',  ( 14.92337183194729988, 59.34226448433412315, -8.527530157486177487 ) ) ;
#23216=CARTESIAN_POINT ( 'NONE',  ( 18.52753015748618282, 3.925597817667451306, -4.923371831947291888 ) ) ;
#23217=CARTESIAN_POINT ( 'NONE',  ( 19.38216949554541557, 47.24863466993041783, -9.382169495545420901 ) ) ;
#23218=VECTOR ( 'NONE', #63283, 1000.000000000000000 ) ;
#23219=CARTESIAN_POINT ( 'NONE',  ( 18.52753015748618282, 48.92559781766745886, -4.923371831947291888 ) ) ;
#23220=CARTESIAN_POINT ( 'NONE',  ( 12.91533473730993009, 56.60535201082151247, -10.88017736071109987 ) ) ;
#23221=CARTESIAN_POINT ( 'NONE',  ( 17.20831665107776587, 47.88393115100078745, 7.208316651077764980 ) ) ;
#23225=CARTESIAN_POINT ( 'NONE',  ( 4.559911319644449179, 57.23035201082150536, -9.422509992056141925 ) ) ;
#23228=CARTESIAN_POINT ( 'NONE',  ( 4.559911319644449179, 28.89701867748817321, 9.422509992056141925 ) ) ;
#23229=CARTESIAN_POINT ( 'NONE',  ( -2.816281873526471635, -1.084698663402913210, -3.434112377981056508 ) ) ;
#23230=CARTESIAN_POINT ( 'NONE',  ( -0.8801773607110991993, 52.85535201082151247, -2.915334737309923874 ) ) ;
#23232=CARTESIAN_POINT ( 'NONE',  ( 17.39651004071842166, 12.93575266056827822, 6.499999999999998224 ) ) ;
#23234=CARTESIAN_POINT ( 'NONE',  ( 20.88017736071110164, 40.35535201082150536, 2.915334737309930979 ) ) ;
#23236=CARTESIAN_POINT ( 'NONE',  ( 17.20831665107776587, 17.88393115100078745, 7.208316651077764980 ) ) ;
#23238=CARTESIAN_POINT ( 'NONE',  ( 0.1532563361054082862, 41.21726448433411605, 2.638427012816831674 ) ) ;
#23239=FACE_OUTER_BOUND ( 'NONE', #6650, .T. ) ;
#23241=CARTESIAN_POINT ( 'NONE',  ( 19.84674366389459621, 58.50893115100078745, 7.409399052514197653E-17 ) ) ;
#23242=CARTESIAN_POINT ( 'NONE',  ( 10.00000000000000178, 63.05374883491396076, 14.16423886937410082 ) ) ;
#23244=CARTESIAN_POINT ( 'NONE',  ( 20.36894250292379738, 19.92874883491396787, -10.36894250292379027 ) ) ;
#23245=CARTESIAN_POINT ( 'NONE',  ( 24.16423886937410614, 49.30374883491396787, 8.672049930838204340E-16 ) ) ;
#23246=AXIS2_PLACEMENT_3D ( 'NONE', #48957, #62478, #1528 ) ;
#23247=CARTESIAN_POINT ( 'NONE',  ( 19.84674366389459621, 28.50893115100078745, 7.409399052514197653E-17 ) ) ;
#23248=CARTESIAN_POINT ( 'NONE',  ( 18.52753015748617571, 13.09226448433411960, 4.923371831947298993 ) ) ;
#23249=CARTESIAN_POINT ( 'NONE',  ( 19.42250999205614193, 5.147018677488171434, 5.440088680355555262 ) ) ;
#23251=CARTESIAN_POINT ( 'NONE',  ( 0.1532563361054100626, 30.80059781766744820, -2.638427012816831230 ) ) ;
#23252=CARTESIAN_POINT ( 'NONE',  ( 15.44008868035555260, 29.73035201082150891, 9.422509992056143702 ) ) ;
#23253=CARTESIAN_POINT ( 'NONE',  ( 0.1532563361054082862, 61.21726448433412315, 2.638427012816831674 ) ) ;
#23254=CARTESIAN_POINT ( 'NONE',  ( 24.16423886937410614, 4.303748834913967869, 8.672049930838204340E-16 ) ) ;
#23257=CARTESIAN_POINT ( 'NONE',  ( 1.472469842513823179, 6.425597817667451750, 4.923371831947296329 ) ) ;
#23258=CARTESIAN_POINT ( 'NONE',  ( 21.09922568453594849, 41.20696800326375353, 6.408140936763242479 ) ) ;
#23259=CARTESIAN_POINT ( 'NONE',  ( 2.791683348922240793, 36.63393115100078035, 7.208316651077764092 ) ) ;
#23261=CARTESIAN_POINT ( 'NONE',  ( 19.84674366389459266, 23.30059781766745530, 2.638427012816836559 ) ) ;
#23263=CARTESIAN_POINT ( 'NONE',  ( 20.36894250292379382, 58.67874883491396076, 10.36894250292379205 ) ) ;
#23264=CARTESIAN_POINT ( 'NONE',  ( 0.5774900079438590739, 52.64701867748817676, -5.440088680355550821 ) ) ;
#23266=CARTESIAN_POINT ( 'NONE',  ( 12.63842701281683034, 37.46726448433411605, 9.846743663894596210 ) ) ;
#23267=CARTESIAN_POINT ( 'NONE',  ( 15.44008868035555260, 9.730352010821505360, 9.422509992056143702 ) ) ;
#23268=CARTESIAN_POINT ( 'NONE',  ( 18.52753015748617571, 38.09226448433412315, 4.923371831947298993 ) ) ;
#23269=CARTESIAN_POINT ( 'NONE',  ( 17.84635730667654840, 38.63791097397319163, 6.500000000000047073 ) ) ;
#23270=CARTESIAN_POINT ( 'NONE',  ( 2.791683348922237240, 45.38393115100079456, -7.208316651077763204 ) ) ;
#23272=CARTESIAN_POINT ( 'NONE',  ( 4.559911319644449179, 48.89701867748817676, 9.422509992056141925 ) ) ;
#23274=ORIENTED_EDGE ( 'NONE', *, *, #72107, .F. ) ;
#23279=CARTESIAN_POINT ( 'NONE',  ( 17.20831665107776587, 2.883931151000785231, 7.208316651077764980 ) ) ;
#23280=CARTESIAN_POINT ( 'NONE',  ( 10.00000000000000000, 57.87363466993042493, -12.81628187352647608 ) ) ;
#23281=CARTESIAN_POINT ( 'NONE',  ( 0.5774900079438590739, 2.647018677488171434, -5.440088680355550821 ) ) ;
#23282=CARTESIAN_POINT ( 'NONE',  ( 0.1532563361054083140, 51.00893115100078745, 1.131784320476157264E-15 ) ) ;
#23284=CARTESIAN_POINT ( 'NONE',  ( -2.266590686148945544, 31.38708216824730002, -7.082119434687050408 ) ) ;
#23285=CARTESIAN_POINT ( 'NONE',  ( 24.16423886937410614, 64.30374883491396076, 8.672049930838204340E-16 ) ) ;
#23286=CARTESIAN_POINT ( 'NONE',  ( 2.791683348922240793, 51.63393115100078745, 7.208316651077764092 ) ) ;
#23288=CARTESIAN_POINT ( 'NONE',  ( 10.00000000000000178, 49.31368534415484106, 10.88017736071110342 ) ) ;
#23289=CARTESIAN_POINT ( 'NONE',  ( 4.559911319644449179, 67.23035201082150536, -9.422509992056141925 ) ) ;
#23293=CARTESIAN_POINT ( 'NONE',  ( 21.09922568453594849, 56.20696800326375353, 6.408140936763242479 ) ) ;
#23294=CARTESIAN_POINT ( 'NONE',  ( 14.92337183194729988, 9.342264484334119601, -8.527530157486177487 ) ) ;
#23297=CARTESIAN_POINT ( 'NONE',  ( 10.00000000000000000, 20.55374883491396787, -14.16423886937410082 ) ) ;
#23298=CARTESIAN_POINT ( 'NONE',  ( 18.52753015748617571, 18.09226448433411960, 4.923371831947298993 ) ) ;
#23299=CARTESIAN_POINT ( 'NONE',  ( 12.91533473730993009, 31.60535201082150891, -10.88017736071109987 ) ) ;
#23302=CARTESIAN_POINT ( 'NONE',  ( 10.00000000000000000, 21.81368534415484106, -10.88017736071110342 ) ) ;
#23307=CARTESIAN_POINT ( 'NONE',  ( 19.42250999205614548, 35.98035201082151247, -5.440088680355545492 ) ) ;
#23308=SURFACE_SIDE_STYLE ('',( #53285 ) ) ;
#23310=CARTESIAN_POINT ( 'NONE',  ( 19.38216949554541202, 15.99863466993042138, 9.382169495545424454 ) ) ;
#23311=CARTESIAN_POINT ( 'NONE',  ( 14.92337183194729633, 7.675597817667451750, 8.527530157486181039 ) ) ;
#23313=CARTESIAN_POINT ( 'NONE',  ( 17.20831665107776587, 22.88393115100078745, 7.208316651077764980 ) ) ;
#23314=CARTESIAN_POINT ( 'NONE',  ( 7.084665262690076126, 34.10535201082151247, 10.88017736071109987 ) ) ;
#23315=CIRCLE ( 'NONE', #26495, 62.50000000000000000 ) ;
#23319=CARTESIAN_POINT ( 'NONE',  ( 3.591859063236763294, 63.29030133659708923, -11.09922568453595026 ) ) ;
#23320=CARTESIAN_POINT ( 'NONE',  ( 17.96484262340118221, 51.18868534415483396, -7.964842623401177768 ) ) ;
#23323=CARTESIAN_POINT ( 'NONE',  ( 0.6178305044545838731, 59.74863466993041783, 9.382169495545420901 ) ) ;
#23324=CARTESIAN_POINT ( 'NONE',  ( 20.88017736071110519, 65.56368534415483396, 2.639326808657452039E-16 ) ) ;
#23325=CARTESIAN_POINT ( 'NONE',  ( -1.099225684535947600, 4.540301336597087456, 6.408140936763237150 ) ) ;
#23327=CARTESIAN_POINT ( 'NONE',  ( 2.791683348922240793, 31.63393115100078745, 7.208316651077764092 ) ) ;
#23328=CARTESIAN_POINT ( 'NONE',  ( -1.099225684535947600, 48.70696800326375353, -6.408140936763238038 ) ) ;
#23330=CARTESIAN_POINT ( 'NONE',  ( 17.20831665107776587, 24.13393115100078035, -7.208316651077762316 ) ) ;
#23331=CARTESIAN_POINT ( 'NONE',  ( 16.40814093676324603, 17.45696800326375353, -11.09922568453594671 ) ) ;
#23334=CARTESIAN_POINT ( 'NONE',  ( 12.91533473730993009, 36.60535201082151247, -10.88017736071109987 ) ) ;
#23335=CARTESIAN_POINT ( 'NONE',  ( 7.361572987183169658, 64.96726448433412315, -9.846743663894592657 ) ) ;
#23336=CARTESIAN_POINT ( 'NONE',  ( -1.926860441876562247, 32.45379003517447813, -3.195792623639530650 ) ) ;
#23337=CARTESIAN_POINT ( 'NONE',  ( 19.84674366389459621, 23.50893115100078390, 7.409399052514197653E-17 ) ) ;
#23338=CARTESIAN_POINT ( 'NONE',  ( 19.84674366389459621, 13.50893115100078568, 7.409399052514197653E-17 ) ) ;
#23339=CARTESIAN_POINT ( 'NONE',  ( 4.559911319644449179, 13.89701867748817143, 9.422509992056141925 ) ) ;
#23340=CARTESIAN_POINT ( 'NONE',  ( 6.565887622018943937, 13.08196800326374998, -12.81628187352647608 ) ) ;
#23341=CARTESIAN_POINT ( 'NONE',  ( 0.1532563361054100626, 65.80059781766745175, -2.638427012816831230 ) ) ;
#23343=CARTESIAN_POINT ( 'NONE',  ( 19.42250999205614548, 5.980352010821504471, -5.440088680355545492 ) ) ;
#23344=CARTESIAN_POINT ( 'NONE',  ( 17.20831665107776587, 42.88393115100077324, 7.208316651077764980 ) ) ;
#23346=CARTESIAN_POINT ( 'NONE',  ( 0.5774900079438590739, 17.64701867748817321, -5.440088680355550821 ) ) ;
#23348=B_SPLINE_CURVE_WITH_KNOTS ( 'NONE', 3,
 ( #85960, #24480, #77449, #32448, #63436, #17469 ),
 .UNSPECIFIED., .F., .F.,
 ( 4, 2, 4 ),
 ( 0.000000000000000000, 0.0002565770811490879037, 0.0005131541622981758075 ),
 .UNSPECIFIED. ) ;
#23349=CARTESIAN_POINT ( 'NONE',  ( 20.88017736071110875, 30.77201867748816966, -2.915334737309920765 ) ) ;
#23350=CARTESIAN_POINT ( 'NONE',  ( -0.8801773607111008646, 3.272018677488171434, 2.915334737309923430 ) ) ;
#23352=FILL_AREA_STYLE ('',( #84346 ) ) ;
#23353=CARTESIAN_POINT ( 'NONE',  ( 19.84674366389459621, 18.50893115100078745, 7.409399052514197653E-17 ) ) ;
#23354=CARTESIAN_POINT ( 'NONE',  ( 22.81628187352648496, 11.83196800326375531, -3.434112377981050290 ) ) ;
#23355=CIRCLE ( 'NONE', #17003, 62.00000000000000000 ) ;
#23357=CARTESIAN_POINT ( 'NONE',  ( 19.84674366389459266, 63.30059781766745886, 2.638427012816836559 ) ) ;
#23360=CARTESIAN_POINT ( 'NONE',  ( 17.08211943468705840, 5.137082168247300906, -12.26659068614894466 ) ) ;
#23361=CARTESIAN_POINT ( 'NONE',  ( 19.84674366389459621, 33.50893115100078745, 7.409399052514197653E-17 ) ) ;
#23364=CARTESIAN_POINT ( 'NONE',  ( 17.08211943468705840, 60.13708216824729647, -12.26659068614894466 ) ) ;
#23365=CARTESIAN_POINT ( 'NONE',  ( 19.84674366389459266, 13.71726448433411782, -2.638427012816827677 ) ) ;
#23367=CARTESIAN_POINT ( 'NONE',  ( 19.42250999205614193, 45.14701867748817676, 5.440088680355555262 ) ) ;
#23368=CARTESIAN_POINT ( 'NONE',  ( -2.816281873526473856, 49.12363466993042493, 9.499525473075851096E-16 ) ) ;
#23369=CARTESIAN_POINT ( 'NONE',  ( 2.035157376598824452, 13.68868534415483751, 7.964842623401179544 ) ) ;
#23370=CARTESIAN_POINT ( 'NONE',  ( 3.591859063236763294, 43.29030133659708923, -11.09922568453595026 ) ) ;
#23371=CARTESIAN_POINT ( 'NONE',  ( 22.81628187352647785, 1.415301336597087012, 3.434112377981063169 ) ) ;
#23372=( NAMED_UNIT ( * ) SI_UNIT ( $, .STERADIAN. ) SOLID_ANGLE_UNIT ( ) );
#23373=ORIENTED_EDGE ( 'NONE', *, *, #2422, .F. ) ;
#23377=CARTESIAN_POINT ( 'NONE',  ( -2.266590686148945544, 42.22041550158063217, 7.082119434687048631 ) ) ;
#23378=CARTESIAN_POINT ( 'NONE',  ( 20.36894250292379738, 14.92874883491396432, -10.36894250292379027 ) ) ;
#23379=CARTESIAN_POINT ( 'NONE',  ( 4.559911319644449179, 23.89701867748817321, 9.422509992056141925 ) ) ;
#23380=CARTESIAN_POINT ( 'NONE',  ( 17.96484262340118221, 36.18868534415484106, -7.964842623401177768 ) ) ;
#23383=CARTESIAN_POINT ( 'NONE',  ( 19.42250999205614193, 60.14701867748817676, 5.440088680355555262 ) ) ;
#23384=CARTESIAN_POINT ( 'NONE',  ( -0.8801773607110991993, 62.85535201082150536, -2.915334737309923874 ) ) ;
#23385=CARTESIAN_POINT ( 'NONE',  ( 16.40814093676324603, 27.45696800326375708, -11.09922568453594671 ) ) ;
#23388=CARTESIAN_POINT ( 'NONE',  ( 2.791683348922237240, 5.383931151000785675, -7.208316651077763204 ) ) ;
#23389=CARTESIAN_POINT ( 'NONE',  ( 1.472469842513823179, 41.42559781766745886, 4.923371831947296329 ) ) ;
#23391=CARTESIAN_POINT ( 'NONE',  ( 2.035157376598822676, 7.438685344154837509, -7.964842623401177768 ) ) ;
#23392=AXIS2_PLACEMENT_3D ( 'NONE', #28740, #98762, #38236 ) ;
#23393=( BOUNDED_SURFACE ( )  B_SPLINE_SURFACE ( 1, 2, ( 
 ( #51323, #80349, #88828, #87354, #64829, #26845, #95347, #36324, #94852, #12824, #43810, #19837, #95851, #50326, #50836, #81807, #13326, #5830, #26353, #27334, #11353, #81329, #80838, #12338, #4368, #28326, #19353, #34833, #41873, #65821, #42843, #18868, #56854, #65326, #49349, #73327, #43323, #4852, #11846, #35327, #49837, #96355, #34333, #27826, #87834, #20339, #58312, #73816, #5350, #35828, #66314, #3869, #96850, #89325, #20834, #79851, #72337, #57341, #42355, #72830, #62133, #14325, #52797, #92641, #69657, #67819, #29793, #52311, #46650, #16660, #36822, #83301, #37329, #82803, #44796, #8655, #75301, #70158, #47643, #90291, #6813, #6315, #24165, #98335, #67314, #39168, #47135, #60304, #90797, #78139, #24659, #31641, #97839, #54636, #85154, #51818, #22323, #1183, #28811, #55128, #74809, #59310, #66817, #32128, #97339, #44307, #77632, #77146, #9149, #29304, #59799, #21828, #16166, #1675, #39666, #62627, #17163, #93132, #85644, #9649, #89808, #21329, #82304, #13826, #48616, #94615, #11605, #33119, #4122, #57101, #95096, #79617, #32630, #10147, #78640, #34097, #55641, #88089, #71140, #42122, #2173, #19107, #79120, #87110, #33602, #10633, #87597, #18625, #72588, #63613, #63129, #34585, #49587, #3140, #49116, #27089, #40642, #80602, #41145, #56139, #18144, #11118, #86634, #65079, #19602, #94119, #71630, #2668, #64588, #64099, #25646, #41637, #80100, #26130, #56621, #50097, #95603, #3630, #72103, #26604, #57592, #25166, #40146, #70650, #93631, #86141, #48125, #17655, #12100, #75065, #42603, #88583, #82071, #21087, #29064, #50595, #73573, #5098, #66583, #14087, #13081, #96605, #60056, #81087, #28581, #67583, #73081, #52080, #98092, #52561, #20596, #97110, #82573, #35589, #6572, #59572, #67075, #51585, #4617, #12588, #43088, #6086, #27589, #90557, #66077, #44567, #35078, #90065, #51082, #59072, #5601, #81574, #21589, #89576, #37084, #28082, #65578, #29551, #22086, #74069, #13581, #96105, #58580, #58079, #43576, #20091, #89082, #36080, #44065, #74572, #97603, #36588, #68565, #69055, #38074, #591, #22577, #54040, #76056, #77039, #31034, #76545, #8552, #46058, #8063, #91049, #38560, #84550, #15578, #61534, #92043, #16049, #23571, #83567, #39051, #30543, #46538, #69546, #1064, #84057, #31529, #96, #62024, #92525, #53048, #24052, #53544, #54522, #32011, #68073, #85038, #39550, #61043, #16550, #75565, #15087, #45558, #7585, #24555, #83065, #47025, #62513, #77516, #9033, #70039, #1562, #93018, #14586, #45055, #7078, #37580, #98600, #30050, #60559, #91556, #23075, #87487, #78513, #63507, #2053, #26012, #56022, #85530, #71027, #17538 ),
 ( #48993, #18018, #79002, #63013, #48501, #56505, #86521, #10507, #41022, #86997, #71524, #55526, #79503, #2550, #3033, #11002, #18503, #33482, #63979, #40529, #94492, #3512, #25041, #41521, #25530, #33007, #94007, #71989, #33971, #56982, #34470, #10028, #64475, #93516, #94981, #26487, #86023, #19002, #49478, #79986, #11488, #64963, #42008, #72475, #48006, #4007, #95489, #40028, #55013, #17042, #47521, #78024, #9527, #70531, #32516, #13459, #26980, #4499, #43455, #81458, #28464, #34964, #57964, #88468, #58452, #43943, #4984, #50468, #97475, #65462, #20476, #36461, #57479, #81948, #28939, #87975, #35464, #50963, #74441, #19970, #5967, #80485, #49978, #12960, #65961, #66452, #73957, #27471, #96987, #19486, #5485, #58959, #66956, #11984, #89458, #72968, #80973, #12472, #73456, #42976, #59443, #20975, #96488, #35956, #42487, #95990, #27959, #51459, #88967, #72789, #2865, #11317, #9858, #86342, #48330, #17845, #57794, #17365, #34292, #65288, #41356, #18338, #10837, #72303, #4326, #34798, #95815, #47834, #48818, #32828, #3833, #79327, #71825, #25842, #49800, #40845, #56340, #63327, #87313, #3334, #78337, #33316, #78834, #10345, #71347, #40357, #63811, #27295, #41836, #93835, #19314, #86834, #80308, #64303, #94321, #64789, #33796, #95306, #94814, #26317, #55847, #26810, #56815, #18831, #49311, #70858, #79813, #2373, #57304, #87796, #11808, #42316, #25361, #8945, #503, #16459, #977, #46456, #8460, #69953, #76949, #32429, #9943, #53959, #38965, #68971, #54927, #31440, #30951, #1472, #77934, #92442, #23965, #40446, #85943, #92929, #61450, #85443, #24462, #15492, #54439, #31926, #91466, #17454, #38478, #22991, #30457, #93432, #47921, #91957, #53457, #60956, #24954, #83965, #7979, #62426, #39463, #47436, #23487, #84466, #15964, #84948, #62930, #61941, #69458, #78426, #46939, #77432, #70947, #45974, #70446, #76464, #16951, #9442, #39943, #1963, #55439, #65378, #19402, #57394, #41927, #93926, #71437, #40939, #95400, #17934, #50381, #33399, #72882, #63423, #80399, #41444, #49397, #94902, #71904, #49888, #79898, #34883, #94411, #25452, #4419, #11903, #64392, #11404, #88390, #2951, #42893, #10919, #55935, #2465, #3428, #19889, #72389, #87884, #56900, #86915, #87405, #56428, #18921, #63898, #3917, #25926, #26899, #34386, #26400, #42405, #64874, #95906, #10431, #27387, #57878, #33887, #80890, #12388, #32921, #86435, #18424, #48419, #48907, #78921, #79423, #74861, #74352, #89372, #51872, #75350, #82355, #43371, #59358, #43857, #20884, #51373, #13876, #81860, #6864, #52845, #96901, #13372, #12873, #97890, #5878, #73871, #44359, #21878, #36374 ) ),
 .UNSPECIFIED., .F., .F., .T. ) 
 B_SPLINE_SURFACE_WITH_KNOTS ( ( 2, 2 ),
 ( 3, 2, 2, 2, 2, 2, 2, 2, 2, 2, 2, 2, 2, 2, 2, 2, 2, 2, 2, 2, 2, 2, 2, 2, 2, 2, 2, 2, 2, 2, 2, 2, 2, 2, 2, 2, 2, 2, 2, 2, 2, 2, 2, 2, 2, 2, 2, 2, 2, 2, 2, 2, 2, 2, 2, 2, 2, 2, 2, 2, 2, 2, 2, 2, 2, 2, 2, 2, 2, 2, 2, 2, 2, 2, 2, 2, 2, 2, 2, 2, 2, 2, 2, 2, 2, 2, 2, 2, 2, 2, 2, 2, 2, 2, 2, 2, 2, 2, 2, 2, 2, 2, 2, 2, 2, 2, 2, 2, 2, 2, 2, 2, 2, 2, 2, 2, 2, 2, 2, 2, 2, 2, 2, 2, 2, 2, 2, 2, 2, 2, 2, 2, 2, 2, 2, 2, 2, 2, 2, 2, 2, 2, 2, 2, 2, 2, 2, 2, 2, 2, 2, 2, 2, 2, 2, 2, 2, 2, 2, 2, 2, 2, 3 ),
 ( 0.000000000000000000, 1.000000000000000000 ),
 ( 0.000000000000000000, 0.005952380952380952051, 0.01190476190476190410, 0.01785714285714285615, 0.02380952380952380820, 0.02976190476190476025, 0.03571428571428571230, 0.04166666666666666435, 0.04761904761904761640, 0.05357142857142856845, 0.05952380952380952051, 0.06547619047619047949, 0.07142857142857142461, 0.07738095238095238360, 0.08333333333333332871, 0.08928571428571428770, 0.09523809523809523281, 0.1011904761904761918, 0.1071428571428571369, 0.1130952380952380959, 0.1190476190476190410, 0.1250000000000000000, 0.1309523809523809590, 0.1369047619047619180, 0.1428571428571428492, 0.1488095238095238082, 0.1547619047619047672, 0.1607142857142857262, 0.1666666666666666574, 0.1726190476190476164, 0.1785714285714285754, 0.1845238095238095344, 0.1904761904761904656, 0.1964285714285714246, 0.2023809523809523836, 0.2083333333333333426, 0.2142857142857142738, 0.2202380952380952328, 0.2261904761904761918, 0.2321428571428571508, 0.2380952380952380820, 0.2440476190476190410, 0.2500000000000000000, 0.2559523809523809312, 0.2619047619047619180, 0.2678571428571428492, 0.2738095238095238360, 0.2797619047619047672, 0.2857142857142856984, 0.2916666666666666852, 0.2976190476190476164, 0.3035714285714285476, 0.3095238095238095344, 0.3154761904761904656, 0.3214285714285714524, 0.3273809523809523836, 0.3333333333333333148, 0.3392857142857143016, 0.3452380952380952328, 0.3511904761904761640, 0.3571428571428571508, 0.3630952380952380820, 0.3690476190476190688, 0.3750000000000000000, 0.3809523809523809312, 0.3869047619047619180, 0.3928571428571428492, 0.3988095238095238360, 0.4047619047619047672, 0.4107142857142856984, 0.4166666666666666852, 0.4226190476190476164, 0.4285714285714285476, 0.4345238095238095344, 0.4404761904761904656, 0.4464285714285714524, 0.4523809523809523836, 0.4583333333333333148, 0.4642857142857143016, 0.4702380952380952328, 0.4761904761904761640, 0.4821428571428571508, 0.4880952380952380820, 0.4940476190476190688, 0.5000000000000000000, 0.5059523809523809312, 0.5119047619047618625, 0.5178571428571429047, 0.5238095238095238360, 0.5297619047619047672, 0.5357142857142856984, 0.5416666666666666297, 0.5476190476190476719, 0.5535714285714286031, 0.5595238095238095344, 0.5654761904761904656, 0.5714285714285713969, 0.5773809523809523281, 0.5833333333333333703, 0.5892857142857143016, 0.5952380952380952328, 0.6011904761904761640, 0.6071428571428570953, 0.6130952380952381375, 0.6190476190476190688, 0.6250000000000000000, 0.6309523809523809312, 0.6369047619047618625, 0.6428571428571429047, 0.6488095238095238360, 0.6547619047619047672, 0.6607142857142856984, 0.6666666666666666297, 0.6726190476190476719, 0.6785714285714286031, 0.6845238095238095344, 0.6904761904761904656, 0.6964285714285713969, 0.7023809523809523281, 0.7083333333333333703, 0.7142857142857143016, 0.7202380952380952328, 0.7261904761904761640, 0.7321428571428570953, 0.7380952380952381375, 0.7440476190476190688, 0.7500000000000000000, 0.7559523809523809312, 0.7619047619047618625, 0.7678571428571429047, 0.7738095238095238360, 0.7797619047619047672, 0.7857142857142856984, 0.7916666666666666297, 0.7976190476190476719, 0.8035714285714286031, 0.8095238095238095344, 0.8154761904761904656, 0.8214285714285713969, 0.8273809523809523281, 0.8333333333333333703, 0.8392857142857143016, 0.8452380952380952328, 0.8511904761904761640, 0.8571428571428570953, 0.8630952380952381375, 0.8690476190476190688, 0.8750000000000000000, 0.8809523809523809312, 0.8869047619047618625, 0.8928571428571429047, 0.8988095238095238360, 0.9047619047619047672, 0.9107142857142856984, 0.9166666666666666297, 0.9226190476190476719, 0.9285714285714286031, 0.9345238095238095344, 0.9404761904761904656, 0.9464285714285713969, 0.9523809523809523281, 0.9583333333333333703, 0.9642857142857143016 ),
 .UNSPECIFIED. ) 
 GEOMETRIC_REPRESENTATION_ITEM ( )  RATIONAL_B_SPLINE_SURFACE ( (
 ( 1.000000000000000000, 0.9659258262890683122, 1.000000000000000000, 0.9659258262890683122, 1.000000000000000000, 0.9659258262890683122, 1.000000000000000000, 0.9659258262890683122, 1.000000000000000000, 0.9659258262890683122, 1.000000000000000000, 0.9659258262890683122, 1.000000000000000000, 0.9659258262890683122, 1.000000000000000000, 0.9659258262890683122, 1.000000000000000000, 0.9659258262890683122, 1.000000000000000000, 0.9659258262890683122, 1.000000000000000000, 0.9659258262890683122, 1.000000000000000000, 0.9659258262890683122, 1.000000000000000000, 0.9659258262890683122, 1.000000000000000000, 0.9659258262890683122, 1.000000000000000000, 0.9659258262890683122, 1.000000000000000000, 0.9659258262890683122, 1.000000000000000000, 0.9659258262890683122, 1.000000000000000000, 0.9659258262890683122, 1.000000000000000000, 0.9659258262890683122, 1.000000000000000000, 0.9659258262890683122, 1.000000000000000000, 0.9659258262890683122, 1.000000000000000000, 0.9659258262890683122, 1.000000000000000000, 0.9659258262890683122, 1.000000000000000000, 0.9659258262890683122, 1.000000000000000000, 0.9659258262890683122, 1.000000000000000000, 0.9659258262890683122, 1.000000000000000000, 0.9659258262890683122, 1.000000000000000000, 0.9659258262890683122, 1.000000000000000000, 0.9659258262890683122, 1.000000000000000000, 0.9659258262890683122, 1.000000000000000000, 0.9659258262890683122, 1.000000000000000000, 0.9659258262890683122, 1.000000000000000000, 0.9659258262890683122, 1.000000000000000000, 0.9659258262890683122, 1.000000000000000000, 0.9659258262890683122, 1.000000000000000000, 0.9659258262890683122, 1.000000000000000000, 0.9659258262890683122, 1.000000000000000000, 0.9659258262890683122, 1.000000000000000000, 0.9659258262890683122, 1.000000000000000000, 0.9659258262890683122, 1.000000000000000000, 0.9659258262890683122, 1.000000000000000000, 0.9659258262890683122, 1.000000000000000000, 0.9659258262890683122, 1.000000000000000000, 0.9659258262890683122, 1.000000000000000000, 0.9659258262890683122, 1.000000000000000000, 0.9659258262890683122, 1.000000000000000000, 0.9659258262890683122, 1.000000000000000000, 0.9659258262890683122, 1.000000000000000000, 0.9659258262890683122, 1.000000000000000000, 0.9659258262890683122, 1.000000000000000000, 0.9659258262890683122, 1.000000000000000000, 0.9659258262890683122, 1.000000000000000000, 0.9659258262890683122, 1.000000000000000000, 0.9659258262890683122, 1.000000000000000000, 0.9659258262890683122, 1.000000000000000000, 0.9659258262890683122, 1.000000000000000000, 0.9659258262890683122, 1.000000000000000000, 0.9659258262890683122, 1.000000000000000000, 0.9659258262890683122, 1.000000000000000000, 0.9659258262890683122, 1.000000000000000000, 0.9659258262890683122, 1.000000000000000000, 0.9659258262890683122, 1.000000000000000000, 0.9659258262890683122, 1.000000000000000000, 0.9659258262890683122, 1.000000000000000000, 0.9659258262890683122, 1.000000000000000000, 0.9659258262890683122, 1.000000000000000000, 0.9659258262890683122, 1.000000000000000000, 0.9659258262890683122, 1.000000000000000000, 0.9659258262890683122, 1.000000000000000000, 0.9659258262890683122, 1.000000000000000000, 0.9659258262890683122, 1.000000000000000000, 0.9659258262890683122, 1.000000000000000000, 0.9659258262890683122, 1.000000000000000000, 0.9659258262890683122, 1.000000000000000000, 0.9659258262890683122, 1.000000000000000000, 0.9659258262890683122, 1.000000000000000000, 0.9659258262890683122, 1.000000000000000000, 0.9659258262890683122, 1.000000000000000000, 0.9659258262890683122, 1.000000000000000000, 0.9659258262890683122, 1.000000000000000000, 0.9659258262890683122, 1.000000000000000000, 0.9659258262890683122, 1.000000000000000000, 0.9659258262890683122, 1.000000000000000000, 0.9659258262890683122, 1.000000000000000000, 0.9659258262890683122, 1.000000000000000000, 0.9659258262890683122, 1.000000000000000000, 0.9659258262890683122, 1.000000000000000000, 0.9659258262890683122, 1.000000000000000000, 0.9659258262890683122, 1.000000000000000000, 0.9659258262890683122, 1.000000000000000000, 0.9659258262890683122, 1.000000000000000000, 0.9659258262890683122, 1.000000000000000000, 0.9659258262890683122, 1.000000000000000000, 0.9659258262890683122, 1.000000000000000000, 0.9659258262890683122, 1.000000000000000000, 0.9659258262890683122, 1.000000000000000000, 0.9659258262890683122, 1.000000000000000000, 0.9659258262890683122, 1.000000000000000000, 0.9659258262890683122, 1.000000000000000000, 0.9659258262890683122, 1.000000000000000000, 0.9659258262890683122, 1.000000000000000000, 0.9659258262890683122, 1.000000000000000000, 0.9659258262890683122, 1.000000000000000000, 0.9659258262890683122, 1.000000000000000000, 0.9659258262890683122, 1.000000000000000000, 0.9659258262890683122, 1.000000000000000000, 0.9659258262890683122, 1.000000000000000000, 0.9659258262890683122, 1.000000000000000000, 0.9659258262890683122, 1.000000000000000000, 0.9659258262890683122, 1.000000000000000000, 0.9659258262890683122, 1.000000000000000000, 0.9659258262890683122, 1.000000000000000000, 0.9659258262890683122, 1.000000000000000000, 0.9659258262890683122, 1.000000000000000000, 0.9659258262890683122, 1.000000000000000000, 0.9659258262890683122, 1.000000000000000000, 0.9659258262890683122, 1.000000000000000000, 0.9659258262890683122, 1.000000000000000000, 0.9659258262890683122, 1.000000000000000000, 0.9659258262890683122, 1.000000000000000000, 0.9659258262890683122, 1.000000000000000000, 0.9659258262890683122, 1.000000000000000000, 0.9659258262890683122, 1.000000000000000000, 0.9659258262890683122, 1.000000000000000000, 0.9659258262890683122, 1.000000000000000000, 0.9659258262890683122, 1.000000000000000000, 0.9659258262890683122, 1.000000000000000000, 0.9659258262890683122, 1.000000000000000000, 0.9659258262890683122, 1.000000000000000000, 0.9659258262890683122, 1.000000000000000000, 0.9659258262890683122, 1.000000000000000000, 0.9659258262890683122, 1.000000000000000000, 0.9659258262890683122, 1.000000000000000000, 0.9659258262890683122, 1.000000000000000000, 0.9659258262890683122, 1.000000000000000000, 0.9659258262890683122, 1.000000000000000000, 0.9659258262890683122, 1.000000000000000000, 0.9659258262890683122, 1.000000000000000000, 0.9659258262890683122, 1.000000000000000000, 0.9659258262890683122, 1.000000000000000000, 0.9659258262890683122, 1.000000000000000000, 0.9659258262890683122, 1.000000000000000000, 0.9659258262890683122, 1.000000000000000000, 0.9659258262890683122, 1.000000000000000000, 0.9659258262890683122, 1.000000000000000000, 0.9659258262890683122, 1.000000000000000000, 0.9659258262890683122, 1.000000000000000000, 0.9659258262890683122, 1.000000000000000000, 0.9659258262890683122, 1.000000000000000000, 0.9659258262890683122, 1.000000000000000000, 0.9659258262890683122, 1.000000000000000000, 0.9659258262890683122, 1.000000000000000000, 0.9659258262890683122, 1.000000000000000000, 0.9659258262890683122, 1.000000000000000000, 0.9659258262890683122, 1.000000000000000000, 0.9659258262890683122, 1.000000000000000000, 0.9659258262890683122, 1.000000000000000000, 0.9659258262890683122, 1.000000000000000000, 0.9659258262890683122, 1.000000000000000000, 0.9659258262890683122, 1.000000000000000000, 0.9659258262890683122, 1.000000000000000000, 0.9659258262890683122, 1.000000000000000000),
 ( 1.000000000000000000, 0.9659258262890683122, 1.000000000000000000, 0.9659258262890683122, 1.000000000000000000, 0.9659258262890683122, 1.000000000000000000, 0.9659258262890683122, 1.000000000000000000, 0.9659258262890683122, 1.000000000000000000, 0.9659258262890683122, 1.000000000000000000, 0.9659258262890683122, 1.000000000000000000, 0.9659258262890683122, 1.000000000000000000, 0.9659258262890683122, 1.000000000000000000, 0.9659258262890683122, 1.000000000000000000, 0.9659258262890683122, 1.000000000000000000, 0.9659258262890683122, 1.000000000000000000, 0.9659258262890683122, 1.000000000000000000, 0.9659258262890683122, 1.000000000000000000, 0.9659258262890683122, 1.000000000000000000, 0.9659258262890683122, 1.000000000000000000, 0.9659258262890683122, 1.000000000000000000, 0.9659258262890683122, 1.000000000000000000, 0.9659258262890683122, 1.000000000000000000, 0.9659258262890683122, 1.000000000000000000, 0.9659258262890683122, 1.000000000000000000, 0.9659258262890683122, 1.000000000000000000, 0.9659258262890683122, 1.000000000000000000, 0.9659258262890683122, 1.000000000000000000, 0.9659258262890683122, 1.000000000000000000, 0.9659258262890683122, 1.000000000000000000, 0.9659258262890683122, 1.000000000000000000, 0.9659258262890683122, 1.000000000000000000, 0.9659258262890683122, 1.000000000000000000, 0.9659258262890683122, 1.000000000000000000, 0.9659258262890683122, 1.000000000000000000, 0.9659258262890683122, 1.000000000000000000, 0.9659258262890683122, 1.000000000000000000, 0.9659258262890683122, 1.000000000000000000, 0.9659258262890683122, 1.000000000000000000, 0.9659258262890683122, 1.000000000000000000, 0.9659258262890683122, 1.000000000000000000, 0.9659258262890683122, 1.000000000000000000, 0.9659258262890683122, 1.000000000000000000, 0.9659258262890683122, 1.000000000000000000, 0.9659258262890683122, 1.000000000000000000, 0.9659258262890683122, 1.000000000000000000, 0.9659258262890683122, 1.000000000000000000, 0.9659258262890683122, 1.000000000000000000, 0.9659258262890683122, 1.000000000000000000, 0.9659258262890683122, 1.000000000000000000, 0.9659258262890683122, 1.000000000000000000, 0.9659258262890683122, 1.000000000000000000, 0.9659258262890683122, 1.000000000000000000, 0.9659258262890683122, 1.000000000000000000, 0.9659258262890683122, 1.000000000000000000, 0.9659258262890683122, 1.000000000000000000, 0.9659258262890683122, 1.000000000000000000, 0.9659258262890683122, 1.000000000000000000, 0.9659258262890683122, 1.000000000000000000, 0.9659258262890683122, 1.000000000000000000, 0.9659258262890683122, 1.000000000000000000, 0.9659258262890683122, 1.000000000000000000, 0.9659258262890683122, 1.000000000000000000, 0.9659258262890683122, 1.000000000000000000, 0.9659258262890683122, 1.000000000000000000, 0.9659258262890683122, 1.000000000000000000, 0.9659258262890683122, 1.000000000000000000, 0.9659258262890683122, 1.000000000000000000, 0.9659258262890683122, 1.000000000000000000, 0.9659258262890683122, 1.000000000000000000, 0.9659258262890683122, 1.000000000000000000, 0.9659258262890683122, 1.000000000000000000, 0.9659258262890683122, 1.000000000000000000, 0.9659258262890683122, 1.000000000000000000, 0.9659258262890683122, 1.000000000000000000, 0.9659258262890683122, 1.000000000000000000, 0.9659258262890683122, 1.000000000000000000, 0.9659258262890683122, 1.000000000000000000, 0.9659258262890683122, 1.000000000000000000, 0.9659258262890683122, 1.000000000000000000, 0.9659258262890683122, 1.000000000000000000, 0.9659258262890683122, 1.000000000000000000, 0.9659258262890683122, 1.000000000000000000, 0.9659258262890683122, 1.000000000000000000, 0.9659258262890683122, 1.000000000000000000, 0.9659258262890683122, 1.000000000000000000, 0.9659258262890683122, 1.000000000000000000, 0.9659258262890683122, 1.000000000000000000, 0.9659258262890683122, 1.000000000000000000, 0.9659258262890683122, 1.000000000000000000, 0.9659258262890683122, 1.000000000000000000, 0.9659258262890683122, 1.000000000000000000, 0.9659258262890683122, 1.000000000000000000, 0.9659258262890683122, 1.000000000000000000, 0.9659258262890683122, 1.000000000000000000, 0.9659258262890683122, 1.000000000000000000, 0.9659258262890683122, 1.000000000000000000, 0.9659258262890683122, 1.000000000000000000, 0.9659258262890683122, 1.000000000000000000, 0.9659258262890683122, 1.000000000000000000, 0.9659258262890683122, 1.000000000000000000, 0.9659258262890683122, 1.000000000000000000, 0.9659258262890683122, 1.000000000000000000, 0.9659258262890683122, 1.000000000000000000, 0.9659258262890683122, 1.000000000000000000, 0.9659258262890683122, 1.000000000000000000, 0.9659258262890683122, 1.000000000000000000, 0.9659258262890683122, 1.000000000000000000, 0.9659258262890683122, 1.000000000000000000, 0.9659258262890683122, 1.000000000000000000, 0.9659258262890683122, 1.000000000000000000, 0.9659258262890683122, 1.000000000000000000, 0.9659258262890683122, 1.000000000000000000, 0.9659258262890683122, 1.000000000000000000, 0.9659258262890683122, 1.000000000000000000, 0.9659258262890683122, 1.000000000000000000, 0.9659258262890683122, 1.000000000000000000, 0.9659258262890683122, 1.000000000000000000, 0.9659258262890683122, 1.000000000000000000, 0.9659258262890683122, 1.000000000000000000, 0.9659258262890683122, 1.000000000000000000, 0.9659258262890683122, 1.000000000000000000, 0.9659258262890683122, 1.000000000000000000, 0.9659258262890683122, 1.000000000000000000, 0.9659258262890683122, 1.000000000000000000, 0.9659258262890683122, 1.000000000000000000, 0.9659258262890683122, 1.000000000000000000, 0.9659258262890683122, 1.000000000000000000, 0.9659258262890683122, 1.000000000000000000, 0.9659258262890683122, 1.000000000000000000, 0.9659258262890683122, 1.000000000000000000, 0.9659258262890683122, 1.000000000000000000, 0.9659258262890683122, 1.000000000000000000, 0.9659258262890683122, 1.000000000000000000, 0.9659258262890683122, 1.000000000000000000, 0.9659258262890683122, 1.000000000000000000, 0.9659258262890683122, 1.000000000000000000, 0.9659258262890683122, 1.000000000000000000, 0.9659258262890683122, 1.000000000000000000, 0.9659258262890683122, 1.000000000000000000, 0.9659258262890683122, 1.000000000000000000, 0.9659258262890683122, 1.000000000000000000, 0.9659258262890683122, 1.000000000000000000, 0.9659258262890683122, 1.000000000000000000, 0.9659258262890683122, 1.000000000000000000, 0.9659258262890683122, 1.000000000000000000, 0.9659258262890683122, 1.000000000000000000, 0.9659258262890683122, 1.000000000000000000, 0.9659258262890683122, 1.000000000000000000, 0.9659258262890683122, 1.000000000000000000, 0.9659258262890683122, 1.000000000000000000, 0.9659258262890683122, 1.000000000000000000, 0.9659258262890683122, 1.000000000000000000, 0.9659258262890683122, 1.000000000000000000, 0.9659258262890683122, 1.000000000000000000, 0.9659258262890683122, 1.000000000000000000, 0.9659258262890683122, 1.000000000000000000, 0.9659258262890683122, 1.000000000000000000, 0.9659258262890683122, 1.000000000000000000, 0.9659258262890683122, 1.000000000000000000, 0.9659258262890683122, 1.000000000000000000, 0.9659258262890683122, 1.000000000000000000, 0.9659258262890683122, 1.000000000000000000, 0.9659258262890683122, 1.000000000000000000, 0.9659258262890683122, 1.000000000000000000, 0.9659258262890683122, 1.000000000000000000) ) ) 
 REPRESENTATION_ITEM ( '' )  SURFACE ( )  );
#23395=CARTESIAN_POINT ( 'NONE',  ( 19.38216949554541557, 27.24863466993041783, -9.382169495545420901 ) ) ;
#23396=CARTESIAN_POINT ( 'NONE',  ( 10.00000000000000000, 9.758931151000785675, -9.846743663894594434 ) ) ;
#23397=CARTESIAN_POINT ( 'NONE',  ( -0.8801773607111009756, 8.063685344154837509, 1.068504757029289695E-15 ) ) ;
#23399=CARTESIAN_POINT ( 'NONE',  ( 18.52753015748617571, 33.09226448433411605, 4.923371831947298993 ) ) ;
#23400=CARTESIAN_POINT ( 'NONE',  ( 14.92337183194729988, 29.34226448433411960, -8.527530157486177487 ) ) ;
#23402=CARTESIAN_POINT ( 'NONE',  ( -2.266590686148945544, 16.38708216824730357, -7.082119434687050408 ) ) ;
#23403=CARTESIAN_POINT ( 'NONE',  ( 20.88017736071110519, 35.56368534415484106, 2.639326808657452039E-16 ) ) ;
#23404=CARTESIAN_POINT ( 'NONE',  ( 20.88017736071110164, 5.355352010821502695, 2.915334737309930979 ) ) ;
#23405=CARTESIAN_POINT ( 'NONE',  ( 10.00000000000000178, 34.31368534415484106, 10.88017736071110342 ) ) ;
#23406=CARTESIAN_POINT ( 'NONE',  ( 7.084665262690076126, 34.10535201082151247, 10.88017736071109987 ) ) ;
#23408=CARTESIAN_POINT ( 'NONE',  ( 2.035157376598824452, 33.68868534415484106, 7.964842623401179544 ) ) ;
#23409=CARTESIAN_POINT ( 'NONE',  ( 22.81628187352647785, 61.41530133659709634, 3.434112377981063169 ) ) ;
#23410=CARTESIAN_POINT ( 'NONE',  ( 0.5774900079438607392, 43.48035201082151247, 5.440088680355550821 ) ) ;
#23412=CARTESIAN_POINT ( 'NONE',  ( 7.084665262690076126, 47.02201867748818387, -10.88017736071110164 ) ) ;
#23415=CARTESIAN_POINT ( 'NONE',  ( 15.44008868035555260, 44.73035201082151247, 9.422509992056143702 ) ) ;
#23420=CARTESIAN_POINT ( 'NONE',  ( -0.3689425029237898834, 66.17874883491396076, -10.36894250292378850 ) ) ;
#23421=CARTESIAN_POINT ( 'NONE',  ( 12.63842701281683034, 2.467264484334118269, 9.846743663894596210 ) ) ;
#23423=DIRECTION ( 'NONE',  ( 0.8320502943378436100, -0.5547001962252291474, 0.000000000000000000 ) ) ;
#23425=CARTESIAN_POINT ( 'NONE',  ( 14.92337183194729633, 37.67559781766745175, 8.527530157486181039 ) ) ;
#23427=CARTESIAN_POINT ( 'NONE',  ( 17.20831665107776587, 32.88393115100078745, 7.208316651077764980 ) ) ;
#23428=CARTESIAN_POINT ( 'NONE',  ( 17.96484262340118221, 44.93868534415483396, 7.964842623401181321 ) ) ;
#23429=CARTESIAN_POINT ( 'NONE',  ( 10.00000000000000178, 42.25893115100078745, 9.846743663894594434 ) ) ;
#23430=CARTESIAN_POINT ( 'NONE',  ( 19.38216949554541202, 20.99863466993042138, 9.382169495545424454 ) ) ;
#23431=DIRECTION ( 'NONE',  ( 0.000000000000000000, -1.000000000000000000, 0.000000000000000000 ) ) ;
#23432=CARTESIAN_POINT ( 'NONE',  ( 7.084665262690076126, 59.10535201082150536, 10.88017736071109987 ) ) ;
#23433=CARTESIAN_POINT ( 'NONE',  ( -0.8801773607111008646, 48.27201867748816966, 2.915334737309923430 ) ) ;
#23434=CARTESIAN_POINT ( 'NONE',  ( 17.96484262340118221, 6.188685344154836621, -7.964842623401177768 ) ) ;
#23435=CARTESIAN_POINT ( 'NONE',  ( 24.16423886937410614, 59.51208216824728936, -3.795296366450302550 ) ) ;
#23436=COLOUR_RGB ( '', 0.72549020, 0.75294118, 0.79215686) ;
#23437=CARTESIAN_POINT ( 'NONE',  ( -1.099225684535947600, 24.54030133659708923, 6.408140936763237150 ) ) ;
#23438=CARTESIAN_POINT ( 'NONE',  ( 1.959929470562281395, 50.51528370094808196, -5.767676674365853629 ) ) ;
#23440=CARTESIAN_POINT ( 'NONE',  ( 13.43411237798105340, 20.58196800326374643, 12.81628187352647963 ) ) ;
#23441=CARTESIAN_POINT ( 'NONE',  ( 17.96484262340118221, 24.93868534415484461, 7.964842623401181321 ) ) ;
#23443=CARTESIAN_POINT ( 'NONE',  ( 20.88017736071110519, 55.56368534415484817, 2.639326808657452039E-16 ) ) ;
#23445=EDGE_CURVE ( 'NONE', #95671, #83096, #75072, .T. ) ;
#23446=CARTESIAN_POINT ( 'NONE',  ( 7.361572987183169658, 4.967264484334119601, -9.846743663894592657 ) ) ;
#23447=CARTESIAN_POINT ( 'NONE',  ( 12.63842701281683034, 47.46726448433412315, 9.846743663894596210 ) ) ;
#23448=CARTESIAN_POINT ( 'NONE',  ( 18.52753015748618282, 38.92559781766745175, -4.923371831947291888 ) ) ;
#23451=CARTESIAN_POINT ( 'NONE',  ( 18.52753015748617571, 33.09226448433411605, 4.923371831947298993 ) ) ;
#23452=CARTESIAN_POINT ( 'NONE',  ( 19.72487221294571569, 54.78217586085238366, 6.499999999999995559 ) ) ;
#23454=CARTESIAN_POINT ( 'NONE',  ( 0.6178305044545818747, 43.49863466993042493, -9.382169495545419124 ) ) ;
#23455=EDGE_CURVE ( 'NONE', #37561, #86252, #46060, .T. ) ;
#23456=CARTESIAN_POINT ( 'NONE',  ( 0.1532563361054100626, 20.80059781766744464, -2.638427012816831230 ) ) ;
#23459=CARTESIAN_POINT ( 'NONE',  ( 2.791683348922240793, 51.63393115100078745, 7.208316651077764092 ) ) ;
#23461=CARTESIAN_POINT ( 'NONE',  ( 10.00000000000000000, 62.87363466993042493, -12.81628187352647608 ) ) ;
#23463=CARTESIAN_POINT ( 'NONE',  ( 19.38216949554541202, 5.998634669930420493, 9.382169495545424454 ) ) ;
#23464=CARTESIAN_POINT ( 'NONE',  ( 4.559911319644449179, 53.89701867748817676, 9.422509992056141925 ) ) ;
#23466=CARTESIAN_POINT ( 'NONE',  ( 10.00000000000000178, 38.05374883491396787, 14.16423886937410082 ) ) ;
#23467=CARTESIAN_POINT ( 'NONE',  ( 2.791683348922237240, 0.3839311510007847872, -7.208316651077763204 ) ) ;
#23469=CARTESIAN_POINT ( 'NONE',  ( 22.26659068614894466, 33.88708216824730357, 7.082119434687054849 ) ) ;
#23471=CARTESIAN_POINT ( 'NONE',  ( 10.00000000000000178, 53.05374883491396787, 14.16423886937410082 ) ) ;
#23472=CARTESIAN_POINT ( 'NONE',  ( 24.16423886937409904, 29.09541550158063572, 3.795296366450317205 ) ) ;
#23473=CARTESIAN_POINT ( 'NONE',  ( 6.204703633549690345, 25.76208216824730712, -14.16423886937410259 ) ) ;
#23474=CARTESIAN_POINT ( 'NONE',  ( 19.05866839779138644, 35.95508385108959004, -6.499999999999965361 ) ) ;
#23477=CARTESIAN_POINT ( 'NONE',  ( 0.1532563361054083140, 46.00893115100079456, 1.131784320476157264E-15 ) ) ;
#23480=CARTESIAN_POINT ( 'NONE',  ( 12.91533473730993009, 21.60535201082150536, -10.88017736071109987 ) ) ;
#23481=CARTESIAN_POINT ( 'NONE',  ( -12.69000000000001371, 93.50000000000000000, -10.09898361729590199 ) ) ;
#23482=CARTESIAN_POINT ( 'NONE',  ( 7.361572987183169658, 59.96726448433410894, -9.846743663894592657 ) ) ;
#23483=CARTESIAN_POINT ( 'NONE',  ( 0.1532563361054082862, 36.21726448433410894, 2.638427012816831674 ) ) ;
#23484=CARTESIAN_POINT ( 'NONE',  ( -2.816281873526471635, 53.91530133659709634, -3.434112377981056508 ) ) ;
#23487=CARTESIAN_POINT ( 'NONE',  ( 5.076628168052704559, 45.17559781766745175, -8.527530157486179263 ) ) ;
#23488=CARTESIAN_POINT ( 'NONE',  ( 1.472469842513823179, 56.42559781766745886, 4.923371831947296329 ) ) ;
#23489=CARTESIAN_POINT ( 'NONE',  ( -0.3689425029237898834, 41.17874883491397497, -10.36894250292378850 ) ) ;
#23492=CARTESIAN_POINT ( 'NONE',  ( 20.36894250292379738, 9.928748834913966093, -10.36894250292379027 ) ) ;
#23493=CARTESIAN_POINT ( 'NONE',  ( 12.91533473730992121, 59.52201867748816966, 10.88017736071110164 ) ) ;
#23494=CARTESIAN_POINT ( 'NONE',  ( -4.164238869374098151, 61.59541550158063217, -3.795296366450310543 ) ) ;
#23495=CARTESIAN_POINT ( 'NONE',  ( 10.00000000000000000, 17.87363466993041783, -12.81628187352647608 ) ) ;
#23496=CARTESIAN_POINT ( 'NONE',  ( 15.44008868035555793, 61.39701867748817676, -9.422509992056140149 ) ) ;
#23499=CARTESIAN_POINT ( 'NONE',  ( 6.565887622018943937, 30.16530133659708568, 12.81628187352647430 ) ) ;
#23500=CARTESIAN_POINT ( 'NONE',  ( 17.08211943468705840, 65.13708216824730357, -12.26659068614894466 ) ) ;
#23502=CARTESIAN_POINT ( 'NONE',  ( 2.035157376598824452, 28.68868534415484106, 7.964842623401179544 ) ) ;
#23503=CARTESIAN_POINT ( 'NONE',  ( 15.44008868035555260, 24.73035201082150891, 9.422509992056143702 ) ) ;
#23504=CARTESIAN_POINT ( 'NONE',  ( 12.63842701281683034, 57.46726448433411605, 9.846743663894596210 ) ) ;
#23505=CARTESIAN_POINT ( 'NONE',  ( 10.00000000000000178, 57.25893115100078745, 9.846743663894594434 ) ) ;
#23506=CARTESIAN_POINT ( 'NONE',  ( -2.816281873526471635, 48.91530133659708213, -3.434112377981056508 ) ) ;
#23507=PRESENTATION_STYLE_ASSIGNMENT (( #69482 ) ) ;
#23509=CARTESIAN_POINT ( 'NONE',  ( 4.559911319644449179, 22.23035201082150536, -9.422509992056141925 ) ) ;
#23511=CARTESIAN_POINT ( 'NONE',  ( 3.591859063236763294, 13.29030133659708746, -11.09922568453595026 ) ) ;
#23513=CARTESIAN_POINT ( 'NONE',  ( 7.361572987183169658, 49.96726448433410894, -9.846743663894592657 ) ) ;
#23515=CARTESIAN_POINT ( 'NONE',  ( 19.42250999205614193, 45.14701867748817676, 5.440088680355555262 ) ) ;
#23517=CARTESIAN_POINT ( 'NONE',  ( -2.816281873526471635, 23.91530133659708568, -3.434112377981056508 ) ) ;
#23518=CARTESIAN_POINT ( 'NONE',  ( 17.96484262340118221, 66.18868534415483396, -7.964842623401177768 ) ) ;
#23520=SURFACE_STYLE_USAGE ( .BOTH. , #39497 ) ;
#23523=CARTESIAN_POINT ( 'NONE',  ( 10.00000000000000178, 44.31368534415484106, 10.88017736071110342 ) ) ;
#23524=CARTESIAN_POINT ( 'NONE',  ( 3.591859063236763294, 48.29030133659708923, -11.09922568453595026 ) ) ;
#23525=CARTESIAN_POINT ( 'NONE',  ( 2.917880565312948704, 12.63708216824730179, 12.26659068614894643 ) ) ;
#23526=CARTESIAN_POINT ( 'NONE',  ( 5.076628168052704559, 10.17559781766745175, -8.527530157486179263 ) ) ;
#23527=CARTESIAN_POINT ( 'NONE',  ( 10.00000000000000178, 67.25893115100079456, 9.846743663894594434 ) ) ;
#23528=CARTESIAN_POINT ( 'NONE',  ( 7.361572987183169658, 4.967264484334119601, -9.846743663894592657 ) ) ;
#23530=CARTESIAN_POINT ( 'NONE',  ( -4.164238869374098151, 41.59541550158061796, -3.795296366450310543 ) ) ;
#23532=CARTESIAN_POINT ( 'NONE',  ( 20.88017736071110875, 5.772018677488170546, -2.915334737309920765 ) ) ;
#23536=CARTESIAN_POINT ( 'NONE',  ( 17.96484262340118221, 4.938685344154837509, 7.964842623401181321 ) ) ;
#23537=CARTESIAN_POINT ( 'NONE',  ( 19.42250999205614548, 5.980352010821504471, -5.440088680355545492 ) ) ;
#23538=CARTESIAN_POINT ( 'NONE',  ( 14.92337183194729633, 37.67559781766745175, 8.527530157486181039 ) ) ;
#23539=EDGE_CURVE ( 'NONE', #46963, #19684, #94493, .T. ) ;
#23540=CARTESIAN_POINT ( 'NONE',  ( 13.43411237798106583, 32.66530133659708213, -12.81628187352647252 ) ) ;
#23543=CARTESIAN_POINT ( 'NONE',  ( 10.00000000000000178, 3.053748834913967425, 14.16423886937410082 ) ) ;
#23544=CARTESIAN_POINT ( 'NONE',  ( 0.5774900079438590739, 27.64701867748817676, -5.440088680355550821 ) ) ;
#23545=CARTESIAN_POINT ( 'NONE',  ( 7.084665262690076126, 7.022018677488170546, -10.88017736071110164 ) ) ;
#23546=CARTESIAN_POINT ( 'NONE',  ( 17.20831665107776587, 37.88393115100078745, 7.208316651077764980 ) ) ;
#23548=CARTESIAN_POINT ( 'NONE',  ( 12.63842701281683922, 19.55059781766745175, -9.846743663894590881 ) ) ;
#23551=CARTESIAN_POINT ( 'NONE',  ( 10.00000000000000000, -0.2410688489992152128, -9.846743663894594434 ) ) ;
#23556=CARTESIAN_POINT ( 'NONE',  ( 19.84674366389459621, 53.50893115100078745, 7.409399052514197653E-17 ) ) ;
#23557=CARTESIAN_POINT ( 'NONE',  ( -0.8801773607110991993, 32.85535201082151247, -2.915334737309923874 ) ) ;
#23558=CARTESIAN_POINT ( 'NONE',  ( 12.91533473730993009, 41.60535201082149825, -10.88017736071109987 ) ) ;
#23559=CARTESIAN_POINT ( 'NONE',  ( 2.035157376598822676, 2.438685344154837953, -7.964842623401177768 ) ) ;
#23560=CARTESIAN_POINT ( 'NONE',  ( -2.816281873526471635, 33.91530133659708213, -3.434112377981056508 ) ) ;
#23561=CARTESIAN_POINT ( 'NONE',  ( 20.36894250292379738, 14.92874883491396432, -10.36894250292379027 ) ) ;
#23562=VECTOR ( 'NONE', #84679, 1000.000000000000000 ) ;
#23564=CARTESIAN_POINT ( 'NONE',  ( 3.591859063236763294, 48.29030133659708923, -11.09922568453595026 ) ) ;
#23566=CARTESIAN_POINT ( 'NONE',  ( 17.20831665107776587, 42.88393115100077324, 7.208316651077764980 ) ) ;
#23567=CARTESIAN_POINT ( 'NONE',  ( 15.44008868035555260, 24.73035201082150891, 9.422509992056143702 ) ) ;
#23569=CARTESIAN_POINT ( 'NONE',  ( 2.035157376598822676, 17.43868534415483751, -7.964842623401177768 ) ) ;
#23571=CARTESIAN_POINT ( 'NONE',  ( 0.5774900079438607392, 58.48035201082151247, 5.440088680355550821 ) ) ;
#23572=CARTESIAN_POINT ( 'NONE',  ( -0.8801773607110991993, 67.85535201082151957, -2.915334737309923874 ) ) ;
#23573=CARTESIAN_POINT ( 'NONE',  ( -0.8801773607111008646, 68.27201867748817676, 2.915334737309923430 ) ) ;
#23574=CARTESIAN_POINT ( 'NONE',  ( 1.472469842513823179, 10.59226448433411782, -4.923371831947296329 ) ) ;
#23575=CARTESIAN_POINT ( 'NONE',  ( 14.92337183194729988, 4.342264484334117824, -8.527530157486177487 ) ) ;
#23578=CARTESIAN_POINT ( 'NONE',  ( 10.00000000000000000, 9.758931151000785675, -9.846743663894594434 ) ) ;
#23580=CARTESIAN_POINT ( 'NONE',  ( 1.472469842513823179, 45.59226448433412315, -4.923371831947296329 ) ) ;
#23584=DIRECTION ( 'NONE',  ( -1.000000000000000000, -0.000000000000000000, 0.000000000000000000 ) ) ;
#23587=CARTESIAN_POINT ( 'NONE',  ( 10.00000000000000000, 15.55374883491396787, -14.16423886937410082 ) ) ;
#23589=CARTESIAN_POINT ( 'NONE',  ( -0.1503990784575328643, 35.12777174578612716, 6.262539305110068177 ) ) ;
#23590=CARTESIAN_POINT ( 'NONE',  ( 0.000000000000000000, 0.5000000000000000000, 6.500000000000000888 ) ) ;
#23591=CARTESIAN_POINT ( 'NONE',  ( 19.42250999205614548, 60.98035201082151247, -5.440088680355545492 ) ) ;
#23592=CARTESIAN_POINT ( 'NONE',  ( 19.42250999205614193, 20.14701867748817321, 5.440088680355555262 ) ) ;
#23595=CARTESIAN_POINT ( 'NONE',  ( 18.52753015748618282, 3.925597817667451306, -4.923371831947291888 ) ) ;
#23596=CARTESIAN_POINT ( 'NONE',  ( 1.472469842513823179, 0.5922644843341181575, -4.923371831947296329 ) ) ;
#23597=CARTESIAN_POINT ( 'NONE',  ( -2.816281873526473856, 29.12363466993041783, 9.499525473075851096E-16 ) ) ;
#23598=CARTESIAN_POINT ( 'NONE',  ( 0.1532563361054083140, 26.00893115100078745, 1.131784320476157264E-15 ) ) ;
#23600=CARTESIAN_POINT ( 'NONE',  ( -2.816281873526471635, 18.91530133659708213, -3.434112377981056508 ) ) ;
#23601=MECHANICAL_DESIGN_GEOMETRIC_PRESENTATION_REPRESENTATION('',(#74682),#12434);
#23602=CARTESIAN_POINT ( 'NONE',  ( 19.84674366389459621, 3.508931151000785231, 7.409399052514197653E-17 ) ) ;
#23604=VERTEX_POINT ( 'NONE', #20976 ) ;
#23605=CARTESIAN_POINT ( 'NONE',  ( 4.559911319644449179, 17.23035201082150536, -9.422509992056141925 ) ) ;
#23606=CARTESIAN_POINT ( 'NONE',  ( 2.917880565312948704, 12.63708216824730179, 12.26659068614894643 ) ) ;
#23607=CARTESIAN_POINT ( 'NONE',  ( 10.00000000000000000, 34.75893115100078745, -9.846743663894594434 ) ) ;
#23609=CARTESIAN_POINT ( 'NONE',  ( 20.88017736071110164, 65.35535201082150536, 2.915334737309930979 ) ) ;
#23610=CARTESIAN_POINT ( 'NONE',  ( 22.81628187352647785, 41.41530133659708923, 3.434112377981063169 ) ) ;
#23612=CARTESIAN_POINT ( 'NONE',  ( -0.8801773607110991993, 22.85535201082150181, -2.915334737309923874 ) ) ;
#23615=CARTESIAN_POINT ( 'NONE',  ( 6.565887622018943937, 15.16530133659708568, 12.81628187352647430 ) ) ;
#23616=CARTESIAN_POINT ( 'NONE',  ( -2.816281873526473856, 14.33196800326375531, 3.434112377981055619 ) ) ;
#23617=CARTESIAN_POINT ( 'NONE',  ( 5.076628168052703671, 46.84226448433412315, 8.527530157486179263 ) ) ;
#23619=CARTESIAN_POINT ( 'NONE',  ( -2.816281873526473856, 54.12363466993041783, 9.499525473075851096E-16 ) ) ;
#23621=CARTESIAN_POINT ( 'NONE',  ( 12.91533473730992121, 54.52201867748816255, 10.88017736071110164 ) ) ;
#23628=CARTESIAN_POINT ( 'NONE',  ( 0.5774900079438607392, 43.48035201082151247, 5.440088680355550821 ) ) ;
#23629=CARTESIAN_POINT ( 'NONE',  ( 20.88017736071110519, 50.56368534415484106, 2.639326808657452039E-16 ) ) ;
#23630=CARTESIAN_POINT ( 'NONE',  ( 2.791683348922237240, 65.38393115100078035, -7.208316651077763204 ) ) ;
#23631=CARTESIAN_POINT ( 'NONE',  ( 19.42250999205614193, 65.14701867748817676, 5.440088680355555262 ) ) ;
#23633=EDGE_CURVE ( 'NONE', #20168, #89098, #24019, .T. ) ;
#23634=CARTESIAN_POINT ( 'NONE',  ( 1.472469842513823179, 56.42559781766745886, 4.923371831947296329 ) ) ;
#23635=CARTESIAN_POINT ( 'NONE',  ( 17.96484262340118221, 11.18868534415483929, -7.964842623401177768 ) ) ;
#23637=CARTESIAN_POINT ( 'NONE',  ( 22.81628187352647785, 11.62363466993042138, 6.195893100308588602E-16 ) ) ;
#23639=CARTESIAN_POINT ( 'NONE',  ( 4.559911319644449179, 38.89701867748817676, 9.422509992056141925 ) ) ;
#23640=CARTESIAN_POINT ( 'NONE',  ( 0.6178305044545838731, 9.748634669930416052, 9.382169495545420901 ) ) ;
#23642=CARTESIAN_POINT ( 'NONE',  ( 20.88017736071110875, 15.77201867748817143, -2.915334737309920765 ) ) ;
#23643=CARTESIAN_POINT ( 'NONE',  ( 10.00000000000000178, 29.31368534415483751, 10.88017736071110342 ) ) ;
#23644=CARTESIAN_POINT ( 'NONE',  ( -2.266590686148945544, 31.38708216824730002, -7.082119434687050408 ) ) ;
#23645=CARTESIAN_POINT ( 'NONE',  ( 14.92337183194729633, 27.67559781766745530, 8.527530157486181039 ) ) ;
#23646=CARTESIAN_POINT ( 'NONE',  ( 17.96484262340118221, 61.18868534415482685, -7.964842623401177768 ) ) ;
#23648=CARTESIAN_POINT ( 'NONE',  ( 17.08211943468705130, 8.470415501580635720, 12.26659068614894998 ) ) ;
#23649=CARTESIAN_POINT ( 'NONE',  ( -46.91882540200030860, 103.2386372682362179, 5.912220560523961055 ) ) ;
#23650=CARTESIAN_POINT ( 'NONE',  ( 10.00000000000000000, 59.75893115100078745, -9.846743663894594434 ) ) ;
#23652=B_SPLINE_CURVE_WITH_KNOTS ( 'NONE', 3,
 ( #48971, #79479, #65441, #95965 ),
 .UNSPECIFIED., .F., .F.,
 ( 4, 4 ),
 ( 1.876390332415650501E-16, 0.001060528352562002848 ),
 .UNSPECIFIED. ) ;
#23653=CARTESIAN_POINT ( 'NONE',  ( 24.16423886937410614, 29.51208216824729647, -3.795296366450302550 ) ) ;
#23654=CARTESIAN_POINT ( 'NONE',  ( -4.164238869374099039, 36.80374883491396787, 8.674139862899312516E-16 ) ) ;
#23655=CARTESIAN_POINT ( 'NONE',  ( 10.00000000000000178, 7.258931151000785675, 9.846743663894594434 ) ) ;
#23656=CARTESIAN_POINT ( 'NONE',  ( 5.076628168052703671, 56.84226448433412315, 8.527530157486179263 ) ) ;
#23658=CARTESIAN_POINT ( 'NONE',  ( 17.96484262340118221, 59.93868534415484106, 7.964842623401181321 ) ) ;
#23659=CARTESIAN_POINT ( 'NONE',  ( 0.6178305044545838731, 24.74863466993042493, 9.382169495545420901 ) ) ;
#23660=CARTESIAN_POINT ( 'NONE',  ( -2.266590686148945544, 32.22041550158063927, 7.082119434687048631 ) ) ;
#23661=CARTESIAN_POINT ( 'NONE',  ( 7.084665262690076126, 12.02201867748817321, -10.88017736071110164 ) ) ;
#23662=CARTESIAN_POINT ( 'NONE',  ( -0.8801773607110991993, 32.85535201082151247, -2.915334737309923874 ) ) ;
#23663=CARTESIAN_POINT ( 'NONE',  ( -0.1503990784575328643, 70.00000000000000000, -6.262539305110068177 ) ) ;
#23664=CARTESIAN_POINT ( 'NONE',  ( 10.00000000000000000, 51.81368534415484106, -10.88017736071110342 ) ) ;
#23667=ORIENTED_EDGE ( 'NONE', *, *, #90758, .T. ) ;
#23669=CARTESIAN_POINT ( 'NONE',  ( -0.2418659066527787949, 12.23410085661204150, -6.114288769123032985 ) ) ;
#23670=ORIENTED_EDGE ( 'NONE', *, *, #24292, .T. ) ;
#23671=CARTESIAN_POINT ( 'NONE',  ( 10.00000000000000000, 0.5537488349139675359, -14.16423886937410082 ) ) ;
#23672=CARTESIAN_POINT ( 'NONE',  ( 13.79529636645030344, 58.26208216824728936, 14.16423886937410614 ) ) ;
#23673=CARTESIAN_POINT ( 'NONE',  ( -4.164238869374098151, 61.59541550158063217, -3.795296366450310543 ) ) ;
#23674=CARTESIAN_POINT ( 'NONE',  ( 1.472469842513823179, 31.42559781766745530, 4.923371831947296329 ) ) ;
#23675=CARTESIAN_POINT ( 'NONE',  ( 0.1532563361054082862, 61.21726448433412315, 2.638427012816831674 ) ) ;
#23676=CARTESIAN_POINT ( 'NONE',  ( 21.92686044187657046, 60.16212336850780673, 4.562052436263912550E-16 ) ) ;
#23679=CARTESIAN_POINT ( 'NONE',  ( 22.81628187352648496, 6.831968003263753531, -3.434112377981050290 ) ) ;
#23681=ORIENTED_EDGE ( 'NONE', *, *, #27099, .T. ) ;
#23682=CARTESIAN_POINT ( 'NONE',  ( 6.204703633549690345, 47.84541550158064638, 14.16423886937410082 ) ) ;
#23683=CARTESIAN_POINT ( 'NONE',  ( 24.16423886937409904, 44.09541550158063927, 3.795296366450317205 ) ) ;
#23685=CARTESIAN_POINT ( 'NONE',  ( 21.09922568453594849, 61.20696800326376064, 6.408140936763242479 ) ) ;
#23686=COLOUR_RGB ( '', 0.31764706, 0.68627451, 0.89019608) ;
#23687=CARTESIAN_POINT ( 'NONE',  ( 0.5774900079438607392, 23.48035201082150536, 5.440088680355550821 ) ) ;
#23688=CARTESIAN_POINT ( 'NONE',  ( 14.92337183194729633, 47.67559781766745175, 8.527530157486181039 ) ) ;
#23689=CARTESIAN_POINT ( 'NONE',  ( 12.91533473730993009, 31.60535201082150891, -10.88017736071109987 ) ) ;
#23691=CARTESIAN_POINT ( 'NONE',  ( 7.361572987183170547, 52.05059781766745175, 9.846743663894590881 ) ) ;
#23692=LINE ( 'NONE', #17658, #90492 ) ;
#23696=DIRECTION ( 'NONE',  ( -0.000000000000000000, 1.000000000000000000, -0.000000000000000000 ) ) ;
#23699=CARTESIAN_POINT ( 'NONE',  ( 12.63842701281683034, 7.467264484334118713, 9.846743663894596210 ) ) ;
#23703=CARTESIAN_POINT ( 'NONE',  ( 0.1532563361054082862, 31.21726448433412315, 2.638427012816831674 ) ) ;
#23707=EDGE_LOOP ( 'NONE', ( #69622, #30924, #98727, #27975 ) ) ;
#23710=CARTESIAN_POINT ( 'NONE',  ( 12.63842701281683922, 59.55059781766744464, -9.846743663894590881 ) ) ;
#23711=CARTESIAN_POINT ( 'NONE',  ( 13.79529636645030344, 33.26208216824730357, 14.16423886937410614 ) ) ;
#23712=CARTESIAN_POINT ( 'NONE',  ( 18.52753015748617571, 53.09226448433412315, 4.923371831947298993 ) ) ;
#23714=CARTESIAN_POINT ( 'NONE',  ( 2.791683348922237240, 25.38393115100078390, -7.208316651077763204 ) ) ;
#23715=CARTESIAN_POINT ( 'NONE',  ( 19.38216949554541557, 57.24863466993042493, -9.382169495545420901 ) ) ;
#23716=CARTESIAN_POINT ( 'NONE',  ( 22.26659068614895176, 4.720415501580633943, -7.082119434687042414 ) ) ;
#23718=CARTESIAN_POINT ( 'NONE',  ( 2.791683348922240793, 66.63393115100079456, 7.208316651077764092 ) ) ;
#23719=CARTESIAN_POINT ( 'NONE',  ( -0.8801773607110991993, 47.85535201082150536, -2.915334737309923874 ) ) ;
#23720=CARTESIAN_POINT ( 'NONE',  ( 19.84674366389459621, 38.50893115100078745, 7.409399052514197653E-17 ) ) ;
#23723=CARTESIAN_POINT ( 'NONE',  ( 2.603489959281614308, 51.58210964143330557, 6.500000000000031086 ) ) ;
#23724=CARTESIAN_POINT ( 'NONE',  ( 20.88017736071110875, 25.77201867748816966, -2.915334737309920765 ) ) ;
#23725=CARTESIAN_POINT ( 'NONE',  ( 0.1532563361054100626, 65.80059781766745175, -2.638427012816831230 ) ) ;
#23726=CARTESIAN_POINT ( 'NONE',  ( 12.91533473730993009, 56.60535201082151247, -10.88017736071109987 ) ) ;
#23727=CARTESIAN_POINT ( 'NONE',  ( 20.88017736071110519, 65.56368534415483396, 2.639326808657452039E-16 ) ) ;
#23729=DIRECTION ( 'NONE',  ( 0.000000000000000000, 0.000000000000000000, -1.000000000000000000 ) ) ;
#23730=CARTESIAN_POINT ( 'NONE',  ( 0.5774900079438607392, 33.48035201082150536, 5.440088680355550821 ) ) ;
#23732=CARTESIAN_POINT ( 'NONE',  ( 18.52753015748618282, 43.92559781766745175, -4.923371831947291888 ) ) ;
#23733=SURFACE_STYLE_FILL_AREA ( #29721 ) ;
#23735=CARTESIAN_POINT ( 'NONE',  ( 13.43411237798106583, 7.665301336597086568, -12.81628187352647252 ) ) ;
#23737=CARTESIAN_POINT ( 'NONE',  ( 17.96484262340118221, 19.93868534415484106, 7.964842623401181321 ) ) ;
#23739=CARTESIAN_POINT ( 'NONE',  ( 10.00000000000000000, 20.55374883491396787, -14.16423886937410082 ) ) ;
#23740=CARTESIAN_POINT ( 'NONE',  ( 22.26659068614895176, 64.72041550158064638, -7.082119434687042414 ) ) ;
#23742=CARTESIAN_POINT ( 'NONE',  ( 10.00000000000000178, 12.25893115100078568, 9.846743663894594434 ) ) ;
#23743=CARTESIAN_POINT ( 'NONE',  ( 20.10239578412225114, 32.63377557478297319, -6.340343622311915617 ) ) ;
#23746=CARTESIAN_POINT ( 'NONE',  ( 7.361572987183169658, 19.96726448433411960, -9.846743663894592657 ) ) ;
#23747=CARTESIAN_POINT ( 'NONE',  ( 17.96484262340118221, 26.18868534415483396, -7.964842623401177768 ) ) ;
#23748=CARTESIAN_POINT ( 'NONE',  ( 2.791683348922237240, 65.38393115100078035, -7.208316651077763204 ) ) ;
#23749=CARTESIAN_POINT ( 'NONE',  ( 2.917880565312948704, 12.63708216824730179, 12.26659068614894643 ) ) ;
#23752=CARTESIAN_POINT ( 'NONE',  ( 17.20831665107776587, 12.88393115100078390, 7.208316651077764980 ) ) ;
#23753=CARTESIAN_POINT ( 'NONE',  ( 3.591859063236763294, 43.29030133659708923, -11.09922568453595026 ) ) ;
#23754=CARTESIAN_POINT ( 'NONE',  ( 7.361572987183170547, 42.05059781766745886, 9.846743663894590881 ) ) ;
#23756=CARTESIAN_POINT ( 'NONE',  ( 7.361572987183170547, 17.05059781766745530, 9.846743663894590881 ) ) ;
#23758=CARTESIAN_POINT ( 'NONE',  ( 24.16423886937410614, 49.30374883491396787, 8.672049930838204340E-16 ) ) ;
#23759=CARTESIAN_POINT ( 'NONE',  ( 17.96484262340118221, 54.93868534415484106, 7.964842623401181321 ) ) ;
#23761=CARTESIAN_POINT ( 'NONE',  ( 10.00000000000000178, 3.053748834913967425, 14.16423886937410082 ) ) ;
#23762=CARTESIAN_POINT ( 'NONE',  ( 17.96484262340118221, 56.18868534415484817, -7.964842623401177768 ) ) ;
#23763=CARTESIAN_POINT ( 'NONE',  ( 0.1532563361054082862, 36.21726448433410894, 2.638427012816831674 ) ) ;
#23764=CARTESIAN_POINT ( 'NONE',  ( 10.00000000000000000, 6.813685344154838397, -10.88017736071110342 ) ) ;
#23765=CARTESIAN_POINT ( 'NONE',  ( 19.84674366389459266, 48.30059781766745175, 2.638427012816836559 ) ) ;
#23766=CARTESIAN_POINT ( 'NONE',  ( -0.8801773607110991993, 47.85535201082150536, -2.915334737309923874 ) ) ;
#23767=ORIENTED_EDGE ( 'NONE', *, *, #39425, .T. ) ;
#23768=VECTOR ( 'NONE', #23423, 1000.000000000000000 ) ;
#23770=VERTEX_POINT ( 'NONE', #42856 ) ;
#23773=CARTESIAN_POINT ( 'NONE',  ( 7.361572987183169658, 39.96726448433411605, -9.846743663894592657 ) ) ;
#23774=CARTESIAN_POINT ( 'NONE',  ( 19.84674366389459621, 28.50893115100078745, 7.409399052514197653E-17 ) ) ;
#23775=CARTESIAN_POINT ( 'NONE',  ( -1.099225684535947600, 58.70696800326375353, -6.408140936763238038 ) ) ;
#23776=CARTESIAN_POINT ( 'NONE',  ( -0.8801773607111008646, 13.27201867748817321, 2.915334737309923430 ) ) ;
#23777=CARTESIAN_POINT ( 'NONE',  ( 1.472469842513823179, 50.59226448433411605, -4.923371831947296329 ) ) ;
#23779=CARTESIAN_POINT ( 'NONE',  ( 10.00000000000000178, 53.05374883491396787, 14.16423886937410082 ) ) ;
#23780=CARTESIAN_POINT ( 'NONE',  ( 14.92337183194729988, 59.34226448433412315, -8.527530157486177487 ) ) ;
#23782=CARTESIAN_POINT ( 'NONE',  ( 12.91533473730993009, 46.60535201082150536, -10.88017736071109987 ) ) ;
#23784=CARTESIAN_POINT ( 'NONE',  ( 5.076628168052703671, 11.84226448433411960, 8.527530157486179263 ) ) ;
#23789=ORIENTED_EDGE ( 'NONE', *, *, #16094, .T. ) ;
#23790=CARTESIAN_POINT ( 'NONE',  ( 17.20831665107776587, 14.13393115100078568, -7.208316651077762316 ) ) ;
#23792=CARTESIAN_POINT ( 'NONE',  ( 6.204703633549690345, 22.84541550158062861, 14.16423886937410082 ) ) ;
#23793=CARTESIAN_POINT ( 'NONE',  ( 7.361572987183170547, 22.05059781766745530, 9.846743663894590881 ) ) ;
#23794=CARTESIAN_POINT ( 'NONE',  ( 7.084665262690076126, 42.02201867748816966, -10.88017736071110164 ) ) ;
#23798=CARTESIAN_POINT ( 'NONE',  ( 7.084665262690076126, 27.02201867748817676, -10.88017736071110164 ) ) ;
#23801=( NAMED_UNIT ( * ) PLANE_ANGLE_UNIT ( ) SI_UNIT ( $, .RADIAN. ) );
#23804=CARTESIAN_POINT ( 'NONE',  ( 10.00000000000000000, 17.87363466993041783, -12.81628187352647608 ) ) ;
#23805=CARTESIAN_POINT ( 'NONE',  ( 2.791683348922237240, 10.38393115100078390, -7.208316651077763204 ) ) ;
#23807=CARTESIAN_POINT ( 'NONE',  ( -10.44000000000001194, 92.00000000000000000, -10.09898361729590199 ) ) ;
#23808=CARTESIAN_POINT ( 'NONE',  ( 5.076628168052704559, 20.17559781766745175, -8.527530157486179263 ) ) ;
#23809=CARTESIAN_POINT ( 'NONE',  ( 15.44008868035555260, 29.73035201082150891, 9.422509992056143702 ) ) ;
#23812=CARTESIAN_POINT ( 'NONE',  ( 10.00000000000000178, 54.31368534415484106, 10.88017736071110342 ) ) ;
#23813=CARTESIAN_POINT ( 'NONE',  ( -0.1503990784575280903, 23.10158574516642815, 6.262539305110076171 ) ) ;
#23815=CARTESIAN_POINT ( 'NONE',  ( 17.96484262340118221, 64.93868534415483396, 7.964842623401181321 ) ) ;
#23816=CARTESIAN_POINT ( 'NONE',  ( 21.09922568453595559, 2.040301336597086568, -6.408140936763230044 ) ) ;
#23819=CARTESIAN_POINT ( 'NONE',  ( 10.00000000000000178, 27.25893115100078390, 9.846743663894594434 ) ) ;
#23820=CARTESIAN_POINT ( 'NONE',  ( 19.38216949554541557, 52.24863466993041072, -9.382169495545420901 ) ) ;
#23821=CARTESIAN_POINT ( 'NONE',  ( -0.000000000000000000, 78.19920772666813491, 8.807240371166628279 ) ) ;
#23822=CARTESIAN_POINT ( 'NONE',  ( 0.1532563361054100626, 25.80059781766744820, -2.638427012816831230 ) ) ;
#23823=CARTESIAN_POINT ( 'NONE',  ( 22.81628187352647785, 21.62363466993041783, 6.195893100308588602E-16 ) ) ;
#23825=DIRECTION ( 'NONE',  ( 0.000000000000000000, 1.000000000000000000, -0.000000000000000000 ) ) ;
#23826=CARTESIAN_POINT ( 'NONE',  ( 20.88017736071110164, 50.35535201082151247, 2.915334737309930979 ) ) ;
#23828=CARTESIAN_POINT ( 'NONE',  ( 17.20831665107776587, 57.88393115100078745, 7.208316651077764980 ) ) ;
#23830=ADVANCED_FACE ( 'NONE', ( #91804 ), #98349, .T. ) ;
#23832=CARTESIAN_POINT ( 'NONE',  ( 19.84674366389459621, 23.50893115100078390, 7.409399052514197653E-17 ) ) ;
#23833=CARTESIAN_POINT ( 'NONE',  ( -0.8801773607110991993, 12.85535201082150358, -2.915334737309923874 ) ) ;
#23834=CARTESIAN_POINT ( 'NONE',  ( -2.816281873526473856, 19.33196800326375708, 3.434112377981055619 ) ) ;
#23835=( NAMED_UNIT ( * ) SI_UNIT ( $, .STERADIAN. ) SOLID_ANGLE_UNIT ( ) );
#23836=DIRECTION ( 'NONE',  ( 0.000000000000000000, -1.000000000000000000, 0.000000000000000000 ) ) ;
#23837=CARTESIAN_POINT ( 'NONE',  ( 20.88017736071110519, 25.56368534415483751, 2.639326808657452039E-16 ) ) ;
#23839=CARTESIAN_POINT ( 'NONE',  ( 2.035157376598822676, 22.43868534415483396, -7.964842623401177768 ) ) ;
#23841=CARTESIAN_POINT ( 'NONE',  ( 20.88017736071110875, 35.77201867748816966, -2.915334737309920765 ) ) ;
#23842=CARTESIAN_POINT ( 'NONE',  ( 20.88017736071110875, 5.772018677488170546, -2.915334737309920765 ) ) ;
#23844=PRESENTATION_STYLE_ASSIGNMENT (( #91834 ) ) ;
#23845=CARTESIAN_POINT ( 'NONE',  ( 10.00000000000000000, 29.75893115100078745, -9.846743663894594434 ) ) ;
#23846=CARTESIAN_POINT ( 'NONE',  ( -2.816281873526471635, 8.915301336597083903, -3.434112377981056508 ) ) ;
#23848=CARTESIAN_POINT ( 'NONE',  ( 19.84674366389459266, 63.71726448433412315, -2.638427012816827677 ) ) ;
#23851=CARTESIAN_POINT ( 'NONE',  ( -2.266590686148945544, 27.22041550158063572, 7.082119434687048631 ) ) ;
#23852=CARTESIAN_POINT ( 'NONE',  ( 7.361572987183169658, 34.96726448433411605, -9.846743663894592657 ) ) ;
#23853=EDGE_CURVE ( 'NONE', #97012, #48470, #97784, .T. ) ;
#23855=ORIENTED_EDGE ( 'NONE', *, *, #49225, .T. ) ;
#23856=CARTESIAN_POINT ( 'NONE',  ( -4.164238869374098151, 56.59541550158063927, -3.795296366450310543 ) ) ;
#23857=CARTESIAN_POINT ( 'NONE',  ( 19.84674366389459266, 28.71726448433411960, -2.638427012816827677 ) ) ;
#23860=CARTESIAN_POINT ( 'NONE',  ( 2.035157376598822676, 47.43868534415484817, -7.964842623401177768 ) ) ;
#23861=CARTESIAN_POINT ( 'NONE',  ( 22.81628187352647785, 46.62363466993041783, 6.195893100308588602E-16 ) ) ;
#23863=CARTESIAN_POINT ( 'NONE',  ( -0.8801773607111008646, 18.27201867748817321, 2.915334737309923430 ) ) ;
#23864=CARTESIAN_POINT ( 'NONE',  ( -2.816281873526471635, 48.91530133659708213, -3.434112377981056508 ) ) ;
#23866=CARTESIAN_POINT ( 'NONE',  ( 7.361572987183170547, 67.05059781766746596, 9.846743663894590881 ) ) ;
#23867=CARTESIAN_POINT ( 'NONE',  ( 17.20831665107776587, 2.883931151000785231, 7.208316651077764980 ) ) ;
#23868=EDGE_LOOP ( 'NONE', ( #28339, #36665, #25052, #71727 ) ) ;
#23871=CARTESIAN_POINT ( 'NONE',  ( 10.00000000000000000, 55.55374883491396787, -14.16423886937410082 ) ) ;
#23872=CARTESIAN_POINT ( 'NONE',  ( 20.36894250292379382, 18.67874883491397142, 10.36894250292379205 ) ) ;
#23873=CARTESIAN_POINT ( 'NONE',  ( 15.44008868035555260, 19.73035201082150536, 9.422509992056143702 ) ) ;
#23874=CARTESIAN_POINT ( 'NONE',  ( 12.91533473730993009, 41.60535201082149825, -10.88017736071109987 ) ) ;
#23878=CARTESIAN_POINT ( 'NONE',  ( -0.8801773607111009756, 63.06368534415484106, 1.068504757029289695E-15 ) ) ;
#23879=CARTESIAN_POINT ( 'NONE',  ( 15.44008868035555793, 66.39701867748817676, -9.422509992056140149 ) ) ;
#23880=CARTESIAN_POINT ( 'NONE',  ( 19.84674366389459266, 23.71726448433412315, -2.638427012816827677 ) ) ;
#23883=CARTESIAN_POINT ( 'NONE',  ( 5.076628168052703671, 11.84226448433411960, 8.527530157486179263 ) ) ;
#23884=CARTESIAN_POINT ( 'NONE',  ( 14.92337183194729988, 34.34226448433411605, -8.527530157486177487 ) ) ;
#23885=CARTESIAN_POINT ( 'NONE',  ( 17.96484262340118221, 19.93868534415484106, 7.964842623401181321 ) ) ;
#23886=CARTESIAN_POINT ( 'NONE',  ( 0.6178305044545838731, 34.74863466993042493, 9.382169495545420901 ) ) ;
#23887=CARTESIAN_POINT ( 'NONE',  ( 19.84674366389459621, 3.508931151000785231, 7.409399052514197653E-17 ) ) ;
#23890=CARTESIAN_POINT ( 'NONE',  ( 2.791683348922237240, 45.38393115100079456, -7.208316651077763204 ) ) ;
#23891=CARTESIAN_POINT ( 'NONE',  ( 10.00000000000000178, 32.25893115100078745, 9.846743663894594434 ) ) ;
#23892=CARTESIAN_POINT ( 'NONE',  ( -4.164238869374099927, 17.01208216824730357, 3.795296366450308767 ) ) ;
#23893=CARTESIAN_POINT ( 'NONE',  ( -0.8801773607111009756, 38.06368534415484106, 1.068504757029289695E-15 ) ) ;
#23894=CARTESIAN_POINT ( 'NONE',  ( 17.96484262340118221, 6.188685344154836621, -7.964842623401177768 ) ) ;
#23895=CARTESIAN_POINT ( 'NONE',  ( 20.88017736071110875, 50.77201867748817676, -2.915334737309920765 ) ) ;
#23896=CARTESIAN_POINT ( 'NONE',  ( 17.96484262340118221, 34.93868534415482685, 7.964842623401181321 ) ) ;
#23898=CARTESIAN_POINT ( 'NONE',  ( 16.40814093676324603, 32.45696800326375353, -11.09922568453594671 ) ) ;
#23899=CARTESIAN_POINT ( 'NONE',  ( 20.88017736071110164, 40.35535201082150536, 2.915334737309930979 ) ) ;
#23901=CARTESIAN_POINT ( 'NONE',  ( -2.816281873526473856, 54.12363466993041783, 9.499525473075851096E-16 ) ) ;
#23902=CARTESIAN_POINT ( 'NONE',  ( 15.44008868035555793, 51.39701867748816966, -9.422509992056140149 ) ) ;
#23903=ORIENTED_EDGE ( 'NONE', *, *, #49841, .T. ) ;
#23904=CARTESIAN_POINT ( 'NONE',  ( 20.88017736071110875, 50.77201867748817676, -2.915334737309920765 ) ) ;
#23907=CARTESIAN_POINT ( 'NONE',  ( -4.164238869374099927, 57.01208216824731068, 3.795296366450308767 ) ) ;
#23908=CARTESIAN_POINT ( 'NONE',  ( 19.42250999205614548, 65.98035201082151957, -5.440088680355545492 ) ) ;
#23909=CARTESIAN_POINT ( 'NONE',  ( 19.42250999205614548, 55.98035201082150536, -5.440088680355545492 ) ) ;
#23912=CARTESIAN_POINT ( 'NONE',  ( 19.84674366389459266, 28.71726448433411960, -2.638427012816827677 ) ) ;
#23914=CARTESIAN_POINT ( 'NONE',  ( 12.63842701281683922, 29.55059781766745175, -9.846743663894590881 ) ) ;
#23915=CARTESIAN_POINT ( 'NONE',  ( 2.035157376598824452, 33.68868534415484106, 7.964842623401179544 ) ) ;
#23916=CARTESIAN_POINT ( 'NONE',  ( 5.076628168052703671, 41.84226448433411605, 8.527530157486179263 ) ) ;
#23917=CARTESIAN_POINT ( 'NONE',  ( 13.43411237798105340, 20.58196800326374643, 12.81628187352647963 ) ) ;
#23919=CARTESIAN_POINT ( 'NONE',  ( 19.80448550324508616, 1.827036817733421081, 6.500000000002772893 ) ) ;
#23920=CARTESIAN_POINT ( 'NONE',  ( 19.42250999205614193, 45.14701867748817676, 5.440088680355555262 ) ) ;
#23921=CARTESIAN_POINT ( 'NONE',  ( 22.26659068614895176, 54.72041550158063217, -7.082119434687042414 ) ) ;
#23923=CARTESIAN_POINT ( 'NONE',  ( 10.00000000000000178, 25.37363466993041783, 12.81628187352647608 ) ) ;
#23924=FACE_OUTER_BOUND ( 'NONE', #30389, .T. ) ;
#23926=CARTESIAN_POINT ( 'NONE',  ( 19.38216949554541202, 30.99863466993042138, 9.382169495545424454 ) ) ;
#23927=CARTESIAN_POINT ( 'NONE',  ( 12.91533473730993009, 21.60535201082150536, -10.88017736071109987 ) ) ;
#23928=CARTESIAN_POINT ( 'NONE',  ( 17.96484262340118221, 56.18868534415484817, -7.964842623401177768 ) ) ;
#23930=ORIENTED_EDGE ( 'NONE', *, *, #74909, .T. ) ;
#23933=CARTESIAN_POINT ( 'NONE',  ( 19.42250999205614548, 65.98035201082151957, -5.440088680355545492 ) ) ;
#23934=CARTESIAN_POINT ( 'NONE',  ( 19.84674366389459266, 53.30059781766744464, 2.638427012816836559 ) ) ;
#23935=CARTESIAN_POINT ( 'NONE',  ( 0.1532563361054100626, 40.80059781766745886, -2.638427012816831230 ) ) ;
#23936=CARTESIAN_POINT ( 'NONE',  ( 18.72515096720568906, 15.05509018479935612, 6.500000000000002665 ) ) ;
#23937=CARTESIAN_POINT ( 'NONE',  ( 18.52753015748617571, 28.09226448433411960, 4.923371831947298993 ) ) ;
#23938=CARTESIAN_POINT ( 'NONE',  ( 20.15039907845753220, 54.72266099184918886, 6.262539305110078836 ) ) ;
#23939=LINE ( 'NONE', #69924, #557 ) ;
#23940=ADVANCED_FACE ( 'NONE', ( #60800 ), #14336, .F. ) ;
#23941=CARTESIAN_POINT ( 'NONE',  ( 12.63842701281683034, 17.46726448433411250, 9.846743663894596210 ) ) ;
#23944=CARTESIAN_POINT ( 'NONE',  ( 0.1532563361054100626, 50.80059781766745175, -2.638427012816831230 ) ) ;
#23945=EDGE_LOOP ( 'NONE', ( #3041, #27074, #55701, #82438, #59144, #38686 ) ) ;
#23947=CARTESIAN_POINT ( 'NONE',  ( -1.099225684535947600, 18.70696800326375353, -6.408140936763238038 ) ) ;
#23948=CARTESIAN_POINT ( 'NONE',  ( 0.5774900079438607392, 48.48035201082150536, 5.440088680355550821 ) ) ;
#23949=CARTESIAN_POINT ( 'NONE',  ( -0.3689425029237898834, 51.17874883491397497, -10.36894250292378850 ) ) ;
#23951=CARTESIAN_POINT ( 'NONE',  ( 13.79529636645031943, 40.34541550158063217, -14.16423886937409904 ) ) ;
#23952=CARTESIAN_POINT ( 'NONE',  ( 20.36894250292379382, 58.67874883491396076, 10.36894250292379205 ) ) ;
#23953=CARTESIAN_POINT ( 'NONE',  ( -4.164238869374098151, 21.59541550158063217, -3.795296366450310543 ) ) ;
#23954=CARTESIAN_POINT ( 'NONE',  ( -4.164238869374099927, 27.01208216824730357, 3.795296366450308767 ) ) ;
#23955=CARTESIAN_POINT ( 'NONE',  ( 20.15039907845753220, 24.72266099184919241, 6.262539305110077947 ) ) ;
#23957=CARTESIAN_POINT ( 'NONE',  ( 14.92337183194729633, 37.67559781766745175, 8.527530157486181039 ) ) ;
#23958=CARTESIAN_POINT ( 'NONE',  ( -0.8801773607111009756, 23.06368534415484106, 1.068504757029289695E-15 ) ) ;
#23961=CARTESIAN_POINT ( 'NONE',  ( 20.00000000000000711, 90.60731807131610083, -5.318367326097200198 ) ) ;
#23962=CARTESIAN_POINT ( 'NONE',  ( 0.1532563361054082862, 41.21726448433411605, 2.638427012816831674 ) ) ;
#23963=CARTESIAN_POINT ( 'NONE',  ( 21.09922568453594849, 61.20696800326376064, 6.408140936763242479 ) ) ;
#23965=CARTESIAN_POINT ( 'NONE',  ( 10.00000000000000000, 39.75893115100078745, -9.846743663894594434 ) ) ;
#23966=CARTESIAN_POINT ( 'NONE',  ( 18.52753015748618282, 58.92559781766745886, -4.923371831947291888 ) ) ;
#23967=CARTESIAN_POINT ( 'NONE',  ( 6.204703633549690345, 35.76208216824729647, -14.16423886937410259 ) ) ;
#23970=CARTESIAN_POINT ( 'NONE',  ( 24.16423886937410614, 14.51208216824730179, -3.795296366450302550 ) ) ;
#23971=CARTESIAN_POINT ( 'NONE',  ( 0.2751277870542967463, 70.00000000000000000, -6.500000000000000888 ) ) ;
#23973=CARTESIAN_POINT ( 'NONE',  ( 1.274849032794324932, 22.55509018479936145, -6.500000000000021316 ) ) ;
#23974=CARTESIAN_POINT ( 'NONE',  ( -2.266590686148945544, 66.38708216824730357, -7.082119434687050408 ) ) ;
#23975=CARTESIAN_POINT ( 'NONE',  ( 10.00000000000000178, 5.373634669930420493, 12.81628187352647608 ) ) ;
#23978=CARTESIAN_POINT ( 'NONE',  ( 2.035157376598822676, 67.43868534415484817, -7.964842623401177768 ) ) ;
#23980=VECTOR ( 'NONE', #31833, 1000.000000000000000 ) ;
#23981=CARTESIAN_POINT ( 'NONE',  ( 1.472469842513823179, 30.59226448433411960, -4.923371831947296329 ) ) ;
#23983=CARTESIAN_POINT ( 'NONE',  ( -4.164238869374099039, 66.80374883491396076, 8.674139862899312516E-16 ) ) ;
#23984=CARTESIAN_POINT ( 'NONE',  ( 1.274849032794102888, 3.572280503510291361, 6.499999999999721112 ) ) ;
#23985=CARTESIAN_POINT ( 'NONE',  ( 15.44008868035555260, 29.73035201082150891, 9.422509992056143702 ) ) ;
#23986=CARTESIAN_POINT ( 'NONE',  ( -0.8801773607110991993, 22.85535201082150181, -2.915334737309923874 ) ) ;
#23987=CARTESIAN_POINT ( 'NONE',  ( 5.076628168052704559, 60.17559781766745175, -8.527530157486179263 ) ) ;
#23988=CARTESIAN_POINT ( 'NONE',  ( 18.52753015748617571, 53.09226448433412315, 4.923371831947298993 ) ) ;
#23989=CARTESIAN_POINT ( 'NONE',  ( -43.84582565093677431, 106.6410155927914332, -4.576759396000646518 ) ) ;
#23990=SURFACE_STYLE_FILL_AREA ( #77957 ) ;
#23993=CARTESIAN_POINT ( 'NONE',  ( 10.00000000000000000, 26.81368534415484106, -10.88017736071110342 ) ) ;
#23994=CARTESIAN_POINT ( 'NONE',  ( -2.816281873526473856, 24.12363466993042138, 9.499525473075851096E-16 ) ) ;
#23995=CARTESIAN_POINT ( 'NONE',  ( -0.3289641300568005855, 55.10497603579417358, 5.963430220938281678 ) ) ;
#23996=CARTESIAN_POINT ( 'NONE',  ( 10.00000000000000178, 62.25893115100078745, 9.846743663894594434 ) ) ;
#23997=CARTESIAN_POINT ( 'NONE',  ( 19.42250999205614548, 50.98035201082151247, -5.440088680355545492 ) ) ;
#23998=CARTESIAN_POINT ( 'NONE',  ( 6.565887622018943937, 20.16530133659708213, 12.81628187352647430 ) ) ;
#23999=CARTESIAN_POINT ( 'NONE',  ( 20.88017736071110875, 60.77201867748817676, -2.915334737309920765 ) ) ;
#24000=CARTESIAN_POINT ( 'NONE',  ( 19.42250999205614193, 15.14701867748817143, 5.440088680355555262 ) ) ;
#24001=CARTESIAN_POINT ( 'NONE',  ( -0.1503990784575328643, 50.12777174578613426, 6.262539305110068177 ) ) ;
#24004=CARTESIAN_POINT ( 'NONE',  ( 2.035157376598822676, 52.43868534415483396, -7.964842623401177768 ) ) ;
#24005=CARTESIAN_POINT ( 'NONE',  ( 0.6178305044545838731, 44.74863466993042493, 9.382169495545420901 ) ) ;
#24006=CARTESIAN_POINT ( 'NONE',  ( 22.26659068614895176, 9.720415501580633943, -7.082119434687042414 ) ) ;
#24007=CARTESIAN_POINT ( 'NONE',  ( 1.472469842513823179, 21.42559781766745175, 4.923371831947296329 ) ) ;
#24008=CARTESIAN_POINT ( 'NONE',  ( 18.52753015748617571, 63.09226448433412315, 4.923371831947298993 ) ) ;
#24010=EDGE_CURVE ( 'NONE', #12669, #71776, #44809, .T. ) ;
#24011=CARTESIAN_POINT ( 'NONE',  ( 12.63842701281683034, 22.46726448433411605, 9.846743663894596210 ) ) ;
#24013=CARTESIAN_POINT ( 'NONE',  ( 13.79529636645030344, 63.26208216824730357, 14.16423886937410614 ) ) ;
#24015=CARTESIAN_POINT ( 'NONE',  ( 10.00000000000000178, 4.313685344154837509, 10.88017736071110342 ) ) ;
#24017=CARTESIAN_POINT ( 'NONE',  ( 19.42250999205614548, 5.980352010821504471, -5.440088680355545492 ) ) ;
#24018=CARTESIAN_POINT ( 'NONE',  ( 1.959929470562273179, 15.51528370094808018, -5.767676674365838529 ) ) ;
#24019=B_SPLINE_CURVE_WITH_KNOTS ( 'NONE', 3,
 ( #27839, #88844, #4866, #5844, #96864, #26366 ),
 .UNSPECIFIED., .F., .F.,
 ( 4, 2, 4 ),
 ( 7.840110604351616646E-18, 0.0002626113303185972870, 0.0005252226606371866594 ),
 .UNSPECIFIED. ) ;
#24020=ORIENTED_EDGE ( 'NONE', *, *, #75995, .F. ) ;
#24022=CARTESIAN_POINT ( 'NONE',  ( 10.00000000000000178, 4.313685344154837509, 10.88017736071110342 ) ) ;
#24023=CARTESIAN_POINT ( 'NONE',  ( 15.44008868035555260, 9.730352010821505360, 9.422509992056143702 ) ) ;
#24024=CARTESIAN_POINT ( 'NONE',  ( 0.1532563361054083140, 46.00893115100079456, 1.131784320476157264E-15 ) ) ;
#24025=CARTESIAN_POINT ( 'NONE',  ( 3.591859063236763294, 43.29030133659708923, -11.09922568453595026 ) ) ;
#24028=CARTESIAN_POINT ( 'NONE',  ( 22.26659068614894466, 23.88708216824730357, 7.082119434687054849 ) ) ;
#24029=CARTESIAN_POINT ( 'NONE',  ( 12.91533473730992121, 24.52201867748816966, 10.88017736071110164 ) ) ;
#24030=CARTESIAN_POINT ( 'NONE',  ( 2.035157376598824452, 3.688685344154837953, 7.964842623401179544 ) ) ;
#24031=CARTESIAN_POINT ( 'NONE',  ( 0.1532563361054082862, 41.21726448433411605, 2.638427012816831674 ) ) ;
#24033=CARTESIAN_POINT ( 'NONE',  ( 17.20831665107776587, 39.13393115100079456, -7.208316651077762316 ) ) ;
#24037=CARTESIAN_POINT ( 'NONE',  ( -0.8801773607111008646, 3.272018677488171434, 2.915334737309923430 ) ) ;
#24038=CARTESIAN_POINT ( 'NONE',  ( 20.88017736071110164, 65.35535201082150536, 2.915334737309930979 ) ) ;
#24039=CARTESIAN_POINT ( 'NONE',  ( 19.42250999205614548, 30.98035201082150536, -5.440088680355545492 ) ) ;
#24040=CARTESIAN_POINT ( 'NONE',  ( 10.00000000000000000, 32.87363466993042493, -12.81628187352647608 ) ) ;
#24041=CARTESIAN_POINT ( 'NONE',  ( -4.164238869374099039, 16.80374883491396787, 8.674139862899312516E-16 ) ) ;
#24043=B_SPLINE_CURVE_WITH_KNOTS ( 'NONE', 3,
 ( #7271, #61238, #38262, #8728, #22277, #83752 ),
 .UNSPECIFIED., .F., .F.,
 ( 4, 2, 4 ),
 ( 0.000000000000000000, 0.0002565770811490928911, 0.0005131541622981857821 ),
 .UNSPECIFIED. ) ;
#24044=CARTESIAN_POINT ( 'NONE',  ( 16.40814093676324603, 47.45696800326375353, -11.09922568453594671 ) ) ;
#24046=CARTESIAN_POINT ( 'NONE',  ( 2.791683348922237240, 45.38393115100079456, -7.208316651077763204 ) ) ;
#24047=CARTESIAN_POINT ( 'NONE',  ( 20.88017736071110519, 20.56368534415484106, 2.639326808657452039E-16 ) ) ;
#24048=VERTEX_POINT ( 'NONE', #24796 ) ;
#24050=CARTESIAN_POINT ( 'NONE',  ( 15.44008868035555260, 14.73035201082150536, 9.422509992056143702 ) ) ;
#24051=ORIENTED_EDGE ( 'NONE', *, *, #29948, .F. ) ;
#24052=CARTESIAN_POINT ( 'NONE',  ( 17.96484262340118221, 61.18868534415482685, -7.964842623401177768 ) ) ;
#24055=CARTESIAN_POINT ( 'NONE',  ( 19.84674366389459621, 8.508931151000785675, 7.409399052514197653E-17 ) ) ;
#24056=CARTESIAN_POINT ( 'NONE',  ( 10.00000000000000000, 61.81368534415484106, -10.88017736071110342 ) ) ;
#24060=CARTESIAN_POINT ( 'NONE',  ( -46.94000000000000483, 102.2681967859571870, 7.165875991462780092 ) ) ;
#24061=CARTESIAN_POINT ( 'NONE',  ( 7.361572987183170547, 12.05059781766744997, 9.846743663894590881 ) ) ;
#24063=CARTESIAN_POINT ( 'NONE',  ( 5.076628168052703671, 36.84226448433412315, 8.527530157486179263 ) ) ;
#24064=VERTEX_POINT ( 'NONE', #17783 ) ;
#24068=CARTESIAN_POINT ( 'NONE',  ( 10.00000000000000000, 57.87363466993042493, -12.81628187352647608 ) ) ;
#24069=CARTESIAN_POINT ( 'NONE',  ( 20.36894250292379382, 8.678748834913967869, 10.36894250292379205 ) ) ;
#24070=CARTESIAN_POINT ( 'NONE',  ( 13.79529636645031943, 25.34541550158063572, -14.16423886937409904 ) ) ;
#24073=CARTESIAN_POINT ( 'NONE',  ( -0.8801773607110991993, 57.85535201082149825, -2.915334737309923874 ) ) ;
#24074=CARTESIAN_POINT ( 'NONE',  ( 10.00000000000000178, 19.31368534415484106, 10.88017736071110342 ) ) ;
#24076=ORIENTED_EDGE ( 'NONE', *, *, #16094, .F. ) ;
#24077=CARTESIAN_POINT ( 'NONE',  ( 19.84674366389459266, 8.300597817667451750, 2.638427012816836559 ) ) ;
#24078=CARTESIAN_POINT ( 'NONE',  ( 5.076628168052704559, 5.175597817667451750, -8.527530157486179263 ) ) ;
#24079=CARTESIAN_POINT ( 'NONE',  ( 0.6178305044545818747, 38.49863466993042493, -9.382169495545419124 ) ) ;
#24080=CARTESIAN_POINT ( 'NONE',  ( 14.92337183194729988, 29.34226448433411960, -8.527530157486177487 ) ) ;
#24082=CARTESIAN_POINT ( 'NONE',  ( -1.099225684535947600, 19.54030133659708568, 6.408140936763237150 ) ) ;
#24085=CARTESIAN_POINT ( 'NONE',  ( 10.00000000000000000, 9.758931151000785675, -9.846743663894594434 ) ) ;
#24086=EDGE_CURVE ( 'NONE', #89063, #30064, #39308, .T. ) ;
#24088=CARTESIAN_POINT ( 'NONE',  ( 7.084665262690076126, 19.10535201082150181, 10.88017736071109987 ) ) ;
#24089=CARTESIAN_POINT ( 'NONE',  ( 24.16423886937410614, 34.30374883491396787, 8.672049930838204340E-16 ) ) ;
#24090=CARTESIAN_POINT ( 'NONE',  ( 0.1532563361054100626, 40.80059781766745886, -2.638427012816831230 ) ) ;
#24091=CARTESIAN_POINT ( 'NONE',  ( 19.42250999205614193, 65.14701867748817676, 5.440088680355555262 ) ) ;
#24092=CARTESIAN_POINT ( 'NONE',  ( 16.40814093676323893, 55.79030133659708923, 11.09922568453595026 ) ) ;
#24094=CARTESIAN_POINT ( 'NONE',  ( 15.44008868035555793, 26.39701867748817321, -9.422509992056140149 ) ) ;
#24097=CARTESIAN_POINT ( 'NONE',  ( 16.40814093676323893, 5.790301336597087456, 11.09922568453595026 ) ) ;
#24098=CARTESIAN_POINT ( 'NONE',  ( 12.63842701281683034, 37.46726448433411605, 9.846743663894596210 ) ) ;
#24100=CARTESIAN_POINT ( 'NONE',  ( 16.40814093676323893, 50.79030133659708923, 11.09922568453595026 ) ) ;
#24101=DIRECTION ( 'NONE',  ( 0.5547001962252290364, 0.8320502943378437211, 0.000000000000000000 ) ) ;
#24102=CARTESIAN_POINT ( 'NONE',  ( 15.44008868035555260, 49.73035201082150536, 9.422509992056143702 ) ) ;
#24106=CARTESIAN_POINT ( 'NONE',  ( 4.559911319644449179, 57.23035201082150536, -9.422509992056141925 ) ) ;
#24108=CARTESIAN_POINT ( 'NONE',  ( 7.084665262690076126, 54.10535201082151247, 10.88017736071109987 ) ) ;
#24109=CARTESIAN_POINT ( 'NONE',  ( 20.15039907845753930, 70.00000000000000000, -6.262539305110068177 ) ) ;
#24110=CARTESIAN_POINT ( 'NONE',  ( 2.035157376598822676, 62.43868534415483396, -7.964842623401177768 ) ) ;
#24111=CARTESIAN_POINT ( 'NONE',  ( 10.00000000000000178, 14.31368534415483929, 10.88017736071110342 ) ) ;
#24112=CARTESIAN_POINT ( 'NONE',  ( 1.472469842513823179, 45.59226448433412315, -4.923371831947296329 ) ) ;
#24113=CARTESIAN_POINT ( 'NONE',  ( 7.084665262690076126, 22.02201867748817321, -10.88017736071110164 ) ) ;
#24116=CARTESIAN_POINT ( 'NONE',  ( 3.591859063236761518, 19.95696800326375353, 11.09922568453594849 ) ) ;
#24118=CARTESIAN_POINT ( 'NONE',  ( 0.5774900079438607392, 38.48035201082150536, 5.440088680355550821 ) ) ;
#24119=CARTESIAN_POINT ( 'NONE',  ( 19.38216949554541202, 10.99863466993042138, 9.382169495545424454 ) ) ;
#24121=CARTESIAN_POINT ( 'NONE',  ( 2.035157376598822676, 17.43868534415483751, -7.964842623401177768 ) ) ;
#24123=CARTESIAN_POINT ( 'NONE',  ( 0.5774900079438590739, 37.64701867748817676, -5.440088680355550821 ) ) ;
#24124=CARTESIAN_POINT ( 'NONE',  ( 22.26659068614894466, 48.88708216824730357, 7.082119434687054849 ) ) ;
#24125=CARTESIAN_POINT ( 'NONE',  ( 0.1532563361054082862, 26.21726448433411605, 2.638427012816831674 ) ) ;
#24126=CARTESIAN_POINT ( 'NONE',  ( 0.5774900079438590739, 62.64701867748817676, -5.440088680355550821 ) ) ;
#24128=CARTESIAN_POINT ( 'NONE',  ( 13.79529636645031943, 20.34541550158063572, -14.16423886937409904 ) ) ;
#24131=CARTESIAN_POINT ( 'NONE',  ( 14.92337183194729988, 64.34226448433412315, -8.527530157486177487 ) ) ;
#24133=ORIENTED_EDGE ( 'NONE', *, *, #731, .T. ) ;
#24134=CARTESIAN_POINT ( 'NONE',  ( -2.266590686148945544, 37.22041550158063217, 7.082119434687048631 ) ) ;
#24135=CARTESIAN_POINT ( 'NONE',  ( 24.16423886937410614, 34.30374883491396787, 8.672049930838204340E-16 ) ) ;
#24136=CARTESIAN_POINT ( 'NONE',  ( 14.92337183194729988, 4.342264484334117824, -8.527530157486177487 ) ) ;
#24137=CARTESIAN_POINT ( 'NONE',  ( 0.1532563361054100626, 65.80059781766745175, -2.638427012816831230 ) ) ;
#24139=CARTESIAN_POINT ( 'NONE',  ( 4.559911319644449179, 58.89701867748817676, 9.422509992056141925 ) ) ;
#24140=CARTESIAN_POINT ( 'NONE',  ( 13.43411237798105340, 20.58196800326374643, 12.81628187352647963 ) ) ;
#24141=CARTESIAN_POINT ( 'NONE',  ( -0.3689425029237881626, 27.42874883491397142, 10.36894250292379027 ) ) ;
#24142=CARTESIAN_POINT ( 'NONE',  ( 17.96484262340118221, 26.18868534415483396, -7.964842623401177768 ) ) ;
#24144=CARTESIAN_POINT ( 'NONE',  ( 20.88017736071110875, 50.77201867748817676, -2.915334737309920765 ) ) ;
#24150=CARTESIAN_POINT ( 'NONE',  ( 24.16423886937410614, 9.512082168247301794, -3.795296366450302550 ) ) ;
#24151=CARTESIAN_POINT ( 'NONE',  ( -4.164238869374098151, 61.59541550158063217, -3.795296366450310543 ) ) ;
#24152=CARTESIAN_POINT ( 'NONE',  ( 24.16423886937410614, 59.30374883491397497, 8.672049930838204340E-16 ) ) ;
#24153=CARTESIAN_POINT ( 'NONE',  ( 1.472469842513823179, 40.59226448433411605, -4.923371831947296329 ) ) ;
#24154=CARTESIAN_POINT ( 'NONE',  ( 18.52753015748617571, 58.09226448433411605, 4.923371831947298993 ) ) ;
#24160=CARTESIAN_POINT ( 'NONE',  ( 6.565887622018943937, 8.081968003263751754, -12.81628187352647608 ) ) ;
#24162=CARTESIAN_POINT ( 'NONE',  ( 20.36894250292379738, 44.92874883491396787, -10.36894250292379027 ) ) ;
#24163=CARTESIAN_POINT ( 'NONE',  ( 6.204703633549690345, 45.76208216824729647, -14.16423886937410259 ) ) ;
#24164=ORIENTED_EDGE ( 'NONE', *, *, #70002, .F. ) ;
#24165=CARTESIAN_POINT ( 'NONE',  ( 4.559911319644449179, 18.89701867748817321, 9.422509992056141925 ) ) ;
#24167=CARTESIAN_POINT ( 'NONE',  ( 20.88017736071110164, 35.35535201082150536, 2.915334737309930979 ) ) ;
#24168=CARTESIAN_POINT ( 'NONE',  ( 17.20831665107776587, 54.13393115100079456, -7.208316651077762316 ) ) ;
#24169=CARTESIAN_POINT ( 'NONE',  ( 20.88017736071110519, 35.56368534415484106, 2.639326808657452039E-16 ) ) ;
#24170=( BOUNDED_CURVE ( )  B_SPLINE_CURVE ( 3, ( #34810, #11820, #96825, #28302 ),
 .UNSPECIFIED., .F., .T. ) 
 B_SPLINE_CURVE_WITH_KNOTS ( ( 4, 4 ),
 ( 0.5528074785697332238, 0.7738571667627152095 ),
 .UNSPECIFIED. ) 
 CURVE ( )  GEOMETRIC_REPRESENTATION_ITEM ( )  RATIONAL_B_SPLINE_CURVE ( ( 1.000000000000000000, 0.9959322297119970191, 0.9959322297119970191, 1.000000000000000000 ) ) 
 REPRESENTATION_ITEM ( '' )  );
#24171=CARTESIAN_POINT ( 'NONE',  ( 10.00000000000000178, 64.31368534415483396, 10.88017736071110342 ) ) ;
#24172=CARTESIAN_POINT ( 'NONE',  ( -0.8801773607111008646, 33.27201867748817676, 2.915334737309923430 ) ) ;
#24173=EDGE_CURVE ( 'NONE', #86034, #82667, #17295, .T. ) ;
#24174=( BOUNDED_SURFACE ( )  B_SPLINE_SURFACE ( 1, 2, ( 
 ( #46256, #32707, #8735, #40717, #24735, #62712, #63203, #39254, #76740, #32210, #93211, #17241, #8256, #38756, #55212, #85728, #78214, #69744, #69257, #9725, #93707, #778, #31229, #61726, #25242, #40224, #82349, #81855, #72874, #42396, #27870, #88876, #13366, #4409, #20384, #58354, #96894, #50373, #34876, #66861, #50875, #59350, #12866, #65370, #96394, #97380, #35868, #73864, #43851, #95900, #28847, #81368, #43365, #28371, #26891, #74855, #35376, #5393, #66357, #80881, #51865, #58861, #74345, #89853, #57386, #13870, #19880, #27380, #5873, #36366, #89365, #44350, #12380, #42885, #21369, #6356, #57871, #20876, #65867, #64867, #95389, #88382, #87877, #51368, #19394, #49880, #73368, #80391, #11895, #4895, #23353, #61325, #68845, #83839, #75344, #91333, #54312, #97883, #16332, #37862, #46334, #22858, #98380, #38839, #38351, #6857, #7851, #14369, #15364, #53330, #69331, #45849, #855, #29343, #53835, #37368, #76335, #59845, #84347, #84825, #378, #91836, #90334, #30826, #44837, #30330, #14871, #98874, #67860, #90837, #31313, #29836, #60344, #76819, #15848, #45342, #60831, #22366, #46815, #8336, #61815, #77307, #92320, #21873, #23845, #83348, #36866, #67358, #52351, #52839, #82849, #75843, #7362, #68356, #86303, #48289, #93301, #33279, #17807, #55302, #18793, #10796, #71307, #92808, #2335, #10308, #2826, #78798, #87272, #79287, #49276, #25801, #1839, #8821, #63770, #39335, #40807, #85812, #25324, #56303, #70324, #17325, #40316, #32790, #86796, #94280, #24825, #77800, #69830, #78297, #33759, #63287, #47798, #18297, #93794, #48780, #55809, #1352, #31803, #9813, #41314, #70820, #71786, #32297, #64263, #3295, #94775, #62301, #9312, #39819, #26275, #24338, #56777, #54799, #85314, #16823, #47298, #62800, #4776, #96774, #19274, #35250, #42767, #12750, #65247, #49757, #81735, #65746, #74228, #27750, #80270, #12259, #66239, #97271, #20759, #28742, #73249, #5762, #79776, #26769, #42279, #28250, #34251, #96276, #58234, #20264, #51248, #13251, #59233, #43249, #88754, #11770, #19763, #72750, #50763, #57264, #95773, #4283, #58745, #43742, #64752, #27254, #73744, #34757, #81252, #11275, #5275, #89249, #36250, #57754, #88257, #66747, #89734, #50248, #35752, #21253, #87759, #80764, #41795, #72268, #3796, #95264, #23241, #53713, #44732, #61217, #44233, #74737, #90228, #30705, #60229, #69222, #76708, #29723, #22249, #8228, #7744, #68246, #38722, #747, #90724, #84232, #14251, #22742, #75727, #59732, #52725, #31200, #61693, #98266, #83231, #15740, #46223, #75229, #91720, #6250, #36754, #21759, #92209, #14755, #51751, #82235, #45229, #7242, #13750 ),
 ( #67244, #15251, #97769, #37748, #53225, #45728, #30214, #29233, #52240, #82732, #68728, #6742, #37259, #83728, #60717, #256, #67746, #98764, #91214, #76230, #38238, #84713, #33648, #93180, #2216, #17212, #9201, #10677, #47689, #2712, #18182, #16215, #71672, #77686, #54683, #40686, #71187, #78182, #41192, #70202, #39713, #56184, #48662, #24217, #9695, #24706, #64144, #23735, #62182, #54198, #25211, #40189, #70697, #92692, #86677, #32675, #63169, #10193, #48170, #55691, #93676, #85205, #86189, #3182, #46700, #77199, #55177, #33164, #17699, #16709, #25693, #78682, #47182, #63658, #1237, #94164, #79164, #8704, #39221, #69707, #31692, #1721, #32177, #62680, #85692, #43132, #43626, #27636, #50642, #56661, #58121, #72149, #88136, #72633, #87150, #12633, #34139, #50141, #18675, #73624, #74112, #88629, #81131, #49161, #20138, #3677, #19649, #4165, #57641, #64631, #49637, #28131, #95140, #26651, #35637, #5147, #34633, #80650, #57147, #5646, #12144, #66123, #36122, #42649, #79664, #96153, #42170, #51130, #94661, #73125, #87644, #4667, #58631, #96652, #89130, #35129, #65628, #80145, #20641, #81620, #65132, #26170, #13129, #11160, #41680, #19158, #11655, #95653, #27137, #46107, #38123, #8109, #83613, #59614, #68611, #37624, #75609, #15128, #6133, #140, #29598, #90601, #30095, #28627, #76591, #37133, #45102, #60100, #52122, #53592, #22128, #45603, #61094, #59114, #15622, #21636, #97647, #76101, #7632, #52609, #84106, #14132, #82616, #30589, #91604, #67122, #83110, #67628, #66630, #97159, #36639, #89624, #68120, #14639, #7120, #29111, #23120, #98646, #60602, #53103, #91097, #22624, #21136, #90111, #51637, #82116, #13626, #44108, #98137, #74619, #44617, #75113, #6619, #40077, #8594, #9577, #16098, #85580, #24597, #71074, #93066, #2599, #48052, #55062, #1112, #40577, #70578, #39101, #2105, #46585, #17094, #47576, #34397, #78072, #64885, #637, #55577, #77083, #32564, #31085, #86075, #87896, #63062, #93560, #61580, #25094, #69592, #32059, #16593, #1610, #31575, #92576, #95413, #62069, #24100, #78566, #17587, #47070, #62562, #54569, #19412, #10076, #26908, #80413, #57405, #92091, #49903, #85085, #38604, #69103, #23619, #77568, #54084, #84600, #9084, #39598, #70086, #51388, #96412, #36387, #20899, #58375, #21891, #13890, #74366, #95917, #5413, #13386, #5895, #89385, #90353, #82367, #52369, #28868, #4912, #44374, #81874, #43870, #59371, #50393, #74872, #73883, #35884, #66882, #72895, #11913, #81386, #97399, #66380, #27888, #97905, #96913, #89875, #6372, #4429, #59866, #65884, #42903, #21389, #51886, #28390, #29363, #88896, #20405, #36886 ) ),
 .UNSPECIFIED., .F., .F., .T. ) 
 B_SPLINE_SURFACE_WITH_KNOTS ( ( 2, 2 ),
 ( 3, 2, 2, 2, 2, 2, 2, 2, 2, 2, 2, 2, 2, 2, 2, 2, 2, 2, 2, 2, 2, 2, 2, 2, 2, 2, 2, 2, 2, 2, 2, 2, 2, 2, 2, 2, 2, 2, 2, 2, 2, 2, 2, 2, 2, 2, 2, 2, 2, 2, 2, 2, 2, 2, 2, 2, 2, 2, 2, 2, 2, 2, 2, 2, 2, 2, 2, 2, 2, 2, 2, 2, 2, 2, 2, 2, 2, 2, 2, 2, 2, 2, 2, 2, 2, 2, 2, 2, 2, 2, 2, 2, 2, 2, 2, 2, 2, 2, 2, 2, 2, 2, 2, 2, 2, 2, 2, 2, 2, 2, 2, 2, 2, 2, 2, 2, 2, 2, 2, 2, 2, 2, 2, 2, 2, 2, 2, 2, 2, 2, 2, 2, 2, 2, 2, 2, 2, 2, 2, 2, 2, 2, 2, 2, 2, 2, 2, 2, 2, 2, 2, 2, 2, 2, 2, 2, 2, 2, 2, 2, 2, 2, 3 ),
 ( 0.000000000000000000, 1.000000000000000000 ),
 ( 0.000000000000000000, 0.005952380952380952051, 0.01190476190476190410, 0.01785714285714285615, 0.02380952380952380820, 0.02976190476190476025, 0.03571428571428571230, 0.04166666666666666435, 0.04761904761904761640, 0.05357142857142856845, 0.05952380952380952051, 0.06547619047619047949, 0.07142857142857142461, 0.07738095238095238360, 0.08333333333333332871, 0.08928571428571428770, 0.09523809523809523281, 0.1011904761904761918, 0.1071428571428571369, 0.1130952380952380959, 0.1190476190476190410, 0.1250000000000000000, 0.1309523809523809590, 0.1369047619047619180, 0.1428571428571428492, 0.1488095238095238082, 0.1547619047619047672, 0.1607142857142857262, 0.1666666666666666574, 0.1726190476190476164, 0.1785714285714285754, 0.1845238095238095344, 0.1904761904761904656, 0.1964285714285714246, 0.2023809523809523836, 0.2083333333333333426, 0.2142857142857142738, 0.2202380952380952328, 0.2261904761904761918, 0.2321428571428571508, 0.2380952380952380820, 0.2440476190476190410, 0.2500000000000000000, 0.2559523809523809312, 0.2619047619047619180, 0.2678571428571428492, 0.2738095238095238360, 0.2797619047619047672, 0.2857142857142856984, 0.2916666666666666852, 0.2976190476190476164, 0.3035714285714285476, 0.3095238095238095344, 0.3154761904761904656, 0.3214285714285714524, 0.3273809523809523836, 0.3333333333333333148, 0.3392857142857143016, 0.3452380952380952328, 0.3511904761904761640, 0.3571428571428571508, 0.3630952380952380820, 0.3690476190476190688, 0.3750000000000000000, 0.3809523809523809312, 0.3869047619047619180, 0.3928571428571428492, 0.3988095238095238360, 0.4047619047619047672, 0.4107142857142856984, 0.4166666666666666852, 0.4226190476190476164, 0.4285714285714285476, 0.4345238095238095344, 0.4404761904761904656, 0.4464285714285714524, 0.4523809523809523836, 0.4583333333333333148, 0.4642857142857143016, 0.4702380952380952328, 0.4761904761904761640, 0.4821428571428571508, 0.4880952380952380820, 0.4940476190476190688, 0.5000000000000000000, 0.5059523809523809312, 0.5119047619047618625, 0.5178571428571429047, 0.5238095238095238360, 0.5297619047619047672, 0.5357142857142856984, 0.5416666666666666297, 0.5476190476190476719, 0.5535714285714286031, 0.5595238095238095344, 0.5654761904761904656, 0.5714285714285713969, 0.5773809523809523281, 0.5833333333333333703, 0.5892857142857143016, 0.5952380952380952328, 0.6011904761904761640, 0.6071428571428570953, 0.6130952380952381375, 0.6190476190476190688, 0.6250000000000000000, 0.6309523809523809312, 0.6369047619047618625, 0.6428571428571429047, 0.6488095238095238360, 0.6547619047619047672, 0.6607142857142856984, 0.6666666666666666297, 0.6726190476190476719, 0.6785714285714286031, 0.6845238095238095344, 0.6904761904761904656, 0.6964285714285713969, 0.7023809523809523281, 0.7083333333333333703, 0.7142857142857143016, 0.7202380952380952328, 0.7261904761904761640, 0.7321428571428570953, 0.7380952380952381375, 0.7440476190476190688, 0.7500000000000000000, 0.7559523809523809312, 0.7619047619047618625, 0.7678571428571429047, 0.7738095238095238360, 0.7797619047619047672, 0.7857142857142856984, 0.7916666666666666297, 0.7976190476190476719, 0.8035714285714286031, 0.8095238095238095344, 0.8154761904761904656, 0.8214285714285713969, 0.8273809523809523281, 0.8333333333333333703, 0.8392857142857143016, 0.8452380952380952328, 0.8511904761904761640, 0.8571428571428570953, 0.8630952380952381375, 0.8690476190476190688, 0.8750000000000000000, 0.8809523809523809312, 0.8869047619047618625, 0.8928571428571429047, 0.8988095238095238360, 0.9047619047619047672, 0.9107142857142856984, 0.9166666666666666297, 0.9226190476190476719, 0.9285714285714286031, 0.9345238095238095344, 0.9404761904761904656, 0.9464285714285713969, 0.9523809523809523281, 0.9583333333333333703, 0.9642857142857143016 ),
 .UNSPECIFIED. ) 
 GEOMETRIC_REPRESENTATION_ITEM ( )  RATIONAL_B_SPLINE_SURFACE ( (
 ( 1.000000000000000000, 0.9659258262890683122, 1.000000000000000000, 0.9659258262890683122, 1.000000000000000000, 0.9659258262890683122, 1.000000000000000000, 0.9659258262890683122, 1.000000000000000000, 0.9659258262890683122, 1.000000000000000000, 0.9659258262890683122, 1.000000000000000000, 0.9659258262890683122, 1.000000000000000000, 0.9659258262890683122, 1.000000000000000000, 0.9659258262890683122, 1.000000000000000000, 0.9659258262890683122, 1.000000000000000000, 0.9659258262890683122, 1.000000000000000000, 0.9659258262890683122, 1.000000000000000000, 0.9659258262890683122, 1.000000000000000000, 0.9659258262890683122, 1.000000000000000000, 0.9659258262890683122, 1.000000000000000000, 0.9659258262890683122, 1.000000000000000000, 0.9659258262890683122, 1.000000000000000000, 0.9659258262890683122, 1.000000000000000000, 0.9659258262890683122, 1.000000000000000000, 0.9659258262890683122, 1.000000000000000000, 0.9659258262890683122, 1.000000000000000000, 0.9659258262890683122, 1.000000000000000000, 0.9659258262890683122, 1.000000000000000000, 0.9659258262890683122, 1.000000000000000000, 0.9659258262890683122, 1.000000000000000000, 0.9659258262890683122, 1.000000000000000000, 0.9659258262890683122, 1.000000000000000000, 0.9659258262890683122, 1.000000000000000000, 0.9659258262890683122, 1.000000000000000000, 0.9659258262890683122, 1.000000000000000000, 0.9659258262890683122, 1.000000000000000000, 0.9659258262890683122, 1.000000000000000000, 0.9659258262890683122, 1.000000000000000000, 0.9659258262890683122, 1.000000000000000000, 0.9659258262890683122, 1.000000000000000000, 0.9659258262890683122, 1.000000000000000000, 0.9659258262890683122, 1.000000000000000000, 0.9659258262890683122, 1.000000000000000000, 0.9659258262890683122, 1.000000000000000000, 0.9659258262890683122, 1.000000000000000000, 0.9659258262890683122, 1.000000000000000000, 0.9659258262890683122, 1.000000000000000000, 0.9659258262890683122, 1.000000000000000000, 0.9659258262890683122, 1.000000000000000000, 0.9659258262890683122, 1.000000000000000000, 0.9659258262890683122, 1.000000000000000000, 0.9659258262890683122, 1.000000000000000000, 0.9659258262890683122, 1.000000000000000000, 0.9659258262890683122, 1.000000000000000000, 0.9659258262890683122, 1.000000000000000000, 0.9659258262890683122, 1.000000000000000000, 0.9659258262890683122, 1.000000000000000000, 0.9659258262890683122, 1.000000000000000000, 0.9659258262890683122, 1.000000000000000000, 0.9659258262890683122, 1.000000000000000000, 0.9659258262890683122, 1.000000000000000000, 0.9659258262890683122, 1.000000000000000000, 0.9659258262890683122, 1.000000000000000000, 0.9659258262890683122, 1.000000000000000000, 0.9659258262890683122, 1.000000000000000000, 0.9659258262890683122, 1.000000000000000000, 0.9659258262890683122, 1.000000000000000000, 0.9659258262890683122, 1.000000000000000000, 0.9659258262890683122, 1.000000000000000000, 0.9659258262890683122, 1.000000000000000000, 0.9659258262890683122, 1.000000000000000000, 0.9659258262890683122, 1.000000000000000000, 0.9659258262890683122, 1.000000000000000000, 0.9659258262890683122, 1.000000000000000000, 0.9659258262890683122, 1.000000000000000000, 0.9659258262890683122, 1.000000000000000000, 0.9659258262890683122, 1.000000000000000000, 0.9659258262890683122, 1.000000000000000000, 0.9659258262890683122, 1.000000000000000000, 0.9659258262890683122, 1.000000000000000000, 0.9659258262890683122, 1.000000000000000000, 0.9659258262890683122, 1.000000000000000000, 0.9659258262890683122, 1.000000000000000000, 0.9659258262890683122, 1.000000000000000000, 0.9659258262890683122, 1.000000000000000000, 0.9659258262890683122, 1.000000000000000000, 0.9659258262890683122, 1.000000000000000000, 0.9659258262890683122, 1.000000000000000000, 0.9659258262890683122, 1.000000000000000000, 0.9659258262890683122, 1.000000000000000000, 0.9659258262890683122, 1.000000000000000000, 0.9659258262890683122, 1.000000000000000000, 0.9659258262890683122, 1.000000000000000000, 0.9659258262890683122, 1.000000000000000000, 0.9659258262890683122, 1.000000000000000000, 0.9659258262890683122, 1.000000000000000000, 0.9659258262890683122, 1.000000000000000000, 0.9659258262890683122, 1.000000000000000000, 0.9659258262890683122, 1.000000000000000000, 0.9659258262890683122, 1.000000000000000000, 0.9659258262890683122, 1.000000000000000000, 0.9659258262890683122, 1.000000000000000000, 0.9659258262890683122, 1.000000000000000000, 0.9659258262890683122, 1.000000000000000000, 0.9659258262890683122, 1.000000000000000000, 0.9659258262890683122, 1.000000000000000000, 0.9659258262890683122, 1.000000000000000000, 0.9659258262890683122, 1.000000000000000000, 0.9659258262890683122, 1.000000000000000000, 0.9659258262890683122, 1.000000000000000000, 0.9659258262890683122, 1.000000000000000000, 0.9659258262890683122, 1.000000000000000000, 0.9659258262890683122, 1.000000000000000000, 0.9659258262890683122, 1.000000000000000000, 0.9659258262890683122, 1.000000000000000000, 0.9659258262890683122, 1.000000000000000000, 0.9659258262890683122, 1.000000000000000000, 0.9659258262890683122, 1.000000000000000000, 0.9659258262890683122, 1.000000000000000000, 0.9659258262890683122, 1.000000000000000000, 0.9659258262890683122, 1.000000000000000000, 0.9659258262890683122, 1.000000000000000000, 0.9659258262890683122, 1.000000000000000000, 0.9659258262890683122, 1.000000000000000000, 0.9659258262890683122, 1.000000000000000000, 0.9659258262890683122, 1.000000000000000000, 0.9659258262890683122, 1.000000000000000000, 0.9659258262890683122, 1.000000000000000000, 0.9659258262890683122, 1.000000000000000000, 0.9659258262890683122, 1.000000000000000000, 0.9659258262890683122, 1.000000000000000000, 0.9659258262890683122, 1.000000000000000000, 0.9659258262890683122, 1.000000000000000000, 0.9659258262890683122, 1.000000000000000000, 0.9659258262890683122, 1.000000000000000000, 0.9659258262890683122, 1.000000000000000000, 0.9659258262890683122, 1.000000000000000000, 0.9659258262890683122, 1.000000000000000000, 0.9659258262890683122, 1.000000000000000000, 0.9659258262890683122, 1.000000000000000000, 0.9659258262890683122, 1.000000000000000000, 0.9659258262890683122, 1.000000000000000000, 0.9659258262890683122, 1.000000000000000000, 0.9659258262890683122, 1.000000000000000000, 0.9659258262890683122, 1.000000000000000000, 0.9659258262890683122, 1.000000000000000000, 0.9659258262890683122, 1.000000000000000000, 0.9659258262890683122, 1.000000000000000000, 0.9659258262890683122, 1.000000000000000000, 0.9659258262890683122, 1.000000000000000000, 0.9659258262890683122, 1.000000000000000000, 0.9659258262890683122, 1.000000000000000000, 0.9659258262890683122, 1.000000000000000000, 0.9659258262890683122, 1.000000000000000000, 0.9659258262890683122, 1.000000000000000000, 0.9659258262890683122, 1.000000000000000000, 0.9659258262890683122, 1.000000000000000000, 0.9659258262890683122, 1.000000000000000000, 0.9659258262890683122, 1.000000000000000000, 0.9659258262890683122, 1.000000000000000000, 0.9659258262890683122, 1.000000000000000000, 0.9659258262890683122, 1.000000000000000000, 0.9659258262890683122, 1.000000000000000000, 0.9659258262890683122, 1.000000000000000000, 0.9659258262890683122, 1.000000000000000000, 0.9659258262890683122, 1.000000000000000000, 0.9659258262890683122, 1.000000000000000000),
 ( 1.000000000000000000, 0.9659258262890683122, 1.000000000000000000, 0.9659258262890683122, 1.000000000000000000, 0.9659258262890683122, 1.000000000000000000, 0.9659258262890683122, 1.000000000000000000, 0.9659258262890683122, 1.000000000000000000, 0.9659258262890683122, 1.000000000000000000, 0.9659258262890683122, 1.000000000000000000, 0.9659258262890683122, 1.000000000000000000, 0.9659258262890683122, 1.000000000000000000, 0.9659258262890683122, 1.000000000000000000, 0.9659258262890683122, 1.000000000000000000, 0.9659258262890683122, 1.000000000000000000, 0.9659258262890683122, 1.000000000000000000, 0.9659258262890683122, 1.000000000000000000, 0.9659258262890683122, 1.000000000000000000, 0.9659258262890683122, 1.000000000000000000, 0.9659258262890683122, 1.000000000000000000, 0.9659258262890683122, 1.000000000000000000, 0.9659258262890683122, 1.000000000000000000, 0.9659258262890683122, 1.000000000000000000, 0.9659258262890683122, 1.000000000000000000, 0.9659258262890683122, 1.000000000000000000, 0.9659258262890683122, 1.000000000000000000, 0.9659258262890683122, 1.000000000000000000, 0.9659258262890683122, 1.000000000000000000, 0.9659258262890683122, 1.000000000000000000, 0.9659258262890683122, 1.000000000000000000, 0.9659258262890683122, 1.000000000000000000, 0.9659258262890683122, 1.000000000000000000, 0.9659258262890683122, 1.000000000000000000, 0.9659258262890683122, 1.000000000000000000, 0.9659258262890683122, 1.000000000000000000, 0.9659258262890683122, 1.000000000000000000, 0.9659258262890683122, 1.000000000000000000, 0.9659258262890683122, 1.000000000000000000, 0.9659258262890683122, 1.000000000000000000, 0.9659258262890683122, 1.000000000000000000, 0.9659258262890683122, 1.000000000000000000, 0.9659258262890683122, 1.000000000000000000, 0.9659258262890683122, 1.000000000000000000, 0.9659258262890683122, 1.000000000000000000, 0.9659258262890683122, 1.000000000000000000, 0.9659258262890683122, 1.000000000000000000, 0.9659258262890683122, 1.000000000000000000, 0.9659258262890683122, 1.000000000000000000, 0.9659258262890683122, 1.000000000000000000, 0.9659258262890683122, 1.000000000000000000, 0.9659258262890683122, 1.000000000000000000, 0.9659258262890683122, 1.000000000000000000, 0.9659258262890683122, 1.000000000000000000, 0.9659258262890683122, 1.000000000000000000, 0.9659258262890683122, 1.000000000000000000, 0.9659258262890683122, 1.000000000000000000, 0.9659258262890683122, 1.000000000000000000, 0.9659258262890683122, 1.000000000000000000, 0.9659258262890683122, 1.000000000000000000, 0.9659258262890683122, 1.000000000000000000, 0.9659258262890683122, 1.000000000000000000, 0.9659258262890683122, 1.000000000000000000, 0.9659258262890683122, 1.000000000000000000, 0.9659258262890683122, 1.000000000000000000, 0.9659258262890683122, 1.000000000000000000, 0.9659258262890683122, 1.000000000000000000, 0.9659258262890683122, 1.000000000000000000, 0.9659258262890683122, 1.000000000000000000, 0.9659258262890683122, 1.000000000000000000, 0.9659258262890683122, 1.000000000000000000, 0.9659258262890683122, 1.000000000000000000, 0.9659258262890683122, 1.000000000000000000, 0.9659258262890683122, 1.000000000000000000, 0.9659258262890683122, 1.000000000000000000, 0.9659258262890683122, 1.000000000000000000, 0.9659258262890683122, 1.000000000000000000, 0.9659258262890683122, 1.000000000000000000, 0.9659258262890683122, 1.000000000000000000, 0.9659258262890683122, 1.000000000000000000, 0.9659258262890683122, 1.000000000000000000, 0.9659258262890683122, 1.000000000000000000, 0.9659258262890683122, 1.000000000000000000, 0.9659258262890683122, 1.000000000000000000, 0.9659258262890683122, 1.000000000000000000, 0.9659258262890683122, 1.000000000000000000, 0.9659258262890683122, 1.000000000000000000, 0.9659258262890683122, 1.000000000000000000, 0.9659258262890683122, 1.000000000000000000, 0.9659258262890683122, 1.000000000000000000, 0.9659258262890683122, 1.000000000000000000, 0.9659258262890683122, 1.000000000000000000, 0.9659258262890683122, 1.000000000000000000, 0.9659258262890683122, 1.000000000000000000, 0.9659258262890683122, 1.000000000000000000, 0.9659258262890683122, 1.000000000000000000, 0.9659258262890683122, 1.000000000000000000, 0.9659258262890683122, 1.000000000000000000, 0.9659258262890683122, 1.000000000000000000, 0.9659258262890683122, 1.000000000000000000, 0.9659258262890683122, 1.000000000000000000, 0.9659258262890683122, 1.000000000000000000, 0.9659258262890683122, 1.000000000000000000, 0.9659258262890683122, 1.000000000000000000, 0.9659258262890683122, 1.000000000000000000, 0.9659258262890683122, 1.000000000000000000, 0.9659258262890683122, 1.000000000000000000, 0.9659258262890683122, 1.000000000000000000, 0.9659258262890683122, 1.000000000000000000, 0.9659258262890683122, 1.000000000000000000, 0.9659258262890683122, 1.000000000000000000, 0.9659258262890683122, 1.000000000000000000, 0.9659258262890683122, 1.000000000000000000, 0.9659258262890683122, 1.000000000000000000, 0.9659258262890683122, 1.000000000000000000, 0.9659258262890683122, 1.000000000000000000, 0.9659258262890683122, 1.000000000000000000, 0.9659258262890683122, 1.000000000000000000, 0.9659258262890683122, 1.000000000000000000, 0.9659258262890683122, 1.000000000000000000, 0.9659258262890683122, 1.000000000000000000, 0.9659258262890683122, 1.000000000000000000, 0.9659258262890683122, 1.000000000000000000, 0.9659258262890683122, 1.000000000000000000, 0.9659258262890683122, 1.000000000000000000, 0.9659258262890683122, 1.000000000000000000, 0.9659258262890683122, 1.000000000000000000, 0.9659258262890683122, 1.000000000000000000, 0.9659258262890683122, 1.000000000000000000, 0.9659258262890683122, 1.000000000000000000, 0.9659258262890683122, 1.000000000000000000, 0.9659258262890683122, 1.000000000000000000, 0.9659258262890683122, 1.000000000000000000, 0.9659258262890683122, 1.000000000000000000, 0.9659258262890683122, 1.000000000000000000, 0.9659258262890683122, 1.000000000000000000, 0.9659258262890683122, 1.000000000000000000, 0.9659258262890683122, 1.000000000000000000, 0.9659258262890683122, 1.000000000000000000, 0.9659258262890683122, 1.000000000000000000, 0.9659258262890683122, 1.000000000000000000, 0.9659258262890683122, 1.000000000000000000, 0.9659258262890683122, 1.000000000000000000, 0.9659258262890683122, 1.000000000000000000, 0.9659258262890683122, 1.000000000000000000, 0.9659258262890683122, 1.000000000000000000, 0.9659258262890683122, 1.000000000000000000, 0.9659258262890683122, 1.000000000000000000, 0.9659258262890683122, 1.000000000000000000, 0.9659258262890683122, 1.000000000000000000, 0.9659258262890683122, 1.000000000000000000, 0.9659258262890683122, 1.000000000000000000, 0.9659258262890683122, 1.000000000000000000, 0.9659258262890683122, 1.000000000000000000, 0.9659258262890683122, 1.000000000000000000, 0.9659258262890683122, 1.000000000000000000, 0.9659258262890683122, 1.000000000000000000, 0.9659258262890683122, 1.000000000000000000, 0.9659258262890683122, 1.000000000000000000, 0.9659258262890683122, 1.000000000000000000, 0.9659258262890683122, 1.000000000000000000, 0.9659258262890683122, 1.000000000000000000, 0.9659258262890683122, 1.000000000000000000, 0.9659258262890683122, 1.000000000000000000, 0.9659258262890683122, 1.000000000000000000, 0.9659258262890683122, 1.000000000000000000) ) ) 
 REPRESENTATION_ITEM ( '' )  SURFACE ( )  );
#24176=AXIS2_PLACEMENT_3D ( 'NONE', #84320, #75317, #83814 ) ;
#24181=CARTESIAN_POINT ( 'NONE',  ( 1.472469842513823179, 36.42559781766745175, 4.923371831947296329 ) ) ;
#24190=CARTESIAN_POINT ( 'NONE',  ( 0.1532563361054082862, 51.21726448433412315, 2.638427012816831674 ) ) ;
#24191=CARTESIAN_POINT ( 'NONE',  ( 10.00000000000000178, 53.05374883491396787, 14.16423886937410082 ) ) ;
#24192=CARTESIAN_POINT ( 'NONE',  ( 10.00000000000000000, 64.75893115100078035, -9.846743663894594434 ) ) ;
#24194=CARTESIAN_POINT ( 'NONE',  ( 1.472469842513823179, 20.59226448433411960, -4.923371831947296329 ) ) ;
#24195=EDGE_CURVE ( 'NONE', #80952, #87032, #61058, .T. ) ;
#24196=CARTESIAN_POINT ( 'NONE',  ( 19.38216949554541202, 45.99863466993041072, 9.382169495545424454 ) ) ;
#24197=CARTESIAN_POINT ( 'NONE',  ( 14.92337183194729633, 62.67559781766745886, 8.527530157486181039 ) ) ;
#24198=CARTESIAN_POINT ( 'NONE',  ( 15.44008868035555260, 59.73035201082151247, 9.422509992056143702 ) ) ;
#24199=DIRECTION ( 'NONE',  ( 0.000000000000000000, 1.000000000000000000, 0.000000000000000000 ) ) ;
#24201=CARTESIAN_POINT ( 'NONE',  ( 12.91533473730992121, 54.52201867748816255, 10.88017736071110164 ) ) ;
#24202=VERTEX_POINT ( 'NONE', #79257 ) ;
#24203=CARTESIAN_POINT ( 'NONE',  ( -2.266590686148945544, 51.38708216824730357, -7.082119434687050408 ) ) ;
#24204=DIRECTION ( 'NONE',  ( 1.000000000000000000, 0.000000000000000000, 0.000000000000000000 ) ) ;
#24205=CARTESIAN_POINT ( 'NONE',  ( -0.8801773607111008646, 23.27201867748817676, 2.915334737309923430 ) ) ;
#24206=CARTESIAN_POINT ( 'NONE',  ( -2.816281873526473856, 14.33196800326375531, 3.434112377981055619 ) ) ;
#24207=CARTESIAN_POINT ( 'NONE',  ( 7.084665262690076126, 62.02201867748816966, -10.88017736071110164 ) ) ;
#24209=EDGE_CURVE ( 'NONE', #13653, #61453, #55777, .T. ) ;
#24210=CARTESIAN_POINT ( 'NONE',  ( 15.44008868035555793, 66.39701867748817676, -9.422509992056140149 ) ) ;
#24212=CARTESIAN_POINT ( 'NONE',  ( 10.00000000000000178, 54.31368534415484106, 10.88017736071110342 ) ) ;
#24214=CARTESIAN_POINT ( 'NONE',  ( 12.63842701281683922, 44.55059781766745175, -9.846743663894590881 ) ) ;
#24215=CARTESIAN_POINT ( 'NONE',  ( 12.63842701281683034, 7.467264484334118713, 9.846743663894596210 ) ) ;
#24217=CARTESIAN_POINT ( 'NONE',  ( 22.81628187352648496, 6.831968003263753531, -3.434112377981050290 ) ) ;
#24218=CARTESIAN_POINT ( 'NONE',  ( -0.8801773607111009756, 8.063685344154837509, 1.068504757029289695E-15 ) ) ;
#24219=CARTESIAN_POINT ( 'NONE',  ( -0.05723567505238445763, 69.83236346210669865, -6.413539670616451360 ) ) ;
#24220=CARTESIAN_POINT ( 'NONE',  ( 0.2751277870542967463, 70.00000000000000000, -6.000000000000000000 ) ) ;
#24221=CARTESIAN_POINT ( 'NONE',  ( 24.16423886937409904, 39.09541550158062506, 3.795296366450317205 ) ) ;
#24222=CARTESIAN_POINT ( 'NONE',  ( -0.3689425029237898834, 66.17874883491396076, -10.36894250292378850 ) ) ;
#24223=CARTESIAN_POINT ( 'NONE',  ( 0.1532563361054083140, 36.00893115100078745, 1.131784320476157264E-15 ) ) ;
#24224=CARTESIAN_POINT ( 'NONE',  ( 5.076628168052703671, 16.84226448433411960, 8.527530157486179263 ) ) ;
#24225=CARTESIAN_POINT ( 'NONE',  ( 15.44008868035555793, 11.39701867748817143, -9.422509992056140149 ) ) ;
#24226=MECHANICAL_DESIGN_GEOMETRIC_PRESENTATION_REPRESENTATION('',(#64092),#80093);
#24227=ORIENTED_EDGE ( 'NONE', *, *, #83791, .T. ) ;
#24228=CARTESIAN_POINT ( 'NONE',  ( 19.84674366389459621, 43.50893115100078745, 7.409399052514197653E-17 ) ) ;
#24229=CARTESIAN_POINT ( 'NONE',  ( 10.00000000000000000, 26.81368534415484106, -10.88017736071110342 ) ) ;
#24230=CARTESIAN_POINT ( 'NONE',  ( 2.791683348922240793, 56.63393115100078035, 7.208316651077764092 ) ) ;
#24231=CARTESIAN_POINT ( 'NONE',  ( -4.164238869374098151, 11.59541550158063217, -3.795296366450310543 ) ) ;
#24235=CARTESIAN_POINT ( 'NONE',  ( 14.92337183194729633, 17.67559781766745175, 8.527530157486181039 ) ) ;
#24236=CARTESIAN_POINT ( 'NONE',  ( -2.816281873526473856, 54.12363466993041783, 9.499525473075851096E-16 ) ) ;
#24237=CARTESIAN_POINT ( 'NONE',  ( 0.1532563361054083140, 51.00893115100078745, 1.131784320476157264E-15 ) ) ;
#24239=CARTESIAN_POINT ( 'NONE',  ( 17.20831665107776587, 19.13393115100078035, -7.208316651077762316 ) ) ;
#24242=CARTESIAN_POINT ( 'NONE',  ( -2.266590686148945544, 57.22041550158063217, 7.082119434687048631 ) ) ;
#24243=CARTESIAN_POINT ( 'NONE',  ( 19.42250999205614193, 55.14701867748817676, 5.440088680355555262 ) ) ;
#24244=SURFACE_STYLE_USAGE ( .BOTH. , #98789 ) ;
#24245=CARTESIAN_POINT ( 'NONE',  ( 7.084665262690076126, 62.02201867748816966, -10.88017736071110164 ) ) ;
#24246=CARTESIAN_POINT ( 'NONE',  ( 17.20831665107776587, 34.13393115100078745, -7.208316651077762316 ) ) ;
#24247=CARTESIAN_POINT ( 'NONE',  ( 2.035157376598824452, 13.68868534415483751, 7.964842623401179544 ) ) ;
#24248=CARTESIAN_POINT ( 'NONE',  ( 18.39792806157248251, 39.52224192338641728, 6.500000000000040856 ) ) ;
#24249=CARTESIAN_POINT ( 'NONE',  ( 1.472469842513823179, 56.42559781766745886, 4.923371831947296329 ) ) ;
#24250=CARTESIAN_POINT ( 'NONE',  ( 20.88017736071110519, 55.56368534415484817, 2.639326808657452039E-16 ) ) ;
#24252=SURFACE_STYLE_USAGE ( .BOTH. , #46733 ) ;
#24253=CIRCLE ( 'NONE', #70560, 0.5000000000000004441 ) ;
#24258=CARTESIAN_POINT ( 'NONE',  ( 14.92337183194729988, 49.34226448433411605, -8.527530157486177487 ) ) ;
#24259=CARTESIAN_POINT ( 'NONE',  ( 17.20831665107776587, 22.88393115100078745, 7.208316651077764980 ) ) ;
#24260=CARTESIAN_POINT ( 'NONE',  ( 21.09922568453594849, 61.20696800326376064, 6.408140936763242479 ) ) ;
#24261=CARTESIAN_POINT ( 'NONE',  ( 0.5774900079438590739, 17.64701867748817321, -5.440088680355550821 ) ) ;
#24262=CARTESIAN_POINT ( 'NONE',  ( 12.63842701281683034, 42.46726448433412315, 9.846743663894596210 ) ) ;
#24264=CARTESIAN_POINT ( 'NONE',  ( 10.00000000000000000, 45.55374883491397497, -14.16423886937410082 ) ) ;
#24265=CARTESIAN_POINT ( 'NONE',  ( 6.204703633549690345, 62.84541550158063927, 14.16423886937410082 ) ) ;
#24268=CARTESIAN_POINT ( 'NONE',  ( 4.559911319644449179, 53.89701867748817676, 9.422509992056141925 ) ) ;
#24269=CARTESIAN_POINT ( 'NONE',  ( 7.361572987183170547, 22.05059781766745530, 9.846743663894590881 ) ) ;
#24273=STYLED_ITEM ( 'NONE', ( #18527 ), #75423 ) ;
#24275=CARTESIAN_POINT ( 'NONE',  ( 1.472469842513823179, 10.59226448433411782, -4.923371831947296329 ) ) ;
#24277=CARTESIAN_POINT ( 'NONE',  ( -4.164238869374099039, 16.80374883491396787, 8.674139862899312516E-16 ) ) ;
#24278=CARTESIAN_POINT ( 'NONE',  ( 1.472469842513823179, 16.42559781766745175, 4.923371831947296329 ) ) ;
#24279=CARTESIAN_POINT ( 'NONE',  ( 7.084665262690076126, 47.02201867748818387, -10.88017736071110164 ) ) ;
#24281=VERTEX_POINT ( 'NONE', #48258 ) ;
#24282=CARTESIAN_POINT ( 'NONE',  ( 0.5774900079438607392, 43.48035201082151247, 5.440088680355550821 ) ) ;
#24283=VERTEX_POINT ( 'NONE', #78770 ) ;
#24284=CARTESIAN_POINT ( 'NONE',  ( -0.8801773607111009756, 43.06368534415484106, 1.068504757029289695E-15 ) ) ;
#24285=CARTESIAN_POINT ( 'NONE',  ( 2.917880565312948704, 2.637082168247300906, 12.26659068614894643 ) ) ;
#24287=ORIENTED_EDGE ( 'NONE', *, *, #82743, .T. ) ;
#24288=CARTESIAN_POINT ( 'NONE',  ( 6.565887622018943937, 20.16530133659708213, 12.81628187352647430 ) ) ;
#24290=CARTESIAN_POINT ( 'NONE',  ( 1.472469842513823179, 6.425597817667451750, 4.923371831947296329 ) ) ;
#24292=EDGE_CURVE ( 'NONE', #15989, #38758, #33252, .T. ) ;
#24294=CARTESIAN_POINT ( 'NONE',  ( 1.472469842513823179, 10.59226448433411782, -4.923371831947296329 ) ) ;
#24295=CARTESIAN_POINT ( 'NONE',  ( 0.5774900079438607392, 38.48035201082150536, 5.440088680355550821 ) ) ;
#24300=B_SPLINE_CURVE_WITH_KNOTS ( 'NONE', 3,
 ( #29130, #37642, #68139, #68629 ),
 .UNSPECIFIED., .F., .F.,
 ( 4, 4 ),
 ( 1.097135458930219133E-17, 0.001060528352561998294 ),
 .UNSPECIFIED. ) ;
#24302=CARTESIAN_POINT ( 'NONE',  ( 17.96484262340118221, 54.93868534415484106, 7.964842623401181321 ) ) ;
#24305=CARTESIAN_POINT ( 'NONE',  ( 0.5774900079438607392, 58.48035201082151247, 5.440088680355550821 ) ) ;
#24307=CARTESIAN_POINT ( 'NONE',  ( 6.565887622018943937, 8.081968003263751754, -12.81628187352647608 ) ) ;
#24308=CARTESIAN_POINT ( 'NONE',  ( -37.92076923076924544, 94.65384615384614619, -9.500000000000000000 ) ) ;
#24309=CARTESIAN_POINT ( 'NONE',  ( 14.92337183194729988, 29.34226448433411960, -8.527530157486177487 ) ) ;
#24310=CARTESIAN_POINT ( 'NONE',  ( 19.38216949554541202, 50.99863466993042493, 9.382169495545424454 ) ) ;
#24311=CARTESIAN_POINT ( 'NONE',  ( 22.26659068614894466, 8.887082168247300018, 7.082119434687054849 ) ) ;
#24312=CARTESIAN_POINT ( 'NONE',  ( 12.63842701281683034, 17.46726448433411250, 9.846743663894596210 ) ) ;
#24313=CARTESIAN_POINT ( 'NONE',  ( 13.43411237798105340, 25.58196800326374998, 12.81628187352647963 ) ) ;
#24316=CARTESIAN_POINT ( 'NONE',  ( 15.44008868035555260, 44.73035201082151247, 9.422509992056143702 ) ) ;
#24317=CARTESIAN_POINT ( 'NONE',  ( 2.791683348922240793, 61.63393115100079456, 7.208316651077764092 ) ) ;
#24319=CARTESIAN_POINT ( 'NONE',  ( 12.63842701281683922, 24.55059781766745175, -9.846743663894590881 ) ) ;
#24320=CARTESIAN_POINT ( 'NONE',  ( 12.91533473730993009, 11.60535201082150536, -10.88017736071109987 ) ) ;
#24321=CARTESIAN_POINT ( 'NONE',  ( 22.81628187352647785, 21.41530133659708923, 3.434112377981063169 ) ) ;
#24323=CARTESIAN_POINT ( 'NONE',  ( 17.96484262340118221, 4.938685344154837509, 7.964842623401181321 ) ) ;
#24326=CARTESIAN_POINT ( 'NONE',  ( 17.96484262340118221, 14.93868534415484106, 7.964842623401181321 ) ) ;
#24329=CARTESIAN_POINT ( 'NONE',  ( 17.20831665107776587, 37.88393115100078745, 7.208316651077764980 ) ) ;
#24330=CARTESIAN_POINT ( 'NONE',  ( 20.88017736071110164, 15.35535201082150358, 2.915334737309930979 ) ) ;
#24331=CARTESIAN_POINT ( 'NONE',  ( 5.500000000000000000, 60.50000000000000000, -5.000000000000000000 ) ) ;
#24334=CARTESIAN_POINT ( 'NONE',  ( -0.8801773607111008646, 38.27201867748816255, 2.915334737309923430 ) ) ;
#24335=CARTESIAN_POINT ( 'NONE',  ( -2.266590686148945544, 66.38708216824730357, -7.082119434687050408 ) ) ;
#24337=CARTESIAN_POINT ( 'NONE',  ( 14.92337183194729633, 12.67559781766745353, 8.527530157486181039 ) ) ;
#24338=CARTESIAN_POINT ( 'NONE',  ( 19.84674366389459266, 43.71726448433410894, -2.638427012816827677 ) ) ;
#24344=CARTESIAN_POINT ( 'NONE',  ( 17.08211943468705840, 20.13708216824730357, -12.26659068614894466 ) ) ;
#24345=CARTESIAN_POINT ( 'NONE',  ( 1.472469842513823179, 40.59226448433411605, -4.923371831947296329 ) ) ;
#24346=DIRECTION ( 'NONE',  ( 0.000000000000000000, -1.000000000000000000, 0.000000000000000000 ) ) ;
#24348=CARTESIAN_POINT ( 'NONE',  ( 22.26659068614895176, 54.72041550158063217, -7.082119434687042414 ) ) ;
#24349=CARTESIAN_POINT ( 'NONE',  ( 14.92337183194729633, 17.67559781766745175, 8.527530157486181039 ) ) ;
#24351=CARTESIAN_POINT ( 'NONE',  ( -0.8801773607111008646, 43.27201867748817676, 2.915334737309923430 ) ) ;
#24353=CARTESIAN_POINT ( 'NONE',  ( 22.81628187352647785, 56.62363466993042493, 6.195893100308588602E-16 ) ) ;
#24354=CARTESIAN_POINT ( 'NONE',  ( 7.084665262690076126, 14.10535201082150358, 10.88017736071109987 ) ) ;
#24355=CARTESIAN_POINT ( 'NONE',  ( 16.40814093676324603, 47.45696800326375353, -11.09922568453594671 ) ) ;
#24356=CARTESIAN_POINT ( 'NONE',  ( 7.361572987183170547, 62.05059781766745886, 9.846743663894590881 ) ) ;
#24357=CARTESIAN_POINT ( 'NONE',  ( 17.20831665107776587, 4.133931151000785675, -7.208316651077762316 ) ) ;
#24360=CARTESIAN_POINT ( 'NONE',  ( 0.6076426042653192416, 17.37576471608601381, -6.500000000000002665 ) ) ;
#24361=CARTESIAN_POINT ( 'NONE',  ( 24.16423886937410614, 54.51208216824730357, -3.795296366450302550 ) ) ;
#24362=CARTESIAN_POINT ( 'NONE',  ( 13.79529636645030344, 8.262082168247300018, 14.16423886937410614 ) ) ;
#24363=CARTESIAN_POINT ( 'NONE',  ( 12.91533473730992121, 14.52201867748817143, 10.88017736071110164 ) ) ;
#24364=CARTESIAN_POINT ( 'NONE',  ( 2.035157376598822676, 32.43868534415483396, -7.964842623401177768 ) ) ;
#24367=CARTESIAN_POINT ( 'NONE',  ( 0.1532563361054083140, 1.008931151000784787, 1.131784320476157264E-15 ) ) ;
#24368=( NAMED_UNIT ( * ) SI_UNIT ( $, .STERADIAN. ) SOLID_ANGLE_UNIT ( ) );
#24369=CARTESIAN_POINT ( 'NONE',  ( 10.00000000000000000, 19.75893115100078390, -9.846743663894594434 ) ) ;
#24370=CARTESIAN_POINT ( 'NONE',  ( 19.72487221294570858, 70.00000000000000000, 6.500000000000000888 ) ) ;
#24371=CARTESIAN_POINT ( 'NONE',  ( 10.00000000000000000, 14.75893115100078568, -9.846743663894594434 ) ) ;
#24372=CARTESIAN_POINT ( 'NONE',  ( 18.52753015748617571, 38.09226448433412315, 4.923371831947298993 ) ) ;
#24373=CARTESIAN_POINT ( 'NONE',  ( 4.559911319644449179, 18.89701867748817321, 9.422509992056141925 ) ) ;
#24374=CARTESIAN_POINT ( 'NONE',  ( 16.40814093676324603, 27.45696800326375708, -11.09922568453594671 ) ) ;
#24375=CARTESIAN_POINT ( 'NONE',  ( 10.00000000000000000, 40.55374883491397497, -14.16423886937410082 ) ) ;
#24376=CARTESIAN_POINT ( 'NONE',  ( 18.52753015748617571, 13.09226448433411960, 4.923371831947298993 ) ) ;
#24378=CARTESIAN_POINT ( 'NONE',  ( 0.1532563361054100626, 45.80059781766745886, -2.638427012816831230 ) ) ;
#24379=CARTESIAN_POINT ( 'NONE',  ( 0.1532563361054082862, 36.21726448433410894, 2.638427012816831674 ) ) ;
#24380=CARTESIAN_POINT ( 'NONE',  ( 6.204703633549690345, 12.84541550158063572, 14.16423886937410082 ) ) ;
#24381=CARTESIAN_POINT ( 'NONE',  ( 15.44008868035555793, 41.39701867748817676, -9.422509992056140149 ) ) ;
#24382=CARTESIAN_POINT ( 'NONE',  ( -0.8801773607110991993, 12.85535201082150358, -2.915334737309923874 ) ) ;
#24383=CARTESIAN_POINT ( 'NONE',  ( 10.00000000000000178, 39.31368534415484106, 10.88017736071110342 ) ) ;
#24384=EDGE_CURVE ( 'NONE', #11511, #83368, #84978, .T. ) ;
#24385=CARTESIAN_POINT ( 'NONE',  ( 0.5774900079438607392, 28.48035201082150891, 5.440088680355550821 ) ) ;
#24386=ORIENTED_EDGE ( 'NONE', *, *, #41465, .T. ) ;
#24387=CARTESIAN_POINT ( 'NONE',  ( -1.099225684535947600, 33.70696800326375353, -6.408140936763238038 ) ) ;
#24388=CARTESIAN_POINT ( 'NONE',  ( 0.5774900079438607392, 43.48035201082151247, 5.440088680355550821 ) ) ;
#24391=CARTESIAN_POINT ( 'NONE',  ( 13.43411237798106583, 62.66530133659708923, -12.81628187352647252 ) ) ;
#24392=CARTESIAN_POINT ( 'NONE',  ( 20.88017736071110875, 55.77201867748816966, -2.915334737309920765 ) ) ;
#24393=VECTOR ( 'NONE', #5624, 1000.000000000000000 ) ;
#24395=CARTESIAN_POINT ( 'NONE',  ( 10.00000000000000000, 46.81368534415484106, -10.88017736071110342 ) ) ;
#24396=CARTESIAN_POINT ( 'NONE',  ( 7.084665262690076126, 7.022018677488169658, -10.88017736071110164 ) ) ;
#24397=CARTESIAN_POINT ( 'NONE',  ( 18.52753015748617571, 8.092264484334117824, 4.923371831947298993 ) ) ;
#24398=CARTESIAN_POINT ( 'NONE',  ( -0.3289641300568005855, 24.27164270246084143, -5.963430220938281678 ) ) ;
#24399=CARTESIAN_POINT ( 'NONE',  ( 22.26659068614894466, 53.88708216824731068, 7.082119434687054849 ) ) ;
#24400=CARTESIAN_POINT ( 'NONE',  ( 7.084665262690076126, 67.02201867748817676, -10.88017736071110164 ) ) ;
#24401=CARTESIAN_POINT ( 'NONE',  ( 22.26659068614894466, 3.887082168247300906, 7.082119434687054849 ) ) ;
#24403=AXIS2_PLACEMENT_3D ( 'NONE', #25916, #64866, #94893 ) ;
#24404=CARTESIAN_POINT ( 'NONE',  ( 17.96484262340118221, 14.93868534415483751, 7.964842623401181321 ) ) ;
#24405=CARTESIAN_POINT ( 'NONE',  ( 12.63842701281683034, 52.46726448433413026, 9.846743663894596210 ) ) ;
#24406=B_SPLINE_CURVE_WITH_KNOTS ( 'NONE', 3,
 ( #16080, #32041, #71058, #84088, #78548, #2582 ),
 .UNSPECIFIED., .F., .F.,
 ( 4, 2, 4 ),
 ( 5.553824967135426632E-18, 0.0002605067024380933443, 0.0005210134048761811592 ),
 .UNSPECIFIED. ) ;
#24408=( GEOMETRIC_REPRESENTATION_CONTEXT ( 3 ) GLOBAL_UNCERTAINTY_ASSIGNED_CONTEXT ( ( #87505 ) ) GLOBAL_UNIT_ASSIGNED_CONTEXT ( ( #40885, #24413, #85391 ) ) REPRESENTATION_CONTEXT ( 'NONE', 'WORKASPACE' ) );
#24409=CARTESIAN_POINT ( 'NONE',  ( 2.791683348922240793, 41.63393115100078745, 7.208316651077764092 ) ) ;
#24411=CARTESIAN_POINT ( 'NONE',  ( 0.5774900079438590739, 37.64701867748817676, -5.440088680355550821 ) ) ;
#24412=CARTESIAN_POINT ( 'NONE',  ( 2.791683348922237240, 35.38393115100079456, -7.208316651077763204 ) ) ;
#24413=( NAMED_UNIT ( * ) PLANE_ANGLE_UNIT ( ) SI_UNIT ( $, .RADIAN. ) );
#24415=CARTESIAN_POINT ( 'NONE',  ( 20.88017736071110519, 40.56368534415484106, 2.639326808657452039E-16 ) ) ;
#24416=CARTESIAN_POINT ( 'NONE',  ( 10.00000000000000000, 60.55374883491397497, -14.16423886937410082 ) ) ;
#24418=CARTESIAN_POINT ( 'NONE',  ( 21.09922568453594849, 21.20696800326375353, 6.408140936763242479 ) ) ;
#24421=CARTESIAN_POINT ( 'NONE',  ( -2.816281873526473856, 24.12363466993042138, 9.499525473075851096E-16 ) ) ;
#24422=CARTESIAN_POINT ( 'NONE',  ( 7.084665262690076126, 17.02201867748817676, -10.88017736071110164 ) ) ;
#24425=AXIS2_PLACEMENT_3D ( 'NONE', #94423, #31939, #92943 ) ;
#24426=CARTESIAN_POINT ( 'NONE',  ( 18.52753015748617571, 3.092264484334118269, 4.923371831947298993 ) ) ;
#24427=CARTESIAN_POINT ( 'NONE',  ( 18.52753015748617571, 53.09226448433412315, 4.923371831947298993 ) ) ;
#24428=CARTESIAN_POINT ( 'NONE',  ( 19.84674366389459266, 8.717264484334116048, -2.638427012816827677 ) ) ;
#24429=CARTESIAN_POINT ( 'NONE',  ( 10.00000000000000000, 34.75893115100078745, -9.846743663894594434 ) ) ;
#24431=CARTESIAN_POINT ( 'NONE',  ( 19.72487221294571569, 14.78217586085237656, 6.499999999999995559 ) ) ;
#24432=CARTESIAN_POINT ( 'NONE',  ( 0.1532563361054083140, 26.00893115100078745, 1.131784320476157264E-15 ) ) ;
#24435=CARTESIAN_POINT ( 'NONE',  ( 1.472469842513823179, 16.42559781766745175, 4.923371831947296329 ) ) ;
#24436=CARTESIAN_POINT ( 'NONE',  ( 0.1532563361054083140, 46.00893115100079456, 1.131784320476157264E-15 ) ) ;
#24439=CARTESIAN_POINT ( 'NONE',  ( 20.24186590665278018, 17.61633188102327097, -6.114288769123028544 ) ) ;
#24440=CARTESIAN_POINT ( 'NONE',  ( 13.43411237798105340, 30.58196800326374998, 12.81628187352647963 ) ) ;
#24441=CARTESIAN_POINT ( 'NONE',  ( 0.2751277870542981341, 8.218334437839383000, 6.500000000000002665 ) ) ;
#24442=CARTESIAN_POINT ( 'NONE',  ( 24.16423886937410614, 39.51208216824731068, -3.795296366450302550 ) ) ;
#24443=CARTESIAN_POINT ( 'NONE',  ( 17.20831665107776587, 2.883931151000785231, 7.208316651077764980 ) ) ;
#24445=CARTESIAN_POINT ( 'NONE',  ( 20.36894250292379382, 48.67874883491396076, 10.36894250292379205 ) ) ;
#24447=CARTESIAN_POINT ( 'NONE',  ( -0.3689425029237881626, 62.42874883491396787, 10.36894250292379027 ) ) ;
#24448=CARTESIAN_POINT ( 'NONE',  ( 17.08211943468705130, 18.47041550158063572, 12.26659068614894998 ) ) ;
#24449=CARTESIAN_POINT ( 'NONE',  ( -4.164238869374099927, 32.01208216824730357, 3.795296366450308767 ) ) ;
#24450=DIRECTION ( 'NONE',  ( 0.000000000000000000, 0.000000000000000000, -1.000000000000000000 ) ) ;
#24453=CARTESIAN_POINT ( 'NONE',  ( 10.00000000000000178, 47.25893115100078745, 9.846743663894594434 ) ) ;
#24455=CARTESIAN_POINT ( 'NONE',  ( 7.084665262690076126, 42.02201867748816966, -10.88017736071110164 ) ) ;
#24456=CARTESIAN_POINT ( 'NONE',  ( 19.72487221294571214, 22.80223176428831877, -6.499999999999988454 ) ) ;
#24458=CARTESIAN_POINT ( 'NONE',  ( 10.00000000000000000, 39.75893115100078745, -9.846743663894594434 ) ) ;
#24459=CARTESIAN_POINT ( 'NONE',  ( 21.09922568453594849, 56.20696800326375353, 6.408140936763242479 ) ) ;
#24462=CARTESIAN_POINT ( 'NONE',  ( 0.1532563361054083140, 41.00893115100078745, 1.131784320476157264E-15 ) ) ;
#24463=CARTESIAN_POINT ( 'NONE',  ( 18.52753015748618282, 63.92559781766745886, -4.923371831947291888 ) ) ;
#24465=CARTESIAN_POINT ( 'NONE',  ( 10.00000000000000178, 18.05374883491396787, 14.16423886937410082 ) ) ;
#24469=CARTESIAN_POINT ( 'NONE',  ( 20.88017736071110519, 5.563685344154838397, 2.639326808657452039E-16 ) ) ;
#24471=CARTESIAN_POINT ( 'NONE',  ( -1.099225684535947600, 13.70696800326375353, -6.408140936763238038 ) ) ;
#24474=CARTESIAN_POINT ( 'NONE',  ( 10.00000000000000178, 64.31368534415483396, 10.88017736071110342 ) ) ;
#24477=CARTESIAN_POINT ( 'NONE',  ( -46.94000000000001194, 101.2919103424992358, -7.700697297268528807 ) ) ;
#24479=CARTESIAN_POINT ( 'NONE',  ( 6.204703633549690345, 57.84541550158063927, 14.16423886937410082 ) ) ;
#24480=CARTESIAN_POINT ( 'NONE',  ( 0.1916775849787236141, 42.25868815902070708, -6.499999999999983125 ) ) ;
#24481=CARTESIAN_POINT ( 'NONE',  ( -0.8801773607111008646, 23.27201867748817676, 2.915334737309923430 ) ) ;
#24482=CARTESIAN_POINT ( 'NONE',  ( 4.559911319644449179, 23.89701867748817321, 9.422509992056141925 ) ) ;
#24483=CARTESIAN_POINT ( 'NONE',  ( 21.09922568453594849, 6.206968003263753531, 6.408140936763242479 ) ) ;
#24484=CARTESIAN_POINT ( 'NONE',  ( 1.472469842513823179, 56.42559781766745886, 4.923371831947296329 ) ) ;
#24485=CARTESIAN_POINT ( 'NONE',  ( 22.81628187352647785, 61.41530133659709634, 3.434112377981063169 ) ) ;
#24486=CARTESIAN_POINT ( 'NONE',  ( 10.00000000000000178, 2.258931151000784787, 9.846743663894594434 ) ) ;
#24488=CARTESIAN_POINT ( 'NONE',  ( 4.559911319644449179, 23.89701867748817321, 9.422509992056141925 ) ) ;
#24489=CARTESIAN_POINT ( 'NONE',  ( -2.816281873526473856, 29.12363466993041783, 9.499525473075851096E-16 ) ) ;
#24490=DIRECTION ( 'NONE',  ( -0.000000000000000000, -0.000000000000000000, 1.000000000000000000 ) ) ;
#24491=CARTESIAN_POINT ( 'NONE',  ( 5.076628168052704559, 55.17559781766745175, -8.527530157486179263 ) ) ;
#24492=CARTESIAN_POINT ( 'NONE',  ( -0.8801773607110991993, 52.85535201082151247, -2.915334737309923874 ) ) ;
#24493=CARTESIAN_POINT ( 'NONE',  ( 14.92337183194729988, 14.34226448433411782, -8.527530157486177487 ) ) ;
#24494=CARTESIAN_POINT ( 'NONE',  ( 3.591859063236761518, 29.95696800326375708, 11.09922568453594849 ) ) ;
#24495=CARTESIAN_POINT ( 'NONE',  ( 20.88017736071110875, 65.77201867748817676, -2.915334737309920765 ) ) ;
#24498=CARTESIAN_POINT ( 'NONE',  ( 19.38216949554541202, 60.99863466993042493, 9.382169495545424454 ) ) ;
#24499=EDGE_LOOP ( 'NONE', ( #14390, #8463, #70262, #22571 ) ) ;
#24502=CARTESIAN_POINT ( 'NONE',  ( -0.8801773607111009756, 3.063685344154837509, 1.068504757029289695E-15 ) ) ;
#24503=CARTESIAN_POINT ( 'NONE',  ( 16.40814093676323893, 50.79030133659708923, 11.09922568453595026 ) ) ;
#24504=CARTESIAN_POINT ( 'NONE',  ( -4.164238869374099039, 11.80374883491396965, 8.674139862899312516E-16 ) ) ;
#24505=CARTESIAN_POINT ( 'NONE',  ( 14.92337183194729633, 12.67559781766745353, 8.527530157486181039 ) ) ;
#24506=CARTESIAN_POINT ( 'NONE',  ( 15.44008868035555793, 11.39701867748817143, -9.422509992056140149 ) ) ;
#24507=CARTESIAN_POINT ( 'NONE',  ( 0.1532563361054083140, 26.00893115100078745, 1.131784320476157264E-15 ) ) ;
#24509=CARTESIAN_POINT ( 'NONE',  ( 6.204703633549690345, 62.84541550158063927, 14.16423886937410082 ) ) ;
#24510=ORIENTED_EDGE ( 'NONE', *, *, #45945, .F. ) ;
#24512=( NAMED_UNIT ( * ) PLANE_ANGLE_UNIT ( ) SI_UNIT ( $, .RADIAN. ) );
#24515=CARTESIAN_POINT ( 'NONE',  ( 10.00000000000000000, 1.813685344154837731, -10.88017736071110342 ) ) ;
#24520=CARTESIAN_POINT ( 'NONE',  ( 7.084665262690076126, 12.02201867748817321, -10.88017736071110164 ) ) ;
#24521=CARTESIAN_POINT ( 'NONE',  ( 17.96484262340118221, 9.938685344154839285, 7.964842623401181321 ) ) ;
#24522=CARTESIAN_POINT ( 'NONE',  ( 1.472469842513823179, 41.42559781766745886, 4.923371831947296329 ) ) ;
#24523=CARTESIAN_POINT ( 'NONE',  ( -2.816281873526471635, 53.91530133659709634, -3.434112377981056508 ) ) ;
#24525=FACE_OUTER_BOUND ( 'NONE', #41264, .T. ) ;
#24526=CARTESIAN_POINT ( 'NONE',  ( 6.204703633549690345, 22.84541550158062861, 14.16423886937410082 ) ) ;
#24527=CARTESIAN_POINT ( 'NONE',  ( 17.96484262340118221, 19.93868534415484106, 7.964842623401181321 ) ) ;
#24528=CARTESIAN_POINT ( 'NONE',  ( 7.084665262690076126, 9.105352010821503583, 10.88017736071109987 ) ) ;
#24529=CARTESIAN_POINT ( 'NONE',  ( 0.1532563361054100626, 60.80059781766744464, -2.638427012816831230 ) ) ;
#24530=DIRECTION ( 'NONE',  ( 0.000000000000000000, 0.000000000000000000, 1.000000000000000000 ) ) ;
#24531=CARTESIAN_POINT ( 'NONE',  ( 10.00000000000000178, 32.25893115100078745, 9.846743663894594434 ) ) ;
#24532=CARTESIAN_POINT ( 'NONE',  ( -45.94000000000000483, 92.00000000000000000, 5.000000000000000000 ) ) ;
#24537=CARTESIAN_POINT ( 'NONE',  ( -0.8801773607111008646, 68.27201867748817676, 2.915334737309923430 ) ) ;
#24538=CARTESIAN_POINT ( 'NONE',  ( 0.1532563361054100626, 55.80059781766745175, -2.638427012816831230 ) ) ;
#24539=CARTESIAN_POINT ( 'NONE',  ( 7.084665262690076126, 42.02201867748816966, -10.88017736071110164 ) ) ;
#24540=CARTESIAN_POINT ( 'NONE',  ( 4.559911319644449179, 3.897018677488170990, 9.422509992056141925 ) ) ;
#24541=CARTESIAN_POINT ( 'NONE',  ( -1.099225684535947600, 43.70696800326375353, -6.408140936763238038 ) ) ;
#24542=CARTESIAN_POINT ( 'NONE',  ( 24.16423886937410614, 24.51208216824730002, -3.795296366450302550 ) ) ;
#24543=B_SPLINE_CURVE_WITH_KNOTS ( 'NONE', 3,
 ( #51246, #97269, #34756, #80763 ),
 .UNSPECIFIED., .F., .F.,
 ( 4, 4 ),
 ( 0.000000000000000000, 0.0006109242138661622953 ),
 .UNSPECIFIED. ) ;
#24546=CARTESIAN_POINT ( 'NONE',  ( 21.09922568453594849, 51.20696800326375353, 6.408140936763242479 ) ) ;
#24549=CARTESIAN_POINT ( 'NONE',  ( 2.791683348922237240, 60.38393115100078745, -7.208316651077763204 ) ) ;
#24551=CARTESIAN_POINT ( 'NONE',  ( 17.96484262340118221, 21.18868534415483396, -7.964842623401177768 ) ) ;
#24552=MECHANICAL_DESIGN_GEOMETRIC_PRESENTATION_REPRESENTATION('',(#26108),#35720);
#24553=CARTESIAN_POINT ( 'NONE',  ( -0.8801773607110991993, 32.85535201082151247, -2.915334737309923874 ) ) ;
#24555=CARTESIAN_POINT ( 'NONE',  ( 4.559911319644449179, 63.89701867748817676, 9.422509992056141925 ) ) ;
#24556=CARTESIAN_POINT ( 'NONE',  ( -46.07478503777810630, 103.8690650836416722, 6.036883934524849948 ) ) ;
#24557=CARTESIAN_POINT ( 'NONE',  ( 0.1532563361054100626, 10.80059781766745175, -2.638427012816831230 ) ) ;
#24558=CARTESIAN_POINT ( 'NONE',  ( 19.42250999205614548, 60.98035201082151247, -5.440088680355545492 ) ) ;
#24560=CARTESIAN_POINT ( 'NONE',  ( 17.96484262340118221, 59.93868534415484106, 7.964842623401181321 ) ) ;
#24561=CARTESIAN_POINT ( 'NONE',  ( 0.1532563361054082862, 1.217264484334117824, 2.638427012816831674 ) ) ;
#24563=CARTESIAN_POINT ( 'NONE',  ( 7.361572987183169658, 44.96726448433412315, -9.846743663894592657 ) ) ;
#24565=ORIENTED_EDGE ( 'NONE', *, *, #71911, .T. ) ;
#24567=CARTESIAN_POINT ( 'NONE',  ( 10.00000000000000178, 3.053748834913967425, 14.16423886937410082 ) ) ;
#24568=( BOUNDED_CURVE ( )  B_SPLINE_CURVE ( 2, ( #59330, #11379, #19859, #35355, #51349, #72855, #43832, #96874, #80373 ),
 .UNSPECIFIED., .F., .F. ) 
 B_SPLINE_CURVE_WITH_KNOTS ( ( 3, 2, 2, 2, 3 ),
 ( 0.4025141644748393976, 0.4047619047619047672, 0.4107142857142856984, 0.4166666666666666852, 0.4189144069537312220 ),
 .UNSPECIFIED. ) 
 CURVE ( )  GEOMETRIC_REPRESENTATION_ITEM ( )  RATIONAL_B_SPLINE_CURVE ( ( 0.9839835555609424134, 0.9871328979762477029, 1.000000000000000000, 0.9659258262890683122, 1.000000000000000000, 0.9659258262890683122, 1.000000000000000000, 0.9871328979762525879, 0.9839835555609448559 ) ) 
 REPRESENTATION_ITEM ( '' )  );
#24569=CARTESIAN_POINT ( 'NONE',  ( 0.6178305044545818747, 63.49863466993043204, -9.382169495545419124 ) ) ;
#24570=CARTESIAN_POINT ( 'NONE',  ( -4.164238869374099039, 6.803748834913967869, 8.674139862899312516E-16 ) ) ;
#24571=CARTESIAN_POINT ( 'NONE',  ( -0.3689425029237898834, 21.17874883491396432, -10.36894250292378850 ) ) ;
#24574=CARTESIAN_POINT ( 'NONE',  ( 7.084665262690076126, 57.02201867748817676, -10.88017736071110164 ) ) ;
#24575=CARTESIAN_POINT ( 'NONE',  ( 17.96484262340118221, 19.93868534415484106, 7.964842623401181321 ) ) ;
#24578=SURFACE_STYLE_FILL_AREA ( #76076 ) ;
#24579=CARTESIAN_POINT ( 'NONE',  ( 16.40814093676323893, 25.79030133659708923, 11.09922568453595026 ) ) ;
#24580=CARTESIAN_POINT ( 'NONE',  ( 19.84674366389459621, 33.50893115100078745, 7.409399052514197653E-17 ) ) ;
#24581=EDGE_CURVE ( 'NONE', #24283, #76727, #65906, .T. ) ;
#24582=CARTESIAN_POINT ( 'NONE',  ( 22.81628187352647785, 21.62363466993041783, 6.195893100308588602E-16 ) ) ;
#24584=CARTESIAN_POINT ( 'NONE',  ( 7.361572987183169658, 19.96726448433411960, -9.846743663894592657 ) ) ;
#24585=CARTESIAN_POINT ( 'NONE',  ( 7.361572987183170547, 12.05059781766744997, 9.846743663894590881 ) ) ;
#24587=CARTESIAN_POINT ( 'NONE',  ( -0.8801773607110991993, 37.85535201082151247, -2.915334737309923874 ) ) ;
#24588=CARTESIAN_POINT ( 'NONE',  ( 17.08211943468705130, 28.47041550158063572, 12.26659068614894998 ) ) ;
#24589=CARTESIAN_POINT ( 'NONE',  ( 10.00000000000000178, 37.25893115100078745, 9.846743663894594434 ) ) ;
#24590=CARTESIAN_POINT ( 'NONE',  ( -0.8801773607111008646, 63.27201867748817676, 2.915334737309923430 ) ) ;
#24591=CARTESIAN_POINT ( 'NONE',  ( 22.81628187352647785, 51.62363466993042493, 6.195893100308588602E-16 ) ) ;
#24593=CARTESIAN_POINT ( 'NONE',  ( -0.8801773607110991993, 32.85535201082151247, -2.915334737309923874 ) ) ;
#24594=CARTESIAN_POINT ( 'NONE',  ( 19.38216949554541557, 22.24863466993041428, -9.382169495545420901 ) ) ;
#24595=CARTESIAN_POINT ( 'NONE',  ( 19.84674366389459621, 43.50893115100078745, 7.409399052514197653E-17 ) ) ;
#24597=CARTESIAN_POINT ( 'NONE',  ( 3.591859063236763294, 43.29030133659708923, -11.09922568453595026 ) ) ;
#24599=CARTESIAN_POINT ( 'NONE',  ( 20.88017736071110519, 50.56368534415484106, 2.639326808657452039E-16 ) ) ;
#24603=CARTESIAN_POINT ( 'NONE',  ( 2.035157376598822676, 47.43868534415484817, -7.964842623401177768 ) ) ;
#24604=CARTESIAN_POINT ( 'NONE',  ( 15.44008868035555793, 61.39701867748817676, -9.422509992056140149 ) ) ;
#24605=DIRECTION ( 'NONE',  ( 0.000000000000000000, 1.000000000000000000, -0.000000000000000000 ) ) ;
#24607=CARTESIAN_POINT ( 'NONE',  ( 2.035157376598822676, 12.43868534415483751, -7.964842623401177768 ) ) ;
#24608=CARTESIAN_POINT ( 'NONE',  ( 0.1532563361054082862, 46.21726448433411605, 2.638427012816831674 ) ) ;
#24609=CARTESIAN_POINT ( 'NONE',  ( 0.5774900079438607392, 23.48035201082150536, 5.440088680355550821 ) ) ;
#24611=CARTESIAN_POINT ( 'NONE',  ( 16.40814093676324603, 22.45696800326375353, -11.09922568453594671 ) ) ;
#24613=CARTESIAN_POINT ( 'NONE',  ( 15.44008868035555260, 34.73035201082151247, 9.422509992056143702 ) ) ;
#24615=CARTESIAN_POINT ( 'NONE',  ( 22.81628187352648496, 6.831968003263753531, -3.434112377981050290 ) ) ;
#24616=CARTESIAN_POINT ( 'NONE',  ( 20.03447792253739834, 47.65514106990689669, -6.401564815979719825 ) ) ;
#24617=CARTESIAN_POINT ( 'NONE',  ( 7.084665262690076126, 14.10535201082150358, 10.88017736071109987 ) ) ;
#24618=CARTESIAN_POINT ( 'NONE',  ( 15.44008868035555793, 36.39701867748816966, -9.422509992056140149 ) ) ;
#24619=CARTESIAN_POINT ( 'NONE',  ( 17.08211943468705840, 45.13708216824730357, -12.26659068614894466 ) ) ;
#24620=CARTESIAN_POINT ( 'NONE',  ( 0.1532563361054083140, 36.00893115100078745, 1.131784320476157264E-15 ) ) ;
#24621=CARTESIAN_POINT ( 'NONE',  ( 17.96484262340118221, 56.18868534415484817, -7.964842623401177768 ) ) ;
#24622=CARTESIAN_POINT ( 'NONE',  ( 19.72487221294570858, 70.00000000000000000, -6.000000000000000000 ) ) ;
#24623=CARTESIAN_POINT ( 'NONE',  ( 24.16423886937410614, 19.30374883491397142, 8.672049930838204340E-16 ) ) ;
#24626=CARTESIAN_POINT ( 'NONE',  ( 2.153642693323440493, 21.13791097397318453, -6.500000000000008882 ) ) ;
#24628=CARTESIAN_POINT ( 'NONE',  ( -4.164238869374099039, 31.80374883491396432, 8.674139862899312516E-16 ) ) ;
#24629=CARTESIAN_POINT ( 'NONE',  ( 2.917880565312950480, 35.97041550158063217, -12.26659068614894821 ) ) ;
#24630=CARTESIAN_POINT ( 'NONE',  ( 14.92337183194729633, 7.675597817667451750, 8.527530157486181039 ) ) ;
#24631=CARTESIAN_POINT ( 'NONE',  ( 14.92337183194729633, 57.67559781766745886, 8.527530157486181039 ) ) ;
#24633=CARTESIAN_POINT ( 'NONE',  ( 2.035157376598822676, 62.43868534415483396, -7.964842623401177768 ) ) ;
#24634=CARTESIAN_POINT ( 'NONE',  ( -1.099225684535947600, 33.70696800326375353, -6.408140936763238038 ) ) ;
#24635=CARTESIAN_POINT ( 'NONE',  ( 2.917880565312948704, 27.63708216824730357, 12.26659068614894643 ) ) ;
#24636=CARTESIAN_POINT ( 'NONE',  ( 17.96484262340118221, 21.18868534415483396, -7.964842623401177768 ) ) ;
#24638=CARTESIAN_POINT ( 'NONE',  ( 0.1532563361054083140, 1.008931151000784787, 1.131784320476157264E-15 ) ) ;
#24644=CARTESIAN_POINT ( 'NONE',  ( 20.36894250292379382, 3.678748834913967869, 10.36894250292379205 ) ) ;
#24645=CARTESIAN_POINT ( 'NONE',  ( -0.8801773607111009756, 8.063685344154837509, 1.068504757029289695E-15 ) ) ;
#24646=CARTESIAN_POINT ( 'NONE',  ( -0.8801773607110991993, 17.85535201082150536, -2.915334737309923874 ) ) ;
#24647=CARTESIAN_POINT ( 'NONE',  ( 7.361572987183170547, 42.05059781766745886, 9.846743663894590881 ) ) ;
#24648=CARTESIAN_POINT ( 'NONE',  ( 7.361572987183169658, 59.96726448433410894, -9.846743663894592657 ) ) ;
#24652=CARTESIAN_POINT ( 'NONE',  ( 16.40814093676324603, 7.456968003263754419, -11.09922568453594671 ) ) ;
#24654=CARTESIAN_POINT ( 'NONE',  ( 22.26659068614895176, 49.72041550158063927, -7.082119434687042414 ) ) ;
#24657=CARTESIAN_POINT ( 'NONE',  ( 13.79529636645031943, 50.34541550158064638, -14.16423886937409904 ) ) ;
#24658=ORIENTED_EDGE ( 'NONE', *, *, #70514, .T. ) ;
#24659=CARTESIAN_POINT ( 'NONE',  ( 20.88017736071110519, 20.56368534415484106, 2.639326808657452039E-16 ) ) ;
#24660=CARTESIAN_POINT ( 'NONE',  ( 10.00000000000000178, 65.37363466993042493, 12.81628187352647608 ) ) ;
#24661=CARTESIAN_POINT ( 'NONE',  ( 12.91533473730993009, 31.60535201082150891, -10.88017736071109987 ) ) ;
#24662=CARTESIAN_POINT ( 'NONE',  ( 2.791683348922237240, 55.38393115100078745, -7.208316651077763204 ) ) ;
#24663=CARTESIAN_POINT ( 'NONE',  ( 2.035157376598822676, 37.43868534415484106, -7.964842623401177768 ) ) ;
#24664=CARTESIAN_POINT ( 'NONE',  ( 17.96484262340118221, 64.93868534415483396, 7.964842623401181321 ) ) ;
#24665=CARTESIAN_POINT ( 'NONE',  ( 4.559911319644449179, 32.23035201082150536, -9.422509992056141925 ) ) ;
#24666=CARTESIAN_POINT ( 'NONE',  ( -0.03932841506543420518, 33.12161441960502373, 6.397827110478944590 ) ) ;
#24669=CARTESIAN_POINT ( 'NONE',  ( 2.791683348922240793, 6.633931151000785675, 7.208316651077764092 ) ) ;
#24672=CARTESIAN_POINT ( 'NONE',  ( 12.63842701281683922, 39.55059781766744464, -9.846743663894590881 ) ) ;
#24673=CARTESIAN_POINT ( 'NONE',  ( 21.09922568453594849, 46.20696800326376064, 6.408140936763242479 ) ) ;
#24678=CARTESIAN_POINT ( 'NONE',  ( 1.472469842513823179, 66.42559781766745175, 4.923371831947296329 ) ) ;
#24679=CARTESIAN_POINT ( 'NONE',  ( 0.5774900079438590739, 52.64701867748817676, -5.440088680355550821 ) ) ;
#24680=CARTESIAN_POINT ( 'NONE',  ( 19.84674366389459266, 48.30059781766745175, 2.638427012816836559 ) ) ;
#24681=CARTESIAN_POINT ( 'NONE',  ( -0.3689425029237881626, 47.42874883491396787, 10.36894250292379027 ) ) ;
#24682=CARTESIAN_POINT ( 'NONE',  ( 0.1532563361054100626, 60.80059781766744464, -2.638427012816831230 ) ) ;
#24685=CARTESIAN_POINT ( 'NONE',  ( 5.076628168052703671, 16.84226448433411960, 8.527530157486179263 ) ) ;
#24686=CARTESIAN_POINT ( 'NONE',  ( 10.00000000000000000, 57.87363466993042493, -12.81628187352647608 ) ) ;
#24687=CARTESIAN_POINT ( 'NONE',  ( 19.84674366389459266, 58.71726448433411605, -2.638427012816827677 ) ) ;
#24688=CARTESIAN_POINT ( 'NONE',  ( 20.88017736071110164, 50.35535201082151247, 2.915334737309930979 ) ) ;
#24690=CARTESIAN_POINT ( 'NONE',  ( 20.24186590665275531, 15.59014588040357374, -6.114288769123077394 ) ) ;
#24692=CARTESIAN_POINT ( 'NONE',  ( -2.266590686148945544, 67.22041550158063217, 7.082119434687048631 ) ) ;
#24694=CARTESIAN_POINT ( 'NONE',  ( 0.5774900079438607392, 33.48035201082150536, 5.440088680355550821 ) ) ;
#24695=CARTESIAN_POINT ( 'NONE',  ( 19.38216949554541202, 15.99863466993042138, 9.382169495545424454 ) ) ;
#24696=CARTESIAN_POINT ( 'NONE',  ( 4.559911319644449179, 63.89701867748817676, 9.422509992056141925 ) ) ;
#24697=CARTESIAN_POINT ( 'NONE',  ( 19.42250999205614548, 65.98035201082151957, -5.440088680355545492 ) ) ;
#24701=CARTESIAN_POINT ( 'NONE',  ( 20.88017736071110519, 55.56368534415484817, 2.639326808657452039E-16 ) ) ;
#24703=CARTESIAN_POINT ( 'NONE',  ( 10.00000000000000000, 39.75893115100078745, -9.846743663894594434 ) ) ;
#24704=CARTESIAN_POINT ( 'NONE',  ( 0.1532563361054083140, 6.008931151000784787, 1.131784320476157264E-15 ) ) ;
#24706=CARTESIAN_POINT ( 'NONE',  ( 19.38216949554541557, 7.248634669930421381, -9.382169495545420901 ) ) ;
#24707=CARTESIAN_POINT ( 'NONE',  ( 10.00000000000000178, 14.31368534415483929, 10.88017736071110342 ) ) ;
#24710=CARTESIAN_POINT ( 'NONE',  ( -0.3689425029237881626, 32.42874883491395366, 10.36894250292379027 ) ) ;
#24711=CARTESIAN_POINT ( 'NONE',  ( 10.00000000000000178, 33.05374883491396787, 14.16423886937410082 ) ) ;
#24712=CARTESIAN_POINT ( 'NONE',  ( -0.8801773607110991993, 2.855352010821504471, -2.915334737309923874 ) ) ;
#24713=CARTESIAN_POINT ( 'NONE',  ( 17.20831665107776587, 29.13393115100078390, -7.208316651077762316 ) ) ;
#24714=CARTESIAN_POINT ( 'NONE',  ( 19.84674366389459266, 13.71726448433411782, -2.638427012816827677 ) ) ;
#24715=CARTESIAN_POINT ( 'NONE',  ( 10.00000000000000178, 9.313685344154839285, 10.88017736071110342 ) ) ;
#24717=CARTESIAN_POINT ( 'NONE',  ( 0.1532563361054100626, 35.80059781766745175, -2.638427012816831230 ) ) ;
#24718=CARTESIAN_POINT ( 'NONE',  ( 19.42250999205614548, 45.98035201082150536, -5.440088680355545492 ) ) ;
#24719=CARTESIAN_POINT ( 'NONE',  ( 1.472469842513823179, 56.42559781766745886, 4.923371831947296329 ) ) ;
#24720=CARTESIAN_POINT ( 'NONE',  ( 24.16423886937410614, 24.51208216824730002, -3.795296366450302550 ) ) ;
#24721=CARTESIAN_POINT ( 'NONE',  ( 2.603489959281614308, 61.58210964143329846, 6.500000000000031086 ) ) ;
#24723=CARTESIAN_POINT ( 'NONE',  ( 17.20831665107776587, 14.13393115100078568, -7.208316651077762316 ) ) ;
#24724=CARTESIAN_POINT ( 'NONE',  ( 16.40814093676323893, 50.79030133659708923, 11.09922568453595026 ) ) ;
#24725=CARTESIAN_POINT ( 'NONE',  ( 19.84674366389459266, 58.71726448433411605, -2.638427012816827677 ) ) ;
#24727=CARTESIAN_POINT ( 'NONE',  ( -0.8801773607110991993, 2.855352010821504471, -2.915334737309923874 ) ) ;
#24728=CARTESIAN_POINT ( 'NONE',  ( 6.204703633549690345, 15.76208216824730179, -14.16423886937410259 ) ) ;
#24729=CARTESIAN_POINT ( 'NONE',  ( 0.5774900079438590739, 62.64701867748817676, -5.440088680355550821 ) ) ;
#24730=CARTESIAN_POINT ( 'NONE',  ( 18.52753015748617571, 43.09226448433412315, 4.923371831947298993 ) ) ;
#24731=CARTESIAN_POINT ( 'NONE',  ( 10.00000000000000000, 16.81368534415483751, -10.88017736071110342 ) ) ;
#24733=CARTESIAN_POINT ( 'NONE',  ( 2.791683348922237240, 60.38393115100078745, -7.208316651077763204 ) ) ;
#24735=CARTESIAN_POINT ( 'NONE',  ( 1.472469842513823179, 0.5922644843341181575, -4.923371831947296329 ) ) ;
#24736=CARTESIAN_POINT ( 'NONE',  ( 22.81628187352647785, 56.62363466993042493, 6.195893100308588602E-16 ) ) ;
#24740=CARTESIAN_POINT ( 'NONE',  ( 19.72487221294570858, 41.86607318730076344, 6.500000000000000888 ) ) ;
#24742=CARTESIAN_POINT ( 'NONE',  ( 17.08211943468705130, 48.47041550158063927, 12.26659068614894998 ) ) ;
#24743=CARTESIAN_POINT ( 'NONE',  ( 7.361572987183169658, 49.96726448433410894, -9.846743663894592657 ) ) ;
#24744=CARTESIAN_POINT ( 'NONE',  ( 12.63842701281683922, 24.55059781766745175, -9.846743663894590881 ) ) ;
#24746=CARTESIAN_POINT ( 'NONE',  ( 12.91533473730992121, 19.52201867748816611, 10.88017736071110164 ) ) ;
#24747=CARTESIAN_POINT ( 'NONE',  ( 19.84674366389459621, 48.50893115100078745, 7.409399052514197653E-17 ) ) ;
#24749=ADVANCED_FACE ( 'NONE', ( #45693 ), #52696, .T. ) ;
#24750=CARTESIAN_POINT ( 'NONE',  ( 17.08211943468705130, 43.47041550158063927, 12.26659068614894998 ) ) ;
#24752=CARTESIAN_POINT ( 'NONE',  ( -2.266590686148945544, 57.22041550158063217, 7.082119434687048631 ) ) ;
#24755=CARTESIAN_POINT ( 'NONE',  ( 2.035157376598822676, 67.43868534415484817, -7.964842623401177768 ) ) ;
#24756=CARTESIAN_POINT ( 'NONE',  ( 10.00000000000000178, 22.25893115100078745, 9.846743663894594434 ) ) ;
#24759=CARTESIAN_POINT ( 'NONE',  ( 1.274849032794164172, 18.57228050351029935, 6.499999999999802824 ) ) ;
#24760=( BOUNDED_CURVE ( )  B_SPLINE_CURVE ( 2, ( #29952, #68470, #58318, #53444, #10421, #25915, #71894, #56417, #48896 ),
 .UNSPECIFIED., .F., .F. ) 
 B_SPLINE_CURVE_WITH_KNOTS ( ( 3, 2, 2, 2, 3 ),
 ( 0.4739427359034107945, 0.4761904761904761640, 0.4821428571428571508, 0.4880952380952380820, 0.4903429783823025079 ),
 .UNSPECIFIED. ) 
 CURVE ( )  GEOMETRIC_REPRESENTATION_ITEM ( )  RATIONAL_B_SPLINE_CURVE ( ( 0.9839835555609424134, 0.9871328979762477029, 1.000000000000000000, 0.9659258262890683122, 1.000000000000000000, 0.9659258262890683122, 1.000000000000000000, 0.9871328979762533651, 0.9839835555609452999 ) ) 
 REPRESENTATION_ITEM ( '' )  );
#24762=CARTESIAN_POINT ( 'NONE',  ( 1.472469842513823179, 15.59226448433411960, -4.923371831947296329 ) ) ;
#24764=CARTESIAN_POINT ( 'NONE',  ( -4.164238869374099927, 17.01208216824730357, 3.795296366450308767 ) ) ;
#24765=CARTESIAN_POINT ( 'NONE',  ( 19.84674366389459266, 23.30059781766745530, 2.638427012816836559 ) ) ;
#24766=CARTESIAN_POINT ( 'NONE',  ( -0.8801773607110991993, 47.85535201082150536, -2.915334737309923874 ) ) ;
#24769=CARTESIAN_POINT ( 'NONE',  ( 20.88017736071110875, 45.77201867748816966, -2.915334737309920765 ) ) ;
#24774=VERTEX_POINT ( 'NONE', #91185 ) ;
#24775=CARTESIAN_POINT ( 'NONE',  ( 12.91533473730993009, 41.60535201082149825, -10.88017736071109987 ) ) ;
#24776=CARTESIAN_POINT ( 'NONE',  ( 24.16423886937410614, 4.303748834913967869, 8.672049930838204340E-16 ) ) ;
#24779=CARTESIAN_POINT ( 'NONE',  ( 16.40814093676323893, 30.79030133659708923, 11.09922568453595026 ) ) ;
#24780=CARTESIAN_POINT ( 'NONE',  ( -4.164238869374098151, 1.595415501580634388, -3.795296366450310543 ) ) ;
#24781=CARTESIAN_POINT ( 'NONE',  ( 19.84674366389459621, 13.50893115100078568, 7.409399052514197653E-17 ) ) ;
#24783=CARTESIAN_POINT ( 'NONE',  ( -1.099225684535947600, 44.54030133659708923, 6.408140936763237150 ) ) ;
#24785=CARTESIAN_POINT ( 'NONE',  ( 2.791683348922237240, 10.38393115100078390, -7.208316651077763204 ) ) ;
#24786=CARTESIAN_POINT ( 'NONE',  ( 7.084665262690076126, 42.02201867748816966, -10.88017736071110164 ) ) ;
#24789=ORIENTED_EDGE ( 'NONE', *, *, #75730, .T. ) ;
#24790=CARTESIAN_POINT ( 'NONE',  ( 20.32896413005680358, 64.74545670184114954, 5.963430220938287007 ) ) ;
#24791=CARTESIAN_POINT ( 'NONE',  ( 0.5774900079438590739, 52.64701867748817676, -5.440088680355550821 ) ) ;
#24792=CARTESIAN_POINT ( 'NONE',  ( -42.84429281707037518, 107.5921494319837706, 4.500000000000002665 ) ) ;
#24793=CARTESIAN_POINT ( 'NONE',  ( 13.99999999999999822, 61.00000000000000711, -6.000000000000000000 ) ) ;
#24794=CARTESIAN_POINT ( 'NONE',  ( 12.91533473730993009, 61.60535201082150536, -10.88017736071109987 ) ) ;
#24795=CARTESIAN_POINT ( 'NONE',  ( 10.00000000000000178, 10.37363466993041961, 12.81628187352647608 ) ) ;
#24796=CARTESIAN_POINT ( 'NONE',  ( -23.44000000000001194, 92.00000000000000000, -9.500000000000000000 ) ) ;
#24797=CARTESIAN_POINT ( 'NONE',  ( 1.472469842513823179, 31.42559781766745530, 4.923371831947296329 ) ) ;
#24799=CARTESIAN_POINT ( 'NONE',  ( -4.164238869374099039, 6.803748834913967869, 8.674139862899312516E-16 ) ) ;
#24800=CARTESIAN_POINT ( 'NONE',  ( 5.076628168052704559, 20.17559781766745175, -8.527530157486179263 ) ) ;
#24801=CARTESIAN_POINT ( 'NONE',  ( 16.40814093676323893, 15.79030133659708746, 11.09922568453595026 ) ) ;
#24803=CARTESIAN_POINT ( 'NONE',  ( 0.2751277870542981341, 18.21833443783937767, 6.500000000000002665 ) ) ;
#24804=CARTESIAN_POINT ( 'NONE',  ( 2.035157376598824452, 48.68868534415483396, 7.964842623401179544 ) ) ;
#24805=CARTESIAN_POINT ( 'NONE',  ( 10.00000000000000000, -2.126365330069579951, -12.81628187352647608 ) ) ;
#24806=CARTESIAN_POINT ( 'NONE',  ( -0.3289641300568009741, 32.24545670184113533, -5.963430220938281678 ) ) ;
#24807=CARTESIAN_POINT ( 'NONE',  ( 7.361572987183169658, 34.96726448433411605, -9.846743663894592657 ) ) ;
#24808=CARTESIAN_POINT ( 'NONE',  ( 18.52753015748617571, 23.09226448433411960, 4.923371831947298993 ) ) ;
#24809=CARTESIAN_POINT ( 'NONE',  ( 0.5774900079438607392, 18.48035201082150536, 5.440088680355550821 ) ) ;
#24811=CARTESIAN_POINT ( 'NONE',  ( 6.565887622018943937, 10.16530133659708746, 12.81628187352647430 ) ) ;
#24812=CARTESIAN_POINT ( 'NONE',  ( 12.63842701281683034, 22.46726448433411605, 9.846743663894596210 ) ) ;
#24813=DIRECTION ( 'NONE',  ( 1.000000000000000000, 0.000000000000000000, 0.000000000000000000 ) ) ;
#24814=CARTESIAN_POINT ( 'NONE',  ( 17.96484262340118221, 16.18868534415483396, -7.964842623401177768 ) ) ;
#24816=CARTESIAN_POINT ( 'NONE',  ( 4.559911319644449179, 67.23035201082150536, -9.422509992056141925 ) ) ;
#24818=CARTESIAN_POINT ( 'NONE',  ( 10.00000000000000178, 42.25893115100078745, 9.846743663894594434 ) ) ;
#24819=CARTESIAN_POINT ( 'NONE',  ( 15.44008868035555793, 11.39701867748817143, -9.422509992056140149 ) ) ;
#24821=CARTESIAN_POINT ( 'NONE',  ( 15.44008868035555793, 51.39701867748816966, -9.422509992056140149 ) ) ;
#24822=CARTESIAN_POINT ( 'NONE',  ( 12.91533473730992121, 14.52201867748817143, 10.88017736071110164 ) ) ;
#24824=CARTESIAN_POINT ( 'NONE',  ( 7.361572987183169658, 14.96726448433411960, -9.846743663894592657 ) ) ;
#24825=CARTESIAN_POINT ( 'NONE',  ( 19.84674366389459621, 38.50893115100078745, 7.409399052514197653E-17 ) ) ;
#24828=CARTESIAN_POINT ( 'NONE',  ( 0.6178305044545818747, -1.501365330069579951, -9.382169495545419124 ) ) ;
#24829=CARTESIAN_POINT ( 'NONE',  ( -2.266590686148945544, 2.220415501580634388, 7.082119434687048631 ) ) ;
#24830=CARTESIAN_POINT ( 'NONE',  ( 20.36894250292379382, 23.67874883491397142, 10.36894250292379205 ) ) ;
#24831=CARTESIAN_POINT ( 'NONE',  ( 14.92337183194729988, 39.34226448433412315, -8.527530157486177487 ) ) ;
#24833=CARTESIAN_POINT ( 'NONE',  ( 2.917880565312950480, 55.97041550158063217, -12.26659068614894821 ) ) ;
#24834=CARTESIAN_POINT ( 'NONE',  ( 5.076628168052704559, 20.17559781766745175, -8.527530157486179263 ) ) ;
#24836=CARTESIAN_POINT ( 'NONE',  ( 20.88017736071110164, 40.35535201082150536, 2.915334737309930979 ) ) ;
#24838=CARTESIAN_POINT ( 'NONE',  ( 12.91533473730993009, 21.60535201082150536, -10.88017736071109987 ) ) ;
#24839=CARTESIAN_POINT ( 'NONE',  ( 0.6178305044545838731, 54.74863466993042493, 9.382169495545420901 ) ) ;
#24840=CARTESIAN_POINT ( 'NONE',  ( 10.00000000000000000, 17.87363466993041783, -12.81628187352647608 ) ) ;
#24841=CARTESIAN_POINT ( 'NONE',  ( 19.72487221294570148, 35.71833443783938833, -6.500000000000010658 ) ) ;
#24842=CARTESIAN_POINT ( 'NONE',  ( 2.791683348922237240, 10.38393115100078390, -7.208316651077763204 ) ) ;
#24846=CARTESIAN_POINT ( 'NONE',  ( 24.16423886937409904, 49.09541550158063217, 3.795296366450317205 ) ) ;
#24847=CARTESIAN_POINT ( 'NONE',  ( 24.16423886937410614, 29.51208216824729647, -3.795296366450302550 ) ) ;
#24848=CARTESIAN_POINT ( 'NONE',  ( 2.035157376598822676, 17.43868534415483751, -7.964842623401177768 ) ) ;
#24849=CARTESIAN_POINT ( 'NONE',  ( 20.88017736071110164, 55.35535201082149825, 2.915334737309930979 ) ) ;
#24850=DIRECTION ( 'NONE',  ( 0.000000000000000000, -1.000000000000000000, 0.000000000000000000 ) ) ;
#24852=CARTESIAN_POINT ( 'NONE',  ( 10.00000000000000178, 64.31368534415483396, 10.88017736071110342 ) ) ;
#24853=CARTESIAN_POINT ( 'NONE',  ( 19.84674366389459266, 13.71726448433411782, -2.638427012816827677 ) ) ;
#24854=FACE_OUTER_BOUND ( 'NONE', #26124, .T. ) ;
#24856=CARTESIAN_POINT ( 'NONE',  ( 17.20831665107776587, 27.88393115100078390, 7.208316651077764980 ) ) ;
#24857=CARTESIAN_POINT ( 'NONE',  ( 19.84674366389459621, 48.50893115100078745, 7.409399052514197653E-17 ) ) ;
#24858=B_SPLINE_CURVE_WITH_KNOTS ( 'NONE', 3,
 ( #91056, #60564, #45061, #36595, #52567, #8068, #59076, #66588, #29557, #38081 ),
 .UNSPECIFIED., .F., .F.,
 ( 4, 2, 2, 2, 4 ),
 ( 0.009575373339651055415, 0.01007433173322977958, 0.01057329012680850548, 0.01157120691396595381, 0.01356704048828087997 ),
 .UNSPECIFIED. ) ;
#24860=CARTESIAN_POINT ( 'NONE',  ( 17.96484262340118221, 16.18868534415483396, -7.964842623401177768 ) ) ;
#24861=CARTESIAN_POINT ( 'NONE',  ( 22.81628187352647785, 31.62363466993042138, 6.195893100308588602E-16 ) ) ;
#24863=CARTESIAN_POINT ( 'NONE',  ( 20.88017736071110519, 55.56368534415484817, 2.639326808657452039E-16 ) ) ;
#24864=CARTESIAN_POINT ( 'NONE',  ( 13.79529636645031943, 40.34541550158063217, -14.16423886937409904 ) ) ;
#24865=CARTESIAN_POINT ( 'NONE',  ( 14.92337183194729633, 12.67559781766745353, 8.527530157486181039 ) ) ;
#24867=EDGE_CURVE ( 'NONE', #49115, #95793, #97865, .T. ) ;
#24869=CARTESIAN_POINT ( 'NONE',  ( 18.52753015748618282, 48.92559781766745886, -4.923371831947291888 ) ) ;
#24870=CARTESIAN_POINT ( 'NONE',  ( 10.00000000000000178, 27.25893115100078390, 9.846743663894594434 ) ) ;
#24871=CARTESIAN_POINT ( 'NONE',  ( 10.00000000000000000, 5.553748834913967869, -14.16423886937410082 ) ) ;
#24872=CARTESIAN_POINT ( 'NONE',  ( -0.3689425029237898834, 21.17874883491396432, -10.36894250292378850 ) ) ;
#24873=CARTESIAN_POINT ( 'NONE',  ( 17.20831665107776587, 29.13393115100078390, -7.208316651077762316 ) ) ;
#24874=CARTESIAN_POINT ( 'NONE',  ( -0.8801773607110991993, 42.85535201082150536, -2.915334737309923874 ) ) ;
#24875=CARTESIAN_POINT ( 'NONE',  ( 12.91533473730993009, 16.60535201082150891, -10.88017736071109987 ) ) ;
#24876=CARTESIAN_POINT ( 'NONE',  ( 2.035157376598822676, 42.43868534415483396, -7.964842623401177768 ) ) ;
#24877=CARTESIAN_POINT ( 'NONE',  ( 10.00000000000000178, 24.31368534415484106, 10.88017736071110342 ) ) ;
#24879=B_SPLINE_CURVE_WITH_KNOTS ( 'NONE', 3,
 ( #30907, #31394, #61403, #61894 ),
 .UNSPECIFIED., .F., .F.,
 ( 4, 4 ),
 ( 0.000000000000000000, 0.002657014572711312479 ),
 .UNSPECIFIED. ) ;
#24880=CARTESIAN_POINT ( 'NONE',  ( 10.00000000000000000, 41.81368534415484106, -10.88017736071110342 ) ) ;
#24882=CARTESIAN_POINT ( 'NONE',  ( 19.38216949554541557, 57.24863466993042493, -9.382169495545420901 ) ) ;
#24886=CARTESIAN_POINT ( 'NONE',  ( 17.96484262340118221, 46.18868534415484106, -7.964842623401177768 ) ) ;
#24887=CARTESIAN_POINT ( 'NONE',  ( 7.084665262690076126, 4.105352010821503583, 10.88017736071109987 ) ) ;
#24892=CARTESIAN_POINT ( 'NONE',  ( 20.36894250292379738, 64.92874883491397497, -10.36894250292379027 ) ) ;
#24893=CARTESIAN_POINT ( 'NONE',  ( 10.00000000000000178, 2.258931151000784787, 9.846743663894594434 ) ) ;
#24894=MECHANICAL_DESIGN_GEOMETRIC_PRESENTATION_REPRESENTATION('',(#98345),#32859);
#24895=CARTESIAN_POINT ( 'NONE',  ( 0.1532563361054082862, 6.217264484334118713, 2.638427012816831674 ) ) ;
#24896=CARTESIAN_POINT ( 'NONE',  ( 20.88017736071110164, 5.355352010821502695, 2.915334737309930979 ) ) ;
#24897=CARTESIAN_POINT ( 'NONE',  ( 0.1532563361054083140, 46.00893115100079456, 1.131784320476157264E-15 ) ) ;
#24900=CARTESIAN_POINT ( 'NONE',  ( 17.20831665107776587, 44.13393115100078745, -7.208316651077762316 ) ) ;
#24902=CARTESIAN_POINT ( 'NONE',  ( 0.5774900079438607392, 43.48035201082151247, 5.440088680355550821 ) ) ;
#24903=CARTESIAN_POINT ( 'NONE',  ( 10.00000000000000000, 54.75893115100078745, -9.846743663894594434 ) ) ;
#24904=CARTESIAN_POINT ( 'NONE',  ( 0.6178305044545838731, 29.74863466993042138, 9.382169495545420901 ) ) ;
#24905=CARTESIAN_POINT ( 'NONE',  ( 10.00000000000000178, 69.31368534415484817, 10.88017736071110342 ) ) ;
#24906=CARTESIAN_POINT ( 'NONE',  ( 2.035157376598824452, 48.68868534415483396, 7.964842623401179544 ) ) ;
#24907=CARTESIAN_POINT ( 'NONE',  ( 22.26659068614895176, 59.72041550158063927, -7.082119434687042414 ) ) ;
#24909=CARTESIAN_POINT ( 'NONE',  ( 22.81628187352648496, 21.83196800326374643, -3.434112377981050290 ) ) ;
#24912=CARTESIAN_POINT ( 'NONE',  ( 19.38216949554541557, 27.24863466993041783, -9.382169495545420901 ) ) ;
#24913=CARTESIAN_POINT ( 'NONE',  ( 2.035157376598822676, 17.43868534415483751, -7.964842623401177768 ) ) ;
#24916=CARTESIAN_POINT ( 'NONE',  ( 7.361572987183169658, -0.03273551566588185635, -9.846743663894592657 ) ) ;
#24917=CARTESIAN_POINT ( 'NONE',  ( 17.20831665107776587, 52.88393115100078035, 7.208316651077764980 ) ) ;
#24918=CARTESIAN_POINT ( 'NONE',  ( 2.791683348922240793, 16.63393115100078745, 7.208316651077764092 ) ) ;
#24919=CARTESIAN_POINT ( 'NONE',  ( 17.20831665107776587, 34.13393115100078745, -7.208316651077762316 ) ) ;
#24922=CARTESIAN_POINT ( 'NONE',  ( 7.361572987183169658, 24.96726448433412315, -9.846743663894592657 ) ) ;
#24923=CARTESIAN_POINT ( 'NONE',  ( 18.72515096720577787, 46.07228050351031357, -6.499999999999891642 ) ) ;
#24924=MECHANICAL_DESIGN_GEOMETRIC_PRESENTATION_REPRESENTATION('',(#98462),#50457);
#24926=CARTESIAN_POINT ( 'NONE',  ( 14.92337183194729633, 22.67559781766745175, 8.527530157486181039 ) ) ;
#24927=CARTESIAN_POINT ( 'NONE',  ( 5.076628168052704559, 0.1755978176674514724, -8.527530157486179263 ) ) ;
#24929=CARTESIAN_POINT ( 'NONE',  ( 17.20831665107776587, 49.13393115100078745, -7.208316651077762316 ) ) ;
#24930=ORIENTED_EDGE ( 'NONE', *, *, #37641, .T. ) ;
#24932=CARTESIAN_POINT ( 'NONE',  ( 19.38216949554541202, 25.99863466993042138, 9.382169495545424454 ) ) ;
#24934=CARTESIAN_POINT ( 'NONE',  ( 10.00000000000000000, 45.55374883491397497, -14.16423886937410082 ) ) ;
#24935=CARTESIAN_POINT ( 'NONE',  ( 17.20831665107776587, 14.13393115100078568, -7.208316651077762316 ) ) ;
#24936=CARTESIAN_POINT ( 'NONE',  ( 10.00000000000000000, 4.758931151000784787, -9.846743663894594434 ) ) ;
#24937=CARTESIAN_POINT ( 'NONE',  ( 19.64201483648647439, 93.04323334508872279, 5.303713241053674921 ) ) ;
#24938=CARTESIAN_POINT ( 'NONE',  ( 24.16423886937410614, 49.51208216824730357, -3.795296366450302550 ) ) ;
#24939=CARTESIAN_POINT ( 'NONE',  ( 18.52753015748618282, 53.92559781766745175, -4.923371831947291888 ) ) ;
#24940=CARTESIAN_POINT ( 'NONE',  ( 10.00000000000000178, 63.05374883491396076, 14.16423886937410082 ) ) ;
#24941=CARTESIAN_POINT ( 'NONE',  ( 13.79529636645031943, 25.34541550158063572, -14.16423886937409904 ) ) ;
#24942=CARTESIAN_POINT ( 'NONE',  ( 20.36894250292379382, 38.67874883491396076, 10.36894250292379205 ) ) ;
#24943=DIRECTION ( 'NONE',  ( -1.000000000000000000, 0.000000000000000000, 0.000000000000000000 ) ) ;
#24945=CARTESIAN_POINT ( 'NONE',  ( 5.076628168052703671, 56.84226448433412315, 8.527530157486179263 ) ) ;
#24947=CARTESIAN_POINT ( 'NONE',  ( 4.559911319644449179, 33.89701867748817676, 9.422509992056141925 ) ) ;
#24948=DIRECTION ( 'NONE',  ( 0.000000000000000000, 0.000000000000000000, -1.000000000000000000 ) ) ;
#24951=CARTESIAN_POINT ( 'NONE',  ( 7.361572987183169658, 39.96726448433411605, -9.846743663894592657 ) ) ;
#24954=CARTESIAN_POINT ( 'NONE',  ( 18.52753015748618282, 43.92559781766745175, -4.923371831947291888 ) ) ;
#24956=VECTOR ( 'NONE', #13358, 1000.000000000000000 ) ;
#24958=ORIENTED_EDGE ( 'NONE', *, *, #1701, .T. ) ;
#24959=CARTESIAN_POINT ( 'NONE',  ( 13.79529636645031943, 15.34541550158063750, -14.16423886937409904 ) ) ;
#24960=AXIS2_PLACEMENT_3D ( 'NONE', #26936, #80441, #33926 ) ;
#24963=FACE_OUTER_BOUND ( 'NONE', #90079, .T. ) ;
#24964=CARTESIAN_POINT ( 'NONE',  ( 20.88017736071110875, 5.772018677488170546, -2.915334737309920765 ) ) ;
#24965=CARTESIAN_POINT ( 'NONE',  ( 6.565887622018943937, 25.16530133659708213, 12.81628187352647430 ) ) ;
#24966=CARTESIAN_POINT ( 'NONE',  ( 20.15039907845753930, 2.627771745786128044, -6.262539305110069954 ) ) ;
#24967=CARTESIAN_POINT ( 'NONE',  ( -0.8801773607111008646, 63.27201867748817676, 2.915334737309923430 ) ) ;
#24969=CARTESIAN_POINT ( 'NONE',  ( -46.82586484710777341, 100.5857744218339036, -9.343464521776596143 ) ) ;
#24971=CARTESIAN_POINT ( 'NONE',  ( -0.3689425029237898834, 56.17874883491396076, -10.36894250292378850 ) ) ;
#24973=CARTESIAN_POINT ( 'NONE',  ( 2.035157376598824452, 23.68868534415484461, 7.964842623401179544 ) ) ;
#24974=CARTESIAN_POINT ( 'NONE',  ( 17.96484262340118221, 36.18868534415484106, -7.964842623401177768 ) ) ;
#24975=CARTESIAN_POINT ( 'NONE',  ( 0.6178305044545818747, -1.501365330069579951, -9.382169495545419124 ) ) ;
#24976=CARTESIAN_POINT ( 'NONE',  ( 10.00000000000000000, 49.75893115100078745, -9.846743663894594434 ) ) ;
#24977=CARTESIAN_POINT ( 'NONE',  ( 0.6178305044545818747, 63.49863466993043204, -9.382169495545419124 ) ) ;
#24978=CARTESIAN_POINT ( 'NONE',  ( 1.042145700049420309, 54.74216108172002748, -6.499999999999917399 ) ) ;
#24979=ADVANCED_FACE ( 'NONE', ( #54654 ), #46193, .T. ) ;
#24981=CARTESIAN_POINT ( 'NONE',  ( 17.96484262340118221, 26.18868534415483396, -7.964842623401177768 ) ) ;
#24982=CARTESIAN_POINT ( 'NONE',  ( 22.81628187352648496, 36.83196800326376064, -3.434112377981050290 ) ) ;
#24984=CARTESIAN_POINT ( 'NONE',  ( -0.000000000000000000, 75.65410658971823921, 6.567011432196594889 ) ) ;
#24986=CARTESIAN_POINT ( 'NONE',  ( 0.6178305044545818747, -1.501365330069579951, -9.382169495545419124 ) ) ;
#24987=CARTESIAN_POINT ( 'NONE',  ( 12.91533473730992121, 49.52201867748817676, 10.88017736071110164 ) ) ;
#24989=CARTESIAN_POINT ( 'NONE',  ( 18.52753015748618282, 8.925597817667451750, -4.923371831947291888 ) ) ;
#24990=CARTESIAN_POINT ( 'NONE',  ( -2.816281873526473856, 39.33196800326374643, 3.434112377981055619 ) ) ;
#24991=CARTESIAN_POINT ( 'NONE',  ( -0.8801773607111009756, 63.06368534415484106, 1.068504757029289695E-15 ) ) ;
#24993=CARTESIAN_POINT ( 'NONE',  ( 18.06765999051789251, 53.99127512925452521, 6.499999999999959144 ) ) ;
#24994=CARTESIAN_POINT ( 'NONE',  ( 22.81628187352647785, 61.62363466993041783, 6.195893100308588602E-16 ) ) ;
#24998=CARTESIAN_POINT ( 'NONE',  ( 10.00000000000000178, 4.313685344154837509, 10.88017736071110342 ) ) ;
#24999=CARTESIAN_POINT ( 'NONE',  ( 13.43411237798106583, 42.66530133659707502, -12.81628187352647252 ) ) ;
#25000=CARTESIAN_POINT ( 'NONE',  ( 19.84674366389459266, 18.30059781766745175, 2.638427012816836559 ) ) ;
#25001=CARTESIAN_POINT ( 'NONE',  ( 12.91533473730993009, 6.605352010821504471, -10.88017736071109987 ) ) ;
#25002=CARTESIAN_POINT ( 'NONE',  ( 2.791683348922237240, 20.38393115100078745, -7.208316651077763204 ) ) ;
#25003=CARTESIAN_POINT ( 'NONE',  ( 2.917880565312948704, 57.63708216824731068, 12.26659068614894643 ) ) ;
#25006=CARTESIAN_POINT ( 'NONE',  ( 2.035157376598822676, 27.43868534415483396, -7.964842623401177768 ) ) ;
#25007=CARTESIAN_POINT ( 'NONE',  ( 0.000000000000000000, 70.80332830338373640, 5.000000000000000000 ) ) ;
#25008=VERTEX_POINT ( 'NONE', #46669 ) ;
#25009=CARTESIAN_POINT ( 'NONE',  ( 7.084665262690076126, 17.02201867748817676, -10.88017736071110164 ) ) ;
#25010=CARTESIAN_POINT ( 'NONE',  ( 7.084665262690076126, 17.02201867748817676, -10.88017736071110164 ) ) ;
#25011=CARTESIAN_POINT ( 'NONE',  ( 10.00000000000000000, 59.75893115100078745, -9.846743663894594434 ) ) ;
#25012=SURFACE_SIDE_STYLE ('',( #47490 ) ) ;
#25014=CARTESIAN_POINT ( 'NONE',  ( -4.164238869374099039, 16.80374883491396787, 8.674139862899312516E-16 ) ) ;
#25015=CARTESIAN_POINT ( 'NONE',  ( 20.88017736071110164, 20.35535201082150891, 2.915334737309930979 ) ) ;
#25016=CARTESIAN_POINT ( 'NONE',  ( 0.5774900079438607392, 23.48035201082150536, 5.440088680355550821 ) ) ;
#25017=CARTESIAN_POINT ( 'NONE',  ( 17.20831665107776587, 59.13393115100078745, -7.208316651077762316 ) ) ;
#25018=STYLED_ITEM ( 'NONE', ( #56395 ), #30487 ) ;
#25020=CARTESIAN_POINT ( 'NONE',  ( 1.472469842513823179, 31.42559781766745530, 4.923371831947296329 ) ) ;
#25021=ADVANCED_FACE ( 'NONE', ( #84678 ), #39055, .T. ) ;
#25023=CARTESIAN_POINT ( 'NONE',  ( 12.63842701281683922, 9.550597817667449974, -9.846743663894590881 ) ) ;
#25026=CARTESIAN_POINT ( 'NONE',  ( 15.44008868035555793, 6.397018677488170546, -9.422509992056140149 ) ) ;
#25027=CARTESIAN_POINT ( 'NONE',  ( 14.92337183194729633, 2.675597817667451750, 8.527530157486181039 ) ) ;
#25028=CARTESIAN_POINT ( 'NONE',  ( 12.91533473730992121, 49.52201867748817676, 10.88017736071110164 ) ) ;
#25029=CARTESIAN_POINT ( 'NONE',  ( 20.88017736071110875, 45.77201867748816966, -2.915334737309920765 ) ) ;
#25030=CARTESIAN_POINT ( 'NONE',  ( 22.81628187352647785, 41.62363466993042493, 6.195893100308588602E-16 ) ) ;
#25032=CARTESIAN_POINT ( 'NONE',  ( 2.917880565312950480, 15.97041550158063217, -12.26659068614894821 ) ) ;
#25034=EDGE_CURVE ( 'NONE', #32525, #50081, #20208, .T. ) ;
#25035=CIRCLE ( 'NONE', #39373, 0.4999999999999961142 ) ;
#25036=CARTESIAN_POINT ( 'NONE',  ( 0.6178305044545818747, 63.49863466993043204, -9.382169495545419124 ) ) ;
#25038=CARTESIAN_POINT ( 'NONE',  ( 19.84674366389459621, 58.50893115100078745, 7.409399052514197653E-17 ) ) ;
#25039=CARTESIAN_POINT ( 'NONE',  ( 10.00000000000000000, 21.81368534415484106, -10.88017736071110342 ) ) ;
#25041=CARTESIAN_POINT ( 'NONE',  ( 14.92337183194729988, 4.342264484334117824, -8.527530157486177487 ) ) ;
#25042=CARTESIAN_POINT ( 'NONE',  ( 10.00000000000000000, 1.813685344154837731, -10.88017736071110342 ) ) ;
#25044=CARTESIAN_POINT ( 'NONE',  ( 12.63842701281683922, 14.55059781766744997, -9.846743663894590881 ) ) ;
#25045=CARTESIAN_POINT ( 'NONE',  ( 20.88017736071110519, 65.56368534415483396, 2.639326808657452039E-16 ) ) ;
#25047=CARTESIAN_POINT ( 'NONE',  ( -0.8801773607111009756, 58.06368534415484106, 1.068504757029289695E-15 ) ) ;
#25050=CARTESIAN_POINT ( 'NONE',  ( 10.00000000000000178, 59.31368534415484106, 10.88017736071110342 ) ) ;
#25051=CARTESIAN_POINT ( 'NONE',  ( 18.52753015748618282, 8.925597817667451750, -4.923371831947291888 ) ) ;
#25052=ORIENTED_EDGE ( 'NONE', *, *, #12204, .T. ) ;
#25056=CARTESIAN_POINT ( 'NONE',  ( 18.52753015748618282, 48.92559781766745886, -4.923371831947291888 ) ) ;
#25057=ORIENTED_EDGE ( 'NONE', *, *, #56791, .T. ) ;
#25059=CARTESIAN_POINT ( 'NONE',  ( 6.204703633549690345, 0.7620821682473009062, -14.16423886937410259 ) ) ;
#25060=CARTESIAN_POINT ( 'NONE',  ( 16.40814093676323893, 60.79030133659709634, 11.09922568453595026 ) ) ;
#25061=CARTESIAN_POINT ( 'NONE',  ( 24.16423886937410614, 19.30374883491397142, 8.672049930838204340E-16 ) ) ;
#25064=CARTESIAN_POINT ( 'NONE',  ( 0.5774900079438590739, 22.64701867748817321, -5.440088680355550821 ) ) ;
#25065=CARTESIAN_POINT ( 'NONE',  ( -45.94000000000001194, 99.99999999999998579, 9.500000000000000000 ) ) ;
#25067=SURFACE_STYLE_USAGE ( .BOTH. , #47046 ) ;
#25069=CARTESIAN_POINT ( 'NONE',  ( 0.1532563361054082862, 21.21726448433412315, 2.638427012816831674 ) ) ;
#25070=CARTESIAN_POINT ( 'NONE',  ( 0.6178305044545838731, 34.74863466993042493, 9.382169495545420901 ) ) ;
#25071=CARTESIAN_POINT ( 'NONE',  ( 1.472469842513823179, 40.59226448433411605, -4.923371831947296329 ) ) ;
#25072=ADVANCED_FACE ( 'NONE', ( #75068 ), #89895, .T. ) ;
#25074=CARTESIAN_POINT ( 'NONE',  ( 22.81628187352647785, 11.41530133659708390, 3.434112377981063169 ) ) ;
#25077=CARTESIAN_POINT ( 'NONE',  ( 17.20831665107776587, 24.13393115100078035, -7.208316651077762316 ) ) ;
#25078=CARTESIAN_POINT ( 'NONE',  ( 17.20831665107776587, 7.883931151000784787, 7.208316651077764980 ) ) ;
#25079=ORIENTED_EDGE ( 'NONE', *, *, #42368, .T. ) ;
#25082=CARTESIAN_POINT ( 'NONE',  ( 19.42250999205614193, 30.14701867748817321, 5.440088680355555262 ) ) ;
#25083=CARTESIAN_POINT ( 'NONE',  ( 2.917880565312948704, 32.63708216824730357, 12.26659068614894643 ) ) ;
#25084=CARTESIAN_POINT ( 'NONE',  ( 17.20831665107776587, 39.13393115100079456, -7.208316651077762316 ) ) ;
#25085=CARTESIAN_POINT ( 'NONE',  ( 18.52753015748618282, 18.92559781766745175, -4.923371831947291888 ) ) ;
#25086=CARTESIAN_POINT ( 'NONE',  ( 13.43411237798105340, 50.58196800326375353, 12.81628187352647963 ) ) ;
#25088=CARTESIAN_POINT ( 'NONE',  ( 15.44008868035555793, 21.39701867748817321, -9.422509992056140149 ) ) ;
#25090=CARTESIAN_POINT ( 'NONE',  ( 19.38216949554541557, 17.24863466993041783, -9.382169495545420901 ) ) ;
#25091=CARTESIAN_POINT ( 'NONE',  ( 21.09922568453595559, 17.04030133659708923, -6.408140936763230044 ) ) ;
#25092=CARTESIAN_POINT ( 'NONE',  ( 5.076628168052704559, 45.17559781766745175, -8.527530157486179263 ) ) ;
#25094=CARTESIAN_POINT ( 'NONE',  ( -2.816281873526471635, 48.91530133659708213, -3.434112377981056508 ) ) ;
#25095=SURFACE_STYLE_FILL_AREA ( #2106 ) ;
#25096=CARTESIAN_POINT ( 'NONE',  ( -0.8801773607111009756, 53.06368534415484106, 1.068504757029289695E-15 ) ) ;
#25099=DIRECTION ( 'NONE',  ( 0.000000000000000000, 0.000000000000000000, -1.000000000000000000 ) ) ;
#25100=CARTESIAN_POINT ( 'NONE',  ( -0.8801773607111009756, 48.06368534415484817, 1.068504757029289695E-15 ) ) ;
#25101=CARTESIAN_POINT ( 'NONE',  ( 4.559911319644449179, 53.89701867748817676, 9.422509992056141925 ) ) ;
#25103=EDGE_CURVE ( 'NONE', #45739, #70278, #85532, .T. ) ;
#25106=CARTESIAN_POINT ( 'NONE',  ( 19.42250999205614193, 15.14701867748817143, 5.440088680355555262 ) ) ;
#25107=EDGE_CURVE ( 'NONE', #83096, #10733, #98075, .T. ) ;
#25108=CARTESIAN_POINT ( 'NONE',  ( 10.00000000000000000, -2.126365330069579951, -12.81628187352647608 ) ) ;
#25109=CARTESIAN_POINT ( 'NONE',  ( 20.88017736071110875, 25.77201867748816966, -2.915334737309920765 ) ) ;
#25112=CARTESIAN_POINT ( 'NONE',  ( 21.09922568453595559, 27.04030133659708568, -6.408140936763230044 ) ) ;
#25114=CARTESIAN_POINT ( 'NONE',  ( 20.88017736071110875, 55.77201867748816966, -2.915334737309920765 ) ) ;
#25115=CARTESIAN_POINT ( 'NONE',  ( 19.84674366389459266, 38.30059781766745175, 2.638427012816836559 ) ) ;
#25116=CARTESIAN_POINT ( 'NONE',  ( 0.6178305044545838731, 4.748634669930420493, 9.382169495545420901 ) ) ;
#25117=DIRECTION ( 'NONE',  ( -0.8320502943378436100, 0.5547001962252291474, -0.000000000000000000 ) ) ;
#25118=CARTESIAN_POINT ( 'NONE',  ( 10.00000000000000000, 11.81368534415483751, -10.88017736071110342 ) ) ;
#25119=CARTESIAN_POINT ( 'NONE',  ( 19.42250999205614193, 40.14701867748817676, 5.440088680355555262 ) ) ;
#25120=CARTESIAN_POINT ( 'NONE',  ( 24.16423886937410614, 54.51208216824730357, -3.795296366450302550 ) ) ;
#25122=CARTESIAN_POINT ( 'NONE',  ( 19.84674366389459621, 43.50893115100078745, 7.409399052514197653E-17 ) ) ;
#25123=CARTESIAN_POINT ( 'NONE',  ( 10.00000000000000000, 66.81368534415484817, -10.88017736071110342 ) ) ;
#25125=CARTESIAN_POINT ( 'NONE',  ( -4.164238869374099927, 17.01208216824730357, 3.795296366450308767 ) ) ;
#25129=CARTESIAN_POINT ( 'NONE',  ( 0.1532563361054100626, 65.80059781766745175, -2.638427012816831230 ) ) ;
#25133=CARTESIAN_POINT ( 'NONE',  ( 10.00000000000000000, 50.55374883491396787, -14.16423886937410082 ) ) ;
#25134=CARTESIAN_POINT ( 'NONE',  ( 10.00000000000000178, 38.05374883491396787, 14.16423886937410082 ) ) ;
#25135=CARTESIAN_POINT ( 'NONE',  ( 0.1532563361054082862, 16.21726448433411960, 2.638427012816831674 ) ) ;
#25136=CARTESIAN_POINT ( 'NONE',  ( 16.40814093676324603, 12.45696800326375353, -11.09922568453594671 ) ) ;
#25137=CARTESIAN_POINT ( 'NONE',  ( 2.791683348922237240, 60.38393115100078745, -7.208316651077763204 ) ) ;
#25139=CARTESIAN_POINT ( 'NONE',  ( 4.559911319644449179, 57.23035201082150536, -9.422509992056141925 ) ) ;
#25140=CARTESIAN_POINT ( 'NONE',  ( -2.816281873526473856, 39.12363466993041783, 9.499525473075851096E-16 ) ) ;
#25142=CARTESIAN_POINT ( 'NONE',  ( 24.16423886937409904, 24.09541550158063927, 3.795296366450317205 ) ) ;
#25143=CARTESIAN_POINT ( 'NONE',  ( 10.00000000000000000, 26.81368534415484106, -10.88017736071110342 ) ) ;
#25145=CARTESIAN_POINT ( 'NONE',  ( 14.92337183194729633, 2.675597817667451750, 8.527530157486181039 ) ) ;
#25148=DIRECTION ( 'NONE',  ( 0.000000000000000000, 0.000000000000000000, -1.000000000000000000 ) ) ;
#25149=CARTESIAN_POINT ( 'NONE',  ( 19.72487221294570858, 70.00000000000000000, -6.000000000000000000 ) ) ;
#25151=CARTESIAN_POINT ( 'NONE',  ( 2.035157376598824452, 3.688685344154837953, 7.964842623401179544 ) ) ;
#25152=CARTESIAN_POINT ( 'NONE',  ( 2.035157376598824452, 8.688685344154839285, 7.964842623401179544 ) ) ;
#25153=CARTESIAN_POINT ( 'NONE',  ( 18.52753015748617571, 43.09226448433412315, 4.923371831947298993 ) ) ;
#25154=CARTESIAN_POINT ( 'NONE',  ( 19.38216949554541202, 0.9986346699304200492, 9.382169495545424454 ) ) ;
#25155=CARTESIAN_POINT ( 'NONE',  ( 21.92686044187656691, 59.95379003517448524, 3.195792623639537755 ) ) ;
#25158=CARTESIAN_POINT ( 'NONE',  ( 16.40814093676323893, 5.790301336597087456, 11.09922568453595026 ) ) ;
#25159=MECHANICAL_DESIGN_GEOMETRIC_PRESENTATION_REPRESENTATION('',(#21941),#93783);
#25161=( BOUNDED_SURFACE ( )  B_SPLINE_SURFACE ( 1, 2, ( 
 ( #48211, #2749, #70245, #78221, #63698, #94201, #56223, #86717, #18221, #64183, #16255, #46737, #39260, #1277, #31730, #56701, #27672, #72188, #88173, #72670, #57678, #3717, #49677, #94704, #96691, #95691, #50680, #19687, #80182, #73165, #43172, #57184, #34178, #81172, #35674, #50174, #87192, #96189, #42204, #51171, #43662, #4704, #64669, #81655, #11695, #27175, #95180, #73660, #80684, #12180, #74148, #13164, #58158, #26688, #12672, #88668, #79701, #42686, #20176, #5187, #35167, #5681, #66157, #26209, #58664, #18715, #87681, #65667, #28170, #89166, #19195, #4205, #34675, #20677, #36166, #65171, #49198, #11198, #41719, #83146, #23154, #66667, #7664, #53629, #8144, #75145, #22159, #68156, #14671, #6655, #37658, #52642, #90141, #30127, #29630, #37171, #67157, #21169, #84147, #67664, #97192, #28660, #6165, #60137, #59152, #59650, #21671, #83645, #45137, #171, #52156, #82649, #98678, #14166, #75643, #15655, #29144, #38155, #68642, #44650, #98174, #7154, #22659, #36669, #60632, #51672, #97682, #91134, #53136, #46138, #90635, #15160, #45640, #76137, #76624, #30620, #89659, #61127, #82150, #91636, #13662, #44144, #74654, #1643, #47104, #39136, #92128, #56106, #9117, #79086, #38636, #77113, #32095, #69138, #31609, #62101, #55612, #17132, #71108, #92610, #54602, #40112, #24135, #47611, #86601, #1148, #78602, #40611, #85118, #70121, #24629, #93596, #8627, #93099, #23654, #69625, #32598, #2140, #18108, #16627, #25134, #77603, #39631, #48585, #62594, #94092, #17620, #666, #86109, #31116, #70614, #48090, #61611, #63096, #16131, #55095, #85615, #78106, #46617, #9612, #54115, #2636, #10112, #33089, #63583, #25613, #84628, #58048, #72076, #49086, #96074, #50561, #34553, #3116, #12066, #57074, #66045, #58545, #88058, #79589, #96572, #64557, #42090, #11089, #88555, #72557, #4089, #89052, #28049, #73053, #41607, #65548, #4586, #94581, #65048, #42569, #35048, #19570, #20563, #81056, #10599, #73544, #41113, #87082, #80571, #50068, #27555, #3602, #34061, #95065, #95574, #12560, #26571, #49557, #20058, #87570, #27061, #51049, #71603, #43063, #33572, #64066, #19082, #57560, #5069, #35556, #80070, #26097, #11576, #56592, #18593, #44033, #22546, #83531, #36554, #14054, #67546, #37547, #21057, #37048, #66550, #51550, #75529, #45022, #63, #82038, #68038, #97566, #74535, #91525, #44536, #38042, #60522, #30511, #30018, #61014, #14553, #98564, #43543, #7042, #59042, #75032, #59538, #6539, #89548, #67044, #81539, #15049, #82535, #91013, #98059, #29030, #60024, #53016, #6056, #13549, #45521, #76021, #29516, #74038, #83036, #90032, #68533, #23039, #90519 ),
 ( #21555, #13049, #22054, #52528, #7552, #52045, #5570, #36046, #97078, #28550, #31977, #39019, #69025, #85006, #46030, #84023, #8999, #92494, #85498, #39515, #23537, #47487, #32971, #70008, #1030, #39996, #16518, #8030, #15545, #54010, #84519, #77004, #31004, #85998, #54979, #61500, #78483, #62980, #24023, #24521, #54491, #46993, #77487, #9998, #76514, #38528, #40501, #92008, #17009, #69514, #16015, #55497, #77990, #559, #46505, #62483, #9495, #70995, #2518, #63477, #8517, #17509, #31491, #70501, #2023, #47974, #61994, #1532, #93980, #53512, #92987, #32486, #93484, #25010, #64930, #26451, #49949, #95457, #26948, #4468, #25978, #73427, #4951, #95956, #48472, #63948, #34935, #33939, #42945, #50434, #3482, #94950, #78970, #41490, #87454, #40992, #56474, #10480, #65432, #19456, #64443, #65926, #11458, #57449, #42456, #86961, #56952, #18969, #49447, #72937, #3968, #10968, #71489, #79952, #17989, #55988, #41976, #72439, #87939, #34436, #94460, #80454, #35432, #11952, #71959, #27437, #57932, #3004, #86490, #18475, #48960, #79470, #33453, #88441, #19941, #80943, #12437, #25502, #66922, #67418, #97443, #28907, #21429, #22425, #27927, #20444, #52898, #35926, #29403, #81917, #66423, #98440, #90395, #43426, #81427, #6415, #52413, #83409, #14930, #45396, #58926, #29897, #5938, #67919, #82913, #59409, #58419, #44413, #74916, #75902, #97945, #14431, #89915, #5453, #7428, #89426, #36430, #88934, #51926, #37924, #96455, #28428, #90897, #50933, #96956, #36927, #12930, #73927, #20939, #59905, #13427, #21932, #44900, #51428, #43910, #75403, #37430, #82410, #74410, #6921, #13936, #60400, #17385, #46876, #38407, #55371, #23415, #912, #68908, #16887, #31375, #61873, #47854, #24886, #31861, #437, #24395, #62360, #53390, #92378, #69888, #92864, #77366, #78359, #39876, #68413, #32358, #98935, #45909, #39395, #8877, #85374, #7912, #30888, #61383, #23904, #70383, #84404, #8394, #54862, #91893, #84884, #85873, #30390, #9374, #9879, #60893, #76879, #54373, #1408, #16392, #38903, #47364, #77863, #53897, #1902, #62865, #69390, #15902, #22921, #91393, #93360, #83899, #15431, #46393, #76397, #40379, #33336, #63831, #57323, #18851, #72811, #94344, #56359, #41856, #25862, #49331, #57814, #2885, #80330, #42337, #86854, #71844, #26338, #95330, #78855, #94834, #25383, #10367, #34312, #3854, #88323, #40867, #26829, #18360, #48838, #50310, #3354, #95834, #19337, #19821, #87816, #80825, #72321, #49820, #2396, #64811, #17865, #33816, #79349, #64323, #48350, #10856, #70879, #4352, #41377, #11829, #56838, #87336, #71372, #34818, #32850, #79833, #11337, #65308 ) ),
 .UNSPECIFIED., .F., .F., .F. ) 
 B_SPLINE_SURFACE_WITH_KNOTS ( ( 2, 2 ),
 ( 3, 2, 2, 2, 2, 2, 2, 2, 2, 2, 2, 2, 2, 2, 2, 2, 2, 2, 2, 2, 2, 2, 2, 2, 2, 2, 2, 2, 2, 2, 2, 2, 2, 2, 2, 2, 2, 2, 2, 2, 2, 2, 2, 2, 2, 2, 2, 2, 2, 2, 2, 2, 2, 2, 2, 2, 2, 2, 2, 2, 2, 2, 2, 2, 2, 2, 2, 2, 2, 2, 2, 2, 2, 2, 2, 2, 2, 2, 2, 2, 2, 2, 2, 2, 2, 2, 2, 2, 2, 2, 2, 2, 2, 2, 2, 2, 2, 2, 2, 2, 2, 2, 2, 2, 2, 2, 2, 2, 2, 2, 2, 2, 2, 2, 2, 2, 2, 2, 2, 2, 2, 2, 2, 2, 2, 2, 2, 2, 2, 2, 2, 2, 2, 2, 2, 2, 2, 2, 2, 2, 2, 2, 2, 2, 2, 2, 2, 2, 2, 2, 2, 2, 2, 2, 2, 2, 2, 2, 2, 2, 2, 2, 3 ),
 ( 0.000000000000000000, 1.000000000000000000 ),
 ( 0.000000000000000000, 0.005952380952380952051, 0.01190476190476190410, 0.01785714285714285615, 0.02380952380952380820, 0.02976190476190476025, 0.03571428571428571230, 0.04166666666666666435, 0.04761904761904761640, 0.05357142857142856845, 0.05952380952380952051, 0.06547619047619047949, 0.07142857142857142461, 0.07738095238095238360, 0.08333333333333332871, 0.08928571428571428770, 0.09523809523809523281, 0.1011904761904761918, 0.1071428571428571369, 0.1130952380952380959, 0.1190476190476190410, 0.1250000000000000000, 0.1309523809523809590, 0.1369047619047619180, 0.1428571428571428492, 0.1488095238095238082, 0.1547619047619047672, 0.1607142857142857262, 0.1666666666666666574, 0.1726190476190476164, 0.1785714285714285754, 0.1845238095238095344, 0.1904761904761904656, 0.1964285714285714246, 0.2023809523809523836, 0.2083333333333333426, 0.2142857142857142738, 0.2202380952380952328, 0.2261904761904761918, 0.2321428571428571508, 0.2380952380952380820, 0.2440476190476190410, 0.2500000000000000000, 0.2559523809523809312, 0.2619047619047619180, 0.2678571428571428492, 0.2738095238095238360, 0.2797619047619047672, 0.2857142857142856984, 0.2916666666666666852, 0.2976190476190476164, 0.3035714285714285476, 0.3095238095238095344, 0.3154761904761904656, 0.3214285714285714524, 0.3273809523809523836, 0.3333333333333333148, 0.3392857142857143016, 0.3452380952380952328, 0.3511904761904761640, 0.3571428571428571508, 0.3630952380952380820, 0.3690476190476190688, 0.3750000000000000000, 0.3809523809523809312, 0.3869047619047619180, 0.3928571428571428492, 0.3988095238095238360, 0.4047619047619047672, 0.4107142857142856984, 0.4166666666666666852, 0.4226190476190476164, 0.4285714285714285476, 0.4345238095238095344, 0.4404761904761904656, 0.4464285714285714524, 0.4523809523809523836, 0.4583333333333333148, 0.4642857142857143016, 0.4702380952380952328, 0.4761904761904761640, 0.4821428571428571508, 0.4880952380952380820, 0.4940476190476190688, 0.5000000000000000000, 0.5059523809523809312, 0.5119047619047618625, 0.5178571428571429047, 0.5238095238095238360, 0.5297619047619047672, 0.5357142857142856984, 0.5416666666666666297, 0.5476190476190476719, 0.5535714285714286031, 0.5595238095238095344, 0.5654761904761904656, 0.5714285714285713969, 0.5773809523809523281, 0.5833333333333333703, 0.5892857142857143016, 0.5952380952380952328, 0.6011904761904761640, 0.6071428571428570953, 0.6130952380952381375, 0.6190476190476190688, 0.6250000000000000000, 0.6309523809523809312, 0.6369047619047618625, 0.6428571428571429047, 0.6488095238095238360, 0.6547619047619047672, 0.6607142857142856984, 0.6666666666666666297, 0.6726190476190476719, 0.6785714285714286031, 0.6845238095238095344, 0.6904761904761904656, 0.6964285714285713969, 0.7023809523809523281, 0.7083333333333333703, 0.7142857142857143016, 0.7202380952380952328, 0.7261904761904761640, 0.7321428571428570953, 0.7380952380952381375, 0.7440476190476190688, 0.7500000000000000000, 0.7559523809523809312, 0.7619047619047618625, 0.7678571428571429047, 0.7738095238095238360, 0.7797619047619047672, 0.7857142857142856984, 0.7916666666666666297, 0.7976190476190476719, 0.8035714285714286031, 0.8095238095238095344, 0.8154761904761904656, 0.8214285714285713969, 0.8273809523809523281, 0.8333333333333333703, 0.8392857142857143016, 0.8452380952380952328, 0.8511904761904761640, 0.8571428571428570953, 0.8630952380952381375, 0.8690476190476190688, 0.8750000000000000000, 0.8809523809523809312, 0.8869047619047618625, 0.8928571428571429047, 0.8988095238095238360, 0.9047619047619047672, 0.9107142857142856984, 0.9166666666666666297, 0.9226190476190476719, 0.9285714285714286031, 0.9345238095238095344, 0.9404761904761904656, 0.9464285714285713969, 0.9523809523809523281, 0.9583333333333333703, 0.9642857142857143016 ),
 .UNSPECIFIED. ) 
 GEOMETRIC_REPRESENTATION_ITEM ( )  RATIONAL_B_SPLINE_SURFACE ( (
 ( 1.000000000000000000, 0.9659258262890683122, 1.000000000000000000, 0.9659258262890683122, 1.000000000000000000, 0.9659258262890683122, 1.000000000000000000, 0.9659258262890683122, 1.000000000000000000, 0.9659258262890683122, 1.000000000000000000, 0.9659258262890683122, 1.000000000000000000, 0.9659258262890683122, 1.000000000000000000, 0.9659258262890683122, 1.000000000000000000, 0.9659258262890683122, 1.000000000000000000, 0.9659258262890683122, 1.000000000000000000, 0.9659258262890683122, 1.000000000000000000, 0.9659258262890683122, 1.000000000000000000, 0.9659258262890683122, 1.000000000000000000, 0.9659258262890683122, 1.000000000000000000, 0.9659258262890683122, 1.000000000000000000, 0.9659258262890683122, 1.000000000000000000, 0.9659258262890683122, 1.000000000000000000, 0.9659258262890683122, 1.000000000000000000, 0.9659258262890683122, 1.000000000000000000, 0.9659258262890683122, 1.000000000000000000, 0.9659258262890683122, 1.000000000000000000, 0.9659258262890683122, 1.000000000000000000, 0.9659258262890683122, 1.000000000000000000, 0.9659258262890683122, 1.000000000000000000, 0.9659258262890683122, 1.000000000000000000, 0.9659258262890683122, 1.000000000000000000, 0.9659258262890683122, 1.000000000000000000, 0.9659258262890683122, 1.000000000000000000, 0.9659258262890683122, 1.000000000000000000, 0.9659258262890683122, 1.000000000000000000, 0.9659258262890683122, 1.000000000000000000, 0.9659258262890683122, 1.000000000000000000, 0.9659258262890683122, 1.000000000000000000, 0.9659258262890683122, 1.000000000000000000, 0.9659258262890683122, 1.000000000000000000, 0.9659258262890683122, 1.000000000000000000, 0.9659258262890683122, 1.000000000000000000, 0.9659258262890683122, 1.000000000000000000, 0.9659258262890683122, 1.000000000000000000, 0.9659258262890683122, 1.000000000000000000, 0.9659258262890683122, 1.000000000000000000, 0.9659258262890683122, 1.000000000000000000, 0.9659258262890683122, 1.000000000000000000, 0.9659258262890683122, 1.000000000000000000, 0.9659258262890683122, 1.000000000000000000, 0.9659258262890683122, 1.000000000000000000, 0.9659258262890683122, 1.000000000000000000, 0.9659258262890683122, 1.000000000000000000, 0.9659258262890683122, 1.000000000000000000, 0.9659258262890683122, 1.000000000000000000, 0.9659258262890683122, 1.000000000000000000, 0.9659258262890683122, 1.000000000000000000, 0.9659258262890683122, 1.000000000000000000, 0.9659258262890683122, 1.000000000000000000, 0.9659258262890683122, 1.000000000000000000, 0.9659258262890683122, 1.000000000000000000, 0.9659258262890683122, 1.000000000000000000, 0.9659258262890683122, 1.000000000000000000, 0.9659258262890683122, 1.000000000000000000, 0.9659258262890683122, 1.000000000000000000, 0.9659258262890683122, 1.000000000000000000, 0.9659258262890683122, 1.000000000000000000, 0.9659258262890683122, 1.000000000000000000, 0.9659258262890683122, 1.000000000000000000, 0.9659258262890683122, 1.000000000000000000, 0.9659258262890683122, 1.000000000000000000, 0.9659258262890683122, 1.000000000000000000, 0.9659258262890683122, 1.000000000000000000, 0.9659258262890683122, 1.000000000000000000, 0.9659258262890683122, 1.000000000000000000, 0.9659258262890683122, 1.000000000000000000, 0.9659258262890683122, 1.000000000000000000, 0.9659258262890683122, 1.000000000000000000, 0.9659258262890683122, 1.000000000000000000, 0.9659258262890683122, 1.000000000000000000, 0.9659258262890683122, 1.000000000000000000, 0.9659258262890683122, 1.000000000000000000, 0.9659258262890683122, 1.000000000000000000, 0.9659258262890683122, 1.000000000000000000, 0.9659258262890683122, 1.000000000000000000, 0.9659258262890683122, 1.000000000000000000, 0.9659258262890683122, 1.000000000000000000, 0.9659258262890683122, 1.000000000000000000, 0.9659258262890683122, 1.000000000000000000, 0.9659258262890683122, 1.000000000000000000, 0.9659258262890683122, 1.000000000000000000, 0.9659258262890683122, 1.000000000000000000, 0.9659258262890683122, 1.000000000000000000, 0.9659258262890683122, 1.000000000000000000, 0.9659258262890683122, 1.000000000000000000, 0.9659258262890683122, 1.000000000000000000, 0.9659258262890683122, 1.000000000000000000, 0.9659258262890683122, 1.000000000000000000, 0.9659258262890683122, 1.000000000000000000, 0.9659258262890683122, 1.000000000000000000, 0.9659258262890683122, 1.000000000000000000, 0.9659258262890683122, 1.000000000000000000, 0.9659258262890683122, 1.000000000000000000, 0.9659258262890683122, 1.000000000000000000, 0.9659258262890683122, 1.000000000000000000, 0.9659258262890683122, 1.000000000000000000, 0.9659258262890683122, 1.000000000000000000, 0.9659258262890683122, 1.000000000000000000, 0.9659258262890683122, 1.000000000000000000, 0.9659258262890683122, 1.000000000000000000, 0.9659258262890683122, 1.000000000000000000, 0.9659258262890683122, 1.000000000000000000, 0.9659258262890683122, 1.000000000000000000, 0.9659258262890683122, 1.000000000000000000, 0.9659258262890683122, 1.000000000000000000, 0.9659258262890683122, 1.000000000000000000, 0.9659258262890683122, 1.000000000000000000, 0.9659258262890683122, 1.000000000000000000, 0.9659258262890683122, 1.000000000000000000, 0.9659258262890683122, 1.000000000000000000, 0.9659258262890683122, 1.000000000000000000, 0.9659258262890683122, 1.000000000000000000, 0.9659258262890683122, 1.000000000000000000, 0.9659258262890683122, 1.000000000000000000, 0.9659258262890683122, 1.000000000000000000, 0.9659258262890683122, 1.000000000000000000, 0.9659258262890683122, 1.000000000000000000, 0.9659258262890683122, 1.000000000000000000, 0.9659258262890683122, 1.000000000000000000, 0.9659258262890683122, 1.000000000000000000, 0.9659258262890683122, 1.000000000000000000, 0.9659258262890683122, 1.000000000000000000, 0.9659258262890683122, 1.000000000000000000, 0.9659258262890683122, 1.000000000000000000, 0.9659258262890683122, 1.000000000000000000, 0.9659258262890683122, 1.000000000000000000, 0.9659258262890683122, 1.000000000000000000, 0.9659258262890683122, 1.000000000000000000, 0.9659258262890683122, 1.000000000000000000, 0.9659258262890683122, 1.000000000000000000, 0.9659258262890683122, 1.000000000000000000, 0.9659258262890683122, 1.000000000000000000, 0.9659258262890683122, 1.000000000000000000, 0.9659258262890683122, 1.000000000000000000, 0.9659258262890683122, 1.000000000000000000, 0.9659258262890683122, 1.000000000000000000, 0.9659258262890683122, 1.000000000000000000, 0.9659258262890683122, 1.000000000000000000, 0.9659258262890683122, 1.000000000000000000, 0.9659258262890683122, 1.000000000000000000, 0.9659258262890683122, 1.000000000000000000, 0.9659258262890683122, 1.000000000000000000, 0.9659258262890683122, 1.000000000000000000, 0.9659258262890683122, 1.000000000000000000, 0.9659258262890683122, 1.000000000000000000, 0.9659258262890683122, 1.000000000000000000, 0.9659258262890683122, 1.000000000000000000, 0.9659258262890683122, 1.000000000000000000, 0.9659258262890683122, 1.000000000000000000, 0.9659258262890683122, 1.000000000000000000, 0.9659258262890683122, 1.000000000000000000, 0.9659258262890683122, 1.000000000000000000, 0.9659258262890683122, 1.000000000000000000, 0.9659258262890683122, 1.000000000000000000, 0.9659258262890683122, 1.000000000000000000, 0.9659258262890683122, 1.000000000000000000, 0.9659258262890683122, 1.000000000000000000),
 ( 1.000000000000000000, 0.9659258262890683122, 1.000000000000000000, 0.9659258262890683122, 1.000000000000000000, 0.9659258262890683122, 1.000000000000000000, 0.9659258262890683122, 1.000000000000000000, 0.9659258262890683122, 1.000000000000000000, 0.9659258262890683122, 1.000000000000000000, 0.9659258262890683122, 1.000000000000000000, 0.9659258262890683122, 1.000000000000000000, 0.9659258262890683122, 1.000000000000000000, 0.9659258262890683122, 1.000000000000000000, 0.9659258262890683122, 1.000000000000000000, 0.9659258262890683122, 1.000000000000000000, 0.9659258262890683122, 1.000000000000000000, 0.9659258262890683122, 1.000000000000000000, 0.9659258262890683122, 1.000000000000000000, 0.9659258262890683122, 1.000000000000000000, 0.9659258262890683122, 1.000000000000000000, 0.9659258262890683122, 1.000000000000000000, 0.9659258262890683122, 1.000000000000000000, 0.9659258262890683122, 1.000000000000000000, 0.9659258262890683122, 1.000000000000000000, 0.9659258262890683122, 1.000000000000000000, 0.9659258262890683122, 1.000000000000000000, 0.9659258262890683122, 1.000000000000000000, 0.9659258262890683122, 1.000000000000000000, 0.9659258262890683122, 1.000000000000000000, 0.9659258262890683122, 1.000000000000000000, 0.9659258262890683122, 1.000000000000000000, 0.9659258262890683122, 1.000000000000000000, 0.9659258262890683122, 1.000000000000000000, 0.9659258262890683122, 1.000000000000000000, 0.9659258262890683122, 1.000000000000000000, 0.9659258262890683122, 1.000000000000000000, 0.9659258262890683122, 1.000000000000000000, 0.9659258262890683122, 1.000000000000000000, 0.9659258262890683122, 1.000000000000000000, 0.9659258262890683122, 1.000000000000000000, 0.9659258262890683122, 1.000000000000000000, 0.9659258262890683122, 1.000000000000000000, 0.9659258262890683122, 1.000000000000000000, 0.9659258262890683122, 1.000000000000000000, 0.9659258262890683122, 1.000000000000000000, 0.9659258262890683122, 1.000000000000000000, 0.9659258262890683122, 1.000000000000000000, 0.9659258262890683122, 1.000000000000000000, 0.9659258262890683122, 1.000000000000000000, 0.9659258262890683122, 1.000000000000000000, 0.9659258262890683122, 1.000000000000000000, 0.9659258262890683122, 1.000000000000000000, 0.9659258262890683122, 1.000000000000000000, 0.9659258262890683122, 1.000000000000000000, 0.9659258262890683122, 1.000000000000000000, 0.9659258262890683122, 1.000000000000000000, 0.9659258262890683122, 1.000000000000000000, 0.9659258262890683122, 1.000000000000000000, 0.9659258262890683122, 1.000000000000000000, 0.9659258262890683122, 1.000000000000000000, 0.9659258262890683122, 1.000000000000000000, 0.9659258262890683122, 1.000000000000000000, 0.9659258262890683122, 1.000000000000000000, 0.9659258262890683122, 1.000000000000000000, 0.9659258262890683122, 1.000000000000000000, 0.9659258262890683122, 1.000000000000000000, 0.9659258262890683122, 1.000000000000000000, 0.9659258262890683122, 1.000000000000000000, 0.9659258262890683122, 1.000000000000000000, 0.9659258262890683122, 1.000000000000000000, 0.9659258262890683122, 1.000000000000000000, 0.9659258262890683122, 1.000000000000000000, 0.9659258262890683122, 1.000000000000000000, 0.9659258262890683122, 1.000000000000000000, 0.9659258262890683122, 1.000000000000000000, 0.9659258262890683122, 1.000000000000000000, 0.9659258262890683122, 1.000000000000000000, 0.9659258262890683122, 1.000000000000000000, 0.9659258262890683122, 1.000000000000000000, 0.9659258262890683122, 1.000000000000000000, 0.9659258262890683122, 1.000000000000000000, 0.9659258262890683122, 1.000000000000000000, 0.9659258262890683122, 1.000000000000000000, 0.9659258262890683122, 1.000000000000000000, 0.9659258262890683122, 1.000000000000000000, 0.9659258262890683122, 1.000000000000000000, 0.9659258262890683122, 1.000000000000000000, 0.9659258262890683122, 1.000000000000000000, 0.9659258262890683122, 1.000000000000000000, 0.9659258262890683122, 1.000000000000000000, 0.9659258262890683122, 1.000000000000000000, 0.9659258262890683122, 1.000000000000000000, 0.9659258262890683122, 1.000000000000000000, 0.9659258262890683122, 1.000000000000000000, 0.9659258262890683122, 1.000000000000000000, 0.9659258262890683122, 1.000000000000000000, 0.9659258262890683122, 1.000000000000000000, 0.9659258262890683122, 1.000000000000000000, 0.9659258262890683122, 1.000000000000000000, 0.9659258262890683122, 1.000000000000000000, 0.9659258262890683122, 1.000000000000000000, 0.9659258262890683122, 1.000000000000000000, 0.9659258262890683122, 1.000000000000000000, 0.9659258262890683122, 1.000000000000000000, 0.9659258262890683122, 1.000000000000000000, 0.9659258262890683122, 1.000000000000000000, 0.9659258262890683122, 1.000000000000000000, 0.9659258262890683122, 1.000000000000000000, 0.9659258262890683122, 1.000000000000000000, 0.9659258262890683122, 1.000000000000000000, 0.9659258262890683122, 1.000000000000000000, 0.9659258262890683122, 1.000000000000000000, 0.9659258262890683122, 1.000000000000000000, 0.9659258262890683122, 1.000000000000000000, 0.9659258262890683122, 1.000000000000000000, 0.9659258262890683122, 1.000000000000000000, 0.9659258262890683122, 1.000000000000000000, 0.9659258262890683122, 1.000000000000000000, 0.9659258262890683122, 1.000000000000000000, 0.9659258262890683122, 1.000000000000000000, 0.9659258262890683122, 1.000000000000000000, 0.9659258262890683122, 1.000000000000000000, 0.9659258262890683122, 1.000000000000000000, 0.9659258262890683122, 1.000000000000000000, 0.9659258262890683122, 1.000000000000000000, 0.9659258262890683122, 1.000000000000000000, 0.9659258262890683122, 1.000000000000000000, 0.9659258262890683122, 1.000000000000000000, 0.9659258262890683122, 1.000000000000000000, 0.9659258262890683122, 1.000000000000000000, 0.9659258262890683122, 1.000000000000000000, 0.9659258262890683122, 1.000000000000000000, 0.9659258262890683122, 1.000000000000000000, 0.9659258262890683122, 1.000000000000000000, 0.9659258262890683122, 1.000000000000000000, 0.9659258262890683122, 1.000000000000000000, 0.9659258262890683122, 1.000000000000000000, 0.9659258262890683122, 1.000000000000000000, 0.9659258262890683122, 1.000000000000000000, 0.9659258262890683122, 1.000000000000000000, 0.9659258262890683122, 1.000000000000000000, 0.9659258262890683122, 1.000000000000000000, 0.9659258262890683122, 1.000000000000000000, 0.9659258262890683122, 1.000000000000000000, 0.9659258262890683122, 1.000000000000000000, 0.9659258262890683122, 1.000000000000000000, 0.9659258262890683122, 1.000000000000000000, 0.9659258262890683122, 1.000000000000000000, 0.9659258262890683122, 1.000000000000000000, 0.9659258262890683122, 1.000000000000000000, 0.9659258262890683122, 1.000000000000000000, 0.9659258262890683122, 1.000000000000000000, 0.9659258262890683122, 1.000000000000000000, 0.9659258262890683122, 1.000000000000000000, 0.9659258262890683122, 1.000000000000000000, 0.9659258262890683122, 1.000000000000000000, 0.9659258262890683122, 1.000000000000000000, 0.9659258262890683122, 1.000000000000000000, 0.9659258262890683122, 1.000000000000000000, 0.9659258262890683122, 1.000000000000000000, 0.9659258262890683122, 1.000000000000000000, 0.9659258262890683122, 1.000000000000000000, 0.9659258262890683122, 1.000000000000000000, 0.9659258262890683122, 1.000000000000000000, 0.9659258262890683122, 1.000000000000000000) ) ) 
 REPRESENTATION_ITEM ( '' )  SURFACE ( )  );
#25162=CARTESIAN_POINT ( 'NONE',  ( 2.917880565312948704, 47.63708216824730357, 12.26659068614894643 ) ) ;
#25164=CARTESIAN_POINT ( 'NONE',  ( 10.00000000000000000, 55.55374883491396787, -14.16423886937410082 ) ) ;
#25165=ORIENTED_EDGE ( 'NONE', *, *, #8268, .T. ) ;
#25166=CARTESIAN_POINT ( 'NONE',  ( 12.91533473730992121, 39.52201867748817676, 10.88017736071110164 ) ) ;
#25167=CARTESIAN_POINT ( 'NONE',  ( -0.8801773607110991993, 42.85535201082150536, -2.915334737309923874 ) ) ;
#25168=CARTESIAN_POINT ( 'NONE',  ( 17.96484262340118221, 36.18868534415484106, -7.964842623401177768 ) ) ;
#25169=CARTESIAN_POINT ( 'NONE',  ( 17.96484262340118221, 66.18868534415483396, -7.964842623401177768 ) ) ;
#25170=CARTESIAN_POINT ( 'NONE',  ( 12.91533473730992121, 24.52201867748816966, 10.88017736071110164 ) ) ;
#25174=CARTESIAN_POINT ( 'NONE',  ( 19.84674366389459266, 18.71726448433411960, -2.638427012816827677 ) ) ;
#25175=VERTEX_POINT ( 'NONE', #47523 ) ;
#25176=CARTESIAN_POINT ( 'NONE',  ( 17.20831665107776587, 42.88393115100077324, 7.208316651077764980 ) ) ;
#25178=CARTESIAN_POINT ( 'NONE',  ( -2.816281873526473856, 44.12363466993042493, 9.499525473075851096E-16 ) ) ;
#25181=ORIENTED_EDGE ( 'NONE', *, *, #90304, .F. ) ;
#25182=CARTESIAN_POINT ( 'NONE',  ( -46.07360246527841952, 103.8701977390176552, 6.036219926076657138 ) ) ;
#25183=CARTESIAN_POINT ( 'NONE',  ( 5.076628168052703671, 56.84226448433412315, 8.527530157486179263 ) ) ;
#25184=CARTESIAN_POINT ( 'NONE',  ( -2.266590686148945544, 51.38708216824730357, -7.082119434687050408 ) ) ;
#25185=CARTESIAN_POINT ( 'NONE',  ( 0.1532563361054083140, 66.00893115100079456, 1.131784320476157264E-15 ) ) ;
#25188=CARTESIAN_POINT ( 'NONE',  ( 2.791683348922237240, 20.38393115100078745, -7.208316651077763204 ) ) ;
#25190=CARTESIAN_POINT ( 'NONE',  ( 21.09922568453594849, 46.20696800326376064, 6.408140936763242479 ) ) ;
#25191=CARTESIAN_POINT ( 'NONE',  ( 5.076628168052704559, 65.17559781766745175, -8.527530157486179263 ) ) ;
#25192=CARTESIAN_POINT ( 'NONE',  ( 19.42250999205614548, 60.98035201082151247, -5.440088680355545492 ) ) ;
#25195=CARTESIAN_POINT ( 'NONE',  ( 5.076628168052704559, 50.17559781766745886, -8.527530157486179263 ) ) ;
#25197=CARTESIAN_POINT ( 'NONE',  ( 21.92686044187657401, 15.37045670184114243, -3.195792623639525765 ) ) ;
#25199=CARTESIAN_POINT ( 'NONE',  ( -0.3689425029237898834, 66.17874883491396076, -10.36894250292378850 ) ) ;
#25200=CARTESIAN_POINT ( 'NONE',  ( -0.1503990784575328643, 0.07447313448805115144, 6.262539305110068177 ) ) ;
#25201=CARTESIAN_POINT ( 'NONE',  ( 7.084665262690076126, 44.10535201082151247, 10.88017736071109987 ) ) ;
#25202=CARTESIAN_POINT ( 'NONE',  ( 10.00000000000000000, 7.873634669930421381, -12.81628187352647608 ) ) ;
#25203=CARTESIAN_POINT ( 'NONE',  ( 20.88017736071110875, 60.77201867748817676, -2.915334737309920765 ) ) ;
#25204=CARTESIAN_POINT ( 'NONE',  ( -0.2418659066527716062, 62.23410085661205216, -6.114288769123046308 ) ) ;
#25207=CARTESIAN_POINT ( 'NONE',  ( 18.72515096720568906, 36.07228050351032778, -6.500000000000007105 ) ) ;
#25208=CARTESIAN_POINT ( 'NONE',  ( 7.361572987183170547, 47.05059781766745175, 9.846743663894590881 ) ) ;
#25209=( NAMED_UNIT ( * ) PLANE_ANGLE_UNIT ( ) SI_UNIT ( $, .RADIAN. ) );
#25211=CARTESIAN_POINT ( 'NONE',  ( 3.591859063236763294, 8.290301336597087456, -11.09922568453595026 ) ) ;
#25212=CARTESIAN_POINT ( 'NONE',  ( 4.559911319644449179, 7.230352010821505360, -9.422509992056141925 ) ) ;
#25214=CARTESIAN_POINT ( 'NONE',  ( -2.266590686148945544, 36.38708216824730357, -7.082119434687050408 ) ) ;
#25215=CARTESIAN_POINT ( 'NONE',  ( 24.16423886937409904, 34.09541550158064638, 3.795296366450317205 ) ) ;
#25216=CARTESIAN_POINT ( 'NONE',  ( 4.559911319644449179, 2.230352010821504916, -9.422509992056141925 ) ) ;
#25217=CARTESIAN_POINT ( 'NONE',  ( 19.84674366389459266, 28.30059781766745886, 2.638427012816836559 ) ) ;
#25218=CARTESIAN_POINT ( 'NONE',  ( 6.565887622018943937, 40.16530133659708923, 12.81628187352647430 ) ) ;
#25219=CARTESIAN_POINT ( 'NONE',  ( 20.88017736071110164, 10.35535201082150714, 2.915334737309930979 ) ) ;
#25221=CARTESIAN_POINT ( 'NONE',  ( 19.84674366389459621, 38.50893115100078745, 7.409399052514197653E-17 ) ) ;
#25223=CARTESIAN_POINT ( 'NONE',  ( 12.91533473730993009, 36.60535201082151247, -10.88017736071109987 ) ) ;
#25224=CARTESIAN_POINT ( 'NONE',  ( 17.20831665107776587, 62.88393115100078745, 7.208316651077764980 ) ) ;
#25225=CARTESIAN_POINT ( 'NONE',  ( 6.204703633549690345, 25.76208216824730712, -14.16423886937410259 ) ) ;
#25229=CARTESIAN_POINT ( 'NONE',  ( 14.92337183194729633, 22.67559781766745175, 8.527530157486181039 ) ) ;
#25230=CARTESIAN_POINT ( 'NONE',  ( 21.09922568453595559, 57.04030133659708923, -6.408140936763230044 ) ) ;
#25231=CARTESIAN_POINT ( 'NONE',  ( 19.84674366389459266, 48.30059781766745175, 2.638427012816836559 ) ) ;
#25232=ORIENTED_EDGE ( 'NONE', *, *, #39854, .T. ) ;
#25234=DIRECTION ( 'NONE',  ( 0.000000000000000000, 0.000000000000000000, -1.000000000000000000 ) ) ;
#25235=CARTESIAN_POINT ( 'NONE',  ( 4.559911319644449179, 2.230352010821504916, -9.422509992056141925 ) ) ;
#25236=CARTESIAN_POINT ( 'NONE',  ( 2.917880565312950480, 15.97041550158063217, -12.26659068614894821 ) ) ;
#25237=CARTESIAN_POINT ( 'NONE',  ( -0.8801773607111008646, 68.27201867748817676, 2.915334737309923430 ) ) ;
#25238=CARTESIAN_POINT ( 'NONE',  ( 2.791683348922240793, 56.63393115100078035, 7.208316651077764092 ) ) ;
#25239=CARTESIAN_POINT ( 'NONE',  ( 2.035157376598822676, 17.43868534415483751, -7.964842623401177768 ) ) ;
#25241=CARTESIAN_POINT ( 'NONE',  ( 0.2751277870542967463, 70.00000000000000000, 6.000000000000000000 ) ) ;
#25242=CARTESIAN_POINT ( 'NONE',  ( 10.00000000000000000, 4.758931151000784787, -9.846743663894594434 ) ) ;
#25243=CARTESIAN_POINT ( 'NONE',  ( -1.099225684535947600, 58.70696800326375353, -6.408140936763238038 ) ) ;
#25247=CARTESIAN_POINT ( 'NONE',  ( 18.95785429995052240, 42.24216108172005590, 6.499999999999943157 ) ) ;
#25248=FILL_AREA_STYLE_COLOUR ( '', #34929 ) ;
#25249=CARTESIAN_POINT ( 'NONE',  ( 22.26659068614894466, 38.88708216824731068, 7.082119434687054849 ) ) ;
#25250=CARTESIAN_POINT ( 'NONE',  ( 2.791683348922237240, 55.38393115100078745, -7.208316651077763204 ) ) ;
#25251=CARTESIAN_POINT ( 'NONE',  ( 19.84674366389459266, 18.30059781766745175, 2.638427012816836559 ) ) ;
#25252=CARTESIAN_POINT ( 'NONE',  ( 17.96484262340118221, 26.18868534415483396, -7.964842623401177768 ) ) ;
#25253=CARTESIAN_POINT ( 'NONE',  ( 14.92337183194729988, 59.34226448433412315, -8.527530157486177487 ) ) ;
#25255=CARTESIAN_POINT ( 'NONE',  ( -0.3689425029237898834, 36.17874883491396787, -10.36894250292378850 ) ) ;
#25256=CARTESIAN_POINT ( 'NONE',  ( 7.084665262690076126, 9.105352010821503583, 10.88017736071109987 ) ) ;
#25258=CARTESIAN_POINT ( 'NONE',  ( 2.035157376598824452, 63.68868534415484106, 7.964842623401179544 ) ) ;
#25259=CARTESIAN_POINT ( 'NONE',  ( 19.84674366389459266, 18.71726448433411960, -2.638427012816827677 ) ) ;
#25260=AXIS2_PLACEMENT_3D ( 'NONE', #62650, #68697, #92182 ) ;
#25265=CARTESIAN_POINT ( 'NONE',  ( 6.565887622018943937, 65.16530133659709634, 12.81628187352647430 ) ) ;
#25267=CARTESIAN_POINT ( 'NONE',  ( 0.1532563361054082862, 26.21726448433411605, 2.638427012816831674 ) ) ;
#25268=ORIENTED_EDGE ( 'NONE', *, *, #86597, .F. ) ;
#25269=CARTESIAN_POINT ( 'NONE',  ( 2.917880565312948704, 37.63708216824731068, 12.26659068614894643 ) ) ;
#25270=CARTESIAN_POINT ( 'NONE',  ( 0.1532563361054100626, 35.80059781766745175, -2.638427012816831230 ) ) ;
#25271=CARTESIAN_POINT ( 'NONE',  ( 2.035157376598822676, 37.43868534415484106, -7.964842623401177768 ) ) ;
#25273=STYLED_ITEM ( 'NONE', ( #36999 ), #58465 ) ;
#25274=PLANE ( 'NONE',  #32015 ) ;
#25277=CARTESIAN_POINT ( 'NONE',  ( 20.88017736071110164, 40.35535201082150536, 2.915334737309930979 ) ) ;
#25280=CARTESIAN_POINT ( 'NONE',  ( 2.917880565312950480, 10.97041550158063572, -12.26659068614894821 ) ) ;
#25282=CARTESIAN_POINT ( 'NONE',  ( 21.09922568453594849, 36.20696800326375353, 6.408140936763242479 ) ) ;
#25283=CARTESIAN_POINT ( 'NONE',  ( 14.92337183194729633, 27.67559781766745530, 8.527530157486181039 ) ) ;
#25284=CARTESIAN_POINT ( 'NONE',  ( -0.8801773607111008646, 3.272018677488171434, 2.915334737309923430 ) ) ;
#25286=CARTESIAN_POINT ( 'NONE',  ( 17.20831665107776587, 34.13393115100078745, -7.208316651077762316 ) ) ;
#25287=ORIENTED_EDGE ( 'NONE', *, *, #34413, .F. ) ;
#25289=CARTESIAN_POINT ( 'NONE',  ( 12.91533473730992121, 54.52201867748816255, 10.88017736071110164 ) ) ;
#25291=CARTESIAN_POINT ( 'NONE',  ( 5.076628168052704559, 0.1755978176674514724, -8.527530157486179263 ) ) ;
#25293=CARTESIAN_POINT ( 'NONE',  ( 10.00000000000000178, 42.25893115100078745, 9.846743663894594434 ) ) ;
#25295=CARTESIAN_POINT ( 'NONE',  ( -4.164238869374099927, 2.012082168247300906, 3.795296366450308767 ) ) ;
#25296=CARTESIAN_POINT ( 'NONE',  ( 12.63842701281683922, 14.55059781766744997, -9.846743663894590881 ) ) ;
#25297=CARTESIAN_POINT ( 'NONE',  ( -2.816281873526473856, 34.12363466993042493, 9.499525473075851096E-16 ) ) ;
#25298=CARTESIAN_POINT ( 'NONE',  ( 1.274849032794164172, 18.57228050351029935, 6.499999999999802824 ) ) ;
#25300=CARTESIAN_POINT ( 'NONE',  ( 17.96484262340118221, 49.93868534415484106, 7.964842623401181321 ) ) ;
#25301=CARTESIAN_POINT ( 'NONE',  ( 6.565887622018943937, 3.081968003263753531, -12.81628187352647608 ) ) ;
#25302=DIRECTION ( 'NONE',  ( -0.000000000000000000, -0.000000000000000000, 1.000000000000000000 ) ) ;
#25303=CARTESIAN_POINT ( 'NONE',  ( 10.00000000000000178, 27.25893115100078390, 9.846743663894594434 ) ) ;
#25304=CARTESIAN_POINT ( 'NONE',  ( 5.076628168052703671, 26.84226448433411960, 8.527530157486179263 ) ) ;
#25305=CARTESIAN_POINT ( 'NONE',  ( 15.44008868035555260, 24.73035201082150891, 9.422509992056143702 ) ) ;
#25307=CARTESIAN_POINT ( 'NONE',  ( 0.6178305044545818747, 33.49863466993042493, -9.382169495545419124 ) ) ;
#25309=CARTESIAN_POINT ( 'NONE',  ( 2.791683348922240793, 21.63393115100078745, 7.208316651077764092 ) ) ;
#25311=CARTESIAN_POINT ( 'NONE',  ( 17.39651004071838969, 44.08210964143329846, -6.500000000000027534 ) ) ;
#25312=CARTESIAN_POINT ( 'NONE',  ( 12.91533473730992121, 19.52201867748816611, 10.88017736071110164 ) ) ;
#25314=CARTESIAN_POINT ( 'NONE',  ( 17.96484262340118221, 61.18868534415482685, -7.964842623401177768 ) ) ;
#25315=B_SPLINE_CURVE_WITH_KNOTS ( 'NONE', 3,
 ( #23125, #39108, #37139, #60108, #69597, #52615, #76598, #30100, #75614, #16104 ),
 .UNSPECIFIED., .F., .F.,
 ( 4, 3, 3, 4 ),
 ( 7.796612332912425077E-17, 0.0006253016069560803211, 0.001250604074564920856, 0.002501455912506534394 ),
 .UNSPECIFIED. ) ;
#25316=CARTESIAN_POINT ( 'NONE',  ( 18.52753015748617571, 38.09226448433412315, 4.923371831947298993 ) ) ;
#25317=CARTESIAN_POINT ( 'NONE',  ( 10.00000000000000178, 19.31368534415484106, 10.88017736071110342 ) ) ;
#25318=FILL_AREA_STYLE ('',( #85807 ) ) ;
#25319=CARTESIAN_POINT ( 'NONE',  ( 2.035157376598822676, 52.43868534415483396, -7.964842623401177768 ) ) ;
#25321=CARTESIAN_POINT ( 'NONE',  ( 0.5774900079438590739, 17.64701867748817321, -5.440088680355550821 ) ) ;
#25322=CARTESIAN_POINT ( 'NONE',  ( 19.80832241502127289, 59.75868815902069997, 6.499999999999984901 ) ) ;
#25324=CARTESIAN_POINT ( 'NONE',  ( 5.076628168052703671, 36.84226448433412315, 8.527530157486179263 ) ) ;
#25328=CARTESIAN_POINT ( 'NONE',  ( -0.3689425029237898834, 1.178748834913967869, -10.36894250292378850 ) ) ;
#25329=VECTOR ( 'NONE', #16026, 1000.000000000000000 ) ;
#25330=CARTESIAN_POINT ( 'NONE',  ( -4.164238869374099927, 22.01208216824730357, 3.795296366450308767 ) ) ;
#25334=CARTESIAN_POINT ( 'NONE',  ( 7.084665262690076126, 7.022018677488170546, -10.88017736071110164 ) ) ;
#25335=CARTESIAN_POINT ( 'NONE',  ( 12.63842701281683034, 27.46726448433411250, 9.846743663894596210 ) ) ;
#25338=CARTESIAN_POINT ( 'NONE',  ( 15.44008868035555793, 41.39701867748817676, -9.422509992056140149 ) ) ;
#25340=CARTESIAN_POINT ( 'NONE',  ( 4.559911319644449179, 18.89701867748817321, 9.422509992056141925 ) ) ;
#25341=CARTESIAN_POINT ( 'NONE',  ( 3.591859063236763294, 48.29030133659708923, -11.09922568453595026 ) ) ;
#25342=CARTESIAN_POINT ( 'NONE',  ( 10.00000000000000000, 12.87363466993042138, -12.81628187352647608 ) ) ;
#25343=CARTESIAN_POINT ( 'NONE',  ( 0.1532563361054082862, 21.21726448433412315, 2.638427012816831674 ) ) ;
#25348=CARTESIAN_POINT ( 'NONE',  ( -0.3689425029237898834, 56.17874883491396076, -10.36894250292378850 ) ) ;
#25349=CARTESIAN_POINT ( 'NONE',  ( 10.00000000000000178, 28.05374883491396787, 14.16423886937410082 ) ) ;
#25350=CARTESIAN_POINT ( 'NONE',  ( 7.084665262690076126, 14.10535201082150358, 10.88017736071109987 ) ) ;
#25351=CARTESIAN_POINT ( 'NONE',  ( 19.42250999205614193, 55.14701867748817676, 5.440088680355555262 ) ) ;
#25354=CARTESIAN_POINT ( 'NONE',  ( 12.63842701281683922, 9.550597817667449974, -9.846743663894590881 ) ) ;
#25355=CARTESIAN_POINT ( 'NONE',  ( 14.92337183194729633, 22.67559781766745175, 8.527530157486181039 ) ) ;
#25356=CARTESIAN_POINT ( 'NONE',  ( 7.361572987183169658, 24.96726448433412315, -9.846743663894592657 ) ) ;
#25357=CARTESIAN_POINT ( 'NONE',  ( 19.84674366389459266, 43.71726448433410894, -2.638427012816827677 ) ) ;
#25358=UNCERTAINTY_MEASURE_WITH_UNIT (LENGTH_MEASURE( 1.000000000000000082E-05 ), #93751, 'distance_accuracy_value', 'NONE');
#25359=CARTESIAN_POINT ( 'NONE',  ( 19.38216949554541202, 35.99863466993041072, 9.382169495545424454 ) ) ;
#25360=CARTESIAN_POINT ( 'NONE',  ( 17.96484262340118221, 56.18868534415484817, -7.964842623401177768 ) ) ;
#25361=CARTESIAN_POINT ( 'NONE',  ( 1.472469842513823179, 35.59226448433412315, -4.923371831947296329 ) ) ;
#25362=CARTESIAN_POINT ( 'NONE',  ( 13.79529636645030344, 43.26208216824730357, 14.16423886937410614 ) ) ;
#25363=CARTESIAN_POINT ( 'NONE',  ( 19.84674366389459266, 28.30059781766745886, 2.638427012816836559 ) ) ;
#25365=CARTESIAN_POINT ( 'NONE',  ( 7.361572987183169658, 54.96726448433413026, -9.846743663894592657 ) ) ;
#25367=CARTESIAN_POINT ( 'NONE',  ( 0.1532563361054100626, 30.80059781766744820, -2.638427012816831230 ) ) ;
#25368=CARTESIAN_POINT ( 'NONE',  ( 20.36894250292379738, 4.928748834913967869, -10.36894250292379027 ) ) ;
#25369=CARTESIAN_POINT ( 'NONE',  ( 20.36894250292379738, 19.92874883491396787, -10.36894250292379027 ) ) ;
#25370=CARTESIAN_POINT ( 'NONE',  ( 5.076628168052703671, 36.84226448433412315, 8.527530157486179263 ) ) ;
#25371=CARTESIAN_POINT ( 'NONE',  ( 19.42250999205614193, 50.14701867748817676, 5.440088680355555262 ) ) ;
#25372=CARTESIAN_POINT ( 'NONE',  ( -0.8801773607111008646, 18.27201867748817321, 2.915334737309923430 ) ) ;
#25373=CARTESIAN_POINT ( 'NONE',  ( 7.084665262690076126, 49.10535201082149825, 10.88017736071109987 ) ) ;
#25374=AXIS2_PLACEMENT_3D ( 'NONE', #92715, #77709, #40215 ) ;
#25375=CARTESIAN_POINT ( 'NONE',  ( -0.8801773607111009756, 33.06368534415484106, 1.068504757029289695E-15 ) ) ;
#25377=CARTESIAN_POINT ( 'NONE',  ( 4.559911319644449179, 52.23035201082151247, -9.422509992056141925 ) ) ;
#25379=CARTESIAN_POINT ( 'NONE',  ( 13.43411237798105340, 60.58196800326376064, 12.81628187352647963 ) ) ;
#25381=CARTESIAN_POINT ( 'NONE',  ( 20.88017736071110164, 60.35535201082151957, 2.915334737309930979 ) ) ;
#25383=CARTESIAN_POINT ( 'NONE',  ( 12.91533473730993009, 61.60535201082150536, -10.88017736071109987 ) ) ;
#25384=CARTESIAN_POINT ( 'NONE',  ( 2.035157376598824452, 3.688685344154837953, 7.964842623401179544 ) ) ;
#25385=CARTESIAN_POINT ( 'NONE',  ( 1.492507162822227951, 27.19955587570481015, -6.499999999999968914 ) ) ;
#25387=CARTESIAN_POINT ( 'NONE',  ( -4.164238869374098151, 61.59541550158063217, -3.795296366450310543 ) ) ;
#25388=CARTESIAN_POINT ( 'NONE',  ( 7.361572987183169658, 4.967264484334119601, -9.846743663894592657 ) ) ;
#25389=CARTESIAN_POINT ( 'NONE',  ( 20.36894250292379382, 8.678748834913967869, 10.36894250292379205 ) ) ;
#25390=CARTESIAN_POINT ( 'NONE',  ( 0.1532563361054083140, 11.00893115100078568, 1.131784320476157264E-15 ) ) ;
#25391=CARTESIAN_POINT ( 'NONE',  ( 0.5774900079438607392, 13.48035201082150358, 5.440088680355550821 ) ) ;
#25392=CARTESIAN_POINT ( 'NONE',  ( 7.361572987183169658, 39.96726448433411605, -9.846743663894592657 ) ) ;
#25393=CARTESIAN_POINT ( 'NONE',  ( 18.52753015748617571, 53.09226448433412315, 4.923371831947298993 ) ) ;
#25396=CARTESIAN_POINT ( 'NONE',  ( 10.00000000000000000, 41.81368534415484106, -10.88017736071110342 ) ) ;
#25397=CARTESIAN_POINT ( 'NONE',  ( 2.791683348922237240, 55.38393115100078745, -7.208316651077763204 ) ) ;
#25398=CARTESIAN_POINT ( 'NONE',  ( 22.81628187352647785, 31.41530133659709279, 3.434112377981063169 ) ) ;
#25399=CARTESIAN_POINT ( 'NONE',  ( 19.72487221294570858, 1.866073187300754110, 6.500000000000000888 ) ) ;
#25400=CARTESIAN_POINT ( 'NONE',  ( -0.8801773607111008646, 58.27201867748816966, 2.915334737309923430 ) ) ;
#25401=CARTESIAN_POINT ( 'NONE',  ( 7.084665262690076126, 7.022018677488170546, -10.88017736071110164 ) ) ;
#25404=CARTESIAN_POINT ( 'NONE',  ( 6.565887622018943937, 48.08196800326375353, -12.81628187352647608 ) ) ;
#25407=CARTESIAN_POINT ( 'NONE',  ( -1.099225684535947600, 24.54030133659708923, 6.408140936763237150 ) ) ;
#25408=CARTESIAN_POINT ( 'NONE',  ( 15.44008868035555260, 34.73035201082151247, 9.422509992056143702 ) ) ;
#25410=ORIENTED_EDGE ( 'NONE', *, *, #87309, .F. ) ;
#25413=CARTESIAN_POINT ( 'NONE',  ( 14.92337183194729988, 4.342264484334117824, -8.527530157486177487 ) ) ;
#25414=CARTESIAN_POINT ( 'NONE',  ( 14.92337183194729988, 59.34226448433412315, -8.527530157486177487 ) ) ;
#25415=CARTESIAN_POINT ( 'NONE',  ( 17.20831665107776587, 12.88393115100078390, 7.208316651077764980 ) ) ;
#25416=CARTESIAN_POINT ( 'NONE',  ( 0.1532563361054082862, 36.21726448433410894, 2.638427012816831674 ) ) ;
#25422=CARTESIAN_POINT ( 'NONE',  ( 12.63842701281683034, 32.46726448433412315, 9.846743663894596210 ) ) ;
#25423=( LENGTH_UNIT ( ) NAMED_UNIT ( * ) SI_UNIT ( .MILLI., .METRE. ) );
#25426=CARTESIAN_POINT ( 'NONE',  ( 18.52753015748618282, 48.92559781766745886, -4.923371831947291888 ) ) ;
#25427=ORIENTED_EDGE ( 'NONE', *, *, #22327, .F. ) ;
#25428=CARTESIAN_POINT ( 'NONE',  ( 22.81628187352648496, 31.83196800326375353, -3.434112377981050290 ) ) ;
#25429=CARTESIAN_POINT ( 'NONE',  ( 12.63842701281683922, 49.55059781766744464, -9.846743663894590881 ) ) ;
#25430=DIRECTION ( 'NONE',  ( 1.000000000000000000, 0.000000000000000000, 0.000000000000000000 ) ) ;
#25431=CARTESIAN_POINT ( 'NONE',  ( 6.204703633549690345, 45.76208216824729647, -14.16423886937410259 ) ) ;
#25433=CARTESIAN_POINT ( 'NONE',  ( 7.361572987183170547, 22.05059781766745530, 9.846743663894590881 ) ) ;
#25434=VERTEX_POINT ( 'NONE', #83198 ) ;
#25437=CARTESIAN_POINT ( 'NONE',  ( -0.3689425029237881626, 37.42874883491396787, 10.36894250292379027 ) ) ;
#25438=CARTESIAN_POINT ( 'NONE',  ( 0.1532563361054083140, 61.00893115100078745, 1.131784320476157264E-15 ) ) ;
#25439=CARTESIAN_POINT ( 'NONE',  ( -4.164238869374099039, 66.80374883491396076, 8.674139862899312516E-16 ) ) ;
#25440=CARTESIAN_POINT ( 'NONE',  ( 6.204703633549690345, 20.76208216824730357, -14.16423886937410259 ) ) ;
#25441=CARTESIAN_POINT ( 'NONE',  ( -0.3689425029237881626, 37.42874883491396787, 10.36894250292379027 ) ) ;
#25444=CARTESIAN_POINT ( 'NONE',  ( 2.791683348922237240, 55.38393115100078745, -7.208316651077763204 ) ) ;
#25446=CARTESIAN_POINT ( 'NONE',  ( 7.084665262690076126, 37.02201867748817676, -10.88017736071110164 ) ) ;
#25447=DIRECTION ( 'NONE',  ( 1.000000000000000000, 0.000000000000000000, -0.000000000000000000 ) ) ;
#25449=CARTESIAN_POINT ( 'NONE',  ( 1.472469842513823179, 41.42559781766745886, 4.923371831947296329 ) ) ;
#25452=CARTESIAN_POINT ( 'NONE',  ( 19.84674366389459266, 53.71726448433411605, -2.638427012816827677 ) ) ;
#25456=CARTESIAN_POINT ( 'NONE',  ( -0.3689425029237898834, 31.17874883491396787, -10.36894250292378850 ) ) ;
#25457=CARTESIAN_POINT ( 'NONE',  ( -46.44000000000001194, 102.9999999999998863, -5.997726559847190053 ) ) ;
#25460=CARTESIAN_POINT ( 'NONE',  ( 20.88017736071110875, 10.77201867748817143, -2.915334737309920765 ) ) ;
#25461=CARTESIAN_POINT ( 'NONE',  ( 16.40814093676323893, 30.79030133659708923, 11.09922568453595026 ) ) ;
#25463=CARTESIAN_POINT ( 'NONE',  ( 2.791683348922237240, 15.38393115100078212, -7.208316651077763204 ) ) ;
#25467=CARTESIAN_POINT ( 'NONE',  ( 20.20021275402706706, 0.02465945891864474576, -6.181800700214930444 ) ) ;
#25469=CARTESIAN_POINT ( 'NONE',  ( 15.44008868035555260, 14.73035201082150536, 9.422509992056143702 ) ) ;
#25471=CARTESIAN_POINT ( 'NONE',  ( 10.00000000000000000, 21.81368534415484106, -10.88017736071110342 ) ) ;
#25472=CARTESIAN_POINT ( 'NONE',  ( 4.559911319644449179, 32.23035201082150536, -9.422509992056141925 ) ) ;
#25473=CARTESIAN_POINT ( 'NONE',  ( 10.00000000000000000, 64.75893115100078035, -9.846743663894594434 ) ) ;
#25474=CARTESIAN_POINT ( 'NONE',  ( 12.63842701281683922, 64.55059781766745175, -9.846743663894590881 ) ) ;
#25475=CARTESIAN_POINT ( 'NONE',  ( 13.43411237798105340, 60.58196800326376064, 12.81628187352647963 ) ) ;
#25476=CARTESIAN_POINT ( 'NONE',  ( 7.361572987183169658, 14.96726448433411960, -9.846743663894592657 ) ) ;
#25477=VERTEX_POINT ( 'NONE', #1203 ) ;
#25478=CARTESIAN_POINT ( 'NONE',  ( 20.88017736071110875, 35.77201867748816966, -2.915334737309920765 ) ) ;
#25479=CARTESIAN_POINT ( 'NONE',  ( 21.09922568453595559, 32.04030133659708923, -6.408140936763230044 ) ) ;
#25480=CARTESIAN_POINT ( 'NONE',  ( -1.926860441876564023, 54.68830936912750929, 1.004413902775740781E-15 ) ) ;
#25481=CARTESIAN_POINT ( 'NONE',  ( 7.361572987183170547, 62.05059781766745886, 9.846743663894590881 ) ) ;
#25482=CARTESIAN_POINT ( 'NONE',  ( 10.00000000000000000, 66.81368534415484817, -10.88017736071110342 ) ) ;
#25483=CARTESIAN_POINT ( 'NONE',  ( 17.20831665107776587, 12.88393115100078390, 7.208316651077764980 ) ) ;
#25484=CARTESIAN_POINT ( 'NONE',  ( 0.6178305044545838731, 34.74863466993042493, 9.382169495545420901 ) ) ;
#25485=CARTESIAN_POINT ( 'NONE',  ( 20.88017736071110519, 55.56368534415484817, 2.639326808657452039E-16 ) ) ;
#25487=CARTESIAN_POINT ( 'NONE',  ( 3.640395162852214650, 101.0000000000000000, -9.500000000000000000 ) ) ;
#25489=CARTESIAN_POINT ( 'NONE',  ( 4.559911319644449179, 8.897018677488171434, 9.422509992056141925 ) ) ;
#25490=CARTESIAN_POINT ( 'NONE',  ( -1.099225684535947600, 59.54030133659708923, 6.408140936763237150 ) ) ;
#25491=CARTESIAN_POINT ( 'NONE',  ( 17.08211943468705840, 25.13708216824730357, -12.26659068614894466 ) ) ;
#25492=CARTESIAN_POINT ( 'NONE',  ( 5.076628168052703671, 21.84226448433411960, 8.527530157486179263 ) ) ;
#25493=CARTESIAN_POINT ( 'NONE',  ( 19.84674366389459266, 13.30059781766745353, 2.638427012816836559 ) ) ;
#25494=CARTESIAN_POINT ( 'NONE',  ( -4.164238869374098151, 61.59541550158063217, -3.795296366450310543 ) ) ;
#25498=CARTESIAN_POINT ( 'NONE',  ( 4.559911319644449179, 17.23035201082150536, -9.422509992056141925 ) ) ;
#25501=ORIENTED_EDGE ( 'NONE', *, *, #53059, .T. ) ;
#25502=CARTESIAN_POINT ( 'NONE',  ( 20.88017736071110164, 30.35535201082151247, 2.915334737309930979 ) ) ;
#25503=CARTESIAN_POINT ( 'NONE',  ( 12.63842701281683034, 57.46726448433411605, 9.846743663894596210 ) ) ;
#25504=CARTESIAN_POINT ( 'NONE',  ( 10.00000000000000000, 47.87363466993042493, -12.81628187352647608 ) ) ;
#25507=CARTESIAN_POINT ( 'NONE',  ( 6.204703633549690345, 17.84541550158063217, 14.16423886937410082 ) ) ;
#25508=CARTESIAN_POINT ( 'NONE',  ( 17.96484262340118221, 34.93868534415482685, 7.964842623401181321 ) ) ;
#25509=CARTESIAN_POINT ( 'NONE',  ( 12.91533473730993009, 16.60535201082150891, -10.88017736071109987 ) ) ;
#25510=CARTESIAN_POINT ( 'NONE',  ( 0.1532563361054100626, 50.80059781766745175, -2.638427012816831230 ) ) ;
#25512=CARTESIAN_POINT ( 'NONE',  ( 10.00000000000000000, 29.75893115100078745, -9.846743663894594434 ) ) ;
#25514=CARTESIAN_POINT ( 'NONE',  ( 17.20831665107776587, 14.13393115100078568, -7.208316651077762316 ) ) ;
#25518=CARTESIAN_POINT ( 'NONE',  ( 5.076628168052704559, 10.17559781766745175, -8.527530157486179263 ) ) ;
#25519=CARTESIAN_POINT ( 'NONE',  ( 0.1532563361054082862, 66.21726448433413736, 2.638427012816831674 ) ) ;
#25520=CARTESIAN_POINT ( 'NONE',  ( 4.559911319644449179, 48.89701867748817676, 9.422509992056141925 ) ) ;
#25521=CARTESIAN_POINT ( 'NONE',  ( 17.96484262340118221, 46.18868534415484106, -7.964842623401177768 ) ) ;
#25522=CARTESIAN_POINT ( 'NONE',  ( 19.42250999205614193, 10.14701867748816966, 5.440088680355555262 ) ) ;
#25523=CARTESIAN_POINT ( 'NONE',  ( 19.38216949554541557, 42.24863466993041783, -9.382169495545420901 ) ) ;
#25524=CARTESIAN_POINT ( 'NONE',  ( -4.164238869374098151, 26.59541550158063217, -3.795296366450310543 ) ) ;
#25525=CARTESIAN_POINT ( 'NONE',  ( -1.099225684535947600, 53.70696800326376064, -6.408140936763238038 ) ) ;
#25527=CARTESIAN_POINT ( 'NONE',  ( 2.791683348922237240, 55.38393115100078745, -7.208316651077763204 ) ) ;
#25528=CARTESIAN_POINT ( 'NONE',  ( 2.035157376598822676, 22.43868534415483396, -7.964842623401177768 ) ) ;
#25530=CARTESIAN_POINT ( 'NONE',  ( 10.00000000000000000, 4.758931151000784787, -9.846743663894594434 ) ) ;
#25532=CARTESIAN_POINT ( 'NONE',  ( 17.20831665107776587, 14.13393115100078568, -7.208316651077762316 ) ) ;
#25534=CARTESIAN_POINT ( 'NONE',  ( 17.96484262340118221, 66.18868534415483396, -7.964842623401177768 ) ) ;
#25536=CARTESIAN_POINT ( 'NONE',  ( 10.00000000000000000, 56.81368534415484106, -10.88017736071110342 ) ) ;
#25538=CARTESIAN_POINT ( 'NONE',  ( 2.035157376598824452, 63.68868534415484106, 7.964842623401179544 ) ) ;
#25539=CARTESIAN_POINT ( 'NONE',  ( 12.63842701281683922, 9.550597817667449974, -9.846743663894590881 ) ) ;
#25543=CARTESIAN_POINT ( 'NONE',  ( 14.92337183194729633, 57.67559781766745886, 8.527530157486181039 ) ) ;
#25546=CARTESIAN_POINT ( 'NONE',  ( 24.16423886937410614, 9.303748834913967869, 8.672049930838204340E-16 ) ) ;
#25547=EDGE_CURVE ( 'NONE', #10733, #32140, #82448, .T. ) ;
#25548=CARTESIAN_POINT ( 'NONE',  ( -2.816281873526471635, 58.91530133659707502, -3.434112377981056508 ) ) ;
#25549=CARTESIAN_POINT ( 'NONE',  ( -4.164238869374099927, 7.012082168247302683, 3.795296366450308767 ) ) ;
#25550=CARTESIAN_POINT ( 'NONE',  ( -2.266590686148945544, 32.22041550158063927, 7.082119434687048631 ) ) ;
#25552=CARTESIAN_POINT ( 'NONE',  ( 10.00000000000000000, 5.553748834913967869, -14.16423886937410082 ) ) ;
#25553=CARTESIAN_POINT ( 'NONE',  ( 7.084665262690076126, 22.02201867748817321, -10.88017736071110164 ) ) ;
#25554=LINE ( 'NONE', #17561, #81899 ) ;
#25556=CARTESIAN_POINT ( 'NONE',  ( 5.076628168052704559, 0.1755978176674514724, -8.527530157486179263 ) ) ;
#25557=CARTESIAN_POINT ( 'NONE',  ( 0.1532563361054100626, 10.80059781766745175, -2.638427012816831230 ) ) ;
#25558=CARTESIAN_POINT ( 'NONE',  ( 22.81628187352647785, 41.41530133659708923, 3.434112377981063169 ) ) ;
#25559=CARTESIAN_POINT ( 'NONE',  ( 0.1532563361054100626, 35.80059781766745175, -2.638427012816831230 ) ) ;
#25562=CARTESIAN_POINT ( 'NONE',  ( 1.472469842513823179, 21.42559781766745175, 4.923371831947296329 ) ) ;
#25563=CARTESIAN_POINT ( 'NONE',  ( 3.591859063236761518, 34.95696800326375353, 11.09922568453594849 ) ) ;
#25565=CARTESIAN_POINT ( 'NONE',  ( 17.20831665107776587, 29.13393115100078390, -7.208316651077762316 ) ) ;
#25566=CARTESIAN_POINT ( 'NONE',  ( 20.36894250292379738, 19.92874883491396787, -10.36894250292379027 ) ) ;
#25568=CARTESIAN_POINT ( 'NONE',  ( 4.559911319644449179, 32.23035201082150536, -9.422509992056141925 ) ) ;
#25569=CARTESIAN_POINT ( 'NONE',  ( 24.16423886937410614, 29.51208216824729647, -3.795296366450302550 ) ) ;
#25570=CARTESIAN_POINT ( 'NONE',  ( 10.00000000000000000, 59.75893115100078745, -9.846743663894594434 ) ) ;
#25571=CARTESIAN_POINT ( 'NONE',  ( 0.1532563361054082862, 6.217264484334118713, 2.638427012816831674 ) ) ;
#25572=CARTESIAN_POINT ( 'NONE',  ( 6.565887622018943937, 58.08196800326376064, -12.81628187352647608 ) ) ;
#25574=CARTESIAN_POINT ( 'NONE',  ( 20.88017736071110875, 25.77201867748816966, -2.915334737309920765 ) ) ;
#25577=CARTESIAN_POINT ( 'NONE',  ( 10.00000000000000178, 15.37363466993042138, 12.81628187352647608 ) ) ;
#25578=CARTESIAN_POINT ( 'NONE',  ( 12.63842701281683034, 42.46726448433412315, 9.846743663894596210 ) ) ;
#25581=CARTESIAN_POINT ( 'NONE',  ( -0.8801773607110991993, 62.85535201082150536, -2.915334737309923874 ) ) ;
#25583=CARTESIAN_POINT ( 'NONE',  ( 0.2751277870542876425, 45.30223176428830811, 6.499999999999984901 ) ) ;
#25585=EDGE_CURVE ( 'NONE', #14086, #98205, #22709, .T. ) ;
#25586=CARTESIAN_POINT ( 'NONE',  ( 19.42250999205614193, 55.14701867748817676, 5.440088680355555262 ) ) ;
#25587=CARTESIAN_POINT ( 'NONE',  ( 20.88017736071110519, 55.56368534415484817, 2.639326808657452039E-16 ) ) ;
#25590=CARTESIAN_POINT ( 'NONE',  ( 15.44008868035555260, 9.730352010821505360, 9.422509992056143702 ) ) ;
#25591=CARTESIAN_POINT ( 'NONE',  ( 14.92337183194729633, 62.67559781766745886, 8.527530157486181039 ) ) ;
#25592=CARTESIAN_POINT ( 'NONE',  ( 0.5774900079438590739, 17.64701867748817321, -5.440088680355550821 ) ) ;
#25595=CARTESIAN_POINT ( 'NONE',  ( 3.591859063236763294, 28.29030133659708568, -11.09922568453595026 ) ) ;
#25597=CARTESIAN_POINT ( 'NONE',  ( 17.96484262340118221, 44.93868534415483396, 7.964842623401181321 ) ) ;
#25598=CARTESIAN_POINT ( 'NONE',  ( 19.84674366389459266, 43.71726448433410894, -2.638427012816827677 ) ) ;
#25599=CARTESIAN_POINT ( 'NONE',  ( 19.38216949554541202, 5.998634669930420493, 9.382169495545424454 ) ) ;
#25601=CARTESIAN_POINT ( 'NONE',  ( 2.035157376598822676, 32.43868534415483396, -7.964842623401177768 ) ) ;
#25602=CARTESIAN_POINT ( 'NONE',  ( 4.559911319644449179, 38.89701867748817676, 9.422509992056141925 ) ) ;
#25603=CARTESIAN_POINT ( 'NONE',  ( 6.204703633549690345, 47.84541550158064638, 14.16423886937410082 ) ) ;
#25604=CARTESIAN_POINT ( 'NONE',  ( 19.84674366389459621, 38.50893115100078745, 7.409399052514197653E-17 ) ) ;
#25605=CARTESIAN_POINT ( 'NONE',  ( 17.96484262340118221, 64.93868534415483396, 7.964842623401181321 ) ) ;
#25607=CARTESIAN_POINT ( 'NONE',  ( 10.00000000000000000, 20.55374883491396787, -14.16423886937410082 ) ) ;
#25612=CARTESIAN_POINT ( 'NONE',  ( 22.26659068614894466, 48.88708216824730357, 7.082119434687054849 ) ) ;
#25613=CARTESIAN_POINT ( 'NONE',  ( 13.79529636645030344, 43.26208216824730357, 14.16423886937410614 ) ) ;
#25614=CARTESIAN_POINT ( 'NONE',  ( 10.00000000000000178, 17.25893115100078745, 9.846743663894594434 ) ) ;
#25615=CARTESIAN_POINT ( 'NONE',  ( 10.00000000000000178, 20.37363466993042138, 12.81628187352647608 ) ) ;
#25616=DIRECTION ( 'NONE',  ( 0.000000000000000000, 0.5943319733993890353, 0.8042198116156974441 ) ) ;
#25617=FACE_OUTER_BOUND ( 'NONE', #13707, .T. ) ;
#25618=CARTESIAN_POINT ( 'NONE',  ( 4.559911319644449179, 3.897018677488170990, 9.422509992056141925 ) ) ;
#25619=CARTESIAN_POINT ( 'NONE',  ( 16.40814093676324603, 32.45696800326375353, -11.09922568453594671 ) ) ;
#25620=CARTESIAN_POINT ( 'NONE',  ( 24.16423886937410614, 49.30374883491396787, 8.672049930838204340E-16 ) ) ;
#25622=CARTESIAN_POINT ( 'NONE',  ( 10.00000000000000178, 64.31368534415483396, 10.88017736071110342 ) ) ;
#25627=DIRECTION ( 'NONE',  ( -1.000000000000000000, 0.000000000000000000, -0.000000000000000000 ) ) ;
#25628=CARTESIAN_POINT ( 'NONE',  ( 2.791683348922240793, 16.63393115100078745, 7.208316651077764092 ) ) ;
#25633=CARTESIAN_POINT ( 'NONE',  ( 6.204703633549690345, 2.845415501580634388, 14.16423886937410082 ) ) ;
#25634=CARTESIAN_POINT ( 'NONE',  ( 20.88017736071110164, 10.35535201082150714, 2.915334737309930979 ) ) ;
#25635=CARTESIAN_POINT ( 'NONE',  ( 15.44008868035555260, 9.730352010821505360, 9.422509992056143702 ) ) ;
#25636=CARTESIAN_POINT ( 'NONE',  ( 2.791683348922240793, 31.63393115100078745, 7.208316651077764092 ) ) ;
#25637=CARTESIAN_POINT ( 'NONE',  ( 21.09922568453594849, 1.206968003263753531, 6.408140936763242479 ) ) ;
#25640=CARTESIAN_POINT ( 'NONE',  ( -1.099225684535947600, 18.70696800326375353, -6.408140936763238038 ) ) ;
#25641=VERTEX_POINT ( 'NONE', #75694 ) ;
#25642=CARTESIAN_POINT ( 'NONE',  ( 10.00000000000000000, 40.55374883491397497, -14.16423886937410082 ) ) ;
#25643=ORIENTED_EDGE ( 'NONE', *, *, #34358, .F. ) ;
#25644=CARTESIAN_POINT ( 'NONE',  ( 6.204703633549690345, 57.84541550158063927, 14.16423886937410082 ) ) ;
#25646=CARTESIAN_POINT ( 'NONE',  ( 4.559911319644449179, 37.23035201082150536, -9.422509992056141925 ) ) ;
#25647=CARTESIAN_POINT ( 'NONE',  ( 10.00000000000000178, 34.31368534415484106, 10.88017736071110342 ) ) ;
#25648=CARTESIAN_POINT ( 'NONE',  ( 15.44008868035555793, 41.39701867748817676, -9.422509992056140149 ) ) ;
#25649=CARTESIAN_POINT ( 'NONE',  ( -0.8801773607111009756, 68.06368534415484817, 1.068504757029289695E-15 ) ) ;
#25650=CARTESIAN_POINT ( 'NONE',  ( 12.91533473730993009, 26.60535201082150536, -10.88017736071109987 ) ) ;
#25655=CARTESIAN_POINT ( 'NONE',  ( 14.92337183194729988, 19.34226448433411960, -8.527530157486177487 ) ) ;
#25658=CARTESIAN_POINT ( 'NONE',  ( 7.361572987183169658, 49.96726448433410894, -9.846743663894592657 ) ) ;
#25659=DIRECTION ( 'NONE',  ( 0.000000000000000000, 0.000000000000000000, 1.000000000000000000 ) ) ;
#25660=ADVANCED_FACE ( 'NONE', ( #30672 ), #7206, .T. ) ;
#25661=CARTESIAN_POINT ( 'NONE',  ( -2.816281873526471635, 43.91530133659708923, -3.434112377981056508 ) ) ;
#25664=CARTESIAN_POINT ( 'NONE',  ( -46.20769938831636381, 103.7415672121642274, 6.113268130406499523 ) ) ;
#25665=CARTESIAN_POINT ( 'NONE',  ( 20.15039907845753930, 69.92552686551195507, 6.262539305110068177 ) ) ;
#25667=CARTESIAN_POINT ( 'NONE',  ( -4.164238869374099039, 41.80374883491397497, 8.674139862899312516E-16 ) ) ;
#25668=CARTESIAN_POINT ( 'NONE',  ( 7.361572987183170547, 67.05059781766746596, 9.846743663894590881 ) ) ;
#25671=CARTESIAN_POINT ( 'NONE',  ( 10.00000000000000178, 17.25893115100078745, 9.846743663894594434 ) ) ;
#25672=CARTESIAN_POINT ( 'NONE',  ( 13.43411237798106583, 62.66530133659708923, -12.81628187352647252 ) ) ;
#25673=CARTESIAN_POINT ( 'NONE',  ( 18.52753015748617571, 58.09226448433411605, 4.923371831947298993 ) ) ;
#25674=CARTESIAN_POINT ( 'NONE',  ( 12.91533473730993009, 61.60535201082150536, -10.88017736071109987 ) ) ;
#25676=CARTESIAN_POINT ( 'NONE',  ( 5.076628168052703671, 61.84226448433412315, 8.527530157486179263 ) ) ;
#25677=CARTESIAN_POINT ( 'NONE',  ( 21.92686044187656691, 14.95379003517447458, 3.195792623639537755 ) ) ;
#25680=CARTESIAN_POINT ( 'NONE',  ( 10.00000000000000178, 58.05374883491397497, 14.16423886937410082 ) ) ;
#25681=LINE ( 'NONE', #10182, #53718 ) ;
#25682=CARTESIAN_POINT ( 'NONE',  ( 20.88017736071110519, 45.56368534415484106, 2.639326808657452039E-16 ) ) ;
#25683=CARTESIAN_POINT ( 'NONE',  ( 22.81628187352647785, 16.62363466993042138, 6.195893100308588602E-16 ) ) ;
#25685=CARTESIAN_POINT ( 'NONE',  ( 20.88017736071110875, 65.77201867748817676, -2.915334737309920321 ) ) ;
#25688=AXIS2_PLACEMENT_3D ( 'NONE', #26078, #34041, #49066 ) ;
#25689=CARTESIAN_POINT ( 'NONE',  ( 0.1129803114748720444, 54.29427333184091253, -6.480634945678676928 ) ) ;
#25690=CARTESIAN_POINT ( 'NONE',  ( 7.361572987183169658, 44.96726448433412315, -9.846743663894592657 ) ) ;
#25691=CARTESIAN_POINT ( 'NONE',  ( 1.472469842513823179, 1.425597817667451528, 4.923371831947296329 ) ) ;
#25693=CARTESIAN_POINT ( 'NONE',  ( 16.40814093676324603, 12.45696800326375353, -11.09922568453594671 ) ) ;
#25695=CARTESIAN_POINT ( 'NONE',  ( 15.44008868035555793, 16.39701867748817321, -9.422509992056140149 ) ) ;
#25698=CARTESIAN_POINT ( 'NONE',  ( 2.917880565312948704, 37.63708216824731068, 12.26659068614894643 ) ) ;
#25699=CARTESIAN_POINT ( 'NONE',  ( 10.00000000000000178, 28.05374883491396787, 14.16423886937410082 ) ) ;
#25700=CARTESIAN_POINT ( 'NONE',  ( 6.204703633549690345, 62.84541550158063927, 14.16423886937410082 ) ) ;
#25701=CARTESIAN_POINT ( 'NONE',  ( 0.1532563361054082862, 41.21726448433411605, 2.638427012816831674 ) ) ;
#25702=CARTESIAN_POINT ( 'NONE',  ( 3.591859063236763294, 33.29030133659708213, -11.09922568453595026 ) ) ;
#25703=CARTESIAN_POINT ( 'NONE',  ( 17.96484262340118221, 9.938685344154837509, 7.964842623401181321 ) ) ;
#25705=CARTESIAN_POINT ( 'NONE',  ( 17.20831665107776587, 34.13393115100078745, -7.208316651077762316 ) ) ;
#25706=CARTESIAN_POINT ( 'NONE',  ( 12.91533473730993009, 41.60535201082149825, -10.88017736071109987 ) ) ;
#25707=CARTESIAN_POINT ( 'NONE',  ( -2.816281873526473856, 9.331968003263753531, 3.434112377981055619 ) ) ;
#25708=CARTESIAN_POINT ( 'NONE',  ( -0.3689425029237881626, 17.42874883491397142, 10.36894250292379027 ) ) ;
#25710=CARTESIAN_POINT ( 'NONE',  ( 12.63842701281683922, 29.55059781766745175, -9.846743663894590881 ) ) ;
#25711=CARTESIAN_POINT ( 'NONE',  ( 0.6178305044545838731, 44.74863466993042493, 9.382169495545420901 ) ) ;
#25712=CARTESIAN_POINT ( 'NONE',  ( 19.84674366389459266, 58.30059781766745886, 2.638427012816836559 ) ) ;
#25715=CARTESIAN_POINT ( 'NONE',  ( 24.16423886937409904, 64.09541550158064638, 3.795296366450317205 ) ) ;
#25716=CARTESIAN_POINT ( 'NONE',  ( 12.91533473730993009, 61.60535201082150536, -10.88017736071109987 ) ) ;
#25717=CARTESIAN_POINT ( 'NONE',  ( 10.00000000000000178, 13.05374883491396787, 14.16423886937410082 ) ) ;
#25718=CARTESIAN_POINT ( 'NONE',  ( 12.63842701281683922, 4.550597817667451750, -9.846743663894590881 ) ) ;
#25719=CARTESIAN_POINT ( 'NONE',  ( 0.1532563361054083140, 51.00893115100078745, 1.131784320476157264E-15 ) ) ;
#25720=CARTESIAN_POINT ( 'NONE',  ( 19.42250999205614193, 15.14701867748817143, 5.440088680355555262 ) ) ;
#25722=CARTESIAN_POINT ( 'NONE',  ( 10.00000000000000178, 67.25893115100079456, 9.846743663894594434 ) ) ;
#25724=EDGE_LOOP ( 'NONE', ( #68549, #10254, #6257, #16227 ) ) ;
#25731=CARTESIAN_POINT ( 'NONE',  ( 17.08211943468705840, 10.13708216824730179, -12.26659068614894466 ) ) ;
#25732=CARTESIAN_POINT ( 'NONE',  ( -2.266590686148945544, 47.22041550158063927, 7.082119434687048631 ) ) ;
#25733=CARTESIAN_POINT ( 'NONE',  ( 0.1532563361054082862, 61.21726448433412315, 2.638427012816831674 ) ) ;
#25734=CARTESIAN_POINT ( 'NONE',  ( 17.20831665107776587, 27.88393115100078390, 7.208316651077764980 ) ) ;
#25735=CARTESIAN_POINT ( 'NONE',  ( -0.1042174387088608406, 38.10736173766201773, 6.337391062633419558 ) ) ;
#25736=CARTESIAN_POINT ( 'NONE',  ( -0.8801773607111008646, 18.27201867748817321, 2.915334737309923430 ) ) ;
#25737=CARTESIAN_POINT ( 'NONE',  ( 6.565887622018943937, -1.918031996736246692, -12.81628187352647608 ) ) ;
#25738=CARTESIAN_POINT ( 'NONE',  ( 24.16423886937410614, 9.512082168247301794, -3.795296366450302550 ) ) ;
#25739=CARTESIAN_POINT ( 'NONE',  ( 24.16423886937410614, 39.30374883491396787, 8.672049930838204340E-16 ) ) ;
#25740=CARTESIAN_POINT ( 'NONE',  ( 0.5774900079438590739, 2.647018677488171434, -5.440088680355550821 ) ) ;
#25741=CARTESIAN_POINT ( 'NONE',  ( 0.1532563361054100626, 65.80059781766745175, -2.638427012816831230 ) ) ;
#25744=CARTESIAN_POINT ( 'NONE',  ( 10.00000000000000000, 61.81368534415484106, -10.88017736071110342 ) ) ;
#25745=CARTESIAN_POINT ( 'NONE',  ( 7.361572987183169658, 14.96726448433411960, -9.846743663894592657 ) ) ;
#25747=ORIENTED_EDGE ( 'NONE', *, *, #60048, .T. ) ;
#25750=CARTESIAN_POINT ( 'NONE',  ( 19.84674366389459621, 18.50893115100078745, 7.409399052514197653E-17 ) ) ;
#25751=VERTEX_POINT ( 'NONE', #85169 ) ;
#25752=CARTESIAN_POINT ( 'NONE',  ( 6.204703633549690345, 37.84541550158063927, 14.16423886937410082 ) ) ;
#25753=CARTESIAN_POINT ( 'NONE',  ( 14.92337183194729633, 32.67559781766745175, 8.527530157486181039 ) ) ;
#25754=CARTESIAN_POINT ( 'NONE',  ( 7.084665262690076126, 44.10535201082151247, 10.88017736071109987 ) ) ;
#25757=CARTESIAN_POINT ( 'NONE',  ( 17.96484262340118221, 46.18868534415484106, -7.964842623401177768 ) ) ;
#25758=CARTESIAN_POINT ( 'NONE',  ( 20.03447792253738768, 37.65514106990689669, -6.401564815979734036 ) ) ;
#25761=CARTESIAN_POINT ( 'NONE',  ( 20.36894250292379382, 8.678748834913967869, 10.36894250292379205 ) ) ;
#25764=CARTESIAN_POINT ( 'NONE',  ( 5.076628168052703671, 1.842264484334118047, 8.527530157486179263 ) ) ;
#25765=CARTESIAN_POINT ( 'NONE',  ( 10.00000000000000000, 37.87363466993041783, -12.81628187352647608 ) ) ;
#25766=CARTESIAN_POINT ( 'NONE',  ( 0.1532563361054100626, 25.80059781766744820, -2.638427012816831230 ) ) ;
#25767=CARTESIAN_POINT ( 'NONE',  ( -2.816281873526473856, 44.12363466993042493, 9.499525473075851096E-16 ) ) ;
#25769=CARTESIAN_POINT ( 'NONE',  ( 1.472469842513823179, 25.59226448433412315, -4.923371831947296329 ) ) ;
#25770=CARTESIAN_POINT ( 'NONE',  ( 20.88017736071110875, 55.77201867748816966, -2.915334737309920765 ) ) ;
#25772=CARTESIAN_POINT ( 'NONE',  ( 12.91533473730992121, 64.52201867748817676, 10.88017736071110164 ) ) ;
#25775=CARTESIAN_POINT ( 'NONE',  ( 0.1532563361054082862, 11.21726448433411605, 2.638427012816831674 ) ) ;
#25777=CARTESIAN_POINT ( 'NONE',  ( -1.099225684535947600, 8.706968003263753531, -6.408140936763238038 ) ) ;
#25779=CARTESIAN_POINT ( 'NONE',  ( 19.84674366389459266, 48.71726448433413026, -2.638427012816827677 ) ) ;
#25781=CARTESIAN_POINT ( 'NONE',  ( 6.204703633549690345, 2.845415501580634388, 14.16423886937410082 ) ) ;
#25782=CARTESIAN_POINT ( 'NONE',  ( 0.1532563361054100626, 35.80059781766745175, -2.638427012816831230 ) ) ;
#25783=CARTESIAN_POINT ( 'NONE',  ( 0.6178305044545838731, 29.74863466993042138, 9.382169495545420901 ) ) ;
#25784=CARTESIAN_POINT ( 'NONE',  ( -0.8801773607110990882, 22.85535201082150181, -2.915334737309924318 ) ) ;
#25785=CARTESIAN_POINT ( 'NONE',  ( -0.8801773607111008646, 48.27201867748816966, 2.915334737309923430 ) ) ;
#25786=CARTESIAN_POINT ( 'NONE',  ( 0.6178305044545838731, 9.748634669930416052, 9.382169495545420901 ) ) ;
#25788=CARTESIAN_POINT ( 'NONE',  ( 7.361572987183170547, 17.05059781766745530, 9.846743663894590881 ) ) ;
#25789=CARTESIAN_POINT ( 'NONE',  ( 0.5774900079438607392, 33.48035201082150536, 5.440088680355550821 ) ) ;
#25790=CARTESIAN_POINT ( 'NONE',  ( 3.591859063236761518, 34.95696800326375353, 11.09922568453594849 ) ) ;
#25792=CARTESIAN_POINT ( 'NONE',  ( 4.559911319644449179, 22.23035201082150536, -9.422509992056141925 ) ) ;
#25794=CARTESIAN_POINT ( 'NONE',  ( 10.00000000000000000, 61.81368534415484106, -10.88017736071110342 ) ) ;
#25795=CARTESIAN_POINT ( 'NONE',  ( 0.1532563361054083140, 41.00893115100078745, 1.131784320476157264E-15 ) ) ;
#25796=CARTESIAN_POINT ( 'NONE',  ( 19.42250999205614548, 25.98035201082150891, -5.440088680355545492 ) ) ;
#25797=CARTESIAN_POINT ( 'NONE',  ( 20.00000000000000000, 0.000000000000000000, -4.500000000000001776 ) ) ;
#25798=CARTESIAN_POINT ( 'NONE',  ( 12.91533473730993009, 41.60535201082149825, -10.88017736071109987 ) ) ;
#25799=CARTESIAN_POINT ( 'NONE',  ( -0.8801773607110991993, 7.855352010821506248, -2.915334737309923874 ) ) ;
#25801=CARTESIAN_POINT ( 'NONE',  ( 2.791683348922237240, 35.38393115100079456, -7.208316651077763204 ) ) ;
#25802=CARTESIAN_POINT ( 'NONE',  ( 2.917880565312950480, 45.97041550158063927, -12.26659068614894821 ) ) ;
#25806=CARTESIAN_POINT ( 'NONE',  ( 6.565887622018943937, 0.1653013365970866511, 12.81628187352647430 ) ) ;
#25808=CARTESIAN_POINT ( 'NONE',  ( 10.00000000000000000, 30.55374883491397142, -14.16423886937410082 ) ) ;
#25810=STYLED_ITEM ( 'NONE', ( #7445 ), #32648 ) ;
#25813=CARTESIAN_POINT ( 'NONE',  ( -0.3689425029237898834, 66.17874883491396076, -10.36894250292378850 ) ) ;
#25814=CARTESIAN_POINT ( 'NONE',  ( 10.00000000000000000, 19.75893115100078390, -9.846743663894594434 ) ) ;
#25815=DIRECTION ( 'NONE',  ( -0.000000000000000000, -0.000000000000000000, 1.000000000000000000 ) ) ;
#25816=CARTESIAN_POINT ( 'NONE',  ( 2.035157376598822676, 62.43868534415483396, -7.964842623401177768 ) ) ;
#25817=CARTESIAN_POINT ( 'NONE',  ( -2.816281873526473856, 64.33196800326376774, 3.434112377981055619 ) ) ;
#25818=CARTESIAN_POINT ( 'NONE',  ( -0.8801773607110991993, 27.85535201082150181, -2.915334737309923874 ) ) ;
#25819=CARTESIAN_POINT ( 'NONE',  ( 10.00000000000000178, 55.37363466993042493, 12.81628187352647608 ) ) ;
#25820=CARTESIAN_POINT ( 'NONE',  ( 6.565887622018943937, 5.165301336597086568, 12.81628187352647430 ) ) ;
#25821=CARTESIAN_POINT ( 'NONE',  ( 1.472469842513823179, 10.59226448433411782, -4.923371831947296329 ) ) ;
#25823=CARTESIAN_POINT ( 'NONE',  ( 0.1532563361054083140, 1.008931151000784787, 1.131784320476157264E-15 ) ) ;
#25824=CARTESIAN_POINT ( 'NONE',  ( 0.1143410931637250938, 20.21691075486302580, 6.480892540919863443 ) ) ;
#25825=CARTESIAN_POINT ( 'NONE',  ( -4.164238869374098151, 51.59541550158063217, -3.795296366450310543 ) ) ;
#25826=CARTESIAN_POINT ( 'NONE',  ( -2.266590686148945544, 26.38708216824730357, -7.082119434687050408 ) ) ;
#25827=CARTESIAN_POINT ( 'NONE',  ( 0.5774900079438607392, 33.48035201082150536, 5.440088680355550821 ) ) ;
#25828=CARTESIAN_POINT ( 'NONE',  ( 17.96484262340118221, 46.18868534415484106, -7.964842623401177768 ) ) ;
#25831=CARTESIAN_POINT ( 'NONE',  ( 5.076628168052703671, 11.84226448433411960, 8.527530157486179263 ) ) ;
#25833=CARTESIAN_POINT ( 'NONE',  ( 10.00000000000000000, 14.75893115100078568, -9.846743663894594434 ) ) ;
#25837=CARTESIAN_POINT ( 'NONE',  ( 17.20831665107776587, 29.13393115100078390, -7.208316651077762316 ) ) ;
#25838=CARTESIAN_POINT ( 'NONE',  ( 2.791683348922237240, 45.38393115100079456, -7.208316651077763204 ) ) ;
#25839=CARTESIAN_POINT ( 'NONE',  ( 12.91533473730993009, 26.60535201082150536, -10.88017736071109987 ) ) ;
#25840=CARTESIAN_POINT ( 'NONE',  ( -2.816281873526473856, 39.12363466993041783, 9.499525473075851096E-16 ) ) ;
#25841=CARTESIAN_POINT ( 'NONE',  ( 4.559911319644449179, 52.23035201082151247, -9.422509992056141925 ) ) ;
#25842=CARTESIAN_POINT ( 'NONE',  ( 12.63842701281683034, 27.46726448433411250, 9.846743663894596210 ) ) ;
#25843=CARTESIAN_POINT ( 'NONE',  ( 17.08211943468705840, 50.13708216824730357, -12.26659068614894466 ) ) ;
#25844=CARTESIAN_POINT ( 'NONE',  ( 17.20831665107776587, 22.88393115100078745, 7.208316651077764980 ) ) ;
#25846=CARTESIAN_POINT ( 'NONE',  ( 1.472469842513823179, 51.42559781766745886, 4.923371831947296329 ) ) ;
#25847=CARTESIAN_POINT ( 'NONE',  ( 0.1532563361054082862, 51.21726448433412315, 2.638427012816831674 ) ) ;
#25848=CARTESIAN_POINT ( 'NONE',  ( 24.16423886937410614, 4.512082168247300906, -3.795296366450302550 ) ) ;
#25849=CARTESIAN_POINT ( 'NONE',  ( -4.164238869374099927, 32.01208216824730357, 3.795296366450308767 ) ) ;
#25850=CARTESIAN_POINT ( 'NONE',  ( 0.1532563361054100626, 25.80059781766744820, -2.638427012816831230 ) ) ;
#25851=CARTESIAN_POINT ( 'NONE',  ( 10.00000000000000000, 26.81368534415484106, -10.88017736071110342 ) ) ;
#25852=CARTESIAN_POINT ( 'NONE',  ( 15.44008868035555260, 39.73035201082150536, 9.422509992056143702 ) ) ;
#25853=CARTESIAN_POINT ( 'NONE',  ( 17.96484262340118221, 44.93868534415483396, 7.964842623401181321 ) ) ;
#25855=CARTESIAN_POINT ( 'NONE',  ( 0.6178305044545838731, 34.74863466993042493, 9.382169495545420901 ) ) ;
#25856=CARTESIAN_POINT ( 'NONE',  ( 15.44008868035555793, 56.39701867748817676, -9.422509992056140149 ) ) ;
#25858=CARTESIAN_POINT ( 'NONE',  ( -28.94000000000001549, 93.50000000000000000, -10.09898361729590199 ) ) ;
#25859=EDGE_CURVE ( 'NONE', #40989, #61441, #81966, .T. ) ;
#25860=CARTESIAN_POINT ( 'NONE',  ( -0.8801773607111008646, 63.27201867748817676, 2.915334737309923430 ) ) ;
#25862=CARTESIAN_POINT ( 'NONE',  ( 7.084665262690076126, 59.10535201082150536, 10.88017736071109987 ) ) ;
#25865=CARTESIAN_POINT ( 'NONE',  ( 19.42250999205614193, 40.14701867748817676, 5.440088680355555262 ) ) ;
#25866=CARTESIAN_POINT ( 'NONE',  ( -0.1503990784575328643, 70.00000000000000000, -6.262539305110068177 ) ) ;
#25867=CARTESIAN_POINT ( 'NONE',  ( -2.266590686148945544, 67.22041550158063217, 7.082119434687048631 ) ) ;
#25868=CARTESIAN_POINT ( 'NONE',  ( 0.1532563361054082862, 11.21726448433411605, 2.638427012816831674 ) ) ;
#25869=CARTESIAN_POINT ( 'NONE',  ( -2.266590686148945544, 6.387082168247300906, -7.082119434687050408 ) ) ;
#25870=CARTESIAN_POINT ( 'NONE',  ( 5.076628168052704559, 10.17559781766745175, -8.527530157486179263 ) ) ;
#25871=CARTESIAN_POINT ( 'NONE',  ( 2.791683348922237240, 45.38393115100079456, -7.208316651077763204 ) ) ;
#25873=CARTESIAN_POINT ( 'NONE',  ( 18.52753015748618282, 53.92559781766745175, -4.923371831947291888 ) ) ;
#25876=CARTESIAN_POINT ( 'NONE',  ( 4.559911319644449179, 47.23035201082150536, -9.422509992056141925 ) ) ;
#25877=CARTESIAN_POINT ( 'NONE',  ( 2.791683348922237240, 50.38393115100078035, -7.208316651077763204 ) ) ;
#25879=CARTESIAN_POINT ( 'NONE',  ( 12.91533473730993009, 66.60535201082150536, -10.88017736071109987 ) ) ;
#25880=CARTESIAN_POINT ( 'NONE',  ( 20.88017736071110164, 55.35535201082149825, 2.915334737309930979 ) ) ;
#25881=CARTESIAN_POINT ( 'NONE',  ( 10.00000000000000178, 4.313685344154837509, 10.88017736071110342 ) ) ;
#25884=CARTESIAN_POINT ( 'NONE',  ( 10.00000000000000178, 45.37363466993041783, 12.81628187352647608 ) ) ;
#25885=CARTESIAN_POINT ( 'NONE',  ( 0.1957200283969147692, 10.25733960839544068, 6.500000000000001776 ) ) ;
#25887=CARTESIAN_POINT ( 'NONE',  ( 10.00000000000000000, 32.87363466993042493, -12.81628187352647608 ) ) ;
#25888=CARTESIAN_POINT ( 'NONE',  ( 2.035157376598822676, 32.43868534415483396, -7.964842623401177768 ) ) ;
#25892=CARTESIAN_POINT ( 'NONE',  ( 19.84674366389459266, 58.71726448433411605, -2.638427012816827677 ) ) ;
#25893=CARTESIAN_POINT ( 'NONE',  ( 14.92337183194729988, 14.34226448433411782, -8.527530157486177487 ) ) ;
#25894=CARTESIAN_POINT ( 'NONE',  ( 2.791683348922240793, 56.63393115100078035, 7.208316651077764092 ) ) ;
#25896=SURFACE_STYLE_FILL_AREA ( #64361 ) ;
#25897=CARTESIAN_POINT ( 'NONE',  ( 19.84674366389459266, 38.71726448433412315, -2.638427012816827677 ) ) ;
#25899=CARTESIAN_POINT ( 'NONE',  ( 10.00000000000000178, 32.25893115100078745, 9.846743663894594434 ) ) ;
#25900=CARTESIAN_POINT ( 'NONE',  ( 19.84674366389459266, 58.30059781766745886, 2.638427012816836559 ) ) ;
#25902=CARTESIAN_POINT ( 'NONE',  ( -0.8801773607111009756, 8.272018677488171434, 2.915334737309923874 ) ) ;
#25903=CARTESIAN_POINT ( 'NONE',  ( 3.591859063236763294, 23.29030133659708568, -11.09922568453595026 ) ) ;
#25904=CARTESIAN_POINT ( 'NONE',  ( 5.076628168052704559, 40.17559781766745175, -8.527530157486179263 ) ) ;
#25906=CARTESIAN_POINT ( 'NONE',  ( 13.79529636645031943, 50.34541550158064638, -14.16423886937409904 ) ) ;
#25907=CARTESIAN_POINT ( 'NONE',  ( 0.1532563361054083140, 21.00893115100078745, 1.131784320476157264E-15 ) ) ;
#25910=CARTESIAN_POINT ( 'NONE',  ( 2.917880565312950480, 60.97041550158063927, -12.26659068614894821 ) ) ;
#25911=CARTESIAN_POINT ( 'NONE',  ( 0.1532563361054082862, 56.21726448433411605, 2.638427012816831674 ) ) ;
#25912=CARTESIAN_POINT ( 'NONE',  ( 2.035157376598822676, 7.438685344154837509, -7.964842623401177768 ) ) ;
#25913=CARTESIAN_POINT ( 'NONE',  ( 13.79529636645030344, 33.26208216824730357, 14.16423886937410614 ) ) ;
#25914=CARTESIAN_POINT ( 'NONE',  ( 22.26659068614894466, 43.88708216824729647, 7.082119434687054849 ) ) ;
#25915=CARTESIAN_POINT ( 'NONE',  ( 19.84674366389459266, 33.71726448433410894, -2.638427012816827677 ) ) ;
#25916=CARTESIAN_POINT ( 'NONE',  ( 6.000000000000000000, 11.50000000000000000, 6.500000000000000888 ) ) ;
#25918=CARTESIAN_POINT ( 'NONE',  ( 2.791683348922237240, 50.38393115100078035, -7.208316651077763204 ) ) ;
#25919=CARTESIAN_POINT ( 'NONE',  ( -0.8801773607110991993, 37.85535201082151247, -2.915334737309923874 ) ) ;
#25922=EDGE_CURVE ( 'NONE', #53414, #12692, #69370, .T. ) ;
#25923=CARTESIAN_POINT ( 'NONE',  ( 0.1532563361054082862, 51.21726448433412315, 2.638427012816831674 ) ) ;
#25926=CARTESIAN_POINT ( 'NONE',  ( 19.84674366389459266, 58.30059781766745886, 2.638427012816836559 ) ) ;
#25927=CARTESIAN_POINT ( 'NONE',  ( 0.2751277870542967463, 70.00000000000000000, -6.500000000000000888 ) ) ;
#25930=CARTESIAN_POINT ( 'NONE',  ( -2.266590686148945544, 32.22041550158063927, 7.082119434687048631 ) ) ;
#25931=CARTESIAN_POINT ( 'NONE',  ( 0.5600000000000083800, 105.0000000000000000, 4.500000000000000888 ) ) ;
#25933=CARTESIAN_POINT ( 'NONE',  ( 10.00000000000000178, 14.31368534415483929, 10.88017736071110342 ) ) ;
#25934=CARTESIAN_POINT ( 'NONE',  ( 22.81628187352647785, 21.41530133659708923, 3.434112377981063169 ) ) ;
#25936=CARTESIAN_POINT ( 'NONE',  ( 19.84674366389459266, 8.300597817667451750, 2.638427012816836559 ) ) ;
#25940=CARTESIAN_POINT ( 'NONE',  ( 19.42250999205614548, 10.98035201082150536, -5.440088680355545492 ) ) ;
#25942=CARTESIAN_POINT ( 'NONE',  ( 10.00000000000000178, 44.31368534415484106, 10.88017736071110342 ) ) ;
#25943=CARTESIAN_POINT ( 'NONE',  ( 12.91533473730993009, 36.60535201082151247, -10.88017736071109987 ) ) ;
#25944=CARTESIAN_POINT ( 'NONE',  ( 18.52753015748618282, 63.92559781766745886, -4.923371831947291888 ) ) ;
#25945=CARTESIAN_POINT ( 'NONE',  ( 1.472469842513823179, 66.42559781766745175, 4.923371831947296329 ) ) ;
#25946=CARTESIAN_POINT ( 'NONE',  ( -1.099225684535947600, 58.70696800326375353, -6.408140936763238038 ) ) ;
#25947=CARTESIAN_POINT ( 'NONE',  ( 1.472469842513823179, 16.42559781766745175, 4.923371831947296329 ) ) ;
#25949=CARTESIAN_POINT ( 'NONE',  ( 17.96484262340118221, 24.93868534415484461, 7.964842623401181321 ) ) ;
#25950=CARTESIAN_POINT ( 'NONE',  ( 13.43411237798105340, 30.58196800326374998, 12.81628187352647963 ) ) ;
#25952=CARTESIAN_POINT ( 'NONE',  ( 12.63842701281683922, 64.55059781766745175, -9.846743663894590881 ) ) ;
#25953=CARTESIAN_POINT ( 'NONE',  ( 2.035157376598824452, 68.68868534415484817, 7.964842623401179544 ) ) ;
#25954=CARTESIAN_POINT ( 'NONE',  ( 14.92337183194729633, 7.675597817667451750, 8.527530157486181039 ) ) ;
#25955=CARTESIAN_POINT ( 'NONE',  ( 21.09922568453594849, 36.20696800326375353, 6.408140936763242479 ) ) ;
#25956=CARTESIAN_POINT ( 'NONE',  ( 7.361572987183170547, 12.05059781766744997, 9.846743663894590881 ) ) ;
#25960=CARTESIAN_POINT ( 'NONE',  ( 0.2751277870542967463, 70.00000000000000000, 6.000000000000000000 ) ) ;
#25961=CARTESIAN_POINT ( 'NONE',  ( -0.8801773607110991993, 12.85535201082150358, -2.915334737309923874 ) ) ;
#25962=CARTESIAN_POINT ( 'NONE',  ( 13.43411237798105340, 60.58196800326376064, 12.81628187352647963 ) ) ;
#25963=CARTESIAN_POINT ( 'NONE',  ( 24.16423886937410614, 24.30374883491396787, 8.672049930838204340E-16 ) ) ;
#25964=CARTESIAN_POINT ( 'NONE',  ( 18.52753015748618282, 13.92559781766745175, -4.923371831947291888 ) ) ;
#25966=CARTESIAN_POINT ( 'NONE',  ( 15.44008868035555260, 4.730352010821504471, 9.422509992056143702 ) ) ;
#25967=CARTESIAN_POINT ( 'NONE',  ( 7.361572987183169658, 14.96726448433411960, -9.846743663894592657 ) ) ;
#25968=CARTESIAN_POINT ( 'NONE',  ( 24.16423886937409904, 59.09541550158063217, 3.795296366450317205 ) ) ;
#25970=AXIS2_PLACEMENT_3D ( 'NONE', #87771, #25815, #86807 ) ;
#25971=CARTESIAN_POINT ( 'NONE',  ( 17.96484262340118221, 19.93868534415484106, 7.964842623401181321 ) ) ;
#25972=ADVANCED_FACE ( 'NONE', ( #2187 ), #64112, .T. ) ;
#25973=CARTESIAN_POINT ( 'NONE',  ( 20.88017736071110875, 25.77201867748816966, -2.915334737309920765 ) ) ;
#25974=CARTESIAN_POINT ( 'NONE',  ( -0.04068437667224622523, 7.219743609177202259, -6.396802510829698640 ) ) ;
#25975=MECHANICAL_DESIGN_GEOMETRIC_PRESENTATION_REPRESENTATION('',(#11545),#86639);
#25977=CARTESIAN_POINT ( 'NONE',  ( 12.63842701281683922, 64.55059781766745175, -9.846743663894590881 ) ) ;
#25978=CARTESIAN_POINT ( 'NONE',  ( 0.5774900079438607392, 18.48035201082150536, 5.440088680355550821 ) ) ;
#25979=CARTESIAN_POINT ( 'NONE',  ( 5.076628168052703671, 61.84226448433412315, 8.527530157486179263 ) ) ;
#25980=LINE ( 'NONE', #57451, #48889 ) ;
#25981=CARTESIAN_POINT ( 'NONE',  ( 16.40814093676323893, 45.79030133659708923, 11.09922568453595026 ) ) ;
#25982=CARTESIAN_POINT ( 'NONE',  ( 19.72487221294571924, 62.80223176428831522, -6.499999999999984901 ) ) ;
#25983=CARTESIAN_POINT ( 'NONE',  ( 20.36894250292379738, 19.92874883491396787, -10.36894250292379027 ) ) ;
#25984=CARTESIAN_POINT ( 'NONE',  ( -0.8801773607111008646, 43.27201867748817676, 2.915334737309923430 ) ) ;
#25985=CARTESIAN_POINT ( 'NONE',  ( 2.035157376598824452, 18.68868534415484106, 7.964842623401179544 ) ) ;
#25987=CARTESIAN_POINT ( 'NONE',  ( 5.076628168052704559, 60.17559781766745175, -8.527530157486179263 ) ) ;
#25989=CARTESIAN_POINT ( 'NONE',  ( 17.20831665107776587, 32.88393115100078745, 7.208316651077764980 ) ) ;
#25991=MECHANICAL_DESIGN_GEOMETRIC_PRESENTATION_REPRESENTATION('',(#67533),#73860);
#25992=CARTESIAN_POINT ( 'NONE',  ( 0.1532563361054100626, 5.800597817667452638, -2.638427012816831230 ) ) ;
#25995=CARTESIAN_POINT ( 'NONE',  ( 20.88017736071110875, 10.77201867748817143, -2.915334737309920765 ) ) ;
#25996=CARTESIAN_POINT ( 'NONE',  ( 17.20831665107776587, 17.88393115100078745, 7.208316651077764980 ) ) ;
#25997=CARTESIAN_POINT ( 'NONE',  ( 0.1532563361054083140, 66.00893115100079456, 1.131784320476157264E-15 ) ) ;
#25998=CARTESIAN_POINT ( 'NONE',  ( 20.88017736071110519, 40.56368534415484106, 2.639326808657452039E-16 ) ) ;
#25999=CARTESIAN_POINT ( 'NONE',  ( 10.00000000000000000, 16.81368534415483751, -10.88017736071110342 ) ) ;
#26000=CARTESIAN_POINT ( 'NONE',  ( 21.09922568453595559, 47.04030133659708923, -6.408140936763230044 ) ) ;
#26001=CARTESIAN_POINT ( 'NONE',  ( -4.164238869374098151, 36.59541550158063217, -3.795296366450310543 ) ) ;
#26003=CARTESIAN_POINT ( 'NONE',  ( 6.000000000000000000, 60.50000000000000000, -6.000000000000000000 ) ) ;
#26005=CARTESIAN_POINT ( 'NONE',  ( -2.816281873526473856, 59.12363466993042493, 9.499525473075851096E-16 ) ) ;
#26007=CARTESIAN_POINT ( 'NONE',  ( 12.63842701281683034, 62.46726448433410894, 9.846743663894596210 ) ) ;
#26008=CARTESIAN_POINT ( 'NONE',  ( 10.00000000000000000, 31.81368534415483751, -10.88017736071110342 ) ) ;
#26012=CARTESIAN_POINT ( 'NONE',  ( 0.5774900079438607392, 68.48035201082150536, 5.440088680355550821 ) ) ;
#26013=CARTESIAN_POINT ( 'NONE',  ( -45.94000000000001194, 100.9999999999999858, -9.500000000000000000 ) ) ;
#26014=CARTESIAN_POINT ( 'NONE',  ( 18.52753015748618282, 28.92559781766745175, -4.923371831947291888 ) ) ;
#26015=CARTESIAN_POINT ( 'NONE',  ( 18.52753015748618282, 13.92559781766745175, -4.923371831947291888 ) ) ;
#26016=CARTESIAN_POINT ( 'NONE',  ( 5.076628168052703671, 6.842264484334118713, 8.527530157486179263 ) ) ;
#26017=CARTESIAN_POINT ( 'NONE',  ( 2.035157376598822676, 62.43868534415483396, -7.964842623401177768 ) ) ;
#26019=CARTESIAN_POINT ( 'NONE',  ( 17.96484262340118221, 61.18868534415482685, -7.964842623401177768 ) ) ;
#26020=CARTESIAN_POINT ( 'NONE',  ( 19.84674366389459621, 18.50893115100078745, 7.409399052514197653E-17 ) ) ;
#26024=CARTESIAN_POINT ( 'NONE',  ( 0.1532563361054083140, 56.00893115100078745, 1.131784320476157264E-15 ) ) ;
#26025=ORIENTED_EDGE ( 'NONE', *, *, #16399, .F. ) ;
#26029=CARTESIAN_POINT ( 'NONE',  ( -2.266590686148945544, 2.220415501580634388, 7.082119434687048631 ) ) ;
#26030=MECHANICAL_DESIGN_GEOMETRIC_PRESENTATION_REPRESENTATION('',(#70717),#64252);
#26031=CARTESIAN_POINT ( 'NONE',  ( 3.591859063236763294, 63.29030133659708923, -11.09922568453595026 ) ) ;
#26032=CARTESIAN_POINT ( 'NONE',  ( 24.16423886937409904, 4.095415501580634832, 3.795296366450317205 ) ) ;
#26033=CARTESIAN_POINT ( 'NONE',  ( 6.204703633549690345, 37.84541550158063927, 14.16423886937410082 ) ) ;
#26035=( LENGTH_UNIT ( ) NAMED_UNIT ( * ) SI_UNIT ( .MILLI., .METRE. ) );
#26036=CARTESIAN_POINT ( 'NONE',  ( 7.084665262690076126, 29.10535201082150181, 10.88017736071109987 ) ) ;
#26037=ORIENTED_EDGE ( 'NONE', *, *, #94333, .T. ) ;
#26038=CARTESIAN_POINT ( 'NONE',  ( 1.472469842513823179, 20.59226448433411960, -4.923371831947296329 ) ) ;
#26040=CARTESIAN_POINT ( 'NONE',  ( -0.8801773607111009756, 58.06368534415484106, 1.068504757029289695E-15 ) ) ;
#26041=CARTESIAN_POINT ( 'NONE',  ( 5.076628168052704559, 10.17559781766745175, -8.527530157486179263 ) ) ;
#26042=CARTESIAN_POINT ( 'NONE',  ( -2.816281873526473856, 39.33196800326374643, 3.434112377981055619 ) ) ;
#26043=CARTESIAN_POINT ( 'NONE',  ( 12.63842701281683034, 37.46726448433411605, 9.846743663894596210 ) ) ;
#26046=CARTESIAN_POINT ( 'NONE',  ( 0.5774900079438590739, 57.64701867748817676, -5.440088680355550821 ) ) ;
#26047=CARTESIAN_POINT ( 'NONE',  ( 6.565887622018943937, 23.08196800326375708, -12.81628187352647608 ) ) ;
#26049=CARTESIAN_POINT ( 'NONE',  ( 12.63842701281683034, 27.46726448433411250, 9.846743663894596210 ) ) ;
#26050=CARTESIAN_POINT ( 'NONE',  ( 22.26659068614895176, 9.720415501580633943, -7.082119434687042414 ) ) ;
#26052=CARTESIAN_POINT ( 'NONE',  ( 2.035157376598822676, 37.43868534415484106, -7.964842623401177768 ) ) ;
#26053=CARTESIAN_POINT ( 'NONE',  ( 13.79529636645030344, 33.26208216824730357, 14.16423886937410614 ) ) ;
#26054=CARTESIAN_POINT ( 'NONE',  ( 5.076628168052704559, 55.17559781766745175, -8.527530157486179263 ) ) ;
#26055=CARTESIAN_POINT ( 'NONE',  ( 17.20831665107776587, 9.133931151000787452, -7.208316651077762316 ) ) ;
#26056=CARTESIAN_POINT ( 'NONE',  ( 3.591859063236761518, 64.95696800326376774, 11.09922568453594849 ) ) ;
#26058=CARTESIAN_POINT ( 'NONE',  ( 15.44008868035555260, 44.73035201082151247, 9.422509992056143702 ) ) ;
#26060=CARTESIAN_POINT ( 'NONE',  ( 22.81628187352647785, 26.62363466993042138, 6.195893100308588602E-16 ) ) ;
#26061=CARTESIAN_POINT ( 'NONE',  ( 19.84674366389459621, 58.50893115100078745, 7.409399052514197653E-17 ) ) ;
#26063=SURFACE_STYLE_FILL_AREA ( #58510 ) ;
#26064=CARTESIAN_POINT ( 'NONE',  ( 0.5774900079438590739, 62.64701867748817676, -5.440088680355550821 ) ) ;
#26069=CARTESIAN_POINT ( 'NONE',  ( 0.5774900079438590739, 47.64701867748817676, -5.440088680355550821 ) ) ;
#26071=CARTESIAN_POINT ( 'NONE',  ( 17.96484262340118221, 59.93868534415484106, 7.964842623401181321 ) ) ;
#26073=CARTESIAN_POINT ( 'NONE',  ( 0.2751277870542914172, 58.21833443783938833, 6.499999999999992006 ) ) ;
#26074=CARTESIAN_POINT ( 'NONE',  ( 5.076628168052703671, 21.84226448433411960, 8.527530157486179263 ) ) ;
#26075=CARTESIAN_POINT ( 'NONE',  ( 7.084665262690076126, 29.10535201082150181, 10.88017736071109987 ) ) ;
#26076=CARTESIAN_POINT ( 'NONE',  ( 2.791683348922237240, 60.38393115100078745, -7.208316651077763204 ) ) ;
#26077=CARTESIAN_POINT ( 'NONE',  ( 19.42250999205614548, 15.98035201082150714, -5.440088680355545492 ) ) ;
#26078=CARTESIAN_POINT ( 'NONE',  ( 0.2751277870542967463, 70.00000000000000000, 6.000000000000000000 ) ) ;
#26080=CARTESIAN_POINT ( 'NONE',  ( 13.43411237798106583, 27.66530133659708568, -12.81628187352647252 ) ) ;
#26081=ORIENTED_EDGE ( 'NONE', *, *, #88312, .T. ) ;
#26082=CARTESIAN_POINT ( 'NONE',  ( 19.42250999205614548, 55.98035201082150536, -5.440088680355545492 ) ) ;
#26083=CARTESIAN_POINT ( 'NONE',  ( 12.63842701281683034, 47.46726448433412315, 9.846743663894596210 ) ) ;
#26084=CARTESIAN_POINT ( 'NONE',  ( 22.81628187352647785, 26.62363466993042138, 6.195893100308588602E-16 ) ) ;
#26085=( NAMED_UNIT ( * ) PLANE_ANGLE_UNIT ( ) SI_UNIT ( $, .RADIAN. ) );
#26086=CARTESIAN_POINT ( 'NONE',  ( -0.8801773607111009756, 33.06368534415484106, 1.068504757029289695E-15 ) ) ;
#26087=CARTESIAN_POINT ( 'NONE',  ( -4.164238869374099927, 47.01208216824729647, 3.795296366450308767 ) ) ;
#26088=CARTESIAN_POINT ( 'NONE',  ( 12.63842701281683034, 37.46726448433411605, 9.846743663894596210 ) ) ;
#26089=CARTESIAN_POINT ( 'NONE',  ( 14.92337183194729988, 4.342264484334117824, -8.527530157486177487 ) ) ;
#26090=CARTESIAN_POINT ( 'NONE',  ( 4.559911319644449179, 52.23035201082151247, -9.422509992056141925 ) ) ;
#26091=CARTESIAN_POINT ( 'NONE',  ( -2.266590686148945544, 21.38708216824730357, -7.082119434687050408 ) ) ;
#26093=CARTESIAN_POINT ( 'NONE',  ( 1.383448333479231795, 22.37718327197428891, -6.499999999999977796 ) ) ;
#26094=EDGE_CURVE ( 'NONE', #91043, #91555, #87231, .T. ) ;
#26095=EDGE_LOOP ( 'NONE', ( #3148, #39189, #73184, #23903 ) ) ;
#26096=CARTESIAN_POINT ( 'NONE',  ( 2.917880565312950480, 50.97041550158064638, -12.26659068614894821 ) ) ;
#26097=CARTESIAN_POINT ( 'NONE',  ( -0.3689425029237898834, 56.17874883491396076, -10.36894250292378850 ) ) ;
#26098=CARTESIAN_POINT ( 'NONE',  ( 1.472469842513823179, 10.59226448433411782, -4.923371831947296329 ) ) ;
#26102=CARTESIAN_POINT ( 'NONE',  ( 6.565887622018943937, 30.16530133659708568, 12.81628187352647430 ) ) ;
#26103=CARTESIAN_POINT ( 'NONE',  ( 10.00000000000000178, 38.05374883491396787, 14.16423886937410082 ) ) ;
#26104=EDGE_CURVE ( 'NONE', #31822, #83562, #78654, .T. ) ;
#26107=CARTESIAN_POINT ( 'NONE',  ( 7.084665262690076126, 67.02201867748817676, -10.88017736071110164 ) ) ;
#26108=STYLED_ITEM ( 'NONE', ( #72425 ), #93637 ) ;
#26111=SURFACE_STYLE_USAGE ( .BOTH. , #680 ) ;
#26112=CARTESIAN_POINT ( 'NONE',  ( 17.20831665107776587, 19.13393115100078035, -7.208316651077762316 ) ) ;
#26114=B_SPLINE_CURVE_WITH_KNOTS ( 'NONE', 3,
 ( #65712, #50216, #79253, #71753, #58711, #11242 ),
 .UNSPECIFIED., .F., .F.,
 ( 4, 2, 4 ),
 ( 0.000000000000000000, 0.0002565770811491099672, 0.0005131541622982199345 ),
 .UNSPECIFIED. ) ;
#26115=ORIENTED_EDGE ( 'NONE', *, *, #3962, .F. ) ;
#26116=CARTESIAN_POINT ( 'NONE',  ( 0.5774900079438590739, 2.647018677488171434, -5.440088680355550821 ) ) ;
#26117=CARTESIAN_POINT ( 'NONE',  ( 12.91533473730993009, 16.60535201082150891, -10.88017736071109987 ) ) ;
#26118=CARTESIAN_POINT ( 'NONE',  ( 2.791683348922237240, 45.38393115100079456, -7.208316651077763204 ) ) ;
#26119=CARTESIAN_POINT ( 'NONE',  ( 6.565887622018943937, 5.165301336597086568, 12.81628187352647430 ) ) ;
#26123=CARTESIAN_POINT ( 'NONE',  ( 13.43411237798106583, 22.66530133659708923, -12.81628187352647252 ) ) ;
#26124=EDGE_LOOP ( 'NONE', ( #70241, #36701, #32318, #88098 ) ) ;
#26125=CARTESIAN_POINT ( 'NONE',  ( -2.266590686148945544, 61.38708216824730357, -7.082119434687050408 ) ) ;
#26126=ORIENTED_EDGE ( 'NONE', *, *, #36189, .F. ) ;
#26128=CARTESIAN_POINT ( 'NONE',  ( 2.917880565312948704, 52.63708216824730357, 12.26659068614894643 ) ) ;
#26130=CARTESIAN_POINT ( 'NONE',  ( -0.8801773607110991993, 37.85535201082151247, -2.915334737309923874 ) ) ;
#26131=CARTESIAN_POINT ( 'NONE',  ( 0.5774900079438607392, 33.48035201082150536, 5.440088680355550821 ) ) ;
#26132=CARTESIAN_POINT ( 'NONE',  ( 19.72487221294570858, 5.718334437839381224, -6.500000000000000888 ) ) ;
#26133=CARTESIAN_POINT ( 'NONE',  ( 2.035157376598822676, 22.43868534415483396, -7.964842623401177768 ) ) ;
#26135=CARTESIAN_POINT ( 'NONE',  ( 19.84674366389459266, 13.71726448433411782, -2.638427012816827677 ) ) ;
#26138=CARTESIAN_POINT ( 'NONE',  ( 1.472469842513823179, 45.59226448433412315, -4.923371831947296329 ) ) ;
#26139=CARTESIAN_POINT ( 'NONE',  ( 18.72515096720570327, 11.07228050351031712, -6.499999999999992006 ) ) ;
#26140=CARTESIAN_POINT ( 'NONE',  ( 21.09922568453594849, 51.20696800326375353, 6.408140936763242479 ) ) ;
#26143=CARTESIAN_POINT ( 'NONE',  ( -46.59701958359877239, 103.7651961684614577, 6.068442458532170569 ) ) ;
#26144=CARTESIAN_POINT ( 'NONE',  ( -0.8801773607111009756, 53.27201867748818387, 2.915334737309923874 ) ) ;
#26145=CARTESIAN_POINT ( 'NONE',  ( 19.84674366389459621, 63.50893115100078745, 7.409399052514197653E-17 ) ) ;
#26146=CARTESIAN_POINT ( 'NONE',  ( -4.164238869374098151, 41.59541550158061796, -3.795296366450310543 ) ) ;
#26147=CARTESIAN_POINT ( 'NONE',  ( 13.99999999999999822, 10.49999999999999822, 6.000000000000000000 ) ) ;
#26150=CARTESIAN_POINT ( 'NONE',  ( 14.92337183194729633, 37.67559781766745175, 8.527530157486181039 ) ) ;
#26151=CARTESIAN_POINT ( 'NONE',  ( 10.00000000000000178, 60.37363466993041783, 12.81628187352647608 ) ) ;
#26152=CARTESIAN_POINT ( 'NONE',  ( -2.816281873526471635, -1.084698663402913210, -3.434112377981056508 ) ) ;
#26153=CARTESIAN_POINT ( 'NONE',  ( 1.472469842513823179, 0.5922644843341181575, -4.923371831947296329 ) ) ;
#26154=CARTESIAN_POINT ( 'NONE',  ( 0.1955144967548901602, 4.327036817733407759, -6.500000000002763123 ) ) ;
#26155=CARTESIAN_POINT ( 'NONE',  ( 7.361572987183170547, 62.05059781766745886, 9.846743663894590881 ) ) ;
#26157=EDGE_LOOP ( 'NONE', ( #6727, #23670, #16162, #81668 ) ) ;
#26158=CARTESIAN_POINT ( 'NONE',  ( 20.36894250292379382, 63.67874883491396787, 10.36894250292379205 ) ) ;
#26160=CARTESIAN_POINT ( 'NONE',  ( 4.559911319644449179, 37.23035201082150536, -9.422509992056141925 ) ) ;
#26161=CARTESIAN_POINT ( 'NONE',  ( -1.099225684535947600, 19.54030133659708568, 6.408140936763237150 ) ) ;
#26162=CARTESIAN_POINT ( 'NONE',  ( 0.5774900079438590739, 67.64701867748817676, -5.440088680355550821 ) ) ;
#26163=CARTESIAN_POINT ( 'NONE',  ( -0.8801773607110991993, 2.855352010821504471, -2.915334737309923874 ) ) ;
#26167=CARTESIAN_POINT ( 'NONE',  ( 17.20831665107776587, 57.88393115100078745, 7.208316651077764980 ) ) ;
#26168=PRESENTATION_STYLE_ASSIGNMENT (( #55688 ) ) ;
#26170=CARTESIAN_POINT ( 'NONE',  ( 19.38216949554541557, 27.24863466993041783, -9.382169495545420901 ) ) ;
#26172=CARTESIAN_POINT ( 'NONE',  ( 19.42250999205614548, 20.98035201082150891, -5.440088680355545492 ) ) ;
#26175=CARTESIAN_POINT ( 'NONE',  ( 13.79529636645031943, 40.34541550158063217, -14.16423886937409904 ) ) ;
#26176=CARTESIAN_POINT ( 'NONE',  ( 24.16423886937409904, 24.09541550158063927, 3.795296366450317205 ) ) ;
#26177=B_SPLINE_CURVE_WITH_KNOTS ( 'NONE', 3,
 ( #91967, #1975, #16471, #84958, #68981, #2475 ),
 .UNSPECIFIED., .F., .F.,
 ( 4, 2, 4 ),
 ( 0.000000000000000000, 0.0002701661927229442807, 0.0005403323854458885614 ),
 .UNSPECIFIED. ) ;
#26178=CARTESIAN_POINT ( 'NONE',  ( 10.00000000000000000, 16.81368534415483751, -10.88017736071110342 ) ) ;
#26179=CARTESIAN_POINT ( 'NONE',  ( 1.472469842513823179, 40.59226448433411605, -4.923371831947296329 ) ) ;
#26180=CARTESIAN_POINT ( 'NONE',  ( 16.40814093676323893, 40.79030133659708923, 11.09922568453595026 ) ) ;
#26181=CARTESIAN_POINT ( 'NONE',  ( -0.8801773607110991993, 12.85535201082150358, -2.915334737309923874 ) ) ;
#26182=CARTESIAN_POINT ( 'NONE',  ( 17.20831665107776587, 32.88393115100078745, 7.208316651077764980 ) ) ;
#26183=CARTESIAN_POINT ( 'NONE',  ( -0.8801773607111008646, 38.27201867748816255, 2.915334737309923430 ) ) ;
#26184=CARTESIAN_POINT ( 'NONE',  ( -2.816281873526471635, 8.915301336597083903, -3.434112377981056508 ) ) ;
#26185=CARTESIAN_POINT ( 'NONE',  ( 13.79529636645030344, 23.26208216824730002, 14.16423886937410614 ) ) ;
#26188=CARTESIAN_POINT ( 'NONE',  ( 10.00000000000000000, 24.75893115100078745, -9.846743663894594434 ) ) ;
#26189=CARTESIAN_POINT ( 'NONE',  ( 21.09922568453594849, 46.20696800326376064, 6.408140936763242479 ) ) ;
#26190=CARTESIAN_POINT ( 'NONE',  ( 2.791683348922237240, 50.38393115100078035, -7.208316651077763204 ) ) ;
#26192=CARTESIAN_POINT ( 'NONE',  ( 10.00000000000000178, 70.00000000000000000, 0.000000000000000000 ) ) ;
#26194=CARTESIAN_POINT ( 'NONE',  ( 10.00000000000000178, 63.05374883491396076, 14.16423886937410082 ) ) ;
#26195=CARTESIAN_POINT ( 'NONE',  ( -4.164238869374098151, 11.59541550158063217, -3.795296366450310543 ) ) ;
#26196=CARTESIAN_POINT ( 'NONE',  ( 0.1532563361054100626, 5.800597817667452638, -2.638427012816831230 ) ) ;
#26197=CARTESIAN_POINT ( 'NONE',  ( 1.472469842513823179, 45.59226448433412315, -4.923371831947296329 ) ) ;
#26198=CARTESIAN_POINT ( 'NONE',  ( 7.084665262690076126, 17.02201867748817676, -10.88017736071110164 ) ) ;
#26199=CARTESIAN_POINT ( 'NONE',  ( 17.39651004071841456, 14.08210964143329669, -6.500000000000003553 ) ) ;
#26200=CARTESIAN_POINT ( 'NONE',  ( 0.1532563361054100626, 60.80059781766744464, -2.638427012816831230 ) ) ;
#26202=VERTEX_POINT ( 'NONE', #12111 ) ;
#26203=DIRECTION ( 'NONE',  ( 0.000000000000000000, 0.000000000000000000, -1.000000000000000000 ) ) ;
#26206=VERTEX_POINT ( 'NONE', #97617 ) ;
#26208=CARTESIAN_POINT ( 'NONE',  ( 6.204703633549690345, 7.845415501580634832, 14.16423886937410082 ) ) ;
#26209=CARTESIAN_POINT ( 'NONE',  ( 20.36894250292379382, 13.67874883491396965, 10.36894250292379205 ) ) ;
#26210=CARTESIAN_POINT ( 'NONE',  ( 17.08211943468705130, 38.47041550158063217, 12.26659068614894998 ) ) ;
#26211=CARTESIAN_POINT ( 'NONE',  ( 2.791683348922240793, 61.63393115100079456, 7.208316651077764092 ) ) ;
#26212=CARTESIAN_POINT ( 'NONE',  ( 0.1532563361054082862, 41.21726448433411605, 2.638427012816831674 ) ) ;
#26213=CARTESIAN_POINT ( 'NONE',  ( -0.8801773607111008646, 38.27201867748816255, 2.915334737309923430 ) ) ;
#26214=CARTESIAN_POINT ( 'NONE',  ( 5.076628168052703671, 66.84226448433412315, 8.527530157486179263 ) ) ;
#26215=CARTESIAN_POINT ( 'NONE',  ( 6.204703633549690345, 0.7620821682473009062, -14.16423886937410259 ) ) ;
#26217=CARTESIAN_POINT ( 'NONE',  ( 19.42250999205614193, 5.147018677488171434, 5.440088680355555262 ) ) ;
#26220=CARTESIAN_POINT ( 'NONE',  ( 19.42250999205614193, 65.14701867748817676, 5.440088680355555262 ) ) ;
#26221=CARTESIAN_POINT ( 'NONE',  ( 1.472469842513823179, 25.59226448433412315, -4.923371831947296329 ) ) ;
#26223=EDGE_LOOP ( 'NONE', ( #98227, #14051, #30554, #72363 ) ) ;
#26226=CARTESIAN_POINT ( 'NONE',  ( 5.076628168052704559, 20.17559781766745175, -8.527530157486179263 ) ) ;
#26227=ORIENTED_EDGE ( 'NONE', *, *, #45515, .T. ) ;
#26228=CARTESIAN_POINT ( 'NONE',  ( 22.26659068614894466, 38.88708216824731068, 7.082119434687054849 ) ) ;
#26229=CARTESIAN_POINT ( 'NONE',  ( 14.92337183194729988, 29.34226448433411960, -8.527530157486177487 ) ) ;
#26230=CARTESIAN_POINT ( 'NONE',  ( 15.44008868035555260, 54.73035201082150536, 9.422509992056143702 ) ) ;
#26232=CARTESIAN_POINT ( 'NONE',  ( 15.44008868035555793, 46.39701867748817676, -9.422509992056140149 ) ) ;
#26233=ADVANCED_FACE ( 'NONE', ( #42134 ), #67642, .F. ) ;
#26236=CARTESIAN_POINT ( 'NONE',  ( -0.3689425029237881626, 7.428748834913967869, 10.36894250292379027 ) ) ;
#26237=VERTEX_POINT ( 'NONE', #65093 ) ;
#26241=CARTESIAN_POINT ( 'NONE',  ( 16.40814093676324603, 27.45696800326375708, -11.09922568453594671 ) ) ;
#26242=CARTESIAN_POINT ( 'NONE',  ( 19.84674366389459621, 18.50893115100078745, 7.409399052514197653E-17 ) ) ;
#26244=CARTESIAN_POINT ( 'NONE',  ( 18.52753015748617571, 33.09226448433411605, 4.923371831947298993 ) ) ;
#26245=CARTESIAN_POINT ( 'NONE',  ( 15.44008868035555260, 64.73035201082151957, 9.422509992056143702 ) ) ;
#26248=CARTESIAN_POINT ( 'NONE',  ( 19.72487221294570858, 29.78217586085238366, 6.499999999999992895 ) ) ;
#26250=CARTESIAN_POINT ( 'NONE',  ( -0.8801773607110991993, 67.85535201082151957, -2.915334737309923874 ) ) ;
#26251=CARTESIAN_POINT ( 'NONE',  ( 21.09922568453595559, 7.040301336597086568, -6.408140936763230044 ) ) ;
#26252=CARTESIAN_POINT ( 'NONE',  ( 5.054308323419867577, 70.51564955044841554, 12.00000000000000000 ) ) ;
#26253=CARTESIAN_POINT ( 'NONE',  ( 2.791683348922240793, 41.63393115100078745, 7.208316651077764092 ) ) ;
#26254=CARTESIAN_POINT ( 'NONE',  ( 13.79529636645031943, 5.345415501580634832, -14.16423886937409904 ) ) ;
#26255=CARTESIAN_POINT ( 'NONE',  ( 5.076628168052703671, 36.84226448433412315, 8.527530157486179263 ) ) ;
#26256=CARTESIAN_POINT ( 'NONE',  ( 22.81628187352647785, 31.41530133659709279, 3.434112377981063169 ) ) ;
#26258=CARTESIAN_POINT ( 'NONE',  ( 17.96484262340118221, 64.93868534415483396, 7.964842623401181321 ) ) ;
#26259=CARTESIAN_POINT ( 'NONE',  ( 19.72487221294570858, 10.71833443783938655, -6.500000000000000888 ) ) ;
#26261=CARTESIAN_POINT ( 'NONE',  ( 0.1532563361054082862, 36.21726448433410894, 2.638427012816831674 ) ) ;
#26262=CARTESIAN_POINT ( 'NONE',  ( 12.91533473730992121, 29.52201867748817321, 10.88017736071110164 ) ) ;
#26263=CARTESIAN_POINT ( 'NONE',  ( 3.591859063236763294, 23.29030133659708568, -11.09922568453595026 ) ) ;
#26264=CARTESIAN_POINT ( 'NONE',  ( 2.791683348922237240, 20.38393115100078745, -7.208316651077763204 ) ) ;
#26266=CARTESIAN_POINT ( 'NONE',  ( 7.084665262690076126, 27.02201867748817676, -10.88017736071110164 ) ) ;
#26267=CARTESIAN_POINT ( 'NONE',  ( -0.8801773607110991993, 62.85535201082150536, -2.915334737309923874 ) ) ;
#26269=CARTESIAN_POINT ( 'NONE',  ( 17.20831665107776587, 49.13393115100078745, -7.208316651077762316 ) ) ;
#26270=CARTESIAN_POINT ( 'NONE',  ( 15.44008868035555260, 29.73035201082150891, 9.422509992056143702 ) ) ;
#26271=CARTESIAN_POINT ( 'NONE',  ( -0.8801773607111009756, 48.06368534415484817, 1.068504757029289695E-15 ) ) ;
#26272=CARTESIAN_POINT ( 'NONE',  ( 19.42250999205614548, 15.98035201082150714, -5.440088680355545492 ) ) ;
#26274=LINE ( 'NONE', #87271, #92053 ) ;
#26275=CARTESIAN_POINT ( 'NONE',  ( 19.84674366389459621, 43.50893115100078745, 7.409399052514197653E-17 ) ) ;
#26276=CARTESIAN_POINT ( 'NONE',  ( 10.00000000000000000, 55.55374883491396787, -14.16423886937410082 ) ) ;
#26278=CARTESIAN_POINT ( 'NONE',  ( 2.153642693323438717, 6.137910973973185413, -6.500000000000002665 ) ) ;
#26279=ADVANCED_FACE ( 'NONE', ( #5111 ), #66088, .T. ) ;
#26281=CARTESIAN_POINT ( 'NONE',  ( 13.79529636645030344, 43.26208216824730357, 14.16423886937410614 ) ) ;
#26283=ORIENTED_EDGE ( 'NONE', *, *, #98842, .T. ) ;
#26284=CARTESIAN_POINT ( 'NONE',  ( -0.3689425029237898834, 61.17874883491396076, -10.36894250292378850 ) ) ;
#26285=CARTESIAN_POINT ( 'NONE',  ( 17.20831665107776587, 29.13393115100078390, -7.208316651077762316 ) ) ;
#26286=LINE ( 'NONE', #17338, #37191 ) ;
#26288=CARTESIAN_POINT ( 'NONE',  ( 4.559911319644449179, 63.89701867748817676, 9.422509992056141925 ) ) ;
#26291=CARTESIAN_POINT ( 'NONE',  ( -0.8801773607110991993, 32.85535201082151247, -2.915334737309923874 ) ) ;
#26292=( BOUNDED_SURFACE ( )  B_SPLINE_SURFACE ( 1, 2, ( 
 ( #97145, #96141, #51118, #58109, #80637, #73611, #43614, #57628, #65121, #81609, #36112, #20125, #87633, #96640, #42636, #51624, #44096, #5135, #95640, #58617, #72622, #27126, #73113, #74101, #88618, #50629, #74607, #6120, #89118, #88125, #13118, #20629, #11644, #81120, #28117, #5634, #35626, #36626, #66618, #95130, #59103, #26641, #19637, #66111, #50130, #28616, #89612, #21125, #4655, #35116, #65615, #12621, #57137, #27624, #43123, #19147, #49624, #42157, #23606, #67110, #8098, #54072, #8584, #75598, #22613, #68601, #83602, #7110, #38112, #53090, #90589, #30578, #30084, #37614, #67616, #21626, #84587, #68108, #97635, #29100, #6607, #60591, #59602, #60087, #22116, #84094, #45592, #626, #52596, #83099, #129, #14627, #76090, #16086, #29585, #38594, #69092, #45092, #98633, #15116, #23109, #37120, #7620, #52111, #98124, #61083, #91593, #46573, #91086, #53581, #15610, #46094, #77072, #76578, #90098, #31072, #82603, #44605, #61570, #14121, #92081, #75100, #71063, #16583, #32552, #17084, #2093, #47059, #93055, #39090, #41062, #40066, #94048, #63053, #24588, #17576, #86555, #1597, #77557, #25569, #79038, #93550, #31564, #40565, #85570, #94534, #87037, #48042, #9073, #2588, #39586, #70077, #55051, #18059, #25083, #55566, #18547, #26053, #33043, #32048, #56061, #63538, #24089, #86065, #48539, #10551, #78554, #49039, #71559, #69581, #3071, #1101, #47564, #62550, #62059, #33527, #64022, #78062, #79543, #10066, #56542, #92563, #9565, #70567, #54557, #85074, #28006, #88514, #95531, #26529, #42526, #3558, #41564, #65507, #50026, #43017, #96029, #80026, #5025, #89504, #27511, #57521, #96531, #73010, #64515, #72031, #11530, #42051, #34511, #87527, #43499, #12515, #19041, #36004, #20519, #80528, #81014, #12027, #4542, #35004, #66507, #34018, #95021, #97032, #49517, #73499, #27021, #72515, #13004, #35509, #57026, #4049, #20016, #66003, #28508, #59002, #21015, #65004, #73998, #19529, #81499, #58502, #58005, #88017, #50517, #89012, #51503, #51004, #5524, #11043, #89991, #68979, #74991, #90475, #43990, #37503, #513, #81997, #14010, #76471, #13508, #52005, #22501, #74492, #36508, #15005, #75977, #37997, #91965, #30464, #7986, #44491, #59981, #38485, #83975, #6494, #52972, #15500, #83484, #45475, #82991, #7506, #68489, #16, #60965, #82494, #30959, #61457, #53465, #6016, #21507, #91473, #22009, #23494, #67001, #52483, #14509, #97523, #28985, #37002, #22998, #29473, #59491, #67498, #60478, #98019, #45982, #44979, #75485, #6998, #67995, #98520, #29973, #90967, #10439, #17461, #23974, #9950, #47928, #38975, #47444, #55449, #78434, #32437, #33408 ),
 ( #54447, #40454, #63906, #39950, #1480, #70953, #85451, #8467, #15974, #84956, #16467, #77442, #31447, #86442, #85951, #61949, #78929, #63429, #24469, #24964, #54934, #16963, #77943, #40946, #84474, #76957, #71444, #92450, #2473, #39471, #46947, #55943, #32929, #987, #69466, #62937, #93935, #2958, #94417, #53965, #8954, #17941, #62433, #25460, #48426, #9449, #46464, #1972, #93439, #69961, #31933, #92937, #70453, #33895, #12881, #18927, #34394, #86922, #80408, #43380, #25933, #56908, #20401, #56433, #94909, #65386, #18433, #79429, #57885, #19896, #80898, #35880, #73382, #50888, #87410, #3924, #81382, #27884, #49404, #95913, #58371, #27393, #88399, #26904, #50389, #12394, #42900, #4908, #26408, #73879, #5409, #96408, #48916, #88892, #35389, #65880, #57401, #66376, #10925, #41451, #71915, #79904, #3436, #64400, #11413, #41934, #72395, #64881, #95408, #87891, #19408, #49899, #11909, #42411, #72891, #4425, #34890, #97395, #20894, #37879, #90850, #36881, #38363, #82870, #37385, #14886, #59367, #6368, #29359, #21887, #45355, #75360, #82363, #13383, #59862, #89381, #28387, #52365, #67371, #29853, #14384, #66878, #22381, #76353, #44854, #44370, #83363, #90349, #51383, #58879, #28863, #89870, #21385, #74362, #30342, #98396, #5890, #22875, #7380, #97901, #67875, #6874, #60356, #52855, #53346, #81870, #43866, #83854, #36383, #75860, #13886, #51882, #98891, #68372, #74869, #60849, #91348, #15378, #45862, #7868, #96910, #31329, #70834, #77321, #40330, #24836, #39349, #30843, #16840, #47313, #25338, #70337, #55318, #62315, #76834, #55822, #61829, #8835, #61341, #24351, #86316, #68861, #870, #63298, #393, #38857, #9328, #91852, #23367, #1853, #62816, #85825, #78809, #17340, #93808, #92337, #46829, #17820, #2346, #23860, #39831, #8349, #32311, #54325, #69346, #32803, #93314, #15862, #53853, #77813, #47809, #48302, #10318, #84361, #84839, #46347, #69843, #16347, #78310, #1367, #31818, #9829, #92822, #54815, #85326, #27269, #34264, #48793, #27765, #33769, #49288, #2837, #95278, #58248, #40820, #71801, #35264, #71319, #10810, #80282, #33293, #94293, #72763, #34772, #95788, #52127, #88272, #65761, #3306, #18805, #96286, #42782, #64276, #11782, #73266, #42290, #4298, #41810, #65259, #57767, #19774, #50261, #41328, #90116, #21643, #12271, #63784, #79301, #80778, #79788, #82623, #25816, #11291, #72278, #56313, #86809, #94788, #3808, #26288, #18311, #4788, #56789, #64766, #87284, #26781, #57279, #87773, #19288, #49775, #45610, #38129, #31090, #91609, #98654, #29604, #76108, #6625, #44623, #68617, #53108, #46112, #146, #83115, #8114, #92582 ) ),
 .UNSPECIFIED., .F., .F., .F. ) 
 B_SPLINE_SURFACE_WITH_KNOTS ( ( 2, 2 ),
 ( 3, 2, 2, 2, 2, 2, 2, 2, 2, 2, 2, 2, 2, 2, 2, 2, 2, 2, 2, 2, 2, 2, 2, 2, 2, 2, 2, 2, 2, 2, 2, 2, 2, 2, 2, 2, 2, 2, 2, 2, 2, 2, 2, 2, 2, 2, 2, 2, 2, 2, 2, 2, 2, 2, 2, 2, 2, 2, 2, 2, 2, 2, 2, 2, 2, 2, 2, 2, 2, 2, 2, 2, 2, 2, 2, 2, 2, 2, 2, 2, 2, 2, 2, 2, 2, 2, 2, 2, 2, 2, 2, 2, 2, 2, 2, 2, 2, 2, 2, 2, 2, 2, 2, 2, 2, 2, 2, 2, 2, 2, 2, 2, 2, 2, 2, 2, 2, 2, 2, 2, 2, 2, 2, 2, 2, 2, 2, 2, 2, 2, 2, 2, 2, 2, 2, 2, 2, 2, 2, 2, 2, 2, 2, 2, 2, 2, 2, 2, 2, 2, 2, 2, 2, 2, 2, 2, 2, 2, 2, 2, 2, 2, 3 ),
 ( 0.000000000000000000, 1.000000000000000000 ),
 ( 0.000000000000000000, 0.005952380952380952051, 0.01190476190476190410, 0.01785714285714285615, 0.02380952380952380820, 0.02976190476190476025, 0.03571428571428571230, 0.04166666666666666435, 0.04761904761904761640, 0.05357142857142856845, 0.05952380952380952051, 0.06547619047619047949, 0.07142857142857142461, 0.07738095238095238360, 0.08333333333333332871, 0.08928571428571428770, 0.09523809523809523281, 0.1011904761904761918, 0.1071428571428571369, 0.1130952380952380959, 0.1190476190476190410, 0.1250000000000000000, 0.1309523809523809590, 0.1369047619047619180, 0.1428571428571428492, 0.1488095238095238082, 0.1547619047619047672, 0.1607142857142857262, 0.1666666666666666574, 0.1726190476190476164, 0.1785714285714285754, 0.1845238095238095344, 0.1904761904761904656, 0.1964285714285714246, 0.2023809523809523836, 0.2083333333333333426, 0.2142857142857142738, 0.2202380952380952328, 0.2261904761904761918, 0.2321428571428571508, 0.2380952380952380820, 0.2440476190476190410, 0.2500000000000000000, 0.2559523809523809312, 0.2619047619047619180, 0.2678571428571428492, 0.2738095238095238360, 0.2797619047619047672, 0.2857142857142856984, 0.2916666666666666852, 0.2976190476190476164, 0.3035714285714285476, 0.3095238095238095344, 0.3154761904761904656, 0.3214285714285714524, 0.3273809523809523836, 0.3333333333333333148, 0.3392857142857143016, 0.3452380952380952328, 0.3511904761904761640, 0.3571428571428571508, 0.3630952380952380820, 0.3690476190476190688, 0.3750000000000000000, 0.3809523809523809312, 0.3869047619047619180, 0.3928571428571428492, 0.3988095238095238360, 0.4047619047619047672, 0.4107142857142856984, 0.4166666666666666852, 0.4226190476190476164, 0.4285714285714285476, 0.4345238095238095344, 0.4404761904761904656, 0.4464285714285714524, 0.4523809523809523836, 0.4583333333333333148, 0.4642857142857143016, 0.4702380952380952328, 0.4761904761904761640, 0.4821428571428571508, 0.4880952380952380820, 0.4940476190476190688, 0.5000000000000000000, 0.5059523809523809312, 0.5119047619047618625, 0.5178571428571429047, 0.5238095238095238360, 0.5297619047619047672, 0.5357142857142856984, 0.5416666666666666297, 0.5476190476190476719, 0.5535714285714286031, 0.5595238095238095344, 0.5654761904761904656, 0.5714285714285713969, 0.5773809523809523281, 0.5833333333333333703, 0.5892857142857143016, 0.5952380952380952328, 0.6011904761904761640, 0.6071428571428570953, 0.6130952380952381375, 0.6190476190476190688, 0.6250000000000000000, 0.6309523809523809312, 0.6369047619047618625, 0.6428571428571429047, 0.6488095238095238360, 0.6547619047619047672, 0.6607142857142856984, 0.6666666666666666297, 0.6726190476190476719, 0.6785714285714286031, 0.6845238095238095344, 0.6904761904761904656, 0.6964285714285713969, 0.7023809523809523281, 0.7083333333333333703, 0.7142857142857143016, 0.7202380952380952328, 0.7261904761904761640, 0.7321428571428570953, 0.7380952380952381375, 0.7440476190476190688, 0.7500000000000000000, 0.7559523809523809312, 0.7619047619047618625, 0.7678571428571429047, 0.7738095238095238360, 0.7797619047619047672, 0.7857142857142856984, 0.7916666666666666297, 0.7976190476190476719, 0.8035714285714286031, 0.8095238095238095344, 0.8154761904761904656, 0.8214285714285713969, 0.8273809523809523281, 0.8333333333333333703, 0.8392857142857143016, 0.8452380952380952328, 0.8511904761904761640, 0.8571428571428570953, 0.8630952380952381375, 0.8690476190476190688, 0.8750000000000000000, 0.8809523809523809312, 0.8869047619047618625, 0.8928571428571429047, 0.8988095238095238360, 0.9047619047619047672, 0.9107142857142856984, 0.9166666666666666297, 0.9226190476190476719, 0.9285714285714286031, 0.9345238095238095344, 0.9404761904761904656, 0.9464285714285713969, 0.9523809523809523281, 0.9583333333333333703, 0.9642857142857143016 ),
 .UNSPECIFIED. ) 
 GEOMETRIC_REPRESENTATION_ITEM ( )  RATIONAL_B_SPLINE_SURFACE ( (
 ( 1.000000000000000000, 0.9659258262890683122, 1.000000000000000000, 0.9659258262890683122, 1.000000000000000000, 0.9659258262890683122, 1.000000000000000000, 0.9659258262890683122, 1.000000000000000000, 0.9659258262890683122, 1.000000000000000000, 0.9659258262890683122, 1.000000000000000000, 0.9659258262890683122, 1.000000000000000000, 0.9659258262890683122, 1.000000000000000000, 0.9659258262890683122, 1.000000000000000000, 0.9659258262890683122, 1.000000000000000000, 0.9659258262890683122, 1.000000000000000000, 0.9659258262890683122, 1.000000000000000000, 0.9659258262890683122, 1.000000000000000000, 0.9659258262890683122, 1.000000000000000000, 0.9659258262890683122, 1.000000000000000000, 0.9659258262890683122, 1.000000000000000000, 0.9659258262890683122, 1.000000000000000000, 0.9659258262890683122, 1.000000000000000000, 0.9659258262890683122, 1.000000000000000000, 0.9659258262890683122, 1.000000000000000000, 0.9659258262890683122, 1.000000000000000000, 0.9659258262890683122, 1.000000000000000000, 0.9659258262890683122, 1.000000000000000000, 0.9659258262890683122, 1.000000000000000000, 0.9659258262890683122, 1.000000000000000000, 0.9659258262890683122, 1.000000000000000000, 0.9659258262890683122, 1.000000000000000000, 0.9659258262890683122, 1.000000000000000000, 0.9659258262890683122, 1.000000000000000000, 0.9659258262890683122, 1.000000000000000000, 0.9659258262890683122, 1.000000000000000000, 0.9659258262890683122, 1.000000000000000000, 0.9659258262890683122, 1.000000000000000000, 0.9659258262890683122, 1.000000000000000000, 0.9659258262890683122, 1.000000000000000000, 0.9659258262890683122, 1.000000000000000000, 0.9659258262890683122, 1.000000000000000000, 0.9659258262890683122, 1.000000000000000000, 0.9659258262890683122, 1.000000000000000000, 0.9659258262890683122, 1.000000000000000000, 0.9659258262890683122, 1.000000000000000000, 0.9659258262890683122, 1.000000000000000000, 0.9659258262890683122, 1.000000000000000000, 0.9659258262890683122, 1.000000000000000000, 0.9659258262890683122, 1.000000000000000000, 0.9659258262890683122, 1.000000000000000000, 0.9659258262890683122, 1.000000000000000000, 0.9659258262890683122, 1.000000000000000000, 0.9659258262890683122, 1.000000000000000000, 0.9659258262890683122, 1.000000000000000000, 0.9659258262890683122, 1.000000000000000000, 0.9659258262890683122, 1.000000000000000000, 0.9659258262890683122, 1.000000000000000000, 0.9659258262890683122, 1.000000000000000000, 0.9659258262890683122, 1.000000000000000000, 0.9659258262890683122, 1.000000000000000000, 0.9659258262890683122, 1.000000000000000000, 0.9659258262890683122, 1.000000000000000000, 0.9659258262890683122, 1.000000000000000000, 0.9659258262890683122, 1.000000000000000000, 0.9659258262890683122, 1.000000000000000000, 0.9659258262890683122, 1.000000000000000000, 0.9659258262890683122, 1.000000000000000000, 0.9659258262890683122, 1.000000000000000000, 0.9659258262890683122, 1.000000000000000000, 0.9659258262890683122, 1.000000000000000000, 0.9659258262890683122, 1.000000000000000000, 0.9659258262890683122, 1.000000000000000000, 0.9659258262890683122, 1.000000000000000000, 0.9659258262890683122, 1.000000000000000000, 0.9659258262890683122, 1.000000000000000000, 0.9659258262890683122, 1.000000000000000000, 0.9659258262890683122, 1.000000000000000000, 0.9659258262890683122, 1.000000000000000000, 0.9659258262890683122, 1.000000000000000000, 0.9659258262890683122, 1.000000000000000000, 0.9659258262890683122, 1.000000000000000000, 0.9659258262890683122, 1.000000000000000000, 0.9659258262890683122, 1.000000000000000000, 0.9659258262890683122, 1.000000000000000000, 0.9659258262890683122, 1.000000000000000000, 0.9659258262890683122, 1.000000000000000000, 0.9659258262890683122, 1.000000000000000000, 0.9659258262890683122, 1.000000000000000000, 0.9659258262890683122, 1.000000000000000000, 0.9659258262890683122, 1.000000000000000000, 0.9659258262890683122, 1.000000000000000000, 0.9659258262890683122, 1.000000000000000000, 0.9659258262890683122, 1.000000000000000000, 0.9659258262890683122, 1.000000000000000000, 0.9659258262890683122, 1.000000000000000000, 0.9659258262890683122, 1.000000000000000000, 0.9659258262890683122, 1.000000000000000000, 0.9659258262890683122, 1.000000000000000000, 0.9659258262890683122, 1.000000000000000000, 0.9659258262890683122, 1.000000000000000000, 0.9659258262890683122, 1.000000000000000000, 0.9659258262890683122, 1.000000000000000000, 0.9659258262890683122, 1.000000000000000000, 0.9659258262890683122, 1.000000000000000000, 0.9659258262890683122, 1.000000000000000000, 0.9659258262890683122, 1.000000000000000000, 0.9659258262890683122, 1.000000000000000000, 0.9659258262890683122, 1.000000000000000000, 0.9659258262890683122, 1.000000000000000000, 0.9659258262890683122, 1.000000000000000000, 0.9659258262890683122, 1.000000000000000000, 0.9659258262890683122, 1.000000000000000000, 0.9659258262890683122, 1.000000000000000000, 0.9659258262890683122, 1.000000000000000000, 0.9659258262890683122, 1.000000000000000000, 0.9659258262890683122, 1.000000000000000000, 0.9659258262890683122, 1.000000000000000000, 0.9659258262890683122, 1.000000000000000000, 0.9659258262890683122, 1.000000000000000000, 0.9659258262890683122, 1.000000000000000000, 0.9659258262890683122, 1.000000000000000000, 0.9659258262890683122, 1.000000000000000000, 0.9659258262890683122, 1.000000000000000000, 0.9659258262890683122, 1.000000000000000000, 0.9659258262890683122, 1.000000000000000000, 0.9659258262890683122, 1.000000000000000000, 0.9659258262890683122, 1.000000000000000000, 0.9659258262890683122, 1.000000000000000000, 0.9659258262890683122, 1.000000000000000000, 0.9659258262890683122, 1.000000000000000000, 0.9659258262890683122, 1.000000000000000000, 0.9659258262890683122, 1.000000000000000000, 0.9659258262890683122, 1.000000000000000000, 0.9659258262890683122, 1.000000000000000000, 0.9659258262890683122, 1.000000000000000000, 0.9659258262890683122, 1.000000000000000000, 0.9659258262890683122, 1.000000000000000000, 0.9659258262890683122, 1.000000000000000000, 0.9659258262890683122, 1.000000000000000000, 0.9659258262890683122, 1.000000000000000000, 0.9659258262890683122, 1.000000000000000000, 0.9659258262890683122, 1.000000000000000000, 0.9659258262890683122, 1.000000000000000000, 0.9659258262890683122, 1.000000000000000000, 0.9659258262890683122, 1.000000000000000000, 0.9659258262890683122, 1.000000000000000000, 0.9659258262890683122, 1.000000000000000000, 0.9659258262890683122, 1.000000000000000000, 0.9659258262890683122, 1.000000000000000000, 0.9659258262890683122, 1.000000000000000000, 0.9659258262890683122, 1.000000000000000000, 0.9659258262890683122, 1.000000000000000000, 0.9659258262890683122, 1.000000000000000000, 0.9659258262890683122, 1.000000000000000000, 0.9659258262890683122, 1.000000000000000000, 0.9659258262890683122, 1.000000000000000000, 0.9659258262890683122, 1.000000000000000000, 0.9659258262890683122, 1.000000000000000000, 0.9659258262890683122, 1.000000000000000000, 0.9659258262890683122, 1.000000000000000000, 0.9659258262890683122, 1.000000000000000000, 0.9659258262890683122, 1.000000000000000000, 0.9659258262890683122, 1.000000000000000000, 0.9659258262890683122, 1.000000000000000000, 0.9659258262890683122, 1.000000000000000000, 0.9659258262890683122, 1.000000000000000000),
 ( 1.000000000000000000, 0.9659258262890683122, 1.000000000000000000, 0.9659258262890683122, 1.000000000000000000, 0.9659258262890683122, 1.000000000000000000, 0.9659258262890683122, 1.000000000000000000, 0.9659258262890683122, 1.000000000000000000, 0.9659258262890683122, 1.000000000000000000, 0.9659258262890683122, 1.000000000000000000, 0.9659258262890683122, 1.000000000000000000, 0.9659258262890683122, 1.000000000000000000, 0.9659258262890683122, 1.000000000000000000, 0.9659258262890683122, 1.000000000000000000, 0.9659258262890683122, 1.000000000000000000, 0.9659258262890683122, 1.000000000000000000, 0.9659258262890683122, 1.000000000000000000, 0.9659258262890683122, 1.000000000000000000, 0.9659258262890683122, 1.000000000000000000, 0.9659258262890683122, 1.000000000000000000, 0.9659258262890683122, 1.000000000000000000, 0.9659258262890683122, 1.000000000000000000, 0.9659258262890683122, 1.000000000000000000, 0.9659258262890683122, 1.000000000000000000, 0.9659258262890683122, 1.000000000000000000, 0.9659258262890683122, 1.000000000000000000, 0.9659258262890683122, 1.000000000000000000, 0.9659258262890683122, 1.000000000000000000, 0.9659258262890683122, 1.000000000000000000, 0.9659258262890683122, 1.000000000000000000, 0.9659258262890683122, 1.000000000000000000, 0.9659258262890683122, 1.000000000000000000, 0.9659258262890683122, 1.000000000000000000, 0.9659258262890683122, 1.000000000000000000, 0.9659258262890683122, 1.000000000000000000, 0.9659258262890683122, 1.000000000000000000, 0.9659258262890683122, 1.000000000000000000, 0.9659258262890683122, 1.000000000000000000, 0.9659258262890683122, 1.000000000000000000, 0.9659258262890683122, 1.000000000000000000, 0.9659258262890683122, 1.000000000000000000, 0.9659258262890683122, 1.000000000000000000, 0.9659258262890683122, 1.000000000000000000, 0.9659258262890683122, 1.000000000000000000, 0.9659258262890683122, 1.000000000000000000, 0.9659258262890683122, 1.000000000000000000, 0.9659258262890683122, 1.000000000000000000, 0.9659258262890683122, 1.000000000000000000, 0.9659258262890683122, 1.000000000000000000, 0.9659258262890683122, 1.000000000000000000, 0.9659258262890683122, 1.000000000000000000, 0.9659258262890683122, 1.000000000000000000, 0.9659258262890683122, 1.000000000000000000, 0.9659258262890683122, 1.000000000000000000, 0.9659258262890683122, 1.000000000000000000, 0.9659258262890683122, 1.000000000000000000, 0.9659258262890683122, 1.000000000000000000, 0.9659258262890683122, 1.000000000000000000, 0.9659258262890683122, 1.000000000000000000, 0.9659258262890683122, 1.000000000000000000, 0.9659258262890683122, 1.000000000000000000, 0.9659258262890683122, 1.000000000000000000, 0.9659258262890683122, 1.000000000000000000, 0.9659258262890683122, 1.000000000000000000, 0.9659258262890683122, 1.000000000000000000, 0.9659258262890683122, 1.000000000000000000, 0.9659258262890683122, 1.000000000000000000, 0.9659258262890683122, 1.000000000000000000, 0.9659258262890683122, 1.000000000000000000, 0.9659258262890683122, 1.000000000000000000, 0.9659258262890683122, 1.000000000000000000, 0.9659258262890683122, 1.000000000000000000, 0.9659258262890683122, 1.000000000000000000, 0.9659258262890683122, 1.000000000000000000, 0.9659258262890683122, 1.000000000000000000, 0.9659258262890683122, 1.000000000000000000, 0.9659258262890683122, 1.000000000000000000, 0.9659258262890683122, 1.000000000000000000, 0.9659258262890683122, 1.000000000000000000, 0.9659258262890683122, 1.000000000000000000, 0.9659258262890683122, 1.000000000000000000, 0.9659258262890683122, 1.000000000000000000, 0.9659258262890683122, 1.000000000000000000, 0.9659258262890683122, 1.000000000000000000, 0.9659258262890683122, 1.000000000000000000, 0.9659258262890683122, 1.000000000000000000, 0.9659258262890683122, 1.000000000000000000, 0.9659258262890683122, 1.000000000000000000, 0.9659258262890683122, 1.000000000000000000, 0.9659258262890683122, 1.000000000000000000, 0.9659258262890683122, 1.000000000000000000, 0.9659258262890683122, 1.000000000000000000, 0.9659258262890683122, 1.000000000000000000, 0.9659258262890683122, 1.000000000000000000, 0.9659258262890683122, 1.000000000000000000, 0.9659258262890683122, 1.000000000000000000, 0.9659258262890683122, 1.000000000000000000, 0.9659258262890683122, 1.000000000000000000, 0.9659258262890683122, 1.000000000000000000, 0.9659258262890683122, 1.000000000000000000, 0.9659258262890683122, 1.000000000000000000, 0.9659258262890683122, 1.000000000000000000, 0.9659258262890683122, 1.000000000000000000, 0.9659258262890683122, 1.000000000000000000, 0.9659258262890683122, 1.000000000000000000, 0.9659258262890683122, 1.000000000000000000, 0.9659258262890683122, 1.000000000000000000, 0.9659258262890683122, 1.000000000000000000, 0.9659258262890683122, 1.000000000000000000, 0.9659258262890683122, 1.000000000000000000, 0.9659258262890683122, 1.000000000000000000, 0.9659258262890683122, 1.000000000000000000, 0.9659258262890683122, 1.000000000000000000, 0.9659258262890683122, 1.000000000000000000, 0.9659258262890683122, 1.000000000000000000, 0.9659258262890683122, 1.000000000000000000, 0.9659258262890683122, 1.000000000000000000, 0.9659258262890683122, 1.000000000000000000, 0.9659258262890683122, 1.000000000000000000, 0.9659258262890683122, 1.000000000000000000, 0.9659258262890683122, 1.000000000000000000, 0.9659258262890683122, 1.000000000000000000, 0.9659258262890683122, 1.000000000000000000, 0.9659258262890683122, 1.000000000000000000, 0.9659258262890683122, 1.000000000000000000, 0.9659258262890683122, 1.000000000000000000, 0.9659258262890683122, 1.000000000000000000, 0.9659258262890683122, 1.000000000000000000, 0.9659258262890683122, 1.000000000000000000, 0.9659258262890683122, 1.000000000000000000, 0.9659258262890683122, 1.000000000000000000, 0.9659258262890683122, 1.000000000000000000, 0.9659258262890683122, 1.000000000000000000, 0.9659258262890683122, 1.000000000000000000, 0.9659258262890683122, 1.000000000000000000, 0.9659258262890683122, 1.000000000000000000, 0.9659258262890683122, 1.000000000000000000, 0.9659258262890683122, 1.000000000000000000, 0.9659258262890683122, 1.000000000000000000, 0.9659258262890683122, 1.000000000000000000, 0.9659258262890683122, 1.000000000000000000, 0.9659258262890683122, 1.000000000000000000, 0.9659258262890683122, 1.000000000000000000, 0.9659258262890683122, 1.000000000000000000, 0.9659258262890683122, 1.000000000000000000, 0.9659258262890683122, 1.000000000000000000, 0.9659258262890683122, 1.000000000000000000, 0.9659258262890683122, 1.000000000000000000, 0.9659258262890683122, 1.000000000000000000, 0.9659258262890683122, 1.000000000000000000, 0.9659258262890683122, 1.000000000000000000, 0.9659258262890683122, 1.000000000000000000, 0.9659258262890683122, 1.000000000000000000, 0.9659258262890683122, 1.000000000000000000, 0.9659258262890683122, 1.000000000000000000, 0.9659258262890683122, 1.000000000000000000, 0.9659258262890683122, 1.000000000000000000, 0.9659258262890683122, 1.000000000000000000, 0.9659258262890683122, 1.000000000000000000, 0.9659258262890683122, 1.000000000000000000, 0.9659258262890683122, 1.000000000000000000, 0.9659258262890683122, 1.000000000000000000, 0.9659258262890683122, 1.000000000000000000, 0.9659258262890683122, 1.000000000000000000, 0.9659258262890683122, 1.000000000000000000) ) ) 
 REPRESENTATION_ITEM ( '' )  SURFACE ( )  );
#26293=CARTESIAN_POINT ( 'NONE',  ( 6.565887622018943937, 63.08196800326376064, -12.81628187352647608 ) ) ;
#26294=CARTESIAN_POINT ( 'NONE',  ( 19.38216949554541557, 7.248634669930421381, -9.382169495545420901 ) ) ;
#26295=CARTESIAN_POINT ( 'NONE',  ( 14.92337183194729988, 19.34226448433411960, -8.527530157486177487 ) ) ;
#26297=AXIS2_PLACEMENT_3D ( 'NONE', #10929, #41455, #30349 ) ;
#26299=CARTESIAN_POINT ( 'NONE',  ( 10.00000000000000178, 68.05374883491397497, 14.16423886937410082 ) ) ;
#26300=CARTESIAN_POINT ( 'NONE',  ( -4.164238869374099927, 32.01208216824730357, 3.795296366450308767 ) ) ;
#26301=CARTESIAN_POINT ( 'NONE',  ( -0.8801773607111009756, 38.06368534415484106, 1.068504757029289695E-15 ) ) ;
#26302=CARTESIAN_POINT ( 'NONE',  ( 0.5774900079438607392, 48.48035201082150536, 5.440088680355550821 ) ) ;
#26303=CARTESIAN_POINT ( 'NONE',  ( 0.000000000000000000, 70.00000000000000000, 6.500000000000000888 ) ) ;
#26305=CARTESIAN_POINT ( 'NONE',  ( 10.00000000000000178, 7.258931151000785675, 9.846743663894594434 ) ) ;
#26306=CARTESIAN_POINT ( 'NONE',  ( 17.20831665107776587, 27.88393115100078390, 7.208316651077764980 ) ) ;
#26307=FILL_AREA_STYLE_COLOUR ( '', #34685 ) ;
#26308=MECHANICAL_DESIGN_GEOMETRIC_PRESENTATION_REPRESENTATION('',(#45431),#82190);
#26309=CARTESIAN_POINT ( 'NONE',  ( 14.92337183194729633, 17.67559781766745175, 8.527530157486181039 ) ) ;
#26310=CARTESIAN_POINT ( 'NONE',  ( 17.20831665107776587, 54.13393115100079456, -7.208316651077762316 ) ) ;
#26311=CARTESIAN_POINT ( 'NONE',  ( 7.084665262690076126, 27.02201867748817676, -10.88017736071110164 ) ) ;
#26312=UNCERTAINTY_MEASURE_WITH_UNIT (LENGTH_MEASURE( 1.000000000000000082E-05 ), #27681, 'distance_accuracy_value', 'NONE');
#26314=CARTESIAN_POINT ( 'NONE',  ( -1.099225684535947600, 44.54030133659708923, 6.408140936763237150 ) ) ;
#26316=CARTESIAN_POINT ( 'NONE',  ( 17.96484262340118221, 61.18868534415482685, -7.964842623401177768 ) ) ;
#26317=CARTESIAN_POINT ( 'NONE',  ( 17.20831665107776587, 32.88393115100078745, 7.208316651077764980 ) ) ;
#26318=CARTESIAN_POINT ( 'NONE',  ( 6.204703633549690345, 60.76208216824730357, -14.16423886937410259 ) ) ;
#26319=CARTESIAN_POINT ( 'NONE',  ( 0.1532563361054083140, 21.00893115100078745, 1.131784320476157264E-15 ) ) ;
#26322=CARTESIAN_POINT ( 'NONE',  ( 6.204703633549690345, 12.84541550158063572, 14.16423886937410082 ) ) ;
#26324=CARTESIAN_POINT ( 'NONE',  ( 2.917880565312950480, 25.97041550158063572, -12.26659068614894821 ) ) ;
#26325=CARTESIAN_POINT ( 'NONE',  ( 0.1532563361054100626, 30.80059781766744820, -2.638427012816831230 ) ) ;
#26327=CARTESIAN_POINT ( 'NONE',  ( 20.88017736071110519, 20.56368534415484106, 2.639326808657452039E-16 ) ) ;
#26328=CARTESIAN_POINT ( 'NONE',  ( 7.084665262690076126, 59.10535201082150536, 10.88017736071109987 ) ) ;
#26329=CARTESIAN_POINT ( 'NONE',  ( 4.559911319644449179, 43.89701867748816966, 9.422509992056141925 ) ) ;
#26331=CARTESIAN_POINT ( 'NONE',  ( 21.09922568453595559, 47.04030133659708923, -6.408140936763230044 ) ) ;
#26332=CARTESIAN_POINT ( 'NONE',  ( 19.42250999205614548, 50.98035201082151247, -5.440088680355545492 ) ) ;
#26333=ORIENTED_EDGE ( 'NONE', *, *, #46207, .F. ) ;
#26335=CARTESIAN_POINT ( 'NONE',  ( -0.1503990784575328643, 50.12777174578613426, 6.262539305110068177 ) ) ;
#26336=CARTESIAN_POINT ( 'NONE',  ( 17.96484262340118221, 64.93868534415483396, 7.964842623401181321 ) ) ;
#26338=CARTESIAN_POINT ( 'NONE',  ( 20.88017736071110875, 60.77201867748817676, -2.915334737309920765 ) ) ;
#26341=CARTESIAN_POINT ( 'NONE',  ( 17.96484262340118221, 4.938685344154837509, 7.964842623401181321 ) ) ;
#26342=CARTESIAN_POINT ( 'NONE',  ( 5.076628168052704559, 10.17559781766745175, -8.527530157486179263 ) ) ;
#26343=CARTESIAN_POINT ( 'NONE',  ( 24.16423886937410614, 9.512082168247301794, -3.795296366450302550 ) ) ;
#26344=CARTESIAN_POINT ( 'NONE',  ( 19.84674366389459266, 3.300597817667451750, 2.638427012816836559 ) ) ;
#26345=CARTESIAN_POINT ( 'NONE',  ( 2.035157376598822676, 12.43868534415483751, -7.964842623401177768 ) ) ;
#26346=CARTESIAN_POINT ( 'NONE',  ( 1.472469842513823179, 51.42559781766745886, 4.923371831947296329 ) ) ;
#26347=VERTEX_POINT ( 'NONE', #28593 ) ;
#26348=CARTESIAN_POINT ( 'NONE',  ( 14.92337183194729633, 42.67559781766745886, 8.527530157486181039 ) ) ;
#26350=CARTESIAN_POINT ( 'NONE',  ( 4.559911319644449179, 57.23035201082150536, -9.422509992056141925 ) ) ;
#26351=CARTESIAN_POINT ( 'NONE',  ( 18.52753015748618282, 53.92559781766745175, -4.923371831947291888 ) ) ;
#26352=CARTESIAN_POINT ( 'NONE',  ( -1.099225684535947600, 28.70696800326375353, -6.408140936763238038 ) ) ;
#26353=CARTESIAN_POINT ( 'NONE',  ( 20.88017736071110519, 5.563685344154837509, 2.639326808657452039E-16 ) ) ;
#26355=CARTESIAN_POINT ( 'NONE',  ( 12.91533473730993009, 61.60535201082150536, -10.88017736071109987 ) ) ;
#26356=CARTESIAN_POINT ( 'NONE',  ( 10.00000000000000000, 65.55374883491396076, -14.16423886937410082 ) ) ;
#26358=CARTESIAN_POINT ( 'NONE',  ( 13.43411237798106583, 37.66530133659708923, -12.81628187352647252 ) ) ;
#26359=CARTESIAN_POINT ( 'NONE',  ( 15.44008868035555260, 34.73035201082151247, 9.422509992056143702 ) ) ;
#26363=CARTESIAN_POINT ( 'NONE',  ( 21.09922568453595559, 47.04030133659708923, -6.408140936763230044 ) ) ;
#26364=CARTESIAN_POINT ( 'NONE',  ( 12.91533473730992121, 39.52201867748817676, 10.88017736071110164 ) ) ;
#26365=EDGE_LOOP ( 'NONE', ( #87678, #78358, #24076, #69259, #35841, #71868 ) ) ;
#26366=CARTESIAN_POINT ( 'NONE',  ( 0.2751277870542913062, 49.36607318730131055, -6.499999999999992006 ) ) ;
#26367=CARTESIAN_POINT ( 'NONE',  ( 18.52753015748617571, 63.09226448433412315, 4.923371831947298993 ) ) ;
#26368=CARTESIAN_POINT ( 'NONE',  ( 19.84674366389459621, 13.50893115100078568, 7.409399052514197653E-17 ) ) ;
#26369=CARTESIAN_POINT ( 'NONE',  ( 5.076628168052703671, 46.84226448433412315, 8.527530157486179263 ) ) ;
#26371=PLANE ( 'NONE',  #77652 ) ;
#26372=CARTESIAN_POINT ( 'NONE',  ( 7.361572987183170547, 37.05059781766744464, 9.846743663894590881 ) ) ;
#26374=DIRECTION ( 'NONE',  ( -0.8320502943378436100, 0.5547001962252291474, -0.000000000000000000 ) ) ;
#26375=CARTESIAN_POINT ( 'NONE',  ( 10.00000000000000178, 22.25893115100078745, 9.846743663894594434 ) ) ;
#26376=CARTESIAN_POINT ( 'NONE',  ( 0.1532563361054082862, 1.217264484334117824, 2.638427012816831674 ) ) ;
#26377=CARTESIAN_POINT ( 'NONE',  ( 17.20831665107776587, 64.13393115100079456, -7.208316651077762316 ) ) ;
#26378=ORIENTED_EDGE ( 'NONE', *, *, #38881, .T. ) ;
#26380=CARTESIAN_POINT ( 'NONE',  ( -1.099225684535947600, 29.54030133659708923, 6.408140936763237150 ) ) ;
#26381=CARTESIAN_POINT ( 'NONE',  ( 1.472469842513823179, 45.59226448433412315, -4.923371831947296329 ) ) ;
#26383=CARTESIAN_POINT ( 'NONE',  ( -0.3689425029237898834, 61.17874883491396076, -10.36894250292378850 ) ) ;
#26384=CARTESIAN_POINT ( 'NONE',  ( 17.20831665107776587, 17.88393115100078745, 7.208316651077764980 ) ) ;
#26385=CARTESIAN_POINT ( 'NONE',  ( 19.67862543671680697, 88.20241052560767514, 5.461907810393946683 ) ) ;
#26386=CARTESIAN_POINT ( 'NONE',  ( -0.3689425029237881626, 62.42874883491396787, 10.36894250292379027 ) ) ;
#26387=CARTESIAN_POINT ( 'NONE',  ( 5.076628168052704559, 55.17559781766745175, -8.527530157486179263 ) ) ;
#26388=CARTESIAN_POINT ( 'NONE',  ( 7.084665262690076126, 4.105352010821503583, 10.88017736071109987 ) ) ;
#26389=CARTESIAN_POINT ( 'NONE',  ( 13.79529636645031943, 35.34541550158063927, -14.16423886937409904 ) ) ;
#26390=CARTESIAN_POINT ( 'NONE',  ( 24.16423886937409904, 44.09541550158063927, 3.795296366450317205 ) ) ;
#26393=CARTESIAN_POINT ( 'NONE',  ( 5.076628168052704559, 55.17559781766745175, -8.527530157486179263 ) ) ;
#26394=CARTESIAN_POINT ( 'NONE',  ( 4.559911319644449179, 37.23035201082150536, -9.422509992056141925 ) ) ;
#26396=CARTESIAN_POINT ( 'NONE',  ( 20.00000000000000711, 96.99164844389140683, -4.500000004094268036 ) ) ;
#26398=CARTESIAN_POINT ( 'NONE',  ( 3.591859063236763294, 63.29030133659708923, -11.09922568453595026 ) ) ;
#26400=CARTESIAN_POINT ( 'NONE',  ( 18.52753015748618282, 58.92559781766745886, -4.923371831947291888 ) ) ;
#26401=DIRECTION ( 'NONE',  ( -0.000000000000000000, -0.000000000000000000, 1.000000000000000000 ) ) ;
#26404=CARTESIAN_POINT ( 'NONE',  ( -2.266590686148945544, 22.22041550158063572, 7.082119434687048631 ) ) ;
#26407=CARTESIAN_POINT ( 'NONE',  ( 18.72515096720577787, 46.07228050351031357, -6.499999999999891642 ) ) ;
#26408=CARTESIAN_POINT ( 'NONE',  ( 19.42250999205614193, 20.14701867748817321, 5.440088680355555262 ) ) ;
#26409=CARTESIAN_POINT ( 'NONE',  ( -2.816281873526471635, 18.91530133659708213, -3.434112377981056508 ) ) ;
#26410=CARTESIAN_POINT ( 'NONE',  ( -46.94000000000001194, 92.00000000000000000, -8.999999999999998224 ) ) ;
#26411=CARTESIAN_POINT ( 'NONE',  ( 10.00000000000000178, 7.258931151000785675, 9.846743663894594434 ) ) ;
#26413=CARTESIAN_POINT ( 'NONE',  ( -2.266590686148945544, 32.22041550158063927, 7.082119434687048631 ) ) ;
#26414=DIRECTION ( 'NONE',  ( 0.000000000000000000, 0.000000000000000000, -1.000000000000000000 ) ) ;
#26415=CARTESIAN_POINT ( 'NONE',  ( -0.1503990784575407469, 17.22266099184918531, -6.262539305110056631 ) ) ;
#26416=CARTESIAN_POINT ( 'NONE',  ( 19.42250999205614193, 10.14701867748816966, 5.440088680355555262 ) ) ;
#26418=CARTESIAN_POINT ( 'NONE',  ( 2.035157376598824452, 38.68868534415483396, 7.964842623401179544 ) ) ;
#26419=CARTESIAN_POINT ( 'NONE',  ( 0.5774900079438607392, 38.48035201082150536, 5.440088680355550821 ) ) ;
#26420=CARTESIAN_POINT ( 'NONE',  ( -1.099225684535947600, -1.293031996736246469, -6.408140936763238038 ) ) ;
#26421=CARTESIAN_POINT ( 'NONE',  ( 0.1532563361054083140, 61.00893115100078745, 1.131784320476157264E-15 ) ) ;
#26423=CARTESIAN_POINT ( 'NONE',  ( 2.791683348922240793, 11.63393115100078568, 7.208316651077764092 ) ) ;
#26424=CARTESIAN_POINT ( 'NONE',  ( 18.72515096720571037, 50.05509018479936856, 6.499999999999982236 ) ) ;
#26425=CARTESIAN_POINT ( 'NONE',  ( -0.8801773607111009756, 48.06368534415484817, 1.068504757029289695E-15 ) ) ;
#26427=UNCERTAINTY_MEASURE_WITH_UNIT (LENGTH_MEASURE( 1.000000000000000082E-05 ), #64001, 'distance_accuracy_value', 'NONE');
#26428=AXIS2_PLACEMENT_3D ( 'NONE', #81968, #76446, #97992 ) ;
#26429=EDGE_CURVE ( 'NONE', #31758, #34270, #40951, .T. ) ;
#26430=CARTESIAN_POINT ( 'NONE',  ( -2.816281873526473856, -0.6680319967362464695, 3.434112377981055619 ) ) ;
#26431=CARTESIAN_POINT ( 'NONE',  ( 15.44008868035555260, 59.73035201082151247, 9.422509992056143702 ) ) ;
#26432=B_SPLINE_CURVE_WITH_KNOTS ( 'NONE', 3,
 ( #59255, #89756, #74760, #6268, #53738, #46244, #768, #70725, #69733, #10217, #48194, #31714 ),
 .UNSPECIFIED., .F., .F.,
 ( 4, 2, 2, 2, 2, 4 ),
 ( 0.0003200197625851165816, 0.0008213128228309329870, 0.001322605883076749230, 0.002325192003568404050, 0.003327778124060059087, 0.004330364244551714557 ),
 .UNSPECIFIED. ) ;
#26434=CARTESIAN_POINT ( 'NONE',  ( 19.84674366389459266, 28.30059781766745886, 2.638427012816836559 ) ) ;
#26435=CARTESIAN_POINT ( 'NONE',  ( 6.565887622018943937, 38.08196800326376064, -12.81628187352647608 ) ) ;
#26436=CARTESIAN_POINT ( 'NONE',  ( 1.472469842513823179, 5.592264484334118713, -4.923371831947296329 ) ) ;
#26439=CARTESIAN_POINT ( 'NONE',  ( 1.821708436314924962, 16.66792564121896802, -6.500000000000007105 ) ) ;
#26440=CARTESIAN_POINT ( 'NONE',  ( 12.91533473730993009, 11.60535201082150536, -10.88017736071109987 ) ) ;
#26442=CARTESIAN_POINT ( 'NONE',  ( 17.20831665107776587, 34.13393115100078745, -7.208316651077762316 ) ) ;
#26443=( NAMED_UNIT ( * ) PLANE_ANGLE_UNIT ( ) SI_UNIT ( $, .RADIAN. ) );
#26444=CARTESIAN_POINT ( 'NONE',  ( -0.3689425029237898834, 66.17874883491396076, -10.36894250292378850 ) ) ;
#26446=CARTESIAN_POINT ( 'NONE',  ( 2.035157376598824452, 18.68868534415484106, 7.964842623401179544 ) ) ;
#26447=CARTESIAN_POINT ( 'NONE',  ( 20.88017736071110519, 15.56368534415483751, 2.639326808657452039E-16 ) ) ;
#26448=FACE_OUTER_BOUND ( 'NONE', #64651, .T. ) ;
#26450=CARTESIAN_POINT ( 'NONE',  ( 1.472469842513823179, 61.42559781766745175, 4.923371831947296329 ) ) ;
#26451=CARTESIAN_POINT ( 'NONE',  ( 2.035157376598822676, 17.43868534415483751, -7.964842623401177768 ) ) ;
#26452=CARTESIAN_POINT ( 'NONE',  ( 19.84674366389459621, 58.50893115100078745, 7.409399052514197653E-17 ) ) ;
#26455=CARTESIAN_POINT ( 'NONE',  ( 19.38216949554541557, 52.24863466993041072, -9.382169495545420901 ) ) ;
#26457=CARTESIAN_POINT ( 'NONE',  ( -2.266590686148945544, 36.38708216824730357, -7.082119434687050408 ) ) ;
#26458=CARTESIAN_POINT ( 'NONE',  ( 0.5774900079438590739, 37.64701867748817676, -5.440088680355550821 ) ) ;
#26459=CARTESIAN_POINT ( 'NONE',  ( -0.8801773607111009756, 18.06368534415484106, 1.068504757029289695E-15 ) ) ;
#26460=CARTESIAN_POINT ( 'NONE',  ( 12.63842701281683034, 57.46726448433411605, 9.846743663894596210 ) ) ;
#26461=CARTESIAN_POINT ( 'NONE',  ( 5.500000000000000000, 60.50000000000000711, 6.500000000000000888 ) ) ;
#26462=CARTESIAN_POINT ( 'NONE',  ( 7.361572987183169658, 49.96726448433410894, -9.846743663894592657 ) ) ;
#26464=CARTESIAN_POINT ( 'NONE',  ( 10.00000000000000178, 2.258931151000784787, 9.846743663894594434 ) ) ;
#26466=VERTEX_POINT ( 'NONE', #69561 ) ;
#26468=CARTESIAN_POINT ( 'NONE',  ( 4.559911319644449179, 18.89701867748817321, 9.422509992056141925 ) ) ;
#26469=CARTESIAN_POINT ( 'NONE',  ( 7.361572987183170547, 17.05059781766745530, 9.846743663894590881 ) ) ;
#26470=CARTESIAN_POINT ( 'NONE',  ( 22.81628187352648496, 1.831968003263753753, -3.434112377981050290 ) ) ;
#26471=CARTESIAN_POINT ( 'NONE',  ( 2.035157376598822676, 47.43868534415484817, -7.964842623401177768 ) ) ;
#26472=CARTESIAN_POINT ( 'NONE',  ( -0.8801773607110991993, 52.85535201082151247, -2.915334737309923874 ) ) ;
#26473=CARTESIAN_POINT ( 'NONE',  ( 2.035157376598822676, 17.43868534415483751, -7.964842623401177768 ) ) ;
#26474=CARTESIAN_POINT ( 'NONE',  ( 16.40814093676324603, 47.45696800326375353, -11.09922568453594671 ) ) ;
#26475=CARTESIAN_POINT ( 'NONE',  ( 22.26659068614895176, 34.72041550158063927, -7.082119434687042414 ) ) ;
#26477=EDGE_CURVE ( 'NONE', #27464, #66913, #79191, .T. ) ;
#26479=CARTESIAN_POINT ( 'NONE',  ( 21.09922568453595559, 52.04030133659708923, -6.408140936763230044 ) ) ;
#26481=CARTESIAN_POINT ( 'NONE',  ( 10.00000000000000178, 62.25893115100078745, 9.846743663894594434 ) ) ;
#26482=CARTESIAN_POINT ( 'NONE',  ( -1.926860441876562025, 14.47997603579417536, -3.195792623639529761 ) ) ;
#26483=CARTESIAN_POINT ( 'NONE',  ( 20.88017736071110519, 35.56368534415484106, 2.639326808657452039E-16 ) ) ;
#26487=CARTESIAN_POINT ( 'NONE',  ( 7.361572987183170547, 7.050597817667451750, 9.846743663894590881 ) ) ;
#26489=CARTESIAN_POINT ( 'NONE',  ( 1.472469842513823179, 11.42559781766745175, 4.923371831947296329 ) ) ;
#26490=CARTESIAN_POINT ( 'NONE',  ( 17.20831665107776587, 27.88393115100078390, 7.208316651077764980 ) ) ;
#26491=CARTESIAN_POINT ( 'NONE',  ( 18.52753015748617571, 8.092264484334117824, 4.923371831947298993 ) ) ;
#26492=CARTESIAN_POINT ( 'NONE',  ( 0.1532563361054100626, 5.800597817667452638, -2.638427012816831230 ) ) ;
#26493=CARTESIAN_POINT ( 'NONE',  ( 4.559911319644449179, 63.89701867748817676, 9.422509992056141925 ) ) ;
#26494=CARTESIAN_POINT ( 'NONE',  ( -0.8801773607110991993, 57.85535201082149825, -2.915334737309923874 ) ) ;
#26495=AXIS2_PLACEMENT_3D ( 'NONE', #78404, #18403, #25430 ) ;
#26496=CARTESIAN_POINT ( 'NONE',  ( 1.472469842513823179, 20.59226448433411960, -4.923371831947296329 ) ) ;
#26500=CARTESIAN_POINT ( 'NONE',  ( 10.00000000000000000, 59.75893115100078745, -9.846743663894594434 ) ) ;
#26501=EDGE_LOOP ( 'NONE', ( #40752, #10524, #98098, #35603, #5438, #73377 ) ) ;
#26505=CARTESIAN_POINT ( 'NONE',  ( 22.26659068614895176, 4.720415501580633943, -7.082119434687042414 ) ) ;
#26508=CARTESIAN_POINT ( 'NONE',  ( 2.917880565312948704, 17.63708216824730357, 12.26659068614894643 ) ) ;
#26509=CARTESIAN_POINT ( 'NONE',  ( -2.266590686148945544, 26.38708216824730357, -7.082119434687050408 ) ) ;
#26511=CARTESIAN_POINT ( 'NONE',  ( -0.1503990784575242878, 59.24884699246888431, -6.262539305110083276 ) ) ;
#26512=CARTESIAN_POINT ( 'NONE',  ( 2.035157376598822676, 32.43868534415483396, -7.964842623401177768 ) ) ;
#26514=CARTESIAN_POINT ( 'NONE',  ( 5.076628168052704559, 20.17559781766745175, -8.527530157486179263 ) ) ;
#26515=CARTESIAN_POINT ( 'NONE',  ( 20.88017736071110519, 55.56368534415484817, 2.639326808657452039E-16 ) ) ;
#26516=CARTESIAN_POINT ( 'NONE',  ( 19.84674366389459621, 13.50893115100078568, 7.409399052514197653E-17 ) ) ;
#26517=CARTESIAN_POINT ( 'NONE',  ( 6.565887622018943937, 48.08196800326375353, -12.81628187352647608 ) ) ;
#26518=CARTESIAN_POINT ( 'NONE',  ( 0.1532563361054100626, 40.80059781766745886, -2.638427012816831230 ) ) ;
#26520=EDGE_CURVE ( 'NONE', #55863, #92145, #14604, .T. ) ;
#26521=CARTESIAN_POINT ( 'NONE',  ( 10.00000000000000000, 27.87363466993042138, -12.81628187352647608 ) ) ;
#26523=CARTESIAN_POINT ( 'NONE',  ( 1.472469842513823179, 30.59226448433411960, -4.923371831947296329 ) ) ;
#26524=CARTESIAN_POINT ( 'NONE',  ( 13.79529636645031943, 10.34541550158063394, -14.16423886937409904 ) ) ;
#26527=CARTESIAN_POINT ( 'NONE',  ( 12.91533473730992121, 44.52201867748816966, 10.88017736071110164 ) ) ;
#26528=CARTESIAN_POINT ( 'NONE',  ( 7.084665262690076126, 54.10535201082151247, 10.88017736071109987 ) ) ;
#26529=CARTESIAN_POINT ( 'NONE',  ( 20.36894250292379738, 39.92874883491396787, -10.36894250292379027 ) ) ;
#26530=CARTESIAN_POINT ( 'NONE',  ( 19.84674366389459621, 58.50893115100078745, 7.409399052514197653E-17 ) ) ;
#26531=CARTESIAN_POINT ( 'NONE',  ( 10.00000000000000000, 9.758931151000785675, -9.846743663894594434 ) ) ;
#26533=CARTESIAN_POINT ( 'NONE',  ( 22.81628187352647785, 61.62363466993041783, 6.195893100308588602E-16 ) ) ;
#26535=CARTESIAN_POINT ( 'NONE',  ( 10.00000000000000000, 46.81368534415484106, -10.88017736071110342 ) ) ;
#26536=DIRECTION ( 'NONE',  ( -1.000000000000000000, 0.000000000000000000, 0.000000000000000000 ) ) ;
#26537=CARTESIAN_POINT ( 'NONE',  ( 22.81628187352647785, 26.41530133659708923, 3.434112377981063169 ) ) ;
#26538=CARTESIAN_POINT ( 'NONE',  ( 17.20831665107776587, 54.13393115100079456, -7.208316651077762316 ) ) ;
#26540=CARTESIAN_POINT ( 'NONE',  ( 7.084665262690076126, 2.022018677488170990, -10.88017736071110164 ) ) ;
#26541=CARTESIAN_POINT ( 'NONE',  ( 15.44008868035555793, 66.39701867748817676, -9.422509992056140149 ) ) ;
#26544=CARTESIAN_POINT ( 'NONE',  ( 1.274849032794305170, 12.55509018479935968, -6.499999999999995559 ) ) ;
#26545=CARTESIAN_POINT ( 'NONE',  ( 17.96484262340118221, 64.93868534415483396, 7.964842623401181321 ) ) ;
#26546=CARTESIAN_POINT ( 'NONE',  ( -0.8801773607110991993, 67.85535201082151957, -2.915334737309923874 ) ) ;
#26549=CARTESIAN_POINT ( 'NONE',  ( 2.791683348922240793, 36.63393115100078035, 7.208316651077764092 ) ) ;
#26550=CARTESIAN_POINT ( 'NONE',  ( 17.96484262340118221, 24.93868534415484461, 7.964842623401181321 ) ) ;
#26551=CARTESIAN_POINT ( 'NONE',  ( 19.38216949554541202, 0.9986346699304200492, 9.382169495545424454 ) ) ;
#26552=CARTESIAN_POINT ( 'NONE',  ( 17.96484262340118221, 31.18868534415483751, -7.964842623401177768 ) ) ;
#26553=CARTESIAN_POINT ( 'NONE',  ( 18.72515096720583827, 56.07228050351029225, -6.499999999999802824 ) ) ;
#26554=CARTESIAN_POINT ( 'NONE',  ( 0.6178305044545818747, 33.49863466993042493, -9.382169495545419124 ) ) ;
#26556=CARTESIAN_POINT ( 'NONE',  ( -0.8801773607111008646, 53.27201867748816966, 2.915334737309923430 ) ) ;
#26558=CARTESIAN_POINT ( 'NONE',  ( 6.565887622018943937, 23.08196800326375708, -12.81628187352647608 ) ) ;
#26560=CARTESIAN_POINT ( 'NONE',  ( 7.084665262690076126, 22.02201867748817321, -10.88017736071110164 ) ) ;
#26561=CARTESIAN_POINT ( 'NONE',  ( 13.79529636645031943, 60.34541550158063927, -14.16423886937409904 ) ) ;
#26562=CARTESIAN_POINT ( 'NONE',  ( 5.076628168052703671, 46.84226448433412315, 8.527530157486179263 ) ) ;
#26563=CARTESIAN_POINT ( 'NONE',  ( 12.63842701281683922, 4.550597817667451750, -9.846743663894590881 ) ) ;
#26564=CARTESIAN_POINT ( 'NONE',  ( 4.559911319644449179, 57.23035201082150536, -9.422509992056141925 ) ) ;
#26566=CARTESIAN_POINT ( 'NONE',  ( 22.26659068614894466, 33.88708216824730357, 7.082119434687054849 ) ) ;
#26569=ORIENTED_EDGE ( 'NONE', *, *, #88174, .F. ) ;
#26570=CARTESIAN_POINT ( 'NONE',  ( 6.204703633549690345, 47.84541550158064638, 14.16423886937410082 ) ) ;
#26571=CARTESIAN_POINT ( 'NONE',  ( 10.00000000000000178, 53.05374883491396787, 14.16423886937410082 ) ) ;
#26572=CARTESIAN_POINT ( 'NONE',  ( 0.1532563361054083140, 16.00893115100078390, 1.131784320476157264E-15 ) ) ;
#26573=CARTESIAN_POINT ( 'NONE',  ( 22.81628187352648496, 16.83196800326374998, -3.434112377981050290 ) ) ;
#26576=CARTESIAN_POINT ( 'NONE',  ( 15.44008868035555793, 66.39701867748817676, -9.422509992056140149 ) ) ;
#26577=CARTESIAN_POINT ( 'NONE',  ( 0.6178305044545818747, 33.49863466993042493, -9.382169495545419124 ) ) ;
#26578=CARTESIAN_POINT ( 'NONE',  ( 22.26659068614894466, 38.88708216824731068, 7.082119434687054849 ) ) ;
#26581=( BOUNDED_SURFACE ( )  B_SPLINE_SURFACE ( 1, 2, ( 
 ( #74364, #91350, #52857, #68374, #67373, #45357, #5893, #58881, #83365, #6876, #51884, #53348, #97903, #52367, #90852, #36385, #21387, #59864, #66880, #14888, #98893, #81872, #89383, #90351, #5411, #43382, #21889, #13888, #44856, #82872, #97397, #37387, #22877, #14386, #98398, #59369, #22383, #12885, #73881, #75862, #7383, #30344, #20896, #60851, #51386, #61343, #69845, #32805, #32313, #63301, #62818, #31820, #84841, #15380, #45865, #7870, #9831, #23369, #62318, #24354, #16842, #54817, #77816, #30845, #68863, #92824, #39833, #70836, #40333, #93810, #83856, #16349, #395, #70339, #46831, #77323, #92339, #17342, #8351, #23863, #91854, #85328, #25340, #78312, #76355, #47316, #9331, #8837, #39351, #1369, #1856, #93316, #46349, #76836, #2349, #24838, #47812, #38365, #55321, #85827, #69348, #53855, #84365, #15864, #38859, #54327, #872, #31331, #61831, #57281, #3308, #63786, #74626, #19290, #86811, #80284, #56792, #56315, #95282, #5655, #18807, #49290, #36643, #13633, #49777, #25818, #11784, #42292, #40822, #79790, #87775, #17822, #44117, #94295, #48304, #55824, #21142, #86318, #33295, #26783, #64768, #74119, #18315, #48795, #79304, #11293, #59122, #6140, #41330, #26291, #41812, #72280, #67128, #78812, #97165, #97655, #10320, #64278, #3810, #28633, #10812, #51642, #36133, #66641, #89631, #71322, #82123, #94790, #71803, #2840, #33771, #87287, #34266, #37142, #44625, #22632, #29119, #22135, #52617, #46114, #7641, #61587, #83118, #21645, #31092, #8117, #91105, #38131, #16106, #98145, #69600, #37631, #52129, #59620, #98656, #60110, #69110, #82626, #6628, #23127, #91611, #46592, #67636, #14140, #14647, #84605, #75120, #15136, #53112, #53601, #83620, #29606, #76110, #77091, #84115, #15631, #8600, #90611, #45110, #75616, #39110, #7126, #45612, #68619, #76600, #149, #68128, #30596, #90118, #38612, #60610, #61102, #643, #92098, #23629, #30102, #54090, #94553, #17593, #64040, #92584, #71081, #63068, #85588, #78575, #48555, #70095, #86082, #70586, #17101, #25101, #24108, #2607, #47586, #9091, #18566, #63556, #32067, #25587, #2113, #1618, #40584, #79056, #93568, #55586, #79562, #56561, #94065, #62570, #56079, #86573, #85093, #48061, #33061, #62076, #87055, #39607, #54578, #1121, #26071, #31583, #77576, #18078, #10085, #10571, #93075, #24604, #55070, #41079, #3087, #49058, #78080, #32571, #71577, #33544, #11061, #16602, #41581, #47078, #9584, #40085, #73023, #96544, #72527, #58518, #43033, #5043, #28020, #34035, #58020, #57534, #80041, #95037, #81513, #35526, #19543, #19056, #26546, #12039, #72049, #4061, #34524, #66020, #96045, #89027 ),
 ( #64530, #3578, #4557, #27035, #51021, #11547, #65018, #50039, #13020, #5541, #95547, #42067, #35021, #49534, #87545, #88528, #65522, #20537, #20030, #88031, #43518, #57042, #74013, #80542, #50532, #42539, #27529, #12533, #81027, #73514, #85904, #39909, #94867, #63860, #70412, #48382, #11370, #10885, #41892, #41409, #10395, #63383, #92897, #24428, #85407, #87368, #1932, #40899, #2916, #94374, #33366, #56392, #9407, #47393, #71400, #18389, #49364, #18883, #72352, #62389, #93887, #77895, #48868, #25415, #55899, #70907, #26368, #17418, #2427, #32389, #25893, #3884, #56867, #54892, #86879, #32884, #16917, #17899, #79866, #62894, #93393, #24918, #79380, #86396, #55403, #71873, #47887, #3385, #33850, #64358, #78389, #78884, #9910, #40412, #98048, #34504, #72023, #24584, #10546, #57019, #85564, #64017, #56056, #78550, #71555, #41559, #63048, #79033, #63535, #10061, #18055, #17076, #94530, #40559, #2087, #11522, #56539, #25077, #18541, #94042, #93544, #33521, #3553, #86550, #48533, #72509, #49512, #87029, #55559, #49033, #79538, #78057, #41057, #26049, #55045, #3068, #42045, #34013, #4042, #64510, #11037, #25565, #47559, #9559, #40060, #19036, #32547, #95014, #26523, #87521, #80019, #93050, #70561, #86060, #17571, #48038, #71059, #2583, #33038, #64996, #65997, #80522, #51496, #96525, #27997, #73492, #97517, #88506, #5019, #12020, #35997, #14005, #59484, #27015, #66499, #35503, #57514, #20513, #82488, #51998, #65501, #27505, #97025, #58496, #28980, #12996, #96023, #28502, #58996, #21009, #74985, #50998, #4535, #74485, #81493, #58000, #43982, #89984, #42520, #20009, #89006, #43493, #89498, #81991, #13502, #6007, #36502, #73003, #50511, #19523, #43010, #88010, #34998, #66994, #73993, #50018, #81008, #12509, #44483, #21501, #6488, #5519, #95523, #37497, #59974, #76950, #30952, #75970, #77433, #22992, #76465, #53960, #98513, #45469, #68483, #90961, #8461, #61942, #6993, #52478, #10, #29467, #67492, #91467, #7498, #68972, #53458, #67986, #61451, #16460, #83966, #30458, #29966, #60957, #46940, #98013, #60472, #22493, #52966, #14503, #69459, #38479, #44973, #37991, #504, #15493, #83478, #91958, #36995, #45975, #7980, #14999, #23488, #90468, #22003, #84467, #15965, #46457, #75479, #978, #38966, #31441, #92443, #84949, #23966, #82983, #54440, #55936, #9944, #39464, #69954, #31927, #33888, #47437, #86436, #48420, #40940, #78922, #2952, #54928, #92930, #17935, #63899, #94904, #64393, #56901, #8946, #40447, #24463, #94412, #70948, #2466, #17455, #41445, #32430, #47922, #85444, #10432, #87406, #3429, #1473, #71438, #78427, #62427, #63424 ) ),
 .UNSPECIFIED., .F., .F., .F. ) 
 B_SPLINE_SURFACE_WITH_KNOTS ( ( 2, 2 ),
 ( 3, 2, 2, 2, 2, 2, 2, 2, 2, 2, 2, 2, 2, 2, 2, 2, 2, 2, 2, 2, 2, 2, 2, 2, 2, 2, 2, 2, 2, 2, 2, 2, 2, 2, 2, 2, 2, 2, 2, 2, 2, 2, 2, 2, 2, 2, 2, 2, 2, 2, 2, 2, 2, 2, 2, 2, 2, 2, 2, 2, 2, 2, 2, 2, 2, 2, 2, 2, 2, 2, 2, 2, 2, 2, 2, 2, 2, 2, 2, 2, 2, 2, 2, 2, 2, 2, 2, 2, 2, 2, 2, 2, 2, 2, 2, 2, 2, 2, 2, 2, 2, 2, 2, 2, 2, 2, 2, 2, 2, 2, 2, 2, 2, 2, 2, 2, 2, 2, 2, 2, 2, 2, 2, 2, 2, 2, 2, 2, 2, 2, 2, 2, 2, 2, 2, 2, 2, 2, 2, 2, 2, 2, 2, 2, 2, 2, 2, 2, 2, 2, 2, 2, 2, 2, 2, 2, 2, 2, 2, 2, 2, 2, 3 ),
 ( 0.000000000000000000, 1.000000000000000000 ),
 ( 0.000000000000000000, 0.005952380952380952051, 0.01190476190476190410, 0.01785714285714285615, 0.02380952380952380820, 0.02976190476190476025, 0.03571428571428571230, 0.04166666666666666435, 0.04761904761904761640, 0.05357142857142856845, 0.05952380952380952051, 0.06547619047619047949, 0.07142857142857142461, 0.07738095238095238360, 0.08333333333333332871, 0.08928571428571428770, 0.09523809523809523281, 0.1011904761904761918, 0.1071428571428571369, 0.1130952380952380959, 0.1190476190476190410, 0.1250000000000000000, 0.1309523809523809590, 0.1369047619047619180, 0.1428571428571428492, 0.1488095238095238082, 0.1547619047619047672, 0.1607142857142857262, 0.1666666666666666574, 0.1726190476190476164, 0.1785714285714285754, 0.1845238095238095344, 0.1904761904761904656, 0.1964285714285714246, 0.2023809523809523836, 0.2083333333333333426, 0.2142857142857142738, 0.2202380952380952328, 0.2261904761904761918, 0.2321428571428571508, 0.2380952380952380820, 0.2440476190476190410, 0.2500000000000000000, 0.2559523809523809312, 0.2619047619047619180, 0.2678571428571428492, 0.2738095238095238360, 0.2797619047619047672, 0.2857142857142856984, 0.2916666666666666852, 0.2976190476190476164, 0.3035714285714285476, 0.3095238095238095344, 0.3154761904761904656, 0.3214285714285714524, 0.3273809523809523836, 0.3333333333333333148, 0.3392857142857143016, 0.3452380952380952328, 0.3511904761904761640, 0.3571428571428571508, 0.3630952380952380820, 0.3690476190476190688, 0.3750000000000000000, 0.3809523809523809312, 0.3869047619047619180, 0.3928571428571428492, 0.3988095238095238360, 0.4047619047619047672, 0.4107142857142856984, 0.4166666666666666852, 0.4226190476190476164, 0.4285714285714285476, 0.4345238095238095344, 0.4404761904761904656, 0.4464285714285714524, 0.4523809523809523836, 0.4583333333333333148, 0.4642857142857143016, 0.4702380952380952328, 0.4761904761904761640, 0.4821428571428571508, 0.4880952380952380820, 0.4940476190476190688, 0.5000000000000000000, 0.5059523809523809312, 0.5119047619047618625, 0.5178571428571429047, 0.5238095238095238360, 0.5297619047619047672, 0.5357142857142856984, 0.5416666666666666297, 0.5476190476190476719, 0.5535714285714286031, 0.5595238095238095344, 0.5654761904761904656, 0.5714285714285713969, 0.5773809523809523281, 0.5833333333333333703, 0.5892857142857143016, 0.5952380952380952328, 0.6011904761904761640, 0.6071428571428570953, 0.6130952380952381375, 0.6190476190476190688, 0.6250000000000000000, 0.6309523809523809312, 0.6369047619047618625, 0.6428571428571429047, 0.6488095238095238360, 0.6547619047619047672, 0.6607142857142856984, 0.6666666666666666297, 0.6726190476190476719, 0.6785714285714286031, 0.6845238095238095344, 0.6904761904761904656, 0.6964285714285713969, 0.7023809523809523281, 0.7083333333333333703, 0.7142857142857143016, 0.7202380952380952328, 0.7261904761904761640, 0.7321428571428570953, 0.7380952380952381375, 0.7440476190476190688, 0.7500000000000000000, 0.7559523809523809312, 0.7619047619047618625, 0.7678571428571429047, 0.7738095238095238360, 0.7797619047619047672, 0.7857142857142856984, 0.7916666666666666297, 0.7976190476190476719, 0.8035714285714286031, 0.8095238095238095344, 0.8154761904761904656, 0.8214285714285713969, 0.8273809523809523281, 0.8333333333333333703, 0.8392857142857143016, 0.8452380952380952328, 0.8511904761904761640, 0.8571428571428570953, 0.8630952380952381375, 0.8690476190476190688, 0.8750000000000000000, 0.8809523809523809312, 0.8869047619047618625, 0.8928571428571429047, 0.8988095238095238360, 0.9047619047619047672, 0.9107142857142856984, 0.9166666666666666297, 0.9226190476190476719, 0.9285714285714286031, 0.9345238095238095344, 0.9404761904761904656, 0.9464285714285713969, 0.9523809523809523281, 0.9583333333333333703, 0.9642857142857143016 ),
 .UNSPECIFIED. ) 
 GEOMETRIC_REPRESENTATION_ITEM ( )  RATIONAL_B_SPLINE_SURFACE ( (
 ( 1.000000000000000000, 0.9659258262890683122, 1.000000000000000000, 0.9659258262890683122, 1.000000000000000000, 0.9659258262890683122, 1.000000000000000000, 0.9659258262890683122, 1.000000000000000000, 0.9659258262890683122, 1.000000000000000000, 0.9659258262890683122, 1.000000000000000000, 0.9659258262890683122, 1.000000000000000000, 0.9659258262890683122, 1.000000000000000000, 0.9659258262890683122, 1.000000000000000000, 0.9659258262890683122, 1.000000000000000000, 0.9659258262890683122, 1.000000000000000000, 0.9659258262890683122, 1.000000000000000000, 0.9659258262890683122, 1.000000000000000000, 0.9659258262890683122, 1.000000000000000000, 0.9659258262890683122, 1.000000000000000000, 0.9659258262890683122, 1.000000000000000000, 0.9659258262890683122, 1.000000000000000000, 0.9659258262890683122, 1.000000000000000000, 0.9659258262890683122, 1.000000000000000000, 0.9659258262890683122, 1.000000000000000000, 0.9659258262890683122, 1.000000000000000000, 0.9659258262890683122, 1.000000000000000000, 0.9659258262890683122, 1.000000000000000000, 0.9659258262890683122, 1.000000000000000000, 0.9659258262890683122, 1.000000000000000000, 0.9659258262890683122, 1.000000000000000000, 0.9659258262890683122, 1.000000000000000000, 0.9659258262890683122, 1.000000000000000000, 0.9659258262890683122, 1.000000000000000000, 0.9659258262890683122, 1.000000000000000000, 0.9659258262890683122, 1.000000000000000000, 0.9659258262890683122, 1.000000000000000000, 0.9659258262890683122, 1.000000000000000000, 0.9659258262890683122, 1.000000000000000000, 0.9659258262890683122, 1.000000000000000000, 0.9659258262890683122, 1.000000000000000000, 0.9659258262890683122, 1.000000000000000000, 0.9659258262890683122, 1.000000000000000000, 0.9659258262890683122, 1.000000000000000000, 0.9659258262890683122, 1.000000000000000000, 0.9659258262890683122, 1.000000000000000000, 0.9659258262890683122, 1.000000000000000000, 0.9659258262890683122, 1.000000000000000000, 0.9659258262890683122, 1.000000000000000000, 0.9659258262890683122, 1.000000000000000000, 0.9659258262890683122, 1.000000000000000000, 0.9659258262890683122, 1.000000000000000000, 0.9659258262890683122, 1.000000000000000000, 0.9659258262890683122, 1.000000000000000000, 0.9659258262890683122, 1.000000000000000000, 0.9659258262890683122, 1.000000000000000000, 0.9659258262890683122, 1.000000000000000000, 0.9659258262890683122, 1.000000000000000000, 0.9659258262890683122, 1.000000000000000000, 0.9659258262890683122, 1.000000000000000000, 0.9659258262890683122, 1.000000000000000000, 0.9659258262890683122, 1.000000000000000000, 0.9659258262890683122, 1.000000000000000000, 0.9659258262890683122, 1.000000000000000000, 0.9659258262890683122, 1.000000000000000000, 0.9659258262890683122, 1.000000000000000000, 0.9659258262890683122, 1.000000000000000000, 0.9659258262890683122, 1.000000000000000000, 0.9659258262890683122, 1.000000000000000000, 0.9659258262890683122, 1.000000000000000000, 0.9659258262890683122, 1.000000000000000000, 0.9659258262890683122, 1.000000000000000000, 0.9659258262890683122, 1.000000000000000000, 0.9659258262890683122, 1.000000000000000000, 0.9659258262890683122, 1.000000000000000000, 0.9659258262890683122, 1.000000000000000000, 0.9659258262890683122, 1.000000000000000000, 0.9659258262890683122, 1.000000000000000000, 0.9659258262890683122, 1.000000000000000000, 0.9659258262890683122, 1.000000000000000000, 0.9659258262890683122, 1.000000000000000000, 0.9659258262890683122, 1.000000000000000000, 0.9659258262890683122, 1.000000000000000000, 0.9659258262890683122, 1.000000000000000000, 0.9659258262890683122, 1.000000000000000000, 0.9659258262890683122, 1.000000000000000000, 0.9659258262890683122, 1.000000000000000000, 0.9659258262890683122, 1.000000000000000000, 0.9659258262890683122, 1.000000000000000000, 0.9659258262890683122, 1.000000000000000000, 0.9659258262890683122, 1.000000000000000000, 0.9659258262890683122, 1.000000000000000000, 0.9659258262890683122, 1.000000000000000000, 0.9659258262890683122, 1.000000000000000000, 0.9659258262890683122, 1.000000000000000000, 0.9659258262890683122, 1.000000000000000000, 0.9659258262890683122, 1.000000000000000000, 0.9659258262890683122, 1.000000000000000000, 0.9659258262890683122, 1.000000000000000000, 0.9659258262890683122, 1.000000000000000000, 0.9659258262890683122, 1.000000000000000000, 0.9659258262890683122, 1.000000000000000000, 0.9659258262890683122, 1.000000000000000000, 0.9659258262890683122, 1.000000000000000000, 0.9659258262890683122, 1.000000000000000000, 0.9659258262890683122, 1.000000000000000000, 0.9659258262890683122, 1.000000000000000000, 0.9659258262890683122, 1.000000000000000000, 0.9659258262890683122, 1.000000000000000000, 0.9659258262890683122, 1.000000000000000000, 0.9659258262890683122, 1.000000000000000000, 0.9659258262890683122, 1.000000000000000000, 0.9659258262890683122, 1.000000000000000000, 0.9659258262890683122, 1.000000000000000000, 0.9659258262890683122, 1.000000000000000000, 0.9659258262890683122, 1.000000000000000000, 0.9659258262890683122, 1.000000000000000000, 0.9659258262890683122, 1.000000000000000000, 0.9659258262890683122, 1.000000000000000000, 0.9659258262890683122, 1.000000000000000000, 0.9659258262890683122, 1.000000000000000000, 0.9659258262890683122, 1.000000000000000000, 0.9659258262890683122, 1.000000000000000000, 0.9659258262890683122, 1.000000000000000000, 0.9659258262890683122, 1.000000000000000000, 0.9659258262890683122, 1.000000000000000000, 0.9659258262890683122, 1.000000000000000000, 0.9659258262890683122, 1.000000000000000000, 0.9659258262890683122, 1.000000000000000000, 0.9659258262890683122, 1.000000000000000000, 0.9659258262890683122, 1.000000000000000000, 0.9659258262890683122, 1.000000000000000000, 0.9659258262890683122, 1.000000000000000000, 0.9659258262890683122, 1.000000000000000000, 0.9659258262890683122, 1.000000000000000000, 0.9659258262890683122, 1.000000000000000000, 0.9659258262890683122, 1.000000000000000000, 0.9659258262890683122, 1.000000000000000000, 0.9659258262890683122, 1.000000000000000000, 0.9659258262890683122, 1.000000000000000000, 0.9659258262890683122, 1.000000000000000000, 0.9659258262890683122, 1.000000000000000000, 0.9659258262890683122, 1.000000000000000000, 0.9659258262890683122, 1.000000000000000000, 0.9659258262890683122, 1.000000000000000000, 0.9659258262890683122, 1.000000000000000000, 0.9659258262890683122, 1.000000000000000000, 0.9659258262890683122, 1.000000000000000000, 0.9659258262890683122, 1.000000000000000000, 0.9659258262890683122, 1.000000000000000000, 0.9659258262890683122, 1.000000000000000000, 0.9659258262890683122, 1.000000000000000000, 0.9659258262890683122, 1.000000000000000000, 0.9659258262890683122, 1.000000000000000000, 0.9659258262890683122, 1.000000000000000000, 0.9659258262890683122, 1.000000000000000000, 0.9659258262890683122, 1.000000000000000000, 0.9659258262890683122, 1.000000000000000000, 0.9659258262890683122, 1.000000000000000000, 0.9659258262890683122, 1.000000000000000000, 0.9659258262890683122, 1.000000000000000000, 0.9659258262890683122, 1.000000000000000000, 0.9659258262890683122, 1.000000000000000000, 0.9659258262890683122, 1.000000000000000000, 0.9659258262890683122, 1.000000000000000000, 0.9659258262890683122, 1.000000000000000000, 0.9659258262890683122, 1.000000000000000000),
 ( 1.000000000000000000, 0.9659258262890683122, 1.000000000000000000, 0.9659258262890683122, 1.000000000000000000, 0.9659258262890683122, 1.000000000000000000, 0.9659258262890683122, 1.000000000000000000, 0.9659258262890683122, 1.000000000000000000, 0.9659258262890683122, 1.000000000000000000, 0.9659258262890683122, 1.000000000000000000, 0.9659258262890683122, 1.000000000000000000, 0.9659258262890683122, 1.000000000000000000, 0.9659258262890683122, 1.000000000000000000, 0.9659258262890683122, 1.000000000000000000, 0.9659258262890683122, 1.000000000000000000, 0.9659258262890683122, 1.000000000000000000, 0.9659258262890683122, 1.000000000000000000, 0.9659258262890683122, 1.000000000000000000, 0.9659258262890683122, 1.000000000000000000, 0.9659258262890683122, 1.000000000000000000, 0.9659258262890683122, 1.000000000000000000, 0.9659258262890683122, 1.000000000000000000, 0.9659258262890683122, 1.000000000000000000, 0.9659258262890683122, 1.000000000000000000, 0.9659258262890683122, 1.000000000000000000, 0.9659258262890683122, 1.000000000000000000, 0.9659258262890683122, 1.000000000000000000, 0.9659258262890683122, 1.000000000000000000, 0.9659258262890683122, 1.000000000000000000, 0.9659258262890683122, 1.000000000000000000, 0.9659258262890683122, 1.000000000000000000, 0.9659258262890683122, 1.000000000000000000, 0.9659258262890683122, 1.000000000000000000, 0.9659258262890683122, 1.000000000000000000, 0.9659258262890683122, 1.000000000000000000, 0.9659258262890683122, 1.000000000000000000, 0.9659258262890683122, 1.000000000000000000, 0.9659258262890683122, 1.000000000000000000, 0.9659258262890683122, 1.000000000000000000, 0.9659258262890683122, 1.000000000000000000, 0.9659258262890683122, 1.000000000000000000, 0.9659258262890683122, 1.000000000000000000, 0.9659258262890683122, 1.000000000000000000, 0.9659258262890683122, 1.000000000000000000, 0.9659258262890683122, 1.000000000000000000, 0.9659258262890683122, 1.000000000000000000, 0.9659258262890683122, 1.000000000000000000, 0.9659258262890683122, 1.000000000000000000, 0.9659258262890683122, 1.000000000000000000, 0.9659258262890683122, 1.000000000000000000, 0.9659258262890683122, 1.000000000000000000, 0.9659258262890683122, 1.000000000000000000, 0.9659258262890683122, 1.000000000000000000, 0.9659258262890683122, 1.000000000000000000, 0.9659258262890683122, 1.000000000000000000, 0.9659258262890683122, 1.000000000000000000, 0.9659258262890683122, 1.000000000000000000, 0.9659258262890683122, 1.000000000000000000, 0.9659258262890683122, 1.000000000000000000, 0.9659258262890683122, 1.000000000000000000, 0.9659258262890683122, 1.000000000000000000, 0.9659258262890683122, 1.000000000000000000, 0.9659258262890683122, 1.000000000000000000, 0.9659258262890683122, 1.000000000000000000, 0.9659258262890683122, 1.000000000000000000, 0.9659258262890683122, 1.000000000000000000, 0.9659258262890683122, 1.000000000000000000, 0.9659258262890683122, 1.000000000000000000, 0.9659258262890683122, 1.000000000000000000, 0.9659258262890683122, 1.000000000000000000, 0.9659258262890683122, 1.000000000000000000, 0.9659258262890683122, 1.000000000000000000, 0.9659258262890683122, 1.000000000000000000, 0.9659258262890683122, 1.000000000000000000, 0.9659258262890683122, 1.000000000000000000, 0.9659258262890683122, 1.000000000000000000, 0.9659258262890683122, 1.000000000000000000, 0.9659258262890683122, 1.000000000000000000, 0.9659258262890683122, 1.000000000000000000, 0.9659258262890683122, 1.000000000000000000, 0.9659258262890683122, 1.000000000000000000, 0.9659258262890683122, 1.000000000000000000, 0.9659258262890683122, 1.000000000000000000, 0.9659258262890683122, 1.000000000000000000, 0.9659258262890683122, 1.000000000000000000, 0.9659258262890683122, 1.000000000000000000, 0.9659258262890683122, 1.000000000000000000, 0.9659258262890683122, 1.000000000000000000, 0.9659258262890683122, 1.000000000000000000, 0.9659258262890683122, 1.000000000000000000, 0.9659258262890683122, 1.000000000000000000, 0.9659258262890683122, 1.000000000000000000, 0.9659258262890683122, 1.000000000000000000, 0.9659258262890683122, 1.000000000000000000, 0.9659258262890683122, 1.000000000000000000, 0.9659258262890683122, 1.000000000000000000, 0.9659258262890683122, 1.000000000000000000, 0.9659258262890683122, 1.000000000000000000, 0.9659258262890683122, 1.000000000000000000, 0.9659258262890683122, 1.000000000000000000, 0.9659258262890683122, 1.000000000000000000, 0.9659258262890683122, 1.000000000000000000, 0.9659258262890683122, 1.000000000000000000, 0.9659258262890683122, 1.000000000000000000, 0.9659258262890683122, 1.000000000000000000, 0.9659258262890683122, 1.000000000000000000, 0.9659258262890683122, 1.000000000000000000, 0.9659258262890683122, 1.000000000000000000, 0.9659258262890683122, 1.000000000000000000, 0.9659258262890683122, 1.000000000000000000, 0.9659258262890683122, 1.000000000000000000, 0.9659258262890683122, 1.000000000000000000, 0.9659258262890683122, 1.000000000000000000, 0.9659258262890683122, 1.000000000000000000, 0.9659258262890683122, 1.000000000000000000, 0.9659258262890683122, 1.000000000000000000, 0.9659258262890683122, 1.000000000000000000, 0.9659258262890683122, 1.000000000000000000, 0.9659258262890683122, 1.000000000000000000, 0.9659258262890683122, 1.000000000000000000, 0.9659258262890683122, 1.000000000000000000, 0.9659258262890683122, 1.000000000000000000, 0.9659258262890683122, 1.000000000000000000, 0.9659258262890683122, 1.000000000000000000, 0.9659258262890683122, 1.000000000000000000, 0.9659258262890683122, 1.000000000000000000, 0.9659258262890683122, 1.000000000000000000, 0.9659258262890683122, 1.000000000000000000, 0.9659258262890683122, 1.000000000000000000, 0.9659258262890683122, 1.000000000000000000, 0.9659258262890683122, 1.000000000000000000, 0.9659258262890683122, 1.000000000000000000, 0.9659258262890683122, 1.000000000000000000, 0.9659258262890683122, 1.000000000000000000, 0.9659258262890683122, 1.000000000000000000, 0.9659258262890683122, 1.000000000000000000, 0.9659258262890683122, 1.000000000000000000, 0.9659258262890683122, 1.000000000000000000, 0.9659258262890683122, 1.000000000000000000, 0.9659258262890683122, 1.000000000000000000, 0.9659258262890683122, 1.000000000000000000, 0.9659258262890683122, 1.000000000000000000, 0.9659258262890683122, 1.000000000000000000, 0.9659258262890683122, 1.000000000000000000, 0.9659258262890683122, 1.000000000000000000, 0.9659258262890683122, 1.000000000000000000, 0.9659258262890683122, 1.000000000000000000, 0.9659258262890683122, 1.000000000000000000, 0.9659258262890683122, 1.000000000000000000, 0.9659258262890683122, 1.000000000000000000, 0.9659258262890683122, 1.000000000000000000, 0.9659258262890683122, 1.000000000000000000, 0.9659258262890683122, 1.000000000000000000, 0.9659258262890683122, 1.000000000000000000, 0.9659258262890683122, 1.000000000000000000, 0.9659258262890683122, 1.000000000000000000, 0.9659258262890683122, 1.000000000000000000, 0.9659258262890683122, 1.000000000000000000, 0.9659258262890683122, 1.000000000000000000, 0.9659258262890683122, 1.000000000000000000, 0.9659258262890683122, 1.000000000000000000, 0.9659258262890683122, 1.000000000000000000, 0.9659258262890683122, 1.000000000000000000, 0.9659258262890683122, 1.000000000000000000, 0.9659258262890683122, 1.000000000000000000) ) ) 
 REPRESENTATION_ITEM ( '' )  SURFACE ( )  );
#26585=CARTESIAN_POINT ( 'NONE',  ( 18.52753015748618282, 18.92559781766745175, -4.923371831947291888 ) ) ;
#26588=CARTESIAN_POINT ( 'NONE',  ( 12.91533473730992121, 4.522018677488170546, 10.88017736071110164 ) ) ;
#26589=CARTESIAN_POINT ( 'NONE',  ( 4.559911319644449179, 7.230352010821505360, -9.422509992056141925 ) ) ;
#26590=CARTESIAN_POINT ( 'NONE',  ( 10.00000000000000000, 54.75893115100078745, -9.846743663894594434 ) ) ;
#26591=CARTESIAN_POINT ( 'NONE',  ( 10.00000000000000000, 2.873634669930420049, -12.81628187352647608 ) ) ;
#26594=ADVANCED_FACE ( 'NONE', ( #45571 ), #77285, .T. ) ;
#26595=MECHANICAL_DESIGN_GEOMETRIC_PRESENTATION_REPRESENTATION('',(#28587),#76060);
#26598=CARTESIAN_POINT ( 'NONE',  ( 21.09922568453594849, 16.20696800326375353, 6.408140936763242479 ) ) ;
#26600=CARTESIAN_POINT ( 'NONE',  ( 6.204703633549690345, 62.84541550158063927, 14.16423886937410082 ) ) ;
#26602=CARTESIAN_POINT ( 'NONE',  ( 2.917880565312950480, 60.97041550158063927, -12.26659068614894821 ) ) ;
#26604=CARTESIAN_POINT ( 'NONE',  ( 7.084665262690076126, 39.10535201082150536, 10.88017736071109987 ) ) ;
#26605=CARTESIAN_POINT ( 'NONE',  ( 4.559911319644449179, 48.89701867748817676, 9.422509992056141925 ) ) ;
#26606=CARTESIAN_POINT ( 'NONE',  ( 7.084665262690076126, 57.02201867748817676, -10.88017736071110164 ) ) ;
#26607=CARTESIAN_POINT ( 'NONE',  ( 4.559911319644449179, 47.23035201082150536, -9.422509992056141925 ) ) ;
#26608=( GEOMETRIC_REPRESENTATION_CONTEXT ( 3 ) GLOBAL_UNCERTAINTY_ASSIGNED_CONTEXT ( ( #79324 ) ) GLOBAL_UNIT_ASSIGNED_CONTEXT ( ( #79597, #41616, #95075 ) ) REPRESENTATION_CONTEXT ( 'NONE', 'WORKASPACE' ) );
#26612=CARTESIAN_POINT ( 'NONE',  ( 18.52753015748618282, 8.925597817667451750, -4.923371831947291888 ) ) ;
#26614=CARTESIAN_POINT ( 'NONE',  ( 19.84674366389459621, 43.50893115100078745, 7.409399052514197653E-17 ) ) ;
#26617=VECTOR ( 'NONE', #2486, 1000.000000000000000 ) ;
#26618=CARTESIAN_POINT ( 'NONE',  ( 19.38216949554541557, 52.24863466993041072, -9.382169495545420901 ) ) ;
#26621=FACE_OUTER_BOUND ( 'NONE', #43435, .T. ) ;
#26622=CARTESIAN_POINT ( 'NONE',  ( 18.52753015748617571, 63.09226448433412315, 4.923371831947298993 ) ) ;
#26623=CARTESIAN_POINT ( 'NONE',  ( 2.917880565312950480, 65.97041550158063217, -12.26659068614894821 ) ) ;
#26624=CARTESIAN_POINT ( 'NONE',  ( 10.00000000000000178, 67.25893115100079456, 9.846743663894594434 ) ) ;
#26625=ORIENTED_EDGE ( 'NONE', *, *, #35481, .F. ) ;
#26627=CARTESIAN_POINT ( 'NONE',  ( 18.52753015748617571, 38.09226448433412315, 4.923371831947298993 ) ) ;
#26628=CARTESIAN_POINT ( 'NONE',  ( 6.565887622018943937, 65.16530133659709634, 12.81628187352647430 ) ) ;
#26629=CARTESIAN_POINT ( 'NONE',  ( 21.09922568453594849, 11.20696800326375531, 6.408140936763242479 ) ) ;
#26630=CARTESIAN_POINT ( 'NONE',  ( 19.84674366389459266, 3.717264484334118713, -2.638427012816827677 ) ) ;
#26633=CARTESIAN_POINT ( 'NONE',  ( 0.1532563361054100626, 15.80059781766745353, -2.638427012816831230 ) ) ;
#26634=CARTESIAN_POINT ( 'NONE',  ( 18.52753015748617571, 53.09226448433412315, 4.923371831947298993 ) ) ;
#26638=EDGE_CURVE ( 'NONE', #66014, #68558, #34328, .T. ) ;
#26639=EDGE_LOOP ( 'NONE', ( #83580, #79698, #39770, #63779 ) ) ;
#26640=CARTESIAN_POINT ( 'NONE',  ( -0.3689425029237881626, 62.42874883491396787, 10.36894250292379027 ) ) ;
#26641=CARTESIAN_POINT ( 'NONE',  ( 24.16423886937409904, 9.095415501580633943, 3.795296366450317205 ) ) ;
#26642=CARTESIAN_POINT ( 'NONE',  ( 5.076628168052704559, 10.17559781766745175, -8.527530157486179263 ) ) ;
#26643=CARTESIAN_POINT ( 'NONE',  ( -0.8801773607111009756, 38.06368534415484106, 1.068504757029289695E-15 ) ) ;
#26644=CARTESIAN_POINT ( 'NONE',  ( 0.6178305044545838731, 29.74863466993042138, 9.382169495545420901 ) ) ;
#26648=CARTESIAN_POINT ( 'NONE',  ( 0.1532563361054083140, 56.00893115100078745, 1.131784320476157264E-15 ) ) ;
#26649=CARTESIAN_POINT ( 'NONE',  ( 14.92337183194729988, 14.34226448433411782, -8.527530157486177487 ) ) ;
#26651=CARTESIAN_POINT ( 'NONE',  ( 22.81628187352647785, 21.41530133659708923, 3.434112377981063169 ) ) ;
#26653=CARTESIAN_POINT ( 'NONE',  ( 19.42250999205614548, 25.98035201082150891, -5.440088680355545492 ) ) ;
#26656=CARTESIAN_POINT ( 'NONE',  ( 17.08211943468705840, 55.13708216824731068, -12.26659068614894466 ) ) ;
#26657=AXIS2_PLACEMENT_3D ( 'NONE', #94997, #9540, #16562 ) ;
#26658=CARTESIAN_POINT ( 'NONE',  ( 17.08211943468705130, 23.47041550158063572, 12.26659068614894998 ) ) ;
#26659=CARTESIAN_POINT ( 'NONE',  ( 10.00000000000000178, 42.25893115100078745, 9.846743663894594434 ) ) ;
#26661=CARTESIAN_POINT ( 'NONE',  ( 19.38216949554541557, 32.24863466993041783, -9.382169495545420901 ) ) ;
#26662=CARTESIAN_POINT ( 'NONE',  ( 19.42250999205614548, 25.98035201082150891, -5.440088680355545492 ) ) ;
#26663=CARTESIAN_POINT ( 'NONE',  ( 5.076628168052703671, 56.84226448433412315, 8.527530157486179263 ) ) ;
#26664=CARTESIAN_POINT ( 'NONE',  ( 15.44008868035555260, 44.73035201082151247, 9.422509992056143702 ) ) ;
#26665=CARTESIAN_POINT ( 'NONE',  ( 3.591859063236761518, -0.04303199673624671928, 11.09922568453594849 ) ) ;
#26666=CARTESIAN_POINT ( 'NONE',  ( 10.00000000000000178, 23.05374883491397142, 14.16423886937410082 ) ) ;
#26668=CARTESIAN_POINT ( 'NONE',  ( 18.52753015748617571, 23.09226448433411960, 4.923371831947298993 ) ) ;
#26669=CARTESIAN_POINT ( 'NONE',  ( 0.1532563361054083140, 66.00893115100079456, 1.131784320476157264E-15 ) ) ;
#26674=CARTESIAN_POINT ( 'NONE',  ( 10.00000000000000000, 16.81368534415483751, -10.88017736071110342 ) ) ;
#26675=CARTESIAN_POINT ( 'NONE',  ( -2.266590686148945544, 16.38708216824730357, -7.082119434687050408 ) ) ;
#26676=CARTESIAN_POINT ( 'NONE',  ( 7.361572987183169658, 4.967264484334119601, -9.846743663894592657 ) ) ;
#26677=CARTESIAN_POINT ( 'NONE',  ( 0.1532563361054100626, 50.80059781766745175, -2.638427012816831230 ) ) ;
#26678=CARTESIAN_POINT ( 'NONE',  ( 20.88017736071110519, 35.56368534415484106, 2.639326808657452039E-16 ) ) ;
#26679=FACE_OUTER_BOUND ( 'NONE', #12220, .T. ) ;
#26680=CARTESIAN_POINT ( 'NONE',  ( 5.076628168052703671, 61.84226448433412315, 8.527530157486179263 ) ) ;
#26681=MECHANICAL_DESIGN_GEOMETRIC_PRESENTATION_REPRESENTATION('',(#69809),#18707);
#26683=CYLINDRICAL_SURFACE ( 'NONE', #92842, 0.5000000000000004441 ) ;
#26687=CARTESIAN_POINT ( 'NONE',  ( -2.266590686148945544, 12.22041550158063394, 7.082119434687048631 ) ) ;
#26688=CARTESIAN_POINT ( 'NONE',  ( -4.164238869374098151, 11.59541550158063217, -3.795296366450310543 ) ) ;
#26689=CARTESIAN_POINT ( 'NONE',  ( 24.16423886937410614, 59.30374883491397497, 8.672049930838204340E-16 ) ) ;
#26690=CARTESIAN_POINT ( 'NONE',  ( 19.84674366389459621, 63.50893115100078745, 7.409399052514197653E-17 ) ) ;
#26691=CARTESIAN_POINT ( 'NONE',  ( 12.63842701281683922, 29.55059781766745175, -9.846743663894590881 ) ) ;
#26693=CARTESIAN_POINT ( 'NONE',  ( 2.035157376598822676, 37.43868534415484106, -7.964842623401177768 ) ) ;
#26694=CARTESIAN_POINT ( 'NONE',  ( 10.00000000000000000, 64.75893115100078035, -9.846743663894594434 ) ) ;
#26695=CARTESIAN_POINT ( 'NONE',  ( 13.79529636645030344, 3.262082168247301350, 14.16423886937410614 ) ) ;
#26696=CARTESIAN_POINT ( 'NONE',  ( 13.79529636645030344, 48.26208216824728936, 14.16423886937410614 ) ) ;
#26697=CARTESIAN_POINT ( 'NONE',  ( -2.266590686148945544, 67.22041550158063217, 7.082119434687048631 ) ) ;
#26700=CARTESIAN_POINT ( 'NONE',  ( 0.5774900079438590739, 67.64701867748817676, -5.440088680355550821 ) ) ;
#26705=CARTESIAN_POINT ( 'NONE',  ( 7.361572987183169658, 19.96726448433411960, -9.846743663894592657 ) ) ;
#26707=CARTESIAN_POINT ( 'NONE',  ( -4.164238869374099927, 27.01208216824730357, 3.795296366450308767 ) ) ;
#26708=CARTESIAN_POINT ( 'NONE',  ( 18.52753015748617571, 38.09226448433412315, 4.923371831947298993 ) ) ;
#26709=CARTESIAN_POINT ( 'NONE',  ( -0.8801773607111008646, 58.27201867748816966, 2.915334737309923430 ) ) ;
#26711=CARTESIAN_POINT ( 'NONE',  ( 19.42250999205614548, 60.98035201082151247, -5.440088680355545492 ) ) ;
#26712=CARTESIAN_POINT ( 'NONE',  ( 1.472469842513823179, 51.42559781766745886, 4.923371831947296329 ) ) ;
#26713=AXIS2_PLACEMENT_3D ( 'NONE', #69564, #3051, #85055 ) ;
#26714=CARTESIAN_POINT ( 'NONE',  ( 10.00000000000000178, 55.37363466993042493, 12.81628187352647608 ) ) ;
#26716=ORIENTED_EDGE ( 'NONE', *, *, #86681, .F. ) ;
#26717=CARTESIAN_POINT ( 'NONE',  ( 2.917880565312950480, 15.97041550158063217, -12.26659068614894821 ) ) ;
#26718=VERTEX_POINT ( 'NONE', #49832 ) ;
#26720=CARTESIAN_POINT ( 'NONE',  ( 13.43411237798105340, 25.58196800326374998, 12.81628187352647963 ) ) ;
#26722=FACE_OUTER_BOUND ( 'NONE', #7570, .T. ) ;
#26723=CARTESIAN_POINT ( 'NONE',  ( 18.52753015748618282, 18.92559781766745175, -4.923371831947291888 ) ) ;
#26724=SURFACE_STYLE_USAGE ( .BOTH. , #3754 ) ;
#26725=CARTESIAN_POINT ( 'NONE',  ( -1.099225684535947600, 54.54030133659708923, 6.408140936763237150 ) ) ;
#26726=CARTESIAN_POINT ( 'NONE',  ( -46.56032334906440440, 103.8061263278352016, -5.692785474544873381 ) ) ;
#26727=CARTESIAN_POINT ( 'NONE',  ( 2.791683348922237240, 35.38393115100079456, -7.208316651077763204 ) ) ;
#26728=ADVANCED_FACE ( 'NONE', ( #55880 ), #72333, .T. ) ;
#26734=CYLINDRICAL_SURFACE ( 'NONE', #46640, 0.5000000000000004441 ) ;
#26735=CARTESIAN_POINT ( 'NONE',  ( 1.274849032794102888, 3.572280503510291361, 6.499999999999721112 ) ) ;
#26736=CARTESIAN_POINT ( 'NONE',  ( 14.92337183194729988, 4.342264484334117824, -8.527530157486177487 ) ) ;
#26737=CARTESIAN_POINT ( 'NONE',  ( 10.00000000000000178, 30.37363466993042138, 12.81628187352647608 ) ) ;
#26739=CARTESIAN_POINT ( 'NONE',  ( 18.52753015748617571, 38.09226448433412315, 4.923371831947298993 ) ) ;
#26741=CARTESIAN_POINT ( 'NONE',  ( -0.3689425029237898834, 26.17874883491396432, -10.36894250292378850 ) ) ;
#26742=CARTESIAN_POINT ( 'NONE',  ( 14.92337183194729633, 32.67559781766745175, 8.527530157486181039 ) ) ;
#26743=CARTESIAN_POINT ( 'NONE',  ( 13.43411237798106583, 32.66530133659708213, -12.81628187352647252 ) ) ;
#26744=CARTESIAN_POINT ( 'NONE',  ( 20.00000000000000711, 97.71973001530635372, 4.500000000000000888 ) ) ;
#26746=CARTESIAN_POINT ( 'NONE',  ( 12.91533473730993009, 66.60535201082150536, -10.88017736071109987 ) ) ;
#26747=EDGE_CURVE ( 'NONE', #65300, #89307, #6402, .T. ) ;
#26748=CARTESIAN_POINT ( 'NONE',  ( -1.099225684535947600, 4.540301336597087456, 6.408140936763237150 ) ) ;
#26749=CARTESIAN_POINT ( 'NONE',  ( 1.959929470562272291, 40.51528370094807485, -5.767676674365837641 ) ) ;
#26750=CARTESIAN_POINT ( 'NONE',  ( 10.00000000000000178, 32.25893115100078745, 9.846743663894594434 ) ) ;
#26751=CARTESIAN_POINT ( 'NONE',  ( -0.8801773607111009756, 23.06368534415484106, 1.068504757029289695E-15 ) ) ;
#26752=CARTESIAN_POINT ( 'NONE',  ( 21.09922568453594849, 31.20696800326375353, 6.408140936763242479 ) ) ;
#26753=CARTESIAN_POINT ( 'NONE',  ( 19.84674366389459266, 33.71726448433410894, -2.638427012816827677 ) ) ;
#26757=CARTESIAN_POINT ( 'NONE',  ( -0.8801773607110991993, 32.85535201082151247, -2.915334737309923874 ) ) ;
#26760=CARTESIAN_POINT ( 'NONE',  ( 15.44008868035555793, 66.39701867748817676, -9.422509992056140149 ) ) ;
#26761=( NAMED_UNIT ( * ) SI_UNIT ( $, .STERADIAN. ) SOLID_ANGLE_UNIT ( ) );
#26762=CARTESIAN_POINT ( 'NONE',  ( 5.076628168052704559, 55.17559781766745175, -8.527530157486179263 ) ) ;
#26763=CARTESIAN_POINT ( 'NONE',  ( -0.8801773607110991993, 32.85535201082151247, -2.915334737309923874 ) ) ;
#26765=CARTESIAN_POINT ( 'NONE',  ( 20.88017736071110875, 50.77201867748817676, -2.915334737309920765 ) ) ;
#26766=CARTESIAN_POINT ( 'NONE',  ( 10.00000000000000178, 14.31368534415483929, 10.88017736071110342 ) ) ;
#26767=CARTESIAN_POINT ( 'NONE',  ( 20.00000000000000711, 79.40087001978915282, -4.500000000000000000 ) ) ;
#26769=CARTESIAN_POINT ( 'NONE',  ( 12.63842701281683922, 49.55059781766744464, -9.846743663894590881 ) ) ;
#26770=CARTESIAN_POINT ( 'NONE',  ( 2.917880565312948704, 52.63708216824730357, 12.26659068614894643 ) ) ;
#26771=FACE_OUTER_BOUND ( 'NONE', #21068, .T. ) ;
#26772=CARTESIAN_POINT ( 'NONE',  ( 10.00000000000000178, 33.05374883491396787, 14.16423886937410082 ) ) ;
#26774=CARTESIAN_POINT ( 'NONE',  ( 22.81628187352647785, 1.415301336597087012, 3.434112377981063169 ) ) ;
#26777=CARTESIAN_POINT ( 'NONE',  ( -2.266590686148945544, 67.22041550158063217, 7.082119434687048631 ) ) ;
#26778=CARTESIAN_POINT ( 'NONE',  ( 7.361572987183170547, 37.05059781766744464, 9.846743663894590881 ) ) ;
#26781=CARTESIAN_POINT ( 'NONE',  ( 19.42250999205614193, 65.14701867748817676, 5.440088680355555262 ) ) ;
#26782=CARTESIAN_POINT ( 'NONE',  ( -1.099225684535947600, 64.54030133659709634, 6.408140936763237150 ) ) ;
#26783=CARTESIAN_POINT ( 'NONE',  ( 20.88017736071110875, 30.77201867748816966, -2.915334737309920765 ) ) ;
#26784=CARTESIAN_POINT ( 'NONE',  ( -1.099225684535947600, 63.70696800326376774, -6.408140936763238038 ) ) ;
#26785=CARTESIAN_POINT ( 'NONE',  ( 21.09922568453595559, 7.040301336597086568, -6.408140936763230044 ) ) ;
#26786=CARTESIAN_POINT ( 'NONE',  ( 5.076628168052704559, 30.17559781766745175, -8.527530157486179263 ) ) ;
#26789=EDGE_CURVE ( 'NONE', #43815, #67057, #95633, .T. ) ;
#26791=CARTESIAN_POINT ( 'NONE',  ( 2.035157376598822676, 2.438685344154838397, -7.964842623401177768 ) ) ;
#26792=CARTESIAN_POINT ( 'NONE',  ( -4.164238869374099039, 26.80374883491397142, 8.674139862899312516E-16 ) ) ;
#26793=CARTESIAN_POINT ( 'NONE',  ( 20.88017736071110875, 30.77201867748816966, -2.915334737309920765 ) ) ;
#26795=CARTESIAN_POINT ( 'NONE',  ( 0.5774900079438590739, 52.64701867748817676, -5.440088680355550821 ) ) ;
#26798=B_SPLINE_CURVE_WITH_KNOTS ( 'NONE', 3,
 ( #33427, #92467, #1992, #32458, #93458, #24984, #55468, #46790, #92297, #52812, #61298, #23821, #91807, #30798, #91303, #15821 ),
 .UNSPECIFIED., .F., .F.,
 ( 4, 2, 2, 2, 2, 2, 2, 4 ),
 ( 0.000000000000000000, 0.002379327621847403523, 0.004758655243694807045, 0.005948319054618508156, 0.007137982865542210134, 0.008327646676465913847, 0.008922478581927750091, 0.009517310487389588070 ),
 .UNSPECIFIED. ) ;
#26799=CARTESIAN_POINT ( 'NONE',  ( 18.52753015748617571, 8.092264484334117824, 4.923371831947298993 ) ) ;
#26802=CARTESIAN_POINT ( 'NONE',  ( 19.84674366389459266, 28.30059781766745886, 2.638427012816836559 ) ) ;
#26803=CARTESIAN_POINT ( 'NONE',  ( 19.84674366389459266, 53.30059781766744464, 2.638427012816836559 ) ) ;
#26805=CARTESIAN_POINT ( 'NONE',  ( 7.084665262690076126, 29.10535201082150181, 10.88017736071109987 ) ) ;
#26806=AXIS2_PLACEMENT_3D ( 'NONE', #55621, #46626, #48101 ) ;
#26807=CARTESIAN_POINT ( 'NONE',  ( -2.816281873526473856, 44.12363466993042493, 9.499525473075851096E-16 ) ) ;
#26809=CARTESIAN_POINT ( 'NONE',  ( 20.88017736071110164, 65.35535201082150536, 2.915334737309930979 ) ) ;
#26810=CARTESIAN_POINT ( 'NONE',  ( 19.84674366389459266, 33.30059781766744464, 2.638427012816836559 ) ) ;
#26811=CARTESIAN_POINT ( 'NONE',  ( 2.917880565312950480, 55.97041550158063217, -12.26659068614894821 ) ) ;
#26812=CARTESIAN_POINT ( 'NONE',  ( 17.20831665107776587, 27.88393115100078390, 7.208316651077764980 ) ) ;
#26813=CARTESIAN_POINT ( 'NONE',  ( 2.603489959281614308, 51.58210964143330557, 6.500000000000031086 ) ) ;
#26815=CARTESIAN_POINT ( 'NONE',  ( -4.164238869374099039, 11.80374883491396965, 8.674139862899312516E-16 ) ) ;
#26816=CARTESIAN_POINT ( 'NONE',  ( -4.164238869374098151, 36.59541550158063217, -3.795296366450310543 ) ) ;
#26817=CARTESIAN_POINT ( 'NONE',  ( 2.791683348922237240, 35.38393115100079456, -7.208316651077763204 ) ) ;
#26818=CARTESIAN_POINT ( 'NONE',  ( 17.62281668512002852, 8.285933195168226462, 6.500000000000004441 ) ) ;
#26819=CARTESIAN_POINT ( 'NONE',  ( 15.44008868035555793, 26.39701867748817321, -9.422509992056140149 ) ) ;
#26820=CARTESIAN_POINT ( 'NONE',  ( 20.88017736071110519, 55.56368534415484817, 2.639326808657452039E-16 ) ) ;
#26821=CARTESIAN_POINT ( 'NONE',  ( 20.88017736071110164, 50.35535201082151247, 2.915334737309930979 ) ) ;
#26823=CARTESIAN_POINT ( 'NONE',  ( 0.6178305044545818747, 38.49863466993042493, -9.382169495545419124 ) ) ;
#26824=CARTESIAN_POINT ( 'NONE',  ( 17.96484262340118221, 49.93868534415484106, 7.964842623401181321 ) ) ;
#26826=( NAMED_UNIT ( * ) PLANE_ANGLE_UNIT ( ) SI_UNIT ( $, .RADIAN. ) );
#26827=CARTESIAN_POINT ( 'NONE',  ( 17.96484262340118221, 66.18868534415483396, -7.964842623401177768 ) ) ;
#26829=CARTESIAN_POINT ( 'NONE',  ( -0.8801773607110991993, 62.85535201082150536, -2.915334737309923874 ) ) ;
#26830=CARTESIAN_POINT ( 'NONE',  ( 20.88017736071110875, 20.77201867748816611, -2.915334737309920765 ) ) ;
#26833=CARTESIAN_POINT ( 'NONE',  ( -0.8801773607110991993, 7.855352010821506248, -2.915334737309923874 ) ) ;
#26834=CARTESIAN_POINT ( 'NONE',  ( 0.1532563361054100626, 15.80059781766745353, -2.638427012816831230 ) ) ;
#26835=CARTESIAN_POINT ( 'NONE',  ( 10.00000000000000178, 23.05374883491397142, 14.16423886937410082 ) ) ;
#26836=CARTESIAN_POINT ( 'NONE',  ( 10.00000000000000178, 24.31368534415484106, 10.88017736071110342 ) ) ;
#26837=CARTESIAN_POINT ( 'NONE',  ( 19.84674366389459266, 63.30059781766745886, 2.638427012816836559 ) ) ;
#26838=ORIENTED_EDGE ( 'NONE', *, *, #96884, .F. ) ;
#26839=CARTESIAN_POINT ( 'NONE',  ( 19.84674366389459621, 63.50893115100078745, 7.409399052514197653E-17 ) ) ;
#26842=CARTESIAN_POINT ( 'NONE',  ( -0.8801773607111008646, 58.27201867748816966, 2.915334737309923430 ) ) ;
#26843=CARTESIAN_POINT ( 'NONE',  ( 2.791683348922240793, 46.63393115100077324, 7.208316651077764092 ) ) ;
#26844=CARTESIAN_POINT ( 'NONE',  ( 13.43411237798106583, 32.66530133659708213, -12.81628187352647252 ) ) ;
#26845=CARTESIAN_POINT ( 'NONE',  ( -0.8801773607110991993, 2.855352010821504471, -2.915334737309923874 ) ) ;
#26847=CARTESIAN_POINT ( 'NONE',  ( 10.00000000000000000, 61.81368534415484106, -10.88017736071110342 ) ) ;
#26848=CARTESIAN_POINT ( 'NONE',  ( -0.8801773607110991993, 2.855352010821504471, -2.915334737309923874 ) ) ;
#26849=EDGE_CURVE ( 'NONE', #19080, #14105, #55273, .T. ) ;
#26851=CARTESIAN_POINT ( 'NONE',  ( 0.6178305044545838731, 39.74863466993041072, 9.382169495545420901 ) ) ;
#26852=CARTESIAN_POINT ( 'NONE',  ( 19.42250999205614548, 35.98035201082151247, -5.440088680355545492 ) ) ;
#26855=CARTESIAN_POINT ( 'NONE',  ( 0.6178305044545838731, 44.74863466993042493, 9.382169495545420901 ) ) ;
#26856=CARTESIAN_POINT ( 'NONE',  ( 20.88017736071110164, 35.35535201082150536, 2.915334737309930979 ) ) ;
#26857=CARTESIAN_POINT ( 'NONE',  ( 10.00000000000000000, 54.75893115100078745, -9.846743663894594434 ) ) ;
#26859=AXIS2_PLACEMENT_3D ( 'NONE', #56637, #71647, #63629 ) ;
#26860=CARTESIAN_POINT ( 'NONE',  ( 1.472469842513823179, 60.59226448433412315, -4.923371831947296329 ) ) ;
#26861=CYLINDRICAL_SURFACE ( 'NONE', #18126, 0.5000000000000004441 ) ;
#26862=CARTESIAN_POINT ( 'NONE',  ( 18.52753015748617571, 53.09226448433412315, 4.923371831947298993 ) ) ;
#26863=CARTESIAN_POINT ( 'NONE',  ( 10.00000000000000000, 21.81368534415484106, -10.88017736071110342 ) ) ;
#26864=CARTESIAN_POINT ( 'NONE',  ( 1.472469842513823179, 41.42559781766745886, 4.923371831947296329 ) ) ;
#26867=CARTESIAN_POINT ( 'NONE',  ( 5.076628168052704559, 45.17559781766745175, -8.527530157486179263 ) ) ;
#26869=CARTESIAN_POINT ( 'NONE',  ( 10.00000000000000000, 14.75893115100078568, -9.846743663894594434 ) ) ;
#26871=CARTESIAN_POINT ( 'NONE',  ( 0.1532563361054083140, 61.00893115100078745, 1.131784320476157264E-15 ) ) ;
#26874=CARTESIAN_POINT ( 'NONE',  ( -2.816281873526473856, 64.33196800326376774, 3.434112377981055619 ) ) ;
#26875=CARTESIAN_POINT ( 'NONE',  ( 20.03447792253739124, 7.655141069906896689, -6.401564815979731371 ) ) ;
#26877=CARTESIAN_POINT ( 'NONE',  ( 10.00000000000000178, 45.37363466993041783, 12.81628187352647608 ) ) ;
#26878=CARTESIAN_POINT ( 'NONE',  ( 18.52753015748617571, 48.09226448433412315, 4.923371831947298993 ) ) ;
#26880=CARTESIAN_POINT ( 'NONE',  ( 20.36894250292379382, 63.67874883491396787, 10.36894250292379205 ) ) ;
#26881=CARTESIAN_POINT ( 'NONE',  ( 12.63842701281683922, 19.55059781766745175, -9.846743663894590881 ) ) ;
#26882=EDGE_CURVE ( 'NONE', #97286, #24048, #71745, .T. ) ;
#26884=CARTESIAN_POINT ( 'NONE',  ( 22.26659068614895176, 54.72041550158063217, -7.082119434687042414 ) ) ;
#26885=CARTESIAN_POINT ( 'NONE',  ( 5.076628168052703671, 66.84226448433412315, 8.527530157486179263 ) ) ;
#26886=CARTESIAN_POINT ( 'NONE',  ( 12.91533473730993009, 6.605352010821504471, -10.88017736071109987 ) ) ;
#26887=CARTESIAN_POINT ( 'NONE',  ( -4.164238869374098151, 31.59541550158063927, -3.795296366450310543 ) ) ;
#26888=CARTESIAN_POINT ( 'NONE',  ( 2.917880565312950480, 45.97041550158063927, -12.26659068614894821 ) ) ;
#26891=CARTESIAN_POINT ( 'NONE',  ( 0.1532563361054083140, 11.00893115100078568, 1.131784320476157264E-15 ) ) ;
#26893=CARTESIAN_POINT ( 'NONE',  ( 10.00000000000000178, 57.25893115100078745, 9.846743663894594434 ) ) ;
#26895=CARTESIAN_POINT ( 'NONE',  ( 7.084665262690076126, 44.10535201082151247, 10.88017736071109987 ) ) ;
#26896=CARTESIAN_POINT ( 'NONE',  ( 19.67858290521088804, 89.00000000000000000, -5.461713021790605360 ) ) ;
#26897=CARTESIAN_POINT ( 'NONE',  ( 19.84674366389459266, 48.71726448433413026, -2.638427012816827677 ) ) ;
#26898=CARTESIAN_POINT ( 'NONE',  ( -1.099225684535947600, 64.54030133659709634, 6.408140936763237150 ) ) ;
#26899=CARTESIAN_POINT ( 'NONE',  ( 19.84674366389459621, 58.50893115100078745, 7.409399052514197653E-17 ) ) ;
#26900=CARTESIAN_POINT ( 'NONE',  ( -4.164238869374099039, 21.80374883491396787, 8.674139862899312516E-16 ) ) ;
#26901=EDGE_CURVE ( 'NONE', #10866, #54718, #78757, .T. ) ;
#26902=CARTESIAN_POINT ( 'NONE',  ( 7.361572987183170547, 2.050597817667451750, 9.846743663894590881 ) ) ;
#26904=CARTESIAN_POINT ( 'NONE',  ( 7.084665262690076126, 19.10535201082150181, 10.88017736071109987 ) ) ;
#26905=CARTESIAN_POINT ( 'NONE',  ( -2.816281873526473856, 29.12363466993041783, 9.499525473075851096E-16 ) ) ;
#26907=CARTESIAN_POINT ( 'NONE',  ( 5.076628168052703671, 6.842264484334118713, 8.527530157486179263 ) ) ;
#26908=CARTESIAN_POINT ( 'NONE',  ( 16.40814093676324603, 52.45696800326375353, -11.09922568453594671 ) ) ;
#26911=ADVANCED_FACE ( 'NONE', ( #26722 ), #49254, .T. ) ;
#26912=CARTESIAN_POINT ( 'NONE',  ( -2.266590686148945544, 22.22041550158063572, 7.082119434687048631 ) ) ;
#26913=CARTESIAN_POINT ( 'NONE',  ( 6.000000000000000000, 11.50000000000000000, 6.000000000000000000 ) ) ;
#26914=CARTESIAN_POINT ( 'NONE',  ( -0.8801773607111008646, 13.27201867748817321, 2.915334737309923430 ) ) ;
#26917=CARTESIAN_POINT ( 'NONE',  ( 15.44008868035555260, 44.73035201082151247, 9.422509992056143702 ) ) ;
#26918=CARTESIAN_POINT ( 'NONE',  ( 0.5774900079438607392, 53.48035201082151247, 5.440088680355550821 ) ) ;
#26919=CARTESIAN_POINT ( 'NONE',  ( 0.6178305044545818747, 18.49863466993041428, -9.382169495545419124 ) ) ;
#26922=CARTESIAN_POINT ( 'NONE',  ( 0.1532563361054082862, 16.21726448433411960, 2.638427012816831674 ) ) ;
#26924=CARTESIAN_POINT ( 'NONE',  ( -0.8801773607111008646, 48.27201867748816966, 2.915334737309923430 ) ) ;
#26926=CARTESIAN_POINT ( 'NONE',  ( 22.81628187352648496, 1.831968003263753753, -3.434112377981050290 ) ) ;
#26927=CARTESIAN_POINT ( 'NONE',  ( 19.42250999205614193, 65.14701867748817676, 5.440088680355555262 ) ) ;
#26928=CARTESIAN_POINT ( 'NONE',  ( 14.92337183194729988, 24.34226448433411960, -8.527530157486177487 ) ) ;
#26929=CARTESIAN_POINT ( 'NONE',  ( 10.00000000000000000, 47.87363466993042493, -12.81628187352647608 ) ) ;
#26930=CARTESIAN_POINT ( 'NONE',  ( 0.1532563361054100626, 0.8005978176674514168, -2.638427012816831230 ) ) ;
#26932=ORIENTED_EDGE ( 'NONE', *, *, #39658, .T. ) ;
#26933=CARTESIAN_POINT ( 'NONE',  ( 2.153642693323453816, 56.13791097397319163, -6.500000000000043521 ) ) ;
#26935=CARTESIAN_POINT ( 'NONE',  ( 12.91533473730992121, 24.52201867748816966, 10.88017736071110164 ) ) ;
#26936=CARTESIAN_POINT ( 'NONE',  ( 0.000000000000000000, 61.50000000000000711, -6.000000000000000000 ) ) ;
#26937=CARTESIAN_POINT ( 'NONE',  ( 1.472469842513823179, 35.59226448433412315, -4.923371831947296329 ) ) ;
#26938=CARTESIAN_POINT ( 'NONE',  ( 0.5774900079438607392, 13.48035201082150358, 5.440088680355550821 ) ) ;
#26939=CARTESIAN_POINT ( 'NONE',  ( 12.91533473730992121, 4.522018677488170546, 10.88017736071110164 ) ) ;
#26940=EDGE_LOOP ( 'NONE', ( #33116, #86123, #17198, #12691 ) ) ;
#26941=CARTESIAN_POINT ( 'NONE',  ( 19.42250999205614548, 10.98035201082150358, -5.440088680355545492 ) ) ;
#26943=CARTESIAN_POINT ( 'NONE',  ( 0.5774900079438590739, 17.64701867748817321, -5.440088680355550821 ) ) ;
#26945=CARTESIAN_POINT ( 'NONE',  ( -0.8801773607110991993, 22.85535201082150181, -2.915334737309923874 ) ) ;
#26947=CARTESIAN_POINT ( 'NONE',  ( 21.92686044187656336, 26.97997603579417714, 3.195792623639536423 ) ) ;
#26948=CARTESIAN_POINT ( 'NONE',  ( -0.8801773607111009756, 18.06368534415484106, 1.068504757029289695E-15 ) ) ;
#26949=CARTESIAN_POINT ( 'NONE',  ( 19.84674366389459266, 58.71726448433411605, -2.638427012816827677 ) ) ;
#26951=CARTESIAN_POINT ( 'NONE',  ( 0.6178305044545818747, 58.49863466993042493, -9.382169495545419124 ) ) ;
#26953=CARTESIAN_POINT ( 'NONE',  ( 6.204703633549690345, 35.76208216824729647, -14.16423886937410259 ) ) ;
#26954=CARTESIAN_POINT ( 'NONE',  ( 19.42250999205614548, 45.98035201082150536, -5.440088680355545492 ) ) ;
#26955=CARTESIAN_POINT ( 'NONE',  ( 17.96484262340118221, 21.18868534415483396, -7.964842623401177768 ) ) ;
#26956=CARTESIAN_POINT ( 'NONE',  ( 19.88565890683628368, 42.71691075486305067, -6.480892540919849232 ) ) ;
#26958=CARTESIAN_POINT ( 'NONE',  ( 14.92337183194729988, 44.34226448433412315, -8.527530157486177487 ) ) ;
#26959=DIRECTION ( 'NONE',  ( -0.000000000000000000, 1.000000000000000000, -0.000000000000000000 ) ) ;
#26960=CARTESIAN_POINT ( 'NONE',  ( 14.92337183194729633, 12.67559781766745353, 8.527530157486181039 ) ) ;
#26962=CARTESIAN_POINT ( 'NONE',  ( 19.42250999205614193, 15.14701867748817143, 5.440088680355555262 ) ) ;
#26963=CARTESIAN_POINT ( 'NONE',  ( 17.20831665107776587, 14.13393115100078568, -7.208316651077762316 ) ) ;
#26964=CARTESIAN_POINT ( 'NONE',  ( 15.44008868035555793, 66.39701867748817676, -9.422509992056140149 ) ) ;
#26965=CARTESIAN_POINT ( 'NONE',  ( 20.88017736071110875, 25.77201867748816966, -2.915334737309920765 ) ) ;
#26966=CARTESIAN_POINT ( 'NONE',  ( 22.81628187352647785, 51.41530133659708923, 3.434112377981063169 ) ) ;
#26967=CARTESIAN_POINT ( 'NONE',  ( -4.164238869374098151, 31.59541550158063927, -3.795296366450310543 ) ) ;
#26969=ADVANCED_FACE ( 'NONE', ( #12049 ), #73034, .T. ) ;
#26973=CARTESIAN_POINT ( 'NONE',  ( -2.816281873526473856, 59.33196800326374643, 3.434112377981055619 ) ) ;
#26975=CARTESIAN_POINT ( 'NONE',  ( 13.43411237798106583, 7.665301336597086568, -12.81628187352647252 ) ) ;
#26977=CARTESIAN_POINT ( 'NONE',  ( 20.88017736071110164, 35.35535201082150536, 2.915334737309930979 ) ) ;
#26978=CARTESIAN_POINT ( 'NONE',  ( 2.791683348922237240, 65.38393115100078035, -7.208316651077763204 ) ) ;
#26979=ORIENTED_EDGE ( 'NONE', *, *, #71412, .F. ) ;
#26980=CARTESIAN_POINT ( 'NONE',  ( 1.472469842513823179, 11.42559781766745175, 4.923371831947296329 ) ) ;
#26982=CARTESIAN_POINT ( 'NONE',  ( 7.361572987183170547, 12.05059781766744997, 9.846743663894590881 ) ) ;
#26984=CARTESIAN_POINT ( 'NONE',  ( 19.84674366389459266, 18.30059781766745175, 2.638427012816836559 ) ) ;
#26985=CARTESIAN_POINT ( 'NONE',  ( 14.92337183194729988, 9.342264484334119601, -8.527530157486177487 ) ) ;
#26986=CARTESIAN_POINT ( 'NONE',  ( 4.559911319644449179, 52.23035201082151247, -9.422509992056141925 ) ) ;
#26988=CARTESIAN_POINT ( 'NONE',  ( 19.84674366389459266, 3.717264484334118713, -2.638427012816827677 ) ) ;
#26989=CARTESIAN_POINT ( 'NONE',  ( 0.1532563361054100626, 15.80059781766745353, -2.638427012816831230 ) ) ;
#26992=EDGE_CURVE ( 'NONE', #63612, #80095, #77472, .T. ) ;
#26993=CARTESIAN_POINT ( 'NONE',  ( 0.1532563361054100626, 60.80059781766744464, -2.638427012816831230 ) ) ;
#26996=CARTESIAN_POINT ( 'NONE',  ( 24.16423886937410614, 14.30374883491396787, 8.672049930838204340E-16 ) ) ;
#26999=CARTESIAN_POINT ( 'NONE',  ( -0.3689425029237881626, 17.42874883491397142, 10.36894250292379027 ) ) ;
#27000=CARTESIAN_POINT ( 'NONE',  ( 17.08211943468705840, 35.13708216824730357, -12.26659068614894466 ) ) ;
#27002=FACE_OUTER_BOUND ( 'NONE', #13387, .T. ) ;
#27003=FILL_AREA_STYLE ('',( #11509 ) ) ;
#27004=CARTESIAN_POINT ( 'NONE',  ( 19.42250999205614193, 30.14701867748817321, 5.440088680355555262 ) ) ;
#27005=DIRECTION ( 'NONE',  ( 0.000000000000000000, 0.000000000000000000, 1.000000000000000000 ) ) ;
#27006=CARTESIAN_POINT ( 'NONE',  ( 1.472469842513823179, 15.59226448433411960, -4.923371831947296329 ) ) ;
#27007=CARTESIAN_POINT ( 'NONE',  ( 10.00000000000000178, 59.31368534415484106, 10.88017736071110342 ) ) ;
#27008=CARTESIAN_POINT ( 'NONE',  ( 0.1532563361054100626, 20.80059781766744464, -2.638427012816831230 ) ) ;
#27009=CARTESIAN_POINT ( 'NONE',  ( 4.559911319644449179, 17.23035201082150536, -9.422509992056141925 ) ) ;
#27010=CARTESIAN_POINT ( 'NONE',  ( -1.099225684535947600, 43.70696800326375353, -6.408140936763238038 ) ) ;
#27011=CARTESIAN_POINT ( 'NONE',  ( 18.52753015748617571, 48.09226448433412315, 4.923371831947298993 ) ) ;
#27012=CARTESIAN_POINT ( 'NONE',  ( 18.52753015748618282, 58.92559781766745886, -4.923371831947291888 ) ) ;
#27013=CARTESIAN_POINT ( 'NONE',  ( -2.816281873526471635, 23.91530133659708568, -3.434112377981056508 ) ) ;
#27015=CARTESIAN_POINT ( 'NONE',  ( 0.1532563361054100626, 35.80059781766745175, -2.638427012816831230 ) ) ;
#27016=CARTESIAN_POINT ( 'NONE',  ( 10.00000000000000178, 8.053748834913967869, 14.16423886937410082 ) ) ;
#27017=ORIENTED_EDGE ( 'NONE', *, *, #28711, .F. ) ;
#27019=CARTESIAN_POINT ( 'NONE',  ( -0.8801773607111009756, 53.06368534415484106, 1.068504757029289695E-15 ) ) ;
#27020=CARTESIAN_POINT ( 'NONE',  ( 17.96484262340118221, 51.18868534415483396, -7.964842623401177768 ) ) ;
#27021=CARTESIAN_POINT ( 'NONE',  ( 2.917880565312948704, 47.63708216824730357, 12.26659068614894643 ) ) ;
#27022=CARTESIAN_POINT ( 'NONE',  ( 14.92337183194729988, 49.34226448433411605, -8.527530157486177487 ) ) ;
#27024=CARTESIAN_POINT ( 'NONE',  ( 7.084665262690076126, 42.02201867748816966, -10.88017736071110164 ) ) ;
#27027=CARTESIAN_POINT ( 'NONE',  ( 21.09922568453595559, 22.04030133659708923, -6.408140936763230044 ) ) ;
#27028=CARTESIAN_POINT ( 'NONE',  ( 2.791683348922237240, 50.38393115100078035, -7.208316651077763204 ) ) ;
#27030=CARTESIAN_POINT ( 'NONE',  ( 4.559911319644449179, 3.897018677488170990, 9.422509992056141925 ) ) ;
#27033=CARTESIAN_POINT ( 'NONE',  ( 12.91533473730993009, 6.605352010821504471, -10.88017736071109987 ) ) ;
#27034=CARTESIAN_POINT ( 'NONE',  ( 19.42250999205614548, 60.98035201082151247, -5.440088680355545492 ) ) ;
#27035=CARTESIAN_POINT ( 'NONE',  ( 2.791683348922237240, 0.3839311510007847872, -7.208316651077763204 ) ) ;
#27037=CARTESIAN_POINT ( 'NONE',  ( 18.52753015748618282, 38.92559781766745175, -4.923371831947291888 ) ) ;
#27038=CARTESIAN_POINT ( 'NONE',  ( 20.88017736071110164, 25.35535201082150891, 2.915334737309930979 ) ) ;
#27039=CARTESIAN_POINT ( 'NONE',  ( 18.52753015748618282, 63.92559781766745886, -4.923371831947291888 ) ) ;
#27040=CARTESIAN_POINT ( 'NONE',  ( 4.559911319644449179, 38.89701867748817676, 9.422509992056141925 ) ) ;
#27043=CARTESIAN_POINT ( 'NONE',  ( 22.81628187352647785, 36.62363466993041783, 6.195893100308588602E-16 ) ) ;
#27045=CARTESIAN_POINT ( 'NONE',  ( 20.88017736071110164, 45.35535201082149115, 2.915334737309930979 ) ) ;
#27046=CARTESIAN_POINT ( 'NONE',  ( 10.00000000000000000, 17.87363466993041783, -12.81628187352647608 ) ) ;
#27048=CARTESIAN_POINT ( 'NONE',  ( 18.52753015748617571, 3.092264484334118269, 4.923371831947298993 ) ) ;
#27049=CARTESIAN_POINT ( 'NONE',  ( -0.8801773607111009756, 23.06368534415484106, 1.068504757029289695E-15 ) ) ;
#27050=CARTESIAN_POINT ( 'NONE',  ( 24.16423886937409904, 64.09541550158064638, 3.795296366450317205 ) ) ;
#27051=CARTESIAN_POINT ( 'NONE',  ( 5.076628168052704559, 55.17559781766745175, -8.527530157486179263 ) ) ;
#27052=CARTESIAN_POINT ( 'NONE',  ( 12.63842701281683034, 2.467264484334118269, 9.846743663894596210 ) ) ;
#27053=CARTESIAN_POINT ( 'NONE',  ( 17.96484262340118221, 59.93868534415484106, 7.964842623401181321 ) ) ;
#27055=CARTESIAN_POINT ( 'NONE',  ( 6.204703633549690345, 35.76208216824729647, -14.16423886937410259 ) ) ;
#27060=CARTESIAN_POINT ( 'NONE',  ( -2.266590686148945544, 51.38708216824730357, -7.082119434687050408 ) ) ;
#27061=CARTESIAN_POINT ( 'NONE',  ( 22.26659068614894466, 53.88708216824731068, 7.082119434687054849 ) ) ;
#27062=CARTESIAN_POINT ( 'NONE',  ( 17.20831665107776587, 19.13393115100078035, -7.208316651077762316 ) ) ;
#27063=CARTESIAN_POINT ( 'NONE',  ( 0.6178305044545838731, 29.74863466993042138, 9.382169495545420901 ) ) ;
#27065=CARTESIAN_POINT ( 'NONE',  ( -0.2418659066527659718, 42.23410085661204505, -6.114288769123055189 ) ) ;
#27067=CARTESIAN_POINT ( 'NONE',  ( 0.6178305044545838731, 44.74863466993042493, 9.382169495545420901 ) ) ;
#27068=CARTESIAN_POINT ( 'NONE',  ( 22.26659068614895176, 44.72041550158063927, -7.082119434687042414 ) ) ;
#27070=CARTESIAN_POINT ( 'NONE',  ( 10.00000000000000000, 14.75893115100078568, -9.846743663894594434 ) ) ;
#27072=VERTEX_POINT ( 'NONE', #52511 ) ;
#27073=CARTESIAN_POINT ( 'NONE',  ( 5.076628168052703671, 21.84226448433411960, 8.527530157486179263 ) ) ;
#27074=ORIENTED_EDGE ( 'NONE', *, *, #57176, .F. ) ;
#27077=CARTESIAN_POINT ( 'NONE',  ( 7.084665262690076126, 19.10535201082150181, 10.88017736071109987 ) ) ;
#27078=CARTESIAN_POINT ( 'NONE',  ( 12.91533473730992121, 19.52201867748816611, 10.88017736071110164 ) ) ;
#27079=CARTESIAN_POINT ( 'NONE',  ( 12.63842701281683922, 49.55059781766744464, -9.846743663894590881 ) ) ;
#27080=CARTESIAN_POINT ( 'NONE',  ( 22.81628187352647785, 6.623634669930420493, 6.195893100308588602E-16 ) ) ;
#27083=CARTESIAN_POINT ( 'NONE',  ( 13.43411237798105340, 15.58196800326374998, 12.81628187352647963 ) ) ;
#27085=CARTESIAN_POINT ( 'NONE',  ( 2.791683348922240793, 31.63393115100078745, 7.208316651077764092 ) ) ;
#27086=CARTESIAN_POINT ( 'NONE',  ( 13.79529636645030344, 58.26208216824728936, 14.16423886937410614 ) ) ;
#27087=CARTESIAN_POINT ( 'NONE',  ( 4.559911319644449179, 8.897018677488173211, 9.422509992056141925 ) ) ;
#27088=ORIENTED_EDGE ( 'NONE', *, *, #70808, .T. ) ;
#27089=CARTESIAN_POINT ( 'NONE',  ( 7.084665262690076126, 34.10535201082151247, 10.88017736071109987 ) ) ;
#27090=CARTESIAN_POINT ( 'NONE',  ( 19.42250999205614548, 45.98035201082150536, -5.440088680355545492 ) ) ;
#27091=CARTESIAN_POINT ( 'NONE',  ( -0.8801773607111008646, 53.27201867748816966, 2.915334737309923430 ) ) ;
#27093=CARTESIAN_POINT ( 'NONE',  ( 2.035157376598824452, 43.68868534415484106, 7.964842623401179544 ) ) ;
#27095=CARTESIAN_POINT ( 'NONE',  ( 1.274849032794292736, 47.55509018479936856, -6.499999999999977796 ) ) ;
#27096=AXIS2_PLACEMENT_3D ( 'NONE', #24532, #55999, #68660 ) ;
#27099=EDGE_CURVE ( 'NONE', #31960, #85529, #57749, .T. ) ;
#27100=CARTESIAN_POINT ( 'NONE',  ( 2.791683348922240793, 11.63393115100078568, 7.208316651077764092 ) ) ;
#27101=VERTEX_POINT ( 'NONE', #1015 ) ;
#27103=CARTESIAN_POINT ( 'NONE',  ( 1.472469842513823179, 60.59226448433412315, -4.923371831947296329 ) ) ;
#27105=CARTESIAN_POINT ( 'NONE',  ( 3.591859063236763294, 53.29030133659708923, -11.09922568453595026 ) ) ;
#27109=CARTESIAN_POINT ( 'NONE',  ( -46.21538524526006597, 104.1852450480875660, 5.851526435683386040 ) ) ;
#27112=CARTESIAN_POINT ( 'NONE',  ( 17.20831665107776587, 29.13393115100078390, -7.208316651077762316 ) ) ;
#27113=CARTESIAN_POINT ( 'NONE',  ( 6.204703633549690345, 62.84541550158063927, 14.16423886937410082 ) ) ;
#27115=ORIENTED_EDGE ( 'NONE', *, *, #53334, .F. ) ;
#27117=CARTESIAN_POINT ( 'NONE',  ( 7.361572987183169658, 29.96726448433411960, -9.846743663894592657 ) ) ;
#27118=CARTESIAN_POINT ( 'NONE',  ( 10.00000000000000178, 65.37363466993042493, 12.81628187352647608 ) ) ;
#27119=CARTESIAN_POINT ( 'NONE',  ( 21.09922568453595559, 2.040301336597086568, -6.408140936763230044 ) ) ;
#27120=CARTESIAN_POINT ( 'NONE',  ( 0.1532563361054083140, 1.008931151000784787, 1.131784320476157264E-15 ) ) ;
#27121=CARTESIAN_POINT ( 'NONE',  ( 0.1532563361054083140, 6.008931151000784787, 1.131784320476157264E-15 ) ) ;
#27122=CARTESIAN_POINT ( 'NONE',  ( 18.52753015748617571, 63.09226448433412315, 4.923371831947298993 ) ) ;
#27125=CARTESIAN_POINT ( 'NONE',  ( 19.42250999205614193, 5.147018677488171434, 5.440088680355555262 ) ) ;
#27126=CARTESIAN_POINT ( 'NONE',  ( 20.36894250292379738, 4.928748834913967869, -10.36894250292379027 ) ) ;
#27127=CARTESIAN_POINT ( 'NONE',  ( 0.1532563361054083140, 11.00893115100078568, 1.131784320476157264E-15 ) ) ;
#27128=CARTESIAN_POINT ( 'NONE',  ( 17.96484262340118221, 46.18868534415484106, -7.964842623401177768 ) ) ;
#27129=CARTESIAN_POINT ( 'NONE',  ( 19.38216949554541557, 32.24863466993041783, -9.382169495545420901 ) ) ;
#27130=CARTESIAN_POINT ( 'NONE',  ( 2.035157376598822676, 67.43868534415484817, -7.964842623401177768 ) ) ;
#27131=FILL_AREA_STYLE_COLOUR ( '', #20052 ) ;
#27132=CARTESIAN_POINT ( 'NONE',  ( 19.72487221294571569, 17.80223176428831522, -6.499999999999990230 ) ) ;
#27134=CARTESIAN_POINT ( 'NONE',  ( -1.099225684535947600, -1.293031996736246469, -6.408140936763238038 ) ) ;
#27135=CARTESIAN_POINT ( 'NONE',  ( 2.791683348922240793, 16.63393115100078745, 7.208316651077764092 ) ) ;
#27137=CARTESIAN_POINT ( 'NONE',  ( -1.099225684535947600, 28.70696800326375353, -6.408140936763238038 ) ) ;
#27139=CARTESIAN_POINT ( 'NONE',  ( 2.035157376598822676, 22.43868534415483396, -7.964842623401177768 ) ) ;
#27142=CARTESIAN_POINT ( 'NONE',  ( 20.36894250292379738, 44.92874883491396787, -10.36894250292379027 ) ) ;
#27143=EDGE_CURVE ( 'NONE', #23604, #53783, #93531, .T. ) ;
#27145=CARTESIAN_POINT ( 'NONE',  ( 0.1532563361054083140, 46.00893115100079456, 1.131784320476157264E-15 ) ) ;
#27146=CARTESIAN_POINT ( 'NONE',  ( 10.00000000000000000, 37.87363466993041783, -12.81628187352647608 ) ) ;
#27147=CARTESIAN_POINT ( 'NONE',  ( 0.5774900079438607392, 23.48035201082150536, 5.440088680355550821 ) ) ;
#27148=CARTESIAN_POINT ( 'NONE',  ( 18.52753015748617571, 58.09226448433411605, 4.923371831947298993 ) ) ;
#27149=CARTESIAN_POINT ( 'NONE',  ( 0.5774900079438590739, 47.64701867748817676, -5.440088680355550821 ) ) ;
#27150=CARTESIAN_POINT ( 'NONE',  ( 0.6178305044545838731, 4.748634669930420493, 9.382169495545420901 ) ) ;
#27151=CARTESIAN_POINT ( 'NONE',  ( 22.26659068614895176, 34.72041550158063927, -7.082119434687042414 ) ) ;
#27154=CARTESIAN_POINT ( 'NONE',  ( 0.1532563361054083140, 21.00893115100078745, 1.131784320476157264E-15 ) ) ;
#27155=CARTESIAN_POINT ( 'NONE',  ( 22.81628187352647785, 61.62363466993041783, 6.195893100308588602E-16 ) ) ;
#27156=CARTESIAN_POINT ( 'NONE',  ( 10.00000000000000000, 2.873634669930420049, -12.81628187352647608 ) ) ;
#27158=CARTESIAN_POINT ( 'NONE',  ( 19.80448550324508616, 11.82703681773342907, 6.500000000002751577 ) ) ;
#27160=CARTESIAN_POINT ( 'NONE',  ( 19.42250999205614548, 10.98035201082150536, -5.440088680355545492 ) ) ;
#27161=CARTESIAN_POINT ( 'NONE',  ( -0.3689425029237881626, 22.42874883491397142, 10.36894250292379027 ) ) ;
#27163=CARTESIAN_POINT ( 'NONE',  ( 19.42250999205614193, 65.14701867748817676, 5.440088680355555262 ) ) ;
#27164=CARTESIAN_POINT ( 'NONE',  ( 14.92337183194729988, 54.34226448433412315, -8.527530157486177487 ) ) ;
#27165=CARTESIAN_POINT ( 'NONE',  ( 17.96484262340118221, 29.93868534415484106, 7.964842623401181321 ) ) ;
#27166=DIRECTION ( 'NONE',  ( -0.000000000000000000, -0.000000000000000000, -1.000000000000000000 ) ) ;
#27168=VECTOR ( 'NONE', #67702, 1000.000000000000000 ) ;
#27169=ORIENTED_EDGE ( 'NONE', *, *, #62861, .F. ) ;
#27174=CARTESIAN_POINT ( 'NONE',  ( -0.3689425029237898834, 6.178748834913968757, -10.36894250292378850 ) ) ;
#27175=CARTESIAN_POINT ( 'NONE',  ( 20.36894250292379738, 9.928748834913966093, -10.36894250292379027 ) ) ;
#27176=CARTESIAN_POINT ( 'NONE',  ( 17.96484262340118221, 41.18868534415484106, -7.964842623401177768 ) ) ;
#27177=CARTESIAN_POINT ( 'NONE',  ( 24.16423886937410614, 49.51208216824730357, -3.795296366450302550 ) ) ;
#27178=CARTESIAN_POINT ( 'NONE',  ( 7.361572987183170547, 62.05059781766745886, 9.846743663894590881 ) ) ;
#27179=CARTESIAN_POINT ( 'NONE',  ( 17.20831665107776587, 29.13393115100078390, -7.208316651077762316 ) ) ;
#27181=CARTESIAN_POINT ( 'NONE',  ( 15.44008868035555260, 34.73035201082151247, 9.422509992056143702 ) ) ;
#27182=CARTESIAN_POINT ( 'NONE',  ( 21.09922568453594849, 11.20696800326375531, 6.408140936763242479 ) ) ;
#27183=CARTESIAN_POINT ( 'NONE',  ( 2.917880565312948704, 2.637082168247300906, 12.26659068614894643 ) ) ;
#27184=CARTESIAN_POINT ( 'NONE',  ( 17.08211943468705840, 50.13708216824730357, -12.26659068614894466 ) ) ;
#27185=CARTESIAN_POINT ( 'NONE',  ( 15.44008868035555793, 6.397018677488171434, -9.422509992056140149 ) ) ;
#27186=CARTESIAN_POINT ( 'NONE',  ( 18.04007052943772038, 39.00257860105349295, -5.767676674365850076 ) ) ;
#27187=CARTESIAN_POINT ( 'NONE',  ( -0.1503990784575328643, 15.12777174578612538, 6.262539305110068177 ) ) ;
#27191=EDGE_LOOP ( 'NONE', ( #98122, #87094, #10157, #17112, #16238, #62590 ) ) ;
#27192=CARTESIAN_POINT ( 'NONE',  ( 18.52753015748617571, 18.09226448433411960, 4.923371831947298993 ) ) ;
#27193=VERTEX_POINT ( 'NONE', #93470 ) ;
#27194=CARTESIAN_POINT ( 'NONE',  ( 13.79529636645030344, 33.26208216824730357, 14.16423886937410614 ) ) ;
#27195=CARTESIAN_POINT ( 'NONE',  ( 19.84674366389459266, 38.30059781766745175, 2.638427012816836559 ) ) ;
#27196=CARTESIAN_POINT ( 'NONE',  ( 7.084665262690076126, 52.02201867748816255, -10.88017736071110164 ) ) ;
#27199=CARTESIAN_POINT ( 'NONE',  ( 17.96484262340118221, 59.93868534415484106, 7.964842623401181321 ) ) ;
#27202=CARTESIAN_POINT ( 'NONE',  ( 3.591859063236761518, 54.95696800326376064, 11.09922568453594849 ) ) ;
#27205=CARTESIAN_POINT ( 'NONE',  ( -2.266590686148945544, 16.38708216824730357, -7.082119434687050408 ) ) ;
#27207=CARTESIAN_POINT ( 'NONE',  ( 0.6178305044545838731, 49.74863466993041072, 9.382169495545420901 ) ) ;
#27208=CARTESIAN_POINT ( 'NONE',  ( 19.42250999205614548, 20.98035201082150891, -5.440088680355545492 ) ) ;
#27209=CARTESIAN_POINT ( 'NONE',  ( 14.92337183194729988, 29.34226448433411960, -8.527530157486177487 ) ) ;
#27210=CARTESIAN_POINT ( 'NONE',  ( 15.44008868035555793, 16.39701867748817321, -9.422509992056140149 ) ) ;
#27211=CARTESIAN_POINT ( 'NONE',  ( 22.81628187352648496, 51.83196800326376064, -3.434112377981050290 ) ) ;
#27214=CARTESIAN_POINT ( 'NONE',  ( 1.472469842513823179, 26.42559781766745175, 4.923371831947296329 ) ) ;
#27215=CARTESIAN_POINT ( 'NONE',  ( 21.92686044187656336, 21.97997603579417358, 3.195792623639536423 ) ) ;
#27219=CARTESIAN_POINT ( 'NONE',  ( 4.559911319644449179, 67.23035201082150536, -9.422509992056141925 ) ) ;
#27222=CARTESIAN_POINT ( 'NONE',  ( 18.52753015748617571, 18.09226448433411960, 4.923371831947298993 ) ) ;
#27223=CARTESIAN_POINT ( 'NONE',  ( 22.81628187352647785, 21.41530133659708923, 3.434112377981063169 ) ) ;
#27228=CARTESIAN_POINT ( 'NONE',  ( 1.472469842513823179, 41.42559781766745886, 4.923371831947296329 ) ) ;
#27230=CARTESIAN_POINT ( 'NONE',  ( 20.36894250292379738, 14.92874883491396432, -10.36894250292379027 ) ) ;
#27231=CARTESIAN_POINT ( 'NONE',  ( 14.92337183194729633, 37.67559781766745175, 8.527530157486181039 ) ) ;
#27232=CARTESIAN_POINT ( 'NONE',  ( 21.09922568453595559, 27.04030133659708568, -6.408140936763230044 ) ) ;
#27235=CARTESIAN_POINT ( 'NONE',  ( 7.084665262690076126, 59.10535201082150536, 10.88017736071109987 ) ) ;
#27236=CARTESIAN_POINT ( 'NONE',  ( 22.81628187352648496, 11.83196800326375531, -3.434112377981050290 ) ) ;
#27238=CARTESIAN_POINT ( 'NONE',  ( 5.076628168052703671, 31.84226448433412315, 8.527530157486179263 ) ) ;
#27239=CARTESIAN_POINT ( 'NONE',  ( 20.88017736071110875, 25.77201867748816966, -2.915334737309920765 ) ) ;
#27240=CARTESIAN_POINT ( 'NONE',  ( 6.565887622018943937, 33.08196800326374643, -12.81628187352647608 ) ) ;
#27241=CARTESIAN_POINT ( 'NONE',  ( 2.791683348922237240, 30.38393115100078390, -7.208316651077763204 ) ) ;
#27243=DIRECTION ( 'NONE',  ( 0.000000000000000000, 0.000000000000000000, 1.000000000000000000 ) ) ;
#27244=CARTESIAN_POINT ( 'NONE',  ( 4.559911319644449179, 32.23035201082150536, -9.422509992056141925 ) ) ;
#27247=CARTESIAN_POINT ( 'NONE',  ( 7.361572987183169658, 49.96726448433410894, -9.846743663894592657 ) ) ;
#27248=CARTESIAN_POINT ( 'NONE',  ( 20.88017736071110875, 35.77201867748816966, -2.915334737309920765 ) ) ;
#27250=CARTESIAN_POINT ( 'NONE',  ( 20.88017736071110875, 65.77201867748817676, -2.915334737309920765 ) ) ;
#27251=CARTESIAN_POINT ( 'NONE',  ( -0.8801773607111009756, 23.06368534415484106, 1.068504757029289695E-15 ) ) ;
#27252=DIRECTION ( 'NONE',  ( 2.478176394252579169E-16, -1.000000000000000000, 0.000000000000000000 ) ) ;
#27254=CARTESIAN_POINT ( 'NONE',  ( 17.20831665107776587, 54.13393115100079456, -7.208316651077762316 ) ) ;
#27255=CARTESIAN_POINT ( 'NONE',  ( 6.204703633549690345, 52.84541550158062506, 14.16423886937410082 ) ) ;
#27258=CARTESIAN_POINT ( 'NONE',  ( 24.16423886937410614, 4.303748834913967869, 8.672049930838204340E-16 ) ) ;
#27260=CARTESIAN_POINT ( 'NONE',  ( -4.164238869374099039, 41.80374883491397497, 8.674139862899312516E-16 ) ) ;
#27261=CARTESIAN_POINT ( 'NONE',  ( 16.40814093676323893, 0.7903013365970867898, 11.09922568453595026 ) ) ;
#27262=AXIS2_PLACEMENT_3D ( 'NONE', #67221, #52215, #61669 ) ;
#27265=CARTESIAN_POINT ( 'NONE',  ( -0.3689425029237881626, 67.42874883491396076, 10.36894250292379027 ) ) ;
#27266=CARTESIAN_POINT ( 'NONE',  ( 14.92337183194729988, 34.34226448433411605, -8.527530157486177487 ) ) ;
#27269=CARTESIAN_POINT ( 'NONE',  ( -0.8801773607110991993, 52.85535201082151247, -2.915334737309923874 ) ) ;
#27271=CARTESIAN_POINT ( 'NONE',  ( 6.565887622018943937, 60.16530133659707502, 12.81628187352647430 ) ) ;
#27272=CARTESIAN_POINT ( 'NONE',  ( 19.38216949554541202, 30.99863466993042138, 9.382169495545424454 ) ) ;
#27273=CARTESIAN_POINT ( 'NONE',  ( 17.20831665107776587, 29.13393115100078390, -7.208316651077762316 ) ) ;
#27275=CARTESIAN_POINT ( 'NONE',  ( 1.472469842513823179, 1.425597817667451528, 4.923371831947296329 ) ) ;
#27277=CARTESIAN_POINT ( 'NONE',  ( 10.00000000000000000, 65.55374883491396076, -14.16423886937410082 ) ) ;
#27278=CARTESIAN_POINT ( 'NONE',  ( 7.084665262690076126, 19.10535201082150181, 10.88017736071109987 ) ) ;
#27279=CARTESIAN_POINT ( 'NONE',  ( 22.26659068614895176, 44.72041550158063927, -7.082119434687042414 ) ) ;
#27280=CARTESIAN_POINT ( 'NONE',  ( 20.88017736071110519, 30.56368534415484106, 2.639326808657452039E-16 ) ) ;
#27281=CARTESIAN_POINT ( 'NONE',  ( 10.00000000000000178, 69.31368534415484817, 10.88017736071110342 ) ) ;
#27283=CARTESIAN_POINT ( 'NONE',  ( 19.84674366389459621, 48.50893115100078745, 7.409399052514197653E-17 ) ) ;
#27284=CARTESIAN_POINT ( 'NONE',  ( 1.472469842513823179, 10.59226448433411782, -4.923371831947296329 ) ) ;
#27286=CARTESIAN_POINT ( 'NONE',  ( 5.076628168052703671, 36.84226448433412315, 8.527530157486179263 ) ) ;
#27287=CARTESIAN_POINT ( 'NONE',  ( 19.84674366389459266, 58.71726448433411605, -2.638427012816827677 ) ) ;
#27288=CARTESIAN_POINT ( 'NONE',  ( 17.96484262340118221, 21.18868534415483396, -7.964842623401177768 ) ) ;
#27289=UNCERTAINTY_MEASURE_WITH_UNIT (LENGTH_MEASURE( 1.000000000000000082E-05 ), #80642, 'distance_accuracy_value', 'NONE');
#27292=CARTESIAN_POINT ( 'NONE',  ( -2.816281873526473856, 39.33196800326374643, 3.434112377981055619 ) ) ;
#27294=CARTESIAN_POINT ( 'NONE',  ( 17.96484262340118221, 59.93868534415484106, 7.964842623401181321 ) ) ;
#27295=CARTESIAN_POINT ( 'NONE',  ( 2.791683348922237240, 30.38393115100078390, -7.208316651077763204 ) ) ;
#27296=CARTESIAN_POINT ( 'NONE',  ( 10.00000000000000000, 65.55374883491396076, -14.16423886937410082 ) ) ;
#27297=CARTESIAN_POINT ( 'NONE',  ( 12.63842701281683922, 24.55059781766745175, -9.846743663894590881 ) ) ;
#27299=CARTESIAN_POINT ( 'NONE',  ( 2.791683348922237240, 65.38393115100078035, -7.208316651077763204 ) ) ;
#27300=CARTESIAN_POINT ( 'NONE',  ( -4.164238869374099039, 31.80374883491396432, 8.674139862899312516E-16 ) ) ;
#27301=CARTESIAN_POINT ( 'NONE',  ( 1.472469842513823179, 40.59226448433411605, -4.923371831947296329 ) ) ;
#27304=CARTESIAN_POINT ( 'NONE',  ( 15.44008868035555793, 31.39701867748817676, -9.422509992056140149 ) ) ;
#27305=CARTESIAN_POINT ( 'NONE',  ( -0.8801773607111009756, 58.06368534415484106, 1.068504757029289695E-15 ) ) ;
#27308=CARTESIAN_POINT ( 'NONE',  ( -2.816281873526473856, 39.33196800326374643, 3.434112377981055619 ) ) ;
#27311=CARTESIAN_POINT ( 'NONE',  ( 7.084665262690076126, 52.02201867748816255, -10.88017736071110164 ) ) ;
#27312=ORIENTED_EDGE ( 'NONE', *, *, #93766, .T. ) ;
#27313=PRESENTATION_STYLE_ASSIGNMENT (( #10002 ) ) ;
#27315=ORIENTED_EDGE ( 'NONE', *, *, #85593, .F. ) ;
#27318=CARTESIAN_POINT ( 'NONE',  ( 12.91533473730992121, 14.52201867748817143, 10.88017736071110164 ) ) ;
#27320=FACE_OUTER_BOUND ( 'NONE', #96071, .T. ) ;
#27321=CARTESIAN_POINT ( 'NONE',  ( 2.035157376598824452, 3.688685344154837953, 7.964842623401179544 ) ) ;
#27322=CARTESIAN_POINT ( 'NONE',  ( 2.791683348922240793, 26.63393115100078745, 7.208316651077764092 ) ) ;
#27323=CARTESIAN_POINT ( 'NONE',  ( 6.204703633549690345, 12.84541550158063572, 14.16423886937410082 ) ) ;
#27326=CARTESIAN_POINT ( 'NONE',  ( 10.00000000000000178, 29.31368534415483751, 10.88017736071110342 ) ) ;
#27327=CARTESIAN_POINT ( 'NONE',  ( 14.92337183194729988, 64.34226448433412315, -8.527530157486177487 ) ) ;
#27329=CARTESIAN_POINT ( 'NONE',  ( 10.00000000000000000, -2.126365330069579951, -12.81628187352647608 ) ) ;
#27331=CARTESIAN_POINT ( 'NONE',  ( 0.5774900079438590739, 47.64701867748817676, -5.440088680355550821 ) ) ;
#27332=CARTESIAN_POINT ( 'NONE',  ( 5.076628168052703671, 61.84226448433412315, 8.527530157486179263 ) ) ;
#27333=CARTESIAN_POINT ( 'NONE',  ( 16.40814093676324603, 42.45696800326375353, -11.09922568453594671 ) ) ;
#27334=CARTESIAN_POINT ( 'NONE',  ( 20.88017736071110875, 5.772018677488170546, -2.915334737309920765 ) ) ;
#27335=DIRECTION ( 'NONE',  ( -1.000000000000000000, 0.000000000000000000, 0.000000000000000000 ) ) ;
#27336=CARTESIAN_POINT ( 'NONE',  ( 19.42250999205614548, 65.98035201082151957, -5.440088680355545492 ) ) ;
#27337=CARTESIAN_POINT ( 'NONE',  ( 17.08211943468705840, 65.13708216824730357, -12.26659068614894466 ) ) ;
#27338=B_SPLINE_CURVE_WITH_KNOTS ( 'NONE', 3,
 ( #20225, #94744, #34220, #26735 ),
 .UNSPECIFIED., .F., .F.,
 ( 4, 4 ),
 ( 3.127317220692750759E-18, 0.002392975128318519749 ),
 .UNSPECIFIED. ) ;
#27339=ADVANCED_FACE ( 'NONE', ( #73409 ), #54230, .F. ) ;
#27342=CARTESIAN_POINT ( 'NONE',  ( 3.591859063236761518, 39.95696800326375353, 11.09922568453594849 ) ) ;
#27343=CARTESIAN_POINT ( 'NONE',  ( 0.5774900079438590739, 27.64701867748817676, -5.440088680355550821 ) ) ;
#27345=CARTESIAN_POINT ( 'NONE',  ( 6.565887622018943937, 40.16530133659708923, 12.81628187352647430 ) ) ;
#27346=CARTESIAN_POINT ( 'NONE',  ( 7.084665262690076126, 34.10535201082151247, 10.88017736071109987 ) ) ;
#27347=CARTESIAN_POINT ( 'NONE',  ( 17.20831665107776587, 54.13393115100079456, -7.208316651077762316 ) ) ;
#27348=EDGE_CURVE ( 'NONE', #50944, #90628, #35825, .T. ) ;
#27351=CARTESIAN_POINT ( 'NONE',  ( 10.00000000000000178, 57.25893115100078745, 9.846743663894594434 ) ) ;
#27352=DIRECTION ( 'NONE',  ( 0.000000000000000000, -1.000000000000000000, 0.000000000000000000 ) ) ;
#27353=CARTESIAN_POINT ( 'NONE',  ( 2.791683348922237240, 50.38393115100078035, -7.208316651077763204 ) ) ;
#27354=CARTESIAN_POINT ( 'NONE',  ( 20.88017736071110164, 25.35535201082150891, 2.915334737309930979 ) ) ;
#27355=CARTESIAN_POINT ( 'NONE',  ( 18.52753015748617571, 38.09226448433412315, 4.923371831947298993 ) ) ;
#27357=CARTESIAN_POINT ( 'NONE',  ( -26.69000000000001194, 92.00000000000000000, -9.500000000000000000 ) ) ;
#27358=CARTESIAN_POINT ( 'NONE',  ( 10.00000000000000000, 34.75893115100078745, -9.846743663894594434 ) ) ;
#27359=CARTESIAN_POINT ( 'NONE',  ( 0.1532563361054082862, 6.217264484334118713, 2.638427012816831674 ) ) ;
#27360=CARTESIAN_POINT ( 'NONE',  ( 1.472469842513823179, 1.425597817667451528, 4.923371831947296329 ) ) ;
#27361=CARTESIAN_POINT ( 'NONE',  ( 19.84674366389459266, 63.30059781766745886, 2.638427012816836559 ) ) ;
#27364=AXIS2_PLACEMENT_3D ( 'NONE', #43137, #5155, #42656 ) ;
#27365=CARTESIAN_POINT ( 'NONE',  ( 6.565887622018943937, 38.08196800326376064, -12.81628187352647608 ) ) ;
#27366=CARTESIAN_POINT ( 'NONE',  ( 19.84674366389459266, 48.30059781766745175, 2.638427012816836559 ) ) ;
#27367=CARTESIAN_POINT ( 'NONE',  ( -0.8801773607110990882, 57.85535201082150536, -2.915334737309924318 ) ) ;
#27368=CARTESIAN_POINT ( 'NONE',  ( 24.16423886937410614, 54.51208216824730357, -3.795296366450302550 ) ) ;
#27369=CARTESIAN_POINT ( 'NONE',  ( 19.84674366389459266, 33.71726448433410894, -2.638427012816827677 ) ) ;
#27372=CARTESIAN_POINT ( 'NONE',  ( 24.16423886937410614, 59.51208216824728936, -3.795296366450302550 ) ) ;
#27374=CARTESIAN_POINT ( 'NONE',  ( 15.44008868035555260, 9.730352010821505360, 9.422509992056143702 ) ) ;
#27375=CARTESIAN_POINT ( 'NONE',  ( 22.26659068614894466, 33.88708216824730357, 7.082119434687054849 ) ) ;
#27376=CARTESIAN_POINT ( 'NONE',  ( 17.08211943468705130, 58.47041550158063927, 12.26659068614894998 ) ) ;
#27380=CARTESIAN_POINT ( 'NONE',  ( 19.84674366389459266, 13.71726448433411782, -2.638427012816827677 ) ) ;
#27382=CARTESIAN_POINT ( 'NONE',  ( 6.565887622018943937, 5.165301336597086568, 12.81628187352647430 ) ) ;
#27384=CARTESIAN_POINT ( 'NONE',  ( 17.96484262340118221, 49.93868534415484106, 7.964842623401181321 ) ) ;
#27385=CARTESIAN_POINT ( 'NONE',  ( 5.076628168052704559, 50.17559781766745886, -8.527530157486179263 ) ) ;
#27387=CARTESIAN_POINT ( 'NONE',  ( 7.361572987183169658, 59.96726448433410894, -9.846743663894592657 ) ) ;
#27388=CARTESIAN_POINT ( 'NONE',  ( -0.3689425029237881626, 2.428748834913967869, 10.36894250292379027 ) ) ;
#27389=CARTESIAN_POINT ( 'NONE',  ( 20.36894250292379738, 29.92874883491396432, -10.36894250292379027 ) ) ;
#27393=CARTESIAN_POINT ( 'NONE',  ( 2.035157376598824452, 18.68868534415484106, 7.964842623401179544 ) ) ;
#27394=CARTESIAN_POINT ( 'NONE',  ( 22.81628187352648496, 36.83196800326376064, -3.434112377981050290 ) ) ;
#27396=CARTESIAN_POINT ( 'NONE',  ( 0.1532563361054083140, 6.008931151000784787, 1.131784320476157264E-15 ) ) ;
#27400=CARTESIAN_POINT ( 'NONE',  ( 13.79529636645030344, 28.26208216824729647, 14.16423886937410614 ) ) ;
#27401=( NAMED_UNIT ( * ) PLANE_ANGLE_UNIT ( ) SI_UNIT ( $, .RADIAN. ) );
#27402=EDGE_CURVE ( 'NONE', #87105, #31762, #59767, .T. ) ;
#27404=CARTESIAN_POINT ( 'NONE',  ( 12.91533473730992121, 9.522018677488171434, 10.88017736071110164 ) ) ;
#27406=CARTESIAN_POINT ( 'NONE',  ( 17.96484262340118221, 39.93868534415484106, 7.964842623401181321 ) ) ;
#27407=CARTESIAN_POINT ( 'NONE',  ( 12.91533473730993009, 46.60535201082150536, -10.88017736071109987 ) ) ;
#27408=CARTESIAN_POINT ( 'NONE',  ( -1.099225684535947600, 18.70696800326375353, -6.408140936763238038 ) ) ;
#27409=FILL_AREA_STYLE_COLOUR ( '', #50607 ) ;
#27410=CARTESIAN_POINT ( 'NONE',  ( 1.611620712799448185, 1.046791834471127114, 6.500000000000002665 ) ) ;
#27411=CARTESIAN_POINT ( 'NONE',  ( 2.791683348922237240, 10.38393115100078390, -7.208316651077763204 ) ) ;
#27413=EDGE_CURVE ( 'NONE', #71943, #13653, #81412, .T. ) ;
#27414=CARTESIAN_POINT ( 'NONE',  ( 2.035157376598822676, 47.43868534415484817, -7.964842623401177768 ) ) ;
#27415=VECTOR ( 'NONE', #89277, 1000.000000000000000 ) ;
#27416=CARTESIAN_POINT ( 'NONE',  ( 22.81628187352648496, 6.831968003263753531, -3.434112377981050290 ) ) ;
#27417=CARTESIAN_POINT ( 'NONE',  ( 2.035157376598822676, 57.43868534415484106, -7.964842623401177768 ) ) ;
#27418=CARTESIAN_POINT ( 'NONE',  ( 5.076628168052703671, 21.84226448433411960, 8.527530157486179263 ) ) ;
#27419=CARTESIAN_POINT ( 'NONE',  ( 22.81628187352647785, 46.62363466993041783, 6.195893100308588602E-16 ) ) ;
#27420=CARTESIAN_POINT ( 'NONE',  ( 18.52753015748617571, 3.092264484334118269, 4.923371831947298993 ) ) ;
#27421=PRESENTATION_STYLE_ASSIGNMENT (( #96938 ) ) ;
#27422=ORIENTED_EDGE ( 'NONE', *, *, #47570, .T. ) ;
#27425=CARTESIAN_POINT ( 'NONE',  ( 10.00000000000000178, 14.31368534415483751, 10.88017736071110342 ) ) ;
#27426=CARTESIAN_POINT ( 'NONE',  ( 22.81628187352647785, 61.41530133659709634, 3.434112377981063169 ) ) ;
#27427=CARTESIAN_POINT ( 'NONE',  ( 10.00000000000000178, 37.25893115100078745, 9.846743663894594434 ) ) ;
#27428=CARTESIAN_POINT ( 'NONE',  ( -0.8801773607111009756, 13.06368534415483929, 1.068504757029289695E-15 ) ) ;
#27429=CARTESIAN_POINT ( 'NONE',  ( 2.035157376598822676, 7.438685344154837509, -7.964842623401177768 ) ) ;
#27431=CARTESIAN_POINT ( 'NONE',  ( 10.00000000000000178, 9.313685344154839285, 10.88017736071110342 ) ) ;
#27432=CARTESIAN_POINT ( 'NONE',  ( 20.88017736071110519, 35.56368534415484106, 2.639326808657452039E-16 ) ) ;
#27434=CARTESIAN_POINT ( 'NONE',  ( 12.91533473730993009, 26.60535201082150536, -10.88017736071109987 ) ) ;
#27435=ORIENTED_EDGE ( 'NONE', *, *, #93798, .F. ) ;
#27436=CARTESIAN_POINT ( 'NONE',  ( 21.92686044187656691, 9.953790035174472806, 3.195792623639537755 ) ) ;
#27437=CARTESIAN_POINT ( 'NONE',  ( -0.8801773607110991993, 27.85535201082150181, -2.915334737309923874 ) ) ;
#27440=CARTESIAN_POINT ( 'NONE',  ( 20.15039907845753930, 5.601585745166425490, -6.262539305110069954 ) ) ;
#27441=CARTESIAN_POINT ( 'NONE',  ( -1.099225684535947600, 64.54030133659709634, 6.408140936763237150 ) ) ;
#27443=CARTESIAN_POINT ( 'NONE',  ( 22.26659068614895176, 29.72041550158063572, -7.082119434687042414 ) ) ;
#27444=CARTESIAN_POINT ( 'NONE',  ( 7.084665262690076126, 44.10535201082151247, 10.88017736071109987 ) ) ;
#27445=CARTESIAN_POINT ( 'NONE',  ( -0.8801773607111008646, 33.27201867748817676, 2.915334737309923430 ) ) ;
#27446=CARTESIAN_POINT ( 'NONE',  ( 0.1532563361054082862, 66.21726448433413736, 2.638427012816831674 ) ) ;
#27449=CARTESIAN_POINT ( 'NONE',  ( 19.84674366389459266, 48.30059781766745175, 2.638427012816836559 ) ) ;
#27452=CARTESIAN_POINT ( 'NONE',  ( 17.20831665107776587, 22.88393115100078745, 7.208316651077764980 ) ) ;
#27455=CARTESIAN_POINT ( 'NONE',  ( 17.96484262340118221, 16.18868534415483396, -7.964842623401177768 ) ) ;
#27456=CARTESIAN_POINT ( 'NONE',  ( 7.361572987183170547, 22.05059781766745530, 9.846743663894590881 ) ) ;
#27457=CARTESIAN_POINT ( 'NONE',  ( 17.96484262340118221, 56.18868534415484817, -7.964842623401177768 ) ) ;
#27458=CARTESIAN_POINT ( 'NONE',  ( 20.88017736071110519, 15.56368534415483751, 2.639326808657452039E-16 ) ) ;
#27459=CARTESIAN_POINT ( 'NONE',  ( -1.099225684535947600, 63.70696800326376774, -6.408140936763238038 ) ) ;
#27460=CARTESIAN_POINT ( 'NONE',  ( 17.08211943468705130, 28.47041550158063572, 12.26659068614894998 ) ) ;
#27461=SURFACE_STYLE_USAGE ( .BOTH. , #34955 ) ;
#27462=ADVANCED_FACE ( 'NONE', ( #81902 ), #66906, .T. ) ;
#27464=VERTEX_POINT ( 'NONE', #74396 ) ;
#27465=CARTESIAN_POINT ( 'NONE',  ( 3.591859063236763294, 8.290301336597087456, -11.09922568453595026 ) ) ;
#27466=CARTESIAN_POINT ( 'NONE',  ( -0.3289641300568005855, 15.10497603579417181, 5.963430220938281678 ) ) ;
#27467=CARTESIAN_POINT ( 'NONE',  ( 7.084665262690076126, 29.10535201082150181, 10.88017736071109987 ) ) ;
#27470=ORIENTED_EDGE ( 'NONE', *, *, #45376, .F. ) ;
#27471=CARTESIAN_POINT ( 'NONE',  ( 17.20831665107776587, 17.88393115100078745, 7.208316651077764980 ) ) ;
#27472=CARTESIAN_POINT ( 'NONE',  ( 10.00000000000000000, 9.758931151000785675, -9.846743663894594434 ) ) ;
#27473=CARTESIAN_POINT ( 'NONE',  ( 12.63842701281683034, 17.46726448433411250, 9.846743663894596210 ) ) ;
#27474=CARTESIAN_POINT ( 'NONE',  ( 1.472469842513823179, 16.42559781766745175, 4.923371831947296329 ) ) ;
#27475=CARTESIAN_POINT ( 'NONE',  ( 1.472469842513823179, 0.5922644843341181575, -4.923371831947296329 ) ) ;
#27477=CARTESIAN_POINT ( 'NONE',  ( 17.96484262340118221, 66.18868534415483396, -7.964842623401177768 ) ) ;
#27478=DIRECTION ( 'NONE',  ( -1.000000000000000000, 0.000000000000000000, 0.000000000000000000 ) ) ;
#27479=CARTESIAN_POINT ( 'NONE',  ( 0.1532563361054100626, 0.8005978176674514168, -2.638427012816831230 ) ) ;
#27480=CARTESIAN_POINT ( 'NONE',  ( 7.361572987183170547, 17.05059781766745530, 9.846743663894590881 ) ) ;
#27484=CARTESIAN_POINT ( 'NONE',  ( 18.52753015748617571, 63.09226448433412315, 4.923371831947298993 ) ) ;
#27485=ORIENTED_EDGE ( 'NONE', *, *, #48131, .F. ) ;
#27486=CARTESIAN_POINT ( 'NONE',  ( -4.164238869374098151, 21.59541550158063217, -3.795296366450310543 ) ) ;
#27489=CARTESIAN_POINT ( 'NONE',  ( 6.204703633549690345, 20.76208216824730357, -14.16423886937410259 ) ) ;
#27490=CARTESIAN_POINT ( 'NONE',  ( 10.00000000000000000, 35.55374883491396787, -14.16423886937410082 ) ) ;
#27491=( NAMED_UNIT ( * ) PLANE_ANGLE_UNIT ( ) SI_UNIT ( $, .RADIAN. ) );
#27492=CARTESIAN_POINT ( 'NONE',  ( 20.36894250292379382, 3.678748834913967869, 10.36894250292379205 ) ) ;
#27493=CARTESIAN_POINT ( 'NONE',  ( 12.91533473730993009, 66.60535201082150536, -10.88017736071109987 ) ) ;
#27494=CARTESIAN_POINT ( 'NONE',  ( 10.00000000000000178, 29.31368534415483751, 10.88017736071110342 ) ) ;
#27496=CARTESIAN_POINT ( 'NONE',  ( 14.92337183194729988, 19.34226448433411960, -8.527530157486177487 ) ) ;
#27497=CARTESIAN_POINT ( 'NONE',  ( 2.035157376598822676, 57.43868534415484106, -7.964842623401177768 ) ) ;
#27498=CARTESIAN_POINT ( 'NONE',  ( 12.63842701281683034, 32.46726448433412315, 9.846743663894596210 ) ) ;
#27499=CARTESIAN_POINT ( 'NONE',  ( 20.88017736071110519, 15.56368534415483751, 2.639326808657452039E-16 ) ) ;
#27500=CARTESIAN_POINT ( 'NONE',  ( 10.00000000000000000, 47.87363466993042493, -12.81628187352647608 ) ) ;
#27501=CARTESIAN_POINT ( 'NONE',  ( 5.076628168052703671, 51.84226448433412315, 8.527530157486179263 ) ) ;
#27502=CARTESIAN_POINT ( 'NONE',  ( 13.43411237798106583, 27.66530133659708568, -12.81628187352647252 ) ) ;
#27504=( GEOMETRIC_REPRESENTATION_CONTEXT ( 3 ) GLOBAL_UNCERTAINTY_ASSIGNED_CONTEXT ( ( #64176 ) ) GLOBAL_UNIT_ASSIGNED_CONTEXT ( ( #83414, #2402, #17872 ) ) REPRESENTATION_CONTEXT ( 'NONE', 'WORKASPACE' ) );
#27505=CARTESIAN_POINT ( 'NONE',  ( 12.63842701281683034, 37.46726448433411605, 9.846743663894596210 ) ) ;
#27506=CARTESIAN_POINT ( 'NONE',  ( 20.36894250292379738, 9.928748834913966093, -10.36894250292379027 ) ) ;
#27507=ORIENTED_EDGE ( 'NONE', *, *, #83340, .F. ) ;
#27509=CARTESIAN_POINT ( 'NONE',  ( 10.00000000000000178, 54.31368534415484106, 10.88017736071110342 ) ) ;
#27510=CARTESIAN_POINT ( 'NONE',  ( 7.084665262690076126, 57.02201867748817676, -10.88017736071110164 ) ) ;
#27511=CARTESIAN_POINT ( 'NONE',  ( -2.266590686148945544, 42.22041550158063217, 7.082119434687048631 ) ) ;
#27512=COLOUR_RGB ( '', 0.09019608, 0.27058824, 0.51372549) ;
#27513=CARTESIAN_POINT ( 'NONE',  ( 2.791683348922237240, 50.38393115100078035, -7.208316651077763204 ) ) ;
#27514=COLOUR_RGB ( '', 0.40784314, 0.44705882, 0.49803922) ;
#27516=CARTESIAN_POINT ( 'NONE',  ( -0.8801773607111009756, 43.06368534415484106, 1.068504757029289695E-15 ) ) ;
#27519=CARTESIAN_POINT ( 'NONE',  ( 1.472469842513823179, 51.42559781766745886, 4.923371831947296329 ) ) ;
#27522=CARTESIAN_POINT ( 'NONE',  ( 2.035157376598824452, 68.68868534415484817, 7.964842623401179544 ) ) ;
#27524=EDGE_CURVE ( 'NONE', #45856, #13800, #65911, .T. ) ;
#27525=CARTESIAN_POINT ( 'NONE',  ( 2.035157376598824452, 8.688685344154839285, 7.964842623401179544 ) ) ;
#27526=CARTESIAN_POINT ( 'NONE',  ( 19.89103541497710737, 65.66234555792573246, -6.479102184480822757 ) ) ;
#27528=CARTESIAN_POINT ( 'NONE',  ( 19.42250999205614193, 65.14701867748817676, 5.440088680355555262 ) ) ;
#27529=CARTESIAN_POINT ( 'NONE',  ( 5.076628168052704559, 5.175597817667451750, -8.527530157486179263 ) ) ;
#27531=CARTESIAN_POINT ( 'NONE',  ( 19.84674366389459621, 33.50893115100078745, 7.409399052514197653E-17 ) ) ;
#27532=CARTESIAN_POINT ( 'NONE',  ( 17.96484262340118221, 21.18868534415483396, -7.964842623401177768 ) ) ;
#27533=CARTESIAN_POINT ( 'NONE',  ( 19.38216949554541557, 12.24863466993041961, -9.382169495545420901 ) ) ;
#27534=CARTESIAN_POINT ( 'NONE',  ( 17.96484262340118221, 39.93868534415484106, 7.964842623401181321 ) ) ;
#27535=CARTESIAN_POINT ( 'NONE',  ( 2.599899806584774264, 0.4361964623231012195, -6.495912400107028084 ) ) ;
#27537=CARTESIAN_POINT ( 'NONE',  ( -1.099225684535947600, 34.54030133659708923, 6.408140936763237150 ) ) ;
#27539=CARTESIAN_POINT ( 'NONE',  ( -0.8801773607110991993, 67.85535201082151957, -2.915334737309923874 ) ) ;
#27540=CARTESIAN_POINT ( 'NONE',  ( 22.81628187352647785, 21.41530133659708923, 3.434112377981063169 ) ) ;
#27542=CARTESIAN_POINT ( 'NONE',  ( 19.42250999205614193, 30.14701867748817321, 5.440088680355555262 ) ) ;
#27543=CARTESIAN_POINT ( 'NONE',  ( -0.3689425029237898834, 61.17874883491396076, -10.36894250292378850 ) ) ;
#27544=CARTESIAN_POINT ( 'NONE',  ( 19.84674366389459621, 53.50893115100078745, 7.409399052514197653E-17 ) ) ;
#27545=CARTESIAN_POINT ( 'NONE',  ( 7.361572987183170547, 2.050597817667451750, 9.846743663894590881 ) ) ;
#27546=CARTESIAN_POINT ( 'NONE',  ( 4.559911319644449179, 63.89701867748817676, 9.422509992056141925 ) ) ;
#27548=CARTESIAN_POINT ( 'NONE',  ( 10.00000000000000178, 28.05374883491396787, 14.16423886937410082 ) ) ;
#27554=CARTESIAN_POINT ( 'NONE',  ( 2.917880565312948704, 67.63708216824730357, 12.26659068614894643 ) ) ;
#27555=CARTESIAN_POINT ( 'NONE',  ( -4.164238869374099039, 51.80374883491396787, 8.674139862899312516E-16 ) ) ;
#27557=CARTESIAN_POINT ( 'NONE',  ( 0.1532563361054082862, 31.21726448433412315, 2.638427012816831674 ) ) ;
#27560=CARTESIAN_POINT ( 'NONE',  ( -0.8801773607111008646, 68.27201867748817676, 2.915334737309923430 ) ) ;
#27561=CARTESIAN_POINT ( 'NONE',  ( 6.204703633549690345, 42.84541550158063217, 14.16423886937410082 ) ) ;
#27562=EDGE_CURVE ( 'NONE', #29895, #76186, #31068, .T. ) ;
#27564=CARTESIAN_POINT ( 'NONE',  ( 17.20831665107776587, 4.133931151000785675, -7.208316651077762316 ) ) ;
#27565=CARTESIAN_POINT ( 'NONE',  ( -32.19000000000001194, 93.50000000000000000, 9.500000000000000000 ) ) ;
#27569=VERTEX_POINT ( 'NONE', #95441 ) ;
#27571=ORIENTED_EDGE ( 'NONE', *, *, #48371, .T. ) ;
#27572=CARTESIAN_POINT ( 'NONE',  ( 15.44008868035555793, 21.39701867748817321, -9.422509992056140149 ) ) ;
#27573=CARTESIAN_POINT ( 'NONE',  ( 17.96484262340118221, 19.93868534415484106, 7.964842623401181321 ) ) ;
#27574=CARTESIAN_POINT ( 'NONE',  ( 18.52753015748618282, 48.92559781766745886, -4.923371831947291888 ) ) ;
#27575=CARTESIAN_POINT ( 'NONE',  ( 6.565887622018943937, 13.08196800326374998, -12.81628187352647608 ) ) ;
#27577=CARTESIAN_POINT ( 'NONE',  ( 19.84674366389459621, 43.50893115100078745, 7.409399052514197653E-17 ) ) ;
#27579=CARTESIAN_POINT ( 'NONE',  ( 10.00000000000000178, 15.37363466993042138, 12.81628187352647608 ) ) ;
#27582=CARTESIAN_POINT ( 'NONE',  ( 5.076628168052703671, 36.84226448433412315, 8.527530157486179263 ) ) ;
#27584=CARTESIAN_POINT ( 'NONE',  ( -2.266590686148945544, 56.38708216824731068, -7.082119434687050408 ) ) ;
#27585=ORIENTED_EDGE ( 'NONE', *, *, #262, .T. ) ;
#27587=CARTESIAN_POINT ( 'NONE',  ( -4.164238869374099927, 67.01208216824728936, 3.795296366450308767 ) ) ;
#27588=ORIENTED_EDGE ( 'NONE', *, *, #83791, .F. ) ;
#27589=CARTESIAN_POINT ( 'NONE',  ( -0.8801773607111009756, 48.06368534415484817, 1.068504757029289695E-15 ) ) ;
#27590=CARTESIAN_POINT ( 'NONE',  ( 10.00000000000000000, 41.81368534415484106, -10.88017736071110342 ) ) ;
#27591=CARTESIAN_POINT ( 'NONE',  ( 12.91533473730992121, 49.52201867748817676, 10.88017736071110164 ) ) ;
#27594=CARTESIAN_POINT ( 'NONE',  ( 10.00000000000000000, 36.81368534415484106, -10.88017736071110342 ) ) ;
#27597=CARTESIAN_POINT ( 'NONE',  ( 19.72487221294570858, 7.802231764288317883, -6.499999999999999112 ) ) ;
#27599=CARTESIAN_POINT ( 'NONE',  ( 14.92337183194729988, 24.34226448433411960, -8.527530157486177487 ) ) ;
#27601=CARTESIAN_POINT ( 'NONE',  ( 2.791683348922240793, 61.63393115100079456, 7.208316651077764092 ) ) ;
#27607=CARTESIAN_POINT ( 'NONE',  ( 12.63842701281683922, 64.55059781766745175, -9.846743663894590881 ) ) ;
#27608=CARTESIAN_POINT ( 'NONE',  ( -2.266590686148945544, 57.22041550158063217, 7.082119434687048631 ) ) ;
#27612=CARTESIAN_POINT ( 'NONE',  ( 0.1532563361054083140, 36.00893115100078745, 1.131784320476157264E-15 ) ) ;
#27613=CARTESIAN_POINT ( 'NONE',  ( -2.816281873526471635, 63.91530133659708923, -3.434112377981056508 ) ) ;
#27614=CARTESIAN_POINT ( 'NONE',  ( 19.38216949554541557, 2.248634669930420049, -9.382169495545420901 ) ) ;
#27615=CARTESIAN_POINT ( 'NONE',  ( 12.63842701281683034, 7.467264484334118713, 9.846743663894596210 ) ) ;
#27617=CARTESIAN_POINT ( 'NONE',  ( 5.076628168052703671, 6.842264484334118713, 8.527530157486179263 ) ) ;
#27618=CARTESIAN_POINT ( 'NONE',  ( 0.1532563361054083140, 56.00893115100078745, 1.131784320476157264E-15 ) ) ;
#27619=CARTESIAN_POINT ( 'NONE',  ( 20.00000000000000711, 98.59912998021083297, 4.500000000000000888 ) ) ;
#27620=CIRCLE ( 'NONE', #83529, 18.53834841531100608 ) ;
#27621=B_SPLINE_CURVE_WITH_KNOTS ( 'NONE', 3,
 ( #90198, #88721, #42252, #49729 ),
 .UNSPECIFIED., .F., .F.,
 ( 4, 4 ),
 ( 0.000000000000000000, 0.002657014572710868390 ),
 .UNSPECIFIED. ) ;
#27623=CARTESIAN_POINT ( 'NONE',  ( 0.5774900079438590739, 7.647018677488171434, -5.440088680355550821 ) ) ;
#27624=CARTESIAN_POINT ( 'NONE',  ( -4.164238869374098151, 11.59541550158063217, -3.795296366450310543 ) ) ;
#27625=CARTESIAN_POINT ( 'NONE',  ( 19.84674366389459266, 13.71726448433411782, -2.638427012816827677 ) ) ;
#27626=CARTESIAN_POINT ( 'NONE',  ( 15.44008868035555260, 49.73035201082150536, 9.422509992056143702 ) ) ;
#27627=CARTESIAN_POINT ( 'NONE',  ( -2.816281873526473856, 24.33196800326375353, 3.434112377981055619 ) ) ;
#27630=CARTESIAN_POINT ( 'NONE',  ( 17.39651004071838969, 59.08210964143329846, -6.500000000000027534 ) ) ;
#27632=CARTESIAN_POINT ( 'NONE',  ( 10.00000000000000000, 7.873634669930421381, -12.81628187352647608 ) ) ;
#27633=CARTESIAN_POINT ( 'NONE',  ( 10.00000000000000000, 59.75893115100078745, -9.846743663894594434 ) ) ;
#27634=CARTESIAN_POINT ( 'NONE',  ( 7.361572987183169658, 14.96726448433411960, -9.846743663894592657 ) ) ;
#27636=CARTESIAN_POINT ( 'NONE',  ( 19.38216949554541202, 15.99863466993042138, 9.382169495545424454 ) ) ;
#27638=CARTESIAN_POINT ( 'NONE',  ( 10.00000000000000000, 31.81368534415483751, -10.88017736071110342 ) ) ;
#27640=CARTESIAN_POINT ( 'NONE',  ( 6.204703633549690345, 47.84541550158064638, 14.16423886937410082 ) ) ;
#27643=CARTESIAN_POINT ( 'NONE',  ( 2.035157376598824452, 33.68868534415484106, 7.964842623401179544 ) ) ;
#27644=CARTESIAN_POINT ( 'NONE',  ( 2.791683348922240793, 56.63393115100078035, 7.208316651077764092 ) ) ;
#27645=CARTESIAN_POINT ( 'NONE',  ( 2.035157376598822676, 57.43868534415484106, -7.964842623401177768 ) ) ;
#27646=CARTESIAN_POINT ( 'NONE',  ( 20.36894250292379382, 28.67874883491396787, 10.36894250292379205 ) ) ;
#27649=CARTESIAN_POINT ( 'NONE',  ( 14.92337183194729988, 39.34226448433412315, -8.527530157486177487 ) ) ;
#27650=CARTESIAN_POINT ( 'NONE',  ( 0.6178305044545818747, 58.49863466993042493, -9.382169495545419124 ) ) ;
#27651=CARTESIAN_POINT ( 'NONE',  ( 22.81628187352647785, 1.623634669930420271, 6.195893100308588602E-16 ) ) ;
#27653=CARTESIAN_POINT ( 'NONE',  ( -0.8801773607111009756, 23.06368534415484106, 1.068504757029289695E-15 ) ) ;
#27654=STYLED_ITEM ( 'NONE', ( #54570 ), #93062 ) ;
#27655=FACE_OUTER_BOUND ( 'NONE', #89145, .T. ) ;
#27656=CARTESIAN_POINT ( 'NONE',  ( 19.42250999205614548, 20.98035201082150891, -5.440088680355545492 ) ) ;
#27657=CARTESIAN_POINT ( 'NONE',  ( -4.164238869374099927, 27.01208216824730357, 3.795296366450308767 ) ) ;
#27658=CARTESIAN_POINT ( 'NONE',  ( 18.52753015748617571, 18.09226448433411960, 4.923371831947298993 ) ) ;
#27659=CARTESIAN_POINT ( 'NONE',  ( 0.1532563361054082862, 61.21726448433412315, 2.638427012816831674 ) ) ;
#27660=CARTESIAN_POINT ( 'NONE',  ( 4.559911319644449179, 28.89701867748817321, 9.422509992056141925 ) ) ;
#27661=AXIS2_PLACEMENT_3D ( 'NONE', #59324, #44324, #74825 ) ;
#27662=CYLINDRICAL_SURFACE ( 'NONE', #71906, 2.999999999999999556 ) ;
#27665=B_SPLINE_CURVE_WITH_KNOTS ( 'NONE', 3,
 ( #59593, #90583, #44596, #90091 ),
 .UNSPECIFIED., .F., .F.,
 ( 4, 4 ),
 ( 0.000000000000000000, 0.002562518741975322069 ),
 .UNSPECIFIED. ) ;
#27667=CARTESIAN_POINT ( 'NONE',  ( 5.076628168052703671, 46.84226448433412315, 8.527530157486179263 ) ) ;
#27669=ORIENTED_EDGE ( 'NONE', *, *, #70155, .T. ) ;
#27671=CARTESIAN_POINT ( 'NONE',  ( 20.36894250292379382, 3.678748834913967869, 10.36894250292379205 ) ) ;
#27672=CARTESIAN_POINT ( 'NONE',  ( 22.26659068614894466, 3.887082168247300906, 7.082119434687054849 ) ) ;
#27674=CARTESIAN_POINT ( 'NONE',  ( -0.8801773607111008646, 43.27201867748817676, 2.915334737309923430 ) ) ;
#27675=CARTESIAN_POINT ( 'NONE',  ( 10.00000000000000178, 58.05374883491397497, 14.16423886937410082 ) ) ;
#27676=CARTESIAN_POINT ( 'NONE',  ( -1.099225684535947600, 3.706968003263753531, -6.408140936763238038 ) ) ;
#27677=CARTESIAN_POINT ( 'NONE',  ( 18.52753015748617571, 33.09226448433411605, 4.923371831947298993 ) ) ;
#27679=CARTESIAN_POINT ( 'NONE',  ( 15.44008868035555793, 36.39701867748816966, -9.422509992056140149 ) ) ;
#27680=CARTESIAN_POINT ( 'NONE',  ( 3.591859063236763294, 8.290301336597087456, -11.09922568453595026 ) ) ;
#27681=( LENGTH_UNIT ( ) NAMED_UNIT ( * ) SI_UNIT ( .MILLI., .METRE. ) );
#27682=CARTESIAN_POINT ( 'NONE',  ( 10.00000000000000000, 55.55374883491396787, -14.16423886937410082 ) ) ;
#27683=CARTESIAN_POINT ( 'NONE',  ( -0.8801773607110991993, 12.85535201082150358, -2.915334737309923874 ) ) ;
#27684=CARTESIAN_POINT ( 'NONE',  ( 18.04007052943772749, 38.01528370094808196, 5.767676674365840306 ) ) ;
#27685=CARTESIAN_POINT ( 'NONE',  ( -32.19000000000001194, 93.50000000000000000, -10.09898361729590199 ) ) ;
#27689=CARTESIAN_POINT ( 'NONE',  ( 20.15039907845753220, 20.60158574516643171, -6.262539305110077947 ) ) ;
#27692=CARTESIAN_POINT ( 'NONE',  ( 6.204703633549690345, 52.84541550158062506, 14.16423886937410082 ) ) ;
#27693=CARTESIAN_POINT ( 'NONE',  ( 10.00000000000000000, 49.75893115100078745, -9.846743663894594434 ) ) ;
#27694=CARTESIAN_POINT ( 'NONE',  ( -0.8801773607111008646, 53.27201867748816966, 2.915334737309923430 ) ) ;
#27697=CARTESIAN_POINT ( 'NONE',  ( 19.42250999205614548, 50.98035201082151247, -5.440088680355545492 ) ) ;
#27698=VECTOR ( 'NONE', #11376, 1000.000000000000000 ) ;
#27701=CARTESIAN_POINT ( 'NONE',  ( 24.16423886937409904, 19.09541550158063927, 3.795296366450317205 ) ) ;
#27702=CARTESIAN_POINT ( 'NONE',  ( 10.00000000000000178, 30.37363466993042138, 12.81628187352647608 ) ) ;
#27703=ORIENTED_EDGE ( 'NONE', *, *, #32410, .T. ) ;
#27704=CARTESIAN_POINT ( 'NONE',  ( 19.38216949554541202, 50.99863466993042493, 9.382169495545424454 ) ) ;
#27706=CARTESIAN_POINT ( 'NONE',  ( 12.91533473730993009, 21.60535201082150536, -10.88017736071109987 ) ) ;
#27707=CARTESIAN_POINT ( 'NONE',  ( 14.92337183194729633, 42.67559781766745886, 8.527530157486181039 ) ) ;
#27708=CARTESIAN_POINT ( 'NONE',  ( 0.5774900079438607392, 8.480352010821505360, 5.440088680355550821 ) ) ;
#27709=CARTESIAN_POINT ( 'NONE',  ( 13.43411237798105340, 50.58196800326375353, 12.81628187352647963 ) ) ;
#27711=CARTESIAN_POINT ( 'NONE',  ( 18.52753015748617571, 38.09226448433412315, 4.923371831947298993 ) ) ;
#27719=CARTESIAN_POINT ( 'NONE',  ( 12.63842701281683034, 17.46726448433411250, 9.846743663894596210 ) ) ;
#27720=CARTESIAN_POINT ( 'NONE',  ( 19.38216949554541557, 22.24863466993041428, -9.382169495545420901 ) ) ;
#27723=CARTESIAN_POINT ( 'NONE',  ( 14.92337183194729633, 57.67559781766745886, 8.527530157486181039 ) ) ;
#27725=CARTESIAN_POINT ( 'NONE',  ( -0.3689425029237881626, 22.42874883491397142, 10.36894250292379027 ) ) ;
#27726=CARTESIAN_POINT ( 'NONE',  ( 18.52753015748618282, 38.92559781766745175, -4.923371831947291888 ) ) ;
#27727=CARTESIAN_POINT ( 'NONE',  ( -2.816281873526473856, 44.33196800326375353, 3.434112377981055619 ) ) ;
#27729=CARTESIAN_POINT ( 'NONE',  ( 2.035157376598824452, 58.68868534415482685, 7.964842623401179544 ) ) ;
#27730=CARTESIAN_POINT ( 'NONE',  ( 3.591859063236761518, 14.95696800326375531, 11.09922568453594849 ) ) ;
#27732=CARTESIAN_POINT ( 'NONE',  ( 5.076628168052703671, 36.84226448433412315, 8.527530157486179263 ) ) ;
#27733=CARTESIAN_POINT ( 'NONE',  ( 2.035157376598822676, 42.43868534415483396, -7.964842623401177768 ) ) ;
#27734=CARTESIAN_POINT ( 'NONE',  ( 13.43411237798106583, 42.66530133659707502, -12.81628187352647252 ) ) ;
#27735=CARTESIAN_POINT ( 'NONE',  ( 14.92337183194729633, 37.67559781766745175, 8.527530157486181039 ) ) ;
#27737=FACE_OUTER_BOUND ( 'NONE', #86153, .T. ) ;
#27738=CARTESIAN_POINT ( 'NONE',  ( 17.96484262340118221, 29.93868534415484106, 7.964842623401181321 ) ) ;
#27740=CARTESIAN_POINT ( 'NONE',  ( 19.42250999205614548, 5.980352010821504471, -5.440088680355545492 ) ) ;
#27741=CARTESIAN_POINT ( 'NONE',  ( 0.1532563361054100626, 50.80059781766745175, -2.638427012816831230 ) ) ;
#27742=CARTESIAN_POINT ( 'NONE',  ( 7.084665262690076126, 34.10535201082151247, 10.88017736071109987 ) ) ;
#27743=CARTESIAN_POINT ( 'NONE',  ( -39.69000000000001194, 92.00000000000000000, -10.09898361729590199 ) ) ;
#27744=CARTESIAN_POINT ( 'NONE',  ( -0.8801773607111008646, 58.27201867748816966, 2.915334737309923430 ) ) ;
#27745=CARTESIAN_POINT ( 'NONE',  ( 12.91533473730993009, 26.60535201082150536, -10.88017736071109987 ) ) ;
#27746=CARTESIAN_POINT ( 'NONE',  ( 0.000000000000000000, 78.20247855283322735, -8.810553791401492418 ) ) ;
#27747=( LENGTH_UNIT ( ) NAMED_UNIT ( * ) SI_UNIT ( .MILLI., .METRE. ) );
#27748=CARTESIAN_POINT ( 'NONE',  ( 5.076628168052703671, 26.84226448433411960, 8.527530157486179263 ) ) ;
#27750=CARTESIAN_POINT ( 'NONE',  ( 12.63842701281683034, 47.46726448433412315, 9.846743663894596210 ) ) ;
#27751=CARTESIAN_POINT ( 'NONE',  ( 24.16423886937410614, 59.30374883491397497, 8.672049930838204340E-16 ) ) ;
#27754=CARTESIAN_POINT ( 'NONE',  ( 24.16423886937410614, 4.512082168247300906, -3.795296366450302550 ) ) ;
#27756=CARTESIAN_POINT ( 'NONE',  ( 13.79529636645030344, 33.26208216824730357, 14.16423886937410614 ) ) ;
#27757=CARTESIAN_POINT ( 'NONE',  ( -2.816281873526473856, 4.331968003263754419, 3.434112377981055619 ) ) ;
#27760=CARTESIAN_POINT ( 'NONE',  ( 20.88017736071110875, 10.77201867748817143, -2.915334737309920765 ) ) ;
#27761=EDGE_CURVE ( 'NONE', #74710, #63139, #66848, .T. ) ;
#27762=CARTESIAN_POINT ( 'NONE',  ( 0.1532563361054100626, 40.80059781766745886, -2.638427012816831230 ) ) ;
#27763=DIRECTION ( 'NONE',  ( -1.000000000000000000, 0.000000000000000000, 0.000000000000000000 ) ) ;
#27765=CARTESIAN_POINT ( 'NONE',  ( 0.5774900079438607392, 53.48035201082151247, 5.440088680355550821 ) ) ;
#27767=CARTESIAN_POINT ( 'NONE',  ( 3.591859063236763294, 63.29030133659708923, -11.09922568453595026 ) ) ;
#27768=CARTESIAN_POINT ( 'NONE',  ( 10.00000000000000178, 30.37363466993042138, 12.81628187352647608 ) ) ;
#27769=CARTESIAN_POINT ( 'NONE',  ( 10.00000000000000000, 34.75893115100078745, -9.846743663894594434 ) ) ;
#27773=CARTESIAN_POINT ( 'NONE',  ( 0.5774900079438607392, 3.480352010821504916, 5.440088680355550821 ) ) ;
#27774=CARTESIAN_POINT ( 'NONE',  ( 7.084665262690076126, 9.105352010821503583, 10.88017736071109987 ) ) ;
#27775=CARTESIAN_POINT ( 'NONE',  ( -0.3689425029237881626, 47.42874883491396787, 10.36894250292379027 ) ) ;
#27776=CARTESIAN_POINT ( 'NONE',  ( 4.559911319644449179, 28.89701867748817321, 9.422509992056141925 ) ) ;
#27777=CARTESIAN_POINT ( 'NONE',  ( 0.5774900079438590739, 57.64701867748817676, -5.440088680355550821 ) ) ;
#27780=CARTESIAN_POINT ( 'NONE',  ( 2.791683348922237240, 20.38393115100078745, -7.208316651077763204 ) ) ;
#27781=LINE ( 'NONE', #95805, #27415 ) ;
#27782=CARTESIAN_POINT ( 'NONE',  ( 5.076628168052704559, 5.175597817667451750, -8.527530157486179263 ) ) ;
#27783=CARTESIAN_POINT ( 'NONE',  ( 5.076628168052704559, 40.17559781766745175, -8.527530157486179263 ) ) ;
#27784=CARTESIAN_POINT ( 'NONE',  ( 10.00000000000000178, 0.3736346699304200492, 12.81628187352647608 ) ) ;
#27785=CARTESIAN_POINT ( 'NONE',  ( 10.00000000000000000, 41.81368534415484106, -10.88017736071110342 ) ) ;
#27787=CARTESIAN_POINT ( 'NONE',  ( -2.816281873526473856, 44.33196800326375353, 3.434112377981055619 ) ) ;
#27788=DIRECTION ( 'NONE',  ( 0.8320502943378436100, -0.5547001962252291474, 0.000000000000000000 ) ) ;
#27791=CARTESIAN_POINT ( 'NONE',  ( 2.035157376598822676, 62.43868534415483396, -7.964842623401177768 ) ) ;
#27792=CARTESIAN_POINT ( 'NONE',  ( 6.565887622018943937, 48.08196800326375353, -12.81628187352647608 ) ) ;
#27793=CARTESIAN_POINT ( 'NONE',  ( 24.16423886937410614, 59.30374883491397497, 8.672049930838204340E-16 ) ) ;
#27794=CARTESIAN_POINT ( 'NONE',  ( 7.361572987183169658, 39.96726448433411605, -9.846743663894592657 ) ) ;
#27797=CARTESIAN_POINT ( 'NONE',  ( 24.16423886937410614, 34.30374883491396787, 8.672049930838204340E-16 ) ) ;
#27798=CARTESIAN_POINT ( 'NONE',  ( 5.076628168052704559, 45.17559781766745175, -8.527530157486179263 ) ) ;
#27800=CARTESIAN_POINT ( 'NONE',  ( -0.8801773607110991993, 32.85535201082151247, -2.915334737309923874 ) ) ;
#27803=CARTESIAN_POINT ( 'NONE',  ( 4.559911319644449179, 53.89701867748817676, 9.422509992056141925 ) ) ;
#27806=CARTESIAN_POINT ( 'NONE',  ( 22.81628187352647785, 41.62363466993042493, 6.195893100308588602E-16 ) ) ;
#27808=CARTESIAN_POINT ( 'NONE',  ( 10.00000000000000178, 64.31368534415483396, 10.88017736071110342 ) ) ;
#27809=VERTEX_POINT ( 'NONE', #40231 ) ;
#27810=CARTESIAN_POINT ( 'NONE',  ( -4.164238869374098151, 1.595415501580634388, -3.795296366450310543 ) ) ;
#27815=CARTESIAN_POINT ( 'NONE',  ( -0.8801773607110991993, 17.85535201082150536, -2.915334737309923874 ) ) ;
#27816=CARTESIAN_POINT ( 'NONE',  ( 20.88017736071110164, 60.35535201082150536, 2.915334737309930979 ) ) ;
#27817=CARTESIAN_POINT ( 'NONE',  ( -4.164238869374099927, 22.01208216824730357, 3.795296366450308767 ) ) ;
#27818=CARTESIAN_POINT ( 'NONE',  ( -0.8801773607110991993, 17.85535201082150536, -2.915334737309923874 ) ) ;
#27819=CARTESIAN_POINT ( 'NONE',  ( 19.84674366389459621, 63.50893115100078745, 7.409399052514197653E-17 ) ) ;
#27821=CARTESIAN_POINT ( 'NONE',  ( 14.92337183194729633, 57.67559781766745886, 8.527530157486181039 ) ) ;
#27823=CARTESIAN_POINT ( 'NONE',  ( 15.44008868035555260, 54.73035201082150536, 9.422509992056143702 ) ) ;
#27825=CARTESIAN_POINT ( 'NONE',  ( 19.38216949554541557, 37.24863466993041783, -9.382169495545420901 ) ) ;
#27826=CARTESIAN_POINT ( 'NONE',  ( 20.88017736071110875, 10.77201867748817143, -2.915334737309920765 ) ) ;
#27828=CARTESIAN_POINT ( 'NONE',  ( 10.00000000000000000, -0.2410688489992152128, -9.846743663894594434 ) ) ;
#27829=CARTESIAN_POINT ( 'NONE',  ( 15.44008868035555793, 16.39701867748817321, -9.422509992056140149 ) ) ;
#27833=CARTESIAN_POINT ( 'NONE',  ( 6.565887622018943937, 60.16530133659707502, 12.81628187352647430 ) ) ;
#27834=CARTESIAN_POINT ( 'NONE',  ( 20.88017736071110875, 25.77201867748816966, -2.915334737309920765 ) ) ;
#27835=CARTESIAN_POINT ( 'NONE',  ( -46.94000000000001194, 102.4632489371167452, -6.394394627233738859 ) ) ;
#27836=CARTESIAN_POINT ( 'NONE',  ( 16.40814093676324603, 37.45696800326376064, -11.09922568453594671 ) ) ;
#27837=CARTESIAN_POINT ( 'NONE',  ( -0.8801773607110991993, 47.85535201082150536, -2.915334737309923874 ) ) ;
#27838=EDGE_LOOP ( 'NONE', ( #51547, #35114, #65796, #8071 ) ) ;
#27839=CARTESIAN_POINT ( 'NONE',  ( -0.1503990784575242878, 49.24884699246889141, -6.262539305110083276 ) ) ;
#27840=CARTESIAN_POINT ( 'NONE',  ( 14.92337183194729988, 9.342264484334119601, -8.527530157486177487 ) ) ;
#27841=CARTESIAN_POINT ( 'NONE',  ( 13.43411237798105340, 0.5819680032637533085, 12.81628187352647963 ) ) ;
#27843=CARTESIAN_POINT ( 'NONE',  ( 17.20831665107776587, 49.13393115100078745, -7.208316651077762316 ) ) ;
#27844=CARTESIAN_POINT ( 'NONE',  ( 19.42250999205614548, 25.98035201082150891, -5.440088680355545492 ) ) ;
#27845=CARTESIAN_POINT ( 'NONE',  ( 19.84674366389459266, 53.71726448433411605, -2.638427012816827677 ) ) ;
#27848=CARTESIAN_POINT ( 'NONE',  ( 0.1532563361054100626, 5.800597817667452638, -2.638427012816831230 ) ) ;
#27849=CARTESIAN_POINT ( 'NONE',  ( 0.1532563361054082862, 56.21726448433411605, 2.638427012816831674 ) ) ;
#27850=ORIENTED_EDGE ( 'NONE', *, *, #3759, .T. ) ;
#27852=CARTESIAN_POINT ( 'NONE',  ( 13.43411237798106583, 32.66530133659708213, -12.81628187352647252 ) ) ;
#27853=CARTESIAN_POINT ( 'NONE',  ( 19.84674366389459266, 33.71726448433410894, -2.638427012816827677 ) ) ;
#27855=CARTESIAN_POINT ( 'NONE',  ( 0.5774900079438607392, 58.48035201082151247, 5.440088680355550821 ) ) ;
#27856=CARTESIAN_POINT ( 'NONE',  ( 13.79529636645031943, 60.34541550158063927, -14.16423886937409904 ) ) ;
#27857=CARTESIAN_POINT ( 'NONE',  ( 19.84674366389459621, 28.50893115100078745, 7.409399052514197653E-17 ) ) ;
#27859=( GEOMETRIC_REPRESENTATION_CONTEXT ( 3 ) GLOBAL_UNCERTAINTY_ASSIGNED_CONTEXT ( ( #3533 ) ) GLOBAL_UNIT_ASSIGNED_CONTEXT ( ( #4520, #27491, #20495 ) ) REPRESENTATION_CONTEXT ( 'NONE', 'WORKASPACE' ) );
#27860=CARTESIAN_POINT ( 'NONE',  ( -0.1503990784575247319, 47.22266099184918886, -6.262539305110083276 ) ) ;
#27861=AXIS2_PLACEMENT_3D ( 'NONE', #64521, #95027, #26536 ) ;
#27862=CARTESIAN_POINT ( 'NONE',  ( -2.266590686148945544, 51.38708216824730357, -7.082119434687050408 ) ) ;
#27864=CARTESIAN_POINT ( 'NONE',  ( 20.88017736071110519, 15.56368534415483751, 2.639326808657452039E-16 ) ) ;
#27865=CARTESIAN_POINT ( 'NONE',  ( -4.164238869374099927, 37.01208216824731068, 3.795296366450308767 ) ) ;
#27866=CARTESIAN_POINT ( 'NONE',  ( 13.79529636645031943, 55.34541550158062506, -14.16423886937409904 ) ) ;
#27868=CARTESIAN_POINT ( 'NONE',  ( -45.94000000000000483, 92.50000000000000000, -9.500000000000000000 ) ) ;
#27869=AXIS2_PLACEMENT_3D ( 'NONE', #67342, #23836, #37850 ) ;
#27870=CARTESIAN_POINT ( 'NONE',  ( 0.1532563361054083140, 6.008931151000784787, 1.131784320476157264E-15 ) ) ;
#27871=CARTESIAN_POINT ( 'NONE',  ( 10.00000000000000000, 2.873634669930420049, -12.81628187352647608 ) ) ;
#27872=CARTESIAN_POINT ( 'NONE',  ( 18.50749283717776805, 14.69955587570481192, 6.500000000000000888 ) ) ;
#27873=CARTESIAN_POINT ( 'NONE',  ( -0.8801773607111008646, 53.27201867748816966, 2.915334737309923430 ) ) ;
#27875=CARTESIAN_POINT ( 'NONE',  ( 18.52753015748618282, 48.92559781766745886, -4.923371831947291888 ) ) ;
#27879=CARTESIAN_POINT ( 'NONE',  ( 6.204703633549690345, 45.76208216824729647, -14.16423886937410259 ) ) ;
#27883=DIRECTION ( 'NONE',  ( 0.000000000000000000, 1.000000000000000000, -0.000000000000000000 ) ) ;
#27884=CARTESIAN_POINT ( 'NONE',  ( -0.8801773607110991993, 17.85535201082150536, -2.915334737309923874 ) ) ;
#27885=CARTESIAN_POINT ( 'NONE',  ( 22.81628187352647785, 41.62363466993042493, 6.195893100308588602E-16 ) ) ;
#27886=LINE ( 'NONE', #26410, #22518 ) ;
#27887=CARTESIAN_POINT ( 'NONE',  ( 22.81628187352647785, 21.41530133659708923, 3.434112377981063169 ) ) ;
#27888=CARTESIAN_POINT ( 'NONE',  ( 19.38216949554541557, 62.24863466993041072, -9.382169495545420901 ) ) ;
#27892=CARTESIAN_POINT ( 'NONE',  ( -0.3689425029237898834, 1.178748834913967869, -10.36894250292378850 ) ) ;
#27894=CARTESIAN_POINT ( 'NONE',  ( 0.5774900079438607392, 23.48035201082150536, 5.440088680355550821 ) ) ;
#27897=CARTESIAN_POINT ( 'NONE',  ( 12.91533473730993009, 36.60535201082151247, -10.88017736071109987 ) ) ;
#27898=CARTESIAN_POINT ( 'NONE',  ( 19.42250999205614193, 50.14701867748817676, 5.440088680355555262 ) ) ;
#27899=CARTESIAN_POINT ( 'NONE',  ( -1.099225684535947600, 8.706968003263753531, -6.408140936763238038 ) ) ;
#27900=CARTESIAN_POINT ( 'NONE',  ( -0.1042174387088625198, 48.10736173766201773, 6.337391062633416894 ) ) ;
#27902=CARTESIAN_POINT ( 'NONE',  ( 10.00000000000000000, 29.75893115100078745, -9.846743663894594434 ) ) ;
#27904=CARTESIAN_POINT ( 'NONE',  ( 0.5774900079438590739, 42.64701867748816966, -5.440088680355550821 ) ) ;
#27905=CARTESIAN_POINT ( 'NONE',  ( -2.816281873526473856, 9.123634669930421381, 9.499525473075851096E-16 ) ) ;
#27906=CARTESIAN_POINT ( 'NONE',  ( 2.791683348922237240, 20.38393115100078745, -7.208316651077763204 ) ) ;
#27907=CARTESIAN_POINT ( 'NONE',  ( 6.565887622018943937, 53.08196800326374643, -12.81628187352647608 ) ) ;
#27908=CARTESIAN_POINT ( 'NONE',  ( 7.361572987183169658, 9.967264484334119601, -9.846743663894592657 ) ) ;
#27912=CARTESIAN_POINT ( 'NONE',  ( 2.035157376598822676, 17.43868534415483751, -7.964842623401177768 ) ) ;
#27913=CARTESIAN_POINT ( 'NONE',  ( 20.15039907845753930, 70.00000000000000000, 6.262539305110068177 ) ) ;
#27914=CARTESIAN_POINT ( 'NONE',  ( 10.00000000000000178, 28.05374883491396787, 14.16423886937410082 ) ) ;
#27915=EDGE_CURVE ( 'NONE', #74651, #89307, #22416, .T. ) ;
#27916=CARTESIAN_POINT ( 'NONE',  ( 14.92337183194729988, 24.34226448433411960, -8.527530157486177487 ) ) ;
#27917=CARTESIAN_POINT ( 'NONE',  ( 0.5774900079438590739, 17.64701867748817321, -5.440088680355550821 ) ) ;
#27918=CARTESIAN_POINT ( 'NONE',  ( 10.00000000000000178, 68.05374883491397497, 14.16423886937410082 ) ) ;
#27921=CARTESIAN_POINT ( 'NONE',  ( 19.42250999205614193, 10.14701867748816966, 5.440088680355555262 ) ) ;
#27922=CARTESIAN_POINT ( 'NONE',  ( 20.88017736071110519, 40.56368534415484106, 2.639326808657452039E-16 ) ) ;
#27924=CARTESIAN_POINT ( 'NONE',  ( 19.42250999205614548, 35.98035201082151247, -5.440088680355545492 ) ) ;
#27925=ORIENTED_EDGE ( 'NONE', *, *, #41663, .F. ) ;
#27926=CARTESIAN_POINT ( 'NONE',  ( 7.361572987183170547, 67.05059781766746596, 9.846743663894590881 ) ) ;
#27927=CARTESIAN_POINT ( 'NONE',  ( 10.00000000000000000, 31.81368534415483751, -10.88017736071110342 ) ) ;
#27929=CARTESIAN_POINT ( 'NONE',  ( 19.38216949554541557, 62.24863466993041072, -9.382169495545420901 ) ) ;
#27931=AXIS2_PLACEMENT_3D ( 'NONE', #67341, #59335, #50356 ) ;
#27932=CARTESIAN_POINT ( 'NONE',  ( 13.79529636645030344, 38.26208216824729647, 14.16423886937410614 ) ) ;
#27933=CARTESIAN_POINT ( 'NONE',  ( 19.42250999205614193, 50.14701867748817676, 5.440088680355555262 ) ) ;
#27934=CARTESIAN_POINT ( 'NONE',  ( 4.559911319644449179, 27.23035201082150536, -9.422509992056141925 ) ) ;
#27935=CARTESIAN_POINT ( 'NONE',  ( 19.72487221294571569, 42.80223176428830811, -6.499999999999990230 ) ) ;
#27938=CARTESIAN_POINT ( 'NONE',  ( 5.076628168052704559, 50.17559781766745886, -8.527530157486179263 ) ) ;
#27941=CARTESIAN_POINT ( 'NONE',  ( 5.076628168052703671, 16.84226448433411960, 8.527530157486179263 ) ) ;
#27943=CARTESIAN_POINT ( 'NONE',  ( 10.00000000000000178, 19.31368534415484106, 10.88017736071110342 ) ) ;
#27944=CARTESIAN_POINT ( 'NONE',  ( 1.472469842513823179, 21.42559781766745175, 4.923371831947296329 ) ) ;
#27945=CARTESIAN_POINT ( 'NONE',  ( -2.816281873526473856, 9.123634669930421381, 9.499525473075851096E-16 ) ) ;
#27946=CARTESIAN_POINT ( 'NONE',  ( 2.035157376598824452, 63.68868534415484106, 7.964842623401179544 ) ) ;
#27947=CARTESIAN_POINT ( 'NONE',  ( 17.96484262340118221, 49.93868534415484106, 7.964842623401181321 ) ) ;
#27948=CARTESIAN_POINT ( 'NONE',  ( 10.00000000000000178, 14.31368534415483751, 10.88017736071110342 ) ) ;
#27949=CARTESIAN_POINT ( 'NONE',  ( 22.81628187352647785, 56.41530133659708213, 3.434112377981063169 ) ) ;
#27950=CARTESIAN_POINT ( 'NONE',  ( 10.00000000000000000, 45.55374883491397497, -14.16423886937410082 ) ) ;
#27953=ORIENTED_EDGE ( 'NONE', *, *, #90389, .T. ) ;
#27954=CARTESIAN_POINT ( 'NONE',  ( 22.81628187352647785, 1.415301336597087012, 3.434112377981063169 ) ) ;
#27955=CARTESIAN_POINT ( 'NONE',  ( 4.559911319644449179, 13.89701867748817143, 9.422509992056141925 ) ) ;
#27956=CARTESIAN_POINT ( 'NONE',  ( 12.91533473730992121, 29.52201867748817321, 10.88017736071110164 ) ) ;
#27957=CARTESIAN_POINT ( 'NONE',  ( 1.472469842513823179, 60.59226448433412315, -4.923371831947296329 ) ) ;
#27959=CARTESIAN_POINT ( 'NONE',  ( 5.076628168052703671, 21.84226448433411960, 8.527530157486179263 ) ) ;
#27960=CARTESIAN_POINT ( 'NONE',  ( 0.1532563361054100626, 15.80059781766745353, -2.638427012816831230 ) ) ;
#27961=CARTESIAN_POINT ( 'NONE',  ( 2.791683348922237240, 20.38393115100078745, -7.208316651077763204 ) ) ;
#27962=CARTESIAN_POINT ( 'NONE',  ( 0.1532563361054082862, 6.217264484334118713, 2.638427012816831674 ) ) ;
#27963=PRESENTATION_STYLE_ASSIGNMENT (( #65965 ) ) ;
#27964=MECHANICAL_DESIGN_GEOMETRIC_PRESENTATION_REPRESENTATION('',(#31181),#91871);
#27967=CARTESIAN_POINT ( 'NONE',  ( 18.52753015748618282, 3.925597817667451306, -4.923371831947291888 ) ) ;
#27968=CARTESIAN_POINT ( 'NONE',  ( -0.1042174387088609239, 23.10736173766202839, 6.337391062633419558 ) ) ;
#27969=CARTESIAN_POINT ( 'NONE',  ( 7.361572987183169658, -0.03273551566588185635, -9.846743663894592657 ) ) ;
#27970=CARTESIAN_POINT ( 'NONE',  ( 17.20831665107776587, 24.13393115100078035, -7.208316651077762316 ) ) ;
#27973=CARTESIAN_POINT ( 'NONE',  ( 0.6178305044545838731, -0.2513653300695798953, 9.382169495545420901 ) ) ;
#27975=ORIENTED_EDGE ( 'NONE', *, *, #43388, .T. ) ;
#27977=CARTESIAN_POINT ( 'NONE',  ( 24.16423886937410614, 19.51208216824729647, -3.795296366450302550 ) ) ;
#27979=CARTESIAN_POINT ( 'NONE',  ( 20.36894250292379382, 13.67874883491396965, 10.36894250292379205 ) ) ;
#27980=CARTESIAN_POINT ( 'NONE',  ( 24.16423886937410614, 49.30374883491396787, 8.672049930838204340E-16 ) ) ;
#27981=SURFACE_SIDE_STYLE ('',( #57006 ) ) ;
#27982=CARTESIAN_POINT ( 'NONE',  ( 10.00000000000000000, 10.55374883491396787, -14.16423886937410082 ) ) ;
#27983=CARTESIAN_POINT ( 'NONE',  ( -0.8801773607111009756, 38.06368534415484106, 1.068504757029289695E-15 ) ) ;
#27985=STYLED_ITEM ( 'NONE', ( #29555 ), #41388 ) ;
#27987=CARTESIAN_POINT ( 'NONE',  ( 0.1532563361054100626, 15.80059781766745353, -2.638427012816831230 ) ) ;
#27989=CARTESIAN_POINT ( 'NONE',  ( 12.91533473730992121, 54.52201867748816255, 10.88017736071110164 ) ) ;
#27990=CARTESIAN_POINT ( 'NONE',  ( 17.20831665107776587, 32.88393115100078745, 7.208316651077764980 ) ) ;
#27991=CARTESIAN_POINT ( 'NONE',  ( 2.035157376598822676, 7.438685344154837509, -7.964842623401177768 ) ) ;
#27992=CARTESIAN_POINT ( 'NONE',  ( -2.816281873526473856, 64.12363466993042493, 9.499525473075851096E-16 ) ) ;
#27993=CARTESIAN_POINT ( 'NONE',  ( 0.1532563361054082862, 56.21726448433411605, 2.638427012816831674 ) ) ;
#27995=CARTESIAN_POINT ( 'NONE',  ( 21.09922568453595559, 37.04030133659708923, -6.408140936763230044 ) ) ;
#27997=CARTESIAN_POINT ( 'NONE',  ( 18.52753015748618282, 33.92559781766745886, -4.923371831947291888 ) ) ;
#27998=EDGE_CURVE ( 'NONE', #38297, #60237, #62494, .T. ) ;
#27999=CARTESIAN_POINT ( 'NONE',  ( 6.204703633549690345, 32.84541550158063927, 14.16423886937410082 ) ) ;
#28004=CARTESIAN_POINT ( 'NONE',  ( 0.5774900079438607392, 43.48035201082151247, 5.440088680355550821 ) ) ;
#28005=CARTESIAN_POINT ( 'NONE',  ( 2.035157376598822676, 62.43868534415483396, -7.964842623401177768 ) ) ;
#28006=CARTESIAN_POINT ( 'NONE',  ( 24.16423886937410614, 39.30374883491396787, 8.672049930838204340E-16 ) ) ;
#28007=CARTESIAN_POINT ( 'NONE',  ( 7.361572987183170547, 67.05059781766746596, 9.846743663894590881 ) ) ;
#28008=CARTESIAN_POINT ( 'NONE',  ( -2.816281873526473856, 64.33196800326376774, 3.434112377981055619 ) ) ;
#28009=CARTESIAN_POINT ( 'NONE',  ( 20.88017736071110164, 40.35535201082150536, 2.915334737309930979 ) ) ;
#28011=CARTESIAN_POINT ( 'NONE',  ( 0.6178305044545818747, 28.49863466993041783, -9.382169495545419124 ) ) ;
#28012=CARTESIAN_POINT ( 'NONE',  ( 7.361572987183169658, 59.96726448433410894, -9.846743663894592657 ) ) ;
#28014=CARTESIAN_POINT ( 'NONE',  ( 15.44008868035555793, 6.397018677488171434, -9.422509992056140149 ) ) ;
#28016=( NAMED_UNIT ( * ) SI_UNIT ( $, .STERADIAN. ) SOLID_ANGLE_UNIT ( ) );
#28018=( BOUNDED_CURVE ( )  B_SPLINE_CURVE ( 2, ( #92421, #24439, #54415, #85418, #90937, #16439, #1451, #30433, #31903 ),
 .UNSPECIFIED., .F., .F. ) 
 B_SPLINE_CURVE_WITH_KNOTS ( ( 3, 2, 2, 2, 3 ),
 ( 0.6901409369402313754, 0.6904761904761904656, 0.6964285714285713969, 0.7023809523809523281, 0.7027162059169114183 ),
 .UNSPECIFIED. ) 
 CURVE ( )  GEOMETRIC_REPRESENTATION_ITEM ( )  RATIONAL_B_SPLINE_CURVE ( ( 0.9963778908391764944, 0.9980808541467923733, 1.000000000000000000, 0.9659258262890683122, 1.000000000000000000, 0.9659258262890683122, 1.000000000000000000, 0.9980808541467923733, 0.9963778908391766054 ) ) 
 REPRESENTATION_ITEM ( '' )  );
#28019=CARTESIAN_POINT ( 'NONE',  ( 2.791683348922240793, 1.633931151000784565, 7.208316651077764092 ) ) ;
#28020=CARTESIAN_POINT ( 'NONE',  ( 20.88017736071110875, 65.77201867748817676, -2.915334737309920765 ) ) ;
#28023=CARTESIAN_POINT ( 'NONE',  ( 0.1532563361054100626, 35.80059781766745175, -2.638427012816831230 ) ) ;
#28025=CARTESIAN_POINT ( 'NONE',  ( 19.42250999205614193, 20.14701867748817321, 5.440088680355555262 ) ) ;
#28026=CARTESIAN_POINT ( 'NONE',  ( 16.40814093676324603, 2.456968003263753531, -11.09922568453594671 ) ) ;
#28027=CARTESIAN_POINT ( 'NONE',  ( 10.00000000000000178, 29.31368534415483751, 10.88017736071110342 ) ) ;
#28030=CARTESIAN_POINT ( 'NONE',  ( -2.816281873526473856, 39.33196800326374643, 3.434112377981055619 ) ) ;
#28031=ORIENTED_EDGE ( 'NONE', *, *, #63010, .T. ) ;
#28032=CARTESIAN_POINT ( 'NONE',  ( 15.44008868035555793, 66.39701867748817676, -9.422509992056140149 ) ) ;
#28033=CARTESIAN_POINT ( 'NONE',  ( 6.565887622018943937, 18.08196800326375708, -12.81628187352647608 ) ) ;
#28034=CARTESIAN_POINT ( 'NONE',  ( 19.80448550324509682, 51.82703681773345039, 6.500000000002705391 ) ) ;
#28035=ADVANCED_FACE ( 'NONE', ( #75662 ), #7173, .F. ) ;
#28036=CARTESIAN_POINT ( 'NONE',  ( 10.00000000000000000, 36.81368534415484106, -10.88017736071110342 ) ) ;
#28038=CARTESIAN_POINT ( 'NONE',  ( 22.26659068614895176, 64.72041550158064638, -7.082119434687042414 ) ) ;
#28039=CARTESIAN_POINT ( 'NONE',  ( 0.1532563361054100626, 55.80059781766745175, -2.638427012816831230 ) ) ;
#28040=CARTESIAN_POINT ( 'NONE',  ( 19.84674366389459266, 8.300597817667451750, 2.638427012816836559 ) ) ;
#28041=CARTESIAN_POINT ( 'NONE',  ( 12.91533473730993009, 61.60535201082150536, -10.88017736071109987 ) ) ;
#28043=CARTESIAN_POINT ( 'NONE',  ( 17.08211943468705840, 25.13708216824730357, -12.26659068614894466 ) ) ;
#28046=CARTESIAN_POINT ( 'NONE',  ( 19.54819611545891789, 81.00370271165274971, -4.999999999999999112 ) ) ;
#28048=CARTESIAN_POINT ( 'NONE',  ( 10.00000000000000178, 63.05374883491396076, 14.16423886937410082 ) ) ;
#28049=CARTESIAN_POINT ( 'NONE',  ( 10.00000000000000178, 48.05374883491396787, 14.16423886937410082 ) ) ;
#28050=CARTESIAN_POINT ( 'NONE',  ( 18.52753015748617571, 28.09226448433411960, 4.923371831947298993 ) ) ;
#28052=CARTESIAN_POINT ( 'NONE',  ( 21.09922568453595559, 27.04030133659708568, -6.408140936763230044 ) ) ;
#28054=CARTESIAN_POINT ( 'NONE',  ( 15.44008868035555793, 11.39701867748817143, -9.422509992056140149 ) ) ;
#28055=CARTESIAN_POINT ( 'NONE',  ( 17.08211943468705130, 63.47041550158063927, 12.26659068614894998 ) ) ;
#28056=CARTESIAN_POINT ( 'NONE',  ( 5.076628168052704559, 35.17559781766745175, -8.527530157486179263 ) ) ;
#28058=CARTESIAN_POINT ( 'NONE',  ( 0.1532563361054100626, 5.800597817667452638, -2.638427012816831230 ) ) ;
#28059=CARTESIAN_POINT ( 'NONE',  ( 20.10493008474208310, 14.71697413083878914, 6.336235997365745831 ) ) ;
#28065=CARTESIAN_POINT ( 'NONE',  ( 2.917880565312948704, 12.63708216824730179, 12.26659068614894643 ) ) ;
#28066=CARTESIAN_POINT ( 'NONE',  ( 10.00000000000000000, 16.81368534415483751, -10.88017736071110342 ) ) ;
#28067=CARTESIAN_POINT ( 'NONE',  ( 0.5774900079438607392, 23.48035201082150536, 5.440088680355550821 ) ) ;
#28068=CARTESIAN_POINT ( 'NONE',  ( 7.361572987183170547, 47.05059781766745175, 9.846743663894590881 ) ) ;
#28069=CARTESIAN_POINT ( 'NONE',  ( 0.6178305044545838731, 19.74863466993042138, 9.382169495545420901 ) ) ;
#28070=CARTESIAN_POINT ( 'NONE',  ( 13.79529636645031943, 10.34541550158063394, -14.16423886937409904 ) ) ;
#28075=CARTESIAN_POINT ( 'NONE',  ( 0.6178305044545818747, 28.49863466993041783, -9.382169495545419124 ) ) ;
#28076=ORIENTED_EDGE ( 'NONE', *, *, #84212, .F. ) ;
#28077=CARTESIAN_POINT ( 'NONE',  ( 12.63842701281683034, 27.46726448433411250, 9.846743663894596210 ) ) ;
#28078=CARTESIAN_POINT ( 'NONE',  ( -4.164238869374099039, 56.80374883491397497, 8.674139862899312516E-16 ) ) ;
#28080=CARTESIAN_POINT ( 'NONE',  ( 2.035157376598824452, 3.688685344154837953, 7.964842623401179544 ) ) ;
#28081=ORIENTED_EDGE ( 'NONE', *, *, #62664, .F. ) ;
#28082=CARTESIAN_POINT ( 'NONE',  ( 20.88017736071110875, 50.77201867748817676, -2.915334737309920765 ) ) ;
#28083=CARTESIAN_POINT ( 'NONE',  ( 0.5774900079438590739, 47.64701867748817676, -5.440088680355550821 ) ) ;
#28084=CARTESIAN_POINT ( 'NONE',  ( 12.91533473730993009, 51.60535201082149825, -10.88017736071109987 ) ) ;
#28086=CARTESIAN_POINT ( 'NONE',  ( 12.91533473730993009, 41.60535201082149825, -10.88017736071109987 ) ) ;
#28088=ADVANCED_FACE ( 'NONE', ( #78496 ), #37676, .T. ) ;
#28089=ORIENTED_EDGE ( 'NONE', *, *, #91027, .F. ) ;
#28091=CARTESIAN_POINT ( 'NONE',  ( 19.84674366389459266, 23.30059781766745530, 2.638427012816836559 ) ) ;
#28093=CARTESIAN_POINT ( 'NONE',  ( 5.076628168052703671, 61.84226448433412315, 8.527530157486179263 ) ) ;
#28094=CARTESIAN_POINT ( 'NONE',  ( -45.94000000000001194, 99.99999999999998579, -12.00000000000000000 ) ) ;
#28095=CARTESIAN_POINT ( 'NONE',  ( 22.26659068614894466, 3.887082168247300906, 7.082119434687054849 ) ) ;
#28099=CARTESIAN_POINT ( 'NONE',  ( 22.26659068614895176, 64.72041550158064638, -7.082119434687042414 ) ) ;
#28103=CARTESIAN_POINT ( 'NONE',  ( 0.1532563361054082862, 36.21726448433410894, 2.638427012816831674 ) ) ;
#28107=CARTESIAN_POINT ( 'NONE',  ( 13.43411237798105340, 0.5819680032637533085, 12.81628187352647963 ) ) ;
#28108=CARTESIAN_POINT ( 'NONE',  ( 18.52753015748617571, 13.09226448433411960, 4.923371831947298993 ) ) ;
#28110=CARTESIAN_POINT ( 'NONE',  ( 7.361572987183169658, 4.967264484334119601, -9.846743663894592657 ) ) ;
#28111=CARTESIAN_POINT ( 'NONE',  ( 10.00000000000000000, -2.126365330069579951, -12.81628187352647608 ) ) ;
#28112=CARTESIAN_POINT ( 'NONE',  ( 19.10478245763047056, 21.02576239577082262, -5.990408912944402253 ) ) ;
#28114=ORIENTED_EDGE ( 'NONE', *, *, #98201, .T. ) ;
#28116=CARTESIAN_POINT ( 'NONE',  ( 15.44008868035555793, 11.39701867748817143, -9.422509992056140149 ) ) ;
#28117=CARTESIAN_POINT ( 'NONE',  ( 2.917880565312948704, 7.637082168247301794, 12.26659068614894643 ) ) ;
#28118=CARTESIAN_POINT ( 'NONE',  ( 2.791683348922240793, 21.63393115100078745, 7.208316651077764092 ) ) ;
#28119=CARTESIAN_POINT ( 'NONE',  ( 2.035157376598822676, 52.43868534415483396, -7.964842623401177768 ) ) ;
#28120=CARTESIAN_POINT ( 'NONE',  ( 10.00000000000000178, 30.37363466993042138, 12.81628187352647608 ) ) ;
#28127=CARTESIAN_POINT ( 'NONE',  ( 10.00000000000000000, 2.873634669930420049, -12.81628187352647608 ) ) ;
#28128=CARTESIAN_POINT ( 'NONE',  ( 19.38216949554541202, 0.9986346699304200492, 9.382169495545424454 ) ) ;
#28129=CARTESIAN_POINT ( 'NONE',  ( 14.92337183194729988, 9.342264484334119601, -8.527530157486177487 ) ) ;
#28131=CARTESIAN_POINT ( 'NONE',  ( 19.38216949554541202, 20.99863466993042138, 9.382169495545424454 ) ) ;
#28133=CARTESIAN_POINT ( 'NONE',  ( 2.035157376598824452, 28.68868534415484106, 7.964842623401179544 ) ) ;
#28134=STYLED_ITEM ( 'NONE', ( #16217 ), #848 ) ;
#28136=CARTESIAN_POINT ( 'NONE',  ( 24.16423886937410614, 49.51208216824730357, -3.795296366450302550 ) ) ;
#28139=CARTESIAN_POINT ( 'NONE',  ( 15.44008868035555793, 26.39701867748817321, -9.422509992056140149 ) ) ;
#28141=CARTESIAN_POINT ( 'NONE',  ( 5.076628168052703671, 51.84226448433412315, 8.527530157486179263 ) ) ;
#28142=CARTESIAN_POINT ( 'NONE',  ( 19.42250999205614193, 55.14701867748817676, 5.440088680355555262 ) ) ;
#28143=EDGE_CURVE ( 'NONE', #11978, #95286, #72451, .T. ) ;
#28144=CARTESIAN_POINT ( 'NONE',  ( 20.36894250292379382, 33.67874883491396076, 10.36894250292379205 ) ) ;
#28145=CARTESIAN_POINT ( 'NONE',  ( 17.39651004071842166, 32.93575266056827644, 6.499999999999998224 ) ) ;
#28147=UNCERTAINTY_MEASURE_WITH_UNIT (LENGTH_MEASURE( 1.000000000000000082E-05 ), #33557, 'distance_accuracy_value', 'NONE');
#28148=CARTESIAN_POINT ( 'NONE',  ( 19.84674366389459266, 43.30059781766744464, 2.638427012816836559 ) ) ;
#28149=CARTESIAN_POINT ( 'NONE',  ( 16.40814093676324603, 2.456968003263753531, -11.09922568453594671 ) ) ;
#28151=CARTESIAN_POINT ( 'NONE',  ( 2.035157376598824452, 18.68868534415484106, 7.964842623401179544 ) ) ;
#28152=LINE ( 'NONE', #3700, #12572 ) ;
#28153=CARTESIAN_POINT ( 'NONE',  ( 0.5774900079438607392, 13.48035201082150358, 5.440088680355550821 ) ) ;
#28154=CARTESIAN_POINT ( 'NONE',  ( 2.791683348922240793, 1.633931151000784565, 7.208316651077764092 ) ) ;
#28155=CARTESIAN_POINT ( 'NONE',  ( 24.16423886937410614, 29.51208216824729647, -3.795296366450302550 ) ) ;
#28156=CARTESIAN_POINT ( 'NONE',  ( 18.52753015748617571, 13.09226448433411960, 4.923371831947298993 ) ) ;
#28157=CARTESIAN_POINT ( 'NONE',  ( 5.076628168052704559, 65.17559781766745175, -8.527530157486179263 ) ) ;
#28158=CARTESIAN_POINT ( 'NONE',  ( 15.44008868035555793, 36.39701867748816966, -9.422509992056140149 ) ) ;
#28164=CARTESIAN_POINT ( 'NONE',  ( 14.92337183194729633, 47.67559781766745175, 8.527530157486181039 ) ) ;
#28166=VERTEX_POINT ( 'NONE', #18980 ) ;
#28167=VERTEX_POINT ( 'NONE', #88451 ) ;
#28169=CARTESIAN_POINT ( 'NONE',  ( -2.266590686148945544, 27.22041550158063572, 7.082119434687048631 ) ) ;
#28170=CARTESIAN_POINT ( 'NONE',  ( 22.26659068614895176, 14.72041550158063572, -7.082119434687042414 ) ) ;
#28172=CARTESIAN_POINT ( 'NONE',  ( 19.42250999205614193, 65.14701867748817676, 5.440088680355555262 ) ) ;
#28173=CARTESIAN_POINT ( 'NONE',  ( 6.204703633549690345, 55.76208216824730357, -14.16423886937410259 ) ) ;
#28174=CARTESIAN_POINT ( 'NONE',  ( 2.791683348922240793, 36.63393115100078035, 7.208316651077764092 ) ) ;
#28176=CARTESIAN_POINT ( 'NONE',  ( 0.5774900079438607392, 28.48035201082150891, 5.440088680355550821 ) ) ;
#28177=CARTESIAN_POINT ( 'NONE',  ( 21.09922568453594849, 6.206968003263753531, 6.408140936763242479 ) ) ;
#28178=CARTESIAN_POINT ( 'NONE',  ( -2.266590686148945544, 21.38708216824730357, -7.082119434687050408 ) ) ;
#28179=CARTESIAN_POINT ( 'NONE',  ( 6.204703633549690345, 57.84541550158063927, 14.16423886937410082 ) ) ;
#28180=CARTESIAN_POINT ( 'NONE',  ( -0.8801773607111008646, 18.27201867748817321, 2.915334737309923430 ) ) ;
#28182=CARTESIAN_POINT ( 'NONE',  ( -0.3289641300567998083, 3.078790035174471029, 5.963430220938281678 ) ) ;
#28183=CARTESIAN_POINT ( 'NONE',  ( 17.96484262340118221, 41.18868534415484106, -7.964842623401177768 ) ) ;
#28189=CARTESIAN_POINT ( 'NONE',  ( 2.917880565312950480, 50.97041550158064638, -12.26659068614894821 ) ) ;
#28190=CARTESIAN_POINT ( 'NONE',  ( 14.92337183194729633, 52.67559781766745175, 8.527530157486181039 ) ) ;
#28191=CARTESIAN_POINT ( 'NONE',  ( 20.88017736071110164, 55.35535201082149825, 2.915334737309930979 ) ) ;
#28193=CARTESIAN_POINT ( 'NONE',  ( 12.91533473730993009, 51.60535201082149825, -10.88017736071109987 ) ) ;
#28194=CARTESIAN_POINT ( 'NONE',  ( 13.43411237798105340, 60.58196800326376064, 12.81628187352647963 ) ) ;
#28197=CARTESIAN_POINT ( 'NONE',  ( 20.36894250292379738, 24.92874883491396787, -10.36894250292379027 ) ) ;
#28198=CARTESIAN_POINT ( 'NONE',  ( 10.00000000000000178, 25.37363466993041783, 12.81628187352647608 ) ) ;
#28200=CARTESIAN_POINT ( 'NONE',  ( 0.6178305044545818747, 38.49863466993042493, -9.382169495545419124 ) ) ;
#28201=CARTESIAN_POINT ( 'NONE',  ( 10.00000000000000000, 16.81368534415483751, -10.88017736071110342 ) ) ;
#28202=CARTESIAN_POINT ( 'NONE',  ( 1.472469842513823179, 31.42559781766745530, 4.923371831947296329 ) ) ;
#28203=CARTESIAN_POINT ( 'NONE',  ( -0.8801773607111009756, 13.06368534415483929, 1.068504757029289695E-15 ) ) ;
#28204=CARTESIAN_POINT ( 'NONE',  ( 6.565887622018943937, 58.08196800326376064, -12.81628187352647608 ) ) ;
#28206=CARTESIAN_POINT ( 'NONE',  ( 14.92337183194729633, 42.67559781766745886, 8.527530157486181039 ) ) ;
#28207=EDGE_CURVE ( 'NONE', #34886, #21097, #95468, .T. ) ;
#28209=CARTESIAN_POINT ( 'NONE',  ( 0.1089645850228891377, 3.162345557925709372, 6.479102184480797000 ) ) ;
#28214=CARTESIAN_POINT ( 'NONE',  ( 0.1532563361054083140, 21.00893115100078745, 1.131784320476157264E-15 ) ) ;
#28215=CARTESIAN_POINT ( 'NONE',  ( 10.00000000000000178, 20.37363466993042138, 12.81628187352647608 ) ) ;
#28217=ORIENTED_EDGE ( 'NONE', *, *, #74833, .F. ) ;
#28218=CARTESIAN_POINT ( 'NONE',  ( 1.472469842513823179, 55.59226448433412315, -4.923371831947296329 ) ) ;
#28220=CARTESIAN_POINT ( 'NONE',  ( 17.08211943468705130, 18.47041550158063572, 12.26659068614894998 ) ) ;
#28221=CARTESIAN_POINT ( 'NONE',  ( 2.791683348922240793, 51.63393115100078745, 7.208316651077764092 ) ) ;
#28222=CARTESIAN_POINT ( 'NONE',  ( 0.6178305044545838731, 44.74863466993042493, 9.382169495545420901 ) ) ;
#28224=CARTESIAN_POINT ( 'NONE',  ( 15.44008868035555260, 64.73035201082151957, 9.422509992056143702 ) ) ;
#28225=CARTESIAN_POINT ( 'NONE',  ( 0.1077916266722774852, 67.24062864464239908, -6.478736007406002528 ) ) ;
#28226=CARTESIAN_POINT ( 'NONE',  ( 7.361572987183170547, 32.05059781766745175, 9.846743663894590881 ) ) ;
#28227=CARTESIAN_POINT ( 'NONE',  ( 7.084665262690076126, 37.02201867748817676, -10.88017736071110164 ) ) ;
#28228=CARTESIAN_POINT ( 'NONE',  ( 21.09922568453595559, 37.04030133659708923, -6.408140936763230044 ) ) ;
#28230=CARTESIAN_POINT ( 'NONE',  ( 19.84674366389459266, 28.71726448433411960, -2.638427012816827677 ) ) ;
#28236=CARTESIAN_POINT ( 'NONE',  ( -0.8801773607111008646, 38.27201867748816255, 2.915334737309923430 ) ) ;
#28239=CARTESIAN_POINT ( 'NONE',  ( 7.084665262690076126, 12.02201867748817143, -10.88017736071110164 ) ) ;
#28240=CARTESIAN_POINT ( 'NONE',  ( 0.1532563361054100626, 55.80059781766745175, -2.638427012816831230 ) ) ;
#28241=CARTESIAN_POINT ( 'NONE',  ( 7.084665262690076126, 42.02201867748816966, -10.88017736071110164 ) ) ;
#28243=CARTESIAN_POINT ( 'NONE',  ( 19.42250999205614548, 60.98035201082151247, -5.440088680355545492 ) ) ;
#28244=CARTESIAN_POINT ( 'NONE',  ( 7.084665262690076126, 32.02201867748816966, -10.88017736071110164 ) ) ;
#28246=CARTESIAN_POINT ( 'NONE',  ( 10.00000000000000000, 4.758931151000784787, -9.846743663894594434 ) ) ;
#28247=CARTESIAN_POINT ( 'NONE',  ( 17.20831665107776587, 29.13393115100078390, -7.208316651077762316 ) ) ;
#28250=CARTESIAN_POINT ( 'NONE',  ( 7.361572987183169658, 49.96726448433410894, -9.846743663894592657 ) ) ;
#28252=CARTESIAN_POINT ( 'NONE',  ( 2.917880565312950480, 55.97041550158063217, -12.26659068614894821 ) ) ;
#28253=CARTESIAN_POINT ( 'NONE',  ( 1.602071938427537923, 62.02224192338640307, -6.500000000000073719 ) ) ;
#28254=CARTESIAN_POINT ( 'NONE',  ( 17.08211943468705840, 10.13708216824730179, -12.26659068614894466 ) ) ;
#28255=CARTESIAN_POINT ( 'NONE',  ( 2.917880565312948704, 42.63708216824729647, 12.26659068614894643 ) ) ;
#28256=CARTESIAN_POINT ( 'NONE',  ( 13.43411237798106583, 2.665301336597086568, -12.81628187352647252 ) ) ;
#28258=CARTESIAN_POINT ( 'NONE',  ( 19.42250999205614193, 20.14701867748817321, 5.440088680355555262 ) ) ;
#28259=CARTESIAN_POINT ( 'NONE',  ( 18.52753015748617571, 48.09226448433412315, 4.923371831947298993 ) ) ;
#28260=FILL_AREA_STYLE_COLOUR ( '', #78713 ) ;
#28265=CARTESIAN_POINT ( 'NONE',  ( 13.43411237798106583, 27.66530133659708568, -12.81628187352647252 ) ) ;
#28266=CARTESIAN_POINT ( 'NONE',  ( 17.20831665107776587, 22.88393115100078745, 7.208316651077764980 ) ) ;
#28268=CARTESIAN_POINT ( 'NONE',  ( 7.361572987183169658, 14.96726448433411960, -9.846743663894592657 ) ) ;
#28270=CARTESIAN_POINT ( 'NONE',  ( 12.91533473730992121, 4.522018677488170546, 10.88017736071110164 ) ) ;
#28271=CARTESIAN_POINT ( 'NONE',  ( 12.91533473730992121, 14.52201867748817143, 10.88017736071110164 ) ) ;
#28272=CARTESIAN_POINT ( 'NONE',  ( 20.36894250292379382, 38.67874883491396076, 10.36894250292379205 ) ) ;
#28273=CARTESIAN_POINT ( 'NONE',  ( 7.084665262690076126, 44.10535201082151247, 10.88017736071109987 ) ) ;
#28274=CARTESIAN_POINT ( 'NONE',  ( 4.559911319644449179, 58.89701867748817676, 9.422509992056141925 ) ) ;
#28277=CARTESIAN_POINT ( 'NONE',  ( 20.32896413005680358, 39.74545670184114243, 5.963430220938287007 ) ) ;
#28278=CARTESIAN_POINT ( 'NONE',  ( 5.076628168052704559, 20.17559781766745175, -8.527530157486179263 ) ) ;
#28279=PRESENTATION_STYLE_ASSIGNMENT (( #96803 ) ) ;
#28280=CARTESIAN_POINT ( 'NONE',  ( 2.791683348922240793, 6.633931151000785675, 7.208316651077764092 ) ) ;
#28282=CARTESIAN_POINT ( 'NONE',  ( 0.1532563361054083140, 31.00893115100078390, 1.131784320476157264E-15 ) ) ;
#28283=CARTESIAN_POINT ( 'NONE',  ( -1.099225684535947600, -1.293031996736246469, -6.408140936763238038 ) ) ;
#28284=EDGE_CURVE ( 'NONE', #39981, #63027, #73937, .T. ) ;
#28285=CARTESIAN_POINT ( 'NONE',  ( 20.88017736071110875, 35.77201867748816966, -2.915334737309920765 ) ) ;
#28287=CARTESIAN_POINT ( 'NONE',  ( -2.816281873526473856, 59.12363466993042493, 9.499525473075851096E-16 ) ) ;
#28289=CARTESIAN_POINT ( 'NONE',  ( 0.1532563361054083140, 1.008931151000784787, 1.131784320476157264E-15 ) ) ;
#28290=CARTESIAN_POINT ( 'NONE',  ( 6.565887622018943937, 43.08196800326374643, -12.81628187352647608 ) ) ;
#28291=CARTESIAN_POINT ( 'NONE',  ( 24.16423886937410614, 64.30374883491396076, 8.672049930838204340E-16 ) ) ;
#28292=CARTESIAN_POINT ( 'NONE',  ( 7.361572987183170547, 37.05059781766744464, 9.846743663894590881 ) ) ;
#28293=CARTESIAN_POINT ( 'NONE',  ( -0.03447792253739352664, 60.15514106990690379, 6.401564815979744694 ) ) ;
#28295=CARTESIAN_POINT ( 'NONE',  ( 19.84674366389459621, 63.50893115100078745, 7.409399052514197653E-17 ) ) ;
#28296=CARTESIAN_POINT ( 'NONE',  ( -4.164238869374099927, 47.01208216824729647, 3.795296366450308767 ) ) ;
#28297=CARTESIAN_POINT ( 'NONE',  ( 0.1532563361054083140, 41.00893115100078745, 1.131784320476157264E-15 ) ) ;
#28299=CARTESIAN_POINT ( 'NONE',  ( 15.44008868035555793, 41.39701867748817676, -9.422509992056140149 ) ) ;
#28300=CARTESIAN_POINT ( 'NONE',  ( 19.42250999205614193, 60.14701867748817676, 5.440088680355555262 ) ) ;
#28302=CARTESIAN_POINT ( 'NONE',  ( -0.08248232600719085372, 0.1423898869303599768, 6.349449577244200782 ) ) ;
#28304=CARTESIAN_POINT ( 'NONE',  ( 19.38216949554541557, 47.24863466993041783, -9.382169495545420901 ) ) ;
#28306=CARTESIAN_POINT ( 'NONE',  ( 10.00000000000000000, -0.2410688489992152128, -9.846743663894594434 ) ) ;
#28307=ORIENTED_EDGE ( 'NONE', *, *, #80156, .T. ) ;
#28308=CARTESIAN_POINT ( 'NONE',  ( 10.00000000000000178, 8.053748834913967869, 14.16423886937410082 ) ) ;
#28309=CARTESIAN_POINT ( 'NONE',  ( 17.20831665107776587, 9.133931151000787452, -7.208316651077762316 ) ) ;
#28314=CARTESIAN_POINT ( 'NONE',  ( 0.5774900079438607392, 8.480352010821505360, 5.440088680355550821 ) ) ;
#28315=CARTESIAN_POINT ( 'NONE',  ( 20.36894250292379738, 14.92874883491396432, -10.36894250292379027 ) ) ;
#28317=CARTESIAN_POINT ( 'NONE',  ( 17.96484262340118221, 24.93868534415484461, 7.964842623401181321 ) ) ;
#28318=CARTESIAN_POINT ( 'NONE',  ( 12.63842701281683034, 57.46726448433411605, 9.846743663894596210 ) ) ;
#28319=EDGE_LOOP ( 'NONE', ( #9267, #8654, #38863, #48401 ) ) ;
#28320=B_SPLINE_CURVE_WITH_KNOTS ( 'NONE', 3,
 ( #89040, #5057, #36033, #7030, #35541, #36544 ),
 .UNSPECIFIED., .F., .F.,
 ( 4, 2, 4 ),
 ( 0.000000000000000000, 0.0002701661927229369623, 0.0005403323854458739247 ),
 .UNSPECIFIED. ) ;
#28321=CARTESIAN_POINT ( 'NONE',  ( 0.1532563361054100626, 55.80059781766745175, -2.638427012816831230 ) ) ;
#28323=CARTESIAN_POINT ( 'NONE',  ( 15.44008868035555793, 61.39701867748817676, -9.422509992056140149 ) ) ;
#28324=CARTESIAN_POINT ( 'NONE',  ( 2.791683348922240793, 61.63393115100079456, 7.208316651077764092 ) ) ;
#28325=CARTESIAN_POINT ( 'NONE',  ( -2.816281873526471635, 38.91530133659708213, -3.434112377981056508 ) ) ;
#28326=CARTESIAN_POINT ( 'NONE',  ( 7.084665262690076126, 7.022018677488169658, -10.88017736071110164 ) ) ;
#28328=CARTESIAN_POINT ( 'NONE',  ( 18.52753015748618282, 3.925597817667451306, -4.923371831947291888 ) ) ;
#28329=CARTESIAN_POINT ( 'NONE',  ( 0.5774900079438607392, 23.48035201082150536, 5.440088680355550821 ) ) ;
#28330=EDGE_CURVE ( 'NONE', #49375, #9043, #97088, .T. ) ;
#28332=CARTESIAN_POINT ( 'NONE',  ( 3.591859063236763294, 48.29030133659708923, -11.09922568453595026 ) ) ;
#28333=CARTESIAN_POINT ( 'NONE',  ( 20.88017736071110875, 45.77201867748816966, -2.915334737309920765 ) ) ;
#28335=CARTESIAN_POINT ( 'NONE',  ( -2.816281873526471635, 43.91530133659708923, -3.434112377981056508 ) ) ;
#28336=CARTESIAN_POINT ( 'NONE',  ( 2.035157376598822676, 47.43868534415484817, -7.964842623401177768 ) ) ;
#28338=CARTESIAN_POINT ( 'NONE',  ( 19.84674366389459266, 58.71726448433411605, -2.638427012816827677 ) ) ;
#28339=ORIENTED_EDGE ( 'NONE', *, *, #51194, .T. ) ;
#28341=CARTESIAN_POINT ( 'NONE',  ( 18.52753015748618282, 23.92559781766745530, -4.923371831947291888 ) ) ;
#28342=CARTESIAN_POINT ( 'NONE',  ( 22.81628187352647785, 1.415301336597087012, 3.434112377981063169 ) ) ;
#28343=CARTESIAN_POINT ( 'NONE',  ( 10.00000000000000178, 70.00000000000000000, 0.000000000000000000 ) ) ;
#28345=CARTESIAN_POINT ( 'NONE',  ( 20.88017736071110164, 20.35535201082150891, 2.915334737309930979 ) ) ;
#28346=CARTESIAN_POINT ( 'NONE',  ( 7.361572987183170547, 52.05059781766745175, 9.846743663894590881 ) ) ;
#28348=PLANE ( 'NONE',  #35934 ) ;
#28350=CARTESIAN_POINT ( 'NONE',  ( 19.84674366389459266, 8.300597817667451750, 2.638427012816836559 ) ) ;
#28351=( NAMED_UNIT ( * ) SI_UNIT ( $, .STERADIAN. ) SOLID_ANGLE_UNIT ( ) );
#28352=CARTESIAN_POINT ( 'NONE',  ( 6.565887622018943937, 0.1653013365970866511, 12.81628187352647430 ) ) ;
#28356=CARTESIAN_POINT ( 'NONE',  ( -2.816281873526473856, 34.12363466993042493, 9.499525473075851096E-16 ) ) ;
#28358=CARTESIAN_POINT ( 'NONE',  ( 12.63842701281683922, 34.55059781766745886, -9.846743663894590881 ) ) ;
#28360=CARTESIAN_POINT ( 'NONE',  ( 22.26659068614894466, 63.88708216824730357, 7.082119434687054849 ) ) ;
#28361=CARTESIAN_POINT ( 'NONE',  ( 1.472469842513823179, 26.42559781766745175, 4.923371831947296329 ) ) ;
#28364=CARTESIAN_POINT ( 'NONE',  ( 12.91533473730992121, 9.522018677488171434, 10.88017736071110164 ) ) ;
#28366=CARTESIAN_POINT ( 'NONE',  ( 2.035157376598822676, 17.43868534415483751, -7.964842623401177768 ) ) ;
#28367=CARTESIAN_POINT ( 'NONE',  ( -2.266590686148945544, 56.38708216824731068, -7.082119434687050408 ) ) ;
#28368=STYLED_ITEM ( 'NONE', ( #51937 ), #12766 ) ;
#28369=CARTESIAN_POINT ( 'NONE',  ( -2.266590686148945544, 51.38708216824730357, -7.082119434687050408 ) ) ;
#28371=CARTESIAN_POINT ( 'NONE',  ( 0.1532563361054100626, 10.80059781766745175, -2.638427012816831230 ) ) ;
#28372=CARTESIAN_POINT ( 'NONE',  ( 7.361572987183169658, 64.96726448433412315, -9.846743663894592657 ) ) ;
#28375=CARTESIAN_POINT ( 'NONE',  ( 2.035157376598822676, 47.43868534415484817, -7.964842623401177768 ) ) ;
#28376=CARTESIAN_POINT ( 'NONE',  ( 0.5774900079438607392, 18.48035201082150536, 5.440088680355550821 ) ) ;
#28377=COLOUR_RGB ( '', 0.08235294, 0.09019608, 0.10196078) ;
#28381=CARTESIAN_POINT ( 'NONE',  ( 19.84674366389459621, 13.50893115100078568, 7.409399052514197653E-17 ) ) ;
#28382=CARTESIAN_POINT ( 'NONE',  ( 17.39651004071838614, 47.93575266056826933, 6.500000000000032863 ) ) ;
#28383=CARTESIAN_POINT ( 'NONE',  ( 10.00000000000000178, 38.05374883491396787, 14.16423886937410082 ) ) ;
#28386=( NAMED_UNIT ( * ) SI_UNIT ( $, .STERADIAN. ) SOLID_ANGLE_UNIT ( ) );
#28387=CARTESIAN_POINT ( 'NONE',  ( 19.42250999205614193, 30.14701867748817321, 5.440088680355555262 ) ) ;
#28388=CARTESIAN_POINT ( 'NONE',  ( 10.00000000000000000, 32.87363466993042493, -12.81628187352647608 ) ) ;
#28389=CARTESIAN_POINT ( 'NONE',  ( 3.591859063236761518, 29.95696800326375708, 11.09922568453594849 ) ) ;
#28390=CARTESIAN_POINT ( 'NONE',  ( -1.099225684535947600, 64.54030133659709634, 6.408140936763237150 ) ) ;
#28394=CARTESIAN_POINT ( 'NONE',  ( 10.00000000000000000, 30.55374883491397142, -14.16423886937410082 ) ) ;
#28395=CARTESIAN_POINT ( 'NONE',  ( -2.266590686148945544, 7.220415501580634832, 7.082119434687048631 ) ) ;
#28396=CARTESIAN_POINT ( 'NONE',  ( 10.00000000000000178, 4.313685344154837509, 10.88017736071110342 ) ) ;
#28397=CARTESIAN_POINT ( 'NONE',  ( 4.559911319644449179, 28.89701867748817321, 9.422509992056141925 ) ) ;
#28398=LINE ( 'NONE', #34901, #12744 ) ;
#28400=CARTESIAN_POINT ( 'NONE',  ( 2.035157376598824452, 58.68868534415482685, 7.964842623401179544 ) ) ;
#28401=CARTESIAN_POINT ( 'NONE',  ( 0.5774900079438607392, 48.48035201082150536, 5.440088680355550821 ) ) ;
#28402=CARTESIAN_POINT ( 'NONE',  ( 16.40814093676323893, 10.79030133659708923, 11.09922568453595026 ) ) ;
#28405=CARTESIAN_POINT ( 'NONE',  ( 10.00000000000000000, 19.75893115100078390, -9.846743663894594434 ) ) ;
#28406=CARTESIAN_POINT ( 'NONE',  ( 2.035157376598822676, 37.43868534415484106, -7.964842623401177768 ) ) ;
#28408=B_SPLINE_CURVE_WITH_KNOTS ( 'NONE', 3,
 ( #5377, #35852, #21352, #51844 ),
 .UNSPECIFIED., .F., .F.,
 ( 4, 4 ),
 ( 0.000000000000000000, 0.001060528352562004799 ),
 .UNSPECIFIED. ) ;
#28409=CARTESIAN_POINT ( 'NONE',  ( 6.565887622018943937, 0.1653013365970866511, 12.81628187352647430 ) ) ;
#28410=CARTESIAN_POINT ( 'NONE',  ( 17.20831665107776587, 19.13393115100078035, -7.208316651077762316 ) ) ;
#28411=CARTESIAN_POINT ( 'NONE',  ( 3.591859063236763294, 53.29030133659708923, -11.09922568453595026 ) ) ;
#28412=CARTESIAN_POINT ( 'NONE',  ( 0.1532563361054082862, 21.21726448433412315, 2.638427012816831674 ) ) ;
#28414=CARTESIAN_POINT ( 'NONE',  ( 6.204703633549690345, 10.76208216824729824, -14.16423886937410259 ) ) ;
#28415=CARTESIAN_POINT ( 'NONE',  ( 0.5774900079438590739, 22.64701867748817321, -5.440088680355550821 ) ) ;
#28416=SURFACE_SIDE_STYLE ('',( #44886 ) ) ;
#28417=CARTESIAN_POINT ( 'NONE',  ( 24.16423886937409904, 29.09541550158063572, 3.795296366450317205 ) ) ;
#28418=CARTESIAN_POINT ( 'NONE',  ( 0.1532563361054100626, 25.80059781766744820, -2.638427012816831230 ) ) ;
#28419=CARTESIAN_POINT ( 'NONE',  ( 15.44008868035555793, 21.39701867748817321, -9.422509992056140149 ) ) ;
#28420=CARTESIAN_POINT ( 'NONE',  ( 4.559911319644449179, 7.230352010821505360, -9.422509992056141925 ) ) ;
#28422=CARTESIAN_POINT ( 'NONE',  ( 0.5774900079438590739, 22.64701867748817321, -5.440088680355550821 ) ) ;
#28423=CARTESIAN_POINT ( 'NONE',  ( 10.00000000000000000, 31.81368534415483751, -10.88017736071110342 ) ) ;
#28424=CARTESIAN_POINT ( 'NONE',  ( 0.2751277870542967463, 70.00000000000000000, -6.000000000000000000 ) ) ;
#28425=CARTESIAN_POINT ( 'NONE',  ( 12.91533473730992121, 39.52201867748817676, 10.88017736071110164 ) ) ;
#28427=CARTESIAN_POINT ( 'NONE',  ( 7.361572987183169658, 54.96726448433413026, -9.846743663894592657 ) ) ;
#28428=CARTESIAN_POINT ( 'NONE',  ( 12.91533473730992121, 39.52201867748817676, 10.88017736071110164 ) ) ;
#28431=CARTESIAN_POINT ( 'NONE',  ( 3.591859063236761518, 59.95696800326375353, 11.09922568453594849 ) ) ;
#28432=CARTESIAN_POINT ( 'NONE',  ( 0.2751277870542980231, 9.366073187301308778, -6.500000000000002665 ) ) ;
#28433=CARTESIAN_POINT ( 'NONE',  ( -4.164238869374099927, 37.01208216824731068, 3.795296366450308767 ) ) ;
#28434=CARTESIAN_POINT ( 'NONE',  ( 17.96484262340118221, 56.18868534415484817, -7.964842623401177768 ) ) ;
#28435=B_SPLINE_CURVE_WITH_KNOTS ( 'NONE', 3,
 ( #82305, #89809, #15323, #44797, #90798, #21829 ),
 .UNSPECIFIED., .F., .F.,
 ( 4, 2, 4 ),
 ( 0.000000000000000000, 0.0002626113303184787295, 0.0005252226606369574590 ),
 .UNSPECIFIED. ) ;
#28437=FACE_OUTER_BOUND ( 'NONE', #44516, .T. ) ;
#28438=CARTESIAN_POINT ( 'NONE',  ( 10.00000000000000178, 52.25893115100078745, 9.846743663894594434 ) ) ;
#28440=CARTESIAN_POINT ( 'NONE',  ( 17.20831665107776587, 2.883931151000785231, 7.208316651077764980 ) ) ;
#28442=CARTESIAN_POINT ( 'NONE',  ( 17.20831665107776587, 24.13393115100078035, -7.208316651077762316 ) ) ;
#28445=CARTESIAN_POINT ( 'NONE',  ( 20.88017736071110519, 25.56368534415483751, 2.639326808657452039E-16 ) ) ;
#28446=CARTESIAN_POINT ( 'NONE',  ( 14.92337183194729633, 27.67559781766745530, 8.527530157486181039 ) ) ;
#28447=CARTESIAN_POINT ( 'NONE',  ( -1.099225684535947600, 9.540301336597087456, 6.408140936763237150 ) ) ;
#28448=CARTESIAN_POINT ( 'NONE',  ( 15.44008868035555260, 54.73035201082150536, 9.422509992056143702 ) ) ;
#28449=CARTESIAN_POINT ( 'NONE',  ( 7.084665262690076126, 32.02201867748816966, -10.88017736071110164 ) ) ;
#28450=CARTESIAN_POINT ( 'NONE',  ( -1.099225684535947600, 53.70696800326376064, -6.408140936763238038 ) ) ;
#28451=CARTESIAN_POINT ( 'NONE',  ( 20.36894250292379738, 44.92874883491396787, -10.36894250292379027 ) ) ;
#28459=CARTESIAN_POINT ( 'NONE',  ( 3.591859063236763294, 3.290301336597087012, -11.09922568453595026 ) ) ;
#28460=CARTESIAN_POINT ( 'NONE',  ( 0.5774900079438607392, 8.480352010821505360, 5.440088680355550821 ) ) ;
#28461=CARTESIAN_POINT ( 'NONE',  ( 0.5774900079438590739, 47.64701867748817676, -5.440088680355550821 ) ) ;
#28462=CARTESIAN_POINT ( 'NONE',  ( 17.20831665107776587, 64.13393115100079456, -7.208316651077762316 ) ) ;
#28464=CARTESIAN_POINT ( 'NONE',  ( 10.00000000000000178, 12.25893115100078568, 9.846743663894594434 ) ) ;
#28466=CARTESIAN_POINT ( 'NONE',  ( 4.559911319644449179, 57.23035201082150536, -9.422509992056141925 ) ) ;
#28467=CARTESIAN_POINT ( 'NONE',  ( 0.1532563361054083140, 31.00893115100078390, 1.131784320476157264E-15 ) ) ;
#28468=CARTESIAN_POINT ( 'NONE',  ( 19.84674366389459266, 18.30059781766745175, 2.638427012816836559 ) ) ;
#28469=CARTESIAN_POINT ( 'NONE',  ( 1.472469842513823179, 20.59226448433411960, -4.923371831947296329 ) ) ;
#28470=CARTESIAN_POINT ( 'NONE',  ( 0.2751277870542875315, 65.30223176428830811, 6.499999999999984901 ) ) ;
#28471=CARTESIAN_POINT ( 'NONE',  ( 15.44008868035555793, 66.39701867748817676, -9.422509992056140149 ) ) ;
#28472=CARTESIAN_POINT ( 'NONE',  ( -0.1503990784575280903, 23.10158574516642815, 6.262539305110076171 ) ) ;
#28473=CARTESIAN_POINT ( 'NONE',  ( 1.472469842513823179, 30.59226448433411960, -4.923371831947296329 ) ) ;
#28476=CARTESIAN_POINT ( 'NONE',  ( 19.38216949554541557, 2.248634669930420049, -9.382169495545420901 ) ) ;
#28478=CARTESIAN_POINT ( 'NONE',  ( 2.035157376598822676, 2.438685344154837953, -7.964842623401177768 ) ) ;
#28479=CARTESIAN_POINT ( 'NONE',  ( 17.08211943468705130, 18.47041550158063572, 12.26659068614894998 ) ) ;
#28480=UNCERTAINTY_MEASURE_WITH_UNIT (LENGTH_MEASURE( 1.000000000000000082E-05 ), #90379, 'distance_accuracy_value', 'NONE');
#28483=CARTESIAN_POINT ( 'NONE',  ( 6.204703633549690345, 15.76208216824730179, -14.16423886937410259 ) ) ;
#28484=CARTESIAN_POINT ( 'NONE',  ( -0.3689425029237881626, 42.42874883491396787, 10.36894250292379027 ) ) ;
#28485=CARTESIAN_POINT ( 'NONE',  ( -4.164238869374098151, 1.595415501580634388, -3.795296366450310543 ) ) ;
#28486=CARTESIAN_POINT ( 'NONE',  ( -4.164238869374099039, 11.80374883491396965, 8.674139862899312516E-16 ) ) ;
#28488=CARTESIAN_POINT ( 'NONE',  ( 12.91533473730993009, 46.60535201082150536, -10.88017736071109987 ) ) ;
#28490=ORIENTED_EDGE ( 'NONE', *, *, #39969, .F. ) ;
#28491=CARTESIAN_POINT ( 'NONE',  ( 5.076628168052703671, 26.84226448433411960, 8.527530157486179263 ) ) ;
#28492=CARTESIAN_POINT ( 'NONE',  ( 0.5774900079438607392, 68.48035201082150536, 5.440088680355550821 ) ) ;
#28493=CARTESIAN_POINT ( 'NONE',  ( 1.472469842513823179, 25.59226448433412315, -4.923371831947296329 ) ) ;
#28494=CARTESIAN_POINT ( 'NONE',  ( 0.5774900079438607392, 8.480352010821505360, 5.440088680355550821 ) ) ;
#28495=CARTESIAN_POINT ( 'NONE',  ( 6.565887622018943937, 55.16530133659709634, 12.81628187352647430 ) ) ;
#28496=CARTESIAN_POINT ( 'NONE',  ( 12.63842701281683034, 52.46726448433413026, 9.846743663894596210 ) ) ;
#28498=CARTESIAN_POINT ( 'NONE',  ( 2.791683348922240793, 26.63393115100078745, 7.208316651077764092 ) ) ;
#28499=CARTESIAN_POINT ( 'NONE',  ( -1.099225684535947600, 43.70696800326375353, -6.408140936763238038 ) ) ;
#28501=CARTESIAN_POINT ( 'NONE',  ( 12.91533473730993009, 41.60535201082149825, -10.88017736071109987 ) ) ;
#28502=CARTESIAN_POINT ( 'NONE',  ( 19.84674366389459266, 38.71726448433412315, -2.638427012816827677 ) ) ;
#28503=CARTESIAN_POINT ( 'NONE',  ( 10.00000000000000000, 25.55374883491396787, -14.16423886937410082 ) ) ;
#28505=CARTESIAN_POINT ( 'NONE',  ( -2.266590686148945544, 6.387082168247300906, -7.082119434687050408 ) ) ;
#28506=CARTESIAN_POINT ( 'NONE',  ( 10.00000000000000000, 46.81368534415484106, -10.88017736071110342 ) ) ;
#28507=CARTESIAN_POINT ( 'NONE',  ( 20.88017736071110164, 65.35535201082150536, 2.915334737309930979 ) ) ;
#28508=CARTESIAN_POINT ( 'NONE',  ( 24.16423886937410614, 49.30374883491396787, 8.672049930838204340E-16 ) ) ;
#28509=CARTESIAN_POINT ( 'NONE',  ( 17.20831665107776587, 62.88393115100078745, 7.208316651077764980 ) ) ;
#28511=CARTESIAN_POINT ( 'NONE',  ( 20.88017736071110875, 60.77201867748817676, -2.915334737309920765 ) ) ;
#28513=CARTESIAN_POINT ( 'NONE',  ( 19.38216949554541557, 22.24863466993041428, -9.382169495545420901 ) ) ;
#28514=CARTESIAN_POINT ( 'NONE',  ( 18.52753015748618282, 63.92559781766745886, -4.923371831947291888 ) ) ;
#28516=CARTESIAN_POINT ( 'NONE',  ( 4.559911319644449179, 18.89701867748817321, 9.422509992056141925 ) ) ;
#28517=CARTESIAN_POINT ( 'NONE',  ( 19.42250999205614548, 5.980352010821504471, -5.440088680355545492 ) ) ;
#28520=CARTESIAN_POINT ( 'NONE',  ( 20.88017736071110164, 5.355352010821502695, 2.915334737309930979 ) ) ;
#28521=EDGE_CURVE ( 'NONE', #24774, #3863, #30174, .T. ) ;
#28523=CARTESIAN_POINT ( 'NONE',  ( 1.472469842513823179, 6.425597817667451750, 4.923371831947296329 ) ) ;
#28524=CARTESIAN_POINT ( 'NONE',  ( 2.791683348922237240, 35.38393115100079456, -7.208316651077763204 ) ) ;
#28525=CARTESIAN_POINT ( 'NONE',  ( 17.96484262340118221, 41.18868534415484106, -7.964842623401177768 ) ) ;
#28526=CARTESIAN_POINT ( 'NONE',  ( 6.565887622018943937, 3.081968003263753531, -12.81628187352647608 ) ) ;
#28527=CARTESIAN_POINT ( 'NONE',  ( 10.00000000000000178, 39.31368534415484106, 10.88017736071110342 ) ) ;
#28529=CARTESIAN_POINT ( 'NONE',  ( 13.43411237798105340, 55.58196800326374643, 12.81628187352647963 ) ) ;
#28531=CARTESIAN_POINT ( 'NONE',  ( -0.8801773607110991993, 62.85535201082150536, -2.915334737309923874 ) ) ;
#28532=CARTESIAN_POINT ( 'NONE',  ( -2.816281873526473856, 29.12363466993041783, 9.499525473075851096E-16 ) ) ;
#28533=CARTESIAN_POINT ( 'NONE',  ( 17.08211943468705130, 8.470415501580635720, 12.26659068614894998 ) ) ;
#28534=CARTESIAN_POINT ( 'NONE',  ( 1.472469842513823179, 1.425597817667451528, 4.923371831947296329 ) ) ;
#28535=CARTESIAN_POINT ( 'NONE',  ( -0.8801773607111008646, 38.27201867748816255, 2.915334737309923430 ) ) ;
#28537=CARTESIAN_POINT ( 'NONE',  ( -4.164238869374098151, 61.59541550158063217, -3.795296366450310543 ) ) ;
#28538=CARTESIAN_POINT ( 'NONE',  ( 17.20831665107776587, 59.13393115100078745, -7.208316651077762316 ) ) ;
#28539=CARTESIAN_POINT ( 'NONE',  ( 14.92337183194729988, 19.34226448433411960, -8.527530157486177487 ) ) ;
#28541=CARTESIAN_POINT ( 'NONE',  ( 2.035157376598824452, 68.68868534415484817, 7.964842623401179544 ) ) ;
#28543=CARTESIAN_POINT ( 'NONE',  ( 22.26659068614895176, 34.72041550158063927, -7.082119434687042414 ) ) ;
#28545=LINE ( 'NONE', #89542, #5863 ) ;
#28547=CARTESIAN_POINT ( 'NONE',  ( 19.67388390623025529, 87.39738367702956623, -5.439653449514034733 ) ) ;
#28549=CARTESIAN_POINT ( 'NONE',  ( -4.164238869374099927, 57.01208216824731068, 3.795296366450308767 ) ) ;
#28550=CARTESIAN_POINT ( 'NONE',  ( 2.035157376598824452, 3.688685344154837953, 7.964842623401179544 ) ) ;
#28551=CARTESIAN_POINT ( 'NONE',  ( 19.84674366389459621, 33.50893115100078745, 7.409399052514197653E-17 ) ) ;
#28553=CARTESIAN_POINT ( 'NONE',  ( -0.2418659066527630297, 43.09014588040357552, 6.114288769123057854 ) ) ;
#28554=CARTESIAN_POINT ( 'NONE',  ( 2.035157376598822676, 12.43868534415483751, -7.964842623401177768 ) ) ;
#28555=CARTESIAN_POINT ( 'NONE',  ( -4.164238869374099927, 57.01208216824731068, 3.795296366450308767 ) ) ;
#28556=CARTESIAN_POINT ( 'NONE',  ( 18.52753015748617571, 33.09226448433411605, 4.923371831947298993 ) ) ;
#28557=CARTESIAN_POINT ( 'NONE',  ( 13.99999999999999822, 60.50000000000000000, 5.000000000000000000 ) ) ;
#28558=CARTESIAN_POINT ( 'NONE',  ( 19.84674366389459266, 3.300597817667451750, 2.638427012816836559 ) ) ;
#28559=CARTESIAN_POINT ( 'NONE',  ( 18.04007052943773104, 4.002578601053487617, -5.767676674365832312 ) ) ;
#28561=VERTEX_POINT ( 'NONE', #66711 ) ;
#28565=CARTESIAN_POINT ( 'NONE',  ( 12.63842701281683034, 42.46726448433412315, 9.846743663894596210 ) ) ;
#28566=CARTESIAN_POINT ( 'NONE',  ( 10.00000000000000178, 18.05374883491396787, 14.16423886937410082 ) ) ;
#28567=CARTESIAN_POINT ( 'NONE',  ( 0.5774900079438590739, 17.64701867748817321, -5.440088680355550821 ) ) ;
#28568=CARTESIAN_POINT ( 'NONE',  ( 2.035157376598824452, 28.68868534415484106, 7.964842623401179544 ) ) ;
#28569=CARTESIAN_POINT ( 'NONE',  ( 14.92337183194729633, 57.67559781766745886, 8.527530157486181039 ) ) ;
#28570=CARTESIAN_POINT ( 'NONE',  ( 3.591859063236763294, 18.29030133659708568, -11.09922568453595026 ) ) ;
#28571=CARTESIAN_POINT ( 'NONE',  ( -2.266590686148945544, 2.220415501580634388, 7.082119434687048631 ) ) ;
#28573=CARTESIAN_POINT ( 'NONE',  ( 16.40814093676324603, 37.45696800326376064, -11.09922568453594671 ) ) ;
#28576=CARTESIAN_POINT ( 'NONE',  ( 7.361572987183170547, 27.05059781766745175, 9.846743663894590881 ) ) ;
#28577=CARTESIAN_POINT ( 'NONE',  ( 4.559911319644449179, 3.897018677488171434, 9.422509992056141925 ) ) ;
#28579=CARTESIAN_POINT ( 'NONE',  ( 10.00000000000000178, 68.05374883491397497, 14.16423886937410082 ) ) ;
#28580=ORIENTED_EDGE ( 'NONE', *, *, #73737, .T. ) ;
#28581=CARTESIAN_POINT ( 'NONE',  ( 10.00000000000000178, 44.31368534415484106, 10.88017736071110342 ) ) ;
#28582=CARTESIAN_POINT ( 'NONE',  ( 2.035157376598822676, 62.43868534415483396, -7.964842623401177768 ) ) ;
#28584=CARTESIAN_POINT ( 'NONE',  ( 2.035157376598824452, 53.68868534415484817, 7.964842623401179544 ) ) ;
#28585=CARTESIAN_POINT ( 'NONE',  ( 7.084665262690076126, 37.02201867748817676, -10.88017736071110164 ) ) ;
#28586=CARTESIAN_POINT ( 'NONE',  ( -1.926860441876562025, 29.47997603579417358, -3.195792623639529761 ) ) ;
#28587=STYLED_ITEM ( 'NONE', ( #84534 ), #60633 ) ;
#28590=CARTESIAN_POINT ( 'NONE',  ( 5.076628168052704559, 35.17559781766745175, -8.527530157486179263 ) ) ;
#28592=CARTESIAN_POINT ( 'NONE',  ( 19.84674366389459621, 58.50893115100078745, 7.409399052514197653E-17 ) ) ;
#28593=CARTESIAN_POINT ( 'NONE',  ( 20.15039907845753220, 40.60158574516643171, -6.262539305110077947 ) ) ;
#28595=CARTESIAN_POINT ( 'NONE',  ( -4.164238869374099927, 7.012082168247302683, 3.795296366450308767 ) ) ;
#28597=CARTESIAN_POINT ( 'NONE',  ( 19.39188664607695856, 50.83703382326398668, -6.499999999999941380 ) ) ;
#28599=CARTESIAN_POINT ( 'NONE',  ( 0.1532563361054082862, 36.21726448433410894, 2.638427012816831674 ) ) ;
#28600=CARTESIAN_POINT ( 'NONE',  ( 17.08211943468705130, 58.47041550158063927, 12.26659068614894998 ) ) ;
#28604=CARTESIAN_POINT ( 'NONE',  ( 12.63842701281683922, 49.55059781766744464, -9.846743663894590881 ) ) ;
#28606=CARTESIAN_POINT ( 'NONE',  ( 3.591859063236761518, 24.95696800326375353, 11.09922568453594849 ) ) ;
#28607=CARTESIAN_POINT ( 'NONE',  ( 5.076628168052703671, 6.842264484334118713, 8.527530157486179263 ) ) ;
#28608=CYLINDRICAL_SURFACE ( 'NONE', #32948, 11.92686044187656513 ) ;
#28609=CARTESIAN_POINT ( 'NONE',  ( 19.84674366389459621, 13.50893115100078568, 7.409399052514197653E-17 ) ) ;
#28610=CARTESIAN_POINT ( 'NONE',  ( 10.00000000000000000, 7.873634669930421381, -12.81628187352647608 ) ) ;
#28615=CARTESIAN_POINT ( 'NONE',  ( 19.42250999205614548, 10.98035201082150536, -5.440088680355545492 ) ) ;
#28616=CARTESIAN_POINT ( 'NONE',  ( 20.36894250292379738, 9.928748834913966093, -10.36894250292379027 ) ) ;
#28617=CARTESIAN_POINT ( 'NONE',  ( 7.361572987183169658, 24.96726448433412315, -9.846743663894592657 ) ) ;
#28618=CARTESIAN_POINT ( 'NONE',  ( 10.00000000000000178, 59.31368534415484106, 10.88017736071110342 ) ) ;
#28619=CARTESIAN_POINT ( 'NONE',  ( 3.591859063236763294, 33.29030133659708213, -11.09922568453595026 ) ) ;
#28621=CARTESIAN_POINT ( 'NONE',  ( 17.96484262340118221, 19.93868534415484106, 7.964842623401181321 ) ) ;
#28624=CARTESIAN_POINT ( 'NONE',  ( 5.076628168052704559, 60.17559781766745175, -8.527530157486179263 ) ) ;
#28625=CARTESIAN_POINT ( 'NONE',  ( 19.84674366389459266, 13.30059781766745353, 2.638427012816836559 ) ) ;
#28627=CARTESIAN_POINT ( 'NONE',  ( 22.81628187352648496, 31.83196800326375353, -3.434112377981050290 ) ) ;
#28628=CARTESIAN_POINT ( 'NONE',  ( 1.821708436314909196, 51.66792564121896447, -6.499999999999929834 ) ) ;
#28629=CARTESIAN_POINT ( 'NONE',  ( 20.88017736071110164, 35.35535201082150536, 2.915334737309930979 ) ) ;
#28632=CARTESIAN_POINT ( 'NONE',  ( 19.42250999205614193, 25.14701867748817321, 5.440088680355555262 ) ) ;
#28633=CARTESIAN_POINT ( 'NONE',  ( 17.96484262340118221, 34.93868534415482685, 7.964842623401181321 ) ) ;
#28634=CARTESIAN_POINT ( 'NONE',  ( 7.361572987183169658, 49.96726448433410894, -9.846743663894592657 ) ) ;
#28635=CARTESIAN_POINT ( 'NONE',  ( 17.96484262340118221, 54.93868534415484106, 7.964842623401181321 ) ) ;
#28636=CARTESIAN_POINT ( 'NONE',  ( 2.917880565312948704, 37.63708216824731068, 12.26659068614894643 ) ) ;
#28637=CARTESIAN_POINT ( 'NONE',  ( 12.63842701281683922, 39.55059781766744464, -9.846743663894590881 ) ) ;
#28638=FACE_OUTER_BOUND ( 'NONE', #52712, .T. ) ;
#28639=CARTESIAN_POINT ( 'NONE',  ( 3.591859063236763294, 3.290301336597087012, -11.09922568453595026 ) ) ;
#28641=CARTESIAN_POINT ( 'NONE',  ( 12.91533473730992121, 19.52201867748816611, 10.88017736071110164 ) ) ;
#28643=CARTESIAN_POINT ( 'NONE',  ( 7.084665262690076126, 17.02201867748817676, -10.88017736071110164 ) ) ;
#28644=CARTESIAN_POINT ( 'NONE',  ( 19.42250999205614193, 65.14701867748817676, 5.440088680355555262 ) ) ;
#28645=CARTESIAN_POINT ( 'NONE',  ( 6.204703633549690345, 22.84541550158062861, 14.16423886937410082 ) ) ;
#28647=CARTESIAN_POINT ( 'NONE',  ( 7.361572987183169658, 14.96726448433411960, -9.846743663894592657 ) ) ;
#28648=CARTESIAN_POINT ( 'NONE',  ( 0.1532563361054082862, 66.21726448433413736, 2.638427012816831674 ) ) ;
#28649=CARTESIAN_POINT ( 'NONE',  ( 4.559911319644449179, 48.89701867748817676, 9.422509992056141925 ) ) ;
#28651=CARTESIAN_POINT ( 'NONE',  ( 20.00000000000000000, 0.000000000000000000, 5.000000000000000000 ) ) ;
#28655=CARTESIAN_POINT ( 'NONE',  ( 1.472469842513823179, 45.59226448433412315, -4.923371831947296329 ) ) ;
#28659=CARTESIAN_POINT ( 'NONE',  ( 24.16423886937410614, 24.30374883491396787, 8.672049930838204340E-16 ) ) ;
#28660=CARTESIAN_POINT ( 'NONE',  ( -4.164238869374098151, 21.59541550158063217, -3.795296366450310543 ) ) ;
#28661=CARTESIAN_POINT ( 'NONE',  ( 19.42250999205614193, 60.14701867748817676, 5.440088680355555262 ) ) ;
#28662=CARTESIAN_POINT ( 'NONE',  ( 20.36894250292379738, 49.92874883491396787, -10.36894250292379027 ) ) ;
#28663=CARTESIAN_POINT ( 'NONE',  ( 7.361572987183169658, 64.96726448433412315, -9.846743663894592657 ) ) ;
#28664=CARTESIAN_POINT ( 'NONE',  ( 2.791683348922237240, 45.38393115100079456, -7.208316651077763204 ) ) ;
#28666=CARTESIAN_POINT ( 'NONE',  ( 20.88017736071110875, 50.77201867748817676, -2.915334737309920765 ) ) ;
#28667=CARTESIAN_POINT ( 'NONE',  ( 16.40814093676324603, 7.456968003263754419, -11.09922568453594671 ) ) ;
#28668=CARTESIAN_POINT ( 'NONE',  ( 2.917880565312950480, 20.97041550158063217, -12.26659068614894821 ) ) ;
#28669=CARTESIAN_POINT ( 'NONE',  ( 17.08211943468705840, 55.13708216824731068, -12.26659068614894466 ) ) ;
#28670=CARTESIAN_POINT ( 'NONE',  ( -0.8801773607110991993, 17.85535201082150536, -2.915334737309923874 ) ) ;
#28671=B_SPLINE_CURVE_WITH_KNOTS ( 'NONE', 3,
 ( #97182, #14159, #75136, #37159 ),
 .UNSPECIFIED., .F., .F.,
 ( 4, 4 ),
 ( 6.254634441385501671E-17, 0.001060528352562000462 ),
 .UNSPECIFIED. ) ;
#28672=CARTESIAN_POINT ( 'NONE',  ( 20.32896413005680714, 5.578790035174471029, -5.963430220938276349 ) ) ;
#28673=CARTESIAN_POINT ( 'NONE',  ( 0.5774900079438590739, 47.64701867748817676, -5.440088680355550821 ) ) ;
#28678=ORIENTED_EDGE ( 'NONE', *, *, #44876, .F. ) ;
#28679=CARTESIAN_POINT ( 'NONE',  ( 22.26659068614895176, 39.72041550158063217, -7.082119434687042414 ) ) ;
#28680=CARTESIAN_POINT ( 'NONE',  ( 18.52753015748617571, 48.09226448433412315, 4.923371831947298993 ) ) ;
#28683=CARTESIAN_POINT ( 'NONE',  ( 4.559911319644449179, 48.89701867748817676, 9.422509992056141925 ) ) ;
#28684=EDGE_CURVE ( 'NONE', #21166, #51739, #73115, .T. ) ;
#28685=B_SPLINE_CURVE_WITH_KNOTS ( 'NONE', 3,
 ( #47615, #33576, #10603, #32098, #33094, #48588 ),
 .UNSPECIFIED., .F., .F.,
 ( 4, 2, 4 ),
 ( 0.000000000000000000, 0.0002701661927229335471, 0.0005403323854458670942 ),
 .UNSPECIFIED. ) ;
#28686=CARTESIAN_POINT ( 'NONE',  ( 19.38216949554541202, 60.99863466993042493, 9.382169495545424454 ) ) ;
#28690=CARTESIAN_POINT ( 'NONE',  ( -0.3689425029237881626, 37.42874883491396787, 10.36894250292379027 ) ) ;
#28691=CARTESIAN_POINT ( 'NONE',  ( 21.09922568453594849, 26.20696800326375353, 6.408140936763242479 ) ) ;
#28692=ORIENTED_EDGE ( 'NONE', *, *, #18588, .F. ) ;
#28693=CARTESIAN_POINT ( 'NONE',  ( 21.09922568453594849, 41.20696800326375353, 6.408140936763242479 ) ) ;
#28695=CARTESIAN_POINT ( 'NONE',  ( 0.1532563361054083140, 36.00893115100078745, 1.131784320476157264E-15 ) ) ;
#28696=CARTESIAN_POINT ( 'NONE',  ( -0.8801773607110991993, 12.85535201082150358, -2.915334737309923874 ) ) ;
#28697=CARTESIAN_POINT ( 'NONE',  ( 16.40814093676324603, 57.45696800326375353, -11.09922568453594671 ) ) ;
#28699=CARTESIAN_POINT ( 'NONE',  ( 19.84674366389459266, 48.71726448433413026, -2.638427012816827677 ) ) ;
#28700=CARTESIAN_POINT ( 'NONE',  ( 20.24186590665277663, 21.76028685723174050, 6.114288769123037426 ) ) ;
#28701=ORIENTED_EDGE ( 'NONE', *, *, #70808, .F. ) ;
#28703=CARTESIAN_POINT ( 'NONE',  ( 19.72487221294571569, 17.80223176428831522, -6.499999999999990230 ) ) ;
#28708=CARTESIAN_POINT ( 'NONE',  ( 19.84674366389459266, 13.30059781766745353, 2.638427012816836559 ) ) ;
#28709=CARTESIAN_POINT ( 'NONE',  ( -2.816281873526471635, 28.91530133659708213, -3.434112377981056508 ) ) ;
#28711=EDGE_CURVE ( 'NONE', #56832, #19862, #91026, .T. ) ;
#28713=CARTESIAN_POINT ( 'NONE',  ( 18.52753015748618282, 53.92559781766745175, -4.923371831947291888 ) ) ;
#28715=CARTESIAN_POINT ( 'NONE',  ( 10.00000000000000000, 25.55374883491396787, -14.16423886937410082 ) ) ;
#28716=CARTESIAN_POINT ( 'NONE',  ( 18.52753015748617571, 48.09226448433412315, 4.923371831947298993 ) ) ;
#28717=CARTESIAN_POINT ( 'NONE',  ( 6.565887622018943937, 50.16530133659708213, 12.81628187352647430 ) ) ;
#28720=CARTESIAN_POINT ( 'NONE',  ( 0.1532563361054100626, 10.80059781766745175, -2.638427012816831230 ) ) ;
#28721=CARTESIAN_POINT ( 'NONE',  ( 20.15039907845753575, 47.62777174578613426, -6.262539305110073506 ) ) ;
#28722=CARTESIAN_POINT ( 'NONE',  ( 17.20831665107776587, 52.88393115100078035, 7.208316651077764980 ) ) ;
#28723=CARTESIAN_POINT ( 'NONE',  ( 20.88017736071110519, 45.56368534415484106, 2.639326808657452039E-16 ) ) ;
#28724=CARTESIAN_POINT ( 'NONE',  ( 10.00000000000000178, 32.25893115100078745, 9.846743663894594434 ) ) ;
#28727=CARTESIAN_POINT ( 'NONE',  ( 0.5774900079438590739, 42.64701867748816966, -5.440088680355550821 ) ) ;
#28728=VERTEX_POINT ( 'NONE', #46184 ) ;
#28729=CARTESIAN_POINT ( 'NONE',  ( 10.00000000000000178, 69.31368534415484817, 10.88017736071110342 ) ) ;
#28730=CARTESIAN_POINT ( 'NONE',  ( 4.559911319644449179, 13.89701867748817143, 9.422509992056141925 ) ) ;
#28731=CARTESIAN_POINT ( 'NONE',  ( 0.1532563361054083140, 51.00893115100078745, 1.131784320476157264E-15 ) ) ;
#28732=CARTESIAN_POINT ( 'NONE',  ( 2.035157376598822676, 47.43868534415484817, -7.964842623401177768 ) ) ;
#28734=CARTESIAN_POINT ( 'NONE',  ( 10.00000000000000178, 54.31368534415484106, 10.88017736071110342 ) ) ;
#28736=CARTESIAN_POINT ( 'NONE',  ( 0.5774900079438590739, 27.64701867748817676, -5.440088680355550821 ) ) ;
#28738=CARTESIAN_POINT ( 'NONE',  ( 7.361572987183169658, -0.03273551566588185635, -9.846743663894592657 ) ) ;
#28739=CARTESIAN_POINT ( 'NONE',  ( 1.472469842513823179, 20.59226448433411960, -4.923371831947296329 ) ) ;
#28740=CARTESIAN_POINT ( 'NONE',  ( 2.831191079880678085, 79.91181047996344944, 5.000000000000000000 ) ) ;
#28742=CARTESIAN_POINT ( 'NONE',  ( 19.84674366389459266, 48.71726448433413026, -2.638427012816827677 ) ) ;
#28744=CARTESIAN_POINT ( 'NONE',  ( 0.5774900079438590739, 2.647018677488171434, -5.440088680355550821 ) ) ;
#28745=CARTESIAN_POINT ( 'NONE',  ( -0.1503990784575359729, 18.10158574516642460, 6.262539305110062848 ) ) ;
#28748=CARTESIAN_POINT ( 'NONE',  ( -0.3689425029237898834, 6.178748834913968757, -10.36894250292378850 ) ) ;
#28749=CARTESIAN_POINT ( 'NONE',  ( 2.917880565312950480, 50.97041550158064638, -12.26659068614894821 ) ) ;
#28750=CARTESIAN_POINT ( 'NONE',  ( -2.816281873526473856, -0.6680319967362464695, 3.434112377981055619 ) ) ;
#28752=CARTESIAN_POINT ( 'NONE',  ( 17.96484262340118221, 14.93868534415484106, 7.964842623401181321 ) ) ;
#28753=CARTESIAN_POINT ( 'NONE',  ( 19.84674366389459266, 43.71726448433410894, -2.638427012816827677 ) ) ;
#28757=CARTESIAN_POINT ( 'NONE',  ( 5.500000000000000000, 11.00000000000000000, 5.000000000000000000 ) ) ;
#28758=CARTESIAN_POINT ( 'NONE',  ( 19.38216949554541557, 22.24863466993041428, -9.382169495545420901 ) ) ;
#28759=CARTESIAN_POINT ( 'NONE',  ( 7.361572987183170547, 22.05059781766745530, 9.846743663894590881 ) ) ;
#28760=ORIENTED_EDGE ( 'NONE', *, *, #93915, .T. ) ;
#28761=CARTESIAN_POINT ( 'NONE',  ( 19.84674366389459266, 8.300597817667451750, 2.638427012816836559 ) ) ;
#28764=CARTESIAN_POINT ( 'NONE',  ( 2.035157376598824452, 18.68868534415484106, 7.964842623401179544 ) ) ;
#28765=CARTESIAN_POINT ( 'NONE',  ( 6.204703633549690345, 37.84541550158063927, 14.16423886937410082 ) ) ;
#28766=CARTESIAN_POINT ( 'NONE',  ( 10.00000000000000000, 66.81368534415484817, -10.88017736071110342 ) ) ;
#28768=CARTESIAN_POINT ( 'NONE',  ( 17.20831665107776587, 19.13393115100078035, -7.208316651077762316 ) ) ;
#28769=CARTESIAN_POINT ( 'NONE',  ( 12.63842701281683922, 4.550597817667451750, -9.846743663894590881 ) ) ;
#28770=CARTESIAN_POINT ( 'NONE',  ( 10.00000000000000178, 42.25893115100078745, 9.846743663894594434 ) ) ;
#28771=CARTESIAN_POINT ( 'NONE',  ( 14.92337183194729988, 64.34226448433412315, -8.527530157486177487 ) ) ;
#28773=CARTESIAN_POINT ( 'NONE',  ( 15.44008868035555793, 31.39701867748817676, -9.422509992056140149 ) ) ;
#28775=CARTESIAN_POINT ( 'NONE',  ( -1.099225684535947600, 59.54030133659708923, 6.408140936763237150 ) ) ;
#28777=CARTESIAN_POINT ( 'NONE',  ( 19.84674366389459266, 3.717264484334118713, -2.638427012816827677 ) ) ;
#28778=CARTESIAN_POINT ( 'NONE',  ( 10.00000000000000000, 47.87363466993042493, -12.81628187352647608 ) ) ;
#28779=CARTESIAN_POINT ( 'NONE',  ( -4.164238869374098151, 66.59541550158060375, -3.795296366450310543 ) ) ;
#28780=CARTESIAN_POINT ( 'NONE',  ( 1.472469842513823179, 36.42559781766745175, 4.923371831947296329 ) ) ;
#28781=( NAMED_UNIT ( * ) SI_UNIT ( $, .STERADIAN. ) SOLID_ANGLE_UNIT ( ) );
#28782=( NAMED_UNIT ( * ) SI_UNIT ( $, .STERADIAN. ) SOLID_ANGLE_UNIT ( ) );
#28783=CARTESIAN_POINT ( 'NONE',  ( 22.26659068614895176, 19.72041550158063572, -7.082119434687042414 ) ) ;
#28784=CARTESIAN_POINT ( 'NONE',  ( 22.26659068614895176, 49.72041550158063927, -7.082119434687042414 ) ) ;
#28785=CARTESIAN_POINT ( 'NONE',  ( 17.20831665107776587, 49.13393115100078745, -7.208316651077762316 ) ) ;
#28787=CARTESIAN_POINT ( 'NONE',  ( 2.035157376598824452, 33.68868534415484106, 7.964842623401179544 ) ) ;
#28788=CARTESIAN_POINT ( 'NONE',  ( 15.44008868035555793, 66.39701867748817676, -9.422509992056140149 ) ) ;
#28791=CARTESIAN_POINT ( 'NONE',  ( -1.099225684535947600, 63.70696800326376774, -6.408140936763238038 ) ) ;
#28792=CARTESIAN_POINT ( 'NONE',  ( 17.96484262340118221, 64.93868534415483396, 7.964842623401181321 ) ) ;
#28794=CARTESIAN_POINT ( 'NONE',  ( 18.52753015748618282, 3.925597817667451306, -4.923371831947291888 ) ) ;
#28795=CARTESIAN_POINT ( 'NONE',  ( -46.31228368244003946, 103.3337736655113588, -5.775421524742657020 ) ) ;
#28798=CARTESIAN_POINT ( 'NONE',  ( 17.96484262340118221, 9.938685344154837509, 7.964842623401181321 ) ) ;
#28802=CARTESIAN_POINT ( 'NONE',  ( 20.88017736071110164, 20.35535201082150891, 2.915334737309930979 ) ) ;
#28804=CARTESIAN_POINT ( 'NONE',  ( 0.1532563361054082862, 56.21726448433411605, 2.638427012816831674 ) ) ;
#28807=CARTESIAN_POINT ( 'NONE',  ( 5.076628168052703671, 66.84226448433412315, 8.527530157486179263 ) ) ;
#28809=CARTESIAN_POINT ( 'NONE',  ( 5.076628168052704559, 0.1755978176674514724, -8.527530157486179263 ) ) ;
#28810=CARTESIAN_POINT ( 'NONE',  ( 12.63842701281683034, 62.46726448433410894, 9.846743663894596210 ) ) ;
#28811=CARTESIAN_POINT ( 'NONE',  ( 4.559911319644449179, 22.23035201082150536, -9.422509992056141925 ) ) ;
#28813=CARTESIAN_POINT ( 'NONE',  ( 1.472469842513823179, 5.592264484334118713, -4.923371831947296329 ) ) ;
#28815=CARTESIAN_POINT ( 'NONE',  ( 12.91533473730992121, 19.52201867748816611, 10.88017736071110164 ) ) ;
#28816=CARTESIAN_POINT ( 'NONE',  ( 3.591859063236761518, 49.95696800326375353, 11.09922568453594849 ) ) ;
#28817=CARTESIAN_POINT ( 'NONE',  ( 0.5774900079438607392, 48.48035201082150536, 5.440088680355550821 ) ) ;
#28819=CARTESIAN_POINT ( 'NONE',  ( -1.099225684535947600, 59.54030133659708923, 6.408140936763237150 ) ) ;
#28820=CARTESIAN_POINT ( 'NONE',  ( 20.88017736071110519, 50.56368534415484106, 2.639326808657452039E-16 ) ) ;
#28821=CARTESIAN_POINT ( 'NONE',  ( 14.92337183194729633, 52.67559781766745175, 8.527530157486181039 ) ) ;
#28822=CARTESIAN_POINT ( 'NONE',  ( 18.52753015748617571, 23.09226448433411960, 4.923371831947298993 ) ) ;
#28823=CARTESIAN_POINT ( 'NONE',  ( 22.81628187352647785, 6.623634669930420493, 6.195893100308588602E-16 ) ) ;
#28825=CARTESIAN_POINT ( 'NONE',  ( 1.472469842513823179, 61.42559781766745175, 4.923371831947296329 ) ) ;
#28826=CARTESIAN_POINT ( 'NONE',  ( 20.88017736071110875, 25.77201867748816966, -2.915334737309920765 ) ) ;
#28827=CARTESIAN_POINT ( 'NONE',  ( 1.472469842513823179, 56.42559781766745886, 4.923371831947296329 ) ) ;
#28829=CARTESIAN_POINT ( 'NONE',  ( 12.63842701281683922, 9.550597817667449974, -9.846743663894590881 ) ) ;
#28831=CARTESIAN_POINT ( 'NONE',  ( 6.565887622018943937, 5.165301336597086568, 12.81628187352647430 ) ) ;
#28834=CARTESIAN_POINT ( 'NONE',  ( 22.81628187352647785, 41.62363466993042493, 6.195893100308588602E-16 ) ) ;
#28835=CARTESIAN_POINT ( 'NONE',  ( 0.1532563361054100626, 30.80059781766744820, -2.638427012816831230 ) ) ;
#28837=CARTESIAN_POINT ( 'NONE',  ( -0.8801773607111009756, 8.063685344154837509, 1.068504757029289695E-15 ) ) ;
#28838=CARTESIAN_POINT ( 'NONE',  ( 2.791683348922237240, 25.38393115100078390, -7.208316651077763204 ) ) ;
#28840=CARTESIAN_POINT ( 'NONE',  ( 10.00000000000000178, 68.05374883491397497, 14.16423886937410082 ) ) ;
#28842=CARTESIAN_POINT ( 'NONE',  ( 0.5774900079438590739, 17.64701867748817321, -5.440088680355550821 ) ) ;
#28843=CARTESIAN_POINT ( 'NONE',  ( 22.26659068614895176, 49.72041550158063927, -7.082119434687042414 ) ) ;
#28844=CARTESIAN_POINT ( 'NONE',  ( 22.26659068614894466, 53.88708216824731068, 7.082119434687054849 ) ) ;
#28847=CARTESIAN_POINT ( 'NONE',  ( 5.076628168052704559, 10.17559781766745175, -8.527530157486179263 ) ) ;
#28848=CARTESIAN_POINT ( 'NONE',  ( 0.6178305044545838731, 4.748634669930420493, 9.382169495545420901 ) ) ;
#28849=ORIENTED_EDGE ( 'NONE', *, *, #31158, .T. ) ;
#28850=CARTESIAN_POINT ( 'NONE',  ( -46.34323875807881166, 103.6109741468810483, 6.190393423093142999 ) ) ;
#28851=CARTESIAN_POINT ( 'NONE',  ( 5.076628168052703671, 56.84226448433412315, 8.527530157486179263 ) ) ;
#28854=CARTESIAN_POINT ( 'NONE',  ( 24.16423886937409904, 4.095415501580634832, 3.795296366450317205 ) ) ;
#28856=CARTESIAN_POINT ( 'NONE',  ( 17.20831665107776587, 24.13393115100078035, -7.208316651077762316 ) ) ;
#28859=CARTESIAN_POINT ( 'NONE',  ( -0.3689425029237881626, 42.42874883491396787, 10.36894250292379027 ) ) ;
#28860=CARTESIAN_POINT ( 'NONE',  ( 7.361572987183169658, 9.967264484334119601, -9.846743663894592657 ) ) ;
#28862=FACE_OUTER_BOUND ( 'NONE', #80753, .T. ) ;
#28863=CARTESIAN_POINT ( 'NONE',  ( -0.8801773607111009756, 33.06368534415484106, 1.068504757029289695E-15 ) ) ;
#28864=CARTESIAN_POINT ( 'NONE',  ( -1.099225684535947600, 33.70696800326375353, -6.408140936763238038 ) ) ;
#28865=SURFACE_STYLE_FILL_AREA ( #66378 ) ;
#28867=CARTESIAN_POINT ( 'NONE',  ( 13.43411237798106583, 37.66530133659708923, -12.81628187352647252 ) ) ;
#28868=CARTESIAN_POINT ( 'NONE',  ( -2.816281873526471635, 58.91530133659707502, -3.434112377981056508 ) ) ;
#28872=CARTESIAN_POINT ( 'NONE',  ( 6.204703633549690345, 42.84541550158063217, 14.16423886937410082 ) ) ;
#28873=CARTESIAN_POINT ( 'NONE',  ( 0.5774900079438607392, 3.480352010821504027, 5.440088680355550821 ) ) ;
#28874=CARTESIAN_POINT ( 'NONE',  ( 7.084665262690076126, 17.02201867748817676, -10.88017736071110164 ) ) ;
#28875=DIRECTION ( 'NONE',  ( 0.9970872288863209532, 0.07626964003977952655, -0.000000000000000000 ) ) ;
#28876=CARTESIAN_POINT ( 'NONE',  ( 19.72487221294570858, 70.00000000000000000, 6.000000000000000000 ) ) ;
#28877=CARTESIAN_POINT ( 'NONE',  ( 12.91533473730993009, 51.60535201082149825, -10.88017736071109987 ) ) ;
#28878=CARTESIAN_POINT ( 'NONE',  ( 7.084665262690076126, 57.02201867748817676, -10.88017736071110164 ) ) ;
#28879=CARTESIAN_POINT ( 'NONE',  ( 19.38216949554541202, 10.99863466993042138, 9.382169495545424454 ) ) ;
#28881=CARTESIAN_POINT ( 'NONE',  ( 10.00000000000000178, 17.25893115100078745, 9.846743663894594434 ) ) ;
#28882=CARTESIAN_POINT ( 'NONE',  ( -0.8801773607111009756, 63.06368534415484106, 1.068504757029289695E-15 ) ) ;
#28884=CARTESIAN_POINT ( 'NONE',  ( 16.40814093676323893, 15.79030133659708746, 11.09922568453595026 ) ) ;
#28886=CARTESIAN_POINT ( 'NONE',  ( 20.88017736071110519, 5.563685344154837509, 2.639326808657452039E-16 ) ) ;
#28887=CARTESIAN_POINT ( 'NONE',  ( 12.63842701281683922, 44.55059781766745175, -9.846743663894590881 ) ) ;
#28888=CARTESIAN_POINT ( 'NONE',  ( -1.099225684535947600, 49.54030133659708923, 6.408140936763237150 ) ) ;
#28889=CARTESIAN_POINT ( 'NONE',  ( 1.472469842513823179, 16.42559781766745175, 4.923371831947296329 ) ) ;
#28890=CARTESIAN_POINT ( 'NONE',  ( 24.16423886937409904, 9.095415501580633943, 3.795296366450317205 ) ) ;
#28891=DIRECTION ( 'NONE',  ( -0.000000000000000000, -1.000000000000000000, 0.000000000000000000 ) ) ;
#28892=CARTESIAN_POINT ( 'NONE',  ( 17.96484262340118221, 26.18868534415483396, -7.964842623401177768 ) ) ;
#28893=DIRECTION ( 'NONE',  ( -0.000000000000000000, 1.000000000000000000, -0.000000000000000000 ) ) ;
#28894=CARTESIAN_POINT ( 'NONE',  ( -4.164238869374099927, 32.01208216824730357, 3.795296366450308767 ) ) ;
#28895=CARTESIAN_POINT ( 'NONE',  ( 1.472469842513823179, 45.59226448433412315, -4.923371831947296329 ) ) ;
#28896=CARTESIAN_POINT ( 'NONE',  ( 10.00000000000000000, 21.81368534415484106, -10.88017736071110342 ) ) ;
#28897=CARTESIAN_POINT ( 'NONE',  ( 2.035157376598822676, 12.43868534415483751, -7.964842623401177768 ) ) ;
#28900=CARTESIAN_POINT ( 'NONE',  ( 0.5774900079438607392, 28.48035201082150891, 5.440088680355550821 ) ) ;
#28901=CIRCLE ( 'NONE', #32118, 0.5000000000000004441 ) ;
#28902=CARTESIAN_POINT ( 'NONE',  ( 19.38216949554541202, 40.99863466993042493, 9.382169495545424454 ) ) ;
#28903=CARTESIAN_POINT ( 'NONE',  ( -0.8801773607111008646, 28.27201867748817321, 2.915334737309923430 ) ) ;
#28904=CARTESIAN_POINT ( 'NONE',  ( 0.5774900079438590739, 37.64701867748817676, -5.440088680355550821 ) ) ;
#28906=CARTESIAN_POINT ( 'NONE',  ( 17.20831665107776587, 54.13393115100079456, -7.208316651077762316 ) ) ;
#28907=CARTESIAN_POINT ( 'NONE',  ( 17.96484262340118221, 31.18868534415483751, -7.964842623401177768 ) ) ;
#28908=CARTESIAN_POINT ( 'NONE',  ( 0.1532563361054100626, 65.80059781766745175, -2.638427012816831230 ) ) ;
#28912=CARTESIAN_POINT ( 'NONE',  ( 10.00000000000000178, 53.05374883491396787, 14.16423886937410082 ) ) ;
#28913=CARTESIAN_POINT ( 'NONE',  ( -0.8801773607111009756, 58.06368534415484106, 1.068504757029289695E-15 ) ) ;
#28915=( BOUNDED_CURVE ( )  B_SPLINE_CURVE ( 2, ( #77962, #93954, #23995, #9469, #25480, #10457, #40966, #61968, #71464 ),
 .UNSPECIFIED., .F., .F. ) 
 B_SPLINE_CURVE_WITH_KNOTS ( ( 3, 2, 2, 2, 3 ),
 ( 0.1544266512259456492, 0.1547619047619047672, 0.1607142857142856984, 0.1666666666666666297, 0.1670019202026257477 ),
 .UNSPECIFIED. ) 
 CURVE ( )  GEOMETRIC_REPRESENTATION_ITEM ( )  RATIONAL_B_SPLINE_CURVE ( ( 0.9963778908391762723, 0.9980808541467921513, 1.000000000000000000, 0.9659258262890683122, 1.000000000000000000, 0.9659258262890683122, 1.000000000000000000, 0.9980808541467922623, 0.9963778908391764944 ) ) 
 REPRESENTATION_ITEM ( '' )  );
#28917=CARTESIAN_POINT ( 'NONE',  ( 12.63842701281683922, 64.55059781766745175, -9.846743663894590881 ) ) ;
#28918=CARTESIAN_POINT ( 'NONE',  ( 10.00000000000000000, 14.75893115100078568, -9.846743663894594434 ) ) ;
#28920=ORIENTED_EDGE ( 'NONE', *, *, #78578, .F. ) ;
#28921=CARTESIAN_POINT ( 'NONE',  ( 1.472469842513823179, 26.42559781766745175, 4.923371831947296329 ) ) ;
#28923=CARTESIAN_POINT ( 'NONE',  ( 0.5774900079438590739, 22.64701867748817321, -5.440088680355550821 ) ) ;
#28924=CARTESIAN_POINT ( 'NONE',  ( 19.84674366389459266, 23.30059781766745530, 2.638427012816836559 ) ) ;
#28925=CARTESIAN_POINT ( 'NONE',  ( 19.42250999205614548, 65.98035201082151957, -5.440088680355545492 ) ) ;
#28926=CARTESIAN_POINT ( 'NONE',  ( 17.96484262340118221, 59.93868534415484106, 7.964842623401181321 ) ) ;
#28927=CARTESIAN_POINT ( 'NONE',  ( 19.42250999205614548, 30.98035201082150536, -5.440088680355545492 ) ) ;
#28928=CARTESIAN_POINT ( 'NONE',  ( 16.40814093676324603, 52.45696800326375353, -11.09922568453594671 ) ) ;
#28929=CARTESIAN_POINT ( 'NONE',  ( 2.917880565312950480, 40.97041550158063217, -12.26659068614894821 ) ) ;
#28933=CARTESIAN_POINT ( 'NONE',  ( 19.38216949554541202, 5.998634669930420493, 9.382169495545424454 ) ) ;
#28934=CARTESIAN_POINT ( 'NONE',  ( 12.91533473730993009, 6.605352010821504471, -10.88017736071109987 ) ) ;
#28935=CARTESIAN_POINT ( 'NONE',  ( 4.559911319644449179, 43.89701867748816966, 9.422509992056141925 ) ) ;
#28939=CARTESIAN_POINT ( 'NONE',  ( 5.076628168052704559, 15.17559781766745175, -8.527530157486179263 ) ) ;
#28941=CARTESIAN_POINT ( 'NONE',  ( 15.44008868035555793, 61.39701867748817676, -9.422509992056140149 ) ) ;
#28943=CARTESIAN_POINT ( 'NONE',  ( 10.00000000000000178, 37.25893115100078745, 9.846743663894594434 ) ) ;
#28944=CARTESIAN_POINT ( 'NONE',  ( 17.20831665107776587, 17.88393115100078745, 7.208316651077764980 ) ) ;
#28945=CARTESIAN_POINT ( 'NONE',  ( 19.84674366389459266, 18.30059781766745175, 2.638427012816836559 ) ) ;
#28946=CARTESIAN_POINT ( 'NONE',  ( 19.72487221294571924, 62.80223176428831522, -6.499999999999984901 ) ) ;
#28947=CARTESIAN_POINT ( 'NONE',  ( -2.816281873526473856, 44.12363466993042493, 9.499525473075851096E-16 ) ) ;
#28949=CARTESIAN_POINT ( 'NONE',  ( 19.42250999205614548, 65.98035201082151957, -5.440088680355545492 ) ) ;
#28952=CARTESIAN_POINT ( 'NONE',  ( 12.63842701281683922, 34.55059781766745886, -9.846743663894590881 ) ) ;
#28953=ORIENTED_EDGE ( 'NONE', *, *, #80003, .F. ) ;
#28954=CARTESIAN_POINT ( 'NONE',  ( 21.09922568453595559, 57.04030133659708923, -6.408140936763230044 ) ) ;
#28956=CARTESIAN_POINT ( 'NONE',  ( 10.00000000000000178, 67.25893115100079456, 9.846743663894594434 ) ) ;
#28957=CARTESIAN_POINT ( 'NONE',  ( -0.8801773607111009756, 18.06368534415484106, 1.068504757029289695E-15 ) ) ;
#28958=CARTESIAN_POINT ( 'NONE',  ( -4.164238869374098151, 26.59541550158063217, -3.795296366450310543 ) ) ;
#28959=CYLINDRICAL_SURFACE ( 'NONE', #26428, 11.92686044187656513 ) ;
#28960=CARTESIAN_POINT ( 'NONE',  ( -4.164238869374099039, 36.80374883491396787, 8.674139862899312516E-16 ) ) ;
#28961=EDGE_CURVE ( 'NONE', #32737, #2953, #47388, .T. ) ;
#28962=CARTESIAN_POINT ( 'NONE',  ( 10.00000000000000000, 40.55374883491397497, -14.16423886937410082 ) ) ;
#28963=CARTESIAN_POINT ( 'NONE',  ( -2.266590686148945544, 11.38708216824730179, -7.082119434687050408 ) ) ;
#28964=CARTESIAN_POINT ( 'NONE',  ( 17.08211943468705130, 8.470415501580635720, 12.26659068614894998 ) ) ;
#28966=CARTESIAN_POINT ( 'NONE',  ( 10.00000000000000000, 46.81368534415484106, -10.88017736071110342 ) ) ;
#28969=CARTESIAN_POINT ( 'NONE',  ( 10.00000000000000000, 34.75893115100078745, -9.846743663894594434 ) ) ;
#28970=CARTESIAN_POINT ( 'NONE',  ( 3.640395162852215538, 107.5383484153110203, 5.000000000000000000 ) ) ;
#28971=CARTESIAN_POINT ( 'NONE',  ( 14.92337183194729633, 22.67559781766745175, 8.527530157486181039 ) ) ;
#28972=CARTESIAN_POINT ( 'NONE',  ( 20.88017736071110875, 15.77201867748817143, -2.915334737309920765 ) ) ;
#28973=CARTESIAN_POINT ( 'NONE',  ( 3.591859063236761518, 54.95696800326376064, 11.09922568453594849 ) ) ;
#28974=CARTESIAN_POINT ( 'NONE',  ( 19.84674366389459266, 53.71726448433411605, -2.638427012816827677 ) ) ;
#28976=CARTESIAN_POINT ( 'NONE',  ( 19.84674366389459621, 23.50893115100078390, 7.409399052514197653E-17 ) ) ;
#28977=CARTESIAN_POINT ( 'NONE',  ( 19.38216949554541557, 42.24863466993041783, -9.382169495545420901 ) ) ;
#28979=CARTESIAN_POINT ( 'NONE',  ( 7.084665262690076126, 42.02201867748816966, -10.88017736071110164 ) ) ;
#28980=CARTESIAN_POINT ( 'NONE',  ( 18.52753015748617571, 38.09226448433412315, 4.923371831947298993 ) ) ;
#28981=CARTESIAN_POINT ( 'NONE',  ( 24.16423886937410614, 24.51208216824730002, -3.795296366450302550 ) ) ;
#28983=CARTESIAN_POINT ( 'NONE',  ( 17.96484262340118221, 59.93868534415484106, 7.964842623401181321 ) ) ;
#28985=CARTESIAN_POINT ( 'NONE',  ( 2.917880565312948704, 62.63708216824730357, 12.26659068614894643 ) ) ;
#28986=CARTESIAN_POINT ( 'NONE',  ( 1.472469842513823179, 65.59226448433412315, -4.923371831947296329 ) ) ;
#28988=CARTESIAN_POINT ( 'NONE',  ( 19.42250999205614548, 50.98035201082151247, -5.440088680355545492 ) ) ;
#28990=CARTESIAN_POINT ( 'NONE',  ( 7.084665262690076126, 14.10535201082150358, 10.88017736071109987 ) ) ;
#28991=CARTESIAN_POINT ( 'NONE',  ( 2.035157376598824452, 13.68868534415483751, 7.964842623401179544 ) ) ;
#28992=CARTESIAN_POINT ( 'NONE',  ( 17.20831665107776587, 39.13393115100079456, -7.208316651077762316 ) ) ;
#28993=CARTESIAN_POINT ( 'NONE',  ( 6.565887622018943937, 55.16530133659709634, 12.81628187352647430 ) ) ;
#28996=CARTESIAN_POINT ( 'NONE',  ( 2.035157376598822676, 12.43868534415483751, -7.964842623401177768 ) ) ;
#28998=CARTESIAN_POINT ( 'NONE',  ( 6.565887622018943937, 5.165301336597086568, 12.81628187352647430 ) ) ;
#29000=CARTESIAN_POINT ( 'NONE',  ( 0.1532563361054082862, 11.21726448433411605, 2.638427012816831674 ) ) ;
#29002=CARTESIAN_POINT ( 'NONE',  ( 19.84674366389459266, 43.71726448433410894, -2.638427012816827677 ) ) ;
#29004=CARTESIAN_POINT ( 'NONE',  ( 17.96484262340118221, 29.93868534415484106, 7.964842623401181321 ) ) ;
#29005=CARTESIAN_POINT ( 'NONE',  ( -2.816281873526473856, 14.12363466993041961, 9.499525473075851096E-16 ) ) ;
#29006=CARTESIAN_POINT ( 'NONE',  ( -0.8801773607111009756, 53.06368534415484106, 1.068504757029289695E-15 ) ) ;
#29009=MECHANICAL_DESIGN_GEOMETRIC_PRESENTATION_REPRESENTATION('',(#11468),#96119);
#29010=CARTESIAN_POINT ( 'NONE',  ( 22.81628187352647785, 51.62363466993042493, 6.195893100308588602E-16 ) ) ;
#29012=CARTESIAN_POINT ( 'NONE',  ( 0.5774900079438607392, 58.48035201082151247, 5.440088680355550821 ) ) ;
#29013=CARTESIAN_POINT ( 'NONE',  ( 3.591859063236763294, 38.29030133659708923, -11.09922568453595026 ) ) ;
#29014=CARTESIAN_POINT ( 'NONE',  ( 22.26659068614894466, 8.887082168247300018, 7.082119434687054849 ) ) ;
#29015=CARTESIAN_POINT ( 'NONE',  ( -0.8801773607111009756, 43.06368534415484106, 1.068504757029289695E-15 ) ) ;
#29017=CARTESIAN_POINT ( 'NONE',  ( 1.472469842513823179, 60.59226448433412315, -4.923371831947296329 ) ) ;
#29018=CARTESIAN_POINT ( 'NONE',  ( 10.00000000000000178, 17.25893115100078745, 9.846743663894594434 ) ) ;
#29019=CARTESIAN_POINT ( 'NONE',  ( 0.1532563361054083140, 11.00893115100078568, 1.131784320476157264E-15 ) ) ;
#29020=DIRECTION ( 'NONE',  ( 0.000000000000000000, -1.000000000000000000, -0.000000000000000000 ) ) ;
#29021=CARTESIAN_POINT ( 'NONE',  ( 22.26659068614895176, 39.72041550158063217, -7.082119434687042414 ) ) ;
#29022=VECTOR ( 'NONE', #49017, 1000.000000000000114 ) ;
#29028=VERTEX_POINT ( 'NONE', #45017 ) ;
#29029=CARTESIAN_POINT ( 'NONE',  ( 24.16423886937410614, 59.30374883491397497, 8.672049930838204340E-16 ) ) ;
#29030=CARTESIAN_POINT ( 'NONE',  ( 13.79529636645031943, 65.34541550158063217, -14.16423886937409904 ) ) ;
#29031=CARTESIAN_POINT ( 'NONE',  ( 0.1532563361054100626, 35.80059781766745175, -2.638427012816831230 ) ) ;
#29033=CARTESIAN_POINT ( 'NONE',  ( -0.3289641300568009741, 42.24545670184114243, -5.963430220938281678 ) ) ;
#29034=CARTESIAN_POINT ( 'NONE',  ( 10.00000000000000178, 8.053748834913967869, 14.16423886937410082 ) ) ;
#29035=CARTESIAN_POINT ( 'NONE',  ( 7.084665262690076126, 7.022018677488169658, -10.88017736071110164 ) ) ;
#29036=CARTESIAN_POINT ( 'NONE',  ( 24.16423886937410614, 59.51208216824728936, -3.795296366450302550 ) ) ;
#29037=CARTESIAN_POINT ( 'NONE',  ( 19.84674366389459266, 33.71726448433410894, -2.638427012816827677 ) ) ;
#29039=CARTESIAN_POINT ( 'NONE',  ( 2.791683348922240793, 11.63393115100078568, 7.208316651077764092 ) ) ;
#29046=CARTESIAN_POINT ( 'NONE',  ( 17.20831665107776587, 47.88393115100078745, 7.208316651077764980 ) ) ;
#29047=CARTESIAN_POINT ( 'NONE',  ( 2.917880565312950480, 15.97041550158063217, -12.26659068614894821 ) ) ;
#29048=CARTESIAN_POINT ( 'NONE',  ( 19.42250999205614193, 20.14701867748817321, 5.440088680355555262 ) ) ;
#29049=CARTESIAN_POINT ( 'NONE',  ( 2.035157376598822676, 22.43868534415483396, -7.964842623401177768 ) ) ;
#29050=CARTESIAN_POINT ( 'NONE',  ( 7.361572987183170547, 62.05059781766745886, 9.846743663894590881 ) ) ;
#29051=CARTESIAN_POINT ( 'NONE',  ( 19.38216949554541202, 15.99863466993042138, 9.382169495545424454 ) ) ;
#29052=CARTESIAN_POINT ( 'NONE',  ( -4.164238869374098151, 6.595415501580634832, -3.795296366450310543 ) ) ;
#29054=CARTESIAN_POINT ( 'NONE',  ( 15.44008868035555793, 66.39701867748817676, -9.422509992056140149 ) ) ;
#29056=B_SPLINE_CURVE_WITH_KNOTS ( 'NONE', 3,
 ( #98908, #46365, #54345, #84858, #85345, #53871, #76853, #69366, #39849, #45882 ),
 .UNSPECIFIED., .F., .F.,
 ( 4, 3, 3, 4 ),
 ( 1.734723475976807094E-17, 0.0006253016069560725148, 0.001250604074564909364, 0.002501455912506525721 ),
 .UNSPECIFIED. ) ;
#29057=CARTESIAN_POINT ( 'NONE',  ( 19.38216949554541557, 37.24863466993041783, -9.382169495545420901 ) ) ;
#29059=CARTESIAN_POINT ( 'NONE',  ( 7.361572987183169658, 34.96726448433411605, -9.846743663894592657 ) ) ;
#29060=CARTESIAN_POINT ( 'NONE',  ( 15.44008868035555793, 11.39701867748817143, -9.422509992056140149 ) ) ;
#29062=CARTESIAN_POINT ( 'NONE',  ( 19.42250999205614193, 5.147018677488171434, 5.440088680355555262 ) ) ;
#29064=CARTESIAN_POINT ( 'NONE',  ( 4.559911319644449179, 42.23035201082151247, -9.422509992056141925 ) ) ;
#29065=CARTESIAN_POINT ( 'NONE',  ( 12.91533473730992121, 64.52201867748817676, 10.88017736071110164 ) ) ;
#29066=CARTESIAN_POINT ( 'NONE',  ( 7.084665262690076126, 69.10535201082151957, 10.88017736071109987 ) ) ;
#29068=CARTESIAN_POINT ( 'NONE',  ( 15.44008868035555260, 59.73035201082151247, 9.422509992056143702 ) ) ;
#29069=CARTESIAN_POINT ( 'NONE',  ( -0.3289641300567998083, 53.07879003517447813, 5.963430220938281678 ) ) ;
#29070=EDGE_CURVE ( 'NONE', #64436, #93697, #1494, .T. ) ;
#29073=ORIENTED_EDGE ( 'NONE', *, *, #83340, .T. ) ;
#29074=CARTESIAN_POINT ( 'NONE',  ( 17.20831665107776587, 27.88393115100078390, 7.208316651077764980 ) ) ;
#29075=ORIENTED_EDGE ( 'NONE', *, *, #98332, .F. ) ;
#29076=CARTESIAN_POINT ( 'NONE',  ( 10.00000000000000178, 62.25893115100078745, 9.846743663894594434 ) ) ;
#29078=AXIS2_PLACEMENT_3D ( 'NONE', #46305, #21841, #37341 ) ;
#29079=( GEOMETRIC_REPRESENTATION_CONTEXT ( 3 ) GLOBAL_UNCERTAINTY_ASSIGNED_CONTEXT ( ( #25358 ) ) GLOBAL_UNIT_ASSIGNED_CONTEXT ( ( #93751, #40760, #70777 ) ) REPRESENTATION_CONTEXT ( 'NONE', 'WORKASPACE' ) );
#29081=CARTESIAN_POINT ( 'NONE',  ( 10.00000000000000000, 0.5537488349139675359, -14.16423886937410082 ) ) ;
#29083=CARTESIAN_POINT ( 'NONE',  ( 15.00000000000000000, 60.50000000000000000, 6.000000000000000000 ) ) ;
#29084=CARTESIAN_POINT ( 'NONE',  ( 10.00000000000000000, 39.75893115100078745, -9.846743663894594434 ) ) ;
#29085=CARTESIAN_POINT ( 'NONE',  ( -0.8801773607110991993, 12.85535201082150358, -2.915334737309923874 ) ) ;
#29089=CARTESIAN_POINT ( 'NONE',  ( 14.92337183194729633, 52.67559781766745175, 8.527530157486181039 ) ) ;
#29091=CARTESIAN_POINT ( 'NONE',  ( 3.591859063236761518, 19.95696800326375353, 11.09922568453594849 ) ) ;
#29092=CARTESIAN_POINT ( 'NONE',  ( 5.076628168052704559, 15.17559781766745175, -8.527530157486179263 ) ) ;
#29093=FACE_OUTER_BOUND ( 'NONE', #26095, .T. ) ;
#29094=CARTESIAN_POINT ( 'NONE',  ( 12.63842701281683922, 19.55059781766745175, -9.846743663894590881 ) ) ;
#29095=CARTESIAN_POINT ( 'NONE',  ( 1.472469842513823179, 66.42559781766745175, 4.923371831947296329 ) ) ;
#29099=CARTESIAN_POINT ( 'NONE',  ( 12.91533473730992121, 14.52201867748817143, 10.88017736071110164 ) ) ;
#29100=CARTESIAN_POINT ( 'NONE',  ( -4.164238869374099927, 17.01208216824730357, 3.795296366450308767 ) ) ;
#29101=CARTESIAN_POINT ( 'NONE',  ( 0.1532563361054100626, 30.80059781766744820, -2.638427012816831230 ) ) ;
#29102=CARTESIAN_POINT ( 'NONE',  ( 15.44008868035555793, 61.39701867748817676, -9.422509992056140149 ) ) ;
#29103=CARTESIAN_POINT ( 'NONE',  ( 6.565887622018943937, 45.16530133659708923, 12.81628187352647430 ) ) ;
#29105=CARTESIAN_POINT ( 'NONE',  ( -0.8801773607111008646, 13.27201867748817143, 2.915334737309923430 ) ) ;
#29108=CARTESIAN_POINT ( 'NONE',  ( 0.6178305044545818747, -1.501365330069579951, -9.382169495545419124 ) ) ;
#29109=CARTESIAN_POINT ( 'NONE',  ( 14.92337183194729988, 29.34226448433411960, -8.527530157486177487 ) ) ;
#29111=CARTESIAN_POINT ( 'NONE',  ( 0.6178305044545818747, 38.49863466993042493, -9.382169495545419124 ) ) ;
#29113=CARTESIAN_POINT ( 'NONE',  ( 10.00000000000000000, 46.81368534415484106, -10.88017736071110342 ) ) ;
#29116=CARTESIAN_POINT ( 'NONE',  ( 4.559911319644449179, 38.89701867748817676, 9.422509992056141925 ) ) ;
#29119=CARTESIAN_POINT ( 'NONE',  ( 0.5774900079438607392, 38.48035201082150536, 5.440088680355550821 ) ) ;
#29121=CARTESIAN_POINT ( 'NONE',  ( 20.88017736071110519, 60.56368534415484106, 2.639326808657452039E-16 ) ) ;
#29124=UNCERTAINTY_MEASURE_WITH_UNIT (LENGTH_MEASURE( 1.000000000000000082E-05 ), #59871, 'distance_accuracy_value', 'NONE');
#29125=CARTESIAN_POINT ( 'NONE',  ( 7.361572987183169658, 34.96726448433411605, -9.846743663894592657 ) ) ;
#29126=CARTESIAN_POINT ( 'NONE',  ( 2.035157376598824452, 8.688685344154839285, 7.964842623401179544 ) ) ;
#29127=CARTESIAN_POINT ( 'NONE',  ( 10.00000000000000000, 17.87363466993041783, -12.81628187352647608 ) ) ;
#29128=ORIENTED_EDGE ( 'NONE', *, *, #42368, .F. ) ;
#29129=CARTESIAN_POINT ( 'NONE',  ( 0.5774900079438590739, 27.64701867748817676, -5.440088680355550821 ) ) ;
#29130=CARTESIAN_POINT ( 'NONE',  ( 18.72515096720570327, 16.07228050351031712, -6.499999999999992006 ) ) ;
#29131=CARTESIAN_POINT ( 'NONE',  ( 15.44008868035555260, 24.73035201082150891, 9.422509992056143702 ) ) ;
#29132=CARTESIAN_POINT ( 'NONE',  ( -0.8801773607111009756, 63.06368534415484106, 1.068504757029289695E-15 ) ) ;
#29133=CARTESIAN_POINT ( 'NONE',  ( 10.00000000000000000, 20.55374883491396787, -14.16423886937410082 ) ) ;
#29134=CARTESIAN_POINT ( 'NONE',  ( 17.20831665107776587, 19.13393115100078035, -7.208316651077762316 ) ) ;
#29135=CARTESIAN_POINT ( 'NONE',  ( 17.96484262340118221, 44.93868534415483396, 7.964842623401181321 ) ) ;
#29137=DIRECTION ( 'NONE',  ( -6.608470384673550777E-17, -1.000000000000000000, 0.000000000000000000 ) ) ;
#29140=CARTESIAN_POINT ( 'NONE',  ( 14.92337183194729988, 49.34226448433411605, -8.527530157486177487 ) ) ;
#29143=CARTESIAN_POINT ( 'NONE',  ( 10.00000000000000178, 23.05374883491397142, 14.16423886937410082 ) ) ;
#29144=CARTESIAN_POINT ( 'NONE',  ( 22.26659068614895176, 24.72041550158063572, -7.082119434687042414 ) ) ;
#29145=CARTESIAN_POINT ( 'NONE',  ( 20.88017736071110164, 65.35535201082150536, 2.915334737309930979 ) ) ;
#29146=CARTESIAN_POINT ( 'NONE',  ( 22.26659068614894466, 63.88708216824730357, 7.082119434687054849 ) ) ;
#29147=CARTESIAN_POINT ( 'NONE',  ( 5.076628168052704559, 65.17559781766745175, -8.527530157486179263 ) ) ;
#29148=CARTESIAN_POINT ( 'NONE',  ( 14.92337183194729988, 49.34226448433411605, -8.527530157486177487 ) ) ;
#29149=CARTESIAN_POINT ( 'NONE',  ( 10.00000000000000000, 51.81368534415484106, -10.88017736071110342 ) ) ;
#29150=CARTESIAN_POINT ( 'NONE',  ( -1.099225684535947600, 3.706968003263753531, -6.408140936763238038 ) ) ;
#29151=CARTESIAN_POINT ( 'NONE',  ( 2.917880565312950480, 15.97041550158063217, -12.26659068614894821 ) ) ;
#29152=CARTESIAN_POINT ( 'NONE',  ( 4.559911319644449179, 13.89701867748817321, 9.422509992056141925 ) ) ;
#29154=CARTESIAN_POINT ( 'NONE',  ( -0.8801773607111009756, 13.06368534415483929, 1.068504757029289695E-15 ) ) ;
#29155=AXIS2_PLACEMENT_3D ( 'NONE', #25065, #27005, #71050 ) ;
#29157=CARTESIAN_POINT ( 'NONE',  ( 2.035157376598824452, 48.68868534415483396, 7.964842623401179544 ) ) ;
#29164=ORIENTED_EDGE ( 'NONE', *, *, #98936, .T. ) ;
#29165=CARTESIAN_POINT ( 'NONE',  ( 0.1532563361054082862, 31.21726448433412315, 2.638427012816831674 ) ) ;
#29166=EDGE_LOOP ( 'NONE', ( #73609, #23930, #30669, #67153 ) ) ;
#29167=CARTESIAN_POINT ( 'NONE',  ( 3.640395162852214650, 89.00000000000000000, -9.500000000000000000 ) ) ;
#29168=CARTESIAN_POINT ( 'NONE',  ( 6.204703633549690345, 40.76208216824731778, -14.16423886937410259 ) ) ;
#29169=CARTESIAN_POINT ( 'NONE',  ( 4.559911319644449179, 8.897018677488173211, 9.422509992056141925 ) ) ;
#29170=CARTESIAN_POINT ( 'NONE',  ( 17.20831665107776587, 17.88393115100078745, 7.208316651077764980 ) ) ;
#29171=CARTESIAN_POINT ( 'NONE',  ( 0.1532563361054082862, 46.21726448433411605, 2.638427012816831674 ) ) ;
#29174=EDGE_CURVE ( 'NONE', #84535, #94230, #87512, .T. ) ;
#29176=CARTESIAN_POINT ( 'NONE',  ( 14.92337183194729988, 4.342264484334117824, -8.527530157486177487 ) ) ;
#29179=CARTESIAN_POINT ( 'NONE',  ( 20.36894250292379738, 29.92874883491396432, -10.36894250292379027 ) ) ;
#29180=CARTESIAN_POINT ( 'NONE',  ( -1.099225684535947600, 24.54030133659708923, 6.408140936763237150 ) ) ;
#29181=VERTEX_POINT ( 'NONE', #45516 ) ;
#29182=STYLED_ITEM ( 'NONE', ( #35539 ), #9315 ) ;
#29183=CARTESIAN_POINT ( 'NONE',  ( 10.00000000000000000, 42.87363466993042493, -12.81628187352647608 ) ) ;
#29184=CARTESIAN_POINT ( 'NONE',  ( 10.00000000000000178, 19.31368534415484106, 10.88017736071110342 ) ) ;
#29185=CARTESIAN_POINT ( 'NONE',  ( 17.20831665107776587, 34.13393115100078745, -7.208316651077762316 ) ) ;
#29186=CARTESIAN_POINT ( 'NONE',  ( 4.559911319644449179, 32.23035201082150536, -9.422509992056141925 ) ) ;
#29187=CARTESIAN_POINT ( 'NONE',  ( 16.40814093676324603, 62.45696800326376064, -11.09922568453594671 ) ) ;
#29189=CARTESIAN_POINT ( 'NONE',  ( 14.92337183194729988, 49.34226448433411605, -8.527530157486177487 ) ) ;
#29190=CARTESIAN_POINT ( 'NONE',  ( 0.1532563361054083140, 56.00893115100078745, 1.131784320476157264E-15 ) ) ;
#29195=DIRECTION ( 'NONE',  ( 0.000000000000000000, 0.000000000000000000, -1.000000000000000000 ) ) ;
#29197=CARTESIAN_POINT ( 'NONE',  ( 0.1532563361054083140, 16.00893115100078390, 1.131784320476157264E-15 ) ) ;
#29198=CARTESIAN_POINT ( 'NONE',  ( -1.099225684535947600, 33.70696800326375353, -6.408140936763238038 ) ) ;
#29201=CARTESIAN_POINT ( 'NONE',  ( 19.84674366389459621, 53.50893115100078745, 7.409399052514197653E-17 ) ) ;
#29203=CARTESIAN_POINT ( 'NONE',  ( 12.63842701281683922, 44.55059781766745175, -9.846743663894590881 ) ) ;
#29204=CARTESIAN_POINT ( 'NONE',  ( 17.08211943468705840, 40.13708216824731068, -12.26659068614894466 ) ) ;
#29205=CARTESIAN_POINT ( 'NONE',  ( 5.076628168052704559, 45.17559781766745175, -8.527530157486179263 ) ) ;
#29206=CARTESIAN_POINT ( 'NONE',  ( 21.09922568453594849, 41.20696800326375353, 6.408140936763242479 ) ) ;
#29209=CARTESIAN_POINT ( 'NONE',  ( 12.63842701281683922, 9.550597817667449974, -9.846743663894590881 ) ) ;
#29212=CARTESIAN_POINT ( 'NONE',  ( 10.00000000000000178, 47.25893115100078745, 9.846743663894594434 ) ) ;
#29213=CARTESIAN_POINT ( 'NONE',  ( 15.44008868035555260, 39.73035201082150536, 9.422509992056143702 ) ) ;
#29214=CARTESIAN_POINT ( 'NONE',  ( 5.076628168052703671, 41.84226448433411605, 8.527530157486179263 ) ) ;
#29216=CARTESIAN_POINT ( 'NONE',  ( -0.8801773607111009756, 43.06368534415484106, 1.068504757029289695E-15 ) ) ;
#29221=CARTESIAN_POINT ( 'NONE',  ( 7.084665262690076126, 14.10535201082150358, 10.88017736071109987 ) ) ;
#29222=CARTESIAN_POINT ( 'NONE',  ( 22.81628187352647785, 6.623634669930420493, 6.195893100308588602E-16 ) ) ;
#29223=CARTESIAN_POINT ( 'NONE',  ( 7.084665262690076126, 44.10535201082151247, 10.88017736071109987 ) ) ;
#29224=CARTESIAN_POINT ( 'NONE',  ( 20.88017736071110164, 55.35535201082149825, 2.915334737309930979 ) ) ;
#29226=CARTESIAN_POINT ( 'NONE',  ( 0.5774900079438590739, 22.64701867748817321, -5.440088680355550821 ) ) ;
#29227=CARTESIAN_POINT ( 'NONE',  ( -46.51330368012592942, 100.8237035043309504, 9.500000000000191847 ) ) ;
#29228=CARTESIAN_POINT ( 'NONE',  ( 18.52753015748617571, 8.092264484334117824, 4.923371831947298993 ) ) ;
#29229=CARTESIAN_POINT ( 'NONE',  ( 19.84674366389459266, 28.30059781766745886, 2.638427012816836559 ) ) ;
#29233=CARTESIAN_POINT ( 'NONE',  ( -2.816281873526473856, -0.6680319967362464695, 3.434112377981055619 ) ) ;
#29235=CARTESIAN_POINT ( 'NONE',  ( 17.96484262340118221, 4.938685344154837509, 7.964842623401181321 ) ) ;
#29236=CARTESIAN_POINT ( 'NONE',  ( -0.03932841506544072774, 18.12161441960501662, 6.397827110478939261 ) ) ;
#29238=CARTESIAN_POINT ( 'NONE',  ( 20.36894250292379738, 9.928748834913966093, -10.36894250292379027 ) ) ;
#29239=CARTESIAN_POINT ( 'NONE',  ( 22.26659068614895176, 49.72041550158063927, -7.082119434687042414 ) ) ;
#29240=CARTESIAN_POINT ( 'NONE',  ( 10.00000000000000000, 1.813685344154837731, -10.88017736071110342 ) ) ;
#29241=EDGE_CURVE ( 'NONE', #14567, #96338, #28545, .T. ) ;
#29243=CARTESIAN_POINT ( 'NONE',  ( 2.791683348922240793, 21.63393115100078745, 7.208316651077764092 ) ) ;
#29244=CARTESIAN_POINT ( 'NONE',  ( 0.5774900079438590739, 12.64701867748817321, -5.440088680355550821 ) ) ;
#29245=CARTESIAN_POINT ( 'NONE',  ( 18.52753015748618282, 48.92559781766745886, -4.923371831947291888 ) ) ;
#29246=( NAMED_UNIT ( * ) SI_UNIT ( $, .STERADIAN. ) SOLID_ANGLE_UNIT ( ) );
#29250=CARTESIAN_POINT ( 'NONE',  ( 0.6178305044545818747, 28.49863466993041783, -9.382169495545419124 ) ) ;
#29251=CARTESIAN_POINT ( 'NONE',  ( 1.472469842513823179, 36.42559781766745175, 4.923371831947296329 ) ) ;
#29253=CARTESIAN_POINT ( 'NONE',  ( 10.00000000000000000, 9.758931151000785675, -9.846743663894594434 ) ) ;
#29256=CARTESIAN_POINT ( 'NONE',  ( 17.96484262340118221, 16.18868534415483396, -7.964842623401177768 ) ) ;
#29257=CARTESIAN_POINT ( 'NONE',  ( 10.00000000000000000, 35.55374883491396787, -14.16423886937410082 ) ) ;
#29258=CARTESIAN_POINT ( 'NONE',  ( 12.91533473730992121, 44.52201867748816966, 10.88017736071110164 ) ) ;
#29259=CARTESIAN_POINT ( 'NONE',  ( 17.96484262340118221, 64.93868534415483396, 7.964842623401181321 ) ) ;
#29261=CARTESIAN_POINT ( 'NONE',  ( 10.00000000000000178, 17.25893115100078745, 9.846743663894594434 ) ) ;
#29262=CARTESIAN_POINT ( 'NONE',  ( -0.8801773607111009756, 3.063685344154837509, 1.068504757029289695E-15 ) ) ;
#29263=CARTESIAN_POINT ( 'NONE',  ( 19.84674366389459621, 3.508931151000785231, 7.409399052514197653E-17 ) ) ;
#29264=CARTESIAN_POINT ( 'NONE',  ( -46.78776334578036256, 100.7330867235808114, 9.217280700845517316 ) ) ;
#29265=CARTESIAN_POINT ( 'NONE',  ( 18.52753015748618282, 33.92559781766745886, -4.923371831947291888 ) ) ;
#29267=CARTESIAN_POINT ( 'NONE',  ( 0.5774900079438607392, 33.48035201082150536, 5.440088680355550821 ) ) ;
#29269=ORIENTED_EDGE ( 'NONE', *, *, #81676, .F. ) ;
#29270=CARTESIAN_POINT ( 'NONE',  ( 16.40814093676323893, 55.79030133659708923, 11.09922568453595026 ) ) ;
#29272=CARTESIAN_POINT ( 'NONE',  ( 17.20831665107776587, 7.883931151000784787, 7.208316651077764980 ) ) ;
#29273=CARTESIAN_POINT ( 'NONE',  ( -2.816281873526471635, 48.91530133659708213, -3.434112377981056508 ) ) ;
#29274=CARTESIAN_POINT ( 'NONE',  ( -0.8801773607111009756, 8.063685344154837509, 1.068504757029289695E-15 ) ) ;
#29275=CARTESIAN_POINT ( 'NONE',  ( 0.1532563361054083140, 36.00893115100078745, 1.131784320476157264E-15 ) ) ;
#29276=DIRECTION ( 'NONE',  ( 0.5547001962252290364, 0.8320502943378437211, 0.000000000000000000 ) ) ;
#29278=CARTESIAN_POINT ( 'NONE',  ( 20.36894250292379382, 43.67874883491397497, 10.36894250292379205 ) ) ;
#29279=CARTESIAN_POINT ( 'NONE',  ( 0.1532563361054100626, 45.80059781766745886, -2.638427012816831230 ) ) ;
#29281=CARTESIAN_POINT ( 'NONE',  ( 15.44008868035555260, 39.73035201082150536, 9.422509992056143702 ) ) ;
#29283=CARTESIAN_POINT ( 'NONE',  ( 19.84674366389459621, 3.508931151000785231, 7.409399052514197653E-17 ) ) ;
#29285=CARTESIAN_POINT ( 'NONE',  ( 16.40814093676324603, 52.45696800326375353, -11.09922568453594671 ) ) ;
#29286=CARTESIAN_POINT ( 'NONE',  ( 5.076628168052704559, 0.1755978176674514724, -8.527530157486179263 ) ) ;
#29287=ORIENTED_EDGE ( 'NONE', *, *, #60048, .F. ) ;
#29288=CARTESIAN_POINT ( 'NONE',  ( -2.266590686148945544, 1.387082168247301128, -7.082119434687050408 ) ) ;
#29289=CARTESIAN_POINT ( 'NONE',  ( 0.1532563361054082862, 6.217264484334118713, 2.638427012816831674 ) ) ;
#29292=CARTESIAN_POINT ( 'NONE',  ( 7.084665262690076126, 22.02201867748817321, -10.88017736071110164 ) ) ;
#29297=CARTESIAN_POINT ( 'NONE',  ( 10.00000000000000000, 36.81368534415484106, -10.88017736071110342 ) ) ;
#29298=CARTESIAN_POINT ( 'NONE',  ( 5.076628168052703671, 66.84226448433412315, 8.527530157486179263 ) ) ;
#29300=ORIENTED_EDGE ( 'NONE', *, *, #71911, .F. ) ;
#29302=CARTESIAN_POINT ( 'NONE',  ( 12.91533473730993009, 66.60535201082150536, -10.88017736071109987 ) ) ;
#29304=CARTESIAN_POINT ( 'NONE',  ( 12.91533473730992121, 24.52201867748816966, 10.88017736071110164 ) ) ;
#29306=CARTESIAN_POINT ( 'NONE',  ( 2.791683348922240793, 6.633931151000785675, 7.208316651077764092 ) ) ;
#29307=CARTESIAN_POINT ( 'NONE',  ( 20.88017736071110519, 20.56368534415484106, 2.639326808657452039E-16 ) ) ;
#29309=CARTESIAN_POINT ( 'NONE',  ( 0.6178305044545838731, 54.74863466993042493, 9.382169495545420901 ) ) ;
#29310=CARTESIAN_POINT ( 'NONE',  ( 19.42250999205614193, 45.14701867748817676, 5.440088680355555262 ) ) ;
#29312=CARTESIAN_POINT ( 'NONE',  ( 21.09922568453595559, 52.04030133659708923, -6.408140936763230044 ) ) ;
#29313=CARTESIAN_POINT ( 'NONE',  ( 15.44008868035555260, 49.73035201082150536, 9.422509992056143702 ) ) ;
#29314=CARTESIAN_POINT ( 'NONE',  ( 14.92337183194729988, 64.34226448433412315, -8.527530157486177487 ) ) ;
#29316=CARTESIAN_POINT ( 'NONE',  ( 19.84674366389459621, 13.50893115100078568, 7.409399052514197653E-17 ) ) ;
#29317=CARTESIAN_POINT ( 'NONE',  ( 6.565887622018943937, 10.16530133659708746, 12.81628187352647430 ) ) ;
#29319=CARTESIAN_POINT ( 'NONE',  ( 7.361572987183170547, 62.05059781766745886, 9.846743663894590881 ) ) ;
#29320=CARTESIAN_POINT ( 'NONE',  ( 7.084665262690076126, 32.02201867748816966, -10.88017736071110164 ) ) ;
#29321=CARTESIAN_POINT ( 'NONE',  ( 17.20831665107776587, 47.88393115100078745, 7.208316651077764980 ) ) ;
#29322=( LENGTH_UNIT ( ) NAMED_UNIT ( * ) SI_UNIT ( .MILLI., .METRE. ) );
#29324=CARTESIAN_POINT ( 'NONE',  ( 14.92337183194729988, 9.342264484334119601, -8.527530157486177487 ) ) ;
#29325=CARTESIAN_POINT ( 'NONE',  ( 22.81628187352647785, 1.623634669930420271, 6.195893100308588602E-16 ) ) ;
#29329=CARTESIAN_POINT ( 'NONE',  ( 22.81628187352648496, 56.83196800326374643, -3.434112377981050290 ) ) ;
#29330=CARTESIAN_POINT ( 'NONE',  ( 17.20831665107776587, 27.88393115100078390, 7.208316651077764980 ) ) ;
#29332=CARTESIAN_POINT ( 'NONE',  ( 2.035157376598824452, 3.688685344154837953, 7.964842623401179544 ) ) ;
#29333=CARTESIAN_POINT ( 'NONE',  ( 7.361572987183170547, 47.05059781766745175, 9.846743663894590881 ) ) ;
#29335=CARTESIAN_POINT ( 'NONE',  ( 1.816707512666849045, 25.10290668512023871, -6.499999999999981348 ) ) ;
#29336=CARTESIAN_POINT ( 'NONE',  ( -2.266590686148945544, 67.22041550158063217, 7.082119434687048631 ) ) ;
#29338=CARTESIAN_POINT ( 'NONE',  ( 0.5774900079438590739, 22.64701867748817321, -5.440088680355550821 ) ) ;
#29339=CARTESIAN_POINT ( 'NONE',  ( -4.164238869374099927, 52.01208216824729647, 3.795296366450308767 ) ) ;
#29340=CARTESIAN_POINT ( 'NONE',  ( -2.266590686148945544, 57.22041550158063217, 7.082119434687048631 ) ) ;
#29342=CARTESIAN_POINT ( 'NONE',  ( 18.52753015748618282, 3.925597817667451306, -4.923371831947291888 ) ) ;
#29343=CARTESIAN_POINT ( 'NONE',  ( 19.84674366389459266, 23.30059781766745530, 2.638427012816836559 ) ) ;
#29344=CARTESIAN_POINT ( 'NONE',  ( 19.38216949554541557, 2.248634669930420049, -9.382169495545420901 ) ) ;
#29348=CARTESIAN_POINT ( 'NONE',  ( 1.816707512666854818, 40.10290668512022449, -6.500000000000003553 ) ) ;
#29349=CARTESIAN_POINT ( 'NONE',  ( 0.1532563361054083140, 56.00893115100078745, 1.131784320476157264E-15 ) ) ;
#29350=CARTESIAN_POINT ( 'NONE',  ( 20.36894250292379738, 9.928748834913966093, -10.36894250292379027 ) ) ;
#29351=CARTESIAN_POINT ( 'NONE',  ( 7.361572987183169658, 24.96726448433412315, -9.846743663894592657 ) ) ;
#29352=ADVANCED_FACE ( 'NONE', ( #54003 ), #39510, .T. ) ;
#29354=ORIENTED_EDGE ( 'NONE', *, *, #5213, .F. ) ;
#29355=CARTESIAN_POINT ( 'NONE',  ( 13.79529636645031943, 40.34541550158063217, -14.16423886937409904 ) ) ;
#29356=CARTESIAN_POINT ( 'NONE',  ( 17.20831665107776587, 2.883931151000785231, 7.208316651077764980 ) ) ;
#29357=CARTESIAN_POINT ( 'NONE',  ( 2.831191079880678085, 79.91181047996344944, 9.500000000000000000 ) ) ;
#29359=CARTESIAN_POINT ( 'NONE',  ( 0.5774900079438607392, 28.48035201082150891, 5.440088680355550821 ) ) ;
#29360=CARTESIAN_POINT ( 'NONE',  ( 16.40814093676324603, 42.45696800326375353, -11.09922568453594671 ) ) ;
#29361=ADVANCED_FACE ( 'NONE', ( #16009 ), #32613, .T. ) ;
#29362=CARTESIAN_POINT ( 'NONE',  ( -2.816281873526473856, 29.12363466993041783, 9.499525473075851096E-16 ) ) ;
#29363=CARTESIAN_POINT ( 'NONE',  ( 0.6178305044545838731, 64.74863466993043914, 9.382169495545420901 ) ) ;
#29368=CARTESIAN_POINT ( 'NONE',  ( 24.16423886937409904, 44.09541550158063927, 3.795296366450317205 ) ) ;
#29369=CARTESIAN_POINT ( 'NONE',  ( 24.16423886937410614, 4.512082168247300906, -3.795296366450302550 ) ) ;
#29370=CARTESIAN_POINT ( 'NONE',  ( -0.8801773607111008646, 8.272018677488171434, 2.915334737309923430 ) ) ;
#29371=CARTESIAN_POINT ( 'NONE',  ( 2.035157376598824452, 28.68868534415484106, 7.964842623401179544 ) ) ;
#29372=DIRECTION ( 'NONE',  ( 0.000000000000000000, 0.000000000000000000, 1.000000000000000000 ) ) ;
#29374=CARTESIAN_POINT ( 'NONE',  ( -0.8801773607110991993, 57.85535201082149825, -2.915334737309923874 ) ) ;
#29376=CARTESIAN_POINT ( 'NONE',  ( 3.591859063236763294, 33.29030133659708213, -11.09922568453595026 ) ) ;
#29377=CYLINDRICAL_SURFACE ( 'NONE', #17157, 0.5000000000000004441 ) ;
#29379=CARTESIAN_POINT ( 'NONE',  ( 17.20831665107776587, 27.88393115100078390, 7.208316651077764980 ) ) ;
#29380=CARTESIAN_POINT ( 'NONE',  ( 10.00000000000000178, 59.31368534415484106, 10.88017736071110342 ) ) ;
#29381=CARTESIAN_POINT ( 'NONE',  ( 3.591859063236763294, 23.29030133659708568, -11.09922568453595026 ) ) ;
#29383=CARTESIAN_POINT ( 'NONE',  ( -0.8801773607110991993, 7.855352010821504471, -2.915334737309923874 ) ) ;
#29384=CARTESIAN_POINT ( 'NONE',  ( 19.84674366389459266, 33.30059781766744464, 2.638427012816836559 ) ) ;
#29385=CARTESIAN_POINT ( 'NONE',  ( 3.591859063236763294, 63.29030133659708923, -11.09922568453595026 ) ) ;
#29386=CARTESIAN_POINT ( 'NONE',  ( 5.076628168052703671, 16.84226448433411960, 8.527530157486179263 ) ) ;
#29387=CARTESIAN_POINT ( 'NONE',  ( -4.164238869374099039, 6.803748834913967869, 8.674139862899312516E-16 ) ) ;
#29389=CARTESIAN_POINT ( 'NONE',  ( 7.084665262690076126, 39.10535201082150536, 10.88017736071109987 ) ) ;
#29390=CARTESIAN_POINT ( 'NONE',  ( 13.79529636645030344, 33.26208216824730357, 14.16423886937410614 ) ) ;
#29391=CARTESIAN_POINT ( 'NONE',  ( 18.52753015748617571, 43.09226448433412315, 4.923371831947298993 ) ) ;
#29392=CARTESIAN_POINT ( 'NONE',  ( -0.8801773607110991993, 32.85535201082151247, -2.915334737309923874 ) ) ;
#29393=CARTESIAN_POINT ( 'NONE',  ( 4.559911319644449179, 22.23035201082150536, -9.422509992056141925 ) ) ;
#29395=( BOUNDED_SURFACE ( )  B_SPLINE_SURFACE ( 1, 2, ( 
 ( #1843, #11280, #32301, #25328, #41799, #2338, #62805, #93305, #24829, #55306, #55814, #50252, #96278, #74741, #21257, #80769, #89253, #43254, #27258, #27754, #36757, #97773, #65750, #58238, #89738, #51754, #12263, #28748, #11774, #42282, #57758, #97274, #88757, #67249, #44237, #20269, #50766, #12756, #96778, #66750, #43746, #81258, #74232, #6253, #36254, #29238, #28254, #73748, #35756, #59239, #42773, #5279, #66243, #58749, #82238, #20765, #4781, #13752, #59736, #72754, #51253, #81739, #13254, #5765, #19278, #49762, #80273, #4288, #34761, #65250, #95779, #88261, #19766, #73255, #35254, #61220, #30217, #44735, #60233, #90728, #46703, #75235, #52243, #92213, #77202, #98270, #67750, #53228, #15255, #8232, #29726, #45732, #83732, #23244, #75731, #22254, #23739, #84236, #54201, #8708, #39224, #22745, #76712, #69712, #31203, #52729, #68733, #83236, #6745, #37263, #14759, #38725, #45232, #76233, #261, #30708, #61697, #84717, #98767, #7246, #16220, #37751, #60721, #68249, #7747, #1240, #91218, #38241, #91724, #53717, #751, #82736, #14255, #15743, #69225, #46227, #31696, #90231, #21763, #32679, #55695, #40691, #10681, #86682, #2220, #18186, #49165, #79168, #41684, #71191, #40194, #78686, #41197, #24710, #70701, #93680, #86192, #71676, #2714, #47693, #64148, #87155, #54686, #33168, #17704, #63173, #94167, #48174, #56188, #10197, #72154, #85209, #25214, #3187, #9698, #63662, #55180, #18680, #25698, #48667, #16713, #32181, #62683, #79668, #47186, #24221, #94666, #11164, #70207, #39717, #33653, #26175, #56667, #1726, #3682, #62187, #92697, #78185, #93183, #77689, #9204, #85697, #17215, #52979, #65633, #22016, #83493, #75491, #65137, #12639, #95658, #87649, #80149, #27142, #52490, #19163, #96157, #43136, #73629, #7003, #29980, #42654, #42174, #37508, #57645, #73130, #34639, #27640, #15012, #4171, #58125, #4672, #68001, #49641, #80655, #28136, #72638, #5153, #64638, #58635, #82997, #60485, #88140, #12149, #90974, #98527, #19653, #35641, #88635, #50145, #35133, #45481, #75983, #20142, #50647, #22507, #34144, #66127, #81137, #96657, #95146, #89136, #26656, #57152, #11660, #14515, #44984, #24971, #47451, #38491, #84962, #68985, #60971, #53472, #520, #24479, #91483, #38982, #16478, #46954, #77950, #1980, #15981, #15507, #9457, #30967, #46468, #7992, #69474, #85958, #76478, #31454, #76964, #39958, #23004, #53971, #1487, #45989, #77448, #38003, #31940, #54942, #32446, #61464, #84480, #62943, #70459, #91971, #8961, #61956, #23500, #8476, #55456, #17468, #993, #92455, #93446, #47935, #23983, #16971, #23, #30470, #54454, #85457, #39478 ),
 ( #69968, #7512, #62441, #92944, #68496, #83982, #41943, #63435, #71924, #79914, #72406, #56917, #57894, #49910, #78440, #33903, #40954, #11422, #49413, #87418, #95418, #17948, #80421, #41457, #3445, #3933, #40462, #88408, #48923, #18935, #64411, #63914, #65397, #94917, #57411, #72901, #70960, #27404, #42421, #86928, #26416, #79435, #34402, #95923, #25940, #33415, #11917, #4435, #78936, #64891, #18440, #19908, #34900, #56442, #10933, #26914, #87904, #19418, #9956, #2479, #32934, #93941, #25469, #55951, #86450, #48435, #10446, #71451, #2965, #94424, #81882, #74373, #67382, #28874, #35891, #52375, #75369, #42909, #21398, #5900, #89390, #82374, #36395, #44381, #97407, #29863, #73391, #51395, #90360, #96920, #58891, #43392, #6884, #51892, #20906, #4920, #20412, #50898, #37397, #35397, #12403, #82879, #67885, #58383, #27894, #13394, #66888, #97911, #88902, #59376, #43877, #13896, #66386, #81393, #14395, #74879, #44866, #98407, #60365, #89880, #36894, #90861, #21898, #12895, #6379, #73890, #65890, #96420, #5421, #29371, #28397, #59872, #50399, #80909, #92836, #16852, #30856, #30354, #62328, #53359, #61353, #22887, #53865, #1867, #91361, #46359, #91862, #24364, #75871, #68874, #16359, #60861, #881, #52868, #46840, #69856, #47327, #83866, #404, #77827, #54827, #15390, #92348, #76847, #45876, #23380, #39843, #32325, #84375, #15874, #85339, #9341, #76366, #31832, #14896, #45367, #7880, #1378, #8361, #38373, #38869, #70349, #62828, #69360, #31341, #22392, #83374, #61842, #7392, #37891, #68382, #23874, #98902, #54338, #84852, #77335, #8847, #39361, #86821, #71812, #41823, #18818, #33305, #49299, #80295, #11303, #72773, #3318, #71331, #10822, #72289, #55834, #2851, #25828, #18324, #3820, #33781, #78822, #95292, #19301, #85839, #64288, #48805, #63797, #26302, #79314, #87298, #41341, #4310, #17352, #94304, #34275, #40831, #56326, #86328, #49787, #94800, #56802, #47822, #63310, #93821, #11793, #78322, #55331, #26795, #42301, #2359, #70846, #79801, #64776, #57291, #32814, #87785, #34784, #93328, #10332, #25351, #24849, #9842, #40343, #17832, #48314, #96799, #51773, #82758, #6271, #96301, #43765, #27777, #19785, #12287, #58262, #82256, #50273, #28274, #74254, #5785, #36777, #59755, #73769, #73279, #67269, #88777, #5298, #65772, #58770, #44753, #35277, #89273, #35775, #97797, #80790, #12777, #59259, #4801, #36274, #95800, #89760, #13773, #90251, #20288, #43274, #21783, #29259, #50787, #66770, #44259, #97293, #81277, #52262, #14280, #57779, #28766, #20784, #66264, #21277, #51275, #74764, #13272, #75255, #88286, #81760, #6768, #65272, #27281 ) ),
 .UNSPECIFIED., .F., .F., .T. ) 
 B_SPLINE_SURFACE_WITH_KNOTS ( ( 2, 2 ),
 ( 3, 2, 2, 2, 2, 2, 2, 2, 2, 2, 2, 2, 2, 2, 2, 2, 2, 2, 2, 2, 2, 2, 2, 2, 2, 2, 2, 2, 2, 2, 2, 2, 2, 2, 2, 2, 2, 2, 2, 2, 2, 2, 2, 2, 2, 2, 2, 2, 2, 2, 2, 2, 2, 2, 2, 2, 2, 2, 2, 2, 2, 2, 2, 2, 2, 2, 2, 2, 2, 2, 2, 2, 2, 2, 2, 2, 2, 2, 2, 2, 2, 2, 2, 2, 2, 2, 2, 2, 2, 2, 2, 2, 2, 2, 2, 2, 2, 2, 2, 2, 2, 2, 2, 2, 2, 2, 2, 2, 2, 2, 2, 2, 2, 2, 2, 2, 2, 2, 2, 2, 2, 2, 2, 2, 2, 2, 2, 2, 2, 2, 2, 2, 2, 2, 2, 2, 2, 2, 2, 2, 2, 2, 2, 2, 2, 2, 2, 2, 2, 2, 2, 2, 2, 2, 2, 2, 2, 2, 2, 2, 2, 2, 3 ),
 ( 0.000000000000000000, 1.000000000000000000 ),
 ( 0.000000000000000000, 0.005952380952380952051, 0.01190476190476190410, 0.01785714285714285615, 0.02380952380952380820, 0.02976190476190476025, 0.03571428571428571230, 0.04166666666666666435, 0.04761904761904761640, 0.05357142857142856845, 0.05952380952380952051, 0.06547619047619047949, 0.07142857142857142461, 0.07738095238095238360, 0.08333333333333332871, 0.08928571428571428770, 0.09523809523809523281, 0.1011904761904761918, 0.1071428571428571369, 0.1130952380952380959, 0.1190476190476190410, 0.1250000000000000000, 0.1309523809523809590, 0.1369047619047619180, 0.1428571428571428492, 0.1488095238095238082, 0.1547619047619047672, 0.1607142857142857262, 0.1666666666666666574, 0.1726190476190476164, 0.1785714285714285754, 0.1845238095238095344, 0.1904761904761904656, 0.1964285714285714246, 0.2023809523809523836, 0.2083333333333333426, 0.2142857142857142738, 0.2202380952380952328, 0.2261904761904761918, 0.2321428571428571508, 0.2380952380952380820, 0.2440476190476190410, 0.2500000000000000000, 0.2559523809523809312, 0.2619047619047619180, 0.2678571428571428492, 0.2738095238095238360, 0.2797619047619047672, 0.2857142857142856984, 0.2916666666666666852, 0.2976190476190476164, 0.3035714285714285476, 0.3095238095238095344, 0.3154761904761904656, 0.3214285714285714524, 0.3273809523809523836, 0.3333333333333333148, 0.3392857142857143016, 0.3452380952380952328, 0.3511904761904761640, 0.3571428571428571508, 0.3630952380952380820, 0.3690476190476190688, 0.3750000000000000000, 0.3809523809523809312, 0.3869047619047619180, 0.3928571428571428492, 0.3988095238095238360, 0.4047619047619047672, 0.4107142857142856984, 0.4166666666666666852, 0.4226190476190476164, 0.4285714285714285476, 0.4345238095238095344, 0.4404761904761904656, 0.4464285714285714524, 0.4523809523809523836, 0.4583333333333333148, 0.4642857142857143016, 0.4702380952380952328, 0.4761904761904761640, 0.4821428571428571508, 0.4880952380952380820, 0.4940476190476190688, 0.5000000000000000000, 0.5059523809523809312, 0.5119047619047618625, 0.5178571428571429047, 0.5238095238095238360, 0.5297619047619047672, 0.5357142857142856984, 0.5416666666666666297, 0.5476190476190476719, 0.5535714285714286031, 0.5595238095238095344, 0.5654761904761904656, 0.5714285714285713969, 0.5773809523809523281, 0.5833333333333333703, 0.5892857142857143016, 0.5952380952380952328, 0.6011904761904761640, 0.6071428571428570953, 0.6130952380952381375, 0.6190476190476190688, 0.6250000000000000000, 0.6309523809523809312, 0.6369047619047618625, 0.6428571428571429047, 0.6488095238095238360, 0.6547619047619047672, 0.6607142857142856984, 0.6666666666666666297, 0.6726190476190476719, 0.6785714285714286031, 0.6845238095238095344, 0.6904761904761904656, 0.6964285714285713969, 0.7023809523809523281, 0.7083333333333333703, 0.7142857142857143016, 0.7202380952380952328, 0.7261904761904761640, 0.7321428571428570953, 0.7380952380952381375, 0.7440476190476190688, 0.7500000000000000000, 0.7559523809523809312, 0.7619047619047618625, 0.7678571428571429047, 0.7738095238095238360, 0.7797619047619047672, 0.7857142857142856984, 0.7916666666666666297, 0.7976190476190476719, 0.8035714285714286031, 0.8095238095238095344, 0.8154761904761904656, 0.8214285714285713969, 0.8273809523809523281, 0.8333333333333333703, 0.8392857142857143016, 0.8452380952380952328, 0.8511904761904761640, 0.8571428571428570953, 0.8630952380952381375, 0.8690476190476190688, 0.8750000000000000000, 0.8809523809523809312, 0.8869047619047618625, 0.8928571428571429047, 0.8988095238095238360, 0.9047619047619047672, 0.9107142857142856984, 0.9166666666666666297, 0.9226190476190476719, 0.9285714285714286031, 0.9345238095238095344, 0.9404761904761904656, 0.9464285714285713969, 0.9523809523809523281, 0.9583333333333333703, 0.9642857142857143016 ),
 .UNSPECIFIED. ) 
 GEOMETRIC_REPRESENTATION_ITEM ( )  RATIONAL_B_SPLINE_SURFACE ( (
 ( 1.000000000000000000, 0.9659258262890683122, 1.000000000000000000, 0.9659258262890683122, 1.000000000000000000, 0.9659258262890683122, 1.000000000000000000, 0.9659258262890683122, 1.000000000000000000, 0.9659258262890683122, 1.000000000000000000, 0.9659258262890683122, 1.000000000000000000, 0.9659258262890683122, 1.000000000000000000, 0.9659258262890683122, 1.000000000000000000, 0.9659258262890683122, 1.000000000000000000, 0.9659258262890683122, 1.000000000000000000, 0.9659258262890683122, 1.000000000000000000, 0.9659258262890683122, 1.000000000000000000, 0.9659258262890683122, 1.000000000000000000, 0.9659258262890683122, 1.000000000000000000, 0.9659258262890683122, 1.000000000000000000, 0.9659258262890683122, 1.000000000000000000, 0.9659258262890683122, 1.000000000000000000, 0.9659258262890683122, 1.000000000000000000, 0.9659258262890683122, 1.000000000000000000, 0.9659258262890683122, 1.000000000000000000, 0.9659258262890683122, 1.000000000000000000, 0.9659258262890683122, 1.000000000000000000, 0.9659258262890683122, 1.000000000000000000, 0.9659258262890683122, 1.000000000000000000, 0.9659258262890683122, 1.000000000000000000, 0.9659258262890683122, 1.000000000000000000, 0.9659258262890683122, 1.000000000000000000, 0.9659258262890683122, 1.000000000000000000, 0.9659258262890683122, 1.000000000000000000, 0.9659258262890683122, 1.000000000000000000, 0.9659258262890683122, 1.000000000000000000, 0.9659258262890683122, 1.000000000000000000, 0.9659258262890683122, 1.000000000000000000, 0.9659258262890683122, 1.000000000000000000, 0.9659258262890683122, 1.000000000000000000, 0.9659258262890683122, 1.000000000000000000, 0.9659258262890683122, 1.000000000000000000, 0.9659258262890683122, 1.000000000000000000, 0.9659258262890683122, 1.000000000000000000, 0.9659258262890683122, 1.000000000000000000, 0.9659258262890683122, 1.000000000000000000, 0.9659258262890683122, 1.000000000000000000, 0.9659258262890683122, 1.000000000000000000, 0.9659258262890683122, 1.000000000000000000, 0.9659258262890683122, 1.000000000000000000, 0.9659258262890683122, 1.000000000000000000, 0.9659258262890683122, 1.000000000000000000, 0.9659258262890683122, 1.000000000000000000, 0.9659258262890683122, 1.000000000000000000, 0.9659258262890683122, 1.000000000000000000, 0.9659258262890683122, 1.000000000000000000, 0.9659258262890683122, 1.000000000000000000, 0.9659258262890683122, 1.000000000000000000, 0.9659258262890683122, 1.000000000000000000, 0.9659258262890683122, 1.000000000000000000, 0.9659258262890683122, 1.000000000000000000, 0.9659258262890683122, 1.000000000000000000, 0.9659258262890683122, 1.000000000000000000, 0.9659258262890683122, 1.000000000000000000, 0.9659258262890683122, 1.000000000000000000, 0.9659258262890683122, 1.000000000000000000, 0.9659258262890683122, 1.000000000000000000, 0.9659258262890683122, 1.000000000000000000, 0.9659258262890683122, 1.000000000000000000, 0.9659258262890683122, 1.000000000000000000, 0.9659258262890683122, 1.000000000000000000, 0.9659258262890683122, 1.000000000000000000, 0.9659258262890683122, 1.000000000000000000, 0.9659258262890683122, 1.000000000000000000, 0.9659258262890683122, 1.000000000000000000, 0.9659258262890683122, 1.000000000000000000, 0.9659258262890683122, 1.000000000000000000, 0.9659258262890683122, 1.000000000000000000, 0.9659258262890683122, 1.000000000000000000, 0.9659258262890683122, 1.000000000000000000, 0.9659258262890683122, 1.000000000000000000, 0.9659258262890683122, 1.000000000000000000, 0.9659258262890683122, 1.000000000000000000, 0.9659258262890683122, 1.000000000000000000, 0.9659258262890683122, 1.000000000000000000, 0.9659258262890683122, 1.000000000000000000, 0.9659258262890683122, 1.000000000000000000, 0.9659258262890683122, 1.000000000000000000, 0.9659258262890683122, 1.000000000000000000, 0.9659258262890683122, 1.000000000000000000, 0.9659258262890683122, 1.000000000000000000, 0.9659258262890683122, 1.000000000000000000, 0.9659258262890683122, 1.000000000000000000, 0.9659258262890683122, 1.000000000000000000, 0.9659258262890683122, 1.000000000000000000, 0.9659258262890683122, 1.000000000000000000, 0.9659258262890683122, 1.000000000000000000, 0.9659258262890683122, 1.000000000000000000, 0.9659258262890683122, 1.000000000000000000, 0.9659258262890683122, 1.000000000000000000, 0.9659258262890683122, 1.000000000000000000, 0.9659258262890683122, 1.000000000000000000, 0.9659258262890683122, 1.000000000000000000, 0.9659258262890683122, 1.000000000000000000, 0.9659258262890683122, 1.000000000000000000, 0.9659258262890683122, 1.000000000000000000, 0.9659258262890683122, 1.000000000000000000, 0.9659258262890683122, 1.000000000000000000, 0.9659258262890683122, 1.000000000000000000, 0.9659258262890683122, 1.000000000000000000, 0.9659258262890683122, 1.000000000000000000, 0.9659258262890683122, 1.000000000000000000, 0.9659258262890683122, 1.000000000000000000, 0.9659258262890683122, 1.000000000000000000, 0.9659258262890683122, 1.000000000000000000, 0.9659258262890683122, 1.000000000000000000, 0.9659258262890683122, 1.000000000000000000, 0.9659258262890683122, 1.000000000000000000, 0.9659258262890683122, 1.000000000000000000, 0.9659258262890683122, 1.000000000000000000, 0.9659258262890683122, 1.000000000000000000, 0.9659258262890683122, 1.000000000000000000, 0.9659258262890683122, 1.000000000000000000, 0.9659258262890683122, 1.000000000000000000, 0.9659258262890683122, 1.000000000000000000, 0.9659258262890683122, 1.000000000000000000, 0.9659258262890683122, 1.000000000000000000, 0.9659258262890683122, 1.000000000000000000, 0.9659258262890683122, 1.000000000000000000, 0.9659258262890683122, 1.000000000000000000, 0.9659258262890683122, 1.000000000000000000, 0.9659258262890683122, 1.000000000000000000, 0.9659258262890683122, 1.000000000000000000, 0.9659258262890683122, 1.000000000000000000, 0.9659258262890683122, 1.000000000000000000, 0.9659258262890683122, 1.000000000000000000, 0.9659258262890683122, 1.000000000000000000, 0.9659258262890683122, 1.000000000000000000, 0.9659258262890683122, 1.000000000000000000, 0.9659258262890683122, 1.000000000000000000, 0.9659258262890683122, 1.000000000000000000, 0.9659258262890683122, 1.000000000000000000, 0.9659258262890683122, 1.000000000000000000, 0.9659258262890683122, 1.000000000000000000, 0.9659258262890683122, 1.000000000000000000, 0.9659258262890683122, 1.000000000000000000, 0.9659258262890683122, 1.000000000000000000, 0.9659258262890683122, 1.000000000000000000, 0.9659258262890683122, 1.000000000000000000, 0.9659258262890683122, 1.000000000000000000, 0.9659258262890683122, 1.000000000000000000, 0.9659258262890683122, 1.000000000000000000, 0.9659258262890683122, 1.000000000000000000, 0.9659258262890683122, 1.000000000000000000, 0.9659258262890683122, 1.000000000000000000, 0.9659258262890683122, 1.000000000000000000, 0.9659258262890683122, 1.000000000000000000, 0.9659258262890683122, 1.000000000000000000, 0.9659258262890683122, 1.000000000000000000, 0.9659258262890683122, 1.000000000000000000, 0.9659258262890683122, 1.000000000000000000, 0.9659258262890683122, 1.000000000000000000, 0.9659258262890683122, 1.000000000000000000, 0.9659258262890683122, 1.000000000000000000, 0.9659258262890683122, 1.000000000000000000, 0.9659258262890683122, 1.000000000000000000, 0.9659258262890683122, 1.000000000000000000),
 ( 1.000000000000000000, 0.9659258262890683122, 1.000000000000000000, 0.9659258262890683122, 1.000000000000000000, 0.9659258262890683122, 1.000000000000000000, 0.9659258262890683122, 1.000000000000000000, 0.9659258262890683122, 1.000000000000000000, 0.9659258262890683122, 1.000000000000000000, 0.9659258262890683122, 1.000000000000000000, 0.9659258262890683122, 1.000000000000000000, 0.9659258262890683122, 1.000000000000000000, 0.9659258262890683122, 1.000000000000000000, 0.9659258262890683122, 1.000000000000000000, 0.9659258262890683122, 1.000000000000000000, 0.9659258262890683122, 1.000000000000000000, 0.9659258262890683122, 1.000000000000000000, 0.9659258262890683122, 1.000000000000000000, 0.9659258262890683122, 1.000000000000000000, 0.9659258262890683122, 1.000000000000000000, 0.9659258262890683122, 1.000000000000000000, 0.9659258262890683122, 1.000000000000000000, 0.9659258262890683122, 1.000000000000000000, 0.9659258262890683122, 1.000000000000000000, 0.9659258262890683122, 1.000000000000000000, 0.9659258262890683122, 1.000000000000000000, 0.9659258262890683122, 1.000000000000000000, 0.9659258262890683122, 1.000000000000000000, 0.9659258262890683122, 1.000000000000000000, 0.9659258262890683122, 1.000000000000000000, 0.9659258262890683122, 1.000000000000000000, 0.9659258262890683122, 1.000000000000000000, 0.9659258262890683122, 1.000000000000000000, 0.9659258262890683122, 1.000000000000000000, 0.9659258262890683122, 1.000000000000000000, 0.9659258262890683122, 1.000000000000000000, 0.9659258262890683122, 1.000000000000000000, 0.9659258262890683122, 1.000000000000000000, 0.9659258262890683122, 1.000000000000000000, 0.9659258262890683122, 1.000000000000000000, 0.9659258262890683122, 1.000000000000000000, 0.9659258262890683122, 1.000000000000000000, 0.9659258262890683122, 1.000000000000000000, 0.9659258262890683122, 1.000000000000000000, 0.9659258262890683122, 1.000000000000000000, 0.9659258262890683122, 1.000000000000000000, 0.9659258262890683122, 1.000000000000000000, 0.9659258262890683122, 1.000000000000000000, 0.9659258262890683122, 1.000000000000000000, 0.9659258262890683122, 1.000000000000000000, 0.9659258262890683122, 1.000000000000000000, 0.9659258262890683122, 1.000000000000000000, 0.9659258262890683122, 1.000000000000000000, 0.9659258262890683122, 1.000000000000000000, 0.9659258262890683122, 1.000000000000000000, 0.9659258262890683122, 1.000000000000000000, 0.9659258262890683122, 1.000000000000000000, 0.9659258262890683122, 1.000000000000000000, 0.9659258262890683122, 1.000000000000000000, 0.9659258262890683122, 1.000000000000000000, 0.9659258262890683122, 1.000000000000000000, 0.9659258262890683122, 1.000000000000000000, 0.9659258262890683122, 1.000000000000000000, 0.9659258262890683122, 1.000000000000000000, 0.9659258262890683122, 1.000000000000000000, 0.9659258262890683122, 1.000000000000000000, 0.9659258262890683122, 1.000000000000000000, 0.9659258262890683122, 1.000000000000000000, 0.9659258262890683122, 1.000000000000000000, 0.9659258262890683122, 1.000000000000000000, 0.9659258262890683122, 1.000000000000000000, 0.9659258262890683122, 1.000000000000000000, 0.9659258262890683122, 1.000000000000000000, 0.9659258262890683122, 1.000000000000000000, 0.9659258262890683122, 1.000000000000000000, 0.9659258262890683122, 1.000000000000000000, 0.9659258262890683122, 1.000000000000000000, 0.9659258262890683122, 1.000000000000000000, 0.9659258262890683122, 1.000000000000000000, 0.9659258262890683122, 1.000000000000000000, 0.9659258262890683122, 1.000000000000000000, 0.9659258262890683122, 1.000000000000000000, 0.9659258262890683122, 1.000000000000000000, 0.9659258262890683122, 1.000000000000000000, 0.9659258262890683122, 1.000000000000000000, 0.9659258262890683122, 1.000000000000000000, 0.9659258262890683122, 1.000000000000000000, 0.9659258262890683122, 1.000000000000000000, 0.9659258262890683122, 1.000000000000000000, 0.9659258262890683122, 1.000000000000000000, 0.9659258262890683122, 1.000000000000000000, 0.9659258262890683122, 1.000000000000000000, 0.9659258262890683122, 1.000000000000000000, 0.9659258262890683122, 1.000000000000000000, 0.9659258262890683122, 1.000000000000000000, 0.9659258262890683122, 1.000000000000000000, 0.9659258262890683122, 1.000000000000000000, 0.9659258262890683122, 1.000000000000000000, 0.9659258262890683122, 1.000000000000000000, 0.9659258262890683122, 1.000000000000000000, 0.9659258262890683122, 1.000000000000000000, 0.9659258262890683122, 1.000000000000000000, 0.9659258262890683122, 1.000000000000000000, 0.9659258262890683122, 1.000000000000000000, 0.9659258262890683122, 1.000000000000000000, 0.9659258262890683122, 1.000000000000000000, 0.9659258262890683122, 1.000000000000000000, 0.9659258262890683122, 1.000000000000000000, 0.9659258262890683122, 1.000000000000000000, 0.9659258262890683122, 1.000000000000000000, 0.9659258262890683122, 1.000000000000000000, 0.9659258262890683122, 1.000000000000000000, 0.9659258262890683122, 1.000000000000000000, 0.9659258262890683122, 1.000000000000000000, 0.9659258262890683122, 1.000000000000000000, 0.9659258262890683122, 1.000000000000000000, 0.9659258262890683122, 1.000000000000000000, 0.9659258262890683122, 1.000000000000000000, 0.9659258262890683122, 1.000000000000000000, 0.9659258262890683122, 1.000000000000000000, 0.9659258262890683122, 1.000000000000000000, 0.9659258262890683122, 1.000000000000000000, 0.9659258262890683122, 1.000000000000000000, 0.9659258262890683122, 1.000000000000000000, 0.9659258262890683122, 1.000000000000000000, 0.9659258262890683122, 1.000000000000000000, 0.9659258262890683122, 1.000000000000000000, 0.9659258262890683122, 1.000000000000000000, 0.9659258262890683122, 1.000000000000000000, 0.9659258262890683122, 1.000000000000000000, 0.9659258262890683122, 1.000000000000000000, 0.9659258262890683122, 1.000000000000000000, 0.9659258262890683122, 1.000000000000000000, 0.9659258262890683122, 1.000000000000000000, 0.9659258262890683122, 1.000000000000000000, 0.9659258262890683122, 1.000000000000000000, 0.9659258262890683122, 1.000000000000000000, 0.9659258262890683122, 1.000000000000000000, 0.9659258262890683122, 1.000000000000000000, 0.9659258262890683122, 1.000000000000000000, 0.9659258262890683122, 1.000000000000000000, 0.9659258262890683122, 1.000000000000000000, 0.9659258262890683122, 1.000000000000000000, 0.9659258262890683122, 1.000000000000000000, 0.9659258262890683122, 1.000000000000000000, 0.9659258262890683122, 1.000000000000000000, 0.9659258262890683122, 1.000000000000000000, 0.9659258262890683122, 1.000000000000000000, 0.9659258262890683122, 1.000000000000000000, 0.9659258262890683122, 1.000000000000000000, 0.9659258262890683122, 1.000000000000000000, 0.9659258262890683122, 1.000000000000000000, 0.9659258262890683122, 1.000000000000000000, 0.9659258262890683122, 1.000000000000000000, 0.9659258262890683122, 1.000000000000000000, 0.9659258262890683122, 1.000000000000000000, 0.9659258262890683122, 1.000000000000000000, 0.9659258262890683122, 1.000000000000000000, 0.9659258262890683122, 1.000000000000000000, 0.9659258262890683122, 1.000000000000000000, 0.9659258262890683122, 1.000000000000000000, 0.9659258262890683122, 1.000000000000000000, 0.9659258262890683122, 1.000000000000000000, 0.9659258262890683122, 1.000000000000000000, 0.9659258262890683122, 1.000000000000000000) ) ) 
 REPRESENTATION_ITEM ( '' )  SURFACE ( )  );
#29396=CARTESIAN_POINT ( 'NONE',  ( -0.8801773607110991993, 27.85535201082150181, -2.915334737309923874 ) ) ;
#29397=CARTESIAN_POINT ( 'NONE',  ( 3.591859063236761518, 44.95696800326376064, 11.09922568453594849 ) ) ;
#29398=CARTESIAN_POINT ( 'NONE',  ( 2.035157376598824452, 38.68868534415483396, 7.964842623401179544 ) ) ;
#29400=CARTESIAN_POINT ( 'NONE',  ( 7.084665262690076126, 44.10535201082151247, 10.88017736071109987 ) ) ;
#29402=CARTESIAN_POINT ( 'NONE',  ( 10.00000000000000178, 57.25893115100078745, 9.846743663894594434 ) ) ;
#29403=CARTESIAN_POINT ( 'NONE',  ( 0.5774900079438590739, 32.64701867748816966, -5.440088680355550821 ) ) ;
#29405=CARTESIAN_POINT ( 'NONE',  ( -0.3689425029237898834, 41.17874883491397497, -10.36894250292378850 ) ) ;
#29406=CARTESIAN_POINT ( 'NONE',  ( 20.88017736071110519, 55.56368534415484817, 2.639326808657452039E-16 ) ) ;
#29407=CARTESIAN_POINT ( 'NONE',  ( 20.10421743870886857, 25.60736173766202839, -6.337391062633416006 ) ) ;
#29409=CARTESIAN_POINT ( 'NONE',  ( 2.791683348922240793, 66.63393115100079456, 7.208316651077764092 ) ) ;
#29410=CARTESIAN_POINT ( 'NONE',  ( 17.20831665107776587, 29.13393115100078390, -7.208316651077762316 ) ) ;
#29411=ORIENTED_EDGE ( 'NONE', *, *, #75409, .T. ) ;
#29412=CARTESIAN_POINT ( 'NONE',  ( 0.1532563361054082862, 21.21726448433412315, 2.638427012816831674 ) ) ;
#29414=CARTESIAN_POINT ( 'NONE',  ( 7.084665262690076126, 29.10535201082150181, 10.88017736071109987 ) ) ;
#29415=CARTESIAN_POINT ( 'NONE',  ( 7.361572987183169658, 19.96726448433411960, -9.846743663894592657 ) ) ;
#29416=CARTESIAN_POINT ( 'NONE',  ( 6.565887622018943937, 15.16530133659708568, 12.81628187352647430 ) ) ;
#29417=CARTESIAN_POINT ( 'NONE',  ( 7.084665262690076126, 69.10535201082151957, 10.88017736071109987 ) ) ;
#29418=CARTESIAN_POINT ( 'NONE',  ( 20.88017736071110875, 55.77201867748816966, -2.915334737309920765 ) ) ;
#29419=CARTESIAN_POINT ( 'NONE',  ( 19.42250999205614193, 35.14701867748816966, 5.440088680355555262 ) ) ;
#29420=CARTESIAN_POINT ( 'NONE',  ( 0.5774900079438590739, 2.647018677488170990, -5.440088680355550821 ) ) ;
#29421=CARTESIAN_POINT ( 'NONE',  ( -0.3689425029237898834, 46.17874883491397497, -10.36894250292378850 ) ) ;
#29422=B_SPLINE_CURVE_WITH_KNOTS ( 'NONE', 3,
 ( #79137, #78657, #10648, #57608 ),
 .UNSPECIFIED., .F., .F.,
 ( 4, 4 ),
 ( 3.469446951953614189E-18, 0.002562518741975320334 ),
 .UNSPECIFIED. ) ;
#29425=ORIENTED_EDGE ( 'NONE', *, *, #4975, .T. ) ;
#29426=CARTESIAN_POINT ( 'NONE',  ( 16.40814093676324603, 12.45696800326375353, -11.09922568453594671 ) ) ;
#29427=CARTESIAN_POINT ( 'NONE',  ( 7.084665262690076126, 9.105352010821503583, 10.88017736071109987 ) ) ;
#29428=CARTESIAN_POINT ( 'NONE',  ( 10.00000000000000000, 41.81368534415484106, -10.88017736071110342 ) ) ;
#29431=CARTESIAN_POINT ( 'NONE',  ( 4.559911319644449179, 58.89701867748817676, 9.422509992056141925 ) ) ;
#29432=CARTESIAN_POINT ( 'NONE',  ( 0.1532563361054082862, 41.21726448433411605, 2.638427012816831674 ) ) ;
#29433=CARTESIAN_POINT ( 'NONE',  ( 5.076628168052704559, 20.17559781766745175, -8.527530157486179263 ) ) ;
#29434=CARTESIAN_POINT ( 'NONE',  ( 7.361572987183169658, 9.967264484334119601, -9.846743663894592657 ) ) ;
#29436=CARTESIAN_POINT ( 'NONE',  ( 19.38216949554541557, 37.24863466993041783, -9.382169495545420901 ) ) ;
#29437=EDGE_CURVE ( 'NONE', #91084, #87032, #12409, .T. ) ;
#29438=CARTESIAN_POINT ( 'NONE',  ( 10.00000000000000178, 64.31368534415483396, 10.88017736071110342 ) ) ;
#29439=DIRECTION ( 'NONE',  ( 0.000000000000000000, 0.000000000000000000, 1.000000000000000000 ) ) ;
#29441=CARTESIAN_POINT ( 'NONE',  ( 19.84674366389459266, 38.71726448433412315, -2.638427012816827677 ) ) ;
#29443=CARTESIAN_POINT ( 'NONE',  ( 3.591859063236761518, 49.95696800326375353, 11.09922568453594849 ) ) ;
#29444=LINE ( 'NONE', #65973, #10257 ) ;
#29445=CARTESIAN_POINT ( 'NONE',  ( 21.09922568453595559, 17.04030133659708923, -6.408140936763230044 ) ) ;
#29446=CARTESIAN_POINT ( 'NONE',  ( 24.16423886937410614, 29.51208216824729647, -3.795296366450302550 ) ) ;
#29447=UNCERTAINTY_MEASURE_WITH_UNIT (LENGTH_MEASURE( 1.000000000000000082E-05 ), #97388, 'distance_accuracy_value', 'NONE');
#29448=CARTESIAN_POINT ( 'NONE',  ( 1.711636803080561098, 41.84492782695770785, -6.500000000000035527 ) ) ;
#29449=CARTESIAN_POINT ( 'NONE',  ( 24.16423886937410614, 29.51208216824729647, -3.795296366450302550 ) ) ;
#29450=CARTESIAN_POINT ( 'NONE',  ( 13.79529636645031943, 45.34541550158062506, -14.16423886937409904 ) ) ;
#29451=CARTESIAN_POINT ( 'NONE',  ( 20.36894250292379738, 4.928748834913967869, -10.36894250292379027 ) ) ;
#29452=CARTESIAN_POINT ( 'NONE',  ( 17.08211943468705840, 10.13708216824730179, -12.26659068614894466 ) ) ;
#29453=CARTESIAN_POINT ( 'NONE',  ( 15.44008868035555793, 46.39701867748817676, -9.422509992056140149 ) ) ;
#29455=CARTESIAN_POINT ( 'NONE',  ( 2.791683348922237240, 30.38393115100078390, -7.208316651077763204 ) ) ;
#29456=CARTESIAN_POINT ( 'NONE',  ( 10.00000000000000178, 64.31368534415483396, 10.88017736071110342 ) ) ;
#29457=CARTESIAN_POINT ( 'NONE',  ( 5.076628168052704559, 35.17559781766745175, -8.527530157486179263 ) ) ;
#29458=CARTESIAN_POINT ( 'NONE',  ( 0.5774900079438590739, 27.64701867748817676, -5.440088680355550821 ) ) ;
#29459=CARTESIAN_POINT ( 'NONE',  ( 13.43411237798105340, 60.58196800326376064, 12.81628187352647963 ) ) ;
#29460=CARTESIAN_POINT ( 'NONE',  ( 19.84674366389459266, 63.71726448433412315, -2.638427012816827677 ) ) ;
#29463=CARTESIAN_POINT ( 'NONE',  ( 5.076628168052704559, 25.17559781766745175, -8.527530157486179263 ) ) ;
#29464=CARTESIAN_POINT ( 'NONE',  ( 3.591859063236761518, 39.95696800326375353, 11.09922568453594849 ) ) ;
#29466=CARTESIAN_POINT ( 'NONE',  ( -0.8801773607111009756, 38.06368534415484106, 1.068504757029289695E-15 ) ) ;
#29467=CARTESIAN_POINT ( 'NONE',  ( 7.361572987183169658, 49.96726448433410894, -9.846743663894592657 ) ) ;
#29468=CARTESIAN_POINT ( 'NONE',  ( 13.79529636645031943, 20.34541550158063572, -14.16423886937409904 ) ) ;
#29471=CARTESIAN_POINT ( 'NONE',  ( 17.96484262340118221, 61.18868534415482685, -7.964842623401177768 ) ) ;
#29473=CARTESIAN_POINT ( 'NONE',  ( 13.79529636645030344, 63.26208216824730357, 14.16423886937410614 ) ) ;
#29474=CARTESIAN_POINT ( 'NONE',  ( 0.6178305044545818747, -1.501365330069579951, -9.382169495545419124 ) ) ;
#29475=CARTESIAN_POINT ( 'NONE',  ( 0.1922240491738437529, 53.18878173731740588, 6.499999999999968026 ) ) ;
#29476=CARTESIAN_POINT ( 'NONE',  ( 19.42250999205614548, 55.98035201082150536, -5.440088680355545492 ) ) ;
#29477=CARTESIAN_POINT ( 'NONE',  ( 2.603489959281614308, 56.58210964143329846, 6.500000000000031086 ) ) ;
#29479=CARTESIAN_POINT ( 'NONE',  ( -0.8801773607111009756, 8.063685344154837509, 1.068504757029289695E-15 ) ) ;
#29480=CARTESIAN_POINT ( 'NONE',  ( 0.5774900079438590739, 7.647018677488171434, -5.440088680355550821 ) ) ;
#29481=AXIS2_PLACEMENT_3D ( 'NONE', #82778, #90770, #98308 ) ;
#29482=CARTESIAN_POINT ( 'NONE',  ( 0.1532563361054100626, 50.80059781766745175, -2.638427012816831230 ) ) ;
#29483=CARTESIAN_POINT ( 'NONE',  ( -2.816281873526473856, 49.33196800326374643, 3.434112377981055619 ) ) ;
#29486=CARTESIAN_POINT ( 'NONE',  ( 12.91533473730993009, 16.60535201082150891, -10.88017736071109987 ) ) ;
#29487=CARTESIAN_POINT ( 'NONE',  ( -2.816281873526471635, 13.91530133659708746, -3.434112377981056508 ) ) ;
#29489=CARTESIAN_POINT ( 'NONE',  ( 5.076628168052703671, 6.842264484334118713, 8.527530157486179263 ) ) ;
#29490=CARTESIAN_POINT ( 'NONE',  ( 14.92337183194729633, 42.67559781766745886, 8.527530157486181039 ) ) ;
#29491=CARTESIAN_POINT ( 'NONE',  ( -0.8801773607111008646, 38.27201867748816255, 2.915334737309923430 ) ) ;
#29493=CARTESIAN_POINT ( 'NONE',  ( 13.43411237798106583, 2.665301336597086568, -12.81628187352647252 ) ) ;
#29494=CARTESIAN_POINT ( 'NONE',  ( 2.035157376598822676, 42.43868534415483396, -7.964842623401177768 ) ) ;
#29496=( BOUNDED_SURFACE ( )  B_SPLINE_SURFACE ( 1, 2, ( 
 ( #97537, #57038, #95543, #50529, #87542, #80538, #12036, #74010, #66017, #51517, #42536, #73019, #89023, #4552, #20533, #74505, #35018, #28520, #82011, #65519, #88525, #43030, #13016, #27033, #5039, #72525, #57531, #51017, #81511, #36524, #88027, #43514, #96041, #27525, #19053, #81024, #13521, #66519, #80037, #58016, #5538, #44003, #23013, #46479, #38992, #75004, #53481, #7011, #90984, #37015, #83007, #28996, #30976, #29988, #83991, #22515, #14524, #7520, #76488, #90488, #67512, #15516, #68994, #52987, #21523, #30480, #75500, #84489, #53980, #60495, #61473, #29486, #52017, #529, #45998, #68009, #69484, #15020, #68503, #8002, #22025, #37517, #83502, #45489, #38500, #38011, #44992, #44504, #75991, #82508, #59507, #34, #98536, #60980, #91493, #98031, #91980, #8487, #23509, #15991, #76974, #90003, #14024, #6508, #59995, #52497, #24488, #77458, #33425, #2490, #8971, #25949, #10455, #70470, #70970, #1990, #32456, #24981, #56451, #31464, #23993, #86938, #39487, #32944, #85469, #69977, #2975, #93952, #46964, #84970, #9966, #55961, #18450, #48932, #79444, #62451, #63923, #9467, #71462, #86461, #62952, #61965, #47945, #78451, #10943, #63445, #17958, #93456, #1498, #41467, #92953, #39968, #92465, #55466, #1002, #54465, #31949, #94435, #16489, #54952, #40472, #16981, #47459, #25478, #48445, #78945, #77959, #85968, #17477, #40963, #35902, #28406, #73899, #34412, #42920, #5432, #73401, #12412, #72913, #96431, #4929, #35408, #50907, #72415, #20915, #51404, #43402, #94927, #11433, #81403, #80430, #89399, #96930, #49919, #42430, #12906, #27904, #34911, #57421, #50409, #20422, #64902, #41953, #58393, #66396, #95933, #64420, #65901, #19429, #58902, #81891, #80919, #3943, #88911, #4445, #95428, #13403, #71936, #65408, #27414, #3457, #33912, #26425, #26924, #56926, #87429, #18946, #57905, #49423, #79925, #87916, #11928, #88418, #19919, #9227, #74383, #21406, #16243, #54224, #62214, #82384, #6386, #36902, #771, #47213, #59882, #82888, #69737, #44390, #61720, #1750, #43888, #85233, #32205, #85722, #52385, #31223, #46725, #92235, #14404, #77224, #23762, #67391, #8729, #6893, #44875, #74888, #97416, #62706, #75378, #5909, #36404, #13907, #37406, #66897, #97919, #29380, #92720, #84739, #77714, #90370, #21910, #39247, #69251, #1263, #93206, #31718, #16736, #39736, #24245, #54711, #70231, #24729, #55207, #28882, #59385, #89889, #51902, #79688, #34662, #55718, #72176, #33192, #78710, #27163, #48690, #72657, #95169, #65159, #93702, #64170, #95677, #11186, #57663, #17235, #63197, #41706, #94188, #79193, #25237, #71215, #47713, #19181, #18211, #86213 ),
 ( #32701, #10705, #9720, #78208, #71697, #56210, #49186, #3211, #17724, #3705, #40219, #33673, #63685, #34166, #41220, #70728, #2243, #48197, #10221, #40710, #2736, #49662, #18702, #25718, #42193, #26676, #86705, #87181, #94691, #26196, #56688, #4192, #64656, #57171, #87668, #80172, #11683, #73645, #58146, #90129, #82137, #35153, #73150, #97179, #44131, #75134, #44640, #37157, #50667, #21659, #96677, #59638, #74642, #58652, #50163, #36151, #66655, #6640, #89645, #6152, #81642, #96175, #67653, #81155, #28156, #80672, #43649, #98163, #88160, #20163, #82639, #19674, #88655, #28647, #12167, #42672, #21157, #13646, #36657, #29619, #35659, #4691, #12660, #52143, #65652, #14156, #43159, #59137, #27658, #51658, #67144, #89152, #97668, #29134, #5174, #66144, #20662, #51158, #13150, #74134, #5669, #98670, #39127, #68633, #77592, #85107, #38147, #30612, #1136, #16618, #91627, #92601, #60623, #83134, #31598, #54105, #163, #659, #52631, #14659, #92114, #84618, #16122, #70110, #7654, #45125, #91124, #24125, #47094, #62092, #22647, #31107, #54594, #61600, #23645, #61118, #46606, #77105, #8618, #69614, #53127, #9107, #39621, #1635, #75631, #30117, #60125, #23143, #90623, #22147, #53616, #84134, #7143, #37647, #15646, #68144, #83635, #15150, #45629, #76128, #46128, #76616, #8133, #38626, #69127, #93585, #40601, #63575, #56096, #49075, #10587, #17609, #47603, #94084, #24620, #62584, #86589, #71098, #64057, #18098, #2130, #26088, #11564, #48575, #78592, #18582, #25604, #85606, #93089, #32590, #63085, #55604, #9600, #64546, #33561, #40103, #57059, #41598, #2624, #3106, #33079, #79074, #41099, #87560, #55086, #17121, #19069, #70604, #94569, #48079, #25122, #34050, #56583, #78097, #86098, #71595, #87073, #49548, #80060, #42082, #10104, #95053, #79577, #3591, #11077, #72066, #26562, #72545, #32086, #59527, #5559, #89537, #96564, #12055, #90020, #96061, #12551, #65036, #58534, #21542, #4078, #35035, #97556, #34541, #73040, #20553, #52033, #95562, #44022, #82526, #44523, #43053, #89042, #36035, #51038, #73532, #74028, #81531, #27544, #66538, #66035, #5059, #4575, #57549, #14042, #35544, #27051, #88048, #42556, #28039, #19561, #58038, #88546, #21047, #13037, #36545, #20047, #50549, #97066, #81044, #43534, #50057, #65538, #74525, #6046, #28538, #59031, #51537, #82028, #13538, #67034, #80561, #29017, #69014, #38516, #92482, #14541, #30992, #91003, #37537, #84991, #7538, #31479, #53999, #24008, #52518, #23029, #54480, #545, #16506, #75022, #22043, #61490, #53005, #38030, #83024, #30005, #6527, #76994, #76010, #91996, #68521, #60511, #53501, #23527 ) ),
 .UNSPECIFIED., .F., .F., .F. ) 
 B_SPLINE_SURFACE_WITH_KNOTS ( ( 2, 2 ),
 ( 3, 2, 2, 2, 2, 2, 2, 2, 2, 2, 2, 2, 2, 2, 2, 2, 2, 2, 2, 2, 2, 2, 2, 2, 2, 2, 2, 2, 2, 2, 2, 2, 2, 2, 2, 2, 2, 2, 2, 2, 2, 2, 2, 2, 2, 2, 2, 2, 2, 2, 2, 2, 2, 2, 2, 2, 2, 2, 2, 2, 2, 2, 2, 2, 2, 2, 2, 2, 2, 2, 2, 2, 2, 2, 2, 2, 2, 2, 2, 2, 2, 2, 2, 2, 2, 2, 2, 2, 2, 2, 2, 2, 2, 2, 2, 2, 2, 2, 2, 2, 2, 2, 2, 2, 2, 2, 2, 2, 2, 2, 2, 2, 2, 2, 2, 2, 2, 2, 2, 2, 2, 2, 2, 2, 2, 2, 2, 2, 2, 2, 2, 2, 2, 2, 2, 2, 2, 2, 2, 2, 2, 2, 2, 2, 2, 2, 2, 2, 2, 2, 2, 2, 2, 2, 2, 2, 2, 2, 2, 2, 2, 2, 3 ),
 ( 0.000000000000000000, 1.000000000000000000 ),
 ( 0.000000000000000000, 0.005952380952380952051, 0.01190476190476190410, 0.01785714285714285615, 0.02380952380952380820, 0.02976190476190476025, 0.03571428571428571230, 0.04166666666666666435, 0.04761904761904761640, 0.05357142857142856845, 0.05952380952380952051, 0.06547619047619047949, 0.07142857142857142461, 0.07738095238095238360, 0.08333333333333332871, 0.08928571428571428770, 0.09523809523809523281, 0.1011904761904761918, 0.1071428571428571369, 0.1130952380952380959, 0.1190476190476190410, 0.1250000000000000000, 0.1309523809523809590, 0.1369047619047619180, 0.1428571428571428492, 0.1488095238095238082, 0.1547619047619047672, 0.1607142857142857262, 0.1666666666666666574, 0.1726190476190476164, 0.1785714285714285754, 0.1845238095238095344, 0.1904761904761904656, 0.1964285714285714246, 0.2023809523809523836, 0.2083333333333333426, 0.2142857142857142738, 0.2202380952380952328, 0.2261904761904761918, 0.2321428571428571508, 0.2380952380952380820, 0.2440476190476190410, 0.2500000000000000000, 0.2559523809523809312, 0.2619047619047619180, 0.2678571428571428492, 0.2738095238095238360, 0.2797619047619047672, 0.2857142857142856984, 0.2916666666666666852, 0.2976190476190476164, 0.3035714285714285476, 0.3095238095238095344, 0.3154761904761904656, 0.3214285714285714524, 0.3273809523809523836, 0.3333333333333333148, 0.3392857142857143016, 0.3452380952380952328, 0.3511904761904761640, 0.3571428571428571508, 0.3630952380952380820, 0.3690476190476190688, 0.3750000000000000000, 0.3809523809523809312, 0.3869047619047619180, 0.3928571428571428492, 0.3988095238095238360, 0.4047619047619047672, 0.4107142857142856984, 0.4166666666666666852, 0.4226190476190476164, 0.4285714285714285476, 0.4345238095238095344, 0.4404761904761904656, 0.4464285714285714524, 0.4523809523809523836, 0.4583333333333333148, 0.4642857142857143016, 0.4702380952380952328, 0.4761904761904761640, 0.4821428571428571508, 0.4880952380952380820, 0.4940476190476190688, 0.5000000000000000000, 0.5059523809523809312, 0.5119047619047618625, 0.5178571428571429047, 0.5238095238095238360, 0.5297619047619047672, 0.5357142857142856984, 0.5416666666666666297, 0.5476190476190476719, 0.5535714285714286031, 0.5595238095238095344, 0.5654761904761904656, 0.5714285714285713969, 0.5773809523809523281, 0.5833333333333333703, 0.5892857142857143016, 0.5952380952380952328, 0.6011904761904761640, 0.6071428571428570953, 0.6130952380952381375, 0.6190476190476190688, 0.6250000000000000000, 0.6309523809523809312, 0.6369047619047618625, 0.6428571428571429047, 0.6488095238095238360, 0.6547619047619047672, 0.6607142857142856984, 0.6666666666666666297, 0.6726190476190476719, 0.6785714285714286031, 0.6845238095238095344, 0.6904761904761904656, 0.6964285714285713969, 0.7023809523809523281, 0.7083333333333333703, 0.7142857142857143016, 0.7202380952380952328, 0.7261904761904761640, 0.7321428571428570953, 0.7380952380952381375, 0.7440476190476190688, 0.7500000000000000000, 0.7559523809523809312, 0.7619047619047618625, 0.7678571428571429047, 0.7738095238095238360, 0.7797619047619047672, 0.7857142857142856984, 0.7916666666666666297, 0.7976190476190476719, 0.8035714285714286031, 0.8095238095238095344, 0.8154761904761904656, 0.8214285714285713969, 0.8273809523809523281, 0.8333333333333333703, 0.8392857142857143016, 0.8452380952380952328, 0.8511904761904761640, 0.8571428571428570953, 0.8630952380952381375, 0.8690476190476190688, 0.8750000000000000000, 0.8809523809523809312, 0.8869047619047618625, 0.8928571428571429047, 0.8988095238095238360, 0.9047619047619047672, 0.9107142857142856984, 0.9166666666666666297, 0.9226190476190476719, 0.9285714285714286031, 0.9345238095238095344, 0.9404761904761904656, 0.9464285714285713969, 0.9523809523809523281, 0.9583333333333333703, 0.9642857142857143016 ),
 .UNSPECIFIED. ) 
 GEOMETRIC_REPRESENTATION_ITEM ( )  RATIONAL_B_SPLINE_SURFACE ( (
 ( 1.000000000000000000, 0.9659258262890683122, 1.000000000000000000, 0.9659258262890683122, 1.000000000000000000, 0.9659258262890683122, 1.000000000000000000, 0.9659258262890683122, 1.000000000000000000, 0.9659258262890683122, 1.000000000000000000, 0.9659258262890683122, 1.000000000000000000, 0.9659258262890683122, 1.000000000000000000, 0.9659258262890683122, 1.000000000000000000, 0.9659258262890683122, 1.000000000000000000, 0.9659258262890683122, 1.000000000000000000, 0.9659258262890683122, 1.000000000000000000, 0.9659258262890683122, 1.000000000000000000, 0.9659258262890683122, 1.000000000000000000, 0.9659258262890683122, 1.000000000000000000, 0.9659258262890683122, 1.000000000000000000, 0.9659258262890683122, 1.000000000000000000, 0.9659258262890683122, 1.000000000000000000, 0.9659258262890683122, 1.000000000000000000, 0.9659258262890683122, 1.000000000000000000, 0.9659258262890683122, 1.000000000000000000, 0.9659258262890683122, 1.000000000000000000, 0.9659258262890683122, 1.000000000000000000, 0.9659258262890683122, 1.000000000000000000, 0.9659258262890683122, 1.000000000000000000, 0.9659258262890683122, 1.000000000000000000, 0.9659258262890683122, 1.000000000000000000, 0.9659258262890683122, 1.000000000000000000, 0.9659258262890683122, 1.000000000000000000, 0.9659258262890683122, 1.000000000000000000, 0.9659258262890683122, 1.000000000000000000, 0.9659258262890683122, 1.000000000000000000, 0.9659258262890683122, 1.000000000000000000, 0.9659258262890683122, 1.000000000000000000, 0.9659258262890683122, 1.000000000000000000, 0.9659258262890683122, 1.000000000000000000, 0.9659258262890683122, 1.000000000000000000, 0.9659258262890683122, 1.000000000000000000, 0.9659258262890683122, 1.000000000000000000, 0.9659258262890683122, 1.000000000000000000, 0.9659258262890683122, 1.000000000000000000, 0.9659258262890683122, 1.000000000000000000, 0.9659258262890683122, 1.000000000000000000, 0.9659258262890683122, 1.000000000000000000, 0.9659258262890683122, 1.000000000000000000, 0.9659258262890683122, 1.000000000000000000, 0.9659258262890683122, 1.000000000000000000, 0.9659258262890683122, 1.000000000000000000, 0.9659258262890683122, 1.000000000000000000, 0.9659258262890683122, 1.000000000000000000, 0.9659258262890683122, 1.000000000000000000, 0.9659258262890683122, 1.000000000000000000, 0.9659258262890683122, 1.000000000000000000, 0.9659258262890683122, 1.000000000000000000, 0.9659258262890683122, 1.000000000000000000, 0.9659258262890683122, 1.000000000000000000, 0.9659258262890683122, 1.000000000000000000, 0.9659258262890683122, 1.000000000000000000, 0.9659258262890683122, 1.000000000000000000, 0.9659258262890683122, 1.000000000000000000, 0.9659258262890683122, 1.000000000000000000, 0.9659258262890683122, 1.000000000000000000, 0.9659258262890683122, 1.000000000000000000, 0.9659258262890683122, 1.000000000000000000, 0.9659258262890683122, 1.000000000000000000, 0.9659258262890683122, 1.000000000000000000, 0.9659258262890683122, 1.000000000000000000, 0.9659258262890683122, 1.000000000000000000, 0.9659258262890683122, 1.000000000000000000, 0.9659258262890683122, 1.000000000000000000, 0.9659258262890683122, 1.000000000000000000, 0.9659258262890683122, 1.000000000000000000, 0.9659258262890683122, 1.000000000000000000, 0.9659258262890683122, 1.000000000000000000, 0.9659258262890683122, 1.000000000000000000, 0.9659258262890683122, 1.000000000000000000, 0.9659258262890683122, 1.000000000000000000, 0.9659258262890683122, 1.000000000000000000, 0.9659258262890683122, 1.000000000000000000, 0.9659258262890683122, 1.000000000000000000, 0.9659258262890683122, 1.000000000000000000, 0.9659258262890683122, 1.000000000000000000, 0.9659258262890683122, 1.000000000000000000, 0.9659258262890683122, 1.000000000000000000, 0.9659258262890683122, 1.000000000000000000, 0.9659258262890683122, 1.000000000000000000, 0.9659258262890683122, 1.000000000000000000, 0.9659258262890683122, 1.000000000000000000, 0.9659258262890683122, 1.000000000000000000, 0.9659258262890683122, 1.000000000000000000, 0.9659258262890683122, 1.000000000000000000, 0.9659258262890683122, 1.000000000000000000, 0.9659258262890683122, 1.000000000000000000, 0.9659258262890683122, 1.000000000000000000, 0.9659258262890683122, 1.000000000000000000, 0.9659258262890683122, 1.000000000000000000, 0.9659258262890683122, 1.000000000000000000, 0.9659258262890683122, 1.000000000000000000, 0.9659258262890683122, 1.000000000000000000, 0.9659258262890683122, 1.000000000000000000, 0.9659258262890683122, 1.000000000000000000, 0.9659258262890683122, 1.000000000000000000, 0.9659258262890683122, 1.000000000000000000, 0.9659258262890683122, 1.000000000000000000, 0.9659258262890683122, 1.000000000000000000, 0.9659258262890683122, 1.000000000000000000, 0.9659258262890683122, 1.000000000000000000, 0.9659258262890683122, 1.000000000000000000, 0.9659258262890683122, 1.000000000000000000, 0.9659258262890683122, 1.000000000000000000, 0.9659258262890683122, 1.000000000000000000, 0.9659258262890683122, 1.000000000000000000, 0.9659258262890683122, 1.000000000000000000, 0.9659258262890683122, 1.000000000000000000, 0.9659258262890683122, 1.000000000000000000, 0.9659258262890683122, 1.000000000000000000, 0.9659258262890683122, 1.000000000000000000, 0.9659258262890683122, 1.000000000000000000, 0.9659258262890683122, 1.000000000000000000, 0.9659258262890683122, 1.000000000000000000, 0.9659258262890683122, 1.000000000000000000, 0.9659258262890683122, 1.000000000000000000, 0.9659258262890683122, 1.000000000000000000, 0.9659258262890683122, 1.000000000000000000, 0.9659258262890683122, 1.000000000000000000, 0.9659258262890683122, 1.000000000000000000, 0.9659258262890683122, 1.000000000000000000, 0.9659258262890683122, 1.000000000000000000, 0.9659258262890683122, 1.000000000000000000, 0.9659258262890683122, 1.000000000000000000, 0.9659258262890683122, 1.000000000000000000, 0.9659258262890683122, 1.000000000000000000, 0.9659258262890683122, 1.000000000000000000, 0.9659258262890683122, 1.000000000000000000, 0.9659258262890683122, 1.000000000000000000, 0.9659258262890683122, 1.000000000000000000, 0.9659258262890683122, 1.000000000000000000, 0.9659258262890683122, 1.000000000000000000, 0.9659258262890683122, 1.000000000000000000, 0.9659258262890683122, 1.000000000000000000, 0.9659258262890683122, 1.000000000000000000, 0.9659258262890683122, 1.000000000000000000, 0.9659258262890683122, 1.000000000000000000, 0.9659258262890683122, 1.000000000000000000, 0.9659258262890683122, 1.000000000000000000, 0.9659258262890683122, 1.000000000000000000, 0.9659258262890683122, 1.000000000000000000, 0.9659258262890683122, 1.000000000000000000, 0.9659258262890683122, 1.000000000000000000, 0.9659258262890683122, 1.000000000000000000, 0.9659258262890683122, 1.000000000000000000, 0.9659258262890683122, 1.000000000000000000, 0.9659258262890683122, 1.000000000000000000, 0.9659258262890683122, 1.000000000000000000, 0.9659258262890683122, 1.000000000000000000, 0.9659258262890683122, 1.000000000000000000, 0.9659258262890683122, 1.000000000000000000, 0.9659258262890683122, 1.000000000000000000, 0.9659258262890683122, 1.000000000000000000, 0.9659258262890683122, 1.000000000000000000, 0.9659258262890683122, 1.000000000000000000, 0.9659258262890683122, 1.000000000000000000, 0.9659258262890683122, 1.000000000000000000),
 ( 1.000000000000000000, 0.9659258262890683122, 1.000000000000000000, 0.9659258262890683122, 1.000000000000000000, 0.9659258262890683122, 1.000000000000000000, 0.9659258262890683122, 1.000000000000000000, 0.9659258262890683122, 1.000000000000000000, 0.9659258262890683122, 1.000000000000000000, 0.9659258262890683122, 1.000000000000000000, 0.9659258262890683122, 1.000000000000000000, 0.9659258262890683122, 1.000000000000000000, 0.9659258262890683122, 1.000000000000000000, 0.9659258262890683122, 1.000000000000000000, 0.9659258262890683122, 1.000000000000000000, 0.9659258262890683122, 1.000000000000000000, 0.9659258262890683122, 1.000000000000000000, 0.9659258262890683122, 1.000000000000000000, 0.9659258262890683122, 1.000000000000000000, 0.9659258262890683122, 1.000000000000000000, 0.9659258262890683122, 1.000000000000000000, 0.9659258262890683122, 1.000000000000000000, 0.9659258262890683122, 1.000000000000000000, 0.9659258262890683122, 1.000000000000000000, 0.9659258262890683122, 1.000000000000000000, 0.9659258262890683122, 1.000000000000000000, 0.9659258262890683122, 1.000000000000000000, 0.9659258262890683122, 1.000000000000000000, 0.9659258262890683122, 1.000000000000000000, 0.9659258262890683122, 1.000000000000000000, 0.9659258262890683122, 1.000000000000000000, 0.9659258262890683122, 1.000000000000000000, 0.9659258262890683122, 1.000000000000000000, 0.9659258262890683122, 1.000000000000000000, 0.9659258262890683122, 1.000000000000000000, 0.9659258262890683122, 1.000000000000000000, 0.9659258262890683122, 1.000000000000000000, 0.9659258262890683122, 1.000000000000000000, 0.9659258262890683122, 1.000000000000000000, 0.9659258262890683122, 1.000000000000000000, 0.9659258262890683122, 1.000000000000000000, 0.9659258262890683122, 1.000000000000000000, 0.9659258262890683122, 1.000000000000000000, 0.9659258262890683122, 1.000000000000000000, 0.9659258262890683122, 1.000000000000000000, 0.9659258262890683122, 1.000000000000000000, 0.9659258262890683122, 1.000000000000000000, 0.9659258262890683122, 1.000000000000000000, 0.9659258262890683122, 1.000000000000000000, 0.9659258262890683122, 1.000000000000000000, 0.9659258262890683122, 1.000000000000000000, 0.9659258262890683122, 1.000000000000000000, 0.9659258262890683122, 1.000000000000000000, 0.9659258262890683122, 1.000000000000000000, 0.9659258262890683122, 1.000000000000000000, 0.9659258262890683122, 1.000000000000000000, 0.9659258262890683122, 1.000000000000000000, 0.9659258262890683122, 1.000000000000000000, 0.9659258262890683122, 1.000000000000000000, 0.9659258262890683122, 1.000000000000000000, 0.9659258262890683122, 1.000000000000000000, 0.9659258262890683122, 1.000000000000000000, 0.9659258262890683122, 1.000000000000000000, 0.9659258262890683122, 1.000000000000000000, 0.9659258262890683122, 1.000000000000000000, 0.9659258262890683122, 1.000000000000000000, 0.9659258262890683122, 1.000000000000000000, 0.9659258262890683122, 1.000000000000000000, 0.9659258262890683122, 1.000000000000000000, 0.9659258262890683122, 1.000000000000000000, 0.9659258262890683122, 1.000000000000000000, 0.9659258262890683122, 1.000000000000000000, 0.9659258262890683122, 1.000000000000000000, 0.9659258262890683122, 1.000000000000000000, 0.9659258262890683122, 1.000000000000000000, 0.9659258262890683122, 1.000000000000000000, 0.9659258262890683122, 1.000000000000000000, 0.9659258262890683122, 1.000000000000000000, 0.9659258262890683122, 1.000000000000000000, 0.9659258262890683122, 1.000000000000000000, 0.9659258262890683122, 1.000000000000000000, 0.9659258262890683122, 1.000000000000000000, 0.9659258262890683122, 1.000000000000000000, 0.9659258262890683122, 1.000000000000000000, 0.9659258262890683122, 1.000000000000000000, 0.9659258262890683122, 1.000000000000000000, 0.9659258262890683122, 1.000000000000000000, 0.9659258262890683122, 1.000000000000000000, 0.9659258262890683122, 1.000000000000000000, 0.9659258262890683122, 1.000000000000000000, 0.9659258262890683122, 1.000000000000000000, 0.9659258262890683122, 1.000000000000000000, 0.9659258262890683122, 1.000000000000000000, 0.9659258262890683122, 1.000000000000000000, 0.9659258262890683122, 1.000000000000000000, 0.9659258262890683122, 1.000000000000000000, 0.9659258262890683122, 1.000000000000000000, 0.9659258262890683122, 1.000000000000000000, 0.9659258262890683122, 1.000000000000000000, 0.9659258262890683122, 1.000000000000000000, 0.9659258262890683122, 1.000000000000000000, 0.9659258262890683122, 1.000000000000000000, 0.9659258262890683122, 1.000000000000000000, 0.9659258262890683122, 1.000000000000000000, 0.9659258262890683122, 1.000000000000000000, 0.9659258262890683122, 1.000000000000000000, 0.9659258262890683122, 1.000000000000000000, 0.9659258262890683122, 1.000000000000000000, 0.9659258262890683122, 1.000000000000000000, 0.9659258262890683122, 1.000000000000000000, 0.9659258262890683122, 1.000000000000000000, 0.9659258262890683122, 1.000000000000000000, 0.9659258262890683122, 1.000000000000000000, 0.9659258262890683122, 1.000000000000000000, 0.9659258262890683122, 1.000000000000000000, 0.9659258262890683122, 1.000000000000000000, 0.9659258262890683122, 1.000000000000000000, 0.9659258262890683122, 1.000000000000000000, 0.9659258262890683122, 1.000000000000000000, 0.9659258262890683122, 1.000000000000000000, 0.9659258262890683122, 1.000000000000000000, 0.9659258262890683122, 1.000000000000000000, 0.9659258262890683122, 1.000000000000000000, 0.9659258262890683122, 1.000000000000000000, 0.9659258262890683122, 1.000000000000000000, 0.9659258262890683122, 1.000000000000000000, 0.9659258262890683122, 1.000000000000000000, 0.9659258262890683122, 1.000000000000000000, 0.9659258262890683122, 1.000000000000000000, 0.9659258262890683122, 1.000000000000000000, 0.9659258262890683122, 1.000000000000000000, 0.9659258262890683122, 1.000000000000000000, 0.9659258262890683122, 1.000000000000000000, 0.9659258262890683122, 1.000000000000000000, 0.9659258262890683122, 1.000000000000000000, 0.9659258262890683122, 1.000000000000000000, 0.9659258262890683122, 1.000000000000000000, 0.9659258262890683122, 1.000000000000000000, 0.9659258262890683122, 1.000000000000000000, 0.9659258262890683122, 1.000000000000000000, 0.9659258262890683122, 1.000000000000000000, 0.9659258262890683122, 1.000000000000000000, 0.9659258262890683122, 1.000000000000000000, 0.9659258262890683122, 1.000000000000000000, 0.9659258262890683122, 1.000000000000000000, 0.9659258262890683122, 1.000000000000000000, 0.9659258262890683122, 1.000000000000000000, 0.9659258262890683122, 1.000000000000000000, 0.9659258262890683122, 1.000000000000000000, 0.9659258262890683122, 1.000000000000000000, 0.9659258262890683122, 1.000000000000000000, 0.9659258262890683122, 1.000000000000000000, 0.9659258262890683122, 1.000000000000000000, 0.9659258262890683122, 1.000000000000000000, 0.9659258262890683122, 1.000000000000000000, 0.9659258262890683122, 1.000000000000000000, 0.9659258262890683122, 1.000000000000000000, 0.9659258262890683122, 1.000000000000000000, 0.9659258262890683122, 1.000000000000000000, 0.9659258262890683122, 1.000000000000000000, 0.9659258262890683122, 1.000000000000000000, 0.9659258262890683122, 1.000000000000000000, 0.9659258262890683122, 1.000000000000000000, 0.9659258262890683122, 1.000000000000000000, 0.9659258262890683122, 1.000000000000000000) ) ) 
 REPRESENTATION_ITEM ( '' )  SURFACE ( )  );
#29498=CARTESIAN_POINT ( 'NONE',  ( 13.43411237798105340, 45.58196800326374643, 12.81628187352647963 ) ) ;
#29499=ORIENTED_EDGE ( 'NONE', *, *, #8806, .F. ) ;
#29500=CARTESIAN_POINT ( 'NONE',  ( 4.559911319644449179, 62.23035201082150536, -9.422509992056141925 ) ) ;
#29501=CARTESIAN_POINT ( 'NONE',  ( 10.00000000000000000, 37.87363466993041783, -12.81628187352647608 ) ) ;
#29502=CARTESIAN_POINT ( 'NONE',  ( 7.361572987183169658, 4.967264484334119601, -9.846743663894592657 ) ) ;
#29503=CARTESIAN_POINT ( 'NONE',  ( 15.44008868035555793, 41.39701867748817676, -9.422509992056140149 ) ) ;
#29506=CARTESIAN_POINT ( 'NONE',  ( 10.00000000000000178, 22.25893115100078745, 9.846743663894594434 ) ) ;
#29508=CARTESIAN_POINT ( 'NONE',  ( 10.00000000000000178, 12.25893115100078568, 9.846743663894594434 ) ) ;
#29509=CARTESIAN_POINT ( 'NONE',  ( 2.917880565312948704, 37.63708216824731068, 12.26659068614894643 ) ) ;
#29510=CARTESIAN_POINT ( 'NONE',  ( 2.603489959281614308, 56.58210964143329846, 6.500000000000031086 ) ) ;
#29512=FILL_AREA_STYLE_COLOUR ( '', #1930 ) ;
#29515=CARTESIAN_POINT ( 'NONE',  ( -0.3689425029237898834, 66.17874883491396076, -10.36894250292378850 ) ) ;
#29516=CARTESIAN_POINT ( 'NONE',  ( -4.164238869374099039, 66.80374883491396076, 8.674139862899312516E-16 ) ) ;
#29517=CARTESIAN_POINT ( 'NONE',  ( 2.791683348922237240, 35.38393115100079456, -7.208316651077763204 ) ) ;
#29518=VECTOR ( 'NONE', #72762, 1000.000000000000000 ) ;
#29519=CARTESIAN_POINT ( 'NONE',  ( -1.099225684535947600, 44.54030133659708923, 6.408140936763237150 ) ) ;
#29522=CARTESIAN_POINT ( 'NONE',  ( 17.08211943468705840, 5.137082168247300906, -12.26659068614894466 ) ) ;
#29523=CARTESIAN_POINT ( 'NONE',  ( 7.084665262690076126, 12.02201867748817143, -10.88017736071110164 ) ) ;
#29524=CARTESIAN_POINT ( 'NONE',  ( -2.266590686148945544, 51.38708216824730357, -7.082119434687050408 ) ) ;
#29525=CARTESIAN_POINT ( 'NONE',  ( 19.84674366389459621, 23.50893115100078390, 7.409399052514197653E-17 ) ) ;
#29527=CARTESIAN_POINT ( 'NONE',  ( 14.92337183194729988, 29.34226448433411960, -8.527530157486177487 ) ) ;
#29528=B_SPLINE_CURVE_WITH_KNOTS ( 'NONE', 3,
 ( #94619, #58082, #12103, #65083, #88586, #26132 ),
 .UNSPECIFIED., .F., .F.,
 ( 4, 2, 4 ),
 ( 0.000000000000000000, 0.0002605067024380892785, 0.0005210134048761785571 ),
 .UNSPECIFIED. ) ;
#29529=EDGE_CURVE ( 'NONE', #38580, #58843, #94922, .T. ) ;
#29536=CARTESIAN_POINT ( 'NONE',  ( 5.076628168052704559, 45.17559781766745175, -8.527530157486179263 ) ) ;
#29537=CARTESIAN_POINT ( 'NONE',  ( -0.3689425029237881626, 17.42874883491397142, 10.36894250292379027 ) ) ;
#29538=CARTESIAN_POINT ( 'NONE',  ( 17.96484262340118221, 29.93868534415484106, 7.964842623401181321 ) ) ;
#29539=CARTESIAN_POINT ( 'NONE',  ( 17.96484262340118221, 39.93868534415484106, 7.964842623401181321 ) ) ;
#29540=CARTESIAN_POINT ( 'NONE',  ( 7.361572987183169658, 64.96726448433412315, -9.846743663894592657 ) ) ;
#29541=CARTESIAN_POINT ( 'NONE',  ( 10.00000000000000178, 20.37363466993042138, 12.81628187352647608 ) ) ;
#29542=CARTESIAN_POINT ( 'NONE',  ( -0.8801773607111008646, 68.27201867748817676, 2.915334737309923430 ) ) ;
#29543=CARTESIAN_POINT ( 'NONE',  ( -1.099225684535947600, 33.70696800326375353, -6.408140936763238038 ) ) ;
#29545=CARTESIAN_POINT ( 'NONE',  ( 10.00000000000000000, 49.75893115100078745, -9.846743663894594434 ) ) ;
#29546=CARTESIAN_POINT ( 'NONE',  ( 7.084665262690076126, 9.105352010821503583, 10.88017736071109987 ) ) ;
#29548=CARTESIAN_POINT ( 'NONE',  ( 12.91533473730993009, 11.60535201082150714, -10.88017736071109987 ) ) ;
#29549=B_SPLINE_CURVE_WITH_KNOTS ( 'NONE', 3,
 ( #62046, #85058, #39572, #15593 ),
 .UNSPECIFIED., .F., .F.,
 ( 4, 4 ),
 ( 4.336808689942017736E-18, 0.001060528352561992006 ),
 .UNSPECIFIED. ) ;
#29551=CARTESIAN_POINT ( 'NONE',  ( 17.96484262340118221, 51.18868534415483396, -7.964842623401177768 ) ) ;
#29552=CARTESIAN_POINT ( 'NONE',  ( 0.5774900079438590739, 52.64701867748817676, -5.440088680355550821 ) ) ;
#29553=B_SPLINE_CURVE_WITH_KNOTS ( 'NONE', 3,
 ( #45981, #85449, #61947, #9447 ),
 .UNSPECIFIED., .F., .F.,
 ( 4, 4 ),
 ( 0.000000000000000000, 0.001036303429213364206 ),
 .UNSPECIFIED. ) ;
#29554=CARTESIAN_POINT ( 'NONE',  ( 4.559911319644449179, 62.23035201082150536, -9.422509992056141925 ) ) ;
#29555=PRESENTATION_STYLE_ASSIGNMENT (( #52565 ) ) ;
#29556=CARTESIAN_POINT ( 'NONE',  ( 19.42250999205614548, 50.98035201082151247, -5.440088680355545492 ) ) ;
#29557=CARTESIAN_POINT ( 'NONE',  ( -46.94000000000001194, 102.4632489371144146, 6.394394627235429951 ) ) ;
#29558=ADVANCED_FACE ( 'NONE', ( #65403 ), #63440, .F. ) ;
#29559=FILL_AREA_STYLE ('',( #37090 ) ) ;
#29560=CARTESIAN_POINT ( 'NONE',  ( 7.361572987183169658, 24.96726448433412315, -9.846743663894592657 ) ) ;
#29562=CARTESIAN_POINT ( 'NONE',  ( 0.000000000000000000, 70.00000000000000000, -5.000000000000000000 ) ) ;
#29564=( NAMED_UNIT ( * ) PLANE_ANGLE_UNIT ( ) SI_UNIT ( $, .RADIAN. ) );
#29565=CARTESIAN_POINT ( 'NONE',  ( 6.204703633549690345, 2.845415501580634388, 14.16423886937410082 ) ) ;
#29566=CARTESIAN_POINT ( 'NONE',  ( 20.10493008474206178, 29.71697413083880335, 6.336235997365763595 ) ) ;
#29568=CARTESIAN_POINT ( 'NONE',  ( 14.92337183194729633, 37.67559781766745175, 8.527530157486181039 ) ) ;
#29569=CARTESIAN_POINT ( 'NONE',  ( -0.8801773607111008646, 8.272018677488171434, 2.915334737309923430 ) ) ;
#29573=CARTESIAN_POINT ( 'NONE',  ( 14.92337183194729633, 42.67559781766745886, 8.527530157486181039 ) ) ;
#29574=CYLINDRICAL_SURFACE ( 'NONE', #96257, 11.92686044187656513 ) ;
#29575=CARTESIAN_POINT ( 'NONE',  ( 22.81628187352648496, 21.83196800326374643, -3.434112377981050290 ) ) ;
#29576=CARTESIAN_POINT ( 'NONE',  ( 19.84674366389459621, 13.50893115100078568, 7.409399052514197653E-17 ) ) ;
#29577=CARTESIAN_POINT ( 'NONE',  ( 0.2751277870542911397, 35.30223176428830811, 6.499999999999992006 ) ) ;
#29578=CARTESIAN_POINT ( 'NONE',  ( 16.40814093676323893, 5.790301336597087456, 11.09922568453595026 ) ) ;
#29581=EDGE_CURVE ( 'NONE', #21351, #46284, #9907, .T. ) ;
#29583=ORIENTED_EDGE ( 'NONE', *, *, #84676, .T. ) ;
#29584=CARTESIAN_POINT ( 'NONE',  ( 12.91533473730992121, 29.52201867748817321, 10.88017736071110164 ) ) ;
#29585=CARTESIAN_POINT ( 'NONE',  ( 17.08211943468705840, 20.13708216824730357, -12.26659068614894466 ) ) ;
#29586=CARTESIAN_POINT ( 'NONE',  ( 2.791683348922240793, 26.63393115100078745, 7.208316651077764092 ) ) ;
#29587=CARTESIAN_POINT ( 'NONE',  ( 12.91533473730993009, 56.60535201082151247, -10.88017736071109987 ) ) ;
#29588=CARTESIAN_POINT ( 'NONE',  ( 21.09922568453595559, 42.04030133659708213, -6.408140936763230044 ) ) ;
#29590=CARTESIAN_POINT ( 'NONE',  ( 19.42250999205614548, 10.98035201082150358, -5.440088680355545492 ) ) ;
#29594=CARTESIAN_POINT ( 'NONE',  ( 0.6178305044545838731, 14.74863466993041783, 9.382169495545420901 ) ) ;
#29595=CARTESIAN_POINT ( 'NONE',  ( 6.565887622018943937, 5.165301336597086568, 12.81628187352647430 ) ) ;
#29596=CARTESIAN_POINT ( 'NONE',  ( 17.20831665107776587, 22.88393115100078745, 7.208316651077764980 ) ) ;
#29598=CARTESIAN_POINT ( 'NONE',  ( 21.09922568453594849, 31.20696800326375353, 6.408140936763242479 ) ) ;
#29601=CARTESIAN_POINT ( 'NONE',  ( 15.44008868035555793, 41.39701867748817676, -9.422509992056140149 ) ) ;
#29604=CARTESIAN_POINT ( 'NONE',  ( 4.559911319644449179, 67.23035201082150536, -9.422509992056141925 ) ) ;
#29605=CARTESIAN_POINT ( 'NONE',  ( 0.5774900079438607392, 38.48035201082150536, 5.440088680355550821 ) ) ;
#29606=CARTESIAN_POINT ( 'NONE',  ( 20.88017736071110875, 45.77201867748816966, -2.915334737309920765 ) ) ;
#29607=CARTESIAN_POINT ( 'NONE',  ( 5.076628168052703671, 66.84226448433412315, 8.527530157486179263 ) ) ;
#29610=CARTESIAN_POINT ( 'NONE',  ( 2.791683348922237240, 35.38393115100079456, -7.208316651077763204 ) ) ;
#29611=CARTESIAN_POINT ( 'NONE',  ( 20.88017736071110875, 10.77201867748817143, -2.915334737309920765 ) ) ;
#29612=CARTESIAN_POINT ( 'NONE',  ( 3.591859063236763294, 13.29030133659708746, -11.09922568453595026 ) ) ;
#29614=CARTESIAN_POINT ( 'NONE',  ( 15.44008868035555260, 29.73035201082150891, 9.422509992056143702 ) ) ;
#29616=CARTESIAN_POINT ( 'NONE',  ( 20.88017736071110875, 25.77201867748816966, -2.915334737309920765 ) ) ;
#29617=CARTESIAN_POINT ( 'NONE',  ( 2.035157376598824452, 68.68868534415484817, 7.964842623401179544 ) ) ;
#29618=CARTESIAN_POINT ( 'NONE',  ( 24.16423886937410614, 39.30374883491396787, 8.672049930838204340E-16 ) ) ;
#29619=CARTESIAN_POINT ( 'NONE',  ( 0.1532563361054082862, 16.21726448433411960, 2.638427012816831674 ) ) ;
#29620=CARTESIAN_POINT ( 'NONE',  ( 12.91533473730992121, 49.52201867748817676, 10.88017736071110164 ) ) ;
#29621=CARTESIAN_POINT ( 'NONE',  ( 19.72487221294571214, 37.80223176428831522, -6.499999999999988454 ) ) ;
#29622=CARTESIAN_POINT ( 'NONE',  ( 24.16423886937410614, 4.303748834913967869, 8.672049930838204340E-16 ) ) ;
#29626=CARTESIAN_POINT ( 'NONE',  ( 1.472469842513823179, 65.59226448433412315, -4.923371831947296329 ) ) ;
#29627=VERTEX_POINT ( 'NONE', #75375 ) ;
#29629=CARTESIAN_POINT ( 'NONE',  ( 6.204703633549690345, 17.84541550158063217, 14.16423886937410082 ) ) ;
#29630=CARTESIAN_POINT ( 'NONE',  ( 17.08211943468705840, 20.13708216824730357, -12.26659068614894466 ) ) ;
#29631=CARTESIAN_POINT ( 'NONE',  ( 0.5774900079438607392, 63.48035201082149825, 5.440088680355550821 ) ) ;
#29632=CARTESIAN_POINT ( 'NONE',  ( -4.164238869374098151, 66.59541550158060375, -3.795296366450310543 ) ) ;
#29633=CARTESIAN_POINT ( 'NONE',  ( 21.09922568453594849, 1.206968003263753531, 6.408140936763242479 ) ) ;
#29634=CARTESIAN_POINT ( 'NONE',  ( 10.00000000000000178, 47.25893115100078745, 9.846743663894594434 ) ) ;
#29636=CARTESIAN_POINT ( 'NONE',  ( 15.44008868035555793, 46.39701867748817676, -9.422509992056140149 ) ) ;
#29637=CARTESIAN_POINT ( 'NONE',  ( 3.591859063236761518, 19.95696800326375353, 11.09922568453594849 ) ) ;
#29638=CARTESIAN_POINT ( 'NONE',  ( -4.164238869374099039, 11.80374883491396965, 8.674139862899312516E-16 ) ) ;
#29639=CARTESIAN_POINT ( 'NONE',  ( 19.42250999205614193, 10.14701867748816966, 5.440088680355555262 ) ) ;
#29641=CARTESIAN_POINT ( 'NONE',  ( -0.8801773607111009756, 18.06368534415484106, 1.068504757029289695E-15 ) ) ;
#29643=CARTESIAN_POINT ( 'NONE',  ( 20.88017736071110519, 60.56368534415484106, 2.639326808657452039E-16 ) ) ;
#29644=CARTESIAN_POINT ( 'NONE',  ( 16.40814093676324603, 47.45696800326375353, -11.09922568453594671 ) ) ;
#29646=ORIENTED_EDGE ( 'NONE', *, *, #5217, .T. ) ;
#29649=CARTESIAN_POINT ( 'NONE',  ( 12.63842701281683034, 32.46726448433412315, 9.846743663894596210 ) ) ;
#29651=CARTESIAN_POINT ( 'NONE',  ( -0.1038446121089042773, 19.24302437010793199, -6.337995344473781323 ) ) ;
#29652=CARTESIAN_POINT ( 'NONE',  ( 10.00000000000000000, 50.55374883491396787, -14.16423886937410082 ) ) ;
#29653=CARTESIAN_POINT ( 'NONE',  ( 17.08211943468705130, 58.47041550158063927, 12.26659068614894998 ) ) ;
#29654=CARTESIAN_POINT ( 'NONE',  ( 1.472469842513823179, 25.59226448433412315, -4.923371831947296329 ) ) ;
#29655=CARTESIAN_POINT ( 'NONE',  ( 12.63842701281683922, 49.55059781766744464, -9.846743663894590881 ) ) ;
#29656=CARTESIAN_POINT ( 'NONE',  ( 21.92686044187657401, 50.37045670184115664, -3.195792623639525765 ) ) ;
#29658=CARTESIAN_POINT ( 'NONE',  ( 7.084665262690076126, 62.02201867748816966, -10.88017736071110164 ) ) ;
#29659=CIRCLE ( 'NONE', #93545, 6.999999999999995559 ) ;
#29662=ORIENTED_EDGE ( 'NONE', *, *, #75684, .T. ) ;
#29664=CARTESIAN_POINT ( 'NONE',  ( 20.36894250292379382, 38.67874883491396076, 10.36894250292379205 ) ) ;
#29665=CARTESIAN_POINT ( 'NONE',  ( -2.816281873526473856, 29.12363466993041783, 9.499525473075851096E-16 ) ) ;
#29666=ORIENTED_EDGE ( 'NONE', *, *, #71019, .F. ) ;
#29667=CARTESIAN_POINT ( 'NONE',  ( -2.816281873526473856, 59.33196800326374643, 3.434112377981055619 ) ) ;
#29668=CARTESIAN_POINT ( 'NONE',  ( 15.44008868035555793, 31.39701867748817676, -9.422509992056140149 ) ) ;
#29669=CARTESIAN_POINT ( 'NONE',  ( 5.076628168052703671, 36.84226448433412315, 8.527530157486179263 ) ) ;
#29670=CARTESIAN_POINT ( 'NONE',  ( 0.5774900079438607392, 28.48035201082150891, 5.440088680355550821 ) ) ;
#29673=CARTESIAN_POINT ( 'NONE',  ( 10.00000000000000178, 47.25893115100078745, 9.846743663894594434 ) ) ;
#29674=CARTESIAN_POINT ( 'NONE',  ( 7.361572987183170547, 57.05059781766744464, 9.846743663894590881 ) ) ;
#29676=ADVANCED_FACE ( 'NONE', ( #5906 ), #29377, .T. ) ;
#29681=CARTESIAN_POINT ( 'NONE',  ( 17.85158348494334746, 59.73726573380444194, -6.500000000000027534 ) ) ;
#29683=CARTESIAN_POINT ( 'NONE',  ( 6.000000000000000000, 11.00000000000000000, -6.000000000000000000 ) ) ;
#29684=CARTESIAN_POINT ( 'NONE',  ( 5.076628168052703671, 36.84226448433412315, 8.527530157486179263 ) ) ;
#29689=CARTESIAN_POINT ( 'NONE',  ( 12.63842701281683922, 59.55059781766744464, -9.846743663894590881 ) ) ;
#29691=CARTESIAN_POINT ( 'NONE',  ( 19.84674366389459621, 38.50893115100078745, 7.409399052514197653E-17 ) ) ;
#29692=CARTESIAN_POINT ( 'NONE',  ( -4.164238869374099927, 32.01208216824730357, 3.795296366450308767 ) ) ;
#29693=CARTESIAN_POINT ( 'NONE',  ( 0.1532563361054083140, 51.00893115100078745, 1.131784320476157264E-15 ) ) ;
#29694=CARTESIAN_POINT ( 'NONE',  ( 19.38216949554541557, 47.24863466993041783, -9.382169495545420901 ) ) ;
#29697=CARTESIAN_POINT ( 'NONE',  ( 1.472469842513823179, 0.5922644843341181575, -4.923371831947296329 ) ) ;
#29698=SURFACE_SIDE_STYLE ('',( #14230 ) ) ;
#29699=CARTESIAN_POINT ( 'NONE',  ( 17.20831665107776587, 42.88393115100077324, 7.208316651077764980 ) ) ;
#29700=CARTESIAN_POINT ( 'NONE',  ( 0.5774900079438590739, 37.64701867748817676, -5.440088680355550821 ) ) ;
#29702=CARTESIAN_POINT ( 'NONE',  ( 14.92337183194729988, 39.34226448433412315, -8.527530157486177487 ) ) ;
#29704=CIRCLE ( 'NONE', #74385, 11.99999999999999645 ) ;
#29706=CARTESIAN_POINT ( 'NONE',  ( 15.44008868035555793, 46.39701867748817676, -9.422509992056140149 ) ) ;
#29708=ORIENTED_EDGE ( 'NONE', *, *, #59796, .F. ) ;
#29709=CARTESIAN_POINT ( 'NONE',  ( 0.6076426042653109150, 22.37576471608601381, -6.499999999999992006 ) ) ;
#29710=CARTESIAN_POINT ( 'NONE',  ( 7.084665262690076126, 9.105352010821503583, 10.88017736071109987 ) ) ;
#29711=CARTESIAN_POINT ( 'NONE',  ( 16.40814093676323893, 0.7903013365970867898, 11.09922568453595026 ) ) ;
#29712=CARTESIAN_POINT ( 'NONE',  ( 2.035157376598824452, 43.68868534415484106, 7.964842623401179544 ) ) ;
#29713=CARTESIAN_POINT ( 'NONE',  ( 0.2751277870542969683, 2.282175860852373894, -6.500000000000000888 ) ) ;
#29717=CARTESIAN_POINT ( 'NONE',  ( 19.42250999205614193, 35.14701867748816966, 5.440088680355555262 ) ) ;
#29718=CARTESIAN_POINT ( 'NONE',  ( -46.58287598127274975, 100.7776474196661525, 9.484240826427258853 ) ) ;
#29719=CARTESIAN_POINT ( 'NONE',  ( 1.472469842513823179, 15.59226448433411960, -4.923371831947296329 ) ) ;
#29720=CARTESIAN_POINT ( 'NONE',  ( 7.361572987183169658, 19.96726448433411960, -9.846743663894592657 ) ) ;
#29721=FILL_AREA_STYLE ('',( #59730 ) ) ;
#29723=CARTESIAN_POINT ( 'NONE',  ( 0.1532563361054100626, 60.80059781766744464, -2.638427012816831230 ) ) ;
#29724=CARTESIAN_POINT ( 'NONE',  ( 10.00000000000000000, 60.55374883491397497, -14.16423886937410082 ) ) ;
#29725=CARTESIAN_POINT ( 'NONE',  ( 20.15039907845753575, 35.60158574516643171, -6.262539305110076171 ) ) ;
#29726=CARTESIAN_POINT ( 'NONE',  ( 24.16423886937410614, 19.30374883491397142, 8.672049930838204340E-16 ) ) ;
#29727=CARTESIAN_POINT ( 'NONE',  ( 24.16423886937410614, 44.30374883491397497, 8.672049930838204340E-16 ) ) ;
#29728=CARTESIAN_POINT ( 'NONE',  ( 12.91533473730992121, 4.522018677488169658, 10.88017736071110164 ) ) ;
#29730=CARTESIAN_POINT ( 'NONE',  ( 19.84674366389459266, 18.71726448433411960, -2.638427012816827677 ) ) ;
#29731=CARTESIAN_POINT ( 'NONE',  ( 0.5774900079438590739, 7.647018677488171434, -5.440088680355550821 ) ) ;
#29732=CARTESIAN_POINT ( 'NONE',  ( 17.20831665107776587, 54.13393115100079456, -7.208316651077762316 ) ) ;
#29733=CARTESIAN_POINT ( 'NONE',  ( 17.08211943468705130, 8.470415501580635720, 12.26659068614894998 ) ) ;
#29735=CARTESIAN_POINT ( 'NONE',  ( 17.20831665107776587, 2.883931151000785231, 7.208316651077764980 ) ) ;
#29736=CARTESIAN_POINT ( 'NONE',  ( -2.816281873526471635, 43.91530133659708923, -3.434112377981056508 ) ) ;
#29737=CARTESIAN_POINT ( 'NONE',  ( 10.00000000000000178, 37.25893115100078745, 9.846743663894594434 ) ) ;
#29739=CARTESIAN_POINT ( 'NONE',  ( 14.92337183194729633, 2.675597817667451750, 8.527530157486181039 ) ) ;
#29742=CARTESIAN_POINT ( 'NONE',  ( 0.5774900079438607392, 8.480352010821505360, 5.440088680355550821 ) ) ;
#29743=CARTESIAN_POINT ( 'NONE',  ( -2.266590686148945544, 51.38708216824730357, -7.082119434687050408 ) ) ;
#29744=CARTESIAN_POINT ( 'NONE',  ( 20.88017736071110519, 45.56368534415484106, 2.639326808657452039E-16 ) ) ;
#29745=CARTESIAN_POINT ( 'NONE',  ( 24.16423886937409904, 4.095415501580634832, 3.795296366450317205 ) ) ;
#29747=CARTESIAN_POINT ( 'NONE',  ( 12.63842701281683034, 27.46726448433411250, 9.846743663894596210 ) ) ;
#29748=CARTESIAN_POINT ( 'NONE',  ( 2.035157376598822676, 12.43868534415483751, -7.964842623401177768 ) ) ;
#29749=CARTESIAN_POINT ( 'NONE',  ( 18.52753015748618282, 38.92559781766745175, -4.923371831947291888 ) ) ;
#29751=CARTESIAN_POINT ( 'NONE',  ( 14.92337183194729988, 49.34226448433411605, -8.527530157486177487 ) ) ;
#29753=CARTESIAN_POINT ( 'NONE',  ( 20.88017736071110519, 35.56368534415484106, 2.639326808657452039E-16 ) ) ;
#29755=CARTESIAN_POINT ( 'NONE',  ( 0.6178305044545818747, 63.49863466993043204, -9.382169495545419124 ) ) ;
#29757=CARTESIAN_POINT ( 'NONE',  ( 12.63842701281683034, 2.467264484334118269, 9.846743663894596210 ) ) ;
#29758=CARTESIAN_POINT ( 'NONE',  ( -2.816281873526471635, 38.91530133659708213, -3.434112377981056508 ) ) ;
#29759=CARTESIAN_POINT ( 'NONE',  ( 2.035157376598824452, 3.688685344154837953, 7.964842623401179544 ) ) ;
#29760=CARTESIAN_POINT ( 'NONE',  ( 7.361572987183169658, 34.96726448433411605, -9.846743663894592657 ) ) ;
#29761=CARTESIAN_POINT ( 'NONE',  ( 20.00000000000000711, 85.81090550034849684, 4.886738312308601451 ) ) ;
#29763=CARTESIAN_POINT ( 'NONE',  ( 24.16423886937409904, 34.09541550158064638, 3.795296366450317205 ) ) ;
#29764=CARTESIAN_POINT ( 'NONE',  ( 17.08211943468705130, 43.47041550158063927, 12.26659068614894998 ) ) ;
#29765=CARTESIAN_POINT ( 'NONE',  ( 10.00000000000000178, 52.25893115100078745, 9.846743663894594434 ) ) ;
#29767=CARTESIAN_POINT ( 'NONE',  ( 12.91533473730992121, 39.52201867748817676, 10.88017736071110164 ) ) ;
#29768=CARTESIAN_POINT ( 'NONE',  ( 7.361572987183170547, 7.050597817667451750, 9.846743663894590881 ) ) ;
#29770=CARTESIAN_POINT ( 'NONE',  ( 6.565887622018943937, 55.16530133659709634, 12.81628187352647430 ) ) ;
#29772=CARTESIAN_POINT ( 'NONE',  ( 1.472469842513823179, 1.425597817667451528, 4.923371831947296329 ) ) ;
#29775=CARTESIAN_POINT ( 'NONE',  ( -2.266590686148945544, 12.22041550158063394, 7.082119434687048631 ) ) ;
#29776=CARTESIAN_POINT ( 'NONE',  ( 1.472469842513823179, 1.425597817667451528, 4.923371831947296329 ) ) ;
#29777=CARTESIAN_POINT ( 'NONE',  ( 20.88017736071110519, 25.56368534415483751, 2.639326808657452039E-16 ) ) ;
#29778=DIRECTION ( 'NONE',  ( -0.6776733583268385042, 0.7353630527936689809, 0.000000000000000000 ) ) ;
#29780=( BOUNDED_SURFACE ( )  B_SPLINE_SURFACE ( 1, 2, ( 
 ( #69975, #60978, #84968, #92951, #30477, #91491, #83989, #23011, #53479, #70466, #46475, #76971, #24486, #16486, #54949, #8484, #85466, #9464, #3453, #49918, #4443, #33422, #18448, #71932, #64417, #34909, #47942, #87912, #65405, #88416, #56449, #33910, #19426, #80429, #72910, #79442, #11925, #48443, #70968, #42429, #41950, #86935, #78448, #94924, #87426, #64898, #10453, #48930, #10940, #2972, #95931, #27411, #17956, #63442, #41464, #40470, #9964, #26423, #56924, #79921, #18943, #78942, #72413, #57902, #49420, #11430, #40961, #3940, #2488, #32941, #71458, #63921, #94432, #25476, #93949, #34409, #55958, #95426, #86458, #26922, #25947, #57419, #96927, #90369, #28881, #13904, #12411, #88909, #50906, #73399, #20420, #66394, #21907, #20914, #73898, #52383, #28405, #74887, #6892, #75377, #67894, #19916, #51403, #35405, #6385, #81890, #13402, #58900, #82887, #43400, #89398, #65898, #89888, #98415, #14403, #80916, #21405, #43885, #42918, #74381, #37405, #5429, #29871, #36403, #5908, #66896, #44874, #97415, #81401, #51900, #44389, #36901, #60373, #59384, #58391, #29379, #82382, #12903, #97918, #50407, #96428, #4927, #67390, #59880, #27902, #35898, #61850, #92357, #69865, #7400, #45884, #45375, #68882, #37898, #14904, #16368, #84862, #91369, #76374, #46849, #9348, #53874, #61361, #54835, #38878, #22895, #23884, #77344, #8855, #1876, #46368, #30361, #1386, #76857, #53367, #31840, #85348, #68390, #75879, #412, #39370, #62337, #92845, #54348, #24372, #16860, #98910, #7889, #60869, #30864, #83874, #15398, #47335, #77836, #38381, #91870, #39852, #70357, #32332, #90870, #23389, #22399, #84384, #15884, #52876, #83382, #8370, #69369, #889, #31350, #79808, #25357, #71340, #94313, #17840, #34283, #87792, #32822, #78330, #25838, #55340, #93337, #18334, #2858, #94808, #48814, #63319, #56810, #42308, #79321, #56334, #93828, #86828, #72781, #24857, #55842, #86336, #48323, #40352, #95300, #64297, #70853, #10831, #11801, #11311, #4317, #40839, #33312, #64783, #71820, #87307, #85847, #78831, #10341, #17360, #63806, #41351, #26803, #3327, #33792, #57299, #26310, #18826, #49795, #19307, #62837, #47830, #49307, #9852, #41831, #72297, #3828, #80302, #2366, #58270, #43282, #80798, #5790, #84129, #30607, #95809, #36281, #73777, #27287, #89282, #53611, #88786, #91622, #51282, #68628, #20296, #5306, #12294, #66778, #15641, #61112, #57787, #97299, #35783, #88293, #20793, #46123, #50794, #23138, #81768, #96806, #66272, #158, #13280, #35283, #28771, #59266, #89768, #76611, #43771, #73286, #45624, #74261, #65779, #15146, #34790, #42802, #19793, #12783, #22641 ),
 ( #53122, #81285, #38142, #65279, #28283, #58777, #4810, #83631, #76123, #96308, #7650, #50282, #27784, #1630, #86584, #63570, #70600, #77100, #63080, #2125, #92109, #32080, #9595, #69122, #94078, #16117, #653, #8127, #71093, #38621, #84614, #78092, #17115, #25116, #46601, #69610, #1131, #62580, #10099, #25599, #92596, #77586, #93084, #24615, #56092, #31102, #48074, #18093, #48570, #16613, #55081, #78587, #31593, #2619, #55598, #33074, #61596, #23640, #40596, #8613, #32585, #54100, #39121, #24119, #62088, #47090, #54589, #85103, #9102, #39616, #70105, #86093, #85601, #47598, #40099, #93581, #17604, #58033, #42078, #57544, #66030, #49071, #20547, #73035, #42551, #96559, #18578, #50544, #95557, #34046, #41093, #65031, #72540, #4570, #4073, #56579, #27046, #28033, #35031, #11558, #34536, #88043, #50051, #96056, #79069, #88540, #10583, #19555, #65533, #80556, #80055, #12050, #64543, #27540, #20042, #79574, #81038, #49545, #95050, #57054, #12545, #26558, #43047, #58528, #3588, #87556, #11073, #73526, #5054, #41594, #35537, #89036, #71590, #3102, #33556, #64054, #94566, #72061, #26084, #87069, #19066, #44518, #52513, #13033, #7533, #59026, #43527, #51032, #15033, #81526, #28532, #22038, #60009, #68023, #89532, #13534, #44017, #6522, #53001, #38024, #36540, #21537, #75017, #67528, #68518, #74023, #90998, #47, #91507, #59523, #37032, #22529, #74520, #45506, #98549, #76006, #30496, #5553, #83515, #21042, #45007, #66532, #60995, #67029, #51531, #90016, #36030, #97059, #52029, #82023, #6040, #30001, #29501, #97551, #29013, #82522, #14039, #60508, #98046, #90504, #83020, #14537, #75513, #7027, #37533, #23026, #92480, #53996, #62967, #76502, #542, #1519, #55482, #16003, #15532, #24999, #2007, #84987, #31965, #9983, #91993, #63463, #31477, #46013, #53498, #24005, #84503, #93472, #8016, #30989, #16996, #85487, #40486, #61488, #85983, #39502, #76990, #84008, #8985, #16503, #47475, #46980, #23524, #69991, #70984, #77975, #54477, #77474, #62466, #92971, #39985, #38513, #32472, #69011, #24503, #9482, #54965, #70487, #17494, #8503, #47959, #78469, #46491, #2506, #32959, #39006, #1017, #69501, #61980, #95943, #73411, #18462, #10954, #33438, #19444, #94939, #94449, #34425, #42444, #56939, #87441, #4939, #50423, #57434, #63935, #49933, #87927, #78958, #18957, #95443, #55975, #80931, #2990, #86476, #93964, #57919, #25490, #71475, #64917, #3954, #11939, #25962, #56463, #86949, #49434, #27426, #12424, #79455, #64432, #79938, #11445, #42930, #17975, #34921, #35419, #48459, #3470, #41963, #65418, #48947, #88429, #72926, #19929, #10469, #40977 ) ),
 .UNSPECIFIED., .F., .F., .T. ) 
 B_SPLINE_SURFACE_WITH_KNOTS ( ( 2, 2 ),
 ( 3, 2, 2, 2, 2, 2, 2, 2, 2, 2, 2, 2, 2, 2, 2, 2, 2, 2, 2, 2, 2, 2, 2, 2, 2, 2, 2, 2, 2, 2, 2, 2, 2, 2, 2, 2, 2, 2, 2, 2, 2, 2, 2, 2, 2, 2, 2, 2, 2, 2, 2, 2, 2, 2, 2, 2, 2, 2, 2, 2, 2, 2, 2, 2, 2, 2, 2, 2, 2, 2, 2, 2, 2, 2, 2, 2, 2, 2, 2, 2, 2, 2, 2, 2, 2, 2, 2, 2, 2, 2, 2, 2, 2, 2, 2, 2, 2, 2, 2, 2, 2, 2, 2, 2, 2, 2, 2, 2, 2, 2, 2, 2, 2, 2, 2, 2, 2, 2, 2, 2, 2, 2, 2, 2, 2, 2, 2, 2, 2, 2, 2, 2, 2, 2, 2, 2, 2, 2, 2, 2, 2, 2, 2, 2, 2, 2, 2, 2, 2, 2, 2, 2, 2, 2, 2, 2, 2, 2, 2, 2, 2, 2, 3 ),
 ( 0.000000000000000000, 1.000000000000000000 ),
 ( 0.000000000000000000, 0.005952380952380952051, 0.01190476190476190410, 0.01785714285714285615, 0.02380952380952380820, 0.02976190476190476025, 0.03571428571428571230, 0.04166666666666666435, 0.04761904761904761640, 0.05357142857142856845, 0.05952380952380952051, 0.06547619047619047949, 0.07142857142857142461, 0.07738095238095238360, 0.08333333333333332871, 0.08928571428571428770, 0.09523809523809523281, 0.1011904761904761918, 0.1071428571428571369, 0.1130952380952380959, 0.1190476190476190410, 0.1250000000000000000, 0.1309523809523809590, 0.1369047619047619180, 0.1428571428571428492, 0.1488095238095238082, 0.1547619047619047672, 0.1607142857142857262, 0.1666666666666666574, 0.1726190476190476164, 0.1785714285714285754, 0.1845238095238095344, 0.1904761904761904656, 0.1964285714285714246, 0.2023809523809523836, 0.2083333333333333426, 0.2142857142857142738, 0.2202380952380952328, 0.2261904761904761918, 0.2321428571428571508, 0.2380952380952380820, 0.2440476190476190410, 0.2500000000000000000, 0.2559523809523809312, 0.2619047619047619180, 0.2678571428571428492, 0.2738095238095238360, 0.2797619047619047672, 0.2857142857142856984, 0.2916666666666666852, 0.2976190476190476164, 0.3035714285714285476, 0.3095238095238095344, 0.3154761904761904656, 0.3214285714285714524, 0.3273809523809523836, 0.3333333333333333148, 0.3392857142857143016, 0.3452380952380952328, 0.3511904761904761640, 0.3571428571428571508, 0.3630952380952380820, 0.3690476190476190688, 0.3750000000000000000, 0.3809523809523809312, 0.3869047619047619180, 0.3928571428571428492, 0.3988095238095238360, 0.4047619047619047672, 0.4107142857142856984, 0.4166666666666666852, 0.4226190476190476164, 0.4285714285714285476, 0.4345238095238095344, 0.4404761904761904656, 0.4464285714285714524, 0.4523809523809523836, 0.4583333333333333148, 0.4642857142857143016, 0.4702380952380952328, 0.4761904761904761640, 0.4821428571428571508, 0.4880952380952380820, 0.4940476190476190688, 0.5000000000000000000, 0.5059523809523809312, 0.5119047619047618625, 0.5178571428571429047, 0.5238095238095238360, 0.5297619047619047672, 0.5357142857142856984, 0.5416666666666666297, 0.5476190476190476719, 0.5535714285714286031, 0.5595238095238095344, 0.5654761904761904656, 0.5714285714285713969, 0.5773809523809523281, 0.5833333333333333703, 0.5892857142857143016, 0.5952380952380952328, 0.6011904761904761640, 0.6071428571428570953, 0.6130952380952381375, 0.6190476190476190688, 0.6250000000000000000, 0.6309523809523809312, 0.6369047619047618625, 0.6428571428571429047, 0.6488095238095238360, 0.6547619047619047672, 0.6607142857142856984, 0.6666666666666666297, 0.6726190476190476719, 0.6785714285714286031, 0.6845238095238095344, 0.6904761904761904656, 0.6964285714285713969, 0.7023809523809523281, 0.7083333333333333703, 0.7142857142857143016, 0.7202380952380952328, 0.7261904761904761640, 0.7321428571428570953, 0.7380952380952381375, 0.7440476190476190688, 0.7500000000000000000, 0.7559523809523809312, 0.7619047619047618625, 0.7678571428571429047, 0.7738095238095238360, 0.7797619047619047672, 0.7857142857142856984, 0.7916666666666666297, 0.7976190476190476719, 0.8035714285714286031, 0.8095238095238095344, 0.8154761904761904656, 0.8214285714285713969, 0.8273809523809523281, 0.8333333333333333703, 0.8392857142857143016, 0.8452380952380952328, 0.8511904761904761640, 0.8571428571428570953, 0.8630952380952381375, 0.8690476190476190688, 0.8750000000000000000, 0.8809523809523809312, 0.8869047619047618625, 0.8928571428571429047, 0.8988095238095238360, 0.9047619047619047672, 0.9107142857142856984, 0.9166666666666666297, 0.9226190476190476719, 0.9285714285714286031, 0.9345238095238095344, 0.9404761904761904656, 0.9464285714285713969, 0.9523809523809523281, 0.9583333333333333703, 0.9642857142857143016 ),
 .UNSPECIFIED. ) 
 GEOMETRIC_REPRESENTATION_ITEM ( )  RATIONAL_B_SPLINE_SURFACE ( (
 ( 1.000000000000000000, 0.9659258262890683122, 1.000000000000000000, 0.9659258262890683122, 1.000000000000000000, 0.9659258262890683122, 1.000000000000000000, 0.9659258262890683122, 1.000000000000000000, 0.9659258262890683122, 1.000000000000000000, 0.9659258262890683122, 1.000000000000000000, 0.9659258262890683122, 1.000000000000000000, 0.9659258262890683122, 1.000000000000000000, 0.9659258262890683122, 1.000000000000000000, 0.9659258262890683122, 1.000000000000000000, 0.9659258262890683122, 1.000000000000000000, 0.9659258262890683122, 1.000000000000000000, 0.9659258262890683122, 1.000000000000000000, 0.9659258262890683122, 1.000000000000000000, 0.9659258262890683122, 1.000000000000000000, 0.9659258262890683122, 1.000000000000000000, 0.9659258262890683122, 1.000000000000000000, 0.9659258262890683122, 1.000000000000000000, 0.9659258262890683122, 1.000000000000000000, 0.9659258262890683122, 1.000000000000000000, 0.9659258262890683122, 1.000000000000000000, 0.9659258262890683122, 1.000000000000000000, 0.9659258262890683122, 1.000000000000000000, 0.9659258262890683122, 1.000000000000000000, 0.9659258262890683122, 1.000000000000000000, 0.9659258262890683122, 1.000000000000000000, 0.9659258262890683122, 1.000000000000000000, 0.9659258262890683122, 1.000000000000000000, 0.9659258262890683122, 1.000000000000000000, 0.9659258262890683122, 1.000000000000000000, 0.9659258262890683122, 1.000000000000000000, 0.9659258262890683122, 1.000000000000000000, 0.9659258262890683122, 1.000000000000000000, 0.9659258262890683122, 1.000000000000000000, 0.9659258262890683122, 1.000000000000000000, 0.9659258262890683122, 1.000000000000000000, 0.9659258262890683122, 1.000000000000000000, 0.9659258262890683122, 1.000000000000000000, 0.9659258262890683122, 1.000000000000000000, 0.9659258262890683122, 1.000000000000000000, 0.9659258262890683122, 1.000000000000000000, 0.9659258262890683122, 1.000000000000000000, 0.9659258262890683122, 1.000000000000000000, 0.9659258262890683122, 1.000000000000000000, 0.9659258262890683122, 1.000000000000000000, 0.9659258262890683122, 1.000000000000000000, 0.9659258262890683122, 1.000000000000000000, 0.9659258262890683122, 1.000000000000000000, 0.9659258262890683122, 1.000000000000000000, 0.9659258262890683122, 1.000000000000000000, 0.9659258262890683122, 1.000000000000000000, 0.9659258262890683122, 1.000000000000000000, 0.9659258262890683122, 1.000000000000000000, 0.9659258262890683122, 1.000000000000000000, 0.9659258262890683122, 1.000000000000000000, 0.9659258262890683122, 1.000000000000000000, 0.9659258262890683122, 1.000000000000000000, 0.9659258262890683122, 1.000000000000000000, 0.9659258262890683122, 1.000000000000000000, 0.9659258262890683122, 1.000000000000000000, 0.9659258262890683122, 1.000000000000000000, 0.9659258262890683122, 1.000000000000000000, 0.9659258262890683122, 1.000000000000000000, 0.9659258262890683122, 1.000000000000000000, 0.9659258262890683122, 1.000000000000000000, 0.9659258262890683122, 1.000000000000000000, 0.9659258262890683122, 1.000000000000000000, 0.9659258262890683122, 1.000000000000000000, 0.9659258262890683122, 1.000000000000000000, 0.9659258262890683122, 1.000000000000000000, 0.9659258262890683122, 1.000000000000000000, 0.9659258262890683122, 1.000000000000000000, 0.9659258262890683122, 1.000000000000000000, 0.9659258262890683122, 1.000000000000000000, 0.9659258262890683122, 1.000000000000000000, 0.9659258262890683122, 1.000000000000000000, 0.9659258262890683122, 1.000000000000000000, 0.9659258262890683122, 1.000000000000000000, 0.9659258262890683122, 1.000000000000000000, 0.9659258262890683122, 1.000000000000000000, 0.9659258262890683122, 1.000000000000000000, 0.9659258262890683122, 1.000000000000000000, 0.9659258262890683122, 1.000000000000000000, 0.9659258262890683122, 1.000000000000000000, 0.9659258262890683122, 1.000000000000000000, 0.9659258262890683122, 1.000000000000000000, 0.9659258262890683122, 1.000000000000000000, 0.9659258262890683122, 1.000000000000000000, 0.9659258262890683122, 1.000000000000000000, 0.9659258262890683122, 1.000000000000000000, 0.9659258262890683122, 1.000000000000000000, 0.9659258262890683122, 1.000000000000000000, 0.9659258262890683122, 1.000000000000000000, 0.9659258262890683122, 1.000000000000000000, 0.9659258262890683122, 1.000000000000000000, 0.9659258262890683122, 1.000000000000000000, 0.9659258262890683122, 1.000000000000000000, 0.9659258262890683122, 1.000000000000000000, 0.9659258262890683122, 1.000000000000000000, 0.9659258262890683122, 1.000000000000000000, 0.9659258262890683122, 1.000000000000000000, 0.9659258262890683122, 1.000000000000000000, 0.9659258262890683122, 1.000000000000000000, 0.9659258262890683122, 1.000000000000000000, 0.9659258262890683122, 1.000000000000000000, 0.9659258262890683122, 1.000000000000000000, 0.9659258262890683122, 1.000000000000000000, 0.9659258262890683122, 1.000000000000000000, 0.9659258262890683122, 1.000000000000000000, 0.9659258262890683122, 1.000000000000000000, 0.9659258262890683122, 1.000000000000000000, 0.9659258262890683122, 1.000000000000000000, 0.9659258262890683122, 1.000000000000000000, 0.9659258262890683122, 1.000000000000000000, 0.9659258262890683122, 1.000000000000000000, 0.9659258262890683122, 1.000000000000000000, 0.9659258262890683122, 1.000000000000000000, 0.9659258262890683122, 1.000000000000000000, 0.9659258262890683122, 1.000000000000000000, 0.9659258262890683122, 1.000000000000000000, 0.9659258262890683122, 1.000000000000000000, 0.9659258262890683122, 1.000000000000000000, 0.9659258262890683122, 1.000000000000000000, 0.9659258262890683122, 1.000000000000000000, 0.9659258262890683122, 1.000000000000000000, 0.9659258262890683122, 1.000000000000000000, 0.9659258262890683122, 1.000000000000000000, 0.9659258262890683122, 1.000000000000000000, 0.9659258262890683122, 1.000000000000000000, 0.9659258262890683122, 1.000000000000000000, 0.9659258262890683122, 1.000000000000000000, 0.9659258262890683122, 1.000000000000000000, 0.9659258262890683122, 1.000000000000000000, 0.9659258262890683122, 1.000000000000000000, 0.9659258262890683122, 1.000000000000000000, 0.9659258262890683122, 1.000000000000000000, 0.9659258262890683122, 1.000000000000000000, 0.9659258262890683122, 1.000000000000000000, 0.9659258262890683122, 1.000000000000000000, 0.9659258262890683122, 1.000000000000000000, 0.9659258262890683122, 1.000000000000000000, 0.9659258262890683122, 1.000000000000000000, 0.9659258262890683122, 1.000000000000000000, 0.9659258262890683122, 1.000000000000000000, 0.9659258262890683122, 1.000000000000000000, 0.9659258262890683122, 1.000000000000000000, 0.9659258262890683122, 1.000000000000000000, 0.9659258262890683122, 1.000000000000000000, 0.9659258262890683122, 1.000000000000000000, 0.9659258262890683122, 1.000000000000000000, 0.9659258262890683122, 1.000000000000000000, 0.9659258262890683122, 1.000000000000000000, 0.9659258262890683122, 1.000000000000000000, 0.9659258262890683122, 1.000000000000000000, 0.9659258262890683122, 1.000000000000000000, 0.9659258262890683122, 1.000000000000000000, 0.9659258262890683122, 1.000000000000000000, 0.9659258262890683122, 1.000000000000000000, 0.9659258262890683122, 1.000000000000000000, 0.9659258262890683122, 1.000000000000000000, 0.9659258262890683122, 1.000000000000000000, 0.9659258262890683122, 1.000000000000000000),
 ( 1.000000000000000000, 0.9659258262890683122, 1.000000000000000000, 0.9659258262890683122, 1.000000000000000000, 0.9659258262890683122, 1.000000000000000000, 0.9659258262890683122, 1.000000000000000000, 0.9659258262890683122, 1.000000000000000000, 0.9659258262890683122, 1.000000000000000000, 0.9659258262890683122, 1.000000000000000000, 0.9659258262890683122, 1.000000000000000000, 0.9659258262890683122, 1.000000000000000000, 0.9659258262890683122, 1.000000000000000000, 0.9659258262890683122, 1.000000000000000000, 0.9659258262890683122, 1.000000000000000000, 0.9659258262890683122, 1.000000000000000000, 0.9659258262890683122, 1.000000000000000000, 0.9659258262890683122, 1.000000000000000000, 0.9659258262890683122, 1.000000000000000000, 0.9659258262890683122, 1.000000000000000000, 0.9659258262890683122, 1.000000000000000000, 0.9659258262890683122, 1.000000000000000000, 0.9659258262890683122, 1.000000000000000000, 0.9659258262890683122, 1.000000000000000000, 0.9659258262890683122, 1.000000000000000000, 0.9659258262890683122, 1.000000000000000000, 0.9659258262890683122, 1.000000000000000000, 0.9659258262890683122, 1.000000000000000000, 0.9659258262890683122, 1.000000000000000000, 0.9659258262890683122, 1.000000000000000000, 0.9659258262890683122, 1.000000000000000000, 0.9659258262890683122, 1.000000000000000000, 0.9659258262890683122, 1.000000000000000000, 0.9659258262890683122, 1.000000000000000000, 0.9659258262890683122, 1.000000000000000000, 0.9659258262890683122, 1.000000000000000000, 0.9659258262890683122, 1.000000000000000000, 0.9659258262890683122, 1.000000000000000000, 0.9659258262890683122, 1.000000000000000000, 0.9659258262890683122, 1.000000000000000000, 0.9659258262890683122, 1.000000000000000000, 0.9659258262890683122, 1.000000000000000000, 0.9659258262890683122, 1.000000000000000000, 0.9659258262890683122, 1.000000000000000000, 0.9659258262890683122, 1.000000000000000000, 0.9659258262890683122, 1.000000000000000000, 0.9659258262890683122, 1.000000000000000000, 0.9659258262890683122, 1.000000000000000000, 0.9659258262890683122, 1.000000000000000000, 0.9659258262890683122, 1.000000000000000000, 0.9659258262890683122, 1.000000000000000000, 0.9659258262890683122, 1.000000000000000000, 0.9659258262890683122, 1.000000000000000000, 0.9659258262890683122, 1.000000000000000000, 0.9659258262890683122, 1.000000000000000000, 0.9659258262890683122, 1.000000000000000000, 0.9659258262890683122, 1.000000000000000000, 0.9659258262890683122, 1.000000000000000000, 0.9659258262890683122, 1.000000000000000000, 0.9659258262890683122, 1.000000000000000000, 0.9659258262890683122, 1.000000000000000000, 0.9659258262890683122, 1.000000000000000000, 0.9659258262890683122, 1.000000000000000000, 0.9659258262890683122, 1.000000000000000000, 0.9659258262890683122, 1.000000000000000000, 0.9659258262890683122, 1.000000000000000000, 0.9659258262890683122, 1.000000000000000000, 0.9659258262890683122, 1.000000000000000000, 0.9659258262890683122, 1.000000000000000000, 0.9659258262890683122, 1.000000000000000000, 0.9659258262890683122, 1.000000000000000000, 0.9659258262890683122, 1.000000000000000000, 0.9659258262890683122, 1.000000000000000000, 0.9659258262890683122, 1.000000000000000000, 0.9659258262890683122, 1.000000000000000000, 0.9659258262890683122, 1.000000000000000000, 0.9659258262890683122, 1.000000000000000000, 0.9659258262890683122, 1.000000000000000000, 0.9659258262890683122, 1.000000000000000000, 0.9659258262890683122, 1.000000000000000000, 0.9659258262890683122, 1.000000000000000000, 0.9659258262890683122, 1.000000000000000000, 0.9659258262890683122, 1.000000000000000000, 0.9659258262890683122, 1.000000000000000000, 0.9659258262890683122, 1.000000000000000000, 0.9659258262890683122, 1.000000000000000000, 0.9659258262890683122, 1.000000000000000000, 0.9659258262890683122, 1.000000000000000000, 0.9659258262890683122, 1.000000000000000000, 0.9659258262890683122, 1.000000000000000000, 0.9659258262890683122, 1.000000000000000000, 0.9659258262890683122, 1.000000000000000000, 0.9659258262890683122, 1.000000000000000000, 0.9659258262890683122, 1.000000000000000000, 0.9659258262890683122, 1.000000000000000000, 0.9659258262890683122, 1.000000000000000000, 0.9659258262890683122, 1.000000000000000000, 0.9659258262890683122, 1.000000000000000000, 0.9659258262890683122, 1.000000000000000000, 0.9659258262890683122, 1.000000000000000000, 0.9659258262890683122, 1.000000000000000000, 0.9659258262890683122, 1.000000000000000000, 0.9659258262890683122, 1.000000000000000000, 0.9659258262890683122, 1.000000000000000000, 0.9659258262890683122, 1.000000000000000000, 0.9659258262890683122, 1.000000000000000000, 0.9659258262890683122, 1.000000000000000000, 0.9659258262890683122, 1.000000000000000000, 0.9659258262890683122, 1.000000000000000000, 0.9659258262890683122, 1.000000000000000000, 0.9659258262890683122, 1.000000000000000000, 0.9659258262890683122, 1.000000000000000000, 0.9659258262890683122, 1.000000000000000000, 0.9659258262890683122, 1.000000000000000000, 0.9659258262890683122, 1.000000000000000000, 0.9659258262890683122, 1.000000000000000000, 0.9659258262890683122, 1.000000000000000000, 0.9659258262890683122, 1.000000000000000000, 0.9659258262890683122, 1.000000000000000000, 0.9659258262890683122, 1.000000000000000000, 0.9659258262890683122, 1.000000000000000000, 0.9659258262890683122, 1.000000000000000000, 0.9659258262890683122, 1.000000000000000000, 0.9659258262890683122, 1.000000000000000000, 0.9659258262890683122, 1.000000000000000000, 0.9659258262890683122, 1.000000000000000000, 0.9659258262890683122, 1.000000000000000000, 0.9659258262890683122, 1.000000000000000000, 0.9659258262890683122, 1.000000000000000000, 0.9659258262890683122, 1.000000000000000000, 0.9659258262890683122, 1.000000000000000000, 0.9659258262890683122, 1.000000000000000000, 0.9659258262890683122, 1.000000000000000000, 0.9659258262890683122, 1.000000000000000000, 0.9659258262890683122, 1.000000000000000000, 0.9659258262890683122, 1.000000000000000000, 0.9659258262890683122, 1.000000000000000000, 0.9659258262890683122, 1.000000000000000000, 0.9659258262890683122, 1.000000000000000000, 0.9659258262890683122, 1.000000000000000000, 0.9659258262890683122, 1.000000000000000000, 0.9659258262890683122, 1.000000000000000000, 0.9659258262890683122, 1.000000000000000000, 0.9659258262890683122, 1.000000000000000000, 0.9659258262890683122, 1.000000000000000000, 0.9659258262890683122, 1.000000000000000000, 0.9659258262890683122, 1.000000000000000000, 0.9659258262890683122, 1.000000000000000000, 0.9659258262890683122, 1.000000000000000000, 0.9659258262890683122, 1.000000000000000000, 0.9659258262890683122, 1.000000000000000000, 0.9659258262890683122, 1.000000000000000000, 0.9659258262890683122, 1.000000000000000000, 0.9659258262890683122, 1.000000000000000000, 0.9659258262890683122, 1.000000000000000000, 0.9659258262890683122, 1.000000000000000000, 0.9659258262890683122, 1.000000000000000000, 0.9659258262890683122, 1.000000000000000000, 0.9659258262890683122, 1.000000000000000000, 0.9659258262890683122, 1.000000000000000000, 0.9659258262890683122, 1.000000000000000000, 0.9659258262890683122, 1.000000000000000000, 0.9659258262890683122, 1.000000000000000000, 0.9659258262890683122, 1.000000000000000000, 0.9659258262890683122, 1.000000000000000000) ) ) 
 REPRESENTATION_ITEM ( '' )  SURFACE ( )  );
#29782=CARTESIAN_POINT ( 'NONE',  ( 0.5774900079438607392, 28.48035201082150891, 5.440088680355550821 ) ) ;
#29784=( BOUNDED_CURVE ( )  B_SPLINE_CURVE ( 2, ( #61512, #69036, #45535, #38541, #54993, #37559, #76032, #7565, #76 ),
 .UNSPECIFIED., .F., .F. ) 
 B_SPLINE_CURVE_WITH_KNOTS ( ( 3, 2, 2, 2, 3 ),
 ( 0.4391432315068939940, 0.4404761904761904656, 0.4464285714285714524, 0.4523809523809523836, 0.4537139113502488552 ),
 .UNSPECIFIED. ) 
 CURVE ( )  GEOMETRIC_REPRESENTATION_ITEM ( )  RATIONAL_B_SPLINE_CURVE ( ( 0.9881565478350728959, 0.9923695281211487584, 1.000000000000000000, 0.9659258262890683122, 1.000000000000000000, 0.9659258262890683122, 1.000000000000000000, 0.9923695281211487584, 0.9881565478350728959 ) ) 
 REPRESENTATION_ITEM ( '' )  );
#29786=CARTESIAN_POINT ( 'NONE',  ( 7.084665262690076126, 37.02201867748817676, -10.88017736071110164 ) ) ;
#29789=CARTESIAN_POINT ( 'NONE',  ( 6.565887622018943937, 13.08196800326374998, -12.81628187352647608 ) ) ;
#29790=CARTESIAN_POINT ( 'NONE',  ( 20.88017736071110519, 65.56368534415483396, 2.639326808657452039E-16 ) ) ;
#29793=CARTESIAN_POINT ( 'NONE',  ( 20.88017736071110519, 15.56368534415483751, 2.639326808657452039E-16 ) ) ;
#29795=CARTESIAN_POINT ( 'NONE',  ( 14.92337183194729988, 4.342264484334117824, -8.527530157486177487 ) ) ;
#29796=CARTESIAN_POINT ( 'NONE',  ( 0.5774900079438590739, 37.64701867748817676, -5.440088680355550821 ) ) ;
#29799=ORIENTED_EDGE ( 'NONE', *, *, #8524, .T. ) ;
#29800=CARTESIAN_POINT ( 'NONE',  ( 6.565887622018943937, 50.16530133659708213, 12.81628187352647430 ) ) ;
#29801=CARTESIAN_POINT ( 'NONE',  ( 15.44008868035555793, 46.39701867748817676, -9.422509992056140149 ) ) ;
#29803=CARTESIAN_POINT ( 'NONE',  ( -1.099225684535947600, 54.54030133659708923, 6.408140936763237150 ) ) ;
#29804=CARTESIAN_POINT ( 'NONE',  ( 15.44008868035555793, 46.39701867748817676, -9.422509992056140149 ) ) ;
#29805=EDGE_CURVE ( 'NONE', #156, #11511, #73007, .T. ) ;
#29806=CARTESIAN_POINT ( 'NONE',  ( 0.6178305044545818747, -1.501365330069579951, -9.382169495545419124 ) ) ;
#29808=CARTESIAN_POINT ( 'NONE',  ( 5.076628168052703671, 11.84226448433411960, 8.527530157486179263 ) ) ;
#29809=CARTESIAN_POINT ( 'NONE',  ( 6.565887622018943937, 60.16530133659707502, 12.81628187352647430 ) ) ;
#29810=CARTESIAN_POINT ( 'NONE',  ( 1.492507162822266809, 37.19955587570481015, -6.500000000000066613 ) ) ;
#29811=CARTESIAN_POINT ( 'NONE',  ( 12.63842701281683922, 4.550597817667451750, -9.846743663894590881 ) ) ;
#29812=CARTESIAN_POINT ( 'NONE',  ( -2.816281873526473856, 9.331968003263753531, 3.434112377981055619 ) ) ;
#29814=CARTESIAN_POINT ( 'NONE',  ( 1.472469842513823179, 60.59226448433412315, -4.923371831947296329 ) ) ;
#29815=CARTESIAN_POINT ( 'NONE',  ( -0.8801773607111008646, 33.27201867748817676, 2.915334737309923430 ) ) ;
#29816=CARTESIAN_POINT ( 'NONE',  ( 12.63842701281683034, 47.46726448433412315, 9.846743663894596210 ) ) ;
#29818=CARTESIAN_POINT ( 'NONE',  ( 5.076628168052703671, 21.84226448433411960, 8.527530157486179263 ) ) ;
#29819=CARTESIAN_POINT ( 'NONE',  ( 14.92337183194729633, 12.67559781766745353, 8.527530157486181039 ) ) ;
#29820=CARTESIAN_POINT ( 'NONE',  ( -1.099225684535947600, 8.706968003263753531, -6.408140936763238038 ) ) ;
#29821=ORIENTED_EDGE ( 'NONE', *, *, #95041, .F. ) ;
#29822=CARTESIAN_POINT ( 'NONE',  ( 10.00000000000000000, 64.75893115100078035, -9.846743663894594434 ) ) ;
#29824=CARTESIAN_POINT ( 'NONE',  ( 15.44008868035555260, 4.730352010821505360, 9.422509992056143702 ) ) ;
#29825=CARTESIAN_POINT ( 'NONE',  ( 10.00000000000000000, 44.75893115100078745, -9.846743663894594434 ) ) ;
#29827=CARTESIAN_POINT ( 'NONE',  ( 0.2751277870542967463, 0.000000000000000000, 6.500000000000000888 ) ) ;
#29828=CARTESIAN_POINT ( 'NONE',  ( 10.00000000000000000, 65.55374883491396076, -14.16423886937410082 ) ) ;
#29829=DIRECTION ( 'NONE',  ( 1.000000000000000000, 0.000000000000000000, 0.000000000000000000 ) ) ;
#29830=ADVANCED_FACE ( 'NONE', ( #24854 ), #8367, .T. ) ;
#29831=CARTESIAN_POINT ( 'NONE',  ( 19.42250999205614193, 30.14701867748817321, 5.440088680355555262 ) ) ;
#29832=CARTESIAN_POINT ( 'NONE',  ( 2.917880565312950480, 55.97041550158063217, -12.26659068614894821 ) ) ;
#29833=CARTESIAN_POINT ( 'NONE',  ( -0.8801773607110991993, 2.855352010821504471, -2.915334737309923874 ) ) ;
#29835=CARTESIAN_POINT ( 'NONE',  ( 12.63842701281683922, 4.550597817667451750, -9.846743663894590881 ) ) ;
#29836=CARTESIAN_POINT ( 'NONE',  ( 7.361572987183170547, 27.05059781766745175, 9.846743663894590881 ) ) ;
#29837=CARTESIAN_POINT ( 'NONE',  ( 10.00000000000000178, 15.37363466993042138, 12.81628187352647608 ) ) ;
#29840=CARTESIAN_POINT ( 'NONE',  ( 19.84674366389459266, 58.30059781766745886, 2.638427012816836559 ) ) ;
#29844=CARTESIAN_POINT ( 'NONE',  ( -4.164238869374098151, 16.59541550158063927, -3.795296366450310543 ) ) ;
#29845=CARTESIAN_POINT ( 'NONE',  ( 19.84674366389459266, 23.30059781766745530, 2.638427012816836559 ) ) ;
#29848=CARTESIAN_POINT ( 'NONE',  ( 20.36894250292379738, 44.92874883491396787, -10.36894250292379027 ) ) ;
#29850=CARTESIAN_POINT ( 'NONE',  ( 17.20831665107776587, 14.13393115100078568, -7.208316651077762316 ) ) ;
#29853=CARTESIAN_POINT ( 'NONE',  ( 20.88017736071110875, 30.77201867748816966, -2.915334737309920765 ) ) ;
#29854=CARTESIAN_POINT ( 'NONE',  ( 10.00000000000000178, 50.37363466993042493, 12.81628187352647608 ) ) ;
#29855=CARTESIAN_POINT ( 'NONE',  ( 10.00000000000000178, 40.37363466993042493, 12.81628187352647608 ) ) ;
#29856=CARTESIAN_POINT ( 'NONE',  ( 12.63842701281683034, 7.467264484334118713, 9.846743663894596210 ) ) ;
#29857=ORIENTED_EDGE ( 'NONE', *, *, #37822, .F. ) ;
#29858=LINE ( 'NONE', #8357, #68615 ) ;
#29859=CARTESIAN_POINT ( 'NONE',  ( -2.266590686148945544, 37.22041550158063217, 7.082119434687048631 ) ) ;
#29860=CARTESIAN_POINT ( 'NONE',  ( 2.917880565312948704, 12.63708216824730179, 12.26659068614894643 ) ) ;
#29861=CARTESIAN_POINT ( 'NONE',  ( 10.00000000000000178, 9.313685344154839285, 10.88017736071110342 ) ) ;
#29863=CARTESIAN_POINT ( 'NONE',  ( 12.91533473730992121, 19.52201867748816611, 10.88017736071110164 ) ) ;
#29866=CARTESIAN_POINT ( 'NONE',  ( 10.00000000000000178, 59.31368534415484106, 10.88017736071110342 ) ) ;
#29867=CARTESIAN_POINT ( 'NONE',  ( 10.00000000000000178, 59.31368534415484106, 10.88017736071110342 ) ) ;
#29868=CARTESIAN_POINT ( 'NONE',  ( 3.591859063236761518, 24.95696800326375353, 11.09922568453594849 ) ) ;
#29871=CARTESIAN_POINT ( 'NONE',  ( 5.076628168052704559, 25.17559781766745175, -8.527530157486179263 ) ) ;
#29873=AXIS2_PLACEMENT_3D ( 'NONE', #38088, #37094, #67593 ) ;
#29874=CARTESIAN_POINT ( 'NONE',  ( -2.816281873526471635, 23.91530133659708568, -3.434112377981056508 ) ) ;
#29875=CARTESIAN_POINT ( 'NONE',  ( 1.707155281725168061, 27.90189080397291477, 6.500000000000023093 ) ) ;
#29876=CARTESIAN_POINT ( 'NONE',  ( 19.42250999205614193, 15.14701867748817143, 5.440088680355555262 ) ) ;
#29877=CARTESIAN_POINT ( 'NONE',  ( 1.472469842513823179, 35.59226448433412315, -4.923371831947296329 ) ) ;
#29878=CARTESIAN_POINT ( 'NONE',  ( 10.00000000000000178, 65.37363466993042493, 12.81628187352647608 ) ) ;
#29879=CARTESIAN_POINT ( 'NONE',  ( 17.20831665107776587, 17.88393115100078745, 7.208316651077764980 ) ) ;
#29880=CARTESIAN_POINT ( 'NONE',  ( -4.164238869374099927, 2.012082168247300906, 3.795296366450308767 ) ) ;
#29882=CARTESIAN_POINT ( 'NONE',  ( 20.88017736071110519, 30.56368534415484106, 2.639326808657452039E-16 ) ) ;
#29883=CARTESIAN_POINT ( 'NONE',  ( 20.15039907845753930, 70.00000000000000000, -6.262539305110068177 ) ) ;
#29884=CARTESIAN_POINT ( 'NONE',  ( 24.16423886937410614, 34.30374883491396787, 8.672049930838204340E-16 ) ) ;
#29885=CARTESIAN_POINT ( 'NONE',  ( 19.84674366389459621, 48.50893115100078745, 7.409399052514197653E-17 ) ) ;
#29886=CARTESIAN_POINT ( 'NONE',  ( 2.035157376598822676, 27.43868534415483396, -7.964842623401177768 ) ) ;
#29888=CARTESIAN_POINT ( 'NONE',  ( 20.88017736071110875, 20.77201867748816611, -2.915334737309920765 ) ) ;
#29889=ORIENTED_EDGE ( 'NONE', *, *, #38991, .T. ) ;
#29890=CARTESIAN_POINT ( 'NONE',  ( 20.88017736071110519, 25.56368534415483751, 2.639326808657452039E-16 ) ) ;
#29891=EDGE_CURVE ( 'NONE', #53231, #97016, #29056, .T. ) ;
#29892=CARTESIAN_POINT ( 'NONE',  ( 13.43411237798106583, 42.66530133659707502, -12.81628187352647252 ) ) ;
#29893=CARTESIAN_POINT ( 'NONE',  ( 17.96484262340118221, 44.93868534415483396, 7.964842623401181321 ) ) ;
#29894=CARTESIAN_POINT ( 'NONE',  ( 12.91533473730992121, 34.52201867748817676, 10.88017736071110164 ) ) ;
#29895=VERTEX_POINT ( 'NONE', #39367 ) ;
#29896=CARTESIAN_POINT ( 'NONE',  ( 19.84674366389459266, 53.71726448433411605, -2.638427012816827677 ) ) ;
#29897=CARTESIAN_POINT ( 'NONE',  ( 20.88017736071110164, 35.35535201082150536, 2.915334737309930979 ) ) ;
#29900=CARTESIAN_POINT ( 'NONE',  ( 24.16423886937409904, 44.09541550158063927, 3.795296366450317205 ) ) ;
#29901=CARTESIAN_POINT ( 'NONE',  ( 2.035157376598824452, 53.68868534415484817, 7.964842623401179544 ) ) ;
#29902=CARTESIAN_POINT ( 'NONE',  ( 0.9408516040111476464, 52.46693863883976405, -6.499999999999953815 ) ) ;
#29904=CARTESIAN_POINT ( 'NONE',  ( 14.92337183194729988, 59.34226448433412315, -8.527530157486177487 ) ) ;
#29905=FACE_OUTER_BOUND ( 'NONE', #67448, .T. ) ;
#29906=CARTESIAN_POINT ( 'NONE',  ( 2.791683348922237240, 30.38393115100078390, -7.208316651077763204 ) ) ;
#29908=CARTESIAN_POINT ( 'NONE',  ( 7.361572987183169658, 34.96726448433411605, -9.846743663894592657 ) ) ;
#29910=CARTESIAN_POINT ( 'NONE',  ( 17.96484262340118221, 26.18868534415483396, -7.964842623401177768 ) ) ;
#29911=CARTESIAN_POINT ( 'NONE',  ( 12.63842701281683922, 44.55059781766745175, -9.846743663894590881 ) ) ;
#29912=CARTESIAN_POINT ( 'NONE',  ( 19.38216949554541202, 15.99863466993042138, 9.382169495545424454 ) ) ;
#29914=CARTESIAN_POINT ( 'NONE',  ( 7.084665262690076126, 54.10535201082151247, 10.88017736071109987 ) ) ;
#29915=CARTESIAN_POINT ( 'NONE',  ( 10.00000000000000178, 29.31368534415483751, 10.88017736071110342 ) ) ;
#29916=CARTESIAN_POINT ( 'NONE',  ( 2.917880565312948704, 42.63708216824729647, 12.26659068614894643 ) ) ;
#29918=CARTESIAN_POINT ( 'NONE',  ( 0.2751277870542967463, 70.00000000000000000, -6.000000000000000000 ) ) ;
#29920=CARTESIAN_POINT ( 'NONE',  ( -1.099225684535947600, 13.70696800326375353, -6.408140936763238038 ) ) ;
#29921=CARTESIAN_POINT ( 'NONE',  ( 4.559911319644449179, 12.23035201082150536, -9.422509992056141925 ) ) ;
#29923=CARTESIAN_POINT ( 'NONE',  ( 19.42250999205614548, 45.98035201082150536, -5.440088680355545492 ) ) ;
#29926=CARTESIAN_POINT ( 'NONE',  ( 10.00000000000000000, 61.81368534415484106, -10.88017736071110342 ) ) ;
#29927=CARTESIAN_POINT ( 'NONE',  ( 10.00000000000000000, 34.75893115100078745, -9.846743663894594434 ) ) ;
#29928=CARTESIAN_POINT ( 'NONE',  ( 0.1532563361054083140, 26.00893115100078745, 1.131784320476157264E-15 ) ) ;
#29929=AXIS2_PLACEMENT_3D ( 'NONE', #91337, #39339, #69335 ) ;
#29930=CARTESIAN_POINT ( 'NONE',  ( 14.92337183194729988, 14.34226448433411782, -8.527530157486177487 ) ) ;
#29933=CARTESIAN_POINT ( 'NONE',  ( 21.09922568453594849, 36.20696800326375353, 6.408140936763242479 ) ) ;
#29934=CARTESIAN_POINT ( 'NONE',  ( 14.92337183194729988, 19.34226448433411960, -8.527530157486177487 ) ) ;
#29936=CARTESIAN_POINT ( 'NONE',  ( -46.44000000000001194, 93.00000000000000000, -9.000000000000000000 ) ) ;
#29938=CARTESIAN_POINT ( 'NONE',  ( 0.1532563361054082862, 36.21726448433410894, 2.638427012816831674 ) ) ;
#29942=CARTESIAN_POINT ( 'NONE',  ( 13.43411237798106583, 7.665301336597086568, -12.81628187352647252 ) ) ;
#29943=EDGE_CURVE ( 'NONE', #31636, #30124, #61848, .T. ) ;
#29944=CARTESIAN_POINT ( 'NONE',  ( -0.8801773607111008646, 48.27201867748816966, 2.915334737309923430 ) ) ;
#29945=CARTESIAN_POINT ( 'NONE',  ( 20.36894250292379382, 28.67874883491396787, 10.36894250292379205 ) ) ;
#29947=CARTESIAN_POINT ( 'NONE',  ( 17.08211943468705130, 33.47041550158063927, 12.26659068614894998 ) ) ;
#29948=EDGE_CURVE ( 'NONE', #9403, #37993, #15968, .T. ) ;
#29949=CARTESIAN_POINT ( 'NONE',  ( 22.26659068614895176, 49.72041550158063927, -7.082119434687042414 ) ) ;
#29950=CARTESIAN_POINT ( 'NONE',  ( 20.36894250292379382, 3.678748834913967869, 10.36894250292379205 ) ) ;
#29951=CARTESIAN_POINT ( 'NONE',  ( 20.36894250292379382, 28.67874883491396787, 10.36894250292379205 ) ) ;
#29952=CARTESIAN_POINT ( 'NONE',  ( 17.39651004071842166, 32.93575266056828355, 6.499999999999998224 ) ) ;
#29953=CARTESIAN_POINT ( 'NONE',  ( 20.88017736071110875, 50.77201867748817676, -2.915334737309920765 ) ) ;
#29955=CARTESIAN_POINT ( 'NONE',  ( 19.84674366389459266, 33.71726448433410894, -2.638427012816827677 ) ) ;
#29956=CARTESIAN_POINT ( 'NONE',  ( 0.000000000000000000, 0.000000000000000000, 6.000000000000000000 ) ) ;
#29957=CARTESIAN_POINT ( 'NONE',  ( 12.63842701281683034, 47.46726448433412315, 9.846743663894596210 ) ) ;
#29958=CARTESIAN_POINT ( 'NONE',  ( 12.91533473730992121, 29.52201867748817321, 10.88017736071110164 ) ) ;
#29959=CARTESIAN_POINT ( 'NONE',  ( 16.40814093676324603, 52.45696800326375353, -11.09922568453594671 ) ) ;
#29960=CARTESIAN_POINT ( 'NONE',  ( 7.361572987183170547, 67.05059781766746596, 9.846743663894590881 ) ) ;
#29962=CARTESIAN_POINT ( 'NONE',  ( 14.92337183194729988, 24.34226448433411960, -8.527530157486177487 ) ) ;
#29963=CARTESIAN_POINT ( 'NONE',  ( 6.565887622018943937, 45.16530133659708923, 12.81628187352647430 ) ) ;
#29965=CARTESIAN_POINT ( 'NONE',  ( 17.96484262340118221, 44.93868534415483396, 7.964842623401181321 ) ) ;
#29966=CARTESIAN_POINT ( 'NONE',  ( 10.00000000000000178, 52.25893115100078745, 9.846743663894594434 ) ) ;
#29967=CARTESIAN_POINT ( 'NONE',  ( -4.164238869374098151, 46.59541550158063927, -3.795296366450310543 ) ) ;
#29969=CARTESIAN_POINT ( 'NONE',  ( -2.266590686148945544, 1.387082168247301128, -7.082119434687050408 ) ) ;
#29971=CARTESIAN_POINT ( 'NONE',  ( 19.42250999205614548, 65.98035201082151957, -5.440088680355545492 ) ) ;
#29972=CARTESIAN_POINT ( 'NONE',  ( 2.035157376598824452, 68.68868534415484817, 7.964842623401179544 ) ) ;
#29973=CARTESIAN_POINT ( 'NONE',  ( 10.00000000000000000, 65.55374883491396076, -14.16423886937410082 ) ) ;
#29974=CARTESIAN_POINT ( 'NONE',  ( 0.6178305044545838731, -0.2513653300695798953, 9.382169495545420901 ) ) ;
#29976=CARTESIAN_POINT ( 'NONE',  ( 0.5774900079438590739, 52.64701867748817676, -5.440088680355550821 ) ) ;
#29979=CARTESIAN_POINT ( 'NONE',  ( 10.00000000000000178, 30.37363466993042138, 12.81628187352647608 ) ) ;
#29980=CARTESIAN_POINT ( 'NONE',  ( -2.266590686148945544, 46.38708216824730357, -7.082119434687050408 ) ) ;
#29982=CARTESIAN_POINT ( 'NONE',  ( 0.5774900079438590739, 7.647018677488171434, -5.440088680355550821 ) ) ;
#29983=CARTESIAN_POINT ( 'NONE',  ( 20.88017736071110875, 25.77201867748816966, -2.915334737309920765 ) ) ;
#29984=CARTESIAN_POINT ( 'NONE',  ( 5.076628168052703671, 56.84226448433412315, 8.527530157486179263 ) ) ;
#29985=CARTESIAN_POINT ( 'NONE',  ( 0.6178305044545818747, 48.49863466993042493, -9.382169495545419124 ) ) ;
#29988=CARTESIAN_POINT ( 'NONE',  ( -0.8801773607110991993, 12.85535201082150358, -2.915334737309923874 ) ) ;
#29989=CARTESIAN_POINT ( 'NONE',  ( 16.40814093676324603, 17.45696800326375353, -11.09922568453594671 ) ) ;
#29990=FACE_OUTER_BOUND ( 'NONE', #6490, .T. ) ;
#29991=CIRCLE ( 'NONE', #68339, 0.5000000000000027756 ) ;
#29992=CARTESIAN_POINT ( 'NONE',  ( 18.52753015748617571, 53.09226448433412315, 4.923371831947298993 ) ) ;
#29993=CARTESIAN_POINT ( 'NONE',  ( 0.5774900079438607392, 33.48035201082150536, 5.440088680355550821 ) ) ;
#29994=CARTESIAN_POINT ( 'NONE',  ( 19.38216949554541202, 25.99863466993042138, 9.382169495545424454 ) ) ;
#29995=CARTESIAN_POINT ( 'NONE',  ( -0.8801773607111009756, 43.06368534415484106, 1.068504757029289695E-15 ) ) ;
#29998=CARTESIAN_POINT ( 'NONE',  ( 22.81628187352647785, 46.62363466993041783, 6.195893100308588602E-16 ) ) ;
#29999=ORIENTED_EDGE ( 'NONE', *, *, #72345, .F. ) ;
#30000=CARTESIAN_POINT ( 'NONE',  ( 20.88017736071110519, 45.56368534415484106, 2.639326808657452039E-16 ) ) ;
#30001=CARTESIAN_POINT ( 'NONE',  ( 13.43411237798106583, 37.66530133659708923, -12.81628187352647252 ) ) ;
#30002=CARTESIAN_POINT ( 'NONE',  ( 20.88017736071110875, 40.77201867748818387, -2.915334737309920765 ) ) ;
#30004=CIRCLE ( 'NONE', #22042, 9.999999999999994671 ) ;
#30005=CARTESIAN_POINT ( 'NONE',  ( 1.472469842513823179, 65.59226448433412315, -4.923371831947296329 ) ) ;
#30006=CARTESIAN_POINT ( 'NONE',  ( 19.84674366389459266, 23.71726448433412315, -2.638427012816827677 ) ) ;
#30007=CARTESIAN_POINT ( 'NONE',  ( 18.52753015748618282, 8.925597817667451750, -4.923371831947291888 ) ) ;
#30008=CARTESIAN_POINT ( 'NONE',  ( 19.05914839598886346, 39.96693863883975695, 6.499999999999922728 ) ) ;
#30009=CARTESIAN_POINT ( 'NONE',  ( 20.36894250292379382, 38.67874883491396076, 10.36894250292379205 ) ) ;
#30013=CARTESIAN_POINT ( 'NONE',  ( 7.084665262690076126, 9.105352010821503583, 10.88017736071109987 ) ) ;
#30017=CARTESIAN_POINT ( 'NONE',  ( 0.5774900079438590739, 2.647018677488171434, -5.440088680355550821 ) ) ;
#30018=CARTESIAN_POINT ( 'NONE',  ( -4.164238869374099039, 61.80374883491397497, 8.674139862899312516E-16 ) ) ;
#30019=CARTESIAN_POINT ( 'NONE',  ( 2.791683348922240793, 46.63393115100077324, 7.208316651077764092 ) ) ;
#30020=CARTESIAN_POINT ( 'NONE',  ( 13.43411237798106583, 37.66530133659708923, -12.81628187352647252 ) ) ;
#30022=CARTESIAN_POINT ( 'NONE',  ( -0.3689425029237881626, 2.428748834913967869, 10.36894250292379027 ) ) ;
#30023=CARTESIAN_POINT ( 'NONE',  ( 4.559911319644449179, 7.230352010821504471, -9.422509992056141925 ) ) ;
#30024=CARTESIAN_POINT ( 'NONE',  ( -0.3689425029237898834, 51.17874883491397497, -10.36894250292378850 ) ) ;
#30025=CARTESIAN_POINT ( 'NONE',  ( 18.52753015748618282, 48.92559781766745886, -4.923371831947291888 ) ) ;
#30027=CARTESIAN_POINT ( 'NONE',  ( 19.84674366389459266, 23.30059781766745530, 2.638427012816836559 ) ) ;
#30030=ORIENTED_EDGE ( 'NONE', *, *, #34970, .F. ) ;
#30033=CARTESIAN_POINT ( 'NONE',  ( 5.076628168052703671, 56.84226448433412315, 8.527530157486179263 ) ) ;
#30034=CARTESIAN_POINT ( 'NONE',  ( -4.164238869374099927, 22.01208216824730357, 3.795296366450308767 ) ) ;
#30035=CARTESIAN_POINT ( 'NONE',  ( 15.44008868035555260, 29.73035201082150891, 9.422509992056143702 ) ) ;
#30036=CARTESIAN_POINT ( 'NONE',  ( -0.8801773607110991993, 32.85535201082151247, -2.915334737309923874 ) ) ;
#30037=CARTESIAN_POINT ( 'NONE',  ( 14.92337183194729988, 64.34226448433412315, -8.527530157486177487 ) ) ;
#30038=CARTESIAN_POINT ( 'NONE',  ( 22.81628187352647785, 36.62363466993041783, 6.195893100308588602E-16 ) ) ;
#30039=CARTESIAN_POINT ( 'NONE',  ( 2.917880565312948704, 2.637082168247300906, 12.26659068614894643 ) ) ;
#30040=CARTESIAN_POINT ( 'NONE',  ( 19.42250999205614193, 65.14701867748817676, 5.440088680355555262 ) ) ;
#30041=EDGE_CURVE ( 'NONE', #26237, #32664, #38379, .T. ) ;
#30042=CARTESIAN_POINT ( 'NONE',  ( 21.09922568453595559, 32.04030133659708923, -6.408140936763230044 ) ) ;
#30044=CARTESIAN_POINT ( 'NONE',  ( 17.20831665107776587, 44.13393115100078745, -7.208316651077762316 ) ) ;
#30045=ADVANCED_FACE ( 'NONE', ( #45373 ), #30359, .F. ) ;
#30046=CARTESIAN_POINT ( 'NONE',  ( -0.8801773607111009756, 13.06368534415483929, 1.068504757029289695E-15 ) ) ;
#30048=CARTESIAN_POINT ( 'NONE',  ( -0.8801773607111008646, 18.27201867748817321, 2.915334737309923430 ) ) ;
#30050=CARTESIAN_POINT ( 'NONE',  ( 10.00000000000000000, 66.81368534415484817, -10.88017736071110342 ) ) ;
#30051=CARTESIAN_POINT ( 'NONE',  ( 0.5774900079438607392, 53.48035201082151247, 5.440088680355550821 ) ) ;
#30053=( LENGTH_UNIT ( ) NAMED_UNIT ( * ) SI_UNIT ( .MILLI., .METRE. ) );
#30054=CARTESIAN_POINT ( 'NONE',  ( 20.88017736071110875, 55.77201867748816966, -2.915334737309920765 ) ) ;
#30056=ORIENTED_EDGE ( 'NONE', *, *, #65937, .F. ) ;
#30057=CARTESIAN_POINT ( 'NONE',  ( 10.00000000000000178, 42.25893115100078745, 9.846743663894594434 ) ) ;
#30060=SURFACE_STYLE_FILL_AREA ( #90568 ) ;
#30062=CARTESIAN_POINT ( 'NONE',  ( 10.00000000000000000, 5.553748834913967869, -14.16423886937410082 ) ) ;
#30064=VERTEX_POINT ( 'NONE', #41348 ) ;
#30065=CARTESIAN_POINT ( 'NONE',  ( -28.92076923076924544, 88.65384615384614619, -9.500000000000000000 ) ) ;
#30067=CARTESIAN_POINT ( 'NONE',  ( 15.44008868035555260, 4.730352010821505360, 9.422509992056143702 ) ) ;
#30069=CARTESIAN_POINT ( 'NONE',  ( -2.816281873526473856, 39.12363466993041783, 9.499525473075851096E-16 ) ) ;
#30070=ORIENTED_EDGE ( 'NONE', *, *, #1938, .F. ) ;
#30072=CARTESIAN_POINT ( 'NONE',  ( 12.63842701281683034, 47.46726448433412315, 9.846743663894596210 ) ) ;
#30074=CARTESIAN_POINT ( 'NONE',  ( 22.81628187352647785, 16.62363466993042138, 6.195893100308588602E-16 ) ) ;
#30075=CARTESIAN_POINT ( 'NONE',  ( 5.076628168052703671, 21.84226448433411960, 8.527530157486179263 ) ) ;
#30079=CARTESIAN_POINT ( 'NONE',  ( 6.565887622018943937, 0.1653013365970866511, 12.81628187352647430 ) ) ;
#30083=CARTESIAN_POINT ( 'NONE',  ( 0.5774900079438590739, 27.64701867748817676, -5.440088680355550821 ) ) ;
#30084=CARTESIAN_POINT ( 'NONE',  ( 10.00000000000000000, 15.55374883491396787, -14.16423886937410082 ) ) ;
#30085=CARTESIAN_POINT ( 'NONE',  ( 19.84674366389459266, 23.30059781766745530, 2.638427012816836559 ) ) ;
#30086=CARTESIAN_POINT ( 'NONE',  ( 2.791683348922237240, 0.3839311510007847872, -7.208316651077763204 ) ) ;
#30087=CARTESIAN_POINT ( 'NONE',  ( 0.6178305044545838731, 34.74863466993042493, 9.382169495545420901 ) ) ;
#30089=CARTESIAN_POINT ( 'NONE',  ( 12.91533473730993009, 16.60535201082150891, -10.88017736071109987 ) ) ;
#30091=CARTESIAN_POINT ( 'NONE',  ( 3.591859063236761518, 14.95696800326375531, 11.09922568453594849 ) ) ;
#30092=CARTESIAN_POINT ( 'NONE',  ( 16.40814093676324603, 2.456968003263753531, -11.09922568453594671 ) ) ;
#30093=CARTESIAN_POINT ( 'NONE',  ( 10.00000000000000000, 29.75893115100078745, -9.846743663894594434 ) ) ;
#30095=CARTESIAN_POINT ( 'NONE',  ( 22.81628187352647785, 31.62363466993042138, 6.195893100308588602E-16 ) ) ;
#30096=CARTESIAN_POINT ( 'NONE',  ( -46.94000000000001194, 93.00000000000000000, 9.000000000000000000 ) ) ;
#30097=CARTESIAN_POINT ( 'NONE',  ( 7.084665262690076126, 34.10535201082151247, 10.88017736071109987 ) ) ;
#30099=CARTESIAN_POINT ( 'NONE',  ( 0.6261916924966959286, 0.5000000000000002220, 6.500000000000003553 ) ) ;
#30100=CARTESIAN_POINT ( 'NONE',  ( 17.84635730667656262, 28.63791097397319163, 6.500000000000019540 ) ) ;
#30101=CARTESIAN_POINT ( 'NONE',  ( 4.559911319644449179, 42.23035201082151247, -9.422509992056141925 ) ) ;
#30102=CARTESIAN_POINT ( 'NONE',  ( 20.88017736071110875, 50.77201867748817676, -2.915334737309920765 ) ) ;
#30103=CARTESIAN_POINT ( 'NONE',  ( 7.361572987183169658, 64.96726448433412315, -9.846743663894592657 ) ) ;
#30105=UNCERTAINTY_MEASURE_WITH_UNIT (LENGTH_MEASURE( 1.000000000000000082E-05 ), #11867, 'distance_accuracy_value', 'NONE');
#30106=( BOUNDED_SURFACE ( )  B_SPLINE_SURFACE ( 1, 2, ( 
 ( #98379, #31311, #52838, #37367, #854, #38349, #46332, #77306, #8820, #39334, #52350, #14367, #69828, #38838, #92319, #98873, #21872, #68844, #68355, #54311, #29342, #59843, #22857, #29835, #82847, #22364, #30328, #44836, #75341, #6856, #60343, #61323, #14869, #45341, #7361, #91331, #83838, #15363, #45848, #80135, #31802, #95641, #50131, #96142, #32295, #78295, #58110, #4656, #62799, #72623, #26642, #9310, #9812, #20126, #27127, #4156, #34623, #80638, #50630, #65122, #57138, #49625, #24337, #39818, #12134, #40314, #81121, #27625, #70819, #2334, #57629, #35117, #93300, #24824, #11645, #42637, #42158, #87634, #32789, #43124, #19148, #88126, #19638, #55300, #63286, #93793, #73114, #65616, #88619, #85811, #12622, #1351, #62300, #17324, #92807, #54797, #85313, #16822, #47297, #77799, #70323, #1838, #47797, #60088, #6121, #28118, #35627, #43615, #5635, #97146, #58618, #74102, #36113, #30085, #98634, #83100, #44097, #44606, #97636, #74608, #83603, #28617, #5136, #96641, #60592, #13119, #81610, #14628, #52112, #29586, #91087, #22614, #53091, #89119, #20630, #15117, #90590, #22117, #36627, #66112, #21627, #13616, #45093, #52597, #75599, #67111, #66619, #73612, #59104, #29101, #51119, #98125, #89613, #21126, #14122, #7111, #51625, #82105, #75101, #59603, #90099, #82604, #6608, #37121, #67617, #37615, #68109, #76579, #23607, #2094, #47565, #8099, #16584, #69582, #53582, #54073, #63054, #70078, #47060, #77558, #24589, #93551, #9074, #1102, #92564, #68602, #84095, #55052, #84588, #25084, #70568, #16087, #46574, #39587, #78063, #38595, #69093, #24090, #85571, #54558, #31565, #77073, #86066, #62060, #85075, #62551, #627, #8585, #39091, #1598, #93056, #32049, #31073, #17085, #32553, #9566, #61571, #40067, #55567, #45593, #76091, #7621, #38113, #130, #30579, #92082, #61084, #91594, #23110, #15611, #46095, #48540, #41063, #71064, #86556, #18060, #73011, #42527, #27022, #87038, #87528, #41565, #18548, #27513, #71560, #48043, #40566, #4543, #56062, #49518, #3072, #79039, #19530, #33528, #72032, #11531, #64516, #96030, #10067, #64023, #4050, #49040, #2589, #78555, #10552, #94535, #26054, #33044, #56543, #79544, #35005, #65508, #57522, #11044, #19042, #3559, #34019, #58006, #95022, #63539, #94049, #17577, #26530, #80027, #57027, #42052, #50027, #72516, #25570, #88018, #34512, #65005, #95532, #80529, #12028, #12516, #73500, #6999, #74992, #44492, #59003, #50518, #36509, #28509, #59982, #6495, #37003, #81998, #96532, #75487, #81500, #89505, #81015, #14011, #43018, #66004, #28986, #67499, #20017, #58503, #59493, #5026, #35511, #28007, #67002 ),
 ( #22010, #89013, #20520, #29474, #51504, #73999, #97524, #98020, #13509, #29974, #43991, #37504, #74493, #51005, #89992, #36005, #44980, #67996, #21508, #13005, #43500, #90476, #5525, #66508, #21016, #6017, #52006, #82495, #98521, #52484, #97033, #82992, #14510, #88515, #53966, #61950, #23975, #38976, #39951, #31934, #988, #77944, #69962, #9450, #31448, #69467, #77443, #17, #60479, #1481, #39472, #54935, #52973, #70454, #92451, #76958, #68980, #54448, #90968, #62434, #84957, #53466, #514, #60966, #15006, #1973, #30960, #22502, #83486, #30465, #46465, #61458, #92938, #45476, #8955, #16469, #24471, #83976, #47445, #46948, #8468, #68490, #75978, #22999, #85452, #16964, #15501, #7507, #38486, #45983, #91475, #15975, #37998, #76472, #7987, #91966, #23495, #84475, #78930, #64402, #64882, #26409, #63907, #87892, #11414, #80410, #79905, #11910, #94910, #87411, #93440, #56909, #9951, #25934, #10440, #94418, #40455, #86443, #95409, #2474, #70954, #72397, #56435, #17942, #10926, #41935, #86923, #72892, #18434, #49900, #48917, #24965, #33896, #40947, #19409, #42412, #41452, #32930, #55450, #3925, #55944, #47929, #33409, #79430, #18928, #71916, #32439, #49405, #63430, #34395, #26905, #17462, #3437, #57402, #62938, #85952, #78435, #93936, #25461, #48428, #71445, #2959, #74363, #13384, #21386, #42901, #6369, #66377, #28388, #66879, #20402, #43381, #28864, #4909, #20895, #59863, #65387, #80899, #43867, #82364, #34891, #73383, #5891, #95914, #57886, #35390, #81871, #27394, #97396, #51883, #97902, #65882, #81383, #90350, #36882, #96409, #36384, #58880, #12395, #12882, #21888, #59368, #89871, #13887, #44371, #52366, #74870, #89382, #51384, #88400, #27885, #67372, #73880, #82871, #29360, #5410, #35881, #14385, #44855, #58372, #88893, #4426, #19897, #50390, #50889, #96911, #16841, #61342, #15863, #92338, #37880, #83855, #7869, #394, #23861, #53854, #60850, #54326, #31819, #84840, #7381, #30844, #15379, #8350, #91853, #69347, #23368, #54816, #67876, #22876, #61830, #38364, #29854, #37386, #45356, #68373, #98892, #60357, #75861, #30343, #62316, #1368, #16348, #45863, #46348, #84362, #76354, #85327, #91349, #6875, #98397, #92823, #14887, #38858, #53347, #68862, #77322, #76835, #83364, #46830, #871, #31330, #24353, #75361, #90851, #22382, #52856, #8836, #39350, #69844, #17821, #9329, #94294, #86317, #18806, #3307, #94789, #40821, #55320, #34265, #40331, #48303, #39832, #71802, #70835, #62817, #78810, #33294, #79302, #2838, #3809, #10811, #17341, #33770, #41329, #32312, #71320, #48794, #64277, #25817, #26782, #49289, #86810, #64767, #56790 ) ),
 .UNSPECIFIED., .F., .F., .F. ) 
 B_SPLINE_SURFACE_WITH_KNOTS ( ( 2, 2 ),
 ( 3, 2, 2, 2, 2, 2, 2, 2, 2, 2, 2, 2, 2, 2, 2, 2, 2, 2, 2, 2, 2, 2, 2, 2, 2, 2, 2, 2, 2, 2, 2, 2, 2, 2, 2, 2, 2, 2, 2, 2, 2, 2, 2, 2, 2, 2, 2, 2, 2, 2, 2, 2, 2, 2, 2, 2, 2, 2, 2, 2, 2, 2, 2, 2, 2, 2, 2, 2, 2, 2, 2, 2, 2, 2, 2, 2, 2, 2, 2, 2, 2, 2, 2, 2, 2, 2, 2, 2, 2, 2, 2, 2, 2, 2, 2, 2, 2, 2, 2, 2, 2, 2, 2, 2, 2, 2, 2, 2, 2, 2, 2, 2, 2, 2, 2, 2, 2, 2, 2, 2, 2, 2, 2, 2, 2, 2, 2, 2, 2, 2, 2, 2, 2, 2, 2, 2, 2, 2, 2, 2, 2, 2, 2, 2, 2, 2, 2, 2, 2, 2, 2, 2, 2, 2, 2, 2, 2, 2, 2, 2, 2, 2, 3 ),
 ( 0.000000000000000000, 1.000000000000000000 ),
 ( 0.000000000000000000, 0.005952380952380952051, 0.01190476190476190410, 0.01785714285714285615, 0.02380952380952380820, 0.02976190476190476025, 0.03571428571428571230, 0.04166666666666666435, 0.04761904761904761640, 0.05357142857142856845, 0.05952380952380952051, 0.06547619047619047949, 0.07142857142857142461, 0.07738095238095238360, 0.08333333333333332871, 0.08928571428571428770, 0.09523809523809523281, 0.1011904761904761918, 0.1071428571428571369, 0.1130952380952380959, 0.1190476190476190410, 0.1250000000000000000, 0.1309523809523809590, 0.1369047619047619180, 0.1428571428571428492, 0.1488095238095238082, 0.1547619047619047672, 0.1607142857142857262, 0.1666666666666666574, 0.1726190476190476164, 0.1785714285714285754, 0.1845238095238095344, 0.1904761904761904656, 0.1964285714285714246, 0.2023809523809523836, 0.2083333333333333426, 0.2142857142857142738, 0.2202380952380952328, 0.2261904761904761918, 0.2321428571428571508, 0.2380952380952380820, 0.2440476190476190410, 0.2500000000000000000, 0.2559523809523809312, 0.2619047619047619180, 0.2678571428571428492, 0.2738095238095238360, 0.2797619047619047672, 0.2857142857142856984, 0.2916666666666666852, 0.2976190476190476164, 0.3035714285714285476, 0.3095238095238095344, 0.3154761904761904656, 0.3214285714285714524, 0.3273809523809523836, 0.3333333333333333148, 0.3392857142857143016, 0.3452380952380952328, 0.3511904761904761640, 0.3571428571428571508, 0.3630952380952380820, 0.3690476190476190688, 0.3750000000000000000, 0.3809523809523809312, 0.3869047619047619180, 0.3928571428571428492, 0.3988095238095238360, 0.4047619047619047672, 0.4107142857142856984, 0.4166666666666666852, 0.4226190476190476164, 0.4285714285714285476, 0.4345238095238095344, 0.4404761904761904656, 0.4464285714285714524, 0.4523809523809523836, 0.4583333333333333148, 0.4642857142857143016, 0.4702380952380952328, 0.4761904761904761640, 0.4821428571428571508, 0.4880952380952380820, 0.4940476190476190688, 0.5000000000000000000, 0.5059523809523809312, 0.5119047619047618625, 0.5178571428571429047, 0.5238095238095238360, 0.5297619047619047672, 0.5357142857142856984, 0.5416666666666666297, 0.5476190476190476719, 0.5535714285714286031, 0.5595238095238095344, 0.5654761904761904656, 0.5714285714285713969, 0.5773809523809523281, 0.5833333333333333703, 0.5892857142857143016, 0.5952380952380952328, 0.6011904761904761640, 0.6071428571428570953, 0.6130952380952381375, 0.6190476190476190688, 0.6250000000000000000, 0.6309523809523809312, 0.6369047619047618625, 0.6428571428571429047, 0.6488095238095238360, 0.6547619047619047672, 0.6607142857142856984, 0.6666666666666666297, 0.6726190476190476719, 0.6785714285714286031, 0.6845238095238095344, 0.6904761904761904656, 0.6964285714285713969, 0.7023809523809523281, 0.7083333333333333703, 0.7142857142857143016, 0.7202380952380952328, 0.7261904761904761640, 0.7321428571428570953, 0.7380952380952381375, 0.7440476190476190688, 0.7500000000000000000, 0.7559523809523809312, 0.7619047619047618625, 0.7678571428571429047, 0.7738095238095238360, 0.7797619047619047672, 0.7857142857142856984, 0.7916666666666666297, 0.7976190476190476719, 0.8035714285714286031, 0.8095238095238095344, 0.8154761904761904656, 0.8214285714285713969, 0.8273809523809523281, 0.8333333333333333703, 0.8392857142857143016, 0.8452380952380952328, 0.8511904761904761640, 0.8571428571428570953, 0.8630952380952381375, 0.8690476190476190688, 0.8750000000000000000, 0.8809523809523809312, 0.8869047619047618625, 0.8928571428571429047, 0.8988095238095238360, 0.9047619047619047672, 0.9107142857142856984, 0.9166666666666666297, 0.9226190476190476719, 0.9285714285714286031, 0.9345238095238095344, 0.9404761904761904656, 0.9464285714285713969, 0.9523809523809523281, 0.9583333333333333703, 0.9642857142857143016 ),
 .UNSPECIFIED. ) 
 GEOMETRIC_REPRESENTATION_ITEM ( )  RATIONAL_B_SPLINE_SURFACE ( (
 ( 1.000000000000000000, 0.9659258262890683122, 1.000000000000000000, 0.9659258262890683122, 1.000000000000000000, 0.9659258262890683122, 1.000000000000000000, 0.9659258262890683122, 1.000000000000000000, 0.9659258262890683122, 1.000000000000000000, 0.9659258262890683122, 1.000000000000000000, 0.9659258262890683122, 1.000000000000000000, 0.9659258262890683122, 1.000000000000000000, 0.9659258262890683122, 1.000000000000000000, 0.9659258262890683122, 1.000000000000000000, 0.9659258262890683122, 1.000000000000000000, 0.9659258262890683122, 1.000000000000000000, 0.9659258262890683122, 1.000000000000000000, 0.9659258262890683122, 1.000000000000000000, 0.9659258262890683122, 1.000000000000000000, 0.9659258262890683122, 1.000000000000000000, 0.9659258262890683122, 1.000000000000000000, 0.9659258262890683122, 1.000000000000000000, 0.9659258262890683122, 1.000000000000000000, 0.9659258262890683122, 1.000000000000000000, 0.9659258262890683122, 1.000000000000000000, 0.9659258262890683122, 1.000000000000000000, 0.9659258262890683122, 1.000000000000000000, 0.9659258262890683122, 1.000000000000000000, 0.9659258262890683122, 1.000000000000000000, 0.9659258262890683122, 1.000000000000000000, 0.9659258262890683122, 1.000000000000000000, 0.9659258262890683122, 1.000000000000000000, 0.9659258262890683122, 1.000000000000000000, 0.9659258262890683122, 1.000000000000000000, 0.9659258262890683122, 1.000000000000000000, 0.9659258262890683122, 1.000000000000000000, 0.9659258262890683122, 1.000000000000000000, 0.9659258262890683122, 1.000000000000000000, 0.9659258262890683122, 1.000000000000000000, 0.9659258262890683122, 1.000000000000000000, 0.9659258262890683122, 1.000000000000000000, 0.9659258262890683122, 1.000000000000000000, 0.9659258262890683122, 1.000000000000000000, 0.9659258262890683122, 1.000000000000000000, 0.9659258262890683122, 1.000000000000000000, 0.9659258262890683122, 1.000000000000000000, 0.9659258262890683122, 1.000000000000000000, 0.9659258262890683122, 1.000000000000000000, 0.9659258262890683122, 1.000000000000000000, 0.9659258262890683122, 1.000000000000000000, 0.9659258262890683122, 1.000000000000000000, 0.9659258262890683122, 1.000000000000000000, 0.9659258262890683122, 1.000000000000000000, 0.9659258262890683122, 1.000000000000000000, 0.9659258262890683122, 1.000000000000000000, 0.9659258262890683122, 1.000000000000000000, 0.9659258262890683122, 1.000000000000000000, 0.9659258262890683122, 1.000000000000000000, 0.9659258262890683122, 1.000000000000000000, 0.9659258262890683122, 1.000000000000000000, 0.9659258262890683122, 1.000000000000000000, 0.9659258262890683122, 1.000000000000000000, 0.9659258262890683122, 1.000000000000000000, 0.9659258262890683122, 1.000000000000000000, 0.9659258262890683122, 1.000000000000000000, 0.9659258262890683122, 1.000000000000000000, 0.9659258262890683122, 1.000000000000000000, 0.9659258262890683122, 1.000000000000000000, 0.9659258262890683122, 1.000000000000000000, 0.9659258262890683122, 1.000000000000000000, 0.9659258262890683122, 1.000000000000000000, 0.9659258262890683122, 1.000000000000000000, 0.9659258262890683122, 1.000000000000000000, 0.9659258262890683122, 1.000000000000000000, 0.9659258262890683122, 1.000000000000000000, 0.9659258262890683122, 1.000000000000000000, 0.9659258262890683122, 1.000000000000000000, 0.9659258262890683122, 1.000000000000000000, 0.9659258262890683122, 1.000000000000000000, 0.9659258262890683122, 1.000000000000000000, 0.9659258262890683122, 1.000000000000000000, 0.9659258262890683122, 1.000000000000000000, 0.9659258262890683122, 1.000000000000000000, 0.9659258262890683122, 1.000000000000000000, 0.9659258262890683122, 1.000000000000000000, 0.9659258262890683122, 1.000000000000000000, 0.9659258262890683122, 1.000000000000000000, 0.9659258262890683122, 1.000000000000000000, 0.9659258262890683122, 1.000000000000000000, 0.9659258262890683122, 1.000000000000000000, 0.9659258262890683122, 1.000000000000000000, 0.9659258262890683122, 1.000000000000000000, 0.9659258262890683122, 1.000000000000000000, 0.9659258262890683122, 1.000000000000000000, 0.9659258262890683122, 1.000000000000000000, 0.9659258262890683122, 1.000000000000000000, 0.9659258262890683122, 1.000000000000000000, 0.9659258262890683122, 1.000000000000000000, 0.9659258262890683122, 1.000000000000000000, 0.9659258262890683122, 1.000000000000000000, 0.9659258262890683122, 1.000000000000000000, 0.9659258262890683122, 1.000000000000000000, 0.9659258262890683122, 1.000000000000000000, 0.9659258262890683122, 1.000000000000000000, 0.9659258262890683122, 1.000000000000000000, 0.9659258262890683122, 1.000000000000000000, 0.9659258262890683122, 1.000000000000000000, 0.9659258262890683122, 1.000000000000000000, 0.9659258262890683122, 1.000000000000000000, 0.9659258262890683122, 1.000000000000000000, 0.9659258262890683122, 1.000000000000000000, 0.9659258262890683122, 1.000000000000000000, 0.9659258262890683122, 1.000000000000000000, 0.9659258262890683122, 1.000000000000000000, 0.9659258262890683122, 1.000000000000000000, 0.9659258262890683122, 1.000000000000000000, 0.9659258262890683122, 1.000000000000000000, 0.9659258262890683122, 1.000000000000000000, 0.9659258262890683122, 1.000000000000000000, 0.9659258262890683122, 1.000000000000000000, 0.9659258262890683122, 1.000000000000000000, 0.9659258262890683122, 1.000000000000000000, 0.9659258262890683122, 1.000000000000000000, 0.9659258262890683122, 1.000000000000000000, 0.9659258262890683122, 1.000000000000000000, 0.9659258262890683122, 1.000000000000000000, 0.9659258262890683122, 1.000000000000000000, 0.9659258262890683122, 1.000000000000000000, 0.9659258262890683122, 1.000000000000000000, 0.9659258262890683122, 1.000000000000000000, 0.9659258262890683122, 1.000000000000000000, 0.9659258262890683122, 1.000000000000000000, 0.9659258262890683122, 1.000000000000000000, 0.9659258262890683122, 1.000000000000000000, 0.9659258262890683122, 1.000000000000000000, 0.9659258262890683122, 1.000000000000000000, 0.9659258262890683122, 1.000000000000000000, 0.9659258262890683122, 1.000000000000000000, 0.9659258262890683122, 1.000000000000000000, 0.9659258262890683122, 1.000000000000000000, 0.9659258262890683122, 1.000000000000000000, 0.9659258262890683122, 1.000000000000000000, 0.9659258262890683122, 1.000000000000000000, 0.9659258262890683122, 1.000000000000000000, 0.9659258262890683122, 1.000000000000000000, 0.9659258262890683122, 1.000000000000000000, 0.9659258262890683122, 1.000000000000000000, 0.9659258262890683122, 1.000000000000000000, 0.9659258262890683122, 1.000000000000000000, 0.9659258262890683122, 1.000000000000000000, 0.9659258262890683122, 1.000000000000000000, 0.9659258262890683122, 1.000000000000000000, 0.9659258262890683122, 1.000000000000000000, 0.9659258262890683122, 1.000000000000000000, 0.9659258262890683122, 1.000000000000000000, 0.9659258262890683122, 1.000000000000000000, 0.9659258262890683122, 1.000000000000000000, 0.9659258262890683122, 1.000000000000000000, 0.9659258262890683122, 1.000000000000000000, 0.9659258262890683122, 1.000000000000000000, 0.9659258262890683122, 1.000000000000000000, 0.9659258262890683122, 1.000000000000000000, 0.9659258262890683122, 1.000000000000000000, 0.9659258262890683122, 1.000000000000000000, 0.9659258262890683122, 1.000000000000000000, 0.9659258262890683122, 1.000000000000000000),
 ( 1.000000000000000000, 0.9659258262890683122, 1.000000000000000000, 0.9659258262890683122, 1.000000000000000000, 0.9659258262890683122, 1.000000000000000000, 0.9659258262890683122, 1.000000000000000000, 0.9659258262890683122, 1.000000000000000000, 0.9659258262890683122, 1.000000000000000000, 0.9659258262890683122, 1.000000000000000000, 0.9659258262890683122, 1.000000000000000000, 0.9659258262890683122, 1.000000000000000000, 0.9659258262890683122, 1.000000000000000000, 0.9659258262890683122, 1.000000000000000000, 0.9659258262890683122, 1.000000000000000000, 0.9659258262890683122, 1.000000000000000000, 0.9659258262890683122, 1.000000000000000000, 0.9659258262890683122, 1.000000000000000000, 0.9659258262890683122, 1.000000000000000000, 0.9659258262890683122, 1.000000000000000000, 0.9659258262890683122, 1.000000000000000000, 0.9659258262890683122, 1.000000000000000000, 0.9659258262890683122, 1.000000000000000000, 0.9659258262890683122, 1.000000000000000000, 0.9659258262890683122, 1.000000000000000000, 0.9659258262890683122, 1.000000000000000000, 0.9659258262890683122, 1.000000000000000000, 0.9659258262890683122, 1.000000000000000000, 0.9659258262890683122, 1.000000000000000000, 0.9659258262890683122, 1.000000000000000000, 0.9659258262890683122, 1.000000000000000000, 0.9659258262890683122, 1.000000000000000000, 0.9659258262890683122, 1.000000000000000000, 0.9659258262890683122, 1.000000000000000000, 0.9659258262890683122, 1.000000000000000000, 0.9659258262890683122, 1.000000000000000000, 0.9659258262890683122, 1.000000000000000000, 0.9659258262890683122, 1.000000000000000000, 0.9659258262890683122, 1.000000000000000000, 0.9659258262890683122, 1.000000000000000000, 0.9659258262890683122, 1.000000000000000000, 0.9659258262890683122, 1.000000000000000000, 0.9659258262890683122, 1.000000000000000000, 0.9659258262890683122, 1.000000000000000000, 0.9659258262890683122, 1.000000000000000000, 0.9659258262890683122, 1.000000000000000000, 0.9659258262890683122, 1.000000000000000000, 0.9659258262890683122, 1.000000000000000000, 0.9659258262890683122, 1.000000000000000000, 0.9659258262890683122, 1.000000000000000000, 0.9659258262890683122, 1.000000000000000000, 0.9659258262890683122, 1.000000000000000000, 0.9659258262890683122, 1.000000000000000000, 0.9659258262890683122, 1.000000000000000000, 0.9659258262890683122, 1.000000000000000000, 0.9659258262890683122, 1.000000000000000000, 0.9659258262890683122, 1.000000000000000000, 0.9659258262890683122, 1.000000000000000000, 0.9659258262890683122, 1.000000000000000000, 0.9659258262890683122, 1.000000000000000000, 0.9659258262890683122, 1.000000000000000000, 0.9659258262890683122, 1.000000000000000000, 0.9659258262890683122, 1.000000000000000000, 0.9659258262890683122, 1.000000000000000000, 0.9659258262890683122, 1.000000000000000000, 0.9659258262890683122, 1.000000000000000000, 0.9659258262890683122, 1.000000000000000000, 0.9659258262890683122, 1.000000000000000000, 0.9659258262890683122, 1.000000000000000000, 0.9659258262890683122, 1.000000000000000000, 0.9659258262890683122, 1.000000000000000000, 0.9659258262890683122, 1.000000000000000000, 0.9659258262890683122, 1.000000000000000000, 0.9659258262890683122, 1.000000000000000000, 0.9659258262890683122, 1.000000000000000000, 0.9659258262890683122, 1.000000000000000000, 0.9659258262890683122, 1.000000000000000000, 0.9659258262890683122, 1.000000000000000000, 0.9659258262890683122, 1.000000000000000000, 0.9659258262890683122, 1.000000000000000000, 0.9659258262890683122, 1.000000000000000000, 0.9659258262890683122, 1.000000000000000000, 0.9659258262890683122, 1.000000000000000000, 0.9659258262890683122, 1.000000000000000000, 0.9659258262890683122, 1.000000000000000000, 0.9659258262890683122, 1.000000000000000000, 0.9659258262890683122, 1.000000000000000000, 0.9659258262890683122, 1.000000000000000000, 0.9659258262890683122, 1.000000000000000000, 0.9659258262890683122, 1.000000000000000000, 0.9659258262890683122, 1.000000000000000000, 0.9659258262890683122, 1.000000000000000000, 0.9659258262890683122, 1.000000000000000000, 0.9659258262890683122, 1.000000000000000000, 0.9659258262890683122, 1.000000000000000000, 0.9659258262890683122, 1.000000000000000000, 0.9659258262890683122, 1.000000000000000000, 0.9659258262890683122, 1.000000000000000000, 0.9659258262890683122, 1.000000000000000000, 0.9659258262890683122, 1.000000000000000000, 0.9659258262890683122, 1.000000000000000000, 0.9659258262890683122, 1.000000000000000000, 0.9659258262890683122, 1.000000000000000000, 0.9659258262890683122, 1.000000000000000000, 0.9659258262890683122, 1.000000000000000000, 0.9659258262890683122, 1.000000000000000000, 0.9659258262890683122, 1.000000000000000000, 0.9659258262890683122, 1.000000000000000000, 0.9659258262890683122, 1.000000000000000000, 0.9659258262890683122, 1.000000000000000000, 0.9659258262890683122, 1.000000000000000000, 0.9659258262890683122, 1.000000000000000000, 0.9659258262890683122, 1.000000000000000000, 0.9659258262890683122, 1.000000000000000000, 0.9659258262890683122, 1.000000000000000000, 0.9659258262890683122, 1.000000000000000000, 0.9659258262890683122, 1.000000000000000000, 0.9659258262890683122, 1.000000000000000000, 0.9659258262890683122, 1.000000000000000000, 0.9659258262890683122, 1.000000000000000000, 0.9659258262890683122, 1.000000000000000000, 0.9659258262890683122, 1.000000000000000000, 0.9659258262890683122, 1.000000000000000000, 0.9659258262890683122, 1.000000000000000000, 0.9659258262890683122, 1.000000000000000000, 0.9659258262890683122, 1.000000000000000000, 0.9659258262890683122, 1.000000000000000000, 0.9659258262890683122, 1.000000000000000000, 0.9659258262890683122, 1.000000000000000000, 0.9659258262890683122, 1.000000000000000000, 0.9659258262890683122, 1.000000000000000000, 0.9659258262890683122, 1.000000000000000000, 0.9659258262890683122, 1.000000000000000000, 0.9659258262890683122, 1.000000000000000000, 0.9659258262890683122, 1.000000000000000000, 0.9659258262890683122, 1.000000000000000000, 0.9659258262890683122, 1.000000000000000000, 0.9659258262890683122, 1.000000000000000000, 0.9659258262890683122, 1.000000000000000000, 0.9659258262890683122, 1.000000000000000000, 0.9659258262890683122, 1.000000000000000000, 0.9659258262890683122, 1.000000000000000000, 0.9659258262890683122, 1.000000000000000000, 0.9659258262890683122, 1.000000000000000000, 0.9659258262890683122, 1.000000000000000000, 0.9659258262890683122, 1.000000000000000000, 0.9659258262890683122, 1.000000000000000000, 0.9659258262890683122, 1.000000000000000000, 0.9659258262890683122, 1.000000000000000000, 0.9659258262890683122, 1.000000000000000000, 0.9659258262890683122, 1.000000000000000000, 0.9659258262890683122, 1.000000000000000000, 0.9659258262890683122, 1.000000000000000000, 0.9659258262890683122, 1.000000000000000000, 0.9659258262890683122, 1.000000000000000000, 0.9659258262890683122, 1.000000000000000000, 0.9659258262890683122, 1.000000000000000000, 0.9659258262890683122, 1.000000000000000000, 0.9659258262890683122, 1.000000000000000000, 0.9659258262890683122, 1.000000000000000000, 0.9659258262890683122, 1.000000000000000000, 0.9659258262890683122, 1.000000000000000000, 0.9659258262890683122, 1.000000000000000000, 0.9659258262890683122, 1.000000000000000000, 0.9659258262890683122, 1.000000000000000000) ) ) 
 REPRESENTATION_ITEM ( '' )  SURFACE ( )  );
#30107=CARTESIAN_POINT ( 'NONE',  ( 12.63842701281683922, 54.55059781766745175, -9.846743663894590881 ) ) ;
#30108=CARTESIAN_POINT ( 'NONE',  ( 10.00000000000000178, 9.313685344154839285, 10.88017736071110342 ) ) ;
#30110=CARTESIAN_POINT ( 'NONE',  ( 21.09922568453595559, 12.04030133659708746, -6.408140936763230044 ) ) ;
#30112=CARTESIAN_POINT ( 'NONE',  ( 7.084665262690076126, 39.10535201082150536, 10.88017736071109987 ) ) ;
#30114=CARTESIAN_POINT ( 'NONE',  ( 2.035157376598822676, 27.43868534415483396, -7.964842623401177768 ) ) ;
#30115=CARTESIAN_POINT ( 'NONE',  ( 17.20831665107776587, 7.883931151000784787, 7.208316651077764980 ) ) ;
#30116=CARTESIAN_POINT ( 'NONE',  ( 20.36894250292379382, 33.67874883491396076, 10.36894250292379205 ) ) ;
#30117=CARTESIAN_POINT ( 'NONE',  ( 7.361572987183169658, 29.96726448433411960, -9.846743663894592657 ) ) ;
#30119=CARTESIAN_POINT ( 'NONE',  ( -0.8801773607110991993, 47.85535201082150536, -2.915334737309923874 ) ) ;
#30123=CARTESIAN_POINT ( 'NONE',  ( 17.20831665107776587, 62.88393115100078745, 7.208316651077764980 ) ) ;
#30124=VERTEX_POINT ( 'NONE', #87304 ) ;
#30126=CARTESIAN_POINT ( 'NONE',  ( 13.79529636645030344, 23.26208216824730002, 14.16423886937410614 ) ) ;
#30127=CARTESIAN_POINT ( 'NONE',  ( 20.36894250292379738, 19.92874883491396787, -10.36894250292379027 ) ) ;
#30128=CARTESIAN_POINT ( 'NONE',  ( 2.035157376598824452, 63.68868534415484106, 7.964842623401179544 ) ) ;
#30129=CARTESIAN_POINT ( 'NONE',  ( 7.084665262690076126, 2.022018677488171434, -10.88017736071110164 ) ) ;
#30130=CARTESIAN_POINT ( 'NONE',  ( 0.1532563361054083140, 51.00893115100078745, 1.131784320476157264E-15 ) ) ;
#30132=CARTESIAN_POINT ( 'NONE',  ( 12.91533473730992121, 49.52201867748817676, 10.88017736071110164 ) ) ;
#30133=CARTESIAN_POINT ( 'NONE',  ( -1.099225684535947600, 13.70696800326375353, -6.408140936763238038 ) ) ;
#30134=CARTESIAN_POINT ( 'NONE',  ( 22.26659068614895176, 19.72041550158063572, -7.082119434687042414 ) ) ;
#30135=CARTESIAN_POINT ( 'NONE',  ( 7.084665262690076126, 14.10535201082150358, 10.88017736071109987 ) ) ;
#30136=CARTESIAN_POINT ( 'NONE',  ( 0.5774900079438607392, 28.48035201082150891, 5.440088680355550821 ) ) ;
#30137=CARTESIAN_POINT ( 'NONE',  ( 4.559911319644449179, 58.89701867748817676, 9.422509992056141925 ) ) ;
#30138=CARTESIAN_POINT ( 'NONE',  ( -2.816281873526473856, 49.33196800326374643, 3.434112377981055619 ) ) ;
#30146=CARTESIAN_POINT ( 'NONE',  ( 6.204703633549690345, 57.84541550158063927, 14.16423886937410082 ) ) ;
#30147=CARTESIAN_POINT ( 'NONE',  ( -4.164238869374099927, 67.01208216824728936, 3.795296366450308767 ) ) ;
#30148=CARTESIAN_POINT ( 'NONE',  ( 10.00000000000000178, 17.25893115100078745, 9.846743663894594434 ) ) ;
#30149=CARTESIAN_POINT ( 'NONE',  ( 12.63842701281683034, 62.46726448433410894, 9.846743663894596210 ) ) ;
#30152=CARTESIAN_POINT ( 'NONE',  ( 19.80832241502127999, 44.75868815902068576, 6.499999999999992895 ) ) ;
#30158=CARTESIAN_POINT ( 'NONE',  ( 20.36894250292379382, 33.67874883491396076, 10.36894250292379205 ) ) ;
#30159=VERTEX_POINT ( 'NONE', #32819 ) ;
#30161=CARTESIAN_POINT ( 'NONE',  ( 2.917880565312948704, 47.63708216824730357, 12.26659068614894643 ) ) ;
#30163=CARTESIAN_POINT ( 'NONE',  ( 0.6178305044545838731, 59.74863466993041783, 9.382169495545420901 ) ) ;
#30164=CARTESIAN_POINT ( 'NONE',  ( 7.084665262690076126, 22.02201867748817321, -10.88017736071110164 ) ) ;
#30165=CARTESIAN_POINT ( 'NONE',  ( 10.00000000000000000, 54.75893115100078745, -9.846743663894594434 ) ) ;
#30166=CARTESIAN_POINT ( 'NONE',  ( 12.91533473730993009, 26.60535201082150536, -10.88017736071109987 ) ) ;
#30169=CARTESIAN_POINT ( 'NONE',  ( 0.1532563361054083140, 56.00893115100078745, 1.131784320476157264E-15 ) ) ;
#30170=CARTESIAN_POINT ( 'NONE',  ( 19.84674366389459266, 53.71726448433411605, -2.638427012816827677 ) ) ;
#30174=LINE ( 'NONE', #81698, #65426 ) ;
#30176=CYLINDRICAL_SURFACE ( 'NONE', #30768, 0.5000000000000004441 ) ;
#30178=CARTESIAN_POINT ( 'NONE',  ( 19.67858290521088804, 89.00000000000000000, 5.461713021790605360 ) ) ;
#30179=CARTESIAN_POINT ( 'NONE',  ( 7.361572987183170547, 37.05059781766744464, 9.846743663894590881 ) ) ;
#30181=CARTESIAN_POINT ( 'NONE',  ( 16.40814093676324603, 37.45696800326376064, -11.09922568453594671 ) ) ;
#30186=DIRECTION ( 'NONE',  ( 0.000000000000000000, -1.000000000000000000, 0.000000000000000000 ) ) ;
#30187=CARTESIAN_POINT ( 'NONE',  ( -0.03447792253739477564, 65.15514106990688958, 6.401564815979731371 ) ) ;
#30188=CARTESIAN_POINT ( 'NONE',  ( 2.791683348922240793, 41.63393115100078745, 7.208316651077764092 ) ) ;
#30189=CARTESIAN_POINT ( 'NONE',  ( -2.266590686148945544, 36.38708216824730357, -7.082119434687050408 ) ) ;
#30190=CARTESIAN_POINT ( 'NONE',  ( 7.361572987183169658, 44.96726448433412315, -9.846743663894592657 ) ) ;
#30192=CARTESIAN_POINT ( 'NONE',  ( 2.791683348922237240, 5.383931151000785675, -7.208316651077763204 ) ) ;
#30193=CARTESIAN_POINT ( 'NONE',  ( -4.164238869374098151, 6.595415501580634832, -3.795296366450310543 ) ) ;
#30194=CARTESIAN_POINT ( 'NONE',  ( 19.84674366389459621, 48.50893115100078745, 7.409399052514197653E-17 ) ) ;
#30195=CARTESIAN_POINT ( 'NONE',  ( 17.96484262340118221, 54.93868534415484106, 7.964842623401181321 ) ) ;
#30196=ADVANCED_FACE ( 'NONE', ( #40349 ), #93943, .T. ) ;
#30197=CARTESIAN_POINT ( 'NONE',  ( 0.1532563361054083140, 46.00893115100079456, 1.131784320476157264E-15 ) ) ;
#30199=CARTESIAN_POINT ( 'NONE',  ( 17.96484262340118221, 39.93868534415484106, 7.964842623401181321 ) ) ;
#30202=CARTESIAN_POINT ( 'NONE',  ( -0.8801773607111009756, 33.06368534415484106, 1.068504757029289695E-15 ) ) ;
#30203=CARTESIAN_POINT ( 'NONE',  ( 5.076628168052703671, 66.84226448433412315, 8.527530157486179263 ) ) ;
#30204=CARTESIAN_POINT ( 'NONE',  ( 20.88017736071110875, 45.77201867748816966, -2.915334737309920765 ) ) ;
#30205=CARTESIAN_POINT ( 'NONE',  ( -0.2418659066527647783, 48.09014588040356841, 6.114288769123054301 ) ) ;
#30208=CARTESIAN_POINT ( 'NONE',  ( 20.88017736071110519, 40.56368534415484106, 2.639326808657452039E-16 ) ) ;
#30210=CARTESIAN_POINT ( 'NONE',  ( 17.20831665107776587, 12.88393115100078390, 7.208316651077764980 ) ) ;
#30211=CARTESIAN_POINT ( 'NONE',  ( 19.84674366389459621, 38.50893115100078745, 7.409399052514197653E-17 ) ) ;
#30214=CARTESIAN_POINT ( 'NONE',  ( -2.816281873526473856, -0.8763653300695799508, 9.499525473075851096E-16 ) ) ;
#30215=CARTESIAN_POINT ( 'NONE',  ( 2.035157376598824452, 3.688685344154837953, 7.964842623401179544 ) ) ;
#30216=CARTESIAN_POINT ( 'NONE',  ( 20.03447792253739124, 27.65514106990690735, -6.401564815979737588 ) ) ;
#30217=CARTESIAN_POINT ( 'NONE',  ( -2.266590686148945544, 16.38708216824730357, -7.082119434687050408 ) ) ;
#30218=CARTESIAN_POINT ( 'NONE',  ( -2.266590686148945544, 47.22041550158063927, 7.082119434687048631 ) ) ;
#30221=CARTESIAN_POINT ( 'NONE',  ( 5.076628168052704559, 25.17559781766745175, -8.527530157486179263 ) ) ;
#30222=CARTESIAN_POINT ( 'NONE',  ( 19.42250999205614548, 20.98035201082150891, -5.440088680355545492 ) ) ;
#30223=CARTESIAN_POINT ( 'NONE',  ( 1.472469842513823179, 46.42559781766745175, 4.923371831947296329 ) ) ;
#30224=CARTESIAN_POINT ( 'NONE',  ( 2.917880565312950480, 5.970415501580634832, -12.26659068614894821 ) ) ;
#30227=CARTESIAN_POINT ( 'NONE',  ( 19.84674366389459266, 8.300597817667451750, 2.638427012816836559 ) ) ;
#30228=CARTESIAN_POINT ( 'NONE',  ( 6.565887622018943937, 33.08196800326374643, -12.81628187352647608 ) ) ;
#30229=CARTESIAN_POINT ( 'NONE',  ( 10.00000000000000178, 42.25893115100078745, 9.846743663894594434 ) ) ;
#30231=CARTESIAN_POINT ( 'NONE',  ( 14.92337183194729988, 9.342264484334119601, -8.527530157486177487 ) ) ;
#30234=CARTESIAN_POINT ( 'NONE',  ( 13.79529636645031943, 55.34541550158062506, -14.16423886937409904 ) ) ;
#30235=CARTESIAN_POINT ( 'NONE',  ( 20.88017736071110875, 45.77201867748816966, -2.915334737309920765 ) ) ;
#30236=CARTESIAN_POINT ( 'NONE',  ( -2.266590686148945544, 2.220415501580634388, 7.082119434687048631 ) ) ;
#30238=CARTESIAN_POINT ( 'NONE',  ( 2.791683348922240793, 36.63393115100078035, 7.208316651077764092 ) ) ;
#30239=CARTESIAN_POINT ( 'NONE',  ( 17.96484262340118221, 9.938685344154837509, 7.964842623401181321 ) ) ;
#30240=CARTESIAN_POINT ( 'NONE',  ( 1.472469842513823179, 35.59226448433412315, -4.923371831947296329 ) ) ;
#30241=CARTESIAN_POINT ( 'NONE',  ( -0.1772112516523293435, 6.298283880980280717E-16, -4.084223281690102958 ) ) ;
#30242=CARTESIAN_POINT ( 'NONE',  ( 2.791683348922237240, 55.38393115100078745, -7.208316651077763204 ) ) ;
#30243=AXIS2_PLACEMENT_3D ( 'NONE', #43411, #13411, #89408 ) ;
#30244=CARTESIAN_POINT ( 'NONE',  ( 15.44008868035555793, 46.39701867748817676, -9.422509992056140149 ) ) ;
#30246=ORIENTED_EDGE ( 'NONE', *, *, #87706, .F. ) ;
#30248=CARTESIAN_POINT ( 'NONE',  ( 16.40814093676324603, 52.45696800326375353, -11.09922568453594671 ) ) ;
#30250=CARTESIAN_POINT ( 'NONE',  ( 12.63842701281683034, 12.46726448433411782, 9.846743663894596210 ) ) ;
#30251=CARTESIAN_POINT ( 'NONE',  ( -2.816281873526473856, 54.33196800326376064, 3.434112377981055619 ) ) ;
#30252=CARTESIAN_POINT ( 'NONE',  ( 4.559911319644449179, 8.897018677488173211, 9.422509992056141925 ) ) ;
#30253=CARTESIAN_POINT ( 'NONE',  ( 18.52753015748618282, 53.92559781766745175, -4.923371831947291888 ) ) ;
#30254=CARTESIAN_POINT ( 'NONE',  ( 20.00000000000001066, 87.41133749857198154, 4.971011743019353446 ) ) ;
#30257=( LENGTH_UNIT ( ) NAMED_UNIT ( * ) SI_UNIT ( .MILLI., .METRE. ) );
#30258=CARTESIAN_POINT ( 'NONE',  ( -4.164238869374098151, 41.59541550158061796, -3.795296366450310543 ) ) ;
#30259=CARTESIAN_POINT ( 'NONE',  ( 19.84674366389459266, 58.71726448433411605, -2.638427012816827677 ) ) ;
#30261=CARTESIAN_POINT ( 'NONE',  ( 4.559911319644449179, 48.89701867748817676, 9.422509992056141925 ) ) ;
#30262=CARTESIAN_POINT ( 'NONE',  ( 19.84674366389459266, 3.300597817667451750, 2.638427012816836559 ) ) ;
#30265=ORIENTED_EDGE ( 'NONE', *, *, #23455, .F. ) ;
#30266=CARTESIAN_POINT ( 'NONE',  ( 13.43411237798106583, 57.66530133659708923, -12.81628187352647252 ) ) ;
#30268=EDGE_CURVE ( 'NONE', #34211, #96219, #50485, .T. ) ;
#30269=CARTESIAN_POINT ( 'NONE',  ( 12.63842701281683922, 4.550597817667451750, -9.846743663894590881 ) ) ;
#30271=CARTESIAN_POINT ( 'NONE',  ( 6.204703633549690345, 15.76208216824730179, -14.16423886937410259 ) ) ;
#30272=CARTESIAN_POINT ( 'NONE',  ( 2.791683348922240793, 26.63393115100078745, 7.208316651077764092 ) ) ;
#30273=CARTESIAN_POINT ( 'NONE',  ( -0.8801773607110991993, 27.85535201082150181, -2.915334737309923874 ) ) ;
#30277=CARTESIAN_POINT ( 'NONE',  ( -0.8801773607111009756, 23.06368534415484106, 1.068504757029289695E-15 ) ) ;
#30278=ORIENTED_EDGE ( 'NONE', *, *, #94153, .F. ) ;
#30279=DIRECTION ( 'NONE',  ( 0.000000000000000000, -1.000000000000000000, 0.000000000000000000 ) ) ;
#30282=VERTEX_POINT ( 'NONE', #93396 ) ;
#30283=CARTESIAN_POINT ( 'NONE',  ( 13.43411237798105340, 15.58196800326374998, 12.81628187352647963 ) ) ;
#30284=CARTESIAN_POINT ( 'NONE',  ( 0.2751277870542912507, 20.30223176428831167, 6.499999999999992006 ) ) ;
#30285=CARTESIAN_POINT ( 'NONE',  ( 17.20831665107776587, 9.133931151000787452, -7.208316651077762316 ) ) ;
#30287=CARTESIAN_POINT ( 'NONE',  ( 19.84674366389459621, 13.50893115100078568, 7.409399052514197653E-17 ) ) ;
#30288=CARTESIAN_POINT ( 'NONE',  ( 2.035157376598822676, 32.43868534415483396, -7.964842623401177768 ) ) ;
#30293=CARTESIAN_POINT ( 'NONE',  ( 7.084665262690076126, 42.02201867748816966, -10.88017736071110164 ) ) ;
#30294=CARTESIAN_POINT ( 'NONE',  ( 21.09922568453594849, 56.20696800326375353, 6.408140936763242479 ) ) ;
#30295=CARTESIAN_POINT ( 'NONE',  ( 4.559911319644449179, 63.89701867748817676, 9.422509992056141925 ) ) ;
#30296=CARTESIAN_POINT ( 'NONE',  ( 6.565887622018943937, 3.081968003263753531, -12.81628187352647608 ) ) ;
#30299=CARTESIAN_POINT ( 'NONE',  ( 18.52753015748618282, 13.92559781766745175, -4.923371831947291888 ) ) ;
#30300=CARTESIAN_POINT ( 'NONE',  ( 22.81628187352647785, 56.62363466993042493, 6.195893100308588602E-16 ) ) ;
#30302=CARTESIAN_POINT ( 'NONE',  ( 18.52753015748618282, 8.925597817667451750, -4.923371831947291888 ) ) ;
#30303=CARTESIAN_POINT ( 'NONE',  ( -2.816281873526473856, 14.33196800326375531, 3.434112377981055619 ) ) ;
#30305=CARTESIAN_POINT ( 'NONE',  ( 19.84674366389459621, 63.50893115100078745, 7.409399052514197653E-17 ) ) ;
#30306=CARTESIAN_POINT ( 'NONE',  ( 20.88017736071110519, 30.56368534415484106, 2.639326808657452039E-16 ) ) ;
#30307=CARTESIAN_POINT ( 'NONE',  ( 19.84674366389459266, 58.30059781766745886, 2.638427012816836559 ) ) ;
#30310=CARTESIAN_POINT ( 'NONE',  ( 10.00000000000000000, 19.75893115100078390, -9.846743663894594434 ) ) ;
#30311=CARTESIAN_POINT ( 'NONE',  ( 17.20831665107776587, 4.133931151000785675, -7.208316651077762316 ) ) ;
#30313=CARTESIAN_POINT ( 'NONE',  ( 0.6178305044545838731, 4.748634669930420493, 9.382169495545420901 ) ) ;
#30315=CARTESIAN_POINT ( 'NONE',  ( 10.00000000000000000, 6.813685344154838397, -10.88017736071110342 ) ) ;
#30318=CARTESIAN_POINT ( 'NONE',  ( 10.00000000000000178, 9.313685344154839285, 10.88017736071110342 ) ) ;
#30319=CARTESIAN_POINT ( 'NONE',  ( 1.472469842513823179, 50.59226448433411605, -4.923371831947296329 ) ) ;
#30321=CARTESIAN_POINT ( 'NONE',  ( 19.05866839779140776, 65.95508385108959715, -6.499999999999956479 ) ) ;
#30322=CARTESIAN_POINT ( 'NONE',  ( -4.164238869374098151, 66.59541550158060375, -3.795296366450310543 ) ) ;
#30323=CARTESIAN_POINT ( 'NONE',  ( 0.8952175423694470613, 13.52576239577081019, 5.990408912944253927 ) ) ;
#30324=CARTESIAN_POINT ( 'NONE',  ( 10.00000000000000178, 29.31368534415483751, 10.88017736071110342 ) ) ;
#30325=CARTESIAN_POINT ( 'NONE',  ( 17.08211943468705840, 50.13708216824730357, -12.26659068614894466 ) ) ;
#30326=CARTESIAN_POINT ( 'NONE',  ( 0.5774900079438590739, 2.647018677488171434, -5.440088680355550821 ) ) ;
#30328=CARTESIAN_POINT ( 'NONE',  ( 5.076628168052704559, 5.175597817667451750, -8.527530157486179263 ) ) ;
#30330=CARTESIAN_POINT ( 'NONE',  ( 0.1532563361054100626, 25.80059781766744820, -2.638427012816831230 ) ) ;
#30331=CARTESIAN_POINT ( 'NONE',  ( -2.816281873526471635, 13.91530133659708746, -3.434112377981056508 ) ) ;
#30332=CARTESIAN_POINT ( 'NONE',  ( 19.72487221294570858, 26.86607318730131055, 6.500000000000000888 ) ) ;
#30334=CARTESIAN_POINT ( 'NONE',  ( -4.164238869374099039, 11.80374883491396965, 8.674139862899312516E-16 ) ) ;
#30335=CARTESIAN_POINT ( 'NONE',  ( 5.076628168052704559, 20.17559781766745175, -8.527530157486179263 ) ) ;
#30338=CARTESIAN_POINT ( 'NONE',  ( 22.26659068614894466, 58.88708216824729647, 7.082119434687054849 ) ) ;
#30339=CARTESIAN_POINT ( 'NONE',  ( 17.20831665107776587, 9.133931151000787452, -7.208316651077762316 ) ) ;
#30341=FACE_OUTER_BOUND ( 'NONE', #22319, .T. ) ;
#30342=CARTESIAN_POINT ( 'NONE',  ( 4.559911319644449179, 33.89701867748817676, 9.422509992056141925 ) ) ;
#30343=CARTESIAN_POINT ( 'NONE',  ( 22.81628187352648496, 51.83196800326376064, -3.434112377981050290 ) ) ;
#30344=CARTESIAN_POINT ( 'NONE',  ( 20.88017736071110164, 10.35535201082150714, 2.915334737309930979 ) ) ;
#30345=CARTESIAN_POINT ( 'NONE',  ( 10.00000000000000000, 37.87363466993041783, -12.81628187352647608 ) ) ;
#30346=CARTESIAN_POINT ( 'NONE',  ( -2.816281873526471635, 3.915301336597087456, -3.434112377981056508 ) ) ;
#30347=CARTESIAN_POINT ( 'NONE',  ( 19.84674366389459621, 3.508931151000785231, 7.409399052514197653E-17 ) ) ;
#30349=DIRECTION ( 'NONE',  ( 1.000000000000000000, 0.000000000000000000, 0.000000000000000000 ) ) ;
#30351=CARTESIAN_POINT ( 'NONE',  ( 2.917880565312950480, 40.97041550158063217, -12.26659068614894821 ) ) ;
#30352=CARTESIAN_POINT ( 'NONE',  ( 10.00000000000000000, 15.55374883491396787, -14.16423886937410082 ) ) ;
#30353=CARTESIAN_POINT ( 'NONE',  ( 7.084665262690076126, 9.105352010821503583, 10.88017736071109987 ) ) ;
#30354=CARTESIAN_POINT ( 'NONE',  ( 20.88017736071110164, 30.35535201082151247, 2.915334737309930979 ) ) ;
#30356=CARTESIAN_POINT ( 'NONE',  ( 17.96484262340118221, 54.93868534415484106, 7.964842623401181321 ) ) ;
#30357=CARTESIAN_POINT ( 'NONE',  ( 12.91533473730993009, 66.60535201082150536, -10.88017736071109987 ) ) ;
#30358=CARTESIAN_POINT ( 'NONE',  ( -1.099225684535947600, 23.70696800326375708, -6.408140936763238038 ) ) ;
#30359=PLANE ( 'NONE',  #9143 ) ;
#30361=CARTESIAN_POINT ( 'NONE',  ( 2.791683348922237240, 35.38393115100079456, -7.208316651077763204 ) ) ;
#30365=CARTESIAN_POINT ( 'NONE',  ( -2.816281873526473856, 24.33196800326375353, 3.434112377981055619 ) ) ;
#30366=CARTESIAN_POINT ( 'NONE',  ( 0.1532563361054100626, 5.800597817667452638, -2.638427012816831230 ) ) ;
#30367=CARTESIAN_POINT ( 'NONE',  ( 17.96484262340118221, 4.938685344154837509, 7.964842623401181321 ) ) ;
#30370=CARTESIAN_POINT ( 'NONE',  ( 18.52753015748617571, 43.09226448433412315, 4.923371831947298993 ) ) ;
#30371=CARTESIAN_POINT ( 'NONE',  ( 13.43411237798105340, 60.58196800326376064, 12.81628187352647963 ) ) ;
#30372=CARTESIAN_POINT ( 'NONE',  ( 17.20831665107776587, 24.13393115100078035, -7.208316651077762316 ) ) ;
#30373=CARTESIAN_POINT ( 'NONE',  ( -4.164238869374099927, 7.012082168247302683, 3.795296366450308767 ) ) ;
#30376=CARTESIAN_POINT ( 'NONE',  ( -0.8801773607111009756, 28.06368534415484106, 1.068504757029289695E-15 ) ) ;
#30377=CARTESIAN_POINT ( 'NONE',  ( 0.5774900079438590739, 17.64701867748817321, -5.440088680355550821 ) ) ;
#30378=CARTESIAN_POINT ( 'NONE',  ( -2.266590686148945544, 46.38708216824730357, -7.082119434687050408 ) ) ;
#30380=CARTESIAN_POINT ( 'NONE',  ( 7.084665262690076126, 34.10535201082151247, 10.88017736071109987 ) ) ;
#30381=CARTESIAN_POINT ( 'NONE',  ( 17.96484262340118221, 11.18868534415484106, -7.964842623401177768 ) ) ;
#30384=CARTESIAN_POINT ( 'NONE',  ( 2.035157376598822676, 32.43868534415483396, -7.964842623401177768 ) ) ;
#30385=CARTESIAN_POINT ( 'NONE',  ( 6.565887622018943937, 50.16530133659708213, 12.81628187352647430 ) ) ;
#30386=CARTESIAN_POINT ( 'NONE',  ( 0.5774900079438607392, 48.48035201082150536, 5.440088680355550821 ) ) ;
#30388=CARTESIAN_POINT ( 'NONE',  ( 7.084665262690076126, 49.10535201082149825, 10.88017736071109987 ) ) ;
#30389=EDGE_LOOP ( 'NONE', ( #69158, #97829, #96114, #81800, #5568, #78316 ) ) ;
#30390=CARTESIAN_POINT ( 'NONE',  ( 2.035157376598822676, 52.43868534415483396, -7.964842623401177768 ) ) ;
#30391=SURFACE_STYLE_USAGE ( .BOTH. , #52899 ) ;
#30393=CARTESIAN_POINT ( 'NONE',  ( 2.917880565312950480, 45.97041550158063927, -12.26659068614894821 ) ) ;
#30394=CARTESIAN_POINT ( 'NONE',  ( 1.472469842513823179, 1.425597817667451528, 4.923371831947296329 ) ) ;
#30397=CARTESIAN_POINT ( 'NONE',  ( 5.076628168052703671, 61.84226448433412315, 8.527530157486179263 ) ) ;
#30399=CARTESIAN_POINT ( 'NONE',  ( 5.076628168052704559, 35.17559781766745175, -8.527530157486179263 ) ) ;
#30402=CARTESIAN_POINT ( 'NONE',  ( 7.361572987183169658, 29.96726448433411960, -9.846743663894592657 ) ) ;
#30405=CARTESIAN_POINT ( 'NONE',  ( 7.084665262690076126, 22.02201867748817321, -10.88017736071110164 ) ) ;
#30406=CARTESIAN_POINT ( 'NONE',  ( 0.1532563361054100626, 35.80059781766745175, -2.638427012816831230 ) ) ;
#30407=CARTESIAN_POINT ( 'NONE',  ( 22.81628187352647785, 26.62363466993042138, 6.195893100308588602E-16 ) ) ;
#30409=CARTESIAN_POINT ( 'NONE',  ( 12.91533473730992121, 54.52201867748816255, 10.88017736071110164 ) ) ;
#30410=CARTESIAN_POINT ( 'NONE',  ( 4.559911319644449179, 42.23035201082151247, -9.422509992056141925 ) ) ;
#30411=CARTESIAN_POINT ( 'NONE',  ( -0.8801773607111008646, 3.272018677488171434, 2.915334737309923430 ) ) ;
#30412=CARTESIAN_POINT ( 'NONE',  ( 22.26659068614894466, 63.88708216824730357, 7.082119434687054849 ) ) ;
#30413=EDGE_CURVE ( 'NONE', #5496, #32549, #49367, .T. ) ;
#30414=CARTESIAN_POINT ( 'NONE',  ( 16.40814093676324603, 27.45696800326375708, -11.09922568453594671 ) ) ;
#30417=CARTESIAN_POINT ( 'NONE',  ( 22.81628187352647785, 21.41530133659708923, 3.434112377981063169 ) ) ;
#30418=CARTESIAN_POINT ( 'NONE',  ( 7.084665262690076126, 19.10535201082150181, 10.88017736071109987 ) ) ;
#30419=CARTESIAN_POINT ( 'NONE',  ( -0.8801773607111009756, 63.06368534415484106, 1.068504757029289695E-15 ) ) ;
#30420=SURFACE_STYLE_USAGE ( .BOTH. , #13456 ) ;
#30422=CARTESIAN_POINT ( 'NONE',  ( 7.084665262690076126, 52.02201867748816255, -10.88017736071110164 ) ) ;
#30423=CARTESIAN_POINT ( 'NONE',  ( 5.076628168052704559, 40.17559781766745175, -8.527530157486179263 ) ) ;
#30424=CARTESIAN_POINT ( 'NONE',  ( 1.472469842513823179, 30.59226448433411960, -4.923371831947296329 ) ) ;
#30425=CARTESIAN_POINT ( 'NONE',  ( 12.63842701281683922, 14.55059781766744997, -9.846743663894590881 ) ) ;
#30427=CARTESIAN_POINT ( 'NONE',  ( 19.38216949554541202, 40.99863466993042493, 9.382169495545424454 ) ) ;
#30428=CARTESIAN_POINT ( 'NONE',  ( 5.076628168052704559, 20.17559781766745175, -8.527530157486179263 ) ) ;
#30431=CARTESIAN_POINT ( 'NONE',  ( 7.361572987183169658, 34.96726448433411605, -9.846743663894592657 ) ) ;
#30433=CARTESIAN_POINT ( 'NONE',  ( 20.24186590665277663, 16.76028685723174405, 6.114288769123035649 ) ) ;
#30434=CARTESIAN_POINT ( 'NONE',  ( 3.591859063236761518, 9.956968003263753531, 11.09922568453594849 ) ) ;
#30435=CARTESIAN_POINT ( 'NONE',  ( 12.91533473730993009, 46.60535201082150536, -10.88017736071109987 ) ) ;
#30436=CARTESIAN_POINT ( 'NONE',  ( 17.08211943468705840, 30.13708216824730357, -12.26659068614894466 ) ) ;
#30439=CARTESIAN_POINT ( 'NONE',  ( -4.164238869374099039, 26.80374883491397142, 8.674139862899312516E-16 ) ) ;
#30441=CARTESIAN_POINT ( 'NONE',  ( 17.08211943468705130, 63.47041550158063927, 12.26659068614894998 ) ) ;
#30442=CARTESIAN_POINT ( 'NONE',  ( -0.3689425029237881626, 7.428748834913967869, 10.36894250292379027 ) ) ;
#30443=CARTESIAN_POINT ( 'NONE',  ( 24.16423886937410614, 24.30374883491396787, 8.672049930838204340E-16 ) ) ;
#30444=CARTESIAN_POINT ( 'NONE',  ( 0.5774900079438607392, 53.48035201082151247, 5.440088680355550821 ) ) ;
#30446=CARTESIAN_POINT ( 'NONE',  ( 18.18329248733322601, 62.60290668512021028, 6.499999999999960920 ) ) ;
#30447=CARTESIAN_POINT ( 'NONE',  ( 17.20831665107776587, 42.88393115100077324, 7.208316651077764980 ) ) ;
#30449=CARTESIAN_POINT ( 'NONE',  ( 4.559911319644449179, 23.89701867748817321, 9.422509992056141925 ) ) ;
#30450=LINE ( 'NONE', #23481, #48935 ) ;
#30451=CARTESIAN_POINT ( 'NONE',  ( 17.20831665107776587, 57.88393115100078745, 7.208316651077764980 ) ) ;
#30453=CARTESIAN_POINT ( 'NONE',  ( 0.2751277870542967463, 69.50000000000000000, 6.500000000000000888 ) ) ;
#30454=CARTESIAN_POINT ( 'NONE',  ( 1.472469842513823179, 31.42559781766745530, 4.923371831947296329 ) ) ;
#30455=CARTESIAN_POINT ( 'NONE',  ( 21.09922568453595559, 52.04030133659708923, -6.408140936763230044 ) ) ;
#30457=CARTESIAN_POINT ( 'NONE',  ( 14.92337183194729633, 42.67559781766745886, 8.527530157486181039 ) ) ;
#30458=CARTESIAN_POINT ( 'NONE',  ( 7.361572987183170547, 52.05059781766745175, 9.846743663894590881 ) ) ;
#30459=CARTESIAN_POINT ( 'NONE',  ( 2.917880565312950480, 35.97041550158063217, -12.26659068614894821 ) ) ;
#30460=ORIENTED_EDGE ( 'NONE', *, *, #53184, .T. ) ;
#30461=CARTESIAN_POINT ( 'NONE',  ( 10.00000000000000000, 5.553748834913967869, -14.16423886937410082 ) ) ;
#30462=CARTESIAN_POINT ( 'NONE',  ( -0.8801773607111009756, 68.06368534415484817, 1.068504757029289695E-15 ) ) ;
#30464=CARTESIAN_POINT ( 'NONE',  ( -4.164238869374098151, 56.59541550158063927, -3.795296366450310543 ) ) ;
#30465=CARTESIAN_POINT ( 'NONE',  ( 19.38216949554541557, 12.24863466993041961, -9.382169495545420901 ) ) ;
#30467=CARTESIAN_POINT ( 'NONE',  ( 2.035157376598822676, 52.43868534415483396, -7.964842623401177768 ) ) ;
#30468=CARTESIAN_POINT ( 'NONE',  ( -1.926860441876562247, 27.45379003517447813, -3.195792623639530650 ) ) ;
#30469=CARTESIAN_POINT ( 'NONE',  ( -46.78604402846880106, 100.7423487049318140, -9.213902555517821114 ) ) ;
#30470=CARTESIAN_POINT ( 'NONE',  ( -0.3689425029237881626, 67.42874883491396076, 10.36894250292379027 ) ) ;
#30472=CARTESIAN_POINT ( 'NONE',  ( 19.42250999205614548, 15.98035201082150714, -5.440088680355545492 ) ) ;
#30473=CARTESIAN_POINT ( 'NONE',  ( 20.88017736071110164, 30.35535201082151247, 2.915334737309930979 ) ) ;
#30474=CARTESIAN_POINT ( 'NONE',  ( 5.076628168052704559, 55.17559781766745175, -8.527530157486179263 ) ) ;
#30475=CARTESIAN_POINT ( 'NONE',  ( 5.076628168052704559, 60.17559781766745175, -8.527530157486179263 ) ) ;
#30476=CARTESIAN_POINT ( 'NONE',  ( 0.6178305044545838731, 49.74863466993041072, 9.382169495545420901 ) ) ;
#30477=CARTESIAN_POINT ( 'NONE',  ( 1.472469842513823179, 0.5922644843341181575, -4.923371831947296329 ) ) ;
#30478=ORIENTED_EDGE ( 'NONE', *, *, #32742, .T. ) ;
#30480=CARTESIAN_POINT ( 'NONE',  ( 20.88017736071110164, 15.35535201082150358, 2.915334737309930979 ) ) ;
#30481=CARTESIAN_POINT ( 'NONE',  ( 10.00000000000000000, 12.87363466993042138, -12.81628187352647608 ) ) ;
#30484=STYLED_ITEM ( 'NONE', ( #40053 ), #79132 ) ;
#30485=CARTESIAN_POINT ( 'NONE',  ( 14.92337183194729988, 44.34226448433412315, -8.527530157486177487 ) ) ;
#30486=CARTESIAN_POINT ( 'NONE',  ( 4.559911319644449179, 32.23035201082150536, -9.422509992056141925 ) ) ;
#30487=ADVANCED_FACE ( 'NONE', ( #64845 ), #26371, .F. ) ;
#30488=CARTESIAN_POINT ( 'NONE',  ( 3.591859063236761518, 19.95696800326375353, 11.09922568453594849 ) ) ;
#30489=CARTESIAN_POINT ( 'NONE',  ( 20.88017736071110164, 45.35535201082149115, 2.915334737309930979 ) ) ;
#30491=LINE ( 'NONE', #22034, #1857 ) ;
#30492=CARTESIAN_POINT ( 'NONE',  ( 22.81628187352647785, 46.41530133659708213, 3.434112377981063169 ) ) ;
#30494=CARTESIAN_POINT ( 'NONE',  ( 0.1532563361054083140, 66.00893115100079456, 1.131784320476157264E-15 ) ) ;
#30495=CARTESIAN_POINT ( 'NONE',  ( 0.5774900079438607392, 48.48035201082150536, 5.440088680355550821 ) ) ;
#30496=CARTESIAN_POINT ( 'NONE',  ( -1.099225684535947600, 34.54030133659708923, 6.408140936763237150 ) ) ;
#30497=CARTESIAN_POINT ( 'NONE',  ( 7.361572987183169658, 9.967264484334119601, -9.846743663894592657 ) ) ;
#30498=CARTESIAN_POINT ( 'NONE',  ( 22.26659068614894466, 43.88708216824729647, 7.082119434687054849 ) ) ;
#30500=CARTESIAN_POINT ( 'NONE',  ( 2.791683348922240793, 11.63393115100078568, 7.208316651077764092 ) ) ;
#30501=CARTESIAN_POINT ( 'NONE',  ( 10.00000000000000178, 7.258931151000785675, 9.846743663894594434 ) ) ;
#30503=CARTESIAN_POINT ( 'NONE',  ( 13.79529636645030344, 38.26208216824729647, 14.16423886937410614 ) ) ;
#30505=CARTESIAN_POINT ( 'NONE',  ( 0.5774900079438607392, 13.48035201082150358, 5.440088680355550821 ) ) ;
#30508=EDGE_LOOP ( 'NONE', ( #50956, #7420, #12297, #80227 ) ) ;
#30510=CARTESIAN_POINT ( 'NONE',  ( 20.88017736071110164, 10.35535201082150714, 2.915334737309930979 ) ) ;
#30511=CARTESIAN_POINT ( 'NONE',  ( -4.164238869374098151, 61.59541550158063217, -3.795296366450310543 ) ) ;
#30512=CARTESIAN_POINT ( 'NONE',  ( 17.20831665107776587, 37.88393115100078745, 7.208316651077764980 ) ) ;
#30513=CARTESIAN_POINT ( 'NONE',  ( 22.81628187352647785, 36.62363466993041783, 6.195893100308588602E-16 ) ) ;
#30515=CARTESIAN_POINT ( 'NONE',  ( -4.164238869374099039, 1.803748834913967647, 8.674139862899312516E-16 ) ) ;
#30516=CARTESIAN_POINT ( 'NONE',  ( 2.035157376598824452, 23.68868534415484461, 7.964842623401179544 ) ) ;
#30517=CARTESIAN_POINT ( 'NONE',  ( 2.035157376598824452, 8.688685344154839285, 7.964842623401179544 ) ) ;
#30518=CARTESIAN_POINT ( 'NONE',  ( 19.84674366389459621, 43.50893115100078745, 7.409399052514197653E-17 ) ) ;
#30520=CARTESIAN_POINT ( 'NONE',  ( 1.472469842513823179, 25.59226448433412315, -4.923371831947296329 ) ) ;
#30528=CARTESIAN_POINT ( 'NONE',  ( 5.076628168052703671, 61.84226448433412315, 8.527530157486179263 ) ) ;
#30529=CARTESIAN_POINT ( 'NONE',  ( 2.035157376598824452, 28.68868534415484106, 7.964842623401179544 ) ) ;
#30530=CARTESIAN_POINT ( 'NONE',  ( 10.00000000000000000, 31.81368534415483751, -10.88017736071110342 ) ) ;
#30531=CARTESIAN_POINT ( 'NONE',  ( 19.84674366389459621, 58.50893115100078745, 7.409399052514197653E-17 ) ) ;
#30532=CARTESIAN_POINT ( 'NONE',  ( 13.43411237798106583, 27.66530133659708568, -12.81628187352647252 ) ) ;
#30533=CARTESIAN_POINT ( 'NONE',  ( 2.917880565312948704, 17.63708216824730357, 12.26659068614894643 ) ) ;
#30535=B_SPLINE_CURVE_WITH_KNOTS ( 'NONE', 3,
 ( #75617, #38132, #22633, #68620, #53113, #54091 ),
 .UNSPECIFIED., .F., .F.,
 ( 4, 2, 4 ),
 ( 5.553824967135426632E-18, 0.0002605067024380923143, 0.0005210134048761790992 ),
 .UNSPECIFIED. ) ;
#30536=CARTESIAN_POINT ( 'NONE',  ( -1.099225684535947600, 43.70696800326375353, -6.408140936763238038 ) ) ;
#30538=CARTESIAN_POINT ( 'NONE',  ( 14.92337183194729988, 39.34226448433412315, -8.527530157486177487 ) ) ;
#30539=CARTESIAN_POINT ( 'NONE',  ( 15.44008868035555260, 4.730352010821505360, 9.422509992056143702 ) ) ;
#30541=CARTESIAN_POINT ( 'NONE',  ( 10.00000000000000178, 14.31368534415483929, 10.88017736071110342 ) ) ;
#30543=CARTESIAN_POINT ( 'NONE',  ( 7.084665262690076126, 59.10535201082150536, 10.88017736071109987 ) ) ;
#30544=CARTESIAN_POINT ( 'NONE',  ( -0.8801773607110991993, 52.85535201082151247, -2.915334737309923874 ) ) ;
#30545=CARTESIAN_POINT ( 'NONE',  ( 4.559911319644449179, 63.89701867748817676, 9.422509992056141925 ) ) ;
#30546=CARTESIAN_POINT ( 'NONE',  ( 12.91533473730992121, 49.52201867748817676, 10.88017736071110164 ) ) ;
#30549=CARTESIAN_POINT ( 'NONE',  ( -46.94000000000000483, 100.4746355719282320, 9.260812147861324561 ) ) ;
#30552=VECTOR ( 'NONE', #86916, 1000.000000000000000 ) ;
#30553=CARTESIAN_POINT ( 'NONE',  ( 19.84674366389459266, 43.30059781766744464, 2.638427012816836559 ) ) ;
#30554=ORIENTED_EDGE ( 'NONE', *, *, #52621, .T. ) ;
#30556=CARTESIAN_POINT ( 'NONE',  ( -2.266590686148945544, 17.22041550158063572, 7.082119434687048631 ) ) ;
#30557=CARTESIAN_POINT ( 'NONE',  ( 0.1957200283969098842, 35.25733960839543357, 6.499999999999991118 ) ) ;
#30558=CARTESIAN_POINT ( 'NONE',  ( 13.99999999999999822, 11.50000000000000000, -6.000000000000000000 ) ) ;
#30559=CARTESIAN_POINT ( 'NONE',  ( -0.8801773607110991993, 62.85535201082150536, -2.915334737309923874 ) ) ;
#30560=CARTESIAN_POINT ( 'NONE',  ( -0.8801773607111008646, 13.27201867748817321, 2.915334737309923430 ) ) ;
#30562=CARTESIAN_POINT ( 'NONE',  ( 16.40814093676323893, 45.79030133659708923, 11.09922568453595026 ) ) ;
#30565=CARTESIAN_POINT ( 'NONE',  ( 19.84674366389459266, 48.71726448433413026, -2.638427012816827677 ) ) ;
#30566=( LENGTH_UNIT ( ) NAMED_UNIT ( * ) SI_UNIT ( .MILLI., .METRE. ) );
#30567=CARTESIAN_POINT ( 'NONE',  ( 3.591859063236763294, 18.29030133659708568, -11.09922568453595026 ) ) ;
#30568=CARTESIAN_POINT ( 'NONE',  ( 7.361572987183170547, 27.05059781766745175, 9.846743663894590881 ) ) ;
#30571=CARTESIAN_POINT ( 'NONE',  ( 18.52753015748617571, 18.09226448433411960, 4.923371831947298993 ) ) ;
#30572=CARTESIAN_POINT ( 'NONE',  ( -2.816281873526473856, 14.33196800326375531, 3.434112377981055619 ) ) ;
#30574=CARTESIAN_POINT ( 'NONE',  ( 10.00000000000000000, 4.758931151000784787, -9.846743663894594434 ) ) ;
#30577=CARTESIAN_POINT ( 'NONE',  ( 2.035157376598824452, 23.68868534415484461, 7.964842623401179544 ) ) ;
#30578=CARTESIAN_POINT ( 'NONE',  ( 13.79529636645031943, 15.34541550158063750, -14.16423886937409904 ) ) ;
#30579=CARTESIAN_POINT ( 'NONE',  ( 1.472469842513823179, 46.42559781766745175, 4.923371831947296329 ) ) ;
#30580=CARTESIAN_POINT ( 'NONE',  ( 20.88017736071110519, 65.56368534415483396, 2.639326808657452039E-16 ) ) ;
#30581=AXIS2_PLACEMENT_3D ( 'NONE', #75013, #6518, #45003 ) ;
#30582=CARTESIAN_POINT ( 'NONE',  ( -1.099225684535947600, 43.70696800326375353, -6.408140936763238038 ) ) ;
#30584=CARTESIAN_POINT ( 'NONE',  ( 2.035157376598824452, 18.68868534415484106, 7.964842623401179544 ) ) ;
#30585=LINE ( 'NONE', #7116, #90044 ) ;
#30586=CARTESIAN_POINT ( 'NONE',  ( -1.099225684535947600, 9.540301336597087456, 6.408140936763237150 ) ) ;
#30587=CARTESIAN_POINT ( 'NONE',  ( 10.00000000000000178, 32.25893115100078745, 9.846743663894594434 ) ) ;
#30589=CARTESIAN_POINT ( 'NONE',  ( 19.38216949554541202, 35.99863466993041072, 9.382169495545424454 ) ) ;
#30591=CARTESIAN_POINT ( 'NONE',  ( 4.559911319644449179, 43.89701867748816966, 9.422509992056141925 ) ) ;
#30595=CARTESIAN_POINT ( 'NONE',  ( 20.88017736071110875, 40.77201867748818387, -2.915334737309920765 ) ) ;
#30596=CARTESIAN_POINT ( 'NONE',  ( 7.084665262690076126, 49.10535201082149825, 10.88017736071109987 ) ) ;
#30597=CARTESIAN_POINT ( 'NONE',  ( 19.84674366389459621, 58.50893115100078745, 7.409399052514197653E-17 ) ) ;
#30599=CARTESIAN_POINT ( 'NONE',  ( -0.8801773607110991993, 67.85535201082151957, -2.915334737309923874 ) ) ;
#30601=CARTESIAN_POINT ( 'NONE',  ( 5.076628168052704559, 55.17559781766745175, -8.527530157486179263 ) ) ;
#30602=CARTESIAN_POINT ( 'NONE',  ( 0.5774900079438590739, 7.647018677488171434, -5.440088680355550821 ) ) ;
#30603=FACE_OUTER_BOUND ( 'NONE', #91421, .T. ) ;
#30604=CARTESIAN_POINT ( 'NONE',  ( 19.38216949554541202, 5.998634669930420493, 9.382169495545424454 ) ) ;
#30606=CARTESIAN_POINT ( 'NONE',  ( 0.5774900079438590739, 32.64701867748816966, -5.440088680355550821 ) ) ;
#30607=CARTESIAN_POINT ( 'NONE',  ( 17.20831665107776587, 57.88393115100078745, 7.208316651077764980 ) ) ;
#30609=CARTESIAN_POINT ( 'NONE',  ( 0.5774900079438607392, 13.48035201082150358, 5.440088680355550821 ) ) ;
#30610=CARTESIAN_POINT ( 'NONE',  ( 19.42250999205614193, 25.14701867748817321, 5.440088680355555262 ) ) ;
#30611=CARTESIAN_POINT ( 'NONE',  ( 24.16423886937410614, 34.30374883491396787, 8.672049930838204340E-16 ) ) ;
#30612=CARTESIAN_POINT ( 'NONE',  ( 7.361572987183170547, 22.05059781766745530, 9.846743663894590881 ) ) ;
#30613=CARTESIAN_POINT ( 'NONE',  ( 4.559911319644449179, 52.23035201082151247, -9.422509992056141925 ) ) ;
#30615=CARTESIAN_POINT ( 'NONE',  ( 18.52753015748617571, 58.09226448433411605, 4.923371831947298993 ) ) ;
#30617=VERTEX_POINT ( 'NONE', #33941 ) ;
#30618=TOROIDAL_SURFACE ( 'NONE', #89721, 18.53834841531100608, 7.000000000000000000 ) ;
#30619=CARTESIAN_POINT ( 'NONE',  ( 22.26659068614895176, 39.72041550158063217, -7.082119434687042414 ) ) ;
#30620=CARTESIAN_POINT ( 'NONE',  ( 20.36894250292379382, 28.67874883491396787, 10.36894250292379205 ) ) ;
#30621=CARTESIAN_POINT ( 'NONE',  ( -0.8801773607111008646, 68.27201867748817676, 2.915334737309923430 ) ) ;
#30622=CARTESIAN_POINT ( 'NONE',  ( 19.84674366389459621, 43.50893115100078745, 7.409399052514197653E-17 ) ) ;
#30624=CARTESIAN_POINT ( 'NONE',  ( 10.00000000000000178, 49.31368534415484106, 10.88017736071110342 ) ) ;
#30625=CARTESIAN_POINT ( 'NONE',  ( 10.00000000000000000, 12.87363466993042138, -12.81628187352647608 ) ) ;
#30626=CARTESIAN_POINT ( 'NONE',  ( 13.79529636645031943, 35.34541550158063927, -14.16423886937409904 ) ) ;
#30627=CARTESIAN_POINT ( 'NONE',  ( 10.00000000000000000, 11.81368534415483751, -10.88017736071110342 ) ) ;
#30628=CARTESIAN_POINT ( 'NONE',  ( 7.084665262690076126, 32.02201867748816966, -10.88017736071110164 ) ) ;
#30629=CARTESIAN_POINT ( 'NONE',  ( 21.92686044187656691, 4.953790035174471917, 3.195792623639537755 ) ) ;
#30630=CARTESIAN_POINT ( 'NONE',  ( 0.5774900079438590739, 52.64701867748817676, -5.440088680355550821 ) ) ;
#30631=CARTESIAN_POINT ( 'NONE',  ( 21.09922568453595559, 47.04030133659708923, -6.408140936763230044 ) ) ;
#30634=DIRECTION ( 'NONE',  ( 1.000000000000000000, 0.000000000000000000, 0.000000000000000000 ) ) ;
#30638=CARTESIAN_POINT ( 'NONE',  ( 17.08211943468705130, 53.47041550158063217, 12.26659068614894998 ) ) ;
#30639=CARTESIAN_POINT ( 'NONE',  ( 17.08211943468705130, 63.47041550158063927, 12.26659068614894998 ) ) ;
#30640=CARTESIAN_POINT ( 'NONE',  ( 2.791683348922240793, 21.63393115100078745, 7.208316651077764092 ) ) ;
#30641=CARTESIAN_POINT ( 'NONE',  ( 7.361572987183170547, 57.05059781766744464, 9.846743663894590881 ) ) ;
#30643=EDGE_CURVE ( 'NONE', #8562, #45049, #25980, .T. ) ;
#30644=CARTESIAN_POINT ( 'NONE',  ( 17.20831665107776587, 9.133931151000787452, -7.208316651077762316 ) ) ;
#30645=VECTOR ( 'NONE', #13210, 1000.000000000000000 ) ;
#30647=CARTESIAN_POINT ( 'NONE',  ( -2.816281873526473856, 4.331968003263754419, 3.434112377981055619 ) ) ;
#30651=CARTESIAN_POINT ( 'NONE',  ( 24.16423886937409904, 29.09541550158063572, 3.795296366450317205 ) ) ;
#30653=CARTESIAN_POINT ( 'NONE',  ( -2.266590686148945544, 37.22041550158063217, 7.082119434687048631 ) ) ;
#30655=CARTESIAN_POINT ( 'NONE',  ( 22.81628187352647785, 51.62363466993042493, 6.195893100308588602E-16 ) ) ;
#30656=CARTESIAN_POINT ( 'NONE',  ( 12.91533473730993009, 26.60535201082150536, -10.88017736071109987 ) ) ;
#30657=CARTESIAN_POINT ( 'NONE',  ( 0.1532563361054100626, 50.80059781766745175, -2.638427012816831230 ) ) ;
#30658=CARTESIAN_POINT ( 'NONE',  ( 12.91533473730992121, 29.52201867748817321, 10.88017736071110164 ) ) ;
#30662=CARTESIAN_POINT ( 'NONE',  ( 19.84674366389459621, 58.50893115100078745, 7.409399052514197653E-17 ) ) ;
#30663=CARTESIAN_POINT ( 'NONE',  ( 14.92337183194729633, 47.67559781766745175, 8.527530157486181039 ) ) ;
#30665=B_SPLINE_CURVE_WITH_KNOTS ( 'NONE', 3,
 ( #28472, #27968, #21469, #13977, #43462, #65468 ),
 .UNSPECIFIED., .F., .F.,
 ( 4, 2, 4 ),
 ( 0.000000000000000000, 0.0002605067024380854296, 0.0005210134048761708592 ),
 .UNSPECIFIED. ) ;
#30667=CARTESIAN_POINT ( 'NONE',  ( 0.1532563361054082862, 1.217264484334117824, 2.638427012816831674 ) ) ;
#30668=CARTESIAN_POINT ( 'NONE',  ( -10.00000000000000000, 82.00000000000000000, -9.500000000000000000 ) ) ;
#30669=ORIENTED_EDGE ( 'NONE', *, *, #5107, .F. ) ;
#30670=CARTESIAN_POINT ( 'NONE',  ( 19.67858290521089160, 88.19931278102706074, 5.461713021790606248 ) ) ;
#30671=CARTESIAN_POINT ( 'NONE',  ( 0.1532563361054082862, 26.21726448433411605, 2.638427012816831674 ) ) ;
#30672=FACE_OUTER_BOUND ( 'NONE', #9997, .T. ) ;
#30673=CARTESIAN_POINT ( 'NONE',  ( 16.40814093676323893, 35.79030133659708923, 11.09922568453595026 ) ) ;
#30677=LINE ( 'NONE', #69678, #98713 ) ;
#30679=CARTESIAN_POINT ( 'NONE',  ( 18.52753015748617571, 58.09226448433411605, 4.923371831947298993 ) ) ;
#30680=CARTESIAN_POINT ( 'NONE',  ( 22.26659068614894466, 28.88708216824730357, 7.082119434687054849 ) ) ;
#30681=CARTESIAN_POINT ( 'NONE',  ( 17.20831665107776587, 62.88393115100078745, 7.208316651077764980 ) ) ;
#30682=CARTESIAN_POINT ( 'NONE',  ( 20.15039907845753575, 36.74884699246889141, 6.262539305110075283 ) ) ;
#30683=CARTESIAN_POINT ( 'NONE',  ( 2.791683348922237240, 10.38393115100078390, -7.208316651077763204 ) ) ;
#30684=CARTESIAN_POINT ( 'NONE',  ( -2.266590686148945544, 2.220415501580634388, 7.082119434687048631 ) ) ;
#30685=CARTESIAN_POINT ( 'NONE',  ( 0.1532563361054100626, 45.80059781766745886, -2.638427012816831230 ) ) ;
#30686=CARTESIAN_POINT ( 'NONE',  ( -0.8801773607111009756, 48.06368534415484817, 1.068504757029289695E-15 ) ) ;
#30690=CARTESIAN_POINT ( 'NONE',  ( 12.91533473730993009, 61.60535201082150536, -10.88017736071109987 ) ) ;
#30693=CARTESIAN_POINT ( 'NONE',  ( 20.88017736071110875, 30.77201867748816966, -2.915334737309920765 ) ) ;
#30694=CARTESIAN_POINT ( 'NONE',  ( 10.00000000000000000, 64.75893115100078035, -9.846743663894594434 ) ) ;
#30695=CARTESIAN_POINT ( 'NONE',  ( 20.88017736071110164, 60.35535201082151957, 2.915334737309930979 ) ) ;
#30697=CARTESIAN_POINT ( 'NONE',  ( 18.04007052943773104, 14.00257860105348762, -5.767676674365834977 ) ) ;
#30699=CARTESIAN_POINT ( 'NONE',  ( 4.559911319644449179, 33.89701867748817676, 9.422509992056141925 ) ) ;
#30700=CARTESIAN_POINT ( 'NONE',  ( 20.00000000000000711, 98.59912998021083297, -4.500000000000001776 ) ) ;
#30701=CARTESIAN_POINT ( 'NONE',  ( 14.92337183194729633, 17.67559781766745175, 8.527530157486181039 ) ) ;
#30702=CARTESIAN_POINT ( 'NONE',  ( 12.63842701281683034, 32.46726448433412315, 9.846743663894596210 ) ) ;
#30703=PLANE ( 'NONE',  #98482 ) ;
#30705=CARTESIAN_POINT ( 'NONE',  ( 7.361572987183169658, 59.96726448433410894, -9.846743663894592657 ) ) ;
#30706=CARTESIAN_POINT ( 'NONE',  ( 13.79529636645031943, 65.34541550158063217, -14.16423886937409904 ) ) ;
#30707=CARTESIAN_POINT ( 'NONE',  ( 20.15039907845753220, 27.62777174578613071, -6.262539305110077947 ) ) ;
#30708=CARTESIAN_POINT ( 'NONE',  ( 24.16423886937410614, 24.51208216824730002, -3.795296366450302550 ) ) ;
#30709=CARTESIAN_POINT ( 'NONE',  ( -4.164238869374099927, 52.01208216824729647, 3.795296366450308767 ) ) ;
#30711=CARTESIAN_POINT ( 'NONE',  ( 2.791683348922240793, 16.63393115100078745, 7.208316651077764092 ) ) ;
#30712=CARTESIAN_POINT ( 'NONE',  ( 0.5774900079438590739, 2.647018677488170990, -5.440088680355550821 ) ) ;
#30713=ORIENTED_EDGE ( 'NONE', *, *, #37166, .F. ) ;
#30714=CARTESIAN_POINT ( 'NONE',  ( 19.84674366389459266, 23.30059781766745530, 2.638427012816836559 ) ) ;
#30716=CARTESIAN_POINT ( 'NONE',  ( 4.559911319644449179, 22.23035201082150536, -9.422509992056141925 ) ) ;
#30717=CARTESIAN_POINT ( 'NONE',  ( -2.816281873526471635, -1.084698663402913210, -3.434112377981056508 ) ) ;
#30718=CARTESIAN_POINT ( 'NONE',  ( 10.00000000000000178, 13.05374883491396787, 14.16423886937410082 ) ) ;
#30719=CARTESIAN_POINT ( 'NONE',  ( 1.821158202401527593, 6.166888798595236310, 6.499999999999993783 ) ) ;
#30723=CARTESIAN_POINT ( 'NONE',  ( 14.92337183194729633, 7.675597817667451750, 8.527530157486181039 ) ) ;
#30724=CARTESIAN_POINT ( 'NONE',  ( 22.81628187352647785, 41.62363466993042493, 6.195893100308588602E-16 ) ) ;
#30725=CARTESIAN_POINT ( 'NONE',  ( 1.472469842513823179, 46.42559781766745175, 4.923371831947296329 ) ) ;
#30727=CARTESIAN_POINT ( 'NONE',  ( 14.92337183194729633, 22.67559781766745175, 8.527530157486181039 ) ) ;
#30730=CARTESIAN_POINT ( 'NONE',  ( 24.16423886937410614, 59.51208216824728936, -3.795296366450302550 ) ) ;
#30731=CARTESIAN_POINT ( 'NONE',  ( -0.8801773607111009756, 58.06368534415484106, 1.068504757029289695E-15 ) ) ;
#30733=CARTESIAN_POINT ( 'NONE',  ( 18.52753015748617571, 38.09226448433412315, 4.923371831947298993 ) ) ;
#30734=CARTESIAN_POINT ( 'NONE',  ( 2.035157376598824452, 8.688685344154839285, 7.964842623401179544 ) ) ;
#30735=CARTESIAN_POINT ( 'NONE',  ( 10.00000000000000000, 44.75893115100078745, -9.846743663894594434 ) ) ;
#30737=CARTESIAN_POINT ( 'NONE',  ( 19.84674366389459621, 53.50893115100078745, 7.409399052514197653E-17 ) ) ;
#30738=CARTESIAN_POINT ( 'NONE',  ( -0.8801773607110991993, 52.85535201082151247, -2.915334737309923874 ) ) ;
#30744=CARTESIAN_POINT ( 'NONE',  ( 19.84674366389459621, 3.508931151000785231, 7.409399052514197653E-17 ) ) ;
#30745=CARTESIAN_POINT ( 'NONE',  ( 0.6178305044545838731, 54.74863466993042493, 9.382169495545420901 ) ) ;
#30746=CARTESIAN_POINT ( 'NONE',  ( 20.88017736071110519, 5.563685344154838397, 2.639326808657452039E-16 ) ) ;
#30747=CARTESIAN_POINT ( 'NONE',  ( 7.361572987183170547, 47.05059781766745175, 9.846743663894590881 ) ) ;
#30749=CARTESIAN_POINT ( 'NONE',  ( -0.3689425029237898834, 31.17874883491396787, -10.36894250292378850 ) ) ;
#30750=CARTESIAN_POINT ( 'NONE',  ( 22.26659068614894466, 58.88708216824729647, 7.082119434687054849 ) ) ;
#30751=CARTESIAN_POINT ( 'NONE',  ( 14.92337183194729633, 52.67559781766745175, 8.527530157486181039 ) ) ;
#30752=CARTESIAN_POINT ( 'NONE',  ( -0.8801773607110991993, 52.85535201082151247, -2.915334737309923874 ) ) ;
#30753=CARTESIAN_POINT ( 'NONE',  ( 2.035157376598822676, 67.43868534415484817, -7.964842623401177768 ) ) ;
#30755=ADVANCED_FACE ( 'NONE', ( #79955 ), #19458, .T. ) ;
#30757=CARTESIAN_POINT ( 'NONE',  ( 19.38216949554541202, 55.99863466993041072, 9.382169495545424454 ) ) ;
#30758=EDGE_LOOP ( 'NONE', ( #87066, #78968, #89034, #33842 ) ) ;
#30759=CARTESIAN_POINT ( 'NONE',  ( 1.472469842513823179, 6.425597817667451750, 4.923371831947296329 ) ) ;
#30761=CARTESIAN_POINT ( 'NONE',  ( 20.36894250292379738, 24.92874883491396787, -10.36894250292379027 ) ) ;
#30762=CARTESIAN_POINT ( 'NONE',  ( 14.92337183194729988, 19.34226448433411960, -8.527530157486177487 ) ) ;
#30763=CARTESIAN_POINT ( 'NONE',  ( 20.88017736071110519, 35.56368534415484106, 2.639326808657452039E-16 ) ) ;
#30767=CARTESIAN_POINT ( 'NONE',  ( 4.559911319644449179, 22.23035201082150536, -9.422509992056141925 ) ) ;
#30768=AXIS2_PLACEMENT_3D ( 'NONE', #61652, #98221, #90190 ) ;
#30769=ORIENTED_EDGE ( 'NONE', *, *, #39054, .F. ) ;
#30770=CARTESIAN_POINT ( 'NONE',  ( 2.035157376598824452, 38.68868534415483396, 7.964842623401179544 ) ) ;
#30771=CARTESIAN_POINT ( 'NONE',  ( 1.821158202401528481, 66.16688879859523809, 6.500000000000007105 ) ) ;
#30774=ORIENTED_EDGE ( 'NONE', *, *, #29581, .F. ) ;
#30775=CARTESIAN_POINT ( 'NONE',  ( 10.00000000000000000, 22.87363466993042138, -12.81628187352647608 ) ) ;
#30777=CARTESIAN_POINT ( 'NONE',  ( 7.361572987183170547, 7.050597817667451750, 9.846743663894590881 ) ) ;
#30780=CARTESIAN_POINT ( 'NONE',  ( 12.63842701281683034, 12.46726448433411782, 9.846743663894596210 ) ) ;
#30781=CARTESIAN_POINT ( 'NONE',  ( 0.5774900079438607392, 33.48035201082150536, 5.440088680355550821 ) ) ;
#30783=VERTEX_POINT ( 'NONE', #27440 ) ;
#30785=CARTESIAN_POINT ( 'NONE',  ( -0.8801773607111009756, 63.06368534415484106, 1.068504757029289695E-15 ) ) ;
#30786=CARTESIAN_POINT ( 'NONE',  ( -46.94000000000016826, 103.2691844435149733, -6.361973263950634561 ) ) ;
#30787=CARTESIAN_POINT ( 'NONE',  ( 22.81628187352647785, 61.41530133659709634, 3.434112377981063169 ) ) ;
#30788=CARTESIAN_POINT ( 'NONE',  ( 19.42250999205614193, 65.14701867748817676, 5.440088680355555262 ) ) ;
#30791=CARTESIAN_POINT ( 'NONE',  ( 0.6178305044545838731, -0.2513653300695798953, 9.382169495545420901 ) ) ;
#30792=COLOUR_RGB ( '', 0.08235294, 0.09019608, 0.10196078) ;
#30793=( NAMED_UNIT ( * ) SI_UNIT ( $, .STERADIAN. ) SOLID_ANGLE_UNIT ( ) );
#30796=CARTESIAN_POINT ( 'NONE',  ( 19.84674366389459266, 28.30059781766745886, 2.638427012816836559 ) ) ;
#30797=CARTESIAN_POINT ( 'NONE',  ( 22.81628187352647785, 51.62363466993042493, 6.195893100308588602E-16 ) ) ;
#30798=CARTESIAN_POINT ( 'NONE',  ( -0.000000000000000000, 78.62409777033050773, 9.230451250305735655 ) ) ;
#30799=CARTESIAN_POINT ( 'NONE',  ( 19.84674366389459266, 23.71726448433412315, -2.638427012816827677 ) ) ;
#30800=MECHANICAL_DESIGN_GEOMETRIC_PRESENTATION_REPRESENTATION('',(#18047),#56302);
#30801=CARTESIAN_POINT ( 'NONE',  ( 13.43411237798105340, 15.58196800326374998, 12.81628187352647963 ) ) ;
#30804=CARTESIAN_POINT ( 'NONE',  ( 12.91533473730992121, 34.52201867748817676, 10.88017736071110164 ) ) ;
#30805=CARTESIAN_POINT ( 'NONE',  ( 0.1532563361054082862, 66.21726448433413736, 2.638427012816831674 ) ) ;
#30807=CARTESIAN_POINT ( 'NONE',  ( 0.1532563361054100626, 20.80059781766744464, -2.638427012816831230 ) ) ;
#30808=CARTESIAN_POINT ( 'NONE',  ( 2.791683348922237240, 5.383931151000785675, -7.208316651077763204 ) ) ;
#30809=CARTESIAN_POINT ( 'NONE',  ( 4.559911319644449179, 18.89701867748817321, 9.422509992056141925 ) ) ;
#30811=CARTESIAN_POINT ( 'NONE',  ( 13.43411237798105340, 20.58196800326374643, 12.81628187352647963 ) ) ;
#30812=CARTESIAN_POINT ( 'NONE',  ( 14.92337183194729633, 57.67559781766745886, 8.527530157486181039 ) ) ;
#30814=CARTESIAN_POINT ( 'NONE',  ( 2.035157376598822676, 7.438685344154837509, -7.964842623401177768 ) ) ;
#30816=CARTESIAN_POINT ( 'NONE',  ( 19.84674366389459266, 43.71726448433410894, -2.638427012816827677 ) ) ;
#30819=CARTESIAN_POINT ( 'NONE',  ( -0.8801773607110991993, 17.85535201082150536, -2.915334737309923874 ) ) ;
#30821=CARTESIAN_POINT ( 'NONE',  ( 17.96484262340118221, 29.93868534415484106, 7.964842623401181321 ) ) ;
#30823=CARTESIAN_POINT ( 'NONE',  ( -2.266590686148945544, 62.22041550158063927, 7.082119434687048631 ) ) ;
#30825=CARTESIAN_POINT ( 'NONE',  ( 19.42250999205614548, 5.980352010821504471, -5.440088680355545492 ) ) ;
#30826=CARTESIAN_POINT ( 'NONE',  ( 2.791683348922237240, 25.38393115100078390, -7.208316651077763204 ) ) ;
#30827=CARTESIAN_POINT ( 'NONE',  ( -2.816281873526473856, 9.331968003263753531, 3.434112377981055619 ) ) ;
#30828=CARTESIAN_POINT ( 'NONE',  ( -46.88208652658967424, 103.4388194638874694, 6.247021903621933880 ) ) ;
#30833=CARTESIAN_POINT ( 'NONE',  ( -4.164238869374098151, 11.59541550158063217, -3.795296366450310543 ) ) ;
#30835=CARTESIAN_POINT ( 'NONE',  ( 7.361572987183170547, 32.05059781766745175, 9.846743663894590881 ) ) ;
#30839=CARTESIAN_POINT ( 'NONE',  ( 6.204703633549690345, 47.84541550158064638, 14.16423886937410082 ) ) ;
#30840=CARTESIAN_POINT ( 'NONE',  ( 10.00000000000000178, 12.25893115100078568, 9.846743663894594434 ) ) ;
#30843=CARTESIAN_POINT ( 'NONE',  ( 20.88017736071110875, 40.77201867748818387, -2.915334737309920765 ) ) ;
#30844=CARTESIAN_POINT ( 'NONE',  ( 6.565887622018943937, 48.08196800326375353, -12.81628187352647608 ) ) ;
#30845=CARTESIAN_POINT ( 'NONE',  ( 17.96484262340118221, 14.93868534415483751, 7.964842623401181321 ) ) ;
#30846=CARTESIAN_POINT ( 'NONE',  ( 22.81628187352647785, 51.41530133659708923, 3.434112377981063169 ) ) ;
#30847=CARTESIAN_POINT ( 'NONE',  ( 1.472469842513823179, 61.42559781766745175, 4.923371831947296329 ) ) ;
#30848=FILL_AREA_STYLE_COLOUR ( '', #49022 ) ;
#30853=CARTESIAN_POINT ( 'NONE',  ( 2.917880565312950480, 45.97041550158063927, -12.26659068614894821 ) ) ;
#30854=CARTESIAN_POINT ( 'NONE',  ( 22.26659068614895176, 14.72041550158063572, -7.082119434687042414 ) ) ;
#30855=CARTESIAN_POINT ( 'NONE',  ( 20.88017736071110519, 25.56368534415483751, 2.639326808657452039E-16 ) ) ;
#30856=CARTESIAN_POINT ( 'NONE',  ( 19.42250999205614193, 30.14701867748817321, 5.440088680355555262 ) ) ;
#30859=CARTESIAN_POINT ( 'NONE',  ( 19.84674366389459266, 3.300597817667451750, 2.638427012816836559 ) ) ;
#30860=CARTESIAN_POINT ( 'NONE',  ( 12.91533473730992121, 59.52201867748816966, 10.88017736071110164 ) ) ;
#30861=CARTESIAN_POINT ( 'NONE',  ( -2.816281873526471635, 28.91530133659708213, -3.434112377981056508 ) ) ;
#30864=CARTESIAN_POINT ( 'NONE',  ( 17.20831665107776587, 39.13393115100079456, -7.208316651077762316 ) ) ;
#30865=CARTESIAN_POINT ( 'NONE',  ( 17.96484262340118221, 9.938685344154837509, 7.964842623401181321 ) ) ;
#30866=CARTESIAN_POINT ( 'NONE',  ( 16.40814093676324603, 12.45696800326375353, -11.09922568453594671 ) ) ;
#30868=CARTESIAN_POINT ( 'NONE',  ( 19.84674366389459266, 3.717264484334118713, -2.638427012816827677 ) ) ;
#30869=CARTESIAN_POINT ( 'NONE',  ( 17.96484262340118221, 14.93868534415483751, 7.964842623401181321 ) ) ;
#30870=CARTESIAN_POINT ( 'NONE',  ( 17.20831665107776587, 44.13393115100078745, -7.208316651077762316 ) ) ;
#30871=CARTESIAN_POINT ( 'NONE',  ( 22.81628187352647785, 61.62363466993041783, 6.195893100308588602E-16 ) ) ;
#30873=CARTESIAN_POINT ( 'NONE',  ( 19.84674366389459266, 33.30059781766744464, 2.638427012816836559 ) ) ;
#30874=CARTESIAN_POINT ( 'NONE',  ( -0.3689425029237881626, 17.42874883491397142, 10.36894250292379027 ) ) ;
#30875=CARTESIAN_POINT ( 'NONE',  ( 2.035157376598824452, 33.68868534415484106, 7.964842623401179544 ) ) ;
#30876=CARTESIAN_POINT ( 'NONE',  ( 17.96484262340118221, 14.93868534415483751, 7.964842623401181321 ) ) ;
#30878=CARTESIAN_POINT ( 'NONE',  ( 17.96484262340118221, 26.18868534415483396, -7.964842623401177768 ) ) ;
#30879=CARTESIAN_POINT ( 'NONE',  ( 12.91533473730993009, 21.60535201082150536, -10.88017736071109987 ) ) ;
#30880=ORIENTED_EDGE ( 'NONE', *, *, #97594, .T. ) ;
#30881=CARTESIAN_POINT ( 'NONE',  ( 12.91533473730992121, 44.52201867748816966, 10.88017736071110164 ) ) ;
#30882=CARTESIAN_POINT ( 'NONE',  ( -1.099225684535947600, 64.54030133659709634, 6.408140936763237150 ) ) ;
#30884=CARTESIAN_POINT ( 'NONE',  ( 4.559911319644449179, 42.23035201082151247, -9.422509992056141925 ) ) ;
#30885=CARTESIAN_POINT ( 'NONE',  ( -0.8801773607110991993, 57.85535201082149825, -2.915334737309923874 ) ) ;
#30886=ORIENTED_EDGE ( 'NONE', *, *, #67539, .F. ) ;
#30887=( BOUNDED_CURVE ( )  B_SPLINE_CURVE ( 2, ( #17466, #71448, #11420, #56440, #78439, #85956, #55949, #40952, #2963 ),
 .UNSPECIFIED., .F., .F. ) 
 B_SPLINE_CURVE_WITH_KNOTS ( ( 3, 2, 2, 2, 3 ),
 ( 0.7972837940830885817, 0.7976190476190476719, 0.8035714285714286031, 0.8095238095238095344, 0.8098590630597686246 ),
 .UNSPECIFIED. ) 
 CURVE ( )  GEOMETRIC_REPRESENTATION_ITEM ( )  RATIONAL_B_SPLINE_CURVE ( ( 0.9963778908391764944, 0.9980808541467923733, 1.000000000000000000, 0.9659258262890683122, 1.000000000000000000, 0.9659258262890683122, 1.000000000000000000, 0.9980808541467922623, 0.9963778908391764944 ) ) 
 REPRESENTATION_ITEM ( '' )  );
#30888=CARTESIAN_POINT ( 'NONE',  ( 20.88017736071110164, 50.35535201082151247, 2.915334737309930979 ) ) ;
#30892=CARTESIAN_POINT ( 'NONE',  ( -2.266590686148945544, 51.38708216824730357, -7.082119434687050408 ) ) ;
#30893=CARTESIAN_POINT ( 'NONE',  ( -0.8801773607110991993, 67.85535201082151957, -2.915334737309923874 ) ) ;
#30894=CARTESIAN_POINT ( 'NONE',  ( 18.72515096720571037, 55.05509018479936145, 6.499999999999982236 ) ) ;
#30896=CARTESIAN_POINT ( 'NONE',  ( 18.52753015748618282, 38.92559781766745175, -4.923371831947291888 ) ) ;
#30898=CARTESIAN_POINT ( 'NONE',  ( 0.1532563361054083140, 41.00893115100078745, 1.131784320476157264E-15 ) ) ;
#30899=CARTESIAN_POINT ( 'NONE',  ( 20.88017736071110164, 45.35535201082149115, 2.915334737309930979 ) ) ;
#30900=CARTESIAN_POINT ( 'NONE',  ( 5.076628168052704559, 35.17559781766745175, -8.527530157486179263 ) ) ;
#30902=CARTESIAN_POINT ( 'NONE',  ( 7.084665262690076126, 57.02201867748817676, -10.88017736071110164 ) ) ;
#30903=CARTESIAN_POINT ( 'NONE',  ( 10.00000000000000178, 44.31368534415484106, 10.88017736071110342 ) ) ;
#30904=CARTESIAN_POINT ( 'NONE',  ( 10.00000000000000178, 65.37363466993042493, 12.81628187352647608 ) ) ;
#30905=CARTESIAN_POINT ( 'NONE',  ( -4.164238869374099039, 61.80374883491397497, 8.674139862899312516E-16 ) ) ;
#30906=CARTESIAN_POINT ( 'NONE',  ( 19.38216949554541557, 17.24863466993041783, -9.382169495545420901 ) ) ;
#30907=CARTESIAN_POINT ( 'NONE',  ( 19.72487221294571214, 22.80223176428831877, -6.499999999999988454 ) ) ;
#30909=CARTESIAN_POINT ( 'NONE',  ( 3.591859063236761518, 14.95696800326375531, 11.09922568453594849 ) ) ;
#30910=CARTESIAN_POINT ( 'NONE',  ( -0.8801773607110991993, 22.85535201082150181, -2.915334737309923874 ) ) ;
#30911=CARTESIAN_POINT ( 'NONE',  ( 20.88017736071110875, 60.77201867748817676, -2.915334737309920765 ) ) ;
#30914=CARTESIAN_POINT ( 'NONE',  ( 12.63842701281683034, 2.467264484334118269, 9.846743663894596210 ) ) ;
#30915=CARTESIAN_POINT ( 'NONE',  ( 0.1532563361054083140, 46.00893115100079456, 1.131784320476157264E-15 ) ) ;
#30916=CARTESIAN_POINT ( 'NONE',  ( 19.84674366389459266, 43.71726448433410894, -2.638427012816827677 ) ) ;
#30917=CARTESIAN_POINT ( 'NONE',  ( 12.63842701281683034, 32.46726448433412315, 9.846743663894596210 ) ) ;
#30919=CARTESIAN_POINT ( 'NONE',  ( 6.565887622018943937, 43.08196800326374643, -12.81628187352647608 ) ) ;
#30920=CARTESIAN_POINT ( 'NONE',  ( 2.791683348922240793, 11.63393115100078568, 7.208316651077764092 ) ) ;
#30922=CARTESIAN_POINT ( 'NONE',  ( 20.15039907845753220, 45.60158574516643881, -6.262539305110077947 ) ) ;
#30923=CARTESIAN_POINT ( 'NONE',  ( 1.472469842513823179, 50.59226448433411605, -4.923371831947296329 ) ) ;
#30924=ORIENTED_EDGE ( 'NONE', *, *, #89439, .T. ) ;
#30925=CARTESIAN_POINT ( 'NONE',  ( 0.2751277870542967463, 0.000000000000000000, 6.500000000000000888 ) ) ;
#30926=CARTESIAN_POINT ( 'NONE',  ( -1.099225684535947600, 8.706968003263753531, -6.408140936763238038 ) ) ;
#30928=CARTESIAN_POINT ( 'NONE',  ( 15.44008868035555260, 49.73035201082150536, 9.422509992056143702 ) ) ;
#30929=CARTESIAN_POINT ( 'NONE',  ( 2.917880565312948704, 37.63708216824731068, 12.26659068614894643 ) ) ;
#30932=CARTESIAN_POINT ( 'NONE',  ( 19.65543155966242139, 92.23967373577187345, 5.359767647080724728 ) ) ;
#30934=CARTESIAN_POINT ( 'NONE',  ( -4.164238869374099039, 31.80374883491396432, 8.674139862899312516E-16 ) ) ;
#30935=CARTESIAN_POINT ( 'NONE',  ( 13.79529636645031943, 65.34541550158063217, -14.16423886937409904 ) ) ;
#30936=CARTESIAN_POINT ( 'NONE',  ( 6.204703633549690345, 5.762082168247301794, -14.16423886937410259 ) ) ;
#30937=CARTESIAN_POINT ( 'NONE',  ( -0.3689425029237881626, 22.42874883491397142, 10.36894250292379027 ) ) ;
#30938=FACE_OUTER_BOUND ( 'NONE', #31677, .T. ) ;
#30939=CARTESIAN_POINT ( 'NONE',  ( 19.42250999205614193, 65.14701867748817676, 5.440088680355555262 ) ) ;
#30940=CARTESIAN_POINT ( 'NONE',  ( -0.1503990784575242878, 29.24884699246888786, -6.262539305110083276 ) ) ;
#30942=CARTESIAN_POINT ( 'NONE',  ( 18.52753015748617571, 43.09226448433412315, 4.923371831947298993 ) ) ;
#30944=CARTESIAN_POINT ( 'NONE',  ( 7.084665262690076126, 24.10535201082150181, 10.88017736071109987 ) ) ;
#30945=CARTESIAN_POINT ( 'NONE',  ( 20.32896413005680714, 55.57879003517447103, -5.963430220938276349 ) ) ;
#30946=CARTESIAN_POINT ( 'NONE',  ( 2.791683348922240793, 66.63393115100079456, 7.208316651077764092 ) ) ;
#30948=CARTESIAN_POINT ( 'NONE',  ( 5.076628168052704559, 40.17559781766745175, -8.527530157486179263 ) ) ;
#30949=CARTESIAN_POINT ( 'NONE',  ( 10.00000000000000178, 60.37363466993041783, 12.81628187352647608 ) ) ;
#30951=CARTESIAN_POINT ( 'NONE',  ( 18.52753015748618282, 38.92559781766745175, -4.923371831947291888 ) ) ;
#30952=CARTESIAN_POINT ( 'NONE',  ( 5.076628168052703671, 46.84226448433412315, 8.527530157486179263 ) ) ;
#30953=CARTESIAN_POINT ( 'NONE',  ( 22.26659068614895176, 44.72041550158063927, -7.082119434687042414 ) ) ;
#30954=ORIENTED_EDGE ( 'NONE', *, *, #41014, .F. ) ;
#30955=EDGE_CURVE ( 'NONE', #72980, #43200, #3027, .T. ) ;
#30956=CARTESIAN_POINT ( 'NONE',  ( 6.204703633549690345, 7.845415501580634832, 14.16423886937410082 ) ) ;
#30957=CARTESIAN_POINT ( 'NONE',  ( 15.44008868035555793, 61.39701867748817676, -9.422509992056140149 ) ) ;
#30959=CARTESIAN_POINT ( 'NONE',  ( 17.08211943468705840, 60.13708216824729647, -12.26659068614894466 ) ) ;
#30960=CARTESIAN_POINT ( 'NONE',  ( 22.81628187352647785, 11.62363466993042138, 6.195893100308588602E-16 ) ) ;
#30961=CARTESIAN_POINT ( 'NONE',  ( 21.92686044187656336, 1.979976035794174472, 3.195792623639536423 ) ) ;
#30962=CARTESIAN_POINT ( 'NONE',  ( 12.63842701281683034, 2.467264484334118269, 9.846743663894596210 ) ) ;
#30965=CARTESIAN_POINT ( 'NONE',  ( -46.94000000000247752, 100.6180954154858398, -9.128675877383326309 ) ) ;
#30966=CARTESIAN_POINT ( 'NONE',  ( 0.6178305044545838731, 29.74863466993042138, 9.382169495545420901 ) ) ;
#30967=CARTESIAN_POINT ( 'NONE',  ( 20.36894250292379738, 59.92874883491397497, -10.36894250292379027 ) ) ;
#30969=CARTESIAN_POINT ( 'NONE',  ( -0.8801773607111008646, 28.27201867748817321, 2.915334737309923430 ) ) ;
#30970=CARTESIAN_POINT ( 'NONE',  ( 19.42250999205614548, 30.98035201082150536, -5.440088680355545492 ) ) ;
#30971=CARTESIAN_POINT ( 'NONE',  ( 2.791683348922237240, 55.38393115100078745, -7.208316651077763204 ) ) ;
#30972=CARTESIAN_POINT ( 'NONE',  ( 19.84674366389459266, 48.30059781766745175, 2.638427012816836559 ) ) ;
#30973=CARTESIAN_POINT ( 'NONE',  ( 22.81628187352647785, 56.41530133659708213, 3.434112377981063169 ) ) ;
#30974=DIRECTION ( 'NONE',  ( -1.000000000000000000, -0.000000000000000000, 0.000000000000000000 ) ) ;
#30976=CARTESIAN_POINT ( 'NONE',  ( 0.5774900079438590739, 12.64701867748817143, -5.440088680355550821 ) ) ;
#30977=CARTESIAN_POINT ( 'NONE',  ( 22.81628187352648496, 16.83196800326374998, -3.434112377981050290 ) ) ;
#30979=CARTESIAN_POINT ( 'NONE',  ( 19.84674366389459266, 48.30059781766745175, 2.638427012816836559 ) ) ;
#30980=CARTESIAN_POINT ( 'NONE',  ( -0.8801773607111008646, 43.27201867748817676, 2.915334737309923430 ) ) ;
#30981=CARTESIAN_POINT ( 'NONE',  ( 6.565887622018943937, 18.08196800326375708, -12.81628187352647608 ) ) ;
#30982=CARTESIAN_POINT ( 'NONE',  ( 12.91533473730992121, 44.52201867748816966, 10.88017736071110164 ) ) ;
#30984=DIRECTION ( 'NONE',  ( 1.000000000000000000, 1.465447498185264965E-15, 0.000000000000000000 ) ) ;
#30986=CARTESIAN_POINT ( 'NONE',  ( 0.1532563361054100626, 60.80059781766744464, -2.638427012816831230 ) ) ;
#30988=CARTESIAN_POINT ( 'NONE',  ( 17.96484262340118221, 44.93868534415483396, 7.964842623401181321 ) ) ;
#30989=CARTESIAN_POINT ( 'NONE',  ( 13.43411237798105340, 45.58196800326374643, 12.81628187352647963 ) ) ;
#30990=CARTESIAN_POINT ( 'NONE',  ( 24.16423886937409904, 9.095415501580633943, 3.795296366450317205 ) ) ;
#30991=CARTESIAN_POINT ( 'NONE',  ( 1.472469842513823179, 5.592264484334118713, -4.923371831947296329 ) ) ;
#30992=CARTESIAN_POINT ( 'NONE',  ( 2.791683348922240793, 61.63393115100079456, 7.208316651077764092 ) ) ;
#30993=CARTESIAN_POINT ( 'NONE',  ( 0.1532563361054100626, 10.80059781766745175, -2.638427012816831230 ) ) ;
#30995=CARTESIAN_POINT ( 'NONE',  ( -0.3689425029237898834, 41.17874883491397497, -10.36894250292378850 ) ) ;
#30997=CARTESIAN_POINT ( 'NONE',  ( 17.96484262340118221, 6.188685344154836621, -7.964842623401177768 ) ) ;
#30998=EDGE_CURVE ( 'NONE', #73080, #45005, #61851, .T. ) ;
#30999=CARTESIAN_POINT ( 'NONE',  ( 17.96484262340118221, 4.938685344154837509, 7.964842623401181321 ) ) ;
#31003=CARTESIAN_POINT ( 'NONE',  ( 4.559911319644449179, 3.897018677488171434, 9.422509992056141925 ) ) ;
#31004=CARTESIAN_POINT ( 'NONE',  ( 0.5774900079438607392, 8.480352010821505360, 5.440088680355550821 ) ) ;
#31005=CARTESIAN_POINT ( 'NONE',  ( 5.076628168052704559, 40.17559781766745175, -8.527530157486179263 ) ) ;
#31006=CARTESIAN_POINT ( 'NONE',  ( 10.00000000000000000, 32.87363466993042493, -12.81628187352647608 ) ) ;
#31007=SURFACE_STYLE_USAGE ( .BOTH. , #25012 ) ;
#31010=CARTESIAN_POINT ( 'NONE',  ( 20.36894250292379382, 8.678748834913967869, 10.36894250292379205 ) ) ;
#31011=CARTESIAN_POINT ( 'NONE',  ( 20.88017736071110164, 25.35535201082150891, 2.915334737309930979 ) ) ;
#31012=CARTESIAN_POINT ( 'NONE',  ( 2.917880565312950480, 65.97041550158063217, -12.26659068614894821 ) ) ;
#31013=CARTESIAN_POINT ( 'NONE',  ( 7.361572987183169658, 39.96726448433411605, -9.846743663894592657 ) ) ;
#31014=CARTESIAN_POINT ( 'NONE',  ( 18.72515096720571037, 45.05509018479935435, 6.499999999999982236 ) ) ;
#31015=CARTESIAN_POINT ( 'NONE',  ( 18.52753015748617571, 23.09226448433411960, 4.923371831947298993 ) ) ;
#31018=ORIENTED_EDGE ( 'NONE', *, *, #86712, .F. ) ;
#31020=CARTESIAN_POINT ( 'NONE',  ( 7.361572987183169658, 59.96726448433410894, -9.846743663894592657 ) ) ;
#31021=CARTESIAN_POINT ( 'NONE',  ( 10.00000000000000000, 26.81368534415484106, -10.88017736071110342 ) ) ;
#31022=CARTESIAN_POINT ( 'NONE',  ( 17.96484262340118221, 41.18868534415484106, -7.964842623401177768 ) ) ;
#31023=CARTESIAN_POINT ( 'NONE',  ( 4.559911319644449179, 7.230352010821504471, -9.422509992056141925 ) ) ;
#31024=CARTESIAN_POINT ( 'NONE',  ( -2.816281873526473856, 24.33196800326375353, 3.434112377981055619 ) ) ;
#31025=CARTESIAN_POINT ( 'NONE',  ( 22.26659068614895176, 14.72041550158063572, -7.082119434687042414 ) ) ;
#31026=EDGE_CURVE ( 'NONE', #98109, #66548, #83726, .T. ) ;
#31027=CARTESIAN_POINT ( 'NONE',  ( -1.099225684535947600, 39.54030133659708923, 6.408140936763237150 ) ) ;
#31029=CARTESIAN_POINT ( 'NONE',  ( 19.84674366389459621, 43.50893115100078745, 7.409399052514197653E-17 ) ) ;
#31030=CARTESIAN_POINT ( 'NONE',  ( 17.96484262340118221, 26.18868534415483396, -7.964842623401177768 ) ) ;
#31032=CARTESIAN_POINT ( 'NONE',  ( 20.88017736071110164, 20.35535201082150891, 2.915334737309930979 ) ) ;
#31034=CARTESIAN_POINT ( 'NONE',  ( 19.42250999205614548, 55.98035201082150536, -5.440088680355545492 ) ) ;
#31035=DIRECTION ( 'NONE',  ( 0.000000000000000000, 0.000000000000000000, -1.000000000000000000 ) ) ;
#31036=CARTESIAN_POINT ( 'NONE',  ( 10.00000000000000000, 66.81368534415484817, -10.88017736071110342 ) ) ;
#31037=CARTESIAN_POINT ( 'NONE',  ( 1.472469842513823179, 6.425597817667451750, 4.923371831947296329 ) ) ;
#31039=CARTESIAN_POINT ( 'NONE',  ( 20.88017736071110519, 50.56368534415484106, 2.639326808657452039E-16 ) ) ;
#31042=CARTESIAN_POINT ( 'NONE',  ( 2.603489959281592991, 11.58210964143329313, 6.500000000000006217 ) ) ;
#31043=FACE_OUTER_BOUND ( 'NONE', #42380, .T. ) ;
#31045=ADVANCED_FACE ( 'NONE', ( #56011 ), #97767, .T. ) ;
#31046=CARTESIAN_POINT ( 'NONE',  ( 17.20831665107776587, 44.13393115100078745, -7.208316651077762316 ) ) ;
#31047=ORIENTED_EDGE ( 'NONE', *, *, #81064, .F. ) ;
#31052=CARTESIAN_POINT ( 'NONE',  ( -4.164238869374099039, 16.80374883491396787, 8.674139862899312516E-16 ) ) ;
#31054=CARTESIAN_POINT ( 'NONE',  ( 19.72487221294570858, 10.71833443783938655, -6.500000000000000888 ) ) ;
#31055=CARTESIAN_POINT ( 'NONE',  ( 0.5774900079438607392, 58.48035201082151247, 5.440088680355550821 ) ) ;
#31056=CARTESIAN_POINT ( 'NONE',  ( 12.91533473730992121, 14.52201867748817143, 10.88017736071110164 ) ) ;
#31057=CARTESIAN_POINT ( 'NONE',  ( 2.603489959281590771, 66.58210964143327715, 6.500000000000003553 ) ) ;
#31059=CARTESIAN_POINT ( 'NONE',  ( 12.63842701281683034, 2.467264484334118269, 9.846743663894596210 ) ) ;
#31060=CARTESIAN_POINT ( 'NONE',  ( 19.84674366389459266, 3.717264484334118713, -2.638427012816827677 ) ) ;
#31062=CARTESIAN_POINT ( 'NONE',  ( -2.816281873526473856, 34.12363466993042493, 9.499525473075851096E-16 ) ) ;
#31063=CARTESIAN_POINT ( 'NONE',  ( 12.63842701281683034, 27.46726448433411250, 9.846743663894596210 ) ) ;
#31065=CARTESIAN_POINT ( 'NONE',  ( -2.816281873526473856, 9.123634669930421381, 9.499525473075851096E-16 ) ) ;
#31067=CARTESIAN_POINT ( 'NONE',  ( 19.84674366389459266, 8.300597817667451750, 2.638427012816836559 ) ) ;
#31068=B_SPLINE_CURVE_WITH_KNOTS ( 'NONE', 3,
 ( #49931, #88427, #80439, #11937 ),
 .UNSPECIFIED., .F., .F.,
 ( 4, 4 ),
 ( 6.234190775262425670E-17, 0.001060528352561999378 ),
 .UNSPECIFIED. ) ;
#31069=VERTEX_POINT ( 'NONE', #57393 ) ;
#31071=CARTESIAN_POINT ( 'NONE',  ( 7.084665262690076126, 27.02201867748817676, -10.88017736071110164 ) ) ;
#31072=CARTESIAN_POINT ( 'NONE',  ( 24.16423886937410614, 24.51208216824730002, -3.795296366450302550 ) ) ;
#31073=CARTESIAN_POINT ( 'NONE',  ( 18.52753015748618282, 43.92559781766745175, -4.923371831947291888 ) ) ;
#31074=CARTESIAN_POINT ( 'NONE',  ( 4.559911319644449179, 67.23035201082150536, -9.422509992056141925 ) ) ;
#31075=CARTESIAN_POINT ( 'NONE',  ( 0.6178305044545818747, 43.49863466993042493, -9.382169495545419124 ) ) ;
#31077=CARTESIAN_POINT ( 'NONE',  ( 17.96484262340118221, 29.93868534415484106, 7.964842623401181321 ) ) ;
#31081=CARTESIAN_POINT ( 'NONE',  ( 6.565887622018943937, 10.16530133659708746, 12.81628187352647430 ) ) ;
#31082=CARTESIAN_POINT ( 'NONE',  ( 21.09922568453594849, 6.206968003263753531, 6.408140936763242479 ) ) ;
#31083=CARTESIAN_POINT ( 'NONE',  ( 7.361572987183170547, 32.05059781766745175, 9.846743663894590881 ) ) ;
#31085=CARTESIAN_POINT ( 'NONE',  ( 13.43411237798106583, 47.66530133659709634, -12.81628187352647252 ) ) ;
#31086=CARTESIAN_POINT ( 'NONE',  ( 17.39651004071842166, 22.93575266056828355, 6.499999999999998224 ) ) ;
#31087=CARTESIAN_POINT ( 'NONE',  ( 20.88017736071110875, 50.77201867748817676, -2.915334737309920765 ) ) ;
#31090=CARTESIAN_POINT ( 'NONE',  ( 12.91533473730993009, 66.60535201082150536, -10.88017736071109987 ) ) ;
#31091=CARTESIAN_POINT ( 'NONE',  ( 2.035157376598822676, 37.43868534415484106, -7.964842623401177768 ) ) ;
#31092=CARTESIAN_POINT ( 'NONE',  ( 19.42250999205614193, 40.14701867748817676, 5.440088680355555262 ) ) ;
#31093=CARTESIAN_POINT ( 'NONE',  ( 0.1532563361054082862, 66.21726448433413736, 2.638427012816831674 ) ) ;
#31095=CARTESIAN_POINT ( 'NONE',  ( 20.88017736071110519, 65.56368534415483396, 2.639326808657452039E-16 ) ) ;
#31096=CARTESIAN_POINT ( 'NONE',  ( 14.92337183194729988, 49.34226448433411605, -8.527530157486177487 ) ) ;
#31097=CARTESIAN_POINT ( 'NONE',  ( 12.91533473730992121, 14.52201867748817143, 10.88017736071110164 ) ) ;
#31099=CARTESIAN_POINT ( 'NONE',  ( 0.6178305044545818747, 8.498634669930421381, -9.382169495545419124 ) ) ;
#31100=EDGE_LOOP ( 'NONE', ( #65320, #35393, #91619, #18846, #44533, #67014 ) ) ;
#31101=CARTESIAN_POINT ( 'NONE',  ( 20.88017736071110875, 40.77201867748818387, -2.915334737309920765 ) ) ;
#31102=CARTESIAN_POINT ( 'NONE',  ( 19.38216949554541557, 7.248634669930421381, -9.382169495545420901 ) ) ;
#31104=CARTESIAN_POINT ( 'NONE',  ( 20.88017736071110164, 15.35535201082150358, 2.915334737309930979 ) ) ;
#31105=CARTESIAN_POINT ( 'NONE',  ( -0.8801773607111009756, 33.06368534415484106, 1.068504757029289695E-15 ) ) ;
#31106=CARTESIAN_POINT ( 'NONE',  ( 6.204703633549690345, 32.84541550158063927, 14.16423886937410082 ) ) ;
#31107=CARTESIAN_POINT ( 'NONE',  ( 7.361572987183170547, 27.05059781766745175, 9.846743663894590881 ) ) ;
#31108=CARTESIAN_POINT ( 'NONE',  ( -0.8801773607110991993, 57.85535201082149825, -2.915334737309923874 ) ) ;
#31109=CARTESIAN_POINT ( 'NONE',  ( 10.00000000000000178, 8.053748834913967869, 14.16423886937410082 ) ) ;
#31112=CARTESIAN_POINT ( 'NONE',  ( 5.076628168052704559, 60.17559781766745175, -8.527530157486179263 ) ) ;
#31115=CARTESIAN_POINT ( 'NONE',  ( -4.164238869374098151, 41.59541550158061796, -3.795296366450310543 ) ) ;
#31116=CARTESIAN_POINT ( 'NONE',  ( 20.36894250292379738, 39.92874883491396787, -10.36894250292379027 ) ) ;
#31117=CARTESIAN_POINT ( 'NONE',  ( 5.076628168052703671, 6.842264484334118713, 8.527530157486179263 ) ) ;
#31118=CARTESIAN_POINT ( 'NONE',  ( 18.52753015748617571, 58.09226448433411605, 4.923371831947298993 ) ) ;
#31120=CARTESIAN_POINT ( 'NONE',  ( 10.00000000000000178, 64.31368534415483396, 10.88017736071110342 ) ) ;
#31121=CARTESIAN_POINT ( 'NONE',  ( -2.816281873526471635, 23.91530133659708568, -3.434112377981056508 ) ) ;
#31122=CARTESIAN_POINT ( 'NONE',  ( 22.26659068614894466, 23.88708216824730357, 7.082119434687054849 ) ) ;
#31123=CARTESIAN_POINT ( 'NONE',  ( 12.91533473730992121, 19.52201867748816611, 10.88017736071110164 ) ) ;
#31124=CARTESIAN_POINT ( 'NONE',  ( 10.00000000000000000, 31.81368534415483751, -10.88017736071110342 ) ) ;
#31126=CARTESIAN_POINT ( 'NONE',  ( 0.5774900079438607392, 53.48035201082151247, 5.440088680355550821 ) ) ;
#31131=TOROIDAL_SURFACE ( 'NONE', #29481, 1.000000000000000000, 0.5000000000000000000 ) ;
#31133=DIRECTION ( 'NONE',  ( 0.000000000000000000, -1.000000000000000000, 0.000000000000000000 ) ) ;
#31135=CARTESIAN_POINT ( 'NONE',  ( 10.00000000000000178, 58.05374883491397497, 14.16423886937410082 ) ) ;
#31136=CARTESIAN_POINT ( 'NONE',  ( 6.204703633549690345, 60.76208216824730357, -14.16423886937410259 ) ) ;
#31137=CARTESIAN_POINT ( 'NONE',  ( 0.1532563361054083140, 31.00893115100078390, 1.131784320476157264E-15 ) ) ;
#31138=CARTESIAN_POINT ( 'NONE',  ( 17.20831665107776587, 57.88393115100078745, 7.208316651077764980 ) ) ;
#31142=CARTESIAN_POINT ( 'NONE',  ( 0.1532563361054083140, 11.00893115100078568, 1.131784320476157264E-15 ) ) ;
#31143=VECTOR ( 'NONE', #25302, 1000.000000000000000 ) ;
#31144=CARTESIAN_POINT ( 'NONE',  ( 6.565887622018943937, 5.165301336597086568, 12.81628187352647430 ) ) ;
#31147=CARTESIAN_POINT ( 'NONE',  ( -4.164238869374098151, 41.59541550158061796, -3.795296366450310543 ) ) ;
#31148=CARTESIAN_POINT ( 'NONE',  ( 2.917880565312948704, 37.63708216824731068, 12.26659068614894643 ) ) ;
#31149=EDGE_LOOP ( 'NONE', ( #80204, #68907, #61485, #84516 ) ) ;
#31150=CARTESIAN_POINT ( 'NONE',  ( 13.43411237798106583, 57.66530133659708923, -12.81628187352647252 ) ) ;
#31151=CARTESIAN_POINT ( 'NONE',  ( 20.88017736071110875, 30.77201867748816966, -2.915334737309920765 ) ) ;
#31152=CARTESIAN_POINT ( 'NONE',  ( 2.791683348922240793, 46.63393115100077324, 7.208316651077764092 ) ) ;
#31153=CARTESIAN_POINT ( 'NONE',  ( 10.00000000000000178, 29.31368534415483751, 10.88017736071110342 ) ) ;
#31155=CARTESIAN_POINT ( 'NONE',  ( 17.20831665107776587, 54.13393115100079456, -7.208316651077762316 ) ) ;
#31156=CARTESIAN_POINT ( 'NONE',  ( 2.791683348922237240, 55.38393115100078745, -7.208316651077763204 ) ) ;
#31158=EDGE_CURVE ( 'NONE', #84056, #55863, #71902, .T. ) ;
#31161=CARTESIAN_POINT ( 'NONE',  ( 5.076628168052703671, 1.842264484334118047, 8.527530157486179263 ) ) ;
#31165=CARTESIAN_POINT ( 'NONE',  ( 1.472469842513823179, 30.59226448433411960, -4.923371831947296329 ) ) ;
#31166=B_SPLINE_CURVE_WITH_KNOTS ( 'NONE', 3,
 ( #46556, #30557, #91574, #75083, #53560, #23589 ),
 .UNSPECIFIED., .F., .F.,
 ( 4, 2, 4 ),
 ( 0.000000000000000000, 0.0002701661927229427628, 0.0005403323854458855257 ),
 .UNSPECIFIED. ) ;
#31169=CARTESIAN_POINT ( 'NONE',  ( 22.81628187352647785, 36.62363466993041783, 6.195893100308588602E-16 ) ) ;
#31171=ORIENTED_EDGE ( 'NONE', *, *, #15058, .T. ) ;
#31174=CARTESIAN_POINT ( 'NONE',  ( 18.52753015748618282, 58.92559781766745886, -4.923371831947291888 ) ) ;
#31175=CARTESIAN_POINT ( 'NONE',  ( 24.16423886937410614, 39.51208216824731068, -3.795296366450302550 ) ) ;
#31176=CARTESIAN_POINT ( 'NONE',  ( 12.63842701281683922, 54.55059781766745175, -9.846743663894590881 ) ) ;
#31177=CARTESIAN_POINT ( 'NONE',  ( 21.92686044187656336, 36.97997603579418069, 3.195792623639536423 ) ) ;
#31178=CARTESIAN_POINT ( 'NONE',  ( 19.84674366389459621, 13.50893115100078568, 7.409399052514197653E-17 ) ) ;
#31179=CARTESIAN_POINT ( 'NONE',  ( 0.6178305044545838731, 54.74863466993042493, 9.382169495545420901 ) ) ;
#31180=SURFACE_STYLE_USAGE ( .BOTH. , #29698 ) ;
#31181=STYLED_ITEM ( 'NONE', ( #58071 ), #52588 ) ;
#31182=CARTESIAN_POINT ( 'NONE',  ( 12.63842701281683034, 62.46726448433410894, 9.846743663894596210 ) ) ;
#31183=CARTESIAN_POINT ( 'NONE',  ( 15.44008868035555260, 49.73035201082150536, 9.422509992056143702 ) ) ;
#31186=CARTESIAN_POINT ( 'NONE',  ( -0.8801773607111008646, 58.27201867748816966, 2.915334737309923430 ) ) ;
#31189=CARTESIAN_POINT ( 'NONE',  ( -0.8801773607110991993, 32.85535201082151247, -2.915334737309923874 ) ) ;
#31190=CARTESIAN_POINT ( 'NONE',  ( 10.00000000000000178, 5.373634669930420493, 12.81628187352647608 ) ) ;
#31191=CARTESIAN_POINT ( 'NONE',  ( 15.44008868035555793, 56.39701867748817676, -9.422509992056140149 ) ) ;
#31192=CARTESIAN_POINT ( 'NONE',  ( 1.046131998949919373, 15.73810908735719494, 6.500000000000002665 ) ) ;
#31195=CARTESIAN_POINT ( 'NONE',  ( 17.96484262340118221, 46.18868534415484106, -7.964842623401177768 ) ) ;
#31197=CARTESIAN_POINT ( 'NONE',  ( 0.1532563361054083140, 36.00893115100078745, 1.131784320476157264E-15 ) ) ;
#31198=SURFACE_SIDE_STYLE ('',( #23733 ) ) ;
#31200=CARTESIAN_POINT ( 'NONE',  ( 19.84674366389459266, 63.71726448433412315, -2.638427012816827677 ) ) ;
#31201=CARTESIAN_POINT ( 'NONE',  ( 19.42250999205614548, 10.98035201082150536, -5.440088680355545492 ) ) ;
#31203=CARTESIAN_POINT ( 'NONE',  ( -2.266590686148945544, 22.22041550158063572, 7.082119434687048631 ) ) ;
#31204=CARTESIAN_POINT ( 'NONE',  ( -4.164238869374099039, 61.80374883491397497, 8.674139862899312516E-16 ) ) ;
#31205=CARTESIAN_POINT ( 'NONE',  ( 7.361572987183170547, 22.05059781766745530, 9.846743663894590881 ) ) ;
#31206=CARTESIAN_POINT ( 'NONE',  ( 19.80427997160308351, 32.75733960839544068, -6.500000000000010658 ) ) ;
#31207=VERTEX_POINT ( 'NONE', #42404 ) ;
#31208=CARTESIAN_POINT ( 'NONE',  ( 10.00000000000000178, 27.25893115100078390, 9.846743663894594434 ) ) ;
#31209=CARTESIAN_POINT ( 'NONE',  ( 20.88017736071110164, 30.35535201082151247, 2.915334737309930979 ) ) ;
#31210=CARTESIAN_POINT ( 'NONE',  ( 14.92337183194729633, 57.67559781766745886, 8.527530157486181039 ) ) ;
#31211=CARTESIAN_POINT ( 'NONE',  ( 24.16423886937410614, 4.512082168247300906, -3.795296366450302550 ) ) ;
#31215=CARTESIAN_POINT ( 'NONE',  ( 7.361572987183170547, 12.05059781766744997, 9.846743663894590881 ) ) ;
#31216=CARTESIAN_POINT ( 'NONE',  ( 21.09922568453594849, 36.20696800326375353, 6.408140936763242479 ) ) ;
#31217=CARTESIAN_POINT ( 'NONE',  ( 5.076628168052704559, 40.17559781766745175, -8.527530157486179263 ) ) ;
#31219=CARTESIAN_POINT ( 'NONE',  ( 2.791683348922240793, 21.63393115100078745, 7.208316651077764092 ) ) ;
#31221=CARTESIAN_POINT ( 'NONE',  ( -0.3689425029237881626, 52.42874883491396076, 10.36894250292379027 ) ) ;
#31222=CARTESIAN_POINT ( 'NONE',  ( 20.88017736071110164, 55.35535201082149825, 2.915334737309930979 ) ) ;
#31223=CARTESIAN_POINT ( 'NONE',  ( 19.42250999205614193, 55.14701867748817676, 5.440088680355555262 ) ) ;
#31224=CARTESIAN_POINT ( 'NONE',  ( 2.791683348922240793, 41.63393115100078745, 7.208316651077764092 ) ) ;
#31225=CARTESIAN_POINT ( 'NONE',  ( 12.91533473730993009, 6.605352010821504471, -10.88017736071109987 ) ) ;
#31227=CARTESIAN_POINT ( 'NONE',  ( 14.92337183194729988, 44.34226448433412315, -8.527530157486177487 ) ) ;
#31228=CARTESIAN_POINT ( 'NONE',  ( 20.88017736071110875, 45.77201867748816966, -2.915334737309920765 ) ) ;
#31229=CARTESIAN_POINT ( 'NONE',  ( 14.92337183194729988, 4.342264484334117824, -8.527530157486177487 ) ) ;
#31231=VERTEX_POINT ( 'NONE', #32427 ) ;
#31232=VERTEX_POINT ( 'NONE', #17452 ) ;
#31233=CARTESIAN_POINT ( 'NONE',  ( -0.1503990784575287842, 28.10158574516642815, 6.262539305110075283 ) ) ;
#31235=LINE ( 'NONE', #7282, #20532 ) ;
#31236=CARTESIAN_POINT ( 'NONE',  ( 18.52753015748617571, 28.09226448433411960, 4.923371831947298993 ) ) ;
#31237=CARTESIAN_POINT ( 'NONE',  ( 13.43411237798105340, 50.58196800326375353, 12.81628187352647963 ) ) ;
#31238=CARTESIAN_POINT ( 'NONE',  ( 12.91533473730992121, 14.52201867748817143, 10.88017736071110164 ) ) ;
#31239=CARTESIAN_POINT ( 'NONE',  ( 18.52753015748617571, 48.09226448433412315, 4.923371831947298993 ) ) ;
#31241=CARTESIAN_POINT ( 'NONE',  ( 24.16423886937409904, 29.09541550158063572, 3.795296366450317205 ) ) ;
#31242=CARTESIAN_POINT ( 'NONE',  ( -4.164238869374098151, 56.59541550158063927, -3.795296366450310543 ) ) ;
#31243=CARTESIAN_POINT ( 'NONE',  ( 0.1532563361054100626, 55.80059781766745175, -2.638427012816831230 ) ) ;
#31245=CARTESIAN_POINT ( 'NONE',  ( 0.5774900079438590739, 57.64701867748817676, -5.440088680355550821 ) ) ;
#31246=CARTESIAN_POINT ( 'NONE',  ( 19.84674366389459266, 18.30059781766745175, 2.638427012816836559 ) ) ;
#31251=CARTESIAN_POINT ( 'NONE',  ( 10.00000000000000178, 12.25893115100078568, 9.846743663894594434 ) ) ;
#31254=CARTESIAN_POINT ( 'NONE',  ( 13.79529636645031943, 25.34541550158063572, -14.16423886937409904 ) ) ;
#31255=CARTESIAN_POINT ( 'NONE',  ( 7.361572987183170547, 27.05059781766745175, 9.846743663894590881 ) ) ;
#31256=CARTESIAN_POINT ( 'NONE',  ( -0.8801773607110991993, 37.85535201082151247, -2.915334737309923874 ) ) ;
#31259=VERTEX_POINT ( 'NONE', #56426 ) ;
#31260=CARTESIAN_POINT ( 'NONE',  ( 10.00000000000000000, 31.81368534415483751, -10.88017736071110342 ) ) ;
#31262=AXIS2_PLACEMENT_3D ( 'NONE', #75274, #29276, #14297 ) ;
#31263=VERTEX_POINT ( 'NONE', #86912 ) ;
#31264=CARTESIAN_POINT ( 'NONE',  ( 2.035157376598822676, 37.43868534415484106, -7.964842623401177768 ) ) ;
#31266=CARTESIAN_POINT ( 'NONE',  ( -2.816281873526473856, 14.12363466993041961, 9.499525473075851096E-16 ) ) ;
#31267=CARTESIAN_POINT ( 'NONE',  ( 5.076628168052703671, 11.84226448433411960, 8.527530157486179263 ) ) ;
#31270=CARTESIAN_POINT ( 'NONE',  ( 1.472469842513823179, 21.42559781766745175, 4.923371831947296329 ) ) ;
#31271=CARTESIAN_POINT ( 'NONE',  ( 4.559911319644449179, 33.89701867748817676, 9.422509992056141925 ) ) ;
#31272=CIRCLE ( 'NONE', #48835, 6.999999999999999112 ) ;
#31278=CARTESIAN_POINT ( 'NONE',  ( 10.00000000000000178, 59.31368534415484106, 10.88017736071110342 ) ) ;
#31282=CARTESIAN_POINT ( 'NONE',  ( 17.96484262340118221, 61.18868534415482685, -7.964842623401177768 ) ) ;
#31283=ADVANCED_FACE ( 'NONE', ( #55933 ), #18422, .T. ) ;
#31284=CARTESIAN_POINT ( 'NONE',  ( 16.40814093676323893, 5.790301336597087456, 11.09922568453595026 ) ) ;
#31287=CARTESIAN_POINT ( 'NONE',  ( 0.1532563361054082862, 36.21726448433410894, 2.638427012816831674 ) ) ;
#31288=CARTESIAN_POINT ( 'NONE',  ( 6.565887622018943937, 50.16530133659708213, 12.81628187352647430 ) ) ;
#31289=CARTESIAN_POINT ( 'NONE',  ( 7.361572987183169658, 14.96726448433411960, -9.846743663894592657 ) ) ;
#31290=CARTESIAN_POINT ( 'NONE',  ( 6.565887622018943937, 20.16530133659708213, 12.81628187352647430 ) ) ;
#31293=CARTESIAN_POINT ( 'NONE',  ( -0.8801773607110991993, 37.85535201082151247, -2.915334737309923874 ) ) ;
#31294=CARTESIAN_POINT ( 'NONE',  ( 14.92337183194729988, 59.34226448433412315, -8.527530157486177487 ) ) ;
#31296=CARTESIAN_POINT ( 'NONE',  ( 0.1532563361054083140, 16.00893115100078390, 1.131784320476157264E-15 ) ) ;
#31297=CARTESIAN_POINT ( 'NONE',  ( 0.1532563361054083140, 6.008931151000784787, 1.131784320476157264E-15 ) ) ;
#31298=CARTESIAN_POINT ( 'NONE',  ( 10.00000000000000178, 14.31368534415483751, 10.88017736071110342 ) ) ;
#31299=CARTESIAN_POINT ( 'NONE',  ( 19.38216949554541202, 15.99863466993042138, 9.382169495545424454 ) ) ;
#31301=CARTESIAN_POINT ( 'NONE',  ( 0.1532563361054083140, 66.00893115100079456, 1.131784320476157264E-15 ) ) ;
#31303=CARTESIAN_POINT ( 'NONE',  ( 19.42250999205614193, 25.14701867748817321, 5.440088680355555262 ) ) ;
#31304=CARTESIAN_POINT ( 'NONE',  ( 10.00000000000000178, 47.25893115100078745, 9.846743663894594434 ) ) ;
#31306=CARTESIAN_POINT ( 'NONE',  ( -0.8801773607111009756, 13.06368534415483929, 1.068504757029289695E-15 ) ) ;
#31308=CARTESIAN_POINT ( 'NONE',  ( 2.035157376598822676, 27.43868534415483396, -7.964842623401177768 ) ) ;
#31309=CARTESIAN_POINT ( 'NONE',  ( 20.88017736071110519, 5.563685344154838397, 2.639326808657452039E-16 ) ) ;
#31310=CARTESIAN_POINT ( 'NONE',  ( -0.1503990784575328643, 70.00000000000000000, 6.262539305110068177 ) ) ;
#31311=CARTESIAN_POINT ( 'NONE',  ( 7.361572987183169658, -0.03273551566588185635, -9.846743663894592657 ) ) ;
#31312=EDGE_CURVE ( 'NONE', #57285, #21583, #77167, .T. ) ;
#31313=CARTESIAN_POINT ( 'NONE',  ( 5.076628168052703671, 26.84226448433411960, 8.527530157486179263 ) ) ;
#31314=CARTESIAN_POINT ( 'NONE',  ( 22.81628187352647785, 6.415301336597088344, 3.434112377981063169 ) ) ;
#31316=VECTOR ( 'NONE', #24605, 1000.000000000000000 ) ;
#31318=CARTESIAN_POINT ( 'NONE',  ( 0.1532563361054083140, 66.00893115100079456, 1.131784320476157264E-15 ) ) ;
#31321=CARTESIAN_POINT ( 'NONE',  ( 6.204703633549690345, 7.845415501580634832, 14.16423886937410082 ) ) ;
#31322=CARTESIAN_POINT ( 'NONE',  ( 2.791683348922240793, 36.63393115100078035, 7.208316651077764092 ) ) ;
#31325=CARTESIAN_POINT ( 'NONE',  ( 24.16423886937409904, 49.09541550158063217, 3.795296366450317205 ) ) ;
#31326=CARTESIAN_POINT ( 'NONE',  ( 7.361572987183170547, 22.05059781766745530, 9.846743663894590881 ) ) ;
#31328=CARTESIAN_POINT ( 'NONE',  ( 10.00000000000000178, 70.00000000000000000, 0.000000000000000000 ) ) ;
#31329=CARTESIAN_POINT ( 'NONE',  ( 12.91533473730992121, 39.52201867748817676, 10.88017736071110164 ) ) ;
#31330=CARTESIAN_POINT ( 'NONE',  ( 22.81628187352647785, 56.41530133659708213, 3.434112377981063169 ) ) ;
#31331=CARTESIAN_POINT ( 'NONE',  ( 7.084665262690076126, 24.10535201082150181, 10.88017736071109987 ) ) ;
#31332=CARTESIAN_POINT ( 'NONE',  ( 16.40814093676324603, 52.45696800326375353, -11.09922568453594671 ) ) ;
#31333=CARTESIAN_POINT ( 'NONE',  ( 0.1532563361054082862, 66.21726448433413736, 2.638427012816831674 ) ) ;
#31334=CARTESIAN_POINT ( 'NONE',  ( 14.92337183194729633, 2.675597817667451750, 8.527530157486181039 ) ) ;
#31337=DIRECTION ( 'NONE',  ( 1.000000000000000000, 0.000000000000000000, -0.000000000000000000 ) ) ;
#31338=CARTESIAN_POINT ( 'NONE',  ( 17.08211943468705840, 60.13708216824729647, -12.26659068614894466 ) ) ;
#31339=CARTESIAN_POINT ( 'NONE',  ( 10.00000000000000178, 18.05374883491396787, 14.16423886937410082 ) ) ;
#31340=CARTESIAN_POINT ( 'NONE',  ( 17.96484262340118221, 16.18868534415483396, -7.964842623401177768 ) ) ;
#31341=CARTESIAN_POINT ( 'NONE',  ( 19.42250999205614193, 40.14701867748817676, 5.440088680355555262 ) ) ;
#31343=DIRECTION ( 'NONE',  ( 0.000000000000000000, 0.000000000000000000, 1.000000000000000000 ) ) ;
#31344=CARTESIAN_POINT ( 'NONE',  ( 15.44008868035555260, 64.73035201082151957, 9.422509992056143702 ) ) ;
#31345=CARTESIAN_POINT ( 'NONE',  ( 10.00000000000000000, 66.81368534415484817, -10.88017736071110342 ) ) ;
#31346=CARTESIAN_POINT ( 'NONE',  ( 22.81628187352648496, 21.83196800326374643, -3.434112377981050290 ) ) ;
#31348=CARTESIAN_POINT ( 'NONE',  ( 19.72487221294570858, 70.00000000000000000, 6.000000000000000000 ) ) ;
#31349=CARTESIAN_POINT ( 'NONE',  ( 14.92337183194729988, 9.342264484334119601, -8.527530157486177487 ) ) ;
#31350=CARTESIAN_POINT ( 'NONE',  ( 19.84674366389459266, 43.30059781766744464, 2.638427012816836559 ) ) ;
#31351=CARTESIAN_POINT ( 'NONE',  ( 20.88017736071110164, 10.35535201082150714, 2.915334737309930979 ) ) ;
#31352=VECTOR ( 'NONE', #87278, 1000.000000000000000 ) ;
#31355=CARTESIAN_POINT ( 'NONE',  ( 21.09922568453594849, 31.20696800326375353, 6.408140936763242479 ) ) ;
#31356=CARTESIAN_POINT ( 'NONE',  ( 5.076628168052704559, 5.175597817667451750, -8.527530157486179263 ) ) ;
#31359=CARTESIAN_POINT ( 'NONE',  ( 14.92337183194729988, 54.34226448433412315, -8.527530157486177487 ) ) ;
#31360=CARTESIAN_POINT ( 'NONE',  ( 18.52753015748618282, 28.92559781766745175, -4.923371831947291888 ) ) ;
#31361=CARTESIAN_POINT ( 'NONE',  ( 6.204703633549690345, 17.84541550158063217, 14.16423886937410082 ) ) ;
#31362=CARTESIAN_POINT ( 'NONE',  ( 2.035157376598822676, 37.43868534415484106, -7.964842623401177768 ) ) ;
#31363=CARTESIAN_POINT ( 'NONE',  ( 12.91533473730992121, 9.522018677488171434, 10.88017736071110164 ) ) ;
#31364=CARTESIAN_POINT ( 'NONE',  ( 7.084665262690076126, 29.10535201082150181, 10.88017736071109987 ) ) ;
#31365=CARTESIAN_POINT ( 'NONE',  ( 12.91533473730992121, 24.52201867748816966, 10.88017736071110164 ) ) ;
#31366=ORIENTED_EDGE ( 'NONE', *, *, #37731, .T. ) ;
#31367=CARTESIAN_POINT ( 'NONE',  ( 16.40814093676323893, 35.79030133659708923, 11.09922568453595026 ) ) ;
#31368=CARTESIAN_POINT ( 'NONE',  ( 4.559911319644449179, 37.23035201082150536, -9.422509992056141925 ) ) ;
#31369=VERTEX_POINT ( 'NONE', #66867 ) ;
#31373=CARTESIAN_POINT ( 'NONE',  ( 19.42250999205614193, 45.14701867748817676, 5.440088680355555262 ) ) ;
#31374=ORIENTED_EDGE ( 'NONE', *, *, #78458, .F. ) ;
#31375=CARTESIAN_POINT ( 'NONE',  ( 20.88017736071110519, 45.56368534415484106, 2.639326808657452039E-16 ) ) ;
#31378=CARTESIAN_POINT ( 'NONE',  ( 24.16423886937410614, 54.51208216824730357, -3.795296366450302550 ) ) ;
#31379=CARTESIAN_POINT ( 'NONE',  ( 2.035157376598822676, 62.43868534415483396, -7.964842623401177768 ) ) ;
#31382=CARTESIAN_POINT ( 'NONE',  ( 1.472469842513823179, 30.59226448433411960, -4.923371831947296329 ) ) ;
#31384=CARTESIAN_POINT ( 'NONE',  ( 14.92337183194729633, 37.67559781766745175, 8.527530157486181039 ) ) ;
#31385=CARTESIAN_POINT ( 'NONE',  ( 7.084665262690076126, 37.02201867748817676, -10.88017736071110164 ) ) ;
#31386=CARTESIAN_POINT ( 'NONE',  ( 14.92337183194729988, 39.34226448433412315, -8.527530157486177487 ) ) ;
#31387=CARTESIAN_POINT ( 'NONE',  ( 10.00000000000000178, 20.37363466993042138, 12.81628187352647608 ) ) ;
#31388=CARTESIAN_POINT ( 'NONE',  ( 7.084665262690076126, 67.02201867748817676, -10.88017736071110164 ) ) ;
#31390=CARTESIAN_POINT ( 'NONE',  ( 2.035157376598822676, 42.43868534415483396, -7.964842623401177768 ) ) ;
#31391=CARTESIAN_POINT ( 'NONE',  ( 24.16423886937409904, 59.09541550158063217, 3.795296366450317205 ) ) ;
#31393=CARTESIAN_POINT ( 'NONE',  ( 6.565887622018943937, 18.08196800326375708, -12.81628187352647608 ) ) ;
#31394=CARTESIAN_POINT ( 'NONE',  ( 18.95386800104996183, 23.23810908735726599, -6.499999999999988454 ) ) ;
#31396=CARTESIAN_POINT ( 'NONE',  ( 10.00000000000000178, 15.37363466993042138, 12.81628187352647608 ) ) ;
#31397=CARTESIAN_POINT ( 'NONE',  ( 4.559911319644449179, 27.23035201082150536, -9.422509992056141925 ) ) ;
#31399=CARTESIAN_POINT ( 'NONE',  ( 7.084665262690076126, 67.02201867748817676, -10.88017736071110164 ) ) ;
#31402=CARTESIAN_POINT ( 'NONE',  ( 0.1532563361054100626, 5.800597817667452638, -2.638427012816831230 ) ) ;
#31403=CARTESIAN_POINT ( 'NONE',  ( 1.472469842513823179, 46.42559781766745175, 4.923371831947296329 ) ) ;
#31404=CARTESIAN_POINT ( 'NONE',  ( 19.84674366389459621, 38.50893115100078745, 7.409399052514197653E-17 ) ) ;
#31406=CARTESIAN_POINT ( 'NONE',  ( 1.472469842513823179, 31.42559781766745530, 4.923371831947296329 ) ) ;
#31407=DIRECTION ( 'NONE',  ( 0.000000000000000000, 0.000000000000000000, -1.000000000000000000 ) ) ;
#31409=CARTESIAN_POINT ( 'NONE',  ( 0.1532563361054100626, 15.80059781766745353, -2.638427012816831230 ) ) ;
#31412=CARTESIAN_POINT ( 'NONE',  ( 17.20831665107776587, 42.88393115100077324, 7.208316651077764980 ) ) ;
#31415=CARTESIAN_POINT ( 'NONE',  ( 19.38216949554541557, 12.24863466993041961, -9.382169495545420901 ) ) ;
#31416=CARTESIAN_POINT ( 'NONE',  ( 15.44008868035555793, 56.39701867748817676, -9.422509992056140149 ) ) ;
#31418=CARTESIAN_POINT ( 'NONE',  ( 13.79529636645030344, 48.26208216824728936, 14.16423886937410614 ) ) ;
#31419=CARTESIAN_POINT ( 'NONE',  ( 7.361572987183169658, -0.03273551566588185635, -9.846743663894592657 ) ) ;
#31420=CARTESIAN_POINT ( 'NONE',  ( 20.00000000000000711, 98.59912998021083297, 5.000000000000000888 ) ) ;
#31421=CARTESIAN_POINT ( 'NONE',  ( 6.204703633549690345, 42.84541550158063217, 14.16423886937410082 ) ) ;
#31422=CARTESIAN_POINT ( 'NONE',  ( 2.917880565312950480, 65.97041550158063217, -12.26659068614894821 ) ) ;
#31423=CARTESIAN_POINT ( 'NONE',  ( 24.16423886937409904, 24.09541550158063927, 3.795296366450317205 ) ) ;
#31424=CARTESIAN_POINT ( 'NONE',  ( 6.204703633549690345, 20.76208216824730357, -14.16423886937410259 ) ) ;
#31428=CARTESIAN_POINT ( 'NONE',  ( 17.20831665107776587, 39.13393115100079456, -7.208316651077762316 ) ) ;
#31429=VECTOR ( 'NONE', #48833, 1000.000000000000000 ) ;
#31430=CARTESIAN_POINT ( 'NONE',  ( 10.00000000000000000, 26.81368534415484106, -10.88017736071110342 ) ) ;
#31431=CARTESIAN_POINT ( 'NONE',  ( 20.15039907845753220, 55.60158574516643171, -6.262539305110077947 ) ) ;
#31433=CARTESIAN_POINT ( 'NONE',  ( 19.67862543671680697, 89.79758947439231065, -5.461907810393946683 ) ) ;
#31435=CARTESIAN_POINT ( 'NONE',  ( 18.52753015748617571, 38.09226448433412315, 4.923371831947298993 ) ) ;
#31437=CARTESIAN_POINT ( 'NONE',  ( 22.81628187352647785, 51.41530133659708923, 3.434112377981063169 ) ) ;
#31440=CARTESIAN_POINT ( 'NONE',  ( 19.84674366389459266, 38.71726448433412315, -2.638427012816827677 ) ) ;
#31441=CARTESIAN_POINT ( 'NONE',  ( 19.84674366389459266, 58.30059781766745886, 2.638427012816836559 ) ) ;
#31442=CARTESIAN_POINT ( 'NONE',  ( 22.26659068614894466, 33.88708216824730357, 7.082119434687054849 ) ) ;
#31445=CARTESIAN_POINT ( 'NONE',  ( 2.917880565312950480, 10.97041550158063572, -12.26659068614894821 ) ) ;
#31446=DIRECTION ( 'NONE',  ( 0.000000000000000000, 0.000000000000000000, 1.000000000000000000 ) ) ;
#31447=CARTESIAN_POINT ( 'NONE',  ( 10.00000000000000178, 4.313685344154837509, 10.88017736071110342 ) ) ;
#31448=CARTESIAN_POINT ( 'NONE',  ( 21.09922568453595559, 7.040301336597086568, -6.408140936763230044 ) ) ;
#31450=CARTESIAN_POINT ( 'NONE',  ( 12.63842701281683922, 4.550597817667451750, -9.846743663894590881 ) ) ;
#31453=CARTESIAN_POINT ( 'NONE',  ( 2.603489959281581889, 30.43575266056827999, -6.499999999999995559 ) ) ;
#31454=CARTESIAN_POINT ( 'NONE',  ( -0.3689425029237898834, 61.17874883491396076, -10.36894250292378850 ) ) ;
#31456=CARTESIAN_POINT ( 'NONE',  ( 4.559911319644449179, 23.89701867748817321, 9.422509992056141925 ) ) ;
#31457=CARTESIAN_POINT ( 'NONE',  ( 17.96484262340118221, 19.93868534415484106, 7.964842623401181321 ) ) ;
#31458=CARTESIAN_POINT ( 'NONE',  ( 0.1532563361054082862, 61.21726448433412315, 2.638427012816831674 ) ) ;
#31459=CARTESIAN_POINT ( 'NONE',  ( 17.20831665107776587, 52.88393115100078035, 7.208316651077764980 ) ) ;
#31461=CARTESIAN_POINT ( 'NONE',  ( -45.03864103619531534, 105.4358411858499380, -5.309474494509486497 ) ) ;
#31464=CARTESIAN_POINT ( 'NONE',  ( 12.91533473730993009, 26.60535201082150536, -10.88017736071109987 ) ) ;
#31465=CARTESIAN_POINT ( 'NONE',  ( 22.81628187352647785, 21.62363466993041783, 6.195893100308588602E-16 ) ) ;
#31466=LINE ( 'NONE', #69979, #56078 ) ;
#31467=COLOUR_RGB ( '', 0.09019608, 0.27058824, 0.51372549) ;
#31468=CARTESIAN_POINT ( 'NONE',  ( 19.84674366389459266, 63.30059781766745886, 2.638427012816836559 ) ) ;
#31469=CARTESIAN_POINT ( 'NONE',  ( -0.8801773607111008646, 53.27201867748816966, 2.915334737309923430 ) ) ;
#31470=CARTESIAN_POINT ( 'NONE',  ( 13.43411237798105340, 25.58196800326374998, 12.81628187352647963 ) ) ;
#31471=CARTESIAN_POINT ( 'NONE',  ( 15.44008868035555260, 59.73035201082151247, 9.422509992056143702 ) ) ;
#31473=CARTESIAN_POINT ( 'NONE',  ( 0.2751277870542911397, 50.30223176428831522, 6.499999999999992006 ) ) ;
#31475=CARTESIAN_POINT ( 'NONE',  ( -0.8801773607111009756, 48.06368534415484817, 1.068504757029289695E-15 ) ) ;
#31476=CARTESIAN_POINT ( 'NONE',  ( 17.96484262340118221, 49.93868534415484106, 7.964842623401181321 ) ) ;
#31477=CARTESIAN_POINT ( 'NONE',  ( -2.816281873526473856, 44.12363466993042493, 9.499525473075851096E-16 ) ) ;
#31478=CARTESIAN_POINT ( 'NONE',  ( 20.36894250292379738, 14.92874883491396432, -10.36894250292379027 ) ) ;
#31479=CARTESIAN_POINT ( 'NONE',  ( 14.92337183194729633, 62.67559781766745886, 8.527530157486181039 ) ) ;
#31480=CARTESIAN_POINT ( 'NONE',  ( 7.361572987183169658, 24.96726448433412315, -9.846743663894592657 ) ) ;
#31482=CARTESIAN_POINT ( 'NONE',  ( -0.3689425029237898834, 61.17874883491396076, -10.36894250292378850 ) ) ;
#31484=CARTESIAN_POINT ( 'NONE',  ( 15.44008868035555260, 4.730352010821504471, 9.422509992056143702 ) ) ;
#31486=CARTESIAN_POINT ( 'NONE',  ( 12.91533473730992121, 4.522018677488169658, 10.88017736071110164 ) ) ;
#31487=CARTESIAN_POINT ( 'NONE',  ( 1.472469842513823179, 16.42559781766745175, 4.923371831947296329 ) ) ;
#31488=VECTOR ( 'NONE', #76730, 1000.000000000000000 ) ;
#31490=CARTESIAN_POINT ( 'NONE',  ( 15.44008868035555793, 6.397018677488171434, -9.422509992056140149 ) ) ;
#31491=CARTESIAN_POINT ( 'NONE',  ( 15.44008868035555260, 14.73035201082150536, 9.422509992056143702 ) ) ;
#31492=CARTESIAN_POINT ( 'NONE',  ( 0.1532563361054100626, 45.80059781766745886, -2.638427012816831230 ) ) ;
#31493=CARTESIAN_POINT ( 'NONE',  ( 16.40814093676323893, 40.79030133659708923, 11.09922568453595026 ) ) ;
#31496=CARTESIAN_POINT ( 'NONE',  ( -0.3689425029237898834, 26.17874883491396432, -10.36894250292378850 ) ) ;
#31497=CARTESIAN_POINT ( 'NONE',  ( 10.00000000000000000, 21.81368534415484106, -10.88017736071110342 ) ) ;
#31498=CARTESIAN_POINT ( 'NONE',  ( 24.16423886937409904, 64.09541550158064638, 3.795296366450317205 ) ) ;
#31501=CARTESIAN_POINT ( 'NONE',  ( 2.791683348922237240, 45.38393115100079456, -7.208316651077763204 ) ) ;
#31503=CARTESIAN_POINT ( 'NONE',  ( 18.52753015748617571, 28.09226448433411960, 4.923371831947298993 ) ) ;
#31504=CARTESIAN_POINT ( 'NONE',  ( 1.472469842513823179, 1.425597817667451528, 4.923371831947296329 ) ) ;
#31508=CARTESIAN_POINT ( 'NONE',  ( 10.00000000000000000, 1.813685344154837731, -10.88017736071110342 ) ) ;
#31509=CARTESIAN_POINT ( 'NONE',  ( 0.1532563361054082862, 1.217264484334117824, 2.638427012816831674 ) ) ;
#31511=ORIENTED_EDGE ( 'NONE', *, *, #79843, .T. ) ;
#31512=CARTESIAN_POINT ( 'NONE',  ( 19.84674366389459266, 63.30059781766745886, 2.638427012816836559 ) ) ;
#31513=CARTESIAN_POINT ( 'NONE',  ( 7.084665262690076126, 37.02201867748817676, -10.88017736071110164 ) ) ;
#31514=CARTESIAN_POINT ( 'NONE',  ( -0.8801773607111008646, 43.27201867748817676, 2.915334737309923430 ) ) ;
#31515=CARTESIAN_POINT ( 'NONE',  ( 20.88017736071110519, 5.563685344154837509, 2.639326808657452039E-16 ) ) ;
#31516=CARTESIAN_POINT ( 'NONE',  ( 19.38216949554541202, 25.99863466993042138, 9.382169495545424454 ) ) ;
#31517=CARTESIAN_POINT ( 'NONE',  ( 22.26659068614894466, 13.88708216824730179, 7.082119434687054849 ) ) ;
#31519=CIRCLE ( 'NONE', #47584, 0.5000000000000004441 ) ;
#31522=CARTESIAN_POINT ( 'NONE',  ( 21.09922568453594849, 46.20696800326376064, 6.408140936763242479 ) ) ;
#31524=CARTESIAN_POINT ( 'NONE',  ( 0.1532563361054100626, 40.80059781766745886, -2.638427012816831230 ) ) ;
#31525=CARTESIAN_POINT ( 'NONE',  ( 7.084665262690076126, 19.10535201082150181, 10.88017736071109987 ) ) ;
#31527=CARTESIAN_POINT ( 'NONE',  ( 0.5774900079438607392, 18.48035201082150536, 5.440088680355550821 ) ) ;
#31529=CARTESIAN_POINT ( 'NONE',  ( 19.42250999205614193, 60.14701867748817676, 5.440088680355555262 ) ) ;
#31531=CARTESIAN_POINT ( 'NONE',  ( 0.1532563361054100626, 5.800597817667452638, -2.638427012816831230 ) ) ;
#31532=CARTESIAN_POINT ( 'NONE',  ( 17.96484262340118221, 64.93868534415483396, 7.964842623401181321 ) ) ;
#31534=CARTESIAN_POINT ( 'NONE',  ( 2.603489959281591659, 10.43575266056827644, -6.500000000000006217 ) ) ;
#31535=CARTESIAN_POINT ( 'NONE',  ( 5.076628168052703671, 1.842264484334118047, 8.527530157486179263 ) ) ;
#31537=CARTESIAN_POINT ( 'NONE',  ( 1.472469842513823179, 40.59226448433411605, -4.923371831947296329 ) ) ;
#31540=CARTESIAN_POINT ( 'NONE',  ( 10.00000000000000178, 67.25893115100079456, 9.846743663894594434 ) ) ;
#31543=CARTESIAN_POINT ( 'NONE',  ( 3.591859063236761518, 59.95696800326375353, 11.09922568453594849 ) ) ;
#31544=CARTESIAN_POINT ( 'NONE',  ( 2.917880565312950480, 0.9704155015806342766, -12.26659068614894821 ) ) ;
#31545=CARTESIAN_POINT ( 'NONE',  ( 24.16423886937410614, 24.51208216824730002, -3.795296366450302550 ) ) ;
#31548=CARTESIAN_POINT ( 'NONE',  ( 18.72515096720569616, 10.05509018479935968, 6.500000000000001776 ) ) ;
#31549=CARTESIAN_POINT ( 'NONE',  ( 20.88017736071110519, 20.56368534415484106, 2.639326808657452039E-16 ) ) ;
#31550=DIRECTION ( 'NONE',  ( -0.000000000000000000, -0.000000000000000000, -1.000000000000000000 ) ) ;
#31552=CARTESIAN_POINT ( 'NONE',  ( 2.791683348922240793, 6.633931151000785675, 7.208316651077764092 ) ) ;
#31553=CARTESIAN_POINT ( 'NONE',  ( 22.81628187352647785, 36.62363466993041783, 6.195893100308588602E-16 ) ) ;
#31554=CARTESIAN_POINT ( 'NONE',  ( 19.84674366389459266, 28.71726448433411960, -2.638427012816827677 ) ) ;
#31556=EDGE_CURVE ( 'NONE', #6459, #10733, #39602, .T. ) ;
#31557=CARTESIAN_POINT ( 'NONE',  ( 16.40814093676323893, 10.79030133659708923, 11.09922568453595026 ) ) ;
#31560=CARTESIAN_POINT ( 'NONE',  ( 0.1532563361054082862, 6.217264484334118713, 2.638427012816831674 ) ) ;
#31563=CARTESIAN_POINT ( 'NONE',  ( 4.559911319644449179, 28.89701867748817321, 9.422509992056141925 ) ) ;
#31564=CARTESIAN_POINT ( 'NONE',  ( 17.08211943468705840, 30.13708216824730357, -12.26659068614894466 ) ) ;
#31565=CARTESIAN_POINT ( 'NONE',  ( 1.472469842513823179, 41.42559781766745886, 4.923371831947296329 ) ) ;
#31566=CARTESIAN_POINT ( 'NONE',  ( 0.5774900079438607392, 68.48035201082150536, 5.440088680355550821 ) ) ;
#31567=CARTESIAN_POINT ( 'NONE',  ( 22.81628187352647785, 56.41530133659708213, 3.434112377981063169 ) ) ;
#31569=CARTESIAN_POINT ( 'NONE',  ( 12.91533473730993009, 26.60535201082150536, -10.88017736071109987 ) ) ;
#31571=CARTESIAN_POINT ( 'NONE',  ( 6.565887622018943937, 3.081968003263753531, -12.81628187352647608 ) ) ;
#31572=CARTESIAN_POINT ( 'NONE',  ( 5.076628168052703671, 36.84226448433412315, 8.527530157486179263 ) ) ;
#31575=CARTESIAN_POINT ( 'NONE',  ( 3.591859063236761518, 49.95696800326375353, 11.09922568453594849 ) ) ;
#31577=CARTESIAN_POINT ( 'NONE',  ( 20.88017736071110875, 55.77201867748816966, -2.915334737309920765 ) ) ;
#31581=VECTOR ( 'NONE', #42700, 1000.000000000000000 ) ;
#31582=CARTESIAN_POINT ( 'NONE',  ( 20.88017736071110164, 60.35535201082151957, 2.915334737309930979 ) ) ;
#31583=CARTESIAN_POINT ( 'NONE',  ( 19.42250999205614193, 60.14701867748817676, 5.440088680355555262 ) ) ;
#31586=CARTESIAN_POINT ( 'NONE',  ( -0.8801773607111009756, 8.063685344154837509, 1.068504757029289695E-15 ) ) ;
#31587=CARTESIAN_POINT ( 'NONE',  ( 17.20831665107776587, 54.13393115100079456, -7.208316651077762316 ) ) ;
#31588=CARTESIAN_POINT ( 'NONE',  ( 7.084665262690076126, 27.02201867748817676, -10.88017736071110164 ) ) ;
#31590=CARTESIAN_POINT ( 'NONE',  ( 13.43411237798105340, 30.58196800326374998, 12.81628187352647963 ) ) ;
#31592=CARTESIAN_POINT ( 'NONE',  ( -0.8801773607111008646, 43.27201867748817676, 2.915334737309923430 ) ) ;
#31593=CARTESIAN_POINT ( 'NONE',  ( -1.099225684535947600, 8.706968003263753531, -6.408140936763238038 ) ) ;
#31594=DIRECTION ( 'NONE',  ( -0.000000000000000000, -0.000000000000000000, 1.000000000000000000 ) ) ;
#31595=CARTESIAN_POINT ( 'NONE',  ( 17.96484262340118221, 9.938685344154837509, 7.964842623401181321 ) ) ;
#31596=CARTESIAN_POINT ( 'NONE',  ( 20.88017736071110519, 35.56368534415484106, 2.639326808657452039E-16 ) ) ;
#31597=CARTESIAN_POINT ( 'NONE',  ( 6.204703633549690345, 35.76208216824729647, -14.16423886937410259 ) ) ;
#31598=CARTESIAN_POINT ( 'NONE',  ( 19.84674366389459621, 23.50893115100078390, 7.409399052514197653E-17 ) ) ;
#31599=CARTESIAN_POINT ( 'NONE',  ( 15.44008868035555260, 64.73035201082151957, 9.422509992056143702 ) ) ;
#31600=CARTESIAN_POINT ( 'NONE',  ( 1.274849032794324932, 32.55509018479936145, -6.500000000000021316 ) ) ;
#31601=CARTESIAN_POINT ( 'NONE',  ( 2.917880565312948704, 17.63708216824730357, 12.26659068614894643 ) ) ;
#31604=CARTESIAN_POINT ( 'NONE',  ( 7.361572987183169658, 59.96726448433410894, -9.846743663894592657 ) ) ;
#31608=CARTESIAN_POINT ( 'NONE',  ( 22.26659068614895176, 29.72041550158063572, -7.082119434687042414 ) ) ;
#31609=CARTESIAN_POINT ( 'NONE',  ( 2.917880565312948704, 32.63708216824730357, 12.26659068614894643 ) ) ;
#31610=CARTESIAN_POINT ( 'NONE',  ( 0.1532563361054100626, 5.800597817667452638, -2.638427012816831230 ) ) ;
#31611=CARTESIAN_POINT ( 'NONE',  ( -2.816281873526473856, 9.331968003263753531, 3.434112377981055619 ) ) ;
#31612=CARTESIAN_POINT ( 'NONE',  ( 1.472469842513823179, 65.59226448433412315, -4.923371831947296329 ) ) ;
#31614=CARTESIAN_POINT ( 'NONE',  ( 17.96484262340118221, 66.18868534415483396, -7.964842623401177768 ) ) ;
#31615=CARTESIAN_POINT ( 'NONE',  ( -2.816281873526473856, 19.33196800326375708, 3.434112377981055619 ) ) ;
#31616=CARTESIAN_POINT ( 'NONE',  ( -2.266590686148945544, 31.38708216824730002, -7.082119434687050408 ) ) ;
#31617=CARTESIAN_POINT ( 'NONE',  ( -0.8801773607111009756, 33.06368534415484106, 1.068504757029289695E-15 ) ) ;
#31619=CARTESIAN_POINT ( 'NONE',  ( 15.44008868035555260, 29.73035201082150891, 9.422509992056143702 ) ) ;
#31620=CARTESIAN_POINT ( 'NONE',  ( 21.92686044187657401, 5.370456701841137992, -3.195792623639525765 ) ) ;
#31621=CARTESIAN_POINT ( 'NONE',  ( -0.8801773607110991993, 57.85535201082149825, -2.915334737309923874 ) ) ;
#31628=CARTESIAN_POINT ( 'NONE',  ( -0.3689425029237881626, 2.428748834913967869, 10.36894250292379027 ) ) ;
#31629=CARTESIAN_POINT ( 'NONE',  ( 10.00000000000000000, 60.55374883491397497, -14.16423886937410082 ) ) ;
#31630=CARTESIAN_POINT ( 'NONE',  ( 24.16423886937410614, 59.51208216824728936, -3.795296366450302550 ) ) ;
#31631=CARTESIAN_POINT ( 'NONE',  ( 5.076628168052704559, 40.17559781766745175, -8.527530157486179263 ) ) ;
#31632=CARTESIAN_POINT ( 'NONE',  ( 2.791683348922240793, 66.63393115100079456, 7.208316651077764092 ) ) ;
#31635=CARTESIAN_POINT ( 'NONE',  ( 10.00000000000000178, 10.37363466993041961, 12.81628187352647608 ) ) ;
#31636=VERTEX_POINT ( 'NONE', #16336 ) ;
#31637=CARTESIAN_POINT ( 'NONE',  ( 20.36894250292379382, 43.67874883491397497, 10.36894250292379205 ) ) ;
#31639=CARTESIAN_POINT ( 'NONE',  ( 10.00000000000000000, 45.55374883491397497, -14.16423886937410082 ) ) ;
#31641=CARTESIAN_POINT ( 'NONE',  ( 20.88017736071110875, 20.77201867748816611, -2.915334737309920765 ) ) ;
#31642=CARTESIAN_POINT ( 'NONE',  ( 10.00000000000000000, 57.87363466993042493, -12.81628187352647608 ) ) ;
#31644=CARTESIAN_POINT ( 'NONE',  ( 12.91533473730992121, 24.52201867748816966, 10.88017736071110164 ) ) ;
#31645=CARTESIAN_POINT ( 'NONE',  ( 19.84674366389459266, 53.71726448433411605, -2.638427012816827677 ) ) ;
#31646=CARTESIAN_POINT ( 'NONE',  ( 0.5774900079438590739, 37.64701867748817676, -5.440088680355550821 ) ) ;
#31647=CARTESIAN_POINT ( 'NONE',  ( -1.926860441876562025, 64.47997603579416648, -3.195792623639529761 ) ) ;
#31648=CARTESIAN_POINT ( 'NONE',  ( 0.1532563361054100626, 50.80059781766745175, -2.638427012816831230 ) ) ;
#31650=CARTESIAN_POINT ( 'NONE',  ( 10.00000000000000000, 31.81368534415483751, -10.88017736071110342 ) ) ;
#31654=CARTESIAN_POINT ( 'NONE',  ( -0.1503990784575247319, 37.22266099184918176, -6.262539305110083276 ) ) ;
#31656=CARTESIAN_POINT ( 'NONE',  ( 7.361572987183170547, 2.050597817667451750, 9.846743663894590881 ) ) ;
#31660=CARTESIAN_POINT ( 'NONE',  ( 1.472469842513823179, 35.59226448433412315, -4.923371831947296329 ) ) ;
#31662=CARTESIAN_POINT ( 'NONE',  ( -45.94000000000000483, 92.50000000000000000, 9.000000000000000000 ) ) ;
#31666=CARTESIAN_POINT ( 'NONE',  ( 0.1532563361054083140, 51.00893115100078745, 1.131784320476157264E-15 ) ) ;
#31667=CARTESIAN_POINT ( 'NONE',  ( 2.917880565312948704, 52.63708216824730357, 12.26659068614894643 ) ) ;
#31668=CARTESIAN_POINT ( 'NONE',  ( 18.52753015748618282, 53.92559781766745175, -4.923371831947291888 ) ) ;
#31670=CARTESIAN_POINT ( 'NONE',  ( 18.52753015748617571, 18.09226448433411960, 4.923371831947298993 ) ) ;
#31671=CARTESIAN_POINT ( 'NONE',  ( 16.40814093676323893, 50.79030133659708923, 11.09922568453595026 ) ) ;
#31672=CARTESIAN_POINT ( 'NONE',  ( 0.1532563361054100626, 55.80059781766745175, -2.638427012816831230 ) ) ;
#31673=CARTESIAN_POINT ( 'NONE',  ( 19.42250999205614548, 50.98035201082151247, -5.440088680355545492 ) ) ;
#31674=CARTESIAN_POINT ( 'NONE',  ( 7.361572987183169658, 49.96726448433410894, -9.846743663894592657 ) ) ;
#31676=CARTESIAN_POINT ( 'NONE',  ( 20.88017736071110875, 55.77201867748816966, -2.915334737309920765 ) ) ;
#31677=EDGE_LOOP ( 'NONE', ( #3032, #26227, #11016, #50884 ) ) ;
#31678=DIRECTION ( 'NONE',  ( 0.01646788341559294114, 0.9998643952135761737, 0.000000000000000000 ) ) ;
#31679=CARTESIAN_POINT ( 'NONE',  ( 7.084665262690076126, 29.10535201082150181, 10.88017736071109987 ) ) ;
#31680=CARTESIAN_POINT ( 'NONE',  ( 0.6178305044545838731, 19.74863466993042138, 9.382169495545420901 ) ) ;
#31681=CARTESIAN_POINT ( 'NONE',  ( 15.44008868035555793, 61.39701867748817676, -9.422509992056140149 ) ) ;
#31682=CARTESIAN_POINT ( 'NONE',  ( 19.42250999205614193, 65.14701867748817676, 5.440088680355555262 ) ) ;
#31683=CARTESIAN_POINT ( 'NONE',  ( 18.52753015748617571, 13.09226448433411960, 4.923371831947298993 ) ) ;
#31685=CARTESIAN_POINT ( 'NONE',  ( 12.91533473730993009, 56.60535201082151247, -10.88017736071109987 ) ) ;
#31686=CARTESIAN_POINT ( 'NONE',  ( -0.03743638938522819704, 54.25197528031017669, -6.399506433553964868 ) ) ;
#31688=VECTOR ( 'NONE', #77331, 1000.000000000000000 ) ;
#31689=CARTESIAN_POINT ( 'NONE',  ( 2.791683348922237240, 35.38393115100079456, -7.208316651077763204 ) ) ;
#31690=CARTESIAN_POINT ( 'NONE',  ( 5.076628168052704559, 5.175597817667451750, -8.527530157486179263 ) ) ;
#31692=CARTESIAN_POINT ( 'NONE',  ( -1.099225684535947600, 14.54030133659708568, 6.408140936763237150 ) ) ;
#31693=CARTESIAN_POINT ( 'NONE',  ( 10.00000000000000178, 9.313685344154839285, 10.88017736071110342 ) ) ;
#31696=CARTESIAN_POINT ( 'NONE',  ( 22.26659068614894466, 28.88708216824730357, 7.082119434687054849 ) ) ;
#31697=CARTESIAN_POINT ( 'NONE',  ( 10.00000000000000000, 60.55374883491397497, -14.16423886937410082 ) ) ;
#31698=CARTESIAN_POINT ( 'NONE',  ( 0.1532563361054100626, 35.80059781766745175, -2.638427012816831230 ) ) ;
#31699=CARTESIAN_POINT ( 'NONE',  ( 17.20831665107776587, 24.13393115100078035, -7.208316651077762316 ) ) ;
#31700=CARTESIAN_POINT ( 'NONE',  ( 10.00000000000000178, 14.31368534415483751, 10.88017736071110342 ) ) ;
#31702=CARTESIAN_POINT ( 'NONE',  ( 14.92337183194729988, 34.34226448433411605, -8.527530157486177487 ) ) ;
#31703=CARTESIAN_POINT ( 'NONE',  ( 0.5774900079438607392, 23.48035201082150536, 5.440088680355550821 ) ) ;
#31704=CARTESIAN_POINT ( 'NONE',  ( 18.52753015748617571, 63.09226448433412315, 4.923371831947298993 ) ) ;
#31705=CARTESIAN_POINT ( 'NONE',  ( -4.164238869374098151, 1.595415501580634388, -3.795296366450310543 ) ) ;
#31708=CARTESIAN_POINT ( 'NONE',  ( 0.1532563361054083140, 11.00893115100078568, 1.131784320476157264E-15 ) ) ;
#31709=CARTESIAN_POINT ( 'NONE',  ( -2.816281873526473856, 39.12363466993041783, 9.499525473075851096E-16 ) ) ;
#31710=CARTESIAN_POINT ( 'NONE',  ( 0.1532563361054082862, 61.21726448433412315, 2.638427012816831674 ) ) ;
#31711=ORIENTED_EDGE ( 'NONE', *, *, #83558, .F. ) ;
#31712=CARTESIAN_POINT ( 'NONE',  ( 10.00000000000000000, 19.75893115100078390, -9.846743663894594434 ) ) ;
#31714=CARTESIAN_POINT ( 'NONE',  ( -46.48928645636213730, 103.2957187381727238, -6.397878122524045530 ) ) ;
#31715=CARTESIAN_POINT ( 'NONE',  ( -2.266590686148945544, 52.22041550158064638, 7.082119434687048631 ) ) ;
#31716=CARTESIAN_POINT ( 'NONE',  ( -0.8801773607110991993, 52.85535201082151247, -2.915334737309923874 ) ) ;
#31717=CARTESIAN_POINT ( 'NONE',  ( 13.79529636645030344, 3.262082168247301350, 14.16423886937410614 ) ) ;
#31718=CARTESIAN_POINT ( 'NONE',  ( 15.44008868035555793, 61.39701867748817676, -9.422509992056140149 ) ) ;
#31719=CARTESIAN_POINT ( 'NONE',  ( 10.00000000000000178, 42.25893115100078745, 9.846743663894594434 ) ) ;
#31720=CARTESIAN_POINT ( 'NONE',  ( 17.96484262340118221, 24.93868534415484461, 7.964842623401181321 ) ) ;
#31721=CARTESIAN_POINT ( 'NONE',  ( 2.791683348922240793, 46.63393115100077324, 7.208316651077764092 ) ) ;
#31722=CARTESIAN_POINT ( 'NONE',  ( -0.8801773607111009756, 43.06368534415484106, 1.068504757029289695E-15 ) ) ;
#31730=CARTESIAN_POINT ( 'NONE',  ( 17.08211943468705130, 3.470415501580634388, 12.26659068614894998 ) ) ;
#31731=CARTESIAN_POINT ( 'NONE',  ( 17.20831665107776587, 47.88393115100078745, 7.208316651077764980 ) ) ;
#31732=CARTESIAN_POINT ( 'NONE',  ( 5.076628168052703671, 21.84226448433411960, 8.527530157486179263 ) ) ;
#31733=CARTESIAN_POINT ( 'NONE',  ( 3.591859063236761518, 59.95696800326375353, 11.09922568453594849 ) ) ;
#31734=CARTESIAN_POINT ( 'NONE',  ( 12.91533473730993009, 16.60535201082150891, -10.88017736071109987 ) ) ;
#31735=CARTESIAN_POINT ( 'NONE',  ( 7.361572987183169658, 54.96726448433413026, -9.846743663894592657 ) ) ;
#31737=CARTESIAN_POINT ( 'NONE',  ( 17.08211943468705840, 45.13708216824730357, -12.26659068614894466 ) ) ;
#31739=CARTESIAN_POINT ( 'NONE',  ( 2.917880565312948704, 57.63708216824731068, 12.26659068614894643 ) ) ;
#31740=CARTESIAN_POINT ( 'NONE',  ( 1.274849032794292736, 67.55509018479936856, -6.499999999999977796 ) ) ;
#31742=CARTESIAN_POINT ( 'NONE',  ( 7.084665262690076126, 52.02201867748816255, -10.88017736071110164 ) ) ;
#31743=CARTESIAN_POINT ( 'NONE',  ( 1.472469842513823179, 21.42559781766745175, 4.923371831947296329 ) ) ;
#31747=( BOUNDED_SURFACE ( )  B_SPLINE_SURFACE ( 1, 2, ( 
 ( #94875, #3394, #24927, #78893, #18396, #16926, #47894, #26376, #87376, #85913, #9918, #56875, #1448, #40421, #31899, #54900, #85415, #80372, #58840, #88363, #97360, #5852, #19858, #50352, #36343, #66336, #96376, #66839, #12361, #27848, #89832, #27359, #59329, #88854, #80863, #58335, #96873, #42378, #42867, #73351, #4876, #28350, #20362, #65350, #11872, #79874, #35354, #28829, #65846, #50857, #12846, #81350, #73843, #43345, #11378, #72360, #5372, #20857, #89347, #51348, #72854, #41898, #81832, #13347, #34360, #34856, #95878, #43831, #74327, #3892, #64851, #95370, #26869, #57365, #87860, #7344, #69314, #13848, #31296, #52819, #61305, #37844, #14346, #53817, #53314, #21852, #22839, #59820, #98856, #68335, #83327, #14853, #52332, #38334, #68827, #90314, #30310, #74831, #358, #836, #15347, #30807, #6335, #45831, #82826, #45325, #29818, #75822, #75324, #37351, #84329, #98360, #60327, #91816, #23337, #90817, #60811, #22347, #61796, #91310, #76317, #92304, #15829, #67335, #76802, #8319, #38823, #51840, #82327, #97860, #85793, #88110, #25303, #65102, #80118, #47783, #87617, #84809, #32772, #70307, #65598, #27112, #19130, #8803, #40294, #11626, #42142, #2319, #4636, #95623, #54294, #57611, #47282, #19619, #50113, #80623, #12117, #62285, #42619, #70802, #16315, #77291, #1335, #92789, #93283, #54784, #85300, #39806, #1823, #24807, #55284, #52579, #88599, #75581, #51103, #28599, #37102, #98106, #89597, #37595, #51605, #74590, #29568, #96126, #96623, #36609, #67096, #50613, #43106, #35608, #73593, #66094, #29084, #21609, #34204, #81558, #36065, #97094, #90050, #51569, #57209, #41746, #71735, #43557, #98077, #28565, #74054, #6072, #89564, #67061, #82055, #52547, #64211, #66566, #14073, #19220, #13564, #64695, #29536, #74555, #36572, #56727, #72215, #3746, #60042, #87218, #97586, #90539, #21573, #79726, #49224, #29046, #59555, #82556, #11226, #44553, #75048, #6557, #87705, #95207, #37067, #67565, #22072, #14571, #3245, #33712, #94727, #18741, #26712, #49702, #76531, #39533, #75547, #91034, #7571, #62011, #98585, #38546, #23556, #84536, #47012, #85022, #62501, #77022, #61516, #76038, #84040, #45540, #69041, #24538, #15071, #575, #15561, #9015, #30033, #91541, #39037, #83549, #54025, #7063, #69531, #92511, #70025, #68550, #23058, #1549, #31994, #81, #16033, #31020, #53033, #53527, #93004, #54998, #46046, #92026, #85516, #60542, #30528, #54509, #22564, #61029, #46522, #8536, #1045, #31512, #41993, #93996, #86510, #72457, #3500, #33470, #3990, #48487, #63966, #57464, #63494, #95475, #25997, #25519, #56492, #86981, #3021, #78989, #10495 ),
 ( #10988, #64462, #11476, #47992, #56007, #34455, #18986, #78503, #18491, #41007, #55514, #18006, #17027, #47506, #71508, #48979, #87472, #49464, #10016, #26470, #9514, #40014, #86013, #94968, #79488, #78007, #2040, #41508, #33957, #32501, #56969, #79970, #62999, #93503, #17526, #40517, #71014, #2536, #32990, #65946, #5471, #36447, #50451, #96473, #20460, #12946, #66939, #66439, #73444, #57949, #87957, #58437, #13954, #35943, #27945, #20959, #28447, #13442, #58944, #67441, #80468, #88952, #89931, #50950, #81445, #80958, #44428, #89445, #51446, #72954, #88456, #12457, #74932, #34950, #43929, #6432, #21447, #95973, #42963, #74427, #51944, #82429, #4970, #29416, #11967, #91905, #45413, #29912, #61887, #53909, #92392, #77380, #8893, #91412, #46406, #39409, #925, #69903, #22938, #54386, #59921, #6938, #22441, #8409, #14446, #53406, #38424, #450, #31387, #23917, #1423, #23430, #76412, #52913, #16411, #90409, #15443, #46889, #21951, #37445, #14944, #38916, #44916, #45923, #68922, #61395, #52430, #82928, #75424, #84418, #7927, #75918, #98951, #37939, #15915, #67936, #68429, #69404, #30407, #98456, #60910, #9894, #86868, #1915, #40884, #92879, #18376, #79364, #26352, #62879, #40398, #79850, #64341, #24904, #48855, #41393, #32374, #70893, #31875, #85390, #93871, #25398, #3372, #16903, #55387, #17402, #95346, #26844, #42354, #81806, #42842, #21328, #59309, #73326, #4851, #89807, #58816, #50835, #51817, #35326, #81328, #13825, #50325, #82303, #12823, #65820, #43322, #20833, #65325, #27825, #58311, #88827, #51322, #5349, #88339, #72829, #34332, #28325, #44306, #13325, #43809, #74304, #5829, #36323, #66816, #64828, #57340, #97338, #19352, #49836, #80348, #95850, #11845, #4367, #27333, #57830, #19836, #70282, #3254, #54758, #85773, #64221, #25767, #93259, #24783, #40270, #48249, #56261, #17283, #10267, #86754, #18259, #47760, #78258, #48736, #79242, #10755, #94737, #56736, #46773, #35708, #36204, #96230, #4242, #87718, #18752, #88212, #43698, #35200, #57712, #50718, #65704, #12711, #27709, #97230, #11235, #19720, #58700, #65207, #27211, #11727, #74185, #88704, #50209, #72225, #19232, #49713, #5716, #3755, #80720, #66702, #66196, #26725, #95218, #12216, #42724, #96728, #57220, #58193, #20214, #81211, #34712, #80223, #20717, #43205, #51208, #28697, #59189, #73696, #28204, #49236, #89204, #79738, #81692, #13205, #41755, #42240, #72706, #95727, #13700, #67701, #83183, #45182, #15197, #83682, #209, #37697, #22203, #59685, #6695, #29187, #98213, #61166, #97724, #60180, #37213, #45679, #44185, #44687, #68195, #67198, #14708, #89695, #98716, #53176 ) ),
 .UNSPECIFIED., .F., .F., .F. ) 
 B_SPLINE_SURFACE_WITH_KNOTS ( ( 2, 2 ),
 ( 3, 2, 2, 2, 2, 2, 2, 2, 2, 2, 2, 2, 2, 2, 2, 2, 2, 2, 2, 2, 2, 2, 2, 2, 2, 2, 2, 2, 2, 2, 2, 2, 2, 2, 2, 2, 2, 2, 2, 2, 2, 2, 2, 2, 2, 2, 2, 2, 2, 2, 2, 2, 2, 2, 2, 2, 2, 2, 2, 2, 2, 2, 2, 2, 2, 2, 2, 2, 2, 2, 2, 2, 2, 2, 2, 2, 2, 2, 2, 2, 2, 2, 2, 2, 2, 2, 2, 2, 2, 2, 2, 2, 2, 2, 2, 2, 2, 2, 2, 2, 2, 2, 2, 2, 2, 2, 2, 2, 2, 2, 2, 2, 2, 2, 2, 2, 2, 2, 2, 2, 2, 2, 2, 2, 2, 2, 2, 2, 2, 2, 2, 2, 2, 2, 2, 2, 2, 2, 2, 2, 2, 2, 2, 2, 2, 2, 2, 2, 2, 2, 2, 2, 2, 2, 2, 2, 2, 2, 2, 2, 2, 2, 3 ),
 ( 0.000000000000000000, 1.000000000000000000 ),
 ( 0.000000000000000000, 0.005952380952380952051, 0.01190476190476190410, 0.01785714285714285615, 0.02380952380952380820, 0.02976190476190476025, 0.03571428571428571230, 0.04166666666666666435, 0.04761904761904761640, 0.05357142857142856845, 0.05952380952380952051, 0.06547619047619047949, 0.07142857142857142461, 0.07738095238095238360, 0.08333333333333332871, 0.08928571428571428770, 0.09523809523809523281, 0.1011904761904761918, 0.1071428571428571369, 0.1130952380952380959, 0.1190476190476190410, 0.1250000000000000000, 0.1309523809523809590, 0.1369047619047619180, 0.1428571428571428492, 0.1488095238095238082, 0.1547619047619047672, 0.1607142857142857262, 0.1666666666666666574, 0.1726190476190476164, 0.1785714285714285754, 0.1845238095238095344, 0.1904761904761904656, 0.1964285714285714246, 0.2023809523809523836, 0.2083333333333333426, 0.2142857142857142738, 0.2202380952380952328, 0.2261904761904761918, 0.2321428571428571508, 0.2380952380952380820, 0.2440476190476190410, 0.2500000000000000000, 0.2559523809523809312, 0.2619047619047619180, 0.2678571428571428492, 0.2738095238095238360, 0.2797619047619047672, 0.2857142857142856984, 0.2916666666666666852, 0.2976190476190476164, 0.3035714285714285476, 0.3095238095238095344, 0.3154761904761904656, 0.3214285714285714524, 0.3273809523809523836, 0.3333333333333333148, 0.3392857142857143016, 0.3452380952380952328, 0.3511904761904761640, 0.3571428571428571508, 0.3630952380952380820, 0.3690476190476190688, 0.3750000000000000000, 0.3809523809523809312, 0.3869047619047619180, 0.3928571428571428492, 0.3988095238095238360, 0.4047619047619047672, 0.4107142857142856984, 0.4166666666666666852, 0.4226190476190476164, 0.4285714285714285476, 0.4345238095238095344, 0.4404761904761904656, 0.4464285714285714524, 0.4523809523809523836, 0.4583333333333333148, 0.4642857142857143016, 0.4702380952380952328, 0.4761904761904761640, 0.4821428571428571508, 0.4880952380952380820, 0.4940476190476190688, 0.5000000000000000000, 0.5059523809523809312, 0.5119047619047618625, 0.5178571428571429047, 0.5238095238095238360, 0.5297619047619047672, 0.5357142857142856984, 0.5416666666666666297, 0.5476190476190476719, 0.5535714285714286031, 0.5595238095238095344, 0.5654761904761904656, 0.5714285714285713969, 0.5773809523809523281, 0.5833333333333333703, 0.5892857142857143016, 0.5952380952380952328, 0.6011904761904761640, 0.6071428571428570953, 0.6130952380952381375, 0.6190476190476190688, 0.6250000000000000000, 0.6309523809523809312, 0.6369047619047618625, 0.6428571428571429047, 0.6488095238095238360, 0.6547619047619047672, 0.6607142857142856984, 0.6666666666666666297, 0.6726190476190476719, 0.6785714285714286031, 0.6845238095238095344, 0.6904761904761904656, 0.6964285714285713969, 0.7023809523809523281, 0.7083333333333333703, 0.7142857142857143016, 0.7202380952380952328, 0.7261904761904761640, 0.7321428571428570953, 0.7380952380952381375, 0.7440476190476190688, 0.7500000000000000000, 0.7559523809523809312, 0.7619047619047618625, 0.7678571428571429047, 0.7738095238095238360, 0.7797619047619047672, 0.7857142857142856984, 0.7916666666666666297, 0.7976190476190476719, 0.8035714285714286031, 0.8095238095238095344, 0.8154761904761904656, 0.8214285714285713969, 0.8273809523809523281, 0.8333333333333333703, 0.8392857142857143016, 0.8452380952380952328, 0.8511904761904761640, 0.8571428571428570953, 0.8630952380952381375, 0.8690476190476190688, 0.8750000000000000000, 0.8809523809523809312, 0.8869047619047618625, 0.8928571428571429047, 0.8988095238095238360, 0.9047619047619047672, 0.9107142857142856984, 0.9166666666666666297, 0.9226190476190476719, 0.9285714285714286031, 0.9345238095238095344, 0.9404761904761904656, 0.9464285714285713969, 0.9523809523809523281, 0.9583333333333333703, 0.9642857142857143016 ),
 .UNSPECIFIED. ) 
 GEOMETRIC_REPRESENTATION_ITEM ( )  RATIONAL_B_SPLINE_SURFACE ( (
 ( 1.000000000000000000, 0.9659258262890683122, 1.000000000000000000, 0.9659258262890683122, 1.000000000000000000, 0.9659258262890683122, 1.000000000000000000, 0.9659258262890683122, 1.000000000000000000, 0.9659258262890683122, 1.000000000000000000, 0.9659258262890683122, 1.000000000000000000, 0.9659258262890683122, 1.000000000000000000, 0.9659258262890683122, 1.000000000000000000, 0.9659258262890683122, 1.000000000000000000, 0.9659258262890683122, 1.000000000000000000, 0.9659258262890683122, 1.000000000000000000, 0.9659258262890683122, 1.000000000000000000, 0.9659258262890683122, 1.000000000000000000, 0.9659258262890683122, 1.000000000000000000, 0.9659258262890683122, 1.000000000000000000, 0.9659258262890683122, 1.000000000000000000, 0.9659258262890683122, 1.000000000000000000, 0.9659258262890683122, 1.000000000000000000, 0.9659258262890683122, 1.000000000000000000, 0.9659258262890683122, 1.000000000000000000, 0.9659258262890683122, 1.000000000000000000, 0.9659258262890683122, 1.000000000000000000, 0.9659258262890683122, 1.000000000000000000, 0.9659258262890683122, 1.000000000000000000, 0.9659258262890683122, 1.000000000000000000, 0.9659258262890683122, 1.000000000000000000, 0.9659258262890683122, 1.000000000000000000, 0.9659258262890683122, 1.000000000000000000, 0.9659258262890683122, 1.000000000000000000, 0.9659258262890683122, 1.000000000000000000, 0.9659258262890683122, 1.000000000000000000, 0.9659258262890683122, 1.000000000000000000, 0.9659258262890683122, 1.000000000000000000, 0.9659258262890683122, 1.000000000000000000, 0.9659258262890683122, 1.000000000000000000, 0.9659258262890683122, 1.000000000000000000, 0.9659258262890683122, 1.000000000000000000, 0.9659258262890683122, 1.000000000000000000, 0.9659258262890683122, 1.000000000000000000, 0.9659258262890683122, 1.000000000000000000, 0.9659258262890683122, 1.000000000000000000, 0.9659258262890683122, 1.000000000000000000, 0.9659258262890683122, 1.000000000000000000, 0.9659258262890683122, 1.000000000000000000, 0.9659258262890683122, 1.000000000000000000, 0.9659258262890683122, 1.000000000000000000, 0.9659258262890683122, 1.000000000000000000, 0.9659258262890683122, 1.000000000000000000, 0.9659258262890683122, 1.000000000000000000, 0.9659258262890683122, 1.000000000000000000, 0.9659258262890683122, 1.000000000000000000, 0.9659258262890683122, 1.000000000000000000, 0.9659258262890683122, 1.000000000000000000, 0.9659258262890683122, 1.000000000000000000, 0.9659258262890683122, 1.000000000000000000, 0.9659258262890683122, 1.000000000000000000, 0.9659258262890683122, 1.000000000000000000, 0.9659258262890683122, 1.000000000000000000, 0.9659258262890683122, 1.000000000000000000, 0.9659258262890683122, 1.000000000000000000, 0.9659258262890683122, 1.000000000000000000, 0.9659258262890683122, 1.000000000000000000, 0.9659258262890683122, 1.000000000000000000, 0.9659258262890683122, 1.000000000000000000, 0.9659258262890683122, 1.000000000000000000, 0.9659258262890683122, 1.000000000000000000, 0.9659258262890683122, 1.000000000000000000, 0.9659258262890683122, 1.000000000000000000, 0.9659258262890683122, 1.000000000000000000, 0.9659258262890683122, 1.000000000000000000, 0.9659258262890683122, 1.000000000000000000, 0.9659258262890683122, 1.000000000000000000, 0.9659258262890683122, 1.000000000000000000, 0.9659258262890683122, 1.000000000000000000, 0.9659258262890683122, 1.000000000000000000, 0.9659258262890683122, 1.000000000000000000, 0.9659258262890683122, 1.000000000000000000, 0.9659258262890683122, 1.000000000000000000, 0.9659258262890683122, 1.000000000000000000, 0.9659258262890683122, 1.000000000000000000, 0.9659258262890683122, 1.000000000000000000, 0.9659258262890683122, 1.000000000000000000, 0.9659258262890683122, 1.000000000000000000, 0.9659258262890683122, 1.000000000000000000, 0.9659258262890683122, 1.000000000000000000, 0.9659258262890683122, 1.000000000000000000, 0.9659258262890683122, 1.000000000000000000, 0.9659258262890683122, 1.000000000000000000, 0.9659258262890683122, 1.000000000000000000, 0.9659258262890683122, 1.000000000000000000, 0.9659258262890683122, 1.000000000000000000, 0.9659258262890683122, 1.000000000000000000, 0.9659258262890683122, 1.000000000000000000, 0.9659258262890683122, 1.000000000000000000, 0.9659258262890683122, 1.000000000000000000, 0.9659258262890683122, 1.000000000000000000, 0.9659258262890683122, 1.000000000000000000, 0.9659258262890683122, 1.000000000000000000, 0.9659258262890683122, 1.000000000000000000, 0.9659258262890683122, 1.000000000000000000, 0.9659258262890683122, 1.000000000000000000, 0.9659258262890683122, 1.000000000000000000, 0.9659258262890683122, 1.000000000000000000, 0.9659258262890683122, 1.000000000000000000, 0.9659258262890683122, 1.000000000000000000, 0.9659258262890683122, 1.000000000000000000, 0.9659258262890683122, 1.000000000000000000, 0.9659258262890683122, 1.000000000000000000, 0.9659258262890683122, 1.000000000000000000, 0.9659258262890683122, 1.000000000000000000, 0.9659258262890683122, 1.000000000000000000, 0.9659258262890683122, 1.000000000000000000, 0.9659258262890683122, 1.000000000000000000, 0.9659258262890683122, 1.000000000000000000, 0.9659258262890683122, 1.000000000000000000, 0.9659258262890683122, 1.000000000000000000, 0.9659258262890683122, 1.000000000000000000, 0.9659258262890683122, 1.000000000000000000, 0.9659258262890683122, 1.000000000000000000, 0.9659258262890683122, 1.000000000000000000, 0.9659258262890683122, 1.000000000000000000, 0.9659258262890683122, 1.000000000000000000, 0.9659258262890683122, 1.000000000000000000, 0.9659258262890683122, 1.000000000000000000, 0.9659258262890683122, 1.000000000000000000, 0.9659258262890683122, 1.000000000000000000, 0.9659258262890683122, 1.000000000000000000, 0.9659258262890683122, 1.000000000000000000, 0.9659258262890683122, 1.000000000000000000, 0.9659258262890683122, 1.000000000000000000, 0.9659258262890683122, 1.000000000000000000, 0.9659258262890683122, 1.000000000000000000, 0.9659258262890683122, 1.000000000000000000, 0.9659258262890683122, 1.000000000000000000, 0.9659258262890683122, 1.000000000000000000, 0.9659258262890683122, 1.000000000000000000, 0.9659258262890683122, 1.000000000000000000, 0.9659258262890683122, 1.000000000000000000, 0.9659258262890683122, 1.000000000000000000, 0.9659258262890683122, 1.000000000000000000, 0.9659258262890683122, 1.000000000000000000, 0.9659258262890683122, 1.000000000000000000, 0.9659258262890683122, 1.000000000000000000, 0.9659258262890683122, 1.000000000000000000, 0.9659258262890683122, 1.000000000000000000, 0.9659258262890683122, 1.000000000000000000, 0.9659258262890683122, 1.000000000000000000, 0.9659258262890683122, 1.000000000000000000, 0.9659258262890683122, 1.000000000000000000, 0.9659258262890683122, 1.000000000000000000, 0.9659258262890683122, 1.000000000000000000, 0.9659258262890683122, 1.000000000000000000, 0.9659258262890683122, 1.000000000000000000, 0.9659258262890683122, 1.000000000000000000, 0.9659258262890683122, 1.000000000000000000, 0.9659258262890683122, 1.000000000000000000, 0.9659258262890683122, 1.000000000000000000, 0.9659258262890683122, 1.000000000000000000, 0.9659258262890683122, 1.000000000000000000, 0.9659258262890683122, 1.000000000000000000, 0.9659258262890683122, 1.000000000000000000, 0.9659258262890683122, 1.000000000000000000),
 ( 1.000000000000000000, 0.9659258262890683122, 1.000000000000000000, 0.9659258262890683122, 1.000000000000000000, 0.9659258262890683122, 1.000000000000000000, 0.9659258262890683122, 1.000000000000000000, 0.9659258262890683122, 1.000000000000000000, 0.9659258262890683122, 1.000000000000000000, 0.9659258262890683122, 1.000000000000000000, 0.9659258262890683122, 1.000000000000000000, 0.9659258262890683122, 1.000000000000000000, 0.9659258262890683122, 1.000000000000000000, 0.9659258262890683122, 1.000000000000000000, 0.9659258262890683122, 1.000000000000000000, 0.9659258262890683122, 1.000000000000000000, 0.9659258262890683122, 1.000000000000000000, 0.9659258262890683122, 1.000000000000000000, 0.9659258262890683122, 1.000000000000000000, 0.9659258262890683122, 1.000000000000000000, 0.9659258262890683122, 1.000000000000000000, 0.9659258262890683122, 1.000000000000000000, 0.9659258262890683122, 1.000000000000000000, 0.9659258262890683122, 1.000000000000000000, 0.9659258262890683122, 1.000000000000000000, 0.9659258262890683122, 1.000000000000000000, 0.9659258262890683122, 1.000000000000000000, 0.9659258262890683122, 1.000000000000000000, 0.9659258262890683122, 1.000000000000000000, 0.9659258262890683122, 1.000000000000000000, 0.9659258262890683122, 1.000000000000000000, 0.9659258262890683122, 1.000000000000000000, 0.9659258262890683122, 1.000000000000000000, 0.9659258262890683122, 1.000000000000000000, 0.9659258262890683122, 1.000000000000000000, 0.9659258262890683122, 1.000000000000000000, 0.9659258262890683122, 1.000000000000000000, 0.9659258262890683122, 1.000000000000000000, 0.9659258262890683122, 1.000000000000000000, 0.9659258262890683122, 1.000000000000000000, 0.9659258262890683122, 1.000000000000000000, 0.9659258262890683122, 1.000000000000000000, 0.9659258262890683122, 1.000000000000000000, 0.9659258262890683122, 1.000000000000000000, 0.9659258262890683122, 1.000000000000000000, 0.9659258262890683122, 1.000000000000000000, 0.9659258262890683122, 1.000000000000000000, 0.9659258262890683122, 1.000000000000000000, 0.9659258262890683122, 1.000000000000000000, 0.9659258262890683122, 1.000000000000000000, 0.9659258262890683122, 1.000000000000000000, 0.9659258262890683122, 1.000000000000000000, 0.9659258262890683122, 1.000000000000000000, 0.9659258262890683122, 1.000000000000000000, 0.9659258262890683122, 1.000000000000000000, 0.9659258262890683122, 1.000000000000000000, 0.9659258262890683122, 1.000000000000000000, 0.9659258262890683122, 1.000000000000000000, 0.9659258262890683122, 1.000000000000000000, 0.9659258262890683122, 1.000000000000000000, 0.9659258262890683122, 1.000000000000000000, 0.9659258262890683122, 1.000000000000000000, 0.9659258262890683122, 1.000000000000000000, 0.9659258262890683122, 1.000000000000000000, 0.9659258262890683122, 1.000000000000000000, 0.9659258262890683122, 1.000000000000000000, 0.9659258262890683122, 1.000000000000000000, 0.9659258262890683122, 1.000000000000000000, 0.9659258262890683122, 1.000000000000000000, 0.9659258262890683122, 1.000000000000000000, 0.9659258262890683122, 1.000000000000000000, 0.9659258262890683122, 1.000000000000000000, 0.9659258262890683122, 1.000000000000000000, 0.9659258262890683122, 1.000000000000000000, 0.9659258262890683122, 1.000000000000000000, 0.9659258262890683122, 1.000000000000000000, 0.9659258262890683122, 1.000000000000000000, 0.9659258262890683122, 1.000000000000000000, 0.9659258262890683122, 1.000000000000000000, 0.9659258262890683122, 1.000000000000000000, 0.9659258262890683122, 1.000000000000000000, 0.9659258262890683122, 1.000000000000000000, 0.9659258262890683122, 1.000000000000000000, 0.9659258262890683122, 1.000000000000000000, 0.9659258262890683122, 1.000000000000000000, 0.9659258262890683122, 1.000000000000000000, 0.9659258262890683122, 1.000000000000000000, 0.9659258262890683122, 1.000000000000000000, 0.9659258262890683122, 1.000000000000000000, 0.9659258262890683122, 1.000000000000000000, 0.9659258262890683122, 1.000000000000000000, 0.9659258262890683122, 1.000000000000000000, 0.9659258262890683122, 1.000000000000000000, 0.9659258262890683122, 1.000000000000000000, 0.9659258262890683122, 1.000000000000000000, 0.9659258262890683122, 1.000000000000000000, 0.9659258262890683122, 1.000000000000000000, 0.9659258262890683122, 1.000000000000000000, 0.9659258262890683122, 1.000000000000000000, 0.9659258262890683122, 1.000000000000000000, 0.9659258262890683122, 1.000000000000000000, 0.9659258262890683122, 1.000000000000000000, 0.9659258262890683122, 1.000000000000000000, 0.9659258262890683122, 1.000000000000000000, 0.9659258262890683122, 1.000000000000000000, 0.9659258262890683122, 1.000000000000000000, 0.9659258262890683122, 1.000000000000000000, 0.9659258262890683122, 1.000000000000000000, 0.9659258262890683122, 1.000000000000000000, 0.9659258262890683122, 1.000000000000000000, 0.9659258262890683122, 1.000000000000000000, 0.9659258262890683122, 1.000000000000000000, 0.9659258262890683122, 1.000000000000000000, 0.9659258262890683122, 1.000000000000000000, 0.9659258262890683122, 1.000000000000000000, 0.9659258262890683122, 1.000000000000000000, 0.9659258262890683122, 1.000000000000000000, 0.9659258262890683122, 1.000000000000000000, 0.9659258262890683122, 1.000000000000000000, 0.9659258262890683122, 1.000000000000000000, 0.9659258262890683122, 1.000000000000000000, 0.9659258262890683122, 1.000000000000000000, 0.9659258262890683122, 1.000000000000000000, 0.9659258262890683122, 1.000000000000000000, 0.9659258262890683122, 1.000000000000000000, 0.9659258262890683122, 1.000000000000000000, 0.9659258262890683122, 1.000000000000000000, 0.9659258262890683122, 1.000000000000000000, 0.9659258262890683122, 1.000000000000000000, 0.9659258262890683122, 1.000000000000000000, 0.9659258262890683122, 1.000000000000000000, 0.9659258262890683122, 1.000000000000000000, 0.9659258262890683122, 1.000000000000000000, 0.9659258262890683122, 1.000000000000000000, 0.9659258262890683122, 1.000000000000000000, 0.9659258262890683122, 1.000000000000000000, 0.9659258262890683122, 1.000000000000000000, 0.9659258262890683122, 1.000000000000000000, 0.9659258262890683122, 1.000000000000000000, 0.9659258262890683122, 1.000000000000000000, 0.9659258262890683122, 1.000000000000000000, 0.9659258262890683122, 1.000000000000000000, 0.9659258262890683122, 1.000000000000000000, 0.9659258262890683122, 1.000000000000000000, 0.9659258262890683122, 1.000000000000000000, 0.9659258262890683122, 1.000000000000000000, 0.9659258262890683122, 1.000000000000000000, 0.9659258262890683122, 1.000000000000000000, 0.9659258262890683122, 1.000000000000000000, 0.9659258262890683122, 1.000000000000000000, 0.9659258262890683122, 1.000000000000000000, 0.9659258262890683122, 1.000000000000000000, 0.9659258262890683122, 1.000000000000000000, 0.9659258262890683122, 1.000000000000000000, 0.9659258262890683122, 1.000000000000000000, 0.9659258262890683122, 1.000000000000000000, 0.9659258262890683122, 1.000000000000000000, 0.9659258262890683122, 1.000000000000000000, 0.9659258262890683122, 1.000000000000000000, 0.9659258262890683122, 1.000000000000000000, 0.9659258262890683122, 1.000000000000000000, 0.9659258262890683122, 1.000000000000000000, 0.9659258262890683122, 1.000000000000000000, 0.9659258262890683122, 1.000000000000000000, 0.9659258262890683122, 1.000000000000000000) ) ) 
 REPRESENTATION_ITEM ( '' )  SURFACE ( )  );
#31749=CARTESIAN_POINT ( 'NONE',  ( 0.1532563361054083140, 16.00893115100078390, 1.131784320476157264E-15 ) ) ;
#31751=CARTESIAN_POINT ( 'NONE',  ( 22.26659068614894466, 13.88708216824730179, 7.082119434687054849 ) ) ;
#31752=CARTESIAN_POINT ( 'NONE',  ( 19.84674366389459621, 18.50893115100078745, 7.409399052514197653E-17 ) ) ;
#31753=CARTESIAN_POINT ( 'NONE',  ( 12.91533473730992121, 44.52201867748816966, 10.88017736071110164 ) ) ;
#31756=CARTESIAN_POINT ( 'NONE',  ( 12.91533473730993009, 36.60535201082151247, -10.88017736071109987 ) ) ;
#31758=VERTEX_POINT ( 'NONE', #45851 ) ;
#31759=CARTESIAN_POINT ( 'NONE',  ( 10.00000000000000178, 13.05374883491396787, 14.16423886937410082 ) ) ;
#31760=ORIENTED_EDGE ( 'NONE', *, *, #36308, .T. ) ;
#31762=VERTEX_POINT ( 'NONE', #30332 ) ;
#31763=CARTESIAN_POINT ( 'NONE',  ( 19.38216949554541557, 12.24863466993041961, -9.382169495545420901 ) ) ;
#31764=CARTESIAN_POINT ( 'NONE',  ( 14.92337183194729988, 14.34226448433411782, -8.527530157486177487 ) ) ;
#31765=DIRECTION ( 'NONE',  ( -0.000000000000000000, -0.000000000000000000, 1.000000000000000000 ) ) ;
#31767=CARTESIAN_POINT ( 'NONE',  ( 2.791683348922237240, 15.38393115100078212, -7.208316651077763204 ) ) ;
#31768=CARTESIAN_POINT ( 'NONE',  ( 17.96484262340118221, 36.18868534415484106, -7.964842623401177768 ) ) ;
#31772=CARTESIAN_POINT ( 'NONE',  ( -0.8801773607111008646, 58.27201867748816966, 2.915334737309923430 ) ) ;
#31774=CARTESIAN_POINT ( 'NONE',  ( 7.084665262690076126, 62.02201867748816966, -10.88017736071110164 ) ) ;
#31775=CARTESIAN_POINT ( 'NONE',  ( 16.40814093676324603, 17.45696800326375353, -11.09922568453594671 ) ) ;
#31777=CARTESIAN_POINT ( 'NONE',  ( 19.84674366389459266, 33.30059781766744464, 2.638427012816836559 ) ) ;
#31778=CARTESIAN_POINT ( 'NONE',  ( 6.565887622018943937, 58.08196800326376064, -12.81628187352647608 ) ) ;
#31780=CARTESIAN_POINT ( 'NONE',  ( 2.791683348922240793, 21.63393115100078745, 7.208316651077764092 ) ) ;
#31781=CARTESIAN_POINT ( 'NONE',  ( -2.816281873526473856, 24.33196800326375353, 3.434112377981055619 ) ) ;
#31784=CARTESIAN_POINT ( 'NONE',  ( 10.00000000000000000, 46.81368534415484106, -10.88017736071110342 ) ) ;
#31785=CARTESIAN_POINT ( 'NONE',  ( 18.52753015748617571, 63.09226448433412315, 4.923371831947298993 ) ) ;
#31787=CARTESIAN_POINT ( 'NONE',  ( 1.472469842513823179, 26.42559781766745175, 4.923371831947296329 ) ) ;
#31788=CARTESIAN_POINT ( 'NONE',  ( 20.88017736071110164, 15.35535201082150358, 2.915334737309930979 ) ) ;
#31789=CARTESIAN_POINT ( 'NONE',  ( 21.09922568453595559, 17.04030133659708923, -6.408140936763230044 ) ) ;
#31793=CARTESIAN_POINT ( 'NONE',  ( 17.96484262340118221, 26.18868534415483396, -7.964842623401177768 ) ) ;
#31794=ORIENTED_EDGE ( 'NONE', *, *, #26747, .T. ) ;
#31796=CARTESIAN_POINT ( 'NONE',  ( 19.84674366389459621, 23.50893115100078390, 7.409399052514197653E-17 ) ) ;
#31797=CARTESIAN_POINT ( 'NONE',  ( 2.035157376598822676, 17.43868534415483751, -7.964842623401177768 ) ) ;
#31798=CARTESIAN_POINT ( 'NONE',  ( 18.72515096720568550, 20.05509018479935790, 6.500000000000015099 ) ) ;
#31799=CARTESIAN_POINT ( 'NONE',  ( 4.559911319644449179, 33.89701867748817676, 9.422509992056141925 ) ) ;
#31801=CARTESIAN_POINT ( 'NONE',  ( 20.88017736071110164, 5.355352010821503583, 2.915334737309930979 ) ) ;
#31802=CARTESIAN_POINT ( 'NONE',  ( 18.52753015748617571, 8.092264484334117824, 4.923371831947298993 ) ) ;
#31803=CARTESIAN_POINT ( 'NONE',  ( 0.1532563361054083140, 41.00893115100078745, 1.131784320476157264E-15 ) ) ;
#31806=ADVANCED_FACE ( 'NONE', ( #98881 ), #60837, .F. ) ;
#31807=CARTESIAN_POINT ( 'NONE',  ( 7.361572987183169658, 64.96726448433412315, -9.846743663894592657 ) ) ;
#31810=CARTESIAN_POINT ( 'NONE',  ( -2.266590686148945544, 22.22041550158063572, 7.082119434687048631 ) ) ;
#31811=CARTESIAN_POINT ( 'NONE',  ( 12.63842701281683922, 34.55059781766745886, -9.846743663894590881 ) ) ;
#31814=CARTESIAN_POINT ( 'NONE',  ( 20.36894250292379738, 49.92874883491396787, -10.36894250292379027 ) ) ;
#31815=CARTESIAN_POINT ( 'NONE',  ( 0.1532563361054100626, 25.80059781766744820, -2.638427012816831230 ) ) ;
#31816=CARTESIAN_POINT ( 'NONE',  ( 20.00000000000000000, 0.000000000000000000, -4.500000000000001776 ) ) ;
#31818=CARTESIAN_POINT ( 'NONE',  ( 10.00000000000000000, 51.81368534415484106, -10.88017736071110342 ) ) ;
#31819=CARTESIAN_POINT ( 'NONE',  ( 16.40814093676324603, 47.45696800326375353, -11.09922568453594671 ) ) ;
#31820=CARTESIAN_POINT ( 'NONE',  ( 2.035157376598822676, 12.43868534415483751, -7.964842623401177768 ) ) ;
#31821=CARTESIAN_POINT ( 'NONE',  ( -1.099225684535947600, 53.70696800326376064, -6.408140936763238038 ) ) ;
#31822=VERTEX_POINT ( 'NONE', #15852 ) ;
#31823=CARTESIAN_POINT ( 'NONE',  ( 7.361572987183169658, 64.96726448433412315, -9.846743663894592657 ) ) ;
#31824=CARTESIAN_POINT ( 'NONE',  ( 7.361572987183170547, 2.050597817667451750, 9.846743663894590881 ) ) ;
#31827=B_SPLINE_CURVE_WITH_KNOTS ( 'NONE', 3,
 ( #69472, #61954, #1485, #77446, #53970, #8959 ),
 .UNSPECIFIED., .F., .F.,
 ( 4, 2, 4 ),
 ( 7.755077673624249124E-18, 0.0002626113303185991302, 0.0005252226606371905625 ),
 .UNSPECIFIED. ) ;
#31829=CARTESIAN_POINT ( 'NONE',  ( 24.16423886937410614, 49.30374883491396787, 8.672049930838204340E-16 ) ) ;
#31830=CARTESIAN_POINT ( 'NONE',  ( 22.26659068614895176, 9.720415501580633943, -7.082119434687042414 ) ) ;
#31831=CARTESIAN_POINT ( 'NONE',  ( 15.44008868035555793, 21.39701867748817321, -9.422509992056140149 ) ) ;
#31832=CARTESIAN_POINT ( 'NONE',  ( -0.8801773607110991993, 37.85535201082151247, -2.915334737309923874 ) ) ;
#31833=DIRECTION ( 'NONE',  ( -0.000000000000000000, 1.000000000000000000, -0.000000000000000000 ) ) ;
#31835=CARTESIAN_POINT ( 'NONE',  ( 0.1532563361054100626, 0.8005978176674514168, -2.638427012816831230 ) ) ;
#31836=CARTESIAN_POINT ( 'NONE',  ( 18.52753015748618282, 18.92559781766745175, -4.923371831947291888 ) ) ;
#31837=CARTESIAN_POINT ( 'NONE',  ( 3.640395162852214650, 89.00000000000000000, 5.000000000000000000 ) ) ;
#31839=CARTESIAN_POINT ( 'NONE',  ( 2.791683348922240793, 6.633931151000785675, 7.208316651077764092 ) ) ;
#31840=CARTESIAN_POINT ( 'NONE',  ( 0.1532563361054082862, 36.21726448433410894, 2.638427012816831674 ) ) ;
#31842=CARTESIAN_POINT ( 'NONE',  ( 17.96484262340118221, 14.93868534415483751, 7.964842623401181321 ) ) ;
#31844=CARTESIAN_POINT ( 'NONE',  ( 22.81628187352648496, 26.83196800326374998, -3.434112377981050290 ) ) ;
#31845=CARTESIAN_POINT ( 'NONE',  ( 12.63842701281683034, 2.467264484334118269, 9.846743663894596210 ) ) ;
#31847=CARTESIAN_POINT ( 'NONE',  ( 17.20831665107776587, 49.13393115100078745, -7.208316651077762316 ) ) ;
#31848=CARTESIAN_POINT ( 'NONE',  ( 2.791683348922237240, 30.38393115100078390, -7.208316651077763204 ) ) ;
#31850=CARTESIAN_POINT ( 'NONE',  ( 24.16423886937410614, 19.51208216824729647, -3.795296366450302550 ) ) ;
#31851=CARTESIAN_POINT ( 'NONE',  ( 0.5774900079438590739, 52.64701867748817676, -5.440088680355550821 ) ) ;
#31852=CARTESIAN_POINT ( 'NONE',  ( -0.8801773607111009756, 13.06368534415483929, 1.068504757029289695E-15 ) ) ;
#31853=CARTESIAN_POINT ( 'NONE',  ( 7.084665262690076126, 47.02201867748818387, -10.88017736071110164 ) ) ;
#31854=CARTESIAN_POINT ( 'NONE',  ( 15.44008868035555793, 31.39701867748817676, -9.422509992056140149 ) ) ;
#31856=CARTESIAN_POINT ( 'NONE',  ( 4.559911319644449179, 33.89701867748817676, 9.422509992056141925 ) ) ;
#31858=CARTESIAN_POINT ( 'NONE',  ( 0.6178305044545818747, 58.49863466993042493, -9.382169495545419124 ) ) ;
#31859=CARTESIAN_POINT ( 'NONE',  ( 20.88017736071110164, 55.35535201082149825, 2.915334737309930979 ) ) ;
#31861=CARTESIAN_POINT ( 'NONE',  ( 15.44008868035555793, 46.39701867748817676, -9.422509992056140149 ) ) ;
#31862=CARTESIAN_POINT ( 'NONE',  ( -32.19000000000001194, 93.50000000000000000, -9.500000000000000000 ) ) ;
#31863=DIRECTION ( 'NONE',  ( -0.000000000000000000, 1.000000000000000000, -0.000000000000000000 ) ) ;
#31865=CARTESIAN_POINT ( 'NONE',  ( 17.08211943468705840, 60.13708216824729647, -12.26659068614894466 ) ) ;
#31866=CARTESIAN_POINT ( 'NONE',  ( 17.96484262340118221, 66.18868534415483396, -7.964842623401177768 ) ) ;
#31867=CARTESIAN_POINT ( 'NONE',  ( -0.3689425029237898834, 11.17874883491396787, -10.36894250292378850 ) ) ;
#31868=PRESENTATION_STYLE_ASSIGNMENT (( #1415 ) ) ;
#31869=CARTESIAN_POINT ( 'NONE',  ( 10.00000000000000178, 14.31368534415483751, 10.88017736071110342 ) ) ;
#31870=CARTESIAN_POINT ( 'NONE',  ( 12.63842701281683034, 47.46726448433412315, 9.846743663894596210 ) ) ;
#31871=ORIENTED_EDGE ( 'NONE', *, *, #80905, .F. ) ;
#31872=CARTESIAN_POINT ( 'NONE',  ( 0.1532563361054100626, 40.80059781766745886, -2.638427012816831230 ) ) ;
#31873=CARTESIAN_POINT ( 'NONE',  ( 10.00000000000000178, 44.31368534415484106, 10.88017736071110342 ) ) ;
#31874=CARTESIAN_POINT ( 'NONE',  ( 12.63842701281683922, 39.55059781766744464, -9.846743663894590881 ) ) ;
#31875=CARTESIAN_POINT ( 'NONE',  ( 16.40814093676323893, 30.79030133659708923, 11.09922568453595026 ) ) ;
#31878=CARTESIAN_POINT ( 'NONE',  ( 20.88017736071110164, 45.35535201082149115, 2.915334737309930979 ) ) ;
#31880=CARTESIAN_POINT ( 'NONE',  ( 17.08211943468705840, 60.13708216824729647, -12.26659068614894466 ) ) ;
#31883=CARTESIAN_POINT ( 'NONE',  ( 10.00000000000000178, 20.37363466993042138, 12.81628187352647608 ) ) ;
#31884=DIRECTION ( 'NONE',  ( 0.000000000000000000, 0.000000000000000000, -1.000000000000000000 ) ) ;
#31886=CARTESIAN_POINT ( 'NONE',  ( 19.38216949554541557, 22.24863466993041428, -9.382169495545420901 ) ) ;
#31887=CARTESIAN_POINT ( 'NONE',  ( 19.42250999205614548, 25.98035201082150891, -5.440088680355545492 ) ) ;
#31890=CARTESIAN_POINT ( 'NONE',  ( 7.084665262690076126, 67.02201867748817676, -10.88017736071110164 ) ) ;
#31891=CARTESIAN_POINT ( 'NONE',  ( 17.20831665107776587, 49.13393115100078745, -7.208316651077762316 ) ) ;
#31892=CARTESIAN_POINT ( 'NONE',  ( 18.52753015748618282, 33.92559781766745886, -4.923371831947291888 ) ) ;
#31894=CARTESIAN_POINT ( 'NONE',  ( 10.00000000000000178, 65.37363466993042493, 12.81628187352647608 ) ) ;
#31895=CARTESIAN_POINT ( 'NONE',  ( 12.63842701281683922, 24.55059781766745175, -9.846743663894590881 ) ) ;
#31896=CARTESIAN_POINT ( 'NONE',  ( 20.32896413005680003, 56.77164270246083788, 5.963430220938287007 ) ) ;
#31898=CARTESIAN_POINT ( 'NONE',  ( 19.84674366389459266, 8.717264484334116048, -2.638427012816827677 ) ) ;
#31899=CARTESIAN_POINT ( 'NONE',  ( 14.92337183194729633, 2.675597817667451750, 8.527530157486181039 ) ) ;
#31901=CARTESIAN_POINT ( 'NONE',  ( 12.63842701281683922, 44.55059781766745175, -9.846743663894590881 ) ) ;
#31902=EDGE_LOOP ( 'NONE', ( #59791, #49718, #13350, #72317 ) ) ;
#31903=CARTESIAN_POINT ( 'NONE',  ( 20.15039907845753575, 16.74884699246888431, 6.262539305110077059 ) ) ;
#31904=CARTESIAN_POINT ( 'NONE',  ( 10.00000000000000000, 27.87363466993042138, -12.81628187352647608 ) ) ;
#31906=CARTESIAN_POINT ( 'NONE',  ( 20.36894250292379738, 39.92874883491396787, -10.36894250292379027 ) ) ;
#31907=CARTESIAN_POINT ( 'NONE',  ( 5.076628168052704559, 0.1755978176674514724, -8.527530157486179263 ) ) ;
#31909=CARTESIAN_POINT ( 'NONE',  ( 17.08211943468705130, 48.47041550158063927, 12.26659068614894998 ) ) ;
#31910=CARTESIAN_POINT ( 'NONE',  ( -4.164238869374099927, 62.01208216824728936, 3.795296366450308767 ) ) ;
#31911=CARTESIAN_POINT ( 'NONE',  ( -2.266590686148945544, 17.22041550158063572, 7.082119434687048631 ) ) ;
#31912=CARTESIAN_POINT ( 'NONE',  ( 2.917880565312950480, 30.97041550158063572, -12.26659068614894821 ) ) ;
#31915=B_SPLINE_CURVE_WITH_KNOTS ( 'NONE', 3,
 ( #19362, #25885, #86388, #18875, #56384, #40892 ),
 .UNSPECIFIED., .F., .F.,
 ( 4, 2, 4 ),
 ( 0.000000000000000000, 0.0002701661927229362576, 0.0005403323854458725152 ),
 .UNSPECIFIED. ) ;
#31917=CARTESIAN_POINT ( 'NONE',  ( 19.84674366389459621, 38.50893115100078745, 7.409399052514197653E-17 ) ) ;
#31918=B_SPLINE_CURVE_WITH_KNOTS ( 'NONE', 3,
 ( #36344, #87861, #72361, #79875 ),
 .UNSPECIFIED., .F., .F.,
 ( 4, 4 ),
 ( 1.644748632280675619E-16, 0.001060528352561984416 ),
 .UNSPECIFIED. ) ;
#31920=CARTESIAN_POINT ( 'NONE',  ( 0.5774900079438607392, 43.48035201082151247, 5.440088680355550821 ) ) ;
#31921=CARTESIAN_POINT ( 'NONE',  ( 20.00000000000000711, 89.78870847431471702, -4.994901225416799484 ) ) ;
#31923=CARTESIAN_POINT ( 'NONE',  ( 1.472469842513823179, 36.42559781766745175, 4.923371831947296329 ) ) ;
#31924=CARTESIAN_POINT ( 'NONE',  ( 16.40814093676324603, 57.45696800326375353, -11.09922568453594671 ) ) ;
#31926=CARTESIAN_POINT ( 'NONE',  ( 2.791683348922240793, 41.63393115100078745, 7.208316651077764092 ) ) ;
#31927=CARTESIAN_POINT ( 'NONE',  ( 2.791683348922237240, 60.38393115100078745, -7.208316651077763204 ) ) ;
#31928=CARTESIAN_POINT ( 'NONE',  ( 13.79529636645031943, 40.34541550158063217, -14.16423886937409904 ) ) ;
#31930=CARTESIAN_POINT ( 'NONE',  ( 22.26659068614894466, 18.88708216824730002, 7.082119434687054849 ) ) ;
#31933=CARTESIAN_POINT ( 'NONE',  ( 4.559911319644449179, 12.23035201082150714, -9.422509992056141925 ) ) ;
#31934=CARTESIAN_POINT ( 'NONE',  ( 19.38216949554541202, 5.998634669930420493, 9.382169495545424454 ) ) ;
#31936=CARTESIAN_POINT ( 'NONE',  ( -0.8801773607110991993, 62.85535201082150536, -2.915334737309923874 ) ) ;
#31938=CARTESIAN_POINT ( 'NONE',  ( -46.50435961404672014, 102.7681846068616238, -6.785878169524574233 ) ) ;
#31939=DIRECTION ( 'NONE',  ( -0.000000000000000000, -0.000000000000000000, -1.000000000000000000 ) ) ;
#31940=CARTESIAN_POINT ( 'NONE',  ( 10.00000000000000178, 63.05374883491396076, 14.16423886937410082 ) ) ;
#31942=CARTESIAN_POINT ( 'NONE',  ( 19.42250999205614548, 20.98035201082150891, -5.440088680355545492 ) ) ;
#31943=CARTESIAN_POINT ( 'NONE',  ( 12.91533473730993009, 26.60535201082150536, -10.88017736071109987 ) ) ;
#31944=CARTESIAN_POINT ( 'NONE',  ( -1.099225684535947600, -0.4596986634029132657, 6.408140936763237150 ) ) ;
#31945=CARTESIAN_POINT ( 'NONE',  ( 5.076628168052704559, 55.17559781766745175, -8.527530157486179263 ) ) ;
#31946=CARTESIAN_POINT ( 'NONE',  ( 10.00000000000000178, 60.37363466993041783, 12.81628187352647608 ) ) ;
#31949=CARTESIAN_POINT ( 'NONE',  ( 10.00000000000000178, 34.31368534415484106, 10.88017736071110342 ) ) ;
#31950=CARTESIAN_POINT ( 'NONE',  ( 22.81628187352647785, 26.41530133659708923, 3.434112377981063169 ) ) ;
#31953=CARTESIAN_POINT ( 'NONE',  ( 1.472469842513823179, 65.59226448433412315, -4.923371831947296329 ) ) ;
#31954=CARTESIAN_POINT ( 'NONE',  ( 2.035157376598822676, 47.43868534415484817, -7.964842623401177768 ) ) ;
#31955=CARTESIAN_POINT ( 'NONE',  ( 0.1532563361054083140, 11.00893115100078568, 1.131784320476157264E-15 ) ) ;
#31956=CARTESIAN_POINT ( 'NONE',  ( 10.00000000000000000, 37.87363466993041783, -12.81628187352647608 ) ) ;
#31957=CARTESIAN_POINT ( 'NONE',  ( 20.88017736071110519, 65.56368534415483396, 2.639326808657452039E-16 ) ) ;
#31960=VERTEX_POINT ( 'NONE', #57267 ) ;
#31962=CARTESIAN_POINT ( 'NONE',  ( 18.72515096720609051, 25.05509018479941119, 6.499999999999470646 ) ) ;
#31964=CARTESIAN_POINT ( 'NONE',  ( 15.44008868035555793, 51.39701867748816966, -9.422509992056140149 ) ) ;
#31965=CARTESIAN_POINT ( 'NONE',  ( 3.591859063236763294, 43.29030133659708923, -11.09922568453595026 ) ) ;
#31966=CARTESIAN_POINT ( 'NONE',  ( 12.63842701281683034, 17.46726448433411250, 9.846743663894596210 ) ) ;
#31968=CARTESIAN_POINT ( 'NONE',  ( 0.1532563361054100626, 15.80059781766745353, -2.638427012816831230 ) ) ;
#31969=CARTESIAN_POINT ( 'NONE',  ( 2.575439399273669938, 0.4791814250636889927, -6.500000000000363265 ) ) ;
#31970=CARTESIAN_POINT ( 'NONE',  ( -2.266590686148945544, 61.38708216824730357, -7.082119434687050408 ) ) ;
#31973=CARTESIAN_POINT ( 'NONE',  ( 10.00000000000000000, 11.81368534415483751, -10.88017736071110342 ) ) ;
#31974=CARTESIAN_POINT ( 'NONE',  ( 19.72487221294570858, 46.86607318730077054, 6.500000000000000888 ) ) ;
#31975=VERTEX_POINT ( 'NONE', #40811 ) ;
#31976=CARTESIAN_POINT ( 'NONE',  ( -0.8801773607111009756, 8.063685344154837509, 1.068504757029289695E-15 ) ) ;
#31977=CARTESIAN_POINT ( 'NONE',  ( 4.559911319644449179, 3.897018677488171434, 9.422509992056141925 ) ) ;
#31978=CARTESIAN_POINT ( 'NONE',  ( 0.1532563361054082862, 46.21726448433411605, 2.638427012816831674 ) ) ;
#31979=CARTESIAN_POINT ( 'NONE',  ( 22.81628187352647785, 46.41530133659708213, 3.434112377981063169 ) ) ;
#31980=FACE_OUTER_BOUND ( 'NONE', #23868, .T. ) ;
#31982=CARTESIAN_POINT ( 'NONE',  ( -2.266590686148945544, 17.22041550158063572, 7.082119434687048631 ) ) ;
#31983=CARTESIAN_POINT ( 'NONE',  ( 12.91533473730993009, 26.60535201082150536, -10.88017736071109987 ) ) ;
#31984=CARTESIAN_POINT ( 'NONE',  ( 20.88017736071110164, 5.355352010821503583, 2.915334737309930979 ) ) ;
#31985=CARTESIAN_POINT ( 'NONE',  ( 19.84674366389459621, 38.50893115100078745, 7.409399052514197653E-17 ) ) ;
#31987=CARTESIAN_POINT ( 'NONE',  ( 10.00000000000000000, 34.75893115100078745, -9.846743663894594434 ) ) ;
#31989=CARTESIAN_POINT ( 'NONE',  ( 3.640395162852214650, 89.00000000000000000, -12.00000000000000000 ) ) ;
#31993=CARTESIAN_POINT ( 'NONE',  ( 1.472469842513823179, 1.425597817667451528, 4.923371831947296329 ) ) ;
#31994=CARTESIAN_POINT ( 'NONE',  ( 14.92337183194729988, 59.34226448433412315, -8.527530157486177487 ) ) ;
#31995=CARTESIAN_POINT ( 'NONE',  ( 17.96484262340118221, 44.93868534415483396, 7.964842623401181321 ) ) ;
#31996=CARTESIAN_POINT ( 'NONE',  ( 7.084665262690076126, 49.10535201082149825, 10.88017736071109987 ) ) ;
#31997=CARTESIAN_POINT ( 'NONE',  ( 17.96484262340118221, 6.188685344154836621, -7.964842623401177768 ) ) ;
#31998=CARTESIAN_POINT ( 'NONE',  ( -1.099225684535947600, 49.54030133659708923, 6.408140936763237150 ) ) ;
#31999=CARTESIAN_POINT ( 'NONE',  ( -2.266590686148945544, 12.22041550158063394, 7.082119434687048631 ) ) ;
#32002=CARTESIAN_POINT ( 'NONE',  ( 3.591859063236761518, 49.95696800326375353, 11.09922568453594849 ) ) ;
#32003=ORIENTED_EDGE ( 'NONE', *, *, #49247, .T. ) ;
#32004=CARTESIAN_POINT ( 'NONE',  ( 18.52753015748618282, 58.92559781766745886, -4.923371831947291888 ) ) ;
#32005=CARTESIAN_POINT ( 'NONE',  ( 2.035157376598824452, 18.68868534415484106, 7.964842623401179544 ) ) ;
#32008=CARTESIAN_POINT ( 'NONE',  ( 0.5774900079438590739, 32.64701867748816966, -5.440088680355550821 ) ) ;
#32011=CARTESIAN_POINT ( 'NONE',  ( 10.00000000000000000, 61.81368534415484106, -10.88017736071110342 ) ) ;
#32012=( BOUNDED_CURVE ( )  B_SPLINE_CURVE ( 2, ( #61592, #77582, #93080, #76606, #92105, #70101, #85596, #17109, #47592 ),
 .UNSPECIFIED., .F., .T. ) 
 B_SPLINE_CURVE_WITH_KNOTS ( ( 3, 2, 2, 2, 3 ),
 ( 0.3310855930462679453, 0.3333333333333333148, 0.3392857142857143016, 0.3452380952380952328, 0.3474858355251606024 ),
 .UNSPECIFIED. ) 
 CURVE ( )  GEOMETRIC_REPRESENTATION_ITEM ( )  RATIONAL_B_SPLINE_CURVE ( ( 0.9839835555609424134, 0.9871328979762477029, 1.000000000000000000, 0.9659258262890683122, 1.000000000000000000, 0.9659258262890683122, 1.000000000000000000, 0.9871328979762477029, 0.9839835555609424134 ) ) 
 REPRESENTATION_ITEM ( '' )  );
#32013=CARTESIAN_POINT ( 'NONE',  ( 7.361572987183169658, 4.967264484334119601, -9.846743663894592657 ) ) ;
#32014=CARTESIAN_POINT ( 'NONE',  ( 0.1532563361054100626, 0.8005978176674514168, -2.638427012816831230 ) ) ;
#32015=AXIS2_PLACEMENT_3D ( 'NONE', #79229, #62742, #71733 ) ;
#32017=CARTESIAN_POINT ( 'NONE',  ( -46.94000000000001194, 101.0890360526157252, 7.984865333617746863 ) ) ;
#32018=CARTESIAN_POINT ( 'NONE',  ( 17.20831665107776587, 2.883931151000785231, 7.208316651077764980 ) ) ;
#32020=CARTESIAN_POINT ( 'NONE',  ( 10.00000000000000178, 37.25893115100078745, 9.846743663894594434 ) ) ;
#32021=ORIENTED_EDGE ( 'NONE', *, *, #92033, .F. ) ;
#32024=CARTESIAN_POINT ( 'NONE',  ( 2.917880565312948704, 12.63708216824730179, 12.26659068614894643 ) ) ;
#32025=CARTESIAN_POINT ( 'NONE',  ( 22.81628187352647785, 61.41530133659709634, 3.434112377981063169 ) ) ;
#32026=CARTESIAN_POINT ( 'NONE',  ( 10.00000000000000000, 0.5537488349139675359, -14.16423886937410082 ) ) ;
#32027=CARTESIAN_POINT ( 'NONE',  ( 10.00000000000000000, 20.55374883491396787, -14.16423886937410082 ) ) ;
#32029=CARTESIAN_POINT ( 'NONE',  ( 19.05866839779138644, 10.95508385108958826, -6.499999999999970690 ) ) ;
#32030=CARTESIAN_POINT ( 'NONE',  ( 0.5774900079438607392, 63.48035201082149825, 5.440088680355550821 ) ) ;
#32031=CARTESIAN_POINT ( 'NONE',  ( 19.42250999205614193, 15.14701867748817143, 5.440088680355555262 ) ) ;
#32032=CARTESIAN_POINT ( 'NONE',  ( 0.1955144967548754498, 59.32703681773342907, -6.500000000002697398 ) ) ;
#32034=CARTESIAN_POINT ( 'NONE',  ( 10.00000000000000000, -0.2410688489992152128, -9.846743663894594434 ) ) ;
#32035=CARTESIAN_POINT ( 'NONE',  ( 19.84674366389459266, 8.300597817667451750, 2.638427012816836559 ) ) ;
#32037=CARTESIAN_POINT ( 'NONE',  ( 22.81628187352647785, 26.41530133659708923, 3.434112377981063169 ) ) ;
#32038=CARTESIAN_POINT ( 'NONE',  ( 0.1532563361054100626, 30.80059781766744820, -2.638427012816831230 ) ) ;
#32040=CARTESIAN_POINT ( 'NONE',  ( 3.591859063236761518, 19.95696800326375353, 11.09922568453594849 ) ) ;
#32041=CARTESIAN_POINT ( 'NONE',  ( 20.10421743870886857, 40.60736173766202484, -6.337391062633416894 ) ) ;
#32043=CARTESIAN_POINT ( 'NONE',  ( 18.52753015748617571, 3.092264484334118269, 4.923371831947298993 ) ) ;
#32044=ORIENTED_EDGE ( 'NONE', *, *, #46756, .F. ) ;
#32047=CARTESIAN_POINT ( 'NONE',  ( -0.8801773607111008646, 43.27201867748817676, 2.915334737309923430 ) ) ;
#32048=CARTESIAN_POINT ( 'NONE',  ( 20.36894250292379382, 33.67874883491396076, 10.36894250292379205 ) ) ;
#32049=CARTESIAN_POINT ( 'NONE',  ( 19.84674366389459266, 43.71726448433410894, -2.638427012816827677 ) ) ;
#32050=CARTESIAN_POINT ( 'NONE',  ( -0.8801773607110991993, 62.85535201082150536, -2.915334737309923874 ) ) ;
#32051=CARTESIAN_POINT ( 'NONE',  ( -2.816281873526471635, 58.91530133659707502, -3.434112377981056508 ) ) ;
#32053=CARTESIAN_POINT ( 'NONE',  ( 17.96484262340118221, 31.18868534415483751, -7.964842623401177768 ) ) ;
#32055=CARTESIAN_POINT ( 'NONE',  ( 6.565887622018943937, 20.16530133659708213, 12.81628187352647430 ) ) ;
#32056=CARTESIAN_POINT ( 'NONE',  ( 16.40814093676324603, 27.45696800326375708, -11.09922568453594671 ) ) ;
#32057=CARTESIAN_POINT ( 'NONE',  ( 10.00000000000000178, 37.25893115100078745, 9.846743663894594434 ) ) ;
#32059=CARTESIAN_POINT ( 'NONE',  ( -2.816281873526473856, 49.33196800326374643, 3.434112377981055619 ) ) ;
#32061=CARTESIAN_POINT ( 'NONE',  ( 10.00000000000000178, 49.31368534415484106, 10.88017736071110342 ) ) ;
#32065=CARTESIAN_POINT ( 'NONE',  ( 2.035157376598822676, 52.43868534415483396, -7.964842623401177768 ) ) ;
#32067=CARTESIAN_POINT ( 'NONE',  ( 20.88017736071110164, 55.35535201082149825, 2.915334737309930979 ) ) ;
#32071=CARTESIAN_POINT ( 'NONE',  ( 20.88017736071110164, 10.35535201082150714, 2.915334737309930979 ) ) ;
#32072=CARTESIAN_POINT ( 'NONE',  ( 10.00000000000000178, 57.25893115100078745, 9.846743663894594434 ) ) ;
#32073=CARTESIAN_POINT ( 'NONE',  ( 12.91533473730992121, 19.52201867748816611, 10.88017736071110164 ) ) ;
#32075=ADVANCED_FACE ( 'NONE', ( #26771 ), #29395, .T. ) ;
#32076=CARTESIAN_POINT ( 'NONE',  ( 0.6178305044545818747, 28.49863466993041783, -9.382169495545419124 ) ) ;
#32078=CARTESIAN_POINT ( 'NONE',  ( 4.559911319644449179, 43.89701867748816966, 9.422509992056141925 ) ) ;
#32080=CARTESIAN_POINT ( 'NONE',  ( 19.38216949554541557, 2.248634669930420049, -9.382169495545420901 ) ) ;
#32082=CARTESIAN_POINT ( 'NONE',  ( -0.8801773607111009756, 8.063685344154837509, 1.068504757029289695E-15 ) ) ;
#32083=COLOUR_RGB ( '', 0.66274510, 0.83137255, 0.94901961) ;
#32084=CARTESIAN_POINT ( 'NONE',  ( 12.91533473730992121, 44.52201867748816966, 10.88017736071110164 ) ) ;
#32085=CARTESIAN_POINT ( 'NONE',  ( 6.204703633549690345, 57.84541550158063927, 14.16423886937410082 ) ) ;
#32086=CARTESIAN_POINT ( 'NONE',  ( 10.00000000000000178, 47.25893115100078745, 9.846743663894594434 ) ) ;
#32087=CARTESIAN_POINT ( 'NONE',  ( 15.44008868035555793, 66.39701867748817676, -9.422509992056140149 ) ) ;
#32088=FACE_OUTER_BOUND ( 'NONE', #94878, .T. ) ;
#32089=CARTESIAN_POINT ( 'NONE',  ( -4.164238869374098151, 21.59541550158063217, -3.795296366450310543 ) ) ;
#32091=CARTESIAN_POINT ( 'NONE',  ( 19.67858290521088804, 89.00000000000000000, -5.461713021790605360 ) ) ;
#32094=CARTESIAN_POINT ( 'NONE',  ( 6.204703633549690345, 30.76208216824730357, -14.16423886937410259 ) ) ;
#32095=CARTESIAN_POINT ( 'NONE',  ( -2.266590686148945544, 32.22041550158063927, 7.082119434687048631 ) ) ;
#32096=CARTESIAN_POINT ( 'NONE',  ( 0.1532563361054082862, 6.217264484334118713, 2.638427012816831674 ) ) ;
#32097=CARTESIAN_POINT ( 'NONE',  ( 17.20831665107776587, 57.88393115100078745, 7.208316651077764980 ) ) ;
#32098=CARTESIAN_POINT ( 'NONE',  ( 20.03447792253738768, 52.65514106990692511, -6.401564815979734924 ) ) ;
#32099=CARTESIAN_POINT ( 'NONE',  ( 12.91533473730993009, 61.60535201082150536, -10.88017736071109987 ) ) ;
#32100=CARTESIAN_POINT ( 'NONE',  ( 6.565887622018943937, 38.08196800326376064, -12.81628187352647608 ) ) ;
#32101=CARTESIAN_POINT ( 'NONE',  ( 22.26659068614894466, 28.88708216824730357, 7.082119434687054849 ) ) ;
#32102=CARTESIAN_POINT ( 'NONE',  ( 15.44008868035555793, 31.39701867748817676, -9.422509992056140149 ) ) ;
#32103=CARTESIAN_POINT ( 'NONE',  ( 20.15039907845753930, 4.722660991849187972, 6.262539305110067289 ) ) ;
#32104=CARTESIAN_POINT ( 'NONE',  ( 0.1532563361054100626, 0.8005978176674514168, -2.638427012816831230 ) ) ;
#32106=VERTEX_POINT ( 'NONE', #68269 ) ;
#32112=CARTESIAN_POINT ( 'NONE',  ( 22.26659068614895176, 4.720415501580633943, -7.082119434687042414 ) ) ;
#32113=CARTESIAN_POINT ( 'NONE',  ( 24.16423886937410614, 64.51208216824728936, -3.795296366450302550 ) ) ;
#32114=CARTESIAN_POINT ( 'NONE',  ( 4.559911319644449179, 17.23035201082150536, -9.422509992056141925 ) ) ;
#32115=CARTESIAN_POINT ( 'NONE',  ( 10.00000000000000000, 34.75893115100078745, -9.846743663894594434 ) ) ;
#32116=CARTESIAN_POINT ( 'NONE',  ( 7.361572987183169658, 54.96726448433413026, -9.846743663894592657 ) ) ;
#32118=AXIS2_PLACEMENT_3D ( 'NONE', #2828, #70822, #10310 ) ;
#32122=CARTESIAN_POINT ( 'NONE',  ( 13.43411237798106583, 2.665301336597086568, -12.81628187352647252 ) ) ;
#32124=CARTESIAN_POINT ( 'NONE',  ( -0.3689425029237898834, 41.17874883491397497, -10.36894250292378850 ) ) ;
#32126=CARTESIAN_POINT ( 'NONE',  ( 17.08211943468705130, 43.47041550158063927, 12.26659068614894998 ) ) ;
#32128=CARTESIAN_POINT ( 'NONE',  ( -0.8801773607111008646, 23.27201867748817676, 2.915334737309923430 ) ) ;
#32129=( LENGTH_UNIT ( ) NAMED_UNIT ( * ) SI_UNIT ( .MILLI., .METRE. ) );
#32130=CARTESIAN_POINT ( 'NONE',  ( 15.44008868035555260, 44.73035201082151247, 9.422509992056143702 ) ) ;
#32131=CARTESIAN_POINT ( 'NONE',  ( 0.1532563361054083140, 46.00893115100079456, 1.131784320476157264E-15 ) ) ;
#32132=CARTESIAN_POINT ( 'NONE',  ( 15.44008868035555260, 39.73035201082150536, 9.422509992056143702 ) ) ;
#32133=CARTESIAN_POINT ( 'NONE',  ( 20.88017736071110519, 60.56368534415484106, 2.639326808657452039E-16 ) ) ;
#32134=CARTESIAN_POINT ( 'NONE',  ( 4.559911319644449179, 28.89701867748817321, 9.422509992056141925 ) ) ;
#32138=CARTESIAN_POINT ( 'NONE',  ( 10.00000000000000178, 7.258931151000785675, 9.846743663894594434 ) ) ;
#32140=VERTEX_POINT ( 'NONE', #60740 ) ;
#32142=CARTESIAN_POINT ( 'NONE',  ( 10.00000000000000000, 39.75893115100078745, -9.846743663894594434 ) ) ;
#32144=CARTESIAN_POINT ( 'NONE',  ( 22.81628187352648496, 46.83196800326376064, -3.434112377981050290 ) ) ;
#32148=CARTESIAN_POINT ( 'NONE',  ( 1.472469842513823179, 65.59226448433412315, -4.923371831947296329 ) ) ;
#32149=CARTESIAN_POINT ( 'NONE',  ( 19.72487221294569792, 32.80223176428832232, -6.500000000000008882 ) ) ;
#32150=CARTESIAN_POINT ( 'NONE',  ( 19.84674366389459621, 53.50893115100078745, 7.409399052514197653E-17 ) ) ;
#32151=CARTESIAN_POINT ( 'NONE',  ( 24.16423886937409904, 44.09541550158063927, 3.795296366450317205 ) ) ;
#32152=CARTESIAN_POINT ( 'NONE',  ( 19.84674366389459266, 63.30059781766745886, 2.638427012816836559 ) ) ;
#32153=ORIENTED_EDGE ( 'NONE', *, *, #87703, .F. ) ;
#32156=CARTESIAN_POINT ( 'NONE',  ( 17.20831665107776587, 19.13393115100078035, -7.208316651077762316 ) ) ;
#32157=CARTESIAN_POINT ( 'NONE',  ( 13.43411237798106583, 52.66530133659708213, -12.81628187352647252 ) ) ;
#32158=CARTESIAN_POINT ( 'NONE',  ( 10.00000000000000178, 62.25893115100078745, 9.846743663894594434 ) ) ;
#32159=CARTESIAN_POINT ( 'NONE',  ( 0.5774900079438590739, 57.64701867748817676, -5.440088680355550821 ) ) ;
#32160=CARTESIAN_POINT ( 'NONE',  ( 19.72487221294571569, 30.71833443783938122, -6.499999999999989342 ) ) ;
#32162=EDGE_CURVE ( 'NONE', #97093, #45049, #24043, .T. ) ;
#32165=CARTESIAN_POINT ( 'NONE',  ( 20.36894250292379738, 59.92874883491397497, -10.36894250292379027 ) ) ;
#32166=CARTESIAN_POINT ( 'NONE',  ( 6.000000000000000000, 11.50000000000000000, -6.000000000000000000 ) ) ;
#32167=CARTESIAN_POINT ( 'NONE',  ( -0.8801773607111008646, 33.27201867748817676, 2.915334737309923430 ) ) ;
#32168=CARTESIAN_POINT ( 'NONE',  ( 0.6178305044545838731, 14.74863466993041783, 9.382169495545420901 ) ) ;
#32169=CARTESIAN_POINT ( 'NONE',  ( 2.035157376598824452, 53.68868534415484817, 7.964842623401179544 ) ) ;
#32172=CARTESIAN_POINT ( 'NONE',  ( 4.559911319644449179, 47.23035201082150536, -9.422509992056141925 ) ) ;
#32173=CARTESIAN_POINT ( 'NONE',  ( 17.85158348494331904, 34.73726573380434957, -6.499999999999977796 ) ) ;
#32174=CARTESIAN_POINT ( 'NONE',  ( 5.076628168052704559, 35.17559781766745175, -8.527530157486179263 ) ) ;
#32175=CARTESIAN_POINT ( 'NONE',  ( 2.791683348922237240, 5.383931151000785675, -7.208316651077763204 ) ) ;
#32177=CARTESIAN_POINT ( 'NONE',  ( 3.591859063236761518, 14.95696800326375531, 11.09922568453594849 ) ) ;
#32178=CARTESIAN_POINT ( 'NONE',  ( 0.5774900079438607392, 13.48035201082150358, 5.440088680355550821 ) ) ;
#32179=CARTESIAN_POINT ( 'NONE',  ( 1.492507162822266142, 67.19955587570481725, -6.500000000000075495 ) ) ;
#32181=CARTESIAN_POINT ( 'NONE',  ( 13.79529636645030344, 38.26208216824729647, 14.16423886937410614 ) ) ;
#32182=CARTESIAN_POINT ( 'NONE',  ( 22.26659068614895176, 29.72041550158063572, -7.082119434687042414 ) ) ;
#32183=CARTESIAN_POINT ( 'NONE',  ( 17.08211943468705840, 60.13708216824729647, -12.26659068614894466 ) ) ;
#32184=CARTESIAN_POINT ( 'NONE',  ( 10.00000000000000000, 24.75893115100078745, -9.846743663894594434 ) ) ;
#32185=CARTESIAN_POINT ( 'NONE',  ( 2.035157376598824452, 8.688685344154839285, 7.964842623401179544 ) ) ;
#32186=AXIS2_PLACEMENT_3D ( 'NONE', #16855, #56330, #2363 ) ;
#32188=CARTESIAN_POINT ( 'NONE',  ( 14.92337183194729633, 37.67559781766745175, 8.527530157486181039 ) ) ;
#32189=CARTESIAN_POINT ( 'NONE',  ( 4.559911319644449179, 23.89701867748817321, 9.422509992056141925 ) ) ;
#32190=CARTESIAN_POINT ( 'NONE',  ( 3.591859063236763294, -1.709698663402913210, -11.09922568453595026 ) ) ;
#32191=CARTESIAN_POINT ( 'NONE',  ( -0.3689425029237898834, 21.17874883491396432, -10.36894250292378850 ) ) ;
#32195=CARTESIAN_POINT ( 'NONE',  ( 5.076628168052703671, 6.842264484334118713, 8.527530157486179263 ) ) ;
#32196=CARTESIAN_POINT ( 'NONE',  ( 22.81628187352647785, 46.62363466993041783, 6.195893100308588602E-16 ) ) ;
#32197=CARTESIAN_POINT ( 'NONE',  ( 2.791683348922237240, 55.38393115100078745, -7.208316651077763204 ) ) ;
#32198=EDGE_LOOP ( 'NONE', ( #41111, #18850, #7307, #15867, #32539, #27315 ) ) ;
#32199=ADVANCED_FACE ( 'NONE', ( #62213 ), #53051, .T. ) ;
#32200=CYLINDRICAL_SURFACE ( 'NONE', #55686, 11.92686044187656513 ) ;
#32201=LINE ( 'NONE', #85229, #31488 ) ;
#32202=CARTESIAN_POINT ( 'NONE',  ( 15.44008868035555793, 6.397018677488171434, -9.422509992056140149 ) ) ;
#32203=CARTESIAN_POINT ( 'NONE',  ( 20.88017736071110519, 50.56368534415484106, 2.639326808657452039E-16 ) ) ;
#32204=CARTESIAN_POINT ( 'NONE',  ( -4.164238869374099927, 12.01208216824730357, 3.795296366450308767 ) ) ;
#32205=CARTESIAN_POINT ( 'NONE',  ( 12.91533473730992121, 54.52201867748816255, 10.88017736071110164 ) ) ;
#32206=CARTESIAN_POINT ( 'NONE',  ( 12.63842701281683034, 42.46726448433412315, 9.846743663894596210 ) ) ;
#32207=CARTESIAN_POINT ( 'NONE',  ( -0.8801773607111008646, 23.27201867748817676, 2.915334737309923430 ) ) ;
#32209=CARTESIAN_POINT ( 'NONE',  ( 0.1532563361054100626, 65.80059781766745175, -2.638427012816831230 ) ) ;
#32210=CARTESIAN_POINT ( 'NONE',  ( 2.791683348922240793, 1.633931151000784565, 7.208316651077764092 ) ) ;
#32211=UNCERTAINTY_MEASURE_WITH_UNIT (LENGTH_MEASURE( 1.000000000000000082E-05 ), #85381, 'distance_accuracy_value', 'NONE');
#32217=CARTESIAN_POINT ( 'NONE',  ( 2.917880565312950480, 45.97041550158063927, -12.26659068614894821 ) ) ;
#32218=CARTESIAN_POINT ( 'NONE',  ( 19.84674366389459621, 43.50893115100078745, 7.409399052514197653E-17 ) ) ;
#32219=CARTESIAN_POINT ( 'NONE',  ( 19.84674366389459266, 18.71726448433411960, -2.638427012816827677 ) ) ;
#32220=CARTESIAN_POINT ( 'NONE',  ( 0.6178305044545838731, 64.74863466993043914, 9.382169495545420901 ) ) ;
#32221=CARTESIAN_POINT ( 'NONE',  ( 0.5774900079438607392, 13.48035201082150358, 5.440088680355550821 ) ) ;
#32222=CARTESIAN_POINT ( 'NONE',  ( 1.472469842513823179, 45.59226448433412315, -4.923371831947296329 ) ) ;
#32224=CARTESIAN_POINT ( 'NONE',  ( -4.164238869374099927, 42.01208216824728936, 3.795296366450308767 ) ) ;
#32225=CARTESIAN_POINT ( 'NONE',  ( -0.3689425029237881626, 57.42874883491397497, 10.36894250292379027 ) ) ;
#32226=CARTESIAN_POINT ( 'NONE',  ( 5.076628168052704559, 65.17559781766745175, -8.527530157486179263 ) ) ;
#32229=CARTESIAN_POINT ( 'NONE',  ( 0.5774900079438607392, 48.48035201082150536, 5.440088680355550821 ) ) ;
#32230=CARTESIAN_POINT ( 'NONE',  ( 2.791683348922240793, 21.63393115100078745, 7.208316651077764092 ) ) ;
#32235=AXIS2_PLACEMENT_3D ( 'NONE', #46075, #76563, #55033 ) ;
#32237=CARTESIAN_POINT ( 'NONE',  ( 1.472469842513823179, 11.42559781766745175, 4.923371831947296329 ) ) ;
#32239=CARTESIAN_POINT ( 'NONE',  ( -0.3689425029237881626, 17.42874883491397142, 10.36894250292379027 ) ) ;
#32240=CARTESIAN_POINT ( 'NONE',  ( 10.00000000000000000, 14.75893115100078568, -9.846743663894594434 ) ) ;
#32241=CARTESIAN_POINT ( 'NONE',  ( 17.96484262340118221, 46.18868534415484106, -7.964842623401177768 ) ) ;
#32243=CARTESIAN_POINT ( 'NONE',  ( 0.5774900079438607392, 38.48035201082150536, 5.440088680355550821 ) ) ;
#32246=CARTESIAN_POINT ( 'NONE',  ( 12.91533473730993009, 46.60535201082150536, -10.88017736071109987 ) ) ;
#32247=CARTESIAN_POINT ( 'NONE',  ( 13.79529636645030344, 13.26208216824729824, 14.16423886937410614 ) ) ;
#32248=VERTEX_POINT ( 'NONE', #96434 ) ;
#32250=CARTESIAN_POINT ( 'NONE',  ( 6.565887622018943937, 25.16530133659708213, 12.81628187352647430 ) ) ;
#32251=CARTESIAN_POINT ( 'NONE',  ( 10.00000000000000000, 0.5537488349139675359, -14.16423886937410082 ) ) ;
#32252=CARTESIAN_POINT ( 'NONE',  ( 14.92337183194729988, 4.342264484334117824, -8.527530157486177487 ) ) ;
#32253=CARTESIAN_POINT ( 'NONE',  ( 17.96484262340118221, 6.188685344154836621, -7.964842623401177768 ) ) ;
#32254=CARTESIAN_POINT ( 'NONE',  ( 19.10478245763048477, 11.02576239577082262, -5.990408912944377384 ) ) ;
#32255=CARTESIAN_POINT ( 'NONE',  ( 17.20831665107776587, 14.13393115100078568, -7.208316651077762316 ) ) ;
#32256=CARTESIAN_POINT ( 'NONE',  ( -0.8801773607110991993, 42.85535201082150536, -2.915334737309923874 ) ) ;
#32261=CARTESIAN_POINT ( 'NONE',  ( 17.96484262340118221, 56.18868534415484817, -7.964842623401177768 ) ) ;
#32263=CARTESIAN_POINT ( 'NONE',  ( 16.40814093676324603, 62.45696800326376064, -11.09922568453594671 ) ) ;
#32264=CARTESIAN_POINT ( 'NONE',  ( 12.91533473730992121, 59.52201867748816966, 10.88017736071110164 ) ) ;
#32266=CARTESIAN_POINT ( 'NONE',  ( 7.361572987183170547, 32.05059781766745175, 9.846743663894590881 ) ) ;
#32268=CARTESIAN_POINT ( 'NONE',  ( 10.00000000000000178, 3.053748834913967425, 14.16423886937410082 ) ) ;
#32269=CARTESIAN_POINT ( 'NONE',  ( 10.00000000000000178, 17.25893115100078745, 9.846743663894594434 ) ) ;
#32270=CARTESIAN_POINT ( 'NONE',  ( 19.38216949554541202, 25.99863466993042138, 9.382169495545424454 ) ) ;
#32273=CARTESIAN_POINT ( 'NONE',  ( 20.88017736071110875, 55.77201867748816966, -2.915334737309920765 ) ) ;
#32275=CARTESIAN_POINT ( 'NONE',  ( 0.1532563361054100626, 65.80059781766745175, -2.638427012816831230 ) ) ;
#32277=CARTESIAN_POINT ( 'NONE',  ( 14.92337183194729988, 19.34226448433411960, -8.527530157486177487 ) ) ;
#32278=CARTESIAN_POINT ( 'NONE',  ( 7.084665262690076126, 14.10535201082150358, 10.88017736071109987 ) ) ;
#32279=CARTESIAN_POINT ( 'NONE',  ( 3.591859063236763294, 13.29030133659708746, -11.09922568453595026 ) ) ;
#32281=CARTESIAN_POINT ( 'NONE',  ( 12.63842701281683922, 24.55059781766745175, -9.846743663894590881 ) ) ;
#32284=CARTESIAN_POINT ( 'NONE',  ( -0.8801773607111008646, 18.27201867748817321, 2.915334737309923430 ) ) ;
#32285=EDGE_CURVE ( 'NONE', #50081, #74944, #39646, .T. ) ;
#32289=CARTESIAN_POINT ( 'NONE',  ( 17.20831665107776587, 47.88393115100078745, 7.208316651077764980 ) ) ;
#32290=CARTESIAN_POINT ( 'NONE',  ( 12.91533473730992121, 14.52201867748817143, 10.88017736071110164 ) ) ;
#32292=CARTESIAN_POINT ( 'NONE',  ( 7.084665262690076126, 49.10535201082149825, 10.88017736071109987 ) ) ;
#32293=CARTESIAN_POINT ( 'NONE',  ( 2.035157376598824452, 18.68868534415484106, 7.964842623401179544 ) ) ;
#32295=CARTESIAN_POINT ( 'NONE',  ( 18.52753015748618282, 8.925597817667451750, -4.923371831947291888 ) ) ;
#32297=CARTESIAN_POINT ( 'NONE',  ( 7.361572987183170547, 42.05059781766745886, 9.846743663894590881 ) ) ;
#32300=CARTESIAN_POINT ( 'NONE',  ( 10.00000000000000178, 67.25893115100079456, 9.846743663894594434 ) ) ;
#32301=CARTESIAN_POINT ( 'NONE',  ( 2.917880565312950480, 0.9704155015806342766, -12.26659068614894821 ) ) ;
#32302=CARTESIAN_POINT ( 'NONE',  ( 20.36894250292379382, 28.67874883491396787, 10.36894250292379205 ) ) ;
#32304=CARTESIAN_POINT ( 'NONE',  ( 0.1532563361054083140, 36.00893115100078745, 1.131784320476157264E-15 ) ) ;
#32306=ORIENTED_EDGE ( 'NONE', *, *, #64407, .T. ) ;
#32307=CARTESIAN_POINT ( 'NONE',  ( 24.16423886937410614, 49.30374883491396787, 8.672049930838204340E-16 ) ) ;
#32308=CARTESIAN_POINT ( 'NONE',  ( 7.361572987183169658, 19.96726448433411960, -9.846743663894592657 ) ) ;
#32309=CARTESIAN_POINT ( 'NONE',  ( 0.2751277870542889192, 28.21833443783938122, 6.499999999999990230 ) ) ;
#32311=CARTESIAN_POINT ( 'NONE',  ( -0.8801773607111009756, 48.06368534415484817, 1.068504757029289695E-15 ) ) ;
#32312=CARTESIAN_POINT ( 'NONE',  ( 0.6178305044545818747, 63.49863466993043204, -9.382169495545419124 ) ) ;
#32313=CARTESIAN_POINT ( 'NONE',  ( 10.00000000000000000, 11.81368534415483751, -10.88017736071110342 ) ) ;
#32314=CARTESIAN_POINT ( 'NONE',  ( -1.099225684535947600, 54.54030133659708923, 6.408140936763237150 ) ) ;
#32315=CARTESIAN_POINT ( 'NONE',  ( 16.40814093676324603, 17.45696800326375353, -11.09922568453594671 ) ) ;
#32316=CARTESIAN_POINT ( 'NONE',  ( 17.39651004071842166, 12.93575266056827822, 6.499999999999998224 ) ) ;
#32317=CARTESIAN_POINT ( 'NONE',  ( 0.1532563361054100626, 10.80059781766745175, -2.638427012816831230 ) ) ;
#32318=ORIENTED_EDGE ( 'NONE', *, *, #47770, .T. ) ;
#32322=CARTESIAN_POINT ( 'NONE',  ( 2.917880565312950480, 50.97041550158064638, -12.26659068614894821 ) ) ;
#32323=CARTESIAN_POINT ( 'NONE',  ( 24.16423886937410614, 29.30374883491396787, 8.672049930838204340E-16 ) ) ;
#32324=CARTESIAN_POINT ( 'NONE',  ( 0.5774900079438590739, 17.64701867748817321, -5.440088680355550821 ) ) ;
#32325=CARTESIAN_POINT ( 'NONE',  ( 12.91533473730993009, 36.60535201082151247, -10.88017736071109987 ) ) ;
#32326=CARTESIAN_POINT ( 'NONE',  ( -46.58162315985163815, 100.7785275715626057, -9.484706478859457945 ) ) ;
#32327=CARTESIAN_POINT ( 'NONE',  ( 5.076628168052703671, 1.842264484334118047, 8.527530157486179263 ) ) ;
#32328=CARTESIAN_POINT ( 'NONE',  ( 0.1532563361054082862, 21.21726448433412315, 2.638427012816831674 ) ) ;
#32329=CARTESIAN_POINT ( 'NONE',  ( 5.500000000000000000, 10.49999999999999822, 6.000000000000000000 ) ) ;
#32331=CARTESIAN_POINT ( 'NONE',  ( 1.472469842513823179, 20.59226448433411960, -4.923371831947296329 ) ) ;
#32332=CARTESIAN_POINT ( 'NONE',  ( 0.1532563361054083140, 41.00893115100078745, 1.131784320476157264E-15 ) ) ;
#32333=CARTESIAN_POINT ( 'NONE',  ( 7.084665262690076126, 12.02201867748817143, -10.88017736071110164 ) ) ;
#32334=EDGE_CURVE ( 'NONE', #1572, #29895, #18609, .T. ) ;
#32335=UNCERTAINTY_MEASURE_WITH_UNIT (LENGTH_MEASURE( 1.000000000000000082E-05 ), #55165, 'distance_accuracy_value', 'NONE');
#32336=( BOUNDED_CURVE ( )  B_SPLINE_CURVE ( 3, ( #22852, #76330, #53830, #98374 ),
 .UNSPECIFIED., .F., .F. ) 
 B_SPLINE_CURVE_WITH_KNOTS ( ( 4, 4 ),
 ( 1.570796326794896558, 2.588785175020066109 ),
 .UNSPECIFIED. ) 
 CURVE ( )  GEOMETRIC_REPRESENTATION_ITEM ( )  RATIONAL_B_SPLINE_CURVE ( ( 1.000000000000000000, 0.9154899770527740177, 0.9154899770527740177, 1.000000000000000000 ) ) 
 REPRESENTATION_ITEM ( '' )  );
#32337=AXIS2_PLACEMENT_3D ( 'NONE', #94858, #70405, #55394 ) ;
#32338=CARTESIAN_POINT ( 'NONE',  ( 19.38216949554541202, 30.99863466993042138, 9.382169495545424454 ) ) ;
#32339=CARTESIAN_POINT ( 'NONE',  ( 20.88017736071110519, 50.56368534415484106, 2.639326808657452039E-16 ) ) ;
#32340=CARTESIAN_POINT ( 'NONE',  ( 13.79529636645031943, 45.34541550158062506, -14.16423886937409904 ) ) ;
#32341=CARTESIAN_POINT ( 'NONE',  ( 19.84674366389459266, 8.300597817667451750, 2.638427012816836559 ) ) ;
#32343=CARTESIAN_POINT ( 'NONE',  ( 0.1532563361054100626, 50.80059781766745175, -2.638427012816831230 ) ) ;
#32344=CARTESIAN_POINT ( 'NONE',  ( 0.1532563361054082862, 26.21726448433411605, 2.638427012816831674 ) ) ;
#32345=CARTESIAN_POINT ( 'NONE',  ( 22.26659068614894466, 13.88708216824730179, 7.082119434687054849 ) ) ;
#32346=CARTESIAN_POINT ( 'NONE',  ( -0.3689425029237881626, 12.42874883491396609, 10.36894250292379027 ) ) ;
#32347=CARTESIAN_POINT ( 'NONE',  ( 1.472469842513823179, 35.59226448433412315, -4.923371831947296329 ) ) ;
#32348=CARTESIAN_POINT ( 'NONE',  ( 19.42250999205614193, 45.14701867748817676, 5.440088680355555262 ) ) ;
#32349=CARTESIAN_POINT ( 'NONE',  ( 15.44008868035555793, 16.39701867748817321, -9.422509992056140149 ) ) ;
#32350=CARTESIAN_POINT ( 'NONE',  ( 7.084665262690076126, 52.02201867748816255, -10.88017736071110164 ) ) ;
#32351=CARTESIAN_POINT ( 'NONE',  ( 2.035157376598822676, 27.43868534415483396, -7.964842623401177768 ) ) ;
#32353=CARTESIAN_POINT ( 'NONE',  ( 20.88017736071110519, 35.56368534415484106, 2.639326808657452039E-16 ) ) ;
#32354=ORIENTED_EDGE ( 'NONE', *, *, #86519, .F. ) ;
#32355=CARTESIAN_POINT ( 'NONE',  ( 6.565887622018943937, 65.16530133659709634, 12.81628187352647430 ) ) ;
#32356=CARTESIAN_POINT ( 'NONE',  ( 0.5774900079438607392, 68.48035201082150536, 5.440088680355550821 ) ) ;
#32358=CARTESIAN_POINT ( 'NONE',  ( 4.559911319644449179, 48.89701867748817676, 9.422509992056141925 ) ) ;
#32359=CARTESIAN_POINT ( 'NONE',  ( 2.035157376598822676, 7.438685344154837509, -7.964842623401177768 ) ) ;
#32361=CARTESIAN_POINT ( 'NONE',  ( 2.917880565312948704, 62.63708216824730357, 12.26659068614894643 ) ) ;
#32362=CARTESIAN_POINT ( 'NONE',  ( 0.5774900079438590739, 62.64701867748817676, -5.440088680355550821 ) ) ;
#32365=CARTESIAN_POINT ( 'NONE',  ( 7.361572987183169658, 9.967264484334119601, -9.846743663894592657 ) ) ;
#32366=COLOUR_RGB ( '', 0.66274510, 0.83137255, 0.94901961) ;
#32367=CARTESIAN_POINT ( 'NONE',  ( 0.5774900079438590739, 12.64701867748817143, -5.440088680355550821 ) ) ;
#32368=CARTESIAN_POINT ( 'NONE',  ( 12.63842701281683922, 49.55059781766744464, -9.846743663894590881 ) ) ;
#32369=ORIENTED_EDGE ( 'NONE', *, *, #30268, .F. ) ;
#32370=CARTESIAN_POINT ( 'NONE',  ( 2.791683348922237240, 50.38393115100078035, -7.208316651077763204 ) ) ;
#32372=CARTESIAN_POINT ( 'NONE',  ( 17.96484262340118221, 36.18868534415484106, -7.964842623401177768 ) ) ;
#32373=CARTESIAN_POINT ( 'NONE',  ( 19.84674366389459266, 53.71726448433411605, -2.638427012816827677 ) ) ;
#32374=CARTESIAN_POINT ( 'NONE',  ( 10.00000000000000178, 30.37363466993042138, 12.81628187352647608 ) ) ;
#32375=DIRECTION ( 'NONE',  ( 0.5547001962252290364, 0.8320502943378437211, 0.000000000000000000 ) ) ;
#32377=CARTESIAN_POINT ( 'NONE',  ( 20.88017736071110164, 40.35535201082150536, 2.915334737309930979 ) ) ;
#32378=CARTESIAN_POINT ( 'NONE',  ( -4.164238869374099039, 56.80374883491397497, 8.674139862899312516E-16 ) ) ;
#32379=ADVANCED_FACE ( 'NONE', ( #83388 ), #49833, .T. ) ;
#32380=CARTESIAN_POINT ( 'NONE',  ( 13.43411237798106583, 22.66530133659708923, -12.81628187352647252 ) ) ;
#32383=CARTESIAN_POINT ( 'NONE',  ( 3.591859063236763294, 33.29030133659708213, -11.09922568453595026 ) ) ;
#32384=CARTESIAN_POINT ( 'NONE',  ( 0.5774900079438590739, 27.64701867748817676, -5.440088680355550821 ) ) ;
#32387=CARTESIAN_POINT ( 'NONE',  ( 17.96484262340118221, 64.93868534415483396, 7.964842623401181321 ) ) ;
#32388=CARTESIAN_POINT ( 'NONE',  ( 14.92337183194729988, 44.34226448433412315, -8.527530157486177487 ) ) ;
#32389=CARTESIAN_POINT ( 'NONE',  ( 17.20831665107776587, 14.13393115100078568, -7.208316651077762316 ) ) ;
#32390=CARTESIAN_POINT ( 'NONE',  ( 17.20831665107776587, 42.88393115100077324, 7.208316651077764980 ) ) ;
#32393=CARTESIAN_POINT ( 'NONE',  ( 1.472469842513823179, 26.42559781766745175, 4.923371831947296329 ) ) ;
#32395=DIRECTION ( 'NONE',  ( 0.000000000000000000, -1.000000000000000000, 0.000000000000000000 ) ) ;
#32396=CIRCLE ( 'NONE', #11714, 11.99999999999999645 ) ;
#32397=CARTESIAN_POINT ( 'NONE',  ( 19.84674366389459266, 23.30059781766745530, 2.638427012816836559 ) ) ;
#32399=CARTESIAN_POINT ( 'NONE',  ( 2.791683348922237240, 50.38393115100078035, -7.208316651077763204 ) ) ;
#32401=( BOUNDED_SURFACE ( )  B_SPLINE_SURFACE ( 1, 2, ( 
 ( #78523, #40039, #94017, #54526, #54047, #63513, #40538, #24561, #70540, #48508, #31535, #61542, #70045, #84558, #92051, #32018, #92531, #2558, #16058, #39062, #47031, #47531, #16557, #78033, #1072, #32524, #85042, #55537, #9535, #55022, #86033, #62031, #63023, #77525, #17546, #2062, #85539, #48014, #17051, #69555, #93523, #79011, #10035, #93025, #25051, #71036, #33014, #25539, #23578, #56030, #46546, #86527, #18027, #10516, #62521, #41030, #9042, #71532, #77046, #24061, #8559, #39556, #1569, #11497, #72979, #79994, #35474, #12971, #56993, #49487, #71997, #57973, #34479, #33980, #4508, #80982, #95498, #26989, #43464, #88978, #95997, #3522, #88479, #27480, #18514, #57488, #34974, #94501, #20485, #41529, #26020, #33493, #96497, #63991, #11012, #65471, #42494, #50479, #64483, #94991, #26496, #87982, #65970, #50973, #19011, #4017, #19493, #49988, #81466, #56515, #73466, #73966, #87005, #42018, #80495, #4993, #87496, #27970, #12482, #58463, #49003, #79510, #72483, #64972, #19981, #11993, #42985, #36472, #75943, #66466, #83449, #44454, #52453, #97984, #74955, #22463, #82956, #37966, #97485, #96996, #7469, #14971, #67463, #14469, #91439, #74452, #45949, #13979, #28473, #5495, #6458, #66966, #45441, #58970, #81958, #89955, #90435, #59454, #21976, #37470, #98483, #60442, #15468, #59945, #43953, #68456, #44944, #28952, #98978, #30431, #13472, #89467, #82456, #90935, #60933, #29938, #75449, #6962, #22965, #20983, #21471, #51469, #36967, #5980, #51970, #52939, #53431, #29441, #67960, #83940, #35967, #17427, #2437, #8920, #9919, #76924, #476, #47896, #70422, #16434, #17909, #62398, #16927, #93403, #38941, #84924, #39435, #31412, #78399, #32895, #46430, #91932, #69929, #68945, #7954, #31901, #46912, #9417, #92906, #8434, #1941, #55908, #24436, #1449, #69430, #54902, #86407, #38449, #951, #61915, #92419, #53935, #40423, #77906, #84443, #85416, #25426, #24929, #76438, #54412, #77405, #70917, #47404, #32399, #30923, #23944, #39919, #62903, #61422, #23459, #55410, #15940, #85916, #63393, #93898, #4390, #35356, #4877, #96378, #48393, #49374, #63871, #34857, #79876, #11380, #56876, #80865, #71881, #87378, #94383, #19379, #27849, #42869, #10404, #49862, #41420, #18397, #88855, #64368, #58337, #72856, #25900, #50354, #18894, #12363, #95372, #48879, #94877, #78895, #65352, #56401, #73353, #41901, #65848, #26871, #79389, #80375, #42379, #95880, #40911, #3894, #86887, #57854, #34362, #10895, #27361, #71410, #3397, #33375, #26377, #88365, #19861, #2927, #11874, #33859, #72362, #64853, #57367, #87862, #97362, #66338, #43346, #44819, #14349, #20859 ),
 ( #98858, #75824, #82828, #89349, #75326, #6839, #5374, #13851, #21854, #81352, #7346, #28352, #12848, #20364, #83329, #50858, #96876, #90316, #29325, #37353, #58842, #81833, #13349, #74834, #22349, #37846, #5854, #89834, #44329, #36847, #68337, #73845, #60329, #30313, #60813, #28831, #6337, #90820, #43833, #14855, #67844, #45327, #35850, #51350, #52822, #74329, #98362, #36346, #66841, #59331, #21350, #51842, #29820, #82329, #67337, #97862, #59822, #52335, #69815, #24811, #84332, #83824, #93286, #70310, #54297, #1338, #78283, #61308, #32775, #839, #15350, #91313, #61799, #23340, #32279, #45834, #68831, #76805, #77294, #46319, #8807, #7838, #40297, #53820, #62787, #53316, #1826, #31299, #39319, #84812, #92307, #9299, #31789, #55287, #15832, #76320, #85797, #17309, #16318, #62288, #9798, #91819, #22841, #23834, #38337, #361, #46802, #8323, #47786, #30811, #38826, #69318, #92792, #24321, #54787, #85304, #16810, #47286, #77787, #39809, #70805, #2322, #26263, #40790, #11261, #80746, #57247, #94763, #56761, #18780, #34237, #80249, #4760, #42264, #93779, #49262, #87744, #64733, #64245, #87255, #48763, #41780, #11755, #33266, #79763, #33744, #79270, #41297, #3783, #10780, #65230, #42751, #86781, #71770, #2814, #19257, #72249, #63759, #95245, #72733, #26752, #49741, #73232, #19748, #4266, #94264, #34739, #95756, #48271, #27240, #57736, #25307, #50232, #71289, #55793, #63271, #88239, #86288, #25790, #12241, #17796, #78785, #56285, #18284, #3281, #10292, #91578, #15594, #28228, #81717, #7096, #98620, #46077, #35231, #61067, #76566, #65729, #14612, #30069, #23095, #96754, #84079, #68585, #8083, #38579, #96256, #53565, #5256, #7602, #53073, #38098, #88732, #35735, #58727, #66223, #27734, #58217, #69076, #20244, #22596, #60578, #91070, #50747, #81235, #12734, #43231, #73725, #116, #75584, #89231, #30562, #20740, #51233, #45079, #37598, #68092, #83585, #15102, #45578, #76072, #61297, #91302, #91806, #60802, #23328, #45315, #76794, #98846, #828, #53809, #350, #31288, #68817, #83318, #84319, #24310, #61786, #38323, #30797, #15820, #8310, #23820, #47274, #84798, #37343, #46308, #92296, #38813, #7827, #69306, #22829, #54283, #16307, #75812, #46789, #76309, #53305, #83813, #77282, #15339, #8793, #85291, #30300, #45822, #7334, #39310, #69803, #37835, #1326, #31778, #62273, #92779, #16798, #54775, #6829, #68326, #67833, #98351, #90809, #29809, #60318, #22337, #52811, #14843, #70297, #77775, #41767, #9288, #55275, #48751, #86769, #94751, #17298, #40284, #70792, #33256, #79751, #34225, #63259, #48260, #2801, #94252, #64722, #39797, #18769 ) ),
 .UNSPECIFIED., .F., .F., .T. ) 
 B_SPLINE_SURFACE_WITH_KNOTS ( ( 2, 2 ),
 ( 3, 2, 2, 2, 2, 2, 2, 2, 2, 2, 2, 2, 2, 2, 2, 2, 2, 2, 2, 2, 2, 2, 2, 2, 2, 2, 2, 2, 2, 2, 2, 2, 2, 2, 2, 2, 2, 2, 2, 2, 2, 2, 2, 2, 2, 2, 2, 2, 2, 2, 2, 2, 2, 2, 2, 2, 2, 2, 2, 2, 2, 2, 2, 2, 2, 2, 2, 2, 2, 2, 2, 2, 2, 2, 2, 2, 2, 2, 2, 2, 2, 2, 2, 2, 2, 2, 2, 2, 2, 2, 2, 2, 2, 2, 2, 2, 2, 2, 2, 2, 2, 2, 2, 2, 2, 2, 2, 2, 2, 2, 2, 2, 2, 2, 2, 2, 2, 2, 2, 2, 2, 2, 2, 2, 2, 2, 2, 2, 2, 2, 2, 2, 2, 2, 2, 2, 2, 2, 2, 2, 2, 2, 2, 2, 2, 2, 2, 2, 2, 2, 2, 2, 2, 2, 2, 2, 2, 2, 2, 2, 2, 2, 3 ),
 ( 0.000000000000000000, 1.000000000000000000 ),
 ( 0.000000000000000000, 0.005952380952380952051, 0.01190476190476190410, 0.01785714285714285615, 0.02380952380952380820, 0.02976190476190476025, 0.03571428571428571230, 0.04166666666666666435, 0.04761904761904761640, 0.05357142857142856845, 0.05952380952380952051, 0.06547619047619047949, 0.07142857142857142461, 0.07738095238095238360, 0.08333333333333332871, 0.08928571428571428770, 0.09523809523809523281, 0.1011904761904761918, 0.1071428571428571369, 0.1130952380952380959, 0.1190476190476190410, 0.1250000000000000000, 0.1309523809523809590, 0.1369047619047619180, 0.1428571428571428492, 0.1488095238095238082, 0.1547619047619047672, 0.1607142857142857262, 0.1666666666666666574, 0.1726190476190476164, 0.1785714285714285754, 0.1845238095238095344, 0.1904761904761904656, 0.1964285714285714246, 0.2023809523809523836, 0.2083333333333333426, 0.2142857142857142738, 0.2202380952380952328, 0.2261904761904761918, 0.2321428571428571508, 0.2380952380952380820, 0.2440476190476190410, 0.2500000000000000000, 0.2559523809523809312, 0.2619047619047619180, 0.2678571428571428492, 0.2738095238095238360, 0.2797619047619047672, 0.2857142857142856984, 0.2916666666666666852, 0.2976190476190476164, 0.3035714285714285476, 0.3095238095238095344, 0.3154761904761904656, 0.3214285714285714524, 0.3273809523809523836, 0.3333333333333333148, 0.3392857142857143016, 0.3452380952380952328, 0.3511904761904761640, 0.3571428571428571508, 0.3630952380952380820, 0.3690476190476190688, 0.3750000000000000000, 0.3809523809523809312, 0.3869047619047619180, 0.3928571428571428492, 0.3988095238095238360, 0.4047619047619047672, 0.4107142857142856984, 0.4166666666666666852, 0.4226190476190476164, 0.4285714285714285476, 0.4345238095238095344, 0.4404761904761904656, 0.4464285714285714524, 0.4523809523809523836, 0.4583333333333333148, 0.4642857142857143016, 0.4702380952380952328, 0.4761904761904761640, 0.4821428571428571508, 0.4880952380952380820, 0.4940476190476190688, 0.5000000000000000000, 0.5059523809523809312, 0.5119047619047618625, 0.5178571428571429047, 0.5238095238095238360, 0.5297619047619047672, 0.5357142857142856984, 0.5416666666666666297, 0.5476190476190476719, 0.5535714285714286031, 0.5595238095238095344, 0.5654761904761904656, 0.5714285714285713969, 0.5773809523809523281, 0.5833333333333333703, 0.5892857142857143016, 0.5952380952380952328, 0.6011904761904761640, 0.6071428571428570953, 0.6130952380952381375, 0.6190476190476190688, 0.6250000000000000000, 0.6309523809523809312, 0.6369047619047618625, 0.6428571428571429047, 0.6488095238095238360, 0.6547619047619047672, 0.6607142857142856984, 0.6666666666666666297, 0.6726190476190476719, 0.6785714285714286031, 0.6845238095238095344, 0.6904761904761904656, 0.6964285714285713969, 0.7023809523809523281, 0.7083333333333333703, 0.7142857142857143016, 0.7202380952380952328, 0.7261904761904761640, 0.7321428571428570953, 0.7380952380952381375, 0.7440476190476190688, 0.7500000000000000000, 0.7559523809523809312, 0.7619047619047618625, 0.7678571428571429047, 0.7738095238095238360, 0.7797619047619047672, 0.7857142857142856984, 0.7916666666666666297, 0.7976190476190476719, 0.8035714285714286031, 0.8095238095238095344, 0.8154761904761904656, 0.8214285714285713969, 0.8273809523809523281, 0.8333333333333333703, 0.8392857142857143016, 0.8452380952380952328, 0.8511904761904761640, 0.8571428571428570953, 0.8630952380952381375, 0.8690476190476190688, 0.8750000000000000000, 0.8809523809523809312, 0.8869047619047618625, 0.8928571428571429047, 0.8988095238095238360, 0.9047619047619047672, 0.9107142857142856984, 0.9166666666666666297, 0.9226190476190476719, 0.9285714285714286031, 0.9345238095238095344, 0.9404761904761904656, 0.9464285714285713969, 0.9523809523809523281, 0.9583333333333333703, 0.9642857142857143016 ),
 .UNSPECIFIED. ) 
 GEOMETRIC_REPRESENTATION_ITEM ( )  RATIONAL_B_SPLINE_SURFACE ( (
 ( 1.000000000000000000, 0.9659258262890683122, 1.000000000000000000, 0.9659258262890683122, 1.000000000000000000, 0.9659258262890683122, 1.000000000000000000, 0.9659258262890683122, 1.000000000000000000, 0.9659258262890683122, 1.000000000000000000, 0.9659258262890683122, 1.000000000000000000, 0.9659258262890683122, 1.000000000000000000, 0.9659258262890683122, 1.000000000000000000, 0.9659258262890683122, 1.000000000000000000, 0.9659258262890683122, 1.000000000000000000, 0.9659258262890683122, 1.000000000000000000, 0.9659258262890683122, 1.000000000000000000, 0.9659258262890683122, 1.000000000000000000, 0.9659258262890683122, 1.000000000000000000, 0.9659258262890683122, 1.000000000000000000, 0.9659258262890683122, 1.000000000000000000, 0.9659258262890683122, 1.000000000000000000, 0.9659258262890683122, 1.000000000000000000, 0.9659258262890683122, 1.000000000000000000, 0.9659258262890683122, 1.000000000000000000, 0.9659258262890683122, 1.000000000000000000, 0.9659258262890683122, 1.000000000000000000, 0.9659258262890683122, 1.000000000000000000, 0.9659258262890683122, 1.000000000000000000, 0.9659258262890683122, 1.000000000000000000, 0.9659258262890683122, 1.000000000000000000, 0.9659258262890683122, 1.000000000000000000, 0.9659258262890683122, 1.000000000000000000, 0.9659258262890683122, 1.000000000000000000, 0.9659258262890683122, 1.000000000000000000, 0.9659258262890683122, 1.000000000000000000, 0.9659258262890683122, 1.000000000000000000, 0.9659258262890683122, 1.000000000000000000, 0.9659258262890683122, 1.000000000000000000, 0.9659258262890683122, 1.000000000000000000, 0.9659258262890683122, 1.000000000000000000, 0.9659258262890683122, 1.000000000000000000, 0.9659258262890683122, 1.000000000000000000, 0.9659258262890683122, 1.000000000000000000, 0.9659258262890683122, 1.000000000000000000, 0.9659258262890683122, 1.000000000000000000, 0.9659258262890683122, 1.000000000000000000, 0.9659258262890683122, 1.000000000000000000, 0.9659258262890683122, 1.000000000000000000, 0.9659258262890683122, 1.000000000000000000, 0.9659258262890683122, 1.000000000000000000, 0.9659258262890683122, 1.000000000000000000, 0.9659258262890683122, 1.000000000000000000, 0.9659258262890683122, 1.000000000000000000, 0.9659258262890683122, 1.000000000000000000, 0.9659258262890683122, 1.000000000000000000, 0.9659258262890683122, 1.000000000000000000, 0.9659258262890683122, 1.000000000000000000, 0.9659258262890683122, 1.000000000000000000, 0.9659258262890683122, 1.000000000000000000, 0.9659258262890683122, 1.000000000000000000, 0.9659258262890683122, 1.000000000000000000, 0.9659258262890683122, 1.000000000000000000, 0.9659258262890683122, 1.000000000000000000, 0.9659258262890683122, 1.000000000000000000, 0.9659258262890683122, 1.000000000000000000, 0.9659258262890683122, 1.000000000000000000, 0.9659258262890683122, 1.000000000000000000, 0.9659258262890683122, 1.000000000000000000, 0.9659258262890683122, 1.000000000000000000, 0.9659258262890683122, 1.000000000000000000, 0.9659258262890683122, 1.000000000000000000, 0.9659258262890683122, 1.000000000000000000, 0.9659258262890683122, 1.000000000000000000, 0.9659258262890683122, 1.000000000000000000, 0.9659258262890683122, 1.000000000000000000, 0.9659258262890683122, 1.000000000000000000, 0.9659258262890683122, 1.000000000000000000, 0.9659258262890683122, 1.000000000000000000, 0.9659258262890683122, 1.000000000000000000, 0.9659258262890683122, 1.000000000000000000, 0.9659258262890683122, 1.000000000000000000, 0.9659258262890683122, 1.000000000000000000, 0.9659258262890683122, 1.000000000000000000, 0.9659258262890683122, 1.000000000000000000, 0.9659258262890683122, 1.000000000000000000, 0.9659258262890683122, 1.000000000000000000, 0.9659258262890683122, 1.000000000000000000, 0.9659258262890683122, 1.000000000000000000, 0.9659258262890683122, 1.000000000000000000, 0.9659258262890683122, 1.000000000000000000, 0.9659258262890683122, 1.000000000000000000, 0.9659258262890683122, 1.000000000000000000, 0.9659258262890683122, 1.000000000000000000, 0.9659258262890683122, 1.000000000000000000, 0.9659258262890683122, 1.000000000000000000, 0.9659258262890683122, 1.000000000000000000, 0.9659258262890683122, 1.000000000000000000, 0.9659258262890683122, 1.000000000000000000, 0.9659258262890683122, 1.000000000000000000, 0.9659258262890683122, 1.000000000000000000, 0.9659258262890683122, 1.000000000000000000, 0.9659258262890683122, 1.000000000000000000, 0.9659258262890683122, 1.000000000000000000, 0.9659258262890683122, 1.000000000000000000, 0.9659258262890683122, 1.000000000000000000, 0.9659258262890683122, 1.000000000000000000, 0.9659258262890683122, 1.000000000000000000, 0.9659258262890683122, 1.000000000000000000, 0.9659258262890683122, 1.000000000000000000, 0.9659258262890683122, 1.000000000000000000, 0.9659258262890683122, 1.000000000000000000, 0.9659258262890683122, 1.000000000000000000, 0.9659258262890683122, 1.000000000000000000, 0.9659258262890683122, 1.000000000000000000, 0.9659258262890683122, 1.000000000000000000, 0.9659258262890683122, 1.000000000000000000, 0.9659258262890683122, 1.000000000000000000, 0.9659258262890683122, 1.000000000000000000, 0.9659258262890683122, 1.000000000000000000, 0.9659258262890683122, 1.000000000000000000, 0.9659258262890683122, 1.000000000000000000, 0.9659258262890683122, 1.000000000000000000, 0.9659258262890683122, 1.000000000000000000, 0.9659258262890683122, 1.000000000000000000, 0.9659258262890683122, 1.000000000000000000, 0.9659258262890683122, 1.000000000000000000, 0.9659258262890683122, 1.000000000000000000, 0.9659258262890683122, 1.000000000000000000, 0.9659258262890683122, 1.000000000000000000, 0.9659258262890683122, 1.000000000000000000, 0.9659258262890683122, 1.000000000000000000, 0.9659258262890683122, 1.000000000000000000, 0.9659258262890683122, 1.000000000000000000, 0.9659258262890683122, 1.000000000000000000, 0.9659258262890683122, 1.000000000000000000, 0.9659258262890683122, 1.000000000000000000, 0.9659258262890683122, 1.000000000000000000, 0.9659258262890683122, 1.000000000000000000, 0.9659258262890683122, 1.000000000000000000, 0.9659258262890683122, 1.000000000000000000, 0.9659258262890683122, 1.000000000000000000, 0.9659258262890683122, 1.000000000000000000, 0.9659258262890683122, 1.000000000000000000, 0.9659258262890683122, 1.000000000000000000, 0.9659258262890683122, 1.000000000000000000, 0.9659258262890683122, 1.000000000000000000, 0.9659258262890683122, 1.000000000000000000, 0.9659258262890683122, 1.000000000000000000, 0.9659258262890683122, 1.000000000000000000, 0.9659258262890683122, 1.000000000000000000, 0.9659258262890683122, 1.000000000000000000, 0.9659258262890683122, 1.000000000000000000, 0.9659258262890683122, 1.000000000000000000, 0.9659258262890683122, 1.000000000000000000, 0.9659258262890683122, 1.000000000000000000, 0.9659258262890683122, 1.000000000000000000, 0.9659258262890683122, 1.000000000000000000, 0.9659258262890683122, 1.000000000000000000, 0.9659258262890683122, 1.000000000000000000, 0.9659258262890683122, 1.000000000000000000, 0.9659258262890683122, 1.000000000000000000, 0.9659258262890683122, 1.000000000000000000, 0.9659258262890683122, 1.000000000000000000, 0.9659258262890683122, 1.000000000000000000, 0.9659258262890683122, 1.000000000000000000, 0.9659258262890683122, 1.000000000000000000),
 ( 1.000000000000000000, 0.9659258262890683122, 1.000000000000000000, 0.9659258262890683122, 1.000000000000000000, 0.9659258262890683122, 1.000000000000000000, 0.9659258262890683122, 1.000000000000000000, 0.9659258262890683122, 1.000000000000000000, 0.9659258262890683122, 1.000000000000000000, 0.9659258262890683122, 1.000000000000000000, 0.9659258262890683122, 1.000000000000000000, 0.9659258262890683122, 1.000000000000000000, 0.9659258262890683122, 1.000000000000000000, 0.9659258262890683122, 1.000000000000000000, 0.9659258262890683122, 1.000000000000000000, 0.9659258262890683122, 1.000000000000000000, 0.9659258262890683122, 1.000000000000000000, 0.9659258262890683122, 1.000000000000000000, 0.9659258262890683122, 1.000000000000000000, 0.9659258262890683122, 1.000000000000000000, 0.9659258262890683122, 1.000000000000000000, 0.9659258262890683122, 1.000000000000000000, 0.9659258262890683122, 1.000000000000000000, 0.9659258262890683122, 1.000000000000000000, 0.9659258262890683122, 1.000000000000000000, 0.9659258262890683122, 1.000000000000000000, 0.9659258262890683122, 1.000000000000000000, 0.9659258262890683122, 1.000000000000000000, 0.9659258262890683122, 1.000000000000000000, 0.9659258262890683122, 1.000000000000000000, 0.9659258262890683122, 1.000000000000000000, 0.9659258262890683122, 1.000000000000000000, 0.9659258262890683122, 1.000000000000000000, 0.9659258262890683122, 1.000000000000000000, 0.9659258262890683122, 1.000000000000000000, 0.9659258262890683122, 1.000000000000000000, 0.9659258262890683122, 1.000000000000000000, 0.9659258262890683122, 1.000000000000000000, 0.9659258262890683122, 1.000000000000000000, 0.9659258262890683122, 1.000000000000000000, 0.9659258262890683122, 1.000000000000000000, 0.9659258262890683122, 1.000000000000000000, 0.9659258262890683122, 1.000000000000000000, 0.9659258262890683122, 1.000000000000000000, 0.9659258262890683122, 1.000000000000000000, 0.9659258262890683122, 1.000000000000000000, 0.9659258262890683122, 1.000000000000000000, 0.9659258262890683122, 1.000000000000000000, 0.9659258262890683122, 1.000000000000000000, 0.9659258262890683122, 1.000000000000000000, 0.9659258262890683122, 1.000000000000000000, 0.9659258262890683122, 1.000000000000000000, 0.9659258262890683122, 1.000000000000000000, 0.9659258262890683122, 1.000000000000000000, 0.9659258262890683122, 1.000000000000000000, 0.9659258262890683122, 1.000000000000000000, 0.9659258262890683122, 1.000000000000000000, 0.9659258262890683122, 1.000000000000000000, 0.9659258262890683122, 1.000000000000000000, 0.9659258262890683122, 1.000000000000000000, 0.9659258262890683122, 1.000000000000000000, 0.9659258262890683122, 1.000000000000000000, 0.9659258262890683122, 1.000000000000000000, 0.9659258262890683122, 1.000000000000000000, 0.9659258262890683122, 1.000000000000000000, 0.9659258262890683122, 1.000000000000000000, 0.9659258262890683122, 1.000000000000000000, 0.9659258262890683122, 1.000000000000000000, 0.9659258262890683122, 1.000000000000000000, 0.9659258262890683122, 1.000000000000000000, 0.9659258262890683122, 1.000000000000000000, 0.9659258262890683122, 1.000000000000000000, 0.9659258262890683122, 1.000000000000000000, 0.9659258262890683122, 1.000000000000000000, 0.9659258262890683122, 1.000000000000000000, 0.9659258262890683122, 1.000000000000000000, 0.9659258262890683122, 1.000000000000000000, 0.9659258262890683122, 1.000000000000000000, 0.9659258262890683122, 1.000000000000000000, 0.9659258262890683122, 1.000000000000000000, 0.9659258262890683122, 1.000000000000000000, 0.9659258262890683122, 1.000000000000000000, 0.9659258262890683122, 1.000000000000000000, 0.9659258262890683122, 1.000000000000000000, 0.9659258262890683122, 1.000000000000000000, 0.9659258262890683122, 1.000000000000000000, 0.9659258262890683122, 1.000000000000000000, 0.9659258262890683122, 1.000000000000000000, 0.9659258262890683122, 1.000000000000000000, 0.9659258262890683122, 1.000000000000000000, 0.9659258262890683122, 1.000000000000000000, 0.9659258262890683122, 1.000000000000000000, 0.9659258262890683122, 1.000000000000000000, 0.9659258262890683122, 1.000000000000000000, 0.9659258262890683122, 1.000000000000000000, 0.9659258262890683122, 1.000000000000000000, 0.9659258262890683122, 1.000000000000000000, 0.9659258262890683122, 1.000000000000000000, 0.9659258262890683122, 1.000000000000000000, 0.9659258262890683122, 1.000000000000000000, 0.9659258262890683122, 1.000000000000000000, 0.9659258262890683122, 1.000000000000000000, 0.9659258262890683122, 1.000000000000000000, 0.9659258262890683122, 1.000000000000000000, 0.9659258262890683122, 1.000000000000000000, 0.9659258262890683122, 1.000000000000000000, 0.9659258262890683122, 1.000000000000000000, 0.9659258262890683122, 1.000000000000000000, 0.9659258262890683122, 1.000000000000000000, 0.9659258262890683122, 1.000000000000000000, 0.9659258262890683122, 1.000000000000000000, 0.9659258262890683122, 1.000000000000000000, 0.9659258262890683122, 1.000000000000000000, 0.9659258262890683122, 1.000000000000000000, 0.9659258262890683122, 1.000000000000000000, 0.9659258262890683122, 1.000000000000000000, 0.9659258262890683122, 1.000000000000000000, 0.9659258262890683122, 1.000000000000000000, 0.9659258262890683122, 1.000000000000000000, 0.9659258262890683122, 1.000000000000000000, 0.9659258262890683122, 1.000000000000000000, 0.9659258262890683122, 1.000000000000000000, 0.9659258262890683122, 1.000000000000000000, 0.9659258262890683122, 1.000000000000000000, 0.9659258262890683122, 1.000000000000000000, 0.9659258262890683122, 1.000000000000000000, 0.9659258262890683122, 1.000000000000000000, 0.9659258262890683122, 1.000000000000000000, 0.9659258262890683122, 1.000000000000000000, 0.9659258262890683122, 1.000000000000000000, 0.9659258262890683122, 1.000000000000000000, 0.9659258262890683122, 1.000000000000000000, 0.9659258262890683122, 1.000000000000000000, 0.9659258262890683122, 1.000000000000000000, 0.9659258262890683122, 1.000000000000000000, 0.9659258262890683122, 1.000000000000000000, 0.9659258262890683122, 1.000000000000000000, 0.9659258262890683122, 1.000000000000000000, 0.9659258262890683122, 1.000000000000000000, 0.9659258262890683122, 1.000000000000000000, 0.9659258262890683122, 1.000000000000000000, 0.9659258262890683122, 1.000000000000000000, 0.9659258262890683122, 1.000000000000000000, 0.9659258262890683122, 1.000000000000000000, 0.9659258262890683122, 1.000000000000000000, 0.9659258262890683122, 1.000000000000000000, 0.9659258262890683122, 1.000000000000000000, 0.9659258262890683122, 1.000000000000000000, 0.9659258262890683122, 1.000000000000000000, 0.9659258262890683122, 1.000000000000000000, 0.9659258262890683122, 1.000000000000000000, 0.9659258262890683122, 1.000000000000000000, 0.9659258262890683122, 1.000000000000000000, 0.9659258262890683122, 1.000000000000000000, 0.9659258262890683122, 1.000000000000000000, 0.9659258262890683122, 1.000000000000000000, 0.9659258262890683122, 1.000000000000000000, 0.9659258262890683122, 1.000000000000000000, 0.9659258262890683122, 1.000000000000000000, 0.9659258262890683122, 1.000000000000000000, 0.9659258262890683122, 1.000000000000000000, 0.9659258262890683122, 1.000000000000000000, 0.9659258262890683122, 1.000000000000000000, 0.9659258262890683122, 1.000000000000000000, 0.9659258262890683122, 1.000000000000000000) ) ) 
 REPRESENTATION_ITEM ( '' )  SURFACE ( )  );
#32405=B_SPLINE_CURVE_WITH_KNOTS ( 'NONE', 3,
 ( #77305, #8819, #39333, #97881 ),
 .UNSPECIFIED., .F., .F.,
 ( 4, 4 ),
 ( 2.168404344971008868E-19, 0.002657014572711346306 ),
 .UNSPECIFIED. ) ;
#32406=CARTESIAN_POINT ( 'NONE',  ( 21.09922568453594849, 31.20696800326375353, 6.408140936763242479 ) ) ;
#32408=CARTESIAN_POINT ( 'NONE',  ( -2.266590686148945544, 52.22041550158064638, 7.082119434687048631 ) ) ;
#32409=CARTESIAN_POINT ( 'NONE',  ( 5.076628168052704559, 25.17559781766745175, -8.527530157486179263 ) ) ;
#32410=EDGE_CURVE ( 'NONE', #40991, #56450, #40862, .T. ) ;
#32411=CARTESIAN_POINT ( 'NONE',  ( 18.52753015748618282, 3.925597817667451306, -4.923371831947291888 ) ) ;
#32412=CARTESIAN_POINT ( 'NONE',  ( 20.00000000000000711, 97.09902325089555575, 4.954892789985619217 ) ) ;
#32413=CARTESIAN_POINT ( 'NONE',  ( 2.917880565312950480, 45.97041550158063927, -12.26659068614894821 ) ) ;
#32414=CARTESIAN_POINT ( 'NONE',  ( 17.20831665107776587, 57.88393115100078745, 7.208316651077764980 ) ) ;
#32415=CARTESIAN_POINT ( 'NONE',  ( -4.164238869374098151, 56.59541550158063927, -3.795296366450310543 ) ) ;
#32416=CARTESIAN_POINT ( 'NONE',  ( 6.204703633549690345, 27.84541550158063217, 14.16423886937410082 ) ) ;
#32417=CARTESIAN_POINT ( 'NONE',  ( -4.164238869374098151, 36.59541550158063217, -3.795296366450310543 ) ) ;
#32418=PLANE ( 'NONE',  #21181 ) ;
#32421=CARTESIAN_POINT ( 'NONE',  ( 18.52753015748618282, 53.92559781766745175, -4.923371831947291888 ) ) ;
#32423=CARTESIAN_POINT ( 'NONE',  ( 15.44008868035555793, 31.39701867748817676, -9.422509992056140149 ) ) ;
#32425=CARTESIAN_POINT ( 'NONE',  ( 19.99999999998935607, 97.09160088439429614, -4.954669604078111966 ) ) ;
#32426=CARTESIAN_POINT ( 'NONE',  ( 0.1532563361054083140, 36.00893115100078745, 1.131784320476157264E-15 ) ) ;
#32427=CARTESIAN_POINT ( 'NONE',  ( 19.50000000000000355, 98.59912998021083297, 5.000000000000000000 ) ) ;
#32429=CARTESIAN_POINT ( 'NONE',  ( 12.63842701281683034, 37.46726448433411605, 9.846743663894596210 ) ) ;
#32430=CARTESIAN_POINT ( 'NONE',  ( 5.076628168052704559, 65.17559781766745175, -8.527530157486179263 ) ) ;
#32432=CARTESIAN_POINT ( 'NONE',  ( 10.00000000000000000, 10.55374883491396787, -14.16423886937410082 ) ) ;
#32434=DIRECTION ( 'NONE',  ( 0.000000000000000000, 0.000000000000000000, -1.000000000000000000 ) ) ;
#32437=CARTESIAN_POINT ( 'NONE',  ( 6.204703633549690345, 67.84541550158060375, 14.16423886937410082 ) ) ;
#32439=CARTESIAN_POINT ( 'NONE',  ( 3.591859063236763294, 28.29030133659708568, -11.09922568453595026 ) ) ;
#32441=CARTESIAN_POINT ( 'NONE',  ( 7.361572987183169658, -0.03273551566588185635, -9.846743663894592657 ) ) ;
#32443=DIRECTION ( 'NONE',  ( 0.000000000000000000, 0.000000000000000000, 1.000000000000000000 ) ) ;
#32444=CARTESIAN_POINT ( 'NONE',  ( 1.959929470562270071, 31.50257860105348939, 5.767676674365832312 ) ) ;
#32446=CARTESIAN_POINT ( 'NONE',  ( 17.08211943468705130, 63.47041550158063927, 12.26659068614894998 ) ) ;
#32447=CARTESIAN_POINT ( 'NONE',  ( 18.04007052943772038, 44.00257860105348584, -5.767676674365850076 ) ) ;
#32448=CARTESIAN_POINT ( 'NONE',  ( -0.04068437667222732368, 42.21974360917722180, -6.396802510829763477 ) ) ;
#32449=CARTESIAN_POINT ( 'NONE',  ( 12.91533473730993009, 26.60535201082150536, -10.88017736071109987 ) ) ;
#32450=CARTESIAN_POINT ( 'NONE',  ( 20.88017736071110164, 35.35535201082150536, 2.915334737309930979 ) ) ;
#32451=CARTESIAN_POINT ( 'NONE',  ( 16.40814093676323893, 5.790301336597087456, 11.09922568453595026 ) ) ;
#32452=CARTESIAN_POINT ( 'NONE',  ( 18.52753015748618282, 53.92559781766745175, -4.923371831947291888 ) ) ;
#32453=CARTESIAN_POINT ( 'NONE',  ( -43.49625190214930370, 106.3671137969544986, -5.071642103756534681 ) ) ;
#32454=CARTESIAN_POINT ( 'NONE',  ( 1.816707512666855928, 55.10290668512021739, -6.500000000000003553 ) ) ;
#32455=ORIENTED_EDGE ( 'NONE', *, *, #68114, .F. ) ;
#32456=CARTESIAN_POINT ( 'NONE',  ( 19.42250999205614548, 25.98035201082150891, -5.440088680355545492 ) ) ;
#32457=CARTESIAN_POINT ( 'NONE',  ( -2.816281873526471635, 33.91530133659708213, -3.434112377981056508 ) ) ;
#32458=CARTESIAN_POINT ( 'NONE',  ( -0.000000000000000000, 73.92154906606739928, 5.594368090432983109 ) ) ;
#32459=CARTESIAN_POINT ( 'NONE',  ( 19.84674366389459266, 58.71726448433411605, -2.638427012816827677 ) ) ;
#32460=B_SPLINE_CURVE_WITH_KNOTS ( 'NONE', 3,
 ( #39839, #24360, #54823, #70345 ),
 .UNSPECIFIED., .F., .F.,
 ( 4, 4 ),
 ( 0.000000000000000000, 0.001036303429213370061 ),
 .UNSPECIFIED. ) ;
#32461=CARTESIAN_POINT ( 'NONE',  ( 7.084665262690076126, 54.10535201082151247, 10.88017736071109987 ) ) ;
#32462=CARTESIAN_POINT ( 'NONE',  ( 0.1532563361054083140, 16.00893115100078390, 1.131784320476157264E-15 ) ) ;
#32463=CARTESIAN_POINT ( 'NONE',  ( -2.816281873526473856, 34.12363466993042493, 9.499525473075851096E-16 ) ) ;
#32464=CARTESIAN_POINT ( 'NONE',  ( 4.559911319644449179, 58.89701867748817676, 9.422509992056141925 ) ) ;
#32467=CARTESIAN_POINT ( 'NONE',  ( 22.81628187352648496, 61.83196800326376774, -3.434112377981050290 ) ) ;
#32470=CARTESIAN_POINT ( 'NONE',  ( 2.153642693323435164, 16.13791097397318808, -6.500000000000007105 ) ) ;
#32471=CARTESIAN_POINT ( 'NONE',  ( -0.8801773607111008646, 3.272018677488171434, 2.915334737309923430 ) ) ;
#32472=CARTESIAN_POINT ( 'NONE',  ( 10.00000000000000178, 50.37363466993042493, 12.81628187352647608 ) ) ;
#32473=CARTESIAN_POINT ( 'NONE',  ( 24.16423886937410614, 14.51208216824730179, -3.795296366450302550 ) ) ;
#32474=CARTESIAN_POINT ( 'NONE',  ( 14.92337183194729633, 17.67559781766745175, 8.527530157486181039 ) ) ;
#32475=CARTESIAN_POINT ( 'NONE',  ( 20.88017736071110164, 5.355352010821502695, 2.915334737309930979 ) ) ;
#32476=CARTESIAN_POINT ( 'NONE',  ( 18.52753015748617571, 23.09226448433411960, 4.923371831947298993 ) ) ;
#32477=CARTESIAN_POINT ( 'NONE',  ( -4.164238869374098151, 56.59541550158063927, -3.795296366450310543 ) ) ;
#32479=CARTESIAN_POINT ( 'NONE',  ( -0.8801773607111008646, 3.272018677488171434, 2.915334737309923430 ) ) ;
#32480=CARTESIAN_POINT ( 'NONE',  ( 17.96484262340118221, 26.18868534415483396, -7.964842623401177768 ) ) ;
#32481=CARTESIAN_POINT ( 'NONE',  ( 19.80448550324509327, 46.82703681773345039, 6.500000000002693845 ) ) ;
#32485=CARTESIAN_POINT ( 'NONE',  ( 17.96484262340118221, 16.18868534415483396, -7.964842623401177768 ) ) ;
#32486=CARTESIAN_POINT ( 'NONE',  ( 12.91533473730993009, 16.60535201082150891, -10.88017736071109987 ) ) ;
#32487=CARTESIAN_POINT ( 'NONE',  ( 0.1532563361054083140, 56.00893115100078745, 1.131784320476157264E-15 ) ) ;
#32488=PLANE ( 'NONE',  #69980 ) ;
#32489=CARTESIAN_POINT ( 'NONE',  ( -0.1503990784575328643, 20.12777174578613071, 6.262539305110068177 ) ) ;
#32490=CARTESIAN_POINT ( 'NONE',  ( 2.917880565312948704, 17.63708216824730357, 12.26659068614894643 ) ) ;
#32491=CARTESIAN_POINT ( 'NONE',  ( 19.42250999205614548, 25.98035201082150891, -5.440088680355545492 ) ) ;
#32492=CARTESIAN_POINT ( 'NONE',  ( 4.559911319644449179, 7.230352010821505360, -9.422509992056141925 ) ) ;
#32493=CARTESIAN_POINT ( 'NONE',  ( 1.472469842513823179, 51.42559781766745886, 4.923371831947296329 ) ) ;
#32494=CARTESIAN_POINT ( 'NONE',  ( 17.62281668512000010, 43.28593319516822646, 6.500000000000063061 ) ) ;
#32495=CARTESIAN_POINT ( 'NONE',  ( 0.1532563361054083140, 36.00893115100078745, 1.131784320476157264E-15 ) ) ;
#32496=CARTESIAN_POINT ( 'NONE',  ( 14.92337183194729988, 9.342264484334119601, -8.527530157486177487 ) ) ;
#32500=CARTESIAN_POINT ( 'NONE',  ( 7.084665262690076126, 69.10535201082151957, 10.88017736071109987 ) ) ;
#32501=CARTESIAN_POINT ( 'NONE',  ( -2.816281873526471635, 3.915301336597087456, -3.434112377981056508 ) ) ;
#32502=CARTESIAN_POINT ( 'NONE',  ( 15.44008868035555260, 44.73035201082151247, 9.422509992056143702 ) ) ;
#32503=CARTESIAN_POINT ( 'NONE',  ( 10.00000000000000000, 46.81368534415484106, -10.88017736071110342 ) ) ;
#32504=CARTESIAN_POINT ( 'NONE',  ( 7.084665262690076126, 4.105352010821503583, 10.88017736071109987 ) ) ;
#32505=CARTESIAN_POINT ( 'NONE',  ( -2.816281873526473856, 44.33196800326375353, 3.434112377981055619 ) ) ;
#32506=CARTESIAN_POINT ( 'NONE',  ( 13.79529636645030344, 23.26208216824730002, 14.16423886937410614 ) ) ;
#32509=CARTESIAN_POINT ( 'NONE',  ( -1.099225684535947600, 48.70696800326375353, -6.408140936763238038 ) ) ;
#32510=ORIENTED_EDGE ( 'NONE', *, *, #64347, .T. ) ;
#32511=CARTESIAN_POINT ( 'NONE',  ( 1.472469842513823179, 56.42559781766745886, 4.923371831947296329 ) ) ;
#32512=CARTESIAN_POINT ( 'NONE',  ( 19.42250999205614548, 15.98035201082150714, -5.440088680355545492 ) ) ;
#32514=CARTESIAN_POINT ( 'NONE',  ( 4.559911319644449179, 33.89701867748817676, 9.422509992056141925 ) ) ;
#32516=CARTESIAN_POINT ( 'NONE',  ( 0.1532563361054083140, 11.00893115100078568, 1.131784320476157264E-15 ) ) ;
#32517=CARTESIAN_POINT ( 'NONE',  ( -45.94000000000001194, 103.9981609152045507, 5.961202730336935041 ) ) ;
#32518=CARTESIAN_POINT ( 'NONE',  ( 0.1532563361054083140, 11.00893115100078568, 1.131784320476157264E-15 ) ) ;
#32519=CARTESIAN_POINT ( 'NONE',  ( 1.472469842513823179, 0.5922644843341181575, -4.923371831947296329 ) ) ;
#32521=CARTESIAN_POINT ( 'NONE',  ( 19.42250999205614548, 55.98035201082150536, -5.440088680355545492 ) ) ;
#32523=CARTESIAN_POINT ( 'NONE',  ( 10.00000000000000178, 69.31368534415484817, 10.88017736071110342 ) ) ;
#32524=CARTESIAN_POINT ( 'NONE',  ( 7.361572987183169658, 4.967264484334119601, -9.846743663894592657 ) ) ;
#32525=VERTEX_POINT ( 'NONE', #65802 ) ;
#32528=CARTESIAN_POINT ( 'NONE',  ( 5.076628168052703671, 61.84226448433412315, 8.527530157486179263 ) ) ;
#32532=CARTESIAN_POINT ( 'NONE',  ( 2.917880565312948704, 2.637082168247300906, 12.26659068614894643 ) ) ;
#32533=CARTESIAN_POINT ( 'NONE',  ( -1.099225684535947600, 53.70696800326376064, -6.408140936763238038 ) ) ;
#32534=CARTESIAN_POINT ( 'NONE',  ( 6.204703633549690345, 2.845415501580634388, 14.16423886937410082 ) ) ;
#32535=CARTESIAN_POINT ( 'NONE',  ( 6.204703633549690345, 20.76208216824730357, -14.16423886937410259 ) ) ;
#32538=CARTESIAN_POINT ( 'NONE',  ( 10.00000000000000178, 24.31368534415484106, 10.88017736071110342 ) ) ;
#32539=ORIENTED_EDGE ( 'NONE', *, *, #80905, .T. ) ;
#32540=CARTESIAN_POINT ( 'NONE',  ( 12.63842701281683922, 9.550597817667449974, -9.846743663894590881 ) ) ;
#32541=CARTESIAN_POINT ( 'NONE',  ( 19.84674366389459621, 18.50893115100078745, 7.409399052514197653E-17 ) ) ;
#32542=CARTESIAN_POINT ( 'NONE',  ( 6.565887622018943937, 30.16530133659708568, 12.81628187352647430 ) ) ;
#32543=CARTESIAN_POINT ( 'NONE',  ( 1.472469842513823179, 35.59226448433412315, -4.923371831947296329 ) ) ;
#32545=CARTESIAN_POINT ( 'NONE',  ( -2.816281873526473856, 14.12363466993041961, 9.499525473075851096E-16 ) ) ;
#32547=CARTESIAN_POINT ( 'NONE',  ( 5.076628168052704559, 30.17559781766745175, -8.527530157486179263 ) ) ;
#32548=CARTESIAN_POINT ( 'NONE',  ( 2.791683348922237240, 0.3839311510007847872, -7.208316651077763204 ) ) ;
#32549=VERTEX_POINT ( 'NONE', #18357 ) ;
#32550=ORIENTED_EDGE ( 'NONE', *, *, #2179, .F. ) ;
#32551=CARTESIAN_POINT ( 'NONE',  ( 2.035157376598824452, 38.68868534415483396, 7.964842623401179544 ) ) ;
#32552=CARTESIAN_POINT ( 'NONE',  ( -2.266590686148945544, 26.38708216824730357, -7.082119434687050408 ) ) ;
#32553=CARTESIAN_POINT ( 'NONE',  ( 14.92337183194729988, 44.34226448433412315, -8.527530157486177487 ) ) ;
#32554=CARTESIAN_POINT ( 'NONE',  ( 18.52753015748617571, 18.09226448433411960, 4.923371831947298993 ) ) ;
#32555=CARTESIAN_POINT ( 'NONE',  ( 22.81628187352648496, 56.83196800326374643, -3.434112377981050290 ) ) ;
#32557=CARTESIAN_POINT ( 'NONE',  ( 4.559911319644449179, 33.89701867748817676, 9.422509992056141925 ) ) ;
#32560=CARTESIAN_POINT ( 'NONE',  ( 10.00000000000000178, 20.37363466993042138, 12.81628187352647608 ) ) ;
#32561=CARTESIAN_POINT ( 'NONE',  ( 21.09922568453595559, 22.04030133659708923, -6.408140936763230044 ) ) ;
#32562=CARTESIAN_POINT ( 'NONE',  ( 14.92337183194729633, 37.67559781766745175, 8.527530157486181039 ) ) ;
#32564=CARTESIAN_POINT ( 'NONE',  ( 16.40814093676324603, 47.45696800326375353, -11.09922568453594671 ) ) ;
#32565=CARTESIAN_POINT ( 'NONE',  ( -0.8801773607110991993, 57.85535201082149825, -2.915334737309923874 ) ) ;
#32570=CARTESIAN_POINT ( 'NONE',  ( 10.00000000000000000, 51.81368534415484106, -10.88017736071110342 ) ) ;
#32571=CARTESIAN_POINT ( 'NONE',  ( 0.5774900079438590739, 62.64701867748817676, -5.440088680355550821 ) ) ;
#32575=CARTESIAN_POINT ( 'NONE',  ( 10.00000000000000178, 4.313685344154837509, 10.88017736071110342 ) ) ;
#32576=CARTESIAN_POINT ( 'NONE',  ( 5.076628168052703671, 61.84226448433412315, 8.527530157486179263 ) ) ;
#32577=CARTESIAN_POINT ( 'NONE',  ( 20.88017736071110164, 20.35535201082150891, 2.915334737309930979 ) ) ;
#32580=CARTESIAN_POINT ( 'NONE',  ( -1.099225684535947600, 23.70696800326375708, -6.408140936763238038 ) ) ;
#32581=ORIENTED_EDGE ( 'NONE', *, *, #89065, .F. ) ;
#32582=CARTESIAN_POINT ( 'NONE',  ( 10.00000000000000000, 56.81368534415484106, -10.88017736071110342 ) ) ;
#32583=CARTESIAN_POINT ( 'NONE',  ( 18.52753015748618282, 33.92559781766745886, -4.923371831947291888 ) ) ;
#32585=CARTESIAN_POINT ( 'NONE',  ( 10.00000000000000178, 10.37363466993041961, 12.81628187352647608 ) ) ;
#32586=CARTESIAN_POINT ( 'NONE',  ( 19.88565890683629078, 47.71691075486302935, -6.480892540919839462 ) ) ;
#32587=CARTESIAN_POINT ( 'NONE',  ( 0.5774900079438590739, 7.647018677488171434, -5.440088680355550821 ) ) ;
#32588=CARTESIAN_POINT ( 'NONE',  ( 17.96484262340118221, 41.18868534415484106, -7.964842623401177768 ) ) ;
#32589=CARTESIAN_POINT ( 'NONE',  ( 24.16423886937409904, 54.09541550158063217, 3.795296366450317205 ) ) ;
#32590=CARTESIAN_POINT ( 'NONE',  ( 17.20831665107776587, 39.13393115100079456, -7.208316651077762316 ) ) ;
#32591=CARTESIAN_POINT ( 'NONE',  ( 4.559911319644449179, 63.89701867748817676, 9.422509992056141925 ) ) ;
#32593=CARTESIAN_POINT ( 'NONE',  ( 22.26659068614895176, 14.72041550158063572, -7.082119434687042414 ) ) ;
#32595=CARTESIAN_POINT ( 'NONE',  ( 1.274849032794306947, 7.555090184799359676, -6.499999999999997335 ) ) ;
#32597=CARTESIAN_POINT ( 'NONE',  ( -4.164238869374099927, 37.01208216824731068, 3.795296366450308767 ) ) ;
#32598=CARTESIAN_POINT ( 'NONE',  ( -2.266590686148945544, 37.22041550158063217, 7.082119434687048631 ) ) ;
#32599=CARTESIAN_POINT ( 'NONE',  ( 7.361572987183170547, 7.050597817667451750, 9.846743663894590881 ) ) ;
#32601=CARTESIAN_POINT ( 'NONE',  ( 22.81628187352647785, 11.62363466993042138, 6.195893100308588602E-16 ) ) ;
#32602=CARTESIAN_POINT ( 'NONE',  ( 7.361572987183170547, 67.05059781766746596, 9.846743663894590881 ) ) ;
#32603=LINE ( 'NONE', #63099, #22761 ) ;
#32604=CARTESIAN_POINT ( 'NONE',  ( 19.42250999205614193, 65.14701867748817676, 5.440088680355555262 ) ) ;
#32605=CARTESIAN_POINT ( 'NONE',  ( 22.81628187352648496, 31.83196800326375353, -3.434112377981050290 ) ) ;
#32606=CARTESIAN_POINT ( 'NONE',  ( -0.3689425029237881626, 32.42874883491395366, 10.36894250292379027 ) ) ;
#32607=CARTESIAN_POINT ( 'NONE',  ( 4.559911319644449179, 27.23035201082150536, -9.422509992056141925 ) ) ;
#32608=CARTESIAN_POINT ( 'NONE',  ( 20.15039907845753930, 70.00000000000000000, -6.262539305110068177 ) ) ;
#32609=CARTESIAN_POINT ( 'NONE',  ( 12.63842701281683034, 2.467264484334118269, 9.846743663894596210 ) ) ;
#32613=( BOUNDED_SURFACE ( )  B_SPLINE_SURFACE ( 1, 2, ( 
 ( #85990, #84511, #47482, #69020, #17502, #93972, #70495, #32479, #551, #47967, #1025, #78477, #24015, #9993, #31484, #61988, #40493, #92488, #77482, #2513, #63470, #30997, #61494, #92000, #96449, #79947, #49942, #58412, #41969, #10475, #19449, #64437, #73419, #65921, #95450, #86956, #27431, #41485, #18469, #48955, #27921, #56470, #79463, #57926, #26941, #94945, #17983, #19934, #80447, #2997, #11451, #11946, #42449, #57442, #48466, #88435, #78963, #72434, #10961, #72932, #87933, #4461, #34927, #71954, #50429, #3961, #34430, #65425, #40985, #71481, #87448, #95949, #64923, #3475, #4945, #80936, #12430, #33447, #63942, #18962, #42937, #26446, #56946, #33933, #35425, #94454, #49442, #25971, #58918, #89418, #45391, #20932, #51420, #81910, #75394, #96950, #66418, #51918, #13928, #6914, #28422, #44405, #82403, #21926, #74404, #13419, #90889, #82905, #22418, #7421, #37918, #21423, #37424, #68406, #29890, #43905, #67410, #5930, #43419, #35920, #36421, #67912, #73920, #74906, #97939, #29396, #60393, #66914, #28900, #97435, #14923, #59404, #89909, #6407, #36918, #98928, #59897, #90388, #52404, #52891, #5448, #14423, #44892, #98434, #83402, #20437, #75896, #30384, #88928, #50925, #81421, #12923, #62859, #23408, #31856, #84877, #68902, #69383, #78354, #40373, #8388, #906, #32353, #93355, #53892, #70378, #53382, #83893, #431, #39871, #31368, #9874, #85867, #38898, #61868, #54368, #39388, #9368, #85368, #92373, #16880, #47848, #77858, #70874, #69882, #23899, #77360, #1896, #84398, #16386, #46870, #8870, #24880, #1402, #46386, #55364, #17380, #15423, #62355, #92859, #24388, #54856, #47356, #2390, #60886, #30881, #15897, #91385, #22915, #45904, #76391, #7906, #38402, #61377, #91886, #76872, #95323, #11333, #12317, #4345, #32844, #87329, #94339, #64804, #3848, #41850, #49815, #71365, #34813, #94829, #56831, #26824, #93850, #42823, #3348, #72316, #26332, #18354, #19815, #18845, #11823, #27311, #25377, #80816, #57809, #65302, #33811, #78850, #49326, #50304, #79341, #86849, #95828, #88317, #33331, #79828, #64317, #73308, #63344, #2881, #42330, #17859, #25856, #63825, #56353, #55862, #34306, #57317, #87811, #71839, #86359, #19331, #48831, #80322, #48345, #10360, #40859, #72803, #10851, #41372, #66800, #14812, #6796, #65799, #74793, #81309, #51800, #89790, #36304, #97320, #73796, #59783, #21808, #43304, #59293, #96333, #52292, #52778, #36803, #90274, #27808, #67297, #12804, #28792, #81787, #21308, #5327, #58798, #37310, #35808, #66294, #44780, #82788, #13303, #82285, #96829, #83287, #13804, #97824, #45283, #44289, #58291, #6301, #51305, #60283 ),
 ( #28306, #89306, #29286, #14310, #75286, #20814, #67799, #98318, #29772, #43790, #74283, #90780, #22306, #4831, #35306, #88808, #20320, #50816, #5812, #16767, #7794, #54255, #38290, #30269, #22795, #68785, #92750, #60771, #8281, #84766, #16275, #47241, #30759, #15788, #91773, #1779, #317, #46276, #76279, #38778, #55239, #45788, #799, #76761, #77743, #91273, #23294, #69766, #15303, #46757, #7300, #1296, #24275, #70263, #61265, #53772, #32237, #9256, #84289, #77252, #31251, #83780, #69277, #93236, #85754, #61747, #92266, #39763, #62736, #23790, #85260, #68297, #98816, #8761, #54739, #39277, #24762, #17265, #31749, #62244, #75778, #37800, #53273, #72208, #86737, #3736, #34694, #64689, #27192, #56719, #25750, #64204, #95199, #10248, #56244, #79223, #71728, #26705, #26226, #33222, #49694, #72687, #40253, #18734, #3238, #18239, #79718, #33704, #41737, #94719, #57694, #70760, #48720, #87697, #94220, #10734, #40741, #4223, #49214, #41253, #2274, #17754, #48231, #65187, #78740, #71244, #11218, #25267, #87210, #34196, #57200, #19213, #2768, #80203, #11709, #86241, #42221, #9751, #95709, #88194, #47740, #78237, #32730, #63229, #55750, #93733, #63717, #82167, #6184, #36687, #82668, #29165, #90158, #14184, #44667, #75161, #67683, #29649, #60158, #42705, #63079, #71589, #53744, #22280, #32583, #76254, #86583, #79068, #9594, #98793, #40595, #53250, #30240, #60744, #10582, #68273, #91245, #71092, #40098, #7771, #41092, #33073, #93580, #14786, #23268, #25115, #55597, #70599, #29749, #2618, #60258, #85600, #22769, #86092, #2124, #17603, #48073, #83755, #63569, #91748, #17114, #78586, #90752, #52754, #289, #10098, #47597, #15279, #18092, #78091, #94077, #25598, #83262, #45256, #56091, #48568, #30735, #75753, #7275, #37776, #38265, #45760, #68758, #61242, #33555, #64053, #94565, #56577, #3101, #26083, #77955, #83987, #91976, #30972, #38495, #62948, #92460, #39483, #69480, #38987, #24976, #69973, #68990, #54459, #47940, #60976, #78446, #998, #9462, #84967, #61961, #9962, #1986, #91489, #8482, #31459, #23988, #16976, #77453, #84485, #32452, #55461, #23009, #1492, #16484, #46959, #31945, #8967, #92949, #62446, #40468, #53477, #24484, #39963, #46473, #54947, #23505, #85964, #85464, #47456, #15512, #61469, #53976, #28, #15986, #76969, #70464, #93451, #7997, #76483, #30475, #45994, #87910, #10451, #26421, #33908, #3938, #56447, #40959, #72908, #64896, #4441, #88414, #19914, #3451, #57417, #50405, #11923, #2970, #49418, #33420, #25474, #17954, #63919, #19424, #55956, #64416, #79919, #11428, #42427, #25945, #10938, #86933, #95929, #94430 ) ),
 .UNSPECIFIED., .F., .F., .T. ) 
 B_SPLINE_SURFACE_WITH_KNOTS ( ( 2, 2 ),
 ( 3, 2, 2, 2, 2, 2, 2, 2, 2, 2, 2, 2, 2, 2, 2, 2, 2, 2, 2, 2, 2, 2, 2, 2, 2, 2, 2, 2, 2, 2, 2, 2, 2, 2, 2, 2, 2, 2, 2, 2, 2, 2, 2, 2, 2, 2, 2, 2, 2, 2, 2, 2, 2, 2, 2, 2, 2, 2, 2, 2, 2, 2, 2, 2, 2, 2, 2, 2, 2, 2, 2, 2, 2, 2, 2, 2, 2, 2, 2, 2, 2, 2, 2, 2, 2, 2, 2, 2, 2, 2, 2, 2, 2, 2, 2, 2, 2, 2, 2, 2, 2, 2, 2, 2, 2, 2, 2, 2, 2, 2, 2, 2, 2, 2, 2, 2, 2, 2, 2, 2, 2, 2, 2, 2, 2, 2, 2, 2, 2, 2, 2, 2, 2, 2, 2, 2, 2, 2, 2, 2, 2, 2, 2, 2, 2, 2, 2, 2, 2, 2, 2, 2, 2, 2, 2, 2, 2, 2, 2, 2, 2, 2, 3 ),
 ( 0.000000000000000000, 1.000000000000000000 ),
 ( 0.000000000000000000, 0.005952380952380952051, 0.01190476190476190410, 0.01785714285714285615, 0.02380952380952380820, 0.02976190476190476025, 0.03571428571428571230, 0.04166666666666666435, 0.04761904761904761640, 0.05357142857142856845, 0.05952380952380952051, 0.06547619047619047949, 0.07142857142857142461, 0.07738095238095238360, 0.08333333333333332871, 0.08928571428571428770, 0.09523809523809523281, 0.1011904761904761918, 0.1071428571428571369, 0.1130952380952380959, 0.1190476190476190410, 0.1250000000000000000, 0.1309523809523809590, 0.1369047619047619180, 0.1428571428571428492, 0.1488095238095238082, 0.1547619047619047672, 0.1607142857142857262, 0.1666666666666666574, 0.1726190476190476164, 0.1785714285714285754, 0.1845238095238095344, 0.1904761904761904656, 0.1964285714285714246, 0.2023809523809523836, 0.2083333333333333426, 0.2142857142857142738, 0.2202380952380952328, 0.2261904761904761918, 0.2321428571428571508, 0.2380952380952380820, 0.2440476190476190410, 0.2500000000000000000, 0.2559523809523809312, 0.2619047619047619180, 0.2678571428571428492, 0.2738095238095238360, 0.2797619047619047672, 0.2857142857142856984, 0.2916666666666666852, 0.2976190476190476164, 0.3035714285714285476, 0.3095238095238095344, 0.3154761904761904656, 0.3214285714285714524, 0.3273809523809523836, 0.3333333333333333148, 0.3392857142857143016, 0.3452380952380952328, 0.3511904761904761640, 0.3571428571428571508, 0.3630952380952380820, 0.3690476190476190688, 0.3750000000000000000, 0.3809523809523809312, 0.3869047619047619180, 0.3928571428571428492, 0.3988095238095238360, 0.4047619047619047672, 0.4107142857142856984, 0.4166666666666666852, 0.4226190476190476164, 0.4285714285714285476, 0.4345238095238095344, 0.4404761904761904656, 0.4464285714285714524, 0.4523809523809523836, 0.4583333333333333148, 0.4642857142857143016, 0.4702380952380952328, 0.4761904761904761640, 0.4821428571428571508, 0.4880952380952380820, 0.4940476190476190688, 0.5000000000000000000, 0.5059523809523809312, 0.5119047619047618625, 0.5178571428571429047, 0.5238095238095238360, 0.5297619047619047672, 0.5357142857142856984, 0.5416666666666666297, 0.5476190476190476719, 0.5535714285714286031, 0.5595238095238095344, 0.5654761904761904656, 0.5714285714285713969, 0.5773809523809523281, 0.5833333333333333703, 0.5892857142857143016, 0.5952380952380952328, 0.6011904761904761640, 0.6071428571428570953, 0.6130952380952381375, 0.6190476190476190688, 0.6250000000000000000, 0.6309523809523809312, 0.6369047619047618625, 0.6428571428571429047, 0.6488095238095238360, 0.6547619047619047672, 0.6607142857142856984, 0.6666666666666666297, 0.6726190476190476719, 0.6785714285714286031, 0.6845238095238095344, 0.6904761904761904656, 0.6964285714285713969, 0.7023809523809523281, 0.7083333333333333703, 0.7142857142857143016, 0.7202380952380952328, 0.7261904761904761640, 0.7321428571428570953, 0.7380952380952381375, 0.7440476190476190688, 0.7500000000000000000, 0.7559523809523809312, 0.7619047619047618625, 0.7678571428571429047, 0.7738095238095238360, 0.7797619047619047672, 0.7857142857142856984, 0.7916666666666666297, 0.7976190476190476719, 0.8035714285714286031, 0.8095238095238095344, 0.8154761904761904656, 0.8214285714285713969, 0.8273809523809523281, 0.8333333333333333703, 0.8392857142857143016, 0.8452380952380952328, 0.8511904761904761640, 0.8571428571428570953, 0.8630952380952381375, 0.8690476190476190688, 0.8750000000000000000, 0.8809523809523809312, 0.8869047619047618625, 0.8928571428571429047, 0.8988095238095238360, 0.9047619047619047672, 0.9107142857142856984, 0.9166666666666666297, 0.9226190476190476719, 0.9285714285714286031, 0.9345238095238095344, 0.9404761904761904656, 0.9464285714285713969, 0.9523809523809523281, 0.9583333333333333703, 0.9642857142857143016 ),
 .UNSPECIFIED. ) 
 GEOMETRIC_REPRESENTATION_ITEM ( )  RATIONAL_B_SPLINE_SURFACE ( (
 ( 1.000000000000000000, 0.9659258262890683122, 1.000000000000000000, 0.9659258262890683122, 1.000000000000000000, 0.9659258262890683122, 1.000000000000000000, 0.9659258262890683122, 1.000000000000000000, 0.9659258262890683122, 1.000000000000000000, 0.9659258262890683122, 1.000000000000000000, 0.9659258262890683122, 1.000000000000000000, 0.9659258262890683122, 1.000000000000000000, 0.9659258262890683122, 1.000000000000000000, 0.9659258262890683122, 1.000000000000000000, 0.9659258262890683122, 1.000000000000000000, 0.9659258262890683122, 1.000000000000000000, 0.9659258262890683122, 1.000000000000000000, 0.9659258262890683122, 1.000000000000000000, 0.9659258262890683122, 1.000000000000000000, 0.9659258262890683122, 1.000000000000000000, 0.9659258262890683122, 1.000000000000000000, 0.9659258262890683122, 1.000000000000000000, 0.9659258262890683122, 1.000000000000000000, 0.9659258262890683122, 1.000000000000000000, 0.9659258262890683122, 1.000000000000000000, 0.9659258262890683122, 1.000000000000000000, 0.9659258262890683122, 1.000000000000000000, 0.9659258262890683122, 1.000000000000000000, 0.9659258262890683122, 1.000000000000000000, 0.9659258262890683122, 1.000000000000000000, 0.9659258262890683122, 1.000000000000000000, 0.9659258262890683122, 1.000000000000000000, 0.9659258262890683122, 1.000000000000000000, 0.9659258262890683122, 1.000000000000000000, 0.9659258262890683122, 1.000000000000000000, 0.9659258262890683122, 1.000000000000000000, 0.9659258262890683122, 1.000000000000000000, 0.9659258262890683122, 1.000000000000000000, 0.9659258262890683122, 1.000000000000000000, 0.9659258262890683122, 1.000000000000000000, 0.9659258262890683122, 1.000000000000000000, 0.9659258262890683122, 1.000000000000000000, 0.9659258262890683122, 1.000000000000000000, 0.9659258262890683122, 1.000000000000000000, 0.9659258262890683122, 1.000000000000000000, 0.9659258262890683122, 1.000000000000000000, 0.9659258262890683122, 1.000000000000000000, 0.9659258262890683122, 1.000000000000000000, 0.9659258262890683122, 1.000000000000000000, 0.9659258262890683122, 1.000000000000000000, 0.9659258262890683122, 1.000000000000000000, 0.9659258262890683122, 1.000000000000000000, 0.9659258262890683122, 1.000000000000000000, 0.9659258262890683122, 1.000000000000000000, 0.9659258262890683122, 1.000000000000000000, 0.9659258262890683122, 1.000000000000000000, 0.9659258262890683122, 1.000000000000000000, 0.9659258262890683122, 1.000000000000000000, 0.9659258262890683122, 1.000000000000000000, 0.9659258262890683122, 1.000000000000000000, 0.9659258262890683122, 1.000000000000000000, 0.9659258262890683122, 1.000000000000000000, 0.9659258262890683122, 1.000000000000000000, 0.9659258262890683122, 1.000000000000000000, 0.9659258262890683122, 1.000000000000000000, 0.9659258262890683122, 1.000000000000000000, 0.9659258262890683122, 1.000000000000000000, 0.9659258262890683122, 1.000000000000000000, 0.9659258262890683122, 1.000000000000000000, 0.9659258262890683122, 1.000000000000000000, 0.9659258262890683122, 1.000000000000000000, 0.9659258262890683122, 1.000000000000000000, 0.9659258262890683122, 1.000000000000000000, 0.9659258262890683122, 1.000000000000000000, 0.9659258262890683122, 1.000000000000000000, 0.9659258262890683122, 1.000000000000000000, 0.9659258262890683122, 1.000000000000000000, 0.9659258262890683122, 1.000000000000000000, 0.9659258262890683122, 1.000000000000000000, 0.9659258262890683122, 1.000000000000000000, 0.9659258262890683122, 1.000000000000000000, 0.9659258262890683122, 1.000000000000000000, 0.9659258262890683122, 1.000000000000000000, 0.9659258262890683122, 1.000000000000000000, 0.9659258262890683122, 1.000000000000000000, 0.9659258262890683122, 1.000000000000000000, 0.9659258262890683122, 1.000000000000000000, 0.9659258262890683122, 1.000000000000000000, 0.9659258262890683122, 1.000000000000000000, 0.9659258262890683122, 1.000000000000000000, 0.9659258262890683122, 1.000000000000000000, 0.9659258262890683122, 1.000000000000000000, 0.9659258262890683122, 1.000000000000000000, 0.9659258262890683122, 1.000000000000000000, 0.9659258262890683122, 1.000000000000000000, 0.9659258262890683122, 1.000000000000000000, 0.9659258262890683122, 1.000000000000000000, 0.9659258262890683122, 1.000000000000000000, 0.9659258262890683122, 1.000000000000000000, 0.9659258262890683122, 1.000000000000000000, 0.9659258262890683122, 1.000000000000000000, 0.9659258262890683122, 1.000000000000000000, 0.9659258262890683122, 1.000000000000000000, 0.9659258262890683122, 1.000000000000000000, 0.9659258262890683122, 1.000000000000000000, 0.9659258262890683122, 1.000000000000000000, 0.9659258262890683122, 1.000000000000000000, 0.9659258262890683122, 1.000000000000000000, 0.9659258262890683122, 1.000000000000000000, 0.9659258262890683122, 1.000000000000000000, 0.9659258262890683122, 1.000000000000000000, 0.9659258262890683122, 1.000000000000000000, 0.9659258262890683122, 1.000000000000000000, 0.9659258262890683122, 1.000000000000000000, 0.9659258262890683122, 1.000000000000000000, 0.9659258262890683122, 1.000000000000000000, 0.9659258262890683122, 1.000000000000000000, 0.9659258262890683122, 1.000000000000000000, 0.9659258262890683122, 1.000000000000000000, 0.9659258262890683122, 1.000000000000000000, 0.9659258262890683122, 1.000000000000000000, 0.9659258262890683122, 1.000000000000000000, 0.9659258262890683122, 1.000000000000000000, 0.9659258262890683122, 1.000000000000000000, 0.9659258262890683122, 1.000000000000000000, 0.9659258262890683122, 1.000000000000000000, 0.9659258262890683122, 1.000000000000000000, 0.9659258262890683122, 1.000000000000000000, 0.9659258262890683122, 1.000000000000000000, 0.9659258262890683122, 1.000000000000000000, 0.9659258262890683122, 1.000000000000000000, 0.9659258262890683122, 1.000000000000000000, 0.9659258262890683122, 1.000000000000000000, 0.9659258262890683122, 1.000000000000000000, 0.9659258262890683122, 1.000000000000000000, 0.9659258262890683122, 1.000000000000000000, 0.9659258262890683122, 1.000000000000000000, 0.9659258262890683122, 1.000000000000000000, 0.9659258262890683122, 1.000000000000000000, 0.9659258262890683122, 1.000000000000000000, 0.9659258262890683122, 1.000000000000000000, 0.9659258262890683122, 1.000000000000000000, 0.9659258262890683122, 1.000000000000000000, 0.9659258262890683122, 1.000000000000000000, 0.9659258262890683122, 1.000000000000000000, 0.9659258262890683122, 1.000000000000000000, 0.9659258262890683122, 1.000000000000000000, 0.9659258262890683122, 1.000000000000000000, 0.9659258262890683122, 1.000000000000000000, 0.9659258262890683122, 1.000000000000000000, 0.9659258262890683122, 1.000000000000000000, 0.9659258262890683122, 1.000000000000000000, 0.9659258262890683122, 1.000000000000000000, 0.9659258262890683122, 1.000000000000000000, 0.9659258262890683122, 1.000000000000000000, 0.9659258262890683122, 1.000000000000000000, 0.9659258262890683122, 1.000000000000000000, 0.9659258262890683122, 1.000000000000000000, 0.9659258262890683122, 1.000000000000000000, 0.9659258262890683122, 1.000000000000000000, 0.9659258262890683122, 1.000000000000000000, 0.9659258262890683122, 1.000000000000000000, 0.9659258262890683122, 1.000000000000000000, 0.9659258262890683122, 1.000000000000000000, 0.9659258262890683122, 1.000000000000000000, 0.9659258262890683122, 1.000000000000000000),
 ( 1.000000000000000000, 0.9659258262890683122, 1.000000000000000000, 0.9659258262890683122, 1.000000000000000000, 0.9659258262890683122, 1.000000000000000000, 0.9659258262890683122, 1.000000000000000000, 0.9659258262890683122, 1.000000000000000000, 0.9659258262890683122, 1.000000000000000000, 0.9659258262890683122, 1.000000000000000000, 0.9659258262890683122, 1.000000000000000000, 0.9659258262890683122, 1.000000000000000000, 0.9659258262890683122, 1.000000000000000000, 0.9659258262890683122, 1.000000000000000000, 0.9659258262890683122, 1.000000000000000000, 0.9659258262890683122, 1.000000000000000000, 0.9659258262890683122, 1.000000000000000000, 0.9659258262890683122, 1.000000000000000000, 0.9659258262890683122, 1.000000000000000000, 0.9659258262890683122, 1.000000000000000000, 0.9659258262890683122, 1.000000000000000000, 0.9659258262890683122, 1.000000000000000000, 0.9659258262890683122, 1.000000000000000000, 0.9659258262890683122, 1.000000000000000000, 0.9659258262890683122, 1.000000000000000000, 0.9659258262890683122, 1.000000000000000000, 0.9659258262890683122, 1.000000000000000000, 0.9659258262890683122, 1.000000000000000000, 0.9659258262890683122, 1.000000000000000000, 0.9659258262890683122, 1.000000000000000000, 0.9659258262890683122, 1.000000000000000000, 0.9659258262890683122, 1.000000000000000000, 0.9659258262890683122, 1.000000000000000000, 0.9659258262890683122, 1.000000000000000000, 0.9659258262890683122, 1.000000000000000000, 0.9659258262890683122, 1.000000000000000000, 0.9659258262890683122, 1.000000000000000000, 0.9659258262890683122, 1.000000000000000000, 0.9659258262890683122, 1.000000000000000000, 0.9659258262890683122, 1.000000000000000000, 0.9659258262890683122, 1.000000000000000000, 0.9659258262890683122, 1.000000000000000000, 0.9659258262890683122, 1.000000000000000000, 0.9659258262890683122, 1.000000000000000000, 0.9659258262890683122, 1.000000000000000000, 0.9659258262890683122, 1.000000000000000000, 0.9659258262890683122, 1.000000000000000000, 0.9659258262890683122, 1.000000000000000000, 0.9659258262890683122, 1.000000000000000000, 0.9659258262890683122, 1.000000000000000000, 0.9659258262890683122, 1.000000000000000000, 0.9659258262890683122, 1.000000000000000000, 0.9659258262890683122, 1.000000000000000000, 0.9659258262890683122, 1.000000000000000000, 0.9659258262890683122, 1.000000000000000000, 0.9659258262890683122, 1.000000000000000000, 0.9659258262890683122, 1.000000000000000000, 0.9659258262890683122, 1.000000000000000000, 0.9659258262890683122, 1.000000000000000000, 0.9659258262890683122, 1.000000000000000000, 0.9659258262890683122, 1.000000000000000000, 0.9659258262890683122, 1.000000000000000000, 0.9659258262890683122, 1.000000000000000000, 0.9659258262890683122, 1.000000000000000000, 0.9659258262890683122, 1.000000000000000000, 0.9659258262890683122, 1.000000000000000000, 0.9659258262890683122, 1.000000000000000000, 0.9659258262890683122, 1.000000000000000000, 0.9659258262890683122, 1.000000000000000000, 0.9659258262890683122, 1.000000000000000000, 0.9659258262890683122, 1.000000000000000000, 0.9659258262890683122, 1.000000000000000000, 0.9659258262890683122, 1.000000000000000000, 0.9659258262890683122, 1.000000000000000000, 0.9659258262890683122, 1.000000000000000000, 0.9659258262890683122, 1.000000000000000000, 0.9659258262890683122, 1.000000000000000000, 0.9659258262890683122, 1.000000000000000000, 0.9659258262890683122, 1.000000000000000000, 0.9659258262890683122, 1.000000000000000000, 0.9659258262890683122, 1.000000000000000000, 0.9659258262890683122, 1.000000000000000000, 0.9659258262890683122, 1.000000000000000000, 0.9659258262890683122, 1.000000000000000000, 0.9659258262890683122, 1.000000000000000000, 0.9659258262890683122, 1.000000000000000000, 0.9659258262890683122, 1.000000000000000000, 0.9659258262890683122, 1.000000000000000000, 0.9659258262890683122, 1.000000000000000000, 0.9659258262890683122, 1.000000000000000000, 0.9659258262890683122, 1.000000000000000000, 0.9659258262890683122, 1.000000000000000000, 0.9659258262890683122, 1.000000000000000000, 0.9659258262890683122, 1.000000000000000000, 0.9659258262890683122, 1.000000000000000000, 0.9659258262890683122, 1.000000000000000000, 0.9659258262890683122, 1.000000000000000000, 0.9659258262890683122, 1.000000000000000000, 0.9659258262890683122, 1.000000000000000000, 0.9659258262890683122, 1.000000000000000000, 0.9659258262890683122, 1.000000000000000000, 0.9659258262890683122, 1.000000000000000000, 0.9659258262890683122, 1.000000000000000000, 0.9659258262890683122, 1.000000000000000000, 0.9659258262890683122, 1.000000000000000000, 0.9659258262890683122, 1.000000000000000000, 0.9659258262890683122, 1.000000000000000000, 0.9659258262890683122, 1.000000000000000000, 0.9659258262890683122, 1.000000000000000000, 0.9659258262890683122, 1.000000000000000000, 0.9659258262890683122, 1.000000000000000000, 0.9659258262890683122, 1.000000000000000000, 0.9659258262890683122, 1.000000000000000000, 0.9659258262890683122, 1.000000000000000000, 0.9659258262890683122, 1.000000000000000000, 0.9659258262890683122, 1.000000000000000000, 0.9659258262890683122, 1.000000000000000000, 0.9659258262890683122, 1.000000000000000000, 0.9659258262890683122, 1.000000000000000000, 0.9659258262890683122, 1.000000000000000000, 0.9659258262890683122, 1.000000000000000000, 0.9659258262890683122, 1.000000000000000000, 0.9659258262890683122, 1.000000000000000000, 0.9659258262890683122, 1.000000000000000000, 0.9659258262890683122, 1.000000000000000000, 0.9659258262890683122, 1.000000000000000000, 0.9659258262890683122, 1.000000000000000000, 0.9659258262890683122, 1.000000000000000000, 0.9659258262890683122, 1.000000000000000000, 0.9659258262890683122, 1.000000000000000000, 0.9659258262890683122, 1.000000000000000000, 0.9659258262890683122, 1.000000000000000000, 0.9659258262890683122, 1.000000000000000000, 0.9659258262890683122, 1.000000000000000000, 0.9659258262890683122, 1.000000000000000000, 0.9659258262890683122, 1.000000000000000000, 0.9659258262890683122, 1.000000000000000000, 0.9659258262890683122, 1.000000000000000000, 0.9659258262890683122, 1.000000000000000000, 0.9659258262890683122, 1.000000000000000000, 0.9659258262890683122, 1.000000000000000000, 0.9659258262890683122, 1.000000000000000000, 0.9659258262890683122, 1.000000000000000000, 0.9659258262890683122, 1.000000000000000000, 0.9659258262890683122, 1.000000000000000000, 0.9659258262890683122, 1.000000000000000000, 0.9659258262890683122, 1.000000000000000000, 0.9659258262890683122, 1.000000000000000000, 0.9659258262890683122, 1.000000000000000000, 0.9659258262890683122, 1.000000000000000000, 0.9659258262890683122, 1.000000000000000000, 0.9659258262890683122, 1.000000000000000000, 0.9659258262890683122, 1.000000000000000000, 0.9659258262890683122, 1.000000000000000000, 0.9659258262890683122, 1.000000000000000000, 0.9659258262890683122, 1.000000000000000000, 0.9659258262890683122, 1.000000000000000000, 0.9659258262890683122, 1.000000000000000000, 0.9659258262890683122, 1.000000000000000000, 0.9659258262890683122, 1.000000000000000000, 0.9659258262890683122, 1.000000000000000000, 0.9659258262890683122, 1.000000000000000000, 0.9659258262890683122, 1.000000000000000000, 0.9659258262890683122, 1.000000000000000000, 0.9659258262890683122, 1.000000000000000000) ) ) 
 REPRESENTATION_ITEM ( '' )  SURFACE ( )  );
#32614=CARTESIAN_POINT ( 'NONE',  ( 4.555630843329476320, 77.03495325336415078, -9.500000000000000000 ) ) ;
#32616=CARTESIAN_POINT ( 'NONE',  ( 17.96484262340118221, 4.938685344154837509, 7.964842623401181321 ) ) ;
#32617=CARTESIAN_POINT ( 'NONE',  ( 4.559911319644449179, 8.897018677488173211, 9.422509992056141925 ) ) ;
#32618=CARTESIAN_POINT ( 'NONE',  ( 7.361572987183170547, 32.05059781766745175, 9.846743663894590881 ) ) ;
#32619=CARTESIAN_POINT ( 'NONE',  ( 0.6178305044545838731, 9.748634669930416052, 9.382169495545420901 ) ) ;
#32624=CARTESIAN_POINT ( 'NONE',  ( 21.09922568453594849, 6.206968003263753531, 6.408140936763242479 ) ) ;
#32625=ORIENTED_EDGE ( 'NONE', *, *, #91027, .T. ) ;
#32626=CARTESIAN_POINT ( 'NONE',  ( -2.266590686148945544, 42.22041550158063217, 7.082119434687048631 ) ) ;
#32628=CARTESIAN_POINT ( 'NONE',  ( 13.79529636645031943, 60.34541550158063927, -14.16423886937409904 ) ) ;
#32629=VERTEX_POINT ( 'NONE', #26335 ) ;
#32630=CARTESIAN_POINT ( 'NONE',  ( 10.00000000000000178, 29.31368534415483751, 10.88017736071110342 ) ) ;
#32631=CARTESIAN_POINT ( 'NONE',  ( 7.084665262690076126, 44.10535201082151247, 10.88017736071109987 ) ) ;
#32633=CARTESIAN_POINT ( 'NONE',  ( 1.472469842513823179, 66.42559781766745175, 4.923371831947296329 ) ) ;
#32634=CARTESIAN_POINT ( 'NONE',  ( 7.084665262690076126, 42.02201867748816966, -10.88017736071110164 ) ) ;
#32635=CARTESIAN_POINT ( 'NONE',  ( 0.5774900079438607392, 63.48035201082149825, 5.440088680355550821 ) ) ;
#32636=CARTESIAN_POINT ( 'NONE',  ( 20.88017736071110875, 25.77201867748816966, -2.915334737309920765 ) ) ;
#32638=ADVANCED_FACE ( 'NONE', ( #3850 ), #5177, .T. ) ;
#32639=VECTOR ( 'NONE', #72858, 1000.000000000000000 ) ;
#32640=CARTESIAN_POINT ( 'NONE',  ( 18.52753015748618282, 18.92559781766745175, -4.923371831947291888 ) ) ;
#32644=CARTESIAN_POINT ( 'NONE',  ( 7.361572987183169658, 44.96726448433412315, -9.846743663894592657 ) ) ;
#32645=AXIS2_PLACEMENT_3D ( 'NONE', #87888, #43377, #20891 ) ;
#32646=DIRECTION ( 'NONE',  ( 0.000000000000000000, 0.000000000000000000, -1.000000000000000000 ) ) ;
#32647=CARTESIAN_POINT ( 'NONE',  ( -2.816281873526473856, 44.33196800326375353, 3.434112377981055619 ) ) ;
#32648=ADVANCED_FACE ( 'NONE', ( #21955 ), #6649, .T. ) ;
#32649=AXIS2_PLACEMENT_3D ( 'NONE', #79549, #58507, #11049 ) ;
#32650=LINE ( 'NONE', #63144, #23562 ) ;
#32651=CARTESIAN_POINT ( 'NONE',  ( 18.72515096720569616, 10.05509018479935968, 6.500000000000001776 ) ) ;
#32653=CARTESIAN_POINT ( 'NONE',  ( 5.076628168052703671, 51.84226448433412315, 8.527530157486179263 ) ) ;
#32654=CARTESIAN_POINT ( 'NONE',  ( -4.164238869374099039, 46.80374883491397497, 8.674139862899312516E-16 ) ) ;
#32655=CARTESIAN_POINT ( 'NONE',  ( 7.361572987183169658, 64.96726448433412315, -9.846743663894592657 ) ) ;
#32657=LINE ( 'NONE', #56163, #55990 ) ;
#32658=CARTESIAN_POINT ( 'NONE',  ( 19.84674366389459266, 18.71726448433411960, -2.638427012816827677 ) ) ;
#32659=CARTESIAN_POINT ( 'NONE',  ( 22.81628187352647785, 56.41530133659708213, 3.434112377981063169 ) ) ;
#32660=CARTESIAN_POINT ( 'NONE',  ( 10.00000000000000178, 67.25893115100079456, 9.846743663894594434 ) ) ;
#32661=CARTESIAN_POINT ( 'NONE',  ( 0.1532563361054082862, 1.217264484334117824, 2.638427012816831674 ) ) ;
#32662=CARTESIAN_POINT ( 'NONE',  ( 19.05866839779139355, 30.95508385108959004, -6.499999999999974243 ) ) ;
#32664=VERTEX_POINT ( 'NONE', #52328 ) ;
#32665=CARTESIAN_POINT ( 'NONE',  ( 10.00000000000000000, 60.55374883491397497, -14.16423886937410082 ) ) ;
#32666=CARTESIAN_POINT ( 'NONE',  ( 19.42250999205614548, 40.98035201082150536, -5.440088680355545492 ) ) ;
#32667=CARTESIAN_POINT ( 'NONE',  ( -2.816281873526471635, 8.915301336597083903, -3.434112377981056508 ) ) ;
#32668=CARTESIAN_POINT ( 'NONE',  ( 20.88017736071110519, 60.56368534415484106, 2.639326808657452039E-16 ) ) ;
#32669=CARTESIAN_POINT ( 'NONE',  ( -1.926860441876562247, 62.45379003517448524, -3.195792623639530650 ) ) ;
#32671=CARTESIAN_POINT ( 'NONE',  ( 0.2751277870542980231, 10.30223176428831522, 6.500000000000002665 ) ) ;
#32672=CARTESIAN_POINT ( 'NONE',  ( 12.63842701281683922, 49.55059781766744464, -9.846743663894590881 ) ) ;
#32673=CARTESIAN_POINT ( 'NONE',  ( 12.63842701281683922, 4.550597817667451750, -9.846743663894590881 ) ) ;
#32675=CARTESIAN_POINT ( 'NONE',  ( -2.816281873526473856, 9.331968003263753531, 3.434112377981055619 ) ) ;
#32676=CARTESIAN_POINT ( 'NONE',  ( 15.44008868035555793, 11.39701867748817143, -9.422509992056140149 ) ) ;
#32677=CARTESIAN_POINT ( 'NONE',  ( 2.603489959281613420, 65.43575266056828355, -6.500000000000031086 ) ) ;
#32679=CARTESIAN_POINT ( 'NONE',  ( 24.16423886937410614, 29.51208216824729647, -3.795296366450302550 ) ) ;
#32681=CARTESIAN_POINT ( 'NONE',  ( 2.917880565312948704, 27.63708216824730357, 12.26659068614894643 ) ) ;
#32682=CARTESIAN_POINT ( 'NONE',  ( 17.08211943468705840, 65.13708216824730357, -12.26659068614894466 ) ) ;
#32683=CARTESIAN_POINT ( 'NONE',  ( 10.00000000000000178, 22.25893115100078745, 9.846743663894594434 ) ) ;
#32684=CARTESIAN_POINT ( 'NONE',  ( 0.5774900079438590739, 12.64701867748817143, -5.440088680355550821 ) ) ;
#32685=EDGE_LOOP ( 'NONE', ( #8904, #95196, #20071, #17507 ) ) ;
#32686=CARTESIAN_POINT ( 'NONE',  ( 2.791683348922237240, 35.38393115100079456, -7.208316651077763204 ) ) ;
#32687=CARTESIAN_POINT ( 'NONE',  ( 15.44008868035555260, 39.73035201082150536, 9.422509992056143702 ) ) ;
#32688=CARTESIAN_POINT ( 'NONE',  ( 14.92337183194729633, 62.67559781766745886, 8.527530157486181039 ) ) ;
#32689=CARTESIAN_POINT ( 'NONE',  ( -4.164238869374099039, 21.80374883491396787, 8.674139862899312516E-16 ) ) ;
#32692=CARTESIAN_POINT ( 'NONE',  ( 1.472469842513823179, 26.42559781766745175, 4.923371831947296329 ) ) ;
#32693=CARTESIAN_POINT ( 'NONE',  ( 19.38216949554541557, 52.24863466993041072, -9.382169495545420901 ) ) ;
#32694=CARTESIAN_POINT ( 'NONE',  ( 18.52753015748618282, 53.92559781766745175, -4.923371831947291888 ) ) ;
#32695=ORIENTED_EDGE ( 'NONE', *, *, #54565, .F. ) ;
#32697=CARTESIAN_POINT ( 'NONE',  ( 0.2751277870542967463, 70.00000000000000000, -6.000000000000000000 ) ) ;
#32698=CARTESIAN_POINT ( 'NONE',  ( 0.5774900079438590739, 7.647018677488171434, -5.440088680355550821 ) ) ;
#32699=CARTESIAN_POINT ( 'NONE',  ( 0.5774900079438590739, 57.64701867748817676, -5.440088680355550821 ) ) ;
#32700=CARTESIAN_POINT ( 'NONE',  ( -2.266590686148945544, 6.387082168247300906, -7.082119434687050408 ) ) ;
#32701=CARTESIAN_POINT ( 'NONE',  ( 10.00000000000000000, -0.2410688489992152128, -9.846743663894594434 ) ) ;
#32702=CARTESIAN_POINT ( 'NONE',  ( 0.1532563361054083140, 56.00893115100078745, 1.131784320476157264E-15 ) ) ;
#32703=CARTESIAN_POINT ( 'NONE',  ( 12.91533473730993009, 21.60535201082150536, -10.88017736071109987 ) ) ;
#32705=CARTESIAN_POINT ( 'NONE',  ( 18.52753015748618282, 63.92559781766745886, -4.923371831947291888 ) ) ;
#32706=( GEOMETRIC_REPRESENTATION_CONTEXT ( 3 ) GLOBAL_UNCERTAINTY_ASSIGNED_CONTEXT ( ( #5162 ) ) GLOBAL_UNIT_ASSIGNED_CONTEXT ( ( #13393, #91360, #45874 ) ) REPRESENTATION_CONTEXT ( 'NONE', 'WORKASPACE' ) );
#32707=CARTESIAN_POINT ( 'NONE',  ( 7.361572987183169658, -0.03273551566588185635, -9.846743663894592657 ) ) ;
#32708=CARTESIAN_POINT ( 'NONE',  ( 0.6178305044545818747, 58.49863466993042493, -9.382169495545419124 ) ) ;
#32710=ORIENTED_EDGE ( 'NONE', *, *, #35578, .F. ) ;
#32711=CARTESIAN_POINT ( 'NONE',  ( -0.1503990784575328643, 70.00000000000000000, 6.262539305110068177 ) ) ;
#32712=CARTESIAN_POINT ( 'NONE',  ( 13.79529636645031943, 40.34541550158063217, -14.16423886937409904 ) ) ;
#32713=CARTESIAN_POINT ( 'NONE',  ( 0.1532563361054100626, 60.80059781766744464, -2.638427012816831230 ) ) ;
#32714=CARTESIAN_POINT ( 'NONE',  ( 10.00000000000000000, 24.75893115100078745, -9.846743663894594434 ) ) ;
#32715=CARTESIAN_POINT ( 'NONE',  ( 2.603489959281614308, 36.58210964143329136, 6.500000000000031086 ) ) ;
#32716=CARTESIAN_POINT ( 'NONE',  ( 20.88017736071110519, 25.56368534415483751, 2.639326808657452039E-16 ) ) ;
#32717=CARTESIAN_POINT ( 'NONE',  ( 17.20831665107776587, 57.88393115100078745, 7.208316651077764980 ) ) ;
#32719=STYLED_ITEM ( 'NONE', ( #12358 ), #85111 ) ;
#32720=CARTESIAN_POINT ( 'NONE',  ( -2.266590686148945544, 52.22041550158064638, 7.082119434687048631 ) ) ;
#32722=ADVANCED_FACE ( 'NONE', ( #37347 ), #51342, .T. ) ;
#32724=CARTESIAN_POINT ( 'NONE',  ( 20.88017736071110875, 60.77201867748817676, -2.915334737309920765 ) ) ;
#32725=CARTESIAN_POINT ( 'NONE',  ( 0.1532563361054083140, 11.00893115100078568, 1.131784320476157264E-15 ) ) ;
#32729=VERTEX_POINT ( 'NONE', #91307 ) ;
#32730=CARTESIAN_POINT ( 'NONE',  ( 14.92337183194729988, 29.34226448433411960, -8.527530157486177487 ) ) ;
#32732=CARTESIAN_POINT ( 'NONE',  ( -4.164238869374098151, 36.59541550158063217, -3.795296366450310543 ) ) ;
#32733=CARTESIAN_POINT ( 'NONE',  ( 14.92337183194729633, 27.67559781766745530, 8.527530157486181039 ) ) ;
#32734=CARTESIAN_POINT ( 'NONE',  ( 10.00000000000000178, 49.31368534415484106, 10.88017736071110342 ) ) ;
#32737=VERTEX_POINT ( 'NONE', #58834 ) ;
#32738=CARTESIAN_POINT ( 'NONE',  ( 12.91533473730993009, 41.60535201082149825, -10.88017736071109987 ) ) ;
#32742=EDGE_CURVE ( 'NONE', #61441, #50256, #93279, .T. ) ;
#32745=CARTESIAN_POINT ( 'NONE',  ( 24.16423886937410614, 4.512082168247300906, -3.795296366450302550 ) ) ;
#32747=CARTESIAN_POINT ( 'NONE',  ( 6.565887622018943937, 33.08196800326374643, -12.81628187352647608 ) ) ;
#32748=CARTESIAN_POINT ( 'NONE',  ( 5.076628168052704559, 20.17559781766745175, -8.527530157486179263 ) ) ;
#32750=CARTESIAN_POINT ( 'NONE',  ( 5.076628168052704559, 25.17559781766745175, -8.527530157486179263 ) ) ;
#32753=EDGE_CURVE ( 'NONE', #80833, #68278, #13021, .T. ) ;
#32756=CARTESIAN_POINT ( 'NONE',  ( 20.88017736071110164, 50.35535201082151247, 2.915334737309930979 ) ) ;
#32759=CARTESIAN_POINT ( 'NONE',  ( 1.472469842513823179, 10.59226448433411782, -4.923371831947296329 ) ) ;
#32760=ADVANCED_FACE ( 'NONE', ( #16311 ), #84802, .T. ) ;
#32763=CARTESIAN_POINT ( 'NONE',  ( 18.52753015748617571, 33.09226448433411605, 4.923371831947298993 ) ) ;
#32765=CARTESIAN_POINT ( 'NONE',  ( 10.00000000000000000, 10.55374883491396787, -14.16423886937410082 ) ) ;
#32766=CARTESIAN_POINT ( 'NONE',  ( 17.20831665107776587, 22.88393115100078745, 7.208316651077764980 ) ) ;
#32767=CARTESIAN_POINT ( 'NONE',  ( 19.38216949554541557, 32.24863466993041783, -9.382169495545420901 ) ) ;
#32768=DIRECTION ( 'NONE',  ( 0.000000000000000000, 0.000000000000000000, -1.000000000000000000 ) ) ;
#32769=CARTESIAN_POINT ( 'NONE',  ( -0.8801773607111008646, 53.27201867748816966, 2.915334737309923430 ) ) ;
#32770=CARTESIAN_POINT ( 'NONE',  ( 13.43411237798106583, 7.665301336597086568, -12.81628187352647252 ) ) ;
#32772=CARTESIAN_POINT ( 'NONE',  ( 19.84674366389459621, 28.50893115100078745, 7.409399052514197653E-17 ) ) ;
#32773=CARTESIAN_POINT ( 'NONE',  ( 17.20831665107776587, 17.88393115100078745, 7.208316651077764980 ) ) ;
#32774=CARTESIAN_POINT ( 'NONE',  ( 17.96484262340118221, 31.18868534415483751, -7.964842623401177768 ) ) ;
#32775=CARTESIAN_POINT ( 'NONE',  ( 21.09922568453595559, 12.04030133659708746, -6.408140936763230044 ) ) ;
#32776=CARTESIAN_POINT ( 'NONE',  ( 7.361572987183169658, 24.96726448433412315, -9.846743663894592657 ) ) ;
#32779=CARTESIAN_POINT ( 'NONE',  ( 2.035157376598822676, 17.43868534415483751, -7.964842623401177768 ) ) ;
#32780=STYLED_ITEM ( 'NONE', ( #22719 ), #85915 ) ;
#32782=CARTESIAN_POINT ( 'NONE',  ( 20.88017736071110164, 65.35535201082150536, 2.915334737309930979 ) ) ;
#32784=CARTESIAN_POINT ( 'NONE',  ( 17.20831665107776587, 39.13393115100079456, -7.208316651077762316 ) ) ;
#32785=CARTESIAN_POINT ( 'NONE',  ( 0.5774900079438590739, 22.64701867748817321, -5.440088680355550821 ) ) ;
#32787=CARTESIAN_POINT ( 'NONE',  ( 7.084665262690076126, 47.02201867748818387, -10.88017736071110164 ) ) ;
#32788=CARTESIAN_POINT ( 'NONE',  ( 10.00000000000000000, 16.81368534415483751, -10.88017736071110342 ) ) ;
#32789=CARTESIAN_POINT ( 'NONE',  ( 0.1532563361054083140, 16.00893115100078390, 1.131784320476157264E-15 ) ) ;
#32790=CARTESIAN_POINT ( 'NONE',  ( 17.20831665107776587, 37.88393115100078745, 7.208316651077764980 ) ) ;
#32793=SURFACE_STYLE_FILL_AREA ( #48293 ) ;
#32794=CARTESIAN_POINT ( 'NONE',  ( 20.36894250292379738, 24.92874883491396787, -10.36894250292379027 ) ) ;
#32795=CARTESIAN_POINT ( 'NONE',  ( 19.84674366389459266, 38.71726448433412315, -2.638427012816827677 ) ) ;
#32796=CARTESIAN_POINT ( 'NONE',  ( 19.72487221294570858, 0.000000000000000000, -6.500000000000000888 ) ) ;
#32799=CARTESIAN_POINT ( 'NONE',  ( 22.26659068614895176, 64.72041550158064638, -7.082119434687042414 ) ) ;
#32800=CARTESIAN_POINT ( 'NONE',  ( 7.361572987183169658, 24.96726448433412315, -9.846743663894592657 ) ) ;
#32803=CARTESIAN_POINT ( 'NONE',  ( 2.035157376598824452, 48.68868534415483396, 7.964842623401179544 ) ) ;
#32805=CARTESIAN_POINT ( 'NONE',  ( 12.91533473730993009, 11.60535201082150536, -10.88017736071109987 ) ) ;
#32806=CARTESIAN_POINT ( 'NONE',  ( 6.565887622018943937, 50.16530133659708213, 12.81628187352647430 ) ) ;
#32807=CARTESIAN_POINT ( 'NONE',  ( -1.099225684535947600, 9.540301336597087456, 6.408140936763237150 ) ) ;
#32808=CARTESIAN_POINT ( 'NONE',  ( 10.00000000000000000, 14.75893115100078568, -9.846743663894594434 ) ) ;
#32810=PLANE ( 'NONE',  #7740 ) ;
#32811=CARTESIAN_POINT ( 'NONE',  ( -4.164238869374099039, 56.80374883491397497, 8.674139862899312516E-16 ) ) ;
#32812=CARTESIAN_POINT ( 'NONE',  ( -4.164238869374099927, 27.01208216824730357, 3.795296366450308767 ) ) ;
#32813=CARTESIAN_POINT ( 'NONE',  ( 4.559911319644449179, 13.89701867748817143, 9.422509992056141925 ) ) ;
#32814=CARTESIAN_POINT ( 'NONE',  ( 7.084665262690076126, 54.10535201082151247, 10.88017736071109987 ) ) ;
#32817=CARTESIAN_POINT ( 'NONE',  ( 20.88017736071110519, 60.56368534415484106, 2.639326808657452039E-16 ) ) ;
#32818=CARTESIAN_POINT ( 'NONE',  ( 1.472469842513823179, 21.42559781766745175, 4.923371831947296329 ) ) ;
#32819=CARTESIAN_POINT ( 'NONE',  ( 2.603489959281614308, 51.58210964143330557, 6.500000000000031086 ) ) ;
#32821=CARTESIAN_POINT ( 'NONE',  ( 2.791683348922240793, 21.63393115100078745, 7.208316651077764092 ) ) ;
#32822=CARTESIAN_POINT ( 'NONE',  ( 7.361572987183169658, 44.96726448433412315, -9.846743663894592657 ) ) ;
#32824=CARTESIAN_POINT ( 'NONE',  ( -0.8801773607110991993, 12.85535201082150358, -2.915334737309923874 ) ) ;
#32825=CARTESIAN_POINT ( 'NONE',  ( 6.565887622018943937, 35.16530133659708923, 12.81628187352647430 ) ) ;
#32827=CARTESIAN_POINT ( 'NONE',  ( 19.42250999205614193, 55.14701867748817676, 5.440088680355555262 ) ) ;
#32828=CARTESIAN_POINT ( 'NONE',  ( 2.791683348922240793, 26.63393115100078745, 7.208316651077764092 ) ) ;
#32829=CARTESIAN_POINT ( 'NONE',  ( 22.26659068614895176, 49.72041550158063927, -7.082119434687042414 ) ) ;
#32830=CARTESIAN_POINT ( 'NONE',  ( 19.84674366389459266, 23.30059781766745530, 2.638427012816836559 ) ) ;
#32832=CARTESIAN_POINT ( 'NONE',  ( 0.1532563361054082862, 56.21726448433411605, 2.638427012816831674 ) ) ;
#32833=CARTESIAN_POINT ( 'NONE',  ( 10.00000000000000000, 34.75893115100078745, -9.846743663894594434 ) ) ;
#32834=CARTESIAN_POINT ( 'NONE',  ( 13.79529636645031943, 15.34541550158063750, -14.16423886937409904 ) ) ;
#32835=CARTESIAN_POINT ( 'NONE',  ( -4.164238869374099927, 22.01208216824730357, 3.795296366450308767 ) ) ;
#32836=CARTESIAN_POINT ( 'NONE',  ( 18.52753015748617571, 28.09226448433411960, 4.923371831947298993 ) ) ;
#32837=CARTESIAN_POINT ( 'NONE',  ( 4.559911319644449179, 42.23035201082151247, -9.422509992056141925 ) ) ;
#32838=CARTESIAN_POINT ( 'NONE',  ( 19.42250999205614193, 25.14701867748817321, 5.440088680355555262 ) ) ;
#32839=CARTESIAN_POINT ( 'NONE',  ( 10.00000000000000000, 46.81368534415484106, -10.88017736071110342 ) ) ;
#32840=CARTESIAN_POINT ( 'NONE',  ( 15.44008868035555793, 26.39701867748817321, -9.422509992056140149 ) ) ;
#32842=CARTESIAN_POINT ( 'NONE',  ( 21.09922568453595559, 37.04030133659708923, -6.408140936763230044 ) ) ;
#32844=CARTESIAN_POINT ( 'NONE',  ( 0.5774900079438590739, 47.64701867748817676, -5.440088680355550821 ) ) ;
#32846=CARTESIAN_POINT ( 'NONE',  ( 3.591859063236761518, 54.95696800326376064, 11.09922568453594849 ) ) ;
#32847=CARTESIAN_POINT ( 'NONE',  ( -0.8801773607111009756, 63.06368534415484106, 1.068504757029289695E-15 ) ) ;
#32849=VECTOR ( 'NONE', #4835, 1000.000000000000000 ) ;
#32850=CARTESIAN_POINT ( 'NONE',  ( 2.035157376598824452, 68.68868534415484817, 7.964842623401179544 ) ) ;
#32851=EDGE_CURVE ( 'NONE', #2953, #45712, #69808, .T. ) ;
#32856=CARTESIAN_POINT ( 'NONE',  ( 22.26659068614894466, 58.88708216824729647, 7.082119434687054849 ) ) ;
#32857=CARTESIAN_POINT ( 'NONE',  ( 1.472469842513823179, 5.592264484334118713, -4.923371831947296329 ) ) ;
#32858=CARTESIAN_POINT ( 'NONE',  ( -0.3689425029237881626, 2.428748834913967869, 10.36894250292379027 ) ) ;
#32859=( GEOMETRIC_REPRESENTATION_CONTEXT ( 3 ) GLOBAL_UNCERTAINTY_ASSIGNED_CONTEXT ( ( #90445 ) ) GLOBAL_UNIT_ASSIGNED_CONTEXT ( ( #16978, #68992, #53978 ) ) REPRESENTATION_CONTEXT ( 'NONE', 'WORKASPACE' ) );
#32861=CARTESIAN_POINT ( 'NONE',  ( 17.20831665107776587, 7.883931151000784787, 7.208316651077764980 ) ) ;
#32862=CARTESIAN_POINT ( 'NONE',  ( 15.44008868035555260, 9.730352010821505360, 9.422509992056143702 ) ) ;
#32863=CARTESIAN_POINT ( 'NONE',  ( 7.361572987183170547, 42.05059781766745886, 9.846743663894590881 ) ) ;
#32865=CARTESIAN_POINT ( 'NONE',  ( 2.791683348922237240, 45.38393115100079456, -7.208316651077763204 ) ) ;
#32866=CARTESIAN_POINT ( 'NONE',  ( 5.500000000000000000, 11.50000000000000000, 5.000000000000000000 ) ) ;
#32867=CARTESIAN_POINT ( 'NONE',  ( 10.00000000000000178, 34.31368534415484106, 10.88017736071110342 ) ) ;
#32868=CARTESIAN_POINT ( 'NONE',  ( 19.84674366389459266, 48.71726448433413026, -2.638427012816827677 ) ) ;
#32871=CARTESIAN_POINT ( 'NONE',  ( 17.96484262340118221, 54.93868534415484106, 7.964842623401181321 ) ) ;
#32872=CARTESIAN_POINT ( 'NONE',  ( 20.88017736071110164, 10.35535201082150714, 2.915334737309930979 ) ) ;
#32874=CARTESIAN_POINT ( 'NONE',  ( 3.591859063236761518, 44.95696800326376064, 11.09922568453594849 ) ) ;
#32877=CARTESIAN_POINT ( 'NONE',  ( -2.816281873526473856, 34.33196800326376064, 3.434112377981055619 ) ) ;
#32878=CARTESIAN_POINT ( 'NONE',  ( 19.42250999205614548, 35.98035201082151247, -5.440088680355545492 ) ) ;
#32882=CARTESIAN_POINT ( 'NONE',  ( 19.84674366389459266, 3.717264484334118713, -2.638427012816827677 ) ) ;
#32883=CARTESIAN_POINT ( 'NONE',  ( 7.361572987183169658, 44.96726448433412315, -9.846743663894592657 ) ) ;
#32884=CARTESIAN_POINT ( 'NONE',  ( 2.791683348922237240, 15.38393115100078212, -7.208316651077763204 ) ) ;
#32885=CARTESIAN_POINT ( 'NONE',  ( 18.52753015748617571, 43.09226448433412315, 4.923371831947298993 ) ) ;
#32887=CARTESIAN_POINT ( 'NONE',  ( -2.816281873526473856, 64.12363466993042493, 9.499525473075851096E-16 ) ) ;
#32888=CARTESIAN_POINT ( 'NONE',  ( 10.00000000000000000, 24.75893115100078745, -9.846743663894594434 ) ) ;
#32892=CARTESIAN_POINT ( 'NONE',  ( 18.52753015748617571, 33.09226448433411605, 4.923371831947298993 ) ) ;
#32895=CARTESIAN_POINT ( 'NONE',  ( 19.84674366389459266, 43.30059781766744464, 2.638427012816836559 ) ) ;
#32896=VERTEX_POINT ( 'NONE', #24803 ) ;
#32897=ADVANCED_FACE ( 'NONE', ( #77780 ), #9293, .T. ) ;
#32899=CARTESIAN_POINT ( 'NONE',  ( 16.40814093676324603, 27.45696800326375708, -11.09922568453594671 ) ) ;
#32900=CARTESIAN_POINT ( 'NONE',  ( 24.16423886937409904, 44.09541550158063927, 3.795296366450317205 ) ) ;
#32901=CARTESIAN_POINT ( 'NONE',  ( 2.791683348922237240, 20.38393115100078745, -7.208316651077763204 ) ) ;
#32903=CARTESIAN_POINT ( 'NONE',  ( 5.076628168052703671, 1.842264484334118047, 8.527530157486179263 ) ) ;
#32904=CARTESIAN_POINT ( 'NONE',  ( 19.99999999999861089, 92.23760269512273169, 5.246947360776563762 ) ) ;
#32905=CARTESIAN_POINT ( 'NONE',  ( 10.00000000000000178, 48.05374883491396787, 14.16423886937410082 ) ) ;
#32906=CARTESIAN_POINT ( 'NONE',  ( 18.52753015748618282, 58.92559781766745886, -4.923371831947291888 ) ) ;
#32907=CARTESIAN_POINT ( 'NONE',  ( 7.084665262690076126, 12.02201867748817321, -10.88017736071110164 ) ) ;
#32908=CARTESIAN_POINT ( 'NONE',  ( 10.00000000000000178, 23.05374883491397142, 14.16423886937410082 ) ) ;
#32909=CARTESIAN_POINT ( 'NONE',  ( -0.3689425029237898834, 41.17874883491397497, -10.36894250292378850 ) ) ;
#32910=DIRECTION ( 'NONE',  ( -0.5547001962252291474, -0.8320502943378437211, -0.000000000000000000 ) ) ;
#32912=CARTESIAN_POINT ( 'NONE',  ( 1.472469842513823179, 51.42559781766745886, 4.923371831947296329 ) ) ;
#32915=CARTESIAN_POINT ( 'NONE',  ( -0.8801773607111008646, 33.27201867748817676, 2.915334737309923430 ) ) ;
#32917=CARTESIAN_POINT ( 'NONE',  ( 2.603489959281613420, 65.43575266056828355, -6.500000000000031086 ) ) ;
#32918=CARTESIAN_POINT ( 'NONE',  ( 7.361572987183170547, 42.05059781766745886, 9.846743663894590881 ) ) ;
#32921=CARTESIAN_POINT ( 'NONE',  ( 0.1532563361054083140, 61.00893115100078745, 1.131784320476157264E-15 ) ) ;
#32922=LINE ( 'NONE', #48908, #92866 ) ;
#32925=ORIENTED_EDGE ( 'NONE', *, *, #95741, .F. ) ;
#32926=CARTESIAN_POINT ( 'NONE',  ( 17.08211943468705130, 23.47041550158063572, 12.26659068614894998 ) ) ;
#32929=CARTESIAN_POINT ( 'NONE',  ( 0.5774900079438607392, 8.480352010821505360, 5.440088680355550821 ) ) ;
#32930=CARTESIAN_POINT ( 'NONE',  ( 22.81628187352647785, 26.41530133659708923, 3.434112377981063169 ) ) ;
#32932=CARTESIAN_POINT ( 'NONE',  ( -0.8801773607111009756, 63.06368534415484106, 1.068504757029289695E-15 ) ) ;
#32933=EDGE_CURVE ( 'NONE', #28166, #9012, #63264, .T. ) ;
#32934=CARTESIAN_POINT ( 'NONE',  ( 10.00000000000000178, 14.31368534415483929, 10.88017736071110342 ) ) ;
#32936=CARTESIAN_POINT ( 'NONE',  ( 2.035157376598822676, 22.43868534415483396, -7.964842623401177768 ) ) ;
#32937=CARTESIAN_POINT ( 'NONE',  ( -0.8801773607110991993, 37.85535201082151247, -2.915334737309923874 ) ) ;
#32938=CARTESIAN_POINT ( 'NONE',  ( 0.1532563361054100626, 65.80059781766745175, -2.638427012816831230 ) ) ;
#32940=CARTESIAN_POINT ( 'NONE',  ( 3.591859063236761518, 64.95696800326376774, 11.09922568453594849 ) ) ;
#32941=CARTESIAN_POINT ( 'NONE',  ( 17.20831665107776587, 14.13393115100078568, -7.208316651077762316 ) ) ;
#32944=CARTESIAN_POINT ( 'NONE',  ( 2.035157376598822676, 27.43868534415483396, -7.964842623401177768 ) ) ;
#32945=CARTESIAN_POINT ( 'NONE',  ( 6.565887622018943937, 30.16530133659708568, 12.81628187352647430 ) ) ;
#32948=AXIS2_PLACEMENT_3D ( 'NONE', #59097, #89606, #6114 ) ;
#32949=CARTESIAN_POINT ( 'NONE',  ( 2.791683348922240793, 56.63393115100078035, 7.208316651077764092 ) ) ;
#32950=CARTESIAN_POINT ( 'NONE',  ( 10.00000000000000000, 46.81368534415484106, -10.88017736071110342 ) ) ;
#32951=CARTESIAN_POINT ( 'NONE',  ( -2.816281873526471635, 33.91530133659708213, -3.434112377981056508 ) ) ;
#32952=CARTESIAN_POINT ( 'NONE',  ( 2.035157376598822676, 67.43868534415484817, -7.964842623401177768 ) ) ;
#32954=CARTESIAN_POINT ( 'NONE',  ( 17.84635730667659104, 53.63791097397319874, 6.499999999999959144 ) ) ;
#32955=ORIENTED_EDGE ( 'NONE', *, *, #49106, .F. ) ;
#32958=CARTESIAN_POINT ( 'NONE',  ( 19.42250999205614193, 5.147018677488171434, 5.440088680355555262 ) ) ;
#32959=CARTESIAN_POINT ( 'NONE',  ( 10.00000000000000000, 52.87363466993041783, -12.81628187352647608 ) ) ;
#32960=CARTESIAN_POINT ( 'NONE',  ( 7.361572987183169658, 14.96726448433411960, -9.846743663894592657 ) ) ;
#32961=CARTESIAN_POINT ( 'NONE',  ( 0.5774900079438590739, 7.647018677488171434, -5.440088680355550821 ) ) ;
#32962=CARTESIAN_POINT ( 'NONE',  ( 0.1532563361054082862, 21.21726448433412315, 2.638427012816831674 ) ) ;
#32963=CARTESIAN_POINT ( 'NONE',  ( 10.00000000000000000, 60.55374883491397497, -14.16423886937410082 ) ) ;
#32965=AXIS2_PLACEMENT_3D ( 'NONE', #28651, #74646, #29137 ) ;
#32966=FILL_AREA_STYLE ('',( #8510 ) ) ;
#32967=CARTESIAN_POINT ( 'NONE',  ( 10.00000000000000178, 24.31368534415484106, 10.88017736071110342 ) ) ;
#32971=CARTESIAN_POINT ( 'NONE',  ( 15.44008868035555793, 6.397018677488171434, -9.422509992056140149 ) ) ;
#32973=CARTESIAN_POINT ( 'NONE',  ( 18.52753015748617571, 53.09226448433412315, 4.923371831947298993 ) ) ;
#32974=CARTESIAN_POINT ( 'NONE',  ( 19.38216949554541202, 50.99863466993042493, 9.382169495545424454 ) ) ;
#32977=CARTESIAN_POINT ( 'NONE',  ( 10.00000000000000178, 23.05374883491397142, 14.16423886937410082 ) ) ;
#32978=CARTESIAN_POINT ( 'NONE',  ( 19.42250999205614193, 40.14701867748817676, 5.440088680355555262 ) ) ;
#32979=CARTESIAN_POINT ( 'NONE',  ( 0.5774900079438607392, 18.48035201082150536, 5.440088680355550821 ) ) ;
#32980=CARTESIAN_POINT ( 'NONE',  ( 19.84674366389459266, 58.30059781766745886, 2.638427012816836559 ) ) ;
#32981=ADVANCED_FACE ( 'NONE', ( #95237 ), #41290, .T. ) ;
#32984=CARTESIAN_POINT ( 'NONE',  ( 0.1532563361054100626, 40.80059781766745886, -2.638427012816831230 ) ) ;
#32985=CARTESIAN_POINT ( 'NONE',  ( 0.1532563361054082862, 6.217264484334118713, 2.638427012816831674 ) ) ;
#32989=CARTESIAN_POINT ( 'NONE',  ( 19.84674366389459266, 8.717264484334116048, -2.638427012816827677 ) ) ;
#32990=CARTESIAN_POINT ( 'NONE',  ( 16.40814093676323893, 5.790301336597087456, 11.09922568453595026 ) ) ;
#32991=CARTESIAN_POINT ( 'NONE',  ( 19.42250999205614193, 50.14701867748817676, 5.440088680355555262 ) ) ;
#32992=CARTESIAN_POINT ( 'NONE',  ( 19.42250999205614548, 45.98035201082150536, -5.440088680355545492 ) ) ;
#32993=CARTESIAN_POINT ( 'NONE',  ( 7.084665262690076126, 7.022018677488169658, -10.88017736071110164 ) ) ;
#32994=CARTESIAN_POINT ( 'NONE',  ( 10.00000000000000178, 45.37363466993041783, 12.81628187352647608 ) ) ;
#32996=CARTESIAN_POINT ( 'NONE',  ( -2.266590686148945544, 27.22041550158063572, 7.082119434687048631 ) ) ;
#32997=PRESENTATION_STYLE_ASSIGNMENT (( #27461 ) ) ;
#32999=( BOUNDED_SURFACE ( )  B_SPLINE_SURFACE ( 3, 2, ( 
 ( #56158, #17671, #33135 ),
 ( #41164, #71648, #40165 ),
 ( #3156, #79635, #11134 ),
 ( #72120, #3648, #34113 ),
 ( #92661, #85174, #16684 ),
 ( #47154, #39689, #13100 ) ),
 .UNSPECIFIED., .F., .F., .F. ) 
 B_SPLINE_SURFACE_WITH_KNOTS ( ( 4, 2, 4 ),
 ( 3, 3 ),
 ( -1.734723475976807094E-17, 0.002729166040780114846, 0.005458332081560247039 ),
 ( 0.000000000000000000, 1.000000000000000000 ),
 .UNSPECIFIED. ) 
 GEOMETRIC_REPRESENTATION_ITEM ( )  RATIONAL_B_SPLINE_SURFACE ( (
 ( 1.000000000000000000, 0.8188293140827536121, 1.000000000000000000),
 ( 1.000000000000000000, 0.8032367185880369131, 1.000000000000000000),
 ( 1.000000000000000000, 0.7862107325766692911, 1.000000000000000000),
 ( 1.000000000000000000, 0.7489714018702576803, 1.000000000000000000),
 ( 1.000000000000000000, 0.7286611199003509842, 1.000000000000000000),
 ( 1.000000000000000000, 0.7071067811865507924, 1.000000000000000000) ) ) 
 REPRESENTATION_ITEM ( '' )  SURFACE ( )  );
#33001=CARTESIAN_POINT ( 'NONE',  ( 6.565887622018943937, 53.08196800326374643, -12.81628187352647608 ) ) ;
#33003=CARTESIAN_POINT ( 'NONE',  ( 0.1532563361054083140, 61.00893115100078745, 1.131784320476157264E-15 ) ) ;
#33004=CARTESIAN_POINT ( 'NONE',  ( 15.44008868035555260, 14.73035201082150536, 9.422509992056143702 ) ) ;
#33007=CARTESIAN_POINT ( 'NONE',  ( 7.361572987183169658, 4.967264484334119601, -9.846743663894592657 ) ) ;
#33009=CARTESIAN_POINT ( 'NONE',  ( 19.84674366389459266, 13.30059781766745353, 2.638427012816836559 ) ) ;
#33010=CARTESIAN_POINT ( 'NONE',  ( -0.8801773607110991993, 67.85535201082151957, -2.915334737309923874 ) ) ;
#33012=CARTESIAN_POINT ( 'NONE',  ( 20.88017736071110875, 50.77201867748817676, -2.915334737309920765 ) ) ;
#33013=CARTESIAN_POINT ( 'NONE',  ( 12.91533473730993009, 61.60535201082150536, -10.88017736071109987 ) ) ;
#33014=CARTESIAN_POINT ( 'NONE',  ( 14.92337183194729988, 9.342264484334119601, -8.527530157486177487 ) ) ;
#33019=CARTESIAN_POINT ( 'NONE',  ( 12.63842701281683034, 52.46726448433413026, 9.846743663894596210 ) ) ;
#33020=ORIENTED_EDGE ( 'NONE', *, *, #14994, .F. ) ;
#33023=CARTESIAN_POINT ( 'NONE',  ( 6.204703633549690345, 5.762082168247301794, -14.16423886937410259 ) ) ;
#33024=CARTESIAN_POINT ( 'NONE',  ( 16.40814093676323893, 55.79030133659708923, 11.09922568453595026 ) ) ;
#33025=CARTESIAN_POINT ( 'NONE',  ( -4.164238869374098151, 6.595415501580634832, -3.795296366450310543 ) ) ;
#33026=CARTESIAN_POINT ( 'NONE',  ( -0.3689425029237881626, 32.42874883491395366, 10.36894250292379027 ) ) ;
#33028=CARTESIAN_POINT ( 'NONE',  ( -4.164238869374098151, 1.595415501580634388, -3.795296366450310543 ) ) ;
#33029=CARTESIAN_POINT ( 'NONE',  ( 15.44008868035555793, 16.39701867748817321, -9.422509992056140149 ) ) ;
#33030=ORIENTED_EDGE ( 'NONE', *, *, #73216, .T. ) ;
#33031=CARTESIAN_POINT ( 'NONE',  ( 7.361572987183170547, 7.050597817667451750, 9.846743663894590881 ) ) ;
#33032=CARTESIAN_POINT ( 'NONE',  ( 17.20831665107776587, 14.13393115100078568, -7.208316651077762316 ) ) ;
#33033=CARTESIAN_POINT ( 'NONE',  ( 16.40814093676323893, 30.79030133659708923, 11.09922568453595026 ) ) ;
#33034=CARTESIAN_POINT ( 'NONE',  ( 0.1532563361054082862, 31.21726448433412315, 2.638427012816831674 ) ) ;
#33036=CARTESIAN_POINT ( 'NONE',  ( -2.816281873526471635, 33.91530133659708213, -3.434112377981056508 ) ) ;
#33038=CARTESIAN_POINT ( 'NONE',  ( 14.92337183194729633, 32.67559781766745175, 8.527530157486181039 ) ) ;
#33039=CARTESIAN_POINT ( 'NONE',  ( 22.26659068614895176, 19.72041550158063572, -7.082119434687042414 ) ) ;
#33042=CARTESIAN_POINT ( 'NONE',  ( -0.8801773607110991993, 32.85535201082151247, -2.915334737309923874 ) ) ;
#33043=CARTESIAN_POINT ( 'NONE',  ( 17.08211943468705130, 33.47041550158063927, 12.26659068614894998 ) ) ;
#33044=CARTESIAN_POINT ( 'NONE',  ( 2.791683348922237240, 55.38393115100078745, -7.208316651077763204 ) ) ;
#33045=CARTESIAN_POINT ( 'NONE',  ( 17.20831665107776587, 19.13393115100078035, -7.208316651077762316 ) ) ;
#33046=CARTESIAN_POINT ( 'NONE',  ( 13.43411237798106583, 57.66530133659708923, -12.81628187352647252 ) ) ;
#33048=CARTESIAN_POINT ( 'NONE',  ( 12.91533473730992121, 34.52201867748817676, 10.88017736071110164 ) ) ;
#33050=CARTESIAN_POINT ( 'NONE',  ( 19.38216949554541557, 17.24863466993041783, -9.382169495545420901 ) ) ;
#33051=CARTESIAN_POINT ( 'NONE',  ( 10.00000000000000000, 34.75893115100078745, -9.846743663894594434 ) ) ;
#33054=CARTESIAN_POINT ( 'NONE',  ( 17.96484262340118221, 64.93868534415483396, 7.964842623401181321 ) ) ;
#33059=CARTESIAN_POINT ( 'NONE',  ( 10.00000000000000178, 49.31368534415484106, 10.88017736071110342 ) ) ;
#33060=STYLED_ITEM ( 'NONE', ( #34201 ), #18110 ) ;
#33061=CARTESIAN_POINT ( 'NONE',  ( 2.035157376598824452, 58.68868534415482685, 7.964842623401179544 ) ) ;
#33065=CARTESIAN_POINT ( 'NONE',  ( 15.44008868035555260, 4.730352010821505360, 9.422509992056143702 ) ) ;
#33066=CARTESIAN_POINT ( 'NONE',  ( -2.816281873526473856, -0.8763653300695799508, 9.499525473075851096E-16 ) ) ;
#33067=CARTESIAN_POINT ( 'NONE',  ( 2.035157376598822676, 27.43868534415483396, -7.964842623401177768 ) ) ;
#33068=CARTESIAN_POINT ( 'NONE',  ( 19.05866839779139355, 55.95508385108959715, -6.499999999999974243 ) ) ;
#33070=CARTESIAN_POINT ( 'NONE',  ( 3.591859063236761518, 24.95696800326375353, 11.09922568453594849 ) ) ;
#33072=CARTESIAN_POINT ( 'NONE',  ( 12.91533473730993009, 51.60535201082149825, -10.88017736071109987 ) ) ;
#33073=CARTESIAN_POINT ( 'NONE',  ( 12.63842701281683034, 37.46726448433411605, 9.846743663894596210 ) ) ;
#33074=CARTESIAN_POINT ( 'NONE',  ( -2.816281873526473856, 9.331968003263753531, 3.434112377981055619 ) ) ;
#33076=CARTESIAN_POINT ( 'NONE',  ( 2.035157376598822676, 27.43868534415483396, -7.964842623401177768 ) ) ;
#33077=CARTESIAN_POINT ( 'NONE',  ( 7.084665262690076126, 39.10535201082150536, 10.88017736071109987 ) ) ;
#33078=CARTESIAN_POINT ( 'NONE',  ( -2.266590686148945544, 46.38708216824730357, -7.082119434687050408 ) ) ;
#33079=CARTESIAN_POINT ( 'NONE',  ( 1.472469842513823179, 41.42559781766745886, 4.923371831947296329 ) ) ;
#33080=CARTESIAN_POINT ( 'NONE',  ( 0.5774900079438607392, 63.48035201082149825, 5.440088680355550821 ) ) ;
#33081=CARTESIAN_POINT ( 'NONE',  ( 17.08211943468705130, 18.47041550158063572, 12.26659068614894998 ) ) ;
#33084=DIRECTION ( 'NONE',  ( -1.000000000000000000, 0.000000000000000000, 0.000000000000000000 ) ) ;
#33085=CARTESIAN_POINT ( 'NONE',  ( 0.1532563361054082862, 66.21726448433413736, 2.638427012816831674 ) ) ;
#33088=CARTESIAN_POINT ( 'NONE',  ( 24.16423886937410614, 44.51208216824730357, -3.795296366450302550 ) ) ;
#33089=CARTESIAN_POINT ( 'NONE',  ( 6.204703633549690345, 42.84541550158063217, 14.16423886937410082 ) ) ;
#33091=CARTESIAN_POINT ( 'NONE',  ( 5.076628168052703671, 11.84226448433411960, 8.527530157486179263 ) ) ;
#33092=CARTESIAN_POINT ( 'NONE',  ( 22.81628187352647785, 21.41530133659708923, 3.434112377981063169 ) ) ;
#33093=CARTESIAN_POINT ( 'NONE',  ( 1.472469842513823179, 66.42559781766745175, 4.923371831947296329 ) ) ;
#33094=CARTESIAN_POINT ( 'NONE',  ( 20.10239578412224404, 52.63377557478296609, -6.340343622311915617 ) ) ;
#33095=CARTESIAN_POINT ( 'NONE',  ( 20.88017736071110875, 55.77201867748816966, -2.915334737309920765 ) ) ;
#33096=CARTESIAN_POINT ( 'NONE',  ( 21.09922568453595559, 32.04030133659708923, -6.408140936763230044 ) ) ;
#33097=CARTESIAN_POINT ( 'NONE',  ( 24.16423886937410614, 44.51208216824730357, -3.795296366450302550 ) ) ;
#33100=CARTESIAN_POINT ( 'NONE',  ( 17.96484262340118221, 64.93868534415483396, 7.964842623401181321 ) ) ;
#33103=DIRECTION ( 'NONE',  ( 0.000000000000000000, -1.000000000000000000, 0.000000000000000000 ) ) ;
#33105=CARTESIAN_POINT ( 'NONE',  ( 17.08211943468705840, 5.137082168247300906, -12.26659068614894466 ) ) ;
#33106=CARTESIAN_POINT ( 'NONE',  ( 15.44008868035555793, 11.39701867748817143, -9.422509992056140149 ) ) ;
#33107=CARTESIAN_POINT ( 'NONE',  ( -0.8801773607111009756, 8.063685344154837509, 1.068504757029289695E-15 ) ) ;
#33108=CARTESIAN_POINT ( 'NONE',  ( 12.63842701281683034, 37.46726448433411605, 9.846743663894596210 ) ) ;
#33109=CARTESIAN_POINT ( 'NONE',  ( 16.40814093676323893, 10.79030133659708923, 11.09922568453595026 ) ) ;
#33112=CARTESIAN_POINT ( 'NONE',  ( 6.565887622018943937, 20.16530133659708213, 12.81628187352647430 ) ) ;
#33115=CARTESIAN_POINT ( 'NONE',  ( 13.79529636645031943, 45.34541550158062506, -14.16423886937409904 ) ) ;
#33116=ORIENTED_EDGE ( 'NONE', *, *, #15058, .F. ) ;
#33117=CARTESIAN_POINT ( 'NONE',  ( -4.164238869374099927, 57.01208216824731068, 3.795296366450308767 ) ) ;
#33119=CARTESIAN_POINT ( 'NONE',  ( -0.8801773607111008646, 28.27201867748817321, 2.915334737309923430 ) ) ;
#33120=CARTESIAN_POINT ( 'NONE',  ( -0.8801773607110991993, 32.85535201082151247, -2.915334737309923874 ) ) ;
#33121=CARTESIAN_POINT ( 'NONE',  ( 7.084665262690076126, 37.02201867748817676, -10.88017736071110164 ) ) ;
#33122=CARTESIAN_POINT ( 'NONE',  ( 7.084665262690076126, 62.02201867748816966, -10.88017736071110164 ) ) ;
#33123=CARTESIAN_POINT ( 'NONE',  ( 20.88017736071110519, 25.56368534415483751, 2.639326808657452039E-16 ) ) ;
#33126=CARTESIAN_POINT ( 'NONE',  ( 19.72487221294571214, 22.80223176428831877, -6.499999999999988454 ) ) ;
#33128=CARTESIAN_POINT ( 'NONE',  ( 7.361572987183169658, 9.967264484334119601, -9.846743663894592657 ) ) ;
#33130=CARTESIAN_POINT ( 'NONE',  ( 12.63842701281683034, 47.46726448433412315, 9.846743663894596210 ) ) ;
#33132=CARTESIAN_POINT ( 'NONE',  ( 0.6178305044545818747, 43.49863466993042493, -9.382169495545419124 ) ) ;
#33135=CARTESIAN_POINT ( 'NONE',  ( -46.30928139467842186, 104.0823827281712397, 5.529860068218138025 ) ) ;
#33136=CARTESIAN_POINT ( 'NONE',  ( 10.00000000000000000, 64.75893115100078035, -9.846743663894594434 ) ) ;
#33137=CARTESIAN_POINT ( 'NONE',  ( -0.3689425029237881626, 42.42874883491396787, 10.36894250292379027 ) ) ;
#33141=CARTESIAN_POINT ( 'NONE',  ( 17.20831665107776587, 24.13393115100078035, -7.208316651077762316 ) ) ;
#33144=CARTESIAN_POINT ( 'NONE',  ( 7.361572987183169658, 59.96726448433410894, -9.846743663894592657 ) ) ;
#33145=CARTESIAN_POINT ( 'NONE',  ( 10.00000000000000178, 2.258931151000784787, 9.846743663894594434 ) ) ;
#33148=CARTESIAN_POINT ( 'NONE',  ( 0.1532563361054100626, 60.80059781766744464, -2.638427012816831230 ) ) ;
#33151=EDGE_LOOP ( 'NONE', ( #17522, #21569, #26333, #36061 ) ) ;
#33152=CARTESIAN_POINT ( 'NONE',  ( -4.164238869374099927, 62.01208216824728936, 3.795296366450308767 ) ) ;
#33154=CARTESIAN_POINT ( 'NONE',  ( 7.084665262690076126, 42.02201867748816966, -10.88017736071110164 ) ) ;
#33155=CARTESIAN_POINT ( 'NONE',  ( 3.591859063236763294, 8.290301336597087456, -11.09922568453595026 ) ) ;
#33159=CARTESIAN_POINT ( 'NONE',  ( 1.046131998950040831, 30.73810908735726244, 6.499999999999992006 ) ) ;
#33160=CARTESIAN_POINT ( 'NONE',  ( 10.00000000000000178, 57.25893115100078745, 9.846743663894594434 ) ) ;
#33161=CARTESIAN_POINT ( 'NONE',  ( 7.361572987183170547, 7.050597817667451750, 9.846743663894590881 ) ) ;
#33164=CARTESIAN_POINT ( 'NONE',  ( 22.81628187352648496, 11.83196800326375531, -3.434112377981050290 ) ) ;
#33165=CARTESIAN_POINT ( 'NONE',  ( 2.035157376598824452, 13.68868534415483751, 7.964842623401179544 ) ) ;
#33166=FACE_OUTER_BOUND ( 'NONE', #92756, .T. ) ;
#33168=CARTESIAN_POINT ( 'NONE',  ( 24.16423886937410614, 34.51208216824731068, -3.795296366450302550 ) ) ;
#33169=EDGE_CURVE ( 'NONE', #6101, #34568, #57738, .T. ) ;
#33170=CARTESIAN_POINT ( 'NONE',  ( -0.3689425029237881626, 32.42874883491395366, 10.36894250292379027 ) ) ;
#33171=CARTESIAN_POINT ( 'NONE',  ( -0.8801773607111008646, 3.272018677488171434, 2.915334737309923430 ) ) ;
#33172=CARTESIAN_POINT ( 'NONE',  ( 19.84674366389459621, 33.50893115100078745, 7.409399052514197653E-17 ) ) ;
#33173=CARTESIAN_POINT ( 'NONE',  ( 3.591859063236763294, 43.29030133659708923, -11.09922568453595026 ) ) ;
#33174=CARTESIAN_POINT ( 'NONE',  ( 4.559911319644449179, 13.89701867748817143, 9.422509992056141925 ) ) ;
#33177=CARTESIAN_POINT ( 'NONE',  ( 18.52753015748618282, 33.92559781766745886, -4.923371831947291888 ) ) ;
#33178=CARTESIAN_POINT ( 'NONE',  ( 19.42250999205614548, 40.98035201082150536, -5.440088680355545492 ) ) ;
#33179=CARTESIAN_POINT ( 'NONE',  ( 13.43411237798105340, 5.581968003263753531, 12.81628187352647963 ) ) ;
#33180=CARTESIAN_POINT ( 'NONE',  ( 6.204703633549690345, 15.76208216824730179, -14.16423886937410259 ) ) ;
#33184=CARTESIAN_POINT ( 'NONE',  ( 12.63842701281683034, 27.46726448433411250, 9.846743663894596210 ) ) ;
#33185=CARTESIAN_POINT ( 'NONE',  ( -2.816281873526471635, 53.91530133659709634, -3.434112377981056508 ) ) ;
#33186=CARTESIAN_POINT ( 'NONE',  ( 18.52753015748617571, 58.09226448433411605, 4.923371831947298993 ) ) ;
#33187=ORIENTED_EDGE ( 'NONE', *, *, #73132, .T. ) ;
#33189=FILL_AREA_STYLE ('',( #11182 ) ) ;
#33190=CARTESIAN_POINT ( 'NONE',  ( 2.917880565312948704, 62.63708216824730357, 12.26659068614894643 ) ) ;
#33191=CARTESIAN_POINT ( 'NONE',  ( 2.917880565312948704, 17.63708216824730357, 12.26659068614894643 ) ) ;
#33192=CARTESIAN_POINT ( 'NONE',  ( 15.44008868035555260, 64.73035201082151957, 9.422509992056143702 ) ) ;
#33193=CARTESIAN_POINT ( 'NONE',  ( 2.791683348922240793, 46.63393115100077324, 7.208316651077764092 ) ) ;
#33194=CARTESIAN_POINT ( 'NONE',  ( 15.44008868035555260, 24.73035201082150891, 9.422509992056143702 ) ) ;
#33196=DIRECTION ( 'NONE',  ( 0.000000000000000000, -1.000000000000000000, 0.000000000000000000 ) ) ;
#33202=CARTESIAN_POINT ( 'NONE',  ( 20.36894250292379738, 14.92874883491396432, -10.36894250292379027 ) ) ;
#33203=SURFACE_SIDE_STYLE ('',( #40232 ) ) ;
#33204=EDGE_CURVE ( 'NONE', #4701, #68203, #71105, .T. ) ;
#33205=CARTESIAN_POINT ( 'NONE',  ( -2.266590686148945544, 41.38708216824729647, -7.082119434687050408 ) ) ;
#33206=CARTESIAN_POINT ( 'NONE',  ( 10.00000000000000178, 57.25893115100078745, 9.846743663894594434 ) ) ;
#33207=CARTESIAN_POINT ( 'NONE',  ( 12.63842701281683034, 27.46726448433411250, 9.846743663894596210 ) ) ;
#33209=CARTESIAN_POINT ( 'NONE',  ( 19.42250999205614193, 20.14701867748817321, 5.440088680355555262 ) ) ;
#33210=CARTESIAN_POINT ( 'NONE',  ( 19.84674366389459266, 58.30059781766745886, 2.638427012816836559 ) ) ;
#33212=CARTESIAN_POINT ( 'NONE',  ( 12.91533473730993009, 11.60535201082150714, -10.88017736071109987 ) ) ;
#33215=CARTESIAN_POINT ( 'NONE',  ( 17.96484262340118221, 59.93868534415484106, 7.964842623401181321 ) ) ;
#33216=ADVANCED_FACE ( 'NONE', ( #3777 ), #34230, .T. ) ;
#33217=CARTESIAN_POINT ( 'NONE',  ( 7.361572987183170547, 12.05059781766744997, 9.846743663894590881 ) ) ;
#33218=( GEOMETRIC_REPRESENTATION_CONTEXT ( 3 ) GLOBAL_UNCERTAINTY_ASSIGNED_CONTEXT ( ( #81144 ) ) GLOBAL_UNIT_ASSIGNED_CONTEXT ( ( #82421, #79101, #13945 ) ) REPRESENTATION_CONTEXT ( 'NONE', 'WORKASPACE' ) );
#33222=CARTESIAN_POINT ( 'NONE',  ( 2.791683348922237240, 20.38393115100078745, -7.208316651077763204 ) ) ;
#33224=CARTESIAN_POINT ( 'NONE',  ( -4.164238869374099039, 36.80374883491396787, 8.674139862899312516E-16 ) ) ;
#33225=CARTESIAN_POINT ( 'NONE',  ( 12.63842701281683034, 27.46726448433411250, 9.846743663894596210 ) ) ;
#33226=CARTESIAN_POINT ( 'NONE',  ( 4.559911319644449179, 48.89701867748817676, 9.422509992056141925 ) ) ;
#33228=SURFACE_STYLE_USAGE ( .BOTH. , #78746 ) ;
#33231=CARTESIAN_POINT ( 'NONE',  ( 4.559911319644449179, 43.89701867748816966, 9.422509992056141925 ) ) ;
#33235=CARTESIAN_POINT ( 'NONE',  ( 4.559911319644449179, 43.89701867748816966, 9.422509992056141925 ) ) ;
#33236=CARTESIAN_POINT ( 'NONE',  ( 17.08211943468705840, 5.137082168247300906, -12.26659068614894466 ) ) ;
#33238=ORIENTED_EDGE ( 'NONE', *, *, #82890, .T. ) ;
#33239=CARTESIAN_POINT ( 'NONE',  ( 16.40814093676324603, 37.45696800326376064, -11.09922568453594671 ) ) ;
#33240=CARTESIAN_POINT ( 'NONE',  ( 2.791683348922240793, 26.63393115100078745, 7.208316651077764092 ) ) ;
#33241=CARTESIAN_POINT ( 'NONE',  ( 7.084665262690076126, 4.105352010821503583, 10.88017736071109987 ) ) ;
#33243=CARTESIAN_POINT ( 'NONE',  ( 10.00000000000000000, 34.75893115100078745, -9.846743663894594434 ) ) ;
#33245=CARTESIAN_POINT ( 'NONE',  ( -0.8801773607111008646, 58.27201867748816966, 2.915334737309923430 ) ) ;
#33247=CARTESIAN_POINT ( 'NONE',  ( 0.2751277870542967463, 0.000000000000000000, 6.500000000000000888 ) ) ;
#33249=CARTESIAN_POINT ( 'NONE',  ( -2.816281873526471635, 63.91530133659708923, -3.434112377981056508 ) ) ;
#33250=CARTESIAN_POINT ( 'NONE',  ( 5.076628168052704559, 5.175597817667451750, -8.527530157486179263 ) ) ;
#33251=CARTESIAN_POINT ( 'NONE',  ( -2.816281873526471635, 13.91530133659708746, -3.434112377981056508 ) ) ;
#33252=LINE ( 'NONE', #63745, #16400 ) ;
#33253=B_SPLINE_CURVE_WITH_KNOTS ( 'NONE', 3,
 ( #22524, #83511, #47954, #70480, #1513, #70979, #24993, #32954, #55476, #63457 ),
 .UNSPECIFIED., .F., .F.,
 ( 4, 3, 3, 4 ),
 ( 0.000000000000000000, 0.0006253016069560473613, 0.001250604074564875320, 0.002501455912506565619 ),
 .UNSPECIFIED. ) ;
#33255=CARTESIAN_POINT ( 'NONE',  ( 17.20831665107776587, 47.88393115100078745, 7.208316651077764980 ) ) ;
#33256=CARTESIAN_POINT ( 'NONE',  ( 0.6178305044545818747, 63.49863466993043204, -9.382169495545419124 ) ) ;
#33257=CARTESIAN_POINT ( 'NONE',  ( 2.917880565312950480, 5.970415501580634832, -12.26659068614894821 ) ) ;
#33258=CARTESIAN_POINT ( 'NONE',  ( 18.52753015748618282, 28.92559781766745175, -4.923371831947291888 ) ) ;
#33259=CARTESIAN_POINT ( 'NONE',  ( -1.099225684535947600, 34.54030133659708923, 6.408140936763237150 ) ) ;
#33262=CARTESIAN_POINT ( 'NONE',  ( 19.42250999205614193, 50.14701867748817676, 5.440088680355555262 ) ) ;
#33263=CARTESIAN_POINT ( 'NONE',  ( 3.591859063236763294, 3.290301336597087012, -11.09922568453595026 ) ) ;
#33264=CARTESIAN_POINT ( 'NONE',  ( 19.84674366389459266, 23.71726448433412315, -2.638427012816827677 ) ) ;
#33265=CARTESIAN_POINT ( 'NONE',  ( 19.42250999205614548, 20.98035201082150891, -5.440088680355545492 ) ) ;
#33266=CARTESIAN_POINT ( 'NONE',  ( 13.43411237798106583, 27.66530133659708568, -12.81628187352647252 ) ) ;
#33268=CARTESIAN_POINT ( 'NONE',  ( 0.5774900079438607392, 13.48035201082150358, 5.440088680355550821 ) ) ;
#33269=CARTESIAN_POINT ( 'NONE',  ( 4.559911319644449179, 57.23035201082150536, -9.422509992056141925 ) ) ;
#33270=CARTESIAN_POINT ( 'NONE',  ( 0.5774900079438607392, 8.480352010821505360, 5.440088680355550821 ) ) ;
#33271=CARTESIAN_POINT ( 'NONE',  ( 5.076628168052703671, 36.84226448433412315, 8.527530157486179263 ) ) ;
#33272=CARTESIAN_POINT ( 'NONE',  ( 0.5774900079438590739, 27.64701867748817676, -5.440088680355550821 ) ) ;
#33274=CARTESIAN_POINT ( 'NONE',  ( 20.88017736071110164, 45.35535201082149115, 2.915334737309930979 ) ) ;
#33276=CARTESIAN_POINT ( 'NONE',  ( 7.084665262690076126, 17.02201867748817676, -10.88017736071110164 ) ) ;
#33278=CARTESIAN_POINT ( 'NONE',  ( 20.24186590665277663, 54.73410085661204505, 6.114288769123050749 ) ) ;
#33279=CARTESIAN_POINT ( 'NONE',  ( 12.63842701281683034, 32.46726448433412315, 9.846743663894596210 ) ) ;
#33280=CARTESIAN_POINT ( 'NONE',  ( -46.68456736488006698, 103.6675473310227176, 5.775421524742653467 ) ) ;
#33281=CARTESIAN_POINT ( 'NONE',  ( 10.00000000000000178, 5.373634669930420493, 12.81628187352647608 ) ) ;
#33282=VECTOR ( 'NONE', #94103, 1000.000000000000000 ) ;
#33286=CARTESIAN_POINT ( 'NONE',  ( 13.79529636645030344, 28.26208216824729647, 14.16423886937410614 ) ) ;
#33287=CARTESIAN_POINT ( 'NONE',  ( 10.00000000000000178, 0.000000000000000000, 0.000000000000000000 ) ) ;
#33289=CARTESIAN_POINT ( 'NONE',  ( -2.266590686148945544, 62.22041550158063927, 7.082119434687048631 ) ) ;
#33291=CARTESIAN_POINT ( 'NONE',  ( 10.00000000000000178, 27.25893115100078390, 9.846743663894594434 ) ) ;
#33293=CARTESIAN_POINT ( 'NONE',  ( 19.42250999205614548, 55.98035201082150536, -5.440088680355545492 ) ) ;
#33294=CARTESIAN_POINT ( 'NONE',  ( 22.81628187352648496, 61.83196800326376774, -3.434112377981050290 ) ) ;
#33295=CARTESIAN_POINT ( 'NONE',  ( 20.88017736071110519, 30.56368534415484106, 2.639326808657452039E-16 ) ) ;
#33297=CARTESIAN_POINT ( 'NONE',  ( -2.816281873526473856, 9.123634669930421381, 9.499525473075851096E-16 ) ) ;
#33298=CARTESIAN_POINT ( 'NONE',  ( 2.791683348922240793, 11.63393115100078568, 7.208316651077764092 ) ) ;
#33302=CARTESIAN_POINT ( 'NONE',  ( 24.16423886937410614, 54.30374883491396787, 8.672049930838204340E-16 ) ) ;
#33303=CARTESIAN_POINT ( 'NONE',  ( -4.164238869374099927, 22.01208216824730357, 3.795296366450308767 ) ) ;
#33304=CARTESIAN_POINT ( 'NONE',  ( 17.96484262340118221, 31.18868534415483751, -7.964842623401177768 ) ) ;
#33305=CARTESIAN_POINT ( 'NONE',  ( 4.559911319644449179, 43.89701867748816966, 9.422509992056141925 ) ) ;
#33306=( NAMED_UNIT ( * ) PLANE_ANGLE_UNIT ( ) SI_UNIT ( $, .RADIAN. ) );
#33308=CARTESIAN_POINT ( 'NONE',  ( 19.84674366389459266, 8.300597817667451750, 2.638427012816836559 ) ) ;
#33310=CARTESIAN_POINT ( 'NONE',  ( 18.52753015748618282, 13.92559781766745175, -4.923371831947291888 ) ) ;
#33311=CARTESIAN_POINT ( 'NONE',  ( 19.84674366389459266, 23.30059781766745530, 2.638427012816836559 ) ) ;
#33312=CARTESIAN_POINT ( 'NONE',  ( 0.1532563361054082862, 51.21726448433412315, 2.638427012816831674 ) ) ;
#33314=CARTESIAN_POINT ( 'NONE',  ( 13.43411237798106583, 37.66530133659708923, -12.81628187352647252 ) ) ;
#33315=CARTESIAN_POINT ( 'NONE',  ( 0.5774900079438590739, 57.64701867748817676, -5.440088680355550821 ) ) ;
#33316=CARTESIAN_POINT ( 'NONE',  ( 17.20831665107776587, 29.13393115100078390, -7.208316651077762316 ) ) ;
#33317=CARTESIAN_POINT ( 'NONE',  ( -2.266590686148945544, 47.22041550158063927, 7.082119434687048631 ) ) ;
#33318=CARTESIAN_POINT ( 'NONE',  ( 10.00000000000000000, 19.75893115100078390, -9.846743663894594434 ) ) ;
#33320=CARTESIAN_POINT ( 'NONE',  ( 17.20831665107776587, 54.13393115100079456, -7.208316651077762316 ) ) ;
#33321=CARTESIAN_POINT ( 'NONE',  ( 2.791683348922237240, 50.38393115100078035, -7.208316651077763204 ) ) ;
#33322=CARTESIAN_POINT ( 'NONE',  ( 17.08211943468705130, 8.470415501580635720, 12.26659068614894998 ) ) ;
#33323=CARTESIAN_POINT ( 'NONE',  ( 10.00000000000000178, 33.05374883491396787, 14.16423886937410082 ) ) ;
#33324=CARTESIAN_POINT ( 'NONE',  ( 14.92337183194729633, 27.67559781766745530, 8.527530157486181039 ) ) ;
#33325=CARTESIAN_POINT ( 'NONE',  ( 4.559911319644449179, 22.23035201082150536, -9.422509992056141925 ) ) ;
#33327=CARTESIAN_POINT ( 'NONE',  ( 15.44008868035555260, 49.73035201082150536, 9.422509992056143702 ) ) ;
#33328=CARTESIAN_POINT ( 'NONE',  ( 4.559911319644449179, 42.23035201082151247, -9.422509992056141925 ) ) ;
#33329=ORIENTED_EDGE ( 'NONE', *, *, #64090, .T. ) ;
#33330=CARTESIAN_POINT ( 'NONE',  ( 19.38216949554541557, 32.24863466993041783, -9.382169495545420901 ) ) ;
#33331=CARTESIAN_POINT ( 'NONE',  ( 15.44008868035555260, 54.73035201082150536, 9.422509992056143702 ) ) ;
#33333=CARTESIAN_POINT ( 'NONE',  ( 10.00000000000000000, -0.2410688489992152128, -9.846743663894594434 ) ) ;
#33334=CARTESIAN_POINT ( 'NONE',  ( 7.084665262690076126, 64.10535201082150536, 10.88017736071109987 ) ) ;
#33336=CARTESIAN_POINT ( 'NONE',  ( 2.035157376598822676, 57.43868534415484106, -7.964842623401177768 ) ) ;
#33337=( NAMED_UNIT ( * ) PLANE_ANGLE_UNIT ( ) SI_UNIT ( $, .RADIAN. ) );
#33339=CARTESIAN_POINT ( 'NONE',  ( 20.20024927138663884, 0.02462294155896342304, 6.181741512439034913 ) ) ;
#33340=CARTESIAN_POINT ( 'NONE',  ( 12.91533473730992121, 4.522018677488170546, 10.88017736071110164 ) ) ;
#33341=CARTESIAN_POINT ( 'NONE',  ( 0.1532563361054083140, 16.00893115100078390, 1.131784320476157264E-15 ) ) ;
#33342=CARTESIAN_POINT ( 'NONE',  ( -0.3689425029237898834, 1.178748834913967869, -10.36894250292378850 ) ) ;
#33343=CARTESIAN_POINT ( 'NONE',  ( 10.00000000000000178, 7.258931151000785675, 9.846743663894594434 ) ) ;
#33344=CARTESIAN_POINT ( 'NONE',  ( 10.00000000000000178, 4.313685344154837509, 10.88017736071110342 ) ) ;
#33345=CARTESIAN_POINT ( 'NONE',  ( 19.84674366389459266, 48.30059781766745175, 2.638427012816836559 ) ) ;
#33346=ORIENTED_EDGE ( 'NONE', *, *, #36104, .F. ) ;
#33347=CARTESIAN_POINT ( 'NONE',  ( 19.84674366389459266, 43.30059781766744464, 2.638427012816836559 ) ) ;
#33350=CARTESIAN_POINT ( 'NONE',  ( 15.44008868035555260, 59.73035201082151247, 9.422509992056143702 ) ) ;
#33351=CARTESIAN_POINT ( 'NONE',  ( 7.361572987183169658, 44.96726448433412315, -9.846743663894592657 ) ) ;
#33352=CARTESIAN_POINT ( 'NONE',  ( 20.88017736071110875, 65.77201867748817676, -2.915334737309920765 ) ) ;
#33353=CARTESIAN_POINT ( 'NONE',  ( 4.559911319644449179, 58.89701867748817676, 9.422509992056141925 ) ) ;
#33354=CARTESIAN_POINT ( 'NONE',  ( 20.88017736071110519, 10.56368534415483929, 2.639326808657452039E-16 ) ) ;
#33355=EDGE_CURVE ( 'NONE', #68797, #27569, #94993, .T. ) ;
#33357=CARTESIAN_POINT ( 'NONE',  ( 21.09922568453595559, 42.04030133659708213, -6.408140936763230044 ) ) ;
#33360=CARTESIAN_POINT ( 'NONE',  ( 21.09922568453595559, 32.04030133659708923, -6.408140936763230044 ) ) ;
#33361=CARTESIAN_POINT ( 'NONE',  ( 2.035157376598822676, 37.43868534415484106, -7.964842623401177768 ) ) ;
#33362=ORIENTED_EDGE ( 'NONE', *, *, #57470, .F. ) ;
#33364=CARTESIAN_POINT ( 'NONE',  ( 0.1532563361054083140, 11.00893115100078568, 1.131784320476157264E-15 ) ) ;
#33365=CARTESIAN_POINT ( 'NONE',  ( 0.6178305044545838731, -0.2513653300695798953, 9.382169495545420901 ) ) ;
#33366=CARTESIAN_POINT ( 'NONE',  ( 5.076628168052704559, 10.17559781766745175, -8.527530157486179263 ) ) ;
#33367=CARTESIAN_POINT ( 'NONE',  ( 12.63842701281683922, 54.55059781766745175, -9.846743663894590881 ) ) ;
#33373=CARTESIAN_POINT ( 'NONE',  ( 19.84674366389459621, 33.50893115100078745, 7.409399052514197653E-17 ) ) ;
#33375=CARTESIAN_POINT ( 'NONE',  ( 18.52753015748618282, 63.92559781766745886, -4.923371831947291888 ) ) ;
#33377=CARTESIAN_POINT ( 'NONE',  ( 0.5774900079438590739, 7.647018677488171434, -5.440088680355550821 ) ) ;
#33378=CARTESIAN_POINT ( 'NONE',  ( 3.591859063236761518, 19.95696800326375353, 11.09922568453594849 ) ) ;
#33379=CARTESIAN_POINT ( 'NONE',  ( 19.84674366389459266, 43.30059781766744464, 2.638427012816836559 ) ) ;
#33381=CARTESIAN_POINT ( 'NONE',  ( 17.08211943468705840, 45.13708216824730357, -12.26659068614894466 ) ) ;
#33382=CARTESIAN_POINT ( 'NONE',  ( 14.92337183194729633, 12.67559781766745353, 8.527530157486181039 ) ) ;
#33385=CARTESIAN_POINT ( 'NONE',  ( 22.26659068614894466, 38.88708216824731068, 7.082119434687054849 ) ) ;
#33386=CARTESIAN_POINT ( 'NONE',  ( 1.472469842513823179, 55.59226448433412315, -4.923371831947296329 ) ) ;
#33387=CARTESIAN_POINT ( 'NONE',  ( -0.8801773607111009756, 8.063685344154837509, 1.068504757029289695E-15 ) ) ;
#33388=CARTESIAN_POINT ( 'NONE',  ( 20.36894250292379382, 28.67874883491396787, 10.36894250292379205 ) ) ;
#33389=CARTESIAN_POINT ( 'NONE',  ( 2.917880565312950480, 40.97041550158063217, -12.26659068614894821 ) ) ;
#33390=SURFACE_STYLE_FILL_AREA ( #2942 ) ;
#33392=CARTESIAN_POINT ( 'NONE',  ( 5.076628168052703671, 51.84226448433412315, 8.527530157486179263 ) ) ;
#33394=CARTESIAN_POINT ( 'NONE',  ( 20.88017736071110875, 30.77201867748816966, -2.915334737309920765 ) ) ;
#33396=CARTESIAN_POINT ( 'NONE',  ( 20.00000000000000711, 93.02849646088141355, -5.197973391108903662 ) ) ;
#33399=CARTESIAN_POINT ( 'NONE',  ( 0.1532563361054082862, 51.21726448433412315, 2.638427012816831674 ) ) ;
#33400=LINE ( 'NONE', #25927, #30552 ) ;
#33403=CARTESIAN_POINT ( 'NONE',  ( -4.164238869374098151, 26.59541550158063217, -3.795296366450310543 ) ) ;
#33405=ADVANCED_FACE ( 'NONE', ( #21734 ), #81989, .T. ) ;
#33408=CARTESIAN_POINT ( 'NONE',  ( 10.00000000000000178, 68.05374883491397497, 14.16423886937410082 ) ) ;
#33409=CARTESIAN_POINT ( 'NONE',  ( 16.40814093676324603, 27.45696800326375708, -11.09922568453594671 ) ) ;
#33411=CARTESIAN_POINT ( 'NONE',  ( 14.92337183194729633, 17.67559781766745175, 8.527530157486181039 ) ) ;
#33415=CARTESIAN_POINT ( 'NONE',  ( 17.96484262340118221, 11.18868534415484106, -7.964842623401177768 ) ) ;
#33417=CARTESIAN_POINT ( 'NONE',  ( 20.88017736071110164, 40.35535201082150536, 2.915334737309930979 ) ) ;
#33418=CARTESIAN_POINT ( 'NONE',  ( 2.035157376598824452, 43.68868534415484106, 7.964842623401179544 ) ) ;
#33419=CARTESIAN_POINT ( 'NONE',  ( 18.52753015748617571, 63.09226448433412315, 4.923371831947298993 ) ) ;
#33420=CARTESIAN_POINT ( 'NONE',  ( 14.92337183194729988, 64.34226448433412315, -8.527530157486177487 ) ) ;
#33421=CARTESIAN_POINT ( 'NONE',  ( -45.65418601736590176, 104.2903935945944056, -5.789884099738774381 ) ) ;
#33422=CARTESIAN_POINT ( 'NONE',  ( 17.20831665107776587, 4.133931151000785675, -7.208316651077762316 ) ) ;
#33425=CARTESIAN_POINT ( 'NONE',  ( 10.00000000000000178, 24.31368534415484106, 10.88017736071110342 ) ) ;
#33426=CARTESIAN_POINT ( 'NONE',  ( 22.81628187352647785, 31.41530133659709279, 3.434112377981063169 ) ) ;
#33427=CARTESIAN_POINT ( 'NONE',  ( 0.000000000000000000, 70.80332830338373640, 5.000000000000000000 ) ) ;
#33428=CARTESIAN_POINT ( 'NONE',  ( 10.00000000000000000, 64.75893115100078035, -9.846743663894594434 ) ) ;
#33429=CARTESIAN_POINT ( 'NONE',  ( -0.8801773607111008646, 68.27201867748817676, 2.915334737309923430 ) ) ;
#33430=CARTESIAN_POINT ( 'NONE',  ( 10.00000000000000000, 9.758931151000785675, -9.846743663894594434 ) ) ;
#33431=CARTESIAN_POINT ( 'NONE',  ( 16.40814093676324603, 32.45696800326375353, -11.09922568453594671 ) ) ;
#33432=CARTESIAN_POINT ( 'NONE',  ( 17.96484262340118221, 61.18868534415482685, -7.964842623401177768 ) ) ;
#33435=B_SPLINE_CURVE_WITH_KNOTS ( 'NONE', 3,
 ( #81766, #37777, #36783, #68274, #30241, #36279, #60745, #13278, #91246, #13777, #53251, #43769, #74259, #5788, #59264, #89766, #82261, #44263 ),
 .UNSPECIFIED., .F., .F.,
 ( 4, 2, 2, 2, 2, 2, 2, 2, 4 ),
 ( 0.000000000000000000, 0.001396361802156549344, 0.002792723604313098688, 0.004189085406469648248, 0.005585447208626197375, 0.006981809010782746502, 0.008378170812939296497, 0.009774532615095844756, 0.01117089441725239475 ),
 .UNSPECIFIED. ) ;
#33437=CARTESIAN_POINT ( 'NONE',  ( 20.88017736071110164, 5.355352010821502695, 2.915334737309930979 ) ) ;
#33438=CARTESIAN_POINT ( 'NONE',  ( 0.6178305044545838731, 54.74863466993042493, 9.382169495545420901 ) ) ;
#33439=CARTESIAN_POINT ( 'NONE',  ( 6.204703633549690345, 25.76208216824730712, -14.16423886937410259 ) ) ;
#33441=CARTESIAN_POINT ( 'NONE',  ( 14.92337183194729988, 19.34226448433411960, -8.527530157486177487 ) ) ;
#33443=CARTESIAN_POINT ( 'NONE',  ( 7.084665262690076126, 9.105352010821503583, 10.88017736071109987 ) ) ;
#33444=CARTESIAN_POINT ( 'NONE',  ( 0.1532563361054082862, 16.21726448433411960, 2.638427012816831674 ) ) ;
#33445=CARTESIAN_POINT ( 'NONE',  ( -0.3689425029237881626, 52.42874883491396076, 10.36894250292379027 ) ) ;
#33446=ORIENTED_EDGE ( 'NONE', *, *, #75055, .T. ) ;
#33447=CARTESIAN_POINT ( 'NONE',  ( -0.8801773607110991993, 17.85535201082150536, -2.915334737309923874 ) ) ;
#33449=CARTESIAN_POINT ( 'NONE',  ( 12.91533473730992121, 19.52201867748816611, 10.88017736071110164 ) ) ;
#33452=CARTESIAN_POINT ( 'NONE',  ( 21.92686044187657401, 10.37045670184113888, -3.195792623639525765 ) ) ;
#33453=CARTESIAN_POINT ( 'NONE',  ( 10.00000000000000178, 29.31368534415483751, 10.88017736071110342 ) ) ;
#33454=CARTESIAN_POINT ( 'NONE',  ( 7.361572987183169658, 54.96726448433413026, -9.846743663894592657 ) ) ;
#33457=CARTESIAN_POINT ( 'NONE',  ( -0.3689425029237881626, 17.42874883491397142, 10.36894250292379027 ) ) ;
#33458=CARTESIAN_POINT ( 'NONE',  ( -0.8801773607111008646, 38.27201867748816255, 2.915334737309923430 ) ) ;
#33459=CARTESIAN_POINT ( 'NONE',  ( 19.42250999205614548, 10.98035201082150536, -5.440088680355545492 ) ) ;
#33460=CARTESIAN_POINT ( 'NONE',  ( 17.20831665107776587, 54.13393115100079456, -7.208316651077762316 ) ) ;
#33462=CARTESIAN_POINT ( 'NONE',  ( 10.00000000000000178, 37.25893115100078745, 9.846743663894594434 ) ) ;
#33464=CARTESIAN_POINT ( 'NONE',  ( 1.472469842513823179, 11.42559781766745175, 4.923371831947296329 ) ) ;
#33466=ORIENTED_EDGE ( 'NONE', *, *, #78683, .T. ) ;
#33468=CARTESIAN_POINT ( 'NONE',  ( -0.8801773607111008646, 18.27201867748817321, 2.915334737309923430 ) ) ;
#33469=CARTESIAN_POINT ( 'NONE',  ( 17.20831665107776587, 9.133931151000787452, -7.208316651077762316 ) ) ;
#33470=CARTESIAN_POINT ( 'NONE',  ( 12.63842701281683922, 64.55059781766745175, -9.846743663894590881 ) ) ;
#33471=CARTESIAN_POINT ( 'NONE',  ( 15.44008868035555260, 49.73035201082150536, 9.422509992056143702 ) ) ;
#33472=CARTESIAN_POINT ( 'NONE',  ( 0.5774900079438590739, 17.64701867748817321, -5.440088680355550821 ) ) ;
#33473=CARTESIAN_POINT ( 'NONE',  ( -1.099225684535947600, 48.70696800326375353, -6.408140936763238038 ) ) ;
#33474=CARTESIAN_POINT ( 'NONE',  ( 22.26659068614894466, 28.88708216824730357, 7.082119434687054849 ) ) ;
#33477=CARTESIAN_POINT ( 'NONE',  ( 10.00000000000000178, 60.37363466993041783, 12.81628187352647608 ) ) ;
#33479=CARTESIAN_POINT ( 'NONE',  ( 5.076628168052704559, 60.17559781766745175, -8.527530157486179263 ) ) ;
#33480=CARTESIAN_POINT ( 'NONE',  ( 17.96484262340118221, 39.93868534415484106, 7.964842623401181321 ) ) ;
#33482=CARTESIAN_POINT ( 'NONE',  ( 19.84674366389459266, 3.300597817667451750, 2.638427012816836559 ) ) ;
#33485=CARTESIAN_POINT ( 'NONE',  ( 19.84674366389459266, 8.300597817667451750, 2.638427012816836559 ) ) ;
#33486=CARTESIAN_POINT ( 'NONE',  ( 7.361572987183170547, 27.05059781766745175, 9.846743663894590881 ) ) ;
#33487=CARTESIAN_POINT ( 'NONE',  ( 10.00000000000000178, 2.258931151000784787, 9.846743663894594434 ) ) ;
#33488=CARTESIAN_POINT ( 'NONE',  ( 2.791683348922237240, 5.383931151000785675, -7.208316651077763204 ) ) ;
#33490=CARTESIAN_POINT ( 'NONE',  ( 15.44008868035555793, 56.39701867748817676, -9.422509992056140149 ) ) ;
#33492=CARTESIAN_POINT ( 'NONE',  ( 4.559911319644449179, 57.23035201082150536, -9.422509992056141925 ) ) ;
#33493=CARTESIAN_POINT ( 'NONE',  ( 19.84674366389459266, 18.71726448433411960, -2.638427012816827677 ) ) ;
#33495=CARTESIAN_POINT ( 'NONE',  ( 0.5774900079438607392, 63.48035201082149825, 5.440088680355550821 ) ) ;
#33496=CARTESIAN_POINT ( 'NONE',  ( 5.076628168052703671, 56.84226448433412315, 8.527530157486179263 ) ) ;
#33500=CARTESIAN_POINT ( 'NONE',  ( 6.204703633549690345, 7.845415501580634832, 14.16423886937410082 ) ) ;
#33502=CARTESIAN_POINT ( 'NONE',  ( 13.43411237798105340, 55.58196800326374643, 12.81628187352647963 ) ) ;
#33503=CARTESIAN_POINT ( 'NONE',  ( 10.00000000000000178, 8.053748834913967869, 14.16423886937410082 ) ) ;
#33504=CARTESIAN_POINT ( 'NONE',  ( 2.917880565312948704, 27.63708216824730357, 12.26659068614894643 ) ) ;
#33506=CARTESIAN_POINT ( 'NONE',  ( 2.917880565312950480, 5.970415501580634832, -12.26659068614894821 ) ) ;
#33507=CARTESIAN_POINT ( 'NONE',  ( 10.00000000000000000, 16.81368534415483751, -10.88017736071110342 ) ) ;
#33510=CARTESIAN_POINT ( 'NONE',  ( 12.63842701281683034, 12.46726448433411782, 9.846743663894596210 ) ) ;
#33511=CARTESIAN_POINT ( 'NONE',  ( 12.91533473730993009, 51.60535201082149825, -10.88017736071109987 ) ) ;
#33512=CARTESIAN_POINT ( 'NONE',  ( 1.472469842513823179, 15.59226448433411960, -4.923371831947296329 ) ) ;
#33514=CARTESIAN_POINT ( 'NONE',  ( 13.43411237798105340, 50.58196800326375353, 12.81628187352647963 ) ) ;
#33515=CARTESIAN_POINT ( 'NONE',  ( 19.84674366389459266, 33.71726448433410894, -2.638427012816827677 ) ) ;
#33518=CARTESIAN_POINT ( 'NONE',  ( 10.00000000000000178, 54.31368534415484106, 10.88017736071110342 ) ) ;
#33519=CARTESIAN_POINT ( 'NONE',  ( 13.43411237798105340, 35.58196800326375353, 12.81628187352647963 ) ) ;
#33521=CARTESIAN_POINT ( 'NONE',  ( 7.361572987183169658, 24.96726448433412315, -9.846743663894592657 ) ) ;
#33523=CARTESIAN_POINT ( 'NONE',  ( 2.917880565312950480, 15.97041550158063217, -12.26659068614894821 ) ) ;
#33524=ORIENTED_EDGE ( 'NONE', *, *, #13416, .F. ) ;
#33526=CARTESIAN_POINT ( 'NONE',  ( 20.88017736071110875, 35.77201867748816966, -2.915334737309920765 ) ) ;
#33527=CARTESIAN_POINT ( 'NONE',  ( -4.164238869374099927, 37.01208216824731068, 3.795296366450308767 ) ) ;
#33528=CARTESIAN_POINT ( 'NONE',  ( 12.63842701281683034, 52.46726448433413026, 9.846743663894596210 ) ) ;
#33529=CARTESIAN_POINT ( 'NONE',  ( 12.63842701281683922, 9.550597817667449974, -9.846743663894590881 ) ) ;
#33530=CARTESIAN_POINT ( 'NONE',  ( 16.40814093676323893, 50.79030133659708923, 11.09922568453595026 ) ) ;
#33532=CARTESIAN_POINT ( 'NONE',  ( 12.91533473730992121, 39.52201867748817676, 10.88017736071110164 ) ) ;
#33535=CARTESIAN_POINT ( 'NONE',  ( 22.81628187352647785, 26.41530133659708923, 3.434112377981063169 ) ) ;
#33536=CARTESIAN_POINT ( 'NONE',  ( 1.472469842513823179, 60.59226448433412315, -4.923371831947296329 ) ) ;
#33538=SURFACE_STYLE_USAGE ( .BOTH. , #3571 ) ;
#33539=CARTESIAN_POINT ( 'NONE',  ( 4.559911319644449179, 67.23035201082150536, -9.422509992056141925 ) ) ;
#33543=CARTESIAN_POINT ( 'NONE',  ( 12.91533473730992121, 59.52201867748816966, 10.88017736071110164 ) ) ;
#33544=CARTESIAN_POINT ( 'NONE',  ( -0.8801773607111009756, 63.06368534415484106, 1.068504757029289695E-15 ) ) ;
#33547=CARTESIAN_POINT ( 'NONE',  ( 18.52753015748617571, 23.09226448433411960, 4.923371831947298993 ) ) ;
#33548=CARTESIAN_POINT ( 'NONE',  ( -0.8801773607111008646, 28.27201867748817321, 2.915334737309923430 ) ) ;
#33549=CARTESIAN_POINT ( 'NONE',  ( 6.565887622018943937, -1.918031996736246692, -12.81628187352647608 ) ) ;
#33550=CARTESIAN_POINT ( 'NONE',  ( -0.8801773607111008646, 28.27201867748817321, 2.915334737309923430 ) ) ;
#33551=CARTESIAN_POINT ( 'NONE',  ( -0.1503990784575277573, 33.10158574516643171, 6.262539305110076171 ) ) ;
#33552=CARTESIAN_POINT ( 'NONE',  ( 19.38216949554541557, 22.24863466993041428, -9.382169495545420901 ) ) ;
#33554=CARTESIAN_POINT ( 'NONE',  ( 20.88017736071110164, 50.35535201082151247, 2.915334737309930979 ) ) ;
#33555=CARTESIAN_POINT ( 'NONE',  ( 1.472469842513823179, 46.42559781766745175, 4.923371831947296329 ) ) ;
#33556=CARTESIAN_POINT ( 'NONE',  ( 16.40814093676323893, 25.79030133659708923, 11.09922568453595026 ) ) ;
#33557=( LENGTH_UNIT ( ) NAMED_UNIT ( * ) SI_UNIT ( .MILLI., .METRE. ) );
#33559=CARTESIAN_POINT ( 'NONE',  ( 2.035157376598822676, 22.43868534415483396, -7.964842623401177768 ) ) ;
#33560=CARTESIAN_POINT ( 'NONE',  ( 22.26659068614895176, 44.72041550158063927, -7.082119434687042414 ) ) ;
#33561=CARTESIAN_POINT ( 'NONE',  ( 5.076628168052704559, 40.17559781766745175, -8.527530157486179263 ) ) ;
#33562=CARTESIAN_POINT ( 'NONE',  ( 7.361572987183169658, 9.967264484334119601, -9.846743663894592657 ) ) ;
#33563=CARTESIAN_POINT ( 'NONE',  ( 20.88017736071110519, 50.56368534415484106, 2.639326808657452039E-16 ) ) ;
#33565=CARTESIAN_POINT ( 'NONE',  ( 6.204703633549690345, 17.84541550158063217, 14.16423886937410082 ) ) ;
#33567=CARTESIAN_POINT ( 'NONE',  ( 2.377183314879970588, 20.78593319516822646, -6.499999999999988454 ) ) ;
#33571=CARTESIAN_POINT ( 'NONE',  ( 2.917880565312950480, 45.97041550158063927, -12.26659068614894821 ) ) ;
#33572=CARTESIAN_POINT ( 'NONE',  ( 22.26659068614895176, 54.72041550158063217, -7.082119434687042414 ) ) ;
#33573=CARTESIAN_POINT ( 'NONE',  ( 18.52753015748617571, 13.09226448433411960, 4.923371831947298993 ) ) ;
#33574=CARTESIAN_POINT ( 'NONE',  ( 0.6178305044545838731, 14.74863466993041783, 9.382169495545420901 ) ) ;
#33576=CARTESIAN_POINT ( 'NONE',  ( 19.80427997160309417, 52.75733960839545489, -6.499999999999988454 ) ) ;
#33577=CARTESIAN_POINT ( 'NONE',  ( 15.44008868035555260, 4.730352010821504471, 9.422509992056143702 ) ) ;
#33578=CARTESIAN_POINT ( 'NONE',  ( 6.565887622018943937, 35.16530133659708923, 12.81628187352647430 ) ) ;
#33579=CARTESIAN_POINT ( 'NONE',  ( 13.79529636645031943, 45.34541550158062506, -14.16423886937409904 ) ) ;
#33581=SURFACE_STYLE_USAGE ( .BOTH. , #3123 ) ;
#33583=ORIENTED_EDGE ( 'NONE', *, *, #40774, .F. ) ;
#33585=CARTESIAN_POINT ( 'NONE',  ( 12.63842701281683034, 22.46726448433411605, 9.846743663894596210 ) ) ;
#33586=DIRECTION ( 'NONE',  ( 0.000000000000000000, 0.000000000000000000, -1.000000000000000000 ) ) ;
#33589=CARTESIAN_POINT ( 'NONE',  ( 0.5774900079438590739, 12.64701867748817321, -5.440088680355550821 ) ) ;
#33590=CARTESIAN_POINT ( 'NONE',  ( 20.88017736071110875, 15.77201867748817143, -2.915334737309920765 ) ) ;
#33591=CARTESIAN_POINT ( 'NONE',  ( 0.1532563361054082862, 56.21726448433411605, 2.638427012816831674 ) ) ;
#33592=CARTESIAN_POINT ( 'NONE',  ( 19.38216949554541557, 7.248634669930421381, -9.382169495545420901 ) ) ;
#33595=CARTESIAN_POINT ( 'NONE',  ( 22.81628187352648496, 21.83196800326374643, -3.434112377981050290 ) ) ;
#33597=CARTESIAN_POINT ( 'NONE',  ( 17.08211943468705840, 60.13708216824729647, -12.26659068614894466 ) ) ;
#33600=CARTESIAN_POINT ( 'NONE',  ( 10.00000000000000178, 53.05374883491396787, 14.16423886937410082 ) ) ;
#33602=CARTESIAN_POINT ( 'NONE',  ( 10.00000000000000000, 31.81368534415483751, -10.88017736071110342 ) ) ;
#33604=CARTESIAN_POINT ( 'NONE',  ( 0.5774900079438590739, 32.64701867748816966, -5.440088680355550821 ) ) ;
#33605=CARTESIAN_POINT ( 'NONE',  ( 2.035157376598822676, 67.43868534415484817, -7.964842623401177768 ) ) ;
#33606=CARTESIAN_POINT ( 'NONE',  ( 17.96484262340118221, 21.18868534415483396, -7.964842623401177768 ) ) ;
#33611=CARTESIAN_POINT ( 'NONE',  ( 17.20831665107776587, 9.133931151000787452, -7.208316651077762316 ) ) ;
#33615=CARTESIAN_POINT ( 'NONE',  ( 19.84674366389459621, 48.50893115100078745, 7.409399052514197653E-17 ) ) ;
#33619=CARTESIAN_POINT ( 'NONE',  ( 14.92337183194729633, 62.67559781766745886, 8.527530157486181039 ) ) ;
#33620=CARTESIAN_POINT ( 'NONE',  ( -0.3689425029237898834, 41.17874883491397497, -10.36894250292378850 ) ) ;
#33624=CARTESIAN_POINT ( 'NONE',  ( 19.84674366389459621, 33.50893115100078745, 7.409399052514197653E-17 ) ) ;
#33626=CARTESIAN_POINT ( 'NONE',  ( 10.00000000000000178, 5.373634669930420493, 12.81628187352647608 ) ) ;
#33627=CARTESIAN_POINT ( 'NONE',  ( 0.5774900079438607392, 68.48035201082150536, 5.440088680355550821 ) ) ;
#33629=CARTESIAN_POINT ( 'NONE',  ( 18.52753015748617571, 58.09226448433411605, 4.923371831947298993 ) ) ;
#33633=B_SPLINE_CURVE_WITH_KNOTS ( 'NONE', 3,
 ( #94657, #32173, #64140, #25207 ),
 .UNSPECIFIED., .F., .F.,
 ( 4, 4 ),
 ( 2.521264072383755851E-16, 0.002392975128318428242 ),
 .UNSPECIFIED. ) ;
#33636=CARTESIAN_POINT ( 'NONE',  ( 22.26659068614895176, 59.72041550158063927, -7.082119434687042414 ) ) ;
#33637=CARTESIAN_POINT ( 'NONE',  ( 2.035157376598824452, 43.68868534415484106, 7.964842623401179544 ) ) ;
#33639=CARTESIAN_POINT ( 'NONE',  ( -2.816281873526473856, 19.33196800326375708, 3.434112377981055619 ) ) ;
#33644=CARTESIAN_POINT ( 'NONE',  ( 0.1077916266722764582, 62.24062864464239908, -6.478736007406002528 ) ) ;
#33645=CARTESIAN_POINT ( 'NONE',  ( 1.472469842513823179, 51.42559781766745886, 4.923371831947296329 ) ) ;
#33646=FILL_AREA_STYLE ('',( #9199 ) ) ;
#33648=CARTESIAN_POINT ( 'NONE',  ( 16.40814093676324603, 2.456968003263753531, -11.09922568453594671 ) ) ;
#33650=CARTESIAN_POINT ( 'NONE',  ( 0.5774900079438607392, 28.48035201082150891, 5.440088680355550821 ) ) ;
#33652=DIRECTION ( 'NONE',  ( 0.000000000000000000, 0.000000000000000000, -1.000000000000000000 ) ) ;
#33653=CARTESIAN_POINT ( 'NONE',  ( 17.08211943468705840, 40.13708216824731068, -12.26659068614894466 ) ) ;
#33654=CARTESIAN_POINT ( 'NONE',  ( 20.36894250292379382, 23.67874883491397142, 10.36894250292379205 ) ) ;
#33655=CARTESIAN_POINT ( 'NONE',  ( 4.559911319644449179, 12.23035201082150714, -9.422509992056141925 ) ) ;
#33656=CARTESIAN_POINT ( 'NONE',  ( 18.52753015748618282, 38.92559781766745175, -4.923371831947291888 ) ) ;
#33657=CARTESIAN_POINT ( 'NONE',  ( 13.43411237798106583, 37.66530133659708923, -12.81628187352647252 ) ) ;
#33658=CARTESIAN_POINT ( 'NONE',  ( 20.88017736071110875, 15.77201867748817143, -2.915334737309920765 ) ) ;
#33659=CARTESIAN_POINT ( 'NONE',  ( 1.472469842513823179, 41.42559781766745886, 4.923371831947296329 ) ) ;
#33660=CARTESIAN_POINT ( 'NONE',  ( 10.00000000000000000, 36.81368534415484106, -10.88017736071110342 ) ) ;
#33661=CARTESIAN_POINT ( 'NONE',  ( -1.099225684535947600, 8.706968003263753531, -6.408140936763238038 ) ) ;
#33662=CARTESIAN_POINT ( 'NONE',  ( 22.26659068614894466, 23.88708216824730357, 7.082119434687054849 ) ) ;
#33663=CARTESIAN_POINT ( 'NONE',  ( 1.472469842513823179, 60.59226448433412315, -4.923371831947296329 ) ) ;
#33665=CARTESIAN_POINT ( 'NONE',  ( 7.361572987183170547, 22.05059781766745530, 9.846743663894590881 ) ) ;
#33666=CARTESIAN_POINT ( 'NONE',  ( 22.81628187352648496, 46.83196800326376064, -3.434112377981050290 ) ) ;
#33667=CARTESIAN_POINT ( 'NONE',  ( 1.472469842513823179, 60.59226448433412315, -4.923371831947296329 ) ) ;
#33669=CARTESIAN_POINT ( 'NONE',  ( 20.15039907845753220, 60.60158574516643881, -6.262539305110077947 ) ) ;
#33671=CARTESIAN_POINT ( 'NONE',  ( -0.3689425029237881626, 67.42874883491396076, 10.36894250292379027 ) ) ;
#33672=CARTESIAN_POINT ( 'NONE',  ( 2.917880565312950480, 10.97041550158063572, -12.26659068614894821 ) ) ;
#33673=CARTESIAN_POINT ( 'NONE',  ( 7.361572987183170547, 2.050597817667451750, 9.846743663894590881 ) ) ;
#33674=CARTESIAN_POINT ( 'NONE',  ( 0.1532563361054083140, 46.00893115100079456, 1.131784320476157264E-15 ) ) ;
#33675=CARTESIAN_POINT ( 'NONE',  ( 12.91533473730992121, 24.52201867748816966, 10.88017736071110164 ) ) ;
#33677=CARTESIAN_POINT ( 'NONE',  ( 0.1532563361054082862, 66.21726448433413736, 2.638427012816831674 ) ) ;
#33679=ORIENTED_EDGE ( 'NONE', *, *, #17005, .F. ) ;
#33684=DIRECTION ( 'NONE',  ( 0.000000000000000000, -1.000000000000000000, -0.000000000000000000 ) ) ;
#33685=CARTESIAN_POINT ( 'NONE',  ( 13.79529636645030344, 8.262082168247300018, 14.16423886937410614 ) ) ;
#33686=CARTESIAN_POINT ( 'NONE',  ( 10.00000000000000000, 45.55374883491397497, -14.16423886937410082 ) ) ;
#33687=CARTESIAN_POINT ( 'NONE',  ( 10.00000000000000000, 59.75893115100078745, -9.846743663894594434 ) ) ;
#33688=CARTESIAN_POINT ( 'NONE',  ( 5.076628168052704559, 40.17559781766745175, -8.527530157486179263 ) ) ;
#33689=CARTESIAN_POINT ( 'NONE',  ( -0.03932841506541377707, 38.12161441960502373, 6.397827110479010315 ) ) ;
#33690=CARTESIAN_POINT ( 'NONE',  ( 19.42250999205614548, 30.98035201082150536, -5.440088680355545492 ) ) ;
#33691=CARTESIAN_POINT ( 'NONE',  ( 17.20831665107776587, 62.88393115100078745, 7.208316651077764980 ) ) ;
#33692=SURFACE_SIDE_STYLE ('',( #64190 ) ) ;
#33693=CARTESIAN_POINT ( 'NONE',  ( 22.26659068614894466, 43.88708216824729647, 7.082119434687054849 ) ) ;
#33694=CARTESIAN_POINT ( 'NONE',  ( 10.00000000000000000, 11.81368534415483751, -10.88017736071110342 ) ) ;
#33697=CARTESIAN_POINT ( 'NONE',  ( -0.8801773607110991993, 62.85535201082150536, -2.915334737309923874 ) ) ;
#33698=CARTESIAN_POINT ( 'NONE',  ( 5.076628168052704559, 30.17559781766745175, -8.527530157486179263 ) ) ;
#33704=CARTESIAN_POINT ( 'NONE',  ( 7.361572987183170547, 22.05059781766745530, 9.846743663894590881 ) ) ;
#33706=CARTESIAN_POINT ( 'NONE',  ( -0.3689425029237881626, 32.42874883491395366, 10.36894250292379027 ) ) ;
#33707=CARTESIAN_POINT ( 'NONE',  ( 19.84674366389459266, 28.71726448433411960, -2.638427012816827677 ) ) ;
#33708=CARTESIAN_POINT ( 'NONE',  ( -0.8801773607110991993, 52.85535201082151247, -2.915334737309923874 ) ) ;
#33711=CARTESIAN_POINT ( 'NONE',  ( 15.44008868035555793, 36.39701867748816966, -9.422509992056140149 ) ) ;
#33712=CARTESIAN_POINT ( 'NONE',  ( 0.1532563361054100626, 50.80059781766745175, -2.638427012816831230 ) ) ;
#33716=CARTESIAN_POINT ( 'NONE',  ( 13.79529636645030344, 3.262082168247301350, 14.16423886937410614 ) ) ;
#33718=CARTESIAN_POINT ( 'NONE',  ( -2.816281873526473856, 34.33196800326376064, 3.434112377981055619 ) ) ;
#33719=CARTESIAN_POINT ( 'NONE',  ( -0.3689425029237898834, 1.178748834913967869, -10.36894250292378850 ) ) ;
#33720=CARTESIAN_POINT ( 'NONE',  ( 10.00000000000000178, 27.25893115100078390, 9.846743663894594434 ) ) ;
#33721=FILL_AREA_STYLE_COLOUR ( '', #27514 ) ;
#33723=CARTESIAN_POINT ( 'NONE',  ( 0.1532563361054083140, 31.00893115100078390, 1.131784320476157264E-15 ) ) ;
#33725=CARTESIAN_POINT ( 'NONE',  ( 12.91533473730993009, 61.60535201082150536, -10.88017736071109987 ) ) ;
#33727=CARTESIAN_POINT ( 'NONE',  ( -0.8801773607110991993, 67.85535201082151957, -2.915334737309923874 ) ) ;
#33728=CARTESIAN_POINT ( 'NONE',  ( 19.39235739573469175, 29.87576471608601381, 6.499999999999992895 ) ) ;
#33730=CARTESIAN_POINT ( 'NONE',  ( 7.361572987183169658, -0.03273551566588185635, -9.846743663894592657 ) ) ;
#33731=CARTESIAN_POINT ( 'NONE',  ( 13.43411237798105340, 10.58196800326375353, 12.81628187352647963 ) ) ;
#33732=CARTESIAN_POINT ( 'NONE',  ( 14.92337183194729633, 42.67559781766745886, 8.527530157486181039 ) ) ;
#33734=CARTESIAN_POINT ( 'NONE',  ( 20.36894250292379738, 4.928748834913967869, -10.36894250292379027 ) ) ;
#33735=CARTESIAN_POINT ( 'NONE',  ( 0.1532563361054100626, 30.80059781766744820, -2.638427012816831230 ) ) ;
#33736=CARTESIAN_POINT ( 'NONE',  ( 10.00000000000000178, 35.37363466993042493, 12.81628187352647608 ) ) ;
#33738=CARTESIAN_POINT ( 'NONE',  ( 7.084665262690076126, 64.10535201082150536, 10.88017736071109987 ) ) ;
#33739=CARTESIAN_POINT ( 'NONE',  ( 10.00000000000000178, 0.3736346699304200492, 12.81628187352647608 ) ) ;
#33742=CARTESIAN_POINT ( 'NONE',  ( 1.472469842513823179, 21.42559781766745175, 4.923371831947296329 ) ) ;
#33743=CARTESIAN_POINT ( 'NONE',  ( -0.8801773607111009756, 28.06368534415484106, 1.068504757029289695E-15 ) ) ;
#33744=CARTESIAN_POINT ( 'NONE',  ( 6.565887622018943937, 28.08196800326375353, -12.81628187352647608 ) ) ;
#33745=CARTESIAN_POINT ( 'NONE',  ( 18.52753015748618282, 23.92559781766745530, -4.923371831947291888 ) ) ;
#33747=VECTOR ( 'NONE', #46844, 1000.000000000000000 ) ;
#33749=CARTESIAN_POINT ( 'NONE',  ( 19.42250999205614548, 30.98035201082150536, -5.440088680355545492 ) ) ;
#33751=CARTESIAN_POINT ( 'NONE',  ( -0.8801773607111009756, 63.06368534415484106, 1.068504757029289695E-15 ) ) ;
#33752=CARTESIAN_POINT ( 'NONE',  ( 7.084665262690076126, 7.022018677488169658, -10.88017736071110164 ) ) ;
#33753=CARTESIAN_POINT ( 'NONE',  ( 7.361572987183169658, 44.96726448433412315, -9.846743663894592657 ) ) ;
#33754=CARTESIAN_POINT ( 'NONE',  ( 20.88017736071110519, 25.56368534415483751, 2.639326808657452039E-16 ) ) ;
#33755=CARTESIAN_POINT ( 'NONE',  ( 17.96484262340118221, 46.18868534415484106, -7.964842623401177768 ) ) ;
#33756=CARTESIAN_POINT ( 'NONE',  ( 20.88017736071110875, 15.77201867748817143, -2.915334737309920765 ) ) ;
#33759=CARTESIAN_POINT ( 'NONE',  ( 14.92337183194729988, 39.34226448433412315, -8.527530157486177487 ) ) ;
#33760=CARTESIAN_POINT ( 'NONE',  ( 6.204703633549690345, 55.76208216824730357, -14.16423886937410259 ) ) ;
#33762=CARTESIAN_POINT ( 'NONE',  ( 10.00000000000000000, 20.55374883491396787, -14.16423886937410082 ) ) ;
#33765=CARTESIAN_POINT ( 'NONE',  ( 22.26659068614894466, 63.88708216824730357, 7.082119434687054849 ) ) ;
#33766=CARTESIAN_POINT ( 'NONE',  ( 2.791683348922240793, 36.63393115100078035, 7.208316651077764092 ) ) ;
#33769=CARTESIAN_POINT ( 'NONE',  ( 2.035157376598824452, 53.68868534415484817, 7.964842623401179544 ) ) ;
#33770=CARTESIAN_POINT ( 'NONE',  ( 6.565887622018943937, 63.08196800326376064, -12.81628187352647608 ) ) ;
#33771=CARTESIAN_POINT ( 'NONE',  ( 4.559911319644449179, 37.23035201082150536, -9.422509992056141925 ) ) ;
#33773=CARTESIAN_POINT ( 'NONE',  ( 21.09922568453594849, 6.206968003263753531, 6.408140936763242479 ) ) ;
#33774=CARTESIAN_POINT ( 'NONE',  ( 1.472469842513823179, 16.42559781766745175, 4.923371831947296329 ) ) ;
#33775=ORIENTED_EDGE ( 'NONE', *, *, #3643, .T. ) ;
#33778=CARTESIAN_POINT ( 'NONE',  ( 12.91533473730993009, 6.605352010821504471, -10.88017736071109987 ) ) ;
#33779=CARTESIAN_POINT ( 'NONE',  ( 17.08211943468705840, 25.13708216824730357, -12.26659068614894466 ) ) ;
#33780=CARTESIAN_POINT ( 'NONE',  ( 7.084665262690076126, 27.02201867748817676, -10.88017736071110164 ) ) ;
#33781=CARTESIAN_POINT ( 'NONE',  ( 10.00000000000000000, 46.81368534415484106, -10.88017736071110342 ) ) ;
#33782=FACE_BOUND ( 'NONE', #74144, .T. ) ;
#33785=CARTESIAN_POINT ( 'NONE',  ( 7.361572987183169658, 14.96726448433411960, -9.846743663894592657 ) ) ;
#33787=CARTESIAN_POINT ( 'NONE',  ( 12.63842701281683922, 14.55059781766744997, -9.846743663894590881 ) ) ;
#33791=CARTESIAN_POINT ( 'NONE',  ( 0.1532563361054083140, 21.00893115100078745, 1.131784320476157264E-15 ) ) ;
#33792=CARTESIAN_POINT ( 'NONE',  ( 19.84674366389459266, 53.71726448433411605, -2.638427012816827677 ) ) ;
#33794=CARTESIAN_POINT ( 'NONE',  ( 3.591859063236761518, 49.95696800326375353, 11.09922568453594849 ) ) ;
#33795=CARTESIAN_POINT ( 'NONE',  ( -0.8801773607111008646, 53.27201867748816966, 2.915334737309923430 ) ) ;
#33796=CARTESIAN_POINT ( 'NONE',  ( 10.00000000000000178, 32.25893115100078745, 9.846743663894594434 ) ) ;
#33797=CARTESIAN_POINT ( 'NONE',  ( -0.3689425029237881626, 47.42874883491396787, 10.36894250292379027 ) ) ;
#33798=CARTESIAN_POINT ( 'NONE',  ( 10.00000000000000000, 24.75893115100078745, -9.846743663894594434 ) ) ;
#33799=CARTESIAN_POINT ( 'NONE',  ( 0.1955144967548765322, 44.32703681773342907, -6.500000000002692957 ) ) ;
#33800=CARTESIAN_POINT ( 'NONE',  ( -42.93999999999999773, 92.00000000000000000, -9.292893218813450318 ) ) ;
#33801=CARTESIAN_POINT ( 'NONE',  ( 10.00000000000000000, 10.55374883491396787, -14.16423886937410082 ) ) ;
#33802=CARTESIAN_POINT ( 'NONE',  ( 13.79529636645031943, 35.34541550158063927, -14.16423886937409904 ) ) ;
#33803=CARTESIAN_POINT ( 'NONE',  ( 7.361572987183169658, 24.96726448433412315, -9.846743663894592657 ) ) ;
#33804=CARTESIAN_POINT ( 'NONE',  ( 18.50749283717776805, 9.699555875704810148, 6.499999999999995559 ) ) ;
#33805=CARTESIAN_POINT ( 'NONE',  ( 0.5774900079438607392, 28.48035201082150891, 5.440088680355550821 ) ) ;
#33807=CARTESIAN_POINT ( 'NONE',  ( 15.44008868035555260, 59.73035201082151247, 9.422509992056143702 ) ) ;
#33808=CARTESIAN_POINT ( 'NONE',  ( 17.96484262340118221, 46.18868534415484106, -7.964842623401177768 ) ) ;
#33810=CARTESIAN_POINT ( 'NONE',  ( 0.6178305044545838731, 49.74863466993041072, 9.382169495545420901 ) ) ;
#33811=CARTESIAN_POINT ( 'NONE',  ( -0.8801773607111009756, 53.06368534415484106, 1.068504757029289695E-15 ) ) ;
#33812=ORIENTED_EDGE ( 'NONE', *, *, #63228, .F. ) ;
#33814=CARTESIAN_POINT ( 'NONE',  ( 2.035157376598822676, 67.43868534415484817, -7.964842623401177768 ) ) ;
#33816=CARTESIAN_POINT ( 'NONE',  ( 19.42250999205614548, 65.98035201082151957, -5.440088680355545492 ) ) ;
#33817=CARTESIAN_POINT ( 'NONE',  ( 19.42250999205614193, 5.147018677488171434, 5.440088680355555262 ) ) ;
#33821=CARTESIAN_POINT ( 'NONE',  ( 12.91533473730993009, 11.60535201082150714, -10.88017736071109987 ) ) ;
#33822=CARTESIAN_POINT ( 'NONE',  ( 19.84674366389459266, 13.30059781766745353, 2.638427012816836559 ) ) ;
#33824=CARTESIAN_POINT ( 'NONE',  ( 10.00000000000000000, 10.55374883491396787, -14.16423886937410082 ) ) ;
#33825=CARTESIAN_POINT ( 'NONE',  ( 12.63842701281683034, 2.467264484334118269, 9.846743663894596210 ) ) ;
#33826=CARTESIAN_POINT ( 'NONE',  ( -0.8801773607111009756, 13.06368534415483929, 1.068504757029289695E-15 ) ) ;
#33827=CARTESIAN_POINT ( 'NONE',  ( 0.1532563361054100626, 50.80059781766745175, -2.638427012816831230 ) ) ;
#33829=CARTESIAN_POINT ( 'NONE',  ( 12.63842701281683034, 47.46726448433412315, 9.846743663894596210 ) ) ;
#33830=ORIENTED_EDGE ( 'NONE', *, *, #52976, .T. ) ;
#33831=CARTESIAN_POINT ( 'NONE',  ( 0.5774900079438607392, 48.48035201082150536, 5.440088680355550821 ) ) ;
#33832=CARTESIAN_POINT ( 'NONE',  ( 7.361572987183169658, 49.96726448433410894, -9.846743663894592657 ) ) ;
#33833=FILL_AREA_STYLE ('',( #3373 ) ) ;
#33835=CARTESIAN_POINT ( 'NONE',  ( -0.8801773607111009756, 63.06368534415484106, 1.068504757029289695E-15 ) ) ;
#33836=CARTESIAN_POINT ( 'NONE',  ( 7.084665262690076126, 4.105352010821503583, 10.88017736071109987 ) ) ;
#33838=MECHANICAL_DESIGN_GEOMETRIC_PRESENTATION_REPRESENTATION('',(#43423),#5257);
#33839=CARTESIAN_POINT ( 'NONE',  ( 3.591859063236761518, 34.95696800326375353, 11.09922568453594849 ) ) ;
#33842=ORIENTED_EDGE ( 'NONE', *, *, #48415, .T. ) ;
#33843=CARTESIAN_POINT ( 'NONE',  ( -1.099225684535947600, 44.54030133659708923, 6.408140936763237150 ) ) ;
#33844=CARTESIAN_POINT ( 'NONE',  ( 4.559911319644449179, 37.23035201082150536, -9.422509992056141925 ) ) ;
#33846=ORIENTED_EDGE ( 'NONE', *, *, #25034, .F. ) ;
#33847=AXIS2_PLACEMENT_3D ( 'NONE', #63480, #39519, #47978 ) ;
#33849=CARTESIAN_POINT ( 'NONE',  ( 0.1532563361054083140, 61.00893115100078745, 1.131784320476157264E-15 ) ) ;
#33850=CARTESIAN_POINT ( 'NONE',  ( 18.52753015748617571, 18.09226448433411960, 4.923371831947298993 ) ) ;
#33851=CARTESIAN_POINT ( 'NONE',  ( 12.63842701281683034, 57.46726448433411605, 9.846743663894596210 ) ) ;
#33852=CARTESIAN_POINT ( 'NONE',  ( 19.72487221294569792, 32.80223176428832232, -6.500000000000008882 ) ) ;
#33856=CARTESIAN_POINT ( 'NONE',  ( 7.361572987183169658, 24.96726448433412315, -9.846743663894592657 ) ) ;
#33859=CARTESIAN_POINT ( 'NONE',  ( 5.076628168052704559, 65.17559781766745175, -8.527530157486179263 ) ) ;
#33860=ORIENTED_EDGE ( 'NONE', *, *, #89863, .F. ) ;
#33864=CARTESIAN_POINT ( 'NONE',  ( 16.40814093676324603, 22.45696800326375353, -11.09922568453594671 ) ) ;
#33866=CARTESIAN_POINT ( 'NONE',  ( 19.84674366389459266, 43.71726448433410894, -2.638427012816827677 ) ) ;
#33868=CARTESIAN_POINT ( 'NONE',  ( 20.36894250292379738, 54.92874883491396076, -10.36894250292379027 ) ) ;
#33869=CARTESIAN_POINT ( 'NONE',  ( 10.00000000000000000, 14.75893115100078568, -9.846743663894594434 ) ) ;
#33871=CARTESIAN_POINT ( 'NONE',  ( 0.2751277870542980231, 5.302231764288316107, 6.500000000000002665 ) ) ;
#33873=CARTESIAN_POINT ( 'NONE',  ( 17.08211943468705130, 63.47041550158063927, 12.26659068614894998 ) ) ;
#33874=CARTESIAN_POINT ( 'NONE',  ( 2.791683348922237240, 60.38393115100078745, -7.208316651077763204 ) ) ;
#33875=CARTESIAN_POINT ( 'NONE',  ( 2.035157376598824452, 8.688685344154839285, 7.964842623401179544 ) ) ;
#33876=CARTESIAN_POINT ( 'NONE',  ( 10.00000000000000178, 43.05374883491397497, 14.16423886937410082 ) ) ;
#33877=CARTESIAN_POINT ( 'NONE',  ( 10.00000000000000000, 45.55374883491397497, -14.16423886937410082 ) ) ;
#33880=CARTESIAN_POINT ( 'NONE',  ( 7.361572987183170547, 52.05059781766745175, 9.846743663894590881 ) ) ;
#33882=CARTESIAN_POINT ( 'NONE',  ( 20.88017736071110519, 40.56368534415484106, 2.639326808657452039E-16 ) ) ;
#33884=CARTESIAN_POINT ( 'NONE',  ( 10.00000000000000178, 52.25893115100078745, 9.846743663894594434 ) ) ;
#33887=CARTESIAN_POINT ( 'NONE',  ( 2.791683348922237240, 60.38393115100078745, -7.208316651077763204 ) ) ;
#33888=CARTESIAN_POINT ( 'NONE',  ( 1.472469842513823179, 60.59226448433412315, -4.923371831947296329 ) ) ;
#33891=CARTESIAN_POINT ( 'NONE',  ( 17.08211943468705840, 30.13708216824730357, -12.26659068614894466 ) ) ;
#33892=CARTESIAN_POINT ( 'NONE',  ( 1.472469842513823179, 1.425597817667451528, 4.923371831947296329 ) ) ;
#33895=CARTESIAN_POINT ( 'NONE',  ( -0.8801773607110991993, 12.85535201082150358, -2.915334737309923874 ) ) ;
#33896=CARTESIAN_POINT ( 'NONE',  ( 10.00000000000000178, 25.37363466993041783, 12.81628187352647608 ) ) ;
#33898=CARTESIAN_POINT ( 'NONE',  ( 10.00000000000000000, 9.758931151000785675, -9.846743663894594434 ) ) ;
#33900=CARTESIAN_POINT ( 'NONE',  ( 2.917880565312950480, 30.97041550158063572, -12.26659068614894821 ) ) ;
#33902=CARTESIAN_POINT ( 'NONE',  ( 19.72487221294571569, 50.71833443783938122, -6.499999999999983125 ) ) ;
#33903=CARTESIAN_POINT ( 'NONE',  ( 17.96484262340118221, 4.938685344154837509, 7.964842623401181321 ) ) ;
#33905=CARTESIAN_POINT ( 'NONE',  ( 19.42250999205614548, 40.98035201082150536, -5.440088680355545492 ) ) ;
#33906=CARTESIAN_POINT ( 'NONE',  ( 17.96484262340118221, 34.93868534415482685, 7.964842623401181321 ) ) ;
#33907=CARTESIAN_POINT ( 'NONE',  ( 5.076628168052703671, 66.84226448433412315, 8.527530157486179263 ) ) ;
#33908=CARTESIAN_POINT ( 'NONE',  ( 0.1532563361054082862, 61.21726448433412315, 2.638427012816831674 ) ) ;
#33909=CARTESIAN_POINT ( 'NONE',  ( 1.274849032793998305, 2.555090184799397424, -6.499999999999581668 ) ) ;
#33910=CARTESIAN_POINT ( 'NONE',  ( 0.1532563361054082862, 6.217264484334118713, 2.638427012816831674 ) ) ;
#33912=CARTESIAN_POINT ( 'NONE',  ( -0.8801773607110991993, 47.85535201082150536, -2.915334737309923874 ) ) ;
#33915=CARTESIAN_POINT ( 'NONE',  ( 22.81628187352647785, 11.41530133659708390, 3.434112377981063169 ) ) ;
#33916=CARTESIAN_POINT ( 'NONE',  ( 17.96484262340118221, 56.18868534415484817, -7.964842623401177768 ) ) ;
#33917=CARTESIAN_POINT ( 'NONE',  ( 17.20831665107776587, 27.88393115100078390, 7.208316651077764980 ) ) ;
#33918=CARTESIAN_POINT ( 'NONE',  ( -2.816281873526471635, 38.91530133659708213, -3.434112377981056508 ) ) ;
#33919=AXIS2_PLACEMENT_3D ( 'NONE', #26252, #42250, #81221 ) ;
#33920=CARTESIAN_POINT ( 'NONE',  ( 19.84674366389459266, 8.717264484334116048, -2.638427012816827677 ) ) ;
#33924=CARTESIAN_POINT ( 'NONE',  ( 1.711636803080560432, 56.84492782695772917, -6.500000000000039080 ) ) ;
#33925=CARTESIAN_POINT ( 'NONE',  ( 2.377183314879977249, 15.78593319516823001, -6.500000000000010658 ) ) ;
#33926=DIRECTION ( 'NONE',  ( 0.000000000000000000, 0.000000000000000000, 1.000000000000000000 ) ) ;
#33927=CARTESIAN_POINT ( 'NONE',  ( 18.52753015748617571, 18.09226448433411960, 4.923371831947298993 ) ) ;
#33929=CARTESIAN_POINT ( 'NONE',  ( 12.91533473730993009, 11.60535201082150536, -10.88017736071109987 ) ) ;
#33930=CARTESIAN_POINT ( 'NONE',  ( 4.559911319644449179, 8.897018677488173211, 9.422509992056141925 ) ) ;
#33933=CARTESIAN_POINT ( 'NONE',  ( 7.084665262690076126, 19.10535201082150181, 10.88017736071109987 ) ) ;
#33934=CARTESIAN_POINT ( 'NONE',  ( 20.88017736071110519, 20.56368534415484106, 2.639326808657452039E-16 ) ) ;
#33936=COLOUR_RGB ( '', 0.08235294, 0.09019608, 0.10196078) ;
#33937=VERTEX_POINT ( 'NONE', #53094 ) ;
#33938=CARTESIAN_POINT ( 'NONE',  ( 18.52753015748618282, 63.92559781766745886, -4.923371831947291888 ) ) ;
#33939=CARTESIAN_POINT ( 'NONE',  ( 17.96484262340118221, 19.93868534415484106, 7.964842623401181321 ) ) ;
#33940=CARTESIAN_POINT ( 'NONE',  ( 14.92337183194729633, 62.67559781766745886, 8.527530157486181039 ) ) ;
#33941=CARTESIAN_POINT ( 'NONE',  ( 20.15039907845753220, 49.72266099184918176, 6.262539305110078836 ) ) ;
#33942=CARTESIAN_POINT ( 'NONE',  ( 0.6178305044545838731, 49.74863466993041072, 9.382169495545420901 ) ) ;
#33944=CARTESIAN_POINT ( 'NONE',  ( 10.00000000000000178, 33.05374883491396787, 14.16423886937410082 ) ) ;
#33945=CARTESIAN_POINT ( 'NONE',  ( 17.96484262340118221, 39.93868534415484106, 7.964842623401181321 ) ) ;
#33946=CARTESIAN_POINT ( 'NONE',  ( 17.96484262340118221, 19.93868534415484106, 7.964842623401181321 ) ) ;
#33947=CARTESIAN_POINT ( 'NONE',  ( 5.076628168052704559, 50.17559781766745886, -8.527530157486179263 ) ) ;
#33949=CARTESIAN_POINT ( 'NONE',  ( 14.92337183194729633, 37.67559781766745175, 8.527530157486181039 ) ) ;
#33952=CARTESIAN_POINT ( 'NONE',  ( 10.00000000000000000, 14.75893115100078568, -9.846743663894594434 ) ) ;
#33954=ORIENTED_EDGE ( 'NONE', *, *, #19291, .T. ) ;
#33955=CARTESIAN_POINT ( 'NONE',  ( 0.5774900079438607392, 13.48035201082150358, 5.440088680355550821 ) ) ;
#33956=CARTESIAN_POINT ( 'NONE',  ( 0.1532563361054082862, 11.21726448433411605, 2.638427012816831674 ) ) ;
#33957=CARTESIAN_POINT ( 'NONE',  ( -1.099225684535947600, 3.706968003263753531, -6.408140936763238038 ) ) ;
#33958=CARTESIAN_POINT ( 'NONE',  ( 20.88017736071110875, 50.77201867748817676, -2.915334737309920765 ) ) ;
#33959=CARTESIAN_POINT ( 'NONE',  ( 19.42250999205614548, 25.98035201082150891, -5.440088680355545492 ) ) ;
#33960=CARTESIAN_POINT ( 'NONE',  ( 3.591859063236763294, 38.29030133659708923, -11.09922568453595026 ) ) ;
#33961=CARTESIAN_POINT ( 'NONE',  ( 24.16423886937410614, 34.51208216824731068, -3.795296366450302550 ) ) ;
#33963=AXIS2_PLACEMENT_3D ( 'NONE', #67207, #8189, #16180 ) ;
#33964=EDGE_CURVE ( 'NONE', #71557, #37014, #91152, .T. ) ;
#33965=CARTESIAN_POINT ( 'NONE',  ( 19.38216949554541202, 60.99863466993042493, 9.382169495545424454 ) ) ;
#33968=CARTESIAN_POINT ( 'NONE',  ( 7.361572987183170547, 57.05059781766744464, 9.846743663894590881 ) ) ;
#33969=CARTESIAN_POINT ( 'NONE',  ( 17.96484262340118221, 34.93868534415482685, 7.964842623401181321 ) ) ;
#33971=CARTESIAN_POINT ( 'NONE',  ( 1.472469842513823179, 5.592264484334118713, -4.923371831947296329 ) ) ;
#33973=CARTESIAN_POINT ( 'NONE',  ( 12.63842701281683034, 12.46726448433411782, 9.846743663894596210 ) ) ;
#33974=CARTESIAN_POINT ( 'NONE',  ( 17.20831665107776587, 24.13393115100078035, -7.208316651077762316 ) ) ;
#33975=CARTESIAN_POINT ( 'NONE',  ( 10.00000000000000000, 4.758931151000784787, -9.846743663894594434 ) ) ;
#33976=CARTESIAN_POINT ( 'NONE',  ( 1.472469842513823179, 6.425597817667451750, 4.923371831947296329 ) ) ;
#33977=CARTESIAN_POINT ( 'NONE',  ( 15.44008868035555793, 61.39701867748817676, -9.422509992056140149 ) ) ;
#33979=CARTESIAN_POINT ( 'NONE',  ( 12.91533473730993009, 56.60535201082151247, -10.88017736071109987 ) ) ;
#33980=CARTESIAN_POINT ( 'NONE',  ( 7.361572987183169658, 14.96726448433411960, -9.846743663894592657 ) ) ;
#33982=ORIENTED_EDGE ( 'NONE', *, *, #510, .F. ) ;
#33984=CARTESIAN_POINT ( 'NONE',  ( 10.00000000000000178, 52.25893115100078745, 9.846743663894594434 ) ) ;
#33986=VERTEX_POINT ( 'NONE', #28382 ) ;
#33988=TOROIDAL_SURFACE ( 'NONE', #59562, 18.53834841531100608, 7.000000000000000000 ) ;
#33989=CARTESIAN_POINT ( 'NONE',  ( 10.00000000000000178, 8.053748834913967869, 14.16423886937410082 ) ) ;
#33995=CARTESIAN_POINT ( 'NONE',  ( 20.36894250292379382, 23.67874883491397142, 10.36894250292379205 ) ) ;
#33996=CARTESIAN_POINT ( 'NONE',  ( 24.16423886937410614, 29.30374883491396787, 8.672049930838204340E-16 ) ) ;
#33997=CARTESIAN_POINT ( 'NONE',  ( 6.204703633549690345, 2.845415501580634388, 14.16423886937410082 ) ) ;
#33999=CARTESIAN_POINT ( 'NONE',  ( 15.44008868035555260, 34.73035201082151247, 9.422509992056143702 ) ) ;
#34000=FILL_AREA_STYLE ('',( #3054 ) ) ;
#34002=CARTESIAN_POINT ( 'NONE',  ( 5.076628168052703671, 21.84226448433411960, 8.527530157486179263 ) ) ;
#34004=CARTESIAN_POINT ( 'NONE',  ( 20.88017736071110164, 55.35535201082149825, 2.915334737309930979 ) ) ;
#34005=CARTESIAN_POINT ( 'NONE',  ( 10.00000000000000000, 9.758931151000785675, -9.846743663894594434 ) ) ;
#34006=ORIENTED_EDGE ( 'NONE', *, *, #84469, .F. ) ;
#34007=CARTESIAN_POINT ( 'NONE',  ( 6.565887622018943937, 40.16530133659708923, 12.81628187352647430 ) ) ;
#34008=CARTESIAN_POINT ( 'NONE',  ( 0.1532563361054083140, 31.00893115100078390, 1.131784320476157264E-15 ) ) ;
#34009=DIRECTION ( 'NONE',  ( 0.000000000000000000, -1.000000000000000000, 0.000000000000000000 ) ) ;
#34010=CARTESIAN_POINT ( 'NONE',  ( 7.084665262690076126, 57.02201867748817676, -10.88017736071110164 ) ) ;
#34011=CARTESIAN_POINT ( 'NONE',  ( 3.591859063236763294, 28.29030133659708568, -11.09922568453595026 ) ) ;
#34013=CARTESIAN_POINT ( 'NONE',  ( 19.84674366389459266, 28.30059781766745886, 2.638427012816836559 ) ) ;
#34014=CARTESIAN_POINT ( 'NONE',  ( 24.16423886937410614, 14.51208216824730179, -3.795296366450302550 ) ) ;
#34016=CARTESIAN_POINT ( 'NONE',  ( 12.91533473730992121, 39.52201867748817676, 10.88017736071110164 ) ) ;
#34017=CARTESIAN_POINT ( 'NONE',  ( 0.5774900079438590739, 52.64701867748817676, -5.440088680355550821 ) ) ;
#34018=CARTESIAN_POINT ( 'NONE',  ( -4.164238869374098151, 46.59541550158063927, -3.795296366450310543 ) ) ;
#34019=CARTESIAN_POINT ( 'NONE',  ( 10.00000000000000178, 57.25893115100078745, 9.846743663894594434 ) ) ;
#34020=CARTESIAN_POINT ( 'NONE',  ( 19.84674366389459266, 8.717264484334116048, -2.638427012816827677 ) ) ;
#34023=CARTESIAN_POINT ( 'NONE',  ( 2.035157376598824452, 43.68868534415484106, 7.964842623401179544 ) ) ;
#34025=CARTESIAN_POINT ( 'NONE',  ( 19.38216949554541202, 20.99863466993042138, 9.382169495545424454 ) ) ;
#34026=CARTESIAN_POINT ( 'NONE',  ( 22.81628187352648496, 21.83196800326374643, -3.434112377981050290 ) ) ;
#34027=CARTESIAN_POINT ( 'NONE',  ( 14.92337183194729633, 47.67559781766745175, 8.527530157486181039 ) ) ;
#34029=CARTESIAN_POINT ( 'NONE',  ( 0.5774900079438607392, 3.480352010821504027, 5.440088680355550821 ) ) ;
#34030=CARTESIAN_POINT ( 'NONE',  ( 19.42250999205614193, 65.14701867748817676, 5.440088680355555262 ) ) ;
#34033=CARTESIAN_POINT ( 'NONE',  ( 7.084665262690076126, 64.10535201082150536, 10.88017736071109987 ) ) ;
#34035=CARTESIAN_POINT ( 'NONE',  ( 19.42250999205614548, 65.98035201082151957, -5.440088680355545492 ) ) ;
#34037=CARTESIAN_POINT ( 'NONE',  ( 0.1532563361054083140, 26.00893115100078745, 1.131784320476157264E-15 ) ) ;
#34038=CARTESIAN_POINT ( 'NONE',  ( 4.559911319644449179, 23.89701867748817321, 9.422509992056141925 ) ) ;
#34039=CARTESIAN_POINT ( 'NONE',  ( 19.84674366389459621, 63.50893115100078745, 7.409399052514197653E-17 ) ) ;
#34040=CARTESIAN_POINT ( 'NONE',  ( 19.42250999205614548, 30.98035201082150536, -5.440088680355545492 ) ) ;
#34041=DIRECTION ( 'NONE',  ( 0.000000000000000000, -1.000000000000000000, 0.000000000000000000 ) ) ;
#34043=CARTESIAN_POINT ( 'NONE',  ( 0.6178305044545838731, 44.74863466993042493, 9.382169495545420901 ) ) ;
#34044=ORIENTED_EDGE ( 'NONE', *, *, #27761, .F. ) ;
#34045=CARTESIAN_POINT ( 'NONE',  ( 17.96484262340118221, 51.18868534415483396, -7.964842623401177768 ) ) ;
#34046=CARTESIAN_POINT ( 'NONE',  ( 22.81628187352647785, 16.41530133659708923, 3.434112377981063169 ) ) ;
#34047=SURFACE_STYLE_USAGE ( .BOTH. , #3589 ) ;
#34048=CARTESIAN_POINT ( 'NONE',  ( -0.8801773607110991993, 22.85535201082150181, -2.915334737309923874 ) ) ;
#34049=CARTESIAN_POINT ( 'NONE',  ( -4.164238869374099039, 46.80374883491397497, 8.674139862899312516E-16 ) ) ;
#34050=CARTESIAN_POINT ( 'NONE',  ( 19.84674366389459266, 43.71726448433410894, -2.638427012816827677 ) ) ;
#34051=CARTESIAN_POINT ( 'NONE',  ( 2.791683348922237240, 0.3839311510007847872, -7.208316651077763204 ) ) ;
#34052=CARTESIAN_POINT ( 'NONE',  ( 10.00000000000000178, 69.31368534415484817, 10.88017736071110342 ) ) ;
#34054=CARTESIAN_POINT ( 'NONE',  ( -4.164238869374099039, 31.80374883491396432, 8.674139862899312516E-16 ) ) ;
#34060=CARTESIAN_POINT ( 'NONE',  ( 17.08211943468705130, 53.47041550158063217, 12.26659068614894998 ) ) ;
#34061=CARTESIAN_POINT ( 'NONE',  ( -2.266590686148945544, 52.22041550158064638, 7.082119434687048631 ) ) ;
#34062=CARTESIAN_POINT ( 'NONE',  ( 5.076628168052704559, 20.17559781766745175, -8.527530157486179263 ) ) ;
#34063=CARTESIAN_POINT ( 'NONE',  ( 19.38216949554541557, 12.24863466993041961, -9.382169495545420901 ) ) ;
#34066=CARTESIAN_POINT ( 'NONE',  ( 0.6081133539230537677, 58.33703382326400799, 6.499999999999968914 ) ) ;
#34067=( NAMED_UNIT ( * ) PLANE_ANGLE_UNIT ( ) SI_UNIT ( $, .RADIAN. ) );
#34068=CARTESIAN_POINT ( 'NONE',  ( 3.591859063236763294, 33.29030133659708213, -11.09922568453595026 ) ) ;
#34069=CARTESIAN_POINT ( 'NONE',  ( 2.917880565312948704, 37.63708216824731068, 12.26659068614894643 ) ) ;
#34072=CARTESIAN_POINT ( 'NONE',  ( -0.8801773607110991993, 67.85535201082151957, -2.915334737309923874 ) ) ;
#34077=CARTESIAN_POINT ( 'NONE',  ( 0.1532563361054082862, 16.21726448433411960, 2.638427012816831674 ) ) ;
#34081=VERTEX_POINT ( 'NONE', #5401 ) ;
#34082=CARTESIAN_POINT ( 'NONE',  ( 10.00000000000000000, 10.55374883491396787, -14.16423886937410082 ) ) ;
#34083=CARTESIAN_POINT ( 'NONE',  ( -0.8801773607110991993, 2.855352010821504471, -2.915334737309923874 ) ) ;
#34084=CARTESIAN_POINT ( 'NONE',  ( -0.8801773607110991993, 12.85535201082150358, -2.915334737309923874 ) ) ;
#34085=CARTESIAN_POINT ( 'NONE',  ( 12.63842701281683034, 52.46726448433413026, 9.846743663894596210 ) ) ;
#34086=CARTESIAN_POINT ( 'NONE',  ( 22.81628187352647785, 6.415301336597088344, 3.434112377981063169 ) ) ;
#34090=CARTESIAN_POINT ( 'NONE',  ( 21.09922568453594849, 21.20696800326375353, 6.408140936763242479 ) ) ;
#34091=ADVANCED_FACE ( 'NONE', ( #12877 ), #71067, .T. ) ;
#34093=CARTESIAN_POINT ( 'NONE',  ( 6.204703633549690345, 60.76208216824730357, -14.16423886937410259 ) ) ;
#34094=EDGE_LOOP ( 'NONE', ( #58155, #18633, #93929, #64555 ) ) ;
#34095=CARTESIAN_POINT ( 'NONE',  ( -0.3689425029237898834, 61.17874883491396076, -10.36894250292378850 ) ) ;
#34096=ORIENTED_EDGE ( 'NONE', *, *, #5720, .T. ) ;
#34097=CARTESIAN_POINT ( 'NONE',  ( 17.96484262340118221, 29.93868534415484106, 7.964842623401181321 ) ) ;
#34098=CARTESIAN_POINT ( 'NONE',  ( 2.035157376598822676, 47.43868534415484817, -7.964842623401177768 ) ) ;
#34099=CARTESIAN_POINT ( 'NONE',  ( -0.8801773607111008646, 33.27201867748817676, 2.915334737309923430 ) ) ;
#34101=CARTESIAN_POINT ( 'NONE',  ( 19.42250999205614548, 35.98035201082151247, -5.440088680355545492 ) ) ;
#34103=CARTESIAN_POINT ( 'NONE',  ( 14.92337183194729988, 14.34226448433411782, -8.527530157486177487 ) ) ;
#34106=CARTESIAN_POINT ( 'NONE',  ( 0.1532563361054082862, 51.21726448433412315, 2.638427012816831674 ) ) ;
#34108=CARTESIAN_POINT ( 'NONE',  ( 22.81628187352647785, 51.41530133659708923, 3.434112377981063169 ) ) ;
#34111=ORIENTED_EDGE ( 'NONE', *, *, #4795, .F. ) ;
#34112=CARTESIAN_POINT ( 'NONE',  ( 0.2751277870542967463, 70.00000000000000000, -6.500000000000000888 ) ) ;
#34113=CARTESIAN_POINT ( 'NONE',  ( -43.85366042784433205, 106.6334074295720313, 4.577838255903318831 ) ) ;
#34115=CARTESIAN_POINT ( 'NONE',  ( -4.164238869374099039, 61.80374883491397497, 8.674139862899312516E-16 ) ) ;
#34119=CARTESIAN_POINT ( 'NONE',  ( 19.84674366389459621, 38.50893115100078745, 7.409399052514197653E-17 ) ) ;
#34120=CARTESIAN_POINT ( 'NONE',  ( 3.591859063236761518, 64.95696800326376774, 11.09922568453594849 ) ) ;
#34121=CARTESIAN_POINT ( 'NONE',  ( 16.40814093676323893, 10.79030133659708923, 11.09922568453595026 ) ) ;
#34122=CARTESIAN_POINT ( 'NONE',  ( 12.63842701281683034, 2.467264484334118269, 9.846743663894596210 ) ) ;
#34123=CARTESIAN_POINT ( 'NONE',  ( 17.20831665107776587, 12.88393115100078390, 7.208316651077764980 ) ) ;
#34124=CARTESIAN_POINT ( 'NONE',  ( 2.791683348922240793, 56.63393115100078035, 7.208316651077764092 ) ) ;
#34126=MECHANICAL_DESIGN_GEOMETRIC_PRESENTATION_REPRESENTATION('',(#56498),#40522);
#34128=CARTESIAN_POINT ( 'NONE',  ( -0.8801773607110991993, 2.855352010821504471, -2.915334737309923874 ) ) ;
#34130=CARTESIAN_POINT ( 'NONE',  ( 20.88017736071110875, 40.77201867748818387, -2.915334737309920765 ) ) ;
#34131=CARTESIAN_POINT ( 'NONE',  ( 21.09922568453594849, 26.20696800326375353, 6.408140936763242479 ) ) ;
#34132=CARTESIAN_POINT ( 'NONE',  ( 20.88017736071110164, 65.35535201082150536, 2.915334737309930979 ) ) ;
#34134=CARTESIAN_POINT ( 'NONE',  ( 19.80427997160309417, 17.75733960839544778, -6.499999999999988454 ) ) ;
#34135=CARTESIAN_POINT ( 'NONE',  ( 20.15039907845753930, 0.07447313448805115144, -6.262539305110068177 ) ) ;
#34136=CARTESIAN_POINT ( 'NONE',  ( 0.1532563361054082862, 51.21726448433412315, 2.638427012816831674 ) ) ;
#34137=CARTESIAN_POINT ( 'NONE',  ( 1.472469842513823179, 20.59226448433411960, -4.923371831947296329 ) ) ;
#34139=CARTESIAN_POINT ( 'NONE',  ( 10.00000000000000000, 17.87363466993041783, -12.81628187352647608 ) ) ;
#34141=CARTESIAN_POINT ( 'NONE',  ( 4.559911319644449179, 28.89701867748817321, 9.422509992056141925 ) ) ;
#34144=CARTESIAN_POINT ( 'NONE',  ( 22.26659068614894466, 53.88708216824731068, 7.082119434687054849 ) ) ;
#34145=CARTESIAN_POINT ( 'NONE',  ( -0.3689425029237898834, 26.17874883491396432, -10.36894250292378850 ) ) ;
#34146=CARTESIAN_POINT ( 'NONE',  ( 10.00000000000000178, 37.25893115100078745, 9.846743663894594434 ) ) ;
#34147=CARTESIAN_POINT ( 'NONE',  ( 0.6178305044545818747, 33.49863466993042493, -9.382169495545419124 ) ) ;
#34148=CARTESIAN_POINT ( 'NONE',  ( 10.00000000000000178, 29.31368534415483751, 10.88017736071110342 ) ) ;
#34149=CARTESIAN_POINT ( 'NONE',  ( 0.1532563361054083140, 56.00893115100078745, 1.131784320476157264E-15 ) ) ;
#34150=CARTESIAN_POINT ( 'NONE',  ( 10.00000000000000178, 39.31368534415484106, 10.88017736071110342 ) ) ;
#34151=CARTESIAN_POINT ( 'NONE',  ( 22.81628187352647785, 6.415301336597088344, 3.434112377981063169 ) ) ;
#34152=CARTESIAN_POINT ( 'NONE',  ( -0.3689425029237881626, 27.42874883491397142, 10.36894250292379027 ) ) ;
#34155=( BOUNDED_CURVE ( )  B_SPLINE_CURVE ( 2, ( #67168, #68652, #14177, #67675, #75655, #89669, #36680, #59661, #13674 ),
 .UNSPECIFIED., .F., .T. ) 
 B_SPLINE_CURVE_WITH_KNOTS ( ( 3, 2, 2, 2, 3 ),
 ( 0.7596570216176964374, 0.7619047619047618625, 0.7678571428571429047, 0.7738095238095238360, 0.7760572640965892610 ),
 .UNSPECIFIED. ) 
 CURVE ( )  GEOMETRIC_REPRESENTATION_ITEM ( )  RATIONAL_B_SPLINE_CURVE ( ( 0.9839835555609424134, 0.9871328979762474809, 1.000000000000000000, 0.9659258262890683122, 1.000000000000000000, 0.9659258262890683122, 1.000000000000000000, 0.9871328979762474809, 0.9839835555609424134 ) ) 
 REPRESENTATION_ITEM ( '' )  );
#34156=CARTESIAN_POINT ( 'NONE',  ( 7.361572987183170547, 27.05059781766745175, 9.846743663894590881 ) ) ;
#34157=CARTESIAN_POINT ( 'NONE',  ( 0.6178305044545818747, 48.49863466993042493, -9.382169495545419124 ) ) ;
#34158=CARTESIAN_POINT ( 'NONE',  ( 6.565887622018943937, 0.1653013365970866511, 12.81628187352647430 ) ) ;
#34162=CARTESIAN_POINT ( 'NONE',  ( 6.204703633549690345, 62.84541550158063927, 14.16423886937410082 ) ) ;
#34163=CARTESIAN_POINT ( 'NONE',  ( 2.035157376598822676, 62.43868534415483396, -7.964842623401177768 ) ) ;
#34164=CARTESIAN_POINT ( 'NONE',  ( 6.204703633549690345, 17.84541550158063217, 14.16423886937410082 ) ) ;
#34166=CARTESIAN_POINT ( 'NONE',  ( 12.63842701281683034, 2.467264484334118269, 9.846743663894596210 ) ) ;
#34167=CARTESIAN_POINT ( 'NONE',  ( 5.076628168052704559, 50.17559781766745886, -8.527530157486179263 ) ) ;
#34168=CARTESIAN_POINT ( 'NONE',  ( 15.44008868035555260, 34.73035201082151247, 9.422509992056143702 ) ) ;
#34170=CARTESIAN_POINT ( 'NONE',  ( 5.076628168052704559, 65.17559781766745175, -8.527530157486179263 ) ) ;
#34177=CARTESIAN_POINT ( 'NONE',  ( 22.26659068614894466, 8.887082168247300018, 7.082119434687054849 ) ) ;
#34178=CARTESIAN_POINT ( 'NONE',  ( -2.266590686148945544, 7.220415501580634832, 7.082119434687048631 ) ) ;
#34179=CARTESIAN_POINT ( 'NONE',  ( 22.26659068614894466, 58.88708216824729647, 7.082119434687054849 ) ) ;
#34180=CARTESIAN_POINT ( 'NONE',  ( 0.1532563361054100626, 55.80059781766745175, -2.638427012816831230 ) ) ;
#34181=CARTESIAN_POINT ( 'NONE',  ( 19.84674366389459266, 38.30059781766745175, 2.638427012816836559 ) ) ;
#34182=CARTESIAN_POINT ( 'NONE',  ( -0.1503990784575328643, 0.1277717457861260453, 6.262539305110068177 ) ) ;
#34183=CARTESIAN_POINT ( 'NONE',  ( 7.084665262690076126, 29.10535201082150181, 10.88017736071109987 ) ) ;
#34184=CARTESIAN_POINT ( 'NONE',  ( 2.791683348922240793, 66.63393115100079456, 7.208316651077764092 ) ) ;
#34185=CARTESIAN_POINT ( 'NONE',  ( -0.3689425029237881626, 7.428748834913967869, 10.36894250292379027 ) ) ;
#34186=CARTESIAN_POINT ( 'NONE',  ( -0.3689425029237881626, 57.42874883491397497, 10.36894250292379027 ) ) ;
#34187=CARTESIAN_POINT ( 'NONE',  ( 7.084665262690076126, 7.022018677488170546, -10.88017736071110164 ) ) ;
#34188=CARTESIAN_POINT ( 'NONE',  ( -0.3289641300567998083, 68.07879003517447813, 5.963430220938281678 ) ) ;
#34190=CARTESIAN_POINT ( 'NONE',  ( 19.42250999205614548, 65.98035201082151957, -5.440088680355545492 ) ) ;
#34191=CARTESIAN_POINT ( 'NONE',  ( 17.20831665107776587, 29.13393115100078390, -7.208316651077762316 ) ) ;
#34194=CARTESIAN_POINT ( 'NONE',  ( 15.00000000000000000, 0.000000000000000000, -6.000000000000000000 ) ) ;
#34195=EDGE_LOOP ( 'NONE', ( #81072, #90169, #49004, #32955, #23681, #20579 ) ) ;
#34196=CARTESIAN_POINT ( 'NONE',  ( 2.791683348922240793, 26.63393115100078745, 7.208316651077764092 ) ) ;
#34198=CARTESIAN_POINT ( 'NONE',  ( 17.08211943468705130, 28.47041550158063572, 12.26659068614894998 ) ) ;
#34199=CARTESIAN_POINT ( 'NONE',  ( 12.63842701281683034, 37.46726448433411605, 9.846743663894596210 ) ) ;
#34200=CARTESIAN_POINT ( 'NONE',  ( 19.42250999205614193, 55.14701867748817676, 5.440088680355555262 ) ) ;
#34201=PRESENTATION_STYLE_ASSIGNMENT (( #33228 ) ) ;
#34202=CARTESIAN_POINT ( 'NONE',  ( 2.035157376598824452, 58.68868534415482685, 7.964842623401179544 ) ) ;
#34204=CARTESIAN_POINT ( 'NONE',  ( 5.076628168052704559, 40.17559781766745175, -8.527530157486179263 ) ) ;
#34206=CARTESIAN_POINT ( 'NONE',  ( 22.81628187352647785, 61.41530133659709634, 3.434112377981063169 ) ) ;
#34210=CARTESIAN_POINT ( 'NONE',  ( -4.164238869374098151, 26.59541550158063217, -3.795296366450310543 ) ) ;
#34211=VERTEX_POINT ( 'NONE', #73875 ) ;
#34212=CARTESIAN_POINT ( 'NONE',  ( 21.09922568453595559, 32.04030133659708923, -6.408140936763230044 ) ) ;
#34213=CARTESIAN_POINT ( 'NONE',  ( 10.00000000000000000, 24.75893115100078745, -9.846743663894594434 ) ) ;
#34214=CARTESIAN_POINT ( 'NONE',  ( 17.96484262340118221, 4.938685344154837509, 7.964842623401181321 ) ) ;
#34215=CARTESIAN_POINT ( 'NONE',  ( 17.20831665107776587, 29.13393115100078390, -7.208316651077762316 ) ) ;
#34217=CARTESIAN_POINT ( 'NONE',  ( -0.8801773607111008646, 68.27201867748817676, 2.915334737309923430 ) ) ;
#34218=CARTESIAN_POINT ( 'NONE',  ( -45.94000000000001194, 103.9981609152045507, 5.961202730336935041 ) ) ;
#34219=EDGE_CURVE ( 'NONE', #86126, #14329, #58873, .T. ) ;
#34220=CARTESIAN_POINT ( 'NONE',  ( 1.707155281725210916, 2.901890803972826394, 6.499999999999999112 ) ) ;
#34221=CARTESIAN_POINT ( 'NONE',  ( 19.84674366389459266, 3.717264484334118713, -2.638427012816827677 ) ) ;
#34222=CARTESIAN_POINT ( 'NONE',  ( 22.81628187352647785, 26.41530133659708923, 3.434112377981063169 ) ) ;
#34224=CARTESIAN_POINT ( 'NONE',  ( 1.472469842513823179, 40.59226448433411605, -4.923371831947296329 ) ) ;
#34225=CARTESIAN_POINT ( 'NONE',  ( -2.816281873526471635, 63.91530133659708923, -3.434112377981056508 ) ) ;
#34226=CARTESIAN_POINT ( 'NONE',  ( 17.08211943468705130, 23.47041550158063572, 12.26659068614894998 ) ) ;
#34227=CARTESIAN_POINT ( 'NONE',  ( 18.52753015748618282, 33.92559781766745886, -4.923371831947291888 ) ) ;
#34228=CARTESIAN_POINT ( 'NONE',  ( 22.81628187352647785, 31.62363466993042138, 6.195893100308588602E-16 ) ) ;
#34230=CYLINDRICAL_SURFACE ( 'NONE', #59267, 0.5000000000000004441 ) ;
#34231=CARTESIAN_POINT ( 'NONE',  ( 10.00000000000000000, 56.81368534415484106, -10.88017736071110342 ) ) ;
#34232=CARTESIAN_POINT ( 'NONE',  ( -2.816281873526471635, 8.915301336597083903, -3.434112377981056508 ) ) ;
#34235=CARTESIAN_POINT ( 'NONE',  ( 7.361572987183169658, 29.96726448433411960, -9.846743663894592657 ) ) ;
#34236=CARTESIAN_POINT ( 'NONE',  ( -0.8801773607111008646, 23.27201867748817676, 2.915334737309923430 ) ) ;
#34237=CARTESIAN_POINT ( 'NONE',  ( 3.591859063236761518, 24.95696800326375353, 11.09922568453594849 ) ) ;
#34238=CARTESIAN_POINT ( 'NONE',  ( 14.92337183194729633, 17.67559781766745175, 8.527530157486181039 ) ) ;
#34241=CARTESIAN_POINT ( 'NONE',  ( 12.91533473730992121, 34.52201867748817676, 10.88017736071110164 ) ) ;
#34242=CARTESIAN_POINT ( 'NONE',  ( 19.42250999205614548, 65.98035201082151957, -5.440088680355545492 ) ) ;
#34243=CARTESIAN_POINT ( 'NONE',  ( 4.559911319644449179, 7.230352010821504471, -9.422509992056141925 ) ) ;
#34244=CARTESIAN_POINT ( 'NONE',  ( 7.361572987183170547, 42.05059781766745886, 9.846743663894590881 ) ) ;
#34245=CARTESIAN_POINT ( 'NONE',  ( 0.5774900079438590739, 32.64701867748816966, -5.440088680355550821 ) ) ;
#34247=CARTESIAN_POINT ( 'NONE',  ( 19.42250999205614193, 50.14701867748817676, 5.440088680355555262 ) ) ;
#34248=CARTESIAN_POINT ( 'NONE',  ( 2.035157376598822676, 12.43868534415483751, -7.964842623401177768 ) ) ;
#34249=CARTESIAN_POINT ( 'NONE',  ( -0.000000000000000000, 74.64896322088237923, -5.938123570160299458 ) ) ;
#34250=CARTESIAN_POINT ( 'NONE',  ( 14.92337183194729988, 4.342264484334117824, -8.527530157486177487 ) ) ;
#34251=CARTESIAN_POINT ( 'NONE',  ( 5.076628168052704559, 50.17559781766745886, -8.527530157486179263 ) ) ;
#34252=CARTESIAN_POINT ( 'NONE',  ( 13.79529636645030344, 48.26208216824728936, 14.16423886937410614 ) ) ;
#34255=PRESENTATION_STYLE_ASSIGNMENT (( #63289 ) ) ;
#34256=CARTESIAN_POINT ( 'NONE',  ( 24.16423886937410614, 34.30374883491396787, 8.672049930838204340E-16 ) ) ;
#34258=ORIENTED_EDGE ( 'NONE', *, *, #3234, .T. ) ;
#34260=CARTESIAN_POINT ( 'NONE',  ( 2.917880565312950480, 65.97041550158063217, -12.26659068614894821 ) ) ;
#34261=CARTESIAN_POINT ( 'NONE',  ( 18.52753015748617571, 38.09226448433412315, 4.923371831947298993 ) ) ;
#34264=CARTESIAN_POINT ( 'NONE',  ( -0.8801773607111009756, 53.06368534415484106, 1.068504757029289695E-15 ) ) ;
#34265=CARTESIAN_POINT ( 'NONE',  ( 6.565887622018943937, 60.16530133659707502, 12.81628187352647430 ) ) ;
#34266=CARTESIAN_POINT ( 'NONE',  ( 0.5774900079438590739, 37.64701867748817676, -5.440088680355550821 ) ) ;
#34267=CARTESIAN_POINT ( 'NONE',  ( 22.81628187352648496, 56.83196800326374643, -3.434112377981050290 ) ) ;
#34268=CARTESIAN_POINT ( 'NONE',  ( 22.81628187352647785, 6.623634669930420493, 6.195893100308588602E-16 ) ) ;
#34269=CARTESIAN_POINT ( 'NONE',  ( 18.52753015748618282, 8.925597817667451750, -4.923371831947291888 ) ) ;
#34270=VERTEX_POINT ( 'NONE', #56065 ) ;
#34272=CARTESIAN_POINT ( 'NONE',  ( -0.3689425029237881626, 62.42874883491396787, 10.36894250292379027 ) ) ;
#34273=CARTESIAN_POINT ( 'NONE',  ( 6.204703633549690345, 30.76208216824730357, -14.16423886937410259 ) ) ;
#34274=CARTESIAN_POINT ( 'NONE',  ( 10.00000000000000000, 26.81368534415484106, -10.88017736071110342 ) ) ;
#34275=CARTESIAN_POINT ( 'NONE',  ( 17.96484262340118221, 49.93868534415484106, 7.964842623401181321 ) ) ;
#34278=CARTESIAN_POINT ( 'NONE',  ( 10.00000000000000000, 4.758931151000784787, -9.846743663894594434 ) ) ;
#34281=CARTESIAN_POINT ( 'NONE',  ( -46.58925734348296999, 101.6427229076536491, 8.029849069859604782 ) ) ;
#34282=CARTESIAN_POINT ( 'NONE',  ( 2.791683348922237240, 25.38393115100078390, -7.208316651077763204 ) ) ;
#34283=CARTESIAN_POINT ( 'NONE',  ( 12.63842701281683922, 44.55059781766745175, -9.846743663894590881 ) ) ;
#34285=CARTESIAN_POINT ( 'NONE',  ( -0.8801773607111008646, 28.27201867748817321, 2.915334737309923430 ) ) ;
#34286=UNCERTAINTY_MEASURE_WITH_UNIT (LENGTH_MEASURE( 1.000000000000000082E-05 ), #74458, 'distance_accuracy_value', 'NONE');
#34287=CARTESIAN_POINT ( 'NONE',  ( 13.43411237798105340, 45.58196800326374643, 12.81628187352647963 ) ) ;
#34291=CARTESIAN_POINT ( 'NONE',  ( 19.42250999205614193, 60.14701867748817676, 5.440088680355555262 ) ) ;
#34292=CARTESIAN_POINT ( 'NONE',  ( 14.92337183194729988, 24.34226448433411960, -8.527530157486177487 ) ) ;
#34293=CARTESIAN_POINT ( 'NONE',  ( 22.26659068614894466, 53.88708216824731068, 7.082119434687054849 ) ) ;
#34294=CARTESIAN_POINT ( 'NONE',  ( 17.20831665107776587, 19.13393115100078035, -7.208316651077762316 ) ) ;
#34297=CARTESIAN_POINT ( 'NONE',  ( 6.204703633549690345, 10.76208216824729824, -14.16423886937410259 ) ) ;
#34298=CARTESIAN_POINT ( 'NONE',  ( 17.08211943468705130, 28.47041550158063572, 12.26659068614894998 ) ) ;
#34299=CARTESIAN_POINT ( 'NONE',  ( 14.92337183194729988, 29.34226448433411960, -8.527530157486177487 ) ) ;
#34300=CARTESIAN_POINT ( 'NONE',  ( 18.39792806157249672, 9.522241923386404849, 6.499999999999995559 ) ) ;
#34301=CARTESIAN_POINT ( 'NONE',  ( 17.96484262340118221, 24.93868534415484461, 7.964842623401181321 ) ) ;
#34302=CARTESIAN_POINT ( 'NONE',  ( 2.035157376598824452, 63.68868534415484106, 7.964842623401179544 ) ) ;
#34305=CARTESIAN_POINT ( 'NONE',  ( -2.816281873526471635, 38.91530133659708213, -3.434112377981056508 ) ) ;
#34306=CARTESIAN_POINT ( 'NONE',  ( 4.559911319644449179, 57.23035201082150536, -9.422509992056141925 ) ) ;
#34309=( LENGTH_UNIT ( ) NAMED_UNIT ( * ) SI_UNIT ( .MILLI., .METRE. ) );
#34310=CARTESIAN_POINT ( 'NONE',  ( 10.00000000000000178, 64.31368534415483396, 10.88017736071110342 ) ) ;
#34312=CARTESIAN_POINT ( 'NONE',  ( 7.084665262690076126, 62.02201867748816966, -10.88017736071110164 ) ) ;
#34315=CARTESIAN_POINT ( 'NONE',  ( 2.603489959281588106, 1.582109641433292690, 6.500000000000000888 ) ) ;
#34317=CARTESIAN_POINT ( 'NONE',  ( 7.084665262690076126, 12.02201867748817321, -10.88017736071110164 ) ) ;
#34318=CARTESIAN_POINT ( 'NONE',  ( 10.00000000000000178, 7.258931151000785675, 9.846743663894594434 ) ) ;
#34319=CARTESIAN_POINT ( 'NONE',  ( 2.917880565312950480, 20.97041550158063217, -12.26659068614894821 ) ) ;
#34320=CARTESIAN_POINT ( 'NONE',  ( 7.361572987183170547, 7.050597817667451750, 9.846743663894590881 ) ) ;
#34322=CARTESIAN_POINT ( 'NONE',  ( -0.8801773607111008646, 23.27201867748817676, 2.915334737309923430 ) ) ;
#34323=CARTESIAN_POINT ( 'NONE',  ( 19.84674366389459266, 53.71726448433411605, -2.638427012816827677 ) ) ;
#34326=CARTESIAN_POINT ( 'NONE',  ( 2.791683348922240793, 66.63393115100079456, 7.208316651077764092 ) ) ;
#34328=LINE ( 'NONE', #32866, #20622 ) ;
#34330=CARTESIAN_POINT ( 'NONE',  ( 10.00000000000000000, 56.81368534415484106, -10.88017736071110342 ) ) ;
#34331=CARTESIAN_POINT ( 'NONE',  ( 7.361572987183169658, 54.96726448433413026, -9.846743663894592657 ) ) ;
#34332=CARTESIAN_POINT ( 'NONE',  ( -1.099225684535947600, 38.70696800326375353, -6.408140936763238038 ) ) ;
#34333=CARTESIAN_POINT ( 'NONE',  ( 20.88017736071110519, 10.56368534415483751, 2.639326808657452039E-16 ) ) ;
#34335=CARTESIAN_POINT ( 'NONE',  ( 15.44008868035555260, 64.73035201082151957, 9.422509992056143702 ) ) ;
#34336=CARTESIAN_POINT ( 'NONE',  ( -4.164238869374099039, 66.80374883491396076, 8.674139862899312516E-16 ) ) ;
#34337=CARTESIAN_POINT ( 'NONE',  ( -0.8801773607111009756, 53.06368534415484106, 1.068504757029289695E-15 ) ) ;
#34338=CARTESIAN_POINT ( 'NONE',  ( -1.099225684535947600, 38.70696800326375353, -6.408140936763238038 ) ) ;
#34339=CARTESIAN_POINT ( 'NONE',  ( 20.88017736071110164, 35.35535201082150536, 2.915334737309930979 ) ) ;
#34343=CARTESIAN_POINT ( 'NONE',  ( 21.09922568453595559, 37.04030133659708923, -6.408140936763230044 ) ) ;
#34344=CARTESIAN_POINT ( 'NONE',  ( 19.42250999205614193, 40.14701867748817676, 5.440088680355555262 ) ) ;
#34349=( BOUNDED_CURVE ( )  B_SPLINE_CURVE ( 2, ( #35804, #5808, #66796, #42326, #19812, #41847, #72313, #72800, #81305 ),
 .UNSPECIFIED., .F., .T. ) 
 B_SPLINE_CURVE_WITH_KNOTS ( ( 3, 2, 2, 2, 3 ),
 ( 0.7953713073319822469, 0.7976190476190476719, 0.8035714285714286031, 0.8095238095238095344, 0.8117715498108749594 ),
 .UNSPECIFIED. ) 
 CURVE ( )  GEOMETRIC_REPRESENTATION_ITEM ( )  RATIONAL_B_SPLINE_CURVE ( ( 0.9839835555609424134, 0.9871328979762477029, 1.000000000000000000, 0.9659258262890683122, 1.000000000000000000, 0.9659258262890683122, 1.000000000000000000, 0.9871328979762474809, 0.9839835555609424134 ) ) 
 REPRESENTATION_ITEM ( '' )  );
#34350=CARTESIAN_POINT ( 'NONE',  ( 2.791683348922240793, 56.63393115100078035, 7.208316651077764092 ) ) ;
#34351=LINE ( 'NONE', #64842, #524 ) ;
#34352=CARTESIAN_POINT ( 'NONE',  ( 7.361572987183170547, 52.05059781766745175, 9.846743663894590881 ) ) ;
#34353=CARTESIAN_POINT ( 'NONE',  ( -0.8801773607111008646, 28.27201867748817321, 2.915334737309923430 ) ) ;
#34355=CARTESIAN_POINT ( 'NONE',  ( 0.1532563361054083140, 41.00893115100078745, 1.131784320476157264E-15 ) ) ;
#34358=EDGE_CURVE ( 'NONE', #16203, #32248, #3376, .T. ) ;
#34359=CARTESIAN_POINT ( 'NONE',  ( 10.00000000000000000, 24.75893115100078745, -9.846743663894594434 ) ) ;
#34360=CARTESIAN_POINT ( 'NONE',  ( 18.52753015748617571, 13.09226448433411960, 4.923371831947298993 ) ) ;
#34362=CARTESIAN_POINT ( 'NONE',  ( 17.20831665107776587, 62.88393115100078745, 7.208316651077764980 ) ) ;
#34365=CARTESIAN_POINT ( 'NONE',  ( 0.6178305044545838731, 44.74863466993042493, 9.382169495545420901 ) ) ;
#34367=CARTESIAN_POINT ( 'NONE',  ( 2.791683348922237240, 40.38393115100078035, -7.208316651077763204 ) ) ;
#34369=CARTESIAN_POINT ( 'NONE',  ( 24.16423886937409904, 64.09541550158064638, 3.795296366450317205 ) ) ;
#34370=CARTESIAN_POINT ( 'NONE',  ( 7.361572987183169658, 14.96726448433411960, -9.846743663894592657 ) ) ;
#34371=CARTESIAN_POINT ( 'NONE',  ( 20.00000000000000711, 89.81050759285638208, 4.994480956907769276 ) ) ;
#34372=CARTESIAN_POINT ( 'NONE',  ( 2.917880565312950480, 50.97041550158064638, -12.26659068614894821 ) ) ;
#34373=CARTESIAN_POINT ( 'NONE',  ( 0.1532563361054082862, 61.21726448433412315, 2.638427012816831674 ) ) ;
#34374=CARTESIAN_POINT ( 'NONE',  ( 7.084665262690076126, 2.022018677488171434, -10.88017736071110164 ) ) ;
#34375=CARTESIAN_POINT ( 'NONE',  ( 17.08211943468705840, 30.13708216824730357, -12.26659068614894466 ) ) ;
#34376=CARTESIAN_POINT ( 'NONE',  ( 13.79529636645030344, 38.26208216824729647, 14.16423886937410614 ) ) ;
#34377=CARTESIAN_POINT ( 'NONE',  ( -43.18635350015717478, 107.2769236248421549, -4.500000000000000888 ) ) ;
#34379=CARTESIAN_POINT ( 'NONE',  ( 3.640395162852214650, 107.5383484153110061, 5.000000000000000000 ) ) ;
#34380=CARTESIAN_POINT ( 'NONE',  ( 0.1532563361054083140, 61.00893115100078745, 1.131784320476157264E-15 ) ) ;
#34382=CARTESIAN_POINT ( 'NONE',  ( 19.42250999205614548, 55.98035201082150536, -5.440088680355545492 ) ) ;
#34383=AXIS2_PLACEMENT_3D ( 'NONE', #17539, #92526, #78514 ) ;
#34384=CARTESIAN_POINT ( 'NONE',  ( 19.54820696779682976, 96.99593637789192258, -5.000000000000000000 ) ) ;
#34385=CARTESIAN_POINT ( 'NONE',  ( 10.00000000000000178, 65.37363466993042493, 12.81628187352647608 ) ) ;
#34386=CARTESIAN_POINT ( 'NONE',  ( 19.84674366389459266, 58.71726448433411605, -2.638427012816827677 ) ) ;
#34390=CARTESIAN_POINT ( 'NONE',  ( -0.3689425029237881626, 22.42874883491397142, 10.36894250292379027 ) ) ;
#34394=CARTESIAN_POINT ( 'NONE',  ( 0.5774900079438607392, 13.48035201082150358, 5.440088680355550821 ) ) ;
#34395=CARTESIAN_POINT ( 'NONE',  ( -2.816281873526471635, 28.91530133659708213, -3.434112377981056508 ) ) ;
#34396=CARTESIAN_POINT ( 'NONE',  ( 12.63842701281683922, 14.55059781766744997, -9.846743663894590881 ) ) ;
#34397=CARTESIAN_POINT ( 'NONE',  ( 21.09922568453594849, 46.20696800326376064, 6.408140936763242479 ) ) ;
#34400=CARTESIAN_POINT ( 'NONE',  ( -0.3689425029237881626, 22.42874883491397142, 10.36894250292379027 ) ) ;
#34401=CARTESIAN_POINT ( 'NONE',  ( 20.15039907845753220, 61.74884699246888431, 6.262539305110078836 ) ) ;
#34402=CARTESIAN_POINT ( 'NONE',  ( 20.88017736071110519, 10.56368534415483929, 2.639326808657452039E-16 ) ) ;
#34404=CARTESIAN_POINT ( 'NONE',  ( 19.42250999205614548, 35.98035201082151247, -5.440088680355545492 ) ) ;
#34405=CARTESIAN_POINT ( 'NONE',  ( 12.91533473730992121, 39.52201867748817676, 10.88017736071110164 ) ) ;
#34406=CARTESIAN_POINT ( 'NONE',  ( 3.591859063236763294, 18.29030133659708568, -11.09922568453595026 ) ) ;
#34407=DIRECTION ( 'NONE',  ( -0.000000000000000000, 1.000000000000000000, -0.000000000000000000 ) ) ;
#34409=CARTESIAN_POINT ( 'NONE',  ( 2.791683348922237240, 15.38393115100078212, -7.208316651077763204 ) ) ;
#34412=CARTESIAN_POINT ( 'NONE',  ( -0.8801773607110991993, 37.85535201082151247, -2.915334737309923874 ) ) ;
#34413=EDGE_CURVE ( 'NONE', #42198, #19862, #7862, .T. ) ;
#34416=CARTESIAN_POINT ( 'NONE',  ( 10.00000000000000178, 5.373634669930420493, 12.81628187352647608 ) ) ;
#34417=CARTESIAN_POINT ( 'NONE',  ( 10.00000000000000000, 61.81368534415484106, -10.88017736071110342 ) ) ;
#34419=CARTESIAN_POINT ( 'NONE',  ( 10.00000000000000000, 24.75893115100078745, -9.846743663894594434 ) ) ;
#34420=CARTESIAN_POINT ( 'NONE',  ( 16.40814093676323893, 45.79030133659708923, 11.09922568453595026 ) ) ;
#34421=CARTESIAN_POINT ( 'NONE',  ( 1.472469842513823179, 0.5922644843341181575, -4.923371831947296329 ) ) ;
#34424=CARTESIAN_POINT ( 'NONE',  ( 2.035157376598824452, 13.68868534415483751, 7.964842623401179544 ) ) ;
#34425=CARTESIAN_POINT ( 'NONE',  ( 13.43411237798105340, 55.58196800326374643, 12.81628187352647963 ) ) ;
#34426=CARTESIAN_POINT ( 'NONE',  ( 0.1532563361054082862, 26.21726448433411605, 2.638427012816831674 ) ) ;
#34427=CARTESIAN_POINT ( 'NONE',  ( 19.42250999205614193, 25.14701867748817321, 5.440088680355555262 ) ) ;
#34428=CARTESIAN_POINT ( 'NONE',  ( 2.035157376598822676, 2.438685344154838397, -7.964842623401177768 ) ) ;
#34429=ORIENTED_EDGE ( 'NONE', *, *, #20593, .F. ) ;
#34430=CARTESIAN_POINT ( 'NONE',  ( 20.88017736071110519, 15.56368534415483751, 2.639326808657452039E-16 ) ) ;
#34431=CARTESIAN_POINT ( 'NONE',  ( 2.035157376598822676, 17.43868534415483751, -7.964842623401177768 ) ) ;
#34433=CARTESIAN_POINT ( 'NONE',  ( 15.44008868035555793, 26.39701867748817321, -9.422509992056140149 ) ) ;
#34435=CARTESIAN_POINT ( 'NONE',  ( 1.472469842513823179, 65.59226448433412315, -4.923371831947296329 ) ) ;
#34436=CARTESIAN_POINT ( 'NONE',  ( 12.91533473730993009, 26.60535201082150536, -10.88017736071109987 ) ) ;
#34437=CARTESIAN_POINT ( 'NONE',  ( 17.20831665107776587, 54.13393115100079456, -7.208316651077762316 ) ) ;
#34441=CARTESIAN_POINT ( 'NONE',  ( 22.81628187352647785, 61.41530133659709634, 3.434112377981063169 ) ) ;
#34443=CARTESIAN_POINT ( 'NONE',  ( 6.204703633549690345, 30.76208216824730357, -14.16423886937410259 ) ) ;
#34444=CARTESIAN_POINT ( 'NONE',  ( 7.084665262690076126, 37.02201867748817676, -10.88017736071110164 ) ) ;
#34445=CARTESIAN_POINT ( 'NONE',  ( 0.5774900079438590739, 12.64701867748817321, -5.440088680355550821 ) ) ;
#34446=CARTESIAN_POINT ( 'NONE',  ( 5.076628168052704559, 55.17559781766745175, -8.527530157486179263 ) ) ;
#34447=CARTESIAN_POINT ( 'NONE',  ( 1.472469842513823179, 46.42559781766745175, 4.923371831947296329 ) ) ;
#34449=CARTESIAN_POINT ( 'NONE',  ( 0.1916775849787266117, 22.25868815902069286, -6.499999999999991118 ) ) ;
#34450=CARTESIAN_POINT ( 'NONE',  ( 12.63842701281683034, 7.467264484334118713, 9.846743663894596210 ) ) ;
#34453=CARTESIAN_POINT ( 'NONE',  ( 17.96484262340118221, 11.18868534415483929, -7.964842623401177768 ) ) ;
#34454=CARTESIAN_POINT ( 'NONE',  ( 7.361572987183170547, 7.050597817667451750, 9.846743663894590881 ) ) ;
#34455=CARTESIAN_POINT ( 'NONE',  ( -2.816281873526471635, -1.084698663402913210, -3.434112377981056508 ) ) ;
#34456=CARTESIAN_POINT ( 'NONE',  ( 20.88017736071110519, 65.56368534415483396, 2.639326808657452039E-16 ) ) ;
#34457=CARTESIAN_POINT ( 'NONE',  ( 19.42250999205614548, 50.98035201082151247, -5.440088680355545492 ) ) ;
#34458=CARTESIAN_POINT ( 'NONE',  ( 19.42250999205614548, 20.98035201082150891, -5.440088680355545492 ) ) ;
#34459=CARTESIAN_POINT ( 'NONE',  ( 0.6178305044545818747, 63.49863466993043204, -9.382169495545419124 ) ) ;
#34460=CARTESIAN_POINT ( 'NONE',  ( 10.00000000000000000, 30.55374883491397142, -14.16423886937410082 ) ) ;
#34462=CARTESIAN_POINT ( 'NONE',  ( 20.32896413005680003, 11.77164270246084143, 5.963430220938287007 ) ) ;
#34463=CARTESIAN_POINT ( 'NONE',  ( 19.38216949554541202, 55.99863466993041072, 9.382169495545424454 ) ) ;
#34465=CARTESIAN_POINT ( 'NONE',  ( 16.40814093676324603, 2.456968003263753531, -11.09922568453594671 ) ) ;
#34467=CARTESIAN_POINT ( 'NONE',  ( 12.91533473730992121, 34.52201867748817676, 10.88017736071110164 ) ) ;
#34468=CARTESIAN_POINT ( 'NONE',  ( 2.791683348922240793, 66.63393115100079456, 7.208316651077764092 ) ) ;
#34470=CARTESIAN_POINT ( 'NONE',  ( 0.1532563361054083140, 6.008931151000784787, 1.131784320476157264E-15 ) ) ;
#34471=CARTESIAN_POINT ( 'NONE',  ( 1.472469842513823179, 10.59226448433411782, -4.923371831947296329 ) ) ;
#34472=CARTESIAN_POINT ( 'NONE',  ( 14.92337183194729988, 19.34226448433411960, -8.527530157486177487 ) ) ;
#34473=CARTESIAN_POINT ( 'NONE',  ( 5.076628168052704559, 10.17559781766745175, -8.527530157486179263 ) ) ;
#34475=CARTESIAN_POINT ( 'NONE',  ( 0.5774900079438590739, 57.64701867748817676, -5.440088680355550821 ) ) ;
#34477=CARTESIAN_POINT ( 'NONE',  ( 0.5774900079438607392, 63.48035201082149825, 5.440088680355550821 ) ) ;
#34479=CARTESIAN_POINT ( 'NONE',  ( 10.00000000000000000, 14.75893115100078568, -9.846743663894594434 ) ) ;
#34482=CARTESIAN_POINT ( 'NONE',  ( 1.472469842513823179, 56.42559781766745886, 4.923371831947296329 ) ) ;
#34485=CARTESIAN_POINT ( 'NONE',  ( 13.79529636645031943, 25.34541550158063572, -14.16423886937409904 ) ) ;
#34486=B_SPLINE_CURVE_WITH_KNOTS ( 'NONE', 3,
 ( #12554, #43537, #58537, #7034, #13541, #21050 ),
 .UNSPECIFIED., .F., .F.,
 ( 4, 2, 4 ),
 ( 0.000000000000000000, 0.0002701661927229383718, 0.0005403323854458767436 ),
 .UNSPECIFIED. ) ;
#34487=UNCERTAINTY_MEASURE_WITH_UNIT (LENGTH_MEASURE( 1.000000000000000082E-05 ), #88319, 'distance_accuracy_value', 'NONE');
#34489=CARTESIAN_POINT ( 'NONE',  ( 2.917880565312950480, 10.97041550158063572, -12.26659068614894821 ) ) ;
#34490=CARTESIAN_POINT ( 'NONE',  ( 22.26659068614895176, 34.72041550158063927, -7.082119434687042414 ) ) ;
#34491=FILL_AREA_STYLE ('',( #5005 ) ) ;
#34492=CARTESIAN_POINT ( 'NONE',  ( -4.164238869374099039, 1.803748834913967647, 8.674139862899312516E-16 ) ) ;
#34493=CARTESIAN_POINT ( 'NONE',  ( 20.88017736071110519, 40.56368534415484106, 2.639326808657452039E-16 ) ) ;
#34495=CARTESIAN_POINT ( 'NONE',  ( 1.472469842513823179, 16.42559781766745175, 4.923371831947296329 ) ) ;
#34496=CARTESIAN_POINT ( 'NONE',  ( 7.084665262690076126, 59.10535201082150536, 10.88017736071109987 ) ) ;
#34497=CARTESIAN_POINT ( 'NONE',  ( 19.84674366389459266, 18.71726448433411960, -2.638427012816827677 ) ) ;
#34498=CARTESIAN_POINT ( 'NONE',  ( 7.084665262690076126, 14.10535201082150358, 10.88017736071109987 ) ) ;
#34499=CARTESIAN_POINT ( 'NONE',  ( -2.816281873526473856, 44.12363466993042493, 9.499525473075851096E-16 ) ) ;
#34500=CARTESIAN_POINT ( 'NONE',  ( 7.361572987183170547, 47.05059781766745175, 9.846743663894590881 ) ) ;
#34502=CARTESIAN_POINT ( 'NONE',  ( 16.40814093676324603, 27.45696800326375708, -11.09922568453594671 ) ) ;
#34504=CARTESIAN_POINT ( 'NONE',  ( 12.63842701281683922, 19.55059781766745175, -9.846743663894590881 ) ) ;
#34505=CARTESIAN_POINT ( 'NONE',  ( 24.16423886937409904, 14.09541550158063217, 3.795296366450317205 ) ) ;
#34506=ORIENTED_EDGE ( 'NONE', *, *, #94333, .F. ) ;
#34507=ORIENTED_EDGE ( 'NONE', *, *, #88960, .F. ) ;
#34508=CARTESIAN_POINT ( 'NONE',  ( 6.000000000000000000, 61.00000000000000711, 5.000000000000000000 ) ) ;
#34509=CARTESIAN_POINT ( 'NONE',  ( 7.084665262690076126, 44.10535201082151247, 10.88017736071109987 ) ) ;
#34510=CARTESIAN_POINT ( 'NONE',  ( 10.00000000000000000, 46.81368534415484106, -10.88017736071110342 ) ) ;
#34511=CARTESIAN_POINT ( 'NONE',  ( 22.26659068614894466, 43.88708216824729647, 7.082119434687054849 ) ) ;
#34512=CARTESIAN_POINT ( 'NONE',  ( 5.076628168052704559, 60.17559781766745175, -8.527530157486179263 ) ) ;
#34513=CARTESIAN_POINT ( 'NONE',  ( 1.472469842513823179, 6.425597817667451750, 4.923371831947296329 ) ) ;
#34514=CARTESIAN_POINT ( 'NONE',  ( -1.099225684535947600, 63.70696800326376774, -6.408140936763238038 ) ) ;
#34515=CARTESIAN_POINT ( 'NONE',  ( 0.5774900079438590739, 47.64701867748817676, -5.440088680355550821 ) ) ;
#34517=CARTESIAN_POINT ( 'NONE',  ( 19.84674366389459266, 58.71726448433411605, -2.638427012816827677 ) ) ;
#34519=CARTESIAN_POINT ( 'NONE',  ( -0.8801773607111008646, 68.27201867748817676, 2.915334737309923430 ) ) ;
#34521=PRESENTATION_STYLE_ASSIGNMENT (( #11543 ) ) ;
#34523=CARTESIAN_POINT ( 'NONE',  ( 4.559911319644449179, 67.23035201082150536, -9.422509992056141925 ) ) ;
#34524=CARTESIAN_POINT ( 'NONE',  ( 2.035157376598824452, 68.68868534415484817, 7.964842623401179544 ) ) ;
#34525=CARTESIAN_POINT ( 'NONE',  ( 0.1532563361054100626, 30.80059781766744820, -2.638427012816831230 ) ) ;
#34527=CARTESIAN_POINT ( 'NONE',  ( 19.42250999205614548, 20.98035201082150891, -5.440088680355545492 ) ) ;
#34528=( GEOMETRIC_REPRESENTATION_CONTEXT ( 3 ) GLOBAL_UNCERTAINTY_ASSIGNED_CONTEXT ( ( #30105 ) ) GLOBAL_UNIT_ASSIGNED_CONTEXT ( ( #11867, #10888, #34849 ) ) REPRESENTATION_CONTEXT ( 'NONE', 'WORKASPACE' ) );
#34529=CARTESIAN_POINT ( 'NONE',  ( 18.52753015748617571, 63.09226448433412315, 4.923371831947298993 ) ) ;
#34530=CARTESIAN_POINT ( 'NONE',  ( 20.88017736071110164, 35.35535201082150536, 2.915334737309930979 ) ) ;
#34531=CARTESIAN_POINT ( 'NONE',  ( 0.6081133539230650920, 13.33703382326400089, 6.500000000000005329 ) ) ;
#34533=CARTESIAN_POINT ( 'NONE',  ( 6.565887622018943937, 40.16530133659708923, 12.81628187352647430 ) ) ;
#34535=CARTESIAN_POINT ( 'NONE',  ( 19.42250999205614193, 45.14701867748817676, 5.440088680355555262 ) ) ;
#34536=CARTESIAN_POINT ( 'NONE',  ( -1.099225684535947600, 18.70696800326375353, -6.408140936763238038 ) ) ;
#34537=CARTESIAN_POINT ( 'NONE',  ( 20.10384461210892582, 51.74302437010795330, 6.337995344473751125 ) ) ;
#34538=CARTESIAN_POINT ( 'NONE',  ( 14.92337183194729633, 2.675597817667451750, 8.527530157486181039 ) ) ;
#34539=CARTESIAN_POINT ( 'NONE',  ( 20.88017736071110875, 30.77201867748816966, -2.915334737309920765 ) ) ;
#34540=CARTESIAN_POINT ( 'NONE',  ( -4.164238869374099039, 61.80374883491397497, 8.674139862899312516E-16 ) ) ;
#34541=CARTESIAN_POINT ( 'NONE',  ( 2.791683348922237240, 50.38393115100078035, -7.208316651077763204 ) ) ;
#34542=CARTESIAN_POINT ( 'NONE',  ( -0.8801773607111009756, 68.06368534415484817, 1.068504757029289695E-15 ) ) ;
#34543=CARTESIAN_POINT ( 'NONE',  ( 0.5774900079438590739, 62.64701867748817676, -5.440088680355550821 ) ) ;
#34545=CARTESIAN_POINT ( 'NONE',  ( 6.204703633549690345, 32.84541550158063927, 14.16423886937410082 ) ) ;
#34546=EDGE_CURVE ( 'NONE', #56832, #96185, #59856, .T. ) ;
#34547=STYLED_ITEM ( 'NONE', ( #90225 ), #35455 ) ;
#34552=CARTESIAN_POINT ( 'NONE',  ( 24.16423886937409904, 49.09541550158063217, 3.795296366450317205 ) ) ;
#34553=CARTESIAN_POINT ( 'NONE',  ( 22.26659068614895176, 44.72041550158063927, -7.082119434687042414 ) ) ;
#34554=CARTESIAN_POINT ( 'NONE',  ( 14.92337183194729988, 14.34226448433411782, -8.527530157486177487 ) ) ;
#34556=CARTESIAN_POINT ( 'NONE',  ( 6.565887622018943937, 15.16530133659708568, 12.81628187352647430 ) ) ;
#34558=CARTESIAN_POINT ( 'NONE',  ( 7.084665262690076126, 69.10535201082151957, 10.88017736071109987 ) ) ;
#34559=CARTESIAN_POINT ( 'NONE',  ( 22.81628187352647785, 51.62363466993042493, 6.195893100308588602E-16 ) ) ;
#34560=CARTESIAN_POINT ( 'NONE',  ( 17.08211943468705130, 38.47041550158063217, 12.26659068614894998 ) ) ;
#34562=CARTESIAN_POINT ( 'NONE',  ( 5.076628168052703671, 11.84226448433411960, 8.527530157486179263 ) ) ;
#34567=CARTESIAN_POINT ( 'NONE',  ( 2.791683348922237240, 15.38393115100078212, -7.208316651077763204 ) ) ;
#34568=VERTEX_POINT ( 'NONE', #47307 ) ;
#34570=CARTESIAN_POINT ( 'NONE',  ( 20.88017736071110875, 5.772018677488170546, -2.915334737309920765 ) ) ;
#34571=CARTESIAN_POINT ( 'NONE',  ( 17.96484262340118221, 31.18868534415483751, -7.964842623401177768 ) ) ;
#34572=CARTESIAN_POINT ( 'NONE',  ( 18.52753015748617571, 48.09226448433412315, 4.923371831947298993 ) ) ;
#34573=CARTESIAN_POINT ( 'NONE',  ( 22.81628187352647785, 1.415301336597087012, 3.434112377981063169 ) ) ;
#34578=CARTESIAN_POINT ( 'NONE',  ( -2.816281873526473856, 19.33196800326375708, 3.434112377981055619 ) ) ;
#34580=CARTESIAN_POINT ( 'NONE',  ( 0.1532563361054083140, 36.00893115100078745, 1.131784320476157264E-15 ) ) ;
#34581=CARTESIAN_POINT ( 'NONE',  ( 10.00000000000000178, 58.05374883491397497, 14.16423886937410082 ) ) ;
#34583=CARTESIAN_POINT ( 'NONE',  ( -2.266590686148945544, 57.22041550158063217, 7.082119434687048631 ) ) ;
#34585=CARTESIAN_POINT ( 'NONE',  ( -0.8801773607111008646, 33.27201867748817676, 2.915334737309923430 ) ) ;
#34586=CARTESIAN_POINT ( 'NONE',  ( 2.035157376598824452, 43.68868534415484106, 7.964842623401179544 ) ) ;
#34587=CARTESIAN_POINT ( 'NONE',  ( 17.96484262340118221, 46.18868534415484106, -7.964842623401177768 ) ) ;
#34590=CARTESIAN_POINT ( 'NONE',  ( 17.96484262340118221, 46.18868534415484106, -7.964842623401177768 ) ) ;
#34592=ADVANCED_FACE ( 'NONE', ( #16832 ), #55816, .T. ) ;
#34595=CARTESIAN_POINT ( 'NONE',  ( 19.84674366389459621, 18.50893115100078745, 7.409399052514197653E-17 ) ) ;
#34598=CARTESIAN_POINT ( 'NONE',  ( 5.076628168052703671, 51.84226448433412315, 8.527530157486179263 ) ) ;
#34599=DIRECTION ( 'NONE',  ( 1.000000000000000000, 0.000000000000000000, 0.000000000000000000 ) ) ;
#34601=CARTESIAN_POINT ( 'NONE',  ( 0.6178305044545818747, 53.49863466993041072, -9.382169495545419124 ) ) ;
#34604=FACE_OUTER_BOUND ( 'NONE', #4653, .T. ) ;
#34606=CARTESIAN_POINT ( 'NONE',  ( 0.2751277870542967463, 70.00000000000000000, -6.000000000000000000 ) ) ;
#34607=CARTESIAN_POINT ( 'NONE',  ( -0.3689425029237898834, 66.17874883491396076, -10.36894250292378850 ) ) ;
#34608=CARTESIAN_POINT ( 'NONE',  ( 2.791683348922240793, 66.63393115100079456, 7.208316651077764092 ) ) ;
#34611=CARTESIAN_POINT ( 'NONE',  ( 18.52753015748618282, 28.92559781766745175, -4.923371831947291888 ) ) ;
#34613=CARTESIAN_POINT ( 'NONE',  ( 21.09922568453594849, 1.206968003263753531, 6.408140936763242479 ) ) ;
#34614=CARTESIAN_POINT ( 'NONE',  ( 4.559911319644449179, 62.23035201082150536, -9.422509992056141925 ) ) ;
#34616=CARTESIAN_POINT ( 'NONE',  ( 0.1532563361054083140, 16.00893115100078390, 1.131784320476157264E-15 ) ) ;
#34617=CARTESIAN_POINT ( 'NONE',  ( 1.472469842513823179, 61.42559781766745175, 4.923371831947296329 ) ) ;
#34618=CARTESIAN_POINT ( 'NONE',  ( 2.603489959281581889, 20.43575266056827999, -6.499999999999995559 ) ) ;
#34622=CARTESIAN_POINT ( 'NONE',  ( 20.88017736071110875, 15.77201867748817143, -2.915334737309920765 ) ) ;
#34623=CARTESIAN_POINT ( 'NONE',  ( 1.472469842513823179, 11.42559781766745175, 4.923371831947296329 ) ) ;
#34624=CARTESIAN_POINT ( 'NONE',  ( 4.559911319644449179, 43.89701867748816966, 9.422509992056141925 ) ) ;
#34625=CARTESIAN_POINT ( 'NONE',  ( 3.591859063236763294, 23.29030133659708568, -11.09922568453595026 ) ) ;
#34627=CARTESIAN_POINT ( 'NONE',  ( 20.88017736071110164, 5.355352010821502695, 2.915334737309930979 ) ) ;
#34629=CARTESIAN_POINT ( 'NONE',  ( 19.72487221294571569, 59.78217586085237656, 6.499999999999986677 ) ) ;
#34630=CARTESIAN_POINT ( 'NONE',  ( 12.63842701281683034, 47.46726448433412315, 9.846743663894596210 ) ) ;
#34631=CARTESIAN_POINT ( 'NONE',  ( 12.63842701281683922, 19.55059781766745175, -9.846743663894590881 ) ) ;
#34633=CARTESIAN_POINT ( 'NONE',  ( 21.09922568453595559, 22.04030133659708923, -6.408140936763230044 ) ) ;
#34635=EDGE_CURVE ( 'NONE', #22152, #84653, #40131, .T. ) ;
#34636=CARTESIAN_POINT ( 'NONE',  ( 15.44008868035555260, 24.73035201082150891, 9.422509992056143702 ) ) ;
#34639=CARTESIAN_POINT ( 'NONE',  ( 2.917880565312948704, 47.63708216824730357, 12.26659068614894643 ) ) ;
#34640=VECTOR ( 'NONE', #65478, 1000.000000000000000 ) ;
#34641=CARTESIAN_POINT ( 'NONE',  ( 0.2751277870542909176, 64.36607318730132477, -6.499999999999992006 ) ) ;
#34642=CARTESIAN_POINT ( 'NONE',  ( 2.791683348922237240, 40.38393115100078035, -7.208316651077763204 ) ) ;
#34644=CARTESIAN_POINT ( 'NONE',  ( 19.38216949554541202, 35.99863466993041072, 9.382169495545424454 ) ) ;
#34645=CARTESIAN_POINT ( 'NONE',  ( 4.559911319644449179, 28.89701867748817321, 9.422509992056141925 ) ) ;
#34647=CARTESIAN_POINT ( 'NONE',  ( 12.63842701281683034, 52.46726448433413026, 9.846743663894596210 ) ) ;
#34648=CARTESIAN_POINT ( 'NONE',  ( 15.44008868035555793, 56.39701867748817676, -9.422509992056140149 ) ) ;
#34649=CARTESIAN_POINT ( 'NONE',  ( 21.09922568453595559, 12.04030133659708746, -6.408140936763230044 ) ) ;
#34650=CARTESIAN_POINT ( 'NONE',  ( 13.79529636645030344, 28.26208216824729647, 14.16423886937410614 ) ) ;
#34654=CARTESIAN_POINT ( 'NONE',  ( 10.00000000000000178, 22.25893115100078745, 9.846743663894594434 ) ) ;
#34655=CARTESIAN_POINT ( 'NONE',  ( -2.816281873526473856, 59.12363466993042493, 9.499525473075851096E-16 ) ) ;
#34656=CARTESIAN_POINT ( 'NONE',  ( 10.00000000000000000, -2.126365330069579951, -12.81628187352647608 ) ) ;
#34659=CARTESIAN_POINT ( 'NONE',  ( 20.88017736071110875, 20.77201867748816611, -2.915334737309920765 ) ) ;
#34660=CARTESIAN_POINT ( 'NONE',  ( 17.96484262340118221, 61.18868534415482685, -7.964842623401177768 ) ) ;
#34661=CARTESIAN_POINT ( 'NONE',  ( -2.266590686148945544, 22.22041550158063572, 7.082119434687048631 ) ) ;
#34662=CARTESIAN_POINT ( 'NONE',  ( 7.084665262690076126, 64.10535201082150536, 10.88017736071109987 ) ) ;
#34663=CARTESIAN_POINT ( 'NONE',  ( 17.20831665107776587, 54.13393115100079456, -7.208316651077762316 ) ) ;
#34664=CARTESIAN_POINT ( 'NONE',  ( 4.559911319644449179, 37.23035201082150536, -9.422509992056141925 ) ) ;
#34665=LINE ( 'NONE', #65162, #60701 ) ;
#34666=CARTESIAN_POINT ( 'NONE',  ( -42.16485527613927076, 107.5383484153110061, -5.000000000000000000 ) ) ;
#34671=ORIENTED_EDGE ( 'NONE', *, *, #41465, .F. ) ;
#34674=CARTESIAN_POINT ( 'NONE',  ( 10.00000000000000000, 10.55374883491396787, -14.16423886937410082 ) ) ;
#34675=CARTESIAN_POINT ( 'NONE',  ( 10.00000000000000000, 15.55374883491396787, -14.16423886937410082 ) ) ;
#34676=CARTESIAN_POINT ( 'NONE',  ( 0.5774900079438607392, 48.48035201082150536, 5.440088680355550821 ) ) ;
#34677=CARTESIAN_POINT ( 'NONE',  ( 22.26659068614895176, 59.72041550158063927, -7.082119434687042414 ) ) ;
#34678=CARTESIAN_POINT ( 'NONE',  ( 7.361572987183170547, 57.05059781766744464, 9.846743663894590881 ) ) ;
#34679=CARTESIAN_POINT ( 'NONE',  ( 5.076628168052704559, 35.17559781766745175, -8.527530157486179263 ) ) ;
#34681=CARTESIAN_POINT ( 'NONE',  ( 4.559911319644449179, 38.89701867748817676, 9.422509992056141925 ) ) ;
#34682=CARTESIAN_POINT ( 'NONE',  ( 0.1532563361054100626, 60.80059781766744464, -2.638427012816831230 ) ) ;
#34683=CARTESIAN_POINT ( 'NONE',  ( -4.164238869374099927, 7.012082168247302683, 3.795296366450308767 ) ) ;
#34684=CARTESIAN_POINT ( 'NONE',  ( 10.00000000000000178, 48.05374883491396787, 14.16423886937410082 ) ) ;
#34685=COLOUR_RGB ( '', 0.09019608, 0.27058824, 0.51372549) ;
#34686=CARTESIAN_POINT ( 'NONE',  ( 12.91533473730993009, 6.605352010821504471, -10.88017736071109987 ) ) ;
#34687=CARTESIAN_POINT ( 'NONE',  ( 19.84674366389459621, 38.50893115100078745, 7.409399052514197653E-17 ) ) ;
#34692=FACE_OUTER_BOUND ( 'NONE', #26223, .T. ) ;
#34694=CARTESIAN_POINT ( 'NONE',  ( 14.92337183194729633, 17.67559781766745175, 8.527530157486181039 ) ) ;
#34696=CARTESIAN_POINT ( 'NONE',  ( 6.204703633549690345, 27.84541550158063217, 14.16423886937410082 ) ) ;
#34697=CARTESIAN_POINT ( 'NONE',  ( 2.791683348922237240, 30.38393115100078390, -7.208316651077763204 ) ) ;
#34698=CARTESIAN_POINT ( 'NONE',  ( 4.559911319644449179, 62.23035201082150536, -9.422509992056141925 ) ) ;
#34700=CARTESIAN_POINT ( 'NONE',  ( 10.00000000000000178, 49.31368534415484106, 10.88017736071110342 ) ) ;
#34704=CARTESIAN_POINT ( 'NONE',  ( -4.164238869374099039, 16.80374883491396787, 8.674139862899312516E-16 ) ) ;
#34706=CARTESIAN_POINT ( 'NONE',  ( -2.816281873526473856, 49.33196800326374643, 3.434112377981055619 ) ) ;
#34708=CARTESIAN_POINT ( 'NONE',  ( 20.88017736071110164, 20.35535201082150891, 2.915334737309930979 ) ) ;
#34709=CARTESIAN_POINT ( 'NONE',  ( 18.52753015748618282, 28.92559781766745175, -4.923371831947291888 ) ) ;
#34711=CARTESIAN_POINT ( 'NONE',  ( 10.00000000000000178, 19.31368534415484106, 10.88017736071110342 ) ) ;
#34712=CARTESIAN_POINT ( 'NONE',  ( 22.81628187352647785, 56.41530133659708213, 3.434112377981063169 ) ) ;
#34714=CARTESIAN_POINT ( 'NONE',  ( 0.1532563361054082862, 36.21726448433410894, 2.638427012816831674 ) ) ;
#34718=CARTESIAN_POINT ( 'NONE',  ( 21.92686044187656691, 22.18830936912750929, 4.562052436263911564E-16 ) ) ;
#34719=DIRECTION ( 'NONE',  ( 0.000000000000000000, 0.000000000000000000, -1.000000000000000000 ) ) ;
#34721=CARTESIAN_POINT ( 'NONE',  ( -0.1503990784575327533, 7.222660991849186196, -6.262539305110070842 ) ) ;
#34722=CARTESIAN_POINT ( 'NONE',  ( 17.20831665107776587, 4.133931151000785675, -7.208316651077762316 ) ) ;
#34723=CARTESIAN_POINT ( 'NONE',  ( 13.43411237798105340, 30.58196800326374998, 12.81628187352647963 ) ) ;
#34726=CARTESIAN_POINT ( 'NONE',  ( 12.63842701281683922, 39.55059781766744464, -9.846743663894590881 ) ) ;
#34728=CARTESIAN_POINT ( 'NONE',  ( 24.16423886937409904, 19.09541550158063927, 3.795296366450317205 ) ) ;
#34729=CARTESIAN_POINT ( 'NONE',  ( 7.361572987183169658, 34.96726448433411605, -9.846743663894592657 ) ) ;
#34730=CARTESIAN_POINT ( 'NONE',  ( -2.816281873526471635, 38.91530133659708213, -3.434112377981056508 ) ) ;
#34731=CARTESIAN_POINT ( 'NONE',  ( 17.85158348494336522, 14.73726573380441174, -6.499999999999984901 ) ) ;
#34733=CARTESIAN_POINT ( 'NONE',  ( 7.084665262690076126, 57.02201867748817676, -10.88017736071110164 ) ) ;
#34734=CARTESIAN_POINT ( 'NONE',  ( 19.38216949554541202, 10.99863466993042138, 9.382169495545424454 ) ) ;
#34736=EDGE_CURVE ( 'NONE', #52255, #5105, #78305, .T. ) ;
#34737=CARTESIAN_POINT ( 'NONE',  ( 18.52753015748617571, 33.09226448433411605, 4.923371831947298993 ) ) ;
#34738=CARTESIAN_POINT ( 'NONE',  ( 4.559911319644449179, 22.23035201082150536, -9.422509992056141925 ) ) ;
#34739=CARTESIAN_POINT ( 'NONE',  ( 16.40814093676324603, 32.45696800326375353, -11.09922568453594671 ) ) ;
#34740=CARTESIAN_POINT ( 'NONE',  ( 0.1532563361054100626, 35.80059781766745175, -2.638427012816831230 ) ) ;
#34742=DIRECTION ( 'NONE',  ( 1.000000000000000000, 0.000000000000000000, 0.000000000000000000 ) ) ;
#34743=CARTESIAN_POINT ( 'NONE',  ( 15.44008868035555260, 34.73035201082151247, 9.422509992056143702 ) ) ;
#34748=CARTESIAN_POINT ( 'NONE',  ( 4.559911319644449179, 2.230352010821504471, -9.422509992056141925 ) ) ;
#34749=CARTESIAN_POINT ( 'NONE',  ( 10.00000000000000178, 62.25893115100078745, 9.846743663894594434 ) ) ;
#34750=CARTESIAN_POINT ( 'NONE',  ( 19.42250999205614548, 30.98035201082150536, -5.440088680355545492 ) ) ;
#34752=CARTESIAN_POINT ( 'NONE',  ( 10.00000000000000000, 56.81368534415484106, -10.88017736071110342 ) ) ;
#34753=CARTESIAN_POINT ( 'NONE',  ( -0.8801773607110991993, 27.85535201082150181, -2.915334737309923874 ) ) ;
#34755=CARTESIAN_POINT ( 'NONE',  ( 19.84674366389459266, 3.717264484334118713, -2.638427012816827677 ) ) ;
#34756=CARTESIAN_POINT ( 'NONE',  ( -46.56032276184168239, 103.8061269828102837, -5.692785089662786291 ) ) ;
#34757=CARTESIAN_POINT ( 'NONE',  ( 12.63842701281683922, 54.55059781766745175, -9.846743663894590881 ) ) ;
#34758=CARTESIAN_POINT ( 'NONE',  ( -0.3689425029237898834, 51.17874883491397497, -10.36894250292378850 ) ) ;
#34759=CARTESIAN_POINT ( 'NONE',  ( 21.92686044187657046, 20.16212336850780673, 4.562052436263912550E-16 ) ) ;
#34761=CARTESIAN_POINT ( 'NONE',  ( 22.26659068614895176, 14.72041550158063572, -7.082119434687042414 ) ) ;
#34762=CARTESIAN_POINT ( 'NONE',  ( 22.26659068614894466, 43.88708216824729647, 7.082119434687054849 ) ) ;
#34764=CARTESIAN_POINT ( 'NONE',  ( 3.591859063236763294, 8.290301336597087456, -11.09922568453595026 ) ) ;
#34767=ORIENTED_EDGE ( 'NONE', *, *, #38798, .T. ) ;
#34768=CARTESIAN_POINT ( 'NONE',  ( 17.96484262340118221, 4.938685344154837509, 7.964842623401181321 ) ) ;
#34769=CARTESIAN_POINT ( 'NONE',  ( 19.84674366389459266, 38.71726448433412315, -2.638427012816827677 ) ) ;
#34772=CARTESIAN_POINT ( 'NONE',  ( 12.91533473730993009, 56.60535201082151247, -10.88017736071109987 ) ) ;
#34775=LINE ( 'NONE', #28757, #21119 ) ;
#34776=CARTESIAN_POINT ( 'NONE',  ( 22.81628187352647785, 26.62363466993042138, 6.195893100308588602E-16 ) ) ;
#34777=CARTESIAN_POINT ( 'NONE',  ( 0.1532563361054083140, 26.00893115100078745, 1.131784320476157264E-15 ) ) ;
#34779=PRESENTATION_STYLE_ASSIGNMENT (( #10326 ) ) ;
#34781=CARTESIAN_POINT ( 'NONE',  ( 4.559911319644449179, 3.897018677488171434, 9.422509992056141925 ) ) ;
#34782=CARTESIAN_POINT ( 'NONE',  ( 22.26659068614895176, 34.72041550158063927, -7.082119434687042414 ) ) ;
#34783=CARTESIAN_POINT ( 'NONE',  ( 19.42250999205614548, 30.98035201082150536, -5.440088680355545492 ) ) ;
#34784=CARTESIAN_POINT ( 'NONE',  ( 12.91533473730992121, 54.52201867748816255, 10.88017736071110164 ) ) ;
#34786=CARTESIAN_POINT ( 'NONE',  ( 17.39651004071841456, 49.08210964143329136, -6.500000000000001776 ) ) ;
#34787=CARTESIAN_POINT ( 'NONE',  ( 2.791683348922237240, 15.38393115100078212, -7.208316651077763204 ) ) ;
#34789=CARTESIAN_POINT ( 'NONE',  ( 7.361572987183170547, 37.05059781766744464, 9.846743663894590881 ) ) ;
#34790=CARTESIAN_POINT ( 'NONE',  ( 1.472469842513823179, 66.42559781766745175, 4.923371831947296329 ) ) ;
#34792=CARTESIAN_POINT ( 'NONE',  ( 17.96484262340118221, 24.93868534415484461, 7.964842623401181321 ) ) ;
#34796=CARTESIAN_POINT ( 'NONE',  ( -2.816281873526471635, 38.91530133659708213, -3.434112377981056508 ) ) ;
#34797=CARTESIAN_POINT ( 'NONE',  ( 7.084665262690076126, 69.10535201082151957, 10.88017736071109987 ) ) ;
#34798=CARTESIAN_POINT ( 'NONE',  ( 0.1532563361054100626, 25.80059781766744820, -2.638427012816831230 ) ) ;
#34799=CARTESIAN_POINT ( 'NONE',  ( 13.79529636645030344, 63.26208216824730357, 14.16423886937410614 ) ) ;
#34800=CARTESIAN_POINT ( 'NONE',  ( 12.63842701281683922, 19.55059781766745175, -9.846743663894590881 ) ) ;
#34802=CARTESIAN_POINT ( 'NONE',  ( 12.63842701281683034, 62.46726448433410894, 9.846743663894596210 ) ) ;
#34803=CARTESIAN_POINT ( 'NONE',  ( 22.26659068614894466, 23.88708216824730357, 7.082119434687054849 ) ) ;
#34804=CARTESIAN_POINT ( 'NONE',  ( -2.266590686148945544, 26.38708216824730357, -7.082119434687050408 ) ) ;
#34805=CARTESIAN_POINT ( 'NONE',  ( 5.076628168052703671, 41.84226448433411605, 8.527530157486179263 ) ) ;
#34806=CARTESIAN_POINT ( 'NONE',  ( 18.61655166652077753, 9.877183271974288914, 6.499999999999968914 ) ) ;
#34807=CARTESIAN_POINT ( 'NONE',  ( 19.42250999205614548, 30.98035201082150536, -5.440088680355545492 ) ) ;
#34809=CARTESIAN_POINT ( 'NONE',  ( 12.91533473730992121, 64.52201867748817676, 10.88017736071110164 ) ) ;
#34810=CARTESIAN_POINT ( 'NONE',  ( -0.1503990784575328643, 0.07447313448805115144, 6.262539305110068177 ) ) ;
#34812=CARTESIAN_POINT ( 'NONE',  ( 0.6178305044545818747, 48.49863466993042493, -9.382169495545419124 ) ) ;
#34813=CARTESIAN_POINT ( 'NONE',  ( 10.00000000000000178, 49.31368534415484106, 10.88017736071110342 ) ) ;
#34815=FILL_AREA_STYLE_COLOUR ( '', #43504 ) ;
#34817=ORIENTED_EDGE ( 'NONE', *, *, #13929, .T. ) ;
#34818=CARTESIAN_POINT ( 'NONE',  ( 0.5774900079438607392, 68.48035201082150536, 5.440088680355550821 ) ) ;
#34819=CARTESIAN_POINT ( 'NONE',  ( 20.88017736071110164, 10.35535201082150714, 2.915334737309930979 ) ) ;
#34822=CARTESIAN_POINT ( 'NONE',  ( 0.5774900079438607392, 3.480352010821504916, 5.440088680355550821 ) ) ;
#34823=CARTESIAN_POINT ( 'NONE',  ( 19.84674366389459621, 3.508931151000785231, 7.409399052514197653E-17 ) ) ;
#34824=CARTESIAN_POINT ( 'NONE',  ( 6.204703633549690345, 15.76208216824730179, -14.16423886937410259 ) ) ;
#34825=CARTESIAN_POINT ( 'NONE',  ( -0.8801773607111009756, 18.06368534415484106, 1.068504757029289695E-15 ) ) ;
#34826=CARTESIAN_POINT ( 'NONE',  ( 5.076628168052704559, 60.17559781766745175, -8.527530157486179263 ) ) ;
#34828=CARTESIAN_POINT ( 'NONE',  ( 10.00000000000000000, 64.75893115100078035, -9.846743663894594434 ) ) ;
#34831=CARTESIAN_POINT ( 'NONE',  ( 10.00000000000000000, 46.81368534415484106, -10.88017736071110342 ) ) ;
#34832=CARTESIAN_POINT ( 'NONE',  ( 1.472469842513823179, 65.59226448433412315, -4.923371831947296329 ) ) ;
#34833=CARTESIAN_POINT ( 'NONE',  ( 2.035157376598822676, 7.438685344154837509, -7.964842623401177768 ) ) ;
#34835=CARTESIAN_POINT ( 'NONE',  ( 19.42250999205614548, 55.98035201082150536, -5.440088680355545492 ) ) ;
#34836=CARTESIAN_POINT ( 'NONE',  ( 2.035157376598824452, 3.688685344154837953, 7.964842623401179544 ) ) ;
#34837=CARTESIAN_POINT ( 'NONE',  ( 13.43411237798105340, 45.58196800326374643, 12.81628187352647963 ) ) ;
#34838=CARTESIAN_POINT ( 'NONE',  ( 10.00000000000000178, 24.31368534415484106, 10.88017736071110342 ) ) ;
#34840=ORIENTED_EDGE ( 'NONE', *, *, #54391, .T. ) ;
#34841=CARTESIAN_POINT ( 'NONE',  ( 22.81628187352647785, 36.41530133659707502, 3.434112377981063169 ) ) ;
#34842=CARTESIAN_POINT ( 'NONE',  ( 10.00000000000000178, 39.31368534415484106, 10.88017736071110342 ) ) ;
#34843=CARTESIAN_POINT ( 'NONE',  ( 12.63842701281683034, 52.46726448433413026, 9.846743663894596210 ) ) ;
#34845=CARTESIAN_POINT ( 'NONE',  ( 5.076628168052703671, 66.84226448433412315, 8.527530157486179263 ) ) ;
#34847=CARTESIAN_POINT ( 'NONE',  ( 0.1532563361054083140, 51.00893115100078745, 1.131784320476157264E-15 ) ) ;
#34848=CARTESIAN_POINT ( 'NONE',  ( 12.91533473730993009, 26.60535201082150536, -10.88017736071109987 ) ) ;
#34849=( NAMED_UNIT ( * ) SI_UNIT ( $, .STERADIAN. ) SOLID_ANGLE_UNIT ( ) );
#34850=CARTESIAN_POINT ( 'NONE',  ( 10.00000000000000178, 37.25893115100078745, 9.846743663894594434 ) ) ;
#34854=CARTESIAN_POINT ( 'NONE',  ( 10.00000000000000178, 47.25893115100078745, 9.846743663894594434 ) ) ;
#34856=CARTESIAN_POINT ( 'NONE',  ( 19.84674366389459266, 13.30059781766745353, 2.638427012816836559 ) ) ;
#34857=CARTESIAN_POINT ( 'NONE',  ( 14.92337183194729988, 54.34226448433412315, -8.527530157486177487 ) ) ;
#34860=VECTOR ( 'NONE', #8039, 1000.000000000000000 ) ;
#34861=SURFACE_STYLE_USAGE ( .BOTH. , #97866 ) ;
#34863=CARTESIAN_POINT ( 'NONE',  ( -1.099225684535947600, 34.54030133659708923, 6.408140936763237150 ) ) ;
#34864=CARTESIAN_POINT ( 'NONE',  ( 7.361572987183170547, 42.05059781766745886, 9.846743663894590881 ) ) ;
#34866=CARTESIAN_POINT ( 'NONE',  ( 2.917880565312950480, 55.97041550158063217, -12.26659068614894821 ) ) ;
#34867=CARTESIAN_POINT ( 'NONE',  ( 19.84674366389459266, 38.30059781766745175, 2.638427012816836559 ) ) ;
#34869=CARTESIAN_POINT ( 'NONE',  ( 6.204703633549690345, 55.76208216824730357, -14.16423886937410259 ) ) ;
#34870=CARTESIAN_POINT ( 'NONE',  ( 7.361572987183170547, 67.05059781766746596, 9.846743663894590881 ) ) ;
#34871=CARTESIAN_POINT ( 'NONE',  ( 20.88017736071110519, 5.563685344154838397, 2.639326808657452039E-16 ) ) ;
#34872=CARTESIAN_POINT ( 'NONE',  ( 6.204703633549690345, 30.76208216824730357, -14.16423886937410259 ) ) ;
#34873=CARTESIAN_POINT ( 'NONE',  ( 10.00000000000000000, 50.55374883491396787, -14.16423886937410082 ) ) ;
#34876=CARTESIAN_POINT ( 'NONE',  ( 14.92337183194729633, 7.675597817667451750, 8.527530157486181039 ) ) ;
#34877=CARTESIAN_POINT ( 'NONE',  ( 0.5774900079438607392, 28.48035201082150891, 5.440088680355550821 ) ) ;
#34878=CARTESIAN_POINT ( 'NONE',  ( 19.38216949554541202, 5.998634669930420493, 9.382169495545424454 ) ) ;
#34879=ORIENTED_EDGE ( 'NONE', *, *, #83431, .T. ) ;
#34880=CARTESIAN_POINT ( 'NONE',  ( 2.035157376598822676, 52.43868534415483396, -7.964842623401177768 ) ) ;
#34883=CARTESIAN_POINT ( 'NONE',  ( 19.84674366389459266, 53.30059781766744464, 2.638427012816836559 ) ) ;
#34884=SURFACE_STYLE_FILL_AREA ( #58364 ) ;
#34886=VERTEX_POINT ( 'NONE', #65755 ) ;
#34887=CARTESIAN_POINT ( 'NONE',  ( 17.08211943468705840, 25.13708216824730357, -12.26659068614894466 ) ) ;
#34888=CARTESIAN_POINT ( 'NONE',  ( 0.2751277870542906956, 37.28217586085238366, -6.499999999999992006 ) ) ;
#34889=SURFACE_STYLE_USAGE ( .BOTH. , #97394 ) ;
#34890=CARTESIAN_POINT ( 'NONE',  ( 19.42250999205614548, 25.98035201082150891, -5.440088680355545492 ) ) ;
#34891=CARTESIAN_POINT ( 'NONE',  ( 10.00000000000000178, 35.37363466993042493, 12.81628187352647608 ) ) ;
#34894=CARTESIAN_POINT ( 'NONE',  ( 12.63842701281683922, 9.550597817667449974, -9.846743663894590881 ) ) ;
#34898=CARTESIAN_POINT ( 'NONE',  ( 20.36894250292379382, 33.67874883491396076, 10.36894250292379205 ) ) ;
#34900=CARTESIAN_POINT ( 'NONE',  ( 0.5774900079438590739, 12.64701867748817321, -5.440088680355550821 ) ) ;
#34901=CARTESIAN_POINT ( 'NONE',  ( -26.69000000000001194, 92.00000000000000000, 9.500000000000000000 ) ) ;
#34904=CARTESIAN_POINT ( 'NONE',  ( 19.42250999205614193, 45.14701867748817676, 5.440088680355555262 ) ) ;
#34905=CARTESIAN_POINT ( 'NONE',  ( 2.035157376598824452, 48.68868534415483396, 7.964842623401179544 ) ) ;
#34906=CARTESIAN_POINT ( 'NONE',  ( 6.565887622018943937, 13.08196800326374998, -12.81628187352647608 ) ) ;
#34909=CARTESIAN_POINT ( 'NONE',  ( 7.361572987183169658, 4.967264484334119601, -9.846743663894592657 ) ) ;
#34911=CARTESIAN_POINT ( 'NONE',  ( -0.8801773607110991993, 42.85535201082150536, -2.915334737309923874 ) ) ;
#34912=CARTESIAN_POINT ( 'NONE',  ( -2.816281873526471635, 8.915301336597083903, -3.434112377981056508 ) ) ;
#34913=CARTESIAN_POINT ( 'NONE',  ( -0.8801773607110991993, 57.85535201082149825, -2.915334737309923874 ) ) ;
#34914=CARTESIAN_POINT ( 'NONE',  ( 1.472469842513823179, 20.59226448433411960, -4.923371831947296329 ) ) ;
#34915=CARTESIAN_POINT ( 'NONE',  ( 0.6178305044545838731, 49.74863466993041072, 9.382169495545420901 ) ) ;
#34916=CARTESIAN_POINT ( 'NONE',  ( 19.84674366389459266, 8.300597817667451750, 2.638427012816836559 ) ) ;
#34918=DIRECTION ( 'NONE',  ( 0.000000000000000000, -1.000000000000000000, 0.000000000000000000 ) ) ;
#34919=CARTESIAN_POINT ( 'NONE',  ( 19.72487221294570858, 26.86607318730131055, 6.500000000000000888 ) ) ;
#34920=CARTESIAN_POINT ( 'NONE',  ( 15.44008868035555260, 14.73035201082150536, 9.422509992056143702 ) ) ;
#34921=CARTESIAN_POINT ( 'NONE',  ( 6.565887622018943937, 63.08196800326376064, -12.81628187352647608 ) ) ;
#34922=CARTESIAN_POINT ( 'NONE',  ( 5.076628168052703671, 31.84226448433412315, 8.527530157486179263 ) ) ;
#34924=CARTESIAN_POINT ( 'NONE',  ( 0.5774900079438590739, 12.64701867748817143, -5.440088680355550821 ) ) ;
#34925=CARTESIAN_POINT ( 'NONE',  ( -0.8801773607111008646, 3.272018677488171434, 2.915334737309923430 ) ) ;
#34927=CARTESIAN_POINT ( 'NONE',  ( 15.44008868035555260, 14.73035201082150536, 9.422509992056143702 ) ) ;
#34929=COLOUR_RGB ( '', 0.31764706, 0.68627451, 0.89019608) ;
#34930=CARTESIAN_POINT ( 'NONE',  ( 20.88017736071110164, 35.35535201082150536, 2.915334737309930979 ) ) ;
#34932=CARTESIAN_POINT ( 'NONE',  ( 15.44008868035555793, 21.39701867748817321, -9.422509992056140149 ) ) ;
#34935=CARTESIAN_POINT ( 'NONE',  ( 15.44008868035555260, 19.73035201082150536, 9.422509992056143702 ) ) ;
#34936=CARTESIAN_POINT ( 'NONE',  ( 10.00000000000000000, 64.75893115100078035, -9.846743663894594434 ) ) ;
#34937=CARTESIAN_POINT ( 'NONE',  ( -1.099225684535947600, 58.70696800326375353, -6.408140936763238038 ) ) ;
#34939=CARTESIAN_POINT ( 'NONE',  ( -2.266590686148945544, 37.22041550158063217, 7.082119434687048631 ) ) ;
#34940=CARTESIAN_POINT ( 'NONE',  ( -0.8801773607110991993, 42.85535201082150536, -2.915334737309923874 ) ) ;
#34941=CARTESIAN_POINT ( 'NONE',  ( 10.00000000000000000, 21.81368534415484106, -10.88017736071110342 ) ) ;
#34944=CARTESIAN_POINT ( 'NONE',  ( 1.472469842513823179, 55.59226448433412315, -4.923371831947296329 ) ) ;
#34945=CARTESIAN_POINT ( 'NONE',  ( 18.52753015748617571, 18.09226448433411960, 4.923371831947298993 ) ) ;
#34947=( BOUNDED_CURVE ( )  B_SPLINE_CURVE ( 2, ( #31534, #23082, #8069, #38566, #22092, #69061, #77045, #52569, #31042 ),
 .UNSPECIFIED., .F., .F. ) 
 B_SPLINE_CURVE_WITH_KNOTS ( ( 3, 2, 2, 2, 3 ),
 ( 0.1525141644748393699, 0.1547619047619047672, 0.1607142857142857262, 0.1666666666666666574, 0.1689144069537320547 ),
 .UNSPECIFIED. ) 
 CURVE ( )  GEOMETRIC_REPRESENTATION_ITEM ( )  RATIONAL_B_SPLINE_CURVE ( ( 0.9839835555609424134, 0.9871328979762477029, 1.000000000000000000, 0.9659258262890683122, 1.000000000000000000, 0.9659258262890683122, 1.000000000000000000, 0.9871328979762477029, 0.9839835555609424134 ) ) 
 REPRESENTATION_ITEM ( '' )  );
#34948=CARTESIAN_POINT ( 'NONE',  ( -0.8801773607111009756, 13.06368534415483929, 1.068504757029289695E-15 ) ) ;
#34949=CARTESIAN_POINT ( 'NONE',  ( 14.92337183194729633, 7.675597817667451750, 8.527530157486181039 ) ) ;
#34950=CARTESIAN_POINT ( 'NONE',  ( 6.565887622018943937, 13.08196800326374998, -12.81628187352647608 ) ) ;
#34951=CARTESIAN_POINT ( 'NONE',  ( 0.5774900079438607392, 63.48035201082149825, 5.440088680355550821 ) ) ;
#34952=CARTESIAN_POINT ( 'NONE',  ( 15.44008868035555260, 24.73035201082150891, 9.422509992056143702 ) ) ;
#34953=CARTESIAN_POINT ( 'NONE',  ( 3.591859063236763294, 63.29030133659708923, -11.09922568453595026 ) ) ;
#34954=CARTESIAN_POINT ( 'NONE',  ( 20.36894250292379382, 33.67874883491396076, 10.36894250292379205 ) ) ;
#34955=SURFACE_SIDE_STYLE ('',( #11972 ) ) ;
#34956=( BOUNDED_CURVE ( )  B_SPLINE_CURVE ( 3, ( #50367, #13360, #51857, #74340 ),
 .UNSPECIFIED., .F., .F. ) 
 B_SPLINE_CURVE_WITH_KNOTS ( ( 4, 4 ),
 ( 4.712388980384689674, 6.283185307179586232 ),
 .UNSPECIFIED. ) 
 CURVE ( )  GEOMETRIC_REPRESENTATION_ITEM ( )  RATIONAL_B_SPLINE_CURVE ( ( 1.000000000000000000, 0.8047378541243649375, 0.8047378541243649375, 1.000000000000000000 ) ) 
 REPRESENTATION_ITEM ( '' )  );
#34957=CARTESIAN_POINT ( 'NONE',  ( 13.43411237798105340, 60.58196800326376064, 12.81628187352647963 ) ) ;
#34958=ORIENTED_EDGE ( 'NONE', *, *, #91567, .F. ) ;
#34959=CARTESIAN_POINT ( 'NONE',  ( -1.099225684535947600, 3.706968003263753531, -6.408140936763238038 ) ) ;
#34960=CARTESIAN_POINT ( 'NONE',  ( -0.3289641300568005855, 14.27164270246084143, -5.963430220938281678 ) ) ;
#34961=CARTESIAN_POINT ( 'NONE',  ( 7.084665262690076126, 34.10535201082151247, 10.88017736071109987 ) ) ;
#34964=CARTESIAN_POINT ( 'NONE',  ( 12.63842701281683034, 12.46726448433411782, 9.846743663894596210 ) ) ;
#34965=VECTOR ( 'NONE', #31594, 1000.000000000000000 ) ;
#34966=CARTESIAN_POINT ( 'NONE',  ( 5.076628168052703671, 11.84226448433411960, 8.527530157486179263 ) ) ;
#34967=CARTESIAN_POINT ( 'NONE',  ( 2.791683348922240793, 16.63393115100078745, 7.208316651077764092 ) ) ;
#34968=CARTESIAN_POINT ( 'NONE',  ( 19.84674366389459266, 13.71726448433411782, -2.638427012816827677 ) ) ;
#34969=CARTESIAN_POINT ( 'NONE',  ( 12.63842701281683034, 2.467264484334118269, 9.846743663894596210 ) ) ;
#34970=EDGE_CURVE ( 'NONE', #93851, #54718, #4784, .T. ) ;
#34971=CARTESIAN_POINT ( 'NONE',  ( 17.20831665107776587, 2.883931151000785231, 7.208316651077764980 ) ) ;
#34973=CARTESIAN_POINT ( 'NONE',  ( 14.92337183194729988, 4.342264484334117824, -8.527530157486177487 ) ) ;
#34974=CARTESIAN_POINT ( 'NONE',  ( 14.92337183194729633, 17.67559781766745175, 8.527530157486181039 ) ) ;
#34975=CARTESIAN_POINT ( 'NONE',  ( -23.44000000000000838, 92.00000000000000000, 9.500000000000000000 ) ) ;
#34976=CARTESIAN_POINT ( 'NONE',  ( 0.6178305044545838731, 4.748634669930420493, 9.382169495545420901 ) ) ;
#34977=ORIENTED_EDGE ( 'NONE', *, *, #83021, .F. ) ;
#34978=ORIENTED_EDGE ( 'NONE', *, *, #51562, .F. ) ;
#34979=CARTESIAN_POINT ( 'NONE',  ( 20.88017736071110164, 5.355352010821502695, 2.915334737309930979 ) ) ;
#34980=CARTESIAN_POINT ( 'NONE',  ( -2.266590686148945544, 16.38708216824730357, -7.082119434687050408 ) ) ;
#34982=CARTESIAN_POINT ( 'NONE',  ( 17.08211943468705130, 13.47041550158063572, 12.26659068614894998 ) ) ;
#34983=CARTESIAN_POINT ( 'NONE',  ( 10.00000000000000178, 38.05374883491396787, 14.16423886937410082 ) ) ;
#34984=CARTESIAN_POINT ( 'NONE',  ( -4.164238869374099927, 2.012082168247300906, 3.795296366450308767 ) ) ;
#34985=CARTESIAN_POINT ( 'NONE',  ( 19.42250999205614193, 40.14701867748817676, 5.440088680355555262 ) ) ;
#34987=CARTESIAN_POINT ( 'NONE',  ( 0.1532563361054083140, 16.00893115100078390, 1.131784320476157264E-15 ) ) ;
#34988=CARTESIAN_POINT ( 'NONE',  ( -0.8801773607111009756, 63.06368534415484106, 1.068504757029289695E-15 ) ) ;
#34989=CARTESIAN_POINT ( 'NONE',  ( 10.00000000000000178, 27.25893115100078390, 9.846743663894594434 ) ) ;
#34991=CARTESIAN_POINT ( 'NONE',  ( 12.91533473730993009, 11.60535201082150714, -10.88017736071109987 ) ) ;
#34992=CARTESIAN_POINT ( 'NONE',  ( 21.09922568453595559, 52.04030133659708923, -6.408140936763230044 ) ) ;
#34993=CARTESIAN_POINT ( 'NONE',  ( 10.00000000000000000, 49.75893115100078745, -9.846743663894594434 ) ) ;
#34994=( GEOMETRIC_REPRESENTATION_CONTEXT ( 3 ) GLOBAL_UNCERTAINTY_ASSIGNED_CONTEXT ( ( #35285 ) ) GLOBAL_UNIT_ASSIGNED_CONTEXT ( ( #67058, #69039, #37563 ) ) REPRESENTATION_CONTEXT ( 'NONE', 'WORKASPACE' ) );
#34995=CARTESIAN_POINT ( 'NONE',  ( 5.500000000000000000, 11.00000000000000000, 6.500000000000000888 ) ) ;
#34996=CARTESIAN_POINT ( 'NONE',  ( 16.40814093676324603, 22.45696800326375353, -11.09922568453594671 ) ) ;
#34998=CARTESIAN_POINT ( 'NONE',  ( 18.52753015748618282, 43.92559781766745175, -4.923371831947291888 ) ) ;
#34999=CARTESIAN_POINT ( 'NONE',  ( -0.3689425029237881626, 17.42874883491397142, 10.36894250292379027 ) ) ;
#35001=ORIENTED_EDGE ( 'NONE', *, *, #26901, .F. ) ;
#35002=CARTESIAN_POINT ( 'NONE',  ( 7.084665262690076126, 49.10535201082149825, 10.88017736071109987 ) ) ;
#35003=CARTESIAN_POINT ( 'NONE',  ( 19.42250999205614548, 50.98035201082151247, -5.440088680355545492 ) ) ;
#35004=CARTESIAN_POINT ( 'NONE',  ( -0.3689425029237898834, 46.17874883491397497, -10.36894250292378850 ) ) ;
#35005=CARTESIAN_POINT ( 'NONE',  ( 0.1532563361054083140, 56.00893115100078745, 1.131784320476157264E-15 ) ) ;
#35007=CARTESIAN_POINT ( 'NONE',  ( -0.8801773607110991993, 37.85535201082151247, -2.915334737309923874 ) ) ;
#35009=CYLINDRICAL_SURFACE ( 'NONE', #32649, 0.5000000000000004441 ) ;
#35011=CARTESIAN_POINT ( 'NONE',  ( 22.81628187352648496, 21.83196800326374643, -3.434112377981050290 ) ) ;
#35012=CARTESIAN_POINT ( 'NONE',  ( 19.84674366389459266, 58.30059781766745886, 2.638427012816836559 ) ) ;
#35014=CARTESIAN_POINT ( 'NONE',  ( 17.96484262340118221, 6.188685344154836621, -7.964842623401177768 ) ) ;
#35015=CARTESIAN_POINT ( 'NONE',  ( -0.8801773607111009756, 63.06368534415484106, 1.068504757029289695E-15 ) ) ;
#35018=CARTESIAN_POINT ( 'NONE',  ( 19.42250999205614193, 5.147018677488171434, 5.440088680355555262 ) ) ;
#35019=CARTESIAN_POINT ( 'NONE',  ( 20.03932841506542673, 65.62161441960505215, -6.397827110478995216 ) ) ;
#35020=CARTESIAN_POINT ( 'NONE',  ( 12.91533473730993009, 61.60535201082150536, -10.88017736071109987 ) ) ;
#35021=CARTESIAN_POINT ( 'NONE',  ( 10.00000000000000178, 2.258931151000784787, 9.846743663894594434 ) ) ;
#35023=CARTESIAN_POINT ( 'NONE',  ( 0.1532563361054082862, 31.21726448433412315, 2.638427012816831674 ) ) ;
#35024=CARTESIAN_POINT ( 'NONE',  ( -0.8801773607110991993, 22.85535201082150181, -2.915334737309923874 ) ) ;
#35025=CARTESIAN_POINT ( 'NONE',  ( 22.81628187352648496, 11.83196800326375531, -3.434112377981050290 ) ) ;
#35026=CARTESIAN_POINT ( 'NONE',  ( 17.96484262340118221, 34.93868534415482685, 7.964842623401181321 ) ) ;
#35028=CARTESIAN_POINT ( 'NONE',  ( 22.81628187352648496, 36.83196800326376064, -3.434112377981050290 ) ) ;
#35030=CARTESIAN_POINT ( 'NONE',  ( 2.035157376598824452, 58.68868534415482685, 7.964842623401179544 ) ) ;
#35031=CARTESIAN_POINT ( 'NONE',  ( 3.591859063236763294, 18.29030133659708568, -11.09922568453595026 ) ) ;
#35032=CARTESIAN_POINT ( 'NONE',  ( 19.84674366389459266, 18.71726448433411960, -2.638427012816827677 ) ) ;
#35033=CARTESIAN_POINT ( 'NONE',  ( 0.5774900079438590739, 22.64701867748817321, -5.440088680355550821 ) ) ;
#35034=CARTESIAN_POINT ( 'NONE',  ( 17.08211943468705130, 58.47041550158063927, 12.26659068614894998 ) ) ;
#35035=CARTESIAN_POINT ( 'NONE',  ( 7.361572987183169658, 49.96726448433410894, -9.846743663894592657 ) ) ;
#35037=CARTESIAN_POINT ( 'NONE',  ( 17.20831665107776587, 4.133931151000785675, -7.208316651077762316 ) ) ;
#35039=CARTESIAN_POINT ( 'NONE',  ( 12.91533473730992121, 59.52201867748816966, 10.88017736071110164 ) ) ;
#35041=CARTESIAN_POINT ( 'NONE',  ( 17.08211943468705130, 33.47041550158063927, 12.26659068614894998 ) ) ;
#35042=EDGE_CURVE ( 'NONE', #6459, #56172, #65745, .T. ) ;
#35043=CARTESIAN_POINT ( 'NONE',  ( 20.15039907845753575, 7.627771745786129820, -6.262539305110077059 ) ) ;
#35045=VERTEX_POINT ( 'NONE', #95263 ) ;
#35047=CARTESIAN_POINT ( 'NONE',  ( 17.08211943468705130, 48.47041550158063927, 12.26659068614894998 ) ) ;
#35048=CARTESIAN_POINT ( 'NONE',  ( 22.26659068614895176, 49.72041550158063927, -7.082119434687042414 ) ) ;
#35049=CARTESIAN_POINT ( 'NONE',  ( 18.52753015748617571, 18.09226448433411960, 4.923371831947298993 ) ) ;
#35050=CARTESIAN_POINT ( 'NONE',  ( -2.816281873526473856, 24.12363466993042138, 9.499525473075851096E-16 ) ) ;
#35053=( NAMED_UNIT ( * ) SI_UNIT ( $, .STERADIAN. ) SOLID_ANGLE_UNIT ( ) );
#35054=CARTESIAN_POINT ( 'NONE',  ( -4.164238869374099039, 46.80374883491397497, 8.674139862899312516E-16 ) ) ;
#35056=CARTESIAN_POINT ( 'NONE',  ( 12.63842701281683922, 9.550597817667449974, -9.846743663894590881 ) ) ;
#35061=SURFACE_STYLE_USAGE ( .BOTH. , #72567 ) ;
#35062=ORIENTED_EDGE ( 'NONE', *, *, #18270, .T. ) ;
#35065=CARTESIAN_POINT ( 'NONE',  ( -0.8801773607111008646, 13.27201867748817321, 2.915334737309923430 ) ) ;
#35066=CARTESIAN_POINT ( 'NONE',  ( 0.5774900079438590739, 27.64701867748817676, -5.440088680355550821 ) ) ;
#35067=CARTESIAN_POINT ( 'NONE',  ( 0.1532563361054083140, 46.00893115100079456, 1.131784320476157264E-15 ) ) ;
#35068=CARTESIAN_POINT ( 'NONE',  ( 21.09922568453595559, 17.04030133659708923, -6.408140936763230044 ) ) ;
#35069=SURFACE_STYLE_FILL_AREA ( #71622 ) ;
#35071=CARTESIAN_POINT ( 'NONE',  ( 0.6178305044545838731, 19.74863466993042138, 9.382169495545420901 ) ) ;
#35073=CARTESIAN_POINT ( 'NONE',  ( 5.076628168052704559, 35.17559781766745175, -8.527530157486179263 ) ) ;
#35074=CARTESIAN_POINT ( 'NONE',  ( -4.164238869374098151, 66.59541550158060375, -3.795296366450310543 ) ) ;
#35076=CARTESIAN_POINT ( 'NONE',  ( 19.42250999205614193, 10.14701867748816966, 5.440088680355555262 ) ) ;
#35078=CARTESIAN_POINT ( 'NONE',  ( 4.559911319644449179, 48.89701867748817676, 9.422509992056141925 ) ) ;
#35080=CARTESIAN_POINT ( 'NONE',  ( -0.8801773607111009756, 43.06368534415484106, 1.068504757029289695E-15 ) ) ;
#35081=CARTESIAN_POINT ( 'NONE',  ( 20.88017736071110519, 45.56368534415484106, 2.639326808657452039E-16 ) ) ;
#35083=CARTESIAN_POINT ( 'NONE',  ( -0.8801773607110991993, 42.85535201082150536, -2.915334737309923874 ) ) ;
#35085=CARTESIAN_POINT ( 'NONE',  ( 21.92686044187656691, 64.95379003517449235, 3.195792623639537755 ) ) ;
#35086=VECTOR ( 'NONE', #45158, 1000.000000000000000 ) ;
#35090=CARTESIAN_POINT ( 'NONE',  ( 2.791683348922240793, 26.63393115100078745, 7.208316651077764092 ) ) ;
#35092=CARTESIAN_POINT ( 'NONE',  ( 12.63842701281683034, 57.46726448433411605, 9.846743663894596210 ) ) ;
#35098=CARTESIAN_POINT ( 'NONE',  ( 18.72515096720579209, 51.07228050351030646, -6.499999999999869438 ) ) ;
#35100=CARTESIAN_POINT ( 'NONE',  ( 0.1532563361054082862, 61.21726448433412315, 2.638427012816831674 ) ) ;
#35101=CARTESIAN_POINT ( 'NONE',  ( -0.3689425029237881626, 67.42874883491396076, 10.36894250292379027 ) ) ;
#35105=CARTESIAN_POINT ( 'NONE',  ( 17.20831665107776587, 34.13393115100078745, -7.208316651077762316 ) ) ;
#35106=CARTESIAN_POINT ( 'NONE',  ( 22.81628187352648496, 61.83196800326376774, -3.434112377981050290 ) ) ;
#35107=CARTESIAN_POINT ( 'NONE',  ( 16.40814093676323893, 0.7903013365970867898, 11.09922568453595026 ) ) ;
#35108=CARTESIAN_POINT ( 'NONE',  ( 10.00000000000000000, 14.75893115100078568, -9.846743663894594434 ) ) ;
#35110=CARTESIAN_POINT ( 'NONE',  ( 17.20831665107776587, 9.133931151000787452, -7.208316651077762316 ) ) ;
#35111=CARTESIAN_POINT ( 'NONE',  ( 0.1532563361054100626, 55.80059781766745175, -2.638427012816831230 ) ) ;
#35114=ORIENTED_EDGE ( 'NONE', *, *, #85593, .T. ) ;
#35115=CARTESIAN_POINT ( 'NONE',  ( 15.44008868035555793, 6.397018677488171434, -9.422509992056140149 ) ) ;
#35116=CARTESIAN_POINT ( 'NONE',  ( 6.204703633549690345, 10.76208216824729824, -14.16423886937410259 ) ) ;
#35117=CARTESIAN_POINT ( 'NONE',  ( 12.63842701281683922, 14.55059781766744997, -9.846743663894590881 ) ) ;
#35118=CARTESIAN_POINT ( 'NONE',  ( 20.88017736071110164, 55.35535201082149825, 2.915334737309930979 ) ) ;
#35119=CARTESIAN_POINT ( 'NONE',  ( 6.565887622018943937, 30.16530133659708568, 12.81628187352647430 ) ) ;
#35120=CARTESIAN_POINT ( 'NONE',  ( 10.00000000000000178, 69.31368534415484817, 10.88017736071110342 ) ) ;
#35121=CARTESIAN_POINT ( 'NONE',  ( 2.035157376598822676, 2.438685344154837953, -7.964842623401177768 ) ) ;
#35122=EDGE_CURVE ( 'NONE', #87107, #56172, #24543, .T. ) ;
#35125=CARTESIAN_POINT ( 'NONE',  ( 16.40814093676324603, 7.456968003263754419, -11.09922568453594671 ) ) ;
#35126=CARTESIAN_POINT ( 'NONE',  ( 3.591859063236761518, -0.04303199673624671928, 11.09922568453594849 ) ) ;
#35127=CARTESIAN_POINT ( 'NONE',  ( 7.361572987183169658, 9.967264484334119601, -9.846743663894592657 ) ) ;
#35129=CARTESIAN_POINT ( 'NONE',  ( 19.38216949554541202, 25.99863466993042138, 9.382169495545424454 ) ) ;
#35131=CARTESIAN_POINT ( 'NONE',  ( 0.5774900079438590739, 22.64701867748817321, -5.440088680355550821 ) ) ;
#35133=CARTESIAN_POINT ( 'NONE',  ( 2.917880565312948704, 52.63708216824730357, 12.26659068614894643 ) ) ;
#35135=CARTESIAN_POINT ( 'NONE',  ( 22.81628187352647785, 51.41530133659708923, 3.434112377981063169 ) ) ;
#35136=CARTESIAN_POINT ( 'NONE',  ( -0.8801773607111008646, 28.27201867748817321, 2.915334737309923430 ) ) ;
#35138=CARTESIAN_POINT ( 'NONE',  ( 2.791683348922237240, 55.38393115100078745, -7.208316651077763204 ) ) ;
#35139=CARTESIAN_POINT ( 'NONE',  ( 20.88017736071110519, 55.56368534415484817, 2.639326808657452039E-16 ) ) ;
#35140=CARTESIAN_POINT ( 'NONE',  ( 24.16423886937409904, 29.09541550158063572, 3.795296366450317205 ) ) ;
#35143=CARTESIAN_POINT ( 'NONE',  ( 12.63842701281683034, 32.46726448433412315, 9.846743663894596210 ) ) ;
#35144=SURFACE_STYLE_USAGE ( .BOTH. , #66136 ) ;
#35145=CARTESIAN_POINT ( 'NONE',  ( -1.099225684535947600, -1.293031996736246469, -6.408140936763238038 ) ) ;
#35147=CARTESIAN_POINT ( 'NONE',  ( 20.88017736071110519, 30.56368534415484106, 2.639326808657452039E-16 ) ) ;
#35148=LINE ( 'NONE', #5169, #78027 ) ;
#35151=CARTESIAN_POINT ( 'NONE',  ( 12.91533473730993009, 11.60535201082150714, -10.88017736071109987 ) ) ;
#35152=CARTESIAN_POINT ( 'NONE',  ( 2.917880565312950480, 25.97041550158063572, -12.26659068614894821 ) ) ;
#35153=CARTESIAN_POINT ( 'NONE',  ( 19.84674366389459266, 8.300597817667451750, 2.638427012816836559 ) ) ;
#35154=CARTESIAN_POINT ( 'NONE',  ( 7.361572987183169658, 64.96726448433412315, -9.846743663894592657 ) ) ;
#35155=CARTESIAN_POINT ( 'NONE',  ( 12.91533473730992121, 39.52201867748817676, 10.88017736071110164 ) ) ;
#35156=CARTESIAN_POINT ( 'NONE',  ( 19.72487221294570858, 64.78217586085237656, 6.499999999999992895 ) ) ;
#35162=CARTESIAN_POINT ( 'NONE',  ( 2.791683348922237240, 40.38393115100078035, -7.208316651077763204 ) ) ;
#35166=CARTESIAN_POINT ( 'NONE',  ( 10.00000000000000178, 8.053748834913967869, 14.16423886937410082 ) ) ;
#35167=CARTESIAN_POINT ( 'NONE',  ( 10.00000000000000178, 13.05374883491396787, 14.16423886937410082 ) ) ;
#35168=CARTESIAN_POINT ( 'NONE',  ( -0.8801773607111009756, 43.06368534415484106, 1.068504757029289695E-15 ) ) ;
#35169=CARTESIAN_POINT ( 'NONE',  ( -4.164238869374098151, 51.59541550158063217, -3.795296366450310543 ) ) ;
#35170=CARTESIAN_POINT ( 'NONE',  ( 10.00000000000000178, 37.25893115100078745, 9.846743663894594434 ) ) ;
#35172=CARTESIAN_POINT ( 'NONE',  ( -0.8801773607111008646, 33.27201867748817676, 2.915334737309923430 ) ) ;
#35173=CARTESIAN_POINT ( 'NONE',  ( -1.099225684535947600, 9.540301336597087456, 6.408140936763237150 ) ) ;
#35174=CARTESIAN_POINT ( 'NONE',  ( -2.266590686148945544, 6.387082168247300906, -7.082119434687050408 ) ) ;
#35175=CARTESIAN_POINT ( 'NONE',  ( 24.16423886937410614, 49.30374883491396787, 8.672049930838204340E-16 ) ) ;
#35176=CARTESIAN_POINT ( 'NONE',  ( 0.5774900079438607392, 3.480352010821504916, 5.440088680355550821 ) ) ;
#35177=CARTESIAN_POINT ( 'NONE',  ( -0.3289641300568009741, 67.24545670184114954, -5.963430220938281678 ) ) ;
#35184=CARTESIAN_POINT ( 'NONE',  ( -4.164238869374099927, 52.01208216824729647, 3.795296366450308767 ) ) ;
#35185=CARTESIAN_POINT ( 'NONE',  ( 7.361572987183170547, 52.05059781766745175, 9.846743663894590881 ) ) ;
#35186=CARTESIAN_POINT ( 'NONE',  ( 4.559911319644449179, 52.23035201082151247, -9.422509992056141925 ) ) ;
#35187=CARTESIAN_POINT ( 'NONE',  ( 19.80448550324510038, 36.82703681773342907, 6.500000000002679634 ) ) ;
#35188=CARTESIAN_POINT ( 'NONE',  ( 10.00000000000000000, 56.81368534415484106, -10.88017736071110342 ) ) ;
#35190=CARTESIAN_POINT ( 'NONE',  ( 21.09922568453594849, 56.20696800326375353, 6.408140936763242479 ) ) ;
#35192=ORIENTED_EDGE ( 'NONE', *, *, #36865, .F. ) ;
#35193=CARTESIAN_POINT ( 'NONE',  ( 10.00000000000000000, 15.55374883491396787, -14.16423886937410082 ) ) ;
#35194=EDGE_LOOP ( 'NONE', ( #78004, #14791, #71061, #57122 ) ) ;
#35195=CARTESIAN_POINT ( 'NONE',  ( 16.40814093676324603, 22.45696800326375353, -11.09922568453594671 ) ) ;
#35197=CARTESIAN_POINT ( 'NONE',  ( 16.40814093676323893, 50.79030133659708923, 11.09922568453595026 ) ) ;
#35198=CARTESIAN_POINT ( 'NONE',  ( 7.361572987183170547, 42.05059781766745886, 9.846743663894590881 ) ) ;
#35199=CARTESIAN_POINT ( 'NONE',  ( -0.8801773607111008646, 8.272018677488171434, 2.915334737309923430 ) ) ;
#35200=CARTESIAN_POINT ( 'NONE',  ( -1.099225684535947600, 49.54030133659708923, 6.408140936763237150 ) ) ;
#35201=CARTESIAN_POINT ( 'NONE',  ( -45.94000000000000483, 103.9981609152045650, -5.961202730336930600 ) ) ;
#35202=CARTESIAN_POINT ( 'NONE',  ( 14.92337183194729988, 39.34226448433412315, -8.527530157486177487 ) ) ;
#35204=VECTOR ( 'NONE', #62667, 1000.000000000000000 ) ;
#35207=DIRECTION ( 'NONE',  ( 0.000000000000000000, -1.000000000000000000, 0.000000000000000000 ) ) ;
#35210=CARTESIAN_POINT ( 'NONE',  ( 19.84674366389459621, 23.50893115100078390, 7.409399052514197653E-17 ) ) ;
#35212=CARTESIAN_POINT ( 'NONE',  ( -1.099225684535947600, 24.54030133659708923, 6.408140936763237150 ) ) ;
#35217=CARTESIAN_POINT ( 'NONE',  ( 17.20831665107776587, 57.88393115100078745, 7.208316651077764980 ) ) ;
#35219=CARTESIAN_POINT ( 'NONE',  ( 22.26659068614894466, 23.88708216824730357, 7.082119434687054849 ) ) ;
#35220=CARTESIAN_POINT ( 'NONE',  ( 19.84674366389459266, 28.71726448433411960, -2.638427012816827677 ) ) ;
#35221=( BOUNDED_SURFACE ( )  B_SPLINE_SURFACE ( 1, 2, ( 
 ( #36653, #59634, #83130, #82635, #67139, #74129, #5170, #97664, #91119, #14152, #44636, #37153, #98159, #45120, #37643, #45626, #96673, #68140, #98667, #20658, #51154, #97175, #13146, #43645, #5665, #36147, #66651, #76613, #32587, #54102, #32082, #47091, #85104, #84131, #53613, #39124, #1133, #93086, #15643, #31595, #69611, #9104, #92111, #46125, #78094, #70107, #9597, #93582, #25118, #8615, #62581, #55601, #17118, #8129, #54591, #38623, #30609, #23140, #69124, #24617, #61115, #62089, #16615, #77589, #47600, #31104, #16119, #23642, #2127, #656, #46603, #84615, #92598, #86095, #77102, #24121, #39618, #40100, #91624, #1632, #55083, #85603, #70601, #7651, #63082, #17606, #76125, #38144, #68630, #160, #50055, #11075, #72064, #11561, #10101, #58036, #18580, #26560, #41596, #33559, #35033, #34048, #27049, #42554, #40598, #96059, #87071, #64544, #72543, #95051, #57056, #65536, #94567, #3103, #80559, #73037, #48572, #87558, #49072, #88544, #48076, #86586, #57547, #33076, #41095, #79071, #18095, #12053, #19067, #49546, #79575, #80058, #4573, #42080, #71592, #4076, #27542, #71095, #78589, #34539, #88046, #65033, #95560, #2621, #63572, #94081, #19558, #25601, #56093, #64055, #26086, #56581, #89039, #75020, #37034, #58531, #74523, #81040, #67531, #68024, #52031, #6525, #12548, #82524, #96561, #13536, #97062, #82026, #28036, #74025, #52516, #20550, #51035, #60011, #98047, #28535, #44020, #81528, #98552, #6043, #14040, #60509, #36543, #43050, #21540, #66535, #75515, #30002, #97554, #13034, #29503, #43530, #5556, #36032, #59029, #89535, #21045, #67032, #29015, #51534, #20045, #22040, #44521, #5056, #59525, #90506, #83022, #90018, #50546, #14539, #73529, #45009, #7029, #37535, #35540, #66032, #10344, #60998, #94320, #55346, #17364, #55846, #53003, #3333, #62841, #70857, #85853, #77843, #79326, #47833, #71346, #86833, #83517, #41355, #32339, #78336, #17844, #9857, #40356, #10836, #39857, #47340, #25841, #18337, #91509, #2372, #93341, #33795, #91001, #23028, #2864, #76008, #85352, #53500, #16866, #56339, #32827, #63326, #24863, #93834, #48817, #25360, #9352, #86341, #71824, #15036, #22532, #48329, #33315, #78833, #40844, #7536, #38027, #50, #63810, #70363, #1880, #50290, #95814, #27294, #34291, #20302, #81291, #3832, #19799, #26316, #12787, #13288, #96316, #50802, #87312, #27791, #41835, #57793, #42315, #88301, #72302, #19313, #96813, #64788, #95305, #5312, #43287, #72788, #80803, #26809, #43776, #12300, #58276, #5798, #42808, #49310, #65783, #11807, #51288, #64302, #73292, #57303, #73782, #87795, #49799, #80307, #4325, #34797, #65287 ),
 ( #4816, #35790, #35290, #88794, #66278, #94813, #28289, #89289, #58783, #81773, #79812, #11316, #14794, #29757, #21794, #23279, #60265, #15288, #30744, #28777, #84273, #75270, #22289, #60754, #90764, #52762, #53755, #82773, #90261, #68768, #61251, #36789, #83270, #6780, #76746, #36288, #74777, #45770, #21291, #29272, #67283, #6286, #300, #45267, #75762, #37294, #67781, #91756, #7283, #97811, #37784, #15772, #97305, #46261, #98303, #76263, #68281, #98802, #66786, #38275, #59275, #30250, #13785, #91254, #22780, #53259, #83765, #59768, #7780, #89774, #52274, #51784, #82270, #44272, #14293, #44765, #63212, #69263, #40235, #84752, #1763, #85243, #70247, #16257, #62228, #40726, #77237, #46739, #48213, #25251, #16749, #32219, #69751, #86720, #62720, #70743, #48704, #93220, #783, #9735, #54723, #63701, #56226, #85737, #8741, #17738, #31732, #39262, #1279, #92735, #47224, #24259, #55223, #17250, #77727, #18224, #10233, #2259, #92249, #24744, #32714, #93716, #47726, #8263, #78723, #38763, #55735, #9239, #71228, #78224, #86227, #2751, #39750, #33207, #94204, #25734, #31236, #61731, #23774, #54239, #49200, #27179, #88178, #26691, #89170, #81176, #42690, #64186, #72674, #80688, #73169, #57682, #58668, #50684, #20681, #96192, #72191, #12676, #50178, #19691, #27677, #18718, #43176, #42207, #4209, #4708, #41235, #79208, #49681, #12184, #34679, #64673, #66162, #65175, #58162, #73663, #71713, #28174, #19198, #95695, #35170, #65671, #88673, #96695, #57187, #34181, #5190, #35678, #79704, #20181, #80185, #10718, #3224, #11202, #33688, #94706, #3720, #41722, #95183, #26212, #56705, #87195, #11698, #87684, #76141, #22164, #89663, #6659, #68644, #13168, #30622, #52161, #60636, #37175, #14170, #61129, #53139, #43666, #52646, #28664, #98178, #67668, #82654, #44654, #21173, #7158, #68161, #51676, #29634, #74152, #98681, #174, #83149, #37661, #5686, #14674, #59156, #75149, #29148, #60142, #82154, #6169, #83648, #13666, #44150, #91137, #30130, #59654, #90639, #74658, #91639, #45140, #75646, #51175, #22663, #36171, #15163, #97686, #7667, #81659, #45644, #36673, #38158, #67161, #90145, #21675, #66671, #97196, #16133, #78606, #93101, #62103, #76627, #92131, #23656, #10115, #1152, #78109, #24631, #32097, #31118, #668, #85120, #47106, #40116, #61613, #77606, #16631, #55098, #8629, #54118, #25137, #17135, #55615, #40613, #71112, #54604, #9615, #2639, #63098, #84631, #1645, #46619, #8146, #69140, #77117, #70617, #38639, #9119, #62596, #85618, #93600, #39138, #92613, #69628, #48093, #31612, #24137, #39634, #70123, #33093, #47614, #2142, #32602, #86112 ) ),
 .UNSPECIFIED., .F., .F., .T. ) 
 B_SPLINE_SURFACE_WITH_KNOTS ( ( 2, 2 ),
 ( 3, 2, 2, 2, 2, 2, 2, 2, 2, 2, 2, 2, 2, 2, 2, 2, 2, 2, 2, 2, 2, 2, 2, 2, 2, 2, 2, 2, 2, 2, 2, 2, 2, 2, 2, 2, 2, 2, 2, 2, 2, 2, 2, 2, 2, 2, 2, 2, 2, 2, 2, 2, 2, 2, 2, 2, 2, 2, 2, 2, 2, 2, 2, 2, 2, 2, 2, 2, 2, 2, 2, 2, 2, 2, 2, 2, 2, 2, 2, 2, 2, 2, 2, 2, 2, 2, 2, 2, 2, 2, 2, 2, 2, 2, 2, 2, 2, 2, 2, 2, 2, 2, 2, 2, 2, 2, 2, 2, 2, 2, 2, 2, 2, 2, 2, 2, 2, 2, 2, 2, 2, 2, 2, 2, 2, 2, 2, 2, 2, 2, 2, 2, 2, 2, 2, 2, 2, 2, 2, 2, 2, 2, 2, 2, 2, 2, 2, 2, 2, 2, 2, 2, 2, 2, 2, 2, 2, 2, 2, 2, 2, 2, 3 ),
 ( 0.000000000000000000, 1.000000000000000000 ),
 ( 0.000000000000000000, 0.005952380952380952051, 0.01190476190476190410, 0.01785714285714285615, 0.02380952380952380820, 0.02976190476190476025, 0.03571428571428571230, 0.04166666666666666435, 0.04761904761904761640, 0.05357142857142856845, 0.05952380952380952051, 0.06547619047619047949, 0.07142857142857142461, 0.07738095238095238360, 0.08333333333333332871, 0.08928571428571428770, 0.09523809523809523281, 0.1011904761904761918, 0.1071428571428571369, 0.1130952380952380959, 0.1190476190476190410, 0.1250000000000000000, 0.1309523809523809590, 0.1369047619047619180, 0.1428571428571428492, 0.1488095238095238082, 0.1547619047619047672, 0.1607142857142857262, 0.1666666666666666574, 0.1726190476190476164, 0.1785714285714285754, 0.1845238095238095344, 0.1904761904761904656, 0.1964285714285714246, 0.2023809523809523836, 0.2083333333333333426, 0.2142857142857142738, 0.2202380952380952328, 0.2261904761904761918, 0.2321428571428571508, 0.2380952380952380820, 0.2440476190476190410, 0.2500000000000000000, 0.2559523809523809312, 0.2619047619047619180, 0.2678571428571428492, 0.2738095238095238360, 0.2797619047619047672, 0.2857142857142856984, 0.2916666666666666852, 0.2976190476190476164, 0.3035714285714285476, 0.3095238095238095344, 0.3154761904761904656, 0.3214285714285714524, 0.3273809523809523836, 0.3333333333333333148, 0.3392857142857143016, 0.3452380952380952328, 0.3511904761904761640, 0.3571428571428571508, 0.3630952380952380820, 0.3690476190476190688, 0.3750000000000000000, 0.3809523809523809312, 0.3869047619047619180, 0.3928571428571428492, 0.3988095238095238360, 0.4047619047619047672, 0.4107142857142856984, 0.4166666666666666852, 0.4226190476190476164, 0.4285714285714285476, 0.4345238095238095344, 0.4404761904761904656, 0.4464285714285714524, 0.4523809523809523836, 0.4583333333333333148, 0.4642857142857143016, 0.4702380952380952328, 0.4761904761904761640, 0.4821428571428571508, 0.4880952380952380820, 0.4940476190476190688, 0.5000000000000000000, 0.5059523809523809312, 0.5119047619047618625, 0.5178571428571429047, 0.5238095238095238360, 0.5297619047619047672, 0.5357142857142856984, 0.5416666666666666297, 0.5476190476190476719, 0.5535714285714286031, 0.5595238095238095344, 0.5654761904761904656, 0.5714285714285713969, 0.5773809523809523281, 0.5833333333333333703, 0.5892857142857143016, 0.5952380952380952328, 0.6011904761904761640, 0.6071428571428570953, 0.6130952380952381375, 0.6190476190476190688, 0.6250000000000000000, 0.6309523809523809312, 0.6369047619047618625, 0.6428571428571429047, 0.6488095238095238360, 0.6547619047619047672, 0.6607142857142856984, 0.6666666666666666297, 0.6726190476190476719, 0.6785714285714286031, 0.6845238095238095344, 0.6904761904761904656, 0.6964285714285713969, 0.7023809523809523281, 0.7083333333333333703, 0.7142857142857143016, 0.7202380952380952328, 0.7261904761904761640, 0.7321428571428570953, 0.7380952380952381375, 0.7440476190476190688, 0.7500000000000000000, 0.7559523809523809312, 0.7619047619047618625, 0.7678571428571429047, 0.7738095238095238360, 0.7797619047619047672, 0.7857142857142856984, 0.7916666666666666297, 0.7976190476190476719, 0.8035714285714286031, 0.8095238095238095344, 0.8154761904761904656, 0.8214285714285713969, 0.8273809523809523281, 0.8333333333333333703, 0.8392857142857143016, 0.8452380952380952328, 0.8511904761904761640, 0.8571428571428570953, 0.8630952380952381375, 0.8690476190476190688, 0.8750000000000000000, 0.8809523809523809312, 0.8869047619047618625, 0.8928571428571429047, 0.8988095238095238360, 0.9047619047619047672, 0.9107142857142856984, 0.9166666666666666297, 0.9226190476190476719, 0.9285714285714286031, 0.9345238095238095344, 0.9404761904761904656, 0.9464285714285713969, 0.9523809523809523281, 0.9583333333333333703, 0.9642857142857143016 ),
 .UNSPECIFIED. ) 
 GEOMETRIC_REPRESENTATION_ITEM ( )  RATIONAL_B_SPLINE_SURFACE ( (
 ( 1.000000000000000000, 0.9659258262890683122, 1.000000000000000000, 0.9659258262890683122, 1.000000000000000000, 0.9659258262890683122, 1.000000000000000000, 0.9659258262890683122, 1.000000000000000000, 0.9659258262890683122, 1.000000000000000000, 0.9659258262890683122, 1.000000000000000000, 0.9659258262890683122, 1.000000000000000000, 0.9659258262890683122, 1.000000000000000000, 0.9659258262890683122, 1.000000000000000000, 0.9659258262890683122, 1.000000000000000000, 0.9659258262890683122, 1.000000000000000000, 0.9659258262890683122, 1.000000000000000000, 0.9659258262890683122, 1.000000000000000000, 0.9659258262890683122, 1.000000000000000000, 0.9659258262890683122, 1.000000000000000000, 0.9659258262890683122, 1.000000000000000000, 0.9659258262890683122, 1.000000000000000000, 0.9659258262890683122, 1.000000000000000000, 0.9659258262890683122, 1.000000000000000000, 0.9659258262890683122, 1.000000000000000000, 0.9659258262890683122, 1.000000000000000000, 0.9659258262890683122, 1.000000000000000000, 0.9659258262890683122, 1.000000000000000000, 0.9659258262890683122, 1.000000000000000000, 0.9659258262890683122, 1.000000000000000000, 0.9659258262890683122, 1.000000000000000000, 0.9659258262890683122, 1.000000000000000000, 0.9659258262890683122, 1.000000000000000000, 0.9659258262890683122, 1.000000000000000000, 0.9659258262890683122, 1.000000000000000000, 0.9659258262890683122, 1.000000000000000000, 0.9659258262890683122, 1.000000000000000000, 0.9659258262890683122, 1.000000000000000000, 0.9659258262890683122, 1.000000000000000000, 0.9659258262890683122, 1.000000000000000000, 0.9659258262890683122, 1.000000000000000000, 0.9659258262890683122, 1.000000000000000000, 0.9659258262890683122, 1.000000000000000000, 0.9659258262890683122, 1.000000000000000000, 0.9659258262890683122, 1.000000000000000000, 0.9659258262890683122, 1.000000000000000000, 0.9659258262890683122, 1.000000000000000000, 0.9659258262890683122, 1.000000000000000000, 0.9659258262890683122, 1.000000000000000000, 0.9659258262890683122, 1.000000000000000000, 0.9659258262890683122, 1.000000000000000000, 0.9659258262890683122, 1.000000000000000000, 0.9659258262890683122, 1.000000000000000000, 0.9659258262890683122, 1.000000000000000000, 0.9659258262890683122, 1.000000000000000000, 0.9659258262890683122, 1.000000000000000000, 0.9659258262890683122, 1.000000000000000000, 0.9659258262890683122, 1.000000000000000000, 0.9659258262890683122, 1.000000000000000000, 0.9659258262890683122, 1.000000000000000000, 0.9659258262890683122, 1.000000000000000000, 0.9659258262890683122, 1.000000000000000000, 0.9659258262890683122, 1.000000000000000000, 0.9659258262890683122, 1.000000000000000000, 0.9659258262890683122, 1.000000000000000000, 0.9659258262890683122, 1.000000000000000000, 0.9659258262890683122, 1.000000000000000000, 0.9659258262890683122, 1.000000000000000000, 0.9659258262890683122, 1.000000000000000000, 0.9659258262890683122, 1.000000000000000000, 0.9659258262890683122, 1.000000000000000000, 0.9659258262890683122, 1.000000000000000000, 0.9659258262890683122, 1.000000000000000000, 0.9659258262890683122, 1.000000000000000000, 0.9659258262890683122, 1.000000000000000000, 0.9659258262890683122, 1.000000000000000000, 0.9659258262890683122, 1.000000000000000000, 0.9659258262890683122, 1.000000000000000000, 0.9659258262890683122, 1.000000000000000000, 0.9659258262890683122, 1.000000000000000000, 0.9659258262890683122, 1.000000000000000000, 0.9659258262890683122, 1.000000000000000000, 0.9659258262890683122, 1.000000000000000000, 0.9659258262890683122, 1.000000000000000000, 0.9659258262890683122, 1.000000000000000000, 0.9659258262890683122, 1.000000000000000000, 0.9659258262890683122, 1.000000000000000000, 0.9659258262890683122, 1.000000000000000000, 0.9659258262890683122, 1.000000000000000000, 0.9659258262890683122, 1.000000000000000000, 0.9659258262890683122, 1.000000000000000000, 0.9659258262890683122, 1.000000000000000000, 0.9659258262890683122, 1.000000000000000000, 0.9659258262890683122, 1.000000000000000000, 0.9659258262890683122, 1.000000000000000000, 0.9659258262890683122, 1.000000000000000000, 0.9659258262890683122, 1.000000000000000000, 0.9659258262890683122, 1.000000000000000000, 0.9659258262890683122, 1.000000000000000000, 0.9659258262890683122, 1.000000000000000000, 0.9659258262890683122, 1.000000000000000000, 0.9659258262890683122, 1.000000000000000000, 0.9659258262890683122, 1.000000000000000000, 0.9659258262890683122, 1.000000000000000000, 0.9659258262890683122, 1.000000000000000000, 0.9659258262890683122, 1.000000000000000000, 0.9659258262890683122, 1.000000000000000000, 0.9659258262890683122, 1.000000000000000000, 0.9659258262890683122, 1.000000000000000000, 0.9659258262890683122, 1.000000000000000000, 0.9659258262890683122, 1.000000000000000000, 0.9659258262890683122, 1.000000000000000000, 0.9659258262890683122, 1.000000000000000000, 0.9659258262890683122, 1.000000000000000000, 0.9659258262890683122, 1.000000000000000000, 0.9659258262890683122, 1.000000000000000000, 0.9659258262890683122, 1.000000000000000000, 0.9659258262890683122, 1.000000000000000000, 0.9659258262890683122, 1.000000000000000000, 0.9659258262890683122, 1.000000000000000000, 0.9659258262890683122, 1.000000000000000000, 0.9659258262890683122, 1.000000000000000000, 0.9659258262890683122, 1.000000000000000000, 0.9659258262890683122, 1.000000000000000000, 0.9659258262890683122, 1.000000000000000000, 0.9659258262890683122, 1.000000000000000000, 0.9659258262890683122, 1.000000000000000000, 0.9659258262890683122, 1.000000000000000000, 0.9659258262890683122, 1.000000000000000000, 0.9659258262890683122, 1.000000000000000000, 0.9659258262890683122, 1.000000000000000000, 0.9659258262890683122, 1.000000000000000000, 0.9659258262890683122, 1.000000000000000000, 0.9659258262890683122, 1.000000000000000000, 0.9659258262890683122, 1.000000000000000000, 0.9659258262890683122, 1.000000000000000000, 0.9659258262890683122, 1.000000000000000000, 0.9659258262890683122, 1.000000000000000000, 0.9659258262890683122, 1.000000000000000000, 0.9659258262890683122, 1.000000000000000000, 0.9659258262890683122, 1.000000000000000000, 0.9659258262890683122, 1.000000000000000000, 0.9659258262890683122, 1.000000000000000000, 0.9659258262890683122, 1.000000000000000000, 0.9659258262890683122, 1.000000000000000000, 0.9659258262890683122, 1.000000000000000000, 0.9659258262890683122, 1.000000000000000000, 0.9659258262890683122, 1.000000000000000000, 0.9659258262890683122, 1.000000000000000000, 0.9659258262890683122, 1.000000000000000000, 0.9659258262890683122, 1.000000000000000000, 0.9659258262890683122, 1.000000000000000000, 0.9659258262890683122, 1.000000000000000000, 0.9659258262890683122, 1.000000000000000000, 0.9659258262890683122, 1.000000000000000000, 0.9659258262890683122, 1.000000000000000000, 0.9659258262890683122, 1.000000000000000000, 0.9659258262890683122, 1.000000000000000000, 0.9659258262890683122, 1.000000000000000000, 0.9659258262890683122, 1.000000000000000000, 0.9659258262890683122, 1.000000000000000000, 0.9659258262890683122, 1.000000000000000000, 0.9659258262890683122, 1.000000000000000000, 0.9659258262890683122, 1.000000000000000000, 0.9659258262890683122, 1.000000000000000000, 0.9659258262890683122, 1.000000000000000000, 0.9659258262890683122, 1.000000000000000000),
 ( 1.000000000000000000, 0.9659258262890683122, 1.000000000000000000, 0.9659258262890683122, 1.000000000000000000, 0.9659258262890683122, 1.000000000000000000, 0.9659258262890683122, 1.000000000000000000, 0.9659258262890683122, 1.000000000000000000, 0.9659258262890683122, 1.000000000000000000, 0.9659258262890683122, 1.000000000000000000, 0.9659258262890683122, 1.000000000000000000, 0.9659258262890683122, 1.000000000000000000, 0.9659258262890683122, 1.000000000000000000, 0.9659258262890683122, 1.000000000000000000, 0.9659258262890683122, 1.000000000000000000, 0.9659258262890683122, 1.000000000000000000, 0.9659258262890683122, 1.000000000000000000, 0.9659258262890683122, 1.000000000000000000, 0.9659258262890683122, 1.000000000000000000, 0.9659258262890683122, 1.000000000000000000, 0.9659258262890683122, 1.000000000000000000, 0.9659258262890683122, 1.000000000000000000, 0.9659258262890683122, 1.000000000000000000, 0.9659258262890683122, 1.000000000000000000, 0.9659258262890683122, 1.000000000000000000, 0.9659258262890683122, 1.000000000000000000, 0.9659258262890683122, 1.000000000000000000, 0.9659258262890683122, 1.000000000000000000, 0.9659258262890683122, 1.000000000000000000, 0.9659258262890683122, 1.000000000000000000, 0.9659258262890683122, 1.000000000000000000, 0.9659258262890683122, 1.000000000000000000, 0.9659258262890683122, 1.000000000000000000, 0.9659258262890683122, 1.000000000000000000, 0.9659258262890683122, 1.000000000000000000, 0.9659258262890683122, 1.000000000000000000, 0.9659258262890683122, 1.000000000000000000, 0.9659258262890683122, 1.000000000000000000, 0.9659258262890683122, 1.000000000000000000, 0.9659258262890683122, 1.000000000000000000, 0.9659258262890683122, 1.000000000000000000, 0.9659258262890683122, 1.000000000000000000, 0.9659258262890683122, 1.000000000000000000, 0.9659258262890683122, 1.000000000000000000, 0.9659258262890683122, 1.000000000000000000, 0.9659258262890683122, 1.000000000000000000, 0.9659258262890683122, 1.000000000000000000, 0.9659258262890683122, 1.000000000000000000, 0.9659258262890683122, 1.000000000000000000, 0.9659258262890683122, 1.000000000000000000, 0.9659258262890683122, 1.000000000000000000, 0.9659258262890683122, 1.000000000000000000, 0.9659258262890683122, 1.000000000000000000, 0.9659258262890683122, 1.000000000000000000, 0.9659258262890683122, 1.000000000000000000, 0.9659258262890683122, 1.000000000000000000, 0.9659258262890683122, 1.000000000000000000, 0.9659258262890683122, 1.000000000000000000, 0.9659258262890683122, 1.000000000000000000, 0.9659258262890683122, 1.000000000000000000, 0.9659258262890683122, 1.000000000000000000, 0.9659258262890683122, 1.000000000000000000, 0.9659258262890683122, 1.000000000000000000, 0.9659258262890683122, 1.000000000000000000, 0.9659258262890683122, 1.000000000000000000, 0.9659258262890683122, 1.000000000000000000, 0.9659258262890683122, 1.000000000000000000, 0.9659258262890683122, 1.000000000000000000, 0.9659258262890683122, 1.000000000000000000, 0.9659258262890683122, 1.000000000000000000, 0.9659258262890683122, 1.000000000000000000, 0.9659258262890683122, 1.000000000000000000, 0.9659258262890683122, 1.000000000000000000, 0.9659258262890683122, 1.000000000000000000, 0.9659258262890683122, 1.000000000000000000, 0.9659258262890683122, 1.000000000000000000, 0.9659258262890683122, 1.000000000000000000, 0.9659258262890683122, 1.000000000000000000, 0.9659258262890683122, 1.000000000000000000, 0.9659258262890683122, 1.000000000000000000, 0.9659258262890683122, 1.000000000000000000, 0.9659258262890683122, 1.000000000000000000, 0.9659258262890683122, 1.000000000000000000, 0.9659258262890683122, 1.000000000000000000, 0.9659258262890683122, 1.000000000000000000, 0.9659258262890683122, 1.000000000000000000, 0.9659258262890683122, 1.000000000000000000, 0.9659258262890683122, 1.000000000000000000, 0.9659258262890683122, 1.000000000000000000, 0.9659258262890683122, 1.000000000000000000, 0.9659258262890683122, 1.000000000000000000, 0.9659258262890683122, 1.000000000000000000, 0.9659258262890683122, 1.000000000000000000, 0.9659258262890683122, 1.000000000000000000, 0.9659258262890683122, 1.000000000000000000, 0.9659258262890683122, 1.000000000000000000, 0.9659258262890683122, 1.000000000000000000, 0.9659258262890683122, 1.000000000000000000, 0.9659258262890683122, 1.000000000000000000, 0.9659258262890683122, 1.000000000000000000, 0.9659258262890683122, 1.000000000000000000, 0.9659258262890683122, 1.000000000000000000, 0.9659258262890683122, 1.000000000000000000, 0.9659258262890683122, 1.000000000000000000, 0.9659258262890683122, 1.000000000000000000, 0.9659258262890683122, 1.000000000000000000, 0.9659258262890683122, 1.000000000000000000, 0.9659258262890683122, 1.000000000000000000, 0.9659258262890683122, 1.000000000000000000, 0.9659258262890683122, 1.000000000000000000, 0.9659258262890683122, 1.000000000000000000, 0.9659258262890683122, 1.000000000000000000, 0.9659258262890683122, 1.000000000000000000, 0.9659258262890683122, 1.000000000000000000, 0.9659258262890683122, 1.000000000000000000, 0.9659258262890683122, 1.000000000000000000, 0.9659258262890683122, 1.000000000000000000, 0.9659258262890683122, 1.000000000000000000, 0.9659258262890683122, 1.000000000000000000, 0.9659258262890683122, 1.000000000000000000, 0.9659258262890683122, 1.000000000000000000, 0.9659258262890683122, 1.000000000000000000, 0.9659258262890683122, 1.000000000000000000, 0.9659258262890683122, 1.000000000000000000, 0.9659258262890683122, 1.000000000000000000, 0.9659258262890683122, 1.000000000000000000, 0.9659258262890683122, 1.000000000000000000, 0.9659258262890683122, 1.000000000000000000, 0.9659258262890683122, 1.000000000000000000, 0.9659258262890683122, 1.000000000000000000, 0.9659258262890683122, 1.000000000000000000, 0.9659258262890683122, 1.000000000000000000, 0.9659258262890683122, 1.000000000000000000, 0.9659258262890683122, 1.000000000000000000, 0.9659258262890683122, 1.000000000000000000, 0.9659258262890683122, 1.000000000000000000, 0.9659258262890683122, 1.000000000000000000, 0.9659258262890683122, 1.000000000000000000, 0.9659258262890683122, 1.000000000000000000, 0.9659258262890683122, 1.000000000000000000, 0.9659258262890683122, 1.000000000000000000, 0.9659258262890683122, 1.000000000000000000, 0.9659258262890683122, 1.000000000000000000, 0.9659258262890683122, 1.000000000000000000, 0.9659258262890683122, 1.000000000000000000, 0.9659258262890683122, 1.000000000000000000, 0.9659258262890683122, 1.000000000000000000, 0.9659258262890683122, 1.000000000000000000, 0.9659258262890683122, 1.000000000000000000, 0.9659258262890683122, 1.000000000000000000, 0.9659258262890683122, 1.000000000000000000, 0.9659258262890683122, 1.000000000000000000, 0.9659258262890683122, 1.000000000000000000, 0.9659258262890683122, 1.000000000000000000, 0.9659258262890683122, 1.000000000000000000, 0.9659258262890683122, 1.000000000000000000, 0.9659258262890683122, 1.000000000000000000, 0.9659258262890683122, 1.000000000000000000, 0.9659258262890683122, 1.000000000000000000, 0.9659258262890683122, 1.000000000000000000, 0.9659258262890683122, 1.000000000000000000, 0.9659258262890683122, 1.000000000000000000, 0.9659258262890683122, 1.000000000000000000, 0.9659258262890683122, 1.000000000000000000, 0.9659258262890683122, 1.000000000000000000) ) ) 
 REPRESENTATION_ITEM ( '' )  SURFACE ( )  );
#35222=CARTESIAN_POINT ( 'NONE',  ( -2.816281873526471635, 48.91530133659708213, -3.434112377981056508 ) ) ;
#35224=CARTESIAN_POINT ( 'NONE',  ( 19.80777595082615861, 15.68878173731740766, -6.500000000000005329 ) ) ;
#35225=CARTESIAN_POINT ( 'NONE',  ( 10.00000000000000178, 59.31368534415484106, 10.88017736071110342 ) ) ;
#35227=CARTESIAN_POINT ( 'NONE',  ( -2.816281873526471635, 13.91530133659708746, -3.434112377981056508 ) ) ;
#35229=CARTESIAN_POINT ( 'NONE',  ( 19.84674366389459266, 33.71726448433410894, -2.638427012816827677 ) ) ;
#35230=CARTESIAN_POINT ( 'NONE',  ( 4.559911319644449179, 33.89701867748817676, 9.422509992056141925 ) ) ;
#35231=CARTESIAN_POINT ( 'NONE',  ( 6.565887622018943937, 38.08196800326376064, -12.81628187352647608 ) ) ;
#35232=CARTESIAN_POINT ( 'NONE',  ( 10.00000000000000178, 37.25893115100078745, 9.846743663894594434 ) ) ;
#35236=CARTESIAN_POINT ( 'NONE',  ( 15.44008868035555793, 31.39701867748817676, -9.422509992056140149 ) ) ;
#35240=CARTESIAN_POINT ( 'NONE',  ( 7.361572987183170547, 52.05059781766745175, 9.846743663894590881 ) ) ;
#35241=CARTESIAN_POINT ( 'NONE',  ( 15.44008868035555793, 31.39701867748817676, -9.422509992056140149 ) ) ;
#35243=EDGE_CURVE ( 'NONE', #6299, #5362, #95772, .T. ) ;
#35244=CARTESIAN_POINT ( 'NONE',  ( 15.44008868035555260, 54.73035201082150536, 9.422509992056143702 ) ) ;
#35245=CARTESIAN_POINT ( 'NONE',  ( 15.44008868035555260, 29.73035201082150891, 9.422509992056143702 ) ) ;
#35247=FILL_AREA_STYLE ('',( #42764 ) ) ;
#35248=CARTESIAN_POINT ( 'NONE',  ( 17.20831665107776587, 24.13393115100078035, -7.208316651077762316 ) ) ;
#35250=CARTESIAN_POINT ( 'NONE',  ( 0.1532563361054100626, 45.80059781766745886, -2.638427012816831230 ) ) ;
#35251=CARTESIAN_POINT ( 'NONE',  ( -4.164238869374098151, 56.59541550158063927, -3.795296366450310543 ) ) ;
#35254=CARTESIAN_POINT ( 'NONE',  ( 2.917880565312950480, 15.97041550158063217, -12.26659068614894821 ) ) ;
#35255=CARTESIAN_POINT ( 'NONE',  ( -2.266590686148945544, 42.22041550158063217, 7.082119434687048631 ) ) ;
#35256=CARTESIAN_POINT ( 'NONE',  ( 19.38216949554541557, 2.248634669930420049, -9.382169495545420901 ) ) ;
#35257=AXIS2_PLACEMENT_3D ( 'NONE', #22598, #67100, #53075 ) ;
#35260=CARTESIAN_POINT ( 'NONE',  ( 12.91533473730992121, 19.52201867748816611, 10.88017736071110164 ) ) ;
#35261=CARTESIAN_POINT ( 'NONE',  ( 19.84674366389459266, 38.30059781766745175, 2.638427012816836559 ) ) ;
#35264=CARTESIAN_POINT ( 'NONE',  ( 19.42250999205614193, 55.14701867748817676, 5.440088680355555262 ) ) ;
#35267=CARTESIAN_POINT ( 'NONE',  ( -2.816281873526473856, 59.12363466993042493, 9.499525473075851096E-16 ) ) ;
#35268=CARTESIAN_POINT ( 'NONE',  ( -2.816281873526473856, 29.33196800326376064, 3.434112377981055619 ) ) ;
#35269=CARTESIAN_POINT ( 'NONE',  ( 12.63842701281683922, 34.55059781766745886, -9.846743663894590881 ) ) ;
#35273=CARTESIAN_POINT ( 'NONE',  ( 20.88017736071110519, 5.563685344154838397, 2.639326808657452039E-16 ) ) ;
#35274=CARTESIAN_POINT ( 'NONE',  ( 19.42250999205614193, 20.14701867748817321, 5.440088680355555262 ) ) ;
#35275=CARTESIAN_POINT ( 'NONE',  ( 24.16423886937410614, 44.51208216824730357, -3.795296366450302550 ) ) ;
#35276=CARTESIAN_POINT ( 'NONE',  ( 20.88017736071110519, 35.56368534415484106, 2.639326808657452039E-16 ) ) ;
#35277=CARTESIAN_POINT ( 'NONE',  ( 12.91533473730993009, 61.60535201082150536, -10.88017736071109987 ) ) ;
#35280=CARTESIAN_POINT ( 'NONE',  ( 12.63842701281683034, 22.46726448433411605, 9.846743663894596210 ) ) ;
#35281=CARTESIAN_POINT ( 'NONE',  ( 19.84674366389459266, 13.30059781766745353, 2.638427012816836559 ) ) ;
#35282=CARTESIAN_POINT ( 'NONE',  ( 10.00000000000000178, 32.25893115100078745, 9.846743663894594434 ) ) ;
#35283=CARTESIAN_POINT ( 'NONE',  ( 17.20831665107776587, 64.13393115100079456, -7.208316651077762316 ) ) ;
#35284=CARTESIAN_POINT ( 'NONE',  ( 4.559911319644449179, 22.23035201082150536, -9.422509992056141925 ) ) ;
#35285=UNCERTAINTY_MEASURE_WITH_UNIT (LENGTH_MEASURE( 1.000000000000000082E-05 ), #67058, 'distance_accuracy_value', 'NONE');
#35288=CARTESIAN_POINT ( 'NONE',  ( 6.565887622018943937, 40.16530133659708923, 12.81628187352647430 ) ) ;
#35290=CARTESIAN_POINT ( 'NONE',  ( 5.076628168052704559, 0.1755978176674514724, -8.527530157486179263 ) ) ;
#35291=CARTESIAN_POINT ( 'NONE',  ( 3.591859063236763294, 43.29030133659708923, -11.09922568453595026 ) ) ;
#35292=CARTESIAN_POINT ( 'NONE',  ( -4.164238869374099039, 56.80374883491397497, 8.674139862899312516E-16 ) ) ;
#35293=CARTESIAN_POINT ( 'NONE',  ( 2.791683348922240793, 31.63393115100078745, 7.208316651077764092 ) ) ;
#35295=CARTESIAN_POINT ( 'NONE',  ( 1.472469842513823179, 60.59226448433412315, -4.923371831947296329 ) ) ;
#35296=CARTESIAN_POINT ( 'NONE',  ( 17.08211943468705130, 18.47041550158063572, 12.26659068614894998 ) ) ;
#35297=CARTESIAN_POINT ( 'NONE',  ( 24.16423886937410614, 34.51208216824731068, -3.795296366450302550 ) ) ;
#35298=CARTESIAN_POINT ( 'NONE',  ( 5.076628168052704559, 50.17559781766745886, -8.527530157486179263 ) ) ;
#35301=CARTESIAN_POINT ( 'NONE',  ( 4.559911319644449179, 42.23035201082151247, -9.422509992056141925 ) ) ;
#35302=CARTESIAN_POINT ( 'NONE',  ( 0.5774900079438590739, 57.64701867748817676, -5.440088680355550821 ) ) ;
#35305=CARTESIAN_POINT ( 'NONE',  ( 13.43411237798105340, 45.58196800326374643, 12.81628187352647963 ) ) ;
#35306=CARTESIAN_POINT ( 'NONE',  ( 14.92337183194729633, 2.675597817667451750, 8.527530157486181039 ) ) ;
#35308=EDGE_CURVE ( 'NONE', #30282, #58661, #10661, .T. ) ;
#35309=CARTESIAN_POINT ( 'NONE',  ( 2.917880565312948704, 2.637082168247300906, 12.26659068614894643 ) ) ;
#35314=CARTESIAN_POINT ( 'NONE',  ( 7.084665262690076126, 17.02201867748817676, -10.88017736071110164 ) ) ;
#35317=CARTESIAN_POINT ( 'NONE',  ( 22.26659068614895176, 14.72041550158063572, -7.082119434687042414 ) ) ;
#35318=CARTESIAN_POINT ( 'NONE',  ( 15.44008868035555260, 19.73035201082150536, 9.422509992056143702 ) ) ;
#35319=CARTESIAN_POINT ( 'NONE',  ( 0.1532563361054100626, 55.80059781766745175, -2.638427012816831230 ) ) ;
#35320=VERTEX_POINT ( 'NONE', #75725 ) ;
#35321=CARTESIAN_POINT ( 'NONE',  ( 5.076628168052704559, 65.17559781766745175, -8.527530157486179263 ) ) ;
#35323=CARTESIAN_POINT ( 'NONE',  ( 4.559911319644449179, 48.89701867748817676, 9.422509992056141925 ) ) ;
#35326=CARTESIAN_POINT ( 'NONE',  ( 6.565887622018943937, 35.16530133659708923, 12.81628187352647430 ) ) ;
#35327=CARTESIAN_POINT ( 'NONE',  ( 17.96484262340118221, 9.938685344154837509, 7.964842623401181321 ) ) ;
#35329=CARTESIAN_POINT ( 'NONE',  ( 12.63842701281683034, 7.467264484334118713, 9.846743663894596210 ) ) ;
#35330=CARTESIAN_POINT ( 'NONE',  ( 19.42250999205614548, 15.98035201082150714, -5.440088680355545492 ) ) ;
#35332=EDGE_CURVE ( 'NONE', #9539, #59946, #63808, .T. ) ;
#35335=CARTESIAN_POINT ( 'NONE',  ( -2.816281873526473856, 49.12363466993042493, 9.499525473075851096E-16 ) ) ;
#35336=CARTESIAN_POINT ( 'NONE',  ( 20.88017736071110875, 30.77201867748816966, -2.915334737309920765 ) ) ;
#35337=CARTESIAN_POINT ( 'NONE',  ( 19.64275500434244748, 93.00187409791189452, 5.306653671078411350 ) ) ;
#35338=CARTESIAN_POINT ( 'NONE',  ( 16.40814093676323893, 40.79030133659708923, 11.09922568453595026 ) ) ;
#35339=CARTESIAN_POINT ( 'NONE',  ( 20.88017736071110519, 45.56368534415484106, 2.639326808657452039E-16 ) ) ;
#35340=ADVANCED_FACE ( 'NONE', ( #23239 ), #46221, .F. ) ;
#35341=( BOUNDED_CURVE ( )  B_SPLINE_CURVE ( 2, ( #58721, #20735, #13224, #43720, #74205, #31177, #75706, #59706, #30682 ),
 .UNSPECIFIED., .F., .F. ) 
 B_SPLINE_CURVE_WITH_KNOTS ( ( 3, 2, 2, 2, 3 ),
 ( 0.4044266512259456214, 0.4047619047619047672, 0.4107142857142856984, 0.4166666666666666297, 0.4170019202026257754 ),
 .UNSPECIFIED. ) 
 CURVE ( )  GEOMETRIC_REPRESENTATION_ITEM ( )  RATIONAL_B_SPLINE_CURVE ( ( 0.9963778908391760503, 0.9980808541467920403, 1.000000000000000000, 0.9659258262890683122, 1.000000000000000000, 0.9659258262890683122, 1.000000000000000000, 0.9980808541467920403, 0.9963778908391760503 ) ) 
 REPRESENTATION_ITEM ( '' )  );
#35342=CARTESIAN_POINT ( 'NONE',  ( 0.1532563361054100626, 50.80059781766745175, -2.638427012816831230 ) ) ;
#35344=CARTESIAN_POINT ( 'NONE',  ( 12.63842701281683922, 9.550597817667449974, -9.846743663894590881 ) ) ;
#35345=CARTESIAN_POINT ( 'NONE',  ( 3.591859063236763294, -1.709698663402913210, -11.09922568453595026 ) ) ;
#35347=CARTESIAN_POINT ( 'NONE',  ( 7.361572987183169658, 44.96726448433412315, -9.846743663894592657 ) ) ;
#35348=CARTESIAN_POINT ( 'NONE',  ( 4.559911319644449179, 17.23035201082150536, -9.422509992056141925 ) ) ;
#35350=CARTESIAN_POINT ( 'NONE',  ( 17.20831665107776587, 37.88393115100078745, 7.208316651077764980 ) ) ;
#35351=CARTESIAN_POINT ( 'NONE',  ( -0.1503990784575277295, 39.24884699246889141, -6.262539305110077947 ) ) ;
#35353=CARTESIAN_POINT ( 'NONE',  ( 1.472469842513823179, 40.59226448433411605, -4.923371831947296329 ) ) ;
#35354=CARTESIAN_POINT ( 'NONE',  ( 14.92337183194729988, 9.342264484334119601, -8.527530157486177487 ) ) ;
#35355=CARTESIAN_POINT ( 'NONE',  ( 19.84674366389459266, 28.30059781766745530, 2.638427012816836559 ) ) ;
#35356=CARTESIAN_POINT ( 'NONE',  ( 18.52753015748617571, 53.09226448433412315, 4.923371831947298993 ) ) ;
#35360=CARTESIAN_POINT ( 'NONE',  ( 13.43411237798106583, 37.66530133659708923, -12.81628187352647252 ) ) ;
#35361=CARTESIAN_POINT ( 'NONE',  ( 18.52753015748618282, 28.92559781766745175, -4.923371831947291888 ) ) ;
#35363=CARTESIAN_POINT ( 'NONE',  ( 20.36894250292379738, 59.92874883491397497, -10.36894250292379027 ) ) ;
#35364=CARTESIAN_POINT ( 'NONE',  ( 7.361572987183170547, 37.05059781766744464, 9.846743663894590881 ) ) ;
#35365=ORIENTED_EDGE ( 'NONE', *, *, #29805, .T. ) ;
#35367=CARTESIAN_POINT ( 'NONE',  ( 19.99999999998935607, 80.90839911560571807, 4.954669604078111966 ) ) ;
#35368=CARTESIAN_POINT ( 'NONE',  ( -4.164238869374099039, 51.80374883491396787, 8.674139862899312516E-16 ) ) ;
#35371=CARTESIAN_POINT ( 'NONE',  ( 17.96484262340118221, 16.18868534415483396, -7.964842623401177768 ) ) ;
#35372=CARTESIAN_POINT ( 'NONE',  ( -2.266590686148945544, 42.22041550158063217, 7.082119434687048631 ) ) ;
#35373=CARTESIAN_POINT ( 'NONE',  ( 20.36894250292379382, 48.67874883491396076, 10.36894250292379205 ) ) ;
#35376=CARTESIAN_POINT ( 'NONE',  ( 1.472469842513823179, 11.42559781766745175, 4.923371831947296329 ) ) ;
#35377=CARTESIAN_POINT ( 'NONE',  ( 1.472469842513823179, 66.42559781766745175, 4.923371831947296329 ) ) ;
#35378=CARTESIAN_POINT ( 'NONE',  ( 7.084665262690076126, 47.02201867748818387, -10.88017736071110164 ) ) ;
#35380=CARTESIAN_POINT ( 'NONE',  ( 12.63842701281683922, 54.55059781766745175, -9.846743663894590881 ) ) ;
#35386=CARTESIAN_POINT ( 'NONE',  ( 17.08211943468705130, 43.47041550158063927, 12.26659068614894998 ) ) ;
#35388=( LENGTH_UNIT ( ) NAMED_UNIT ( * ) SI_UNIT ( .MILLI., .METRE. ) );
#35389=CARTESIAN_POINT ( 'NONE',  ( 15.44008868035555793, 21.39701867748817321, -9.422509992056140149 ) ) ;
#35390=CARTESIAN_POINT ( 'NONE',  ( 22.81628187352647785, 36.41530133659707502, 3.434112377981063169 ) ) ;
#35392=CARTESIAN_POINT ( 'NONE',  ( 1.274849032794294290, 53.57228050351032067, 6.499999999999979572 ) ) ;
#35393=ORIENTED_EDGE ( 'NONE', *, *, #57943, .F. ) ;
#35397=CARTESIAN_POINT ( 'NONE',  ( 2.035157376598822676, 22.43868534415483396, -7.964842623401177768 ) ) ;
#35400=CARTESIAN_POINT ( 'NONE',  ( 4.559911319644449179, 43.89701867748816966, 9.422509992056141925 ) ) ;
#35401=CARTESIAN_POINT ( 'NONE',  ( 17.96484262340118221, 54.93868534415484106, 7.964842623401181321 ) ) ;
#35402=CARTESIAN_POINT ( 'NONE',  ( 19.38216949554541557, 7.248634669930421381, -9.382169495545420901 ) ) ;
#35403=( NAMED_UNIT ( * ) PLANE_ANGLE_UNIT ( ) SI_UNIT ( $, .RADIAN. ) );
#35404=DIRECTION ( 'NONE',  ( 1.000000000000000000, 0.000000000000000000, 0.000000000000000000 ) ) ;
#35405=CARTESIAN_POINT ( 'NONE',  ( 0.1532563361054082862, 21.21726448433412315, 2.638427012816831674 ) ) ;
#35408=CARTESIAN_POINT ( 'NONE',  ( 12.91533473730992121, 39.52201867748817676, 10.88017736071110164 ) ) ;
#35409=COLOUR_RGB ( '', 0.31764706, 0.68627451, 0.89019608) ;
#35410=CARTESIAN_POINT ( 'NONE',  ( 6.565887622018943937, 3.081968003263753531, -12.81628187352647608 ) ) ;
#35411=CARTESIAN_POINT ( 'NONE',  ( 12.91533473730993009, 61.60535201082150536, -10.88017736071109987 ) ) ;
#35412=CARTESIAN_POINT ( 'NONE',  ( 7.361572987183170547, 22.05059781766745530, 9.846743663894590881 ) ) ;
#35413=CARTESIAN_POINT ( 'NONE',  ( 3.591859063236761518, 49.95696800326375353, 11.09922568453594849 ) ) ;
#35414=CARTESIAN_POINT ( 'NONE',  ( 0.1532563361054082862, 11.21726448433411605, 2.638427012816831674 ) ) ;
#35417=CARTESIAN_POINT ( 'NONE',  ( 1.959929470562281395, 35.51528370094808196, -5.767676674365853629 ) ) ;
#35418=CARTESIAN_POINT ( 'NONE',  ( -0.8801773607110991993, 17.85535201082150536, -2.915334737309923874 ) ) ;
#35419=CARTESIAN_POINT ( 'NONE',  ( 3.591859063236763294, 63.29030133659708923, -11.09922568453595026 ) ) ;
#35420=CARTESIAN_POINT ( 'NONE',  ( -0.3689425029237898834, 31.17874883491396787, -10.36894250292378850 ) ) ;
#35421=CARTESIAN_POINT ( 'NONE',  ( 17.20831665107776587, 32.88393115100078745, 7.208316651077764980 ) ) ;
#35422=CARTESIAN_POINT ( 'NONE',  ( 19.42250999205614548, 20.98035201082150891, -5.440088680355545492 ) ) ;
#35423=CARTESIAN_POINT ( 'NONE',  ( 17.96484262340118221, 6.188685344154837509, -7.964842623401177768 ) ) ;
#35425=CARTESIAN_POINT ( 'NONE',  ( 10.00000000000000178, 19.31368534415484106, 10.88017736071110342 ) ) ;
#35427=CARTESIAN_POINT ( 'NONE',  ( 17.96484262340118221, 34.93868534415482685, 7.964842623401181321 ) ) ;
#35431=CARTESIAN_POINT ( 'NONE',  ( 20.15039907845753930, 9.722660991849181755, 6.262539305110064625 ) ) ;
#35432=CARTESIAN_POINT ( 'NONE',  ( 4.559911319644449179, 27.23035201082150536, -9.422509992056141925 ) ) ;
#35434=DIRECTION ( 'NONE',  ( 0.000000000000000000, 0.000000000000000000, -1.000000000000000000 ) ) ;
#35435=CARTESIAN_POINT ( 'NONE',  ( 22.81628187352647785, 56.41530133659708213, 3.434112377981063169 ) ) ;
#35436=CARTESIAN_POINT ( 'NONE',  ( 0.1955144967548966828, 9.327036817733409535, -6.500000000002781775 ) ) ;
#35437=CARTESIAN_POINT ( 'NONE',  ( 24.16423886937409904, 29.09541550158063572, 3.795296366450317205 ) ) ;
#35438=CARTESIAN_POINT ( 'NONE',  ( 12.91533473730993009, 46.60535201082150536, -10.88017736071109987 ) ) ;
#35439=CARTESIAN_POINT ( 'NONE',  ( 4.559911319644449179, 33.89701867748817676, 9.422509992056141925 ) ) ;
#35440=CARTESIAN_POINT ( 'NONE',  ( 14.92337183194729633, 62.67559781766745886, 8.527530157486181039 ) ) ;
#35442=CARTESIAN_POINT ( 'NONE',  ( 17.20831665107776587, 54.13393115100079456, -7.208316651077762316 ) ) ;
#35446=CARTESIAN_POINT ( 'NONE',  ( 2.791683348922240793, 26.63393115100078745, 7.208316651077764092 ) ) ;
#35448=AXIS2_PLACEMENT_3D ( 'NONE', #91575, #47546, #16568 ) ;
#35449=CARTESIAN_POINT ( 'NONE',  ( 0.5774900079438590739, 17.64701867748817321, -5.440088680355550821 ) ) ;
#35450=CARTESIAN_POINT ( 'NONE',  ( 1.472469842513823179, 30.59226448433411960, -4.923371831947296329 ) ) ;
#35451=CARTESIAN_POINT ( 'NONE',  ( 20.88017736071110164, 60.35535201082151957, 2.915334737309930979 ) ) ;
#35452=CARTESIAN_POINT ( 'NONE',  ( -0.8801773607111009756, 18.06368534415484106, 1.068504757029289695E-15 ) ) ;
#35453=CARTESIAN_POINT ( 'NONE',  ( 19.38216949554541202, 55.99863466993041072, 9.382169495545424454 ) ) ;
#35454=CARTESIAN_POINT ( 'NONE',  ( 2.917880565312950480, 50.97041550158064638, -12.26659068614894821 ) ) ;
#35455=ADVANCED_FACE ( 'NONE', ( #6740 ), #30703, .F. ) ;
#35458=CARTESIAN_POINT ( 'NONE',  ( 21.09922568453594849, 1.206968003263753531, 6.408140936763242479 ) ) ;
#35459=SURFACE_SIDE_STYLE ('',( #19966 ) ) ;
#35461=CARTESIAN_POINT ( 'NONE',  ( 2.035157376598822676, 32.43868534415483396, -7.964842623401177768 ) ) ;
#35462=CARTESIAN_POINT ( 'NONE',  ( 19.84674366389459621, 63.50893115100078745, 7.409399052514197653E-17 ) ) ;
#35464=CARTESIAN_POINT ( 'NONE',  ( 1.472469842513823179, 15.59226448433411960, -4.923371831947296329 ) ) ;
#35466=CARTESIAN_POINT ( 'NONE',  ( 2.791683348922237240, 15.38393115100078212, -7.208316651077763204 ) ) ;
#35467=CARTESIAN_POINT ( 'NONE',  ( 5.076628168052704559, 25.17559781766745175, -8.527530157486179263 ) ) ;
#35468=CARTESIAN_POINT ( 'NONE',  ( 12.63842701281683034, 7.467264484334118713, 9.846743663894596210 ) ) ;
#35469=CARTESIAN_POINT ( 'NONE',  ( 7.361572987183169658, 4.967264484334119601, -9.846743663894592657 ) ) ;
#35471=CARTESIAN_POINT ( 'NONE',  ( 5.076628168052704559, 0.1755978176674514724, -8.527530157486179263 ) ) ;
#35473=CARTESIAN_POINT ( 'NONE',  ( 19.84674366389459266, 8.717264484334116048, -2.638427012816827677 ) ) ;
#35474=CARTESIAN_POINT ( 'NONE',  ( 19.84674366389459621, 13.50893115100078568, 7.409399052514197653E-17 ) ) ;
#35478=CARTESIAN_POINT ( 'NONE',  ( -1.099225684535947600, -0.4596986634029132657, 6.408140936763237150 ) ) ;
#35480=CARTESIAN_POINT ( 'NONE',  ( 12.91533473730993009, 6.605352010821504471, -10.88017736071109987 ) ) ;
#35481=EDGE_CURVE ( 'NONE', #16271, #14086, #17697, .T. ) ;
#35482=CARTESIAN_POINT ( 'NONE',  ( 24.16423886937409904, 14.09541550158063217, 3.795296366450317205 ) ) ;
#35483=UNCERTAINTY_MEASURE_WITH_UNIT (LENGTH_MEASURE( 1.000000000000000082E-05 ), #40834, 'distance_accuracy_value', 'NONE');
#35485=CARTESIAN_POINT ( 'NONE',  ( -4.164238869374099039, 21.80374883491396787, 8.674139862899312516E-16 ) ) ;
#35486=CARTESIAN_POINT ( 'NONE',  ( 10.00000000000000178, 43.05374883491397497, 14.16423886937410082 ) ) ;
#35488=CARTESIAN_POINT ( 'NONE',  ( 24.16423886937409904, 19.09541550158063927, 3.795296366450317205 ) ) ;
#35489=CARTESIAN_POINT ( 'NONE',  ( 0.5774900079438590739, 67.64701867748817676, -5.440088680355550821 ) ) ;
#35490=CARTESIAN_POINT ( 'NONE',  ( 4.559911319644449179, 37.23035201082150536, -9.422509992056141925 ) ) ;
#35493=CARTESIAN_POINT ( 'NONE',  ( 17.20831665107776587, 14.13393115100078568, -7.208316651077762316 ) ) ;
#35494=CARTESIAN_POINT ( 'NONE',  ( -0.8801773607110991993, 52.85535201082151247, -2.915334737309923874 ) ) ;
#35495=CARTESIAN_POINT ( 'NONE',  ( 7.361572987183169658, 29.96726448433411960, -9.846743663894592657 ) ) ;
#35496=CARTESIAN_POINT ( 'NONE',  ( 20.88017736071110875, 5.772018677488170546, -2.915334737309920765 ) ) ;
#35497=CARTESIAN_POINT ( 'NONE',  ( -2.816281873526471635, 48.91530133659708213, -3.434112377981056508 ) ) ;
#35498=CARTESIAN_POINT ( 'NONE',  ( 17.20831665107776587, 52.88393115100078035, 7.208316651077764980 ) ) ;
#35500=CARTESIAN_POINT ( 'NONE',  ( 19.38216949554541202, 40.99863466993042493, 9.382169495545424454 ) ) ;
#35502=CIRCLE ( 'NONE', #54626, 0.5000000000000004441 ) ;
#35503=CARTESIAN_POINT ( 'NONE',  ( 0.1532563361054082862, 36.21726448433410894, 2.638427012816831674 ) ) ;
#35504=CARTESIAN_POINT ( 'NONE',  ( -2.266590686148945544, 32.22041550158063927, 7.082119434687048631 ) ) ;
#35507=CARTESIAN_POINT ( 'NONE',  ( 20.88017736071110519, 45.56368534415484106, 2.639326808657452039E-16 ) ) ;
#35508=CARTESIAN_POINT ( 'NONE',  ( 20.88017736071110164, 60.35535201082151957, 2.915334737309930979 ) ) ;
#35509=CARTESIAN_POINT ( 'NONE',  ( 13.79529636645030344, 48.26208216824728936, 14.16423886937410614 ) ) ;
#35511=CARTESIAN_POINT ( 'NONE',  ( 5.076628168052703671, 66.84226448433412315, 8.527530157486179263 ) ) ;
#35513=CARTESIAN_POINT ( 'NONE',  ( -0.1049300847420659016, 57.21697413083879269, -6.336235997365754713 ) ) ;
#35514=CARTESIAN_POINT ( 'NONE',  ( 17.96484262340118221, 41.18868534415484106, -7.964842623401177768 ) ) ;
#35517=CARTESIAN_POINT ( 'NONE',  ( 6.565887622018943937, 28.08196800326375353, -12.81628187352647608 ) ) ;
#35518=CARTESIAN_POINT ( 'NONE',  ( 19.84674366389459621, 48.50893115100078745, 7.409399052514197653E-17 ) ) ;
#35520=CARTESIAN_POINT ( 'NONE',  ( 7.084665262690076126, 14.10535201082150358, 10.88017736071109987 ) ) ;
#35522=VERTEX_POINT ( 'NONE', #94659 ) ;
#35524=CARTESIAN_POINT ( 'NONE',  ( 12.91533473730992121, 64.52201867748817676, 10.88017736071110164 ) ) ;
#35526=CARTESIAN_POINT ( 'NONE',  ( 4.559911319644449179, 67.23035201082150536, -9.422509992056141925 ) ) ;
#35528=CARTESIAN_POINT ( 'NONE',  ( 18.52753015748618282, 33.92559781766745886, -4.923371831947291888 ) ) ;
#35529=CARTESIAN_POINT ( 'NONE',  ( 17.96484262340118221, 26.18868534415483396, -7.964842623401177768 ) ) ;
#35530=CARTESIAN_POINT ( 'NONE',  ( 16.40814093676324603, 7.456968003263754419, -11.09922568453594671 ) ) ;
#35531=CARTESIAN_POINT ( 'NONE',  ( 17.96484262340118221, 29.93868534415484106, 7.964842623401181321 ) ) ;
#35534=CARTESIAN_POINT ( 'NONE',  ( 3.591859063236761518, 34.95696800326375353, 11.09922568453594849 ) ) ;
#35536=CARTESIAN_POINT ( 'NONE',  ( 19.42250999205614193, 65.14701867748817676, 5.440088680355555262 ) ) ;
#35537=CARTESIAN_POINT ( 'NONE',  ( 3.591859063236761518, 24.95696800326375353, 11.09922568453594849 ) ) ;
#35539=PRESENTATION_STYLE_ASSIGNMENT (( #67031 ) ) ;
#35540=CARTESIAN_POINT ( 'NONE',  ( 15.44008868035555793, 46.39701867748817676, -9.422509992056140149 ) ) ;
#35541=CARTESIAN_POINT ( 'NONE',  ( -0.1023957841222607745, 15.13377557478295898, 6.340343622311898741 ) ) ;
#35542=CARTESIAN_POINT ( 'NONE',  ( 20.36894250292379382, 63.67874883491396787, 10.36894250292379205 ) ) ;
#35544=CARTESIAN_POINT ( 'NONE',  ( 7.361572987183169658, 54.96726448433413026, -9.846743663894592657 ) ) ;
#35545=CARTESIAN_POINT ( 'NONE',  ( 0.1532563361054083140, 1.008931151000784787, 1.131784320476157264E-15 ) ) ;
#35546=CARTESIAN_POINT ( 'NONE',  ( 20.88017736071110519, 60.56368534415484106, 2.639326808657452039E-16 ) ) ;
#35548=CARTESIAN_POINT ( 'NONE',  ( 2.917880565312950480, 30.97041550158063572, -12.26659068614894821 ) ) ;
#35549=( BOUNDED_CURVE ( )  B_SPLINE_CURVE ( 2, ( #55374, #92867, #24397, #1904, #85875, #78362, #49334, #57817, #96839 ),
 .UNSPECIFIED., .F., .F. ) 
 B_SPLINE_CURVE_WITH_KNOTS ( ( 3, 2, 2, 2, 3 ),
 ( 0.1167998787605536576, 0.1190476190476190410, 0.1250000000000000000, 0.1309523809523809590, 0.1332001212394463563 ),
 .UNSPECIFIED. ) 
 CURVE ( )  GEOMETRIC_REPRESENTATION_ITEM ( )  RATIONAL_B_SPLINE_CURVE ( ( 0.9839835555609424134, 0.9871328979762477029, 1.000000000000000000, 0.9659258262890683122, 1.000000000000000000, 0.9659258262890683122, 1.000000000000000000, 0.9871328979762477029, 0.9839835555609424134 ) ) 
 REPRESENTATION_ITEM ( '' )  );
#35550=ADVANCED_FACE ( 'NONE', ( #16707 ), #36563, .T. ) ;
#35553=( BOUNDED_CURVE ( )  B_SPLINE_CURVE ( 2, ( #23232, #14748, #31683, #98756, #76222, #45221, #45720, #30697, #76701 ),
 .UNSPECIFIED., .F., .T. ) 
 B_SPLINE_CURVE_WITH_KNOTS ( ( 3, 2, 2, 2, 3 ),
 ( 0.1882284501891250961, 0.1904761904761904656, 0.1964285714285714246, 0.2023809523809523836, 0.2046286926680177809 ),
 .UNSPECIFIED. ) 
 CURVE ( )  GEOMETRIC_REPRESENTATION_ITEM ( )  RATIONAL_B_SPLINE_CURVE ( ( 0.9839835555609424134, 0.9871328979762477029, 1.000000000000000000, 0.9659258262890683122, 1.000000000000000000, 0.9659258262890683122, 1.000000000000000000, 0.9871328979762477029, 0.9839835555609424134 ) ) 
 REPRESENTATION_ITEM ( '' )  );
#35555=CARTESIAN_POINT ( 'NONE',  ( 20.36894250292379738, 64.92874883491397497, -10.36894250292379027 ) ) ;
#35556=CARTESIAN_POINT ( 'NONE',  ( 6.204703633549690345, 55.76208216824730357, -14.16423886937410259 ) ) ;
#35557=CARTESIAN_POINT ( 'NONE',  ( 1.472469842513823179, 25.59226448433412315, -4.923371831947296329 ) ) ;
#35558=CARTESIAN_POINT ( 'NONE',  ( -2.816281873526473856, 24.33196800326375353, 3.434112377981055619 ) ) ;
#35560=CARTESIAN_POINT ( 'NONE',  ( 2.035157376598824452, 3.688685344154837953, 7.964842623401179544 ) ) ;
#35561=CARTESIAN_POINT ( 'NONE',  ( 2.917880565312950480, 60.97041550158063927, -12.26659068614894821 ) ) ;
#35564=CARTESIAN_POINT ( 'NONE',  ( 2.791683348922240793, 6.633931151000785675, 7.208316651077764092 ) ) ;
#35567=ORIENTED_EDGE ( 'NONE', *, *, #32162, .F. ) ;
#35571=CARTESIAN_POINT ( 'NONE',  ( 24.16423886937410614, 14.51208216824730179, -3.795296366450302550 ) ) ;
#35572=CARTESIAN_POINT ( 'NONE',  ( 2.035157376598824452, 13.68868534415483751, 7.964842623401179544 ) ) ;
#35573=CARTESIAN_POINT ( 'NONE',  ( 20.88017736071110875, 25.77201867748816966, -2.915334737309920765 ) ) ;
#35574=CARTESIAN_POINT ( 'NONE',  ( 0.1532563361054083140, 51.00893115100078745, 1.131784320476157264E-15 ) ) ;
#35575=CARTESIAN_POINT ( 'NONE',  ( 22.81628187352647785, 11.62363466993042138, 6.195893100308588602E-16 ) ) ;
#35578=EDGE_CURVE ( 'NONE', #18635, #71943, #12650, .T. ) ;
#35579=CARTESIAN_POINT ( 'NONE',  ( 22.81628187352647785, 26.41530133659708923, 3.434112377981063169 ) ) ;
#35580=ORIENTED_EDGE ( 'NONE', *, *, #69556, .F. ) ;
#35582=CARTESIAN_POINT ( 'NONE',  ( 10.00000000000000178, 27.25893115100078390, 9.846743663894594434 ) ) ;
#35584=CARTESIAN_POINT ( 'NONE',  ( -0.3689425029237881626, 62.42874883491396787, 10.36894250292379027 ) ) ;
#35587=CARTESIAN_POINT ( 'NONE',  ( 10.00000000000000000, 1.813685344154838175, -10.88017736071110342 ) ) ;
#35589=CARTESIAN_POINT ( 'NONE',  ( 17.96484262340118221, 46.18868534415484106, -7.964842623401177768 ) ) ;
#35590=CARTESIAN_POINT ( 'NONE',  ( -0.8801773607111008646, 43.27201867748817676, 2.915334737309923430 ) ) ;
#35591=CARTESIAN_POINT ( 'NONE',  ( 19.42250999205614193, 45.14701867748817676, 5.440088680355555262 ) ) ;
#35592=MECHANICAL_DESIGN_GEOMETRIC_PRESENTATION_REPRESENTATION('',(#21188),#67507);
#35594=CARTESIAN_POINT ( 'NONE',  ( 15.44008868035555260, 44.73035201082151247, 9.422509992056143702 ) ) ;
#35596=ORIENTED_EDGE ( 'NONE', *, *, #49470, .F. ) ;
#35597=CARTESIAN_POINT ( 'NONE',  ( 19.84674366389459266, 28.71726448433411960, -2.638427012816827677 ) ) ;
#35599=CARTESIAN_POINT ( 'NONE',  ( 17.20831665107776587, 64.13393115100079456, -7.208316651077762316 ) ) ;
#35603=ORIENTED_EDGE ( 'NONE', *, *, #94153, .T. ) ;
#35604=ADVANCED_FACE ( 'NONE', ( #28638 ), #16886, .T. ) ;
#35607=CARTESIAN_POINT ( 'NONE',  ( 20.15039907845753930, 2.627771745786128044, -6.262539305110069954 ) ) ;
#35608=CARTESIAN_POINT ( 'NONE',  ( 17.20831665107776587, 39.13393115100079456, -7.208316651077762316 ) ) ;
#35609=CARTESIAN_POINT ( 'NONE',  ( -2.266590686148945544, 56.38708216824731068, -7.082119434687050408 ) ) ;
#35613=CARTESIAN_POINT ( 'NONE',  ( 1.472469842513823179, 30.59226448433411960, -4.923371831947296329 ) ) ;
#35615=CARTESIAN_POINT ( 'NONE',  ( -1.099225684535947600, 8.706968003263753531, -6.408140936763238038 ) ) ;
#35617=CARTESIAN_POINT ( 'NONE',  ( 10.00000000000000178, 17.25893115100078745, 9.846743663894594434 ) ) ;
#35618=EDGE_CURVE ( 'NONE', #19780, #85989, #80475, .T. ) ;
#35620=CARTESIAN_POINT ( 'NONE',  ( 0.1532563361054082862, 11.21726448433411605, 2.638427012816831674 ) ) ;
#35621=CARTESIAN_POINT ( 'NONE',  ( 1.472469842513823179, 65.59226448433412315, -4.923371831947296329 ) ) ;
#35624=VERTEX_POINT ( 'NONE', #48581 ) ;
#35625=CARTESIAN_POINT ( 'NONE',  ( 20.88017736071110875, 5.772018677488170546, -2.915334737309920765 ) ) ;
#35626=CARTESIAN_POINT ( 'NONE',  ( 10.00000000000000178, 8.053748834913967869, 14.16423886937410082 ) ) ;
#35627=CARTESIAN_POINT ( 'NONE',  ( 5.076628168052703671, 21.84226448433411960, 8.527530157486179263 ) ) ;
#35628=CARTESIAN_POINT ( 'NONE',  ( 12.91533473730992121, 49.52201867748817676, 10.88017736071110164 ) ) ;
#35629=CARTESIAN_POINT ( 'NONE',  ( 13.43411237798106583, 27.66530133659708568, -12.81628187352647252 ) ) ;
#35631=CARTESIAN_POINT ( 'NONE',  ( 15.44008868035555260, 4.730352010821504471, 9.422509992056143702 ) ) ;
#35634=CARTESIAN_POINT ( 'NONE',  ( 19.84674366389459266, 58.71726448433411605, -2.638427012816827677 ) ) ;
#35635=CARTESIAN_POINT ( 'NONE',  ( 1.472469842513823179, 16.42559781766745175, 4.923371831947296329 ) ) ;
#35637=CARTESIAN_POINT ( 'NONE',  ( 22.81628187352647785, 21.62363466993041783, 6.195893100308588602E-16 ) ) ;
#35639=CARTESIAN_POINT ( 'NONE',  ( 17.96484262340118221, 24.93868534415484461, 7.964842623401181321 ) ) ;
#35641=CARTESIAN_POINT ( 'NONE',  ( -4.164238869374099927, 52.01208216824729647, 3.795296366450308767 ) ) ;
#35643=CARTESIAN_POINT ( 'NONE',  ( 10.00000000000000000, 31.81368534415483751, -10.88017736071110342 ) ) ;
#35644=CARTESIAN_POINT ( 'NONE',  ( 18.52753015748618282, 48.92559781766745886, -4.923371831947291888 ) ) ;
#35645=CARTESIAN_POINT ( 'NONE',  ( 17.96484262340118221, 51.18868534415483396, -7.964842623401177768 ) ) ;
#35646=CARTESIAN_POINT ( 'NONE',  ( 17.08211943468705840, 30.13708216824730357, -12.26659068614894466 ) ) ;
#35649=CARTESIAN_POINT ( 'NONE',  ( 2.791683348922237240, 40.38393115100078035, -7.208316651077763204 ) ) ;
#35651=CARTESIAN_POINT ( 'NONE',  ( 1.472469842513823179, 66.42559781766745175, 4.923371831947296329 ) ) ;
#35653=CARTESIAN_POINT ( 'NONE',  ( 20.88017736071110875, 20.77201867748816611, -2.915334737309920765 ) ) ;
#35654=AXIS2_PLACEMENT_3D ( 'NONE', #72150, #11656, #64632 ) ;
#35656=CARTESIAN_POINT ( 'NONE',  ( 10.00000000000000178, 14.31368534415483929, 10.88017736071110342 ) ) ;
#35657=CARTESIAN_POINT ( 'NONE',  ( 19.84674366389459266, 3.300597817667451750, 2.638427012816836559 ) ) ;
#35658=CARTESIAN_POINT ( 'NONE',  ( 20.36894250292379382, 18.67874883491397142, 10.36894250292379205 ) ) ;
#35659=CARTESIAN_POINT ( 'NONE',  ( 1.472469842513823179, 16.42559781766745175, 4.923371831947296329 ) ) ;
#35660=CARTESIAN_POINT ( 'NONE',  ( 5.076628168052703671, 66.84226448433412315, 8.527530157486179263 ) ) ;
#35661=CARTESIAN_POINT ( 'NONE',  ( 10.00000000000000178, 34.31368534415484106, 10.88017736071110342 ) ) ;
#35664=DIRECTION ( 'NONE',  ( -1.000000000000000000, 0.000000000000000000, 0.000000000000000000 ) ) ;
#35668=CARTESIAN_POINT ( 'NONE',  ( 1.472469842513823179, 46.42559781766745175, 4.923371831947296329 ) ) ;
#35669=VERTEX_POINT ( 'NONE', #56103 ) ;
#35671=B_SPLINE_CURVE_WITH_KNOTS ( 'NONE', 3,
 ( #87803, #19325, #88802, #80811, #5321, #80316 ),
 .UNSPECIFIED., .F., .F.,
 ( 4, 2, 4 ),
 ( 0.000000000000000000, 0.0002701661927229266624, 0.0005403323854458533249 ),
 .UNSPECIFIED. ) ;
#35673=CARTESIAN_POINT ( 'NONE',  ( -4.164238869374099927, 22.01208216824730357, 3.795296366450308767 ) ) ;
#35674=CARTESIAN_POINT ( 'NONE',  ( 2.917880565312948704, 7.637082168247301794, 12.26659068614894643 ) ) ;
#35675=CARTESIAN_POINT ( 'NONE',  ( 19.42250999205614548, 60.98035201082151247, -5.440088680355545492 ) ) ;
#35676=CARTESIAN_POINT ( 'NONE',  ( -2.266590686148945544, 51.38708216824730357, -7.082119434687050408 ) ) ;
#35677=CARTESIAN_POINT ( 'NONE',  ( 2.791683348922237240, 65.38393115100078035, -7.208316651077763204 ) ) ;
#35678=CARTESIAN_POINT ( 'NONE',  ( 19.84674366389459266, 38.71726448433412315, -2.638427012816827677 ) ) ;
#35680=CARTESIAN_POINT ( 'NONE',  ( 17.96484262340118221, 34.93868534415482685, 7.964842623401181321 ) ) ;
#35681=CARTESIAN_POINT ( 'NONE',  ( 16.40814093676324603, 2.456968003263753531, -11.09922568453594671 ) ) ;
#35682=CARTESIAN_POINT ( 'NONE',  ( 24.16423886937410614, 9.303748834913967869, 8.672049930838204340E-16 ) ) ;
#35683=CARTESIAN_POINT ( 'NONE',  ( -2.266590686148945544, 57.22041550158063217, 7.082119434687048631 ) ) ;
#35684=CARTESIAN_POINT ( 'NONE',  ( 12.91533473730992121, 24.52201867748816966, 10.88017736071110164 ) ) ;
#35687=CARTESIAN_POINT ( 'NONE',  ( 0.5774900079438590739, 42.64701867748816966, -5.440088680355550821 ) ) ;
#35693=CARTESIAN_POINT ( 'NONE',  ( 20.36894250292379382, 43.67874883491397497, 10.36894250292379205 ) ) ;
#35694=CARTESIAN_POINT ( 'NONE',  ( 1.472469842513823179, 40.59226448433411605, -4.923371831947296329 ) ) ;
#35695=CARTESIAN_POINT ( 'NONE',  ( -0.8801773607110991993, 62.85535201082150536, -2.915334737309923874 ) ) ;
#35697=CARTESIAN_POINT ( 'NONE',  ( 12.91533473730992121, 54.52201867748816255, 10.88017736071110164 ) ) ;
#35700=ORIENTED_EDGE ( 'NONE', *, *, #8806, .T. ) ;
#35701=CARTESIAN_POINT ( 'NONE',  ( 22.26659068614894466, 13.88708216824730179, 7.082119434687054849 ) ) ;
#35702=EDGE_CURVE ( 'NONE', #6101, #83218, #76926, .T. ) ;
#35703=CARTESIAN_POINT ( 'NONE',  ( -2.816281873526473856, 24.33196800326375353, 3.434112377981055619 ) ) ;
#35705=CARTESIAN_POINT ( 'NONE',  ( -2.816281873526473856, 39.12363466993041783, 9.499525473075851096E-16 ) ) ;
#35706=CARTESIAN_POINT ( 'NONE',  ( 0.1532563361054100626, 30.80059781766744820, -2.638427012816831230 ) ) ;
#35707=CARTESIAN_POINT ( 'NONE',  ( 4.559911319644449179, 8.897018677488171434, 9.422509992056141925 ) ) ;
#35708=CARTESIAN_POINT ( 'NONE',  ( 10.00000000000000000, 47.87363466993042493, -12.81628187352647608 ) ) ;
#35710=CARTESIAN_POINT ( 'NONE',  ( 17.20831665107776587, 49.13393115100078745, -7.208316651077762316 ) ) ;
#35713=CARTESIAN_POINT ( 'NONE',  ( -0.1042174387088653925, 3.107361737662015955, 6.337391062633415117 ) ) ;
#35718=CARTESIAN_POINT ( 'NONE',  ( 18.52753015748618282, 18.92559781766745175, -4.923371831947291888 ) ) ;
#35719=CARTESIAN_POINT ( 'NONE',  ( 22.81628187352647785, 26.62363466993042138, 6.195893100308588602E-16 ) ) ;
#35720=( GEOMETRIC_REPRESENTATION_CONTEXT ( 3 ) GLOBAL_UNCERTAINTY_ASSIGNED_CONTEXT ( ( #28480 ) ) GLOBAL_UNIT_ASSIGNED_CONTEXT ( ( #90379, #97930, #52396 ) ) REPRESENTATION_CONTEXT ( 'NONE', 'WORKASPACE' ) );
#35723=CARTESIAN_POINT ( 'NONE',  ( 1.472469842513823179, 51.42559781766745886, 4.923371831947296329 ) ) ;
#35725=CARTESIAN_POINT ( 'NONE',  ( 13.79529636645031943, 15.34541550158063750, -14.16423886937409904 ) ) ;
#35726=CARTESIAN_POINT ( 'NONE',  ( 1.472469842513823179, 50.59226448433411605, -4.923371831947296329 ) ) ;
#35727=CARTESIAN_POINT ( 'NONE',  ( 6.565887622018943937, 43.08196800326374643, -12.81628187352647608 ) ) ;
#35730=CARTESIAN_POINT ( 'NONE',  ( 7.084665262690076126, 62.02201867748816966, -10.88017736071110164 ) ) ;
#35732=CARTESIAN_POINT ( 'NONE',  ( 1.472469842513823179, 31.42559781766745530, 4.923371831947296329 ) ) ;
#35733=CARTESIAN_POINT ( 'NONE',  ( 7.084665262690076126, 39.10535201082150536, 10.88017736071109987 ) ) ;
#35734=EDGE_CURVE ( 'NONE', #85215, #30617, #17615, .T. ) ;
#35735=CARTESIAN_POINT ( 'NONE',  ( 21.09922568453595559, 42.04030133659708213, -6.408140936763230044 ) ) ;
#35738=CARTESIAN_POINT ( 'NONE',  ( 7.084665262690076126, 29.10535201082150181, 10.88017736071109987 ) ) ;
#35740=CARTESIAN_POINT ( 'NONE',  ( 6.000000000000000000, 11.00000000000000000, 6.500000000000000888 ) ) ;
#35741=CARTESIAN_POINT ( 'NONE',  ( 7.084665262690076126, 22.02201867748817321, -10.88017736071110164 ) ) ;
#35742=CARTESIAN_POINT ( 'NONE',  ( 14.92337183194729633, 52.67559781766745175, 8.527530157486181039 ) ) ;
#35743=CARTESIAN_POINT ( 'NONE',  ( 4.559911319644449179, 42.23035201082151247, -9.422509992056141925 ) ) ;
#35744=PLANE ( 'NONE',  #56811 ) ;
#35745=CARTESIAN_POINT ( 'NONE',  ( -0.8801773607110991993, 57.85535201082149825, -2.915334737309923874 ) ) ;
#35746=CARTESIAN_POINT ( 'NONE',  ( 19.42250999205614548, 30.98035201082150536, -5.440088680355545492 ) ) ;
#35747=CARTESIAN_POINT ( 'NONE',  ( 0.000000000000000000, 72.39124140214553904, -5.153078942141819496 ) ) ;
#35748=SURFACE_SIDE_STYLE ('',( #36246 ) ) ;
#35749=CARTESIAN_POINT ( 'NONE',  ( 0.1532563361054083140, 31.00893115100078390, 1.131784320476157264E-15 ) ) ;
#35752=CARTESIAN_POINT ( 'NONE',  ( 5.076628168052703671, 56.84226448433412315, 8.527530157486179263 ) ) ;
#35753=CARTESIAN_POINT ( 'NONE',  ( 22.26659068614895176, 49.72041550158063927, -7.082119434687042414 ) ) ;
#35755=CARTESIAN_POINT ( 'NONE',  ( 1.274849032794292736, 62.55509018479936145, -6.499999999999977796 ) ) ;
#35756=CARTESIAN_POINT ( 'NONE',  ( 10.00000000000000000, 10.55374883491396787, -14.16423886937410082 ) ) ;
#35757=CARTESIAN_POINT ( 'NONE',  ( -2.266590686148945544, 37.22041550158063217, 7.082119434687048631 ) ) ;
#35758=CARTESIAN_POINT ( 'NONE',  ( -1.099225684535947600, -1.293031996736246469, -6.408140936763238038 ) ) ;
#35760=CARTESIAN_POINT ( 'NONE',  ( 20.88017736071110519, 15.56368534415483751, 2.639326808657452039E-16 ) ) ;
#35761=CARTESIAN_POINT ( 'NONE',  ( 5.076628168052703671, 31.84226448433412315, 8.527530157486179263 ) ) ;
#35764=DIRECTION ( 'NONE',  ( 0.000000000000000000, -1.000000000000000000, 0.000000000000000000 ) ) ;
#35767=CARTESIAN_POINT ( 'NONE',  ( 10.00000000000000178, 25.37363466993041783, 12.81628187352647608 ) ) ;
#35768=CARTESIAN_POINT ( 'NONE',  ( 7.361572987183169658, 24.96726448433412315, -9.846743663894592657 ) ) ;
#35770=CARTESIAN_POINT ( 'NONE',  ( 12.63842701281683034, 7.467264484334118713, 9.846743663894596210 ) ) ;
#35772=CARTESIAN_POINT ( 'NONE',  ( 19.42250999205614548, 5.980352010821504471, -5.440088680355545492 ) ) ;
#35773=CARTESIAN_POINT ( 'NONE',  ( 0.5774900079438590739, 12.64701867748817143, -5.440088680355550821 ) ) ;
#35774=CARTESIAN_POINT ( 'NONE',  ( 22.26659068614895176, 39.72041550158063217, -7.082119434687042414 ) ) ;
#35775=CARTESIAN_POINT ( 'NONE',  ( 7.084665262690076126, 62.02201867748816966, -10.88017736071110164 ) ) ;
#35777=CARTESIAN_POINT ( 'NONE',  ( 20.24186590665277308, 40.59014588040356131, -6.114288769123051637 ) ) ;
#35778=CARTESIAN_POINT ( 'NONE',  ( 12.63842701281683922, 24.55059781766745175, -9.846743663894590881 ) ) ;
#35780=CARTESIAN_POINT ( 'NONE',  ( 18.52753015748617571, 8.092264484334117824, 4.923371831947298993 ) ) ;
#35782=CARTESIAN_POINT ( 'NONE',  ( 2.791683348922240793, 36.63393115100078035, 7.208316651077764092 ) ) ;
#35783=CARTESIAN_POINT ( 'NONE',  ( 5.076628168052703671, 61.84226448433412315, 8.527530157486179263 ) ) ;
#35784=CARTESIAN_POINT ( 'NONE',  ( 2.035157376598822676, 32.43868534415483396, -7.964842623401177768 ) ) ;
#35787=CARTESIAN_POINT ( 'NONE',  ( 16.40814093676323893, 50.79030133659708923, 11.09922568453595026 ) ) ;
#35790=CARTESIAN_POINT ( 'NONE',  ( 7.361572987183169658, -0.03273551566588185635, -9.846743663894592657 ) ) ;
#35791=CARTESIAN_POINT ( 'NONE',  ( 6.565887622018943937, 45.16530133659708923, 12.81628187352647430 ) ) ;
#35792=CARTESIAN_POINT ( 'NONE',  ( 24.16423886937410614, 54.30374883491396787, 8.672049930838204340E-16 ) ) ;
#35793=CARTESIAN_POINT ( 'NONE',  ( 10.00000000000000000, 39.75893115100078745, -9.846743663894594434 ) ) ;
#35794=LINE ( 'NONE', #96817, #21496 ) ;
#35796=CARTESIAN_POINT ( 'NONE',  ( 18.52753015748618282, 58.92559781766745886, -4.923371831947291888 ) ) ;
#35797=CARTESIAN_POINT ( 'NONE',  ( 24.16423886937409904, 19.09541550158063927, 3.795296366450317205 ) ) ;
#35798=CARTESIAN_POINT ( 'NONE',  ( -4.164238869374098151, 46.59541550158063927, -3.795296366450310543 ) ) ;
#35799=CARTESIAN_POINT ( 'NONE',  ( 14.92337183194729988, 39.34226448433412315, -8.527530157486177487 ) ) ;
#35801=CARTESIAN_POINT ( 'NONE',  ( -0.8801773607111008646, 38.27201867748816255, 2.915334737309923430 ) ) ;
#35803=CARTESIAN_POINT ( 'NONE',  ( 2.035157376598824452, 53.68868534415484817, 7.964842623401179544 ) ) ;
#35804=CARTESIAN_POINT ( 'NONE',  ( 2.603489959281588995, 55.43575266056826933, -6.500000000000003553 ) ) ;
#35806=CARTESIAN_POINT ( 'NONE',  ( 6.565887622018943937, 43.08196800326374643, -12.81628187352647608 ) ) ;
#35808=CARTESIAN_POINT ( 'NONE',  ( 17.96484262340118221, 66.18868534415483396, -7.964842623401177768 ) ) ;
#35810=CARTESIAN_POINT ( 'NONE',  ( -2.266590686148945544, 2.220415501580634388, 7.082119434687048631 ) ) ;
#35811=CARTESIAN_POINT ( 'NONE',  ( 5.076628168052703671, 11.84226448433411960, 8.527530157486179263 ) ) ;
#35812=CARTESIAN_POINT ( 'NONE',  ( -1.926860441876564023, 59.68830936912751639, 1.004413902775740781E-15 ) ) ;
#35814=CARTESIAN_POINT ( 'NONE',  ( -0.1503990784575407469, 12.22266099184918531, -6.262539305110056631 ) ) ;
#35815=CARTESIAN_POINT ( 'NONE',  ( 20.88017736071110875, 15.77201867748817143, -2.915334737309920765 ) ) ;
#35818=CARTESIAN_POINT ( 'NONE',  ( -4.164238869374098151, 16.59541550158063927, -3.795296366450310543 ) ) ;
#35819=CARTESIAN_POINT ( 'NONE',  ( 2.035157376598822676, 27.43868534415483396, -7.964842623401177768 ) ) ;
#35820=CARTESIAN_POINT ( 'NONE',  ( 19.84674366389459621, 53.50893115100078745, 7.409399052514197653E-17 ) ) ;
#35821=VERTEX_POINT ( 'NONE', #32595 ) ;
#35823=CARTESIAN_POINT ( 'NONE',  ( 14.92337183194729633, 62.67559781766745886, 8.527530157486181039 ) ) ;
#35825=( BOUNDED_CURVE ( )  B_SPLINE_CURVE ( 2, ( #74897, #35417, #73911, #58404, #50421, #51910, #20429, #43897, #59396 ),
 .UNSPECIFIED., .F., .F. ) 
 B_SPLINE_CURVE_WITH_KNOTS ( ( 3, 2, 2, 2, 3 ),
 ( 0.5096570216176964374, 0.5119047619047618625, 0.5178571428571429047, 0.5238095238095238360, 0.5260572640965892610 ),
 .UNSPECIFIED. ) 
 CURVE ( )  GEOMETRIC_REPRESENTATION_ITEM ( )  RATIONAL_B_SPLINE_CURVE ( ( 0.9839835555609424134, 0.9871328979762474809, 1.000000000000000000, 0.9659258262890683122, 1.000000000000000000, 0.9659258262890683122, 1.000000000000000000, 0.9871328979762474809, 0.9839835555609424134 ) ) 
 REPRESENTATION_ITEM ( '' )  );
#35826=CARTESIAN_POINT ( 'NONE',  ( 15.44008868035555793, 66.39701867748817676, -9.422509992056140149 ) ) ;
#35827=CARTESIAN_POINT ( 'NONE',  ( 19.84674366389459621, 58.50893115100078745, 7.409399052514197653E-17 ) ) ;
#35828=CARTESIAN_POINT ( 'NONE',  ( 7.084665262690076126, 12.02201867748817143, -10.88017736071110164 ) ) ;
#35829=CARTESIAN_POINT ( 'NONE',  ( -0.3077640640441539621, 0.000000000000000000, 5.999999999999999112 ) ) ;
#35830=CARTESIAN_POINT ( 'NONE',  ( 5.076628168052704559, 0.1755978176674514724, -8.527530157486179263 ) ) ;
#35831=CARTESIAN_POINT ( 'NONE',  ( 2.035157376598824452, 18.68868534415484106, 7.964842623401179544 ) ) ;
#35834=CARTESIAN_POINT ( 'NONE',  ( -2.816281873526473856, 54.12363466993041783, 9.499525473075851096E-16 ) ) ;
#35835=CARTESIAN_POINT ( 'NONE',  ( 7.084665262690076126, 37.02201867748817676, -10.88017736071110164 ) ) ;
#35837=CARTESIAN_POINT ( 'NONE',  ( 13.43411237798106583, 42.66530133659707502, -12.81628187352647252 ) ) ;
#35838=CARTESIAN_POINT ( 'NONE',  ( 20.88017736071110164, 50.35535201082151247, 2.915334737309930979 ) ) ;
#35839=CARTESIAN_POINT ( 'NONE',  ( 18.52753015748618282, 53.92559781766745175, -4.923371831947291888 ) ) ;
#35841=ORIENTED_EDGE ( 'NONE', *, *, #7702, .T. ) ;
#35842=CARTESIAN_POINT ( 'NONE',  ( 17.20831665107776587, 22.88393115100078745, 7.208316651077764980 ) ) ;
#35843=CARTESIAN_POINT ( 'NONE',  ( 6.565887622018943937, 0.1653013365970866511, 12.81628187352647430 ) ) ;
#35845=CARTESIAN_POINT ( 'NONE',  ( 1.472469842513823179, 66.42559781766745175, 4.923371831947296329 ) ) ;
#35846=CARTESIAN_POINT ( 'NONE',  ( -0.8801773607110991993, 17.85535201082150536, -2.915334737309923874 ) ) ;
#35847=CARTESIAN_POINT ( 'NONE',  ( 19.84674366389459266, 48.30059781766745175, 2.638427012816836559 ) ) ;
#35849=CARTESIAN_POINT ( 'NONE',  ( 10.00000000000000000, -0.2410688489992152128, -9.846743663894594434 ) ) ;
#35850=CARTESIAN_POINT ( 'NONE',  ( 22.81628187352647785, 6.623634669930420493, 6.195893100308588602E-16 ) ) ;
#35852=CARTESIAN_POINT ( 'NONE',  ( 0.9413316022086133383, 63.45508385108958294, 6.499999999999978684 ) ) ;
#35853=CARTESIAN_POINT ( 'NONE',  ( 0.6178305044545818747, 33.49863466993042493, -9.382169495545419124 ) ) ;
#35854=CARTESIAN_POINT ( 'NONE',  ( 10.00000000000000000, 29.75893115100078745, -9.846743663894594434 ) ) ;
#35856=CARTESIAN_POINT ( 'NONE',  ( 6.204703633549690345, 52.84541550158062506, 14.16423886937410082 ) ) ;
#35857=CARTESIAN_POINT ( 'NONE',  ( 19.84674366389459266, 28.71726448433411960, -2.638427012816827677 ) ) ;
#35859=CARTESIAN_POINT ( 'NONE',  ( 19.39188664607695856, 65.83703382326400799, -6.499999999999937828 ) ) ;
#35861=CARTESIAN_POINT ( 'NONE',  ( 10.00000000000000000, 55.55374883491396787, -14.16423886937410082 ) ) ;
#35863=CARTESIAN_POINT ( 'NONE',  ( 17.96484262340118221, 26.18868534415483396, -7.964842623401177768 ) ) ;
#35864=CARTESIAN_POINT ( 'NONE',  ( 13.79529636645031943, 30.34541550158063927, -14.16423886937409904 ) ) ;
#35865=CARTESIAN_POINT ( 'NONE',  ( 6.204703633549690345, 47.84541550158064638, 14.16423886937410082 ) ) ;
#35868=CARTESIAN_POINT ( 'NONE',  ( 14.92337183194729988, 9.342264484334119601, -8.527530157486177487 ) ) ;
#35869=CARTESIAN_POINT ( 'NONE',  ( 10.00000000000000178, 67.25893115100079456, 9.846743663894594434 ) ) ;
#35870=CARTESIAN_POINT ( 'NONE',  ( 18.17829156368507171, 14.16792564121896270, 6.500000000000019540 ) ) ;
#35871=CARTESIAN_POINT ( 'NONE',  ( 15.44008868035555793, 56.39701867748817676, -9.422509992056140149 ) ) ;
#35872=CARTESIAN_POINT ( 'NONE',  ( 2.791683348922237240, 60.38393115100078745, -7.208316651077763204 ) ) ;
#35877=CARTESIAN_POINT ( 'NONE',  ( 10.00000000000000178, 43.05374883491397497, 14.16423886937410082 ) ) ;
#35880=CARTESIAN_POINT ( 'NONE',  ( 12.91533473730993009, 16.60535201082150891, -10.88017736071109987 ) ) ;
#35881=CARTESIAN_POINT ( 'NONE',  ( 10.00000000000000000, 42.87363466993042493, -12.81628187352647608 ) ) ;
#35882=PRESENTATION_STYLE_ASSIGNMENT (( #36883 ) ) ;
#35883=CARTESIAN_POINT ( 'NONE',  ( -2.816281873526471635, 38.91530133659708213, -3.434112377981056508 ) ) ;
#35884=CARTESIAN_POINT ( 'NONE',  ( 16.40814093676323893, 60.79030133659709634, 11.09922568453595026 ) ) ;
#35885=ORIENTED_EDGE ( 'NONE', *, *, #62162, .F. ) ;
#35888=CARTESIAN_POINT ( 'NONE',  ( -4.164238869374099039, 26.80374883491397142, 8.674139862899312516E-16 ) ) ;
#35889=CARTESIAN_POINT ( 'NONE',  ( -4.164238869374099927, 7.012082168247302683, 3.795296366450308767 ) ) ;
#35891=CARTESIAN_POINT ( 'NONE',  ( 4.559911319644449179, 17.23035201082150536, -9.422509992056141925 ) ) ;
#35892=CARTESIAN_POINT ( 'NONE',  ( -22.17076923076924189, 84.15384615384614619, -9.500000000000000000 ) ) ;
#35894=CARTESIAN_POINT ( 'NONE',  ( -0.8801773607110991993, 52.85535201082151247, -2.915334737309923874 ) ) ;
#35895=CARTESIAN_POINT ( 'NONE',  ( 17.96484262340118221, 51.18868534415483396, -7.964842623401177768 ) ) ;
#35896=CARTESIAN_POINT ( 'NONE',  ( 0.6178305044545838731, 9.748634669930416052, 9.382169495545420901 ) ) ;
#35897=DIRECTION ( 'NONE',  ( 0.000000000000000000, 0.000000000000000000, -1.000000000000000000 ) ) ;
#35898=CARTESIAN_POINT ( 'NONE',  ( 7.361572987183169658, 29.96726448433411960, -9.846743663894592657 ) ) ;
#35900=CARTESIAN_POINT ( 'NONE',  ( 18.61655166652076687, 49.87718327197428891, 6.499999999999981348 ) ) ;
#35901=CIRCLE ( 'NONE', #16787, 0.5000000000000004441 ) ;
#35902=CARTESIAN_POINT ( 'NONE',  ( 4.559911319644449179, 37.23035201082150536, -9.422509992056141925 ) ) ;
#35903=EDGE_CURVE ( 'NONE', #71629, #2953, #39921, .T. ) ;
#35904=CARTESIAN_POINT ( 'NONE',  ( 10.00000000000000178, 10.37363466993041961, 12.81628187352647608 ) ) ;
#35907=CARTESIAN_POINT ( 'NONE',  ( 18.52753015748618282, 28.92559781766745175, -4.923371831947291888 ) ) ;
#35908=CARTESIAN_POINT ( 'NONE',  ( 3.591859063236761518, 54.95696800326376064, 11.09922568453594849 ) ) ;
#35909=CARTESIAN_POINT ( 'NONE',  ( 1.472469842513823179, 11.42559781766745175, 4.923371831947296329 ) ) ;
#35911=FACE_OUTER_BOUND ( 'NONE', #8157, .T. ) ;
#35913=CARTESIAN_POINT ( 'NONE',  ( 7.084665262690076126, 14.10535201082150358, 10.88017736071109987 ) ) ;
#35915=CARTESIAN_POINT ( 'NONE',  ( 1.472469842513823179, 26.42559781766745175, 4.923371831947296329 ) ) ;
#35916=CARTESIAN_POINT ( 'NONE',  ( 20.88017736071110164, 20.35535201082150891, 2.915334737309930979 ) ) ;
#35917=CARTESIAN_POINT ( 'NONE',  ( 7.084665262690076126, 4.105352010821503583, 10.88017736071109987 ) ) ;
#35919=AXIS2_PLACEMENT_3D ( 'NONE', #17467, #77447, #8960 ) ;
#35920=CARTESIAN_POINT ( 'NONE',  ( 12.91533473730993009, 26.60535201082150536, -10.88017736071109987 ) ) ;
#35921=CARTESIAN_POINT ( 'NONE',  ( 2.035157376598822676, 37.43868534415484106, -7.964842623401177768 ) ) ;
#35923=CARTESIAN_POINT ( 'NONE',  ( 20.88017736071110875, 40.77201867748818387, -2.915334737309920765 ) ) ;
#35925=CARTESIAN_POINT ( 'NONE',  ( 18.52753015748618282, 53.92559781766745175, -4.923371831947291888 ) ) ;
#35926=CARTESIAN_POINT ( 'NONE',  ( 2.035157376598822676, 32.43868534415483396, -7.964842623401177768 ) ) ;
#35931=CARTESIAN_POINT ( 'NONE',  ( -0.3689425029237881626, 27.42874883491397142, 10.36894250292379027 ) ) ;
#35932=CARTESIAN_POINT ( 'NONE',  ( 15.44008868035555793, 51.39701867748816966, -9.422509992056140149 ) ) ;
#35933=CARTESIAN_POINT ( 'NONE',  ( 17.85158348494335812, 49.73726573380442773, -6.500000000000001776 ) ) ;
#35934=AXIS2_PLACEMENT_3D ( 'NONE', #58838, #81831, #36845 ) ;
#35936=CARTESIAN_POINT ( 'NONE',  ( 10.00000000000000000, 49.75893115100078745, -9.846743663894594434 ) ) ;
#35939=CARTESIAN_POINT ( 'NONE',  ( 12.63842701281683922, 19.55059781766745175, -9.846743663894590881 ) ) ;
#35941=CARTESIAN_POINT ( 'NONE',  ( 20.88017736071110875, 30.77201867748816966, -2.915334737309920765 ) ) ;
#35942=CARTESIAN_POINT ( 'NONE',  ( 19.84674366389459266, 23.71726448433412315, -2.638427012816827677 ) ) ;
#35943=CARTESIAN_POINT ( 'NONE',  ( -2.816281873526471635, 8.915301336597083903, -3.434112377981056508 ) ) ;
#35944=CARTESIAN_POINT ( 'NONE',  ( 2.035157376598822676, 57.43868534415484106, -7.964842623401177768 ) ) ;
#35945=CARTESIAN_POINT ( 'NONE',  ( 15.44008868035555793, 36.39701867748816966, -9.422509992056140149 ) ) ;
#35946=CARTESIAN_POINT ( 'NONE',  ( 0.6178305044545818747, 58.49863466993042493, -9.382169495545419124 ) ) ;
#35947=CARTESIAN_POINT ( 'NONE',  ( 24.16423886937409904, 39.09541550158062506, 3.795296366450317205 ) ) ;
#35952=CARTESIAN_POINT ( 'NONE',  ( 19.38216949554541557, 2.248634669930420049, -9.382169495545420901 ) ) ;
#35953=CARTESIAN_POINT ( 'NONE',  ( 12.91533473730993009, 41.60535201082149825, -10.88017736071109987 ) ) ;
#35954=CARTESIAN_POINT ( 'NONE',  ( 1.472469842513823179, 65.59226448433412315, -4.923371831947296329 ) ) ;
#35955=ORIENTED_EDGE ( 'NONE', *, *, #8756, .F. ) ;
#35956=CARTESIAN_POINT ( 'NONE',  ( 0.1532563361054082862, 21.21726448433412315, 2.638427012816831674 ) ) ;
#35957=CARTESIAN_POINT ( 'NONE',  ( 0.5774900079438607392, 63.48035201082149825, 5.440088680355550821 ) ) ;
#35959=CARTESIAN_POINT ( 'NONE',  ( 0.1532563361054100626, 30.80059781766744820, -2.638427012816831230 ) ) ;
#35960=CARTESIAN_POINT ( 'NONE',  ( 0.1532563361054100626, 30.80059781766744820, -2.638427012816831230 ) ) ;
#35961=CARTESIAN_POINT ( 'NONE',  ( 12.63842701281683922, 19.55059781766745175, -9.846743663894590881 ) ) ;
#35962=VECTOR ( 'NONE', #46327, 1000.000000000000000 ) ;
#35964=CARTESIAN_POINT ( 'NONE',  ( 20.88017736071110875, 65.77201867748817676, -2.915334737309920765 ) ) ;
#35966=CARTESIAN_POINT ( 'NONE',  ( 0.1532563361054082862, 11.21726448433411605, 2.638427012816831674 ) ) ;
#35967=CARTESIAN_POINT ( 'NONE',  ( 14.92337183194729988, 39.34226448433412315, -8.527530157486177487 ) ) ;
#35970=CARTESIAN_POINT ( 'NONE',  ( 17.20831665107776587, 62.88393115100078745, 7.208316651077764980 ) ) ;
#35972=CARTESIAN_POINT ( 'NONE',  ( 10.00000000000000000, 1.813685344154837731, -10.88017736071110342 ) ) ;
#35973=CARTESIAN_POINT ( 'NONE',  ( 6.204703633549690345, 22.84541550158062861, 14.16423886937410082 ) ) ;
#35975=CARTESIAN_POINT ( 'NONE',  ( -0.3689425029237881626, 22.42874883491397142, 10.36894250292379027 ) ) ;
#35976=CARTESIAN_POINT ( 'NONE',  ( -0.3689425029237898834, 51.17874883491397497, -10.36894250292378850 ) ) ;
#35978=CARTESIAN_POINT ( 'NONE',  ( 2.917880565312950480, 0.9704155015806342766, -12.26659068614894821 ) ) ;
#35979=CARTESIAN_POINT ( 'NONE',  ( -4.164238869374098151, 11.59541550158063217, -3.795296366450310543 ) ) ;
#35980=CARTESIAN_POINT ( 'NONE',  ( 10.00000000000000000, 41.81368534415484106, -10.88017736071110342 ) ) ;
#35982=AXIS2_PLACEMENT_3D ( 'NONE', #57003, #58476, #80506 ) ;
#35984=CARTESIAN_POINT ( 'NONE',  ( 10.00000000000000000, 24.75893115100078745, -9.846743663894594434 ) ) ;
#35985=CARTESIAN_POINT ( 'NONE',  ( 10.00000000000000000, 66.81368534415484817, -10.88017736071110342 ) ) ;
#35986=CARTESIAN_POINT ( 'NONE',  ( 14.92337183194729988, 34.34226448433411605, -8.527530157486177487 ) ) ;
#35987=ORIENTED_EDGE ( 'NONE', *, *, #5720, .F. ) ;
#35988=CARTESIAN_POINT ( 'NONE',  ( 10.00000000000000000, 11.81368534415483751, -10.88017736071110342 ) ) ;
#35989=CARTESIAN_POINT ( 'NONE',  ( 22.81628187352648496, 56.83196800326374643, -3.434112377981050290 ) ) ;
#35990=CARTESIAN_POINT ( 'NONE',  ( 2.791683348922237240, 45.38393115100079456, -7.208316651077763204 ) ) ;
#35993=CARTESIAN_POINT ( 'NONE',  ( 21.09922568453594849, 46.20696800326376064, 6.408140936763242479 ) ) ;
#35996=CARTESIAN_POINT ( 'NONE',  ( 4.559911319644449179, 48.89701867748817676, 9.422509992056141925 ) ) ;
#35997=CARTESIAN_POINT ( 'NONE',  ( 5.076628168052704559, 35.17559781766745175, -8.527530157486179263 ) ) ;
#35998=CARTESIAN_POINT ( 'NONE',  ( -0.3689425029237898834, 21.17874883491396432, -10.36894250292378850 ) ) ;
#36000=CARTESIAN_POINT ( 'NONE',  ( -0.3689425029237898834, 6.178748834913968757, -10.36894250292378850 ) ) ;
#36002=CARTESIAN_POINT ( 'NONE',  ( 12.91533473730993009, 56.60535201082151247, -10.88017736071109987 ) ) ;
#36004=CARTESIAN_POINT ( 'NONE',  ( 20.36894250292379738, 44.92874883491396787, -10.36894250292379027 ) ) ;
#36005=CARTESIAN_POINT ( 'NONE',  ( 19.38216949554541202, 0.9986346699304200492, 9.382169495545424454 ) ) ;
#36007=CARTESIAN_POINT ( 'NONE',  ( 20.88017736071110519, 50.56368534415484106, 2.639326808657452039E-16 ) ) ;
#36009=CARTESIAN_POINT ( 'NONE',  ( 10.00000000000000000, 22.87363466993042138, -12.81628187352647608 ) ) ;
#36010=CARTESIAN_POINT ( 'NONE',  ( 22.81628187352648496, 1.831968003263753753, -3.434112377981050290 ) ) ;
#36012=CARTESIAN_POINT ( 'NONE',  ( -0.8801773607111008646, 18.27201867748817321, 2.915334737309923430 ) ) ;
#36013=CARTESIAN_POINT ( 'NONE',  ( 12.91533473730993009, 6.605352010821504471, -10.88017736071109987 ) ) ;
#36016=FILL_AREA_STYLE ('',( #96541 ) ) ;
#36017=CARTESIAN_POINT ( 'NONE',  ( 14.92337183194729633, 2.675597817667451750, 8.527530157486181039 ) ) ;
#36019=VECTOR ( 'NONE', #50136, 1000.000000000000000 ) ;
#36020=CARTESIAN_POINT ( 'NONE',  ( 10.00000000000000000, 39.75893115100078745, -9.846743663894594434 ) ) ;
#36021=CARTESIAN_POINT ( 'NONE',  ( 0.5774900079438590739, 37.64701867748817676, -5.440088680355550821 ) ) ;
#36023=CARTESIAN_POINT ( 'NONE',  ( 19.38216949554541557, 7.248634669930421381, -9.382169495545420901 ) ) ;
#36024=CARTESIAN_POINT ( 'NONE',  ( -0.8801773607110991993, 37.85535201082151247, -2.915334737309923874 ) ) ;
#36027=CARTESIAN_POINT ( 'NONE',  ( 0.6178305044545818747, 43.49863466993042493, -9.382169495545419124 ) ) ;
#36029=CARTESIAN_POINT ( 'NONE',  ( 12.91533473730993009, 66.60535201082150536, -10.88017736071109987 ) ) ;
#36030=CARTESIAN_POINT ( 'NONE',  ( 22.81628187352647785, 36.62363466993041783, 6.195893100308588602E-16 ) ) ;
#36031=CARTESIAN_POINT ( 'NONE',  ( 6.204703633549690345, 7.845415501580634832, 14.16423886937410082 ) ) ;
#36032=CARTESIAN_POINT ( 'NONE',  ( 7.084665262690076126, 42.02201867748816966, -10.88017736071110164 ) ) ;
#36033=CARTESIAN_POINT ( 'NONE',  ( 0.1143410931637255656, 15.21691075486302580, 6.480892540919855449 ) ) ;
#36034=CARTESIAN_POINT ( 'NONE',  ( 20.36894250292379738, 64.92874883491397497, -10.36894250292379027 ) ) ;
#36035=CARTESIAN_POINT ( 'NONE',  ( 12.63842701281683034, 52.46726448433413026, 9.846743663894596210 ) ) ;
#36036=CARTESIAN_POINT ( 'NONE',  ( 12.63842701281683034, 17.46726448433411250, 9.846743663894596210 ) ) ;
#36037=CARTESIAN_POINT ( 'NONE',  ( -0.8801773607111008646, 68.27201867748817676, 2.915334737309923430 ) ) ;
#36039=CARTESIAN_POINT ( 'NONE',  ( -4.164238869374099927, 32.01208216824730357, 3.795296366450308767 ) ) ;
#36041=PRESENTATION_STYLE_ASSIGNMENT (( #81050 ) ) ;
#36044=ORIENTED_EDGE ( 'NONE', *, *, #46962, .T. ) ;
#36045=CARTESIAN_POINT ( 'NONE',  ( 24.16423886937409904, 59.09541550158063217, 3.795296366450317205 ) ) ;
#36046=CARTESIAN_POINT ( 'NONE',  ( -0.8801773607111008646, 3.272018677488171434, 2.915334737309923430 ) ) ;
#36047=CARTESIAN_POINT ( 'NONE',  ( 19.84674366389459266, 23.71726448433412315, -2.638427012816827677 ) ) ;
#36049=CARTESIAN_POINT ( 'NONE',  ( 3.591859063236761518, 29.95696800326375708, 11.09922568453594849 ) ) ;
#36052=CARTESIAN_POINT ( 'NONE',  ( 0.5774900079438590739, 17.64701867748817321, -5.440088680355550821 ) ) ;
#36053=CARTESIAN_POINT ( 'NONE',  ( 20.36894250292379382, 53.67874883491397497, 10.36894250292379205 ) ) ;
#36055=CARTESIAN_POINT ( 'NONE',  ( 19.84674366389459266, 23.71726448433412315, -2.638427012816827677 ) ) ;
#36057=CARTESIAN_POINT ( 'NONE',  ( 12.63842701281683034, 12.46726448433411782, 9.846743663894596210 ) ) ;
#36058=EDGE_CURVE ( 'NONE', #98100, #71776, #70919, .T. ) ;
#36061=ORIENTED_EDGE ( 'NONE', *, *, #30998, .T. ) ;
#36065=CARTESIAN_POINT ( 'NONE',  ( 1.472469842513823179, 40.59226448433411605, -4.923371831947296329 ) ) ;
#36066=CARTESIAN_POINT ( 'NONE',  ( 15.44008868035555793, 16.39701867748817321, -9.422509992056140149 ) ) ;
#36067=CARTESIAN_POINT ( 'NONE',  ( 20.88017736071110519, 30.56368534415484106, 2.639326808657452039E-16 ) ) ;
#36068=CARTESIAN_POINT ( 'NONE',  ( 18.52753015748618282, 58.92559781766745886, -4.923371831947291888 ) ) ;
#36069=CARTESIAN_POINT ( 'NONE',  ( 19.38216949554541202, 10.99863466993042138, 9.382169495545424454 ) ) ;
#36070=CARTESIAN_POINT ( 'NONE',  ( -4.164238869374098151, 11.59541550158063217, -3.795296366450310543 ) ) ;
#36072=VECTOR ( 'NONE', #23696, 1000.000000000000000 ) ;
#36073=CARTESIAN_POINT ( 'NONE',  ( 13.43411237798105340, 30.58196800326374998, 12.81628187352647963 ) ) ;
#36074=ORIENTED_EDGE ( 'NONE', *, *, #13960, .F. ) ;
#36075=CARTESIAN_POINT ( 'NONE',  ( 1.472469842513823179, 31.42559781766745530, 4.923371831947296329 ) ) ;
#36076=CARTESIAN_POINT ( 'NONE',  ( 19.42250999205614193, 5.147018677488171434, 5.440088680355555262 ) ) ;
#36078=CARTESIAN_POINT ( 'NONE',  ( 10.00000000000000000, 65.55374883491396076, -14.16423886937410082 ) ) ;
#36080=CARTESIAN_POINT ( 'NONE',  ( -0.8801773607111008646, 53.27201867748816966, 2.915334737309923430 ) ) ;
#36081=CARTESIAN_POINT ( 'NONE',  ( 0.5774900079438590739, 62.64701867748817676, -5.440088680355550821 ) ) ;
#36082=CARTESIAN_POINT ( 'NONE',  ( 10.00000000000000178, 54.31368534415484106, 10.88017736071110342 ) ) ;
#36084=CARTESIAN_POINT ( 'NONE',  ( 10.00000000000000178, 44.31368534415484106, 10.88017736071110342 ) ) ;
#36087=CARTESIAN_POINT ( 'NONE',  ( 18.52753015748617571, 28.09226448433411960, 4.923371831947298993 ) ) ;
#36088=VERTEX_POINT ( 'NONE', #62977 ) ;
#36089=CARTESIAN_POINT ( 'NONE',  ( 17.20831665107776587, 52.88393115100078035, 7.208316651077764980 ) ) ;
#36091=CARTESIAN_POINT ( 'NONE',  ( -4.164238869374098151, 11.59541550158063217, -3.795296366450310543 ) ) ;
#36094=CARTESIAN_POINT ( 'NONE',  ( 18.18329248733322956, 47.60290668512021739, 6.499999999999960920 ) ) ;
#36095=CARTESIAN_POINT ( 'NONE',  ( 20.36894250292379738, 54.92874883491396076, -10.36894250292379027 ) ) ;
#36099=CARTESIAN_POINT ( 'NONE',  ( 2.791683348922240793, 51.63393115100078745, 7.208316651077764092 ) ) ;
#36102=CARTESIAN_POINT ( 'NONE',  ( 6.565887622018943937, 18.08196800326375708, -12.81628187352647608 ) ) ;
#36103=CARTESIAN_POINT ( 'NONE',  ( 7.361572987183169658, 14.96726448433411960, -9.846743663894592657 ) ) ;
#36104=EDGE_CURVE ( 'NONE', #53783, #800, #53782, .T. ) ;
#36105=CARTESIAN_POINT ( 'NONE',  ( 0.6261916924966959286, 0.5000000000000002220, 6.500000000000003553 ) ) ;
#36106=CARTESIAN_POINT ( 'NONE',  ( 14.92337183194729988, 9.342264484334119601, -8.527530157486177487 ) ) ;
#36107=CARTESIAN_POINT ( 'NONE',  ( 13.43411237798105340, 0.5819680032637533085, 12.81628187352647963 ) ) ;
#36111=CARTESIAN_POINT ( 'NONE',  ( 7.084665262690076126, 9.105352010821503583, 10.88017736071109987 ) ) ;
#36112=CARTESIAN_POINT ( 'NONE',  ( 2.917880565312948704, 2.637082168247300906, 12.26659068614894643 ) ) ;
#36113=CARTESIAN_POINT ( 'NONE',  ( 18.52753015748617571, 23.09226448433411960, 4.923371831947298993 ) ) ;
#36114=CARTESIAN_POINT ( 'NONE',  ( -0.8801773607111009756, 53.06368534415484106, 1.068504757029289695E-15 ) ) ;
#36115=CARTESIAN_POINT ( 'NONE',  ( 22.81628187352647785, 26.41530133659708923, 3.434112377981063169 ) ) ;
#36119=CARTESIAN_POINT ( 'NONE',  ( 22.81628187352647785, 1.415301336597087012, 3.434112377981063169 ) ) ;
#36120=CARTESIAN_POINT ( 'NONE',  ( 19.84674366389459621, 8.508931151000785675, 7.409399052514197653E-17 ) ) ;
#36122=CARTESIAN_POINT ( 'NONE',  ( 3.591859063236763294, 23.29030133659708568, -11.09922568453595026 ) ) ;
#36124=CARTESIAN_POINT ( 'NONE',  ( 20.88017736071110164, 45.35535201082149115, 2.915334737309930979 ) ) ;
#36130=CARTESIAN_POINT ( 'NONE',  ( 0.5774900079438590739, 32.64701867748816966, -5.440088680355550821 ) ) ;
#36133=CARTESIAN_POINT ( 'NONE',  ( 20.88017736071110519, 35.56368534415484106, 2.639326808657452039E-16 ) ) ;
#36134=CARTESIAN_POINT ( 'NONE',  ( 14.92337183194729988, 49.34226448433411605, -8.527530157486177487 ) ) ;
#36135=ADVANCED_FACE ( 'NONE', ( #39992 ), #77484, .F. ) ;
#36136=CARTESIAN_POINT ( 'NONE',  ( 17.96484262340118221, 49.93868534415484106, 7.964842623401181321 ) ) ;
#36137=CARTESIAN_POINT ( 'NONE',  ( 10.00000000000000178, 33.05374883491396787, 14.16423886937410082 ) ) ;
#36140=UNCERTAINTY_MEASURE_WITH_UNIT (LENGTH_MEASURE( 1.000000000000000082E-05 ), #35388, 'distance_accuracy_value', 'NONE');
#36142=CARTESIAN_POINT ( 'NONE',  ( 2.791683348922240793, 36.63393115100078035, 7.208316651077764092 ) ) ;
#36143=CARTESIAN_POINT ( 'NONE',  ( 0.6178305044545818747, 63.49863466993043204, -9.382169495545419124 ) ) ;
#36144=CARTESIAN_POINT ( 'NONE',  ( 13.43411237798106583, 2.665301336597086568, -12.81628187352647252 ) ) ;
#36145=EDGE_LOOP ( 'NONE', ( #42787, #59867, #58811, #18138 ) ) ;
#36146=CARTESIAN_POINT ( 'NONE',  ( 10.00000000000000000, 21.81368534415484106, -10.88017736071110342 ) ) ;
#36147=CARTESIAN_POINT ( 'NONE',  ( 7.084665262690076126, 7.022018677488169658, -10.88017736071110164 ) ) ;
#36148=CARTESIAN_POINT ( 'NONE',  ( 15.44008868035555260, 14.73035201082150536, 9.422509992056143702 ) ) ;
#36149=CARTESIAN_POINT ( 'NONE',  ( 5.076628168052704559, 0.1755978176674514724, -8.527530157486179263 ) ) ;
#36150=CARTESIAN_POINT ( 'NONE',  ( 10.00000000000000178, 28.05374883491396787, 14.16423886937410082 ) ) ;
#36151=CARTESIAN_POINT ( 'NONE',  ( 0.1532563361054082862, 11.21726448433411605, 2.638427012816831674 ) ) ;
#36152=CARTESIAN_POINT ( 'NONE',  ( 18.52753015748618282, 63.92559781766745886, -4.923371831947291888 ) ) ;
#36153=CARTESIAN_POINT ( 'NONE',  ( 4.559911319644449179, 38.89701867748817676, 9.422509992056141925 ) ) ;
#36155=CARTESIAN_POINT ( 'NONE',  ( 20.88017736071110519, 25.56368534415483751, 2.639326808657452039E-16 ) ) ;
#36159=LINE ( 'NONE', #97186, #36959 ) ;
#36160=CARTESIAN_POINT ( 'NONE',  ( 2.791683348922240793, 46.63393115100077324, 7.208316651077764092 ) ) ;
#36163=ORIENTED_EDGE ( 'NONE', *, *, #30955, .F. ) ;
#36165=CARTESIAN_POINT ( 'NONE',  ( 13.79529636645030344, 28.26208216824729647, 14.16423886937410614 ) ) ;
#36166=CARTESIAN_POINT ( 'NONE',  ( 2.917880565312950480, 15.97041550158063217, -12.26659068614894821 ) ) ;
#36168=CARTESIAN_POINT ( 'NONE',  ( 17.96484262340118221, 61.18868534415482685, -7.964842623401177768 ) ) ;
#36169=CARTESIAN_POINT ( 'NONE',  ( 22.26659068614895176, 49.72041550158063927, -7.082119434687042414 ) ) ;
#36170=CARTESIAN_POINT ( 'NONE',  ( 0.1532563361054083140, 66.00893115100079456, 1.131784320476157264E-15 ) ) ;
#36171=CARTESIAN_POINT ( 'NONE',  ( 17.20831665107776587, 52.88393115100078035, 7.208316651077764980 ) ) ;
#36173=CARTESIAN_POINT ( 'NONE',  ( 15.44008868035555260, 49.73035201082150536, 9.422509992056143702 ) ) ;
#36174=CARTESIAN_POINT ( 'NONE',  ( 22.81628187352647785, 1.415301336597087012, 3.434112377981063169 ) ) ;
#36175=CARTESIAN_POINT ( 'NONE',  ( -4.164238869374099927, 12.01208216824730357, 3.795296366450308767 ) ) ;
#36176=CARTESIAN_POINT ( 'NONE',  ( 2.917880565312948704, 52.63708216824730357, 12.26659068614894643 ) ) ;
#36177=CARTESIAN_POINT ( 'NONE',  ( 7.084665262690076126, 19.10535201082150181, 10.88017736071109987 ) ) ;
#36179=CARTESIAN_POINT ( 'NONE',  ( 19.42250999205614193, 45.14701867748817676, 5.440088680355555262 ) ) ;
#36180=CARTESIAN_POINT ( 'NONE',  ( 19.50000000000000711, 105.0000000000000000, 5.000000000000000000 ) ) ;
#36181=VERTEX_POINT ( 'NONE', #79466 ) ;
#36185=COLOUR_RGB ( '', 0.08235294, 0.09019608, 0.10196078) ;
#36186=CARTESIAN_POINT ( 'NONE',  ( 22.26659068614894466, 43.88708216824729647, 7.082119434687054849 ) ) ;
#36187=CARTESIAN_POINT ( 'NONE',  ( 10.00000000000000178, 47.25893115100078745, 9.846743663894594434 ) ) ;
#36188=CARTESIAN_POINT ( 'NONE',  ( 19.42250999205614548, 65.98035201082151957, -5.440088680355545492 ) ) ;
#36189=EDGE_CURVE ( 'NONE', #86614, #1529, #1878, .T. ) ;
#36191=CARTESIAN_POINT ( 'NONE',  ( -0.8801773607111009756, 48.06368534415484817, 1.068504757029289695E-15 ) ) ;
#36194=CARTESIAN_POINT ( 'NONE',  ( 0.6178305044545838731, 54.74863466993042493, 9.382169495545420901 ) ) ;
#36198=CARTESIAN_POINT ( 'NONE',  ( 2.917880565312948704, 17.63708216824730357, 12.26659068614894643 ) ) ;
#36199=CARTESIAN_POINT ( 'NONE',  ( 6.565887622018943937, 20.16530133659708213, 12.81628187352647430 ) ) ;
#36200=ORIENTED_EDGE ( 'NONE', *, *, #49123, .F. ) ;
#36201=CARTESIAN_POINT ( 'NONE',  ( 19.38216949554541557, 47.24863466993041783, -9.382169495545420901 ) ) ;
#36202=CARTESIAN_POINT ( 'NONE',  ( 17.20831665107776587, 32.88393115100078745, 7.208316651077764980 ) ) ;
#36203=CARTESIAN_POINT ( 'NONE',  ( 2.035157376598822676, 7.438685344154837509, -7.964842623401177768 ) ) ;
#36204=CARTESIAN_POINT ( 'NONE',  ( 6.565887622018943937, 48.08196800326375353, -12.81628187352647608 ) ) ;
#36205=DIRECTION ( 'NONE',  ( 0.000000000000000000, 0.000000000000000000, -1.000000000000000000 ) ) ;
#36206=CARTESIAN_POINT ( 'NONE',  ( 5.076628168052703671, 36.84226448433412315, 8.527530157486179263 ) ) ;
#36208=( BOUNDED_CURVE ( )  B_SPLINE_CURVE ( 2, ( #28721, #81714, #13226, #59211, #89715, #45209, #98744, #98238, #236 ),
 .UNSPECIFIED., .F., .T. ) 
 B_SPLINE_CURVE_WITH_KNOTS ( ( 3, 2, 2, 2, 3 ),
 ( 0.2615695083688028277, 0.2619047619047619735, 0.2678571428571429047, 0.2738095238095238360, 0.2741447773454829817 ),
 .UNSPECIFIED. ) 
 CURVE ( )  GEOMETRIC_REPRESENTATION_ITEM ( )  RATIONAL_B_SPLINE_CURVE ( ( 0.9963778908391760503, 0.9980808541467920403, 1.000000000000000000, 0.9659258262890683122, 1.000000000000000000, 0.9659258262890683122, 1.000000000000000000, 0.9980808541467920403, 0.9963778908391759392 ) ) 
 REPRESENTATION_ITEM ( '' )  );
#36209=CARTESIAN_POINT ( 'NONE',  ( 4.559911319644449179, 68.89701867748817676, 9.422509992056141925 ) ) ;
#36211=CARTESIAN_POINT ( 'NONE',  ( 1.274849032794231007, 33.57228050351031357, 6.499999999999895195 ) ) ;
#36214=CARTESIAN_POINT ( 'NONE',  ( 1.274849032794292736, 67.55509018479936856, -6.499999999999977796 ) ) ;
#36215=CARTESIAN_POINT ( 'NONE',  ( 2.791683348922237240, 15.38393115100078212, -7.208316651077763204 ) ) ;
#36216=CARTESIAN_POINT ( 'NONE',  ( 0.6178305044545838731, 24.74863466993042493, 9.382169495545420901 ) ) ;
#36219=CARTESIAN_POINT ( 'NONE',  ( 10.00000000000000178, 62.25893115100078745, 9.846743663894594434 ) ) ;
#36221=CARTESIAN_POINT ( 'NONE',  ( -4.164238869374098151, 16.59541550158063927, -3.795296366450310543 ) ) ;
#36222=CARTESIAN_POINT ( 'NONE',  ( 7.361572987183170547, 47.05059781766745175, 9.846743663894590881 ) ) ;
#36223=CARTESIAN_POINT ( 'NONE',  ( -1.099225684535947600, 49.54030133659708923, 6.408140936763237150 ) ) ;
#36226=CARTESIAN_POINT ( 'NONE',  ( 5.076628168052704559, 10.17559781766745175, -8.527530157486179263 ) ) ;
#36227=STYLED_ITEM ( 'NONE', ( #46724 ), #32199 ) ;
#36229=CARTESIAN_POINT ( 'NONE',  ( 19.84674366389459266, 33.30059781766744464, 2.638427012816836559 ) ) ;
#36230=CARTESIAN_POINT ( 'NONE',  ( 4.559911319644449179, 43.89701867748816966, 9.422509992056141925 ) ) ;
#36232=AXIS2_PLACEMENT_3D ( 'NONE', #15587, #7089, #22590 ) ;
#36237=CARTESIAN_POINT ( 'NONE',  ( 2.035157376598822676, 52.43868534415483396, -7.964842623401177768 ) ) ;
#36238=ORIENTED_EDGE ( 'NONE', *, *, #74721, .F. ) ;
#36239=CARTESIAN_POINT ( 'NONE',  ( 0.5774900079438607392, 68.48035201082150536, 5.440088680355550821 ) ) ;
#36240=CARTESIAN_POINT ( 'NONE',  ( 0.5774900079438607392, 18.48035201082150536, 5.440088680355550821 ) ) ;
#36241=CARTESIAN_POINT ( 'NONE',  ( 2.791683348922237240, 50.38393115100078035, -7.208316651077763204 ) ) ;
#36242=CARTESIAN_POINT ( 'NONE',  ( 19.42250999205614548, 40.98035201082150536, -5.440088680355545492 ) ) ;
#36244=CARTESIAN_POINT ( 'NONE',  ( 2.035157376598824452, 53.68868534415484817, 7.964842623401179544 ) ) ;
#36245=CARTESIAN_POINT ( 'NONE',  ( 7.084665262690076126, 24.10535201082150181, 10.88017736071109987 ) ) ;
#36246=SURFACE_STYLE_FILL_AREA ( #35247 ) ;
#36247=CARTESIAN_POINT ( 'NONE',  ( 5.076628168052703671, 21.84226448433411960, 8.527530157486179263 ) ) ;
#36248=CARTESIAN_POINT ( 'NONE',  ( 5.500000000000000000, 61.00000000000000711, 6.000000000000000000 ) ) ;
#36250=CARTESIAN_POINT ( 'NONE',  ( 1.472469842513823179, 55.59226448433412315, -4.923371831947296329 ) ) ;
#36252=CARTESIAN_POINT ( 'NONE',  ( 6.204703633549690345, 67.84541550158060375, 14.16423886937410082 ) ) ;
#36254=CARTESIAN_POINT ( 'NONE',  ( 22.26659068614895176, 9.720415501580633943, -7.082119434687042414 ) ) ;
#36255=CARTESIAN_POINT ( 'NONE',  ( 6.204703633549690345, 42.84541550158063217, 14.16423886937410082 ) ) ;
#36256=CARTESIAN_POINT ( 'NONE',  ( 6.565887622018943937, -1.918031996736246692, -12.81628187352647608 ) ) ;
#36257=VERTEX_POINT ( 'NONE', #25007 ) ;
#36259=CARTESIAN_POINT ( 'NONE',  ( 17.96484262340118221, 16.18868534415483396, -7.964842623401177768 ) ) ;
#36260=CARTESIAN_POINT ( 'NONE',  ( 18.52753015748618282, 53.92559781766745175, -4.923371831947291888 ) ) ;
#36261=CARTESIAN_POINT ( 'NONE',  ( 22.17874357816322117, 89.00000000000000000, 12.00000000000000000 ) ) ;
#36265=CARTESIAN_POINT ( 'NONE',  ( 12.63842701281683922, 4.550597817667451750, -9.846743663894590881 ) ) ;
#36266=CARTESIAN_POINT ( 'NONE',  ( -1.099225684535947600, 18.70696800326375353, -6.408140936763238038 ) ) ;
#36267=CARTESIAN_POINT ( 'NONE',  ( 1.472469842513823179, 31.42559781766745530, 4.923371831947296329 ) ) ;
#36270=CARTESIAN_POINT ( 'NONE',  ( 14.92337183194729988, 4.342264484334117824, -8.527530157486177487 ) ) ;
#36272=CARTESIAN_POINT ( 'NONE',  ( 10.00000000000000178, 9.313685344154839285, 10.88017736071110342 ) ) ;
#36273=CARTESIAN_POINT ( 'NONE',  ( -4.164238869374099927, 37.01208216824731068, 3.795296366450308767 ) ) ;
#36274=CARTESIAN_POINT ( 'NONE',  ( -0.8801773607111008646, 63.27201867748817676, 2.915334737309923430 ) ) ;
#36276=CARTESIAN_POINT ( 'NONE',  ( 14.92337183194729633, 22.67559781766745175, 8.527530157486181039 ) ) ;
#36278=CARTESIAN_POINT ( 'NONE',  ( 18.52753015748617571, 3.092264484334118269, 4.923371831947298993 ) ) ;
#36279=CARTESIAN_POINT ( 'NONE',  ( -0.5867979546742444485, 6.298283880980277759E-16, -3.244044026693988059 ) ) ;
#36280=CARTESIAN_POINT ( 'NONE',  ( 12.63842701281683922, 39.55059781766744464, -9.846743663894590881 ) ) ;
#36281=CARTESIAN_POINT ( 'NONE',  ( 19.84674366389459266, 58.30059781766745886, 2.638427012816836559 ) ) ;
#36282=CARTESIAN_POINT ( 'NONE',  ( 20.88017736071110164, 40.35535201082150536, 2.915334737309930979 ) ) ;
#36283=UNCERTAINTY_MEASURE_WITH_UNIT (LENGTH_MEASURE( 1.000000000000000082E-05 ), #16551, 'distance_accuracy_value', 'NONE');
#36286=CARTESIAN_POINT ( 'NONE',  ( 3.591859063236761518, 54.95696800326376064, 11.09922568453594849 ) ) ;
#36288=CARTESIAN_POINT ( 'NONE',  ( 7.361572987183170547, 7.050597817667451750, 9.846743663894590881 ) ) ;
#36289=CARTESIAN_POINT ( 'NONE',  ( 22.81628187352647785, 46.62363466993041783, 6.195893100308588602E-16 ) ) ;
#36290=CARTESIAN_POINT ( 'NONE',  ( 22.26659068614895176, 64.72041550158064638, -7.082119434687042414 ) ) ;
#36291=CARTESIAN_POINT ( 'NONE',  ( 0.1532563361054100626, 35.80059781766745175, -2.638427012816831230 ) ) ;
#36293=CARTESIAN_POINT ( 'NONE',  ( 1.472469842513823179, 0.5922644843341181575, -4.923371831947296329 ) ) ;
#36294=CARTESIAN_POINT ( 'NONE',  ( 2.917880565312950480, 45.97041550158063927, -12.26659068614894821 ) ) ;
#36295=CARTESIAN_POINT ( 'NONE',  ( 19.84674366389459266, 38.71726448433412315, -2.638427012816827677 ) ) ;
#36297=CARTESIAN_POINT ( 'NONE',  ( 17.96484262340118221, 34.93868534415482685, 7.964842623401181321 ) ) ;
#36298=CARTESIAN_POINT ( 'NONE',  ( 0.1532563361054100626, 0.8005978176674514168, -2.638427012816831230 ) ) ;
#36301=ORIENTED_EDGE ( 'NONE', *, *, #24867, .F. ) ;
#36302=CARTESIAN_POINT ( 'NONE',  ( 3.591859063236763294, 58.29030133659708923, -11.09922568453595026 ) ) ;
#36304=CARTESIAN_POINT ( 'NONE',  ( 10.00000000000000000, 61.81368534415484106, -10.88017736071110342 ) ) ;
#36306=CARTESIAN_POINT ( 'NONE',  ( 6.204703633549690345, 0.7620821682473009062, -14.16423886937410259 ) ) ;
#36307=CARTESIAN_POINT ( 'NONE',  ( 19.84674366389459266, 3.717264484334118713, -2.638427012816827677 ) ) ;
#36308=EDGE_CURVE ( 'NONE', #43937, #31231, #56762, .T. ) ;
#36310=ORIENTED_EDGE ( 'NONE', *, *, #44603, .T. ) ;
#36312=CARTESIAN_POINT ( 'NONE',  ( 20.88017736071110519, 10.56368534415483751, 2.639326808657452039E-16 ) ) ;
#36314=ORIENTED_EDGE ( 'NONE', *, *, #52943, .F. ) ;
#36315=CARTESIAN_POINT ( 'NONE',  ( -0.8801773607111009756, 23.06368534415484106, 1.068504757029289695E-15 ) ) ;
#36316=CARTESIAN_POINT ( 'NONE',  ( 12.63842701281683922, 59.55059781766744464, -9.846743663894590881 ) ) ;
#36319=CARTESIAN_POINT ( 'NONE',  ( 0.1532563361054100626, 65.80059781766745175, -2.638427012816831230 ) ) ;
#36321=CARTESIAN_POINT ( 'NONE',  ( 5.076628168052703671, 1.842264484334118047, 8.527530157486179263 ) ) ;
#36322=CARTESIAN_POINT ( 'NONE',  ( 19.84674366389459266, 63.71726448433412315, -2.638427012816827677 ) ) ;
#36323=CARTESIAN_POINT ( 'NONE',  ( 6.565887622018943937, 40.16530133659708923, 12.81628187352647430 ) ) ;
#36324=CARTESIAN_POINT ( 'NONE',  ( -0.8801773607111008646, 3.272018677488171434, 2.915334737309923430 ) ) ;
#36325=CARTESIAN_POINT ( 'NONE',  ( 19.84674366389459266, 3.717264484334118713, -2.638427012816827677 ) ) ;
#36326=CARTESIAN_POINT ( 'NONE',  ( 2.035157376598822676, 17.43868534415483751, -7.964842623401177768 ) ) ;
#36328=CARTESIAN_POINT ( 'NONE',  ( -1.099225684535947600, 54.54030133659708923, 6.408140936763237150 ) ) ;
#36329=CARTESIAN_POINT ( 'NONE',  ( 0.5774900079438590739, 47.64701867748817676, -5.440088680355550821 ) ) ;
#36331=CARTESIAN_POINT ( 'NONE',  ( -1.099225684535947600, 48.70696800326375353, -6.408140936763238038 ) ) ;
#36332=CARTESIAN_POINT ( 'NONE',  ( 20.88017736071110875, 50.77201867748817676, -2.915334737309920765 ) ) ;
#36334=CARTESIAN_POINT ( 'NONE',  ( 0.1532563361054083140, 61.00893115100078745, 1.131784320476157264E-15 ) ) ;
#36337=CARTESIAN_POINT ( 'NONE',  ( 12.63842701281683034, 22.46726448433411605, 9.846743663894596210 ) ) ;
#36338=CARTESIAN_POINT ( 'NONE',  ( -2.816281873526471635, 3.915301336597087456, -3.434112377981056508 ) ) ;
#36339=CYLINDRICAL_SURFACE ( 'NONE', #27661, 0.5000000000000004441 ) ;
#36340=CARTESIAN_POINT ( 'NONE',  ( 0.1532563361054100626, 65.80059781766745175, -2.638427012816831230 ) ) ;
#36341=CARTESIAN_POINT ( 'NONE',  ( 15.44008868035555793, 26.39701867748817321, -9.422509992056140149 ) ) ;
#36342=CARTESIAN_POINT ( 'NONE',  ( 0.1532563361054082862, 56.21726448433411605, 2.638427012816831674 ) ) ;
#36343=CARTESIAN_POINT ( 'NONE',  ( 10.00000000000000000, 4.758931151000784787, -9.846743663894594434 ) ) ;
#36344=CARTESIAN_POINT ( 'NONE',  ( 1.274849032794116210, 8.572280503510292249, 6.499999999999738876 ) ) ;
#36346=CARTESIAN_POINT ( 'NONE',  ( 13.43411237798106583, 7.665301336597086568, -12.81628187352647252 ) ) ;
#36347=VERTEX_POINT ( 'NONE', #16514 ) ;
#36351=CARTESIAN_POINT ( 'NONE',  ( 3.591859063236761518, 34.95696800326375353, 11.09922568453594849 ) ) ;
#36352=CARTESIAN_POINT ( 'NONE',  ( 19.84674366389459266, 33.30059781766744464, 2.638427012816836559 ) ) ;
#36354=CARTESIAN_POINT ( 'NONE',  ( -4.164238869374098151, 66.59541550158060375, -3.795296366450310543 ) ) ;
#36355=EDGE_CURVE ( 'NONE', #55640, #10095, #61332, .T. ) ;
#36356=CARTESIAN_POINT ( 'NONE',  ( 10.00000000000000000, 29.75893115100078745, -9.846743663894594434 ) ) ;
#36358=CARTESIAN_POINT ( 'NONE',  ( 20.36894250292379738, 64.92874883491397497, -10.36894250292379027 ) ) ;
#36360=CARTESIAN_POINT ( 'NONE',  ( 0.5774900079438607392, 23.48035201082150536, 5.440088680355550821 ) ) ;
#36361=CARTESIAN_POINT ( 'NONE',  ( 6.204703633549690345, 52.84541550158062506, 14.16423886937410082 ) ) ;
#36363=CARTESIAN_POINT ( 'NONE',  ( -0.3689425029237881626, 52.42874883491396076, 10.36894250292379027 ) ) ;
#36366=CARTESIAN_POINT ( 'NONE',  ( 17.20831665107776587, 14.13393115100078568, -7.208316651077762316 ) ) ;
#36368=CARTESIAN_POINT ( 'NONE',  ( 5.076628168052704559, 65.17559781766745175, -8.527530157486179263 ) ) ;
#36370=CARTESIAN_POINT ( 'NONE',  ( -0.8801773607110991993, 47.85535201082150536, -2.915334737309923874 ) ) ;
#36372=CARTESIAN_POINT ( 'NONE',  ( -46.94000000000001194, 100.4376529975800025, -8.999999999986080468 ) ) ;
#36373=VECTOR ( 'NONE', #9126, 1000.000000000000000 ) ;
#36374=CARTESIAN_POINT ( 'NONE',  ( 10.00000000000000178, 67.25893115100079456, 9.846743663894594434 ) ) ;
#36375=CARTESIAN_POINT ( 'NONE',  ( 6.204703633549690345, 2.845415501580634388, 14.16423886937410082 ) ) ;
#36377=CARTESIAN_POINT ( 'NONE',  ( 10.00000000000000178, 22.25893115100078745, 9.846743663894594434 ) ) ;
#36379=CARTESIAN_POINT ( 'NONE',  ( 13.79529636645031943, 35.34541550158063927, -14.16423886937409904 ) ) ;
#36380=CARTESIAN_POINT ( 'NONE',  ( 0.1532563361054083140, 11.00893115100078568, 1.131784320476157264E-15 ) ) ;
#36381=CARTESIAN_POINT ( 'NONE',  ( -0.1042174387088605353, 63.10736173766204615, 6.337391062633419558 ) ) ;
#36383=CARTESIAN_POINT ( 'NONE',  ( 10.00000000000000000, 36.81368534415484106, -10.88017736071110342 ) ) ;
#36384=CARTESIAN_POINT ( 'NONE',  ( -1.099225684535947600, 38.70696800326375353, -6.408140936763238038 ) ) ;
#36385=CARTESIAN_POINT ( 'NONE',  ( 17.96484262340118221, 4.938685344154837509, 7.964842623401181321 ) ) ;
#36386=CARTESIAN_POINT ( 'NONE',  ( 21.09922568453595559, 37.04030133659708923, -6.408140936763230044 ) ) ;
#36387=CARTESIAN_POINT ( 'NONE',  ( 19.38216949554541202, 55.99863466993041072, 9.382169495545424454 ) ) ;
#36388=ORIENTED_EDGE ( 'NONE', *, *, #94607, .T. ) ;
#36392=CARTESIAN_POINT ( 'NONE',  ( 2.917880565312948704, 37.63708216824731068, 12.26659068614894643 ) ) ;
#36393=CARTESIAN_POINT ( 'NONE',  ( -2.266590686148945544, 2.220415501580634388, 7.082119434687048631 ) ) ;
#36394=CARTESIAN_POINT ( 'NONE',  ( -0.8801773607110991993, 12.85535201082150358, -2.915334737309923874 ) ) ;
#36395=CARTESIAN_POINT ( 'NONE',  ( 4.559911319644449179, 18.89701867748817321, 9.422509992056141925 ) ) ;
#36396=LINE ( 'NONE', #35892, #82996 ) ;
#36398=CARTESIAN_POINT ( 'NONE',  ( 2.035157376598822676, 47.43868534415484817, -7.964842623401177768 ) ) ;
#36399=CARTESIAN_POINT ( 'NONE',  ( 15.44008868035555260, 54.73035201082150536, 9.422509992056143702 ) ) ;
#36400=CARTESIAN_POINT ( 'NONE',  ( 10.00000000000000000, 17.87363466993041783, -12.81628187352647608 ) ) ;
#36402=CARTESIAN_POINT ( 'NONE',  ( 0.000000000000000000, 70.80332830338373640, -5.000000000000000000 ) ) ;
#36403=CARTESIAN_POINT ( 'NONE',  ( 2.791683348922237240, 25.38393115100078390, -7.208316651077763204 ) ) ;
#36404=CARTESIAN_POINT ( 'NONE',  ( -0.8801773607111008646, 58.27201867748816966, 2.915334737309923430 ) ) ;
#36405=CARTESIAN_POINT ( 'NONE',  ( -1.099225684535947600, 13.70696800326375353, -6.408140936763238038 ) ) ;
#36406=( LENGTH_UNIT ( ) NAMED_UNIT ( * ) SI_UNIT ( .MILLI., .METRE. ) );
#36407=CARTESIAN_POINT ( 'NONE',  ( 4.559911319644449179, 13.89701867748817143, 9.422509992056141925 ) ) ;
#36408=CARTESIAN_POINT ( 'NONE',  ( 10.00000000000000000, 39.75893115100078745, -9.846743663894594434 ) ) ;
#36409=CARTESIAN_POINT ( 'NONE',  ( 16.40814093676324603, 47.45696800326375353, -11.09922568453594671 ) ) ;
#36410=CARTESIAN_POINT ( 'NONE',  ( 1.472469842513823179, 21.42559781766745175, 4.923371831947296329 ) ) ;
#36411=( LENGTH_UNIT ( ) NAMED_UNIT ( * ) SI_UNIT ( .MILLI., .METRE. ) );
#36412=CARTESIAN_POINT ( 'NONE',  ( 13.79529636645031943, 10.34541550158063394, -14.16423886937409904 ) ) ;
#36414=CARTESIAN_POINT ( 'NONE',  ( 15.44008868035555260, 24.73035201082150891, 9.422509992056143702 ) ) ;
#36416=CARTESIAN_POINT ( 'NONE',  ( 13.79529636645030344, 28.26208216824729647, 14.16423886937410614 ) ) ;
#36417=CARTESIAN_POINT ( 'NONE',  ( 18.52753015748617571, 28.09226448433411960, 4.923371831947298993 ) ) ;
#36418=CARTESIAN_POINT ( 'NONE',  ( 0.5774900079438607392, 23.48035201082150536, 5.440088680355550821 ) ) ;
#36419=CARTESIAN_POINT ( 'NONE',  ( 0.5774900079438607392, 23.48035201082150536, 5.440088680355550821 ) ) ;
#36421=CARTESIAN_POINT ( 'NONE',  ( 10.00000000000000000, 26.81368534415484106, -10.88017736071110342 ) ) ;
#36422=CARTESIAN_POINT ( 'NONE',  ( -2.816281873526473856, 44.33196800326375353, 3.434112377981055619 ) ) ;
#36423=ADVANCED_FACE ( 'NONE', ( #64440 ), #73923, .T. ) ;
#36424=CARTESIAN_POINT ( 'NONE',  ( 19.42250999205614193, 40.14701867748817676, 5.440088680355555262 ) ) ;
#36426=CARTESIAN_POINT ( 'NONE',  ( 15.44008868035555260, 39.73035201082150536, 9.422509992056143702 ) ) ;
#36429=CARTESIAN_POINT ( 'NONE',  ( 5.076628168052703671, 51.84226448433412315, 8.527530157486179263 ) ) ;
#36430=CARTESIAN_POINT ( 'NONE',  ( 0.5774900079438607392, 38.48035201082150536, 5.440088680355550821 ) ) ;
#36433=CARTESIAN_POINT ( 'NONE',  ( -0.1038446121089122015, 9.243024370107935539, -6.337995344473772441 ) ) ;
#36434=CARTESIAN_POINT ( 'NONE',  ( 6.204703633549690345, 52.84541550158062506, 14.16423886937410082 ) ) ;
#36435=CARTESIAN_POINT ( 'NONE',  ( 15.44008868035555260, 54.73035201082150536, 9.422509992056143702 ) ) ;
#36438=CARTESIAN_POINT ( 'NONE',  ( 19.84674366389459266, 63.30059781766745886, 2.638427012816836559 ) ) ;
#36439=CARTESIAN_POINT ( 'NONE',  ( 10.00000000000000178, 2.258931151000784787, 9.846743663894594434 ) ) ;
#36440=CARTESIAN_POINT ( 'NONE',  ( 17.20831665107776587, 24.13393115100078035, -7.208316651077762316 ) ) ;
#36441=ORIENTED_EDGE ( 'NONE', *, *, #31312, .T. ) ;
#36442=CARTESIAN_POINT ( 'NONE',  ( 1.472469842513823179, 16.42559781766745175, 4.923371831947296329 ) ) ;
#36445=CARTESIAN_POINT ( 'NONE',  ( 4.559911319644449179, 28.89701867748817321, 9.422509992056141925 ) ) ;
#36446=CARTESIAN_POINT ( 'NONE',  ( 14.92337183194729988, 19.34226448433411960, -8.527530157486177487 ) ) ;
#36447=CARTESIAN_POINT ( 'NONE',  ( 22.81628187352647785, 6.415301336597088344, 3.434112377981063169 ) ) ;
#36448=CARTESIAN_POINT ( 'NONE',  ( 7.084665262690076126, 59.10535201082150536, 10.88017736071109987 ) ) ;
#36449=CARTESIAN_POINT ( 'NONE',  ( -0.8801773607111009756, 58.06368534415484106, 1.068504757029289695E-15 ) ) ;
#36450=CARTESIAN_POINT ( 'NONE',  ( 2.035157376598824452, 38.68868534415483396, 7.964842623401179544 ) ) ;
#36451=CARTESIAN_POINT ( 'NONE',  ( 19.38216949554541202, 60.99863466993042493, 9.382169495545424454 ) ) ;
#36452=CARTESIAN_POINT ( 'NONE',  ( 20.36894250292379738, 49.92874883491396787, -10.36894250292379027 ) ) ;
#36457=CARTESIAN_POINT ( 'NONE',  ( 13.43411237798105340, 0.5819680032637533085, 12.81628187352647963 ) ) ;
#36458=CARTESIAN_POINT ( 'NONE',  ( 4.559911319644449179, 52.23035201082151247, -9.422509992056141925 ) ) ;
#36459=CARTESIAN_POINT ( 'NONE',  ( 6.204703633549690345, 0.7620821682473009062, -14.16423886937410259 ) ) ;
#36460=VERTEX_POINT ( 'NONE', #79949 ) ;
#36461=CARTESIAN_POINT ( 'NONE',  ( 12.63842701281683922, 14.55059781766744997, -9.846743663894590881 ) ) ;
#36463=CARTESIAN_POINT ( 'NONE',  ( 12.91533473730992121, 59.52201867748816966, 10.88017736071110164 ) ) ;
#36464=CARTESIAN_POINT ( 'NONE',  ( 19.84674366389459621, 33.50893115100078745, 7.409399052514197653E-17 ) ) ;
#36465=CARTESIAN_POINT ( 'NONE',  ( 19.84674366389459266, 28.71726448433411960, -2.638427012816827677 ) ) ;
#36466=CARTESIAN_POINT ( 'NONE',  ( 2.791683348922240793, 16.63393115100078745, 7.208316651077764092 ) ) ;
#36468=CARTESIAN_POINT ( 'NONE',  ( 0.6178305044545818747, 38.49863466993042493, -9.382169495545419124 ) ) ;
#36469=CARTESIAN_POINT ( 'NONE',  ( 19.84674366389459266, 3.717264484334118713, -2.638427012816827677 ) ) ;
#36472=CARTESIAN_POINT ( 'NONE',  ( 0.1532563361054082862, 26.21726448433411605, 2.638427012816831674 ) ) ;
#36475=CARTESIAN_POINT ( 'NONE',  ( 6.565887622018943937, 53.08196800326374643, -12.81628187352647608 ) ) ;
#36477=CARTESIAN_POINT ( 'NONE',  ( -1.099225684535947600, -1.293031996736246469, -6.408140936763238038 ) ) ;
#36478=CARTESIAN_POINT ( 'NONE',  ( 2.035157376598824452, 3.688685344154837953, 7.964842623401179544 ) ) ;
#36480=CARTESIAN_POINT ( 'NONE',  ( 13.79529636645031943, 15.34541550158063750, -14.16423886937409904 ) ) ;
#36484=CARTESIAN_POINT ( 'NONE',  ( 2.917880565312950480, 35.97041550158063217, -12.26659068614894821 ) ) ;
#36485=CARTESIAN_POINT ( 'NONE',  ( 10.00000000000000000, 45.55374883491397497, -14.16423886937410082 ) ) ;
#36486=CARTESIAN_POINT ( 'NONE',  ( 24.16423886937410614, 9.303748834913967869, 8.672049930838204340E-16 ) ) ;
#36487=CARTESIAN_POINT ( 'NONE',  ( -4.164238869374099927, 17.01208216824730357, 3.795296366450308767 ) ) ;
#36489=CARTESIAN_POINT ( 'NONE',  ( 17.96484262340118221, 44.93868534415483396, 7.964842623401181321 ) ) ;
#36491=CARTESIAN_POINT ( 'NONE',  ( 18.52753015748618282, 28.92559781766745175, -4.923371831947291888 ) ) ;
#36492=CARTESIAN_POINT ( 'NONE',  ( 2.035157376598824452, 68.68868534415484817, 7.964842623401179544 ) ) ;
#36493=CARTESIAN_POINT ( 'NONE',  ( 14.92337183194729633, 32.67559781766745175, 8.527530157486181039 ) ) ;
#36494=CARTESIAN_POINT ( 'NONE',  ( 17.96484262340118221, 14.93868534415484106, 7.964842623401181321 ) ) ;
#36495=CARTESIAN_POINT ( 'NONE',  ( 3.591859063236761518, 64.95696800326376774, 11.09922568453594849 ) ) ;
#36496=CARTESIAN_POINT ( 'NONE',  ( 19.84674366389459266, 48.71726448433413026, -2.638427012816827677 ) ) ;
#36498=CARTESIAN_POINT ( 'NONE',  ( 18.52753015748617571, 23.09226448433411960, 4.923371831947298993 ) ) ;
#36499=CARTESIAN_POINT ( 'NONE',  ( 0.6178305044545838731, 44.74863466993042493, 9.382169495545420901 ) ) ;
#36501=CARTESIAN_POINT ( 'NONE',  ( 4.559911319644449179, 42.23035201082151247, -9.422509992056141925 ) ) ;
#36502=CARTESIAN_POINT ( 'NONE',  ( 14.92337183194729633, 42.67559781766745886, 8.527530157486181039 ) ) ;
#36503=CARTESIAN_POINT ( 'NONE',  ( 22.26659068614894466, 28.88708216824730357, 7.082119434687054849 ) ) ;
#36504=ORIENTED_EDGE ( 'NONE', *, *, #46255, .F. ) ;
#36505=CARTESIAN_POINT ( 'NONE',  ( -0.3689425029237881626, 2.428748834913967869, 10.36894250292379027 ) ) ;
#36506=CARTESIAN_POINT ( 'NONE',  ( 10.00000000000000000, 51.81368534415484106, -10.88017736071110342 ) ) ;
#36507=CARTESIAN_POINT ( 'NONE',  ( -0.1491070598754174470, 61.94583914210339515, 4.500000000000000888 ) ) ;
#36508=CARTESIAN_POINT ( 'NONE',  ( 10.00000000000000000, 55.55374883491396787, -14.16423886937410082 ) ) ;
#36509=CARTESIAN_POINT ( 'NONE',  ( 14.92337183194729633, 62.67559781766745886, 8.527530157486181039 ) ) ;
#36511=CARTESIAN_POINT ( 'NONE',  ( 0.5774900079438607392, 48.48035201082150536, 5.440088680355550821 ) ) ;
#36513=CARTESIAN_POINT ( 'NONE',  ( 0.2751277870542911952, 38.21833443783937412, 6.499999999999992006 ) ) ;
#36514=MECHANICAL_DESIGN_GEOMETRIC_PRESENTATION_REPRESENTATION('',(#20524),#6178);
#36515=CARTESIAN_POINT ( 'NONE',  ( 3.591859063236761518, 29.95696800326375708, 11.09922568453594849 ) ) ;
#36516=CARTESIAN_POINT ( 'NONE',  ( 19.38216949554541557, 2.248634669930420049, -9.382169495545420901 ) ) ;
#36518=CARTESIAN_POINT ( 'NONE',  ( 19.42250999205614193, 15.14701867748817143, 5.440088680355555262 ) ) ;
#36519=CARTESIAN_POINT ( 'NONE',  ( -0.8801773607111008646, 8.272018677488171434, 2.915334737309923430 ) ) ;
#36520=CARTESIAN_POINT ( 'NONE',  ( 19.84674366389459266, 48.71726448433413026, -2.638427012816827677 ) ) ;
#36522=B_SPLINE_CURVE_WITH_KNOTS ( 'NONE', 3,
 ( #13183, #97208, #44162, #74672, #6182, #67174 ),
 .UNSPECIFIED., .F., .F.,
 ( 4, 2, 4 ),
 ( 0.000000000000000000, 0.0002565770811490990168, 0.0005131541622981980336 ),
 .UNSPECIFIED. ) ;
#36524=CARTESIAN_POINT ( 'NONE',  ( -0.8801773607110991993, 7.855352010821504471, -2.915334737309923874 ) ) ;
#36525=CARTESIAN_POINT ( 'NONE',  ( 13.43411237798105340, 0.5819680032637533085, 12.81628187352647963 ) ) ;
#36527=ADVANCED_FACE ( 'NONE', ( #26448 ), #18513, .T. ) ;
#36529=CARTESIAN_POINT ( 'NONE',  ( 0.1532563361054083140, 6.008931151000784787, 1.131784320476157264E-15 ) ) ;
#36531=CARTESIAN_POINT ( 'NONE',  ( 12.63842701281683922, 49.55059781766744464, -9.846743663894590881 ) ) ;
#36532=CARTESIAN_POINT ( 'NONE',  ( 2.035157376598822676, 42.43868534415483396, -7.964842623401177768 ) ) ;
#36533=CARTESIAN_POINT ( 'NONE',  ( 10.00000000000000178, 10.37363466993041961, 12.81628187352647608 ) ) ;
#36534=CARTESIAN_POINT ( 'NONE',  ( 17.96484262340118221, 51.18868534415483396, -7.964842623401177768 ) ) ;
#36536=CARTESIAN_POINT ( 'NONE',  ( 2.831191079880678085, 79.91181047996344944, -9.500000000000000000 ) ) ;
#36537=CARTESIAN_POINT ( 'NONE',  ( 16.40814093676323893, 50.79030133659708923, 11.09922568453595026 ) ) ;
#36539=CARTESIAN_POINT ( 'NONE',  ( 7.084665262690076126, 62.02201867748816966, -10.88017736071110164 ) ) ;
#36540=CARTESIAN_POINT ( 'NONE',  ( 21.09922568453594849, 31.20696800326375353, 6.408140936763242479 ) ) ;
#36541=CARTESIAN_POINT ( 'NONE',  ( -4.164238869374099927, 2.012082168247300906, 3.795296366450308767 ) ) ;
#36542=CARTESIAN_POINT ( 'NONE',  ( -16.94000000000001549, 92.00000000000000000, 9.500000000000000000 ) ) ;
#36543=CARTESIAN_POINT ( 'NONE',  ( 15.44008868035555260, 39.73035201082150536, 9.422509992056143702 ) ) ;
#36544=CARTESIAN_POINT ( 'NONE',  ( -0.1503990784575328643, 15.12777174578612538, 6.262539305110068177 ) ) ;
#36545=CARTESIAN_POINT ( 'NONE',  ( 7.361572987183170547, 57.05059781766744464, 9.846743663894590881 ) ) ;
#36546=CARTESIAN_POINT ( 'NONE',  ( 14.92337183194729633, 12.67559781766745353, 8.527530157486181039 ) ) ;
#36547=CARTESIAN_POINT ( 'NONE',  ( 7.361572987183169658, 9.967264484334119601, -9.846743663894592657 ) ) ;
#36548=CARTESIAN_POINT ( 'NONE',  ( 2.917880565312948704, 42.63708216824729647, 12.26659068614894643 ) ) ;
#36551=CARTESIAN_POINT ( 'NONE',  ( 19.67858290521088449, 88.19818180006032549, -5.461713021790604472 ) ) ;
#36553=CARTESIAN_POINT ( 'NONE',  ( 24.16423886937410614, 64.51208216824728936, -3.795296366450302550 ) ) ;
#36554=CARTESIAN_POINT ( 'NONE',  ( 2.917880565312948704, 57.63708216824731068, 12.26659068614894643 ) ) ;
#36555=CARTESIAN_POINT ( 'NONE',  ( 17.20831665107776587, 32.88393115100078745, 7.208316651077764980 ) ) ;
#36556=CARTESIAN_POINT ( 'NONE',  ( 19.38216949554541202, 25.99863466993042138, 9.382169495545424454 ) ) ;
#36557=FACE_OUTER_BOUND ( 'NONE', #53134, .T. ) ;
#36559=CARTESIAN_POINT ( 'NONE',  ( 2.917880565312948704, 2.637082168247300906, 12.26659068614894643 ) ) ;
#36560=CARTESIAN_POINT ( 'NONE',  ( -0.8801773607111008646, 8.272018677488171434, 2.915334737309923430 ) ) ;
#36561=CARTESIAN_POINT ( 'NONE',  ( -2.266590686148945544, 56.38708216824731068, -7.082119434687050408 ) ) ;
#36562=CARTESIAN_POINT ( 'NONE',  ( 17.20831665107776587, 24.13393115100078035, -7.208316651077762316 ) ) ;
#36563=( BOUNDED_SURFACE ( )  B_SPLINE_SURFACE ( 1, 2, ( 
 ( #62678, #85690, #71185, #47180, #63167, #3180, #46698, #86675, #25691, #41190, #39219, #77196, #10675, #17210, #70695, #47687, #2214, #8702, #93178, #1719, #71670, #69705, #70200, #32673, #78180, #1235, #31690, #32175, #18180, #62180, #24704, #86187, #48168, #92690, #2710, #33161, #48660, #24215, #43624, #88627, #57145, #73123, #36120, #79662, #97157, #19647, #28129, #4665, #87642, #35127, #3675, #19156, #20136, #95138, #65626, #96151, #50139, #80648, #49635, #73622, #12142, #74110, #96650, #66628, #66121, #28625, #50640, #5145, #11158, #81129, #26649, #42647, #95651, #27634, #80143, #72631, #51128, #11653, #42168, #58629, #35635, #27135, #58119, #4163, #59112, #12631, #43130, #18673, #89127, #41678, #20639, #65130, #5644, #49159, #81618, #34631, #13127, #57639, #88134, #72147, #34137, #64629, #52120, #98135, #22126, #14637, #7630, #68118, #75111, #53101, #8107, #29596, #61092, #45100, #60098, #22622, #75607, #83611, #37622, #69101, #82114, #37131, #76099, #52607, #44106, #51635, #59612, #21634, #14130, #74617, #90109, #82614, #46105, #6131, #13624, #91602, #76589, #97645, #67120, #83108, #7118, #38121, #29109, #98644, #30093, #15126, #6617, #44615, #23118, #45601, #53590, #38602, #635, #60600, #68609, #31083, #30587, #67626, #91095, #90599, #36637, #138, #84104, #15620, #89622, #21134, #40075, #2103, #33051, #55060, #69590, #48547, #54567, #92574, #1608, #62067, #93064, #41071, #31572, #85578, #32057, #24098, #32562, #54082, #16096, #1110, #70576, #92089, #55575, #10074, #56070, #85083, #39596, #18068, #63547, #16591, #63060, #17092, #47068, #70084, #79047, #71566, #9082, #62560, #94056, #25578, #77566, #71072, #84598, #46583, #24595, #40575, #47574, #10560, #86565, #78070, #9575, #93558, #25092, #2597, #86073, #17585, #48050, #3078, #78564, #61578, #23617, #77081, #8592, #39099, #34027, #89017, #87046, #94543, #35518, #20526, #41572, #11052, #95538, #57527, #50523, #72039, #88022, #27028, #65513, #19049, #3569, #66009, #27519, #96537, #51011, #81505, #65010, #20023, #13010, #73507, #64524, #12033, #95029, #18557, #79553, #26538, #81020, #49049, #19535, #42531, #73015, #5031, #50031, #57034, #43507, #87536, #49526, #72522, #80033, #80534, #74005, #11538, #4548, #4056, #42059, #35012, #26061, #34517, #96035, #58010, #64031, #88520, #12522, #28012, #43024, #58508, #33536, #56551, #67008, #76839, #30847, #13514, #15382, #24356, #85330, #53350, #45867, #77326, #8839, #97529, #16351, #97039, #28514, #43995, #84844, #76357, #54819, #31823, #83858, #7872, #397, #84367, #54329, #31333, #38367, #61833, #92827, #23866, #16844 ),
 ( #39353, #46833, #53857, #47318, #92341, #8353, #15866, #69847, #74497, #1371, #68866, #61345, #69350, #22879, #91856, #62320, #6020, #23371, #5530, #36010, #66512, #36516, #46351, #59008, #89511, #21021, #38861, #51510, #874, #30346, #82002, #60853, #91352, #48797, #55323, #25820, #63788, #10322, #40824, #47814, #33773, #71324, #34268, #56794, #26785, #26294, #57283, #10814, #64280, #39835, #41333, #85829, #2842, #55826, #33297, #17344, #32807, #11295, #78314, #9834, #18809, #94792, #86320, #94297, #40335, #87777, #56317, #71805, #19293, #86813, #70341, #79306, #25342, #64770, #77818, #18317, #70838, #87289, #2351, #63303, #93812, #9333, #17825, #48306, #49292, #3310, #78814, #1859, #79793, #41815, #62820, #72282, #3812, #95284, #32315, #93318, #24840, #59250, #96789, #90243, #36266, #20775, #58760, #66761, #88276, #51764, #12768, #73759, #13264, #65764, #88768, #74245, #50265, #66255, #6263, #49780, #89750, #28758, #44251, #42294, #97787, #13763, #58252, #5290, #50776, #43264, #67260, #96291, #4791, #82248, #74754, #80781, #35767, #20279, #80286, #11786, #19777, #21267, #34776, #42785, #12278, #73270, #36768, #28265, #89264, #81268, #51266, #29250, #81750, #43756, #97284, #35268, #59746, #5777, #72766, #4302, #27768, #65262, #95791, #27272, #57771, #77216, #21774, #61711, #763, #16236, #14270, #69727, #84730, #30228, #45748, #22757, #15267, #39239, #68260, #75740, #54213, #46716, #22267, #76244, #91233, #62204, #52253, #60246, #31216, #6759, #14771, #52740, #90739, #8721, #7760, #61231, #53239, #60732, #1254, #91737, #83249, #38253, #31709, #82749, #44744, #83743, #92227, #68745, #45244, #277, #37273, #7261, #23258, #98281, #30724, #53733, #84252, #15754, #37763, #76725, #46239, #75246, #23753, #67762, #69241, #29736, #8244, #38741, #98780, #25711, #70223, #86206, #70719, #55709, #1742, #47706, #26189, #62697, #32196, #33666, #10699, #2235, #17717, #55200, #72169, #48190, #56204, #34157, #78703, #85224, #94182, #40212, #49179, #41698, #71208, #93198, #3203, #17229, #24724, #85714, #3696, #78200, #9712, #64163, #2730, #32693, #92710, #94681, #86697, #77705, #10212, #18203, #48682, #33185, #24236, #56681, #87172, #40704, #54703, #79185, #63677, #63190, #93695, #79680, #47204, #16727, #18695, #11178, #25230, #41213, #71691, #9217, #39729, #4184, #20154, #27650, #96668, #50156, #34655, #66647, #58645, #97171, #82129, #13638, #96167, #51148, #44123, #5661, #95669, #43147, #27155, #19174, #11675, #57656, #81634, #49654, #58137, #73636, #5164, #36143, #88646, #72649, #51649, #88153, #19667, #4681, #65150, #50657, #74633 ) ),
 .UNSPECIFIED., .F., .F., .F. ) 
 B_SPLINE_SURFACE_WITH_KNOTS ( ( 2, 2 ),
 ( 3, 2, 2, 2, 2, 2, 2, 2, 2, 2, 2, 2, 2, 2, 2, 2, 2, 2, 2, 2, 2, 2, 2, 2, 2, 2, 2, 2, 2, 2, 2, 2, 2, 2, 2, 2, 2, 2, 2, 2, 2, 2, 2, 2, 2, 2, 2, 2, 2, 2, 2, 2, 2, 2, 2, 2, 2, 2, 2, 2, 2, 2, 2, 2, 2, 2, 2, 2, 2, 2, 2, 2, 2, 2, 2, 2, 2, 2, 2, 2, 2, 2, 2, 2, 2, 2, 2, 2, 2, 2, 2, 2, 2, 2, 2, 2, 2, 2, 2, 2, 2, 2, 2, 2, 2, 2, 2, 2, 2, 2, 2, 2, 2, 2, 2, 2, 2, 2, 2, 2, 2, 2, 2, 2, 2, 2, 2, 2, 2, 2, 2, 2, 2, 2, 2, 2, 2, 2, 2, 2, 2, 2, 2, 2, 2, 2, 2, 2, 2, 2, 2, 2, 2, 2, 2, 2, 2, 2, 2, 2, 2, 2, 3 ),
 ( 0.000000000000000000, 1.000000000000000000 ),
 ( 0.000000000000000000, 0.005952380952380952051, 0.01190476190476190410, 0.01785714285714285615, 0.02380952380952380820, 0.02976190476190476025, 0.03571428571428571230, 0.04166666666666666435, 0.04761904761904761640, 0.05357142857142856845, 0.05952380952380952051, 0.06547619047619047949, 0.07142857142857142461, 0.07738095238095238360, 0.08333333333333332871, 0.08928571428571428770, 0.09523809523809523281, 0.1011904761904761918, 0.1071428571428571369, 0.1130952380952380959, 0.1190476190476190410, 0.1250000000000000000, 0.1309523809523809590, 0.1369047619047619180, 0.1428571428571428492, 0.1488095238095238082, 0.1547619047619047672, 0.1607142857142857262, 0.1666666666666666574, 0.1726190476190476164, 0.1785714285714285754, 0.1845238095238095344, 0.1904761904761904656, 0.1964285714285714246, 0.2023809523809523836, 0.2083333333333333426, 0.2142857142857142738, 0.2202380952380952328, 0.2261904761904761918, 0.2321428571428571508, 0.2380952380952380820, 0.2440476190476190410, 0.2500000000000000000, 0.2559523809523809312, 0.2619047619047619180, 0.2678571428571428492, 0.2738095238095238360, 0.2797619047619047672, 0.2857142857142856984, 0.2916666666666666852, 0.2976190476190476164, 0.3035714285714285476, 0.3095238095238095344, 0.3154761904761904656, 0.3214285714285714524, 0.3273809523809523836, 0.3333333333333333148, 0.3392857142857143016, 0.3452380952380952328, 0.3511904761904761640, 0.3571428571428571508, 0.3630952380952380820, 0.3690476190476190688, 0.3750000000000000000, 0.3809523809523809312, 0.3869047619047619180, 0.3928571428571428492, 0.3988095238095238360, 0.4047619047619047672, 0.4107142857142856984, 0.4166666666666666852, 0.4226190476190476164, 0.4285714285714285476, 0.4345238095238095344, 0.4404761904761904656, 0.4464285714285714524, 0.4523809523809523836, 0.4583333333333333148, 0.4642857142857143016, 0.4702380952380952328, 0.4761904761904761640, 0.4821428571428571508, 0.4880952380952380820, 0.4940476190476190688, 0.5000000000000000000, 0.5059523809523809312, 0.5119047619047618625, 0.5178571428571429047, 0.5238095238095238360, 0.5297619047619047672, 0.5357142857142856984, 0.5416666666666666297, 0.5476190476190476719, 0.5535714285714286031, 0.5595238095238095344, 0.5654761904761904656, 0.5714285714285713969, 0.5773809523809523281, 0.5833333333333333703, 0.5892857142857143016, 0.5952380952380952328, 0.6011904761904761640, 0.6071428571428570953, 0.6130952380952381375, 0.6190476190476190688, 0.6250000000000000000, 0.6309523809523809312, 0.6369047619047618625, 0.6428571428571429047, 0.6488095238095238360, 0.6547619047619047672, 0.6607142857142856984, 0.6666666666666666297, 0.6726190476190476719, 0.6785714285714286031, 0.6845238095238095344, 0.6904761904761904656, 0.6964285714285713969, 0.7023809523809523281, 0.7083333333333333703, 0.7142857142857143016, 0.7202380952380952328, 0.7261904761904761640, 0.7321428571428570953, 0.7380952380952381375, 0.7440476190476190688, 0.7500000000000000000, 0.7559523809523809312, 0.7619047619047618625, 0.7678571428571429047, 0.7738095238095238360, 0.7797619047619047672, 0.7857142857142856984, 0.7916666666666666297, 0.7976190476190476719, 0.8035714285714286031, 0.8095238095238095344, 0.8154761904761904656, 0.8214285714285713969, 0.8273809523809523281, 0.8333333333333333703, 0.8392857142857143016, 0.8452380952380952328, 0.8511904761904761640, 0.8571428571428570953, 0.8630952380952381375, 0.8690476190476190688, 0.8750000000000000000, 0.8809523809523809312, 0.8869047619047618625, 0.8928571428571429047, 0.8988095238095238360, 0.9047619047619047672, 0.9107142857142856984, 0.9166666666666666297, 0.9226190476190476719, 0.9285714285714286031, 0.9345238095238095344, 0.9404761904761904656, 0.9464285714285713969, 0.9523809523809523281, 0.9583333333333333703, 0.9642857142857143016 ),
 .UNSPECIFIED. ) 
 GEOMETRIC_REPRESENTATION_ITEM ( )  RATIONAL_B_SPLINE_SURFACE ( (
 ( 1.000000000000000000, 0.9659258262890683122, 1.000000000000000000, 0.9659258262890683122, 1.000000000000000000, 0.9659258262890683122, 1.000000000000000000, 0.9659258262890683122, 1.000000000000000000, 0.9659258262890683122, 1.000000000000000000, 0.9659258262890683122, 1.000000000000000000, 0.9659258262890683122, 1.000000000000000000, 0.9659258262890683122, 1.000000000000000000, 0.9659258262890683122, 1.000000000000000000, 0.9659258262890683122, 1.000000000000000000, 0.9659258262890683122, 1.000000000000000000, 0.9659258262890683122, 1.000000000000000000, 0.9659258262890683122, 1.000000000000000000, 0.9659258262890683122, 1.000000000000000000, 0.9659258262890683122, 1.000000000000000000, 0.9659258262890683122, 1.000000000000000000, 0.9659258262890683122, 1.000000000000000000, 0.9659258262890683122, 1.000000000000000000, 0.9659258262890683122, 1.000000000000000000, 0.9659258262890683122, 1.000000000000000000, 0.9659258262890683122, 1.000000000000000000, 0.9659258262890683122, 1.000000000000000000, 0.9659258262890683122, 1.000000000000000000, 0.9659258262890683122, 1.000000000000000000, 0.9659258262890683122, 1.000000000000000000, 0.9659258262890683122, 1.000000000000000000, 0.9659258262890683122, 1.000000000000000000, 0.9659258262890683122, 1.000000000000000000, 0.9659258262890683122, 1.000000000000000000, 0.9659258262890683122, 1.000000000000000000, 0.9659258262890683122, 1.000000000000000000, 0.9659258262890683122, 1.000000000000000000, 0.9659258262890683122, 1.000000000000000000, 0.9659258262890683122, 1.000000000000000000, 0.9659258262890683122, 1.000000000000000000, 0.9659258262890683122, 1.000000000000000000, 0.9659258262890683122, 1.000000000000000000, 0.9659258262890683122, 1.000000000000000000, 0.9659258262890683122, 1.000000000000000000, 0.9659258262890683122, 1.000000000000000000, 0.9659258262890683122, 1.000000000000000000, 0.9659258262890683122, 1.000000000000000000, 0.9659258262890683122, 1.000000000000000000, 0.9659258262890683122, 1.000000000000000000, 0.9659258262890683122, 1.000000000000000000, 0.9659258262890683122, 1.000000000000000000, 0.9659258262890683122, 1.000000000000000000, 0.9659258262890683122, 1.000000000000000000, 0.9659258262890683122, 1.000000000000000000, 0.9659258262890683122, 1.000000000000000000, 0.9659258262890683122, 1.000000000000000000, 0.9659258262890683122, 1.000000000000000000, 0.9659258262890683122, 1.000000000000000000, 0.9659258262890683122, 1.000000000000000000, 0.9659258262890683122, 1.000000000000000000, 0.9659258262890683122, 1.000000000000000000, 0.9659258262890683122, 1.000000000000000000, 0.9659258262890683122, 1.000000000000000000, 0.9659258262890683122, 1.000000000000000000, 0.9659258262890683122, 1.000000000000000000, 0.9659258262890683122, 1.000000000000000000, 0.9659258262890683122, 1.000000000000000000, 0.9659258262890683122, 1.000000000000000000, 0.9659258262890683122, 1.000000000000000000, 0.9659258262890683122, 1.000000000000000000, 0.9659258262890683122, 1.000000000000000000, 0.9659258262890683122, 1.000000000000000000, 0.9659258262890683122, 1.000000000000000000, 0.9659258262890683122, 1.000000000000000000, 0.9659258262890683122, 1.000000000000000000, 0.9659258262890683122, 1.000000000000000000, 0.9659258262890683122, 1.000000000000000000, 0.9659258262890683122, 1.000000000000000000, 0.9659258262890683122, 1.000000000000000000, 0.9659258262890683122, 1.000000000000000000, 0.9659258262890683122, 1.000000000000000000, 0.9659258262890683122, 1.000000000000000000, 0.9659258262890683122, 1.000000000000000000, 0.9659258262890683122, 1.000000000000000000, 0.9659258262890683122, 1.000000000000000000, 0.9659258262890683122, 1.000000000000000000, 0.9659258262890683122, 1.000000000000000000, 0.9659258262890683122, 1.000000000000000000, 0.9659258262890683122, 1.000000000000000000, 0.9659258262890683122, 1.000000000000000000, 0.9659258262890683122, 1.000000000000000000, 0.9659258262890683122, 1.000000000000000000, 0.9659258262890683122, 1.000000000000000000, 0.9659258262890683122, 1.000000000000000000, 0.9659258262890683122, 1.000000000000000000, 0.9659258262890683122, 1.000000000000000000, 0.9659258262890683122, 1.000000000000000000, 0.9659258262890683122, 1.000000000000000000, 0.9659258262890683122, 1.000000000000000000, 0.9659258262890683122, 1.000000000000000000, 0.9659258262890683122, 1.000000000000000000, 0.9659258262890683122, 1.000000000000000000, 0.9659258262890683122, 1.000000000000000000, 0.9659258262890683122, 1.000000000000000000, 0.9659258262890683122, 1.000000000000000000, 0.9659258262890683122, 1.000000000000000000, 0.9659258262890683122, 1.000000000000000000, 0.9659258262890683122, 1.000000000000000000, 0.9659258262890683122, 1.000000000000000000, 0.9659258262890683122, 1.000000000000000000, 0.9659258262890683122, 1.000000000000000000, 0.9659258262890683122, 1.000000000000000000, 0.9659258262890683122, 1.000000000000000000, 0.9659258262890683122, 1.000000000000000000, 0.9659258262890683122, 1.000000000000000000, 0.9659258262890683122, 1.000000000000000000, 0.9659258262890683122, 1.000000000000000000, 0.9659258262890683122, 1.000000000000000000, 0.9659258262890683122, 1.000000000000000000, 0.9659258262890683122, 1.000000000000000000, 0.9659258262890683122, 1.000000000000000000, 0.9659258262890683122, 1.000000000000000000, 0.9659258262890683122, 1.000000000000000000, 0.9659258262890683122, 1.000000000000000000, 0.9659258262890683122, 1.000000000000000000, 0.9659258262890683122, 1.000000000000000000, 0.9659258262890683122, 1.000000000000000000, 0.9659258262890683122, 1.000000000000000000, 0.9659258262890683122, 1.000000000000000000, 0.9659258262890683122, 1.000000000000000000, 0.9659258262890683122, 1.000000000000000000, 0.9659258262890683122, 1.000000000000000000, 0.9659258262890683122, 1.000000000000000000, 0.9659258262890683122, 1.000000000000000000, 0.9659258262890683122, 1.000000000000000000, 0.9659258262890683122, 1.000000000000000000, 0.9659258262890683122, 1.000000000000000000, 0.9659258262890683122, 1.000000000000000000, 0.9659258262890683122, 1.000000000000000000, 0.9659258262890683122, 1.000000000000000000, 0.9659258262890683122, 1.000000000000000000, 0.9659258262890683122, 1.000000000000000000, 0.9659258262890683122, 1.000000000000000000, 0.9659258262890683122, 1.000000000000000000, 0.9659258262890683122, 1.000000000000000000, 0.9659258262890683122, 1.000000000000000000, 0.9659258262890683122, 1.000000000000000000, 0.9659258262890683122, 1.000000000000000000, 0.9659258262890683122, 1.000000000000000000, 0.9659258262890683122, 1.000000000000000000, 0.9659258262890683122, 1.000000000000000000, 0.9659258262890683122, 1.000000000000000000, 0.9659258262890683122, 1.000000000000000000, 0.9659258262890683122, 1.000000000000000000, 0.9659258262890683122, 1.000000000000000000, 0.9659258262890683122, 1.000000000000000000, 0.9659258262890683122, 1.000000000000000000, 0.9659258262890683122, 1.000000000000000000, 0.9659258262890683122, 1.000000000000000000, 0.9659258262890683122, 1.000000000000000000, 0.9659258262890683122, 1.000000000000000000, 0.9659258262890683122, 1.000000000000000000, 0.9659258262890683122, 1.000000000000000000, 0.9659258262890683122, 1.000000000000000000, 0.9659258262890683122, 1.000000000000000000, 0.9659258262890683122, 1.000000000000000000, 0.9659258262890683122, 1.000000000000000000),
 ( 1.000000000000000000, 0.9659258262890683122, 1.000000000000000000, 0.9659258262890683122, 1.000000000000000000, 0.9659258262890683122, 1.000000000000000000, 0.9659258262890683122, 1.000000000000000000, 0.9659258262890683122, 1.000000000000000000, 0.9659258262890683122, 1.000000000000000000, 0.9659258262890683122, 1.000000000000000000, 0.9659258262890683122, 1.000000000000000000, 0.9659258262890683122, 1.000000000000000000, 0.9659258262890683122, 1.000000000000000000, 0.9659258262890683122, 1.000000000000000000, 0.9659258262890683122, 1.000000000000000000, 0.9659258262890683122, 1.000000000000000000, 0.9659258262890683122, 1.000000000000000000, 0.9659258262890683122, 1.000000000000000000, 0.9659258262890683122, 1.000000000000000000, 0.9659258262890683122, 1.000000000000000000, 0.9659258262890683122, 1.000000000000000000, 0.9659258262890683122, 1.000000000000000000, 0.9659258262890683122, 1.000000000000000000, 0.9659258262890683122, 1.000000000000000000, 0.9659258262890683122, 1.000000000000000000, 0.9659258262890683122, 1.000000000000000000, 0.9659258262890683122, 1.000000000000000000, 0.9659258262890683122, 1.000000000000000000, 0.9659258262890683122, 1.000000000000000000, 0.9659258262890683122, 1.000000000000000000, 0.9659258262890683122, 1.000000000000000000, 0.9659258262890683122, 1.000000000000000000, 0.9659258262890683122, 1.000000000000000000, 0.9659258262890683122, 1.000000000000000000, 0.9659258262890683122, 1.000000000000000000, 0.9659258262890683122, 1.000000000000000000, 0.9659258262890683122, 1.000000000000000000, 0.9659258262890683122, 1.000000000000000000, 0.9659258262890683122, 1.000000000000000000, 0.9659258262890683122, 1.000000000000000000, 0.9659258262890683122, 1.000000000000000000, 0.9659258262890683122, 1.000000000000000000, 0.9659258262890683122, 1.000000000000000000, 0.9659258262890683122, 1.000000000000000000, 0.9659258262890683122, 1.000000000000000000, 0.9659258262890683122, 1.000000000000000000, 0.9659258262890683122, 1.000000000000000000, 0.9659258262890683122, 1.000000000000000000, 0.9659258262890683122, 1.000000000000000000, 0.9659258262890683122, 1.000000000000000000, 0.9659258262890683122, 1.000000000000000000, 0.9659258262890683122, 1.000000000000000000, 0.9659258262890683122, 1.000000000000000000, 0.9659258262890683122, 1.000000000000000000, 0.9659258262890683122, 1.000000000000000000, 0.9659258262890683122, 1.000000000000000000, 0.9659258262890683122, 1.000000000000000000, 0.9659258262890683122, 1.000000000000000000, 0.9659258262890683122, 1.000000000000000000, 0.9659258262890683122, 1.000000000000000000, 0.9659258262890683122, 1.000000000000000000, 0.9659258262890683122, 1.000000000000000000, 0.9659258262890683122, 1.000000000000000000, 0.9659258262890683122, 1.000000000000000000, 0.9659258262890683122, 1.000000000000000000, 0.9659258262890683122, 1.000000000000000000, 0.9659258262890683122, 1.000000000000000000, 0.9659258262890683122, 1.000000000000000000, 0.9659258262890683122, 1.000000000000000000, 0.9659258262890683122, 1.000000000000000000, 0.9659258262890683122, 1.000000000000000000, 0.9659258262890683122, 1.000000000000000000, 0.9659258262890683122, 1.000000000000000000, 0.9659258262890683122, 1.000000000000000000, 0.9659258262890683122, 1.000000000000000000, 0.9659258262890683122, 1.000000000000000000, 0.9659258262890683122, 1.000000000000000000, 0.9659258262890683122, 1.000000000000000000, 0.9659258262890683122, 1.000000000000000000, 0.9659258262890683122, 1.000000000000000000, 0.9659258262890683122, 1.000000000000000000, 0.9659258262890683122, 1.000000000000000000, 0.9659258262890683122, 1.000000000000000000, 0.9659258262890683122, 1.000000000000000000, 0.9659258262890683122, 1.000000000000000000, 0.9659258262890683122, 1.000000000000000000, 0.9659258262890683122, 1.000000000000000000, 0.9659258262890683122, 1.000000000000000000, 0.9659258262890683122, 1.000000000000000000, 0.9659258262890683122, 1.000000000000000000, 0.9659258262890683122, 1.000000000000000000, 0.9659258262890683122, 1.000000000000000000, 0.9659258262890683122, 1.000000000000000000, 0.9659258262890683122, 1.000000000000000000, 0.9659258262890683122, 1.000000000000000000, 0.9659258262890683122, 1.000000000000000000, 0.9659258262890683122, 1.000000000000000000, 0.9659258262890683122, 1.000000000000000000, 0.9659258262890683122, 1.000000000000000000, 0.9659258262890683122, 1.000000000000000000, 0.9659258262890683122, 1.000000000000000000, 0.9659258262890683122, 1.000000000000000000, 0.9659258262890683122, 1.000000000000000000, 0.9659258262890683122, 1.000000000000000000, 0.9659258262890683122, 1.000000000000000000, 0.9659258262890683122, 1.000000000000000000, 0.9659258262890683122, 1.000000000000000000, 0.9659258262890683122, 1.000000000000000000, 0.9659258262890683122, 1.000000000000000000, 0.9659258262890683122, 1.000000000000000000, 0.9659258262890683122, 1.000000000000000000, 0.9659258262890683122, 1.000000000000000000, 0.9659258262890683122, 1.000000000000000000, 0.9659258262890683122, 1.000000000000000000, 0.9659258262890683122, 1.000000000000000000, 0.9659258262890683122, 1.000000000000000000, 0.9659258262890683122, 1.000000000000000000, 0.9659258262890683122, 1.000000000000000000, 0.9659258262890683122, 1.000000000000000000, 0.9659258262890683122, 1.000000000000000000, 0.9659258262890683122, 1.000000000000000000, 0.9659258262890683122, 1.000000000000000000, 0.9659258262890683122, 1.000000000000000000, 0.9659258262890683122, 1.000000000000000000, 0.9659258262890683122, 1.000000000000000000, 0.9659258262890683122, 1.000000000000000000, 0.9659258262890683122, 1.000000000000000000, 0.9659258262890683122, 1.000000000000000000, 0.9659258262890683122, 1.000000000000000000, 0.9659258262890683122, 1.000000000000000000, 0.9659258262890683122, 1.000000000000000000, 0.9659258262890683122, 1.000000000000000000, 0.9659258262890683122, 1.000000000000000000, 0.9659258262890683122, 1.000000000000000000, 0.9659258262890683122, 1.000000000000000000, 0.9659258262890683122, 1.000000000000000000, 0.9659258262890683122, 1.000000000000000000, 0.9659258262890683122, 1.000000000000000000, 0.9659258262890683122, 1.000000000000000000, 0.9659258262890683122, 1.000000000000000000, 0.9659258262890683122, 1.000000000000000000, 0.9659258262890683122, 1.000000000000000000, 0.9659258262890683122, 1.000000000000000000, 0.9659258262890683122, 1.000000000000000000, 0.9659258262890683122, 1.000000000000000000, 0.9659258262890683122, 1.000000000000000000, 0.9659258262890683122, 1.000000000000000000, 0.9659258262890683122, 1.000000000000000000, 0.9659258262890683122, 1.000000000000000000, 0.9659258262890683122, 1.000000000000000000, 0.9659258262890683122, 1.000000000000000000, 0.9659258262890683122, 1.000000000000000000, 0.9659258262890683122, 1.000000000000000000, 0.9659258262890683122, 1.000000000000000000, 0.9659258262890683122, 1.000000000000000000, 0.9659258262890683122, 1.000000000000000000, 0.9659258262890683122, 1.000000000000000000, 0.9659258262890683122, 1.000000000000000000, 0.9659258262890683122, 1.000000000000000000, 0.9659258262890683122, 1.000000000000000000, 0.9659258262890683122, 1.000000000000000000, 0.9659258262890683122, 1.000000000000000000, 0.9659258262890683122, 1.000000000000000000, 0.9659258262890683122, 1.000000000000000000, 0.9659258262890683122, 1.000000000000000000) ) ) 
 REPRESENTATION_ITEM ( '' )  SURFACE ( )  );
#36565=CARTESIAN_POINT ( 'NONE',  ( 0.1532563361054082862, 11.21726448433411605, 2.638427012816831674 ) ) ;
#36566=CARTESIAN_POINT ( 'NONE',  ( 18.17829156368505750, 59.16792564121895026, 6.500000000000043521 ) ) ;
#36571=ORIENTED_EDGE ( 'NONE', *, *, #93681, .F. ) ;
#36572=CARTESIAN_POINT ( 'NONE',  ( 1.472469842513823179, 45.59226448433412315, -4.923371831947296329 ) ) ;
#36573=CARTESIAN_POINT ( 'NONE',  ( 10.00000000000000000, 20.55374883491396787, -14.16423886937410082 ) ) ;
#36574=CARTESIAN_POINT ( 'NONE',  ( 17.96484262340118221, 24.93868534415484461, 7.964842623401181321 ) ) ;
#36575=CARTESIAN_POINT ( 'NONE',  ( 20.88017736071110164, 30.35535201082151247, 2.915334737309930979 ) ) ;
#36576=CARTESIAN_POINT ( 'NONE',  ( 0.1532563361054083140, 61.00893115100078745, 1.131784320476157264E-15 ) ) ;
#36577=CARTESIAN_POINT ( 'NONE',  ( 13.43411237798105340, 15.58196800326374998, 12.81628187352647963 ) ) ;
#36579=CARTESIAN_POINT ( 'NONE',  ( 20.88017736071110519, 65.56368534415483396, 2.639326808657452039E-16 ) ) ;
#36580=CARTESIAN_POINT ( 'NONE',  ( 13.43411237798106583, 32.66530133659708213, -12.81628187352647252 ) ) ;
#36582=CARTESIAN_POINT ( 'NONE',  ( 18.52753015748617571, 28.09226448433411960, 4.923371831947298993 ) ) ;
#36583=CARTESIAN_POINT ( 'NONE',  ( -0.8801773607111008646, 8.272018677488171434, 2.915334737309923430 ) ) ;
#36584=VERTEX_POINT ( 'NONE', #41487 ) ;
#36586=CARTESIAN_POINT ( 'NONE',  ( 19.42250999205614548, 5.980352010821504471, -5.440088680355545492 ) ) ;
#36588=CARTESIAN_POINT ( 'NONE',  ( 7.084665262690076126, 54.10535201082151247, 10.88017736071109987 ) ) ;
#36589=CARTESIAN_POINT ( 'NONE',  ( 0.5774900079438607392, 63.48035201082149825, 5.440088680355550821 ) ) ;
#36591=CARTESIAN_POINT ( 'NONE',  ( 20.88017736071110164, 55.35535201082149825, 2.915334737309930979 ) ) ;
#36594=CARTESIAN_POINT ( 'NONE',  ( 7.084665262690076126, 59.10535201082150536, 10.88017736071109987 ) ) ;
#36595=CARTESIAN_POINT ( 'NONE',  ( -46.94000000000001904, 100.7935499705848486, 8.437539667958747103 ) ) ;
#36599=CARTESIAN_POINT ( 'NONE',  ( 18.52753015748618282, 23.92559781766745530, -4.923371831947291888 ) ) ;
#36600=ORIENTED_EDGE ( 'NONE', *, *, #30041, .F. ) ;
#36601=CARTESIAN_POINT ( 'NONE',  ( 19.84674366389459266, 53.30059781766744464, 2.638427012816836559 ) ) ;
#36604=CARTESIAN_POINT ( 'NONE',  ( 17.08211943468705130, 8.470415501580635720, 12.26659068614894998 ) ) ;
#36605=ORIENTED_EDGE ( 'NONE', *, *, #75923, .F. ) ;
#36609=CARTESIAN_POINT ( 'NONE',  ( 19.84674366389459266, 38.30059781766745175, 2.638427012816836559 ) ) ;
#36610=CARTESIAN_POINT ( 'NONE',  ( 12.91533473730993009, 11.60535201082150714, -10.88017736071109987 ) ) ;
#36613=CARTESIAN_POINT ( 'NONE',  ( 2.831191079880678085, 79.91181047996344944, 9.500000000000000000 ) ) ;
#36614=CARTESIAN_POINT ( 'NONE',  ( 10.00000000000000178, 52.25893115100078745, 9.846743663894594434 ) ) ;
#36616=CARTESIAN_POINT ( 'NONE',  ( 10.00000000000000000, 17.87363466993041783, -12.81628187352647608 ) ) ;
#36617=CARTESIAN_POINT ( 'NONE',  ( 19.84674366389459266, 8.300597817667451750, 2.638427012816836559 ) ) ;
#36618=COLOUR_RGB ( '', 0.31764706, 0.68627451, 0.89019608) ;
#36619=CARTESIAN_POINT ( 'NONE',  ( 0.5069705099446313312, 0.4330826616539849572, 6.500000000000002665 ) ) ;
#36620=CARTESIAN_POINT ( 'NONE',  ( 0.6178305044545838731, 4.748634669930420493, 9.382169495545420901 ) ) ;
#36625=CARTESIAN_POINT ( 'NONE',  ( 4.559911319644449179, 13.89701867748817321, 9.422509992056141925 ) ) ;
#36626=CARTESIAN_POINT ( 'NONE',  ( 13.79529636645030344, 8.262082168247300018, 14.16423886937410614 ) ) ;
#36627=CARTESIAN_POINT ( 'NONE',  ( 19.84674366389459621, 28.50893115100078745, 7.409399052514197653E-17 ) ) ;
#36628=CARTESIAN_POINT ( 'NONE',  ( 4.559911319644449179, 57.23035201082150536, -9.422509992056141925 ) ) ;
#36629=CARTESIAN_POINT ( 'NONE',  ( 0.6178305044545838731, 44.74863466993042493, 9.382169495545420901 ) ) ;
#36630=CARTESIAN_POINT ( 'NONE',  ( 20.88017736071110875, 20.77201867748816611, -2.915334737309920765 ) ) ;
#36635=CARTESIAN_POINT ( 'NONE',  ( 22.81628187352648496, 1.831968003263753753, -3.434112377981050290 ) ) ;
#36636=CARTESIAN_POINT ( 'NONE',  ( 12.63842701281683034, 62.46726448433410894, 9.846743663894596210 ) ) ;
#36637=CARTESIAN_POINT ( 'NONE',  ( 18.52753015748617571, 33.09226448433411605, 4.923371831947298993 ) ) ;
#36639=CARTESIAN_POINT ( 'NONE',  ( 16.40814093676324603, 37.45696800326376064, -11.09922568453594671 ) ) ;
#36640=CARTESIAN_POINT ( 'NONE',  ( 19.42250999205614548, 45.98035201082150536, -5.440088680355545492 ) ) ;
#36642=CARTESIAN_POINT ( 'NONE',  ( 12.91533473730993009, 36.60535201082151247, -10.88017736071109987 ) ) ;
#36643=CARTESIAN_POINT ( 'NONE',  ( 4.559911319644449179, 27.23035201082150536, -9.422509992056141925 ) ) ;
#36644=CARTESIAN_POINT ( 'NONE',  ( 0.1532563361054083140, 66.00893115100079456, 1.131784320476157264E-15 ) ) ;
#36645=CARTESIAN_POINT ( 'NONE',  ( 19.42250999205614193, 60.14701867748817676, 5.440088680355555262 ) ) ;
#36646=CARTESIAN_POINT ( 'NONE',  ( 2.791683348922240793, 41.63393115100078745, 7.208316651077764092 ) ) ;
#36647=CARTESIAN_POINT ( 'NONE',  ( 17.96484262340118221, 14.93868534415483751, 7.964842623401181321 ) ) ;
#36648=CARTESIAN_POINT ( 'NONE',  ( 22.81628187352647785, 16.62363466993042138, 6.195893100308588602E-16 ) ) ;
#36650=CARTESIAN_POINT ( 'NONE',  ( -0.8801773607111008646, 23.27201867748817676, 2.915334737309923430 ) ) ;
#36652=CARTESIAN_POINT ( 'NONE',  ( 18.18329248733322245, 7.602906685120198738, 6.499999999999993783 ) ) ;
#36653=CARTESIAN_POINT ( 'NONE',  ( 10.00000000000000000, 1.813685344154837731, -10.88017736071110342 ) ) ;
#36654=CARTESIAN_POINT ( 'NONE',  ( 20.88017736071110519, 15.56368534415483751, 2.639326808657452039E-16 ) ) ;
#36655=CARTESIAN_POINT ( 'NONE',  ( 20.88017736071110164, 65.35535201082150536, 2.915334737309930979 ) ) ;
#36656=CARTESIAN_POINT ( 'NONE',  ( 17.08211943468705130, 28.47041550158063572, 12.26659068614894998 ) ) ;
#36657=CARTESIAN_POINT ( 'NONE',  ( 0.1532563361054083140, 16.00893115100078390, 1.131784320476157264E-15 ) ) ;
#36658=CARTESIAN_POINT ( 'NONE',  ( 2.791683348922237240, 65.38393115100078035, -7.208316651077763204 ) ) ;
#36659=CARTESIAN_POINT ( 'NONE',  ( -0.8801773607111009756, 48.06368534415484817, 1.068504757029289695E-15 ) ) ;
#36661=CARTESIAN_POINT ( 'NONE',  ( 20.88017736071110875, 25.77201867748816966, -2.915334737309920321 ) ) ;
#36664=CARTESIAN_POINT ( 'NONE',  ( 19.84674366389459266, 48.71726448433413026, -2.638427012816827677 ) ) ;
#36665=ORIENTED_EDGE ( 'NONE', *, *, #72974, .T. ) ;
#36666=ORIENTED_EDGE ( 'NONE', *, *, #62916, .F. ) ;
#36668=CARTESIAN_POINT ( 'NONE',  ( -0.3689425029237881626, 22.42874883491397142, 10.36894250292379027 ) ) ;
#36669=CARTESIAN_POINT ( 'NONE',  ( -0.3689425029237898834, 26.17874883491396432, -10.36894250292378850 ) ) ;
#36670=CARTESIAN_POINT ( 'NONE',  ( 15.44008868035555793, 56.39701867748817676, -9.422509992056140149 ) ) ;
#36671=CARTESIAN_POINT ( 'NONE',  ( -0.8801773607111008646, 3.272018677488171434, 2.915334737309923430 ) ) ;
#36672=CARTESIAN_POINT ( 'NONE',  ( -1.099225684535947600, 4.540301336597087456, 6.408140936763237150 ) ) ;
#36673=CARTESIAN_POINT ( 'NONE',  ( 17.20831665107776587, 54.13393115100079456, -7.208316651077762316 ) ) ;
#36675=CARTESIAN_POINT ( 'NONE',  ( -0.8801773607111008646, 43.27201867748817676, 2.915334737309923430 ) ) ;
#36676=CARTESIAN_POINT ( 'NONE',  ( 6.565887622018943937, 3.081968003263753531, -12.81628187352647608 ) ) ;
#36677=CARTESIAN_POINT ( 'NONE',  ( 6.204703633549690345, 20.76208216824730357, -14.16423886937410259 ) ) ;
#36678=CARTESIAN_POINT ( 'NONE',  ( 19.42250999205614193, 20.14701867748817321, 5.440088680355555262 ) ) ;
#36679=CARTESIAN_POINT ( 'NONE',  ( 0.5774900079438590739, 12.64701867748817321, -5.440088680355550821 ) ) ;
#36680=CARTESIAN_POINT ( 'NONE',  ( 18.52753015748618282, 53.92559781766745175, -4.923371831947291888 ) ) ;
#36681=CARTESIAN_POINT ( 'NONE',  ( 2.035157376598822676, 42.43868534415483396, -7.964842623401177768 ) ) ;
#36684=ORIENTED_EDGE ( 'NONE', *, *, #40889, .T. ) ;
#36687=CARTESIAN_POINT ( 'NONE',  ( 0.1532563361054100626, 30.80059781766744820, -2.638427012816831230 ) ) ;
#36691=CARTESIAN_POINT ( 'NONE',  ( 13.79529636645030344, 43.26208216824730357, 14.16423886937410614 ) ) ;
#36692=CARTESIAN_POINT ( 'NONE',  ( -0.8801773607110991993, 2.855352010821504471, -2.915334737309923874 ) ) ;
#36693=CARTESIAN_POINT ( 'NONE',  ( 19.84674366389459266, 28.71726448433411960, -2.638427012816827677 ) ) ;
#36694=CARTESIAN_POINT ( 'NONE',  ( 2.791683348922237240, 50.38393115100078035, -7.208316651077763204 ) ) ;
#36699=CARTESIAN_POINT ( 'NONE',  ( 19.84674366389459621, 3.508931151000785231, 7.409399052514197653E-17 ) ) ;
#36701=ORIENTED_EDGE ( 'NONE', *, *, #21603, .F. ) ;
#36702=CARTESIAN_POINT ( 'NONE',  ( 17.08211943468705840, 35.13708216824730357, -12.26659068614894466 ) ) ;
#36703=CARTESIAN_POINT ( 'NONE',  ( 13.43411237798106583, 27.66530133659708568, -12.81628187352647252 ) ) ;
#36705=CARTESIAN_POINT ( 'NONE',  ( 21.09922568453595559, 42.04030133659708213, -6.408140936763230044 ) ) ;
#36706=CARTESIAN_POINT ( 'NONE',  ( 12.63842701281683922, 39.55059781766744464, -9.846743663894590881 ) ) ;
#36707=CARTESIAN_POINT ( 'NONE',  ( 20.88017736071110164, 10.35535201082150714, 2.915334737309930979 ) ) ;
#36709=CARTESIAN_POINT ( 'NONE',  ( 7.361572987183170547, 47.05059781766745175, 9.846743663894590881 ) ) ;
#36710=CARTESIAN_POINT ( 'NONE',  ( 12.63842701281683034, 52.46726448433413026, 9.846743663894596210 ) ) ;
#36715=B_SPLINE_CURVE_WITH_KNOTS ( 'NONE', 3,
 ( #38939, #69428, #54410, #474, #53429, #67958 ),
 .UNSPECIFIED., .F., .F.,
 ( 4, 2, 4 ),
 ( 4.906538933386797396E-18, 0.0002605067024380951332, 0.0005210134048761852791 ),
 .UNSPECIFIED. ) ;
#36717=DIRECTION ( 'NONE',  ( -0.000000000000000000, -0.000000000000000000, -1.000000000000000000 ) ) ;
#36720=CARTESIAN_POINT ( 'NONE',  ( 10.00000000000000000, 14.75893115100078568, -9.846743663894594434 ) ) ;
#36721=EDGE_CURVE ( 'NONE', #87224, #54365, #37146, .T. ) ;
#36722=CARTESIAN_POINT ( 'NONE',  ( 22.81628187352648496, 41.83196800326375353, -3.434112377981050290 ) ) ;
#36725=CARTESIAN_POINT ( 'NONE',  ( 17.20831665107776587, 54.13393115100079456, -7.208316651077762316 ) ) ;
#36727=CARTESIAN_POINT ( 'NONE',  ( 20.36894250292379382, 33.67874883491396076, 10.36894250292379205 ) ) ;
#36728=CARTESIAN_POINT ( 'NONE',  ( 19.84674366389459621, 43.50893115100078745, 7.409399052514197653E-17 ) ) ;
#36729=CARTESIAN_POINT ( 'NONE',  ( 19.38216949554541202, 50.99863466993042493, 9.382169495545424454 ) ) ;
#36731=CARTESIAN_POINT ( 'NONE',  ( 0.2751277870542980231, 9.366073187301308778, -6.500000000000002665 ) ) ;
#36732=CARTESIAN_POINT ( 'NONE',  ( 14.92337183194729988, 4.342264484334117824, -8.527530157486177487 ) ) ;
#36733=CARTESIAN_POINT ( 'NONE',  ( -0.1503990784575247319, 67.22266099184919597, -6.262539305110083276 ) ) ;
#36734=CARTESIAN_POINT ( 'NONE',  ( 12.63842701281683922, 49.55059781766744464, -9.846743663894590881 ) ) ;
#36735=CARTESIAN_POINT ( 'NONE',  ( 19.42250999205614548, 40.98035201082150536, -5.440088680355545492 ) ) ;
#36736=CARTESIAN_POINT ( 'NONE',  ( 14.92337183194729988, 29.34226448433411960, -8.527530157486177487 ) ) ;
#36737=CARTESIAN_POINT ( 'NONE',  ( 20.88017736071110519, 45.56368534415484106, 2.639326808657452039E-16 ) ) ;
#36741=CARTESIAN_POINT ( 'NONE',  ( 2.035157376598822676, 17.43868534415483751, -7.964842623401177768 ) ) ;
#36742=CARTESIAN_POINT ( 'NONE',  ( 10.00000000000000178, 52.25893115100078745, 9.846743663894594434 ) ) ;
#36743=CARTESIAN_POINT ( 'NONE',  ( 0.5774900079438607392, 43.48035201082151247, 5.440088680355550821 ) ) ;
#36745=CARTESIAN_POINT ( 'NONE',  ( 12.91533473730992121, 64.52201867748817676, 10.88017736071110164 ) ) ;
#36748=CARTESIAN_POINT ( 'NONE',  ( 2.035157376598824452, 28.68868534415484106, 7.964842623401179544 ) ) ;
#36750=CARTESIAN_POINT ( 'NONE',  ( 7.361572987183170547, 7.050597817667451750, 9.846743663894590881 ) ) ;
#36751=CARTESIAN_POINT ( 'NONE',  ( 5.076628168052704559, 20.17559781766745175, -8.527530157486179263 ) ) ;
#36754=CARTESIAN_POINT ( 'NONE',  ( 1.472469842513823179, 65.59226448433412315, -4.923371831947296329 ) ) ;
#36755=CARTESIAN_POINT ( 'NONE',  ( 10.00000000000000178, 4.313685344154837509, 10.88017736071110342 ) ) ;
#36757=CARTESIAN_POINT ( 'NONE',  ( 22.26659068614895176, 4.720415501580633943, -7.082119434687042414 ) ) ;
#36758=CARTESIAN_POINT ( 'NONE',  ( 17.08211943468705840, 45.13708216824730357, -12.26659068614894466 ) ) ;
#36759=CARTESIAN_POINT ( 'NONE',  ( 0.6178305044545818747, 8.498634669930421381, -9.382169495545419124 ) ) ;
#36761=CARTESIAN_POINT ( 'NONE',  ( 5.076628168052704559, 15.17559781766745175, -8.527530157486179263 ) ) ;
#36762=CARTESIAN_POINT ( 'NONE',  ( -0.8801773607111008646, 13.27201867748817321, 2.915334737309923430 ) ) ;
#36763=CARTESIAN_POINT ( 'NONE',  ( 0.1532563361054083140, 46.00893115100079456, 1.131784320476157264E-15 ) ) ;
#36767=CARTESIAN_POINT ( 'NONE',  ( 7.361572987183169658, -0.03273551566588185635, -9.846743663894592657 ) ) ;
#36768=CARTESIAN_POINT ( 'NONE',  ( 16.40814093676324603, 27.45696800326375708, -11.09922568453594671 ) ) ;
#36769=CARTESIAN_POINT ( 'NONE',  ( 5.076628168052703671, 21.84226448433411960, 8.527530157486179263 ) ) ;
#36770=ORIENTED_EDGE ( 'NONE', *, *, #35332, .T. ) ;
#36771=CARTESIAN_POINT ( 'NONE',  ( 7.361572987183170547, 12.05059781766744997, 9.846743663894590881 ) ) ;
#36774=CARTESIAN_POINT ( 'NONE',  ( 19.42250999205614548, 10.98035201082150358, -5.440088680355545492 ) ) ;
#36775=CARTESIAN_POINT ( 'NONE',  ( 6.204703633549690345, 35.76208216824729647, -14.16423886937410259 ) ) ;
#36776=CARTESIAN_POINT ( 'NONE',  ( 15.44008868035555793, 41.39701867748817676, -9.422509992056140149 ) ) ;
#36777=CARTESIAN_POINT ( 'NONE',  ( 12.91533473730992121, 59.52201867748816966, 10.88017736071110164 ) ) ;
#36778=AXIS2_PLACEMENT_3D ( 'NONE', #4773, #5270, #27252 ) ;
#36780=CARTESIAN_POINT ( 'NONE',  ( 2.791683348922237240, 25.38393115100078390, -7.208316651077763204 ) ) ;
#36781=CARTESIAN_POINT ( 'NONE',  ( 7.084665262690076126, 9.105352010821503583, 10.88017736071109987 ) ) ;
#36782=CARTESIAN_POINT ( 'NONE',  ( 5.076628168052704559, 10.17559781766745175, -8.527530157486179263 ) ) ;
#36783=CARTESIAN_POINT ( 'NONE',  ( 0.5636945946910000282, 8.154255672638645939E-15, -5.268011858241770540 ) ) ;
#36784=CARTESIAN_POINT ( 'NONE',  ( 14.92337183194729633, 42.67559781766745886, 8.527530157486181039 ) ) ;
#36785=CARTESIAN_POINT ( 'NONE',  ( -0.8801773607111009756, 38.06368534415484106, 1.068504757029289695E-15 ) ) ;
#36787=CARTESIAN_POINT ( 'NONE',  ( -2.816281873526471635, 53.91530133659709634, -3.434112377981056508 ) ) ;
#36789=CARTESIAN_POINT ( 'NONE',  ( 0.1532563361054082862, 6.217264484334118713, 2.638427012816831674 ) ) ;
#36790=CARTESIAN_POINT ( 'NONE',  ( 21.09922568453595559, 47.04030133659708923, -6.408140936763230044 ) ) ;
#36791=CARTESIAN_POINT ( 'NONE',  ( 15.44008868035555260, 9.730352010821505360, 9.422509992056143702 ) ) ;
#36792=CARTESIAN_POINT ( 'NONE',  ( 14.92337183194729633, 37.67559781766745175, 8.527530157486181039 ) ) ;
#36794=CARTESIAN_POINT ( 'NONE',  ( -2.266590686148945544, 17.22041550158063572, 7.082119434687048631 ) ) ;
#36795=CARTESIAN_POINT ( 'NONE',  ( 24.16423886937410614, 39.51208216824731068, -3.795296366450302550 ) ) ;
#36796=CARTESIAN_POINT ( 'NONE',  ( 19.84674366389459621, 38.50893115100078745, 7.409399052514197653E-17 ) ) ;
#36798=CARTESIAN_POINT ( 'NONE',  ( 12.91533473730992121, 34.52201867748817676, 10.88017736071110164 ) ) ;
#36799=CARTESIAN_POINT ( 'NONE',  ( 4.559911319644449179, 68.89701867748817676, 9.422509992056141925 ) ) ;
#36802=CARTESIAN_POINT ( 'NONE',  ( -2.816281873526473856, 54.12363466993041783, 9.499525473075851096E-16 ) ) ;
#36803=CARTESIAN_POINT ( 'NONE',  ( 4.559911319644449179, 63.89701867748817676, 9.422509992056141925 ) ) ;
#36804=ORIENTED_EDGE ( 'NONE', *, *, #14144, .T. ) ;
#36805=CARTESIAN_POINT ( 'NONE',  ( 6.204703633549690345, 10.76208216824729824, -14.16423886937410259 ) ) ;
#36806=CARTESIAN_POINT ( 'NONE',  ( 1.472469842513823179, 10.59226448433411782, -4.923371831947296329 ) ) ;
#36808=CARTESIAN_POINT ( 'NONE',  ( 1.197528957823066786, 8.576208590949788468E-17, -6.052460312987175683 ) ) ;
#36809=ORIENTED_EDGE ( 'NONE', *, *, #60105, .T. ) ;
#36810=( BOUNDED_CURVE ( )  B_SPLINE_CURVE ( 2, ( #2943, #49390, #40930, #79890, #63889, #10423, #34877, #65371, #86904 ),
 .UNSPECIFIED., .F., .T. ) 
 B_SPLINE_CURVE_WITH_KNOTS ( ( 3, 2, 2, 2, 3 ),
 ( 0.3677146600783225971, 0.3690476190476190688, 0.3750000000000000000, 0.3809523809523809312, 0.3822853399216774029 ),
 .UNSPECIFIED. ) 
 CURVE ( )  GEOMETRIC_REPRESENTATION_ITEM ( )  RATIONAL_B_SPLINE_CURVE ( ( 0.9881565478350731180, 0.9923695281211488695, 1.000000000000000000, 0.9659258262890683122, 1.000000000000000000, 0.9659258262890683122, 1.000000000000000000, 0.9923695281211488695, 0.9881565478350731180 ) ) 
 REPRESENTATION_ITEM ( '' )  );
#36812=CARTESIAN_POINT ( 'NONE',  ( 10.00000000000000000, 11.81368534415483751, -10.88017736071110342 ) ) ;
#36814=CARTESIAN_POINT ( 'NONE',  ( 19.42250999205614548, 40.98035201082150536, -5.440088680355545492 ) ) ;
#36816=EDGE_LOOP ( 'NONE', ( #97843, #73101, #86473, #30460 ) ) ;
#36818=CARTESIAN_POINT ( 'NONE',  ( 16.40814093676323893, 10.79030133659708923, 11.09922568453595026 ) ) ;
#36819=ORIENTED_EDGE ( 'NONE', *, *, #67334, .T. ) ;
#36820=CARTESIAN_POINT ( 'NONE',  ( 17.96484262340118221, 61.18868534415482685, -7.964842623401177768 ) ) ;
#36821=CARTESIAN_POINT ( 'NONE',  ( 10.00000000000000178, 67.25893115100079456, 9.846743663894594434 ) ) ;
#36822=CARTESIAN_POINT ( 'NONE',  ( 15.44008868035555793, 16.39701867748817321, -9.422509992056140149 ) ) ;
#36824=CARTESIAN_POINT ( 'NONE',  ( 0.5774900079438607392, 68.48035201082150536, 5.440088680355550821 ) ) ;
#36826=CARTESIAN_POINT ( 'NONE',  ( 10.00000000000000178, 14.31368534415483929, 10.88017736071110342 ) ) ;
#36828=EDGE_CURVE ( 'NONE', #96626, #67947, #67184, .T. ) ;
#36829=CARTESIAN_POINT ( 'NONE',  ( -1.099225684535947600, 59.54030133659708923, 6.408140936763237150 ) ) ;
#36830=CARTESIAN_POINT ( 'NONE',  ( 17.96484262340118221, 49.93868534415484106, 7.964842623401181321 ) ) ;
#36833=CARTESIAN_POINT ( 'NONE',  ( 22.81628187352648496, 51.83196800326376064, -3.434112377981050290 ) ) ;
#36834=CARTESIAN_POINT ( 'NONE',  ( 4.559911319644449179, 43.89701867748816966, 9.422509992056141925 ) ) ;
#36835=CARTESIAN_POINT ( 'NONE',  ( -1.099225684535947600, -1.293031996736246469, -6.408140936763238038 ) ) ;
#36836=DIRECTION ( 'NONE',  ( 0.000000000000000000, 0.000000000000000000, -1.000000000000000000 ) ) ;
#36837=B_SPLINE_CURVE_WITH_KNOTS ( 'NONE', 3,
 ( #70159, #4980, #11980, #80480 ),
 .UNSPECIFIED., .F., .F.,
 ( 4, 4 ),
 ( 3.291406376790657244E-17, 0.001060528352562001547 ),
 .UNSPECIFIED. ) ;
#36839=CARTESIAN_POINT ( 'NONE',  ( 7.361572987183169658, 19.96726448433411960, -9.846743663894592657 ) ) ;
#36840=CARTESIAN_POINT ( 'NONE',  ( -1.099225684535947600, 8.706968003263753531, -6.408140936763238038 ) ) ;
#36842=CARTESIAN_POINT ( 'NONE',  ( 5.076628168052703671, 66.84226448433412315, 8.527530157486179263 ) ) ;
#36843=CARTESIAN_POINT ( 'NONE',  ( 19.42250999205614548, 40.98035201082150536, -5.440088680355545492 ) ) ;
#36845=DIRECTION ( 'NONE',  ( 1.000000000000000000, 0.000000000000000000, 0.000000000000000000 ) ) ;
#36846=CARTESIAN_POINT ( 'NONE',  ( 10.00000000000000178, 7.258931151000785675, 9.846743663894594434 ) ) ;
#36847=CARTESIAN_POINT ( 'NONE',  ( -2.816281873526471635, 3.915301336597087456, -3.434112377981056508 ) ) ;
#36851=CARTESIAN_POINT ( 'NONE',  ( 0.1532563361054083140, 61.00893115100078745, 1.131784320476157264E-15 ) ) ;
#36852=CARTESIAN_POINT ( 'NONE',  ( 3.591859063236763294, 53.29030133659708923, -11.09922568453595026 ) ) ;
#36853=CARTESIAN_POINT ( 'NONE',  ( 5.076628168052703671, 36.84226448433412315, 8.527530157486179263 ) ) ;
#36855=CARTESIAN_POINT ( 'NONE',  ( 4.559911319644449179, 7.230352010821505360, -9.422509992056141925 ) ) ;
#36856=CARTESIAN_POINT ( 'NONE',  ( 0.1532563361054083140, 36.00893115100078745, 1.131784320476157264E-15 ) ) ;
#36858=CARTESIAN_POINT ( 'NONE',  ( 7.084665262690076126, 2.022018677488171434, -10.88017736071110164 ) ) ;
#36859=CARTESIAN_POINT ( 'NONE',  ( 2.603489959281584998, 6.582109641433292246, 6.499999999999998224 ) ) ;
#36860=CARTESIAN_POINT ( 'NONE',  ( 10.00000000000000178, 24.31368534415484106, 10.88017736071110342 ) ) ;
#36861=CARTESIAN_POINT ( 'NONE',  ( -4.164238869374099039, 51.80374883491396787, 8.674139862899312516E-16 ) ) ;
#36862=CARTESIAN_POINT ( 'NONE',  ( -2.266590686148945544, 47.22041550158063927, 7.082119434687048631 ) ) ;
#36865=EDGE_CURVE ( 'NONE', #24048, #1911, #48398, .T. ) ;
#36866=CARTESIAN_POINT ( 'NONE',  ( 5.076628168052704559, 30.17559781766745175, -8.527530157486179263 ) ) ;
#36867=CARTESIAN_POINT ( 'NONE',  ( 22.81628187352648496, 1.831968003263753753, -3.434112377981050290 ) ) ;
#36870=EDGE_CURVE ( 'NONE', #10425, #94783, #23315, .T. ) ;
#36873=CARTESIAN_POINT ( 'NONE',  ( 2.917880565312948704, 12.63708216824730179, 12.26659068614894643 ) ) ;
#36875=CARTESIAN_POINT ( 'NONE',  ( 14.92337183194729633, 27.67559781766745530, 8.527530157486181039 ) ) ;
#36878=CARTESIAN_POINT ( 'NONE',  ( 22.26659068614895176, 39.72041550158063217, -7.082119434687042414 ) ) ;
#36879=CARTESIAN_POINT ( 'NONE',  ( 2.791683348922240793, 11.63393115100078568, 7.208316651077764092 ) ) ;
#36881=CARTESIAN_POINT ( 'NONE',  ( 7.084665262690076126, 27.02201867748817676, -10.88017736071110164 ) ) ;
#36882=CARTESIAN_POINT ( 'NONE',  ( 3.591859063236763294, 38.29030133659708923, -11.09922568453595026 ) ) ;
#36883=SURFACE_STYLE_USAGE ( .BOTH. , #89873 ) ;
#36885=CARTESIAN_POINT ( 'NONE',  ( 13.43411237798105340, 30.58196800326374998, 12.81628187352647963 ) ) ;
#36886=CARTESIAN_POINT ( 'NONE',  ( 10.00000000000000178, 65.37363466993042493, 12.81628187352647608 ) ) ;
#36887=ORIENTED_EDGE ( 'NONE', *, *, #88268, .F. ) ;
#36890=CARTESIAN_POINT ( 'NONE',  ( 20.15039907845753575, 35.60158574516643171, -6.262539305110076171 ) ) ;
#36891=CARTESIAN_POINT ( 'NONE',  ( 6.204703633549690345, 40.76208216824731778, -14.16423886937410259 ) ) ;
#36892=CARTESIAN_POINT ( 'NONE',  ( -4.164238869374099927, 2.012082168247300906, 3.795296366450308767 ) ) ;
#36893=CARTESIAN_POINT ( 'NONE',  ( 19.42250999205614548, 10.98035201082150358, -5.440088680355545492 ) ) ;
#36894=CARTESIAN_POINT ( 'NONE',  ( 10.00000000000000000, 26.81368534415484106, -10.88017736071110342 ) ) ;
#36897=CARTESIAN_POINT ( 'NONE',  ( 10.00000000000000178, 54.31368534415484106, 10.88017736071110342 ) ) ;
#36898=CARTESIAN_POINT ( 'NONE',  ( 7.084665262690076126, 47.02201867748818387, -10.88017736071110164 ) ) ;
#36899=CARTESIAN_POINT ( 'NONE',  ( 13.43411237798106583, 32.66530133659708213, -12.81628187352647252 ) ) ;
#36900=CARTESIAN_POINT ( 'NONE',  ( 19.88701968852511826, 26.79427333184090898, 6.480634945678690251 ) ) ;
#36901=CARTESIAN_POINT ( 'NONE',  ( 7.361572987183170547, 27.05059781766745175, 9.846743663894590881 ) ) ;
#36902=CARTESIAN_POINT ( 'NONE',  ( 4.559911319644449179, 52.23035201082151247, -9.422509992056141925 ) ) ;
#36903=CARTESIAN_POINT ( 'NONE',  ( 10.00000000000000000, 17.87363466993041783, -12.81628187352647608 ) ) ;
#36905=CARTESIAN_POINT ( 'NONE',  ( 0.5774900079438590739, 7.647018677488171434, -5.440088680355550821 ) ) ;
#36906=CARTESIAN_POINT ( 'NONE',  ( 10.00000000000000178, 37.25893115100078745, 9.846743663894594434 ) ) ;
#36907=CARTESIAN_POINT ( 'NONE',  ( 13.43411237798106583, 62.66530133659708923, -12.81628187352647252 ) ) ;
#36908=CARTESIAN_POINT ( 'NONE',  ( 19.84674366389459621, 13.50893115100078568, 7.409399052514197653E-17 ) ) ;
#36909=CARTESIAN_POINT ( 'NONE',  ( 24.16423886937410614, 9.303748834913967869, 8.672049930838204340E-16 ) ) ;
#36910=CARTESIAN_POINT ( 'NONE',  ( 19.10478245763057714, 30.10160829253887371, 5.990408912944228170 ) ) ;
#36911=CARTESIAN_POINT ( 'NONE',  ( 0.5774900079438607392, 38.48035201082150536, 5.440088680355550821 ) ) ;
#36912=CARTESIAN_POINT ( 'NONE',  ( -0.8801773607110991993, 2.855352010821504471, -2.915334737309923874 ) ) ;
#36913=CARTESIAN_POINT ( 'NONE',  ( 19.84674366389459266, 43.30059781766744464, 2.638427012816836559 ) ) ;
#36914=CARTESIAN_POINT ( 'NONE',  ( -0.8801773607111008646, 38.27201867748816255, 2.915334737309923430 ) ) ;
#36915=CARTESIAN_POINT ( 'NONE',  ( 10.00000000000000178, 19.31368534415484106, 10.88017736071110342 ) ) ;
#36918=CARTESIAN_POINT ( 'NONE',  ( 15.44008868035555260, 29.73035201082150891, 9.422509992056143702 ) ) ;
#36920=CARTESIAN_POINT ( 'NONE',  ( 13.43411237798105340, 40.58196800326375353, 12.81628187352647963 ) ) ;
#36922=CARTESIAN_POINT ( 'NONE',  ( 0.5774900079438607392, 33.48035201082150536, 5.440088680355550821 ) ) ;
#36923=CARTESIAN_POINT ( 'NONE',  ( 1.959929470562273179, 46.50257860105348584, 5.767676674365838529 ) ) ;
#36924=CARTESIAN_POINT ( 'NONE',  ( 20.88017736071110875, 35.77201867748816966, -2.915334737309920765 ) ) ;
#36925=ORIENTED_EDGE ( 'NONE', *, *, #68556, .F. ) ;
#36926=CARTESIAN_POINT ( 'NONE',  ( 14.92337183194729633, 52.67559781766745175, 8.527530157486181039 ) ) ;
#36927=CARTESIAN_POINT ( 'NONE',  ( 20.88017736071110164, 40.35535201082150536, 2.915334737309930979 ) ) ;
#36928=CARTESIAN_POINT ( 'NONE',  ( 2.791683348922240793, 66.63393115100079456, 7.208316651077764092 ) ) ;
#36931=CARTESIAN_POINT ( 'NONE',  ( 24.16423886937410614, 49.51208216824730357, -3.795296366450302550 ) ) ;
#36932=CARTESIAN_POINT ( 'NONE',  ( 2.035157376598824452, 58.68868534415482685, 7.964842623401179544 ) ) ;
#36936=CARTESIAN_POINT ( 'NONE',  ( 19.84674366389459266, 63.71726448433412315, -2.638427012816827677 ) ) ;
#36937=CARTESIAN_POINT ( 'NONE',  ( 0.1532563361054082862, 26.21726448433411605, 2.638427012816831674 ) ) ;
#36939=CARTESIAN_POINT ( 'NONE',  ( 14.92337183194729633, 27.67559781766745530, 8.527530157486181039 ) ) ;
#36941=CARTESIAN_POINT ( 'NONE',  ( 7.084665262690076126, 24.10535201082150181, 10.88017736071109987 ) ) ;
#36942=CARTESIAN_POINT ( 'NONE',  ( 0.1532563361054082862, 26.21726448433411605, 2.638427012816831674 ) ) ;
#36945=CARTESIAN_POINT ( 'NONE',  ( 19.05866839779139355, 25.95508385108958649, -6.499999999999974243 ) ) ;
#36946=CARTESIAN_POINT ( 'NONE',  ( 4.559911319644449179, 37.23035201082150536, -9.422509992056141925 ) ) ;
#36947=CARTESIAN_POINT ( 'NONE',  ( -0.3689425029237881626, 47.42874883491396787, 10.36894250292379027 ) ) ;
#36949=EDGE_CURVE ( 'NONE', #71629, #35522, #31272, .T. ) ;
#36950=CARTESIAN_POINT ( 'NONE',  ( 20.15039907845753575, 35.60158574516643171, -6.262539305110076171 ) ) ;
#36952=CARTESIAN_POINT ( 'NONE',  ( -2.816281873526471635, 18.91530133659708213, -3.434112377981056508 ) ) ;
#36953=CARTESIAN_POINT ( 'NONE',  ( 19.42250999205614548, 5.980352010821504471, -5.440088680355545492 ) ) ;
#36954=CARTESIAN_POINT ( 'NONE',  ( 20.88017736071110164, 50.35535201082151247, 2.915334737309930979 ) ) ;
#36956=ADVANCED_FACE ( 'NONE', ( #39924 ), #92912, .T. ) ;
#36958=CARTESIAN_POINT ( 'NONE',  ( 20.88017736071110875, 55.77201867748816966, -2.915334737309920765 ) ) ;
#36959=VECTOR ( 'NONE', #98168, 1000.000000000000000 ) ;
#36960=CARTESIAN_POINT ( 'NONE',  ( 10.00000000000000000, 39.75893115100078745, -9.846743663894594434 ) ) ;
#36961=CARTESIAN_POINT ( 'NONE',  ( 10.00000000000000178, 22.25893115100078745, 9.846743663894594434 ) ) ;
#36962=CARTESIAN_POINT ( 'NONE',  ( 2.791683348922237240, 10.38393115100078390, -7.208316651077763204 ) ) ;
#36964=CARTESIAN_POINT ( 'NONE',  ( 1.472469842513823179, 0.5922644843341181575, -4.923371831947296329 ) ) ;
#36967=CARTESIAN_POINT ( 'NONE',  ( 14.92337183194729633, 37.67559781766745175, 8.527530157486181039 ) ) ;
#36969=CARTESIAN_POINT ( 'NONE',  ( -2.816281873526473856, 59.12363466993042493, 9.499525473075851096E-16 ) ) ;
#36971=CARTESIAN_POINT ( 'NONE',  ( 10.00000000000000000, 64.75893115100078035, -9.846743663894594434 ) ) ;
#36972=CARTESIAN_POINT ( 'NONE',  ( 22.26659068614894466, 33.88708216824730357, 7.082119434687054849 ) ) ;
#36974=CARTESIAN_POINT ( 'NONE',  ( -0.3689425029237898834, 31.17874883491396787, -10.36894250292378850 ) ) ;
#36975=CARTESIAN_POINT ( 'NONE',  ( 24.16423886937410614, 44.30374883491397497, 8.672049930838204340E-16 ) ) ;
#36976=CARTESIAN_POINT ( 'NONE',  ( 17.08211943468705130, 3.470415501580634388, 12.26659068614894998 ) ) ;
#36977=CARTESIAN_POINT ( 'NONE',  ( 24.16423886937410614, 9.303748834913967869, 8.672049930838204340E-16 ) ) ;
#36978=CARTESIAN_POINT ( 'NONE',  ( 17.96484262340118221, 64.93868534415483396, 7.964842623401181321 ) ) ;
#36979=CARTESIAN_POINT ( 'NONE',  ( 20.88017736071110519, 45.56368534415484106, 2.639326808657452039E-16 ) ) ;
#36981=CARTESIAN_POINT ( 'NONE',  ( 14.92337183194729988, 29.34226448433411960, -8.527530157486177487 ) ) ;
#36982=CARTESIAN_POINT ( 'NONE',  ( 2.603489959281588106, 1.582109641433292690, 6.500000000000000888 ) ) ;
#36983=CARTESIAN_POINT ( 'NONE',  ( 10.00000000000000178, 32.25893115100078745, 9.846743663894594434 ) ) ;
#36986=CARTESIAN_POINT ( 'NONE',  ( 4.559911319644449179, 27.23035201082150536, -9.422509992056141925 ) ) ;
#36987=CARTESIAN_POINT ( 'NONE',  ( -1.099225684535947600, 53.70696800326376064, -6.408140936763238038 ) ) ;
#36988=CARTESIAN_POINT ( 'NONE',  ( 18.52753015748618282, 63.92559781766745886, -4.923371831947291888 ) ) ;
#36991=CARTESIAN_POINT ( 'NONE',  ( 0.1532563361054100626, 30.80059781766744820, -2.638427012816831230 ) ) ;
#36992=CARTESIAN_POINT ( 'NONE',  ( 22.81628187352647785, 41.41530133659708923, 3.434112377981063169 ) ) ;
#36994=CARTESIAN_POINT ( 'NONE',  ( 7.084665262690076126, 39.10535201082150536, 10.88017736071109987 ) ) ;
#36995=CARTESIAN_POINT ( 'NONE',  ( 1.472469842513823179, 55.59226448433412315, -4.923371831947296329 ) ) ;
#36997=CARTESIAN_POINT ( 'NONE',  ( -4.164238869374098151, 31.59541550158063927, -3.795296366450310543 ) ) ;
#36999=PRESENTATION_STYLE_ASSIGNMENT (( #6491 ) ) ;
#37000=CARTESIAN_POINT ( 'NONE',  ( 20.88017736071110164, 60.35535201082151957, 2.915334737309930979 ) ) ;
#37001=CARTESIAN_POINT ( 'NONE',  ( 7.084665262690076126, 69.10535201082151957, 10.88017736071109987 ) ) ;
#37002=CARTESIAN_POINT ( 'NONE',  ( 6.204703633549690345, 62.84541550158063927, 14.16423886937410082 ) ) ;
#37003=CARTESIAN_POINT ( 'NONE',  ( 19.84674366389459621, 63.50893115100078745, 7.409399052514197653E-17 ) ) ;
#37004=CARTESIAN_POINT ( 'NONE',  ( 0.1089645850229084695, 53.16234555792572536, 6.479102184480833415 ) ) ;
#37005=CARTESIAN_POINT ( 'NONE',  ( 12.91533473730992121, 49.52201867748817676, 10.88017736071110164 ) ) ;
#37007=CARTESIAN_POINT ( 'NONE',  ( 19.38216949554541202, 30.99863466993042138, 9.382169495545424454 ) ) ;
#37009=CARTESIAN_POINT ( 'NONE',  ( 4.559911319644449179, 8.897018677488171434, 9.422509992056141925 ) ) ;
#37010=CARTESIAN_POINT ( 'NONE',  ( 15.44008868035555260, 4.730352010821505360, 9.422509992056143702 ) ) ;
#37011=CARTESIAN_POINT ( 'NONE',  ( 14.92337183194729988, 54.34226448433412315, -8.527530157486177487 ) ) ;
#37012=CARTESIAN_POINT ( 'NONE',  ( 21.09922568453595559, 47.04030133659708923, -6.408140936763230044 ) ) ;
#37014=VERTEX_POINT ( 'NONE', #2933 ) ;
#37015=CARTESIAN_POINT ( 'NONE',  ( 7.084665262690076126, 12.02201867748817143, -10.88017736071110164 ) ) ;
#37016=CARTESIAN_POINT ( 'NONE',  ( 13.43411237798106583, 22.66530133659708923, -12.81628187352647252 ) ) ;
#37017=CARTESIAN_POINT ( 'NONE',  ( 20.04068437667223890, 39.71974360917720048, 6.396802510829769695 ) ) ;
#37018=CARTESIAN_POINT ( 'NONE',  ( 7.361572987183170547, 17.05059781766745530, 9.846743663894590881 ) ) ;
#37021=CARTESIAN_POINT ( 'NONE',  ( 19.84674366389459621, 48.50893115100078745, 7.409399052514197653E-17 ) ) ;
#37022=CARTESIAN_POINT ( 'NONE',  ( 15.44008868035555793, 36.39701867748816966, -9.422509992056140149 ) ) ;
#37024=CARTESIAN_POINT ( 'NONE',  ( 6.565887622018943937, 10.16530133659708746, 12.81628187352647430 ) ) ;
#37025=CARTESIAN_POINT ( 'NONE',  ( 10.00000000000000000, 46.81368534415484106, -10.88017736071110342 ) ) ;
#37029=CARTESIAN_POINT ( 'NONE',  ( 6.565887622018943937, 53.08196800326374643, -12.81628187352647608 ) ) ;
#37032=CARTESIAN_POINT ( 'NONE',  ( 3.591859063236763294, 33.29030133659708213, -11.09922568453595026 ) ) ;
#37033=CARTESIAN_POINT ( 'NONE',  ( 24.16423886937410614, 4.303748834913967869, 8.672049930838204340E-16 ) ) ;
#37034=CARTESIAN_POINT ( 'NONE',  ( 4.559911319644449179, 33.89701867748817676, 9.422509992056141925 ) ) ;
#37035=CARTESIAN_POINT ( 'NONE',  ( 5.076628168052703671, 61.84226448433412315, 8.527530157486179263 ) ) ;
#37037=CARTESIAN_POINT ( 'NONE',  ( 0.1532563361054100626, 15.80059781766745353, -2.638427012816831230 ) ) ;
#37038=CARTESIAN_POINT ( 'NONE',  ( 18.52753015748617571, 3.092264484334118269, 4.923371831947298993 ) ) ;
#37039=CARTESIAN_POINT ( 'NONE',  ( -4.164238869374099927, 37.01208216824731068, 3.795296366450308767 ) ) ;
#37047=CARTESIAN_POINT ( 'NONE',  ( 6.204703633549690345, 60.76208216824730357, -14.16423886937410259 ) ) ;
#37048=CARTESIAN_POINT ( 'NONE',  ( 20.36894250292379382, 58.67874883491396076, 10.36894250292379205 ) ) ;
#37049=CARTESIAN_POINT ( 'NONE',  ( 12.63842701281683034, 27.46726448433411250, 9.846743663894596210 ) ) ;
#37050=CARTESIAN_POINT ( 'NONE',  ( -1.099225684535947600, 28.70696800326375353, -6.408140936763238038 ) ) ;
#37053=CARTESIAN_POINT ( 'NONE',  ( 6.204703633549690345, 5.762082168247301794, -14.16423886937410259 ) ) ;
#37054=CARTESIAN_POINT ( 'NONE',  ( 4.559911319644449179, 8.897018677488171434, 9.422509992056141925 ) ) ;
#37055=CARTESIAN_POINT ( 'NONE',  ( -4.164238869374099927, 52.01208216824729647, 3.795296366450308767 ) ) ;
#37058=CARTESIAN_POINT ( 'NONE',  ( 19.84674366389459621, 28.50893115100078745, 7.409399052514197653E-17 ) ) ;
#37060=CARTESIAN_POINT ( 'NONE',  ( 7.361572987183169658, 24.96726448433412315, -9.846743663894592657 ) ) ;
#37064=ORIENTED_EDGE ( 'NONE', *, *, #31158, .F. ) ;
#37067=CARTESIAN_POINT ( 'NONE',  ( 10.00000000000000000, 49.75893115100078745, -9.846743663894594434 ) ) ;
#37068=CARTESIAN_POINT ( 'NONE',  ( 2.917880565312948704, 17.63708216824730357, 12.26659068614894643 ) ) ;
#37069=CARTESIAN_POINT ( 'NONE',  ( 7.084665262690076126, 32.02201867748816966, -10.88017736071110164 ) ) ;
#37070=CARTESIAN_POINT ( 'NONE',  ( 15.44008868035555260, 44.73035201082151247, 9.422509992056143702 ) ) ;
#37071=CARTESIAN_POINT ( 'NONE',  ( 17.20831665107776587, 57.88393115100078745, 7.208316651077764980 ) ) ;
#37072=CARTESIAN_POINT ( 'NONE',  ( 6.565887622018943937, 15.16530133659708568, 12.81628187352647430 ) ) ;
#37073=CARTESIAN_POINT ( 'NONE',  ( -4.164238869374098151, 1.595415501580634388, -3.795296366450310543 ) ) ;
#37074=CARTESIAN_POINT ( 'NONE',  ( 0.5774900079438590739, 62.64701867748817676, -5.440088680355550821 ) ) ;
#37076=CARTESIAN_POINT ( 'NONE',  ( 0.6178305044545818747, 38.49863466993042493, -9.382169495545419124 ) ) ;
#37078=CARTESIAN_POINT ( 'NONE',  ( 5.076628168052704559, 45.17559781766745175, -8.527530157486179263 ) ) ;
#37079=CARTESIAN_POINT ( 'NONE',  ( 2.035157376598822676, 2.438685344154838397, -7.964842623401177768 ) ) ;
#37080=ORIENTED_EDGE ( 'NONE', *, *, #79343, .T. ) ;
#37082=CARTESIAN_POINT ( 'NONE',  ( 12.91533473730992121, 9.522018677488171434, 10.88017736071110164 ) ) ;
#37084=CARTESIAN_POINT ( 'NONE',  ( 20.88017736071110519, 50.56368534415484106, 2.639326808657452039E-16 ) ) ;
#37085=CARTESIAN_POINT ( 'NONE',  ( 4.559911319644449179, 57.23035201082150536, -9.422509992056141925 ) ) ;
#37086=CARTESIAN_POINT ( 'NONE',  ( 2.035157376598824452, 58.68868534415482685, 7.964842623401179544 ) ) ;
#37088=CARTESIAN_POINT ( 'NONE',  ( 20.88017736071110875, 60.77201867748817676, -2.915334737309920765 ) ) ;
#37090=FILL_AREA_STYLE_COLOUR ( '', #79252 ) ;
#37091=VECTOR ( 'NONE', #80229, 1000.000000000000000 ) ;
#37092=CARTESIAN_POINT ( 'NONE',  ( 5.076628168052704559, 30.17559781766745175, -8.527530157486179263 ) ) ;
#37094=DIRECTION ( 'NONE',  ( 0.9970872288863210642, 0.07626964003977955431, 0.000000000000000000 ) ) ;
#37095=AXIS2_PLACEMENT_3D ( 'NONE', #74821, #59811, #45820 ) ;
#37100=LINE ( 'NONE', #30065, #50626 ) ;
#37101=LINE ( 'NONE', #82588, #38605 ) ;
#37102=CARTESIAN_POINT ( 'NONE',  ( 1.472469842513823179, 36.42559781766745175, 4.923371831947296329 ) ) ;
#37103=CARTESIAN_POINT ( 'NONE',  ( 17.96484262340118221, 6.188685344154837509, -7.964842623401177768 ) ) ;
#37105=ORIENTED_EDGE ( 'NONE', *, *, #86035, .T. ) ;
#37106=CARTESIAN_POINT ( 'NONE',  ( 20.03447792253739834, 62.65514106990689669, -6.401564815979719825 ) ) ;
#37108=CARTESIAN_POINT ( 'NONE',  ( 14.92337183194729988, 49.34226448433411605, -8.527530157486177487 ) ) ;
#37110=CARTESIAN_POINT ( 'NONE',  ( 6.565887622018943937, 13.08196800326374998, -12.81628187352647608 ) ) ;
#37111=CARTESIAN_POINT ( 'NONE',  ( 5.076628168052703671, 11.84226448433411960, 8.527530157486179263 ) ) ;
#37113=CARTESIAN_POINT ( 'NONE',  ( 1.472469842513823179, 16.42559781766745175, 4.923371831947296329 ) ) ;
#37114=CARTESIAN_POINT ( 'NONE',  ( 3.591859063236763294, 8.290301336597087456, -11.09922568453595026 ) ) ;
#37119=CARTESIAN_POINT ( 'NONE',  ( 20.88017736071110875, 25.77201867748816966, -2.915334737309920765 ) ) ;
#37120=CARTESIAN_POINT ( 'NONE',  ( -4.164238869374098151, 21.59541550158063217, -3.795296366450310543 ) ) ;
#37121=CARTESIAN_POINT ( 'NONE',  ( 19.84674366389459266, 33.71726448433410894, -2.638427012816827677 ) ) ;
#37122=CARTESIAN_POINT ( 'NONE',  ( 10.00000000000000000, 61.81368534415484106, -10.88017736071110342 ) ) ;
#37123=CARTESIAN_POINT ( 'NONE',  ( 13.43411237798106583, 37.66530133659708923, -12.81628187352647252 ) ) ;
#37125=CARTESIAN_POINT ( 'NONE',  ( 20.88017736071110164, 10.35535201082150714, 2.915334737309930979 ) ) ;
#37129=CARTESIAN_POINT ( 'NONE',  ( 13.43411237798105340, 10.58196800326375353, 12.81628187352647963 ) ) ;
#37130=CARTESIAN_POINT ( 'NONE',  ( 5.076628168052703671, 61.84226448433412315, 8.527530157486179263 ) ) ;
#37131=CARTESIAN_POINT ( 'NONE',  ( 7.361572987183169658, 24.96726448433412315, -9.846743663894592657 ) ) ;
#37133=CARTESIAN_POINT ( 'NONE',  ( 19.38216949554541557, 32.24863466993041783, -9.382169495545420901 ) ) ;
#37135=CARTESIAN_POINT ( 'NONE',  ( 2.035157376598822676, 37.43868534415484106, -7.964842623401177768 ) ) ;
#37139=CARTESIAN_POINT ( 'NONE',  ( 18.50749283717776805, 29.69955587570480660, 6.499999999999997335 ) ) ;
#37140=CARTESIAN_POINT ( 'NONE',  ( 10.00000000000000000, 46.81368534415484106, -10.88017736071110342 ) ) ;
#37142=CARTESIAN_POINT ( 'NONE',  ( -0.8801773607110991993, 37.85535201082151247, -2.915334737309923874 ) ) ;
#37143=CARTESIAN_POINT ( 'NONE',  ( 18.52753015748617571, 63.09226448433412315, 4.923371831947298993 ) ) ;
#37145=UNCERTAINTY_MEASURE_WITH_UNIT (LENGTH_MEASURE( 1.000000000000000082E-05 ), #97413, 'distance_accuracy_value', 'NONE');
#37146=( BOUNDED_CURVE ( )  B_SPLINE_CURVE ( 2, ( #75899, #51922, #68410, #74911, #13932, #6411, #22918, #36923, #98932 ),
 .UNSPECIFIED., .F., .T. ) 
 B_SPLINE_CURVE_WITH_KNOTS ( ( 3, 2, 2, 2, 3 ),
 ( 0.6525141644748393421, 0.6547619047619047672, 0.6607142857142856984, 0.6666666666666666297, 0.6689144069537320547 ),
 .UNSPECIFIED. ) 
 CURVE ( )  GEOMETRIC_REPRESENTATION_ITEM ( )  RATIONAL_B_SPLINE_CURVE ( ( 0.9839835555609424134, 0.9871328979762474809, 1.000000000000000000, 0.9659258262890683122, 1.000000000000000000, 0.9659258262890683122, 1.000000000000000000, 0.9871328979762477029, 0.9839835555609425244 ) ) 
 REPRESENTATION_ITEM ( '' )  );
#37147=CARTESIAN_POINT ( 'NONE',  ( 0.1532563361054083140, 41.00893115100078745, 1.131784320476157264E-15 ) ) ;
#37148=CARTESIAN_POINT ( 'NONE',  ( 17.96484262340118221, 9.938685344154837509, 7.964842623401181321 ) ) ;
#37149=CARTESIAN_POINT ( 'NONE',  ( 0.6178305044545838731, 14.74863466993041783, 9.382169495545420901 ) ) ;
#37150=EDGE_LOOP ( 'NONE', ( #4628, #85417, #45918, #72620 ) ) ;
#37151=CARTESIAN_POINT ( 'NONE',  ( -0.8801773607110991993, 22.85535201082150181, -2.915334737309923874 ) ) ;
#37153=CARTESIAN_POINT ( 'NONE',  ( 7.084665262690076126, 4.105352010821503583, 10.88017736071109987 ) ) ;
#37154=CARTESIAN_POINT ( 'NONE',  ( 7.084665262690076126, 27.02201867748817676, -10.88017736071110164 ) ) ;
#37155=CARTESIAN_POINT ( 'NONE',  ( 17.20831665107776587, 2.883931151000785231, 7.208316651077764980 ) ) ;
#37156=CARTESIAN_POINT ( 'NONE',  ( 17.08211943468705130, 43.47041550158063927, 12.26659068614894998 ) ) ;
#37157=CARTESIAN_POINT ( 'NONE',  ( 12.63842701281683922, 9.550597817667449974, -9.846743663894590881 ) ) ;
#37158=CARTESIAN_POINT ( 'NONE',  ( 7.084665262690076126, 42.02201867748816966, -10.88017736071110164 ) ) ;
#37159=CARTESIAN_POINT ( 'NONE',  ( 19.72487221294571569, 45.71833443783938122, -6.499999999999989342 ) ) ;
#37162=UNCERTAINTY_MEASURE_WITH_UNIT (LENGTH_MEASURE( 1.000000000000000082E-05 ), #27747, 'distance_accuracy_value', 'NONE');
#37165=CARTESIAN_POINT ( 'NONE',  ( 2.791683348922237240, 65.38393115100078035, -7.208316651077763204 ) ) ;
#37166=EDGE_CURVE ( 'NONE', #47944, #39498, #265, .T. ) ;
#37170=CARTESIAN_POINT ( 'NONE',  ( 17.08211943468705130, 18.47041550158063572, 12.26659068614894998 ) ) ;
#37171=CARTESIAN_POINT ( 'NONE',  ( 13.79529636645031943, 20.34541550158063572, -14.16423886937409904 ) ) ;
#37172=CARTESIAN_POINT ( 'NONE',  ( 12.91533473730993009, 61.60535201082150536, -10.88017736071109987 ) ) ;
#37173=CARTESIAN_POINT ( 'NONE',  ( -4.164238869374099927, 62.01208216824728936, 3.795296366450308767 ) ) ;
#37174=CARTESIAN_POINT ( 'NONE',  ( 21.09922568453595559, 2.040301336597086568, -6.408140936763230044 ) ) ;
#37175=CARTESIAN_POINT ( 'NONE',  ( 17.20831665107776587, 44.13393115100078745, -7.208316651077762316 ) ) ;
#37177=CARTESIAN_POINT ( 'NONE',  ( 17.96484262340118221, 44.93868534415483396, 7.964842623401181321 ) ) ;
#37178=CARTESIAN_POINT ( 'NONE',  ( 16.40814093676323893, 5.790301336597087456, 11.09922568453595026 ) ) ;
#37179=CARTESIAN_POINT ( 'NONE',  ( 20.36894250292379738, 14.92874883491396432, -10.36894250292379027 ) ) ;
#37180=CARTESIAN_POINT ( 'NONE',  ( 0.5774900079438607392, 13.48035201082150358, 5.440088680355550821 ) ) ;
#37182=CARTESIAN_POINT ( 'NONE',  ( 4.559911319644449179, 13.89701867748817321, 9.422509992056141925 ) ) ;
#37185=CARTESIAN_POINT ( 'NONE',  ( 20.88017736071110875, 55.77201867748816966, -2.915334737309920765 ) ) ;
#37187=CARTESIAN_POINT ( 'NONE',  ( 13.43411237798106583, 47.66530133659709634, -12.81628187352647252 ) ) ;
#37191=VECTOR ( 'NONE', #79786, 1000.000000000000000 ) ;
#37193=ORIENTED_EDGE ( 'NONE', *, *, #29891, .F. ) ;
#37194=CARTESIAN_POINT ( 'NONE',  ( 0.2751277870542911952, 19.36607318730131055, -6.499999999999992006 ) ) ;
#37195=CARTESIAN_POINT ( 'NONE',  ( -2.266590686148945544, 41.38708216824729647, -7.082119434687050408 ) ) ;
#37196=CARTESIAN_POINT ( 'NONE',  ( 7.084665262690076126, 2.022018677488171434, -10.88017736071110164 ) ) ;
#37197=CARTESIAN_POINT ( 'NONE',  ( 14.92337183194729988, 19.34226448433411960, -8.527530157486177487 ) ) ;
#37198=CARTESIAN_POINT ( 'NONE',  ( 14.92337183194729988, 49.34226448433411605, -8.527530157486177487 ) ) ;
#37199=CARTESIAN_POINT ( 'NONE',  ( 4.559911319644449179, 68.89701867748817676, 9.422509992056141925 ) ) ;
#37200=CARTESIAN_POINT ( 'NONE',  ( 18.52753015748618282, 3.925597817667451306, -4.923371831947291888 ) ) ;
#37203=CARTESIAN_POINT ( 'NONE',  ( 20.36894250292379738, 34.92874883491396076, -10.36894250292379027 ) ) ;
#37205=EDGE_CURVE ( 'NONE', #80817, #87107, #16950, .T. ) ;
#37206=CARTESIAN_POINT ( 'NONE',  ( 0.6178305044545838731, 29.74863466993042138, 9.382169495545420901 ) ) ;
#37209=CARTESIAN_POINT ( 'NONE',  ( 6.565887622018943937, 55.16530133659709634, 12.81628187352647430 ) ) ;
#37210=CARTESIAN_POINT ( 'NONE',  ( 15.44008868035555260, 29.73035201082150891, 9.422509992056143702 ) ) ;
#37211=CARTESIAN_POINT ( 'NONE',  ( 0.1532563361054083140, 41.00893115100078745, 1.131784320476157264E-15 ) ) ;
#37212=CARTESIAN_POINT ( 'NONE',  ( 0.5774900079438590739, 32.64701867748816966, -5.440088680355550821 ) ) ;
#37213=CARTESIAN_POINT ( 'NONE',  ( 0.6178305044545818747, 63.49863466993043204, -9.382169495545419124 ) ) ;
#37215=CARTESIAN_POINT ( 'NONE',  ( 1.472469842513823179, 40.59226448433411605, -4.923371831947296329 ) ) ;
#37216=CARTESIAN_POINT ( 'NONE',  ( 2.791683348922240793, 56.63393115100078035, 7.208316651077764092 ) ) ;
#37217=EDGE_CURVE ( 'NONE', #76154, #80095, #11224, .T. ) ;
#37220=CIRCLE ( 'NONE', #59536, 9.999999999999994671 ) ;
#37225=CARTESIAN_POINT ( 'NONE',  ( 19.84674366389459621, 18.50893115100078745, 7.409399052514197653E-17 ) ) ;
#37228=CARTESIAN_POINT ( 'NONE',  ( 19.84674366389459266, 53.30059781766744464, 2.638427012816836559 ) ) ;
#37229=CARTESIAN_POINT ( 'NONE',  ( 0.1532563361054083140, 46.00893115100079456, 1.131784320476157264E-15 ) ) ;
#37230=CARTESIAN_POINT ( 'NONE',  ( 6.204703633549690345, 32.84541550158063927, 14.16423886937410082 ) ) ;
#37231=CARTESIAN_POINT ( 'NONE',  ( 7.361572987183169658, 49.96726448433410894, -9.846743663894592657 ) ) ;
#37232=CARTESIAN_POINT ( 'NONE',  ( 10.00000000000000178, 50.37363466993042493, 12.81628187352647608 ) ) ;
#37233=DIRECTION ( 'NONE',  ( 0.000000000000000000, 0.000000000000000000, -1.000000000000000000 ) ) ;
#37234=CARTESIAN_POINT ( 'NONE',  ( 14.92337183194729633, 2.675597817667451750, 8.527530157486181039 ) ) ;
#37235=CARTESIAN_POINT ( 'NONE',  ( 20.36894250292379382, 3.678748834913967869, 10.36894250292379205 ) ) ;
#37236=CARTESIAN_POINT ( 'NONE',  ( 7.361572987183169658, 54.96726448433413026, -9.846743663894592657 ) ) ;
#37237=CARTESIAN_POINT ( 'NONE',  ( -0.8801773607110991993, 42.85535201082150536, -2.915334737309923874 ) ) ;
#37239=CARTESIAN_POINT ( 'NONE',  ( 10.00000000000000178, 42.25893115100078745, 9.846743663894594434 ) ) ;
#37240=CARTESIAN_POINT ( 'NONE',  ( 20.03743638938529159, 31.75197528031016603, 6.399506433553909801 ) ) ;
#37241=CARTESIAN_POINT ( 'NONE',  ( 10.00000000000000178, 44.31368534415484106, 10.88017736071110342 ) ) ;
#37245=CARTESIAN_POINT ( 'NONE',  ( 10.00000000000000000, 21.81368534415484106, -10.88017736071110342 ) ) ;
#37246=CARTESIAN_POINT ( 'NONE',  ( 10.00000000000000000, -2.126365330069579951, -12.81628187352647608 ) ) ;
#37247=CARTESIAN_POINT ( 'NONE',  ( 20.88017736071110164, 45.35535201082149115, 2.915334737309930979 ) ) ;
#37251=CARTESIAN_POINT ( 'NONE',  ( 10.00000000000000178, 39.31368534415484106, 10.88017736071110342 ) ) ;
#37253=CARTESIAN_POINT ( 'NONE',  ( 12.63842701281683922, 14.55059781766744997, -9.846743663894590881 ) ) ;
#37255=CARTESIAN_POINT ( 'NONE',  ( 5.076628168052704559, 25.17559781766745175, -8.527530157486179263 ) ) ;
#37259=CARTESIAN_POINT ( 'NONE',  ( 10.00000000000000178, 0.3736346699304200492, 12.81628187352647608 ) ) ;
#37260=CARTESIAN_POINT ( 'NONE',  ( -2.266590686148945544, 66.38708216824730357, -7.082119434687050408 ) ) ;
#37263=CARTESIAN_POINT ( 'NONE',  ( 13.79529636645030344, 23.26208216824730002, 14.16423886937410614 ) ) ;
#37264=CARTESIAN_POINT ( 'NONE',  ( 10.00000000000000000, 45.55374883491397497, -14.16423886937410082 ) ) ;
#37265=CARTESIAN_POINT ( 'NONE',  ( 20.88017736071110875, 5.772018677488170546, -2.915334737309920765 ) ) ;
#37267=CARTESIAN_POINT ( 'NONE',  ( 0.1532563361054100626, 25.80059781766744820, -2.638427012816831230 ) ) ;
#37268=CARTESIAN_POINT ( 'NONE',  ( 20.88017736071110164, 15.35535201082150358, 2.915334737309930979 ) ) ;
#37269=CARTESIAN_POINT ( 'NONE',  ( 2.791683348922240793, 46.63393115100077324, 7.208316651077764092 ) ) ;
#37270=CARTESIAN_POINT ( 'NONE',  ( 2.917880565312948704, 2.637082168247300906, 12.26659068614894643 ) ) ;
#37272=CARTESIAN_POINT ( 'NONE',  ( 0.1532563361054082862, 1.217264484334117824, 2.638427012816831674 ) ) ;
#37273=CARTESIAN_POINT ( 'NONE',  ( 16.40814093676323893, 40.79030133659708923, 11.09922568453595026 ) ) ;
#37274=CARTESIAN_POINT ( 'NONE',  ( 0.1532563361054083140, 36.00893115100078745, 1.131784320476157264E-15 ) ) ;
#37276=CARTESIAN_POINT ( 'NONE',  ( 0.1532563361054083140, 6.008931151000784787, 1.131784320476157264E-15 ) ) ;
#37278=CARTESIAN_POINT ( 'NONE',  ( 19.88701968852526036, 16.79427333184085569, 6.480634945678614756 ) ) ;
#37279=CARTESIAN_POINT ( 'NONE',  ( -0.8801773607110991993, 12.85535201082150358, -2.915334737309923874 ) ) ;
#37280=CARTESIAN_POINT ( 'NONE',  ( -0.3689425029237898834, 51.17874883491397497, -10.36894250292378850 ) ) ;
#37281=CARTESIAN_POINT ( 'NONE',  ( 1.472469842513823179, 20.59226448433411960, -4.923371831947296329 ) ) ;
#37282=CARTESIAN_POINT ( 'NONE',  ( 10.00000000000000178, 4.313685344154837509, 10.88017736071110342 ) ) ;
#37283=CARTESIAN_POINT ( 'NONE',  ( 19.84674366389459266, 3.300597817667451750, 2.638427012816836559 ) ) ;
#37285=CARTESIAN_POINT ( 'NONE',  ( 10.00000000000000178, 47.25893115100078745, 9.846743663894594434 ) ) ;
#37287=CARTESIAN_POINT ( 'NONE',  ( 17.96484262340118221, 36.18868534415484106, -7.964842623401177768 ) ) ;
#37288=UNCERTAINTY_MEASURE_WITH_UNIT (LENGTH_MEASURE( 1.000000000000000082E-05 ), #30566, 'distance_accuracy_value', 'NONE');
#37292=CARTESIAN_POINT ( 'NONE',  ( 10.00000000000000178, 65.37363466993042493, 12.81628187352647608 ) ) ;
#37294=CARTESIAN_POINT ( 'NONE',  ( 17.20831665107776587, 9.133931151000787452, -7.208316651077762316 ) ) ;
#37295=CARTESIAN_POINT ( 'NONE',  ( -1.099225684535947600, 39.54030133659708923, 6.408140936763237150 ) ) ;
#37296=CARTESIAN_POINT ( 'NONE',  ( 6.204703633549690345, 67.84541550158060375, 14.16423886937410082 ) ) ;
#37297=CARTESIAN_POINT ( 'NONE',  ( 12.63842701281683922, 29.55059781766745175, -9.846743663894590881 ) ) ;
#37299=CARTESIAN_POINT ( 'NONE',  ( 22.26659068614895176, 34.72041550158063927, -7.082119434687042414 ) ) ;
#37301=CARTESIAN_POINT ( 'NONE',  ( 6.204703633549690345, 47.84541550158064638, 14.16423886937410082 ) ) ;
#37302=CARTESIAN_POINT ( 'NONE',  ( 1.472469842513823179, 51.42559781766745886, 4.923371831947296329 ) ) ;
#37304=CARTESIAN_POINT ( 'NONE',  ( -0.8801773607111009756, 43.06368534415484106, 1.068504757029289695E-15 ) ) ;
#37305=CARTESIAN_POINT ( 'NONE',  ( 0.5774900079438607392, 68.48035201082150536, 5.440088680355550821 ) ) ;
#37308=CARTESIAN_POINT ( 'NONE',  ( 21.09922568453595559, 52.04030133659708923, -6.408140936763230044 ) ) ;
#37310=CARTESIAN_POINT ( 'NONE',  ( 19.42250999205614548, 65.98035201082151957, -5.440088680355545492 ) ) ;
#37312=CARTESIAN_POINT ( 'NONE',  ( 24.16423886937410614, 9.512082168247301794, -3.795296366450302550 ) ) ;
#37313=CARTESIAN_POINT ( 'NONE',  ( 17.20831665107776587, 2.883931151000785231, 7.208316651077764980 ) ) ;
#37314=CARTESIAN_POINT ( 'NONE',  ( 7.084665262690076126, 24.10535201082150181, 10.88017736071109987 ) ) ;
#37316=CARTESIAN_POINT ( 'NONE',  ( 4.559911319644449179, 23.89701867748817321, 9.422509992056141925 ) ) ;
#37319=CARTESIAN_POINT ( 'NONE',  ( 17.96484262340118221, 31.18868534415483751, -7.964842623401177768 ) ) ;
#37320=CARTESIAN_POINT ( 'NONE',  ( 0.2751277870542875315, 65.30223176428830811, 6.499999999999984901 ) ) ;
#37325=CARTESIAN_POINT ( 'NONE',  ( 22.81628187352648496, 11.83196800326375531, -3.434112377981050290 ) ) ;
#37327=CARTESIAN_POINT ( 'NONE',  ( 10.00000000000000000, -0.2410688489992152128, -9.846743663894594434 ) ) ;
#37329=CARTESIAN_POINT ( 'NONE',  ( 10.00000000000000000, 16.81368534415483751, -10.88017736071110342 ) ) ;
#37330=CARTESIAN_POINT ( 'NONE',  ( -0.1503990784575328643, 70.00000000000000000, -6.262539305110068177 ) ) ;
#37331=CARTESIAN_POINT ( 'NONE',  ( 17.20831665107776587, 7.883931151000784787, 7.208316651077764980 ) ) ;
#37332=CARTESIAN_POINT ( 'NONE',  ( 17.96484262340118221, 14.93868534415484106, 7.964842623401181321 ) ) ;
#37333=( BOUNDED_SURFACE ( )  B_SPLINE_SURFACE ( 1, 2, ( 
 ( #6377, #50896, #96418, #27892, #37395, #58381, #81391, #36892, #36393, #73888, #19906, #97909, #82372, #80907, #20904, #97405, #67380, #74371, #12401, #29369, #90358, #43875, #42907, #21896, #66887, #73390, #4918, #12893, #5419, #58889, #51393, #35889, #28395, #81880, #92346, #68381, #84373, #24362, #67883, #8845, #46838, #62326, #60363, #16850, #31830, #76364, #91860, #68872, #98405, #39359, #69358, #60859, #7878, #98900, #22390, #85337, #38371, #9339, #29860, #7390, #53862, #402, #69853, #90859, #37888, #92834, #61351, #8359, #30854, #23378, #54825, #38867, #30352, #15872, #47325, #52866, #77824, #46357, #77333, #76845, #91359, #879, #83372, #22885, #31339, #45365, #61839, #23872, #54336, #84850, #16357, #1376, #14895, #75869, #53357, #83864, #15388, #45873, #71810, #94798, #1865, #3316, #17350, #33303, #17830, #2849, #47820, #93818, #72287, #9840, #78320, #79799, #56800, #48312, #63795, #2357, #19299, #94303, #33779, #80293, #71330, #18322, #79312, #11301, #25826, #40341, #26792, #32812, #70844, #78820, #63308, #56324, #25349, #93326, #87296, #55832, #86326, #10819, #32323, #24847, #10330, #48803, #70347, #64286, #18815, #34273, #40829, #86819, #95290, #41821, #41339, #26300, #49297, #3818, #64774, #57289, #49785, #87783, #39841, #62826, #55329, #85836, #21275, #4308, #34782, #50271, #89758, #20286, #29257, #36775, #88775, #81275, #5297, #89271, #59257, #36273, #50784, #66768, #97795, #28765, #90249, #20782, #12775, #28272, #51771, #73277, #43272, #73767, #35774, #82255, #51273, #96299, #74252, #59754, #66262, #13771, #96797, #58767, #43763, #81759, #5784, #13271, #21781, #65270, #58260, #97291, #44258, #95798, #72771, #80788, #42792, #35275, #27279, #12285, #4799, #67267, #57777, #88284, #74762, #52260, #6270, #11791, #42299, #65770, #19783, #27775, #8726, #22275, #15760, #68267, #52747, #84736, #7269, #90746, #23758, #61236, #15273, #69248, #1259, #54221, #14779, #91743, #45251, #37280, #29743, #75747, #769, #67769, #31715, #31221, #62211, #46246, #38747, #44751, #76731, #60253, #76251, #60738, #45754, #83256, #37771, #16241, #98786, #30234, #46723, #61717, #91240, #7765, #22764, #92716, #38260, #8249, #24242, #68751, #75254, #84257, #53245, #39244, #82755, #23263, #83750, #92232, #283, #30730, #53739, #14278, #77222, #69734, #6767, #98289, #2240, #64654, #56686, #18208, #39733, #48195, #56208, #48688, #33190, #34162, #26194, #64168, #2734, #95167, #41218, #25715, #63682, #71695, #93203, #87178, #17721, #78708, #79190, #70726, #93700, #10703, #55205, #71213, #11184, #54708, #94687, #33671, #49183, #47210, #3702 ),
 ( #9223, #72173, #25235, #85230, #16733, #24727, #40708, #63194, #18700, #77711, #85719, #79685, #10218, #94186, #55714, #86211, #41703, #86703, #17233, #3209, #70228, #1747, #32202, #62703, #47710, #78205, #9717, #40216, #32698, #65155, #96674, #4189, #73642, #12656, #88652, #13147, #50663, #81152, #58143, #82134, #5666, #80670, #59134, #95673, #27160, #66652, #43646, #35151, #20160, #88158, #6149, #43156, #58649, #67140, #5171, #19179, #28153, #73148, #13643, #74638, #35656, #57660, #36148, #50161, #19672, #12164, #36654, #42670, #4687, #97176, #66141, #65650, #26674, #28643, #89148, #11681, #20659, #51155, #81639, #74130, #57168, #89642, #21154, #51655, #87665, #44128, #49659, #80169, #42190, #96173, #72654, #34659, #27656, #61116, #14656, #37644, #23141, #98160, #15148, #54103, #97665, #38624, #76614, #92112, #90126, #46604, #161, #45627, #7140, #68631, #29131, #69125, #30610, #90620, #68141, #29616, #52140, #16120, #98668, #39125, #59635, #37154, #83633, #30114, #657, #21656, #67650, #61598, #91121, #38145, #60620, #22644, #23643, #91625, #60122, #53124, #77103, #82636, #8616, #76126, #8131, #7652, #22144, #53614, #14153, #52628, #84132, #75131, #15644, #46126, #31105, #84616, #44637, #6636, #83131, #45121, #75628, #10585, #2622, #41096, #17607, #10102, #31596, #86096, #16616, #9598, #24618, #40101, #47092, #71593, #94082, #48077, #24123, #70602, #55602, #78590, #63083, #3104, #25602, #33077, #93583, #69612, #71096, #40599, #25119, #63573, #77590, #56094, #2128, #32588, #86587, #55084, #17119, #18096, #9105, #48573, #79072, #1134, #62090, #92599, #54592, #39619, #85105, #70108, #1633, #32084, #62582, #93087, #85604, #47601, #78095, #68461, #60448, #14477, #77410, #30435, #1453, #59952, #98488, #45955, #98983, #956, #82961, #29944, #23948, #53437, #481, #60936, #91445, #84929, #30928, #90939, #15472, #8925, #21983, #39440, #22970, #69436, #76443, #22467, #7959, #44950, #52944, #61428, #37475, #38455, #68950, #83946, #46436, #91936, #23464, #53940, #16441, #38945, #69934, #8439, #90442, #84447, #15944, #52457, #76929, #67965, #31416, #37972, #61920, #83454, #14976, #92423, #45446, #75949, #54418, #46917, #75454, #6968, #7474, #9653, #16667, #71143, #79122, #46658, #62139, #2671, #32133, #41147, #48618, #1681, #93137, #17168, #2177, #33122, #48128, #62633, #78644, #10635, #40645, #3143, #32635, #77638, #56142, #92647, #24171, #63616, #94123, #24664, #85648, #85159, #69664, #47648, #47141, #25169, #78143, #16173, #55645, #70164, #71632, #33605, #63133, #54642, #25649, #9155, #39673, #55134, #64101, #40150, #70655 ) ),
 .UNSPECIFIED., .F., .F., .F. ) 
 B_SPLINE_SURFACE_WITH_KNOTS ( ( 2, 2 ),
 ( 3, 2, 2, 2, 2, 2, 2, 2, 2, 2, 2, 2, 2, 2, 2, 2, 2, 2, 2, 2, 2, 2, 2, 2, 2, 2, 2, 2, 2, 2, 2, 2, 2, 2, 2, 2, 2, 2, 2, 2, 2, 2, 2, 2, 2, 2, 2, 2, 2, 2, 2, 2, 2, 2, 2, 2, 2, 2, 2, 2, 2, 2, 2, 2, 2, 2, 2, 2, 2, 2, 2, 2, 2, 2, 2, 2, 2, 2, 2, 2, 2, 2, 2, 2, 2, 2, 2, 2, 2, 2, 2, 2, 2, 2, 2, 2, 2, 2, 2, 2, 2, 2, 2, 2, 2, 2, 2, 2, 2, 2, 2, 2, 2, 2, 2, 2, 2, 2, 2, 2, 2, 2, 2, 2, 2, 2, 2, 2, 2, 2, 2, 2, 2, 2, 2, 2, 2, 2, 2, 2, 2, 2, 2, 2, 2, 2, 2, 2, 2, 2, 2, 2, 2, 2, 2, 2, 2, 2, 2, 2, 2, 2, 3 ),
 ( 0.000000000000000000, 1.000000000000000000 ),
 ( 0.000000000000000000, 0.005952380952380952051, 0.01190476190476190410, 0.01785714285714285615, 0.02380952380952380820, 0.02976190476190476025, 0.03571428571428571230, 0.04166666666666666435, 0.04761904761904761640, 0.05357142857142856845, 0.05952380952380952051, 0.06547619047619047949, 0.07142857142857142461, 0.07738095238095238360, 0.08333333333333332871, 0.08928571428571428770, 0.09523809523809523281, 0.1011904761904761918, 0.1071428571428571369, 0.1130952380952380959, 0.1190476190476190410, 0.1250000000000000000, 0.1309523809523809590, 0.1369047619047619180, 0.1428571428571428492, 0.1488095238095238082, 0.1547619047619047672, 0.1607142857142857262, 0.1666666666666666574, 0.1726190476190476164, 0.1785714285714285754, 0.1845238095238095344, 0.1904761904761904656, 0.1964285714285714246, 0.2023809523809523836, 0.2083333333333333426, 0.2142857142857142738, 0.2202380952380952328, 0.2261904761904761918, 0.2321428571428571508, 0.2380952380952380820, 0.2440476190476190410, 0.2500000000000000000, 0.2559523809523809312, 0.2619047619047619180, 0.2678571428571428492, 0.2738095238095238360, 0.2797619047619047672, 0.2857142857142856984, 0.2916666666666666852, 0.2976190476190476164, 0.3035714285714285476, 0.3095238095238095344, 0.3154761904761904656, 0.3214285714285714524, 0.3273809523809523836, 0.3333333333333333148, 0.3392857142857143016, 0.3452380952380952328, 0.3511904761904761640, 0.3571428571428571508, 0.3630952380952380820, 0.3690476190476190688, 0.3750000000000000000, 0.3809523809523809312, 0.3869047619047619180, 0.3928571428571428492, 0.3988095238095238360, 0.4047619047619047672, 0.4107142857142856984, 0.4166666666666666852, 0.4226190476190476164, 0.4285714285714285476, 0.4345238095238095344, 0.4404761904761904656, 0.4464285714285714524, 0.4523809523809523836, 0.4583333333333333148, 0.4642857142857143016, 0.4702380952380952328, 0.4761904761904761640, 0.4821428571428571508, 0.4880952380952380820, 0.4940476190476190688, 0.5000000000000000000, 0.5059523809523809312, 0.5119047619047618625, 0.5178571428571429047, 0.5238095238095238360, 0.5297619047619047672, 0.5357142857142856984, 0.5416666666666666297, 0.5476190476190476719, 0.5535714285714286031, 0.5595238095238095344, 0.5654761904761904656, 0.5714285714285713969, 0.5773809523809523281, 0.5833333333333333703, 0.5892857142857143016, 0.5952380952380952328, 0.6011904761904761640, 0.6071428571428570953, 0.6130952380952381375, 0.6190476190476190688, 0.6250000000000000000, 0.6309523809523809312, 0.6369047619047618625, 0.6428571428571429047, 0.6488095238095238360, 0.6547619047619047672, 0.6607142857142856984, 0.6666666666666666297, 0.6726190476190476719, 0.6785714285714286031, 0.6845238095238095344, 0.6904761904761904656, 0.6964285714285713969, 0.7023809523809523281, 0.7083333333333333703, 0.7142857142857143016, 0.7202380952380952328, 0.7261904761904761640, 0.7321428571428570953, 0.7380952380952381375, 0.7440476190476190688, 0.7500000000000000000, 0.7559523809523809312, 0.7619047619047618625, 0.7678571428571429047, 0.7738095238095238360, 0.7797619047619047672, 0.7857142857142856984, 0.7916666666666666297, 0.7976190476190476719, 0.8035714285714286031, 0.8095238095238095344, 0.8154761904761904656, 0.8214285714285713969, 0.8273809523809523281, 0.8333333333333333703, 0.8392857142857143016, 0.8452380952380952328, 0.8511904761904761640, 0.8571428571428570953, 0.8630952380952381375, 0.8690476190476190688, 0.8750000000000000000, 0.8809523809523809312, 0.8869047619047618625, 0.8928571428571429047, 0.8988095238095238360, 0.9047619047619047672, 0.9107142857142856984, 0.9166666666666666297, 0.9226190476190476719, 0.9285714285714286031, 0.9345238095238095344, 0.9404761904761904656, 0.9464285714285713969, 0.9523809523809523281, 0.9583333333333333703, 0.9642857142857143016 ),
 .UNSPECIFIED. ) 
 GEOMETRIC_REPRESENTATION_ITEM ( )  RATIONAL_B_SPLINE_SURFACE ( (
 ( 1.000000000000000000, 0.9659258262890683122, 1.000000000000000000, 0.9659258262890683122, 1.000000000000000000, 0.9659258262890683122, 1.000000000000000000, 0.9659258262890683122, 1.000000000000000000, 0.9659258262890683122, 1.000000000000000000, 0.9659258262890683122, 1.000000000000000000, 0.9659258262890683122, 1.000000000000000000, 0.9659258262890683122, 1.000000000000000000, 0.9659258262890683122, 1.000000000000000000, 0.9659258262890683122, 1.000000000000000000, 0.9659258262890683122, 1.000000000000000000, 0.9659258262890683122, 1.000000000000000000, 0.9659258262890683122, 1.000000000000000000, 0.9659258262890683122, 1.000000000000000000, 0.9659258262890683122, 1.000000000000000000, 0.9659258262890683122, 1.000000000000000000, 0.9659258262890683122, 1.000000000000000000, 0.9659258262890683122, 1.000000000000000000, 0.9659258262890683122, 1.000000000000000000, 0.9659258262890683122, 1.000000000000000000, 0.9659258262890683122, 1.000000000000000000, 0.9659258262890683122, 1.000000000000000000, 0.9659258262890683122, 1.000000000000000000, 0.9659258262890683122, 1.000000000000000000, 0.9659258262890683122, 1.000000000000000000, 0.9659258262890683122, 1.000000000000000000, 0.9659258262890683122, 1.000000000000000000, 0.9659258262890683122, 1.000000000000000000, 0.9659258262890683122, 1.000000000000000000, 0.9659258262890683122, 1.000000000000000000, 0.9659258262890683122, 1.000000000000000000, 0.9659258262890683122, 1.000000000000000000, 0.9659258262890683122, 1.000000000000000000, 0.9659258262890683122, 1.000000000000000000, 0.9659258262890683122, 1.000000000000000000, 0.9659258262890683122, 1.000000000000000000, 0.9659258262890683122, 1.000000000000000000, 0.9659258262890683122, 1.000000000000000000, 0.9659258262890683122, 1.000000000000000000, 0.9659258262890683122, 1.000000000000000000, 0.9659258262890683122, 1.000000000000000000, 0.9659258262890683122, 1.000000000000000000, 0.9659258262890683122, 1.000000000000000000, 0.9659258262890683122, 1.000000000000000000, 0.9659258262890683122, 1.000000000000000000, 0.9659258262890683122, 1.000000000000000000, 0.9659258262890683122, 1.000000000000000000, 0.9659258262890683122, 1.000000000000000000, 0.9659258262890683122, 1.000000000000000000, 0.9659258262890683122, 1.000000000000000000, 0.9659258262890683122, 1.000000000000000000, 0.9659258262890683122, 1.000000000000000000, 0.9659258262890683122, 1.000000000000000000, 0.9659258262890683122, 1.000000000000000000, 0.9659258262890683122, 1.000000000000000000, 0.9659258262890683122, 1.000000000000000000, 0.9659258262890683122, 1.000000000000000000, 0.9659258262890683122, 1.000000000000000000, 0.9659258262890683122, 1.000000000000000000, 0.9659258262890683122, 1.000000000000000000, 0.9659258262890683122, 1.000000000000000000, 0.9659258262890683122, 1.000000000000000000, 0.9659258262890683122, 1.000000000000000000, 0.9659258262890683122, 1.000000000000000000, 0.9659258262890683122, 1.000000000000000000, 0.9659258262890683122, 1.000000000000000000, 0.9659258262890683122, 1.000000000000000000, 0.9659258262890683122, 1.000000000000000000, 0.9659258262890683122, 1.000000000000000000, 0.9659258262890683122, 1.000000000000000000, 0.9659258262890683122, 1.000000000000000000, 0.9659258262890683122, 1.000000000000000000, 0.9659258262890683122, 1.000000000000000000, 0.9659258262890683122, 1.000000000000000000, 0.9659258262890683122, 1.000000000000000000, 0.9659258262890683122, 1.000000000000000000, 0.9659258262890683122, 1.000000000000000000, 0.9659258262890683122, 1.000000000000000000, 0.9659258262890683122, 1.000000000000000000, 0.9659258262890683122, 1.000000000000000000, 0.9659258262890683122, 1.000000000000000000, 0.9659258262890683122, 1.000000000000000000, 0.9659258262890683122, 1.000000000000000000, 0.9659258262890683122, 1.000000000000000000, 0.9659258262890683122, 1.000000000000000000, 0.9659258262890683122, 1.000000000000000000, 0.9659258262890683122, 1.000000000000000000, 0.9659258262890683122, 1.000000000000000000, 0.9659258262890683122, 1.000000000000000000, 0.9659258262890683122, 1.000000000000000000, 0.9659258262890683122, 1.000000000000000000, 0.9659258262890683122, 1.000000000000000000, 0.9659258262890683122, 1.000000000000000000, 0.9659258262890683122, 1.000000000000000000, 0.9659258262890683122, 1.000000000000000000, 0.9659258262890683122, 1.000000000000000000, 0.9659258262890683122, 1.000000000000000000, 0.9659258262890683122, 1.000000000000000000, 0.9659258262890683122, 1.000000000000000000, 0.9659258262890683122, 1.000000000000000000, 0.9659258262890683122, 1.000000000000000000, 0.9659258262890683122, 1.000000000000000000, 0.9659258262890683122, 1.000000000000000000, 0.9659258262890683122, 1.000000000000000000, 0.9659258262890683122, 1.000000000000000000, 0.9659258262890683122, 1.000000000000000000, 0.9659258262890683122, 1.000000000000000000, 0.9659258262890683122, 1.000000000000000000, 0.9659258262890683122, 1.000000000000000000, 0.9659258262890683122, 1.000000000000000000, 0.9659258262890683122, 1.000000000000000000, 0.9659258262890683122, 1.000000000000000000, 0.9659258262890683122, 1.000000000000000000, 0.9659258262890683122, 1.000000000000000000, 0.9659258262890683122, 1.000000000000000000, 0.9659258262890683122, 1.000000000000000000, 0.9659258262890683122, 1.000000000000000000, 0.9659258262890683122, 1.000000000000000000, 0.9659258262890683122, 1.000000000000000000, 0.9659258262890683122, 1.000000000000000000, 0.9659258262890683122, 1.000000000000000000, 0.9659258262890683122, 1.000000000000000000, 0.9659258262890683122, 1.000000000000000000, 0.9659258262890683122, 1.000000000000000000, 0.9659258262890683122, 1.000000000000000000, 0.9659258262890683122, 1.000000000000000000, 0.9659258262890683122, 1.000000000000000000, 0.9659258262890683122, 1.000000000000000000, 0.9659258262890683122, 1.000000000000000000, 0.9659258262890683122, 1.000000000000000000, 0.9659258262890683122, 1.000000000000000000, 0.9659258262890683122, 1.000000000000000000, 0.9659258262890683122, 1.000000000000000000, 0.9659258262890683122, 1.000000000000000000, 0.9659258262890683122, 1.000000000000000000, 0.9659258262890683122, 1.000000000000000000, 0.9659258262890683122, 1.000000000000000000, 0.9659258262890683122, 1.000000000000000000, 0.9659258262890683122, 1.000000000000000000, 0.9659258262890683122, 1.000000000000000000, 0.9659258262890683122, 1.000000000000000000, 0.9659258262890683122, 1.000000000000000000, 0.9659258262890683122, 1.000000000000000000, 0.9659258262890683122, 1.000000000000000000, 0.9659258262890683122, 1.000000000000000000, 0.9659258262890683122, 1.000000000000000000, 0.9659258262890683122, 1.000000000000000000, 0.9659258262890683122, 1.000000000000000000, 0.9659258262890683122, 1.000000000000000000, 0.9659258262890683122, 1.000000000000000000, 0.9659258262890683122, 1.000000000000000000, 0.9659258262890683122, 1.000000000000000000, 0.9659258262890683122, 1.000000000000000000, 0.9659258262890683122, 1.000000000000000000, 0.9659258262890683122, 1.000000000000000000, 0.9659258262890683122, 1.000000000000000000, 0.9659258262890683122, 1.000000000000000000, 0.9659258262890683122, 1.000000000000000000, 0.9659258262890683122, 1.000000000000000000, 0.9659258262890683122, 1.000000000000000000, 0.9659258262890683122, 1.000000000000000000, 0.9659258262890683122, 1.000000000000000000),
 ( 1.000000000000000000, 0.9659258262890683122, 1.000000000000000000, 0.9659258262890683122, 1.000000000000000000, 0.9659258262890683122, 1.000000000000000000, 0.9659258262890683122, 1.000000000000000000, 0.9659258262890683122, 1.000000000000000000, 0.9659258262890683122, 1.000000000000000000, 0.9659258262890683122, 1.000000000000000000, 0.9659258262890683122, 1.000000000000000000, 0.9659258262890683122, 1.000000000000000000, 0.9659258262890683122, 1.000000000000000000, 0.9659258262890683122, 1.000000000000000000, 0.9659258262890683122, 1.000000000000000000, 0.9659258262890683122, 1.000000000000000000, 0.9659258262890683122, 1.000000000000000000, 0.9659258262890683122, 1.000000000000000000, 0.9659258262890683122, 1.000000000000000000, 0.9659258262890683122, 1.000000000000000000, 0.9659258262890683122, 1.000000000000000000, 0.9659258262890683122, 1.000000000000000000, 0.9659258262890683122, 1.000000000000000000, 0.9659258262890683122, 1.000000000000000000, 0.9659258262890683122, 1.000000000000000000, 0.9659258262890683122, 1.000000000000000000, 0.9659258262890683122, 1.000000000000000000, 0.9659258262890683122, 1.000000000000000000, 0.9659258262890683122, 1.000000000000000000, 0.9659258262890683122, 1.000000000000000000, 0.9659258262890683122, 1.000000000000000000, 0.9659258262890683122, 1.000000000000000000, 0.9659258262890683122, 1.000000000000000000, 0.9659258262890683122, 1.000000000000000000, 0.9659258262890683122, 1.000000000000000000, 0.9659258262890683122, 1.000000000000000000, 0.9659258262890683122, 1.000000000000000000, 0.9659258262890683122, 1.000000000000000000, 0.9659258262890683122, 1.000000000000000000, 0.9659258262890683122, 1.000000000000000000, 0.9659258262890683122, 1.000000000000000000, 0.9659258262890683122, 1.000000000000000000, 0.9659258262890683122, 1.000000000000000000, 0.9659258262890683122, 1.000000000000000000, 0.9659258262890683122, 1.000000000000000000, 0.9659258262890683122, 1.000000000000000000, 0.9659258262890683122, 1.000000000000000000, 0.9659258262890683122, 1.000000000000000000, 0.9659258262890683122, 1.000000000000000000, 0.9659258262890683122, 1.000000000000000000, 0.9659258262890683122, 1.000000000000000000, 0.9659258262890683122, 1.000000000000000000, 0.9659258262890683122, 1.000000000000000000, 0.9659258262890683122, 1.000000000000000000, 0.9659258262890683122, 1.000000000000000000, 0.9659258262890683122, 1.000000000000000000, 0.9659258262890683122, 1.000000000000000000, 0.9659258262890683122, 1.000000000000000000, 0.9659258262890683122, 1.000000000000000000, 0.9659258262890683122, 1.000000000000000000, 0.9659258262890683122, 1.000000000000000000, 0.9659258262890683122, 1.000000000000000000, 0.9659258262890683122, 1.000000000000000000, 0.9659258262890683122, 1.000000000000000000, 0.9659258262890683122, 1.000000000000000000, 0.9659258262890683122, 1.000000000000000000, 0.9659258262890683122, 1.000000000000000000, 0.9659258262890683122, 1.000000000000000000, 0.9659258262890683122, 1.000000000000000000, 0.9659258262890683122, 1.000000000000000000, 0.9659258262890683122, 1.000000000000000000, 0.9659258262890683122, 1.000000000000000000, 0.9659258262890683122, 1.000000000000000000, 0.9659258262890683122, 1.000000000000000000, 0.9659258262890683122, 1.000000000000000000, 0.9659258262890683122, 1.000000000000000000, 0.9659258262890683122, 1.000000000000000000, 0.9659258262890683122, 1.000000000000000000, 0.9659258262890683122, 1.000000000000000000, 0.9659258262890683122, 1.000000000000000000, 0.9659258262890683122, 1.000000000000000000, 0.9659258262890683122, 1.000000000000000000, 0.9659258262890683122, 1.000000000000000000, 0.9659258262890683122, 1.000000000000000000, 0.9659258262890683122, 1.000000000000000000, 0.9659258262890683122, 1.000000000000000000, 0.9659258262890683122, 1.000000000000000000, 0.9659258262890683122, 1.000000000000000000, 0.9659258262890683122, 1.000000000000000000, 0.9659258262890683122, 1.000000000000000000, 0.9659258262890683122, 1.000000000000000000, 0.9659258262890683122, 1.000000000000000000, 0.9659258262890683122, 1.000000000000000000, 0.9659258262890683122, 1.000000000000000000, 0.9659258262890683122, 1.000000000000000000, 0.9659258262890683122, 1.000000000000000000, 0.9659258262890683122, 1.000000000000000000, 0.9659258262890683122, 1.000000000000000000, 0.9659258262890683122, 1.000000000000000000, 0.9659258262890683122, 1.000000000000000000, 0.9659258262890683122, 1.000000000000000000, 0.9659258262890683122, 1.000000000000000000, 0.9659258262890683122, 1.000000000000000000, 0.9659258262890683122, 1.000000000000000000, 0.9659258262890683122, 1.000000000000000000, 0.9659258262890683122, 1.000000000000000000, 0.9659258262890683122, 1.000000000000000000, 0.9659258262890683122, 1.000000000000000000, 0.9659258262890683122, 1.000000000000000000, 0.9659258262890683122, 1.000000000000000000, 0.9659258262890683122, 1.000000000000000000, 0.9659258262890683122, 1.000000000000000000, 0.9659258262890683122, 1.000000000000000000, 0.9659258262890683122, 1.000000000000000000, 0.9659258262890683122, 1.000000000000000000, 0.9659258262890683122, 1.000000000000000000, 0.9659258262890683122, 1.000000000000000000, 0.9659258262890683122, 1.000000000000000000, 0.9659258262890683122, 1.000000000000000000, 0.9659258262890683122, 1.000000000000000000, 0.9659258262890683122, 1.000000000000000000, 0.9659258262890683122, 1.000000000000000000, 0.9659258262890683122, 1.000000000000000000, 0.9659258262890683122, 1.000000000000000000, 0.9659258262890683122, 1.000000000000000000, 0.9659258262890683122, 1.000000000000000000, 0.9659258262890683122, 1.000000000000000000, 0.9659258262890683122, 1.000000000000000000, 0.9659258262890683122, 1.000000000000000000, 0.9659258262890683122, 1.000000000000000000, 0.9659258262890683122, 1.000000000000000000, 0.9659258262890683122, 1.000000000000000000, 0.9659258262890683122, 1.000000000000000000, 0.9659258262890683122, 1.000000000000000000, 0.9659258262890683122, 1.000000000000000000, 0.9659258262890683122, 1.000000000000000000, 0.9659258262890683122, 1.000000000000000000, 0.9659258262890683122, 1.000000000000000000, 0.9659258262890683122, 1.000000000000000000, 0.9659258262890683122, 1.000000000000000000, 0.9659258262890683122, 1.000000000000000000, 0.9659258262890683122, 1.000000000000000000, 0.9659258262890683122, 1.000000000000000000, 0.9659258262890683122, 1.000000000000000000, 0.9659258262890683122, 1.000000000000000000, 0.9659258262890683122, 1.000000000000000000, 0.9659258262890683122, 1.000000000000000000, 0.9659258262890683122, 1.000000000000000000, 0.9659258262890683122, 1.000000000000000000, 0.9659258262890683122, 1.000000000000000000, 0.9659258262890683122, 1.000000000000000000, 0.9659258262890683122, 1.000000000000000000, 0.9659258262890683122, 1.000000000000000000, 0.9659258262890683122, 1.000000000000000000, 0.9659258262890683122, 1.000000000000000000, 0.9659258262890683122, 1.000000000000000000, 0.9659258262890683122, 1.000000000000000000, 0.9659258262890683122, 1.000000000000000000, 0.9659258262890683122, 1.000000000000000000, 0.9659258262890683122, 1.000000000000000000, 0.9659258262890683122, 1.000000000000000000, 0.9659258262890683122, 1.000000000000000000, 0.9659258262890683122, 1.000000000000000000, 0.9659258262890683122, 1.000000000000000000, 0.9659258262890683122, 1.000000000000000000) ) ) 
 REPRESENTATION_ITEM ( '' )  SURFACE ( )  );
#37335=CARTESIAN_POINT ( 'NONE',  ( -2.816281873526473856, 54.33196800326376064, 3.434112377981055619 ) ) ;
#37336=CARTESIAN_POINT ( 'NONE',  ( 17.96484262340118221, 46.18868534415484106, -7.964842623401177768 ) ) ;
#37338=CARTESIAN_POINT ( 'NONE',  ( 19.38216949554541202, 50.99863466993042493, 9.382169495545424454 ) ) ;
#37339=CARTESIAN_POINT ( 'NONE',  ( 12.91533473730993009, 46.60535201082150536, -10.88017736071109987 ) ) ;
#37340=CARTESIAN_POINT ( 'NONE',  ( 0.1532563361054082862, 66.21726448433413736, 2.638427012816831674 ) ) ;
#37341=DIRECTION ( 'NONE',  ( -0.5547001962252290364, -0.8320502943378437211, 0.000000000000000000 ) ) ;
#37342=CARTESIAN_POINT ( 'NONE',  ( 0.1532563361054082862, 16.21726448433411960, 2.638427012816831674 ) ) ;
#37343=CARTESIAN_POINT ( 'NONE',  ( 10.00000000000000000, 52.87363466993041783, -12.81628187352647608 ) ) ;
#37345=CARTESIAN_POINT ( 'NONE',  ( 19.38216949554541557, 7.248634669930421381, -9.382169495545420901 ) ) ;
#37347=FACE_OUTER_BOUND ( 'NONE', #94859, .T. ) ;
#37348=CARTESIAN_POINT ( 'NONE',  ( 4.559911319644449179, 42.23035201082151247, -9.422509992056141925 ) ) ;
#37349=CARTESIAN_POINT ( 'NONE',  ( 10.00000000000000178, 52.25893115100078745, 9.846743663894594434 ) ) ;
#37351=CARTESIAN_POINT ( 'NONE',  ( 12.63842701281683034, 22.46726448433411605, 9.846743663894596210 ) ) ;
#37352=CARTESIAN_POINT ( 'NONE',  ( 12.63842701281683034, 12.46726448433411782, 9.846743663894596210 ) ) ;
#37353=CARTESIAN_POINT ( 'NONE',  ( 22.81628187352648496, 1.831968003263753753, -3.434112377981050290 ) ) ;
#37355=CARTESIAN_POINT ( 'NONE',  ( 20.88017736071110875, 5.772018677488170546, -2.915334737309920765 ) ) ;
#37356=CARTESIAN_POINT ( 'NONE',  ( 18.52753015748618282, 63.92559781766745886, -4.923371831947291888 ) ) ;
#37357=CARTESIAN_POINT ( 'NONE',  ( -0.8801773607110991993, 7.855352010821506248, -2.915334737309923874 ) ) ;
#37358=CARTESIAN_POINT ( 'NONE',  ( 2.791683348922237240, 40.38393115100078035, -7.208316651077763204 ) ) ;
#37360=DIRECTION ( 'NONE',  ( -1.000000000000000000, 0.000000000000000000, 0.000000000000000000 ) ) ;
#37361=CARTESIAN_POINT ( 'NONE',  ( 2.035157376598824452, 3.688685344154837953, 7.964842623401179544 ) ) ;
#37363=CARTESIAN_POINT ( 'NONE',  ( 7.084665262690076126, 14.10535201082150358, 10.88017736071109987 ) ) ;
#37364=CARTESIAN_POINT ( 'NONE',  ( 6.204703633549690345, 45.76208216824729647, -14.16423886937410259 ) ) ;
#37365=CARTESIAN_POINT ( 'NONE',  ( 22.26659068614895176, 64.72041550158064638, -7.082119434687042414 ) ) ;
#37367=CARTESIAN_POINT ( 'NONE',  ( 2.791683348922237240, 0.3839311510007847872, -7.208316651077763204 ) ) ;
#37368=CARTESIAN_POINT ( 'NONE',  ( 19.84674366389459266, 23.71726448433412315, -2.638427012816827677 ) ) ;
#37369=CARTESIAN_POINT ( 'NONE',  ( -1.099225684535947600, 9.540301336597087456, 6.408140936763237150 ) ) ;
#37373=CARTESIAN_POINT ( 'NONE',  ( 10.00000000000000178, 57.25893115100078745, 9.846743663894594434 ) ) ;
#37376=CARTESIAN_POINT ( 'NONE',  ( 22.26659068614895176, 9.720415501580633943, -7.082119434687042414 ) ) ;
#37377=CARTESIAN_POINT ( 'NONE',  ( 2.791683348922237240, 30.38393115100078390, -7.208316651077763204 ) ) ;
#37380=VECTOR ( 'NONE', #4702, 1000.000000000000000 ) ;
#37381=CARTESIAN_POINT ( 'NONE',  ( -4.164238869374099927, 42.01208216824728936, 3.795296366450308767 ) ) ;
#37382=CARTESIAN_POINT ( 'NONE',  ( 1.472469842513823179, 6.425597817667451750, 4.923371831947296329 ) ) ;
#37384=DIRECTION ( 'NONE',  ( 0.000000000000000000, -1.000000000000000000, 0.000000000000000000 ) ) ;
#37385=CARTESIAN_POINT ( 'NONE',  ( 0.5774900079438590739, 27.64701867748817676, -5.440088680355550821 ) ) ;
#37386=CARTESIAN_POINT ( 'NONE',  ( 13.43411237798105340, 50.58196800326375353, 12.81628187352647963 ) ) ;
#37387=CARTESIAN_POINT ( 'NONE',  ( -0.8801773607111008646, 8.272018677488171434, 2.915334737309923430 ) ) ;
#37388=CARTESIAN_POINT ( 'NONE',  ( 16.40814093676323893, 35.79030133659708923, 11.09922568453595026 ) ) ;
#37389=CARTESIAN_POINT ( 'NONE',  ( 1.472469842513823179, 5.592264484334118713, -4.923371831947296329 ) ) ;
#37394=CARTESIAN_POINT ( 'NONE',  ( 20.36894250292379382, 38.67874883491396076, 10.36894250292379205 ) ) ;
#37395=CARTESIAN_POINT ( 'NONE',  ( -2.266590686148945544, 1.387082168247301128, -7.082119434687050408 ) ) ;
#37396=CARTESIAN_POINT ( 'NONE',  ( 19.42250999205614193, 10.14701867748816966, 5.440088680355555262 ) ) ;
#37397=CARTESIAN_POINT ( 'NONE',  ( 4.559911319644449179, 22.23035201082150536, -9.422509992056141925 ) ) ;
#37400=CARTESIAN_POINT ( 'NONE',  ( 17.96484262340118221, 51.18868534415483396, -7.964842623401177768 ) ) ;
#37401=CARTESIAN_POINT ( 'NONE',  ( 20.88017736071110519, 60.56368534415484106, 2.639326808657452039E-16 ) ) ;
#37402=CARTESIAN_POINT ( 'NONE',  ( -1.099225684535947600, 28.70696800326375353, -6.408140936763238038 ) ) ;
#37405=CARTESIAN_POINT ( 'NONE',  ( 10.00000000000000000, 24.75893115100078745, -9.846743663894594434 ) ) ;
#37406=CARTESIAN_POINT ( 'NONE',  ( 2.035157376598824452, 58.68868534415482685, 7.964842623401179544 ) ) ;
#37408=CARTESIAN_POINT ( 'NONE',  ( -2.816281873526473856, 19.33196800326375708, 3.434112377981055619 ) ) ;
#37410=CARTESIAN_POINT ( 'NONE',  ( 0.8952175423694819223, 43.52576239577081907, 5.990408912944316100 ) ) ;
#37411=CARTESIAN_POINT ( 'NONE',  ( 10.00000000000000178, 9.313685344154839285, 10.88017736071110342 ) ) ;
#37412=CARTESIAN_POINT ( 'NONE',  ( 14.92337183194729633, 42.67559781766745886, 8.527530157486181039 ) ) ;
#37413=CARTESIAN_POINT ( 'NONE',  ( 22.81628187352648496, 56.83196800326374643, -3.434112377981050290 ) ) ;
#37414=CARTESIAN_POINT ( 'NONE',  ( 14.92337183194729988, 19.34226448433411960, -8.527530157486177487 ) ) ;
#37415=EDGE_CURVE ( 'NONE', #85865, #2342, #20795, .T. ) ;
#37417=CARTESIAN_POINT ( 'NONE',  ( 19.42250999205614548, 30.98035201082150536, -5.440088680355545492 ) ) ;
#37418=CARTESIAN_POINT ( 'NONE',  ( 7.084665262690076126, 4.105352010821503583, 10.88017736071109987 ) ) ;
#37419=CARTESIAN_POINT ( 'NONE',  ( 22.26659068614894466, 33.88708216824730357, 7.082119434687054849 ) ) ;
#37420=CARTESIAN_POINT ( 'NONE',  ( 2.791683348922240793, 41.63393115100078745, 7.208316651077764092 ) ) ;
#37421=CARTESIAN_POINT ( 'NONE',  ( 12.91533473730992121, 34.52201867748817676, 10.88017736071110164 ) ) ;
#37422=CARTESIAN_POINT ( 'NONE',  ( 20.88017736071110164, 10.35535201082150714, 2.915334737309930979 ) ) ;
#37423=ORIENTED_EDGE ( 'NONE', *, *, #15028, .F. ) ;
#37424=CARTESIAN_POINT ( 'NONE',  ( 19.42250999205614193, 25.14701867748817321, 5.440088680355555262 ) ) ;
#37425=CARTESIAN_POINT ( 'NONE',  ( 22.81628187352647785, 41.62363466993042493, 6.195893100308588602E-16 ) ) ;
#37426=CARTESIAN_POINT ( 'NONE',  ( 19.42250999205614193, 50.14701867748817676, 5.440088680355555262 ) ) ;
#37429=CARTESIAN_POINT ( 'NONE',  ( 1.472469842513823179, 60.59226448433412315, -4.923371831947296329 ) ) ;
#37430=CARTESIAN_POINT ( 'NONE',  ( 0.5774900079438590739, 42.64701867748816966, -5.440088680355550821 ) ) ;
#37432=CARTESIAN_POINT ( 'NONE',  ( 19.89103541497711447, 30.66234555792570049, -6.479102184480773907 ) ) ;
#37433=CARTESIAN_POINT ( 'NONE',  ( 10.00000000000000178, 48.05374883491396787, 14.16423886937410082 ) ) ;
#37434=CARTESIAN_POINT ( 'NONE',  ( 10.00000000000000000, 46.81368534415484106, -10.88017736071110342 ) ) ;
#37437=CARTESIAN_POINT ( 'NONE',  ( 10.00000000000000178, 57.25893115100078745, 9.846743663894594434 ) ) ;
#37438=CARTESIAN_POINT ( 'NONE',  ( 0.5774900079438607392, 3.480352010821504027, 5.440088680355550821 ) ) ;
#37439=CARTESIAN_POINT ( 'NONE',  ( 12.63842701281683922, 29.55059781766745175, -9.846743663894590881 ) ) ;
#37441=CARTESIAN_POINT ( 'NONE',  ( 5.076628168052704559, 30.17559781766745175, -8.527530157486179263 ) ) ;
#37443=CARTESIAN_POINT ( 'NONE',  ( -0.8801773607111008646, 23.27201867748817676, 2.915334737309923430 ) ) ;
#37444=CARTESIAN_POINT ( 'NONE',  ( 18.52753015748618282, 28.92559781766745175, -4.923371831947291888 ) ) ;
#37445=CARTESIAN_POINT ( 'NONE',  ( 13.43411237798106583, 22.66530133659708923, -12.81628187352647252 ) ) ;
#37446=CARTESIAN_POINT ( 'NONE',  ( 1.707155281725177609, 37.90189080397285437, 6.499999999999955591 ) ) ;
#37447=CARTESIAN_POINT ( 'NONE',  ( -0.8801773607110991993, 62.85535201082150536, -2.915334737309923874 ) ) ;
#37448=CARTESIAN_POINT ( 'NONE',  ( 10.00000000000000000, 26.81368534415484106, -10.88017736071110342 ) ) ;
#37449=CARTESIAN_POINT ( 'NONE',  ( -2.266590686148945544, 47.22041550158063927, 7.082119434687048631 ) ) ;
#37453=ORIENTED_EDGE ( 'NONE', *, *, #19004, .F. ) ;
#37455=CARTESIAN_POINT ( 'NONE',  ( -1.099225684535947600, 19.54030133659708568, 6.408140936763237150 ) ) ;
#37456=CARTESIAN_POINT ( 'NONE',  ( -0.8801773607110991993, 7.855352010821504471, -2.915334737309923874 ) ) ;
#37457=CARTESIAN_POINT ( 'NONE',  ( 7.084665262690076126, 49.10535201082149825, 10.88017736071109987 ) ) ;
#37458=SURFACE_STYLE_FILL_AREA ( #6446 ) ;
#37460=ORIENTED_EDGE ( 'NONE', *, *, #34736, .F. ) ;
#37461=CARTESIAN_POINT ( 'NONE',  ( -0.8801773607110991993, 57.85535201082149825, -2.915334737309923874 ) ) ;
#37462=CARTESIAN_POINT ( 'NONE',  ( 1.472469842513823179, 41.42559781766745886, 4.923371831947296329 ) ) ;
#37463=CARTESIAN_POINT ( 'NONE',  ( 0.1532563361054082862, 26.21726448433411605, 2.638427012816831674 ) ) ;
#37464=CARTESIAN_POINT ( 'NONE',  ( 19.84674366389459266, 13.30059781766745353, 2.638427012816836559 ) ) ;
#37466=CARTESIAN_POINT ( 'NONE',  ( 6.565887622018943937, 35.16530133659708923, 12.81628187352647430 ) ) ;
#37467=CARTESIAN_POINT ( 'NONE',  ( 18.52753015748617571, 18.09226448433411960, 4.923371831947298993 ) ) ;
#37470=CARTESIAN_POINT ( 'NONE',  ( 17.20831665107776587, 32.88393115100078745, 7.208316651077764980 ) ) ;
#37472=CARTESIAN_POINT ( 'NONE',  ( 19.38216949554541202, 50.99863466993042493, 9.382169495545424454 ) ) ;
#37474=CARTESIAN_POINT ( 'NONE',  ( -2.816281873526471635, 8.915301336597083903, -3.434112377981056508 ) ) ;
#37475=CARTESIAN_POINT ( 'NONE',  ( 0.5774900079438590739, 52.64701867748817676, -5.440088680355550821 ) ) ;
#37476=CARTESIAN_POINT ( 'NONE',  ( -0.3689425029237898834, 36.17874883491396787, -10.36894250292378850 ) ) ;
#37479=CARTESIAN_POINT ( 'NONE',  ( 10.00000000000000000, 25.55374883491396787, -14.16423886937410082 ) ) ;
#37480=CARTESIAN_POINT ( 'NONE',  ( -4.164238869374098151, 51.59541550158063217, -3.795296366450310543 ) ) ;
#37481=CARTESIAN_POINT ( 'NONE',  ( 24.16423886937410614, 4.303748834913967869, 8.672049930838204340E-16 ) ) ;
#37482=CARTESIAN_POINT ( 'NONE',  ( 20.36894250292379738, 9.928748834913966093, -10.36894250292379027 ) ) ;
#37484=CARTESIAN_POINT ( 'NONE',  ( -0.8801773607111009756, 43.06368534415484106, 1.068504757029289695E-15 ) ) ;
#37486=CARTESIAN_POINT ( 'NONE',  ( 18.52753015748618282, 33.92559781766745886, -4.923371831947291888 ) ) ;
#37487=CARTESIAN_POINT ( 'NONE',  ( 2.035157376598824452, 63.68868534415484106, 7.964842623401179544 ) ) ;
#37488=CARTESIAN_POINT ( 'NONE',  ( 10.00000000000000000, 44.75893115100078745, -9.846743663894594434 ) ) ;
#37489=CARTESIAN_POINT ( 'NONE',  ( 7.084665262690076126, 29.10535201082150181, 10.88017736071109987 ) ) ;
#37490=CARTESIAN_POINT ( 'NONE',  ( 13.43411237798105340, 55.58196800326374643, 12.81628187352647963 ) ) ;
#37491=CARTESIAN_POINT ( 'NONE',  ( 17.20831665107776587, 59.13393115100078745, -7.208316651077762316 ) ) ;
#37494=CARTESIAN_POINT ( 'NONE',  ( -2.816281873526473856, 39.12363466993041783, 9.499525473075851096E-16 ) ) ;
#37496=CARTESIAN_POINT ( 'NONE',  ( 7.084665262690076126, 44.10535201082151247, 10.88017736071109987 ) ) ;
#37497=CARTESIAN_POINT ( 'NONE',  ( 0.1532563361054082862, 46.21726448433411605, 2.638427012816831674 ) ) ;
#37498=CARTESIAN_POINT ( 'NONE',  ( 22.26659068614895176, 24.72041550158063572, -7.082119434687042414 ) ) ;
#37500=( NAMED_UNIT ( * ) PLANE_ANGLE_UNIT ( ) SI_UNIT ( $, .RADIAN. ) );
#37501=CARTESIAN_POINT ( 'NONE',  ( 7.084665262690076126, 62.02201867748816966, -10.88017736071110164 ) ) ;
#37502=CARTESIAN_POINT ( 'NONE',  ( 0.5774900079438590739, 67.64701867748817676, -5.440088680355550821 ) ) ;
#37503=CARTESIAN_POINT ( 'NONE',  ( 20.36894250292379382, 53.67874883491397497, 10.36894250292379205 ) ) ;
#37504=CARTESIAN_POINT ( 'NONE',  ( 6.565887622018943937, 0.1653013365970866511, 12.81628187352647430 ) ) ;
#37506=CARTESIAN_POINT ( 'NONE',  ( 7.084665262690076126, 49.10535201082149825, 10.88017736071109987 ) ) ;
#37507=CARTESIAN_POINT ( 'NONE',  ( 2.148416515056622789, 57.23726573380439930, 6.499999999999959144 ) ) ;
#37508=CARTESIAN_POINT ( 'NONE',  ( -4.164238869374099927, 47.01208216824729647, 3.795296366450308767 ) ) ;
#37510=CARTESIAN_POINT ( 'NONE',  ( 19.42250999205614548, 10.98035201082150358, -5.440088680355545492 ) ) ;
#37511=CARTESIAN_POINT ( 'NONE',  ( 12.91533473730992121, 19.52201867748816611, 10.88017736071110164 ) ) ;
#37513=CARTESIAN_POINT ( 'NONE',  ( 14.92337183194729633, 52.67559781766745175, 8.527530157486181039 ) ) ;
#37514=CARTESIAN_POINT ( 'NONE',  ( 16.40814093676324603, 47.45696800326375353, -11.09922568453594671 ) ) ;
#37515=CARTESIAN_POINT ( 'NONE',  ( -35.44000000000001194, 93.50000000000000000, -9.500000000000000000 ) ) ;
#37517=CARTESIAN_POINT ( 'NONE',  ( 2.035157376598824452, 18.68868534415484106, 7.964842623401179544 ) ) ;
#37518=CARTESIAN_POINT ( 'NONE',  ( 16.40814093676323893, 20.79030133659708923, 11.09922568453595026 ) ) ;
#37522=CARTESIAN_POINT ( 'NONE',  ( 10.00000000000000000, 49.75893115100078745, -9.846743663894594434 ) ) ;
#37523=CARTESIAN_POINT ( 'NONE',  ( 7.084665262690076126, 34.10535201082151247, 10.88017736071109987 ) ) ;
#37525=CARTESIAN_POINT ( 'NONE',  ( 22.81628187352648496, 16.83196800326374998, -3.434112377981050290 ) ) ;
#37526=CARTESIAN_POINT ( 'NONE',  ( -0.8801773607111009756, 48.06368534415484817, 1.068504757029289695E-15 ) ) ;
#37529=CARTESIAN_POINT ( 'NONE',  ( -2.816281873526471635, 53.91530133659709634, -3.434112377981056508 ) ) ;
#37532=CARTESIAN_POINT ( 'NONE',  ( 7.084665262690076126, 54.10535201082151247, 10.88017736071109987 ) ) ;
#37533=CARTESIAN_POINT ( 'NONE',  ( 10.00000000000000178, 40.37363466993042493, 12.81628187352647608 ) ) ;
#37534=CARTESIAN_POINT ( 'NONE',  ( 2.791683348922240793, 6.633931151000785675, 7.208316651077764092 ) ) ;
#37535=CARTESIAN_POINT ( 'NONE',  ( 17.96484262340118221, 46.18868534415484106, -7.964842623401177768 ) ) ;
#37536=CARTESIAN_POINT ( 'NONE',  ( 2.791683348922237240, 65.38393115100078035, -7.208316651077763204 ) ) ;
#37537=CARTESIAN_POINT ( 'NONE',  ( 7.361572987183170547, 62.05059781766745886, 9.846743663894590881 ) ) ;
#37538=CARTESIAN_POINT ( 'NONE',  ( 0.1532563361054100626, 20.80059781766744464, -2.638427012816831230 ) ) ;
#37539=CARTESIAN_POINT ( 'NONE',  ( 0.1532563361054082862, 1.217264484334117824, 2.638427012816831674 ) ) ;
#37541=CARTESIAN_POINT ( 'NONE',  ( 2.917880565312950480, 40.97041550158063217, -12.26659068614894821 ) ) ;
#37543=CARTESIAN_POINT ( 'NONE',  ( -0.8801773607110991993, 12.85535201082150358, -2.915334737309923874 ) ) ;
#37546=CARTESIAN_POINT ( 'NONE',  ( -2.266590686148945544, 67.22041550158063217, 7.082119434687048631 ) ) ;
#37547=CARTESIAN_POINT ( 'NONE',  ( 13.79529636645030344, 58.26208216824728936, 14.16423886937410614 ) ) ;
#37548=CARTESIAN_POINT ( 'NONE',  ( 10.00000000000000178, 47.25893115100078745, 9.846743663894594434 ) ) ;
#37549=( GEOMETRIC_REPRESENTATION_CONTEXT ( 3 ) GLOBAL_UNCERTAINTY_ASSIGNED_CONTEXT ( ( #36140 ) ) GLOBAL_UNIT_ASSIGNED_CONTEXT ( ( #35388, #81381, #28386 ) ) REPRESENTATION_CONTEXT ( 'NONE', 'WORKASPACE' ) );
#37550=CARTESIAN_POINT ( 'NONE',  ( 3.591859063236763294, 33.29030133659708213, -11.09922568453595026 ) ) ;
#37553=CARTESIAN_POINT ( 'NONE',  ( -2.266590686148945544, 1.387082168247301128, -7.082119434687050408 ) ) ;
#37554=CARTESIAN_POINT ( 'NONE',  ( 12.91533473730993009, 6.605352010821504471, -10.88017736071109987 ) ) ;
#37555=CARTESIAN_POINT ( 'NONE',  ( 6.204703633549690345, 50.76208216824730357, -14.16423886937410259 ) ) ;
#37556=CARTESIAN_POINT ( 'NONE',  ( 12.63842701281683034, 47.46726448433412315, 9.846743663894596210 ) ) ;
#37558=CARTESIAN_POINT ( 'NONE',  ( 12.63842701281683922, 24.55059781766745175, -9.846743663894590881 ) ) ;
#37559=CARTESIAN_POINT ( 'NONE',  ( -0.8801773607111009756, 33.27201867748817676, 2.915334737309923874 ) ) ;
#37561=VERTEX_POINT ( 'NONE', #94148 ) ;
#37563=( NAMED_UNIT ( * ) SI_UNIT ( $, .STERADIAN. ) SOLID_ANGLE_UNIT ( ) );
#37564=ORIENTED_EDGE ( 'NONE', *, *, #3122, .T. ) ;
#37565=CARTESIAN_POINT ( 'NONE',  ( 7.084665262690076126, 34.10535201082151247, 10.88017736071109987 ) ) ;
#37566=CARTESIAN_POINT ( 'NONE',  ( 10.00000000000000000, 41.81368534415484106, -10.88017736071110342 ) ) ;
#37567=CARTESIAN_POINT ( 'NONE',  ( 12.63842701281683034, 57.46726448433411605, 9.846743663894596210 ) ) ;
#37568=CARTESIAN_POINT ( 'NONE',  ( 22.81628187352647785, 36.41530133659707502, 3.434112377981063169 ) ) ;
#37569=CARTESIAN_POINT ( 'NONE',  ( 6.204703633549690345, 7.845415501580634832, 14.16423886937410082 ) ) ;
#37572=CARTESIAN_POINT ( 'NONE',  ( 10.00000000000000178, 69.31368534415484817, 10.88017736071110342 ) ) ;
#37573=CARTESIAN_POINT ( 'NONE',  ( 19.38216949554541557, 27.24863466993041783, -9.382169495545420901 ) ) ;
#37575=CARTESIAN_POINT ( 'NONE',  ( 18.52753015748618282, 38.92559781766745175, -4.923371831947291888 ) ) ;
#37576=CARTESIAN_POINT ( 'NONE',  ( 2.035157376598824452, 3.688685344154837953, 7.964842623401179544 ) ) ;
#37578=CARTESIAN_POINT ( 'NONE',  ( 10.00000000000000000, 11.81368534415483751, -10.88017736071110342 ) ) ;
#37580=CARTESIAN_POINT ( 'NONE',  ( 15.44008868035555793, 66.39701867748817676, -9.422509992056140149 ) ) ;
#37581=CARTESIAN_POINT ( 'NONE',  ( -0.8801773607111009756, 53.06368534415484106, 1.068504757029289695E-15 ) ) ;
#37582=CARTESIAN_POINT ( 'NONE',  ( 20.88017736071110164, 65.35535201082150536, 2.915334737309930979 ) ) ;
#37583=CARTESIAN_POINT ( 'NONE',  ( 20.88017736071110164, 50.35535201082151247, 2.915334737309930979 ) ) ;
#37584=CARTESIAN_POINT ( 'NONE',  ( -1.926860441876564023, 52.87045670184114954, 3.195792623639529761 ) ) ;
#37586=ORIENTED_EDGE ( 'NONE', *, *, #86646, .F. ) ;
#37587=CARTESIAN_POINT ( 'NONE',  ( 1.472469842513823179, 36.42559781766745175, 4.923371831947296329 ) ) ;
#37592=CARTESIAN_POINT ( 'NONE',  ( 22.26659068614894466, 8.887082168247300018, 7.082119434687054849 ) ) ;
#37593=CARTESIAN_POINT ( 'NONE',  ( -0.2418659066527775181, 8.090145880403570189, 6.114288769123032985 ) ) ;
#37594=CARTESIAN_POINT ( 'NONE',  ( 2.603489959281060973, 26.58210964143323096, 6.499999999999401368 ) ) ;
#37595=CARTESIAN_POINT ( 'NONE',  ( 7.361572987183170547, 37.05059781766744464, 9.846743663894590881 ) ) ;
#37596=CARTESIAN_POINT ( 'NONE',  ( 7.084665262690076126, 7.022018677488170546, -10.88017736071110164 ) ) ;
#37598=CARTESIAN_POINT ( 'NONE',  ( 22.81628187352647785, 46.62363466993041783, 6.195893100308588602E-16 ) ) ;
#37601=CARTESIAN_POINT ( 'NONE',  ( 2.791683348922237240, 45.38393115100079456, -7.208316651077763204 ) ) ;
#37603=CARTESIAN_POINT ( 'NONE',  ( 19.38216949554541557, 17.24863466993041783, -9.382169495545420901 ) ) ;
#37604=CARTESIAN_POINT ( 'NONE',  ( 12.63842701281683922, 29.55059781766745175, -9.846743663894590881 ) ) ;
#37607=CARTESIAN_POINT ( 'NONE',  ( 13.43411237798105340, 5.581968003263753531, 12.81628187352647963 ) ) ;
#37611=EDGE_CURVE ( 'NONE', #81206, #88856, #13610, .T. ) ;
#37613=CARTESIAN_POINT ( 'NONE',  ( 20.88017736071110519, 20.56368534415484106, 2.639326808657452039E-16 ) ) ;
#37614=CARTESIAN_POINT ( 'NONE',  ( 6.204703633549690345, 15.76208216824730179, -14.16423886937410259 ) ) ;
#37615=CARTESIAN_POINT ( 'NONE',  ( 17.20831665107776587, 34.13393115100078745, -7.208316651077762316 ) ) ;
#37616=CARTESIAN_POINT ( 'NONE',  ( -0.8801773607111009756, 68.06368534415484817, 1.068504757029289695E-15 ) ) ;
#37617=CARTESIAN_POINT ( 'NONE',  ( 19.38216949554541202, 35.99863466993041072, 9.382169495545424454 ) ) ;
#37619=CARTESIAN_POINT ( 'NONE',  ( 20.88017736071110875, 15.77201867748817143, -2.915334737309920765 ) ) ;
#37621=CARTESIAN_POINT ( 'NONE',  ( 22.81628187352648496, 1.831968003263753753, -3.434112377981050290 ) ) ;
#37622=CARTESIAN_POINT ( 'NONE',  ( 14.92337183194729988, 24.34226448433411960, -8.527530157486177487 ) ) ;
#37624=CARTESIAN_POINT ( 'NONE',  ( 6.565887622018943937, 30.16530133659708568, 12.81628187352647430 ) ) ;
#37626=CARTESIAN_POINT ( 'NONE',  ( 12.91533473730993009, 41.60535201082149825, -10.88017736071109987 ) ) ;
#37630=CARTESIAN_POINT ( 'NONE',  ( 12.91533473730993009, 41.60535201082149825, -10.88017736071109987 ) ) ;
#37631=CARTESIAN_POINT ( 'NONE',  ( 12.91533473730993009, 41.60535201082149825, -10.88017736071109987 ) ) ;
#37632=CARTESIAN_POINT ( 'NONE',  ( 19.84674366389459266, 58.30059781766745886, 2.638427012816836559 ) ) ;
#37633=CARTESIAN_POINT ( 'NONE',  ( 4.559911319644449179, 68.89701867748817676, 9.422509992056141925 ) ) ;
#37635=CARTESIAN_POINT ( 'NONE',  ( 5.076628168052703671, 51.84226448433412315, 8.527530157486179263 ) ) ;
#37636=CARTESIAN_POINT ( 'NONE',  ( 10.00000000000000178, 14.31368534415483751, 10.88017736071110342 ) ) ;
#37638=CARTESIAN_POINT ( 'NONE',  ( 19.38216949554541557, 7.248634669930421381, -9.382169495545420901 ) ) ;
#37640=CARTESIAN_POINT ( 'NONE',  ( 12.91533473730992121, 39.52201867748817676, 10.88017736071110164 ) ) ;
#37641=EDGE_CURVE ( 'NONE', #63345, #31263, #6439, .T. ) ;
#37642=CARTESIAN_POINT ( 'NONE',  ( 19.05866839779138999, 15.95508385108959004, -6.499999999999970690 ) ) ;
#37643=CARTESIAN_POINT ( 'NONE',  ( 15.44008868035555260, 4.730352010821504471, 9.422509992056143702 ) ) ;
#37644=CARTESIAN_POINT ( 'NONE',  ( 12.91533473730993009, 21.60535201082150536, -10.88017736071109987 ) ) ;
#37645=CARTESIAN_POINT ( 'NONE',  ( 0.5774900079438607392, 68.48035201082150536, 5.440088680355550821 ) ) ;
#37646=CARTESIAN_POINT ( 'NONE',  ( 10.00000000000000178, 38.05374883491396787, 14.16423886937410082 ) ) ;
#37647=CARTESIAN_POINT ( 'NONE',  ( 2.791683348922240793, 31.63393115100078745, 7.208316651077764092 ) ) ;
#37648=CARTESIAN_POINT ( 'NONE',  ( 10.00000000000000178, 49.31368534415484106, 10.88017736071110342 ) ) ;
#37649=CARTESIAN_POINT ( 'NONE',  ( 18.95386800104995118, 38.23810908735726599, -6.499999999999988454 ) ) ;
#37650=CARTESIAN_POINT ( 'NONE',  ( -4.164238869374098151, 6.595415501580634832, -3.795296366450310543 ) ) ;
#37653=CARTESIAN_POINT ( 'NONE',  ( 18.52753015748618282, 58.92559781766745886, -4.923371831947291888 ) ) ;
#37655=EDGE_LOOP ( 'NONE', ( #91707, #90234, #75141, #74216 ) ) ;
#37657=CARTESIAN_POINT ( 'NONE',  ( -4.164238869374099039, 21.80374883491396787, 8.674139862899312516E-16 ) ) ;
#37658=CARTESIAN_POINT ( 'NONE',  ( 24.16423886937410614, 19.30374883491397142, 8.672049930838204340E-16 ) ) ;
#37659=CARTESIAN_POINT ( 'NONE',  ( 12.91533473730993009, 66.60535201082150536, -10.88017736071109987 ) ) ;
#37660=CARTESIAN_POINT ( 'NONE',  ( 22.26659068614895176, 64.72041550158064638, -7.082119434687042414 ) ) ;
#37661=CARTESIAN_POINT ( 'NONE',  ( 19.84674366389459266, 48.30059781766745175, 2.638427012816836559 ) ) ;
#37663=CARTESIAN_POINT ( 'NONE',  ( 12.91533473730993009, 46.60535201082150536, -10.88017736071109987 ) ) ;
#37664=CARTESIAN_POINT ( 'NONE',  ( -1.099225684535947600, 19.54030133659708568, 6.408140936763237150 ) ) ;
#37665=CARTESIAN_POINT ( 'NONE',  ( 22.26659068614894466, 13.88708216824730179, 7.082119434687054849 ) ) ;
#37666=CARTESIAN_POINT ( 'NONE',  ( 15.44008868035555260, 9.730352010821505360, 9.422509992056143702 ) ) ;
#37667=CARTESIAN_POINT ( 'NONE',  ( 10.00000000000000178, 19.31368534415484106, 10.88017736071110342 ) ) ;
#37669=CARTESIAN_POINT ( 'NONE',  ( 20.88017736071110164, 55.35535201082149825, 2.915334737309930979 ) ) ;
#37670=CARTESIAN_POINT ( 'NONE',  ( 3.591859063236761518, 44.95696800326376064, 11.09922568453594849 ) ) ;
#37676=CYLINDRICAL_SURFACE ( 'NONE', #71864, 0.5000000000000004441 ) ;
#37679=CARTESIAN_POINT ( 'NONE',  ( 6.204703633549690345, 65.76208216824731778, -14.16423886937410259 ) ) ;
#37680=CARTESIAN_POINT ( 'NONE',  ( -2.266590686148945544, 67.22041550158063217, 7.082119434687048631 ) ) ;
#37681=CARTESIAN_POINT ( 'NONE',  ( 10.00000000000000000, 29.75893115100078745, -9.846743663894594434 ) ) ;
#37682=CARTESIAN_POINT ( 'NONE',  ( 19.84674366389459621, 58.50893115100078745, 7.409399052514197653E-17 ) ) ;
#37683=CARTESIAN_POINT ( 'NONE',  ( 10.00000000000000178, 64.31368534415483396, 10.88017736071110342 ) ) ;
#37684=CARTESIAN_POINT ( 'NONE',  ( 19.89220837332778657, 44.74062864464239908, 6.478736007405907493 ) ) ;
#37685=EDGE_CURVE ( 'NONE', #31232, #90628, #45765, .T. ) ;
#37686=CARTESIAN_POINT ( 'NONE',  ( 15.44008868035555793, 66.39701867748817676, -9.422509992056140149 ) ) ;
#37690=CARTESIAN_POINT ( 'NONE',  ( 17.08211943468705840, 40.13708216824731068, -12.26659068614894466 ) ) ;
#37691=CARTESIAN_POINT ( 'NONE',  ( -2.266590686148945544, 46.38708216824730357, -7.082119434687050408 ) ) ;
#37692=EDGE_LOOP ( 'NONE', ( #61279, #19593, #67056, #93166 ) ) ;
#37693=CARTESIAN_POINT ( 'NONE',  ( 10.00000000000000178, 60.37363466993041783, 12.81628187352647608 ) ) ;
#37694=CARTESIAN_POINT ( 'NONE',  ( 4.559911319644449179, 27.23035201082150536, -9.422509992056141925 ) ) ;
#37695=CARTESIAN_POINT ( 'NONE',  ( 2.791683348922237240, 50.38393115100078035, -7.208316651077763204 ) ) ;
#37696=CARTESIAN_POINT ( 'NONE',  ( -0.8801773607110991993, 22.85535201082150181, -2.915334737309923874 ) ) ;
#37697=CARTESIAN_POINT ( 'NONE',  ( 22.81628187352647785, 61.62363466993041783, 6.195893100308588602E-16 ) ) ;
#37699=CARTESIAN_POINT ( 'NONE',  ( 5.076628168052703671, 51.84226448433412315, 8.527530157486179263 ) ) ;
#37700=CARTESIAN_POINT ( 'NONE',  ( 5.076628168052703671, 51.84226448433412315, 8.527530157486179263 ) ) ;
#37705=CARTESIAN_POINT ( 'NONE',  ( 19.64275089555620113, 84.99790889484839340, 5.306638067702549755 ) ) ;
#37706=CARTESIAN_POINT ( 'NONE',  ( 5.076628168052703671, 26.84226448433411960, 8.527530157486179263 ) ) ;
#37708=CARTESIAN_POINT ( 'NONE',  ( -2.816281873526473856, 34.33196800326376064, 3.434112377981055619 ) ) ;
#37710=CARTESIAN_POINT ( 'NONE',  ( 0.1129803114748731130, 39.29427333184090543, -6.480634945678677816 ) ) ;
#37711=VERTEX_POINT ( 'NONE', #58609 ) ;
#37714=CARTESIAN_POINT ( 'NONE',  ( 0.1532563361054082862, 36.21726448433410894, 2.638427012816831674 ) ) ;
#37715=CARTESIAN_POINT ( 'NONE',  ( 17.08211943468705130, 33.47041550158063927, 12.26659068614894998 ) ) ;
#37716=CARTESIAN_POINT ( 'NONE',  ( 1.472469842513823179, 51.42559781766745886, 4.923371831947296329 ) ) ;
#37718=CARTESIAN_POINT ( 'NONE',  ( 19.84674366389459621, 3.508931151000785231, 7.409399052514197653E-17 ) ) ;
#37720=CARTESIAN_POINT ( 'NONE',  ( -0.3689425029237898834, 6.178748834913968757, -10.36894250292378850 ) ) ;
#37721=CARTESIAN_POINT ( 'NONE',  ( 12.63842701281683922, 44.55059781766745175, -9.846743663894590881 ) ) ;
#37722=CARTESIAN_POINT ( 'NONE',  ( 2.035157376598824452, 48.68868534415483396, 7.964842623401179544 ) ) ;
#37724=CARTESIAN_POINT ( 'NONE',  ( 14.92337183194729988, 44.34226448433412315, -8.527530157486177487 ) ) ;
#37728=ADVANCED_FACE ( 'NONE', ( #29093 ), #28608, .T. ) ;
#37730=CARTESIAN_POINT ( 'NONE',  ( 15.44008868035555793, 41.39701867748817676, -9.422509992056140149 ) ) ;
#37731=EDGE_CURVE ( 'NONE', #10095, #28167, #27665, .T. ) ;
#37732=VECTOR ( 'NONE', #53181, 1000.000000000000000 ) ;
#37736=CARTESIAN_POINT ( 'NONE',  ( 20.88017736071110519, 10.56368534415483751, 2.639326808657452039E-16 ) ) ;
#37737=CARTESIAN_POINT ( 'NONE',  ( 19.84674366389459621, 63.50893115100078745, 7.409399052514197653E-17 ) ) ;
#37738=CARTESIAN_POINT ( 'NONE',  ( 19.42250999205614193, 50.14701867748817676, 5.440088680355555262 ) ) ;
#37739=CARTESIAN_POINT ( 'NONE',  ( -0.2418659066527643342, 47.23410085661203084, -6.114288769123057854 ) ) ;
#37740=CARTESIAN_POINT ( 'NONE',  ( 19.89103541497709671, 10.66234555792571115, -6.479102184480792559 ) ) ;
#37742=CARTESIAN_POINT ( 'NONE',  ( 15.44008868035555793, 46.39701867748817676, -9.422509992056140149 ) ) ;
#37744=CARTESIAN_POINT ( 'NONE',  ( 0.1532563361054100626, 15.80059781766745353, -2.638427012816831230 ) ) ;
#37745=CARTESIAN_POINT ( 'NONE',  ( 18.52753015748617571, 33.09226448433411605, 4.923371831947298993 ) ) ;
#37746=( LENGTH_UNIT ( ) NAMED_UNIT ( * ) SI_UNIT ( .MILLI., .METRE. ) );
#37748=CARTESIAN_POINT ( 'NONE',  ( 0.6178305044545818747, -1.501365330069579951, -9.382169495545419124 ) ) ;
#37749=CARTESIAN_POINT ( 'NONE',  ( 20.88017736071110875, 5.772018677488170546, -2.915334737309920765 ) ) ;
#37751=CARTESIAN_POINT ( 'NONE',  ( 6.204703633549690345, 25.76208216824730712, -14.16423886937410259 ) ) ;
#37753=CARTESIAN_POINT ( 'NONE',  ( 2.917880565312948704, 52.63708216824730357, 12.26659068614894643 ) ) ;
#37754=CARTESIAN_POINT ( 'NONE',  ( 4.559911319644449179, 2.230352010821504471, -9.422509992056141925 ) ) ;
#37756=CARTESIAN_POINT ( 'NONE',  ( 14.92337183194729988, 24.34226448433411960, -8.527530157486177487 ) ) ;
#37758=CARTESIAN_POINT ( 'NONE',  ( 4.559911319644449179, 27.23035201082150536, -9.422509992056141925 ) ) ;
#37759=CARTESIAN_POINT ( 'NONE',  ( 12.63842701281683922, 54.55059781766745175, -9.846743663894590881 ) ) ;
#37760=CARTESIAN_POINT ( 'NONE',  ( 10.00000000000000000, 5.553748834913967869, -14.16423886937410082 ) ) ;
#37761=CARTESIAN_POINT ( 'NONE',  ( 18.17884179759846930, 48.66688879859523809, -6.500000000000002665 ) ) ;
#37763=CARTESIAN_POINT ( 'NONE',  ( 16.40814093676324603, 42.45696800326375353, -11.09922568453594671 ) ) ;
#37764=CARTESIAN_POINT ( 'NONE',  ( 12.63842701281683922, 39.55059781766744464, -9.846743663894590881 ) ) ;
#37766=CARTESIAN_POINT ( 'NONE',  ( 19.84674366389459266, 8.717264484334116048, -2.638427012816827677 ) ) ;
#37770=CARTESIAN_POINT ( 'NONE',  ( -0.8801773607111009756, 3.063685344154838397, 1.068504757029289695E-15 ) ) ;
#37771=CARTESIAN_POINT ( 'NONE',  ( 22.26659068614895176, 54.72041550158063217, -7.082119434687042414 ) ) ;
#37772=CARTESIAN_POINT ( 'NONE',  ( 17.96484262340118221, 39.93868534415484106, 7.964842623401181321 ) ) ;
#37773=CARTESIAN_POINT ( 'NONE',  ( 21.92686044187656336, 51.97997603579418069, 3.195792623639536423 ) ) ;
#37774=CARTESIAN_POINT ( 'NONE',  ( 19.84674366389459266, 33.30059781766744464, 2.638427012816836559 ) ) ;
#37775=CARTESIAN_POINT ( 'NONE',  ( 0.5774900079438590739, 7.647018677488171434, -5.440088680355550821 ) ) ;
#37776=CARTESIAN_POINT ( 'NONE',  ( 2.791683348922237240, 45.38393115100079456, -7.208316651077763204 ) ) ;
#37777=CARTESIAN_POINT ( 'NONE',  ( 0.8438640652791046248, 1.024801820426205776E-17, -5.642539323548857233 ) ) ;
#37778=CARTESIAN_POINT ( 'NONE',  ( 5.076628168052703671, 46.84226448433412315, 8.527530157486179263 ) ) ;
#37779=CARTESIAN_POINT ( 'NONE',  ( -0.8801773607110991993, 37.85535201082151247, -2.915334737309923874 ) ) ;
#37781=ORIENTED_EDGE ( 'NONE', *, *, #19309, .F. ) ;
#37782=CARTESIAN_POINT ( 'NONE',  ( -2.816281873526473856, 59.33196800326374643, 3.434112377981055619 ) ) ;
#37784=CARTESIAN_POINT ( 'NONE',  ( 5.076628168052704559, 10.17559781766745175, -8.527530157486179263 ) ) ;
#37785=CARTESIAN_POINT ( 'NONE',  ( 22.81628187352647785, 61.62363466993041783, 6.195893100308588602E-16 ) ) ;
#37786=CARTESIAN_POINT ( 'NONE',  ( -4.164238869374099039, 66.80374883491396076, 8.674139862899312516E-16 ) ) ;
#37787=CARTESIAN_POINT ( 'NONE',  ( 12.63842701281683034, 52.46726448433413026, 9.846743663894596210 ) ) ;
#37788=CARTESIAN_POINT ( 'NONE',  ( 20.00000000000000711, 93.00652443313859408, 4.825407044038334980 ) ) ;
#37789=CARTESIAN_POINT ( 'NONE',  ( 24.16423886937410614, 24.51208216824730002, -3.795296366450302550 ) ) ;
#37791=CARTESIAN_POINT ( 'NONE',  ( 20.36894250292379738, 44.92874883491396787, -10.36894250292379027 ) ) ;
#37792=CARTESIAN_POINT ( 'NONE',  ( 18.52753015748618282, 53.92559781766745175, -4.923371831947291888 ) ) ;
#37793=CARTESIAN_POINT ( 'NONE',  ( 0.5774900079438590739, 52.64701867748817676, -5.440088680355550821 ) ) ;
#37794=CARTESIAN_POINT ( 'NONE',  ( 0.1532563361054083140, 6.008931151000784787, 1.131784320476157264E-15 ) ) ;
#37797=B_SPLINE_CURVE_WITH_KNOTS ( 'NONE', 3,
 ( #87858, #78890, #63866, #2433 ),
 .UNSPECIFIED., .F., .F.,
 ( 4, 4 ),
 ( 0.000000000000000000, 0.002657014572711350643 ),
 .UNSPECIFIED. ) ;
#37798=CARTESIAN_POINT ( 'NONE',  ( 6.565887622018943937, 58.08196800326376064, -12.81628187352647608 ) ) ;
#37800=CARTESIAN_POINT ( 'NONE',  ( 2.791683348922240793, 16.63393115100078745, 7.208316651077764092 ) ) ;
#37802=CARTESIAN_POINT ( 'NONE',  ( -4.164238869374099927, 22.01208216824730357, 3.795296366450308767 ) ) ;
#37803=CARTESIAN_POINT ( 'NONE',  ( 0.1532563361054100626, 0.8005978176674514168, -2.638427012816831230 ) ) ;
#37804=CARTESIAN_POINT ( 'NONE',  ( 15.44008868035555260, 24.73035201082150891, 9.422509992056143702 ) ) ;
#37809=CARTESIAN_POINT ( 'NONE',  ( 0.5774900079438607392, 33.48035201082150536, 5.440088680355550821 ) ) ;
#37811=CARTESIAN_POINT ( 'NONE',  ( 0.5774900079438590739, 37.64701867748817676, -5.440088680355550821 ) ) ;
#37812=CARTESIAN_POINT ( 'NONE',  ( 1.821158202401529369, 46.16688879859523098, 6.500000000000007105 ) ) ;
#37814=CARTESIAN_POINT ( 'NONE',  ( -1.099225684535947600, 18.70696800326375353, -6.408140936763238038 ) ) ;
#37817=CARTESIAN_POINT ( 'NONE',  ( -0.8801773607111009756, 63.06368534415484106, 1.068504757029289695E-15 ) ) ;
#37820=CARTESIAN_POINT ( 'NONE',  ( 14.92337183194729633, 17.67559781766745175, 8.527530157486181039 ) ) ;
#37821=CARTESIAN_POINT ( 'NONE',  ( 12.91533473730993009, 36.60535201082151247, -10.88017736071109987 ) ) ;
#37822=EDGE_CURVE ( 'NONE', #9521, #98326, #96633, .T. ) ;
#37823=MECHANICAL_DESIGN_GEOMETRIC_PRESENTATION_REPRESENTATION('',(#5910),#50583);
#37825=VERTEX_POINT ( 'NONE', #15108 ) ;
#37828=CARTESIAN_POINT ( 'NONE',  ( 4.559911319644449179, 37.23035201082150536, -9.422509992056141925 ) ) ;
#37829=CARTESIAN_POINT ( 'NONE',  ( -46.43955761922751435, 103.5181700978648820, -6.245201398087227851 ) ) ;
#37830=CARTESIAN_POINT ( 'NONE',  ( -2.816281873526473856, 49.33196800326374643, 3.434112377981055619 ) ) ;
#37831=CARTESIAN_POINT ( 'NONE',  ( 15.44008868035555260, 59.73035201082151247, 9.422509992056143702 ) ) ;
#37832=CARTESIAN_POINT ( 'NONE',  ( 19.38216949554541202, 0.9986346699304200492, 9.382169495545424454 ) ) ;
#37834=CARTESIAN_POINT ( 'NONE',  ( 7.361572987183170547, 22.05059781766745530, 9.846743663894590881 ) ) ;
#37835=CARTESIAN_POINT ( 'NONE',  ( 13.43411237798106583, 57.66530133659708923, -12.81628187352647252 ) ) ;
#37836=CARTESIAN_POINT ( 'NONE',  ( 2.377183314880002563, 35.78593319516821225, -6.500000000000057732 ) ) ;
#37837=CARTESIAN_POINT ( 'NONE',  ( 0.1532563361054100626, 5.800597817667452638, -2.638427012816831230 ) ) ;
#37838=CARTESIAN_POINT ( 'NONE',  ( 0.6178305044545818747, 8.498634669930421381, -9.382169495545419124 ) ) ;
#37840=CARTESIAN_POINT ( 'NONE',  ( 18.52753015748617571, 63.09226448433412315, 4.923371831947298993 ) ) ;
#37841=CARTESIAN_POINT ( 'NONE',  ( 20.88017736071110875, 35.77201867748816966, -2.915334737309920765 ) ) ;
#37842=CARTESIAN_POINT ( 'NONE',  ( 5.076628168052703671, 46.84226448433412315, 8.527530157486179263 ) ) ;
#37844=CARTESIAN_POINT ( 'NONE',  ( 2.791683348922240793, 16.63393115100078745, 7.208316651077764092 ) ) ;
#37845=CARTESIAN_POINT ( 'NONE',  ( 0.1532563361054100626, 10.80059781766745175, -2.638427012816831230 ) ) ;
#37846=CARTESIAN_POINT ( 'NONE',  ( 6.565887622018943937, 3.081968003263753531, -12.81628187352647608 ) ) ;
#37848=MECHANICAL_DESIGN_GEOMETRIC_PRESENTATION_REPRESENTATION('',(#12265),#77722);
#37849=CARTESIAN_POINT ( 'NONE',  ( 17.96484262340118221, 6.188685344154836621, -7.964842623401177768 ) ) ;
#37850=DIRECTION ( 'NONE',  ( 0.000000000000000000, 0.000000000000000000, -1.000000000000000000 ) ) ;
#37853=CARTESIAN_POINT ( 'NONE',  ( 20.88017736071110519, 5.563685344154838397, 2.639326808657452039E-16 ) ) ;
#37854=CARTESIAN_POINT ( 'NONE',  ( 5.076628168052703671, 41.84226448433411605, 8.527530157486179263 ) ) ;
#37857=CARTESIAN_POINT ( 'NONE',  ( 6.204703633549690345, 67.84541550158060375, 14.16423886937410082 ) ) ;
#37859=CARTESIAN_POINT ( 'NONE',  ( 12.91533473730992121, 39.52201867748817676, 10.88017736071110164 ) ) ;
#37860=CARTESIAN_POINT ( 'NONE',  ( -0.3689425029237898834, 46.17874883491397497, -10.36894250292378850 ) ) ;
#37861=CARTESIAN_POINT ( 'NONE',  ( 6.204703633549690345, 67.84541550158060375, 14.16423886937410082 ) ) ;
#37862=CARTESIAN_POINT ( 'NONE',  ( 2.791683348922237240, 20.38393115100078745, -7.208316651077763204 ) ) ;
#37863=CARTESIAN_POINT ( 'NONE',  ( 22.81628187352648496, 16.83196800326374998, -3.434112377981050290 ) ) ;
#37867=CARTESIAN_POINT ( 'NONE',  ( 14.92337183194729988, 59.34226448433412315, -8.527530157486177487 ) ) ;
#37870=CARTESIAN_POINT ( 'NONE',  ( -2.266590686148945544, 7.220415501580634832, 7.082119434687048631 ) ) ;
#37871=CARTESIAN_POINT ( 'NONE',  ( 0.1532563361054083140, 31.00893115100078390, 1.131784320476157264E-15 ) ) ;
#37874=CARTESIAN_POINT ( 'NONE',  ( 10.00000000000000000, 55.55374883491396787, -14.16423886937410082 ) ) ;
#37876=CARTESIAN_POINT ( 'NONE',  ( 14.92337183194729988, 4.342264484334117824, -8.527530157486177487 ) ) ;
#37878=DIRECTION ( 'NONE',  ( 0.000000000000000000, 0.000000000000000000, 1.000000000000000000 ) ) ;
#37879=CARTESIAN_POINT ( 'NONE',  ( 12.91533473730993009, 26.60535201082150536, -10.88017736071109987 ) ) ;
#37880=CARTESIAN_POINT ( 'NONE',  ( 16.40814093676323893, 45.79030133659708923, 11.09922568453595026 ) ) ;
#37881=CARTESIAN_POINT ( 'NONE',  ( 13.43411237798105340, 35.58196800326375353, 12.81628187352647963 ) ) ;
#37882=CARTESIAN_POINT ( 'NONE',  ( 10.00000000000000178, 2.258931151000784787, 9.846743663894594434 ) ) ;
#37885=EDGE_CURVE ( 'NONE', #47405, #46987, #69487, .T. ) ;
#37887=CARTESIAN_POINT ( 'NONE',  ( 10.00000000000000178, 43.05374883491397497, 14.16423886937410082 ) ) ;
#37888=CARTESIAN_POINT ( 'NONE',  ( 22.26659068614894466, 13.88708216824730179, 7.082119434687054849 ) ) ;
#37889=CARTESIAN_POINT ( 'NONE',  ( 15.44008868035555793, 6.397018677488170546, -9.422509992056140149 ) ) ;
#37890=AXIS2_PLACEMENT_3D ( 'NONE', #77250, #85257, #8758 ) ;
#37891=CARTESIAN_POINT ( 'NONE',  ( 17.96484262340118221, 41.18868534415484106, -7.964842623401177768 ) ) ;
#37892=CARTESIAN_POINT ( 'NONE',  ( -45.94000000000001194, 100.9999999999999858, -9.500000000000000000 ) ) ;
#37893=CARTESIAN_POINT ( 'NONE',  ( 17.96484262340118221, 59.93868534415484106, 7.964842623401181321 ) ) ;
#37894=CARTESIAN_POINT ( 'NONE',  ( -0.8801773607110991993, 67.85535201082151957, -2.915334737309923874 ) ) ;
#37895=CARTESIAN_POINT ( 'NONE',  ( -2.816281873526473856, 29.12363466993041783, 9.499525473075851096E-16 ) ) ;
#37898=CARTESIAN_POINT ( 'NONE',  ( 2.791683348922240793, 31.63393115100078745, 7.208316651077764092 ) ) ;
#37902=CARTESIAN_POINT ( 'NONE',  ( 10.00000000000000000, 22.87363466993042138, -12.81628187352647608 ) ) ;
#37904=CARTESIAN_POINT ( 'NONE',  ( 20.88017736071110519, 15.56368534415483751, 2.639326808657452039E-16 ) ) ;
#37905=CARTESIAN_POINT ( 'NONE',  ( 10.00000000000000178, 42.25893115100078745, 9.846743663894594434 ) ) ;
#37906=CARTESIAN_POINT ( 'NONE',  ( 19.38216949554541202, 55.99863466993041072, 9.382169495545424454 ) ) ;
#37907=CARTESIAN_POINT ( 'NONE',  ( 19.84674366389459621, 18.50893115100078745, 7.409399052514197653E-17 ) ) ;
#37908=CARTESIAN_POINT ( 'NONE',  ( 13.79529636645030344, 3.262082168247301350, 14.16423886937410614 ) ) ;
#37909=CARTESIAN_POINT ( 'NONE',  ( 6.204703633549690345, 2.845415501580634388, 14.16423886937410082 ) ) ;
#37911=CARTESIAN_POINT ( 'NONE',  ( 15.44008868035555260, 34.73035201082151247, 9.422509992056143702 ) ) ;
#37912=CARTESIAN_POINT ( 'NONE',  ( 7.084665262690076126, 17.02201867748817676, -10.88017736071110164 ) ) ;
#37913=CARTESIAN_POINT ( 'NONE',  ( -4.164238869374099927, 42.01208216824728936, 3.795296366450308767 ) ) ;
#37915=CARTESIAN_POINT ( 'NONE',  ( -0.8801773607111009756, 28.06368534415484106, 1.068504757029289695E-15 ) ) ;
#37916=CARTESIAN_POINT ( 'NONE',  ( 7.084665262690076126, 14.10535201082150358, 10.88017736071109987 ) ) ;
#37918=CARTESIAN_POINT ( 'NONE',  ( 15.44008868035555260, 24.73035201082150891, 9.422509992056143702 ) ) ;
#37919=CARTESIAN_POINT ( 'NONE',  ( 16.40814093676323893, 45.79030133659708923, 11.09922568453595026 ) ) ;
#37920=CARTESIAN_POINT ( 'NONE',  ( 7.084665262690076126, 47.02201867748818387, -10.88017736071110164 ) ) ;
#37922=CARTESIAN_POINT ( 'NONE',  ( -0.8801773607111009756, 48.06368534415484817, 1.068504757029289695E-15 ) ) ;
#37924=CARTESIAN_POINT ( 'NONE',  ( 7.084665262690076126, 39.10535201082150536, 10.88017736071109987 ) ) ;
#37927=CARTESIAN_POINT ( 'NONE',  ( 6.204703633549690345, 40.76208216824731778, -14.16423886937410259 ) ) ;
#37928=CARTESIAN_POINT ( 'NONE',  ( 20.88017736071110519, 60.56368534415484106, 2.639326808657452039E-16 ) ) ;
#37930=CARTESIAN_POINT ( 'NONE',  ( 5.076628168052704559, 0.1755978176674514724, -8.527530157486179263 ) ) ;
#37931=CARTESIAN_POINT ( 'NONE',  ( 0.1532563361054082862, 61.21726448433412315, 2.638427012816831674 ) ) ;
#37933=CARTESIAN_POINT ( 'NONE',  ( 0.1532563361054082862, 31.21726448433412315, 2.638427012816831674 ) ) ;
#37935=CARTESIAN_POINT ( 'NONE',  ( 10.00000000000000000, 39.75893115100078745, -9.846743663894594434 ) ) ;
#37937=CARTESIAN_POINT ( 'NONE',  ( 19.42250999205614548, 30.98035201082150536, -5.440088680355545492 ) ) ;
#37938=CARTESIAN_POINT ( 'NONE',  ( 18.52753015748617571, 33.09226448433411605, 4.923371831947298993 ) ) ;
#37939=CARTESIAN_POINT ( 'NONE',  ( 13.43411237798105340, 25.58196800326374998, 12.81628187352647963 ) ) ;
#37940=CARTESIAN_POINT ( 'NONE',  ( 4.559911319644449179, 67.23035201082150536, -9.422509992056141925 ) ) ;
#37941=CARTESIAN_POINT ( 'NONE',  ( 10.00000000000000178, 54.31368534415484106, 10.88017736071110342 ) ) ;
#37942=CARTESIAN_POINT ( 'NONE',  ( -0.8801773607110991993, 27.85535201082150181, -2.915334737309923874 ) ) ;
#37943=CARTESIAN_POINT ( 'NONE',  ( 15.44008868035555260, 4.730352010821504471, 9.422509992056143702 ) ) ;
#37944=CARTESIAN_POINT ( 'NONE',  ( -4.164238869374098151, 61.59541550158063217, -3.795296366450310543 ) ) ;
#37946=CARTESIAN_POINT ( 'NONE',  ( 21.09922568453595559, 27.04030133659708568, -6.408140936763230044 ) ) ;
#37948=ORIENTED_EDGE ( 'NONE', *, *, #19309, .T. ) ;
#37949=CARTESIAN_POINT ( 'NONE',  ( 19.38216949554541202, 20.99863466993042138, 9.382169495545424454 ) ) ;
#37950=CARTESIAN_POINT ( 'NONE',  ( 20.88017736071110519, 5.563685344154837509, 2.639326808657452039E-16 ) ) ;
#37951=CARTESIAN_POINT ( 'NONE',  ( -0.8801773607111008646, 48.27201867748816966, 2.915334737309923430 ) ) ;
#37953=MECHANICAL_DESIGN_GEOMETRIC_PRESENTATION_REPRESENTATION('',(#28368),#33218);
#37954=CARTESIAN_POINT ( 'NONE',  ( 17.96484262340118221, 59.93868534415484106, 7.964842623401181321 ) ) ;
#37955=CARTESIAN_POINT ( 'NONE',  ( 14.92337183194729633, 37.67559781766745175, 8.527530157486181039 ) ) ;
#37956=CARTESIAN_POINT ( 'NONE',  ( 14.92337183194729988, 24.34226448433411960, -8.527530157486177487 ) ) ;
#37959=CARTESIAN_POINT ( 'NONE',  ( 18.52753015748618282, 18.92559781766745175, -4.923371831947291888 ) ) ;
#37962=CARTESIAN_POINT ( 'NONE',  ( 12.63842701281683922, 14.55059781766744997, -9.846743663894590881 ) ) ;
#37966=CARTESIAN_POINT ( 'NONE',  ( 19.84674366389459266, 28.30059781766745886, 2.638427012816836559 ) ) ;
#37967=ORIENTED_EDGE ( 'NONE', *, *, #96884, .T. ) ;
#37971=CARTESIAN_POINT ( 'NONE',  ( -1.099225684535947600, 14.54030133659708568, 6.408140936763237150 ) ) ;
#37972=CARTESIAN_POINT ( 'NONE',  ( 12.91533473730993009, 56.60535201082151247, -10.88017736071109987 ) ) ;
#37973=CARTESIAN_POINT ( 'NONE',  ( -2.266590686148945544, 36.38708216824730357, -7.082119434687050408 ) ) ;
#37975=CARTESIAN_POINT ( 'NONE',  ( 1.821708436314945612, 41.66792564121896447, -6.500000000000040856 ) ) ;
#37976=CARTESIAN_POINT ( 'NONE',  ( 20.36894250292379382, 33.67874883491396076, 10.36894250292379205 ) ) ;
#37977=CARTESIAN_POINT ( 'NONE',  ( 10.00000000000000178, 58.05374883491397497, 14.16423886937410082 ) ) ;
#37978=CARTESIAN_POINT ( 'NONE',  ( 24.16423886937410614, 14.51208216824730179, -3.795296366450302550 ) ) ;
#37979=CARTESIAN_POINT ( 'NONE',  ( 2.917880565312950480, 20.97041550158063217, -12.26659068614894821 ) ) ;
#37981=CARTESIAN_POINT ( 'NONE',  ( 12.91533473730992121, 49.52201867748817676, 10.88017736071110164 ) ) ;
#37982=CARTESIAN_POINT ( 'NONE',  ( 17.39651004071838614, 62.93575266056827644, 6.500000000000032863 ) ) ;
#37983=CARTESIAN_POINT ( 'NONE',  ( 14.92337183194729633, 42.67559781766745886, 8.527530157486181039 ) ) ;
#37984=CARTESIAN_POINT ( 'NONE',  ( 10.00000000000000178, 19.31368534415484106, 10.88017736071110342 ) ) ;
#37985=CARTESIAN_POINT ( 'NONE',  ( -2.816281873526473856, 54.33196800326376064, 3.434112377981055619 ) ) ;
#37986=CARTESIAN_POINT ( 'NONE',  ( 0.1532563361054100626, 60.80059781766744464, -2.638427012816831230 ) ) ;
#37987=CARTESIAN_POINT ( 'NONE',  ( 20.00000000000286349, 82.51979501594313149, -5.046714348924735027 ) ) ;
#37988=CARTESIAN_POINT ( 'NONE',  ( -1.099225684535947600, 53.70696800326376064, -6.408140936763238038 ) ) ;
#37990=CARTESIAN_POINT ( 'NONE',  ( -0.8801773607111008646, 43.27201867748817676, 2.915334737309923430 ) ) ;
#37991=CARTESIAN_POINT ( 'NONE',  ( 12.63842701281683922, 54.55059781766745175, -9.846743663894590881 ) ) ;
#37992=CARTESIAN_POINT ( 'NONE',  ( 17.08211943468705840, 45.13708216824730357, -12.26659068614894466 ) ) ;
#37993=VERTEX_POINT ( 'NONE', #45585 ) ;
#37994=CARTESIAN_POINT ( 'NONE',  ( 20.36894250292379738, 4.928748834913967869, -10.36894250292379027 ) ) ;
#37995=CARTESIAN_POINT ( 'NONE',  ( 15.44008868035555793, 66.39701867748817676, -9.422509992056140149 ) ) ;
#37997=CARTESIAN_POINT ( 'NONE',  ( -0.3689425029237898834, 56.17874883491396076, -10.36894250292378850 ) ) ;
#37998=CARTESIAN_POINT ( 'NONE',  ( 21.09922568453595559, 17.04030133659708923, -6.408140936763230044 ) ) ;
#38000=CARTESIAN_POINT ( 'NONE',  ( 7.084665262690076126, 52.02201867748816255, -10.88017736071110164 ) ) ;
#38001=CYLINDRICAL_SURFACE ( 'NONE', #78982, 0.5000000000000004441 ) ;
#38002=CARTESIAN_POINT ( 'NONE',  ( -46.94000000000001194, 100.7103534007538883, -8.569772222592094479 ) ) ;
#38003=CARTESIAN_POINT ( 'NONE',  ( 6.204703633549690345, 62.84541550158063927, 14.16423886937410082 ) ) ;
#38005=CARTESIAN_POINT ( 'NONE',  ( 2.035157376598824452, 13.68868534415483751, 7.964842623401179544 ) ) ;
#38006=CARTESIAN_POINT ( 'NONE',  ( 4.559911319644449179, 22.23035201082150536, -9.422509992056141925 ) ) ;
#38007=CARTESIAN_POINT ( 'NONE',  ( 10.00000000000000178, 62.25893115100078745, 9.846743663894594434 ) ) ;
#38008=CARTESIAN_POINT ( 'NONE',  ( 19.38216949554541202, 45.99863466993041072, 9.382169495545424454 ) ) ;
#38011=CARTESIAN_POINT ( 'NONE',  ( 12.91533473730992121, 19.52201867748816611, 10.88017736071110164 ) ) ;
#38012=CARTESIAN_POINT ( 'NONE',  ( 16.40814093676324603, 22.45696800326375353, -11.09922568453594671 ) ) ;
#38014=CARTESIAN_POINT ( 'NONE',  ( 10.00000000000000178, 42.25893115100078745, 9.846743663894594434 ) ) ;
#38015=CARTESIAN_POINT ( 'NONE',  ( 2.035157376598822676, 37.43868534415484106, -7.964842623401177768 ) ) ;
#38016=CARTESIAN_POINT ( 'NONE',  ( 21.09922568453595559, 27.04030133659708568, -6.408140936763230044 ) ) ;
#38017=CARTESIAN_POINT ( 'NONE',  ( 15.44008868035555260, 49.73035201082150536, 9.422509992056143702 ) ) ;
#38019=DIRECTION ( 'NONE',  ( 0.000000000000000000, 0.000000000000000000, -1.000000000000000000 ) ) ;
#38020=CARTESIAN_POINT ( 'NONE',  ( 16.40814093676323893, 45.79030133659708923, 11.09922568453595026 ) ) ;
#38022=DIRECTION ( 'NONE',  ( 0.000000000000000000, 0.000000000000000000, -1.000000000000000000 ) ) ;
#38023=CARTESIAN_POINT ( 'NONE',  ( 20.88017736071110875, 55.77201867748816966, -2.915334737309920765 ) ) ;
#38024=CARTESIAN_POINT ( 'NONE',  ( 19.38216949554541202, 30.99863466993042138, 9.382169495545424454 ) ) ;
#38025=CARTESIAN_POINT ( 'NONE',  ( -4.164238869374098151, 1.595415501580634388, -3.795296366450310543 ) ) ;
#38026=CARTESIAN_POINT ( 'NONE',  ( 0.1532563361054083140, 6.008931151000784787, 1.131784320476157264E-15 ) ) ;
#38027=CARTESIAN_POINT ( 'NONE',  ( 0.5774900079438607392, 58.48035201082151247, 5.440088680355550821 ) ) ;
#38028=CARTESIAN_POINT ( 'NONE',  ( 6.204703633549690345, 47.84541550158064638, 14.16423886937410082 ) ) ;
#38030=CARTESIAN_POINT ( 'NONE',  ( 5.076628168052704559, 65.17559781766745175, -8.527530157486179263 ) ) ;
#38031=CARTESIAN_POINT ( 'NONE',  ( 14.92337183194729633, 17.67559781766745175, 8.527530157486181039 ) ) ;
#38032=CARTESIAN_POINT ( 'NONE',  ( 0.1532563361054083140, 6.008931151000784787, 1.131784320476157264E-15 ) ) ;
#38034=CARTESIAN_POINT ( 'NONE',  ( 6.204703633549690345, 42.84541550158063217, 14.16423886937410082 ) ) ;
#38037=CARTESIAN_POINT ( 'NONE',  ( 19.42250999205614548, 10.98035201082150358, -5.440088680355545492 ) ) ;
#38039=VECTOR ( 'NONE', #70133, 1000.000000000000000 ) ;
#38040=ORIENTED_EDGE ( 'NONE', *, *, #37641, .F. ) ;
#38041=CARTESIAN_POINT ( 'NONE',  ( 7.084665262690076126, 4.105352010821503583, 10.88017736071109987 ) ) ;
#38042=CARTESIAN_POINT ( 'NONE',  ( -0.3689425029237898834, 61.17874883491396076, -10.36894250292378850 ) ) ;
#38043=CARTESIAN_POINT ( 'NONE',  ( 10.00000000000000000, 49.75893115100078745, -9.846743663894594434 ) ) ;
#38044=CARTESIAN_POINT ( 'NONE',  ( 0.6178305044545838731, 44.74863466993042493, 9.382169495545420901 ) ) ;
#38046=CARTESIAN_POINT ( 'NONE',  ( 22.26659068614894466, 3.887082168247300906, 7.082119434687054849 ) ) ;
#38047=CARTESIAN_POINT ( 'NONE',  ( 0.5774900079438607392, 8.480352010821505360, 5.440088680355550821 ) ) ;
#38048=CARTESIAN_POINT ( 'NONE',  ( -4.164238869374099039, 66.80374883491396076, 8.674139862899312516E-16 ) ) ;
#38049=CARTESIAN_POINT ( 'NONE',  ( 1.472469842513823179, 41.42559781766745886, 4.923371831947296329 ) ) ;
#38050=CARTESIAN_POINT ( 'NONE',  ( 17.84635730667658393, 43.63791097397316321, 6.499999999999926281 ) ) ;
#38051=CARTESIAN_POINT ( 'NONE',  ( 14.92337183194729633, 27.67559781766745530, 8.527530157486181039 ) ) ;
#38052=CARTESIAN_POINT ( 'NONE',  ( 19.50000000000000711, 105.0000000000000000, 4.500000000000000888 ) ) ;
#38058=CARTESIAN_POINT ( 'NONE',  ( 4.559911319644449179, 32.23035201082150536, -9.422509992056141925 ) ) ;
#38059=CARTESIAN_POINT ( 'NONE',  ( 4.559911319644449179, 32.23035201082150536, -9.422509992056141925 ) ) ;
#38060=CARTESIAN_POINT ( 'NONE',  ( 19.84674366389459621, 63.50893115100078745, 7.409399052514197653E-17 ) ) ;
#38061=CARTESIAN_POINT ( 'NONE',  ( 3.591859063236763294, 28.29030133659708568, -11.09922568453595026 ) ) ;
#38062=CARTESIAN_POINT ( 'NONE',  ( 17.08211943468705840, 10.13708216824730179, -12.26659068614894466 ) ) ;
#38063=CARTESIAN_POINT ( 'NONE',  ( 10.00000000000000178, 64.31368534415483396, 10.88017736071110342 ) ) ;
#38066=CARTESIAN_POINT ( 'NONE',  ( 13.43411237798106583, 42.66530133659707502, -12.81628187352647252 ) ) ;
#38067=EDGE_LOOP ( 'NONE', ( #81036, #80376, #98299, #15351, #78962, #84021 ) ) ;
#38068=CARTESIAN_POINT ( 'NONE',  ( 1.472469842513823179, 50.59226448433411605, -4.923371831947296329 ) ) ;
#38069=CARTESIAN_POINT ( 'NONE',  ( 17.96484262340118221, 11.18868534415484106, -7.964842623401177768 ) ) ;
#38071=CARTESIAN_POINT ( 'NONE',  ( 2.035157376598824452, 13.68868534415483751, 7.964842623401179544 ) ) ;
#38072=B_SPLINE_CURVE_WITH_KNOTS ( 'NONE', 3,
 ( #31473, #85481, #61976, #15999, #76983, #24001 ),
 .UNSPECIFIED., .F., .F.,
 ( 4, 2, 4 ),
 ( 0.000000000000000000, 0.0002701661927229447686, 0.0005403323854458895372 ),
 .UNSPECIFIED. ) ;
#38074=CARTESIAN_POINT ( 'NONE',  ( 15.44008868035555260, 54.73035201082150536, 9.422509992056143702 ) ) ;
#38075=CARTESIAN_POINT ( 'NONE',  ( 19.42250999205614548, 60.98035201082151247, -5.440088680355545492 ) ) ;
#38076=CARTESIAN_POINT ( 'NONE',  ( 2.035157376598824452, 63.68868534415484106, 7.964842623401179544 ) ) ;
#38080=CARTESIAN_POINT ( 'NONE',  ( 20.88017736071110164, 55.35535201082149825, 2.915334737309930979 ) ) ;
#38081=CARTESIAN_POINT ( 'NONE',  ( -46.94000000000001194, 103.0000000000000000, 5.997726559847112782 ) ) ;
#38082=CARTESIAN_POINT ( 'NONE',  ( -46.94000000000001194, 100.4344880109628093, 9.014049137172644777 ) ) ;
#38084=ORIENTED_EDGE ( 'NONE', *, *, #47570, .F. ) ;
#38085=EDGE_CURVE ( 'NONE', #65595, #94683, #51329, .T. ) ;
#38086=CARTESIAN_POINT ( 'NONE',  ( 14.92337183194729633, 42.67559781766745886, 8.527530157486181039 ) ) ;
#38088=CARTESIAN_POINT ( 'NONE',  ( 3.558677480090427725, 70.40124509038875544, 12.00000000000000000 ) ) ;
#38089=CARTESIAN_POINT ( 'NONE',  ( 0.2751277870542891413, 24.36607318730131411, -6.499999999999989342 ) ) ;
#38090=ADVANCED_FACE ( 'NONE', ( #94039 ), #48033, .F. ) ;
#38091=CARTESIAN_POINT ( 'NONE',  ( 17.08211943468705130, 3.470415501580634388, 12.26659068614894998 ) ) ;
#38095=CARTESIAN_POINT ( 'NONE',  ( 10.00000000000000000, 61.81368534415484106, -10.88017736071110342 ) ) ;
#38096=CARTESIAN_POINT ( 'NONE',  ( 17.96484262340118221, 4.938685344154837509, 7.964842623401181321 ) ) ;
#38098=CARTESIAN_POINT ( 'NONE',  ( 22.81628187352647785, 41.62363466993042493, 6.195893100308588602E-16 ) ) ;
#38101=CARTESIAN_POINT ( 'NONE',  ( 10.00000000000000000, 44.75893115100078745, -9.846743663894594434 ) ) ;
#38102=CARTESIAN_POINT ( 'NONE',  ( -1.099225684535947600, 14.54030133659708568, 6.408140936763237150 ) ) ;
#38103=CARTESIAN_POINT ( 'NONE',  ( 1.472469842513823179, 26.42559781766745175, 4.923371831947296329 ) ) ;
#38105=CARTESIAN_POINT ( 'NONE',  ( 0.6178305044545838731, 9.748634669930416052, 9.382169495545420901 ) ) ;
#38108=CARTESIAN_POINT ( 'NONE',  ( 2.791683348922240793, 1.633931151000784565, 7.208316651077764092 ) ) ;
#38111=CARTESIAN_POINT ( 'NONE',  ( 4.559911319644449179, 22.23035201082150536, -9.422509992056141925 ) ) ;
#38112=CARTESIAN_POINT ( 'NONE',  ( 22.26659068614895176, 14.72041550158063572, -7.082119434687042414 ) ) ;
#38113=CARTESIAN_POINT ( 'NONE',  ( 0.1532563361054083140, 46.00893115100079456, 1.131784320476157264E-15 ) ) ;
#38114=CARTESIAN_POINT ( 'NONE',  ( 14.92337183194729633, 2.675597817667451750, 8.527530157486181039 ) ) ;
#38115=CARTESIAN_POINT ( 'NONE',  ( 13.43411237798105340, 35.58196800326375353, 12.81628187352647963 ) ) ;
#38117=CARTESIAN_POINT ( 'NONE',  ( 2.035157376598824452, 8.688685344154839285, 7.964842623401179544 ) ) ;
#38120=CARTESIAN_POINT ( 'NONE',  ( 3.591859063236761518, 9.956968003263753531, 11.09922568453594849 ) ) ;
#38121=CARTESIAN_POINT ( 'NONE',  ( 17.20831665107776587, 29.13393115100078390, -7.208316651077762316 ) ) ;
#38123=CARTESIAN_POINT ( 'NONE',  ( -2.816281873526473856, 29.12363466993041783, 9.499525473075851096E-16 ) ) ;
#38124=LINE ( 'NONE', #53593, #19670 ) ;
#38125=CARTESIAN_POINT ( 'NONE',  ( 0.5774900079438590739, 37.64701867748817676, -5.440088680355550821 ) ) ;
#38129=CARTESIAN_POINT ( 'NONE',  ( 15.44008868035555793, 66.39701867748817676, -9.422509992056140149 ) ) ;
#38130=CARTESIAN_POINT ( 'NONE',  ( 17.96484262340118221, 34.93868534415482685, 7.964842623401181321 ) ) ;
#38131=CARTESIAN_POINT ( 'NONE',  ( 20.88017736071110875, 40.77201867748818387, -2.915334737309920765 ) ) ;
#38132=CARTESIAN_POINT ( 'NONE',  ( 20.10421743870887212, 60.60736173766203194, -6.337391062633416006 ) ) ;
#38133=CARTESIAN_POINT ( 'NONE',  ( 2.035157376598824452, 63.68868534415484106, 7.964842623401179544 ) ) ;
#38135=CARTESIAN_POINT ( 'NONE',  ( 18.52753015748617571, 53.09226448433412315, 4.923371831947298993 ) ) ;
#38136=CARTESIAN_POINT ( 'NONE',  ( 0.5774900079438607392, 13.48035201082150358, 5.440088680355550821 ) ) ;
#38138=CARTESIAN_POINT ( 'NONE',  ( 10.00000000000000178, 15.37363466993042138, 12.81628187352647608 ) ) ;
#38140=CARTESIAN_POINT ( 'NONE',  ( -0.8801773607111009756, 33.06368534415484106, 1.068504757029289695E-15 ) ) ;
#38142=CARTESIAN_POINT ( 'NONE',  ( 3.591859063236763294, -1.709698663402913210, -11.09922568453595026 ) ) ;
#38144=CARTESIAN_POINT ( 'NONE',  ( 17.96484262340118221, 19.93868534415484106, 7.964842623401181321 ) ) ;
#38145=CARTESIAN_POINT ( 'NONE',  ( 2.035157376598824452, 28.68868534415484106, 7.964842623401179544 ) ) ;
#38146=CARTESIAN_POINT ( 'NONE',  ( 22.26659068614895176, 39.72041550158063217, -7.082119434687042414 ) ) ;
#38147=CARTESIAN_POINT ( 'NONE',  ( 5.076628168052703671, 21.84226448433411960, 8.527530157486179263 ) ) ;
#38149=CARTESIAN_POINT ( 'NONE',  ( 12.91533473730993009, 51.60535201082149825, -10.88017736071109987 ) ) ;
#38150=CARTESIAN_POINT ( 'NONE',  ( 2.917880565312950480, 0.9704155015806342766, -12.26659068614894821 ) ) ;
#38151=CARTESIAN_POINT ( 'NONE',  ( 2.791683348922237240, 55.38393115100078745, -7.208316651077763204 ) ) ;
#38152=ORIENTED_EDGE ( 'NONE', *, *, #66289, .T. ) ;
#38154=CARTESIAN_POINT ( 'NONE',  ( 17.08211943468705840, 35.13708216824730357, -12.26659068614894466 ) ) ;
#38155=CARTESIAN_POINT ( 'NONE',  ( 20.36894250292379738, 24.92874883491396787, -10.36894250292379027 ) ) ;
#38156=CARTESIAN_POINT ( 'NONE',  ( 5.076628168052704559, 10.17559781766745175, -8.527530157486179263 ) ) ;
#38157=CARTESIAN_POINT ( 'NONE',  ( 6.565887622018943937, 10.16530133659708746, 12.81628187352647430 ) ) ;
#38158=CARTESIAN_POINT ( 'NONE',  ( 14.92337183194729988, 54.34226448433412315, -8.527530157486177487 ) ) ;
#38160=CARTESIAN_POINT ( 'NONE',  ( 2.035157376598824452, 43.68868534415484106, 7.964842623401179544 ) ) ;
#38161=CARTESIAN_POINT ( 'NONE',  ( 19.38216949554541557, 17.24863466993041783, -9.382169495545420901 ) ) ;
#38162=CARTESIAN_POINT ( 'NONE',  ( 22.26659068614895176, 34.72041550158063927, -7.082119434687042414 ) ) ;
#38163=CARTESIAN_POINT ( 'NONE',  ( 20.88017736071110875, 10.77201867748817143, -2.915334737309920765 ) ) ;
#38164=CARTESIAN_POINT ( 'NONE',  ( 20.88017736071110164, 25.35535201082150891, 2.915334737309930979 ) ) ;
#38165=CARTESIAN_POINT ( 'NONE',  ( 20.15039907845753930, 5.601585745166425490, -6.262539305110069954 ) ) ;
#38166=CARTESIAN_POINT ( 'NONE',  ( 0.5774900079438590739, 62.64701867748817676, -5.440088680355550821 ) ) ;
#38174=CARTESIAN_POINT ( 'NONE',  ( -0.3689425029237898834, 61.17874883491396076, -10.36894250292378850 ) ) ;
#38175=CARTESIAN_POINT ( 'NONE',  ( 10.00000000000000178, 63.05374883491396076, 14.16423886937410082 ) ) ;
#38176=CARTESIAN_POINT ( 'NONE',  ( 17.20831665107776587, 19.13393115100078035, -7.208316651077762316 ) ) ;
#38177=CARTESIAN_POINT ( 'NONE',  ( 14.92337183194729633, 62.67559781766745886, 8.527530157486181039 ) ) ;
#38183=CARTESIAN_POINT ( 'NONE',  ( 1.472469842513823179, 11.42559781766745175, 4.923371831947296329 ) ) ;
#38184=EDGE_CURVE ( 'NONE', #31822, #6951, #15834, .T. ) ;
#38187=CARTESIAN_POINT ( 'NONE',  ( -2.266590686148945544, 31.38708216824730002, -7.082119434687050408 ) ) ;
#38188=CARTESIAN_POINT ( 'NONE',  ( 24.16423886937410614, 49.30374883491396787, 8.672049930838204340E-16 ) ) ;
#38190=CARTESIAN_POINT ( 'NONE',  ( -2.816281873526473856, 54.33196800326376064, 3.434112377981055619 ) ) ;
#38191=CARTESIAN_POINT ( 'NONE',  ( 20.88017736071110164, 25.35535201082150891, 2.915334737309930979 ) ) ;
#38192=CARTESIAN_POINT ( 'NONE',  ( 19.84674366389459266, 43.71726448433410894, -2.638427012816827677 ) ) ;
#38193=CARTESIAN_POINT ( 'NONE',  ( 10.00000000000000000, 21.81368534415484106, -10.88017736071110342 ) ) ;
#38196=CARTESIAN_POINT ( 'NONE',  ( 0.1532563361054100626, 60.80059781766744464, -2.638427012816831230 ) ) ;
#38197=CARTESIAN_POINT ( 'NONE',  ( 17.20831665107776587, 44.13393115100078745, -7.208316651077762316 ) ) ;
#38200=EDGE_CURVE ( 'NONE', #73080, #71557, #88007, .T. ) ;
#38204=CARTESIAN_POINT ( 'NONE',  ( 18.52753015748618282, 33.92559781766745886, -4.923371831947291888 ) ) ;
#38206=CARTESIAN_POINT ( 'NONE',  ( 6.565887622018943937, 33.08196800326374643, -12.81628187352647608 ) ) ;
#38208=CARTESIAN_POINT ( 'NONE',  ( 0.6081133539230532126, 38.33703382326400089, 6.499999999999970690 ) ) ;
#38209=CARTESIAN_POINT ( 'NONE',  ( 0.2751277870542874204, 39.36607318730131055, -6.499999999999984901 ) ) ;
#38210=ORIENTED_EDGE ( 'NONE', *, *, #9970, .F. ) ;
#38212=CARTESIAN_POINT ( 'NONE',  ( 17.20831665107776587, 64.13393115100079456, -7.208316651077762316 ) ) ;
#38214=CARTESIAN_POINT ( 'NONE',  ( 1.472469842513823179, 35.59226448433412315, -4.923371831947296329 ) ) ;
#38215=CARTESIAN_POINT ( 'NONE',  ( -0.3689425029237898834, 36.17874883491396787, -10.36894250292378850 ) ) ;
#38216=CARTESIAN_POINT ( 'NONE',  ( 5.076628168052704559, 55.17559781766745175, -8.527530157486179263 ) ) ;
#38218=CARTESIAN_POINT ( 'NONE',  ( 18.52753015748617571, 8.092264484334117824, 4.923371831947298993 ) ) ;
#38219=CARTESIAN_POINT ( 'NONE',  ( -0.3689425029237898834, 1.178748834913967869, -10.36894250292378850 ) ) ;
#38220=CARTESIAN_POINT ( 'NONE',  ( 1.472469842513823179, 50.59226448433411605, -4.923371831947296329 ) ) ;
#38221=CARTESIAN_POINT ( 'NONE',  ( -0.8801773607111008646, 58.27201867748816966, 2.915334737309923430 ) ) ;
#38222=CARTESIAN_POINT ( 'NONE',  ( 18.52753015748618282, 43.92559781766745175, -4.923371831947291888 ) ) ;
#38224=CARTESIAN_POINT ( 'NONE',  ( 2.035157376598822676, 42.43868534415483396, -7.964842623401177768 ) ) ;
#38226=CARTESIAN_POINT ( 'NONE',  ( -0.1503990784575277573, 63.10158574516643171, 6.262539305110076171 ) ) ;
#38227=CARTESIAN_POINT ( 'NONE',  ( 15.44008868035555793, 26.39701867748817321, -9.422509992056140149 ) ) ;
#38228=CARTESIAN_POINT ( 'NONE',  ( -1.099225684535947600, -1.293031996736246469, -6.408140936763238038 ) ) ;
#38229=CARTESIAN_POINT ( 'NONE',  ( -0.8801773607111008646, 58.27201867748816966, 2.915334737309923430 ) ) ;
#38230=CARTESIAN_POINT ( 'NONE',  ( -0.1503990784575247319, 47.22266099184918886, -6.262539305110083276 ) ) ;
#38232=CARTESIAN_POINT ( 'NONE',  ( 12.91533473730992121, 44.52201867748816966, 10.88017736071110164 ) ) ;
#38234=CARTESIAN_POINT ( 'NONE',  ( 7.361572987183169658, 14.96726448433411960, -9.846743663894592657 ) ) ;
#38235=CARTESIAN_POINT ( 'NONE',  ( 5.076628168052703671, 41.84226448433411605, 8.527530157486179263 ) ) ;
#38236=DIRECTION ( 'NONE',  ( -1.000000000000000000, 0.000000000000000000, 0.000000000000000000 ) ) ;
#38238=CARTESIAN_POINT ( 'NONE',  ( 21.09922568453595559, 2.040301336597086568, -6.408140936763230044 ) ) ;
#38239=CARTESIAN_POINT ( 'NONE',  ( -0.3689425029237898834, 61.17874883491396076, -10.36894250292378850 ) ) ;
#38241=CARTESIAN_POINT ( 'NONE',  ( -4.164238869374099927, 27.01208216824730357, 3.795296366450308767 ) ) ;
#38243=CARTESIAN_POINT ( 'NONE',  ( 6.204703633549690345, 55.76208216824730357, -14.16423886937410259 ) ) ;
#38244=CARTESIAN_POINT ( 'NONE',  ( 14.92337183194729988, 19.34226448433411960, -8.527530157486177487 ) ) ;
#38245=CARTESIAN_POINT ( 'NONE',  ( 10.00000000000000178, 4.313685344154837509, 10.88017736071110342 ) ) ;
#38247=CARTESIAN_POINT ( 'NONE',  ( 10.00000000000000000, 29.75893115100078745, -9.846743663894594434 ) ) ;
#38248=CARTESIAN_POINT ( 'NONE',  ( 2.035157376598824452, 33.68868534415484106, 7.964842623401179544 ) ) ;
#38249=CARTESIAN_POINT ( 'NONE',  ( 14.92337183194729988, 54.34226448433412315, -8.527530157486177487 ) ) ;
#38250=CARTESIAN_POINT ( 'NONE',  ( -2.266590686148945544, 2.220415501580634388, 7.082119434687048631 ) ) ;
#38252=CARTESIAN_POINT ( 'NONE',  ( 10.00000000000000178, 17.25893115100078745, 9.846743663894594434 ) ) ;
#38253=CARTESIAN_POINT ( 'NONE',  ( -2.816281873526471635, 38.91530133659708213, -3.434112377981056508 ) ) ;
#38254=CARTESIAN_POINT ( 'NONE',  ( 0.1532563361054100626, 45.80059781766745886, -2.638427012816831230 ) ) ;
#38256=CARTESIAN_POINT ( 'NONE',  ( 18.52753015748617571, 28.09226448433411960, 4.923371831947298993 ) ) ;
#38260=CARTESIAN_POINT ( 'NONE',  ( -4.164238869374099039, 56.80374883491397497, 8.674139862899312516E-16 ) ) ;
#38261=CARTESIAN_POINT ( 'NONE',  ( 4.559911319644449179, 52.23035201082151247, -9.422509992056141925 ) ) ;
#38262=CARTESIAN_POINT ( 'NONE',  ( 0.1077916266722474814, 32.24062864464239198, -6.478736007405950126 ) ) ;
#38263=CARTESIAN_POINT ( 'NONE',  ( 14.92337183194729988, 39.34226448433412315, -8.527530157486177487 ) ) ;
#38264=CARTESIAN_POINT ( 'NONE',  ( 0.5774900079438607392, 8.480352010821505360, 5.440088680355550821 ) ) ;
#38265=CARTESIAN_POINT ( 'NONE',  ( 1.472469842513823179, 45.59226448433412315, -4.923371831947296329 ) ) ;
#38267=CARTESIAN_POINT ( 'NONE',  ( 0.1532563361054082862, 46.21726448433411605, 2.638427012816831674 ) ) ;
#38268=AXIS2_PLACEMENT_3D ( 'NONE', #58032, #53993, #38022 ) ;
#38269=CARTESIAN_POINT ( 'NONE',  ( 7.084665262690076126, 52.02201867748816255, -10.88017736071110164 ) ) ;
#38270=( BOUNDED_CURVE ( )  B_SPLINE_CURVE ( 2, ( #18899, #2930, #33377, #63873, #70920, #25902, #47898, #11383, #56404 ),
 .UNSPECIFIED., .F., .F. ) 
 B_SPLINE_CURVE_WITH_KNOTS ( ( 3, 2, 2, 2, 3 ),
 ( 0.08200037436403688484, 0.08333333333333332871, 0.08928571428571428770, 0.09523809523809523281, 0.09657105420739148238 ),
 .UNSPECIFIED. ) 
 CURVE ( )  GEOMETRIC_REPRESENTATION_ITEM ( )  RATIONAL_B_SPLINE_CURVE ( ( 0.9881565478350731180, 0.9923695281211489805, 1.000000000000000000, 0.9659258262890683122, 1.000000000000000000, 0.9659258262890683122, 1.000000000000000000, 0.9923695281211499797, 0.9881565478350742282 ) ) 
 REPRESENTATION_ITEM ( '' )  );
#38272=ORIENTED_EDGE ( 'NONE', *, *, #7405, .F. ) ;
#38275=CARTESIAN_POINT ( 'NONE',  ( 7.361572987183170547, 12.05059781766744997, 9.846743663894590881 ) ) ;
#38276=CARTESIAN_POINT ( 'NONE',  ( 22.81628187352648496, 51.83196800326376064, -3.434112377981050290 ) ) ;
#38277=CARTESIAN_POINT ( 'NONE',  ( 20.88017736071110519, 10.56368534415483929, 2.639326808657452039E-16 ) ) ;
#38278=CARTESIAN_POINT ( 'NONE',  ( 10.00000000000000178, 47.25893115100078745, 9.846743663894594434 ) ) ;
#38279=FACE_OUTER_BOUND ( 'NONE', #20777, .T. ) ;
#38280=CARTESIAN_POINT ( 'NONE',  ( -0.3689425029237881626, 27.42874883491397142, 10.36894250292379027 ) ) ;
#38281=CARTESIAN_POINT ( 'NONE',  ( -2.266590686148945544, 56.38708216824731068, -7.082119434687050408 ) ) ;
#38282=CARTESIAN_POINT ( 'NONE',  ( 2.791683348922240793, 61.63393115100079456, 7.208316651077764092 ) ) ;
#38284=CARTESIAN_POINT ( 'NONE',  ( 19.42250999205614548, 55.98035201082150536, -5.440088680355545492 ) ) ;
#38285=CARTESIAN_POINT ( 'NONE',  ( 2.035157376598824452, 68.68868534415484817, 7.964842623401179544 ) ) ;
#38288=CARTESIAN_POINT ( 'NONE',  ( 22.81628187352647785, 61.62363466993041783, 6.195893100308588602E-16 ) ) ;
#38289=ORIENTED_EDGE ( 'NONE', *, *, #72108, .T. ) ;
#38290=CARTESIAN_POINT ( 'NONE',  ( 14.92337183194729988, 4.342264484334117824, -8.527530157486177487 ) ) ;
#38292=CARTESIAN_POINT ( 'NONE',  ( 10.00000000000000178, 18.05374883491396787, 14.16423886937410082 ) ) ;
#38293=CARTESIAN_POINT ( 'NONE',  ( 1.472469842513823179, 20.59226448433411960, -4.923371831947296329 ) ) ;
#38294=CARTESIAN_POINT ( 'NONE',  ( 10.00000000000000000, 31.81368534415483751, -10.88017736071110342 ) ) ;
#38297=VERTEX_POINT ( 'NONE', #93541 ) ;
#38298=CARTESIAN_POINT ( 'NONE',  ( 15.44008868035555793, 31.39701867748817676, -9.422509992056140149 ) ) ;
#38301=ORIENTED_EDGE ( 'NONE', *, *, #67956, .T. ) ;
#38302=CARTESIAN_POINT ( 'NONE',  ( 20.88017736071110164, 40.35535201082150536, 2.915334737309930979 ) ) ;
#38303=CARTESIAN_POINT ( 'NONE',  ( 19.89103541497709315, 55.66234555792568983, -6.479102184480829862 ) ) ;
#38305=CARTESIAN_POINT ( 'NONE',  ( 21.09922568453594849, 21.20696800326375353, 6.408140936763242479 ) ) ;
#38306=CARTESIAN_POINT ( 'NONE',  ( 1.821158202401629067, 21.16688879859529138, 6.499999999999990230 ) ) ;
#38307=CARTESIAN_POINT ( 'NONE',  ( 0.1532563361054083140, 11.00893115100078568, 1.131784320476157264E-15 ) ) ;
#38309=CARTESIAN_POINT ( 'NONE',  ( 0.1532563361054082862, 21.21726448433412315, 2.638427012816831674 ) ) ;
#38310=CARTESIAN_POINT ( 'NONE',  ( 10.00000000000000000, 26.81368534415484106, -10.88017736071110342 ) ) ;
#38312=VERTEX_POINT ( 'NONE', #72019 ) ;
#38314=CARTESIAN_POINT ( 'NONE',  ( 2.035157376598824452, 53.68868534415484817, 7.964842623401179544 ) ) ;
#38315=CARTESIAN_POINT ( 'NONE',  ( 2.603489959281584998, 6.582109641433292246, 6.499999999999998224 ) ) ;
#38316=CARTESIAN_POINT ( 'NONE',  ( 16.40814093676324603, 52.45696800326375353, -11.09922568453594671 ) ) ;
#38317=CARTESIAN_POINT ( 'NONE',  ( -0.8801773607111009756, 58.06368534415484106, 1.068504757029289695E-15 ) ) ;
#38318=CARTESIAN_POINT ( 'NONE',  ( 12.63842701281683922, 64.55059781766745175, -9.846743663894590881 ) ) ;
#38322=CARTESIAN_POINT ( 'NONE',  ( 14.92337183194729633, 37.67559781766745175, 8.527530157486181039 ) ) ;
#38323=CARTESIAN_POINT ( 'NONE',  ( 22.81628187352647785, 51.41530133659708923, 3.434112377981063169 ) ) ;
#38324=DIRECTION ( 'NONE',  ( -0.000000000000000000, -0.000000000000000000, -1.000000000000000000 ) ) ;
#38325=CARTESIAN_POINT ( 'NONE',  ( 14.92337183194729633, 12.67559781766745353, 8.527530157486181039 ) ) ;
#38326=CARTESIAN_POINT ( 'NONE',  ( -1.099225684535947600, 14.54030133659708568, 6.408140936763237150 ) ) ;
#38329=CARTESIAN_POINT ( 'NONE',  ( 10.00000000000000178, 39.31368534415484106, 10.88017736071110342 ) ) ;
#38331=CARTESIAN_POINT ( 'NONE',  ( 1.472469842513823179, 61.42559781766745175, 4.923371831947296329 ) ) ;
#38333=VECTOR ( 'NONE', #87465, 1000.000000000000000 ) ;
#38334=CARTESIAN_POINT ( 'NONE',  ( 17.20831665107776587, 19.13393115100078035, -7.208316651077762316 ) ) ;
#38335=CARTESIAN_POINT ( 'NONE',  ( 12.63842701281683034, 2.467264484334118269, 9.846743663894596210 ) ) ;
#38336=CARTESIAN_POINT ( 'NONE',  ( 12.91533473730993009, 16.60535201082150891, -10.88017736071109987 ) ) ;
#38337=CARTESIAN_POINT ( 'NONE',  ( -1.099225684535947600, 19.54030133659708568, 6.408140936763237150 ) ) ;
#38338=CARTESIAN_POINT ( 'NONE',  ( 12.63842701281683034, 57.46726448433411605, 9.846743663894596210 ) ) ;
#38340=CARTESIAN_POINT ( 'NONE',  ( 19.42250999205614548, 10.98035201082150536, -5.440088680355545492 ) ) ;
#38341=CARTESIAN_POINT ( 'NONE',  ( 2.791683348922240793, 46.63393115100077324, 7.208316651077764092 ) ) ;
#38344=CARTESIAN_POINT ( 'NONE',  ( 10.00000000000000000, 6.813685344154838397, -10.88017736071110342 ) ) ;
#38345=CARTESIAN_POINT ( 'NONE',  ( -25.69000000000001194, 93.50000000000000000, 9.500000000000000000 ) ) ;
#38346=CARTESIAN_POINT ( 'NONE',  ( 7.084665262690076126, 27.02201867748817676, -10.88017736071110164 ) ) ;
#38347=CARTESIAN_POINT ( 'NONE',  ( 24.16423886937410614, 64.51208216824728936, -3.795296366450302550 ) ) ;
#38349=CARTESIAN_POINT ( 'NONE',  ( 0.1532563361054100626, 0.8005978176674514168, -2.638427012816831230 ) ) ;
#38351=CARTESIAN_POINT ( 'NONE',  ( 1.472469842513823179, 21.42559781766745175, 4.923371831947296329 ) ) ;
#38352=CARTESIAN_POINT ( 'NONE',  ( 19.38216949554541202, 10.99863466993042138, 9.382169495545424454 ) ) ;
#38353=CARTESIAN_POINT ( 'NONE',  ( -46.94000000000001194, 103.0000000000000000, 5.997726559847112782 ) ) ;
#38355=CARTESIAN_POINT ( 'NONE',  ( 10.00000000000000000, -2.126365330069579951, -12.81628187352647608 ) ) ;
#38358=CARTESIAN_POINT ( 'NONE',  ( -2.266590686148945544, 17.22041550158063572, 7.082119434687048631 ) ) ;
#38359=CARTESIAN_POINT ( 'NONE',  ( 18.52753015748617571, 28.09226448433411960, 4.923371831947298993 ) ) ;
#38360=CARTESIAN_POINT ( 'NONE',  ( 20.36894250292379738, 54.92874883491396076, -10.36894250292379027 ) ) ;
#38361=CARTESIAN_POINT ( 'NONE',  ( 7.361572987183170547, 12.05059781766744997, 9.846743663894590881 ) ) ;
#38363=CARTESIAN_POINT ( 'NONE',  ( 4.559911319644449179, 27.23035201082150536, -9.422509992056141925 ) ) ;
#38364=CARTESIAN_POINT ( 'NONE',  ( 6.565887622018943937, 50.16530133659708213, 12.81628187352647430 ) ) ;
#38365=CARTESIAN_POINT ( 'NONE',  ( 7.084665262690076126, 22.02201867748817321, -10.88017736071110164 ) ) ;
#38366=CARTESIAN_POINT ( 'NONE',  ( 10.00000000000000178, 45.37363466993041783, 12.81628187352647608 ) ) ;
#38367=CARTESIAN_POINT ( 'NONE',  ( 1.472469842513823179, 66.42559781766745175, 4.923371831947296329 ) ) ;
#38368=ORIENTED_EDGE ( 'NONE', *, *, #27143, .T. ) ;
#38370=CARTESIAN_POINT ( 'NONE',  ( 10.00000000000000000, 35.55374883491396787, -14.16423886937410082 ) ) ;
#38371=CARTESIAN_POINT ( 'NONE',  ( -2.266590686148945544, 12.22041550158063394, 7.082119434687048631 ) ) ;
#38372=CARTESIAN_POINT ( 'NONE',  ( -0.8801773607111009756, 8.063685344154837509, 1.068504757029289695E-15 ) ) ;
#38373=CARTESIAN_POINT ( 'NONE',  ( 7.084665262690076126, 39.10535201082150536, 10.88017736071109987 ) ) ;
#38374=CARTESIAN_POINT ( 'NONE',  ( 18.72515096720572458, 40.05509018479936145, 6.499999999999964473 ) ) ;
#38376=CARTESIAN_POINT ( 'NONE',  ( 17.96484262340118221, 64.93868534415483396, 7.964842623401181321 ) ) ;
#38377=CARTESIAN_POINT ( 'NONE',  ( 0.5774900079438607392, 68.48035201082150536, 5.440088680355550821 ) ) ;
#38378=CARTESIAN_POINT ( 'NONE',  ( 21.09922568453594849, 31.20696800326375353, 6.408140936763242479 ) ) ;
#38379=LINE ( 'NONE', #70354, #89009 ) ;
#38381=CARTESIAN_POINT ( 'NONE',  ( 5.076628168052704559, 40.17559781766745175, -8.527530157486179263 ) ) ;
#38383=CARTESIAN_POINT ( 'NONE',  ( -0.8801773607111009756, 18.06368534415484106, 1.068504757029289695E-15 ) ) ;
#38385=CARTESIAN_POINT ( 'NONE',  ( 3.591859063236763294, 13.29030133659708746, -11.09922568453595026 ) ) ;
#38386=CARTESIAN_POINT ( 'NONE',  ( 1.472469842513823179, 11.42559781766745175, 4.923371831947296329 ) ) ;
#38387=CARTESIAN_POINT ( 'NONE',  ( 15.44008868035555793, 11.39701867748817143, -9.422509992056140149 ) ) ;
#38388=CARTESIAN_POINT ( 'NONE',  ( 14.92337183194729633, 37.67559781766745175, 8.527530157486181039 ) ) ;
#38389=CARTESIAN_POINT ( 'NONE',  ( 21.09922568453594849, 61.20696800326376064, 6.408140936763242479 ) ) ;
#38390=CARTESIAN_POINT ( 'NONE',  ( 7.361572987183170547, 37.05059781766744464, 9.846743663894590881 ) ) ;
#38391=CARTESIAN_POINT ( 'NONE',  ( 10.00000000000000000, 0.5537488349139675359, -14.16423886937410082 ) ) ;
#38392=CARTESIAN_POINT ( 'NONE',  ( 13.79529636645030344, 18.26208216824730002, 14.16423886937410614 ) ) ;
#38394=CARTESIAN_POINT ( 'NONE',  ( 7.084665262690076126, 29.10535201082150181, 10.88017736071109987 ) ) ;
#38395=CARTESIAN_POINT ( 'NONE',  ( 4.559911319644449179, 8.897018677488171434, 9.422509992056141925 ) ) ;
#38396=CARTESIAN_POINT ( 'NONE',  ( 24.16423886937409904, 39.09541550158062506, 3.795296366450317205 ) ) ;
#38397=CARTESIAN_POINT ( 'NONE',  ( 10.00000000000000000, 36.81368534415484106, -10.88017736071110342 ) ) ;
#38398=CARTESIAN_POINT ( 'NONE',  ( 20.88017736071110519, 15.56368534415483751, 2.639326808657452039E-16 ) ) ;
#38402=CARTESIAN_POINT ( 'NONE',  ( 19.42250999205614548, 45.98035201082150536, -5.440088680355545492 ) ) ;
#38403=CARTESIAN_POINT ( 'NONE',  ( 21.09922568453595559, 62.04030133659709634, -6.408140936763230044 ) ) ;
#38404=CARTESIAN_POINT ( 'NONE',  ( 15.44008868035555793, 41.39701867748817676, -9.422509992056140149 ) ) ;
#38405=CARTESIAN_POINT ( 'NONE',  ( 7.084665262690076126, 52.02201867748816255, -10.88017736071110164 ) ) ;
#38407=CARTESIAN_POINT ( 'NONE',  ( 10.00000000000000178, 44.31368534415484106, 10.88017736071110342 ) ) ;
#38409=( LENGTH_UNIT ( ) NAMED_UNIT ( * ) SI_UNIT ( .MILLI., .METRE. ) );
#38411=CARTESIAN_POINT ( 'NONE',  ( 10.00000000000000000, 50.55374883491396787, -14.16423886937410082 ) ) ;
#38412=CARTESIAN_POINT ( 'NONE',  ( 1.472469842513823179, 0.5922644843341181575, -4.923371831947296329 ) ) ;
#38414=ADVANCED_FACE ( 'NONE', ( #21998 ), #75472, .T. ) ;
#38415=FILL_AREA_STYLE ('',( #8886 ) ) ;
#38416=CARTESIAN_POINT ( 'NONE',  ( 17.20831665107776587, 62.88393115100078745, 7.208316651077764980 ) ) ;
#38418=CARTESIAN_POINT ( 'NONE',  ( 17.20831665107776587, 37.88393115100078745, 7.208316651077764980 ) ) ;
#38419=ORIENTED_EDGE ( 'NONE', *, *, #26094, .F. ) ;
#38420=CARTESIAN_POINT ( 'NONE',  ( 19.84674366389459621, 33.50893115100078745, 7.409399052514197653E-17 ) ) ;
#38422=CARTESIAN_POINT ( 'NONE',  ( 2.035157376598824452, 43.68868534415484106, 7.964842623401179544 ) ) ;
#38423=CARTESIAN_POINT ( 'NONE',  ( 19.84674366389459621, 33.50893115100078745, 7.409399052514197653E-17 ) ) ;
#38424=CARTESIAN_POINT ( 'NONE',  ( 3.591859063236761518, 19.95696800326375353, 11.09922568453594849 ) ) ;
#38425=DIRECTION ( 'NONE',  ( 0.000000000000000000, 0.000000000000000000, -1.000000000000000000 ) ) ;
#38426=CARTESIAN_POINT ( 'NONE',  ( 0.5774900079438607392, 53.48035201082151247, 5.440088680355550821 ) ) ;
#38427=CARTESIAN_POINT ( 'NONE',  ( 19.42250999205614548, 45.98035201082150536, -5.440088680355545492 ) ) ;
#38428=CARTESIAN_POINT ( 'NONE',  ( 6.204703633549690345, 60.76208216824730357, -14.16423886937410259 ) ) ;
#38430=CARTESIAN_POINT ( 'NONE',  ( 13.43411237798106583, 17.66530133659708923, -12.81628187352647252 ) ) ;
#38433=CARTESIAN_POINT ( 'NONE',  ( 22.81628187352647785, 16.62363466993042138, 6.195893100308588602E-16 ) ) ;
#38434=CARTESIAN_POINT ( 'NONE',  ( 20.88017736071110875, 15.77201867748817143, -2.915334737309920765 ) ) ;
#38435=CARTESIAN_POINT ( 'NONE',  ( 10.00000000000000000, 56.81368534415484106, -10.88017736071110342 ) ) ;
#38439=CARTESIAN_POINT ( 'NONE',  ( 20.88017736071110519, 65.56368534415483396, 2.639326808657452039E-16 ) ) ;
#38440=CARTESIAN_POINT ( 'NONE',  ( 17.20831665107776587, 54.13393115100079456, -7.208316651077762316 ) ) ;
#38441=CARTESIAN_POINT ( 'NONE',  ( 2.791683348922237240, 40.38393115100078035, -7.208316651077763204 ) ) ;
#38442=CARTESIAN_POINT ( 'NONE',  ( 19.84674366389459266, 23.71726448433412315, -2.638427012816827677 ) ) ;
#38443=CARTESIAN_POINT ( 'NONE',  ( -0.1023957841222409432, 40.13377557478296609, 6.340343622311920058 ) ) ;
#38445=CARTESIAN_POINT ( 'NONE',  ( 10.00000000000000000, 37.87363466993041783, -12.81628187352647608 ) ) ;
#38446=CARTESIAN_POINT ( 'NONE',  ( 7.361572987183169658, 9.967264484334119601, -9.846743663894592657 ) ) ;
#38449=CARTESIAN_POINT ( 'NONE',  ( 7.361572987183170547, 47.05059781766745175, 9.846743663894590881 ) ) ;
#38453=B_SPLINE_CURVE_WITH_KNOTS ( 'NONE', 3,
 ( #46696, #63653, #33644, #17695, #71183, #8700 ),
 .UNSPECIFIED., .F., .F.,
 ( 4, 2, 4 ),
 ( 0.000000000000000000, 0.0002565770811490921863, 0.0005131541622981843727 ),
 .UNSPECIFIED. ) ;
#38454=CARTESIAN_POINT ( 'NONE',  ( 6.565887622018943937, 13.08196800326374998, -12.81628187352647608 ) ) ;
#38455=CARTESIAN_POINT ( 'NONE',  ( -0.8801773607110991993, 52.85535201082151247, -2.915334737309923874 ) ) ;
#38456=CARTESIAN_POINT ( 'NONE',  ( 2.917880565312950480, 35.97041550158063217, -12.26659068614894821 ) ) ;
#38460=CARTESIAN_POINT ( 'NONE',  ( 2.917880565312948704, 27.63708216824730357, 12.26659068614894643 ) ) ;
#38462=CARTESIAN_POINT ( 'NONE',  ( 10.00000000000000000, 60.55374883491397497, -14.16423886937410082 ) ) ;
#38463=CARTESIAN_POINT ( 'NONE',  ( 17.08211943468705840, 10.13708216824730179, -12.26659068614894466 ) ) ;
#38464=CARTESIAN_POINT ( 'NONE',  ( -0.3689425029237898834, 31.17874883491396787, -10.36894250292378850 ) ) ;
#38466=CARTESIAN_POINT ( 'NONE',  ( 15.44008868035555260, 64.73035201082151957, 9.422509992056143702 ) ) ;
#38467=CARTESIAN_POINT ( 'NONE',  ( 20.10493008474206178, 24.71697413083879624, 6.336235997365763595 ) ) ;
#38469=CARTESIAN_POINT ( 'NONE',  ( 17.20831665107776587, 37.88393115100078745, 7.208316651077764980 ) ) ;
#38470=AXIS2_PLACEMENT_3D ( 'NONE', #21194, #49699, #97216 ) ;
#38471=CARTESIAN_POINT ( 'NONE',  ( 4.559911319644449179, 22.23035201082150536, -9.422509992056141925 ) ) ;
#38472=CARTESIAN_POINT ( 'NONE',  ( 17.39651004071838969, 44.08210964143329846, -6.500000000000027534 ) ) ;
#38473=CARTESIAN_POINT ( 'NONE',  ( 0.1532563361054082862, 66.21726448433413736, 2.638427012816831674 ) ) ;
#38474=CARTESIAN_POINT ( 'NONE',  ( 20.00000000000000711, 85.76239730488823909, -5.246947360776204050 ) ) ;
#38475=CARTESIAN_POINT ( 'NONE',  ( 14.92337183194729633, 37.67559781766745175, 8.527530157486181039 ) ) ;
#38476=CARTESIAN_POINT ( 'NONE',  ( 13.43411237798105340, 60.58196800326376064, 12.81628187352647963 ) ) ;
#38478=CARTESIAN_POINT ( 'NONE',  ( 10.00000000000000178, 42.25893115100078745, 9.846743663894594434 ) ) ;
#38479=CARTESIAN_POINT ( 'NONE',  ( 17.20831665107776587, 54.13393115100079456, -7.208316651077762316 ) ) ;
#38480=CARTESIAN_POINT ( 'NONE',  ( 22.26659068614895176, 39.72041550158063217, -7.082119434687042414 ) ) ;
#38482=CARTESIAN_POINT ( 'NONE',  ( 13.79529636645031943, 20.34541550158063572, -14.16423886937409904 ) ) ;
#38483=CARTESIAN_POINT ( 'NONE',  ( 0.5774900079438590739, 57.64701867748817676, -5.440088680355550821 ) ) ;
#38485=CARTESIAN_POINT ( 'NONE',  ( -0.3689425029237881626, 57.42874883491397497, 10.36894250292379027 ) ) ;
#38486=CARTESIAN_POINT ( 'NONE',  ( 21.09922568453594849, 16.20696800326375353, 6.408140936763242479 ) ) ;
#38488=CARTESIAN_POINT ( 'NONE',  ( 7.084665262690076126, 62.02201867748816966, -10.88017736071110164 ) ) ;
#38489=DIRECTION ( 'NONE',  ( 0.000000000000000000, -1.000000000000000000, 0.000000000000000000 ) ) ;
#38490=CARTESIAN_POINT ( 'NONE',  ( -46.94000000000000483, 100.7316555907688809, -8.991040189367279112 ) ) ;
#38491=CARTESIAN_POINT ( 'NONE',  ( -4.164238869374098151, 56.59541550158063927, -3.795296366450310543 ) ) ;
#38492=CARTESIAN_POINT ( 'NONE',  ( 4.559911319644449179, 32.23035201082150536, -9.422509992056141925 ) ) ;
#38493=CARTESIAN_POINT ( 'NONE',  ( 0.5774900079438607392, 28.48035201082150891, 5.440088680355550821 ) ) ;
#38494=CARTESIAN_POINT ( 'NONE',  ( 0.1532563361054083140, 51.00893115100078745, 1.131784320476157264E-15 ) ) ;
#38495=CARTESIAN_POINT ( 'NONE',  ( 19.84674366389459621, 48.50893115100078745, 7.409399052514197653E-17 ) ) ;
#38496=CARTESIAN_POINT ( 'NONE',  ( -1.099225684535947600, 53.70696800326376064, -6.408140936763238038 ) ) ;
#38497=ORIENTED_EDGE ( 'NONE', *, *, #92478, .F. ) ;
#38500=CARTESIAN_POINT ( 'NONE',  ( 10.00000000000000178, 19.31368534415484106, 10.88017736071110342 ) ) ;
#38501=CARTESIAN_POINT ( 'NONE',  ( 21.09922568453595559, 17.04030133659708923, -6.408140936763230044 ) ) ;
#38503=CARTESIAN_POINT ( 'NONE',  ( 14.92337183194729633, 47.67559781766745175, 8.527530157486181039 ) ) ;
#38504=CARTESIAN_POINT ( 'NONE',  ( 2.035157376598824452, 48.68868534415483396, 7.964842623401179544 ) ) ;
#38505=CARTESIAN_POINT ( 'NONE',  ( 10.00000000000000000, 22.87363466993042138, -12.81628187352647608 ) ) ;
#38506=CARTESIAN_POINT ( 'NONE',  ( 7.084665262690076126, 44.10535201082151247, 10.88017736071109987 ) ) ;
#38509=CARTESIAN_POINT ( 'NONE',  ( -1.099225684535947600, 53.70696800326376064, -6.408140936763238038 ) ) ;
#38512=CARTESIAN_POINT ( 'NONE',  ( 15.44008868035555260, 44.73035201082151247, 9.422509992056143702 ) ) ;
#38513=CARTESIAN_POINT ( 'NONE',  ( 6.565887622018943937, 50.16530133659708213, 12.81628187352647430 ) ) ;
#38514=CARTESIAN_POINT ( 'NONE',  ( 22.26659068614895176, 19.72041550158063572, -7.082119434687042414 ) ) ;
#38515=CARTESIAN_POINT ( 'NONE',  ( 19.84674366389459266, 8.300597817667451750, 2.638427012816836559 ) ) ;
#38516=CARTESIAN_POINT ( 'NONE',  ( 0.1532563361054083140, 61.00893115100078745, 1.131784320476157264E-15 ) ) ;
#38517=CARTESIAN_POINT ( 'NONE',  ( 18.52753015748618282, 33.92559781766745886, -4.923371831947291888 ) ) ;
#38518=CARTESIAN_POINT ( 'NONE',  ( 5.076628168052704559, 10.17559781766745175, -8.527530157486179263 ) ) ;
#38520=CARTESIAN_POINT ( 'NONE',  ( -4.164238869374098151, 46.59541550158063927, -3.795296366450310543 ) ) ;
#38523=CARTESIAN_POINT ( 'NONE',  ( 15.44008868035555260, 4.730352010821504471, 9.422509992056143702 ) ) ;
#38527=CARTESIAN_POINT ( 'NONE',  ( -0.8801773607110991993, 12.85535201082150358, -2.915334737309923874 ) ) ;
#38528=CARTESIAN_POINT ( 'NONE',  ( 17.96484262340118221, 11.18868534415484106, -7.964842623401177768 ) ) ;
#38530=CARTESIAN_POINT ( 'NONE',  ( 10.00000000000000178, 42.25893115100078745, 9.846743663894594434 ) ) ;
#38531=CARTESIAN_POINT ( 'NONE',  ( 21.09922568453595559, 42.04030133659708213, -6.408140936763230044 ) ) ;
#38533=CARTESIAN_POINT ( 'NONE',  ( -4.164238869374099927, 12.01208216824730357, 3.795296366450308767 ) ) ;
#38534=CARTESIAN_POINT ( 'NONE',  ( 0.5774900079438590739, 32.64701867748816966, -5.440088680355550821 ) ) ;
#38535=CARTESIAN_POINT ( 'NONE',  ( 0.5774900079438607392, 3.480352010821504916, 5.440088680355550821 ) ) ;
#38536=CARTESIAN_POINT ( 'NONE',  ( 10.00000000000000178, 42.25893115100078745, 9.846743663894594434 ) ) ;
#38539=CARTESIAN_POINT ( 'NONE',  ( 5.076628168052703671, 26.84226448433411960, 8.527530157486179263 ) ) ;
#38541=CARTESIAN_POINT ( 'NONE',  ( -0.8801773607110990882, 32.85535201082150536, -2.915334737309924318 ) ) ;
#38545=VERTEX_POINT ( 'NONE', #89979 ) ;
#38546=CARTESIAN_POINT ( 'NONE',  ( 19.84674366389459266, 53.30059781766744464, 2.638427012816836559 ) ) ;
#38547=CARTESIAN_POINT ( 'NONE',  ( 17.96484262340118221, 34.93868534415482685, 7.964842623401181321 ) ) ;
#38548=CARTESIAN_POINT ( 'NONE',  ( 2.035157376598822676, 32.43868534415483396, -7.964842623401177768 ) ) ;
#38549=CARTESIAN_POINT ( 'NONE',  ( 0.5774900079438590739, 2.647018677488170990, -5.440088680355550821 ) ) ;
#38550=CARTESIAN_POINT ( 'NONE',  ( -2.816281873526471635, 28.91530133659708213, -3.434112377981056508 ) ) ;
#38551=CARTESIAN_POINT ( 'NONE',  ( 13.79529636645030344, 18.26208216824730002, 14.16423886937410614 ) ) ;
#38553=CARTESIAN_POINT ( 'NONE',  ( 19.38216949554541557, 47.24863466993041783, -9.382169495545420901 ) ) ;
#38555=CARTESIAN_POINT ( 'NONE',  ( 14.92337183194729988, 44.34226448433412315, -8.527530157486177487 ) ) ;
#38556=CARTESIAN_POINT ( 'NONE',  ( 20.88017736071110519, 25.56368534415483751, 2.639326808657452039E-16 ) ) ;
#38558=CARTESIAN_POINT ( 'NONE',  ( 4.559911319644449179, 13.89701867748817321, 9.422509992056141925 ) ) ;
#38559=ORIENTED_EDGE ( 'NONE', *, *, #90955, .T. ) ;
#38560=CARTESIAN_POINT ( 'NONE',  ( 4.559911319644449179, 57.23035201082150536, -9.422509992056141925 ) ) ;
#38561=CARTESIAN_POINT ( 'NONE',  ( 7.084665262690076126, 64.10535201082150536, 10.88017736071109987 ) ) ;
#38562=CARTESIAN_POINT ( 'NONE',  ( 14.92337183194729633, 12.67559781766745353, 8.527530157486181039 ) ) ;
#38563=CARTESIAN_POINT ( 'NONE',  ( 2.035157376598824452, 48.68868534415483396, 7.964842623401179544 ) ) ;
#38566=CARTESIAN_POINT ( 'NONE',  ( 0.1532563361054100626, 10.80059781766745175, -2.638427012816831230 ) ) ;
#38569=( GEOMETRIC_REPRESENTATION_CONTEXT ( 3 ) GLOBAL_UNCERTAINTY_ASSIGNED_CONTEXT ( ( #96288 ) ) GLOBAL_UNIT_ASSIGNED_CONTEXT ( ( #43868, #44372, #6370 ) ) REPRESENTATION_CONTEXT ( 'NONE', 'WORKASPACE' ) );
#38570=CARTESIAN_POINT ( 'NONE',  ( 1.472469842513823179, 41.42559781766745886, 4.923371831947296329 ) ) ;
#38572=FACE_OUTER_BOUND ( 'NONE', #21958, .T. ) ;
#38573=CARTESIAN_POINT ( 'NONE',  ( 0.000000000000000000, 0.5000000000000000000, -6.500000000000000888 ) ) ;
#38574=CARTESIAN_POINT ( 'NONE',  ( 13.79529636645030344, 18.26208216824730002, 14.16423886937410614 ) ) ;
#38575=CARTESIAN_POINT ( 'NONE',  ( -0.3289641300568009741, 7.245456701841137992, -5.963430220938281678 ) ) ;
#38576=CARTESIAN_POINT ( 'NONE',  ( 19.39235739573468820, 9.875764716086008477, 6.500000000000000000 ) ) ;
#38577=CARTESIAN_POINT ( 'NONE',  ( 19.42250999205614548, 10.98035201082150536, -5.440088680355545492 ) ) ;
#38579=CARTESIAN_POINT ( 'NONE',  ( 10.00000000000000178, 40.37363466993042493, 12.81628187352647608 ) ) ;
#38580=VERTEX_POINT ( 'NONE', #30453 ) ;
#38581=CARTESIAN_POINT ( 'NONE',  ( 19.84674366389459266, 3.300597817667451750, 2.638427012816836559 ) ) ;
#38582=CARTESIAN_POINT ( 'NONE',  ( 5.076628168052704559, 0.1755978176674514724, -8.527530157486179263 ) ) ;
#38583=CARTESIAN_POINT ( 'NONE',  ( 21.09922568453595559, 32.04030133659708923, -6.408140936763230044 ) ) ;
#38584=CARTESIAN_POINT ( 'NONE',  ( 17.20831665107776587, 17.88393115100078745, 7.208316651077764980 ) ) ;
#38586=CARTESIAN_POINT ( 'NONE',  ( 17.20831665107776587, 19.13393115100078035, -7.208316651077762316 ) ) ;
#38587=CARTESIAN_POINT ( 'NONE',  ( 13.43411237798106583, 12.66530133659708746, -12.81628187352647252 ) ) ;
#38590=CARTESIAN_POINT ( 'NONE',  ( 12.63842701281683034, 7.467264484334118713, 9.846743663894596210 ) ) ;
#38593=CARTESIAN_POINT ( 'NONE',  ( -0.8801773607111008646, 23.27201867748817676, 2.915334737309923430 ) ) ;
#38594=CARTESIAN_POINT ( 'NONE',  ( 13.79529636645031943, 20.34541550158063572, -14.16423886937409904 ) ) ;
#38595=CARTESIAN_POINT ( 'NONE',  ( 2.791683348922237240, 40.38393115100078035, -7.208316651077763204 ) ) ;
#38596=CARTESIAN_POINT ( 'NONE',  ( 7.361572987183170547, 2.050597817667451750, 9.846743663894590881 ) ) ;
#38597=CARTESIAN_POINT ( 'NONE',  ( 22.81628187352647785, 46.41530133659708213, 3.434112377981063169 ) ) ;
#38599=CARTESIAN_POINT ( 'NONE',  ( 20.88017736071110519, 30.56368534415484106, 2.639326808657452039E-16 ) ) ;
#38601=CARTESIAN_POINT ( 'NONE',  ( -2.816281873526473856, 14.12363466993041961, 9.499525473075851096E-16 ) ) ;
#38602=CARTESIAN_POINT ( 'NONE',  ( 0.1532563361054082862, 31.21726448433412315, 2.638427012816831674 ) ) ;
#38604=CARTESIAN_POINT ( 'NONE',  ( -1.099225684535947600, 53.70696800326376064, -6.408140936763238038 ) ) ;
#38605=VECTOR ( 'NONE', #59088, 1000.000000000000000 ) ;
#38606=CARTESIAN_POINT ( 'NONE',  ( 0.5774900079438607392, 53.48035201082151247, 5.440088680355550821 ) ) ;
#38611=CARTESIAN_POINT ( 'NONE',  ( 0.5774900079438590739, 37.64701867748817676, -5.440088680355550821 ) ) ;
#38612=CARTESIAN_POINT ( 'NONE',  ( 12.91533473730992121, 49.52201867748817676, 10.88017736071110164 ) ) ;
#38613=CARTESIAN_POINT ( 'NONE',  ( 17.20831665107776587, 64.13393115100079456, -7.208316651077762316 ) ) ;
#38614=CARTESIAN_POINT ( 'NONE',  ( 17.96484262340118221, 64.93868534415483396, 7.964842623401181321 ) ) ;
#38615=CARTESIAN_POINT ( 'NONE',  ( 2.791683348922240793, 51.63393115100078745, 7.208316651077764092 ) ) ;
#38616=CARTESIAN_POINT ( 'NONE',  ( 10.00000000000000000, 11.81368534415483751, -10.88017736071110342 ) ) ;
#38618=CARTESIAN_POINT ( 'NONE',  ( -2.816281873526473856, 9.331968003263753531, 3.434112377981055619 ) ) ;
#38619=EDGE_LOOP ( 'NONE', ( #57763, #29662, #8173, #35596 ) ) ;
#38620=CARTESIAN_POINT ( 'NONE',  ( 0.5774900079438590739, 37.64701867748817676, -5.440088680355550821 ) ) ;
#38621=CARTESIAN_POINT ( 'NONE',  ( -2.816281873526471635, 3.915301336597087456, -3.434112377981056508 ) ) ;
#38623=CARTESIAN_POINT ( 'NONE',  ( -0.8801773607111008646, 13.27201867748817143, 2.915334737309923430 ) ) ;
#38624=CARTESIAN_POINT ( 'NONE',  ( -0.8801773607110991993, 22.85535201082150181, -2.915334737309923874 ) ) ;
#38625=CARTESIAN_POINT ( 'NONE',  ( 20.36894250292379382, 38.67874883491396076, 10.36894250292379205 ) ) ;
#38626=CARTESIAN_POINT ( 'NONE',  ( 19.84674366389459266, 33.71726448433410894, -2.638427012816827677 ) ) ;
#38627=CARTESIAN_POINT ( 'NONE',  ( 15.44008868035555793, 46.39701867748817676, -9.422509992056140149 ) ) ;
#38629=CARTESIAN_POINT ( 'NONE',  ( -0.3689425029237881626, 7.428748834913967869, 10.36894250292379027 ) ) ;
#38631=CARTESIAN_POINT ( 'NONE',  ( 17.20831665107776587, 59.13393115100078745, -7.208316651077762316 ) ) ;
#38635=CARTESIAN_POINT ( 'NONE',  ( 17.08211943468705840, 30.13708216824730357, -12.26659068614894466 ) ) ;
#38636=CARTESIAN_POINT ( 'NONE',  ( -4.164238869374099039, 31.80374883491396432, 8.674139862899312516E-16 ) ) ;
#38638=CARTESIAN_POINT ( 'NONE',  ( 1.472469842513823179, 6.425597817667451750, 4.923371831947296329 ) ) ;
#38639=CARTESIAN_POINT ( 'NONE',  ( 19.84674366389459266, 63.71726448433412315, -2.638427012816827677 ) ) ;
#38641=CARTESIAN_POINT ( 'NONE',  ( 20.88017736071110164, 65.35535201082150536, 2.915334737309930979 ) ) ;
#38642=CARTESIAN_POINT ( 'NONE',  ( 16.40814093676323893, 15.79030133659708746, 11.09922568453595026 ) ) ;
#38643=CARTESIAN_POINT ( 'NONE',  ( -4.164238869374099927, 32.01208216824730357, 3.795296366450308767 ) ) ;
#38644=CARTESIAN_POINT ( 'NONE',  ( 7.084665262690076126, 19.10535201082150181, 10.88017736071109987 ) ) ;
#38645=CARTESIAN_POINT ( 'NONE',  ( 20.88017736071110519, 30.56368534415484106, 2.639326808657452039E-16 ) ) ;
#38647=CARTESIAN_POINT ( 'NONE',  ( 7.084665262690076126, 59.10535201082150536, 10.88017736071109987 ) ) ;
#38650=FILL_AREA_STYLE ('',( #8158 ) ) ;
#38652=CARTESIAN_POINT ( 'NONE',  ( -1.926860441876564023, 12.87045670184114066, 3.195792623639529761 ) ) ;
#38655=CARTESIAN_POINT ( 'NONE',  ( 6.204703633549690345, 55.76208216824730357, -14.16423886937410259 ) ) ;
#38656=CARTESIAN_POINT ( 'NONE',  ( 22.26659068614895176, 64.72041550158064638, -7.082119434687042414 ) ) ;
#38657=CARTESIAN_POINT ( 'NONE',  ( 5.076628168052704559, 20.17559781766745175, -8.527530157486179263 ) ) ;
#38658=CARTESIAN_POINT ( 'NONE',  ( 2.791683348922240793, 56.63393115100078035, 7.208316651077764092 ) ) ;
#38661=CARTESIAN_POINT ( 'NONE',  ( 18.52753015748618282, 8.925597817667451750, -4.923371831947291888 ) ) ;
#38662=MECHANICAL_DESIGN_GEOMETRIC_PRESENTATION_REPRESENTATION('',(#97775),#27504);
#38663=CARTESIAN_POINT ( 'NONE',  ( 19.38216949554541202, 0.9986346699304200492, 9.382169495545424454 ) ) ;
#38665=ORIENTED_EDGE ( 'NONE', *, *, #40774, .T. ) ;
#38667=CARTESIAN_POINT ( 'NONE',  ( 6.204703633549690345, 30.76208216824730357, -14.16423886937410259 ) ) ;
#38670=CARTESIAN_POINT ( 'NONE',  ( 13.79529636645030344, 48.26208216824728936, 14.16423886937410614 ) ) ;
#38672=CARTESIAN_POINT ( 'NONE',  ( 22.81628187352647785, 56.41530133659708213, 3.434112377981063169 ) ) ;
#38675=CARTESIAN_POINT ( 'NONE',  ( 5.076628168052704559, 50.17559781766745886, -8.527530157486179263 ) ) ;
#38676=CARTESIAN_POINT ( 'NONE',  ( 0.5774900079438607392, 23.48035201082150536, 5.440088680355550821 ) ) ;
#38679=CARTESIAN_POINT ( 'NONE',  ( 18.52753015748617571, 53.09226448433412315, 4.923371831947298993 ) ) ;
#38680=CARTESIAN_POINT ( 'NONE',  ( 10.00000000000000000, 54.75893115100078745, -9.846743663894594434 ) ) ;
#38684=CARTESIAN_POINT ( 'NONE',  ( 5.076628168052703671, 6.842264484334118713, 8.527530157486179263 ) ) ;
#38686=ORIENTED_EDGE ( 'NONE', *, *, #85357, .F. ) ;
#38689=CARTESIAN_POINT ( 'NONE',  ( 14.92337183194729988, 34.34226448433411605, -8.527530157486177487 ) ) ;
#38691=CARTESIAN_POINT ( 'NONE',  ( 19.38216949554541557, 42.24863466993041783, -9.382169495545420901 ) ) ;
#38694=FACE_OUTER_BOUND ( 'NONE', #13458, .T. ) ;
#38696=CARTESIAN_POINT ( 'NONE',  ( 12.63842701281683922, 54.55059781766745175, -9.846743663894590881 ) ) ;
#38697=CARTESIAN_POINT ( 'NONE',  ( 10.00000000000000000, 35.55374883491396787, -14.16423886937410082 ) ) ;
#38698=CARTESIAN_POINT ( 'NONE',  ( 19.84674366389459621, 58.50893115100078745, 7.409399052514197653E-17 ) ) ;
#38700=CARTESIAN_POINT ( 'NONE',  ( 7.361572987183169658, 24.96726448433412315, -9.846743663894592657 ) ) ;
#38701=CARTESIAN_POINT ( 'NONE',  ( 0.6178305044545818747, 48.49863466993042493, -9.382169495545419124 ) ) ;
#38702=CARTESIAN_POINT ( 'NONE',  ( 17.08211943468705130, 3.470415501580634388, 12.26659068614894998 ) ) ;
#38703=CARTESIAN_POINT ( 'NONE',  ( 14.92337183194729633, 57.67559781766745886, 8.527530157486181039 ) ) ;
#38704=CARTESIAN_POINT ( 'NONE',  ( 17.96484262340118221, 51.18868534415483396, -7.964842623401177768 ) ) ;
#38705=CARTESIAN_POINT ( 'NONE',  ( 12.63842701281683034, 42.46726448433412315, 9.846743663894596210 ) ) ;
#38708=CARTESIAN_POINT ( 'NONE',  ( 10.00000000000000178, 59.31368534415484106, 10.88017736071110342 ) ) ;
#38711=CARTESIAN_POINT ( 'NONE',  ( -0.8801773607110991993, 27.85535201082150181, -2.915334737309923874 ) ) ;
#38712=CARTESIAN_POINT ( 'NONE',  ( 19.38216949554541557, 2.248634669930420049, -9.382169495545420901 ) ) ;
#38713=CARTESIAN_POINT ( 'NONE',  ( -0.8801773607111009756, 58.06368534415484106, 1.068504757029289695E-15 ) ) ;
#38715=CARTESIAN_POINT ( 'NONE',  ( 19.72487221294570858, 10.71833443783938655, -6.500000000000000888 ) ) ;
#38716=FACE_OUTER_BOUND ( 'NONE', #41168, .T. ) ;
#38717=CARTESIAN_POINT ( 'NONE',  ( 0.5774900079438607392, 43.48035201082151247, 5.440088680355550821 ) ) ;
#38719=CARTESIAN_POINT ( 'NONE',  ( 1.472469842513823179, 31.42559781766745530, 4.923371831947296329 ) ) ;
#38720=SURFACE_STYLE_USAGE ( .BOTH. , #31198 ) ;
#38722=CARTESIAN_POINT ( 'NONE',  ( 5.076628168052703671, 61.84226448433412315, 8.527530157486179263 ) ) ;
#38723=CARTESIAN_POINT ( 'NONE',  ( 15.44008868035555260, 19.73035201082150536, 9.422509992056143702 ) ) ;
#38724=CARTESIAN_POINT ( 'NONE',  ( 19.88565890683628368, 27.71691075486304001, -6.480892540919854561 ) ) ;
#38725=CARTESIAN_POINT ( 'NONE',  ( 20.36894250292379382, 23.67874883491397142, 10.36894250292379205 ) ) ;
#38727=CARTESIAN_POINT ( 'NONE',  ( 13.79529636645031943, 60.34541550158063927, -14.16423886937409904 ) ) ;
#38728=CARTESIAN_POINT ( 'NONE',  ( 17.20831665107776587, 34.13393115100078745, -7.208316651077762316 ) ) ;
#38729=CARTESIAN_POINT ( 'NONE',  ( 5.076628168052703671, 11.84226448433411960, 8.527530157486179263 ) ) ;
#38730=CARTESIAN_POINT ( 'NONE',  ( 2.035157376598824452, 3.688685344154837953, 7.964842623401179544 ) ) ;
#38732=CARTESIAN_POINT ( 'NONE',  ( 19.84674366389459266, 23.71726448433412315, -2.638427012816827677 ) ) ;
#38733=CARTESIAN_POINT ( 'NONE',  ( 15.44008868035555260, 24.73035201082150891, 9.422509992056143702 ) ) ;
#38734=CARTESIAN_POINT ( 'NONE',  ( 7.361572987183170547, 57.05059781766744464, 9.846743663894590881 ) ) ;
#38735=CARTESIAN_POINT ( 'NONE',  ( 13.79529636645030344, 3.262082168247301350, 14.16423886937410614 ) ) ;
#38736=LINE ( 'NONE', #84727, #53514 ) ;
#38738=VECTOR ( 'NONE', #39794, 1000.000000000000000 ) ;
#38740=CARTESIAN_POINT ( 'NONE',  ( 17.20831665107776587, 9.133931151000787452, -7.208316651077762316 ) ) ;
#38741=CARTESIAN_POINT ( 'NONE',  ( -2.816281873526473856, 44.33196800326375353, 3.434112377981055619 ) ) ;
#38742=CARTESIAN_POINT ( 'NONE',  ( 5.076628168052704559, 35.17559781766745175, -8.527530157486179263 ) ) ;
#38744=CARTESIAN_POINT ( 'NONE',  ( 19.84674366389459621, 18.50893115100078745, 7.409399052514197653E-17 ) ) ;
#38747=CARTESIAN_POINT ( 'NONE',  ( 10.00000000000000178, 53.05374883491396787, 14.16423886937410082 ) ) ;
#38748=CARTESIAN_POINT ( 'NONE',  ( 7.084665262690076126, 54.10535201082151247, 10.88017736071109987 ) ) ;
#38750=CARTESIAN_POINT ( 'NONE',  ( 5.076628168052703671, 41.84226448433411605, 8.527530157486179263 ) ) ;
#38751=CARTESIAN_POINT ( 'NONE',  ( 20.88017736071110519, 10.56368534415483751, 2.639326808657452039E-16 ) ) ;
#38752=AXIS2_PLACEMENT_3D ( 'NONE', #36261, #73755, #95786 ) ;
#38754=CARTESIAN_POINT ( 'NONE',  ( 19.84674366389459266, 53.71726448433411605, -2.638427012816827677 ) ) ;
#38755=CARTESIAN_POINT ( 'NONE',  ( 10.00000000000000000, 46.81368534415484106, -10.88017736071110342 ) ) ;
#38756=CARTESIAN_POINT ( 'NONE',  ( 12.63842701281683034, 2.467264484334118269, 9.846743663894596210 ) ) ;
#38758=VERTEX_POINT ( 'NONE', #15960 ) ;
#38763=CARTESIAN_POINT ( 'NONE',  ( 0.1532563361054100626, 25.80059781766744820, -2.638427012816831230 ) ) ;
#38764=CARTESIAN_POINT ( 'NONE',  ( -1.099225684535947600, 63.70696800326376774, -6.408140936763238038 ) ) ;
#38765=CARTESIAN_POINT ( 'NONE',  ( 15.44008868035555260, 14.73035201082150536, 9.422509992056143702 ) ) ;
#38766=CARTESIAN_POINT ( 'NONE',  ( 10.00000000000000000, 44.75893115100078745, -9.846743663894594434 ) ) ;
#38767=CARTESIAN_POINT ( 'NONE',  ( 13.79529636645030344, 58.26208216824728936, 14.16423886937410614 ) ) ;
#38768=CARTESIAN_POINT ( 'NONE',  ( 0.1532563361054083140, 51.00893115100078745, 1.131784320476157264E-15 ) ) ;
#38770=CARTESIAN_POINT ( 'NONE',  ( 12.91533473730993009, 51.60535201082149825, -10.88017736071109987 ) ) ;
#38771=ADVANCED_FACE ( 'NONE', ( #16455 ), #78787, .T. ) ;
#38772=CARTESIAN_POINT ( 'NONE',  ( 2.791683348922237240, 10.38393115100078390, -7.208316651077763204 ) ) ;
#38778=CARTESIAN_POINT ( 'NONE',  ( 17.20831665107776587, 7.883931151000784787, 7.208316651077764980 ) ) ;
#38780=CARTESIAN_POINT ( 'NONE',  ( 2.917880565312948704, 17.63708216824730357, 12.26659068614894643 ) ) ;
#38781=CARTESIAN_POINT ( 'NONE',  ( 0.1532563361054082862, 26.21726448433411605, 2.638427012816831674 ) ) ;
#38782=CARTESIAN_POINT ( 'NONE',  ( 10.00000000000000178, 24.31368534415484106, 10.88017736071110342 ) ) ;
#38784=CARTESIAN_POINT ( 'NONE',  ( 10.00000000000000178, 29.31368534415483751, 10.88017736071110342 ) ) ;
#38786=ORIENTED_EDGE ( 'NONE', *, *, #62767, .T. ) ;
#38787=CARTESIAN_POINT ( 'NONE',  ( 4.559911319644449179, 37.23035201082150536, -9.422509992056141925 ) ) ;
#38788=CARTESIAN_POINT ( 'NONE',  ( 2.603489959281590771, 66.58210964143327715, 6.500000000000003553 ) ) ;
#38792=CARTESIAN_POINT ( 'NONE',  ( 0.6178305044545838731, 19.74863466993042138, 9.382169495545420901 ) ) ;
#38793=CARTESIAN_POINT ( 'NONE',  ( 12.63842701281683922, 4.550597817667451750, -9.846743663894590881 ) ) ;
#38796=CARTESIAN_POINT ( 'NONE',  ( 0.1532563361054100626, 15.80059781766745353, -2.638427012816831230 ) ) ;
#38797=CARTESIAN_POINT ( 'NONE',  ( 17.96484262340118221, 29.93868534415484106, 7.964842623401181321 ) ) ;
#38798=EDGE_CURVE ( 'NONE', #61558, #63207, #74234, .T. ) ;
#38800=ORIENTED_EDGE ( 'NONE', *, *, #91919, .F. ) ;
#38802=CARTESIAN_POINT ( 'NONE',  ( -0.8801773607111008646, 63.27201867748817676, 2.915334737309923430 ) ) ;
#38806=CARTESIAN_POINT ( 'NONE',  ( 0.5774900079438607392, 63.48035201082149825, 5.440088680355550821 ) ) ;
#38807=COLOUR_RGB ( '', 0.72549020, 0.75294118, 0.79215686) ;
#38809=CARTESIAN_POINT ( 'NONE',  ( 6.565887622018943937, 5.165301336597086568, 12.81628187352647430 ) ) ;
#38811=CARTESIAN_POINT ( 'NONE',  ( 10.00000000000000178, 70.00000000000000000, 0.000000000000000000 ) ) ;
#38812=CARTESIAN_POINT ( 'NONE',  ( 12.63842701281683922, 34.55059781766745886, -9.846743663894590881 ) ) ;
#38813=CARTESIAN_POINT ( 'NONE',  ( 0.6178305044545818747, 53.49863466993041072, -9.382169495545419124 ) ) ;
#38814=CARTESIAN_POINT ( 'NONE',  ( 1.602071938427540809, 37.02224192338639597, -6.500000000000066613 ) ) ;
#38815=CARTESIAN_POINT ( 'NONE',  ( 2.791683348922237240, 25.38393115100078390, -7.208316651077763204 ) ) ;
#38817=CARTESIAN_POINT ( 'NONE',  ( 22.81628187352647785, 16.41530133659708923, 3.434112377981063169 ) ) ;
#38818=CARTESIAN_POINT ( 'NONE',  ( -46.30928139467842897, 104.0823827281712255, 5.529860068218143354 ) ) ;
#38819=DIRECTION ( 'NONE',  ( 0.000000000000000000, 0.000000000000000000, 1.000000000000000000 ) ) ;
#38820=CARTESIAN_POINT ( 'NONE',  ( 17.96484262340118221, 31.18868534415483751, -7.964842623401177768 ) ) ;
#38821=CARTESIAN_POINT ( 'NONE',  ( 2.791683348922240793, 66.63393115100079456, 7.208316651077764092 ) ) ;
#38823=CARTESIAN_POINT ( 'NONE',  ( 0.1532563361054083140, 26.00893115100078745, 1.131784320476157264E-15 ) ) ;
#38824=CARTESIAN_POINT ( 'NONE',  ( 0.1532563361054082862, 6.217264484334118713, 2.638427012816831674 ) ) ;
#38825=CARTESIAN_POINT ( 'NONE',  ( 2.035157376598824452, 8.688685344154839285, 7.964842623401179544 ) ) ;
#38826=CARTESIAN_POINT ( 'NONE',  ( 16.40814093676323893, 20.79030133659708923, 11.09922568453595026 ) ) ;
#38828=CARTESIAN_POINT ( 'NONE',  ( 17.20831665107776587, 62.88393115100078745, 7.208316651077764980 ) ) ;
#38830=CARTESIAN_POINT ( 'NONE',  ( 2.035157376598822676, 22.43868534415483396, -7.964842623401177768 ) ) ;
#38831=CARTESIAN_POINT ( 'NONE',  ( 7.361572987183169658, 44.96726448433412315, -9.846743663894592657 ) ) ;
#38833=CARTESIAN_POINT ( 'NONE',  ( -0.8801773607111009756, 18.06368534415484106, 1.068504757029289695E-15 ) ) ;
#38835=CARTESIAN_POINT ( 'NONE',  ( -0.8801773607111009756, 33.06368534415484106, 1.068504757029289695E-15 ) ) ;
#38836=CARTESIAN_POINT ( 'NONE',  ( -4.164238869374098151, 61.59541550158063217, -3.795296366450310543 ) ) ;
#38838=CARTESIAN_POINT ( 'NONE',  ( 12.63842701281683034, 2.467264484334118269, 9.846743663894596210 ) ) ;
#38839=CARTESIAN_POINT ( 'NONE',  ( 0.1532563361054082862, 21.21726448433412315, 2.638427012816831674 ) ) ;
#38840=CARTESIAN_POINT ( 'NONE',  ( 21.09922568453595559, 7.040301336597086568, -6.408140936763230044 ) ) ;
#38841=FACE_OUTER_BOUND ( 'NONE', #68993, .T. ) ;
#38847=CARTESIAN_POINT ( 'NONE',  ( 17.08211943468705130, 13.47041550158063572, 12.26659068614894998 ) ) ;
#38849=CARTESIAN_POINT ( 'NONE',  ( 10.00000000000000000, 34.75893115100078745, -9.846743663894594434 ) ) ;
#38852=CARTESIAN_POINT ( 'NONE',  ( 20.36894250292379382, 53.67874883491397497, 10.36894250292379205 ) ) ;
#38854=CARTESIAN_POINT ( 'NONE',  ( 2.791683348922237240, 25.38393115100078390, -7.208316651077763204 ) ) ;
#38856=CYLINDRICAL_SURFACE ( 'NONE', #75786, 11.92686044187656513 ) ;
#38857=CARTESIAN_POINT ( 'NONE',  ( 12.91533473730992121, 44.52201867748816966, 10.88017736071110164 ) ) ;
#38858=CARTESIAN_POINT ( 'NONE',  ( 0.6178305044545838731, 54.74863466993042493, 9.382169495545420901 ) ) ;
#38859=CARTESIAN_POINT ( 'NONE',  ( 0.5774900079438607392, 23.48035201082150536, 5.440088680355550821 ) ) ;
#38860=CARTESIAN_POINT ( 'NONE',  ( 16.40814093676324603, 42.45696800326375353, -11.09922568453594671 ) ) ;
#38861=CARTESIAN_POINT ( 'NONE',  ( 3.591859063236763294, 3.290301336597087012, -11.09922568453595026 ) ) ;
#38862=CARTESIAN_POINT ( 'NONE',  ( 0.1532563361054083140, 6.008931151000784787, 1.131784320476157264E-15 ) ) ;
#38863=ORIENTED_EDGE ( 'NONE', *, *, #62916, .T. ) ;
#38866=CARTESIAN_POINT ( 'NONE',  ( -4.164238869374099039, 51.80374883491396787, 8.674139862899312516E-16 ) ) ;
#38867=CARTESIAN_POINT ( 'NONE',  ( 13.79529636645031943, 15.34541550158063750, -14.16423886937409904 ) ) ;
#38868=CARTESIAN_POINT ( 'NONE',  ( 20.88017736071110164, 15.35535201082150358, 2.915334737309930979 ) ) ;
#38869=CARTESIAN_POINT ( 'NONE',  ( 10.00000000000000178, 39.31368534415484106, 10.88017736071110342 ) ) ;
#38872=CARTESIAN_POINT ( 'NONE',  ( 10.00000000000000000, 66.81368534415484817, -10.88017736071110342 ) ) ;
#38873=CARTESIAN_POINT ( 'NONE',  ( 0.5774900079438607392, 63.48035201082149825, 5.440088680355550821 ) ) ;
#38874=CARTESIAN_POINT ( 'NONE',  ( -1.099225684535947600, 29.54030133659708923, 6.408140936763237150 ) ) ;
#38877=CARTESIAN_POINT ( 'NONE',  ( 5.076628168052704559, 10.17559781766745175, -8.527530157486179263 ) ) ;
#38878=CARTESIAN_POINT ( 'NONE',  ( 18.52753015748618282, 33.92559781766745886, -4.923371831947291888 ) ) ;
#38879=CARTESIAN_POINT ( 'NONE',  ( 20.88017736071110875, 15.77201867748817143, -2.915334737309920765 ) ) ;
#38880=CARTESIAN_POINT ( 'NONE',  ( -1.099225684535947600, 38.70696800326375353, -6.408140936763238038 ) ) ;
#38881=EDGE_CURVE ( 'NONE', #87349, #71629, #62379, .T. ) ;
#38882=TOROIDAL_SURFACE ( 'NONE', #26297, 0.5000000000000043299, 0.5000000000000000000 ) ;
#38883=B_SPLINE_CURVE_WITH_KNOTS ( 'NONE', 3,
 ( #98755, #31192, #44224, #98255 ),
 .UNSPECIFIED., .F., .F.,
 ( 4, 4 ),
 ( 9.215718466126787689E-19, 0.002657014572710872727 ),
 .UNSPECIFIED. ) ;
#38884=CARTESIAN_POINT ( 'NONE',  ( 0.1532563361054082862, 6.217264484334118713, 2.638427012816831674 ) ) ;
#38886=CARTESIAN_POINT ( 'NONE',  ( 2.791683348922240793, 51.63393115100078745, 7.208316651077764092 ) ) ;
#38888=CARTESIAN_POINT ( 'NONE',  ( 2.791683348922240793, 31.63393115100078745, 7.208316651077764092 ) ) ;
#38889=CARTESIAN_POINT ( 'NONE',  ( 24.16423886937409904, 14.09541550158063217, 3.795296366450317205 ) ) ;
#38890=CARTESIAN_POINT ( 'NONE',  ( 10.00000000000000178, 34.31368534415484106, 10.88017736071110342 ) ) ;
#38891=CARTESIAN_POINT ( 'NONE',  ( 17.96484262340118221, 4.938685344154837509, 7.964842623401181321 ) ) ;
#38894=CARTESIAN_POINT ( 'NONE',  ( 4.559911319644449179, 28.89701867748817321, 9.422509992056141925 ) ) ;
#38895=CARTESIAN_POINT ( 'NONE',  ( 20.88017736071110164, 35.35535201082150536, 2.915334737309930979 ) ) ;
#38898=CARTESIAN_POINT ( 'NONE',  ( -0.8801773607110991993, 37.85535201082151247, -2.915334737309923874 ) ) ;
#38900=CARTESIAN_POINT ( 'NONE',  ( 22.81628187352648496, 61.83196800326376774, -3.434112377981050290 ) ) ;
#38901=CARTESIAN_POINT ( 'NONE',  ( 17.96484262340118221, 49.93868534415484106, 7.964842623401181321 ) ) ;
#38903=CARTESIAN_POINT ( 'NONE',  ( 7.084665262690076126, 54.10535201082151247, 10.88017736071109987 ) ) ;
#38905=CARTESIAN_POINT ( 'NONE',  ( -0.3289641300568005855, 25.10497603579417358, 5.963430220938281678 ) ) ;
#38906=CARTESIAN_POINT ( 'NONE',  ( -4.164238869374099039, 66.80374883491396076, 8.674139862899312516E-16 ) ) ;
#38907=CARTESIAN_POINT ( 'NONE',  ( 0.5774900079438607392, 63.48035201082149825, 5.440088680355550821 ) ) ;
#38908=CARTESIAN_POINT ( 'NONE',  ( 18.72515096720583827, 56.07228050351029225, -6.499999999999803713 ) ) ;
#38910=CARTESIAN_POINT ( 'NONE',  ( 10.00000000000000000, 1.813685344154837731, -10.88017736071110342 ) ) ;
#38911=CARTESIAN_POINT ( 'NONE',  ( 5.076628168052703671, 26.84226448433411960, 8.527530157486179263 ) ) ;
#38913=CARTESIAN_POINT ( 'NONE',  ( 12.63842701281683034, 37.46726448433411605, 9.846743663894596210 ) ) ;
#38914=CARTESIAN_POINT ( 'NONE',  ( 19.42250999205614548, 35.98035201082151247, -5.440088680355545492 ) ) ;
#38915=CARTESIAN_POINT ( 'NONE',  ( 10.00000000000000000, 34.75893115100078745, -9.846743663894594434 ) ) ;
#38916=CARTESIAN_POINT ( 'NONE',  ( 6.565887622018943937, 23.08196800326375708, -12.81628187352647608 ) ) ;
#38918=CARTESIAN_POINT ( 'NONE',  ( 20.10384461210894003, 1.743024370107933319, 6.337995344473744019 ) ) ;
#38919=CARTESIAN_POINT ( 'NONE',  ( 0.5774900079438607392, 43.48035201082151247, 5.440088680355550821 ) ) ;
#38920=CARTESIAN_POINT ( 'NONE',  ( 17.08211943468705130, 53.47041550158063217, 12.26659068614894998 ) ) ;
#38923=CARTESIAN_POINT ( 'NONE',  ( 22.81628187352647785, 26.62363466993042138, 6.195893100308588602E-16 ) ) ;
#38924=CARTESIAN_POINT ( 'NONE',  ( 1.472469842513823179, 50.59226448433411605, -4.923371831947296329 ) ) ;
#38926=CARTESIAN_POINT ( 'NONE',  ( 16.40814093676324603, 17.45696800326375353, -11.09922568453594671 ) ) ;
#38927=CARTESIAN_POINT ( 'NONE',  ( 4.559911319644449179, 18.89701867748817321, 9.422509992056141925 ) ) ;
#38928=CARTESIAN_POINT ( 'NONE',  ( 4.559911319644449179, 63.89701867748817676, 9.422509992056141925 ) ) ;
#38931=CARTESIAN_POINT ( 'NONE',  ( 2.791683348922237240, 5.383931151000785675, -7.208316651077763204 ) ) ;
#38932=CARTESIAN_POINT ( 'NONE',  ( 7.361572987183170547, 52.05059781766745175, 9.846743663894590881 ) ) ;
#38933=CARTESIAN_POINT ( 'NONE',  ( 2.791683348922237240, 35.38393115100079456, -7.208316651077763204 ) ) ;
#38935=CARTESIAN_POINT ( 'NONE',  ( 19.84674366389459266, 28.71726448433411960, -2.638427012816827677 ) ) ;
#38936=CARTESIAN_POINT ( 'NONE',  ( -0.1503990784575328643, 40.12777174578613426, 6.262539305110068177 ) ) ;
#38938=CARTESIAN_POINT ( 'NONE',  ( 19.84674366389459266, 8.300597817667451750, 2.638427012816836559 ) ) ;
#38939=CARTESIAN_POINT ( 'NONE',  ( 20.15039907845753575, 50.60158574516642460, -6.262539305110073506 ) ) ;
#38941=CARTESIAN_POINT ( 'NONE',  ( 10.00000000000000178, 42.25893115100078745, 9.846743663894594434 ) ) ;
#38944=CARTESIAN_POINT ( 'NONE',  ( -2.816281873526473856, 9.331968003263753531, 3.434112377981055619 ) ) ;
#38945=CARTESIAN_POINT ( 'NONE',  ( 12.91533473730992121, 54.52201867748816255, 10.88017736071110164 ) ) ;
#38946=CARTESIAN_POINT ( 'NONE',  ( 20.36894250292379382, 38.67874883491396076, 10.36894250292379205 ) ) ;
#38949=CARTESIAN_POINT ( 'NONE',  ( 2.917880565312950480, 40.97041550158063217, -12.26659068614894821 ) ) ;
#38950=CARTESIAN_POINT ( 'NONE',  ( 20.36894250292379738, 64.92874883491397497, -10.36894250292379027 ) ) ;
#38951=CARTESIAN_POINT ( 'NONE',  ( 2.917880565312950480, 25.97041550158063572, -12.26659068614894821 ) ) ;
#38952=CARTESIAN_POINT ( 'NONE',  ( 22.26659068614895176, 29.72041550158063572, -7.082119434687042414 ) ) ;
#38953=CARTESIAN_POINT ( 'NONE',  ( 20.04068437667225311, 24.71974360917720759, 6.396802510829709298 ) ) ;
#38956=CARTESIAN_POINT ( 'NONE',  ( 19.84674366389459266, 38.71726448433412315, -2.638427012816827677 ) ) ;
#38958=CARTESIAN_POINT ( 'NONE',  ( 20.88017736071110875, 25.77201867748816966, -2.915334737309920765 ) ) ;
#38962=CARTESIAN_POINT ( 'NONE',  ( 18.52753015748618282, 33.92559781766745886, -4.923371831947291888 ) ) ;
#38963=CARTESIAN_POINT ( 'NONE',  ( 10.00000000000000000, 57.87363466993042493, -12.81628187352647608 ) ) ;
#38965=CARTESIAN_POINT ( 'NONE',  ( 18.52753015748617571, 38.09226448433412315, 4.923371831947298993 ) ) ;
#38966=CARTESIAN_POINT ( 'NONE',  ( 18.52753015748617571, 58.09226448433411605, 4.923371831947298993 ) ) ;
#38968=CARTESIAN_POINT ( 'NONE',  ( 20.36894250292379738, 44.92874883491396787, -10.36894250292379027 ) ) ;
#38970=CARTESIAN_POINT ( 'NONE',  ( 13.79529636645030344, 18.26208216824730002, 14.16423886937410614 ) ) ;
#38971=ADVANCED_FACE ( 'NONE', ( #5398 ), #59354, .T. ) ;
#38972=CARTESIAN_POINT ( 'NONE',  ( -0.8801773607111009756, 58.06368534415484106, 1.068504757029289695E-15 ) ) ;
#38975=CARTESIAN_POINT ( 'NONE',  ( -4.164238869374099927, 67.01208216824728936, 3.795296366450308767 ) ) ;
#38976=CARTESIAN_POINT ( 'NONE',  ( 13.43411237798105340, 5.581968003263753531, 12.81628187352647963 ) ) ;
#38978=CARTESIAN_POINT ( 'NONE',  ( 17.20831665107776587, 4.133931151000785675, -7.208316651077762316 ) ) ;
#38979=CARTESIAN_POINT ( 'NONE',  ( 13.99999999999999822, 60.50000000000000000, 6.500000000000000888 ) ) ;
#38982=CARTESIAN_POINT ( 'NONE',  ( 13.79529636645030344, 58.26208216824728936, 14.16423886937410614 ) ) ;
#38983=DIRECTION ( 'NONE',  ( 1.000000000000000000, -0.000000000000000000, -0.000000000000000000 ) ) ;
#38984=CARTESIAN_POINT ( 'NONE',  ( 20.88017736071110519, 20.56368534415484106, 2.639326808657452039E-16 ) ) ;
#38985=CARTESIAN_POINT ( 'NONE',  ( 15.44008868035555793, 26.39701867748817321, -9.422509992056140149 ) ) ;
#38986=CARTESIAN_POINT ( 'NONE',  ( 12.63842701281683922, 54.55059781766745175, -9.846743663894590881 ) ) ;
#38987=CARTESIAN_POINT ( 'NONE',  ( 12.63842701281683922, 49.55059781766744464, -9.846743663894590881 ) ) ;
#38988=CARTESIAN_POINT ( 'NONE',  ( 3.591859063236761518, 59.95696800326375353, 11.09922568453594849 ) ) ;
#38991=EDGE_CURVE ( 'NONE', #86252, #63207, #48037, .T. ) ;
#38992=CARTESIAN_POINT ( 'NONE',  ( 19.42250999205614548, 10.98035201082150358, -5.440088680355545492 ) ) ;
#38993=CARTESIAN_POINT ( 'NONE',  ( 0.6178305044545818747, 13.49863466993041783, -9.382169495545419124 ) ) ;
#38994=CYLINDRICAL_SURFACE ( 'NONE', #54488, 9.999999999999996447 ) ;
#38995=CARTESIAN_POINT ( 'NONE',  ( 5.076628168052704559, 60.17559781766745175, -8.527530157486179263 ) ) ;
#38996=CARTESIAN_POINT ( 'NONE',  ( 17.96484262340118221, 44.93868534415483396, 7.964842623401181321 ) ) ;
#38997=CARTESIAN_POINT ( 'NONE',  ( -1.099225684535947600, 24.54030133659708923, 6.408140936763237150 ) ) ;
#38998=CARTESIAN_POINT ( 'NONE',  ( 0.5774900079438590739, 62.64701867748817676, -5.440088680355550821 ) ) ;
#39001=CARTESIAN_POINT ( 'NONE',  ( 13.43411237798105340, 60.58196800326376064, 12.81628187352647963 ) ) ;
#39002=ORIENTED_EDGE ( 'NONE', *, *, #9021, .T. ) ;
#39003=CARTESIAN_POINT ( 'NONE',  ( 0.8952175423694801459, 47.60160829253886305, -5.990408912944315212 ) ) ;
#39005=CARTESIAN_POINT ( 'NONE',  ( 15.44008868035555793, 46.39701867748817676, -9.422509992056140149 ) ) ;
#39006=CARTESIAN_POINT ( 'NONE',  ( 6.565887622018943937, 53.08196800326374643, -12.81628187352647608 ) ) ;
#39007=CARTESIAN_POINT ( 'NONE',  ( -4.164238869374099927, 17.01208216824730357, 3.795296366450308767 ) ) ;
#39008=EDGE_CURVE ( 'NONE', #37711, #35624, #2743, .T. ) ;
#39010=CARTESIAN_POINT ( 'NONE',  ( 19.84674366389459266, 23.71726448433412315, -2.638427012816827677 ) ) ;
#39012=CARTESIAN_POINT ( 'NONE',  ( -0.3689425029237898834, 56.17874883491396076, -10.36894250292378850 ) ) ;
#39014=CARTESIAN_POINT ( 'NONE',  ( 4.559911319644449179, 8.897018677488171434, 9.422509992056141925 ) ) ;
#39016=ORIENTED_EDGE ( 'NONE', *, *, #7405, .T. ) ;
#39018=CARTESIAN_POINT ( 'NONE',  ( -0.8801773607110991993, 2.855352010821504471, -2.915334737309923874 ) ) ;
#39019=CARTESIAN_POINT ( 'NONE',  ( 7.084665262690076126, 4.105352010821503583, 10.88017736071109987 ) ) ;
#39020=CARTESIAN_POINT ( 'NONE',  ( 10.00000000000000178, 37.25893115100078745, 9.846743663894594434 ) ) ;
#39021=CARTESIAN_POINT ( 'NONE',  ( 22.81628187352647785, 41.41530133659708923, 3.434112377981063169 ) ) ;
#39022=CARTESIAN_POINT ( 'NONE',  ( -0.1503990784575279516, 43.10158574516643171, 6.262539305110076171 ) ) ;
#39024=CARTESIAN_POINT ( 'NONE',  ( 0.6076426042653170212, 2.375764716086009365, -6.500000000000000888 ) ) ;
#39025=CARTESIAN_POINT ( 'NONE',  ( 13.79529636645030344, 18.26208216824730002, 14.16423886937410614 ) ) ;
#39026=CARTESIAN_POINT ( 'NONE',  ( 7.084665262690076126, 24.10535201082150181, 10.88017736071109987 ) ) ;
#39027=CARTESIAN_POINT ( 'NONE',  ( -2.266590686148945544, 67.22041550158063217, 7.082119434687048631 ) ) ;
#39028=CARTESIAN_POINT ( 'NONE',  ( 5.076628168052704559, 40.17559781766745175, -8.527530157486179263 ) ) ;
#39030=CARTESIAN_POINT ( 'NONE',  ( 19.84674366389459621, 23.50893115100078390, 7.409399052514197653E-17 ) ) ;
#39035=B_SPLINE_CURVE_WITH_KNOTS ( 'NONE', 3,
 ( #92062, #54055, #17064, #68581 ),
 .UNSPECIFIED., .F., .F.,
 ( 4, 4 ),
 ( 5.553824967135426632E-18, 0.0003153927346766718259 ),
 .UNSPECIFIED. ) ;
#39037=CARTESIAN_POINT ( 'NONE',  ( 10.00000000000000178, 57.25893115100078745, 9.846743663894594434 ) ) ;
#39038=CARTESIAN_POINT ( 'NONE',  ( 19.42250999205614193, 30.14701867748817321, 5.440088680355555262 ) ) ;
#39039=CARTESIAN_POINT ( 'NONE',  ( -0.8801773607110991993, 42.85535201082150536, -2.915334737309923874 ) ) ;
#39040=CARTESIAN_POINT ( 'NONE',  ( 15.44008868035555260, 4.730352010821504471, 9.422509992056143702 ) ) ;
#39041=CARTESIAN_POINT ( 'NONE',  ( 16.40814093676324603, 27.45696800326375708, -11.09922568453594671 ) ) ;
#39042=CARTESIAN_POINT ( 'NONE',  ( -4.164238869374099927, 12.01208216824730357, 3.795296366450308767 ) ) ;
#39044=CARTESIAN_POINT ( 'NONE',  ( 22.81628187352647785, 46.62363466993041783, 6.195893100308588602E-16 ) ) ;
#39045=ORIENTED_EDGE ( 'NONE', *, *, #25034, .T. ) ;
#39046=CARTESIAN_POINT ( 'NONE',  ( 14.92337183194729633, 42.67559781766745886, 8.527530157486181039 ) ) ;
#39047=CARTESIAN_POINT ( 'NONE',  ( 20.88017736071110164, 20.35535201082150891, 2.915334737309930979 ) ) ;
#39049=CARTESIAN_POINT ( 'NONE',  ( 4.559911319644449179, 18.89701867748817321, 9.422509992056141925 ) ) ;
#39051=CARTESIAN_POINT ( 'NONE',  ( 4.559911319644449179, 58.89701867748817676, 9.422509992056141925 ) ) ;
#39052=DIRECTION ( 'NONE',  ( 0.000000000000000000, -1.000000000000000000, 0.000000000000000000 ) ) ;
#39054=EDGE_CURVE ( 'NONE', #23604, #11760, #71023, .T. ) ;
#39055=( BOUNDED_SURFACE ( )  B_SPLINE_SURFACE ( 1, 2, ( 
 ( #52050, #22551, #60528, #7049, #37553, #44541, #30515, #91530, #14058, #30022, #36559, #23045, #23543, #7557, #61018, #97571, #38046, #82541, #68043, #52533, #98569, #75037, #29522, #8035, #6543, #37053, #15549, #53517, #83041, #91018, #67552, #54015, #53021, #68538, #16021, #83536, #29034, #76026, #22059, #31010, #84524, #15055, #98063, #84029, #60029, #90524, #14557, #74540, #45026, #75533, #46034, #45528, #69, #6060, #76519, #38533, #59543, #69029, #564, #61506, #92013, #90038, #21561, #46510, #2028, #9004, #78489, #17513, #55502, #63481, #85011, #48476, #9500, #70504, #10003, #8522, #56480, #17014, #25014, #40002, #31982, #33457, #32490, #25507, #40996, #39025, #47979, #62985, #85504, #40505, #93491, #71001, #86002, #25983, #69520, #47492, #86494, #92992, #54985, #39520, #3008, #2524, #77995, #1035, #16524, #46999, #63954, #24526, #32977, #93985, #55994, #54496, #24028, #17994, #78975, #10485, #77492, #71493, #94466, #86966, #62488, #70012, #77010, #31496, #61999, #92498, #1538, #49953, #4957, #35931, #58425, #49452, #95961, #79958, #71964, #64448, #11462, #35437, #3487, #80458, #27443, #57937, #88939, #72444, #57453, #34443, #43430, #41980, #87946, #18974, #11956, #96961, #87459, #42461, #19461, #20448, #33944, #64934, #12443, #56956, #88445, #48965, #42951, #65932, #12936, #3974, #95462, #73931, #50938, #26953, #19945, #72943, #26457, #4473, #66428, #28433, #34939, #65437, #81432, #5459, #50440, #27932, #10974, #41495, #80945, #96460, #73430, #58931, #18480, #79475, #94955, #82916, #67923, #37927, #14933, #29405, #45400, #76400, #7431, #68911, #98444, #67423, #6926, #68416, #51931, #97948, #21937, #14434, #98939, #29900, #74920, #91396, #15433, #81922, #82415, #59908, #52417, #44905, #30393, #60405, #6418, #22924, #45911, #13430, #90901, #75407, #90398, #22429, #37433, #83412, #52901, #439, #43916, #75906, #60897, #36931, #53393, #13939, #7915, #83903, #38411, #74414, #59414, #89920, #30892, #89431, #20945, #51432, #5943, #97447, #66927, #36434, #28912, #21434, #44416, #16890, #24399, #93364, #46878, #31378, #63355, #55376, #93859, #78859, #10371, #92869, #47858, #40872, #2399, #92381, #39881, #23907, #15906, #8397, #54376, #78364, #46396, #54867, #70387, #1906, #32856, #16396, #1412, #77370, #86369, #84889, #31865, #61876, #85378, #71377, #8881, #47369, #62364, #25387, #76884, #39399, #85877, #915, #32361, #91895, #17389, #9883, #55870, #69892, #77867, #17870, #48353, #9378, #62868, #24892, #69393, #40383, #2889, #61386, #70882, #23420, #53899, #84407, #38906, #42832, #25867, #56364, #71848, #12328, #41861 ),
 ( #94839, #73317, #42341, #79836, #44672, #36692, #95838, #18363, #34822, #27321, #11833, #14188, #6188, #33340, #87821, #26341, #65312, #4356, #72816, #50314, #3358, #67180, #95334, #57327, #57819, #94348, #75166, #3857, #88327, #26833, #18856, #21692, #19341, #97703, #29169, #86857, #82672, #72324, #49824, #19825, #80334, #80828, #52178, #11341, #87341, #59670, #90162, #33821, #63834, #34317, #48842, #79353, #64327, #10860, #41381, #56842, #49336, #64815, #74692, #73692, #20714, #81208, #20211, #6202, #51205, #50206, #96725, #97720, #42237, #90176, #12708, #89691, #28201, #43202, #21706, #82187, #72703, #81688, #57709, #89201, #43695, #5227, #67195, #73202, #29184, #80220, #4734, #11724, #4239, #34708, #65203, #95724, #27208, #88209, #96227, #27706, #45676, #30164, #15194, #60177, #7191, #84660, #22200, #90674, #23687, #69175, #60668, #76174, #45178, #31644, #7695, #15690, #52191, #38191, #44684, #46175, #22694, #8657, #1185, #30656, #52679, #54150, #37694, #83180, #83679, #14203, #68678, #206, #16168, #61163, #91671, #6691, #46652, #76659, #37210, #23190, #698, #39170, #67698, #31151, #69659, #98210, #29668, #24661, #55131, #72105, #62629, #85645, #33604, #33120, #70651, #34099, #26131, #86635, #9151, #17656, #25647, #18145, #2669, #3632, #94616, #24167, #78641, #17164, #56140, #94121, #63614, #41146, #93134, #56622, #86143, #48126, #48617, #85155, #64590, #93632, #79121, #10148, #9650, #11121, #40643, #3142, #18626, #16663, #54637, #63130, #71141, #10634, #71631, #64100, #41640, #2174, #78140, #87111, #49118, #47645, #79620, #25167, #47137, #77634, #40147, #39669, #70160, #32631, #55643, #1677, #32130, #88585, #35591, #65580, #35081, #21089, #66079, #34587, #50597, #13583, #57104, #74574, #96107, #5603, #81089, #58081, #6088, #97112, #87600, #96607, #72590, #43090, #12590, #27591, #20093, #65082, #51085, #13083, #95605, #73575, #19110, #43578, #44067, #28084, #81576, #49590, #58582, #4124, #5100, #73083, #89084, #27091, #50099, #28584, #57594, #88091, #36082, #74071, #4620, #20599, #19604, #36591, #66585, #59074, #95098, #89578, #80102, #51587, #82073, #26606, #11607, #42124, #80604, #12102, #42605, #91052, #84059, #37086, #22579, #60561, #98, #52564, #67585, #69057, #61045, #593, #84552, #16052, #98602, #53546, #46540, #8065, #98094, #45560, #29554, #21591, #44570, #60058, #46059, #52082, #53050, #38076, #30545, #38561, #22088, #7080, #83068, #92045, #90559, #37582, #14588, #83569, #77041, #45057, #15089, #68075, #31036, #82575, #75567, #91558, #23077, #61536, #97605, #23573, #54042, #8554, #67078, #29066, #59574 ) ),
 .UNSPECIFIED., .F., .F., .T. ) 
 B_SPLINE_SURFACE_WITH_KNOTS ( ( 2, 2 ),
 ( 3, 2, 2, 2, 2, 2, 2, 2, 2, 2, 2, 2, 2, 2, 2, 2, 2, 2, 2, 2, 2, 2, 2, 2, 2, 2, 2, 2, 2, 2, 2, 2, 2, 2, 2, 2, 2, 2, 2, 2, 2, 2, 2, 2, 2, 2, 2, 2, 2, 2, 2, 2, 2, 2, 2, 2, 2, 2, 2, 2, 2, 2, 2, 2, 2, 2, 2, 2, 2, 2, 2, 2, 2, 2, 2, 2, 2, 2, 2, 2, 2, 2, 2, 2, 2, 2, 2, 2, 2, 2, 2, 2, 2, 2, 2, 2, 2, 2, 2, 2, 2, 2, 2, 2, 2, 2, 2, 2, 2, 2, 2, 2, 2, 2, 2, 2, 2, 2, 2, 2, 2, 2, 2, 2, 2, 2, 2, 2, 2, 2, 2, 2, 2, 2, 2, 2, 2, 2, 2, 2, 2, 2, 2, 2, 2, 2, 2, 2, 2, 2, 2, 2, 2, 2, 2, 2, 2, 2, 2, 2, 2, 2, 3 ),
 ( 0.000000000000000000, 1.000000000000000000 ),
 ( 0.000000000000000000, 0.005952380952380952051, 0.01190476190476190410, 0.01785714285714285615, 0.02380952380952380820, 0.02976190476190476025, 0.03571428571428571230, 0.04166666666666666435, 0.04761904761904761640, 0.05357142857142856845, 0.05952380952380952051, 0.06547619047619047949, 0.07142857142857142461, 0.07738095238095238360, 0.08333333333333332871, 0.08928571428571428770, 0.09523809523809523281, 0.1011904761904761918, 0.1071428571428571369, 0.1130952380952380959, 0.1190476190476190410, 0.1250000000000000000, 0.1309523809523809590, 0.1369047619047619180, 0.1428571428571428492, 0.1488095238095238082, 0.1547619047619047672, 0.1607142857142857262, 0.1666666666666666574, 0.1726190476190476164, 0.1785714285714285754, 0.1845238095238095344, 0.1904761904761904656, 0.1964285714285714246, 0.2023809523809523836, 0.2083333333333333426, 0.2142857142857142738, 0.2202380952380952328, 0.2261904761904761918, 0.2321428571428571508, 0.2380952380952380820, 0.2440476190476190410, 0.2500000000000000000, 0.2559523809523809312, 0.2619047619047619180, 0.2678571428571428492, 0.2738095238095238360, 0.2797619047619047672, 0.2857142857142856984, 0.2916666666666666852, 0.2976190476190476164, 0.3035714285714285476, 0.3095238095238095344, 0.3154761904761904656, 0.3214285714285714524, 0.3273809523809523836, 0.3333333333333333148, 0.3392857142857143016, 0.3452380952380952328, 0.3511904761904761640, 0.3571428571428571508, 0.3630952380952380820, 0.3690476190476190688, 0.3750000000000000000, 0.3809523809523809312, 0.3869047619047619180, 0.3928571428571428492, 0.3988095238095238360, 0.4047619047619047672, 0.4107142857142856984, 0.4166666666666666852, 0.4226190476190476164, 0.4285714285714285476, 0.4345238095238095344, 0.4404761904761904656, 0.4464285714285714524, 0.4523809523809523836, 0.4583333333333333148, 0.4642857142857143016, 0.4702380952380952328, 0.4761904761904761640, 0.4821428571428571508, 0.4880952380952380820, 0.4940476190476190688, 0.5000000000000000000, 0.5059523809523809312, 0.5119047619047618625, 0.5178571428571429047, 0.5238095238095238360, 0.5297619047619047672, 0.5357142857142856984, 0.5416666666666666297, 0.5476190476190476719, 0.5535714285714286031, 0.5595238095238095344, 0.5654761904761904656, 0.5714285714285713969, 0.5773809523809523281, 0.5833333333333333703, 0.5892857142857143016, 0.5952380952380952328, 0.6011904761904761640, 0.6071428571428570953, 0.6130952380952381375, 0.6190476190476190688, 0.6250000000000000000, 0.6309523809523809312, 0.6369047619047618625, 0.6428571428571429047, 0.6488095238095238360, 0.6547619047619047672, 0.6607142857142856984, 0.6666666666666666297, 0.6726190476190476719, 0.6785714285714286031, 0.6845238095238095344, 0.6904761904761904656, 0.6964285714285713969, 0.7023809523809523281, 0.7083333333333333703, 0.7142857142857143016, 0.7202380952380952328, 0.7261904761904761640, 0.7321428571428570953, 0.7380952380952381375, 0.7440476190476190688, 0.7500000000000000000, 0.7559523809523809312, 0.7619047619047618625, 0.7678571428571429047, 0.7738095238095238360, 0.7797619047619047672, 0.7857142857142856984, 0.7916666666666666297, 0.7976190476190476719, 0.8035714285714286031, 0.8095238095238095344, 0.8154761904761904656, 0.8214285714285713969, 0.8273809523809523281, 0.8333333333333333703, 0.8392857142857143016, 0.8452380952380952328, 0.8511904761904761640, 0.8571428571428570953, 0.8630952380952381375, 0.8690476190476190688, 0.8750000000000000000, 0.8809523809523809312, 0.8869047619047618625, 0.8928571428571429047, 0.8988095238095238360, 0.9047619047619047672, 0.9107142857142856984, 0.9166666666666666297, 0.9226190476190476719, 0.9285714285714286031, 0.9345238095238095344, 0.9404761904761904656, 0.9464285714285713969, 0.9523809523809523281, 0.9583333333333333703, 0.9642857142857143016 ),
 .UNSPECIFIED. ) 
 GEOMETRIC_REPRESENTATION_ITEM ( )  RATIONAL_B_SPLINE_SURFACE ( (
 ( 1.000000000000000000, 0.9659258262890683122, 1.000000000000000000, 0.9659258262890683122, 1.000000000000000000, 0.9659258262890683122, 1.000000000000000000, 0.9659258262890683122, 1.000000000000000000, 0.9659258262890683122, 1.000000000000000000, 0.9659258262890683122, 1.000000000000000000, 0.9659258262890683122, 1.000000000000000000, 0.9659258262890683122, 1.000000000000000000, 0.9659258262890683122, 1.000000000000000000, 0.9659258262890683122, 1.000000000000000000, 0.9659258262890683122, 1.000000000000000000, 0.9659258262890683122, 1.000000000000000000, 0.9659258262890683122, 1.000000000000000000, 0.9659258262890683122, 1.000000000000000000, 0.9659258262890683122, 1.000000000000000000, 0.9659258262890683122, 1.000000000000000000, 0.9659258262890683122, 1.000000000000000000, 0.9659258262890683122, 1.000000000000000000, 0.9659258262890683122, 1.000000000000000000, 0.9659258262890683122, 1.000000000000000000, 0.9659258262890683122, 1.000000000000000000, 0.9659258262890683122, 1.000000000000000000, 0.9659258262890683122, 1.000000000000000000, 0.9659258262890683122, 1.000000000000000000, 0.9659258262890683122, 1.000000000000000000, 0.9659258262890683122, 1.000000000000000000, 0.9659258262890683122, 1.000000000000000000, 0.9659258262890683122, 1.000000000000000000, 0.9659258262890683122, 1.000000000000000000, 0.9659258262890683122, 1.000000000000000000, 0.9659258262890683122, 1.000000000000000000, 0.9659258262890683122, 1.000000000000000000, 0.9659258262890683122, 1.000000000000000000, 0.9659258262890683122, 1.000000000000000000, 0.9659258262890683122, 1.000000000000000000, 0.9659258262890683122, 1.000000000000000000, 0.9659258262890683122, 1.000000000000000000, 0.9659258262890683122, 1.000000000000000000, 0.9659258262890683122, 1.000000000000000000, 0.9659258262890683122, 1.000000000000000000, 0.9659258262890683122, 1.000000000000000000, 0.9659258262890683122, 1.000000000000000000, 0.9659258262890683122, 1.000000000000000000, 0.9659258262890683122, 1.000000000000000000, 0.9659258262890683122, 1.000000000000000000, 0.9659258262890683122, 1.000000000000000000, 0.9659258262890683122, 1.000000000000000000, 0.9659258262890683122, 1.000000000000000000, 0.9659258262890683122, 1.000000000000000000, 0.9659258262890683122, 1.000000000000000000, 0.9659258262890683122, 1.000000000000000000, 0.9659258262890683122, 1.000000000000000000, 0.9659258262890683122, 1.000000000000000000, 0.9659258262890683122, 1.000000000000000000, 0.9659258262890683122, 1.000000000000000000, 0.9659258262890683122, 1.000000000000000000, 0.9659258262890683122, 1.000000000000000000, 0.9659258262890683122, 1.000000000000000000, 0.9659258262890683122, 1.000000000000000000, 0.9659258262890683122, 1.000000000000000000, 0.9659258262890683122, 1.000000000000000000, 0.9659258262890683122, 1.000000000000000000, 0.9659258262890683122, 1.000000000000000000, 0.9659258262890683122, 1.000000000000000000, 0.9659258262890683122, 1.000000000000000000, 0.9659258262890683122, 1.000000000000000000, 0.9659258262890683122, 1.000000000000000000, 0.9659258262890683122, 1.000000000000000000, 0.9659258262890683122, 1.000000000000000000, 0.9659258262890683122, 1.000000000000000000, 0.9659258262890683122, 1.000000000000000000, 0.9659258262890683122, 1.000000000000000000, 0.9659258262890683122, 1.000000000000000000, 0.9659258262890683122, 1.000000000000000000, 0.9659258262890683122, 1.000000000000000000, 0.9659258262890683122, 1.000000000000000000, 0.9659258262890683122, 1.000000000000000000, 0.9659258262890683122, 1.000000000000000000, 0.9659258262890683122, 1.000000000000000000, 0.9659258262890683122, 1.000000000000000000, 0.9659258262890683122, 1.000000000000000000, 0.9659258262890683122, 1.000000000000000000, 0.9659258262890683122, 1.000000000000000000, 0.9659258262890683122, 1.000000000000000000, 0.9659258262890683122, 1.000000000000000000, 0.9659258262890683122, 1.000000000000000000, 0.9659258262890683122, 1.000000000000000000, 0.9659258262890683122, 1.000000000000000000, 0.9659258262890683122, 1.000000000000000000, 0.9659258262890683122, 1.000000000000000000, 0.9659258262890683122, 1.000000000000000000, 0.9659258262890683122, 1.000000000000000000, 0.9659258262890683122, 1.000000000000000000, 0.9659258262890683122, 1.000000000000000000, 0.9659258262890683122, 1.000000000000000000, 0.9659258262890683122, 1.000000000000000000, 0.9659258262890683122, 1.000000000000000000, 0.9659258262890683122, 1.000000000000000000, 0.9659258262890683122, 1.000000000000000000, 0.9659258262890683122, 1.000000000000000000, 0.9659258262890683122, 1.000000000000000000, 0.9659258262890683122, 1.000000000000000000, 0.9659258262890683122, 1.000000000000000000, 0.9659258262890683122, 1.000000000000000000, 0.9659258262890683122, 1.000000000000000000, 0.9659258262890683122, 1.000000000000000000, 0.9659258262890683122, 1.000000000000000000, 0.9659258262890683122, 1.000000000000000000, 0.9659258262890683122, 1.000000000000000000, 0.9659258262890683122, 1.000000000000000000, 0.9659258262890683122, 1.000000000000000000, 0.9659258262890683122, 1.000000000000000000, 0.9659258262890683122, 1.000000000000000000, 0.9659258262890683122, 1.000000000000000000, 0.9659258262890683122, 1.000000000000000000, 0.9659258262890683122, 1.000000000000000000, 0.9659258262890683122, 1.000000000000000000, 0.9659258262890683122, 1.000000000000000000, 0.9659258262890683122, 1.000000000000000000, 0.9659258262890683122, 1.000000000000000000, 0.9659258262890683122, 1.000000000000000000, 0.9659258262890683122, 1.000000000000000000, 0.9659258262890683122, 1.000000000000000000, 0.9659258262890683122, 1.000000000000000000, 0.9659258262890683122, 1.000000000000000000, 0.9659258262890683122, 1.000000000000000000, 0.9659258262890683122, 1.000000000000000000, 0.9659258262890683122, 1.000000000000000000, 0.9659258262890683122, 1.000000000000000000, 0.9659258262890683122, 1.000000000000000000, 0.9659258262890683122, 1.000000000000000000, 0.9659258262890683122, 1.000000000000000000, 0.9659258262890683122, 1.000000000000000000, 0.9659258262890683122, 1.000000000000000000, 0.9659258262890683122, 1.000000000000000000, 0.9659258262890683122, 1.000000000000000000, 0.9659258262890683122, 1.000000000000000000, 0.9659258262890683122, 1.000000000000000000, 0.9659258262890683122, 1.000000000000000000, 0.9659258262890683122, 1.000000000000000000, 0.9659258262890683122, 1.000000000000000000, 0.9659258262890683122, 1.000000000000000000, 0.9659258262890683122, 1.000000000000000000, 0.9659258262890683122, 1.000000000000000000, 0.9659258262890683122, 1.000000000000000000, 0.9659258262890683122, 1.000000000000000000, 0.9659258262890683122, 1.000000000000000000, 0.9659258262890683122, 1.000000000000000000, 0.9659258262890683122, 1.000000000000000000, 0.9659258262890683122, 1.000000000000000000, 0.9659258262890683122, 1.000000000000000000, 0.9659258262890683122, 1.000000000000000000, 0.9659258262890683122, 1.000000000000000000, 0.9659258262890683122, 1.000000000000000000, 0.9659258262890683122, 1.000000000000000000, 0.9659258262890683122, 1.000000000000000000, 0.9659258262890683122, 1.000000000000000000, 0.9659258262890683122, 1.000000000000000000, 0.9659258262890683122, 1.000000000000000000, 0.9659258262890683122, 1.000000000000000000, 0.9659258262890683122, 1.000000000000000000, 0.9659258262890683122, 1.000000000000000000),
 ( 1.000000000000000000, 0.9659258262890683122, 1.000000000000000000, 0.9659258262890683122, 1.000000000000000000, 0.9659258262890683122, 1.000000000000000000, 0.9659258262890683122, 1.000000000000000000, 0.9659258262890683122, 1.000000000000000000, 0.9659258262890683122, 1.000000000000000000, 0.9659258262890683122, 1.000000000000000000, 0.9659258262890683122, 1.000000000000000000, 0.9659258262890683122, 1.000000000000000000, 0.9659258262890683122, 1.000000000000000000, 0.9659258262890683122, 1.000000000000000000, 0.9659258262890683122, 1.000000000000000000, 0.9659258262890683122, 1.000000000000000000, 0.9659258262890683122, 1.000000000000000000, 0.9659258262890683122, 1.000000000000000000, 0.9659258262890683122, 1.000000000000000000, 0.9659258262890683122, 1.000000000000000000, 0.9659258262890683122, 1.000000000000000000, 0.9659258262890683122, 1.000000000000000000, 0.9659258262890683122, 1.000000000000000000, 0.9659258262890683122, 1.000000000000000000, 0.9659258262890683122, 1.000000000000000000, 0.9659258262890683122, 1.000000000000000000, 0.9659258262890683122, 1.000000000000000000, 0.9659258262890683122, 1.000000000000000000, 0.9659258262890683122, 1.000000000000000000, 0.9659258262890683122, 1.000000000000000000, 0.9659258262890683122, 1.000000000000000000, 0.9659258262890683122, 1.000000000000000000, 0.9659258262890683122, 1.000000000000000000, 0.9659258262890683122, 1.000000000000000000, 0.9659258262890683122, 1.000000000000000000, 0.9659258262890683122, 1.000000000000000000, 0.9659258262890683122, 1.000000000000000000, 0.9659258262890683122, 1.000000000000000000, 0.9659258262890683122, 1.000000000000000000, 0.9659258262890683122, 1.000000000000000000, 0.9659258262890683122, 1.000000000000000000, 0.9659258262890683122, 1.000000000000000000, 0.9659258262890683122, 1.000000000000000000, 0.9659258262890683122, 1.000000000000000000, 0.9659258262890683122, 1.000000000000000000, 0.9659258262890683122, 1.000000000000000000, 0.9659258262890683122, 1.000000000000000000, 0.9659258262890683122, 1.000000000000000000, 0.9659258262890683122, 1.000000000000000000, 0.9659258262890683122, 1.000000000000000000, 0.9659258262890683122, 1.000000000000000000, 0.9659258262890683122, 1.000000000000000000, 0.9659258262890683122, 1.000000000000000000, 0.9659258262890683122, 1.000000000000000000, 0.9659258262890683122, 1.000000000000000000, 0.9659258262890683122, 1.000000000000000000, 0.9659258262890683122, 1.000000000000000000, 0.9659258262890683122, 1.000000000000000000, 0.9659258262890683122, 1.000000000000000000, 0.9659258262890683122, 1.000000000000000000, 0.9659258262890683122, 1.000000000000000000, 0.9659258262890683122, 1.000000000000000000, 0.9659258262890683122, 1.000000000000000000, 0.9659258262890683122, 1.000000000000000000, 0.9659258262890683122, 1.000000000000000000, 0.9659258262890683122, 1.000000000000000000, 0.9659258262890683122, 1.000000000000000000, 0.9659258262890683122, 1.000000000000000000, 0.9659258262890683122, 1.000000000000000000, 0.9659258262890683122, 1.000000000000000000, 0.9659258262890683122, 1.000000000000000000, 0.9659258262890683122, 1.000000000000000000, 0.9659258262890683122, 1.000000000000000000, 0.9659258262890683122, 1.000000000000000000, 0.9659258262890683122, 1.000000000000000000, 0.9659258262890683122, 1.000000000000000000, 0.9659258262890683122, 1.000000000000000000, 0.9659258262890683122, 1.000000000000000000, 0.9659258262890683122, 1.000000000000000000, 0.9659258262890683122, 1.000000000000000000, 0.9659258262890683122, 1.000000000000000000, 0.9659258262890683122, 1.000000000000000000, 0.9659258262890683122, 1.000000000000000000, 0.9659258262890683122, 1.000000000000000000, 0.9659258262890683122, 1.000000000000000000, 0.9659258262890683122, 1.000000000000000000, 0.9659258262890683122, 1.000000000000000000, 0.9659258262890683122, 1.000000000000000000, 0.9659258262890683122, 1.000000000000000000, 0.9659258262890683122, 1.000000000000000000, 0.9659258262890683122, 1.000000000000000000, 0.9659258262890683122, 1.000000000000000000, 0.9659258262890683122, 1.000000000000000000, 0.9659258262890683122, 1.000000000000000000, 0.9659258262890683122, 1.000000000000000000, 0.9659258262890683122, 1.000000000000000000, 0.9659258262890683122, 1.000000000000000000, 0.9659258262890683122, 1.000000000000000000, 0.9659258262890683122, 1.000000000000000000, 0.9659258262890683122, 1.000000000000000000, 0.9659258262890683122, 1.000000000000000000, 0.9659258262890683122, 1.000000000000000000, 0.9659258262890683122, 1.000000000000000000, 0.9659258262890683122, 1.000000000000000000, 0.9659258262890683122, 1.000000000000000000, 0.9659258262890683122, 1.000000000000000000, 0.9659258262890683122, 1.000000000000000000, 0.9659258262890683122, 1.000000000000000000, 0.9659258262890683122, 1.000000000000000000, 0.9659258262890683122, 1.000000000000000000, 0.9659258262890683122, 1.000000000000000000, 0.9659258262890683122, 1.000000000000000000, 0.9659258262890683122, 1.000000000000000000, 0.9659258262890683122, 1.000000000000000000, 0.9659258262890683122, 1.000000000000000000, 0.9659258262890683122, 1.000000000000000000, 0.9659258262890683122, 1.000000000000000000, 0.9659258262890683122, 1.000000000000000000, 0.9659258262890683122, 1.000000000000000000, 0.9659258262890683122, 1.000000000000000000, 0.9659258262890683122, 1.000000000000000000, 0.9659258262890683122, 1.000000000000000000, 0.9659258262890683122, 1.000000000000000000, 0.9659258262890683122, 1.000000000000000000, 0.9659258262890683122, 1.000000000000000000, 0.9659258262890683122, 1.000000000000000000, 0.9659258262890683122, 1.000000000000000000, 0.9659258262890683122, 1.000000000000000000, 0.9659258262890683122, 1.000000000000000000, 0.9659258262890683122, 1.000000000000000000, 0.9659258262890683122, 1.000000000000000000, 0.9659258262890683122, 1.000000000000000000, 0.9659258262890683122, 1.000000000000000000, 0.9659258262890683122, 1.000000000000000000, 0.9659258262890683122, 1.000000000000000000, 0.9659258262890683122, 1.000000000000000000, 0.9659258262890683122, 1.000000000000000000, 0.9659258262890683122, 1.000000000000000000, 0.9659258262890683122, 1.000000000000000000, 0.9659258262890683122, 1.000000000000000000, 0.9659258262890683122, 1.000000000000000000, 0.9659258262890683122, 1.000000000000000000, 0.9659258262890683122, 1.000000000000000000, 0.9659258262890683122, 1.000000000000000000, 0.9659258262890683122, 1.000000000000000000, 0.9659258262890683122, 1.000000000000000000, 0.9659258262890683122, 1.000000000000000000, 0.9659258262890683122, 1.000000000000000000, 0.9659258262890683122, 1.000000000000000000, 0.9659258262890683122, 1.000000000000000000, 0.9659258262890683122, 1.000000000000000000, 0.9659258262890683122, 1.000000000000000000, 0.9659258262890683122, 1.000000000000000000, 0.9659258262890683122, 1.000000000000000000, 0.9659258262890683122, 1.000000000000000000, 0.9659258262890683122, 1.000000000000000000, 0.9659258262890683122, 1.000000000000000000, 0.9659258262890683122, 1.000000000000000000, 0.9659258262890683122, 1.000000000000000000, 0.9659258262890683122, 1.000000000000000000, 0.9659258262890683122, 1.000000000000000000, 0.9659258262890683122, 1.000000000000000000, 0.9659258262890683122, 1.000000000000000000, 0.9659258262890683122, 1.000000000000000000, 0.9659258262890683122, 1.000000000000000000) ) ) 
 REPRESENTATION_ITEM ( '' )  SURFACE ( )  );
#39056=CARTESIAN_POINT ( 'NONE',  ( 14.92337183194729633, 7.675597817667451750, 8.527530157486181039 ) ) ;
#39057=CARTESIAN_POINT ( 'NONE',  ( 2.035157376598824452, 68.68868534415484817, 7.964842623401179544 ) ) ;
#39058=CARTESIAN_POINT ( 'NONE',  ( 5.054308323419867577, 70.51564955044841554, 5.000000000000000000 ) ) ;
#39061=CARTESIAN_POINT ( 'NONE',  ( -46.94000000000001194, 103.0000000000000000, 5.997726559847112782 ) ) ;
#39062=CARTESIAN_POINT ( 'NONE',  ( 19.84674366389459266, 3.717264484334118713, -2.638427012816827677 ) ) ;
#39064=CARTESIAN_POINT ( 'NONE',  ( 19.84674366389459266, 43.71726448433410894, -2.638427012816827677 ) ) ;
#39069=CARTESIAN_POINT ( 'NONE',  ( -2.266590686148945544, 7.220415501580634832, 7.082119434687048631 ) ) ;
#39070=CARTESIAN_POINT ( 'NONE',  ( 22.26659068614894466, 23.88708216824730357, 7.082119434687054849 ) ) ;
#39073=CARTESIAN_POINT ( 'NONE',  ( 17.96484262340118221, 61.18868534415482685, -7.964842623401177768 ) ) ;
#39074=CARTESIAN_POINT ( 'NONE',  ( 2.035157376598822676, 27.43868534415483396, -7.964842623401177768 ) ) ;
#39075=ORIENTED_EDGE ( 'NONE', *, *, #10286, .T. ) ;
#39076=CARTESIAN_POINT ( 'NONE',  ( 12.63842701281683034, 7.467264484334118713, 9.846743663894596210 ) ) ;
#39077=CARTESIAN_POINT ( 'NONE',  ( 1.472469842513823179, 5.592264484334118713, -4.923371831947296329 ) ) ;
#39078=CARTESIAN_POINT ( 'NONE',  ( 21.09922568453594849, 26.20696800326375353, 6.408140936763242479 ) ) ;
#39079=CARTESIAN_POINT ( 'NONE',  ( 17.20831665107776587, 27.88393115100078390, 7.208316651077764980 ) ) ;
#39081=CARTESIAN_POINT ( 'NONE',  ( 22.81628187352647785, 16.62363466993042138, 6.195893100308588602E-16 ) ) ;
#39084=CARTESIAN_POINT ( 'NONE',  ( 10.00000000000000178, 7.258931151000785675, 9.846743663894594434 ) ) ;
#39086=ORIENTED_EDGE ( 'NONE', *, *, #26992, .F. ) ;
#39089=CARTESIAN_POINT ( 'NONE',  ( 19.42250999205614548, 20.98035201082150891, -5.440088680355545492 ) ) ;
#39090=CARTESIAN_POINT ( 'NONE',  ( -0.3689425029237881626, 27.42874883491397142, 10.36894250292379027 ) ) ;
#39091=CARTESIAN_POINT ( 'NONE',  ( 18.52753015748617571, 43.09226448433412315, 4.923371831947298993 ) ) ;
#39092=CARTESIAN_POINT ( 'NONE',  ( 2.035157376598822676, 67.43868534415484817, -7.964842623401177768 ) ) ;
#39093=CARTESIAN_POINT ( 'NONE',  ( 21.09922568453595559, 47.04030133659708923, -6.408140936763230044 ) ) ;
#39095=CARTESIAN_POINT ( 'NONE',  ( -0.8801773607111009756, 23.06368534415484106, 1.068504757029289695E-15 ) ) ;
#39097=CARTESIAN_POINT ( 'NONE',  ( 22.81628187352648496, 11.83196800326375531, -3.434112377981050290 ) ) ;
#39098=CARTESIAN_POINT ( 'NONE',  ( 3.591859063236761518, 14.95696800326375531, 11.09922568453594849 ) ) ;
#39099=CARTESIAN_POINT ( 'NONE',  ( 12.63842701281683034, 47.46726448433412315, 9.846743663894596210 ) ) ;
#39101=CARTESIAN_POINT ( 'NONE',  ( 6.565887622018943937, 45.16530133659708923, 12.81628187352647430 ) ) ;
#39103=SURFACE_STYLE_USAGE ( .BOTH. , #78567 ) ;
#39104=CARTESIAN_POINT ( 'NONE',  ( 7.084665262690076126, 47.02201867748818387, -10.88017736071110164 ) ) ;
#39105=CARTESIAN_POINT ( 'NONE',  ( 19.80832241502127644, 9.758688159020689312, 6.499999999999999112 ) ) ;
#39108=CARTESIAN_POINT ( 'NONE',  ( 18.61655166652077042, 29.87718327197428891, 6.499999999999981348 ) ) ;
#39109=CARTESIAN_POINT ( 'NONE',  ( -0.8801773607111009756, 53.06368534415484106, 1.068504757029289695E-15 ) ) ;
#39110=CARTESIAN_POINT ( 'NONE',  ( 0.5774900079438590739, 47.64701867748817676, -5.440088680355550821 ) ) ;
#39113=CARTESIAN_POINT ( 'NONE',  ( 10.00000000000000178, 69.31368534415484817, 10.88017736071110342 ) ) ;
#39114=CARTESIAN_POINT ( 'NONE',  ( 19.84674366389459266, 48.71726448433413026, -2.638427012816827677 ) ) ;
#39115=CARTESIAN_POINT ( 'NONE',  ( 0.5774900079438590739, 22.64701867748817321, -5.440088680355550821 ) ) ;
#39117=CARTESIAN_POINT ( 'NONE',  ( 10.00000000000000000, 27.87363466993042138, -12.81628187352647608 ) ) ;
#39119=CARTESIAN_POINT ( 'NONE',  ( 15.44008868035555260, 39.73035201082150536, 9.422509992056143702 ) ) ;
#39121=CARTESIAN_POINT ( 'NONE',  ( 16.40814093676323893, 10.79030133659708923, 11.09922568453595026 ) ) ;
#39124=CARTESIAN_POINT ( 'NONE',  ( 7.084665262690076126, 9.105352010821503583, 10.88017736071109987 ) ) ;
#39125=CARTESIAN_POINT ( 'NONE',  ( 12.91533473730993009, 26.60535201082150536, -10.88017736071109987 ) ) ;
#39126=CARTESIAN_POINT ( 'NONE',  ( 13.79529636645031943, 35.34541550158063927, -14.16423886937409904 ) ) ;
#39127=CARTESIAN_POINT ( 'NONE',  ( 0.1532563361054083140, 21.00893115100078745, 1.131784320476157264E-15 ) ) ;
#39128=CARTESIAN_POINT ( 'NONE',  ( 4.559911319644449179, 58.89701867748817676, 9.422509992056141925 ) ) ;
#39130=CARTESIAN_POINT ( 'NONE',  ( 20.36894250292379382, 8.678748834913967869, 10.36894250292379205 ) ) ;
#39133=CARTESIAN_POINT ( 'NONE',  ( 12.63842701281683922, 59.55059781766744464, -9.846743663894590881 ) ) ;
#39135=CARTESIAN_POINT ( 'NONE',  ( -0.3689425029237881626, 32.42874883491395366, 10.36894250292379027 ) ) ;
#39136=CARTESIAN_POINT ( 'NONE',  ( 6.204703633549690345, 30.76208216824730357, -14.16423886937410259 ) ) ;
#39137=CARTESIAN_POINT ( 'NONE',  ( 12.63842701281683922, 4.550597817667451750, -9.846743663894590881 ) ) ;
#39138=CARTESIAN_POINT ( 'NONE',  ( 10.00000000000000000, 64.75893115100078035, -9.846743663894594434 ) ) ;
#39140=CARTESIAN_POINT ( 'NONE',  ( 4.559911319644449179, 63.89701867748817676, 9.422509992056141925 ) ) ;
#39141=CARTESIAN_POINT ( 'NONE',  ( 0.6178305044545818747, 13.49863466993041783, -9.382169495545419124 ) ) ;
#39142=CARTESIAN_POINT ( 'NONE',  ( -4.164238869374098151, 36.59541550158063217, -3.795296366450310543 ) ) ;
#39143=CARTESIAN_POINT ( 'NONE',  ( -0.8801773607111008646, 23.27201867748817676, 2.915334737309923430 ) ) ;
#39144=CARTESIAN_POINT ( 'NONE',  ( 20.88017736071110875, 30.77201867748816966, -2.915334737309920765 ) ) ;
#39145=CARTESIAN_POINT ( 'NONE',  ( 20.24186590665275176, 4.734100856612036168, 6.114288769123088052 ) ) ;
#39146=CARTESIAN_POINT ( 'NONE',  ( 2.035157376598824452, 58.68868534415482685, 7.964842623401179544 ) ) ;
#39147=B_SPLINE_CURVE_WITH_KNOTS ( 'NONE', 3,
 ( #52578, #90573, #53069, #89101, #14609, #20614 ),
 .UNSPECIFIED., .F., .F.,
 ( 4, 2, 4 ),
 ( 0.000000000000000000, 0.0003802939046624577652, 0.0007605878093249155304 ),
 .UNSPECIFIED. ) ;
#39149=VERTEX_POINT ( 'NONE', #22861 ) ;
#39150=CARTESIAN_POINT ( 'NONE',  ( 20.15039907845753930, 0.07447313448805115144, 6.262539305110068177 ) ) ;
#39151=ORIENTED_EDGE ( 'NONE', *, *, #96468, .F. ) ;
#39154=CARTESIAN_POINT ( 'NONE',  ( -2.266590686148945544, 6.387082168247300906, -7.082119434687050408 ) ) ;
#39155=CARTESIAN_POINT ( 'NONE',  ( 22.26659068614895176, 59.72041550158063927, -7.082119434687042414 ) ) ;
#39156=CARTESIAN_POINT ( 'NONE',  ( 0.5774900079438590739, 2.647018677488171434, -5.440088680355550821 ) ) ;
#39157=CARTESIAN_POINT ( 'NONE',  ( 5.076628168052703671, 31.84226448433412315, 8.527530157486179263 ) ) ;
#39158=CARTESIAN_POINT ( 'NONE',  ( 0.1532563361054100626, 65.80059781766745175, -2.638427012816831230 ) ) ;
#39161=MECHANICAL_DESIGN_GEOMETRIC_PRESENTATION_REPRESENTATION('',(#32719),#45497);
#39162=CARTESIAN_POINT ( 'NONE',  ( 22.81628187352647785, 6.415301336597088344, 3.434112377981063169 ) ) ;
#39163=ORIENTED_EDGE ( 'NONE', *, *, #53520, .T. ) ;
#39164=( BOUNDED_SURFACE ( )  B_SPLINE_SURFACE ( 1, 2, ( 
 ( #40054, #8573, #38582, #47048, #23596, #45582, #22601, #91582, #53569, #84082, #68589, #93045, #92549, #119, #15597, #46080, #69080, #77544, #61560, #31060, #84574, #85557, #83589, #7606, #17069, #615, #24078, #54060, #39077, #62539, #54545, #69571, #1090, #31552, #16573, #47552, #78049, #9551, #85062, #55039, #9062, #32035, #39575, #70064, #1586, #70553, #79530, #88001, #34005, #19028, #26041, #40553, #19514, #25557, #18533, #49505, #63528, #80010, #86541, #64009, #49024, #87515, #71053, #87021, #17564, #2576, #26516, #95008, #50011, #33032, #11515, #48525, #94036, #42512, #95515, #41549, #33512, #80514, #10054, #11030, #12013, #57013, #57505, #10539, #79027, #72014, #41049, #94522, #56049, #18048, #32541, #34497, #56532, #42038, #3544, #71548, #64502, #72502, #3058, #4034, #64988, #27008, #72996, #25069, #63041, #93538, #55552, #86053, #48030, #78543, #28971, #5510, #5011, #43972, #51989, #66488, #97015, #82974, #59965, #66985, #73484, #59474, #97506, #88498, #28493, #5999, #89975, #81982, #14492, #74974, #4526, #67482, #34989, #80999, #74474, #13493, #21492, #43001, #65990, #96517, #58986, #6479, #20504, #43484, #82477, #35495, #20999, #90457, #65493, #44475, #21994, #44964, #12988, #89489, #51487, #96013, #36983, #27498, #36493, #27990, #13997, #98004, #73985, #58485, #57992, #52470, #35986, #20001, #50502, #88998, #29457, #12502, #50990, #81484, #92433, #53950, #8936, #68474, #91457, #76940, #98989, #84458, #23957, #38469, #68962, #54919, #31917, #38956, #45460, #31428, #69448, #60463, #494, #8449, #968, #15956, #85434, #46929, #75468, #39453, #6983, #52957, #46449, #61932, #54431, #14989, #37983, #30447, #30942, #77422, #22983, #15483, #84940, #75959, #91946, #62418, #37488, #16451, #92922, #16943, #83957, #61440, #23477, #67977, #69945, #98502, #1465, #60948, #24453, #29957, #45966, #7487, #90951, #22483, #76456, #83468, #53448, #7971, #40931, #47426, #40439, #70939, #64385, #25918, #79891, #2456, #63412, #48900, #32912, #56420, #33392, #33880, #78418, #94895, #93917, #78914, #63890, #3420, #85935, #2944, #32421, #17446, #41436, #10913, #64869, #47912, #26393, #25444, #9935, #57388, #11399, #86905, #48411, #95391, #24945, #94404, #26893, #71897, #72383, #55927, #86426, #18415, #17927, #10424, #55428, #71429, #77926, #49391, #79413, #56893, #87397, #18914, #41922, #3912, #34380, #87879, #9433, #39936, #70438, #1957, #62922, #93423, #74856, #67359, #96895, #88384, #43852, #20385, #19883, #58862, #49882, #95902, #89366, #28372, #36368, #57873, #80883, #12381, #73865, #21370, #35377, #58356, #74346, #50374, #35869 ),
 ( #42886, #5874, #50876, #88877, #43366, #44351, #80394, #42398, #6357, #73369, #51369, #4896, #65868, #51866, #13367, #65372, #4411, #20877, #66862, #36867, #97884, #29344, #96395, #82350, #27871, #89854, #11897, #72876, #81369, #66358, #81856, #59846, #97381, #28848, #12867, #27382, #19396, #5394, #59351, #34878, #13871, #31314, #90335, #60345, #38840, #52352, #53331, #15365, #84348, #82850, #68846, #379, #61326, #23846, #15849, #30827, #37369, #856, #61816, #76820, #90838, #7852, #8337, #38352, #76336, #68357, #91837, #23354, #53836, #46335, #22367, #92321, #21874, #69332, #6858, #52840, #14371, #30331, #44838, #75345, #22859, #45850, #67861, #98381, #29837, #83349, #83840, #7363, #14872, #45343, #75844, #37863, #98875, #60832, #91335, #43199, #89198, #13199, #5710, #97717, #59184, #66188, #96223, #21703, #67695, #22196, #20710, #36199, #66696, #60174, #14200, #90670, #97224, #5223, #44179, #43692, #51202, #81205, #35195, #98207, #81685, #80715, #12211, #20207, #74180, #42718, #73689, #35703, #29180, #89688, #44681, #96722, #28198, #82184, #58694, #21203, #28691, #67192, #12705, #59680, #51702, #13695, #74688, #36703, #50712, #6199, #65698, #90173, #52188, #82682, #29665, #75177, #6688, #37206, #73199, #4730, #27702, #58187, #88699, #79172, #95151, #57155, #19166, #73133, #4174, #26661, #10201, #19656, #50147, #65140, #25702, #34147, #95661, #64641, #3686, #64152, #87653, #49645, #80152, #42177, #63666, #12151, #42658, #34644, #86195, #2720, #72641, #71681, #80657, #88144, #41201, #33657, #27146, #4674, #94671, #57648, #94171, #17707, #63176, #11664, #3191, #93685, #49170, #25218, #55699, #56192, #26180, #56671, #87160, #48178, #41688, #48671, #78690, #18685, #40694, #71196, #79672, #11169, #33173, #72158, #86686, #18190, #10688, #22512, #83002, #23010, #68006, #90001, #96159, #6504, #67509, #38008, #14520, #91977, #84486, #15017, #37012, #60977, #37514, #98028, #75988, #83988, #98532, #29985, #15987, #23506, #29, #29483, #91490, #30476, #21518, #60490, #68501, #53478, #45486, #46474, #7998, #35135, #526, #65636, #14021, #7517, #15513, #45995, #75002, #59991, #90485, #90979, #38496, #52495, #75497, #76484, #22021, #52984, #53977, #28993, #68991, #76970, #59504, #44989, #83499, #30973, #52014, #61470, #82503, #44501, #7008, #70967, #70465, #16977, #8968, #61962, #25946, #77956, #48929, #8483, #46960, #1987, #38988, #1493, #31946, #25475, #85965, #40960, #62447, #24485, #9963, #92950, #17473, #93452, #93948, #39484, #55957, #54948, #39964, #24977, #63441, #77454, #62949, #92461, #69974, #2487, #32940, #56448, #85465 ) ),
 .UNSPECIFIED., .F., .F., .F. ) 
 B_SPLINE_SURFACE_WITH_KNOTS ( ( 2, 2 ),
 ( 3, 2, 2, 2, 2, 2, 2, 2, 2, 2, 2, 2, 2, 2, 2, 2, 2, 2, 2, 2, 2, 2, 2, 2, 2, 2, 2, 2, 2, 2, 2, 2, 2, 2, 2, 2, 2, 2, 2, 2, 2, 2, 2, 2, 2, 2, 2, 2, 2, 2, 2, 2, 2, 2, 2, 2, 2, 2, 2, 2, 2, 2, 2, 2, 2, 2, 2, 2, 2, 2, 2, 2, 2, 2, 2, 2, 2, 2, 2, 2, 2, 2, 2, 2, 2, 2, 2, 2, 2, 2, 2, 2, 2, 2, 2, 2, 2, 2, 2, 2, 2, 2, 2, 2, 2, 2, 2, 2, 2, 2, 2, 2, 2, 2, 2, 2, 2, 2, 2, 2, 2, 2, 2, 2, 2, 2, 2, 2, 2, 2, 2, 2, 2, 2, 2, 2, 2, 2, 2, 2, 2, 2, 2, 2, 2, 2, 2, 2, 2, 2, 2, 2, 2, 2, 2, 2, 2, 2, 2, 2, 2, 2, 3 ),
 ( 0.000000000000000000, 1.000000000000000000 ),
 ( 0.000000000000000000, 0.005952380952380952051, 0.01190476190476190410, 0.01785714285714285615, 0.02380952380952380820, 0.02976190476190476025, 0.03571428571428571230, 0.04166666666666666435, 0.04761904761904761640, 0.05357142857142856845, 0.05952380952380952051, 0.06547619047619047949, 0.07142857142857142461, 0.07738095238095238360, 0.08333333333333332871, 0.08928571428571428770, 0.09523809523809523281, 0.1011904761904761918, 0.1071428571428571369, 0.1130952380952380959, 0.1190476190476190410, 0.1250000000000000000, 0.1309523809523809590, 0.1369047619047619180, 0.1428571428571428492, 0.1488095238095238082, 0.1547619047619047672, 0.1607142857142857262, 0.1666666666666666574, 0.1726190476190476164, 0.1785714285714285754, 0.1845238095238095344, 0.1904761904761904656, 0.1964285714285714246, 0.2023809523809523836, 0.2083333333333333426, 0.2142857142857142738, 0.2202380952380952328, 0.2261904761904761918, 0.2321428571428571508, 0.2380952380952380820, 0.2440476190476190410, 0.2500000000000000000, 0.2559523809523809312, 0.2619047619047619180, 0.2678571428571428492, 0.2738095238095238360, 0.2797619047619047672, 0.2857142857142856984, 0.2916666666666666852, 0.2976190476190476164, 0.3035714285714285476, 0.3095238095238095344, 0.3154761904761904656, 0.3214285714285714524, 0.3273809523809523836, 0.3333333333333333148, 0.3392857142857143016, 0.3452380952380952328, 0.3511904761904761640, 0.3571428571428571508, 0.3630952380952380820, 0.3690476190476190688, 0.3750000000000000000, 0.3809523809523809312, 0.3869047619047619180, 0.3928571428571428492, 0.3988095238095238360, 0.4047619047619047672, 0.4107142857142856984, 0.4166666666666666852, 0.4226190476190476164, 0.4285714285714285476, 0.4345238095238095344, 0.4404761904761904656, 0.4464285714285714524, 0.4523809523809523836, 0.4583333333333333148, 0.4642857142857143016, 0.4702380952380952328, 0.4761904761904761640, 0.4821428571428571508, 0.4880952380952380820, 0.4940476190476190688, 0.5000000000000000000, 0.5059523809523809312, 0.5119047619047618625, 0.5178571428571429047, 0.5238095238095238360, 0.5297619047619047672, 0.5357142857142856984, 0.5416666666666666297, 0.5476190476190476719, 0.5535714285714286031, 0.5595238095238095344, 0.5654761904761904656, 0.5714285714285713969, 0.5773809523809523281, 0.5833333333333333703, 0.5892857142857143016, 0.5952380952380952328, 0.6011904761904761640, 0.6071428571428570953, 0.6130952380952381375, 0.6190476190476190688, 0.6250000000000000000, 0.6309523809523809312, 0.6369047619047618625, 0.6428571428571429047, 0.6488095238095238360, 0.6547619047619047672, 0.6607142857142856984, 0.6666666666666666297, 0.6726190476190476719, 0.6785714285714286031, 0.6845238095238095344, 0.6904761904761904656, 0.6964285714285713969, 0.7023809523809523281, 0.7083333333333333703, 0.7142857142857143016, 0.7202380952380952328, 0.7261904761904761640, 0.7321428571428570953, 0.7380952380952381375, 0.7440476190476190688, 0.7500000000000000000, 0.7559523809523809312, 0.7619047619047618625, 0.7678571428571429047, 0.7738095238095238360, 0.7797619047619047672, 0.7857142857142856984, 0.7916666666666666297, 0.7976190476190476719, 0.8035714285714286031, 0.8095238095238095344, 0.8154761904761904656, 0.8214285714285713969, 0.8273809523809523281, 0.8333333333333333703, 0.8392857142857143016, 0.8452380952380952328, 0.8511904761904761640, 0.8571428571428570953, 0.8630952380952381375, 0.8690476190476190688, 0.8750000000000000000, 0.8809523809523809312, 0.8869047619047618625, 0.8928571428571429047, 0.8988095238095238360, 0.9047619047619047672, 0.9107142857142856984, 0.9166666666666666297, 0.9226190476190476719, 0.9285714285714286031, 0.9345238095238095344, 0.9404761904761904656, 0.9464285714285713969, 0.9523809523809523281, 0.9583333333333333703, 0.9642857142857143016 ),
 .UNSPECIFIED. ) 
 GEOMETRIC_REPRESENTATION_ITEM ( )  RATIONAL_B_SPLINE_SURFACE ( (
 ( 1.000000000000000000, 0.9659258262890683122, 1.000000000000000000, 0.9659258262890683122, 1.000000000000000000, 0.9659258262890683122, 1.000000000000000000, 0.9659258262890683122, 1.000000000000000000, 0.9659258262890683122, 1.000000000000000000, 0.9659258262890683122, 1.000000000000000000, 0.9659258262890683122, 1.000000000000000000, 0.9659258262890683122, 1.000000000000000000, 0.9659258262890683122, 1.000000000000000000, 0.9659258262890683122, 1.000000000000000000, 0.9659258262890683122, 1.000000000000000000, 0.9659258262890683122, 1.000000000000000000, 0.9659258262890683122, 1.000000000000000000, 0.9659258262890683122, 1.000000000000000000, 0.9659258262890683122, 1.000000000000000000, 0.9659258262890683122, 1.000000000000000000, 0.9659258262890683122, 1.000000000000000000, 0.9659258262890683122, 1.000000000000000000, 0.9659258262890683122, 1.000000000000000000, 0.9659258262890683122, 1.000000000000000000, 0.9659258262890683122, 1.000000000000000000, 0.9659258262890683122, 1.000000000000000000, 0.9659258262890683122, 1.000000000000000000, 0.9659258262890683122, 1.000000000000000000, 0.9659258262890683122, 1.000000000000000000, 0.9659258262890683122, 1.000000000000000000, 0.9659258262890683122, 1.000000000000000000, 0.9659258262890683122, 1.000000000000000000, 0.9659258262890683122, 1.000000000000000000, 0.9659258262890683122, 1.000000000000000000, 0.9659258262890683122, 1.000000000000000000, 0.9659258262890683122, 1.000000000000000000, 0.9659258262890683122, 1.000000000000000000, 0.9659258262890683122, 1.000000000000000000, 0.9659258262890683122, 1.000000000000000000, 0.9659258262890683122, 1.000000000000000000, 0.9659258262890683122, 1.000000000000000000, 0.9659258262890683122, 1.000000000000000000, 0.9659258262890683122, 1.000000000000000000, 0.9659258262890683122, 1.000000000000000000, 0.9659258262890683122, 1.000000000000000000, 0.9659258262890683122, 1.000000000000000000, 0.9659258262890683122, 1.000000000000000000, 0.9659258262890683122, 1.000000000000000000, 0.9659258262890683122, 1.000000000000000000, 0.9659258262890683122, 1.000000000000000000, 0.9659258262890683122, 1.000000000000000000, 0.9659258262890683122, 1.000000000000000000, 0.9659258262890683122, 1.000000000000000000, 0.9659258262890683122, 1.000000000000000000, 0.9659258262890683122, 1.000000000000000000, 0.9659258262890683122, 1.000000000000000000, 0.9659258262890683122, 1.000000000000000000, 0.9659258262890683122, 1.000000000000000000, 0.9659258262890683122, 1.000000000000000000, 0.9659258262890683122, 1.000000000000000000, 0.9659258262890683122, 1.000000000000000000, 0.9659258262890683122, 1.000000000000000000, 0.9659258262890683122, 1.000000000000000000, 0.9659258262890683122, 1.000000000000000000, 0.9659258262890683122, 1.000000000000000000, 0.9659258262890683122, 1.000000000000000000, 0.9659258262890683122, 1.000000000000000000, 0.9659258262890683122, 1.000000000000000000, 0.9659258262890683122, 1.000000000000000000, 0.9659258262890683122, 1.000000000000000000, 0.9659258262890683122, 1.000000000000000000, 0.9659258262890683122, 1.000000000000000000, 0.9659258262890683122, 1.000000000000000000, 0.9659258262890683122, 1.000000000000000000, 0.9659258262890683122, 1.000000000000000000, 0.9659258262890683122, 1.000000000000000000, 0.9659258262890683122, 1.000000000000000000, 0.9659258262890683122, 1.000000000000000000, 0.9659258262890683122, 1.000000000000000000, 0.9659258262890683122, 1.000000000000000000, 0.9659258262890683122, 1.000000000000000000, 0.9659258262890683122, 1.000000000000000000, 0.9659258262890683122, 1.000000000000000000, 0.9659258262890683122, 1.000000000000000000, 0.9659258262890683122, 1.000000000000000000, 0.9659258262890683122, 1.000000000000000000, 0.9659258262890683122, 1.000000000000000000, 0.9659258262890683122, 1.000000000000000000, 0.9659258262890683122, 1.000000000000000000, 0.9659258262890683122, 1.000000000000000000, 0.9659258262890683122, 1.000000000000000000, 0.9659258262890683122, 1.000000000000000000, 0.9659258262890683122, 1.000000000000000000, 0.9659258262890683122, 1.000000000000000000, 0.9659258262890683122, 1.000000000000000000, 0.9659258262890683122, 1.000000000000000000, 0.9659258262890683122, 1.000000000000000000, 0.9659258262890683122, 1.000000000000000000, 0.9659258262890683122, 1.000000000000000000, 0.9659258262890683122, 1.000000000000000000, 0.9659258262890683122, 1.000000000000000000, 0.9659258262890683122, 1.000000000000000000, 0.9659258262890683122, 1.000000000000000000, 0.9659258262890683122, 1.000000000000000000, 0.9659258262890683122, 1.000000000000000000, 0.9659258262890683122, 1.000000000000000000, 0.9659258262890683122, 1.000000000000000000, 0.9659258262890683122, 1.000000000000000000, 0.9659258262890683122, 1.000000000000000000, 0.9659258262890683122, 1.000000000000000000, 0.9659258262890683122, 1.000000000000000000, 0.9659258262890683122, 1.000000000000000000, 0.9659258262890683122, 1.000000000000000000, 0.9659258262890683122, 1.000000000000000000, 0.9659258262890683122, 1.000000000000000000, 0.9659258262890683122, 1.000000000000000000, 0.9659258262890683122, 1.000000000000000000, 0.9659258262890683122, 1.000000000000000000, 0.9659258262890683122, 1.000000000000000000, 0.9659258262890683122, 1.000000000000000000, 0.9659258262890683122, 1.000000000000000000, 0.9659258262890683122, 1.000000000000000000, 0.9659258262890683122, 1.000000000000000000, 0.9659258262890683122, 1.000000000000000000, 0.9659258262890683122, 1.000000000000000000, 0.9659258262890683122, 1.000000000000000000, 0.9659258262890683122, 1.000000000000000000, 0.9659258262890683122, 1.000000000000000000, 0.9659258262890683122, 1.000000000000000000, 0.9659258262890683122, 1.000000000000000000, 0.9659258262890683122, 1.000000000000000000, 0.9659258262890683122, 1.000000000000000000, 0.9659258262890683122, 1.000000000000000000, 0.9659258262890683122, 1.000000000000000000, 0.9659258262890683122, 1.000000000000000000, 0.9659258262890683122, 1.000000000000000000, 0.9659258262890683122, 1.000000000000000000, 0.9659258262890683122, 1.000000000000000000, 0.9659258262890683122, 1.000000000000000000, 0.9659258262890683122, 1.000000000000000000, 0.9659258262890683122, 1.000000000000000000, 0.9659258262890683122, 1.000000000000000000, 0.9659258262890683122, 1.000000000000000000, 0.9659258262890683122, 1.000000000000000000, 0.9659258262890683122, 1.000000000000000000, 0.9659258262890683122, 1.000000000000000000, 0.9659258262890683122, 1.000000000000000000, 0.9659258262890683122, 1.000000000000000000, 0.9659258262890683122, 1.000000000000000000, 0.9659258262890683122, 1.000000000000000000, 0.9659258262890683122, 1.000000000000000000, 0.9659258262890683122, 1.000000000000000000, 0.9659258262890683122, 1.000000000000000000, 0.9659258262890683122, 1.000000000000000000, 0.9659258262890683122, 1.000000000000000000, 0.9659258262890683122, 1.000000000000000000, 0.9659258262890683122, 1.000000000000000000, 0.9659258262890683122, 1.000000000000000000, 0.9659258262890683122, 1.000000000000000000, 0.9659258262890683122, 1.000000000000000000, 0.9659258262890683122, 1.000000000000000000, 0.9659258262890683122, 1.000000000000000000, 0.9659258262890683122, 1.000000000000000000, 0.9659258262890683122, 1.000000000000000000, 0.9659258262890683122, 1.000000000000000000, 0.9659258262890683122, 1.000000000000000000),
 ( 1.000000000000000000, 0.9659258262890683122, 1.000000000000000000, 0.9659258262890683122, 1.000000000000000000, 0.9659258262890683122, 1.000000000000000000, 0.9659258262890683122, 1.000000000000000000, 0.9659258262890683122, 1.000000000000000000, 0.9659258262890683122, 1.000000000000000000, 0.9659258262890683122, 1.000000000000000000, 0.9659258262890683122, 1.000000000000000000, 0.9659258262890683122, 1.000000000000000000, 0.9659258262890683122, 1.000000000000000000, 0.9659258262890683122, 1.000000000000000000, 0.9659258262890683122, 1.000000000000000000, 0.9659258262890683122, 1.000000000000000000, 0.9659258262890683122, 1.000000000000000000, 0.9659258262890683122, 1.000000000000000000, 0.9659258262890683122, 1.000000000000000000, 0.9659258262890683122, 1.000000000000000000, 0.9659258262890683122, 1.000000000000000000, 0.9659258262890683122, 1.000000000000000000, 0.9659258262890683122, 1.000000000000000000, 0.9659258262890683122, 1.000000000000000000, 0.9659258262890683122, 1.000000000000000000, 0.9659258262890683122, 1.000000000000000000, 0.9659258262890683122, 1.000000000000000000, 0.9659258262890683122, 1.000000000000000000, 0.9659258262890683122, 1.000000000000000000, 0.9659258262890683122, 1.000000000000000000, 0.9659258262890683122, 1.000000000000000000, 0.9659258262890683122, 1.000000000000000000, 0.9659258262890683122, 1.000000000000000000, 0.9659258262890683122, 1.000000000000000000, 0.9659258262890683122, 1.000000000000000000, 0.9659258262890683122, 1.000000000000000000, 0.9659258262890683122, 1.000000000000000000, 0.9659258262890683122, 1.000000000000000000, 0.9659258262890683122, 1.000000000000000000, 0.9659258262890683122, 1.000000000000000000, 0.9659258262890683122, 1.000000000000000000, 0.9659258262890683122, 1.000000000000000000, 0.9659258262890683122, 1.000000000000000000, 0.9659258262890683122, 1.000000000000000000, 0.9659258262890683122, 1.000000000000000000, 0.9659258262890683122, 1.000000000000000000, 0.9659258262890683122, 1.000000000000000000, 0.9659258262890683122, 1.000000000000000000, 0.9659258262890683122, 1.000000000000000000, 0.9659258262890683122, 1.000000000000000000, 0.9659258262890683122, 1.000000000000000000, 0.9659258262890683122, 1.000000000000000000, 0.9659258262890683122, 1.000000000000000000, 0.9659258262890683122, 1.000000000000000000, 0.9659258262890683122, 1.000000000000000000, 0.9659258262890683122, 1.000000000000000000, 0.9659258262890683122, 1.000000000000000000, 0.9659258262890683122, 1.000000000000000000, 0.9659258262890683122, 1.000000000000000000, 0.9659258262890683122, 1.000000000000000000, 0.9659258262890683122, 1.000000000000000000, 0.9659258262890683122, 1.000000000000000000, 0.9659258262890683122, 1.000000000000000000, 0.9659258262890683122, 1.000000000000000000, 0.9659258262890683122, 1.000000000000000000, 0.9659258262890683122, 1.000000000000000000, 0.9659258262890683122, 1.000000000000000000, 0.9659258262890683122, 1.000000000000000000, 0.9659258262890683122, 1.000000000000000000, 0.9659258262890683122, 1.000000000000000000, 0.9659258262890683122, 1.000000000000000000, 0.9659258262890683122, 1.000000000000000000, 0.9659258262890683122, 1.000000000000000000, 0.9659258262890683122, 1.000000000000000000, 0.9659258262890683122, 1.000000000000000000, 0.9659258262890683122, 1.000000000000000000, 0.9659258262890683122, 1.000000000000000000, 0.9659258262890683122, 1.000000000000000000, 0.9659258262890683122, 1.000000000000000000, 0.9659258262890683122, 1.000000000000000000, 0.9659258262890683122, 1.000000000000000000, 0.9659258262890683122, 1.000000000000000000, 0.9659258262890683122, 1.000000000000000000, 0.9659258262890683122, 1.000000000000000000, 0.9659258262890683122, 1.000000000000000000, 0.9659258262890683122, 1.000000000000000000, 0.9659258262890683122, 1.000000000000000000, 0.9659258262890683122, 1.000000000000000000, 0.9659258262890683122, 1.000000000000000000, 0.9659258262890683122, 1.000000000000000000, 0.9659258262890683122, 1.000000000000000000, 0.9659258262890683122, 1.000000000000000000, 0.9659258262890683122, 1.000000000000000000, 0.9659258262890683122, 1.000000000000000000, 0.9659258262890683122, 1.000000000000000000, 0.9659258262890683122, 1.000000000000000000, 0.9659258262890683122, 1.000000000000000000, 0.9659258262890683122, 1.000000000000000000, 0.9659258262890683122, 1.000000000000000000, 0.9659258262890683122, 1.000000000000000000, 0.9659258262890683122, 1.000000000000000000, 0.9659258262890683122, 1.000000000000000000, 0.9659258262890683122, 1.000000000000000000, 0.9659258262890683122, 1.000000000000000000, 0.9659258262890683122, 1.000000000000000000, 0.9659258262890683122, 1.000000000000000000, 0.9659258262890683122, 1.000000000000000000, 0.9659258262890683122, 1.000000000000000000, 0.9659258262890683122, 1.000000000000000000, 0.9659258262890683122, 1.000000000000000000, 0.9659258262890683122, 1.000000000000000000, 0.9659258262890683122, 1.000000000000000000, 0.9659258262890683122, 1.000000000000000000, 0.9659258262890683122, 1.000000000000000000, 0.9659258262890683122, 1.000000000000000000, 0.9659258262890683122, 1.000000000000000000, 0.9659258262890683122, 1.000000000000000000, 0.9659258262890683122, 1.000000000000000000, 0.9659258262890683122, 1.000000000000000000, 0.9659258262890683122, 1.000000000000000000, 0.9659258262890683122, 1.000000000000000000, 0.9659258262890683122, 1.000000000000000000, 0.9659258262890683122, 1.000000000000000000, 0.9659258262890683122, 1.000000000000000000, 0.9659258262890683122, 1.000000000000000000, 0.9659258262890683122, 1.000000000000000000, 0.9659258262890683122, 1.000000000000000000, 0.9659258262890683122, 1.000000000000000000, 0.9659258262890683122, 1.000000000000000000, 0.9659258262890683122, 1.000000000000000000, 0.9659258262890683122, 1.000000000000000000, 0.9659258262890683122, 1.000000000000000000, 0.9659258262890683122, 1.000000000000000000, 0.9659258262890683122, 1.000000000000000000, 0.9659258262890683122, 1.000000000000000000, 0.9659258262890683122, 1.000000000000000000, 0.9659258262890683122, 1.000000000000000000, 0.9659258262890683122, 1.000000000000000000, 0.9659258262890683122, 1.000000000000000000, 0.9659258262890683122, 1.000000000000000000, 0.9659258262890683122, 1.000000000000000000, 0.9659258262890683122, 1.000000000000000000, 0.9659258262890683122, 1.000000000000000000, 0.9659258262890683122, 1.000000000000000000, 0.9659258262890683122, 1.000000000000000000, 0.9659258262890683122, 1.000000000000000000, 0.9659258262890683122, 1.000000000000000000, 0.9659258262890683122, 1.000000000000000000, 0.9659258262890683122, 1.000000000000000000, 0.9659258262890683122, 1.000000000000000000, 0.9659258262890683122, 1.000000000000000000, 0.9659258262890683122, 1.000000000000000000, 0.9659258262890683122, 1.000000000000000000, 0.9659258262890683122, 1.000000000000000000, 0.9659258262890683122, 1.000000000000000000, 0.9659258262890683122, 1.000000000000000000, 0.9659258262890683122, 1.000000000000000000, 0.9659258262890683122, 1.000000000000000000, 0.9659258262890683122, 1.000000000000000000, 0.9659258262890683122, 1.000000000000000000, 0.9659258262890683122, 1.000000000000000000, 0.9659258262890683122, 1.000000000000000000, 0.9659258262890683122, 1.000000000000000000, 0.9659258262890683122, 1.000000000000000000, 0.9659258262890683122, 1.000000000000000000) ) ) 
 REPRESENTATION_ITEM ( '' )  SURFACE ( )  );
#39165=CARTESIAN_POINT ( 'NONE',  ( -2.266590686148945544, 51.38708216824730357, -7.082119434687050408 ) ) ;
#39166=CARTESIAN_POINT ( 'NONE',  ( 13.79529636645030344, 38.26208216824729647, 14.16423886937410614 ) ) ;
#39168=CARTESIAN_POINT ( 'NONE',  ( 12.91533473730992121, 19.52201867748816611, 10.88017736071110164 ) ) ;
#39169=CARTESIAN_POINT ( 'NONE',  ( 19.38216949554541557, 52.24863466993041072, -9.382169495545420901 ) ) ;
#39170=CARTESIAN_POINT ( 'NONE',  ( 20.88017736071110164, 30.35535201082151247, 2.915334737309930979 ) ) ;
#39171=CARTESIAN_POINT ( 'NONE',  ( 17.20831665107776587, 52.88393115100078035, 7.208316651077764980 ) ) ;
#39172=CARTESIAN_POINT ( 'NONE',  ( 17.96484262340118221, 26.18868534415483396, -7.964842623401177768 ) ) ;
#39173=CARTESIAN_POINT ( 'NONE',  ( 7.361572987183169658, 59.96726448433410894, -9.846743663894592657 ) ) ;
#39175=CARTESIAN_POINT ( 'NONE',  ( 15.44008868035555793, 26.39701867748817321, -9.422509992056140149 ) ) ;
#39180=CARTESIAN_POINT ( 'NONE',  ( 1.472469842513823179, 0.5922644843341181575, -4.923371831947296329 ) ) ;
#39182=EDGE_LOOP ( 'NONE', ( #68277, #36310, #37460, #79219 ) ) ;
#39184=CARTESIAN_POINT ( 'NONE',  ( 1.472469842513823179, 25.59226448433412315, -4.923371831947296329 ) ) ;
#39186=CARTESIAN_POINT ( 'NONE',  ( -2.816281873526473856, 49.12363466993042493, 9.499525473075851096E-16 ) ) ;
#39187=FILL_AREA_STYLE_COLOUR ( '', #38807 ) ;
#39189=ORIENTED_EDGE ( 'NONE', *, *, #19903, .T. ) ;
#39192=CARTESIAN_POINT ( 'NONE',  ( 1.472469842513823179, 60.59226448433412315, -4.923371831947296329 ) ) ;
#39193=CARTESIAN_POINT ( 'NONE',  ( 2.917880565312948704, 42.63708216824729647, 12.26659068614894643 ) ) ;
#39194=CARTESIAN_POINT ( 'NONE',  ( 19.84674366389459621, 53.50893115100078745, 7.409399052514197653E-17 ) ) ;
#39196=CARTESIAN_POINT ( 'NONE',  ( 12.63842701281683034, 17.46726448433411250, 9.846743663894596210 ) ) ;
#39197=CARTESIAN_POINT ( 'NONE',  ( 19.38216949554541202, 55.99863466993041072, 9.382169495545424454 ) ) ;
#39199=CARTESIAN_POINT ( 'NONE',  ( 7.361572987183170547, 57.05059781766744464, 9.846743663894590881 ) ) ;
#39200=CARTESIAN_POINT ( 'NONE',  ( 17.96484262340118221, 49.93868534415484106, 7.964842623401181321 ) ) ;
#39205=CARTESIAN_POINT ( 'NONE',  ( 4.559911319644449179, 53.89701867748817676, 9.422509992056141925 ) ) ;
#39209=CARTESIAN_POINT ( 'NONE',  ( 0.5774900079438590739, 32.64701867748816966, -5.440088680355550821 ) ) ;
#39210=CARTESIAN_POINT ( 'NONE',  ( 21.09922568453595559, 17.04030133659708923, -6.408140936763230044 ) ) ;
#39211=CARTESIAN_POINT ( 'NONE',  ( 2.035157376598822676, 52.43868534415483396, -7.964842623401177768 ) ) ;
#39213=CARTESIAN_POINT ( 'NONE',  ( -42.60666666666668334, 92.50000000000000000, 9.500000000000000000 ) ) ;
#39215=CARTESIAN_POINT ( 'NONE',  ( 15.44008868035555260, 39.73035201082150536, 9.422509992056143702 ) ) ;
#39217=( GEOMETRIC_REPRESENTATION_CONTEXT ( 3 ) GLOBAL_UNCERTAINTY_ASSIGNED_CONTEXT ( ( #52133 ) ) GLOBAL_UNIT_ASSIGNED_CONTEXT ( ( #30053, #60562, #91053 ) ) REPRESENTATION_CONTEXT ( 'NONE', 'WORKASPACE' ) );
#39218=CARTESIAN_POINT ( 'NONE',  ( 17.20831665107776587, 39.13393115100079456, -7.208316651077762316 ) ) ;
#39219=CARTESIAN_POINT ( 'NONE',  ( 5.076628168052703671, 1.842264484334118047, 8.527530157486179263 ) ) ;
#39221=CARTESIAN_POINT ( 'NONE',  ( -2.816281873526473856, 14.12363466993041961, 9.499525473075851096E-16 ) ) ;
#39223=CARTESIAN_POINT ( 'NONE',  ( 10.00000000000000178, 19.31368534415484106, 10.88017736071110342 ) ) ;
#39224=CARTESIAN_POINT ( 'NONE',  ( -2.266590686148945544, 21.38708216824730357, -7.082119434687050408 ) ) ;
#39225=CARTESIAN_POINT ( 'NONE',  ( 20.36894250292379382, 58.67874883491396076, 10.36894250292379205 ) ) ;
#39227=CARTESIAN_POINT ( 'NONE',  ( 7.361572987183170547, 32.05059781766745175, 9.846743663894590881 ) ) ;
#39228=CARTESIAN_POINT ( 'NONE',  ( 0.1532563361054100626, 15.80059781766745353, -2.638427012816831230 ) ) ;
#39229=PRESENTATION_STYLE_ASSIGNMENT (( #8711 ) ) ;
#39232=CARTESIAN_POINT ( 'NONE',  ( 2.791683348922237240, 25.38393115100078390, -7.208316651077763204 ) ) ;
#39233=CARTESIAN_POINT ( 'NONE',  ( 12.91533473730992121, 29.52201867748817321, 10.88017736071110164 ) ) ;
#39234=CARTESIAN_POINT ( 'NONE',  ( 14.92337183194729988, 64.34226448433412315, -8.527530157486177487 ) ) ;
#39235=CARTESIAN_POINT ( 'NONE',  ( -2.266590686148945544, 6.387082168247300906, -7.082119434687050408 ) ) ;
#39237=UNCERTAINTY_MEASURE_WITH_UNIT (LENGTH_MEASURE( 1.000000000000000082E-05 ), #47414, 'distance_accuracy_value', 'NONE');
#39238=CARTESIAN_POINT ( 'NONE',  ( 1.472469842513823179, 5.592264484334118713, -4.923371831947296329 ) ) ;
#39239=CARTESIAN_POINT ( 'NONE',  ( -2.816281873526471635, 33.91530133659708213, -3.434112377981056508 ) ) ;
#39240=CARTESIAN_POINT ( 'NONE',  ( 19.84674366389459621, 43.50893115100078745, 7.409399052514197653E-17 ) ) ;
#39242=CARTESIAN_POINT ( 'NONE',  ( 12.63842701281683034, 17.46726448433411250, 9.846743663894596210 ) ) ;
#39243=CARTESIAN_POINT ( 'NONE',  ( 2.148416515056630338, 12.23726573380443128, 6.499999999999988454 ) ) ;
#39244=CARTESIAN_POINT ( 'NONE',  ( 13.79529636645030344, 58.26208216824728936, 14.16423886937410614 ) ) ;
#39245=CARTESIAN_POINT ( 'NONE',  ( 17.96484262340118221, 49.93868534415484106, 7.964842623401181321 ) ) ;
#39246=( NAMED_UNIT ( * ) SI_UNIT ( $, .STERADIAN. ) SOLID_ANGLE_UNIT ( ) );
#39247=CARTESIAN_POINT ( 'NONE',  ( 20.88017736071110519, 60.56368534415484106, 2.639326808657452039E-16 ) ) ;
#39248=CARTESIAN_POINT ( 'NONE',  ( 14.92337183194729633, 37.67559781766745175, 8.527530157486181039 ) ) ;
#39249=CARTESIAN_POINT ( 'NONE',  ( 10.00000000000000178, 14.31368534415483751, 10.88017736071110342 ) ) ;
#39251=CARTESIAN_POINT ( 'NONE',  ( 0.1532563361054083140, 56.00893115100078745, 1.131784320476157264E-15 ) ) ;
#39253=CARTESIAN_POINT ( 'NONE',  ( 15.44008868035555260, 44.73035201082151247, 9.422509992056143702 ) ) ;
#39254=CARTESIAN_POINT ( 'NONE',  ( 0.1532563361054082862, 1.217264484334117824, 2.638427012816831674 ) ) ;
#39260=CARTESIAN_POINT ( 'NONE',  ( 10.00000000000000178, 3.053748834913967425, 14.16423886937410082 ) ) ;
#39261=CARTESIAN_POINT ( 'NONE',  ( 12.63842701281683034, 47.46726448433412315, 9.846743663894596210 ) ) ;
#39262=CARTESIAN_POINT ( 'NONE',  ( 7.361572987183170547, 22.05059781766745530, 9.846743663894590881 ) ) ;
#39263=CARTESIAN_POINT ( 'NONE',  ( 19.38216949554541202, 50.99863466993042493, 9.382169495545424454 ) ) ;
#39264=CARTESIAN_POINT ( 'NONE',  ( 12.91533473730993009, 21.60535201082150536, -10.88017736071109987 ) ) ;
#39265=CARTESIAN_POINT ( 'NONE',  ( 17.20831665107776587, 54.13393115100079456, -7.208316651077762316 ) ) ;
#39266=CARTESIAN_POINT ( 'NONE',  ( -0.3289641300568005855, 34.27164270246084499, -5.963430220938281678 ) ) ;
#39267=CARTESIAN_POINT ( 'NONE',  ( -4.164238869374099039, 31.80374883491396432, 8.674139862899312516E-16 ) ) ;
#39268=CARTESIAN_POINT ( 'NONE',  ( 13.79529636645031943, 55.34541550158062506, -14.16423886937409904 ) ) ;
#39269=CARTESIAN_POINT ( 'NONE',  ( 1.472469842513823179, 55.59226448433412315, -4.923371831947296329 ) ) ;
#39271=CARTESIAN_POINT ( 'NONE',  ( 17.96484262340118221, 44.93868534415483396, 7.964842623401181321 ) ) ;
#39272=CARTESIAN_POINT ( 'NONE',  ( 14.92337183194729633, 12.67559781766745353, 8.527530157486181039 ) ) ;
#39273=CARTESIAN_POINT ( 'NONE',  ( -35.44000000000001194, 93.50000000000000000, 9.500000000000000000 ) ) ;
#39274=VERTEX_POINT ( 'NONE', #84827 ) ;
#39276=ORIENTED_EDGE ( 'NONE', *, *, #90103, .F. ) ;
#39277=CARTESIAN_POINT ( 'NONE',  ( 2.791683348922237240, 15.38393115100078212, -7.208316651077763204 ) ) ;
#39278=ORIENTED_EDGE ( 'NONE', *, *, #61432, .T. ) ;
#39280=CARTESIAN_POINT ( 'NONE',  ( 2.917880565312948704, 22.63708216824730002, 12.26659068614894643 ) ) ;
#39281=CARTESIAN_POINT ( 'NONE',  ( 5.076628168052703671, 21.84226448433411960, 8.527530157486179263 ) ) ;
#39282=CARTESIAN_POINT ( 'NONE',  ( 12.91533473730993009, 41.60535201082149825, -10.88017736071109987 ) ) ;
#39283=LINE ( 'NONE', #322, #84048 ) ;
#39285=CARTESIAN_POINT ( 'NONE',  ( 20.88017736071110875, 35.77201867748816966, -2.915334737309920765 ) ) ;
#39288=CARTESIAN_POINT ( 'NONE',  ( 10.00000000000000178, 44.31368534415484106, 10.88017736071110342 ) ) ;
#39289=CARTESIAN_POINT ( 'NONE',  ( 22.26659068614894466, 8.887082168247300018, 7.082119434687054849 ) ) ;
#39292=CARTESIAN_POINT ( 'NONE',  ( 10.00000000000000178, 15.37363466993042138, 12.81628187352647608 ) ) ;
#39293=CARTESIAN_POINT ( 'NONE',  ( 5.076628168052704559, 15.17559781766745175, -8.527530157486179263 ) ) ;
#39296=CARTESIAN_POINT ( 'NONE',  ( 18.52753015748617571, 13.09226448433411960, 4.923371831947298993 ) ) ;
#39297=CARTESIAN_POINT ( 'NONE',  ( 0.5774900079438607392, 28.48035201082150891, 5.440088680355550821 ) ) ;
#39303=CARTESIAN_POINT ( 'NONE',  ( 0.5774900079438590739, 57.64701867748817676, -5.440088680355550821 ) ) ;
#39305=CARTESIAN_POINT ( 'NONE',  ( 21.09922568453595559, 62.04030133659709634, -6.408140936763230044 ) ) ;
#39306=CARTESIAN_POINT ( 'NONE',  ( 4.559911319644449179, 58.89701867748817676, 9.422509992056141925 ) ) ;
#39307=CARTESIAN_POINT ( 'NONE',  ( -1.099225684535947600, 13.70696800326375353, -6.408140936763238038 ) ) ;
#39308=LINE ( 'NONE', #77279, #14769 ) ;
#39309=CARTESIAN_POINT ( 'NONE',  ( 5.076628168052703671, 26.84226448433411960, 8.527530157486179263 ) ) ;
#39310=CARTESIAN_POINT ( 'NONE',  ( 19.38216949554541557, 57.24863466993042493, -9.382169495545420901 ) ) ;
#39311=FACE_OUTER_BOUND ( 'NONE', #19095, .T. ) ;
#39312=CARTESIAN_POINT ( 'NONE',  ( 17.20831665107776587, 19.13393115100078035, -7.208316651077762316 ) ) ;
#39313=CARTESIAN_POINT ( 'NONE',  ( 22.81628187352647785, 16.62363466993042138, 6.195893100308588602E-16 ) ) ;
#39315=CARTESIAN_POINT ( 'NONE',  ( 20.88017736071110875, 50.77201867748817676, -2.915334737309920765 ) ) ;
#39316=CARTESIAN_POINT ( 'NONE',  ( 5.076628168052704559, 60.17559781766745175, -8.527530157486179263 ) ) ;
#39317=CARTESIAN_POINT ( 'NONE',  ( 2.791683348922237240, 25.38393115100078390, -7.208316651077763204 ) ) ;
#39318=CARTESIAN_POINT ( 'NONE',  ( 10.00000000000000000, 11.81368534415483751, -10.88017736071110342 ) ) ;
#39319=CARTESIAN_POINT ( 'NONE',  ( 21.09922568453594849, 16.20696800326375353, 6.408140936763242479 ) ) ;
#39323=CARTESIAN_POINT ( 'NONE',  ( 0.5774900079438607392, 23.48035201082150536, 5.440088680355550821 ) ) ;
#39327=CARTESIAN_POINT ( 'NONE',  ( 1.472469842513823179, 25.59226448433412315, -4.923371831947296329 ) ) ;
#39328=CARTESIAN_POINT ( 'NONE',  ( 17.96484262340118221, 14.93868534415484106, 7.964842623401181321 ) ) ;
#39330=B_SPLINE_CURVE_WITH_KNOTS ( 'NONE', 3,
 ( #8118, #86574, #47079, #55587, #18079, #86083 ),
 .UNSPECIFIED., .F., .F.,
 ( 4, 2, 4 ),
 ( 0.000000000000000000, 0.0002626113303184824700, 0.0005252226606369649400 ),
 .UNSPECIFIED. ) ;
#39331=CARTESIAN_POINT ( 'NONE',  ( 2.035157376598822676, 37.43868534415484106, -7.964842623401177768 ) ) ;
#39332=CARTESIAN_POINT ( 'NONE',  ( 10.00000000000000000, 1.813685344154838175, -10.88017736071110342 ) ) ;
#39333=CARTESIAN_POINT ( 'NONE',  ( 1.821158202401484072, 41.16688879859522388, 6.499999999999917399 ) ) ;
#39334=CARTESIAN_POINT ( 'NONE',  ( 2.791683348922240793, 1.633931151000784565, 7.208316651077764092 ) ) ;
#39335=CARTESIAN_POINT ( 'NONE',  ( 0.1532563361054082862, 36.21726448433410894, 2.638427012816831674 ) ) ;
#39339=DIRECTION ( 'NONE',  ( 0.000000000000000000, 0.000000000000000000, -1.000000000000000000 ) ) ;
#39341=CARTESIAN_POINT ( 'NONE',  ( -0.3689425029237898834, 26.17874883491396432, -10.36894250292378850 ) ) ;
#39342=CARTESIAN_POINT ( 'NONE',  ( 2.791683348922237240, 40.38393115100078035, -7.208316651077763204 ) ) ;
#39343=CARTESIAN_POINT ( 'NONE',  ( 19.72487221294570858, 70.00000000000000000, 6.000000000000000000 ) ) ;
#39345=CARTESIAN_POINT ( 'NONE',  ( 24.16423886937410614, 49.51208216824730357, -3.795296366450302550 ) ) ;
#39346=CARTESIAN_POINT ( 'NONE',  ( 0.1532563361054100626, 15.80059781766745353, -2.638427012816831230 ) ) ;
#39349=CARTESIAN_POINT ( 'NONE',  ( 20.88017736071110519, 40.56368534415484106, 2.639326808657452039E-16 ) ) ;
#39350=CARTESIAN_POINT ( 'NONE',  ( 10.00000000000000000, 57.87363466993042493, -12.81628187352647608 ) ) ;
#39351=CARTESIAN_POINT ( 'NONE',  ( 19.42250999205614193, 20.14701867748817321, 5.440088680355555262 ) ) ;
#39352=CARTESIAN_POINT ( 'NONE',  ( 0.6178305044545818747, 53.49863466993041072, -9.382169495545419124 ) ) ;
#39353=CARTESIAN_POINT ( 'NONE',  ( 10.00000000000000000, -2.126365330069579951, -12.81628187352647608 ) ) ;
#39354=CARTESIAN_POINT ( 'NONE',  ( 0.6081133539230503260, 53.33703382326400799, 6.499999999999974243 ) ) ;
#39358=CARTESIAN_POINT ( 'NONE',  ( 6.204703633549690345, 52.84541550158062506, 14.16423886937410082 ) ) ;
#39359=CARTESIAN_POINT ( 'NONE',  ( 6.204703633549690345, 10.76208216824729824, -14.16423886937410259 ) ) ;
#39360=CARTESIAN_POINT ( 'NONE',  ( 19.42250999205614193, 25.14701867748817321, 5.440088680355555262 ) ) ;
#39361=CARTESIAN_POINT ( 'NONE',  ( -0.8801773607110991993, 42.85535201082150536, -2.915334737309923874 ) ) ;
#39364=CARTESIAN_POINT ( 'NONE',  ( -0.8801773607111008646, 68.27201867748817676, 2.915334737309923430 ) ) ;
#39365=CARTESIAN_POINT ( 'NONE',  ( -0.8801773607111009756, 68.06368534415484817, 1.068504757029289695E-15 ) ) ;
#39366=CARTESIAN_POINT ( 'NONE',  ( 2.791683348922240793, 26.63393115100078745, 7.208316651077764092 ) ) ;
#39367=CARTESIAN_POINT ( 'NONE',  ( 1.274849032794223680, 28.57228050351031001, 6.499999999999884537 ) ) ;
#39369=CARTESIAN_POINT ( 'NONE',  ( 18.52753015748617571, 13.09226448433411960, 4.923371831947298993 ) ) ;
#39370=CARTESIAN_POINT ( 'NONE',  ( 10.00000000000000178, 37.25893115100078745, 9.846743663894594434 ) ) ;
#39372=CARTESIAN_POINT ( 'NONE',  ( -0.8801773607111009756, 13.06368534415483929, 1.068504757029289695E-15 ) ) ;
#39373=AXIS2_PLACEMENT_3D ( 'NONE', #28795, #88321, #59297 ) ;
#39374=CARTESIAN_POINT ( 'NONE',  ( -2.816281873526471635, 28.91530133659708213, -3.434112377981056508 ) ) ;
#39375=CARTESIAN_POINT ( 'NONE',  ( 17.20831665107776587, 4.133931151000785675, -7.208316651077762316 ) ) ;
#39378=CARTESIAN_POINT ( 'NONE',  ( 14.92337183194729633, 52.67559781766745175, 8.527530157486181039 ) ) ;
#39379=CARTESIAN_POINT ( 'NONE',  ( 1.472469842513823179, 36.42559781766745175, 4.923371831947296329 ) ) ;
#39380=CARTESIAN_POINT ( 'NONE',  ( 24.16423886937410614, 19.30374883491397142, 8.672049930838204340E-16 ) ) ;
#39381=CARTESIAN_POINT ( 'NONE',  ( 4.559911319644449179, 52.23035201082151247, -9.422509992056141925 ) ) ;
#39382=CARTESIAN_POINT ( 'NONE',  ( 19.42250999205614548, 10.98035201082150358, -5.440088680355545492 ) ) ;
#39384=CARTESIAN_POINT ( 'NONE',  ( 20.88017736071110519, 40.56368534415484106, 2.639326808657452039E-16 ) ) ;
#39385=CARTESIAN_POINT ( 'NONE',  ( 12.91533473730993009, 36.60535201082151247, -10.88017736071109987 ) ) ;
#39387=CARTESIAN_POINT ( 'NONE',  ( 10.00000000000000000, 32.87363466993042493, -12.81628187352647608 ) ) ;
#39388=CARTESIAN_POINT ( 'NONE',  ( 0.5774900079438607392, 38.48035201082150536, 5.440088680355550821 ) ) ;
#39389=ORIENTED_EDGE ( 'NONE', *, *, #52221, .T. ) ;
#39390=CARTESIAN_POINT ( 'NONE',  ( 10.00000000000000000, 52.87363466993041783, -12.81628187352647608 ) ) ;
#39391=AXIS2_PLACEMENT_3D ( 'NONE', #5262, #6238, #11761 ) ;
#39392=CARTESIAN_POINT ( 'NONE',  ( 2.035157376598824452, 53.68868534415484817, 7.964842623401179544 ) ) ;
#39395=CARTESIAN_POINT ( 'NONE',  ( 12.91533473730992121, 49.52201867748817676, 10.88017736071110164 ) ) ;
#39398=CARTESIAN_POINT ( 'NONE',  ( -1.926860441876563801, 24.89664270246083788, 3.195792623639529761 ) ) ;
#39399=CARTESIAN_POINT ( 'NONE',  ( -4.164238869374099927, 62.01208216824728936, 3.795296366450308767 ) ) ;
#39400=CARTESIAN_POINT ( 'NONE',  ( -0.8801773607110991993, 62.85535201082150536, -2.915334737309923874 ) ) ;
#39401=CARTESIAN_POINT ( 'NONE',  ( 6.204703633549690345, 5.762082168247301794, -14.16423886937410259 ) ) ;
#39402=SURFACE_STYLE_FILL_AREA ( #38415 ) ;
#39403=CARTESIAN_POINT ( 'NONE',  ( 17.96484262340118221, 4.938685344154837509, 7.964842623401181321 ) ) ;
#39404=CARTESIAN_POINT ( 'NONE',  ( 10.00000000000000178, 27.25893115100078390, 9.846743663894594434 ) ) ;
#39406=CARTESIAN_POINT ( 'NONE',  ( 1.472469842513823179, 30.59226448433411960, -4.923371831947296329 ) ) ;
#39407=CARTESIAN_POINT ( 'NONE',  ( 7.084665262690076126, 42.02201867748816966, -10.88017736071110164 ) ) ;
#39408=CARTESIAN_POINT ( 'NONE',  ( 19.84674366389459266, 33.71726448433410894, -2.638427012816827677 ) ) ;
#39409=CARTESIAN_POINT ( 'NONE',  ( 13.43411237798106583, 17.66530133659708923, -12.81628187352647252 ) ) ;
#39410=CARTESIAN_POINT ( 'NONE',  ( 10.00000000000000178, 64.31368534415483396, 10.88017736071110342 ) ) ;
#39411=CARTESIAN_POINT ( 'NONE',  ( 17.96484262340118221, 41.18868534415484106, -7.964842623401177768 ) ) ;
#39412=CARTESIAN_POINT ( 'NONE',  ( 20.36894250292379738, 59.92874883491397497, -10.36894250292379027 ) ) ;
#39413=AXIS2_PLACEMENT_3D ( 'NONE', #25241, #33196, #55722 ) ;
#39415=CARTESIAN_POINT ( 'NONE',  ( 6.565887622018943937, 20.16530133659708213, 12.81628187352647430 ) ) ;
#39417=VERTEX_POINT ( 'NONE', #1841 ) ;
#39418=CARTESIAN_POINT ( 'NONE',  ( 10.00000000000000178, 25.37363466993041783, 12.81628187352647608 ) ) ;
#39419=CARTESIAN_POINT ( 'NONE',  ( 10.00000000000000178, 24.31368534415484106, 10.88017736071110342 ) ) ;
#39420=STYLED_ITEM ( 'NONE', ( #46022 ), #29361 ) ;
#39423=CARTESIAN_POINT ( 'NONE',  ( 5.076628168052703671, 1.842264484334118047, 8.527530157486179263 ) ) ;
#39424=CARTESIAN_POINT ( 'NONE',  ( 17.20831665107776587, 42.88393115100077324, 7.208316651077764980 ) ) ;
#39425=EDGE_CURVE ( 'NONE', #71988, #45674, #63288, .T. ) ;
#39426=CARTESIAN_POINT ( 'NONE',  ( 2.791683348922240793, 36.63393115100078035, 7.208316651077764092 ) ) ;
#39428=CARTESIAN_POINT ( 'NONE',  ( -2.816281873526473856, 64.33196800326376774, 3.434112377981055619 ) ) ;
#39429=CARTESIAN_POINT ( 'NONE',  ( 19.84674366389459621, 28.50893115100078745, 7.409399052514197653E-17 ) ) ;
#39432=CARTESIAN_POINT ( 'NONE',  ( 19.84674366389459266, 13.71726448433411782, -2.638427012816827677 ) ) ;
#39433=FACE_OUTER_BOUND ( 'NONE', #21586, .T. ) ;
#39435=CARTESIAN_POINT ( 'NONE',  ( 14.92337183194729633, 42.67559781766745886, 8.527530157486181039 ) ) ;
#39439=CARTESIAN_POINT ( 'NONE',  ( -2.816281873526471635, 13.91530133659708746, -3.434112377981056508 ) ) ;
#39440=CARTESIAN_POINT ( 'NONE',  ( 20.88017736071110875, 50.77201867748817676, -2.915334737309920765 ) ) ;
#39442=CARTESIAN_POINT ( 'NONE',  ( 13.79529636645031943, 40.34541550158063217, -14.16423886937409904 ) ) ;
#39443=( BOUNDED_CURVE ( )  B_SPLINE_CURVE ( 3, ( #4742, #87726, #95225, #96237 ),
 .UNSPECIFIED., .F., .F. ) 
 B_SPLINE_CURVE_WITH_KNOTS ( ( 4, 4 ),
 ( 1.570796326794896558, 2.588785175020066109 ),
 .UNSPECIFIED. ) 
 CURVE ( )  GEOMETRIC_REPRESENTATION_ITEM ( )  RATIONAL_B_SPLINE_CURVE ( ( 1.000000000000000000, 0.9154899770527740177, 0.9154899770527740177, 1.000000000000000000 ) ) 
 REPRESENTATION_ITEM ( '' )  );
#39444=FILL_AREA_STYLE ('',( #55917 ) ) ;
#39446=EDGE_CURVE ( 'NONE', #2953, #34081, #28901, .T. ) ;
#39447=CARTESIAN_POINT ( 'NONE',  ( 24.16423886937410614, 44.51208216824730357, -3.795296366450302550 ) ) ;
#39448=CARTESIAN_POINT ( 'NONE',  ( -4.164238869374099039, 61.80374883491397497, 8.674139862899312516E-16 ) ) ;
#39449=CARTESIAN_POINT ( 'NONE',  ( 22.26659068614894466, 18.88708216824730002, 7.082119434687054849 ) ) ;
#39450=CARTESIAN_POINT ( 'NONE',  ( 13.79529636645031943, 25.34541550158063572, -14.16423886937409904 ) ) ;
#39453=CARTESIAN_POINT ( 'NONE',  ( 0.1532563361054082862, 41.21726448433411605, 2.638427012816831674 ) ) ;
#39456=CARTESIAN_POINT ( 'NONE',  ( 10.00000000000000178, 39.31368534415484106, 10.88017736071110342 ) ) ;
#39458=CARTESIAN_POINT ( 'NONE',  ( 19.65571488900283725, 92.22086433622595791, -5.360955758211049194 ) ) ;
#39459=CARTESIAN_POINT ( 'NONE',  ( 5.076628168052704559, 45.17559781766745175, -8.527530157486179263 ) ) ;
#39461=CARTESIAN_POINT ( 'NONE',  ( 22.81628187352647785, 61.62363466993041783, 6.195893100308588602E-16 ) ) ;
#39463=CARTESIAN_POINT ( 'NONE',  ( 10.00000000000000000, 44.75893115100078745, -9.846743663894594434 ) ) ;
#39464=CARTESIAN_POINT ( 'NONE',  ( 7.361572987183169658, 59.96726448433410894, -9.846743663894592657 ) ) ;
#39465=CARTESIAN_POINT ( 'NONE',  ( 6.204703633549690345, 42.84541550158063217, 14.16423886937410082 ) ) ;
#39467=CARTESIAN_POINT ( 'NONE',  ( -4.164238869374098151, 11.59541550158063217, -3.795296366450310543 ) ) ;
#39469=CARTESIAN_POINT ( 'NONE',  ( 0.2751277870542871984, 68.21833443783938833, 6.499999999999984901 ) ) ;
#39471=CARTESIAN_POINT ( 'NONE',  ( -0.8801773607110991993, 7.855352010821506248, -2.915334737309923874 ) ) ;
#39472=CARTESIAN_POINT ( 'NONE',  ( 3.591859063236763294, 8.290301336597087456, -11.09922568453595026 ) ) ;
#39474=CARTESIAN_POINT ( 'NONE',  ( -0.8801773607111008646, 68.27201867748817676, 2.915334737309923430 ) ) ;
#39476=CARTESIAN_POINT ( 'NONE',  ( -46.94000000000001194, 103.2691844435154422, -6.361973263950303270 ) ) ;
#39478=CARTESIAN_POINT ( 'NONE',  ( 10.00000000000000178, 68.05374883491397497, 14.16423886937410082 ) ) ;
#39480=CARTESIAN_POINT ( 'NONE',  ( 7.084665262690076126, 32.02201867748816966, -10.88017736071110164 ) ) ;
#39481=CARTESIAN_POINT ( 'NONE',  ( 10.00000000000000000, 26.81368534415484106, -10.88017736071110342 ) ) ;
#39482=CARTESIAN_POINT ( 'NONE',  ( 10.00000000000000000, 2.873634669930420049, -12.81628187352647608 ) ) ;
#39483=CARTESIAN_POINT ( 'NONE',  ( 17.20831665107776587, 49.13393115100078745, -7.208316651077762316 ) ) ;
#39484=CARTESIAN_POINT ( 'NONE',  ( 13.43411237798106583, 62.66530133659708923, -12.81628187352647252 ) ) ;
#39486=EDGE_LOOP ( 'NONE', ( #66684, #17769, #78400, #83779, #88648, #46154 ) ) ;
#39487=CARTESIAN_POINT ( 'NONE',  ( 4.559911319644449179, 27.23035201082150536, -9.422509992056141925 ) ) ;
#39489=CARTESIAN_POINT ( 'NONE',  ( 0.6178305044545838731, 34.74863466993042493, 9.382169495545420901 ) ) ;
#39490=CARTESIAN_POINT ( 'NONE',  ( 18.52753015748618282, 63.92559781766745886, -4.923371831947291888 ) ) ;
#39491=CARTESIAN_POINT ( 'NONE',  ( 4.559911319644449179, 48.89701867748817676, 9.422509992056141925 ) ) ;
#39492=CARTESIAN_POINT ( 'NONE',  ( 0.1532563361054100626, 15.80059781766745353, -2.638427012816831230 ) ) ;
#39494=CARTESIAN_POINT ( 'NONE',  ( -2.816281873526473856, 19.12363466993042138, 9.499525473075851096E-16 ) ) ;
#39495=CARTESIAN_POINT ( 'NONE',  ( 7.084665262690076126, 64.10535201082150536, 10.88017736071109987 ) ) ;
#39497=SURFACE_SIDE_STYLE ('',( #91989 ) ) ;
#39498=VERTEX_POINT ( 'NONE', #78299 ) ;
#39501=CARTESIAN_POINT ( 'NONE',  ( 7.084665262690076126, 44.10535201082151247, 10.88017736071109987 ) ) ;
#39502=CARTESIAN_POINT ( 'NONE',  ( 22.81628187352648496, 46.83196800326376064, -3.434112377981050290 ) ) ;
#39503=CARTESIAN_POINT ( 'NONE',  ( 24.16423886937410614, 9.303748834913967869, 8.672049930838204340E-16 ) ) ;
#39504=CARTESIAN_POINT ( 'NONE',  ( 19.84674366389459266, 23.30059781766745530, 2.638427012816836559 ) ) ;
#39505=CARTESIAN_POINT ( 'NONE',  ( 17.96484262340118221, 11.18868534415483929, -7.964842623401177768 ) ) ;
#39506=CARTESIAN_POINT ( 'NONE',  ( 1.472469842513823179, 25.59226448433412315, -4.923371831947296329 ) ) ;
#39507=CARTESIAN_POINT ( 'NONE',  ( 19.39235739573469885, 39.87576471608601025, 6.499999999999986677 ) ) ;
#39508=CARTESIAN_POINT ( 'NONE',  ( 22.26659068614895176, 54.72041550158063217, -7.082119434687042414 ) ) ;
#39509=ORIENTED_EDGE ( 'NONE', *, *, #89584, .F. ) ;
#39510=CYLINDRICAL_SURFACE ( 'NONE', #56960, 0.5000000000000004441 ) ;
#39511=CARTESIAN_POINT ( 'NONE',  ( 20.88017736071110519, 5.563685344154837509, 2.639326808657452039E-16 ) ) ;
#39512=CARTESIAN_POINT ( 'NONE',  ( 1.472469842513823179, 15.59226448433411960, -4.923371831947296329 ) ) ;
#39514=CARTESIAN_POINT ( 'NONE',  ( 15.44008868035555260, 9.730352010821505360, 9.422509992056143702 ) ) ;
#39515=CARTESIAN_POINT ( 'NONE',  ( 20.88017736071110875, 5.772018677488170546, -2.915334737309920765 ) ) ;
#39516=CARTESIAN_POINT ( 'NONE',  ( 19.84674366389459266, 43.71726448433410894, -2.638427012816827677 ) ) ;
#39517=CARTESIAN_POINT ( 'NONE',  ( 6.565887622018943937, 43.08196800326374643, -12.81628187352647608 ) ) ;
#39519=DIRECTION ( 'NONE',  ( 1.000000000000000000, 0.000000000000000000, -0.000000000000000000 ) ) ;
#39520=CARTESIAN_POINT ( 'NONE',  ( -0.3689425029237898834, 21.17874883491396432, -10.36894250292378850 ) ) ;
#39521=CARTESIAN_POINT ( 'NONE',  ( -0.8801773607111009756, 23.06368534415484106, 1.068504757029289695E-15 ) ) ;
#39522=CARTESIAN_POINT ( 'NONE',  ( -0.3689425029237881626, 67.42874883491396076, 10.36894250292379027 ) ) ;
#39523=CARTESIAN_POINT ( 'NONE',  ( 18.52753015748617571, 43.09226448433412315, 4.923371831947298993 ) ) ;
#39525=CARTESIAN_POINT ( 'NONE',  ( 10.00000000000000178, 42.25893115100078745, 9.846743663894594434 ) ) ;
#39529=ORIENTED_EDGE ( 'NONE', *, *, #34736, .T. ) ;
#39530=CARTESIAN_POINT ( 'NONE',  ( 20.88017736071110519, 5.563685344154837509, 2.639326808657452039E-16 ) ) ;
#39531=CARTESIAN_POINT ( 'NONE',  ( 12.91533473730993009, 66.60535201082150536, -10.88017736071109987 ) ) ;
#39533=CARTESIAN_POINT ( 'NONE',  ( 7.361572987183170547, 52.05059781766745175, 9.846743663894590881 ) ) ;
#39534=CARTESIAN_POINT ( 'NONE',  ( 7.084665262690076126, 52.02201867748816255, -10.88017736071110164 ) ) ;
#39535=CARTESIAN_POINT ( 'NONE',  ( 17.96484262340118221, 11.18868534415483929, -7.964842623401177768 ) ) ;
#39536=CARTESIAN_POINT ( 'NONE',  ( 10.00000000000000178, 25.37363466993041783, 12.81628187352647608 ) ) ;
#39537=CARTESIAN_POINT ( 'NONE',  ( 24.16423886937409904, 24.09541550158063927, 3.795296366450317205 ) ) ;
#39542=CARTESIAN_POINT ( 'NONE',  ( 10.00000000000000178, 45.37363466993041783, 12.81628187352647608 ) ) ;
#39545=CARTESIAN_POINT ( 'NONE',  ( 12.63842701281683922, 64.55059781766745175, -9.846743663894590881 ) ) ;
#39546=CARTESIAN_POINT ( 'NONE',  ( 0.5774900079438590739, 17.64701867748817321, -5.440088680355550821 ) ) ;
#39547=ORIENTED_EDGE ( 'NONE', *, *, #84118, .F. ) ;
#39548=CARTESIAN_POINT ( 'NONE',  ( 15.44008868035555793, 31.39701867748817676, -9.422509992056140149 ) ) ;
#39550=CARTESIAN_POINT ( 'NONE',  ( 2.035157376598822676, 62.43868534415483396, -7.964842623401177768 ) ) ;
#39551=CARTESIAN_POINT ( 'NONE',  ( 20.88017736071110519, 65.56368534415483396, 2.639326808657452039E-16 ) ) ;
#39552=CARTESIAN_POINT ( 'NONE',  ( 7.361572987183170547, 12.05059781766744997, 9.846743663894590881 ) ) ;
#39553=EDGE_CURVE ( 'NONE', #35821, #36181, #18136, .T. ) ;
#39554=CARTESIAN_POINT ( 'NONE',  ( 4.559911319644449179, 68.89701867748817676, 9.422509992056141925 ) ) ;
#39556=CARTESIAN_POINT ( 'NONE',  ( 12.63842701281683034, 12.46726448433411782, 9.846743663894596210 ) ) ;
#39558=CARTESIAN_POINT ( 'NONE',  ( 12.63842701281683034, 37.46726448433411605, 9.846743663894596210 ) ) ;
#39562=CARTESIAN_POINT ( 'NONE',  ( -0.3689425029237881626, 2.428748834913967869, 10.36894250292379027 ) ) ;
#39563=CARTESIAN_POINT ( 'NONE',  ( 6.565887622018943937, 58.08196800326376064, -12.81628187352647608 ) ) ;
#39565=CARTESIAN_POINT ( 'NONE',  ( 20.36894250292379738, 9.928748834913966093, -10.36894250292379027 ) ) ;
#39566=CARTESIAN_POINT ( 'NONE',  ( 2.917880565312948704, 17.63708216824730357, 12.26659068614894643 ) ) ;
#39569=CARTESIAN_POINT ( 'NONE',  ( 20.15039907845753220, 55.60158574516643171, -6.262539305110077947 ) ) ;
#39570=CARTESIAN_POINT ( 'NONE',  ( 0.5774900079438590739, 62.64701867748817676, -5.440088680355550821 ) ) ;
#39571=CARTESIAN_POINT ( 'NONE',  ( 2.035157376598822676, 22.43868534415483396, -7.964842623401177768 ) ) ;
#39572=CARTESIAN_POINT ( 'NONE',  ( 0.6081133539230402230, 68.33703382326399378, 6.499999999999953815 ) ) ;
#39574=CARTESIAN_POINT ( 'NONE',  ( 17.20831665107776587, 9.133931151000787452, -7.208316651077762316 ) ) ;
#39575=CARTESIAN_POINT ( 'NONE',  ( 19.84674366389459621, 8.508931151000785675, 7.409399052514197653E-17 ) ) ;
#39576=CARTESIAN_POINT ( 'NONE',  ( 19.38216949554541557, 32.24863466993041783, -9.382169495545420901 ) ) ;
#39577=CARTESIAN_POINT ( 'NONE',  ( 2.791683348922237240, 20.38393115100078745, -7.208316651077763204 ) ) ;
#39578=CARTESIAN_POINT ( 'NONE',  ( 19.38216949554541202, 10.99863466993042138, 9.382169495545424454 ) ) ;
#39582=CARTESIAN_POINT ( 'NONE',  ( 5.076628168052704559, 0.1755978176674514724, -8.527530157486179263 ) ) ;
#39585=CARTESIAN_POINT ( 'NONE',  ( 0.5774900079438590739, 42.64701867748816966, -5.440088680355550821 ) ) ;
#39586=CARTESIAN_POINT ( 'NONE',  ( -4.164238869374099039, 31.80374883491396432, 8.674139862899312516E-16 ) ) ;
#39587=CARTESIAN_POINT ( 'NONE',  ( 7.361572987183169658, 39.96726448433411605, -9.846743663894592657 ) ) ;
#39588=CARTESIAN_POINT ( 'NONE',  ( 2.791683348922240793, 1.633931151000784565, 7.208316651077764092 ) ) ;
#39589=CARTESIAN_POINT ( 'NONE',  ( 0.6178305044545818747, 58.49863466993042493, -9.382169495545419124 ) ) ;
#39591=CARTESIAN_POINT ( 'NONE',  ( 15.44008868035555260, 24.73035201082150891, 9.422509992056143702 ) ) ;
#39594=CARTESIAN_POINT ( 'NONE',  ( 3.591859063236761518, 19.95696800326375353, 11.09922568453594849 ) ) ;
#39595=CARTESIAN_POINT ( 'NONE',  ( 19.38216949554541202, 10.99863466993042138, 9.382169495545424454 ) ) ;
#39596=CARTESIAN_POINT ( 'NONE',  ( 10.00000000000000000, 39.75893115100078745, -9.846743663894594434 ) ) ;
#39598=CARTESIAN_POINT ( 'NONE',  ( 6.565887622018943937, 55.16530133659709634, 12.81628187352647430 ) ) ;
#39600=CARTESIAN_POINT ( 'NONE',  ( 17.96484262340118221, 59.93868534415484106, 7.964842623401181321 ) ) ;
#39602=CIRCLE ( 'NONE', #15626, 0.4999999999999961142 ) ;
#39606=CARTESIAN_POINT ( 'NONE',  ( 15.44008868035555793, 56.39701867748817676, -9.422509992056140149 ) ) ;
#39607=CARTESIAN_POINT ( 'NONE',  ( 10.00000000000000178, 59.31368534415484106, 10.88017736071110342 ) ) ;
#39609=CARTESIAN_POINT ( 'NONE',  ( 17.96484262340118221, 9.938685344154839285, 7.964842623401181321 ) ) ;
#39610=CARTESIAN_POINT ( 'NONE',  ( 0.1532563361054100626, 55.80059781766745175, -2.638427012816831230 ) ) ;
#39611=CARTESIAN_POINT ( 'NONE',  ( 15.44008868035555793, 16.39701867748817321, -9.422509992056140149 ) ) ;
#39613=CARTESIAN_POINT ( 'NONE',  ( 22.81628187352647785, 31.62363466993042138, 6.195893100308588602E-16 ) ) ;
#39614=VERTEX_POINT ( 'NONE', #16825 ) ;
#39615=CARTESIAN_POINT ( 'NONE',  ( 10.00000000000000000, 41.81368534415484106, -10.88017736071110342 ) ) ;
#39616=CARTESIAN_POINT ( 'NONE',  ( 19.38216949554541557, 12.24863466993041961, -9.382169495545420901 ) ) ;
#39618=CARTESIAN_POINT ( 'NONE',  ( 0.5774900079438590739, 17.64701867748817321, -5.440088680355550821 ) ) ;
#39619=CARTESIAN_POINT ( 'NONE',  ( 2.035157376598824452, 43.68868534415484106, 7.964842623401179544 ) ) ;
#39620=CARTESIAN_POINT ( 'NONE',  ( -2.266590686148945544, 57.22041550158063217, 7.082119434687048631 ) ) ;
#39621=CARTESIAN_POINT ( 'NONE',  ( 14.92337183194729988, 29.34226448433411960, -8.527530157486177487 ) ) ;
#39622=CARTESIAN_POINT ( 'NONE',  ( 7.084665262690076126, 64.10535201082150536, 10.88017736071109987 ) ) ;
#39623=CARTESIAN_POINT ( 'NONE',  ( 19.50000000000000711, 105.0000000000000000, -5.000000000000000000 ) ) ;
#39624=CARTESIAN_POINT ( 'NONE',  ( -2.266590686148945544, 17.22041550158063572, 7.082119434687048631 ) ) ;
#39630=CARTESIAN_POINT ( 'NONE',  ( 10.00000000000000000, 40.55374883491397497, -14.16423886937410082 ) ) ;
#39631=CARTESIAN_POINT ( 'NONE',  ( 17.08211943468705130, 38.47041550158063217, 12.26659068614894998 ) ) ;
#39632=CARTESIAN_POINT ( 'NONE',  ( 10.00000000000000000, 66.81368534415484817, -10.88017736071110342 ) ) ;
#39633=CARTESIAN_POINT ( 'NONE',  ( -2.816281873526473856, 9.123634669930421381, 9.499525473075851096E-16 ) ) ;
#39634=CARTESIAN_POINT ( 'NONE',  ( 0.1532563361054083140, 66.00893115100079456, 1.131784320476157264E-15 ) ) ;
#39635=CARTESIAN_POINT ( 'NONE',  ( 1.274849032794294290, 58.57228050351032778, 6.499999999999979572 ) ) ;
#39636=CARTESIAN_POINT ( 'NONE',  ( -0.8801773607111009756, 58.06368534415484106, 1.068504757029289695E-15 ) ) ;
#39637=CARTESIAN_POINT ( 'NONE',  ( 0.6178305044545818747, 23.49863466993041783, -9.382169495545419124 ) ) ;
#39638=CARTESIAN_POINT ( 'NONE',  ( 24.16423886937410614, 34.51208216824731068, -3.795296366450302550 ) ) ;
#39639=CARTESIAN_POINT ( 'NONE',  ( 20.88017736071110519, 30.56368534415484106, 2.639326808657452039E-16 ) ) ;
#39640=CARTESIAN_POINT ( 'NONE',  ( 4.559911319644449179, 27.23035201082150536, -9.422509992056141925 ) ) ;
#39642=CARTESIAN_POINT ( 'NONE',  ( 10.00000000000000000, -0.2410688489992152128, -9.846743663894594434 ) ) ;
#39646=( BOUNDED_CURVE ( )  B_SPLINE_CURVE ( 2, ( #88916, #97922, #43890, #52878, #45378, #74890, #96934, #37410, #20918 ),
 .UNSPECIFIED., .F., .T. ) 
 B_SPLINE_CURVE_WITH_KNOTS ( ( 3, 2, 2, 2, 3 ),
 ( 0.5820003743640369542, 0.5833333333333333703, 0.5892857142857143016, 0.5952380952380952328, 0.5965710542073916489 ),
 .UNSPECIFIED. ) 
 CURVE ( )  GEOMETRIC_REPRESENTATION_ITEM ( )  RATIONAL_B_SPLINE_CURVE ( ( 0.9881565478350734510, 0.9923695281211492025, 1.000000000000000000, 0.9659258262890683122, 1.000000000000000000, 0.9659258262890683122, 1.000000000000000000, 0.9923695281211490915, 0.9881565478350733400 ) ) 
 REPRESENTATION_ITEM ( '' )  );
#39647=DIRECTION ( 'NONE',  ( -1.000000000000000000, 0.000000000000000000, 0.000000000000000000 ) ) ;
#39650=( LENGTH_UNIT ( ) NAMED_UNIT ( * ) SI_UNIT ( .MILLI., .METRE. ) );
#39651=CARTESIAN_POINT ( 'NONE',  ( 22.26659068614894466, 63.88708216824730357, 7.082119434687054849 ) ) ;
#39652=CARTESIAN_POINT ( 'NONE',  ( 4.559911319644449179, 13.89701867748817321, 9.422509992056141925 ) ) ;
#39653=CARTESIAN_POINT ( 'NONE',  ( 17.20831665107776587, 39.13393115100079456, -7.208316651077762316 ) ) ;
#39654=CARTESIAN_POINT ( 'NONE',  ( 19.84674366389459266, 58.30059781766745886, 2.638427012816836559 ) ) ;
#39655=CARTESIAN_POINT ( 'NONE',  ( 19.72487221294571569, 42.80223176428830811, -6.499999999999990230 ) ) ;
#39658=EDGE_CURVE ( 'NONE', #7550, #88366, #51753, .T. ) ;
#39659=CARTESIAN_POINT ( 'NONE',  ( -2.816281873526473856, -0.6680319967362464695, 3.434112377981055619 ) ) ;
#39662=CARTESIAN_POINT ( 'NONE',  ( -4.164238869374099927, 42.01208216824728936, 3.795296366450308767 ) ) ;
#39664=CARTESIAN_POINT ( 'NONE',  ( 22.26659068614894466, 38.88708216824731068, 7.082119434687054849 ) ) ;
#39666=CARTESIAN_POINT ( 'NONE',  ( 20.88017736071110519, 25.56368534415483751, 2.639326808657452039E-16 ) ) ;
#39668=AXIS2_PLACEMENT_3D ( 'NONE', #80115, #72119, #93647 ) ;
#39669=CARTESIAN_POINT ( 'NONE',  ( 2.035157376598824452, 43.68868534415484106, 7.964842623401179544 ) ) ;
#39670=CARTESIAN_POINT ( 'NONE',  ( 7.361572987183169658, 54.96726448433413026, -9.846743663894592657 ) ) ;
#39671=CARTESIAN_POINT ( 'NONE',  ( 19.42250999205614193, 35.14701867748816966, 5.440088680355555262 ) ) ;
#39673=CARTESIAN_POINT ( 'NONE',  ( 0.5774900079438607392, 68.48035201082150536, 5.440088680355550821 ) ) ;
#39674=CARTESIAN_POINT ( 'NONE',  ( 20.88017736071110519, 30.56368534415484106, 2.639326808657452039E-16 ) ) ;
#39677=VERTEX_POINT ( 'NONE', #80272 ) ;
#39678=CARTESIAN_POINT ( 'NONE',  ( 5.076628168052704559, 5.175597817667451750, -8.527530157486179263 ) ) ;
#39682=CARTESIAN_POINT ( 'NONE',  ( 2.791683348922237240, 30.38393115100078390, -7.208316651077763204 ) ) ;
#39684=CARTESIAN_POINT ( 'NONE',  ( -1.099225684535947600, 43.70696800326375353, -6.408140936763238038 ) ) ;
#39689=CARTESIAN_POINT ( 'NONE',  ( -42.50369195530268485, 107.9060299417078426, 4.999999999999996447 ) ) ;
#39690=CARTESIAN_POINT ( 'NONE',  ( 19.84674366389459266, 48.71726448433413026, -2.638427012816827677 ) ) ;
#39691=CARTESIAN_POINT ( 'NONE',  ( 2.917880565312950480, 45.97041550158063927, -12.26659068614894821 ) ) ;
#39692=CARTESIAN_POINT ( 'NONE',  ( 17.20831665107776587, 64.13393115100079456, -7.208316651077762316 ) ) ;
#39693=VERTEX_POINT ( 'NONE', #11773 ) ;
#39695=CARTESIAN_POINT ( 'NONE',  ( 12.63842701281683034, 22.46726448433411605, 9.846743663894596210 ) ) ;
#39696=CARTESIAN_POINT ( 'NONE',  ( 22.81628187352648496, 51.83196800326376064, -3.434112377981050290 ) ) ;
#39697=CARTESIAN_POINT ( 'NONE',  ( 1.472469842513823179, 61.42559781766745175, 4.923371831947296329 ) ) ;
#39698=CARTESIAN_POINT ( 'NONE',  ( 17.96484262340118221, 59.93868534415484106, 7.964842623401181321 ) ) ;
#39702=CARTESIAN_POINT ( 'NONE',  ( 2.917880565312950480, 60.97041550158063927, -12.26659068614894821 ) ) ;
#39703=CARTESIAN_POINT ( 'NONE',  ( 19.42250999205614548, 30.98035201082150536, -5.440088680355545492 ) ) ;
#39704=CARTESIAN_POINT ( 'NONE',  ( -2.816281873526473856, 9.123634669930421381, 9.499525473075851096E-16 ) ) ;
#39705=CARTESIAN_POINT ( 'NONE',  ( -0.8801773607111009756, 63.06368534415484106, 1.068504757029289695E-15 ) ) ;
#39709=CARTESIAN_POINT ( 'NONE',  ( 2.035157376598824452, 58.68868534415482685, 7.964842623401179544 ) ) ;
#39711=CARTESIAN_POINT ( 'NONE',  ( 12.63842701281683922, 39.55059781766744464, -9.846743663894590881 ) ) ;
#39713=CARTESIAN_POINT ( 'NONE',  ( 21.09922568453594849, 6.206968003263753531, 6.408140936763242479 ) ) ;
#39714=CARTESIAN_POINT ( 'NONE',  ( 10.00000000000000000, 16.81368534415483751, -10.88017736071110342 ) ) ;
#39715=CARTESIAN_POINT ( 'NONE',  ( 0.09770025222076776650, 69.67742753483355500, -6.500000000000000000 ) ) ;
#39717=CARTESIAN_POINT ( 'NONE',  ( 20.36894250292379738, 39.92874883491396787, -10.36894250292379027 ) ) ;
#39718=CARTESIAN_POINT ( 'NONE',  ( 24.16423886937409904, 64.09541550158064638, 3.795296366450317205 ) ) ;
#39719=CARTESIAN_POINT ( 'NONE',  ( 10.00000000000000000, 14.75893115100078568, -9.846743663894594434 ) ) ;
#39720=CARTESIAN_POINT ( 'NONE',  ( 20.88017736071110875, 10.77201867748817143, -2.915334737309920765 ) ) ;
#39722=CARTESIAN_POINT ( 'NONE',  ( 7.361572987183169658, 39.96726448433411605, -9.846743663894592657 ) ) ;
#39723=CARTESIAN_POINT ( 'NONE',  ( -0.8801773607111008646, 28.27201867748817321, 2.915334737309923430 ) ) ;
#39724=CARTESIAN_POINT ( 'NONE',  ( 7.361572987183169658, 64.96726448433412315, -9.846743663894592657 ) ) ;
#39725=CARTESIAN_POINT ( 'NONE',  ( 20.36894250292379738, 14.92874883491396432, -10.36894250292379027 ) ) ;
#39727=CARTESIAN_POINT ( 'NONE',  ( 0.8719017118913388043, 123.9374316453451286, -5.000000000000000000 ) ) ;
#39728=CARTESIAN_POINT ( 'NONE',  ( 19.84674366389459266, 13.71726448433411782, -2.638427012816827677 ) ) ;
#39729=CARTESIAN_POINT ( 'NONE',  ( 10.00000000000000000, 57.87363466993042493, -12.81628187352647608 ) ) ;
#39730=CARTESIAN_POINT ( 'NONE',  ( 0.1532563361054082862, 51.21726448433412315, 2.638427012816831674 ) ) ;
#39733=CARTESIAN_POINT ( 'NONE',  ( -4.164238869374099039, 61.80374883491397497, 8.674139862899312516E-16 ) ) ;
#39735=CARTESIAN_POINT ( 'NONE',  ( 20.36894250292379382, 13.67874883491396965, 10.36894250292379205 ) ) ;
#39736=CARTESIAN_POINT ( 'NONE',  ( 10.00000000000000000, 61.81368534415484106, -10.88017736071110342 ) ) ;
#39737=CARTESIAN_POINT ( 'NONE',  ( 1.472469842513823179, 40.59226448433411605, -4.923371831947296329 ) ) ;
#39738=CARTESIAN_POINT ( 'NONE',  ( 0.5774900079438607392, 18.48035201082150536, 5.440088680355550821 ) ) ;
#39740=CARTESIAN_POINT ( 'NONE',  ( 12.63842701281683034, 62.46726448433410894, 9.846743663894596210 ) ) ;
#39741=EDGE_CURVE ( 'NONE', #80524, #663, #49737, .T. ) ;
#39747=CARTESIAN_POINT ( 'NONE',  ( 17.39651004071843232, 17.93575266056828355, 6.499999999999984013 ) ) ;
#39749=CARTESIAN_POINT ( 'NONE',  ( 12.63842701281683922, 49.55059781766744464, -9.846743663894590881 ) ) ;
#39750=CARTESIAN_POINT ( 'NONE',  ( 10.00000000000000178, 27.25893115100078390, 9.846743663894594434 ) ) ;
#39751=CARTESIAN_POINT ( 'NONE',  ( 19.38216949554541202, 55.99863466993041072, 9.382169495545424454 ) ) ;
#39752=CARTESIAN_POINT ( 'NONE',  ( 2.035157376598824452, 23.68868534415484461, 7.964842623401179544 ) ) ;
#39753=CARTESIAN_POINT ( 'NONE',  ( 5.076628168052704559, 50.17559781766745886, -8.527530157486179263 ) ) ;
#39755=CARTESIAN_POINT ( 'NONE',  ( -4.164238869374099039, 56.80374883491397497, 8.674139862899312516E-16 ) ) ;
#39757=CARTESIAN_POINT ( 'NONE',  ( 20.88017736071110519, 55.56368534415484817, 2.639326808657452039E-16 ) ) ;
#39758=CARTESIAN_POINT ( 'NONE',  ( 5.076628168052704559, 20.17559781766745175, -8.527530157486179263 ) ) ;
#39760=ORIENTED_EDGE ( 'NONE', *, *, #41267, .T. ) ;
#39761=CARTESIAN_POINT ( 'NONE',  ( 2.603489959281588995, 55.43575266056826933, -6.500000000000003553 ) ) ;
#39763=CARTESIAN_POINT ( 'NONE',  ( 19.84674366389459266, 13.71726448433411782, -2.638427012816827677 ) ) ;
#39765=CARTESIAN_POINT ( 'NONE',  ( 6.204703633549690345, 17.84541550158063217, 14.16423886937410082 ) ) ;
#39766=CARTESIAN_POINT ( 'NONE',  ( 0.1532563361054083140, 26.00893115100078745, 1.131784320476157264E-15 ) ) ;
#39767=CARTESIAN_POINT ( 'NONE',  ( 0.5774900079438590739, 37.64701867748817676, -5.440088680355550821 ) ) ;
#39768=STYLED_ITEM ( 'NONE', ( #47757 ), #26911 ) ;
#39770=ORIENTED_EDGE ( 'NONE', *, *, #62855, .T. ) ;
#39771=CARTESIAN_POINT ( 'NONE',  ( 19.42250999205614193, 35.14701867748816966, 5.440088680355555262 ) ) ;
#39773=CARTESIAN_POINT ( 'NONE',  ( 19.80427997160309417, 37.75733960839544778, -6.499999999999988454 ) ) ;
#39777=CARTESIAN_POINT ( 'NONE',  ( 22.26659068614895176, 9.720415501580633943, -7.082119434687042414 ) ) ;
#39778=ORIENTED_EDGE ( 'NONE', *, *, #7858, .F. ) ;
#39779=ORIENTED_EDGE ( 'NONE', *, *, #2152, .T. ) ;
#39780=CARTESIAN_POINT ( 'NONE',  ( 3.591859063236761518, 29.95696800326375708, 11.09922568453594849 ) ) ;
#39782=CARTESIAN_POINT ( 'NONE',  ( 12.63842701281683922, 9.550597817667449974, -9.846743663894590881 ) ) ;
#39785=CARTESIAN_POINT ( 'NONE',  ( 12.63842701281683034, 17.46726448433411250, 9.846743663894596210 ) ) ;
#39786=CARTESIAN_POINT ( 'NONE',  ( 10.00000000000000178, 34.31368534415484106, 10.88017736071110342 ) ) ;
#39789=CARTESIAN_POINT ( 'NONE',  ( 4.559911319644449179, 62.23035201082150536, -9.422509992056141925 ) ) ;
#39792=CARTESIAN_POINT ( 'NONE',  ( 10.00000000000000000, 56.81368534415484106, -10.88017736071110342 ) ) ;
#39793=CARTESIAN_POINT ( 'NONE',  ( 16.40814093676324603, 7.456968003263754419, -11.09922568453594671 ) ) ;
#39794=DIRECTION ( 'NONE',  ( 0.8320502943378436100, -0.5547001962252291474, 0.000000000000000000 ) ) ;
#39796=CARTESIAN_POINT ( 'NONE',  ( 18.52753015748618282, 28.92559781766745175, -4.923371831947291888 ) ) ;
#39797=CARTESIAN_POINT ( 'NONE',  ( 6.565887622018943937, 65.16530133659709634, 12.81628187352647430 ) ) ;
#39798=CARTESIAN_POINT ( 'NONE',  ( -0.3689425029237898834, 1.178748834913967869, -10.36894250292378850 ) ) ;
#39799=CARTESIAN_POINT ( 'NONE',  ( 5.076628168052704559, 15.17559781766745175, -8.527530157486179263 ) ) ;
#39800=CARTESIAN_POINT ( 'NONE',  ( 6.565887622018943937, 23.08196800326375708, -12.81628187352647608 ) ) ;
#39802=CARTESIAN_POINT ( 'NONE',  ( 17.96484262340118221, 51.18868534415483396, -7.964842623401177768 ) ) ;
#39803=CARTESIAN_POINT ( 'NONE',  ( 1.472469842513823179, 65.59226448433412315, -4.923371831947296329 ) ) ;
#39806=CARTESIAN_POINT ( 'NONE',  ( 12.63842701281683922, 34.55059781766745886, -9.846743663894590881 ) ) ;
#39807=CARTESIAN_POINT ( 'NONE',  ( 17.20831665107776587, 27.88393115100078390, 7.208316651077764980 ) ) ;
#39808=CARTESIAN_POINT ( 'NONE',  ( 15.44008868035555793, 16.39701867748817321, -9.422509992056140149 ) ) ;
#39809=CARTESIAN_POINT ( 'NONE',  ( 13.43411237798106583, 22.66530133659708923, -12.81628187352647252 ) ) ;
#39810=CARTESIAN_POINT ( 'NONE',  ( 12.63842701281683922, 19.55059781766745175, -9.846743663894590881 ) ) ;
#39812=CARTESIAN_POINT ( 'NONE',  ( 7.084665262690076126, 19.10535201082150181, 10.88017736071109987 ) ) ;
#39813=CARTESIAN_POINT ( 'NONE',  ( 19.84674366389459266, 38.30059781766745175, 2.638427012816836559 ) ) ;
#39814=CARTESIAN_POINT ( 'NONE',  ( 12.91533473730993009, 21.60535201082150536, -10.88017736071109987 ) ) ;
#39815=CARTESIAN_POINT ( 'NONE',  ( 4.559911319644449179, 37.23035201082150536, -9.422509992056141925 ) ) ;
#39816=CARTESIAN_POINT ( 'NONE',  ( 15.44008868035555260, 14.73035201082150536, 9.422509992056143702 ) ) ;
#39817=CARTESIAN_POINT ( 'NONE',  ( 20.04068437667223890, 59.71974360917720048, 6.396802510829770583 ) ) ;
#39818=CARTESIAN_POINT ( 'NONE',  ( 17.20831665107776587, 12.88393115100078390, 7.208316651077764980 ) ) ;
#39819=CARTESIAN_POINT ( 'NONE',  ( 19.84674366389459266, 43.30059781766744464, 2.638427012816836559 ) ) ;
#39822=AXIS2_PLACEMENT_3D ( 'NONE', #19927, #4937, #12422 ) ;
#39824=CARTESIAN_POINT ( 'NONE',  ( 24.16423886937410614, 29.51208216824729647, -3.795296366450302550 ) ) ;
#39825=CARTESIAN_POINT ( 'NONE',  ( 18.52753015748617571, 38.09226448433412315, 4.923371831947298993 ) ) ;
#39827=CARTESIAN_POINT ( 'NONE',  ( -4.164238869374099927, 52.01208216824729647, 3.795296366450308767 ) ) ;
#39828=CARTESIAN_POINT ( 'NONE',  ( 12.63842701281683034, 17.46726448433411250, 9.846743663894596210 ) ) ;
#39829=LINE ( 'NONE', #31816, #69019 ) ;
#39831=CARTESIAN_POINT ( 'NONE',  ( 0.5774900079438590739, 47.64701867748817676, -5.440088680355550821 ) ) ;
#39832=CARTESIAN_POINT ( 'NONE',  ( 16.40814093676323893, 60.79030133659709634, 11.09922568453595026 ) ) ;
#39833=CARTESIAN_POINT ( 'NONE',  ( 20.88017736071110519, 15.56368534415483751, 2.639326808657452039E-16 ) ) ;
#39834=CARTESIAN_POINT ( 'NONE',  ( -2.816281873526473856, 54.33196800326376064, 3.434112377981055619 ) ) ;
#39835=CARTESIAN_POINT ( 'NONE',  ( 6.565887622018943937, 8.081968003263751754, -12.81628187352647608 ) ) ;
#39836=CARTESIAN_POINT ( 'NONE',  ( 19.84674366389459266, 18.30059781766745175, 2.638427012816836559 ) ) ;
#39837=ORIENTED_EDGE ( 'NONE', *, *, #2973, .F. ) ;
#39839=CARTESIAN_POINT ( 'NONE',  ( 0.2751277870542982451, 17.28217586085238011, -6.500000000000002665 ) ) ;
#39840=CARTESIAN_POINT ( 'NONE',  ( 17.08211943468705130, 53.47041550158063217, 12.26659068614894998 ) ) ;
#39841=CARTESIAN_POINT ( 'NONE',  ( 17.08211943468705130, 33.47041550158063927, 12.26659068614894998 ) ) ;
#39842=CARTESIAN_POINT ( 'NONE',  ( 7.084665262690076126, 17.02201867748817676, -10.88017736071110164 ) ) ;
#39843=CARTESIAN_POINT ( 'NONE',  ( 15.44008868035555793, 36.39701867748816966, -9.422509992056140149 ) ) ;
#39844=PRESENTATION_STYLE_ASSIGNMENT (( #17833 ) ) ;
#39845=( GEOMETRIC_REPRESENTATION_CONTEXT ( 3 ) GLOBAL_UNCERTAINTY_ASSIGNED_CONTEXT ( ( #28147 ) ) GLOBAL_UNIT_ASSIGNED_CONTEXT ( ( #33557, #26085, #87557 ) ) REPRESENTATION_CONTEXT ( 'NONE', 'WORKASPACE' ) );
#39846=CARTESIAN_POINT ( 'NONE',  ( 2.035157376598824452, 68.68868534415484817, 7.964842623401179544 ) ) ;
#39848=CARTESIAN_POINT ( 'NONE',  ( 10.00000000000000000, 24.75893115100078745, -9.846743663894594434 ) ) ;
#39849=CARTESIAN_POINT ( 'NONE',  ( 17.62281668512004629, 18.28593319516823001, 6.499999999999968914 ) ) ;
#39850=DIRECTION ( 'NONE',  ( 0.000000000000000000, 0.000000000000000000, -1.000000000000000000 ) ) ;
#39851=CARTESIAN_POINT ( 'NONE',  ( 7.361572987183169658, 14.96726448433411960, -9.846743663894592657 ) ) ;
#39852=CARTESIAN_POINT ( 'NONE',  ( 1.472469842513823179, 40.59226448433411605, -4.923371831947296329 ) ) ;
#39854=EDGE_CURVE ( 'NONE', #26202, #16435, #94438, .T. ) ;
#39855=CARTESIAN_POINT ( 'NONE',  ( 10.00000000000000178, 9.313685344154839285, 10.88017736071110342 ) ) ;
#39856=CARTESIAN_POINT ( 'NONE',  ( -2.816281873526473856, 29.12363466993041783, 9.499525473075851096E-16 ) ) ;
#39857=CARTESIAN_POINT ( 'NONE',  ( 10.00000000000000000, 51.81368534415484106, -10.88017736071110342 ) ) ;
#39858=CARTESIAN_POINT ( 'NONE',  ( -4.164238869374099927, 52.01208216824729647, 3.795296366450308767 ) ) ;
#39859=CARTESIAN_POINT ( 'NONE',  ( 18.52753015748617571, 3.092264484334118269, 4.923371831947298993 ) ) ;
#39861=CARTESIAN_POINT ( 'NONE',  ( 1.472469842513823179, 45.59226448433412315, -4.923371831947296329 ) ) ;
#39862=CARTESIAN_POINT ( 'NONE',  ( 18.52753015748618282, 33.92559781766745886, -4.923371831947291888 ) ) ;
#39863=CARTESIAN_POINT ( 'NONE',  ( 20.36894250292379382, 13.67874883491396965, 10.36894250292379205 ) ) ;
#39864=CARTESIAN_POINT ( 'NONE',  ( 10.00000000000000178, 13.05374883491396787, 14.16423886937410082 ) ) ;
#39865=CARTESIAN_POINT ( 'NONE',  ( 17.96484262340118221, 44.93868534415483396, 7.964842623401181321 ) ) ;
#39866=CARTESIAN_POINT ( 'NONE',  ( 2.035157376598822676, 7.438685344154837509, -7.964842623401177768 ) ) ;
#39867=CARTESIAN_POINT ( 'NONE',  ( 12.91533473730993009, 41.60535201082149825, -10.88017736071109987 ) ) ;
#39868=CARTESIAN_POINT ( 'NONE',  ( 19.42250999205614548, 25.98035201082150891, -5.440088680355545492 ) ) ;
#39870=CARTESIAN_POINT ( 'NONE',  ( 6.565887622018943937, 35.16530133659708923, 12.81628187352647430 ) ) ;
#39871=CARTESIAN_POINT ( 'NONE',  ( 7.084665262690076126, 37.02201867748817676, -10.88017736071110164 ) ) ;
#39873=CARTESIAN_POINT ( 'NONE',  ( -2.816281873526471635, 63.91530133659708923, -3.434112377981056508 ) ) ;
#39874=CARTESIAN_POINT ( 'NONE',  ( 17.96484262340118221, 46.18868534415484106, -7.964842623401177768 ) ) ;
#39876=CARTESIAN_POINT ( 'NONE',  ( 0.5774900079438607392, 48.48035201082150536, 5.440088680355550821 ) ) ;
#39877=CARTESIAN_POINT ( 'NONE',  ( 20.88017736071110164, 5.355352010821502695, 2.915334737309930979 ) ) ;
#39881=CARTESIAN_POINT ( 'NONE',  ( -4.164238869374099039, 56.80374883491397497, 8.674139862899312516E-16 ) ) ;
#39882=CARTESIAN_POINT ( 'NONE',  ( 19.42250999205614548, 60.98035201082151247, -5.440088680355545492 ) ) ;
#39883=CARTESIAN_POINT ( 'NONE',  ( 13.79529636645030344, 3.262082168247301350, 14.16423886937410614 ) ) ;
#39886=CARTESIAN_POINT ( 'NONE',  ( 19.42250999205614548, 15.98035201082150714, -5.440088680355545492 ) ) ;
#39887=CARTESIAN_POINT ( 'NONE',  ( 17.20831665107776587, 42.88393115100077324, 7.208316651077764980 ) ) ;
#39890=CARTESIAN_POINT ( 'NONE',  ( 18.52753015748617571, 43.09226448433412315, 4.923371831947298993 ) ) ;
#39891=CARTESIAN_POINT ( 'NONE',  ( 2.035157376598824452, 63.68868534415484106, 7.964842623401179544 ) ) ;
#39892=CARTESIAN_POINT ( 'NONE',  ( 20.88017736071110519, 40.56368534415484106, 2.639326808657452039E-16 ) ) ;
#39893=CARTESIAN_POINT ( 'NONE',  ( 14.92337183194729633, 32.67559781766745175, 8.527530157486181039 ) ) ;
#39896=CARTESIAN_POINT ( 'NONE',  ( 4.559911319644449179, 52.23035201082151247, -9.422509992056141925 ) ) ;
#39897=CARTESIAN_POINT ( 'NONE',  ( 2.917880565312948704, 62.63708216824730357, 12.26659068614894643 ) ) ;
#39898=CARTESIAN_POINT ( 'NONE',  ( 16.40814093676324603, 22.45696800326375353, -11.09922568453594671 ) ) ;
#39901=CARTESIAN_POINT ( 'NONE',  ( 6.565887622018943937, 33.08196800326374643, -12.81628187352647608 ) ) ;
#39902=CARTESIAN_POINT ( 'NONE',  ( 19.42250999205614193, 25.14701867748817321, 5.440088680355555262 ) ) ;
#39905=VECTOR ( 'NONE', #46331, 1000.000000000000000 ) ;
#39907=CARTESIAN_POINT ( 'NONE',  ( 20.88017736071110164, 65.35535201082150536, 2.915334737309930979 ) ) ;
#39908=CARTESIAN_POINT ( 'NONE',  ( 19.84674366389459266, 43.30059781766744464, 2.638427012816836559 ) ) ;
#39909=CARTESIAN_POINT ( 'NONE',  ( 0.1532563361054082862, 6.217264484334118713, 2.638427012816831674 ) ) ;
#39910=CARTESIAN_POINT ( 'NONE',  ( 5.076628168052703671, 31.84226448433412315, 8.527530157486179263 ) ) ;
#39913=CARTESIAN_POINT ( 'NONE',  ( 12.63842701281683034, 27.46726448433411250, 9.846743663894596210 ) ) ;
#39917=CARTESIAN_POINT ( 'NONE',  ( 17.20831665107776587, 27.88393115100078390, 7.208316651077764980 ) ) ;
#39919=CARTESIAN_POINT ( 'NONE',  ( 0.1532563361054083140, 51.00893115100078745, 1.131784320476157264E-15 ) ) ;
#39921=B_SPLINE_CURVE_WITH_KNOTS ( 'NONE', 3,
 ( #32091, #36551, #28547, #89048, #42087, #20054, #28046, #20559 ),
 .UNSPECIFIED., .F., .F.,
 ( 4, 2, 2, 4 ),
 ( 0.009612260643802141014, 0.01201872016511521847, 0.01442517968642829593, 0.01923809872905445084 ),
 .UNSPECIFIED. ) ;
#39923=CARTESIAN_POINT ( 'NONE',  ( 6.565887622018943937, 28.08196800326375353, -12.81628187352647608 ) ) ;
#39924=FACE_OUTER_BOUND ( 'NONE', #43386, .T. ) ;
#39925=CARTESIAN_POINT ( 'NONE',  ( 17.08211943468705130, 48.47041550158063927, 12.26659068614894998 ) ) ;
#39926=CARTESIAN_POINT ( 'NONE',  ( 10.00000000000000000, 24.75893115100078745, -9.846743663894594434 ) ) ;
#39927=CARTESIAN_POINT ( 'NONE',  ( 10.00000000000000000, -0.2410688489992152128, -9.846743663894594434 ) ) ;
#39928=CARTESIAN_POINT ( 'NONE',  ( 19.59242374975054446, 95.44328903796339603, 5.127491817726292034 ) ) ;
#39929=CARTESIAN_POINT ( 'NONE',  ( 13.79529636645030344, 38.26208216824729647, 14.16423886937410614 ) ) ;
#39930=CARTESIAN_POINT ( 'NONE',  ( 7.361572987183169658, 64.96726448433412315, -9.846743663894592657 ) ) ;
#39931=CARTESIAN_POINT ( 'NONE',  ( 24.16423886937410614, 59.51208216824728936, -3.795296366450302550 ) ) ;
#39932=CARTESIAN_POINT ( 'NONE',  ( -4.164238869374099039, 26.80374883491397142, 8.674139862899312516E-16 ) ) ;
#39933=CARTESIAN_POINT ( 'NONE',  ( 22.26659068614894466, 23.88708216824730357, 7.082119434687054849 ) ) ;
#39935=CARTESIAN_POINT ( 'NONE',  ( 20.00000000000000711, 105.0000000000000000, 5.000000000000000000 ) ) ;
#39936=CARTESIAN_POINT ( 'NONE',  ( 2.791683348922240793, 61.63393115100079456, 7.208316651077764092 ) ) ;
#39937=CARTESIAN_POINT ( 'NONE',  ( 12.91533473730993009, 31.60535201082150891, -10.88017736071109987 ) ) ;
#39938=CYLINDRICAL_SURFACE ( 'NONE', #63420, 11.92686044187656513 ) ;
#39940=CARTESIAN_POINT ( 'NONE',  ( 2.791683348922240793, 36.63393115100078035, 7.208316651077764092 ) ) ;
#39941=CARTESIAN_POINT ( 'NONE',  ( 0.6178305044545838731, 49.74863466993041072, 9.382169495545420901 ) ) ;
#39943=CARTESIAN_POINT ( 'NONE',  ( 19.84674366389459621, 48.50893115100078745, 7.409399052514197653E-17 ) ) ;
#39946=CARTESIAN_POINT ( 'NONE',  ( -4.164238869374098151, 16.59541550158063927, -3.795296366450310543 ) ) ;
#39950=CARTESIAN_POINT ( 'NONE',  ( 2.035157376598822676, 2.438685344154838397, -7.964842623401177768 ) ) ;
#39951=CARTESIAN_POINT ( 'NONE',  ( 16.40814093676323893, 5.790301336597087456, 11.09922568453595026 ) ) ;
#39953=CARTESIAN_POINT ( 'NONE',  ( 15.44008868035555793, 66.39701867748817676, -9.422509992056140149 ) ) ;
#39958=CARTESIAN_POINT ( 'NONE',  ( -4.164238869374098151, 61.59541550158063217, -3.795296366450310543 ) ) ;
#39960=CARTESIAN_POINT ( 'NONE',  ( 0.5774900079438590739, 32.64701867748816966, -5.440088680355550821 ) ) ;
#39961=CARTESIAN_POINT ( 'NONE',  ( 4.559911319644449179, 38.89701867748817676, 9.422509992056141925 ) ) ;
#39962=CARTESIAN_POINT ( 'NONE',  ( -2.816281873526471635, 3.915301336597087456, -3.434112377981056508 ) ) ;
#39963=CARTESIAN_POINT ( 'NONE',  ( 2.791683348922240793, 56.63393115100078035, 7.208316651077764092 ) ) ;
#39964=CARTESIAN_POINT ( 'NONE',  ( 3.591859063236763294, 63.29030133659708923, -11.09922568453595026 ) ) ;
#39968=CARTESIAN_POINT ( 'NONE',  ( -0.8801773607111008646, 33.27201867748817676, 2.915334737309923430 ) ) ;
#39969=EDGE_CURVE ( 'NONE', #34886, #71042, #40792, .T. ) ;
#39970=CARTESIAN_POINT ( 'NONE',  ( 10.00000000000000000, 32.87363466993042493, -12.81628187352647608 ) ) ;
#39972=CARTESIAN_POINT ( 'NONE',  ( 5.076628168052704559, 65.17559781766745175, -8.527530157486179263 ) ) ;
#39974=CARTESIAN_POINT ( 'NONE',  ( 12.91533473730993009, 46.60535201082150536, -10.88017736071109987 ) ) ;
#39975=CARTESIAN_POINT ( 'NONE',  ( 12.63842701281683922, 14.55059781766744997, -9.846743663894590881 ) ) ;
#39976=CARTESIAN_POINT ( 'NONE',  ( 16.40814093676324603, 37.45696800326376064, -11.09922568453594671 ) ) ;
#39977=CARTESIAN_POINT ( 'NONE',  ( 15.44008868035555793, 66.39701867748817676, -9.422509992056140149 ) ) ;
#39979=FILL_AREA_STYLE ('',( #8980 ) ) ;
#39980=CARTESIAN_POINT ( 'NONE',  ( 21.09922568453594849, 61.20696800326376064, 6.408140936763242479 ) ) ;
#39981=VERTEX_POINT ( 'NONE', #29725 ) ;
#39984=CARTESIAN_POINT ( 'NONE',  ( 17.96484262340118221, 11.18868534415483929, -7.964842623401177768 ) ) ;
#39985=CARTESIAN_POINT ( 'NONE',  ( 3.591859063236761518, 49.95696800326375353, 11.09922568453594849 ) ) ;
#39986=CARTESIAN_POINT ( 'NONE',  ( -2.266590686148945544, 11.38708216824730179, -7.082119434687050408 ) ) ;
#39987=CARTESIAN_POINT ( 'NONE',  ( 18.52753015748618282, 23.92559781766745530, -4.923371831947291888 ) ) ;
#39988=CARTESIAN_POINT ( 'NONE',  ( 17.20831665107776587, 17.88393115100078745, 7.208316651077764980 ) ) ;
#39989=CARTESIAN_POINT ( 'NONE',  ( -4.164238869374099039, 56.80374883491397497, 8.674139862899312516E-16 ) ) ;
#39991=CARTESIAN_POINT ( 'NONE',  ( 12.91533473730993009, 21.60535201082150536, -10.88017736071109987 ) ) ;
#39992=FACE_OUTER_BOUND ( 'NONE', #82147, .T. ) ;
#39993=VERTEX_POINT ( 'NONE', #76232 ) ;
#39995=CARTESIAN_POINT ( 'NONE',  ( 10.00000000000000000, 16.81368534415483751, -10.88017736071110342 ) ) ;
#39996=CARTESIAN_POINT ( 'NONE',  ( 7.084665262690076126, 7.022018677488170546, -10.88017736071110164 ) ) ;
#39997=CARTESIAN_POINT ( 'NONE',  ( 0.1532563361054100626, 55.80059781766745175, -2.638427012816831230 ) ) ;
#39999=CARTESIAN_POINT ( 'NONE',  ( 16.40814093676323893, 55.79030133659708923, 11.09922568453595026 ) ) ;
#40000=DIRECTION ( 'NONE',  ( 0.000000000000000000, 0.000000000000000000, -1.000000000000000000 ) ) ;
#40002=CARTESIAN_POINT ( 'NONE',  ( -4.164238869374099927, 17.01208216824730357, 3.795296366450308767 ) ) ;
#40003=CARTESIAN_POINT ( 'NONE',  ( 12.91533473730993009, 31.60535201082150891, -10.88017736071109987 ) ) ;
#40004=CARTESIAN_POINT ( 'NONE',  ( 22.26659068614894466, 63.88708216824730357, 7.082119434687054849 ) ) ;
#40005=CARTESIAN_POINT ( 'NONE',  ( 10.00000000000000178, 62.25893115100078745, 9.846743663894594434 ) ) ;
#40007=CARTESIAN_POINT ( 'NONE',  ( 0.1532563361054083140, 31.00893115100078390, 1.131784320476157264E-15 ) ) ;
#40009=CARTESIAN_POINT ( 'NONE',  ( 1.472469842513823179, 6.425597817667451750, 4.923371831947296329 ) ) ;
#40012=CARTESIAN_POINT ( 'NONE',  ( 0.5774900079438607392, 3.480352010821504027, 5.440088680355550821 ) ) ;
#40013=CARTESIAN_POINT ( 'NONE',  ( -0.8801773607110991993, 67.85535201082151957, -2.915334737309923874 ) ) ;
#40014=CARTESIAN_POINT ( 'NONE',  ( 19.38216949554541557, 2.248634669930420049, -9.382169495545420901 ) ) ;
#40015=CARTESIAN_POINT ( 'NONE',  ( 2.035157376598822676, 42.43868534415483396, -7.964842623401177768 ) ) ;
#40016=CARTESIAN_POINT ( 'NONE',  ( 2.035157376598822676, 12.43868534415483751, -7.964842623401177768 ) ) ;
#40017=CARTESIAN_POINT ( 'NONE',  ( -1.099225684535947600, 38.70696800326375353, -6.408140936763238038 ) ) ;
#40018=CARTESIAN_POINT ( 'NONE',  ( 22.26659068614895176, 19.72041550158063572, -7.082119434687042414 ) ) ;
#40019=( BOUNDED_SURFACE ( )  B_SPLINE_SURFACE ( 1, 2, ( 
 ( #89410, #74899, #83396, #59891, #6397, #36912, #97933, #52399, #75388, #20926, #6906, #37418, #14916, #45386, #75892, #38891, #901, #23404, #16380, #85363, #7900, #23894, #8383, #53888, #15893, #77355, #84394, #39866, #17374, #61372, #46379, #76385, #62350, #69379, #38395, #8866, #16875, #31363, #61863, #47844, #93350, #1397, #68897, #92854, #39382, #69877, #47351, #53378, #91882, #91380, #76867, #83888, #60880, #24382, #31852, #425, #92368, #54849, #55357, #77852, #62852, #54361, #70373, #30876, #22908, #9362, #1890, #84871, #78348, #46863, #32349, #24875, #85862, #37912, #68400, #98921, #30377, #15417, #45899, #25372, #41367, #2384, #40367, #64312, #48826, #41845, #94823, #78844, #3842, #88311, #26327, #3343, #10355, #71834, #19809, #70868, #40854, #71358, #33325, #86353, #42324, #11326, #17855, #56824, #57804, #57312, #50299, #86844, #18348, #80317, #18840, #34301, #32838, #2876, #63820, #94332, #9869, #63340, #26819, #10846, #25851, #72798, #79336, #64799, #95823, #65296, #93845, #55857, #33805, #48341, #95317, #87323, #49320, #79824, #4337, #56348, #72311, #87804, #19326, #49809, #34807, #11817, #27304, #73791, #50811, #22298, #96823, #60275, #6296, #27800, #82783, #51298, #44774, #28787, #81302, #13797, #74787, #36798, #90774, #36297, #20313, #90270, #66794, #12797, #59777, #75280, #58285, #65793, #58792, #67292, #21804, #80812, #42818, #43298, #5322, #35801, #88803, #14303, #82280, #66288, #97314, #29767, #29281, #12310, #89299, #20810, #52284, #89784, #97819, #73302, #28299, #81783, #13297, #4826, #35301, #6790, #43784, #74277, #37304, #5805, #67791, #98313, #96327, #59286, #21301, #51793, #44283, #39271, #84281, #15781, #61259, #85253, #76272, #91766, #98812, #23782, #1772, #47233, #14805, #54248, #45780, #22790, #93230, #68779, #32229, #77245, #30261, #54733, #23288, #16759, #791, #53267, #84760, #46749, #8752, #62729, #8273, #91265, #62237, #38770, #83773, #31742, #77737, #60764, #37793, #30752, #69760, #92744, #1288, #16268, #24268, #9248, #68291, #7789, #7293, #53766, #15297, #75772, #39757, #70257, #38284, #310, #52772, #83281, #45277, #46270, #76755, #69272, #31245, #61741, #92259, #3231, #40735, #57194, #56236, #79216, #94713, #93726, #10242, #33215, #86235, #49208, #72201, #32724, #9744, #2762, #85747, #55232, #25744, #71238, #71721, #86730, #63222, #33697, #95192, #18232, #63710, #25258, #94213, #10728, #55744, #64196, #48714, #41244, #26220, #56713, #70754, #87204, #34190, #18728, #79712, #11211, #41730, #3729, #64683, #24755, #26700, #47734, #17259, #78231, #40245, #2268, #17746, #48223, #78732 ),
 ( #15604, #621, #39582, #32548, #55046, #40062, #46569, #47560, #46089, #38108, #85566, #9069, #54067, #55561, #1097, #54553, #32043, #76574, #23602, #77068, #69088, #17078, #70562, #84090, #30574, #8580, #7615, #45588, #69578, #84581, #47054, #31560, #8094, #70073, #93546, #62056, #39084, #38590, #92558, #25078, #76085, #31067, #61567, #92077, #91589, #78058, #16579, #23103, #24085, #63049, #62545, #15111, #16082, #85070, #9560, #77552, #1593, #68597, #93051, #24585, #2088, #125, #61078, #53576, #72568, #19094, #64570, #43923, #4104, #59421, #18608, #18125, #28918, #5949, #87581, #34567, #13946, #94595, #67431, #34077, #48598, #25628, #95081, #56606, #66933, #79102, #3126, #11103, #11589, #79601, #42106, #64080, #26585, #26112, #65061, #74420, #49574, #80084, #6425, #82422, #89438, #87095, #81928, #20951, #10614, #95588, #27073, #86615, #44421, #33585, #41126, #56118, #89925, #71615, #49097, #58938, #51438, #36440, #41621, #72087, #3612, #13436, #21440, #74926, #57087, #97454, #51938, #36937, #54380, #97954, #38911, #84894, #39404, #7437, #53400, #69398, #90906, #61882, #15910, #23912, #92386, #29410, #920, #37439, #91900, #14440, #46883, #29906, #31382, #59915, #76890, #37933, #45917, #91404, #68422, #46400, #76405, #16404, #22435, #90404, #77375, #8402, #60903, #7921, #8888, #67930, #21945, #98945, #52422, #82922, #30399, #60412, #44910, #75416, #6931, #83418, #83909, #52906, #15438, #98450, #68916, #14938, #23425, #38418, #22932, #53904, #444, #45406, #30896, #75912, #84412, #61390, #2405, #25392, #40877, #86862, #11346, #48849, #1417, #55875, #94353, #71383, #70887, #32863, #55382, #48358, #18368, #39887, #86374, #40390, #85882, #47863, #10375, #17395, #71853, #49342, #93370, #78369, #9382, #25871, #9888, #63361, #24897, #41386, #94845, #70391, #85383, #93864, #62369, #31870, #17876, #78865, #2895, #33345, #1910, #63839, #79841, #56370, #79358, #32368, #10865, #69897, #92873, #62873, #3363, #33827, #47374, #64334, #26346, #77872, #56847, #18861, #87346, #24405, #54873, #16897, #13316, #50829, #35820, #34323, #11838, #72822, #42345, #82297, #41866, #58810, #89800, #65814, #42836, #35319, #96844, #28804, #97332, #21319, #72329, #73320, #57331, #28318, #4843, #96346, #50317, #74296, #65316, #80832, #87827, #12817, #51810, #36316, #3862, #43315, #34826, #4360, #64821, #57823, #95338, #66307, #19345, #43803, #12332, #5823, #88821, #95842, #73809, #89319, #20827, #26837, #27819, #80340, #51316, #58304, #27327, #81799, #66810, #49828, #88332, #19829, #59303, #20333, #81322, #5342, #15315, #91785, #29298, #67812, #67308 ) ),
 .UNSPECIFIED., .F., .F., .F. ) 
 B_SPLINE_SURFACE_WITH_KNOTS ( ( 2, 2 ),
 ( 3, 2, 2, 2, 2, 2, 2, 2, 2, 2, 2, 2, 2, 2, 2, 2, 2, 2, 2, 2, 2, 2, 2, 2, 2, 2, 2, 2, 2, 2, 2, 2, 2, 2, 2, 2, 2, 2, 2, 2, 2, 2, 2, 2, 2, 2, 2, 2, 2, 2, 2, 2, 2, 2, 2, 2, 2, 2, 2, 2, 2, 2, 2, 2, 2, 2, 2, 2, 2, 2, 2, 2, 2, 2, 2, 2, 2, 2, 2, 2, 2, 2, 2, 2, 2, 2, 2, 2, 2, 2, 2, 2, 2, 2, 2, 2, 2, 2, 2, 2, 2, 2, 2, 2, 2, 2, 2, 2, 2, 2, 2, 2, 2, 2, 2, 2, 2, 2, 2, 2, 2, 2, 2, 2, 2, 2, 2, 2, 2, 2, 2, 2, 2, 2, 2, 2, 2, 2, 2, 2, 2, 2, 2, 2, 2, 2, 2, 2, 2, 2, 2, 2, 2, 2, 2, 2, 2, 2, 2, 2, 2, 2, 3 ),
 ( 0.000000000000000000, 1.000000000000000000 ),
 ( 0.000000000000000000, 0.005952380952380952051, 0.01190476190476190410, 0.01785714285714285615, 0.02380952380952380820, 0.02976190476190476025, 0.03571428571428571230, 0.04166666666666666435, 0.04761904761904761640, 0.05357142857142856845, 0.05952380952380952051, 0.06547619047619047949, 0.07142857142857142461, 0.07738095238095238360, 0.08333333333333332871, 0.08928571428571428770, 0.09523809523809523281, 0.1011904761904761918, 0.1071428571428571369, 0.1130952380952380959, 0.1190476190476190410, 0.1250000000000000000, 0.1309523809523809590, 0.1369047619047619180, 0.1428571428571428492, 0.1488095238095238082, 0.1547619047619047672, 0.1607142857142857262, 0.1666666666666666574, 0.1726190476190476164, 0.1785714285714285754, 0.1845238095238095344, 0.1904761904761904656, 0.1964285714285714246, 0.2023809523809523836, 0.2083333333333333426, 0.2142857142857142738, 0.2202380952380952328, 0.2261904761904761918, 0.2321428571428571508, 0.2380952380952380820, 0.2440476190476190410, 0.2500000000000000000, 0.2559523809523809312, 0.2619047619047619180, 0.2678571428571428492, 0.2738095238095238360, 0.2797619047619047672, 0.2857142857142856984, 0.2916666666666666852, 0.2976190476190476164, 0.3035714285714285476, 0.3095238095238095344, 0.3154761904761904656, 0.3214285714285714524, 0.3273809523809523836, 0.3333333333333333148, 0.3392857142857143016, 0.3452380952380952328, 0.3511904761904761640, 0.3571428571428571508, 0.3630952380952380820, 0.3690476190476190688, 0.3750000000000000000, 0.3809523809523809312, 0.3869047619047619180, 0.3928571428571428492, 0.3988095238095238360, 0.4047619047619047672, 0.4107142857142856984, 0.4166666666666666852, 0.4226190476190476164, 0.4285714285714285476, 0.4345238095238095344, 0.4404761904761904656, 0.4464285714285714524, 0.4523809523809523836, 0.4583333333333333148, 0.4642857142857143016, 0.4702380952380952328, 0.4761904761904761640, 0.4821428571428571508, 0.4880952380952380820, 0.4940476190476190688, 0.5000000000000000000, 0.5059523809523809312, 0.5119047619047618625, 0.5178571428571429047, 0.5238095238095238360, 0.5297619047619047672, 0.5357142857142856984, 0.5416666666666666297, 0.5476190476190476719, 0.5535714285714286031, 0.5595238095238095344, 0.5654761904761904656, 0.5714285714285713969, 0.5773809523809523281, 0.5833333333333333703, 0.5892857142857143016, 0.5952380952380952328, 0.6011904761904761640, 0.6071428571428570953, 0.6130952380952381375, 0.6190476190476190688, 0.6250000000000000000, 0.6309523809523809312, 0.6369047619047618625, 0.6428571428571429047, 0.6488095238095238360, 0.6547619047619047672, 0.6607142857142856984, 0.6666666666666666297, 0.6726190476190476719, 0.6785714285714286031, 0.6845238095238095344, 0.6904761904761904656, 0.6964285714285713969, 0.7023809523809523281, 0.7083333333333333703, 0.7142857142857143016, 0.7202380952380952328, 0.7261904761904761640, 0.7321428571428570953, 0.7380952380952381375, 0.7440476190476190688, 0.7500000000000000000, 0.7559523809523809312, 0.7619047619047618625, 0.7678571428571429047, 0.7738095238095238360, 0.7797619047619047672, 0.7857142857142856984, 0.7916666666666666297, 0.7976190476190476719, 0.8035714285714286031, 0.8095238095238095344, 0.8154761904761904656, 0.8214285714285713969, 0.8273809523809523281, 0.8333333333333333703, 0.8392857142857143016, 0.8452380952380952328, 0.8511904761904761640, 0.8571428571428570953, 0.8630952380952381375, 0.8690476190476190688, 0.8750000000000000000, 0.8809523809523809312, 0.8869047619047618625, 0.8928571428571429047, 0.8988095238095238360, 0.9047619047619047672, 0.9107142857142856984, 0.9166666666666666297, 0.9226190476190476719, 0.9285714285714286031, 0.9345238095238095344, 0.9404761904761904656, 0.9464285714285713969, 0.9523809523809523281, 0.9583333333333333703, 0.9642857142857143016 ),
 .UNSPECIFIED. ) 
 GEOMETRIC_REPRESENTATION_ITEM ( )  RATIONAL_B_SPLINE_SURFACE ( (
 ( 1.000000000000000000, 0.9659258262890683122, 1.000000000000000000, 0.9659258262890683122, 1.000000000000000000, 0.9659258262890683122, 1.000000000000000000, 0.9659258262890683122, 1.000000000000000000, 0.9659258262890683122, 1.000000000000000000, 0.9659258262890683122, 1.000000000000000000, 0.9659258262890683122, 1.000000000000000000, 0.9659258262890683122, 1.000000000000000000, 0.9659258262890683122, 1.000000000000000000, 0.9659258262890683122, 1.000000000000000000, 0.9659258262890683122, 1.000000000000000000, 0.9659258262890683122, 1.000000000000000000, 0.9659258262890683122, 1.000000000000000000, 0.9659258262890683122, 1.000000000000000000, 0.9659258262890683122, 1.000000000000000000, 0.9659258262890683122, 1.000000000000000000, 0.9659258262890683122, 1.000000000000000000, 0.9659258262890683122, 1.000000000000000000, 0.9659258262890683122, 1.000000000000000000, 0.9659258262890683122, 1.000000000000000000, 0.9659258262890683122, 1.000000000000000000, 0.9659258262890683122, 1.000000000000000000, 0.9659258262890683122, 1.000000000000000000, 0.9659258262890683122, 1.000000000000000000, 0.9659258262890683122, 1.000000000000000000, 0.9659258262890683122, 1.000000000000000000, 0.9659258262890683122, 1.000000000000000000, 0.9659258262890683122, 1.000000000000000000, 0.9659258262890683122, 1.000000000000000000, 0.9659258262890683122, 1.000000000000000000, 0.9659258262890683122, 1.000000000000000000, 0.9659258262890683122, 1.000000000000000000, 0.9659258262890683122, 1.000000000000000000, 0.9659258262890683122, 1.000000000000000000, 0.9659258262890683122, 1.000000000000000000, 0.9659258262890683122, 1.000000000000000000, 0.9659258262890683122, 1.000000000000000000, 0.9659258262890683122, 1.000000000000000000, 0.9659258262890683122, 1.000000000000000000, 0.9659258262890683122, 1.000000000000000000, 0.9659258262890683122, 1.000000000000000000, 0.9659258262890683122, 1.000000000000000000, 0.9659258262890683122, 1.000000000000000000, 0.9659258262890683122, 1.000000000000000000, 0.9659258262890683122, 1.000000000000000000, 0.9659258262890683122, 1.000000000000000000, 0.9659258262890683122, 1.000000000000000000, 0.9659258262890683122, 1.000000000000000000, 0.9659258262890683122, 1.000000000000000000, 0.9659258262890683122, 1.000000000000000000, 0.9659258262890683122, 1.000000000000000000, 0.9659258262890683122, 1.000000000000000000, 0.9659258262890683122, 1.000000000000000000, 0.9659258262890683122, 1.000000000000000000, 0.9659258262890683122, 1.000000000000000000, 0.9659258262890683122, 1.000000000000000000, 0.9659258262890683122, 1.000000000000000000, 0.9659258262890683122, 1.000000000000000000, 0.9659258262890683122, 1.000000000000000000, 0.9659258262890683122, 1.000000000000000000, 0.9659258262890683122, 1.000000000000000000, 0.9659258262890683122, 1.000000000000000000, 0.9659258262890683122, 1.000000000000000000, 0.9659258262890683122, 1.000000000000000000, 0.9659258262890683122, 1.000000000000000000, 0.9659258262890683122, 1.000000000000000000, 0.9659258262890683122, 1.000000000000000000, 0.9659258262890683122, 1.000000000000000000, 0.9659258262890683122, 1.000000000000000000, 0.9659258262890683122, 1.000000000000000000, 0.9659258262890683122, 1.000000000000000000, 0.9659258262890683122, 1.000000000000000000, 0.9659258262890683122, 1.000000000000000000, 0.9659258262890683122, 1.000000000000000000, 0.9659258262890683122, 1.000000000000000000, 0.9659258262890683122, 1.000000000000000000, 0.9659258262890683122, 1.000000000000000000, 0.9659258262890683122, 1.000000000000000000, 0.9659258262890683122, 1.000000000000000000, 0.9659258262890683122, 1.000000000000000000, 0.9659258262890683122, 1.000000000000000000, 0.9659258262890683122, 1.000000000000000000, 0.9659258262890683122, 1.000000000000000000, 0.9659258262890683122, 1.000000000000000000, 0.9659258262890683122, 1.000000000000000000, 0.9659258262890683122, 1.000000000000000000, 0.9659258262890683122, 1.000000000000000000, 0.9659258262890683122, 1.000000000000000000, 0.9659258262890683122, 1.000000000000000000, 0.9659258262890683122, 1.000000000000000000, 0.9659258262890683122, 1.000000000000000000, 0.9659258262890683122, 1.000000000000000000, 0.9659258262890683122, 1.000000000000000000, 0.9659258262890683122, 1.000000000000000000, 0.9659258262890683122, 1.000000000000000000, 0.9659258262890683122, 1.000000000000000000, 0.9659258262890683122, 1.000000000000000000, 0.9659258262890683122, 1.000000000000000000, 0.9659258262890683122, 1.000000000000000000, 0.9659258262890683122, 1.000000000000000000, 0.9659258262890683122, 1.000000000000000000, 0.9659258262890683122, 1.000000000000000000, 0.9659258262890683122, 1.000000000000000000, 0.9659258262890683122, 1.000000000000000000, 0.9659258262890683122, 1.000000000000000000, 0.9659258262890683122, 1.000000000000000000, 0.9659258262890683122, 1.000000000000000000, 0.9659258262890683122, 1.000000000000000000, 0.9659258262890683122, 1.000000000000000000, 0.9659258262890683122, 1.000000000000000000, 0.9659258262890683122, 1.000000000000000000, 0.9659258262890683122, 1.000000000000000000, 0.9659258262890683122, 1.000000000000000000, 0.9659258262890683122, 1.000000000000000000, 0.9659258262890683122, 1.000000000000000000, 0.9659258262890683122, 1.000000000000000000, 0.9659258262890683122, 1.000000000000000000, 0.9659258262890683122, 1.000000000000000000, 0.9659258262890683122, 1.000000000000000000, 0.9659258262890683122, 1.000000000000000000, 0.9659258262890683122, 1.000000000000000000, 0.9659258262890683122, 1.000000000000000000, 0.9659258262890683122, 1.000000000000000000, 0.9659258262890683122, 1.000000000000000000, 0.9659258262890683122, 1.000000000000000000, 0.9659258262890683122, 1.000000000000000000, 0.9659258262890683122, 1.000000000000000000, 0.9659258262890683122, 1.000000000000000000, 0.9659258262890683122, 1.000000000000000000, 0.9659258262890683122, 1.000000000000000000, 0.9659258262890683122, 1.000000000000000000, 0.9659258262890683122, 1.000000000000000000, 0.9659258262890683122, 1.000000000000000000, 0.9659258262890683122, 1.000000000000000000, 0.9659258262890683122, 1.000000000000000000, 0.9659258262890683122, 1.000000000000000000, 0.9659258262890683122, 1.000000000000000000, 0.9659258262890683122, 1.000000000000000000, 0.9659258262890683122, 1.000000000000000000, 0.9659258262890683122, 1.000000000000000000, 0.9659258262890683122, 1.000000000000000000, 0.9659258262890683122, 1.000000000000000000, 0.9659258262890683122, 1.000000000000000000, 0.9659258262890683122, 1.000000000000000000, 0.9659258262890683122, 1.000000000000000000, 0.9659258262890683122, 1.000000000000000000, 0.9659258262890683122, 1.000000000000000000, 0.9659258262890683122, 1.000000000000000000, 0.9659258262890683122, 1.000000000000000000, 0.9659258262890683122, 1.000000000000000000, 0.9659258262890683122, 1.000000000000000000, 0.9659258262890683122, 1.000000000000000000, 0.9659258262890683122, 1.000000000000000000, 0.9659258262890683122, 1.000000000000000000, 0.9659258262890683122, 1.000000000000000000, 0.9659258262890683122, 1.000000000000000000, 0.9659258262890683122, 1.000000000000000000, 0.9659258262890683122, 1.000000000000000000, 0.9659258262890683122, 1.000000000000000000, 0.9659258262890683122, 1.000000000000000000, 0.9659258262890683122, 1.000000000000000000, 0.9659258262890683122, 1.000000000000000000),
 ( 1.000000000000000000, 0.9659258262890683122, 1.000000000000000000, 0.9659258262890683122, 1.000000000000000000, 0.9659258262890683122, 1.000000000000000000, 0.9659258262890683122, 1.000000000000000000, 0.9659258262890683122, 1.000000000000000000, 0.9659258262890683122, 1.000000000000000000, 0.9659258262890683122, 1.000000000000000000, 0.9659258262890683122, 1.000000000000000000, 0.9659258262890683122, 1.000000000000000000, 0.9659258262890683122, 1.000000000000000000, 0.9659258262890683122, 1.000000000000000000, 0.9659258262890683122, 1.000000000000000000, 0.9659258262890683122, 1.000000000000000000, 0.9659258262890683122, 1.000000000000000000, 0.9659258262890683122, 1.000000000000000000, 0.9659258262890683122, 1.000000000000000000, 0.9659258262890683122, 1.000000000000000000, 0.9659258262890683122, 1.000000000000000000, 0.9659258262890683122, 1.000000000000000000, 0.9659258262890683122, 1.000000000000000000, 0.9659258262890683122, 1.000000000000000000, 0.9659258262890683122, 1.000000000000000000, 0.9659258262890683122, 1.000000000000000000, 0.9659258262890683122, 1.000000000000000000, 0.9659258262890683122, 1.000000000000000000, 0.9659258262890683122, 1.000000000000000000, 0.9659258262890683122, 1.000000000000000000, 0.9659258262890683122, 1.000000000000000000, 0.9659258262890683122, 1.000000000000000000, 0.9659258262890683122, 1.000000000000000000, 0.9659258262890683122, 1.000000000000000000, 0.9659258262890683122, 1.000000000000000000, 0.9659258262890683122, 1.000000000000000000, 0.9659258262890683122, 1.000000000000000000, 0.9659258262890683122, 1.000000000000000000, 0.9659258262890683122, 1.000000000000000000, 0.9659258262890683122, 1.000000000000000000, 0.9659258262890683122, 1.000000000000000000, 0.9659258262890683122, 1.000000000000000000, 0.9659258262890683122, 1.000000000000000000, 0.9659258262890683122, 1.000000000000000000, 0.9659258262890683122, 1.000000000000000000, 0.9659258262890683122, 1.000000000000000000, 0.9659258262890683122, 1.000000000000000000, 0.9659258262890683122, 1.000000000000000000, 0.9659258262890683122, 1.000000000000000000, 0.9659258262890683122, 1.000000000000000000, 0.9659258262890683122, 1.000000000000000000, 0.9659258262890683122, 1.000000000000000000, 0.9659258262890683122, 1.000000000000000000, 0.9659258262890683122, 1.000000000000000000, 0.9659258262890683122, 1.000000000000000000, 0.9659258262890683122, 1.000000000000000000, 0.9659258262890683122, 1.000000000000000000, 0.9659258262890683122, 1.000000000000000000, 0.9659258262890683122, 1.000000000000000000, 0.9659258262890683122, 1.000000000000000000, 0.9659258262890683122, 1.000000000000000000, 0.9659258262890683122, 1.000000000000000000, 0.9659258262890683122, 1.000000000000000000, 0.9659258262890683122, 1.000000000000000000, 0.9659258262890683122, 1.000000000000000000, 0.9659258262890683122, 1.000000000000000000, 0.9659258262890683122, 1.000000000000000000, 0.9659258262890683122, 1.000000000000000000, 0.9659258262890683122, 1.000000000000000000, 0.9659258262890683122, 1.000000000000000000, 0.9659258262890683122, 1.000000000000000000, 0.9659258262890683122, 1.000000000000000000, 0.9659258262890683122, 1.000000000000000000, 0.9659258262890683122, 1.000000000000000000, 0.9659258262890683122, 1.000000000000000000, 0.9659258262890683122, 1.000000000000000000, 0.9659258262890683122, 1.000000000000000000, 0.9659258262890683122, 1.000000000000000000, 0.9659258262890683122, 1.000000000000000000, 0.9659258262890683122, 1.000000000000000000, 0.9659258262890683122, 1.000000000000000000, 0.9659258262890683122, 1.000000000000000000, 0.9659258262890683122, 1.000000000000000000, 0.9659258262890683122, 1.000000000000000000, 0.9659258262890683122, 1.000000000000000000, 0.9659258262890683122, 1.000000000000000000, 0.9659258262890683122, 1.000000000000000000, 0.9659258262890683122, 1.000000000000000000, 0.9659258262890683122, 1.000000000000000000, 0.9659258262890683122, 1.000000000000000000, 0.9659258262890683122, 1.000000000000000000, 0.9659258262890683122, 1.000000000000000000, 0.9659258262890683122, 1.000000000000000000, 0.9659258262890683122, 1.000000000000000000, 0.9659258262890683122, 1.000000000000000000, 0.9659258262890683122, 1.000000000000000000, 0.9659258262890683122, 1.000000000000000000, 0.9659258262890683122, 1.000000000000000000, 0.9659258262890683122, 1.000000000000000000, 0.9659258262890683122, 1.000000000000000000, 0.9659258262890683122, 1.000000000000000000, 0.9659258262890683122, 1.000000000000000000, 0.9659258262890683122, 1.000000000000000000, 0.9659258262890683122, 1.000000000000000000, 0.9659258262890683122, 1.000000000000000000, 0.9659258262890683122, 1.000000000000000000, 0.9659258262890683122, 1.000000000000000000, 0.9659258262890683122, 1.000000000000000000, 0.9659258262890683122, 1.000000000000000000, 0.9659258262890683122, 1.000000000000000000, 0.9659258262890683122, 1.000000000000000000, 0.9659258262890683122, 1.000000000000000000, 0.9659258262890683122, 1.000000000000000000, 0.9659258262890683122, 1.000000000000000000, 0.9659258262890683122, 1.000000000000000000, 0.9659258262890683122, 1.000000000000000000, 0.9659258262890683122, 1.000000000000000000, 0.9659258262890683122, 1.000000000000000000, 0.9659258262890683122, 1.000000000000000000, 0.9659258262890683122, 1.000000000000000000, 0.9659258262890683122, 1.000000000000000000, 0.9659258262890683122, 1.000000000000000000, 0.9659258262890683122, 1.000000000000000000, 0.9659258262890683122, 1.000000000000000000, 0.9659258262890683122, 1.000000000000000000, 0.9659258262890683122, 1.000000000000000000, 0.9659258262890683122, 1.000000000000000000, 0.9659258262890683122, 1.000000000000000000, 0.9659258262890683122, 1.000000000000000000, 0.9659258262890683122, 1.000000000000000000, 0.9659258262890683122, 1.000000000000000000, 0.9659258262890683122, 1.000000000000000000, 0.9659258262890683122, 1.000000000000000000, 0.9659258262890683122, 1.000000000000000000, 0.9659258262890683122, 1.000000000000000000, 0.9659258262890683122, 1.000000000000000000, 0.9659258262890683122, 1.000000000000000000, 0.9659258262890683122, 1.000000000000000000, 0.9659258262890683122, 1.000000000000000000, 0.9659258262890683122, 1.000000000000000000, 0.9659258262890683122, 1.000000000000000000, 0.9659258262890683122, 1.000000000000000000, 0.9659258262890683122, 1.000000000000000000, 0.9659258262890683122, 1.000000000000000000, 0.9659258262890683122, 1.000000000000000000, 0.9659258262890683122, 1.000000000000000000, 0.9659258262890683122, 1.000000000000000000, 0.9659258262890683122, 1.000000000000000000, 0.9659258262890683122, 1.000000000000000000, 0.9659258262890683122, 1.000000000000000000, 0.9659258262890683122, 1.000000000000000000, 0.9659258262890683122, 1.000000000000000000, 0.9659258262890683122, 1.000000000000000000, 0.9659258262890683122, 1.000000000000000000, 0.9659258262890683122, 1.000000000000000000, 0.9659258262890683122, 1.000000000000000000, 0.9659258262890683122, 1.000000000000000000, 0.9659258262890683122, 1.000000000000000000, 0.9659258262890683122, 1.000000000000000000, 0.9659258262890683122, 1.000000000000000000, 0.9659258262890683122, 1.000000000000000000, 0.9659258262890683122, 1.000000000000000000, 0.9659258262890683122, 1.000000000000000000, 0.9659258262890683122, 1.000000000000000000, 0.9659258262890683122, 1.000000000000000000) ) ) 
 REPRESENTATION_ITEM ( '' )  SURFACE ( )  );
#40020=CARTESIAN_POINT ( 'NONE',  ( 22.81628187352647785, 41.62363466993042493, 6.195893100308588602E-16 ) ) ;
#40022=( BOUNDED_SURFACE ( )  B_SPLINE_SURFACE ( 1, 2, ( 
 ( #23551, #17022, #98577, #9010, #46041, #77017, #8531, #69526, #31504, #40512, #11470, #64455, #26464, #49459, #9507, #18486, #56000, #47987, #2035, #64942, #94963, #18002, #55508, #62994, #41002, #47499, #71009, #2531, #56964, #25992, #79965, #32985, #40009, #41988, #87466, #10491, #56487, #34450, #17520, #87953, #86504, #70511, #78002, #48482, #78497, #18981, #32496, #25023, #41503, #10982, #95469, #86008, #93498, #63488, #3983, #10011, #33464, #71502, #71971, #3015, #93991, #94474, #26960, #3494, #78984, #63961, #86975, #57460, #72452, #25514, #48974, #79482, #33952, #42467, #59424, #13438, #58433, #59917, #5467, #58940, #36442, #80954, #27941, #50946, #73439, #89927, #44423, #88452, #34945, #81440, #11963, #49960, #73939, #88948, #51441, #35939, #19953, #43925, #97956, #66435, #12942, #50447, #43438, #29412, #80464, #12452, #42958, #4965, #95968, #51940, #20953, #27452, #96970, #67435, #66935, #19469, #97456, #28442, #20455, #72950, #4478, #65444, #74928, #57945, #89440, #81930, #74423, #5951, #28921, #35446, #65942, #21442, #82424, #6427, #36939, #96469, #13949, #91407, #6934, #76892, #22934, #53402, #98947, #23914, #14940, #30402, #37441, #61392, #39406, #84896, #52425, #91902, #60905, #82924, #45919, #8890, #77377, #90909, #52908, #23427, #83911, #54382, #38420, #22437, #53906, #84414, #46402, #1419, #76407, #29908, #922, #7923, #83421, #69400, #16407, #67932, #15912, #14442, #45409, #60414, #8406, #38913, #31384, #61884, #98452, #75914, #44912, #68424, #75419, #7438, #92389, #15439, #37935, #68919, #46886, #447, #69899, #31872, #30898, #90405, #21947, #24409, #18863, #70393, #54875, #62371, #26348, #92875, #39890, #33347, #71385, #79360, #1912, #24900, #55384, #17878, #64336, #49344, #47866, #32865, #86376, #78867, #79845, #85386, #3367, #11348, #3864, #70889, #48361, #33829, #85884, #56849, #10867, #41389, #94847, #16899, #63842, #2407, #62875, #47376, #41868, #71856, #63364, #32370, #77874, #55878, #9385, #17397, #78371, #87348, #40879, #72331, #9890, #93372, #40393, #93866, #25393, #2898, #10377, #94355, #25873, #56373, #86864, #18370, #48851, #65319, #74299, #87830, #11840, #28321, #96846, #51812, #72824, #19348, #19832, #89802, #49830, #20335, #27821, #58812, #96350, #42347, #81324, #82299, #89321, #65816, #58307, #88823, #5345, #51318, #74805, #13319, #64823, #43317, #21322, #50831, #59305, #12819, #50319, #73811, #81801, #4362, #35823, #4846, #80834, #66309, #26839, #20829, #12334, #13821, #57826, #42838, #34828, #43805, #35321, #95844, #5825, #36319, #66812, #97334, #44302, #34326, #28807, #95340, #57333 ),
 ( #27329, #88334, #80342, #73322, #70641, #54628, #8171, #39659, #1669, #62617, #17648, #62127, #46167, #17156, #92636, #38663, #85638, #2167, #84175, #70151, #197, #690, #76651, #32122, #77626, #9142, #47637, #23181, #61634, #61155, #84652, #30647, #69166, #78132, #16160, #31144, #92154, #93126, #25158, #9641, #32624, #39162, #40140, #23679, #91664, #63122, #24652, #46642, #48118, #24160, #47128, #55122, #54143, #77141, #69652, #8650, #93625, #55634, #1177, #53658, #31635, #15682, #36818, #85147, #16654, #86135, #6311, #67310, #72581, #58072, #64581, #72097, #48610, #41631, #88576, #40636, #79113, #10627, #3134, #56132, #12092, #80094, #86624, #95090, #27579, #27083, #20085, #57585, #26598, #79611, #10141, #71134, #2662, #4610, #18137, #57095, #19101, #11597, #49582, #4113, #25640, #63607, #87591, #34578, #65571, #35071, #78631, #33112, #11112, #94113, #65072, #3622, #34090, #87104, #42595, #33595, #42117, #41138, #95597, #26123, #71625, #64093, #94606, #56615, #88082, #19592, #18619, #50090, #80595, #73074, #96098, #49109, #7071, #14080, #20587, #6564, #44560, #35579, #44058, #52072, #12582, #37573, #58573, #43081, #50587, #14579, #81079, #28075, #21582, #59563, #67573, #89074, #13073, #43566, #6079, #52554, #68065, #36073, #21080, #74565, #67067, #98593, #73566, #90549, #30042, #91042, #59064, #36580, #22079, #74062, #45047, #98085, #29543, #83058, #5091, #82566, #89569, #51074, #66069, #60551, #60049, #51576, #81566, #96597, #97595, #5594, #66575, #97102, #75557, #29057, #28573, #82065, #13573, #90058, #75058, #37076, #1055, #9520, #91548, #63007, #31027, #15079, #22570, #92035, #53536, #62506, #76048, #89, #16543, #85029, #40020, #61036, #7578, #8054, #78015, #38066, #8544, #16041, #47017, #84542, #30536, #69539, #70524, #77509, #54032, #46529, #77032, #92519, #39542, #53041, #1555, #83557, #31522, #2047, #39044, #47515, #62018, #38553, #24044, #70031, #23067, #54515, #23564, #69048, #32509, #17036, #45550, #9026, #61526, #68557, #32002, #84050, #15570, #46051, #76538, #93011, #24546, #85523, #55006, #582, #26479, #87480, #49471, #4492, #48988, #33001, #3999, #79496, #25525, #72466, #87965, #71021, #56975, #86018, #86515, #63502, #18994, #64469, #94976, #34463, #10023, #48495, #47999, #71518, #17532, #94002, #64955, #3028, #56015, #78997, #79978, #11976, #95482, #19479, #26005, #26973, #18013, #78508, #57471, #11481, #33477, #34957, #10995, #33965, #42001, #10502, #63973, #56499, #41016, #49971, #80477, #94486, #40523, #86990, #2544, #25036, #41515, #18497, #42478, #71982, #3506, #72961, #93510, #55521, #58951 ) ),
 .UNSPECIFIED., .F., .F., .F. ) 
 B_SPLINE_SURFACE_WITH_KNOTS ( ( 2, 2 ),
 ( 3, 2, 2, 2, 2, 2, 2, 2, 2, 2, 2, 2, 2, 2, 2, 2, 2, 2, 2, 2, 2, 2, 2, 2, 2, 2, 2, 2, 2, 2, 2, 2, 2, 2, 2, 2, 2, 2, 2, 2, 2, 2, 2, 2, 2, 2, 2, 2, 2, 2, 2, 2, 2, 2, 2, 2, 2, 2, 2, 2, 2, 2, 2, 2, 2, 2, 2, 2, 2, 2, 2, 2, 2, 2, 2, 2, 2, 2, 2, 2, 2, 2, 2, 2, 2, 2, 2, 2, 2, 2, 2, 2, 2, 2, 2, 2, 2, 2, 2, 2, 2, 2, 2, 2, 2, 2, 2, 2, 2, 2, 2, 2, 2, 2, 2, 2, 2, 2, 2, 2, 2, 2, 2, 2, 2, 2, 2, 2, 2, 2, 2, 2, 2, 2, 2, 2, 2, 2, 2, 2, 2, 2, 2, 2, 2, 2, 2, 2, 2, 2, 2, 2, 2, 2, 2, 2, 2, 2, 2, 2, 2, 2, 3 ),
 ( 0.000000000000000000, 1.000000000000000000 ),
 ( 0.000000000000000000, 0.005952380952380952051, 0.01190476190476190410, 0.01785714285714285615, 0.02380952380952380820, 0.02976190476190476025, 0.03571428571428571230, 0.04166666666666666435, 0.04761904761904761640, 0.05357142857142856845, 0.05952380952380952051, 0.06547619047619047949, 0.07142857142857142461, 0.07738095238095238360, 0.08333333333333332871, 0.08928571428571428770, 0.09523809523809523281, 0.1011904761904761918, 0.1071428571428571369, 0.1130952380952380959, 0.1190476190476190410, 0.1250000000000000000, 0.1309523809523809590, 0.1369047619047619180, 0.1428571428571428492, 0.1488095238095238082, 0.1547619047619047672, 0.1607142857142857262, 0.1666666666666666574, 0.1726190476190476164, 0.1785714285714285754, 0.1845238095238095344, 0.1904761904761904656, 0.1964285714285714246, 0.2023809523809523836, 0.2083333333333333426, 0.2142857142857142738, 0.2202380952380952328, 0.2261904761904761918, 0.2321428571428571508, 0.2380952380952380820, 0.2440476190476190410, 0.2500000000000000000, 0.2559523809523809312, 0.2619047619047619180, 0.2678571428571428492, 0.2738095238095238360, 0.2797619047619047672, 0.2857142857142856984, 0.2916666666666666852, 0.2976190476190476164, 0.3035714285714285476, 0.3095238095238095344, 0.3154761904761904656, 0.3214285714285714524, 0.3273809523809523836, 0.3333333333333333148, 0.3392857142857143016, 0.3452380952380952328, 0.3511904761904761640, 0.3571428571428571508, 0.3630952380952380820, 0.3690476190476190688, 0.3750000000000000000, 0.3809523809523809312, 0.3869047619047619180, 0.3928571428571428492, 0.3988095238095238360, 0.4047619047619047672, 0.4107142857142856984, 0.4166666666666666852, 0.4226190476190476164, 0.4285714285714285476, 0.4345238095238095344, 0.4404761904761904656, 0.4464285714285714524, 0.4523809523809523836, 0.4583333333333333148, 0.4642857142857143016, 0.4702380952380952328, 0.4761904761904761640, 0.4821428571428571508, 0.4880952380952380820, 0.4940476190476190688, 0.5000000000000000000, 0.5059523809523809312, 0.5119047619047618625, 0.5178571428571429047, 0.5238095238095238360, 0.5297619047619047672, 0.5357142857142856984, 0.5416666666666666297, 0.5476190476190476719, 0.5535714285714286031, 0.5595238095238095344, 0.5654761904761904656, 0.5714285714285713969, 0.5773809523809523281, 0.5833333333333333703, 0.5892857142857143016, 0.5952380952380952328, 0.6011904761904761640, 0.6071428571428570953, 0.6130952380952381375, 0.6190476190476190688, 0.6250000000000000000, 0.6309523809523809312, 0.6369047619047618625, 0.6428571428571429047, 0.6488095238095238360, 0.6547619047619047672, 0.6607142857142856984, 0.6666666666666666297, 0.6726190476190476719, 0.6785714285714286031, 0.6845238095238095344, 0.6904761904761904656, 0.6964285714285713969, 0.7023809523809523281, 0.7083333333333333703, 0.7142857142857143016, 0.7202380952380952328, 0.7261904761904761640, 0.7321428571428570953, 0.7380952380952381375, 0.7440476190476190688, 0.7500000000000000000, 0.7559523809523809312, 0.7619047619047618625, 0.7678571428571429047, 0.7738095238095238360, 0.7797619047619047672, 0.7857142857142856984, 0.7916666666666666297, 0.7976190476190476719, 0.8035714285714286031, 0.8095238095238095344, 0.8154761904761904656, 0.8214285714285713969, 0.8273809523809523281, 0.8333333333333333703, 0.8392857142857143016, 0.8452380952380952328, 0.8511904761904761640, 0.8571428571428570953, 0.8630952380952381375, 0.8690476190476190688, 0.8750000000000000000, 0.8809523809523809312, 0.8869047619047618625, 0.8928571428571429047, 0.8988095238095238360, 0.9047619047619047672, 0.9107142857142856984, 0.9166666666666666297, 0.9226190476190476719, 0.9285714285714286031, 0.9345238095238095344, 0.9404761904761904656, 0.9464285714285713969, 0.9523809523809523281, 0.9583333333333333703, 0.9642857142857143016 ),
 .UNSPECIFIED. ) 
 GEOMETRIC_REPRESENTATION_ITEM ( )  RATIONAL_B_SPLINE_SURFACE ( (
 ( 1.000000000000000000, 0.9659258262890683122, 1.000000000000000000, 0.9659258262890683122, 1.000000000000000000, 0.9659258262890683122, 1.000000000000000000, 0.9659258262890683122, 1.000000000000000000, 0.9659258262890683122, 1.000000000000000000, 0.9659258262890683122, 1.000000000000000000, 0.9659258262890683122, 1.000000000000000000, 0.9659258262890683122, 1.000000000000000000, 0.9659258262890683122, 1.000000000000000000, 0.9659258262890683122, 1.000000000000000000, 0.9659258262890683122, 1.000000000000000000, 0.9659258262890683122, 1.000000000000000000, 0.9659258262890683122, 1.000000000000000000, 0.9659258262890683122, 1.000000000000000000, 0.9659258262890683122, 1.000000000000000000, 0.9659258262890683122, 1.000000000000000000, 0.9659258262890683122, 1.000000000000000000, 0.9659258262890683122, 1.000000000000000000, 0.9659258262890683122, 1.000000000000000000, 0.9659258262890683122, 1.000000000000000000, 0.9659258262890683122, 1.000000000000000000, 0.9659258262890683122, 1.000000000000000000, 0.9659258262890683122, 1.000000000000000000, 0.9659258262890683122, 1.000000000000000000, 0.9659258262890683122, 1.000000000000000000, 0.9659258262890683122, 1.000000000000000000, 0.9659258262890683122, 1.000000000000000000, 0.9659258262890683122, 1.000000000000000000, 0.9659258262890683122, 1.000000000000000000, 0.9659258262890683122, 1.000000000000000000, 0.9659258262890683122, 1.000000000000000000, 0.9659258262890683122, 1.000000000000000000, 0.9659258262890683122, 1.000000000000000000, 0.9659258262890683122, 1.000000000000000000, 0.9659258262890683122, 1.000000000000000000, 0.9659258262890683122, 1.000000000000000000, 0.9659258262890683122, 1.000000000000000000, 0.9659258262890683122, 1.000000000000000000, 0.9659258262890683122, 1.000000000000000000, 0.9659258262890683122, 1.000000000000000000, 0.9659258262890683122, 1.000000000000000000, 0.9659258262890683122, 1.000000000000000000, 0.9659258262890683122, 1.000000000000000000, 0.9659258262890683122, 1.000000000000000000, 0.9659258262890683122, 1.000000000000000000, 0.9659258262890683122, 1.000000000000000000, 0.9659258262890683122, 1.000000000000000000, 0.9659258262890683122, 1.000000000000000000, 0.9659258262890683122, 1.000000000000000000, 0.9659258262890683122, 1.000000000000000000, 0.9659258262890683122, 1.000000000000000000, 0.9659258262890683122, 1.000000000000000000, 0.9659258262890683122, 1.000000000000000000, 0.9659258262890683122, 1.000000000000000000, 0.9659258262890683122, 1.000000000000000000, 0.9659258262890683122, 1.000000000000000000, 0.9659258262890683122, 1.000000000000000000, 0.9659258262890683122, 1.000000000000000000, 0.9659258262890683122, 1.000000000000000000, 0.9659258262890683122, 1.000000000000000000, 0.9659258262890683122, 1.000000000000000000, 0.9659258262890683122, 1.000000000000000000, 0.9659258262890683122, 1.000000000000000000, 0.9659258262890683122, 1.000000000000000000, 0.9659258262890683122, 1.000000000000000000, 0.9659258262890683122, 1.000000000000000000, 0.9659258262890683122, 1.000000000000000000, 0.9659258262890683122, 1.000000000000000000, 0.9659258262890683122, 1.000000000000000000, 0.9659258262890683122, 1.000000000000000000, 0.9659258262890683122, 1.000000000000000000, 0.9659258262890683122, 1.000000000000000000, 0.9659258262890683122, 1.000000000000000000, 0.9659258262890683122, 1.000000000000000000, 0.9659258262890683122, 1.000000000000000000, 0.9659258262890683122, 1.000000000000000000, 0.9659258262890683122, 1.000000000000000000, 0.9659258262890683122, 1.000000000000000000, 0.9659258262890683122, 1.000000000000000000, 0.9659258262890683122, 1.000000000000000000, 0.9659258262890683122, 1.000000000000000000, 0.9659258262890683122, 1.000000000000000000, 0.9659258262890683122, 1.000000000000000000, 0.9659258262890683122, 1.000000000000000000, 0.9659258262890683122, 1.000000000000000000, 0.9659258262890683122, 1.000000000000000000, 0.9659258262890683122, 1.000000000000000000, 0.9659258262890683122, 1.000000000000000000, 0.9659258262890683122, 1.000000000000000000, 0.9659258262890683122, 1.000000000000000000, 0.9659258262890683122, 1.000000000000000000, 0.9659258262890683122, 1.000000000000000000, 0.9659258262890683122, 1.000000000000000000, 0.9659258262890683122, 1.000000000000000000, 0.9659258262890683122, 1.000000000000000000, 0.9659258262890683122, 1.000000000000000000, 0.9659258262890683122, 1.000000000000000000, 0.9659258262890683122, 1.000000000000000000, 0.9659258262890683122, 1.000000000000000000, 0.9659258262890683122, 1.000000000000000000, 0.9659258262890683122, 1.000000000000000000, 0.9659258262890683122, 1.000000000000000000, 0.9659258262890683122, 1.000000000000000000, 0.9659258262890683122, 1.000000000000000000, 0.9659258262890683122, 1.000000000000000000, 0.9659258262890683122, 1.000000000000000000, 0.9659258262890683122, 1.000000000000000000, 0.9659258262890683122, 1.000000000000000000, 0.9659258262890683122, 1.000000000000000000, 0.9659258262890683122, 1.000000000000000000, 0.9659258262890683122, 1.000000000000000000, 0.9659258262890683122, 1.000000000000000000, 0.9659258262890683122, 1.000000000000000000, 0.9659258262890683122, 1.000000000000000000, 0.9659258262890683122, 1.000000000000000000, 0.9659258262890683122, 1.000000000000000000, 0.9659258262890683122, 1.000000000000000000, 0.9659258262890683122, 1.000000000000000000, 0.9659258262890683122, 1.000000000000000000, 0.9659258262890683122, 1.000000000000000000, 0.9659258262890683122, 1.000000000000000000, 0.9659258262890683122, 1.000000000000000000, 0.9659258262890683122, 1.000000000000000000, 0.9659258262890683122, 1.000000000000000000, 0.9659258262890683122, 1.000000000000000000, 0.9659258262890683122, 1.000000000000000000, 0.9659258262890683122, 1.000000000000000000, 0.9659258262890683122, 1.000000000000000000, 0.9659258262890683122, 1.000000000000000000, 0.9659258262890683122, 1.000000000000000000, 0.9659258262890683122, 1.000000000000000000, 0.9659258262890683122, 1.000000000000000000, 0.9659258262890683122, 1.000000000000000000, 0.9659258262890683122, 1.000000000000000000, 0.9659258262890683122, 1.000000000000000000, 0.9659258262890683122, 1.000000000000000000, 0.9659258262890683122, 1.000000000000000000, 0.9659258262890683122, 1.000000000000000000, 0.9659258262890683122, 1.000000000000000000, 0.9659258262890683122, 1.000000000000000000, 0.9659258262890683122, 1.000000000000000000, 0.9659258262890683122, 1.000000000000000000, 0.9659258262890683122, 1.000000000000000000, 0.9659258262890683122, 1.000000000000000000, 0.9659258262890683122, 1.000000000000000000, 0.9659258262890683122, 1.000000000000000000, 0.9659258262890683122, 1.000000000000000000, 0.9659258262890683122, 1.000000000000000000, 0.9659258262890683122, 1.000000000000000000, 0.9659258262890683122, 1.000000000000000000, 0.9659258262890683122, 1.000000000000000000, 0.9659258262890683122, 1.000000000000000000, 0.9659258262890683122, 1.000000000000000000, 0.9659258262890683122, 1.000000000000000000, 0.9659258262890683122, 1.000000000000000000, 0.9659258262890683122, 1.000000000000000000, 0.9659258262890683122, 1.000000000000000000, 0.9659258262890683122, 1.000000000000000000, 0.9659258262890683122, 1.000000000000000000, 0.9659258262890683122, 1.000000000000000000, 0.9659258262890683122, 1.000000000000000000, 0.9659258262890683122, 1.000000000000000000),
 ( 1.000000000000000000, 0.9659258262890683122, 1.000000000000000000, 0.9659258262890683122, 1.000000000000000000, 0.9659258262890683122, 1.000000000000000000, 0.9659258262890683122, 1.000000000000000000, 0.9659258262890683122, 1.000000000000000000, 0.9659258262890683122, 1.000000000000000000, 0.9659258262890683122, 1.000000000000000000, 0.9659258262890683122, 1.000000000000000000, 0.9659258262890683122, 1.000000000000000000, 0.9659258262890683122, 1.000000000000000000, 0.9659258262890683122, 1.000000000000000000, 0.9659258262890683122, 1.000000000000000000, 0.9659258262890683122, 1.000000000000000000, 0.9659258262890683122, 1.000000000000000000, 0.9659258262890683122, 1.000000000000000000, 0.9659258262890683122, 1.000000000000000000, 0.9659258262890683122, 1.000000000000000000, 0.9659258262890683122, 1.000000000000000000, 0.9659258262890683122, 1.000000000000000000, 0.9659258262890683122, 1.000000000000000000, 0.9659258262890683122, 1.000000000000000000, 0.9659258262890683122, 1.000000000000000000, 0.9659258262890683122, 1.000000000000000000, 0.9659258262890683122, 1.000000000000000000, 0.9659258262890683122, 1.000000000000000000, 0.9659258262890683122, 1.000000000000000000, 0.9659258262890683122, 1.000000000000000000, 0.9659258262890683122, 1.000000000000000000, 0.9659258262890683122, 1.000000000000000000, 0.9659258262890683122, 1.000000000000000000, 0.9659258262890683122, 1.000000000000000000, 0.9659258262890683122, 1.000000000000000000, 0.9659258262890683122, 1.000000000000000000, 0.9659258262890683122, 1.000000000000000000, 0.9659258262890683122, 1.000000000000000000, 0.9659258262890683122, 1.000000000000000000, 0.9659258262890683122, 1.000000000000000000, 0.9659258262890683122, 1.000000000000000000, 0.9659258262890683122, 1.000000000000000000, 0.9659258262890683122, 1.000000000000000000, 0.9659258262890683122, 1.000000000000000000, 0.9659258262890683122, 1.000000000000000000, 0.9659258262890683122, 1.000000000000000000, 0.9659258262890683122, 1.000000000000000000, 0.9659258262890683122, 1.000000000000000000, 0.9659258262890683122, 1.000000000000000000, 0.9659258262890683122, 1.000000000000000000, 0.9659258262890683122, 1.000000000000000000, 0.9659258262890683122, 1.000000000000000000, 0.9659258262890683122, 1.000000000000000000, 0.9659258262890683122, 1.000000000000000000, 0.9659258262890683122, 1.000000000000000000, 0.9659258262890683122, 1.000000000000000000, 0.9659258262890683122, 1.000000000000000000, 0.9659258262890683122, 1.000000000000000000, 0.9659258262890683122, 1.000000000000000000, 0.9659258262890683122, 1.000000000000000000, 0.9659258262890683122, 1.000000000000000000, 0.9659258262890683122, 1.000000000000000000, 0.9659258262890683122, 1.000000000000000000, 0.9659258262890683122, 1.000000000000000000, 0.9659258262890683122, 1.000000000000000000, 0.9659258262890683122, 1.000000000000000000, 0.9659258262890683122, 1.000000000000000000, 0.9659258262890683122, 1.000000000000000000, 0.9659258262890683122, 1.000000000000000000, 0.9659258262890683122, 1.000000000000000000, 0.9659258262890683122, 1.000000000000000000, 0.9659258262890683122, 1.000000000000000000, 0.9659258262890683122, 1.000000000000000000, 0.9659258262890683122, 1.000000000000000000, 0.9659258262890683122, 1.000000000000000000, 0.9659258262890683122, 1.000000000000000000, 0.9659258262890683122, 1.000000000000000000, 0.9659258262890683122, 1.000000000000000000, 0.9659258262890683122, 1.000000000000000000, 0.9659258262890683122, 1.000000000000000000, 0.9659258262890683122, 1.000000000000000000, 0.9659258262890683122, 1.000000000000000000, 0.9659258262890683122, 1.000000000000000000, 0.9659258262890683122, 1.000000000000000000, 0.9659258262890683122, 1.000000000000000000, 0.9659258262890683122, 1.000000000000000000, 0.9659258262890683122, 1.000000000000000000, 0.9659258262890683122, 1.000000000000000000, 0.9659258262890683122, 1.000000000000000000, 0.9659258262890683122, 1.000000000000000000, 0.9659258262890683122, 1.000000000000000000, 0.9659258262890683122, 1.000000000000000000, 0.9659258262890683122, 1.000000000000000000, 0.9659258262890683122, 1.000000000000000000, 0.9659258262890683122, 1.000000000000000000, 0.9659258262890683122, 1.000000000000000000, 0.9659258262890683122, 1.000000000000000000, 0.9659258262890683122, 1.000000000000000000, 0.9659258262890683122, 1.000000000000000000, 0.9659258262890683122, 1.000000000000000000, 0.9659258262890683122, 1.000000000000000000, 0.9659258262890683122, 1.000000000000000000, 0.9659258262890683122, 1.000000000000000000, 0.9659258262890683122, 1.000000000000000000, 0.9659258262890683122, 1.000000000000000000, 0.9659258262890683122, 1.000000000000000000, 0.9659258262890683122, 1.000000000000000000, 0.9659258262890683122, 1.000000000000000000, 0.9659258262890683122, 1.000000000000000000, 0.9659258262890683122, 1.000000000000000000, 0.9659258262890683122, 1.000000000000000000, 0.9659258262890683122, 1.000000000000000000, 0.9659258262890683122, 1.000000000000000000, 0.9659258262890683122, 1.000000000000000000, 0.9659258262890683122, 1.000000000000000000, 0.9659258262890683122, 1.000000000000000000, 0.9659258262890683122, 1.000000000000000000, 0.9659258262890683122, 1.000000000000000000, 0.9659258262890683122, 1.000000000000000000, 0.9659258262890683122, 1.000000000000000000, 0.9659258262890683122, 1.000000000000000000, 0.9659258262890683122, 1.000000000000000000, 0.9659258262890683122, 1.000000000000000000, 0.9659258262890683122, 1.000000000000000000, 0.9659258262890683122, 1.000000000000000000, 0.9659258262890683122, 1.000000000000000000, 0.9659258262890683122, 1.000000000000000000, 0.9659258262890683122, 1.000000000000000000, 0.9659258262890683122, 1.000000000000000000, 0.9659258262890683122, 1.000000000000000000, 0.9659258262890683122, 1.000000000000000000, 0.9659258262890683122, 1.000000000000000000, 0.9659258262890683122, 1.000000000000000000, 0.9659258262890683122, 1.000000000000000000, 0.9659258262890683122, 1.000000000000000000, 0.9659258262890683122, 1.000000000000000000, 0.9659258262890683122, 1.000000000000000000, 0.9659258262890683122, 1.000000000000000000, 0.9659258262890683122, 1.000000000000000000, 0.9659258262890683122, 1.000000000000000000, 0.9659258262890683122, 1.000000000000000000, 0.9659258262890683122, 1.000000000000000000, 0.9659258262890683122, 1.000000000000000000, 0.9659258262890683122, 1.000000000000000000, 0.9659258262890683122, 1.000000000000000000, 0.9659258262890683122, 1.000000000000000000, 0.9659258262890683122, 1.000000000000000000, 0.9659258262890683122, 1.000000000000000000, 0.9659258262890683122, 1.000000000000000000, 0.9659258262890683122, 1.000000000000000000, 0.9659258262890683122, 1.000000000000000000, 0.9659258262890683122, 1.000000000000000000, 0.9659258262890683122, 1.000000000000000000, 0.9659258262890683122, 1.000000000000000000, 0.9659258262890683122, 1.000000000000000000, 0.9659258262890683122, 1.000000000000000000, 0.9659258262890683122, 1.000000000000000000, 0.9659258262890683122, 1.000000000000000000, 0.9659258262890683122, 1.000000000000000000, 0.9659258262890683122, 1.000000000000000000, 0.9659258262890683122, 1.000000000000000000, 0.9659258262890683122, 1.000000000000000000, 0.9659258262890683122, 1.000000000000000000, 0.9659258262890683122, 1.000000000000000000, 0.9659258262890683122, 1.000000000000000000) ) ) 
 REPRESENTATION_ITEM ( '' )  SURFACE ( )  );
#40023=CARTESIAN_POINT ( 'NONE',  ( 10.00000000000000000, 54.75893115100078745, -9.846743663894594434 ) ) ;
#40024=CARTESIAN_POINT ( 'NONE',  ( 17.96484262340118221, 14.93868534415484106, 7.964842623401181321 ) ) ;
#40026=CARTESIAN_POINT ( 'NONE',  ( -0.8801773607111008646, 28.27201867748817321, 2.915334737309923430 ) ) ;
#40028=CARTESIAN_POINT ( 'NONE',  ( 12.63842701281683922, 9.550597817667449974, -9.846743663894590881 ) ) ;
#40030=CARTESIAN_POINT ( 'NONE',  ( 12.91533473730993009, 66.60535201082150536, -10.88017736071109987 ) ) ;
#40032=CARTESIAN_POINT ( 'NONE',  ( 0.1532563361054083140, 6.008931151000784787, 1.131784320476157264E-15 ) ) ;
#40033=CARTESIAN_POINT ( 'NONE',  ( 7.361572987183169658, -0.03273551566588185635, -9.846743663894592657 ) ) ;
#40036=CARTESIAN_POINT ( 'NONE',  ( 10.00000000000000000, 51.81368534415484106, -10.88017736071110342 ) ) ;
#40038=CARTESIAN_POINT ( 'NONE',  ( 0.5774900079438590739, 67.64701867748817676, -5.440088680355550821 ) ) ;
#40039=CARTESIAN_POINT ( 'NONE',  ( 7.361572987183169658, -0.03273551566588185635, -9.846743663894592657 ) ) ;
#40041=CARTESIAN_POINT ( 'NONE',  ( 1.472469842513823179, 61.42559781766745175, 4.923371831947296329 ) ) ;
#40042=ORIENTED_EDGE ( 'NONE', *, *, #87703, .T. ) ;
#40045=CARTESIAN_POINT ( 'NONE',  ( 20.36894250292379738, 9.928748834913966093, -10.36894250292379027 ) ) ;
#40046=CARTESIAN_POINT ( 'NONE',  ( 0.6178305044545838731, 54.74863466993042493, 9.382169495545420901 ) ) ;
#40047=CARTESIAN_POINT ( 'NONE',  ( -2.266590686148945544, 22.22041550158063572, 7.082119434687048631 ) ) ;
#40050=CARTESIAN_POINT ( 'NONE',  ( 0.5774900079438590739, 17.64701867748817321, -5.440088680355550821 ) ) ;
#40053=PRESENTATION_STYLE_ASSIGNMENT (( #25067 ) ) ;
#40054=CARTESIAN_POINT ( 'NONE',  ( 10.00000000000000000, -0.2410688489992152128, -9.846743663894594434 ) ) ;
#40055=CARTESIAN_POINT ( 'NONE',  ( 19.38216949554541557, 27.24863466993041783, -9.382169495545420901 ) ) ;
#40056=CARTESIAN_POINT ( 'NONE',  ( 19.84674366389459266, 43.30059781766744464, 2.638427012816836559 ) ) ;
#40058=CARTESIAN_POINT ( 'NONE',  ( 10.00000000000000000, 17.87363466993041783, -12.81628187352647608 ) ) ;
#40059=DIRECTION ( 'NONE',  ( 1.000000000000000000, 0.000000000000000000, 0.000000000000000000 ) ) ;
#40060=CARTESIAN_POINT ( 'NONE',  ( 10.00000000000000000, 29.75893115100078745, -9.846743663894594434 ) ) ;
#40062=CARTESIAN_POINT ( 'NONE',  ( 0.1532563361054100626, 0.8005978176674514168, -2.638427012816831230 ) ) ;
#40065=CARTESIAN_POINT ( 'NONE',  ( 17.96484262340118221, 31.18868534415483751, -7.964842623401177768 ) ) ;
#40066=CARTESIAN_POINT ( 'NONE',  ( 6.204703633549690345, 27.84541550158063217, 14.16423886937410082 ) ) ;
#40067=CARTESIAN_POINT ( 'NONE',  ( 7.361572987183169658, 44.96726448433412315, -9.846743663894592657 ) ) ;
#40069=CARTESIAN_POINT ( 'NONE',  ( 14.92337183194729633, 17.67559781766745175, 8.527530157486181039 ) ) ;
#40070=CARTESIAN_POINT ( 'NONE',  ( 3.591859063236761518, 54.95696800326376064, 11.09922568453594849 ) ) ;
#40071=DIRECTION ( 'NONE',  ( 1.000000000000000000, 0.000000000000000000, 0.000000000000000000 ) ) ;
#40072=CARTESIAN_POINT ( 'NONE',  ( 20.88017736071110875, 30.77201867748816966, -2.915334737309920765 ) ) ;
#40074=CARTESIAN_POINT ( 'NONE',  ( 0.6178305044545838731, 19.74863466993042138, 9.382169495545420901 ) ) ;
#40075=CARTESIAN_POINT ( 'NONE',  ( 14.92337183194729988, 34.34226448433411605, -8.527530157486177487 ) ) ;
#40077=CARTESIAN_POINT ( 'NONE',  ( 19.38216949554541557, 42.24863466993041783, -9.382169495545420901 ) ) ;
#40079=CARTESIAN_POINT ( 'NONE',  ( 0.5774900079438607392, 58.48035201082151247, 5.440088680355550821 ) ) ;
#40084=CARTESIAN_POINT ( 'NONE',  ( 20.88017736071110875, 50.77201867748817676, -2.915334737309920765 ) ) ;
#40085=CARTESIAN_POINT ( 'NONE',  ( 10.00000000000000178, 64.31368534415483396, 10.88017736071110342 ) ) ;
#40086=DIRECTION ( 'NONE',  ( 0.000000000000000000, 0.000000000000000000, 1.000000000000000000 ) ) ;
#40090=CARTESIAN_POINT ( 'NONE',  ( 0.5774900079438607392, 13.48035201082150358, 5.440088680355550821 ) ) ;
#40091=CARTESIAN_POINT ( 'NONE',  ( 19.84674366389459266, 58.30059781766745886, 2.638427012816836559 ) ) ;
#40092=CARTESIAN_POINT ( 'NONE',  ( 20.88017736071110519, 15.56368534415483751, 2.639326808657452039E-16 ) ) ;
#40093=CARTESIAN_POINT ( 'NONE',  ( 20.15039907845753220, 44.72266099184918176, 6.262539305110078836 ) ) ;
#40095=CARTESIAN_POINT ( 'NONE',  ( 22.81628187352647785, 26.41530133659708923, 3.434112377981063169 ) ) ;
#40097=CARTESIAN_POINT ( 'NONE',  ( 0.5774900079438590739, 52.64701867748817676, -5.440088680355550821 ) ) ;
#40098=CARTESIAN_POINT ( 'NONE',  ( 5.076628168052703671, 36.84226448433412315, 8.527530157486179263 ) ) ;
#40099=CARTESIAN_POINT ( 'NONE',  ( 3.591859063236763294, 13.29030133659708746, -11.09922568453595026 ) ) ;
#40100=CARTESIAN_POINT ( 'NONE',  ( -0.8801773607110991993, 17.85535201082150536, -2.915334737309923874 ) ) ;
#40101=CARTESIAN_POINT ( 'NONE',  ( 12.91533473730993009, 36.60535201082151247, -10.88017736071109987 ) ) ;
#40102=CARTESIAN_POINT ( 'NONE',  ( 2.917880565312950480, 55.97041550158063217, -12.26659068614894821 ) ) ;
#40103=CARTESIAN_POINT ( 'NONE',  ( 2.791683348922237240, 40.38393115100078035, -7.208316651077763204 ) ) ;
#40104=CARTESIAN_POINT ( 'NONE',  ( 12.91533473730993009, 66.60535201082150536, -10.88017736071109987 ) ) ;
#40106=CARTESIAN_POINT ( 'NONE',  ( 6.204703633549690345, 10.76208216824729824, -14.16423886937410259 ) ) ;
#40107=( NAMED_UNIT ( * ) SI_UNIT ( $, .STERADIAN. ) SOLID_ANGLE_UNIT ( ) );
#40110=ORIENTED_EDGE ( 'NONE', *, *, #17867, .T. ) ;
#40111=CARTESIAN_POINT ( 'NONE',  ( 13.79529636645031943, 30.34541550158063927, -14.16423886937409904 ) ) ;
#40112=CARTESIAN_POINT ( 'NONE',  ( 24.16423886937409904, 34.09541550158064638, 3.795296366450317205 ) ) ;
#40113=CARTESIAN_POINT ( 'NONE',  ( 12.63842701281683922, 9.550597817667449974, -9.846743663894590881 ) ) ;
#40115=CARTESIAN_POINT ( 'NONE',  ( 16.40814093676323893, 20.79030133659708923, 11.09922568453595026 ) ) ;
#40116=CARTESIAN_POINT ( 'NONE',  ( 18.52753015748618282, 58.92559781766745886, -4.923371831947291888 ) ) ;
#40118=CARTESIAN_POINT ( 'NONE',  ( 15.44008868035555260, 54.73035201082150536, 9.422509992056143702 ) ) ;
#40119=CARTESIAN_POINT ( 'NONE',  ( 13.43411237798106583, 37.66530133659708923, -12.81628187352647252 ) ) ;
#40120=CARTESIAN_POINT ( 'NONE',  ( 10.00000000000000000, 25.55374883491396787, -14.16423886937410082 ) ) ;
#40121=CARTESIAN_POINT ( 'NONE',  ( 20.88017736071110875, 20.77201867748816611, -2.915334737309920765 ) ) ;
#40123=CARTESIAN_POINT ( 'NONE',  ( 17.96484262340118221, 66.18868534415483396, -7.964842623401177768 ) ) ;
#40126=CARTESIAN_POINT ( 'NONE',  ( 17.20831665107776587, 7.883931151000784787, 7.208316651077764980 ) ) ;
#40131=CIRCLE ( 'NONE', #96014, 11.92686044187656513 ) ;
#40132=CARTESIAN_POINT ( 'NONE',  ( 17.08211943468705130, 3.470415501580634388, 12.26659068614894998 ) ) ;
#40133=CARTESIAN_POINT ( 'NONE',  ( 15.44008868035555260, 9.730352010821505360, 9.422509992056143702 ) ) ;
#40134=CARTESIAN_POINT ( 'NONE',  ( -0.8801773607111008646, 13.27201867748817321, 2.915334737309923430 ) ) ;
#40135=CARTESIAN_POINT ( 'NONE',  ( 12.63842701281683034, 42.46726448433412315, 9.846743663894596210 ) ) ;
#40136=CARTESIAN_POINT ( 'NONE',  ( 3.591859063236763294, 3.290301336597087012, -11.09922568453595026 ) ) ;
#40140=CARTESIAN_POINT ( 'NONE',  ( 22.81628187352647785, 6.623634669930420493, 6.195893100308588602E-16 ) ) ;
#40142=CARTESIAN_POINT ( 'NONE',  ( 20.36894250292379382, 48.67874883491396076, 10.36894250292379205 ) ) ;
#40144=CARTESIAN_POINT ( 'NONE',  ( 10.00000000000000178, 63.05374883491396076, 14.16423886937410082 ) ) ;
#40145=ORIENTED_EDGE ( 'NONE', *, *, #81064, .T. ) ;
#40146=CARTESIAN_POINT ( 'NONE',  ( 15.44008868035555260, 39.73035201082150536, 9.422509992056143702 ) ) ;
#40147=CARTESIAN_POINT ( 'NONE',  ( 0.5774900079438607392, 43.48035201082151247, 5.440088680355550821 ) ) ;
#40148=CARTESIAN_POINT ( 'NONE',  ( 5.076628168052704559, 60.17559781766745175, -8.527530157486179263 ) ) ;
#40149=CARTESIAN_POINT ( 'NONE',  ( 10.00000000000000178, 34.31368534415484106, 10.88017736071110342 ) ) ;
#40150=CARTESIAN_POINT ( 'NONE',  ( 7.084665262690076126, 69.10535201082151957, 10.88017736071109987 ) ) ;
#40151=CARTESIAN_POINT ( 'NONE',  ( 19.42250999205614193, 25.14701867748817321, 5.440088680355555262 ) ) ;
#40154=( LENGTH_UNIT ( ) NAMED_UNIT ( * ) SI_UNIT ( .MILLI., .METRE. ) );
#40158=CARTESIAN_POINT ( 'NONE',  ( 7.361572987183169658, 39.96726448433411605, -9.846743663894592657 ) ) ;
#40160=CARTESIAN_POINT ( 'NONE',  ( 10.00000000000000178, 45.37363466993041783, 12.81628187352647608 ) ) ;
#40162=B_SPLINE_CURVE_WITH_KNOTS ( 'NONE', 3,
 ( #22357, #30321, #35859, #53323 ),
 .UNSPECIFIED., .F., .F.,
 ( 4, 4 ),
 ( 1.854451039242195167E-16, 0.001060528352561992006 ),
 .UNSPECIFIED. ) ;
#40165=CARTESIAN_POINT ( 'NONE',  ( -45.73459272351794169, 104.7119485869564528, 5.163735687858058476 ) ) ;
#40166=CARTESIAN_POINT ( 'NONE',  ( 7.361572987183169658, 54.96726448433413026, -9.846743663894592657 ) ) ;
#40167=CARTESIAN_POINT ( 'NONE',  ( 20.36894250292379382, 43.67874883491397497, 10.36894250292379205 ) ) ;
#40168=CARTESIAN_POINT ( 'NONE',  ( 5.076628168052703671, 56.84226448433412315, 8.527530157486179263 ) ) ;
#40170=CARTESIAN_POINT ( 'NONE',  ( 19.72487221294570858, 41.86607318730076344, 6.500000000000000888 ) ) ;
#40172=CARTESIAN_POINT ( 'NONE',  ( 17.20831665107776587, 22.88393115100078745, 7.208316651077764980 ) ) ;
#40173=CARTESIAN_POINT ( 'NONE',  ( 6.565887622018943937, 58.08196800326376064, -12.81628187352647608 ) ) ;
#40174=CARTESIAN_POINT ( 'NONE',  ( 17.20831665107776587, 64.13393115100079456, -7.208316651077762316 ) ) ;
#40175=CARTESIAN_POINT ( 'NONE',  ( 12.91533473730992121, 64.52201867748817676, 10.88017736071110164 ) ) ;
#40178=CARTESIAN_POINT ( 'NONE',  ( 17.08211943468705840, 60.13708216824729647, -12.26659068614894466 ) ) ;
#40179=SURFACE_SIDE_STYLE ('',( #9188 ) ) ;
#40180=CARTESIAN_POINT ( 'NONE',  ( 20.88017736071110164, 30.35535201082151247, 2.915334737309930979 ) ) ;
#40181=CARTESIAN_POINT ( 'NONE',  ( 6.565887622018943937, 18.08196800326375708, -12.81628187352647608 ) ) ;
#40182=CARTESIAN_POINT ( 'NONE',  ( 12.91533473730992121, 54.52201867748816255, 10.88017736071110164 ) ) ;
#40185=CARTESIAN_POINT ( 'NONE',  ( -0.1503990784575275907, 58.10158574516644592, 6.262539305110076171 ) ) ;
#40187=CARTESIAN_POINT ( 'NONE',  ( 17.20831665107776587, 54.13393115100079456, -7.208316651077762316 ) ) ;
#40189=CARTESIAN_POINT ( 'NONE',  ( 0.6178305044545818747, 8.498634669930421381, -9.382169495545419124 ) ) ;
#40191=CARTESIAN_POINT ( 'NONE',  ( 4.559911319644449179, 8.897018677488173211, 9.422509992056141925 ) ) ;
#40192=CARTESIAN_POINT ( 'NONE',  ( 1.821708436314967372, 66.66792564121897158, -6.500000000000079048 ) ) ;
#40194=CARTESIAN_POINT ( 'NONE',  ( -4.164238869374099039, 31.80374883491396432, 8.674139862899312516E-16 ) ) ;
#40195=CARTESIAN_POINT ( 'NONE',  ( 22.26659068614894466, 23.88708216824730357, 7.082119434687054849 ) ) ;
#40196=CARTESIAN_POINT ( 'NONE',  ( -0.8801773607111009756, 3.063685344154838397, 1.068504757029289695E-15 ) ) ;
#40197=CARTESIAN_POINT ( 'NONE',  ( 0.1532563361054082862, 36.21726448433410894, 2.638427012816831674 ) ) ;
#40198=CARTESIAN_POINT ( 'NONE',  ( 12.63842701281683922, 14.55059781766744997, -9.846743663894590881 ) ) ;
#40199=CARTESIAN_POINT ( 'NONE',  ( 20.88017736071110164, 20.35535201082150891, 2.915334737309930979 ) ) ;
#40200=EDGE_CURVE ( 'NONE', #56195, #36584, #49968, .T. ) ;
#40203=CARTESIAN_POINT ( 'NONE',  ( 10.00000000000000000, 44.75893115100078745, -9.846743663894594434 ) ) ;
#40204=CARTESIAN_POINT ( 'NONE',  ( 20.88017736071110875, 45.77201867748816966, -2.915334737309920765 ) ) ;
#40205=CARTESIAN_POINT ( 'NONE',  ( 17.20831665107776587, 59.13393115100078745, -7.208316651077762316 ) ) ;
#40206=CARTESIAN_POINT ( 'NONE',  ( -4.164238869374098151, 16.59541550158063927, -3.795296366450310543 ) ) ;
#40207=CARTESIAN_POINT ( 'NONE',  ( -1.926860441876562247, 17.45379003517447458, -3.195792623639530650 ) ) ;
#40210=UNCERTAINTY_MEASURE_WITH_UNIT (LENGTH_MEASURE( 1.000000000000000082E-05 ), #97851, 'distance_accuracy_value', 'NONE');
#40211=CARTESIAN_POINT ( 'NONE',  ( 0.1532563361054082862, 16.21726448433411960, 2.638427012816831674 ) ) ;
#40212=CARTESIAN_POINT ( 'NONE',  ( -2.816281873526473856, 49.33196800326374643, 3.434112377981055619 ) ) ;
#40213=CARTESIAN_POINT ( 'NONE',  ( 5.076628168052703671, 51.84226448433412315, 8.527530157486179263 ) ) ;
#40215=DIRECTION ( 'NONE',  ( 0.000000000000000000, 0.000000000000000000, -1.000000000000000000 ) ) ;
#40216=CARTESIAN_POINT ( 'NONE',  ( 2.035157376598822676, 7.438685344154837509, -7.964842623401177768 ) ) ;
#40217=CARTESIAN_POINT ( 'NONE',  ( 10.00000000000000000, 56.81368534415484106, -10.88017736071110342 ) ) ;
#40218=CARTESIAN_POINT ( 'NONE',  ( -4.164238869374099039, 6.803748834913967869, 8.674139862899312516E-16 ) ) ;
#40219=CARTESIAN_POINT ( 'NONE',  ( 5.076628168052703671, 1.842264484334118047, 8.527530157486179263 ) ) ;
#40220=CARTESIAN_POINT ( 'NONE',  ( 1.472469842513823179, 55.59226448433412315, -4.923371831947296329 ) ) ;
#40221=CARTESIAN_POINT ( 'NONE',  ( 19.42250999205614193, 20.14701867748817321, 5.440088680355555262 ) ) ;
#40222=CARTESIAN_POINT ( 'NONE',  ( 20.15039907845753930, 11.74884699246888964, 6.262539305110064625 ) ) ;
#40223=CARTESIAN_POINT ( 'NONE',  ( 12.63842701281683922, 59.55059781766744464, -9.846743663894590881 ) ) ;
#40224=CARTESIAN_POINT ( 'NONE',  ( 7.361572987183169658, 4.967264484334119601, -9.846743663894592657 ) ) ;
#40225=AXIS2_PLACEMENT_3D ( 'NONE', #17591, #77573, #16598 ) ;
#40226=CARTESIAN_POINT ( 'NONE',  ( -1.099225684535947600, 63.70696800326376774, -6.408140936763238038 ) ) ;
#40231=CARTESIAN_POINT ( 'NONE',  ( 18.72515096720573879, 35.05509018479936145, 6.499999999999937828 ) ) ;
#40232=SURFACE_STYLE_FILL_AREA ( #48701 ) ;
#40233=CARTESIAN_POINT ( 'NONE',  ( -0.3689425029237881626, 37.42874883491396787, 10.36894250292379027 ) ) ;
#40234=CARTESIAN_POINT ( 'NONE',  ( 0.1532563361054100626, 50.80059781766745175, -2.638427012816831230 ) ) ;
#40235=CARTESIAN_POINT ( 'NONE',  ( 0.1532563361054083140, 16.00893115100078390, 1.131784320476157264E-15 ) ) ;
#40236=CARTESIAN_POINT ( 'NONE',  ( 0.2751277870542911952, 38.21833443783937412, 6.499999999999992006 ) ) ;
#40237=CARTESIAN_POINT ( 'NONE',  ( 2.035157376598824452, 13.68868534415483751, 7.964842623401179544 ) ) ;
#40238=CARTESIAN_POINT ( 'NONE',  ( 0.1532563361054083140, 66.00893115100079456, 1.131784320476157264E-15 ) ) ;
#40239=CARTESIAN_POINT ( 'NONE',  ( -0.1503990784575328643, 35.12777174578612716, 6.262539305110068177 ) ) ;
#40240=CARTESIAN_POINT ( 'NONE',  ( 20.36894250292379382, 38.67874883491396076, 10.36894250292379205 ) ) ;
#40241=CARTESIAN_POINT ( 'NONE',  ( -0.3689425029237898834, 61.17874883491396076, -10.36894250292378850 ) ) ;
#40242=CARTESIAN_POINT ( 'NONE',  ( 10.00000000000000178, 67.25893115100079456, 9.846743663894594434 ) ) ;
#40243=COLOUR_RGB ( '', 0.31764706, 0.68627451, 0.89019608) ;
#40245=CARTESIAN_POINT ( 'NONE',  ( 0.5774900079438607392, 68.48035201082150536, 5.440088680355550821 ) ) ;
#40246=ADVANCED_FACE ( 'NONE', ( #63661 ), #18185, .T. ) ;
#40247=CARTESIAN_POINT ( 'NONE',  ( 2.791683348922240793, 11.63393115100078568, 7.208316651077764092 ) ) ;
#40252=ORIENTED_EDGE ( 'NONE', *, *, #86646, .T. ) ;
#40253=CARTESIAN_POINT ( 'NONE',  ( 0.1532563361054083140, 21.00893115100078745, 1.131784320476157264E-15 ) ) ;
#40255=CARTESIAN_POINT ( 'NONE',  ( 24.16423886937410614, 29.51208216824729647, -3.795296366450302550 ) ) ;
#40256=CARTESIAN_POINT ( 'NONE',  ( 19.84674366389459266, 23.71726448433412315, -2.638427012816827677 ) ) ;
#40257=CARTESIAN_POINT ( 'NONE',  ( 10.00000000000000000, 41.81368534415484106, -10.88017736071110342 ) ) ;
#40261=CARTESIAN_POINT ( 'NONE',  ( 12.91533473730992121, 39.52201867748817676, 10.88017736071110164 ) ) ;
#40264=CARTESIAN_POINT ( 'NONE',  ( 6.204703633549690345, 0.7620821682473009062, -14.16423886937410259 ) ) ;
#40266=CARTESIAN_POINT ( 'NONE',  ( -1.099225684535947600, 29.54030133659708923, 6.408140936763237150 ) ) ;
#40267=B_SPLINE_CURVE_WITH_KNOTS ( 'NONE', 3,
 ( #3762, #85284, #55268, #85781 ),
 .UNSPECIFIED., .F., .F.,
 ( 4, 4 ),
 ( 0.000000000000000000, 0.002392975128318458600 ),
 .UNSPECIFIED. ) ;
#40268=CARTESIAN_POINT ( 'NONE',  ( 17.20831665107776587, 7.883931151000784787, 7.208316651077764980 ) ) ;
#40270=CARTESIAN_POINT ( 'NONE',  ( 0.6178305044545838731, 44.74863466993042493, 9.382169495545420901 ) ) ;
#40271=CARTESIAN_POINT ( 'NONE',  ( 0.1532563361054083140, 26.00893115100078745, 1.131784320476157264E-15 ) ) ;
#40274=ORIENTED_EDGE ( 'NONE', *, *, #33964, .T. ) ;
#40275=CARTESIAN_POINT ( 'NONE',  ( 1.932340009482123699, 46.49127512925448968, -6.499999999999926281 ) ) ;
#40276=CARTESIAN_POINT ( 'NONE',  ( -0.8801773607110991993, 52.85535201082151247, -2.915334737309923874 ) ) ;
#40279=CARTESIAN_POINT ( 'NONE',  ( 18.52753015748617571, 3.092264484334118269, 4.923371831947298993 ) ) ;
#40280=CARTESIAN_POINT ( 'NONE',  ( -2.816281873526473856, 9.123634669930421381, 9.499525473075851096E-16 ) ) ;
#40283=CARTESIAN_POINT ( 'NONE',  ( 17.20831665107776587, 29.13393115100078390, -7.208316651077762316 ) ) ;
#40284=CARTESIAN_POINT ( 'NONE',  ( 6.565887622018943937, 63.08196800326376064, -12.81628187352647608 ) ) ;
#40285=CARTESIAN_POINT ( 'NONE',  ( 22.26659068614894466, 13.88708216824730179, 7.082119434687054849 ) ) ;
#40286=CARTESIAN_POINT ( 'NONE',  ( 7.361572987183170547, 22.05059781766745530, 9.846743663894590881 ) ) ;
#40287=CARTESIAN_POINT ( 'NONE',  ( -2.816281873526473856, 39.12363466993041783, 9.499525473075851096E-16 ) ) ;
#40290=CARTESIAN_POINT ( 'NONE',  ( -0.8801773607111009756, 43.06368534415484106, 1.068504757029289695E-15 ) ) ;
#40291=CARTESIAN_POINT ( 'NONE',  ( 16.40814093676324603, 2.456968003263753531, -11.09922568453594671 ) ) ;
#40294=CARTESIAN_POINT ( 'NONE',  ( 10.00000000000000000, 29.75893115100078745, -9.846743663894594434 ) ) ;
#40295=CARTESIAN_POINT ( 'NONE',  ( 0.1532563361054082862, 26.21726448433411605, 2.638427012816831674 ) ) ;
#40296=CARTESIAN_POINT ( 'NONE',  ( 20.88017736071110164, 20.35535201082150891, 2.915334737309930979 ) ) ;
#40297=CARTESIAN_POINT ( 'NONE',  ( 3.591859063236761518, 14.95696800326375531, 11.09922568453594849 ) ) ;
#40298=AXIS2_PLACEMENT_3D ( 'NONE', #74192, #36717, #75191 ) ;
#40299=CARTESIAN_POINT ( 'NONE',  ( 5.076628168052703671, 21.84226448433411960, 8.527530157486179263 ) ) ;
#40300=DIRECTION ( 'NONE',  ( 0.000000000000000000, -1.000000000000000000, 0.000000000000000000 ) ) ;
#40301=CARTESIAN_POINT ( 'NONE',  ( 12.91533473730993009, 16.60535201082150891, -10.88017736071109987 ) ) ;
#40305=CARTESIAN_POINT ( 'NONE',  ( 19.42250999205614548, 60.98035201082151247, -5.440088680355545492 ) ) ;
#40307=CARTESIAN_POINT ( 'NONE',  ( 12.63842701281683922, 49.55059781766744464, -9.846743663894590881 ) ) ;
#40308=CARTESIAN_POINT ( 'NONE',  ( 19.42250999205614193, 15.14701867748817143, 5.440088680355555262 ) ) ;
#40310=AXIS2_PLACEMENT_3D ( 'NONE', #55616, #94096, #18597 ) ;
#40311=CARTESIAN_POINT ( 'NONE',  ( 0.5774900079438590739, 42.64701867748816966, -5.440088680355550821 ) ) ;
#40312=CARTESIAN_POINT ( 'NONE',  ( 15.44008868035555793, 16.39701867748817321, -9.422509992056140149 ) ) ;
#40313=CARTESIAN_POINT ( 'NONE',  ( -0.3289641300568005855, 20.10497603579417358, 5.963430220938281678 ) ) ;
#40314=CARTESIAN_POINT ( 'NONE',  ( 19.84674366389459266, 13.30059781766745353, 2.638427012816836559 ) ) ;
#40316=CARTESIAN_POINT ( 'NONE',  ( 14.92337183194729633, 37.67559781766745175, 8.527530157486181039 ) ) ;
#40318=CARTESIAN_POINT ( 'NONE',  ( 6.000000000000000000, 11.00000000000000000, -5.000000000000000000 ) ) ;
#40319=CARTESIAN_POINT ( 'NONE',  ( -2.816281873526471635, -1.084698663402913210, -3.434112377981056508 ) ) ;
#40321=CARTESIAN_POINT ( 'NONE',  ( 22.26659068614895176, 19.72041550158063572, -7.082119434687042414 ) ) ;
#40323=CARTESIAN_POINT ( 'NONE',  ( 19.84674366389459621, 38.50893115100078745, 7.409399052514197653E-17 ) ) ;
#40324=EDGE_CURVE ( 'NONE', #29627, #88696, #32396, .T. ) ;
#40326=CARTESIAN_POINT ( 'NONE',  ( 17.96484262340118221, 6.188685344154837509, -7.964842623401177768 ) ) ;
#40327=CARTESIAN_POINT ( 'NONE',  ( 18.52753015748618282, 23.92559781766745530, -4.923371831947291888 ) ) ;
#40330=CARTESIAN_POINT ( 'NONE',  ( 19.42250999205614193, 40.14701867748817676, 5.440088680355555262 ) ) ;
#40331=CARTESIAN_POINT ( 'NONE',  ( 10.00000000000000178, 60.37363466993041783, 12.81628187352647608 ) ) ;
#40333=CARTESIAN_POINT ( 'NONE',  ( 19.42250999205614548, 15.98035201082150714, -5.440088680355545492 ) ) ;
#40334=CARTESIAN_POINT ( 'NONE',  ( 13.43411237798105340, 45.58196800326374643, 12.81628187352647963 ) ) ;
#40335=CARTESIAN_POINT ( 'NONE',  ( 21.09922568453594849, 11.20696800326375531, 6.408140936763242479 ) ) ;
#40336=CARTESIAN_POINT ( 'NONE',  ( 12.63842701281683922, 19.55059781766745175, -9.846743663894590881 ) ) ;
#40340=CARTESIAN_POINT ( 'NONE',  ( -0.3689425029237898834, 51.17874883491397497, -10.36894250292378850 ) ) ;
#40341=CARTESIAN_POINT ( 'NONE',  ( -4.164238869374098151, 26.59541550158063217, -3.795296366450310543 ) ) ;
#40342=CARTESIAN_POINT ( 'NONE',  ( 2.035157376598824452, 23.68868534415484461, 7.964842623401179544 ) ) ;
#40343=CARTESIAN_POINT ( 'NONE',  ( 20.88017736071110875, 55.77201867748816966, -2.915334737309920765 ) ) ;
#40345=DIRECTION ( 'NONE',  ( -0.8320502943378437211, 0.5547001962252290364, 0.000000000000000000 ) ) ;
#40346=DIRECTION ( 'NONE',  ( -1.000000000000000000, 0.000000000000000000, 0.000000000000000000 ) ) ;
#40347=CARTESIAN_POINT ( 'NONE',  ( 17.96484262340118221, 61.18868534415482685, -7.964842623401177768 ) ) ;
#40348=CARTESIAN_POINT ( 'NONE',  ( 10.00000000000000178, 17.25893115100078745, 9.846743663894594434 ) ) ;
#40349=FACE_OUTER_BOUND ( 'NONE', #14260, .T. ) ;
#40351=CARTESIAN_POINT ( 'NONE',  ( 17.20831665107776587, 22.88393115100078745, 7.208316651077764980 ) ) ;
#40352=CARTESIAN_POINT ( 'NONE',  ( 14.92337183194729988, 49.34226448433411605, -8.527530157486177487 ) ) ;
#40353=CARTESIAN_POINT ( 'NONE',  ( 10.00000000000000178, 19.31368534415484106, 10.88017736071110342 ) ) ;
#40355=CARTESIAN_POINT ( 'NONE',  ( 0.6178305044545818747, 33.49863466993042493, -9.382169495545419124 ) ) ;
#40356=CARTESIAN_POINT ( 'NONE',  ( 15.44008868035555793, 51.39701867748816966, -9.422509992056140149 ) ) ;
#40357=CARTESIAN_POINT ( 'NONE',  ( 7.361572987183169658, 29.96726448433411960, -9.846743663894592657 ) ) ;
#40358=CARTESIAN_POINT ( 'NONE',  ( 22.26659068614894466, 48.88708216824730357, 7.082119434687054849 ) ) ;
#40359=CARTESIAN_POINT ( 'NONE',  ( 5.076628168052703671, 26.84226448433411960, 8.527530157486179263 ) ) ;
#40361=CARTESIAN_POINT ( 'NONE',  ( 0.1532563361054083140, 51.00893115100078745, 1.131784320476157264E-15 ) ) ;
#40362=CARTESIAN_POINT ( 'NONE',  ( 0.1532563361054083140, 26.00893115100078745, 1.131784320476157264E-15 ) ) ;
#40363=CARTESIAN_POINT ( 'NONE',  ( 24.16423886937409904, 14.09541550158063217, 3.795296366450317205 ) ) ;
#40364=CARTESIAN_POINT ( 'NONE',  ( 20.36894250292379738, 24.92874883491396787, -10.36894250292379027 ) ) ;
#40365=CARTESIAN_POINT ( 'NONE',  ( 0.1532563361054082862, 36.21726448433410894, 2.638427012816831674 ) ) ;
#40366=CARTESIAN_POINT ( 'NONE',  ( 20.88017736071110519, 40.56368534415484106, 2.639326808657452039E-16 ) ) ;
#40367=CARTESIAN_POINT ( 'NONE',  ( 4.559911319644449179, 18.89701867748817321, 9.422509992056141925 ) ) ;
#40369=CARTESIAN_POINT ( 'NONE',  ( 7.084665262690076126, 42.02201867748816966, -10.88017736071110164 ) ) ;
#40370=CARTESIAN_POINT ( 'NONE',  ( 19.42250999205614193, 30.14701867748817321, 5.440088680355555262 ) ) ;
#40372=CARTESIAN_POINT ( 'NONE',  ( 19.38216949554541202, 35.99863466993041072, 9.382169495545424454 ) ) ;
#40373=CARTESIAN_POINT ( 'NONE',  ( 17.96484262340118221, 34.93868534415482685, 7.964842623401181321 ) ) ;
#40375=CARTESIAN_POINT ( 'NONE',  ( 16.40814093676323893, 55.79030133659708923, 11.09922568453595026 ) ) ;
#40376=CARTESIAN_POINT ( 'NONE',  ( -0.8801773607110991993, 67.85535201082151957, -2.915334737309923874 ) ) ;
#40377=AXIS2_PLACEMENT_3D ( 'NONE', #58899, #66393, #35404 ) ;
#40379=CARTESIAN_POINT ( 'NONE',  ( 4.559911319644449179, 57.23035201082150536, -9.422509992056141925 ) ) ;
#40380=CARTESIAN_POINT ( 'NONE',  ( -0.8801773607110991993, 7.855352010821504471, -2.915334737309923874 ) ) ;
#40382=CARTESIAN_POINT ( 'NONE',  ( -0.1503990784575328643, 69.92552686551195507, 6.262539305110068177 ) ) ;
#40383=CARTESIAN_POINT ( 'NONE',  ( 13.79529636645031943, 65.34541550158063217, -14.16423886937409904 ) ) ;
#40384=CARTESIAN_POINT ( 'NONE',  ( 1.472469842513823179, 11.42559781766745175, 4.923371831947296329 ) ) ;
#40385=CARTESIAN_POINT ( 'NONE',  ( -2.266590686148945544, 11.38708216824730179, -7.082119434687050408 ) ) ;
#40387=CARTESIAN_POINT ( 'NONE',  ( 14.92337183194729633, 2.675597817667451750, 8.527530157486181039 ) ) ;
#40389=CARTESIAN_POINT ( 'NONE',  ( 12.91533473730992121, 9.522018677488171434, 10.88017736071110164 ) ) ;
#40390=CARTESIAN_POINT ( 'NONE',  ( 19.84674366389459266, 43.30059781766744464, 2.638427012816836559 ) ) ;
#40393=CARTESIAN_POINT ( 'NONE',  ( 14.92337183194729633, 52.67559781766745175, 8.527530157486181039 ) ) ;
#40396=CARTESIAN_POINT ( 'NONE',  ( 19.42250999205614548, 45.98035201082150536, -5.440088680355545492 ) ) ;
#40397=CARTESIAN_POINT ( 'NONE',  ( 10.00000000000000178, 47.25893115100078745, 9.846743663894594434 ) ) ;
#40398=CARTESIAN_POINT ( 'NONE',  ( -2.816281873526473856, 29.12363466993041783, 9.499525473075851096E-16 ) ) ;
#40401=CARTESIAN_POINT ( 'NONE',  ( 17.96484262340118221, 49.93868534415484106, 7.964842623401181321 ) ) ;
#40402=CARTESIAN_POINT ( 'NONE',  ( 19.42250999205614548, 5.980352010821504471, -5.440088680355545492 ) ) ;
#40403=CARTESIAN_POINT ( 'NONE',  ( 10.00000000000000178, 35.37363466993042493, 12.81628187352647608 ) ) ;
#40406=CARTESIAN_POINT ( 'NONE',  ( -2.816281873526471635, 33.91530133659708213, -3.434112377981056508 ) ) ;
#40407=CARTESIAN_POINT ( 'NONE',  ( 0.5774900079438590739, 37.64701867748817676, -5.440088680355550821 ) ) ;
#40411=CARTESIAN_POINT ( 'NONE',  ( 1.472469842513823179, 50.59226448433411605, -4.923371831947296329 ) ) ;
#40412=CARTESIAN_POINT ( 'NONE',  ( 17.20831665107776587, 19.13393115100078035, -7.208316651077762316 ) ) ;
#40413=CARTESIAN_POINT ( 'NONE',  ( 1.472469842513823179, 35.59226448433412315, -4.923371831947296329 ) ) ;
#40415=CARTESIAN_POINT ( 'NONE',  ( 18.52753015748618282, 28.92559781766745175, -4.923371831947291888 ) ) ;
#40418=AXIS2_PLACEMENT_3D ( 'NONE', #48665, #86680, #33652 ) ;
#40420=CARTESIAN_POINT ( 'NONE',  ( 5.076628168052703671, 26.84226448433411960, 8.527530157486179263 ) ) ;
#40421=CARTESIAN_POINT ( 'NONE',  ( 12.63842701281683034, 2.467264484334118269, 9.846743663894596210 ) ) ;
#40423=CARTESIAN_POINT ( 'NONE',  ( 18.52753015748617571, 48.09226448433412315, 4.923371831947298993 ) ) ;
#40426=CARTESIAN_POINT ( 'NONE',  ( 10.00000000000000178, 25.37363466993041783, 12.81628187352647608 ) ) ;
#40428=CARTESIAN_POINT ( 'NONE',  ( 24.16423886937410614, 44.51208216824730357, -3.795296366450302550 ) ) ;
#40429=CARTESIAN_POINT ( 'NONE',  ( 7.361572987183170547, 17.05059781766745530, 9.846743663894590881 ) ) ;
#40432=CARTESIAN_POINT ( 'NONE',  ( 24.16423886937410614, 39.51208216824731068, -3.795296366450302550 ) ) ;
#40433=CARTESIAN_POINT ( 'NONE',  ( 0.1532563361054083140, 66.00893115100079456, 1.131784320476157264E-15 ) ) ;
#40434=CARTESIAN_POINT ( 'NONE',  ( -0.8801773607110991993, 7.855352010821506248, -2.915334737309923874 ) ) ;
#40435=CARTESIAN_POINT ( 'NONE',  ( 22.26659068614895176, 24.72041550158063572, -7.082119434687042414 ) ) ;
#40436=CARTESIAN_POINT ( 'NONE',  ( -4.164238869374099039, 36.80374883491396787, 8.674139862899312516E-16 ) ) ;
#40439=CARTESIAN_POINT ( 'NONE',  ( 10.00000000000000000, 49.75893115100078745, -9.846743663894594434 ) ) ;
#40440=CARTESIAN_POINT ( 'NONE',  ( 19.42250999205614548, 35.98035201082151247, -5.440088680355545492 ) ) ;
#40442=CARTESIAN_POINT ( 'NONE',  ( 19.54746220608152640, 97.02070453147715057, -5.000000000000000000 ) ) ;
#40443=CARTESIAN_POINT ( 'NONE',  ( 0.1532563361054100626, 35.80059781766745175, -2.638427012816831230 ) ) ;
#40446=CARTESIAN_POINT ( 'NONE',  ( 7.361572987183169658, 39.96726448433411605, -9.846743663894592657 ) ) ;
#40447=CARTESIAN_POINT ( 'NONE',  ( 19.84674366389459266, 63.71726448433412315, -2.638427012816827677 ) ) ;
#40450=CARTESIAN_POINT ( 'NONE',  ( 6.204703633549690345, 12.84541550158063572, 14.16423886937410082 ) ) ;
#40453=CARTESIAN_POINT ( 'NONE',  ( 20.88017736071110164, 45.35535201082149825, 2.915334737309930979 ) ) ;
#40454=CARTESIAN_POINT ( 'NONE',  ( 7.084665262690076126, 2.022018677488171434, -10.88017736071110164 ) ) ;
#40455=CARTESIAN_POINT ( 'NONE',  ( 21.09922568453595559, 22.04030133659708923, -6.408140936763230044 ) ) ;
#40458=CARTESIAN_POINT ( 'NONE',  ( 5.076628168052704559, 0.1755978176674514724, -8.527530157486179263 ) ) ;
#40462=CARTESIAN_POINT ( 'NONE',  ( 4.559911319644449179, 7.230352010821505360, -9.422509992056141925 ) ) ;
#40464=CARTESIAN_POINT ( 'NONE',  ( -0.8801773607111009756, 23.06368534415484106, 1.068504757029289695E-15 ) ) ;
#40465=CARTESIAN_POINT ( 'NONE',  ( -0.8801773607111008646, 38.27201867748816255, 2.915334737309923430 ) ) ;
#40466=AXIS2_PLACEMENT_3D ( 'NONE', #65342, #57358, #74322 ) ;
#40467=CARTESIAN_POINT ( 'NONE',  ( 1.472469842513823179, 65.59226448433412315, -4.923371831947296329 ) ) ;
#40468=CARTESIAN_POINT ( 'NONE',  ( 0.1532563361054083140, 56.00893115100078745, 1.131784320476157264E-15 ) ) ;
#40469=CARTESIAN_POINT ( 'NONE',  ( -44.44142132516394383, 105.4794309841216347, -5.302661541405906398 ) ) ;
#40470=CARTESIAN_POINT ( 'NONE',  ( 0.1532563361054082862, 11.21726448433411605, 2.638427012816831674 ) ) ;
#40471=ORIENTED_EDGE ( 'NONE', *, *, #97594, .F. ) ;
#40472=CARTESIAN_POINT ( 'NONE',  ( 19.42250999205614193, 35.14701867748816966, 5.440088680355555262 ) ) ;
#40473=CARTESIAN_POINT ( 'NONE',  ( 3.591859063236763294, 33.29030133659708213, -11.09922568453595026 ) ) ;
#40476=CARTESIAN_POINT ( 'NONE',  ( 2.791683348922237240, 60.38393115100078745, -7.208316651077763204 ) ) ;
#40477=CARTESIAN_POINT ( 'NONE',  ( -0.8801773607111009756, 53.06368534415484106, 1.068504757029289695E-15 ) ) ;
#40478=CARTESIAN_POINT ( 'NONE',  ( 19.84674366389459266, 13.30059781766745353, 2.638427012816836559 ) ) ;
#40479=CARTESIAN_POINT ( 'NONE',  ( 22.81628187352647785, 41.41530133659708923, 3.434112377981063169 ) ) ;
#40480=CARTESIAN_POINT ( 'NONE',  ( -0.8801773607111008646, 58.27201867748816966, 2.915334737309923430 ) ) ;
#40483=ORIENTED_EDGE ( 'NONE', *, *, #79080, .T. ) ;
#40485=CARTESIAN_POINT ( 'NONE',  ( 4.559911319644449179, 2.230352010821504471, -9.422509992056141925 ) ) ;
#40486=CARTESIAN_POINT ( 'NONE',  ( 21.09922568453594849, 46.20696800326376064, 6.408140936763242479 ) ) ;
#40487=CARTESIAN_POINT ( 'NONE',  ( -4.164238869374098151, 11.59541550158063217, -3.795296366450310543 ) ) ;
#40488=CARTESIAN_POINT ( 'NONE',  ( 7.361572987183170547, 12.05059781766744997, 9.846743663894590881 ) ) ;
#40489=( LENGTH_UNIT ( ) NAMED_UNIT ( * ) SI_UNIT ( .MILLI., .METRE. ) );
#40490=CARTESIAN_POINT ( 'NONE',  ( 14.92337183194729633, 17.67559781766745175, 8.527530157486181039 ) ) ;
#40491=CARTESIAN_POINT ( 'NONE',  ( 17.08211943468705840, 60.13708216824729647, -12.26659068614894466 ) ) ;
#40493=CARTESIAN_POINT ( 'NONE',  ( 19.42250999205614193, 5.147018677488171434, 5.440088680355555262 ) ) ;
#40496=CARTESIAN_POINT ( 'NONE',  ( 20.88017736071110875, 15.77201867748817143, -2.915334737309920765 ) ) ;
#40498=ORIENTED_EDGE ( 'NONE', *, *, #42578, .F. ) ;
#40501=CARTESIAN_POINT ( 'NONE',  ( 15.44008868035555793, 11.39701867748817143, -9.422509992056140149 ) ) ;
#40502=CARTESIAN_POINT ( 'NONE',  ( 17.20831665107776587, 52.88393115100078035, 7.208316651077764980 ) ) ;
#40503=CARTESIAN_POINT ( 'NONE',  ( 1.274849032794292736, 67.55509018479936856, -6.499999999999977796 ) ) ;
#40504=FACE_OUTER_BOUND ( 'NONE', #9768, .T. ) ;
#40505=CARTESIAN_POINT ( 'NONE',  ( 24.16423886937409904, 19.09541550158063927, 3.795296366450317205 ) ) ;
#40506=CARTESIAN_POINT ( 'NONE',  ( 10.00000000000000000, 41.81368534415484106, -10.88017736071110342 ) ) ;
#40507=CARTESIAN_POINT ( 'NONE',  ( 20.88017736071110875, 20.77201867748816611, -2.915334737309920765 ) ) ;
#40508=CARTESIAN_POINT ( 'NONE',  ( 0.1532563361054083140, 56.00893115100078745, 1.131784320476157264E-15 ) ) ;
#40510=CARTESIAN_POINT ( 'NONE',  ( 2.791683348922237240, 30.38393115100078390, -7.208316651077763204 ) ) ;
#40512=CARTESIAN_POINT ( 'NONE',  ( 2.791683348922240793, 1.633931151000784565, 7.208316651077764092 ) ) ;
#40516=CARTESIAN_POINT ( 'NONE',  ( 5.076628168052703671, 16.84226448433411960, 8.527530157486179263 ) ) ;
#40517=CARTESIAN_POINT ( 'NONE',  ( 6.565887622018943937, 5.165301336597086568, 12.81628187352647430 ) ) ;
#40518=CARTESIAN_POINT ( 'NONE',  ( 12.91533473730993009, 51.60535201082149825, -10.88017736071109987 ) ) ;
#40519=CARTESIAN_POINT ( 'NONE',  ( -0.8801773607111008646, 8.272018677488171434, 2.915334737309923430 ) ) ;
#40520=CARTESIAN_POINT ( 'NONE',  ( -2.816281873526473856, 49.12363466993042493, 9.499525473075851096E-16 ) ) ;
#40521=CARTESIAN_POINT ( 'NONE',  ( 6.204703633549690345, 20.76208216824730357, -14.16423886937410259 ) ) ;
#40522=( GEOMETRIC_REPRESENTATION_CONTEXT ( 3 ) GLOBAL_UNCERTAINTY_ASSIGNED_CONTEXT ( ( #57495 ) ) GLOBAL_UNIT_ASSIGNED_CONTEXT ( ( #94795, #87780, #3815 ) ) REPRESENTATION_CONTEXT ( 'NONE', 'WORKASPACE' ) );
#40523=CARTESIAN_POINT ( 'NONE',  ( 10.00000000000000000, 62.87363466993042493, -12.81628187352647608 ) ) ;
#40525=CARTESIAN_POINT ( 'NONE',  ( 14.92337183194729988, 54.34226448433412315, -8.527530157486177487 ) ) ;
#40526=CARTESIAN_POINT ( 'NONE',  ( 7.084665262690076126, 24.10535201082150181, 10.88017736071109987 ) ) ;
#40529=CARTESIAN_POINT ( 'NONE',  ( 19.84674366389459266, 3.717264484334118713, -2.638427012816827677 ) ) ;
#40531=CARTESIAN_POINT ( 'NONE',  ( 5.076628168052704559, 10.17559781766745175, -8.527530157486179263 ) ) ;
#40532=CARTESIAN_POINT ( 'NONE',  ( 10.00000000000000178, 69.31368534415484817, 10.88017736071110342 ) ) ;
#40535=CARTESIAN_POINT ( 'NONE',  ( 17.96484262340118221, 54.93868534415484106, 7.964842623401181321 ) ) ;
#40537=CARTESIAN_POINT ( 'NONE',  ( 2.035157376598824452, 58.68868534415482685, 7.964842623401179544 ) ) ;
#40538=CARTESIAN_POINT ( 'NONE',  ( 0.1532563361054083140, 1.008931151000784787, 1.131784320476157264E-15 ) ) ;
#40540=CARTESIAN_POINT ( 'NONE',  ( 0.2751277870542986892, 7.282175860852375671, -6.500000000000003553 ) ) ;
#40541=CARTESIAN_POINT ( 'NONE',  ( 1.472469842513823179, 50.59226448433411605, -4.923371831947296329 ) ) ;
#40544=CARTESIAN_POINT ( 'NONE',  ( 24.16423886937410614, 4.303748834913967869, 8.672049930838204340E-16 ) ) ;
#40545=CARTESIAN_POINT ( 'NONE',  ( 22.81628187352647785, 56.41530133659708213, 3.434112377981063169 ) ) ;
#40546=CARTESIAN_POINT ( 'NONE',  ( 22.26659068614895176, 4.720415501580633943, -7.082119434687042414 ) ) ;
#40547=CARTESIAN_POINT ( 'NONE',  ( 24.16423886937409904, 24.09541550158063927, 3.795296366450317205 ) ) ;
#40548=CARTESIAN_POINT ( 'NONE',  ( 10.00000000000000178, 3.053748834913967425, 14.16423886937410082 ) ) ;
#40549=CARTESIAN_POINT ( 'NONE',  ( 20.88017736071110519, 25.56368534415483751, 2.639326808657452039E-16 ) ) ;
#40552=CARTESIAN_POINT ( 'NONE',  ( 1.472469842513823179, 5.592264484334118713, -4.923371831947296329 ) ) ;
#40553=CARTESIAN_POINT ( 'NONE',  ( 2.791683348922237240, 10.38393115100078390, -7.208316651077763204 ) ) ;
#40554=CARTESIAN_POINT ( 'NONE',  ( 19.38216949554541202, 30.99863466993042138, 9.382169495545424454 ) ) ;
#40555=CARTESIAN_POINT ( 'NONE',  ( 19.84674366389459266, 43.71726448433410894, -2.638427012816827677 ) ) ;
#40556=DIRECTION ( 'NONE',  ( 0.000000000000000000, -0.000000000000000000, -1.000000000000000000 ) ) ;
#40557=CARTESIAN_POINT ( 'NONE',  ( -2.816281873526473856, 24.33196800326375353, 3.434112377981055619 ) ) ;
#40559=CARTESIAN_POINT ( 'NONE',  ( 19.84674366389459266, 23.30059781766745530, 2.638427012816836559 ) ) ;
#40560=CARTESIAN_POINT ( 'NONE',  ( 24.16423886937409904, 19.09541550158063927, 3.795296366450317205 ) ) ;
#40562=ORIENTED_EDGE ( 'NONE', *, *, #25859, .T. ) ;
#40564=CARTESIAN_POINT ( 'NONE',  ( 15.44008868035555793, 31.39701867748817676, -9.422509992056140149 ) ) ;
#40565=CARTESIAN_POINT ( 'NONE',  ( 13.79529636645031943, 30.34541550158063927, -14.16423886937409904 ) ) ;
#40566=CARTESIAN_POINT ( 'NONE',  ( 0.1532563361054083140, 51.00893115100078745, 1.131784320476157264E-15 ) ) ;
#40567=CARTESIAN_POINT ( 'NONE',  ( 2.791683348922237240, 15.38393115100078212, -7.208316651077763204 ) ) ;
#40568=CARTESIAN_POINT ( 'NONE',  ( -2.816281873526471635, 48.91530133659708213, -3.434112377981056508 ) ) ;
#40570=CARTESIAN_POINT ( 'NONE',  ( 10.00000000000000000, 26.81368534415484106, -10.88017736071110342 ) ) ;
#40572=LINE ( 'NONE', #2100, #50203 ) ;
#40573=CARTESIAN_POINT ( 'NONE',  ( -2.816281873526473856, 19.33196800326375708, 3.434112377981055619 ) ) ;
#40574=CARTESIAN_POINT ( 'NONE',  ( 19.38216949554541202, 20.99863466993042138, 9.382169495545424454 ) ) ;
#40575=CARTESIAN_POINT ( 'NONE',  ( 19.84674366389459266, 43.71726448433410894, -2.638427012816827677 ) ) ;
#40577=CARTESIAN_POINT ( 'NONE',  ( 0.6178305044545838731, 44.74863466993042493, 9.382169495545420901 ) ) ;
#40578=FACE_OUTER_BOUND ( 'NONE', #66407, .T. ) ;
#40579=CARTESIAN_POINT ( 'NONE',  ( -0.8801773607110991993, 47.85535201082150536, -2.915334737309923874 ) ) ;
#40580=CARTESIAN_POINT ( 'NONE',  ( 19.89220837332774749, 9.740628644642393752, 6.478736007405950126 ) ) ;
#40583=CARTESIAN_POINT ( 'NONE',  ( 4.559911319644449179, 58.89701867748817676, 9.422509992056141925 ) ) ;
#40584=CARTESIAN_POINT ( 'NONE',  ( 17.96484262340118221, 56.18868534415484817, -7.964842623401177768 ) ) ;
#40588=CARTESIAN_POINT ( 'NONE',  ( 20.88017736071110519, 5.563685344154838397, 2.639326808657452039E-16 ) ) ;
#40589=CARTESIAN_POINT ( 'NONE',  ( 0.6178305044545838731, -0.2513653300695798953, 9.382169495545420901 ) ) ;
#40590=CARTESIAN_POINT ( 'NONE',  ( 12.91533473730992121, 24.52201867748816966, 10.88017736071110164 ) ) ;
#40592=CARTESIAN_POINT ( 'NONE',  ( 22.81628187352647785, 21.62363466993041783, 6.195893100308588602E-16 ) ) ;
#40594=CARTESIAN_POINT ( 'NONE',  ( 4.559911319644449179, 47.23035201082150536, -9.422509992056141925 ) ) ;
#40595=CARTESIAN_POINT ( 'NONE',  ( 5.076628168052704559, 35.17559781766745175, -8.527530157486179263 ) ) ;
#40596=CARTESIAN_POINT ( 'NONE',  ( 3.591859063236761518, 9.956968003263753531, 11.09922568453594849 ) ) ;
#40598=CARTESIAN_POINT ( 'NONE',  ( 0.5774900079438607392, 23.48035201082150536, 5.440088680355550821 ) ) ;
#40599=CARTESIAN_POINT ( 'NONE',  ( 17.96484262340118221, 39.93868534415484106, 7.964842623401181321 ) ) ;
#40600=CARTESIAN_POINT ( 'NONE',  ( 6.204703633549690345, 52.84541550158062506, 14.16423886937410082 ) ) ;
#40601=CARTESIAN_POINT ( 'NONE',  ( 14.92337183194729988, 34.34226448433411605, -8.527530157486177487 ) ) ;
#40602=CARTESIAN_POINT ( 'NONE',  ( 15.44008868035555793, 61.39701867748817676, -9.422509992056140149 ) ) ;
#40604=CARTESIAN_POINT ( 'NONE',  ( 10.00000000000000000, 15.55374883491396787, -14.16423886937410082 ) ) ;
#40610=CARTESIAN_POINT ( 'NONE',  ( 20.36894250292379738, 54.92874883491396076, -10.36894250292379027 ) ) ;
#40611=CARTESIAN_POINT ( 'NONE',  ( 13.79529636645031943, 35.34541550158063927, -14.16423886937409904 ) ) ;
#40612=CARTESIAN_POINT ( 'NONE',  ( 5.076628168052703671, 21.84226448433411960, 8.527530157486179263 ) ) ;
#40613=CARTESIAN_POINT ( 'NONE',  ( 0.1532563361054083140, 61.00893115100078745, 1.131784320476157264E-15 ) ) ;
#40614=CYLINDRICAL_SURFACE ( 'NONE', #83420, 0.5000000000000004441 ) ;
#40615=CARTESIAN_POINT ( 'NONE',  ( 0.5774900079438607392, 53.48035201082151247, 5.440088680355550821 ) ) ;
#40616=CARTESIAN_POINT ( 'NONE',  ( -2.816281873526471635, 28.91530133659708213, -3.434112377981056508 ) ) ;
#40617=CARTESIAN_POINT ( 'NONE',  ( -2.266590686148945544, 41.38708216824729647, -7.082119434687050408 ) ) ;
#40618=CARTESIAN_POINT ( 'NONE',  ( 20.88017736071110519, 25.56368534415483751, 2.639326808657452039E-16 ) ) ;
#40620=CARTESIAN_POINT ( 'NONE',  ( 4.559911319644449179, 63.89701867748817676, 9.422509992056141925 ) ) ;
#40623=CARTESIAN_POINT ( 'NONE',  ( 7.361572987183170547, 7.050597817667451750, 9.846743663894590881 ) ) ;
#40624=EDGE_LOOP ( 'NONE', ( #49673, #9060, #27507, #82572 ) ) ;
#40629=CARTESIAN_POINT ( 'NONE',  ( 17.96484262340118221, 9.938685344154839285, 7.964842623401181321 ) ) ;
#40630=CARTESIAN_POINT ( 'NONE',  ( 0.5774900079438590739, 12.64701867748817321, -5.440088680355550821 ) ) ;
#40631=CARTESIAN_POINT ( 'NONE',  ( 1.472469842513823179, 35.59226448433412315, -4.923371831947296329 ) ) ;
#40632=CARTESIAN_POINT ( 'NONE',  ( 13.43411237798106583, 7.665301336597086568, -12.81628187352647252 ) ) ;
#40636=CARTESIAN_POINT ( 'NONE',  ( 0.6178305044545818747, 13.49863466993041783, -9.382169495545419124 ) ) ;
#40638=CARTESIAN_POINT ( 'NONE',  ( 2.917880565312948704, 52.63708216824730357, 12.26659068614894643 ) ) ;
#40639=VERTEX_POINT ( 'NONE', #43630 ) ;
#40640=CARTESIAN_POINT ( 'NONE',  ( -0.3689425029237881626, 52.42874883491396076, 10.36894250292379027 ) ) ;
#40642=CARTESIAN_POINT ( 'NONE',  ( 10.00000000000000178, 34.31368534415484106, 10.88017736071110342 ) ) ;
#40643=CARTESIAN_POINT ( 'NONE',  ( 10.00000000000000178, 39.31368534415484106, 10.88017736071110342 ) ) ;
#40644=CARTESIAN_POINT ( 'NONE',  ( 2.035157376598824452, 38.68868534415483396, 7.964842623401179544 ) ) ;
#40645=CARTESIAN_POINT ( 'NONE',  ( -0.8801773607111009756, 63.06368534415484106, 1.068504757029289695E-15 ) ) ;
#40646=CARTESIAN_POINT ( 'NONE',  ( 0.5774900079438590739, 27.64701867748817676, -5.440088680355550821 ) ) ;
#40647=EDGE_CURVE ( 'NONE', #10095, #93630, #47347, .T. ) ;
#40650=CARTESIAN_POINT ( 'NONE',  ( 10.00000000000000178, 12.25893115100078568, 9.846743663894594434 ) ) ;
#40655=CARTESIAN_POINT ( 'NONE',  ( 5.076628168052703671, 41.84226448433411605, 8.527530157486179263 ) ) ;
#40662=CARTESIAN_POINT ( 'NONE',  ( 19.84674366389459621, 48.50893115100078745, 7.409399052514197653E-17 ) ) ;
#40663=CARTESIAN_POINT ( 'NONE',  ( 6.204703633549690345, 42.84541550158063217, 14.16423886937410082 ) ) ;
#40664=CARTESIAN_POINT ( 'NONE',  ( -22.44000000000001194, 93.50000000000000000, -10.09898361729590199 ) ) ;
#40667=CARTESIAN_POINT ( 'NONE',  ( 10.00000000000000178, 22.25893115100078745, 9.846743663894594434 ) ) ;
#40669=CARTESIAN_POINT ( 'NONE',  ( 0.6178305044545838731, 64.74863466993043914, 9.382169495545420901 ) ) ;
#40670=CARTESIAN_POINT ( 'NONE',  ( 0.1532563361054082862, 56.21726448433411605, 2.638427012816831674 ) ) ;
#40671=CARTESIAN_POINT ( 'NONE',  ( 17.96484262340118221, 66.18868534415483396, -7.964842623401177768 ) ) ;
#40672=CARTESIAN_POINT ( 'NONE',  ( 0.1532563361054100626, 45.80059781766745886, -2.638427012816831230 ) ) ;
#40675=CARTESIAN_POINT ( 'NONE',  ( -4.164238869374099039, 61.80374883491397497, 8.674139862899312516E-16 ) ) ;
#40677=CARTESIAN_POINT ( 'NONE',  ( 12.91533473730993009, 36.60535201082151247, -10.88017736071109987 ) ) ;
#40678=CARTESIAN_POINT ( 'NONE',  ( 19.38216949554541202, 10.99863466993042138, 9.382169495545424454 ) ) ;
#40679=CARTESIAN_POINT ( 'NONE',  ( 12.91533473730993009, 66.60535201082150536, -10.88017736071109987 ) ) ;
#40680=CARTESIAN_POINT ( 'NONE',  ( -0.2418659066527703572, 63.09014588040356841, 6.114288769123046308 ) ) ;
#40682=CARTESIAN_POINT ( 'NONE',  ( 19.89103541497709315, 45.66234555792569694, -6.479102184480826310 ) ) ;
#40684=CARTESIAN_POINT ( 'NONE',  ( 18.52753015748617571, 53.09226448433412315, 4.923371831947298993 ) ) ;
#40686=CARTESIAN_POINT ( 'NONE',  ( 6.565887622018943937, 5.165301336597086568, 12.81628187352647430 ) ) ;
#40687=CARTESIAN_POINT ( 'NONE',  ( -0.8801773607111009756, 18.06368534415484106, 1.068504757029289695E-15 ) ) ;
#40691=CARTESIAN_POINT ( 'NONE',  ( 20.36894250292379738, 29.92874883491396432, -10.36894250292379027 ) ) ;
#40692=CARTESIAN_POINT ( 'NONE',  ( -2.266590686148945544, 31.38708216824730002, -7.082119434687050408 ) ) ;
#40693=CARTESIAN_POINT ( 'NONE',  ( 6.204703633549690345, 57.84541550158063927, 14.16423886937410082 ) ) ;
#40694=CARTESIAN_POINT ( 'NONE',  ( 16.40814093676324603, 42.45696800326375353, -11.09922568453594671 ) ) ;
#40695=CARTESIAN_POINT ( 'NONE',  ( 4.559911319644449179, 17.23035201082150536, -9.422509992056141925 ) ) ;
#40697=CARTESIAN_POINT ( 'NONE',  ( 18.52753015748617571, 43.09226448433412315, 4.923371831947298993 ) ) ;
#40698=CARTESIAN_POINT ( 'NONE',  ( 19.42250999205614548, 35.98035201082151247, -5.440088680355545492 ) ) ;
#40699=CARTESIAN_POINT ( 'NONE',  ( 12.63842701281683922, 64.55059781766745175, -9.846743663894590881 ) ) ;
#40700=CARTESIAN_POINT ( 'NONE',  ( -4.164238869374098151, 26.59541550158063217, -3.795296366450310543 ) ) ;
#40701=CARTESIAN_POINT ( 'NONE',  ( 1.816707512666842605, 45.10290668512025292, -6.499999999999958256 ) ) ;
#40703=CARTESIAN_POINT ( 'NONE',  ( 19.84674366389459621, 18.50893115100078745, 7.409399052514197653E-17 ) ) ;
#40704=CARTESIAN_POINT ( 'NONE',  ( 0.6178305044545838731, 54.74863466993042493, 9.382169495545420901 ) ) ;
#40705=CARTESIAN_POINT ( 'NONE',  ( 1.472469842513823179, 50.59226448433411605, -4.923371831947296329 ) ) ;
#40707=CARTESIAN_POINT ( 'NONE',  ( 2.603489959281613420, 35.43575266056827644, -6.500000000000031086 ) ) ;
#40708=CARTESIAN_POINT ( 'NONE',  ( -0.8801773607111009756, 3.063685344154838397, 1.068504757029289695E-15 ) ) ;
#40709=CARTESIAN_POINT ( 'NONE',  ( 10.00000000000000000, 15.55374883491396787, -14.16423886937410082 ) ) ;
#40710=CARTESIAN_POINT ( 'NONE',  ( 19.84674366389459266, 3.717264484334118713, -2.638427012816827677 ) ) ;
#40711=CARTESIAN_POINT ( 'NONE',  ( 5.076628168052704559, 55.17559781766745175, -8.527530157486179263 ) ) ;
#40712=CARTESIAN_POINT ( 'NONE',  ( 19.42250999205614548, 25.98035201082150891, -5.440088680355545492 ) ) ;
#40714=CARTESIAN_POINT ( 'NONE',  ( 1.472469842513823179, 61.42559781766745175, 4.923371831947296329 ) ) ;
#40716=EDGE_CURVE ( 'NONE', #63612, #56374, #31827, .T. ) ;
#40717=CARTESIAN_POINT ( 'NONE',  ( 2.791683348922237240, 0.3839311510007847872, -7.208316651077763204 ) ) ;
#40718=CARTESIAN_POINT ( 'NONE',  ( 0.2751277870542967463, 70.00000000000000000, 6.000000000000000000 ) ) ;
#40722=CARTESIAN_POINT ( 'NONE',  ( -0.3689425029237898834, 11.17874883491396787, -10.36894250292378850 ) ) ;
#40723=( GEOMETRIC_REPRESENTATION_CONTEXT ( 3 ) GLOBAL_UNCERTAINTY_ASSIGNED_CONTEXT ( ( #44461 ) ) GLOBAL_UNIT_ASSIGNED_CONTEXT ( ( #75827, #90318, #7840 ) ) REPRESENTATION_CONTEXT ( 'NONE', 'WORKASPACE' ) );
#40724=CARTESIAN_POINT ( 'NONE',  ( 20.36894250292379382, 38.67874883491396076, 10.36894250292379205 ) ) ;
#40725=CARTESIAN_POINT ( 'NONE',  ( 18.52753015748618282, 53.92559781766745175, -4.923371831947291888 ) ) ;
#40726=CARTESIAN_POINT ( 'NONE',  ( 12.63842701281683034, 17.46726448433411250, 9.846743663894596210 ) ) ;
#40728=CARTESIAN_POINT ( 'NONE',  ( 7.084665262690076126, 17.02201867748817676, -10.88017736071110164 ) ) ;
#40729=CARTESIAN_POINT ( 'NONE',  ( 14.92337183194729988, 64.34226448433412315, -8.527530157486177487 ) ) ;
#40730=CARTESIAN_POINT ( 'NONE',  ( 10.00000000000000000, 40.55374883491397497, -14.16423886937410082 ) ) ;
#40732=CARTESIAN_POINT ( 'NONE',  ( -0.8801773607111008646, 3.272018677488171434, 2.915334737309923430 ) ) ;
#40735=CARTESIAN_POINT ( 'NONE',  ( 0.5774900079438607392, 58.48035201082151247, 5.440088680355550821 ) ) ;
#40736=CARTESIAN_POINT ( 'NONE',  ( 0.1532563361054083140, 16.00893115100078390, 1.131784320476157264E-15 ) ) ;
#40739=CARTESIAN_POINT ( 'NONE',  ( 10.00000000000000178, 65.37363466993042493, 12.81628187352647608 ) ) ;
#40741=CARTESIAN_POINT ( 'NONE',  ( 18.52753015748618282, 23.92559781766745530, -4.923371831947291888 ) ) ;
#40743=CARTESIAN_POINT ( 'NONE',  ( -4.164238869374099927, 32.01208216824730357, 3.795296366450308767 ) ) ;
#40744=CARTESIAN_POINT ( 'NONE',  ( 1.472469842513823179, 30.59226448433411960, -4.923371831947296329 ) ) ;
#40745=CARTESIAN_POINT ( 'NONE',  ( 0.5774900079438607392, 38.48035201082150536, 5.440088680355550821 ) ) ;
#40748=CARTESIAN_POINT ( 'NONE',  ( 7.084665262690076126, 37.02201867748817676, -10.88017736071110164 ) ) ;
#40749=CARTESIAN_POINT ( 'NONE',  ( 19.88565890683628368, 37.71691075486301514, -6.480892540919849232 ) ) ;
#40752=ORIENTED_EDGE ( 'NONE', *, *, #41663, .T. ) ;
#40753=CARTESIAN_POINT ( 'NONE',  ( -0.8801773607110991993, 42.85535201082150536, -2.915334737309923874 ) ) ;
#40754=CARTESIAN_POINT ( 'NONE',  ( 6.204703633549690345, 10.76208216824729824, -14.16423886937410259 ) ) ;
#40757=CARTESIAN_POINT ( 'NONE',  ( 21.09922568453595559, 37.04030133659708923, -6.408140936763230044 ) ) ;
#40758=SURFACE_STYLE_FILL_AREA ( #64218 ) ;
#40759=CARTESIAN_POINT ( 'NONE',  ( 0.1532563361054082862, 21.21726448433412315, 2.638427012816831674 ) ) ;
#40760=( NAMED_UNIT ( * ) PLANE_ANGLE_UNIT ( ) SI_UNIT ( $, .RADIAN. ) );
#40761=ADVANCED_FACE ( 'NONE', ( #85455 ), #10458, .T. ) ;
#40762=CARTESIAN_POINT ( 'NONE',  ( 14.92337183194729988, 34.34226448433411605, -8.527530157486177487 ) ) ;
#40763=AXIS2_PLACEMENT_3D ( 'NONE', #61319, #22359, #29829 ) ;
#40764=CARTESIAN_POINT ( 'NONE',  ( 10.00000000000000178, 59.31368534415484106, 10.88017736071110342 ) ) ;
#40769=CARTESIAN_POINT ( 'NONE',  ( 20.88017736071110164, 65.35535201082150536, 2.915334737309930979 ) ) ;
#40770=CARTESIAN_POINT ( 'NONE',  ( 18.72515096720583827, 30.05509018479937566, 6.499999999999810818 ) ) ;
#40773=CARTESIAN_POINT ( 'NONE',  ( 0.1532563361054100626, 5.800597817667452638, -2.638427012816831230 ) ) ;
#40774=EDGE_CURVE ( 'NONE', #24283, #70171, #73618, .T. ) ;
#40775=CARTESIAN_POINT ( 'NONE',  ( 10.00000000000000178, 15.37363466993042138, 12.81628187352647608 ) ) ;
#40776=DIRECTION ( 'NONE',  ( 0.000000000000000000, -1.000000000000000000, 0.000000000000000000 ) ) ;
#40778=CARTESIAN_POINT ( 'NONE',  ( 0.1532563361054100626, 50.80059781766745175, -2.638427012816831230 ) ) ;
#40779=CARTESIAN_POINT ( 'NONE',  ( 19.42250999205614548, 35.98035201082151247, -5.440088680355545492 ) ) ;
#40780=CARTESIAN_POINT ( 'NONE',  ( 24.16423886937410614, 4.512082168247300906, -3.795296366450302550 ) ) ;
#40781=CARTESIAN_POINT ( 'NONE',  ( 18.52753015748617571, 28.09226448433411960, 4.923371831947298993 ) ) ;
#40782=CARTESIAN_POINT ( 'NONE',  ( -2.816281873526473856, 34.33196800326376064, 3.434112377981055619 ) ) ;
#40785=CARTESIAN_POINT ( 'NONE',  ( 7.084665262690076126, 49.10535201082149825, 10.88017736071109987 ) ) ;
#40786=CARTESIAN_POINT ( 'NONE',  ( 22.81628187352647785, 1.623634669930420271, 6.195893100308588602E-16 ) ) ;
#40788=CARTESIAN_POINT ( 'NONE',  ( 5.076628168052704559, 15.17559781766745175, -8.527530157486179263 ) ) ;
#40789=CARTESIAN_POINT ( 'NONE',  ( 17.96484262340118221, 24.93868534415484461, 7.964842623401181321 ) ) ;
#40790=CARTESIAN_POINT ( 'NONE',  ( 0.6178305044545818747, 23.49863466993041783, -9.382169495545419124 ) ) ;
#40792=B_SPLINE_CURVE_WITH_KNOTS ( 'NONE', 3,
 ( #53715, #75233, #38724, #30216, #91216, #30707 ),
 .UNSPECIFIED., .F., .F.,
 ( 4, 2, 4 ),
 ( 0.000000000000000000, 0.0002701661927229225967, 0.0005403323854458451933 ),
 .UNSPECIFIED. ) ;
#40795=CARTESIAN_POINT ( 'NONE',  ( 20.88017736071110164, 15.35535201082150358, 2.915334737309930979 ) ) ;
#40798=CARTESIAN_POINT ( 'NONE',  ( 0.5774900079438590739, 67.64701867748817676, -5.440088680355550821 ) ) ;
#40799=CARTESIAN_POINT ( 'NONE',  ( 5.076628168052704559, 45.17559781766745175, -8.527530157486179263 ) ) ;
#40800=CARTESIAN_POINT ( 'NONE',  ( 17.96484262340118221, 36.18868534415484106, -7.964842623401177768 ) ) ;
#40802=EDGE_CURVE ( 'NONE', #83218, #14105, #20671, .T. ) ;
#40803=CARTESIAN_POINT ( 'NONE',  ( 0.5774900079438590739, 52.64701867748817676, -5.440088680355550821 ) ) ;
#40804=CARTESIAN_POINT ( 'NONE',  ( 7.084665262690076126, 9.105352010821503583, 10.88017736071109987 ) ) ;
#40807=CARTESIAN_POINT ( 'NONE',  ( 1.472469842513823179, 36.42559781766745175, 4.923371831947296329 ) ) ;
#40810=CARTESIAN_POINT ( 'NONE',  ( 16.40814093676324603, 2.456968003263753531, -11.09922568453594671 ) ) ;
#40811=CARTESIAN_POINT ( 'NONE',  ( 20.15039907845753575, 50.60158574516642460, -6.262539305110073506 ) ) ;
#40813=CARTESIAN_POINT ( 'NONE',  ( 10.00000000000000178, 28.05374883491396787, 14.16423886937410082 ) ) ;
#40816=CARTESIAN_POINT ( 'NONE',  ( 10.00000000000000000, 60.55374883491397497, -14.16423886937410082 ) ) ;
#40817=CARTESIAN_POINT ( 'NONE',  ( 2.791683348922240793, 21.63393115100078745, 7.208316651077764092 ) ) ;
#40820=CARTESIAN_POINT ( 'NONE',  ( 15.44008868035555260, 54.73035201082150536, 9.422509992056143702 ) ) ;
#40821=CARTESIAN_POINT ( 'NONE',  ( 0.6178305044545838731, 59.74863466993041783, 9.382169495545420901 ) ) ;
#40822=CARTESIAN_POINT ( 'NONE',  ( 0.5774900079438607392, 28.48035201082150891, 5.440088680355550821 ) ) ;
#40823=CARTESIAN_POINT ( 'NONE',  ( 16.40814093676324603, 62.45696800326376064, -11.09922568453594671 ) ) ;
#40824=CARTESIAN_POINT ( 'NONE',  ( 16.40814093676323893, 5.790301336597087456, 11.09922568453595026 ) ) ;
#40825=CARTESIAN_POINT ( 'NONE',  ( 12.63842701281683922, 9.550597817667449974, -9.846743663894590881 ) ) ;
#40826=ORIENTED_EDGE ( 'NONE', *, *, #27524, .F. ) ;
#40828=CARTESIAN_POINT ( 'NONE',  ( 22.26659068614894466, 58.88708216824729647, 7.082119434687054849 ) ) ;
#40829=CARTESIAN_POINT ( 'NONE',  ( 2.917880565312950480, 30.97041550158063572, -12.26659068614894821 ) ) ;
#40830=CARTESIAN_POINT ( 'NONE',  ( 17.96484262340118221, 14.93868534415483751, 7.964842623401181321 ) ) ;
#40831=CARTESIAN_POINT ( 'NONE',  ( 19.42250999205614193, 50.14701867748817676, 5.440088680355555262 ) ) ;
#40833=CARTESIAN_POINT ( 'NONE',  ( 0.1532563361054083140, 11.00893115100078568, 1.131784320476157264E-15 ) ) ;
#40834=( LENGTH_UNIT ( ) NAMED_UNIT ( * ) SI_UNIT ( .MILLI., .METRE. ) );
#40835=CARTESIAN_POINT ( 'NONE',  ( 5.076628168052703671, 16.84226448433411960, 8.527530157486179263 ) ) ;
#40836=SURFACE_STYLE_USAGE ( .BOTH. , #41827 ) ;
#40837=DIRECTION ( 'NONE',  ( 0.000000000000000000, -1.000000000000000000, 0.000000000000000000 ) ) ;
#40838=CARTESIAN_POINT ( 'NONE',  ( 5.076628168052704559, 20.17559781766745175, -8.527530157486179263 ) ) ;
#40839=CARTESIAN_POINT ( 'NONE',  ( 0.1532563361054083140, 51.00893115100078745, 1.131784320476157264E-15 ) ) ;
#40841=CARTESIAN_POINT ( 'NONE',  ( 0.5774900079438590739, 27.64701867748817676, -5.440088680355550821 ) ) ;
#40842=CARTESIAN_POINT ( 'NONE',  ( 16.40814093676324603, 37.45696800326376064, -11.09922568453594671 ) ) ;
#40844=CARTESIAN_POINT ( 'NONE',  ( -0.8801773607111009756, 58.06368534415484106, 1.068504757029289695E-15 ) ) ;
#40845=CARTESIAN_POINT ( 'NONE',  ( 17.20831665107776587, 27.88393115100078390, 7.208316651077764980 ) ) ;
#40846=CARTESIAN_POINT ( 'NONE',  ( -4.164238869374099927, 47.01208216824729647, 3.795296366450308767 ) ) ;
#40847=CARTESIAN_POINT ( 'NONE',  ( 1.472469842513823179, 16.42559781766745175, 4.923371831947296329 ) ) ;
#40849=CARTESIAN_POINT ( 'NONE',  ( 5.076628168052703671, 56.84226448433412315, 8.527530157486179263 ) ) ;
#40850=CARTESIAN_POINT ( 'NONE',  ( 18.52753015748617571, 48.09226448433412315, 4.923371831947298993 ) ) ;
#40851=CARTESIAN_POINT ( 'NONE',  ( 20.36894250292379738, 29.92874883491396432, -10.36894250292379027 ) ) ;
#40852=CARTESIAN_POINT ( 'NONE',  ( 19.84674366389459266, 28.30059781766745886, 2.638427012816836559 ) ) ;
#40853=CARTESIAN_POINT ( 'NONE',  ( 15.44008868035555793, 46.39701867748817676, -9.422509992056140149 ) ) ;
#40854=CARTESIAN_POINT ( 'NONE',  ( 10.00000000000000000, 21.81368534415484106, -10.88017736071110342 ) ) ;
#40855=CARTESIAN_POINT ( 'NONE',  ( -0.8801773607111009756, 48.06368534415484817, 1.068504757029289695E-15 ) ) ;
#40856=CARTESIAN_POINT ( 'NONE',  ( 17.96484262340118221, 26.18868534415483396, -7.964842623401177768 ) ) ;
#40858=CARTESIAN_POINT ( 'NONE',  ( 16.40814093676323893, 30.79030133659708923, 11.09922568453595026 ) ) ;
#40859=CARTESIAN_POINT ( 'NONE',  ( 10.00000000000000178, 59.31368534415484106, 10.88017736071110342 ) ) ;
#40861=ADVANCED_FACE ( 'NONE', ( #49411 ), #6861, .T. ) ;
#40862=LINE ( 'NONE', #25858, #31429 ) ;
#40863=CARTESIAN_POINT ( 'NONE',  ( 4.559911319644449179, 67.23035201082150536, -9.422509992056141925 ) ) ;
#40867=CARTESIAN_POINT ( 'NONE',  ( 0.5774900079438590739, 62.64701867748817676, -5.440088680355550821 ) ) ;
#40868=( NAMED_UNIT ( * ) SI_UNIT ( $, .STERADIAN. ) SOLID_ANGLE_UNIT ( ) );
#40870=CARTESIAN_POINT ( 'NONE',  ( 2.377183314879983911, 25.78593319516823001, -6.500000000000031974 ) ) ;
#40872=CARTESIAN_POINT ( 'NONE',  ( -0.3689425029237898834, 56.17874883491396076, -10.36894250292378850 ) ) ;
#40873=CARTESIAN_POINT ( 'NONE',  ( 10.00000000000000000, 14.75893115100078568, -9.846743663894594434 ) ) ;
#40874=CARTESIAN_POINT ( 'NONE',  ( -0.3689425029237898834, 6.178748834913968757, -10.36894250292378850 ) ) ;
#40875=CARTESIAN_POINT ( 'NONE',  ( 1.472469842513823179, 1.425597817667451528, 4.923371831947296329 ) ) ;
#40876=CARTESIAN_POINT ( 'NONE',  ( 15.44008868035555260, 4.730352010821504471, 9.422509992056143702 ) ) ;
#40877=CARTESIAN_POINT ( 'NONE',  ( 5.076628168052704559, 40.17559781766745175, -8.527530157486179263 ) ) ;
#40879=CARTESIAN_POINT ( 'NONE',  ( 5.076628168052703671, 51.84226448433412315, 8.527530157486179263 ) ) ;
#40881=DIRECTION ( 'NONE',  ( 0.000000000000000000, 0.000000000000000000, -1.000000000000000000 ) ) ;
#40882=CARTESIAN_POINT ( 'NONE',  ( 10.00000000000000178, 59.31368534415484106, 10.88017736071110342 ) ) ;
#40883=CARTESIAN_POINT ( 'NONE',  ( 1.472469842513823179, 55.59226448433412315, -4.923371831947296329 ) ) ;
#40884=CARTESIAN_POINT ( 'NONE',  ( 10.00000000000000000, 27.87363466993042138, -12.81628187352647608 ) ) ;
#40885=( LENGTH_UNIT ( ) NAMED_UNIT ( * ) SI_UNIT ( .MILLI., .METRE. ) );
#40887=CARTESIAN_POINT ( 'NONE',  ( 12.91533473730992121, 54.52201867748816255, 10.88017736071110164 ) ) ;
#40888=CARTESIAN_POINT ( 'NONE',  ( 2.035157376598824452, 8.688685344154839285, 7.964842623401179544 ) ) ;
#40889=EDGE_CURVE ( 'NONE', #64701, #12669, #30887, .T. ) ;
#40891=CARTESIAN_POINT ( 'NONE',  ( 22.81628187352647785, 36.41530133659707502, 3.434112377981063169 ) ) ;
#40892=CARTESIAN_POINT ( 'NONE',  ( -0.1503990784575328643, 10.12777174578612716, 6.262539305110068177 ) ) ;
#40894=CARTESIAN_POINT ( 'NONE',  ( 0.6178305044545818747, 33.49863466993042493, -9.382169495545419124 ) ) ;
#40895=CARTESIAN_POINT ( 'NONE',  ( 0.5774900079438590739, 32.64701867748816966, -5.440088680355550821 ) ) ;
#40898=CARTESIAN_POINT ( 'NONE',  ( -1.099225684535947600, -1.293031996736246469, -6.408140936763238038 ) ) ;
#40899=CARTESIAN_POINT ( 'NONE',  ( 12.63842701281683922, 9.550597817667449974, -9.846743663894590881 ) ) ;
#40900=CARTESIAN_POINT ( 'NONE',  ( 0.1532563361054083140, 56.00893115100078745, 1.131784320476157264E-15 ) ) ;
#40903=CARTESIAN_POINT ( 'NONE',  ( 17.20831665107776587, 42.88393115100077324, 7.208316651077764980 ) ) ;
#40904=CARTESIAN_POINT ( 'NONE',  ( -0.1503990784575247319, 52.22266099184918176, -6.262539305110083276 ) ) ;
#40908=CARTESIAN_POINT ( 'NONE',  ( 17.20831665107776587, 24.13393115100078035, -7.208316651077762316 ) ) ;
#40909=FILL_AREA_STYLE_COLOUR ( '', #78655 ) ;
#40911=CARTESIAN_POINT ( 'NONE',  ( 7.361572987183170547, 62.05059781766745886, 9.846743663894590881 ) ) ;
#40914=CARTESIAN_POINT ( 'NONE',  ( 10.00000000000000000, 22.87363466993042138, -12.81628187352647608 ) ) ;
#40915=CARTESIAN_POINT ( 'NONE',  ( 1.472469842513823179, 50.59226448433411605, -4.923371831947296329 ) ) ;
#40917=CARTESIAN_POINT ( 'NONE',  ( 22.17874357816322117, 89.00000000000000000, -12.00000000000000000 ) ) ;
#40918=CARTESIAN_POINT ( 'NONE',  ( 24.16423886937410614, 49.30374883491396787, 8.672049930838204340E-16 ) ) ;
#40919=CARTESIAN_POINT ( 'NONE',  ( 14.92337183194729988, 14.34226448433411782, -8.527530157486177487 ) ) ;
#40923=CARTESIAN_POINT ( 'NONE',  ( -0.3689425029237881626, 42.42874883491396787, 10.36894250292379027 ) ) ;
#40924=CARTESIAN_POINT ( 'NONE',  ( 5.076628168052704559, 60.17559781766745175, -8.527530157486179263 ) ) ;
#40926=CARTESIAN_POINT ( 'NONE',  ( -0.8801773607110991993, 12.85535201082150358, -2.915334737309923874 ) ) ;
#40927=CARTESIAN_POINT ( 'NONE',  ( 13.79529636645030344, 28.26208216824729647, 14.16423886937410614 ) ) ;
#40928=CARTESIAN_POINT ( 'NONE',  ( 13.79529636645031943, 35.34541550158063927, -14.16423886937409904 ) ) ;
#40929=FILL_AREA_STYLE_COLOUR ( '', #94679 ) ;
#40930=CARTESIAN_POINT ( 'NONE',  ( 0.5774900079438590739, 27.64701867748817676, -5.440088680355550821 ) ) ;
#40931=CARTESIAN_POINT ( 'NONE',  ( 14.92337183194729988, 49.34226448433411605, -8.527530157486177487 ) ) ;
#40933=CARTESIAN_POINT ( 'NONE',  ( 20.88017736071110164, 40.35535201082150536, 2.915334737309930979 ) ) ;
#40934=CARTESIAN_POINT ( 'NONE',  ( 19.88565890683628012, 22.71691075486302580, -6.480892540919844791 ) ) ;
#40939=CARTESIAN_POINT ( 'NONE',  ( 2.791683348922237240, 50.38393115100078035, -7.208316651077763204 ) ) ;
#40940=CARTESIAN_POINT ( 'NONE',  ( 1.472469842513823179, 61.42559781766745175, 4.923371831947296329 ) ) ;
#40942=CARTESIAN_POINT ( 'NONE',  ( 10.00000000000000178, 33.05374883491396787, 14.16423886937410082 ) ) ;
#40945=DIRECTION ( 'NONE',  ( 0.000000000000000000, -1.000000000000000000, 0.000000000000000000 ) ) ;
#40946=CARTESIAN_POINT ( 'NONE',  ( 12.91533473730993009, 6.605352010821504471, -10.88017736071109987 ) ) ;
#40947=CARTESIAN_POINT ( 'NONE',  ( 13.43411237798105340, 25.58196800326374998, 12.81628187352647963 ) ) ;
#40949=CARTESIAN_POINT ( 'NONE',  ( 1.472469842513823179, 11.42559781766745175, 4.923371831947296329 ) ) ;
#40950=FACE_OUTER_BOUND ( 'NONE', #76925, .T. ) ;
#40951=B_SPLINE_CURVE_WITH_KNOTS ( 'NONE', 3,
 ( #58592, #89094, #20609, #19613, #83079, #38089 ),
 .UNSPECIFIED., .F., .F.,
 ( 4, 2, 4 ),
 ( 6.705420115022808671E-18, 0.0002626113303185853608, 0.0005252226606371639996 ),
 .UNSPECIFIED. ) ;
#40952=CARTESIAN_POINT ( 'NONE',  ( -0.2418659066527783508, 9.260286857231744051, -6.114288769123032985 ) ) ;
#40954=CARTESIAN_POINT ( 'NONE',  ( 19.42250999205614193, 5.147018677488171434, 5.440088680355555262 ) ) ;
#40956=CARTESIAN_POINT ( 'NONE',  ( 17.96484262340118221, 34.93868534415482685, 7.964842623401181321 ) ) ;
#40957=CARTESIAN_POINT ( 'NONE',  ( 12.91533473730992121, 34.52201867748817676, 10.88017736071110164 ) ) ;
#40958=CARTESIAN_POINT ( 'NONE',  ( 0.6178305044545838731, 4.748634669930420493, 9.382169495545420901 ) ) ;
#40959=CARTESIAN_POINT ( 'NONE',  ( 5.076628168052703671, 61.84226448433412315, 8.527530157486179263 ) ) ;
#40960=CARTESIAN_POINT ( 'NONE',  ( 19.38216949554541202, 60.99863466993042493, 9.382169495545424454 ) ) ;
#40961=CARTESIAN_POINT ( 'NONE',  ( 19.84674366389459621, 13.50893115100078568, 7.409399052514197653E-17 ) ) ;
#40962=EDGE_LOOP ( 'NONE', ( #6797, #2517, #90317, #81222 ) ) ;
#40963=CARTESIAN_POINT ( 'NONE',  ( 7.084665262690076126, 37.02201867748817676, -10.88017736071110164 ) ) ;
#40964=CARTESIAN_POINT ( 'NONE',  ( 22.81628187352647785, 36.41530133659707502, 3.434112377981063169 ) ) ;
#40966=CARTESIAN_POINT ( 'NONE',  ( -0.3289641300568005855, 54.27164270246084499, -5.963430220938281678 ) ) ;
#40969=CARTESIAN_POINT ( 'NONE',  ( 19.84674366389459621, 63.50893115100078745, 7.409399052514197653E-17 ) ) ;
#40970=CARTESIAN_POINT ( 'NONE',  ( 0.5774900079438590739, 67.64701867748817676, -5.440088680355550821 ) ) ;
#40971=CARTESIAN_POINT ( 'NONE',  ( 14.92337183194729633, 17.67559781766745175, 8.527530157486181039 ) ) ;
#40972=CARTESIAN_POINT ( 'NONE',  ( 3.591859063236763294, 33.29030133659708213, -11.09922568453595026 ) ) ;
#40973=CARTESIAN_POINT ( 'NONE',  ( 20.88017736071110875, 55.77201867748816966, -2.915334737309920765 ) ) ;
#40976=CARTESIAN_POINT ( 'NONE',  ( 2.035157376598824452, 8.688685344154839285, 7.964842623401179544 ) ) ;
#40977=CARTESIAN_POINT ( 'NONE',  ( 10.00000000000000178, 65.37363466993042493, 12.81628187352647608 ) ) ;
#40978=CARTESIAN_POINT ( 'NONE',  ( -2.266590686148945544, 26.38708216824730357, -7.082119434687050408 ) ) ;
#40979=CARTESIAN_POINT ( 'NONE',  ( 12.63842701281683034, 22.46726448433411605, 9.846743663894596210 ) ) ;
#40980=SURFACE_STYLE_USAGE ( .BOTH. , #98554 ) ;
#40981=CARTESIAN_POINT ( 'NONE',  ( 0.1532563361054083140, 16.00893115100078390, 1.131784320476157264E-15 ) ) ;
#40982=CARTESIAN_POINT ( 'NONE',  ( 22.26659068614895176, 59.72041550158063927, -7.082119434687042414 ) ) ;
#40985=CARTESIAN_POINT ( 'NONE',  ( 19.42250999205614548, 15.98035201082150714, -5.440088680355545492 ) ) ;
#40986=ADVANCED_FACE ( 'NONE', ( #51890 ), #37333, .T. ) ;
#40987=CARTESIAN_POINT ( 'NONE',  ( 17.96484262340118221, 14.93868534415483751, 7.964842623401181321 ) ) ;
#40988=CARTESIAN_POINT ( 'NONE',  ( 20.10384461210892226, 46.74302437010791778, 6.337995344473753789 ) ) ;
#40989=VERTEX_POINT ( 'NONE', #93635 ) ;
#40991=VERTEX_POINT ( 'NONE', #86145 ) ;
#40992=CARTESIAN_POINT ( 'NONE',  ( 12.91533473730993009, 21.60535201082150536, -10.88017736071109987 ) ) ;
#40993=CARTESIAN_POINT ( 'NONE',  ( 7.361572987183170547, 52.05059781766745175, 9.846743663894590881 ) ) ;
#40994=CARTESIAN_POINT ( 'NONE',  ( 3.591859063236761518, 49.95696800326375353, 11.09922568453594849 ) ) ;
#40995=CARTESIAN_POINT ( 'NONE',  ( -0.8801773607111009756, 68.06368534415484817, 1.068504757029289695E-15 ) ) ;
#40996=CARTESIAN_POINT ( 'NONE',  ( 10.00000000000000178, 18.05374883491396787, 14.16423886937410082 ) ) ;
#40997=CARTESIAN_POINT ( 'NONE',  ( -0.8801773607111009756, 33.06368534415484106, 1.068504757029289695E-15 ) ) ;
#40998=CARTESIAN_POINT ( 'NONE',  ( 0.5774900079438590739, 22.64701867748817321, -5.440088680355550821 ) ) ;
#40999=CARTESIAN_POINT ( 'NONE',  ( 7.361572987183169658, 54.96726448433413026, -9.846743663894592657 ) ) ;
#41001=CARTESIAN_POINT ( 'NONE',  ( 18.52753015748618282, 38.92559781766745175, -4.923371831947291888 ) ) ;
#41002=CARTESIAN_POINT ( 'NONE',  ( 10.00000000000000000, 4.758931151000784787, -9.846743663894594434 ) ) ;
#41004=ORIENTED_EDGE ( 'NONE', *, *, #46732, .T. ) ;
#41005=CARTESIAN_POINT ( 'NONE',  ( 4.559911319644449179, 2.230352010821504471, -9.422509992056141925 ) ) ;
#41006=CARTESIAN_POINT ( 'NONE',  ( 0.1532563361054083140, 11.00893115100078568, 1.131784320476157264E-15 ) ) ;
#41007=CARTESIAN_POINT ( 'NONE',  ( 0.6178305044545838731, -0.2513653300695798953, 9.382169495545420901 ) ) ;
#41008=CARTESIAN_POINT ( 'NONE',  ( 17.96484262340118221, 49.93868534415484106, 7.964842623401181321 ) ) ;
#41009=CARTESIAN_POINT ( 'NONE',  ( 20.88017736071110164, 45.35535201082149115, 2.915334737309930979 ) ) ;
#41010=CARTESIAN_POINT ( 'NONE',  ( 20.88017736071110875, 15.77201867748817143, -2.915334737309920765 ) ) ;
#41011=CARTESIAN_POINT ( 'NONE',  ( 16.40814093676324603, 42.45696800326375353, -11.09922568453594671 ) ) ;
#41012=CARTESIAN_POINT ( 'NONE',  ( 2.917880565312950480, 25.97041550158063572, -12.26659068614894821 ) ) ;
#41014=EDGE_CURVE ( 'NONE', #47240, #39693, #23692, .T. ) ;
#41016=CARTESIAN_POINT ( 'NONE',  ( 21.09922568453595559, 62.04030133659709634, -6.408140936763230044 ) ) ;
#41018=CARTESIAN_POINT ( 'NONE',  ( 14.92337183194729988, 59.34226448433412315, -8.527530157486177487 ) ) ;
#41020=CARTESIAN_POINT ( 'NONE',  ( 15.44008868035555260, 39.73035201082150536, 9.422509992056143702 ) ) ;
#41022=CARTESIAN_POINT ( 'NONE',  ( 1.472469842513823179, 1.425597817667451528, 4.923371831947296329 ) ) ;
#41023=DIRECTION ( 'NONE',  ( 0.000000000000000000, -1.000000000000000000, 0.000000000000000000 ) ) ;
#41024=CARTESIAN_POINT ( 'NONE',  ( 5.076628168052703671, 26.84226448433411960, 8.527530157486179263 ) ) ;
#41025=CARTESIAN_POINT ( 'NONE',  ( 7.084665262690076126, 67.02201867748817676, -10.88017736071110164 ) ) ;
#41026=CARTESIAN_POINT ( 'NONE',  ( 7.361572987183170547, 2.050597817667451750, 9.846743663894590881 ) ) ;
#41027=CARTESIAN_POINT ( 'NONE',  ( 7.084665262690076126, 62.02201867748816966, -10.88017736071110164 ) ) ;
#41029=CARTESIAN_POINT ( 'NONE',  ( 12.91533473730992121, 59.52201867748816966, 10.88017736071110164 ) ) ;
#41030=CARTESIAN_POINT ( 'NONE',  ( 0.1532563361054082862, 11.21726448433411605, 2.638427012816831674 ) ) ;
#41035=CARTESIAN_POINT ( 'NONE',  ( 19.84674366389459621, 53.50893115100078745, 7.409399052514197653E-17 ) ) ;
#41038=DIRECTION ( 'NONE',  ( 0.000000000000000000, 0.000000000000000000, -1.000000000000000000 ) ) ;
#41039=CARTESIAN_POINT ( 'NONE',  ( -4.164238869374099039, 6.803748834913967869, 8.674139862899312516E-16 ) ) ;
#41040=CARTESIAN_POINT ( 'NONE',  ( 6.565887622018943937, 55.16530133659709634, 12.81628187352647430 ) ) ;
#41041=CARTESIAN_POINT ( 'NONE',  ( -0.3689425029237881626, 7.428748834913967869, 10.36894250292379027 ) ) ;
#41042=CARTESIAN_POINT ( 'NONE',  ( 2.917880565312948704, 32.63708216824730357, 12.26659068614894643 ) ) ;
#41044=CARTESIAN_POINT ( 'NONE',  ( 24.16423886937409904, 4.095415501580634832, 3.795296366450317205 ) ) ;
#41045=CARTESIAN_POINT ( 'NONE',  ( -0.8801773607111008646, 23.27201867748817676, 2.915334737309923430 ) ) ;
#41047=ORIENTED_EDGE ( 'NONE', *, *, #9761, .F. ) ;
#41048=CARTESIAN_POINT ( 'NONE',  ( 18.52753015748617571, 23.09226448433411960, 4.923371831947298993 ) ) ;
#41049=CARTESIAN_POINT ( 'NONE',  ( 14.92337183194729633, 17.67559781766745175, 8.527530157486181039 ) ) ;
#41050=CARTESIAN_POINT ( 'NONE',  ( 3.591859063236761518, 49.95696800326375353, 11.09922568453594849 ) ) ;
#41051=CARTESIAN_POINT ( 'NONE',  ( 12.63842701281683922, 34.55059781766745886, -9.846743663894590881 ) ) ;
#41053=CARTESIAN_POINT ( 'NONE',  ( 12.91533473730993009, 56.60535201082151247, -10.88017736071109987 ) ) ;
#41054=CARTESIAN_POINT ( 'NONE',  ( 0.6178305044545818747, 33.49863466993042493, -9.382169495545419124 ) ) ;
#41057=CARTESIAN_POINT ( 'NONE',  ( 10.00000000000000178, 27.25893115100078390, 9.846743663894594434 ) ) ;
#41058=CARTESIAN_POINT ( 'NONE',  ( -2.266590686148945544, 11.38708216824730179, -7.082119434687050408 ) ) ;
#41061=CARTESIAN_POINT ( 'NONE',  ( 20.88017736071110875, 30.77201867748816966, -2.915334737309920765 ) ) ;
#41062=CARTESIAN_POINT ( 'NONE',  ( 2.917880565312948704, 27.63708216824730357, 12.26659068614894643 ) ) ;
#41063=CARTESIAN_POINT ( 'NONE',  ( 18.52753015748617571, 48.09226448433412315, 4.923371831947298993 ) ) ;
#41064=CARTESIAN_POINT ( 'NONE',  ( 1.472469842513823179, 10.59226448433411782, -4.923371831947296329 ) ) ;
#41065=CARTESIAN_POINT ( 'NONE',  ( 13.43411237798106583, 47.66530133659709634, -12.81628187352647252 ) ) ;
#41066=DIRECTION ( 'NONE',  ( 0.000000000000000000, -1.000000000000000000, 0.000000000000000000 ) ) ;
#41067=CARTESIAN_POINT ( 'NONE',  ( 17.96484262340118221, 34.93868534415482685, 7.964842623401181321 ) ) ;
#41069=CARTESIAN_POINT ( 'NONE',  ( 3.591859063236763294, 18.29030133659708568, -11.09922568453595026 ) ) ;
#41070=CARTESIAN_POINT ( 'NONE',  ( 13.43411237798106583, 17.66530133659708923, -12.81628187352647252 ) ) ;
#41071=CARTESIAN_POINT ( 'NONE',  ( 2.791683348922240793, 36.63393115100078035, 7.208316651077764092 ) ) ;
#41074=LINE ( 'NONE', #79051, #66324 ) ;
#41077=CARTESIAN_POINT ( 'NONE',  ( 10.00000000000000178, 70.00000000000000000, 0.000000000000000000 ) ) ;
#41078=CARTESIAN_POINT ( 'NONE',  ( 19.42250999205614193, 50.14701867748817676, 5.440088680355555262 ) ) ;
#41079=CARTESIAN_POINT ( 'NONE',  ( 10.00000000000000000, 61.81368534415484106, -10.88017736071110342 ) ) ;
#41082=CARTESIAN_POINT ( 'NONE',  ( 1.472469842513823179, 21.42559781766745175, 4.923371831947296329 ) ) ;
#41084=CARTESIAN_POINT ( 'NONE',  ( 10.00000000000000000, 26.81368534415484106, -10.88017736071110342 ) ) ;
#41085=CARTESIAN_POINT ( 'NONE',  ( 13.43411237798105340, 0.5819680032637533085, 12.81628187352647963 ) ) ;
#41086=CARTESIAN_POINT ( 'NONE',  ( 17.96484262340118221, 26.18868534415483396, -7.964842623401177768 ) ) ;
#41089=CARTESIAN_POINT ( 'NONE',  ( 22.81628187352647785, 21.41530133659708923, 3.434112377981063169 ) ) ;
#41090=EDGE_LOOP ( 'NONE', ( #34111, #18473, #12602, #45200 ) ) ;
#41091=CARTESIAN_POINT ( 'NONE',  ( 7.084665262690076126, 52.02201867748816255, -10.88017736071110164 ) ) ;
#41092=CARTESIAN_POINT ( 'NONE',  ( 10.00000000000000178, 37.25893115100078745, 9.846743663894594434 ) ) ;
#41093=CARTESIAN_POINT ( 'NONE',  ( 22.81628187352647785, 16.62363466993042138, 6.195893100308588602E-16 ) ) ;
#41095=CARTESIAN_POINT ( 'NONE',  ( 0.5774900079438590739, 27.64701867748817676, -5.440088680355550821 ) ) ;
#41096=CARTESIAN_POINT ( 'NONE',  ( 17.96484262340118221, 34.93868534415482685, 7.964842623401181321 ) ) ;
#41097=CARTESIAN_POINT ( 'NONE',  ( 17.08211943468705840, 50.13708216824730357, -12.26659068614894466 ) ) ;
#41099=CARTESIAN_POINT ( 'NONE',  ( 5.076628168052703671, 41.84226448433411605, 8.527530157486179263 ) ) ;
#41100=CARTESIAN_POINT ( 'NONE',  ( 10.00000000000000000, 61.81368534415484106, -10.88017736071110342 ) ) ;
#41101=CARTESIAN_POINT ( 'NONE',  ( 2.035157376598824452, 43.68868534415484106, 7.964842623401179544 ) ) ;
#41103=CARTESIAN_POINT ( 'NONE',  ( 6.204703633549690345, 12.84541550158063572, 14.16423886937410082 ) ) ;
#41111=ORIENTED_EDGE ( 'NONE', *, *, #72012, .T. ) ;
#41112=CARTESIAN_POINT ( 'NONE',  ( -4.164238869374098151, 51.59541550158063217, -3.795296366450310543 ) ) ;
#41113=CARTESIAN_POINT ( 'NONE',  ( 2.917880565312950480, 50.97041550158064638, -12.26659068614894821 ) ) ;
#41114=CARTESIAN_POINT ( 'NONE',  ( 2.791683348922237240, 10.38393115100078390, -7.208316651077763204 ) ) ;
#41115=CARTESIAN_POINT ( 'NONE',  ( 10.00000000000000000, 12.87363466993042138, -12.81628187352647608 ) ) ;
#41117=CARTESIAN_POINT ( 'NONE',  ( 19.72487221294570858, 70.00000000000000000, -6.000000000000000000 ) ) ;
#41118=CARTESIAN_POINT ( 'NONE',  ( 4.559911319644449179, 2.230352010821504471, -9.422509992056141925 ) ) ;
#41119=CARTESIAN_POINT ( 'NONE',  ( -2.816281873526471635, 33.91530133659708213, -3.434112377981056508 ) ) ;
#41120=CARTESIAN_POINT ( 'NONE',  ( -0.3689425029237881626, 42.42874883491396787, 10.36894250292379027 ) ) ;
#41122=FILL_AREA_STYLE_COLOUR ( '', #9063 ) ;
#41124=EDGE_LOOP ( 'NONE', ( #75625, #92174, #16979, #41619 ) ) ;
#41126=CARTESIAN_POINT ( 'NONE',  ( 14.92337183194729633, 22.67559781766745175, 8.527530157486181039 ) ) ;
#41129=CARTESIAN_POINT ( 'NONE',  ( -2.266590686148945544, 12.22041550158063394, 7.082119434687048631 ) ) ;
#41130=CARTESIAN_POINT ( 'NONE',  ( 12.91533473730993009, 11.60535201082150714, -10.88017736071109987 ) ) ;
#41131=CARTESIAN_POINT ( 'NONE',  ( 15.44008868035555260, 14.73035201082150536, 9.422509992056143702 ) ) ;
#41132=CARTESIAN_POINT ( 'NONE',  ( 5.076628168052703671, 36.84226448433412315, 8.527530157486179263 ) ) ;
#41133=CARTESIAN_POINT ( 'NONE',  ( 10.00000000000000000, -2.126365330069579951, -12.81628187352647608 ) ) ;
#41136=( BOUNDED_SURFACE ( )  B_SPLINE_SURFACE ( 1, 2, ( 
 ( #45561, #90561, #83070, #60060, #8066, #61047, #66586, #91560, #97113, #89579, #13585, #14089, #44572, #75069, #67586, #16553, #1564, #46541, #92527, #71029, #8555, #77042, #78516, #55530, #47027, #32013, #1067, #84553, #62516, #31531, #40032, #93021, #31037, #70534, #85040, #94010, #86522, #17046, #39056, #48008, #62027, #69550, #24055, #18020, #54524, #77519, #10030, #47525, #9035, #48502, #40531, #2056, #23574, #24557, #32518, #63016, #78028, #79005, #2552, #39552, #70042, #56024, #38562, #55016, #85533, #33009, #9530, #93517, #86026, #25532, #61538, #25044, #17541, #63508, #69058, #596, #92046, #54043, #16053, #87977, #57966, #34967, #49481, #65464, #96490, #27473, #88970, #19488, #87491, #26984, #88470, #71991, #19005, #42011, #34472, #19972, #49981, #94984, #72971, #27961, #79989, #80975, #64965, #11491, #42489, #95491, #4502, #57482, #20479, #3036, #56984, #95991, #72477, #63984, #71526, #79505, #41523, #33974, #94495, #11007, #3515, #65963, #35467, #50470, #4010, #80488, #11986, #12474, #50965, #64477, #41024, #33486, #58454, #48996, #42978, #26490, #73458, #4986, #10508, #18506, #26014, #56509, #87000, #67949, #98969, #22455, #13463, #59936, #43945, #35959, #28467, #74443, #98473, #66454, #13970, #90426, #21967, #52930, #74947, #89460, #68448, #5970, #36464, #21464, #81951, #44445, #66959, #96990, #29927, #97477, #51461, #52446, #73959, #58964, #20978, #82946, #12962, #75442, #60433, #75934, #28943, #59445, #37955, #83441, #89946, #14461, #6449, #44935, #51962, #82446, #7457, #6954, #36960, #67455, #30423, #43457, #60924, #97976, #90926, #29432, #37462, #14962, #45432, #91429, #22956, #81459, #5488, #39424, #16426, #39908, #77395, #8908, #84915, #9909, #32388, #2426, #1931, #32883, #85406, #9406, #15458, #16916, #30915, #46902, #31403, #69918, #61414, #8425, #85903, #23447, #91922, #93392, #70411, #61904, #1439, #15931, #467, #31891, #46422, #54891, #62388, #45939, #47392, #941, #40411, #63382, #92896, #53924, #62893, #76915, #84434, #38932, #93886, #69421, #92410, #24917, #24427, #23934, #53422, #55402, #77893, #38440, #17417, #47886, #78388, #70906, #83929, #76429, #7944, #68937, #54403, #11862, #95360, #34350, #42370, #63859, #27351, #87367, #49363, #87851, #41408, #64357, #49854, #25892, #41891, #80854, #25414, #65341, #4380, #19850, #17898, #73341, #26860, #72350, #33849, #57357, #55898, #95869, #19369, #18388, #94866, #56391, #78883, #42858, #26367, #65839, #86395, #94373, #11369, #56866, #57844, #48381, #86878, #88354, #18882, #79865, #64841, #3883, #80363, #50343, #72844, #48867, #34845, #4868, #10394 ),
 ( #12351, #79379, #35345, #10884, #40898, #71399, #71872, #3384, #2915, #33365, #50850, #35843, #74824, #27841, #90309, #44812, #90812, #28342, #74321, #52814, #98354, #58832, #67328, #21343, #5364, #5847, #14847, #75815, #43825, #36338, #67835, #82321, #89339, #75318, #83321, #20354, #66330, #6831, #66832, #45318, #22340, #97354, #28823, #89826, #6328, #37345, #21845, #59323, #52326, #7337, #14339, #37838, #36840, #51834, #13841, #29812, #20849, #44323, #97854, #29317, #60321, #59813, #81825, #82819, #96368, #58329, #88846, #81343, #12839, #43339, #73836, #96866, #51340, #13341, #60805, #15823, #54779, #831, #22833, #30303, #38326, #353, #91809, #53308, #68820, #30801, #24801, #93278, #77778, #38817, #39313, #92299, #69309, #78274, #23331, #98849, #91305, #55278, #7830, #1329, #53811, #61300, #70301, #84322, #76312, #9291, #46793, #31290, #46310, #76797, #85788, #1815, #8313, #69806, #23823, #61789, #54286, #17301, #47776, #84801, #16310, #39800, #77286, #8796, #16801, #9788, #83816, #31781, #47277, #62276, #68329, #15342, #92782, #24313, #85294, #32270, #62779, #45825, #79262, #64725, #27232, #57238, #19739, #49255, #18275, #56753, #87736, #2804, #48754, #71762, #64237, #19248, #18772, #25783, #3775, #57727, #10773, #11747, #94755, #41288, #72241, #26256, #34228, #87246, #50224, #32767, #86773, #26743, #3272, #93771, #2312, #10282, #71282, #63750, #25297, #40782, #33259, #95748, #65221, #49732, #33736, #11252, #79754, #41770, #80738, #94255, #70795, #63262, #88230, #78777, #95235, #56277, #80239, #42255, #72725, #48263, #4259, #34730, #40287, #55784, #86279, #17788, #43222, #89711, #73717, #65721, #58207, #5249, #29206, #96247, #43719, #21225, #51729, #82708, #5737, #20235, #98233, #35727, #66215, #51225, #12727, #74203, #96746, #27727, #59705, #28222, #81228, #82211, #4751, #88724, #50739, #13721, #42742, #6225, #90202, #6715, #58720, #29694, #81709, #52703, #12233, #89225, #97248, #20734, #52214, #35222, #13223, #75205, #36223, #44205, #66724, #28717, #37232, #74715, #59208, #36729, #60203, #73223, #90698, #67220, #21732, #97743, #14226, #44705, #67721, #22227, #55544, #62038, #32533, #70546, #47542, #71045, #9542, #40046, #17060, #41040, #63521, #33502, #33024, #64000, #17555, #40545, #45206, #48021, #92538, #78040, #62529, #2072, #24068, #39563, #18039, #54536, #85051, #25548, #2568, #93035, #63031, #47038, #31543, #93529, #77534, #86043, #25060, #75705, #78533, #32025, #71540, #94511, #10046, #16564, #94025, #9052, #70053, #1576, #26031, #24569, #55029, #56039, #86534, #85548, #83208, #48516, #79019, #68219, #10530 ) ),
 .UNSPECIFIED., .F., .F., .T. ) 
 B_SPLINE_SURFACE_WITH_KNOTS ( ( 2, 2 ),
 ( 3, 2, 2, 2, 2, 2, 2, 2, 2, 2, 2, 2, 2, 2, 2, 2, 2, 2, 2, 2, 2, 2, 2, 2, 2, 2, 2, 2, 2, 2, 2, 2, 2, 2, 2, 2, 2, 2, 2, 2, 2, 2, 2, 2, 2, 2, 2, 2, 2, 2, 2, 2, 2, 2, 2, 2, 2, 2, 2, 2, 2, 2, 2, 2, 2, 2, 2, 2, 2, 2, 2, 2, 2, 2, 2, 2, 2, 2, 2, 2, 2, 2, 2, 2, 2, 2, 2, 2, 2, 2, 2, 2, 2, 2, 2, 2, 2, 2, 2, 2, 2, 2, 2, 2, 2, 2, 2, 2, 2, 2, 2, 2, 2, 2, 2, 2, 2, 2, 2, 2, 2, 2, 2, 2, 2, 2, 2, 2, 2, 2, 2, 2, 2, 2, 2, 2, 2, 2, 2, 2, 2, 2, 2, 2, 2, 2, 2, 2, 2, 2, 2, 2, 2, 2, 2, 2, 2, 2, 2, 2, 2, 2, 3 ),
 ( 0.000000000000000000, 1.000000000000000000 ),
 ( 0.000000000000000000, 0.005952380952380952051, 0.01190476190476190410, 0.01785714285714285615, 0.02380952380952380820, 0.02976190476190476025, 0.03571428571428571230, 0.04166666666666666435, 0.04761904761904761640, 0.05357142857142856845, 0.05952380952380952051, 0.06547619047619047949, 0.07142857142857142461, 0.07738095238095238360, 0.08333333333333332871, 0.08928571428571428770, 0.09523809523809523281, 0.1011904761904761918, 0.1071428571428571369, 0.1130952380952380959, 0.1190476190476190410, 0.1250000000000000000, 0.1309523809523809590, 0.1369047619047619180, 0.1428571428571428492, 0.1488095238095238082, 0.1547619047619047672, 0.1607142857142857262, 0.1666666666666666574, 0.1726190476190476164, 0.1785714285714285754, 0.1845238095238095344, 0.1904761904761904656, 0.1964285714285714246, 0.2023809523809523836, 0.2083333333333333426, 0.2142857142857142738, 0.2202380952380952328, 0.2261904761904761918, 0.2321428571428571508, 0.2380952380952380820, 0.2440476190476190410, 0.2500000000000000000, 0.2559523809523809312, 0.2619047619047619180, 0.2678571428571428492, 0.2738095238095238360, 0.2797619047619047672, 0.2857142857142856984, 0.2916666666666666852, 0.2976190476190476164, 0.3035714285714285476, 0.3095238095238095344, 0.3154761904761904656, 0.3214285714285714524, 0.3273809523809523836, 0.3333333333333333148, 0.3392857142857143016, 0.3452380952380952328, 0.3511904761904761640, 0.3571428571428571508, 0.3630952380952380820, 0.3690476190476190688, 0.3750000000000000000, 0.3809523809523809312, 0.3869047619047619180, 0.3928571428571428492, 0.3988095238095238360, 0.4047619047619047672, 0.4107142857142856984, 0.4166666666666666852, 0.4226190476190476164, 0.4285714285714285476, 0.4345238095238095344, 0.4404761904761904656, 0.4464285714285714524, 0.4523809523809523836, 0.4583333333333333148, 0.4642857142857143016, 0.4702380952380952328, 0.4761904761904761640, 0.4821428571428571508, 0.4880952380952380820, 0.4940476190476190688, 0.5000000000000000000, 0.5059523809523809312, 0.5119047619047618625, 0.5178571428571429047, 0.5238095238095238360, 0.5297619047619047672, 0.5357142857142856984, 0.5416666666666666297, 0.5476190476190476719, 0.5535714285714286031, 0.5595238095238095344, 0.5654761904761904656, 0.5714285714285713969, 0.5773809523809523281, 0.5833333333333333703, 0.5892857142857143016, 0.5952380952380952328, 0.6011904761904761640, 0.6071428571428570953, 0.6130952380952381375, 0.6190476190476190688, 0.6250000000000000000, 0.6309523809523809312, 0.6369047619047618625, 0.6428571428571429047, 0.6488095238095238360, 0.6547619047619047672, 0.6607142857142856984, 0.6666666666666666297, 0.6726190476190476719, 0.6785714285714286031, 0.6845238095238095344, 0.6904761904761904656, 0.6964285714285713969, 0.7023809523809523281, 0.7083333333333333703, 0.7142857142857143016, 0.7202380952380952328, 0.7261904761904761640, 0.7321428571428570953, 0.7380952380952381375, 0.7440476190476190688, 0.7500000000000000000, 0.7559523809523809312, 0.7619047619047618625, 0.7678571428571429047, 0.7738095238095238360, 0.7797619047619047672, 0.7857142857142856984, 0.7916666666666666297, 0.7976190476190476719, 0.8035714285714286031, 0.8095238095238095344, 0.8154761904761904656, 0.8214285714285713969, 0.8273809523809523281, 0.8333333333333333703, 0.8392857142857143016, 0.8452380952380952328, 0.8511904761904761640, 0.8571428571428570953, 0.8630952380952381375, 0.8690476190476190688, 0.8750000000000000000, 0.8809523809523809312, 0.8869047619047618625, 0.8928571428571429047, 0.8988095238095238360, 0.9047619047619047672, 0.9107142857142856984, 0.9166666666666666297, 0.9226190476190476719, 0.9285714285714286031, 0.9345238095238095344, 0.9404761904761904656, 0.9464285714285713969, 0.9523809523809523281, 0.9583333333333333703, 0.9642857142857143016 ),
 .UNSPECIFIED. ) 
 GEOMETRIC_REPRESENTATION_ITEM ( )  RATIONAL_B_SPLINE_SURFACE ( (
 ( 1.000000000000000000, 0.9659258262890683122, 1.000000000000000000, 0.9659258262890683122, 1.000000000000000000, 0.9659258262890683122, 1.000000000000000000, 0.9659258262890683122, 1.000000000000000000, 0.9659258262890683122, 1.000000000000000000, 0.9659258262890683122, 1.000000000000000000, 0.9659258262890683122, 1.000000000000000000, 0.9659258262890683122, 1.000000000000000000, 0.9659258262890683122, 1.000000000000000000, 0.9659258262890683122, 1.000000000000000000, 0.9659258262890683122, 1.000000000000000000, 0.9659258262890683122, 1.000000000000000000, 0.9659258262890683122, 1.000000000000000000, 0.9659258262890683122, 1.000000000000000000, 0.9659258262890683122, 1.000000000000000000, 0.9659258262890683122, 1.000000000000000000, 0.9659258262890683122, 1.000000000000000000, 0.9659258262890683122, 1.000000000000000000, 0.9659258262890683122, 1.000000000000000000, 0.9659258262890683122, 1.000000000000000000, 0.9659258262890683122, 1.000000000000000000, 0.9659258262890683122, 1.000000000000000000, 0.9659258262890683122, 1.000000000000000000, 0.9659258262890683122, 1.000000000000000000, 0.9659258262890683122, 1.000000000000000000, 0.9659258262890683122, 1.000000000000000000, 0.9659258262890683122, 1.000000000000000000, 0.9659258262890683122, 1.000000000000000000, 0.9659258262890683122, 1.000000000000000000, 0.9659258262890683122, 1.000000000000000000, 0.9659258262890683122, 1.000000000000000000, 0.9659258262890683122, 1.000000000000000000, 0.9659258262890683122, 1.000000000000000000, 0.9659258262890683122, 1.000000000000000000, 0.9659258262890683122, 1.000000000000000000, 0.9659258262890683122, 1.000000000000000000, 0.9659258262890683122, 1.000000000000000000, 0.9659258262890683122, 1.000000000000000000, 0.9659258262890683122, 1.000000000000000000, 0.9659258262890683122, 1.000000000000000000, 0.9659258262890683122, 1.000000000000000000, 0.9659258262890683122, 1.000000000000000000, 0.9659258262890683122, 1.000000000000000000, 0.9659258262890683122, 1.000000000000000000, 0.9659258262890683122, 1.000000000000000000, 0.9659258262890683122, 1.000000000000000000, 0.9659258262890683122, 1.000000000000000000, 0.9659258262890683122, 1.000000000000000000, 0.9659258262890683122, 1.000000000000000000, 0.9659258262890683122, 1.000000000000000000, 0.9659258262890683122, 1.000000000000000000, 0.9659258262890683122, 1.000000000000000000, 0.9659258262890683122, 1.000000000000000000, 0.9659258262890683122, 1.000000000000000000, 0.9659258262890683122, 1.000000000000000000, 0.9659258262890683122, 1.000000000000000000, 0.9659258262890683122, 1.000000000000000000, 0.9659258262890683122, 1.000000000000000000, 0.9659258262890683122, 1.000000000000000000, 0.9659258262890683122, 1.000000000000000000, 0.9659258262890683122, 1.000000000000000000, 0.9659258262890683122, 1.000000000000000000, 0.9659258262890683122, 1.000000000000000000, 0.9659258262890683122, 1.000000000000000000, 0.9659258262890683122, 1.000000000000000000, 0.9659258262890683122, 1.000000000000000000, 0.9659258262890683122, 1.000000000000000000, 0.9659258262890683122, 1.000000000000000000, 0.9659258262890683122, 1.000000000000000000, 0.9659258262890683122, 1.000000000000000000, 0.9659258262890683122, 1.000000000000000000, 0.9659258262890683122, 1.000000000000000000, 0.9659258262890683122, 1.000000000000000000, 0.9659258262890683122, 1.000000000000000000, 0.9659258262890683122, 1.000000000000000000, 0.9659258262890683122, 1.000000000000000000, 0.9659258262890683122, 1.000000000000000000, 0.9659258262890683122, 1.000000000000000000, 0.9659258262890683122, 1.000000000000000000, 0.9659258262890683122, 1.000000000000000000, 0.9659258262890683122, 1.000000000000000000, 0.9659258262890683122, 1.000000000000000000, 0.9659258262890683122, 1.000000000000000000, 0.9659258262890683122, 1.000000000000000000, 0.9659258262890683122, 1.000000000000000000, 0.9659258262890683122, 1.000000000000000000, 0.9659258262890683122, 1.000000000000000000, 0.9659258262890683122, 1.000000000000000000, 0.9659258262890683122, 1.000000000000000000, 0.9659258262890683122, 1.000000000000000000, 0.9659258262890683122, 1.000000000000000000, 0.9659258262890683122, 1.000000000000000000, 0.9659258262890683122, 1.000000000000000000, 0.9659258262890683122, 1.000000000000000000, 0.9659258262890683122, 1.000000000000000000, 0.9659258262890683122, 1.000000000000000000, 0.9659258262890683122, 1.000000000000000000, 0.9659258262890683122, 1.000000000000000000, 0.9659258262890683122, 1.000000000000000000, 0.9659258262890683122, 1.000000000000000000, 0.9659258262890683122, 1.000000000000000000, 0.9659258262890683122, 1.000000000000000000, 0.9659258262890683122, 1.000000000000000000, 0.9659258262890683122, 1.000000000000000000, 0.9659258262890683122, 1.000000000000000000, 0.9659258262890683122, 1.000000000000000000, 0.9659258262890683122, 1.000000000000000000, 0.9659258262890683122, 1.000000000000000000, 0.9659258262890683122, 1.000000000000000000, 0.9659258262890683122, 1.000000000000000000, 0.9659258262890683122, 1.000000000000000000, 0.9659258262890683122, 1.000000000000000000, 0.9659258262890683122, 1.000000000000000000, 0.9659258262890683122, 1.000000000000000000, 0.9659258262890683122, 1.000000000000000000, 0.9659258262890683122, 1.000000000000000000, 0.9659258262890683122, 1.000000000000000000, 0.9659258262890683122, 1.000000000000000000, 0.9659258262890683122, 1.000000000000000000, 0.9659258262890683122, 1.000000000000000000, 0.9659258262890683122, 1.000000000000000000, 0.9659258262890683122, 1.000000000000000000, 0.9659258262890683122, 1.000000000000000000, 0.9659258262890683122, 1.000000000000000000, 0.9659258262890683122, 1.000000000000000000, 0.9659258262890683122, 1.000000000000000000, 0.9659258262890683122, 1.000000000000000000, 0.9659258262890683122, 1.000000000000000000, 0.9659258262890683122, 1.000000000000000000, 0.9659258262890683122, 1.000000000000000000, 0.9659258262890683122, 1.000000000000000000, 0.9659258262890683122, 1.000000000000000000, 0.9659258262890683122, 1.000000000000000000, 0.9659258262890683122, 1.000000000000000000, 0.9659258262890683122, 1.000000000000000000, 0.9659258262890683122, 1.000000000000000000, 0.9659258262890683122, 1.000000000000000000, 0.9659258262890683122, 1.000000000000000000, 0.9659258262890683122, 1.000000000000000000, 0.9659258262890683122, 1.000000000000000000, 0.9659258262890683122, 1.000000000000000000, 0.9659258262890683122, 1.000000000000000000, 0.9659258262890683122, 1.000000000000000000, 0.9659258262890683122, 1.000000000000000000, 0.9659258262890683122, 1.000000000000000000, 0.9659258262890683122, 1.000000000000000000, 0.9659258262890683122, 1.000000000000000000, 0.9659258262890683122, 1.000000000000000000, 0.9659258262890683122, 1.000000000000000000, 0.9659258262890683122, 1.000000000000000000, 0.9659258262890683122, 1.000000000000000000, 0.9659258262890683122, 1.000000000000000000, 0.9659258262890683122, 1.000000000000000000, 0.9659258262890683122, 1.000000000000000000, 0.9659258262890683122, 1.000000000000000000, 0.9659258262890683122, 1.000000000000000000, 0.9659258262890683122, 1.000000000000000000, 0.9659258262890683122, 1.000000000000000000, 0.9659258262890683122, 1.000000000000000000, 0.9659258262890683122, 1.000000000000000000, 0.9659258262890683122, 1.000000000000000000, 0.9659258262890683122, 1.000000000000000000),
 ( 1.000000000000000000, 0.9659258262890683122, 1.000000000000000000, 0.9659258262890683122, 1.000000000000000000, 0.9659258262890683122, 1.000000000000000000, 0.9659258262890683122, 1.000000000000000000, 0.9659258262890683122, 1.000000000000000000, 0.9659258262890683122, 1.000000000000000000, 0.9659258262890683122, 1.000000000000000000, 0.9659258262890683122, 1.000000000000000000, 0.9659258262890683122, 1.000000000000000000, 0.9659258262890683122, 1.000000000000000000, 0.9659258262890683122, 1.000000000000000000, 0.9659258262890683122, 1.000000000000000000, 0.9659258262890683122, 1.000000000000000000, 0.9659258262890683122, 1.000000000000000000, 0.9659258262890683122, 1.000000000000000000, 0.9659258262890683122, 1.000000000000000000, 0.9659258262890683122, 1.000000000000000000, 0.9659258262890683122, 1.000000000000000000, 0.9659258262890683122, 1.000000000000000000, 0.9659258262890683122, 1.000000000000000000, 0.9659258262890683122, 1.000000000000000000, 0.9659258262890683122, 1.000000000000000000, 0.9659258262890683122, 1.000000000000000000, 0.9659258262890683122, 1.000000000000000000, 0.9659258262890683122, 1.000000000000000000, 0.9659258262890683122, 1.000000000000000000, 0.9659258262890683122, 1.000000000000000000, 0.9659258262890683122, 1.000000000000000000, 0.9659258262890683122, 1.000000000000000000, 0.9659258262890683122, 1.000000000000000000, 0.9659258262890683122, 1.000000000000000000, 0.9659258262890683122, 1.000000000000000000, 0.9659258262890683122, 1.000000000000000000, 0.9659258262890683122, 1.000000000000000000, 0.9659258262890683122, 1.000000000000000000, 0.9659258262890683122, 1.000000000000000000, 0.9659258262890683122, 1.000000000000000000, 0.9659258262890683122, 1.000000000000000000, 0.9659258262890683122, 1.000000000000000000, 0.9659258262890683122, 1.000000000000000000, 0.9659258262890683122, 1.000000000000000000, 0.9659258262890683122, 1.000000000000000000, 0.9659258262890683122, 1.000000000000000000, 0.9659258262890683122, 1.000000000000000000, 0.9659258262890683122, 1.000000000000000000, 0.9659258262890683122, 1.000000000000000000, 0.9659258262890683122, 1.000000000000000000, 0.9659258262890683122, 1.000000000000000000, 0.9659258262890683122, 1.000000000000000000, 0.9659258262890683122, 1.000000000000000000, 0.9659258262890683122, 1.000000000000000000, 0.9659258262890683122, 1.000000000000000000, 0.9659258262890683122, 1.000000000000000000, 0.9659258262890683122, 1.000000000000000000, 0.9659258262890683122, 1.000000000000000000, 0.9659258262890683122, 1.000000000000000000, 0.9659258262890683122, 1.000000000000000000, 0.9659258262890683122, 1.000000000000000000, 0.9659258262890683122, 1.000000000000000000, 0.9659258262890683122, 1.000000000000000000, 0.9659258262890683122, 1.000000000000000000, 0.9659258262890683122, 1.000000000000000000, 0.9659258262890683122, 1.000000000000000000, 0.9659258262890683122, 1.000000000000000000, 0.9659258262890683122, 1.000000000000000000, 0.9659258262890683122, 1.000000000000000000, 0.9659258262890683122, 1.000000000000000000, 0.9659258262890683122, 1.000000000000000000, 0.9659258262890683122, 1.000000000000000000, 0.9659258262890683122, 1.000000000000000000, 0.9659258262890683122, 1.000000000000000000, 0.9659258262890683122, 1.000000000000000000, 0.9659258262890683122, 1.000000000000000000, 0.9659258262890683122, 1.000000000000000000, 0.9659258262890683122, 1.000000000000000000, 0.9659258262890683122, 1.000000000000000000, 0.9659258262890683122, 1.000000000000000000, 0.9659258262890683122, 1.000000000000000000, 0.9659258262890683122, 1.000000000000000000, 0.9659258262890683122, 1.000000000000000000, 0.9659258262890683122, 1.000000000000000000, 0.9659258262890683122, 1.000000000000000000, 0.9659258262890683122, 1.000000000000000000, 0.9659258262890683122, 1.000000000000000000, 0.9659258262890683122, 1.000000000000000000, 0.9659258262890683122, 1.000000000000000000, 0.9659258262890683122, 1.000000000000000000, 0.9659258262890683122, 1.000000000000000000, 0.9659258262890683122, 1.000000000000000000, 0.9659258262890683122, 1.000000000000000000, 0.9659258262890683122, 1.000000000000000000, 0.9659258262890683122, 1.000000000000000000, 0.9659258262890683122, 1.000000000000000000, 0.9659258262890683122, 1.000000000000000000, 0.9659258262890683122, 1.000000000000000000, 0.9659258262890683122, 1.000000000000000000, 0.9659258262890683122, 1.000000000000000000, 0.9659258262890683122, 1.000000000000000000, 0.9659258262890683122, 1.000000000000000000, 0.9659258262890683122, 1.000000000000000000, 0.9659258262890683122, 1.000000000000000000, 0.9659258262890683122, 1.000000000000000000, 0.9659258262890683122, 1.000000000000000000, 0.9659258262890683122, 1.000000000000000000, 0.9659258262890683122, 1.000000000000000000, 0.9659258262890683122, 1.000000000000000000, 0.9659258262890683122, 1.000000000000000000, 0.9659258262890683122, 1.000000000000000000, 0.9659258262890683122, 1.000000000000000000, 0.9659258262890683122, 1.000000000000000000, 0.9659258262890683122, 1.000000000000000000, 0.9659258262890683122, 1.000000000000000000, 0.9659258262890683122, 1.000000000000000000, 0.9659258262890683122, 1.000000000000000000, 0.9659258262890683122, 1.000000000000000000, 0.9659258262890683122, 1.000000000000000000, 0.9659258262890683122, 1.000000000000000000, 0.9659258262890683122, 1.000000000000000000, 0.9659258262890683122, 1.000000000000000000, 0.9659258262890683122, 1.000000000000000000, 0.9659258262890683122, 1.000000000000000000, 0.9659258262890683122, 1.000000000000000000, 0.9659258262890683122, 1.000000000000000000, 0.9659258262890683122, 1.000000000000000000, 0.9659258262890683122, 1.000000000000000000, 0.9659258262890683122, 1.000000000000000000, 0.9659258262890683122, 1.000000000000000000, 0.9659258262890683122, 1.000000000000000000, 0.9659258262890683122, 1.000000000000000000, 0.9659258262890683122, 1.000000000000000000, 0.9659258262890683122, 1.000000000000000000, 0.9659258262890683122, 1.000000000000000000, 0.9659258262890683122, 1.000000000000000000, 0.9659258262890683122, 1.000000000000000000, 0.9659258262890683122, 1.000000000000000000, 0.9659258262890683122, 1.000000000000000000, 0.9659258262890683122, 1.000000000000000000, 0.9659258262890683122, 1.000000000000000000, 0.9659258262890683122, 1.000000000000000000, 0.9659258262890683122, 1.000000000000000000, 0.9659258262890683122, 1.000000000000000000, 0.9659258262890683122, 1.000000000000000000, 0.9659258262890683122, 1.000000000000000000, 0.9659258262890683122, 1.000000000000000000, 0.9659258262890683122, 1.000000000000000000, 0.9659258262890683122, 1.000000000000000000, 0.9659258262890683122, 1.000000000000000000, 0.9659258262890683122, 1.000000000000000000, 0.9659258262890683122, 1.000000000000000000, 0.9659258262890683122, 1.000000000000000000, 0.9659258262890683122, 1.000000000000000000, 0.9659258262890683122, 1.000000000000000000, 0.9659258262890683122, 1.000000000000000000, 0.9659258262890683122, 1.000000000000000000, 0.9659258262890683122, 1.000000000000000000, 0.9659258262890683122, 1.000000000000000000, 0.9659258262890683122, 1.000000000000000000, 0.9659258262890683122, 1.000000000000000000, 0.9659258262890683122, 1.000000000000000000, 0.9659258262890683122, 1.000000000000000000, 0.9659258262890683122, 1.000000000000000000, 0.9659258262890683122, 1.000000000000000000) ) ) 
 REPRESENTATION_ITEM ( '' )  SURFACE ( )  );
#41138=CARTESIAN_POINT ( 'NONE',  ( 19.38216949554541557, 22.24863466993041428, -9.382169495545420901 ) ) ;
#41141=CARTESIAN_POINT ( 'NONE',  ( -4.164238869374098151, 46.59541550158063927, -3.795296366450310543 ) ) ;
#41143=CARTESIAN_POINT ( 'NONE',  ( 24.16423886937410614, 54.51208216824730357, -3.795296366450302550 ) ) ;
#41145=CARTESIAN_POINT ( 'NONE',  ( 15.44008868035555260, 34.73035201082151247, 9.422509992056143702 ) ) ;
#41146=CARTESIAN_POINT ( 'NONE',  ( 12.91533473730993009, 36.60535201082151247, -10.88017736071109987 ) ) ;
#41147=CARTESIAN_POINT ( 'NONE',  ( 20.88017736071110875, 60.77201867748817676, -2.915334737309920765 ) ) ;
#41148=CARTESIAN_POINT ( 'NONE',  ( 0.5774900079438590739, 22.64701867748817321, -5.440088680355550821 ) ) ;
#41153=CARTESIAN_POINT ( 'NONE',  ( 0.1532563361054083140, 21.00893115100078745, 1.131784320476157264E-15 ) ) ;
#41157=CARTESIAN_POINT ( 'NONE',  ( 7.361572987183170547, 42.05059781766745886, 9.846743663894590881 ) ) ;
#41159=CARTESIAN_POINT ( 'NONE',  ( 13.43411237798106583, 47.66530133659709634, -12.81628187352647252 ) ) ;
#41161=VECTOR ( 'NONE', #75659, 1000.000000000000000 ) ;
#41163=CARTESIAN_POINT ( 'NONE',  ( -46.34323875807881166, 103.6109741468810483, 6.190393423093142999 ) ) ;
#41164=CARTESIAN_POINT ( 'NONE',  ( -45.36990007558824800, 104.5810639163623676, 5.619481386446134152 ) ) ;
#41166=CARTESIAN_POINT ( 'NONE',  ( 2.917880565312950480, 50.97041550158064638, -12.26659068614894821 ) ) ;
#41168=EDGE_LOOP ( 'NONE', ( #38272, #79485, #5621, #47385 ) ) ;
#41170=CARTESIAN_POINT ( 'NONE',  ( 18.52753015748618282, 38.92559781766745175, -4.923371831947291888 ) ) ;
#41172=CARTESIAN_POINT ( 'NONE',  ( 0.6178305044545838731, 9.748634669930416052, 9.382169495545420901 ) ) ;
#41173=CARTESIAN_POINT ( 'NONE',  ( 18.52753015748618282, 3.925597817667451306, -4.923371831947291888 ) ) ;
#41177=CARTESIAN_POINT ( 'NONE',  ( 10.00000000000000178, 57.25893115100078745, 9.846743663894594434 ) ) ;
#41180=CARTESIAN_POINT ( 'NONE',  ( 2.917880565312948704, 57.63708216824731068, 12.26659068614894643 ) ) ;
#41182=CARTESIAN_POINT ( 'NONE',  ( -0.8801773607110991993, 37.85535201082151247, -2.915334737309923874 ) ) ;
#41183=CARTESIAN_POINT ( 'NONE',  ( -1.099225684535947600, 18.70696800326375353, -6.408140936763238038 ) ) ;
#41189=CARTESIAN_POINT ( 'NONE',  ( 14.92337183194729633, 47.67559781766745175, 8.527530157486181039 ) ) ;
#41190=CARTESIAN_POINT ( 'NONE',  ( 2.791683348922240793, 1.633931151000784565, 7.208316651077764092 ) ) ;
#41192=CARTESIAN_POINT ( 'NONE',  ( 16.40814093676323893, 5.790301336597087456, 11.09922568453595026 ) ) ;
#41194=CARTESIAN_POINT ( 'NONE',  ( 19.42250999205614193, 25.14701867748817321, 5.440088680355555262 ) ) ;
#41197=CARTESIAN_POINT ( 'NONE',  ( -2.266590686148945544, 32.22041550158063927, 7.082119434687048631 ) ) ;
#41198=CARTESIAN_POINT ( 'NONE',  ( -4.164238869374099039, 26.80374883491397142, 8.674139862899312516E-16 ) ) ;
#41199=CARTESIAN_POINT ( 'NONE',  ( -0.8801773607110991993, 12.85535201082150358, -2.915334737309923874 ) ) ;
#41200=CARTESIAN_POINT ( 'NONE',  ( 19.84674366389459266, 43.30059781766744464, 2.638427012816836559 ) ) ;
#41201=CARTESIAN_POINT ( 'NONE',  ( 16.40814093676324603, 37.45696800326376064, -11.09922568453594671 ) ) ;
#41202=CARTESIAN_POINT ( 'NONE',  ( 19.42250999205614193, 15.14701867748817143, 5.440088680355555262 ) ) ;
#41204=CARTESIAN_POINT ( 'NONE',  ( 19.84674366389459266, 38.30059781766745175, 2.638427012816836559 ) ) ;
#41205=CARTESIAN_POINT ( 'NONE',  ( 15.44008868035555260, 34.73035201082151247, 9.422509992056143702 ) ) ;
#41206=CARTESIAN_POINT ( 'NONE',  ( 13.43411237798106583, 2.665301336597086568, -12.81628187352647252 ) ) ;
#41207=CARTESIAN_POINT ( 'NONE',  ( -0.3689425029237881626, 22.42874883491397142, 10.36894250292379027 ) ) ;
#41208=CARTESIAN_POINT ( 'NONE',  ( -0.3289641300568009741, 17.24545670184113888, -5.963430220938281678 ) ) ;
#41212=CARTESIAN_POINT ( 'NONE',  ( 19.84674366389459266, 23.30059781766745530, 2.638427012816836559 ) ) ;
#41213=CARTESIAN_POINT ( 'NONE',  ( 19.38216949554541557, 57.24863466993042493, -9.382169495545420901 ) ) ;
#41214=CARTESIAN_POINT ( 'NONE',  ( 19.84674366389459621, 53.50893115100078745, 7.409399052514197653E-17 ) ) ;
#41217=SURFACE_STYLE_USAGE ( .BOTH. , #63681 ) ;
#41218=CARTESIAN_POINT ( 'NONE',  ( 22.26659068614894466, 63.88708216824730357, 7.082119434687054849 ) ) ;
#41219=CARTESIAN_POINT ( 'NONE',  ( 24.16423886937410614, 9.303748834913967869, 8.672049930838204340E-16 ) ) ;
#41220=CARTESIAN_POINT ( 'NONE',  ( 14.92337183194729633, 2.675597817667451750, 8.527530157486181039 ) ) ;
#41221=CARTESIAN_POINT ( 'NONE',  ( 19.84674366389459621, 48.50893115100078745, 7.409399052514197653E-17 ) ) ;
#41222=CARTESIAN_POINT ( 'NONE',  ( 4.559911319644449179, 18.89701867748817321, 9.422509992056141925 ) ) ;
#41223=CARTESIAN_POINT ( 'NONE',  ( 19.72487221294571569, 39.78217586085237656, 6.499999999999986677 ) ) ;
#41224=CARTESIAN_POINT ( 'NONE',  ( 19.10478245763068372, 25.10160829253888792, 5.990408912944043429 ) ) ;
#41226=ORIENTED_EDGE ( 'NONE', *, *, #5652, .T. ) ;
#41231=CARTESIAN_POINT ( 'NONE',  ( 20.36894250292379738, 4.928748834913967869, -10.36894250292379027 ) ) ;
#41233=CARTESIAN_POINT ( 'NONE',  ( 17.08211943468705130, 43.47041550158063927, 12.26659068614894998 ) ) ;
#41234=CARTESIAN_POINT ( 'NONE',  ( 12.63842701281683922, 59.55059781766744464, -9.846743663894590881 ) ) ;
#41235=CARTESIAN_POINT ( 'NONE',  ( 14.92337183194729988, 34.34226448433411605, -8.527530157486177487 ) ) ;
#41236=CARTESIAN_POINT ( 'NONE',  ( -0.8801773607110991993, 37.85535201082151247, -2.915334737309923874 ) ) ;
#41237=CARTESIAN_POINT ( 'NONE',  ( 0.1532563361054083140, 61.00893115100078745, 1.131784320476157264E-15 ) ) ;
#41238=CARTESIAN_POINT ( 'NONE',  ( 17.08211943468705840, 10.13708216824730179, -12.26659068614894466 ) ) ;
#41240=CARTESIAN_POINT ( 'NONE',  ( 13.79529636645031943, 40.34541550158063217, -14.16423886937409904 ) ) ;
#41241=CARTESIAN_POINT ( 'NONE',  ( -0.8801773607110991993, 7.855352010821506248, -2.915334737309923874 ) ) ;
#41244=CARTESIAN_POINT ( 'NONE',  ( 17.96484262340118221, 64.93868534415483396, 7.964842623401181321 ) ) ;
#41246=CARTESIAN_POINT ( 'NONE',  ( 14.92337183194729633, 32.67559781766745175, 8.527530157486181039 ) ) ;
#41247=( GEOMETRIC_REPRESENTATION_CONTEXT ( 3 ) GLOBAL_UNCERTAINTY_ASSIGNED_CONTEXT ( ( #43145 ) ) GLOBAL_UNIT_ASSIGNED_CONTEXT ( ( #7920, #75415, #91899 ) ) REPRESENTATION_CONTEXT ( 'NONE', 'WORKASPACE' ) );
#41253=CARTESIAN_POINT ( 'NONE',  ( 12.63842701281683922, 24.55059781766745175, -9.846743663894590881 ) ) ;
#41255=CARTESIAN_POINT ( 'NONE',  ( -2.266590686148945544, 27.22041550158063572, 7.082119434687048631 ) ) ;
#41256=CARTESIAN_POINT ( 'NONE',  ( 19.84674366389459266, 28.30059781766745886, 2.638427012816836559 ) ) ;
#41257=CARTESIAN_POINT ( 'NONE',  ( 20.88017736071110164, 60.35535201082151957, 2.915334737309930979 ) ) ;
#41258=VECTOR ( 'NONE', #27788, 1000.000000000000000 ) ;
#41260=CARTESIAN_POINT ( 'NONE',  ( 20.88017736071110875, 40.77201867748818387, -2.915334737309920765 ) ) ;
#41264=EDGE_LOOP ( 'NONE', ( #94006, #38084, #43309, #26838, #18515, #15798, #17928, #36163, #17384, #33030 ) ) ;
#41265=CARTESIAN_POINT ( 'NONE',  ( 19.42250999205614548, 45.98035201082150536, -5.440088680355545492 ) ) ;
#41266=CARTESIAN_POINT ( 'NONE',  ( 10.00000000000000000, 5.553748834913967869, -14.16423886937410082 ) ) ;
#41267=EDGE_CURVE ( 'NONE', #30783, #98547, #29528, .T. ) ;
#41268=ORIENTED_EDGE ( 'NONE', *, *, #48609, .F. ) ;
#41269=CARTESIAN_POINT ( 'NONE',  ( 7.361572987183170547, 2.050597817667451750, 9.846743663894590881 ) ) ;
#41270=CARTESIAN_POINT ( 'NONE',  ( -1.099225684535947600, 33.70696800326375353, -6.408140936763238038 ) ) ;
#41271=CARTESIAN_POINT ( 'NONE',  ( 12.63842701281683034, 22.46726448433411605, 9.846743663894596210 ) ) ;
#41272=CARTESIAN_POINT ( 'NONE',  ( 10.00000000000000178, 4.313685344154837509, 10.88017736071110342 ) ) ;
#41274=CARTESIAN_POINT ( 'NONE',  ( 7.361572987183169658, 24.96726448433412315, -9.846743663894592657 ) ) ;
#41275=CARTESIAN_POINT ( 'NONE',  ( 0.5774900079438590739, 62.64701867748817676, -5.440088680355550821 ) ) ;
#41277=CARTESIAN_POINT ( 'NONE',  ( 10.00000000000000178, 64.31368534415483396, 10.88017736071110342 ) ) ;
#41280=CARTESIAN_POINT ( 'NONE',  ( 1.472469842513823179, 1.425597817667451528, 4.923371831947296329 ) ) ;
#41281=CARTESIAN_POINT ( 'NONE',  ( 6.565887622018943937, 15.16530133659708568, 12.81628187352647430 ) ) ;
#41284=CARTESIAN_POINT ( 'NONE',  ( 18.52753015748618282, 48.92559781766745886, -4.923371831947291888 ) ) ;
#41286=CARTESIAN_POINT ( 'NONE',  ( 6.204703633549690345, 10.76208216824729824, -14.16423886937410259 ) ) ;
#41287=CARTESIAN_POINT ( 'NONE',  ( 12.63842701281683034, 27.46726448433411250, 9.846743663894596210 ) ) ;
#41288=CARTESIAN_POINT ( 'NONE',  ( 19.38216949554541202, 30.99863466993042138, 9.382169495545424454 ) ) ;
#41290=CYLINDRICAL_SURFACE ( 'NONE', #3328, 0.5000000000000004441 ) ;
#41291=CARTESIAN_POINT ( 'NONE',  ( 15.44008868035555260, 49.73035201082150536, 9.422509992056143702 ) ) ;
#41292=CARTESIAN_POINT ( 'NONE',  ( 22.81628187352647785, 6.415301336597088344, 3.434112377981063169 ) ) ;
#41294=CARTESIAN_POINT ( 'NONE',  ( 1.472469842513823179, 20.59226448433411960, -4.923371831947296329 ) ) ;
#41295=CARTESIAN_POINT ( 'NONE',  ( 19.42250999205614548, 25.98035201082150891, -5.440088680355545492 ) ) ;
#41297=CARTESIAN_POINT ( 'NONE',  ( 0.6178305044545818747, 28.49863466993041783, -9.382169495545419124 ) ) ;
#41299=CARTESIAN_POINT ( 'NONE',  ( 12.63842701281683034, 17.46726448433411250, 9.846743663894596210 ) ) ;
#41302=CARTESIAN_POINT ( 'NONE',  ( 20.88017736071110875, 30.77201867748816966, -2.915334737309920765 ) ) ;
#41303=ORIENTED_EDGE ( 'NONE', *, *, #16597, .T. ) ;
#41304=CARTESIAN_POINT ( 'NONE',  ( 17.96484262340118221, 54.93868534415484106, 7.964842623401181321 ) ) ;
#41305=CARTESIAN_POINT ( 'NONE',  ( 7.084665262690076126, 2.022018677488170990, -10.88017736071110164 ) ) ;
#41306=CARTESIAN_POINT ( 'NONE',  ( 17.20831665107776587, 44.13393115100078745, -7.208316651077762316 ) ) ;
#41307=CARTESIAN_POINT ( 'NONE',  ( -0.8801773607111008646, 28.27201867748817321, 2.915334737309923430 ) ) ;
#41308=SURFACE_STYLE_FILL_AREA ( #25318 ) ;
#41309=CARTESIAN_POINT ( 'NONE',  ( -0.8801773607110991993, 47.85535201082150536, -2.915334737309923874 ) ) ;
#41310=COLOUR_RGB ( '', 0.72549020, 0.75294118, 0.79215686) ;
#41311=CARTESIAN_POINT ( 'NONE',  ( 20.88017736071110875, 10.77201867748817143, -2.915334737309920765 ) ) ;
#41312=CARTESIAN_POINT ( 'NONE',  ( -1.926860441876563801, 19.89664270246084143, 3.195792623639529761 ) ) ;
#41314=CARTESIAN_POINT ( 'NONE',  ( 1.472469842513823179, 41.42559781766745886, 4.923371831947296329 ) ) ;
#41315=CARTESIAN_POINT ( 'NONE',  ( 24.16423886937409904, 44.09541550158063927, 3.795296366450317205 ) ) ;
#41316=CARTESIAN_POINT ( 'NONE',  ( 1.707155281725170060, 47.90189080397283306, 6.499999999999919176 ) ) ;
#41317=CARTESIAN_POINT ( 'NONE',  ( 2.377183314879974585, 5.785933195168225573, -6.499999999999999112 ) ) ;
#41321=CARTESIAN_POINT ( 'NONE',  ( 6.204703633549690345, 30.76208216824730357, -14.16423886937410259 ) ) ;
#41324=CARTESIAN_POINT ( 'NONE',  ( 6.204703633549690345, 67.84541550158060375, 14.16423886937410082 ) ) ;
#41325=CARTESIAN_POINT ( 'NONE',  ( 2.791683348922237240, 40.38393115100078035, -7.208316651077763204 ) ) ;
#41328=CARTESIAN_POINT ( 'NONE',  ( 20.88017736071110519, 60.56368534415484106, 2.639326808657452039E-16 ) ) ;
#41329=CARTESIAN_POINT ( 'NONE',  ( 3.591859063236763294, 63.29030133659708923, -11.09922568453595026 ) ) ;
#41330=CARTESIAN_POINT ( 'NONE',  ( 0.5774900079438590739, 32.64701867748816966, -5.440088680355550821 ) ) ;
#41332=CARTESIAN_POINT ( 'NONE',  ( 19.38216949554541557, 57.24863466993042493, -9.382169495545420901 ) ) ;
#41333=CARTESIAN_POINT ( 'NONE',  ( 3.591859063236763294, 8.290301336597087456, -11.09922568453595026 ) ) ;
#41334=CARTESIAN_POINT ( 'NONE',  ( 19.84674366389459621, 18.50893115100078745, 7.409399052514197653E-17 ) ) ;
#41337=CARTESIAN_POINT ( 'NONE',  ( 0.1957200283969102450, 20.25733960839543712, 6.499999999999992006 ) ) ;
#41338=CARTESIAN_POINT ( 'NONE',  ( 15.44008868035555260, 4.730352010821505360, 9.422509992056143702 ) ) ;
#41339=CARTESIAN_POINT ( 'NONE',  ( -4.164238869374099039, 31.80374883491396432, 8.674139862899312516E-16 ) ) ;
#41340=CARTESIAN_POINT ( 'NONE',  ( 12.91533473730992121, 29.52201867748817321, 10.88017736071110164 ) ) ;
#41341=CARTESIAN_POINT ( 'NONE',  ( 7.084665262690076126, 49.10535201082149825, 10.88017736071109987 ) ) ;
#41345=CARTESIAN_POINT ( 'NONE',  ( 12.63842701281683922, 4.550597817667451750, -9.846743663894590881 ) ) ;
#41347=CARTESIAN_POINT ( 'NONE',  ( 0.1532563361054082862, 26.21726448433411605, 2.638427012816831674 ) ) ;
#41348=CARTESIAN_POINT ( 'NONE',  ( 20.15039907845753220, 64.72266099184918176, 6.262539305110077947 ) ) ;
#41350=CARTESIAN_POINT ( 'NONE',  ( 0.1532563361054100626, 25.80059781766744820, -2.638427012816831230 ) ) ;
#41351=CARTESIAN_POINT ( 'NONE',  ( 18.52753015748617571, 53.09226448433412315, 4.923371831947298993 ) ) ;
#41352=CARTESIAN_POINT ( 'NONE',  ( -0.8801773607111009756, 23.06368534415484106, 1.068504757029289695E-15 ) ) ;
#41353=UNCERTAINTY_MEASURE_WITH_UNIT (LENGTH_MEASURE( 1.000000000000000082E-05 ), #84750, 'distance_accuracy_value', 'NONE');
#41354=CARTESIAN_POINT ( 'NONE',  ( 21.09922568453595559, 42.04030133659708213, -6.408140936763230044 ) ) ;
#41355=CARTESIAN_POINT ( 'NONE',  ( 20.88017736071110164, 50.35535201082151247, 2.915334737309930979 ) ) ;
#41356=CARTESIAN_POINT ( 'NONE',  ( 10.00000000000000000, 24.75893115100078745, -9.846743663894594434 ) ) ;
#41357=CARTESIAN_POINT ( 'NONE',  ( 24.16423886937410614, 39.51208216824731068, -3.795296366450302550 ) ) ;
#41358=CARTESIAN_POINT ( 'NONE',  ( 10.00000000000000178, 22.25893115100078745, 9.846743663894594434 ) ) ;
#41359=CARTESIAN_POINT ( 'NONE',  ( -0.1503990784575242878, 44.24884699246889852, -6.262539305110083276 ) ) ;
#41362=CARTESIAN_POINT ( 'NONE',  ( -42.94000000000001194, 92.00000000000000000, -8.999999999999998224 ) ) ;
#41363=CARTESIAN_POINT ( 'NONE',  ( 24.16423886937410614, 9.512082168247301794, -3.795296366450302550 ) ) ;
#41364=CARTESIAN_POINT ( 'NONE',  ( 20.36894250292379382, 33.67874883491396076, 10.36894250292379205 ) ) ;
#41365=CARTESIAN_POINT ( 'NONE',  ( 7.361572987183169658, 29.96726448433411960, -9.846743663894592657 ) ) ;
#41366=DIRECTION ( 'NONE',  ( 0.000000000000000000, 0.000000000000000000, -1.000000000000000000 ) ) ;
#41367=CARTESIAN_POINT ( 'NONE',  ( 0.5774900079438607392, 18.48035201082150536, 5.440088680355550821 ) ) ;
#41368=CARTESIAN_POINT ( 'NONE',  ( 12.91533473730993009, 46.60535201082150536, -10.88017736071109987 ) ) ;
#41369=CARTESIAN_POINT ( 'NONE',  ( 10.00000000000000000, 41.81368534415484106, -10.88017736071110342 ) ) ;
#41371=CARTESIAN_POINT ( 'NONE',  ( 22.81628187352648496, 31.83196800326375353, -3.434112377981050290 ) ) ;
#41372=CARTESIAN_POINT ( 'NONE',  ( 17.96484262340118221, 59.93868534415484106, 7.964842623401181321 ) ) ;
#41373=ORIENTED_EDGE ( 'NONE', *, *, #82010, .T. ) ;
#41375=CARTESIAN_POINT ( 'NONE',  ( 17.96484262340118221, 61.18868534415482685, -7.964842623401177768 ) ) ;
#41376=VERTEX_POINT ( 'NONE', #76547 ) ;
#41377=CARTESIAN_POINT ( 'NONE',  ( 2.035157376598822676, 67.43868534415484817, -7.964842623401177768 ) ) ;
#41378=FACE_OUTER_BOUND ( 'NONE', #73338, .T. ) ;
#41379=CARTESIAN_POINT ( 'NONE',  ( 20.88017736071110875, 40.77201867748817676, -2.915334737309920321 ) ) ;
#41381=CARTESIAN_POINT ( 'NONE',  ( -0.8801773607111009756, 13.06368534415483929, 1.068504757029289695E-15 ) ) ;
#41382=CARTESIAN_POINT ( 'NONE',  ( 19.84674366389459266, 3.717264484334118713, -2.638427012816827677 ) ) ;
#41383=CARTESIAN_POINT ( 'NONE',  ( 2.917880565312948704, 7.637082168247301794, 12.26659068614894643 ) ) ;
#41384=CARTESIAN_POINT ( 'NONE',  ( 2.791683348922237240, 10.38393115100078390, -7.208316651077763204 ) ) ;
#41385=CARTESIAN_POINT ( 'NONE',  ( 10.00000000000000178, 9.313685344154839285, 10.88017736071110342 ) ) ;
#41386=CARTESIAN_POINT ( 'NONE',  ( 0.1532563361054082862, 46.21726448433411605, 2.638427012816831674 ) ) ;
#41387=ORIENTED_EDGE ( 'NONE', *, *, #43800, .T. ) ;
#41388=ADVANCED_FACE ( 'NONE', ( #68568 ), #41136, .T. ) ;
#41389=CARTESIAN_POINT ( 'NONE',  ( 19.84674366389459266, 48.30059781766745175, 2.638427012816836559 ) ) ;
#41390=VERTEX_POINT ( 'NONE', #3047 ) ;
#41391=CARTESIAN_POINT ( 'NONE',  ( 15.44008868035555260, 49.73035201082150536, 9.422509992056143702 ) ) ;
#41392=CARTESIAN_POINT ( 'NONE',  ( 12.63842701281683922, 54.55059781766745175, -9.846743663894590881 ) ) ;
#41393=CARTESIAN_POINT ( 'NONE',  ( 6.565887622018943937, 30.16530133659708568, 12.81628187352647430 ) ) ;
#41395=CYLINDRICAL_SURFACE ( 'NONE', #97434, 2.999999999999999112 ) ;
#41396=CARTESIAN_POINT ( 'NONE',  ( -0.8801773607111009756, 58.06368534415484106, 1.068504757029289695E-15 ) ) ;
#41397=CARTESIAN_POINT ( 'NONE',  ( 12.91533473730993009, 11.60535201082150714, -10.88017736071109987 ) ) ;
#41399=CIRCLE ( 'NONE', #79696, 7.000000000000005329 ) ;
#41400=CARTESIAN_POINT ( 'NONE',  ( 3.591859063236763294, 38.29030133659708923, -11.09922568453595026 ) ) ;
#41403=CARTESIAN_POINT ( 'NONE',  ( 21.09922568453595559, 27.04030133659708568, -6.408140936763230044 ) ) ;
#41404=CARTESIAN_POINT ( 'NONE',  ( 20.88017736071110875, 30.77201867748816966, -2.915334737309920765 ) ) ;
#41405=ORIENTED_EDGE ( 'NONE', *, *, #7858, .T. ) ;
#41406=CARTESIAN_POINT ( 'NONE',  ( 10.00000000000000178, 7.258931151000785675, 9.846743663894594434 ) ) ;
#41407=( BOUNDED_CURVE ( )  B_SPLINE_CURVE ( 3, ( #9130, #84165, #61143, #39150 ),
 .UNSPECIFIED., .F., .T. ) 
 B_SPLINE_CURVE_WITH_KNOTS ( ( 4, 4 ),
 ( 4.712388980384689674, 5.730377828609853452 ),
 .UNSPECIFIED. ) 
 CURVE ( )  GEOMETRIC_REPRESENTATION_ITEM ( )  RATIONAL_B_SPLINE_CURVE ( ( 1.000000000000000000, 0.9154899770527749059, 0.9154899770527749059, 1.000000000000000000 ) ) 
 REPRESENTATION_ITEM ( '' )  );
#41408=CARTESIAN_POINT ( 'NONE',  ( 18.52753015748617571, 58.09226448433411605, 4.923371831947298993 ) ) ;
#41409=CARTESIAN_POINT ( 'NONE',  ( 17.20831665107776587, 7.883931151000784787, 7.208316651077764980 ) ) ;
#41410=CARTESIAN_POINT ( 'NONE',  ( 2.791683348922237240, 45.38393115100079456, -7.208316651077763204 ) ) ;
#41413=CARTESIAN_POINT ( 'NONE',  ( 12.63842701281683034, 42.46726448433412315, 9.846743663894596210 ) ) ;
#41416=VECTOR ( 'NONE', #87714, 1000.000000000000000 ) ;
#41417=CARTESIAN_POINT ( 'NONE',  ( 10.00000000000000000, 29.75893115100078745, -9.846743663894594434 ) ) ;
#41418=SURFACE_STYLE_FILL_AREA ( #93896 ) ;
#41420=CARTESIAN_POINT ( 'NONE',  ( 7.361572987183170547, 57.05059781766744464, 9.846743663894590881 ) ) ;
#41422=CARTESIAN_POINT ( 'NONE',  ( 16.40814093676323893, 20.79030133659708923, 11.09922568453595026 ) ) ;
#41423=CARTESIAN_POINT ( 'NONE',  ( 12.63842701281683922, 39.55059781766744464, -9.846743663894590881 ) ) ;
#41425=CARTESIAN_POINT ( 'NONE',  ( -0.3689425029237898834, 46.17874883491397497, -10.36894250292378850 ) ) ;
#41426=CARTESIAN_POINT ( 'NONE',  ( 19.84674366389459266, 13.71726448433411782, -2.638427012816827677 ) ) ;
#41427=CARTESIAN_POINT ( 'NONE',  ( 20.00000000000000711, 88.21129152568526877, 4.994901225416799484 ) ) ;
#41428=CARTESIAN_POINT ( 'NONE',  ( -2.266590686148945544, 62.22041550158063927, 7.082119434687048631 ) ) ;
#41429=CARTESIAN_POINT ( 'NONE',  ( 19.84674366389459621, 53.50893115100078745, 7.409399052514197653E-17 ) ) ;
#41430=CARTESIAN_POINT ( 'NONE',  ( -4.164238869374098151, 66.59541550158060375, -3.795296366450310543 ) ) ;
#41431=CARTESIAN_POINT ( 'NONE',  ( 2.917880565312950480, 40.97041550158063217, -12.26659068614894821 ) ) ;
#41432=CARTESIAN_POINT ( 'NONE',  ( 22.26659068614895176, 44.72041550158063927, -7.082119434687042414 ) ) ;
#41435=DIRECTION ( 'NONE',  ( 0.000000000000000000, 0.000000000000000000, -1.000000000000000000 ) ) ;
#41436=CARTESIAN_POINT ( 'NONE',  ( 14.92337183194729988, 54.34226448433412315, -8.527530157486177487 ) ) ;
#41438=CARTESIAN_POINT ( 'NONE',  ( 2.035157376598824452, 38.68868534415483396, 7.964842623401179544 ) ) ;
#41441=CARTESIAN_POINT ( 'NONE',  ( 2.791683348922240793, 46.63393115100077324, 7.208316651077764092 ) ) ;
#41444=CARTESIAN_POINT ( 'NONE',  ( 7.361572987183170547, 52.05059781766745175, 9.846743663894590881 ) ) ;
#41445=CARTESIAN_POINT ( 'NONE',  ( 7.361572987183169658, 64.96726448433412315, -9.846743663894592657 ) ) ;
#41447=CARTESIAN_POINT ( 'NONE',  ( 10.00000000000000178, 28.05374883491396787, 14.16423886937410082 ) ) ;
#41448=CARTESIAN_POINT ( 'NONE',  ( 7.361572987183169658, -0.03273551566588185635, -9.846743663894592657 ) ) ;
#41450=CARTESIAN_POINT ( 'NONE',  ( 20.88017736071110875, 45.77201867748816966, -2.915334737309920321 ) ) ;
#41451=CARTESIAN_POINT ( 'NONE',  ( 2.035157376598822676, 22.43868534415483396, -7.964842623401177768 ) ) ;
#41452=CARTESIAN_POINT ( 'NONE',  ( 21.09922568453594849, 26.20696800326375353, 6.408140936763242479 ) ) ;
#41454=CARTESIAN_POINT ( 'NONE',  ( 0.1532563361054083140, 11.00893115100078568, 1.131784320476157264E-15 ) ) ;
#41455=DIRECTION ( 'NONE',  ( 0.000000000000000000, 0.000000000000000000, 1.000000000000000000 ) ) ;
#41457=CARTESIAN_POINT ( 'NONE',  ( 12.91533473730993009, 6.605352010821504471, -10.88017736071109987 ) ) ;
#41459=CARTESIAN_POINT ( 'NONE',  ( 12.91533473730993009, 41.60535201082149825, -10.88017736071109987 ) ) ;
#41460=CARTESIAN_POINT ( 'NONE',  ( 10.00000000000000000, 36.81368534415484106, -10.88017736071110342 ) ) ;
#41461=CARTESIAN_POINT ( 'NONE',  ( 22.81628187352647785, 1.623634669930420271, 6.195893100308588602E-16 ) ) ;
#41462=CARTESIAN_POINT ( 'NONE',  ( 0.2751277870542967463, 0.000000000000000000, 6.500000000000000888 ) ) ;
#41464=CARTESIAN_POINT ( 'NONE',  ( 0.1532563361054083140, 11.00893115100078568, 1.131784320476157264E-15 ) ) ;
#41465=EDGE_CURVE ( 'NONE', #9539, #21162, #1081, .T. ) ;
#41467=CARTESIAN_POINT ( 'NONE',  ( -0.8801773607110991993, 32.85535201082151247, -2.915334737309923874 ) ) ;
#41469=CARTESIAN_POINT ( 'NONE',  ( 19.38216949554541202, 10.99863466993042138, 9.382169495545424454 ) ) ;
#41470=CARTESIAN_POINT ( 'NONE',  ( 10.00000000000000178, 69.31368534415484817, 10.88017736071110342 ) ) ;
#41472=CARTESIAN_POINT ( 'NONE',  ( 10.00000000000000178, 7.258931151000785675, 9.846743663894594434 ) ) ;
#41473=CARTESIAN_POINT ( 'NONE',  ( -1.099225684535947600, 38.70696800326375353, -6.408140936763238038 ) ) ;
#41474=CARTESIAN_POINT ( 'NONE',  ( 10.00000000000000178, 12.25893115100078568, 9.846743663894594434 ) ) ;
#41477=SURFACE_STYLE_USAGE ( .BOTH. , #79452 ) ;
#41479=CARTESIAN_POINT ( 'NONE',  ( 7.084665262690076126, 12.02201867748817143, -10.88017736071110164 ) ) ;
#41481=CARTESIAN_POINT ( 'NONE',  ( 2.791683348922240793, 11.63393115100078568, 7.208316651077764092 ) ) ;
#41482=CARTESIAN_POINT ( 'NONE',  ( 20.88017736071110519, 10.56368534415483751, 2.639326808657452039E-16 ) ) ;
#41483=CARTESIAN_POINT ( 'NONE',  ( 0.5774900079438590739, 7.647018677488171434, -5.440088680355550821 ) ) ;
#41485=CARTESIAN_POINT ( 'NONE',  ( 12.91533473730992121, 9.522018677488171434, 10.88017736071110164 ) ) ;
#41486=CARTESIAN_POINT ( 'NONE',  ( 19.42250999205614193, 20.14701867748817321, 5.440088680355555262 ) ) ;
#41487=CARTESIAN_POINT ( 'NONE',  ( 13.99999999999999822, 11.00000000000000000, -6.000000000000000000 ) ) ;
#41489=CARTESIAN_POINT ( 'NONE',  ( 20.24186590665275531, 27.61633188102327807, -6.114288769123077394 ) ) ;
#41490=CARTESIAN_POINT ( 'NONE',  ( 17.96484262340118221, 21.18868534415483396, -7.964842623401177768 ) ) ;
#41491=CARTESIAN_POINT ( 'NONE',  ( 2.791683348922237240, 50.38393115100078035, -7.208316651077763204 ) ) ;
#41493=CARTESIAN_POINT ( 'NONE',  ( -2.816281873526471635, 48.91530133659708213, -3.434112377981056508 ) ) ;
#41494=CARTESIAN_POINT ( 'NONE',  ( 2.831191079880678085, 79.91181047996344944, -5.000000000000000000 ) ) ;
#41495=CARTESIAN_POINT ( 'NONE',  ( 20.36894250292379382, 38.67874883491396076, 10.36894250292379205 ) ) ;
#41496=CARTESIAN_POINT ( 'NONE',  ( 20.88017736071110875, 40.77201867748818387, -2.915334737309920765 ) ) ;
#41497=CARTESIAN_POINT ( 'NONE',  ( -0.8801773607111008646, 18.27201867748817321, 2.915334737309923430 ) ) ;
#41498=CARTESIAN_POINT ( 'NONE',  ( 19.84674366389459266, 58.71726448433411605, -2.638427012816827677 ) ) ;
#41500=CARTESIAN_POINT ( 'NONE',  ( 7.361572987183170547, 42.05059781766745886, 9.846743663894590881 ) ) ;
#41503=CARTESIAN_POINT ( 'NONE',  ( 10.00000000000000000, 9.758931151000785675, -9.846743663894594434 ) ) ;
#41506=CARTESIAN_POINT ( 'NONE',  ( 12.91533473730993009, 16.60535201082150891, -10.88017736071109987 ) ) ;
#41507=CARTESIAN_POINT ( 'NONE',  ( 7.361572987183169658, 4.967264484334119601, -9.846743663894592657 ) ) ;
#41508=CARTESIAN_POINT ( 'NONE',  ( 0.6178305044545818747, 3.498634669930420049, -9.382169495545419124 ) ) ;
#41509=CARTESIAN_POINT ( 'NONE',  ( 12.91533473730992121, 44.52201867748816966, 10.88017736071110164 ) ) ;
#41510=CARTESIAN_POINT ( 'NONE',  ( 4.559911319644449179, 47.23035201082150536, -9.422509992056141925 ) ) ;
#41511=CARTESIAN_POINT ( 'NONE',  ( 2.035157376598822676, 22.43868534415483396, -7.964842623401177768 ) ) ;
#41512=CARTESIAN_POINT ( 'NONE',  ( 16.40814093676323893, 50.79030133659708923, 11.09922568453595026 ) ) ;
#41513=CARTESIAN_POINT ( 'NONE',  ( -2.266590686148945544, 37.22041550158063217, 7.082119434687048631 ) ) ;
#41515=CARTESIAN_POINT ( 'NONE',  ( -1.099225684535947600, 63.70696800326376774, -6.408140936763238038 ) ) ;
#41517=CARTESIAN_POINT ( 'NONE',  ( 7.361572987183170547, 52.05059781766745175, 9.846743663894590881 ) ) ;
#41518=( NAMED_UNIT ( * ) PLANE_ANGLE_UNIT ( ) SI_UNIT ( $, .RADIAN. ) );
#41519=CARTESIAN_POINT ( 'NONE',  ( 4.559911319644449179, 38.89701867748817676, 9.422509992056141925 ) ) ;
#41520=ORIENTED_EDGE ( 'NONE', *, *, #48415, .F. ) ;
#41521=CARTESIAN_POINT ( 'NONE',  ( 12.63842701281683922, 4.550597817667451750, -9.846743663894590881 ) ) ;
#41522=CARTESIAN_POINT ( 'NONE',  ( 18.52753015748617571, 13.09226448433411960, 4.923371831947298993 ) ) ;
#41523=CARTESIAN_POINT ( 'NONE',  ( 18.52753015748618282, 23.92559781766745530, -4.923371831947291888 ) ) ;
#41524=CARTESIAN_POINT ( 'NONE',  ( 12.63842701281683034, 17.46726448433411250, 9.846743663894596210 ) ) ;
#41525=CARTESIAN_POINT ( 'NONE',  ( 12.63842701281683922, 4.550597817667451750, -9.846743663894590881 ) ) ;
#41526=CARTESIAN_POINT ( 'NONE',  ( -0.8801773607111009756, 63.06368534415484106, 1.068504757029289695E-15 ) ) ;
#41528=CARTESIAN_POINT ( 'NONE',  ( 2.035157376598822676, 57.43868534415484106, -7.964842623401177768 ) ) ;
#41529=CARTESIAN_POINT ( 'NONE',  ( 19.84674366389459266, 18.30059781766745175, 2.638427012816836559 ) ) ;
#41533=CARTESIAN_POINT ( 'NONE',  ( 18.52753015748617571, 53.09226448433412315, 4.923371831947298993 ) ) ;
#41536=UNCERTAINTY_MEASURE_WITH_UNIT (LENGTH_MEASURE( 1.000000000000000082E-05 ), #51555, 'distance_accuracy_value', 'NONE');
#41538=CARTESIAN_POINT ( 'NONE',  ( 10.00000000000000178, 23.05374883491397142, 14.16423886937410082 ) ) ;
#41540=CARTESIAN_POINT ( 'NONE',  ( 17.08211943468705840, 30.13708216824730357, -12.26659068614894466 ) ) ;
#41541=EDGE_CURVE ( 'NONE', #48470, #10425, #61537, .T. ) ;
#41542=CARTESIAN_POINT ( 'NONE',  ( -2.266590686148945544, 2.220415501580634388, 7.082119434687048631 ) ) ;
#41544=CARTESIAN_POINT ( 'NONE',  ( 12.91533473730992121, 29.52201867748817321, 10.88017736071110164 ) ) ;
#41547=CARTESIAN_POINT ( 'NONE',  ( 10.00000000000000178, 17.25893115100078745, 9.846743663894594434 ) ) ;
#41548=CARTESIAN_POINT ( 'NONE',  ( 17.96484262340118221, 49.93868534415484106, 7.964842623401181321 ) ) ;
#41549=CARTESIAN_POINT ( 'NONE',  ( 2.791683348922237240, 15.38393115100078212, -7.208316651077763204 ) ) ;
#41551=CARTESIAN_POINT ( 'NONE',  ( 0.6178305044545818747, 43.49863466993042493, -9.382169495545419124 ) ) ;
#41552=CARTESIAN_POINT ( 'NONE',  ( 5.076628168052704559, 40.17559781766745175, -8.527530157486179263 ) ) ;
#41556=CARTESIAN_POINT ( 'NONE',  ( 15.44008868035555260, 59.73035201082151247, 9.422509992056143702 ) ) ;
#41557=CARTESIAN_POINT ( 'NONE',  ( -2.816281873526473856, 29.12363466993041783, 9.499525473075851096E-16 ) ) ;
#41559=CARTESIAN_POINT ( 'NONE',  ( 2.791683348922240793, 21.63393115100078745, 7.208316651077764092 ) ) ;
#41560=CARTESIAN_POINT ( 'NONE',  ( 10.00000000000000178, 13.05374883491396787, 14.16423886937410082 ) ) ;
#41562=CARTESIAN_POINT ( 'NONE',  ( 20.88017736071110164, 30.35535201082151247, 2.915334737309930979 ) ) ;
#41563=CARTESIAN_POINT ( 'NONE',  ( 2.035157376598824452, 48.68868534415483396, 7.964842623401179544 ) ) ;
#41564=CARTESIAN_POINT ( 'NONE',  ( 10.00000000000000000, 40.55374883491397497, -14.16423886937410082 ) ) ;
#41565=CARTESIAN_POINT ( 'NONE',  ( 7.361572987183169658, 49.96726448433410894, -9.846743663894592657 ) ) ;
#41566=CARTESIAN_POINT ( 'NONE',  ( 17.20831665107776587, 7.883931151000784787, 7.208316651077764980 ) ) ;
#41569=CARTESIAN_POINT ( 'NONE',  ( 20.88017736071110875, 35.77201867748816966, -2.915334737309920765 ) ) ;
#41571=CARTESIAN_POINT ( 'NONE',  ( -2.816281873526473856, 19.33196800326375708, 3.434112377981055619 ) ) ;
#41572=CARTESIAN_POINT ( 'NONE',  ( 18.52753015748618282, 48.92559781766745886, -4.923371831947291888 ) ) ;
#41574=FILL_AREA_STYLE_COLOUR ( '', #30792 ) ;
#41575=CARTESIAN_POINT ( 'NONE',  ( 15.44008868035555793, 61.39701867748817676, -9.422509992056140149 ) ) ;
#41577=CARTESIAN_POINT ( 'NONE',  ( -0.1503990784575403861, 14.24884699246888964, -6.262539305110056631 ) ) ;
#41579=CARTESIAN_POINT ( 'NONE',  ( 20.88017736071110519, 65.56368534415483396, 2.639326808657452039E-16 ) ) ;
#41581=CARTESIAN_POINT ( 'NONE',  ( 2.035157376598824452, 63.68868534415484106, 7.964842623401179544 ) ) ;
#41584=CARTESIAN_POINT ( 'NONE',  ( 1.472469842513823179, 25.59226448433412315, -4.923371831947296329 ) ) ;
#41585=CARTESIAN_POINT ( 'NONE',  ( 2.035157376598822676, 22.43868534415483396, -7.964842623401177768 ) ) ;
#41587=CARTESIAN_POINT ( 'NONE',  ( -1.099225684535947600, -1.293031996736246469, -6.408140936763238038 ) ) ;
#41588=CARTESIAN_POINT ( 'NONE',  ( 7.084665262690076126, 42.02201867748816966, -10.88017736071110164 ) ) ;
#41589=CARTESIAN_POINT ( 'NONE',  ( 19.72487221294571569, 55.71833443783938833, -6.499999999999990230 ) ) ;
#41591=CARTESIAN_POINT ( 'NONE',  ( -2.816281873526471635, 43.91530133659708923, -3.434112377981056508 ) ) ;
#41592=ORIENTED_EDGE ( 'NONE', *, *, #28207, .T. ) ;
#41593=CARTESIAN_POINT ( 'NONE',  ( 0.5774900079438607392, 48.48035201082150536, 5.440088680355550821 ) ) ;
#41594=CARTESIAN_POINT ( 'NONE',  ( 0.6178305044545838731, 24.74863466993042493, 9.382169495545420901 ) ) ;
#41596=CARTESIAN_POINT ( 'NONE',  ( 4.559911319644449179, 22.23035201082150536, -9.422509992056141925 ) ) ;
#41597=CARTESIAN_POINT ( 'NONE',  ( 20.36894250292379738, 54.92874883491396076, -10.36894250292379027 ) ) ;
#41598=CARTESIAN_POINT ( 'NONE',  ( 0.1532563361054100626, 40.80059781766745886, -2.638427012816831230 ) ) ;
#41599=CARTESIAN_POINT ( 'NONE',  ( 2.035157376598824452, 68.68868534415484817, 7.964842623401179544 ) ) ;
#41600=CARTESIAN_POINT ( 'NONE',  ( 4.559911319644449179, 68.89701867748817676, 9.422509992056141925 ) ) ;
#41602=CARTESIAN_POINT ( 'NONE',  ( -4.164238869374099927, 22.01208216824730357, 3.795296366450308767 ) ) ;
#41604=CARTESIAN_POINT ( 'NONE',  ( 10.00000000000000178, 67.25893115100079456, 9.846743663894594434 ) ) ;
#41606=CARTESIAN_POINT ( 'NONE',  ( -0.3689425029237881626, 47.42874883491396787, 10.36894250292379027 ) ) ;
#41607=CARTESIAN_POINT ( 'NONE',  ( 17.08211943468705130, 48.47041550158063927, 12.26659068614894998 ) ) ;
#41608=CARTESIAN_POINT ( 'NONE',  ( 1.472469842513823179, 15.59226448433411960, -4.923371831947296329 ) ) ;
#41611=CARTESIAN_POINT ( 'NONE',  ( 20.88017736071110164, 5.355352010821502695, 2.915334737309930979 ) ) ;
#41612=CARTESIAN_POINT ( 'NONE',  ( 22.81628187352647785, 26.41530133659708923, 3.434112377981063169 ) ) ;
#41613=CARTESIAN_POINT ( 'NONE',  ( 24.16423886937409904, 44.09541550158063927, 3.795296366450317205 ) ) ;
#41616=( NAMED_UNIT ( * ) PLANE_ANGLE_UNIT ( ) SI_UNIT ( $, .RADIAN. ) );
#41617=AXIS2_PLACEMENT_3D ( 'NONE', #47452, #38983, #16479 ) ;
#41619=ORIENTED_EDGE ( 'NONE', *, *, #37415, .T. ) ;
#41620=CARTESIAN_POINT ( 'NONE',  ( 19.72487221294570858, 70.00000000000000000, 6.500000000000000888 ) ) ;
#41621=CARTESIAN_POINT ( 'NONE',  ( 14.92337183194729988, 24.34226448433411960, -8.527530157486177487 ) ) ;
#41625=CARTESIAN_POINT ( 'NONE',  ( 20.88017736071110519, 5.563685344154838397, 2.639326808657452039E-16 ) ) ;
#41626=CARTESIAN_POINT ( 'NONE',  ( 10.00000000000000000, 11.81368534415483751, -10.88017736071110342 ) ) ;
#41627=CARTESIAN_POINT ( 'NONE',  ( 19.84674366389459266, 43.71726448433410894, -2.638427012816827677 ) ) ;
#41628=CARTESIAN_POINT ( 'NONE',  ( 13.43411237798105340, 5.581968003263753531, 12.81628187352647963 ) ) ;
#41629=LINE ( 'NONE', #87588, #98239 ) ;
#41631=CARTESIAN_POINT ( 'NONE',  ( 6.565887622018943937, 13.08196800326374998, -12.81628187352647608 ) ) ;
#41633=CARTESIAN_POINT ( 'NONE',  ( 24.16423886937410614, 54.30374883491396787, 8.672049930838204340E-16 ) ) ;
#41635=CARTESIAN_POINT ( 'NONE',  ( -4.164238869374098151, 51.59541550158063217, -3.795296366450310543 ) ) ;
#41637=CARTESIAN_POINT ( 'NONE',  ( 2.035157376598822676, 37.43868534415484106, -7.964842623401177768 ) ) ;
#41638=CARTESIAN_POINT ( 'NONE',  ( 20.88017736071110875, 45.77201867748816966, -2.915334737309920765 ) ) ;
#41640=CARTESIAN_POINT ( 'NONE',  ( 15.44008868035555793, 41.39701867748817676, -9.422509992056140149 ) ) ;
#41642=CARTESIAN_POINT ( 'NONE',  ( 7.084665262690076126, 42.02201867748816966, -10.88017736071110164 ) ) ;
#41645=CARTESIAN_POINT ( 'NONE',  ( 7.361572987183170547, 17.05059781766745530, 9.846743663894590881 ) ) ;
#41648=CARTESIAN_POINT ( 'NONE',  ( 0.1532563361054100626, 50.80059781766745175, -2.638427012816831230 ) ) ;
#41650=CARTESIAN_POINT ( 'NONE',  ( 6.565887622018943937, 60.16530133659707502, 12.81628187352647430 ) ) ;
#41654=CYLINDRICAL_SURFACE ( 'NONE', #45016, 0.5000000000000004441 ) ;
#41655=CARTESIAN_POINT ( 'NONE',  ( 24.16423886937409904, 59.09541550158063217, 3.795296366450317205 ) ) ;
#41659=CARTESIAN_POINT ( 'NONE',  ( 7.361572987183170547, 27.05059781766745175, 9.846743663894590881 ) ) ;
#41661=CARTESIAN_POINT ( 'NONE',  ( -2.816281873526471635, 8.915301336597083903, -3.434112377981056508 ) ) ;
#41662=CARTESIAN_POINT ( 'NONE',  ( 4.559911319644449179, 68.89701867748817676, 9.422509992056141925 ) ) ;
#41663=EDGE_CURVE ( 'NONE', #19684, #18045, #12009, .T. ) ;
#41664=CARTESIAN_POINT ( 'NONE',  ( 7.361572987183169658, 14.96726448433411960, -9.846743663894592657 ) ) ;
#41665=CARTESIAN_POINT ( 'NONE',  ( 14.92337183194729988, 59.34226448433412315, -8.527530157486177487 ) ) ;
#41667=COLOUR_RGB ( '', 0.66274510, 0.83137255, 0.94901961) ;
#41670=CARTESIAN_POINT ( 'NONE',  ( 10.00000000000000178, 68.05374883491397497, 14.16423886937410082 ) ) ;
#41671=CARTESIAN_POINT ( 'NONE',  ( 17.96484262340118221, 44.93868534415483396, 7.964842623401181321 ) ) ;
#41673=CARTESIAN_POINT ( 'NONE',  ( 16.40814093676323893, 25.79030133659708923, 11.09922568453595026 ) ) ;
#41675=CARTESIAN_POINT ( 'NONE',  ( 2.035157376598822676, 7.438685344154837509, -7.964842623401177768 ) ) ;
#41677=CARTESIAN_POINT ( 'NONE',  ( 18.52753015748617571, 48.09226448433412315, 4.923371831947298993 ) ) ;
#41678=CARTESIAN_POINT ( 'NONE',  ( 19.84674366389459266, 18.30059781766745175, 2.638427012816836559 ) ) ;
#41680=CARTESIAN_POINT ( 'NONE',  ( 10.00000000000000000, 27.87363466993042138, -12.81628187352647608 ) ) ;
#41682=CARTESIAN_POINT ( 'NONE',  ( 12.91533473730993009, 26.60535201082150536, -10.88017736071109987 ) ) ;
#41684=CARTESIAN_POINT ( 'NONE',  ( -2.266590686148945544, 31.38708216824730002, -7.082119434687050408 ) ) ;
#41685=CARTESIAN_POINT ( 'NONE',  ( 6.204703633549690345, 25.76208216824730712, -14.16423886937410259 ) ) ;
#41686=CARTESIAN_POINT ( 'NONE',  ( -0.8801773607111009756, 8.063685344154837509, 1.068504757029289695E-15 ) ) ;
#41687=CARTESIAN_POINT ( 'NONE',  ( 10.00000000000000178, 47.25893115100078745, 9.846743663894594434 ) ) ;
#41688=CARTESIAN_POINT ( 'NONE',  ( 22.81628187352647785, 41.62363466993042493, 6.195893100308588602E-16 ) ) ;
#41689=CARTESIAN_POINT ( 'NONE',  ( 2.035157376598824452, 28.68868534415484106, 7.964842623401179544 ) ) ;
#41690=CARTESIAN_POINT ( 'NONE',  ( 18.52753015748617571, 48.09226448433412315, 4.923371831947298993 ) ) ;
#41691=ADVANCED_FACE ( 'NONE', ( #66476 ), #72492, .T. ) ;
#41692=CARTESIAN_POINT ( 'NONE',  ( 0.5774900079438607392, 38.48035201082150536, 5.440088680355550821 ) ) ;
#41693=CARTESIAN_POINT ( 'NONE',  ( 22.81628187352648496, 6.831968003263753531, -3.434112377981050290 ) ) ;
#41694=CARTESIAN_POINT ( 'NONE',  ( -2.266590686148945544, 17.22041550158063572, 7.082119434687048631 ) ) ;
#41697=CARTESIAN_POINT ( 'NONE',  ( 18.52753015748618282, 23.92559781766745530, -4.923371831947291888 ) ) ;
#41698=CARTESIAN_POINT ( 'NONE',  ( 0.6178305044545838731, 49.74863466993041072, 9.382169495545420901 ) ) ;
#41699=CARTESIAN_POINT ( 'NONE',  ( -2.816281873526471635, 3.915301336597087456, -3.434112377981056508 ) ) ;
#41703=CARTESIAN_POINT ( 'NONE',  ( 19.42250999205614193, 5.147018677488171434, 5.440088680355555262 ) ) ;
#41704=CARTESIAN_POINT ( 'NONE',  ( 7.084665262690076126, 59.10535201082150536, 10.88017736071109987 ) ) ;
#41705=CARTESIAN_POINT ( 'NONE',  ( 24.16423886937410614, 14.30374883491396787, 8.672049930838204340E-16 ) ) ;
#41706=CARTESIAN_POINT ( 'NONE',  ( 0.5774900079438590739, 67.64701867748817676, -5.440088680355550821 ) ) ;
#41707=CARTESIAN_POINT ( 'NONE',  ( 7.361572987183169658, 49.96726448433410894, -9.846743663894592657 ) ) ;
#41708=CARTESIAN_POINT ( 'NONE',  ( 2.035157376598822676, 37.43868534415484106, -7.964842623401177768 ) ) ;
#41710=CARTESIAN_POINT ( 'NONE',  ( 1.472469842513823179, 60.59226448433412315, -4.923371831947296329 ) ) ;
#41711=VECTOR ( 'NONE', #85819, 1000.000000000000000 ) ;
#41713=EDGE_LOOP ( 'NONE', ( #49069, #34506, #4202, #28692, #80935, #42145 ) ) ;
#41718=CARTESIAN_POINT ( 'NONE',  ( 24.16423886937409904, 4.095415501580634832, 3.795296366450317205 ) ) ;
#41719=CARTESIAN_POINT ( 'NONE',  ( -4.164238869374099039, 16.80374883491396787, 8.674139862899312516E-16 ) ) ;
#41720=CARTESIAN_POINT ( 'NONE',  ( -4.164238869374099927, 52.01208216824729647, 3.795296366450308767 ) ) ;
#41721=CARTESIAN_POINT ( 'NONE',  ( 12.63842701281683034, 62.46726448433410894, 9.846743663894596210 ) ) ;
#41722=CARTESIAN_POINT ( 'NONE',  ( 0.1532563361054100626, 40.80059781766745886, -2.638427012816831230 ) ) ;
#41723=CARTESIAN_POINT ( 'NONE',  ( 4.559911319644449179, 27.23035201082150536, -9.422509992056141925 ) ) ;
#41724=CARTESIAN_POINT ( 'NONE',  ( 1.472469842513823179, 66.42559781766745175, 4.923371831947296329 ) ) ;
#41725=CARTESIAN_POINT ( 'NONE',  ( -0.3689425029237881626, 2.428748834913967869, 10.36894250292379027 ) ) ;
#41726=CARTESIAN_POINT ( 'NONE',  ( 22.26659068614895176, 44.72041550158063927, -7.082119434687042414 ) ) ;
#41727=CARTESIAN_POINT ( 'NONE',  ( -4.164238869374099927, 67.01208216824728936, 3.795296366450308767 ) ) ;
#41730=CARTESIAN_POINT ( 'NONE',  ( 10.00000000000000000, 66.81368534415484817, -10.88017736071110342 ) ) ;
#41731=CARTESIAN_POINT ( 'NONE',  ( 1.472469842513823179, 31.42559781766745530, 4.923371831947296329 ) ) ;
#41733=EDGE_CURVE ( 'NONE', #50081, #37711, #50961, .T. ) ;
#41735=ORIENTED_EDGE ( 'NONE', *, *, #65475, .F. ) ;
#41737=CARTESIAN_POINT ( 'NONE',  ( 10.00000000000000178, 22.25893115100078745, 9.846743663894594434 ) ) ;
#41738=ORIENTED_EDGE ( 'NONE', *, *, #86183, .F. ) ;
#41739=CARTESIAN_POINT ( 'NONE',  ( 10.00000000000000178, 28.05374883491396787, 14.16423886937410082 ) ) ;
#41740=CARTESIAN_POINT ( 'NONE',  ( 12.63842701281683922, 34.55059781766745886, -9.846743663894590881 ) ) ;
#41741=CARTESIAN_POINT ( 'NONE',  ( 17.96484262340118221, 54.93868534415484106, 7.964842623401181321 ) ) ;
#41742=ADVANCED_FACE ( 'NONE', ( #97495 ), #28959, .T. ) ;
#41745=CARTESIAN_POINT ( 'NONE',  ( 20.88017736071110875, 60.77201867748817676, -2.915334737309920765 ) ) ;
#41746=CARTESIAN_POINT ( 'NONE',  ( 2.791683348922240793, 41.63393115100078745, 7.208316651077764092 ) ) ;
#41749=CARTESIAN_POINT ( 'NONE',  ( -0.3689425029237898834, 26.17874883491396432, -10.36894250292378850 ) ) ;
#41751=CARTESIAN_POINT ( 'NONE',  ( 0.6178305044545818747, 33.49863466993042493, -9.382169495545419124 ) ) ;
#41752=CARTESIAN_POINT ( 'NONE',  ( 1.472469842513823179, 25.59226448433412315, -4.923371831947296329 ) ) ;
#41755=CARTESIAN_POINT ( 'NONE',  ( -2.816281873526473856, 59.33196800326374643, 3.434112377981055619 ) ) ;
#41757=CARTESIAN_POINT ( 'NONE',  ( 18.52753015748618282, 23.92559781766745530, -4.923371831947291888 ) ) ;
#41758=CARTESIAN_POINT ( 'NONE',  ( 20.88017736071110164, 65.35535201082150536, 2.915334737309930979 ) ) ;
#41761=CARTESIAN_POINT ( 'NONE',  ( -45.73405099927177986, 104.7125420406077723, 5.163390560272683061 ) ) ;
#41763=CARTESIAN_POINT ( 'NONE',  ( 14.92337183194729633, 2.675597817667451750, 8.527530157486181039 ) ) ;
#41764=CARTESIAN_POINT ( 'NONE',  ( 0.6178305044545838731, 29.74863466993042138, 9.382169495545420901 ) ) ;
#41766=CARTESIAN_POINT ( 'NONE',  ( 17.20831665107776587, 39.13393115100079456, -7.208316651077762316 ) ) ;
#41767=CARTESIAN_POINT ( 'NONE',  ( 22.81628187352647785, 61.62363466993041783, 6.195893100308588602E-16 ) ) ;
#41768=CARTESIAN_POINT ( 'NONE',  ( -0.3689425029237881626, 2.428748834913967869, 10.36894250292379027 ) ) ;
#41769=CARTESIAN_POINT ( 'NONE',  ( 5.076628168052703671, 31.84226448433412315, 8.527530157486179263 ) ) ;
#41770=CARTESIAN_POINT ( 'NONE',  ( 19.38216949554541202, 35.99863466993041072, 9.382169495545424454 ) ) ;
#41772=CARTESIAN_POINT ( 'NONE',  ( 19.72487221294571214, 15.71833443783937589, -6.500000000000001776 ) ) ;
#41773=CARTESIAN_POINT ( 'NONE',  ( -0.8801773607111009756, 68.06368534415484817, 1.068504757029289695E-15 ) ) ;
#41774=CARTESIAN_POINT ( 'NONE',  ( 10.00000000000000000, 7.873634669930421381, -12.81628187352647608 ) ) ;
#41777=CARTESIAN_POINT ( 'NONE',  ( 5.076628168052704559, 40.17559781766745175, -8.527530157486179263 ) ) ;
#41778=CARTESIAN_POINT ( 'NONE',  ( 0.5774900079438590739, 22.64701867748817321, -5.440088680355550821 ) ) ;
#41780=CARTESIAN_POINT ( 'NONE',  ( 19.38216949554541557, 27.24863466993041783, -9.382169495545420901 ) ) ;
#41781=CARTESIAN_POINT ( 'NONE',  ( 14.92337183194729633, 27.67559781766745530, 8.527530157486181039 ) ) ;
#41783=CARTESIAN_POINT ( 'NONE',  ( 0.5774900079438590739, 32.64701867748816966, -5.440088680355550821 ) ) ;
#41786=CARTESIAN_POINT ( 'NONE',  ( 12.91533473730992121, 64.52201867748817676, 10.88017736071110164 ) ) ;
#41787=CARTESIAN_POINT ( 'NONE',  ( 15.44008868035555793, 6.397018677488170546, -9.422509992056140149 ) ) ;
#41788=CARTESIAN_POINT ( 'NONE',  ( 5.076628168052703671, 41.84226448433411605, 8.527530157486179263 ) ) ;
#41789=CARTESIAN_POINT ( 'NONE',  ( 10.00000000000000178, 29.31368534415483751, 10.88017736071110342 ) ) ;
#41790=FACE_OUTER_BOUND ( 'NONE', #36816, .T. ) ;
#41791=CARTESIAN_POINT ( 'NONE',  ( -0.8801773607111009756, 43.06368534415484106, 1.068504757029289695E-15 ) ) ;
#41792=CARTESIAN_POINT ( 'NONE',  ( 15.44008868035555260, 19.73035201082150536, 9.422509992056143702 ) ) ;
#41794=CARTESIAN_POINT ( 'NONE',  ( 0.1532563361054100626, 5.800597817667452638, -2.638427012816831230 ) ) ;
#41795=CARTESIAN_POINT ( 'NONE',  ( 14.92337183194729633, 57.67559781766745886, 8.527530157486181039 ) ) ;
#41796=CARTESIAN_POINT ( 'NONE',  ( -2.266590686148945544, 56.38708216824731068, -7.082119434687050408 ) ) ;
#41797=CARTESIAN_POINT ( 'NONE',  ( 20.32896413005680714, 20.57879003517447458, -5.963430220938276349 ) ) ;
#41799=CARTESIAN_POINT ( 'NONE',  ( -2.266590686148945544, 1.387082168247301128, -7.082119434687050408 ) ) ;
#41800=CARTESIAN_POINT ( 'NONE',  ( 24.16423886937410614, 39.30374883491396787, 8.672049930838204340E-16 ) ) ;
#41806=CARTESIAN_POINT ( 'NONE',  ( 17.08211943468705840, 65.13708216824730357, -12.26659068614894466 ) ) ;
#41807=CARTESIAN_POINT ( 'NONE',  ( 14.92337183194729633, 37.67559781766745175, 8.527530157486181039 ) ) ;
#41810=CARTESIAN_POINT ( 'NONE',  ( 12.91533473730992121, 59.52201867748816966, 10.88017736071110164 ) ) ;
#41812=CARTESIAN_POINT ( 'NONE',  ( -0.8801773607111009756, 33.06368534415484106, 1.068504757029289695E-15 ) ) ;
#41814=CARTESIAN_POINT ( 'NONE',  ( 6.565887622018943937, 55.16530133659709634, 12.81628187352647430 ) ) ;
#41815=CARTESIAN_POINT ( 'NONE',  ( 22.81628187352647785, 16.41530133659708923, 3.434112377981063169 ) ) ;
#41816=CARTESIAN_POINT ( 'NONE',  ( 7.361572987183169658, 19.96726448433411960, -9.846743663894592657 ) ) ;
#41821=CARTESIAN_POINT ( 'NONE',  ( -4.164238869374098151, 31.59541550158063927, -3.795296366450310543 ) ) ;
#41822=CARTESIAN_POINT ( 'NONE',  ( 10.00000000000000000, 36.81368534415484106, -10.88017736071110342 ) ) ;
#41823=CARTESIAN_POINT ( 'NONE',  ( 0.5774900079438607392, 43.48035201082151247, 5.440088680355550821 ) ) ;
#41826=CARTESIAN_POINT ( 'NONE',  ( 1.472469842513823179, 15.59226448433411960, -4.923371831947296329 ) ) ;
#41827=SURFACE_SIDE_STYLE ('',( #87789 ) ) ;
#41828=COLOUR_RGB ( '', 0.66274510, 0.83137255, 0.94901961) ;
#41829=CARTESIAN_POINT ( 'NONE',  ( -46.48928645636215151, 103.2957187381728232, 6.397878122523974476 ) ) ;
#41830=CARTESIAN_POINT ( 'NONE',  ( 19.84674366389459266, 18.71726448433411960, -2.638427012816827677 ) ) ;
#41831=CARTESIAN_POINT ( 'NONE',  ( 0.1532563361054100626, 55.80059781766745175, -2.638427012816831230 ) ) ;
#41832=CARTESIAN_POINT ( 'NONE',  ( 20.88017736071110164, 25.35535201082150891, 2.915334737309930979 ) ) ;
#41833=CARTESIAN_POINT ( 'NONE',  ( 21.09922568453594849, 51.20696800326375353, 6.408140936763242479 ) ) ;
#41835=CARTESIAN_POINT ( 'NONE',  ( 0.5774900079438590739, 62.64701867748817676, -5.440088680355550821 ) ) ;
#41836=CARTESIAN_POINT ( 'NONE',  ( 1.472469842513823179, 30.59226448433411960, -4.923371831947296329 ) ) ;
#41837=CARTESIAN_POINT ( 'NONE',  ( 2.917880565312950480, 65.97041550158063217, -12.26659068614894821 ) ) ;
#41838=CARTESIAN_POINT ( 'NONE',  ( 7.361572987183170547, 27.05059781766745175, 9.846743663894590881 ) ) ;
#41839=CARTESIAN_POINT ( 'NONE',  ( 0.1957200283969099119, 60.25733960839542647, 6.499999999999992006 ) ) ;
#41840=CARTESIAN_POINT ( 'NONE',  ( 10.00000000000000178, 67.25893115100079456, 9.846743663894594434 ) ) ;
#41841=CARTESIAN_POINT ( 'NONE',  ( 24.16423886937410614, 14.30374883491396787, 8.672049930838204340E-16 ) ) ;
#41842=CARTESIAN_POINT ( 'NONE',  ( 20.36894250292379738, 34.92874883491396076, -10.36894250292379027 ) ) ;
#41843=CARTESIAN_POINT ( 'NONE',  ( 1.472469842513823179, 26.42559781766745175, 4.923371831947296329 ) ) ;
#41844=CARTESIAN_POINT ( 'NONE',  ( 5.500000000000000000, 11.50000000000000000, 5.000000000000000000 ) ) ;
#41845=CARTESIAN_POINT ( 'NONE',  ( 12.91533473730992121, 19.52201867748816611, 10.88017736071110164 ) ) ;
#41846=CARTESIAN_POINT ( 'NONE',  ( -0.8801773607111008646, 58.27201867748816966, 2.915334737309923430 ) ) ;
#41847=CARTESIAN_POINT ( 'NONE',  ( 0.1532563361054082862, 56.21726448433411605, 2.638427012816831674 ) ) ;
#41849=CARTESIAN_POINT ( 'NONE',  ( -2.816281873526471635, 43.91530133659708923, -3.434112377981056508 ) ) ;
#41850=CARTESIAN_POINT ( 'NONE',  ( 2.035157376598824452, 48.68868534415483396, 7.964842623401179544 ) ) ;
#41856=CARTESIAN_POINT ( 'NONE',  ( 4.559911319644449179, 58.89701867748817676, 9.422509992056141925 ) ) ;
#41857=SURFACE_SIDE_STYLE ('',( #85874 ) ) ;
#41861=CARTESIAN_POINT ( 'NONE',  ( 10.00000000000000178, 68.05374883491397497, 14.16423886937410082 ) ) ;
#41862=CARTESIAN_POINT ( 'NONE',  ( 18.52753015748618282, 13.92559781766745175, -4.923371831947291888 ) ) ;
#41863=CARTESIAN_POINT ( 'NONE',  ( 24.16423886937409904, 19.09541550158063927, 3.795296366450317205 ) ) ;
#41864=CARTESIAN_POINT ( 'NONE',  ( 17.20831665107776587, 2.883931151000785231, 7.208316651077764980 ) ) ;
#41865=CARTESIAN_POINT ( 'NONE',  ( 20.88017736071110519, 20.56368534415484106, 2.639326808657452039E-16 ) ) ;
#41866=CARTESIAN_POINT ( 'NONE',  ( 10.00000000000000000, 54.75893115100078745, -9.846743663894594434 ) ) ;
#41868=CARTESIAN_POINT ( 'NONE',  ( 10.00000000000000000, 49.75893115100078745, -9.846743663894594434 ) ) ;
#41871=CARTESIAN_POINT ( 'NONE',  ( 10.00000000000000000, 51.81368534415484106, -10.88017736071110342 ) ) ;
#41872=CARTESIAN_POINT ( 'NONE',  ( 1.472469842513823179, 51.42559781766745886, 4.923371831947296329 ) ) ;
#41873=CARTESIAN_POINT ( 'NONE',  ( 0.5774900079438590739, 7.647018677488171434, -5.440088680355550821 ) ) ;
#41875=CARTESIAN_POINT ( 'NONE',  ( 0.5774900079438607392, 63.48035201082149825, 5.440088680355550821 ) ) ;
#41876=CARTESIAN_POINT ( 'NONE',  ( 10.00000000000000178, 9.313685344154839285, 10.88017736071110342 ) ) ;
#41878=EDGE_LOOP ( 'NONE', ( #29269, #10749, #10474, #60159 ) ) ;
#41879=CARTESIAN_POINT ( 'NONE',  ( 16.40814093676323893, 40.79030133659708923, 11.09922568453595026 ) ) ;
#41880=CARTESIAN_POINT ( 'NONE',  ( 4.559911319644449179, 27.23035201082150536, -9.422509992056141925 ) ) ;
#41883=CARTESIAN_POINT ( 'NONE',  ( 3.591859063236763294, 48.29030133659708923, -11.09922568453595026 ) ) ;
#41884=CARTESIAN_POINT ( 'NONE',  ( 10.00000000000000178, 29.31368534415483751, 10.88017736071110342 ) ) ;
#41889=CARTESIAN_POINT ( 'NONE',  ( 18.52753015748618282, 8.925597817667451750, -4.923371831947291888 ) ) ;
#41891=CARTESIAN_POINT ( 'NONE',  ( 18.52753015748618282, 58.92559781766745886, -4.923371831947291888 ) ) ;
#41892=CARTESIAN_POINT ( 'NONE',  ( 14.92337183194729633, 7.675597817667451750, 8.527530157486181039 ) ) ;
#41893=CARTESIAN_POINT ( 'NONE',  ( 0.1532563361054100626, 50.80059781766745175, -2.638427012816831230 ) ) ;
#41894=CARTESIAN_POINT ( 'NONE',  ( -0.8801773607111009756, 28.06368534415484106, 1.068504757029289695E-15 ) ) ;
#41895=CARTESIAN_POINT ( 'NONE',  ( -0.04068437667222125909, 52.21974360917721469, -6.396802510829770583 ) ) ;
#41897=CARTESIAN_POINT ( 'NONE',  ( 19.84674366389459621, 28.50893115100078745, 7.409399052514197653E-17 ) ) ;
#41898=CARTESIAN_POINT ( 'NONE',  ( 12.63842701281683034, 12.46726448433411782, 9.846743663894596210 ) ) ;
#41901=CARTESIAN_POINT ( 'NONE',  ( 1.472469842513823179, 60.59226448433412315, -4.923371831947296329 ) ) ;
#41902=EDGE_LOOP ( 'NONE', ( #15528, #85967, #53991, #33812 ) ) ;
#41903=CARTESIAN_POINT ( 'NONE',  ( -2.816281873526473856, 64.12363466993042493, 9.499525473075851096E-16 ) ) ;
#41904=CARTESIAN_POINT ( 'NONE',  ( 19.72487221294570858, 7.802231764288317883, -6.499999999999999112 ) ) ;
#41905=CARTESIAN_POINT ( 'NONE',  ( -2.816281873526473856, 24.33196800326375353, 3.434112377981055619 ) ) ;
#41906=CARTESIAN_POINT ( 'NONE',  ( 19.84674366389459266, 38.30059781766745175, 2.638427012816836559 ) ) ;
#41908=CARTESIAN_POINT ( 'NONE',  ( 17.08211943468705840, 60.13708216824729647, -12.26659068614894466 ) ) ;
#41910=CARTESIAN_POINT ( 'NONE',  ( 1.472469842513823179, 20.59226448433411960, -4.923371831947296329 ) ) ;
#41911=ORIENTED_EDGE ( 'NONE', *, *, #70927, .F. ) ;
#41912=CARTESIAN_POINT ( 'NONE',  ( 20.00000000000000711, 84.97150353911858645, 5.197973391108559937 ) ) ;
#41913=CARTESIAN_POINT ( 'NONE',  ( 20.36894250292379382, 63.67874883491396787, 10.36894250292379205 ) ) ;
#41914=CARTESIAN_POINT ( 'NONE',  ( 7.361572987183170547, 57.05059781766744464, 9.846743663894590881 ) ) ;
#41915=CARTESIAN_POINT ( 'NONE',  ( 6.204703633549690345, 67.84541550158060375, 14.16423886937410082 ) ) ;
#41916=CARTESIAN_POINT ( 'NONE',  ( 20.36894250292379738, 39.92874883491396787, -10.36894250292379027 ) ) ;
#41917=CARTESIAN_POINT ( 'NONE',  ( -2.266590686148945544, 41.38708216824729647, -7.082119434687050408 ) ) ;
#41922=CARTESIAN_POINT ( 'NONE',  ( 1.472469842513823179, 60.59226448433412315, -4.923371831947296329 ) ) ;
#41923=CARTESIAN_POINT ( 'NONE',  ( 20.88017736071110164, 50.35535201082151247, 2.915334737309930979 ) ) ;
#41925=CARTESIAN_POINT ( 'NONE',  ( 12.63842701281683922, 49.55059781766744464, -9.846743663894590881 ) ) ;
#41926=CARTESIAN_POINT ( 'NONE',  ( 0.2751277870542967463, 70.00000000000000000, -6.000000000000000000 ) ) ;
#41927=CARTESIAN_POINT ( 'NONE',  ( 10.00000000000000000, 49.75893115100078745, -9.846743663894594434 ) ) ;
#41928=CARTESIAN_POINT ( 'NONE',  ( 17.08211943468705130, 3.470415501580634388, 12.26659068614894998 ) ) ;
#41930=CARTESIAN_POINT ( 'NONE',  ( 24.16423886937410614, 24.51208216824730002, -3.795296366450302550 ) ) ;
#41931=SURFACE_STYLE_FILL_AREA ( #4422 ) ;
#41933=LINE ( 'NONE', #19407, #66424 ) ;
#41934=CARTESIAN_POINT ( 'NONE',  ( 2.035157376598824452, 23.68868534415484461, 7.964842623401179544 ) ) ;
#41935=CARTESIAN_POINT ( 'NONE',  ( -2.816281873526471635, 23.91530133659708568, -3.434112377981056508 ) ) ;
#41937=CARTESIAN_POINT ( 'NONE',  ( 17.20831665107776587, 14.13393115100078568, -7.208316651077762316 ) ) ;
#41941=CARTESIAN_POINT ( 'NONE',  ( 10.00000000000000178, 23.05374883491397142, 14.16423886937410082 ) ) ;
#41942=CARTESIAN_POINT ( 'NONE',  ( 2.603489959281581889, 20.43575266056827999, -6.499999999999995559 ) ) ;
#41943=CARTESIAN_POINT ( 'NONE',  ( -0.8801773607111009756, 3.063685344154838397, 1.068504757029289695E-15 ) ) ;
#41945=CARTESIAN_POINT ( 'NONE',  ( 0.5774900079438607392, 43.48035201082151247, 5.440088680355550821 ) ) ;
#41946=CARTESIAN_POINT ( 'NONE',  ( 15.44008868035555793, 31.39701867748817676, -9.422509992056140149 ) ) ;
#41947=CARTESIAN_POINT ( 'NONE',  ( 6.565887622018943937, 8.081968003263751754, -12.81628187352647608 ) ) ;
#41950=CARTESIAN_POINT ( 'NONE',  ( 18.52753015748617571, 8.092264484334117824, 4.923371831947298993 ) ) ;
#41952=CARTESIAN_POINT ( 'NONE',  ( 18.06765999051787830, 48.99127512925448258, 6.499999999999931610 ) ) ;
#41953=CARTESIAN_POINT ( 'NONE',  ( 4.559911319644449179, 43.89701867748816966, 9.422509992056141925 ) ) ;
#41954=CARTESIAN_POINT ( 'NONE',  ( -2.816281873526471635, 3.915301336597087456, -3.434112377981056508 ) ) ;
#41955=CARTESIAN_POINT ( 'NONE',  ( 4.559911319644449179, 62.23035201082150536, -9.422509992056141925 ) ) ;
#41956=CARTESIAN_POINT ( 'NONE',  ( 10.00000000000000000, 29.75893115100078745, -9.846743663894594434 ) ) ;
#41957=CARTESIAN_POINT ( 'NONE',  ( 6.565887622018943937, 40.16530133659708923, 12.81628187352647430 ) ) ;
#41958=AXIS2_PLACEMENT_3D ( 'NONE', #62150, #78154, #8675 ) ;
#41959=CARTESIAN_POINT ( 'NONE',  ( 14.92337183194729988, 4.342264484334117824, -8.527530157486177487 ) ) ;
#41961=FILL_AREA_STYLE_COLOUR ( '', #3768 ) ;
#41963=CARTESIAN_POINT ( 'NONE',  ( -2.816281873526471635, 63.91530133659708923, -3.434112377981056508 ) ) ;
#41964=CARTESIAN_POINT ( 'NONE',  ( 0.1532563361054083140, 36.00893115100078745, 1.131784320476157264E-15 ) ) ;
#41965=CARTESIAN_POINT ( 'NONE',  ( 12.91533473730992121, 24.52201867748816966, 10.88017736071110164 ) ) ;
#41966=CARTESIAN_POINT ( 'NONE',  ( 15.44008868035555260, 9.730352010821505360, 9.422509992056143702 ) ) ;
#41968=CIRCLE ( 'NONE', #70731, 2.999999999999999112 ) ;
#41969=CARTESIAN_POINT ( 'NONE',  ( 0.5774900079438590739, 7.647018677488171434, -5.440088680355550821 ) ) ;
#41971=CARTESIAN_POINT ( 'NONE',  ( 0.5774900079438590739, 22.64701867748817321, -5.440088680355550821 ) ) ;
#41973=AXIS2_PLACEMENT_3D ( 'NONE', #3596, #33084, #87565 ) ;
#41974=EDGE_LOOP ( 'NONE', ( #16671, #85883, #29857, #8142 ) ) ;
#41975=CARTESIAN_POINT ( 'NONE',  ( 2.791683348922240793, 66.63393115100079456, 7.208316651077764092 ) ) ;
#41976=CARTESIAN_POINT ( 'NONE',  ( 19.42250999205614548, 25.98035201082150891, -5.440088680355545492 ) ) ;
#41977=CARTESIAN_POINT ( 'NONE',  ( 0.1532563361054083140, 61.00893115100078745, 1.131784320476157264E-15 ) ) ;
#41979=CARTESIAN_POINT ( 'NONE',  ( 21.09922568453595559, 57.04030133659708923, -6.408140936763230044 ) ) ;
#41980=CARTESIAN_POINT ( 'NONE',  ( -0.3689425029237898834, 31.17874883491396787, -10.36894250292378850 ) ) ;
#41981=CARTESIAN_POINT ( 'NONE',  ( 10.00000000000000178, 44.31368534415484106, 10.88017736071110342 ) ) ;
#41982=CARTESIAN_POINT ( 'NONE',  ( 20.88017736071110519, 10.56368534415483929, 2.639326808657452039E-16 ) ) ;
#41983=CARTESIAN_POINT ( 'NONE',  ( 14.92337183194729633, 52.67559781766745175, 8.527530157486181039 ) ) ;
#41984=LINE ( 'NONE', #26461, #85994 ) ;
#41985=CARTESIAN_POINT ( 'NONE',  ( 2.791683348922237240, 50.38393115100078035, -7.208316651077763204 ) ) ;
#41988=CARTESIAN_POINT ( 'NONE',  ( 2.791683348922240793, 6.633931151000785675, 7.208316651077764092 ) ) ;
#41991=CARTESIAN_POINT ( 'NONE',  ( 20.88017736071110519, 10.56368534415483751, 2.639326808657452039E-16 ) ) ;
#41992=CARTESIAN_POINT ( 'NONE',  ( 18.52753015748617571, 8.092264484334117824, 4.923371831947298993 ) ) ;
#41993=CARTESIAN_POINT ( 'NONE',  ( 19.84674366389459621, 63.50893115100078745, 7.409399052514197653E-17 ) ) ;
#41994=CARTESIAN_POINT ( 'NONE',  ( 20.88017736071110875, 60.77201867748817676, -2.915334737309920765 ) ) ;
#41995=CARTESIAN_POINT ( 'NONE',  ( 10.00000000000000178, 19.31368534415484106, 10.88017736071110342 ) ) ;
#41996=CARTESIAN_POINT ( 'NONE',  ( 0.6178305044545838731, 44.74863466993042493, 9.382169495545420901 ) ) ;
#41997=CARTESIAN_POINT ( 'NONE',  ( -0.3689425029237898834, 26.17874883491396432, -10.36894250292378850 ) ) ;
#41999=( BOUNDED_CURVE ( )  B_SPLINE_CURVE ( 2, ( #67855, #16327, #77302, #8330, #59838, #6850, #15844, #45336, #36859 ),
 .UNSPECIFIED., .F., .T. ) 
 B_SPLINE_CURVE_WITH_KNOTS ( ( 3, 2, 2, 2, 3 ),
 ( 0.08108559304626794528, 0.08333333333333332871, 0.08928571428571428770, 0.09523809523809523281, 0.09748583552516061623 ),
 .UNSPECIFIED. ) 
 CURVE ( )  GEOMETRIC_REPRESENTATION_ITEM ( )  RATIONAL_B_SPLINE_CURVE ( ( 0.9839835555609424134, 0.9871328979762477029, 1.000000000000000000, 0.9659258262890683122, 1.000000000000000000, 0.9659258262890683122, 1.000000000000000000, 0.9871328979762477029, 0.9839835555609424134 ) ) 
 REPRESENTATION_ITEM ( '' )  );
#42001=CARTESIAN_POINT ( 'NONE',  ( 21.09922568453594849, 61.20696800326376064, 6.408140936763242479 ) ) ;
#42003=CARTESIAN_POINT ( 'NONE',  ( 6.565887622018943937, -1.918031996736246692, -12.81628187352647608 ) ) ;
#42005=CARTESIAN_POINT ( 'NONE',  ( 4.559911319644449179, 27.23035201082150536, -9.422509992056141925 ) ) ;
#42006=CARTESIAN_POINT ( 'NONE',  ( 10.00000000000000178, 67.25893115100079456, 9.846743663894594434 ) ) ;
#42008=CARTESIAN_POINT ( 'NONE',  ( 19.84674366389459621, 8.508931151000785675, 7.409399052514197653E-17 ) ) ;
#42009=CARTESIAN_POINT ( 'NONE',  ( 5.076628168052703671, 6.842264484334118713, 8.527530157486179263 ) ) ;
#42011=CARTESIAN_POINT ( 'NONE',  ( 17.20831665107776587, 19.13393115100078035, -7.208316651077762316 ) ) ;
#42013=CARTESIAN_POINT ( 'NONE',  ( 17.20831665107776587, 12.88393115100078390, 7.208316651077764980 ) ) ;
#42014=CARTESIAN_POINT ( 'NONE',  ( 10.00000000000000178, 2.258931151000784787, 9.846743663894594434 ) ) ;
#42015=CARTESIAN_POINT ( 'NONE',  ( -0.8801773607111009756, 53.06368534415484106, 1.068504757029289695E-15 ) ) ;
#42016=CARTESIAN_POINT ( 'NONE',  ( -0.8801773607111009756, 38.27201867748816966, 2.915334737309923874 ) ) ;
#42017=CARTESIAN_POINT ( 'NONE',  ( 15.44008868035555793, 56.39701867748817676, -9.422509992056140149 ) ) ;
#42018=CARTESIAN_POINT ( 'NONE',  ( 19.84674366389459266, 23.30059781766745530, 2.638427012816836559 ) ) ;
#42019=ORIENTED_EDGE ( 'NONE', *, *, #24010, .T. ) ;
#42022=CARTESIAN_POINT ( 'NONE',  ( 2.791683348922237240, 60.38393115100078745, -7.208316651077763204 ) ) ;
#42023=ORIENTED_EDGE ( 'NONE', *, *, #81063, .T. ) ;
#42024=CARTESIAN_POINT ( 'NONE',  ( 7.084665262690076126, 4.105352010821503583, 10.88017736071109987 ) ) ;
#42025=CARTESIAN_POINT ( 'NONE',  ( -2.266590686148945544, 17.22041550158063572, 7.082119434687048631 ) ) ;
#42030=CARTESIAN_POINT ( 'NONE',  ( 6.204703633549690345, 10.76208216824729824, -14.16423886937410259 ) ) ;
#42031=CARTESIAN_POINT ( 'NONE',  ( 2.917880565312950480, 30.97041550158063572, -12.26659068614894821 ) ) ;
#42033=CARTESIAN_POINT ( 'NONE',  ( 17.96484262340118221, 29.93868534415484106, 7.964842623401181321 ) ) ;
#42035=CARTESIAN_POINT ( 'NONE',  ( 5.076628168052704559, 10.17559781766745175, -8.527530157486179263 ) ) ;
#42036=AXIS2_PLACEMENT_3D ( 'NONE', #28343, #12352, #20850 ) ;
#42037=CARTESIAN_POINT ( 'NONE',  ( 10.00000000000000178, 54.31368534415484106, 10.88017736071110342 ) ) ;
#42038=CARTESIAN_POINT ( 'NONE',  ( 17.20831665107776587, 19.13393115100078035, -7.208316651077762316 ) ) ;
#42039=CARTESIAN_POINT ( 'NONE',  ( 15.44008868035555793, 6.397018677488171434, -9.422509992056140149 ) ) ;
#42040=CARTESIAN_POINT ( 'NONE',  ( 10.00000000000000178, 50.37363466993042493, 12.81628187352647608 ) ) ;
#42041=CARTESIAN_POINT ( 'NONE',  ( 1.472469842513823179, 41.42559781766745886, 4.923371831947296329 ) ) ;
#42042=CARTESIAN_POINT ( 'NONE',  ( 18.52753015748617571, 58.09226448433411605, 4.923371831947298993 ) ) ;
#42043=CARTESIAN_POINT ( 'NONE',  ( 22.81628187352647785, 26.62363466993042138, 6.195893100308588602E-16 ) ) ;
#42045=CARTESIAN_POINT ( 'NONE',  ( 18.52753015748617571, 28.09226448433411960, 4.923371831947298993 ) ) ;
#42046=CARTESIAN_POINT ( 'NONE',  ( 2.917880565312948704, 7.637082168247301794, 12.26659068614894643 ) ) ;
#42049=CARTESIAN_POINT ( 'NONE',  ( 12.91533473730993009, 51.60535201082149825, -10.88017736071109987 ) ) ;
#42050=CARTESIAN_POINT ( 'NONE',  ( 15.44008868035555260, 59.73035201082151247, 9.422509992056143702 ) ) ;
#42051=CARTESIAN_POINT ( 'NONE',  ( 20.36894250292379382, 43.67874883491397497, 10.36894250292379205 ) ) ;
#42052=CARTESIAN_POINT ( 'NONE',  ( 17.20831665107776587, 59.13393115100078745, -7.208316651077762316 ) ) ;
#42053=CARTESIAN_POINT ( 'NONE',  ( 2.791683348922240793, 6.633931151000785675, 7.208316651077764092 ) ) ;
#42054=FACE_OUTER_BOUND ( 'NONE', #3368, .T. ) ;
#42055=CARTESIAN_POINT ( 'NONE',  ( 10.00000000000000178, 44.31368534415484106, 10.88017736071110342 ) ) ;
#42058=CARTESIAN_POINT ( 'NONE',  ( 13.43411237798105340, 25.58196800326374998, 12.81628187352647963 ) ) ;
#42059=CARTESIAN_POINT ( 'NONE',  ( 18.52753015748617571, 58.09226448433411605, 4.923371831947298993 ) ) ;
#42061=CARTESIAN_POINT ( 'NONE',  ( 2.035157376598824452, 63.68868534415484106, 7.964842623401179544 ) ) ;
#42065=CARTESIAN_POINT ( 'NONE',  ( 0.1532563361054082862, 1.217264484334117824, 2.638427012816831674 ) ) ;
#42067=CARTESIAN_POINT ( 'NONE',  ( 7.361572987183170547, 2.050597817667451750, 9.846743663894590881 ) ) ;
#42069=CARTESIAN_POINT ( 'NONE',  ( 18.52753015748617571, 38.09226448433412315, 4.923371831947298993 ) ) ;
#42070=CARTESIAN_POINT ( 'NONE',  ( 12.91533473730992121, 24.52201867748816966, 10.88017736071110164 ) ) ;
#42071=CARTESIAN_POINT ( 'NONE',  ( 19.84674366389459621, 58.50893115100078745, 7.409399052514197653E-17 ) ) ;
#42072=CARTESIAN_POINT ( 'NONE',  ( 15.44008868035555793, 31.39701867748817676, -9.422509992056140149 ) ) ;
#42075=CARTESIAN_POINT ( 'NONE',  ( 3.591859063236763294, 33.29030133659708213, -11.09922568453595026 ) ) ;
#42076=ORIENTED_EDGE ( 'NONE', *, *, #8714, .T. ) ;
#42077=CARTESIAN_POINT ( 'NONE',  ( 20.88017736071110164, 55.35535201082149825, 2.915334737309930979 ) ) ;
#42078=CARTESIAN_POINT ( 'NONE',  ( -2.816281873526473856, 14.12363466993041961, 9.499525473075851096E-16 ) ) ;
#42079=CARTESIAN_POINT ( 'NONE',  ( 0.1532563361054083140, 1.008931151000784787, 1.131784320476157264E-15 ) ) ;
#42080=CARTESIAN_POINT ( 'NONE',  ( 12.91533473730992121, 29.52201867748817321, 10.88017736071110164 ) ) ;
#42081=CARTESIAN_POINT ( 'NONE',  ( -2.266590686148945544, 61.38708216824730357, -7.082119434687050408 ) ) ;
#42082=CARTESIAN_POINT ( 'NONE',  ( 2.791683348922237240, 45.38393115100079456, -7.208316651077763204 ) ) ;
#42083=CARTESIAN_POINT ( 'NONE',  ( 0.1532563361054100626, 0.8005978176674514168, -2.638427012816831230 ) ) ;
#42084=CARTESIAN_POINT ( 'NONE',  ( 10.00000000000000000, 56.81368534415484106, -10.88017736071110342 ) ) ;
#42086=CARTESIAN_POINT ( 'NONE',  ( -0.3689425029237881626, 27.42874883491397142, 10.36894250292379027 ) ) ;
#42087=CARTESIAN_POINT ( 'NONE',  ( 19.64275500434244748, 84.99812590208811969, -5.306653671078411350 ) ) ;
#42089=CARTESIAN_POINT ( 'NONE',  ( 6.204703633549690345, 45.76208216824729647, -14.16423886937410259 ) ) ;
#42090=CARTESIAN_POINT ( 'NONE',  ( -4.164238869374099039, 46.80374883491397497, 8.674139862899312516E-16 ) ) ;
#42091=CARTESIAN_POINT ( 'NONE',  ( 1.472469842513823179, 20.59226448433411960, -4.923371831947296329 ) ) ;
#42092=CARTESIAN_POINT ( 'NONE',  ( -1.099225684535947600, 19.54030133659708568, 6.408140936763237150 ) ) ;
#42097=CARTESIAN_POINT ( 'NONE',  ( 19.38216949554541202, 50.99863466993042493, 9.382169495545424454 ) ) ;
#42098=CARTESIAN_POINT ( 'NONE',  ( -4.164238869374099039, 41.80374883491397497, 8.674139862899312516E-16 ) ) ;
#42101=CARTESIAN_POINT ( 'NONE',  ( 19.84674366389459266, 13.71726448433411782, -2.638427012816827677 ) ) ;
#42105=FILL_AREA_STYLE_COLOUR ( '', #23686 ) ;
#42106=CARTESIAN_POINT ( 'NONE',  ( 19.84674366389459621, 18.50893115100078745, 7.409399052514197653E-17 ) ) ;
#42110=CARTESIAN_POINT ( 'NONE',  ( 6.204703633549690345, 10.76208216824729824, -14.16423886937410259 ) ) ;
#42111=CARTESIAN_POINT ( 'NONE',  ( -0.8801773607111009756, 3.063685344154838397, 1.068504757029289695E-15 ) ) ;
#42112=CARTESIAN_POINT ( 'NONE',  ( -0.8801773607111009756, 28.06368534415484106, 1.068504757029289695E-15 ) ) ;
#42113=CARTESIAN_POINT ( 'NONE',  ( 10.00000000000000000, 44.75893115100078745, -9.846743663894594434 ) ) ;
#42114=CARTESIAN_POINT ( 'NONE',  ( -2.816281873526473856, 4.331968003263754419, 3.434112377981055619 ) ) ;
#42117=CARTESIAN_POINT ( 'NONE',  ( 21.09922568453595559, 22.04030133659708923, -6.408140936763230044 ) ) ;
#42119=CARTESIAN_POINT ( 'NONE',  ( -2.266590686148945544, 62.22041550158063927, 7.082119434687048631 ) ) ;
#42120=CARTESIAN_POINT ( 'NONE',  ( -0.3689425029237898834, 56.17874883491396076, -10.36894250292378850 ) ) ;
#42122=CARTESIAN_POINT ( 'NONE',  ( 20.88017736071110875, 30.77201867748816966, -2.915334737309920765 ) ) ;
#42123=CARTESIAN_POINT ( 'NONE',  ( 15.44008868035555260, 39.73035201082150536, 9.422509992056143702 ) ) ;
#42124=CARTESIAN_POINT ( 'NONE',  ( 2.035157376598822676, 57.43868534415484106, -7.964842623401177768 ) ) ;
#42126=CARTESIAN_POINT ( 'NONE',  ( -0.8801773607110991993, 37.85535201082151247, -2.915334737309923874 ) ) ;
#42129=EDGE_CURVE ( 'NONE', #32729, #35669, #79657, .T. ) ;
#42130=CARTESIAN_POINT ( 'NONE',  ( 12.63842701281683034, 17.46726448433411250, 9.846743663894596210 ) ) ;
#42133=CARTESIAN_POINT ( 'NONE',  ( 14.92337183194729988, 59.34226448433412315, -8.527530157486177487 ) ) ;
#42134=FACE_OUTER_BOUND ( 'NONE', #26501, .T. ) ;
#42135=ADVANCED_FACE ( 'NONE', ( #47904 ), #91448, .T. ) ;
#42136=CARTESIAN_POINT ( 'NONE',  ( 19.38216949554541202, 60.99863466993042493, 9.382169495545424454 ) ) ;
#42141=CARTESIAN_POINT ( 'NONE',  ( 5.076628168052703671, 61.84226448433412315, 8.527530157486179263 ) ) ;
#42142=CARTESIAN_POINT ( 'NONE',  ( 5.076628168052704559, 30.17559781766745175, -8.527530157486179263 ) ) ;
#42143=CARTESIAN_POINT ( 'NONE',  ( 20.36894250292379382, 58.67874883491396076, 10.36894250292379205 ) ) ;
#42144=CARTESIAN_POINT ( 'NONE',  ( 19.39188664607694434, 5.837033823263999999, -6.500000000000002665 ) ) ;
#42145=ORIENTED_EDGE ( 'NONE', *, *, #6442, .T. ) ;
#42147=CARTESIAN_POINT ( 'NONE',  ( 17.20831665107776587, 37.88393115100078745, 7.208316651077764980 ) ) ;
#42148=CARTESIAN_POINT ( 'NONE',  ( 19.38216949554541202, 0.9986346699304200492, 9.382169495545424454 ) ) ;
#42149=CARTESIAN_POINT ( 'NONE',  ( 19.42250999205614193, 65.14701867748817676, 5.440088680355555262 ) ) ;
#42151=CARTESIAN_POINT ( 'NONE',  ( 10.00000000000000178, 7.258931151000785675, 9.846743663894594434 ) ) ;
#42152=CARTESIAN_POINT ( 'NONE',  ( 18.52753015748618282, 58.92559781766745886, -4.923371831947291888 ) ) ;
#42153=CARTESIAN_POINT ( 'NONE',  ( 0.2751277870542911952, 19.36607318730131055, -6.499999999999992006 ) ) ;
#42156=CARTESIAN_POINT ( 'NONE',  ( 2.035157376598822676, 7.438685344154837509, -7.964842623401177768 ) ) ;
#42157=CARTESIAN_POINT ( 'NONE',  ( -0.3689425029237881626, 12.42874883491396609, 10.36894250292379027 ) ) ;
#42158=CARTESIAN_POINT ( 'NONE',  ( 1.472469842513823179, 15.59226448433411960, -4.923371831947296329 ) ) ;
#42159=CARTESIAN_POINT ( 'NONE',  ( 7.084665262690076126, 39.10535201082150536, 10.88017736071109987 ) ) ;
#42160=CARTESIAN_POINT ( 'NONE',  ( 10.00000000000000000, 22.87363466993042138, -12.81628187352647608 ) ) ;
#42161=CARTESIAN_POINT ( 'NONE',  ( 12.91533473730992121, 64.52201867748817676, 10.88017736071110164 ) ) ;
#42162=FACE_OUTER_BOUND ( 'NONE', #19982, .T. ) ;
#42165=LINE ( 'NONE', #72628, #69289 ) ;
#42167=CARTESIAN_POINT ( 'NONE',  ( 10.00000000000000000, 54.75893115100078745, -9.846743663894594434 ) ) ;
#42168=CARTESIAN_POINT ( 'NONE',  ( 0.1532563361054083140, 16.00893115100078390, 1.131784320476157264E-15 ) ) ;
#42170=CARTESIAN_POINT ( 'NONE',  ( -2.816281873526473856, 24.12363466993042138, 9.499525473075851096E-16 ) ) ;
#42172=CARTESIAN_POINT ( 'NONE',  ( 12.91533473730992121, 24.52201867748816966, 10.88017736071110164 ) ) ;
#42174=CARTESIAN_POINT ( 'NONE',  ( -4.164238869374099039, 46.80374883491397497, 8.674139862899312516E-16 ) ) ;
#42176=CARTESIAN_POINT ( 'NONE',  ( 18.52753015748618282, 43.92559781766745175, -4.923371831947291888 ) ) ;
#42177=CARTESIAN_POINT ( 'NONE',  ( 6.565887622018943937, 35.16530133659708923, 12.81628187352647430 ) ) ;
#42178=CARTESIAN_POINT ( 'NONE',  ( 0.5774900079438607392, 28.48035201082150891, 5.440088680355550821 ) ) ;
#42179=CARTESIAN_POINT ( 'NONE',  ( 12.63842701281683034, 47.46726448433412315, 9.846743663894596210 ) ) ;
#42180=CARTESIAN_POINT ( 'NONE',  ( 7.084665262690076126, 39.10535201082150536, 10.88017736071109987 ) ) ;
#42181=CARTESIAN_POINT ( 'NONE',  ( 10.00000000000000000, 7.873634669930421381, -12.81628187352647608 ) ) ;
#42182=CARTESIAN_POINT ( 'NONE',  ( -2.266590686148945544, 31.38708216824730002, -7.082119434687050408 ) ) ;
#42183=CARTESIAN_POINT ( 'NONE',  ( 17.84635730667655906, 33.63791097397319163, 6.500000000000019540 ) ) ;
#42184=CARTESIAN_POINT ( 'NONE',  ( 2.791683348922240793, 21.63393115100078745, 7.208316651077764092 ) ) ;
#42185=CARTESIAN_POINT ( 'NONE',  ( 7.084665262690076126, 2.022018677488170990, -10.88017736071110164 ) ) ;
#42186=CARTESIAN_POINT ( 'NONE',  ( 12.63842701281683922, 64.55059781766745175, -9.846743663894590881 ) ) ;
#42188=CYLINDRICAL_SURFACE ( 'NONE', #95649, 11.92686044187656513 ) ;
#42190=CARTESIAN_POINT ( 'NONE',  ( 19.42250999205614193, 20.14701867748817321, 5.440088680355555262 ) ) ;
#42191=CARTESIAN_POINT ( 'NONE',  ( 4.559911319644449179, 58.89701867748817676, 9.422509992056141925 ) ) ;
#42192=CARTESIAN_POINT ( 'NONE',  ( 10.00000000000000000, 30.55374883491397142, -14.16423886937410082 ) ) ;
#42193=CARTESIAN_POINT ( 'NONE',  ( 10.00000000000000000, 4.758931151000784787, -9.846743663894594434 ) ) ;
#42194=CARTESIAN_POINT ( 'NONE',  ( 18.52753015748617571, 53.09226448433412315, 4.923371831947298993 ) ) ;
#42195=CARTESIAN_POINT ( 'NONE',  ( 10.00000000000000000, 36.81368534415484106, -10.88017736071110342 ) ) ;
#42198=VERTEX_POINT ( 'NONE', #33871 ) ;
#42200=VERTEX_POINT ( 'NONE', #27860 ) ;
#42201=ORIENTED_EDGE ( 'NONE', *, *, #36949, .F. ) ;
#42203=CARTESIAN_POINT ( 'NONE',  ( -0.3689425029237881626, 2.428748834913967869, 10.36894250292379027 ) ) ;
#42204=CARTESIAN_POINT ( 'NONE',  ( 17.08211943468705130, 8.470415501580635720, 12.26659068614894998 ) ) ;
#42205=CARTESIAN_POINT ( 'NONE',  ( 10.00000000000000000, 60.55374883491397497, -14.16423886937410082 ) ) ;
#42206=CARTESIAN_POINT ( 'NONE',  ( 5.076628168052704559, 55.17559781766745175, -8.527530157486179263 ) ) ;
#42207=CARTESIAN_POINT ( 'NONE',  ( 19.84674366389459266, 33.71726448433410894, -2.638427012816827677 ) ) ;
#42208=CARTESIAN_POINT ( 'NONE',  ( -0.7262372900963632860, 0.05317965760449581969, 5.275332923266317309 ) ) ;
#42209=CARTESIAN_POINT ( 'NONE',  ( 2.035157376598822676, 32.43868534415483396, -7.964842623401177768 ) ) ;
#42210=CARTESIAN_POINT ( 'NONE',  ( -2.816281873526473856, -0.6680319967362464695, 3.434112377981055619 ) ) ;
#42211=CARTESIAN_POINT ( 'NONE',  ( -4.164238869374098151, 6.595415501580634832, -3.795296366450310543 ) ) ;
#42212=CARTESIAN_POINT ( 'NONE',  ( -4.164238869374099927, 52.01208216824729647, 3.795296366450308767 ) ) ;
#42213=CARTESIAN_POINT ( 'NONE',  ( 10.00000000000000000, 1.813685344154838175, -10.88017736071110342 ) ) ;
#42215=LINE ( 'NONE', #72200, #31581 ) ;
#42218=B_SPLINE_CURVE_WITH_KNOTS ( 'NONE', 3,
 ( #24456, #86429, #40934, #17449, #8939, #63416 ),
 .UNSPECIFIED., .F., .F.,
 ( 4, 2, 4 ),
 ( 0.000000000000000000, 0.0002701661927229247651, 0.0005403323854458495301 ),
 .UNSPECIFIED. ) ;
#42220=ORIENTED_EDGE ( 'NONE', *, *, #92118, .T. ) ;
#42221=CARTESIAN_POINT ( 'NONE',  ( 18.52753015748617571, 28.09226448433411960, 4.923371831947298993 ) ) ;
#42222=ORIENTED_EDGE ( 'NONE', *, *, #97240, .T. ) ;
#42223=CARTESIAN_POINT ( 'NONE',  ( 10.00000000000000000, 30.55374883491397142, -14.16423886937410082 ) ) ;
#42224=CARTESIAN_POINT ( 'NONE',  ( 12.63842701281683034, 32.46726448433412315, 9.846743663894596210 ) ) ;
#42225=CARTESIAN_POINT ( 'NONE',  ( 12.91533473730993009, 56.60535201082151247, -10.88017736071109987 ) ) ;
#42226=EDGE_CURVE ( 'NONE', #79846, #23173, #57567, .T. ) ;
#42228=CARTESIAN_POINT ( 'NONE',  ( 17.96484262340118221, 56.18868534415484817, -7.964842623401177768 ) ) ;
#42230=CARTESIAN_POINT ( 'NONE',  ( 13.43411237798106583, 62.66530133659708923, -12.81628187352647252 ) ) ;
#42233=CARTESIAN_POINT ( 'NONE',  ( 13.79529636645031943, 15.34541550158063750, -14.16423886937409904 ) ) ;
#42235=ORIENTED_EDGE ( 'NONE', *, *, #68466, .T. ) ;
#42236=CARTESIAN_POINT ( 'NONE',  ( 6.565887622018943937, 48.08196800326375353, -12.81628187352647608 ) ) ;
#42237=CARTESIAN_POINT ( 'NONE',  ( 19.42250999205614548, 15.98035201082150714, -5.440088680355545492 ) ) ;
#42238=CARTESIAN_POINT ( 'NONE',  ( 19.84674366389459266, 23.71726448433412315, -2.638427012816827677 ) ) ;
#42239=CARTESIAN_POINT ( 'NONE',  ( 7.084665262690076126, 17.02201867748817676, -10.88017736071110164 ) ) ;
#42240=CARTESIAN_POINT ( 'NONE',  ( -1.099225684535947600, 59.54030133659708923, 6.408140936763237150 ) ) ;
#42241=CARTESIAN_POINT ( 'NONE',  ( -46.20769938831809753, 103.7415672121655348, -6.113268130405502987 ) ) ;
#42242=CARTESIAN_POINT ( 'NONE',  ( 5.076628168052703671, 26.84226448433411960, 8.527530157486179263 ) ) ;
#42243=CARTESIAN_POINT ( 'NONE',  ( 19.05914839598885990, 19.96693863883976405, 6.499999999999943157 ) ) ;
#42245=CARTESIAN_POINT ( 'NONE',  ( 4.559911319644449179, 68.89701867748817676, 9.422509992056141925 ) ) ;
#42246=CARTESIAN_POINT ( 'NONE',  ( -1.926860441876562025, 44.47997603579418069, -3.195792623639529761 ) ) ;
#42247=CARTESIAN_POINT ( 'NONE',  ( 2.791683348922237240, 0.3839311510007847872, -7.208316651077763204 ) ) ;
#42249=CARTESIAN_POINT ( 'NONE',  ( 13.43411237798106583, 22.66530133659708923, -12.81628187352647252 ) ) ;
#42250=DIRECTION ( 'NONE',  ( 0.9970872288863216193, 0.07626964003977222684, 0.000000000000000000 ) ) ;
#42251=CARTESIAN_POINT ( 'NONE',  ( 18.52753015748618282, 43.92559781766745175, -4.923371831947291888 ) ) ;
#42252=CARTESIAN_POINT ( 'NONE',  ( 18.17884179759834851, 28.66688879859530559, -6.499999999999984901 ) ) ;
#42253=CARTESIAN_POINT ( 'NONE',  ( 10.00000000000000178, 23.05374883491397142, 14.16423886937410082 ) ) ;
#42254=CARTESIAN_POINT ( 'NONE',  ( 14.92337183194729988, 29.34226448433411960, -8.527530157486177487 ) ) ;
#42255=CARTESIAN_POINT ( 'NONE',  ( 6.565887622018943937, 38.08196800326376064, -12.81628187352647608 ) ) ;
#42257=CARTESIAN_POINT ( 'NONE',  ( 20.15039907845753575, 15.60158574516642815, -6.262539305110077059 ) ) ;
#42258=CARTESIAN_POINT ( 'NONE',  ( 4.559911319644449179, 68.89701867748817676, 9.422509992056141925 ) ) ;
#42259=CARTESIAN_POINT ( 'NONE',  ( 16.40814093676324603, 7.456968003263754419, -11.09922568453594671 ) ) ;
#42262=CARTESIAN_POINT ( 'NONE',  ( 18.52753015748617571, 38.09226448433412315, 4.923371831947298993 ) ) ;
#42263=CARTESIAN_POINT ( 'NONE',  ( 2.035157376598822676, 27.43868534415483396, -7.964842623401177768 ) ) ;
#42264=CARTESIAN_POINT ( 'NONE',  ( 13.43411237798105340, 25.58196800326374998, 12.81628187352647963 ) ) ;
#42265=CARTESIAN_POINT ( 'NONE',  ( 14.92337183194729633, 32.67559781766745175, 8.527530157486181039 ) ) ;
#42267=CARTESIAN_POINT ( 'NONE',  ( 4.559911319644449179, 27.23035201082150536, -9.422509992056141925 ) ) ;
#42271=CARTESIAN_POINT ( 'NONE',  ( 14.92337183194729988, 59.34226448433412315, -8.527530157486177487 ) ) ;
#42272=CARTESIAN_POINT ( 'NONE',  ( -0.8801773607111009756, 33.06368534415484106, 1.068504757029289695E-15 ) ) ;
#42275=CARTESIAN_POINT ( 'NONE',  ( 17.96484262340118221, 51.18868534415483396, -7.964842623401177768 ) ) ;
#42276=CARTESIAN_POINT ( 'NONE',  ( 7.084665262690076126, 22.02201867748817321, -10.88017736071110164 ) ) ;
#42279=CARTESIAN_POINT ( 'NONE',  ( 10.00000000000000000, 49.75893115100078745, -9.846743663894594434 ) ) ;
#42280=CARTESIAN_POINT ( 'NONE',  ( 20.36894250292379738, 49.92874883491396787, -10.36894250292379027 ) ) ;
#42282=CARTESIAN_POINT ( 'NONE',  ( -4.164238869374098151, 6.595415501580634832, -3.795296366450310543 ) ) ;
#42283=CARTESIAN_POINT ( 'NONE',  ( 2.917880565312950480, 40.97041550158063217, -12.26659068614894821 ) ) ;
#42284=CARTESIAN_POINT ( 'NONE',  ( 10.00000000000000178, 10.37363466993041961, 12.81628187352647608 ) ) ;
#42287=CARTESIAN_POINT ( 'NONE',  ( 10.00000000000000178, 4.313685344154837509, 10.88017736071110342 ) ) ;
#42288=CARTESIAN_POINT ( 'NONE',  ( 12.63842701281683922, 34.55059781766745886, -9.846743663894590881 ) ) ;
#42289=CARTESIAN_POINT ( 'NONE',  ( 19.72487221294570858, 70.00000000000000000, 6.500000000000000888 ) ) ;
#42290=CARTESIAN_POINT ( 'NONE',  ( 7.084665262690076126, 59.10535201082150536, 10.88017736071109987 ) ) ;
#42292=CARTESIAN_POINT ( 'NONE',  ( -0.8801773607111008646, 28.27201867748817321, 2.915334737309923430 ) ) ;
#42293=DIRECTION ( 'NONE',  ( 0.000000000000000000, 0.000000000000000000, -1.000000000000000000 ) ) ;
#42294=CARTESIAN_POINT ( 'NONE',  ( 13.43411237798106583, 22.66530133659708923, -12.81628187352647252 ) ) ;
#42295=CARTESIAN_POINT ( 'NONE',  ( 2.791683348922240793, 31.63393115100078745, 7.208316651077764092 ) ) ;
#42298=CARTESIAN_POINT ( 'NONE',  ( 24.16423886937409904, 64.09541550158064638, 3.795296366450317205 ) ) ;
#42299=CARTESIAN_POINT ( 'NONE',  ( -4.164238869374099039, 46.80374883491397497, 8.674139862899312516E-16 ) ) ;
#42300=CARTESIAN_POINT ( 'NONE',  ( 15.44008868035555260, 34.73035201082151247, 9.422509992056143702 ) ) ;
#42301=CARTESIAN_POINT ( 'NONE',  ( -0.8801773607110991993, 52.85535201082151247, -2.915334737309923874 ) ) ;
#42304=CARTESIAN_POINT ( 'NONE',  ( 5.076628168052704559, 15.17559781766745175, -8.527530157486179263 ) ) ;
#42307=CARTESIAN_POINT ( 'NONE',  ( 17.20831665107776587, 19.13393115100078035, -7.208316651077762316 ) ) ;
#42308=CARTESIAN_POINT ( 'NONE',  ( 10.00000000000000178, 47.25893115100078745, 9.846743663894594434 ) ) ;
#42309=CARTESIAN_POINT ( 'NONE',  ( 20.88017736071110875, 20.77201867748816611, -2.915334737309920765 ) ) ;
#42312=CARTESIAN_POINT ( 'NONE',  ( 16.40814093676323893, 40.79030133659708923, 11.09922568453595026 ) ) ;
#42313=CIRCLE ( 'NONE', #63006, 11.92686044187656513 ) ;
#42315=CARTESIAN_POINT ( 'NONE',  ( -0.8801773607111009756, 63.06368534415484106, 1.068504757029289695E-15 ) ) ;
#42316=CARTESIAN_POINT ( 'NONE',  ( 2.791683348922237240, 35.38393115100079456, -7.208316651077763204 ) ) ;
#42317=CARTESIAN_POINT ( 'NONE',  ( 17.08211943468705840, 55.13708216824731068, -12.26659068614894466 ) ) ;
#42318=CARTESIAN_POINT ( 'NONE',  ( 2.791683348922237240, 20.38393115100078745, -7.208316651077763204 ) ) ;
#42320=CARTESIAN_POINT ( 'NONE',  ( 18.52753015748618282, 63.92559781766745886, -4.923371831947291888 ) ) ;
#42321=CARTESIAN_POINT ( 'NONE',  ( 17.08211943468705840, 30.13708216824730357, -12.26659068614894466 ) ) ;
#42322=CARTESIAN_POINT ( 'NONE',  ( 5.076628168052703671, 46.84226448433412315, 8.527530157486179263 ) ) ;
#42324=CARTESIAN_POINT ( 'NONE',  ( 0.5774900079438590739, 22.64701867748817321, -5.440088680355550821 ) ) ;
#42325=CARTESIAN_POINT ( 'NONE',  ( 19.42250999205614548, 55.98035201082150536, -5.440088680355545492 ) ) ;
#42326=CARTESIAN_POINT ( 'NONE',  ( 0.1532563361054100626, 55.80059781766744464, -2.638427012816831230 ) ) ;
#42328=CARTESIAN_POINT ( 'NONE',  ( 22.81628187352647785, 51.41530133659708923, 3.434112377981063169 ) ) ;
#42330=CARTESIAN_POINT ( 'NONE',  ( 19.42250999205614548, 55.98035201082150536, -5.440088680355545492 ) ) ;
#42331=ORIENTED_EDGE ( 'NONE', *, *, #71019, .T. ) ;
#42333=FILL_AREA_STYLE ('',( #87331 ) ) ;
#42335=CARTESIAN_POINT ( 'NONE',  ( 0.5774900079438607392, 63.48035201082149825, 5.440088680355550821 ) ) ;
#42337=CARTESIAN_POINT ( 'NONE',  ( 19.42250999205614193, 60.14701867748817676, 5.440088680355555262 ) ) ;
#42338=CARTESIAN_POINT ( 'NONE',  ( 17.96484262340118221, 21.18868534415483396, -7.964842623401177768 ) ) ;
#42339=CARTESIAN_POINT ( 'NONE',  ( 18.72515096720578853, 60.05509018479938277, 6.499999999999877431 ) ) ;
#42341=CARTESIAN_POINT ( 'NONE',  ( 4.559911319644449179, 2.230352010821504916, -9.422509992056141925 ) ) ;
#42342=CARTESIAN_POINT ( 'NONE',  ( 7.361572987183170547, 12.05059781766744997, 9.846743663894590881 ) ) ;
#42343=CARTESIAN_POINT ( 'NONE',  ( 24.16423886937409904, 14.09541550158063217, 3.795296366450317205 ) ) ;
#42344=CARTESIAN_POINT ( 'NONE',  ( 12.91533473730993009, 21.60535201082150536, -10.88017736071109987 ) ) ;
#42345=CARTESIAN_POINT ( 'NONE',  ( 14.92337183194729988, 54.34226448433412315, -8.527530157486177487 ) ) ;
#42347=CARTESIAN_POINT ( 'NONE',  ( 19.84674366389459266, 58.30059781766745886, 2.638427012816836559 ) ) ;
#42351=CARTESIAN_POINT ( 'NONE',  ( 15.44008868035555793, 51.39701867748816966, -9.422509992056140149 ) ) ;
#42354=CARTESIAN_POINT ( 'NONE',  ( 10.00000000000000000, 32.87363466993042493, -12.81628187352647608 ) ) ;
#42355=CARTESIAN_POINT ( 'NONE',  ( 4.559911319644449179, 13.89701867748817143, 9.422509992056141925 ) ) ;
#42357=CARTESIAN_POINT ( 'NONE',  ( 7.084665262690076126, 59.10535201082150536, 10.88017736071109987 ) ) ;
#42358=CARTESIAN_POINT ( 'NONE',  ( 2.917880565312948704, 67.63708216824730357, 12.26659068614894643 ) ) ;
#42361=CARTESIAN_POINT ( 'NONE',  ( 19.38216949554541202, 45.99863466993041072, 9.382169495545424454 ) ) ;
#42362=CARTESIAN_POINT ( 'NONE',  ( 10.00000000000000000, 26.81368534415484106, -10.88017736071110342 ) ) ;
#42363=CARTESIAN_POINT ( 'NONE',  ( -33.19000000000001194, 92.00000000000000000, -9.500000000000000000 ) ) ;
#42364=ORIENTED_EDGE ( 'NONE', *, *, #52104, .T. ) ;
#42365=CARTESIAN_POINT ( 'NONE',  ( 10.00000000000000000, 42.87363466993042493, -12.81628187352647608 ) ) ;
#42366=CARTESIAN_POINT ( 'NONE',  ( -0.8801773607110991993, 32.85535201082151247, -2.915334737309923874 ) ) ;
#42367=CARTESIAN_POINT ( 'NONE',  ( 5.076628168052703671, 56.84226448433412315, 8.527530157486179263 ) ) ;
#42368=EDGE_CURVE ( 'NONE', #6749, #34270, #50780, .T. ) ;
#42370=CARTESIAN_POINT ( 'NONE',  ( 5.076628168052703671, 56.84226448433412315, 8.527530157486179263 ) ) ;
#42372=CARTESIAN_POINT ( 'NONE',  ( 7.361572987183169658, 54.96726448433413026, -9.846743663894592657 ) ) ;
#42373=CARTESIAN_POINT ( 'NONE',  ( 0.5774900079438607392, 28.48035201082150891, 5.440088680355550821 ) ) ;
#42374=CARTESIAN_POINT ( 'NONE',  ( 2.791683348922237240, 35.38393115100079456, -7.208316651077763204 ) ) ;
#42377=CARTESIAN_POINT ( 'NONE',  ( 0.1532563361054100626, 45.80059781766745886, -2.638427012816831230 ) ) ;
#42378=CARTESIAN_POINT ( 'NONE',  ( 12.63842701281683034, 7.467264484334118713, 9.846743663894596210 ) ) ;
#42379=CARTESIAN_POINT ( 'NONE',  ( 2.791683348922240793, 61.63393115100079456, 7.208316651077764092 ) ) ;
#42380=EDGE_LOOP ( 'NONE', ( #86874, #64487, #11935, #69528, #44898, #71646 ) ) ;
#42382=CARTESIAN_POINT ( 'NONE',  ( 6.565887622018943937, 33.08196800326374643, -12.81628187352647608 ) ) ;
#42383=CARTESIAN_POINT ( 'NONE',  ( 19.84674366389459621, 43.50893115100078745, 7.409399052514197653E-17 ) ) ;
#42385=CARTESIAN_POINT ( 'NONE',  ( 17.08211943468705130, 53.47041550158063217, 12.26659068614894998 ) ) ;
#42386=CARTESIAN_POINT ( 'NONE',  ( 17.20831665107776587, 34.13393115100078745, -7.208316651077762316 ) ) ;
#42387=CARTESIAN_POINT ( 'NONE',  ( 19.67387888393819750, 87.39346174270656320, 5.439610960095202508 ) ) ;
#42388=CARTESIAN_POINT ( 'NONE',  ( -0.3689425029237898834, 56.17874883491396076, -10.36894250292378850 ) ) ;
#42390=CARTESIAN_POINT ( 'NONE',  ( -0.8801773607110991993, 2.855352010821504471, -2.915334737309923874 ) ) ;
#42391=CARTESIAN_POINT ( 'NONE',  ( 20.36894250292379738, 34.92874883491396076, -10.36894250292379027 ) ) ;
#42392=CARTESIAN_POINT ( 'NONE',  ( 10.00000000000000178, 33.05374883491396787, 14.16423886937410082 ) ) ;
#42394=CARTESIAN_POINT ( 'NONE',  ( 19.72487221294570858, 70.00000000000000000, 6.500000000000000888 ) ) ;
#42396=CARTESIAN_POINT ( 'NONE',  ( 0.1532563361054100626, 5.800597817667452638, -2.638427012816831230 ) ) ;
#42398=CARTESIAN_POINT ( 'NONE',  ( -2.816281873526473856, -0.6680319967362464695, 3.434112377981055619 ) ) ;
#42399=VERTEX_POINT ( 'NONE', #21865 ) ;
#42400=CARTESIAN_POINT ( 'NONE',  ( 20.88017736071110164, 55.35535201082149825, 2.915334737309930979 ) ) ;
#42404=CARTESIAN_POINT ( 'NONE',  ( 1.274849032794294290, 53.57228050351032067, 6.499999999999979572 ) ) ;
#42405=CARTESIAN_POINT ( 'NONE',  ( 17.20831665107776587, 59.13393115100078745, -7.208316651077762316 ) ) ;
#42408=CARTESIAN_POINT ( 'NONE',  ( 24.16423886937409904, 29.09541550158063572, 3.795296366450317205 ) ) ;
#42411=CARTESIAN_POINT ( 'NONE',  ( 20.88017736071110164, 25.35535201082150891, 2.915334737309930979 ) ) ;
#42412=CARTESIAN_POINT ( 'NONE',  ( 19.38216949554541202, 25.99863466993042138, 9.382169495545424454 ) ) ;
#42414=CARTESIAN_POINT ( 'NONE',  ( 19.84674366389459266, 13.30059781766745353, 2.638427012816836559 ) ) ;
#42418=CARTESIAN_POINT ( 'NONE',  ( -0.3689425029237898834, 31.17874883491396787, -10.36894250292378850 ) ) ;
#42420=SURFACE_STYLE_USAGE ( .BOTH. , #56916 ) ;
#42421=CARTESIAN_POINT ( 'NONE',  ( 15.44008868035555260, 9.730352010821505360, 9.422509992056143702 ) ) ;
#42424=CARTESIAN_POINT ( 'NONE',  ( 15.44008868035555793, 36.39701867748816966, -9.422509992056140149 ) ) ;
#42425=CARTESIAN_POINT ( 'NONE',  ( 2.035157376598824452, 53.68868534415484817, 7.964842623401179544 ) ) ;
#42426=CARTESIAN_POINT ( 'NONE',  ( -1.099225684535947600, 13.70696800326375353, -6.408140936763238038 ) ) ;
#42427=CARTESIAN_POINT ( 'NONE',  ( 0.1532563361054082862, 66.21726448433413736, 2.638427012816831674 ) ) ;
#42429=CARTESIAN_POINT ( 'NONE',  ( 17.20831665107776587, 7.883931151000784787, 7.208316651077764980 ) ) ;
#42430=CARTESIAN_POINT ( 'NONE',  ( 4.559911319644449179, 42.23035201082151247, -9.422509992056141925 ) ) ;
#42431=MECHANICAL_DESIGN_GEOMETRIC_PRESENTATION_REPRESENTATION('',(#20080),#75968);
#42434=CARTESIAN_POINT ( 'NONE',  ( 13.43411237798106583, 7.665301336597086568, -12.81628187352647252 ) ) ;
#42435=CARTESIAN_POINT ( 'NONE',  ( 15.44008868035555793, 61.39701867748817676, -9.422509992056140149 ) ) ;
#42436=COLOUR_RGB ( '', 0.08235294, 0.09019608, 0.10196078) ;
#42437=CARTESIAN_POINT ( 'NONE',  ( 0.1532563361054083140, 26.00893115100078745, 1.131784320476157264E-15 ) ) ;
#42438=CARTESIAN_POINT ( 'NONE',  ( 19.38216949554541202, 45.99863466993041072, 9.382169495545424454 ) ) ;
#42439=CARTESIAN_POINT ( 'NONE',  ( 19.84674366389459266, 3.717264484334118713, -2.638427012816827677 ) ) ;
#42441=CARTESIAN_POINT ( 'NONE',  ( 2.377183314879976805, 55.78593319516822646, -6.500000000000005329 ) ) ;
#42443=CARTESIAN_POINT ( 'NONE',  ( 20.88017736071110875, 25.77201867748816966, -2.915334737309920765 ) ) ;
#42444=CARTESIAN_POINT ( 'NONE',  ( 16.40814093676323893, 55.79030133659708923, 11.09922568453595026 ) ) ;
#42445=CARTESIAN_POINT ( 'NONE',  ( 18.52753015748618282, 28.92559781766745175, -4.923371831947291888 ) ) ;
#42446=CARTESIAN_POINT ( 'NONE',  ( 4.559911319644449179, 23.89701867748817321, 9.422509992056141925 ) ) ;
#42447=CARTESIAN_POINT ( 'NONE',  ( -0.3689425029237881626, 67.42874883491396076, 10.36894250292379027 ) ) ;
#42448=ORIENTED_EDGE ( 'NONE', *, *, #66289, .F. ) ;
#42449=CARTESIAN_POINT ( 'NONE',  ( 0.5774900079438590739, 12.64701867748817143, -5.440088680355550821 ) ) ;
#42450=EDGE_CURVE ( 'NONE', #63634, #67813, #13862, .T. ) ;
#42451=CARTESIAN_POINT ( 'NONE',  ( 2.035157376598822676, 32.43868534415483396, -7.964842623401177768 ) ) ;
#42453=CARTESIAN_POINT ( 'NONE',  ( 10.00000000000000178, 24.31368534415484106, 10.88017736071110342 ) ) ;
#42455=CARTESIAN_POINT ( 'NONE',  ( 0.1532563361054083140, 66.00893115100079456, 1.131784320476157264E-15 ) ) ;
#42456=CARTESIAN_POINT ( 'NONE',  ( 0.5774900079438607392, 23.48035201082150536, 5.440088680355550821 ) ) ;
#42457=CARTESIAN_POINT ( 'NONE',  ( 2.791683348922237240, 65.38393115100078035, -7.208316651077763204 ) ) ;
#42459=CARTESIAN_POINT ( 'NONE',  ( -2.816281873526473856, 59.12363466993042493, 9.499525473075851096E-16 ) ) ;
#42460=CARTESIAN_POINT ( 'NONE',  ( 0.8952175423695025724, 68.52576239577081196, 5.990408912944351627 ) ) ;
#42461=CARTESIAN_POINT ( 'NONE',  ( -0.3689425029237881626, 32.42874883491395366, 10.36894250292379027 ) ) ;
#42462=CARTESIAN_POINT ( 'NONE',  ( 10.00000000000000000, 36.81368534415484106, -10.88017736071110342 ) ) ;
#42463=CARTESIAN_POINT ( 'NONE',  ( 4.559911319644449179, 18.89701867748817321, 9.422509992056141925 ) ) ;
#42466=CARTESIAN_POINT ( 'NONE',  ( 0.1532563361054100626, 50.80059781766745175, -2.638427012816831230 ) ) ;
#42467=CARTESIAN_POINT ( 'NONE',  ( 7.361572987183169658, 14.96726448433411960, -9.846743663894592657 ) ) ;
#42469=CARTESIAN_POINT ( 'NONE',  ( 10.00000000000000000, 6.813685344154838397, -10.88017736071110342 ) ) ;
#42470=CARTESIAN_POINT ( 'NONE',  ( 19.84674366389459266, 13.30059781766745353, 2.638427012816836559 ) ) ;
#42471=CARTESIAN_POINT ( 'NONE',  ( -0.8801773607111009756, 63.06368534415484106, 1.068504757029289695E-15 ) ) ;
#42472=CARTESIAN_POINT ( 'NONE',  ( 12.91533473730993009, 21.60535201082150536, -10.88017736071109987 ) ) ;
#42473=CARTESIAN_POINT ( 'NONE',  ( 22.81628187352647785, 51.62363466993042493, 6.195893100308588602E-16 ) ) ;
#42474=CARTESIAN_POINT ( 'NONE',  ( -0.3689425029237881626, 32.42874883491395366, 10.36894250292379027 ) ) ;
#42478=CARTESIAN_POINT ( 'NONE',  ( -2.816281873526473856, 64.12363466993042493, 9.499525473075851096E-16 ) ) ;
#42480=CARTESIAN_POINT ( 'NONE',  ( 19.38216949554541557, 7.248634669930421381, -9.382169495545420901 ) ) ;
#42481=CARTESIAN_POINT ( 'NONE',  ( -1.926860441876564023, 14.68830936912750573, 1.004413902775740781E-15 ) ) ;
#42482=CARTESIAN_POINT ( 'NONE',  ( 10.00000000000000000, 36.81368534415484106, -10.88017736071110342 ) ) ;
#42484=EDGE_CURVE ( 'NONE', #11760, #32896, #43691, .T. ) ;
#42487=CARTESIAN_POINT ( 'NONE',  ( 1.472469842513823179, 21.42559781766745175, 4.923371831947296329 ) ) ;
#42488=CARTESIAN_POINT ( 'NONE',  ( 19.84674366389459266, 13.30059781766745353, 2.638427012816836559 ) ) ;
#42489=CARTESIAN_POINT ( 'NONE',  ( 1.472469842513823179, 21.42559781766745175, 4.923371831947296329 ) ) ;
#42490=CARTESIAN_POINT ( 'NONE',  ( 17.20831665107776587, 7.883931151000784787, 7.208316651077764980 ) ) ;
#42491=CARTESIAN_POINT ( 'NONE',  ( -0.8801773607111008646, 68.27201867748817676, 2.915334737309923430 ) ) ;
#42493=CARTESIAN_POINT ( 'NONE',  ( 17.20831665107776587, 7.883931151000784787, 7.208316651077764980 ) ) ;
#42494=CARTESIAN_POINT ( 'NONE',  ( 10.00000000000000000, 19.75893115100078390, -9.846743663894594434 ) ) ;
#42498=CARTESIAN_POINT ( 'NONE',  ( 0.1532563361054083140, 66.00893115100079456, 1.131784320476157264E-15 ) ) ;
#42501=CARTESIAN_POINT ( 'NONE',  ( 10.00000000000000000, 6.813685344154838397, -10.88017736071110342 ) ) ;
#42503=CARTESIAN_POINT ( 'NONE',  ( -2.266590686148945544, 22.22041550158063572, 7.082119434687048631 ) ) ;
#42506=CARTESIAN_POINT ( 'NONE',  ( -0.3689425029237898834, 16.17874883491396076, -10.36894250292378850 ) ) ;
#42507=CARTESIAN_POINT ( 'NONE',  ( -0.3689425029237881626, 37.42874883491396787, 10.36894250292379027 ) ) ;
#42508=CARTESIAN_POINT ( 'NONE',  ( 7.084665262690076126, 32.02201867748816966, -10.88017736071110164 ) ) ;
#42510=CARTESIAN_POINT ( 'NONE',  ( 18.52753015748617571, 13.09226448433411960, 4.923371831947298993 ) ) ;
#42511=CARTESIAN_POINT ( 'NONE',  ( -0.8801773607110991993, 62.85535201082150536, -2.915334737309923874 ) ) ;
#42512=CARTESIAN_POINT ( 'NONE',  ( 7.361572987183169658, 14.96726448433411960, -9.846743663894592657 ) ) ;
#42513=CARTESIAN_POINT ( 'NONE',  ( 20.88017736071110519, 5.563685344154838397, 2.639326808657452039E-16 ) ) ;
#42514=CARTESIAN_POINT ( 'NONE',  ( -2.816281873526473856, 39.12363466993041783, 9.499525473075851096E-16 ) ) ;
#42515=CARTESIAN_POINT ( 'NONE',  ( 10.00000000000000178, 47.25893115100078745, 9.846743663894594434 ) ) ;
#42516=CARTESIAN_POINT ( 'NONE',  ( 5.500000000000000000, 61.00000000000000711, -6.000000000000000000 ) ) ;
#42518=CARTESIAN_POINT ( 'NONE',  ( 10.00000000000000178, 25.37363466993041783, 12.81628187352647608 ) ) ;
#42520=CARTESIAN_POINT ( 'NONE',  ( 0.1532563361054083140, 41.00893115100078745, 1.131784320476157264E-15 ) ) ;
#42521=CARTESIAN_POINT ( 'NONE',  ( -4.164238869374099039, 11.80374883491396965, 8.674139862899312516E-16 ) ) ;
#42524=CARTESIAN_POINT ( 'NONE',  ( 0.5774900079438607392, 53.48035201082151247, 5.440088680355550821 ) ) ;
#42525=CARTESIAN_POINT ( 'NONE',  ( 0.5774900079438607392, 48.48035201082150536, 5.440088680355550821 ) ) ;
#42526=CARTESIAN_POINT ( 'NONE',  ( 17.08211943468705840, 40.13708216824731068, -12.26659068614894466 ) ) ;
#42527=CARTESIAN_POINT ( 'NONE',  ( 17.20831665107776587, 49.13393115100078745, -7.208316651077762316 ) ) ;
#42529=CARTESIAN_POINT ( 'NONE',  ( -0.8801773607111009756, 38.06368534415484106, 1.068504757029289695E-15 ) ) ;
#42530=CARTESIAN_POINT ( 'NONE',  ( -45.94000000000001194, 99.99999999999998579, 9.500000000000000000 ) ) ;
#42531=CARTESIAN_POINT ( 'NONE',  ( 7.361572987183169658, 54.96726448433413026, -9.846743663894592657 ) ) ;
#42533=CARTESIAN_POINT ( 'NONE',  ( -0.8801773607111009756, 3.063685344154837509, 1.068504757029289695E-15 ) ) ;
#42534=LINE ( 'NONE', #43027, #18455 ) ;
#42536=CARTESIAN_POINT ( 'NONE',  ( 4.559911319644449179, 3.897018677488170990, 9.422509992056141925 ) ) ;
#42538=CARTESIAN_POINT ( 'NONE',  ( 5.076628168052704559, 0.1755978176674514724, -8.527530157486179263 ) ) ;
#42539=CARTESIAN_POINT ( 'NONE',  ( 7.361572987183169658, 4.967264484334119601, -9.846743663894592657 ) ) ;
#42541=CARTESIAN_POINT ( 'NONE',  ( 1.472469842513823179, 31.42559781766745530, 4.923371831947296329 ) ) ;
#42542=CARTESIAN_POINT ( 'NONE',  ( 7.084665262690076126, 22.02201867748817321, -10.88017736071110164 ) ) ;
#42544=CARTESIAN_POINT ( 'NONE',  ( 6.565887622018943937, 8.081968003263751754, -12.81628187352647608 ) ) ;
#42545=CARTESIAN_POINT ( 'NONE',  ( 10.00000000000000178, 34.31368534415484106, 10.88017736071110342 ) ) ;
#42548=CARTESIAN_POINT ( 'NONE',  ( 16.40814093676323893, 35.79030133659708923, 11.09922568453595026 ) ) ;
#42551=CARTESIAN_POINT ( 'NONE',  ( 10.00000000000000178, 15.37363466993042138, 12.81628187352647608 ) ) ;
#42553=FILL_AREA_STYLE_COLOUR ( '', #77079 ) ;
#42554=CARTESIAN_POINT ( 'NONE',  ( -0.8801773607111008646, 23.27201867748817676, 2.915334737309923430 ) ) ;
#42555=CARTESIAN_POINT ( 'NONE',  ( 22.26659068614894466, 58.88708216824729647, 7.082119434687054849 ) ) ;
#42556=CARTESIAN_POINT ( 'NONE',  ( 1.472469842513823179, 55.59226448433412315, -4.923371831947296329 ) ) ;
#42557=CARTESIAN_POINT ( 'NONE',  ( 5.076628168052704559, 5.175597817667451750, -8.527530157486179263 ) ) ;
#42558=CARTESIAN_POINT ( 'NONE',  ( 20.88017736071110875, 65.77201867748817676, -2.915334737309920765 ) ) ;
#42560=CARTESIAN_POINT ( 'NONE',  ( 20.36894250292379382, 28.67874883491396787, 10.36894250292379205 ) ) ;
#42562=( GEOMETRIC_REPRESENTATION_CONTEXT ( 3 ) GLOBAL_UNCERTAINTY_ASSIGNED_CONTEXT ( ( #87430 ) ) GLOBAL_UNIT_ASSIGNED_CONTEXT ( ( #37746, #68726, #74735 ) ) REPRESENTATION_CONTEXT ( 'NONE', 'WORKASPACE' ) );
#42564=( BOUNDED_SURFACE ( )  B_SPLINE_SURFACE ( 1, 2, ( 
 ( #20130, #87144, #72143, #35121, #5140, #26163, #87638, #65621, #18668, #49155, #19152, #58114, #79656, #88623, #35631, #89123, #49630, #34627, #51123, #96645, #80139, #50634, #58622, #20634, #81615, #5639, #94655, #41675, #11649, #65126, #67115, #15615, #46099, #38117, #89618, #6125, #45597, #75105, #84100, #91598, #44609, #37125, #21130, #82608, #29590, #82109, #14632, #76095, #45096, #22121, #6612, #8103, #52601, #7114, #83607, #29105, #67621, #98129, #23114, #60092, #90594, #51629, #14125, #83104, #13620, #75603, #7625, #37619, #68113, #98638, #66623, #30089, #60596, #15121, #59607, #91091, #22619, #53095, #68606, #134, #52116, #30584, #53586, #61088, #97640, #76583, #97150, #28621, #59107, #44101, #74611, #36630, #90102, #21630, #25088, #70082, #92086, #631, #8589, #69586, #62065, #23612, #39095, #1106, #94053, #63543, #48047, #9078, #9570, #62556, #39591, #48544, #92568, #69097, #61575, #25574, #77077, #70573, #24094, #31569, #40570, #54563, #46579, #78561, #17089, #93555, #56066, #86561, #18065, #54077, #84592, #79043, #55571, #86070, #1604, #31077, #85575, #47569, #38599, #40072, #17581, #32053, #85079, #16092, #16588, #77562, #47064, #63058, #93060, #24593, #78067, #10071, #55056, #2098, #32557, #71068, #2593, #33048, #88020, #41067, #4545, #58008, #5028, #41569, #87532, #66006, #12518, #72036, #80531, #43020, #12030, #50029, #11535, #35007, #42529, #73013, #88518, #11048, #58505, #89015, #81017, #33532, #49044, #20019, #19046, #28009, #10556, #50520, #73502, #35514, #3076, #20522, #65510, #27024, #49522, #96032, #71563, #96534, #27516, #3564, #80030, #34023, #64027, #51007, #42055, #94540, #26058, #79548, #95535, #72519, #56548, #87043, #18552, #19533, #64520, #95026, #26535, #57031, #57524, #4053, #34515, #65008, #22504, #83489, #36511, #14013, #67502, #37506, #21018, #37005, #66510, #51507, #98021, #67999, #36007, #98523, #28988, #14512, #15008, #75489, #44494, #38000, #60481, #30467, #29976, #60968, #44982, #90970, #43503, #7001, #59005, #74994, #59496, #6497, #89507, #67004, #81502, #45478, #82497, #52975, #29476, #97525, #59984, #75980, #43993, #82000, #7509, #68492, #90477, #74002, #82994, #89994, #19, #91478, #22012, #13511, #23001, #21510, #52486, #74495, #13007, #5527, #97035, #28511, #6019, #52008, #23496, #9452, #16967, #38488, #46950, #54937, #47446, #31936, #32932, #24967, #92940, #70956, #62940, #2476, #24474, #62437, #70456, #91968, #55452, #16472, #77444, #77946, #69469, #92452, #39953, #53968, #69964, #9952, #63432, #23978, #93938, #53468, #84477, #39474, #61952, #93442, #76474, #1976, #85453 ),
 ( #1483, #32441, #40458, #85953, #17463, #8957, #61460, #83978, #46466, #54450, #15503, #47931, #45985, #30962, #78437, #7989, #68982, #15977, #516, #76960, #8471, #38978, #990, #31450, #84959, #72894, #19900, #56437, #3439, #80901, #27396, #86924, #95412, #57888, #26907, #64884, #26411, #49902, #57404, #87894, #4428, #25936, #74746, #6258, #95916, #48430, #63909, #34894, #33898, #44242, #50392, #64404, #94912, #78932, #41454, #87413, #40949, #72399, #65389, #3927, #79907, #56912, #67254, #11416, #19411, #42414, #18437, #18930, #49407, #41937, #88402, #34396, #10928, #13756, #36761, #25463, #48919, #80412, #11912, #55946, #86445, #17944, #10442, #71447, #2961, #71918, #33411, #94420, #79432, #59740, #67754, #29730, #22259, #52247, #98273, #60238, #54206, #23746, #8238, #68253, #68738, #22749, #98773, #8713, #52733, #29243, #21768, #92218, #90235, #46708, #270, #15259, #7252, #30714, #97778, #38732, #61224, #90733, #37756, #83241, #82741, #16228, #30221, #39232, #14261, #37267, #83737, #60725, #69232, #44739, #15747, #76236, #31208, #14764, #84723, #7753, #45740, #6750, #77208, #45237, #757, #61704, #75734, #91224, #38247, #53726, #53232, #91729, #75240, #23251, #84243, #46233, #76719, #86689, #17221, #2723, #3194, #63669, #2227, #26182, #48674, #18688, #18194, #49172, #33177, #25705, #31702, #94174, #47194, #63181, #47700, #32686, #77697, #24717, #69720, #71684, #70709, #56196, #93688, #55190, #48182, #79176, #32188, #9209, #10691, #41204, #25221, #62194, #71200, #78192, #56674, #79674, #78694, #39722, #87163, #85705, #55702, #70215, #86198, #17710, #33659, #10204, #11171, #64155, #1734, #94673, #1246, #54694, #40697, #92703, #24228, #85216, #16720, #62690, #93190, #9705, #40203, #59123, #12643, #50652, #58640, #80155, #43634, #4676, #65638, #5158, #57650, #80660, #66131, #42179, #58129, #97166, #41690, #81628, #20649, #72161, #35644, #89139, #36134, #72643, #19658, #28634, #74120, #4176, #43140, #5656, #73632, #81140, #42660, #96660, #28141, #51140, #13136, #34647, #89632, #21143, #66642, #64643, #11666, #51643, #50149, #82124, #3688, #12155, #73136, #95154, #88147, #35138, #57157, #88639, #34149, #20147, #96162, #27644, #26663, #87655, #19168, #49648, #65142, #95663, #27148, #37632, #30597, #91106, #98146, #61103, #69111, #91612, #44626, #68129, #52618, #45613, #98657, #7642, #60611, #92099, #6141, #60111, #150, #45111, #67129, #74627, #82627, #75121, #37143, #97656, #14141, #6629, #644, #38613, #23128, #83119, #83621, #30103, #14648, #23630, #67637, #44118, #36644, #31093, #52130, #76111, #29607, #90612, #15632 ) ),
 .UNSPECIFIED., .F., .F., .F. ) 
 B_SPLINE_SURFACE_WITH_KNOTS ( ( 2, 2 ),
 ( 3, 2, 2, 2, 2, 2, 2, 2, 2, 2, 2, 2, 2, 2, 2, 2, 2, 2, 2, 2, 2, 2, 2, 2, 2, 2, 2, 2, 2, 2, 2, 2, 2, 2, 2, 2, 2, 2, 2, 2, 2, 2, 2, 2, 2, 2, 2, 2, 2, 2, 2, 2, 2, 2, 2, 2, 2, 2, 2, 2, 2, 2, 2, 2, 2, 2, 2, 2, 2, 2, 2, 2, 2, 2, 2, 2, 2, 2, 2, 2, 2, 2, 2, 2, 2, 2, 2, 2, 2, 2, 2, 2, 2, 2, 2, 2, 2, 2, 2, 2, 2, 2, 2, 2, 2, 2, 2, 2, 2, 2, 2, 2, 2, 2, 2, 2, 2, 2, 2, 2, 2, 2, 2, 2, 2, 2, 2, 2, 2, 2, 2, 2, 2, 2, 2, 2, 2, 2, 2, 2, 2, 2, 2, 2, 2, 2, 2, 2, 2, 2, 2, 2, 2, 2, 2, 2, 2, 2, 2, 2, 2, 2, 3 ),
 ( 0.000000000000000000, 1.000000000000000000 ),
 ( 0.000000000000000000, 0.005952380952380952051, 0.01190476190476190410, 0.01785714285714285615, 0.02380952380952380820, 0.02976190476190476025, 0.03571428571428571230, 0.04166666666666666435, 0.04761904761904761640, 0.05357142857142856845, 0.05952380952380952051, 0.06547619047619047949, 0.07142857142857142461, 0.07738095238095238360, 0.08333333333333332871, 0.08928571428571428770, 0.09523809523809523281, 0.1011904761904761918, 0.1071428571428571369, 0.1130952380952380959, 0.1190476190476190410, 0.1250000000000000000, 0.1309523809523809590, 0.1369047619047619180, 0.1428571428571428492, 0.1488095238095238082, 0.1547619047619047672, 0.1607142857142857262, 0.1666666666666666574, 0.1726190476190476164, 0.1785714285714285754, 0.1845238095238095344, 0.1904761904761904656, 0.1964285714285714246, 0.2023809523809523836, 0.2083333333333333426, 0.2142857142857142738, 0.2202380952380952328, 0.2261904761904761918, 0.2321428571428571508, 0.2380952380952380820, 0.2440476190476190410, 0.2500000000000000000, 0.2559523809523809312, 0.2619047619047619180, 0.2678571428571428492, 0.2738095238095238360, 0.2797619047619047672, 0.2857142857142856984, 0.2916666666666666852, 0.2976190476190476164, 0.3035714285714285476, 0.3095238095238095344, 0.3154761904761904656, 0.3214285714285714524, 0.3273809523809523836, 0.3333333333333333148, 0.3392857142857143016, 0.3452380952380952328, 0.3511904761904761640, 0.3571428571428571508, 0.3630952380952380820, 0.3690476190476190688, 0.3750000000000000000, 0.3809523809523809312, 0.3869047619047619180, 0.3928571428571428492, 0.3988095238095238360, 0.4047619047619047672, 0.4107142857142856984, 0.4166666666666666852, 0.4226190476190476164, 0.4285714285714285476, 0.4345238095238095344, 0.4404761904761904656, 0.4464285714285714524, 0.4523809523809523836, 0.4583333333333333148, 0.4642857142857143016, 0.4702380952380952328, 0.4761904761904761640, 0.4821428571428571508, 0.4880952380952380820, 0.4940476190476190688, 0.5000000000000000000, 0.5059523809523809312, 0.5119047619047618625, 0.5178571428571429047, 0.5238095238095238360, 0.5297619047619047672, 0.5357142857142856984, 0.5416666666666666297, 0.5476190476190476719, 0.5535714285714286031, 0.5595238095238095344, 0.5654761904761904656, 0.5714285714285713969, 0.5773809523809523281, 0.5833333333333333703, 0.5892857142857143016, 0.5952380952380952328, 0.6011904761904761640, 0.6071428571428570953, 0.6130952380952381375, 0.6190476190476190688, 0.6250000000000000000, 0.6309523809523809312, 0.6369047619047618625, 0.6428571428571429047, 0.6488095238095238360, 0.6547619047619047672, 0.6607142857142856984, 0.6666666666666666297, 0.6726190476190476719, 0.6785714285714286031, 0.6845238095238095344, 0.6904761904761904656, 0.6964285714285713969, 0.7023809523809523281, 0.7083333333333333703, 0.7142857142857143016, 0.7202380952380952328, 0.7261904761904761640, 0.7321428571428570953, 0.7380952380952381375, 0.7440476190476190688, 0.7500000000000000000, 0.7559523809523809312, 0.7619047619047618625, 0.7678571428571429047, 0.7738095238095238360, 0.7797619047619047672, 0.7857142857142856984, 0.7916666666666666297, 0.7976190476190476719, 0.8035714285714286031, 0.8095238095238095344, 0.8154761904761904656, 0.8214285714285713969, 0.8273809523809523281, 0.8333333333333333703, 0.8392857142857143016, 0.8452380952380952328, 0.8511904761904761640, 0.8571428571428570953, 0.8630952380952381375, 0.8690476190476190688, 0.8750000000000000000, 0.8809523809523809312, 0.8869047619047618625, 0.8928571428571429047, 0.8988095238095238360, 0.9047619047619047672, 0.9107142857142856984, 0.9166666666666666297, 0.9226190476190476719, 0.9285714285714286031, 0.9345238095238095344, 0.9404761904761904656, 0.9464285714285713969, 0.9523809523809523281, 0.9583333333333333703, 0.9642857142857143016 ),
 .UNSPECIFIED. ) 
 GEOMETRIC_REPRESENTATION_ITEM ( )  RATIONAL_B_SPLINE_SURFACE ( (
 ( 1.000000000000000000, 0.9659258262890683122, 1.000000000000000000, 0.9659258262890683122, 1.000000000000000000, 0.9659258262890683122, 1.000000000000000000, 0.9659258262890683122, 1.000000000000000000, 0.9659258262890683122, 1.000000000000000000, 0.9659258262890683122, 1.000000000000000000, 0.9659258262890683122, 1.000000000000000000, 0.9659258262890683122, 1.000000000000000000, 0.9659258262890683122, 1.000000000000000000, 0.9659258262890683122, 1.000000000000000000, 0.9659258262890683122, 1.000000000000000000, 0.9659258262890683122, 1.000000000000000000, 0.9659258262890683122, 1.000000000000000000, 0.9659258262890683122, 1.000000000000000000, 0.9659258262890683122, 1.000000000000000000, 0.9659258262890683122, 1.000000000000000000, 0.9659258262890683122, 1.000000000000000000, 0.9659258262890683122, 1.000000000000000000, 0.9659258262890683122, 1.000000000000000000, 0.9659258262890683122, 1.000000000000000000, 0.9659258262890683122, 1.000000000000000000, 0.9659258262890683122, 1.000000000000000000, 0.9659258262890683122, 1.000000000000000000, 0.9659258262890683122, 1.000000000000000000, 0.9659258262890683122, 1.000000000000000000, 0.9659258262890683122, 1.000000000000000000, 0.9659258262890683122, 1.000000000000000000, 0.9659258262890683122, 1.000000000000000000, 0.9659258262890683122, 1.000000000000000000, 0.9659258262890683122, 1.000000000000000000, 0.9659258262890683122, 1.000000000000000000, 0.9659258262890683122, 1.000000000000000000, 0.9659258262890683122, 1.000000000000000000, 0.9659258262890683122, 1.000000000000000000, 0.9659258262890683122, 1.000000000000000000, 0.9659258262890683122, 1.000000000000000000, 0.9659258262890683122, 1.000000000000000000, 0.9659258262890683122, 1.000000000000000000, 0.9659258262890683122, 1.000000000000000000, 0.9659258262890683122, 1.000000000000000000, 0.9659258262890683122, 1.000000000000000000, 0.9659258262890683122, 1.000000000000000000, 0.9659258262890683122, 1.000000000000000000, 0.9659258262890683122, 1.000000000000000000, 0.9659258262890683122, 1.000000000000000000, 0.9659258262890683122, 1.000000000000000000, 0.9659258262890683122, 1.000000000000000000, 0.9659258262890683122, 1.000000000000000000, 0.9659258262890683122, 1.000000000000000000, 0.9659258262890683122, 1.000000000000000000, 0.9659258262890683122, 1.000000000000000000, 0.9659258262890683122, 1.000000000000000000, 0.9659258262890683122, 1.000000000000000000, 0.9659258262890683122, 1.000000000000000000, 0.9659258262890683122, 1.000000000000000000, 0.9659258262890683122, 1.000000000000000000, 0.9659258262890683122, 1.000000000000000000, 0.9659258262890683122, 1.000000000000000000, 0.9659258262890683122, 1.000000000000000000, 0.9659258262890683122, 1.000000000000000000, 0.9659258262890683122, 1.000000000000000000, 0.9659258262890683122, 1.000000000000000000, 0.9659258262890683122, 1.000000000000000000, 0.9659258262890683122, 1.000000000000000000, 0.9659258262890683122, 1.000000000000000000, 0.9659258262890683122, 1.000000000000000000, 0.9659258262890683122, 1.000000000000000000, 0.9659258262890683122, 1.000000000000000000, 0.9659258262890683122, 1.000000000000000000, 0.9659258262890683122, 1.000000000000000000, 0.9659258262890683122, 1.000000000000000000, 0.9659258262890683122, 1.000000000000000000, 0.9659258262890683122, 1.000000000000000000, 0.9659258262890683122, 1.000000000000000000, 0.9659258262890683122, 1.000000000000000000, 0.9659258262890683122, 1.000000000000000000, 0.9659258262890683122, 1.000000000000000000, 0.9659258262890683122, 1.000000000000000000, 0.9659258262890683122, 1.000000000000000000, 0.9659258262890683122, 1.000000000000000000, 0.9659258262890683122, 1.000000000000000000, 0.9659258262890683122, 1.000000000000000000, 0.9659258262890683122, 1.000000000000000000, 0.9659258262890683122, 1.000000000000000000, 0.9659258262890683122, 1.000000000000000000, 0.9659258262890683122, 1.000000000000000000, 0.9659258262890683122, 1.000000000000000000, 0.9659258262890683122, 1.000000000000000000, 0.9659258262890683122, 1.000000000000000000, 0.9659258262890683122, 1.000000000000000000, 0.9659258262890683122, 1.000000000000000000, 0.9659258262890683122, 1.000000000000000000, 0.9659258262890683122, 1.000000000000000000, 0.9659258262890683122, 1.000000000000000000, 0.9659258262890683122, 1.000000000000000000, 0.9659258262890683122, 1.000000000000000000, 0.9659258262890683122, 1.000000000000000000, 0.9659258262890683122, 1.000000000000000000, 0.9659258262890683122, 1.000000000000000000, 0.9659258262890683122, 1.000000000000000000, 0.9659258262890683122, 1.000000000000000000, 0.9659258262890683122, 1.000000000000000000, 0.9659258262890683122, 1.000000000000000000, 0.9659258262890683122, 1.000000000000000000, 0.9659258262890683122, 1.000000000000000000, 0.9659258262890683122, 1.000000000000000000, 0.9659258262890683122, 1.000000000000000000, 0.9659258262890683122, 1.000000000000000000, 0.9659258262890683122, 1.000000000000000000, 0.9659258262890683122, 1.000000000000000000, 0.9659258262890683122, 1.000000000000000000, 0.9659258262890683122, 1.000000000000000000, 0.9659258262890683122, 1.000000000000000000, 0.9659258262890683122, 1.000000000000000000, 0.9659258262890683122, 1.000000000000000000, 0.9659258262890683122, 1.000000000000000000, 0.9659258262890683122, 1.000000000000000000, 0.9659258262890683122, 1.000000000000000000, 0.9659258262890683122, 1.000000000000000000, 0.9659258262890683122, 1.000000000000000000, 0.9659258262890683122, 1.000000000000000000, 0.9659258262890683122, 1.000000000000000000, 0.9659258262890683122, 1.000000000000000000, 0.9659258262890683122, 1.000000000000000000, 0.9659258262890683122, 1.000000000000000000, 0.9659258262890683122, 1.000000000000000000, 0.9659258262890683122, 1.000000000000000000, 0.9659258262890683122, 1.000000000000000000, 0.9659258262890683122, 1.000000000000000000, 0.9659258262890683122, 1.000000000000000000, 0.9659258262890683122, 1.000000000000000000, 0.9659258262890683122, 1.000000000000000000, 0.9659258262890683122, 1.000000000000000000, 0.9659258262890683122, 1.000000000000000000, 0.9659258262890683122, 1.000000000000000000, 0.9659258262890683122, 1.000000000000000000, 0.9659258262890683122, 1.000000000000000000, 0.9659258262890683122, 1.000000000000000000, 0.9659258262890683122, 1.000000000000000000, 0.9659258262890683122, 1.000000000000000000, 0.9659258262890683122, 1.000000000000000000, 0.9659258262890683122, 1.000000000000000000, 0.9659258262890683122, 1.000000000000000000, 0.9659258262890683122, 1.000000000000000000, 0.9659258262890683122, 1.000000000000000000, 0.9659258262890683122, 1.000000000000000000, 0.9659258262890683122, 1.000000000000000000, 0.9659258262890683122, 1.000000000000000000, 0.9659258262890683122, 1.000000000000000000, 0.9659258262890683122, 1.000000000000000000, 0.9659258262890683122, 1.000000000000000000, 0.9659258262890683122, 1.000000000000000000, 0.9659258262890683122, 1.000000000000000000, 0.9659258262890683122, 1.000000000000000000, 0.9659258262890683122, 1.000000000000000000, 0.9659258262890683122, 1.000000000000000000, 0.9659258262890683122, 1.000000000000000000, 0.9659258262890683122, 1.000000000000000000, 0.9659258262890683122, 1.000000000000000000, 0.9659258262890683122, 1.000000000000000000, 0.9659258262890683122, 1.000000000000000000, 0.9659258262890683122, 1.000000000000000000),
 ( 1.000000000000000000, 0.9659258262890683122, 1.000000000000000000, 0.9659258262890683122, 1.000000000000000000, 0.9659258262890683122, 1.000000000000000000, 0.9659258262890683122, 1.000000000000000000, 0.9659258262890683122, 1.000000000000000000, 0.9659258262890683122, 1.000000000000000000, 0.9659258262890683122, 1.000000000000000000, 0.9659258262890683122, 1.000000000000000000, 0.9659258262890683122, 1.000000000000000000, 0.9659258262890683122, 1.000000000000000000, 0.9659258262890683122, 1.000000000000000000, 0.9659258262890683122, 1.000000000000000000, 0.9659258262890683122, 1.000000000000000000, 0.9659258262890683122, 1.000000000000000000, 0.9659258262890683122, 1.000000000000000000, 0.9659258262890683122, 1.000000000000000000, 0.9659258262890683122, 1.000000000000000000, 0.9659258262890683122, 1.000000000000000000, 0.9659258262890683122, 1.000000000000000000, 0.9659258262890683122, 1.000000000000000000, 0.9659258262890683122, 1.000000000000000000, 0.9659258262890683122, 1.000000000000000000, 0.9659258262890683122, 1.000000000000000000, 0.9659258262890683122, 1.000000000000000000, 0.9659258262890683122, 1.000000000000000000, 0.9659258262890683122, 1.000000000000000000, 0.9659258262890683122, 1.000000000000000000, 0.9659258262890683122, 1.000000000000000000, 0.9659258262890683122, 1.000000000000000000, 0.9659258262890683122, 1.000000000000000000, 0.9659258262890683122, 1.000000000000000000, 0.9659258262890683122, 1.000000000000000000, 0.9659258262890683122, 1.000000000000000000, 0.9659258262890683122, 1.000000000000000000, 0.9659258262890683122, 1.000000000000000000, 0.9659258262890683122, 1.000000000000000000, 0.9659258262890683122, 1.000000000000000000, 0.9659258262890683122, 1.000000000000000000, 0.9659258262890683122, 1.000000000000000000, 0.9659258262890683122, 1.000000000000000000, 0.9659258262890683122, 1.000000000000000000, 0.9659258262890683122, 1.000000000000000000, 0.9659258262890683122, 1.000000000000000000, 0.9659258262890683122, 1.000000000000000000, 0.9659258262890683122, 1.000000000000000000, 0.9659258262890683122, 1.000000000000000000, 0.9659258262890683122, 1.000000000000000000, 0.9659258262890683122, 1.000000000000000000, 0.9659258262890683122, 1.000000000000000000, 0.9659258262890683122, 1.000000000000000000, 0.9659258262890683122, 1.000000000000000000, 0.9659258262890683122, 1.000000000000000000, 0.9659258262890683122, 1.000000000000000000, 0.9659258262890683122, 1.000000000000000000, 0.9659258262890683122, 1.000000000000000000, 0.9659258262890683122, 1.000000000000000000, 0.9659258262890683122, 1.000000000000000000, 0.9659258262890683122, 1.000000000000000000, 0.9659258262890683122, 1.000000000000000000, 0.9659258262890683122, 1.000000000000000000, 0.9659258262890683122, 1.000000000000000000, 0.9659258262890683122, 1.000000000000000000, 0.9659258262890683122, 1.000000000000000000, 0.9659258262890683122, 1.000000000000000000, 0.9659258262890683122, 1.000000000000000000, 0.9659258262890683122, 1.000000000000000000, 0.9659258262890683122, 1.000000000000000000, 0.9659258262890683122, 1.000000000000000000, 0.9659258262890683122, 1.000000000000000000, 0.9659258262890683122, 1.000000000000000000, 0.9659258262890683122, 1.000000000000000000, 0.9659258262890683122, 1.000000000000000000, 0.9659258262890683122, 1.000000000000000000, 0.9659258262890683122, 1.000000000000000000, 0.9659258262890683122, 1.000000000000000000, 0.9659258262890683122, 1.000000000000000000, 0.9659258262890683122, 1.000000000000000000, 0.9659258262890683122, 1.000000000000000000, 0.9659258262890683122, 1.000000000000000000, 0.9659258262890683122, 1.000000000000000000, 0.9659258262890683122, 1.000000000000000000, 0.9659258262890683122, 1.000000000000000000, 0.9659258262890683122, 1.000000000000000000, 0.9659258262890683122, 1.000000000000000000, 0.9659258262890683122, 1.000000000000000000, 0.9659258262890683122, 1.000000000000000000, 0.9659258262890683122, 1.000000000000000000, 0.9659258262890683122, 1.000000000000000000, 0.9659258262890683122, 1.000000000000000000, 0.9659258262890683122, 1.000000000000000000, 0.9659258262890683122, 1.000000000000000000, 0.9659258262890683122, 1.000000000000000000, 0.9659258262890683122, 1.000000000000000000, 0.9659258262890683122, 1.000000000000000000, 0.9659258262890683122, 1.000000000000000000, 0.9659258262890683122, 1.000000000000000000, 0.9659258262890683122, 1.000000000000000000, 0.9659258262890683122, 1.000000000000000000, 0.9659258262890683122, 1.000000000000000000, 0.9659258262890683122, 1.000000000000000000, 0.9659258262890683122, 1.000000000000000000, 0.9659258262890683122, 1.000000000000000000, 0.9659258262890683122, 1.000000000000000000, 0.9659258262890683122, 1.000000000000000000, 0.9659258262890683122, 1.000000000000000000, 0.9659258262890683122, 1.000000000000000000, 0.9659258262890683122, 1.000000000000000000, 0.9659258262890683122, 1.000000000000000000, 0.9659258262890683122, 1.000000000000000000, 0.9659258262890683122, 1.000000000000000000, 0.9659258262890683122, 1.000000000000000000, 0.9659258262890683122, 1.000000000000000000, 0.9659258262890683122, 1.000000000000000000, 0.9659258262890683122, 1.000000000000000000, 0.9659258262890683122, 1.000000000000000000, 0.9659258262890683122, 1.000000000000000000, 0.9659258262890683122, 1.000000000000000000, 0.9659258262890683122, 1.000000000000000000, 0.9659258262890683122, 1.000000000000000000, 0.9659258262890683122, 1.000000000000000000, 0.9659258262890683122, 1.000000000000000000, 0.9659258262890683122, 1.000000000000000000, 0.9659258262890683122, 1.000000000000000000, 0.9659258262890683122, 1.000000000000000000, 0.9659258262890683122, 1.000000000000000000, 0.9659258262890683122, 1.000000000000000000, 0.9659258262890683122, 1.000000000000000000, 0.9659258262890683122, 1.000000000000000000, 0.9659258262890683122, 1.000000000000000000, 0.9659258262890683122, 1.000000000000000000, 0.9659258262890683122, 1.000000000000000000, 0.9659258262890683122, 1.000000000000000000, 0.9659258262890683122, 1.000000000000000000, 0.9659258262890683122, 1.000000000000000000, 0.9659258262890683122, 1.000000000000000000, 0.9659258262890683122, 1.000000000000000000, 0.9659258262890683122, 1.000000000000000000, 0.9659258262890683122, 1.000000000000000000, 0.9659258262890683122, 1.000000000000000000, 0.9659258262890683122, 1.000000000000000000, 0.9659258262890683122, 1.000000000000000000, 0.9659258262890683122, 1.000000000000000000, 0.9659258262890683122, 1.000000000000000000, 0.9659258262890683122, 1.000000000000000000, 0.9659258262890683122, 1.000000000000000000, 0.9659258262890683122, 1.000000000000000000, 0.9659258262890683122, 1.000000000000000000, 0.9659258262890683122, 1.000000000000000000, 0.9659258262890683122, 1.000000000000000000, 0.9659258262890683122, 1.000000000000000000, 0.9659258262890683122, 1.000000000000000000, 0.9659258262890683122, 1.000000000000000000, 0.9659258262890683122, 1.000000000000000000, 0.9659258262890683122, 1.000000000000000000, 0.9659258262890683122, 1.000000000000000000, 0.9659258262890683122, 1.000000000000000000, 0.9659258262890683122, 1.000000000000000000, 0.9659258262890683122, 1.000000000000000000, 0.9659258262890683122, 1.000000000000000000, 0.9659258262890683122, 1.000000000000000000, 0.9659258262890683122, 1.000000000000000000, 0.9659258262890683122, 1.000000000000000000) ) ) 
 REPRESENTATION_ITEM ( '' )  SURFACE ( )  );
#42568=CARTESIAN_POINT ( 'NONE',  ( 13.79529636645031943, 50.34541550158064638, -14.16423886937409904 ) ) ;
#42569=CARTESIAN_POINT ( 'NONE',  ( 24.16423886937410614, 49.51208216824730357, -3.795296366450302550 ) ) ;
#42570=CARTESIAN_POINT ( 'NONE',  ( 5.076628168052704559, 15.17559781766745175, -8.527530157486179263 ) ) ;
#42571=CARTESIAN_POINT ( 'NONE',  ( 19.38216949554541202, 30.99863466993042138, 9.382169495545424454 ) ) ;
#42573=( NAMED_UNIT ( * ) SI_UNIT ( $, .STERADIAN. ) SOLID_ANGLE_UNIT ( ) );
#42574=FILL_AREA_STYLE ('',( #65053 ) ) ;
#42575=CARTESIAN_POINT ( 'NONE',  ( 24.16423886937410614, 44.30374883491397497, 8.672049930838204340E-16 ) ) ;
#42576=EDGE_CURVE ( 'NONE', #52625, #48349, #98867, .T. ) ;
#42577=( GEOMETRIC_REPRESENTATION_CONTEXT ( 3 ) GLOBAL_UNCERTAINTY_ASSIGNED_CONTEXT ( ( #58475 ) ) GLOBAL_UNIT_ASSIGNED_CONTEXT ( ( #23083, #52570, #14596 ) ) REPRESENTATION_CONTEXT ( 'NONE', 'WORKASPACE' ) );
#42578=EDGE_CURVE ( 'NONE', #18624, #98326, #40162, .T. ) ;
#42580=CARTESIAN_POINT ( 'NONE',  ( 7.361572987183169658, 14.96726448433411960, -9.846743663894592657 ) ) ;
#42587=MECHANICAL_DESIGN_GEOMETRIC_PRESENTATION_REPRESENTATION('',(#85695),#55363);
#42588=CARTESIAN_POINT ( 'NONE',  ( 20.88017736071110519, 20.56368534415484106, 2.639326808657452039E-16 ) ) ;
#42589=CARTESIAN_POINT ( 'NONE',  ( 20.88017736071110164, 25.35535201082150891, 2.915334737309930979 ) ) ;
#42590=CARTESIAN_POINT ( 'NONE',  ( 10.00000000000000000, 49.75893115100078745, -9.846743663894594434 ) ) ;
#42591=CARTESIAN_POINT ( 'NONE',  ( 19.38216949554541557, 12.24863466993041961, -9.382169495545420901 ) ) ;
#42595=CARTESIAN_POINT ( 'NONE',  ( 22.81628187352647785, 21.62363466993041783, 6.195893100308588602E-16 ) ) ;
#42596=ORIENTED_EDGE ( 'NONE', *, *, #98732, .T. ) ;
#42597=CARTESIAN_POINT ( 'NONE',  ( 0.1532563361054100626, 30.80059781766744820, -2.638427012816831230 ) ) ;
#42598=CARTESIAN_POINT ( 'NONE',  ( 24.16423886937410614, 59.51208216824728936, -3.795296366450302550 ) ) ;
#42599=VERTEX_POINT ( 'NONE', #43358 ) ;
#42601=CARTESIAN_POINT ( 'NONE',  ( 17.96484262340118221, 9.938685344154839285, 7.964842623401181321 ) ) ;
#42603=CARTESIAN_POINT ( 'NONE',  ( 15.44008868035555793, 41.39701867748817676, -9.422509992056140149 ) ) ;
#42604=CARTESIAN_POINT ( 'NONE',  ( 2.035157376598822676, 42.43868534415483396, -7.964842623401177768 ) ) ;
#42605=CARTESIAN_POINT ( 'NONE',  ( -0.8801773607111009756, 58.06368534415484106, 1.068504757029289695E-15 ) ) ;
#42607=CARTESIAN_POINT ( 'NONE',  ( 17.96484262340118221, 36.18868534415484106, -7.964842623401177768 ) ) ;
#42610=CARTESIAN_POINT ( 'NONE',  ( 10.00000000000000000, 29.75893115100078745, -9.846743663894594434 ) ) ;
#42612=CARTESIAN_POINT ( 'NONE',  ( 1.472469842513823179, 56.42559781766745886, 4.923371831947296329 ) ) ;
#42617=CARTESIAN_POINT ( 'NONE',  ( 17.39651004071838614, 47.93575266056826933, 6.500000000000032863 ) ) ;
#42618=CARTESIAN_POINT ( 'NONE',  ( 7.361572987183169658, 64.96726448433412315, -9.846743663894592657 ) ) ;
#42619=CARTESIAN_POINT ( 'NONE',  ( 14.92337183194729633, 32.67559781766745175, 8.527530157486181039 ) ) ;
#42620=CARTESIAN_POINT ( 'NONE',  ( 10.00000000000000178, 58.05374883491397497, 14.16423886937410082 ) ) ;
#42624=CARTESIAN_POINT ( 'NONE',  ( 2.791683348922237240, 35.38393115100079456, -7.208316651077763204 ) ) ;
#42626=CARTESIAN_POINT ( 'NONE',  ( 6.565887622018943937, 5.165301336597086568, 12.81628187352647430 ) ) ;
#42627=CARTESIAN_POINT ( 'NONE',  ( 10.00000000000000178, 7.258931151000785675, 9.846743663894594434 ) ) ;
#42629=CARTESIAN_POINT ( 'NONE',  ( 14.92337183194729633, 7.675597817667451750, 8.527530157486181039 ) ) ;
#42630=CARTESIAN_POINT ( 'NONE',  ( 0.1532563361054082862, 61.21726448433412315, 2.638427012816831674 ) ) ;
#42632=MECHANICAL_DESIGN_GEOMETRIC_PRESENTATION_REPRESENTATION('',(#33060),#87310);
#42634=ORIENTED_EDGE ( 'NONE', *, *, #78578, .T. ) ;
#42635=CARTESIAN_POINT ( 'NONE',  ( 4.559911319644449179, 12.23035201082150714, -9.422509992056141925 ) ) ;
#42636=CARTESIAN_POINT ( 'NONE',  ( 17.08211943468705130, 3.470415501580634388, 12.26659068614894998 ) ) ;
#42637=CARTESIAN_POINT ( 'NONE',  ( 2.791683348922237240, 15.38393115100078212, -7.208316651077763204 ) ) ;
#42638=CARTESIAN_POINT ( 'NONE',  ( -0.8801773607110991993, 42.85535201082150536, -2.915334737309923874 ) ) ;
#42639=CARTESIAN_POINT ( 'NONE',  ( -1.099225684535947600, 29.54030133659708923, 6.408140936763237150 ) ) ;
#42641=PRESENTATION_STYLE_ASSIGNMENT (( #95645 ) ) ;
#42642=CARTESIAN_POINT ( 'NONE',  ( -0.2418659066527731605, 57.23410085661204505, -6.114288769123041867 ) ) ;
#42645=CARTESIAN_POINT ( 'NONE',  ( 21.09922568453595559, 7.040301336597086568, -6.408140936763230044 ) ) ;
#42646=CARTESIAN_POINT ( 'NONE',  ( -2.816281873526471635, -1.084698663402913210, -3.434112377981056508 ) ) ;
#42647=CARTESIAN_POINT ( 'NONE',  ( 12.63842701281683922, 14.55059781766744997, -9.846743663894590881 ) ) ;
#42649=CARTESIAN_POINT ( 'NONE',  ( 0.6178305044545818747, 23.49863466993041783, -9.382169495545419124 ) ) ;
#42651=CARTESIAN_POINT ( 'NONE',  ( -0.8801773607111009756, 33.06368534415484106, 1.068504757029289695E-15 ) ) ;
#42653=EDGE_CURVE ( 'NONE', #71557, #1898, #6848, .T. ) ;
#42654=CARTESIAN_POINT ( 'NONE',  ( -4.164238869374098151, 46.59541550158063927, -3.795296366450310543 ) ) ;
#42656=DIRECTION ( 'NONE',  ( 0.000000000000000000, 0.000000000000000000, -1.000000000000000000 ) ) ;
#42658=CARTESIAN_POINT ( 'NONE',  ( 16.40814093676323893, 35.79030133659708923, 11.09922568453595026 ) ) ;
#42659=CARTESIAN_POINT ( 'NONE',  ( 10.00000000000000000, 21.81368534415484106, -10.88017736071110342 ) ) ;
#42660=CARTESIAN_POINT ( 'NONE',  ( 1.472469842513823179, 51.42559781766745886, 4.923371831947296329 ) ) ;
#42661=CARTESIAN_POINT ( 'NONE',  ( 19.42250999205614193, 50.14701867748817676, 5.440088680355555262 ) ) ;
#42662=CARTESIAN_POINT ( 'NONE',  ( 6.204703633549690345, 37.84541550158063927, 14.16423886937410082 ) ) ;
#42664=CARTESIAN_POINT ( 'NONE',  ( 19.84674366389459621, 23.50893115100078390, 7.409399052514197653E-17 ) ) ;
#42666=CARTESIAN_POINT ( 'NONE',  ( 6.565887622018943937, 5.165301336597086568, 12.81628187352647430 ) ) ;
#42669=( NAMED_UNIT ( * ) SI_UNIT ( $, .STERADIAN. ) SOLID_ANGLE_UNIT ( ) );
#42670=CARTESIAN_POINT ( 'NONE',  ( 20.88017736071110875, 15.77201867748817143, -2.915334737309920765 ) ) ;
#42671=CARTESIAN_POINT ( 'NONE',  ( -4.164238869374099927, 22.01208216824730357, 3.795296366450308767 ) ) ;
#42672=CARTESIAN_POINT ( 'NONE',  ( 2.791683348922237240, 15.38393115100078212, -7.208316651077763204 ) ) ;
#42674=CARTESIAN_POINT ( 'NONE',  ( -0.8801773607111008646, 33.27201867748817676, 2.915334737309923430 ) ) ;
#42675=CARTESIAN_POINT ( 'NONE',  ( 18.17884179759848706, 13.66688879859523276, -6.499999999999968914 ) ) ;
#42677=ADVANCED_FACE ( 'NONE', ( #96887 ), #58851, .T. ) ;
#42680=CARTESIAN_POINT ( 'NONE',  ( 0.1532563361054100626, 40.80059781766745886, -2.638427012816831230 ) ) ;
#42682=ORIENTED_EDGE ( 'NONE', *, *, #56791, .F. ) ;
#42684=CARTESIAN_POINT ( 'NONE',  ( 0.2751277870542967463, 0.000000000000000000, 6.500000000000000888 ) ) ;
#42685=CARTESIAN_POINT ( 'NONE',  ( 17.08211943468705130, 3.470415501580634388, 12.26659068614894998 ) ) ;
#42686=CARTESIAN_POINT ( 'NONE',  ( -0.3689425029237881626, 12.42874883491396609, 10.36894250292379027 ) ) ;
#42687=CARTESIAN_POINT ( 'NONE',  ( 15.44008868035555260, 49.73035201082150536, 9.422509992056143702 ) ) ;
#42688=CARTESIAN_POINT ( 'NONE',  ( 10.00000000000000000, 50.55374883491396787, -14.16423886937410082 ) ) ;
#42689=CARTESIAN_POINT ( 'NONE',  ( 6.565887622018943937, 3.081968003263753531, -12.81628187352647608 ) ) ;
#42690=CARTESIAN_POINT ( 'NONE',  ( 5.076628168052704559, 30.17559781766745175, -8.527530157486179263 ) ) ;
#42692=CARTESIAN_POINT ( 'NONE',  ( 4.559911319644449179, 32.23035201082150536, -9.422509992056141925 ) ) ;
#42693=CARTESIAN_POINT ( 'NONE',  ( 21.09922568453595559, 12.04030133659708746, -6.408140936763230044 ) ) ;
#42694=CARTESIAN_POINT ( 'NONE',  ( -2.266590686148945544, 2.220415501580634388, 7.082119434687048631 ) ) ;
#42695=CARTESIAN_POINT ( 'NONE',  ( -0.3689425029237898834, 51.17874883491397497, -10.36894250292378850 ) ) ;
#42696=EDGE_CURVE ( 'NONE', #32629, #20168, #5892, .T. ) ;
#42698=CARTESIAN_POINT ( 'NONE',  ( 15.44008868035555793, 11.39701867748817143, -9.422509992056140149 ) ) ;
#42700=DIRECTION ( 'NONE',  ( -0.8320502943378436100, 0.5547001962252291474, -0.000000000000000000 ) ) ;
#42703=CARTESIAN_POINT ( 'NONE',  ( -46.44000000000001194, 100.8660254037844339, 9.500000000000000000 ) ) ;
#42705=CARTESIAN_POINT ( 'NONE',  ( 17.20831665107776587, 32.88393115100078745, 7.208316651077764980 ) ) ;
#42707=CARTESIAN_POINT ( 'NONE',  ( 13.79529636645031943, 40.34541550158063217, -14.16423886937409904 ) ) ;
#42708=CARTESIAN_POINT ( 'NONE',  ( 5.076628168052703671, 36.84226448433412315, 8.527530157486179263 ) ) ;
#42709=CARTESIAN_POINT ( 'NONE',  ( 0.5774900079438607392, 63.48035201082149825, 5.440088680355550821 ) ) ;
#42711=CARTESIAN_POINT ( 'NONE',  ( 0.5774900079438590739, 52.64701867748817676, -5.440088680355550821 ) ) ;
#42712=CARTESIAN_POINT ( 'NONE',  ( 0.6178305044545818747, 53.49863466993041072, -9.382169495545419124 ) ) ;
#42714=ORIENTED_EDGE ( 'NONE', *, *, #86519, .T. ) ;
#42715=CARTESIAN_POINT ( 'NONE',  ( 24.16423886937410614, 14.30374883491396787, 8.672049930838204340E-16 ) ) ;
#42716=ORIENTED_EDGE ( 'NONE', *, *, #36058, .F. ) ;
#42718=CARTESIAN_POINT ( 'NONE',  ( -2.816281873526471635, 23.91530133659708568, -3.434112377981056508 ) ) ;
#42719=ORIENTED_EDGE ( 'NONE', *, *, #74909, .F. ) ;
#42720=CARTESIAN_POINT ( 'NONE',  ( 10.00000000000000178, 40.37363466993042493, 12.81628187352647608 ) ) ;
#42722=CARTESIAN_POINT ( 'NONE',  ( 17.20831665107776587, 24.13393115100078035, -7.208316651077762316 ) ) ;
#42723=CARTESIAN_POINT ( 'NONE',  ( 0.5774900079438590739, 12.64701867748817143, -5.440088680355550821 ) ) ;
#42724=CARTESIAN_POINT ( 'NONE',  ( 6.565887622018943937, 55.16530133659709634, 12.81628187352647430 ) ) ;
#42725=CARTESIAN_POINT ( 'NONE',  ( -46.68456736488006698, 103.6675473310227034, -5.775421524742656132 ) ) ;
#42726=CARTESIAN_POINT ( 'NONE',  ( 14.92337183194729988, 44.34226448433412315, -8.527530157486177487 ) ) ;
#42730=CARTESIAN_POINT ( 'NONE',  ( 0.5774900079438590739, 67.64701867748817676, -5.440088680355550821 ) ) ;
#42732=CARTESIAN_POINT ( 'NONE',  ( 19.42250999205614548, 65.98035201082151957, -5.440088680355545492 ) ) ;
#42734=CARTESIAN_POINT ( 'NONE',  ( -1.926860441876563801, 44.89664270246083788, 3.195792623639529761 ) ) ;
#42735=CARTESIAN_POINT ( 'NONE',  ( 17.20831665107776587, 22.88393115100078745, 7.208316651077764980 ) ) ;
#42736=CARTESIAN_POINT ( 'NONE',  ( 6.565887622018943937, 23.08196800326375708, -12.81628187352647608 ) ) ;
#42738=CARTESIAN_POINT ( 'NONE',  ( 14.92337183194729988, 39.34226448433412315, -8.527530157486177487 ) ) ;
#42740=CARTESIAN_POINT ( 'NONE',  ( 13.79529636645030344, 23.26208216824730002, 14.16423886937410614 ) ) ;
#42741=CARTESIAN_POINT ( 'NONE',  ( 18.52753015748617571, 33.09226448433411605, 4.923371831947298993 ) ) ;
#42742=CARTESIAN_POINT ( 'NONE',  ( 21.09922568453594849, 46.20696800326376064, 6.408140936763242479 ) ) ;
#42744=CARTESIAN_POINT ( 'NONE',  ( 15.44008868035555793, 61.39701867748817676, -9.422509992056140149 ) ) ;
#42746=CARTESIAN_POINT ( 'NONE',  ( 13.43411237798105340, 15.58196800326374998, 12.81628187352647963 ) ) ;
#42749=CARTESIAN_POINT ( 'NONE',  ( 17.20831665107776587, 37.88393115100078745, 7.208316651077764980 ) ) ;
#42750=CARTESIAN_POINT ( 'NONE',  ( -0.8801773607111008646, 28.27201867748817321, 2.915334737309923430 ) ) ;
#42751=CARTESIAN_POINT ( 'NONE',  ( -2.816281873526473856, 29.33196800326376064, 3.434112377981055619 ) ) ;
#42752=CARTESIAN_POINT ( 'NONE',  ( 5.076628168052703671, 36.84226448433412315, 8.527530157486179263 ) ) ;
#42754=CARTESIAN_POINT ( 'NONE',  ( 12.91533473730993009, 36.60535201082151247, -10.88017736071109987 ) ) ;
#42757=CARTESIAN_POINT ( 'NONE',  ( 2.035157376598822676, 2.438685344154837953, -7.964842623401177768 ) ) ;
#42758=CARTESIAN_POINT ( 'NONE',  ( 5.076628168052704559, 60.17559781766745175, -8.527530157486179263 ) ) ;
#42759=CARTESIAN_POINT ( 'NONE',  ( 10.00000000000000178, 34.31368534415484106, 10.88017736071110342 ) ) ;
#42761=CARTESIAN_POINT ( 'NONE',  ( 7.084665262690076126, 54.10535201082151247, 10.88017736071109987 ) ) ;
#42762=CARTESIAN_POINT ( 'NONE',  ( 4.559911319644449179, 23.89701867748817321, 9.422509992056141925 ) ) ;
#42763=LINE ( 'NONE', #51747, #84659 ) ;
#42764=FILL_AREA_STYLE_COLOUR ( '', #21196 ) ;
#42765=CARTESIAN_POINT ( 'NONE',  ( 12.63842701281683922, 29.55059781766745175, -9.846743663894590881 ) ) ;
#42767=CARTESIAN_POINT ( 'NONE',  ( 0.1532563361054083140, 46.00893115100079456, 1.131784320476157264E-15 ) ) ;
#42769=CARTESIAN_POINT ( 'NONE',  ( -4.164238869374099039, 56.80374883491397497, 8.674139862899312516E-16 ) ) ;
#42773=CARTESIAN_POINT ( 'NONE',  ( 2.917880565312950480, 10.97041550158063572, -12.26659068614894821 ) ) ;
#42774=CARTESIAN_POINT ( 'NONE',  ( 6.204703633549690345, 32.84541550158063927, 14.16423886937410082 ) ) ;
#42775=CARTESIAN_POINT ( 'NONE',  ( 6.565887622018943937, 0.1653013365970866511, 12.81628187352647430 ) ) ;
#42778=CARTESIAN_POINT ( 'NONE',  ( 7.084665262690076126, 19.10535201082150181, 10.88017736071109987 ) ) ;
#42779=CARTESIAN_POINT ( 'NONE',  ( 14.92337183194729633, 32.67559781766745175, 8.527530157486181039 ) ) ;
#42782=CARTESIAN_POINT ( 'NONE',  ( -0.8801773607111008646, 58.27201867748816966, 2.915334737309923430 ) ) ;
#42784=CARTESIAN_POINT ( 'NONE',  ( 22.81628187352647785, 61.62363466993041783, 6.195893100308588602E-16 ) ) ;
#42785=CARTESIAN_POINT ( 'NONE',  ( 22.81628187352648496, 26.83196800326374998, -3.434112377981050290 ) ) ;
#42786=CARTESIAN_POINT ( 'NONE',  ( 17.20831665107776587, 34.13393115100078745, -7.208316651077762316 ) ) ;
#42787=ORIENTED_EDGE ( 'NONE', *, *, #32753, .T. ) ;
#42788=CARTESIAN_POINT ( 'NONE',  ( 1.472469842513823179, 0.5922644843341181575, -4.923371831947296329 ) ) ;
#42790=CARTESIAN_POINT ( 'NONE',  ( 2.917880565312950480, 65.97041550158063217, -12.26659068614894821 ) ) ;
#42791=CARTESIAN_POINT ( 'NONE',  ( 17.96484262340118221, 19.93868534415484106, 7.964842623401181321 ) ) ;
#42792=CARTESIAN_POINT ( 'NONE',  ( 24.16423886937410614, 44.30374883491397497, 8.672049930838204340E-16 ) ) ;
#42793=CARTESIAN_POINT ( 'NONE',  ( 2.035157376598824452, 33.68868534415484106, 7.964842623401179544 ) ) ;
#42798=CARTESIAN_POINT ( 'NONE',  ( 2.791683348922237240, 5.383931151000785675, -7.208316651077763204 ) ) ;
#42800=CARTESIAN_POINT ( 'NONE',  ( 10.00000000000000178, 2.258931151000784787, 9.846743663894594434 ) ) ;
#42801=CARTESIAN_POINT ( 'NONE',  ( 10.00000000000000178, 37.25893115100078745, 9.846743663894594434 ) ) ;
#42802=CARTESIAN_POINT ( 'NONE',  ( 2.791683348922240793, 66.63393115100079456, 7.208316651077764092 ) ) ;
#42807=CARTESIAN_POINT ( 'NONE',  ( 13.43411237798105340, 40.58196800326375353, 12.81628187352647963 ) ) ;
#42808=CARTESIAN_POINT ( 'NONE',  ( 15.44008868035555793, 66.39701867748817676, -9.422509992056140149 ) ) ;
#42809=CARTESIAN_POINT ( 'NONE',  ( 10.00000000000000178, 50.37363466993042493, 12.81628187352647608 ) ) ;
#42810=CARTESIAN_POINT ( 'NONE',  ( 20.36894250292379382, 63.67874883491396787, 10.36894250292379205 ) ) ;
#42811=CARTESIAN_POINT ( 'NONE',  ( 5.076628168052703671, 41.84226448433411605, 8.527530157486179263 ) ) ;
#42813=CARTESIAN_POINT ( 'NONE',  ( 0.1532563361054100626, 65.80059781766745175, -2.638427012816831230 ) ) ;
#42815=CARTESIAN_POINT ( 'NONE',  ( 13.79529636645030344, 33.26208216824730357, 14.16423886937410614 ) ) ;
#42816=CARTESIAN_POINT ( 'NONE',  ( 7.361572987183169658, 44.96726448433412315, -9.846743663894592657 ) ) ;
#42817=CARTESIAN_POINT ( 'NONE',  ( -0.1503990784575328643, 69.92552686551195507, 6.262539305110068177 ) ) ;
#42818=CARTESIAN_POINT ( 'NONE',  ( 0.5774900079438590739, 37.64701867748817676, -5.440088680355550821 ) ) ;
#42819=CARTESIAN_POINT ( 'NONE',  ( 2.035157376598822676, 52.43868534415483396, -7.964842623401177768 ) ) ;
#42822=CARTESIAN_POINT ( 'NONE',  ( 0.6178305044545818747, 43.49863466993042493, -9.382169495545419124 ) ) ;
#42823=CARTESIAN_POINT ( 'NONE',  ( 20.88017736071110164, 50.35535201082151247, 2.915334737309930979 ) ) ;
#42825=CARTESIAN_POINT ( 'NONE',  ( 18.52753015748617571, 63.09226448433412315, 4.923371831947298993 ) ) ;
#42830=CARTESIAN_POINT ( 'NONE',  ( -0.8801773607111009756, 13.06368534415483929, 1.068504757029289695E-15 ) ) ;
#42832=CARTESIAN_POINT ( 'NONE',  ( -4.164238869374099927, 67.01208216824728936, 3.795296366450308767 ) ) ;
#42834=CARTESIAN_POINT ( 'NONE',  ( 10.00000000000000178, 18.05374883491396787, 14.16423886937410082 ) ) ;
#42835=CARTESIAN_POINT ( 'NONE',  ( 4.559911319644449179, 22.23035201082150536, -9.422509992056141925 ) ) ;
#42836=CARTESIAN_POINT ( 'NONE',  ( 1.472469842513823179, 55.59226448433412315, -4.923371831947296329 ) ) ;
#42838=CARTESIAN_POINT ( 'NONE',  ( 12.63842701281683922, 64.55059781766745175, -9.846743663894590881 ) ) ;
#42840=CARTESIAN_POINT ( 'NONE',  ( 2.035157376598824452, 48.68868534415483396, 7.964842623401179544 ) ) ;
#42841=CARTESIAN_POINT ( 'NONE',  ( 7.361572987183170547, 62.05059781766745886, 9.846743663894590881 ) ) ;
#42842=CARTESIAN_POINT ( 'NONE',  ( 3.591859063236763294, 33.29030133659708213, -11.09922568453595026 ) ) ;
#42843=CARTESIAN_POINT ( 'NONE',  ( -0.8801773607111009756, 8.063685344154837509, 1.068504757029289695E-15 ) ) ;
#42845=CARTESIAN_POINT ( 'NONE',  ( 7.084665262690076126, 54.10535201082151247, 10.88017736071109987 ) ) ;
#42846=CARTESIAN_POINT ( 'NONE',  ( 7.084665262690076126, 17.02201867748817676, -10.88017736071110164 ) ) ;
#42848=CARTESIAN_POINT ( 'NONE',  ( 6.565887622018943937, 55.16530133659709634, 12.81628187352647430 ) ) ;
#42849=CARTESIAN_POINT ( 'NONE',  ( 19.42250999205614548, 25.98035201082150891, -5.440088680355545492 ) ) ;
#42850=CARTESIAN_POINT ( 'NONE',  ( 19.67858290521088804, 89.00000000000000000, 5.461713021790605360 ) ) ;
#42852=CARTESIAN_POINT ( 'NONE',  ( 22.81628187352648496, 46.83196800326376064, -3.434112377981050290 ) ) ;
#42853=CARTESIAN_POINT ( 'NONE',  ( 0.5774900079438590739, 52.64701867748817676, -5.440088680355550821 ) ) ;
#42854=CARTESIAN_POINT ( 'NONE',  ( 0.1532563361054100626, 60.80059781766744464, -2.638427012816831230 ) ) ;
#42856=CARTESIAN_POINT ( 'NONE',  ( -0.1503990784575242878, 44.24884699246889852, -6.262539305110083276 ) ) ;
#42858=CARTESIAN_POINT ( 'NONE',  ( 17.20831665107776587, 62.88393115100078745, 7.208316651077764980 ) ) ;
#42860=CARTESIAN_POINT ( 'NONE',  ( 19.84674366389459621, 53.50893115100078745, 7.409399052514197653E-17 ) ) ;
#42861=CARTESIAN_POINT ( 'NONE',  ( -0.8801773607111009756, 23.06368534415484106, 1.068504757029289695E-15 ) ) ;
#42862=DIRECTION ( 'NONE',  ( 0.5547001962252290364, 0.8320502943378437211, 0.000000000000000000 ) ) ;
#42863=CARTESIAN_POINT ( 'NONE',  ( 1.472469842513823179, 36.42559781766745175, 4.923371831947296329 ) ) ;
#42865=CARTESIAN_POINT ( 'NONE',  ( 1.472469842513823179, 45.59226448433412315, -4.923371831947296329 ) ) ;
#42867=CARTESIAN_POINT ( 'NONE',  ( 14.92337183194729633, 7.675597817667451750, 8.527530157486181039 ) ) ;
#42868=SURFACE_STYLE_FILL_AREA ( #19378 ) ;
#42869=CARTESIAN_POINT ( 'NONE',  ( 1.472469842513823179, 56.42559781766745886, 4.923371831947296329 ) ) ;
#42872=CARTESIAN_POINT ( 'NONE',  ( 10.00000000000000000, 42.87363466993042493, -12.81628187352647608 ) ) ;
#42873=CARTESIAN_POINT ( 'NONE',  ( 1.472469842513823179, 41.42559781766745886, 4.923371831947296329 ) ) ;
#42875=CARTESIAN_POINT ( 'NONE',  ( 24.16423886937409904, 54.09541550158063217, 3.795296366450317205 ) ) ;
#42876=CARTESIAN_POINT ( 'NONE',  ( 17.20831665107776587, 29.13393115100078390, -7.208316651077762316 ) ) ;
#42878=CARTESIAN_POINT ( 'NONE',  ( 13.79529636645031943, 55.34541550158062506, -14.16423886937409904 ) ) ;
#42880=CARTESIAN_POINT ( 'NONE',  ( 20.88017736071110875, 20.77201867748816611, -2.915334737309920765 ) ) ;
#42881=CARTESIAN_POINT ( 'NONE',  ( 10.00000000000000178, 38.05374883491396787, 14.16423886937410082 ) ) ;
#42882=CARTESIAN_POINT ( 'NONE',  ( 24.16423886937410614, 54.51208216824730357, -3.795296366450302550 ) ) ;
#42884=DIRECTION ( 'NONE',  ( -0.000000000000000000, 1.000000000000000000, 0.000000000000000000 ) ) ;
#42885=CARTESIAN_POINT ( 'NONE',  ( 7.361572987183169658, 14.96726448433411960, -9.846743663894592657 ) ) ;
#42886=CARTESIAN_POINT ( 'NONE',  ( 10.00000000000000000, -2.126365330069579951, -12.81628187352647608 ) ) ;
#42888=CARTESIAN_POINT ( 'NONE',  ( 0.5774900079438607392, 53.48035201082151247, 5.440088680355550821 ) ) ;
#42889=CARTESIAN_POINT ( 'NONE',  ( -0.03743638938522213938, 64.25197528031021932, -6.399506433553973750 ) ) ;
#42891=CARTESIAN_POINT ( 'NONE',  ( 2.791683348922240793, 51.63393115100078745, 7.208316651077764092 ) ) ;
#42893=CARTESIAN_POINT ( 'NONE',  ( 5.076628168052704559, 55.17559781766745175, -8.527530157486179263 ) ) ;
#42896=CARTESIAN_POINT ( 'NONE',  ( 2.917880565312948704, 32.63708216824730357, 12.26659068614894643 ) ) ;
#42900=CARTESIAN_POINT ( 'NONE',  ( 15.44008868035555260, 19.73035201082150536, 9.422509992056143702 ) ) ;
#42901=CARTESIAN_POINT ( 'NONE',  ( 19.38216949554541557, 32.24863466993041783, -9.382169495545420901 ) ) ;
#42903=CARTESIAN_POINT ( 'NONE',  ( -2.816281873526471635, 63.91530133659708923, -3.434112377981056508 ) ) ;
#42906=CARTESIAN_POINT ( 'NONE',  ( -2.266590686148945544, 27.22041550158063572, 7.082119434687048631 ) ) ;
#42907=CARTESIAN_POINT ( 'NONE',  ( 17.08211943468705840, 5.137082168247300906, -12.26659068614894466 ) ) ;
#42909=CARTESIAN_POINT ( 'NONE',  ( -0.8801773607110991993, 17.85535201082150536, -2.915334737309923874 ) ) ;
#42913=CARTESIAN_POINT ( 'NONE',  ( 19.42250999205614548, 45.98035201082150536, -5.440088680355545492 ) ) ;
#42914=CARTESIAN_POINT ( 'NONE',  ( 12.91533473730993009, 56.60535201082151247, -10.88017736071109987 ) ) ;
#42915=CARTESIAN_POINT ( 'NONE',  ( 16.40814093676324603, 7.456968003263754419, -11.09922568453594671 ) ) ;
#42918=CARTESIAN_POINT ( 'NONE',  ( 14.92337183194729988, 24.34226448433411960, -8.527530157486177487 ) ) ;
#42920=CARTESIAN_POINT ( 'NONE',  ( -0.8801773607111009756, 38.06368534415484106, 1.068504757029289695E-15 ) ) ;
#42922=CARTESIAN_POINT ( 'NONE',  ( -1.099225684535947600, 8.706968003263753531, -6.408140936763238038 ) ) ;
#42923=CARTESIAN_POINT ( 'NONE',  ( 15.44008868035555793, 56.39701867748817676, -9.422509992056140149 ) ) ;
#42924=CARTESIAN_POINT ( 'NONE',  ( 0.1532563361054100626, 25.80059781766744820, -2.638427012816831230 ) ) ;
#42925=CARTESIAN_POINT ( 'NONE',  ( -1.099225684535947600, 44.54030133659708923, 6.408140936763237150 ) ) ;
#42926=CARTESIAN_POINT ( 'NONE',  ( 0.1532563361054082862, 1.217264484334117824, 2.638427012816831674 ) ) ;
#42928=FACE_OUTER_BOUND ( 'NONE', #3474, .T. ) ;
#42929=CARTESIAN_POINT ( 'NONE',  ( 12.91533473730992121, 14.52201867748817143, 10.88017736071110164 ) ) ;
#42930=CARTESIAN_POINT ( 'NONE',  ( 13.43411237798106583, 62.66530133659708923, -12.81628187352647252 ) ) ;
#42931=CARTESIAN_POINT ( 'NONE',  ( -4.164238869374098151, 21.59541550158063217, -3.795296366450310543 ) ) ;
#42932=CARTESIAN_POINT ( 'NONE',  ( 0.1532563361054083140, 31.00893115100078390, 1.131784320476157264E-15 ) ) ;
#42934=CARTESIAN_POINT ( 'NONE',  ( 15.44008868035555793, 16.39701867748817321, -9.422509992056140149 ) ) ;
#42935=CARTESIAN_POINT ( 'NONE',  ( -0.8801773607110991993, 2.855352010821504471, -2.915334737309923874 ) ) ;
#42937=CARTESIAN_POINT ( 'NONE',  ( 0.5774900079438607392, 18.48035201082150536, 5.440088680355550821 ) ) ;
#42938=CIRCLE ( 'NONE', #18964, 0.5000000000000004441 ) ;
#42939=CARTESIAN_POINT ( 'NONE',  ( 17.96484262340118221, 31.18868534415483751, -7.964842623401177768 ) ) ;
#42941=CARTESIAN_POINT ( 'NONE',  ( 2.035157376598822676, 42.43868534415483396, -7.964842623401177768 ) ) ;
#42944=CARTESIAN_POINT ( 'NONE',  ( 0.1532563361054082862, 61.21726448433412315, 2.638427012816831674 ) ) ;
#42945=CARTESIAN_POINT ( 'NONE',  ( 19.42250999205614193, 20.14701867748817321, 5.440088680355555262 ) ) ;
#42946=CARTESIAN_POINT ( 'NONE',  ( 7.361572987183170547, 67.05059781766746596, 9.846743663894590881 ) ) ;
#42948=DIRECTION ( 'NONE',  ( 0.000000000000000000, -1.000000000000000000, 0.000000000000000000 ) ) ;
#42949=CARTESIAN_POINT ( 'NONE',  ( 16.40814093676324603, 57.45696800326375353, -11.09922568453594671 ) ) ;
#42951=CARTESIAN_POINT ( 'NONE',  ( 24.16423886937410614, 34.30374883491396787, 8.672049930838204340E-16 ) ) ;
#42952=CARTESIAN_POINT ( 'NONE',  ( 15.44008868035555793, 46.39701867748817676, -9.422509992056140149 ) ) ;
#42953=CARTESIAN_POINT ( 'NONE',  ( 12.91533473730993009, 36.60535201082151247, -10.88017736071109987 ) ) ;
#42956=CARTESIAN_POINT ( 'NONE',  ( 19.84674366389459621, 43.50893115100078745, 7.409399052514197653E-17 ) ) ;
#42958=CARTESIAN_POINT ( 'NONE',  ( 5.076628168052703671, 21.84226448433411960, 8.527530157486179263 ) ) ;
#42960=ADVANCED_FACE ( 'NONE', ( #87750 ), #61544, .T. ) ;
#42961=CARTESIAN_POINT ( 'NONE',  ( 4.559911319644449179, 8.897018677488171434, 9.422509992056141925 ) ) ;
#42962=CARTESIAN_POINT ( 'NONE',  ( 7.361572987183169658, 29.96726448433411960, -9.846743663894592657 ) ) ;
#42963=CARTESIAN_POINT ( 'NONE',  ( -2.816281873526473856, 14.12363466993041961, 9.499525473075851096E-16 ) ) ;
#42964=CARTESIAN_POINT ( 'NONE',  ( 7.084665262690076126, 54.10535201082151247, 10.88017736071109987 ) ) ;
#42965=CARTESIAN_POINT ( 'NONE',  ( 20.88017736071110164, 25.35535201082150891, 2.915334737309930979 ) ) ;
#42966=CARTESIAN_POINT ( 'NONE',  ( -2.816281873526471635, 53.91530133659709634, -3.434112377981056508 ) ) ;
#42967=CARTESIAN_POINT ( 'NONE',  ( 17.08211943468705130, 38.47041550158063217, 12.26659068614894998 ) ) ;
#42968=ADVANCED_FACE ( 'NONE', ( #82333 ), #45330, .T. ) ;
#42971=CARTESIAN_POINT ( 'NONE',  ( 5.076628168052703671, 66.84226448433412315, 8.527530157486179263 ) ) ;
#42973=CARTESIAN_POINT ( 'NONE',  ( 0.5774900079438590739, 27.64701867748817676, -5.440088680355550821 ) ) ;
#42974=CARTESIAN_POINT ( 'NONE',  ( 18.52753015748617571, 63.09226448433412315, 4.923371831947298993 ) ) ;
#42976=CARTESIAN_POINT ( 'NONE',  ( 2.791683348922237240, 20.38393115100078745, -7.208316651077763204 ) ) ;
#42977=CARTESIAN_POINT ( 'NONE',  ( 19.84674366389459266, 13.71726448433411782, -2.638427012816827677 ) ) ;
#42978=CARTESIAN_POINT ( 'NONE',  ( 14.92337183194729633, 27.67559781766745530, 8.527530157486181039 ) ) ;
#42979=CARTESIAN_POINT ( 'NONE',  ( 10.00000000000000178, 17.25893115100078745, 9.846743663894594434 ) ) ;
#42980=CARTESIAN_POINT ( 'NONE',  ( 0.1532563361054083140, 1.008931151000784787, 1.131784320476157264E-15 ) ) ;
#42982=CARTESIAN_POINT ( 'NONE',  ( 7.361572987183169658, -0.03273551566588185635, -9.846743663894592657 ) ) ;
#42984=CARTESIAN_POINT ( 'NONE',  ( 7.361572987183170547, 7.050597817667451750, 9.846743663894590881 ) ) ;
#42985=CARTESIAN_POINT ( 'NONE',  ( 0.1532563361054083140, 26.00893115100078745, 1.131784320476157264E-15 ) ) ;
#42988=CARTESIAN_POINT ( 'NONE',  ( -2.816281873526471635, 3.915301336597087456, -3.434112377981056508 ) ) ;
#42989=CARTESIAN_POINT ( 'NONE',  ( 6.204703633549690345, 20.76208216824730357, -14.16423886937410259 ) ) ;
#42991=CARTESIAN_POINT ( 'NONE',  ( 24.16423886937410614, 14.51208216824730179, -3.795296366450302550 ) ) ;
#42992=CARTESIAN_POINT ( 'NONE',  ( -0.3689425029237881626, 52.42874883491396076, 10.36894250292379027 ) ) ;
#42994=CARTESIAN_POINT ( 'NONE',  ( 6.204703633549690345, 0.7620821682473009062, -14.16423886937410259 ) ) ;
#42995=CARTESIAN_POINT ( 'NONE',  ( 2.917880565312948704, 7.637082168247301794, 12.26659068614894643 ) ) ;
#42996=CARTESIAN_POINT ( 'NONE',  ( 4.559911319644449179, 32.23035201082150536, -9.422509992056141925 ) ) ;
#42999=CARTESIAN_POINT ( 'NONE',  ( 18.52753015748617571, 18.09226448433411960, 4.923371831947298993 ) ) ;
#43000=CARTESIAN_POINT ( 'NONE',  ( 10.00000000000000000, 61.81368534415484106, -10.88017736071110342 ) ) ;
#43001=CARTESIAN_POINT ( 'NONE',  ( 19.84674366389459266, 28.30059781766745886, 2.638427012816836559 ) ) ;
#43002=CARTESIAN_POINT ( 'NONE',  ( 20.88017736071110164, 10.35535201082150714, 2.915334737309930979 ) ) ;
#43003=CARTESIAN_POINT ( 'NONE',  ( 16.40814093676323893, 40.79030133659708923, 11.09922568453595026 ) ) ;
#43004=CARTESIAN_POINT ( 'NONE',  ( 0.1532563361054100626, 45.80059781766745886, -2.638427012816831230 ) ) ;
#43008=CARTESIAN_POINT ( 'NONE',  ( 16.40814093676323893, 40.79030133659708923, 11.09922568453595026 ) ) ;
#43010=CARTESIAN_POINT ( 'NONE',  ( 19.84674366389459621, 43.50893115100078745, 7.409399052514197653E-17 ) ) ;
#43011=CARTESIAN_POINT ( 'NONE',  ( 6.204703633549690345, 30.76208216824730357, -14.16423886937410259 ) ) ;
#43015=CARTESIAN_POINT ( 'NONE',  ( -0.8801773607110991993, 47.85535201082150536, -2.915334737309923874 ) ) ;
#43016=CARTESIAN_POINT ( 'NONE',  ( 19.42250999205614548, 55.98035201082150536, -5.440088680355545492 ) ) ;
#43017=CARTESIAN_POINT ( 'NONE',  ( -0.3689425029237898834, 41.17874883491397497, -10.36894250292378850 ) ) ;
#43018=CARTESIAN_POINT ( 'NONE',  ( 5.076628168052704559, 65.17559781766745175, -8.527530157486179263 ) ) ;
#43019=CARTESIAN_POINT ( 'NONE',  ( 3.591859063236763294, 63.29030133659708923, -11.09922568453595026 ) ) ;
#43020=CARTESIAN_POINT ( 'NONE',  ( 7.084665262690076126, 37.02201867748817676, -10.88017736071110164 ) ) ;
#43023=CARTESIAN_POINT ( 'NONE',  ( 19.38216949554541202, 25.99863466993042138, 9.382169495545424454 ) ) ;
#43024=CARTESIAN_POINT ( 'NONE',  ( 5.076628168052704559, 60.17559781766745175, -8.527530157486179263 ) ) ;
#43026=CARTESIAN_POINT ( 'NONE',  ( 19.42250999205614193, 5.147018677488171434, 5.440088680355555262 ) ) ;
#43027=CARTESIAN_POINT ( 'NONE',  ( -0.1503990784575328643, 70.00000000000000000, 6.262539305110068177 ) ) ;
#43028=ORIENTED_EDGE ( 'NONE', *, *, #47684, .T. ) ;
#43030=CARTESIAN_POINT ( 'NONE',  ( 17.96484262340118221, 6.188685344154836621, -7.964842623401177768 ) ) ;
#43032=CARTESIAN_POINT ( 'NONE',  ( 4.559911319644449179, 62.23035201082150536, -9.422509992056141925 ) ) ;
#43033=CARTESIAN_POINT ( 'NONE',  ( 20.88017736071110164, 65.35535201082150536, 2.915334737309930979 ) ) ;
#43036=CARTESIAN_POINT ( 'NONE',  ( 5.076628168052704559, 30.17559781766745175, -8.527530157486179263 ) ) ;
#43037=CARTESIAN_POINT ( 'NONE',  ( 0.5774900079438590739, 22.64701867748817321, -5.440088680355550821 ) ) ;
#43038=B_SPLINE_CURVE_WITH_KNOTS ( 'NONE', 3,
 ( #6222, #13220, #19736, #5734 ),
 .UNSPECIFIED., .F., .F.,
 ( 4, 4 ),
 ( 4.906538933386798166E-18, 0.002392975128318429977 ),
 .UNSPECIFIED. ) ;
#43039=CARTESIAN_POINT ( 'NONE',  ( -2.816281873526473856, 4.123634669930420493, 9.499525473075851096E-16 ) ) ;
#43040=CARTESIAN_POINT ( 'NONE',  ( 20.88017736071110519, 40.56368534415484106, 2.639326808657452039E-16 ) ) ;
#43043=CARTESIAN_POINT ( 'NONE',  ( 3.591859063236763294, 43.29030133659708923, -11.09922568453595026 ) ) ;
#43045=CARTESIAN_POINT ( 'NONE',  ( 4.559911319644449179, 58.89701867748817676, 9.422509992056141925 ) ) ;
#43046=EDGE_CURVE ( 'NONE', #72967, #57072, #66351, .T. ) ;
#43047=CARTESIAN_POINT ( 'NONE',  ( 3.591859063236763294, 23.29030133659708568, -11.09922568453595026 ) ) ;
#43049=CARTESIAN_POINT ( 'NONE',  ( 20.15039907845753220, 31.74884699246888786, 6.262539305110077059 ) ) ;
#43050=CARTESIAN_POINT ( 'NONE',  ( 17.96484262340118221, 39.93868534415484106, 7.964842623401181321 ) ) ;
#43051=CARTESIAN_POINT ( 'NONE',  ( 10.00000000000000000, 64.75893115100078035, -9.846743663894594434 ) ) ;
#43052=CARTESIAN_POINT ( 'NONE',  ( 17.08211943468705840, 65.13708216824730357, -12.26659068614894466 ) ) ;
#43053=CARTESIAN_POINT ( 'NONE',  ( 7.361572987183170547, 52.05059781766745175, 9.846743663894590881 ) ) ;
#43055=CARTESIAN_POINT ( 'NONE',  ( 1.472469842513823179, 5.592264484334118713, -4.923371831947296329 ) ) ;
#43056=CARTESIAN_POINT ( 'NONE',  ( 7.084665262690076126, 67.02201867748817676, -10.88017736071110164 ) ) ;
#43058=CARTESIAN_POINT ( 'NONE',  ( 2.917880565312950480, 25.97041550158063572, -12.26659068614894821 ) ) ;
#43060=ORIENTED_EDGE ( 'NONE', *, *, #19153, .T. ) ;
#43061=ORIENTED_EDGE ( 'NONE', *, *, #17005, .T. ) ;
#43062=CARTESIAN_POINT ( 'NONE',  ( 7.084665262690076126, 2.022018677488171434, -10.88017736071110164 ) ) ;
#43063=CARTESIAN_POINT ( 'NONE',  ( 24.16423886937410614, 54.51208216824730357, -3.795296366450302550 ) ) ;
#43064=CARTESIAN_POINT ( 'NONE',  ( 5.076628168052703671, 31.84226448433412315, 8.527530157486179263 ) ) ;
#43066=SURFACE_STYLE_FILL_AREA ( #96577 ) ;
#43067=CARTESIAN_POINT ( 'NONE',  ( -2.266590686148945544, 52.22041550158064638, 7.082119434687048631 ) ) ;
#43068=CARTESIAN_POINT ( 'NONE',  ( -0.1503990784575328643, 0.1277717457861260453, 6.262539305110068177 ) ) ;
#43069=CARTESIAN_POINT ( 'NONE',  ( 14.92337183194729988, 14.34226448433411782, -8.527530157486177487 ) ) ;
#43075=CARTESIAN_POINT ( 'NONE',  ( 7.084665262690076126, 14.10535201082150358, 10.88017736071109987 ) ) ;
#43076=CARTESIAN_POINT ( 'NONE',  ( 15.44008868035555260, 19.73035201082150536, 9.422509992056143702 ) ) ;
#43077=CARTESIAN_POINT ( 'NONE',  ( 18.52753015748617571, 53.09226448433412315, 4.923371831947298993 ) ) ;
#43078=CARTESIAN_POINT ( 'NONE',  ( -2.816281873526471635, 18.91530133659708213, -3.434112377981056508 ) ) ;
#43079=DIRECTION ( 'NONE',  ( 0.000000000000000000, 0.000000000000000000, -1.000000000000000000 ) ) ;
#43080=EDGE_CURVE ( 'NONE', #75865, #24283, #55795, .T. ) ;
#43081=CARTESIAN_POINT ( 'NONE',  ( 13.43411237798106583, 27.66530133659708568, -12.81628187352647252 ) ) ;
#43083=CARTESIAN_POINT ( 'NONE',  ( 17.20831665107776587, 37.88393115100078745, 7.208316651077764980 ) ) ;
#43084=CARTESIAN_POINT ( 'NONE',  ( 2.917880565312950480, 65.97041550158063217, -12.26659068614894821 ) ) ;
#43086=CARTESIAN_POINT ( 'NONE',  ( 22.26659068614894466, 63.88708216824730357, 7.082119434687054849 ) ) ;
#43088=CARTESIAN_POINT ( 'NONE',  ( 0.5774900079438590739, 47.64701867748817676, -5.440088680355550821 ) ) ;
#43089=CARTESIAN_POINT ( 'NONE',  ( 12.91533473730992121, 44.52201867748816966, 10.88017736071110164 ) ) ;
#43090=CARTESIAN_POINT ( 'NONE',  ( 7.084665262690076126, 49.10535201082149825, 10.88017736071109987 ) ) ;
#43091=CARTESIAN_POINT ( 'NONE',  ( 12.91533473730993009, 36.60535201082151247, -10.88017736071109987 ) ) ;
#43097=CARTESIAN_POINT ( 'NONE',  ( 7.361572987183170547, 32.05059781766745175, 9.846743663894590881 ) ) ;
#43099=CARTESIAN_POINT ( 'NONE',  ( 2.791683348922237240, 55.38393115100078745, -7.208316651077763204 ) ) ;
#43101=EDGE_CURVE ( 'NONE', #49843, #12573, #86291, .T. ) ;
#43102=SURFACE_SIDE_STYLE ('',( #81099 ) ) ;
#43106=CARTESIAN_POINT ( 'NONE',  ( 18.52753015748618282, 38.92559781766745175, -4.923371831947291888 ) ) ;
#43107=CARTESIAN_POINT ( 'NONE',  ( -4.164238869374099927, 62.01208216824728936, 3.795296366450308767 ) ) ;
#43108=CARTESIAN_POINT ( 'NONE',  ( 17.84635730667659104, 63.63791097397319874, 6.499999999999953815 ) ) ;
#43111=CARTESIAN_POINT ( 'NONE',  ( 5.076628168052704559, 35.17559781766745175, -8.527530157486179263 ) ) ;
#43112=CYLINDRICAL_SURFACE ( 'NONE', #8392, 0.5000000000000004441 ) ;
#43113=CARTESIAN_POINT ( 'NONE',  ( 22.81628187352648496, 1.831968003263753753, -3.434112377981050290 ) ) ;
#43114=CARTESIAN_POINT ( 'NONE',  ( 14.92337183194729633, 12.67559781766745353, 8.527530157486181039 ) ) ;
#43117=CARTESIAN_POINT ( 'NONE',  ( 1.472469842513823179, 10.59226448433411782, -4.923371831947296329 ) ) ;
#43118=CARTESIAN_POINT ( 'NONE',  ( 5.076628168052703671, 56.84226448433412315, 8.527530157486179263 ) ) ;
#43122=CARTESIAN_POINT ( 'NONE',  ( 17.96484262340118221, 4.938685344154837509, 7.964842623401181321 ) ) ;
#43123=CARTESIAN_POINT ( 'NONE',  ( -4.164238869374099039, 11.80374883491396965, 8.674139862899312516E-16 ) ) ;
#43124=CARTESIAN_POINT ( 'NONE',  ( 0.1532563361054082862, 16.21726448433411960, 2.638427012816831674 ) ) ;
#43125=CARTESIAN_POINT ( 'NONE',  ( 7.084665262690076126, 54.10535201082151247, 10.88017736071109987 ) ) ;
#43126=CARTESIAN_POINT ( 'NONE',  ( 13.43411237798105340, 20.58196800326374643, 12.81628187352647963 ) ) ;
#43127=CARTESIAN_POINT ( 'NONE',  ( -0.3289641300567998083, 58.07879003517447813, 5.963430220938281678 ) ) ;
#43129=CARTESIAN_POINT ( 'NONE',  ( 10.00000000000000178, 0.3736346699304200492, 12.81628187352647608 ) ) ;
#43130=CARTESIAN_POINT ( 'NONE',  ( 14.92337183194729633, 17.67559781766745175, 8.527530157486181039 ) ) ;
#43132=CARTESIAN_POINT ( 'NONE',  ( 13.43411237798105340, 15.58196800326374998, 12.81628187352647963 ) ) ;
#43134=CARTESIAN_POINT ( 'NONE',  ( 4.559911319644449179, 27.23035201082150536, -9.422509992056141925 ) ) ;
#43136=CARTESIAN_POINT ( 'NONE',  ( 6.204703633549690345, 45.76208216824729647, -14.16423886937410259 ) ) ;
#43137=CARTESIAN_POINT ( 'NONE',  ( 10.00000000000000178, 70.00000000000000000, 0.000000000000000000 ) ) ;
#43138=CARTESIAN_POINT ( 'NONE',  ( -0.8801773607110991993, 27.85535201082150181, -2.915334737309923874 ) ) ;
#43139=VECTOR ( 'NONE', #64295, 1000.000000000000000 ) ;
#43140=CARTESIAN_POINT ( 'NONE',  ( 1.472469842513823179, 50.59226448433411605, -4.923371831947296329 ) ) ;
#43142=CARTESIAN_POINT ( 'NONE',  ( -0.8801773607111008646, 53.27201867748816966, 2.915334737309923430 ) ) ;
#43143=CARTESIAN_POINT ( 'NONE',  ( 13.79529636645030344, 33.26208216824730357, 14.16423886937410614 ) ) ;
#43145=UNCERTAINTY_MEASURE_WITH_UNIT (LENGTH_MEASURE( 1.000000000000000082E-05 ), #7920, 'distance_accuracy_value', 'NONE');
#43146=CARTESIAN_POINT ( 'NONE',  ( 19.84674366389459266, 33.71726448433410894, -2.638427012816827677 ) ) ;
#43147=CARTESIAN_POINT ( 'NONE',  ( 22.81628187352647785, 61.41530133659709634, 3.434112377981063169 ) ) ;
#43149=CARTESIAN_POINT ( 'NONE',  ( 10.00000000000000178, 0.3736346699304200492, 12.81628187352647608 ) ) ;
#43151=CARTESIAN_POINT ( 'NONE',  ( 7.084665262690076126, 27.02201867748817676, -10.88017736071110164 ) ) ;
#43155=STYLED_ITEM ( 'NONE', ( #39844 ), #19831 ) ;
#43156=CARTESIAN_POINT ( 'NONE',  ( 2.035157376598822676, 12.43868534415483751, -7.964842623401177768 ) ) ;
#43157=CARTESIAN_POINT ( 'NONE',  ( 2.035157376598822676, 67.43868534415484817, -7.964842623401177768 ) ) ;
#43158=CARTESIAN_POINT ( 'NONE',  ( 22.26659068614894466, 18.88708216824730002, 7.082119434687054849 ) ) ;
#43159=CARTESIAN_POINT ( 'NONE',  ( 14.92337183194729633, 17.67559781766745175, 8.527530157486181039 ) ) ;
#43160=CARTESIAN_POINT ( 'NONE',  ( 7.361572987183169658, 59.96726448433410894, -9.846743663894592657 ) ) ;
#43161=CARTESIAN_POINT ( 'NONE',  ( 17.96484262340118221, 34.93868534415482685, 7.964842623401181321 ) ) ;
#43162=CARTESIAN_POINT ( 'NONE',  ( 0.2751277870542911952, 34.36607318730131055, -6.499999999999992006 ) ) ;
#43163=FACE_OUTER_BOUND ( 'NONE', #66808, .T. ) ;
#43167=CARTESIAN_POINT ( 'NONE',  ( 1.472469842513823179, 51.42559781766745886, 4.923371831947296329 ) ) ;
#43169=ORIENTED_EDGE ( 'NONE', *, *, #29241, .T. ) ;
#43171=CARTESIAN_POINT ( 'NONE',  ( -4.164238869374098151, 26.59541550158063217, -3.795296366450310543 ) ) ;
#43172=CARTESIAN_POINT ( 'NONE',  ( -4.164238869374099039, 6.803748834913967869, 8.674139862899312516E-16 ) ) ;
#43173=CARTESIAN_POINT ( 'NONE',  ( 15.44008868035555260, 64.73035201082151957, 9.422509992056143702 ) ) ;
#43174=CARTESIAN_POINT ( 'NONE',  ( -4.164238869374099039, 51.80374883491396787, 8.674139862899312516E-16 ) ) ;
#43175=CARTESIAN_POINT ( 'NONE',  ( 10.00000000000000178, 0.3736346699304200492, 12.81628187352647608 ) ) ;
#43176=CARTESIAN_POINT ( 'NONE',  ( 19.84674366389459621, 33.50893115100078745, 7.409399052514197653E-17 ) ) ;
#43177=CARTESIAN_POINT ( 'NONE',  ( 4.559911319644449179, 28.89701867748817321, 9.422509992056141925 ) ) ;
#43178=CARTESIAN_POINT ( 'NONE',  ( 22.81628187352647785, 11.41530133659708390, 3.434112377981063169 ) ) ;
#43179=CARTESIAN_POINT ( 'NONE',  ( 22.26659068614894466, 3.887082168247300906, 7.082119434687054849 ) ) ;
#43180=CARTESIAN_POINT ( 'NONE',  ( 22.26659068614895176, 49.72041550158063927, -7.082119434687042414 ) ) ;
#43181=CARTESIAN_POINT ( 'NONE',  ( 20.88017736071110875, 15.77201867748817143, -2.915334737309920765 ) ) ;
#43182=CARTESIAN_POINT ( 'NONE',  ( 18.72515096720569971, 5.055090184799359676, 6.500000000000000000 ) ) ;
#43184=CARTESIAN_POINT ( 'NONE',  ( 12.91533473730993009, 46.60535201082150536, -10.88017736071109987 ) ) ;
#43186=ORIENTED_EDGE ( 'NONE', *, *, #57470, .T. ) ;
#43189=CARTESIAN_POINT ( 'NONE',  ( 17.08211943468705840, 40.13708216824731068, -12.26659068614894466 ) ) ;
#43190=CARTESIAN_POINT ( 'NONE',  ( 18.52753015748617571, 53.09226448433412315, 4.923371831947298993 ) ) ;
#43191=CARTESIAN_POINT ( 'NONE',  ( 2.035157376598824452, 58.68868534415482685, 7.964842623401179544 ) ) ;
#43193=CARTESIAN_POINT ( 'NONE',  ( 7.084665262690076126, 52.02201867748816255, -10.88017736071110164 ) ) ;
#43195=CARTESIAN_POINT ( 'NONE',  ( -2.816281873526473856, 59.12363466993042493, 9.499525473075851096E-16 ) ) ;
#43198=CARTESIAN_POINT ( 'NONE',  ( 6.204703633549690345, 20.76208216824730357, -14.16423886937410259 ) ) ;
#43199=CARTESIAN_POINT ( 'NONE',  ( 13.43411237798106583, 17.66530133659708923, -12.81628187352647252 ) ) ;
#43200=VERTEX_POINT ( 'NONE', #72253 ) ;
#43201=CARTESIAN_POINT ( 'NONE',  ( 6.565887622018943937, 38.08196800326376064, -12.81628187352647608 ) ) ;
#43202=CARTESIAN_POINT ( 'NONE',  ( 7.084665262690076126, 17.02201867748817676, -10.88017736071110164 ) ) ;
#43203=CARTESIAN_POINT ( 'NONE',  ( 12.63842701281683034, 37.46726448433411605, 9.846743663894596210 ) ) ;
#43204=CARTESIAN_POINT ( 'NONE',  ( 2.035157376598824452, 13.68868534415483751, 7.964842623401179544 ) ) ;
#43205=CARTESIAN_POINT ( 'NONE',  ( 21.09922568453595559, 57.04030133659708923, -6.408140936763230044 ) ) ;
#43206=CARTESIAN_POINT ( 'NONE',  ( 19.84674366389459621, 48.50893115100078745, 7.409399052514197653E-17 ) ) ;
#43212=CARTESIAN_POINT ( 'NONE',  ( 5.076628168052703671, 16.84226448433411960, 8.527530157486179263 ) ) ;
#43213=CARTESIAN_POINT ( 'NONE',  ( 19.38216949554541202, 25.99863466993042138, 9.382169495545424454 ) ) ;
#43216=VECTOR ( 'NONE', #9475, 1000.000000000000000 ) ;
#43218=CARTESIAN_POINT ( 'NONE',  ( 18.52753015748617571, 63.09226448433412315, 4.923371831947298993 ) ) ;
#43220=CARTESIAN_POINT ( 'NONE',  ( 6.204703633549690345, 15.76208216824730179, -14.16423886937410259 ) ) ;
#43221=CARTESIAN_POINT ( 'NONE',  ( 18.52753015748618282, 48.92559781766745886, -4.923371831947291888 ) ) ;
#43222=CARTESIAN_POINT ( 'NONE',  ( 3.591859063236761518, 39.95696800326375353, 11.09922568453594849 ) ) ;
#43225=CARTESIAN_POINT ( 'NONE',  ( 20.88017736071110875, 60.77201867748817676, -2.915334737309920765 ) ) ;
#43227=AXIS2_PLACEMENT_3D ( 'NONE', #88691, #59674, #19218 ) ;
#43229=CARTESIAN_POINT ( 'NONE',  ( 2.791683348922240793, 41.63393115100078745, 7.208316651077764092 ) ) ;
#43230=CARTESIAN_POINT ( 'NONE',  ( 7.084665262690076126, 34.10535201082151247, 10.88017736071109987 ) ) ;
#43231=CARTESIAN_POINT ( 'NONE',  ( 0.6178305044545838731, 44.74863466993042493, 9.382169495545420901 ) ) ;
#43232=DIRECTION ( 'NONE',  ( 0.000000000000000000, -1.000000000000000000, 0.000000000000000000 ) ) ;
#43233=EDGE_CURVE ( 'NONE', #58661, #12573, #66194, .T. ) ;
#43234=CARTESIAN_POINT ( 'NONE',  ( 0.5774900079438590739, 37.64701867748817676, -5.440088680355550821 ) ) ;
#43237=CARTESIAN_POINT ( 'NONE',  ( 2.035157376598824452, 68.68868534415484817, 7.964842623401179544 ) ) ;
#43238=CARTESIAN_POINT ( 'NONE',  ( 0.5774900079438590739, 12.64701867748817143, -5.440088680355550821 ) ) ;
#43239=CARTESIAN_POINT ( 'NONE',  ( 12.63842701281683922, 59.55059781766744464, -9.846743663894590881 ) ) ;
#43240=CARTESIAN_POINT ( 'NONE',  ( 17.96484262340118221, 49.93868534415484106, 7.964842623401181321 ) ) ;
#43242=CARTESIAN_POINT ( 'NONE',  ( 17.96484262340118221, 66.18868534415483396, -7.964842623401177768 ) ) ;
#43243=CARTESIAN_POINT ( 'NONE',  ( 20.88017736071110519, 30.56368534415484106, 2.639326808657452039E-16 ) ) ;
#43245=CARTESIAN_POINT ( 'NONE',  ( 5.076628168052703671, 1.842264484334118047, 8.527530157486179263 ) ) ;
#43246=CARTESIAN_POINT ( 'NONE',  ( 0.1532563361054083140, 21.00893115100078745, 1.131784320476157264E-15 ) ) ;
#43249=CARTESIAN_POINT ( 'NONE',  ( 2.791683348922240793, 51.63393115100078745, 7.208316651077764092 ) ) ;
#43250=CARTESIAN_POINT ( 'NONE',  ( 22.26659068614895176, 59.72041550158063927, -7.082119434687042414 ) ) ;
#43254=CARTESIAN_POINT ( 'NONE',  ( 24.16423886937409904, 4.095415501580634832, 3.795296366450317205 ) ) ;
#43255=CARTESIAN_POINT ( 'NONE',  ( -4.164238869374098151, 41.59541550158061796, -3.795296366450310543 ) ) ;
#43256=CARTESIAN_POINT ( 'NONE',  ( 19.38216949554541202, 0.9986346699304200492, 9.382169495545424454 ) ) ;
#43259=CARTESIAN_POINT ( 'NONE',  ( 17.96484262340118221, 19.93868534415484106, 7.964842623401181321 ) ) ;
#43260=CARTESIAN_POINT ( 'NONE',  ( 1.472469842513823179, 31.42559781766745530, 4.923371831947296329 ) ) ;
#43264=CARTESIAN_POINT ( 'NONE',  ( -2.816281873526471635, 23.91530133659708568, -3.434112377981056508 ) ) ;
#43265=CARTESIAN_POINT ( 'NONE',  ( 19.84674366389459621, 28.50893115100078745, 7.409399052514197653E-17 ) ) ;
#43267=CARTESIAN_POINT ( 'NONE',  ( 2.791683348922237240, 10.38393115100078390, -7.208316651077763204 ) ) ;
#43270=CARTESIAN_POINT ( 'NONE',  ( 2.917880565312948704, 62.63708216824730357, 12.26659068614894643 ) ) ;
#43271=CARTESIAN_POINT ( 'NONE',  ( 0.5774900079438607392, 8.480352010821505360, 5.440088680355550821 ) ) ;
#43272=CARTESIAN_POINT ( 'NONE',  ( 24.16423886937410614, 39.30374883491396787, 8.672049930838204340E-16 ) ) ;
#43273=CARTESIAN_POINT ( 'NONE',  ( 0.5774900079438607392, 43.48035201082151247, 5.440088680355550821 ) ) ;
#43274=CARTESIAN_POINT ( 'NONE',  ( 12.91533473730992121, 64.52201867748817676, 10.88017736071110164 ) ) ;
#43277=CARTESIAN_POINT ( 'NONE',  ( 1.472469842513823179, 26.42559781766745175, 4.923371831947296329 ) ) ;
#43279=CARTESIAN_POINT ( 'NONE',  ( 0.1532563361054100626, 10.80059781766745175, -2.638427012816831230 ) ) ;
#43281=CARTESIAN_POINT ( 'NONE',  ( 10.00000000000000000, 34.75893115100078745, -9.846743663894594434 ) ) ;
#43282=CARTESIAN_POINT ( 'NONE',  ( 7.361572987183170547, 57.05059781766744464, 9.846743663894590881 ) ) ;
#43283=CARTESIAN_POINT ( 'NONE',  ( 0.5774900079438590739, 42.64701867748816966, -5.440088680355550821 ) ) ;
#43284=EDGE_CURVE ( 'NONE', #47816, #93851, #80253, .T. ) ;
#43286=CARTESIAN_POINT ( 'NONE',  ( 0.6178305044545838731, 49.74863466993041072, 9.382169495545420901 ) ) ;
#43287=CARTESIAN_POINT ( 'NONE',  ( 15.44008868035555260, 64.73035201082151957, 9.422509992056143702 ) ) ;
#43288=CARTESIAN_POINT ( 'NONE',  ( 0.6178305044545838731, 44.74863466993042493, 9.382169495545420901 ) ) ;
#43289=CARTESIAN_POINT ( 'NONE',  ( 17.08211943468705130, 53.47041550158063217, 12.26659068614894998 ) ) ;
#43290=CARTESIAN_POINT ( 'NONE',  ( 10.00000000000000178, 37.25893115100078745, 9.846743663894594434 ) ) ;
#43292=CARTESIAN_POINT ( 'NONE',  ( 0.1532563361054082862, 66.21726448433413736, 2.638427012816831674 ) ) ;
#43293=CARTESIAN_POINT ( 'NONE',  ( 6.204703633549690345, 17.84541550158063217, 14.16423886937410082 ) ) ;
#43294=CARTESIAN_POINT ( 'NONE',  ( -4.164238869374099927, 42.01208216824728936, 3.795296366450308767 ) ) ;
#43295=CARTESIAN_POINT ( 'NONE',  ( 7.361572987183170547, 47.05059781766745175, 9.846743663894590881 ) ) ;
#43298=CARTESIAN_POINT ( 'NONE',  ( -0.8801773607110991993, 37.85535201082151247, -2.915334737309923874 ) ) ;
#43299=CARTESIAN_POINT ( 'NONE',  ( 19.42250999205614548, 60.98035201082151247, -5.440088680355545492 ) ) ;
#43300=CARTESIAN_POINT ( 'NONE',  ( 20.88017736071110519, 50.56368534415484106, 2.639326808657452039E-16 ) ) ;
#43302=CARTESIAN_POINT ( 'NONE',  ( 3.591859063236763294, 48.29030133659708923, -11.09922568453595026 ) ) ;
#43304=CARTESIAN_POINT ( 'NONE',  ( -0.8801773607110991993, 62.85535201082150536, -2.915334737309923874 ) ) ;
#43306=CARTESIAN_POINT ( 'NONE',  ( 6.204703633549690345, 12.84541550158063572, 14.16423886937410082 ) ) ;
#43307=CARTESIAN_POINT ( 'NONE',  ( 18.52753015748618282, 8.925597817667451750, -4.923371831947291888 ) ) ;
#43309=ORIENTED_EDGE ( 'NONE', *, *, #62861, .T. ) ;
#43311=CARTESIAN_POINT ( 'NONE',  ( -0.8801773607111009756, 18.06368534415484106, 1.068504757029289695E-15 ) ) ;
#43312=CARTESIAN_POINT ( 'NONE',  ( 18.72515096720590577, 61.07228050351029935, -6.499999999999718447 ) ) ;
#43313=CARTESIAN_POINT ( 'NONE',  ( 24.16423886937410614, 14.51208216824730179, -3.795296366450302550 ) ) ;
#43314=CARTESIAN_POINT ( 'NONE',  ( 17.96484262340118221, 19.93868534415484106, 7.964842623401181321 ) ) ;
#43315=CARTESIAN_POINT ( 'NONE',  ( 7.361572987183169658, 59.96726448433410894, -9.846743663894592657 ) ) ;
#43317=CARTESIAN_POINT ( 'NONE',  ( 0.1532563361054100626, 60.80059781766744464, -2.638427012816831230 ) ) ;
#43320=CARTESIAN_POINT ( 'NONE',  ( 10.00000000000000178, 64.31368534415483396, 10.88017736071110342 ) ) ;
#43322=CARTESIAN_POINT ( 'NONE',  ( 22.81628187352647785, 36.62363466993041783, 6.195893100308588602E-16 ) ) ;
#43323=CARTESIAN_POINT ( 'NONE',  ( 10.00000000000000178, 9.313685344154839285, 10.88017736071110342 ) ) ;
#43325=CARTESIAN_POINT ( 'NONE',  ( 12.63842701281683922, 4.550597817667451750, -9.846743663894590881 ) ) ;
#43326=CARTESIAN_POINT ( 'NONE',  ( 4.559911319644449179, 23.89701867748817321, 9.422509992056141925 ) ) ;
#43327=ADVANCED_FACE ( 'NONE', ( #27737 ), #81236, .T. ) ;
#43330=CARTESIAN_POINT ( 'NONE',  ( 19.38216949554541202, 50.99863466993042493, 9.382169495545424454 ) ) ;
#43331=CARTESIAN_POINT ( 'NONE',  ( 19.42250999205614548, 40.98035201082150536, -5.440088680355545492 ) ) ;
#43333=CARTESIAN_POINT ( 'NONE',  ( 21.09922568453594849, 36.20696800326375353, 6.408140936763242479 ) ) ;
#43334=CARTESIAN_POINT ( 'NONE',  ( 10.00000000000000000, 41.81368534415484106, -10.88017736071110342 ) ) ;
#43335=CARTESIAN_POINT ( 'NONE',  ( 10.00000000000000178, 57.25893115100078745, 9.846743663894594434 ) ) ;
#43338=CARTESIAN_POINT ( 'NONE',  ( 1.472469842513823179, 20.59226448433411960, -4.923371831947296329 ) ) ;
#43339=CARTESIAN_POINT ( 'NONE',  ( 19.38216949554541557, 12.24863466993041961, -9.382169495545420901 ) ) ;
#43341=CARTESIAN_POINT ( 'NONE',  ( 7.361572987183169658, 59.96726448433410894, -9.846743663894592657 ) ) ;
#43342=CARTESIAN_POINT ( 'NONE',  ( 20.88017736071110875, 20.77201867748816611, -2.915334737309920765 ) ) ;
#43343=CARTESIAN_POINT ( 'NONE',  ( 10.00000000000000000, 54.75893115100078745, -9.846743663894594434 ) ) ;
#43345=CARTESIAN_POINT ( 'NONE',  ( 0.1532563361054100626, 10.80059781766745175, -2.638427012816831230 ) ) ;
#43346=CARTESIAN_POINT ( 'NONE',  ( 2.791683348922240793, 66.63393115100079456, 7.208316651077764092 ) ) ;
#43352=CARTESIAN_POINT ( 'NONE',  ( 21.09922568453595559, 42.04030133659708213, -6.408140936763230044 ) ) ;
#43354=CARTESIAN_POINT ( 'NONE',  ( 6.204703633549690345, 62.84541550158063927, 14.16423886937410082 ) ) ;
#43355=CARTESIAN_POINT ( 'NONE',  ( 12.63842701281683922, 29.55059781766745175, -9.846743663894590881 ) ) ;
#43358=CARTESIAN_POINT ( 'NONE',  ( 17.39651004071842166, 22.93575266056828355, 6.499999999999998224 ) ) ;
#43359=CARTESIAN_POINT ( 'NONE',  ( 10.00000000000000178, 53.05374883491396787, 14.16423886937410082 ) ) ;
#43360=CARTESIAN_POINT ( 'NONE',  ( 15.44008868035555260, 19.73035201082150536, 9.422509992056143702 ) ) ;
#43361=CARTESIAN_POINT ( 'NONE',  ( 6.204703633549690345, 37.84541550158063927, 14.16423886937410082 ) ) ;
#43362=CARTESIAN_POINT ( 'NONE',  ( 2.917880565312948704, 52.63708216824730357, 12.26659068614894643 ) ) ;
#43365=CARTESIAN_POINT ( 'NONE',  ( 1.472469842513823179, 10.59226448433411782, -4.923371831947296329 ) ) ;
#43366=CARTESIAN_POINT ( 'NONE',  ( -1.099225684535947600, -1.293031996736246469, -6.408140936763238038 ) ) ;
#43368=CARTESIAN_POINT ( 'NONE',  ( 12.91533473730992121, 44.52201867748816966, 10.88017736071110164 ) ) ;
#43371=CARTESIAN_POINT ( 'NONE',  ( 19.84674366389459266, 63.71726448433412315, -2.638427012816827677 ) ) ;
#43374=CARTESIAN_POINT ( 'NONE',  ( 2.917880565312950480, 35.97041550158063217, -12.26659068614894821 ) ) ;
#43377=DIRECTION ( 'NONE',  ( 0.000000000000000000, 0.000000000000000000, 1.000000000000000000 ) ) ;
#43380=CARTESIAN_POINT ( 'NONE',  ( 7.084665262690076126, 14.10535201082150358, 10.88017736071109987 ) ) ;
#43381=CARTESIAN_POINT ( 'NONE',  ( 0.6178305044545818747, 33.49863466993042493, -9.382169495545419124 ) ) ;
#43382=CARTESIAN_POINT ( 'NONE',  ( 7.084665262690076126, 7.022018677488169658, -10.88017736071110164 ) ) ;
#43384=CARTESIAN_POINT ( 'NONE',  ( 13.43411237798105340, 40.58196800326375353, 12.81628187352647963 ) ) ;
#43386=EDGE_LOOP ( 'NONE', ( #41373, #78059, #11803, #32550 ) ) ;
#43388=EDGE_CURVE ( 'NONE', #52625, #28728, #91326, .T. ) ;
#43390=CARTESIAN_POINT ( 'NONE',  ( 17.08211943468705130, 23.47041550158063572, 12.26659068614894998 ) ) ;
#43391=FILL_AREA_STYLE_COLOUR ( '', #85387 ) ;
#43392=CARTESIAN_POINT ( 'NONE',  ( 20.88017736071110875, 20.77201867748816611, -2.915334737309920765 ) ) ;
#43395=CARTESIAN_POINT ( 'NONE',  ( 15.44008868035555260, 49.73035201082150536, 9.422509992056143702 ) ) ;
#43396=CARTESIAN_POINT ( 'NONE',  ( 17.96484262340118221, 46.18868534415484106, -7.964842623401177768 ) ) ;
#43397=CARTESIAN_POINT ( 'NONE',  ( 22.81628187352648496, 11.83196800326375531, -3.434112377981050290 ) ) ;
#43400=CARTESIAN_POINT ( 'NONE',  ( 12.63842701281683034, 22.46726448433411605, 9.846743663894596210 ) ) ;
#43402=CARTESIAN_POINT ( 'NONE',  ( 20.88017736071110519, 40.56368534415484106, 2.639326808657452039E-16 ) ) ;
#43404=CARTESIAN_POINT ( 'NONE',  ( 13.43411237798106583, 2.665301336597086568, -12.81628187352647252 ) ) ;
#43405=CARTESIAN_POINT ( 'NONE',  ( 10.00000000000000178, 2.258931151000784787, 9.846743663894594434 ) ) ;
#43406=CARTESIAN_POINT ( 'NONE',  ( 17.20831665107776587, 29.13393115100078390, -7.208316651077762316 ) ) ;
#43407=CARTESIAN_POINT ( 'NONE',  ( -1.099225684535947600, 54.54030133659708923, 6.408140936763237150 ) ) ;
#43408=CARTESIAN_POINT ( 'NONE',  ( 1.472469842513823179, 10.59226448433411782, -4.923371831947296329 ) ) ;
#43411=CARTESIAN_POINT ( 'NONE',  ( 2.831191079880678085, 79.91181047996344944, -12.00000000000000000 ) ) ;
#43412=CARTESIAN_POINT ( 'NONE',  ( 20.88017736071110519, 25.56368534415483751, 2.639326808657452039E-16 ) ) ;
#43413=FACE_OUTER_BOUND ( 'NONE', #35194, .T. ) ;
#43414=CARTESIAN_POINT ( 'NONE',  ( -4.164238869374098151, 31.59541550158063927, -3.795296366450310543 ) ) ;
#43415=CARTESIAN_POINT ( 'NONE',  ( 18.52753015748617571, 33.09226448433411605, 4.923371831947298993 ) ) ;
#43416=CARTESIAN_POINT ( 'NONE',  ( -0.8801773607111009756, 18.06368534415484106, 1.068504757029289695E-15 ) ) ;
#43417=CARTESIAN_POINT ( 'NONE',  ( 10.00000000000000000, 1.813685344154838175, -10.88017736071110342 ) ) ;
#43418=ORIENTED_EDGE ( 'NONE', *, *, #30998, .F. ) ;
#43419=CARTESIAN_POINT ( 'NONE',  ( 15.44008868035555793, 26.39701867748817321, -9.422509992056140149 ) ) ;
#43420=CARTESIAN_POINT ( 'NONE',  ( 20.88017736071110875, 30.77201867748816966, -2.915334737309920765 ) ) ;
#43422=CARTESIAN_POINT ( 'NONE',  ( 19.42250999205614548, 40.98035201082150536, -5.440088680355545492 ) ) ;
#43423=STYLED_ITEM ( 'NONE', ( #77160 ), #65030 ) ;
#43425=CARTESIAN_POINT ( 'NONE',  ( 19.84674366389459621, 58.50893115100078745, 7.409399052514197653E-17 ) ) ;
#43426=CARTESIAN_POINT ( 'NONE',  ( 2.035157376598824452, 33.68868534415484106, 7.964842623401179544 ) ) ;
#43428=CARTESIAN_POINT ( 'NONE',  ( 10.00000000000000000, 62.87363466993042493, -12.81628187352647608 ) ) ;
#43429=DIRECTION ( 'NONE',  ( -0.000000000000000000, 1.000000000000000000, 0.000000000000000000 ) ) ;
#43430=CARTESIAN_POINT ( 'NONE',  ( 2.917880565312950480, 30.97041550158063572, -12.26659068614894821 ) ) ;
#43431=CARTESIAN_POINT ( 'NONE',  ( 15.44008868035555793, 56.39701867748817676, -9.422509992056140149 ) ) ;
#43432=CARTESIAN_POINT ( 'NONE',  ( 12.63842701281683922, 64.55059781766745175, -9.846743663894590881 ) ) ;
#43434=CARTESIAN_POINT ( 'NONE',  ( 19.84674366389459266, 48.71726448433413026, -2.638427012816827677 ) ) ;
#43435=EDGE_LOOP ( 'NONE', ( #43186, #76278, #52635, #25501 ) ) ;
#43438=CARTESIAN_POINT ( 'NONE',  ( 0.1532563361054083140, 21.00893115100078745, 1.131784320476157264E-15 ) ) ;
#43440=CARTESIAN_POINT ( 'NONE',  ( 7.084665262690076126, 27.02201867748817676, -10.88017736071110164 ) ) ;
#43441=CARTESIAN_POINT ( 'NONE',  ( 0.1532563361054100626, 20.80059781766744464, -2.638427012816831230 ) ) ;
#43442=CARTESIAN_POINT ( 'NONE',  ( 10.00000000000000178, 59.31368534415484106, 10.88017736071110342 ) ) ;
#43443=CARTESIAN_POINT ( 'NONE',  ( 2.035157376598822676, 27.43868534415483396, -7.964842623401177768 ) ) ;
#43444=CARTESIAN_POINT ( 'NONE',  ( 22.81628187352648496, 56.83196800326374643, -3.434112377981050290 ) ) ;
#43445=CARTESIAN_POINT ( 'NONE',  ( 24.16423886937410614, 39.51208216824731068, -3.795296366450302550 ) ) ;
#43447=FACE_OUTER_BOUND ( 'NONE', #48880, .T. ) ;
#43448=ORIENTED_EDGE ( 'NONE', *, *, #69562, .T. ) ;
#43449=B_SPLINE_CURVE_WITH_KNOTS ( 'NONE', 3,
 ( #50195, #80209, #72692, #4229, #35187, #12201 ),
 .UNSPECIFIED., .F., .F.,
 ( 4, 2, 4 ),
 ( 0.000000000000000000, 0.0002626113303184867526, 0.0005252226606369735052 ),
 .UNSPECIFIED. ) ;
#43450=CARTESIAN_POINT ( 'NONE',  ( 0.6178305044545838731, -0.2513653300695798953, 9.382169495545420901 ) ) ;
#43451=CARTESIAN_POINT ( 'NONE',  ( 7.084665262690076126, 14.10535201082150358, 10.88017736071109987 ) ) ;
#43452=CARTESIAN_POINT ( 'NONE',  ( 20.88017736071110519, 50.56368534415484106, 2.639326808657452039E-16 ) ) ;
#43453=CARTESIAN_POINT ( 'NONE',  ( 0.1532563361054100626, 65.80059781766745175, -2.638427012816831230 ) ) ;
#43455=CARTESIAN_POINT ( 'NONE',  ( 5.076628168052703671, 11.84226448433411960, 8.527530157486179263 ) ) ;
#43456=CARTESIAN_POINT ( 'NONE',  ( 0.1532563361054083140, 16.00893115100078390, 1.131784320476157264E-15 ) ) ;
#43457=CARTESIAN_POINT ( 'NONE',  ( 2.791683348922237240, 40.38393115100078035, -7.208316651077763204 ) ) ;
#43458=CARTESIAN_POINT ( 'NONE',  ( 10.00000000000000178, 7.258931151000785675, 9.846743663894594434 ) ) ;
#43459=CARTESIAN_POINT ( 'NONE',  ( 0.1532563361054100626, 10.80059781766745175, -2.638427012816831230 ) ) ;
#43461=CARTESIAN_POINT ( 'NONE',  ( 15.44008868035555260, 64.73035201082151957, 9.422509992056143702 ) ) ;
#43462=CARTESIAN_POINT ( 'NONE',  ( 0.1922240491738430590, 23.18878173731740588, 6.499999999999968914 ) ) ;
#43463=CARTESIAN_POINT ( 'NONE',  ( 0.1532563361054083140, 11.00893115100078568, 1.131784320476157264E-15 ) ) ;
#43464=CARTESIAN_POINT ( 'NONE',  ( 0.1532563361054083140, 16.00893115100078390, 1.131784320476157264E-15 ) ) ;
#43469=CARTESIAN_POINT ( 'NONE',  ( 21.09922568453595559, 2.040301336597086568, -6.408140936763230044 ) ) ;
#43470=SURFACE_STYLE_USAGE ( .BOTH. , #96002 ) ;
#43471=CARTESIAN_POINT ( 'NONE',  ( 2.917880565312950480, 20.97041550158063217, -12.26659068614894821 ) ) ;
#43475=CARTESIAN_POINT ( 'NONE',  ( 17.08211943468705840, 15.13708216824730179, -12.26659068614894466 ) ) ;
#43476=CARTESIAN_POINT ( 'NONE',  ( 10.00000000000000000, 50.55374883491396787, -14.16423886937410082 ) ) ;
#43478=CARTESIAN_POINT ( 'NONE',  ( 13.79529636645031943, 15.34541550158063750, -14.16423886937409904 ) ) ;
#43479=CARTESIAN_POINT ( 'NONE',  ( 0.5774900079438607392, 28.48035201082150891, 5.440088680355550821 ) ) ;
#43482=CARTESIAN_POINT ( 'NONE',  ( 0.1532563361054083140, 26.00893115100078745, 1.131784320476157264E-15 ) ) ;
#43484=CARTESIAN_POINT ( 'NONE',  ( 12.63842701281683922, 29.55059781766745175, -9.846743663894590881 ) ) ;
#43485=CARTESIAN_POINT ( 'NONE',  ( 7.084665262690076126, 7.022018677488170546, -10.88017736071110164 ) ) ;
#43486=CARTESIAN_POINT ( 'NONE',  ( 19.38216949554541202, 60.99863466993042493, 9.382169495545424454 ) ) ;
#43487=CARTESIAN_POINT ( 'NONE',  ( 17.20831665107776587, 49.13393115100078745, -7.208316651077762316 ) ) ;
#43489=CARTESIAN_POINT ( 'NONE',  ( -2.816281873526471635, 43.91530133659708923, -3.434112377981056508 ) ) ;
#43492=CARTESIAN_POINT ( 'NONE',  ( 10.00000000000000000, 46.81368534415484106, -10.88017736071110342 ) ) ;
#43493=CARTESIAN_POINT ( 'NONE',  ( 2.791683348922240793, 41.63393115100078745, 7.208316651077764092 ) ) ;
#43494=CARTESIAN_POINT ( 'NONE',  ( -2.266590686148945544, 26.38708216824730357, -7.082119434687050408 ) ) ;
#43495=ORIENTED_EDGE ( 'NONE', *, *, #23853, .T. ) ;
#43496=CARTESIAN_POINT ( 'NONE',  ( 10.00000000000000178, 3.053748834913967425, 14.16423886937410082 ) ) ;
#43497=CARTESIAN_POINT ( 'NONE',  ( 20.88017736071110875, 45.77201867748816966, -2.915334737309920765 ) ) ;
#43498=CARTESIAN_POINT ( 'NONE',  ( 7.084665262690076126, 64.10535201082150536, 10.88017736071109987 ) ) ;
#43499=CARTESIAN_POINT ( 'NONE',  ( 24.16423886937410614, 44.30374883491397497, 8.672049930838204340E-16 ) ) ;
#43500=CARTESIAN_POINT ( 'NONE',  ( 21.09922568453595559, 2.040301336597086568, -6.408140936763230044 ) ) ;
#43502=CARTESIAN_POINT ( 'NONE',  ( -0.1503990784575282014, 57.22266099184919597, -6.262539305110077947 ) ) ;
#43503=CARTESIAN_POINT ( 'NONE',  ( 0.5774900079438607392, 53.48035201082151247, 5.440088680355550821 ) ) ;
#43504=COLOUR_RGB ( '', 0.09019608, 0.27058824, 0.51372549) ;
#43506=CARTESIAN_POINT ( 'NONE',  ( 22.81628187352648496, 26.83196800326374998, -3.434112377981050290 ) ) ;
#43507=CARTESIAN_POINT ( 'NONE',  ( 0.1532563361054083140, 56.00893115100078745, 1.131784320476157264E-15 ) ) ;
#43509=( NAMED_UNIT ( * ) SI_UNIT ( $, .STERADIAN. ) SOLID_ANGLE_UNIT ( ) );
#43510=CARTESIAN_POINT ( 'NONE',  ( 20.88017736071110164, 15.35535201082150358, 2.915334737309930979 ) ) ;
#43512=VERTEX_POINT ( 'NONE', #82220 ) ;
#43514=CARTESIAN_POINT ( 'NONE',  ( -0.8801773607111008646, 8.272018677488171434, 2.915334737309923430 ) ) ;
#43517=CARTESIAN_POINT ( 'NONE',  ( -0.8801773607110991993, 62.85535201082150536, -2.915334737309923874 ) ) ;
#43518=CARTESIAN_POINT ( 'NONE',  ( 18.52753015748618282, 3.925597817667451306, -4.923371831947291888 ) ) ;
#43519=CARTESIAN_POINT ( 'NONE',  ( 19.84674366389459621, 38.50893115100078745, 7.409399052514197653E-17 ) ) ;
#43520=CARTESIAN_POINT ( 'NONE',  ( 20.88017736071110875, 40.77201867748818387, -2.915334737309920765 ) ) ;
#43521=CARTESIAN_POINT ( 'NONE',  ( 16.40814093676323893, 5.790301336597087456, 11.09922568453595026 ) ) ;
#43522=CARTESIAN_POINT ( 'NONE',  ( 20.88017736071110164, 40.35535201082150536, 2.915334737309930979 ) ) ;
#43524=CARTESIAN_POINT ( 'NONE',  ( 16.40814093676324603, 37.45696800326376064, -11.09922568453594671 ) ) ;
#43525=ORIENTED_EDGE ( 'NONE', *, *, #68349, .F. ) ;
#43526=CARTESIAN_POINT ( 'NONE',  ( 15.44008868035555260, 59.73035201082151247, 9.422509992056143702 ) ) ;
#43527=CARTESIAN_POINT ( 'NONE',  ( 3.591859063236763294, 28.29030133659708568, -11.09922568453595026 ) ) ;
#43528=CARTESIAN_POINT ( 'NONE',  ( -4.164238869374099927, 7.012082168247302683, 3.795296366450308767 ) ) ;
#43529=CARTESIAN_POINT ( 'NONE',  ( 5.076628168052704559, 0.1755978176674514724, -8.527530157486179263 ) ) ;
#43530=CARTESIAN_POINT ( 'NONE',  ( 12.91533473730993009, 41.60535201082149825, -10.88017736071109987 ) ) ;
#43532=CARTESIAN_POINT ( 'NONE',  ( 24.16423886937410614, 59.30374883491397497, 8.672049930838204340E-16 ) ) ;
#43534=CARTESIAN_POINT ( 'NONE',  ( 18.52753015748617571, 58.09226448433411605, 4.923371831947298993 ) ) ;
#43535=CARTESIAN_POINT ( 'NONE',  ( 0.1532563361054082862, 11.21726448433411605, 2.638427012816831674 ) ) ;
#43536=CARTESIAN_POINT ( 'NONE',  ( 20.88017736071110164, 60.35535201082151957, 2.915334737309930979 ) ) ;
#43537=CARTESIAN_POINT ( 'NONE',  ( 0.1957200283969147692, 5.257339608395445119, 6.500000000000001776 ) ) ;
#43538=CARTESIAN_POINT ( 'NONE',  ( 20.36894250292379738, 29.92874883491396432, -10.36894250292379027 ) ) ;
#43542=CARTESIAN_POINT ( 'NONE',  ( 2.917880565312950480, 60.97041550158063927, -12.26659068614894821 ) ) ;
#43543=CARTESIAN_POINT ( 'NONE',  ( 2.917880565312948704, 62.63708216824730357, 12.26659068614894643 ) ) ;
#43544=CARTESIAN_POINT ( 'NONE',  ( 18.52753015748617571, 33.09226448433411605, 4.923371831947298993 ) ) ;
#43545=CARTESIAN_POINT ( 'NONE',  ( 0.6178305044545818747, 28.49863466993041783, -9.382169495545419124 ) ) ;
#43546=CARTESIAN_POINT ( 'NONE',  ( -45.94000000000001194, 107.5383484153110061, -12.00000000000000000 ) ) ;
#43547=CARTESIAN_POINT ( 'NONE',  ( -23.44000000000001194, 92.00000000000000000, -10.09898361729590199 ) ) ;
#43548=CARTESIAN_POINT ( 'NONE',  ( 2.035157376598822676, 17.43868534415483751, -7.964842623401177768 ) ) ;
#43549=CARTESIAN_POINT ( 'NONE',  ( 6.204703633549690345, 60.76208216824730357, -14.16423886937410259 ) ) ;
#43550=CARTESIAN_POINT ( 'NONE',  ( 12.63842701281683034, 32.46726448433412315, 9.846743663894596210 ) ) ;
#43552=CARTESIAN_POINT ( 'NONE',  ( 18.52753015748618282, 13.92559781766745175, -4.923371831947291888 ) ) ;
#43557=CARTESIAN_POINT ( 'NONE',  ( 7.361572987183170547, 42.05059781766745886, 9.846743663894590881 ) ) ;
#43558=CARTESIAN_POINT ( 'NONE',  ( 15.44008868035555260, 24.73035201082150891, 9.422509992056143702 ) ) ;
#43559=CARTESIAN_POINT ( 'NONE',  ( -0.8801773607111009756, 23.06368534415484106, 1.068504757029289695E-15 ) ) ;
#43560=CARTESIAN_POINT ( 'NONE',  ( 17.20831665107776587, 59.13393115100078745, -7.208316651077762316 ) ) ;
#43561=CARTESIAN_POINT ( 'NONE',  ( 3.591859063236763294, 13.29030133659708746, -11.09922568453595026 ) ) ;
#43562=CARTESIAN_POINT ( 'NONE',  ( -0.3689425029237881626, 7.428748834913967869, 10.36894250292379027 ) ) ;
#43566=CARTESIAN_POINT ( 'NONE',  ( 0.6178305044545838731, 29.74863466993042138, 9.382169495545420901 ) ) ;
#43568=STYLED_ITEM ( 'NONE', ( #85660 ), #25021 ) ;
#43569=CARTESIAN_POINT ( 'NONE',  ( 5.076628168052704559, 30.17559781766745175, -8.527530157486179263 ) ) ;
#43571=CARTESIAN_POINT ( 'NONE',  ( 20.88017736071110164, 5.355352010821503583, 2.915334737309930979 ) ) ;
#43572=VERTEX_POINT ( 'NONE', #6233 ) ;
#43574=CARTESIAN_POINT ( 'NONE',  ( 4.559911319644449179, 7.230352010821505360, -9.422509992056141925 ) ) ;
#43576=CARTESIAN_POINT ( 'NONE',  ( 0.5774900079438590739, 52.64701867748817676, -5.440088680355550821 ) ) ;
#43577=CARTESIAN_POINT ( 'NONE',  ( 10.00000000000000178, 49.31368534415484106, 10.88017736071110342 ) ) ;
#43578=CARTESIAN_POINT ( 'NONE',  ( 17.96484262340118221, 51.18868534415483396, -7.964842623401177768 ) ) ;
#43582=CARTESIAN_POINT ( 'NONE',  ( 10.00000000000000000, 41.81368534415484106, -10.88017736071110342 ) ) ;
#43587=CARTESIAN_POINT ( 'NONE',  ( 14.92337183194729988, 34.34226448433411605, -8.527530157486177487 ) ) ;
#43589=CARTESIAN_POINT ( 'NONE',  ( 7.361572987183169658, 54.96726448433413026, -9.846743663894592657 ) ) ;
#43590=DIRECTION ( 'NONE',  ( 0.000000000000000000, -1.000000000000000000, 0.000000000000000000 ) ) ;
#43593=CARTESIAN_POINT ( 'NONE',  ( -0.3689425029237898834, 11.17874883491396787, -10.36894250292378850 ) ) ;
#43598=CARTESIAN_POINT ( 'NONE',  ( 17.08211943468705840, 60.13708216824729647, -12.26659068614894466 ) ) ;
#43602=CARTESIAN_POINT ( 'NONE',  ( 2.791683348922237240, 50.38393115100078035, -7.208316651077763204 ) ) ;
#43604=CARTESIAN_POINT ( 'NONE',  ( -2.816281873526471635, 18.91530133659708213, -3.434112377981056508 ) ) ;
#43606=CARTESIAN_POINT ( 'NONE',  ( 2.791683348922237240, 5.383931151000785675, -7.208316651077763204 ) ) ;
#43608=CARTESIAN_POINT ( 'NONE',  ( 18.52753015748618282, 13.92559781766745175, -4.923371831947291888 ) ) ;
#43609=CARTESIAN_POINT ( 'NONE',  ( 7.361572987183170547, 67.05059781766746596, 9.846743663894590881 ) ) ;
#43612=ORIENTED_EDGE ( 'NONE', *, *, #3881, .T. ) ;
#43613=CARTESIAN_POINT ( 'NONE',  ( 10.00000000000000178, 14.31368534415483929, 10.88017736071110342 ) ) ;
#43614=CARTESIAN_POINT ( 'NONE',  ( -4.164238869374099039, 1.803748834913967647, 8.674139862899312516E-16 ) ) ;
#43615=CARTESIAN_POINT ( 'NONE',  ( 7.361572987183170547, 22.05059781766745530, 9.846743663894590881 ) ) ;
#43616=CARTESIAN_POINT ( 'NONE',  ( 0.5774900079438607392, 58.48035201082151247, 5.440088680355550821 ) ) ;
#43617=CARTESIAN_POINT ( 'NONE',  ( -1.099225684535947600, 23.70696800326375708, -6.408140936763238038 ) ) ;
#43622=CARTESIAN_POINT ( 'NONE',  ( 6.565887622018943937, 3.081968003263753531, -12.81628187352647608 ) ) ;
#43623=CARTESIAN_POINT ( 'NONE',  ( 14.92337183194729633, 62.67559781766745886, 8.527530157486181039 ) ) ;
#43624=CARTESIAN_POINT ( 'NONE',  ( 14.92337183194729633, 7.675597817667451750, 8.527530157486181039 ) ) ;
#43626=CARTESIAN_POINT ( 'NONE',  ( 16.40814093676323893, 15.79030133659708746, 11.09922568453595026 ) ) ;
#43628=CARTESIAN_POINT ( 'NONE',  ( 10.00000000000000178, 34.31368534415484106, 10.88017736071110342 ) ) ;
#43630=CARTESIAN_POINT ( 'NONE',  ( 17.39651004071842522, 24.08210964143329491, -6.499999999999992895 ) ) ;
#43633=CARTESIAN_POINT ( 'NONE',  ( 4.559911319644449179, 23.89701867748817321, 9.422509992056141925 ) ) ;
#43634=CARTESIAN_POINT ( 'NONE',  ( 0.1532563361054083140, 46.00893115100079456, 1.131784320476157264E-15 ) ) ;
#43635=CARTESIAN_POINT ( 'NONE',  ( 7.084665262690076126, 57.02201867748817676, -10.88017736071110164 ) ) ;
#43636=CARTESIAN_POINT ( 'NONE',  ( -2.266590686148945544, 37.22041550158063217, 7.082119434687048631 ) ) ;
#43638=VECTOR ( 'NONE', #3642, 1000.000000000000000 ) ;
#43639=CARTESIAN_POINT ( 'NONE',  ( 0.1532563361054100626, 40.80059781766745886, -2.638427012816831230 ) ) ;
#43640=CARTESIAN_POINT ( 'NONE',  ( 0.1532563361054100626, 65.80059781766745175, -2.638427012816831230 ) ) ;
#43642=CARTESIAN_POINT ( 'NONE',  ( 10.00000000000000178, 29.31368534415483751, 10.88017736071110342 ) ) ;
#43645=CARTESIAN_POINT ( 'NONE',  ( 12.91533473730993009, 6.605352010821504471, -10.88017736071109987 ) ) ;
#43646=CARTESIAN_POINT ( 'NONE',  ( 15.44008868035555793, 11.39701867748817143, -9.422509992056140149 ) ) ;
#43647=CARTESIAN_POINT ( 'NONE',  ( 20.88017736071110875, 65.77201867748817676, -2.915334737309920765 ) ) ;
#43648=CARTESIAN_POINT ( 'NONE',  ( 20.36894250292379738, 29.92874883491396432, -10.36894250292379027 ) ) ;
#43649=CARTESIAN_POINT ( 'NONE',  ( 19.84674366389459621, 13.50893115100078568, 7.409399052514197653E-17 ) ) ;
#43651=CARTESIAN_POINT ( 'NONE',  ( 20.88017736071110875, 30.77201867748816966, -2.915334737309920765 ) ) ;
#43653=CARTESIAN_POINT ( 'NONE',  ( 17.39651004071838969, 39.08210964143329846, -6.500000000000027534 ) ) ;
#43654=CARTESIAN_POINT ( 'NONE',  ( 19.10478245763047056, 26.02576239577082262, -5.990408912944402253 ) ) ;
#43655=VERTEX_POINT ( 'NONE', #77180 ) ;
#43657=CARTESIAN_POINT ( 'NONE',  ( 2.791683348922237240, 45.38393115100079456, -7.208316651077763204 ) ) ;
#43661=CARTESIAN_POINT ( 'NONE',  ( 17.08211943468705840, 20.13708216824730357, -12.26659068614894466 ) ) ;
#43662=CARTESIAN_POINT ( 'NONE',  ( 22.26659068614894466, 8.887082168247300018, 7.082119434687054849 ) ) ;
#43663=CARTESIAN_POINT ( 'NONE',  ( 12.91533473730992121, 54.52201867748816255, 10.88017736071110164 ) ) ;
#43664=CARTESIAN_POINT ( 'NONE',  ( 6.204703633549690345, 50.76208216824730357, -14.16423886937410259 ) ) ;
#43665=CARTESIAN_POINT ( 'NONE',  ( 0.1532563361054100626, 65.80059781766745175, -2.638427012816831230 ) ) ;
#43666=CARTESIAN_POINT ( 'NONE',  ( 7.361572987183169658, 44.96726448433412315, -9.846743663894592657 ) ) ;
#43667=CARTESIAN_POINT ( 'NONE',  ( 2.035157376598822676, 47.43868534415484817, -7.964842623401177768 ) ) ;
#43668=CARTESIAN_POINT ( 'NONE',  ( 22.81628187352648496, 1.831968003263753753, -3.434112377981050290 ) ) ;
#43669=CARTESIAN_POINT ( 'NONE',  ( -0.3689425029237881626, 22.42874883491397142, 10.36894250292379027 ) ) ;
#43670=CARTESIAN_POINT ( 'NONE',  ( 20.36894250292379738, 49.92874883491396787, -10.36894250292379027 ) ) ;
#43671=CARTESIAN_POINT ( 'NONE',  ( 17.96484262340118221, 24.93868534415484461, 7.964842623401181321 ) ) ;
#43672=CARTESIAN_POINT ( 'NONE',  ( 19.72487221294570858, 4.782175860852374782, 6.500000000000002665 ) ) ;
#43673=CARTESIAN_POINT ( 'NONE',  ( 19.42250999205614548, 45.98035201082150536, -5.440088680355545492 ) ) ;
#43679=CARTESIAN_POINT ( 'NONE',  ( 10.00000000000000000, 45.55374883491397497, -14.16423886937410082 ) ) ;
#43680=CARTESIAN_POINT ( 'NONE',  ( 17.20831665107776587, 44.13393115100078745, -7.208316651077762316 ) ) ;
#43681=CARTESIAN_POINT ( 'NONE',  ( 20.88017736071110164, 65.35535201082150536, 2.915334737309930979 ) ) ;
#43685=CARTESIAN_POINT ( 'NONE',  ( 4.559911319644449179, 52.23035201082151247, -9.422509992056141925 ) ) ;
#43687=CARTESIAN_POINT ( 'NONE',  ( 6.565887622018943937, 55.16530133659709634, 12.81628187352647430 ) ) ;
#43690=CARTESIAN_POINT ( 'NONE',  ( 20.36894250292379382, 23.67874883491397142, 10.36894250292379205 ) ) ;
#43691=B_SPLINE_CURVE_WITH_KNOTS ( 'NONE', 3,
 ( #67349, #51359, #44341, #60823 ),
 .UNSPECIFIED., .F., .F.,
 ( 4, 4 ),
 ( 1.242751103718668000E-16, 0.001060528352561993307 ),
 .UNSPECIFIED. ) ;
#43692=CARTESIAN_POINT ( 'NONE',  ( 22.81628187352648496, 21.83196800326374643, -3.434112377981050290 ) ) ;
#43694=CARTESIAN_POINT ( 'NONE',  ( -1.099225684535947600, 44.54030133659708923, 6.408140936763237150 ) ) ;
#43695=CARTESIAN_POINT ( 'NONE',  ( 0.5774900079438607392, 18.48035201082150536, 5.440088680355550821 ) ) ;
#43696=CARTESIAN_POINT ( 'NONE',  ( 19.84674366389459266, 43.30059781766744464, 2.638427012816836559 ) ) ;
#43697=CARTESIAN_POINT ( 'NONE',  ( 15.44008868035555260, 14.73035201082150536, 9.422509992056143702 ) ) ;
#43698=CARTESIAN_POINT ( 'NONE',  ( -2.816281873526473856, 49.33196800326374643, 3.434112377981055619 ) ) ;
#43699=ADVANCED_FACE ( 'NONE', ( #92672 ), #71172, .T. ) ;
#43701=CARTESIAN_POINT ( 'NONE',  ( 12.63842701281683922, 44.55059781766745175, -9.846743663894590881 ) ) ;
#43708=CARTESIAN_POINT ( 'NONE',  ( 14.92337183194729633, 17.67559781766745175, 8.527530157486181039 ) ) ;
#43709=CARTESIAN_POINT ( 'NONE',  ( 6.565887622018943937, 28.08196800326375353, -12.81628187352647608 ) ) ;
#43712=CARTESIAN_POINT ( 'NONE',  ( 0.2751277870542911952, 38.21833443783937412, 6.499999999999992006 ) ) ;
#43713=B_SPLINE_CURVE_WITH_KNOTS ( 'NONE', 3,
 ( #93693, #55707, #86203, #17715, #10209, #86694, #20652, #42183, #11671, #28145 ),
 .UNSPECIFIED., .F., .F.,
 ( 4, 3, 3, 4 ),
 ( 1.551583845779545699E-17, 0.0006253016069560773937, 0.001250604074564914785, 0.002501455912506532226 ),
 .UNSPECIFIED. ) ;
#43715=CARTESIAN_POINT ( 'NONE',  ( 1.472469842513823179, 61.42559781766745175, 4.923371831947296329 ) ) ;
#43717=CARTESIAN_POINT ( 'NONE',  ( 24.16423886937409904, 24.09541550158063927, 3.795296366450317205 ) ) ;
#43718=CARTESIAN_POINT ( 'NONE',  ( 10.00000000000000178, 47.25893115100078745, 9.846743663894594434 ) ) ;
#43719=CARTESIAN_POINT ( 'NONE',  ( 22.81628187352647785, 41.62363466993042493, 6.195893100308588602E-16 ) ) ;
#43720=CARTESIAN_POINT ( 'NONE',  ( 21.92686044187657046, 37.39664270246084499, -3.195792623639524432 ) ) ;
#43722=CARTESIAN_POINT ( 'NONE',  ( 4.559911319644449179, 63.89701867748817676, 9.422509992056141925 ) ) ;
#43724=CARTESIAN_POINT ( 'NONE',  ( 17.20831665107776587, 29.13393115100078390, -7.208316651077762316 ) ) ;
#43725=CARTESIAN_POINT ( 'NONE',  ( 19.42250999205614548, 35.98035201082151247, -5.440088680355545492 ) ) ;
#43726=CARTESIAN_POINT ( 'NONE',  ( 19.84674366389459266, 33.30059781766744464, 2.638427012816836559 ) ) ;
#43728=CARTESIAN_POINT ( 'NONE',  ( 2.831191079880678085, 79.91181047996344944, 5.000000000000000000 ) ) ;
#43729=CARTESIAN_POINT ( 'NONE',  ( 4.559911319644449179, 48.89701867748817676, 9.422509992056141925 ) ) ;
#43732=CARTESIAN_POINT ( 'NONE',  ( 17.96484262340118221, 16.18868534415483396, -7.964842623401177768 ) ) ;
#43733=CARTESIAN_POINT ( 'NONE',  ( 5.076628168052703671, 56.84226448433412315, 8.527530157486179263 ) ) ;
#43734=CARTESIAN_POINT ( 'NONE',  ( 20.88017736071110875, 40.77201867748818387, -2.915334737309920765 ) ) ;
#43735=CARTESIAN_POINT ( 'NONE',  ( 20.88017736071110519, 65.56368534415483396, 2.639326808657452039E-16 ) ) ;
#43736=CARTESIAN_POINT ( 'NONE',  ( 15.44008868035555793, 31.39701867748817676, -9.422509992056140149 ) ) ;
#43738=CARTESIAN_POINT ( 'NONE',  ( 19.84674366389459266, 3.300597817667451750, 2.638427012816836559 ) ) ;
#43739=CARTESIAN_POINT ( 'NONE',  ( 0.1532563361054082862, 26.21726448433411605, 2.638427012816831674 ) ) ;
#43742=CARTESIAN_POINT ( 'NONE',  ( 19.84674366389459266, 53.71726448433411605, -2.638427012816827677 ) ) ;
#43743=CARTESIAN_POINT ( 'NONE',  ( 13.79529636645030344, 58.26208216824728936, 14.16423886937410614 ) ) ;
#43745=CARTESIAN_POINT ( 'NONE',  ( 1.932340009482124588, 61.49127512925447547, -6.499999999999922728 ) ) ;
#43746=CARTESIAN_POINT ( 'NONE',  ( 22.26659068614894466, 8.887082168247300018, 7.082119434687054849 ) ) ;
#43747=EDGE_CURVE ( 'NONE', #89307, #39417, #54307, .T. ) ;
#43748=CARTESIAN_POINT ( 'NONE',  ( -2.266590686148945544, 41.38708216824729647, -7.082119434687050408 ) ) ;
#43749=CARTESIAN_POINT ( 'NONE',  ( -2.816281873526471635, -1.084698663402913210, -3.434112377981056508 ) ) ;
#43751=CARTESIAN_POINT ( 'NONE',  ( 7.084665262690076126, 12.02201867748817321, -10.88017736071110164 ) ) ;
#43752=CARTESIAN_POINT ( 'NONE',  ( 1.472469842513823179, 50.59226448433411605, -4.923371831947296329 ) ) ;
#43755=DIRECTION ( 'NONE',  ( 1.000000000000000000, 0.000000000000000000, 0.000000000000000000 ) ) ;
#43756=CARTESIAN_POINT ( 'NONE',  ( -2.816281873526471635, 28.91530133659708213, -3.434112377981056508 ) ) ;
#43757=CARTESIAN_POINT ( 'NONE',  ( 17.20831665107776587, 24.13393115100078035, -7.208316651077762316 ) ) ;
#43759=CARTESIAN_POINT ( 'NONE',  ( 19.84674366389459266, 3.717264484334118713, -2.638427012816827677 ) ) ;
#43760=CARTESIAN_POINT ( 'NONE',  ( 18.39792806157249672, 4.522241923386406626, 6.500000000000004441 ) ) ;
#43762=CARTESIAN_POINT ( 'NONE',  ( 4.559911319644449179, 13.89701867748817143, 9.422509992056141925 ) ) ;
#43763=CARTESIAN_POINT ( 'NONE',  ( -4.164238869374099039, 41.80374883491397497, 8.674139862899312516E-16 ) ) ;
#43764=CARTESIAN_POINT ( 'NONE',  ( 0.5774900079438590739, 42.64701867748816966, -5.440088680355550821 ) ) ;
#43765=CARTESIAN_POINT ( 'NONE',  ( 2.035157376598822676, 57.43868534415484106, -7.964842623401177768 ) ) ;
#43766=CARTESIAN_POINT ( 'NONE',  ( 7.361572987183170547, 22.05059781766745530, 9.846743663894590881 ) ) ;
#43767=CARTESIAN_POINT ( 'NONE',  ( 19.72487221294570858, 21.86607318730131411, 6.500000000000000888 ) ) ;
#43768=CARTESIAN_POINT ( 'NONE',  ( 7.361572987183170547, 7.050597817667451750, 9.846743663894590881 ) ) ;
#43769=CARTESIAN_POINT ( 'NONE',  ( -1.504961813935599357, 2.551371850025192809E-18, 0.8438823471837141321 ) ) ;
#43770=CARTESIAN_POINT ( 'NONE',  ( 14.92337183194729988, 39.34226448433412315, -8.527530157486177487 ) ) ;
#43771=CARTESIAN_POINT ( 'NONE',  ( 5.076628168052704559, 65.17559781766745175, -8.527530157486179263 ) ) ;
#43772=CARTESIAN_POINT ( 'NONE',  ( 2.035157376598824452, 38.68868534415483396, 7.964842623401179544 ) ) ;
#43774=CARTESIAN_POINT ( 'NONE',  ( 19.38216949554541202, 60.99863466993042493, 9.382169495545424454 ) ) ;
#43776=CARTESIAN_POINT ( 'NONE',  ( 20.88017736071110519, 65.56368534415483396, 2.639326808657452039E-16 ) ) ;
#43777=CARTESIAN_POINT ( 'NONE',  ( 19.38216949554541557, 42.24863466993041783, -9.382169495545420901 ) ) ;
#43778=CARTESIAN_POINT ( 'NONE',  ( 22.26659068614894466, 63.88708216824730357, 7.082119434687054849 ) ) ;
#43779=CARTESIAN_POINT ( 'NONE',  ( 19.84674366389459621, 38.50893115100078745, 7.409399052514197653E-17 ) ) ;
#43780=CARTESIAN_POINT ( 'NONE',  ( 7.361572987183170547, 2.050597817667451750, 9.846743663894590881 ) ) ;
#43781=CARTESIAN_POINT ( 'NONE',  ( -0.3689425029237881626, 42.42874883491396787, 10.36894250292379027 ) ) ;
#43782=CARTESIAN_POINT ( 'NONE',  ( 12.63842701281683034, 42.46726448433412315, 9.846743663894596210 ) ) ;
#43784=CARTESIAN_POINT ( 'NONE',  ( 0.5774900079438590739, 42.64701867748816966, -5.440088680355550821 ) ) ;
#43786=CARTESIAN_POINT ( 'NONE',  ( 12.91533473730992121, 59.52201867748816966, 10.88017736071110164 ) ) ;
#43788=CARTESIAN_POINT ( 'NONE',  ( 16.40814093676324603, 42.45696800326375353, -11.09922568453594671 ) ) ;
#43789=B_SPLINE_CURVE_WITH_KNOTS ( 'NONE', 3,
 ( #60072, #58599, #59586, #37594 ),
 .UNSPECIFIED., .F., .F.,
 ( 4, 4 ),
 ( 5.811364099686433976E-18, 0.002657014572710831961 ),
 .UNSPECIFIED. ) ;
#43790=CARTESIAN_POINT ( 'NONE',  ( 2.791683348922240793, 1.633931151000784565, 7.208316651077764092 ) ) ;
#43792=CARTESIAN_POINT ( 'NONE',  ( 2.917880565312950480, 5.970415501580634832, -12.26659068614894821 ) ) ;
#43793=CARTESIAN_POINT ( 'NONE',  ( 19.84674366389459266, 13.30059781766745353, 2.638427012816836559 ) ) ;
#43794=CARTESIAN_POINT ( 'NONE',  ( -0.3289641300568005855, 59.27164270246083788, -5.963430220938281678 ) ) ;
#43796=EDGE_CURVE ( 'NONE', #4701, #88366, #13657, .T. ) ;
#43797=CARTESIAN_POINT ( 'NONE',  ( 15.44008868035555793, 11.39701867748817143, -9.422509992056140149 ) ) ;
#43800=EDGE_CURVE ( 'NONE', #53231, #94197, #67809, .T. ) ;
#43802=CARTESIAN_POINT ( 'NONE',  ( 12.91533473730992121, 29.52201867748817321, 10.88017736071110164 ) ) ;
#43803=CARTESIAN_POINT ( 'NONE',  ( 2.791683348922240793, 61.63393115100079456, 7.208316651077764092 ) ) ;
#43805=CARTESIAN_POINT ( 'NONE',  ( 7.361572987183169658, 64.96726448433412315, -9.846743663894592657 ) ) ;
#43806=ORIENTED_EDGE ( 'NONE', *, *, #70842, .F. ) ;
#43807=CARTESIAN_POINT ( 'NONE',  ( 1.472469842513823179, 1.425597817667451528, 4.923371831947296329 ) ) ;
#43809=CARTESIAN_POINT ( 'NONE',  ( -1.099225684535947600, 39.54030133659708923, 6.408140936763237150 ) ) ;
#43810=CARTESIAN_POINT ( 'NONE',  ( 4.559911319644449179, 3.897018677488170990, 9.422509992056141925 ) ) ;
#43812=CARTESIAN_POINT ( 'NONE',  ( 0.1532563361054100626, 5.800597817667452638, -2.638427012816831230 ) ) ;
#43813=CARTESIAN_POINT ( 'NONE',  ( 4.559911319644449179, 12.23035201082150714, -9.422509992056141925 ) ) ;
#43815=VERTEX_POINT ( 'NONE', #65116 ) ;
#43816=CARTESIAN_POINT ( 'NONE',  ( -2.816281873526473856, 49.33196800326374643, 3.434112377981055619 ) ) ;
#43817=CARTESIAN_POINT ( 'NONE',  ( 12.91533473730992121, 44.52201867748816966, 10.88017736071110164 ) ) ;
#43818=DIRECTION ( 'NONE',  ( 0.000000000000000000, -1.000000000000000000, 0.000000000000000000 ) ) ;
#43819=CARTESIAN_POINT ( 'NONE',  ( 10.00000000000000000, 37.87363466993041783, -12.81628187352647608 ) ) ;
#43820=CARTESIAN_POINT ( 'NONE',  ( 4.559911319644449179, 48.89701867748817676, 9.422509992056141925 ) ) ;
#43821=CARTESIAN_POINT ( 'NONE',  ( 2.791683348922240793, 51.63393115100078745, 7.208316651077764092 ) ) ;
#43822=EDGE_CURVE ( 'NONE', #83218, #67137, #13767, .T. ) ;
#43824=CARTESIAN_POINT ( 'NONE',  ( 7.361572987183170547, 12.05059781766744997, 9.846743663894590881 ) ) ;
#43825=CARTESIAN_POINT ( 'NONE',  ( -1.099225684535947600, 3.706968003263753531, -6.408140936763238038 ) ) ;
#43827=CARTESIAN_POINT ( 'NONE',  ( 12.63842701281683922, 59.55059781766744464, -9.846743663894590881 ) ) ;
#43828=CARTESIAN_POINT ( 'NONE',  ( 2.035157376598822676, 27.43868534415483396, -7.964842623401177768 ) ) ;
#43829=CARTESIAN_POINT ( 'NONE',  ( 12.63842701281683922, 44.55059781766745175, -9.846743663894590881 ) ) ;
#43831=CARTESIAN_POINT ( 'NONE',  ( 19.84674366389459266, 13.71726448433411782, -2.638427012816827677 ) ) ;
#43832=CARTESIAN_POINT ( 'NONE',  ( 18.52753015748618282, 28.92559781766745175, -4.923371831947291888 ) ) ;
#43833=CARTESIAN_POINT ( 'NONE',  ( 16.40814093676323893, 5.790301336597087456, 11.09922568453595026 ) ) ;
#43834=ORIENTED_EDGE ( 'NONE', *, *, #3637, .F. ) ;
#43836=DIRECTION ( 'NONE',  ( 0.8320502943378436100, -0.5547001962252291474, 0.000000000000000000 ) ) ;
#43837=CARTESIAN_POINT ( 'NONE',  ( -1.099225684535947600, 43.70696800326375353, -6.408140936763238038 ) ) ;
#43838=CARTESIAN_POINT ( 'NONE',  ( 1.472469842513823179, 30.59226448433411960, -4.923371831947296329 ) ) ;
#43840=CARTESIAN_POINT ( 'NONE',  ( 15.44008868035555793, 11.39701867748817143, -9.422509992056140149 ) ) ;
#43841=CARTESIAN_POINT ( 'NONE',  ( 2.791683348922240793, 36.63393115100078035, 7.208316651077764092 ) ) ;
#43842=MECHANICAL_DESIGN_GEOMETRIC_PRESENTATION_REPRESENTATION('',(#61406),#27859);
#43845=CARTESIAN_POINT ( 'NONE',  ( 20.88017736071110519, 10.56368534415483929, 2.639326808657452039E-16 ) ) ;
#43847=CARTESIAN_POINT ( 'NONE',  ( 12.91533473730992121, 24.52201867748816966, 10.88017736071110164 ) ) ;
#43848=CARTESIAN_POINT ( 'NONE',  ( 24.16423886937410614, 44.51208216824730357, -3.795296366450302550 ) ) ;
#43849=CARTESIAN_POINT ( 'NONE',  ( 2.917880565312948704, 47.63708216824730357, 12.26659068614894643 ) ) ;
#43851=CARTESIAN_POINT ( 'NONE',  ( 10.00000000000000000, 9.758931151000785675, -9.846743663894594434 ) ) ;
#43852=CARTESIAN_POINT ( 'NONE',  ( 19.84674366389459621, 63.50893115100078745, 7.409399052514197653E-17 ) ) ;
#43853=ORIENTED_EDGE ( 'NONE', *, *, #61910, .T. ) ;
#43854=CARTESIAN_POINT ( 'NONE',  ( 0.5774900079438590739, 52.64701867748817676, -5.440088680355550821 ) ) ;
#43855=CARTESIAN_POINT ( 'NONE',  ( 1.274849032794164172, 18.57228050351029935, 6.499999999999802824 ) ) ;
#43857=CARTESIAN_POINT ( 'NONE',  ( 17.20831665107776587, 64.13393115100079456, -7.208316651077762316 ) ) ;
#43859=CARTESIAN_POINT ( 'NONE',  ( 7.361572987183170547, 22.05059781766745530, 9.846743663894590881 ) ) ;
#43860=DIRECTION ( 'NONE',  ( -1.000000000000000000, 0.000000000000000000, 0.000000000000000000 ) ) ;
#43861=ORIENTED_EDGE ( 'NONE', *, *, #64231, .T. ) ;
#43863=CARTESIAN_POINT ( 'NONE',  ( 17.08211943468705840, 45.13708216824730357, -12.26659068614894466 ) ) ;
#43864=CARTESIAN_POINT ( 'NONE',  ( 14.92337183194729633, 2.675597817667451750, 8.527530157486181039 ) ) ;
#43866=CARTESIAN_POINT ( 'NONE',  ( 15.44008868035555793, 36.39701867748816966, -9.422509992056140149 ) ) ;
#43867=CARTESIAN_POINT ( 'NONE',  ( 3.591859063236761518, 34.95696800326375353, 11.09922568453594849 ) ) ;
#43868=( LENGTH_UNIT ( ) NAMED_UNIT ( * ) SI_UNIT ( .MILLI., .METRE. ) );
#43869=CARTESIAN_POINT ( 'NONE',  ( 22.81628187352648496, 31.83196800326375353, -3.434112377981050290 ) ) ;
#43870=CARTESIAN_POINT ( 'NONE',  ( 0.6178305044545838731, 59.74863466993041783, 9.382169495545420901 ) ) ;
#43871=ORIENTED_EDGE ( 'NONE', *, *, #22498, .F. ) ;
#43874=CARTESIAN_POINT ( 'NONE',  ( -0.3689425029237898834, 26.17874883491396432, -10.36894250292378850 ) ) ;
#43875=CARTESIAN_POINT ( 'NONE',  ( 20.36894250292379738, 4.928748834913967869, -10.36894250292379027 ) ) ;
#43876=CARTESIAN_POINT ( 'NONE',  ( 17.96484262340118221, 4.938685344154837509, 7.964842623401181321 ) ) ;
#43877=CARTESIAN_POINT ( 'NONE',  ( 15.44008868035555260, 24.73035201082150891, 9.422509992056143702 ) ) ;
#43879=DIRECTION ( 'NONE',  ( -1.000000000000000000, 0.000000000000000000, 0.000000000000000000 ) ) ;
#43880=CARTESIAN_POINT ( 'NONE',  ( 15.44008868035555793, 51.39701867748816966, -9.422509992056140149 ) ) ;
#43881=CARTESIAN_POINT ( 'NONE',  ( 10.00000000000000178, 54.31368534415484106, 10.88017736071110342 ) ) ;
#43882=CARTESIAN_POINT ( 'NONE',  ( 16.40814093676323893, 15.79030133659708746, 11.09922568453595026 ) ) ;
#43884=CARTESIAN_POINT ( 'NONE',  ( -0.03447792253739217355, 30.15514106990690024, 6.401564815979747358 ) ) ;
#43885=CARTESIAN_POINT ( 'NONE',  ( 17.20831665107776587, 24.13393115100078035, -7.208316651077762316 ) ) ;
#43888=CARTESIAN_POINT ( 'NONE',  ( 7.084665262690076126, 54.10535201082151247, 10.88017736071109987 ) ) ;
#43889=CARTESIAN_POINT ( 'NONE',  ( 3.591859063236761518, 14.95696800326375531, 11.09922568453594849 ) ) ;
#43890=CARTESIAN_POINT ( 'NONE',  ( 0.5774900079438590739, 42.64701867748816966, -5.440088680355550821 ) ) ;
#43891=CARTESIAN_POINT ( 'NONE',  ( 10.00000000000000178, 22.25893115100078745, 9.846743663894594434 ) ) ;
#43892=CARTESIAN_POINT ( 'NONE',  ( 13.43411237798105340, 50.58196800326375353, 12.81628187352647963 ) ) ;
#43893=CARTESIAN_POINT ( 'NONE',  ( 18.52753015748618282, 23.92559781766745530, -4.923371831947291888 ) ) ;
#43894=SURFACE_SIDE_STYLE ('',( #78463 ) ) ;
#43896=CARTESIAN_POINT ( 'NONE',  ( 22.26659068614895176, 4.720415501580633943, -7.082119434687042414 ) ) ;
#43897=CARTESIAN_POINT ( 'NONE',  ( 1.959929470562282283, 36.50257860105348584, 5.767676674365853629 ) ) ;
#43898=CARTESIAN_POINT ( 'NONE',  ( 10.00000000000000178, 24.31368534415484106, 10.88017736071110342 ) ) ;
#43900=CARTESIAN_POINT ( 'NONE',  ( 14.92337183194729988, 29.34226448433411960, -8.527530157486177487 ) ) ;
#43901=CARTESIAN_POINT ( 'NONE',  ( 4.559911319644449179, 12.23035201082150536, -9.422509992056141925 ) ) ;
#43902=CARTESIAN_POINT ( 'NONE',  ( 2.035157376598824452, 13.68868534415483751, 7.964842623401179544 ) ) ;
#43905=CARTESIAN_POINT ( 'NONE',  ( 20.88017736071110875, 25.77201867748816966, -2.915334737309920765 ) ) ;
#43906=CARTESIAN_POINT ( 'NONE',  ( 21.09922568453595559, 47.04030133659708923, -6.408140936763230044 ) ) ;
#43907=CARTESIAN_POINT ( 'NONE',  ( 20.88017736071110875, 35.77201867748816966, -2.915334737309920765 ) ) ;
#43910=CARTESIAN_POINT ( 'NONE',  ( 4.559911319644449179, 42.23035201082151247, -9.422509992056141925 ) ) ;
#43914=CARTESIAN_POINT ( 'NONE',  ( 13.43411237798106583, 62.66530133659708923, -12.81628187352647252 ) ) ;
#43915=FACE_OUTER_BOUND ( 'NONE', #23707, .T. ) ;
#43916=CARTESIAN_POINT ( 'NONE',  ( 22.26659068614894466, 48.88708216824730357, 7.082119434687054849 ) ) ;
#43917=CARTESIAN_POINT ( 'NONE',  ( 20.88017736071110519, 50.56368534415484106, 2.639326808657452039E-16 ) ) ;
#43922=CARTESIAN_POINT ( 'NONE',  ( 14.92337183194729988, 49.34226448433411605, -8.527530157486177487 ) ) ;
#43923=CARTESIAN_POINT ( 'NONE',  ( 19.84674366389459266, 13.71726448433411782, -2.638427012816827677 ) ) ;
#43925=CARTESIAN_POINT ( 'NONE',  ( 7.361572987183169658, 19.96726448433411960, -9.846743663894592657 ) ) ;
#43927=CARTESIAN_POINT ( 'NONE',  ( 17.96484262340118221, 24.93868534415484461, 7.964842623401181321 ) ) ;
#43928=CARTESIAN_POINT ( 'NONE',  ( 2.791683348922240793, 21.63393115100078745, 7.208316651077764092 ) ) ;
#43929=CARTESIAN_POINT ( 'NONE',  ( 3.591859063236763294, 13.29030133659708746, -11.09922568453595026 ) ) ;
#43930=CARTESIAN_POINT ( 'NONE',  ( 10.00000000000000000, 61.81368534415484106, -10.88017736071110342 ) ) ;
#43931=CARTESIAN_POINT ( 'NONE',  ( 7.084665262690076126, 52.02201867748816255, -10.88017736071110164 ) ) ;
#43932=CARTESIAN_POINT ( 'NONE',  ( 19.42250999205614548, 35.98035201082151247, -5.440088680355545492 ) ) ;
#43933=CARTESIAN_POINT ( 'NONE',  ( 13.43411237798105340, 55.58196800326374643, 12.81628187352647963 ) ) ;
#43934=CARTESIAN_POINT ( 'NONE',  ( 17.08211943468705840, 50.13708216824730357, -12.26659068614894466 ) ) ;
#43937=VERTEX_POINT ( 'NONE', #27619 ) ;
#43938=CARTESIAN_POINT ( 'NONE',  ( -2.816281873526473856, 4.123634669930420493, 9.499525473075851096E-16 ) ) ;
#43939=CARTESIAN_POINT ( 'NONE',  ( 20.88017736071110164, 10.35535201082150714, 2.915334737309930979 ) ) ;
#43940=CARTESIAN_POINT ( 'NONE',  ( 2.035157376598824452, 43.68868534415484106, 7.964842623401179544 ) ) ;
#43943=CARTESIAN_POINT ( 'NONE',  ( 19.84674366389459266, 13.30059781766745353, 2.638427012816836559 ) ) ;
#43944=CARTESIAN_POINT ( 'NONE',  ( 2.035157376598822676, 52.43868534415483396, -7.964842623401177768 ) ) ;
#43945=CARTESIAN_POINT ( 'NONE',  ( 1.472469842513823179, 30.59226448433411960, -4.923371831947296329 ) ) ;
#43946=CARTESIAN_POINT ( 'NONE',  ( 12.63842701281683922, 29.55059781766745175, -9.846743663894590881 ) ) ;
#43947=CARTESIAN_POINT ( 'NONE',  ( 19.84674366389459266, 13.71726448433411782, -2.638427012816827677 ) ) ;
#43948=MECHANICAL_DESIGN_GEOMETRIC_PRESENTATION_REPRESENTATION('',(#890),#93427);
#43950=CARTESIAN_POINT ( 'NONE',  ( 2.035157376598824452, 68.68868534415484817, 7.964842623401179544 ) ) ;
#43953=CARTESIAN_POINT ( 'NONE',  ( 18.52753015748618282, 33.92559781766745886, -4.923371831947291888 ) ) ;
#43956=CARTESIAN_POINT ( 'NONE',  ( 2.791683348922240793, 66.63393115100079456, 7.208316651077764092 ) ) ;
#43958=LINE ( 'NONE', #95503, #34640 ) ;
#43959=CARTESIAN_POINT ( 'NONE',  ( -0.3689425029237881626, 22.42874883491397142, 10.36894250292379027 ) ) ;
#43961=CARTESIAN_POINT ( 'NONE',  ( 17.08211943468705840, 35.13708216824730357, -12.26659068614894466 ) ) ;
#43962=CARTESIAN_POINT ( 'NONE',  ( 20.36894250292379382, 43.67874883491397497, 10.36894250292379205 ) ) ;
#43963=CARTESIAN_POINT ( 'NONE',  ( 10.00000000000000000, 10.55374883491396787, -14.16423886937410082 ) ) ;
#43964=CARTESIAN_POINT ( 'NONE',  ( -4.164238869374099039, 6.803748834913967869, 8.674139862899312516E-16 ) ) ;
#43965=CARTESIAN_POINT ( 'NONE',  ( 20.88017736071110519, 65.56368534415483396, 2.639326808657452039E-16 ) ) ;
#43966=CARTESIAN_POINT ( 'NONE',  ( 12.91533473730992121, 54.52201867748816255, 10.88017736071110164 ) ) ;
#43969=EDGE_LOOP ( 'NONE', ( #57135, #69930, #57658, #46055 ) ) ;
#43970=CARTESIAN_POINT ( 'NONE',  ( 18.52753015748617571, 28.09226448433411960, 4.923371831947298993 ) ) ;
#43971=CARTESIAN_POINT ( 'NONE',  ( -0.8801773607111009756, 68.06368534415484817, 1.068504757029289695E-15 ) ) ;
#43972=CARTESIAN_POINT ( 'NONE',  ( 19.84674366389459266, 23.30059781766745530, 2.638427012816836559 ) ) ;
#43973=CARTESIAN_POINT ( 'NONE',  ( 17.96484262340118221, 11.18868534415484106, -7.964842623401177768 ) ) ;
#43974=CARTESIAN_POINT ( 'NONE',  ( 10.00000000000000000, 62.87363466993042493, -12.81628187352647608 ) ) ;
#43975=CARTESIAN_POINT ( 'NONE',  ( 5.076628168052704559, 45.17559781766745175, -8.527530157486179263 ) ) ;
#43977=CARTESIAN_POINT ( 'NONE',  ( 12.63842701281683922, 24.55059781766745175, -9.846743663894590881 ) ) ;
#43978=CARTESIAN_POINT ( 'NONE',  ( 19.38216949554541557, 37.24863466993041783, -9.382169495545420901 ) ) ;
#43981=CARTESIAN_POINT ( 'NONE',  ( 15.44008868035555260, 49.73035201082150536, 9.422509992056143702 ) ) ;
#43982=CARTESIAN_POINT ( 'NONE',  ( 1.472469842513823179, 40.59226448433411605, -4.923371831947296329 ) ) ;
#43983=B_SPLINE_CURVE_WITH_KNOTS ( 'NONE', 3,
 ( #2267, #47232, #8272, #63221 ),
 .UNSPECIFIED., .F., .F.,
 ( 4, 4 ),
 ( 1.532679976604137452E-17, 0.002392975128318449059 ),
 .UNSPECIFIED. ) ;
#43984=CARTESIAN_POINT ( 'NONE',  ( 2.917880565312948704, 27.63708216824730357, 12.26659068614894643 ) ) ;
#43986=CARTESIAN_POINT ( 'NONE',  ( 20.36894250292379382, 3.678748834913967869, 10.36894250292379205 ) ) ;
#43988=CARTESIAN_POINT ( 'NONE',  ( -0.8801773607111009756, 48.06368534415484817, 1.068504757029289695E-15 ) ) ;
#43989=CARTESIAN_POINT ( 'NONE',  ( 10.00000000000000178, 69.31368534415484817, 10.88017736071110342 ) ) ;
#43990=CARTESIAN_POINT ( 'NONE',  ( 17.08211943468705130, 53.47041550158063217, 12.26659068614894998 ) ) ;
#43991=CARTESIAN_POINT ( 'NONE',  ( 3.591859063236761518, -0.04303199673624671928, 11.09922568453594849 ) ) ;
#43993=CARTESIAN_POINT ( 'NONE',  ( 10.00000000000000000, 56.81368534415484106, -10.88017736071110342 ) ) ;
#43995=CARTESIAN_POINT ( 'NONE',  ( 17.20831665107776587, 64.13393115100079456, -7.208316651077762316 ) ) ;
#43997=CARTESIAN_POINT ( 'NONE',  ( 12.91533473730992121, 14.52201867748817143, 10.88017736071110164 ) ) ;
#43998=CARTESIAN_POINT ( 'NONE',  ( 15.44008868035555793, 11.39701867748817143, -9.422509992056140149 ) ) ;
#43999=CARTESIAN_POINT ( 'NONE',  ( 18.52753015748617571, 38.09226448433412315, 4.923371831947298993 ) ) ;
#44001=ORIENTED_EDGE ( 'NONE', *, *, #90571, .T. ) ;
#44003=CARTESIAN_POINT ( 'NONE',  ( 20.88017736071110164, 10.35535201082150714, 2.915334737309930979 ) ) ;
#44004=CARTESIAN_POINT ( 'NONE',  ( 6.565887622018943937, 0.1653013365970866511, 12.81628187352647430 ) ) ;
#44005=CARTESIAN_POINT ( 'NONE',  ( 2.603489959281613420, 60.43575266056826933, -6.500000000000031086 ) ) ;
#44006=CARTESIAN_POINT ( 'NONE',  ( 1.472469842513823179, 16.42559781766745175, 4.923371831947296329 ) ) ;
#44008=CARTESIAN_POINT ( 'NONE',  ( 12.63842701281683034, 32.46726448433412315, 9.846743663894596210 ) ) ;
#44009=CARTESIAN_POINT ( 'NONE',  ( 20.88017736071110875, 35.77201867748816966, -2.915334737309920765 ) ) ;
#44010=CARTESIAN_POINT ( 'NONE',  ( 3.591859063236763294, 13.29030133659708746, -11.09922568453595026 ) ) ;
#44011=CARTESIAN_POINT ( 'NONE',  ( 10.00000000000000178, 49.31368534415484106, 10.88017736071110342 ) ) ;
#44013=DIRECTION ( 'NONE',  ( 6.608470384673550777E-17, 1.000000000000000000, -0.000000000000000000 ) ) ;
#44014=CARTESIAN_POINT ( 'NONE',  ( 13.43411237798106583, 57.66530133659708923, -12.81628187352647252 ) ) ;
#44016=CARTESIAN_POINT ( 'NONE',  ( -0.8801773607111008646, 68.27201867748817676, 2.915334737309923430 ) ) ;
#44017=CARTESIAN_POINT ( 'NONE',  ( 10.00000000000000178, 30.37363466993042138, 12.81628187352647608 ) ) ;
#44018=CARTESIAN_POINT ( 'NONE',  ( 10.00000000000000178, 8.053748834913967869, 14.16423886937410082 ) ) ;
#44020=CARTESIAN_POINT ( 'NONE',  ( 0.5774900079438607392, 38.48035201082150536, 5.440088680355550821 ) ) ;
#44021=CARTESIAN_POINT ( 'NONE',  ( 0.1532563361054082862, 66.21726448433413736, 2.638427012816831674 ) ) ;
#44022=CARTESIAN_POINT ( 'NONE',  ( 1.472469842513823179, 51.42559781766745886, 4.923371831947296329 ) ) ;
#44023=CARTESIAN_POINT ( 'NONE',  ( 14.92337183194729988, 14.34226448433411782, -8.527530157486177487 ) ) ;
#44024=CARTESIAN_POINT ( 'NONE',  ( 7.361572987183170547, 7.050597817667451750, 9.846743663894590881 ) ) ;
#44026=CARTESIAN_POINT ( 'NONE',  ( 13.79529636645031943, 30.34541550158063927, -14.16423886937409904 ) ) ;
#44027=AXIS2_PLACEMENT_3D ( 'NONE', #20256, #58737, #95258 ) ;
#44029=SURFACE_SIDE_STYLE ('',( #90515 ) ) ;
#44031=EDGE_LOOP ( 'NONE', ( #2253, #37080, #91683, #3139 ) ) ;
#44032=CARTESIAN_POINT ( 'NONE',  ( 20.36894250292379738, 59.92874883491397497, -10.36894250292379027 ) ) ;
#44033=CARTESIAN_POINT ( 'NONE',  ( -4.164238869374099927, 57.01208216824731068, 3.795296366450308767 ) ) ;
#44035=CARTESIAN_POINT ( 'NONE',  ( 2.791683348922240793, 26.63393115100078745, 7.208316651077764092 ) ) ;
#44037=CARTESIAN_POINT ( 'NONE',  ( 13.43411237798105340, 30.58196800326374998, 12.81628187352647963 ) ) ;
#44038=DIRECTION ( 'NONE',  ( 0.000000000000000000, -1.000000000000000000, 0.000000000000000000 ) ) ;
#44039=CARTESIAN_POINT ( 'NONE',  ( -1.926860441876563801, 42.66212336850781384, 1.004413902775740978E-15 ) ) ;
#44040=CARTESIAN_POINT ( 'NONE',  ( 0.5774900079438607392, 18.48035201082150536, 5.440088680355550821 ) ) ;
#44041=CARTESIAN_POINT ( 'NONE',  ( 13.79529636645030344, 53.26208216824730357, 14.16423886937410614 ) ) ;
#44042=CARTESIAN_POINT ( 'NONE',  ( 19.84674366389459266, 23.30059781766745530, 2.638427012816836559 ) ) ;
#44043=ADVANCED_FACE ( 'NONE', ( #79649 ), #89115, .T. ) ;
#44045=CARTESIAN_POINT ( 'NONE',  ( 0.1532563361054082862, 16.21726448433411960, 2.638427012816831674 ) ) ;
#44046=CARTESIAN_POINT ( 'NONE',  ( 18.39792806157247895, 59.52224192338640307, 6.500000000000035527 ) ) ;
#44052=CARTESIAN_POINT ( 'NONE',  ( 20.88017736071110519, 25.56368534415483751, 2.639326808657452039E-16 ) ) ;
#44053=CARTESIAN_POINT ( 'NONE',  ( 10.00000000000000178, 24.31368534415484106, 10.88017736071110342 ) ) ;
#44054=CARTESIAN_POINT ( 'NONE',  ( 14.92337183194729633, 62.67559781766745886, 8.527530157486181039 ) ) ;
#44055=CARTESIAN_POINT ( 'NONE',  ( 13.43411237798106583, 22.66530133659708923, -12.81628187352647252 ) ) ;
#44056=CARTESIAN_POINT ( 'NONE',  ( -4.164238869374099927, 7.012082168247302683, 3.795296366450308767 ) ) ;
#44058=CARTESIAN_POINT ( 'NONE',  ( 22.81628187352647785, 26.62363466993042138, 6.195893100308588602E-16 ) ) ;
#44059=ORIENTED_EDGE ( 'NONE', *, *, #7933, .T. ) ;
#44060=CARTESIAN_POINT ( 'NONE',  ( 0.1532563361054082862, 31.21726448433412315, 2.638427012816831674 ) ) ;
#44061=CARTESIAN_POINT ( 'NONE',  ( 15.44008868035555260, 9.730352010821505360, 9.422509992056143702 ) ) ;
#44063=CARTESIAN_POINT ( 'NONE',  ( 6.204703633549690345, 65.76208216824731778, -14.16423886937410259 ) ) ;
#44065=CARTESIAN_POINT ( 'NONE',  ( 0.5774900079438607392, 53.48035201082151247, 5.440088680355550821 ) ) ;
#44066=CARTESIAN_POINT ( 'NONE',  ( -0.8801773607111008646, 53.27201867748816966, 2.915334737309923430 ) ) ;
#44067=CARTESIAN_POINT ( 'NONE',  ( 15.44008868035555793, 51.39701867748816966, -9.422509992056140149 ) ) ;
#44068=FILL_AREA_STYLE_COLOUR ( '', #63108 ) ;
#44069=CARTESIAN_POINT ( 'NONE',  ( 4.559911319644449179, 52.23035201082151247, -9.422509992056141925 ) ) ;
#44071=PRESENTATION_STYLE_ASSIGNMENT (( #13588 ) ) ;
#44072=CARTESIAN_POINT ( 'NONE',  ( 14.92337183194729633, 27.67559781766745530, 8.527530157486181039 ) ) ;
#44074=CARTESIAN_POINT ( 'NONE',  ( 17.20831665107776587, 54.13393115100079456, -7.208316651077762316 ) ) ;
#44075=B_SPLINE_CURVE_WITH_KNOTS ( 'NONE', 3,
 ( #2260, #62721, #78724, #11699 ),
 .UNSPECIFIED., .F., .F.,
 ( 4, 4 ),
 ( 5.284504157781969479E-17, 0.002562518741975526333 ),
 .UNSPECIFIED. ) ;
#44077=EDGE_LOOP ( 'NONE', ( #46613, #71660, #88156, #7075, #52675, #75003, #65517, #65817 ) ) ;
#44081=CARTESIAN_POINT ( 'NONE',  ( 15.44008868035555793, 11.39701867748817143, -9.422509992056140149 ) ) ;
#44085=CARTESIAN_POINT ( 'NONE',  ( 5.076628168052703671, 51.84226448433412315, 8.527530157486179263 ) ) ;
#44086=LINE ( 'NONE', #68096, #24393 ) ;
#44088=CARTESIAN_POINT ( 'NONE',  ( 13.43411237798106583, 12.66530133659708746, -12.81628187352647252 ) ) ;
#44089=CARTESIAN_POINT ( 'NONE',  ( 0.1532563361054082862, 11.21726448433411605, 2.638427012816831674 ) ) ;
#44091=CARTESIAN_POINT ( 'NONE',  ( 19.84674366389459266, 18.71726448433411960, -2.638427012816827677 ) ) ;
#44092=CARTESIAN_POINT ( 'NONE',  ( 19.38216949554541557, 2.248634669930420049, -9.382169495545420901 ) ) ;
#44095=CARTESIAN_POINT ( 'NONE',  ( 17.96484262340118221, 6.188685344154837509, -7.964842623401177768 ) ) ;
#44096=CARTESIAN_POINT ( 'NONE',  ( 22.26659068614894466, 3.887082168247300906, 7.082119434687054849 ) ) ;
#44097=CARTESIAN_POINT ( 'NONE',  ( 18.52753015748618282, 23.92559781766745530, -4.923371831947291888 ) ) ;
#44098=CARTESIAN_POINT ( 'NONE',  ( 0.5774900079438607392, 53.48035201082151247, 5.440088680355550821 ) ) ;
#44099=CARTESIAN_POINT ( 'NONE',  ( -2.816281873526471635, 38.91530133659708213, -3.434112377981056508 ) ) ;
#44101=CARTESIAN_POINT ( 'NONE',  ( 20.88017736071110164, 20.35535201082150891, 2.915334737309930979 ) ) ;
#44102=CARTESIAN_POINT ( 'NONE',  ( 20.10239578412225825, 17.63377557478296609, -6.340343622311919169 ) ) ;
#44104=CARTESIAN_POINT ( 'NONE',  ( 6.565887622018943937, 5.165301336597086568, 12.81628187352647430 ) ) ;
#44105=CARTESIAN_POINT ( 'NONE',  ( 7.361572987183169658, 64.96726448433412315, -9.846743663894592657 ) ) ;
#44106=CARTESIAN_POINT ( 'NONE',  ( 1.472469842513823179, 25.59226448433412315, -4.923371831947296329 ) ) ;
#44108=CARTESIAN_POINT ( 'NONE',  ( 19.38216949554541202, 40.99863466993042493, 9.382169495545424454 ) ) ;
#44109=CARTESIAN_POINT ( 'NONE',  ( 19.42250999205614548, 35.98035201082151247, -5.440088680355545492 ) ) ;
#44115=CARTESIAN_POINT ( 'NONE',  ( 17.96484262340118221, 44.93868534415483396, 7.964842623401181321 ) ) ;
#44117=CARTESIAN_POINT ( 'NONE',  ( 10.00000000000000178, 29.31368534415483751, 10.88017736071110342 ) ) ;
#44118=CARTESIAN_POINT ( 'NONE',  ( 0.1532563361054100626, 65.80059781766745175, -2.638427012816831230 ) ) ;
#44119=CARTESIAN_POINT ( 'NONE',  ( 20.88017736071110519, 50.56368534415484106, 2.639326808657452039E-16 ) ) ;
#44120=AXIS2_PLACEMENT_3D ( 'NONE', #49121, #89088, #57107 ) ;
#44121=UNCERTAINTY_MEASURE_WITH_UNIT (LENGTH_MEASURE( 1.000000000000000082E-05 ), #52749, 'distance_accuracy_value', 'NONE');
#44122=CARTESIAN_POINT ( 'NONE',  ( 18.52753015748618282, 38.92559781766745175, -4.923371831947291888 ) ) ;
#44123=CARTESIAN_POINT ( 'NONE',  ( 16.40814093676323893, 60.79030133659709634, 11.09922568453595026 ) ) ;
#44124=CARTESIAN_POINT ( 'NONE',  ( 6.565887622018943937, 15.16530133659708568, 12.81628187352647430 ) ) ;
#44126=CARTESIAN_POINT ( 'NONE',  ( 4.559911319644449179, 27.23035201082150536, -9.422509992056141925 ) ) ;
#44128=CARTESIAN_POINT ( 'NONE',  ( 12.91533473730992121, 19.52201867748816611, 10.88017736071110164 ) ) ;
#44129=CARTESIAN_POINT ( 'NONE',  ( 19.84674366389459621, 3.508931151000785231, 7.409399052514197653E-17 ) ) ;
#44130=CARTESIAN_POINT ( 'NONE',  ( 22.26659068614895176, 24.72041550158063572, -7.082119434687042414 ) ) ;
#44131=CARTESIAN_POINT ( 'NONE',  ( 18.52753015748618282, 8.925597817667451750, -4.923371831947291888 ) ) ;
#44133=CARTESIAN_POINT ( 'NONE',  ( -0.8801773607111008646, 43.27201867748817676, 2.915334737309923430 ) ) ;
#44139=CARTESIAN_POINT ( 'NONE',  ( 14.92337183194729988, 44.34226448433412315, -8.527530157486177487 ) ) ;
#44143=CARTESIAN_POINT ( 'NONE',  ( 10.00000000000000000, 20.55374883491396787, -14.16423886937410082 ) ) ;
#44144=CARTESIAN_POINT ( 'NONE',  ( 20.36894250292379738, 29.92874883491396432, -10.36894250292379027 ) ) ;
#44147=CARTESIAN_POINT ( 'NONE',  ( 0.5774900079438590739, 57.64701867748817676, -5.440088680355550821 ) ) ;
#44148=CARTESIAN_POINT ( 'NONE',  ( -0.3689425029237898834, 66.17874883491396076, -10.36894250292378850 ) ) ;
#44149=CARTESIAN_POINT ( 'NONE',  ( -2.816281873526471635, 3.915301336597087456, -3.434112377981056508 ) ) ;
#44150=CARTESIAN_POINT ( 'NONE',  ( 1.472469842513823179, 50.59226448433411605, -4.923371831947296329 ) ) ;
#44152=CARTESIAN_POINT ( 'NONE',  ( 0.5774900079438590739, 42.64701867748816966, -5.440088680355550821 ) ) ;
#44153=CARTESIAN_POINT ( 'NONE',  ( 19.38216949554541202, 0.9986346699304200492, 9.382169495545424454 ) ) ;
#44154=CARTESIAN_POINT ( 'NONE',  ( 17.08211943468705130, 23.47041550158063572, 12.26659068614894998 ) ) ;
#44155=CARTESIAN_POINT ( 'NONE',  ( 15.44008868035555260, 19.73035201082150536, 9.422509992056143702 ) ) ;
#44156=CARTESIAN_POINT ( 'NONE',  ( 12.91533473730992121, 14.52201867748817143, 10.88017736071110164 ) ) ;
#44158=CARTESIAN_POINT ( 'NONE',  ( 20.88017736071110164, 40.35535201082150536, 2.915334737309930979 ) ) ;
#44159=CARTESIAN_POINT ( 'NONE',  ( 10.00000000000000178, 45.37363466993041783, 12.81628187352647608 ) ) ;
#44162=CARTESIAN_POINT ( 'NONE',  ( 19.89220837332776526, 4.740628644642391087, 6.478736007405957231 ) ) ;
#44168=CARTESIAN_POINT ( 'NONE',  ( 17.08211943468705840, 45.13708216824730357, -12.26659068614894466 ) ) ;
#44169=CARTESIAN_POINT ( 'NONE',  ( 1.472469842513823179, 21.42559781766745175, 4.923371831947296329 ) ) ;
#44170=CARTESIAN_POINT ( 'NONE',  ( 0.1532563361054100626, 40.80059781766745886, -2.638427012816831230 ) ) ;
#44171=CARTESIAN_POINT ( 'NONE',  ( 0.5774900079438590739, 67.64701867748817676, -5.440088680355550821 ) ) ;
#44173=CARTESIAN_POINT ( 'NONE',  ( 18.52753015748617571, 3.092264484334118269, 4.923371831947298993 ) ) ;
#44174=CARTESIAN_POINT ( 'NONE',  ( -2.816281873526471635, 58.91530133659707502, -3.434112377981056508 ) ) ;
#44176=VERTEX_POINT ( 'NONE', #94647 ) ;
#44177=CARTESIAN_POINT ( 'NONE',  ( 24.16423886937410614, 34.30374883491396787, 8.672049930838204340E-16 ) ) ;
#44179=CARTESIAN_POINT ( 'NONE',  ( 22.81628187352647785, 21.62363466993041783, 6.195893100308588602E-16 ) ) ;
#44181=CARTESIAN_POINT ( 'NONE',  ( 21.09922568453594849, 46.20696800326376064, 6.408140936763242479 ) ) ;
#44183=CARTESIAN_POINT ( 'NONE',  ( 18.52753015748618282, 38.92559781766745175, -4.923371831947291888 ) ) ;
#44184=CARTESIAN_POINT ( 'NONE',  ( 17.96484262340118221, 9.938685344154837509, 7.964842623401181321 ) ) ;
#44185=CARTESIAN_POINT ( 'NONE',  ( -2.816281873526471635, 63.91530133659708923, -3.434112377981056508 ) ) ;
#44187=CARTESIAN_POINT ( 'NONE',  ( 7.361572987183169658, 39.96726448433411605, -9.846743663894592657 ) ) ;
#44188=CARTESIAN_POINT ( 'NONE',  ( 18.52753015748617571, 48.09226448433412315, 4.923371831947298993 ) ) ;
#44193=CARTESIAN_POINT ( 'NONE',  ( 1.274849032794317383, 27.55509018479935790, -6.500000000000010658 ) ) ;
#44196=CARTESIAN_POINT ( 'NONE',  ( 1.472469842513823179, 15.59226448433411960, -4.923371831947296329 ) ) ;
#44197=CARTESIAN_POINT ( 'NONE',  ( 3.591859063236763294, 33.29030133659708213, -11.09922568453595026 ) ) ;
#44201=CARTESIAN_POINT ( 'NONE',  ( 14.92337183194729633, 52.67559781766745175, 8.527530157486181039 ) ) ;
#44203=CARTESIAN_POINT ( 'NONE',  ( 20.36894250292379738, 19.92874883491396787, -10.36894250292379027 ) ) ;
#44204=CARTESIAN_POINT ( 'NONE',  ( 17.20831665107776587, 52.88393115100078035, 7.208316651077764980 ) ) ;
#44205=CARTESIAN_POINT ( 'NONE',  ( 0.6178305044545838731, 49.74863466993041072, 9.382169495545420901 ) ) ;
#44208=CARTESIAN_POINT ( 'NONE',  ( 7.361572987183169658, -0.03273551566588185635, -9.846743663894592657 ) ) ;
#44211=CARTESIAN_POINT ( 'NONE',  ( 18.52753015748617571, 43.09226448433412315, 4.923371831947298993 ) ) ;
#44212=CARTESIAN_POINT ( 'NONE',  ( 17.96484262340118221, 36.18868534415484106, -7.964842623401177768 ) ) ;
#44214=CARTESIAN_POINT ( 'NONE',  ( 5.076628168052704559, 35.17559781766745175, -8.527530157486179263 ) ) ;
#44218=CARTESIAN_POINT ( 'NONE',  ( 0.5774900079438607392, 48.48035201082150536, 5.440088680355550821 ) ) ;
#44221=CARTESIAN_POINT ( 'NONE',  ( 17.96484262340118221, 9.938685344154837509, 7.964842623401181321 ) ) ;
#44222=CARTESIAN_POINT ( 'NONE',  ( 0.1532563361054100626, 60.80059781766744464, -2.638427012816831230 ) ) ;
#44223=CARTESIAN_POINT ( 'NONE',  ( 17.96484262340118221, 39.93868534415484106, 7.964842623401181321 ) ) ;
#44224=CARTESIAN_POINT ( 'NONE',  ( 1.821158202401649051, 16.16688879859530559, 6.499999999999976019 ) ) ;
#44225=CARTESIAN_POINT ( 'NONE',  ( 20.88017736071110875, 60.77201867748817676, -2.915334737309920765 ) ) ;
#44227=CARTESIAN_POINT ( 'NONE',  ( 12.91533473730992121, 29.52201867748817321, 10.88017736071110164 ) ) ;
#44229=CARTESIAN_POINT ( 'NONE',  ( 10.00000000000000178, 7.258931151000785675, 9.846743663894594434 ) ) ;
#44230=CARTESIAN_POINT ( 'NONE',  ( 17.20831665107776587, 22.88393115100078745, 7.208316651077764980 ) ) ;
#44233=CARTESIAN_POINT ( 'NONE',  ( 14.92337183194729988, 59.34226448433412315, -8.527530157486177487 ) ) ;
#44235=CARTESIAN_POINT ( 'NONE',  ( 17.08211943468705130, 63.47041550158063927, 12.26659068614894998 ) ) ;
#44236=DIRECTION ( 'NONE',  ( 0.000000000000000000, -1.000000000000000000, 0.000000000000000000 ) ) ;
#44237=CARTESIAN_POINT ( 'NONE',  ( 2.917880565312948704, 7.637082168247301794, 12.26659068614894643 ) ) ;
#44239=CARTESIAN_POINT ( 'NONE',  ( -0.3689425029237881626, 52.42874883491396076, 10.36894250292379027 ) ) ;
#44240=CARTESIAN_POINT ( 'NONE',  ( 3.591859063236763294, -1.709698663402913210, -11.09922568453595026 ) ) ;
#44242=CARTESIAN_POINT ( 'NONE',  ( 7.361572987183169658, 9.967264484334119601, -9.846743663894592657 ) ) ;
#44243=CARTESIAN_POINT ( 'NONE',  ( 4.559911319644449179, 17.23035201082150536, -9.422509992056141925 ) ) ;
#44244=EDGE_CURVE ( 'NONE', #6749, #1572, #78018, .T. ) ;
#44245=CARTESIAN_POINT ( 'NONE',  ( 18.52753015748617571, 53.09226448433412315, 4.923371831947298993 ) ) ;
#44246=CARTESIAN_POINT ( 'NONE',  ( 20.30776406404399026, 0.000000000000000000, 6.000000000000280664 ) ) ;
#44248=CARTESIAN_POINT ( 'NONE',  ( 20.15039907845753220, 30.60158574516642815, -6.262539305110077947 ) ) ;
#44250=( NAMED_UNIT ( * ) SI_UNIT ( $, .STERADIAN. ) SOLID_ANGLE_UNIT ( ) );
#44251=CARTESIAN_POINT ( 'NONE',  ( 16.40814093676324603, 22.45696800326375353, -11.09922568453594671 ) ) ;
#44252=CARTESIAN_POINT ( 'NONE',  ( 1.472469842513823179, 25.59226448433412315, -4.923371831947296329 ) ) ;
#44254=CARTESIAN_POINT ( 'NONE',  ( 10.00000000000000178, 2.258931151000784787, 9.846743663894594434 ) ) ;
#44256=CARTESIAN_POINT ( 'NONE',  ( 5.500000000000000000, 11.00000000000000000, -6.000000000000000000 ) ) ;
#44257=CARTESIAN_POINT ( 'NONE',  ( 2.035157376598822676, 12.43868534415483751, -7.964842623401177768 ) ) ;
#44258=CARTESIAN_POINT ( 'NONE',  ( 17.08211943468705130, 43.47041550158063927, 12.26659068614894998 ) ) ;
#44259=CARTESIAN_POINT ( 'NONE',  ( 20.88017736071110519, 65.56368534415483396, 2.639326808657452039E-16 ) ) ;
#44260=CARTESIAN_POINT ( 'NONE',  ( 0.1532563361054082862, 21.21726448433412315, 2.638427012816831674 ) ) ;
#44261=CARTESIAN_POINT ( 'NONE',  ( 0.5774900079438590739, 2.647018677488170990, -5.440088680355550821 ) ) ;
#44262=CARTESIAN_POINT ( 'NONE',  ( 1.472469842513823179, 11.42559781766745175, 4.923371831947296329 ) ) ;
#44263=CARTESIAN_POINT ( 'NONE',  ( -1.028725271592155099, -1.208271517246092823E-15, 4.540618777627624780 ) ) ;
#44264=CARTESIAN_POINT ( 'NONE',  ( 12.63842701281683034, 42.46726448433412315, 9.846743663894596210 ) ) ;
#44266=CARTESIAN_POINT ( 'NONE',  ( 19.42250999205614548, 30.98035201082150536, -5.440088680355545492 ) ) ;
#44269=CARTESIAN_POINT ( 'NONE',  ( -1.099225684535947600, 58.70696800326375353, -6.408140936763238038 ) ) ;
#44272=CARTESIAN_POINT ( 'NONE',  ( 7.361572987183169658, 14.96726448433411960, -9.846743663894592657 ) ) ;
#44273=CARTESIAN_POINT ( 'NONE',  ( 10.00000000000000178, 40.37363466993042493, 12.81628187352647608 ) ) ;
#44274=CARTESIAN_POINT ( 'NONE',  ( 4.559911319644449179, 3.897018677488171434, 9.422509992056141925 ) ) ;
#44275=CARTESIAN_POINT ( 'NONE',  ( 1.472469842513823179, 30.59226448433411960, -4.923371831947296329 ) ) ;
#44276=CARTESIAN_POINT ( 'NONE',  ( 20.00000000000001066, 82.60888403405834879, 4.637569772578755689 ) ) ;
#44279=CARTESIAN_POINT ( 'NONE',  ( 2.917880565312948704, 22.63708216824730002, 12.26659068614894643 ) ) ;
#44280=CARTESIAN_POINT ( 'NONE',  ( 22.26659068614894466, 48.88708216824730357, 7.082119434687054849 ) ) ;
#44281=CARTESIAN_POINT ( 'NONE',  ( 17.20831665107776587, 42.88393115100077324, 7.208316651077764980 ) ) ;
#44283=CARTESIAN_POINT ( 'NONE',  ( 15.44008868035555260, 44.73035201082151247, 9.422509992056143702 ) ) ;
#44285=CARTESIAN_POINT ( 'NONE',  ( 12.91533473730993009, 66.60535201082150536, -10.88017736071109987 ) ) ;
#44287=CARTESIAN_POINT ( 'NONE',  ( 10.00000000000000000, 52.87363466993041783, -12.81628187352647608 ) ) ;
#44289=CARTESIAN_POINT ( 'NONE',  ( 0.5774900079438607392, 68.48035201082150536, 5.440088680355550821 ) ) ;
#44290=ORIENTED_EDGE ( 'NONE', *, *, #25922, .F. ) ;
#44291=CARTESIAN_POINT ( 'NONE',  ( 22.26659068614895176, 9.720415501580633943, -7.082119434687042414 ) ) ;
#44292=CARTESIAN_POINT ( 'NONE',  ( 12.63842701281683922, 9.550597817667449974, -9.846743663894590881 ) ) ;
#44294=CARTESIAN_POINT ( 'NONE',  ( -0.1503990784575242878, 59.24884699246888431, -6.262539305110083276 ) ) ;
#44296=CIRCLE ( 'NONE', #90609, 0.5000000000000004441 ) ;
#44297=CARTESIAN_POINT ( 'NONE',  ( 0.5774900079438607392, 13.48035201082150358, 5.440088680355550821 ) ) ;
#44298=VERTEX_POINT ( 'NONE', #52107 ) ;
#44299=CARTESIAN_POINT ( 'NONE',  ( 7.084665262690076126, 39.10535201082150536, 10.88017736071109987 ) ) ;
#44300=CARTESIAN_POINT ( 'NONE',  ( 20.15039907845753220, 55.60158574516643171, -6.262539305110077947 ) ) ;
#44302=CARTESIAN_POINT ( 'NONE',  ( 1.472469842513823179, 66.42559781766745175, 4.923371831947296329 ) ) ;
#44304=CARTESIAN_POINT ( 'NONE',  ( -0.8801773607110991993, 67.85535201082151957, -2.915334737309923874 ) ) ;
#44306=CARTESIAN_POINT ( 'NONE',  ( -2.816281873526473856, 39.12363466993041783, 9.499525473075851096E-16 ) ) ;
#44307=CARTESIAN_POINT ( 'NONE',  ( 2.035157376598824452, 23.68868534415484461, 7.964842623401179544 ) ) ;
#44308=CARTESIAN_POINT ( 'NONE',  ( -0.1042174387088606602, 58.10736173766205326, 6.337391062633418670 ) ) ;
#44309=CARTESIAN_POINT ( 'NONE',  ( 14.92337183194729633, 7.675597817667451750, 8.527530157486181039 ) ) ;
#44310=CARTESIAN_POINT ( 'NONE',  ( 20.88017736071110164, 15.35535201082150358, 2.915334737309930979 ) ) ;
#44314=CARTESIAN_POINT ( 'NONE',  ( 0.6178305044545838731, 49.74863466993041072, 9.382169495545420901 ) ) ;
#44315=CARTESIAN_POINT ( 'NONE',  ( 12.91533473730992121, 49.52201867748817676, 10.88017736071110164 ) ) ;
#44316=CARTESIAN_POINT ( 'NONE',  ( -46.94000000000001904, 100.8832200551275662, -8.297377427090140145 ) ) ;
#44317=CARTESIAN_POINT ( 'NONE',  ( -2.816281873526471635, 53.91530133659709634, -3.434112377981056508 ) ) ;
#44318=CARTESIAN_POINT ( 'NONE',  ( 7.084665262690076126, 44.10535201082151247, 10.88017736071109987 ) ) ;
#44320=CARTESIAN_POINT ( 'NONE',  ( 7.361572987183169658, 54.96726448433413026, -9.846743663894592657 ) ) ;
#44322=CARTESIAN_POINT ( 'NONE',  ( 17.20831665107776587, 12.88393115100078390, 7.208316651077764980 ) ) ;
#44323=CARTESIAN_POINT ( 'NONE',  ( 0.6178305044545838731, 9.748634669930416052, 9.382169495545420901 ) ) ;
#44324=DIRECTION ( 'NONE',  ( -0.000000000000000000, 0.000000000000000000, 1.000000000000000000 ) ) ;
#44325=CARTESIAN_POINT ( 'NONE',  ( 5.076628168052703671, 61.84226448433412315, 8.527530157486179263 ) ) ;
#44326=CARTESIAN_POINT ( 'NONE',  ( 0.5774900079438590739, 37.64701867748817676, -5.440088680355550821 ) ) ;
#44327=CARTESIAN_POINT ( 'NONE',  ( 14.92337183194729633, 52.67559781766745175, 8.527530157486181039 ) ) ;
#44328=CARTESIAN_POINT ( 'NONE',  ( 18.52753015748617571, 3.092264484334118269, 4.923371831947298993 ) ) ;
#44329=CARTESIAN_POINT ( 'NONE',  ( -1.099225684535947600, 3.706968003263753531, -6.408140936763238038 ) ) ;
#44332=FILL_AREA_STYLE_COLOUR ( '', #41310 ) ;
#44334=CARTESIAN_POINT ( 'NONE',  ( 2.791683348922240793, 61.63393115100079456, 7.208316651077764092 ) ) ;
#44335=CARTESIAN_POINT ( 'NONE',  ( 22.81628187352647785, 46.62363466993041783, 6.195893100308588602E-16 ) ) ;
#44336=CARTESIAN_POINT ( 'NONE',  ( 0.1532563361054082862, 36.21726448433410894, 2.638427012816831674 ) ) ;
#44337=DIRECTION ( 'NONE',  ( 0.6186827199538547095, 0.6777609120375008844, 0.3973308925122679969 ) ) ;
#44338=CARTESIAN_POINT ( 'NONE',  ( -0.8801773607111008646, 8.272018677488171434, 2.915334737309923430 ) ) ;
#44339=CARTESIAN_POINT ( 'NONE',  ( 14.92337183194729988, 29.34226448433411960, -8.527530157486177487 ) ) ;
#44341=CARTESIAN_POINT ( 'NONE',  ( 0.6081133539230648699, 18.33703382326400089, 6.500000000000005329 ) ) ;
#44342=CARTESIAN_POINT ( 'NONE',  ( 4.559911319644449179, 7.230352010821505360, -9.422509992056141925 ) ) ;
#44344=CARTESIAN_POINT ( 'NONE',  ( 15.44008868035555260, 14.73035201082150536, 9.422509992056143702 ) ) ;
#44345=CARTESIAN_POINT ( 'NONE',  ( 20.36894250292379738, 44.92874883491396787, -10.36894250292379027 ) ) ;
#44347=CARTESIAN_POINT ( 'NONE',  ( -4.164238869374099039, 56.80374883491397497, 8.674139862899312516E-16 ) ) ;
#44348=FACE_OUTER_BOUND ( 'NONE', #79909, .T. ) ;
#44349=DIRECTION ( 'NONE',  ( 0.000000000000000000, -1.000000000000000000, 0.000000000000000000 ) ) ;
#44350=CARTESIAN_POINT ( 'NONE',  ( 12.63842701281683922, 14.55059781766744997, -9.846743663894590881 ) ) ;
#44351=CARTESIAN_POINT ( 'NONE',  ( -2.816281873526471635, -1.084698663402913210, -3.434112377981056508 ) ) ;
#44354=CARTESIAN_POINT ( 'NONE',  ( 0.2751277870542909176, 64.36607318730132477, -6.499999999999992006 ) ) ;
#44355=CARTESIAN_POINT ( 'NONE',  ( 5.076628168052704559, 55.17559781766745175, -8.527530157486179263 ) ) ;
#44359=CARTESIAN_POINT ( 'NONE',  ( 5.076628168052703671, 66.84226448433412315, 8.527530157486179263 ) ) ;
#44360=CARTESIAN_POINT ( 'NONE',  ( -0.3689425029237898834, 6.178748834913968757, -10.36894250292378850 ) ) ;
#44361=CARTESIAN_POINT ( 'NONE',  ( 12.63842701281683922, 24.55059781766745175, -9.846743663894590881 ) ) ;
#44362=CARTESIAN_POINT ( 'NONE',  ( 13.99999999999999822, 11.50000000000000000, 6.500000000000000888 ) ) ;
#44364=CARTESIAN_POINT ( 'NONE',  ( 2.917880565312950480, 45.97041550158063927, -12.26659068614894821 ) ) ;
#44367=CARTESIAN_POINT ( 'NONE',  ( 12.63842701281683034, 7.467264484334118713, 9.846743663894596210 ) ) ;
#44370=CARTESIAN_POINT ( 'NONE',  ( 7.084665262690076126, 32.02201867748816966, -10.88017736071110164 ) ) ;
#44371=CARTESIAN_POINT ( 'NONE',  ( 10.00000000000000178, 40.37363466993042493, 12.81628187352647608 ) ) ;
#44372=( NAMED_UNIT ( * ) PLANE_ANGLE_UNIT ( ) SI_UNIT ( $, .RADIAN. ) );
#44373=CARTESIAN_POINT ( 'NONE',  ( 19.38216949554541557, 37.24863466993041783, -9.382169495545420901 ) ) ;
#44374=CARTESIAN_POINT ( 'NONE',  ( -2.816281873526473856, 59.33196800326374643, 3.434112377981055619 ) ) ;
#44376=CARTESIAN_POINT ( 'NONE',  ( 1.711636803080557767, 11.84492782695770607, -6.500000000000021316 ) ) ;
#44378=CARTESIAN_POINT ( 'NONE',  ( 13.79529636645031943, 35.34541550158063927, -14.16423886937409904 ) ) ;
#44380=CARTESIAN_POINT ( 'NONE',  ( 4.559911319644449179, 8.897018677488171434, 9.422509992056141925 ) ) ;
#44381=CARTESIAN_POINT ( 'NONE',  ( 7.084665262690076126, 19.10535201082150181, 10.88017736071109987 ) ) ;
#44384=CARTESIAN_POINT ( 'NONE',  ( 10.00000000000000000, 56.81368534415484106, -10.88017736071110342 ) ) ;
#44385=CARTESIAN_POINT ( 'NONE',  ( 2.035157376598822676, 57.43868534415484106, -7.964842623401177768 ) ) ;
#44386=CARTESIAN_POINT ( 'NONE',  ( 3.591859063236763294, 28.29030133659708568, -11.09922568453595026 ) ) ;
#44389=CARTESIAN_POINT ( 'NONE',  ( 5.076628168052703671, 26.84226448433411960, 8.527530157486179263 ) ) ;
#44390=CARTESIAN_POINT ( 'NONE',  ( 0.5774900079438607392, 53.48035201082151247, 5.440088680355550821 ) ) ;
#44391=CARTESIAN_POINT ( 'NONE',  ( 10.00000000000000178, 20.37363466993042138, 12.81628187352647608 ) ) ;
#44392=CARTESIAN_POINT ( 'NONE',  ( 10.00000000000000000, 11.81368534415483751, -10.88017736071110342 ) ) ;
#44393=CARTESIAN_POINT ( 'NONE',  ( 12.63842701281683034, 37.46726448433411605, 9.846743663894596210 ) ) ;
#44394=CARTESIAN_POINT ( 'NONE',  ( 19.38216949554541557, 42.24863466993041783, -9.382169495545420901 ) ) ;
#44395=CARTESIAN_POINT ( 'NONE',  ( 19.84674366389459266, 13.30059781766745353, 2.638427012816836559 ) ) ;
#44396=CARTESIAN_POINT ( 'NONE',  ( -0.3689425029237881626, 2.428748834913967869, 10.36894250292379027 ) ) ;
#44398=CARTESIAN_POINT ( 'NONE',  ( 4.559911319644449179, 23.89701867748817321, 9.422509992056141925 ) ) ;
#44399=CARTESIAN_POINT ( 'NONE',  ( 24.16423886937409904, 34.09541550158064638, 3.795296366450317205 ) ) ;
#44401=CARTESIAN_POINT ( 'NONE',  ( 14.92337183194729633, 47.67559781766745175, 8.527530157486181039 ) ) ;
#44402=CARTESIAN_POINT ( 'NONE',  ( 10.00000000000000000, 31.81368534415483751, -10.88017736071110342 ) ) ;
#44403=CARTESIAN_POINT ( 'NONE',  ( 12.91533473730993009, 11.60535201082150714, -10.88017736071109987 ) ) ;
#44404=ORIENTED_EDGE ( 'NONE', *, *, #44925, .T. ) ;
#44405=CARTESIAN_POINT ( 'NONE',  ( -0.8801773607110991993, 22.85535201082150181, -2.915334737309923874 ) ) ;
#44406=CARTESIAN_POINT ( 'NONE',  ( 13.43411237798105340, 50.58196800326375353, 12.81628187352647963 ) ) ;
#44407=CARTESIAN_POINT ( 'NONE',  ( 17.96484262340118221, 39.93868534415484106, 7.964842623401181321 ) ) ;
#44409=CARTESIAN_POINT ( 'NONE',  ( 20.88017736071110164, 40.35535201082150536, 2.915334737309930979 ) ) ;
#44412=CARTESIAN_POINT ( 'NONE',  ( 14.92337183194729988, 59.34226448433412315, -8.527530157486177487 ) ) ;
#44413=CARTESIAN_POINT ( 'NONE',  ( 12.91533473730993009, 36.60535201082151247, -10.88017736071109987 ) ) ;
#44416=CARTESIAN_POINT ( 'NONE',  ( 17.08211943468705130, 53.47041550158063217, 12.26659068614894998 ) ) ;
#44417=CARTESIAN_POINT ( 'NONE',  ( 4.559911319644449179, 47.23035201082150536, -9.422509992056141925 ) ) ;
#44420=CARTESIAN_POINT ( 'NONE',  ( 17.20831665107776587, 57.88393115100078745, 7.208316651077764980 ) ) ;
#44421=CARTESIAN_POINT ( 'NONE',  ( 10.00000000000000178, 22.25893115100078745, 9.846743663894594434 ) ) ;
#44423=CARTESIAN_POINT ( 'NONE',  ( 14.92337183194729633, 17.67559781766745175, 8.527530157486181039 ) ) ;
#44425=CARTESIAN_POINT ( 'NONE',  ( 20.88017736071110875, 20.77201867748816611, -2.915334737309920765 ) ) ;
#44426=CARTESIAN_POINT ( 'NONE',  ( 12.63842701281683922, 19.55059781766745175, -9.846743663894590881 ) ) ;
#44427=CARTESIAN_POINT ( 'NONE',  ( 17.39651004071838614, 47.93575266056826933, 6.500000000000032863 ) ) ;
#44428=CARTESIAN_POINT ( 'NONE',  ( 22.81628187352647785, 11.62363466993042138, 6.195893100308588602E-16 ) ) ;
#44429=CARTESIAN_POINT ( 'NONE',  ( 2.603489959281614308, 36.58210964143329136, 6.500000000000031086 ) ) ;
#44430=CARTESIAN_POINT ( 'NONE',  ( -0.8801773607111008646, 63.27201867748817676, 2.915334737309923430 ) ) ;
#44431=CARTESIAN_POINT ( 'NONE',  ( 19.42250999205614193, 30.14701867748817321, 5.440088680355555262 ) ) ;
#44432=CARTESIAN_POINT ( 'NONE',  ( 21.09922568453595559, 62.04030133659709634, -6.408140936763230044 ) ) ;
#44433=CARTESIAN_POINT ( 'NONE',  ( 22.26659068614894466, 38.88708216824731068, 7.082119434687054849 ) ) ;
#44436=CARTESIAN_POINT ( 'NONE',  ( -45.36634016833912852, 104.5847037719681936, 5.617347555694320427 ) ) ;
#44438=CARTESIAN_POINT ( 'NONE',  ( 6.565887622018943937, 18.08196800326375708, -12.81628187352647608 ) ) ;
#44439=CARTESIAN_POINT ( 'NONE',  ( 12.91533473730992121, 4.522018677488169658, 10.88017736071110164 ) ) ;
#44440=CARTESIAN_POINT ( 'NONE',  ( 20.88017736071110875, 45.77201867748816966, -2.915334737309920765 ) ) ;
#44444=CARTESIAN_POINT ( 'NONE',  ( 10.00000000000000000, 51.81368534415484106, -10.88017736071110342 ) ) ;
#44445=CARTESIAN_POINT ( 'NONE',  ( 17.20831665107776587, 34.13393115100078745, -7.208316651077762316 ) ) ;
#44446=CARTESIAN_POINT ( 'NONE',  ( 17.20831665107776587, 19.13393115100078035, -7.208316651077762316 ) ) ;
#44447=CARTESIAN_POINT ( 'NONE',  ( 5.076628168052703671, 11.84226448433411960, 8.527530157486179263 ) ) ;
#44448=ADVANCED_FACE ( 'NONE', ( #54550 ), #33988, .F. ) ;
#44450=CARTESIAN_POINT ( 'NONE',  ( -2.816281873526473856, 39.33196800326374643, 3.434112377981055619 ) ) ;
#44451=CARTESIAN_POINT ( 'NONE',  ( 20.88017736071110519, 65.56368534415483396, 2.639326808657452039E-16 ) ) ;
#44452=DIRECTION ( 'NONE',  ( -0.000000000000000000, -1.000000000000000000, -0.000000000000000000 ) ) ;
#44454=CARTESIAN_POINT ( 'NONE',  ( 7.361572987183170547, 27.05059781766745175, 9.846743663894590881 ) ) ;
#44456=CARTESIAN_POINT ( 'NONE',  ( -2.816281873526471635, 58.91530133659707502, -3.434112377981056508 ) ) ;
#44458=CARTESIAN_POINT ( 'NONE',  ( 7.361572987183169658, 64.96726448433412315, -9.846743663894592657 ) ) ;
#44459=CARTESIAN_POINT ( 'NONE',  ( 24.16423886937409904, 39.09541550158062506, 3.795296366450317205 ) ) ;
#44460=B_SPLINE_CURVE_WITH_KNOTS ( 'NONE', 3,
 ( #98328, #14822, #37812, #60783 ),
 .UNSPECIFIED., .F., .F.,
 ( 4, 4 ),
 ( 4.878909776184769953E-19, 0.002657014572711323755 ),
 .UNSPECIFIED. ) ;
#44461=UNCERTAINTY_MEASURE_WITH_UNIT (LENGTH_MEASURE( 1.000000000000000082E-05 ), #75827, 'distance_accuracy_value', 'NONE');
#44463=CARTESIAN_POINT ( 'NONE',  ( -2.266590686148945544, 27.22041550158063572, 7.082119434687048631 ) ) ;
#44464=CARTESIAN_POINT ( 'NONE',  ( -2.266590686148945544, 47.22041550158063927, 7.082119434687048631 ) ) ;
#44465=CARTESIAN_POINT ( 'NONE',  ( -0.3689425029237881626, 12.42874883491396609, 10.36894250292379027 ) ) ;
#44466=CARTESIAN_POINT ( 'NONE',  ( 10.00000000000000178, 18.05374883491396787, 14.16423886937410082 ) ) ;
#44468=CARTESIAN_POINT ( 'NONE',  ( 0.5774900079438590739, 42.64701867748816966, -5.440088680355550821 ) ) ;
#44472=CARTESIAN_POINT ( 'NONE',  ( 19.84674366389459266, 23.30059781766745530, 2.638427012816836559 ) ) ;
#44474=CARTESIAN_POINT ( 'NONE',  ( -46.44000000000001194, 93.00000000000000000, -9.500000000000000000 ) ) ;
#44475=CARTESIAN_POINT ( 'NONE',  ( 0.1532563361054100626, 30.80059781766744820, -2.638427012816831230 ) ) ;
#44476=CARTESIAN_POINT ( 'NONE',  ( 19.42250999205614193, 25.14701867748817321, 5.440088680355555262 ) ) ;
#44477=CARTESIAN_POINT ( 'NONE',  ( -2.816281873526471635, 58.91530133659707502, -3.434112377981056508 ) ) ;
#44478=CARTESIAN_POINT ( 'NONE',  ( 5.076628168052703671, 46.84226448433412315, 8.527530157486179263 ) ) ;
#44479=CARTESIAN_POINT ( 'NONE',  ( 19.38216949554541557, 47.24863466993041783, -9.382169495545420901 ) ) ;
#44482=CARTESIAN_POINT ( 'NONE',  ( 12.91533473730993009, 36.60535201082151247, -10.88017736071109987 ) ) ;
#44483=CARTESIAN_POINT ( 'NONE',  ( 5.076628168052704559, 45.17559781766745175, -8.527530157486179263 ) ) ;
#44485=CARTESIAN_POINT ( 'NONE',  ( 6.204703633549690345, 22.84541550158062861, 14.16423886937410082 ) ) ;
#44489=CARTESIAN_POINT ( 'NONE',  ( 17.96484262340118221, 66.18868534415483396, -7.964842623401177768 ) ) ;
#44491=CARTESIAN_POINT ( 'NONE',  ( -4.164238869374099927, 57.01208216824731068, 3.795296366450308767 ) ) ;
#44492=CARTESIAN_POINT ( 'NONE',  ( 7.361572987183170547, 62.05059781766745886, 9.846743663894590881 ) ) ;
#44494=CARTESIAN_POINT ( 'NONE',  ( 10.00000000000000000, 51.81368534415484106, -10.88017736071110342 ) ) ;
#44495=CARTESIAN_POINT ( 'NONE',  ( 1.707155281725174945, 57.90189080397285437, 6.499999999999955591 ) ) ;
#44498=CARTESIAN_POINT ( 'NONE',  ( 0.5774900079438607392, 13.48035201082150358, 5.440088680355550821 ) ) ;
#44499=CARTESIAN_POINT ( 'NONE',  ( 15.44008868035555793, 16.39701867748817321, -9.422509992056140149 ) ) ;
#44500=CARTESIAN_POINT ( 'NONE',  ( 1.472469842513823179, 41.42559781766745886, 4.923371831947296329 ) ) ;
#44501=CARTESIAN_POINT ( 'NONE',  ( 19.38216949554541557, 57.24863466993042493, -9.382169495545420901 ) ) ;
#44504=CARTESIAN_POINT ( 'NONE',  ( 17.96484262340118221, 19.93868534415484106, 7.964842623401181321 ) ) ;
#44505=CARTESIAN_POINT ( 'NONE',  ( 10.00000000000000178, 25.37363466993041783, 12.81628187352647608 ) ) ;
#44507=CARTESIAN_POINT ( 'NONE',  ( 0.1532563361054100626, 10.80059781766745175, -2.638427012816831230 ) ) ;
#44508=CARTESIAN_POINT ( 'NONE',  ( 19.84674366389459621, 53.50893115100078745, 7.409399052514197653E-17 ) ) ;
#44509=B_SPLINE_CURVE_WITH_KNOTS ( 'NONE', 3,
 ( #8725, #39243, #47208, #71211 ),
 .UNSPECIFIED., .F., .F.,
 ( 4, 4 ),
 ( 8.182674270850422113E-18, 0.002392975128318503269 ),
 .UNSPECIFIED. ) ;
#44510=CARTESIAN_POINT ( 'NONE',  ( 19.42250999205614548, 35.98035201082151247, -5.440088680355545492 ) ) ;
#44511=CARTESIAN_POINT ( 'NONE',  ( 21.09922568453595559, 12.04030133659708746, -6.408140936763230044 ) ) ;
#44512=CARTESIAN_POINT ( 'NONE',  ( 12.91533473730993009, 51.60535201082149825, -10.88017736071109987 ) ) ;
#44515=CARTESIAN_POINT ( 'NONE',  ( 16.40814093676324603, 57.45696800326375353, -11.09922568453594671 ) ) ;
#44516=EDGE_LOOP ( 'NONE', ( #58513, #83642, #86408, #92079, #81053, #33583 ) ) ;
#44518=CARTESIAN_POINT ( 'NONE',  ( 19.38216949554541557, 27.24863466993041783, -9.382169495545420901 ) ) ;
#44519=CARTESIAN_POINT ( 'NONE',  ( -2.266590686148945544, 1.387082168247301128, -7.082119434687050408 ) ) ;
#44521=CARTESIAN_POINT ( 'NONE',  ( 4.559911319644449179, 43.89701867748816966, 9.422509992056141925 ) ) ;
#44522=CARTESIAN_POINT ( 'NONE',  ( 10.00000000000000178, 67.25893115100079456, 9.846743663894594434 ) ) ;
#44523=CARTESIAN_POINT ( 'NONE',  ( 5.076628168052703671, 51.84226448433412315, 8.527530157486179263 ) ) ;
#44524=CARTESIAN_POINT ( 'NONE',  ( 17.20831665107776587, 19.13393115100078035, -7.208316651077762316 ) ) ;
#44525=CARTESIAN_POINT ( 'NONE',  ( 19.84674366389459621, 3.508931151000785231, 7.409399052514197653E-17 ) ) ;
#44527=CARTESIAN_POINT ( 'NONE',  ( 24.16423886937409904, 39.09541550158062506, 3.795296366450317205 ) ) ;
#44529=MECHANICAL_DESIGN_GEOMETRIC_PRESENTATION_REPRESENTATION('',(#39768),#73287);
#44533=ORIENTED_EDGE ( 'NONE', *, *, #75097, .T. ) ;
#44535=CARTESIAN_POINT ( 'NONE',  ( -2.266590686148945544, 56.38708216824731068, -7.082119434687050408 ) ) ;
#44536=CARTESIAN_POINT ( 'NONE',  ( 2.917880565312950480, 60.97041550158063927, -12.26659068614894821 ) ) ;
#44537=CARTESIAN_POINT ( 'NONE',  ( 10.00000000000000178, 32.25893115100078745, 9.846743663894594434 ) ) ;
#44538=CARTESIAN_POINT ( 'NONE',  ( -1.099225684535947600, 24.54030133659708923, 6.408140936763237150 ) ) ;
#44541=CARTESIAN_POINT ( 'NONE',  ( -4.164238869374098151, 1.595415501580634388, -3.795296366450310543 ) ) ;
#44542=CARTESIAN_POINT ( 'NONE',  ( -0.8801773607111009756, 13.06368534415483929, 1.068504757029289695E-15 ) ) ;
#44543=CARTESIAN_POINT ( 'NONE',  ( -0.3689425029237881626, 52.42874883491396076, 10.36894250292379027 ) ) ;
#44544=CARTESIAN_POINT ( 'NONE',  ( 2.791683348922237240, 35.38393115100079456, -7.208316651077763204 ) ) ;
#44546=CARTESIAN_POINT ( 'NONE',  ( 14.92337183194729633, 22.67559781766745175, 8.527530157486181039 ) ) ;
#44549=ORIENTED_EDGE ( 'NONE', *, *, #49046, .F. ) ;
#44553=CARTESIAN_POINT ( 'NONE',  ( 19.84674366389459266, 48.71726448433413026, -2.638427012816827677 ) ) ;
#44554=CARTESIAN_POINT ( 'NONE',  ( 17.96484262340118221, 14.93868534415484106, 7.964842623401181321 ) ) ;
#44555=CARTESIAN_POINT ( 'NONE',  ( 10.00000000000000178, 44.31368534415484106, 10.88017736071110342 ) ) ;
#44556=SURFACE_STYLE_FILL_AREA ( #23061 ) ;
#44557=CARTESIAN_POINT ( 'NONE',  ( 3.591859063236763294, 23.29030133659708568, -11.09922568453595026 ) ) ;
#44558=CARTESIAN_POINT ( 'NONE',  ( 22.26659068614894466, 8.887082168247300018, 7.082119434687054849 ) ) ;
#44559=CARTESIAN_POINT ( 'NONE',  ( 19.42250999205614548, 65.98035201082151957, -5.440088680355545492 ) ) ;
#44560=CARTESIAN_POINT ( 'NONE',  ( 21.09922568453594849, 26.20696800326375353, 6.408140936763242479 ) ) ;
#44562=CARTESIAN_POINT ( 'NONE',  ( 2.791683348922237240, 35.38393115100079456, -7.208316651077763204 ) ) ;
#44563=CARTESIAN_POINT ( 'NONE',  ( 20.88017736071110875, 10.77201867748817143, -2.915334737309920765 ) ) ;
#44564=EDGE_LOOP ( 'NONE', ( #49904, #81834, #52593, #62605, #28953, #18709 ) ) ;
#44565=CARTESIAN_POINT ( 'NONE',  ( 24.16423886937410614, 64.30374883491396076, 8.672049930838204340E-16 ) ) ;
#44567=CARTESIAN_POINT ( 'NONE',  ( 2.035157376598824452, 48.68868534415483396, 7.964842623401179544 ) ) ;
#44568=CARTESIAN_POINT ( 'NONE',  ( 7.084665262690076126, 62.02201867748816966, -10.88017736071110164 ) ) ;
#44570=CARTESIAN_POINT ( 'NONE',  ( 0.5774900079438590739, 62.64701867748817676, -5.440088680355550821 ) ) ;
#44572=CARTESIAN_POINT ( 'NONE',  ( 10.00000000000000178, 2.258931151000784787, 9.846743663894594434 ) ) ;
#44573=CARTESIAN_POINT ( 'NONE',  ( 20.88017736071110164, 60.35535201082151957, 2.915334737309930979 ) ) ;
#44577=CARTESIAN_POINT ( 'NONE',  ( 19.84674366389459266, 23.71726448433412315, -2.638427012816827677 ) ) ;
#44581=CARTESIAN_POINT ( 'NONE',  ( 2.917880565312950480, 5.970415501580634832, -12.26659068614894821 ) ) ;
#44582=ORIENTED_EDGE ( 'NONE', *, *, #37885, .T. ) ;
#44586=CARTESIAN_POINT ( 'NONE',  ( 15.44008868035555260, 9.730352010821505360, 9.422509992056143702 ) ) ;
#44589=( BOUNDED_CURVE ( )  B_SPLINE_CURVE ( 3, ( #41362, #33800, #94818, #3837 ),
 .UNSPECIFIED., .F., .T. ) 
 B_SPLINE_CURVE_WITH_KNOTS ( ( 4, 4 ),
 ( 0.000000000000000000, 1.570796326794896558 ),
 .UNSPECIFIED. ) 
 CURVE ( )  GEOMETRIC_REPRESENTATION_ITEM ( )  RATIONAL_B_SPLINE_CURVE ( ( 1.000000000000000000, 0.8047378541243649375, 0.8047378541243649375, 1.000000000000000000 ) ) 
 REPRESENTATION_ITEM ( '' )  );
#44590=DIRECTION ( 'NONE',  ( -1.000000000000000000, 0.000000000000000000, 0.000000000000000000 ) ) ;
#44591=CARTESIAN_POINT ( 'NONE',  ( 1.472469842513823179, 41.42559781766745886, 4.923371831947296329 ) ) ;
#44593=CARTESIAN_POINT ( 'NONE',  ( 16.40814093676324603, 22.45696800326375353, -11.09922568453594671 ) ) ;
#44594=CARTESIAN_POINT ( 'NONE',  ( 17.20831665107776587, 9.133931151000787452, -7.208316651077762316 ) ) ;
#44596=CARTESIAN_POINT ( 'NONE',  ( 1.042145700049398549, 29.74216108172003459, -6.499999999999841016 ) ) ;
#44597=CARTESIAN_POINT ( 'NONE',  ( 10.00000000000000000, 19.75893115100078390, -9.846743663894594434 ) ) ;
#44598=CARTESIAN_POINT ( 'NONE',  ( 16.40814093676323893, 0.7903013365970867898, 11.09922568453595026 ) ) ;
#44601=ORIENTED_EDGE ( 'NONE', *, *, #24867, .T. ) ;
#44603=EDGE_CURVE ( 'NONE', #26347, #5105, #24406, .T. ) ;
#44604=CARTESIAN_POINT ( 'NONE',  ( 15.44008868035555260, 24.73035201082150891, 9.422509992056143702 ) ) ;
#44605=CARTESIAN_POINT ( 'NONE',  ( 20.36894250292379738, 24.92874883491396787, -10.36894250292379027 ) ) ;
#44606=CARTESIAN_POINT ( 'NONE',  ( 17.20831665107776587, 24.13393115100078035, -7.208316651077762316 ) ) ;
#44607=CARTESIAN_POINT ( 'NONE',  ( 15.44008868035555793, 51.39701867748816966, -9.422509992056140149 ) ) ;
#44608=CARTESIAN_POINT ( 'NONE',  ( -2.816281873526471635, 33.91530133659708213, -3.434112377981056508 ) ) ;
#44609=CARTESIAN_POINT ( 'NONE',  ( 19.42250999205614193, 10.14701867748816966, 5.440088680355555262 ) ) ;
#44610=CARTESIAN_POINT ( 'NONE',  ( 0.6081133539230521023, 43.33703382326400089, 6.499999999999974243 ) ) ;
#44613=CARTESIAN_POINT ( 'NONE',  ( 19.38216949554541202, 15.99863466993042138, 9.382169495545424454 ) ) ;
#44614=CARTESIAN_POINT ( 'NONE',  ( 14.92337183194729988, 59.34226448433412315, -8.527530157486177487 ) ) ;
#44615=CARTESIAN_POINT ( 'NONE',  ( 2.791683348922237240, 30.38393115100078390, -7.208316651077763204 ) ) ;
#44617=CARTESIAN_POINT ( 'NONE',  ( 22.81628187352647785, 41.62363466993042493, 6.195893100308588602E-16 ) ) ;
#44619=CARTESIAN_POINT ( 'NONE',  ( 0.5774900079438607392, 38.48035201082150536, 5.440088680355550821 ) ) ;
#44623=CARTESIAN_POINT ( 'NONE',  ( -0.8801773607110991993, 67.85535201082151957, -2.915334737309923874 ) ) ;
#44624=CARTESIAN_POINT ( 'NONE',  ( -0.8801773607111008646, 43.27201867748817676, 2.915334737309923430 ) ) ;
#44625=CARTESIAN_POINT ( 'NONE',  ( -0.8801773607111009756, 38.06368534415484106, 1.068504757029289695E-15 ) ) ;
#44626=CARTESIAN_POINT ( 'NONE',  ( 10.00000000000000000, 59.75893115100078745, -9.846743663894594434 ) ) ;
#44627=CARTESIAN_POINT ( 'NONE',  ( 12.91533473730992121, 59.52201867748816966, 10.88017736071110164 ) ) ;
#44629=CARTESIAN_POINT ( 'NONE',  ( 10.00000000000000000, 44.75893115100078745, -9.846743663894594434 ) ) ;
#44630=CARTESIAN_POINT ( 'NONE',  ( 4.559911319644449179, 12.23035201082150536, -9.422509992056141925 ) ) ;
#44631=CARTESIAN_POINT ( 'NONE',  ( 19.38216949554541557, 12.24863466993041961, -9.382169495545420901 ) ) ;
#44633=CARTESIAN_POINT ( 'NONE',  ( 7.084665262690076126, 22.02201867748817321, -10.88017736071110164 ) ) ;
#44636=CARTESIAN_POINT ( 'NONE',  ( 4.559911319644449179, 3.897018677488170990, 9.422509992056141925 ) ) ;
#44637=CARTESIAN_POINT ( 'NONE',  ( 0.5774900079438607392, 33.48035201082150536, 5.440088680355550821 ) ) ;
#44638=CARTESIAN_POINT ( 'NONE',  ( 12.63842701281683922, 4.550597817667451750, -9.846743663894590881 ) ) ;
#44639=CARTESIAN_POINT ( 'NONE',  ( -2.266590686148945544, 32.22041550158063927, 7.082119434687048631 ) ) ;
#44640=CARTESIAN_POINT ( 'NONE',  ( 14.92337183194729988, 9.342264484334119601, -8.527530157486177487 ) ) ;
#44641=CARTESIAN_POINT ( 'NONE',  ( 7.084665262690076126, 52.02201867748816255, -10.88017736071110164 ) ) ;
#44643=CARTESIAN_POINT ( 'NONE',  ( 13.79529636645030344, 3.262082168247301350, 14.16423886937410614 ) ) ;
#44645=CARTESIAN_POINT ( 'NONE',  ( -46.94000000000001194, 103.0000000000000000, 5.997726559847112782 ) ) ;
#44646=CARTESIAN_POINT ( 'NONE',  ( 0.1532563361054100626, 55.80059781766745175, -2.638427012816831230 ) ) ;
#44647=ORIENTED_EDGE ( 'NONE', *, *, #26992, .T. ) ;
#44649=CARTESIAN_POINT ( 'NONE',  ( 20.36894250292379738, 24.92874883491396787, -10.36894250292379027 ) ) ;
#44650=CARTESIAN_POINT ( 'NONE',  ( 13.79529636645031943, 25.34541550158063572, -14.16423886937409904 ) ) ;
#44651=CARTESIAN_POINT ( 'NONE',  ( -0.8801773607110991993, 62.85535201082150536, -2.915334737309923874 ) ) ;
#44652=CARTESIAN_POINT ( 'NONE',  ( 0.5774900079438607392, 3.480352010821504916, 5.440088680355550821 ) ) ;
#44653=CARTESIAN_POINT ( 'NONE',  ( 22.81628187352648496, 1.831968003263753753, -3.434112377981050290 ) ) ;
#44654=CARTESIAN_POINT ( 'NONE',  ( 0.1532563361054082862, 46.21726448433411605, 2.638427012816831674 ) ) ;
#44656=CARTESIAN_POINT ( 'NONE',  ( -0.8801773607111009756, 43.06368534415484106, 1.068504757029289695E-15 ) ) ;
#44657=CARTESIAN_POINT ( 'NONE',  ( 0.6178305044545818747, 8.498634669930421381, -9.382169495545419124 ) ) ;
#44658=CARTESIAN_POINT ( 'NONE',  ( 17.08211943468705130, 13.47041550158063572, 12.26659068614894998 ) ) ;
#44659=CARTESIAN_POINT ( 'NONE',  ( 20.88017736071110164, 10.35535201082150714, 2.915334737309930979 ) ) ;
#44660=CARTESIAN_POINT ( 'NONE',  ( 10.00000000000000178, 14.31368534415483929, 10.88017736071110342 ) ) ;
#44661=CARTESIAN_POINT ( 'NONE',  ( 20.15039907845753220, 17.62777174578612716, -6.262539305110077947 ) ) ;
#44662=CARTESIAN_POINT ( 'NONE',  ( 2.035157376598824452, 38.68868534415483396, 7.964842623401179544 ) ) ;
#44667=CARTESIAN_POINT ( 'NONE',  ( 5.076628168052703671, 31.84226448433412315, 8.527530157486179263 ) ) ;
#44669=ORIENTED_EDGE ( 'NONE', *, *, #24173, .F. ) ;
#44671=CARTESIAN_POINT ( 'NONE',  ( 24.16423886937409904, 49.09541550158063217, 3.795296366450317205 ) ) ;
#44672=CARTESIAN_POINT ( 'NONE',  ( 0.5774900079438590739, 2.647018677488171434, -5.440088680355550821 ) ) ;
#44673=CARTESIAN_POINT ( 'NONE',  ( 19.84674366389459266, 28.30059781766745886, 2.638427012816836559 ) ) ;
#44674=CARTESIAN_POINT ( 'NONE',  ( 12.63842701281683034, 42.46726448433412315, 9.846743663894596210 ) ) ;
#44677=CARTESIAN_POINT ( 'NONE',  ( 15.44008868035555793, 61.39701867748817676, -9.422509992056140149 ) ) ;
#44680=CARTESIAN_POINT ( 'NONE',  ( 13.79529636645030344, 28.26208216824729647, 14.16423886937410614 ) ) ;
#44681=CARTESIAN_POINT ( 'NONE',  ( 3.591859063236761518, 24.95696800326375353, 11.09922568453594849 ) ) ;
#44683=CARTESIAN_POINT ( 'NONE',  ( 3.591859063236763294, 63.29030133659708923, -11.09922568453595026 ) ) ;
#44684=CARTESIAN_POINT ( 'NONE',  ( 20.88017736071110519, 25.56368534415483751, 2.639326808657452039E-16 ) ) ;
#44685=CARTESIAN_POINT ( 'NONE',  ( 0.1532563361054100626, 35.80059781766745175, -2.638427012816831230 ) ) ;
#44686=CARTESIAN_POINT ( 'NONE',  ( 2.035157376598822676, 32.43868534415483396, -7.964842623401177768 ) ) ;
#44687=CARTESIAN_POINT ( 'NONE',  ( -2.816281873526473856, 64.12363466993042493, 9.499525473075851096E-16 ) ) ;
#44688=CYLINDRICAL_SURFACE ( 'NONE', #60718, 0.5000000000000004441 ) ;
#44689=CARTESIAN_POINT ( 'NONE',  ( 2.791683348922237240, 40.38393115100078035, -7.208316651077763204 ) ) ;
#44690=CARTESIAN_POINT ( 'NONE',  ( 7.361572987183169658, 49.96726448433410894, -9.846743663894592657 ) ) ;
#44696=CARTESIAN_POINT ( 'NONE',  ( 17.39651004071842522, 19.08210964143329491, -6.499999999999992895 ) ) ;
#44698=CARTESIAN_POINT ( 'NONE',  ( 12.63842701281683922, 14.55059781766744997, -9.846743663894590881 ) ) ;
#44701=CARTESIAN_POINT ( 'NONE',  ( 14.92337183194729988, 59.34226448433412315, -8.527530157486177487 ) ) ;
#44702=CARTESIAN_POINT ( 'NONE',  ( 7.361572987183170547, 37.05059781766744464, 9.846743663894590881 ) ) ;
#44703=CARTESIAN_POINT ( 'NONE',  ( 24.16423886937409904, 34.09541550158064638, 3.795296366450317205 ) ) ;
#44704=CARTESIAN_POINT ( 'NONE',  ( 1.472469842513823179, 40.59226448433411605, -4.923371831947296329 ) ) ;
#44705=CARTESIAN_POINT ( 'NONE',  ( 13.43411237798106583, 52.66530133659708213, -12.81628187352647252 ) ) ;
#44706=CARTESIAN_POINT ( 'NONE',  ( 10.00000000000000178, 70.00000000000000000, 0.000000000000000000 ) ) ;
#44708=CARTESIAN_POINT ( 'NONE',  ( 17.20831665107776587, 9.133931151000787452, -7.208316651077762316 ) ) ;
#44709=CARTESIAN_POINT ( 'NONE',  ( 13.79529636645030344, 3.262082168247301350, 14.16423886937410614 ) ) ;
#44710=CARTESIAN_POINT ( 'NONE',  ( 14.92337183194729988, 54.34226448433412315, -8.527530157486177487 ) ) ;
#44711=CARTESIAN_POINT ( 'NONE',  ( 4.559911319644449179, 42.23035201082151247, -9.422509992056141925 ) ) ;
#44712=CARTESIAN_POINT ( 'NONE',  ( 14.92337183194729633, 42.67559781766745886, 8.527530157486181039 ) ) ;
#44716=CARTESIAN_POINT ( 'NONE',  ( 15.44008868035555260, 49.73035201082150536, 9.422509992056143702 ) ) ;
#44720=CARTESIAN_POINT ( 'NONE',  ( 17.96484262340118221, 11.18868534415483929, -7.964842623401177768 ) ) ;
#44721=CARTESIAN_POINT ( 'NONE',  ( 14.92337183194729988, 64.34226448433412315, -8.527530157486177487 ) ) ;
#44722=CARTESIAN_POINT ( 'NONE',  ( -0.8801773607111008646, 38.27201867748816255, 2.915334737309923430 ) ) ;
#44724=CARTESIAN_POINT ( 'NONE',  ( 10.00000000000000000, 66.81368534415484817, -10.88017736071110342 ) ) ;
#44726=CARTESIAN_POINT ( 'NONE',  ( 19.42250999205614548, 35.98035201082151247, -5.440088680355545492 ) ) ;
#44728=CARTESIAN_POINT ( 'NONE',  ( 17.20831665107776587, 7.883931151000784787, 7.208316651077764980 ) ) ;
#44729=CARTESIAN_POINT ( 'NONE',  ( 0.1532563361054100626, 20.80059781766744464, -2.638427012816831230 ) ) ;
#44732=CARTESIAN_POINT ( 'NONE',  ( 18.52753015748618282, 58.92559781766745886, -4.923371831947291888 ) ) ;
#44734=CARTESIAN_POINT ( 'NONE',  ( 24.16423886937410614, 64.30374883491396076, 8.672049930838204340E-16 ) ) ;
#44735=CARTESIAN_POINT ( 'NONE',  ( -4.164238869374098151, 16.59541550158063927, -3.795296366450310543 ) ) ;
#44736=CARTESIAN_POINT ( 'NONE',  ( 24.16423886937410614, 54.51208216824730357, -3.795296366450302550 ) ) ;
#44737=CARTESIAN_POINT ( 'NONE',  ( 20.88017736071110519, 5.563685344154837509, 2.639326808657452039E-16 ) ) ;
#44739=CARTESIAN_POINT ( 'NONE',  ( 2.791683348922240793, 26.63393115100078745, 7.208316651077764092 ) ) ;
#44740=CARTESIAN_POINT ( 'NONE',  ( 4.559911319644449179, 18.89701867748817321, 9.422509992056141925 ) ) ;
#44741=CARTESIAN_POINT ( 'NONE',  ( 7.361572987183170547, 52.05059781766745175, 9.846743663894590881 ) ) ;
#44744=CARTESIAN_POINT ( 'NONE',  ( -1.099225684535947600, 39.54030133659708923, 6.408140936763237150 ) ) ;
#44745=CARTESIAN_POINT ( 'NONE',  ( 12.63842701281683034, 47.46726448433412315, 9.846743663894596210 ) ) ;
#44747=CARTESIAN_POINT ( 'NONE',  ( 19.84674366389459266, 13.71726448433411782, -2.638427012816827677 ) ) ;
#44750=CARTESIAN_POINT ( 'NONE',  ( 20.88017736071110164, 10.35535201082150714, 2.915334737309930979 ) ) ;
#44751=CARTESIAN_POINT ( 'NONE',  ( 13.79529636645030344, 53.26208216824730357, 14.16423886937410614 ) ) ;
#44752=CARTESIAN_POINT ( 'NONE',  ( 12.91533473730993009, 46.60535201082150536, -10.88017736071109987 ) ) ;
#44753=CARTESIAN_POINT ( 'NONE',  ( 15.44008868035555793, 61.39701867748817676, -9.422509992056140149 ) ) ;
#44755=CARTESIAN_POINT ( 'NONE',  ( 0.1532563361054100626, 20.80059781766744464, -2.638427012816831230 ) ) ;
#44756=CARTESIAN_POINT ( 'NONE',  ( -0.8801773607111008646, 8.272018677488171434, 2.915334737309923430 ) ) ;
#44757=CARTESIAN_POINT ( 'NONE',  ( 12.63842701281683034, 12.46726448433411782, 9.846743663894596210 ) ) ;
#44759=CARTESIAN_POINT ( 'NONE',  ( 5.076628168052703671, 56.84226448433412315, 8.527530157486179263 ) ) ;
#44760=EDGE_CURVE ( 'NONE', #32525, #60007, #23348, .T. ) ;
#44761=CARTESIAN_POINT ( 'NONE',  ( -0.8801773607111009756, 33.06368534415484106, 1.068504757029289695E-15 ) ) ;
#44762=ORIENTED_EDGE ( 'NONE', *, *, #4215, .T. ) ;
#44763=CARTESIAN_POINT ( 'NONE',  ( 0.6178305044545838731, 64.74863466993043914, 9.382169495545420901 ) ) ;
#44765=CARTESIAN_POINT ( 'NONE',  ( 2.791683348922237240, 15.38393115100078212, -7.208316651077763204 ) ) ;
#44766=CARTESIAN_POINT ( 'NONE',  ( 16.40814093676324603, 37.45696800326376064, -11.09922568453594671 ) ) ;
#44767=CARTESIAN_POINT ( 'NONE',  ( 0.5774900079438590739, 12.64701867748817321, -5.440088680355550821 ) ) ;
#44768=CARTESIAN_POINT ( 'NONE',  ( 10.00000000000000000, 34.75893115100078745, -9.846743663894594434 ) ) ;
#44769=CARTESIAN_POINT ( 'NONE',  ( 0.1532563361054100626, 0.8005978176674514168, -2.638427012816831230 ) ) ;
#44770=CARTESIAN_POINT ( 'NONE',  ( 20.36894250292379382, 33.67874883491396076, 10.36894250292379205 ) ) ;
#44771=CARTESIAN_POINT ( 'NONE',  ( -4.164238869374099039, 41.80374883491397497, 8.674139862899312516E-16 ) ) ;
#44772=CARTESIAN_POINT ( 'NONE',  ( 7.361572987183169658, 54.96726448433413026, -9.846743663894592657 ) ) ;
#44774=CARTESIAN_POINT ( 'NONE',  ( 0.5774900079438607392, 33.48035201082150536, 5.440088680355550821 ) ) ;
#44775=CARTESIAN_POINT ( 'NONE',  ( 18.52753015748617571, 3.092264484334118269, 4.923371831947298993 ) ) ;
#44778=CARTESIAN_POINT ( 'NONE',  ( -2.816281873526471635, 63.91530133659708923, -3.434112377981056508 ) ) ;
#44780=CARTESIAN_POINT ( 'NONE',  ( 12.91533473730993009, 66.60535201082150536, -10.88017736071109987 ) ) ;
#44782=CARTESIAN_POINT ( 'NONE',  ( -4.164238869374098151, 11.59541550158063217, -3.795296366450310543 ) ) ;
#44783=CARTESIAN_POINT ( 'NONE',  ( 19.84674366389459621, 13.50893115100078568, 7.409399052514197653E-17 ) ) ;
#44784=CARTESIAN_POINT ( 'NONE',  ( 7.084665262690076126, 29.10535201082150181, 10.88017736071109987 ) ) ;
#44785=CARTESIAN_POINT ( 'NONE',  ( 2.094539387258905538, 0.2439618909456068852, -6.442855573511589995 ) ) ;
#44786=ORIENTED_EDGE ( 'NONE', *, *, #29437, .F. ) ;
#44788=CARTESIAN_POINT ( 'NONE',  ( 2.035157376598822676, 22.43868534415483396, -7.964842623401177768 ) ) ;
#44789=EDGE_LOOP ( 'NONE', ( #93146, #5550, #3985, #89116 ) ) ;
#44791=CARTESIAN_POINT ( 'NONE',  ( 20.03932841506542673, 55.62161441960502373, -6.397827110479002322 ) ) ;
#44794=CARTESIAN_POINT ( 'NONE',  ( 2.035157376598824452, 68.68868534415484817, 7.964842623401179544 ) ) ;
#44796=CARTESIAN_POINT ( 'NONE',  ( 4.559911319644449179, 17.23035201082150536, -9.422509992056141925 ) ) ;
#44797=CARTESIAN_POINT ( 'NONE',  ( 19.88701968852526747, 6.794273331840863683, 6.480634945678607650 ) ) ;
#44798=CARTESIAN_POINT ( 'NONE',  ( 5.076628168052703671, 1.842264484334118047, 8.527530157486179263 ) ) ;
#44800=CARTESIAN_POINT ( 'NONE',  ( 4.559911319644449179, 18.89701867748817321, 9.422509992056141925 ) ) ;
#44801=EDGE_CURVE ( 'NONE', #52823, #19862, #92387, .T. ) ;
#44803=CARTESIAN_POINT ( 'NONE',  ( 19.38216949554541557, 52.24863466993041072, -9.382169495545420901 ) ) ;
#44804=CARTESIAN_POINT ( 'NONE',  ( 0.5774900079438590739, 37.64701867748817676, -5.440088680355550821 ) ) ;
#44806=CARTESIAN_POINT ( 'NONE',  ( -2.816281873526473856, 49.12363466993042493, 9.499525473075851096E-16 ) ) ;
#44807=CARTESIAN_POINT ( 'NONE',  ( -0.8801773607111009756, 43.06368534415484106, 1.068504757029289695E-15 ) ) ;
#44808=CARTESIAN_POINT ( 'NONE',  ( -2.816281873526473856, 4.331968003263754419, 3.434112377981055619 ) ) ;
#44809=LINE ( 'NONE', #62774, #17967 ) ;
#44810=CARTESIAN_POINT ( 'NONE',  ( 5.076628168052704559, 15.17559781766745175, -8.527530157486179263 ) ) ;
#44812=CARTESIAN_POINT ( 'NONE',  ( 19.38216949554541202, 0.9986346699304200492, 9.382169495545424454 ) ) ;
#44814=CARTESIAN_POINT ( 'NONE',  ( 10.00000000000000000, 41.81368534415484106, -10.88017736071110342 ) ) ;
#44815=CARTESIAN_POINT ( 'NONE',  ( 18.52753015748617571, 48.09226448433412315, 4.923371831947298993 ) ) ;
#44818=CARTESIAN_POINT ( 'NONE',  ( 5.076628168052704559, 10.17559781766745175, -8.527530157486179263 ) ) ;
#44819=CARTESIAN_POINT ( 'NONE',  ( 5.076628168052703671, 66.84226448433412315, 8.527530157486179263 ) ) ;
#44820=EDGE_LOOP ( 'NONE', ( #30886, #46078, #15605, #27115 ) ) ;
#44822=CARTESIAN_POINT ( 'NONE',  ( 12.63842701281683034, 62.46726448433410894, 9.846743663894596210 ) ) ;
#44826=CARTESIAN_POINT ( 'NONE',  ( 15.44008868035555793, 6.397018677488171434, -9.422509992056140149 ) ) ;
#44827=CARTESIAN_POINT ( 'NONE',  ( 1.472469842513823179, 51.42559781766745886, 4.923371831947296329 ) ) ;
#44828=DIRECTION ( 'NONE',  ( -0.000000000000000000, 0.000000000000000000, 1.000000000000000000 ) ) ;
#44830=CARTESIAN_POINT ( 'NONE',  ( 0.5774900079438590739, 2.647018677488171434, -5.440088680355550821 ) ) ;
#44832=CARTESIAN_POINT ( 'NONE',  ( 7.084665262690076126, 19.10535201082150181, 10.88017736071109987 ) ) ;
#44834=CARTESIAN_POINT ( 'NONE',  ( 13.79529636645031943, 55.34541550158062506, -14.16423886937409904 ) ) ;
#44835=CARTESIAN_POINT ( 'NONE',  ( -4.164238869374099927, 67.01208216824728936, 3.795296366450308767 ) ) ;
#44836=CARTESIAN_POINT ( 'NONE',  ( 2.791683348922237240, 5.383931151000785675, -7.208316651077763204 ) ) ;
#44837=CARTESIAN_POINT ( 'NONE',  ( 1.472469842513823179, 25.59226448433412315, -4.923371831947296329 ) ) ;
#44838=CARTESIAN_POINT ( 'NONE',  ( -2.816281873526473856, 14.12363466993041961, 9.499525473075851096E-16 ) ) ;
#44842=CARTESIAN_POINT ( 'NONE',  ( 0.1532563361054083140, 61.00893115100078745, 1.131784320476157264E-15 ) ) ;
#44844=FACE_OUTER_BOUND ( 'NONE', #86255, .T. ) ;
#44845=CARTESIAN_POINT ( 'NONE',  ( 24.16423886937410614, 9.303748834913967869, 8.672049930838204340E-16 ) ) ;
#44846=AXIS2_PLACEMENT_3D ( 'NONE', #6029, #51019, #19054 ) ;
#44847=CARTESIAN_POINT ( 'NONE',  ( 17.20831665107776587, 27.88393115100078390, 7.208316651077764980 ) ) ;
#44848=CARTESIAN_POINT ( 'NONE',  ( 0.2751277870542967463, 0.000000000000000000, 6.500000000000000888 ) ) ;
#44850=CARTESIAN_POINT ( 'NONE',  ( 22.26659068614895176, 34.72041550158063927, -7.082119434687042414 ) ) ;
#44851=CARTESIAN_POINT ( 'NONE',  ( 17.20831665107776587, 12.88393115100078390, 7.208316651077764980 ) ) ;
#44854=CARTESIAN_POINT ( 'NONE',  ( 10.00000000000000000, 31.81368534415483751, -10.88017736071110342 ) ) ;
#44855=CARTESIAN_POINT ( 'NONE',  ( 3.591859063236763294, 43.29030133659708923, -11.09922568453595026 ) ) ;
#44856=CARTESIAN_POINT ( 'NONE',  ( 0.5774900079438590739, 7.647018677488171434, -5.440088680355550821 ) ) ;
#44857=AXIS2_PLACEMENT_3D ( 'NONE', #83259, #59260, #66772 ) ;
#44858=CARTESIAN_POINT ( 'NONE',  ( 21.09922568453594849, 31.20696800326375353, 6.408140936763242479 ) ) ;
#44859=( NAMED_UNIT ( * ) PLANE_ANGLE_UNIT ( ) SI_UNIT ( $, .RADIAN. ) );
#44864=CARTESIAN_POINT ( 'NONE',  ( -0.3689425029237898834, 36.17874883491396787, -10.36894250292378850 ) ) ;
#44865=CARTESIAN_POINT ( 'NONE',  ( 2.035157376598822676, 7.438685344154837509, -7.964842623401177768 ) ) ;
#44866=CARTESIAN_POINT ( 'NONE',  ( 19.42250999205614548, 25.98035201082150891, -5.440088680355545492 ) ) ;
#44869=CARTESIAN_POINT ( 'NONE',  ( 4.559911319644449179, 48.89701867748817676, 9.422509992056141925 ) ) ;
#44870=CARTESIAN_POINT ( 'NONE',  ( 20.88017736071110519, 65.56368534415483396, 2.639326808657452039E-16 ) ) ;
#44871=CARTESIAN_POINT ( 'NONE',  ( 13.43411237798105340, 25.58196800326374998, 12.81628187352647963 ) ) ;
#44874=CARTESIAN_POINT ( 'NONE',  ( 0.1532563361054083140, 26.00893115100078745, 1.131784320476157264E-15 ) ) ;
#44875=CARTESIAN_POINT ( 'NONE',  ( 7.084665262690076126, 57.02201867748817676, -10.88017736071110164 ) ) ;
#44876=EDGE_CURVE ( 'NONE', #35320, #95857, #52789, .T. ) ;
#44877=CARTESIAN_POINT ( 'NONE',  ( 19.38216949554541557, 12.24863466993041961, -9.382169495545420901 ) ) ;
#44878=CARTESIAN_POINT ( 'NONE',  ( 2.791683348922240793, 1.633931151000784565, 7.208316651077764092 ) ) ;
#44879=CARTESIAN_POINT ( 'NONE',  ( 12.91533473730993009, 11.60535201082150536, -10.88017736071109987 ) ) ;
#44880=CARTESIAN_POINT ( 'NONE',  ( 0.1532563361054100626, 35.80059781766745175, -2.638427012816831230 ) ) ;
#44881=CARTESIAN_POINT ( 'NONE',  ( -2.816281873526473856, 59.12363466993042493, 9.499525473075851096E-16 ) ) ;
#44882=CARTESIAN_POINT ( 'NONE',  ( 18.52753015748618282, 13.92559781766745175, -4.923371831947291888 ) ) ;
#44883=CARTESIAN_POINT ( 'NONE',  ( -0.3689425029237898834, 1.178748834913967869, -10.36894250292378850 ) ) ;
#44885=CARTESIAN_POINT ( 'NONE',  ( 15.44008868035555793, 31.39701867748817676, -9.422509992056140149 ) ) ;
#44886=SURFACE_STYLE_FILL_AREA ( #14416 ) ;
#44887=CARTESIAN_POINT ( 'NONE',  ( 2.791683348922240793, 46.63393115100077324, 7.208316651077764092 ) ) ;
#44888=CARTESIAN_POINT ( 'NONE',  ( 0.5774900079438607392, 33.48035201082150536, 5.440088680355550821 ) ) ;
#44889=CARTESIAN_POINT ( 'NONE',  ( 0.5774900079438590739, 12.64701867748817321, -5.440088680355550821 ) ) ;
#44891=VECTOR ( 'NONE', #77807, 1000.000000000000000 ) ;
#44892=CARTESIAN_POINT ( 'NONE',  ( 15.44008868035555793, 31.39701867748817676, -9.422509992056140149 ) ) ;
#44894=CARTESIAN_POINT ( 'NONE',  ( -2.816281873526473856, 49.33196800326374643, 3.434112377981055619 ) ) ;
#44895=CARTESIAN_POINT ( 'NONE',  ( 12.91533473730992121, 49.52201867748817676, 10.88017736071110164 ) ) ;
#44897=CARTESIAN_POINT ( 'NONE',  ( 17.96484262340118221, 41.18868534415484106, -7.964842623401177768 ) ) ;
#44898=ORIENTED_EDGE ( 'NONE', *, *, #9194, .F. ) ;
#44899=CARTESIAN_POINT ( 'NONE',  ( 19.84674366389459266, 58.71726448433411605, -2.638427012816827677 ) ) ;
#44900=CARTESIAN_POINT ( 'NONE',  ( 10.00000000000000000, 41.81368534415484106, -10.88017736071110342 ) ) ;
#44905=CARTESIAN_POINT ( 'NONE',  ( 6.204703633549690345, 45.76208216824729647, -14.16423886937410259 ) ) ;
#44906=CARTESIAN_POINT ( 'NONE',  ( 17.96484262340118221, 51.18868534415483396, -7.964842623401177768 ) ) ;
#44907=PLANE ( 'NONE',  #22190 ) ;
#44908=CARTESIAN_POINT ( 'NONE',  ( 17.20831665107776587, 64.13393115100079456, -7.208316651077762316 ) ) ;
#44910=CARTESIAN_POINT ( 'NONE',  ( 1.472469842513823179, 35.59226448433412315, -4.923371831947296329 ) ) ;
#44912=CARTESIAN_POINT ( 'NONE',  ( 19.84674366389459621, 38.50893115100078745, 7.409399052514197653E-17 ) ) ;
#44914=CARTESIAN_POINT ( 'NONE',  ( 19.42250999205614548, 25.98035201082150891, -5.440088680355545492 ) ) ;
#44915=CARTESIAN_POINT ( 'NONE',  ( 19.84674366389459266, 28.30059781766745886, 2.638427012816836559 ) ) ;
#44916=CARTESIAN_POINT ( 'NONE',  ( 3.591859063236763294, 23.29030133659708568, -11.09922568453595026 ) ) ;
#44918=CARTESIAN_POINT ( 'NONE',  ( 7.084665262690076126, 64.10535201082150536, 10.88017736071109987 ) ) ;
#44919=CARTESIAN_POINT ( 'NONE',  ( 7.084665262690076126, 39.10535201082150536, 10.88017736071109987 ) ) ;
#44920=CARTESIAN_POINT ( 'NONE',  ( 4.559911319644449179, 3.897018677488170990, 9.422509992056141925 ) ) ;
#44921=CARTESIAN_POINT ( 'NONE',  ( 22.26659068614894466, 43.88708216824729647, 7.082119434687054849 ) ) ;
#44925=EDGE_CURVE ( 'NONE', #65472, #83178, #521, .T. ) ;
#44927=CARTESIAN_POINT ( 'NONE',  ( 10.00000000000000000, 17.87363466993041783, -12.81628187352647608 ) ) ;
#44928=CARTESIAN_POINT ( 'NONE',  ( 4.559911319644449179, 7.230352010821504471, -9.422509992056141925 ) ) ;
#44929=CARTESIAN_POINT ( 'NONE',  ( 2.035157376598824452, 53.68868534415484817, 7.964842623401179544 ) ) ;
#44930=AXIS2_PLACEMENT_3D ( 'NONE', #537, #44013, #98041 ) ;
#44932=ORIENTED_EDGE ( 'NONE', *, *, #14425, .T. ) ;
#44933=CARTESIAN_POINT ( 'NONE',  ( 15.44008868035555793, 51.39701867748816966, -9.422509992056140149 ) ) ;
#44935=CARTESIAN_POINT ( 'NONE',  ( 19.84674366389459266, 38.71726448433412315, -2.638427012816827677 ) ) ;
#44937=CARTESIAN_POINT ( 'NONE',  ( 7.361572987183170547, 22.05059781766745530, 9.846743663894590881 ) ) ;
#44938=CARTESIAN_POINT ( 'NONE',  ( 10.00000000000000000, 14.75893115100078568, -9.846743663894594434 ) ) ;
#44940=CARTESIAN_POINT ( 'NONE',  ( 13.43411237798105340, 40.58196800326375353, 12.81628187352647963 ) ) ;
#44941=CARTESIAN_POINT ( 'NONE',  ( 17.20831665107776587, 9.133931151000787452, -7.208316651077762316 ) ) ;
#44944=CARTESIAN_POINT ( 'NONE',  ( 14.92337183194729988, 34.34226448433411605, -8.527530157486177487 ) ) ;
#44946=CARTESIAN_POINT ( 'NONE',  ( 3.591859063236761518, 59.95696800326375353, 11.09922568453594849 ) ) ;
#44948=CARTESIAN_POINT ( 'NONE',  ( 6.565887622018943937, 15.16530133659708568, 12.81628187352647430 ) ) ;
#44950=CARTESIAN_POINT ( 'NONE',  ( 7.084665262690076126, 52.02201867748816255, -10.88017736071110164 ) ) ;
#44951=CARTESIAN_POINT ( 'NONE',  ( 13.79529636645031943, 35.34541550158063927, -14.16423886937409904 ) ) ;
#44952=CARTESIAN_POINT ( 'NONE',  ( 2.377183314879979026, 40.78593319516822646, -6.500000000000005329 ) ) ;
#44954=CARTESIAN_POINT ( 'NONE',  ( -2.266590686148945544, 32.22041550158063927, 7.082119434687048631 ) ) ;
#44956=CARTESIAN_POINT ( 'NONE',  ( 6.204703633549690345, 50.76208216824730357, -14.16423886937410259 ) ) ;
#44957=CARTESIAN_POINT ( 'NONE',  ( 2.917880565312948704, 7.637082168247301794, 12.26659068614894643 ) ) ;
#44958=CARTESIAN_POINT ( 'NONE',  ( 10.00000000000000000, 15.55374883491396787, -14.16423886937410082 ) ) ;
#44960=CARTESIAN_POINT ( 'NONE',  ( 2.035157376598824452, 48.68868534415483396, 7.964842623401179544 ) ) ;
#44962=CARTESIAN_POINT ( 'NONE',  ( 12.63842701281683922, 24.55059781766745175, -9.846743663894590881 ) ) ;
#44963=CARTESIAN_POINT ( 'NONE',  ( 4.559911319644449179, 68.89701867748817676, 9.422509992056141925 ) ) ;
#44964=CARTESIAN_POINT ( 'NONE',  ( 0.1532563361054082862, 31.21726448433412315, 2.638427012816831674 ) ) ;
#44966=CARTESIAN_POINT ( 'NONE',  ( 4.559911319644449179, 28.89701867748817321, 9.422509992056141925 ) ) ;
#44967=CARTESIAN_POINT ( 'NONE',  ( 21.09922568453594849, 61.20696800326376064, 6.408140936763242479 ) ) ;
#44968=CARTESIAN_POINT ( 'NONE',  ( 17.20831665107776587, 64.13393115100079456, -7.208316651077762316 ) ) ;
#44970=CARTESIAN_POINT ( 'NONE',  ( 16.40814093676323893, 35.79030133659708923, 11.09922568453595026 ) ) ;
#44972=CARTESIAN_POINT ( 'NONE',  ( 10.00000000000000000, 41.81368534415484106, -10.88017736071110342 ) ) ;
#44973=CARTESIAN_POINT ( 'NONE',  ( 14.92337183194729988, 54.34226448433412315, -8.527530157486177487 ) ) ;
#44975=CARTESIAN_POINT ( 'NONE',  ( -4.164238869374098151, 21.59541550158063217, -3.795296366450310543 ) ) ;
#44977=CARTESIAN_POINT ( 'NONE',  ( -0.3689425029237898834, 1.178748834913967869, -10.36894250292378850 ) ) ;
#44978=CARTESIAN_POINT ( 'NONE',  ( 20.88017736071110875, 65.77201867748817676, -2.915334737309920765 ) ) ;
#44979=CARTESIAN_POINT ( 'NONE',  ( 24.16423886937410614, 64.51208216824728936, -3.795296366450302550 ) ) ;
#44980=CARTESIAN_POINT ( 'NONE',  ( 21.09922568453594849, 1.206968003263753531, 6.408140936763242479 ) ) ;
#44982=CARTESIAN_POINT ( 'NONE',  ( -0.8801773607111009756, 53.06368534415484106, 1.068504757029289695E-15 ) ) ;
#44984=CARTESIAN_POINT ( 'NONE',  ( 2.917880565312950480, 55.97041550158063217, -12.26659068614894821 ) ) ;
#44986=CARTESIAN_POINT ( 'NONE',  ( 12.91533473730993009, 11.60535201082150536, -10.88017736071109987 ) ) ;
#44987=CARTESIAN_POINT ( 'NONE',  ( 2.035157376598824452, 18.68868534415484106, 7.964842623401179544 ) ) ;
#44988=CARTESIAN_POINT ( 'NONE',  ( 14.92337183194729633, 62.67559781766745886, 8.527530157486181039 ) ) ;
#44989=CARTESIAN_POINT ( 'NONE',  ( 19.38216949554541202, 55.99863466993041072, 9.382169495545424454 ) ) ;
#44992=CARTESIAN_POINT ( 'NONE',  ( 15.44008868035555260, 19.73035201082150536, 9.422509992056143702 ) ) ;
#44994=CARTESIAN_POINT ( 'NONE',  ( 19.38216949554541557, 17.24863466993041783, -9.382169495545420901 ) ) ;
#44996=VECTOR ( 'NONE', #8019, 1000.000000000000000 ) ;
#44997=( GEOMETRIC_REPRESENTATION_CONTEXT ( 3 ) GLOBAL_UNCERTAINTY_ASSIGNED_CONTEXT ( ( #17481 ) ) GLOBAL_UNIT_ASSIGNED_CONTEXT ( ( #34309, #26826, #57811 ) ) REPRESENTATION_CONTEXT ( 'NONE', 'WORKASPACE' ) );
#44998=CARTESIAN_POINT ( 'NONE',  ( 2.791683348922237240, 45.38393115100079456, -7.208316651077763204 ) ) ;
#44999=CARTESIAN_POINT ( 'NONE',  ( 7.084665262690076126, 39.10535201082150536, 10.88017736071109987 ) ) ;
#45000=CARTESIAN_POINT ( 'NONE',  ( 6.565887622018943937, 23.08196800326375708, -12.81628187352647608 ) ) ;
#45001=CARTESIAN_POINT ( 'NONE',  ( -0.8801773607110991993, 42.85535201082150536, -2.915334737309923874 ) ) ;
#45003=DIRECTION ( 'NONE',  ( 1.000000000000000000, 0.000000000000000000, 0.000000000000000000 ) ) ;
#45004=CARTESIAN_POINT ( 'NONE',  ( 6.565887622018943937, 48.08196800326375353, -12.81628187352647608 ) ) ;
#45005=VERTEX_POINT ( 'NONE', #70962 ) ;
#45006=CARTESIAN_POINT ( 'NONE',  ( 20.88017736071110164, 45.35535201082149115, 2.915334737309930979 ) ) ;
#45007=CARTESIAN_POINT ( 'NONE',  ( 10.00000000000000178, 35.37363466993042493, 12.81628187352647608 ) ) ;
#45008=CARTESIAN_POINT ( 'NONE',  ( 6.204703633549690345, 5.762082168247301794, -14.16423886937410259 ) ) ;
#45009=CARTESIAN_POINT ( 'NONE',  ( 20.88017736071110875, 45.77201867748816966, -2.915334737309920765 ) ) ;
#45010=CARTESIAN_POINT ( 'NONE',  ( 18.52753015748618282, 63.92559781766745886, -4.923371831947291888 ) ) ;
#45012=CARTESIAN_POINT ( 'NONE',  ( 18.52753015748617571, 23.09226448433411960, 4.923371831947298993 ) ) ;
#45013=CARTESIAN_POINT ( 'NONE',  ( 18.52753015748617571, 13.09226448433411960, 4.923371831947298993 ) ) ;
#45015=CARTESIAN_POINT ( 'NONE',  ( 20.36894250292379738, 49.92874883491396787, -10.36894250292379027 ) ) ;
#45016=AXIS2_PLACEMENT_3D ( 'NONE', #34606, #49608, #18645 ) ;
#45017=CARTESIAN_POINT ( 'NONE',  ( 20.00000000000000711, 79.40087001978915282, 4.500000000000000888 ) ) ;
#45021=CARTESIAN_POINT ( 'NONE',  ( -4.164238869374099927, 67.01208216824728936, 3.795296366450308767 ) ) ;
#45022=CARTESIAN_POINT ( 'NONE',  ( 24.16423886937410614, 59.51208216824728936, -3.795296366450302550 ) ) ;
#45023=CARTESIAN_POINT ( 'NONE',  ( 1.472469842513823179, 36.42559781766745175, 4.923371831947296329 ) ) ;
#45024=CARTESIAN_POINT ( 'NONE',  ( 10.00000000000000178, 45.37363466993041783, 12.81628187352647608 ) ) ;
#45026=CARTESIAN_POINT ( 'NONE',  ( 10.00000000000000000, 10.55374883491396787, -14.16423886937410082 ) ) ;
#45027=CARTESIAN_POINT ( 'NONE',  ( 17.96484262340118221, 16.18868534415483396, -7.964842623401177768 ) ) ;
#45028=CARTESIAN_POINT ( 'NONE',  ( 2.917880565312948704, 62.63708216824730357, 12.26659068614894643 ) ) ;
#45029=CARTESIAN_POINT ( 'NONE',  ( 5.076628168052703671, 46.84226448433412315, 8.527530157486179263 ) ) ;
#45030=DIRECTION ( 'NONE',  ( 1.000000000000000000, 0.000000000000000000, 0.000000000000000000 ) ) ;
#45031=CARTESIAN_POINT ( 'NONE',  ( 7.361572987183170547, 27.05059781766745175, 9.846743663894590881 ) ) ;
#45035=EDGE_LOOP ( 'NONE', ( #80700, #47656, #13156, #37967 ) ) ;
#45036=SURFACE_STYLE_FILL_AREA ( #15069 ) ;
#45039=CARTESIAN_POINT ( 'NONE',  ( 6.204703633549690345, 20.76208216824730357, -14.16423886937410259 ) ) ;
#45040=CARTESIAN_POINT ( 'NONE',  ( 19.42250999205614548, 35.98035201082151247, -5.440088680355545492 ) ) ;
#45041=CARTESIAN_POINT ( 'NONE',  ( 7.084665262690076126, 42.02201867748816966, -10.88017736071110164 ) ) ;
#45042=CARTESIAN_POINT ( 'NONE',  ( 18.52753015748617571, 58.09226448433411605, 4.923371831947298993 ) ) ;
#45043=CARTESIAN_POINT ( 'NONE',  ( 6.565887622018943937, 35.16530133659708923, 12.81628187352647430 ) ) ;
#45044=CARTESIAN_POINT ( 'NONE',  ( 24.16423886937410614, 9.303748834913967869, 8.672049930838204340E-16 ) ) ;
#45047=CARTESIAN_POINT ( 'NONE',  ( 3.591859063236763294, 33.29030133659708213, -11.09922568453595026 ) ) ;
#45049=VERTEX_POINT ( 'NONE', #71452 ) ;
#45050=CARTESIAN_POINT ( 'NONE',  ( 12.63842701281683034, 47.46726448433412315, 9.846743663894596210 ) ) ;
#45051=CARTESIAN_POINT ( 'NONE',  ( 10.00000000000000178, 4.313685344154837509, 10.88017736071110342 ) ) ;
#45053=CARTESIAN_POINT ( 'NONE',  ( 2.035157376598822676, 12.43868534415483751, -7.964842623401177768 ) ) ;
#45055=CARTESIAN_POINT ( 'NONE',  ( 19.42250999205614548, 65.98035201082151957, -5.440088680355545492 ) ) ;
#45056=CARTESIAN_POINT ( 'NONE',  ( 17.96484262340118221, 56.18868534415484817, -7.964842623401177768 ) ) ;
#45057=CARTESIAN_POINT ( 'NONE',  ( 17.96484262340118221, 66.18868534415483396, -7.964842623401177768 ) ) ;
#45059=CARTESIAN_POINT ( 'NONE',  ( 15.44008868035555260, 54.73035201082150536, 9.422509992056143702 ) ) ;
#45061=CARTESIAN_POINT ( 'NONE',  ( -46.94000000000001194, 100.6164469615930841, 8.719320056954199316 ) ) ;
#45062=LINE ( 'NONE', #7084, #75855 ) ;
#45066=CARTESIAN_POINT ( 'NONE',  ( 5.076628168052704559, 45.17559781766745175, -8.527530157486179263 ) ) ;
#45070=MECHANICAL_DESIGN_GEOMETRIC_PRESENTATION_REPRESENTATION('',(#80191),#92961);
#45073=COLOUR_RGB ( '', 0.72549020, 0.75294118, 0.79215686) ;
#45074=CARTESIAN_POINT ( 'NONE',  ( 17.08211943468705840, 5.137082168247300906, -12.26659068614894466 ) ) ;
#45077=CARTESIAN_POINT ( 'NONE',  ( 17.96484262340118221, 11.18868534415484106, -7.964842623401177768 ) ) ;
#45079=CARTESIAN_POINT ( 'NONE',  ( 22.81628187352647785, 46.41530133659708213, 3.434112377981063169 ) ) ;
#45081=CARTESIAN_POINT ( 'NONE',  ( 19.88565890683628723, 62.71691075486300804, -6.480892540919839462 ) ) ;
#45082=CARTESIAN_POINT ( 'NONE',  ( 0.1532563361054082862, 46.21726448433411605, 2.638427012816831674 ) ) ;
#45084=CARTESIAN_POINT ( 'NONE',  ( 10.00000000000000178, 20.37363466993042138, 12.81628187352647608 ) ) ;
#45085=CARTESIAN_POINT ( 'NONE',  ( 2.791683348922237240, 25.38393115100078390, -7.208316651077763204 ) ) ;
#45087=CARTESIAN_POINT ( 'NONE',  ( 16.40814093676324603, 2.456968003263753531, -11.09922568453594671 ) ) ;
#45091=CARTESIAN_POINT ( 'NONE',  ( 17.96484262340118221, 19.93868534415484106, 7.964842623401181321 ) ) ;
#45092=CARTESIAN_POINT ( 'NONE',  ( 6.204703633549690345, 20.76208216824730357, -14.16423886937410259 ) ) ;
#45093=CARTESIAN_POINT ( 'NONE',  ( 14.92337183194729988, 29.34226448433411960, -8.527530157486177487 ) ) ;
#45094=CARTESIAN_POINT ( 'NONE',  ( 10.00000000000000000, -0.2410688489992152128, -9.846743663894594434 ) ) ;
#45095=CARTESIAN_POINT ( 'NONE',  ( 10.00000000000000000, 37.87363466993041783, -12.81628187352647608 ) ) ;
#45096=CARTESIAN_POINT ( 'NONE',  ( 10.00000000000000000, 11.81368534415483751, -10.88017736071110342 ) ) ;
#45099=CARTESIAN_POINT ( 'NONE',  ( 19.38216949554541557, 7.248634669930421381, -9.382169495545420901 ) ) ;
#45100=CARTESIAN_POINT ( 'NONE',  ( 19.84674366389459266, 23.30059781766745530, 2.638427012816836559 ) ) ;
#45102=CARTESIAN_POINT ( 'NONE',  ( 16.40814093676324603, 32.45696800326375353, -11.09922568453594671 ) ) ;
#45104=CARTESIAN_POINT ( 'NONE',  ( -0.8801773607110991993, 37.85535201082151247, -2.915334737309923874 ) ) ;
#45105=DIRECTION ( 'NONE',  ( 0.000000000000000000, 1.000000000000000000, 0.000000000000000000 ) ) ;
#45107=CARTESIAN_POINT ( 'NONE',  ( 19.72487221294571569, 20.71833443783938122, -6.499999999999990230 ) ) ;
#45108=CARTESIAN_POINT ( 'NONE',  ( 17.96484262340118221, 41.18868534415484106, -7.964842623401177768 ) ) ;
#45110=CARTESIAN_POINT ( 'NONE',  ( 4.559911319644449179, 47.23035201082150536, -9.422509992056141925 ) ) ;
#45111=CARTESIAN_POINT ( 'NONE',  ( 7.361572987183170547, 62.05059781766745886, 9.846743663894590881 ) ) ;
#45112=CARTESIAN_POINT ( 'NONE',  ( 17.96484262340118221, 61.18868534415482685, -7.964842623401177768 ) ) ;
#45113=CARTESIAN_POINT ( 'NONE',  ( 2.791683348922240793, 56.63393115100078035, 7.208316651077764092 ) ) ;
#45114=CARTESIAN_POINT ( 'NONE',  ( 19.42250999205614193, 5.147018677488171434, 5.440088680355555262 ) ) ;
#45116=CARTESIAN_POINT ( 'NONE',  ( 6.565887622018943937, 8.081968003263751754, -12.81628187352647608 ) ) ;
#45118=CARTESIAN_POINT ( 'NONE',  ( 0.5774900079438590739, 22.64701867748817321, -5.440088680355550821 ) ) ;
#45120=CARTESIAN_POINT ( 'NONE',  ( 12.91533473730992121, 4.522018677488169658, 10.88017736071110164 ) ) ;
#45121=CARTESIAN_POINT ( 'NONE',  ( 7.084665262690076126, 34.10535201082151247, 10.88017736071109987 ) ) ;
#45122=CARTESIAN_POINT ( 'NONE',  ( 19.42250999205614548, 65.98035201082151957, -5.440088680355545492 ) ) ;
#45123=CARTESIAN_POINT ( 'NONE',  ( -4.164238869374099039, 31.80374883491396432, 8.674139862899312516E-16 ) ) ;
#45125=CARTESIAN_POINT ( 'NONE',  ( 0.1532563361054100626, 25.80059781766744820, -2.638427012816831230 ) ) ;
#45126=CARTESIAN_POINT ( 'NONE',  ( 15.44008868035555260, 44.73035201082151247, 9.422509992056143702 ) ) ;
#45128=CARTESIAN_POINT ( 'NONE',  ( -2.266590686148945544, 7.220415501580634832, 7.082119434687048631 ) ) ;
#45130=EDGE_LOOP ( 'NONE', ( #50171, #66076, #5324, #75641 ) ) ;
#45133=CARTESIAN_POINT ( 'NONE',  ( 5.076628168052703671, 56.84226448433412315, 8.527530157486179263 ) ) ;
#45136=CARTESIAN_POINT ( 'NONE',  ( 22.26659068614895176, 24.72041550158063572, -7.082119434687042414 ) ) ;
#45137=CARTESIAN_POINT ( 'NONE',  ( 10.00000000000000178, 23.05374883491397142, 14.16423886937410082 ) ) ;
#45138=CARTESIAN_POINT ( 'NONE',  ( 19.42250999205614548, 65.98035201082151957, -5.440088680355545492 ) ) ;
#45139=CARTESIAN_POINT ( 'NONE',  ( 17.08211943468705840, 65.13708216824730357, -12.26659068614894466 ) ) ;
#45140=CARTESIAN_POINT ( 'NONE',  ( 7.361572987183170547, 52.05059781766745175, 9.846743663894590881 ) ) ;
#45142=CARTESIAN_POINT ( 'NONE',  ( 12.91533473730993009, 51.60535201082149825, -10.88017736071109987 ) ) ;
#45143=CARTESIAN_POINT ( 'NONE',  ( -1.099225684535947600, 14.54030133659708568, 6.408140936763237150 ) ) ;
#45144=CARTESIAN_POINT ( 'NONE',  ( 13.79529636645030344, 18.26208216824730002, 14.16423886937410614 ) ) ;
#45145=CARTESIAN_POINT ( 'NONE',  ( 4.559911319644449179, 17.23035201082150536, -9.422509992056141925 ) ) ;
#45147=AXIS2_PLACEMENT_3D ( 'NONE', #23206, #15214, #74197 ) ;
#45148=CARTESIAN_POINT ( 'NONE',  ( 0.5774900079438607392, 23.48035201082150536, 5.440088680355550821 ) ) ;
#45149=CARTESIAN_POINT ( 'NONE',  ( -1.926860441876562247, 2.453790035174471473, -3.195792623639530650 ) ) ;
#45150=CARTESIAN_POINT ( 'NONE',  ( 7.084665262690076126, 52.02201867748816255, -10.88017736071110164 ) ) ;
#45158=DIRECTION ( 'NONE',  ( -0.000000000000000000, -0.000000000000000000, 1.000000000000000000 ) ) ;
#45160=DIRECTION ( 'NONE',  ( 0.000000000000000000, -1.000000000000000000, 0.000000000000000000 ) ) ;
#45161=CARTESIAN_POINT ( 'NONE',  ( 17.08211943468705840, 65.13708216824730357, -12.26659068614894466 ) ) ;
#45162=CARTESIAN_POINT ( 'NONE',  ( 20.36894250292379382, 58.67874883491396076, 10.36894250292379205 ) ) ;
#45163=CARTESIAN_POINT ( 'NONE',  ( 0.1532563361054083140, 26.00893115100078745, 1.131784320476157264E-15 ) ) ;
#45164=CARTESIAN_POINT ( 'NONE',  ( 5.076628168052703671, 61.84226448433412315, 8.527530157486179263 ) ) ;
#45165=CARTESIAN_POINT ( 'NONE',  ( 20.32896413005680714, 50.57879003517447103, -5.963430220938276349 ) ) ;
#45166=CARTESIAN_POINT ( 'NONE',  ( 19.72487221294571214, 44.78217586085236945, 6.499999999999993783 ) ) ;
#45167=CARTESIAN_POINT ( 'NONE',  ( 17.96484262340118221, 66.18868534415483396, -7.964842623401177768 ) ) ;
#45172=CARTESIAN_POINT ( 'NONE',  ( 22.26659068614894466, 38.88708216824731068, 7.082119434687054849 ) ) ;
#45174=CARTESIAN_POINT ( 'NONE',  ( -4.164238869374099927, 37.01208216824731068, 3.795296366450308767 ) ) ;
#45177=CARTESIAN_POINT ( 'NONE',  ( 21.09922568453595559, 52.04030133659708923, -6.408140936763230044 ) ) ;
#45178=CARTESIAN_POINT ( 'NONE',  ( 10.00000000000000178, 24.31368534415484106, 10.88017736071110342 ) ) ;
#45179=CARTESIAN_POINT ( 'NONE',  ( 1.472469842513823179, 45.59226448433412315, -4.923371831947296329 ) ) ;
#45180=CARTESIAN_POINT ( 'NONE',  ( 10.00000000000000000, 31.81368534415483751, -10.88017736071110342 ) ) ;
#45181=( BOUNDED_CURVE ( )  B_SPLINE_CURVE ( 2, ( #14206, #75182, #82025, #51034, #89038, #97061, #19557, #13535, #43049 ),
 .UNSPECIFIED., .F., .T. ) 
 B_SPLINE_CURVE_WITH_KNOTS ( ( 3, 2, 2, 2, 3 ),
 ( 0.4758552226545170183, 0.4761904761904762196, 0.4821428571428571508, 0.4880952380952381375, 0.4884304916311972833 ),
 .UNSPECIFIED. ) 
 CURVE ( )  GEOMETRIC_REPRESENTATION_ITEM ( )  RATIONAL_B_SPLINE_CURVE ( ( 0.9963778908391753841, 0.9980808541467917072, 1.000000000000000000, 0.9659258262890683122, 1.000000000000000000, 0.9659258262890683122, 1.000000000000000000, 0.9980808541467920403, 0.9963778908391759392 ) ) 
 REPRESENTATION_ITEM ( '' )  );
#45182=CARTESIAN_POINT ( 'NONE',  ( 16.40814093676323893, 60.79030133659709634, 11.09922568453595026 ) ) ;
#45184=CARTESIAN_POINT ( 'NONE',  ( 14.92337183194729633, 57.67559781766745886, 8.527530157486181039 ) ) ;
#45185=CARTESIAN_POINT ( 'NONE',  ( 18.52753015748617571, 53.09226448433412315, 4.923371831947298993 ) ) ;
#45186=( BOUNDED_SURFACE ( )  B_SPLINE_SURFACE ( 1, 2, ( 
 ( #97100, #66571, #68060, #90056, #13569, #37073, #75553, #89568, #28571, #14577, #30039, #52067, #20586, #60047, #74561, #83554, #76043, #90545, #21077, #15077, #82061, #60547, #51071, #51575, #7069, #97592, #45546, #53038, #6077, #29052, #81563, #44056, #21579, #43562, #75054, #37569, #22077, #82562, #14078, #68554, #44558, #52552, #45044, #83056, #91040, #22569, #38062, #28070, #58567, #89072, #13070, #74060, #5593, #36070, #54513, #39042, #31999, #85026, #93008, #47016, #78507, #91546, #46527, #85521, #31517, #53532, #61034, #69046, #31025, #23561, #84046, #580, #61521, #55518, #25032, #9518, #69536, #70029, #24041, #1049, #10020, #54029, #30533, #23063, #86017, #38551, #62505, #84541, #92031, #2045, #16038, #8051, #40018, #77506, #55003, #17530, #47997, #40521, #15566, #46050, #86, #17032, #47510, #62016, #76536, #9020, #92516, #70522, #78011, #32506, #16539, #77027, #8541, #39537, #1553, #24542, #63004, #93506, #48491, #11480, #49967, #2540, #41012, #41997, #63498, #25524, #10499, #49468, #32996, #64951, #19477, #65452, #3026, #48983, #27460, #72958, #33474, #72461, #94973, #78994, #79492, #88460, #95479, #3995, #34460, #80473, #71512, #19961, #50456, #26967, #57468, #79974, #80962, #42474, #87961, #12462, #11971, #71018, #4487, #34954, #95977, #63971, #57953, #33961, #26475, #94000, #86986, #10992, #56010, #94483, #87476, #86514, #18011, #26001, #56496, #18495, #41513, #71979, #3504, #18991, #64466, #56973, #42967, #82933, #44433, #35947, #51451, #43445, #96477, #60421, #13447, #83430, #73448, #81449, #28929, #81937, #14451, #65950, #59926, #21452, #75429, #66443, #29916, #51949, #89935, #50954, #90915, #5475, #44921, #6943, #96977, #97965, #20963, #28451, #12950, #97464, #27950, #73946, #59433, #29421, #58442, #90414, #89450, #74936, #37449, #36947, #74431, #98461, #21956, #22445, #52435, #52918, #6437, #67940, #4974, #67446, #20465, #36452, #43934, #5959, #58948, #66944, #35454, #82434, #13959, #88956, #76899, #455, #92396, #62377, #76417, #53410, #1427, #54882, #38920, #7446, #16415, #61399, #70400, #62883, #23921, #83918, #1919, #68926, #46410, #15447, #15920, #929, #46892, #69408, #32378, #77383, #45928, #69907, #8896, #98956, #8414, #93380, #16907, #7932, #84902, #31391, #22943, #23435, #24907, #39412, #31880, #92883, #24416, #38428, #55390, #14949, #85394, #37944, #30905, #47382, #53914, #45418, #39897, #91910, #84423, #68434, #61891, #54390, #30412, #77881, #9393, #75922, #60913, #91417, #27337, #71863, #26356, #3872, #48370, #94362, #18380, #10875, #34336, #64345, #71391, #64832, #42358, #95350, #17886 ),
 ( #11356, #86384, #3375, #72833, #85891, #26848, #57344, #80352, #78377, #34836, #87357, #33836, #25881, #56857, #17405, #87838, #18871, #78875, #56382, #10383, #40402, #4371, #86871, #47873, #9898, #25401, #94855, #48859, #19356, #70896, #49840, #49352, #11849, #40888, #65329, #79855, #41876, #93875, #95855, #2904, #2413, #32872, #33354, #72340, #63850, #79368, #55887, #41397, #63371, #96358, #43813, #13829, #12341, #74812, #5353, #89811, #90294, #51821, #89328, #14328, #36826, #6816, #6318, #37332, #21332, #44310, #19840, #82307, #35330, #51326, #27829, #97342, #50329, #42846, #58315, #36326, #88342, #67317, #97842, #52314, #88831, #35831, #44800, #59802, #20342, #28815, #81810, #65824, #66317, #75304, #29307, #59313, #21831, #82806, #50839, #67822, #98338, #57833, #80841, #81332, #73330, #96853, #4856, #12828, #28329, #58819, #43326, #73819, #20838, #13329, #5833, #74308, #66819, #84309, #68807, #70285, #15809, #69296, #46776, #91291, #38310, #61285, #53794, #77269, #8298, #15325, #8780, #85280, #39297, #60791, #46294, #337, #61771, #76782, #23809, #38797, #9276, #22326, #76298, #16295, #91794, #83304, #90800, #98834, #22813, #53294, #14829, #30288, #83802, #16786, #54761, #69788, #30781, #817, #31271, #23314, #39786, #45807, #60307, #52801, #47261, #68314, #92286, #7815, #54270, #31768, #84786, #37821, #1317, #62262, #92768, #77761, #29796, #45305, #75800, #7318, #24295, #88584, #58080, #72589, #62758, #50098, #42123, #73574, #20092, #50596, #95604, #11120, #89083, #95097, #4123, #93262, #27590, #24786, #79618, #42604, #81088, #32256, #35080, #35590, #96106, #34586, #58581, #12589, #51084, #43089, #81575, #65579, #5099, #55261, #66078, #41638, #27090, #80101, #65080, #72104, #57102, #96606, #3631, #34098, #28083, #57593, #87598, #80603, #20597, #64589, #26605, #13082, #43577, #88090, #85776, #4618, #49588, #1801, #17286, #12101, #19109, #49117, #11606, #19603, #73082, #75067, #60057, #7079, #29552, #30544, #37581, #44066, #30051, #68074, #59073, #67584, #75566, #98601, #52562, #53545, #45559, #14587, #91557, #83568, #23076, #45056, #83067, #91051, #13582, #76057, #37085, #98093, #60560, #90066, #14088, #22578, #74573, #90558, #61044, #74070, #15088, #53049, #68566, #66584, #84058, #7586, #22087, #82574, #38075, #5602, #97, #15579, #67077, #44568, #6087, #28582, #36081, #6573, #97111, #89577, #36589, #21088, #51586, #82072, #97604, #29065, #59573, #21590, #52081, #55527, #39551, #70040, #92044, #86024, #46539, #40030, #70532, #77040, #85531, #1065, #16051, #23572, #47026, #592, #54041, #77517, #17043, #69056, #47522 ) ),
 .UNSPECIFIED., .F., .F., .T. ) 
 B_SPLINE_SURFACE_WITH_KNOTS ( ( 2, 2 ),
 ( 3, 2, 2, 2, 2, 2, 2, 2, 2, 2, 2, 2, 2, 2, 2, 2, 2, 2, 2, 2, 2, 2, 2, 2, 2, 2, 2, 2, 2, 2, 2, 2, 2, 2, 2, 2, 2, 2, 2, 2, 2, 2, 2, 2, 2, 2, 2, 2, 2, 2, 2, 2, 2, 2, 2, 2, 2, 2, 2, 2, 2, 2, 2, 2, 2, 2, 2, 2, 2, 2, 2, 2, 2, 2, 2, 2, 2, 2, 2, 2, 2, 2, 2, 2, 2, 2, 2, 2, 2, 2, 2, 2, 2, 2, 2, 2, 2, 2, 2, 2, 2, 2, 2, 2, 2, 2, 2, 2, 2, 2, 2, 2, 2, 2, 2, 2, 2, 2, 2, 2, 2, 2, 2, 2, 2, 2, 2, 2, 2, 2, 2, 2, 2, 2, 2, 2, 2, 2, 2, 2, 2, 2, 2, 2, 2, 2, 2, 2, 2, 2, 2, 2, 2, 2, 2, 2, 2, 2, 2, 2, 2, 2, 3 ),
 ( 0.000000000000000000, 1.000000000000000000 ),
 ( 0.000000000000000000, 0.005952380952380952051, 0.01190476190476190410, 0.01785714285714285615, 0.02380952380952380820, 0.02976190476190476025, 0.03571428571428571230, 0.04166666666666666435, 0.04761904761904761640, 0.05357142857142856845, 0.05952380952380952051, 0.06547619047619047949, 0.07142857142857142461, 0.07738095238095238360, 0.08333333333333332871, 0.08928571428571428770, 0.09523809523809523281, 0.1011904761904761918, 0.1071428571428571369, 0.1130952380952380959, 0.1190476190476190410, 0.1250000000000000000, 0.1309523809523809590, 0.1369047619047619180, 0.1428571428571428492, 0.1488095238095238082, 0.1547619047619047672, 0.1607142857142857262, 0.1666666666666666574, 0.1726190476190476164, 0.1785714285714285754, 0.1845238095238095344, 0.1904761904761904656, 0.1964285714285714246, 0.2023809523809523836, 0.2083333333333333426, 0.2142857142857142738, 0.2202380952380952328, 0.2261904761904761918, 0.2321428571428571508, 0.2380952380952380820, 0.2440476190476190410, 0.2500000000000000000, 0.2559523809523809312, 0.2619047619047619180, 0.2678571428571428492, 0.2738095238095238360, 0.2797619047619047672, 0.2857142857142856984, 0.2916666666666666852, 0.2976190476190476164, 0.3035714285714285476, 0.3095238095238095344, 0.3154761904761904656, 0.3214285714285714524, 0.3273809523809523836, 0.3333333333333333148, 0.3392857142857143016, 0.3452380952380952328, 0.3511904761904761640, 0.3571428571428571508, 0.3630952380952380820, 0.3690476190476190688, 0.3750000000000000000, 0.3809523809523809312, 0.3869047619047619180, 0.3928571428571428492, 0.3988095238095238360, 0.4047619047619047672, 0.4107142857142856984, 0.4166666666666666852, 0.4226190476190476164, 0.4285714285714285476, 0.4345238095238095344, 0.4404761904761904656, 0.4464285714285714524, 0.4523809523809523836, 0.4583333333333333148, 0.4642857142857143016, 0.4702380952380952328, 0.4761904761904761640, 0.4821428571428571508, 0.4880952380952380820, 0.4940476190476190688, 0.5000000000000000000, 0.5059523809523809312, 0.5119047619047618625, 0.5178571428571429047, 0.5238095238095238360, 0.5297619047619047672, 0.5357142857142856984, 0.5416666666666666297, 0.5476190476190476719, 0.5535714285714286031, 0.5595238095238095344, 0.5654761904761904656, 0.5714285714285713969, 0.5773809523809523281, 0.5833333333333333703, 0.5892857142857143016, 0.5952380952380952328, 0.6011904761904761640, 0.6071428571428570953, 0.6130952380952381375, 0.6190476190476190688, 0.6250000000000000000, 0.6309523809523809312, 0.6369047619047618625, 0.6428571428571429047, 0.6488095238095238360, 0.6547619047619047672, 0.6607142857142856984, 0.6666666666666666297, 0.6726190476190476719, 0.6785714285714286031, 0.6845238095238095344, 0.6904761904761904656, 0.6964285714285713969, 0.7023809523809523281, 0.7083333333333333703, 0.7142857142857143016, 0.7202380952380952328, 0.7261904761904761640, 0.7321428571428570953, 0.7380952380952381375, 0.7440476190476190688, 0.7500000000000000000, 0.7559523809523809312, 0.7619047619047618625, 0.7678571428571429047, 0.7738095238095238360, 0.7797619047619047672, 0.7857142857142856984, 0.7916666666666666297, 0.7976190476190476719, 0.8035714285714286031, 0.8095238095238095344, 0.8154761904761904656, 0.8214285714285713969, 0.8273809523809523281, 0.8333333333333333703, 0.8392857142857143016, 0.8452380952380952328, 0.8511904761904761640, 0.8571428571428570953, 0.8630952380952381375, 0.8690476190476190688, 0.8750000000000000000, 0.8809523809523809312, 0.8869047619047618625, 0.8928571428571429047, 0.8988095238095238360, 0.9047619047619047672, 0.9107142857142856984, 0.9166666666666666297, 0.9226190476190476719, 0.9285714285714286031, 0.9345238095238095344, 0.9404761904761904656, 0.9464285714285713969, 0.9523809523809523281, 0.9583333333333333703, 0.9642857142857143016 ),
 .UNSPECIFIED. ) 
 GEOMETRIC_REPRESENTATION_ITEM ( )  RATIONAL_B_SPLINE_SURFACE ( (
 ( 1.000000000000000000, 0.9659258262890683122, 1.000000000000000000, 0.9659258262890683122, 1.000000000000000000, 0.9659258262890683122, 1.000000000000000000, 0.9659258262890683122, 1.000000000000000000, 0.9659258262890683122, 1.000000000000000000, 0.9659258262890683122, 1.000000000000000000, 0.9659258262890683122, 1.000000000000000000, 0.9659258262890683122, 1.000000000000000000, 0.9659258262890683122, 1.000000000000000000, 0.9659258262890683122, 1.000000000000000000, 0.9659258262890683122, 1.000000000000000000, 0.9659258262890683122, 1.000000000000000000, 0.9659258262890683122, 1.000000000000000000, 0.9659258262890683122, 1.000000000000000000, 0.9659258262890683122, 1.000000000000000000, 0.9659258262890683122, 1.000000000000000000, 0.9659258262890683122, 1.000000000000000000, 0.9659258262890683122, 1.000000000000000000, 0.9659258262890683122, 1.000000000000000000, 0.9659258262890683122, 1.000000000000000000, 0.9659258262890683122, 1.000000000000000000, 0.9659258262890683122, 1.000000000000000000, 0.9659258262890683122, 1.000000000000000000, 0.9659258262890683122, 1.000000000000000000, 0.9659258262890683122, 1.000000000000000000, 0.9659258262890683122, 1.000000000000000000, 0.9659258262890683122, 1.000000000000000000, 0.9659258262890683122, 1.000000000000000000, 0.9659258262890683122, 1.000000000000000000, 0.9659258262890683122, 1.000000000000000000, 0.9659258262890683122, 1.000000000000000000, 0.9659258262890683122, 1.000000000000000000, 0.9659258262890683122, 1.000000000000000000, 0.9659258262890683122, 1.000000000000000000, 0.9659258262890683122, 1.000000000000000000, 0.9659258262890683122, 1.000000000000000000, 0.9659258262890683122, 1.000000000000000000, 0.9659258262890683122, 1.000000000000000000, 0.9659258262890683122, 1.000000000000000000, 0.9659258262890683122, 1.000000000000000000, 0.9659258262890683122, 1.000000000000000000, 0.9659258262890683122, 1.000000000000000000, 0.9659258262890683122, 1.000000000000000000, 0.9659258262890683122, 1.000000000000000000, 0.9659258262890683122, 1.000000000000000000, 0.9659258262890683122, 1.000000000000000000, 0.9659258262890683122, 1.000000000000000000, 0.9659258262890683122, 1.000000000000000000, 0.9659258262890683122, 1.000000000000000000, 0.9659258262890683122, 1.000000000000000000, 0.9659258262890683122, 1.000000000000000000, 0.9659258262890683122, 1.000000000000000000, 0.9659258262890683122, 1.000000000000000000, 0.9659258262890683122, 1.000000000000000000, 0.9659258262890683122, 1.000000000000000000, 0.9659258262890683122, 1.000000000000000000, 0.9659258262890683122, 1.000000000000000000, 0.9659258262890683122, 1.000000000000000000, 0.9659258262890683122, 1.000000000000000000, 0.9659258262890683122, 1.000000000000000000, 0.9659258262890683122, 1.000000000000000000, 0.9659258262890683122, 1.000000000000000000, 0.9659258262890683122, 1.000000000000000000, 0.9659258262890683122, 1.000000000000000000, 0.9659258262890683122, 1.000000000000000000, 0.9659258262890683122, 1.000000000000000000, 0.9659258262890683122, 1.000000000000000000, 0.9659258262890683122, 1.000000000000000000, 0.9659258262890683122, 1.000000000000000000, 0.9659258262890683122, 1.000000000000000000, 0.9659258262890683122, 1.000000000000000000, 0.9659258262890683122, 1.000000000000000000, 0.9659258262890683122, 1.000000000000000000, 0.9659258262890683122, 1.000000000000000000, 0.9659258262890683122, 1.000000000000000000, 0.9659258262890683122, 1.000000000000000000, 0.9659258262890683122, 1.000000000000000000, 0.9659258262890683122, 1.000000000000000000, 0.9659258262890683122, 1.000000000000000000, 0.9659258262890683122, 1.000000000000000000, 0.9659258262890683122, 1.000000000000000000, 0.9659258262890683122, 1.000000000000000000, 0.9659258262890683122, 1.000000000000000000, 0.9659258262890683122, 1.000000000000000000, 0.9659258262890683122, 1.000000000000000000, 0.9659258262890683122, 1.000000000000000000, 0.9659258262890683122, 1.000000000000000000, 0.9659258262890683122, 1.000000000000000000, 0.9659258262890683122, 1.000000000000000000, 0.9659258262890683122, 1.000000000000000000, 0.9659258262890683122, 1.000000000000000000, 0.9659258262890683122, 1.000000000000000000, 0.9659258262890683122, 1.000000000000000000, 0.9659258262890683122, 1.000000000000000000, 0.9659258262890683122, 1.000000000000000000, 0.9659258262890683122, 1.000000000000000000, 0.9659258262890683122, 1.000000000000000000, 0.9659258262890683122, 1.000000000000000000, 0.9659258262890683122, 1.000000000000000000, 0.9659258262890683122, 1.000000000000000000, 0.9659258262890683122, 1.000000000000000000, 0.9659258262890683122, 1.000000000000000000, 0.9659258262890683122, 1.000000000000000000, 0.9659258262890683122, 1.000000000000000000, 0.9659258262890683122, 1.000000000000000000, 0.9659258262890683122, 1.000000000000000000, 0.9659258262890683122, 1.000000000000000000, 0.9659258262890683122, 1.000000000000000000, 0.9659258262890683122, 1.000000000000000000, 0.9659258262890683122, 1.000000000000000000, 0.9659258262890683122, 1.000000000000000000, 0.9659258262890683122, 1.000000000000000000, 0.9659258262890683122, 1.000000000000000000, 0.9659258262890683122, 1.000000000000000000, 0.9659258262890683122, 1.000000000000000000, 0.9659258262890683122, 1.000000000000000000, 0.9659258262890683122, 1.000000000000000000, 0.9659258262890683122, 1.000000000000000000, 0.9659258262890683122, 1.000000000000000000, 0.9659258262890683122, 1.000000000000000000, 0.9659258262890683122, 1.000000000000000000, 0.9659258262890683122, 1.000000000000000000, 0.9659258262890683122, 1.000000000000000000, 0.9659258262890683122, 1.000000000000000000, 0.9659258262890683122, 1.000000000000000000, 0.9659258262890683122, 1.000000000000000000, 0.9659258262890683122, 1.000000000000000000, 0.9659258262890683122, 1.000000000000000000, 0.9659258262890683122, 1.000000000000000000, 0.9659258262890683122, 1.000000000000000000, 0.9659258262890683122, 1.000000000000000000, 0.9659258262890683122, 1.000000000000000000, 0.9659258262890683122, 1.000000000000000000, 0.9659258262890683122, 1.000000000000000000, 0.9659258262890683122, 1.000000000000000000, 0.9659258262890683122, 1.000000000000000000, 0.9659258262890683122, 1.000000000000000000, 0.9659258262890683122, 1.000000000000000000, 0.9659258262890683122, 1.000000000000000000, 0.9659258262890683122, 1.000000000000000000, 0.9659258262890683122, 1.000000000000000000, 0.9659258262890683122, 1.000000000000000000, 0.9659258262890683122, 1.000000000000000000, 0.9659258262890683122, 1.000000000000000000, 0.9659258262890683122, 1.000000000000000000, 0.9659258262890683122, 1.000000000000000000, 0.9659258262890683122, 1.000000000000000000, 0.9659258262890683122, 1.000000000000000000, 0.9659258262890683122, 1.000000000000000000, 0.9659258262890683122, 1.000000000000000000, 0.9659258262890683122, 1.000000000000000000, 0.9659258262890683122, 1.000000000000000000, 0.9659258262890683122, 1.000000000000000000, 0.9659258262890683122, 1.000000000000000000, 0.9659258262890683122, 1.000000000000000000, 0.9659258262890683122, 1.000000000000000000, 0.9659258262890683122, 1.000000000000000000, 0.9659258262890683122, 1.000000000000000000, 0.9659258262890683122, 1.000000000000000000, 0.9659258262890683122, 1.000000000000000000, 0.9659258262890683122, 1.000000000000000000, 0.9659258262890683122, 1.000000000000000000),
 ( 1.000000000000000000, 0.9659258262890683122, 1.000000000000000000, 0.9659258262890683122, 1.000000000000000000, 0.9659258262890683122, 1.000000000000000000, 0.9659258262890683122, 1.000000000000000000, 0.9659258262890683122, 1.000000000000000000, 0.9659258262890683122, 1.000000000000000000, 0.9659258262890683122, 1.000000000000000000, 0.9659258262890683122, 1.000000000000000000, 0.9659258262890683122, 1.000000000000000000, 0.9659258262890683122, 1.000000000000000000, 0.9659258262890683122, 1.000000000000000000, 0.9659258262890683122, 1.000000000000000000, 0.9659258262890683122, 1.000000000000000000, 0.9659258262890683122, 1.000000000000000000, 0.9659258262890683122, 1.000000000000000000, 0.9659258262890683122, 1.000000000000000000, 0.9659258262890683122, 1.000000000000000000, 0.9659258262890683122, 1.000000000000000000, 0.9659258262890683122, 1.000000000000000000, 0.9659258262890683122, 1.000000000000000000, 0.9659258262890683122, 1.000000000000000000, 0.9659258262890683122, 1.000000000000000000, 0.9659258262890683122, 1.000000000000000000, 0.9659258262890683122, 1.000000000000000000, 0.9659258262890683122, 1.000000000000000000, 0.9659258262890683122, 1.000000000000000000, 0.9659258262890683122, 1.000000000000000000, 0.9659258262890683122, 1.000000000000000000, 0.9659258262890683122, 1.000000000000000000, 0.9659258262890683122, 1.000000000000000000, 0.9659258262890683122, 1.000000000000000000, 0.9659258262890683122, 1.000000000000000000, 0.9659258262890683122, 1.000000000000000000, 0.9659258262890683122, 1.000000000000000000, 0.9659258262890683122, 1.000000000000000000, 0.9659258262890683122, 1.000000000000000000, 0.9659258262890683122, 1.000000000000000000, 0.9659258262890683122, 1.000000000000000000, 0.9659258262890683122, 1.000000000000000000, 0.9659258262890683122, 1.000000000000000000, 0.9659258262890683122, 1.000000000000000000, 0.9659258262890683122, 1.000000000000000000, 0.9659258262890683122, 1.000000000000000000, 0.9659258262890683122, 1.000000000000000000, 0.9659258262890683122, 1.000000000000000000, 0.9659258262890683122, 1.000000000000000000, 0.9659258262890683122, 1.000000000000000000, 0.9659258262890683122, 1.000000000000000000, 0.9659258262890683122, 1.000000000000000000, 0.9659258262890683122, 1.000000000000000000, 0.9659258262890683122, 1.000000000000000000, 0.9659258262890683122, 1.000000000000000000, 0.9659258262890683122, 1.000000000000000000, 0.9659258262890683122, 1.000000000000000000, 0.9659258262890683122, 1.000000000000000000, 0.9659258262890683122, 1.000000000000000000, 0.9659258262890683122, 1.000000000000000000, 0.9659258262890683122, 1.000000000000000000, 0.9659258262890683122, 1.000000000000000000, 0.9659258262890683122, 1.000000000000000000, 0.9659258262890683122, 1.000000000000000000, 0.9659258262890683122, 1.000000000000000000, 0.9659258262890683122, 1.000000000000000000, 0.9659258262890683122, 1.000000000000000000, 0.9659258262890683122, 1.000000000000000000, 0.9659258262890683122, 1.000000000000000000, 0.9659258262890683122, 1.000000000000000000, 0.9659258262890683122, 1.000000000000000000, 0.9659258262890683122, 1.000000000000000000, 0.9659258262890683122, 1.000000000000000000, 0.9659258262890683122, 1.000000000000000000, 0.9659258262890683122, 1.000000000000000000, 0.9659258262890683122, 1.000000000000000000, 0.9659258262890683122, 1.000000000000000000, 0.9659258262890683122, 1.000000000000000000, 0.9659258262890683122, 1.000000000000000000, 0.9659258262890683122, 1.000000000000000000, 0.9659258262890683122, 1.000000000000000000, 0.9659258262890683122, 1.000000000000000000, 0.9659258262890683122, 1.000000000000000000, 0.9659258262890683122, 1.000000000000000000, 0.9659258262890683122, 1.000000000000000000, 0.9659258262890683122, 1.000000000000000000, 0.9659258262890683122, 1.000000000000000000, 0.9659258262890683122, 1.000000000000000000, 0.9659258262890683122, 1.000000000000000000, 0.9659258262890683122, 1.000000000000000000, 0.9659258262890683122, 1.000000000000000000, 0.9659258262890683122, 1.000000000000000000, 0.9659258262890683122, 1.000000000000000000, 0.9659258262890683122, 1.000000000000000000, 0.9659258262890683122, 1.000000000000000000, 0.9659258262890683122, 1.000000000000000000, 0.9659258262890683122, 1.000000000000000000, 0.9659258262890683122, 1.000000000000000000, 0.9659258262890683122, 1.000000000000000000, 0.9659258262890683122, 1.000000000000000000, 0.9659258262890683122, 1.000000000000000000, 0.9659258262890683122, 1.000000000000000000, 0.9659258262890683122, 1.000000000000000000, 0.9659258262890683122, 1.000000000000000000, 0.9659258262890683122, 1.000000000000000000, 0.9659258262890683122, 1.000000000000000000, 0.9659258262890683122, 1.000000000000000000, 0.9659258262890683122, 1.000000000000000000, 0.9659258262890683122, 1.000000000000000000, 0.9659258262890683122, 1.000000000000000000, 0.9659258262890683122, 1.000000000000000000, 0.9659258262890683122, 1.000000000000000000, 0.9659258262890683122, 1.000000000000000000, 0.9659258262890683122, 1.000000000000000000, 0.9659258262890683122, 1.000000000000000000, 0.9659258262890683122, 1.000000000000000000, 0.9659258262890683122, 1.000000000000000000, 0.9659258262890683122, 1.000000000000000000, 0.9659258262890683122, 1.000000000000000000, 0.9659258262890683122, 1.000000000000000000, 0.9659258262890683122, 1.000000000000000000, 0.9659258262890683122, 1.000000000000000000, 0.9659258262890683122, 1.000000000000000000, 0.9659258262890683122, 1.000000000000000000, 0.9659258262890683122, 1.000000000000000000, 0.9659258262890683122, 1.000000000000000000, 0.9659258262890683122, 1.000000000000000000, 0.9659258262890683122, 1.000000000000000000, 0.9659258262890683122, 1.000000000000000000, 0.9659258262890683122, 1.000000000000000000, 0.9659258262890683122, 1.000000000000000000, 0.9659258262890683122, 1.000000000000000000, 0.9659258262890683122, 1.000000000000000000, 0.9659258262890683122, 1.000000000000000000, 0.9659258262890683122, 1.000000000000000000, 0.9659258262890683122, 1.000000000000000000, 0.9659258262890683122, 1.000000000000000000, 0.9659258262890683122, 1.000000000000000000, 0.9659258262890683122, 1.000000000000000000, 0.9659258262890683122, 1.000000000000000000, 0.9659258262890683122, 1.000000000000000000, 0.9659258262890683122, 1.000000000000000000, 0.9659258262890683122, 1.000000000000000000, 0.9659258262890683122, 1.000000000000000000, 0.9659258262890683122, 1.000000000000000000, 0.9659258262890683122, 1.000000000000000000, 0.9659258262890683122, 1.000000000000000000, 0.9659258262890683122, 1.000000000000000000, 0.9659258262890683122, 1.000000000000000000, 0.9659258262890683122, 1.000000000000000000, 0.9659258262890683122, 1.000000000000000000, 0.9659258262890683122, 1.000000000000000000, 0.9659258262890683122, 1.000000000000000000, 0.9659258262890683122, 1.000000000000000000, 0.9659258262890683122, 1.000000000000000000, 0.9659258262890683122, 1.000000000000000000, 0.9659258262890683122, 1.000000000000000000, 0.9659258262890683122, 1.000000000000000000, 0.9659258262890683122, 1.000000000000000000, 0.9659258262890683122, 1.000000000000000000, 0.9659258262890683122, 1.000000000000000000, 0.9659258262890683122, 1.000000000000000000, 0.9659258262890683122, 1.000000000000000000, 0.9659258262890683122, 1.000000000000000000, 0.9659258262890683122, 1.000000000000000000) ) ) 
 REPRESENTATION_ITEM ( '' )  SURFACE ( )  );
#45195=CARTESIAN_POINT ( 'NONE',  ( 17.20831665107776587, 37.88393115100078745, 7.208316651077764980 ) ) ;
#45200=ORIENTED_EDGE ( 'NONE', *, *, #65693, .T. ) ;
#45201=CARTESIAN_POINT ( 'NONE',  ( 18.52753015748617571, 53.09226448433412315, 4.923371831947298993 ) ) ;
#45202=CARTESIAN_POINT ( 'NONE',  ( 0.2751277870542875315, 65.30223176428830811, 6.499999999999984901 ) ) ;
#45203=CARTESIAN_POINT ( 'NONE',  ( 17.20831665107776587, 44.13393115100078745, -7.208316651077762316 ) ) ;
#45204=CARTESIAN_POINT ( 'NONE',  ( 20.36894250292379382, 28.67874883491396787, 10.36894250292379205 ) ) ;
#45205=CARTESIAN_POINT ( 'NONE',  ( 14.92337183194729633, 42.67559781766745886, 8.527530157486181039 ) ) ;
#45206=CARTESIAN_POINT ( 'NONE',  ( 22.81628187352647785, 56.62363466993042493, 6.195893100308588602E-16 ) ) ;
#45207=FACE_OUTER_BOUND ( 'NONE', #79826, .T. ) ;
#45208=CARTESIAN_POINT ( 'NONE',  ( 1.472469842513823179, 6.425597817667451750, 4.923371831947296329 ) ) ;
#45209=CARTESIAN_POINT ( 'NONE',  ( 21.92686044187656336, 46.97997603579418069, 3.195792623639536423 ) ) ;
#45210=CARTESIAN_POINT ( 'NONE',  ( 1.472469842513823179, 45.59226448433412315, -4.923371831947296329 ) ) ;
#45211=CARTESIAN_POINT ( 'NONE',  ( 20.88017736071110164, 60.35535201082151957, 2.915334737309930979 ) ) ;
#45212=CARTESIAN_POINT ( 'NONE',  ( 2.791683348922237240, 40.38393115100078035, -7.208316651077763204 ) ) ;
#45214=CARTESIAN_POINT ( 'NONE',  ( 10.00000000000000000, 51.81368534415484106, -10.88017736071110342 ) ) ;
#45216=ORIENTED_EDGE ( 'NONE', *, *, #86362, .T. ) ;
#45218=CARTESIAN_POINT ( 'NONE',  ( 20.88017736071110519, 15.56368534415483751, 2.639326808657452039E-16 ) ) ;
#45219=CARTESIAN_POINT ( 'NONE',  ( 10.00000000000000178, 0.3736346699304200492, 12.81628187352647608 ) ) ;
#45220=CARTESIAN_POINT ( 'NONE',  ( 19.42250999205614193, 45.14701867748817676, 5.440088680355555262 ) ) ;
#45221=CARTESIAN_POINT ( 'NONE',  ( 19.84674366389459266, 13.71726448433411782, -2.638427012816827677 ) ) ;
#45222=CARTESIAN_POINT ( 'NONE',  ( -46.34323875807881166, 103.6109741468810483, -6.190393423093146552 ) ) ;
#45223=CARTESIAN_POINT ( 'NONE',  ( 17.96484262340118221, 34.93868534415482685, 7.964842623401181321 ) ) ;
#45225=CARTESIAN_POINT ( 'NONE',  ( 18.52753015748618282, 8.925597817667451750, -4.923371831947291888 ) ) ;
#45226=CARTESIAN_POINT ( 'NONE',  ( 19.84674366389459266, 33.30059781766744464, 2.638427012816836559 ) ) ;
#45229=CARTESIAN_POINT ( 'NONE',  ( 5.076628168052703671, 66.84226448433412315, 8.527530157486179263 ) ) ;
#45230=CARTESIAN_POINT ( 'NONE',  ( 15.44008868035555793, 6.397018677488171434, -9.422509992056140149 ) ) ;
#45232=CARTESIAN_POINT ( 'NONE',  ( 22.26659068614894466, 23.88708216824730357, 7.082119434687054849 ) ) ;
#45233=CARTESIAN_POINT ( 'NONE',  ( 22.26659068614895176, 44.72041550158063927, -7.082119434687042414 ) ) ;
#45234=FILL_AREA_STYLE_COLOUR ( '', #88787 ) ;
#45237=CARTESIAN_POINT ( 'NONE',  ( 19.84674366389459266, 28.71726448433411960, -2.638427012816827677 ) ) ;
#45238=CARTESIAN_POINT ( 'NONE',  ( -0.8801773607110991993, 32.85535201082151247, -2.915334737309923874 ) ) ;
#45239=CARTESIAN_POINT ( 'NONE',  ( 19.84674366389459266, 48.30059781766745175, 2.638427012816836559 ) ) ;
#45240=CARTESIAN_POINT ( 'NONE',  ( 24.16423886937410614, 9.303748834913967869, 8.672049930838204340E-16 ) ) ;
#45241=CARTESIAN_POINT ( 'NONE',  ( 19.72487221294571569, 47.80223176428831522, -6.499999999999982236 ) ) ;
#45243=FILL_AREA_STYLE ('',( #14770 ) ) ;
#45244=CARTESIAN_POINT ( 'NONE',  ( 10.00000000000000178, 40.37363466993042493, 12.81628187352647608 ) ) ;
#45245=CARTESIAN_POINT ( 'NONE',  ( 1.472469842513823179, 35.59226448433412315, -4.923371831947296329 ) ) ;
#45247=CARTESIAN_POINT ( 'NONE',  ( 18.52753015748618282, 13.92559781766745175, -4.923371831947291888 ) ) ;
#45249=CARTESIAN_POINT ( 'NONE',  ( 19.80448550324508261, 16.82703681773341131, 6.500000000002789768 ) ) ;
#45250=CARTESIAN_POINT ( 'NONE',  ( 15.44008868035555793, 6.397018677488171434, -9.422509992056140149 ) ) ;
#45251=CARTESIAN_POINT ( 'NONE',  ( 2.917880565312950480, 50.97041550158064638, -12.26659068614894821 ) ) ;
#45252=CARTESIAN_POINT ( 'NONE',  ( -4.164238869374098151, 1.595415501580634388, -3.795296366450310543 ) ) ;
#45254=CARTESIAN_POINT ( 'NONE',  ( 19.84674366389459266, 28.71726448433411960, -2.638427012816827677 ) ) ;
#45255=CARTESIAN_POINT ( 'NONE',  ( 0.5774900079438607392, 3.480352010821504027, 5.440088680355550821 ) ) ;
#45256=CARTESIAN_POINT ( 'NONE',  ( 17.20831665107776587, 44.13393115100078745, -7.208316651077762316 ) ) ;
#45258=CARTESIAN_POINT ( 'NONE',  ( 7.361572987183170547, 52.05059781766745175, 9.846743663894590881 ) ) ;
#45262=CARTESIAN_POINT ( 'NONE',  ( -0.8801773607111008646, 33.27201867748817676, 2.915334737309923430 ) ) ;
#45265=CARTESIAN_POINT ( 'NONE',  ( 3.591859063236763294, 53.29030133659708923, -11.09922568453595026 ) ) ;
#45267=CARTESIAN_POINT ( 'NONE',  ( 19.84674366389459266, 8.717264484334116048, -2.638427012816827677 ) ) ;
#45268=CARTESIAN_POINT ( 'NONE',  ( -1.099225684535947600, 59.54030133659708923, 6.408140936763237150 ) ) ;
#45269=CARTESIAN_POINT ( 'NONE',  ( 15.44008868035555793, 6.397018677488171434, -9.422509992056140149 ) ) ;
#45270=CARTESIAN_POINT ( 'NONE',  ( 19.84674366389459266, 43.30059781766744464, 2.638427012816836559 ) ) ;
#45273=CARTESIAN_POINT ( 'NONE',  ( 20.36894250292379738, 34.92874883491396076, -10.36894250292379027 ) ) ;
#45274=CARTESIAN_POINT ( 'NONE',  ( 13.79529636645030344, 43.26208216824730357, 14.16423886937410614 ) ) ;
#45275=CARTESIAN_POINT ( 'NONE',  ( 17.20831665107776587, 59.13393115100078745, -7.208316651077762316 ) ) ;
#45277=CARTESIAN_POINT ( 'NONE',  ( 10.00000000000000000, 56.81368534415484106, -10.88017736071110342 ) ) ;
#45278=CARTESIAN_POINT ( 'NONE',  ( 0.1532563361054082862, 6.217264484334118713, 2.638427012816831674 ) ) ;
#45281=CARTESIAN_POINT ( 'NONE',  ( 22.81628187352648496, 61.83196800326376774, -3.434112377981050290 ) ) ;
#45283=CARTESIAN_POINT ( 'NONE',  ( -0.8801773607111008646, 68.27201867748817676, 2.915334737309923430 ) ) ;
#45285=CARTESIAN_POINT ( 'NONE',  ( 22.26659068614894466, 8.887082168247300018, 7.082119434687054849 ) ) ;
#45286=CARTESIAN_POINT ( 'NONE',  ( 18.52753015748617571, 8.092264484334117824, 4.923371831947298993 ) ) ;
#45287=CARTESIAN_POINT ( 'NONE',  ( -0.8801773607111009756, 28.06368534415484106, 1.068504757029289695E-15 ) ) ;
#45290=CARTESIAN_POINT ( 'NONE',  ( -0.8801773607110991993, 22.85535201082150181, -2.915334737309923874 ) ) ;
#45295=CARTESIAN_POINT ( 'NONE',  ( -0.8801773607110991993, 32.85535201082151247, -2.915334737309923874 ) ) ;
#45296=FACE_OUTER_BOUND ( 'NONE', #65201, .T. ) ;
#45299=CARTESIAN_POINT ( 'NONE',  ( 3.591859063236761518, 19.95696800326375353, 11.09922568453594849 ) ) ;
#45301=CARTESIAN_POINT ( 'NONE',  ( 12.91533473730993009, 61.60535201082150536, -10.88017736071109987 ) ) ;
#45304=CARTESIAN_POINT ( 'NONE',  ( 10.00000000000000000, 14.75893115100078568, -9.846743663894594434 ) ) ;
#45305=CARTESIAN_POINT ( 'NONE',  ( -0.8801773607110991993, 37.85535201082151247, -2.915334737309923874 ) ) ;
#45309=CARTESIAN_POINT ( 'NONE',  ( 20.88017736071110164, 40.35535201082150536, 2.915334737309930979 ) ) ;
#45310=CARTESIAN_POINT ( 'NONE',  ( -46.94000000000014694, 103.2291249090730787, -5.913062993056311889 ) ) ;
#45311=CARTESIAN_POINT ( 'NONE',  ( 22.81628187352648496, 56.83196800326374643, -3.434112377981050290 ) ) ;
#45312=CARTESIAN_POINT ( 'NONE',  ( 19.42250999205614548, 60.98035201082151247, -5.440088680355545492 ) ) ;
#45313=CARTESIAN_POINT ( 'NONE',  ( 22.81628187352647785, 1.623634669930420271, 6.195893100308588602E-16 ) ) ;
#45314=CARTESIAN_POINT ( 'NONE',  ( 1.472469842513823179, 21.42559781766745175, 4.923371831947296329 ) ) ;
#45315=CARTESIAN_POINT ( 'NONE',  ( -2.816281873526471635, 48.91530133659708213, -3.434112377981056508 ) ) ;
#45317=CARTESIAN_POINT ( 'NONE',  ( 19.84674366389459266, 8.300597817667451750, 2.638427012816836559 ) ) ;
#45318=CARTESIAN_POINT ( 'NONE',  ( 19.38216949554541202, 5.998634669930420493, 9.382169495545424454 ) ) ;
#45321=CARTESIAN_POINT ( 'NONE',  ( 20.88017736071110164, 40.35535201082150536, 2.915334737309930979 ) ) ;
#45322=CARTESIAN_POINT ( 'NONE',  ( 2.791683348922240793, 51.63393115100078745, 7.208316651077764092 ) ) ;
#45324=ADVANCED_FACE ( 'NONE', ( #20908 ), #81884, .T. ) ;
#45325=CARTESIAN_POINT ( 'NONE',  ( 2.791683348922240793, 21.63393115100078745, 7.208316651077764092 ) ) ;
#45326=CARTESIAN_POINT ( 'NONE',  ( 0.1532563361054100626, 5.800597817667452638, -2.638427012816831230 ) ) ;
#45327=CARTESIAN_POINT ( 'NONE',  ( 22.81628187352647785, 6.415301336597088344, 3.434112377981063169 ) ) ;
#45329=CARTESIAN_POINT ( 'NONE',  ( 10.00000000000000000, 1.813685344154837731, -10.88017736071110342 ) ) ;
#45330=CYLINDRICAL_SURFACE ( 'NONE', #27869, 0.5000000000000004441 ) ;
#45332=CARTESIAN_POINT ( 'NONE',  ( -4.164238869374099039, 66.80374883491396076, 8.674139862899312516E-16 ) ) ;
#45333=CARTESIAN_POINT ( 'NONE',  ( 0.1532563361054082862, 46.21726448433411605, 2.638427012816831674 ) ) ;
#45335=CARTESIAN_POINT ( 'NONE',  ( 19.42250999205614548, 5.980352010821504471, -5.440088680355545492 ) ) ;
#45336=CARTESIAN_POINT ( 'NONE',  ( 1.959929470562270959, 6.502578601053488505, 5.767676674365833200 ) ) ;
#45337=CARTESIAN_POINT ( 'NONE',  ( 4.559911319644449179, 38.89701867748817676, 9.422509992056141925 ) ) ;
#45338=CARTESIAN_POINT ( 'NONE',  ( 24.16423886937409904, 44.09541550158063927, 3.795296366450317205 ) ) ;
#45339=CARTESIAN_POINT ( 'NONE',  ( 2.917880565312950480, 60.97041550158063927, -12.26659068614894821 ) ) ;
#45341=CARTESIAN_POINT ( 'NONE',  ( 2.791683348922240793, 6.633931151000785675, 7.208316651077764092 ) ) ;
#45342=CARTESIAN_POINT ( 'NONE',  ( 17.20831665107776587, 27.88393115100078390, 7.208316651077764980 ) ) ;
#45343=CARTESIAN_POINT ( 'NONE',  ( 22.81628187352647785, 16.41530133659708923, 3.434112377981063169 ) ) ;
#45347=CARTESIAN_POINT ( 'NONE',  ( 13.79529636645030344, 8.262082168247300018, 14.16423886937410614 ) ) ;
#45348=CARTESIAN_POINT ( 'NONE',  ( 0.1532563361054100626, 30.80059781766744820, -2.638427012816831230 ) ) ;
#45349=CARTESIAN_POINT ( 'NONE',  ( -0.1503990784575328643, 70.00000000000000000, 6.262539305110068177 ) ) ;
#45351=CARTESIAN_POINT ( 'NONE',  ( 24.16423886937410614, 39.51208216824731068, -3.795296366450302550 ) ) ;
#45352=CARTESIAN_POINT ( 'NONE',  ( 12.63842701281683922, 9.550597817667449974, -9.846743663894590881 ) ) ;
#45355=CARTESIAN_POINT ( 'NONE',  ( 4.559911319644449179, 28.89701867748817321, 9.422509992056141925 ) ) ;
#45356=CARTESIAN_POINT ( 'NONE',  ( 16.40814093676323893, 50.79030133659708923, 11.09922568453595026 ) ) ;
#45357=CARTESIAN_POINT ( 'NONE',  ( -0.8801773607110991993, 2.855352010821504471, -2.915334737309923874 ) ) ;
#45358=CARTESIAN_POINT ( 'NONE',  ( -2.816281873526473856, 34.33196800326376064, 3.434112377981055619 ) ) ;
#45359=CARTESIAN_POINT ( 'NONE',  ( 14.92337183194729988, 4.342264484334117824, -8.527530157486177487 ) ) ;
#45364=CARTESIAN_POINT ( 'NONE',  ( -4.164238869374099039, 36.80374883491396787, 8.674139862899312516E-16 ) ) ;
#45365=CARTESIAN_POINT ( 'NONE',  ( 13.79529636645030344, 18.26208216824730002, 14.16423886937410614 ) ) ;
#45366=CARTESIAN_POINT ( 'NONE',  ( 10.00000000000000000, 1.813685344154837731, -10.88017736071110342 ) ) ;
#45367=CARTESIAN_POINT ( 'NONE',  ( -0.8801773607111008646, 38.27201867748816255, 2.915334737309923430 ) ) ;
#45370=CARTESIAN_POINT ( 'NONE',  ( 2.035157376598822676, 52.43868534415483396, -7.964842623401177768 ) ) ;
#45371=CARTESIAN_POINT ( 'NONE',  ( 7.084665262690076126, 67.02201867748817676, -10.88017736071110164 ) ) ;
#45372=CARTESIAN_POINT ( 'NONE',  ( 19.38216949554541557, 27.24863466993041783, -9.382169495545420901 ) ) ;
#45373=FACE_OUTER_BOUND ( 'NONE', #73684, .T. ) ;
#45375=CARTESIAN_POINT ( 'NONE',  ( 0.1532563361054082862, 31.21726448433412315, 2.638427012816831674 ) ) ;
#45376=EDGE_CURVE ( 'NONE', #26206, #86034, #82881, .T. ) ;
#45377=CARTESIAN_POINT ( 'NONE',  ( 21.09922568453594849, 21.20696800326375353, 6.408140936763242479 ) ) ;
#45378=CARTESIAN_POINT ( 'NONE',  ( -0.8801773607111009756, 43.06368534415484106, 1.068504757029289695E-15 ) ) ;
#45379=CARTESIAN_POINT ( 'NONE',  ( 4.559911319644449179, 12.23035201082150536, -9.422509992056141925 ) ) ;
#45380=CARTESIAN_POINT ( 'NONE',  ( 2.791683348922240793, 41.63393115100078745, 7.208316651077764092 ) ) ;
#45382=CARTESIAN_POINT ( 'NONE',  ( 12.63842701281683034, 12.46726448433411782, 9.846743663894596210 ) ) ;
#45383=CARTESIAN_POINT ( 'NONE',  ( 2.917880565312950480, 5.970415501580634832, -12.26659068614894821 ) ) ;
#45385=CARTESIAN_POINT ( 'NONE',  ( 4.559911319644449179, 37.23035201082150536, -9.422509992056141925 ) ) ;
#45386=CARTESIAN_POINT ( 'NONE',  ( 12.91533473730992121, 4.522018677488169658, 10.88017736071110164 ) ) ;
#45387=CARTESIAN_POINT ( 'NONE',  ( 10.00000000000000000, 26.81368534415484106, -10.88017736071110342 ) ) ;
#45388=CARTESIAN_POINT ( 'NONE',  ( 4.559911319644449179, 12.23035201082150714, -9.422509992056141925 ) ) ;
#45391=CARTESIAN_POINT ( 'NONE',  ( 20.88017736071110519, 20.56368534415484106, 2.639326808657452039E-16 ) ) ;
#45392=CARTESIAN_POINT ( 'NONE',  ( 22.81628187352647785, 41.41530133659708923, 3.434112377981063169 ) ) ;
#45393=CARTESIAN_POINT ( 'NONE',  ( 4.559911319644449179, 43.89701867748816966, 9.422509992056141925 ) ) ;
#45394=CARTESIAN_POINT ( 'NONE',  ( 20.88017736071110519, 55.56368534415484817, 2.639326808657452039E-16 ) ) ;
#45395=ORIENTED_EDGE ( 'NONE', *, *, #35903, .F. ) ;
#45396=CARTESIAN_POINT ( 'NONE',  ( 17.96484262340118221, 34.93868534415482685, 7.964842623401181321 ) ) ;
#45399=CARTESIAN_POINT ( 'NONE',  ( 0.1077916266722768468, 37.24062864464240619, -6.478736007406001640 ) ) ;
#45400=CARTESIAN_POINT ( 'NONE',  ( -2.266590686148945544, 41.38708216824729647, -7.082119434687050408 ) ) ;
#45401=CARTESIAN_POINT ( 'NONE',  ( 17.20831665107776587, 2.883931151000785231, 7.208316651077764980 ) ) ;
#45404=CARTESIAN_POINT ( 'NONE',  ( 17.20831665107776587, 59.13393115100078745, -7.208316651077762316 ) ) ;
#45406=CARTESIAN_POINT ( 'NONE',  ( 19.84674366389459266, 38.71726448433412315, -2.638427012816827677 ) ) ;
#45409=CARTESIAN_POINT ( 'NONE',  ( 5.076628168052703671, 36.84226448433412315, 8.527530157486179263 ) ) ;
#45411=CARTESIAN_POINT ( 'NONE',  ( -0.8801773607111009756, 23.06368534415484106, 1.068504757029289695E-15 ) ) ;
#45412=CARTESIAN_POINT ( 'NONE',  ( 10.00000000000000000, 44.75893115100078745, -9.846743663894594434 ) ) ;
#45413=CARTESIAN_POINT ( 'NONE',  ( 16.40814093676323893, 15.79030133659708746, 11.09922568453595026 ) ) ;
#45415=CARTESIAN_POINT ( 'NONE',  ( 15.44008868035555793, 56.39701867748817676, -9.422509992056140149 ) ) ;
#45416=CARTESIAN_POINT ( 'NONE',  ( 10.00000000000000178, 39.31368534415484106, 10.88017736071110342 ) ) ;
#45417=FILL_AREA_STYLE_COLOUR ( '', #49767 ) ;
#45418=CARTESIAN_POINT ( 'NONE',  ( -0.3689425029237881626, 62.42874883491396787, 10.36894250292379027 ) ) ;
#45420=EDGE_LOOP ( 'NONE', ( #7591, #62429, #87347, #72010 ) ) ;
#45421=AXIS2_PLACEMENT_3D ( 'NONE', #25931, #31446, #92934 ) ;
#45422=CARTESIAN_POINT ( 'NONE',  ( 6.565887622018943937, 13.08196800326374998, -12.81628187352647608 ) ) ;
#45423=CARTESIAN_POINT ( 'NONE',  ( -0.8801773607111008646, 13.27201867748817143, 2.915334737309923430 ) ) ;
#45424=CARTESIAN_POINT ( 'NONE',  ( 12.91533473730992121, 44.52201867748816966, 10.88017736071110164 ) ) ;
#45426=AXIS2_PLACEMENT_3D ( 'NONE', #42530, #81503, #13008 ) ;
#45430=CARTESIAN_POINT ( 'NONE',  ( 20.88017736071110519, 60.56368534415484106, 2.639326808657452039E-16 ) ) ;
#45431=STYLED_ITEM ( 'NONE', ( #10300 ), #42960 ) ;
#45432=CARTESIAN_POINT ( 'NONE',  ( 5.076628168052703671, 41.84226448433411605, 8.527530157486179263 ) ) ;
#45433=CARTESIAN_POINT ( 'NONE',  ( 18.52753015748617571, 18.09226448433411960, 4.923371831947298993 ) ) ;
#45434=CARTESIAN_POINT ( 'NONE',  ( 19.84674366389459266, 8.717264484334116048, -2.638427012816827677 ) ) ;
#45435=CARTESIAN_POINT ( 'NONE',  ( 0.1957200283969098564, 40.25733960839544778, 6.499999999999992006 ) ) ;
#45438=CARTESIAN_POINT ( 'NONE',  ( 0.1532563361054100626, 10.80059781766745175, -2.638427012816831230 ) ) ;
#45441=CARTESIAN_POINT ( 'NONE',  ( 1.472469842513823179, 31.42559781766745530, 4.923371831947296329 ) ) ;
#45444=CARTESIAN_POINT ( 'NONE',  ( 19.38216949554541557, 17.24863466993041783, -9.382169495545420901 ) ) ;
#45446=CARTESIAN_POINT ( 'NONE',  ( 0.5774900079438590739, 57.64701867748817676, -5.440088680355550821 ) ) ;
#45447=CARTESIAN_POINT ( 'NONE',  ( -2.266590686148945544, 32.22041550158063927, 7.082119434687048631 ) ) ;
#45448=UNCERTAINTY_MEASURE_WITH_UNIT (LENGTH_MEASURE( 1.000000000000000082E-05 ), #4806, 'distance_accuracy_value', 'NONE');
#45450=CARTESIAN_POINT ( 'NONE',  ( 10.00000000000000000, 35.55374883491396787, -14.16423886937410082 ) ) ;
#45452=CARTESIAN_POINT ( 'NONE',  ( -0.3689425029237881626, 57.42874883491397497, 10.36894250292379027 ) ) ;
#45453=CARTESIAN_POINT ( 'NONE',  ( 24.16423886937409904, 9.095415501580633943, 3.795296366450317205 ) ) ;
#45454=CARTESIAN_POINT ( 'NONE',  ( -0.3689425029237881626, 32.42874883491395366, 10.36894250292379027 ) ) ;
#45456=CARTESIAN_POINT ( 'NONE',  ( 0.5774900079438590739, 52.64701867748817676, -5.440088680355550821 ) ) ;
#45458=( BOUNDED_CURVE ( )  B_SPLINE_CURVE ( 2, ( #72443, #70998, #19944, #79474, #87458, #3486, #94465, #57936, #64447 ),
 .UNSPECIFIED., .F., .F. ) 
 B_SPLINE_CURVE_WITH_KNOTS ( ( 3, 2, 2, 2, 3 ),
 ( 0.8687123655116599785, 0.8690476190476190688, 0.8750000000000000000, 0.8809523809523809312, 0.8812876344883400215 ),
 .UNSPECIFIED. ) 
 CURVE ( )  GEOMETRIC_REPRESENTATION_ITEM ( )  RATIONAL_B_SPLINE_CURVE ( ( 0.9963778908391764944, 0.9980808541467923733, 1.000000000000000000, 0.9659258262890683122, 1.000000000000000000, 0.9659258262890683122, 1.000000000000000000, 0.9980808541467922623, 0.9963778908391764944 ) ) 
 REPRESENTATION_ITEM ( '' )  );
#45459=CARTESIAN_POINT ( 'NONE',  ( 7.084665262690076126, 69.10535201082151957, 10.88017736071109987 ) ) ;
#45460=CARTESIAN_POINT ( 'NONE',  ( 18.52753015748618282, 38.92559781766745175, -4.923371831947291888 ) ) ;
#45461=CARTESIAN_POINT ( 'NONE',  ( 19.42250999205614193, 30.14701867748817321, 5.440088680355555262 ) ) ;
#45462=CARTESIAN_POINT ( 'NONE',  ( -2.816281873526473856, 59.12363466993042493, 9.499525473075851096E-16 ) ) ;
#45463=CARTESIAN_POINT ( 'NONE',  ( 2.791683348922240793, 61.63393115100079456, 7.208316651077764092 ) ) ;
#45465=CARTESIAN_POINT ( 'NONE',  ( 5.076628168052704559, 30.17559781766745175, -8.527530157486179263 ) ) ;
#45466=CARTESIAN_POINT ( 'NONE',  ( 13.43411237798106583, 52.66530133659708213, -12.81628187352647252 ) ) ;
#45468=CARTESIAN_POINT ( 'NONE',  ( 15.44008868035555793, 46.39701867748817676, -9.422509992056140149 ) ) ;
#45469=CARTESIAN_POINT ( 'NONE',  ( 19.84674366389459266, 48.30059781766745175, 2.638427012816836559 ) ) ;
#45470=CARTESIAN_POINT ( 'NONE',  ( 24.16423886937410614, 34.30374883491396787, 8.672049930838204340E-16 ) ) ;
#45471=ORIENTED_EDGE ( 'NONE', *, *, #49470, .T. ) ;
#45473=CARTESIAN_POINT ( 'NONE',  ( 4.559911319644449179, 62.23035201082150536, -9.422509992056141925 ) ) ;
#45474=CARTESIAN_POINT ( 'NONE',  ( 7.084665262690076126, 67.02201867748817676, -10.88017736071110164 ) ) ;
#45475=CARTESIAN_POINT ( 'NONE',  ( 20.36894250292379382, 58.67874883491396076, 10.36894250292379205 ) ) ;
#45476=CARTESIAN_POINT ( 'NONE',  ( 6.565887622018943937, 13.08196800326374998, -12.81628187352647608 ) ) ;
#45478=CARTESIAN_POINT ( 'NONE',  ( 20.88017736071110164, 55.35535201082149825, 2.915334737309930979 ) ) ;
#45481=CARTESIAN_POINT ( 'NONE',  ( 6.204703633549690345, 52.84541550158062506, 14.16423886937410082 ) ) ;
#45483=CARTESIAN_POINT ( 'NONE',  ( 17.96484262340118221, 14.93868534415483751, 7.964842623401181321 ) ) ;
#45484=CARTESIAN_POINT ( 'NONE',  ( 17.96484262340118221, 29.93868534415484106, 7.964842623401181321 ) ) ;
#45485=CARTESIAN_POINT ( 'NONE',  ( 1.472469842513823179, 61.42559781766745175, 4.923371831947296329 ) ) ;
#45486=CARTESIAN_POINT ( 'NONE',  ( 16.40814093676323893, 50.79030133659708923, 11.09922568453595026 ) ) ;
#45488=ORIENTED_EDGE ( 'NONE', *, *, #9620, .F. ) ;
#45489=CARTESIAN_POINT ( 'NONE',  ( 7.084665262690076126, 19.10535201082150181, 10.88017736071109987 ) ) ;
#45491=CARTESIAN_POINT ( 'NONE',  ( 3.591859063236763294, 23.29030133659708568, -11.09922568453595026 ) ) ;
#45493=( GEOMETRIC_REPRESENTATION_CONTEXT ( 3 ) GLOBAL_UNCERTAINTY_ASSIGNED_CONTEXT ( ( #13481 ) ) GLOBAL_UNIT_ASSIGNED_CONTEXT ( ( #48766, #77789, #71773 ) ) REPRESENTATION_CONTEXT ( 'NONE', 'WORKASPACE' ) );
#45494=CARTESIAN_POINT ( 'NONE',  ( 5.076628168052703671, 46.84226448433412315, 8.527530157486179263 ) ) ;
#45496=CARTESIAN_POINT ( 'NONE',  ( 4.559911319644449179, 37.23035201082150536, -9.422509992056141925 ) ) ;
#45497=( GEOMETRIC_REPRESENTATION_CONTEXT ( 3 ) GLOBAL_UNCERTAINTY_ASSIGNED_CONTEXT ( ( #11504 ) ) GLOBAL_UNIT_ASSIGNED_CONTEXT ( ( #29322, #5370, #73347 ) ) REPRESENTATION_CONTEXT ( 'NONE', 'WORKASPACE' ) );
#45498=CARTESIAN_POINT ( 'NONE',  ( 6.565887622018943937, 28.08196800326375353, -12.81628187352647608 ) ) ;
#45499=CARTESIAN_POINT ( 'NONE',  ( 2.035157376598824452, 48.68868534415483396, 7.964842623401179544 ) ) ;
#45501=CARTESIAN_POINT ( 'NONE',  ( 19.72487221294570858, 70.00000000000000000, -6.000000000000000000 ) ) ;
#45502=CARTESIAN_POINT ( 'NONE',  ( -1.099225684535947600, 48.70696800326375353, -6.408140936763238038 ) ) ;
#45504=B_SPLINE_CURVE_WITH_KNOTS ( 'NONE', 3,
 ( #89922, #35933, #96964, #58934 ),
 .UNSPECIFIED., .F., .F.,
 ( 4, 4 ),
 ( 0.000000000000000000, 0.002392975128318479416 ),
 .UNSPECIFIED. ) ;
#45505=CARTESIAN_POINT ( 'NONE',  ( 19.42250999205614193, 55.14701867748817676, 5.440088680355555262 ) ) ;
#45506=CARTESIAN_POINT ( 'NONE',  ( -2.816281873526471635, 33.91530133659708213, -3.434112377981056508 ) ) ;
#45507=CARTESIAN_POINT ( 'NONE',  ( -0.3689425029237881626, 2.428748834913967869, 10.36894250292379027 ) ) ;
#45508=CARTESIAN_POINT ( 'NONE',  ( 0.1532563361054082862, 6.217264484334118713, 2.638427012816831674 ) ) ;
#45509=CARTESIAN_POINT ( 'NONE',  ( 20.36894250292379738, 49.92874883491396787, -10.36894250292379027 ) ) ;
#45511=CARTESIAN_POINT ( 'NONE',  ( 19.84674366389459621, 13.50893115100078568, 7.409399052514197653E-17 ) ) ;
#45512=CARTESIAN_POINT ( 'NONE',  ( 0.1532563361054100626, 0.8005978176674514168, -2.638427012816831230 ) ) ;
#45513=CARTESIAN_POINT ( 'NONE',  ( 2.588169541918969419, 0.4578369456018643868, -6.498696640609835207 ) ) ;
#45514=CARTESIAN_POINT ( 'NONE',  ( 2.917880565312948704, 47.63708216824730357, 12.26659068614894643 ) ) ;
#45515=EDGE_CURVE ( 'NONE', #13300, #20878, #59128, .T. ) ;
#45516=CARTESIAN_POINT ( 'NONE',  ( 18.72515096720570327, 16.07228050351031712, -6.499999999999992006 ) ) ;
#45517=CARTESIAN_POINT ( 'NONE',  ( 7.084665262690076126, 2.022018677488170990, -10.88017736071110164 ) ) ;
#45520=CARTESIAN_POINT ( 'NONE',  ( -0.8801773607111009756, 3.063685344154838397, 1.068504757029289695E-15 ) ) ;
#45521=CARTESIAN_POINT ( 'NONE',  ( -2.266590686148945544, 66.38708216824730357, -7.082119434687050408 ) ) ;
#45522=CARTESIAN_POINT ( 'NONE',  ( 14.92337183194729988, 49.34226448433411605, -8.527530157486177487 ) ) ;
#45525=CARTESIAN_POINT ( 'NONE',  ( -2.816281873526471635, 43.91530133659708923, -3.434112377981056508 ) ) ;
#45528=CARTESIAN_POINT ( 'NONE',  ( -0.3689425029237898834, 11.17874883491396787, -10.36894250292378850 ) ) ;
#45529=CARTESIAN_POINT ( 'NONE',  ( 19.42250999205614548, 15.98035201082150714, -5.440088680355545492 ) ) ;
#45530=CARTESIAN_POINT ( 'NONE',  ( 20.88017736071110164, 10.35535201082150714, 2.915334737309930979 ) ) ;
#45531=CARTESIAN_POINT ( 'NONE',  ( 7.361572987183169658, 44.96726448433412315, -9.846743663894592657 ) ) ;
#45533=CARTESIAN_POINT ( 'NONE',  ( 12.63842701281683034, 27.46726448433411250, 9.846743663894596210 ) ) ;
#45535=CARTESIAN_POINT ( 'NONE',  ( 0.5774900079438590739, 32.64701867748816966, -5.440088680355550821 ) ) ;
#45540=CARTESIAN_POINT ( 'NONE',  ( 2.791683348922237240, 55.38393115100078745, -7.208316651077763204 ) ) ;
#45541=CARTESIAN_POINT ( 'NONE',  ( 24.16423886937410614, 19.51208216824729647, -3.795296366450302550 ) ) ;
#45542=CARTESIAN_POINT ( 'NONE',  ( 12.91533473730993009, 31.60535201082150891, -10.88017736071109987 ) ) ;
#45543=CARTESIAN_POINT ( 'NONE',  ( -0.8801773607111008646, 33.27201867748817676, 2.915334737309923430 ) ) ;
#45544=CARTESIAN_POINT ( 'NONE',  ( 1.472469842513823179, 61.42559781766745175, 4.923371831947296329 ) ) ;
#45545=CARTESIAN_POINT ( 'NONE',  ( 13.43411237798106583, 32.66530133659708213, -12.81628187352647252 ) ) ;
#45546=CARTESIAN_POINT ( 'NONE',  ( 2.917880565312950480, 5.970415501580634832, -12.26659068614894821 ) ) ;
#45547=CIRCLE ( 'NONE', #40763, 1.000000000000007772 ) ;
#45548=CARTESIAN_POINT ( 'NONE',  ( -0.8801773607111008646, 63.27201867748817676, 2.915334737309923430 ) ) ;
#45550=CARTESIAN_POINT ( 'NONE',  ( -2.816281873526473856, 49.12363466993042493, 9.499525473075851096E-16 ) ) ;
#45551=ORIENTED_EDGE ( 'NONE', *, *, #78331, .F. ) ;
#45552=CARTESIAN_POINT ( 'NONE',  ( 18.52753015748618282, 43.92559781766745175, -4.923371831947291888 ) ) ;
#45553=CARTESIAN_POINT ( 'NONE',  ( 2.035157376598824452, 8.688685344154839285, 7.964842623401179544 ) ) ;
#45554=VERTEX_POINT ( 'NONE', #73892 ) ;
#45556=CARTESIAN_POINT ( 'NONE',  ( 12.91533473730992121, 19.52201867748816611, 10.88017736071110164 ) ) ;
#45558=CARTESIAN_POINT ( 'NONE',  ( 0.5774900079438607392, 63.48035201082149825, 5.440088680355550821 ) ) ;
#45559=CARTESIAN_POINT ( 'NONE',  ( 19.42250999205614193, 55.14701867748817676, 5.440088680355555262 ) ) ;
#45560=CARTESIAN_POINT ( 'NONE',  ( 7.084665262690076126, 62.02201867748816966, -10.88017736071110164 ) ) ;
#45561=CARTESIAN_POINT ( 'NONE',  ( 10.00000000000000000, -0.2410688489992152128, -9.846743663894594434 ) ) ;
#45562=CARTESIAN_POINT ( 'NONE',  ( 12.91533473730992121, 54.52201867748816255, 10.88017736071110164 ) ) ;
#45565=CARTESIAN_POINT ( 'NONE',  ( -46.93999999999942219, 101.0602049476338777, 8.583117191026476078 ) ) ;
#45567=CARTESIAN_POINT ( 'NONE',  ( 18.52753015748618282, 38.92559781766745175, -4.923371831947291888 ) ) ;
#45569=CARTESIAN_POINT ( 'NONE',  ( 2.791683348922237240, 65.38393115100078035, -7.208316651077763204 ) ) ;
#45571=FACE_OUTER_BOUND ( 'NONE', #1942, .T. ) ;
#45572=( BOUNDED_SURFACE ( )  B_SPLINE_SURFACE ( 1, 2, ( 
 ( #56597, #80075, #41118, #79594, #19086, #49563, #81061, #73548, #5074, #35560, #25618, #87088, #18114, #79092, #33577, #18598, #49091, #41611, #57079, #72080, #3606, #72561, #76027, #37554, #22552, #29035, #30023, #97083, #20569, #68044, #90525, #36560, #38047, #82542, #37054, #14558, #59047, #6061, #59544, #51556, #98570, #53022, #66554, #13054, #90039, #89056, #28054, #52051, #67049, #29523, #14059, #28554, #22060, #7558, #44542, #52534, #96578, #67553, #60529, #58549, #89551, #21061, #82042, #74042, #91019, #98064, #5577, #75038, #45529, #45027, #51054, #75534, #6544, #97572, #81544, #43548, #36052, #83537, #13554, #60030, #44040, #74541, #15056, #83042, #21562, #7050, #77493, #24527, #55503, #25015, #17514, #68539, #69521, #84030, #54986, #1036, #31497, #77011, #2029, #92014, #8523, #15550, #39521, #47980, #62986, #30516, #70013, #39026, #61019, #24029, #86003, #78490, #69030, #31011, #1539, #62000, #32491, #16525, #565, #31983, #62489, #85505, #10004, #61507, #23544, #92993, #92499, #93492, #47000, #54016, #17015, #47493, #77996, #70, #54497, #8036, #9501, #85012, #91531, #84525, #9005, #53518, #16022, #40003, #70505, #23046, #46035, #76520, #38534, #46511, #40997, #88446, #19946, #11957, #63482, #78976, #19462, #48966, #93986, #25508, #71494, #50441, #80459, #65438, #71965, #72944, #3009, #55995, #42462, #34444, #79476, #80946, #26458, #79959, #57454, #33458, #10975, #3488, #94467, #4474, #95962, #10486, #86495, #33945, #32978, #71002, #94956, #41496, #72445, #56957, #63955, #64935, #40506, #87460, #95463, #2525, #11463, #34940, #17995, #25984, #56481, #86967, #48477, #27444, #41981, #18481, #18975, #64449, #87947, #49453, #49954, #3975, #26954, #57938, #42952, #35438, #37434, #50939, #44417, #96962, #81433, #14435, #6419, #58426, #96461, #21435, #67424, #98445, #67924, #60406, #12444, #13431, #27933, #97949, #43917, #74415, #20946, #44906, #35932, #51433, #88940, #82416, #90902, #6927, #73431, #13940, #81923, #4958, #66928, #29901, #5944, #52902, #65933, #12937, #36435, #20449, #5460, #66429, #29406, #89921, #75408, #28434, #43431, #22430, #90399, #97448, #51932, #73932, #58932, #89432, #28913, #59415, #74921, #36932, #59909, #52418, #21938, #82917, #77371, #46879, #1907, #22925, #37928, #68912, #39882, #68417, #69394, #76885, #8882, #46397, #60898, #31379, #32362, #39400, #15907, #8398, #38907, #54377, #16891, #916, #1413, #98940, #61877, #47370, #75907, #84890, #92382, #440, #23908, #31866, #45912, #53394, #69893, #24400, #16397, #7432, #62365, #30893, #91397, #62869, #92870, #15434, #54868, #84408, #83904 ),
 ( #85379, #76401, #91896, #77868, #38412, #9379, #70388, #7916, #30394, #93365, #61387, #14934, #24893, #23421, #83413, #45401, #53900, #49337, #34823, #41382, #79837, #95839, #94840, #57328, #17390, #25388, #86370, #78860, #32857, #87822, #56843, #63356, #71849, #4357, #3858, #65313, #34318, #3359, #56365, #85878, #47859, #78365, #80335, #93860, #18364, #63835, #19342, #10372, #94349, #2400, #26342, #55377, #49825, #9884, #87342, #25868, #40384, #10861, #72817, #42342, #55871, #17871, #18857, #86858, #11834, #33822, #48354, #11342, #41862, #72325, #70883, #64328, #40873, #64816, #95335, #71378, #2890, #26834, #33341, #48843, #79354, #22185, #98699, #53161, #30148, #60657, #7683, #29170, #76645, #8166, #193, #51691, #67181, #38176, #37197, #82170, #13683, #59671, #38657, #68666, #53653, #60163, #61149, #90163, #44169, #30640, #22680, #67688, #69162, #14693, #68180, #45664, #21693, #98197, #90659, #82673, #91658, #84172, #97704, #74677, #52666, #19826, #57820, #83168, #29654, #91156, #45163, #52179, #83666, #27322, #75667, #15184, #88328, #76161, #23176, #6189, #14189, #44673, #75167, #36693, #15677, #46162, #6677, #7178, #37681, #48111, #48604, #78625, #47631, #1666, #31137, #61630, #23674, #25636, #39157, #32618, #85142, #69647, #2656, #93618, #46636, #84649, #9637, #55630, #86621, #56126, #79108, #686, #32115, #16152, #86130, #62613, #40631, #17152, #18132, #92149, #71129, #10620, #41132, #9137, #55116, #33108, #92630, #63603, #17643, #10136, #94108, #54136, #70635, #39653, #1171, #77138, #8647, #70145, #31631, #62122, #24153, #93120, #54621, #16650, #47122, #77622, #78127, #24647, #85634, #40135, #2163, #63116, #25153, #50086, #58565, #41627, #13068, #80089, #64086, #71620, #42113, #3616, #12579, #26118, #49102, #65566, #35067, #89070, #11108, #56610, #57092, #28068, #87099, #57580, #65068, #96092, #34572, #79605, #19588, #20584, #27574, #4108, #95594, #27079, #42590, #5087, #88076, #88572, #18613, #80590, #35574, #94601, #73070, #12085, #87586, #4606, #20076, #34085, #72092, #58069, #43077, #50581, #64576, #81076, #19098, #95085, #51069, #73563, #26590, #66065, #72575, #49579, #96593, #81561, #3131, #33591, #11594, #84, #7067, #13567, #98588, #37567, #28569, #37071, #45042, #5591, #30531, #51573, #36068, #43560, #7574, #74058, #21075, #14575, #52550, #60545, #82059, #6075, #36576, #98081, #45544, #97590, #67064, #29050, #61032, #91544, #44054, #59557, #75551, #14076, #38060, #90543, #74559, #68058, #30037, #91038, #53530, #29540, #90054, #53036, #60045, #76041, #21577, #22075, #59062, #52065, #6561, #67569, #22567 ) ),
 .UNSPECIFIED., .F., .F., .F. ) 
 B_SPLINE_SURFACE_WITH_KNOTS ( ( 2, 2 ),
 ( 3, 2, 2, 2, 2, 2, 2, 2, 2, 2, 2, 2, 2, 2, 2, 2, 2, 2, 2, 2, 2, 2, 2, 2, 2, 2, 2, 2, 2, 2, 2, 2, 2, 2, 2, 2, 2, 2, 2, 2, 2, 2, 2, 2, 2, 2, 2, 2, 2, 2, 2, 2, 2, 2, 2, 2, 2, 2, 2, 2, 2, 2, 2, 2, 2, 2, 2, 2, 2, 2, 2, 2, 2, 2, 2, 2, 2, 2, 2, 2, 2, 2, 2, 2, 2, 2, 2, 2, 2, 2, 2, 2, 2, 2, 2, 2, 2, 2, 2, 2, 2, 2, 2, 2, 2, 2, 2, 2, 2, 2, 2, 2, 2, 2, 2, 2, 2, 2, 2, 2, 2, 2, 2, 2, 2, 2, 2, 2, 2, 2, 2, 2, 2, 2, 2, 2, 2, 2, 2, 2, 2, 2, 2, 2, 2, 2, 2, 2, 2, 2, 2, 2, 2, 2, 2, 2, 2, 2, 2, 2, 2, 2, 3 ),
 ( 0.000000000000000000, 1.000000000000000000 ),
 ( 0.000000000000000000, 0.005952380952380952051, 0.01190476190476190410, 0.01785714285714285615, 0.02380952380952380820, 0.02976190476190476025, 0.03571428571428571230, 0.04166666666666666435, 0.04761904761904761640, 0.05357142857142856845, 0.05952380952380952051, 0.06547619047619047949, 0.07142857142857142461, 0.07738095238095238360, 0.08333333333333332871, 0.08928571428571428770, 0.09523809523809523281, 0.1011904761904761918, 0.1071428571428571369, 0.1130952380952380959, 0.1190476190476190410, 0.1250000000000000000, 0.1309523809523809590, 0.1369047619047619180, 0.1428571428571428492, 0.1488095238095238082, 0.1547619047619047672, 0.1607142857142857262, 0.1666666666666666574, 0.1726190476190476164, 0.1785714285714285754, 0.1845238095238095344, 0.1904761904761904656, 0.1964285714285714246, 0.2023809523809523836, 0.2083333333333333426, 0.2142857142857142738, 0.2202380952380952328, 0.2261904761904761918, 0.2321428571428571508, 0.2380952380952380820, 0.2440476190476190410, 0.2500000000000000000, 0.2559523809523809312, 0.2619047619047619180, 0.2678571428571428492, 0.2738095238095238360, 0.2797619047619047672, 0.2857142857142856984, 0.2916666666666666852, 0.2976190476190476164, 0.3035714285714285476, 0.3095238095238095344, 0.3154761904761904656, 0.3214285714285714524, 0.3273809523809523836, 0.3333333333333333148, 0.3392857142857143016, 0.3452380952380952328, 0.3511904761904761640, 0.3571428571428571508, 0.3630952380952380820, 0.3690476190476190688, 0.3750000000000000000, 0.3809523809523809312, 0.3869047619047619180, 0.3928571428571428492, 0.3988095238095238360, 0.4047619047619047672, 0.4107142857142856984, 0.4166666666666666852, 0.4226190476190476164, 0.4285714285714285476, 0.4345238095238095344, 0.4404761904761904656, 0.4464285714285714524, 0.4523809523809523836, 0.4583333333333333148, 0.4642857142857143016, 0.4702380952380952328, 0.4761904761904761640, 0.4821428571428571508, 0.4880952380952380820, 0.4940476190476190688, 0.5000000000000000000, 0.5059523809523809312, 0.5119047619047618625, 0.5178571428571429047, 0.5238095238095238360, 0.5297619047619047672, 0.5357142857142856984, 0.5416666666666666297, 0.5476190476190476719, 0.5535714285714286031, 0.5595238095238095344, 0.5654761904761904656, 0.5714285714285713969, 0.5773809523809523281, 0.5833333333333333703, 0.5892857142857143016, 0.5952380952380952328, 0.6011904761904761640, 0.6071428571428570953, 0.6130952380952381375, 0.6190476190476190688, 0.6250000000000000000, 0.6309523809523809312, 0.6369047619047618625, 0.6428571428571429047, 0.6488095238095238360, 0.6547619047619047672, 0.6607142857142856984, 0.6666666666666666297, 0.6726190476190476719, 0.6785714285714286031, 0.6845238095238095344, 0.6904761904761904656, 0.6964285714285713969, 0.7023809523809523281, 0.7083333333333333703, 0.7142857142857143016, 0.7202380952380952328, 0.7261904761904761640, 0.7321428571428570953, 0.7380952380952381375, 0.7440476190476190688, 0.7500000000000000000, 0.7559523809523809312, 0.7619047619047618625, 0.7678571428571429047, 0.7738095238095238360, 0.7797619047619047672, 0.7857142857142856984, 0.7916666666666666297, 0.7976190476190476719, 0.8035714285714286031, 0.8095238095238095344, 0.8154761904761904656, 0.8214285714285713969, 0.8273809523809523281, 0.8333333333333333703, 0.8392857142857143016, 0.8452380952380952328, 0.8511904761904761640, 0.8571428571428570953, 0.8630952380952381375, 0.8690476190476190688, 0.8750000000000000000, 0.8809523809523809312, 0.8869047619047618625, 0.8928571428571429047, 0.8988095238095238360, 0.9047619047619047672, 0.9107142857142856984, 0.9166666666666666297, 0.9226190476190476719, 0.9285714285714286031, 0.9345238095238095344, 0.9404761904761904656, 0.9464285714285713969, 0.9523809523809523281, 0.9583333333333333703, 0.9642857142857143016 ),
 .UNSPECIFIED. ) 
 GEOMETRIC_REPRESENTATION_ITEM ( )  RATIONAL_B_SPLINE_SURFACE ( (
 ( 1.000000000000000000, 0.9659258262890683122, 1.000000000000000000, 0.9659258262890683122, 1.000000000000000000, 0.9659258262890683122, 1.000000000000000000, 0.9659258262890683122, 1.000000000000000000, 0.9659258262890683122, 1.000000000000000000, 0.9659258262890683122, 1.000000000000000000, 0.9659258262890683122, 1.000000000000000000, 0.9659258262890683122, 1.000000000000000000, 0.9659258262890683122, 1.000000000000000000, 0.9659258262890683122, 1.000000000000000000, 0.9659258262890683122, 1.000000000000000000, 0.9659258262890683122, 1.000000000000000000, 0.9659258262890683122, 1.000000000000000000, 0.9659258262890683122, 1.000000000000000000, 0.9659258262890683122, 1.000000000000000000, 0.9659258262890683122, 1.000000000000000000, 0.9659258262890683122, 1.000000000000000000, 0.9659258262890683122, 1.000000000000000000, 0.9659258262890683122, 1.000000000000000000, 0.9659258262890683122, 1.000000000000000000, 0.9659258262890683122, 1.000000000000000000, 0.9659258262890683122, 1.000000000000000000, 0.9659258262890683122, 1.000000000000000000, 0.9659258262890683122, 1.000000000000000000, 0.9659258262890683122, 1.000000000000000000, 0.9659258262890683122, 1.000000000000000000, 0.9659258262890683122, 1.000000000000000000, 0.9659258262890683122, 1.000000000000000000, 0.9659258262890683122, 1.000000000000000000, 0.9659258262890683122, 1.000000000000000000, 0.9659258262890683122, 1.000000000000000000, 0.9659258262890683122, 1.000000000000000000, 0.9659258262890683122, 1.000000000000000000, 0.9659258262890683122, 1.000000000000000000, 0.9659258262890683122, 1.000000000000000000, 0.9659258262890683122, 1.000000000000000000, 0.9659258262890683122, 1.000000000000000000, 0.9659258262890683122, 1.000000000000000000, 0.9659258262890683122, 1.000000000000000000, 0.9659258262890683122, 1.000000000000000000, 0.9659258262890683122, 1.000000000000000000, 0.9659258262890683122, 1.000000000000000000, 0.9659258262890683122, 1.000000000000000000, 0.9659258262890683122, 1.000000000000000000, 0.9659258262890683122, 1.000000000000000000, 0.9659258262890683122, 1.000000000000000000, 0.9659258262890683122, 1.000000000000000000, 0.9659258262890683122, 1.000000000000000000, 0.9659258262890683122, 1.000000000000000000, 0.9659258262890683122, 1.000000000000000000, 0.9659258262890683122, 1.000000000000000000, 0.9659258262890683122, 1.000000000000000000, 0.9659258262890683122, 1.000000000000000000, 0.9659258262890683122, 1.000000000000000000, 0.9659258262890683122, 1.000000000000000000, 0.9659258262890683122, 1.000000000000000000, 0.9659258262890683122, 1.000000000000000000, 0.9659258262890683122, 1.000000000000000000, 0.9659258262890683122, 1.000000000000000000, 0.9659258262890683122, 1.000000000000000000, 0.9659258262890683122, 1.000000000000000000, 0.9659258262890683122, 1.000000000000000000, 0.9659258262890683122, 1.000000000000000000, 0.9659258262890683122, 1.000000000000000000, 0.9659258262890683122, 1.000000000000000000, 0.9659258262890683122, 1.000000000000000000, 0.9659258262890683122, 1.000000000000000000, 0.9659258262890683122, 1.000000000000000000, 0.9659258262890683122, 1.000000000000000000, 0.9659258262890683122, 1.000000000000000000, 0.9659258262890683122, 1.000000000000000000, 0.9659258262890683122, 1.000000000000000000, 0.9659258262890683122, 1.000000000000000000, 0.9659258262890683122, 1.000000000000000000, 0.9659258262890683122, 1.000000000000000000, 0.9659258262890683122, 1.000000000000000000, 0.9659258262890683122, 1.000000000000000000, 0.9659258262890683122, 1.000000000000000000, 0.9659258262890683122, 1.000000000000000000, 0.9659258262890683122, 1.000000000000000000, 0.9659258262890683122, 1.000000000000000000, 0.9659258262890683122, 1.000000000000000000, 0.9659258262890683122, 1.000000000000000000, 0.9659258262890683122, 1.000000000000000000, 0.9659258262890683122, 1.000000000000000000, 0.9659258262890683122, 1.000000000000000000, 0.9659258262890683122, 1.000000000000000000, 0.9659258262890683122, 1.000000000000000000, 0.9659258262890683122, 1.000000000000000000, 0.9659258262890683122, 1.000000000000000000, 0.9659258262890683122, 1.000000000000000000, 0.9659258262890683122, 1.000000000000000000, 0.9659258262890683122, 1.000000000000000000, 0.9659258262890683122, 1.000000000000000000, 0.9659258262890683122, 1.000000000000000000, 0.9659258262890683122, 1.000000000000000000, 0.9659258262890683122, 1.000000000000000000, 0.9659258262890683122, 1.000000000000000000, 0.9659258262890683122, 1.000000000000000000, 0.9659258262890683122, 1.000000000000000000, 0.9659258262890683122, 1.000000000000000000, 0.9659258262890683122, 1.000000000000000000, 0.9659258262890683122, 1.000000000000000000, 0.9659258262890683122, 1.000000000000000000, 0.9659258262890683122, 1.000000000000000000, 0.9659258262890683122, 1.000000000000000000, 0.9659258262890683122, 1.000000000000000000, 0.9659258262890683122, 1.000000000000000000, 0.9659258262890683122, 1.000000000000000000, 0.9659258262890683122, 1.000000000000000000, 0.9659258262890683122, 1.000000000000000000, 0.9659258262890683122, 1.000000000000000000, 0.9659258262890683122, 1.000000000000000000, 0.9659258262890683122, 1.000000000000000000, 0.9659258262890683122, 1.000000000000000000, 0.9659258262890683122, 1.000000000000000000, 0.9659258262890683122, 1.000000000000000000, 0.9659258262890683122, 1.000000000000000000, 0.9659258262890683122, 1.000000000000000000, 0.9659258262890683122, 1.000000000000000000, 0.9659258262890683122, 1.000000000000000000, 0.9659258262890683122, 1.000000000000000000, 0.9659258262890683122, 1.000000000000000000, 0.9659258262890683122, 1.000000000000000000, 0.9659258262890683122, 1.000000000000000000, 0.9659258262890683122, 1.000000000000000000, 0.9659258262890683122, 1.000000000000000000, 0.9659258262890683122, 1.000000000000000000, 0.9659258262890683122, 1.000000000000000000, 0.9659258262890683122, 1.000000000000000000, 0.9659258262890683122, 1.000000000000000000, 0.9659258262890683122, 1.000000000000000000, 0.9659258262890683122, 1.000000000000000000, 0.9659258262890683122, 1.000000000000000000, 0.9659258262890683122, 1.000000000000000000, 0.9659258262890683122, 1.000000000000000000, 0.9659258262890683122, 1.000000000000000000, 0.9659258262890683122, 1.000000000000000000, 0.9659258262890683122, 1.000000000000000000, 0.9659258262890683122, 1.000000000000000000, 0.9659258262890683122, 1.000000000000000000, 0.9659258262890683122, 1.000000000000000000, 0.9659258262890683122, 1.000000000000000000, 0.9659258262890683122, 1.000000000000000000, 0.9659258262890683122, 1.000000000000000000, 0.9659258262890683122, 1.000000000000000000, 0.9659258262890683122, 1.000000000000000000, 0.9659258262890683122, 1.000000000000000000, 0.9659258262890683122, 1.000000000000000000, 0.9659258262890683122, 1.000000000000000000, 0.9659258262890683122, 1.000000000000000000, 0.9659258262890683122, 1.000000000000000000, 0.9659258262890683122, 1.000000000000000000, 0.9659258262890683122, 1.000000000000000000, 0.9659258262890683122, 1.000000000000000000, 0.9659258262890683122, 1.000000000000000000, 0.9659258262890683122, 1.000000000000000000, 0.9659258262890683122, 1.000000000000000000, 0.9659258262890683122, 1.000000000000000000, 0.9659258262890683122, 1.000000000000000000, 0.9659258262890683122, 1.000000000000000000, 0.9659258262890683122, 1.000000000000000000),
 ( 1.000000000000000000, 0.9659258262890683122, 1.000000000000000000, 0.9659258262890683122, 1.000000000000000000, 0.9659258262890683122, 1.000000000000000000, 0.9659258262890683122, 1.000000000000000000, 0.9659258262890683122, 1.000000000000000000, 0.9659258262890683122, 1.000000000000000000, 0.9659258262890683122, 1.000000000000000000, 0.9659258262890683122, 1.000000000000000000, 0.9659258262890683122, 1.000000000000000000, 0.9659258262890683122, 1.000000000000000000, 0.9659258262890683122, 1.000000000000000000, 0.9659258262890683122, 1.000000000000000000, 0.9659258262890683122, 1.000000000000000000, 0.9659258262890683122, 1.000000000000000000, 0.9659258262890683122, 1.000000000000000000, 0.9659258262890683122, 1.000000000000000000, 0.9659258262890683122, 1.000000000000000000, 0.9659258262890683122, 1.000000000000000000, 0.9659258262890683122, 1.000000000000000000, 0.9659258262890683122, 1.000000000000000000, 0.9659258262890683122, 1.000000000000000000, 0.9659258262890683122, 1.000000000000000000, 0.9659258262890683122, 1.000000000000000000, 0.9659258262890683122, 1.000000000000000000, 0.9659258262890683122, 1.000000000000000000, 0.9659258262890683122, 1.000000000000000000, 0.9659258262890683122, 1.000000000000000000, 0.9659258262890683122, 1.000000000000000000, 0.9659258262890683122, 1.000000000000000000, 0.9659258262890683122, 1.000000000000000000, 0.9659258262890683122, 1.000000000000000000, 0.9659258262890683122, 1.000000000000000000, 0.9659258262890683122, 1.000000000000000000, 0.9659258262890683122, 1.000000000000000000, 0.9659258262890683122, 1.000000000000000000, 0.9659258262890683122, 1.000000000000000000, 0.9659258262890683122, 1.000000000000000000, 0.9659258262890683122, 1.000000000000000000, 0.9659258262890683122, 1.000000000000000000, 0.9659258262890683122, 1.000000000000000000, 0.9659258262890683122, 1.000000000000000000, 0.9659258262890683122, 1.000000000000000000, 0.9659258262890683122, 1.000000000000000000, 0.9659258262890683122, 1.000000000000000000, 0.9659258262890683122, 1.000000000000000000, 0.9659258262890683122, 1.000000000000000000, 0.9659258262890683122, 1.000000000000000000, 0.9659258262890683122, 1.000000000000000000, 0.9659258262890683122, 1.000000000000000000, 0.9659258262890683122, 1.000000000000000000, 0.9659258262890683122, 1.000000000000000000, 0.9659258262890683122, 1.000000000000000000, 0.9659258262890683122, 1.000000000000000000, 0.9659258262890683122, 1.000000000000000000, 0.9659258262890683122, 1.000000000000000000, 0.9659258262890683122, 1.000000000000000000, 0.9659258262890683122, 1.000000000000000000, 0.9659258262890683122, 1.000000000000000000, 0.9659258262890683122, 1.000000000000000000, 0.9659258262890683122, 1.000000000000000000, 0.9659258262890683122, 1.000000000000000000, 0.9659258262890683122, 1.000000000000000000, 0.9659258262890683122, 1.000000000000000000, 0.9659258262890683122, 1.000000000000000000, 0.9659258262890683122, 1.000000000000000000, 0.9659258262890683122, 1.000000000000000000, 0.9659258262890683122, 1.000000000000000000, 0.9659258262890683122, 1.000000000000000000, 0.9659258262890683122, 1.000000000000000000, 0.9659258262890683122, 1.000000000000000000, 0.9659258262890683122, 1.000000000000000000, 0.9659258262890683122, 1.000000000000000000, 0.9659258262890683122, 1.000000000000000000, 0.9659258262890683122, 1.000000000000000000, 0.9659258262890683122, 1.000000000000000000, 0.9659258262890683122, 1.000000000000000000, 0.9659258262890683122, 1.000000000000000000, 0.9659258262890683122, 1.000000000000000000, 0.9659258262890683122, 1.000000000000000000, 0.9659258262890683122, 1.000000000000000000, 0.9659258262890683122, 1.000000000000000000, 0.9659258262890683122, 1.000000000000000000, 0.9659258262890683122, 1.000000000000000000, 0.9659258262890683122, 1.000000000000000000, 0.9659258262890683122, 1.000000000000000000, 0.9659258262890683122, 1.000000000000000000, 0.9659258262890683122, 1.000000000000000000, 0.9659258262890683122, 1.000000000000000000, 0.9659258262890683122, 1.000000000000000000, 0.9659258262890683122, 1.000000000000000000, 0.9659258262890683122, 1.000000000000000000, 0.9659258262890683122, 1.000000000000000000, 0.9659258262890683122, 1.000000000000000000, 0.9659258262890683122, 1.000000000000000000, 0.9659258262890683122, 1.000000000000000000, 0.9659258262890683122, 1.000000000000000000, 0.9659258262890683122, 1.000000000000000000, 0.9659258262890683122, 1.000000000000000000, 0.9659258262890683122, 1.000000000000000000, 0.9659258262890683122, 1.000000000000000000, 0.9659258262890683122, 1.000000000000000000, 0.9659258262890683122, 1.000000000000000000, 0.9659258262890683122, 1.000000000000000000, 0.9659258262890683122, 1.000000000000000000, 0.9659258262890683122, 1.000000000000000000, 0.9659258262890683122, 1.000000000000000000, 0.9659258262890683122, 1.000000000000000000, 0.9659258262890683122, 1.000000000000000000, 0.9659258262890683122, 1.000000000000000000, 0.9659258262890683122, 1.000000000000000000, 0.9659258262890683122, 1.000000000000000000, 0.9659258262890683122, 1.000000000000000000, 0.9659258262890683122, 1.000000000000000000, 0.9659258262890683122, 1.000000000000000000, 0.9659258262890683122, 1.000000000000000000, 0.9659258262890683122, 1.000000000000000000, 0.9659258262890683122, 1.000000000000000000, 0.9659258262890683122, 1.000000000000000000, 0.9659258262890683122, 1.000000000000000000, 0.9659258262890683122, 1.000000000000000000, 0.9659258262890683122, 1.000000000000000000, 0.9659258262890683122, 1.000000000000000000, 0.9659258262890683122, 1.000000000000000000, 0.9659258262890683122, 1.000000000000000000, 0.9659258262890683122, 1.000000000000000000, 0.9659258262890683122, 1.000000000000000000, 0.9659258262890683122, 1.000000000000000000, 0.9659258262890683122, 1.000000000000000000, 0.9659258262890683122, 1.000000000000000000, 0.9659258262890683122, 1.000000000000000000, 0.9659258262890683122, 1.000000000000000000, 0.9659258262890683122, 1.000000000000000000, 0.9659258262890683122, 1.000000000000000000, 0.9659258262890683122, 1.000000000000000000, 0.9659258262890683122, 1.000000000000000000, 0.9659258262890683122, 1.000000000000000000, 0.9659258262890683122, 1.000000000000000000, 0.9659258262890683122, 1.000000000000000000, 0.9659258262890683122, 1.000000000000000000, 0.9659258262890683122, 1.000000000000000000, 0.9659258262890683122, 1.000000000000000000, 0.9659258262890683122, 1.000000000000000000, 0.9659258262890683122, 1.000000000000000000, 0.9659258262890683122, 1.000000000000000000, 0.9659258262890683122, 1.000000000000000000, 0.9659258262890683122, 1.000000000000000000, 0.9659258262890683122, 1.000000000000000000, 0.9659258262890683122, 1.000000000000000000, 0.9659258262890683122, 1.000000000000000000, 0.9659258262890683122, 1.000000000000000000, 0.9659258262890683122, 1.000000000000000000, 0.9659258262890683122, 1.000000000000000000, 0.9659258262890683122, 1.000000000000000000, 0.9659258262890683122, 1.000000000000000000, 0.9659258262890683122, 1.000000000000000000, 0.9659258262890683122, 1.000000000000000000, 0.9659258262890683122, 1.000000000000000000, 0.9659258262890683122, 1.000000000000000000, 0.9659258262890683122, 1.000000000000000000, 0.9659258262890683122, 1.000000000000000000, 0.9659258262890683122, 1.000000000000000000, 0.9659258262890683122, 1.000000000000000000) ) ) 
 REPRESENTATION_ITEM ( '' )  SURFACE ( )  );
#45573=CARTESIAN_POINT ( 'NONE',  ( 10.00000000000000178, 8.053748834913967869, 14.16423886937410082 ) ) ;
#45575=CARTESIAN_POINT ( 'NONE',  ( -46.94000000000001194, 93.00000000000000000, 9.000000000000000000 ) ) ;
#45576=CARTESIAN_POINT ( 'NONE',  ( 12.91533473730993009, 6.605352010821504471, -10.88017736071109987 ) ) ;
#45578=CARTESIAN_POINT ( 'NONE',  ( 16.40814093676324603, 47.45696800326375353, -11.09922568453594671 ) ) ;
#45579=ORIENTED_EDGE ( 'NONE', *, *, #26477, .T. ) ;
#45581=CARTESIAN_POINT ( 'NONE',  ( 1.472469842513823179, 50.59226448433411605, -4.923371831947296329 ) ) ;
#45582=CARTESIAN_POINT ( 'NONE',  ( 0.1532563361054100626, 0.8005978176674514168, -2.638427012816831230 ) ) ;
#45583=CARTESIAN_POINT ( 'NONE',  ( 22.81628187352647785, 16.41530133659708923, 3.434112377981063169 ) ) ;
#45584=CARTESIAN_POINT ( 'NONE',  ( 18.52753015748617571, 18.09226448433411960, 4.923371831947298993 ) ) ;
#45585=CARTESIAN_POINT ( 'NONE',  ( 1.274849032794294290, 63.57228050351031357, 6.499999999999979572 ) ) ;
#45586=CARTESIAN_POINT ( 'NONE',  ( 19.38216949554541202, 20.99863466993042138, 9.382169495545424454 ) ) ;
#45587=CARTESIAN_POINT ( 'NONE',  ( 2.603489959281060973, 26.58210964143323096, 6.499999999999401368 ) ) ;
#45588=CARTESIAN_POINT ( 'NONE',  ( 2.791683348922237240, 5.383931151000785675, -7.208316651077763204 ) ) ;
#45591=CARTESIAN_POINT ( 'NONE',  ( 20.88017736071110164, 20.35535201082150891, 2.915334737309930979 ) ) ;
#45592=CARTESIAN_POINT ( 'NONE',  ( 17.08211943468705130, 18.47041550158063572, 12.26659068614894998 ) ) ;
#45593=CARTESIAN_POINT ( 'NONE',  ( 2.791683348922237240, 45.38393115100079456, -7.208316651077763204 ) ) ;
#45594=CARTESIAN_POINT ( 'NONE',  ( 2.791683348922237240, 5.383931151000785675, -7.208316651077763204 ) ) ;
#45595=CARTESIAN_POINT ( 'NONE',  ( -1.099225684535947600, 39.54030133659708923, 6.408140936763237150 ) ) ;
#45597=CARTESIAN_POINT ( 'NONE',  ( 10.00000000000000178, 9.313685344154839285, 10.88017736071110342 ) ) ;
#45599=CARTESIAN_POINT ( 'NONE',  ( 10.00000000000000178, 15.37363466993042138, 12.81628187352647608 ) ) ;
#45600=CARTESIAN_POINT ( 'NONE',  ( 13.43411237798106583, 12.66530133659708746, -12.81628187352647252 ) ) ;
#45601=CARTESIAN_POINT ( 'NONE',  ( 0.1532563361054100626, 30.80059781766744820, -2.638427012816831230 ) ) ;
#45603=CARTESIAN_POINT ( 'NONE',  ( 0.6178305044545818747, 33.49863466993042493, -9.382169495545419124 ) ) ;
#45604=LINE ( 'NONE', #30096, #57981 ) ;
#45606=CARTESIAN_POINT ( 'NONE',  ( 7.084665262690076126, 44.10535201082151247, 10.88017736071109987 ) ) ;
#45610=CARTESIAN_POINT ( 'NONE',  ( 17.96484262340118221, 66.18868534415483396, -7.964842623401177768 ) ) ;
#45611=CARTESIAN_POINT ( 'NONE',  ( 20.88017736071110164, 35.35535201082150536, 2.915334737309930979 ) ) ;
#45612=CARTESIAN_POINT ( 'NONE',  ( -0.8801773607111009756, 48.06368534415484817, 1.068504757029289695E-15 ) ) ;
#45613=CARTESIAN_POINT ( 'NONE',  ( 2.791683348922237240, 60.38393115100078745, -7.208316651077763204 ) ) ;
#45618=CARTESIAN_POINT ( 'NONE',  ( 0.1532563361054100626, 45.80059781766745886, -2.638427012816831230 ) ) ;
#45619=CARTESIAN_POINT ( 'NONE',  ( 7.084665262690076126, 4.105352010821503583, 10.88017736071109987 ) ) ;
#45621=CARTESIAN_POINT ( 'NONE',  ( 22.81628187352648496, 11.83196800326375531, -3.434112377981050290 ) ) ;
#45623=CARTESIAN_POINT ( 'NONE',  ( 0.5774900079438607392, 33.48035201082150536, 5.440088680355550821 ) ) ;
#45624=CARTESIAN_POINT ( 'NONE',  ( 1.472469842513823179, 65.59226448433412315, -4.923371831947296329 ) ) ;
#45626=CARTESIAN_POINT ( 'NONE',  ( 17.96484262340118221, 4.938685344154837509, 7.964842623401181321 ) ) ;
#45627=CARTESIAN_POINT ( 'NONE',  ( 7.084665262690076126, 24.10535201082150181, 10.88017736071109987 ) ) ;
#45628=CARTESIAN_POINT ( 'NONE',  ( 24.16423886937409904, 34.09541550158064638, 3.795296366450317205 ) ) ;
#45629=CARTESIAN_POINT ( 'NONE',  ( 14.92337183194729633, 32.67559781766745175, 8.527530157486181039 ) ) ;
#45630=CARTESIAN_POINT ( 'NONE',  ( 12.91533473730993009, 41.60535201082149825, -10.88017736071109987 ) ) ;
#45631=CARTESIAN_POINT ( 'NONE',  ( 22.26659068614895176, 9.720415501580633943, -7.082119434687042414 ) ) ;
#45633=CARTESIAN_POINT ( 'NONE',  ( -46.83212803583222694, 103.4681393821014836, 5.836481404741387102 ) ) ;
#45634=CARTESIAN_POINT ( 'NONE',  ( 19.84674366389459266, 58.71726448433411605, -2.638427012816827677 ) ) ;
#45639=CARTESIAN_POINT ( 'NONE',  ( -0.3689425029237898834, 31.17874883491396787, -10.36894250292378850 ) ) ;
#45640=CARTESIAN_POINT ( 'NONE',  ( 10.00000000000000178, 28.05374883491396787, 14.16423886937410082 ) ) ;
#45641=CARTESIAN_POINT ( 'NONE',  ( 10.00000000000000000, 4.758931151000784787, -9.846743663894594434 ) ) ;
#45643=CARTESIAN_POINT ( 'NONE',  ( -0.3689425029237881626, 62.42874883491396787, 10.36894250292379027 ) ) ;
#45644=CARTESIAN_POINT ( 'NONE',  ( 18.52753015748618282, 53.92559781766745175, -4.923371831947291888 ) ) ;
#45646=CARTESIAN_POINT ( 'NONE',  ( 4.559911319644449179, 47.23035201082150536, -9.422509992056141925 ) ) ;
#45647=CARTESIAN_POINT ( 'NONE',  ( 19.38216949554541557, 22.24863466993041428, -9.382169495545420901 ) ) ;
#45648=CARTESIAN_POINT ( 'NONE',  ( 20.36894250292379382, 13.67874883491396965, 10.36894250292379205 ) ) ;
#45649=CARTESIAN_POINT ( 'NONE',  ( 12.91533473730992121, 14.52201867748817143, 10.88017736071110164 ) ) ;
#45651=CARTESIAN_POINT ( 'NONE',  ( 19.42250999205614548, 35.98035201082151247, -5.440088680355545492 ) ) ;
#45653=CARTESIAN_POINT ( 'NONE',  ( -0.8801773607111008646, 53.27201867748816966, 2.915334737309923430 ) ) ;
#45654=EDGE_CURVE ( 'NONE', #18045, #57285, #8789, .T. ) ;
#45660=EDGE_LOOP ( 'NONE', ( #32710, #65028, #83095, #15811, #27925, #90821, #69507, #90085, #29287, #55154, #98663, #27588, #35001, #41738, #5451, #24020, #70969, #65717, #53896, #76327, #35192, #15496, #79201, #26979, #216, #30954, #75913, #44669, #27470, #19025, #82340, #12010 ) ) ;
#45662=CARTESIAN_POINT ( 'NONE',  ( 20.36894250292379382, 63.67874883491396787, 10.36894250292379205 ) ) ;
#45663=CARTESIAN_POINT ( 'NONE',  ( 2.917880565312950480, 60.97041550158063927, -12.26659068614894821 ) ) ;
#45664=CARTESIAN_POINT ( 'NONE',  ( 17.20831665107776587, 22.88393115100078745, 7.208316651077764980 ) ) ;
#45665=CARTESIAN_POINT ( 'NONE',  ( 18.52753015748618282, 53.92559781766745175, -4.923371831947291888 ) ) ;
#45668=CARTESIAN_POINT ( 'NONE',  ( 19.84674366389459266, 8.717264484334116048, -2.638427012816827677 ) ) ;
#45672=CARTESIAN_POINT ( 'NONE',  ( 17.08211943468705130, 33.47041550158063927, 12.26659068614894998 ) ) ;
#45673=CARTESIAN_POINT ( 'NONE',  ( 24.16423886937409904, 39.09541550158062506, 3.795296366450317205 ) ) ;
#45674=VERTEX_POINT ( 'NONE', #17355 ) ;
#45675=CARTESIAN_POINT ( 'NONE',  ( -1.099225684535947600, 59.54030133659708923, 6.408140936763237150 ) ) ;
#45676=CARTESIAN_POINT ( 'NONE',  ( 10.00000000000000000, 21.81368534415484106, -10.88017736071110342 ) ) ;
#45677=CARTESIAN_POINT ( 'NONE',  ( 7.361572987183169658, 44.96726448433412315, -9.846743663894592657 ) ) ;
#45678=CARTESIAN_POINT ( 'NONE',  ( 4.559911319644449179, 22.23035201082150536, -9.422509992056141925 ) ) ;
#45679=CARTESIAN_POINT ( 'NONE',  ( -1.099225684535947600, 63.70696800326376774, -6.408140936763238038 ) ) ;
#45681=CARTESIAN_POINT ( 'NONE',  ( 2.791683348922237240, 60.38393115100078745, -7.208316651077763204 ) ) ;
#45682=CARTESIAN_POINT ( 'NONE',  ( 10.00000000000000000, 49.75893115100078745, -9.846743663894594434 ) ) ;
#45684=AXIS2_PLACEMENT_3D ( 'NONE', #3168, #64617, #5132 ) ;
#45685=LINE ( 'NONE', #60676, #37732 ) ;
#45690=CARTESIAN_POINT ( 'NONE',  ( 12.63842701281683034, 32.46726448433412315, 9.846743663894596210 ) ) ;
#45692=CARTESIAN_POINT ( 'NONE',  ( 21.09922568453595559, 37.04030133659708923, -6.408140936763230044 ) ) ;
#45693=FACE_OUTER_BOUND ( 'NONE', #29166, .T. ) ;
#45694=CARTESIAN_POINT ( 'NONE',  ( -0.03743638938522799581, 39.25197528031018379, -6.399506433553962204 ) ) ;
#45696=CARTESIAN_POINT ( 'NONE',  ( 14.92337183194729988, 64.34226448433412315, -8.527530157486177487 ) ) ;
#45698=CARTESIAN_POINT ( 'NONE',  ( 0.1532563361054100626, 40.80059781766745886, -2.638427012816831230 ) ) ;
#45699=CARTESIAN_POINT ( 'NONE',  ( -4.164238869374098151, 36.59541550158063217, -3.795296366450310543 ) ) ;
#45700=CARTESIAN_POINT ( 'NONE',  ( 2.791683348922237240, 55.38393115100078745, -7.208316651077763204 ) ) ;
#45702=CARTESIAN_POINT ( 'NONE',  ( 2.791683348922237240, 0.3839311510007847872, -7.208316651077763204 ) ) ;
#45703=( LENGTH_UNIT ( ) NAMED_UNIT ( * ) SI_UNIT ( .MILLI., .METRE. ) );
#45704=EDGE_CURVE ( 'NONE', #5362, #1078, #76774, .T. ) ;
#45705=CARTESIAN_POINT ( 'NONE',  ( 10.00000000000000000, 49.75893115100078745, -9.846743663894594434 ) ) ;
#45706=CARTESIAN_POINT ( 'NONE',  ( 17.96484262340118221, 56.18868534415484817, -7.964842623401177768 ) ) ;
#45707=AXIS2_PLACEMENT_3D ( 'NONE', #13857, #44337, #50361 ) ;
#45708=CARTESIAN_POINT ( 'NONE',  ( 1.472469842513823179, 46.42559781766745175, 4.923371831947296329 ) ) ;
#45712=VERTEX_POINT ( 'NONE', #85841 ) ;
#45713=CARTESIAN_POINT ( 'NONE',  ( 2.035157376598824452, 48.68868534415483396, 7.964842623401179544 ) ) ;
#45716=CARTESIAN_POINT ( 'NONE',  ( 20.88017736071110519, 35.56368534415484106, 2.639326808657452039E-16 ) ) ;
#45717=CARTESIAN_POINT ( 'NONE',  ( -2.816281873526473856, 4.331968003263754419, 3.434112377981055619 ) ) ;
#45718=CARTESIAN_POINT ( 'NONE',  ( 0.5774900079438607392, 58.48035201082151247, 5.440088680355550821 ) ) ;
#45720=CARTESIAN_POINT ( 'NONE',  ( 18.52753015748618282, 13.92559781766745175, -4.923371831947291888 ) ) ;
#45722=CARTESIAN_POINT ( 'NONE',  ( 4.559911319644449179, 43.89701867748816966, 9.422509992056141925 ) ) ;
#45724=CARTESIAN_POINT ( 'NONE',  ( 10.00000000000000000, 9.758931151000785675, -9.846743663894594434 ) ) ;
#45725=CARTESIAN_POINT ( 'NONE',  ( 17.20831665107776587, 37.88393115100078745, 7.208316651077764980 ) ) ;
#45726=CARTESIAN_POINT ( 'NONE',  ( 19.88565890683628012, 57.71691075486304356, -6.480892540919849232 ) ) ;
#45728=CARTESIAN_POINT ( 'NONE',  ( -2.816281873526471635, -1.084698663402913210, -3.434112377981056508 ) ) ;
#45730=CARTESIAN_POINT ( 'NONE',  ( 6.204703633549690345, 60.76208216824730357, -14.16423886937410259 ) ) ;
#45732=CARTESIAN_POINT ( 'NONE',  ( 24.16423886937410614, 19.51208216824729647, -3.795296366450302550 ) ) ;
#45733=AXIS2_PLACEMENT_3D ( 'NONE', #21962, #75437, #60429 ) ;
#45734=CARTESIAN_POINT ( 'NONE',  ( 17.08211943468705130, 48.47041550158063927, 12.26659068614894998 ) ) ;
#45736=CARTESIAN_POINT ( 'NONE',  ( 12.63842701281683034, 12.46726448433411782, 9.846743663894596210 ) ) ;
#45737=CARTESIAN_POINT ( 'NONE',  ( 2.035157376598822676, 2.438685344154837953, -7.964842623401177768 ) ) ;
#45739=VERTEX_POINT ( 'NONE', #9342 ) ;
#45740=CARTESIAN_POINT ( 'NONE',  ( 18.52753015748617571, 28.09226448433411960, 4.923371831947298993 ) ) ;
#45741=CARTESIAN_POINT ( 'NONE',  ( -0.8801773607111009756, 33.06368534415484106, 1.068504757029289695E-15 ) ) ;
#45742=CARTESIAN_POINT ( 'NONE',  ( 14.92337183194729988, 44.34226448433412315, -8.527530157486177487 ) ) ;
#45743=CARTESIAN_POINT ( 'NONE',  ( 10.00000000000000178, 3.053748834913967425, 14.16423886937410082 ) ) ;
#45744=DIRECTION ( 'NONE',  ( -0.000000000000000000, 0.000000000000000000, -1.000000000000000000 ) ) ;
#45747=CARTESIAN_POINT ( 'NONE',  ( 12.63842701281683922, 14.55059781766744997, -9.846743663894590881 ) ) ;
#45748=CARTESIAN_POINT ( 'NONE',  ( 3.591859063236763294, 33.29030133659708213, -11.09922568453595026 ) ) ;
#45749=CARTESIAN_POINT ( 'NONE',  ( 7.361572987183169658, 44.96726448433412315, -9.846743663894592657 ) ) ;
#45750=ORIENTED_EDGE ( 'NONE', *, *, #46498, .F. ) ;
#45751=CARTESIAN_POINT ( 'NONE',  ( 12.63842701281683034, 27.46726448433411250, 9.846743663894596210 ) ) ;
#45754=CARTESIAN_POINT ( 'NONE',  ( 24.16423886937410614, 54.30374883491396787, 8.672049930838204340E-16 ) ) ;
#45758=CARTESIAN_POINT ( 'NONE',  ( 14.92337183194729988, 34.34226448433411605, -8.527530157486177487 ) ) ;
#45759=CARTESIAN_POINT ( 'NONE',  ( 20.88017736071110875, 5.772018677488170546, -2.915334737309920765 ) ) ;
#45760=CARTESIAN_POINT ( 'NONE',  ( 0.1532563361054100626, 45.80059781766745886, -2.638427012816831230 ) ) ;
#45761=CARTESIAN_POINT ( 'NONE',  ( 17.39651004071841811, 2.935752660568277328, 6.500000000000002665 ) ) ;
#45762=CARTESIAN_POINT ( 'NONE',  ( 0.1532563361054082862, 51.21726448433412315, 2.638427012816831674 ) ) ;
#45764=CARTESIAN_POINT ( 'NONE',  ( 20.88017736071110875, 55.77201867748816966, -2.915334737309920765 ) ) ;
#45765=B_SPLINE_CURVE_WITH_KNOTS ( 'NONE', 3,
 ( #29577, #98627, #67609, #51615 ),
 .UNSPECIFIED., .F., .F.,
 ( 4, 4 ),
 ( 5.421010862427522170E-20, 0.002657014572711345439 ),
 .UNSPECIFIED. ) ;
#45768=CARTESIAN_POINT ( 'NONE',  ( 0.6178305044545818747, 53.49863466993041072, -9.382169495545419124 ) ) ;
#45770=CARTESIAN_POINT ( 'NONE',  ( 12.63842701281683034, 7.467264484334118713, 9.846743663894596210 ) ) ;
#45771=CARTESIAN_POINT ( 'NONE',  ( 6.565887622018943937, 53.08196800326374643, -12.81628187352647608 ) ) ;
#45772=CARTESIAN_POINT ( 'NONE',  ( -0.3689425029237898834, 66.17874883491396076, -10.36894250292378850 ) ) ;
#45773=CARTESIAN_POINT ( 'NONE',  ( 2.791683348922240793, 51.63393115100078745, 7.208316651077764092 ) ) ;
#45775=CARTESIAN_POINT ( 'NONE',  ( 6.204703633549690345, 27.84541550158063217, 14.16423886937410082 ) ) ;
#45777=CARTESIAN_POINT ( 'NONE',  ( 24.16423886937409904, 64.09541550158064638, 3.795296366450317205 ) ) ;
#45778=CARTESIAN_POINT ( 'NONE',  ( 1.472469842513823179, 50.59226448433411605, -4.923371831947296329 ) ) ;
#45780=CARTESIAN_POINT ( 'NONE',  ( 0.5774900079438590739, 47.64701867748817676, -5.440088680355550821 ) ) ;
#45782=CARTESIAN_POINT ( 'NONE',  ( -0.8801773607111009756, 68.06368534415484817, 1.068504757029289695E-15 ) ) ;
#45784=EDGE_LOOP ( 'NONE', ( #14160, #33466, #38800, #20797 ) ) ;
#45785=CARTESIAN_POINT ( 'NONE',  ( 16.40814093676323893, 60.79030133659709634, 11.09922568453595026 ) ) ;
#45786=( BOUNDED_CURVE ( )  B_SPLINE_CURVE ( 2, ( #42339, #58806, #96341, #27816, #12813, #72322, #97329, #58301, #43312 ),
 .UNSPECIFIED., .F., .F. ) 
 B_SPLINE_CURVE_WITH_KNOTS ( ( 3, 2, 2, 2, 3 ),
 ( 0.8320003743640370653, 0.8333333333333333703, 0.8392857142857143016, 0.8452380952380952328, 0.8465710542073914269 ),
 .UNSPECIFIED. ) 
 CURVE ( )  GEOMETRIC_REPRESENTATION_ITEM ( )  RATIONAL_B_SPLINE_CURVE ( ( 0.9881565478350742282, 0.9923695281211498687, 1.000000000000000000, 0.9659258262890683122, 1.000000000000000000, 0.9659258262890683122, 1.000000000000000000, 0.9923695281211504238, 0.9881565478350748943 ) ) 
 REPRESENTATION_ITEM ( '' )  );
#45787=ORIENTED_EDGE ( 'NONE', *, *, #21581, .T. ) ;
#45788=CARTESIAN_POINT ( 'NONE',  ( 19.84674366389459266, 8.300597817667451750, 2.638427012816836559 ) ) ;
#45790=CARTESIAN_POINT ( 'NONE',  ( 10.00000000000000000, 25.55374883491396787, -14.16423886937410082 ) ) ;
#45791=CARTESIAN_POINT ( 'NONE',  ( 10.00000000000000000, 19.75893115100078390, -9.846743663894594434 ) ) ;
#45792=CARTESIAN_POINT ( 'NONE',  ( 19.42250999205614548, 25.98035201082150891, -5.440088680355545492 ) ) ;
#45795=CARTESIAN_POINT ( 'NONE',  ( 17.96484262340118221, 24.93868534415484461, 7.964842623401181321 ) ) ;
#45798=CARTESIAN_POINT ( 'NONE',  ( 15.44008868035555260, 34.73035201082151247, 9.422509992056143702 ) ) ;
#45799=CARTESIAN_POINT ( 'NONE',  ( 20.15039907845753220, 46.74884699246888431, 6.262539305110077947 ) ) ;
#45802=CARTESIAN_POINT ( 'NONE',  ( 21.09922568453595559, 22.04030133659708923, -6.408140936763230044 ) ) ;
#45803=CARTESIAN_POINT ( 'NONE',  ( 1.472469842513823179, 15.59226448433411960, -4.923371831947296329 ) ) ;
#45806=CARTESIAN_POINT ( 'NONE',  ( 17.20831665107776587, 19.13393115100078035, -7.208316651077762316 ) ) ;
#45807=CARTESIAN_POINT ( 'NONE',  ( 12.91533473730992121, 34.52201867748817676, 10.88017736071110164 ) ) ;
#45808=MECHANICAL_DESIGN_GEOMETRIC_PRESENTATION_REPRESENTATION('',(#79340),#13906);
#45811=ORIENTED_EDGE ( 'NONE', *, *, #50588, .F. ) ;
#45814=CARTESIAN_POINT ( 'NONE',  ( 17.96484262340118221, 59.93868534415484106, 7.964842623401181321 ) ) ;
#45815=CARTESIAN_POINT ( 'NONE',  ( -46.48621475366246614, 103.4032225623660821, -6.318809327474250281 ) ) ;
#45816=CARTESIAN_POINT ( 'NONE',  ( -2.816281873526473856, 54.33196800326376064, 3.434112377981055619 ) ) ;
#45817=CARTESIAN_POINT ( 'NONE',  ( 12.91533473730992121, 64.52201867748817676, 10.88017736071110164 ) ) ;
#45818=CARTESIAN_POINT ( 'NONE',  ( 6.565887622018943937, -1.918031996736246692, -12.81628187352647608 ) ) ;
#45819=B_SPLINE_CURVE_WITH_KNOTS ( 'NONE', 3,
 ( #72056, #74019, #11554, #81034 ),
 .UNSPECIFIED., .F., .F.,
 ( 4, 4 ),
 ( 0.000000000000000000, 0.002392975128318533193 ),
 .UNSPECIFIED. ) ;
#45820=DIRECTION ( 'NONE',  ( 0.000000000000000000, 0.000000000000000000, -1.000000000000000000 ) ) ;
#45821=CARTESIAN_POINT ( 'NONE',  ( 10.00000000000000000, 29.75893115100078745, -9.846743663894594434 ) ) ;
#45822=CARTESIAN_POINT ( 'NONE',  ( 22.81628187352648496, 56.83196800326374643, -3.434112377981050290 ) ) ;
#45824=CARTESIAN_POINT ( 'NONE',  ( 7.361572987183169658, 9.967264484334119601, -9.846743663894592657 ) ) ;
#45825=CARTESIAN_POINT ( 'NONE',  ( 22.81628187352647785, 26.41530133659708923, 3.434112377981063169 ) ) ;
#45826=CARTESIAN_POINT ( 'NONE',  ( 15.00000000000000000, 0.000000000000000000, -6.500000000000000888 ) ) ;
#45827=CARTESIAN_POINT ( 'NONE',  ( 17.96484262340118221, 36.18868534415484106, -7.964842623401177768 ) ) ;
#45828=CARTESIAN_POINT ( 'NONE',  ( 2.791683348922237240, 60.38393115100078745, -7.208316651077763204 ) ) ;
#45831=CARTESIAN_POINT ( 'NONE',  ( 0.1532563361054082862, 21.21726448433412315, 2.638427012816831674 ) ) ;
#45832=CARTESIAN_POINT ( 'NONE',  ( 7.361572987183170547, 7.050597817667451750, 9.846743663894590881 ) ) ;
#45833=CARTESIAN_POINT ( 'NONE',  ( 17.96484262340118221, 9.938685344154837509, 7.964842623401181321 ) ) ;
#45834=CARTESIAN_POINT ( 'NONE',  ( 0.6178305044545818747, 13.49863466993041783, -9.382169495545419124 ) ) ;
#45840=CARTESIAN_POINT ( 'NONE',  ( 4.559911319644449179, 3.897018677488171434, 9.422509992056141925 ) ) ;
#45841=CARTESIAN_POINT ( 'NONE',  ( 17.20831665107776587, 47.88393115100078745, 7.208316651077764980 ) ) ;
#45842=CARTESIAN_POINT ( 'NONE',  ( -0.1503990784575242878, 49.24884699246889141, -6.262539305110083276 ) ) ;
#45843=CARTESIAN_POINT ( 'NONE',  ( -4.164238869374099927, 67.01208216824728936, 3.795296366450308767 ) ) ;
#45844=CARTESIAN_POINT ( 'NONE',  ( 19.72487221294570858, 64.78217586085237656, 6.499999999999992895 ) ) ;
#45845=CARTESIAN_POINT ( 'NONE',  ( 2.035157376598822676, 32.43868534415483396, -7.964842623401177768 ) ) ;
#45846=CARTESIAN_POINT ( 'NONE',  ( 13.79529636645031943, 65.34541550158063217, -14.16423886937409904 ) ) ;
#45848=CARTESIAN_POINT ( 'NONE',  ( 14.92337183194729633, 7.675597817667451750, 8.527530157486181039 ) ) ;
#45849=CARTESIAN_POINT ( 'NONE',  ( 17.20831665107776587, 22.88393115100078745, 7.208316651077764980 ) ) ;
#45850=CARTESIAN_POINT ( 'NONE',  ( 0.6178305044545838731, 14.74863466993041783, 9.382169495545420901 ) ) ;
#45851=CARTESIAN_POINT ( 'NONE',  ( -0.1503990784575260087, 24.24884699246888786, -6.262539305110081500 ) ) ;
#45853=CARTESIAN_POINT ( 'NONE',  ( 2.917880565312948704, 7.637082168247301794, 12.26659068614894643 ) ) ;
#45854=CARTESIAN_POINT ( 'NONE',  ( 2.791683348922240793, 31.63393115100078745, 7.208316651077764092 ) ) ;
#45856=VERTEX_POINT ( 'NONE', #47824 ) ;
#45857=CARTESIAN_POINT ( 'NONE',  ( -0.3689425029237881626, 47.42874883491396787, 10.36894250292379027 ) ) ;
#45859=CARTESIAN_POINT ( 'NONE',  ( 0.1532563361054082862, 11.21726448433411605, 2.638427012816831674 ) ) ;
#45860=CARTESIAN_POINT ( 'NONE',  ( 5.500000000000000000, 60.50000000000000000, 5.000000000000000000 ) ) ;
#45862=CARTESIAN_POINT ( 'NONE',  ( 4.559911319644449179, 38.89701867748817676, 9.422509992056141925 ) ) ;
#45863=CARTESIAN_POINT ( 'NONE',  ( 13.43411237798106583, 52.66530133659708213, -12.81628187352647252 ) ) ;
#45865=CARTESIAN_POINT ( 'NONE',  ( -0.8801773607111009756, 13.06368534415483929, 1.068504757029289695E-15 ) ) ;
#45866=CARTESIAN_POINT ( 'NONE',  ( 3.591859063236761518, 44.95696800326376064, 11.09922568453594849 ) ) ;
#45867=CARTESIAN_POINT ( 'NONE',  ( 14.92337183194729633, 62.67559781766745886, 8.527530157486181039 ) ) ;
#45868=FACE_OUTER_BOUND ( 'NONE', #89652, .T. ) ;
#45872=CARTESIAN_POINT ( 'NONE',  ( 13.79529636645031943, 45.34541550158062506, -14.16423886937409904 ) ) ;
#45873=CARTESIAN_POINT ( 'NONE',  ( 6.204703633549690345, 20.76208216824730357, -14.16423886937410259 ) ) ;
#45874=( NAMED_UNIT ( * ) SI_UNIT ( $, .STERADIAN. ) SOLID_ANGLE_UNIT ( ) );
#45876=CARTESIAN_POINT ( 'NONE',  ( 19.42250999205614548, 35.98035201082151247, -5.440088680355545492 ) ) ;
#45878=CARTESIAN_POINT ( 'NONE',  ( 6.000000000000000000, 61.50000000000000711, 6.000000000000000000 ) ) ;
#45879=CARTESIAN_POINT ( 'NONE',  ( 17.20831665107776587, 2.883931151000785231, 7.208316651077764980 ) ) ;
#45880=CARTESIAN_POINT ( 'NONE',  ( 7.084665262690076126, 59.10535201082150536, 10.88017736071109987 ) ) ;
#45881=CARTESIAN_POINT ( 'NONE',  ( 3.591859063236763294, 23.29030133659708568, -11.09922568453595026 ) ) ;
#45882=CARTESIAN_POINT ( 'NONE',  ( 17.39651004071843232, 17.93575266056828355, 6.499999999999984013 ) ) ;
#45884=CARTESIAN_POINT ( 'NONE',  ( 0.1532563361054083140, 31.00893115100078390, 1.131784320476157264E-15 ) ) ;
#45886=CARTESIAN_POINT ( 'NONE',  ( 12.91533473730992121, 9.522018677488171434, 10.88017736071110164 ) ) ;
#45887=AXIS2_PLACEMENT_3D ( 'NONE', #57803, #96822, #41366 ) ;
#45888=CARTESIAN_POINT ( 'NONE',  ( 13.43411237798105340, 20.58196800326374643, 12.81628187352647963 ) ) ;
#45889=CARTESIAN_POINT ( 'NONE',  ( 5.076628168052704559, 15.17559781766745175, -8.527530157486179263 ) ) ;
#45891=CARTESIAN_POINT ( 'NONE',  ( 0.5774900079438607392, 8.480352010821505360, 5.440088680355550821 ) ) ;
#45892=CARTESIAN_POINT ( 'NONE',  ( 19.84674366389459266, 43.30059781766744464, 2.638427012816836559 ) ) ;
#45893=CARTESIAN_POINT ( 'NONE',  ( 16.40814093676323893, 55.79030133659708923, 11.09922568453595026 ) ) ;
#45894=CARTESIAN_POINT ( 'NONE',  ( 2.791683348922237240, 15.38393115100078212, -7.208316651077763204 ) ) ;
#45895=CARTESIAN_POINT ( 'NONE',  ( -2.266590686148945544, 2.220415501580634388, 7.082119434687048631 ) ) ;
#45896=CARTESIAN_POINT ( 'NONE',  ( 22.26659068614894466, 8.887082168247300018, 7.082119434687054849 ) ) ;
#45898=CARTESIAN_POINT ( 'NONE',  ( 7.084665262690076126, 32.02201867748816966, -10.88017736071110164 ) ) ;
#45899=CARTESIAN_POINT ( 'NONE',  ( -0.8801773607111009756, 18.06368534415484106, 1.068504757029289695E-15 ) ) ;
#45900=CARTESIAN_POINT ( 'NONE',  ( -4.164238869374098151, 41.59541550158061796, -3.795296366450310543 ) ) ;
#45901=CARTESIAN_POINT ( 'NONE',  ( 15.44008868035555793, 36.39701867748816966, -9.422509992056140149 ) ) ;
#45902=CARTESIAN_POINT ( 'NONE',  ( 19.42250999205614193, 15.14701867748817143, 5.440088680355555262 ) ) ;
#45904=CARTESIAN_POINT ( 'NONE',  ( 20.88017736071110164, 45.35535201082149115, 2.915334737309930979 ) ) ;
#45905=CARTESIAN_POINT ( 'NONE',  ( 22.81628187352647785, 61.62363466993041783, 6.195893100308588602E-16 ) ) ;
#45906=CARTESIAN_POINT ( 'NONE',  ( 20.88017736071110164, 50.35535201082151247, 2.915334737309930979 ) ) ;
#45907=CARTESIAN_POINT ( 'NONE',  ( 10.00000000000000000, 56.81368534415484106, -10.88017736071110342 ) ) ;
#45909=CARTESIAN_POINT ( 'NONE',  ( 10.00000000000000178, 49.31368534415484106, 10.88017736071110342 ) ) ;
#45911=CARTESIAN_POINT ( 'NONE',  ( -4.164238869374099039, 46.80374883491397497, 8.674139862899312516E-16 ) ) ;
#45912=CARTESIAN_POINT ( 'NONE',  ( 15.44008868035555793, 66.39701867748817676, -9.422509992056140149 ) ) ;
#45913=CARTESIAN_POINT ( 'NONE',  ( 0.2751277870542910842, 52.28217586085238366, -6.499999999999992006 ) ) ;
#45915=CARTESIAN_POINT ( 'NONE',  ( 5.076628168052704559, 60.17559781766745175, -8.527530157486179263 ) ) ;
#45916=SURFACE_SIDE_STYLE ('',( #91403 ) ) ;
#45917=CARTESIAN_POINT ( 'NONE',  ( 1.472469842513823179, 31.42559781766745530, 4.923371831947296329 ) ) ;
#45918=ORIENTED_EDGE ( 'NONE', *, *, #65518, .F. ) ;
#45919=CARTESIAN_POINT ( 'NONE',  ( 5.076628168052703671, 31.84226448433412315, 8.527530157486179263 ) ) ;
#45921=CARTESIAN_POINT ( 'NONE',  ( 20.88017736071110519, 35.56368534415484106, 2.639326808657452039E-16 ) ) ;
#45922=CARTESIAN_POINT ( 'NONE',  ( 17.20831665107776587, 39.13393115100079456, -7.208316651077762316 ) ) ;
#45923=CARTESIAN_POINT ( 'NONE',  ( 0.6178305044545818747, 23.49863466993041783, -9.382169495545419124 ) ) ;
#45924=CARTESIAN_POINT ( 'NONE',  ( 10.00000000000000000, 66.81368534415484817, -10.88017736071110342 ) ) ;
#45925=CARTESIAN_POINT ( 'NONE',  ( 12.91533473730993009, 56.60535201082151247, -10.88017736071109987 ) ) ;
#45926=CARTESIAN_POINT ( 'NONE',  ( 0.5774900079438590739, 42.64701867748816966, -5.440088680355550821 ) ) ;
#45927=CARTESIAN_POINT ( 'NONE',  ( 19.42250999205614548, 5.980352010821504471, -5.440088680355545492 ) ) ;
#45928=CARTESIAN_POINT ( 'NONE',  ( -2.266590686148945544, 57.22041550158063217, 7.082119434687048631 ) ) ;
#45929=CARTESIAN_POINT ( 'NONE',  ( -2.816281873526471635, 23.91530133659708568, -3.434112377981056508 ) ) ;
#45932=CARTESIAN_POINT ( 'NONE',  ( -2.816281873526473856, 9.123634669930421381, 9.499525473075851096E-16 ) ) ;
#45933=CARTESIAN_POINT ( 'NONE',  ( 0.5774900079438607392, 23.48035201082150536, 5.440088680355550821 ) ) ;
#45934=CARTESIAN_POINT ( 'NONE',  ( 17.96484262340118221, 66.18868534415483396, -7.964842623401177768 ) ) ;
#45937=B_SPLINE_CURVE_WITH_KNOTS ( 'NONE', 3,
 ( #90986, #83994, #6511, #37017, #52989, #76490 ),
 .UNSPECIFIED., .F., .F.,
 ( 4, 2, 4 ),
 ( 0.000000000000000000, 0.0002565770811490933789, 0.0005131541622981867579 ),
 .UNSPECIFIED. ) ;
#45938=CARTESIAN_POINT ( 'NONE',  ( 12.91533473730993009, 61.60535201082150536, -10.88017736071109987 ) ) ;
#45939=CARTESIAN_POINT ( 'NONE',  ( 7.361572987183169658, 49.96726448433410894, -9.846743663894592657 ) ) ;
#45940=CARTESIAN_POINT ( 'NONE',  ( 1.472469842513823179, 26.42559781766745175, 4.923371831947296329 ) ) ;
#45941=CARTESIAN_POINT ( 'NONE',  ( 14.92337183194729633, 27.67559781766745530, 8.527530157486181039 ) ) ;
#45942=DIRECTION ( 'NONE',  ( 0.000000000000000000, 0.000000000000000000, 1.000000000000000000 ) ) ;
#45943=DIRECTION ( 'NONE',  ( -0.000000000000000000, -0.000000000000000000, -1.000000000000000000 ) ) ;
#45944=CARTESIAN_POINT ( 'NONE',  ( 13.43411237798106583, 42.66530133659707502, -12.81628187352647252 ) ) ;
#45945=EDGE_CURVE ( 'NONE', #33986, #9878, #54528, .T. ) ;
#45946=CARTESIAN_POINT ( 'NONE',  ( 10.00000000000000000, 14.75893115100078568, -9.846743663894594434 ) ) ;
#45949=CARTESIAN_POINT ( 'NONE',  ( 5.076628168052704559, 30.17559781766745175, -8.527530157486179263 ) ) ;
#45954=CARTESIAN_POINT ( 'NONE',  ( 10.00000000000000000, 17.87363466993041783, -12.81628187352647608 ) ) ;
#45955=CARTESIAN_POINT ( 'NONE',  ( 2.035157376598822676, 47.43868534415484817, -7.964842623401177768 ) ) ;
#45956=CARTESIAN_POINT ( 'NONE',  ( -4.164238869374099039, 31.80374883491396432, 8.674139862899312516E-16 ) ) ;
#45957=CARTESIAN_POINT ( 'NONE',  ( 1.383448333479218473, 42.37718327197428181, -6.499999999999959144 ) ) ;
#45958=CARTESIAN_POINT ( 'NONE',  ( 17.08211943468705840, 25.13708216824730357, -12.26659068614894466 ) ) ;
#45959=CARTESIAN_POINT ( 'NONE',  ( -4.164238869374099927, 57.01208216824731068, 3.795296366450308767 ) ) ;
#45960=CARTESIAN_POINT ( 'NONE',  ( 17.08211943468705840, 15.13708216824730179, -12.26659068614894466 ) ) ;
#45961=CARTESIAN_POINT ( 'NONE',  ( 13.79529636645031943, 30.34541550158063927, -14.16423886937409904 ) ) ;
#45963=CARTESIAN_POINT ( 'NONE',  ( -0.8801773607110991993, 52.85535201082151247, -2.915334737309923874 ) ) ;
#45964=CARTESIAN_POINT ( 'NONE',  ( 19.72487221294571214, 24.78217586085238011, 6.499999999999993783 ) ) ;
#45966=CARTESIAN_POINT ( 'NONE',  ( 14.92337183194729633, 47.67559781766745175, 8.527530157486181039 ) ) ;
#45967=CARTESIAN_POINT ( 'NONE',  ( 4.559911319644449179, 18.89701867748817321, 9.422509992056141925 ) ) ;
#45969=CARTESIAN_POINT ( 'NONE',  ( 12.63842701281683034, 62.46726448433410894, 9.846743663894596210 ) ) ;
#45971=CARTESIAN_POINT ( 'NONE',  ( 17.20831665107776587, 22.88393115100078745, 7.208316651077764980 ) ) ;
#45972=CARTESIAN_POINT ( 'NONE',  ( 10.00000000000000178, 55.37363466993042493, 12.81628187352647608 ) ) ;
#45974=CARTESIAN_POINT ( 'NONE',  ( 12.63842701281683034, 47.46726448433412315, 9.846743663894596210 ) ) ;
#45975=CARTESIAN_POINT ( 'NONE',  ( 0.1532563361054100626, 55.80059781766745175, -2.638427012816831230 ) ) ;
#45976=CARTESIAN_POINT ( 'NONE',  ( 17.08211943468705840, 40.13708216824731068, -12.26659068614894466 ) ) ;
#45979=CARTESIAN_POINT ( 'NONE',  ( 20.36894250292379382, 8.678748834913967869, 10.36894250292379205 ) ) ;
#45980=CARTESIAN_POINT ( 'NONE',  ( -0.8801773607110991993, 62.85535201082150536, -2.915334737309923874 ) ) ;
#45981=CARTESIAN_POINT ( 'NONE',  ( 19.72487221294571214, 44.78217586085236945, 6.499999999999993783 ) ) ;
#45982=CARTESIAN_POINT ( 'NONE',  ( 24.16423886937410614, 64.30374883491396076, 8.672049930838204340E-16 ) ) ;
#45983=CARTESIAN_POINT ( 'NONE',  ( 22.81628187352647785, 16.41530133659708923, 3.434112377981063169 ) ) ;
#45985=CARTESIAN_POINT ( 'NONE',  ( 10.00000000000000178, 2.258931151000784787, 9.846743663894594434 ) ) ;
#45986=CARTESIAN_POINT ( 'NONE',  ( -0.1049300847420639449, 27.21697413083879624, -6.336235997365760930 ) ) ;
#45988=CARTESIAN_POINT ( 'NONE',  ( -2.816281873526471635, 33.91530133659708213, -3.434112377981056508 ) ) ;
#45989=CARTESIAN_POINT ( 'NONE',  ( -0.3689425029237881626, 62.42874883491396787, 10.36894250292379027 ) ) ;
#45991=CARTESIAN_POINT ( 'NONE',  ( 0.5774900079438590739, 17.64701867748817321, -5.440088680355550821 ) ) ;
#45992=CARTESIAN_POINT ( 'NONE',  ( -0.8801773607111009756, 23.06368534415484106, 1.068504757029289695E-15 ) ) ;
#45993=CARTESIAN_POINT ( 'NONE',  ( 18.52753015748618282, 53.92559781766745175, -4.923371831947291888 ) ) ;
#45994=CARTESIAN_POINT ( 'NONE',  ( 2.791683348922237240, 60.38393115100078745, -7.208316651077763204 ) ) ;
#45995=CARTESIAN_POINT ( 'NONE',  ( 13.43411237798106583, 52.66530133659708213, -12.81628187352647252 ) ) ;
#45998=CARTESIAN_POINT ( 'NONE',  ( 4.559911319644449179, 17.23035201082150536, -9.422509992056141925 ) ) ;
#45999=CARTESIAN_POINT ( 'NONE',  ( 6.565887622018943937, 15.16530133659708568, 12.81628187352647430 ) ) ;
#46002=CARTESIAN_POINT ( 'NONE',  ( 7.361572987183169658, 44.96726448433412315, -9.846743663894592657 ) ) ;
#46003=CARTESIAN_POINT ( 'NONE',  ( 20.88017736071110519, 55.56368534415484817, 2.639326808657452039E-16 ) ) ;
#46004=CARTESIAN_POINT ( 'NONE',  ( 22.81628187352647785, 21.62363466993041783, 6.195893100308588602E-16 ) ) ;
#46005=CARTESIAN_POINT ( 'NONE',  ( 7.084665262690076126, 54.10535201082151247, 10.88017736071109987 ) ) ;
#46006=CARTESIAN_POINT ( 'NONE',  ( 18.72515096720568906, 15.05509018479935612, 6.500000000000002665 ) ) ;
#46008=CARTESIAN_POINT ( 'NONE',  ( 22.81628187352648496, 56.83196800326374643, -3.434112377981050290 ) ) ;
#46012=CARTESIAN_POINT ( 'NONE',  ( 12.91533473730992121, 44.52201867748816966, 10.88017736071110164 ) ) ;
#46013=CARTESIAN_POINT ( 'NONE',  ( -2.816281873526473856, 44.33196800326375353, 3.434112377981055619 ) ) ;
#46014=CARTESIAN_POINT ( 'NONE',  ( -4.164238869374098151, 16.59541550158063927, -3.795296366450310543 ) ) ;
#46015=MECHANICAL_DESIGN_GEOMETRIC_PRESENTATION_REPRESENTATION('',(#47644),#41247);
#46016=LINE ( 'NONE', #76505, #44996 ) ;
#46017=CARTESIAN_POINT ( 'NONE',  ( 1.472469842513823179, 25.59226448433412315, -4.923371831947296329 ) ) ;
#46019=CARTESIAN_POINT ( 'NONE',  ( 14.92337183194729633, 7.675597817667451750, 8.527530157486181039 ) ) ;
#46021=CARTESIAN_POINT ( 'NONE',  ( -0.3689425029237881626, 42.42874883491396787, 10.36894250292379027 ) ) ;
#46022=PRESENTATION_STYLE_ASSIGNMENT (( #54973 ) ) ;
#46024=CARTESIAN_POINT ( 'NONE',  ( 10.00000000000000178, 14.31368534415483751, 10.88017736071110342 ) ) ;
#46028=EDGE_LOOP ( 'NONE', ( #96540, #67862, #92125, #76439 ) ) ;
#46029=CARTESIAN_POINT ( 'NONE',  ( 7.084665262690076126, 7.022018677488170546, -10.88017736071110164 ) ) ;
#46030=CARTESIAN_POINT ( 'NONE',  ( 15.44008868035555260, 4.730352010821505360, 9.422509992056143702 ) ) ;
#46031=CARTESIAN_POINT ( 'NONE',  ( 17.20831665107776587, 39.13393115100079456, -7.208316651077762316 ) ) ;
#46032=CARTESIAN_POINT ( 'NONE',  ( 6.565887622018943937, 33.08196800326374643, -12.81628187352647608 ) ) ;
#46033=CARTESIAN_POINT ( 'NONE',  ( 1.707155281725155849, 22.90189080397288635, 6.499999999999955591 ) ) ;
#46034=CARTESIAN_POINT ( 'NONE',  ( 2.917880565312950480, 10.97041550158063572, -12.26659068614894821 ) ) ;
#46035=CARTESIAN_POINT ( 'NONE',  ( 4.559911319644449179, 32.23035201082150536, -9.422509992056141925 ) ) ;
#46036=CARTESIAN_POINT ( 'NONE',  ( 20.36894250292379382, 63.67874883491396787, 10.36894250292379205 ) ) ;
#46037=CARTESIAN_POINT ( 'NONE',  ( 14.92337183194729633, 37.67559781766745175, 8.527530157486181039 ) ) ;
#46038=CARTESIAN_POINT ( 'NONE',  ( 18.39792806157246119, 44.52224192338639597, 6.500000000000077272 ) ) ;
#46039=CARTESIAN_POINT ( 'NONE',  ( 0.1532563361054083140, 21.00893115100078745, 1.131784320476157264E-15 ) ) ;
#46040=B_SPLINE_CURVE_WITH_KNOTS ( 'NONE', 3,
 ( #98307, #52278, #22784, #37788, #98806, #67785, #82274, #68772, #30254, #29761, #83769, #44276, #304, #60269 ),
 .UNSPECIFIED., .F., .F.,
 ( 4, 2, 2, 2, 2, 2, 4 ),
 ( 0.000000000000000000, 0.004797171936611957510, 0.007195757904917936265, 0.009594343873223915020, 0.01199292984152989378, 0.01439151580983587253, 0.01918868774644783004 ),
 .UNSPECIFIED. ) ;
#46041=CARTESIAN_POINT ( 'NONE',  ( 1.472469842513823179, 0.5922644843341181575, -4.923371831947296329 ) ) ;
#46046=CARTESIAN_POINT ( 'NONE',  ( 0.1532563361054083140, 61.00893115100078745, 1.131784320476157264E-15 ) ) ;
#46047=CARTESIAN_POINT ( 'NONE',  ( 20.88017736071110875, 30.77201867748816966, -2.915334737309920765 ) ) ;
#46048=CARTESIAN_POINT ( 'NONE',  ( 20.88017736071110164, 40.35535201082150536, 2.915334737309930979 ) ) ;
#46049=CARTESIAN_POINT ( 'NONE',  ( 22.81628187352648496, 31.83196800326375353, -3.434112377981050290 ) ) ;
#46050=CARTESIAN_POINT ( 'NONE',  ( -0.3689425029237898834, 21.17874883491396432, -10.36894250292378850 ) ) ;
#46051=CARTESIAN_POINT ( 'NONE',  ( 13.43411237798105340, 50.58196800326375353, 12.81628187352647963 ) ) ;
#46053=CARTESIAN_POINT ( 'NONE',  ( 5.076628168052703671, 46.84226448433412315, 8.527530157486179263 ) ) ;
#46054=CARTESIAN_POINT ( 'NONE',  ( 12.91533473730993009, 16.60535201082150891, -10.88017736071109987 ) ) ;
#46055=ORIENTED_EDGE ( 'NONE', *, *, #69387, .F. ) ;
#46056=CARTESIAN_POINT ( 'NONE',  ( 17.96484262340118221, 19.93868534415484106, 7.964842623401181321 ) ) ;
#46058=CARTESIAN_POINT ( 'NONE',  ( 12.91533473730993009, 56.60535201082151247, -10.88017736071109987 ) ) ;
#46059=CARTESIAN_POINT ( 'NONE',  ( -0.8801773607111009756, 63.06368534415484106, 1.068504757029289695E-15 ) ) ;
#46060=( BOUNDED_CURVE ( )  B_SPLINE_CURVE ( 2, ( #56506, #46656, #1188, #701, #19003, #31647, #70163, #79987, #62137 ),
 .UNSPECIFIED., .F., .F. ) 
 B_SPLINE_CURVE_WITH_KNOTS ( ( 3, 2, 2, 2, 3 ),
 ( 0.01156950836880285202, 0.01190476190476197349, 0.01785714285714290472, 0.02380952380952383596, 0.02414477734548295743 ),
 .UNSPECIFIED. ) 
 CURVE ( )  GEOMETRIC_REPRESENTATION_ITEM ( )  RATIONAL_B_SPLINE_CURVE ( ( 0.9963778908391762723, 0.9980808541467921513, 1.000000000000000000, 0.9659258262890683122, 1.000000000000000000, 0.9659258262890683122, 1.000000000000000000, 0.9980808541467921513, 0.9963778908391762723 ) ) 
 REPRESENTATION_ITEM ( '' )  );
#46062=CARTESIAN_POINT ( 'NONE',  ( -0.8801773607110991993, 47.85535201082150536, -2.915334737309923874 ) ) ;
#46063=CARTESIAN_POINT ( 'NONE',  ( -0.1503990784575247319, 52.22266099184918176, -6.262539305110083276 ) ) ;
#46065=CARTESIAN_POINT ( 'NONE',  ( -46.94000000000001194, 100.7103534007538883, 8.569772222592094479 ) ) ;
#46069=CARTESIAN_POINT ( 'NONE',  ( 19.84674366389459621, 38.50893115100078745, 7.409399052514197653E-17 ) ) ;
#46073=CARTESIAN_POINT ( 'NONE',  ( 24.16423886937410614, 24.30374883491396787, 8.672049930838204340E-16 ) ) ;
#46075=CARTESIAN_POINT ( 'NONE',  ( 19.72487221294570858, 70.00000000000000000, 6.000000000000000000 ) ) ;
#46076=CARTESIAN_POINT ( 'NONE',  ( 7.084665262690076126, 14.10535201082150358, 10.88017736071109987 ) ) ;
#46077=CARTESIAN_POINT ( 'NONE',  ( 10.00000000000000000, 37.87363466993041783, -12.81628187352647608 ) ) ;
#46078=ORIENTED_EDGE ( 'NONE', *, *, #32851, .F. ) ;
#46080=CARTESIAN_POINT ( 'NONE',  ( 17.20831665107776587, 2.883931151000785231, 7.208316651077764980 ) ) ;
#46081=CARTESIAN_POINT ( 'NONE',  ( 13.43411237798105340, 25.58196800326374998, 12.81628187352647963 ) ) ;
#46082=CARTESIAN_POINT ( 'NONE',  ( 10.00000000000000000, 19.75893115100078390, -9.846743663894594434 ) ) ;
#46084=CARTESIAN_POINT ( 'NONE',  ( 19.72487221294570858, 0.000000000000000000, -6.500000000000000888 ) ) ;
#46085=CARTESIAN_POINT ( 'NONE',  ( 10.00000000000000178, 17.25893115100078745, 9.846743663894594434 ) ) ;
#46086=CARTESIAN_POINT ( 'NONE',  ( -2.816281873526471635, 13.91530133659708746, -3.434112377981056508 ) ) ;
#46087=AXIS2_PLACEMENT_3D ( 'NONE', #28557, #74045, #45030 ) ;
#46089=CARTESIAN_POINT ( 'NONE',  ( 1.472469842513823179, 1.425597817667451528, 4.923371831947296329 ) ) ;
#46093=CARTESIAN_POINT ( 'NONE',  ( 4.559911319644449179, 27.23035201082150536, -9.422509992056141925 ) ) ;
#46094=CARTESIAN_POINT ( 'NONE',  ( 20.36894250292379382, 23.67874883491397142, 10.36894250292379205 ) ) ;
#46095=CARTESIAN_POINT ( 'NONE',  ( 14.92337183194729633, 47.67559781766745175, 8.527530157486181039 ) ) ;
#46096=CARTESIAN_POINT ( 'NONE',  ( 10.00000000000000000, 66.81368534415484817, -10.88017736071110342 ) ) ;
#46097=CARTESIAN_POINT ( 'NONE',  ( -1.099225684535947600, 34.54030133659708923, 6.408140936763237150 ) ) ;
#46099=CARTESIAN_POINT ( 'NONE',  ( 0.5774900079438607392, 8.480352010821505360, 5.440088680355550821 ) ) ;
#46102=CARTESIAN_POINT ( 'NONE',  ( 19.38216949554541202, 10.99863466993042138, 9.382169495545424454 ) ) ;
#46104=CARTESIAN_POINT ( 'NONE',  ( 0.6178305044545838731, 4.748634669930420493, 9.382169495545420901 ) ) ;
#46105=CARTESIAN_POINT ( 'NONE',  ( 10.00000000000000178, 27.25893115100078390, 9.846743663894594434 ) ) ;
#46107=CARTESIAN_POINT ( 'NONE',  ( -2.816281873526471635, 28.91530133659708213, -3.434112377981056508 ) ) ;
#46109=CARTESIAN_POINT ( 'NONE',  ( 15.44008868035555793, 51.39701867748816966, -9.422509992056140149 ) ) ;
#46110=CARTESIAN_POINT ( 'NONE',  ( 1.274849032794292736, 62.55509018479936145, -6.499999999999977796 ) ) ;
#46112=CARTESIAN_POINT ( 'NONE',  ( 0.5774900079438607392, 68.48035201082150536, 5.440088680355550821 ) ) ;
#46113=CARTESIAN_POINT ( 'NONE',  ( -0.8801773607110991993, 42.85535201082150536, -2.915334737309923874 ) ) ;
#46114=CARTESIAN_POINT ( 'NONE',  ( 7.084665262690076126, 39.10535201082150536, 10.88017736071109987 ) ) ;
#46116=LINE ( 'NONE', #76603, #93895 ) ;
#46117=CARTESIAN_POINT ( 'NONE',  ( 14.92337183194729633, 57.67559781766745886, 8.527530157486181039 ) ) ;
#46118=CARTESIAN_POINT ( 'NONE',  ( 20.88017736071110875, 5.772018677488170546, -2.915334737309920765 ) ) ;
#46120=CARTESIAN_POINT ( 'NONE',  ( 21.09922568453595559, 7.040301336597086568, -6.408140936763230044 ) ) ;
#46121=ORIENTED_EDGE ( 'NONE', *, *, #68033, .F. ) ;
#46122=CARTESIAN_POINT ( 'NONE',  ( 7.084665262690076126, 42.02201867748816966, -10.88017736071110164 ) ) ;
#46123=CARTESIAN_POINT ( 'NONE',  ( 12.63842701281683034, 62.46726448433410894, 9.846743663894596210 ) ) ;
#46125=CARTESIAN_POINT ( 'NONE',  ( 20.88017736071110875, 10.77201867748817143, -2.915334737309920765 ) ) ;
#46126=CARTESIAN_POINT ( 'NONE',  ( -0.8801773607110991993, 32.85535201082151247, -2.915334737309923874 ) ) ;
#46127=CARTESIAN_POINT ( 'NONE',  ( 2.917880565312948704, 42.63708216824729647, 12.26659068614894643 ) ) ;
#46128=CARTESIAN_POINT ( 'NONE',  ( 18.52753015748617571, 33.09226448433411605, 4.923371831947298993 ) ) ;
#46129=CARTESIAN_POINT ( 'NONE',  ( -0.8801773607110991993, 52.85535201082151247, -2.915334737309923874 ) ) ;
#46131=SURFACE_STYLE_USAGE ( .BOTH. , #98672 ) ;
#46134=CARTESIAN_POINT ( 'NONE',  ( 0.1532563361054082862, 61.21726448433412315, 2.638427012816831674 ) ) ;
#46136=ORIENTED_EDGE ( 'NONE', *, *, #32334, .F. ) ;
#46137=CARTESIAN_POINT ( 'NONE',  ( 13.79529636645031943, 35.34541550158063927, -14.16423886937409904 ) ) ;
#46138=CARTESIAN_POINT ( 'NONE',  ( -0.3689425029237881626, 27.42874883491397142, 10.36894250292379027 ) ) ;
#46139=CARTESIAN_POINT ( 'NONE',  ( 17.20831665107776587, 4.133931151000785675, -7.208316651077762316 ) ) ;
#46140=CARTESIAN_POINT ( 'NONE',  ( 13.43411237798105340, 10.58196800326375353, 12.81628187352647963 ) ) ;
#46143=CARTESIAN_POINT ( 'NONE',  ( 20.88017736071110519, 60.56368534415484106, 2.639326808657452039E-16 ) ) ;
#46144=CARTESIAN_POINT ( 'NONE',  ( 3.591859063236763294, 23.29030133659708568, -11.09922568453595026 ) ) ;
#46145=CARTESIAN_POINT ( 'NONE',  ( 22.26659068614895176, 24.72041550158063572, -7.082119434687042414 ) ) ;
#46146=CARTESIAN_POINT ( 'NONE',  ( 20.88017736071110519, 10.56368534415483929, 2.639326808657452039E-16 ) ) ;
#46147=CARTESIAN_POINT ( 'NONE',  ( -0.8801773607111008646, 33.27201867748817676, 2.915334737309923430 ) ) ;
#46148=LINE ( 'NONE', #23663, #36373 ) ;
#46149=CARTESIAN_POINT ( 'NONE',  ( 20.88017736071110519, 50.56368534415484106, 2.639326808657452039E-16 ) ) ;
#46150=EDGE_CURVE ( 'NONE', #26347, #43655, #2700, .T. ) ;
#46152=CARTESIAN_POINT ( 'NONE',  ( 19.38216949554541557, 52.24863466993041072, -9.382169495545420901 ) ) ;
#46154=ORIENTED_EDGE ( 'NONE', *, *, #68670, .F. ) ;
#46155=FACE_OUTER_BOUND ( 'NONE', #91772, .T. ) ;
#46160=CARTESIAN_POINT ( 'NONE',  ( 2.917880565312948704, 57.63708216824731068, 12.26659068614894643 ) ) ;
#46161=CARTESIAN_POINT ( 'NONE',  ( 22.26659068614894466, 63.88708216824730357, 7.082119434687054849 ) ) ;
#46162=CARTESIAN_POINT ( 'NONE',  ( 17.20831665107776587, 29.13393115100078390, -7.208316651077762316 ) ) ;
#46163=CARTESIAN_POINT ( 'NONE',  ( 12.63842701281683922, 59.55059781766744464, -9.846743663894590881 ) ) ;
#46166=CARTESIAN_POINT ( 'NONE',  ( 7.361572987183169658, 9.967264484334119601, -9.846743663894592657 ) ) ;
#46167=CARTESIAN_POINT ( 'NONE',  ( 10.00000000000000178, 0.3736346699304200492, 12.81628187352647608 ) ) ;
#46171=CARTESIAN_POINT ( 'NONE',  ( -4.164238869374098151, 36.59541550158063217, -3.795296366450310543 ) ) ;
#46172=CARTESIAN_POINT ( 'NONE',  ( 17.08211943468705130, 38.47041550158063217, 12.26659068614894998 ) ) ;
#46174=CARTESIAN_POINT ( 'NONE',  ( 13.43411237798105340, 55.58196800326374643, 12.81628187352647963 ) ) ;
#46175=CARTESIAN_POINT ( 'NONE',  ( 20.88017736071110875, 25.77201867748816966, -2.915334737309920765 ) ) ;
#46176=CARTESIAN_POINT ( 'NONE',  ( 19.84674366389459621, 48.50893115100078745, 7.409399052514197653E-17 ) ) ;
#46177=CARTESIAN_POINT ( 'NONE',  ( 15.44008868035555793, 21.39701867748817321, -9.422509992056140149 ) ) ;
#46178=CARTESIAN_POINT ( 'NONE',  ( 5.076628168052704559, 50.17559781766745886, -8.527530157486179263 ) ) ;
#46179=CARTESIAN_POINT ( 'NONE',  ( 17.20831665107776587, 47.88393115100078745, 7.208316651077764980 ) ) ;
#46184=CARTESIAN_POINT ( 'NONE',  ( 19.72487221294570858, 31.86607318730074567, 6.500000000000000888 ) ) ;
#46185=CARTESIAN_POINT ( 'NONE',  ( 2.791683348922240793, 1.633931151000784565, 7.208316651077764092 ) ) ;
#46189=CARTESIAN_POINT ( 'NONE',  ( 10.00000000000000000, 24.75893115100078745, -9.846743663894594434 ) ) ;
#46192=CARTESIAN_POINT ( 'NONE',  ( 22.81628187352647785, 41.62363466993042493, 6.195893100308588602E-16 ) ) ;
#46193=CYLINDRICAL_SURFACE ( 'NONE', #41958, 0.5000000000000004441 ) ;
#46196=CARTESIAN_POINT ( 'NONE',  ( 2.791683348922237240, 65.38393115100078035, -7.208316651077763204 ) ) ;
#46197=CARTESIAN_POINT ( 'NONE',  ( 19.84674366389459266, 58.71726448433411605, -2.638427012816827677 ) ) ;
#46198=CARTESIAN_POINT ( 'NONE',  ( 20.36894250292379738, 29.92874883491396432, -10.36894250292379027 ) ) ;
#46199=CARTESIAN_POINT ( 'NONE',  ( 2.791683348922240793, 56.63393115100078035, 7.208316651077764092 ) ) ;
#46201=CARTESIAN_POINT ( 'NONE',  ( 7.361572987183170547, 7.050597817667451750, 9.846743663894590881 ) ) ;
#46202=CARTESIAN_POINT ( 'NONE',  ( 0.6178305044545838731, 49.74863466993041072, 9.382169495545420901 ) ) ;
#46203=CARTESIAN_POINT ( 'NONE',  ( 6.204703633549690345, 2.845415501580634388, 14.16423886937410082 ) ) ;
#46204=CARTESIAN_POINT ( 'NONE',  ( 0.1532563361054082862, 51.21726448433412315, 2.638427012816831674 ) ) ;
#46205=CARTESIAN_POINT ( 'NONE',  ( 10.00000000000000178, 54.31368534415484106, 10.88017736071110342 ) ) ;
#46207=EDGE_CURVE ( 'NONE', #73080, #48374, #54421, .T. ) ;
#46210=CARTESIAN_POINT ( 'NONE',  ( 7.084665262690076126, 32.02201867748816966, -10.88017736071110164 ) ) ;
#46211=CARTESIAN_POINT ( 'NONE',  ( -1.099225684535947600, -0.4596986634029132657, 6.408140936763237150 ) ) ;
#46212=CARTESIAN_POINT ( 'NONE',  ( 7.084665262690076126, 54.10535201082151247, 10.88017736071109987 ) ) ;
#46216=CARTESIAN_POINT ( 'NONE',  ( -46.48608351833326680, 103.4078159519480806, -6.315430899466240255 ) ) ;
#46217=CARTESIAN_POINT ( 'NONE',  ( -0.8801773607110991993, 37.85535201082151247, -2.915334737309923874 ) ) ;
#46219=CARTESIAN_POINT ( 'NONE',  ( 19.84674366389459266, 13.30059781766745353, 2.638427012816836559 ) ) ;
#46220=CARTESIAN_POINT ( 'NONE',  ( 0.1532563361054100626, 40.80059781766745886, -2.638427012816831230 ) ) ;
#46221=CYLINDRICAL_SURFACE ( 'NONE', #79245, 0.5000000000000004441 ) ;
#46223=CARTESIAN_POINT ( 'NONE',  ( 10.00000000000000000, 64.75893115100078035, -9.846743663894594434 ) ) ;
#46224=CARTESIAN_POINT ( 'NONE',  ( 2.035157376598822676, 12.43868534415483751, -7.964842623401177768 ) ) ;
#46225=SURFACE_STYLE_USAGE ( .BOTH. , #62185 ) ;
#46227=CARTESIAN_POINT ( 'NONE',  ( 20.36894250292379382, 28.67874883491396787, 10.36894250292379205 ) ) ;
#46228=CARTESIAN_POINT ( 'NONE',  ( 24.16423886937409904, 49.09541550158063217, 3.795296366450317205 ) ) ;
#46229=CARTESIAN_POINT ( 'NONE',  ( 19.84674366389459266, 33.71726448433410894, -2.638427012816827677 ) ) ;
#46230=CARTESIAN_POINT ( 'NONE',  ( 0.1532563361054100626, 20.80059781766744464, -2.638427012816831230 ) ) ;
#46231=CARTESIAN_POINT ( 'NONE',  ( 17.96484262340118221, 6.188685344154836621, -7.964842623401177768 ) ) ;
#46233=CARTESIAN_POINT ( 'NONE',  ( 0.1532563361054082862, 31.21726448433412315, 2.638427012816831674 ) ) ;
#46234=CARTESIAN_POINT ( 'NONE',  ( 10.00000000000000178, 24.31368534415484106, 10.88017736071110342 ) ) ;
#46235=CARTESIAN_POINT ( 'NONE',  ( 0.1532563361054083140, 61.00893115100078745, 1.131784320476157264E-15 ) ) ;
#46236=CARTESIAN_POINT ( 'NONE',  ( 20.36894250292379738, 4.928748834913967869, -10.36894250292379027 ) ) ;
#46238=CARTESIAN_POINT ( 'NONE',  ( 7.361572987183170547, 7.050597817667451750, 9.846743663894590881 ) ) ;
#46239=CARTESIAN_POINT ( 'NONE',  ( 10.00000000000000000, 42.87363466993042493, -12.81628187352647608 ) ) ;
#46240=CARTESIAN_POINT ( 'NONE',  ( 5.076628168052703671, 36.84226448433412315, 8.527530157486179263 ) ) ;
#46242=CARTESIAN_POINT ( 'NONE',  ( 12.63842701281683922, 24.55059781766745175, -9.846743663894590881 ) ) ;
#46244=CARTESIAN_POINT ( 'NONE',  ( -46.61731745958343254, 101.4415013874591835, -8.301784926884796079 ) ) ;
#46246=CARTESIAN_POINT ( 'NONE',  ( 6.204703633549690345, 52.84541550158062506, 14.16423886937410082 ) ) ;
#46247=CARTESIAN_POINT ( 'NONE',  ( 0.5774900079438607392, 53.48035201082151247, 5.440088680355550821 ) ) ;
#46248=( NAMED_UNIT ( * ) PLANE_ANGLE_UNIT ( ) SI_UNIT ( $, .RADIAN. ) );
#46249=CARTESIAN_POINT ( 'NONE',  ( 0.1532563361054082862, 41.21726448433411605, 2.638427012816831674 ) ) ;
#46250=CARTESIAN_POINT ( 'NONE',  ( 7.084665262690076126, 4.105352010821503583, 10.88017736071109987 ) ) ;
#46252=CARTESIAN_POINT ( 'NONE',  ( 0.1532563361054100626, 45.80059781766745886, -2.638427012816831230 ) ) ;
#46254=CARTESIAN_POINT ( 'NONE',  ( -0.8801773607111009756, 53.06368534415484106, 1.068504757029289695E-15 ) ) ;
#46255=EDGE_CURVE ( 'NONE', #97016, #91796, #98256, .T. ) ;
#46256=CARTESIAN_POINT ( 'NONE',  ( 10.00000000000000000, -0.2410688489992152128, -9.846743663894594434 ) ) ;
#46259=DIRECTION ( 'NONE',  ( 0.000000000000000000, -1.000000000000000000, 0.000000000000000000 ) ) ;
#46261=CARTESIAN_POINT ( 'NONE',  ( 0.1532563361054100626, 10.80059781766745175, -2.638427012816831230 ) ) ;
#46262=CARTESIAN_POINT ( 'NONE',  ( -1.099225684535947600, 54.54030133659708923, 6.408140936763237150 ) ) ;
#46263=CARTESIAN_POINT ( 'NONE',  ( 17.96484262340118221, 9.938685344154839285, 7.964842623401181321 ) ) ;
#46264=CARTESIAN_POINT ( 'NONE',  ( 14.92337183194729633, 42.67559781766745886, 8.527530157486181039 ) ) ;
#46266=CARTESIAN_POINT ( 'NONE',  ( -4.164238869374099927, 27.01208216824730357, 3.795296366450308767 ) ) ;
#46267=CARTESIAN_POINT ( 'NONE',  ( 13.79529636645030344, 63.26208216824730357, 14.16423886937410614 ) ) ;
#46268=CARTESIAN_POINT ( 'NONE',  ( 12.63842701281683034, 62.46726448433410894, 9.846743663894596210 ) ) ;
#46270=CARTESIAN_POINT ( 'NONE',  ( 7.084665262690076126, 57.02201867748817676, -10.88017736071110164 ) ) ;
#46271=CARTESIAN_POINT ( 'NONE',  ( 18.52753015748618282, 3.925597817667451306, -4.923371831947291888 ) ) ;
#46273=ORIENTED_EDGE ( 'NONE', *, *, #61415, .F. ) ;
#46276=CARTESIAN_POINT ( 'NONE',  ( 12.63842701281683034, 7.467264484334118713, 9.846743663894596210 ) ) ;
#46277=ORIENTED_EDGE ( 'NONE', *, *, #81288, .F. ) ;
#46278=CARTESIAN_POINT ( 'NONE',  ( 22.26659068614894466, 18.88708216824730002, 7.082119434687054849 ) ) ;
#46279=CARTESIAN_POINT ( 'NONE',  ( 12.63842701281683034, 22.46726448433411605, 9.846743663894596210 ) ) ;
#46280=CARTESIAN_POINT ( 'NONE',  ( 19.42250999205614548, 35.98035201082151247, -5.440088680355545492 ) ) ;
#46283=CARTESIAN_POINT ( 'NONE',  ( 0.5774900079438590739, 32.64701867748816966, -5.440088680355550821 ) ) ;
#46284=VERTEX_POINT ( 'NONE', #51277 ) ;
#46285=CARTESIAN_POINT ( 'NONE',  ( 15.44008868035555793, 31.39701867748817676, -9.422509992056140149 ) ) ;
#46288=CARTESIAN_POINT ( 'NONE',  ( 6.565887622018943937, 23.08196800326375708, -12.81628187352647608 ) ) ;
#46289=CARTESIAN_POINT ( 'NONE',  ( 12.63842701281683034, 7.467264484334118713, 9.846743663894596210 ) ) ;
#46290=DIRECTION ( 'NONE',  ( -1.000000000000000000, 0.000000000000000000, 0.000000000000000000 ) ) ;
#46291=EDGE_CURVE ( 'NONE', #88480, #85215, #12883, .T. ) ;
#46293=CARTESIAN_POINT ( 'NONE',  ( 0.1532563361054083140, 11.00893115100078568, 1.131784320476157264E-15 ) ) ;
#46294=CARTESIAN_POINT ( 'NONE',  ( 4.559911319644449179, 28.89701867748817321, 9.422509992056141925 ) ) ;
#46297=ORIENTED_EDGE ( 'NONE', *, *, #70514, .F. ) ;
#46299=CARTESIAN_POINT ( 'NONE',  ( 20.88017736071110164, 55.35535201082149825, 2.915334737309930979 ) ) ;
#46300=CARTESIAN_POINT ( 'NONE',  ( -46.59701958359876528, 103.7651961684614861, -6.068442458532165240 ) ) ;
#46301=CARTESIAN_POINT ( 'NONE',  ( 22.81628187352647785, 61.62363466993041783, 6.195893100308588602E-16 ) ) ;
#46302=CARTESIAN_POINT ( 'NONE',  ( 19.42250999205614548, 65.98035201082151957, -5.440088680355545492 ) ) ;
#46304=CARTESIAN_POINT ( 'NONE',  ( 0.1532563361054100626, 65.80059781766745175, -2.638427012816831230 ) ) ;
#46305=CARTESIAN_POINT ( 'NONE',  ( -29.94000000000001549, 92.00000000000000000, -10.09898361729590199 ) ) ;
#46307=CARTESIAN_POINT ( 'NONE',  ( 0.1532563361054082862, 31.21726448433412315, 2.638427012816831674 ) ) ;
#46308=CARTESIAN_POINT ( 'NONE',  ( 6.565887622018943937, 53.08196800326374643, -12.81628187352647608 ) ) ;
#46309=CARTESIAN_POINT ( 'NONE',  ( 5.076628168052704559, 25.17559781766745175, -8.527530157486179263 ) ) ;
#46310=CARTESIAN_POINT ( 'NONE',  ( 10.00000000000000178, 20.37363466993042138, 12.81628187352647608 ) ) ;
#46313=CARTESIAN_POINT ( 'NONE',  ( 7.084665262690076126, 34.10535201082151247, 10.88017736071109987 ) ) ;
#46315=CARTESIAN_POINT ( 'NONE',  ( 14.92337183194729988, 64.34226448433412315, -8.527530157486177487 ) ) ;
#46317=CARTESIAN_POINT ( 'NONE',  ( 14.92337183194729988, 14.34226448433411782, -8.527530157486177487 ) ) ;
#46318=CARTESIAN_POINT ( 'NONE',  ( 12.91533473730992121, 19.52201867748816611, 10.88017736071110164 ) ) ;
#46319=CARTESIAN_POINT ( 'NONE',  ( -2.816281873526473856, 14.33196800326375531, 3.434112377981055619 ) ) ;
#46320=( NAMED_UNIT ( * ) PLANE_ANGLE_UNIT ( ) SI_UNIT ( $, .RADIAN. ) );
#46321=FILL_AREA_STYLE ('',( #54298 ) ) ;
#46322=CARTESIAN_POINT ( 'NONE',  ( 2.791683348922240793, 66.63393115100079456, 7.208316651077764092 ) ) ;
#46324=CARTESIAN_POINT ( 'NONE',  ( 7.084665262690076126, 24.10535201082150181, 10.88017736071109987 ) ) ;
#46325=CARTESIAN_POINT ( 'NONE',  ( 2.791683348922240793, 41.63393115100078745, 7.208316651077764092 ) ) ;
#46326=CARTESIAN_POINT ( 'NONE',  ( 20.88017736071110519, 20.56368534415484106, 2.639326808657452039E-16 ) ) ;
#46327=DIRECTION ( 'NONE',  ( -0.8320502943378436100, 0.5547001962252291474, -0.000000000000000000 ) ) ;
#46329=CARTESIAN_POINT ( 'NONE',  ( 0.5774900079438590739, 27.64701867748817676, -5.440088680355550821 ) ) ;
#46330=CARTESIAN_POINT ( 'NONE',  ( 4.559911319644449179, 2.230352010821504916, -9.422509992056141925 ) ) ;
#46331=DIRECTION ( 'NONE',  ( -0.000000000000000000, 1.000000000000000000, -0.000000000000000000 ) ) ;
#46332=CARTESIAN_POINT ( 'NONE',  ( 0.1532563361054083140, 1.008931151000784787, 1.131784320476157264E-15 ) ) ;
#46334=CARTESIAN_POINT ( 'NONE',  ( 1.472469842513823179, 20.59226448433411960, -4.923371831947296329 ) ) ;
#46335=CARTESIAN_POINT ( 'NONE',  ( 19.38216949554541557, 12.24863466993041961, -9.382169495545420901 ) ) ;
#46339=CARTESIAN_POINT ( 'NONE',  ( -4.164238869374099039, 16.80374883491396787, 8.674139862899312516E-16 ) ) ;
#46340=CARTESIAN_POINT ( 'NONE',  ( 19.84674366389459266, 43.71726448433410894, -2.638427012816827677 ) ) ;
#46343=CARTESIAN_POINT ( 'NONE',  ( -2.266590686148945544, 57.22041550158063217, 7.082119434687048631 ) ) ;
#46344=CARTESIAN_POINT ( 'NONE',  ( 14.92337183194729633, 22.67559781766745175, 8.527530157486181039 ) ) ;
#46345=LINE ( 'NONE', #53344, #21111 ) ;
#46347=CARTESIAN_POINT ( 'NONE',  ( 20.88017736071110875, 50.77201867748817676, -2.915334737309920765 ) ) ;
#46348=CARTESIAN_POINT ( 'NONE',  ( 10.00000000000000000, 52.87363466993041783, -12.81628187352647608 ) ) ;
#46349=CARTESIAN_POINT ( 'NONE',  ( 19.42250999205614548, 20.98035201082150891, -5.440088680355545492 ) ) ;
#46350=CARTESIAN_POINT ( 'NONE',  ( 19.38216949554541557, 42.24863466993041783, -9.382169495545420901 ) ) ;
#46351=CARTESIAN_POINT ( 'NONE',  ( 16.40814093676324603, 2.456968003263753531, -11.09922568453594671 ) ) ;
#46352=CARTESIAN_POINT ( 'NONE',  ( 18.52753015748617571, 3.092264484334118269, 4.923371831947298993 ) ) ;
#46356=CARTESIAN_POINT ( 'NONE',  ( 22.26659068614895176, 49.72041550158063927, -7.082119434687042414 ) ) ;
#46357=CARTESIAN_POINT ( 'NONE',  ( -4.164238869374098151, 16.59541550158063927, -3.795296366450310543 ) ) ;
#46358=CARTESIAN_POINT ( 'NONE',  ( 17.96484262340118221, 26.18868534415483396, -7.964842623401177768 ) ) ;
#46359=CARTESIAN_POINT ( 'NONE',  ( 7.084665262690076126, 32.02201867748816966, -10.88017736071110164 ) ) ;
#46362=CARTESIAN_POINT ( 'NONE',  ( 0.5774900079438607392, 68.48035201082150536, 5.440088680355550821 ) ) ;
#46363=CARTESIAN_POINT ( 'NONE',  ( 2.035157376598824452, 68.68868534415484817, 7.964842623401179544 ) ) ;
#46364=CARTESIAN_POINT ( 'NONE',  ( -1.099225684535947600, 24.54030133659708923, 6.408140936763237150 ) ) ;
#46365=CARTESIAN_POINT ( 'NONE',  ( 18.61655166652077753, 19.87718327197428891, 6.499999999999971578 ) ) ;
#46367=CARTESIAN_POINT ( 'NONE',  ( 2.791683348922240793, 11.63393115100078568, 7.208316651077764092 ) ) ;
#46368=CARTESIAN_POINT ( 'NONE',  ( 5.076628168052704559, 35.17559781766745175, -8.527530157486179263 ) ) ;
#46369=CARTESIAN_POINT ( 'NONE',  ( 19.42250999205614193, 15.14701867748817143, 5.440088680355555262 ) ) ;
#46371=CARTESIAN_POINT ( 'NONE',  ( 6.565887622018943937, 38.08196800326376064, -12.81628187352647608 ) ) ;
#46372=CARTESIAN_POINT ( 'NONE',  ( 1.472469842513823179, 15.59226448433411960, -4.923371831947296329 ) ) ;
#46373=CARTESIAN_POINT ( 'NONE',  ( 12.91533473730992121, 9.522018677488171434, 10.88017736071110164 ) ) ;
#46374=CARTESIAN_POINT ( 'NONE',  ( 12.63842701281683922, 49.55059781766744464, -9.846743663894590881 ) ) ;
#46375=CARTESIAN_POINT ( 'NONE',  ( 1.472469842513823179, 30.59226448433411960, -4.923371831947296329 ) ) ;
#46376=CARTESIAN_POINT ( 'NONE',  ( 24.16423886937409904, 24.09541550158063927, 3.795296366450317205 ) ) ;
#46378=CARTESIAN_POINT ( 'NONE',  ( 10.00000000000000000, 26.81368534415484106, -10.88017736071110342 ) ) ;
#46379=CARTESIAN_POINT ( 'NONE',  ( -0.8801773607111009756, 8.063685344154837509, 1.068504757029289695E-15 ) ) ;
#46380=AXIS2_PLACEMENT_3D ( 'NONE', #53360, #83867, #29372 ) ;
#46381=CARTESIAN_POINT ( 'NONE',  ( 20.88017736071110875, 25.77201867748816966, -2.915334737309920765 ) ) ;
#46383=CARTESIAN_POINT ( 'NONE',  ( 19.42250999205614193, 25.14701867748817321, 5.440088680355555262 ) ) ;
#46384=ORIENTED_EDGE ( 'NONE', *, *, #56512, .F. ) ;
#46386=CARTESIAN_POINT ( 'NONE',  ( 4.559911319644449179, 42.23035201082151247, -9.422509992056141925 ) ) ;
#46389=CARTESIAN_POINT ( 'NONE',  ( 10.00000000000000000, 57.87363466993042493, -12.81628187352647608 ) ) ;
#46390=CARTESIAN_POINT ( 'NONE',  ( 7.084665262690076126, 42.02201867748816966, -10.88017736071110164 ) ) ;
#46391=CARTESIAN_POINT ( 'NONE',  ( 10.00000000000000000, 46.81368534415484106, -10.88017736071110342 ) ) ;
#46393=CARTESIAN_POINT ( 'NONE',  ( 10.00000000000000000, 56.81368534415484106, -10.88017736071110342 ) ) ;
#46394=FACE_OUTER_BOUND ( 'NONE', #16558, .T. ) ;
#46396=CARTESIAN_POINT ( 'NONE',  ( 10.00000000000000178, 58.05374883491397497, 14.16423886937410082 ) ) ;
#46397=CARTESIAN_POINT ( 'NONE',  ( 7.084665262690076126, 62.02201867748816966, -10.88017736071110164 ) ) ;
#46398=CARTESIAN_POINT ( 'NONE',  ( 20.88017736071110519, 55.56368534415484817, 2.639326808657452039E-16 ) ) ;
#46400=CARTESIAN_POINT ( 'NONE',  ( 7.361572987183170547, 32.05059781766745175, 9.846743663894590881 ) ) ;
#46402=CARTESIAN_POINT ( 'NONE',  ( 14.92337183194729988, 34.34226448433411605, -8.527530157486177487 ) ) ;
#46404=CARTESIAN_POINT ( 'NONE',  ( 19.42250999205614193, 40.14701867748817676, 5.440088680355555262 ) ) ;
#46405=CARTESIAN_POINT ( 'NONE',  ( 19.84674366389459266, 38.30059781766745175, 2.638427012816836559 ) ) ;
#46406=CARTESIAN_POINT ( 'NONE',  ( 16.40814093676324603, 17.45696800326375353, -11.09922568453594671 ) ) ;
#46407=CARTESIAN_POINT ( 'NONE',  ( 20.03447792253740189, 2.655141069906897133, -6.401564815979724266 ) ) ;
#46408=CARTESIAN_POINT ( 'NONE',  ( -0.8801773607111008646, 53.27201867748816966, 2.915334737309923430 ) ) ;
#46409=CARTESIAN_POINT ( 'NONE',  ( 10.00000000000000178, 49.31368534415484106, 10.88017736071110342 ) ) ;
#46410=CARTESIAN_POINT ( 'NONE',  ( 10.00000000000000000, 55.55374883491396787, -14.16423886937410082 ) ) ;
#46413=CARTESIAN_POINT ( 'NONE',  ( 0.6178305044545838731, 24.74863466993042493, 9.382169495545420901 ) ) ;
#46414=CARTESIAN_POINT ( 'NONE',  ( 1.959929470562282283, 51.50257860105348584, 5.767676674365853629 ) ) ;
#46415=VERTEX_POINT ( 'NONE', #75750 ) ;
#46416=CARTESIAN_POINT ( 'NONE',  ( 10.00000000000000178, 10.37363466993041961, 12.81628187352647608 ) ) ;
#46417=CARTESIAN_POINT ( 'NONE',  ( 10.00000000000000000, 26.81368534415484106, -10.88017736071110342 ) ) ;
#46418=EDGE_CURVE ( 'NONE', #38545, #6951, #7272, .T. ) ;
#46419=CARTESIAN_POINT ( 'NONE',  ( 7.084665262690076126, 62.02201867748816966, -10.88017736071110164 ) ) ;
#46421=CARTESIAN_POINT ( 'NONE',  ( 18.52753015748618282, 3.925597817667451306, -4.923371831947291888 ) ) ;
#46422=CARTESIAN_POINT ( 'NONE',  ( 14.92337183194729988, 49.34226448433411605, -8.527530157486177487 ) ) ;
#46423=CARTESIAN_POINT ( 'NONE',  ( 0.1532563361054082862, 31.21726448433412315, 2.638427012816831674 ) ) ;
#46424=CARTESIAN_POINT ( 'NONE',  ( 1.472469842513823179, 25.59226448433412315, -4.923371831947296329 ) ) ;
#46426=CARTESIAN_POINT ( 'NONE',  ( 20.15039907845753220, 25.60158574516642815, -6.262539305110077947 ) ) ;
#46427=CARTESIAN_POINT ( 'NONE',  ( 5.076628168052704559, 15.17559781766745175, -8.527530157486179263 ) ) ;
#46428=DIRECTION ( 'NONE',  ( 0.000000000000000000, 1.000000000000000000, 0.000000000000000000 ) ) ;
#46430=CARTESIAN_POINT ( 'NONE',  ( 19.84674366389459621, 43.50893115100078745, 7.409399052514197653E-17 ) ) ;
#46431=ORIENTED_EDGE ( 'NONE', *, *, #21818, .F. ) ;
#46432=( BOUNDED_CURVE ( )  B_SPLINE_CURVE ( 2, ( #54658, #62651, #24679, #17184, #70177, #26144, #94137, #1693, #78658 ),
 .UNSPECIFIED., .F., .F. ) 
 B_SPLINE_CURVE_WITH_KNOTS ( ( 3, 2, 2, 2, 3 ),
 ( 0.7248575172211797479, 0.7261904761904761640, 0.7321428571428570953, 0.7380952380952381375, 0.7394281970645346647 ),
 .UNSPECIFIED. ) 
 CURVE ( )  GEOMETRIC_REPRESENTATION_ITEM ( )  RATIONAL_B_SPLINE_CURVE ( ( 0.9881565478350733400, 0.9923695281211490915, 1.000000000000000000, 0.9659258262890683122, 1.000000000000000000, 0.9659258262890683122, 1.000000000000000000, 0.9923695281211484254, 0.9881565478350726739 ) ) 
 REPRESENTATION_ITEM ( '' )  );
#46434=CARTESIAN_POINT ( 'NONE',  ( 22.81628187352647785, 16.41530133659708923, 3.434112377981063169 ) ) ;
#46436=CARTESIAN_POINT ( 'NONE',  ( 0.5774900079438607392, 53.48035201082151247, 5.440088680355550821 ) ) ;
#46437=CARTESIAN_POINT ( 'NONE',  ( 22.26659068614894466, 38.88708216824731068, 7.082119434687054849 ) ) ;
#46439=SURFACE_STYLE_FILL_AREA ( #39444 ) ;
#46440=CARTESIAN_POINT ( 'NONE',  ( 20.00000000000000711, 89.81725769049432984, 5.338627755225069826 ) ) ;
#46441=CARTESIAN_POINT ( 'NONE',  ( 24.16423886937409904, 39.09541550158062506, 3.795296366450317205 ) ) ;
#46443=CARTESIAN_POINT ( 'NONE',  ( 24.16423886937409904, 64.09541550158064638, 3.795296366450317205 ) ) ;
#46444=CARTESIAN_POINT ( 'NONE',  ( -4.164238869374099927, 27.01208216824730357, 3.795296366450308767 ) ) ;
#46445=CARTESIAN_POINT ( 'NONE',  ( 6.204703633549690345, 30.76208216824730357, -14.16423886937410259 ) ) ;
#46446=CARTESIAN_POINT ( 'NONE',  ( 13.99999999999999822, 11.50000000000000000, 6.000000000000000000 ) ) ;
#46448=CARTESIAN_POINT ( 'NONE',  ( -10.00000000000007105, 92.00000000000000000, 9.500000000000000000 ) ) ;
#46449=CARTESIAN_POINT ( 'NONE',  ( 5.076628168052703671, 41.84226448433411605, 8.527530157486179263 ) ) ;
#46452=CARTESIAN_POINT ( 'NONE',  ( 20.00000000000001066, 87.37138358833496454, -5.317662825072152266 ) ) ;
#46453=CARTESIAN_POINT ( 'NONE',  ( 0.1532563361054083140, 46.00893115100079456, 1.131784320476157264E-15 ) ) ;
#46454=CARTESIAN_POINT ( 'NONE',  ( 0.6178305044545838731, 54.74863466993042493, 9.382169495545420901 ) ) ;
#46456=CARTESIAN_POINT ( 'NONE',  ( 2.791683348922240793, 36.63393115100078035, 7.208316651077764092 ) ) ;
#46457=CARTESIAN_POINT ( 'NONE',  ( 12.63842701281683034, 57.46726448433411605, 9.846743663894596210 ) ) ;
#46458=CARTESIAN_POINT ( 'NONE',  ( -0.3689425029237881626, 42.42874883491396787, 10.36894250292379027 ) ) ;
#46460=CARTESIAN_POINT ( 'NONE',  ( 2.917880565312948704, 7.637082168247301794, 12.26659068614894643 ) ) ;
#46461=CARTESIAN_POINT ( 'NONE',  ( 19.42250999205614548, 60.98035201082151247, -5.440088680355545492 ) ) ;
#46464=CARTESIAN_POINT ( 'NONE',  ( 15.44008868035555793, 11.39701867748817143, -9.422509992056140149 ) ) ;
#46465=CARTESIAN_POINT ( 'NONE',  ( 16.40814093676324603, 12.45696800326375353, -11.09922568453594671 ) ) ;
#46466=CARTESIAN_POINT ( 'NONE',  ( 1.472469842513823179, 1.425597817667451528, 4.923371831947296329 ) ) ;
#46468=CARTESIAN_POINT ( 'NONE',  ( 17.08211943468705840, 60.13708216824729647, -12.26659068614894466 ) ) ;
#46470=CARTESIAN_POINT ( 'NONE',  ( 7.084665262690076126, 22.02201867748817321, -10.88017736071110164 ) ) ;
#46471=CARTESIAN_POINT ( 'NONE',  ( 20.88017736071110164, 25.35535201082150891, 2.915334737309930979 ) ) ;
#46472=CARTESIAN_POINT ( 'NONE',  ( 10.00000000000000178, 52.25893115100078745, 9.846743663894594434 ) ) ;
#46473=CARTESIAN_POINT ( 'NONE',  ( 5.076628168052703671, 56.84226448433412315, 8.527530157486179263 ) ) ;
#46474=CARTESIAN_POINT ( 'NONE',  ( 19.38216949554541202, 50.99863466993042493, 9.382169495545424454 ) ) ;
#46475=CARTESIAN_POINT ( 'NONE',  ( 5.076628168052703671, 1.842264484334118047, 8.527530157486179263 ) ) ;
#46479=CARTESIAN_POINT ( 'NONE',  ( 20.88017736071110875, 10.77201867748817143, -2.915334737309920765 ) ) ;
#46480=CARTESIAN_POINT ( 'NONE',  ( 6.565887622018943937, 18.08196800326375708, -12.81628187352647608 ) ) ;
#46482=CARTESIAN_POINT ( 'NONE',  ( 1.472469842513823179, 46.42559781766745175, 4.923371831947296329 ) ) ;
#46483=CARTESIAN_POINT ( 'NONE',  ( -0.8801773607111008646, 48.27201867748816966, 2.915334737309923430 ) ) ;
#46484=CARTESIAN_POINT ( 'NONE',  ( 13.43411237798105340, 15.58196800326374998, 12.81628187352647963 ) ) ;
#46485=CARTESIAN_POINT ( 'NONE',  ( 0.5774900079438590739, 67.64701867748817676, -5.440088680355550821 ) ) ;
#46490=CARTESIAN_POINT ( 'NONE',  ( 4.559911319644449179, 48.89701867748817676, 9.422509992056141925 ) ) ;
#46491=CARTESIAN_POINT ( 'NONE',  ( 16.40814093676324603, 52.45696800326375353, -11.09922568453594671 ) ) ;
#46492=CARTESIAN_POINT ( 'NONE',  ( 20.36894250292379382, 13.67874883491396965, 10.36894250292379205 ) ) ;
#46493=CARTESIAN_POINT ( 'NONE',  ( 12.63842701281683034, 7.467264484334118713, 9.846743663894596210 ) ) ;
#46494=FACE_OUTER_BOUND ( 'NONE', #14653, .T. ) ;
#46495=CARTESIAN_POINT ( 'NONE',  ( 19.84674366389459266, 18.30059781766745175, 2.638427012816836559 ) ) ;
#46496=DIRECTION ( 'NONE',  ( -0.000000000000000000, -0.000000000000000000, -1.000000000000000000 ) ) ;
#46497=CARTESIAN_POINT ( 'NONE',  ( -4.164238869374099927, 52.01208216824729647, 3.795296366450308767 ) ) ;
#46498=EDGE_CURVE ( 'NONE', #42399, #18624, #45819, .T. ) ;
#46499=CARTESIAN_POINT ( 'NONE',  ( 0.5774900079438590739, 7.647018677488171434, -5.440088680355550821 ) ) ;
#46503=ORIENTED_EDGE ( 'NONE', *, *, #4231, .F. ) ;
#46504=CARTESIAN_POINT ( 'NONE',  ( 10.00000000000000178, 9.313685344154839285, 10.88017736071110342 ) ) ;
#46505=CARTESIAN_POINT ( 'NONE',  ( -0.8801773607111009756, 13.06368534415483929, 1.068504757029289695E-15 ) ) ;
#46506=CARTESIAN_POINT ( 'NONE',  ( 7.361572987183170547, 42.05059781766745886, 9.846743663894590881 ) ) ;
#46507=CARTESIAN_POINT ( 'NONE',  ( 3.591859063236763294, 38.29030133659708923, -11.09922568453595026 ) ) ;
#46508=CARTESIAN_POINT ( 'NONE',  ( 19.72487221294570858, 70.00000000000000000, -6.000000000000000000 ) ) ;
#46509=CARTESIAN_POINT ( 'NONE',  ( 1.274849032793998305, 2.555090184799397424, -6.499999999999581668 ) ) ;
#46510=CARTESIAN_POINT ( 'NONE',  ( 20.36894250292379382, 13.67874883491396965, 10.36894250292379205 ) ) ;
#46511=CARTESIAN_POINT ( 'NONE',  ( -0.8801773607110991993, 32.85535201082151247, -2.915334737309923874 ) ) ;
#46512=CARTESIAN_POINT ( 'NONE',  ( -0.8801773607111008646, 8.272018677488171434, 2.915334737309923430 ) ) ;
#46513=CARTESIAN_POINT ( 'NONE',  ( 18.52753015748617571, 38.09226448433412315, 4.923371831947298993 ) ) ;
#46515=CARTESIAN_POINT ( 'NONE',  ( 19.84674366389459266, 18.71726448433411960, -2.638427012816827677 ) ) ;
#46518=EDGE_LOOP ( 'NONE', ( #40471, #51351, #71983, #583 ) ) ;
#46520=( NAMED_UNIT ( * ) SI_UNIT ( $, .STERADIAN. ) SOLID_ANGLE_UNIT ( ) );
#46521=ORIENTED_EDGE ( 'NONE', *, *, #80080, .T. ) ;
#46522=CARTESIAN_POINT ( 'NONE',  ( 14.92337183194729633, 62.67559781766745886, 8.527530157486181039 ) ) ;
#46523=CARTESIAN_POINT ( 'NONE',  ( 20.88017736071110164, 30.35535201082151247, 2.915334737309930979 ) ) ;
#46524=CARTESIAN_POINT ( 'NONE',  ( 15.44008868035555260, 34.73035201082151247, 9.422509992056143702 ) ) ;
#46525=CARTESIAN_POINT ( 'NONE',  ( 17.96484262340118221, 9.938685344154837509, 7.964842623401181321 ) ) ;
#46526=CARTESIAN_POINT ( 'NONE',  ( -2.816281873526473856, 34.33196800326376064, 3.434112377981055619 ) ) ;
#46527=CARTESIAN_POINT ( 'NONE',  ( 17.08211943468705130, 13.47041550158063572, 12.26659068614894998 ) ) ;
#46529=CARTESIAN_POINT ( 'NONE',  ( 0.6178305044545838731, 44.74863466993042493, 9.382169495545420901 ) ) ;
#46531=CARTESIAN_POINT ( 'NONE',  ( 10.00000000000000178, 42.25893115100078745, 9.846743663894594434 ) ) ;
#46533=CARTESIAN_POINT ( 'NONE',  ( -0.8801773607111009756, 23.06368534415484106, 1.068504757029289695E-15 ) ) ;
#46536=CARTESIAN_POINT ( 'NONE',  ( -0.8801773607111008646, 23.27201867748817676, 2.915334737309923430 ) ) ;
#46538=CARTESIAN_POINT ( 'NONE',  ( 10.00000000000000178, 59.31368534415484106, 10.88017736071110342 ) ) ;
#46539=CARTESIAN_POINT ( 'NONE',  ( 15.44008868035555793, 66.39701867748817676, -9.422509992056140149 ) ) ;
#46540=CARTESIAN_POINT ( 'NONE',  ( 15.44008868035555793, 61.39701867748817676, -9.422509992056140149 ) ) ;
#46541=CARTESIAN_POINT ( 'NONE',  ( 19.84674366389459266, 3.300597817667451750, 2.638427012816836559 ) ) ;
#46542=CARTESIAN_POINT ( 'NONE',  ( 17.96484262340118221, 61.18868534415482685, -7.964842623401177768 ) ) ;
#46545=CARTESIAN_POINT ( 'NONE',  ( -46.94000000000001194, 101.9444105523804893, 6.894162316358291243 ) ) ;
#46546=CARTESIAN_POINT ( 'NONE',  ( 5.076628168052704559, 10.17559781766745175, -8.527530157486179263 ) ) ;
#46549=CARTESIAN_POINT ( 'NONE',  ( 0.1532563361054082862, 46.21726448433411605, 2.638427012816831674 ) ) ;
#46555=CARTESIAN_POINT ( 'NONE',  ( 10.00000000000000000, 25.55374883491396787, -14.16423886937410082 ) ) ;
#46556=CARTESIAN_POINT ( 'NONE',  ( 0.2751277870542911397, 35.30223176428830811, 6.499999999999992006 ) ) ;
#46558=CARTESIAN_POINT ( 'NONE',  ( 12.91533473730992121, 19.52201867748816611, 10.88017736071110164 ) ) ;
#46559=DIRECTION ( 'NONE',  ( 1.000000000000000000, 0.000000000000000000, 0.000000000000000000 ) ) ;
#46561=CARTESIAN_POINT ( 'NONE',  ( 5.076628168052703671, 6.842264484334118713, 8.527530157486179263 ) ) ;
#46562=CARTESIAN_POINT ( 'NONE',  ( 3.591859063236761518, 34.95696800326375353, 11.09922568453594849 ) ) ;
#46563=CARTESIAN_POINT ( 'NONE',  ( 0.1532563361054083140, 21.00893115100078745, 1.131784320476157264E-15 ) ) ;
#46566=CARTESIAN_POINT ( 'NONE',  ( 22.81628187352648496, 11.83196800326375531, -3.434112377981050290 ) ) ;
#46569=CARTESIAN_POINT ( 'NONE',  ( 0.1532563361054083140, 1.008931151000784787, 1.131784320476157264E-15 ) ) ;
#46571=ORIENTED_EDGE ( 'NONE', *, *, #7616, .F. ) ;
#46572=CARTESIAN_POINT ( 'NONE',  ( 2.035157376598822676, 27.43868534415483396, -7.964842623401177768 ) ) ;
#46573=CARTESIAN_POINT ( 'NONE',  ( 6.204703633549690345, 22.84541550158062861, 14.16423886937410082 ) ) ;
#46574=CARTESIAN_POINT ( 'NONE',  ( 10.00000000000000000, 39.75893115100078745, -9.846743663894594434 ) ) ;
#46575=CARTESIAN_POINT ( 'NONE',  ( 5.076628168052704559, 0.1755978176674514724, -8.527530157486179263 ) ) ;
#46577=CARTESIAN_POINT ( 'NONE',  ( 22.81628187352648496, 51.83196800326376064, -3.434112377981050290 ) ) ;
#46579=CARTESIAN_POINT ( 'NONE',  ( 4.559911319644449179, 27.23035201082150536, -9.422509992056141925 ) ) ;
#46581=CARTESIAN_POINT ( 'NONE',  ( -1.099225684535947600, 13.70696800326375353, -6.408140936763238038 ) ) ;
#46582=CARTESIAN_POINT ( 'NONE',  ( -2.816281873526473856, 4.123634669930420493, 9.499525473075851096E-16 ) ) ;
#46583=CARTESIAN_POINT ( 'NONE',  ( 19.84674366389459266, 43.30059781766744464, 2.638427012816836559 ) ) ;
#46585=CARTESIAN_POINT ( 'NONE',  ( 13.43411237798105340, 45.58196800326374643, 12.81628187352647963 ) ) ;
#46587=( GEOMETRIC_REPRESENTATION_CONTEXT ( 3 ) GLOBAL_UNCERTAINTY_ASSIGNED_CONTEXT ( ( #16126 ) ) GLOBAL_UNIT_ASSIGNED_CONTEXT ( ( #21549, #89047, #13045 ) ) REPRESENTATION_CONTEXT ( 'NONE', 'WORKASPACE' ) );
#46588=CARTESIAN_POINT ( 'NONE',  ( 20.88017736071110519, 55.56368534415484817, 2.639326808657452039E-16 ) ) ;
#46591=CARTESIAN_POINT ( 'NONE',  ( -0.8801773607111008646, 53.27201867748816966, 2.915334737309923430 ) ) ;
#46592=CARTESIAN_POINT ( 'NONE',  ( 2.035157376598824452, 43.68868534415484106, 7.964842623401179544 ) ) ;
#46594=CARTESIAN_POINT ( 'NONE',  ( 0.5774900079438607392, 68.48035201082150536, 5.440088680355550821 ) ) ;
#46595=CARTESIAN_POINT ( 'NONE',  ( 2.791683348922237240, 45.38393115100079456, -7.208316651077763204 ) ) ;
#46596=CARTESIAN_POINT ( 'NONE',  ( 0.5774900079438607392, 8.480352010821505360, 5.440088680355550821 ) ) ;
#46598=CARTESIAN_POINT ( 'NONE',  ( -2.816281873526473856, 29.12363466993041783, 9.499525473075851096E-16 ) ) ;
#46600=CARTESIAN_POINT ( 'NONE',  ( 17.96484262340118221, 41.18868534415484106, -7.964842623401177768 ) ) ;
#46601=CARTESIAN_POINT ( 'NONE',  ( 3.591859063236761518, 4.956968003263753531, 11.09922568453594849 ) ) ;
#46603=CARTESIAN_POINT ( 'NONE',  ( 15.44008868035555793, 16.39701867748817321, -9.422509992056140149 ) ) ;
#46604=CARTESIAN_POINT ( 'NONE',  ( 2.035157376598824452, 23.68868534415484461, 7.964842623401179544 ) ) ;
#46605=CARTESIAN_POINT ( 'NONE',  ( 10.00000000000000000, 40.55374883491397497, -14.16423886937410082 ) ) ;
#46606=CARTESIAN_POINT ( 'NONE',  ( 18.52753015748617571, 28.09226448433411960, 4.923371831947298993 ) ) ;
#46607=CARTESIAN_POINT ( 'NONE',  ( 12.91533473730992121, 64.52201867748817676, 10.88017736071110164 ) ) ;
#46609=( LENGTH_UNIT ( ) NAMED_UNIT ( * ) SI_UNIT ( .MILLI., .METRE. ) );
#46612=CARTESIAN_POINT ( 'NONE',  ( 19.84674366389459266, 53.71726448433411605, -2.638427012816827677 ) ) ;
#46613=ORIENTED_EDGE ( 'NONE', *, *, #4287, .T. ) ;
#46616=CARTESIAN_POINT ( 'NONE',  ( 20.36894250292379738, 29.92874883491396432, -10.36894250292379027 ) ) ;
#46617=CARTESIAN_POINT ( 'NONE',  ( -4.164238869374099039, 41.80374883491397497, 8.674139862899312516E-16 ) ) ;
#46618=CARTESIAN_POINT ( 'NONE',  ( 0.1532563361054083140, 1.008931151000784787, 1.131784320476157264E-15 ) ) ;
#46619=CARTESIAN_POINT ( 'NONE',  ( 14.92337183194729633, 62.67559781766745886, 8.527530157486181039 ) ) ;
#46621=CARTESIAN_POINT ( 'NONE',  ( 10.00000000000000000, 61.81368534415484106, -10.88017736071110342 ) ) ;
#46622=CARTESIAN_POINT ( 'NONE',  ( 10.00000000000000178, 20.37363466993042138, 12.81628187352647608 ) ) ;
#46623=CARTESIAN_POINT ( 'NONE',  ( -4.164238869374098151, 31.59541550158063927, -3.795296366450310543 ) ) ;
#46624=CARTESIAN_POINT ( 'NONE',  ( 4.559911319644449179, 32.23035201082150536, -9.422509992056141925 ) ) ;
#46625=CARTESIAN_POINT ( 'NONE',  ( -0.8801773607111008646, 28.27201867748817321, 2.915334737309923430 ) ) ;
#46626=DIRECTION ( 'NONE',  ( -0.000000000000000000, -0.000000000000000000, 1.000000000000000000 ) ) ;
#46627=CARTESIAN_POINT ( 'NONE',  ( 12.91533473730992121, 54.52201867748816255, 10.88017736071110164 ) ) ;
#46631=CYLINDRICAL_SURFACE ( 'NONE', #76487, 0.5000000000000004441 ) ;
#46633=CARTESIAN_POINT ( 'NONE',  ( 24.16423886937409904, 9.095415501580633943, 3.795296366450317205 ) ) ;
#46634=CARTESIAN_POINT ( 'NONE',  ( -2.266590686148945544, 57.22041550158063217, 7.082119434687048631 ) ) ;
#46635=CARTESIAN_POINT ( 'NONE',  ( 20.36894250292379382, 63.67874883491396787, 10.36894250292379205 ) ) ;
#46636=CARTESIAN_POINT ( 'NONE',  ( 18.52753015748617571, 33.09226448433411605, 4.923371831947298993 ) ) ;
#46637=CARTESIAN_POINT ( 'NONE',  ( 7.361572987183169658, 64.96726448433412315, -9.846743663894592657 ) ) ;
#46640=AXIS2_PLACEMENT_3D ( 'NONE', #86759, #34719, #56742 ) ;
#46642=CARTESIAN_POINT ( 'NONE',  ( 13.43411237798106583, 7.665301336597086568, -12.81628187352647252 ) ) ;
#46645=CARTESIAN_POINT ( 'NONE',  ( -0.3689425029237881626, 52.42874883491396076, 10.36894250292379027 ) ) ;
#46648=CARTESIAN_POINT ( 'NONE',  ( -4.164238869374099927, 42.01208216824728936, 3.795296366450308767 ) ) ;
#46650=CARTESIAN_POINT ( 'NONE',  ( 19.42250999205614548, 15.98035201082150714, -5.440088680355545492 ) ) ;
#46651=CARTESIAN_POINT ( 'NONE',  ( 21.09922568453595559, 62.04030133659709634, -6.408140936763230044 ) ) ;
#46652=CARTESIAN_POINT ( 'NONE',  ( 10.00000000000000178, 29.31368534415483751, 10.88017736071110342 ) ) ;
#46653=CARTESIAN_POINT ( 'NONE',  ( 5.076628168052703671, 46.84226448433412315, 8.527530157486179263 ) ) ;
#46654=CARTESIAN_POINT ( 'NONE',  ( 17.96484262340118221, 31.18868534415483751, -7.964842623401177768 ) ) ;
#46656=CARTESIAN_POINT ( 'NONE',  ( -0.2418659066527717449, 65.11633188102328518, 6.114288769123044531 ) ) ;
#46657=CARTESIAN_POINT ( 'NONE',  ( 18.52753015748618282, 58.92559781766745886, -4.923371831947291888 ) ) ;
#46658=CARTESIAN_POINT ( 'NONE',  ( 17.96484262340118221, 59.93868534415484106, 7.964842623401181321 ) ) ;
#46660=DIRECTION ( 'NONE',  ( 0.000000000000000000, -0.000000000000000000, -1.000000000000000000 ) ) ;
#46661=ORIENTED_EDGE ( 'NONE', *, *, #50666, .F. ) ;
#46663=DIRECTION ( 'NONE',  ( 0.000000000000000000, 0.000000000000000000, 1.000000000000000000 ) ) ;
#46664=ORIENTED_EDGE ( 'NONE', *, *, #47660, .T. ) ;
#46666=CARTESIAN_POINT ( 'NONE',  ( 5.076628168052704559, 30.17559781766745175, -8.527530157486179263 ) ) ;
#46668=CARTESIAN_POINT ( 'NONE',  ( 19.38216949554541202, 45.99863466993041072, 9.382169495545424454 ) ) ;
#46669=CARTESIAN_POINT ( 'NONE',  ( 15.00000000000000000, 60.50000000000000000, 6.500000000000000888 ) ) ;
#46671=ORIENTED_EDGE ( 'NONE', *, *, #3565, .F. ) ;
#46672=CARTESIAN_POINT ( 'NONE',  ( 7.361572987183169658, 64.96726448433412315, -9.846743663894592657 ) ) ;
#46674=CARTESIAN_POINT ( 'NONE',  ( 0.1532563361054100626, 55.80059781766745175, -2.638427012816831230 ) ) ;
#46675=CARTESIAN_POINT ( 'NONE',  ( 13.79529636645031943, 30.34541550158063927, -14.16423886937409904 ) ) ;
#46676=CARTESIAN_POINT ( 'NONE',  ( 0.1532563361054082862, 61.21726448433412315, 2.638427012816831674 ) ) ;
#46677=CARTESIAN_POINT ( 'NONE',  ( 2.603489959281586774, 5.435752660568278216, -6.500000000000001776 ) ) ;
#46678=CARTESIAN_POINT ( 'NONE',  ( 18.52753015748618282, 18.92559781766745175, -4.923371831947291888 ) ) ;
#46679=CARTESIAN_POINT ( 'NONE',  ( 10.00000000000000178, 55.37363466993042493, 12.81628187352647608 ) ) ;
#46680=CARTESIAN_POINT ( 'NONE',  ( 24.16423886937409904, 4.095415501580634832, 3.795296366450317205 ) ) ;
#46681=CARTESIAN_POINT ( 'NONE',  ( -1.099225684535947600, -1.293031996736246469, -6.408140936763238038 ) ) ;
#46682=CARTESIAN_POINT ( 'NONE',  ( -0.8801773607110991993, 52.85535201082151247, -2.915334737309923874 ) ) ;
#46683=ADVANCED_FACE ( 'NONE', ( #82518 ), #60005, .T. ) ;
#46684=CARTESIAN_POINT ( 'NONE',  ( 18.52753015748618282, 38.92559781766745175, -4.923371831947291888 ) ) ;
#46687=CARTESIAN_POINT ( 'NONE',  ( -38.69000000000001194, 93.50000000000000000, -9.500000000000000000 ) ) ;
#46688=CARTESIAN_POINT ( 'NONE',  ( 10.00000000000000178, 29.31368534415483751, 10.88017736071110342 ) ) ;
#46689=CARTESIAN_POINT ( 'NONE',  ( 21.09922568453595559, 2.040301336597086568, -6.408140936763230044 ) ) ;
#46690=CARTESIAN_POINT ( 'NONE',  ( 12.91533473730992121, 59.52201867748816966, 10.88017736071110164 ) ) ;
#46692=ADVANCED_FACE ( 'NONE', ( #90499 ), #98545, .T. ) ;
#46693=CARTESIAN_POINT ( 'NONE',  ( 0.5774900079438607392, 68.48035201082150536, 5.440088680355550821 ) ) ;
#46695=CARTESIAN_POINT ( 'NONE',  ( 12.91533473730993009, 36.60535201082151247, -10.88017736071109987 ) ) ;
#46696=CARTESIAN_POINT ( 'NONE',  ( 0.2751277870542909731, 62.28217586085237656, -6.499999999999992006 ) ) ;
#46697=CARTESIAN_POINT ( 'NONE',  ( 17.20831665107776587, 44.13393115100078745, -7.208316651077762316 ) ) ;
#46698=CARTESIAN_POINT ( 'NONE',  ( 0.1532563361054083140, 1.008931151000784787, 1.131784320476157264E-15 ) ) ;
#46700=CARTESIAN_POINT ( 'NONE',  ( 21.09922568453594849, 11.20696800326375531, 6.408140936763242479 ) ) ;
#46701=CARTESIAN_POINT ( 'NONE',  ( 7.084665262690076126, 9.105352010821503583, 10.88017736071109987 ) ) ;
#46703=CARTESIAN_POINT ( 'NONE',  ( -2.266590686148945544, 17.22041550158063572, 7.082119434687048631 ) ) ;
#46704=CARTESIAN_POINT ( 'NONE',  ( 22.26659068614895176, 59.72041550158063927, -7.082119434687042414 ) ) ;
#46705=CARTESIAN_POINT ( 'NONE',  ( 19.84674366389459266, 23.30059781766745530, 2.638427012816836559 ) ) ;
#46706=SURFACE_STYLE_FILL_AREA ( #7249 ) ;
#46708=CARTESIAN_POINT ( 'NONE',  ( 12.63842701281683034, 22.46726448433411605, 9.846743663894596210 ) ) ;
#46709=CARTESIAN_POINT ( 'NONE',  ( 7.084665262690076126, 27.02201867748817676, -10.88017736071110164 ) ) ;
#46710=CARTESIAN_POINT ( 'NONE',  ( 0.1532563361054083140, 66.00893115100079456, 1.131784320476157264E-15 ) ) ;
#46711=CARTESIAN_POINT ( 'NONE',  ( 24.16423886937410614, 14.51208216824730179, -3.795296366450302550 ) ) ;
#46715=CARTESIAN_POINT ( 'NONE',  ( 17.20831665107776587, 7.883931151000784787, 7.208316651077764980 ) ) ;
#46716=CARTESIAN_POINT ( 'NONE',  ( 0.6178305044545838731, 34.74863466993042493, 9.382169495545420901 ) ) ;
#46717=CARTESIAN_POINT ( 'NONE',  ( 5.076628168052703671, 41.84226448433411605, 8.527530157486179263 ) ) ;
#46719=CARTESIAN_POINT ( 'NONE',  ( 2.791683348922240793, 16.63393115100078745, 7.208316651077764092 ) ) ;
#46720=MECHANICAL_DESIGN_GEOMETRIC_PRESENTATION_REPRESENTATION('',(#5267),#93036);
#46723=CARTESIAN_POINT ( 'NONE',  ( 10.00000000000000000, 55.55374883491396787, -14.16423886937410082 ) ) ;
#46724=PRESENTATION_STYLE_ASSIGNMENT (( #24244 ) ) ;
#46725=CARTESIAN_POINT ( 'NONE',  ( 20.88017736071110164, 55.35535201082149825, 2.915334737309930979 ) ) ;
#46726=CARTESIAN_POINT ( 'NONE',  ( 18.52753015748618282, 38.92559781766745175, -4.923371831947291888 ) ) ;
#46727=CARTESIAN_POINT ( 'NONE',  ( 0.5774900079438590739, 22.64701867748817321, -5.440088680355550821 ) ) ;
#46728=COLOUR_RGB ( '', 0.09019608, 0.27058824, 0.51372549) ;
#46730=CARTESIAN_POINT ( 'NONE',  ( 7.361572987183169658, 54.96726448433413026, -9.846743663894592657 ) ) ;
#46731=CARTESIAN_POINT ( 'NONE',  ( -0.8801773607111008646, 43.27201867748817676, 2.915334737309923430 ) ) ;
#46732=EDGE_CURVE ( 'NONE', #13300, #64876, #30491, .T. ) ;
#46733=SURFACE_SIDE_STYLE ('',( #84266 ) ) ;
#46737=CARTESIAN_POINT ( 'NONE',  ( 6.204703633549690345, 2.845415501580634388, 14.16423886937410082 ) ) ;
#46738=CARTESIAN_POINT ( 'NONE',  ( 5.076628168052704559, 45.17559781766745175, -8.527530157486179263 ) ) ;
#46739=CARTESIAN_POINT ( 'NONE',  ( 17.20831665107776587, 17.88393115100078745, 7.208316651077764980 ) ) ;
#46740=CARTESIAN_POINT ( 'NONE',  ( 22.81628187352648496, 56.83196800326374643, -3.434112377981050290 ) ) ;
#46741=CARTESIAN_POINT ( 'NONE',  ( 10.00000000000000178, 14.31368534415483929, 10.88017736071110342 ) ) ;
#46742=CARTESIAN_POINT ( 'NONE',  ( 18.52753015748617571, 43.09226448433412315, 4.923371831947298993 ) ) ;
#46745=CARTESIAN_POINT ( 'NONE',  ( 22.26659068614895176, 24.72041550158063572, -7.082119434687042414 ) ) ;
#46746=CARTESIAN_POINT ( 'NONE',  ( 22.26659068614894466, 63.88708216824730357, 7.082119434687054849 ) ) ;
#46747=CARTESIAN_POINT ( 'NONE',  ( 17.20831665107776587, 62.88393115100078745, 7.208316651077764980 ) ) ;
#46749=CARTESIAN_POINT ( 'NONE',  ( 20.88017736071110164, 50.35535201082151247, 2.915334737309930979 ) ) ;
#46750=CARTESIAN_POINT ( 'NONE',  ( 0.1532563361054100626, 20.80059781766744464, -2.638427012816831230 ) ) ;
#46756=EDGE_CURVE ( 'NONE', #50558, #97012, #60920, .T. ) ;
#46757=CARTESIAN_POINT ( 'NONE',  ( 7.361572987183169658, 9.967264484334119601, -9.846743663894592657 ) ) ;
#46759=CARTESIAN_POINT ( 'NONE',  ( 24.16423886937410614, 19.51208216824729647, -3.795296366450302550 ) ) ;
#46760=CARTESIAN_POINT ( 'NONE',  ( 0.1532563361054082862, 21.21726448433412315, 2.638427012816831674 ) ) ;
#46761=CARTESIAN_POINT ( 'NONE',  ( 20.88017736071110875, 40.77201867748818387, -2.915334737309920765 ) ) ;
#46762=ORIENTED_EDGE ( 'NONE', *, *, #9402, .T. ) ;
#46763=CARTESIAN_POINT ( 'NONE',  ( 4.559911319644449179, 27.23035201082150536, -9.422509992056141925 ) ) ;
#46765=CARTESIAN_POINT ( 'NONE',  ( 7.084665262690076126, 44.10535201082151247, 10.88017736071109987 ) ) ;
#46766=CARTESIAN_POINT ( 'NONE',  ( 22.26659068614894466, 3.887082168247300906, 7.082119434687054849 ) ) ;
#46767=ORIENTED_EDGE ( 'NONE', *, *, #20474, .T. ) ;
#46768=EDGE_CURVE ( 'NONE', #88041, #72980, #73686, .T. ) ;
#46769=ORIENTED_EDGE ( 'NONE', *, *, #92673, .T. ) ;
#46770=CARTESIAN_POINT ( 'NONE',  ( 10.00000000000000178, 20.37363466993042138, 12.81628187352647608 ) ) ;
#46771=CARTESIAN_POINT ( 'NONE',  ( 0.1532563361054100626, 15.80059781766745353, -2.638427012816831230 ) ) ;
#46773=CARTESIAN_POINT ( 'NONE',  ( 13.43411237798106583, 47.66530133659709634, -12.81628187352647252 ) ) ;
#46775=CARTESIAN_POINT ( 'NONE',  ( 17.20831665107776587, 17.88393115100078745, 7.208316651077764980 ) ) ;
#46776=CARTESIAN_POINT ( 'NONE',  ( 15.44008868035555793, 26.39701867748817321, -9.422509992056140149 ) ) ;
#46780=CARTESIAN_POINT ( 'NONE',  ( 20.88017736071110875, 55.77201867748816966, -2.915334737309920765 ) ) ;
#46783=CARTESIAN_POINT ( 'NONE',  ( 20.88017736071110875, 65.77201867748817676, -2.915334737309920765 ) ) ;
#46785=( GEOMETRIC_REPRESENTATION_CONTEXT ( 3 ) GLOBAL_UNCERTAINTY_ASSIGNED_CONTEXT ( ( #47338 ) ) GLOBAL_UNIT_ASSIGNED_CONTEXT ( ( #377, #46814, #8335 ) ) REPRESENTATION_CONTEXT ( 'NONE', 'WORKASPACE' ) );
#46786=CARTESIAN_POINT ( 'NONE',  ( 13.43411237798105340, 0.5819680032637533085, 12.81628187352647963 ) ) ;
#46788=CARTESIAN_POINT ( 'NONE',  ( 2.791683348922237240, 25.38393115100078390, -7.208316651077763204 ) ) ;
#46789=CARTESIAN_POINT ( 'NONE',  ( 3.591859063236761518, 54.95696800326376064, 11.09922568453594849 ) ) ;
#46790=CARTESIAN_POINT ( 'NONE',  ( -0.000000000000000000, 76.60832266181904515, 7.291975907158628090 ) ) ;
#46791=CARTESIAN_POINT ( 'NONE',  ( 14.92337183194729988, 14.34226448433411782, -8.527530157486177487 ) ) ;
#46792=STYLED_ITEM ( 'NONE', ( #84043 ), #76858 ) ;
#46793=CARTESIAN_POINT ( 'NONE',  ( 3.591859063236761518, 19.95696800326375353, 11.09922568453594849 ) ) ;
#46795=CARTESIAN_POINT ( 'NONE',  ( -45.94000000000000483, 92.50000000000000000, -8.999999999999998224 ) ) ;
#46796=CARTESIAN_POINT ( 'NONE',  ( 12.91533473730993009, 46.60535201082150536, -10.88017736071109987 ) ) ;
#46797=CARTESIAN_POINT ( 'NONE',  ( 1.472469842513823179, 60.59226448433412315, -4.923371831947296329 ) ) ;
#46799=CARTESIAN_POINT ( 'NONE',  ( 0.1532563361054100626, 15.80059781766745353, -2.638427012816831230 ) ) ;
#46800=CARTESIAN_POINT ( 'NONE',  ( 20.88017736071110875, 10.77201867748817143, -2.915334737309920765 ) ) ;
#46801=ADVANCED_FACE ( 'NONE', ( #83015 ), #68864, .F. ) ;
#46802=CARTESIAN_POINT ( 'NONE',  ( 3.591859063236761518, 19.95696800326375353, 11.09922568453594849 ) ) ;
#46806=CARTESIAN_POINT ( 'NONE',  ( 4.559911319644449179, 13.89701867748817321, 9.422509992056141925 ) ) ;
#46807=CARTESIAN_POINT ( 'NONE',  ( -1.926860441876564023, 49.68830936912750929, 1.004413902775740781E-15 ) ) ;
#46808=CARTESIAN_POINT ( 'NONE',  ( 0.1532563361054083140, 36.00893115100078745, 1.131784320476157264E-15 ) ) ;
#46809=CARTESIAN_POINT ( 'NONE',  ( 2.035157376598822676, 12.43868534415483751, -7.964842623401177768 ) ) ;
#46811=CARTESIAN_POINT ( 'NONE',  ( 12.91533473730993009, 31.60535201082150891, -10.88017736071109987 ) ) ;
#46812=CARTESIAN_POINT ( 'NONE',  ( 20.36894250292379382, 63.67874883491396787, 10.36894250292379205 ) ) ;
#46814=( NAMED_UNIT ( * ) PLANE_ANGLE_UNIT ( ) SI_UNIT ( $, .RADIAN. ) );
#46815=CARTESIAN_POINT ( 'NONE',  ( 19.84674366389459621, 28.50893115100078745, 7.409399052514197653E-17 ) ) ;
#46821=CARTESIAN_POINT ( 'NONE',  ( 22.26659068614894466, 23.88708216824730357, 7.082119434687054849 ) ) ;
#46823=CARTESIAN_POINT ( 'NONE',  ( 0.1532563361054082862, 36.21726448433410894, 2.638427012816831674 ) ) ;
#46825=CARTESIAN_POINT ( 'NONE',  ( 2.917880565312948704, 52.63708216824730357, 12.26659068614894643 ) ) ;
#46826=CARTESIAN_POINT ( 'NONE',  ( 1.472469842513823179, 20.59226448433411960, -4.923371831947296329 ) ) ;
#46828=DIRECTION ( 'NONE',  ( 1.000000000000000000, 0.000000000000000000, 0.000000000000000000 ) ) ;
#46829=CARTESIAN_POINT ( 'NONE',  ( 10.00000000000000000, 46.81368534415484106, -10.88017736071110342 ) ) ;
#46830=CARTESIAN_POINT ( 'NONE',  ( 19.38216949554541202, 55.99863466993041072, 9.382169495545424454 ) ) ;
#46831=CARTESIAN_POINT ( 'NONE',  ( 4.559911319644449179, 17.23035201082150536, -9.422509992056141925 ) ) ;
#46832=CARTESIAN_POINT ( 'NONE',  ( -2.816281873526473856, 49.33196800326374643, 3.434112377981055619 ) ) ;
#46833=CARTESIAN_POINT ( 'NONE',  ( 6.565887622018943937, -1.918031996736246692, -12.81628187352647608 ) ) ;
#46834=PRESENTATION_STYLE_ASSIGNMENT (( #15383 ) ) ;
#46837=CARTESIAN_POINT ( 'NONE',  ( 22.26659068614894466, 53.88708216824731068, 7.082119434687054849 ) ) ;
#46838=CARTESIAN_POINT ( 'NONE',  ( 22.26659068614894466, 8.887082168247300018, 7.082119434687054849 ) ) ;
#46839=CARTESIAN_POINT ( 'NONE',  ( 0.5774900079438607392, 13.48035201082150358, 5.440088680355550821 ) ) ;
#46840=CARTESIAN_POINT ( 'NONE',  ( 4.559911319644449179, 33.89701867748817676, 9.422509992056141925 ) ) ;
#46842=CARTESIAN_POINT ( 'NONE',  ( -46.71044717097655763, 100.6858870166936413, -9.426445562487726804 ) ) ;
#46843=CARTESIAN_POINT ( 'NONE',  ( 4.559911319644449179, 63.89701867748817676, 9.422509992056141925 ) ) ;
#46844=DIRECTION ( 'NONE',  ( 0.000000000000000000, -1.000000000000000000, 0.000000000000000000 ) ) ;
#46845=CARTESIAN_POINT ( 'NONE',  ( 19.84674366389459621, 18.50893115100078745, 7.409399052514197653E-17 ) ) ;
#46848=CARTESIAN_POINT ( 'NONE',  ( 19.84674366389459621, 8.508931151000785675, 7.409399052514197653E-17 ) ) ;
#46849=CARTESIAN_POINT ( 'NONE',  ( 17.20831665107776587, 32.88393115100078745, 7.208316651077764980 ) ) ;
#46850=CARTESIAN_POINT ( 'NONE',  ( 19.42250999205614193, 10.14701867748816966, 5.440088680355555262 ) ) ;
#46852=CARTESIAN_POINT ( 'NONE',  ( 10.00000000000000000, 32.87363466993042493, -12.81628187352647608 ) ) ;
#46853=CARTESIAN_POINT ( 'NONE',  ( 14.92337183194729633, 2.675597817667451750, 8.527530157486181039 ) ) ;
#46854=CARTESIAN_POINT ( 'NONE',  ( 19.39235739573469530, 54.87576471608601736, 6.499999999999995559 ) ) ;
#46857=CARTESIAN_POINT ( 'NONE',  ( 14.92337183194729988, 49.34226448433411605, -8.527530157486177487 ) ) ;
#46858=AXIS2_PLACEMENT_3D ( 'NONE', #70665, #25659, #48139 ) ;
#46859=CARTESIAN_POINT ( 'NONE',  ( 0.1532563361054100626, 35.80059781766745175, -2.638427012816831230 ) ) ;
#46860=CARTESIAN_POINT ( 'NONE',  ( -2.266590686148945544, 1.387082168247301128, -7.082119434687050408 ) ) ;
#46861=CARTESIAN_POINT ( 'NONE',  ( -4.164238869374099039, 21.80374883491396787, 8.674139862899312516E-16 ) ) ;
#46862=CARTESIAN_POINT ( 'NONE',  ( 7.084665262690076126, 34.10535201082151247, 10.88017736071109987 ) ) ;
#46863=CARTESIAN_POINT ( 'NONE',  ( 17.96484262340118221, 16.18868534415483396, -7.964842623401177768 ) ) ;
#46865=CARTESIAN_POINT ( 'NONE',  ( 17.96484262340118221, 49.93868534415484106, 7.964842623401181321 ) ) ;
#46866=CARTESIAN_POINT ( 'NONE',  ( 19.42250999205614548, 35.98035201082151247, -5.440088680355545492 ) ) ;
#46869=CARTESIAN_POINT ( 'NONE',  ( 3.591859063236763294, 38.29030133659708923, -11.09922568453595026 ) ) ;
#46870=CARTESIAN_POINT ( 'NONE',  ( 15.44008868035555793, 41.39701867748817676, -9.422509992056140149 ) ) ;
#46871=EDGE_CURVE ( 'NONE', #81215, #91132, #33253, .T. ) ;
#46873=CARTESIAN_POINT ( 'NONE',  ( -2.816281873526471635, 58.91530133659707502, -3.434112377981056508 ) ) ;
#46874=CARTESIAN_POINT ( 'NONE',  ( 19.42250999205614548, 50.98035201082151247, -5.440088680355545492 ) ) ;
#46876=CARTESIAN_POINT ( 'NONE',  ( 7.084665262690076126, 44.10535201082151247, 10.88017736071109987 ) ) ;
#46877=CARTESIAN_POINT ( 'NONE',  ( 1.274849032794317383, 27.55509018479935790, -6.500000000000010658 ) ) ;
#46878=CARTESIAN_POINT ( 'NONE',  ( 24.16423886937410614, 54.30374883491396787, 8.672049930838204340E-16 ) ) ;
#46879=CARTESIAN_POINT ( 'NONE',  ( 17.96484262340118221, 59.93868534415484106, 7.964842623401181321 ) ) ;
#46880=CARTESIAN_POINT ( 'NONE',  ( 19.42250999205614193, 55.14701867748817676, 5.440088680355555262 ) ) ;
#46882=FILL_AREA_STYLE ('',( #15437 ) ) ;
#46883=CARTESIAN_POINT ( 'NONE',  ( 5.076628168052704559, 30.17559781766745175, -8.527530157486179263 ) ) ;
#46886=CARTESIAN_POINT ( 'NONE',  ( 5.076628168052704559, 40.17559781766745175, -8.527530157486179263 ) ) ;
#46887=CARTESIAN_POINT ( 'NONE',  ( 4.559911319644449179, 38.89701867748817676, 9.422509992056141925 ) ) ;
#46888=CARTESIAN_POINT ( 'NONE',  ( 0.1532563361054100626, 40.80059781766745886, -2.638427012816831230 ) ) ;
#46889=CARTESIAN_POINT ( 'NONE',  ( 19.38216949554541557, 22.24863466993041428, -9.382169495545420901 ) ) ;
#46890=CARTESIAN_POINT ( 'NONE',  ( 12.91533473730992121, 64.52201867748817676, 10.88017736071110164 ) ) ;
#46891=CARTESIAN_POINT ( 'NONE',  ( 15.44008868035555260, 49.73035201082150536, 9.422509992056143702 ) ) ;
#46892=CARTESIAN_POINT ( 'NONE',  ( -2.266590686148945544, 56.38708216824731068, -7.082119434687050408 ) ) ;
#46894=CARTESIAN_POINT ( 'NONE',  ( 13.43411237798105340, 25.58196800326374998, 12.81628187352647963 ) ) ;
#46897=CARTESIAN_POINT ( 'NONE',  ( -2.816281873526471635, 23.91530133659708568, -3.434112377981056508 ) ) ;
#46898=CARTESIAN_POINT ( 'NONE',  ( 10.00000000000000000, 16.81368534415483751, -10.88017736071110342 ) ) ;
#46899=ORIENTED_EDGE ( 'NONE', *, *, #35578, .T. ) ;
#46901=CARTESIAN_POINT ( 'NONE',  ( 7.361572987183170547, 7.050597817667451750, 9.846743663894590881 ) ) ;
#46902=CARTESIAN_POINT ( 'NONE',  ( 0.1532563361054082862, 46.21726448433411605, 2.638427012816831674 ) ) ;
#46903=CARTESIAN_POINT ( 'NONE',  ( 0.1532563361054083140, 41.00893115100078745, 1.131784320476157264E-15 ) ) ;
#46906=CARTESIAN_POINT ( 'NONE',  ( 18.52753015748618282, 23.92559781766745530, -4.923371831947291888 ) ) ;
#46909=CARTESIAN_POINT ( 'NONE',  ( 1.472469842513823179, 11.42559781766745175, 4.923371831947296329 ) ) ;
#46912=CARTESIAN_POINT ( 'NONE',  ( 10.00000000000000000, 44.75893115100078745, -9.846743663894594434 ) ) ;
#46915=CARTESIAN_POINT ( 'NONE',  ( 0.6178305044545818747, 13.49863466993041783, -9.382169495545419124 ) ) ;
#46917=CARTESIAN_POINT ( 'NONE',  ( -0.8801773607111008646, 58.27201867748816966, 2.915334737309923430 ) ) ;
#46918=CARTESIAN_POINT ( 'NONE',  ( -4.164238869374099927, 52.01208216824729647, 3.795296366450308767 ) ) ;
#46919=CARTESIAN_POINT ( 'NONE',  ( 2.791683348922240793, 1.633931151000784565, 7.208316651077764092 ) ) ;
#46922=CARTESIAN_POINT ( 'NONE',  ( 22.26659068614895176, 44.72041550158063927, -7.082119434687042414 ) ) ;
#46923=CARTESIAN_POINT ( 'NONE',  ( -0.3689425029237898834, 61.17874883491396076, -10.36894250292378850 ) ) ;
#46924=CARTESIAN_POINT ( 'NONE',  ( 2.917880565312948704, 17.63708216824730357, 12.26659068614894643 ) ) ;
#46925=CARTESIAN_POINT ( 'NONE',  ( 20.36894250292379738, 29.92874883491396432, -10.36894250292379027 ) ) ;
#46929=CARTESIAN_POINT ( 'NONE',  ( 0.1532563361054100626, 40.80059781766745886, -2.638427012816831230 ) ) ;
#46931=CARTESIAN_POINT ( 'NONE',  ( 0.5774900079438590739, 42.64701867748816966, -5.440088680355550821 ) ) ;
#46932=DIRECTION ( 'NONE',  ( -0.000000000000000000, -1.000000000000000000, 0.000000000000000000 ) ) ;
#46933=FACE_OUTER_BOUND ( 'NONE', #15957, .T. ) ;
#46935=CARTESIAN_POINT ( 'NONE',  ( 20.00000000000000711, 90.58866250143879029, -4.971011742375100795 ) ) ;
#46936=CARTESIAN_POINT ( 'NONE',  ( 10.00000000000000000, 44.75893115100078745, -9.846743663894594434 ) ) ;
#46937=CARTESIAN_POINT ( 'NONE',  ( 21.09922568453595559, 57.04030133659708923, -6.408140936763230044 ) ) ;
#46939=CARTESIAN_POINT ( 'NONE',  ( 5.076628168052703671, 46.84226448433412315, 8.527530157486179263 ) ) ;
#46940=CARTESIAN_POINT ( 'NONE',  ( 14.92337183194729633, 52.67559781766745175, 8.527530157486181039 ) ) ;
#46941=CARTESIAN_POINT ( 'NONE',  ( 13.79529636645030344, 38.26208216824729647, 14.16423886937410614 ) ) ;
#46943=CARTESIAN_POINT ( 'NONE',  ( 2.917880565312948704, 17.63708216824730357, 12.26659068614894643 ) ) ;
#46945=CARTESIAN_POINT ( 'NONE',  ( -0.03932841506541930043, 68.12161441960500952, 6.397827110479001433 ) ) ;
#46947=CARTESIAN_POINT ( 'NONE',  ( -0.8801773607111009756, 8.063685344154837509, 1.068504757029289695E-15 ) ) ;
#46948=CARTESIAN_POINT ( 'NONE',  ( -2.816281873526473856, 14.33196800326375531, 3.434112377981055619 ) ) ;
#46950=CARTESIAN_POINT ( 'NONE',  ( 4.559911319644449179, 62.23035201082150536, -9.422509992056141925 ) ) ;
#46952=CARTESIAN_POINT ( 'NONE',  ( -46.94000000000000483, 102.2681967859571870, -7.165875991463089179 ) ) ;
#46953=FACE_OUTER_BOUND ( 'NONE', #9628, .T. ) ;
#46954=CARTESIAN_POINT ( 'NONE',  ( 20.36894250292379382, 58.67874883491396076, 10.36894250292379205 ) ) ;
#46956=CARTESIAN_POINT ( 'NONE',  ( -0.8801773607110991993, 22.85535201082150181, -2.915334737309923874 ) ) ;
#46957=CARTESIAN_POINT ( 'NONE',  ( -0.8801773607110991993, 17.85535201082150536, -2.915334737309923874 ) ) ;
#46958=CARTESIAN_POINT ( 'NONE',  ( 18.52753015748617571, 53.09226448433412315, 4.923371831947298993 ) ) ;
#46959=CARTESIAN_POINT ( 'NONE',  ( 7.361572987183169658, 54.96726448433413026, -9.846743663894592657 ) ) ;
#46960=CARTESIAN_POINT ( 'NONE',  ( -1.099225684535947600, 59.54030133659708923, 6.408140936763237150 ) ) ;
#46962=EDGE_CURVE ( 'NONE', #51568, #156, #62961, .T. ) ;
#46963=VERTEX_POINT ( 'NONE', #25487 ) ;
#46964=CARTESIAN_POINT ( 'NONE',  ( 0.5774900079438607392, 28.48035201082150891, 5.440088680355550821 ) ) ;
#46965=CARTESIAN_POINT ( 'NONE',  ( 22.81628187352647785, 31.62363466993042138, 6.195893100308588602E-16 ) ) ;
#46967=EDGE_CURVE ( 'NONE', #63997, #32629, #38072, .T. ) ;
#46968=CARTESIAN_POINT ( 'NONE',  ( 17.20831665107776587, 59.13393115100078745, -7.208316651077762316 ) ) ;
#46969=CARTESIAN_POINT ( 'NONE',  ( 12.91533473730992121, 44.52201867748816966, 10.88017736071110164 ) ) ;
#46971=CARTESIAN_POINT ( 'NONE',  ( 10.00000000000000178, 17.25893115100078745, 9.846743663894594434 ) ) ;
#46972=CARTESIAN_POINT ( 'NONE',  ( 22.81628187352647785, 16.62363466993042138, 6.195893100308588602E-16 ) ) ;
#46973=CARTESIAN_POINT ( 'NONE',  ( 19.42250999205614193, 60.14701867748817676, 5.440088680355555262 ) ) ;
#46977=CARTESIAN_POINT ( 'NONE',  ( -0.8801773607111009756, 48.27201867748816966, 2.915334737309923874 ) ) ;
#46979=CARTESIAN_POINT ( 'NONE',  ( 4.559911319644449179, 47.23035201082150536, -9.422509992056141925 ) ) ;
#46980=CARTESIAN_POINT ( 'NONE',  ( 6.565887622018943937, 48.08196800326375353, -12.81628187352647608 ) ) ;
#46981=CARTESIAN_POINT ( 'NONE',  ( 2.917880565312950480, 10.97041550158063572, -12.26659068614894821 ) ) ;
#46982=CARTESIAN_POINT ( 'NONE',  ( 10.00000000000000000, 19.75893115100078390, -9.846743663894594434 ) ) ;
#46983=CARTESIAN_POINT ( 'NONE',  ( 0.5774900079438607392, 3.480352010821504027, 5.440088680355550821 ) ) ;
#46984=CARTESIAN_POINT ( 'NONE',  ( 17.20831665107776587, 14.13393115100078568, -7.208316651077762316 ) ) ;
#46985=CARTESIAN_POINT ( 'NONE',  ( 19.72487221294571214, 15.71833443783937589, -6.500000000000001776 ) ) ;
#46986=CARTESIAN_POINT ( 'NONE',  ( -2.266590686148945544, 51.38708216824730357, -7.082119434687050408 ) ) ;
#46987=VERTEX_POINT ( 'NONE', #9976 ) ;
#46989=CARTESIAN_POINT ( 'NONE',  ( 2.035157376598824452, 8.688685344154839285, 7.964842623401179544 ) ) ;
#46990=CARTESIAN_POINT ( 'NONE',  ( 1.711636803080549329, 31.84492782695769719, -6.499999999999986677 ) ) ;
#46992=CARTESIAN_POINT ( 'NONE',  ( 20.88017736071110519, 10.56368534415483929, 2.639326808657452039E-16 ) ) ;
#46993=CARTESIAN_POINT ( 'NONE',  ( 20.88017736071110164, 10.35535201082150714, 2.915334737309930979 ) ) ;
#46994=CARTESIAN_POINT ( 'NONE',  ( 18.52753015748618282, 38.92559781766745175, -4.923371831947291888 ) ) ;
#46995=CARTESIAN_POINT ( 'NONE',  ( 0.6178305044545818747, 38.49863466993042493, -9.382169495545419124 ) ) ;
#46999=CARTESIAN_POINT ( 'NONE',  ( -0.3689425029237881626, 22.42874883491397142, 10.36894250292379027 ) ) ;
#47000=CARTESIAN_POINT ( 'NONE',  ( 0.5774900079438607392, 28.48035201082150891, 5.440088680355550821 ) ) ;
#47001=CARTESIAN_POINT ( 'NONE',  ( 7.084665262690076126, 2.022018677488171434, -10.88017736071110164 ) ) ;
#47003=CARTESIAN_POINT ( 'NONE',  ( 19.84674366389459266, 48.30059781766745175, 2.638427012816836559 ) ) ;
#47005=CARTESIAN_POINT ( 'NONE',  ( 2.791683348922240793, 31.63393115100078745, 7.208316651077764092 ) ) ;
#47007=ADVANCED_FACE ( 'NONE', ( #77469 ), #85212, .T. ) ;
#47010=CARTESIAN_POINT ( 'NONE',  ( 7.084665262690076126, 4.105352010821503583, 10.88017736071109987 ) ) ;
#47011=CARTESIAN_POINT ( 'NONE',  ( 0.5774900079438590739, 62.64701867748817676, -5.440088680355550821 ) ) ;
#47012=CARTESIAN_POINT ( 'NONE',  ( 18.52753015748618282, 53.92559781766745175, -4.923371831947291888 ) ) ;
#47013=CARTESIAN_POINT ( 'NONE',  ( -0.8801773607111008646, 38.27201867748816255, 2.915334737309923430 ) ) ;
#47014=CARTESIAN_POINT ( 'NONE',  ( 20.88017736071110519, 10.56368534415483751, 2.639326808657452039E-16 ) ) ;
#47015=CARTESIAN_POINT ( 'NONE',  ( 3.591859063236761518, 29.95696800326375708, 11.09922568453594849 ) ) ;
#47016=CARTESIAN_POINT ( 'NONE',  ( 6.204703633549690345, 12.84541550158063572, 14.16423886937410082 ) ) ;
#47017=CARTESIAN_POINT ( 'NONE',  ( 3.591859063236763294, 43.29030133659708923, -11.09922568453595026 ) ) ;
#47019=( BOUNDED_SURFACE ( )  B_SPLINE_SURFACE ( 1, 2, ( 
 ( #68757, #773, #69253, #61722, #44261, #14785, #29262, #288, #45255, #75752, #52753, #46250, #37282, #83261, #21785, #15278, #92237, #8252, #74767, #45759, #7274, #6275, #68272, #31225, #23764, #14283, #75258, #7770, #37775, #76735, #60743, #44756, #38264, #30734, #61241, #36781, #98792, #52265, #23267, #30239, #6771, #91747, #38751, #82761, #53743, #67272, #67772, #98293, #84262, #15764, #97800, #29748, #60257, #90751, #91244, #22768, #53249, #24247, #63687, #93208, #39249, #8731, #16738, #64172, #25720, #10707, #17237, #18213, #85235, #69739, #56212, #78712, #24731, #26198, #70730, #25239, #2738, #47215, #55209, #47715, #39738, #86707, #41222, #54713, #1265, #78210, #77226, #16245, #40221, #85724, #17726, #2245, #77716, #10223, #94693, #32703, #9722, #9229, #63199, #84741, #46727, #70233, #1752, #32207, #62216, #48692, #86215, #92722, #93704, #33675, #33194, #31720, #94190, #55720, #48199, #62708, #40712, #71217, #71699, #79195, #3213, #96177, #88657, #88162, #19676, #65161, #89154, #80174, #95679, #3707, #27660, #5671, #51160, #18704, #58148, #27165, #49188, #12169, #74136, #43651, #57173, #19183, #20165, #57665, #20664, #4693, #87670, #50669, #81157, #12662, #66657, #42674, #95171, #66146, #73153, #49664, #35661, #81644, #34168, #43161, #79690, #11685, #26678, #73647, #5176, #96679, #28158, #72178, #42195, #11188, #34664, #41708, #72659, #58654, #50165, #64658, #4194, #80674, #36153, #13152, #97181, #35155, #56690, #65654, #87183, #68634, #22648, #67654, #69128, #14660, #68145, #45630, #90130, #37158, #60126, #82640, #164, #53617, #97669, #44133, #90624, #21159, #59139, #83135, #98164, #60624, #45126, #29135, #53128, #8134, #75632, #22149, #59639, #52632, #38627, #89647, #21660, #52144, #14158, #6154, #61119, #30119, #36659, #7144, #76617, #76129, #28649, #7655, #37648, #29620, #51660, #82139, #13648, #84135, #67145, #98671, #91125, #83636, #15151, #38149, #74644, #44641, #30613, #91628, #15647, #46129, #75135, #6641, #23144, #16123, #86100, #48080, #62585, #93090, #79075, #56097, #63086, #69615, #55605, #93586, #84619, #24621, #2131, #61601, #86590, #8619, #92115, #660, #63576, #31108, #77106, #70605, #9601, #17610, #39128, #62094, #92602, #55087, #2625, #18099, #85108, #70111, #85607, #17122, #48576, #23646, #40602, #10588, #41100, #9108, #47604, #71099, #24126, #94086, #78593, #10105, #33080, #54106, #32591, #39622, #1137, #46607, #31599, #25605, #1636, #54595, #16619, #78099, #47095, #77593, #32087, #40104, #25123, #5060, #64547, #64058, #73533, #50550, #34542, #50058, #58535, #41599, #13038, #80061, #94570 ),
 ( #89043, #20554, #72067, #34051, #73041, #42083, #35545, #19562, #3592, #4576, #65539, #27545, #81532, #27052, #11079, #81045, #57550, #95054, #12552, #66036, #49076, #35037, #26089, #26563, #57060, #96062, #42557, #58039, #43055, #87074, #87561, #56584, #49549, #18583, #19071, #96565, #11565, #79578, #72546, #4079, #51039, #28040, #71596, #65037, #95563, #88049, #80562, #12056, #3108, #33562, #88547, #20048, #67535, #60014, #53, #43535, #83521, #30500, #84012, #52034, #98050, #15039, #36546, #7539, #60512, #22535, #45511, #5560, #14542, #82527, #44023, #97067, #61002, #91004, #14043, #51538, #59033, #37037, #74029, #67035, #97557, #53006, #22044, #76011, #29018, #36036, #38031, #68522, #6528, #52519, #91513, #13539, #66539, #44524, #28539, #89538, #75023, #74526, #23030, #21048, #82029, #37538, #7032, #53502, #6047, #59528, #90021, #21543, #29506, #90509, #83026, #68027, #45012, #75517, #98555, #30006, #10844, #48339, #78842, #71356, #86842, #33803, #57310, #94821, #46017, #25850, #72309, #2875, #41843, #10353, #2382, #94330, #64310, #85860, #33324, #86350, #32836, #40852, #8020, #18346, #63338, #24873, #34299, #79335, #47842, #41365, #17853, #17372, #56347, #26325, #63819, #48824, #95315, #3840, #71832, #78345, #3341, #56822, #546, #87321, #18838, #76506, #64797, #55355, #38517, #15535, #79822, #69015, #93348, #49318, #11324, #26817, #32347, #62850, #9867, #40365, #70866, #93843, #25370, #55855, #12308, #65294, #21299, #89297, #95821, #73789, #36796, #36295, #67290, #66792, #35799, #88801, #19323, #49807, #11815, #13795, #27301, #66286, #28297, #20808, #58790, #81781, #34805, #72796, #96821, #43782, #74785, #44281, #97818, #87802, #20311, #4335, #74275, #50809, #81300, #96325, #51791, #42816, #27798, #57802, #51295, #29279, #82278, #80315, #13296, #58283, #42322, #43295, #6294, #88309, #19807, #50297, #5803, #12795, #80810, #97312, #73300, #28785, #59283, #89782, #4824, #5320, #35298, #65791, #45778, #90772, #38768, #54246, #37302, #23286, #52283, #52770, #29765, #84279, #30751, #61258, #69270, #75277, #14803, #14301, #37792, #82781, #98311, #790, #68289, #44772, #6788, #22296, #39269, #31243, #84758, #91262, #92257, #60273, #67789, #61739, #53764, #98810, #1286, #76270, #307, #76752, #83278, #30259, #22788, #45275, #23780, #16264, #75770, #7291, #53266, #60762, #90268, #15296, #83772, #91764, #7787, #38282, #15779, #69758, #68777, #46268, #8271, #46747, #77243, #8750, #59775, #21802, #62727, #11209, #71719, #56711, #63220, #64193, #32226, #54730, #3230, #25741, #70752, #72198, #17744, #71235, #48712, #93227, #40242 ) ),
 .UNSPECIFIED., .F., .F., .F. ) 
 B_SPLINE_SURFACE_WITH_KNOTS ( ( 2, 2 ),
 ( 3, 2, 2, 2, 2, 2, 2, 2, 2, 2, 2, 2, 2, 2, 2, 2, 2, 2, 2, 2, 2, 2, 2, 2, 2, 2, 2, 2, 2, 2, 2, 2, 2, 2, 2, 2, 2, 2, 2, 2, 2, 2, 2, 2, 2, 2, 2, 2, 2, 2, 2, 2, 2, 2, 2, 2, 2, 2, 2, 2, 2, 2, 2, 2, 2, 2, 2, 2, 2, 2, 2, 2, 2, 2, 2, 2, 2, 2, 2, 2, 2, 2, 2, 2, 2, 2, 2, 2, 2, 2, 2, 2, 2, 2, 2, 2, 2, 2, 2, 2, 2, 2, 2, 2, 2, 2, 2, 2, 2, 2, 2, 2, 2, 2, 2, 2, 2, 2, 2, 2, 2, 2, 2, 2, 2, 2, 2, 2, 2, 2, 2, 2, 2, 2, 2, 2, 2, 2, 2, 2, 2, 2, 2, 2, 2, 2, 2, 2, 2, 2, 2, 2, 2, 2, 2, 2, 2, 2, 2, 2, 2, 2, 3 ),
 ( 0.000000000000000000, 1.000000000000000000 ),
 ( 0.000000000000000000, 0.005952380952380952051, 0.01190476190476190410, 0.01785714285714285615, 0.02380952380952380820, 0.02976190476190476025, 0.03571428571428571230, 0.04166666666666666435, 0.04761904761904761640, 0.05357142857142856845, 0.05952380952380952051, 0.06547619047619047949, 0.07142857142857142461, 0.07738095238095238360, 0.08333333333333332871, 0.08928571428571428770, 0.09523809523809523281, 0.1011904761904761918, 0.1071428571428571369, 0.1130952380952380959, 0.1190476190476190410, 0.1250000000000000000, 0.1309523809523809590, 0.1369047619047619180, 0.1428571428571428492, 0.1488095238095238082, 0.1547619047619047672, 0.1607142857142857262, 0.1666666666666666574, 0.1726190476190476164, 0.1785714285714285754, 0.1845238095238095344, 0.1904761904761904656, 0.1964285714285714246, 0.2023809523809523836, 0.2083333333333333426, 0.2142857142857142738, 0.2202380952380952328, 0.2261904761904761918, 0.2321428571428571508, 0.2380952380952380820, 0.2440476190476190410, 0.2500000000000000000, 0.2559523809523809312, 0.2619047619047619180, 0.2678571428571428492, 0.2738095238095238360, 0.2797619047619047672, 0.2857142857142856984, 0.2916666666666666852, 0.2976190476190476164, 0.3035714285714285476, 0.3095238095238095344, 0.3154761904761904656, 0.3214285714285714524, 0.3273809523809523836, 0.3333333333333333148, 0.3392857142857143016, 0.3452380952380952328, 0.3511904761904761640, 0.3571428571428571508, 0.3630952380952380820, 0.3690476190476190688, 0.3750000000000000000, 0.3809523809523809312, 0.3869047619047619180, 0.3928571428571428492, 0.3988095238095238360, 0.4047619047619047672, 0.4107142857142856984, 0.4166666666666666852, 0.4226190476190476164, 0.4285714285714285476, 0.4345238095238095344, 0.4404761904761904656, 0.4464285714285714524, 0.4523809523809523836, 0.4583333333333333148, 0.4642857142857143016, 0.4702380952380952328, 0.4761904761904761640, 0.4821428571428571508, 0.4880952380952380820, 0.4940476190476190688, 0.5000000000000000000, 0.5059523809523809312, 0.5119047619047618625, 0.5178571428571429047, 0.5238095238095238360, 0.5297619047619047672, 0.5357142857142856984, 0.5416666666666666297, 0.5476190476190476719, 0.5535714285714286031, 0.5595238095238095344, 0.5654761904761904656, 0.5714285714285713969, 0.5773809523809523281, 0.5833333333333333703, 0.5892857142857143016, 0.5952380952380952328, 0.6011904761904761640, 0.6071428571428570953, 0.6130952380952381375, 0.6190476190476190688, 0.6250000000000000000, 0.6309523809523809312, 0.6369047619047618625, 0.6428571428571429047, 0.6488095238095238360, 0.6547619047619047672, 0.6607142857142856984, 0.6666666666666666297, 0.6726190476190476719, 0.6785714285714286031, 0.6845238095238095344, 0.6904761904761904656, 0.6964285714285713969, 0.7023809523809523281, 0.7083333333333333703, 0.7142857142857143016, 0.7202380952380952328, 0.7261904761904761640, 0.7321428571428570953, 0.7380952380952381375, 0.7440476190476190688, 0.7500000000000000000, 0.7559523809523809312, 0.7619047619047618625, 0.7678571428571429047, 0.7738095238095238360, 0.7797619047619047672, 0.7857142857142856984, 0.7916666666666666297, 0.7976190476190476719, 0.8035714285714286031, 0.8095238095238095344, 0.8154761904761904656, 0.8214285714285713969, 0.8273809523809523281, 0.8333333333333333703, 0.8392857142857143016, 0.8452380952380952328, 0.8511904761904761640, 0.8571428571428570953, 0.8630952380952381375, 0.8690476190476190688, 0.8750000000000000000, 0.8809523809523809312, 0.8869047619047618625, 0.8928571428571429047, 0.8988095238095238360, 0.9047619047619047672, 0.9107142857142856984, 0.9166666666666666297, 0.9226190476190476719, 0.9285714285714286031, 0.9345238095238095344, 0.9404761904761904656, 0.9464285714285713969, 0.9523809523809523281, 0.9583333333333333703, 0.9642857142857143016 ),
 .UNSPECIFIED. ) 
 GEOMETRIC_REPRESENTATION_ITEM ( )  RATIONAL_B_SPLINE_SURFACE ( (
 ( 1.000000000000000000, 0.9659258262890683122, 1.000000000000000000, 0.9659258262890683122, 1.000000000000000000, 0.9659258262890683122, 1.000000000000000000, 0.9659258262890683122, 1.000000000000000000, 0.9659258262890683122, 1.000000000000000000, 0.9659258262890683122, 1.000000000000000000, 0.9659258262890683122, 1.000000000000000000, 0.9659258262890683122, 1.000000000000000000, 0.9659258262890683122, 1.000000000000000000, 0.9659258262890683122, 1.000000000000000000, 0.9659258262890683122, 1.000000000000000000, 0.9659258262890683122, 1.000000000000000000, 0.9659258262890683122, 1.000000000000000000, 0.9659258262890683122, 1.000000000000000000, 0.9659258262890683122, 1.000000000000000000, 0.9659258262890683122, 1.000000000000000000, 0.9659258262890683122, 1.000000000000000000, 0.9659258262890683122, 1.000000000000000000, 0.9659258262890683122, 1.000000000000000000, 0.9659258262890683122, 1.000000000000000000, 0.9659258262890683122, 1.000000000000000000, 0.9659258262890683122, 1.000000000000000000, 0.9659258262890683122, 1.000000000000000000, 0.9659258262890683122, 1.000000000000000000, 0.9659258262890683122, 1.000000000000000000, 0.9659258262890683122, 1.000000000000000000, 0.9659258262890683122, 1.000000000000000000, 0.9659258262890683122, 1.000000000000000000, 0.9659258262890683122, 1.000000000000000000, 0.9659258262890683122, 1.000000000000000000, 0.9659258262890683122, 1.000000000000000000, 0.9659258262890683122, 1.000000000000000000, 0.9659258262890683122, 1.000000000000000000, 0.9659258262890683122, 1.000000000000000000, 0.9659258262890683122, 1.000000000000000000, 0.9659258262890683122, 1.000000000000000000, 0.9659258262890683122, 1.000000000000000000, 0.9659258262890683122, 1.000000000000000000, 0.9659258262890683122, 1.000000000000000000, 0.9659258262890683122, 1.000000000000000000, 0.9659258262890683122, 1.000000000000000000, 0.9659258262890683122, 1.000000000000000000, 0.9659258262890683122, 1.000000000000000000, 0.9659258262890683122, 1.000000000000000000, 0.9659258262890683122, 1.000000000000000000, 0.9659258262890683122, 1.000000000000000000, 0.9659258262890683122, 1.000000000000000000, 0.9659258262890683122, 1.000000000000000000, 0.9659258262890683122, 1.000000000000000000, 0.9659258262890683122, 1.000000000000000000, 0.9659258262890683122, 1.000000000000000000, 0.9659258262890683122, 1.000000000000000000, 0.9659258262890683122, 1.000000000000000000, 0.9659258262890683122, 1.000000000000000000, 0.9659258262890683122, 1.000000000000000000, 0.9659258262890683122, 1.000000000000000000, 0.9659258262890683122, 1.000000000000000000, 0.9659258262890683122, 1.000000000000000000, 0.9659258262890683122, 1.000000000000000000, 0.9659258262890683122, 1.000000000000000000, 0.9659258262890683122, 1.000000000000000000, 0.9659258262890683122, 1.000000000000000000, 0.9659258262890683122, 1.000000000000000000, 0.9659258262890683122, 1.000000000000000000, 0.9659258262890683122, 1.000000000000000000, 0.9659258262890683122, 1.000000000000000000, 0.9659258262890683122, 1.000000000000000000, 0.9659258262890683122, 1.000000000000000000, 0.9659258262890683122, 1.000000000000000000, 0.9659258262890683122, 1.000000000000000000, 0.9659258262890683122, 1.000000000000000000, 0.9659258262890683122, 1.000000000000000000, 0.9659258262890683122, 1.000000000000000000, 0.9659258262890683122, 1.000000000000000000, 0.9659258262890683122, 1.000000000000000000, 0.9659258262890683122, 1.000000000000000000, 0.9659258262890683122, 1.000000000000000000, 0.9659258262890683122, 1.000000000000000000, 0.9659258262890683122, 1.000000000000000000, 0.9659258262890683122, 1.000000000000000000, 0.9659258262890683122, 1.000000000000000000, 0.9659258262890683122, 1.000000000000000000, 0.9659258262890683122, 1.000000000000000000, 0.9659258262890683122, 1.000000000000000000, 0.9659258262890683122, 1.000000000000000000, 0.9659258262890683122, 1.000000000000000000, 0.9659258262890683122, 1.000000000000000000, 0.9659258262890683122, 1.000000000000000000, 0.9659258262890683122, 1.000000000000000000, 0.9659258262890683122, 1.000000000000000000, 0.9659258262890683122, 1.000000000000000000, 0.9659258262890683122, 1.000000000000000000, 0.9659258262890683122, 1.000000000000000000, 0.9659258262890683122, 1.000000000000000000, 0.9659258262890683122, 1.000000000000000000, 0.9659258262890683122, 1.000000000000000000, 0.9659258262890683122, 1.000000000000000000, 0.9659258262890683122, 1.000000000000000000, 0.9659258262890683122, 1.000000000000000000, 0.9659258262890683122, 1.000000000000000000, 0.9659258262890683122, 1.000000000000000000, 0.9659258262890683122, 1.000000000000000000, 0.9659258262890683122, 1.000000000000000000, 0.9659258262890683122, 1.000000000000000000, 0.9659258262890683122, 1.000000000000000000, 0.9659258262890683122, 1.000000000000000000, 0.9659258262890683122, 1.000000000000000000, 0.9659258262890683122, 1.000000000000000000, 0.9659258262890683122, 1.000000000000000000, 0.9659258262890683122, 1.000000000000000000, 0.9659258262890683122, 1.000000000000000000, 0.9659258262890683122, 1.000000000000000000, 0.9659258262890683122, 1.000000000000000000, 0.9659258262890683122, 1.000000000000000000, 0.9659258262890683122, 1.000000000000000000, 0.9659258262890683122, 1.000000000000000000, 0.9659258262890683122, 1.000000000000000000, 0.9659258262890683122, 1.000000000000000000, 0.9659258262890683122, 1.000000000000000000, 0.9659258262890683122, 1.000000000000000000, 0.9659258262890683122, 1.000000000000000000, 0.9659258262890683122, 1.000000000000000000, 0.9659258262890683122, 1.000000000000000000, 0.9659258262890683122, 1.000000000000000000, 0.9659258262890683122, 1.000000000000000000, 0.9659258262890683122, 1.000000000000000000, 0.9659258262890683122, 1.000000000000000000, 0.9659258262890683122, 1.000000000000000000, 0.9659258262890683122, 1.000000000000000000, 0.9659258262890683122, 1.000000000000000000, 0.9659258262890683122, 1.000000000000000000, 0.9659258262890683122, 1.000000000000000000, 0.9659258262890683122, 1.000000000000000000, 0.9659258262890683122, 1.000000000000000000, 0.9659258262890683122, 1.000000000000000000, 0.9659258262890683122, 1.000000000000000000, 0.9659258262890683122, 1.000000000000000000, 0.9659258262890683122, 1.000000000000000000, 0.9659258262890683122, 1.000000000000000000, 0.9659258262890683122, 1.000000000000000000, 0.9659258262890683122, 1.000000000000000000, 0.9659258262890683122, 1.000000000000000000, 0.9659258262890683122, 1.000000000000000000, 0.9659258262890683122, 1.000000000000000000, 0.9659258262890683122, 1.000000000000000000, 0.9659258262890683122, 1.000000000000000000, 0.9659258262890683122, 1.000000000000000000, 0.9659258262890683122, 1.000000000000000000, 0.9659258262890683122, 1.000000000000000000, 0.9659258262890683122, 1.000000000000000000, 0.9659258262890683122, 1.000000000000000000, 0.9659258262890683122, 1.000000000000000000, 0.9659258262890683122, 1.000000000000000000, 0.9659258262890683122, 1.000000000000000000, 0.9659258262890683122, 1.000000000000000000, 0.9659258262890683122, 1.000000000000000000, 0.9659258262890683122, 1.000000000000000000, 0.9659258262890683122, 1.000000000000000000, 0.9659258262890683122, 1.000000000000000000, 0.9659258262890683122, 1.000000000000000000, 0.9659258262890683122, 1.000000000000000000, 0.9659258262890683122, 1.000000000000000000),
 ( 1.000000000000000000, 0.9659258262890683122, 1.000000000000000000, 0.9659258262890683122, 1.000000000000000000, 0.9659258262890683122, 1.000000000000000000, 0.9659258262890683122, 1.000000000000000000, 0.9659258262890683122, 1.000000000000000000, 0.9659258262890683122, 1.000000000000000000, 0.9659258262890683122, 1.000000000000000000, 0.9659258262890683122, 1.000000000000000000, 0.9659258262890683122, 1.000000000000000000, 0.9659258262890683122, 1.000000000000000000, 0.9659258262890683122, 1.000000000000000000, 0.9659258262890683122, 1.000000000000000000, 0.9659258262890683122, 1.000000000000000000, 0.9659258262890683122, 1.000000000000000000, 0.9659258262890683122, 1.000000000000000000, 0.9659258262890683122, 1.000000000000000000, 0.9659258262890683122, 1.000000000000000000, 0.9659258262890683122, 1.000000000000000000, 0.9659258262890683122, 1.000000000000000000, 0.9659258262890683122, 1.000000000000000000, 0.9659258262890683122, 1.000000000000000000, 0.9659258262890683122, 1.000000000000000000, 0.9659258262890683122, 1.000000000000000000, 0.9659258262890683122, 1.000000000000000000, 0.9659258262890683122, 1.000000000000000000, 0.9659258262890683122, 1.000000000000000000, 0.9659258262890683122, 1.000000000000000000, 0.9659258262890683122, 1.000000000000000000, 0.9659258262890683122, 1.000000000000000000, 0.9659258262890683122, 1.000000000000000000, 0.9659258262890683122, 1.000000000000000000, 0.9659258262890683122, 1.000000000000000000, 0.9659258262890683122, 1.000000000000000000, 0.9659258262890683122, 1.000000000000000000, 0.9659258262890683122, 1.000000000000000000, 0.9659258262890683122, 1.000000000000000000, 0.9659258262890683122, 1.000000000000000000, 0.9659258262890683122, 1.000000000000000000, 0.9659258262890683122, 1.000000000000000000, 0.9659258262890683122, 1.000000000000000000, 0.9659258262890683122, 1.000000000000000000, 0.9659258262890683122, 1.000000000000000000, 0.9659258262890683122, 1.000000000000000000, 0.9659258262890683122, 1.000000000000000000, 0.9659258262890683122, 1.000000000000000000, 0.9659258262890683122, 1.000000000000000000, 0.9659258262890683122, 1.000000000000000000, 0.9659258262890683122, 1.000000000000000000, 0.9659258262890683122, 1.000000000000000000, 0.9659258262890683122, 1.000000000000000000, 0.9659258262890683122, 1.000000000000000000, 0.9659258262890683122, 1.000000000000000000, 0.9659258262890683122, 1.000000000000000000, 0.9659258262890683122, 1.000000000000000000, 0.9659258262890683122, 1.000000000000000000, 0.9659258262890683122, 1.000000000000000000, 0.9659258262890683122, 1.000000000000000000, 0.9659258262890683122, 1.000000000000000000, 0.9659258262890683122, 1.000000000000000000, 0.9659258262890683122, 1.000000000000000000, 0.9659258262890683122, 1.000000000000000000, 0.9659258262890683122, 1.000000000000000000, 0.9659258262890683122, 1.000000000000000000, 0.9659258262890683122, 1.000000000000000000, 0.9659258262890683122, 1.000000000000000000, 0.9659258262890683122, 1.000000000000000000, 0.9659258262890683122, 1.000000000000000000, 0.9659258262890683122, 1.000000000000000000, 0.9659258262890683122, 1.000000000000000000, 0.9659258262890683122, 1.000000000000000000, 0.9659258262890683122, 1.000000000000000000, 0.9659258262890683122, 1.000000000000000000, 0.9659258262890683122, 1.000000000000000000, 0.9659258262890683122, 1.000000000000000000, 0.9659258262890683122, 1.000000000000000000, 0.9659258262890683122, 1.000000000000000000, 0.9659258262890683122, 1.000000000000000000, 0.9659258262890683122, 1.000000000000000000, 0.9659258262890683122, 1.000000000000000000, 0.9659258262890683122, 1.000000000000000000, 0.9659258262890683122, 1.000000000000000000, 0.9659258262890683122, 1.000000000000000000, 0.9659258262890683122, 1.000000000000000000, 0.9659258262890683122, 1.000000000000000000, 0.9659258262890683122, 1.000000000000000000, 0.9659258262890683122, 1.000000000000000000, 0.9659258262890683122, 1.000000000000000000, 0.9659258262890683122, 1.000000000000000000, 0.9659258262890683122, 1.000000000000000000, 0.9659258262890683122, 1.000000000000000000, 0.9659258262890683122, 1.000000000000000000, 0.9659258262890683122, 1.000000000000000000, 0.9659258262890683122, 1.000000000000000000, 0.9659258262890683122, 1.000000000000000000, 0.9659258262890683122, 1.000000000000000000, 0.9659258262890683122, 1.000000000000000000, 0.9659258262890683122, 1.000000000000000000, 0.9659258262890683122, 1.000000000000000000, 0.9659258262890683122, 1.000000000000000000, 0.9659258262890683122, 1.000000000000000000, 0.9659258262890683122, 1.000000000000000000, 0.9659258262890683122, 1.000000000000000000, 0.9659258262890683122, 1.000000000000000000, 0.9659258262890683122, 1.000000000000000000, 0.9659258262890683122, 1.000000000000000000, 0.9659258262890683122, 1.000000000000000000, 0.9659258262890683122, 1.000000000000000000, 0.9659258262890683122, 1.000000000000000000, 0.9659258262890683122, 1.000000000000000000, 0.9659258262890683122, 1.000000000000000000, 0.9659258262890683122, 1.000000000000000000, 0.9659258262890683122, 1.000000000000000000, 0.9659258262890683122, 1.000000000000000000, 0.9659258262890683122, 1.000000000000000000, 0.9659258262890683122, 1.000000000000000000, 0.9659258262890683122, 1.000000000000000000, 0.9659258262890683122, 1.000000000000000000, 0.9659258262890683122, 1.000000000000000000, 0.9659258262890683122, 1.000000000000000000, 0.9659258262890683122, 1.000000000000000000, 0.9659258262890683122, 1.000000000000000000, 0.9659258262890683122, 1.000000000000000000, 0.9659258262890683122, 1.000000000000000000, 0.9659258262890683122, 1.000000000000000000, 0.9659258262890683122, 1.000000000000000000, 0.9659258262890683122, 1.000000000000000000, 0.9659258262890683122, 1.000000000000000000, 0.9659258262890683122, 1.000000000000000000, 0.9659258262890683122, 1.000000000000000000, 0.9659258262890683122, 1.000000000000000000, 0.9659258262890683122, 1.000000000000000000, 0.9659258262890683122, 1.000000000000000000, 0.9659258262890683122, 1.000000000000000000, 0.9659258262890683122, 1.000000000000000000, 0.9659258262890683122, 1.000000000000000000, 0.9659258262890683122, 1.000000000000000000, 0.9659258262890683122, 1.000000000000000000, 0.9659258262890683122, 1.000000000000000000, 0.9659258262890683122, 1.000000000000000000, 0.9659258262890683122, 1.000000000000000000, 0.9659258262890683122, 1.000000000000000000, 0.9659258262890683122, 1.000000000000000000, 0.9659258262890683122, 1.000000000000000000, 0.9659258262890683122, 1.000000000000000000, 0.9659258262890683122, 1.000000000000000000, 0.9659258262890683122, 1.000000000000000000, 0.9659258262890683122, 1.000000000000000000, 0.9659258262890683122, 1.000000000000000000, 0.9659258262890683122, 1.000000000000000000, 0.9659258262890683122, 1.000000000000000000, 0.9659258262890683122, 1.000000000000000000, 0.9659258262890683122, 1.000000000000000000, 0.9659258262890683122, 1.000000000000000000, 0.9659258262890683122, 1.000000000000000000, 0.9659258262890683122, 1.000000000000000000, 0.9659258262890683122, 1.000000000000000000, 0.9659258262890683122, 1.000000000000000000, 0.9659258262890683122, 1.000000000000000000, 0.9659258262890683122, 1.000000000000000000, 0.9659258262890683122, 1.000000000000000000, 0.9659258262890683122, 1.000000000000000000, 0.9659258262890683122, 1.000000000000000000) ) ) 
 REPRESENTATION_ITEM ( '' )  SURFACE ( )  );
#47020=CARTESIAN_POINT ( 'NONE',  ( 18.52753015748618282, 53.92559781766745175, -4.923371831947291888 ) ) ;
#47021=CARTESIAN_POINT ( 'NONE',  ( 19.42250999205614193, 15.14701867748817143, 5.440088680355555262 ) ) ;
#47023=CARTESIAN_POINT ( 'NONE',  ( 20.88017736071110164, 10.35535201082150714, 2.915334737309930979 ) ) ;
#47024=VERTEX_POINT ( 'NONE', #65433 ) ;
#47025=CARTESIAN_POINT ( 'NONE',  ( 10.00000000000000178, 64.31368534415483396, 10.88017736071110342 ) ) ;
#47026=CARTESIAN_POINT ( 'NONE',  ( -0.8801773607111009756, 68.06368534415484817, 1.068504757029289695E-15 ) ) ;
#47027=CARTESIAN_POINT ( 'NONE',  ( 10.00000000000000000, 4.758931151000784787, -9.846743663894594434 ) ) ;
#47028=CARTESIAN_POINT ( 'NONE',  ( -0.8801773607111009756, 68.06368534415484817, 1.068504757029289695E-15 ) ) ;
#47031=CARTESIAN_POINT ( 'NONE',  ( 18.52753015748618282, 3.925597817667451306, -4.923371831947291888 ) ) ;
#47033=CARTESIAN_POINT ( 'NONE',  ( 19.84674366389459266, 38.71726448433412315, -2.638427012816827677 ) ) ;
#47036=DIRECTION ( 'NONE',  ( -1.000000000000000000, 0.000000000000000000, 0.000000000000000000 ) ) ;
#47037=CARTESIAN_POINT ( 'NONE',  ( 17.08211943468705130, 3.470415501580634388, 12.26659068614894998 ) ) ;
#47038=CARTESIAN_POINT ( 'NONE',  ( 0.6178305044545838731, 59.74863466993041783, 9.382169495545420901 ) ) ;
#47039=CARTESIAN_POINT ( 'NONE',  ( 22.26659068614895176, 9.720415501580633943, -7.082119434687042414 ) ) ;
#47040=CARTESIAN_POINT ( 'NONE',  ( 22.26659068614894466, 13.88708216824730179, 7.082119434687054849 ) ) ;
#47041=CARTESIAN_POINT ( 'NONE',  ( -0.1503990784575328643, 70.00000000000000000, -6.262539305110068177 ) ) ;
#47042=LINE ( 'NONE', #62043, #91332 ) ;
#47043=CARTESIAN_POINT ( 'NONE',  ( 15.44008868035555793, 21.39701867748817321, -9.422509992056140149 ) ) ;
#47046=SURFACE_SIDE_STYLE ('',( #6594 ) ) ;
#47048=CARTESIAN_POINT ( 'NONE',  ( 2.791683348922237240, 0.3839311510007847872, -7.208316651077763204 ) ) ;
#47049=CARTESIAN_POINT ( 'NONE',  ( 10.00000000000000178, 30.37363466993042138, 12.81628187352647608 ) ) ;
#47050=CARTESIAN_POINT ( 'NONE',  ( 1.472469842513823179, 30.59226448433411960, -4.923371831947296329 ) ) ;
#47052=CARTESIAN_POINT ( 'NONE',  ( 6.565887622018943937, 13.08196800326374998, -12.81628187352647608 ) ) ;
#47054=CARTESIAN_POINT ( 'NONE',  ( 0.1532563361054083140, 6.008931151000784787, 1.131784320476157264E-15 ) ) ;
#47056=ORIENTED_EDGE ( 'NONE', *, *, #64090, .F. ) ;
#47058=CARTESIAN_POINT ( 'NONE',  ( 10.00000000000000000, 41.81368534415484106, -10.88017736071110342 ) ) ;
#47059=CARTESIAN_POINT ( 'NONE',  ( -4.164238869374099927, 27.01208216824730357, 3.795296366450308767 ) ) ;
#47060=CARTESIAN_POINT ( 'NONE',  ( 5.076628168052703671, 36.84226448433412315, 8.527530157486179263 ) ) ;
#47061=CARTESIAN_POINT ( 'NONE',  ( 12.63842701281683034, 2.467264484334118269, 9.846743663894596210 ) ) ;
#47062=CARTESIAN_POINT ( 'NONE',  ( -2.816281873526473856, 59.33196800326374643, 3.434112377981055619 ) ) ;
#47064=CARTESIAN_POINT ( 'NONE',  ( 4.559911319644449179, 32.23035201082150536, -9.422509992056141925 ) ) ;
#47066=CARTESIAN_POINT ( 'NONE',  ( 21.09922568453595559, 17.04030133659708923, -6.408140936763230044 ) ) ;
#47067=CARTESIAN_POINT ( 'NONE',  ( -2.816281873526471635, 3.915301336597087456, -3.434112377981056508 ) ) ;
#47068=CARTESIAN_POINT ( 'NONE',  ( 0.1532563361054083140, 41.00893115100078745, 1.131784320476157264E-15 ) ) ;
#47070=CARTESIAN_POINT ( 'NONE',  ( 22.81628187352647785, 51.41530133659708923, 3.434112377981063169 ) ) ;
#47072=( LENGTH_UNIT ( ) NAMED_UNIT ( * ) SI_UNIT ( .MILLI., .METRE. ) );
#47073=CARTESIAN_POINT ( 'NONE',  ( 19.42250999205614548, 55.98035201082150536, -5.440088680355545492 ) ) ;
#47077=CARTESIAN_POINT ( 'NONE',  ( 0.5774900079438607392, 48.48035201082150536, 5.440088680355550821 ) ) ;
#47078=CARTESIAN_POINT ( 'NONE',  ( 4.559911319644449179, 63.89701867748817676, 9.422509992056141925 ) ) ;
#47079=CARTESIAN_POINT ( 'NONE',  ( 20.03743638938529870, 56.75197528031016958, 6.399506433553887597 ) ) ;
#47083=CARTESIAN_POINT ( 'NONE',  ( 12.91533473730993009, 6.605352010821504471, -10.88017736071109987 ) ) ;
#47085=CARTESIAN_POINT ( 'NONE',  ( 19.84674366389459621, 48.50893115100078745, 7.409399052514197653E-17 ) ) ;
#47086=CARTESIAN_POINT ( 'NONE',  ( 4.559911319644449179, 22.23035201082150536, -9.422509992056141925 ) ) ;
#47087=CARTESIAN_POINT ( 'NONE',  ( -2.816281873526473856, 24.12363466993042138, 9.499525473075851096E-16 ) ) ;
#47088=ORIENTED_EDGE ( 'NONE', *, *, #68466, .F. ) ;
#47089=CARTESIAN_POINT ( 'NONE',  ( 4.559911319644449179, 33.89701867748817676, 9.422509992056141925 ) ) ;
#47090=CARTESIAN_POINT ( 'NONE',  ( 22.81628187352647785, 11.41530133659708390, 3.434112377981063169 ) ) ;
#47091=CARTESIAN_POINT ( 'NONE',  ( -0.8801773607111008646, 8.272018677488171434, 2.915334737309923430 ) ) ;
#47092=CARTESIAN_POINT ( 'NONE',  ( 10.00000000000000000, 36.81368534415484106, -10.88017736071110342 ) ) ;
#47093=CARTESIAN_POINT ( 'NONE',  ( -4.164238869374098151, 56.59541550158063927, -3.795296366450310543 ) ) ;
#47094=CARTESIAN_POINT ( 'NONE',  ( 1.472469842513823179, 26.42559781766745175, 4.923371831947296329 ) ) ;
#47095=CARTESIAN_POINT ( 'NONE',  ( 19.42250999205614548, 65.98035201082151957, -5.440088680355545492 ) ) ;
#47096=CARTESIAN_POINT ( 'NONE',  ( 0.2751277870542908621, 32.28217586085237656, -6.499999999999992006 ) ) ;
#47097=CARTESIAN_POINT ( 'NONE',  ( -0.3689425029237881626, 12.42874883491396609, 10.36894250292379027 ) ) ;
#47099=( LENGTH_UNIT ( ) NAMED_UNIT ( * ) SI_UNIT ( .MILLI., .METRE. ) );
#47100=CARTESIAN_POINT ( 'NONE',  ( 1.821708436314933843, 21.66792564121896092, -6.500000000000008882 ) ) ;
#47103=CARTESIAN_POINT ( 'NONE',  ( 24.16423886937409904, 39.09541550158062506, 3.795296366450317205 ) ) ;
#47104=CARTESIAN_POINT ( 'NONE',  ( 10.00000000000000000, 30.55374883491397142, -14.16423886937410082 ) ) ;
#47105=CARTESIAN_POINT ( 'NONE',  ( 10.00000000000000178, 69.31368534415484817, 10.88017736071110342 ) ) ;
#47106=CARTESIAN_POINT ( 'NONE',  ( 19.84674366389459266, 58.71726448433411605, -2.638427012816827677 ) ) ;
#47107=FACE_OUTER_BOUND ( 'NONE', #10996, .T. ) ;
#47108=CARTESIAN_POINT ( 'NONE',  ( 15.44008868035555793, 56.39701867748817676, -9.422509992056140149 ) ) ;
#47109=CARTESIAN_POINT ( 'NONE',  ( 13.43411237798106583, 22.66530133659708923, -12.81628187352647252 ) ) ;
#47110=CARTESIAN_POINT ( 'NONE',  ( 20.36894250292379738, 34.92874883491396076, -10.36894250292379027 ) ) ;
#47111=CARTESIAN_POINT ( 'NONE',  ( 20.88017736071110875, 30.77201867748816966, -2.915334737309920765 ) ) ;
#47112=CARTESIAN_POINT ( 'NONE',  ( -0.8801773607110991993, 27.85535201082150181, -2.915334737309923874 ) ) ;
#47114=CARTESIAN_POINT ( 'NONE',  ( 17.96484262340118221, 54.93868534415484106, 7.964842623401181321 ) ) ;
#47120=CARTESIAN_POINT ( 'NONE',  ( 10.00000000000000178, 63.05374883491396076, 14.16423886937410082 ) ) ;
#47121=CARTESIAN_POINT ( 'NONE',  ( 20.36894250292379738, 64.92874883491397497, -10.36894250292379027 ) ) ;
#47122=CARTESIAN_POINT ( 'NONE',  ( 1.472469842513823179, 41.42559781766745886, 4.923371831947296329 ) ) ;
#47123=CARTESIAN_POINT ( 'NONE',  ( 10.00000000000000000, 54.75893115100078745, -9.846743663894594434 ) ) ;
#47124=CARTESIAN_POINT ( 'NONE',  ( 20.32896413005680358, 59.74545670184114243, 5.963430220938287007 ) ) ;
#47128=CARTESIAN_POINT ( 'NONE',  ( 3.591859063236763294, 8.290301336597087456, -11.09922568453595026 ) ) ;
#47131=CARTESIAN_POINT ( 'NONE',  ( 2.917880565312950480, 50.97041550158064638, -12.26659068614894821 ) ) ;
#47133=CARTESIAN_POINT ( 'NONE',  ( 10.00000000000000000, 40.55374883491397497, -14.16423886937410082 ) ) ;
#47135=CARTESIAN_POINT ( 'NONE',  ( 15.44008868035555260, 19.73035201082150536, 9.422509992056143702 ) ) ;
#47137=CARTESIAN_POINT ( 'NONE',  ( -0.8801773607111009756, 43.06368534415484106, 1.068504757029289695E-15 ) ) ;
#47138=CARTESIAN_POINT ( 'NONE',  ( 17.20831665107776587, 44.13393115100078745, -7.208316651077762316 ) ) ;
#47139=CARTESIAN_POINT ( 'NONE',  ( 20.88017736071110164, 40.35535201082150536, 2.915334737309930979 ) ) ;
#47141=CARTESIAN_POINT ( 'NONE',  ( 19.42250999205614548, 65.98035201082151957, -5.440088680355545492 ) ) ;
#47142=CARTESIAN_POINT ( 'NONE',  ( 20.88017736071110164, 25.35535201082150891, 2.915334737309930979 ) ) ;
#47145=CARTESIAN_POINT ( 'NONE',  ( 1.472469842513823179, 1.425597817667451528, 4.923371831947296329 ) ) ;
#47148=CARTESIAN_POINT ( 'NONE',  ( 0.2751277870542967463, 70.00000000000000000, -6.500000000000000888 ) ) ;
#47149=CARTESIAN_POINT ( 'NONE',  ( 18.52753015748617571, 28.09226448433411960, 4.923371831947298993 ) ) ;
#47154=CARTESIAN_POINT ( 'NONE',  ( -42.16485527613926365, 107.5383484153110061, 5.000000000000000888 ) ) ;
#47155=CARTESIAN_POINT ( 'NONE',  ( 2.791683348922237240, 50.38393115100078035, -7.208316651077763204 ) ) ;
#47156=CARTESIAN_POINT ( 'NONE',  ( 13.79529636645030344, 48.26208216824728936, 14.16423886937410614 ) ) ;
#47157=CARTESIAN_POINT ( 'NONE',  ( 12.63842701281683922, 59.55059781766744464, -9.846743663894590881 ) ) ;
#47159=CARTESIAN_POINT ( 'NONE',  ( 18.52753015748618282, 13.92559781766745175, -4.923371831947291888 ) ) ;
#47160=CARTESIAN_POINT ( 'NONE',  ( -1.099225684535947600, 54.54030133659708923, 6.408140936763237150 ) ) ;
#47161=CARTESIAN_POINT ( 'NONE',  ( 19.84674366389459621, 58.50893115100078745, 7.409399052514197653E-17 ) ) ;
#47162=CARTESIAN_POINT ( 'NONE',  ( 15.44008868035555793, 56.39701867748817676, -9.422509992056140149 ) ) ;
#47164=CARTESIAN_POINT ( 'NONE',  ( 18.52753015748618282, 48.92559781766745886, -4.923371831947291888 ) ) ;
#47165=CARTESIAN_POINT ( 'NONE',  ( 18.72515096720568195, 31.07228050351032422, -6.500000000000018652 ) ) ;
#47169=CARTESIAN_POINT ( 'NONE',  ( 20.36894250292379738, 54.92874883491396076, -10.36894250292379027 ) ) ;
#47171=CARTESIAN_POINT ( 'NONE',  ( 0.5774900079438590739, 27.64701867748817676, -5.440088680355550821 ) ) ;
#47172=CARTESIAN_POINT ( 'NONE',  ( 21.09922568453594849, 11.20696800326375531, 6.408140936763242479 ) ) ;
#47173=CARTESIAN_POINT ( 'NONE',  ( 0.5774900079438590739, 62.64701867748817676, -5.440088680355550821 ) ) ;
#47177=CARTESIAN_POINT ( 'NONE',  ( 4.559911319644449179, 53.89701867748817676, 9.422509992056141925 ) ) ;
#47178=CARTESIAN_POINT ( 'NONE',  ( 2.603489959281582777, 31.58210964143329136, 6.499999999999995559 ) ) ;
#47179=CARTESIAN_POINT ( 'NONE',  ( 5.076628168052704559, 40.17559781766745175, -8.527530157486179263 ) ) ;
#47180=CARTESIAN_POINT ( 'NONE',  ( 2.791683348922237240, 0.3839311510007847872, -7.208316651077763204 ) ) ;
#47182=CARTESIAN_POINT ( 'NONE',  ( 10.00000000000000000, 12.87363466993042138, -12.81628187352647608 ) ) ;
#47183=CARTESIAN_POINT ( 'NONE',  ( 19.42250999205614548, 15.98035201082150714, -5.440088680355545492 ) ) ;
#47184=( LENGTH_UNIT ( ) NAMED_UNIT ( * ) SI_UNIT ( .MILLI., .METRE. ) );
#47186=CARTESIAN_POINT ( 'NONE',  ( 22.26659068614894466, 38.88708216824731068, 7.082119434687054849 ) ) ;
#47187=CARTESIAN_POINT ( 'NONE',  ( 17.08211943468705130, 58.47041550158063927, 12.26659068614894998 ) ) ;
#47189=CARTESIAN_POINT ( 'NONE',  ( 19.84674366389459266, 28.71726448433411960, -2.638427012816827677 ) ) ;
#47190=CARTESIAN_POINT ( 'NONE',  ( 7.361572987183169658, 19.96726448433411960, -9.846743663894592657 ) ) ;
#47191=CARTESIAN_POINT ( 'NONE',  ( 15.44008868035555260, 14.73035201082150536, 9.422509992056143702 ) ) ;
#47194=CARTESIAN_POINT ( 'NONE',  ( 10.00000000000000000, 34.75893115100078745, -9.846743663894594434 ) ) ;
#47196=CARTESIAN_POINT ( 'NONE',  ( -0.8801773607111009756, 23.06368534415484106, 1.068504757029289695E-15 ) ) ;
#47197=CARTESIAN_POINT ( 'NONE',  ( 1.472469842513823179, 55.59226448433412315, -4.923371831947296329 ) ) ;
#47198=CARTESIAN_POINT ( 'NONE',  ( 22.26659068614895176, 4.720415501580633943, -7.082119434687042414 ) ) ;
#47202=UNCERTAINTY_MEASURE_WITH_UNIT (LENGTH_MEASURE( 1.000000000000000082E-05 ), #78487, 'distance_accuracy_value', 'NONE');
#47203=CARTESIAN_POINT ( 'NONE',  ( 0.1532563361054100626, 5.800597817667452638, -2.638427012816831230 ) ) ;
#47204=CARTESIAN_POINT ( 'NONE',  ( 21.09922568453594849, 56.20696800326375353, 6.408140936763242479 ) ) ;
#47205=CARTESIAN_POINT ( 'NONE',  ( 5.076628168052703671, 56.84226448433412315, 8.527530157486179263 ) ) ;
#47207=CARTESIAN_POINT ( 'NONE',  ( 19.84674366389459266, 18.30059781766745175, 2.638427012816836559 ) ) ;
#47208=CARTESIAN_POINT ( 'NONE',  ( 1.707155281725204476, 12.90189080397283483, 6.499999999999992006 ) ) ;
#47210=CARTESIAN_POINT ( 'NONE',  ( 6.204703633549690345, 67.84541550158060375, 14.16423886937410082 ) ) ;
#47211=CARTESIAN_POINT ( 'NONE',  ( 10.00000000000000000, 51.81368534415484106, -10.88017736071110342 ) ) ;
#47213=CARTESIAN_POINT ( 'NONE',  ( 0.5774900079438590739, 52.64701867748817676, -5.440088680355550821 ) ) ;
#47214=CARTESIAN_POINT ( 'NONE',  ( 5.076628168052703671, 36.84226448433412315, 8.527530157486179263 ) ) ;
#47215=CARTESIAN_POINT ( 'NONE',  ( -0.8801773607110991993, 17.85535201082150536, -2.915334737309923874 ) ) ;
#47217=CARTESIAN_POINT ( 'NONE',  ( 10.00000000000000178, 62.25893115100078745, 9.846743663894594434 ) ) ;
#47219=ORIENTED_EDGE ( 'NONE', *, *, #72949, .T. ) ;
#47223=CARTESIAN_POINT ( 'NONE',  ( 19.84674366389459266, 38.30059781766745175, 2.638427012816836559 ) ) ;
#47224=CARTESIAN_POINT ( 'NONE',  ( 14.92337183194729633, 22.67559781766745175, 8.527530157486181039 ) ) ;
#47225=CARTESIAN_POINT ( 'NONE',  ( 10.00000000000000178, 60.37363466993041783, 12.81628187352647608 ) ) ;
#47226=CARTESIAN_POINT ( 'NONE',  ( 10.00000000000000178, 19.31368534415484106, 10.88017736071110342 ) ) ;
#47227=CARTESIAN_POINT ( 'NONE',  ( 0.1532563361054100626, 45.80059781766745886, -2.638427012816831230 ) ) ;
#47228=CARTESIAN_POINT ( 'NONE',  ( -1.926860441876564023, 34.68830936912750929, 1.004413902775740781E-15 ) ) ;
#47229=CARTESIAN_POINT ( 'NONE',  ( -0.3689425029237898834, 46.17874883491397497, -10.36894250292378850 ) ) ;
#47230=CARTESIAN_POINT ( 'NONE',  ( 24.16423886937410614, 59.51208216824728936, -3.795296366450302550 ) ) ;
#47231=CARTESIAN_POINT ( 'NONE',  ( -45.94000000000001194, 103.9981609152045650, -5.961202730336927047 ) ) ;
#47232=CARTESIAN_POINT ( 'NONE',  ( 2.148416515056654763, 67.23726573380442062, 6.500000000000004441 ) ) ;
#47233=CARTESIAN_POINT ( 'NONE',  ( 7.084665262690076126, 47.02201867748818387, -10.88017736071110164 ) ) ;
#47235=CARTESIAN_POINT ( 'NONE',  ( 7.361572987183170547, 17.05059781766745530, 9.846743663894590881 ) ) ;
#47239=CARTESIAN_POINT ( 'NONE',  ( 20.32896413005680714, 30.57879003517447103, -5.963430220938276349 ) ) ;
#47240=VERTEX_POINT ( 'NONE', #31862 ) ;
#47241=CARTESIAN_POINT ( 'NONE',  ( 0.1532563361054082862, 6.217264484334118713, 2.638427012816831674 ) ) ;
#47244=CARTESIAN_POINT ( 'NONE',  ( 20.36894250292379382, 13.67874883491396965, 10.36894250292379205 ) ) ;
#47245=CARTESIAN_POINT ( 'NONE',  ( 17.20831665107776587, 14.13393115100078568, -7.208316651077762316 ) ) ;
#47246=CARTESIAN_POINT ( 'NONE',  ( 4.559911319644449179, 43.89701867748816966, 9.422509992056141925 ) ) ;
#47247=ADVANCED_FACE ( 'NONE', ( #46394 ), #84885, .F. ) ;
#47248=SURFACE_STYLE_FILL_AREA ( #3742 ) ;
#47250=CARTESIAN_POINT ( 'NONE',  ( 12.91533473730993009, 46.60535201082150536, -10.88017736071109987 ) ) ;
#47252=CARTESIAN_POINT ( 'NONE',  ( 17.08211943468705130, 8.470415501580635720, 12.26659068614894998 ) ) ;
#47256=CARTESIAN_POINT ( 'NONE',  ( 22.81628187352647785, 21.41530133659708923, 3.434112377981063169 ) ) ;
#47257=CARTESIAN_POINT ( 'NONE',  ( 10.00000000000000178, 7.258931151000785675, 9.846743663894594434 ) ) ;
#47258=CARTESIAN_POINT ( 'NONE',  ( 20.88017736071110875, 5.772018677488170546, -2.915334737309920765 ) ) ;
#47260=CARTESIAN_POINT ( 'NONE',  ( 17.20831665107776587, 12.88393115100078390, 7.208316651077764980 ) ) ;
#47261=CARTESIAN_POINT ( 'NONE',  ( 19.42250999205614193, 35.14701867748816966, 5.440088680355555262 ) ) ;
#47262=AXIS2_PLACEMENT_3D ( 'NONE', #51423, #65428, #95952 ) ;
#47265=CARTESIAN_POINT ( 'NONE',  ( 22.81628187352647785, 61.41530133659709634, 3.434112377981063169 ) ) ;
#47266=CARTESIAN_POINT ( 'NONE',  ( 7.084665262690076126, 62.02201867748816966, -10.88017736071110164 ) ) ;
#47267=CARTESIAN_POINT ( 'NONE',  ( -42.50369195530268485, 107.9060299417078426, 4.500000000000000888 ) ) ;
#47270=CARTESIAN_POINT ( 'NONE',  ( 0.5774900079438590739, 67.64701867748817676, -5.440088680355550821 ) ) ;
#47271=CARTESIAN_POINT ( 'NONE',  ( 13.43411237798106583, 12.66530133659708746, -12.81628187352647252 ) ) ;
#47273=CARTESIAN_POINT ( 'NONE',  ( 17.20831665107776587, 27.88393115100078390, 7.208316651077764980 ) ) ;
#47274=CARTESIAN_POINT ( 'NONE',  ( 16.40814093676324603, 52.45696800326375353, -11.09922568453594671 ) ) ;
#47275=CARTESIAN_POINT ( 'NONE',  ( 20.36894250292379382, 3.678748834913967869, 10.36894250292379205 ) ) ;
#47276=CARTESIAN_POINT ( 'NONE',  ( 18.52753015748617571, 13.09226448433411960, 4.923371831947298993 ) ) ;
#47277=CARTESIAN_POINT ( 'NONE',  ( -1.099225684535947600, 24.54030133659708923, 6.408140936763237150 ) ) ;
#47280=CARTESIAN_POINT ( 'NONE',  ( 10.00000000000000000, 51.81368534415484106, -10.88017736071110342 ) ) ;
#47281=CARTESIAN_POINT ( 'NONE',  ( 19.84674366389459266, 63.30059781766745886, 2.638427012816836559 ) ) ;
#47282=CARTESIAN_POINT ( 'NONE',  ( 1.472469842513823179, 31.42559781766745530, 4.923371831947296329 ) ) ;
#47283=CARTESIAN_POINT ( 'NONE',  ( 7.361572987183170547, 27.05059781766745175, 9.846743663894590881 ) ) ;
#47284=CARTESIAN_POINT ( 'NONE',  ( -0.8801773607111008646, 8.272018677488171434, 2.915334737309923430 ) ) ;
#47285=ADVANCED_FACE ( 'NONE', ( #41378 ), #23131, .T. ) ;
#47286=CARTESIAN_POINT ( 'NONE',  ( 19.38216949554541557, 22.24863466993041428, -9.382169495545420901 ) ) ;
#47287=CARTESIAN_POINT ( 'NONE',  ( 17.20831665107776587, 24.13393115100078035, -7.208316651077762316 ) ) ;
#47290=CARTESIAN_POINT ( 'NONE',  ( -0.8801773607111009756, 13.06368534415483929, 1.068504757029289695E-15 ) ) ;
#47293=CARTESIAN_POINT ( 'NONE',  ( 19.84674366389459266, 48.71726448433413026, -2.638427012816827677 ) ) ;
#47294=CARTESIAN_POINT ( 'NONE',  ( 7.084665262690076126, 14.10535201082150358, 10.88017736071109987 ) ) ;
#47295=CARTESIAN_POINT ( 'NONE',  ( 15.44008868035555260, 29.73035201082150891, 9.422509992056143702 ) ) ;
#47296=CARTESIAN_POINT ( 'NONE',  ( 20.88017736071110164, 15.35535201082150358, 2.915334737309930979 ) ) ;
#47297=CARTESIAN_POINT ( 'NONE',  ( 5.076628168052704559, 20.17559781766745175, -8.527530157486179263 ) ) ;
#47298=CARTESIAN_POINT ( 'NONE',  ( 10.00000000000000000, 44.75893115100078745, -9.846743663894594434 ) ) ;
#47303=FILL_AREA_STYLE_COLOUR ( '', #66565 ) ;
#47305=CARTESIAN_POINT ( 'NONE',  ( -2.266590686148945544, 21.38708216824730357, -7.082119434687050408 ) ) ;
#47306=CARTESIAN_POINT ( 'NONE',  ( 12.63842701281683034, 37.46726448433411605, 9.846743663894596210 ) ) ;
#47307=CARTESIAN_POINT ( 'NONE',  ( 1.274849032794199255, 23.57228050351030646, 6.499999999999850786 ) ) ;
#47310=CARTESIAN_POINT ( 'NONE',  ( -4.164238869374098151, 51.59541550158063217, -3.795296366450310543 ) ) ;
#47311=CARTESIAN_POINT ( 'NONE',  ( 5.076628168052703671, 16.84226448433411960, 8.527530157486179263 ) ) ;
#47313=CARTESIAN_POINT ( 'NONE',  ( 17.96484262340118221, 41.18868534415484106, -7.964842623401177768 ) ) ;
#47316=CARTESIAN_POINT ( 'NONE',  ( 12.91533473730992121, 19.52201867748816611, 10.88017736071110164 ) ) ;
#47317=CARTESIAN_POINT ( 'NONE',  ( 19.38216949554541202, 45.99863466993041072, 9.382169495545424454 ) ) ;
#47318=CARTESIAN_POINT ( 'NONE',  ( 0.6178305044545818747, -1.501365330069579951, -9.382169495545419124 ) ) ;
#47319=CARTESIAN_POINT ( 'NONE',  ( 7.361572987183170547, 12.05059781766744997, 9.846743663894590881 ) ) ;
#47324=CARTESIAN_POINT ( 'NONE',  ( -4.164238869374099927, 52.01208216824729647, 3.795296366450308767 ) ) ;
#47325=CARTESIAN_POINT ( 'NONE',  ( 2.917880565312950480, 15.97041550158063217, -12.26659068614894821 ) ) ;
#47326=CARTESIAN_POINT ( 'NONE',  ( -0.8801773607110991993, 17.85535201082150536, -2.915334737309923874 ) ) ;
#47327=CARTESIAN_POINT ( 'NONE',  ( 10.00000000000000178, 34.31368534415484106, 10.88017736071110342 ) ) ;
#47330=CARTESIAN_POINT ( 'NONE',  ( 7.084665262690076126, 62.02201867748816966, -10.88017736071110164 ) ) ;
#47331=CARTESIAN_POINT ( 'NONE',  ( 17.20831665107776587, 24.13393115100078035, -7.208316651077762316 ) ) ;
#47332=CARTESIAN_POINT ( 'NONE',  ( 1.274849032794294290, 63.57228050351031357, 6.499999999999979572 ) ) ;
#47334=CARTESIAN_POINT ( 'NONE',  ( 10.00000000000000178, 12.25893115100078568, 9.846743663894594434 ) ) ;
#47335=CARTESIAN_POINT ( 'NONE',  ( 10.00000000000000000, 39.75893115100078745, -9.846743663894594434 ) ) ;
#47336=CARTESIAN_POINT ( 'NONE',  ( -0.8801773607111008646, 13.27201867748817143, 2.915334737309923430 ) ) ;
#47338=UNCERTAINTY_MEASURE_WITH_UNIT (LENGTH_MEASURE( 1.000000000000000082E-05 ), #377, 'distance_accuracy_value', 'NONE');
#47339=CARTESIAN_POINT ( 'NONE',  ( 16.40814093676323893, 30.79030133659708923, 11.09922568453595026 ) ) ;
#47340=CARTESIAN_POINT ( 'NONE',  ( 7.084665262690076126, 52.02201867748816255, -10.88017736071110164 ) ) ;
#47341=CARTESIAN_POINT ( 'NONE',  ( 24.16423886937410614, 49.51208216824730357, -3.795296366450302550 ) ) ;
#47342=CARTESIAN_POINT ( 'NONE',  ( 12.63842701281683034, 7.467264484334118713, 9.846743663894596210 ) ) ;
#47343=CARTESIAN_POINT ( 'NONE',  ( 2.603489959281613420, 35.43575266056827644, -6.500000000000031086 ) ) ;
#47344=CARTESIAN_POINT ( 'NONE',  ( 2.791683348922237240, 50.38393115100078035, -7.208316651077763204 ) ) ;
#47345=CARTESIAN_POINT ( 'NONE',  ( 10.00000000000000000, 29.75893115100078745, -9.846743663894594434 ) ) ;
#47346=CARTESIAN_POINT ( 'NONE',  ( -0.3689425029237898834, 6.178748834913968757, -10.36894250292378850 ) ) ;
#47347=( BOUNDED_CURVE ( )  B_SPLINE_CURVE ( 2, ( #54939, #15505, #23981, #76962, #60970, #61462, #70458, #32444, #519 ),
 .UNSPECIFIED., .F., .F. ) 
 B_SPLINE_CURVE_WITH_KNOTS ( ( 3, 2, 2, 2, 3 ),
 ( 0.4382284501891250961, 0.4404761904761904656, 0.4464285714285714524, 0.4523809523809523836, 0.4546286926680177531 ),
 .UNSPECIFIED. ) 
 CURVE ( )  GEOMETRIC_REPRESENTATION_ITEM ( )  RATIONAL_B_SPLINE_CURVE ( ( 0.9839835555609424134, 0.9871328979762477029, 1.000000000000000000, 0.9659258262890683122, 1.000000000000000000, 0.9659258262890683122, 1.000000000000000000, 0.9871328979762477029, 0.9839835555609424134 ) ) 
 REPRESENTATION_ITEM ( '' )  );
#47348=CARTESIAN_POINT ( 'NONE',  ( 10.00000000000000178, 23.05374883491397142, 14.16423886937410082 ) ) ;
#47349=CARTESIAN_POINT ( 'NONE',  ( 2.035157376598824452, 43.68868534415484106, 7.964842623401179544 ) ) ;
#47351=CARTESIAN_POINT ( 'NONE',  ( 15.44008868035555793, 11.39701867748817143, -9.422509992056140149 ) ) ;
#47352=CARTESIAN_POINT ( 'NONE',  ( 7.084665262690076126, 44.10535201082151247, 10.88017736071109987 ) ) ;
#47353=CARTESIAN_POINT ( 'NONE',  ( 2.035157376598824452, 28.68868534415484106, 7.964842623401179544 ) ) ;
#47356=CARTESIAN_POINT ( 'NONE',  ( 4.559911319644449179, 43.89701867748816966, 9.422509992056141925 ) ) ;
#47358=CARTESIAN_POINT ( 'NONE',  ( 10.00000000000000000, 62.87363466993042493, -12.81628187352647608 ) ) ;
#47361=CARTESIAN_POINT ( 'NONE',  ( 7.084665262690076126, 57.02201867748817676, -10.88017736071110164 ) ) ;
#47364=CARTESIAN_POINT ( 'NONE',  ( 10.00000000000000178, 54.31368534415484106, 10.88017736071110342 ) ) ;
#47365=CARTESIAN_POINT ( 'NONE',  ( -0.8801773607111009756, 3.063685344154837509, 1.068504757029289695E-15 ) ) ;
#47367=CARTESIAN_POINT ( 'NONE',  ( 18.72515096720571393, 41.07228050351032778, -6.499999999999974243 ) ) ;
#47369=CARTESIAN_POINT ( 'NONE',  ( -0.3689425029237898834, 61.17874883491396076, -10.36894250292378850 ) ) ;
#47370=CARTESIAN_POINT ( 'NONE',  ( 17.96484262340118221, 64.93868534415483396, 7.964842623401181321 ) ) ;
#47371=CARTESIAN_POINT ( 'NONE',  ( -4.164238869374099039, 6.803748834913967869, 8.674139862899312516E-16 ) ) ;
#47373=CARTESIAN_POINT ( 'NONE',  ( 20.88017736071110875, 15.77201867748817143, -2.915334737309920765 ) ) ;
#47374=CARTESIAN_POINT ( 'NONE',  ( 0.1532563361054083140, 51.00893115100078745, 1.131784320476157264E-15 ) ) ;
#47376=CARTESIAN_POINT ( 'NONE',  ( 12.63842701281683922, 49.55059781766744464, -9.846743663894590881 ) ) ;
#47377=CARTESIAN_POINT ( 'NONE',  ( -0.8801773607111008646, 43.27201867748817676, 2.915334737309923430 ) ) ;
#47378=CARTESIAN_POINT ( 'NONE',  ( 0.1532563361054082862, 36.21726448433410894, 2.638427012816831674 ) ) ;
#47379=SURFACE_STYLE_FILL_AREA ( #94359 ) ;
#47380=CARTESIAN_POINT ( 'NONE',  ( 20.88017736071110519, 65.56368534415483396, 2.639326808657452039E-16 ) ) ;
#47381=CARTESIAN_POINT ( 'NONE',  ( 12.91533473730992121, 44.52201867748816966, 10.88017736071110164 ) ) ;
#47382=CARTESIAN_POINT ( 'NONE',  ( -4.164238869374099927, 62.01208216824728936, 3.795296366450308767 ) ) ;
#47383=CARTESIAN_POINT ( 'NONE',  ( 19.38216949554541202, 25.99863466993042138, 9.382169495545424454 ) ) ;
#47384=CARTESIAN_POINT ( 'NONE',  ( 6.000000000000000000, 61.00000000000000711, 5.000000000000000000 ) ) ;
#47385=ORIENTED_EDGE ( 'NONE', *, *, #83431, .F. ) ;
#47386=CARTESIAN_POINT ( 'NONE',  ( -2.816281873526473856, 29.12363466993041783, 9.499525473075851096E-16 ) ) ;
#47387=CARTESIAN_POINT ( 'NONE',  ( 7.084665262690076126, 24.10535201082150181, 10.88017736071109987 ) ) ;
#47388=CIRCLE ( 'NONE', #72947, 18.53834841531100608 ) ;
#47389=EDGE_CURVE ( 'NONE', #25008, #9131, #9905, .T. ) ;
#47391=CARTESIAN_POINT ( 'NONE',  ( 7.084665262690076126, 69.10535201082151957, 10.88017736071109987 ) ) ;
#47392=CARTESIAN_POINT ( 'NONE',  ( 5.076628168052704559, 50.17559781766745886, -8.527530157486179263 ) ) ;
#47393=CARTESIAN_POINT ( 'NONE',  ( 0.1532563361054100626, 10.80059781766745175, -2.638427012816831230 ) ) ;
#47394=CARTESIAN_POINT ( 'NONE',  ( 12.63842701281683922, 39.55059781766744464, -9.846743663894590881 ) ) ;
#47397=CARTESIAN_POINT ( 'NONE',  ( 19.84674366389459621, 23.50893115100078390, 7.409399052514197653E-17 ) ) ;
#47398=CARTESIAN_POINT ( 'NONE',  ( 20.04068437667226732, 54.71974360917722890, 6.396802510829642685 ) ) ;
#47399=CARTESIAN_POINT ( 'NONE',  ( 5.500000000000000000, 11.00000000000000000, 6.000000000000000000 ) ) ;
#47400=CARTESIAN_POINT ( 'NONE',  ( 1.472469842513823179, 31.42559781766745530, 4.923371831947296329 ) ) ;
#47404=CARTESIAN_POINT ( 'NONE',  ( 5.076628168052704559, 50.17559781766745886, -8.527530157486179263 ) ) ;
#47405=VERTEX_POINT ( 'NONE', #16292 ) ;
#47407=CARTESIAN_POINT ( 'NONE',  ( 21.09922568453594849, 21.20696800326375353, 6.408140936763242479 ) ) ;
#47411=CARTESIAN_POINT ( 'NONE',  ( -0.3689425029237898834, 41.17874883491397497, -10.36894250292378850 ) ) ;
#47413=CARTESIAN_POINT ( 'NONE',  ( 12.63842701281683922, 14.55059781766744997, -9.846743663894590881 ) ) ;
#47414=( LENGTH_UNIT ( ) NAMED_UNIT ( * ) SI_UNIT ( .MILLI., .METRE. ) );
#47415=CARTESIAN_POINT ( 'NONE',  ( 20.00000000000000711, 98.59912998021083297, 4.500000000000000888 ) ) ;
#47416=CARTESIAN_POINT ( 'NONE',  ( 24.16423886937409904, 44.09541550158063927, 3.795296366450317205 ) ) ;
#47417=CARTESIAN_POINT ( 'NONE',  ( 14.92337183194729988, 59.34226448433412315, -8.527530157486177487 ) ) ;
#47419=CARTESIAN_POINT ( 'NONE',  ( 13.79529636645031943, 60.34541550158063927, -14.16423886937409904 ) ) ;
#47420=CARTESIAN_POINT ( 'NONE',  ( -0.3689425029237881626, 22.42874883491397142, 10.36894250292379027 ) ) ;
#47421=CARTESIAN_POINT ( 'NONE',  ( 10.00000000000000178, 28.05374883491396787, 14.16423886937410082 ) ) ;
#47422=CARTESIAN_POINT ( 'NONE',  ( -44.79809994011756658, 105.6827849507685926, -4.824119973700185859 ) ) ;
#47426=CARTESIAN_POINT ( 'NONE',  ( 12.63842701281683922, 49.55059781766744464, -9.846743663894590881 ) ) ;
#47428=CARTESIAN_POINT ( 'NONE',  ( 2.035157376598824452, 33.68868534415484106, 7.964842623401179544 ) ) ;
#47431=CARTESIAN_POINT ( 'NONE',  ( 5.076628168052704559, 35.17559781766745175, -8.527530157486179263 ) ) ;
#47433=CARTESIAN_POINT ( 'NONE',  ( 16.40814093676324603, 52.45696800326375353, -11.09922568453594671 ) ) ;
#47435=CIRCLE ( 'NONE', #64974, 0.4999999999999995559 ) ;
#47436=CARTESIAN_POINT ( 'NONE',  ( 7.361572987183169658, 44.96726448433412315, -9.846743663894592657 ) ) ;
#47437=CARTESIAN_POINT ( 'NONE',  ( 0.1532563361054100626, 60.80059781766744464, -2.638427012816831230 ) ) ;
#47440=CARTESIAN_POINT ( 'NONE',  ( 6.204703633549690345, 10.76208216824729824, -14.16423886937410259 ) ) ;
#47441=DIRECTION ( 'NONE',  ( 0.000000000000000000, 1.000000000000000000, -0.000000000000000000 ) ) ;
#47444=CARTESIAN_POINT ( 'NONE',  ( -2.266590686148945544, 67.22041550158063217, 7.082119434687048631 ) ) ;
#47445=CARTESIAN_POINT ( 'NONE',  ( -2.816281873526473856, 14.12363466993041961, 9.499525473075851096E-16 ) ) ;
#47446=CARTESIAN_POINT ( 'NONE',  ( 0.5774900079438590739, 62.64701867748817676, -5.440088680355550821 ) ) ;
#47449=CARTESIAN_POINT ( 'NONE',  ( -46.94000000000001194, 102.4380508258080198, -6.413016458746108484 ) ) ;
#47451=CARTESIAN_POINT ( 'NONE',  ( -2.266590686148945544, 56.38708216824731068, -7.082119434687050408 ) ) ;
#47452=CARTESIAN_POINT ( 'NONE',  ( 6.000000000000000000, 10.49999999999999822, 6.000000000000000000 ) ) ;
#47453=CARTESIAN_POINT ( 'NONE',  ( 2.035157376598822676, 27.43868534415483396, -7.964842623401177768 ) ) ;
#47454=CARTESIAN_POINT ( 'NONE',  ( 20.88017736071110875, 35.77201867748816966, -2.915334737309920765 ) ) ;
#47455=CARTESIAN_POINT ( 'NONE',  ( 6.565887622018943937, 3.081968003263753531, -12.81628187352647608 ) ) ;
#47456=CARTESIAN_POINT ( 'NONE',  ( 17.20831665107776587, 57.88393115100078745, 7.208316651077764980 ) ) ;
#47457=FACE_OUTER_BOUND ( 'NONE', #55563, .T. ) ;
#47459=CARTESIAN_POINT ( 'NONE',  ( 20.88017736071110519, 35.56368534415484106, 2.639326808657452039E-16 ) ) ;
#47460=CARTESIAN_POINT ( 'NONE',  ( 21.09922568453594849, 26.20696800326375353, 6.408140936763242479 ) ) ;
#47462=CARTESIAN_POINT ( 'NONE',  ( 17.20831665107776587, 64.13393115100079456, -7.208316651077762316 ) ) ;
#47463=CARTESIAN_POINT ( 'NONE',  ( 20.88017736071110519, 45.56368534415484106, 2.639326808657452039E-16 ) ) ;
#47464=CARTESIAN_POINT ( 'NONE',  ( 18.52753015748617571, 18.09226448433411960, 4.923371831947298993 ) ) ;
#47466=CARTESIAN_POINT ( 'NONE',  ( -2.816281873526473856, 29.33196800326376064, 3.434112377981055619 ) ) ;
#47467=CARTESIAN_POINT ( 'NONE',  ( 19.42250999205614548, 60.98035201082151247, -5.440088680355545492 ) ) ;
#47469=DIRECTION ( 'NONE',  ( 6.608470384673550777E-17, 1.000000000000000000, -0.000000000000000000 ) ) ;
#47470=CARTESIAN_POINT ( 'NONE',  ( 21.09922568453595559, 62.04030133659709634, -6.408140936763230044 ) ) ;
#47474=CARTESIAN_POINT ( 'NONE',  ( 4.559911319644449179, 3.897018677488170990, 9.422509992056141925 ) ) ;
#47475=CARTESIAN_POINT ( 'NONE',  ( 10.00000000000000000, 47.87363466993042493, -12.81628187352647608 ) ) ;
#47476=CARTESIAN_POINT ( 'NONE',  ( 13.79529636645031943, 10.34541550158063394, -14.16423886937409904 ) ) ;
#47477=CARTESIAN_POINT ( 'NONE',  ( 17.20831665107776587, 19.13393115100078035, -7.208316651077762316 ) ) ;
#47478=CARTESIAN_POINT ( 'NONE',  ( 2.035157376598822676, 2.438685344154837953, -7.964842623401177768 ) ) ;
#47479=CARTESIAN_POINT ( 'NONE',  ( 18.52753015748618282, 13.92559781766745175, -4.923371831947291888 ) ) ;
#47480=CARTESIAN_POINT ( 'NONE',  ( 20.36894250292379738, 54.92874883491396076, -10.36894250292379027 ) ) ;
#47481=ORIENTED_EDGE ( 'NONE', *, *, #38881, .F. ) ;
#47482=CARTESIAN_POINT ( 'NONE',  ( 4.559911319644449179, 2.230352010821504471, -9.422509992056141925 ) ) ;
#47483=CARTESIAN_POINT ( 'NONE',  ( 4.559911319644449179, 12.23035201082150536, -9.422509992056141925 ) ) ;
#47486=CARTESIAN_POINT ( 'NONE',  ( 12.91533473730992121, 9.522018677488171434, 10.88017736071110164 ) ) ;
#47487=CARTESIAN_POINT ( 'NONE',  ( 17.96484262340118221, 6.188685344154837509, -7.964842623401177768 ) ) ;
#47488=CARTESIAN_POINT ( 'NONE',  ( 1.472469842513823179, 46.42559781766745175, 4.923371831947296329 ) ) ;
#47489=CARTESIAN_POINT ( 'NONE',  ( 3.591859063236761518, 54.95696800326376064, 11.09922568453594849 ) ) ;
#47490=SURFACE_STYLE_FILL_AREA ( #54983 ) ;
#47492=CARTESIAN_POINT ( 'NONE',  ( 13.79529636645031943, 20.34541550158063572, -14.16423886937409904 ) ) ;
#47493=CARTESIAN_POINT ( 'NONE',  ( 7.084665262690076126, 29.10535201082150181, 10.88017736071109987 ) ) ;
#47494=CARTESIAN_POINT ( 'NONE',  ( 2.035157376598822676, 2.438685344154838397, -7.964842623401177768 ) ) ;
#47495=CARTESIAN_POINT ( 'NONE',  ( 5.076628168052703671, 61.84226448433412315, 8.527530157486179263 ) ) ;
#47497=CARTESIAN_POINT ( 'NONE',  ( 1.472469842513823179, 41.42559781766745886, 4.923371831947296329 ) ) ;
#47498=DIRECTION ( 'NONE',  ( 0.000000000000000000, -1.000000000000000000, 0.000000000000000000 ) ) ;
#47499=CARTESIAN_POINT ( 'NONE',  ( 7.361572987183169658, 4.967264484334119601, -9.846743663894592657 ) ) ;
#47503=SURFACE_SIDE_STYLE ('',( #54996 ) ) ;
#47504=CARTESIAN_POINT ( 'NONE',  ( 2.791683348922237240, 0.3839311510007847872, -7.208316651077763204 ) ) ;
#47506=CARTESIAN_POINT ( 'NONE',  ( 13.43411237798105340, 0.5819680032637533085, 12.81628187352647963 ) ) ;
#47507=CARTESIAN_POINT ( 'NONE',  ( 12.91533473730993009, 41.60535201082149825, -10.88017736071109987 ) ) ;
#47508=CARTESIAN_POINT ( 'NONE',  ( 10.00000000000000178, 9.313685344154839285, 10.88017736071110342 ) ) ;
#47509=CARTESIAN_POINT ( 'NONE',  ( 21.09922568453595559, 42.04030133659708213, -6.408140936763230044 ) ) ;
#47510=CARTESIAN_POINT ( 'NONE',  ( -4.164238869374099039, 21.80374883491396787, 8.674139862899312516E-16 ) ) ;
#47513=VECTOR ( 'NONE', #29020, 1000.000000000000000 ) ;
#47515=CARTESIAN_POINT ( 'NONE',  ( 22.81628187352648496, 46.83196800326376064, -3.434112377981050290 ) ) ;
#47517=CARTESIAN_POINT ( 'NONE',  ( 5.076628168052703671, 51.84226448433412315, 8.527530157486179263 ) ) ;
#47518=CARTESIAN_POINT ( 'NONE',  ( 12.91533473730993009, 21.60535201082150536, -10.88017736071109987 ) ) ;
#47519=CARTESIAN_POINT ( 'NONE',  ( 10.00000000000000178, 34.31368534415484106, 10.88017736071110342 ) ) ;
#47521=CARTESIAN_POINT ( 'NONE',  ( 5.076628168052704559, 10.17559781766745175, -8.527530157486179263 ) ) ;
#47522=CARTESIAN_POINT ( 'NONE',  ( 10.00000000000000178, 69.31368534415484817, 10.88017736071110342 ) ) ;
#47523=CARTESIAN_POINT ( 'NONE',  ( -0.1503990784575359729, 18.10158574516642460, 6.262539305110062848 ) ) ;
#47525=CARTESIAN_POINT ( 'NONE',  ( 12.63842701281683922, 9.550597817667449974, -9.846743663894590881 ) ) ;
#47527=CARTESIAN_POINT ( 'NONE',  ( 19.42250999205614193, 65.14701867748817676, 5.440088680355555262 ) ) ;
#47528=CARTESIAN_POINT ( 'NONE',  ( 18.72515096720583827, 65.05509018479936856, 6.499999999999810818 ) ) ;
#47529=CARTESIAN_POINT ( 'NONE',  ( 0.5774900079438607392, 38.48035201082150536, 5.440088680355550821 ) ) ;
#47530=CARTESIAN_POINT ( 'NONE',  ( 19.42250999205614193, 65.14701867748817676, 5.440088680355555262 ) ) ;
#47531=CARTESIAN_POINT ( 'NONE',  ( 17.20831665107776587, 4.133931151000785675, -7.208316651077762316 ) ) ;
#47536=CARTESIAN_POINT ( 'NONE',  ( 17.20831665107776587, 59.13393115100078745, -7.208316651077762316 ) ) ;
#47537=ORIENTED_EDGE ( 'NONE', *, *, #27402, .F. ) ;
#47540=CARTESIAN_POINT ( 'NONE',  ( -4.164238869374098151, 6.595415501580634832, -3.795296366450310543 ) ) ;
#47542=CARTESIAN_POINT ( 'NONE',  ( -2.816281873526473856, 54.12363466993041783, 9.499525473075851096E-16 ) ) ;
#47543=CARTESIAN_POINT ( 'NONE',  ( -4.164238869374099039, 1.803748834913967647, 8.674139862899312516E-16 ) ) ;
#47544=CARTESIAN_POINT ( 'NONE',  ( 24.16423886937409904, 19.09541550158063927, 3.795296366450317205 ) ) ;
#47545=CARTESIAN_POINT ( 'NONE',  ( 0.1143410931637208749, 45.21691075486302935, 6.480892540919845679 ) ) ;
#47546=DIRECTION ( 'NONE',  ( -0.000000000000000000, -0.000000000000000000, -1.000000000000000000 ) ) ;
#47547=CARTESIAN_POINT ( 'NONE',  ( 10.00000000000000178, 59.31368534415484106, 10.88017736071110342 ) ) ;
#47548=CARTESIAN_POINT ( 'NONE',  ( 4.559911319644449179, 17.23035201082150536, -9.422509992056141925 ) ) ;
#47551=CARTESIAN_POINT ( 'NONE',  ( 18.52753015748618282, 8.925597817667451750, -4.923371831947291888 ) ) ;
#47552=CARTESIAN_POINT ( 'NONE',  ( 7.361572987183170547, 7.050597817667451750, 9.846743663894590881 ) ) ;
#47553=CARTESIAN_POINT ( 'NONE',  ( 22.81628187352648496, 31.83196800326375353, -3.434112377981050290 ) ) ;
#47554=CARTESIAN_POINT ( 'NONE',  ( 17.20831665107776587, 42.88393115100077324, 7.208316651077764980 ) ) ;
#47556=CARTESIAN_POINT ( 'NONE',  ( -2.816281873526473856, 9.331968003263753531, 3.434112377981055619 ) ) ;
#47559=CARTESIAN_POINT ( 'NONE',  ( 14.92337183194729988, 29.34226448433411960, -8.527530157486177487 ) ) ;
#47560=CARTESIAN_POINT ( 'NONE',  ( 0.1532563361054082862, 1.217264484334117824, 2.638427012816831674 ) ) ;
#47563=CARTESIAN_POINT ( 'NONE',  ( 2.035157376598822676, 32.43868534415483396, -7.964842623401177768 ) ) ;
#47564=CARTESIAN_POINT ( 'NONE',  ( -2.266590686148945544, 36.38708216824730357, -7.082119434687050408 ) ) ;
#47565=CARTESIAN_POINT ( 'NONE',  ( 5.076628168052704559, 35.17559781766745175, -8.527530157486179263 ) ) ;
#47566=CARTESIAN_POINT ( 'NONE',  ( 12.63842701281683034, 17.46726448433411250, 9.846743663894596210 ) ) ;
#47567=CARTESIAN_POINT ( 'NONE',  ( 3.591859063236763294, 53.29030133659708923, -11.09922568453595026 ) ) ;
#47569=CARTESIAN_POINT ( 'NONE',  ( 20.88017736071110164, 30.35535201082151247, 2.915334737309930979 ) ) ;
#47570=EDGE_CURVE ( 'NONE', #36257, #22305, #55767, .T. ) ;
#47573=CARTESIAN_POINT ( 'NONE',  ( 6.565887622018943937, 28.08196800326375353, -12.81628187352647608 ) ) ;
#47574=CARTESIAN_POINT ( 'NONE',  ( 18.52753015748618282, 43.92559781766745175, -4.923371831947291888 ) ) ;
#47576=CARTESIAN_POINT ( 'NONE',  ( 19.38216949554541202, 45.99863466993041072, 9.382169495545424454 ) ) ;
#47578=CARTESIAN_POINT ( 'NONE',  ( 15.44008868035555260, 59.73035201082151247, 9.422509992056143702 ) ) ;
#47580=STYLED_ITEM ( 'NONE', ( #56155 ), #57825 ) ;
#47584=AXIS2_PLACEMENT_3D ( 'NONE', #2761, #78230, #16758 ) ;
#47585=CARTESIAN_POINT ( 'NONE',  ( -0.8801773607110991993, 52.85535201082151247, -2.915334737309923874 ) ) ;
#47586=CARTESIAN_POINT ( 'NONE',  ( 12.91533473730992121, 54.52201867748816255, 10.88017736071110164 ) ) ;
#47589=CARTESIAN_POINT ( 'NONE',  ( 20.88017736071110519, 10.56368534415483929, 2.639326808657452039E-16 ) ) ;
#47590=CARTESIAN_POINT ( 'NONE',  ( 1.472469842513823179, 65.59226448433412315, -4.923371831947296329 ) ) ;
#47591=CARTESIAN_POINT ( 'NONE',  ( 17.96484262340118221, 19.93868534415484106, 7.964842623401181321 ) ) ;
#47592=CARTESIAN_POINT ( 'NONE',  ( 17.39651004071842522, 24.08210964143329491, -6.499999999999992895 ) ) ;
#47593=CARTESIAN_POINT ( 'NONE',  ( -0.1503990784575328643, 70.00000000000000000, 6.262539305110068177 ) ) ;
#47594=CARTESIAN_POINT ( 'NONE',  ( -1.099225684535947600, 24.54030133659708923, 6.408140936763237150 ) ) ;
#47596=CARTESIAN_POINT ( 'NONE',  ( 19.42250999205614193, 35.14701867748816966, 5.440088680355555262 ) ) ;
#47597=CARTESIAN_POINT ( 'NONE',  ( 14.92337183194729633, 42.67559781766745886, 8.527530157486181039 ) ) ;
#47598=CARTESIAN_POINT ( 'NONE',  ( 6.565887622018943937, 13.08196800326374998, -12.81628187352647608 ) ) ;
#47600=CARTESIAN_POINT ( 'NONE',  ( 19.42250999205614193, 15.14701867748817143, 5.440088680355555262 ) ) ;
#47601=CARTESIAN_POINT ( 'NONE',  ( 20.88017736071110164, 45.35535201082149115, 2.915334737309930979 ) ) ;
#47602=CARTESIAN_POINT ( 'NONE',  ( 20.36894250292379738, 44.92874883491396787, -10.36894250292379027 ) ) ;
#47603=CARTESIAN_POINT ( 'NONE',  ( 1.472469842513823179, 35.59226448433412315, -4.923371831947296329 ) ) ;
#47604=CARTESIAN_POINT ( 'NONE',  ( 4.559911319644449179, 62.23035201082150536, -9.422509992056141925 ) ) ;
#47606=CARTESIAN_POINT ( 'NONE',  ( -4.164238869374099927, 12.01208216824730357, 3.795296366450308767 ) ) ;
#47607=B_SPLINE_CURVE_WITH_KNOTS ( 'NONE', 3,
 ( #88517, #81016, #12517, #5027, #35513, #43502 ),
 .UNSPECIFIED., .F., .F.,
 ( 4, 2, 4 ),
 ( 0.000000000000000000, 0.0002565770811490877411, 0.0005131541622981754822 ),
 .UNSPECIFIED. ) ;
#47608=CARTESIAN_POINT ( 'NONE',  ( 18.18329248733322245, 12.60290668512019963, 6.499999999999997335 ) ) ;
#47610=CARTESIAN_POINT ( 'NONE',  ( 2.917880565312950480, 30.97041550158063572, -12.26659068614894821 ) ) ;
#47611=CARTESIAN_POINT ( 'NONE',  ( 24.16423886937410614, 34.51208216824731068, -3.795296366450302550 ) ) ;
#47612=CARTESIAN_POINT ( 'NONE',  ( 14.92337183194729988, 9.342264484334119601, -8.527530157486177487 ) ) ;
#47613=CARTESIAN_POINT ( 'NONE',  ( 6.565887622018943937, 20.16530133659708213, 12.81628187352647430 ) ) ;
#47614=CARTESIAN_POINT ( 'NONE',  ( 2.791683348922240793, 66.63393115100079456, 7.208316651077764092 ) ) ;
#47615=CARTESIAN_POINT ( 'NONE',  ( 19.72487221294571569, 52.80223176428831522, -6.499999999999990230 ) ) ;
#47616=CARTESIAN_POINT ( 'NONE',  ( 2.035157376598822676, 57.43868534415484106, -7.964842623401177768 ) ) ;
#47617=CARTESIAN_POINT ( 'NONE',  ( 0.6178305044545818747, 38.49863466993042493, -9.382169495545419124 ) ) ;
#47618=CARTESIAN_POINT ( 'NONE',  ( 10.00000000000000000, 30.55374883491397142, -14.16423886937410082 ) ) ;
#47619=CARTESIAN_POINT ( 'NONE',  ( 20.88017736071110875, 25.77201867748816966, -2.915334737309920765 ) ) ;
#47620=FACE_OUTER_BOUND ( 'NONE', #22727, .T. ) ;
#47621=CARTESIAN_POINT ( 'NONE',  ( 5.076628168052703671, 1.842264484334118047, 8.527530157486179263 ) ) ;
#47628=CARTESIAN_POINT ( 'NONE',  ( -2.266590686148945544, 1.387082168247301128, -7.082119434687050408 ) ) ;
#47629=CARTESIAN_POINT ( 'NONE',  ( 0.5774900079438607392, 8.480352010821505360, 5.440088680355550821 ) ) ;
#47630=CARTESIAN_POINT ( 'NONE',  ( 12.91533473730993009, 11.60535201082150714, -10.88017736071109987 ) ) ;
#47631=CARTESIAN_POINT ( 'NONE',  ( 1.472469842513823179, 30.59226448433411960, -4.923371831947296329 ) ) ;
#47632=CARTESIAN_POINT ( 'NONE',  ( -1.099225684535947600, -1.293031996736246469, -6.408140936763238038 ) ) ;
#47637=CARTESIAN_POINT ( 'NONE',  ( 3.591859063236763294, 3.290301336597087012, -11.09922568453595026 ) ) ;
#47639=CARTESIAN_POINT ( 'NONE',  ( 2.917880565312950480, 45.97041550158063927, -12.26659068614894821 ) ) ;
#47641=CARTESIAN_POINT ( 'NONE',  ( 2.917880565312948704, 62.63708216824730357, 12.26659068614894643 ) ) ;
#47643=CARTESIAN_POINT ( 'NONE',  ( -0.8801773607111009756, 18.06368534415484106, 1.068504757029289695E-15 ) ) ;
#47644=STYLED_ITEM ( 'NONE', ( #22931 ), #13115 ) ;
#47645=CARTESIAN_POINT ( 'NONE',  ( 2.035157376598822676, 42.43868534415483396, -7.964842623401177768 ) ) ;
#47646=CARTESIAN_POINT ( 'NONE',  ( 19.84674366389459266, 58.71726448433411605, -2.638427012816827677 ) ) ;
#47647=CARTESIAN_POINT ( 'NONE',  ( 17.96484262340118221, 39.93868534415484106, 7.964842623401181321 ) ) ;
#47648=CARTESIAN_POINT ( 'NONE',  ( 20.88017736071110875, 65.77201867748817676, -2.915334737309920765 ) ) ;
#47649=CARTESIAN_POINT ( 'NONE',  ( 7.084665262690076126, 34.10535201082151247, 10.88017736071109987 ) ) ;
#47651=CIRCLE ( 'NONE', #46087, 0.5000000000000004441 ) ;
#47653=ADVANCED_FACE ( 'NONE', ( #18751 ), #95431, .T. ) ;
#47654=CARTESIAN_POINT ( 'NONE',  ( 1.472469842513823179, 5.592264484334118713, -4.923371831947296329 ) ) ;
#47656=ORIENTED_EDGE ( 'NONE', *, *, #63110, .T. ) ;
#47658=CARTESIAN_POINT ( 'NONE',  ( 1.472469842513823179, 40.59226448433411605, -4.923371831947296329 ) ) ;
#47660=EDGE_CURVE ( 'NONE', #1911, #14086, #72608, .T. ) ;
#47665=CARTESIAN_POINT ( 'NONE',  ( 17.20831665107776587, 54.13393115100079456, -7.208316651077762316 ) ) ;
#47666=CARTESIAN_POINT ( 'NONE',  ( 24.16423886937409904, 54.09541550158063217, 3.795296366450317205 ) ) ;
#47667=CARTESIAN_POINT ( 'NONE',  ( 1.472469842513823179, 65.59226448433412315, -4.923371831947296329 ) ) ;
#47670=CARTESIAN_POINT ( 'NONE',  ( 1.472469842513823179, 21.42559781766745175, 4.923371831947296329 ) ) ;
#47671=CARTESIAN_POINT ( 'NONE',  ( -2.816281873526471635, 48.91530133659708213, -3.434112377981056508 ) ) ;
#47672=CARTESIAN_POINT ( 'NONE',  ( 12.63842701281683922, 64.55059781766745175, -9.846743663894590881 ) ) ;
#47673=CARTESIAN_POINT ( 'NONE',  ( -0.8801773607111009756, 63.06368534415484106, 1.068504757029289695E-15 ) ) ;
#47674=CARTESIAN_POINT ( 'NONE',  ( 5.500000000000000000, 11.00000000000000000, 6.500000000000000888 ) ) ;
#47677=CARTESIAN_POINT ( 'NONE',  ( 6.204703633549690345, 57.84541550158063927, 14.16423886937410082 ) ) ;
#47678=CARTESIAN_POINT ( 'NONE',  ( 2.603489959281613420, 65.43575266056828355, -6.500000000000031086 ) ) ;
#47679=CARTESIAN_POINT ( 'NONE',  ( 10.00000000000000178, 34.31368534415484106, 10.88017736071110342 ) ) ;
#47680=CARTESIAN_POINT ( 'NONE',  ( -2.816281873526473856, 14.12363466993041961, 9.499525473075851096E-16 ) ) ;
#47681=CARTESIAN_POINT ( 'NONE',  ( 7.084665262690076126, 52.02201867748816255, -10.88017736071110164 ) ) ;
#47684=EDGE_CURVE ( 'NONE', #41376, #98547, #10610, .T. ) ;
#47686=CARTESIAN_POINT ( 'NONE',  ( 7.361572987183170547, 52.05059781766745175, 9.846743663894590881 ) ) ;
#47687=CARTESIAN_POINT ( 'NONE',  ( 17.20831665107776587, 2.883931151000785231, 7.208316651077764980 ) ) ;
#47689=CARTESIAN_POINT ( 'NONE',  ( -1.099225684535947600, 3.706968003263753531, -6.408140936763238038 ) ) ;
#47690=CARTESIAN_POINT ( 'NONE',  ( 7.084665262690076126, 7.022018677488170546, -10.88017736071110164 ) ) ;
#47691=FILL_AREA_STYLE ('',( #85207 ) ) ;
#47693=CARTESIAN_POINT ( 'NONE',  ( 20.36894250292379382, 33.67874883491396076, 10.36894250292379205 ) ) ;
#47694=CARTESIAN_POINT ( 'NONE',  ( -4.164238869374098151, 26.59541550158063217, -3.795296366450310543 ) ) ;
#47695=CARTESIAN_POINT ( 'NONE',  ( 2.917880565312948704, 62.63708216824730357, 12.26659068614894643 ) ) ;
#47696=CARTESIAN_POINT ( 'NONE',  ( 0.1532563361054100626, 30.80059781766744820, -2.638427012816831230 ) ) ;
#47697=CARTESIAN_POINT ( 'NONE',  ( 17.20831665107776587, 17.88393115100078745, 7.208316651077764980 ) ) ;
#47698=CARTESIAN_POINT ( 'NONE',  ( -0.8801773607111008646, 18.27201867748817321, 2.915334737309923430 ) ) ;
#47700=CARTESIAN_POINT ( 'NONE',  ( 5.076628168052704559, 35.17559781766745175, -8.527530157486179263 ) ) ;
#47701=CARTESIAN_POINT ( 'NONE',  ( 17.96484262340118221, 41.18868534415484106, -7.964842623401177768 ) ) ;
#47702=CARTESIAN_POINT ( 'NONE',  ( 0.1532563361054083140, 56.00893115100078745, 1.131784320476157264E-15 ) ) ;
#47703=CARTESIAN_POINT ( 'NONE',  ( 2.917880565312948704, 17.63708216824730357, 12.26659068614894643 ) ) ;
#47705=CARTESIAN_POINT ( 'NONE',  ( 5.076628168052703671, 11.84226448433411960, 8.527530157486179263 ) ) ;
#47706=CARTESIAN_POINT ( 'NONE',  ( 19.38216949554541202, 45.99863466993041072, 9.382169495545424454 ) ) ;
#47707=CARTESIAN_POINT ( 'NONE',  ( 19.84674366389459266, 53.71726448433411605, -2.638427012816827677 ) ) ;
#47710=CARTESIAN_POINT ( 'NONE',  ( 10.00000000000000000, 6.813685344154838397, -10.88017736071110342 ) ) ;
#47711=CARTESIAN_POINT ( 'NONE',  ( -0.8801773607111008646, 48.27201867748816966, 2.915334737309923430 ) ) ;
#47712=CARTESIAN_POINT ( 'NONE',  ( -2.266590686148945544, 7.220415501580634832, 7.082119434687048631 ) ) ;
#47713=CARTESIAN_POINT ( 'NONE',  ( 2.035157376598824452, 68.68868534415484817, 7.964842623401179544 ) ) ;
#47714=CARTESIAN_POINT ( 'NONE',  ( 10.00000000000000178, 37.25893115100078745, 9.846743663894594434 ) ) ;
#47715=CARTESIAN_POINT ( 'NONE',  ( -0.8801773607111008646, 18.27201867748817321, 2.915334737309923430 ) ) ;
#47716=CARTESIAN_POINT ( 'NONE',  ( 18.50749283717775384, 39.69955587570481725, 6.500000000000040856 ) ) ;
#47717=CARTESIAN_POINT ( 'NONE',  ( 14.92337183194729988, 59.34226448433412315, -8.527530157486177487 ) ) ;
#47718=AXIS2_PLACEMENT_3D ( 'NONE', #13433, #74923, #73434 ) ;
#47719=CARTESIAN_POINT ( 'NONE',  ( 0.6178305044545838731, 64.74863466993043914, 9.382169495545420901 ) ) ;
#47720=ORIENTED_EDGE ( 'NONE', *, *, #11878, .T. ) ;
#47724=CARTESIAN_POINT ( 'NONE',  ( 24.16423886937410614, 39.30374883491396787, 8.672049930838204340E-16 ) ) ;
#47725=CARTESIAN_POINT ( 'NONE',  ( 2.791683348922237240, 45.38393115100079456, -7.208316651077763204 ) ) ;
#47726=CARTESIAN_POINT ( 'NONE',  ( 5.076628168052704559, 25.17559781766745175, -8.527530157486179263 ) ) ;
#47727=LINE ( 'NONE', #95184, #88533 ) ;
#47728=CARTESIAN_POINT ( 'NONE',  ( 20.88017736071110875, 15.77201867748817143, -2.915334737309920765 ) ) ;
#47729=CARTESIAN_POINT ( 'NONE',  ( 12.63842701281683034, 57.46726448433411605, 9.846743663894596210 ) ) ;
#47731=CARTESIAN_POINT ( 'NONE',  ( 17.08211943468705840, 60.13708216824729647, -12.26659068614894466 ) ) ;
#47734=CARTESIAN_POINT ( 'NONE',  ( -0.8801773607110991993, 67.85535201082151957, -2.915334737309923874 ) ) ;
#47735=CARTESIAN_POINT ( 'NONE',  ( 17.20831665107776587, 12.88393115100078390, 7.208316651077764980 ) ) ;
#47740=CARTESIAN_POINT ( 'NONE',  ( 18.52753015748618282, 28.92559781766745175, -4.923371831947291888 ) ) ;
#47742=CARTESIAN_POINT ( 'NONE',  ( 24.16423886937409904, 19.09541550158063927, 3.795296366450317205 ) ) ;
#47743=CARTESIAN_POINT ( 'NONE',  ( 2.791683348922237240, 20.38393115100078745, -7.208316651077763204 ) ) ;
#47744=CARTESIAN_POINT ( 'NONE',  ( 0.5774900079438590739, 42.64701867748816966, -5.440088680355550821 ) ) ;
#47747=ORIENTED_EDGE ( 'NONE', *, *, #69317, .T. ) ;
#47748=CARTESIAN_POINT ( 'NONE',  ( 2.035157376598822676, 37.43868534415484106, -7.964842623401177768 ) ) ;
#47752=CARTESIAN_POINT ( 'NONE',  ( -4.164238869374098151, 6.595415501580634832, -3.795296366450310543 ) ) ;
#47754=ORIENTED_EDGE ( 'NONE', *, *, #32410, .F. ) ;
#47755=CARTESIAN_POINT ( 'NONE',  ( 19.38216949554541202, 30.99863466993042138, 9.382169495545424454 ) ) ;
#47757=PRESENTATION_STYLE_ASSIGNMENT (( #57217 ) ) ;
#47758=CARTESIAN_POINT ( 'NONE',  ( 5.076628168052703671, 6.842264484334118713, 8.527530157486179263 ) ) ;
#47760=CARTESIAN_POINT ( 'NONE',  ( 21.09922568453594849, 46.20696800326376064, 6.408140936763242479 ) ) ;
#47762=CARTESIAN_POINT ( 'NONE',  ( 1.472469842513823179, 31.42559781766745530, 4.923371831947296329 ) ) ;
#47766=CARTESIAN_POINT ( 'NONE',  ( 19.42250999205614548, 60.98035201082151247, -5.440088680355545492 ) ) ;
#47769=CARTESIAN_POINT ( 'NONE',  ( 19.84674366389459266, 8.717264484334116048, -2.638427012816827677 ) ) ;
#47770=EDGE_CURVE ( 'NONE', #16203, #20878, #13177, .T. ) ;
#47772=CARTESIAN_POINT ( 'NONE',  ( 10.00000000000000000, 34.75893115100078745, -9.846743663894594434 ) ) ;
#47773=CARTESIAN_POINT ( 'NONE',  ( 18.72515096720573879, 35.05509018479936145, 6.499999999999937828 ) ) ;
#47774=CARTESIAN_POINT ( 'NONE',  ( 13.79529636645030344, 13.26208216824729824, 14.16423886937410614 ) ) ;
#47775=CARTESIAN_POINT ( 'NONE',  ( 5.076628168052703671, 16.84226448433411960, 8.527530157486179263 ) ) ;
#47776=CARTESIAN_POINT ( 'NONE',  ( 16.40814093676324603, 22.45696800326375353, -11.09922568453594671 ) ) ;
#47777=CARTESIAN_POINT ( 'NONE',  ( 2.148416515056672083, 17.23726573380437443, 6.499999999999988454 ) ) ;
#47779=CARTESIAN_POINT ( 'NONE',  ( 20.88017736071110875, 45.77201867748816966, -2.915334737309920765 ) ) ;
#47780=CARTESIAN_POINT ( 'NONE',  ( 19.84674366389459621, 58.50893115100078745, 7.409399052514197653E-17 ) ) ;
#47783=CARTESIAN_POINT ( 'NONE',  ( 17.20831665107776587, 27.88393115100078390, 7.208316651077764980 ) ) ;
#47784=CARTESIAN_POINT ( 'NONE',  ( 12.63842701281683034, 27.46726448433411250, 9.846743663894596210 ) ) ;
#47785=CARTESIAN_POINT ( 'NONE',  ( -0.8801773607110991993, 17.85535201082150536, -2.915334737309923874 ) ) ;
#47786=CARTESIAN_POINT ( 'NONE',  ( 10.00000000000000178, 20.37363466993042138, 12.81628187352647608 ) ) ;
#47787=CARTESIAN_POINT ( 'NONE',  ( 17.20831665107776587, 19.13393115100078035, -7.208316651077762316 ) ) ;
#47789=CARTESIAN_POINT ( 'NONE',  ( 15.44008868035555793, 21.39701867748817321, -9.422509992056140149 ) ) ;
#47790=CARTESIAN_POINT ( 'NONE',  ( -0.8801773607111008646, 58.27201867748816966, 2.915334737309923430 ) ) ;
#47792=CARTESIAN_POINT ( 'NONE',  ( 12.63842701281683922, 39.55059781766744464, -9.846743663894590881 ) ) ;
#47793=CARTESIAN_POINT ( 'NONE',  ( -0.8801773607110991993, 12.85535201082150358, -2.915334737309923874 ) ) ;
#47794=CARTESIAN_POINT ( 'NONE',  ( 4.559911319644449179, 52.23035201082151247, -9.422509992056141925 ) ) ;
#47795=CARTESIAN_POINT ( 'NONE',  ( 17.96484262340118221, 11.18868534415484106, -7.964842623401177768 ) ) ;
#47797=CARTESIAN_POINT ( 'NONE',  ( 0.1532563361054083140, 21.00893115100078745, 1.131784320476157264E-15 ) ) ;
#47798=CARTESIAN_POINT ( 'NONE',  ( 10.00000000000000000, 39.75893115100078745, -9.846743663894594434 ) ) ;
#47802=CARTESIAN_POINT ( 'NONE',  ( 2.917880565312948704, 27.63708216824730357, 12.26659068614894643 ) ) ;
#47803=CARTESIAN_POINT ( 'NONE',  ( 5.076628168052704559, 35.17559781766745175, -8.527530157486179263 ) ) ;
#47805=CARTESIAN_POINT ( 'NONE',  ( 19.42250999205614193, 5.147018677488171434, 5.440088680355555262 ) ) ;
#47806=CARTESIAN_POINT ( 'NONE',  ( 19.84674366389459266, 23.30059781766745530, 2.638427012816836559 ) ) ;
#47809=CARTESIAN_POINT ( 'NONE',  ( 15.44008868035555260, 49.73035201082150536, 9.422509992056143702 ) ) ;
#47812=CARTESIAN_POINT ( 'NONE',  ( 10.00000000000000000, 21.81368534415484106, -10.88017736071110342 ) ) ;
#47813=CARTESIAN_POINT ( 'NONE',  ( 10.00000000000000000, 42.87363466993042493, -12.81628187352647608 ) ) ;
#47814=CARTESIAN_POINT ( 'NONE',  ( 19.38216949554541202, 5.998634669930420493, 9.382169495545424454 ) ) ;
#47815=CARTESIAN_POINT ( 'NONE',  ( 0.1532563361054083140, 16.00893115100078390, 1.131784320476157264E-15 ) ) ;
#47816=VERTEX_POINT ( 'NONE', #78661 ) ;
#47819=CARTESIAN_POINT ( 'NONE',  ( 20.36894250292379738, 54.92874883491396076, -10.36894250292379027 ) ) ;
#47820=CARTESIAN_POINT ( 'NONE',  ( 2.917880565312948704, 22.63708216824730002, 12.26659068614894643 ) ) ;
#47821=CARTESIAN_POINT ( 'NONE',  ( -0.8801773607111009756, 23.06368534415484106, 1.068504757029289695E-15 ) ) ;
#47822=CARTESIAN_POINT ( 'NONE',  ( 15.44008868035555793, 51.39701867748816966, -9.422509992056140149 ) ) ;
#47824=CARTESIAN_POINT ( 'NONE',  ( 19.72487221294571569, 47.80223176428831522, -6.499999999999982236 ) ) ;
#47825=CARTESIAN_POINT ( 'NONE',  ( 2.035157376598822676, 62.43868534415483396, -7.964842623401177768 ) ) ;
#47826=CARTESIAN_POINT ( 'NONE',  ( 17.20831665107776587, 19.13393115100078035, -7.208316651077762316 ) ) ;
#47829=CARTESIAN_POINT ( 'NONE',  ( 12.63842701281683922, 29.55059781766745175, -9.846743663894590881 ) ) ;
#47830=CARTESIAN_POINT ( 'NONE',  ( 5.076628168052704559, 55.17559781766745175, -8.527530157486179263 ) ) ;
#47831=CARTESIAN_POINT ( 'NONE',  ( 0.5774900079438607392, 18.48035201082150536, 5.440088680355550821 ) ) ;
#47832=CARTESIAN_POINT ( 'NONE',  ( 13.43411237798105340, 30.58196800326374998, 12.81628187352647963 ) ) ;
#47833=CARTESIAN_POINT ( 'NONE',  ( 12.91533473730992121, 49.52201867748817676, 10.88017736071110164 ) ) ;
#47834=CARTESIAN_POINT ( 'NONE',  ( 0.1532563361054082862, 26.21726448433411605, 2.638427012816831674 ) ) ;
#47835=CARTESIAN_POINT ( 'NONE',  ( 10.00000000000000178, 43.05374883491397497, 14.16423886937410082 ) ) ;
#47836=CARTESIAN_POINT ( 'NONE',  ( 17.20831665107776587, 2.883931151000785231, 7.208316651077764980 ) ) ;
#47838=CARTESIAN_POINT ( 'NONE',  ( 12.63842701281683922, 54.55059781766745175, -9.846743663894590881 ) ) ;
#47839=CARTESIAN_POINT ( 'NONE',  ( 19.84674366389459266, 38.30059781766745175, 2.638427012816836559 ) ) ;
#47840=CARTESIAN_POINT ( 'NONE',  ( 20.36894250292379738, 9.928748834913966093, -10.36894250292379027 ) ) ;
#47841=CARTESIAN_POINT ( 'NONE',  ( 2.917880565312948704, 22.63708216824730002, 12.26659068614894643 ) ) ;
#47842=CARTESIAN_POINT ( 'NONE',  ( 10.00000000000000000, 29.75893115100078745, -9.846743663894594434 ) ) ;
#47843=CARTESIAN_POINT ( 'NONE',  ( 20.88017736071110875, 50.77201867748817676, -2.915334737309920765 ) ) ;
#47844=CARTESIAN_POINT ( 'NONE',  ( 17.96484262340118221, 9.938685344154837509, 7.964842623401181321 ) ) ;
#47845=CARTESIAN_POINT ( 'NONE',  ( -0.8801773607111008646, 48.27201867748816966, 2.915334737309923430 ) ) ;
#47846=CARTESIAN_POINT ( 'NONE',  ( 4.559911319644449179, 28.89701867748817321, 9.422509992056141925 ) ) ;
#47848=CARTESIAN_POINT ( 'NONE',  ( 12.91533473730992121, 39.52201867748817676, 10.88017736071110164 ) ) ;
#47850=CARTESIAN_POINT ( 'NONE',  ( 13.43411237798105340, 55.58196800326374643, 12.81628187352647963 ) ) ;
#47852=CARTESIAN_POINT ( 'NONE',  ( 12.91533473730992121, 64.52201867748817676, 10.88017736071110164 ) ) ;
#47854=CARTESIAN_POINT ( 'NONE',  ( 19.42250999205614548, 45.98035201082150536, -5.440088680355545492 ) ) ;
#47855=CARTESIAN_POINT ( 'NONE',  ( -0.8801773607111008646, 3.272018677488171434, 2.915334737309923430 ) ) ;
#47856=CARTESIAN_POINT ( 'NONE',  ( 1.711636803080536451, 26.84492782695771140, -6.499999999999968914 ) ) ;
#47858=CARTESIAN_POINT ( 'NONE',  ( 2.917880565312950480, 55.97041550158063217, -12.26659068614894821 ) ) ;
#47859=CARTESIAN_POINT ( 'NONE',  ( 18.52753015748617571, 8.092264484334117824, 4.923371831947298993 ) ) ;
#47860=CARTESIAN_POINT ( 'NONE',  ( 10.00000000000000178, 8.053748834913967869, 14.16423886937410082 ) ) ;
#47861=CARTESIAN_POINT ( 'NONE',  ( 1.472469842513823179, 11.42559781766745175, 4.923371831947296329 ) ) ;
#47862=CARTESIAN_POINT ( 'NONE',  ( 20.88017736071110519, 10.56368534415483751, 2.639326808657452039E-16 ) ) ;
#47863=CARTESIAN_POINT ( 'NONE',  ( 19.84674366389459266, 43.71726448433410894, -2.638427012816827677 ) ) ;
#47866=CARTESIAN_POINT ( 'NONE',  ( 5.076628168052704559, 45.17559781766745175, -8.527530157486179263 ) ) ;
#47868=CARTESIAN_POINT ( 'NONE',  ( 12.91533473730993009, 36.60535201082151247, -10.88017736071109987 ) ) ;
#47869=CARTESIAN_POINT ( 'NONE',  ( 2.791683348922240793, 56.63393115100078035, 7.208316651077764092 ) ) ;
#47870=CARTESIAN_POINT ( 'NONE',  ( 19.42250999205614193, 65.14701867748817676, 5.440088680355555262 ) ) ;
#47871=CARTESIAN_POINT ( 'NONE',  ( 4.559911319644449179, 43.89701867748816966, 9.422509992056141925 ) ) ;
#47873=CARTESIAN_POINT ( 'NONE',  ( 12.91533473730993009, 6.605352010821504471, -10.88017736071109987 ) ) ;
#47876=CARTESIAN_POINT ( 'NONE',  ( 0.6178305044545818747, 23.49863466993041783, -9.382169495545419124 ) ) ;
#47879=CARTESIAN_POINT ( 'NONE',  ( 19.38216949554541202, 25.99863466993042138, 9.382169495545424454 ) ) ;
#47880=CARTESIAN_POINT ( 'NONE',  ( 15.44008868035555260, 19.73035201082150536, 9.422509992056143702 ) ) ;
#47882=ORIENTED_EDGE ( 'NONE', *, *, #66971, .T. ) ;
#47885=CARTESIAN_POINT ( 'NONE',  ( -0.8801773607111009756, 68.06368534415484817, 1.068504757029289695E-15 ) ) ;
#47886=CARTESIAN_POINT ( 'NONE',  ( 12.63842701281683922, 54.55059781766745175, -9.846743663894590881 ) ) ;
#47887=CARTESIAN_POINT ( 'NONE',  ( 14.92337183194729633, 17.67559781766745175, 8.527530157486181039 ) ) ;
#47888=CARTESIAN_POINT ( 'NONE',  ( 10.00000000000000178, 37.25893115100078745, 9.846743663894594434 ) ) ;
#47890=CARTESIAN_POINT ( 'NONE',  ( 5.076628168052703671, 26.84226448433411960, 8.527530157486179263 ) ) ;
#47893=CARTESIAN_POINT ( 'NONE',  ( 0.1532563361054083140, 31.00893115100078390, 1.131784320476157264E-15 ) ) ;
#47894=CARTESIAN_POINT ( 'NONE',  ( 0.1532563361054083140, 1.008931151000784787, 1.131784320476157264E-15 ) ) ;
#47896=CARTESIAN_POINT ( 'NONE',  ( 0.1532563361054100626, 40.80059781766745886, -2.638427012816831230 ) ) ;
#47898=CARTESIAN_POINT ( 'NONE',  ( 0.5774900079438607392, 8.480352010821505360, 5.440088680355550821 ) ) ;
#47899=CARTESIAN_POINT ( 'NONE',  ( 10.00000000000000178, 30.37363466993042138, 12.81628187352647608 ) ) ;
#47901=CARTESIAN_POINT ( 'NONE',  ( 20.36894250292379382, 48.67874883491396076, 10.36894250292379205 ) ) ;
#47902=CARTESIAN_POINT ( 'NONE',  ( 14.92337183194729633, 17.67559781766745175, 8.527530157486181039 ) ) ;
#47903=CARTESIAN_POINT ( 'NONE',  ( 12.63842701281683922, 4.550597817667451750, -9.846743663894590881 ) ) ;
#47904=FACE_OUTER_BOUND ( 'NONE', #96224, .T. ) ;
#47905=CARTESIAN_POINT ( 'NONE',  ( 17.08211943468705130, 38.47041550158063217, 12.26659068614894998 ) ) ;
#47906=CARTESIAN_POINT ( 'NONE',  ( 0.1532563361054100626, 65.80059781766745175, -2.638427012816831230 ) ) ;
#47907=CARTESIAN_POINT ( 'NONE',  ( 15.44008868035555793, 11.39701867748817143, -9.422509992056140149 ) ) ;
#47908=CARTESIAN_POINT ( 'NONE',  ( 13.79529636645031943, 20.34541550158063572, -14.16423886937409904 ) ) ;
#47909=CARTESIAN_POINT ( 'NONE',  ( 6.204703633549690345, 40.76208216824731778, -14.16423886937410259 ) ) ;
#47912=CARTESIAN_POINT ( 'NONE',  ( 7.361572987183169658, 54.96726448433413026, -9.846743663894592657 ) ) ;
#47913=ORIENTED_EDGE ( 'NONE', *, *, #12173, .T. ) ;
#47914=CARTESIAN_POINT ( 'NONE',  ( 0.5774900079438590739, 37.64701867748817676, -5.440088680355550821 ) ) ;
#47916=CARTESIAN_POINT ( 'NONE',  ( 19.50000000000000711, 98.59912998021081876, -4.999999999999999112 ) ) ;
#47918=CARTESIAN_POINT ( 'NONE',  ( 18.52753015748617571, 43.09226448433412315, 4.923371831947298993 ) ) ;
#47921=CARTESIAN_POINT ( 'NONE',  ( 18.52753015748617571, 43.09226448433412315, 4.923371831947298993 ) ) ;
#47922=CARTESIAN_POINT ( 'NONE',  ( 2.791683348922237240, 65.38393115100078035, -7.208316651077763204 ) ) ;
#47924=CARTESIAN_POINT ( 'NONE',  ( 24.16423886937410614, 9.303748834913967869, 8.672049930838204340E-16 ) ) ;
#47925=DIRECTION ( 'NONE',  ( -1.000000000000000000, 0.000000000000000000, 0.000000000000000000 ) ) ;
#47928=CARTESIAN_POINT ( 'NONE',  ( -4.164238869374099039, 66.80374883491396076, 8.674139862899312516E-16 ) ) ;
#47929=CARTESIAN_POINT ( 'NONE',  ( 19.38216949554541557, 27.24863466993041783, -9.382169495545420901 ) ) ;
#47931=CARTESIAN_POINT ( 'NONE',  ( 7.361572987183170547, 2.050597817667451750, 9.846743663894590881 ) ) ;
#47933=CIRCLE ( 'NONE', #46380, 6.999999999999999112 ) ;
#47935=CARTESIAN_POINT ( 'NONE',  ( -4.164238869374098151, 66.59541550158060375, -3.795296366450310543 ) ) ;
#47937=CARTESIAN_POINT ( 'NONE',  ( 7.084665262690076126, 27.02201867748817676, -10.88017736071110164 ) ) ;
#47938=CARTESIAN_POINT ( 'NONE',  ( 15.44008868035555260, 34.73035201082151247, 9.422509992056143702 ) ) ;
#47939=CARTESIAN_POINT ( 'NONE',  ( 19.84674366389459266, 63.30059781766745886, 2.638427012816836559 ) ) ;
#47940=CARTESIAN_POINT ( 'NONE',  ( 1.472469842513823179, 50.59226448433411605, -4.923371831947296329 ) ) ;
#47941=CARTESIAN_POINT ( 'NONE',  ( -42.84233569985355672, 106.9556388676848258, -5.000000000000000888 ) ) ;
#47942=CARTESIAN_POINT ( 'NONE',  ( 5.076628168052704559, 5.175597817667451750, -8.527530157486179263 ) ) ;
#47944=VERTEX_POINT ( 'NONE', #3651 ) ;
#47945=CARTESIAN_POINT ( 'NONE',  ( 15.44008868035555793, 31.39701867748817676, -9.422509992056140149 ) ) ;
#47946=CARTESIAN_POINT ( 'NONE',  ( 19.38216949554541557, 27.24863466993041783, -9.382169495545420901 ) ) ;
#47948=CARTESIAN_POINT ( 'NONE',  ( 7.361572987183169658, 59.96726448433410894, -9.846743663894592657 ) ) ;
#47949=CARTESIAN_POINT ( 'NONE',  ( 15.44008868035555260, 49.73035201082150536, 9.422509992056143702 ) ) ;
#47950=CARTESIAN_POINT ( 'NONE',  ( 2.791683348922237240, 10.38393115100078390, -7.208316651077763204 ) ) ;
#47951=CARTESIAN_POINT ( 'NONE',  ( 10.00000000000000178, 40.37363466993042493, 12.81628187352647608 ) ) ;
#47952=CARTESIAN_POINT ( 'NONE',  ( -0.8801773607111009756, 68.06368534415484817, 1.068504757029289695E-15 ) ) ;
#47953=FILL_AREA_STYLE ('',( #17487 ) ) ;
#47954=CARTESIAN_POINT ( 'NONE',  ( 18.50749283717779647, 54.69955587570481725, 6.499999999999920952 ) ) ;
#47955=ORIENTED_EDGE ( 'NONE', *, *, #61757, .F. ) ;
#47956=B_SPLINE_CURVE_WITH_KNOTS ( 'NONE', 3,
 ( #23723, #53212, #67733, #84220 ),
 .UNSPECIFIED., .F., .F.,
 ( 4, 4 ),
 ( 3.227937720230791035E-17, 0.002392975128318423038 ),
 .UNSPECIFIED. ) ;
#47957=CARTESIAN_POINT ( 'NONE',  ( 1.711636803080541558, 16.84492782695771496, -6.499999999999984901 ) ) ;
#47958=CARTESIAN_POINT ( 'NONE',  ( 2.035157376598822676, 7.438685344154837509, -7.964842623401177768 ) ) ;
#47959=CARTESIAN_POINT ( 'NONE',  ( 21.09922568453595559, 52.04030133659708923, -6.408140936763230044 ) ) ;
#47960=CARTESIAN_POINT ( 'NONE',  ( -2.266590686148945544, 17.22041550158063572, 7.082119434687048631 ) ) ;
#47961=CARTESIAN_POINT ( 'NONE',  ( 19.84674366389459621, 13.50893115100078568, 7.409399052514197653E-17 ) ) ;
#47962=CARTESIAN_POINT ( 'NONE',  ( 12.91533473730992121, 9.522018677488171434, 10.88017736071110164 ) ) ;
#47964=CARTESIAN_POINT ( 'NONE',  ( 18.52753015748617571, 18.09226448433411960, 4.923371831947298993 ) ) ;
#47965=CARTESIAN_POINT ( 'NONE',  ( 13.79529636645030344, 53.26208216824730357, 14.16423886937410614 ) ) ;
#47967=CARTESIAN_POINT ( 'NONE',  ( 2.035157376598824452, 3.688685344154837953, 7.964842623401179544 ) ) ;
#47969=CARTESIAN_POINT ( 'NONE',  ( -0.8801773607111009756, 18.06368534415484106, 1.068504757029289695E-15 ) ) ;
#47970=CARTESIAN_POINT ( 'NONE',  ( 1.274849032794324932, 32.55509018479936145, -6.500000000000021316 ) ) ;
#47972=ORIENTED_EDGE ( 'NONE', *, *, #12449, .F. ) ;
#47973=CARTESIAN_POINT ( 'NONE',  ( 12.91533473730993009, 16.60535201082150891, -10.88017736071109987 ) ) ;
#47974=CARTESIAN_POINT ( 'NONE',  ( 20.88017736071110164, 15.35535201082150358, 2.915334737309930979 ) ) ;
#47975=CARTESIAN_POINT ( 'NONE',  ( 1.472469842513823179, 56.42559781766745886, 4.923371831947296329 ) ) ;
#47978=DIRECTION ( 'NONE',  ( -0.000000000000000000, 0.000000000000000000, -1.000000000000000000 ) ) ;
#47979=CARTESIAN_POINT ( 'NONE',  ( 17.08211943468705130, 18.47041550158063572, 12.26659068614894998 ) ) ;
#47980=CARTESIAN_POINT ( 'NONE',  ( -0.8801773607111008646, 23.27201867748817676, 2.915334737309923430 ) ) ;
#47981=CARTESIAN_POINT ( 'NONE',  ( 19.42250999205614193, 20.14701867748817321, 5.440088680355555262 ) ) ;
#47983=CARTESIAN_POINT ( 'NONE',  ( 1.472469842513823179, 50.59226448433411605, -4.923371831947296329 ) ) ;
#47985=CARTESIAN_POINT ( 'NONE',  ( 7.361572987183169658, 29.96726448433411960, -9.846743663894592657 ) ) ;
#47987=CARTESIAN_POINT ( 'NONE',  ( 19.84674366389459266, 3.300597817667451750, 2.638427012816836559 ) ) ;
#47990=( LENGTH_UNIT ( ) NAMED_UNIT ( * ) SI_UNIT ( .MILLI., .METRE. ) );
#47991=CARTESIAN_POINT ( 'NONE',  ( 14.92337183194729633, 12.67559781766745353, 8.527530157486181039 ) ) ;
#47992=CARTESIAN_POINT ( 'NONE',  ( 0.6178305044545818747, -1.501365330069579951, -9.382169495545419124 ) ) ;
#47993=CARTESIAN_POINT ( 'NONE',  ( -0.8801773607111008646, 43.27201867748817676, 2.915334737309923430 ) ) ;
#47994=CARTESIAN_POINT ( 'NONE',  ( -0.8801773607110991993, 47.85535201082150536, -2.915334737309923874 ) ) ;
#47995=CARTESIAN_POINT ( 'NONE',  ( 19.42250999205614193, 5.147018677488171434, 5.440088680355555262 ) ) ;
#47996=CARTESIAN_POINT ( 'NONE',  ( 13.43411237798106583, 47.66530133659709634, -12.81628187352647252 ) ) ;
#47997=CARTESIAN_POINT ( 'NONE',  ( 10.00000000000000000, 20.55374883491396787, -14.16423886937410082 ) ) ;
#47999=CARTESIAN_POINT ( 'NONE',  ( 22.81628187352647785, 56.62363466993042493, 6.195893100308588602E-16 ) ) ;
#48001=B_SPLINE_CURVE_WITH_KNOTS ( 'NONE', 3,
 ( #44300, #84301, #44791, #38303, #90285, #61763 ),
 .UNSPECIFIED., .F., .F.,
 ( 4, 2, 4 ),
 ( 6.992893892674702526E-18, 0.0002605067024381006627, 0.0005210134048761942780 ),
 .UNSPECIFIED. ) ;
#48002=CARTESIAN_POINT ( 'NONE',  ( 7.361572987183169658, 59.96726448433410894, -9.846743663894592657 ) ) ;
#48003=CARTESIAN_POINT ( 'NONE',  ( -0.8801773607111008646, 23.27201867748817676, 2.915334737309923430 ) ) ;
#48006=CARTESIAN_POINT ( 'NONE',  ( 18.52753015748618282, 8.925597817667451750, -4.923371831947291888 ) ) ;
#48008=CARTESIAN_POINT ( 'NONE',  ( 17.20831665107776587, 7.883931151000784787, 7.208316651077764980 ) ) ;
#48009=CARTESIAN_POINT ( 'NONE',  ( 0.1532563361054083140, 1.008931151000784787, 1.131784320476157264E-15 ) ) ;
#48011=CARTESIAN_POINT ( 'NONE',  ( 10.00000000000000000, 61.81368534415484106, -10.88017736071110342 ) ) ;
#48013=CARTESIAN_POINT ( 'NONE',  ( 7.084665262690076126, 67.02201867748817676, -10.88017736071110164 ) ) ;
#48014=CARTESIAN_POINT ( 'NONE',  ( 12.63842701281683034, 7.467264484334118713, 9.846743663894596210 ) ) ;
#48017=CARTESIAN_POINT ( 'NONE',  ( 10.00000000000000000, 54.75893115100078745, -9.846743663894594434 ) ) ;
#48021=CARTESIAN_POINT ( 'NONE',  ( 22.81628187352648496, 56.83196800326374643, -3.434112377981050290 ) ) ;
#48022=( NAMED_UNIT ( * ) SI_UNIT ( $, .STERADIAN. ) SOLID_ANGLE_UNIT ( ) );
#48023=CARTESIAN_POINT ( 'NONE',  ( 20.36894250292379738, 19.92874883491396787, -10.36894250292379027 ) ) ;
#48024=CARTESIAN_POINT ( 'NONE',  ( -0.1503990784575328643, 45.12777174578613426, 6.262539305110068177 ) ) ;
#48025=( NAMED_UNIT ( * ) SI_UNIT ( $, .STERADIAN. ) SOLID_ANGLE_UNIT ( ) );
#48026=CARTESIAN_POINT ( 'NONE',  ( 15.44008868035555260, 64.73035201082151957, 9.422509992056143702 ) ) ;
#48027=CARTESIAN_POINT ( 'NONE',  ( 15.44008868035555260, 24.73035201082150891, 9.422509992056143702 ) ) ;
#48030=CARTESIAN_POINT ( 'NONE',  ( 10.00000000000000178, 22.25893115100078745, 9.846743663894594434 ) ) ;
#48031=CARTESIAN_POINT ( 'NONE',  ( 16.40814093676324603, 37.45696800326376064, -11.09922568453594671 ) ) ;
#48032=CARTESIAN_POINT ( 'NONE',  ( 2.791683348922240793, 41.63393115100078745, 7.208316651077764092 ) ) ;
#48033=PLANE ( 'NONE',  #1149 ) ;
#48035=CARTESIAN_POINT ( 'NONE',  ( 3.591859063236763294, 33.29030133659708213, -11.09922568453595026 ) ) ;
#48037=B_SPLINE_CURVE_WITH_KNOTS ( 'NONE', 3,
 ( #89856, #65375, #42889, #80886, #88387, #44354 ),
 .UNSPECIFIED., .F., .F.,
 ( 4, 2, 4 ),
 ( 7.909150811748204484E-18, 0.0002626113303185971786, 0.0005252226606371864425 ),
 .UNSPECIFIED. ) ;
#48038=CARTESIAN_POINT ( 'NONE',  ( 7.361572987183170547, 32.05059781766745175, 9.846743663894590881 ) ) ;
#48039=CARTESIAN_POINT ( 'NONE',  ( 10.00000000000000000, 15.55374883491396787, -14.16423886937410082 ) ) ;
#48041=CARTESIAN_POINT ( 'NONE',  ( -0.8801773607111009756, 33.06368534415484106, 1.068504757029289695E-15 ) ) ;
#48042=CARTESIAN_POINT ( 'NONE',  ( -0.3689425029237898834, 31.17874883491396787, -10.36894250292378850 ) ) ;
#48043=CARTESIAN_POINT ( 'NONE',  ( 0.1532563361054100626, 50.80059781766745175, -2.638427012816831230 ) ) ;
#48044=CARTESIAN_POINT ( 'NONE',  ( 5.076628168052704559, 15.17559781766745175, -8.527530157486179263 ) ) ;
#48045=CARTESIAN_POINT ( 'NONE',  ( -2.816281873526473856, 54.33196800326376064, 3.434112377981055619 ) ) ;
#48047=CARTESIAN_POINT ( 'NONE',  ( 4.559911319644449179, 23.89701867748817321, 9.422509992056141925 ) ) ;
#48048=CARTESIAN_POINT ( 'NONE',  ( 10.00000000000000000, 17.87363466993041783, -12.81628187352647608 ) ) ;
#48049=CARTESIAN_POINT ( 'NONE',  ( 16.40814093676323893, 20.79030133659708923, 11.09922568453595026 ) ) ;
#48050=CARTESIAN_POINT ( 'NONE',  ( 0.1532563361054083140, 46.00893115100079456, 1.131784320476157264E-15 ) ) ;
#48052=CARTESIAN_POINT ( 'NONE',  ( -2.816281873526473856, 44.12363466993042493, 9.499525473075851096E-16 ) ) ;
#48053=PLANE ( 'NONE',  #517 ) ;
#48054=CARTESIAN_POINT ( 'NONE',  ( 4.559911319644449179, 52.23035201082151247, -9.422509992056141925 ) ) ;
#48059=CARTESIAN_POINT ( 'NONE',  ( 2.035157376598822676, 57.43868534415484106, -7.964842623401177768 ) ) ;
#48061=CARTESIAN_POINT ( 'NONE',  ( 0.5774900079438607392, 58.48035201082151247, 5.440088680355550821 ) ) ;
#48062=DIRECTION ( 'NONE',  ( -1.000000000000000000, 0.000000000000000000, 0.000000000000000000 ) ) ;
#48064=CARTESIAN_POINT ( 'NONE',  ( -0.8801773607111008646, 8.272018677488171434, 2.915334737309923430 ) ) ;
#48065=CARTESIAN_POINT ( 'NONE',  ( 7.361572987183170547, 67.05059781766746596, 9.846743663894590881 ) ) ;
#48066=CARTESIAN_POINT ( 'NONE',  ( 0.5774900079438607392, 18.48035201082150536, 5.440088680355550821 ) ) ;
#48070=CARTESIAN_POINT ( 'NONE',  ( 10.00000000000000000, 22.87363466993042138, -12.81628187352647608 ) ) ;
#48072=CARTESIAN_POINT ( 'NONE',  ( 20.88017736071110875, 45.77201867748816966, -2.915334737309920765 ) ) ;
#48073=CARTESIAN_POINT ( 'NONE',  ( 1.472469842513823179, 40.59226448433411605, -4.923371831947296329 ) ) ;
#48074=CARTESIAN_POINT ( 'NONE',  ( 16.40814093676324603, 7.456968003263754419, -11.09922568453594671 ) ) ;
#48075=LINE ( 'NONE', #92597, #68546 ) ;
#48076=CARTESIAN_POINT ( 'NONE',  ( 10.00000000000000000, 26.81368534415484106, -10.88017736071110342 ) ) ;
#48077=CARTESIAN_POINT ( 'NONE',  ( 2.035157376598822676, 37.43868534415484106, -7.964842623401177768 ) ) ;
#48078=CARTESIAN_POINT ( 'NONE',  ( 2.917880565312950480, 50.97041550158064638, -12.26659068614894821 ) ) ;
#48079=CARTESIAN_POINT ( 'NONE',  ( 19.84674366389459266, 43.30059781766744464, 2.638427012816836559 ) ) ;
#48080=CARTESIAN_POINT ( 'NONE',  ( 7.084665262690076126, 54.10535201082151247, 10.88017736071109987 ) ) ;
#48082=CARTESIAN_POINT ( 'NONE',  ( -4.164238869374099039, 16.80374883491396787, 8.674139862899312516E-16 ) ) ;
#48085=CARTESIAN_POINT ( 'NONE',  ( 0.1532563361054083140, 66.00893115100079456, 1.131784320476157264E-15 ) ) ;
#48086=ADVANCED_FACE ( 'NONE', ( #21108 ), #52096, .F. ) ;
#48089=CARTESIAN_POINT ( 'NONE',  ( 2.917880565312948704, 47.63708216824730357, 12.26659068614894643 ) ) ;
#48090=CARTESIAN_POINT ( 'NONE',  ( 13.79529636645031943, 40.34541550158063217, -14.16423886937409904 ) ) ;
#48091=CARTESIAN_POINT ( 'NONE',  ( 12.63842701281683034, 17.46726448433411250, 9.846743663894596210 ) ) ;
#48092=CARTESIAN_POINT ( 'NONE',  ( -2.816281873526471635, 18.91530133659708213, -3.434112377981056508 ) ) ;
#48093=CARTESIAN_POINT ( 'NONE',  ( 2.791683348922237240, 65.38393115100078035, -7.208316651077763204 ) ) ;
#48095=CARTESIAN_POINT ( 'NONE',  ( 12.91533473730992121, 64.52201867748817676, 10.88017736071110164 ) ) ;
#48096=CARTESIAN_POINT ( 'NONE',  ( -1.099225684535947600, 28.70696800326375353, -6.408140936763238038 ) ) ;
#48097=CARTESIAN_POINT ( 'NONE',  ( 10.00000000000000178, 33.05374883491396787, 14.16423886937410082 ) ) ;
#48099=CARTESIAN_POINT ( 'NONE',  ( 17.96484262340118221, 29.93868534415484106, 7.964842623401181321 ) ) ;
#48101=DIRECTION ( 'NONE',  ( -1.000000000000000000, 0.000000000000000000, 0.000000000000000000 ) ) ;
#48102=CARTESIAN_POINT ( 'NONE',  ( 2.035157376598824452, 68.68868534415484817, 7.964842623401179544 ) ) ;
#48104=CARTESIAN_POINT ( 'NONE',  ( 0.1532563361054082862, 6.217264484334118713, 2.638427012816831674 ) ) ;
#48105=ORIENTED_EDGE ( 'NONE', *, *, #12449, .T. ) ;
#48107=CARTESIAN_POINT ( 'NONE',  ( 20.15039907845753220, 57.62777174578613426, -6.262539305110077947 ) ) ;
#48108=ORIENTED_EDGE ( 'NONE', *, *, #19903, .F. ) ;
#48109=CARTESIAN_POINT ( 'NONE',  ( 2.035157376598822676, 7.438685344154837509, -7.964842623401177768 ) ) ;
#48110=CARTESIAN_POINT ( 'NONE',  ( 20.88017736071110164, 5.355352010821503583, 2.915334737309930979 ) ) ;
#48111=CARTESIAN_POINT ( 'NONE',  ( 7.361572987183169658, 29.96726448433411960, -9.846743663894592657 ) ) ;
#48112=CARTESIAN_POINT ( 'NONE',  ( -1.099225684535947600, -0.4596986634029132657, 6.408140936763237150 ) ) ;
#48118=CARTESIAN_POINT ( 'NONE',  ( 10.00000000000000000, 7.873634669930421381, -12.81628187352647608 ) ) ;
#48119=VERTEX_POINT ( 'NONE', #81106 ) ;
#48120=CARTESIAN_POINT ( 'NONE',  ( -2.266590686148945544, 46.38708216824730357, -7.082119434687050408 ) ) ;
#48123=CARTESIAN_POINT ( 'NONE',  ( -2.266590686148945544, 51.38708216824730357, -7.082119434687050408 ) ) ;
#48125=CARTESIAN_POINT ( 'NONE',  ( 20.88017736071110519, 40.56368534415484106, 2.639326808657452039E-16 ) ) ;
#48126=CARTESIAN_POINT ( 'NONE',  ( 2.035157376598822676, 37.43868534415484106, -7.964842623401177768 ) ) ;
#48127=CARTESIAN_POINT ( 'NONE',  ( -0.8801773607110991993, 37.85535201082151247, -2.915334737309923874 ) ) ;
#48128=CARTESIAN_POINT ( 'NONE',  ( 4.559911319644449179, 62.23035201082150536, -9.422509992056141925 ) ) ;
#48130=CARTESIAN_POINT ( 'NONE',  ( 7.084665262690076126, 24.10535201082150181, 10.88017736071109987 ) ) ;
#48131=EDGE_CURVE ( 'NONE', #11431, #86051, #49906, .T. ) ;
#48134=CARTESIAN_POINT ( 'NONE',  ( 10.00000000000000000, 19.75893115100078390, -9.846743663894594434 ) ) ;
#48135=CARTESIAN_POINT ( 'NONE',  ( 19.72487221294571214, 2.802231764288312998, -6.500000000000001776 ) ) ;
#48136=ORIENTED_EDGE ( 'NONE', *, *, #24195, .F. ) ;
#48138=CARTESIAN_POINT ( 'NONE',  ( 14.92337183194729988, 49.34226448433411605, -8.527530157486177487 ) ) ;
#48139=DIRECTION ( 'NONE',  ( 1.000000000000000000, 0.000000000000000000, 0.000000000000000000 ) ) ;
#48145=CARTESIAN_POINT ( 'NONE',  ( 0.1532563361054082862, 56.21726448433411605, 2.638427012816831674 ) ) ;
#48146=CARTESIAN_POINT ( 'NONE',  ( 17.08211943468705130, 53.47041550158063217, 12.26659068614894998 ) ) ;
#48147=CARTESIAN_POINT ( 'NONE',  ( 18.72515096720570327, 6.072280503510315341, -6.499999999999985789 ) ) ;
#48151=CARTESIAN_POINT ( 'NONE',  ( 14.92337183194729633, 17.67559781766745175, 8.527530157486181039 ) ) ;
#48152=CARTESIAN_POINT ( 'NONE',  ( 16.40814093676323893, 60.79030133659709634, 11.09922568453595026 ) ) ;
#48153=CARTESIAN_POINT ( 'NONE',  ( 10.00000000000000000, -2.126365330069579951, -12.81628187352647608 ) ) ;
#48154=CARTESIAN_POINT ( 'NONE',  ( 0.5774900079438590739, 62.64701867748817676, -5.440088680355550821 ) ) ;
#48155=CARTESIAN_POINT ( 'NONE',  ( 0.1532563361054083140, 51.00893115100078745, 1.131784320476157264E-15 ) ) ;
#48158=CARTESIAN_POINT ( 'NONE',  ( 24.16423886937409904, 59.09541550158063217, 3.795296366450317205 ) ) ;
#48160=CARTESIAN_POINT ( 'NONE',  ( 2.035157376598824452, 48.68868534415483396, 7.964842623401179544 ) ) ;
#48161=CARTESIAN_POINT ( 'NONE',  ( 0.6178305044545818747, 18.49863466993041428, -9.382169495545419124 ) ) ;
#48162=CARTESIAN_POINT ( 'NONE',  ( -0.8801773607111008646, 68.27201867748817676, 2.915334737309923430 ) ) ;
#48167=CARTESIAN_POINT ( 'NONE',  ( 14.92337183194729633, 52.67559781766745175, 8.527530157486181039 ) ) ;
#48168=CARTESIAN_POINT ( 'NONE',  ( 1.472469842513823179, 6.425597817667451750, 4.923371831947296329 ) ) ;
#48170=CARTESIAN_POINT ( 'NONE',  ( 3.591859063236761518, 9.956968003263753531, 11.09922568453594849 ) ) ;
#48171=CARTESIAN_POINT ( 'NONE',  ( 17.96484262340118221, 16.18868534415483396, -7.964842623401177768 ) ) ;
#48174=CARTESIAN_POINT ( 'NONE',  ( 13.79529636645031943, 35.34541550158063927, -14.16423886937409904 ) ) ;
#48175=CARTESIAN_POINT ( 'NONE',  ( 6.204703633549690345, 35.76208216824729647, -14.16423886937410259 ) ) ;
#48176=CARTESIAN_POINT ( 'NONE',  ( -2.266590686148945544, 62.22041550158063927, 7.082119434687048631 ) ) ;
#48177=CARTESIAN_POINT ( 'NONE',  ( 17.20831665107776587, 32.88393115100078745, 7.208316651077764980 ) ) ;
#48178=CARTESIAN_POINT ( 'NONE',  ( 22.81628187352647785, 41.41530133659708923, 3.434112377981063169 ) ) ;
#48179=CARTESIAN_POINT ( 'NONE',  ( -0.8801773607110991993, 7.855352010821504471, -2.915334737309923874 ) ) ;
#48182=CARTESIAN_POINT ( 'NONE',  ( 10.00000000000000178, 37.25893115100078745, 9.846743663894594434 ) ) ;
#48183=CARTESIAN_POINT ( 'NONE',  ( 19.42250999205614193, 45.14701867748817676, 5.440088680355555262 ) ) ;
#48184=CARTESIAN_POINT ( 'NONE',  ( 5.076628168052704559, 65.17559781766745175, -8.527530157486179263 ) ) ;
#48185=CARTESIAN_POINT ( 'NONE',  ( -4.164238869374099927, 17.01208216824730357, 3.795296366450308767 ) ) ;
#48188=( BOUNDED_CURVE ( )  B_SPLINE_CURVE ( 2, ( #38165, #97203, #28672, #31620, #91646, #30629, #54611, #39145, #32103 ),
 .UNSPECIFIED., .F., .F. ) 
 B_SPLINE_CURVE_WITH_KNOTS ( ( 3, 2, 2, 2, 3 ),
 ( 0.9044266512259456769, 0.9047619047619047672, 0.9107142857142856984, 0.9166666666666667407, 0.9170019202026259419 ),
 .UNSPECIFIED. ) 
 CURVE ( )  GEOMETRIC_REPRESENTATION_ITEM ( )  RATIONAL_B_SPLINE_CURVE ( ( 0.9963778908391764944, 0.9980808541467923733, 1.000000000000000000, 0.9659258262890682012, 1.000000000000000000, 0.9659258262890682012, 1.000000000000000000, 0.9980808541467917072, 0.9963778908391753841 ) ) 
 REPRESENTATION_ITEM ( '' )  );
#48189=CARTESIAN_POINT ( 'NONE',  ( 18.52753015748618282, 28.92559781766745175, -4.923371831947291888 ) ) ;
#48190=CARTESIAN_POINT ( 'NONE',  ( 6.565887622018943937, 48.08196800326375353, -12.81628187352647608 ) ) ;
#48191=CARTESIAN_POINT ( 'NONE',  ( 14.92337183194729633, 52.67559781766745175, 8.527530157486181039 ) ) ;
#48193=DIRECTION ( 'NONE',  ( 0.000000000000000000, 0.000000000000000000, -1.000000000000000000 ) ) ;
#48194=CARTESIAN_POINT ( 'NONE',  ( -46.49699363514445594, 103.0259809974584044, -6.596269562656988938 ) ) ;
#48195=CARTESIAN_POINT ( 'NONE',  ( -4.164238869374099927, 62.01208216824728936, 3.795296366450308767 ) ) ;
#48196=CARTESIAN_POINT ( 'NONE',  ( 2.917880565312948704, 12.63708216824730179, 12.26659068614894643 ) ) ;
#48197=CARTESIAN_POINT ( 'NONE',  ( 19.84674366389459266, 3.300597817667451750, 2.638427012816836559 ) ) ;
#48198=CARTESIAN_POINT ( 'NONE',  ( 17.20831665107776587, 44.13393115100078745, -7.208316651077762316 ) ) ;
#48199=CARTESIAN_POINT ( 'NONE',  ( 20.88017736071110519, 25.56368534415483751, 2.639326808657452039E-16 ) ) ;
#48201=CARTESIAN_POINT ( 'NONE',  ( 19.84674366389459621, 58.50893115100078745, 7.409399052514197653E-17 ) ) ;
#48204=FACE_OUTER_BOUND ( 'NONE', #4537, .T. ) ;
#48211=CARTESIAN_POINT ( 'NONE',  ( 10.00000000000000000, 0.5537488349139675359, -14.16423886937410082 ) ) ;
#48212=CARTESIAN_POINT ( 'NONE',  ( 19.84674366389459266, 58.71726448433411605, -2.638427012816827677 ) ) ;
#48213=CARTESIAN_POINT ( 'NONE',  ( 18.52753015748617571, 18.09226448433411960, 4.923371831947298993 ) ) ;
#48215=CARTESIAN_POINT ( 'NONE',  ( 4.559911319644449179, 23.89701867748817321, 9.422509992056141925 ) ) ;
#48216=CARTESIAN_POINT ( 'NONE',  ( 18.52753015748618282, 63.92559781766745886, -4.923371831947291888 ) ) ;
#48219=CARTESIAN_POINT ( 'NONE',  ( 2.035157376598822676, 2.438685344154838397, -7.964842623401177768 ) ) ;
#48223=CARTESIAN_POINT ( 'NONE',  ( 7.084665262690076126, 69.10535201082151957, 10.88017736071109987 ) ) ;
#48224=AXIS2_PLACEMENT_3D ( 'NONE', #2143, #79593, #3605 ) ;
#48225=CARTESIAN_POINT ( 'NONE',  ( 2.791683348922237240, 15.38393115100078212, -7.208316651077763204 ) ) ;
#48229=VECTOR ( 'NONE', #63035, 1000.000000000000000 ) ;
#48231=CARTESIAN_POINT ( 'NONE',  ( 5.076628168052704559, 25.17559781766745175, -8.527530157486179263 ) ) ;
#48232=ORIENTED_EDGE ( 'NONE', *, *, #58957, .T. ) ;
#48233=CARTESIAN_POINT ( 'NONE',  ( 13.79529636645030344, 28.26208216824729647, 14.16423886937410614 ) ) ;
#48234=CARTESIAN_POINT ( 'NONE',  ( 19.84674366389459621, 33.50893115100078745, 7.409399052514197653E-17 ) ) ;
#48235=CARTESIAN_POINT ( 'NONE',  ( 17.96484262340118221, 41.18868534415484106, -7.964842623401177768 ) ) ;
#48238=CARTESIAN_POINT ( 'NONE',  ( 19.42250999205614193, 45.14701867748817676, 5.440088680355555262 ) ) ;
#48241=ORIENTED_EDGE ( 'NONE', *, *, #33355, .T. ) ;
#48242=CARTESIAN_POINT ( 'NONE',  ( 2.917880565312948704, 12.63708216824730179, 12.26659068614894643 ) ) ;
#48244=EDGE_CURVE ( 'NONE', #75354, #14763, #65484, .T. ) ;
#48246=CARTESIAN_POINT ( 'NONE',  ( 22.81628187352647785, 36.62363466993041783, 6.195893100308588602E-16 ) ) ;
#48247=CARTESIAN_POINT ( 'NONE',  ( 10.00000000000000000, 29.75893115100078745, -9.846743663894594434 ) ) ;
#48249=CARTESIAN_POINT ( 'NONE',  ( 3.591859063236761518, 44.95696800326376064, 11.09922568453594849 ) ) ;
#48250=CARTESIAN_POINT ( 'NONE',  ( 0.1532563361054082862, 26.21726448433411605, 2.638427012816831674 ) ) ;
#48251=CARTESIAN_POINT ( 'NONE',  ( 17.96484262340118221, 54.93868534415484106, 7.964842623401181321 ) ) ;
#48252=AXIS2_PLACEMENT_3D ( 'NONE', #11362, #64835, #93878 ) ;
#48253=CARTESIAN_POINT ( 'NONE',  ( 0.5774900079438590739, 67.64701867748817676, -5.440088680355550821 ) ) ;
#48255=CARTESIAN_POINT ( 'NONE',  ( 10.00000000000000178, 65.37363466993042493, 12.81628187352647608 ) ) ;
#48256=CARTESIAN_POINT ( 'NONE',  ( 7.361572987183169658, 9.967264484334119601, -9.846743663894592657 ) ) ;
#48257=CARTESIAN_POINT ( 'NONE',  ( -1.099225684535947600, 9.540301336597087456, 6.408140936763237150 ) ) ;
#48258=CARTESIAN_POINT ( 'NONE',  ( -0.1503990784575328643, 0.1277717457861260453, 6.262539305110068177 ) ) ;
#48259=CARTESIAN_POINT ( 'NONE',  ( 19.84674366389459266, 38.30059781766745175, 2.638427012816836559 ) ) ;
#48260=CARTESIAN_POINT ( 'NONE',  ( -2.816281873526473856, 64.33196800326376774, 3.434112377981055619 ) ) ;
#48261=CARTESIAN_POINT ( 'NONE',  ( 20.36894250292379738, 9.928748834913966093, -10.36894250292379027 ) ) ;
#48262=CARTESIAN_POINT ( 'NONE',  ( 19.84674366389459266, 18.71726448433411960, -2.638427012816827677 ) ) ;
#48263=CARTESIAN_POINT ( 'NONE',  ( 0.6178305044545818747, 38.49863466993042493, -9.382169495545419124 ) ) ;
#48265=CARTESIAN_POINT ( 'NONE',  ( 0.8952175423694934686, 22.60160829253886305, -5.990408912944337416 ) ) ;
#48266=CARTESIAN_POINT ( 'NONE',  ( 4.559911319644449179, 47.23035201082150536, -9.422509992056141925 ) ) ;
#48267=CARTESIAN_POINT ( 'NONE',  ( 22.81628187352647785, 11.62363466993042138, 6.195893100308588602E-16 ) ) ;
#48268=CARTESIAN_POINT ( 'NONE',  ( -0.2418659066527499291, 32.23410085661203084, -6.114288769123083611 ) ) ;
#48269=CARTESIAN_POINT ( 'NONE',  ( 7.361572987183169658, 24.96726448433412315, -9.846743663894592657 ) ) ;
#48270=CARTESIAN_POINT ( 'NONE',  ( 20.88017736071110519, 30.56368534415484106, 2.639326808657452039E-16 ) ) ;
#48271=CARTESIAN_POINT ( 'NONE',  ( 10.00000000000000000, 32.87363466993042493, -12.81628187352647608 ) ) ;
#48273=CARTESIAN_POINT ( 'NONE',  ( 7.361572987183170547, 22.05059781766745530, 9.846743663894590881 ) ) ;
#48276=CARTESIAN_POINT ( 'NONE',  ( 0.5774900079438590739, 22.64701867748817321, -5.440088680355550821 ) ) ;
#48279=CARTESIAN_POINT ( 'NONE',  ( 7.084665262690076126, 67.02201867748817676, -10.88017736071110164 ) ) ;
#48280=CARTESIAN_POINT ( 'NONE',  ( -0.8801773607111009756, 8.063685344154837509, 1.068504757029289695E-15 ) ) ;
#48281=CARTESIAN_POINT ( 'NONE',  ( 1.472469842513823179, 45.59226448433412315, -4.923371831947296329 ) ) ;
#48282=CARTESIAN_POINT ( 'NONE',  ( 7.084665262690076126, 12.02201867748817321, -10.88017736071110164 ) ) ;
#48285=CARTESIAN_POINT ( 'NONE',  ( 4.559911319644449179, 43.89701867748816966, 9.422509992056141925 ) ) ;
#48286=CARTESIAN_POINT ( 'NONE',  ( 12.91533473730992121, 19.52201867748816611, 10.88017736071110164 ) ) ;
#48287=CARTESIAN_POINT ( 'NONE',  ( -0.2418659066527782397, 20.11633188102327452, 6.114288769123032985 ) ) ;
#48289=CARTESIAN_POINT ( 'NONE',  ( 7.361572987183170547, 32.05059781766745175, 9.846743663894590881 ) ) ;
#48293=FILL_AREA_STYLE ('',( #47303 ) ) ;
#48294=CARTESIAN_POINT ( 'NONE',  ( 6.204703633549690345, 25.76208216824730712, -14.16423886937410259 ) ) ;
#48298=CARTESIAN_POINT ( 'NONE',  ( 6.204703633549690345, 65.76208216824731778, -14.16423886937410259 ) ) ;
#48299=CARTESIAN_POINT ( 'NONE',  ( 17.20831665107776587, 27.88393115100078390, 7.208316651077764980 ) ) ;
#48302=CARTESIAN_POINT ( 'NONE',  ( 17.96484262340118221, 49.93868534415484106, 7.964842623401181321 ) ) ;
#48303=CARTESIAN_POINT ( 'NONE',  ( 13.43411237798105340, 60.58196800326376064, 12.81628187352647963 ) ) ;
#48304=CARTESIAN_POINT ( 'NONE',  ( 15.44008868035555260, 29.73035201082150891, 9.422509992056143702 ) ) ;
#48306=CARTESIAN_POINT ( 'NONE',  ( 6.565887622018943937, 15.16530133659708568, 12.81628187352647430 ) ) ;
#48307=CARTESIAN_POINT ( 'NONE',  ( 12.63842701281683922, 14.55059781766744997, -9.846743663894590881 ) ) ;
#48309=CARTESIAN_POINT ( 'NONE',  ( 0.2751277870542909731, 44.36607318730131055, -6.499999999999992006 ) ) ;
#48310=CARTESIAN_POINT ( 'NONE',  ( 2.917880565312948704, 57.63708216824731068, 12.26659068614894643 ) ) ;
#48312=CARTESIAN_POINT ( 'NONE',  ( 24.16423886937409904, 24.09541550158063927, 3.795296366450317205 ) ) ;
#48313=CARTESIAN_POINT ( 'NONE',  ( 0.5774900079438607392, 18.48035201082150536, 5.440088680355550821 ) ) ;
#48314=CARTESIAN_POINT ( 'NONE',  ( 17.96484262340118221, 56.18868534415484817, -7.964842623401177768 ) ) ;
#48315=( LENGTH_UNIT ( ) NAMED_UNIT ( * ) SI_UNIT ( .MILLI., .METRE. ) );
#48317=CARTESIAN_POINT ( 'NONE',  ( 18.52753015748618282, 8.925597817667451750, -4.923371831947291888 ) ) ;
#48319=CARTESIAN_POINT ( 'NONE',  ( 18.52753015748617571, 23.09226448433411960, 4.923371831947298993 ) ) ;
#48322=CARTESIAN_POINT ( 'NONE',  ( 0.1532563361054100626, 30.80059781766744820, -2.638427012816831230 ) ) ;
#48323=CARTESIAN_POINT ( 'NONE',  ( 17.20831665107776587, 49.13393115100078745, -7.208316651077762316 ) ) ;
#48324=CARTESIAN_POINT ( 'NONE',  ( 4.559911319644449179, 27.23035201082150536, -9.422509992056141925 ) ) ;
#48326=AXIS2_PLACEMENT_3D ( 'NONE', #68439, #91420, #22947 ) ;
#48327=EDGE_CURVE ( 'NONE', #74552, #46284, #2307, .T. ) ;
#48328=CARTESIAN_POINT ( 'NONE',  ( 21.09922568453595559, 37.04030133659708923, -6.408140936763230044 ) ) ;
#48329=CARTESIAN_POINT ( 'NONE',  ( 2.035157376598822676, 57.43868534415484106, -7.964842623401177768 ) ) ;
#48330=CARTESIAN_POINT ( 'NONE',  ( 19.84674366389459621, 23.50893115100078390, 7.409399052514197653E-17 ) ) ;
#48331=CARTESIAN_POINT ( 'NONE',  ( 17.08211943468705840, 40.13708216824731068, -12.26659068614894466 ) ) ;
#48332=CARTESIAN_POINT ( 'NONE',  ( 0.1532563361054100626, 15.80059781766745353, -2.638427012816831230 ) ) ;
#48334=CARTESIAN_POINT ( 'NONE',  ( 1.472469842513823179, 56.42559781766745886, 4.923371831947296329 ) ) ;
#48335=CARTESIAN_POINT ( 'NONE',  ( 7.361572987183170547, 32.05059781766745175, 9.846743663894590881 ) ) ;
#48336=CARTESIAN_POINT ( 'NONE',  ( -2.266590686148945544, 7.220415501580634832, 7.082119434687048631 ) ) ;
#48338=CARTESIAN_POINT ( 'NONE',  ( 6.204703633549690345, 15.76208216824730179, -14.16423886937410259 ) ) ;
#48339=CARTESIAN_POINT ( 'NONE',  ( 17.20831665107776587, 24.13393115100078035, -7.208316651077762316 ) ) ;
#48340=CARTESIAN_POINT ( 'NONE',  ( 2.035157376598822676, 47.43868534415484817, -7.964842623401177768 ) ) ;
#48341=CARTESIAN_POINT ( 'NONE',  ( 2.035157376598824452, 28.68868534415484106, 7.964842623401179544 ) ) ;
#48342=CARTESIAN_POINT ( 'NONE',  ( 2.035157376598824452, 43.68868534415484106, 7.964842623401179544 ) ) ;
#48343=CARTESIAN_POINT ( 'NONE',  ( 4.559911319644449179, 33.89701867748817676, 9.422509992056141925 ) ) ;
#48345=CARTESIAN_POINT ( 'NONE',  ( 4.559911319644449179, 58.89701867748817676, 9.422509992056141925 ) ) ;
#48346=EDGE_LOOP ( 'NONE', ( #85071, #37453, #89208, #31374, #55478, #6995 ) ) ;
#48347=CARTESIAN_POINT ( 'NONE',  ( 4.559911319644449179, 62.23035201082150536, -9.422509992056141925 ) ) ;
#48349=VERTEX_POINT ( 'NONE', #91577 ) ;
#48350=CARTESIAN_POINT ( 'NONE',  ( 12.91533473730993009, 66.60535201082150536, -10.88017736071109987 ) ) ;
#48351=CARTESIAN_POINT ( 'NONE',  ( 2.603489959281601873, 25.43575266056827289, -6.500000000000015987 ) ) ;
#48352=CARTESIAN_POINT ( 'NONE',  ( 19.72487221294570858, 70.00000000000000000, 6.500000000000000888 ) ) ;
#48353=CARTESIAN_POINT ( 'NONE',  ( 24.16423886937410614, 64.30374883491396076, 8.672049930838204340E-16 ) ) ;
#48354=CARTESIAN_POINT ( 'NONE',  ( 19.84674366389459621, 13.50893115100078568, 7.409399052514197653E-17 ) ) ;
#48355=CARTESIAN_POINT ( 'NONE',  ( -4.164238869374099039, 1.803748834913967647, 8.674139862899312516E-16 ) ) ;
#48356=CARTESIAN_POINT ( 'NONE',  ( 7.361572987183169658, 4.967264484334119601, -9.846743663894592657 ) ) ;
#48358=CARTESIAN_POINT ( 'NONE',  ( 12.63842701281683034, 42.46726448433412315, 9.846743663894596210 ) ) ;
#48361=CARTESIAN_POINT ( 'NONE',  ( 10.00000000000000178, 47.25893115100078745, 9.846743663894594434 ) ) ;
#48365=CARTESIAN_POINT ( 'NONE',  ( 20.88017736071110875, 55.77201867748816966, -2.915334737309920765 ) ) ;
#48366=CARTESIAN_POINT ( 'NONE',  ( 14.92337183194729988, 49.34226448433411605, -8.527530157486177487 ) ) ;
#48369=CARTESIAN_POINT ( 'NONE',  ( 20.88017736071110519, 60.56368534415484106, 2.639326808657452039E-16 ) ) ;
#48370=CARTESIAN_POINT ( 'NONE',  ( 2.917880565312950480, 65.97041550158063217, -12.26659068614894821 ) ) ;
#48371=EDGE_CURVE ( 'NONE', #61558, #76088, #94649, .T. ) ;
#48372=CARTESIAN_POINT ( 'NONE',  ( 21.09922568453595559, 37.04030133659708923, -6.408140936763230044 ) ) ;
#48374=VERTEX_POINT ( 'NONE', #54542 ) ;
#48375=CARTESIAN_POINT ( 'NONE',  ( 13.43411237798105340, 30.58196800326374998, 12.81628187352647963 ) ) ;
#48376=CARTESIAN_POINT ( 'NONE',  ( 12.91533473730992121, 29.52201867748817321, 10.88017736071110164 ) ) ;
#48379=CARTESIAN_POINT ( 'NONE',  ( 5.076628168052704559, 10.17559781766745175, -8.527530157486179263 ) ) ;
#48381=CARTESIAN_POINT ( 'NONE',  ( 12.63842701281683922, 64.55059781766745175, -9.846743663894590881 ) ) ;
#48382=CARTESIAN_POINT ( 'NONE',  ( 7.361572987183170547, 7.050597817667451750, 9.846743663894590881 ) ) ;
#48383=CARTESIAN_POINT ( 'NONE',  ( 17.20831665107776587, 44.13393115100078745, -7.208316651077762316 ) ) ;
#48385=CARTESIAN_POINT ( 'NONE',  ( 3.591859063236761518, 64.95696800326376774, 11.09922568453594849 ) ) ;
#48386=CARTESIAN_POINT ( 'NONE',  ( 0.1532563361054100626, 40.80059781766745886, -2.638427012816831230 ) ) ;
#48390=CARTESIAN_POINT ( 'NONE',  ( 7.361572987183169658, 29.96726448433411960, -9.846743663894592657 ) ) ;
#48391=LINE ( 'NONE', #17426, #70667 ) ;
#48393=CARTESIAN_POINT ( 'NONE',  ( 19.84674366389459266, 53.71726448433411605, -2.638427012816827677 ) ) ;
#48396=CARTESIAN_POINT ( 'NONE',  ( 6.565887622018943937, 25.16530133659708213, 12.81628187352647430 ) ) ;
#48397=CARTESIAN_POINT ( 'NONE',  ( 7.361572987183169658, 49.96726448433410894, -9.846743663894592657 ) ) ;
#48398=LINE ( 'NONE', #94389, #91956 ) ;
#48399=CARTESIAN_POINT ( 'NONE',  ( 24.16423886937409904, 49.09541550158063217, 3.795296366450317205 ) ) ;
#48400=CARTESIAN_POINT ( 'NONE',  ( 19.84674366389459266, 13.30059781766745353, 2.638427012816836559 ) ) ;
#48401=ORIENTED_EDGE ( 'NONE', *, *, #59426, .T. ) ;
#48402=SURFACE_SIDE_STYLE ('',( #46439 ) ) ;
#48404=CARTESIAN_POINT ( 'NONE',  ( -4.164238869374099927, 47.01208216824729647, 3.795296366450308767 ) ) ;
#48405=CARTESIAN_POINT ( 'NONE',  ( 0.1532563361054100626, 60.80059781766744464, -2.638427012816831230 ) ) ;
#48406=CARTESIAN_POINT ( 'NONE',  ( -0.8801773607111008646, 3.272018677488171434, 2.915334737309923430 ) ) ;
#48407=CARTESIAN_POINT ( 'NONE',  ( 6.204703633549690345, 25.76208216824730712, -14.16423886937410259 ) ) ;
#48408=CARTESIAN_POINT ( 'NONE',  ( 10.00000000000000178, 43.05374883491397497, 14.16423886937410082 ) ) ;
#48409=CARTESIAN_POINT ( 'NONE',  ( 14.49999999999999822, 11.50000000000000000, -6.000000000000000000 ) ) ;
#48410=FACE_OUTER_BOUND ( 'NONE', #41090, .T. ) ;
#48411=CARTESIAN_POINT ( 'NONE',  ( 1.472469842513823179, 56.42559781766745886, 4.923371831947296329 ) ) ;
#48412=CARTESIAN_POINT ( 'NONE',  ( 4.559911319644449179, 38.89701867748817676, 9.422509992056141925 ) ) ;
#48415=EDGE_CURVE ( 'NONE', #28166, #56195, #21100, .T. ) ;
#48416=CARTESIAN_POINT ( 'NONE',  ( 1.472469842513823179, 35.59226448433412315, -4.923371831947296329 ) ) ;
#48419=CARTESIAN_POINT ( 'NONE',  ( 2.791683348922240793, 61.63393115100079456, 7.208316651077764092 ) ) ;
#48420=CARTESIAN_POINT ( 'NONE',  ( 0.1532563361054082862, 61.21726448433412315, 2.638427012816831674 ) ) ;
#48421=EDGE_LOOP ( 'NONE', ( #29164, #65073, #57489, #72684 ) ) ;
#48422=CARTESIAN_POINT ( 'NONE',  ( -4.164238869374099927, 32.01208216824730357, 3.795296366450308767 ) ) ;
#48423=CARTESIAN_POINT ( 'NONE',  ( 13.99999999999999822, 60.50000000000000000, 6.000000000000000000 ) ) ;
#48426=CARTESIAN_POINT ( 'NONE',  ( 19.42250999205614548, 10.98035201082150536, -5.440088680355545492 ) ) ;
#48428=CARTESIAN_POINT ( 'NONE',  ( 19.38216949554541202, 30.99863466993042138, 9.382169495545424454 ) ) ;
#48430=CARTESIAN_POINT ( 'NONE',  ( 17.20831665107776587, 9.133931151000787452, -7.208316651077762316 ) ) ;
#48432=CARTESIAN_POINT ( 'NONE',  ( 20.15039907845753220, 41.74884699246887720, 6.262539305110078836 ) ) ;
#48433=DIRECTION ( 'NONE',  ( -1.000000000000000000, 0.000000000000000000, 0.000000000000000000 ) ) ;
#48435=CARTESIAN_POINT ( 'NONE',  ( 20.88017736071110164, 15.35535201082150358, 2.915334737309930979 ) ) ;
#48437=CARTESIAN_POINT ( 'NONE',  ( 4.559911319644449179, 42.23035201082151247, -9.422509992056141925 ) ) ;
#48438=CARTESIAN_POINT ( 'NONE',  ( -0.8801773607110991993, 42.85535201082150536, -2.915334737309923874 ) ) ;
#48440=CARTESIAN_POINT ( 'NONE',  ( 6.565887622018943937, -1.918031996736246692, -12.81628187352647608 ) ) ;
#48442=CARTESIAN_POINT ( 'NONE',  ( -45.11020673897264999, 105.3618001163576849, -4.929053739391441979 ) ) ;
#48443=CARTESIAN_POINT ( 'NONE',  ( 12.63842701281683034, 7.467264484334118713, 9.846743663894596210 ) ) ;
#48445=CARTESIAN_POINT ( 'NONE',  ( 19.42250999205614548, 35.98035201082151247, -5.440088680355545492 ) ) ;
#48446=CARTESIAN_POINT ( 'NONE',  ( -1.099225684535947600, 34.54030133659708923, 6.408140936763237150 ) ) ;
#48449=EDGE_CURVE ( 'NONE', #6068, #58843, #29549, .T. ) ;
#48450=CARTESIAN_POINT ( 'NONE',  ( 0.1532563361054082862, 61.21726448433412315, 2.638427012816831674 ) ) ;
#48451=CARTESIAN_POINT ( 'NONE',  ( -0.8801773607111008646, 58.27201867748816966, 2.915334737309923430 ) ) ;
#48452=CARTESIAN_POINT ( 'NONE',  ( 19.84674366389459621, 8.508931151000785675, 7.409399052514197653E-17 ) ) ;
#48453=CARTESIAN_POINT ( 'NONE',  ( -1.099225684535947600, 29.54030133659708923, 6.408140936763237150 ) ) ;
#48454=CARTESIAN_POINT ( 'NONE',  ( 7.084665262690076126, 67.02201867748817676, -10.88017736071110164 ) ) ;
#48458=CARTESIAN_POINT ( 'NONE',  ( 20.88017736071110519, 5.563685344154837509, 2.639326808657452039E-16 ) ) ;
#48459=CARTESIAN_POINT ( 'NONE',  ( 0.6178305044545818747, 63.49863466993043204, -9.382169495545419124 ) ) ;
#48460=CARTESIAN_POINT ( 'NONE',  ( -0.3689425029237898834, 26.17874883491396432, -10.36894250292378850 ) ) ;
#48461=CARTESIAN_POINT ( 'NONE',  ( 2.791683348922237240, 15.38393115100078212, -7.208316651077763204 ) ) ;
#48462=CARTESIAN_POINT ( 'NONE',  ( 20.88017736071110875, 5.772018677488170546, -2.915334737309920765 ) ) ;
#48463=CARTESIAN_POINT ( 'NONE',  ( 10.00000000000000178, 22.25893115100078745, 9.846743663894594434 ) ) ;
#48464=CARTESIAN_POINT ( 'NONE',  ( -4.164238869374099927, 57.01208216824731068, 3.795296366450308767 ) ) ;
#48466=CARTESIAN_POINT ( 'NONE',  ( -0.8801773607111009756, 13.06368534415483929, 1.068504757029289695E-15 ) ) ;
#48468=CARTESIAN_POINT ( 'NONE',  ( 0.5774900079438590739, 27.64701867748817676, -5.440088680355550821 ) ) ;
#48469=CARTESIAN_POINT ( 'NONE',  ( 2.153642693323440938, 31.13791097397318097, -6.500000000000005329 ) ) ;
#48470=VERTEX_POINT ( 'NONE', #92546 ) ;
#48472=CARTESIAN_POINT ( 'NONE',  ( 10.00000000000000178, 19.31368534415484106, 10.88017736071110342 ) ) ;
#48473=CARTESIAN_POINT ( 'NONE',  ( 5.076628168052704559, 60.17559781766745175, -8.527530157486179263 ) ) ;
#48474=CARTESIAN_POINT ( 'NONE',  ( 0.6178305044545818747, 48.49863466993042493, -9.382169495545419124 ) ) ;
#48476=CARTESIAN_POINT ( 'NONE',  ( 13.79529636645031943, 15.34541550158063750, -14.16423886937409904 ) ) ;
#48477=CARTESIAN_POINT ( 'NONE',  ( 4.559911319644449179, 43.89701867748816966, 9.422509992056141925 ) ) ;
#48478=CARTESIAN_POINT ( 'NONE',  ( 17.96484262340118221, 16.18868534415483396, -7.964842623401177768 ) ) ;
#48479=CARTESIAN_POINT ( 'NONE',  ( 2.791683348922240793, 51.63393115100078745, 7.208316651077764092 ) ) ;
#48481=CARTESIAN_POINT ( 'NONE',  ( 19.84674366389459266, 38.30059781766745175, 2.638427012816836559 ) ) ;
#48482=CARTESIAN_POINT ( 'NONE',  ( 19.84674366389459266, 8.717264484334116048, -2.638427012816827677 ) ) ;
#48486=CARTESIAN_POINT ( 'NONE',  ( 5.076628168052704559, 15.17559781766745175, -8.527530157486179263 ) ) ;
#48487=CARTESIAN_POINT ( 'NONE',  ( 7.361572987183169658, 64.96726448433412315, -9.846743663894592657 ) ) ;
#48488=CARTESIAN_POINT ( 'NONE',  ( 19.42250999205614548, 40.98035201082150536, -5.440088680355545492 ) ) ;
#48489=CARTESIAN_POINT ( 'NONE',  ( 0.5774900079438607392, 18.48035201082150536, 5.440088680355550821 ) ) ;
#48490=CARTESIAN_POINT ( 'NONE',  ( -2.816281873526471635, 48.91530133659708213, -3.434112377981056508 ) ) ;
#48491=CARTESIAN_POINT ( 'NONE',  ( 17.08211943468705840, 25.13708216824730357, -12.26659068614894466 ) ) ;
#48493=DIRECTION ( 'NONE',  ( -0.000000000000000000, -0.000000000000000000, 1.000000000000000000 ) ) ;
#48495=CARTESIAN_POINT ( 'NONE',  ( 22.81628187352647785, 56.41530133659708213, 3.434112377981063169 ) ) ;
#48497=CARTESIAN_POINT ( 'NONE',  ( 0.1532563361054082862, 56.21726448433411605, 2.638427012816831674 ) ) ;
#48498=CARTESIAN_POINT ( 'NONE',  ( -0.8801773607111008646, 38.27201867748816255, 2.915334737309923430 ) ) ;
#48501=CARTESIAN_POINT ( 'NONE',  ( 1.472469842513823179, 0.5922644843341181575, -4.923371831947296329 ) ) ;
#48502=CARTESIAN_POINT ( 'NONE',  ( 7.361572987183169658, 9.967264484334119601, -9.846743663894592657 ) ) ;
#48503=CARTESIAN_POINT ( 'NONE',  ( -0.8801773607110991993, 62.85535201082150536, -2.915334737309923874 ) ) ;
#48505=CARTESIAN_POINT ( 'NONE',  ( 0.5774900079438590739, 52.64701867748817676, -5.440088680355550821 ) ) ;
#48507=CARTESIAN_POINT ( 'NONE',  ( -0.8801773607111008646, 58.27201867748816966, 2.915334737309923430 ) ) ;
#48508=CARTESIAN_POINT ( 'NONE',  ( 2.791683348922240793, 1.633931151000784565, 7.208316651077764092 ) ) ;
#48510=CARTESIAN_POINT ( 'NONE',  ( -0.8801773607111009756, 63.27201867748817676, 2.915334737309923874 ) ) ;
#48511=CARTESIAN_POINT ( 'NONE',  ( 19.84674366389459266, 58.30059781766745886, 2.638427012816836559 ) ) ;
#48513=ORIENTED_EDGE ( 'NONE', *, *, #32933, .T. ) ;
#48515=CARTESIAN_POINT ( 'NONE',  ( 22.26659068614894466, 8.887082168247300018, 7.082119434687054849 ) ) ;
#48516=CARTESIAN_POINT ( 'NONE',  ( 0.6178305044545838731, 64.74863466993043914, 9.382169495545420901 ) ) ;
#48517=CARTESIAN_POINT ( 'NONE',  ( 6.204703633549690345, 0.7620821682473009062, -14.16423886937410259 ) ) ;
#48518=CARTESIAN_POINT ( 'NONE',  ( 13.79529636645030344, 33.26208216824730357, 14.16423886937410614 ) ) ;
#48519=CARTESIAN_POINT ( 'NONE',  ( 0.2751277870542876425, 45.30223176428830811, 6.499999999999984901 ) ) ;
#48520=CARTESIAN_POINT ( 'NONE',  ( 22.26659068614894466, 3.887082168247300906, 7.082119434687054849 ) ) ;
#48521=CARTESIAN_POINT ( 'NONE',  ( 19.42250999205614548, 15.98035201082150714, -5.440088680355545492 ) ) ;
#48524=CARTESIAN_POINT ( 'NONE',  ( 18.52753015748617571, 3.092264484334118269, 4.923371831947298993 ) ) ;
#48525=CARTESIAN_POINT ( 'NONE',  ( 12.63842701281683922, 14.55059781766744997, -9.846743663894590881 ) ) ;
#48526=CARTESIAN_POINT ( 'NONE',  ( -2.816281873526473856, 49.33196800326374643, 3.434112377981055619 ) ) ;
#48527=CARTESIAN_POINT ( 'NONE',  ( 17.20831665107776587, 37.88393115100078745, 7.208316651077764980 ) ) ;
#48529=CARTESIAN_POINT ( 'NONE',  ( -0.8801773607111009756, 58.06368534415484106, 1.068504757029289695E-15 ) ) ;
#48531=CARTESIAN_POINT ( 'NONE',  ( 6.565887622018943937, 35.16530133659708923, 12.81628187352647430 ) ) ;
#48533=CARTESIAN_POINT ( 'NONE',  ( 1.472469842513823179, 25.59226448433412315, -4.923371831947296329 ) ) ;
#48534=CARTESIAN_POINT ( 'NONE',  ( 6.204703633549690345, 10.76208216824729824, -14.16423886937410259 ) ) ;
#48538=CARTESIAN_POINT ( 'NONE',  ( 0.5774900079438590739, 32.64701867748816966, -5.440088680355550821 ) ) ;
#48539=CARTESIAN_POINT ( 'NONE',  ( 22.26659068614895176, 34.72041550158063927, -7.082119434687042414 ) ) ;
#48540=CARTESIAN_POINT ( 'NONE',  ( 17.20831665107776587, 47.88393115100078745, 7.208316651077764980 ) ) ;
#48541=CARTESIAN_POINT ( 'NONE',  ( 5.076628168052704559, 10.17559781766745175, -8.527530157486179263 ) ) ;
#48542=CARTESIAN_POINT ( 'NONE',  ( 19.38216949554541202, 50.99863466993042493, 9.382169495545424454 ) ) ;
#48544=CARTESIAN_POINT ( 'NONE',  ( 17.96484262340118221, 24.93868534415484461, 7.964842623401181321 ) ) ;
#48546=CARTESIAN_POINT ( 'NONE',  ( 13.43411237798105340, 25.58196800326374998, 12.81628187352647963 ) ) ;
#48547=CARTESIAN_POINT ( 'NONE',  ( 2.791683348922237240, 35.38393115100079456, -7.208316651077763204 ) ) ;
#48549=CARTESIAN_POINT ( 'NONE',  ( -25.69000000000001194, 93.50000000000000000, -10.09898361729590199 ) ) ;
#48550=CARTESIAN_POINT ( 'NONE',  ( 10.00000000000000000, 61.81368534415484106, -10.88017736071110342 ) ) ;
#48551=CARTESIAN_POINT ( 'NONE',  ( 18.95386800105010394, 33.23810908735718783, -6.500000000000008882 ) ) ;
#48554=CARTESIAN_POINT ( 'NONE',  ( 7.084665262690076126, 59.10535201082150536, 10.88017736071109987 ) ) ;
#48555=CARTESIAN_POINT ( 'NONE',  ( -0.8801773607110991993, 52.85535201082151247, -2.915334737309923874 ) ) ;
#48558=ADVANCED_FACE ( 'NONE', ( #10536 ), #93535, .T. ) ;
#48560=CARTESIAN_POINT ( 'NONE',  ( 12.91533473730993009, 11.60535201082150714, -10.88017736071109987 ) ) ;
#48561=CARTESIAN_POINT ( 'NONE',  ( 10.00000000000000178, 62.25893115100078745, 9.846743663894594434 ) ) ;
#48562=CARTESIAN_POINT ( 'NONE',  ( 17.96484262340118221, 16.18868534415483396, -7.964842623401177768 ) ) ;
#48564=CARTESIAN_POINT ( 'NONE',  ( 16.40814093676323893, 30.79030133659708923, 11.09922568453595026 ) ) ;
#48566=CARTESIAN_POINT ( 'NONE',  ( -0.8801773607111009756, 53.06368534415484106, 1.068504757029289695E-15 ) ) ;
#48568=CARTESIAN_POINT ( 'NONE',  ( 12.63842701281683922, 44.55059781766745175, -9.846743663894590881 ) ) ;
#48569=AXIS2_PLACEMENT_3D ( 'NONE', #52233, #59725, #23729 ) ;
#48570=CARTESIAN_POINT ( 'NONE',  ( 10.00000000000000000, 7.873634669930421381, -12.81628187352647608 ) ) ;
#48571=SURFACE_STYLE_FILL_AREA ( #57055 ) ;
#48572=CARTESIAN_POINT ( 'NONE',  ( 19.42250999205614548, 25.98035201082150891, -5.440088680355545492 ) ) ;
#48573=CARTESIAN_POINT ( 'NONE',  ( 2.035157376598822676, 42.43868534415483396, -7.964842623401177768 ) ) ;
#48574=CARTESIAN_POINT ( 'NONE',  ( -0.3689425029237898834, 51.17874883491397497, -10.36894250292378850 ) ) ;
#48575=CARTESIAN_POINT ( 'NONE',  ( 17.20831665107776587, 37.88393115100078745, 7.208316651077764980 ) ) ;
#48576=CARTESIAN_POINT ( 'NONE',  ( 19.42250999205614548, 60.98035201082151247, -5.440088680355545492 ) ) ;
#48577=CARTESIAN_POINT ( 'NONE',  ( -0.8801773607111009756, 48.06368534415484817, 1.068504757029289695E-15 ) ) ;
#48579=CARTESIAN_POINT ( 'NONE',  ( 24.16423886937410614, 14.30374883491396787, 8.672049930838204340E-16 ) ) ;
#48581=CARTESIAN_POINT ( 'NONE',  ( 0.2751277870542874204, 39.36607318730131055, -6.499999999999984901 ) ) ;
#48584=CARTESIAN_POINT ( 'NONE',  ( 24.16423886937410614, 49.30374883491396787, 8.672049930838204340E-16 ) ) ;
#48585=CARTESIAN_POINT ( 'NONE',  ( 20.36894250292379382, 38.67874883491396076, 10.36894250292379205 ) ) ;
#48586=CARTESIAN_POINT ( 'NONE',  ( 1.472469842513823179, 21.42559781766745175, 4.923371831947296329 ) ) ;
#48588=CARTESIAN_POINT ( 'NONE',  ( 20.15039907845753220, 52.62777174578612716, -6.262539305110077947 ) ) ;
#48589=CARTESIAN_POINT ( 'NONE',  ( 7.084665262690076126, 67.02201867748817676, -10.88017736071110164 ) ) ;
#48590=CARTESIAN_POINT ( 'NONE',  ( -2.816281873526473856, 29.33196800326376064, 3.434112377981055619 ) ) ;
#48591=CARTESIAN_POINT ( 'NONE',  ( -4.164238869374099927, 37.01208216824731068, 3.795296366450308767 ) ) ;
#48593=CARTESIAN_POINT ( 'NONE',  ( 7.084665262690076126, 69.10535201082151957, 10.88017736071109987 ) ) ;
#48595=CARTESIAN_POINT ( 'NONE',  ( 14.92337183194729633, 7.675597817667451750, 8.527530157486181039 ) ) ;
#48596=EDGE_LOOP ( 'NONE', ( #25181, #61978, #2545, #95861 ) ) ;
#48597=( NAMED_UNIT ( * ) SI_UNIT ( $, .STERADIAN. ) SOLID_ANGLE_UNIT ( ) );
#48598=CARTESIAN_POINT ( 'NONE',  ( 1.472469842513823179, 16.42559781766745175, 4.923371831947296329 ) ) ;
#48599=FACE_OUTER_BOUND ( 'NONE', #41974, .T. ) ;
#48601=CARTESIAN_POINT ( 'NONE',  ( 24.16423886937410614, 4.512082168247300906, -3.795296366450302550 ) ) ;
#48602=CARTESIAN_POINT ( 'NONE',  ( 7.084665262690076126, 9.105352010821503583, 10.88017736071109987 ) ) ;
#48603=CARTESIAN_POINT ( 'NONE',  ( -0.8801773607111009756, 13.06368534415483929, 1.068504757029289695E-15 ) ) ;
#48604=CARTESIAN_POINT ( 'NONE',  ( 5.076628168052704559, 30.17559781766745175, -8.527530157486179263 ) ) ;
#48605=CARTESIAN_POINT ( 'NONE',  ( 0.6178305044545838731, 4.748634669930420493, 9.382169495545420901 ) ) ;
#48609=EDGE_CURVE ( 'NONE', #24064, #56450, #25554, .T. ) ;
#48610=CARTESIAN_POINT ( 'NONE',  ( 10.00000000000000000, 12.87363466993042138, -12.81628187352647608 ) ) ;
#48612=CARTESIAN_POINT ( 'NONE',  ( -0.3689425029237898834, 46.17874883491397497, -10.36894250292378850 ) ) ;
#48614=CARTESIAN_POINT ( 'NONE',  ( 17.08211943468705840, 60.13708216824729647, -12.26659068614894466 ) ) ;
#48616=CARTESIAN_POINT ( 'NONE',  ( 0.5774900079438590739, 27.64701867748817676, -5.440088680355550821 ) ) ;
#48617=CARTESIAN_POINT ( 'NONE',  ( 0.5774900079438590739, 37.64701867748817676, -5.440088680355550821 ) ) ;
#48618=CARTESIAN_POINT ( 'NONE',  ( 19.42250999205614548, 60.98035201082151247, -5.440088680355545492 ) ) ;
#48619=CARTESIAN_POINT ( 'NONE',  ( 15.44008868035555260, 29.73035201082150891, 9.422509992056143702 ) ) ;
#48623=CARTESIAN_POINT ( 'NONE',  ( 18.52753015748617571, 18.09226448433411960, 4.923371831947298993 ) ) ;
#48627=CARTESIAN_POINT ( 'NONE',  ( 2.791683348922237240, 45.38393115100079456, -7.208316651077763204 ) ) ;
#48628=VECTOR ( 'NONE', #47441, 1000.000000000000000 ) ;
#48630=CARTESIAN_POINT ( 'NONE',  ( 3.591859063236761518, 44.95696800326376064, 11.09922568453594849 ) ) ;
#48633=CYLINDRICAL_SURFACE ( 'NONE', #26859, 1.000000000000007772 ) ;
#48635=CARTESIAN_POINT ( 'NONE',  ( 2.791683348922240793, 61.63393115100079456, 7.208316651077764092 ) ) ;
#48636=CARTESIAN_POINT ( 'NONE',  ( 24.16423886937410614, 49.30374883491396787, 8.672049930838204340E-16 ) ) ;
#48639=CARTESIAN_POINT ( 'NONE',  ( 1.042145700049401436, 4.742161081720030147, -6.499999999999861444 ) ) ;
#48640=CARTESIAN_POINT ( 'NONE',  ( 1.472469842513823179, 26.42559781766745175, 4.923371831947296329 ) ) ;
#48641=CARTESIAN_POINT ( 'NONE',  ( -2.816281873526473856, 64.33196800326376774, 3.434112377981055619 ) ) ;
#48642=CARTESIAN_POINT ( 'NONE',  ( 1.472469842513823179, 65.59226448433412315, -4.923371831947296329 ) ) ;
#48643=CARTESIAN_POINT ( 'NONE',  ( 14.92337183194729633, 2.675597817667451750, 8.527530157486181039 ) ) ;
#48644=CARTESIAN_POINT ( 'NONE',  ( -0.03743638938523734944, 4.251975280310180239, -6.399506433553933782 ) ) ;
#48646=CARTESIAN_POINT ( 'NONE',  ( 12.63842701281683922, 64.55059781766745175, -9.846743663894590881 ) ) ;
#48647=CARTESIAN_POINT ( 'NONE',  ( 20.32896413005680358, 14.74545670184113710, 5.963430220938287007 ) ) ;
#48648=MECHANICAL_DESIGN_GEOMETRIC_PRESENTATION_REPRESENTATION('',(#64618),#37549);
#48652=CARTESIAN_POINT ( 'NONE',  ( 24.16423886937410614, 59.51208216824728936, -3.795296366450302550 ) ) ;
#48654=CARTESIAN_POINT ( 'NONE',  ( 7.084665262690076126, 47.02201867748818387, -10.88017736071110164 ) ) ;
#48655=CARTESIAN_POINT ( 'NONE',  ( -2.816281873526471635, 13.91530133659708746, -3.434112377981056508 ) ) ;
#48656=CARTESIAN_POINT ( 'NONE',  ( 17.96484262340118221, 66.18868534415483396, -7.964842623401177768 ) ) ;
#48658=CARTESIAN_POINT ( 'NONE',  ( 19.80777595082615861, 45.68878173731741299, -6.499999999999961808 ) ) ;
#48659=CARTESIAN_POINT ( 'NONE',  ( 1.472469842513823179, 56.42559781766745886, 4.923371831947296329 ) ) ;
#48660=CARTESIAN_POINT ( 'NONE',  ( 10.00000000000000178, 7.258931151000785675, 9.846743663894594434 ) ) ;
#48662=CARTESIAN_POINT ( 'NONE',  ( 22.81628187352647785, 6.623634669930420493, 6.195893100308588602E-16 ) ) ;
#48663=CARTESIAN_POINT ( 'NONE',  ( 10.00000000000000000, 21.81368534415484106, -10.88017736071110342 ) ) ;
#48665=CARTESIAN_POINT ( 'NONE',  ( 13.99999999999999822, 10.49999999999999822, -6.000000000000000000 ) ) ;
#48667=CARTESIAN_POINT ( 'NONE',  ( 6.204703633549690345, 37.84541550158063927, 14.16423886937410082 ) ) ;
#48668=CARTESIAN_POINT ( 'NONE',  ( 13.79529636645031943, 25.34541550158063572, -14.16423886937409904 ) ) ;
#48669=CARTESIAN_POINT ( 'NONE',  ( 7.084665262690076126, 2.022018677488171434, -10.88017736071110164 ) ) ;
#48670=CARTESIAN_POINT ( 'NONE',  ( 19.84674366389459266, 38.30059781766745175, 2.638427012816836559 ) ) ;
#48671=CARTESIAN_POINT ( 'NONE',  ( 22.81628187352648496, 41.83196800326375353, -3.434112377981050290 ) ) ;
#48672=CARTESIAN_POINT ( 'NONE',  ( -0.8801773607111009756, 13.06368534415483929, 1.068504757029289695E-15 ) ) ;
#48673=ORIENTED_EDGE ( 'NONE', *, *, #40324, .F. ) ;
#48674=CARTESIAN_POINT ( 'NONE',  ( 18.52753015748617571, 33.09226448433411605, 4.923371831947298993 ) ) ;
#48675=CARTESIAN_POINT ( 'NONE',  ( -0.8801773607111008646, 43.27201867748817676, 2.915334737309923430 ) ) ;
#48676=CARTESIAN_POINT ( 'NONE',  ( 6.565887622018943937, 10.16530133659708746, 12.81628187352647430 ) ) ;
#48677=CARTESIAN_POINT ( 'NONE',  ( 17.08211943468705840, 15.13708216824730179, -12.26659068614894466 ) ) ;
#48679=B_SPLINE_CURVE_WITH_KNOTS ( 'NONE', 3,
 ( #87924, #80928, #19441, #49930, #33924, #11936, #65415, #26933, #42441, #72923 ),
 .UNSPECIFIED., .F., .F.,
 ( 4, 3, 3, 4 ),
 ( 7.573910767901059648E-18, 0.0006253016069560791285, 0.001250604074564940806, 0.002501455912506563885 ),
 .UNSPECIFIED. ) ;
#48681=CARTESIAN_POINT ( 'NONE',  ( 19.84674366389459266, 28.30059781766745886, 2.638427012816836559 ) ) ;
#48682=CARTESIAN_POINT ( 'NONE',  ( -1.099225684535947600, 53.70696800326376064, -6.408140936763238038 ) ) ;
#48683=CARTESIAN_POINT ( 'NONE',  ( 12.63842701281683922, 59.55059781766744464, -9.846743663894590881 ) ) ;
#48684=ORIENTED_EDGE ( 'NONE', *, *, #46967, .F. ) ;
#48688=CARTESIAN_POINT ( 'NONE',  ( -0.3689425029237881626, 62.42874883491396787, 10.36894250292379027 ) ) ;
#48689=CARTESIAN_POINT ( 'NONE',  ( 22.26659068614895176, 9.720415501580633943, -7.082119434687042414 ) ) ;
#48690=CARTESIAN_POINT ( 'NONE',  ( 20.88017736071110164, 65.35535201082150536, 2.915334737309930979 ) ) ;
#48691=CARTESIAN_POINT ( 'NONE',  ( 5.076628168052704559, 45.17559781766745175, -8.527530157486179263 ) ) ;
#48692=CARTESIAN_POINT ( 'NONE',  ( 2.035157376598824452, 23.68868534415484461, 7.964842623401179544 ) ) ;
#48694=CARTESIAN_POINT ( 'NONE',  ( 18.52753015748617571, 63.09226448433412315, 4.923371831947298993 ) ) ;
#48695=VECTOR ( 'NONE', #73889, 1000.000000000000000 ) ;
#48696=ORIENTED_EDGE ( 'NONE', *, *, #92118, .F. ) ;
#48700=CARTESIAN_POINT ( 'NONE',  ( 6.204703633549690345, 10.76208216824729824, -14.16423886937410259 ) ) ;
#48701=FILL_AREA_STYLE ('',( #25248 ) ) ;
#48702=CARTESIAN_POINT ( 'NONE',  ( 13.79529636645030344, 38.26208216824729647, 14.16423886937410614 ) ) ;
#48703=CARTESIAN_POINT ( 'NONE',  ( 18.52753015748618282, 58.92559781766745886, -4.923371831947291888 ) ) ;
#48704=CARTESIAN_POINT ( 'NONE',  ( 10.00000000000000000, 19.75893115100078390, -9.846743663894594434 ) ) ;
#48705=CARTESIAN_POINT ( 'NONE',  ( -2.816281873526473856, 64.33196800326376774, 3.434112377981055619 ) ) ;
#48706=CARTESIAN_POINT ( 'NONE',  ( 17.96484262340118221, 24.93868534415484461, 7.964842623401181321 ) ) ;
#48707=CARTESIAN_POINT ( 'NONE',  ( 18.52753015748617571, 58.09226448433411605, 4.923371831947298993 ) ) ;
#48708=CARTESIAN_POINT ( 'NONE',  ( -4.164238869374099927, 2.012082168247300906, 3.795296366450308767 ) ) ;
#48709=CARTESIAN_POINT ( 'NONE',  ( 2.917880565312948704, 42.63708216824729647, 12.26659068614894643 ) ) ;
#48711=CARTESIAN_POINT ( 'NONE',  ( -0.8801773607111008646, 8.272018677488171434, 2.915334737309923430 ) ) ;
#48712=CARTESIAN_POINT ( 'NONE',  ( 5.076628168052703671, 66.84226448433412315, 8.527530157486179263 ) ) ;
#48714=CARTESIAN_POINT ( 'NONE',  ( 15.44008868035555260, 64.73035201082151957, 9.422509992056143702 ) ) ;
#48715=CARTESIAN_POINT ( 'NONE',  ( 14.92337183194729988, 34.34226448433411605, -8.527530157486177487 ) ) ;
#48717=ORIENTED_EDGE ( 'NONE', *, *, #81866, .F. ) ;
#48720=CARTESIAN_POINT ( 'NONE',  ( 18.52753015748617571, 23.09226448433411960, 4.923371831947298993 ) ) ;
#48722=CARTESIAN_POINT ( 'NONE',  ( 24.16423886937410614, 39.30374883491396787, 8.672049930838204340E-16 ) ) ;
#48723=CARTESIAN_POINT ( 'NONE',  ( 0.1532563361054083140, 36.00893115100078745, 1.131784320476157264E-15 ) ) ;
#48724=CARTESIAN_POINT ( 'NONE',  ( 15.44008868035555260, 49.73035201082150536, 9.422509992056143702 ) ) ;
#48725=CARTESIAN_POINT ( 'NONE',  ( 0.5774900079438590739, 47.64701867748817676, -5.440088680355550821 ) ) ;
#48730=CARTESIAN_POINT ( 'NONE',  ( 20.88017736071110519, 45.56368534415484106, 2.639326808657452039E-16 ) ) ;
#48731=CARTESIAN_POINT ( 'NONE',  ( -2.266590686148945544, 1.387082168247301128, -7.082119434687050408 ) ) ;
#48733=CARTESIAN_POINT ( 'NONE',  ( 10.00000000000000178, 30.37363466993042138, 12.81628187352647608 ) ) ;
#48734=CARTESIAN_POINT ( 'NONE',  ( 19.84674366389459266, 28.71726448433411960, -2.638427012816827677 ) ) ;
#48735=PRESENTATION_STYLE_ASSIGNMENT (( #26724 ) ) ;
#48736=CARTESIAN_POINT ( 'NONE',  ( 22.81628187352647785, 46.62363466993041783, 6.195893100308588602E-16 ) ) ;
#48738=CARTESIAN_POINT ( 'NONE',  ( 7.361572987183170547, 27.05059781766745175, 9.846743663894590881 ) ) ;
#48741=CARTESIAN_POINT ( 'NONE',  ( 0.5774900079438607392, 58.48035201082151247, 5.440088680355550821 ) ) ;
#48742=VECTOR ( 'NONE', #12646, 1000.000000000000000 ) ;
#48744=CARTESIAN_POINT ( 'NONE',  ( -46.30928139467842897, 104.0823827281712255, 5.529860068218143354 ) ) ;
#48746=CARTESIAN_POINT ( 'NONE',  ( 19.84674366389459266, 3.300597817667451750, 2.638427012816836559 ) ) ;
#48747=CARTESIAN_POINT ( 'NONE',  ( 19.38216949554541557, 7.248634669930421381, -9.382169495545420901 ) ) ;
#48750=CARTESIAN_POINT ( 'NONE',  ( 19.84674366389459266, 43.30059781766744464, 2.638427012816836559 ) ) ;
#48751=CARTESIAN_POINT ( 'NONE',  ( 19.38216949554541557, 62.24863466993041072, -9.382169495545420901 ) ) ;
#48752=CARTESIAN_POINT ( 'NONE',  ( 10.00000000000000178, 8.053748834913967869, 14.16423886937410082 ) ) ;
#48753=CARTESIAN_POINT ( 'NONE',  ( 12.63842701281683922, 39.55059781766744464, -9.846743663894590881 ) ) ;
#48754=CARTESIAN_POINT ( 'NONE',  ( -1.099225684535947600, 28.70696800326375353, -6.408140936763238038 ) ) ;
#48756=CARTESIAN_POINT ( 'NONE',  ( 19.89103541497710737, 15.66234555792571292, -6.479102184480796112 ) ) ;
#48757=CARTESIAN_POINT ( 'NONE',  ( 2.035157376598824452, 43.68868534415484106, 7.964842623401179544 ) ) ;
#48759=CARTESIAN_POINT ( 'NONE',  ( 13.43411237798106583, 12.66530133659708746, -12.81628187352647252 ) ) ;
#48760=CARTESIAN_POINT ( 'NONE',  ( 1.472469842513823179, 41.42559781766745886, 4.923371831947296329 ) ) ;
#48761=CARTESIAN_POINT ( 'NONE',  ( 0.1532563361054083140, 16.00893115100078390, 1.131784320476157264E-15 ) ) ;
#48762=CARTESIAN_POINT ( 'NONE',  ( -0.8801773607111009756, 33.06368534415484106, 1.068504757029289695E-15 ) ) ;
#48763=CARTESIAN_POINT ( 'NONE',  ( 21.09922568453595559, 27.04030133659708568, -6.408140936763230044 ) ) ;
#48765=CARTESIAN_POINT ( 'NONE',  ( 5.076628168052704559, 25.17559781766745175, -8.527530157486179263 ) ) ;
#48766=( LENGTH_UNIT ( ) NAMED_UNIT ( * ) SI_UNIT ( .MILLI., .METRE. ) );
#48769=CARTESIAN_POINT ( 'NONE',  ( 4.559911319644449179, 38.89701867748817676, 9.422509992056141925 ) ) ;
#48772=CARTESIAN_POINT ( 'NONE',  ( 7.084665262690076126, 64.10535201082150536, 10.88017736071109987 ) ) ;
#48773=CARTESIAN_POINT ( 'NONE',  ( 5.076628168052703671, 46.84226448433412315, 8.527530157486179263 ) ) ;
#48774=CARTESIAN_POINT ( 'NONE',  ( 4.559911319644449179, 37.23035201082150536, -9.422509992056141925 ) ) ;
#48776=CARTESIAN_POINT ( 'NONE',  ( 15.44008868035555793, 46.39701867748817676, -9.422509992056140149 ) ) ;
#48777=CARTESIAN_POINT ( 'NONE',  ( 4.559911319644449179, 13.89701867748817321, 9.422509992056141925 ) ) ;
#48780=CARTESIAN_POINT ( 'NONE',  ( 2.791683348922237240, 40.38393115100078035, -7.208316651077763204 ) ) ;
#48781=CARTESIAN_POINT ( 'NONE',  ( -4.164238869374098151, 36.59541550158063217, -3.795296366450310543 ) ) ;
#48783=CARTESIAN_POINT ( 'NONE',  ( 1.821708436314931845, 6.667925641218958255, -6.500000000000002665 ) ) ;
#48785=CARTESIAN_POINT ( 'NONE',  ( 24.16423886937410614, 24.51208216824730002, -3.795296366450302550 ) ) ;
#48789=CARTESIAN_POINT ( 'NONE',  ( 0.5774900079438590739, 2.647018677488171434, -5.440088680355550821 ) ) ;
#48790=CARTESIAN_POINT ( 'NONE',  ( 18.52753015748618282, 28.92559781766745175, -4.923371831947291888 ) ) ;
#48793=CARTESIAN_POINT ( 'NONE',  ( -0.8801773607111008646, 53.27201867748816966, 2.915334737309923430 ) ) ;
#48794=CARTESIAN_POINT ( 'NONE',  ( -2.816281873526471635, 63.91530133659708923, -3.434112377981056508 ) ) ;
#48795=CARTESIAN_POINT ( 'NONE',  ( 12.91533473730993009, 31.60535201082150891, -10.88017736071109987 ) ) ;
#48796=CARTESIAN_POINT ( 'NONE',  ( 3.591859063236761518, 59.95696800326375353, 11.09922568453594849 ) ) ;
#48797=CARTESIAN_POINT ( 'NONE',  ( 0.6178305044545838731, 4.748634669930420493, 9.382169495545420901 ) ) ;
#48798=CARTESIAN_POINT ( 'NONE',  ( 14.92337183194729633, 17.67559781766745175, 8.527530157486181039 ) ) ;
#48802=CARTESIAN_POINT ( 'NONE',  ( 6.204703633549690345, 65.76208216824731778, -14.16423886937410259 ) ) ;
#48803=CARTESIAN_POINT ( 'NONE',  ( 20.36894250292379738, 29.92874883491396432, -10.36894250292379027 ) ) ;
#48804=CARTESIAN_POINT ( 'NONE',  ( 12.91533473730993009, 36.60535201082151247, -10.88017736071109987 ) ) ;
#48805=CARTESIAN_POINT ( 'NONE',  ( -0.8801773607111009756, 48.06368534415484817, 1.068504757029289695E-15 ) ) ;
#48806=FILL_AREA_STYLE ('',( #9843 ) ) ;
#48808=CARTESIAN_POINT ( 'NONE',  ( 18.52753015748617571, 13.09226448433411960, 4.923371831947298993 ) ) ;
#48810=CARTESIAN_POINT ( 'NONE',  ( 0.1532563361054100626, 25.80059781766744820, -2.638427012816831230 ) ) ;
#48812=CARTESIAN_POINT ( 'NONE',  ( 0.2751277870542967463, 70.00000000000000000, -6.500000000000000888 ) ) ;
#48813=CARTESIAN_POINT ( 'NONE',  ( 7.361572987183169658, 19.96726448433411960, -9.846743663894592657 ) ) ;
#48814=CARTESIAN_POINT ( 'NONE',  ( 2.791683348922240793, 46.63393115100077324, 7.208316651077764092 ) ) ;
#48815=CARTESIAN_POINT ( 'NONE',  ( 22.81628187352647785, 41.62363466993042493, 6.195893100308588602E-16 ) ) ;
#48816=COLOUR_RGB ( '', 0.66274510, 0.83137255, 0.94901961) ;
#48817=CARTESIAN_POINT ( 'NONE',  ( 19.42250999205614548, 55.98035201082150536, -5.440088680355545492 ) ) ;
#48818=CARTESIAN_POINT ( 'NONE',  ( 1.472469842513823179, 26.42559781766745175, 4.923371831947296329 ) ) ;
#48819=CARTESIAN_POINT ( 'NONE',  ( -4.164238869374098151, 51.59541550158063217, -3.795296366450310543 ) ) ;
#48820=CARTESIAN_POINT ( 'NONE',  ( 1.472469842513823179, 21.42559781766745175, 4.923371831947296329 ) ) ;
#48822=CARTESIAN_POINT ( 'NONE',  ( 1.472469842513823179, 65.59226448433412315, -4.923371831947296329 ) ) ;
#48823=CARTESIAN_POINT ( 'NONE',  ( 22.26659068614894466, 28.88708216824730357, 7.082119434687054849 ) ) ;
#48824=CARTESIAN_POINT ( 'NONE',  ( 0.1532563361054082862, 31.21726448433412315, 2.638427012816831674 ) ) ;
#48826=CARTESIAN_POINT ( 'NONE',  ( 10.00000000000000178, 19.31368534415484106, 10.88017736071110342 ) ) ;
#48827=CARTESIAN_POINT ( 'NONE',  ( 4.559911319644449179, 48.89701867748817676, 9.422509992056141925 ) ) ;
#48828=CARTESIAN_POINT ( 'NONE',  ( 12.91533473730992121, 49.52201867748817676, 10.88017736071110164 ) ) ;
#48830=CARTESIAN_POINT ( 'NONE',  ( 16.40814093676324603, 37.45696800326376064, -11.09922568453594671 ) ) ;
#48831=CARTESIAN_POINT ( 'NONE',  ( 0.5774900079438607392, 58.48035201082151247, 5.440088680355550821 ) ) ;
#48833=DIRECTION ( 'NONE',  ( -0.000000000000000000, -0.000000000000000000, 1.000000000000000000 ) ) ;
#48834=CARTESIAN_POINT ( 'NONE',  ( 2.035157376598824452, 68.68868534415484817, 7.964842623401179544 ) ) ;
#48835=AXIS2_PLACEMENT_3D ( 'NONE', #40917, #87383, #62405 ) ;
#48838=CARTESIAN_POINT ( 'NONE',  ( -0.8801773607111008646, 63.27201867748817676, 2.915334737309923430 ) ) ;
#48839=CARTESIAN_POINT ( 'NONE',  ( 17.96484262340118221, 4.938685344154837509, 7.964842623401181321 ) ) ;
#48840=CARTESIAN_POINT ( 'NONE',  ( 1.821708436314921853, 26.66792564121896802, -6.499999999999992006 ) ) ;
#48842=CARTESIAN_POINT ( 'NONE',  ( 4.559911319644449179, 12.23035201082150714, -9.422509992056141925 ) ) ;
#48843=CARTESIAN_POINT ( 'NONE',  ( 0.1532563361054082862, 16.21726448433411960, 2.638427012816831674 ) ) ;
#48844=CARTESIAN_POINT ( 'NONE',  ( 24.16423886937410614, 9.303748834913967869, 8.672049930838204340E-16 ) ) ;
#48846=CARTESIAN_POINT ( 'NONE',  ( 10.00000000000000178, 2.258931151000784787, 9.846743663894594434 ) ) ;
#48847=B_SPLINE_CURVE_WITH_KNOTS ( 'NONE', 3,
 ( #66895, #67893, #15397, #43884, #22398, #14402 ),
 .UNSPECIFIED., .F., .F.,
 ( 4, 2, 4 ),
 ( 0.000000000000000000, 0.0002701661927229319750, 0.0005403323854458639500 ),
 .UNSPECIFIED. ) ;
#48848=CARTESIAN_POINT ( 'NONE',  ( 2.035157376598822676, 7.438685344154837509, -7.964842623401177768 ) ) ;
#48849=CARTESIAN_POINT ( 'NONE',  ( 0.1532563361054100626, 40.80059781766745886, -2.638427012816831230 ) ) ;
#48851=CARTESIAN_POINT ( 'NONE',  ( 10.00000000000000000, 54.75893115100078745, -9.846743663894594434 ) ) ;
#48853=CARTESIAN_POINT ( 'NONE',  ( 7.084665262690076126, 47.02201867748818387, -10.88017736071110164 ) ) ;
#48854=CARTESIAN_POINT ( 'NONE',  ( 7.361572987183170547, 47.05059781766745175, 9.846743663894590881 ) ) ;
#48855=CARTESIAN_POINT ( 'NONE',  ( 3.591859063236761518, 29.95696800326375708, 11.09922568453594849 ) ) ;
#48858=CARTESIAN_POINT ( 'NONE',  ( 12.91533473730992121, 64.52201867748817676, 10.88017736071110164 ) ) ;
#48859=CARTESIAN_POINT ( 'NONE',  ( 2.035157376598822676, 7.438685344154837509, -7.964842623401177768 ) ) ;
#48861=CARTESIAN_POINT ( 'NONE',  ( 22.81628187352648496, 46.83196800326376064, -3.434112377981050290 ) ) ;
#48864=CARTESIAN_POINT ( 'NONE',  ( 21.09922568453595559, 22.04030133659708923, -6.408140936763230044 ) ) ;
#48865=CARTESIAN_POINT ( 'NONE',  ( -0.8801773607111009756, 38.06368534415484106, 1.068504757029289695E-15 ) ) ;
#48867=CARTESIAN_POINT ( 'NONE',  ( 2.791683348922240793, 66.63393115100079456, 7.208316651077764092 ) ) ;
#48868=CARTESIAN_POINT ( 'NONE',  ( 14.92337183194729633, 12.67559781766745353, 8.527530157486181039 ) ) ;
#48869=CARTESIAN_POINT ( 'NONE',  ( 7.361572987183170547, 57.05059781766744464, 9.846743663894590881 ) ) ;
#48871=CARTESIAN_POINT ( 'NONE',  ( 18.52753015748618282, 33.92559781766745886, -4.923371831947291888 ) ) ;
#48873=VECTOR ( 'NONE', #92585, 1000.000000000000000 ) ;
#48876=CARTESIAN_POINT ( 'NONE',  ( 12.63842701281683034, 27.46726448433411250, 9.846743663894596210 ) ) ;
#48877=SURFACE_STYLE_USAGE ( .BOTH. , #70420 ) ;
#48879=CARTESIAN_POINT ( 'NONE',  ( 14.92337183194729988, 59.34226448433412315, -8.527530157486177487 ) ) ;
#48880=EDGE_LOOP ( 'NONE', ( #90888, #71693, #33860, #83048 ) ) ;
#48883=CARTESIAN_POINT ( 'NONE',  ( 3.591859063236761518, 24.95696800326375353, 11.09922568453594849 ) ) ;
#48884=CARTESIAN_POINT ( 'NONE',  ( 19.84674366389459266, 48.71726448433413026, -2.638427012816827677 ) ) ;
#48885=DIRECTION ( 'NONE',  ( 1.000000000000000000, 0.000000000000000000, -0.000000000000000000 ) ) ;
#48886=CARTESIAN_POINT ( 'NONE',  ( 17.08211943468705840, 40.13708216824731068, -12.26659068614894466 ) ) ;
#48887=CARTESIAN_POINT ( 'NONE',  ( 0.1532563361054100626, 15.80059781766745353, -2.638427012816831230 ) ) ;
#48889=VECTOR ( 'NONE', #64445, 1000.000000000000000 ) ;
#48891=CARTESIAN_POINT ( 'NONE',  ( -2.266590686148945544, 52.22041550158064638, 7.082119434687048631 ) ) ;
#48892=CARTESIAN_POINT ( 'NONE',  ( 2.791683348922240793, 61.63393115100079456, 7.208316651077764092 ) ) ;
#48893=CARTESIAN_POINT ( 'NONE',  ( -0.8801773607111008646, 8.272018677488171434, 2.915334737309923430 ) ) ;
#48894=CARTESIAN_POINT ( 'NONE',  ( 13.79529636645031943, 40.34541550158063217, -14.16423886937409904 ) ) ;
#48895=CARTESIAN_POINT ( 'NONE',  ( 24.16423886937410614, 44.51208216824730357, -3.795296366450302550 ) ) ;
#48896=CARTESIAN_POINT ( 'NONE',  ( 17.39651004071897589, 34.08210964143323451, -6.499999999999361400 ) ) ;
#48900=CARTESIAN_POINT ( 'NONE',  ( 0.1532563361054082862, 51.21726448433412315, 2.638427012816831674 ) ) ;
#48901=ORIENTED_EDGE ( 'NONE', *, *, #55426, .T. ) ;
#48902=CARTESIAN_POINT ( 'NONE',  ( 10.00000000000000000, 41.81368534415484106, -10.88017736071110342 ) ) ;
#48903=DIRECTION ( 'NONE',  ( 0.000000000000000000, 0.000000000000000000, -1.000000000000000000 ) ) ;
#48904=CARTESIAN_POINT ( 'NONE',  ( 1.042145700049408319, 64.74216108172002748, -6.499999999999931610 ) ) ;
#48905=DIRECTION ( 'NONE',  ( 0.000000000000000000, 0.000000000000000000, -1.000000000000000000 ) ) ;
#48907=CARTESIAN_POINT ( 'NONE',  ( 5.076628168052703671, 61.84226448433412315, 8.527530157486179263 ) ) ;
#48908=CARTESIAN_POINT ( 'NONE',  ( -41.94000000000001194, 93.50000000000000000, -10.09898361729590199 ) ) ;
#48911=CARTESIAN_POINT ( 'NONE',  ( 2.917880565312950480, 25.97041550158063572, -12.26659068614894821 ) ) ;
#48915=CARTESIAN_POINT ( 'NONE',  ( 19.42250999205614193, 45.14701867748817676, 5.440088680355555262 ) ) ;
#48916=CARTESIAN_POINT ( 'NONE',  ( 19.42250999205614548, 20.98035201082150891, -5.440088680355545492 ) ) ;
#48917=CARTESIAN_POINT ( 'NONE',  ( 3.591859063236761518, 24.95696800326375353, 11.09922568453594849 ) ) ;
#48919=CARTESIAN_POINT ( 'NONE',  ( 1.472469842513823179, 15.59226448433411960, -4.923371831947296329 ) ) ;
#48920=CARTESIAN_POINT ( 'NONE',  ( 20.15039907845753575, 59.72266099184918176, 6.262539305110074395 ) ) ;
#48921=CARTESIAN_POINT ( 'NONE',  ( 2.603489959281199972, 21.58210964143324873, 6.499999999999559464 ) ) ;
#48922=DIRECTION ( 'NONE',  ( 0.000000000000000000, -1.000000000000000000, 0.000000000000000000 ) ) ;
#48923=CARTESIAN_POINT ( 'NONE',  ( 0.5774900079438590739, 7.647018677488171434, -5.440088680355550821 ) ) ;
#48925=CARTESIAN_POINT ( 'NONE',  ( 17.96484262340118221, 36.18868534415484106, -7.964842623401177768 ) ) ;
#48926=CARTESIAN_POINT ( 'NONE',  ( -0.8801773607111008646, 33.27201867748817676, 2.915334737309923430 ) ) ;
#48927=CARTESIAN_POINT ( 'NONE',  ( 3.591859063236763294, 3.290301336597087012, -11.09922568453595026 ) ) ;
#48928=CARTESIAN_POINT ( 'NONE',  ( 4.999999999999999112, 61.00000000000000000, 6.500000000000000888 ) ) ;
#48929=CARTESIAN_POINT ( 'NONE',  ( -2.816281873526473856, 59.12363466993042493, 9.499525473075851096E-16 ) ) ;
#48930=CARTESIAN_POINT ( 'NONE',  ( 12.63842701281683922, 9.550597817667449974, -9.846743663894590881 ) ) ;
#48931=EDGE_LOOP ( 'NONE', ( #62481, #26037, #40826, #33775 ) ) ;
#48932=CARTESIAN_POINT ( 'NONE',  ( 12.91533473730992121, 29.52201867748817321, 10.88017736071110164 ) ) ;
#48933=CARTESIAN_POINT ( 'NONE',  ( -1.099225684535947600, 33.70696800326375353, -6.408140936763238038 ) ) ;
#48934=CIRCLE ( 'NONE', #50507, 0.5000000000000004441 ) ;
#48935=VECTOR ( 'NONE', #76458, 1000.000000000000000 ) ;
#48937=CARTESIAN_POINT ( 'NONE',  ( 0.1532563361054083140, 56.00893115100078745, 1.131784320476157264E-15 ) ) ;
#48938=CARTESIAN_POINT ( 'NONE',  ( 2.035157376598822676, 67.43868534415484817, -7.964842623401177768 ) ) ;
#48939=CARTESIAN_POINT ( 'NONE',  ( 0.1532563361054083140, 6.008931151000784787, 1.131784320476157264E-15 ) ) ;
#48940=CARTESIAN_POINT ( 'NONE',  ( -2.816281873526473856, 29.12363466993041783, 9.499525473075851096E-16 ) ) ;
#48941=CARTESIAN_POINT ( 'NONE',  ( 7.361572987183169658, 4.967264484334119601, -9.846743663894592657 ) ) ;
#48942=LINE ( 'NONE', #3949, #11247 ) ;
#48944=SURFACE_STYLE_FILL_AREA ( #56936 ) ;
#48946=CARTESIAN_POINT ( 'NONE',  ( 2.035157376598822676, 2.438685344154837953, -7.964842623401177768 ) ) ;
#48947=CARTESIAN_POINT ( 'NONE',  ( -2.816281873526473856, 64.33196800326376774, 3.434112377981055619 ) ) ;
#48948=CARTESIAN_POINT ( 'NONE',  ( 10.00000000000000000, 25.55374883491396787, -14.16423886937410082 ) ) ;
#48949=CARTESIAN_POINT ( 'NONE',  ( 18.52753015748618282, 18.92559781766745175, -4.923371831947291888 ) ) ;
#48950=CARTESIAN_POINT ( 'NONE',  ( 7.084665262690076126, 7.022018677488169658, -10.88017736071110164 ) ) ;
#48951=CARTESIAN_POINT ( 'NONE',  ( 12.63842701281683034, 27.46726448433411250, 9.846743663894596210 ) ) ;
#48952=CARTESIAN_POINT ( 'NONE',  ( 2.035157376598824452, 3.688685344154837953, 7.964842623401179544 ) ) ;
#48955=CARTESIAN_POINT ( 'NONE',  ( 17.96484262340118221, 9.938685344154837509, 7.964842623401181321 ) ) ;
#48956=CARTESIAN_POINT ( 'NONE',  ( 15.44008868035555260, 14.73035201082150536, 9.422509992056143702 ) ) ;
#48957=CARTESIAN_POINT ( 'NONE',  ( -45.94000000000000483, 92.00000000000000000, 5.000000000000000000 ) ) ;
#48960=CARTESIAN_POINT ( 'NONE',  ( 4.559911319644449179, 28.89701867748817321, 9.422509992056141925 ) ) ;
#48961=CARTESIAN_POINT ( 'NONE',  ( 10.00000000000000178, 62.25893115100078745, 9.846743663894594434 ) ) ;
#48963=CARTESIAN_POINT ( 'NONE',  ( 3.591859063236763294, 48.29030133659708923, -11.09922568453595026 ) ) ;
#48965=CARTESIAN_POINT ( 'NONE',  ( 24.16423886937409904, 34.09541550158064638, 3.795296366450317205 ) ) ;
#48966=CARTESIAN_POINT ( 'NONE',  ( 12.91533473730992121, 34.52201867748817676, 10.88017736071110164 ) ) ;
#48967=CARTESIAN_POINT ( 'NONE',  ( 15.44008868035555793, 11.39701867748817143, -9.422509992056140149 ) ) ;
#48969=CARTESIAN_POINT ( 'NONE',  ( 0.1532563361054082862, 51.21726448433412315, 2.638427012816831674 ) ) ;
#48971=CARTESIAN_POINT ( 'NONE',  ( 18.72515096720590577, 61.07228050351029935, -6.499999999999718447 ) ) ;
#48972=CARTESIAN_POINT ( 'NONE',  ( 5.076628168052703671, 36.84226448433412315, 8.527530157486179263 ) ) ;
#48974=CARTESIAN_POINT ( 'NONE',  ( 14.92337183194729988, 14.34226448433411782, -8.527530157486177487 ) ) ;
#48976=ORIENTED_EDGE ( 'NONE', *, *, #88312, .F. ) ;
#48977=CARTESIAN_POINT ( 'NONE',  ( -0.8801773607111009756, 18.06368534415484106, 1.068504757029289695E-15 ) ) ;
#48978=CARTESIAN_POINT ( 'NONE',  ( 18.52753015748618282, 8.925597817667451750, -4.923371831947291888 ) ) ;
#48979=CARTESIAN_POINT ( 'NONE',  ( 19.38216949554541202, 0.9986346699304200492, 9.382169495545424454 ) ) ;
#48980=CARTESIAN_POINT ( 'NONE',  ( 20.88017736071110164, 50.35535201082151247, 2.915334737309930979 ) ) ;
#48981=CARTESIAN_POINT ( 'NONE',  ( 19.42250999205614193, 20.14701867748817321, 5.440088680355555262 ) ) ;
#48982=CARTESIAN_POINT ( 'NONE',  ( 22.81628187352648496, 41.83196800326375353, -3.434112377981050290 ) ) ;
#48983=CARTESIAN_POINT ( 'NONE',  ( 13.79529636645030344, 28.26208216824729647, 14.16423886937410614 ) ) ;
#48988=CARTESIAN_POINT ( 'NONE',  ( 10.00000000000000000, 52.87363466993041783, -12.81628187352647608 ) ) ;
#48989=ORIENTED_EDGE ( 'NONE', *, *, #2579, .T. ) ;
#48990=CARTESIAN_POINT ( 'NONE',  ( 14.92337183194729988, 64.34226448433412315, -8.527530157486177487 ) ) ;
#48991=CARTESIAN_POINT ( 'NONE',  ( 4.559911319644449179, 37.23035201082150536, -9.422509992056141925 ) ) ;
#48992=EDGE_LOOP ( 'NONE', ( #67602, #69193, #54762, #15144 ) ) ;
#48993=CARTESIAN_POINT ( 'NONE',  ( 10.00000000000000000, -0.2410688489992152128, -9.846743663894594434 ) ) ;
#48996=CARTESIAN_POINT ( 'NONE',  ( 12.63842701281683034, 27.46726448433411250, 9.846743663894596210 ) ) ;
#48997=CARTESIAN_POINT ( 'NONE',  ( 17.20831665107776587, 9.133931151000787452, -7.208316651077762316 ) ) ;
#48998=CARTESIAN_POINT ( 'NONE',  ( 0.1532563361054100626, 0.8005978176674514168, -2.638427012816831230 ) ) ;
#48999=CARTESIAN_POINT ( 'NONE',  ( 4.559911319644449179, 58.89701867748817676, 9.422509992056141925 ) ) ;
#49002=CARTESIAN_POINT ( 'NONE',  ( 7.084665262690076126, 59.10535201082150536, 10.88017736071109987 ) ) ;
#49003=CARTESIAN_POINT ( 'NONE',  ( 10.00000000000000000, 24.75893115100078745, -9.846743663894594434 ) ) ;
#49004=ORIENTED_EDGE ( 'NONE', *, *, #29174, .T. ) ;
#49009=CARTESIAN_POINT ( 'NONE',  ( 14.92337183194729988, 54.34226448433412315, -8.527530157486177487 ) ) ;
#49012=CARTESIAN_POINT ( 'NONE',  ( -0.3689425029237898834, 11.17874883491396787, -10.36894250292378850 ) ) ;
#49013=DIRECTION ( 'NONE',  ( 0.000000000000000000, 0.000000000000000000, -1.000000000000000000 ) ) ;
#49014=CARTESIAN_POINT ( 'NONE',  ( -4.164238869374099927, 2.012082168247300906, 3.795296366450308767 ) ) ;
#49015=CARTESIAN_POINT ( 'NONE',  ( 24.16423886937409904, 39.09541550158062506, 3.795296366450317205 ) ) ;
#49016=CARTESIAN_POINT ( 'NONE',  ( -0.03447792253739288132, 45.15514106990688958, 6.401564815979726930 ) ) ;
#49017=DIRECTION ( 'NONE',  ( 0.9970872288863208421, 0.07626964003977952655, -0.000000000000000000 ) ) ;
#49018=CARTESIAN_POINT ( 'NONE',  ( 0.5774900079438590739, 37.64701867748817676, -5.440088680355550821 ) ) ;
#49019=SURFACE_SIDE_STYLE ('',( #94518 ) ) ;
#49021=CARTESIAN_POINT ( 'NONE',  ( 0.1532563361054100626, 10.80059781766745175, -2.638427012816831230 ) ) ;
#49022=COLOUR_RGB ( '', 0.72549020, 0.75294118, 0.79215686) ;
#49023=CARTESIAN_POINT ( 'NONE',  ( 2.035157376598824452, 58.68868534415482685, 7.964842623401179544 ) ) ;
#49024=CARTESIAN_POINT ( 'NONE',  ( 10.00000000000000178, 12.25893115100078568, 9.846743663894594434 ) ) ;
#49025=CARTESIAN_POINT ( 'NONE',  ( 16.40814093676324603, 42.45696800326375353, -11.09922568453594671 ) ) ;
#49026=CARTESIAN_POINT ( 'NONE',  ( 10.00000000000000178, 37.25893115100078745, 9.846743663894594434 ) ) ;
#49028=CARTESIAN_POINT ( 'NONE',  ( 20.88017736071110519, 60.56368534415484106, 2.639326808657452039E-16 ) ) ;
#49029=CARTESIAN_POINT ( 'NONE',  ( 12.63842701281683034, 22.46726448433411605, 9.846743663894596210 ) ) ;
#49030=CARTESIAN_POINT ( 'NONE',  ( 6.565887622018943937, 28.08196800326375353, -12.81628187352647608 ) ) ;
#49033=CARTESIAN_POINT ( 'NONE',  ( 2.791683348922240793, 26.63393115100078745, 7.208316651077764092 ) ) ;
#49034=CARTESIAN_POINT ( 'NONE',  ( -0.3689425029237898834, 11.17874883491396787, -10.36894250292378850 ) ) ;
#49037=CARTESIAN_POINT ( 'NONE',  ( 4.559911319644449179, 38.89701867748817676, 9.422509992056141925 ) ) ;
#49038=CARTESIAN_POINT ( 'NONE',  ( -0.8801773607110991993, 57.85535201082149825, -2.915334737309923874 ) ) ;
#49039=CARTESIAN_POINT ( 'NONE',  ( 13.79529636645031943, 35.34541550158063927, -14.16423886937409904 ) ) ;
#49040=CARTESIAN_POINT ( 'NONE',  ( 17.20831665107776587, 54.13393115100079456, -7.208316651077762316 ) ) ;
#49041=CARTESIAN_POINT ( 'NONE',  ( 14.92337183194729633, 12.67559781766745353, 8.527530157486181039 ) ) ;
#49042=CARTESIAN_POINT ( 'NONE',  ( 22.81628187352648496, 61.83196800326376774, -3.434112377981050290 ) ) ;
#49044=CARTESIAN_POINT ( 'NONE',  ( 15.44008868035555260, 39.73035201082150536, 9.422509992056143702 ) ) ;
#49046=EDGE_CURVE ( 'NONE', #4379, #67947, #61930, .T. ) ;
#49047=CARTESIAN_POINT ( 'NONE',  ( 6.565887622018943937, 18.08196800326375708, -12.81628187352647608 ) ) ;
#49048=CARTESIAN_POINT ( 'NONE',  ( 0.6178305044545818747, 18.49863466993041428, -9.382169495545419124 ) ) ;
#49049=CARTESIAN_POINT ( 'NONE',  ( 12.63842701281683922, 54.55059781766745175, -9.846743663894590881 ) ) ;
#49051=PRESENTATION_STYLE_ASSIGNMENT (( #33538 ) ) ;
#49052=CARTESIAN_POINT ( 'NONE',  ( 12.91533473730993009, 66.60535201082150536, -10.88017736071109987 ) ) ;
#49057=CARTESIAN_POINT ( 'NONE',  ( 0.5774900079438607392, 63.48035201082149825, 5.440088680355550821 ) ) ;
#49058=CARTESIAN_POINT ( 'NONE',  ( 4.559911319644449179, 62.23035201082150536, -9.422509992056141925 ) ) ;
#49061=CARTESIAN_POINT ( 'NONE',  ( 14.92337183194729988, 24.34226448433411960, -8.527530157486177487 ) ) ;
#49063=CARTESIAN_POINT ( 'NONE',  ( 15.44008868035555793, 21.39701867748817321, -9.422509992056140149 ) ) ;
#49064=CARTESIAN_POINT ( 'NONE',  ( 18.52753015748618282, 58.92559781766745886, -4.923371831947291888 ) ) ;
#49065=CARTESIAN_POINT ( 'NONE',  ( -0.8801773607111009756, 28.06368534415484106, 1.068504757029289695E-15 ) ) ;
#49066=DIRECTION ( 'NONE',  ( 0.000000000000000000, 0.000000000000000000, -1.000000000000000000 ) ) ;
#49068=CARTESIAN_POINT ( 'NONE',  ( 3.591859063236763294, 38.29030133659708923, -11.09922568453595026 ) ) ;
#49069=ORIENTED_EDGE ( 'NONE', *, *, #66975, .T. ) ;
#49070=CARTESIAN_POINT ( 'NONE',  ( 19.42250999205614548, 50.98035201082151247, -5.440088680355545492 ) ) ;
#49071=CARTESIAN_POINT ( 'NONE',  ( 0.6178305044545838731, 14.74863466993041783, 9.382169495545420901 ) ) ;
#49072=CARTESIAN_POINT ( 'NONE',  ( 15.44008868035555793, 26.39701867748817321, -9.422509992056140149 ) ) ;
#49073=CARTESIAN_POINT ( 'NONE',  ( 10.00000000000000000, 55.55374883491396787, -14.16423886937410082 ) ) ;
#49075=CARTESIAN_POINT ( 'NONE',  ( 7.361572987183169658, 34.96726448433411605, -9.846743663894592657 ) ) ;
#49076=CARTESIAN_POINT ( 'NONE',  ( 18.52753015748618282, 3.925597817667451306, -4.923371831947291888 ) ) ;
#49077=CARTESIAN_POINT ( 'NONE',  ( 0.5774900079438607392, 43.48035201082151247, 5.440088680355550821 ) ) ;
#49079=CARTESIAN_POINT ( 'NONE',  ( 2.917880565312950480, 10.97041550158063572, -12.26659068614894821 ) ) ;
#49080=COLOUR_RGB ( '', 0.08235294, 0.09019608, 0.10196078) ;
#49084=ORIENTED_EDGE ( 'NONE', *, *, #64872, .T. ) ;
#49085=CARTESIAN_POINT ( 'NONE',  ( -0.3689425029237898834, 46.17874883491397497, -10.36894250292378850 ) ) ;
#49086=CARTESIAN_POINT ( 'NONE',  ( 24.16423886937409904, 44.09541550158063927, 3.795296366450317205 ) ) ;
#49087=CARTESIAN_POINT ( 'NONE',  ( 12.63842701281683034, 12.46726448433411782, 9.846743663894596210 ) ) ;
#49088=CARTESIAN_POINT ( 'NONE',  ( -2.816281873526471635, 13.91530133659708746, -3.434112377981056508 ) ) ;
#49091=CARTESIAN_POINT ( 'NONE',  ( 19.42250999205614193, 5.147018677488171434, 5.440088680355555262 ) ) ;
#49092=CARTESIAN_POINT ( 'NONE',  ( 10.00000000000000000, 27.87363466993042138, -12.81628187352647608 ) ) ;
#49093=CARTESIAN_POINT ( 'NONE',  ( 13.79529636645030344, 38.26208216824729647, 14.16423886937410614 ) ) ;
#49097=CARTESIAN_POINT ( 'NONE',  ( 19.84674366389459621, 23.50893115100078390, 7.409399052514197653E-17 ) ) ;
#49100=CARTESIAN_POINT ( 'NONE',  ( -4.164238869374098151, 66.59541550158060375, -3.795296366450310543 ) ) ;
#49101=CARTESIAN_POINT ( 'NONE',  ( 10.00000000000000000, 16.81368534415483751, -10.88017736071110342 ) ) ;
#49102=CARTESIAN_POINT ( 'NONE',  ( 1.472469842513823179, 45.59226448433412315, -4.923371831947296329 ) ) ;
#49103=CARTESIAN_POINT ( 'NONE',  ( 6.565887622018943937, 8.081968003263751754, -12.81628187352647608 ) ) ;
#49104=DIRECTION ( 'NONE',  ( 0.000000000000000000, -1.000000000000000000, 0.000000000000000000 ) ) ;
#49106=EDGE_CURVE ( 'NONE', #31960, #94230, #65318, .T. ) ;
#49109=CARTESIAN_POINT ( 'NONE',  ( 6.565887622018943937, 25.16530133659708213, 12.81628187352647430 ) ) ;
#49112=CARTESIAN_POINT ( 'NONE',  ( -4.164238869374099039, 61.80374883491397497, 8.674139862899312516E-16 ) ) ;
#49113=EDGE_LOOP ( 'NONE', ( #17220, #60703, #74745, #74846 ) ) ;
#49114=CARTESIAN_POINT ( 'NONE',  ( 22.26659068614894466, 58.88708216824729647, 7.082119434687054849 ) ) ;
#49115=VERTEX_POINT ( 'NONE', #491 ) ;
#49116=CARTESIAN_POINT ( 'NONE',  ( 4.559911319644449179, 33.89701867748817676, 9.422509992056141925 ) ) ;
#49117=CARTESIAN_POINT ( 'NONE',  ( 17.96484262340118221, 51.18868534415483396, -7.964842623401177768 ) ) ;
#49118=CARTESIAN_POINT ( 'NONE',  ( 4.559911319644449179, 42.23035201082151247, -9.422509992056141925 ) ) ;
#49120=CARTESIAN_POINT ( 'NONE',  ( 2.035157376598822676, 37.43868534415484106, -7.964842623401177768 ) ) ;
#49121=CARTESIAN_POINT ( 'NONE',  ( 4.999999999999999112, 11.50000000000000000, 6.000000000000000000 ) ) ;
#49122=COLOUR_RGB ( '', 0.08235294, 0.09019608, 0.10196078) ;
#49123=EDGE_CURVE ( 'NONE', #85384, #28167, #58226, .T. ) ;
#49124=CARTESIAN_POINT ( 'NONE',  ( 12.63842701281683922, 9.550597817667449974, -9.846743663894590881 ) ) ;
#49127=CARTESIAN_POINT ( 'NONE',  ( 19.84674366389459266, 48.71726448433413026, -2.638427012816827677 ) ) ;
#49128=CARTESIAN_POINT ( 'NONE',  ( 10.00000000000000178, 70.00000000000000000, 0.000000000000000000 ) ) ;
#49129=CARTESIAN_POINT ( 'NONE',  ( -1.099225684535947600, 59.54030133659708923, 6.408140936763237150 ) ) ;
#49131=( NAMED_UNIT ( * ) PLANE_ANGLE_UNIT ( ) SI_UNIT ( $, .RADIAN. ) );
#49132=VECTOR ( 'NONE', #67680, 1000.000000000000000 ) ;
#49135=CARTESIAN_POINT ( 'NONE',  ( 22.26659068614895176, 59.72041550158063927, -7.082119434687042414 ) ) ;
#49137=ORIENTED_EDGE ( 'NONE', *, *, #64795, .F. ) ;
#49139=CARTESIAN_POINT ( 'NONE',  ( 12.63842701281683034, 27.46726448433411250, 9.846743663894596210 ) ) ;
#49142=CARTESIAN_POINT ( 'NONE',  ( -1.099225684535947600, 4.540301336597087456, 6.408140936763237150 ) ) ;
#49143=CARTESIAN_POINT ( 'NONE',  ( 7.084665262690076126, 67.02201867748817676, -10.88017736071110164 ) ) ;
#49146=CARTESIAN_POINT ( 'NONE',  ( 2.791683348922237240, 55.38393115100078745, -7.208316651077763204 ) ) ;
#49147=AXIS2_PLACEMENT_3D ( 'NONE', #78115, #9623, #70623 ) ;
#49150=CARTESIAN_POINT ( 'NONE',  ( 2.035157376598822676, 2.438685344154838397, -7.964842623401177768 ) ) ;
#49152=CARTESIAN_POINT ( 'NONE',  ( 20.88017736071110164, 40.35535201082150536, 2.915334737309930979 ) ) ;
#49153=CARTESIAN_POINT ( 'NONE',  ( -1.099225684535947600, 9.540301336597087456, 6.408140936763237150 ) ) ;
#49154=CARTESIAN_POINT ( 'NONE',  ( 7.084665262690076126, 69.10535201082151957, 10.88017736071109987 ) ) ;
#49155=CARTESIAN_POINT ( 'NONE',  ( 2.035157376598824452, 3.688685344154837953, 7.964842623401179544 ) ) ;
#49158=CARTESIAN_POINT ( 'NONE',  ( 0.1532563361054083140, 46.00893115100079456, 1.131784320476157264E-15 ) ) ;
#49159=CARTESIAN_POINT ( 'NONE',  ( 17.20831665107776587, 19.13393115100078035, -7.208316651077762316 ) ) ;
#49161=CARTESIAN_POINT ( 'NONE',  ( -2.816281873526473856, 19.33196800326375708, 3.434112377981055619 ) ) ;
#49163=CARTESIAN_POINT ( 'NONE',  ( 19.42250999205614193, 30.14701867748817321, 5.440088680355555262 ) ) ;
#49165=CARTESIAN_POINT ( 'NONE',  ( 2.917880565312950480, 30.97041550158063572, -12.26659068614894821 ) ) ;
#49167=CARTESIAN_POINT ( 'NONE',  ( -2.266590686148945544, 32.22041550158063927, 7.082119434687048631 ) ) ;
#49168=CARTESIAN_POINT ( 'NONE',  ( 7.084665262690076126, 12.02201867748817321, -10.88017736071110164 ) ) ;
#49169=CARTESIAN_POINT ( 'NONE',  ( 14.92337183194729633, 47.67559781766745175, 8.527530157486181039 ) ) ;
#49170=CARTESIAN_POINT ( 'NONE',  ( 3.591859063236761518, 39.95696800326375353, 11.09922568453594849 ) ) ;
#49171=CARTESIAN_POINT ( 'NONE',  ( 2.035157376598824452, 13.68868534415483751, 7.964842623401179544 ) ) ;
#49172=CARTESIAN_POINT ( 'NONE',  ( 19.84674366389459266, 33.71726448433410894, -2.638427012816827677 ) ) ;
#49173=CARTESIAN_POINT ( 'NONE',  ( 17.96484262340118221, 44.93868534415483396, 7.964842623401181321 ) ) ;
#49174=CARTESIAN_POINT ( 'NONE',  ( 22.81628187352647785, 1.415301336597087012, 3.434112377981063169 ) ) ;
#49175=CARTESIAN_POINT ( 'NONE',  ( 10.00000000000000178, 28.05374883491396787, 14.16423886937410082 ) ) ;
#49177=UNCERTAINTY_MEASURE_WITH_UNIT (LENGTH_MEASURE( 1.000000000000000082E-05 ), #49709, 'distance_accuracy_value', 'NONE');
#49178=CARTESIAN_POINT ( 'NONE',  ( 2.791683348922240793, 26.63393115100078745, 7.208316651077764092 ) ) ;
#49179=CARTESIAN_POINT ( 'NONE',  ( -1.099225684535947600, 49.54030133659708923, 6.408140936763237150 ) ) ;
#49180=CARTESIAN_POINT ( 'NONE',  ( 18.52753015748618282, 48.92559781766745886, -4.923371831947291888 ) ) ;
#49183=CARTESIAN_POINT ( 'NONE',  ( 2.917880565312948704, 67.63708216824730357, 12.26659068614894643 ) ) ;
#49184=CARTESIAN_POINT ( 'NONE',  ( 10.00000000000000000, 61.81368534415484106, -10.88017736071110342 ) ) ;
#49185=CARTESIAN_POINT ( 'NONE',  ( 2.917880565312948704, 7.637082168247301794, 12.26659068614894643 ) ) ;
#49186=CARTESIAN_POINT ( 'NONE',  ( 0.1532563361054083140, 1.008931151000784787, 1.131784320476157264E-15 ) ) ;
#49187=CARTESIAN_POINT ( 'NONE',  ( 10.00000000000000178, 47.25893115100078745, 9.846743663894594434 ) ) ;
#49188=CARTESIAN_POINT ( 'NONE',  ( 19.42250999205614193, 30.14701867748817321, 5.440088680355555262 ) ) ;
#49190=CARTESIAN_POINT ( 'NONE',  ( 7.361572987183169658, 59.96726448433410894, -9.846743663894592657 ) ) ;
#49191=ORIENTED_EDGE ( 'NONE', *, *, #59021, .T. ) ;
#49195=ORIENTED_EDGE ( 'NONE', *, *, #11090, .F. ) ;
#49197=CARTESIAN_POINT ( 'NONE',  ( 2.917880565312948704, 7.637082168247301794, 12.26659068614894643 ) ) ;
#49198=CARTESIAN_POINT ( 'NONE',  ( -2.266590686148945544, 16.38708216824730357, -7.082119434687050408 ) ) ;
#49199=CARTESIAN_POINT ( 'NONE',  ( 0.1532563361054082862, 56.21726448433411605, 2.638427012816831674 ) ) ;
#49200=CARTESIAN_POINT ( 'NONE',  ( 18.52753015748618282, 28.92559781766745175, -4.923371831947291888 ) ) ;
#49202=CARTESIAN_POINT ( 'NONE',  ( 2.035157376598824452, 28.68868534415484106, 7.964842623401179544 ) ) ;
#49203=CARTESIAN_POINT ( 'NONE',  ( 0.1532563361054082862, 61.21726448433412315, 2.638427012816831674 ) ) ;
#49204=CARTESIAN_POINT ( 'NONE',  ( 22.26659068614895176, 9.720415501580633943, -7.082119434687042414 ) ) ;
#49205=CARTESIAN_POINT ( 'NONE',  ( 17.96484262340118221, 9.938685344154839285, 7.964842623401181321 ) ) ;
#49207=DIRECTION ( 'NONE',  ( -1.000000000000000000, -0.000000000000000000, -0.000000000000000000 ) ) ;
#49208=CARTESIAN_POINT ( 'NONE',  ( 20.88017736071110164, 60.35535201082151957, 2.915334737309930979 ) ) ;
#49209=CARTESIAN_POINT ( 'NONE',  ( 7.361572987183169658, 24.96726448433412315, -9.846743663894592657 ) ) ;
#49210=AXIS2_PLACEMENT_3D ( 'NONE', #19093, #49573, #94594 ) ;
#49212=EDGE_LOOP ( 'NONE', ( #5981, #36887, #78123, #28849, #61727, #56850, #34958, #5855, #45551, #65645, #29300, #46769, #79222, #39151, #18105, #53188, #35885, #66189, #79100, #87696, #76216, #58014, #75188, #66074, #29128, #61472, #31711, #23186, #21552, #65353, #60934, #63444, #92607, #76911, #56354, #74956, #6605, #77629, #33846, #83139, #16928, #8213, #20055, #83658, #39547, #38497, #53676, #42634, #6670, #63503, #17534, #84547, #55624, #88661, #80082, #28307, #76874, #73675, #96683, #20123, #74635, #16675, #40498, #45750, #28076, #61746, #43806, #7568, #54693, #24386, #34429, #50116, #44290, #84091, #70761, #47056, #46571, #90073, #51529, #92287, #91915, #39529, #46297, #2616, #87362, #80452, #53664, #89593, #30070, #16992, #20952, #81086, #48976, #41592, #32021, #8260, #74436, #92659, #13816, #71245, #93978, #74774, #92770, #15901, #90895, #47219, #91885, #38419, #4512, #68305 ) ) ;
#49214=CARTESIAN_POINT ( 'NONE',  ( 14.92337183194729988, 24.34226448433411960, -8.527530157486177487 ) ) ;
#49216=CARTESIAN_POINT ( 'NONE',  ( -0.3689425029237898834, 31.17874883491396787, -10.36894250292378850 ) ) ;
#49217=CARTESIAN_POINT ( 'NONE',  ( 2.791683348922240793, 36.63393115100078035, 7.208316651077764092 ) ) ;
#49218=CARTESIAN_POINT ( 'NONE',  ( 7.084665262690076126, 59.10535201082150536, 10.88017736071109987 ) ) ;
#49223=CARTESIAN_POINT ( 'NONE',  ( 17.96484262340118221, 44.93868534415483396, 7.964842623401181321 ) ) ;
#49224=CARTESIAN_POINT ( 'NONE',  ( 14.92337183194729633, 47.67559781766745175, 8.527530157486181039 ) ) ;
#49225=EDGE_CURVE ( 'NONE', #91084, #95857, #86695, .T. ) ;
#49229=CARTESIAN_POINT ( 'NONE',  ( -0.3689425029237898834, 21.17874883491396432, -10.36894250292378850 ) ) ;
#49232=CARTESIAN_POINT ( 'NONE',  ( 3.591859063236761518, 34.95696800326375353, 11.09922568453594849 ) ) ;
#49233=SURFACE_SIDE_STYLE ('',( #40758 ) ) ;
#49234=CARTESIAN_POINT ( 'NONE',  ( 7.361572987183169658, 24.96726448433412315, -9.846743663894592657 ) ) ;
#49235=CARTESIAN_POINT ( 'NONE',  ( -0.8801773607110991993, 2.855352010821504471, -2.915334737309923874 ) ) ;
#49236=CARTESIAN_POINT ( 'NONE',  ( 3.591859063236763294, 58.29030133659708923, -11.09922568453595026 ) ) ;
#49237=CARTESIAN_POINT ( 'NONE',  ( 14.92337183194729988, 24.34226448433411960, -8.527530157486177487 ) ) ;
#49238=CARTESIAN_POINT ( 'NONE',  ( 4.559911319644449179, 57.23035201082150536, -9.422509992056141925 ) ) ;
#49240=ADVANCED_FACE ( 'NONE', ( #17925 ), #70936, .T. ) ;
#49242=CARTESIAN_POINT ( 'NONE',  ( 7.084665262690076126, 69.10535201082151957, 10.88017736071109987 ) ) ;
#49243=CARTESIAN_POINT ( 'NONE',  ( -44.17147705133852043, 106.3134523618952869, 4.660915905273111726 ) ) ;
#49245=CARTESIAN_POINT ( 'NONE',  ( 2.791683348922240793, 1.633931151000784565, 7.208316651077764092 ) ) ;
#49246=CARTESIAN_POINT ( 'NONE',  ( 22.81628187352648496, 16.83196800326374998, -3.434112377981050290 ) ) ;
#49247=EDGE_CURVE ( 'NONE', #32664, #57881, #77924, .T. ) ;
#49250=CARTESIAN_POINT ( 'NONE',  ( 19.84674366389459266, 43.71726448433410894, -2.638427012816827677 ) ) ;
#49252=CARTESIAN_POINT ( 'NONE',  ( 20.36894250292379382, 8.678748834913967869, 10.36894250292379205 ) ) ;
#49253=CARTESIAN_POINT ( 'NONE',  ( 10.00000000000000000, 29.75893115100078745, -9.846743663894594434 ) ) ;
#49254=( BOUNDED_SURFACE ( )  B_SPLINE_SURFACE ( 1, 2, ( 
 ( #32251, #78255, #71261, #33719, #93256, #24780, #55256, #64668, #72187, #42203, #94703, #79204, #12179, #4204, #42685, #27671, #58157, #41718, #95690, #88667, #50173, #41231, #87680, #71709, #63697, #56222, #3221, #27174, #94200, #3716, #19194, #49676, #80683, #64182, #49197, #26208, #35166, #33685, #79700, #10714, #34177, #20175, #56700, #95179, #11197, #73164, #25731, #87191, #34674, #48700, #80181, #40722, #65170, #57677, #4703, #18714, #26687, #65666, #96188, #57183, #11694, #72669, #18220, #88172, #50679, #10230, #19686, #71224, #2748, #33202, #86716, #90634, #73659, #5186, #20676, #60136, #89658, #98677, #7153, #59151, #51671, #74653, #59649, #29629, #6654, #21168, #37170, #68155, #98173, #60631, #90140, #82149, #97681, #22158, #43661, #13661, #44143, #6164, #52641, #21670, #66666, #83145, #37657, #35673, #52155, #36668, #67156, #14165, #29143, #30126, #51170, #74147, #14670, #82648, #28659, #91133, #45136, #44649, #66156, #75144, #67663, #75642, #22658, #81171, #12671, #43171, #96690, #5680, #28169, #58663, #89165, #81654, #13163, #36165, #97191, #77112, #16626, #15159, #63095, #23653, #31608, #46616, #38635, #40111, #8626, #32094, #47610, #45639, #2139, #78105, #24628, #54114, #170, #39135, #70613, #665, #8143, #85614, #9611, #53628, #69624, #84627, #93595, #53135, #91635, #62593, #38154, #46137, #84146, #23153, #17131, #1147, #92609, #16130, #92127, #32597, #24134, #15654, #62100, #83644, #76136, #7663, #54601, #93098, #85117, #47103, #68641, #55094, #30619, #77602, #61126, #9116, #39630, #70120, #1642, #76623, #69137, #31115, #61610, #79588, #86108, #72556, #73052, #57073, #80069, #17619, #87569, #2635, #18592, #3115, #87081, #33088, #79085, #57559, #94091, #63582, #65047, #42089, #33571, #49085, #86600, #4585, #11088, #19081, #65547, #41606, #48089, #26570, #71602, #80570, #35047, #3601, #25612, #34552, #48584, #56105, #18107, #10598, #64065, #42568, #25133, #94580, #26096, #95573, #27060, #41112, #88057, #78601, #10111, #56591, #4088, #72075, #55611, #50067, #34060, #64556, #95064, #49556, #19569, #11575, #12065, #40610, #71107, #14053, #75528, #6055, #74037, #13548, #44535, #58544, #5569, #28549, #21056, #75031, #74534, #81538, #98058, #22053, #88554, #67043, #51549, #36045, #29029, #82037, #90031, #44032, #7041, #20057, #97077, #37047, #43542, #66549, #89051, #52527, #97565, #59041, #50560, #66044, #96571, #83035, #28048, #20562, #51048, #82534, #5068, #73543, #89547, #36553, #6538, #35555, #59537, #21554, #52044, #13048, #67545, #29515, #60023, #90518, #14552, #45021, #37546, #96073, #27554, #58047, #81055 ),
 ( #12559, #43062, #77989, #70007, #30017, #39018, #45520, #16014, #54009, #558, #31003, #38041, #24022, #85005, #7551, #23536, #60521, #16517, #17008, #1029, #54490, #91012, #31490, #76020, #61499, #46029, #92007, #68532, #23038, #1531, #31976, #61993, #53015, #84518, #69513, #92493, #46504, #47486, #39514, #68037, #77003, #30510, #46992, #77486, #8516, #8998, #62, #62482, #92986, #24520, #54978, #22545, #9494, #38527, #85497, #98563, #53511, #83530, #15048, #61013, #91524, #84022, #15544, #76513, #8029, #69024, #70500, #93483, #78482, #32485, #62979, #47973, #39995, #25009, #55496, #85997, #2022, #17508, #73639, #14149, #20157, #28151, #66139, #5167, #98156, #28641, #74636, #5664, #74127, #60119, #6148, #35653, #89640, #52626, #96170, #14654, #36146, #44633, #21151, #97174, #45118, #37151, #27653, #36650, #12653, #82132, #51652, #66650, #59131, #96671, #90125, #52138, #58648, #13641, #58140, #82633, #83127, #67138, #21653, #88649, #97662, #43151, #44126, #13145, #29129, #89146, #20657, #67647, #51152, #81637, #75129, #6635, #43642, #59630, #29614, #75626, #90618, #22142, #35147, #65646, #50660, #81149, #53610, #62579, #55080, #84613, #76120, #16611, #30606, #7649, #38140, #85599, #45623, #68627, #47089, #16115, #84128, #17113, #24613, #68138, #47596, #8126, #77585, #61595, #69121, #7138, #9101, #98664, #77099, #83629, #54098, #92108, #38620, #652, #157, #62087, #24118, #61111, #23639, #30112, #54587, #37640, #39119, #92594, #60618, #69609, #15145, #31101, #15639, #46600, #91620, #23137, #39615, #46122, #76609, #70104, #85102, #8611, #1130, #31592, #91117, #1629, #32078, #22640, #93083, #53121, #79573, #25597, #34535, #27045, #56576, #48072, #87555, #2617, #78585, #10096, #57543, #17602, #40594, #19065, #87067, #56090, #88042, #80054, #41593, #63078, #71588, #11072, #72060, #18577, #19554, #49544, #78090, #33554, #71091, #3587, #49070, #34045, #95049, #33072, #11557, #41091, #3100, #64541, #40097, #9593, #48566, #26556, #64052, #63568, #65029, #94564, #57053, #72538, #70597, #2123, #4072, #42077, #79067, #25114, #26082, #95556, #86582, #94076, #32582, #93579, #18091, #55596, #10581, #86091, #50050, #88539, #29012, #35030, #43045, #81037, #20041, #14038, #43526, #89531, #20546, #89035, #75016, #21040, #50543, #5551, #67527, #98044, #81524, #36539, #29500, #90015, #12544, #28531, #73525, #4568, #96055, #5053, #67028, #65532, #13032, #59025, #51530, #21535, #35536, #51031, #66029, #6521, #96557, #74022, #28032, #36029, #60008, #58527, #66531, #97058, #52028, #27539, #82022, #44016, #13533, #74519, #80553, #6039, #97550 ) ),
 .UNSPECIFIED., .F., .F., .T. ) 
 B_SPLINE_SURFACE_WITH_KNOTS ( ( 2, 2 ),
 ( 3, 2, 2, 2, 2, 2, 2, 2, 2, 2, 2, 2, 2, 2, 2, 2, 2, 2, 2, 2, 2, 2, 2, 2, 2, 2, 2, 2, 2, 2, 2, 2, 2, 2, 2, 2, 2, 2, 2, 2, 2, 2, 2, 2, 2, 2, 2, 2, 2, 2, 2, 2, 2, 2, 2, 2, 2, 2, 2, 2, 2, 2, 2, 2, 2, 2, 2, 2, 2, 2, 2, 2, 2, 2, 2, 2, 2, 2, 2, 2, 2, 2, 2, 2, 2, 2, 2, 2, 2, 2, 2, 2, 2, 2, 2, 2, 2, 2, 2, 2, 2, 2, 2, 2, 2, 2, 2, 2, 2, 2, 2, 2, 2, 2, 2, 2, 2, 2, 2, 2, 2, 2, 2, 2, 2, 2, 2, 2, 2, 2, 2, 2, 2, 2, 2, 2, 2, 2, 2, 2, 2, 2, 2, 2, 2, 2, 2, 2, 2, 2, 2, 2, 2, 2, 2, 2, 2, 2, 2, 2, 2, 2, 3 ),
 ( 0.000000000000000000, 1.000000000000000000 ),
 ( 0.000000000000000000, 0.005952380952380952051, 0.01190476190476190410, 0.01785714285714285615, 0.02380952380952380820, 0.02976190476190476025, 0.03571428571428571230, 0.04166666666666666435, 0.04761904761904761640, 0.05357142857142856845, 0.05952380952380952051, 0.06547619047619047949, 0.07142857142857142461, 0.07738095238095238360, 0.08333333333333332871, 0.08928571428571428770, 0.09523809523809523281, 0.1011904761904761918, 0.1071428571428571369, 0.1130952380952380959, 0.1190476190476190410, 0.1250000000000000000, 0.1309523809523809590, 0.1369047619047619180, 0.1428571428571428492, 0.1488095238095238082, 0.1547619047619047672, 0.1607142857142857262, 0.1666666666666666574, 0.1726190476190476164, 0.1785714285714285754, 0.1845238095238095344, 0.1904761904761904656, 0.1964285714285714246, 0.2023809523809523836, 0.2083333333333333426, 0.2142857142857142738, 0.2202380952380952328, 0.2261904761904761918, 0.2321428571428571508, 0.2380952380952380820, 0.2440476190476190410, 0.2500000000000000000, 0.2559523809523809312, 0.2619047619047619180, 0.2678571428571428492, 0.2738095238095238360, 0.2797619047619047672, 0.2857142857142856984, 0.2916666666666666852, 0.2976190476190476164, 0.3035714285714285476, 0.3095238095238095344, 0.3154761904761904656, 0.3214285714285714524, 0.3273809523809523836, 0.3333333333333333148, 0.3392857142857143016, 0.3452380952380952328, 0.3511904761904761640, 0.3571428571428571508, 0.3630952380952380820, 0.3690476190476190688, 0.3750000000000000000, 0.3809523809523809312, 0.3869047619047619180, 0.3928571428571428492, 0.3988095238095238360, 0.4047619047619047672, 0.4107142857142856984, 0.4166666666666666852, 0.4226190476190476164, 0.4285714285714285476, 0.4345238095238095344, 0.4404761904761904656, 0.4464285714285714524, 0.4523809523809523836, 0.4583333333333333148, 0.4642857142857143016, 0.4702380952380952328, 0.4761904761904761640, 0.4821428571428571508, 0.4880952380952380820, 0.4940476190476190688, 0.5000000000000000000, 0.5059523809523809312, 0.5119047619047618625, 0.5178571428571429047, 0.5238095238095238360, 0.5297619047619047672, 0.5357142857142856984, 0.5416666666666666297, 0.5476190476190476719, 0.5535714285714286031, 0.5595238095238095344, 0.5654761904761904656, 0.5714285714285713969, 0.5773809523809523281, 0.5833333333333333703, 0.5892857142857143016, 0.5952380952380952328, 0.6011904761904761640, 0.6071428571428570953, 0.6130952380952381375, 0.6190476190476190688, 0.6250000000000000000, 0.6309523809523809312, 0.6369047619047618625, 0.6428571428571429047, 0.6488095238095238360, 0.6547619047619047672, 0.6607142857142856984, 0.6666666666666666297, 0.6726190476190476719, 0.6785714285714286031, 0.6845238095238095344, 0.6904761904761904656, 0.6964285714285713969, 0.7023809523809523281, 0.7083333333333333703, 0.7142857142857143016, 0.7202380952380952328, 0.7261904761904761640, 0.7321428571428570953, 0.7380952380952381375, 0.7440476190476190688, 0.7500000000000000000, 0.7559523809523809312, 0.7619047619047618625, 0.7678571428571429047, 0.7738095238095238360, 0.7797619047619047672, 0.7857142857142856984, 0.7916666666666666297, 0.7976190476190476719, 0.8035714285714286031, 0.8095238095238095344, 0.8154761904761904656, 0.8214285714285713969, 0.8273809523809523281, 0.8333333333333333703, 0.8392857142857143016, 0.8452380952380952328, 0.8511904761904761640, 0.8571428571428570953, 0.8630952380952381375, 0.8690476190476190688, 0.8750000000000000000, 0.8809523809523809312, 0.8869047619047618625, 0.8928571428571429047, 0.8988095238095238360, 0.9047619047619047672, 0.9107142857142856984, 0.9166666666666666297, 0.9226190476190476719, 0.9285714285714286031, 0.9345238095238095344, 0.9404761904761904656, 0.9464285714285713969, 0.9523809523809523281, 0.9583333333333333703, 0.9642857142857143016 ),
 .UNSPECIFIED. ) 
 GEOMETRIC_REPRESENTATION_ITEM ( )  RATIONAL_B_SPLINE_SURFACE ( (
 ( 1.000000000000000000, 0.9659258262890683122, 1.000000000000000000, 0.9659258262890683122, 1.000000000000000000, 0.9659258262890683122, 1.000000000000000000, 0.9659258262890683122, 1.000000000000000000, 0.9659258262890683122, 1.000000000000000000, 0.9659258262890683122, 1.000000000000000000, 0.9659258262890683122, 1.000000000000000000, 0.9659258262890683122, 1.000000000000000000, 0.9659258262890683122, 1.000000000000000000, 0.9659258262890683122, 1.000000000000000000, 0.9659258262890683122, 1.000000000000000000, 0.9659258262890683122, 1.000000000000000000, 0.9659258262890683122, 1.000000000000000000, 0.9659258262890683122, 1.000000000000000000, 0.9659258262890683122, 1.000000000000000000, 0.9659258262890683122, 1.000000000000000000, 0.9659258262890683122, 1.000000000000000000, 0.9659258262890683122, 1.000000000000000000, 0.9659258262890683122, 1.000000000000000000, 0.9659258262890683122, 1.000000000000000000, 0.9659258262890683122, 1.000000000000000000, 0.9659258262890683122, 1.000000000000000000, 0.9659258262890683122, 1.000000000000000000, 0.9659258262890683122, 1.000000000000000000, 0.9659258262890683122, 1.000000000000000000, 0.9659258262890683122, 1.000000000000000000, 0.9659258262890683122, 1.000000000000000000, 0.9659258262890683122, 1.000000000000000000, 0.9659258262890683122, 1.000000000000000000, 0.9659258262890683122, 1.000000000000000000, 0.9659258262890683122, 1.000000000000000000, 0.9659258262890683122, 1.000000000000000000, 0.9659258262890683122, 1.000000000000000000, 0.9659258262890683122, 1.000000000000000000, 0.9659258262890683122, 1.000000000000000000, 0.9659258262890683122, 1.000000000000000000, 0.9659258262890683122, 1.000000000000000000, 0.9659258262890683122, 1.000000000000000000, 0.9659258262890683122, 1.000000000000000000, 0.9659258262890683122, 1.000000000000000000, 0.9659258262890683122, 1.000000000000000000, 0.9659258262890683122, 1.000000000000000000, 0.9659258262890683122, 1.000000000000000000, 0.9659258262890683122, 1.000000000000000000, 0.9659258262890683122, 1.000000000000000000, 0.9659258262890683122, 1.000000000000000000, 0.9659258262890683122, 1.000000000000000000, 0.9659258262890683122, 1.000000000000000000, 0.9659258262890683122, 1.000000000000000000, 0.9659258262890683122, 1.000000000000000000, 0.9659258262890683122, 1.000000000000000000, 0.9659258262890683122, 1.000000000000000000, 0.9659258262890683122, 1.000000000000000000, 0.9659258262890683122, 1.000000000000000000, 0.9659258262890683122, 1.000000000000000000, 0.9659258262890683122, 1.000000000000000000, 0.9659258262890683122, 1.000000000000000000, 0.9659258262890683122, 1.000000000000000000, 0.9659258262890683122, 1.000000000000000000, 0.9659258262890683122, 1.000000000000000000, 0.9659258262890683122, 1.000000000000000000, 0.9659258262890683122, 1.000000000000000000, 0.9659258262890683122, 1.000000000000000000, 0.9659258262890683122, 1.000000000000000000, 0.9659258262890683122, 1.000000000000000000, 0.9659258262890683122, 1.000000000000000000, 0.9659258262890683122, 1.000000000000000000, 0.9659258262890683122, 1.000000000000000000, 0.9659258262890683122, 1.000000000000000000, 0.9659258262890683122, 1.000000000000000000, 0.9659258262890683122, 1.000000000000000000, 0.9659258262890683122, 1.000000000000000000, 0.9659258262890683122, 1.000000000000000000, 0.9659258262890683122, 1.000000000000000000, 0.9659258262890683122, 1.000000000000000000, 0.9659258262890683122, 1.000000000000000000, 0.9659258262890683122, 1.000000000000000000, 0.9659258262890683122, 1.000000000000000000, 0.9659258262890683122, 1.000000000000000000, 0.9659258262890683122, 1.000000000000000000, 0.9659258262890683122, 1.000000000000000000, 0.9659258262890683122, 1.000000000000000000, 0.9659258262890683122, 1.000000000000000000, 0.9659258262890683122, 1.000000000000000000, 0.9659258262890683122, 1.000000000000000000, 0.9659258262890683122, 1.000000000000000000, 0.9659258262890683122, 1.000000000000000000, 0.9659258262890683122, 1.000000000000000000, 0.9659258262890683122, 1.000000000000000000, 0.9659258262890683122, 1.000000000000000000, 0.9659258262890683122, 1.000000000000000000, 0.9659258262890683122, 1.000000000000000000, 0.9659258262890683122, 1.000000000000000000, 0.9659258262890683122, 1.000000000000000000, 0.9659258262890683122, 1.000000000000000000, 0.9659258262890683122, 1.000000000000000000, 0.9659258262890683122, 1.000000000000000000, 0.9659258262890683122, 1.000000000000000000, 0.9659258262890683122, 1.000000000000000000, 0.9659258262890683122, 1.000000000000000000, 0.9659258262890683122, 1.000000000000000000, 0.9659258262890683122, 1.000000000000000000, 0.9659258262890683122, 1.000000000000000000, 0.9659258262890683122, 1.000000000000000000, 0.9659258262890683122, 1.000000000000000000, 0.9659258262890683122, 1.000000000000000000, 0.9659258262890683122, 1.000000000000000000, 0.9659258262890683122, 1.000000000000000000, 0.9659258262890683122, 1.000000000000000000, 0.9659258262890683122, 1.000000000000000000, 0.9659258262890683122, 1.000000000000000000, 0.9659258262890683122, 1.000000000000000000, 0.9659258262890683122, 1.000000000000000000, 0.9659258262890683122, 1.000000000000000000, 0.9659258262890683122, 1.000000000000000000, 0.9659258262890683122, 1.000000000000000000, 0.9659258262890683122, 1.000000000000000000, 0.9659258262890683122, 1.000000000000000000, 0.9659258262890683122, 1.000000000000000000, 0.9659258262890683122, 1.000000000000000000, 0.9659258262890683122, 1.000000000000000000, 0.9659258262890683122, 1.000000000000000000, 0.9659258262890683122, 1.000000000000000000, 0.9659258262890683122, 1.000000000000000000, 0.9659258262890683122, 1.000000000000000000, 0.9659258262890683122, 1.000000000000000000, 0.9659258262890683122, 1.000000000000000000, 0.9659258262890683122, 1.000000000000000000, 0.9659258262890683122, 1.000000000000000000, 0.9659258262890683122, 1.000000000000000000, 0.9659258262890683122, 1.000000000000000000, 0.9659258262890683122, 1.000000000000000000, 0.9659258262890683122, 1.000000000000000000, 0.9659258262890683122, 1.000000000000000000, 0.9659258262890683122, 1.000000000000000000, 0.9659258262890683122, 1.000000000000000000, 0.9659258262890683122, 1.000000000000000000, 0.9659258262890683122, 1.000000000000000000, 0.9659258262890683122, 1.000000000000000000, 0.9659258262890683122, 1.000000000000000000, 0.9659258262890683122, 1.000000000000000000, 0.9659258262890683122, 1.000000000000000000, 0.9659258262890683122, 1.000000000000000000, 0.9659258262890683122, 1.000000000000000000, 0.9659258262890683122, 1.000000000000000000, 0.9659258262890683122, 1.000000000000000000, 0.9659258262890683122, 1.000000000000000000, 0.9659258262890683122, 1.000000000000000000, 0.9659258262890683122, 1.000000000000000000, 0.9659258262890683122, 1.000000000000000000, 0.9659258262890683122, 1.000000000000000000, 0.9659258262890683122, 1.000000000000000000, 0.9659258262890683122, 1.000000000000000000, 0.9659258262890683122, 1.000000000000000000, 0.9659258262890683122, 1.000000000000000000, 0.9659258262890683122, 1.000000000000000000, 0.9659258262890683122, 1.000000000000000000, 0.9659258262890683122, 1.000000000000000000, 0.9659258262890683122, 1.000000000000000000, 0.9659258262890683122, 1.000000000000000000, 0.9659258262890683122, 1.000000000000000000, 0.9659258262890683122, 1.000000000000000000),
 ( 1.000000000000000000, 0.9659258262890683122, 1.000000000000000000, 0.9659258262890683122, 1.000000000000000000, 0.9659258262890683122, 1.000000000000000000, 0.9659258262890683122, 1.000000000000000000, 0.9659258262890683122, 1.000000000000000000, 0.9659258262890683122, 1.000000000000000000, 0.9659258262890683122, 1.000000000000000000, 0.9659258262890683122, 1.000000000000000000, 0.9659258262890683122, 1.000000000000000000, 0.9659258262890683122, 1.000000000000000000, 0.9659258262890683122, 1.000000000000000000, 0.9659258262890683122, 1.000000000000000000, 0.9659258262890683122, 1.000000000000000000, 0.9659258262890683122, 1.000000000000000000, 0.9659258262890683122, 1.000000000000000000, 0.9659258262890683122, 1.000000000000000000, 0.9659258262890683122, 1.000000000000000000, 0.9659258262890683122, 1.000000000000000000, 0.9659258262890683122, 1.000000000000000000, 0.9659258262890683122, 1.000000000000000000, 0.9659258262890683122, 1.000000000000000000, 0.9659258262890683122, 1.000000000000000000, 0.9659258262890683122, 1.000000000000000000, 0.9659258262890683122, 1.000000000000000000, 0.9659258262890683122, 1.000000000000000000, 0.9659258262890683122, 1.000000000000000000, 0.9659258262890683122, 1.000000000000000000, 0.9659258262890683122, 1.000000000000000000, 0.9659258262890683122, 1.000000000000000000, 0.9659258262890683122, 1.000000000000000000, 0.9659258262890683122, 1.000000000000000000, 0.9659258262890683122, 1.000000000000000000, 0.9659258262890683122, 1.000000000000000000, 0.9659258262890683122, 1.000000000000000000, 0.9659258262890683122, 1.000000000000000000, 0.9659258262890683122, 1.000000000000000000, 0.9659258262890683122, 1.000000000000000000, 0.9659258262890683122, 1.000000000000000000, 0.9659258262890683122, 1.000000000000000000, 0.9659258262890683122, 1.000000000000000000, 0.9659258262890683122, 1.000000000000000000, 0.9659258262890683122, 1.000000000000000000, 0.9659258262890683122, 1.000000000000000000, 0.9659258262890683122, 1.000000000000000000, 0.9659258262890683122, 1.000000000000000000, 0.9659258262890683122, 1.000000000000000000, 0.9659258262890683122, 1.000000000000000000, 0.9659258262890683122, 1.000000000000000000, 0.9659258262890683122, 1.000000000000000000, 0.9659258262890683122, 1.000000000000000000, 0.9659258262890683122, 1.000000000000000000, 0.9659258262890683122, 1.000000000000000000, 0.9659258262890683122, 1.000000000000000000, 0.9659258262890683122, 1.000000000000000000, 0.9659258262890683122, 1.000000000000000000, 0.9659258262890683122, 1.000000000000000000, 0.9659258262890683122, 1.000000000000000000, 0.9659258262890683122, 1.000000000000000000, 0.9659258262890683122, 1.000000000000000000, 0.9659258262890683122, 1.000000000000000000, 0.9659258262890683122, 1.000000000000000000, 0.9659258262890683122, 1.000000000000000000, 0.9659258262890683122, 1.000000000000000000, 0.9659258262890683122, 1.000000000000000000, 0.9659258262890683122, 1.000000000000000000, 0.9659258262890683122, 1.000000000000000000, 0.9659258262890683122, 1.000000000000000000, 0.9659258262890683122, 1.000000000000000000, 0.9659258262890683122, 1.000000000000000000, 0.9659258262890683122, 1.000000000000000000, 0.9659258262890683122, 1.000000000000000000, 0.9659258262890683122, 1.000000000000000000, 0.9659258262890683122, 1.000000000000000000, 0.9659258262890683122, 1.000000000000000000, 0.9659258262890683122, 1.000000000000000000, 0.9659258262890683122, 1.000000000000000000, 0.9659258262890683122, 1.000000000000000000, 0.9659258262890683122, 1.000000000000000000, 0.9659258262890683122, 1.000000000000000000, 0.9659258262890683122, 1.000000000000000000, 0.9659258262890683122, 1.000000000000000000, 0.9659258262890683122, 1.000000000000000000, 0.9659258262890683122, 1.000000000000000000, 0.9659258262890683122, 1.000000000000000000, 0.9659258262890683122, 1.000000000000000000, 0.9659258262890683122, 1.000000000000000000, 0.9659258262890683122, 1.000000000000000000, 0.9659258262890683122, 1.000000000000000000, 0.9659258262890683122, 1.000000000000000000, 0.9659258262890683122, 1.000000000000000000, 0.9659258262890683122, 1.000000000000000000, 0.9659258262890683122, 1.000000000000000000, 0.9659258262890683122, 1.000000000000000000, 0.9659258262890683122, 1.000000000000000000, 0.9659258262890683122, 1.000000000000000000, 0.9659258262890683122, 1.000000000000000000, 0.9659258262890683122, 1.000000000000000000, 0.9659258262890683122, 1.000000000000000000, 0.9659258262890683122, 1.000000000000000000, 0.9659258262890683122, 1.000000000000000000, 0.9659258262890683122, 1.000000000000000000, 0.9659258262890683122, 1.000000000000000000, 0.9659258262890683122, 1.000000000000000000, 0.9659258262890683122, 1.000000000000000000, 0.9659258262890683122, 1.000000000000000000, 0.9659258262890683122, 1.000000000000000000, 0.9659258262890683122, 1.000000000000000000, 0.9659258262890683122, 1.000000000000000000, 0.9659258262890683122, 1.000000000000000000, 0.9659258262890683122, 1.000000000000000000, 0.9659258262890683122, 1.000000000000000000, 0.9659258262890683122, 1.000000000000000000, 0.9659258262890683122, 1.000000000000000000, 0.9659258262890683122, 1.000000000000000000, 0.9659258262890683122, 1.000000000000000000, 0.9659258262890683122, 1.000000000000000000, 0.9659258262890683122, 1.000000000000000000, 0.9659258262890683122, 1.000000000000000000, 0.9659258262890683122, 1.000000000000000000, 0.9659258262890683122, 1.000000000000000000, 0.9659258262890683122, 1.000000000000000000, 0.9659258262890683122, 1.000000000000000000, 0.9659258262890683122, 1.000000000000000000, 0.9659258262890683122, 1.000000000000000000, 0.9659258262890683122, 1.000000000000000000, 0.9659258262890683122, 1.000000000000000000, 0.9659258262890683122, 1.000000000000000000, 0.9659258262890683122, 1.000000000000000000, 0.9659258262890683122, 1.000000000000000000, 0.9659258262890683122, 1.000000000000000000, 0.9659258262890683122, 1.000000000000000000, 0.9659258262890683122, 1.000000000000000000, 0.9659258262890683122, 1.000000000000000000, 0.9659258262890683122, 1.000000000000000000, 0.9659258262890683122, 1.000000000000000000, 0.9659258262890683122, 1.000000000000000000, 0.9659258262890683122, 1.000000000000000000, 0.9659258262890683122, 1.000000000000000000, 0.9659258262890683122, 1.000000000000000000, 0.9659258262890683122, 1.000000000000000000, 0.9659258262890683122, 1.000000000000000000, 0.9659258262890683122, 1.000000000000000000, 0.9659258262890683122, 1.000000000000000000, 0.9659258262890683122, 1.000000000000000000, 0.9659258262890683122, 1.000000000000000000, 0.9659258262890683122, 1.000000000000000000, 0.9659258262890683122, 1.000000000000000000, 0.9659258262890683122, 1.000000000000000000, 0.9659258262890683122, 1.000000000000000000, 0.9659258262890683122, 1.000000000000000000, 0.9659258262890683122, 1.000000000000000000, 0.9659258262890683122, 1.000000000000000000, 0.9659258262890683122, 1.000000000000000000, 0.9659258262890683122, 1.000000000000000000, 0.9659258262890683122, 1.000000000000000000, 0.9659258262890683122, 1.000000000000000000, 0.9659258262890683122, 1.000000000000000000, 0.9659258262890683122, 1.000000000000000000, 0.9659258262890683122, 1.000000000000000000, 0.9659258262890683122, 1.000000000000000000, 0.9659258262890683122, 1.000000000000000000, 0.9659258262890683122, 1.000000000000000000) ) ) 
 REPRESENTATION_ITEM ( '' )  SURFACE ( )  );
#49255=CARTESIAN_POINT ( 'NONE',  ( 13.43411237798106583, 27.66530133659708568, -12.81628187352647252 ) ) ;
#49258=CARTESIAN_POINT ( 'NONE',  ( 0.5774900079438590739, 67.64701867748817676, -5.440088680355550821 ) ) ;
#49259=CARTESIAN_POINT ( 'NONE',  ( 3.591859063236763294, 8.290301336597087456, -11.09922568453595026 ) ) ;
#49260=CARTESIAN_POINT ( 'NONE',  ( 12.63842701281683034, 32.46726448433412315, 9.846743663894596210 ) ) ;
#49261=CARTESIAN_POINT ( 'NONE',  ( 4.559911319644449179, 27.23035201082150536, -9.422509992056141925 ) ) ;
#49262=CARTESIAN_POINT ( 'NONE',  ( 19.38216949554541202, 25.99863466993042138, 9.382169495545424454 ) ) ;
#49264=CARTESIAN_POINT ( 'NONE',  ( 1.472469842513823179, 26.42559781766745175, 4.923371831947296329 ) ) ;
#49266=CARTESIAN_POINT ( 'NONE',  ( 20.88017736071110519, 30.56368534415484106, 2.639326808657452039E-16 ) ) ;
#49267=EDGE_LOOP ( 'NONE', ( #97057, #73585, #41004, #20101 ) ) ;
#49268=CARTESIAN_POINT ( 'NONE',  ( 2.035157376598824452, 58.68868534415482685, 7.964842623401179544 ) ) ;
#49269=CARTESIAN_POINT ( 'NONE',  ( 14.92337183194729988, 49.34226448433411605, -8.527530157486177487 ) ) ;
#49270=CARTESIAN_POINT ( 'NONE',  ( 10.00000000000000000, 31.81368534415483751, -10.88017736071110342 ) ) ;
#49271=( NAMED_UNIT ( * ) SI_UNIT ( $, .STERADIAN. ) SOLID_ANGLE_UNIT ( ) );
#49272=CARTESIAN_POINT ( 'NONE',  ( 4.559911319644449179, 42.23035201082151247, -9.422509992056141925 ) ) ;
#49273=VECTOR ( 'NONE', #5118, 1000.000000000000000 ) ;
#49274=CARTESIAN_POINT ( 'NONE',  ( -0.8801773607111009756, 18.06368534415484106, 1.068504757029289695E-15 ) ) ;
#49276=CARTESIAN_POINT ( 'NONE',  ( 5.076628168052704559, 35.17559781766745175, -8.527530157486179263 ) ) ;
#49277=CARTESIAN_POINT ( 'NONE',  ( 10.00000000000000178, 53.05374883491396787, 14.16423886937410082 ) ) ;
#49282=CARTESIAN_POINT ( 'NONE',  ( 6.204703633549690345, 37.84541550158063927, 14.16423886937410082 ) ) ;
#49285=CARTESIAN_POINT ( 'NONE',  ( -4.164238869374099927, 62.01208216824728936, 3.795296366450308767 ) ) ;
#49286=CARTESIAN_POINT ( 'NONE',  ( 2.791683348922237240, 35.38393115100079456, -7.208316651077763204 ) ) ;
#49288=CARTESIAN_POINT ( 'NONE',  ( 4.559911319644449179, 53.89701867748817676, 9.422509992056141925 ) ) ;
#49289=CARTESIAN_POINT ( 'NONE',  ( 0.6178305044545838731, 64.74863466993043914, 9.382169495545420901 ) ) ;
#49290=CARTESIAN_POINT ( 'NONE',  ( 7.084665262690076126, 27.02201867748817676, -10.88017736071110164 ) ) ;
#49291=CARTESIAN_POINT ( 'NONE',  ( 16.40814093676324603, 57.45696800326375353, -11.09922568453594671 ) ) ;
#49292=CARTESIAN_POINT ( 'NONE',  ( 10.00000000000000178, 15.37363466993042138, 12.81628187352647608 ) ) ;
#49293=CARTESIAN_POINT ( 'NONE',  ( 1.472469842513823179, 15.59226448433411960, -4.923371831947296329 ) ) ;
#49295=CARTESIAN_POINT ( 'NONE',  ( 17.62281668512002142, 3.285933195168227794, 6.500000000000010658 ) ) ;
#49296=CARTESIAN_POINT ( 'NONE',  ( 6.204703633549690345, 62.84541550158063927, 14.16423886937410082 ) ) ;
#49297=CARTESIAN_POINT ( 'NONE',  ( -2.266590686148945544, 32.22041550158063927, 7.082119434687048631 ) ) ;
#49298=CARTESIAN_POINT ( 'NONE',  ( 12.91533473730993009, 31.60535201082150891, -10.88017736071109987 ) ) ;
#49299=CARTESIAN_POINT ( 'NONE',  ( 7.084665262690076126, 44.10535201082151247, 10.88017736071109987 ) ) ;
#49300=DIRECTION ( 'NONE',  ( 0.000000000000000000, -0.000000000000000000, -1.000000000000000000 ) ) ;
#49302=CARTESIAN_POINT ( 'NONE',  ( 17.20831665107776587, 12.88393115100078390, 7.208316651077764980 ) ) ;
#49303=CARTESIAN_POINT ( 'NONE',  ( 14.92337183194729633, 27.67559781766745530, 8.527530157486181039 ) ) ;
#49304=FILL_AREA_STYLE ('',( #26307 ) ) ;
#49306=CARTESIAN_POINT ( 'NONE',  ( 19.84674366389459266, 23.71726448433412315, -2.638427012816827677 ) ) ;
#49307=CARTESIAN_POINT ( 'NONE',  ( 2.791683348922237240, 55.38393115100078745, -7.208316651077763204 ) ) ;
#49308=CARTESIAN_POINT ( 'NONE',  ( 12.91533473730993009, 21.60535201082150536, -10.88017736071109987 ) ) ;
#49309=CARTESIAN_POINT ( 'NONE',  ( 22.81628187352647785, 41.41530133659708923, 3.434112377981063169 ) ) ;
#49310=CARTESIAN_POINT ( 'NONE',  ( 12.91533473730993009, 66.60535201082150536, -10.88017736071109987 ) ) ;
#49311=CARTESIAN_POINT ( 'NONE',  ( 18.52753015748618282, 33.92559781766745886, -4.923371831947291888 ) ) ;
#49312=CARTESIAN_POINT ( 'NONE',  ( 24.16423886937409904, 64.09541550158064638, 3.795296366450317205 ) ) ;
#49313=CARTESIAN_POINT ( 'NONE',  ( 2.791683348922237240, 25.38393115100078390, -7.208316651077763204 ) ) ;
#49314=CARTESIAN_POINT ( 'NONE',  ( -0.1038446121089033475, 44.24302437010793909, -6.337995344473784876 ) ) ;
#49315=CARTESIAN_POINT ( 'NONE',  ( 14.92337183194729633, 62.67559781766745886, 8.527530157486181039 ) ) ;
#49316=CARTESIAN_POINT ( 'NONE',  ( 24.16423886937409904, 4.095415501580634832, 3.795296366450317205 ) ) ;
#49317=CARTESIAN_POINT ( 'NONE',  ( -0.3689425029237898834, 36.17874883491396787, -10.36894250292378850 ) ) ;
#49318=CARTESIAN_POINT ( 'NONE',  ( 7.361572987183169658, 34.96726448433411605, -9.846743663894592657 ) ) ;
#49320=CARTESIAN_POINT ( 'NONE',  ( 10.00000000000000178, 29.31368534415483751, 10.88017736071110342 ) ) ;
#49321=CARTESIAN_POINT ( 'NONE',  ( -0.8801773607111009756, 63.06368534415484106, 1.068504757029289695E-15 ) ) ;
#49324=CARTESIAN_POINT ( 'NONE',  ( 6.565887622018943937, 50.16530133659708213, 12.81628187352647430 ) ) ;
#49326=CARTESIAN_POINT ( 'NONE',  ( 0.5774900079438607392, 53.48035201082151247, 5.440088680355550821 ) ) ;
#49329=CARTESIAN_POINT ( 'NONE',  ( 20.88017736071110519, 60.56368534415484106, 2.639326808657452039E-16 ) ) ;
#49331=CARTESIAN_POINT ( 'NONE',  ( 10.00000000000000178, 59.31368534415484106, 10.88017736071110342 ) ) ;
#49333=CARTESIAN_POINT ( 'NONE',  ( 7.084665262690076126, 2.022018677488170990, -10.88017736071110164 ) ) ;
#49334=CARTESIAN_POINT ( 'NONE',  ( 18.52753015748618282, 8.925597817667451750, -4.923371831947291888 ) ) ;
#49336=CARTESIAN_POINT ( 'NONE',  ( 0.5774900079438607392, 13.48035201082150358, 5.440088680355550821 ) ) ;
#49337=CARTESIAN_POINT ( 'NONE',  ( 19.84674366389459266, 3.300597817667451750, 2.638427012816836559 ) ) ;
#49338=CARTESIAN_POINT ( 'NONE',  ( 22.26659068614895176, 9.720415501580633943, -7.082119434687042414 ) ) ;
#49340=CARTESIAN_POINT ( 'NONE',  ( 12.63842701281683922, 4.550597817667451750, -9.846743663894590881 ) ) ;
#49341=CARTESIAN_POINT ( 'NONE',  ( 0.5774900079438607392, 18.48035201082150536, 5.440088680355550821 ) ) ;
#49342=CARTESIAN_POINT ( 'NONE',  ( 12.63842701281683922, 44.55059781766745175, -9.846743663894590881 ) ) ;
#49344=CARTESIAN_POINT ( 'NONE',  ( 7.361572987183169658, 44.96726448433412315, -9.846743663894592657 ) ) ;
#49347=CARTESIAN_POINT ( 'NONE',  ( 19.42250999205614548, 50.98035201082151247, -5.440088680355545492 ) ) ;
#49348=CARTESIAN_POINT ( 'NONE',  ( 18.52753015748617571, 53.09226448433412315, 4.923371831947298993 ) ) ;
#49349=CARTESIAN_POINT ( 'NONE',  ( 4.559911319644449179, 8.897018677488171434, 9.422509992056141925 ) ) ;
#49350=DIRECTION ( 'NONE',  ( -0.000000000000000000, -0.000000000000000000, -1.000000000000000000 ) ) ;
#49351=CARTESIAN_POINT ( 'NONE',  ( 2.035157376598822676, 62.43868534415483396, -7.964842623401177768 ) ) ;
#49352=CARTESIAN_POINT ( 'NONE',  ( -0.8801773607111008646, 8.272018677488171434, 2.915334737309923430 ) ) ;
#49355=CARTESIAN_POINT ( 'NONE',  ( 19.38216949554541557, 37.24863466993041783, -9.382169495545420901 ) ) ;
#49356=CARTESIAN_POINT ( 'NONE',  ( 15.44008868035555260, 29.73035201082150891, 9.422509992056143702 ) ) ;
#49358=VERTEX_POINT ( 'NONE', #48409 ) ;
#49359=CARTESIAN_POINT ( 'NONE',  ( 16.40814093676324603, 47.45696800326375353, -11.09922568453594671 ) ) ;
#49360=CARTESIAN_POINT ( 'NONE',  ( 15.44008868035555793, 36.39701867748816966, -9.422509992056140149 ) ) ;
#49361=ADVANCED_FACE ( 'NONE', ( #56891 ), #32418, .F. ) ;
#49363=CARTESIAN_POINT ( 'NONE',  ( 14.92337183194729633, 57.67559781766745886, 8.527530157486181039 ) ) ;
#49364=CARTESIAN_POINT ( 'NONE',  ( 1.472469842513823179, 11.42559781766745175, 4.923371831947296329 ) ) ;
#49365=CARTESIAN_POINT ( 'NONE',  ( 18.52753015748618282, 48.92559781766745886, -4.923371831947291888 ) ) ;
#49366=CARTESIAN_POINT ( 'NONE',  ( -0.8801773607110991993, 27.85535201082150181, -2.915334737309923874 ) ) ;
#49367=LINE ( 'NONE', #79869, #79448 ) ;
#49368=CARTESIAN_POINT ( 'NONE',  ( 10.00000000000000000, 39.75893115100078745, -9.846743663894594434 ) ) ;
#49372=CARTESIAN_POINT ( 'NONE',  ( 5.076628168052703671, 31.84226448433412315, 8.527530157486179263 ) ) ;
#49374=CARTESIAN_POINT ( 'NONE',  ( 18.52753015748618282, 53.92559781766745175, -4.923371831947291888 ) ) ;
#49375=VERTEX_POINT ( 'NONE', #73863 ) ;
#49377=CARTESIAN_POINT ( 'NONE',  ( 19.38216949554541557, 27.24863466993041783, -9.382169495545420901 ) ) ;
#49378=CARTESIAN_POINT ( 'NONE',  ( 5.076628168052703671, 46.84226448433412315, 8.527530157486179263 ) ) ;
#49380=CARTESIAN_POINT ( 'NONE',  ( 24.16423886937409904, 59.09541550158063217, 3.795296366450317205 ) ) ;
#49381=CARTESIAN_POINT ( 'NONE',  ( 19.84674366389459266, 23.71726448433412315, -2.638427012816827677 ) ) ;
#49382=CARTESIAN_POINT ( 'NONE',  ( -1.926860441876562025, 39.47997603579417358, -3.195792623639529761 ) ) ;
#49383=CARTESIAN_POINT ( 'NONE',  ( -4.164238869374099927, 62.01208216824728936, 3.795296366450308767 ) ) ;
#49384=CARTESIAN_POINT ( 'NONE',  ( 14.92337183194729988, 54.34226448433412315, -8.527530157486177487 ) ) ;
#49385=CARTESIAN_POINT ( 'NONE',  ( -2.266590686148945544, 67.22041550158063217, 7.082119434687048631 ) ) ;
#49386=CARTESIAN_POINT ( 'NONE',  ( -4.164238869374099039, 31.80374883491396432, 8.674139862899312516E-16 ) ) ;
#49387=CARTESIAN_POINT ( 'NONE',  ( 6.204703633549690345, 37.84541550158063927, 14.16423886937410082 ) ) ;
#49388=CARTESIAN_POINT ( 'NONE',  ( 2.831191079880678085, 79.91181047996344944, 9.500000000000000000 ) ) ;
#49390=CARTESIAN_POINT ( 'NONE',  ( 0.8952175423694904710, 27.60160829253885950, -5.990408912944333863 ) ) ;
#49391=CARTESIAN_POINT ( 'NONE',  ( 12.63842701281683922, 59.55059781766744464, -9.846743663894590881 ) ) ;
#49392=CARTESIAN_POINT ( 'NONE',  ( 17.96484262340118221, 54.93868534415484106, 7.964842623401181321 ) ) ;
#49395=CARTESIAN_POINT ( 'NONE',  ( 7.361572987183169658, 49.96726448433410894, -9.846743663894592657 ) ) ;
#49397=CARTESIAN_POINT ( 'NONE',  ( 10.00000000000000178, 52.25893115100078745, 9.846743663894594434 ) ) ;
#49400=CARTESIAN_POINT ( 'NONE',  ( -4.164238869374099039, 26.80374883491397142, 8.674139862899312516E-16 ) ) ;
#49401=PRESENTATION_STYLE_ASSIGNMENT (( #20398 ) ) ;
#49403=CARTESIAN_POINT ( 'NONE',  ( 19.10478245763052385, 46.02576239577081907, -5.990408912944311659 ) ) ;
#49404=CARTESIAN_POINT ( 'NONE',  ( -0.8801773607111009756, 18.06368534415484106, 1.068504757029289695E-15 ) ) ;
#49405=CARTESIAN_POINT ( 'NONE',  ( 0.6178305044545818747, 28.49863466993041783, -9.382169495545419124 ) ) ;
#49406=CARTESIAN_POINT ( 'NONE',  ( 20.32896413005680003, 61.77164270246083788, 5.963430220938287007 ) ) ;
#49407=CARTESIAN_POINT ( 'NONE',  ( 18.52753015748618282, 13.92559781766745175, -4.923371831947291888 ) ) ;
#49410=CARTESIAN_POINT ( 'NONE',  ( 17.08211943468705130, 33.47041550158063927, 12.26659068614894998 ) ) ;
#49411=FACE_OUTER_BOUND ( 'NONE', #84051, .T. ) ;
#49413=CARTESIAN_POINT ( 'NONE',  ( 20.88017736071110519, 5.563685344154838397, 2.639326808657452039E-16 ) ) ;
#49415=CARTESIAN_POINT ( 'NONE',  ( -0.8801773607111008646, 43.27201867748817676, 2.915334737309923430 ) ) ;
#49416=CARTESIAN_POINT ( 'NONE',  ( 19.42250999205614193, 35.14701867748816966, 5.440088680355555262 ) ) ;
#49417=CARTESIAN_POINT ( 'NONE',  ( 22.81628187352648496, 1.831968003263753753, -3.434112377981050290 ) ) ;
#49418=CARTESIAN_POINT ( 'NONE',  ( 17.20831665107776587, 64.13393115100079456, -7.208316651077762316 ) ) ;
#49420=CARTESIAN_POINT ( 'NONE',  ( 18.52753015748617571, 13.09226448433411960, 4.923371831947298993 ) ) ;
#49421=CARTESIAN_POINT ( 'NONE',  ( 18.39792806157246829, 49.52224192338640307, 6.500000000000079936 ) ) ;
#49423=CARTESIAN_POINT ( 'NONE',  ( 10.00000000000000178, 49.31368534415484106, 10.88017736071110342 ) ) ;
#49424=CARTESIAN_POINT ( 'NONE',  ( -1.099225684535947600, 3.706968003263753531, -6.408140936763238038 ) ) ;
#49425=CARTESIAN_POINT ( 'NONE',  ( -0.8801773607110991993, 62.85535201082150536, -2.915334737309923874 ) ) ;
#49426=CARTESIAN_POINT ( 'NONE',  ( 1.472469842513823179, 30.59226448433411960, -4.923371831947296329 ) ) ;
#49427=CARTESIAN_POINT ( 'NONE',  ( 19.38216949554541557, 37.24863466993041783, -9.382169495545420901 ) ) ;
#49428=CARTESIAN_POINT ( 'NONE',  ( 10.00000000000000000, 9.758931151000785675, -9.846743663894594434 ) ) ;
#49430=ORIENTED_EDGE ( 'NONE', *, *, #44801, .T. ) ;
#49433=CARTESIAN_POINT ( 'NONE',  ( 10.00000000000000000, 6.813685344154838397, -10.88017736071110342 ) ) ;
#49434=CARTESIAN_POINT ( 'NONE',  ( 21.09922568453594849, 61.20696800326376064, 6.408140936763242479 ) ) ;
#49435=CARTESIAN_POINT ( 'NONE',  ( -0.3689425029237881626, 22.42874883491397142, 10.36894250292379027 ) ) ;
#49436=CARTESIAN_POINT ( 'NONE',  ( 2.791683348922237240, 35.38393115100079456, -7.208316651077763204 ) ) ;
#49438=CARTESIAN_POINT ( 'NONE',  ( 4.559911319644449179, 22.23035201082150536, -9.422509992056141925 ) ) ;
#49439=CARTESIAN_POINT ( 'NONE',  ( 10.00000000000000000, 6.813685344154838397, -10.88017736071110342 ) ) ;
#49441=VECTOR ( 'NONE', #67820, 1000.000000000000000 ) ;
#49442=CARTESIAN_POINT ( 'NONE',  ( 15.44008868035555260, 19.73035201082150536, 9.422509992056143702 ) ) ;
#49443=CARTESIAN_POINT ( 'NONE',  ( 2.035157376598824452, 23.68868534415484461, 7.964842623401179544 ) ) ;
#49444=DIRECTION ( 'NONE',  ( 0.000000000000000000, -1.000000000000000000, 0.000000000000000000 ) ) ;
#49446=CARTESIAN_POINT ( 'NONE',  ( 10.00000000000000178, 67.25893115100079456, 9.846743663894594434 ) ) ;
#49447=CARTESIAN_POINT ( 'NONE',  ( 10.00000000000000178, 24.31368534415484106, 10.88017736071110342 ) ) ;
#49449=CARTESIAN_POINT ( 'NONE',  ( 17.20831665107776587, 57.88393115100078745, 7.208316651077764980 ) ) ;
#49452=CARTESIAN_POINT ( 'NONE',  ( 6.204703633549690345, 27.84541550158063217, 14.16423886937410082 ) ) ;
#49453=CARTESIAN_POINT ( 'NONE',  ( 20.88017736071110164, 45.35535201082149115, 2.915334737309930979 ) ) ;
#49454=CARTESIAN_POINT ( 'NONE',  ( 7.084665262690076126, 19.10535201082150181, 10.88017736071109987 ) ) ;
#49455=CARTESIAN_POINT ( 'NONE',  ( 1.472469842513823179, 60.59226448433412315, -4.923371831947296329 ) ) ;
#49458=CARTESIAN_POINT ( 'NONE',  ( 0.1532563361054082862, 46.21726448433411605, 2.638427012816831674 ) ) ;
#49459=CARTESIAN_POINT ( 'NONE',  ( 12.63842701281683034, 2.467264484334118269, 9.846743663894596210 ) ) ;
#49461=ORIENTED_EDGE ( 'NONE', *, *, #35122, .F. ) ;
#49462=CARTESIAN_POINT ( 'NONE',  ( 20.88017736071110164, 10.35535201082150714, 2.915334737309930979 ) ) ;
#49463=CARTESIAN_POINT ( 'NONE',  ( 1.472469842513823179, 6.425597817667451750, 4.923371831947296329 ) ) ;
#49464=CARTESIAN_POINT ( 'NONE',  ( 22.81628187352647785, 1.415301336597087012, 3.434112377981063169 ) ) ;
#49465=CARTESIAN_POINT ( 'NONE',  ( 15.44008868035555793, 46.39701867748817676, -9.422509992056140149 ) ) ;
#49466=CARTESIAN_POINT ( 'NONE',  ( 0.5774900079438607392, 13.48035201082150358, 5.440088680355550821 ) ) ;
#49467=CARTESIAN_POINT ( 'NONE',  ( -2.816281873526473856, 39.33196800326374643, 3.434112377981055619 ) ) ;
#49468=CARTESIAN_POINT ( 'NONE',  ( -4.164238869374099927, 27.01208216824730357, 3.795296366450308767 ) ) ;
#49469=CARTESIAN_POINT ( 'NONE',  ( -2.168404344971008868E-15, 78.91966277462715595, -9.500000000000000000 ) ) ;
#49470=EDGE_CURVE ( 'NONE', #17007, #38580, #9681, .T. ) ;
#49471=CARTESIAN_POINT ( 'NONE',  ( 16.40814093676324603, 52.45696800326375353, -11.09922568453594671 ) ) ;
#49473=CARTESIAN_POINT ( 'NONE',  ( 22.81628187352647785, 6.415301336597088344, 3.434112377981063169 ) ) ;
#49474=CARTESIAN_POINT ( 'NONE',  ( 0.5774900079438607392, 33.48035201082150536, 5.440088680355550821 ) ) ;
#49475=CARTESIAN_POINT ( 'NONE',  ( 0.1532563361054083140, 61.00893115100078745, 1.131784320476157264E-15 ) ) ;
#49476=EDGE_CURVE ( 'NONE', #18635, #8299, #65866, .T. ) ;
#49478=CARTESIAN_POINT ( 'NONE',  ( 14.92337183194729633, 7.675597817667451750, 8.527530157486181039 ) ) ;
#49480=CARTESIAN_POINT ( 'NONE',  ( 17.20831665107776587, 7.883931151000784787, 7.208316651077764980 ) ) ;
#49481=CARTESIAN_POINT ( 'NONE',  ( 5.076628168052703671, 16.84226448433411960, 8.527530157486179263 ) ) ;
#49482=CARTESIAN_POINT ( 'NONE',  ( 2.791683348922237240, 5.383931151000785675, -7.208316651077763204 ) ) ;
#49483=SURFACE_SIDE_STYLE ('',( #56987 ) ) ;
#49484=CARTESIAN_POINT ( 'NONE',  ( 0.5774900079438607392, 58.48035201082151247, 5.440088680355550821 ) ) ;
#49485=CARTESIAN_POINT ( 'NONE',  ( -0.8801773607110990882, 37.85535201082150536, -2.915334737309924318 ) ) ;
#49486=CARTESIAN_POINT ( 'NONE',  ( 12.91533473730993009, 66.60535201082150536, -10.88017736071109987 ) ) ;
#49487=CARTESIAN_POINT ( 'NONE',  ( 17.20831665107776587, 14.13393115100078568, -7.208316651077762316 ) ) ;
#49488=ORIENTED_EDGE ( 'NONE', *, *, #50935, .T. ) ;
#49490=CARTESIAN_POINT ( 'NONE',  ( 0.1532563361054100626, 55.80059781766745175, -2.638427012816831230 ) ) ;
#49494=CARTESIAN_POINT ( 'NONE',  ( 10.00000000000000178, 13.05374883491396787, 14.16423886937410082 ) ) ;
#49497=CARTESIAN_POINT ( 'NONE',  ( 22.26659068614894466, 13.88708216824730179, 7.082119434687054849 ) ) ;
#49499=CARTESIAN_POINT ( 'NONE',  ( -0.3689425029237898834, 26.17874883491396432, -10.36894250292378850 ) ) ;
#49500=CARTESIAN_POINT ( 'NONE',  ( 10.00000000000000000, 31.81368534415483751, -10.88017736071110342 ) ) ;
#49503=CARTESIAN_POINT ( 'NONE',  ( 5.076628168052703671, 11.84226448433411960, 8.527530157486179263 ) ) ;
#49504=CARTESIAN_POINT ( 'NONE',  ( 2.035157376598822676, 52.43868534415483396, -7.964842623401177768 ) ) ;
#49505=CARTESIAN_POINT ( 'NONE',  ( 0.1532563361054082862, 11.21726448433411605, 2.638427012816831674 ) ) ;
#49506=CARTESIAN_POINT ( 'NONE',  ( -1.099225684535947600, 49.54030133659708923, 6.408140936763237150 ) ) ;
#49507=CARTESIAN_POINT ( 'NONE',  ( 2.791683348922240793, 36.63393115100078035, 7.208316651077764092 ) ) ;
#49510=CARTESIAN_POINT ( 'NONE',  ( 22.81628187352647785, 31.41530133659709279, 3.434112377981063169 ) ) ;
#49512=CARTESIAN_POINT ( 'NONE',  ( 0.1532563361054083140, 26.00893115100078745, 1.131784320476157264E-15 ) ) ;
#49513=CARTESIAN_POINT ( 'NONE',  ( 20.36894250292379382, 18.67874883491397142, 10.36894250292379205 ) ) ;
#49514=ORIENTED_EDGE ( 'NONE', *, *, #31312, .F. ) ;
#49515=CARTESIAN_POINT ( 'NONE',  ( -0.8801773607111008646, 48.27201867748816966, 2.915334737309923430 ) ) ;
#49516=CARTESIAN_POINT ( 'NONE',  ( 20.88017736071110164, 55.35535201082149825, 2.915334737309930979 ) ) ;
#49517=CARTESIAN_POINT ( 'NONE',  ( -2.266590686148945544, 47.22041550158063927, 7.082119434687048631 ) ) ;
#49518=CARTESIAN_POINT ( 'NONE',  ( 2.791683348922240793, 51.63393115100078745, 7.208316651077764092 ) ) ;
#49519=CARTESIAN_POINT ( 'NONE',  ( 2.791683348922240793, 16.63393115100078745, 7.208316651077764092 ) ) ;
#49520=CARTESIAN_POINT ( 'NONE',  ( 10.00000000000000178, 65.37363466993042493, 12.81628187352647608 ) ) ;
#49522=CARTESIAN_POINT ( 'NONE',  ( 4.559911319644449179, 42.23035201082151247, -9.422509992056141925 ) ) ;
#49525=CARTESIAN_POINT ( 'NONE',  ( -2.816281873526473856, 29.33196800326376064, 3.434112377981055619 ) ) ;
#49526=CARTESIAN_POINT ( 'NONE',  ( 1.472469842513823179, 56.42559781766745886, 4.923371831947296329 ) ) ;
#49528=CARTESIAN_POINT ( 'NONE',  ( 20.88017736071110519, 5.563685344154837509, 2.639326808657452039E-16 ) ) ;
#49529=CARTESIAN_POINT ( 'NONE',  ( 2.035157376598822676, 67.43868534415484817, -7.964842623401177768 ) ) ;
#49530=EDGE_CURVE ( 'NONE', #31960, #31762, #20875, .T. ) ;
#49531=SURFACE_STYLE_FILL_AREA ( #36016 ) ;
#49532=CARTESIAN_POINT ( 'NONE',  ( 0.2751277870542909176, 59.36607318730130345, -6.499999999999992006 ) ) ;
#49533=CARTESIAN_POINT ( 'NONE',  ( -0.8801773607111009756, 63.06368534415484106, 1.068504757029289695E-15 ) ) ;
#49534=CARTESIAN_POINT ( 'NONE',  ( 12.63842701281683034, 2.467264484334118269, 9.846743663894596210 ) ) ;
#49536=CARTESIAN_POINT ( 'NONE',  ( 0.1532563361054083140, 36.00893115100078745, 1.131784320476157264E-15 ) ) ;
#49537=CARTESIAN_POINT ( 'NONE',  ( 0.5774900079438607392, 18.48035201082150536, 5.440088680355550821 ) ) ;
#49538=CARTESIAN_POINT ( 'NONE',  ( 17.20831665107776587, 62.88393115100078745, 7.208316651077764980 ) ) ;
#49539=CARTESIAN_POINT ( 'NONE',  ( 15.44008868035555260, 34.73035201082151247, 9.422509992056143702 ) ) ;
#49542=CARTESIAN_POINT ( 'NONE',  ( -2.816281873526473856, 34.12363466993042493, 9.499525473075851096E-16 ) ) ;
#49543=ORIENTED_EDGE ( 'NONE', *, *, #14589, .T. ) ;
#49544=CARTESIAN_POINT ( 'NONE',  ( 17.96484262340118221, 49.93868534415484106, 7.964842623401181321 ) ) ;
#49545=CARTESIAN_POINT ( 'NONE',  ( 19.38216949554541557, 22.24863466993041428, -9.382169495545420901 ) ) ;
#49546=CARTESIAN_POINT ( 'NONE',  ( 2.035157376598824452, 28.68868534415484106, 7.964842623401179544 ) ) ;
#49547=CARTESIAN_POINT ( 'NONE',  ( 2.035157376598822676, 2.438685344154838397, -7.964842623401177768 ) ) ;
#49548=CARTESIAN_POINT ( 'NONE',  ( 7.361572987183169658, 44.96726448433412315, -9.846743663894592657 ) ) ;
#49549=CARTESIAN_POINT ( 'NONE',  ( 1.472469842513823179, 6.425597817667451750, 4.923371831947296329 ) ) ;
#49550=CARTESIAN_POINT ( 'NONE',  ( -0.8801773607111009756, 58.06368534415484106, 1.068504757029289695E-15 ) ) ;
#49552=CARTESIAN_POINT ( 'NONE',  ( 17.08211943468705840, 35.13708216824730357, -12.26659068614894466 ) ) ;
#49556=CARTESIAN_POINT ( 'NONE',  ( 24.16423886937409904, 54.09541550158063217, 3.795296366450317205 ) ) ;
#49557=CARTESIAN_POINT ( 'NONE',  ( 13.79529636645030344, 53.26208216824730357, 14.16423886937410614 ) ) ;
#49559=CARTESIAN_POINT ( 'NONE',  ( 19.84674366389459266, 13.30059781766745353, 2.638427012816836559 ) ) ;
#49560=CARTESIAN_POINT ( 'NONE',  ( 19.38216949554541202, 15.99863466993042138, 9.382169495545424454 ) ) ;
#49563=CARTESIAN_POINT ( 'NONE',  ( -0.8801773607110991993, 2.855352010821504471, -2.915334737309923874 ) ) ;
#49564=CARTESIAN_POINT ( 'NONE',  ( 16.40814093676323893, 30.79030133659708923, 11.09922568453595026 ) ) ;
#49565=CARTESIAN_POINT ( 'NONE',  ( 2.917880565312950480, 45.97041550158063927, -12.26659068614894821 ) ) ;
#49566=ADVANCED_FACE ( 'NONE', ( #13869 ), #50874, .T. ) ;
#49568=CARTESIAN_POINT ( 'NONE',  ( 10.00000000000000178, 12.25893115100078568, 9.846743663894594434 ) ) ;
#49572=ORIENTED_EDGE ( 'NONE', *, *, #70799, .T. ) ;
#49573=DIRECTION ( 'NONE',  ( -0.8320502943378437211, 0.5547001962252290364, 0.000000000000000000 ) ) ;
#49574=CARTESIAN_POINT ( 'NONE',  ( 10.00000000000000000, 19.75893115100078390, -9.846743663894594434 ) ) ;
#49576=ORIENTED_EDGE ( 'NONE', *, *, #95041, .T. ) ;
#49577=CARTESIAN_POINT ( 'NONE',  ( 6.204703633549690345, 67.84541550158060375, 14.16423886937410082 ) ) ;
#49578=CARTESIAN_POINT ( 'NONE',  ( 20.88017736071110875, 30.77201867748816966, -2.915334737309920765 ) ) ;
#49579=CARTESIAN_POINT ( 'NONE',  ( 2.791683348922237240, 55.38393115100078745, -7.208316651077763204 ) ) ;
#49580=CARTESIAN_POINT ( 'NONE',  ( 6.565887622018943937, -1.918031996736246692, -12.81628187352647608 ) ) ;
#49582=CARTESIAN_POINT ( 'NONE',  ( 3.591859063236763294, 18.29030133659708568, -11.09922568453595026 ) ) ;
#49584=CARTESIAN_POINT ( 'NONE',  ( 6.204703633549690345, 65.76208216824731778, -14.16423886937410259 ) ) ;
#49585=CARTESIAN_POINT ( 'NONE',  ( 24.16423886937409904, 59.09541550158063217, 3.795296366450317205 ) ) ;
#49587=CARTESIAN_POINT ( 'NONE',  ( 0.5774900079438607392, 33.48035201082150536, 5.440088680355550821 ) ) ;
#49588=CARTESIAN_POINT ( 'NONE',  ( 19.42250999205614193, 50.14701867748817676, 5.440088680355555262 ) ) ;
#49589=AXIS2_PLACEMENT_3D ( 'NONE', #98141, #45105, #83113 ) ;
#49590=CARTESIAN_POINT ( 'NONE',  ( 7.084665262690076126, 52.02201867748816255, -10.88017736071110164 ) ) ;
#49592=CARTESIAN_POINT ( 'NONE',  ( 20.88017736071110519, 40.56368534415484106, 2.639326808657452039E-16 ) ) ;
#49594=VECTOR ( 'NONE', #17580, 1000.000000000000000 ) ;
#49595=EDGE_CURVE ( 'NONE', #91901, #41376, #19898, .T. ) ;
#49598=CARTESIAN_POINT ( 'NONE',  ( 19.84674366389459266, 13.30059781766745353, 2.638427012816836559 ) ) ;
#49601=CARTESIAN_POINT ( 'NONE',  ( 19.84674366389459621, 38.50893115100078745, 7.409399052514197653E-17 ) ) ;
#49603=CARTESIAN_POINT ( 'NONE',  ( 0.6178305044545838731, 49.74863466993041072, 9.382169495545420901 ) ) ;
#49608=DIRECTION ( 'NONE',  ( 0.000000000000000000, -1.000000000000000000, 0.000000000000000000 ) ) ;
#49609=CARTESIAN_POINT ( 'NONE',  ( 10.00000000000000000, 65.55374883491396076, -14.16423886937410082 ) ) ;
#49613=CARTESIAN_POINT ( 'NONE',  ( 14.92337183194729988, 39.34226448433412315, -8.527530157486177487 ) ) ;
#49615=CARTESIAN_POINT ( 'NONE',  ( 22.81628187352648496, 11.83196800326375531, -3.434112377981050290 ) ) ;
#49616=CARTESIAN_POINT ( 'NONE',  ( 12.91533473730993009, 66.60535201082150536, -10.88017736071109987 ) ) ;
#49617=CARTESIAN_POINT ( 'NONE',  ( -0.1038446121089073443, 4.243024370107933763, -6.337995344473778658 ) ) ;
#49618=CARTESIAN_POINT ( 'NONE',  ( 19.84674366389459266, 8.717264484334116048, -2.638427012816827677 ) ) ;
#49619=CARTESIAN_POINT ( 'NONE',  ( 19.84674366389459266, 58.71726448433411605, -2.638427012816827677 ) ) ;
#49623=CARTESIAN_POINT ( 'NONE',  ( -2.266590686148945544, 61.38708216824730357, -7.082119434687050408 ) ) ;
#49624=CARTESIAN_POINT ( 'NONE',  ( -2.266590686148945544, 12.22041550158063394, 7.082119434687048631 ) ) ;
#49625=CARTESIAN_POINT ( 'NONE',  ( 12.63842701281683034, 12.46726448433411782, 9.846743663894596210 ) ) ;
#49626=CARTESIAN_POINT ( 'NONE',  ( -0.8801773607111008646, 48.27201867748816966, 2.915334737309923430 ) ) ;
#49628=CARTESIAN_POINT ( 'NONE',  ( 22.81628187352647785, 26.62363466993042138, 6.195893100308588602E-16 ) ) ;
#49630=CARTESIAN_POINT ( 'NONE',  ( 19.42250999205614193, 5.147018677488171434, 5.440088680355555262 ) ) ;
#49634=CARTESIAN_POINT ( 'NONE',  ( 1.472469842513823179, 55.59226448433412315, -4.923371831947296329 ) ) ;
#49635=CARTESIAN_POINT ( 'NONE',  ( 5.076628168052703671, 11.84226448433411960, 8.527530157486179263 ) ) ;
#49637=CARTESIAN_POINT ( 'NONE',  ( 16.40814093676323893, 20.79030133659708923, 11.09922568453595026 ) ) ;
#49638=CARTESIAN_POINT ( 'NONE',  ( 1.274849032794292736, 52.55509018479936856, -6.499999999999977796 ) ) ;
#49639=CARTESIAN_POINT ( 'NONE',  ( 15.44008868035555793, 31.39701867748817676, -9.422509992056140149 ) ) ;
#49641=CARTESIAN_POINT ( 'NONE',  ( 24.16423886937409904, 49.09541550158063217, 3.795296366450317205 ) ) ;
#49642=ADVANCED_FACE ( 'NONE', ( #60830 ), #30106, .T. ) ;
#49643=CARTESIAN_POINT ( 'NONE',  ( 10.00000000000000000, 25.55374883491396787, -14.16423886937410082 ) ) ;
#49644=CARTESIAN_POINT ( 'NONE',  ( 7.361572987183170547, 42.05059781766745886, 9.846743663894590881 ) ) ;
#49645=CARTESIAN_POINT ( 'NONE',  ( 0.6178305044545838731, 34.74863466993042493, 9.382169495545420901 ) ) ;
#49646=CARTESIAN_POINT ( 'NONE',  ( 10.00000000000000178, 24.31368534415484106, 10.88017736071110342 ) ) ;
#49648=CARTESIAN_POINT ( 'NONE',  ( 12.63842701281683034, 57.46726448433411605, 9.846743663894596210 ) ) ;
#49649=CARTESIAN_POINT ( 'NONE',  ( 20.88017736071110519, 45.56368534415484106, 2.639326808657452039E-16 ) ) ;
#49650=CARTESIAN_POINT ( 'NONE',  ( 13.43411237798105340, 10.58196800326375353, 12.81628187352647963 ) ) ;
#49651=CARTESIAN_POINT ( 'NONE',  ( 13.79529636645030344, 38.26208216824729647, 14.16423886937410614 ) ) ;
#49653=CARTESIAN_POINT ( 'NONE',  ( 1.472469842513823179, 30.59226448433411960, -4.923371831947296329 ) ) ;
#49654=CARTESIAN_POINT ( 'NONE',  ( 13.43411237798106583, 62.66530133659708923, -12.81628187352647252 ) ) ;
#49655=CARTESIAN_POINT ( 'NONE',  ( 3.591859063236761518, 4.956968003263753531, 11.09922568453594849 ) ) ;
#49658=LINE ( 'NONE', #50662, #71485 ) ;
#49659=CARTESIAN_POINT ( 'NONE',  ( 15.44008868035555260, 19.73035201082150536, 9.422509992056143702 ) ) ;
#49660=CARTESIAN_POINT ( 'NONE',  ( 20.36894250292379738, 9.928748834913966093, -10.36894250292379027 ) ) ;
#49662=CARTESIAN_POINT ( 'NONE',  ( 17.20831665107776587, 4.133931151000785675, -7.208316651077762316 ) ) ;
#49663=CARTESIAN_POINT ( 'NONE',  ( 10.00000000000000178, 52.25893115100078745, 9.846743663894594434 ) ) ;
#49664=CARTESIAN_POINT ( 'NONE',  ( 7.084665262690076126, 34.10535201082151247, 10.88017736071109987 ) ) ;
#49666=CARTESIAN_POINT ( 'NONE',  ( 18.72515096720568195, 26.07228050351032778, -6.500000000000018652 ) ) ;
#49673=ORIENTED_EDGE ( 'NONE', *, *, #6708, .F. ) ;
#49676=CARTESIAN_POINT ( 'NONE',  ( -4.164238869374099927, 7.012082168247302683, 3.795296366450308767 ) ) ;
#49677=CARTESIAN_POINT ( 'NONE',  ( 17.08211943468705840, 5.137082168247300906, -12.26659068614894466 ) ) ;
#49679=CARTESIAN_POINT ( 'NONE',  ( 13.79529636645031943, 50.34541550158064638, -14.16423886937409904 ) ) ;
#49680=CARTESIAN_POINT ( 'NONE',  ( 1.472469842513823179, 60.59226448433412315, -4.923371831947296329 ) ) ;
#49681=CARTESIAN_POINT ( 'NONE',  ( 10.00000000000000000, 34.75893115100078745, -9.846743663894594434 ) ) ;
#49682=CARTESIAN_POINT ( 'NONE',  ( 0.1922240491738438917, 38.18878173731739878, 6.499999999999968914 ) ) ;
#49683=CARTESIAN_POINT ( 'NONE',  ( 10.00000000000000178, 29.31368534415483751, 10.88017736071110342 ) ) ;
#49684=CARTESIAN_POINT ( 'NONE',  ( 3.591859063236763294, -1.709698663402913210, -11.09922568453595026 ) ) ;
#49685=CARTESIAN_POINT ( 'NONE',  ( 2.917880565312950480, 0.9704155015806342766, -12.26659068614894821 ) ) ;
#49686=CARTESIAN_POINT ( 'NONE',  ( 13.79529636645030344, 58.26208216824728936, 14.16423886937410614 ) ) ;
#49687=CARTESIAN_POINT ( 'NONE',  ( -0.8801773607111009756, 3.063685344154838397, 1.068504757029289695E-15 ) ) ;
#49694=CARTESIAN_POINT ( 'NONE',  ( 1.472469842513823179, 20.59226448433411960, -4.923371831947296329 ) ) ;
#49696=CARTESIAN_POINT ( 'NONE',  ( 13.79529636645031943, 35.34541550158063927, -14.16423886937409904 ) ) ;
#49697=CARTESIAN_POINT ( 'NONE',  ( 19.84674366389459266, 38.71726448433412315, -2.638427012816827677 ) ) ;
#49698=CARTESIAN_POINT ( 'NONE',  ( 10.00000000000000000, 61.81368534415484106, -10.88017736071110342 ) ) ;
#49699=DIRECTION ( 'NONE',  ( -0.000000000000000000, -0.000000000000000000, -1.000000000000000000 ) ) ;
#49701=CARTESIAN_POINT ( 'NONE',  ( 0.5774900079438607392, 48.48035201082150536, 5.440088680355550821 ) ) ;
#49702=CARTESIAN_POINT ( 'NONE',  ( 2.791683348922240793, 51.63393115100078745, 7.208316651077764092 ) ) ;
#49703=CARTESIAN_POINT ( 'NONE',  ( 19.38216949554541557, 62.24863466993041072, -9.382169495545420901 ) ) ;
#49705=VERTEX_POINT ( 'NONE', #55823 ) ;
#49706=CARTESIAN_POINT ( 'NONE',  ( -4.164238869374098151, 21.59541550158063217, -3.795296366450310543 ) ) ;
#49708=CARTESIAN_POINT ( 'NONE',  ( 13.43411237798106583, 32.66530133659708213, -12.81628187352647252 ) ) ;
#49709=( LENGTH_UNIT ( ) NAMED_UNIT ( * ) SI_UNIT ( .MILLI., .METRE. ) );
#49710=CARTESIAN_POINT ( 'NONE',  ( 2.791683348922237240, 25.38393115100078390, -7.208316651077763204 ) ) ;
#49711=CARTESIAN_POINT ( 'NONE',  ( 19.42250999205614193, 15.14701867748817143, 5.440088680355555262 ) ) ;
#49713=CARTESIAN_POINT ( 'NONE',  ( 3.591859063236763294, 53.29030133659708923, -11.09922568453595026 ) ) ;
#49714=CARTESIAN_POINT ( 'NONE',  ( -46.21538524526005887, 104.1852450480875660, -5.851526435683386040 ) ) ;
#49715=CARTESIAN_POINT ( 'NONE',  ( 10.00000000000000178, 27.25893115100078390, 9.846743663894594434 ) ) ;
#49717=CARTESIAN_POINT ( 'NONE',  ( 19.39235739573469530, 19.87576471608601025, 6.499999999999990230 ) ) ;
#49718=ORIENTED_EDGE ( 'NONE', *, *, #36058, .T. ) ;
#49720=CARTESIAN_POINT ( 'NONE',  ( 17.96484262340118221, 64.93868534415483396, 7.964842623401181321 ) ) ;
#49721=CARTESIAN_POINT ( 'NONE',  ( -0.1503990784575328643, 70.00000000000000000, -6.262539305110068177 ) ) ;
#49722=CARTESIAN_POINT ( 'NONE',  ( 0.2751277870542986892, 7.282175860852375671, -6.500000000000003553 ) ) ;
#49723=CARTESIAN_POINT ( 'NONE',  ( 10.00000000000000178, 7.258931151000785675, 9.846743663894594434 ) ) ;
#49724=CARTESIAN_POINT ( 'NONE',  ( -2.816281873526473856, 24.12363466993042138, 9.499525473075851096E-16 ) ) ;
#49727=B_SPLINE_CURVE_WITH_KNOTS ( 'NONE', 3,
 ( #41359, #49314, #11320, #3836, #33799, #79816 ),
 .UNSPECIFIED., .F., .F.,
 ( 4, 2, 4 ),
 ( 7.944000812428443953E-18, 0.0002626113303185986965, 0.0005252226606371893699 ),
 .UNSPECIFIED. ) ;
#49728=CARTESIAN_POINT ( 'NONE',  ( 2.791683348922237240, 50.38393115100078035, -7.208316651077763204 ) ) ;
#49729=CARTESIAN_POINT ( 'NONE',  ( 17.39651004071890128, 29.08210964143323096, -6.499999999999448441 ) ) ;
#49730=CARTESIAN_POINT ( 'NONE',  ( -0.3689425029237881626, 27.42874883491397142, 10.36894250292379027 ) ) ;
#49731=CARTESIAN_POINT ( 'NONE',  ( 7.361572987183170547, 37.05059781766744464, 9.846743663894590881 ) ) ;
#49732=CARTESIAN_POINT ( 'NONE',  ( 6.565887622018943937, 35.16530133659708923, 12.81628187352647430 ) ) ;
#49733=LINE ( 'NONE', #26744, #72410 ) ;
#49735=CARTESIAN_POINT ( 'NONE',  ( -0.8801773607110991993, 62.85535201082150536, -2.915334737309923874 ) ) ;
#49736=CARTESIAN_POINT ( 'NONE',  ( 22.81628187352647785, 6.623634669930420493, 6.195893100308588602E-16 ) ) ;
#49737=CIRCLE ( 'NONE', #16219, 1.000000000000000000 ) ;
#49739=CARTESIAN_POINT ( 'NONE',  ( 10.00000000000000000, 34.75893115100078745, -9.846743663894594434 ) ) ;
#49740=CARTESIAN_POINT ( 'NONE',  ( 20.88017736071110519, 20.56368534415484106, 2.639326808657452039E-16 ) ) ;
#49741=CARTESIAN_POINT ( 'NONE',  ( 22.81628187352647785, 31.41530133659709279, 3.434112377981063169 ) ) ;
#49742=CARTESIAN_POINT ( 'NONE',  ( 1.472469842513823179, 31.42559781766745530, 4.923371831947296329 ) ) ;
#49745=CARTESIAN_POINT ( 'NONE',  ( 15.44008868035555793, 26.39701867748817321, -9.422509992056140149 ) ) ;
#49747=CARTESIAN_POINT ( 'NONE',  ( 10.00000000000000000, 66.81368534415484817, -10.88017736071110342 ) ) ;
#49748=CARTESIAN_POINT ( 'NONE',  ( 2.035157376598822676, 7.438685344154837509, -7.964842623401177768 ) ) ;
#49749=CARTESIAN_POINT ( 'NONE',  ( 19.84674366389459266, 58.30059781766745886, 2.638427012816836559 ) ) ;
#49750=CARTESIAN_POINT ( 'NONE',  ( 15.44008868035555793, 26.39701867748817321, -9.422509992056140149 ) ) ;
#49752=CARTESIAN_POINT ( 'NONE',  ( 10.00000000000000178, 44.31368534415484106, 10.88017736071110342 ) ) ;
#49753=CARTESIAN_POINT ( 'NONE',  ( 17.96484262340118221, 21.18868534415483396, -7.964842623401177768 ) ) ;
#49754=CARTESIAN_POINT ( 'NONE',  ( 20.00000000000001066, 90.58866250142803267, -4.971011743019353446 ) ) ;
#49755=CARTESIAN_POINT ( 'NONE',  ( 0.1532563361054082862, 6.217264484334118713, 2.638427012816831674 ) ) ;
#49757=CARTESIAN_POINT ( 'NONE',  ( 2.791683348922240793, 46.63393115100077324, 7.208316651077764092 ) ) ;
#49759=CARTESIAN_POINT ( 'NONE',  ( 22.26659068614894466, 48.88708216824730357, 7.082119434687054849 ) ) ;
#49762=CARTESIAN_POINT ( 'NONE',  ( 24.16423886937409904, 14.09541550158063217, 3.795296366450317205 ) ) ;
#49763=EDGE_CURVE ( 'NONE', #25641, #35624, #88273, .T. ) ;
#49764=CARTESIAN_POINT ( 'NONE',  ( 2.917880565312948704, 37.63708216824731068, 12.26659068614894643 ) ) ;
#49765=STYLED_ITEM ( 'NONE', ( #34521 ), #63828 ) ;
#49766=CARTESIAN_POINT ( 'NONE',  ( 22.81628187352647785, 6.623634669930420493, 6.195893100308588602E-16 ) ) ;
#49767=COLOUR_RGB ( '', 0.09019608, 0.27058824, 0.51372549) ;
#49769=VERTEX_POINT ( 'NONE', #44248 ) ;
#49770=CARTESIAN_POINT ( 'NONE',  ( 13.79529636645030344, 63.26208216824730357, 14.16423886937410614 ) ) ;
#49772=CARTESIAN_POINT ( 'NONE',  ( 0.1532563361054083140, 31.00893115100078390, 1.131784320476157264E-15 ) ) ;
#49775=CARTESIAN_POINT ( 'NONE',  ( 19.42250999205614548, 65.98035201082151957, -5.440088680355545492 ) ) ;
#49777=CARTESIAN_POINT ( 'NONE',  ( 0.5774900079438590739, 27.64701867748817676, -5.440088680355550821 ) ) ;
#49780=CARTESIAN_POINT ( 'NONE',  ( 22.81628187352648496, 21.83196800326374643, -3.434112377981050290 ) ) ;
#49781=CARTESIAN_POINT ( 'NONE',  ( 18.52753015748617571, 33.09226448433411605, 4.923371831947298993 ) ) ;
#49784=CARTESIAN_POINT ( 'NONE',  ( -0.3689425029237898834, 61.17874883491396076, -10.36894250292378850 ) ) ;
#49785=CARTESIAN_POINT ( 'NONE',  ( 10.00000000000000178, 33.05374883491396787, 14.16423886937410082 ) ) ;
#49786=CARTESIAN_POINT ( 'NONE',  ( 10.00000000000000178, 29.31368534415483751, 10.88017736071110342 ) ) ;
#49787=CARTESIAN_POINT ( 'NONE',  ( 20.88017736071110875, 50.77201867748817676, -2.915334737309920765 ) ) ;
#49790=CARTESIAN_POINT ( 'NONE',  ( 0.1532563361054082862, 11.21726448433411605, 2.638427012816831674 ) ) ;
#49792=( NAMED_UNIT ( * ) PLANE_ANGLE_UNIT ( ) SI_UNIT ( $, .RADIAN. ) );
#49794=CARTESIAN_POINT ( 'NONE',  ( 12.63842701281683922, 24.55059781766745175, -9.846743663894590881 ) ) ;
#49795=CARTESIAN_POINT ( 'NONE',  ( 12.63842701281683922, 54.55059781766745175, -9.846743663894590881 ) ) ;
#49796=CARTESIAN_POINT ( 'NONE',  ( -1.099225684535947600, 48.70696800326375353, -6.408140936763238038 ) ) ;
#49799=CARTESIAN_POINT ( 'NONE',  ( 0.5774900079438607392, 68.48035201082150536, 5.440088680355550821 ) ) ;
#49800=CARTESIAN_POINT ( 'NONE',  ( 14.92337183194729633, 27.67559781766745530, 8.527530157486181039 ) ) ;
#49801=CARTESIAN_POINT ( 'NONE',  ( -4.164238869374099927, 62.01208216824728936, 3.795296366450308767 ) ) ;
#49802=CARTESIAN_POINT ( 'NONE',  ( 18.52753015748617571, 23.09226448433411960, 4.923371831947298993 ) ) ;
#49803=CARTESIAN_POINT ( 'NONE',  ( -0.1023957841222417897, 60.13377557478297319, 6.340343622311918281 ) ) ;
#49804=CARTESIAN_POINT ( 'NONE',  ( 12.63842701281683922, 59.55059781766744464, -9.846743663894590881 ) ) ;
#49805=CARTESIAN_POINT ( 'NONE',  ( 10.00000000000000178, 23.05374883491397142, 14.16423886937410082 ) ) ;
#49806=CARTESIAN_POINT ( 'NONE',  ( 22.26659068614895176, 29.72041550158063572, -7.082119434687042414 ) ) ;
#49807=CARTESIAN_POINT ( 'NONE',  ( 7.361572987183169658, 39.96726448433411605, -9.846743663894592657 ) ) ;
#49808=CARTESIAN_POINT ( 'NONE',  ( 4.555630843329481650, 77.03495325336413657, -9.500000000000000000 ) ) ;
#49809=CARTESIAN_POINT ( 'NONE',  ( 20.88017736071110875, 30.77201867748816966, -2.915334737309920765 ) ) ;
#49811=CARTESIAN_POINT ( 'NONE',  ( 4.559911319644449179, 63.89701867748817676, 9.422509992056141925 ) ) ;
#49814=CARTESIAN_POINT ( 'NONE',  ( 6.565887622018943937, 40.16530133659708923, 12.81628187352647430 ) ) ;
#49815=CARTESIAN_POINT ( 'NONE',  ( 4.559911319644449179, 48.89701867748817676, 9.422509992056141925 ) ) ;
#49818=CARTESIAN_POINT ( 'NONE',  ( -0.8801773607111009756, 58.06368534415484106, 1.068504757029289695E-15 ) ) ;
#49820=CARTESIAN_POINT ( 'NONE',  ( 19.42250999205614193, 65.14701867748817676, 5.440088680355555262 ) ) ;
#49821=CARTESIAN_POINT ( 'NONE',  ( 7.084665262690076126, 19.10535201082150181, 10.88017736071109987 ) ) ;
#49823=CARTESIAN_POINT ( 'NONE',  ( 20.25387647958508808, 5.218815989627756379E-14, 6.092576751097550591 ) ) ;
#49824=CARTESIAN_POINT ( 'NONE',  ( 15.44008868035555260, 9.730352010821505360, 9.422509992056143702 ) ) ;
#49825=CARTESIAN_POINT ( 'NONE',  ( 1.472469842513823179, 10.59226448433411782, -4.923371831947296329 ) ) ;
#49826=CARTESIAN_POINT ( 'NONE',  ( 6.204703633549690345, 17.84541550158063217, 14.16423886937410082 ) ) ;
#49827=CARTESIAN_POINT ( 'NONE',  ( 0.5774900079438590739, 22.64701867748817321, -5.440088680355550821 ) ) ;
#49828=CARTESIAN_POINT ( 'NONE',  ( 7.361572987183169658, 64.96726448433412315, -9.846743663894592657 ) ) ;
#49829=ORIENTED_EDGE ( 'NONE', *, *, #81811, .F. ) ;
#49830=CARTESIAN_POINT ( 'NONE',  ( 10.00000000000000178, 57.25893115100078745, 9.846743663894594434 ) ) ;
#49832=CARTESIAN_POINT ( 'NONE',  ( 1.274849032794292736, 47.55509018479936856, -6.499999999999977796 ) ) ;
#49833=( BOUNDED_SURFACE ( )  B_SPLINE_SURFACE ( 1, 2, ( 
 ( #89402, #7406, #81894, #13405, #14906, #14407, #5914, #50910, #81406, #44878, #12908, #75380, #43405, #31845, #46853, #47836, #39859, #68392, #23887, #30868, #1390, #39375, #77349, #85354, #7892, #70365, #31356, #92361, #62341, #30366, #78339, #38884, #8860, #61857, #53881, #55348, #54353, #47342, #62843, #60872, #17367, #32341, #76861, #84865, #69373, #16374, #85855, #15887, #23396, #1882, #93343, #68887, #69870, #895, #9860, #98913, #38386, #77845, #53370, #61365, #417, #91875, #24865, #92848, #24376, #54841, #8374, #91372, #16868, #84388, #9354, #22898, #83880, #15406, #45889, #76377, #46372, #48332, #71349, #79329, #40847, #71827, #19802, #10347, #64305, #10839, #4328, #2867, #94816, #72791, #78836, #18833, #70860, #34294, #87798, #34800, #33318, #18340, #95817, #42318, #63813, #11319, #26319, #94323, #48820, #57796, #50293, #86836, #41358, #11810, #65290, #25844, #49802, #32830, #63329, #56342, #19316, #3336, #88304, #27297, #33798, #56817, #87315, #49313, #80310, #64791, #79815, #95308, #80806, #57306, #40359, #41838, #72305, #3835, #2375, #26812, #93837, #25363, #55849, #86344, #17847, #96816, #14296, #37297, #4819, #82273, #66789, #51291, #44275, #97308, #6289, #59278, #90767, #35293, #13291, #52277, #58786, #20802, #5315, #67784, #13788, #81776, #65786, #81294, #12790, #98306, #96319, #73295, #44768, #29760, #20305, #88797, #74270, #36291, #29275, #50805, #28780, #5801, #74780, #28292, #43290, #75273, #36792, #6783, #60268, #22292, #43779, #97814, #52765, #82776, #73785, #89777, #35793, #27794, #58279, #66281, #59771, #89292, #21294, #51787, #67286, #12303, #42811, #90264, #21797, #24262, #46264, #8266, #46742, #45270, #93223, #53758, #61734, #76749, #68771, #70250, #38766, #62231, #77730, #75765, #32222, #47227, #91759, #69266, #84276, #786, #1766, #30747, #38278, #16752, #9242, #83768, #31239, #15775, #24747, #83273, #22783, #92738, #68284, #76266, #15291, #53262, #39753, #92252, #23777, #54242, #23282, #62723, #84755, #45773, #16260, #14797, #7286, #37787, #77240, #54726, #8744, #91257, #98805, #7783, #30253, #39265, #60757, #69754, #1282, #31735, #85246, #303, #61254, #79210, #65177, #64189, #17253, #3723, #4212, #87198, #11205, #47729, #18721, #32717, #48707, #33210, #18227, #63215, #10236, #87687, #25253, #93719, #95186, #72194, #63704, #10720, #17740, #34682, #41237, #49203, #95698, #71715, #78226, #56707, #2754, #11701, #55226, #33691, #55738, #64676, #78726, #86229, #48216, #85740, #40729, #71231, #26694, #94709, #94207, #9738, #57190, #79707, #40238, #3227, #41724, #34184, #26214, #70746, #19201 ),
 ( #2262, #25737, #49684, #56229, #72677, #80188, #86723, #42210, #20684, #5688, #74661, #51678, #66165, #82157, #14173, #44153, #6662, #36174, #5193, #43668, #6172, #88676, #35681, #58671, #51178, #36676, #66674, #12679, #29150, #52164, #19694, #97199, #81661, #96698, #59159, #13171, #21176, #74155, #37178, #50181, #28177, #67164, #73666, #89173, #20184, #82657, #28667, #89665, #80691, #96195, #27680, #44657, #12187, #88180, #59657, #75152, #35173, #4711, #13669, #97688, #90148, #65674, #21678, #67671, #27182, #43178, #58165, #57684, #42693, #73172, #50687, #81179, #30625, #84634, #16634, #39141, #30133, #76630, #60639, #52649, #45143, #91140, #16136, #83152, #61132, #8149, #38642, #69631, #92616, #7670, #7161, #1155, #22666, #38161, #98684, #91642, #77609, #68164, #23160, #68647, #62106, #53142, #53635, #31615, #37664, #69143, #29637, #92134, #46622, #24140, #83651, #76144, #54607, #85123, #15166, #671, #84155, #45647, #177, #47109, #9122, #15661, #46144, #39637, #98181, #31121, #8632, #90642, #61616, #23659, #54121, #77120, #60145, #22167, #14677, #75649, #78609, #41612, #72081, #63101, #79595, #62599, #93104, #9618, #49092, #10118, #87575, #95072, #48096, #40616, #63589, #48590, #18599, #94587, #71115, #26102, #57080, #87089, #49564, #79093, #2642, #86606, #11096, #32605, #33096, #94098, #25619, #3607, #10605, #55618, #34068, #26577, #24634, #41119, #56112, #18115, #3120, #71609, #64072, #33578, #80076, #55101, #56598, #64562, #17626, #19087, #93603, #11582, #70126, #1648, #85621, #40119, #70620, #32100, #17138, #47617, #78112, #2145, #25140, #86115, #6409, #67411, #60394, #81911, #97940, #36920, #75395, #28902, #13421, #45392, #37425, #75897, #60888, #91386, #74908, #29892, #22916, #83403, #74406, #21927, #5931, #95580, #89420, #36422, #90891, #27067, #29397, #52406, #82907, #14924, #37919, #51920, #51421, #7422, #66916, #82404, #43906, #59898, #53384, #97437, #90390, #13930, #68408, #59405, #14424, #98930, #89910, #44894, #72562, #67913, #22419, #30385, #21424, #44406, #83894, #42097, #6915, #4096, #34559, #98435, #52893, #65054, #58919, #20933, #39390, #93357, #9876, #7908, #63346, #78356, #23901, #69884, #16388, #8872, #32846, #61870, #69386, #47850, #40375, #15898, #1404, #84881, #55864, #15424, #53893, #24882, #432, #8390, #46389, #84399, #70876, #31858, #54858, #46873, #54370, #2393, #85371, #76875, #62357, #93852, #76392, #25379, #77363, #55366, #92861, #23409, #45905, #38900, #38403, #16882, #91887, #24391, #47358, #77860, #9370, #908, #70380, #39873, #68904, #1899, #30882, #62862, #61379, #32355, #85869 ) ),
 .UNSPECIFIED., .F., .F., .F. ) 
 B_SPLINE_SURFACE_WITH_KNOTS ( ( 2, 2 ),
 ( 3, 2, 2, 2, 2, 2, 2, 2, 2, 2, 2, 2, 2, 2, 2, 2, 2, 2, 2, 2, 2, 2, 2, 2, 2, 2, 2, 2, 2, 2, 2, 2, 2, 2, 2, 2, 2, 2, 2, 2, 2, 2, 2, 2, 2, 2, 2, 2, 2, 2, 2, 2, 2, 2, 2, 2, 2, 2, 2, 2, 2, 2, 2, 2, 2, 2, 2, 2, 2, 2, 2, 2, 2, 2, 2, 2, 2, 2, 2, 2, 2, 2, 2, 2, 2, 2, 2, 2, 2, 2, 2, 2, 2, 2, 2, 2, 2, 2, 2, 2, 2, 2, 2, 2, 2, 2, 2, 2, 2, 2, 2, 2, 2, 2, 2, 2, 2, 2, 2, 2, 2, 2, 2, 2, 2, 2, 2, 2, 2, 2, 2, 2, 2, 2, 2, 2, 2, 2, 2, 2, 2, 2, 2, 2, 2, 2, 2, 2, 2, 2, 2, 2, 2, 2, 2, 2, 2, 2, 2, 2, 2, 2, 3 ),
 ( 0.000000000000000000, 1.000000000000000000 ),
 ( 0.000000000000000000, 0.005952380952380952051, 0.01190476190476190410, 0.01785714285714285615, 0.02380952380952380820, 0.02976190476190476025, 0.03571428571428571230, 0.04166666666666666435, 0.04761904761904761640, 0.05357142857142856845, 0.05952380952380952051, 0.06547619047619047949, 0.07142857142857142461, 0.07738095238095238360, 0.08333333333333332871, 0.08928571428571428770, 0.09523809523809523281, 0.1011904761904761918, 0.1071428571428571369, 0.1130952380952380959, 0.1190476190476190410, 0.1250000000000000000, 0.1309523809523809590, 0.1369047619047619180, 0.1428571428571428492, 0.1488095238095238082, 0.1547619047619047672, 0.1607142857142857262, 0.1666666666666666574, 0.1726190476190476164, 0.1785714285714285754, 0.1845238095238095344, 0.1904761904761904656, 0.1964285714285714246, 0.2023809523809523836, 0.2083333333333333426, 0.2142857142857142738, 0.2202380952380952328, 0.2261904761904761918, 0.2321428571428571508, 0.2380952380952380820, 0.2440476190476190410, 0.2500000000000000000, 0.2559523809523809312, 0.2619047619047619180, 0.2678571428571428492, 0.2738095238095238360, 0.2797619047619047672, 0.2857142857142856984, 0.2916666666666666852, 0.2976190476190476164, 0.3035714285714285476, 0.3095238095238095344, 0.3154761904761904656, 0.3214285714285714524, 0.3273809523809523836, 0.3333333333333333148, 0.3392857142857143016, 0.3452380952380952328, 0.3511904761904761640, 0.3571428571428571508, 0.3630952380952380820, 0.3690476190476190688, 0.3750000000000000000, 0.3809523809523809312, 0.3869047619047619180, 0.3928571428571428492, 0.3988095238095238360, 0.4047619047619047672, 0.4107142857142856984, 0.4166666666666666852, 0.4226190476190476164, 0.4285714285714285476, 0.4345238095238095344, 0.4404761904761904656, 0.4464285714285714524, 0.4523809523809523836, 0.4583333333333333148, 0.4642857142857143016, 0.4702380952380952328, 0.4761904761904761640, 0.4821428571428571508, 0.4880952380952380820, 0.4940476190476190688, 0.5000000000000000000, 0.5059523809523809312, 0.5119047619047618625, 0.5178571428571429047, 0.5238095238095238360, 0.5297619047619047672, 0.5357142857142856984, 0.5416666666666666297, 0.5476190476190476719, 0.5535714285714286031, 0.5595238095238095344, 0.5654761904761904656, 0.5714285714285713969, 0.5773809523809523281, 0.5833333333333333703, 0.5892857142857143016, 0.5952380952380952328, 0.6011904761904761640, 0.6071428571428570953, 0.6130952380952381375, 0.6190476190476190688, 0.6250000000000000000, 0.6309523809523809312, 0.6369047619047618625, 0.6428571428571429047, 0.6488095238095238360, 0.6547619047619047672, 0.6607142857142856984, 0.6666666666666666297, 0.6726190476190476719, 0.6785714285714286031, 0.6845238095238095344, 0.6904761904761904656, 0.6964285714285713969, 0.7023809523809523281, 0.7083333333333333703, 0.7142857142857143016, 0.7202380952380952328, 0.7261904761904761640, 0.7321428571428570953, 0.7380952380952381375, 0.7440476190476190688, 0.7500000000000000000, 0.7559523809523809312, 0.7619047619047618625, 0.7678571428571429047, 0.7738095238095238360, 0.7797619047619047672, 0.7857142857142856984, 0.7916666666666666297, 0.7976190476190476719, 0.8035714285714286031, 0.8095238095238095344, 0.8154761904761904656, 0.8214285714285713969, 0.8273809523809523281, 0.8333333333333333703, 0.8392857142857143016, 0.8452380952380952328, 0.8511904761904761640, 0.8571428571428570953, 0.8630952380952381375, 0.8690476190476190688, 0.8750000000000000000, 0.8809523809523809312, 0.8869047619047618625, 0.8928571428571429047, 0.8988095238095238360, 0.9047619047619047672, 0.9107142857142856984, 0.9166666666666666297, 0.9226190476190476719, 0.9285714285714286031, 0.9345238095238095344, 0.9404761904761904656, 0.9464285714285713969, 0.9523809523809523281, 0.9583333333333333703, 0.9642857142857143016 ),
 .UNSPECIFIED. ) 
 GEOMETRIC_REPRESENTATION_ITEM ( )  RATIONAL_B_SPLINE_SURFACE ( (
 ( 1.000000000000000000, 0.9659258262890683122, 1.000000000000000000, 0.9659258262890683122, 1.000000000000000000, 0.9659258262890683122, 1.000000000000000000, 0.9659258262890683122, 1.000000000000000000, 0.9659258262890683122, 1.000000000000000000, 0.9659258262890683122, 1.000000000000000000, 0.9659258262890683122, 1.000000000000000000, 0.9659258262890683122, 1.000000000000000000, 0.9659258262890683122, 1.000000000000000000, 0.9659258262890683122, 1.000000000000000000, 0.9659258262890683122, 1.000000000000000000, 0.9659258262890683122, 1.000000000000000000, 0.9659258262890683122, 1.000000000000000000, 0.9659258262890683122, 1.000000000000000000, 0.9659258262890683122, 1.000000000000000000, 0.9659258262890683122, 1.000000000000000000, 0.9659258262890683122, 1.000000000000000000, 0.9659258262890683122, 1.000000000000000000, 0.9659258262890683122, 1.000000000000000000, 0.9659258262890683122, 1.000000000000000000, 0.9659258262890683122, 1.000000000000000000, 0.9659258262890683122, 1.000000000000000000, 0.9659258262890683122, 1.000000000000000000, 0.9659258262890683122, 1.000000000000000000, 0.9659258262890683122, 1.000000000000000000, 0.9659258262890683122, 1.000000000000000000, 0.9659258262890683122, 1.000000000000000000, 0.9659258262890683122, 1.000000000000000000, 0.9659258262890683122, 1.000000000000000000, 0.9659258262890683122, 1.000000000000000000, 0.9659258262890683122, 1.000000000000000000, 0.9659258262890683122, 1.000000000000000000, 0.9659258262890683122, 1.000000000000000000, 0.9659258262890683122, 1.000000000000000000, 0.9659258262890683122, 1.000000000000000000, 0.9659258262890683122, 1.000000000000000000, 0.9659258262890683122, 1.000000000000000000, 0.9659258262890683122, 1.000000000000000000, 0.9659258262890683122, 1.000000000000000000, 0.9659258262890683122, 1.000000000000000000, 0.9659258262890683122, 1.000000000000000000, 0.9659258262890683122, 1.000000000000000000, 0.9659258262890683122, 1.000000000000000000, 0.9659258262890683122, 1.000000000000000000, 0.9659258262890683122, 1.000000000000000000, 0.9659258262890683122, 1.000000000000000000, 0.9659258262890683122, 1.000000000000000000, 0.9659258262890683122, 1.000000000000000000, 0.9659258262890683122, 1.000000000000000000, 0.9659258262890683122, 1.000000000000000000, 0.9659258262890683122, 1.000000000000000000, 0.9659258262890683122, 1.000000000000000000, 0.9659258262890683122, 1.000000000000000000, 0.9659258262890683122, 1.000000000000000000, 0.9659258262890683122, 1.000000000000000000, 0.9659258262890683122, 1.000000000000000000, 0.9659258262890683122, 1.000000000000000000, 0.9659258262890683122, 1.000000000000000000, 0.9659258262890683122, 1.000000000000000000, 0.9659258262890683122, 1.000000000000000000, 0.9659258262890683122, 1.000000000000000000, 0.9659258262890683122, 1.000000000000000000, 0.9659258262890683122, 1.000000000000000000, 0.9659258262890683122, 1.000000000000000000, 0.9659258262890683122, 1.000000000000000000, 0.9659258262890683122, 1.000000000000000000, 0.9659258262890683122, 1.000000000000000000, 0.9659258262890683122, 1.000000000000000000, 0.9659258262890683122, 1.000000000000000000, 0.9659258262890683122, 1.000000000000000000, 0.9659258262890683122, 1.000000000000000000, 0.9659258262890683122, 1.000000000000000000, 0.9659258262890683122, 1.000000000000000000, 0.9659258262890683122, 1.000000000000000000, 0.9659258262890683122, 1.000000000000000000, 0.9659258262890683122, 1.000000000000000000, 0.9659258262890683122, 1.000000000000000000, 0.9659258262890683122, 1.000000000000000000, 0.9659258262890683122, 1.000000000000000000, 0.9659258262890683122, 1.000000000000000000, 0.9659258262890683122, 1.000000000000000000, 0.9659258262890683122, 1.000000000000000000, 0.9659258262890683122, 1.000000000000000000, 0.9659258262890683122, 1.000000000000000000, 0.9659258262890683122, 1.000000000000000000, 0.9659258262890683122, 1.000000000000000000, 0.9659258262890683122, 1.000000000000000000, 0.9659258262890683122, 1.000000000000000000, 0.9659258262890683122, 1.000000000000000000, 0.9659258262890683122, 1.000000000000000000, 0.9659258262890683122, 1.000000000000000000, 0.9659258262890683122, 1.000000000000000000, 0.9659258262890683122, 1.000000000000000000, 0.9659258262890683122, 1.000000000000000000, 0.9659258262890683122, 1.000000000000000000, 0.9659258262890683122, 1.000000000000000000, 0.9659258262890683122, 1.000000000000000000, 0.9659258262890683122, 1.000000000000000000, 0.9659258262890683122, 1.000000000000000000, 0.9659258262890683122, 1.000000000000000000, 0.9659258262890683122, 1.000000000000000000, 0.9659258262890683122, 1.000000000000000000, 0.9659258262890683122, 1.000000000000000000, 0.9659258262890683122, 1.000000000000000000, 0.9659258262890683122, 1.000000000000000000, 0.9659258262890683122, 1.000000000000000000, 0.9659258262890683122, 1.000000000000000000, 0.9659258262890683122, 1.000000000000000000, 0.9659258262890683122, 1.000000000000000000, 0.9659258262890683122, 1.000000000000000000, 0.9659258262890683122, 1.000000000000000000, 0.9659258262890683122, 1.000000000000000000, 0.9659258262890683122, 1.000000000000000000, 0.9659258262890683122, 1.000000000000000000, 0.9659258262890683122, 1.000000000000000000, 0.9659258262890683122, 1.000000000000000000, 0.9659258262890683122, 1.000000000000000000, 0.9659258262890683122, 1.000000000000000000, 0.9659258262890683122, 1.000000000000000000, 0.9659258262890683122, 1.000000000000000000, 0.9659258262890683122, 1.000000000000000000, 0.9659258262890683122, 1.000000000000000000, 0.9659258262890683122, 1.000000000000000000, 0.9659258262890683122, 1.000000000000000000, 0.9659258262890683122, 1.000000000000000000, 0.9659258262890683122, 1.000000000000000000, 0.9659258262890683122, 1.000000000000000000, 0.9659258262890683122, 1.000000000000000000, 0.9659258262890683122, 1.000000000000000000, 0.9659258262890683122, 1.000000000000000000, 0.9659258262890683122, 1.000000000000000000, 0.9659258262890683122, 1.000000000000000000, 0.9659258262890683122, 1.000000000000000000, 0.9659258262890683122, 1.000000000000000000, 0.9659258262890683122, 1.000000000000000000, 0.9659258262890683122, 1.000000000000000000, 0.9659258262890683122, 1.000000000000000000, 0.9659258262890683122, 1.000000000000000000, 0.9659258262890683122, 1.000000000000000000, 0.9659258262890683122, 1.000000000000000000, 0.9659258262890683122, 1.000000000000000000, 0.9659258262890683122, 1.000000000000000000, 0.9659258262890683122, 1.000000000000000000, 0.9659258262890683122, 1.000000000000000000, 0.9659258262890683122, 1.000000000000000000, 0.9659258262890683122, 1.000000000000000000, 0.9659258262890683122, 1.000000000000000000, 0.9659258262890683122, 1.000000000000000000, 0.9659258262890683122, 1.000000000000000000, 0.9659258262890683122, 1.000000000000000000, 0.9659258262890683122, 1.000000000000000000, 0.9659258262890683122, 1.000000000000000000, 0.9659258262890683122, 1.000000000000000000, 0.9659258262890683122, 1.000000000000000000, 0.9659258262890683122, 1.000000000000000000, 0.9659258262890683122, 1.000000000000000000, 0.9659258262890683122, 1.000000000000000000, 0.9659258262890683122, 1.000000000000000000, 0.9659258262890683122, 1.000000000000000000, 0.9659258262890683122, 1.000000000000000000, 0.9659258262890683122, 1.000000000000000000, 0.9659258262890683122, 1.000000000000000000),
 ( 1.000000000000000000, 0.9659258262890683122, 1.000000000000000000, 0.9659258262890683122, 1.000000000000000000, 0.9659258262890683122, 1.000000000000000000, 0.9659258262890683122, 1.000000000000000000, 0.9659258262890683122, 1.000000000000000000, 0.9659258262890683122, 1.000000000000000000, 0.9659258262890683122, 1.000000000000000000, 0.9659258262890683122, 1.000000000000000000, 0.9659258262890683122, 1.000000000000000000, 0.9659258262890683122, 1.000000000000000000, 0.9659258262890683122, 1.000000000000000000, 0.9659258262890683122, 1.000000000000000000, 0.9659258262890683122, 1.000000000000000000, 0.9659258262890683122, 1.000000000000000000, 0.9659258262890683122, 1.000000000000000000, 0.9659258262890683122, 1.000000000000000000, 0.9659258262890683122, 1.000000000000000000, 0.9659258262890683122, 1.000000000000000000, 0.9659258262890683122, 1.000000000000000000, 0.9659258262890683122, 1.000000000000000000, 0.9659258262890683122, 1.000000000000000000, 0.9659258262890683122, 1.000000000000000000, 0.9659258262890683122, 1.000000000000000000, 0.9659258262890683122, 1.000000000000000000, 0.9659258262890683122, 1.000000000000000000, 0.9659258262890683122, 1.000000000000000000, 0.9659258262890683122, 1.000000000000000000, 0.9659258262890683122, 1.000000000000000000, 0.9659258262890683122, 1.000000000000000000, 0.9659258262890683122, 1.000000000000000000, 0.9659258262890683122, 1.000000000000000000, 0.9659258262890683122, 1.000000000000000000, 0.9659258262890683122, 1.000000000000000000, 0.9659258262890683122, 1.000000000000000000, 0.9659258262890683122, 1.000000000000000000, 0.9659258262890683122, 1.000000000000000000, 0.9659258262890683122, 1.000000000000000000, 0.9659258262890683122, 1.000000000000000000, 0.9659258262890683122, 1.000000000000000000, 0.9659258262890683122, 1.000000000000000000, 0.9659258262890683122, 1.000000000000000000, 0.9659258262890683122, 1.000000000000000000, 0.9659258262890683122, 1.000000000000000000, 0.9659258262890683122, 1.000000000000000000, 0.9659258262890683122, 1.000000000000000000, 0.9659258262890683122, 1.000000000000000000, 0.9659258262890683122, 1.000000000000000000, 0.9659258262890683122, 1.000000000000000000, 0.9659258262890683122, 1.000000000000000000, 0.9659258262890683122, 1.000000000000000000, 0.9659258262890683122, 1.000000000000000000, 0.9659258262890683122, 1.000000000000000000, 0.9659258262890683122, 1.000000000000000000, 0.9659258262890683122, 1.000000000000000000, 0.9659258262890683122, 1.000000000000000000, 0.9659258262890683122, 1.000000000000000000, 0.9659258262890683122, 1.000000000000000000, 0.9659258262890683122, 1.000000000000000000, 0.9659258262890683122, 1.000000000000000000, 0.9659258262890683122, 1.000000000000000000, 0.9659258262890683122, 1.000000000000000000, 0.9659258262890683122, 1.000000000000000000, 0.9659258262890683122, 1.000000000000000000, 0.9659258262890683122, 1.000000000000000000, 0.9659258262890683122, 1.000000000000000000, 0.9659258262890683122, 1.000000000000000000, 0.9659258262890683122, 1.000000000000000000, 0.9659258262890683122, 1.000000000000000000, 0.9659258262890683122, 1.000000000000000000, 0.9659258262890683122, 1.000000000000000000, 0.9659258262890683122, 1.000000000000000000, 0.9659258262890683122, 1.000000000000000000, 0.9659258262890683122, 1.000000000000000000, 0.9659258262890683122, 1.000000000000000000, 0.9659258262890683122, 1.000000000000000000, 0.9659258262890683122, 1.000000000000000000, 0.9659258262890683122, 1.000000000000000000, 0.9659258262890683122, 1.000000000000000000, 0.9659258262890683122, 1.000000000000000000, 0.9659258262890683122, 1.000000000000000000, 0.9659258262890683122, 1.000000000000000000, 0.9659258262890683122, 1.000000000000000000, 0.9659258262890683122, 1.000000000000000000, 0.9659258262890683122, 1.000000000000000000, 0.9659258262890683122, 1.000000000000000000, 0.9659258262890683122, 1.000000000000000000, 0.9659258262890683122, 1.000000000000000000, 0.9659258262890683122, 1.000000000000000000, 0.9659258262890683122, 1.000000000000000000, 0.9659258262890683122, 1.000000000000000000, 0.9659258262890683122, 1.000000000000000000, 0.9659258262890683122, 1.000000000000000000, 0.9659258262890683122, 1.000000000000000000, 0.9659258262890683122, 1.000000000000000000, 0.9659258262890683122, 1.000000000000000000, 0.9659258262890683122, 1.000000000000000000, 0.9659258262890683122, 1.000000000000000000, 0.9659258262890683122, 1.000000000000000000, 0.9659258262890683122, 1.000000000000000000, 0.9659258262890683122, 1.000000000000000000, 0.9659258262890683122, 1.000000000000000000, 0.9659258262890683122, 1.000000000000000000, 0.9659258262890683122, 1.000000000000000000, 0.9659258262890683122, 1.000000000000000000, 0.9659258262890683122, 1.000000000000000000, 0.9659258262890683122, 1.000000000000000000, 0.9659258262890683122, 1.000000000000000000, 0.9659258262890683122, 1.000000000000000000, 0.9659258262890683122, 1.000000000000000000, 0.9659258262890683122, 1.000000000000000000, 0.9659258262890683122, 1.000000000000000000, 0.9659258262890683122, 1.000000000000000000, 0.9659258262890683122, 1.000000000000000000, 0.9659258262890683122, 1.000000000000000000, 0.9659258262890683122, 1.000000000000000000, 0.9659258262890683122, 1.000000000000000000, 0.9659258262890683122, 1.000000000000000000, 0.9659258262890683122, 1.000000000000000000, 0.9659258262890683122, 1.000000000000000000, 0.9659258262890683122, 1.000000000000000000, 0.9659258262890683122, 1.000000000000000000, 0.9659258262890683122, 1.000000000000000000, 0.9659258262890683122, 1.000000000000000000, 0.9659258262890683122, 1.000000000000000000, 0.9659258262890683122, 1.000000000000000000, 0.9659258262890683122, 1.000000000000000000, 0.9659258262890683122, 1.000000000000000000, 0.9659258262890683122, 1.000000000000000000, 0.9659258262890683122, 1.000000000000000000, 0.9659258262890683122, 1.000000000000000000, 0.9659258262890683122, 1.000000000000000000, 0.9659258262890683122, 1.000000000000000000, 0.9659258262890683122, 1.000000000000000000, 0.9659258262890683122, 1.000000000000000000, 0.9659258262890683122, 1.000000000000000000, 0.9659258262890683122, 1.000000000000000000, 0.9659258262890683122, 1.000000000000000000, 0.9659258262890683122, 1.000000000000000000, 0.9659258262890683122, 1.000000000000000000, 0.9659258262890683122, 1.000000000000000000, 0.9659258262890683122, 1.000000000000000000, 0.9659258262890683122, 1.000000000000000000, 0.9659258262890683122, 1.000000000000000000, 0.9659258262890683122, 1.000000000000000000, 0.9659258262890683122, 1.000000000000000000, 0.9659258262890683122, 1.000000000000000000, 0.9659258262890683122, 1.000000000000000000, 0.9659258262890683122, 1.000000000000000000, 0.9659258262890683122, 1.000000000000000000, 0.9659258262890683122, 1.000000000000000000, 0.9659258262890683122, 1.000000000000000000, 0.9659258262890683122, 1.000000000000000000, 0.9659258262890683122, 1.000000000000000000, 0.9659258262890683122, 1.000000000000000000, 0.9659258262890683122, 1.000000000000000000, 0.9659258262890683122, 1.000000000000000000, 0.9659258262890683122, 1.000000000000000000, 0.9659258262890683122, 1.000000000000000000, 0.9659258262890683122, 1.000000000000000000, 0.9659258262890683122, 1.000000000000000000, 0.9659258262890683122, 1.000000000000000000, 0.9659258262890683122, 1.000000000000000000) ) ) 
 REPRESENTATION_ITEM ( '' )  SURFACE ( )  );
#49834=CARTESIAN_POINT ( 'NONE',  ( 0.5774900079438590739, 52.64701867748817676, -5.440088680355550821 ) ) ;
#49835=CARTESIAN_POINT ( 'NONE',  ( 19.84674366389459266, 48.30059781766745175, 2.638427012816836559 ) ) ;
#49836=CARTESIAN_POINT ( 'NONE',  ( 22.81628187352647785, 41.41530133659708923, 3.434112377981063169 ) ) ;
#49837=CARTESIAN_POINT ( 'NONE',  ( 19.42250999205614193, 10.14701867748816966, 5.440088680355555262 ) ) ;
#49839=CARTESIAN_POINT ( 'NONE',  ( 10.00000000000000178, 64.31368534415483396, 10.88017736071110342 ) ) ;
#49840=CARTESIAN_POINT ( 'NONE',  ( -0.8801773607111009756, 8.063685344154837509, 1.068504757029289695E-15 ) ) ;
#49841=EDGE_CURVE ( 'NONE', #74297, #87937, #59745, .T. ) ;
#49843=VERTEX_POINT ( 'NONE', #80283 ) ;
#49844=CARTESIAN_POINT ( 'NONE',  ( 6.565887622018943937, 45.16530133659708923, 12.81628187352647430 ) ) ;
#49845=CARTESIAN_POINT ( 'NONE',  ( 10.00000000000000000, 36.81368534415484106, -10.88017736071110342 ) ) ;
#49848=CARTESIAN_POINT ( 'NONE',  ( 10.00000000000000000, 47.87363466993042493, -12.81628187352647608 ) ) ;
#49849=CARTESIAN_POINT ( 'NONE',  ( 17.96484262340118221, 29.93868534415484106, 7.964842623401181321 ) ) ;
#49850=CARTESIAN_POINT ( 'NONE',  ( 5.076628168052703671, 51.84226448433412315, 8.527530157486179263 ) ) ;
#49854=CARTESIAN_POINT ( 'NONE',  ( 19.84674366389459621, 58.50893115100078745, 7.409399052514197653E-17 ) ) ;
#49855=FACE_OUTER_BOUND ( 'NONE', #37692, .T. ) ;
#49856=CARTESIAN_POINT ( 'NONE',  ( 1.472469842513823179, 45.59226448433412315, -4.923371831947296329 ) ) ;
#49857=CARTESIAN_POINT ( 'NONE',  ( 17.96484262340118221, 26.18868534415483396, -7.964842623401177768 ) ) ;
#49860=LINE ( 'NONE', #9916, #86744 ) ;
#49861=CARTESIAN_POINT ( 'NONE',  ( 7.361572987183169658, 39.96726448433411605, -9.846743663894592657 ) ) ;
#49862=CARTESIAN_POINT ( 'NONE',  ( 5.076628168052703671, 56.84226448433412315, 8.527530157486179263 ) ) ;
#49864=B_SPLINE_CURVE_WITH_KNOTS ( 'NONE', 3,
 ( #34401, #72900, #4919, #18934, #95417, #87903 ),
 .UNSPECIFIED., .F., .F.,
 ( 4, 2, 4 ),
 ( 0.000000000000000000, 0.0002626113303184859395, 0.0005252226606369718789 ),
 .UNSPECIFIED. ) ;
#49865=CARTESIAN_POINT ( 'NONE',  ( 16.40814093676323893, 35.79030133659708923, 11.09922568453595026 ) ) ;
#49866=CARTESIAN_POINT ( 'NONE',  ( 19.84674366389459621, 48.50893115100078745, 7.409399052514197653E-17 ) ) ;
#49868=CARTESIAN_POINT ( 'NONE',  ( 10.00000000000000178, 63.05374883491396076, 14.16423886937410082 ) ) ;
#49869=CARTESIAN_POINT ( 'NONE',  ( 5.076628168052704559, 30.17559781766745175, -8.527530157486179263 ) ) ;
#49872=CARTESIAN_POINT ( 'NONE',  ( -4.164238869374099927, 57.01208216824731068, 3.795296366450308767 ) ) ;
#49874=CARTESIAN_POINT ( 'NONE',  ( 4.559911319644449179, 8.897018677488173211, 9.422509992056141925 ) ) ;
#49876=CARTESIAN_POINT ( 'NONE',  ( 17.08211943468705130, 33.47041550158063927, 12.26659068614894998 ) ) ;
#49877=CARTESIAN_POINT ( 'NONE',  ( -0.3689425029237881626, 42.42874883491396787, 10.36894250292379027 ) ) ;
#49878=CARTESIAN_POINT ( 'NONE',  ( 0.2751277870542980231, 10.30223176428831522, 6.500000000000002665 ) ) ;
#49880=CARTESIAN_POINT ( 'NONE',  ( 12.63842701281683034, 17.46726448433411250, 9.846743663894596210 ) ) ;
#49881=CARTESIAN_POINT ( 'NONE',  ( 0.2751277870542967463, 70.00000000000000000, 6.000000000000000000 ) ) ;
#49882=CARTESIAN_POINT ( 'NONE',  ( 14.92337183194729988, 64.34226448433412315, -8.527530157486177487 ) ) ;
#49884=CARTESIAN_POINT ( 'NONE',  ( 12.91533473730992121, 49.52201867748817676, 10.88017736071110164 ) ) ;
#49886=CARTESIAN_POINT ( 'NONE',  ( 12.63842701281683034, 47.46726448433412315, 9.846743663894596210 ) ) ;
#49888=CARTESIAN_POINT ( 'NONE',  ( 17.20831665107776587, 52.88393115100078035, 7.208316651077764980 ) ) ;
#49893=CARTESIAN_POINT ( 'NONE',  ( 22.26659068614895176, 24.72041550158063572, -7.082119434687042414 ) ) ;
#49899=CARTESIAN_POINT ( 'NONE',  ( 17.96484262340118221, 24.93868534415484461, 7.964842623401181321 ) ) ;
#49900=CARTESIAN_POINT ( 'NONE',  ( 0.6178305044545838731, 24.74863466993042493, 9.382169495545420901 ) ) ;
#49902=CARTESIAN_POINT ( 'NONE',  ( 12.63842701281683034, 7.467264484334118713, 9.846743663894596210 ) ) ;
#49903=CARTESIAN_POINT ( 'NONE',  ( 3.591859063236763294, 53.29030133659708923, -11.09922568453595026 ) ) ;
#49904=ORIENTED_EDGE ( 'NONE', *, *, #84212, .T. ) ;
#49906=B_SPLINE_CURVE_WITH_KNOTS ( 'NONE', 3,
 ( #12607, #5122, #67098, #6592, #58096, #96625, #90084, #43108, #73595, #51105 ),
 .UNSPECIFIED., .F., .F.,
 ( 4, 3, 3, 4 ),
 ( 5.003707553108401214E-17, 0.0006253016069560650338, 0.001250604074564886812, 0.002501455912506567354 ),
 .UNSPECIFIED. ) ;
#49907=CARTESIAN_POINT ( 'NONE',  ( 22.26659068614894466, 23.88708216824730357, 7.082119434687054849 ) ) ;
#49910=CARTESIAN_POINT ( 'NONE',  ( 12.91533473730992121, 4.522018677488170546, 10.88017736071110164 ) ) ;
#49913=CARTESIAN_POINT ( 'NONE',  ( 7.084665262690076126, 37.02201867748817676, -10.88017736071110164 ) ) ;
#49914=CARTESIAN_POINT ( 'NONE',  ( 20.88017736071110519, 50.56368534415484106, 2.639326808657452039E-16 ) ) ;
#49915=CARTESIAN_POINT ( 'NONE',  ( -1.099225684535947600, 9.540301336597087456, 6.408140936763237150 ) ) ;
#49917=CARTESIAN_POINT ( 'NONE',  ( 0.5774900079438607392, 3.480352010821504916, 5.440088680355550821 ) ) ;
#49918=CARTESIAN_POINT ( 'NONE',  ( 19.84674366389459266, 3.717264484334118713, -2.638427012816827677 ) ) ;
#49919=CARTESIAN_POINT ( 'NONE',  ( 7.084665262690076126, 42.02201867748816966, -10.88017736071110164 ) ) ;
#49921=CARTESIAN_POINT ( 'NONE',  ( 22.81628187352647785, 6.623634669930420493, 6.195893100308588602E-16 ) ) ;
#49922=CARTESIAN_POINT ( 'NONE',  ( 20.88017736071110519, 60.56368534415484106, 2.639326808657452039E-16 ) ) ;
#49923=CARTESIAN_POINT ( 'NONE',  ( 18.52753015748617571, 23.09226448433411960, 4.923371831947298993 ) ) ;
#49924=CARTESIAN_POINT ( 'NONE',  ( 21.09922568453595559, 52.04030133659708923, -6.408140936763230044 ) ) ;
#49925=AXIS2_PLACEMENT_3D ( 'NONE', #86999, #71028, #94008 ) ;
#49926=CARTESIAN_POINT ( 'NONE',  ( 14.92337183194729633, 2.675597817667451750, 8.527530157486181039 ) ) ;
#49930=CARTESIAN_POINT ( 'NONE',  ( 1.602071938427517495, 57.02224192338643149, -6.500000000000039080 ) ) ;
#49931=CARTESIAN_POINT ( 'NONE',  ( 1.274849032794223680, 28.57228050351031001, 6.499999999999884537 ) ) ;
#49932=CARTESIAN_POINT ( 'NONE',  ( 12.91533473730993009, 21.60535201082150536, -10.88017736071109987 ) ) ;
#49933=CARTESIAN_POINT ( 'NONE',  ( 19.38216949554541557, 57.24863466993042493, -9.382169495545420901 ) ) ;
#49934=CARTESIAN_POINT ( 'NONE',  ( -4.164238869374099039, 21.80374883491396787, 8.674139862899312516E-16 ) ) ;
#49936=CARTESIAN_POINT ( 'NONE',  ( 1.472469842513823179, 25.59226448433412315, -4.923371831947296329 ) ) ;
#49937=AXIS2_PLACEMENT_3D ( 'NONE', #7928, #23431, #38425 ) ;
#49938=CARTESIAN_POINT ( 'NONE',  ( 19.42250999205614193, 20.14701867748817321, 5.440088680355555262 ) ) ;
#49939=CARTESIAN_POINT ( 'NONE',  ( 12.91533473730993009, 6.605352010821504471, -10.88017736071109987 ) ) ;
#49942=CARTESIAN_POINT ( 'NONE',  ( 4.559911319644449179, 7.230352010821504471, -9.422509992056141925 ) ) ;
#49943=CARTESIAN_POINT ( 'NONE',  ( 20.88017736071110164, 30.35535201082151247, 2.915334737309930979 ) ) ;
#49946=CARTESIAN_POINT ( 'NONE',  ( 0.5774900079438607392, 28.48035201082150891, 5.440088680355550821 ) ) ;
#49947=ORIENTED_EDGE ( 'NONE', *, *, #14472, .T. ) ;
#49948=CARTESIAN_POINT ( 'NONE',  ( 17.20831665107776587, 64.13393115100079456, -7.208316651077762316 ) ) ;
#49949=CARTESIAN_POINT ( 'NONE',  ( 0.5774900079438590739, 17.64701867748817321, -5.440088680355550821 ) ) ;
#49950=CARTESIAN_POINT ( 'NONE',  ( 19.84674366389459266, 63.30059781766745886, 2.638427012816836559 ) ) ;
#49953=CARTESIAN_POINT ( 'NONE',  ( -4.164238869374099927, 27.01208216824730357, 3.795296366450308767 ) ) ;
#49954=CARTESIAN_POINT ( 'NONE',  ( 20.88017736071110519, 45.56368534415484106, 2.639326808657452039E-16 ) ) ;
#49955=CARTESIAN_POINT ( 'NONE',  ( 4.559911319644449179, 17.23035201082150536, -9.422509992056141925 ) ) ;
#49956=CARTESIAN_POINT ( 'NONE',  ( 19.72487221294570858, 9.782175860852373006, 6.500000000000000000 ) ) ;
#49958=CARTESIAN_POINT ( 'NONE',  ( 1.472469842513823179, 51.42559781766745886, 4.923371831947296329 ) ) ;
#49960=CARTESIAN_POINT ( 'NONE',  ( 19.84674366389459266, 18.71726448433411960, -2.638427012816827677 ) ) ;
#49962=CARTESIAN_POINT ( 'NONE',  ( 12.91533473730992121, 14.52201867748817143, 10.88017736071110164 ) ) ;
#49963=CARTESIAN_POINT ( 'NONE',  ( 1.472469842513823179, 16.42559781766745175, 4.923371831947296329 ) ) ;
#49964=CARTESIAN_POINT ( 'NONE',  ( 17.96484262340118221, 54.93868534415484106, 7.964842623401181321 ) ) ;
#49965=CARTESIAN_POINT ( 'NONE',  ( 15.44008868035555793, 16.39701867748817321, -9.422509992056140149 ) ) ;
#49966=CARTESIAN_POINT ( 'NONE',  ( 22.81628187352647785, 61.41530133659709634, 3.434112377981063169 ) ) ;
#49967=CARTESIAN_POINT ( 'NONE',  ( 10.00000000000000000, 25.55374883491396787, -14.16423886937410082 ) ) ;
#49968=CIRCLE ( 'NONE', #40418, 0.5000000000000004441 ) ;
#49971=CARTESIAN_POINT ( 'NONE',  ( 19.38216949554541557, 62.24863466993041072, -9.382169495545420901 ) ) ;
#49973=CARTESIAN_POINT ( 'NONE',  ( 22.81628187352647785, 6.623634669930420493, 6.195893100308588602E-16 ) ) ;
#49974=CARTESIAN_POINT ( 'NONE',  ( -1.926860441876563801, 14.89664270246084143, 3.195792623639529761 ) ) ;
#49975=CARTESIAN_POINT ( 'NONE',  ( -0.8801773607111009756, 38.06368534415484106, 1.068504757029289695E-15 ) ) ;
#49976=CARTESIAN_POINT ( 'NONE',  ( 5.076628168052703671, 56.84226448433412315, 8.527530157486179263 ) ) ;
#49978=CARTESIAN_POINT ( 'NONE',  ( 5.076628168052703671, 16.84226448433411960, 8.527530157486179263 ) ) ;
#49980=CARTESIAN_POINT ( 'NONE',  ( 12.63842701281683922, 9.550597817667449974, -9.846743663894590881 ) ) ;
#49981=CARTESIAN_POINT ( 'NONE',  ( 10.00000000000000000, 19.75893115100078390, -9.846743663894594434 ) ) ;
#49982=CARTESIAN_POINT ( 'NONE',  ( 10.00000000000000000, 14.75893115100078568, -9.846743663894594434 ) ) ;
#49983=CARTESIAN_POINT ( 'NONE',  ( 2.791683348922237240, 0.3839311510007847872, -7.208316651077763204 ) ) ;
#49985=CARTESIAN_POINT ( 'NONE',  ( 20.88017736071110875, 60.77201867748817676, -2.915334737309920765 ) ) ;
#49987=CARTESIAN_POINT ( 'NONE',  ( 5.076628168052704559, 0.1755978176674514724, -8.527530157486179263 ) ) ;
#49988=CARTESIAN_POINT ( 'NONE',  ( 7.361572987183170547, 22.05059781766745530, 9.846743663894590881 ) ) ;
#49992=CARTESIAN_POINT ( 'NONE',  ( -2.816281873526473856, 4.331968003263754419, 3.434112377981055619 ) ) ;
#49994=ORIENTED_EDGE ( 'NONE', *, *, #80532, .T. ) ;
#49996=CARTESIAN_POINT ( 'NONE',  ( 24.16423886937409904, 19.09541550158063927, 3.795296366450317205 ) ) ;
#50001=CARTESIAN_POINT ( 'NONE',  ( 17.08211943468705840, 20.13708216824730357, -12.26659068614894466 ) ) ;
#50002=CARTESIAN_POINT ( 'NONE',  ( 13.79529636645031943, 35.34541550158063927, -14.16423886937409904 ) ) ;
#50004=CARTESIAN_POINT ( 'NONE',  ( 19.42250999205614548, 35.98035201082151247, -5.440088680355545492 ) ) ;
#50005=PRESENTATION_STYLE_ASSIGNMENT (( #87510 ) ) ;
#50007=CARTESIAN_POINT ( 'NONE',  ( 5.076628168052703671, 16.84226448433411960, 8.527530157486179263 ) ) ;
#50010=CARTESIAN_POINT ( 'NONE',  ( 12.91533473730993009, 61.60535201082150536, -10.88017736071109987 ) ) ;
#50011=CARTESIAN_POINT ( 'NONE',  ( 18.52753015748618282, 13.92559781766745175, -4.923371831947291888 ) ) ;
#50012=CARTESIAN_POINT ( 'NONE',  ( 17.96484262340118221, 4.938685344154837509, 7.964842623401181321 ) ) ;
#50013=CARTESIAN_POINT ( 'NONE',  ( 22.81628187352648496, 51.83196800326376064, -3.434112377981050290 ) ) ;
#50014=CARTESIAN_POINT ( 'NONE',  ( 1.472469842513823179, 55.59226448433412315, -4.923371831947296329 ) ) ;
#50015=CARTESIAN_POINT ( 'NONE',  ( -0.1503990784575328643, 25.12777174578613426, 6.262539305110068177 ) ) ;
#50016=CARTESIAN_POINT ( 'NONE',  ( -1.099225684535947600, 29.54030133659708923, 6.408140936763237150 ) ) ;
#50018=CARTESIAN_POINT ( 'NONE',  ( 12.63842701281683922, 44.55059781766745175, -9.846743663894590881 ) ) ;
#50020=CARTESIAN_POINT ( 'NONE',  ( -4.164238869374098151, 16.59541550158063927, -3.795296366450310543 ) ) ;
#50024=CARTESIAN_POINT ( 'NONE',  ( 15.44008868035555260, 49.73035201082150536, 9.422509992056143702 ) ) ;
#50025=CARTESIAN_POINT ( 'NONE',  ( 4.559911319644449179, 52.23035201082151247, -9.422509992056141925 ) ) ;
#50026=CARTESIAN_POINT ( 'NONE',  ( 2.917880565312950480, 40.97041550158063217, -12.26659068614894821 ) ) ;
#50027=CARTESIAN_POINT ( 'NONE',  ( 14.92337183194729988, 59.34226448433412315, -8.527530157486177487 ) ) ;
#50029=CARTESIAN_POINT ( 'NONE',  ( 2.035157376598822676, 37.43868534415484106, -7.964842623401177768 ) ) ;
#50031=CARTESIAN_POINT ( 'NONE',  ( 1.472469842513823179, 55.59226448433412315, -4.923371831947296329 ) ) ;
#50033=CARTESIAN_POINT ( 'NONE',  ( 20.88017736071110164, 5.355352010821502695, 2.915334737309930979 ) ) ;
#50034=CARTESIAN_POINT ( 'NONE',  ( 7.084665262690076126, 62.02201867748816966, -10.88017736071110164 ) ) ;
#50036=FACE_OUTER_BOUND ( 'NONE', #12716, .T. ) ;
#50037=CARTESIAN_POINT ( 'NONE',  ( 2.035157376598822676, 62.43868534415483396, -7.964842623401177768 ) ) ;
#50039=CARTESIAN_POINT ( 'NONE',  ( 0.1532563361054082862, 1.217264484334117824, 2.638427012816831674 ) ) ;
#50041=CARTESIAN_POINT ( 'NONE',  ( 5.076628168052704559, 40.17559781766745175, -8.527530157486179263 ) ) ;
#50043=CARTESIAN_POINT ( 'NONE',  ( 12.91533473730993009, 26.60535201082150536, -10.88017736071109987 ) ) ;
#50044=CARTESIAN_POINT ( 'NONE',  ( 3.591859063236763294, 8.290301336597087456, -11.09922568453595026 ) ) ;
#50045=CARTESIAN_POINT ( 'NONE',  ( 4.559911319644449179, 33.89701867748817676, 9.422509992056141925 ) ) ;
#50048=CARTESIAN_POINT ( 'NONE',  ( 13.43411237798105340, 35.58196800326375353, 12.81628187352647963 ) ) ;
#50049=ORIENTED_EDGE ( 'NONE', *, *, #76418, .F. ) ;
#50050=CARTESIAN_POINT ( 'NONE',  ( -0.8801773607111009756, 58.06368534415484106, 1.068504757029289695E-15 ) ) ;
#50051=CARTESIAN_POINT ( 'NONE',  ( -2.816281873526473856, 19.12363466993042138, 9.499525473075851096E-16 ) ) ;
#50055=CARTESIAN_POINT ( 'NONE',  ( 20.88017736071110519, 20.56368534415484106, 2.639326808657452039E-16 ) ) ;
#50056=CARTESIAN_POINT ( 'NONE',  ( -0.3689425029237881626, 67.42874883491396076, 10.36894250292379027 ) ) ;
#50057=CARTESIAN_POINT ( 'NONE',  ( 19.84674366389459266, 58.30059781766745886, 2.638427012816836559 ) ) ;
#50058=CARTESIAN_POINT ( 'NONE',  ( -0.8801773607111008646, 68.27201867748817676, 2.915334737309923430 ) ) ;
#50059=CARTESIAN_POINT ( 'NONE',  ( 19.42250999205614548, 65.98035201082151957, -5.440088680355545492 ) ) ;
#50061=CARTESIAN_POINT ( 'NONE',  ( -2.266590686148945544, 36.38708216824730357, -7.082119434687050408 ) ) ;
#50066=ORIENTED_EDGE ( 'NONE', *, *, #28684, .T. ) ;
#50067=CARTESIAN_POINT ( 'NONE',  ( 13.79529636645030344, 53.26208216824730357, 14.16423886937410614 ) ) ;
#50068=CARTESIAN_POINT ( 'NONE',  ( -4.164238869374098151, 51.59541550158063217, -3.795296366450310543 ) ) ;
#50069=CARTESIAN_POINT ( 'NONE',  ( 18.52753015748618282, 13.92559781766745175, -4.923371831947291888 ) ) ;
#50071=CARTESIAN_POINT ( 'NONE',  ( -0.1503990784575282014, 42.22266099184918886, -6.262539305110077947 ) ) ;
#50073=CARTESIAN_POINT ( 'NONE',  ( 24.16423886937410614, 39.51208216824731068, -3.795296366450302550 ) ) ;
#50076=CARTESIAN_POINT ( 'NONE',  ( 10.00000000000000000, 9.758931151000785675, -9.846743663894594434 ) ) ;
#50081=VERTEX_POINT ( 'NONE', #69725 ) ;
#50083=ORIENTED_EDGE ( 'NONE', *, *, #74320, .T. ) ;
#50084=CARTESIAN_POINT ( 'NONE',  ( 0.5774900079438607392, 18.48035201082150536, 5.440088680355550821 ) ) ;
#50085=CARTESIAN_POINT ( 'NONE',  ( -0.8801773607111008646, 23.27201867748817676, 2.915334737309923430 ) ) ;
#50086=CARTESIAN_POINT ( 'NONE',  ( 19.84674366389459266, 43.30059781766744464, 2.638427012816836559 ) ) ;
#50087=CARTESIAN_POINT ( 'NONE',  ( 16.40814093676324603, 22.45696800326375353, -11.09922568453594671 ) ) ;
#50089=B_SPLINE_CURVE_WITH_KNOTS ( 'NONE', 3,
 ( #62950, #32454, #24978, #75989 ),
 .UNSPECIFIED., .F., .F.,
 ( 4, 4 ),
 ( 4.336808689942017736E-19, 0.002562518741975332043 ),
 .UNSPECIFIED. ) ;
#50090=CARTESIAN_POINT ( 'NONE',  ( -2.816281873526473856, 24.33196800326375353, 3.434112377981055619 ) ) ;
#50091=EDGE_LOOP ( 'NONE', ( #81553, #50204, #93454, #27312, #65090 ) ) ;
#50092=CARTESIAN_POINT ( 'NONE',  ( 19.84674366389459266, 28.71726448433411960, -2.638427012816827677 ) ) ;
#50093=CARTESIAN_POINT ( 'NONE',  ( -2.266590686148945544, 66.38708216824730357, -7.082119434687050408 ) ) ;
#50095=CARTESIAN_POINT ( 'NONE',  ( 4.559911319644449179, 3.897018677488171434, 9.422509992056141925 ) ) ;
#50097=CARTESIAN_POINT ( 'NONE',  ( -0.8801773607111008646, 38.27201867748816255, 2.915334737309923430 ) ) ;
#50098=CARTESIAN_POINT ( 'NONE',  ( 12.91533473730992121, 39.52201867748817676, 10.88017736071110164 ) ) ;
#50099=CARTESIAN_POINT ( 'NONE',  ( 0.5774900079438607392, 53.48035201082151247, 5.440088680355550821 ) ) ;
#50101=CARTESIAN_POINT ( 'NONE',  ( -0.8801773607111009756, 43.06368534415484106, 1.068504757029289695E-15 ) ) ;
#50105=CARTESIAN_POINT ( 'NONE',  ( 18.52753015748618282, 13.92559781766745175, -4.923371831947291888 ) ) ;
#50107=CARTESIAN_POINT ( 'NONE',  ( 19.84674366389459621, 63.50893115100078745, 7.409399052514197653E-17 ) ) ;
#50112=CARTESIAN_POINT ( 'NONE',  ( 5.076628168052703671, 66.84226448433412315, 8.527530157486179263 ) ) ;
#50113=CARTESIAN_POINT ( 'NONE',  ( 5.076628168052703671, 31.84226448433412315, 8.527530157486179263 ) ) ;
#50114=CARTESIAN_POINT ( 'NONE',  ( 24.16423886937410614, 64.51208216824728936, -3.795296366450302550 ) ) ;
#50116=ORIENTED_EDGE ( 'NONE', *, *, #98201, .F. ) ;
#50118=CARTESIAN_POINT ( 'NONE',  ( 5.076628168052703671, 26.84226448433411960, 8.527530157486179263 ) ) ;
#50119=CARTESIAN_POINT ( 'NONE',  ( -2.816281873526471635, 3.915301336597087456, -3.434112377981056508 ) ) ;
#50120=CARTESIAN_POINT ( 'NONE',  ( 5.076628168052704559, 5.175597817667451750, -8.527530157486179263 ) ) ;
#50122=CARTESIAN_POINT ( 'NONE',  ( 14.92337183194729988, 4.342264484334117824, -8.527530157486177487 ) ) ;
#50123=CARTESIAN_POINT ( 'NONE',  ( 14.92337183194729988, 64.34226448433412315, -8.527530157486177487 ) ) ;
#50129=CARTESIAN_POINT ( 'NONE',  ( 12.91533473730993009, 11.60535201082150714, -10.88017736071109987 ) ) ;
#50130=CARTESIAN_POINT ( 'NONE',  ( 22.26659068614895176, 9.720415501580633943, -7.082119434687042414 ) ) ;
#50131=CARTESIAN_POINT ( 'NONE',  ( 19.84674366389459621, 8.508931151000785675, 7.409399052514197653E-17 ) ) ;
#50132=CARTESIAN_POINT ( 'NONE',  ( 17.96484262340118221, 39.93868534415484106, 7.964842623401181321 ) ) ;
#50133=CARTESIAN_POINT ( 'NONE',  ( 10.00000000000000178, 20.37363466993042138, 12.81628187352647608 ) ) ;
#50136=DIRECTION ( 'NONE',  ( 0.000000000000000000, -1.000000000000000000, 0.000000000000000000 ) ) ;
#50137=CARTESIAN_POINT ( 'NONE',  ( 3.591859063236761518, -0.04303199673624671928, 11.09922568453594849 ) ) ;
#50138=CARTESIAN_POINT ( 'NONE',  ( 0.1532563361054082862, 66.21726448433413736, 2.638427012816831674 ) ) ;
#50139=CARTESIAN_POINT ( 'NONE',  ( 1.472469842513823179, 11.42559781766745175, 4.923371831947296329 ) ) ;
#50141=CARTESIAN_POINT ( 'NONE',  ( 6.565887622018943937, 18.08196800326375708, -12.81628187352647608 ) ) ;
#50143=CARTESIAN_POINT ( 'NONE',  ( 0.5774900079438590739, 32.64701867748816966, -5.440088680355550821 ) ) ;
#50144=DIRECTION ( 'NONE',  ( 0.000000000000000000, 0.000000000000000000, 1.000000000000000000 ) ) ;
#50145=CARTESIAN_POINT ( 'NONE',  ( -0.3689425029237881626, 52.42874883491396076, 10.36894250292379027 ) ) ;
#50147=CARTESIAN_POINT ( 'NONE',  ( 10.00000000000000000, 32.87363466993042493, -12.81628187352647608 ) ) ;
#50148=CARTESIAN_POINT ( 'NONE',  ( -0.8801773607110991993, 32.85535201082151247, -2.915334737309923874 ) ) ;
#50149=CARTESIAN_POINT ( 'NONE',  ( 18.52753015748618282, 53.92559781766745175, -4.923371831947291888 ) ) ;
#50150=CARTESIAN_POINT ( 'NONE',  ( 12.91533473730993009, 56.60535201082151247, -10.88017736071109987 ) ) ;
#50151=B_SPLINE_CURVE_WITH_KNOTS ( 'NONE', 3,
 ( #55580, #39105, #40580, #86078, #17590, #15625 ),
 .UNSPECIFIED., .F., .F.,
 ( 4, 2, 4 ),
 ( 0.000000000000000000, 0.0002565770811491039499, 0.0005131541622982078998 ),
 .UNSPECIFIED. ) ;
#50152=CARTESIAN_POINT ( 'NONE',  ( 10.00000000000000000, 35.55374883491396787, -14.16423886937410082 ) ) ;
#50155=CARTESIAN_POINT ( 'NONE',  ( 0.1532563361054100626, 20.80059781766744464, -2.638427012816831230 ) ) ;
#50156=CARTESIAN_POINT ( 'NONE',  ( -2.816281873526471635, 58.91530133659707502, -3.434112377981056508 ) ) ;
#50157=CARTESIAN_POINT ( 'NONE',  ( 0.6178305044545818747, -1.501365330069579951, -9.382169495545419124 ) ) ;
#50159=CARTESIAN_POINT ( 'NONE',  ( 21.92686044187657046, 7.396642702460841434, -3.195792623639524432 ) ) ;
#50161=CARTESIAN_POINT ( 'NONE',  ( 17.96484262340118221, 14.93868534415484106, 7.964842623401181321 ) ) ;
#50162=CARTESIAN_POINT ( 'NONE',  ( 24.16423886937410614, 19.51208216824729647, -3.795296366450302550 ) ) ;
#50163=CARTESIAN_POINT ( 'NONE',  ( 0.1532563361054083140, 11.00893115100078568, 1.131784320476157264E-15 ) ) ;
#50165=CARTESIAN_POINT ( 'NONE',  ( -0.8801773607111009756, 38.06368534415484106, 1.068504757029289695E-15 ) ) ;
#50169=CARTESIAN_POINT ( 'NONE',  ( 0.1532563361054082862, 41.21726448433411605, 2.638427012816831674 ) ) ;
#50171=ORIENTED_EDGE ( 'NONE', *, *, #85272, .F. ) ;
#50173=CARTESIAN_POINT ( 'NONE',  ( 22.26659068614895176, 4.720415501580633943, -7.082119434687042414 ) ) ;
#50174=CARTESIAN_POINT ( 'NONE',  ( 6.204703633549690345, 7.845415501580634832, 14.16423886937410082 ) ) ;
#50175=CARTESIAN_POINT ( 'NONE',  ( 20.88017736071110164, 45.35535201082149115, 2.915334737309930979 ) ) ;
#50176=CARTESIAN_POINT ( 'NONE',  ( 2.917880565312948704, 57.63708216824731068, 12.26659068614894643 ) ) ;
#50177=CARTESIAN_POINT ( 'NONE',  ( 14.92337183194729988, 59.34226448433412315, -8.527530157486177487 ) ) ;
#50178=CARTESIAN_POINT ( 'NONE',  ( 14.92337183194729633, 32.67559781766745175, 8.527530157486181039 ) ) ;
#50180=CARTESIAN_POINT ( 'NONE',  ( 12.91533473730992121, 39.52201867748817676, 10.88017736071110164 ) ) ;
#50181=CARTESIAN_POINT ( 'NONE',  ( 19.38216949554541202, 5.998634669930420493, 9.382169495545424454 ) ) ;
#50182=CARTESIAN_POINT ( 'NONE',  ( -4.164238869374099039, 1.803748834913967647, 8.674139862899312516E-16 ) ) ;
#50183=CARTESIAN_POINT ( 'NONE',  ( 22.26659068614895176, 54.72041550158063217, -7.082119434687042414 ) ) ;
#50184=CARTESIAN_POINT ( 'NONE',  ( 20.88017736071110875, 10.77201867748817143, -2.915334737309920765 ) ) ;
#50186=CARTESIAN_POINT ( 'NONE',  ( 0.000000000000000000, 70.00000000000000000, 5.000000000000000000 ) ) ;
#50190=ORIENTED_EDGE ( 'NONE', *, *, #36721, .F. ) ;
#50192=CARTESIAN_POINT ( 'NONE',  ( -0.3689425029237881626, 42.42874883491396787, 10.36894250292379027 ) ) ;
#50193=CARTESIAN_POINT ( 'NONE',  ( 2.791683348922240793, 31.63393115100078745, 7.208316651077764092 ) ) ;
#50194=CARTESIAN_POINT ( 'NONE',  ( 7.084665262690076126, 62.02201867748816966, -10.88017736071110164 ) ) ;
#50195=CARTESIAN_POINT ( 'NONE',  ( 20.15039907845753575, 36.74884699246889141, 6.262539305110075283 ) ) ;
#50196=CARTESIAN_POINT ( 'NONE',  ( 7.084665262690076126, 59.10535201082150536, 10.88017736071109987 ) ) ;
#50198=TOROIDAL_SURFACE ( 'NONE', #45421, 18.93999999999999773, 0.5000000000000000000 ) ;
#50199=CARTESIAN_POINT ( 'NONE',  ( 3.591859063236763294, 63.29030133659708923, -11.09922568453595026 ) ) ;
#50202=CARTESIAN_POINT ( 'NONE',  ( 24.16423886937410614, 19.51208216824729647, -3.795296366450302550 ) ) ;
#50203=VECTOR ( 'NONE', #9571, 1000.000000000000000 ) ;
#50204=ORIENTED_EDGE ( 'NONE', *, *, #43080, .T. ) ;
#50205=CARTESIAN_POINT ( 'NONE',  ( 10.00000000000000178, 50.37363466993042493, 12.81628187352647608 ) ) ;
#50206=CARTESIAN_POINT ( 'NONE',  ( 20.88017736071110164, 15.35535201082150358, 2.915334737309930979 ) ) ;
#50207=CARTESIAN_POINT ( 'NONE',  ( 7.361572987183170547, 27.05059781766745175, 9.846743663894590881 ) ) ;
#50208=CARTESIAN_POINT ( 'NONE',  ( 2.035157376598822676, 17.43868534415483751, -7.964842623401177768 ) ) ;
#50209=CARTESIAN_POINT ( 'NONE',  ( 13.43411237798106583, 52.66530133659708213, -12.81628187352647252 ) ) ;
#50210=CARTESIAN_POINT ( 'NONE',  ( -46.59701958359876528, 103.7651961684614861, -6.068442458532171457 ) ) ;
#50211=CARTESIAN_POINT ( 'NONE',  ( 12.63842701281683034, 37.46726448433411605, 9.846743663894596210 ) ) ;
#50216=CARTESIAN_POINT ( 'NONE',  ( 0.1916775849787259733, 17.25868815902069642, -6.500000000000001776 ) ) ;
#50217=CARTESIAN_POINT ( 'NONE',  ( 10.00000000000000178, 22.25893115100078745, 9.846743663894594434 ) ) ;
#50218=CARTESIAN_POINT ( 'NONE',  ( 0.6178305044545838731, 19.74863466993042138, 9.382169495545420901 ) ) ;
#50220=CARTESIAN_POINT ( 'NONE',  ( 19.84674366389459621, 43.50893115100078745, 7.409399052514197653E-17 ) ) ;
#50222=CARTESIAN_POINT ( 'NONE',  ( 17.08211943468705840, 15.13708216824730179, -12.26659068614894466 ) ) ;
#50223=CARTESIAN_POINT ( 'NONE',  ( 19.84674366389459621, 38.50893115100078745, 7.409399052514197653E-17 ) ) ;
#50224=CARTESIAN_POINT ( 'NONE',  ( 21.09922568453595559, 32.04030133659708923, -6.408140936763230044 ) ) ;
#50226=CARTESIAN_POINT ( 'NONE',  ( 2.035157376598824452, 63.68868534415484106, 7.964842623401179544 ) ) ;
#50227=CARTESIAN_POINT ( 'NONE',  ( 19.38216949554541557, 7.248634669930421381, -9.382169495545420901 ) ) ;
#50230=CARTESIAN_POINT ( 'NONE',  ( 1.472469842513823179, 36.42559781766745175, 4.923371831947296329 ) ) ;
#50231=CARTESIAN_POINT ( 'NONE',  ( 7.084665262690076126, 24.10535201082150181, 10.88017736071109987 ) ) ;
#50232=CARTESIAN_POINT ( 'NONE',  ( -1.099225684535947600, 33.70696800326375353, -6.408140936763238038 ) ) ;
#50233=CARTESIAN_POINT ( 'NONE',  ( 5.076628168052704559, 30.17559781766745175, -8.527530157486179263 ) ) ;
#50234=SHAPE_DEFINITION_REPRESENTATION ( #21304, #19841 ) ;
#50237=CARTESIAN_POINT ( 'NONE',  ( 2.035157376598822676, 37.43868534415484106, -7.964842623401177768 ) ) ;
#50240=CARTESIAN_POINT ( 'NONE',  ( 20.88017736071110875, 5.772018677488170546, -2.915334737309920765 ) ) ;
#50241=CARTESIAN_POINT ( 'NONE',  ( 19.84674366389459266, 53.71726448433411605, -2.638427012816827677 ) ) ;
#50242=CARTESIAN_POINT ( 'NONE',  ( -0.8801773607111008646, 33.27201867748817676, 2.915334737309923430 ) ) ;
#50243=CARTESIAN_POINT ( 'NONE',  ( 4.559911319644449179, 57.23035201082150536, -9.422509992056141925 ) ) ;
#50244=CARTESIAN_POINT ( 'NONE',  ( 4.559911319644449179, 28.89701867748817321, 9.422509992056141925 ) ) ;
#50246=CARTESIAN_POINT ( 'NONE',  ( 14.92337183194729633, 2.675597817667451750, 8.527530157486181039 ) ) ;
#50248=CARTESIAN_POINT ( 'NONE',  ( 2.791683348922240793, 56.63393115100078035, 7.208316651077764092 ) ) ;
#50249=CARTESIAN_POINT ( 'NONE',  ( 22.26659068614894466, 58.88708216824729647, 7.082119434687054849 ) ) ;
#50251=DIRECTION ( 'NONE',  ( 1.000000000000000000, 0.000000000000000000, 0.000000000000000000 ) ) ;
#50252=CARTESIAN_POINT ( 'NONE',  ( 6.204703633549690345, 2.845415501580634388, 14.16423886937410082 ) ) ;
#50253=CARTESIAN_POINT ( 'NONE',  ( -0.3689425029237898834, 31.17874883491396787, -10.36894250292378850 ) ) ;
#50254=CARTESIAN_POINT ( 'NONE',  ( 16.40814093676324603, 7.456968003263754419, -11.09922568453594671 ) ) ;
#50256=VERTEX_POINT ( 'NONE', #6755 ) ;
#50258=CARTESIAN_POINT ( 'NONE',  ( 7.084665262690076126, 17.02201867748817676, -10.88017736071110164 ) ) ;
#50259=CARTESIAN_POINT ( 'NONE',  ( 7.361572987183170547, 42.05059781766745886, 9.846743663894590881 ) ) ;
#50261=CARTESIAN_POINT ( 'NONE',  ( 20.88017736071110164, 60.35535201082151957, 2.915334737309930979 ) ) ;
#50264=CARTESIAN_POINT ( 'NONE',  ( 21.09922568453595559, 62.04030133659709634, -6.408140936763230044 ) ) ;
#50265=CARTESIAN_POINT ( 'NONE',  ( 21.09922568453594849, 21.20696800326375353, 6.408140936763242479 ) ) ;
#50266=CARTESIAN_POINT ( 'NONE',  ( 19.84674366389459621, 33.50893115100078745, 7.409399052514197653E-17 ) ) ;
#50269=CARTESIAN_POINT ( 'NONE',  ( -0.8801773607111009756, 3.063685344154838397, 1.068504757029289695E-15 ) ) ;
#50270=CARTESIAN_POINT ( 'NONE',  ( 10.00000000000000178, 19.31368534415484106, 10.88017736071110342 ) ) ;
#50271=CARTESIAN_POINT ( 'NONE',  ( 20.36894250292379738, 34.92874883491396076, -10.36894250292379027 ) ) ;
#50272=CARTESIAN_POINT ( 'NONE',  ( 17.96484262340118221, 34.93868534415482685, 7.964842623401181321 ) ) ;
#50273=CARTESIAN_POINT ( 'NONE',  ( 2.035157376598824452, 58.68868534415482685, 7.964842623401179544 ) ) ;
#50277=CARTESIAN_POINT ( 'NONE',  ( 10.00000000000000000, 9.758931151000785675, -9.846743663894594434 ) ) ;
#50278=CARTESIAN_POINT ( 'NONE',  ( 19.88701968852512536, 21.79427333184091964, 6.480634945678691139 ) ) ;
#50279=CARTESIAN_POINT ( 'NONE',  ( 10.00000000000000000, 9.758931151000785675, -9.846743663894594434 ) ) ;
#50281=CARTESIAN_POINT ( 'NONE',  ( 17.20831665107776587, 37.88393115100078745, 7.208316651077764980 ) ) ;
#50282=CARTESIAN_POINT ( 'NONE',  ( 6.565887622018943937, 0.1653013365970866511, 12.81628187352647430 ) ) ;
#50284=CARTESIAN_POINT ( 'NONE',  ( 15.44008868035555793, 26.39701867748817321, -9.422509992056140149 ) ) ;
#50287=CARTESIAN_POINT ( 'NONE',  ( 3.591859063236761518, 39.95696800326375353, 11.09922568453594849 ) ) ;
#50288=AXIS2_PLACEMENT_3D ( 'NONE', #85950, #86441, #17460 ) ;
#50290=CARTESIAN_POINT ( 'NONE',  ( 12.91533473730992121, 59.52201867748816966, 10.88017736071110164 ) ) ;
#50291=CARTESIAN_POINT ( 'NONE',  ( -2.816281873526471635, 43.91530133659708923, -3.434112377981056508 ) ) ;
#50292=CARTESIAN_POINT ( 'NONE',  ( -0.3689425029237881626, 57.42874883491397497, 10.36894250292379027 ) ) ;
#50293=CARTESIAN_POINT ( 'NONE',  ( 5.076628168052703671, 21.84226448433411960, 8.527530157486179263 ) ) ;
#50294=CARTESIAN_POINT ( 'NONE',  ( 0.2751277870542911397, 50.30223176428831522, 6.499999999999992006 ) ) ;
#50295=CARTESIAN_POINT ( 'NONE',  ( 10.00000000000000178, 62.25893115100078745, 9.846743663894594434 ) ) ;
#50296=CARTESIAN_POINT ( 'NONE',  ( 2.917880565312950480, 30.97041550158063572, -12.26659068614894821 ) ) ;
#50297=CARTESIAN_POINT ( 'NONE',  ( 17.20831665107776587, 47.88393115100078745, 7.208316651077764980 ) ) ;
#50299=CARTESIAN_POINT ( 'NONE',  ( 4.559911319644449179, 23.89701867748817321, 9.422509992056141925 ) ) ;
#50300=CARTESIAN_POINT ( 'NONE',  ( 20.88017736071110519, 60.56368534415484106, 2.639326808657452039E-16 ) ) ;
#50303=CARTESIAN_POINT ( 'NONE',  ( 6.565887622018943937, 48.08196800326375353, -12.81628187352647608 ) ) ;
#50304=CARTESIAN_POINT ( 'NONE',  ( 2.035157376598824452, 53.68868534415484817, 7.964842623401179544 ) ) ;
#50306=SURFACE_STYLE_FILL_AREA ( #93490 ) ;
#50310=CARTESIAN_POINT ( 'NONE',  ( 0.5774900079438607392, 63.48035201082149825, 5.440088680355550821 ) ) ;
#50311=CARTESIAN_POINT ( 'NONE',  ( 15.44008868035555260, 9.730352010821505360, 9.422509992056143702 ) ) ;
#50313=SURFACE_STYLE_FILL_AREA ( #84169 ) ;
#50314=CARTESIAN_POINT ( 'NONE',  ( 20.88017736071110875, 5.772018677488170546, -2.915334737309920765 ) ) ;
#50315=CARTESIAN_POINT ( 'NONE',  ( 20.36894250292379382, 13.67874883491396965, 10.36894250292379205 ) ) ;
#50316=CARTESIAN_POINT ( 'NONE',  ( 20.88017736071110875, 20.77201867748816611, -2.915334737309920765 ) ) ;
#50317=CARTESIAN_POINT ( 'NONE',  ( 18.52753015748617571, 58.09226448433411605, 4.923371831947298993 ) ) ;
#50319=CARTESIAN_POINT ( 'NONE',  ( 5.076628168052703671, 61.84226448433412315, 8.527530157486179263 ) ) ;
#50323=CARTESIAN_POINT ( 'NONE',  ( 0.5774900079438590739, 57.64701867748817676, -5.440088680355550821 ) ) ;
#50324=CARTESIAN_POINT ( 'NONE',  ( 5.076628168052703671, 66.84226448433412315, 8.527530157486179263 ) ) ;
#50325=CARTESIAN_POINT ( 'NONE',  ( 16.40814093676323893, 35.79030133659708923, 11.09922568453595026 ) ) ;
#50326=CARTESIAN_POINT ( 'NONE',  ( 12.91533473730992121, 4.522018677488169658, 10.88017736071110164 ) ) ;
#50328=CARTESIAN_POINT ( 'NONE',  ( 19.42250999205614193, 60.14701867748817676, 5.440088680355555262 ) ) ;
#50329=CARTESIAN_POINT ( 'NONE',  ( 10.00000000000000000, 16.81368534415483751, -10.88017736071110342 ) ) ;
#50332=CARTESIAN_POINT ( 'NONE',  ( 3.591859063236763294, 53.29030133659708923, -11.09922568453595026 ) ) ;
#50333=CARTESIAN_POINT ( 'NONE',  ( 2.035157376598824452, 23.68868534415484461, 7.964842623401179544 ) ) ;
#50337=CARTESIAN_POINT ( 'NONE',  ( -2.816281873526473856, 39.33196800326374643, 3.434112377981055619 ) ) ;
#50338=CARTESIAN_POINT ( 'NONE',  ( 19.42250999205614548, 30.98035201082150536, -5.440088680355545492 ) ) ;
#50339=CARTESIAN_POINT ( 'NONE',  ( 0.1532563361054082862, 61.21726448433412315, 2.638427012816831674 ) ) ;
#50342=CARTESIAN_POINT ( 'NONE',  ( 19.84674366389459621, 8.508931151000785675, 7.409399052514197653E-17 ) ) ;
#50343=CARTESIAN_POINT ( 'NONE',  ( 0.1532563361054082862, 66.21726448433413736, 2.638427012816831674 ) ) ;
#50345=CARTESIAN_POINT ( 'NONE',  ( 10.00000000000000178, 47.25893115100078745, 9.846743663894594434 ) ) ;
#50346=CARTESIAN_POINT ( 'NONE',  ( 4.559911319644449179, 18.89701867748817321, 9.422509992056141925 ) ) ;
#50348=CARTESIAN_POINT ( 'NONE',  ( 12.63842701281683922, 34.55059781766745886, -9.846743663894590881 ) ) ;
#50350=FILL_AREA_STYLE ('',( #52331 ) ) ;
#50351=CARTESIAN_POINT ( 'NONE',  ( 14.92337183194729988, 44.34226448433412315, -8.527530157486177487 ) ) ;
#50352=CARTESIAN_POINT ( 'NONE',  ( 12.63842701281683922, 4.550597817667451750, -9.846743663894590881 ) ) ;
#50353=CARTESIAN_POINT ( 'NONE',  ( -20.19000000000000838, 92.00000000000000000, -9.500000000000000000 ) ) ;
#50354=CARTESIAN_POINT ( 'NONE',  ( 19.84674366389459621, 58.50893115100078745, 7.409399052514197653E-17 ) ) ;
#50356=DIRECTION ( 'NONE',  ( 1.000000000000000000, 0.000000000000000000, 0.000000000000000000 ) ) ;
#50357=CARTESIAN_POINT ( 'NONE',  ( 22.81628187352648496, 36.83196800326376064, -3.434112377981050290 ) ) ;
#50360=CARTESIAN_POINT ( 'NONE',  ( 14.92337183194729988, 49.34226448433411605, -8.527530157486177487 ) ) ;
#50361=DIRECTION ( 'NONE',  ( -0.7385627893568607050, 0.6741846973770715401, 0.000000000000000000 ) ) ;
#50362=CARTESIAN_POINT ( 'NONE',  ( 24.16423886937410614, 59.30374883491397497, 8.672049930838204340E-16 ) ) ;
#50363=CARTESIAN_POINT ( 'NONE',  ( 14.92337183194729988, 34.34226448433411605, -8.527530157486177487 ) ) ;
#50364=CARTESIAN_POINT ( 'NONE',  ( -0.3289641300568005855, 40.10497603579417358, 5.963430220938281678 ) ) ;
#50366=CARTESIAN_POINT ( 'NONE',  ( 24.16423886937410614, 54.51208216824730357, -3.795296366450302550 ) ) ;
#50367=CARTESIAN_POINT ( 'NONE',  ( -42.60666666666668334, 92.50000000000000000, 9.500000000000000000 ) ) ;
#50368=CARTESIAN_POINT ( 'NONE',  ( 10.00000000000000178, 14.31368534415483929, 10.88017736071110342 ) ) ;
#50369=CARTESIAN_POINT ( 'NONE',  ( 24.16423886937410614, 39.30374883491396787, 8.672049930838204340E-16 ) ) ;
#50370=CARTESIAN_POINT ( 'NONE',  ( 22.26659068614894466, 58.88708216824729647, 7.082119434687054849 ) ) ;
#50372=CARTESIAN_POINT ( 'NONE',  ( 0.2751277870542967463, 69.50000000000000000, 6.500000000000000888 ) ) ;
#50373=CARTESIAN_POINT ( 'NONE',  ( 12.63842701281683034, 7.467264484334118713, 9.846743663894596210 ) ) ;
#50374=CARTESIAN_POINT ( 'NONE',  ( 7.361572987183170547, 67.05059781766746596, 9.846743663894590881 ) ) ;
#50375=VERTEX_POINT ( 'NONE', #63675 ) ;
#50376=CARTESIAN_POINT ( 'NONE',  ( 10.00000000000000000, 46.81368534415484106, -10.88017736071110342 ) ) ;
#50378=CARTESIAN_POINT ( 'NONE',  ( -0.8801773607111009756, 18.27201867748817321, 2.915334737309923874 ) ) ;
#50380=B_SPLINE_CURVE_WITH_KNOTS ( 'NONE', 3,
 ( #27132, #34134, #88131, #88624, #44102, #19643 ),
 .UNSPECIFIED., .F., .F.,
 ( 4, 2, 4 ),
 ( 0.000000000000000000, 0.0002701661927229229761, 0.0005403323854458459523 ),
 .UNSPECIFIED. ) ;
#50381=CARTESIAN_POINT ( 'NONE',  ( 0.1532563361054083140, 51.00893115100078745, 1.131784320476157264E-15 ) ) ;
#50385=CARTESIAN_POINT ( 'NONE',  ( 2.917880565312948704, 27.63708216824730357, 12.26659068614894643 ) ) ;
#50389=CARTESIAN_POINT ( 'NONE',  ( 10.00000000000000178, 19.31368534415484106, 10.88017736071110342 ) ) ;
#50390=CARTESIAN_POINT ( 'NONE',  ( -2.816281873526473856, 44.33196800326375353, 3.434112377981055619 ) ) ;
#50392=CARTESIAN_POINT ( 'NONE',  ( 5.076628168052704559, 10.17559781766745175, -8.527530157486179263 ) ) ;
#50393=CARTESIAN_POINT ( 'NONE',  ( 6.565887622018943937, 60.16530133659707502, 12.81628187352647430 ) ) ;
#50396=CARTESIAN_POINT ( 'NONE',  ( -4.164238869374099039, 31.80374883491396432, 8.674139862899312516E-16 ) ) ;
#50397=FILL_AREA_STYLE_COLOUR ( '', #31467 ) ;
#50399=CARTESIAN_POINT ( 'NONE',  ( 10.00000000000000178, 29.31368534415483751, 10.88017736071110342 ) ) ;
#50402=CARTESIAN_POINT ( 'NONE',  ( 12.91533473730993009, 46.60535201082150536, -10.88017736071109987 ) ) ;
#50403=CARTESIAN_POINT ( 'NONE',  ( -0.8801773607110991993, 47.85535201082150536, -2.915334737309923874 ) ) ;
#50404=CARTESIAN_POINT ( 'NONE',  ( 3.591859063236761518, 19.95696800326375353, 11.09922568453594849 ) ) ;
#50405=CARTESIAN_POINT ( 'NONE',  ( 19.84674366389459621, 63.50893115100078745, 7.409399052514197653E-17 ) ) ;
#50406=CARTESIAN_POINT ( 'NONE',  ( 1.282179089048214760, 0.8662784883469558661, 6.500000000000002665 ) ) ;
#50407=CARTESIAN_POINT ( 'NONE',  ( 19.84674366389459266, 28.71726448433411960, -2.638427012816827677 ) ) ;
#50409=CARTESIAN_POINT ( 'NONE',  ( -0.8801773607111008646, 43.27201867748817676, 2.915334737309923430 ) ) ;
#50412=CARTESIAN_POINT ( 'NONE',  ( 3.591859063236761518, 4.956968003263753531, 11.09922568453594849 ) ) ;
#50413=CARTESIAN_POINT ( 'NONE',  ( 10.00000000000000178, 59.31368534415484106, 10.88017736071110342 ) ) ;
#50415=CARTESIAN_POINT ( 'NONE',  ( 7.361572987183170547, 27.05059781766745175, 9.846743663894590881 ) ) ;
#50416=CARTESIAN_POINT ( 'NONE',  ( 22.81628187352648496, 51.83196800326376064, -3.434112377981050290 ) ) ;
#50417=CARTESIAN_POINT ( 'NONE',  ( 5.076628168052704559, 10.17559781766745175, -8.527530157486179263 ) ) ;
#50418=( NAMED_UNIT ( * ) PLANE_ANGLE_UNIT ( ) SI_UNIT ( $, .RADIAN. ) );
#50419=EDGE_LOOP ( 'NONE', ( #22597, #47913, #53559 ) ) ;
#50421=CARTESIAN_POINT ( 'NONE',  ( 0.1532563361054083140, 36.00893115100078745, 1.131784320476157264E-15 ) ) ;
#50422=CARTESIAN_POINT ( 'NONE',  ( 19.42250999205614548, 25.98035201082150891, -5.440088680355545492 ) ) ;
#50423=CARTESIAN_POINT ( 'NONE',  ( 22.81628187352647785, 56.62363466993042493, 6.195893100308588602E-16 ) ) ;
#50424=CARTESIAN_POINT ( 'NONE',  ( 2.917880565312950480, 20.97041550158063217, -12.26659068614894821 ) ) ;
#50425=CARTESIAN_POINT ( 'NONE',  ( 14.92337183194729633, 27.67559781766745530, 8.527530157486181039 ) ) ;
#50426=CARTESIAN_POINT ( 'NONE',  ( -0.8801773607111008646, 18.27201867748817321, 2.915334737309923430 ) ) ;
#50427=CARTESIAN_POINT ( 'NONE',  ( 24.16423886937410614, 64.51208216824728936, -3.795296366450302550 ) ) ;
#50429=CARTESIAN_POINT ( 'NONE',  ( 19.42250999205614193, 15.14701867748817143, 5.440088680355555262 ) ) ;
#50430=CARTESIAN_POINT ( 'NONE',  ( 10.00000000000000178, 29.31368534415483751, 10.88017736071110342 ) ) ;
#50431=CARTESIAN_POINT ( 'NONE',  ( 7.084665262690076126, 37.02201867748817676, -10.88017736071110164 ) ) ;
#50434=CARTESIAN_POINT ( 'NONE',  ( 20.88017736071110164, 20.35535201082150891, 2.915334737309930979 ) ) ;
#50435=CARTESIAN_POINT ( 'NONE',  ( 17.20831665107776587, 64.13393115100079456, -7.208316651077762316 ) ) ;
#50440=CARTESIAN_POINT ( 'NONE',  ( 10.00000000000000178, 38.05374883491396787, 14.16423886937410082 ) ) ;
#50441=CARTESIAN_POINT ( 'NONE',  ( 20.88017736071110164, 35.35535201082150536, 2.915334737309930979 ) ) ;
#50442=CARTESIAN_POINT ( 'NONE',  ( 15.44008868035555260, 29.73035201082150891, 9.422509992056143702 ) ) ;
#50443=CARTESIAN_POINT ( 'NONE',  ( 1.472469842513823179, 65.59226448433412315, -4.923371831947296329 ) ) ;
#50445=CARTESIAN_POINT ( 'NONE',  ( 2.791683348922237240, 45.38393115100079456, -7.208316651077763204 ) ) ;
#50447=CARTESIAN_POINT ( 'NONE',  ( 0.1532563361054100626, 20.80059781766744464, -2.638427012816831230 ) ) ;
#50449=CARTESIAN_POINT ( 'NONE',  ( -0.8801773607111009756, 8.063685344154837509, 1.068504757029289695E-15 ) ) ;
#50450=CARTESIAN_POINT ( 'NONE',  ( 14.92337183194729988, 29.34226448433411960, -8.527530157486177487 ) ) ;
#50451=CARTESIAN_POINT ( 'NONE',  ( 22.81628187352647785, 6.623634669930420493, 6.195893100308588602E-16 ) ) ;
#50452=CARTESIAN_POINT ( 'NONE',  ( 20.88017736071110164, 55.35535201082149825, 2.915334737309930979 ) ) ;
#50453=CARTESIAN_POINT ( 'NONE',  ( 19.42250999205614193, 50.14701867748817676, 5.440088680355555262 ) ) ;
#50454=CARTESIAN_POINT ( 'NONE',  ( 20.88017736071110875, 20.77201867748816611, -2.915334737309920765 ) ) ;
#50455=CARTESIAN_POINT ( 'NONE',  ( 0.6178305044545838731, 59.74863466993041783, 9.382169495545420901 ) ) ;
#50456=CARTESIAN_POINT ( 'NONE',  ( -2.266590686148945544, 31.38708216824730002, -7.082119434687050408 ) ) ;
#50457=( GEOMETRIC_REPRESENTATION_CONTEXT ( 3 ) GLOBAL_UNCERTAINTY_ASSIGNED_CONTEXT ( ( #78333 ) ) GLOBAL_UNIT_ASSIGNED_CONTEXT ( ( #14258, #83735, #53724 ) ) REPRESENTATION_CONTEXT ( 'NONE', 'WORKASPACE' ) );
#50460=CARTESIAN_POINT ( 'NONE',  ( 20.32896413005680714, 35.57879003517447103, -5.963430220938276349 ) ) ;
#50463=CARTESIAN_POINT ( 'NONE',  ( 19.38216949554541202, 0.9986346699304200492, 9.382169495545424454 ) ) ;
#50464=FACE_OUTER_BOUND ( 'NONE', #6069, .T. ) ;
#50465=CARTESIAN_POINT ( 'NONE',  ( 20.88017736071110519, 30.56368534415484106, 2.639326808657452039E-16 ) ) ;
#50466=CARTESIAN_POINT ( 'NONE',  ( 18.52753015748617571, 58.09226448433411605, 4.923371831947298993 ) ) ;
#50468=CARTESIAN_POINT ( 'NONE',  ( 19.84674366389459266, 13.71726448433411782, -2.638427012816827677 ) ) ;
#50470=CARTESIAN_POINT ( 'NONE',  ( 2.791683348922237240, 25.38393115100078390, -7.208316651077763204 ) ) ;
#50471=CARTESIAN_POINT ( 'NONE',  ( 7.361572987183170547, 7.050597817667451750, 9.846743663894590881 ) ) ;
#50472=MECHANICAL_DESIGN_GEOMETRIC_PRESENTATION_REPRESENTATION('',(#28134),#60104);
#50473=CARTESIAN_POINT ( 'NONE',  ( 19.84674366389459621, 3.508931151000785231, 7.409399052514197653E-17 ) ) ;
#50475=CARTESIAN_POINT ( 'NONE',  ( 10.00000000000000178, 69.31368534415484817, 10.88017736071110342 ) ) ;
#50477=CARTESIAN_POINT ( 'NONE',  ( 19.84674366389459621, 3.508931151000785231, 7.409399052514197653E-17 ) ) ;
#50479=CARTESIAN_POINT ( 'NONE',  ( 7.361572987183169658, 19.96726448433411960, -9.846743663894592657 ) ) ;
#50483=CARTESIAN_POINT ( 'NONE',  ( 13.43411237798106583, 2.665301336597086568, -12.81628187352647252 ) ) ;
#50485=B_SPLINE_CURVE_WITH_KNOTS ( 'NONE', 3,
 ( #24431, #8911, #17902, #23936 ),
 .UNSPECIFIED., .F., .F.,
 ( 4, 4 ),
 ( 0.000000000000000000, 0.001036303429213384589 ),
 .UNSPECIFIED. ) ;
#50487=CARTESIAN_POINT ( 'NONE',  ( 20.88017736071110519, 5.563685344154837509, 2.639326808657452039E-16 ) ) ;
#50489=CARTESIAN_POINT ( 'NONE',  ( -0.3689425029237881626, 17.42874883491397142, 10.36894250292379027 ) ) ;
#50493=CARTESIAN_POINT ( 'NONE',  ( 24.16423886937409904, 19.09541550158063927, 3.795296366450317205 ) ) ;
#50494=CARTESIAN_POINT ( 'NONE',  ( -0.3689425029237898834, 31.17874883491396787, -10.36894250292378850 ) ) ;
#50495=CARTESIAN_POINT ( 'NONE',  ( -4.164238869374098151, 16.59541550158063927, -3.795296366450310543 ) ) ;
#50496=CARTESIAN_POINT ( 'NONE',  ( 10.00000000000000178, 69.31368534415484817, 10.88017736071110342 ) ) ;
#50497=CARTESIAN_POINT ( 'NONE',  ( 15.44008868035555793, 31.39701867748817676, -9.422509992056140149 ) ) ;
#50500=CARTESIAN_POINT ( 'NONE',  ( 0.1532563361054100626, 20.80059781766744464, -2.638427012816831230 ) ) ;
#50501=CARTESIAN_POINT ( 'NONE',  ( 2.035157376598824452, 53.68868534415484817, 7.964842623401179544 ) ) ;
#50502=CARTESIAN_POINT ( 'NONE',  ( 10.00000000000000000, 34.75893115100078745, -9.846743663894594434 ) ) ;
#50503=CARTESIAN_POINT ( 'NONE',  ( 19.42250999205614193, 5.147018677488171434, 5.440088680355555262 ) ) ;
#50504=CARTESIAN_POINT ( 'NONE',  ( 6.565887622018943937, 45.16530133659708923, 12.81628187352647430 ) ) ;
#50505=CARTESIAN_POINT ( 'NONE',  ( 7.361572987183170547, 57.05059781766744464, 9.846743663894590881 ) ) ;
#50507=AXIS2_PLACEMENT_3D ( 'NONE', #32166, #78172, #24204 ) ;
#50508=CARTESIAN_POINT ( 'NONE',  ( 0.6178305044545818747, 48.49863466993042493, -9.382169495545419124 ) ) ;
#50511=CARTESIAN_POINT ( 'NONE',  ( 18.52753015748617571, 43.09226448433412315, 4.923371831947298993 ) ) ;
#50512=CARTESIAN_POINT ( 'NONE',  ( 6.204703633549690345, 25.76208216824730712, -14.16423886937410259 ) ) ;
#50515=CARTESIAN_POINT ( 'NONE',  ( 0.5774900079438590739, 47.64701867748817676, -5.440088680355550821 ) ) ;
#50516=CARTESIAN_POINT ( 'NONE',  ( 4.559911319644449179, 48.89701867748817676, 9.422509992056141925 ) ) ;
#50517=CARTESIAN_POINT ( 'NONE',  ( -2.266590686148945544, 51.38708216824730357, -7.082119434687050408 ) ) ;
#50518=CARTESIAN_POINT ( 'NONE',  ( 12.63842701281683034, 62.46726448433410894, 9.846743663894596210 ) ) ;
#50520=CARTESIAN_POINT ( 'NONE',  ( 20.88017736071110875, 40.77201867748818387, -2.915334737309920765 ) ) ;
#50522=CARTESIAN_POINT ( 'NONE',  ( 0.6178305044545838731, 24.74863466993042493, 9.382169495545420901 ) ) ;
#50523=CARTESIAN_POINT ( 'NONE',  ( 10.00000000000000000, 49.75893115100078745, -9.846743663894594434 ) ) ;
#50525=FACE_OUTER_BOUND ( 'NONE', #15608, .T. ) ;
#50526=CARTESIAN_POINT ( 'NONE',  ( 17.96484262340118221, 61.18868534415482685, -7.964842623401177768 ) ) ;
#50529=CARTESIAN_POINT ( 'NONE',  ( 2.035157376598822676, 2.438685344154837953, -7.964842623401177768 ) ) ;
#50531=CARTESIAN_POINT ( 'NONE',  ( 15.44008868035555793, 66.39701867748817676, -9.422509992056140149 ) ) ;
#50532=CARTESIAN_POINT ( 'NONE',  ( 10.00000000000000000, 4.758931151000784787, -9.846743663894594434 ) ) ;
#50534=CARTESIAN_POINT ( 'NONE',  ( 17.20831665107776587, 29.13393115100078390, -7.208316651077762316 ) ) ;
#50535=CARTESIAN_POINT ( 'NONE',  ( 4.559911319644449179, 17.23035201082150536, -9.422509992056141925 ) ) ;
#50537=CARTESIAN_POINT ( 'NONE',  ( 0.6178305044545818747, 3.498634669930420049, -9.382169495545419124 ) ) ;
#50538=CARTESIAN_POINT ( 'NONE',  ( 20.88017736071110519, 35.56368534415484106, 2.639326808657452039E-16 ) ) ;
#50541=CARTESIAN_POINT ( 'NONE',  ( 19.38216949554541557, 42.24863466993041783, -9.382169495545420901 ) ) ;
#50543=CARTESIAN_POINT ( 'NONE',  ( 19.42250999205614548, 60.98035201082151247, -5.440088680355545492 ) ) ;
#50544=CARTESIAN_POINT ( 'NONE',  ( 19.38216949554541202, 15.99863466993042138, 9.382169495545424454 ) ) ;
#50546=CARTESIAN_POINT ( 'NONE',  ( 19.42250999205614193, 45.14701867748817676, 5.440088680355555262 ) ) ;
#50547=CARTESIAN_POINT ( 'NONE',  ( 0.1532563361054082862, 61.21726448433412315, 2.638427012816831674 ) ) ;
#50548=CARTESIAN_POINT ( 'NONE',  ( 20.36894250292379382, 58.67874883491396076, 10.36894250292379205 ) ) ;
#50549=CARTESIAN_POINT ( 'NONE',  ( 12.63842701281683034, 57.46726448433411605, 9.846743663894596210 ) ) ;
#50550=CARTESIAN_POINT ( 'NONE',  ( -0.8801773607110991993, 67.85535201082151957, -2.915334737309923874 ) ) ;
#50551=CARTESIAN_POINT ( 'NONE',  ( 7.084665262690076126, 64.10535201082150536, 10.88017736071109987 ) ) ;
#50553=CARTESIAN_POINT ( 'NONE',  ( -0.3689425029237898834, 31.17874883491396787, -10.36894250292378850 ) ) ;
#50558=VERTEX_POINT ( 'NONE', #39727 ) ;
#50559=VERTEX_POINT ( 'NONE', #3692 ) ;
#50560=CARTESIAN_POINT ( 'NONE',  ( -2.266590686148945544, 62.22041550158063927, 7.082119434687048631 ) ) ;
#50561=CARTESIAN_POINT ( 'NONE',  ( 24.16423886937410614, 44.51208216824730357, -3.795296366450302550 ) ) ;
#50562=CARTESIAN_POINT ( 'NONE',  ( 17.20831665107776587, 29.13393115100078390, -7.208316651077762316 ) ) ;
#50563=CARTESIAN_POINT ( 'NONE',  ( 16.40814093676323893, 25.79030133659708923, 11.09922568453595026 ) ) ;
#50565=CARTESIAN_POINT ( 'NONE',  ( 4.559911319644449179, 67.23035201082150536, -9.422509992056141925 ) ) ;
#50566=CARTESIAN_POINT ( 'NONE',  ( 13.79529636645030344, 43.26208216824730357, 14.16423886937410614 ) ) ;
#50570=CARTESIAN_POINT ( 'NONE',  ( 17.20831665107776587, 7.883931151000784787, 7.208316651077764980 ) ) ;
#50574=ORIENTED_EDGE ( 'NONE', *, *, #48327, .T. ) ;
#50578=CARTESIAN_POINT ( 'NONE',  ( -2.266590686148945544, 11.38708216824730179, -7.082119434687050408 ) ) ;
#50579=CARTESIAN_POINT ( 'NONE',  ( 0.5774900079438590739, 22.64701867748817321, -5.440088680355550821 ) ) ;
#50580=CARTESIAN_POINT ( 'NONE',  ( 10.00000000000000000, 26.81368534415484106, -10.88017736071110342 ) ) ;
#50581=CARTESIAN_POINT ( 'NONE',  ( 19.84674366389459266, 53.30059781766744464, 2.638427012816836559 ) ) ;
#50582=CARTESIAN_POINT ( 'NONE',  ( 22.81628187352647785, 16.62363466993042138, 6.195893100308588602E-16 ) ) ;
#50583=( GEOMETRIC_REPRESENTATION_CONTEXT ( 3 ) GLOBAL_UNCERTAINTY_ASSIGNED_CONTEXT ( ( #34286 ) ) GLOBAL_UNIT_ASSIGNED_CONTEXT ( ( #74458, #58470, #12975 ) ) REPRESENTATION_CONTEXT ( 'NONE', 'WORKASPACE' ) );
#50587=CARTESIAN_POINT ( 'NONE',  ( 10.00000000000000000, 27.87363466993042138, -12.81628187352647608 ) ) ;
#50588=EDGE_CURVE ( 'NONE', #27809, #98371, #43713, .T. ) ;
#50590=CARTESIAN_POINT ( 'NONE',  ( 7.361572987183170547, 32.05059781766745175, 9.846743663894590881 ) ) ;
#50591=CARTESIAN_POINT ( 'NONE',  ( 17.08211943468705130, 63.47041550158063927, 12.26659068614894998 ) ) ;
#50592=ORIENTED_EDGE ( 'NONE', *, *, #82133, .F. ) ;
#50593=CARTESIAN_POINT ( 'NONE',  ( 15.44008868035555260, 4.730352010821505360, 9.422509992056143702 ) ) ;
#50595=CARTESIAN_POINT ( 'NONE',  ( 2.035157376598822676, 42.43868534415483396, -7.964842623401177768 ) ) ;
#50596=CARTESIAN_POINT ( 'NONE',  ( 20.88017736071110164, 40.35535201082150536, 2.915334737309930979 ) ) ;
#50597=CARTESIAN_POINT ( 'NONE',  ( 15.44008868035555793, 46.39701867748817676, -9.422509992056140149 ) ) ;
#50599=CARTESIAN_POINT ( 'NONE',  ( 15.44008868035555793, 36.39701867748816966, -9.422509992056140149 ) ) ;
#50603=CARTESIAN_POINT ( 'NONE',  ( 19.84674366389459266, 28.30059781766745886, 2.638427012816836559 ) ) ;
#50605=CARTESIAN_POINT ( 'NONE',  ( 17.20831665107776587, 57.88393115100078745, 7.208316651077764980 ) ) ;
#50607=COLOUR_RGB ( '', 0.72549020, 0.75294118, 0.79215686) ;
#50613=CARTESIAN_POINT ( 'NONE',  ( 19.84674366389459266, 38.71726448433412315, -2.638427012816827677 ) ) ;
#50614=CARTESIAN_POINT ( 'NONE',  ( 2.917880565312948704, 57.63708216824731068, 12.26659068614894643 ) ) ;
#50618=CARTESIAN_POINT ( 'NONE',  ( 5.076628168052703671, 31.84226448433412315, 8.527530157486179263 ) ) ;
#50620=CARTESIAN_POINT ( 'NONE',  ( 3.591859063236761518, 4.956968003263753531, 11.09922568453594849 ) ) ;
#50621=CARTESIAN_POINT ( 'NONE',  ( 19.84674366389459266, 8.717264484334116048, -2.638427012816827677 ) ) ;
#50623=CARTESIAN_POINT ( 'NONE',  ( 10.00000000000000000, 9.758931151000785675, -9.846743663894594434 ) ) ;
#50624=CARTESIAN_POINT ( 'NONE',  ( 18.52753015748618282, 53.92559781766745175, -4.923371831947291888 ) ) ;
#50626=VECTOR ( 'NONE', #92061, 1000.000000000000114 ) ;
#50628=CARTESIAN_POINT ( 'NONE',  ( 12.91533473730993009, 6.605352010821504471, -10.88017736071109987 ) ) ;
#50629=CARTESIAN_POINT ( 'NONE',  ( 6.204703633549690345, 5.762082168247301794, -14.16423886937410259 ) ) ;
#50630=CARTESIAN_POINT ( 'NONE',  ( 5.076628168052703671, 11.84226448433411960, 8.527530157486179263 ) ) ;
#50631=CARTESIAN_POINT ( 'NONE',  ( -0.8801773607111008646, 53.27201867748816966, 2.915334737309923430 ) ) ;
#50632=CARTESIAN_POINT ( 'NONE',  ( 21.09922568453595559, 27.04030133659708568, -6.408140936763230044 ) ) ;
#50634=CARTESIAN_POINT ( 'NONE',  ( 17.96484262340118221, 6.188685344154836621, -7.964842623401177768 ) ) ;
#50636=CARTESIAN_POINT ( 'NONE',  ( 20.05723567505238947, 0.1676365378933190875, -6.413539670616452248 ) ) ;
#50638=CARTESIAN_POINT ( 'NONE',  ( 16.40814093676323893, 0.7903013365970867898, 11.09922568453595026 ) ) ;
#50639=CARTESIAN_POINT ( 'NONE',  ( 2.791683348922237240, 65.38393115100078035, -7.208316651077763204 ) ) ;
#50640=CARTESIAN_POINT ( 'NONE',  ( 19.84674366389459621, 13.50893115100078568, 7.409399052514197653E-17 ) ) ;
#50642=CARTESIAN_POINT ( 'NONE',  ( 21.09922568453594849, 16.20696800326375353, 6.408140936763242479 ) ) ;
#50644=CARTESIAN_POINT ( 'NONE',  ( -0.8801773607110991993, 27.85535201082150181, -2.915334737309923874 ) ) ;
#50647=CARTESIAN_POINT ( 'NONE',  ( 17.08211943468705130, 53.47041550158063217, 12.26659068614894998 ) ) ;
#50651=CARTESIAN_POINT ( 'NONE',  ( 2.035157376598822676, 27.43868534415483396, -7.964842623401177768 ) ) ;
#50652=CARTESIAN_POINT ( 'NONE',  ( 2.791683348922237240, 45.38393115100079456, -7.208316651077763204 ) ) ;
#50653=CARTESIAN_POINT ( 'NONE',  ( 0.5774900079438607392, 58.48035201082151247, 5.440088680355550821 ) ) ;
#50654=CARTESIAN_POINT ( 'NONE',  ( -4.164238869374098151, 31.59541550158063927, -3.795296366450310543 ) ) ;
#50656=CARTESIAN_POINT ( 'NONE',  ( 14.92337183194729633, 37.67559781766745175, 8.527530157486181039 ) ) ;
#50657=CARTESIAN_POINT ( 'NONE',  ( 6.565887622018943937, 65.16530133659709634, 12.81628187352647430 ) ) ;
#50658=CARTESIAN_POINT ( 'NONE',  ( 5.076628168052703671, 66.84226448433412315, 8.527530157486179263 ) ) ;
#50660=CARTESIAN_POINT ( 'NONE',  ( 19.42250999205614548, 30.98035201082150536, -5.440088680355545492 ) ) ;
#50662=CARTESIAN_POINT ( 'NONE',  ( 14.49999999999999822, 11.50000000000000000, -5.000000000000000000 ) ) ;
#50663=CARTESIAN_POINT ( 'NONE',  ( 10.00000000000000178, 9.313685344154839285, 10.88017736071110342 ) ) ;
#50664=CARTESIAN_POINT ( 'NONE',  ( 17.96484262340118221, 66.18868534415483396, -7.964842623401177768 ) ) ;
#50665=CARTESIAN_POINT ( 'NONE',  ( -2.266590686148945544, 26.38708216824730357, -7.082119434687050408 ) ) ;
#50666=EDGE_CURVE ( 'NONE', #45674, #36088, #81143, .T. ) ;
#50667=CARTESIAN_POINT ( 'NONE',  ( 10.00000000000000000, 9.758931151000785675, -9.846743663894594434 ) ) ;
#50668=CARTESIAN_POINT ( 'NONE',  ( 5.076628168052704559, 60.17559781766745175, -8.527530157486179263 ) ) ;
#50669=CARTESIAN_POINT ( 'NONE',  ( 2.035157376598822676, 32.43868534415483396, -7.964842623401177768 ) ) ;
#50670=CARTESIAN_POINT ( 'NONE',  ( 19.05914839598885280, 64.96693863883976405, 6.499999999999962697 ) ) ;
#50675=CARTESIAN_POINT ( 'NONE',  ( 7.361572987183170547, 47.05059781766745175, 9.846743663894590881 ) ) ;
#50679=CARTESIAN_POINT ( 'NONE',  ( 22.26659068614894466, 13.88708216824730179, 7.082119434687054849 ) ) ;
#50680=CARTESIAN_POINT ( 'NONE',  ( 2.917880565312950480, 5.970415501580634832, -12.26659068614894821 ) ) ;
#50681=CARTESIAN_POINT ( 'NONE',  ( 4.559911319644449179, 53.89701867748817676, 9.422509992056141925 ) ) ;
#50682=CARTESIAN_POINT ( 'NONE',  ( 10.00000000000000000, 55.55374883491396787, -14.16423886937410082 ) ) ;
#50683=CARTESIAN_POINT ( 'NONE',  ( 3.591859063236763294, 3.290301336597087012, -11.09922568453595026 ) ) ;
#50684=CARTESIAN_POINT ( 'NONE',  ( 2.791683348922240793, 31.63393115100078745, 7.208316651077764092 ) ) ;
#50686=CARTESIAN_POINT ( 'NONE',  ( 2.035157376598822676, 27.43868534415483396, -7.964842623401177768 ) ) ;
#50687=CARTESIAN_POINT ( 'NONE',  ( 16.40814093676324603, 12.45696800326375353, -11.09922568453594671 ) ) ;
#50688=CARTESIAN_POINT ( 'NONE',  ( 17.08211943468705130, 3.470415501580634388, 12.26659068614894998 ) ) ;
#50689=CARTESIAN_POINT ( 'NONE',  ( 20.88017736071110164, 15.35535201082150358, 2.915334737309930979 ) ) ;
#50690=CARTESIAN_POINT ( 'NONE',  ( -1.926860441876562247, 67.45379003517449235, -3.195792623639530650 ) ) ;
#50692=CARTESIAN_POINT ( 'NONE',  ( -0.8801773607111008646, 38.27201867748816255, 2.915334737309923430 ) ) ;
#50696=EDGE_LOOP ( 'NONE', ( #12120, #65685, #82086, #9630 ) ) ;
#50698=CARTESIAN_POINT ( 'NONE',  ( 10.00000000000000178, 48.05374883491396787, 14.16423886937410082 ) ) ;
#50699=CARTESIAN_POINT ( 'NONE',  ( 17.20831665107776587, 52.88393115100078035, 7.208316651077764980 ) ) ;
#50700=CARTESIAN_POINT ( 'NONE',  ( 20.88017736071110875, 55.77201867748816966, -2.915334737309920765 ) ) ;
#50704=CARTESIAN_POINT ( 'NONE',  ( 0.5774900079438607392, 58.48035201082151247, 5.440088680355550821 ) ) ;
#50706=CARTESIAN_POINT ( 'NONE',  ( -2.816281873526473856, 59.33196800326374643, 3.434112377981055619 ) ) ;
#50710=CARTESIAN_POINT ( 'NONE',  ( 15.44008868035555260, 49.73035201082150536, 9.422509992056143702 ) ) ;
#50711=CARTESIAN_POINT ( 'NONE',  ( 2.917880565312950480, 20.97041550158063217, -12.26659068614894821 ) ) ;
#50712=CARTESIAN_POINT ( 'NONE',  ( 10.00000000000000000, 27.87363466993042138, -12.81628187352647608 ) ) ;
#50714=CARTESIAN_POINT ( 'NONE',  ( 3.591859063236761518, 44.95696800326376064, 11.09922568453594849 ) ) ;
#50716=CARTESIAN_POINT ( 'NONE',  ( 10.00000000000000178, 32.25893115100078745, 9.846743663894594434 ) ) ;
#50717=CARTESIAN_POINT ( 'NONE',  ( 2.035157376598824452, 8.688685344154839285, 7.964842623401179544 ) ) ;
#50718=CARTESIAN_POINT ( 'NONE',  ( 3.591859063236761518, 49.95696800326375353, 11.09922568453594849 ) ) ;
#50720=CARTESIAN_POINT ( 'NONE',  ( 2.791683348922237240, 45.38393115100079456, -7.208316651077763204 ) ) ;
#50724=CARTESIAN_POINT ( 'NONE',  ( -0.8801773607110991993, 67.85535201082151957, -2.915334737309923874 ) ) ;
#50731=CARTESIAN_POINT ( 'NONE',  ( 19.84674366389459266, 23.71726448433412315, -2.638427012816827677 ) ) ;
#50732=CARTESIAN_POINT ( 'NONE',  ( 6.565887622018943937, 25.16530133659708213, 12.81628187352647430 ) ) ;
#50735=EDGE_LOOP ( 'NONE', ( #70035, #69781, #50592, #60022 ) ) ;
#50737=CARTESIAN_POINT ( 'NONE',  ( 24.16423886937410614, 24.30374883491396787, 8.672049930838204340E-16 ) ) ;
#50738=CARTESIAN_POINT ( 'NONE',  ( 17.20831665107776587, 39.13393115100079456, -7.208316651077762316 ) ) ;
#50739=CARTESIAN_POINT ( 'NONE',  ( 16.40814093676323893, 45.79030133659708923, 11.09922568453595026 ) ) ;
#50742=CARTESIAN_POINT ( 'NONE',  ( 12.91533473730993009, 61.60535201082150536, -10.88017736071109987 ) ) ;
#50743=CARTESIAN_POINT ( 'NONE',  ( -1.099225684535947600, 14.54030133659708568, 6.408140936763237150 ) ) ;
#50745=CARTESIAN_POINT ( 'NONE',  ( 1.472469842513823179, 40.59226448433411605, -4.923371831947296329 ) ) ;
#50746=CARTESIAN_POINT ( 'NONE',  ( 15.44008868035555260, 34.73035201082151247, 9.422509992056143702 ) ) ;
#50747=CARTESIAN_POINT ( 'NONE',  ( -2.816281873526473856, 44.12363466993042493, 9.499525473075851096E-16 ) ) ;
#50748=CARTESIAN_POINT ( 'NONE',  ( 0.1532563361054083140, 31.00893115100078390, 1.131784320476157264E-15 ) ) ;
#50751=CARTESIAN_POINT ( 'NONE',  ( 19.42250999205614193, 35.14701867748816966, 5.440088680355555262 ) ) ;
#50753=CYLINDRICAL_SURFACE ( 'NONE', #39391, 7.000000000000006217 ) ;
#50754=CARTESIAN_POINT ( 'NONE',  ( 20.88017736071110875, 10.77201867748817143, -2.915334737309920765 ) ) ;
#50755=CARTESIAN_POINT ( 'NONE',  ( 2.791683348922237240, 55.38393115100078745, -7.208316651077763204 ) ) ;
#50756=CARTESIAN_POINT ( 'NONE',  ( 12.91533473730992121, 34.52201867748817676, 10.88017736071110164 ) ) ;
#50758=CARTESIAN_POINT ( 'NONE',  ( 0.5774900079438590739, 57.64701867748817676, -5.440088680355550821 ) ) ;
#50759=CARTESIAN_POINT ( 'NONE',  ( 20.88017736071110519, 25.56368534415483751, 2.639326808657452039E-16 ) ) ;
#50760=CARTESIAN_POINT ( 'NONE',  ( 14.92337183194729988, 24.34226448433411960, -8.527530157486177487 ) ) ;
#50763=CARTESIAN_POINT ( 'NONE',  ( 14.92337183194729633, 52.67559781766745175, 8.527530157486181039 ) ) ;
#50764=CARTESIAN_POINT ( 'NONE',  ( -4.164238869374099927, 57.01208216824731068, 3.795296366450308767 ) ) ;
#50766=CARTESIAN_POINT ( 'NONE',  ( 10.00000000000000178, 8.053748834913967869, 14.16423886937410082 ) ) ;
#50767=CARTESIAN_POINT ( 'NONE',  ( 20.36894250292379382, 33.67874883491396076, 10.36894250292379205 ) ) ;
#50768=AXIS2_PLACEMENT_3D ( 'NONE', #32697, #93699, #25234 ) ;
#50769=CARTESIAN_POINT ( 'NONE',  ( 0.6178305044545838731, -0.2513653300695798953, 9.382169495545420901 ) ) ;
#50771=CARTESIAN_POINT ( 'NONE',  ( 2.035157376598822676, 17.43868534415483751, -7.964842623401177768 ) ) ;
#50772=CARTESIAN_POINT ( 'NONE',  ( 7.361572987183169658, 39.96726448433411605, -9.846743663894592657 ) ) ;
#50776=CARTESIAN_POINT ( 'NONE',  ( -1.099225684535947600, 23.70696800326375708, -6.408140936763238038 ) ) ;
#50777=CARTESIAN_POINT ( 'NONE',  ( 2.791683348922240793, 26.63393115100078745, 7.208316651077764092 ) ) ;
#50779=CARTESIAN_POINT ( 'NONE',  ( 17.20831665107776587, 4.133931151000785675, -7.208316651077762316 ) ) ;
#50780=B_SPLINE_CURVE_WITH_KNOTS ( 'NONE', 3,
 ( #81845, #29335, #51854, #83339 ),
 .UNSPECIFIED., .F., .F.,
 ( 4, 4 ),
 ( 2.523187944655234921E-17, 0.002562518741975313395 ),
 .UNSPECIFIED. ) ;
#50782=CARTESIAN_POINT ( 'NONE',  ( 19.42250999205614193, 5.147018677488171434, 5.440088680355555262 ) ) ;
#50783=CARTESIAN_POINT ( 'NONE',  ( 0.5774900079438590739, 17.64701867748817321, -5.440088680355550821 ) ) ;
#50784=CARTESIAN_POINT ( 'NONE',  ( -2.266590686148945544, 37.22041550158063217, 7.082119434687048631 ) ) ;
#50785=CARTESIAN_POINT ( 'NONE',  ( 4.559911319644449179, 27.23035201082150536, -9.422509992056141925 ) ) ;
#50787=CARTESIAN_POINT ( 'NONE',  ( 19.42250999205614193, 65.14701867748817676, 5.440088680355555262 ) ) ;
#50790=CARTESIAN_POINT ( 'NONE',  ( 12.63842701281683034, 17.46726448433411250, 9.846743663894596210 ) ) ;
#50791=CARTESIAN_POINT ( 'NONE',  ( 17.20831665107776587, 4.133931151000785675, -7.208316651077762316 ) ) ;
#50793=CARTESIAN_POINT ( 'NONE',  ( 7.361572987183170547, 42.05059781766745886, 9.846743663894590881 ) ) ;
#50794=CARTESIAN_POINT ( 'NONE',  ( 14.92337183194729633, 62.67559781766745886, 8.527530157486181039 ) ) ;
#50796=CARTESIAN_POINT ( 'NONE',  ( -0.8801773607111008646, 38.27201867748816255, 2.915334737309923430 ) ) ;
#50800=CARTESIAN_POINT ( 'NONE',  ( 16.40814093676324603, 47.45696800326375353, -11.09922568453594671 ) ) ;
#50802=CARTESIAN_POINT ( 'NONE',  ( 7.084665262690076126, 62.02201867748816966, -10.88017736071110164 ) ) ;
#50803=CARTESIAN_POINT ( 'NONE',  ( -2.816281873526473856, 44.33196800326375353, 3.434112377981055619 ) ) ;
#50804=CARTESIAN_POINT ( 'NONE',  ( 17.08211943468705130, 58.47041550158063927, 12.26659068614894998 ) ) ;
#50805=CARTESIAN_POINT ( 'NONE',  ( 0.1532563361054082862, 36.21726448433410894, 2.638427012816831674 ) ) ;
#50806=CARTESIAN_POINT ( 'NONE',  ( 19.72487221294571569, 20.71833443783938122, -6.499999999999990230 ) ) ;
#50807=CARTESIAN_POINT ( 'NONE',  ( 14.92337183194729988, 64.34226448433412315, -8.527530157486177487 ) ) ;
#50808=CARTESIAN_POINT ( 'NONE',  ( 6.204703633549690345, 25.76208216824730712, -14.16423886937410259 ) ) ;
#50809=CARTESIAN_POINT ( 'NONE',  ( 17.20831665107776587, 44.13393115100078745, -7.208316651077762316 ) ) ;
#50811=CARTESIAN_POINT ( 'NONE',  ( 10.00000000000000000, 31.81368534415483751, -10.88017736071110342 ) ) ;
#50812=CARTESIAN_POINT ( 'NONE',  ( 0.5774900079438590739, 52.64701867748817676, -5.440088680355550821 ) ) ;
#50814=CARTESIAN_POINT ( 'NONE',  ( -1.099225684535947600, 43.70696800326375353, -6.408140936763238038 ) ) ;
#50816=CARTESIAN_POINT ( 'NONE',  ( 19.84674366389459266, 3.300597817667451750, 2.638427012816836559 ) ) ;
#50817=ORIENTED_EDGE ( 'NONE', *, *, #79658, .T. ) ;
#50818=CARTESIAN_POINT ( 'NONE',  ( 17.08211943468705840, 5.137082168247300906, -12.26659068614894466 ) ) ;
#50819=CARTESIAN_POINT ( 'NONE',  ( 10.00000000000000178, 2.258931151000784787, 9.846743663894594434 ) ) ;
#50820=CARTESIAN_POINT ( 'NONE',  ( 2.599899806584774264, 0.4361964623231012195, -6.495912400107028084 ) ) ;
#50823=CARTESIAN_POINT ( 'NONE',  ( 12.91533473730993009, 11.60535201082150536, -10.88017736071109987 ) ) ;
#50826=CARTESIAN_POINT ( 'NONE',  ( 10.00000000000000000, 20.55374883491396787, -14.16423886937410082 ) ) ;
#50828=CARTESIAN_POINT ( 'NONE',  ( 20.88017736071110164, 25.35535201082150891, 2.915334737309930979 ) ) ;
#50829=CARTESIAN_POINT ( 'NONE',  ( 19.84674366389459266, 53.30059781766744464, 2.638427012816836559 ) ) ;
#50831=CARTESIAN_POINT ( 'NONE',  ( 0.1532563361054082862, 61.21726448433412315, 2.638427012816831674 ) ) ;
#50833=CARTESIAN_POINT ( 'NONE',  ( 19.42250999205614193, 60.14701867748817676, 5.440088680355555262 ) ) ;
#50834=CARTESIAN_POINT ( 'NONE',  ( 1.472469842513823179, 66.42559781766745175, 4.923371831947296329 ) ) ;
#50835=CARTESIAN_POINT ( 'NONE',  ( 0.6178305044545838731, 34.74863466993042493, 9.382169495545420901 ) ) ;
#50836=CARTESIAN_POINT ( 'NONE',  ( 15.44008868035555260, 4.730352010821504471, 9.422509992056143702 ) ) ;
#50838=CARTESIAN_POINT ( 'NONE',  ( 10.00000000000000000, 4.758931151000784787, -9.846743663894594434 ) ) ;
#50839=CARTESIAN_POINT ( 'NONE',  ( 15.44008868035555793, 21.39701867748817321, -9.422509992056140149 ) ) ;
#50841=CARTESIAN_POINT ( 'NONE',  ( 13.43411237798106583, 57.66530133659708923, -12.81628187352647252 ) ) ;
#50842=CARTESIAN_POINT ( 'NONE',  ( 15.44008868035555260, 24.73035201082150891, 9.422509992056143702 ) ) ;
#50844=CARTESIAN_POINT ( 'NONE',  ( 21.09922568453594849, 46.20696800326376064, 6.408140936763242479 ) ) ;
#50845=CARTESIAN_POINT ( 'NONE',  ( 20.88017736071110875, 45.77201867748816966, -2.915334737309920765 ) ) ;
#50846=CARTESIAN_POINT ( 'NONE',  ( 1.472469842513823179, 55.59226448433412315, -4.923371831947296329 ) ) ;
#50849=CARTESIAN_POINT ( 'NONE',  ( 0.1532563361054100626, 20.80059781766744464, -2.638427012816831230 ) ) ;
#50850=CARTESIAN_POINT ( 'NONE',  ( 3.591859063236761518, -0.04303199673624671928, 11.09922568453594849 ) ) ;
#50853=CARTESIAN_POINT ( 'NONE',  ( -0.8801773607111008646, 18.27201867748817321, 2.915334737309923430 ) ) ;
#50854=CARTESIAN_POINT ( 'NONE',  ( 17.20831665107776587, 54.13393115100079456, -7.208316651077762316 ) ) ;
#50857=CARTESIAN_POINT ( 'NONE',  ( 7.361572987183169658, 9.967264484334119601, -9.846743663894592657 ) ) ;
#50858=CARTESIAN_POINT ( 'NONE',  ( 19.38216949554541202, 0.9986346699304200492, 9.382169495545424454 ) ) ;
#50863=CARTESIAN_POINT ( 'NONE',  ( 19.38216949554541557, 37.24863466993041783, -9.382169495545420901 ) ) ;
#50864=CARTESIAN_POINT ( 'NONE',  ( 12.63842701281683034, 37.46726448433411605, 9.846743663894596210 ) ) ;
#50866=CARTESIAN_POINT ( 'NONE',  ( -0.3689425029237881626, 62.42874883491396787, 10.36894250292379027 ) ) ;
#50867=CARTESIAN_POINT ( 'NONE',  ( 18.52753015748618282, 28.92559781766745175, -4.923371831947291888 ) ) ;
#50868=CARTESIAN_POINT ( 'NONE',  ( -0.2418659066527655277, 39.26028685723174050, -6.114288769123055189 ) ) ;
#50869=CARTESIAN_POINT ( 'NONE',  ( 13.79529636645030344, 53.26208216824730357, 14.16423886937410614 ) ) ;
#50871=CARTESIAN_POINT ( 'NONE',  ( 15.44008868035555260, 24.73035201082150891, 9.422509992056143702 ) ) ;
#50872=CARTESIAN_POINT ( 'NONE',  ( -0.3689425029237881626, 42.42874883491396787, 10.36894250292379027 ) ) ;
#50873=CARTESIAN_POINT ( 'NONE',  ( 20.36894250292379382, 58.67874883491396076, 10.36894250292379205 ) ) ;
#50874=CYLINDRICAL_SURFACE ( 'NONE', #8469, 0.5000000000000004441 ) ;
#50875=CARTESIAN_POINT ( 'NONE',  ( 18.52753015748617571, 8.092264484334117824, 4.923371831947298993 ) ) ;
#50876=CARTESIAN_POINT ( 'NONE',  ( 3.591859063236763294, -1.709698663402913210, -11.09922568453595026 ) ) ;
#50877=CARTESIAN_POINT ( 'NONE',  ( 17.84635730667655906, 13.63791097397318985, 6.500000000000019540 ) ) ;
#50879=CARTESIAN_POINT ( 'NONE',  ( 20.88017736071110875, 50.77201867748817676, -2.915334737309920765 ) ) ;
#50881=CARTESIAN_POINT ( 'NONE',  ( 0.1532563361054083140, 51.00893115100078745, 1.131784320476157264E-15 ) ) ;
#50884=ORIENTED_EDGE ( 'NONE', *, *, #34358, .T. ) ;
#50885=CARTESIAN_POINT ( 'NONE',  ( -4.164238869374099927, 47.01208216824729647, 3.795296366450308767 ) ) ;
#50886=DIRECTION ( 'NONE',  ( 0.000000000000000000, 0.000000000000000000, 1.000000000000000000 ) ) ;
#50888=CARTESIAN_POINT ( 'NONE',  ( 7.084665262690076126, 17.02201867748817676, -10.88017736071110164 ) ) ;
#50889=CARTESIAN_POINT ( 'NONE',  ( -1.099225684535947600, 44.54030133659708923, 6.408140936763237150 ) ) ;
#50891=CARTESIAN_POINT ( 'NONE',  ( -2.816281873526473856, 19.12363466993042138, 9.499525473075851096E-16 ) ) ;
#50895=CARTESIAN_POINT ( 'NONE',  ( -0.3689425029237881626, 27.42874883491397142, 10.36894250292379027 ) ) ;
#50896=CARTESIAN_POINT ( 'NONE',  ( 6.204703633549690345, 0.7620821682473009062, -14.16423886937410259 ) ) ;
#50898=CARTESIAN_POINT ( 'NONE',  ( 7.084665262690076126, 22.02201867748817321, -10.88017736071110164 ) ) ;
#50900=DIRECTION ( 'NONE',  ( 0.000000000000000000, -1.000000000000000000, 0.000000000000000000 ) ) ;
#50901=CARTESIAN_POINT ( 'NONE',  ( 4.559911319644449179, 47.23035201082150536, -9.422509992056141925 ) ) ;
#50902=CARTESIAN_POINT ( 'NONE',  ( 12.91533473730992121, 54.52201867748816255, 10.88017736071110164 ) ) ;
#50903=CARTESIAN_POINT ( 'NONE',  ( 3.591859063236763294, 8.290301336597087456, -11.09922568453595026 ) ) ;
#50905=CARTESIAN_POINT ( 'NONE',  ( 1.274849032794102888, 3.572280503510291361, 6.499999999999721112 ) ) ;
#50906=CARTESIAN_POINT ( 'NONE',  ( 18.52753015748617571, 18.09226448433411960, 4.923371831947298993 ) ) ;
#50907=CARTESIAN_POINT ( 'NONE',  ( 15.44008868035555260, 39.73035201082150536, 9.422509992056143702 ) ) ;
#50909=CARTESIAN_POINT ( 'NONE',  ( 19.38216949554541557, 2.248634669930420049, -9.382169495545420901 ) ) ;
#50910=CARTESIAN_POINT ( 'NONE',  ( 0.1532563361054082862, 1.217264484334117824, 2.638427012816831674 ) ) ;
#50911=CARTESIAN_POINT ( 'NONE',  ( 5.076628168052704559, 20.17559781766745175, -8.527530157486179263 ) ) ;
#50912=CARTESIAN_POINT ( 'NONE',  ( -2.816281873526471635, 53.91530133659709634, -3.434112377981056508 ) ) ;
#50913=CARTESIAN_POINT ( 'NONE',  ( 2.791683348922240793, 6.633931151000785675, 7.208316651077764092 ) ) ;
#50917=CARTESIAN_POINT ( 'NONE',  ( 20.88017736071110519, 20.56368534415484106, 2.639326808657452039E-16 ) ) ;
#50919=CARTESIAN_POINT ( 'NONE',  ( 6.204703633549690345, 30.76208216824730357, -14.16423886937410259 ) ) ;
#50920=CARTESIAN_POINT ( 'NONE',  ( 0.1532563361054100626, 30.80059781766744820, -2.638427012816831230 ) ) ;
#50922=CARTESIAN_POINT ( 'NONE',  ( 17.96484262340118221, 21.18868534415483396, -7.964842623401177768 ) ) ;
#50923=CARTESIAN_POINT ( 'NONE',  ( 0.5774900079438607392, 8.480352010821505360, 5.440088680355550821 ) ) ;
#50925=CARTESIAN_POINT ( 'NONE',  ( -0.8801773607110991993, 32.85535201082151247, -2.915334737309923874 ) ) ;
#50927=CARTESIAN_POINT ( 'NONE',  ( 17.96484262340118221, 41.18868534415484106, -7.964842623401177768 ) ) ;
#50929=CARTESIAN_POINT ( 'NONE',  ( 2.035157376598824452, 43.68868534415484106, 7.964842623401179544 ) ) ;
#50932=CARTESIAN_POINT ( 'NONE',  ( 19.84674366389459621, 63.50893115100078745, 7.409399052514197653E-17 ) ) ;
#50933=CARTESIAN_POINT ( 'NONE',  ( 17.96484262340118221, 39.93868534415484106, 7.964842623401181321 ) ) ;
#50935=EDGE_CURVE ( 'NONE', #31636, #81215, #87805, .T. ) ;
#50936=CARTESIAN_POINT ( 'NONE',  ( -2.816281873526473856, 64.33196800326376774, 3.434112377981055619 ) ) ;
#50938=CARTESIAN_POINT ( 'NONE',  ( 10.00000000000000000, 35.55374883491396787, -14.16423886937410082 ) ) ;
#50939=CARTESIAN_POINT ( 'NONE',  ( 7.084665262690076126, 47.02201867748818387, -10.88017736071110164 ) ) ;
#50940=CARTESIAN_POINT ( 'NONE',  ( 10.00000000000000178, 67.25893115100079456, 9.846743663894594434 ) ) ;
#50942=CARTESIAN_POINT ( 'NONE',  ( 5.076628168052703671, 46.84226448433412315, 8.527530157486179263 ) ) ;
#50944=VERTEX_POINT ( 'NONE', #47343 ) ;
#50946=CARTESIAN_POINT ( 'NONE',  ( 7.361572987183170547, 17.05059781766745530, 9.846743663894590881 ) ) ;
#50948=CARTESIAN_POINT ( 'NONE',  ( 2.035157376598824452, 8.688685344154839285, 7.964842623401179544 ) ) ;
#50949=CARTESIAN_POINT ( 'NONE',  ( 0.1532563361054083140, 31.00893115100078390, 1.131784320476157264E-15 ) ) ;
#50950=CARTESIAN_POINT ( 'NONE',  ( 19.38216949554541202, 10.99863466993042138, 9.382169495545424454 ) ) ;
#50951=CARTESIAN_POINT ( 'NONE',  ( -0.8801773607111009756, 58.06368534415484106, 1.068504757029289695E-15 ) ) ;
#50952=CARTESIAN_POINT ( 'NONE',  ( 0.5774900079438590739, 32.64701867748816966, -5.440088680355550821 ) ) ;
#50953=CARTESIAN_POINT ( 'NONE',  ( -1.099225684535947600, 58.70696800326375353, -6.408140936763238038 ) ) ;
#50954=CARTESIAN_POINT ( 'NONE',  ( 13.79529636645030344, 43.26208216824730357, 14.16423886937410614 ) ) ;
#50956=ORIENTED_EDGE ( 'NONE', *, *, #17779, .T. ) ;
#50957=CARTESIAN_POINT ( 'NONE',  ( 22.81628187352647785, 1.623634669930420271, 6.195893100308588602E-16 ) ) ;
#50958=CARTESIAN_POINT ( 'NONE',  ( 2.035157376598824452, 3.688685344154837953, 7.964842623401179544 ) ) ;
#50959=CARTESIAN_POINT ( 'NONE',  ( 20.88017736071110875, 40.77201867748818387, -2.915334737309920765 ) ) ;
#50960=CARTESIAN_POINT ( 'NONE',  ( 10.00000000000000178, 62.25893115100078745, 9.846743663894594434 ) ) ;
#50961=B_SPLINE_CURVE_WITH_KNOTS ( 'NONE', 3,
 ( #82963, #45957, #89477, #7961, #29448, #37975, #14482, #66974, #44952, #13482 ),
 .UNSPECIFIED., .F., .F.,
 ( 4, 3, 3, 4 ),
 ( 7.573910767901059648E-18, 0.0006253016069560859589, 0.001250604074564941890, 0.002501455912506543935 ),
 .UNSPECIFIED. ) ;
#50963=CARTESIAN_POINT ( 'NONE',  ( 0.1532563361054100626, 15.80059781766745353, -2.638427012816831230 ) ) ;
#50964=CARTESIAN_POINT ( 'NONE',  ( 19.84674366389459621, 13.50893115100078568, 7.409399052514197653E-17 ) ) ;
#50965=CARTESIAN_POINT ( 'NONE',  ( 1.472469842513823179, 26.42559781766745175, 4.923371831947296329 ) ) ;
#50966=CARTESIAN_POINT ( 'NONE',  ( 12.63842701281683922, 14.55059781766744997, -9.846743663894590881 ) ) ;
#50967=( NAMED_UNIT ( * ) PLANE_ANGLE_UNIT ( ) SI_UNIT ( $, .RADIAN. ) );
#50970=CARTESIAN_POINT ( 'NONE',  ( 10.00000000000000178, 7.258931151000785675, 9.846743663894594434 ) ) ;
#50972=CARTESIAN_POINT ( 'NONE',  ( 10.00000000000000000, 9.758931151000785675, -9.846743663894594434 ) ) ;
#50973=CARTESIAN_POINT ( 'NONE',  ( 0.1532563361054082862, 21.21726448433412315, 2.638427012816831674 ) ) ;
#50976=CARTESIAN_POINT ( 'NONE',  ( 12.63842701281683922, 64.55059781766745175, -9.846743663894590881 ) ) ;
#50978=CARTESIAN_POINT ( 'NONE',  ( 6.204703633549690345, 17.84541550158063217, 14.16423886937410082 ) ) ;
#50980=CARTESIAN_POINT ( 'NONE',  ( -4.164238869374099039, 16.80374883491396787, 8.674139862899312516E-16 ) ) ;
#50982=CARTESIAN_POINT ( 'NONE',  ( -0.3689425029237881626, 47.42874883491396787, 10.36894250292379027 ) ) ;
#50984=CARTESIAN_POINT ( 'NONE',  ( 22.26659068614895176, 14.72041550158063572, -7.082119434687042414 ) ) ;
#50985=CARTESIAN_POINT ( 'NONE',  ( 20.88017736071110164, 65.35535201082150536, 2.915334737309930979 ) ) ;
#50986=CARTESIAN_POINT ( 'NONE',  ( 12.91533473730993009, 36.60535201082151247, -10.88017736071109987 ) ) ;
#50988=CARTESIAN_POINT ( 'NONE',  ( 0.1532563361054082862, 26.21726448433411605, 2.638427012816831674 ) ) ;
#50989=CARTESIAN_POINT ( 'NONE',  ( 17.96484262340118221, 51.18868534415483396, -7.964842623401177768 ) ) ;
#50990=CARTESIAN_POINT ( 'NONE',  ( 1.472469842513823179, 35.59226448433412315, -4.923371831947296329 ) ) ;
#50991=CARTESIAN_POINT ( 'NONE',  ( 20.88017736071110875, 10.77201867748817143, -2.915334737309920765 ) ) ;
#50992=CARTESIAN_POINT ( 'NONE',  ( 16.40814093676323893, 55.79030133659708923, 11.09922568453595026 ) ) ;
#50993=CARTESIAN_POINT ( 'NONE',  ( 10.00000000000000178, 57.25893115100078745, 9.846743663894594434 ) ) ;
#50995=CARTESIAN_POINT ( 'NONE',  ( 13.43411237798105340, 40.58196800326375353, 12.81628187352647963 ) ) ;
#50997=CARTESIAN_POINT ( 'NONE',  ( -0.8801773607111009756, 48.06368534415484817, 1.068504757029289695E-15 ) ) ;
#50998=CARTESIAN_POINT ( 'NONE',  ( 12.63842701281683922, 39.55059781766744464, -9.846743663894590881 ) ) ;
#50999=CARTESIAN_POINT ( 'NONE',  ( 10.00000000000000178, 33.05374883491396787, 14.16423886937410082 ) ) ;
#51000=VERTEX_POINT ( 'NONE', #86345 ) ;
#51001=CARTESIAN_POINT ( 'NONE',  ( 10.00000000000000000, 0.5537488349139675359, -14.16423886937410082 ) ) ;
#51002=CARTESIAN_POINT ( 'NONE',  ( 19.42250999205614548, 55.98035201082150536, -5.440088680355545492 ) ) ;
#51003=CARTESIAN_POINT ( 'NONE',  ( 4.559911319644449179, 68.89701867748817676, 9.422509992056141925 ) ) ;
#51004=CARTESIAN_POINT ( 'NONE',  ( -4.164238869374099927, 52.01208216824729647, 3.795296366450308767 ) ) ;
#51005=CARTESIAN_POINT ( 'NONE',  ( 13.43411237798105340, 0.5819680032637533085, 12.81628187352647963 ) ) ;
#51006=CARTESIAN_POINT ( 'NONE',  ( 19.38216949554541202, 60.99863466993042493, 9.382169495545424454 ) ) ;
#51007=CARTESIAN_POINT ( 'NONE',  ( 7.084665262690076126, 44.10535201082151247, 10.88017736071109987 ) ) ;
#51010=CARTESIAN_POINT ( 'NONE',  ( -2.816281873526471635, 23.91530133659708568, -3.434112377981056508 ) ) ;
#51011=CARTESIAN_POINT ( 'NONE',  ( 5.076628168052703671, 51.84226448433412315, 8.527530157486179263 ) ) ;
#51013=CARTESIAN_POINT ( 'NONE',  ( 10.00000000000000000, 1.813685344154837731, -10.88017736071110342 ) ) ;
#51014=CARTESIAN_POINT ( 'NONE',  ( 0.5774900079438590739, 17.64701867748817321, -5.440088680355550821 ) ) ;
#51017=CARTESIAN_POINT ( 'NONE',  ( 2.035157376598822676, 7.438685344154837509, -7.964842623401177768 ) ) ;
#51019=DIRECTION ( 'NONE',  ( 0.000000000000000000, 0.000000000000000000, 1.000000000000000000 ) ) ;
#51020=CARTESIAN_POINT ( 'NONE',  ( 10.00000000000000000, 66.81368534415484817, -10.88017736071110342 ) ) ;
#51021=CARTESIAN_POINT ( 'NONE',  ( 1.472469842513823179, 0.5922644843341181575, -4.923371831947296329 ) ) ;
#51022=CARTESIAN_POINT ( 'NONE',  ( 1.472469842513823179, 36.42559781766745175, 4.923371831947296329 ) ) ;
#51024=CARTESIAN_POINT ( 'NONE',  ( 2.035157376598822676, 27.43868534415483396, -7.964842623401177768 ) ) ;
#51025=CARTESIAN_POINT ( 'NONE',  ( 6.565887622018943937, 5.165301336597086568, 12.81628187352647430 ) ) ;
#51026=CARTESIAN_POINT ( 'NONE',  ( 0.5774900079438590739, 32.64701867748816966, -5.440088680355550821 ) ) ;
#51029=CARTESIAN_POINT ( 'NONE',  ( 6.565887622018943937, 38.08196800326376064, -12.81628187352647608 ) ) ;
#51031=CARTESIAN_POINT ( 'NONE',  ( 20.88017736071110164, 65.35535201082150536, 2.915334737309930979 ) ) ;
#51032=CARTESIAN_POINT ( 'NONE',  ( 0.6178305044545818747, 28.49863466993041783, -9.382169495545419124 ) ) ;
#51033=CARTESIAN_POINT ( 'NONE',  ( 22.26659068614894466, 3.887082168247300906, 7.082119434687054849 ) ) ;
#51034=CARTESIAN_POINT ( 'NONE',  ( 21.92686044187657046, 32.39664270246083788, -3.195792623639524432 ) ) ;
#51035=CARTESIAN_POINT ( 'NONE',  ( 0.5774900079438590739, 37.64701867748817676, -5.440088680355550821 ) ) ;
#51036=CARTESIAN_POINT ( 'NONE',  ( 1.472469842513823179, 65.59226448433412315, -4.923371831947296329 ) ) ;
#51037=CARTESIAN_POINT ( 'NONE',  ( 10.00000000000000000, 1.813685344154838175, -10.88017736071110342 ) ) ;
#51038=CARTESIAN_POINT ( 'NONE',  ( 14.92337183194729633, 52.67559781766745175, 8.527530157486181039 ) ) ;
#51039=CARTESIAN_POINT ( 'NONE',  ( 18.52753015748617571, 8.092264484334117824, 4.923371831947298993 ) ) ;
#51040=CARTESIAN_POINT ( 'NONE',  ( -0.8801773607111009756, 68.06368534415484817, 1.068504757029289695E-15 ) ) ;
#51042=CARTESIAN_POINT ( 'NONE',  ( 22.26659068614894466, 28.88708216824730357, 7.082119434687054849 ) ) ;
#51048=CARTESIAN_POINT ( 'NONE',  ( 17.08211943468705130, 63.47041550158063927, 12.26659068614894998 ) ) ;
#51049=CARTESIAN_POINT ( 'NONE',  ( 24.16423886937409904, 54.09541550158063217, 3.795296366450317205 ) ) ;
#51050=CARTESIAN_POINT ( 'NONE',  ( 2.791683348922237240, 25.38393115100078390, -7.208316651077763204 ) ) ;
#51051=CARTESIAN_POINT ( 'NONE',  ( -2.816281873526471635, 23.91530133659708568, -3.434112377981056508 ) ) ;
#51053=DIRECTION ( 'NONE',  ( -0.8320502943378437211, 0.5547001962252290364, 0.000000000000000000 ) ) ;
#51054=CARTESIAN_POINT ( 'NONE',  ( 15.44008868035555793, 16.39701867748817321, -9.422509992056140149 ) ) ;
#51055=CARTESIAN_POINT ( 'NONE',  ( 24.16423886937409904, 54.09541550158063217, 3.795296366450317205 ) ) ;
#51056=CARTESIAN_POINT ( 'NONE',  ( 10.00000000000000178, 27.25893115100078390, 9.846743663894594434 ) ) ;
#51058=CARTESIAN_POINT ( 'NONE',  ( 19.84674366389459266, 13.30059781766745353, 2.638427012816836559 ) ) ;
#51066=CARTESIAN_POINT ( 'NONE',  ( 17.08211943468705840, 15.13708216824730179, -12.26659068614894466 ) ) ;
#51067=CARTESIAN_POINT ( 'NONE',  ( 0.5774900079438607392, 13.48035201082150358, 5.440088680355550821 ) ) ;
#51068=CARTESIAN_POINT ( 'NONE',  ( 19.42250999205614193, 30.14701867748817321, 5.440088680355555262 ) ) ;
#51069=CARTESIAN_POINT ( 'NONE',  ( 14.92337183194729988, 54.34226448433412315, -8.527530157486177487 ) ) ;
#51070=CARTESIAN_POINT ( 'NONE',  ( 0.6178305044545818747, 13.49863466993041783, -9.382169495545419124 ) ) ;
#51071=CARTESIAN_POINT ( 'NONE',  ( 17.08211943468705840, 5.137082168247300906, -12.26659068614894466 ) ) ;
#51072=CARTESIAN_POINT ( 'NONE',  ( 19.84674366389459266, 43.71726448433411605, -2.638427012816827677 ) ) ;
#51073=B_SPLINE_CURVE_WITH_KNOTS ( 'NONE', 3,
 ( #98067, #90530, #22064, #52537 ),
 .UNSPECIFIED., .F., .F.,
 ( 4, 4 ),
 ( 3.469446951953614189E-18, 0.001060528352562002848 ),
 .UNSPECIFIED. ) ;
#51074=CARTESIAN_POINT ( 'NONE',  ( 0.6178305044545838731, 34.74863466993042493, 9.382169495545420901 ) ) ;
#51075=CARTESIAN_POINT ( 'NONE',  ( 10.00000000000000000, -0.2410688489992152128, -9.846743663894594434 ) ) ;
#51077=CARTESIAN_POINT ( 'NONE',  ( 2.791683348922240793, 26.63393115100078745, 7.208316651077764092 ) ) ;
#51078=CARTESIAN_POINT ( 'NONE',  ( -4.164238869374099927, 57.01208216824731068, 3.795296366450308767 ) ) ;
#51080=CARTESIAN_POINT ( 'NONE',  ( 4.559911319644449179, 2.230352010821504916, -9.422509992056141925 ) ) ;
#51082=CARTESIAN_POINT ( 'NONE',  ( 10.00000000000000178, 49.31368534415484106, 10.88017736071110342 ) ) ;
#51084=CARTESIAN_POINT ( 'NONE',  ( 10.00000000000000178, 44.31368534415484106, 10.88017736071110342 ) ) ;
#51085=CARTESIAN_POINT ( 'NONE',  ( 19.42250999205614193, 50.14701867748817676, 5.440088680355555262 ) ) ;
#51087=CARTESIAN_POINT ( 'NONE',  ( 20.88017736071110519, 35.56368534415484106, 2.639326808657452039E-16 ) ) ;
#51092=ORIENTED_EDGE ( 'NONE', *, *, #60105, .F. ) ;
#51093=CARTESIAN_POINT ( 'NONE',  ( 0.1532563361054083140, 26.00893115100078745, 1.131784320476157264E-15 ) ) ;
#51096=CARTESIAN_POINT ( 'NONE',  ( 17.20831665107776587, 62.88393115100078745, 7.208316651077764980 ) ) ;
#51098=CARTESIAN_POINT ( 'NONE',  ( 10.00000000000000000, 10.55374883491396787, -14.16423886937410082 ) ) ;
#51101=CARTESIAN_POINT ( 'NONE',  ( 19.72487221294570858, 46.86607318730077054, 6.500000000000000888 ) ) ;
#51102=CARTESIAN_POINT ( 'NONE',  ( 1.274849032794231007, 43.57228050351031357, 6.499999999999895195 ) ) ;
#51103=CARTESIAN_POINT ( 'NONE',  ( 0.1532563361054083140, 36.00893115100078745, 1.131784320476157264E-15 ) ) ;
#51104=CARTESIAN_POINT ( 'NONE',  ( 6.204703633549690345, 55.76208216824730357, -14.16423886937410259 ) ) ;
#51105=CARTESIAN_POINT ( 'NONE',  ( 17.39651004071838614, 62.93575266056827644, 6.500000000000032863 ) ) ;
#51107=CARTESIAN_POINT ( 'NONE',  ( -16.94000000000001194, 92.00000000000000000, 9.500000000000000000 ) ) ;
#51108=CARTESIAN_POINT ( 'NONE',  ( 1.472469842513823179, 51.42559781766745886, 4.923371831947296329 ) ) ;
#51110=CARTESIAN_POINT ( 'NONE',  ( -2.816281873526473856, 9.123634669930421381, 9.499525473075851096E-16 ) ) ;
#51111=CARTESIAN_POINT ( 'NONE',  ( 12.63842701281683922, 14.55059781766744997, -9.846743663894590881 ) ) ;
#51113=CARTESIAN_POINT ( 'NONE',  ( 5.076628168052703671, 11.84226448433411960, 8.527530157486179263 ) ) ;
#51114=CARTESIAN_POINT ( 'NONE',  ( 0.6178305044545818747, 8.498634669930421381, -9.382169495545419124 ) ) ;
#51117=CARTESIAN_POINT ( 'NONE',  ( 20.88017736071110164, 15.35535201082150358, 2.915334737309930979 ) ) ;
#51118=CARTESIAN_POINT ( 'NONE',  ( 2.917880565312950480, 0.9704155015806342766, -12.26659068614894821 ) ) ;
#51119=CARTESIAN_POINT ( 'NONE',  ( 0.1532563361054083140, 31.00893115100078390, 1.131784320476157264E-15 ) ) ;
#51120=CARTESIAN_POINT ( 'NONE',  ( 15.44008868035555793, 56.39701867748817676, -9.422509992056140149 ) ) ;
#51121=CARTESIAN_POINT ( 'NONE',  ( 16.40814093676324603, 32.45696800326375353, -11.09922568453594671 ) ) ;
#51123=CARTESIAN_POINT ( 'NONE',  ( 20.88017736071110519, 5.563685344154837509, 2.639326808657452039E-16 ) ) ;
#51124=CARTESIAN_POINT ( 'NONE',  ( -1.926860441876564023, 57.87045670184114954, 3.195792623639529761 ) ) ;
#51126=CARTESIAN_POINT ( 'NONE',  ( 19.38216949554541557, 2.248634669930420049, -9.382169495545420901 ) ) ;
#51127=CARTESIAN_POINT ( 'NONE',  ( -2.816281873526473856, -0.8763653300695799508, 9.499525473075851096E-16 ) ) ;
#51128=CARTESIAN_POINT ( 'NONE',  ( 1.472469842513823179, 15.59226448433411960, -4.923371831947296329 ) ) ;
#51130=CARTESIAN_POINT ( 'NONE',  ( -2.816281873526473856, 24.33196800326375353, 3.434112377981055619 ) ) ;
#51132=CARTESIAN_POINT ( 'NONE',  ( 17.96484262340118221, 36.18868534415484106, -7.964842623401177768 ) ) ;
#51137=CARTESIAN_POINT ( 'NONE',  ( 19.42250999205614548, 20.98035201082150891, -5.440088680355545492 ) ) ;
#51140=CARTESIAN_POINT ( 'NONE',  ( 7.361572987183170547, 52.05059781766745175, 9.846743663894590881 ) ) ;
#51141=CARTESIAN_POINT ( 'NONE',  ( 4.559911319644449179, 53.89701867748817676, 9.422509992056141925 ) ) ;
#51142=CARTESIAN_POINT ( 'NONE',  ( -4.164238869374099039, 36.80374883491396787, 8.674139862899312516E-16 ) ) ;
#51146=UNCERTAINTY_MEASURE_WITH_UNIT (LENGTH_MEASURE( 1.000000000000000082E-05 ), #47184, 'distance_accuracy_value', 'NONE');
#51147=CARTESIAN_POINT ( 'NONE',  ( 17.20831665107776587, 44.13393115100078745, -7.208316651077762316 ) ) ;
#51148=CARTESIAN_POINT ( 'NONE',  ( 13.43411237798105340, 60.58196800326376064, 12.81628187352647963 ) ) ;
#51150=CARTESIAN_POINT ( 'NONE',  ( 19.38216949554541557, 2.248634669930420049, -9.382169495545420901 ) ) ;
#51152=CARTESIAN_POINT ( 'NONE',  ( 0.5774900079438607392, 28.48035201082150891, 5.440088680355550821 ) ) ;
#51153=CARTESIAN_POINT ( 'NONE',  ( 21.92686044187656691, 7.188309369127508397, 4.562052436263911564E-16 ) ) ;
#51154=CARTESIAN_POINT ( 'NONE',  ( 19.42250999205614548, 5.980352010821504471, -5.440088680355545492 ) ) ;
#51155=CARTESIAN_POINT ( 'NONE',  ( -0.8801773607110991993, 17.85535201082150536, -2.915334737309923874 ) ) ;
#51156=CARTESIAN_POINT ( 'NONE',  ( 0.5774900079438590739, 62.64701867748817676, -5.440088680355550821 ) ) ;
#51157=CARTESIAN_POINT ( 'NONE',  ( 2.917880565312948704, 27.63708216824730357, 12.26659068614894643 ) ) ;
#51158=CARTESIAN_POINT ( 'NONE',  ( 7.361572987183169658, 19.96726448433411960, -9.846743663894592657 ) ) ;
#51159=CARTESIAN_POINT ( 'NONE',  ( 17.20831665107776587, 59.13393115100078745, -7.208316651077762316 ) ) ;
#51160=CARTESIAN_POINT ( 'NONE',  ( 10.00000000000000178, 29.31368534415483751, 10.88017736071110342 ) ) ;
#51164=ORIENTED_EDGE ( 'NONE', *, *, #83547, .T. ) ;
#51166=CARTESIAN_POINT ( 'NONE',  ( 19.84674366389459266, 43.71726448433410894, -2.638427012816827677 ) ) ;
#51170=CARTESIAN_POINT ( 'NONE',  ( 17.08211943468705130, 23.47041550158063572, 12.26659068614894998 ) ) ;
#51171=CARTESIAN_POINT ( 'NONE',  ( 20.36894250292379382, 8.678748834913967869, 10.36894250292379205 ) ) ;
#51172=CARTESIAN_POINT ( 'NONE',  ( 17.96484262340118221, 54.93868534415484106, 7.964842623401181321 ) ) ;
#51173=CARTESIAN_POINT ( 'NONE',  ( 24.16423886937410614, 54.51208216824730357, -3.795296366450302550 ) ) ;
#51174=CARTESIAN_POINT ( 'NONE',  ( -1.099225684535947600, -1.293031996736246469, -6.408140936763238038 ) ) ;
#51175=CARTESIAN_POINT ( 'NONE',  ( 12.63842701281683034, 52.46726448433413026, 9.846743663894596210 ) ) ;
#51177=CARTESIAN_POINT ( 'NONE',  ( 0.5774900079438590739, 37.64701867748817676, -5.440088680355550821 ) ) ;
#51178=CARTESIAN_POINT ( 'NONE',  ( 10.00000000000000000, 2.873634669930420049, -12.81628187352647608 ) ) ;
#51179=CARTESIAN_POINT ( 'NONE',  ( 2.917880565312948704, 12.63708216824730179, 12.26659068614894643 ) ) ;
#51180=CARTESIAN_POINT ( 'NONE',  ( 24.16423886937410614, 54.30374883491396787, 8.672049930838204340E-16 ) ) ;
#51181=CARTESIAN_POINT ( 'NONE',  ( 19.42250999205614193, 15.14701867748817143, 5.440088680355555262 ) ) ;
#51182=CARTESIAN_POINT ( 'NONE',  ( 19.72487221294571569, 14.78217586085237656, 6.499999999999995559 ) ) ;
#51183=CARTESIAN_POINT ( 'NONE',  ( 10.00000000000000000, 46.81368534415484106, -10.88017736071110342 ) ) ;
#51186=EDGE_LOOP ( 'NONE', ( #9658, #76291, #6447, #38040, #9270, #45488, #20592 ) ) ;
#51190=CARTESIAN_POINT ( 'NONE',  ( 24.16423886937410614, 49.30374883491396787, 8.672049930838204340E-16 ) ) ;
#51191=CARTESIAN_POINT ( 'NONE',  ( 10.00000000000000000, 44.75893115100078745, -9.846743663894594434 ) ) ;
#51192=CARTESIAN_POINT ( 'NONE',  ( 10.00000000000000000, 56.81368534415484106, -10.88017736071110342 ) ) ;
#51194=EDGE_CURVE ( 'NONE', #24774, #51686, #35794, .T. ) ;
#51195=CARTESIAN_POINT ( 'NONE',  ( 12.91533473730993009, 56.60535201082151247, -10.88017736071109987 ) ) ;
#51197=CARTESIAN_POINT ( 'NONE',  ( -1.099225684535947600, 58.70696800326375353, -6.408140936763238038 ) ) ;
#51199=VERTEX_POINT ( 'NONE', #50806 ) ;
#51200=CARTESIAN_POINT ( 'NONE',  ( 6.204703633549690345, 25.76208216824730712, -14.16423886937410259 ) ) ;
#51201=ORIENTED_EDGE ( 'NONE', *, *, #57354, .T. ) ;
#51202=CARTESIAN_POINT ( 'NONE',  ( 21.09922568453595559, 22.04030133659708923, -6.408140936763230044 ) ) ;
#51204=CARTESIAN_POINT ( 'NONE',  ( 6.565887622018943937, 43.08196800326374643, -12.81628187352647608 ) ) ;
#51205=CARTESIAN_POINT ( 'NONE',  ( 19.42250999205614193, 15.14701867748817143, 5.440088680355555262 ) ) ;
#51206=CARTESIAN_POINT ( 'NONE',  ( 14.92337183194729633, 32.67559781766745175, 8.527530157486181039 ) ) ;
#51207=CARTESIAN_POINT ( 'NONE',  ( 12.91533473730992121, 14.52201867748817143, 10.88017736071110164 ) ) ;
#51208=CARTESIAN_POINT ( 'NONE',  ( 19.38216949554541557, 57.24863466993042493, -9.382169495545420901 ) ) ;
#51209=DIRECTION ( 'NONE',  ( -0.000000000000000000, -0.000000000000000000, 1.000000000000000000 ) ) ;
#51210=CARTESIAN_POINT ( 'NONE',  ( 2.791683348922240793, 41.63393115100078745, 7.208316651077764092 ) ) ;
#51216=CARTESIAN_POINT ( 'NONE',  ( 1.472469842513823179, 16.42559781766745175, 4.923371831947296329 ) ) ;
#51217=CARTESIAN_POINT ( 'NONE',  ( 22.81628187352648496, 26.83196800326374998, -3.434112377981050290 ) ) ;
#51221=CARTESIAN_POINT ( 'NONE',  ( 5.076628168052704559, 60.17559781766745175, -8.527530157486179263 ) ) ;
#51223=CARTESIAN_POINT ( 'NONE',  ( -4.164238869374098151, 21.59541550158063217, -3.795296366450310543 ) ) ;
#51224=CARTESIAN_POINT ( 'NONE',  ( 18.52753015748617571, 43.09226448433412315, 4.923371831947298993 ) ) ;
#51225=CARTESIAN_POINT ( 'NONE',  ( 0.6178305044545818747, 43.49863466993042493, -9.382169495545419124 ) ) ;
#51228=CARTESIAN_POINT ( 'NONE',  ( 20.88017736071110519, 60.56368534415484106, 2.639326808657452039E-16 ) ) ;
#51229=CIRCLE ( 'NONE', #17497, 1.000000000000000000 ) ;
#51231=CARTESIAN_POINT ( 'NONE',  ( 2.791683348922240793, 31.63393115100078745, 7.208316651077764092 ) ) ;
#51232=CARTESIAN_POINT ( 'NONE',  ( 2.035157376598824452, 43.68868534415484106, 7.964842623401179544 ) ) ;
#51233=CARTESIAN_POINT ( 'NONE',  ( 21.09922568453594849, 46.20696800326376064, 6.408140936763242479 ) ) ;
#51235=CARTESIAN_POINT ( 'NONE',  ( 20.88017736071110875, 40.77201867748818387, -2.915334737309920765 ) ) ;
#51238=CARTESIAN_POINT ( 'NONE',  ( 15.44008868035555793, 16.39701867748817321, -9.422509992056140149 ) ) ;
#51239=CARTESIAN_POINT ( 'NONE',  ( 17.20831665107776587, 62.88393115100078745, 7.208316651077764980 ) ) ;
#51240=CARTESIAN_POINT ( 'NONE',  ( 4.559911319644449179, 43.89701867748816966, 9.422509992056141925 ) ) ;
#51241=CARTESIAN_POINT ( 'NONE',  ( 15.44008868035555260, 59.73035201082151247, 9.422509992056143702 ) ) ;
#51242=CARTESIAN_POINT ( 'NONE',  ( 0.5774900079438607392, 28.48035201082150891, 5.440088680355550821 ) ) ;
#51243=CARTESIAN_POINT ( 'NONE',  ( -0.000000000000000000, 76.91853713602722564, -7.561724626172516395 ) ) ;
#51244=CARTESIAN_POINT ( 'NONE',  ( 19.39235739573469530, 49.87576471608600315, 6.499999999999993783 ) ) ;
#51245=CARTESIAN_POINT ( 'NONE',  ( 12.63842701281683034, 27.46726448433411250, 9.846743663894596210 ) ) ;
#51246=CARTESIAN_POINT ( 'NONE',  ( -46.30928139467842897, 104.0823827281712255, -5.529860068218142466 ) ) ;
#51248=CARTESIAN_POINT ( 'NONE',  ( 0.1532563361054083140, 51.00893115100078745, 1.131784320476157264E-15 ) ) ;
#51249=B_SPLINE_CURVE_WITH_KNOTS ( 'NONE', 3,
 ( #59198, #7204, #97238, #36214 ),
 .UNSPECIFIED., .F., .F.,
 ( 4, 4 ),
 ( 0.000000000000000000, 0.001036303429213363990 ),
 .UNSPECIFIED. ) ;
#51250=CARTESIAN_POINT ( 'NONE',  ( 6.204703633549690345, 50.76208216824730357, -14.16423886937410259 ) ) ;
#51252=CARTESIAN_POINT ( 'NONE',  ( 1.821708436314909640, 61.66792564121894316, -6.499999999999922728 ) ) ;
#51253=CARTESIAN_POINT ( 'NONE',  ( 10.00000000000000178, 13.05374883491396787, 14.16423886937410082 ) ) ;
#51254=CARTESIAN_POINT ( 'NONE',  ( 22.26659068614895176, 39.72041550158063217, -7.082119434687042414 ) ) ;
#51255=CARTESIAN_POINT ( 'NONE',  ( 13.43411237798105340, 0.5819680032637533085, 12.81628187352647963 ) ) ;
#51259=CARTESIAN_POINT ( 'NONE',  ( -0.8801773607110991993, 7.855352010821506248, -2.915334737309923874 ) ) ;
#51260=CARTESIAN_POINT ( 'NONE',  ( 18.52753015748617571, 43.09226448433412315, 4.923371831947298993 ) ) ;
#51264=EDGE_CURVE ( 'NONE', #23770, #2388, #49727, .T. ) ;
#51265=CARTESIAN_POINT ( 'NONE',  ( 0.1532563361054100626, 0.8005978176674514168, -2.638427012816831230 ) ) ;
#51266=CARTESIAN_POINT ( 'NONE',  ( 3.591859063236763294, 28.29030133659708568, -11.09922568453595026 ) ) ;
#51267=CARTESIAN_POINT ( 'NONE',  ( 5.076628168052703671, 31.84226448433412315, 8.527530157486179263 ) ) ;
#51269=CARTESIAN_POINT ( 'NONE',  ( 7.361572987183170547, 2.050597817667451750, 9.846743663894590881 ) ) ;
#51272=CARTESIAN_POINT ( 'NONE',  ( 12.91533473730993009, 16.60535201082150891, -10.88017736071109987 ) ) ;
#51273=CARTESIAN_POINT ( 'NONE',  ( 17.08211943468705840, 40.13708216824731068, -12.26659068614894466 ) ) ;
#51274=CARTESIAN_POINT ( 'NONE',  ( -0.8801773607110991993, 47.85535201082150536, -2.915334737309923874 ) ) ;
#51275=CARTESIAN_POINT ( 'NONE',  ( 0.5774900079438590739, 67.64701867748817676, -5.440088680355550821 ) ) ;
#51277=CARTESIAN_POINT ( 'NONE',  ( 0.2751277870542876980, 48.21833443783936701, 6.499999999999984901 ) ) ;
#51278=CARTESIAN_POINT ( 'NONE',  ( 12.63842701281683922, 29.55059781766745175, -9.846743663894590881 ) ) ;
#51279=SURFACE_SIDE_STYLE ('',( #66268 ) ) ;
#51280=CARTESIAN_POINT ( 'NONE',  ( 12.63842701281683034, 2.467264484334118269, 9.846743663894596210 ) ) ;
#51281=CARTESIAN_POINT ( 'NONE',  ( 19.84674366389459266, 33.30059781766744464, 2.638427012816836559 ) ) ;
#51282=CARTESIAN_POINT ( 'NONE',  ( 10.00000000000000000, 59.75893115100078745, -9.846743663894594434 ) ) ;
#51283=CARTESIAN_POINT ( 'NONE',  ( 20.88017736071110164, 35.35535201082150536, 2.915334737309930979 ) ) ;
#51287=CARTESIAN_POINT ( 'NONE',  ( -1.099225684535947600, 53.70696800326376064, -6.408140936763238038 ) ) ;
#51288=CARTESIAN_POINT ( 'NONE',  ( 4.559911319644449179, 67.23035201082150536, -9.422509992056141925 ) ) ;
#51289=CARTESIAN_POINT ( 'NONE',  ( 21.09922568453595559, 42.04030133659708213, -6.408140936763230044 ) ) ;
#51290=CARTESIAN_POINT ( 'NONE',  ( 6.204703633549690345, 57.84541550158063927, 14.16423886937410082 ) ) ;
#51291=CARTESIAN_POINT ( 'NONE',  ( 2.791683348922237240, 30.38393115100078390, -7.208316651077763204 ) ) ;
#51294=CARTESIAN_POINT ( 'NONE',  ( 17.08211943468705130, 38.47041550158063217, 12.26659068614894998 ) ) ;
#51295=CARTESIAN_POINT ( 'NONE',  ( 1.472469842513823179, 45.59226448433412315, -4.923371831947296329 ) ) ;
#51298=CARTESIAN_POINT ( 'NONE',  ( -0.8801773607111008646, 33.27201867748817676, 2.915334737309923430 ) ) ;
#51300=CARTESIAN_POINT ( 'NONE',  ( 2.035157376598822676, 57.43868534415484106, -7.964842623401177768 ) ) ;
#51302=ORIENTED_EDGE ( 'NONE', *, *, #841, .F. ) ;
#51303=CARTESIAN_POINT ( 'NONE',  ( -2.816281873526473856, 49.33196800326374643, 3.434112377981055619 ) ) ;
#51305=CARTESIAN_POINT ( 'NONE',  ( 7.084665262690076126, 69.10535201082151957, 10.88017736071109987 ) ) ;
#51307=CARTESIAN_POINT ( 'NONE',  ( 2.917880565312948704, 7.637082168247301794, 12.26659068614894643 ) ) ;
#51308=CARTESIAN_POINT ( 'NONE',  ( 5.076628168052703671, 1.842264484334118047, 8.527530157486179263 ) ) ;
#51309=CARTESIAN_POINT ( 'NONE',  ( 1.420647316330978072, 0.04189720826290899841, -6.202995698450457063 ) ) ;
#51311=CARTESIAN_POINT ( 'NONE',  ( -0.8801773607111009756, 8.063685344154837509, 1.068504757029289695E-15 ) ) ;
#51313=CARTESIAN_POINT ( 'NONE',  ( 2.917880565312948704, 22.63708216824730002, 12.26659068614894643 ) ) ;
#51314=EDGE_LOOP ( 'NONE', ( #36074, #2665, #25410, #59168 ) ) ;
#51315=CARTESIAN_POINT ( 'NONE',  ( 15.44008868035555793, 26.39701867748817321, -9.422509992056140149 ) ) ;
#51316=CARTESIAN_POINT ( 'NONE',  ( 18.52753015748618282, 63.92559781766745886, -4.923371831947291888 ) ) ;
#51318=CARTESIAN_POINT ( 'NONE',  ( 7.361572987183169658, 59.96726448433410894, -9.846743663894592657 ) ) ;
#51320=CARTESIAN_POINT ( 'NONE',  ( 0.5774900079438590739, 67.64701867748817676, -5.440088680355550821 ) ) ;
#51322=CARTESIAN_POINT ( 'NONE',  ( 10.00000000000000000, 37.87363466993041783, -12.81628187352647608 ) ) ;
#51323=CARTESIAN_POINT ( 'NONE',  ( 10.00000000000000000, 1.813685344154837731, -10.88017736071110342 ) ) ;
#51325=CARTESIAN_POINT ( 'NONE',  ( 19.84674366389459266, 8.300597817667451750, 2.638427012816836559 ) ) ;
#51326=CARTESIAN_POINT ( 'NONE',  ( 17.96484262340118221, 16.18868534415483396, -7.964842623401177768 ) ) ;
#51329=( BOUNDED_CURVE ( )  B_SPLINE_CURVE ( 2, ( #63045, #4038, #42042, #57510, #55555, #12017, #27012, #71551, #87024 ),
 .UNSPECIFIED., .F., .F. ) 
 B_SPLINE_CURVE_WITH_KNOTS ( ( 3, 2, 2, 2, 3 ),
 ( 0.8310855930462679453, 0.8333333333333333703, 0.8392857142857143016, 0.8452380952380952328, 0.8474858355251606579 ),
 .UNSPECIFIED. ) 
 CURVE ( )  GEOMETRIC_REPRESENTATION_ITEM ( )  RATIONAL_B_SPLINE_CURVE ( ( 0.9839835555609424134, 0.9871328979762477029, 1.000000000000000000, 0.9659258262890683122, 1.000000000000000000, 0.9659258262890683122, 1.000000000000000000, 0.9871328979762474809, 0.9839835555609424134 ) ) 
 REPRESENTATION_ITEM ( '' )  );
#51332=CARTESIAN_POINT ( 'NONE',  ( 6.565887622018943937, 58.08196800326376064, -12.81628187352647608 ) ) ;
#51333=CARTESIAN_POINT ( 'NONE',  ( 2.035157376598822676, 37.43868534415484106, -7.964842623401177768 ) ) ;
#51334=CARTESIAN_POINT ( 'NONE',  ( -0.1503990784575328643, 70.00000000000000000, -6.262539305110068177 ) ) ;
#51335=CARTESIAN_POINT ( 'NONE',  ( 10.00000000000000178, 35.37363466993042493, 12.81628187352647608 ) ) ;
#51336=CARTESIAN_POINT ( 'NONE',  ( 10.00000000000000000, 46.81368534415484106, -10.88017736071110342 ) ) ;
#51337=CARTESIAN_POINT ( 'NONE',  ( 10.00000000000000000, 59.75893115100078745, -9.846743663894594434 ) ) ;
#51339=CARTESIAN_POINT ( 'NONE',  ( 12.63842701281683034, 12.46726448433411782, 9.846743663894596210 ) ) ;
#51340=CARTESIAN_POINT ( 'NONE',  ( 10.00000000000000000, 12.87363466993042138, -12.81628187352647608 ) ) ;
#51342=CYLINDRICAL_SURFACE ( 'NONE', #76901, 0.5000000000000004441 ) ;
#51343=CARTESIAN_POINT ( 'NONE',  ( 0.5774900079438607392, 18.48035201082150536, 5.440088680355550821 ) ) ;
#51344=CARTESIAN_POINT ( 'NONE',  ( 5.076628168052703671, 51.84226448433412315, 8.527530157486179263 ) ) ;
#51347=EDGE_CURVE ( 'NONE', #20694, #80255, #56825, .T. ) ;
#51348=CARTESIAN_POINT ( 'NONE',  ( 7.361572987183170547, 12.05059781766744997, 9.846743663894590881 ) ) ;
#51349=CARTESIAN_POINT ( 'NONE',  ( 19.84674366389459621, 28.50893115100078745, 7.409399052514197653E-17 ) ) ;
#51350=CARTESIAN_POINT ( 'NONE',  ( 22.81628187352648496, 6.831968003263753531, -3.434112377981050290 ) ) ;
#51351=ORIENTED_EDGE ( 'NONE', *, *, #55912, .T. ) ;
#51353=AXIS2_PLACEMENT_3D ( 'NONE', #46795, #85296, #38819 ) ;
#51354=CARTESIAN_POINT ( 'NONE',  ( 16.40814093676324603, 42.45696800326375353, -11.09922568453594671 ) ) ;
#51355=CARTESIAN_POINT ( 'NONE',  ( 0.1532563361054083140, 31.00893115100078390, 1.131784320476157264E-15 ) ) ;
#51356=CARTESIAN_POINT ( 'NONE',  ( 17.08211943468705840, 55.13708216824731068, -12.26659068614894466 ) ) ;
#51357=CARTESIAN_POINT ( 'NONE',  ( 2.791683348922237240, 35.38393115100079456, -7.208316651077763204 ) ) ;
#51358=STYLED_ITEM ( 'NONE', ( #85375 ), #47285 ) ;
#51359=CARTESIAN_POINT ( 'NONE',  ( 0.9413316022086175572, 18.45508385108958649, 6.499999999999973355 ) ) ;
#51360=CARTESIAN_POINT ( 'NONE',  ( 17.96484262340118221, 9.938685344154839285, 7.964842623401181321 ) ) ;
#51361=CARTESIAN_POINT ( 'NONE',  ( 0.1532563361054082862, 66.21726448433413736, 2.638427012816831674 ) ) ;
#51362=CARTESIAN_POINT ( 'NONE',  ( -0.8801773607111009756, 23.06368534415484106, 1.068504757029289695E-15 ) ) ;
#51363=CARTESIAN_POINT ( 'NONE',  ( 22.26659068614895176, 44.72041550158063927, -7.082119434687042414 ) ) ;
#51364=CARTESIAN_POINT ( 'NONE',  ( 13.79529636645030344, 48.26208216824728936, 14.16423886937410614 ) ) ;
#51366=( NAMED_UNIT ( * ) SI_UNIT ( $, .STERADIAN. ) SOLID_ANGLE_UNIT ( ) );
#51367=AXIS2_PLACEMENT_3D ( 'NONE', #30558, #16069, #1086 ) ;
#51368=CARTESIAN_POINT ( 'NONE',  ( 7.361572987183170547, 17.05059781766745530, 9.846743663894590881 ) ) ;
#51369=CARTESIAN_POINT ( 'NONE',  ( 3.591859063236761518, -0.04303199673624671928, 11.09922568453594849 ) ) ;
#51370=ORIENTED_EDGE ( 'NONE', *, *, #31556, .F. ) ;
#51371=CARTESIAN_POINT ( 'NONE',  ( 2.035157376598824452, 43.68868534415484106, 7.964842623401179544 ) ) ;
#51373=CARTESIAN_POINT ( 'NONE',  ( 12.63842701281683922, 64.55059781766745175, -9.846743663894590881 ) ) ;
#51374=CARTESIAN_POINT ( 'NONE',  ( 19.84674366389459266, 28.30059781766745886, 2.638427012816836559 ) ) ;
#51378=CARTESIAN_POINT ( 'NONE',  ( 24.16423886937410614, 44.51208216824730357, -3.795296366450302550 ) ) ;
#51380=CARTESIAN_POINT ( 'NONE',  ( 0.1532563361054082862, 1.217264484334117824, 2.638427012816831674 ) ) ;
#51383=CARTESIAN_POINT ( 'NONE',  ( 0.5774900079438590739, 32.64701867748816966, -5.440088680355550821 ) ) ;
#51384=CARTESIAN_POINT ( 'NONE',  ( 21.09922568453594849, 41.20696800326375353, 6.408140936763242479 ) ) ;
#51386=CARTESIAN_POINT ( 'NONE',  ( 19.42250999205614548, 10.98035201082150358, -5.440088680355545492 ) ) ;
#51387=CARTESIAN_POINT ( 'NONE',  ( 22.81628187352647785, 41.41530133659708923, 3.434112377981063169 ) ) ;
#51388=CARTESIAN_POINT ( 'NONE',  ( 13.43411237798105340, 55.58196800326374643, 12.81628187352647963 ) ) ;
#51392=CARTESIAN_POINT ( 'NONE',  ( 6.204703633549690345, 22.84541550158062861, 14.16423886937410082 ) ) ;
#51393=CARTESIAN_POINT ( 'NONE',  ( -4.164238869374099039, 6.803748834913967869, 8.674139862899312516E-16 ) ) ;
#51394=CARTESIAN_POINT ( 'NONE',  ( 7.084665262690076126, 12.02201867748817143, -10.88017736071110164 ) ) ;
#51395=CARTESIAN_POINT ( 'NONE',  ( 17.96484262340118221, 19.93868534415484106, 7.964842623401181321 ) ) ;
#51396=DIRECTION ( 'NONE',  ( -1.000000000000000000, -0.000000000000000000, -0.000000000000000000 ) ) ;
#51398=CARTESIAN_POINT ( 'NONE',  ( 0.5774900079438590739, 52.64701867748817676, -5.440088680355550821 ) ) ;
#51399=CARTESIAN_POINT ( 'NONE',  ( 7.084665262690076126, 52.02201867748816255, -10.88017736071110164 ) ) ;
#51400=CARTESIAN_POINT ( 'NONE',  ( 21.09922568453595559, 17.04030133659708923, -6.408140936763230044 ) ) ;
#51403=CARTESIAN_POINT ( 'NONE',  ( 0.1532563361054083140, 21.00893115100078745, 1.131784320476157264E-15 ) ) ;
#51404=CARTESIAN_POINT ( 'NONE',  ( 20.88017736071110164, 40.35535201082150536, 2.915334737309930979 ) ) ;
#51406=CARTESIAN_POINT ( 'NONE',  ( 6.565887622018943937, 15.16530133659708568, 12.81628187352647430 ) ) ;
#51407=CARTESIAN_POINT ( 'NONE',  ( 2.148416515056676523, 27.23726573380435667, 6.499999999999981348 ) ) ;
#51408=CARTESIAN_POINT ( 'NONE',  ( 19.84674366389459621, 23.50893115100078390, 7.409399052514197653E-17 ) ) ;
#51409=CARTESIAN_POINT ( 'NONE',  ( 21.09922568453595559, 47.04030133659708923, -6.408140936763230044 ) ) ;
#51410=CARTESIAN_POINT ( 'NONE',  ( 7.361572987183170547, 22.05059781766745530, 9.846743663894590881 ) ) ;
#51414=CARTESIAN_POINT ( 'NONE',  ( 10.00000000000000000, 21.81368534415484106, -10.88017736071110342 ) ) ;
#51415=CARTESIAN_POINT ( 'NONE',  ( 17.08211943468705130, 33.47041550158063927, 12.26659068614894998 ) ) ;
#51416=CARTESIAN_POINT ( 'NONE',  ( 17.20831665107776587, 29.13393115100078390, -7.208316651077762316 ) ) ;
#51417=CARTESIAN_POINT ( 'NONE',  ( -0.8801773607111009756, 23.06368534415484106, 1.068504757029289695E-15 ) ) ;
#51418=CARTESIAN_POINT ( 'NONE',  ( 12.91533473730993009, 16.60535201082150891, -10.88017736071109987 ) ) ;
#51419=ORIENTED_EDGE ( 'NONE', *, *, #8542, .T. ) ;
#51420=CARTESIAN_POINT ( 'NONE',  ( 19.42250999205614548, 20.98035201082150891, -5.440088680355545492 ) ) ;
#51421=CARTESIAN_POINT ( 'NONE',  ( 21.09922568453594849, 46.20696800326376064, 6.408140936763242479 ) ) ;
#51422=CARTESIAN_POINT ( 'NONE',  ( 12.91533473730992121, 39.52201867748817676, 10.88017736071110164 ) ) ;
#51423=CARTESIAN_POINT ( 'NONE',  ( 13.99999999999999822, 60.50000000000000711, -6.000000000000000000 ) ) ;
#51424=CARTESIAN_POINT ( 'NONE',  ( 15.44008868035555793, 36.39701867748816966, -9.422509992056140149 ) ) ;
#51425=COLOUR_RGB ( '', 0.40784314, 0.44705882, 0.49803922) ;
#51427=CARTESIAN_POINT ( 'NONE',  ( 19.84674366389459621, 53.50893115100078745, 7.409399052514197653E-17 ) ) ;
#51428=CARTESIAN_POINT ( 'NONE',  ( 7.084665262690076126, 42.02201867748816966, -10.88017736071110164 ) ) ;
#51429=CARTESIAN_POINT ( 'NONE',  ( 10.00000000000000178, 67.25893115100079456, 9.846743663894594434 ) ) ;
#51430=CARTESIAN_POINT ( 'NONE',  ( 21.09922568453595559, 62.04030133659709634, -6.408140936763230044 ) ) ;
#51432=CARTESIAN_POINT ( 'NONE',  ( -4.164238869374099927, 52.01208216824729647, 3.795296366450308767 ) ) ;
#51433=CARTESIAN_POINT ( 'NONE',  ( 12.91533473730993009, 51.60535201082149825, -10.88017736071109987 ) ) ;
#51434=CARTESIAN_POINT ( 'NONE',  ( 0.5600000000000083800, 105.0000000000000000, 5.000000000000000000 ) ) ;
#51435=CARTESIAN_POINT ( 'NONE',  ( 19.84674366389459266, 43.30059781766744464, 2.638427012816836559 ) ) ;
#51437=CARTESIAN_POINT ( 'NONE',  ( 10.00000000000000000, 4.758931151000784787, -9.846743663894594434 ) ) ;
#51438=CARTESIAN_POINT ( 'NONE',  ( 18.52753015748618282, 23.92559781766745530, -4.923371831947291888 ) ) ;
#51440=VECTOR ( 'NONE', #74041, 1000.000000000000000 ) ;
#51441=CARTESIAN_POINT ( 'NONE',  ( 14.92337183194729988, 19.34226448433411960, -8.527530157486177487 ) ) ;
#51444=CARTESIAN_POINT ( 'NONE',  ( 2.035157376598822676, 32.43868534415483396, -7.964842623401177768 ) ) ;
#51445=CARTESIAN_POINT ( 'NONE',  ( 18.52753015748618282, 18.92559781766745175, -4.923371831947291888 ) ) ;
#51446=CARTESIAN_POINT ( 'NONE',  ( 21.09922568453595559, 12.04030133659708746, -6.408140936763230044 ) ) ;
#51447=CARTESIAN_POINT ( 'NONE',  ( 15.44008868035555260, 64.73035201082151957, 9.422509992056143702 ) ) ;
#51448=CARTESIAN_POINT ( 'NONE',  ( 20.88017736071110164, 50.35535201082151247, 2.915334737309930979 ) ) ;
#51449=CARTESIAN_POINT ( 'NONE',  ( 4.559911319644449179, 33.89701867748817676, 9.422509992056141925 ) ) ;
#51450=CARTESIAN_POINT ( 'NONE',  ( 0.6178305044545818747, 53.49863466993041072, -9.382169495545419124 ) ) ;
#51451=CARTESIAN_POINT ( 'NONE',  ( 24.16423886937410614, 39.30374883491396787, 8.672049930838204340E-16 ) ) ;
#51452=CARTESIAN_POINT ( 'NONE',  ( -43.81448451332931882, 106.0682908843177614, 5.149235002859532173 ) ) ;
#51453=ORIENTED_EDGE ( 'NONE', *, *, #58506, .T. ) ;
#51454=CARTESIAN_POINT ( 'NONE',  ( 22.81628187352648496, 1.831968003263753753, -3.434112377981050290 ) ) ;
#51455=CARTESIAN_POINT ( 'NONE',  ( 10.00000000000000178, 14.31368534415483751, 10.88017736071110342 ) ) ;
#51456=CARTESIAN_POINT ( 'NONE',  ( -0.8801773607110991993, 42.85535201082150536, -2.915334737309923874 ) ) ;
#51458=ORIENTED_EDGE ( 'NONE', *, *, #7907, .T. ) ;
#51459=CARTESIAN_POINT ( 'NONE',  ( 7.361572987183170547, 22.05059781766745530, 9.846743663894590881 ) ) ;
#51460=CARTESIAN_POINT ( 'NONE',  ( 12.91533473730992121, 64.52201867748817676, 10.88017736071110164 ) ) ;
#51461=CARTESIAN_POINT ( 'NONE',  ( 5.076628168052704559, 35.17559781766745175, -8.527530157486179263 ) ) ;
#51462=CARTESIAN_POINT ( 'NONE',  ( 12.63842701281683034, 27.46726448433411250, 9.846743663894596210 ) ) ;
#51463=CARTESIAN_POINT ( 'NONE',  ( 5.076628168052704559, 10.17559781766745175, -8.527530157486179263 ) ) ;
#51466=CARTESIAN_POINT ( 'NONE',  ( 10.00000000000000178, 2.258931151000784787, 9.846743663894594434 ) ) ;
#51469=CARTESIAN_POINT ( 'NONE',  ( 12.63842701281683034, 37.46726448433411605, 9.846743663894596210 ) ) ;
#51472=CARTESIAN_POINT ( 'NONE',  ( 0.1532563361054100626, 65.80059781766745175, -2.638427012816831230 ) ) ;
#51473=CARTESIAN_POINT ( 'NONE',  ( -0.8801773607110991993, 2.855352010821504471, -2.915334737309923874 ) ) ;
#51474=CARTESIAN_POINT ( 'NONE',  ( 10.00000000000000178, 23.05374883491397142, 14.16423886937410082 ) ) ;
#51477=CARTESIAN_POINT ( 'NONE',  ( 6.204703633549690345, 22.84541550158062861, 14.16423886937410082 ) ) ;
#51478=CARTESIAN_POINT ( 'NONE',  ( 24.16423886937410614, 39.51208216824731068, -3.795296366450302550 ) ) ;
#51479=CARTESIAN_POINT ( 'NONE',  ( 6.204703633549690345, 10.76208216824729824, -14.16423886937410259 ) ) ;
#51480=CARTESIAN_POINT ( 'NONE',  ( 13.79529636645030344, 8.262082168247300018, 14.16423886937410614 ) ) ;
#51482=CARTESIAN_POINT ( 'NONE',  ( 2.035157376598824452, 53.68868534415484817, 7.964842623401179544 ) ) ;
#51485=CARTESIAN_POINT ( 'NONE',  ( 1.472469842513823179, 30.59226448433411960, -4.923371831947296329 ) ) ;
#51487=CARTESIAN_POINT ( 'NONE',  ( 5.076628168052703671, 31.84226448433412315, 8.527530157486179263 ) ) ;
#51488=CARTESIAN_POINT ( 'NONE',  ( 20.88017736071110519, 10.56368534415483929, 2.639326808657452039E-16 ) ) ;
#51489=CARTESIAN_POINT ( 'NONE',  ( -1.099225684535947600, 58.70696800326375353, -6.408140936763238038 ) ) ;
#51490=CARTESIAN_POINT ( 'NONE',  ( 1.472469842513823179, 50.59226448433411605, -4.923371831947296329 ) ) ;
#51492=CARTESIAN_POINT ( 'NONE',  ( 19.84674366389459266, 33.30059781766744464, 2.638427012816836559 ) ) ;
#51493=CARTESIAN_POINT ( 'NONE',  ( 22.81628187352647785, 36.41530133659707502, 3.434112377981063169 ) ) ;
#51495=CARTESIAN_POINT ( 'NONE',  ( -0.8801773607110991993, 47.85535201082150536, -2.915334737309923874 ) ) ;
#51496=CARTESIAN_POINT ( 'NONE',  ( 19.84674366389459621, 33.50893115100078745, 7.409399052514197653E-17 ) ) ;
#51497=CARTESIAN_POINT ( 'NONE',  ( 13.79529636645030344, 23.26208216824730002, 14.16423886937410614 ) ) ;
#51498=EDGE_CURVE ( 'NONE', #63997, #30159, #16288, .T. ) ;
#51499=ORIENTED_EDGE ( 'NONE', *, *, #63790, .F. ) ;
#51501=CARTESIAN_POINT ( 'NONE',  ( 20.88017736071110164, 50.35535201082151247, 2.915334737309930979 ) ) ;
#51503=CARTESIAN_POINT ( 'NONE',  ( -4.164238869374099039, 51.80374883491396787, 8.674139862899312516E-16 ) ) ;
#51504=CARTESIAN_POINT ( 'NONE',  ( -1.099225684535947600, -1.293031996736246469, -6.408140936763238038 ) ) ;
#51505=( GEOMETRIC_REPRESENTATION_CONTEXT ( 3 ) GLOBAL_UNCERTAINTY_ASSIGNED_CONTEXT ( ( #6282 ) ) GLOBAL_UNIT_ASSIGNED_CONTEXT ( ( #74854, #66356, #51366 ) ) REPRESENTATION_CONTEXT ( 'NONE', 'WORKASPACE' ) );
#51507=CARTESIAN_POINT ( 'NONE',  ( 17.96484262340118221, 49.93868534415484106, 7.964842623401181321 ) ) ;
#51508=CARTESIAN_POINT ( 'NONE',  ( -0.04068437667224029941, 27.21974360917721114, -6.396802510829693311 ) ) ;
#51509=CARTESIAN_POINT ( 'NONE',  ( 21.09922568453594849, 21.20696800326375353, 6.408140936763242479 ) ) ;
#51510=CARTESIAN_POINT ( 'NONE',  ( 0.6178305044545818747, 3.498634669930420049, -9.382169495545419124 ) ) ;
#51512=CARTESIAN_POINT ( 'NONE',  ( 15.44008868035555260, 19.73035201082150536, 9.422509992056143702 ) ) ;
#51513=CARTESIAN_POINT ( 'NONE',  ( 4.559911319644449179, 8.897018677488173211, 9.422509992056141925 ) ) ;
#51514=CARTESIAN_POINT ( 'NONE',  ( 0.1532563361054082862, 46.21726448433411605, 2.638427012816831674 ) ) ;
#51517=CARTESIAN_POINT ( 'NONE',  ( 2.035157376598824452, 3.688685344154837953, 7.964842623401179544 ) ) ;
#51518=CARTESIAN_POINT ( 'NONE',  ( -1.099225684535947600, 3.706968003263753531, -6.408140936763238038 ) ) ;
#51520=VECTOR ( 'NONE', #80266, 1000.000000000000000 ) ;
#51521=CARTESIAN_POINT ( 'NONE',  ( 0.1532563361054100626, 15.80059781766745353, -2.638427012816831230 ) ) ;
#51522=CARTESIAN_POINT ( 'NONE',  ( 1.472469842513823179, 35.59226448433412315, -4.923371831947296329 ) ) ;
#51523=CARTESIAN_POINT ( 'NONE',  ( 12.91533473730993009, 41.60535201082149825, -10.88017736071109987 ) ) ;
#51524=CARTESIAN_POINT ( 'NONE',  ( 16.40814093676324603, 12.45696800326375353, -11.09922568453594671 ) ) ;
#51525=CARTESIAN_POINT ( 'NONE',  ( 12.91533473730992121, 54.52201867748816255, 10.88017736071110164 ) ) ;
#51528=CARTESIAN_POINT ( 'NONE',  ( 10.00000000000000178, 50.37363466993042493, 12.81628187352647608 ) ) ;
#51529=ORIENTED_EDGE ( 'NONE', *, *, #66975, .F. ) ;
#51530=CARTESIAN_POINT ( 'NONE',  ( 15.44008868035555260, 64.73035201082151957, 9.422509992056143702 ) ) ;
#51531=CARTESIAN_POINT ( 'NONE',  ( 21.09922568453594849, 36.20696800326375353, 6.408140936763242479 ) ) ;
#51532=CARTESIAN_POINT ( 'NONE',  ( 6.204703633549690345, 0.7620821682473009062, -14.16423886937410259 ) ) ;
#51533=CARTESIAN_POINT ( 'NONE',  ( 2.791683348922240793, 1.633931151000784565, 7.208316651077764092 ) ) ;
#51534=CARTESIAN_POINT ( 'NONE',  ( -0.8801773607111008646, 43.27201867748817676, 2.915334737309923430 ) ) ;
#51535=CARTESIAN_POINT ( 'NONE',  ( 1.472469842513823179, 61.42559781766745175, 4.923371831947296329 ) ) ;
#51537=CARTESIAN_POINT ( 'NONE',  ( 12.63842701281683922, 59.55059781766744464, -9.846743663894590881 ) ) ;
#51538=CARTESIAN_POINT ( 'NONE',  ( 2.791683348922237240, 15.38393115100078212, -7.208316651077763204 ) ) ;
#51540=CARTESIAN_POINT ( 'NONE',  ( 10.00000000000000000, 61.81368534415484106, -10.88017736071110342 ) ) ;
#51542=CARTESIAN_POINT ( 'NONE',  ( -4.164238869374098151, 26.59541550158063217, -3.795296366450310543 ) ) ;
#51547=ORIENTED_EDGE ( 'NONE', *, *, #6464, .F. ) ;
#51548=VECTOR ( 'NONE', #35207, 1000.000000000000000 ) ;
#51549=CARTESIAN_POINT ( 'NONE',  ( 22.26659068614894466, 58.88708216824729647, 7.082119434687054849 ) ) ;
#51550=CARTESIAN_POINT ( 'NONE',  ( 24.16423886937409904, 59.09541550158063217, 3.795296366450317205 ) ) ;
#51551=CARTESIAN_POINT ( 'NONE',  ( 7.361572987183169658, 34.96726448433411605, -9.846743663894592657 ) ) ;
#51552=B_SPLINE_CURVE_WITH_KNOTS ( 'NONE', 3,
 ( #65743, #58229, #20754, #65244, #27746, #88749, #20259, #51243, #81247, #57751, #95770, #34249, #12746, #97267, #35747, #66235, #81730, #13245 ),
 .UNSPECIFIED., .F., .F.,
 ( 4, 2, 2, 2, 2, 2, 2, 2, 4 ),
 ( 1.551583845779545699E-17, 0.0005964982550586688404, 0.001192996510117322285, 0.002385993020234661918, 0.003578989530352000899, 0.004771986040469341182, 0.007157979060703985319, 0.008350975570821308688, 0.009543972080938632058 ),
 .UNSPECIFIED. ) ;
#51553=CARTESIAN_POINT ( 'NONE',  ( 22.81628187352647785, 31.62363466993042138, 6.195893100308588602E-16 ) ) ;
#51555=( LENGTH_UNIT ( ) NAMED_UNIT ( * ) SI_UNIT ( .MILLI., .METRE. ) );
#51556=CARTESIAN_POINT ( 'NONE',  ( 17.96484262340118221, 9.938685344154837509, 7.964842623401181321 ) ) ;
#51557=CARTESIAN_POINT ( 'NONE',  ( 10.00000000000000000, 60.55374883491397497, -14.16423886937410082 ) ) ;
#51558=CARTESIAN_POINT ( 'NONE',  ( 0.1532563361054083140, 26.00893115100078745, 1.131784320476157264E-15 ) ) ;
#51561=CARTESIAN_POINT ( 'NONE',  ( 7.361572987183169658, 9.967264484334119601, -9.846743663894592657 ) ) ;
#51562=EDGE_CURVE ( 'NONE', #53168, #42200, #96147, .T. ) ;
#51565=ORIENTED_EDGE ( 'NONE', *, *, #46291, .F. ) ;
#51568=VERTEX_POINT ( 'NONE', #65787 ) ;
#51569=CARTESIAN_POINT ( 'NONE',  ( 0.1532563361054082862, 41.21726448433411605, 2.638427012816831674 ) ) ;
#51570=CARTESIAN_POINT ( 'NONE',  ( -4.164238869374098151, 16.59541550158063927, -3.795296366450310543 ) ) ;
#51571=CARTESIAN_POINT ( 'NONE',  ( 19.42250999205614193, 25.14701867748817321, 5.440088680355555262 ) ) ;
#51572=CARTESIAN_POINT ( 'NONE',  ( 19.42250999205614193, 25.14701867748817321, 5.440088680355555262 ) ) ;
#51573=CARTESIAN_POINT ( 'NONE',  ( 19.84674366389459266, 58.71726448433411605, -2.638427012816827677 ) ) ;
#51574=CARTESIAN_POINT ( 'NONE',  ( 21.09922568453595559, 22.04030133659708923, -6.408140936763230044 ) ) ;
#51575=CARTESIAN_POINT ( 'NONE',  ( 13.79529636645031943, 5.345415501580634832, -14.16423886937409904 ) ) ;
#51576=CARTESIAN_POINT ( 'NONE',  ( 13.43411237798105340, 35.58196800326375353, 12.81628187352647963 ) ) ;
#51577=ORIENTED_EDGE ( 'NONE', *, *, #14714, .T. ) ;
#51578=CARTESIAN_POINT ( 'NONE',  ( 2.791683348922237240, 30.38393115100078390, -7.208316651077763204 ) ) ;
#51579=MECHANICAL_DESIGN_GEOMETRIC_PRESENTATION_REPRESENTATION('',(#19596),#51505);
#51580=CARTESIAN_POINT ( 'NONE',  ( 17.96484262340118221, 4.938685344154837509, 7.964842623401181321 ) ) ;
#51583=CARTESIAN_POINT ( 'NONE',  ( -2.266590686148945544, 67.22041550158063217, 7.082119434687048631 ) ) ;
#51584=EDGE_LOOP ( 'NONE', ( #28760, #54857, #80677, #49084 ) ) ;
#51585=CARTESIAN_POINT ( 'NONE',  ( 7.084665262690076126, 47.02201867748818387, -10.88017736071110164 ) ) ;
#51586=CARTESIAN_POINT ( 'NONE',  ( 4.559911319644449179, 63.89701867748817676, 9.422509992056141925 ) ) ;
#51587=CARTESIAN_POINT ( 'NONE',  ( 12.91533473730993009, 56.60535201082151247, -10.88017736071109987 ) ) ;
#51591=CARTESIAN_POINT ( 'NONE',  ( 2.035157376598824452, 58.68868534415482685, 7.964842623401179544 ) ) ;
#51592=CARTESIAN_POINT ( 'NONE',  ( 19.72487221294570858, 70.00000000000000000, -6.000000000000000000 ) ) ;
#51596=CARTESIAN_POINT ( 'NONE',  ( 12.63842701281683922, 24.55059781766745175, -9.846743663894590881 ) ) ;
#51598=CARTESIAN_POINT ( 'NONE',  ( 14.92337183194729633, 57.67559781766745886, 8.527530157486181039 ) ) ;
#51601=CARTESIAN_POINT ( 'NONE',  ( 20.36894250292379738, 9.928748834913966093, -10.36894250292379027 ) ) ;
#51605=CARTESIAN_POINT ( 'NONE',  ( 10.00000000000000178, 37.25893115100078745, 9.846743663894594434 ) ) ;
#51606=CARTESIAN_POINT ( 'NONE',  ( 10.00000000000000178, 68.05374883491397497, 14.16423886937410082 ) ) ;
#51609=( BOUNDED_SURFACE ( )  B_SPLINE_SURFACE ( 3, 2, ( 
 ( #41163, #26143, #9667 ),
 ( #25664, #70669, #95620 ),
 ( #25182, #18643, #11133 ),
 ( #94136, #27109, #64604 ) ),
 .UNSPECIFIED., .F., .F., .F. ) 
 B_SPLINE_SURFACE_WITH_KNOTS ( ( 4, 4 ),
 ( 3, 3 ),
 ( -2.168404344971008868E-19, 0.0006068291151710580476 ),
 ( 0.000000000000000000, 1.000000000000000000 ),
 .UNSPECIFIED. ) 
 GEOMETRIC_REPRESENTATION_ITEM ( )  RATIONAL_B_SPLINE_SURFACE ( (
 ( 1.000000000000000000, 0.8414823709351009207, 1.000000000000000000),
 ( 1.000000000000000000, 0.8336435218270028535, 1.000000000000000000),
 ( 1.000000000000000000, 0.8260591074388748956, 1.000000000000000000),
 ( 1.000000000000000000, 0.8188293140827598293, 1.000000000000000000) ) ) 
 REPRESENTATION_ITEM ( '' )  SURFACE ( )  );
#51611=CARTESIAN_POINT ( 'NONE',  ( 5.076628168052704559, 45.17559781766745175, -8.527530157486179263 ) ) ;
#51612=CARTESIAN_POINT ( 'NONE',  ( 0.2751277870542967463, 70.00000000000000000, -6.000000000000000000 ) ) ;
#51613=CARTESIAN_POINT ( 'NONE',  ( -2.816281873526473856, 19.12363466993042138, 9.499525473075851096E-16 ) ) ;
#51614=CARTESIAN_POINT ( 'NONE',  ( 0.1532563361054083140, 11.00893115100078568, 1.131784320476157264E-15 ) ) ;
#51615=CARTESIAN_POINT ( 'NONE',  ( 2.603489959281614308, 36.58210964143329136, 6.500000000000031086 ) ) ;
#51616=CARTESIAN_POINT ( 'NONE',  ( 14.92337183194729633, 17.67559781766745175, 8.527530157486181039 ) ) ;
#51617=CARTESIAN_POINT ( 'NONE',  ( 3.591859063236761518, -0.04303199673624671928, 11.09922568453594849 ) ) ;
#51618=( BOUNDED_SURFACE ( )  B_SPLINE_SURFACE ( 1, 2, ( 
 ( #75363, #92828, #53351, #84368, #76358, #68376, #69848, #7873, #61834, #77327, #6878, #31824, #37882, #14890, #31334, #23867, #46352, #62321, #30347, #98895, #16352, #24357, #45359, #76840, #83859, #82874, #14388, #7386, #37389, #8354, #38862, #69351, #60854, #67879, #54330, #84845, #98400, #29856, #90854, #91353, #22880, #10323, #72283, #16845, #34269, #55827, #64281, #40825, #17345, #56795, #56318, #24842, #25821, #32317, #2844, #71325, #87290, #33298, #18810, #47319, #71806, #93320, #63789, #77819, #3311, #3813, #86814, #10815, #9334, #18318, #62821, #48307, #32808, #17826, #55324, #9835, #49293, #85830, #47815, #94793, #33774, #63304, #78815, #78315, #64771, #94298, #48798, #95285, #79307, #39836, #41334, #2352, #11296, #54820, #26295, #40336, #79794, #41816, #85331, #70342, #1860, #70839, #93813, #25343, #86321, #73271, #36769, #28759, #89265, #11787, #20280, #28266, #20776, #5291, #6264, #97285, #67261, #43757, #19778, #59251, #96790, #35768, #80287, #65765, #44252, #74246, #34777, #4303, #88769, #50777, #5778, #65263, #81269, #12769, #58761, #12279, #95792, #89751, #43265, #21268, #73760, #27273, #58253, #13265, #74755, #66762, #26786, #66256, #51765, #57284, #72767, #88277, #36267, #42295, #51267, #81751, #82249, #13764, #87778, #19294, #49781, #57772, #50266, #96292, #80782, #42786, #4792, #35269, #27769, #76726, #38742, #52254, #45245, #91738, #37274, #76245, #29251, #23259, #46240, #92228, #29737, #75741, #54214, #764, #60247, #68746, #22758, #6760, #7263, #16237, #77217, #37764, #68261, #69243, #31217, #90740, #8245, #90244, #21775, #67763, #61712, #98781, #46717, #23754, #30229, #60733, #84731, #53734, #15268, #8722, #39240, #91234, #97788, #61232, #59747, #7761, #53240, #45749, #15755, #22268, #83745, #38254, #278, #82750, #30725, #83250, #98282, #14271, #84253, #44745, #75248, #52741, #14772, #25231, #63678, #17718, #49180, #62205, #70720, #10700, #17230, #78201, #62698, #26190, #40705, #9713, #24237, #39730, #70224, #56682, #40213, #2731, #55710, #94183, #48191, #79681, #92711, #2236, #41214, #47707, #32694, #93199, #87173, #71209, #63191, #54704, #1743, #32197, #18696, #85225, #93696, #11179, #86698, #77706, #47205, #86207, #78704, #18204, #9218, #10213, #33186, #25712, #55201, #24725, #71692, #56205, #64164, #48683, #85715, #79186, #3204, #69728, #33667, #1255, #94682, #31710, #16728, #87661, #4185, #58646, #95163, #73145, #20155, #81147, #13143, #81635, #59129, #73637, #58138, #72650, #80666, #42186, #4682, #19175, #57657, #80165, #20655, #43640, #26669, #88155, #35651, #11676, #50658, #72170, #66137 ),
 ( #34656, #74125, #89144, #50157, #35145, #65151, #21149, #65644, #5165, #82130, #96168, #34158, #43149, #19668, #97172, #89638, #12651, #95670, #27651, #5662, #96669, #51150, #28149, #36144, #27156, #66648, #28639, #12161, #51650, #41699, #3697, #57164, #88647, #64650, #49655, #42666, #92106, #84125, #54096, #30604, #6633, #15637, #83627, #22638, #46120, #37638, #8124, #60616, #82631, #45116, #155, #31099, #53608, #61593, #75624, #38618, #13639, #59628, #75127, #61109, #67136, #7136, #91115, #53119, #76607, #69119, #23637, #45621, #30110, #44631, #52624, #14147, #68135, #90123, #29612, #52136, #91618, #650, #97660, #60117, #7647, #37149, #15143, #44124, #38138, #23135, #74634, #67645, #90616, #6146, #36648, #98154, #76118, #98662, #21651, #22140, #29127, #83125, #14652, #68625, #56088, #86580, #77583, #94074, #77097, #8609, #24116, #63566, #93081, #3098, #10579, #62577, #55078, #41089, #40592, #2121, #71586, #33552, #24611, #84611, #48070, #64050, #93577, #85597, #32580, #2615, #47087, #17111, #47594, #9591, #33070, #63076, #70102, #54585, #16113, #78088, #94562, #40095, #70595, #17600, #25112, #78583, #55594, #26080, #39117, #86089, #25595, #32076, #10094, #9099, #46598, #71089, #18089, #69607, #85100, #16609, #1128, #31590, #48564, #62085, #79065, #92592, #39613, #1627, #80551, #73523, #95047, #12047, #19552, #88537, #42075, #26554, #97056, #5051, #49542, #58525, #27537, #65530, #35534, #57051, #89033, #50048, #42548, #20039, #18575, #66529, #27043, #35028, #73032, #72536, #43524, #4566, #66027, #51029, #49068, #5549, #11555, #87553, #96555, #28030, #96053, #74020, #4070, #34533, #20544, #81522, #19063, #58030, #57541, #56574, #87065, #80052, #79571, #50541, #81035, #12542, #65027, #13030, #43043, #36027, #11070, #41591, #72058, #3585, #95554, #34043, #64539, #88040, #8011, #29498, #38020, #83016, #90013, #30492, #29998, #97548, #98546, #6037, #75509, #14533, #60991, #45004, #91502, #89529, #45502, #67026, #7023, #21038, #76002, #76498, #60505, #83512, #51528, #90995, #36537, #22035, #6519, #90500, #29010, #82519, #23022, #59519, #21533, #68513, #7530, #37029, #52509, #52026, #38509, #37529, #22525, #69007, #68019, #82020, #52998, #75014, #84003, #28529, #15030, #14036, #43, #53493, #15527, #46008, #59023, #13531, #44515, #44014, #74517, #67525, #98042, #60006, #62962, #84499, #92966, #2002, #93467, #77970, #78954, #70980, #85482, #39001, #63458, #24498, #39980, #85978, #24994, #32467, #47470, #69496, #54960, #17971, #61484, #10465, #1514, #9978, #16991, #61977, #2501, #55477, #1012, #70481, #76985, #9477, #17489 ) ),
 .UNSPECIFIED., .F., .F., .F. ) 
 B_SPLINE_SURFACE_WITH_KNOTS ( ( 2, 2 ),
 ( 3, 2, 2, 2, 2, 2, 2, 2, 2, 2, 2, 2, 2, 2, 2, 2, 2, 2, 2, 2, 2, 2, 2, 2, 2, 2, 2, 2, 2, 2, 2, 2, 2, 2, 2, 2, 2, 2, 2, 2, 2, 2, 2, 2, 2, 2, 2, 2, 2, 2, 2, 2, 2, 2, 2, 2, 2, 2, 2, 2, 2, 2, 2, 2, 2, 2, 2, 2, 2, 2, 2, 2, 2, 2, 2, 2, 2, 2, 2, 2, 2, 2, 2, 2, 2, 2, 2, 2, 2, 2, 2, 2, 2, 2, 2, 2, 2, 2, 2, 2, 2, 2, 2, 2, 2, 2, 2, 2, 2, 2, 2, 2, 2, 2, 2, 2, 2, 2, 2, 2, 2, 2, 2, 2, 2, 2, 2, 2, 2, 2, 2, 2, 2, 2, 2, 2, 2, 2, 2, 2, 2, 2, 2, 2, 2, 2, 2, 2, 2, 2, 2, 2, 2, 2, 2, 2, 2, 2, 2, 2, 2, 2, 3 ),
 ( 0.000000000000000000, 1.000000000000000000 ),
 ( 0.000000000000000000, 0.005952380952380952051, 0.01190476190476190410, 0.01785714285714285615, 0.02380952380952380820, 0.02976190476190476025, 0.03571428571428571230, 0.04166666666666666435, 0.04761904761904761640, 0.05357142857142856845, 0.05952380952380952051, 0.06547619047619047949, 0.07142857142857142461, 0.07738095238095238360, 0.08333333333333332871, 0.08928571428571428770, 0.09523809523809523281, 0.1011904761904761918, 0.1071428571428571369, 0.1130952380952380959, 0.1190476190476190410, 0.1250000000000000000, 0.1309523809523809590, 0.1369047619047619180, 0.1428571428571428492, 0.1488095238095238082, 0.1547619047619047672, 0.1607142857142857262, 0.1666666666666666574, 0.1726190476190476164, 0.1785714285714285754, 0.1845238095238095344, 0.1904761904761904656, 0.1964285714285714246, 0.2023809523809523836, 0.2083333333333333426, 0.2142857142857142738, 0.2202380952380952328, 0.2261904761904761918, 0.2321428571428571508, 0.2380952380952380820, 0.2440476190476190410, 0.2500000000000000000, 0.2559523809523809312, 0.2619047619047619180, 0.2678571428571428492, 0.2738095238095238360, 0.2797619047619047672, 0.2857142857142856984, 0.2916666666666666852, 0.2976190476190476164, 0.3035714285714285476, 0.3095238095238095344, 0.3154761904761904656, 0.3214285714285714524, 0.3273809523809523836, 0.3333333333333333148, 0.3392857142857143016, 0.3452380952380952328, 0.3511904761904761640, 0.3571428571428571508, 0.3630952380952380820, 0.3690476190476190688, 0.3750000000000000000, 0.3809523809523809312, 0.3869047619047619180, 0.3928571428571428492, 0.3988095238095238360, 0.4047619047619047672, 0.4107142857142856984, 0.4166666666666666852, 0.4226190476190476164, 0.4285714285714285476, 0.4345238095238095344, 0.4404761904761904656, 0.4464285714285714524, 0.4523809523809523836, 0.4583333333333333148, 0.4642857142857143016, 0.4702380952380952328, 0.4761904761904761640, 0.4821428571428571508, 0.4880952380952380820, 0.4940476190476190688, 0.5000000000000000000, 0.5059523809523809312, 0.5119047619047618625, 0.5178571428571429047, 0.5238095238095238360, 0.5297619047619047672, 0.5357142857142856984, 0.5416666666666666297, 0.5476190476190476719, 0.5535714285714286031, 0.5595238095238095344, 0.5654761904761904656, 0.5714285714285713969, 0.5773809523809523281, 0.5833333333333333703, 0.5892857142857143016, 0.5952380952380952328, 0.6011904761904761640, 0.6071428571428570953, 0.6130952380952381375, 0.6190476190476190688, 0.6250000000000000000, 0.6309523809523809312, 0.6369047619047618625, 0.6428571428571429047, 0.6488095238095238360, 0.6547619047619047672, 0.6607142857142856984, 0.6666666666666666297, 0.6726190476190476719, 0.6785714285714286031, 0.6845238095238095344, 0.6904761904761904656, 0.6964285714285713969, 0.7023809523809523281, 0.7083333333333333703, 0.7142857142857143016, 0.7202380952380952328, 0.7261904761904761640, 0.7321428571428570953, 0.7380952380952381375, 0.7440476190476190688, 0.7500000000000000000, 0.7559523809523809312, 0.7619047619047618625, 0.7678571428571429047, 0.7738095238095238360, 0.7797619047619047672, 0.7857142857142856984, 0.7916666666666666297, 0.7976190476190476719, 0.8035714285714286031, 0.8095238095238095344, 0.8154761904761904656, 0.8214285714285713969, 0.8273809523809523281, 0.8333333333333333703, 0.8392857142857143016, 0.8452380952380952328, 0.8511904761904761640, 0.8571428571428570953, 0.8630952380952381375, 0.8690476190476190688, 0.8750000000000000000, 0.8809523809523809312, 0.8869047619047618625, 0.8928571428571429047, 0.8988095238095238360, 0.9047619047619047672, 0.9107142857142856984, 0.9166666666666666297, 0.9226190476190476719, 0.9285714285714286031, 0.9345238095238095344, 0.9404761904761904656, 0.9464285714285713969, 0.9523809523809523281, 0.9583333333333333703, 0.9642857142857143016 ),
 .UNSPECIFIED. ) 
 GEOMETRIC_REPRESENTATION_ITEM ( )  RATIONAL_B_SPLINE_SURFACE ( (
 ( 1.000000000000000000, 0.9659258262890683122, 1.000000000000000000, 0.9659258262890683122, 1.000000000000000000, 0.9659258262890683122, 1.000000000000000000, 0.9659258262890683122, 1.000000000000000000, 0.9659258262890683122, 1.000000000000000000, 0.9659258262890683122, 1.000000000000000000, 0.9659258262890683122, 1.000000000000000000, 0.9659258262890683122, 1.000000000000000000, 0.9659258262890683122, 1.000000000000000000, 0.9659258262890683122, 1.000000000000000000, 0.9659258262890683122, 1.000000000000000000, 0.9659258262890683122, 1.000000000000000000, 0.9659258262890683122, 1.000000000000000000, 0.9659258262890683122, 1.000000000000000000, 0.9659258262890683122, 1.000000000000000000, 0.9659258262890683122, 1.000000000000000000, 0.9659258262890683122, 1.000000000000000000, 0.9659258262890683122, 1.000000000000000000, 0.9659258262890683122, 1.000000000000000000, 0.9659258262890683122, 1.000000000000000000, 0.9659258262890683122, 1.000000000000000000, 0.9659258262890683122, 1.000000000000000000, 0.9659258262890683122, 1.000000000000000000, 0.9659258262890683122, 1.000000000000000000, 0.9659258262890683122, 1.000000000000000000, 0.9659258262890683122, 1.000000000000000000, 0.9659258262890683122, 1.000000000000000000, 0.9659258262890683122, 1.000000000000000000, 0.9659258262890683122, 1.000000000000000000, 0.9659258262890683122, 1.000000000000000000, 0.9659258262890683122, 1.000000000000000000, 0.9659258262890683122, 1.000000000000000000, 0.9659258262890683122, 1.000000000000000000, 0.9659258262890683122, 1.000000000000000000, 0.9659258262890683122, 1.000000000000000000, 0.9659258262890683122, 1.000000000000000000, 0.9659258262890683122, 1.000000000000000000, 0.9659258262890683122, 1.000000000000000000, 0.9659258262890683122, 1.000000000000000000, 0.9659258262890683122, 1.000000000000000000, 0.9659258262890683122, 1.000000000000000000, 0.9659258262890683122, 1.000000000000000000, 0.9659258262890683122, 1.000000000000000000, 0.9659258262890683122, 1.000000000000000000, 0.9659258262890683122, 1.000000000000000000, 0.9659258262890683122, 1.000000000000000000, 0.9659258262890683122, 1.000000000000000000, 0.9659258262890683122, 1.000000000000000000, 0.9659258262890683122, 1.000000000000000000, 0.9659258262890683122, 1.000000000000000000, 0.9659258262890683122, 1.000000000000000000, 0.9659258262890683122, 1.000000000000000000, 0.9659258262890683122, 1.000000000000000000, 0.9659258262890683122, 1.000000000000000000, 0.9659258262890683122, 1.000000000000000000, 0.9659258262890683122, 1.000000000000000000, 0.9659258262890683122, 1.000000000000000000, 0.9659258262890683122, 1.000000000000000000, 0.9659258262890683122, 1.000000000000000000, 0.9659258262890683122, 1.000000000000000000, 0.9659258262890683122, 1.000000000000000000, 0.9659258262890683122, 1.000000000000000000, 0.9659258262890683122, 1.000000000000000000, 0.9659258262890683122, 1.000000000000000000, 0.9659258262890683122, 1.000000000000000000, 0.9659258262890683122, 1.000000000000000000, 0.9659258262890683122, 1.000000000000000000, 0.9659258262890683122, 1.000000000000000000, 0.9659258262890683122, 1.000000000000000000, 0.9659258262890683122, 1.000000000000000000, 0.9659258262890683122, 1.000000000000000000, 0.9659258262890683122, 1.000000000000000000, 0.9659258262890683122, 1.000000000000000000, 0.9659258262890683122, 1.000000000000000000, 0.9659258262890683122, 1.000000000000000000, 0.9659258262890683122, 1.000000000000000000, 0.9659258262890683122, 1.000000000000000000, 0.9659258262890683122, 1.000000000000000000, 0.9659258262890683122, 1.000000000000000000, 0.9659258262890683122, 1.000000000000000000, 0.9659258262890683122, 1.000000000000000000, 0.9659258262890683122, 1.000000000000000000, 0.9659258262890683122, 1.000000000000000000, 0.9659258262890683122, 1.000000000000000000, 0.9659258262890683122, 1.000000000000000000, 0.9659258262890683122, 1.000000000000000000, 0.9659258262890683122, 1.000000000000000000, 0.9659258262890683122, 1.000000000000000000, 0.9659258262890683122, 1.000000000000000000, 0.9659258262890683122, 1.000000000000000000, 0.9659258262890683122, 1.000000000000000000, 0.9659258262890683122, 1.000000000000000000, 0.9659258262890683122, 1.000000000000000000, 0.9659258262890683122, 1.000000000000000000, 0.9659258262890683122, 1.000000000000000000, 0.9659258262890683122, 1.000000000000000000, 0.9659258262890683122, 1.000000000000000000, 0.9659258262890683122, 1.000000000000000000, 0.9659258262890683122, 1.000000000000000000, 0.9659258262890683122, 1.000000000000000000, 0.9659258262890683122, 1.000000000000000000, 0.9659258262890683122, 1.000000000000000000, 0.9659258262890683122, 1.000000000000000000, 0.9659258262890683122, 1.000000000000000000, 0.9659258262890683122, 1.000000000000000000, 0.9659258262890683122, 1.000000000000000000, 0.9659258262890683122, 1.000000000000000000, 0.9659258262890683122, 1.000000000000000000, 0.9659258262890683122, 1.000000000000000000, 0.9659258262890683122, 1.000000000000000000, 0.9659258262890683122, 1.000000000000000000, 0.9659258262890683122, 1.000000000000000000, 0.9659258262890683122, 1.000000000000000000, 0.9659258262890683122, 1.000000000000000000, 0.9659258262890683122, 1.000000000000000000, 0.9659258262890683122, 1.000000000000000000, 0.9659258262890683122, 1.000000000000000000, 0.9659258262890683122, 1.000000000000000000, 0.9659258262890683122, 1.000000000000000000, 0.9659258262890683122, 1.000000000000000000, 0.9659258262890683122, 1.000000000000000000, 0.9659258262890683122, 1.000000000000000000, 0.9659258262890683122, 1.000000000000000000, 0.9659258262890683122, 1.000000000000000000, 0.9659258262890683122, 1.000000000000000000, 0.9659258262890683122, 1.000000000000000000, 0.9659258262890683122, 1.000000000000000000, 0.9659258262890683122, 1.000000000000000000, 0.9659258262890683122, 1.000000000000000000, 0.9659258262890683122, 1.000000000000000000, 0.9659258262890683122, 1.000000000000000000, 0.9659258262890683122, 1.000000000000000000, 0.9659258262890683122, 1.000000000000000000, 0.9659258262890683122, 1.000000000000000000, 0.9659258262890683122, 1.000000000000000000, 0.9659258262890683122, 1.000000000000000000, 0.9659258262890683122, 1.000000000000000000, 0.9659258262890683122, 1.000000000000000000, 0.9659258262890683122, 1.000000000000000000, 0.9659258262890683122, 1.000000000000000000, 0.9659258262890683122, 1.000000000000000000, 0.9659258262890683122, 1.000000000000000000, 0.9659258262890683122, 1.000000000000000000, 0.9659258262890683122, 1.000000000000000000, 0.9659258262890683122, 1.000000000000000000, 0.9659258262890683122, 1.000000000000000000, 0.9659258262890683122, 1.000000000000000000, 0.9659258262890683122, 1.000000000000000000, 0.9659258262890683122, 1.000000000000000000, 0.9659258262890683122, 1.000000000000000000, 0.9659258262890683122, 1.000000000000000000, 0.9659258262890683122, 1.000000000000000000, 0.9659258262890683122, 1.000000000000000000, 0.9659258262890683122, 1.000000000000000000, 0.9659258262890683122, 1.000000000000000000, 0.9659258262890683122, 1.000000000000000000, 0.9659258262890683122, 1.000000000000000000, 0.9659258262890683122, 1.000000000000000000, 0.9659258262890683122, 1.000000000000000000, 0.9659258262890683122, 1.000000000000000000, 0.9659258262890683122, 1.000000000000000000, 0.9659258262890683122, 1.000000000000000000),
 ( 1.000000000000000000, 0.9659258262890683122, 1.000000000000000000, 0.9659258262890683122, 1.000000000000000000, 0.9659258262890683122, 1.000000000000000000, 0.9659258262890683122, 1.000000000000000000, 0.9659258262890683122, 1.000000000000000000, 0.9659258262890683122, 1.000000000000000000, 0.9659258262890683122, 1.000000000000000000, 0.9659258262890683122, 1.000000000000000000, 0.9659258262890683122, 1.000000000000000000, 0.9659258262890683122, 1.000000000000000000, 0.9659258262890683122, 1.000000000000000000, 0.9659258262890683122, 1.000000000000000000, 0.9659258262890683122, 1.000000000000000000, 0.9659258262890683122, 1.000000000000000000, 0.9659258262890683122, 1.000000000000000000, 0.9659258262890683122, 1.000000000000000000, 0.9659258262890683122, 1.000000000000000000, 0.9659258262890683122, 1.000000000000000000, 0.9659258262890683122, 1.000000000000000000, 0.9659258262890683122, 1.000000000000000000, 0.9659258262890683122, 1.000000000000000000, 0.9659258262890683122, 1.000000000000000000, 0.9659258262890683122, 1.000000000000000000, 0.9659258262890683122, 1.000000000000000000, 0.9659258262890683122, 1.000000000000000000, 0.9659258262890683122, 1.000000000000000000, 0.9659258262890683122, 1.000000000000000000, 0.9659258262890683122, 1.000000000000000000, 0.9659258262890683122, 1.000000000000000000, 0.9659258262890683122, 1.000000000000000000, 0.9659258262890683122, 1.000000000000000000, 0.9659258262890683122, 1.000000000000000000, 0.9659258262890683122, 1.000000000000000000, 0.9659258262890683122, 1.000000000000000000, 0.9659258262890683122, 1.000000000000000000, 0.9659258262890683122, 1.000000000000000000, 0.9659258262890683122, 1.000000000000000000, 0.9659258262890683122, 1.000000000000000000, 0.9659258262890683122, 1.000000000000000000, 0.9659258262890683122, 1.000000000000000000, 0.9659258262890683122, 1.000000000000000000, 0.9659258262890683122, 1.000000000000000000, 0.9659258262890683122, 1.000000000000000000, 0.9659258262890683122, 1.000000000000000000, 0.9659258262890683122, 1.000000000000000000, 0.9659258262890683122, 1.000000000000000000, 0.9659258262890683122, 1.000000000000000000, 0.9659258262890683122, 1.000000000000000000, 0.9659258262890683122, 1.000000000000000000, 0.9659258262890683122, 1.000000000000000000, 0.9659258262890683122, 1.000000000000000000, 0.9659258262890683122, 1.000000000000000000, 0.9659258262890683122, 1.000000000000000000, 0.9659258262890683122, 1.000000000000000000, 0.9659258262890683122, 1.000000000000000000, 0.9659258262890683122, 1.000000000000000000, 0.9659258262890683122, 1.000000000000000000, 0.9659258262890683122, 1.000000000000000000, 0.9659258262890683122, 1.000000000000000000, 0.9659258262890683122, 1.000000000000000000, 0.9659258262890683122, 1.000000000000000000, 0.9659258262890683122, 1.000000000000000000, 0.9659258262890683122, 1.000000000000000000, 0.9659258262890683122, 1.000000000000000000, 0.9659258262890683122, 1.000000000000000000, 0.9659258262890683122, 1.000000000000000000, 0.9659258262890683122, 1.000000000000000000, 0.9659258262890683122, 1.000000000000000000, 0.9659258262890683122, 1.000000000000000000, 0.9659258262890683122, 1.000000000000000000, 0.9659258262890683122, 1.000000000000000000, 0.9659258262890683122, 1.000000000000000000, 0.9659258262890683122, 1.000000000000000000, 0.9659258262890683122, 1.000000000000000000, 0.9659258262890683122, 1.000000000000000000, 0.9659258262890683122, 1.000000000000000000, 0.9659258262890683122, 1.000000000000000000, 0.9659258262890683122, 1.000000000000000000, 0.9659258262890683122, 1.000000000000000000, 0.9659258262890683122, 1.000000000000000000, 0.9659258262890683122, 1.000000000000000000, 0.9659258262890683122, 1.000000000000000000, 0.9659258262890683122, 1.000000000000000000, 0.9659258262890683122, 1.000000000000000000, 0.9659258262890683122, 1.000000000000000000, 0.9659258262890683122, 1.000000000000000000, 0.9659258262890683122, 1.000000000000000000, 0.9659258262890683122, 1.000000000000000000, 0.9659258262890683122, 1.000000000000000000, 0.9659258262890683122, 1.000000000000000000, 0.9659258262890683122, 1.000000000000000000, 0.9659258262890683122, 1.000000000000000000, 0.9659258262890683122, 1.000000000000000000, 0.9659258262890683122, 1.000000000000000000, 0.9659258262890683122, 1.000000000000000000, 0.9659258262890683122, 1.000000000000000000, 0.9659258262890683122, 1.000000000000000000, 0.9659258262890683122, 1.000000000000000000, 0.9659258262890683122, 1.000000000000000000, 0.9659258262890683122, 1.000000000000000000, 0.9659258262890683122, 1.000000000000000000, 0.9659258262890683122, 1.000000000000000000, 0.9659258262890683122, 1.000000000000000000, 0.9659258262890683122, 1.000000000000000000, 0.9659258262890683122, 1.000000000000000000, 0.9659258262890683122, 1.000000000000000000, 0.9659258262890683122, 1.000000000000000000, 0.9659258262890683122, 1.000000000000000000, 0.9659258262890683122, 1.000000000000000000, 0.9659258262890683122, 1.000000000000000000, 0.9659258262890683122, 1.000000000000000000, 0.9659258262890683122, 1.000000000000000000, 0.9659258262890683122, 1.000000000000000000, 0.9659258262890683122, 1.000000000000000000, 0.9659258262890683122, 1.000000000000000000, 0.9659258262890683122, 1.000000000000000000, 0.9659258262890683122, 1.000000000000000000, 0.9659258262890683122, 1.000000000000000000, 0.9659258262890683122, 1.000000000000000000, 0.9659258262890683122, 1.000000000000000000, 0.9659258262890683122, 1.000000000000000000, 0.9659258262890683122, 1.000000000000000000, 0.9659258262890683122, 1.000000000000000000, 0.9659258262890683122, 1.000000000000000000, 0.9659258262890683122, 1.000000000000000000, 0.9659258262890683122, 1.000000000000000000, 0.9659258262890683122, 1.000000000000000000, 0.9659258262890683122, 1.000000000000000000, 0.9659258262890683122, 1.000000000000000000, 0.9659258262890683122, 1.000000000000000000, 0.9659258262890683122, 1.000000000000000000, 0.9659258262890683122, 1.000000000000000000, 0.9659258262890683122, 1.000000000000000000, 0.9659258262890683122, 1.000000000000000000, 0.9659258262890683122, 1.000000000000000000, 0.9659258262890683122, 1.000000000000000000, 0.9659258262890683122, 1.000000000000000000, 0.9659258262890683122, 1.000000000000000000, 0.9659258262890683122, 1.000000000000000000, 0.9659258262890683122, 1.000000000000000000, 0.9659258262890683122, 1.000000000000000000, 0.9659258262890683122, 1.000000000000000000, 0.9659258262890683122, 1.000000000000000000, 0.9659258262890683122, 1.000000000000000000, 0.9659258262890683122, 1.000000000000000000, 0.9659258262890683122, 1.000000000000000000, 0.9659258262890683122, 1.000000000000000000, 0.9659258262890683122, 1.000000000000000000, 0.9659258262890683122, 1.000000000000000000, 0.9659258262890683122, 1.000000000000000000, 0.9659258262890683122, 1.000000000000000000, 0.9659258262890683122, 1.000000000000000000, 0.9659258262890683122, 1.000000000000000000, 0.9659258262890683122, 1.000000000000000000, 0.9659258262890683122, 1.000000000000000000, 0.9659258262890683122, 1.000000000000000000, 0.9659258262890683122, 1.000000000000000000, 0.9659258262890683122, 1.000000000000000000, 0.9659258262890683122, 1.000000000000000000, 0.9659258262890683122, 1.000000000000000000, 0.9659258262890683122, 1.000000000000000000, 0.9659258262890683122, 1.000000000000000000) ) ) 
 REPRESENTATION_ITEM ( '' )  SURFACE ( )  );
#51621=ADVANCED_FACE ( 'NONE', ( #38279 ), #59279, .F. ) ;
#51623=CARTESIAN_POINT ( 'NONE',  ( 0.5774900079438607392, 13.48035201082150358, 5.440088680355550821 ) ) ;
#51624=CARTESIAN_POINT ( 'NONE',  ( 20.36894250292379382, 3.678748834913967869, 10.36894250292379205 ) ) ;
#51625=CARTESIAN_POINT ( 'NONE',  ( 10.00000000000000178, 32.25893115100078745, 9.846743663894594434 ) ) ;
#51626=CARTESIAN_POINT ( 'NONE',  ( 10.00000000000000178, 49.31368534415484106, 10.88017736071110342 ) ) ;
#51627=CARTESIAN_POINT ( 'NONE',  ( 3.591859063236761518, 24.95696800326375353, 11.09922568453594849 ) ) ;
#51629=CARTESIAN_POINT ( 'NONE',  ( 12.91533473730992121, 14.52201867748817143, 10.88017736071110164 ) ) ;
#51633=CARTESIAN_POINT ( 'NONE',  ( -1.099225684535947600, 4.540301336597087456, 6.408140936763237150 ) ) ;
#51634=CARTESIAN_POINT ( 'NONE',  ( 12.63842701281683922, 64.55059781766745175, -9.846743663894590881 ) ) ;
#51635=CARTESIAN_POINT ( 'NONE',  ( 0.1532563361054100626, 25.80059781766744820, -2.638427012816831230 ) ) ;
#51637=CARTESIAN_POINT ( 'NONE',  ( 10.00000000000000178, 40.37363466993042493, 12.81628187352647608 ) ) ;
#51638=CARTESIAN_POINT ( 'NONE',  ( 2.035157376598824452, 38.68868534415483396, 7.964842623401179544 ) ) ;
#51640=CYLINDRICAL_SURFACE ( 'NONE', #27364, 11.92686044187656513 ) ;
#51641=CARTESIAN_POINT ( 'NONE',  ( 7.084665262690076126, 22.02201867748817321, -10.88017736071110164 ) ) ;
#51642=CARTESIAN_POINT ( 'NONE',  ( 20.88017736071110164, 35.35535201082150536, 2.915334737309930979 ) ) ;
#51643=CARTESIAN_POINT ( 'NONE',  ( 19.84674366389459266, 53.71726448433411605, -2.638427012816827677 ) ) ;
#51644=CARTESIAN_POINT ( 'NONE',  ( -0.8801773607110991993, 57.85535201082149825, -2.915334737309923874 ) ) ;
#51645=AXIS2_PLACEMENT_3D ( 'NONE', #61836, #1862, #93815 ) ;
#51646=CARTESIAN_POINT ( 'NONE',  ( 24.16423886937410614, 34.30374883491396787, 8.672049930838204340E-16 ) ) ;
#51648=CARTESIAN_POINT ( 'NONE',  ( 0.1532563361054082862, 41.21726448433411605, 2.638427012816831674 ) ) ;
#51649=CARTESIAN_POINT ( 'NONE',  ( -2.816281873526473856, 64.12363466993042493, 9.499525473075851096E-16 ) ) ;
#51650=CARTESIAN_POINT ( 'NONE',  ( -1.099225684535947600, 3.706968003263753531, -6.408140936763238038 ) ) ;
#51652=CARTESIAN_POINT ( 'NONE',  ( 4.559911319644449179, 23.89701867748817321, 9.422509992056141925 ) ) ;
#51655=CARTESIAN_POINT ( 'NONE',  ( 7.084665262690076126, 19.10535201082150181, 10.88017736071109987 ) ) ;
#51656=CARTESIAN_POINT ( 'NONE',  ( 20.88017736071110519, 65.56368534415483396, 2.639326808657452039E-16 ) ) ;
#51657=CARTESIAN_POINT ( 'NONE',  ( 22.26659068614894466, 23.88708216824730357, 7.082119434687054849 ) ) ;
#51658=CARTESIAN_POINT ( 'NONE',  ( 19.84674366389459266, 18.30059781766745175, 2.638427012816836559 ) ) ;
#51660=CARTESIAN_POINT ( 'NONE',  ( 15.44008868035555260, 49.73035201082150536, 9.422509992056143702 ) ) ;
#51662=CARTESIAN_POINT ( 'NONE',  ( -0.1503990784575242878, 34.24884699246889141, -6.262539305110083276 ) ) ;
#51663=CARTESIAN_POINT ( 'NONE',  ( -42.83893681340153847, 106.9585622934581721, -5.000000000000000888 ) ) ;
#51664=EDGE_CURVE ( 'NONE', #43937, #29028, #46040, .T. ) ;
#51667=CARTESIAN_POINT ( 'NONE',  ( 2.791683348922240793, 41.63393115100078745, 7.208316651077764092 ) ) ;
#51669=ORIENTED_EDGE ( 'NONE', *, *, #89716, .F. ) ;
#51671=CARTESIAN_POINT ( 'NONE',  ( -2.266590686148945544, 17.22041550158063572, 7.082119434687048631 ) ) ;
#51672=CARTESIAN_POINT ( 'NONE',  ( -4.164238869374098151, 26.59541550158063217, -3.795296366450310543 ) ) ;
#51673=CARTESIAN_POINT ( 'NONE',  ( 12.91533473730993009, 56.60535201082151247, -10.88017736071109987 ) ) ;
#51674=CARTESIAN_POINT ( 'NONE',  ( 2.917880565312948704, 62.63708216824730357, 12.26659068614894643 ) ) ;
#51675=CARTESIAN_POINT ( 'NONE',  ( 3.591859063236763294, -1.709698663402913210, -11.09922568453595026 ) ) ;
#51676=CARTESIAN_POINT ( 'NONE',  ( 7.361572987183170547, 47.05059781766745175, 9.846743663894590881 ) ) ;
#51677=CARTESIAN_POINT ( 'NONE',  ( 4.559911319644449179, 43.89701867748816966, 9.422509992056141925 ) ) ;
#51678=CARTESIAN_POINT ( 'NONE',  ( 6.565887622018943937, 0.1653013365970866511, 12.81628187352647430 ) ) ;
#51679=CARTESIAN_POINT ( 'NONE',  ( 10.00000000000000178, 23.05374883491397142, 14.16423886937410082 ) ) ;
#51680=CARTESIAN_POINT ( 'NONE',  ( -2.266590686148945544, 47.22041550158063927, 7.082119434687048631 ) ) ;
#51681=CARTESIAN_POINT ( 'NONE',  ( 2.035157376598822676, 22.43868534415483396, -7.964842623401177768 ) ) ;
#51682=CARTESIAN_POINT ( 'NONE',  ( -1.926860441876563801, 2.662123368507804511, 1.004413902775740978E-15 ) ) ;
#51683=CARTESIAN_POINT ( 'NONE',  ( -0.8801773607110991993, 37.85535201082151247, -2.915334737309923874 ) ) ;
#51684=CARTESIAN_POINT ( 'NONE',  ( 6.565887622018943937, 53.08196800326374643, -12.81628187352647608 ) ) ;
#51686=VERTEX_POINT ( 'NONE', #90768 ) ;
#51688=VERTEX_POINT ( 'NONE', #97309 ) ;
#51690=CARTESIAN_POINT ( 'NONE',  ( -0.3689425029237898834, 46.17874883491397497, -10.36894250292378850 ) ) ;
#51691=CARTESIAN_POINT ( 'NONE',  ( 19.84674366389459266, 18.71726448433411960, -2.638427012816827677 ) ) ;
#51692=CARTESIAN_POINT ( 'NONE',  ( 2.791683348922237240, 45.38393115100079456, -7.208316651077763204 ) ) ;
#51693=CARTESIAN_POINT ( 'NONE',  ( 15.44008868035555793, 66.39701867748817676, -9.422509992056140149 ) ) ;
#51694=CARTESIAN_POINT ( 'NONE',  ( -0.1503990784575328643, 55.12777174578612716, 6.262539305110068177 ) ) ;
#51696=CARTESIAN_POINT ( 'NONE',  ( -0.8801773607110991993, 57.85535201082149825, -2.915334737309923874 ) ) ;
#51697=CARTESIAN_POINT ( 'NONE',  ( -1.099225684535947600, 53.70696800326376064, -6.408140936763238038 ) ) ;
#51701=CARTESIAN_POINT ( 'NONE',  ( 13.79529636645031943, 35.34541550158063927, -14.16423886937409904 ) ) ;
#51702=CARTESIAN_POINT ( 'NONE',  ( 21.09922568453595559, 27.04030133659708568, -6.408140936763230044 ) ) ;
#51703=ORIENTED_EDGE ( 'NONE', *, *, #90341, .T. ) ;
#51704=CARTESIAN_POINT ( 'NONE',  ( 13.43411237798106583, 42.66530133659707502, -12.81628187352647252 ) ) ;
#51705=CARTESIAN_POINT ( 'NONE',  ( 10.00000000000000000, 34.75893115100078745, -9.846743663894594434 ) ) ;
#51706=CARTESIAN_POINT ( 'NONE',  ( 20.88017736071110875, 15.77201867748817143, -2.915334737309920765 ) ) ;
#51708=DIRECTION ( 'NONE',  ( 0.000000000000000000, -1.000000000000000000, 0.000000000000000000 ) ) ;
#51709=CARTESIAN_POINT ( 'NONE',  ( 1.472469842513823179, 45.59226448433412315, -4.923371831947296329 ) ) ;
#51710=CARTESIAN_POINT ( 'NONE',  ( 10.00000000000000178, 47.25893115100078745, 9.846743663894594434 ) ) ;
#51715=CARTESIAN_POINT ( 'NONE',  ( -15.94000000000001371, 93.50000000000000000, -10.09898361729590199 ) ) ;
#51716=CARTESIAN_POINT ( 'NONE',  ( 0.2751277870543045734, 27.28217586085238011, -6.500000000000012434 ) ) ;
#51718=DIRECTION ( 'NONE',  ( -0.07626964003977219908, 0.9970872288863213972, 0.000000000000000000 ) ) ;
#51719=CARTESIAN_POINT ( 'NONE',  ( 19.84674366389459621, 13.50893115100078568, 7.409399052514197653E-17 ) ) ;
#51721=CARTESIAN_POINT ( 'NONE',  ( 21.09922568453594849, 41.20696800326375353, 6.408140936763242479 ) ) ;
#51725=CARTESIAN_POINT ( 'NONE',  ( 17.20831665107776587, 59.13393115100078745, -7.208316651077762316 ) ) ;
#51727=CARTESIAN_POINT ( 'NONE',  ( 2.917880565312950480, 15.97041550158063217, -12.26659068614894821 ) ) ;
#51728=CARTESIAN_POINT ( 'NONE',  ( 10.00000000000000178, 52.25893115100078745, 9.846743663894594434 ) ) ;
#51729=CARTESIAN_POINT ( 'NONE',  ( 21.09922568453595559, 42.04030133659708213, -6.408140936763230044 ) ) ;
#51732=CARTESIAN_POINT ( 'NONE',  ( 1.472469842513823179, 11.42559781766745175, 4.923371831947296329 ) ) ;
#51733=CARTESIAN_POINT ( 'NONE',  ( 0.1916775849787265840, 67.25868815902069286, -6.499999999999991118 ) ) ;
#51734=CARTESIAN_POINT ( 'NONE',  ( 12.63842701281683034, 52.46726448433413026, 9.846743663894596210 ) ) ;
#51735=CARTESIAN_POINT ( 'NONE',  ( 12.91533473730992121, 39.52201867748817676, 10.88017736071110164 ) ) ;
#51737=CARTESIAN_POINT ( 'NONE',  ( 19.80448550324506840, 31.82703681773341131, 6.500000000002799538 ) ) ;
#51738=CARTESIAN_POINT ( 'NONE',  ( 20.88017736071110164, 40.35535201082150536, 2.915334737309930979 ) ) ;
#51739=VERTEX_POINT ( 'NONE', #76267 ) ;
#51740=CARTESIAN_POINT ( 'NONE',  ( 2.035157376598824452, 18.68868534415484106, 7.964842623401179544 ) ) ;
#51741=CARTESIAN_POINT ( 'NONE',  ( 17.20831665107776587, 54.13393115100079456, -7.208316651077762316 ) ) ;
#51742=CARTESIAN_POINT ( 'NONE',  ( -0.8801773607111009756, 38.06368534415484106, 1.068504757029289695E-15 ) ) ;
#51745=CARTESIAN_POINT ( 'NONE',  ( 20.88017736071110519, 55.56368534415484817, 2.639326808657452039E-16 ) ) ;
#51746=CARTESIAN_POINT ( 'NONE',  ( 20.88017736071110164, 20.35535201082150891, 2.915334737309930979 ) ) ;
#51747=CARTESIAN_POINT ( 'NONE',  ( -46.94000000000001194, 103.0000000000000000, 5.000000000000000000 ) ) ;
#51748=CARTESIAN_POINT ( 'NONE',  ( 2.791683348922237240, 5.383931151000785675, -7.208316651077763204 ) ) ;
#51749=CARTESIAN_POINT ( 'NONE',  ( 18.52753015748617571, 28.09226448433411960, 4.923371831947298993 ) ) ;
#51751=CARTESIAN_POINT ( 'NONE',  ( 1.472469842513823179, 66.42559781766745175, 4.923371831947296329 ) ) ;
#51752=CARTESIAN_POINT ( 'NONE',  ( 4.559911319644449179, 3.897018677488171434, 9.422509992056141925 ) ) ;
#51753=LINE ( 'NONE', #74231, #88079 ) ;
#51754=CARTESIAN_POINT ( 'NONE',  ( 6.204703633549690345, 5.762082168247301794, -14.16423886937410259 ) ) ;
#51755=CARTESIAN_POINT ( 'NONE',  ( 13.79529636645031943, 50.34541550158064638, -14.16423886937409904 ) ) ;
#51756=CARTESIAN_POINT ( 'NONE',  ( -2.816281873526473856, 9.123634669930421381, 9.499525473075851096E-16 ) ) ;
#51758=CARTESIAN_POINT ( 'NONE',  ( 7.084665262690076126, 9.105352010821503583, 10.88017736071109987 ) ) ;
#51759=CARTESIAN_POINT ( 'NONE',  ( 5.076628168052703671, 51.84226448433412315, 8.527530157486179263 ) ) ;
#51760=FILL_AREA_STYLE ('',( #28260 ) ) ;
#51763=CARTESIAN_POINT ( 'NONE',  ( 1.472469842513823179, 0.5922644843341181575, -4.923371831947296329 ) ) ;
#51764=CARTESIAN_POINT ( 'NONE',  ( 0.6178305044545838731, 19.74863466993042138, 9.382169495545420901 ) ) ;
#51765=CARTESIAN_POINT ( 'NONE',  ( 1.472469842513823179, 30.59226448433411960, -4.923371831947296329 ) ) ;
#51767=CARTESIAN_POINT ( 'NONE',  ( 1.472469842513823179, 11.42559781766745175, 4.923371831947296329 ) ) ;
#51770=CARTESIAN_POINT ( 'NONE',  ( 4.559911319644449179, 18.89701867748817321, 9.422509992056141925 ) ) ;
#51771=CARTESIAN_POINT ( 'NONE',  ( 22.26659068614894466, 38.88708216824731068, 7.082119434687054849 ) ) ;
#51772=CARTESIAN_POINT ( 'NONE',  ( 10.00000000000000178, 44.31368534415484106, 10.88017736071110342 ) ) ;
#51773=CARTESIAN_POINT ( 'NONE',  ( 12.91533473730993009, 56.60535201082151247, -10.88017736071109987 ) ) ;
#51775=CARTESIAN_POINT ( 'NONE',  ( 14.92337183194729988, 24.34226448433411960, -8.527530157486177487 ) ) ;
#51777=CARTESIAN_POINT ( 'NONE',  ( 17.20831665107776587, 2.883931151000785231, 7.208316651077764980 ) ) ;
#51778=CARTESIAN_POINT ( 'NONE',  ( 19.84674366389459266, 33.71726448433410894, -2.638427012816827677 ) ) ;
#51779=CARTESIAN_POINT ( 'NONE',  ( 0.5774900079438590739, 32.64701867748816966, -5.440088680355550821 ) ) ;
#51782=CARTESIAN_POINT ( 'NONE',  ( -2.816281873526473856, 54.33196800326376064, 3.434112377981055619 ) ) ;
#51784=CARTESIAN_POINT ( 'NONE',  ( 12.63842701281683922, 14.55059781766744997, -9.846743663894590881 ) ) ;
#51785=CARTESIAN_POINT ( 'NONE',  ( 0.6178305044545838731, 49.74863466993041072, 9.382169495545420901 ) ) ;
#51786=CARTESIAN_POINT ( 'NONE',  ( 4.559911319644449179, 2.230352010821504916, -9.422509992056141925 ) ) ;
#51787=CARTESIAN_POINT ( 'NONE',  ( 0.1532563361054082862, 41.21726448433411605, 2.638427012816831674 ) ) ;
#51788=CARTESIAN_POINT ( 'NONE',  ( 14.92337183194729633, 2.675597817667451750, 8.527530157486181039 ) ) ;
#51789=CARTESIAN_POINT ( 'NONE',  ( 20.36894250292379738, 19.92874883491396787, -10.36894250292379027 ) ) ;
#51790=CARTESIAN_POINT ( 'NONE',  ( 22.26659068614895176, 44.72041550158063927, -7.082119434687042414 ) ) ;
#51791=CARTESIAN_POINT ( 'NONE',  ( 10.00000000000000000, 44.75893115100078745, -9.846743663894594434 ) ) ;
#51793=CARTESIAN_POINT ( 'NONE',  ( 12.91533473730992121, 44.52201867748816966, 10.88017736071110164 ) ) ;
#51795=CARTESIAN_POINT ( 'NONE',  ( 12.63842701281683034, 7.467264484334118713, 9.846743663894596210 ) ) ;
#51798=CARTESIAN_POINT ( 'NONE',  ( 0.6178305044545838731, 64.74863466993043914, 9.382169495545420901 ) ) ;
#51800=CARTESIAN_POINT ( 'NONE',  ( 15.44008868035555793, 61.39701867748817676, -9.422509992056140149 ) ) ;
#51803=CARTESIAN_POINT ( 'NONE',  ( 6.204703633549690345, 5.762082168247301794, -14.16423886937410259 ) ) ;
#51804=CARTESIAN_POINT ( 'NONE',  ( 17.20831665107776587, 4.133931151000785675, -7.208316651077762316 ) ) ;
#51807=CARTESIAN_POINT ( 'NONE',  ( -0.8801773607111008646, 13.27201867748817143, 2.915334737309923430 ) ) ;
#51809=CARTESIAN_POINT ( 'NONE',  ( 12.91533473730992121, 34.52201867748817676, 10.88017736071110164 ) ) ;
#51810=CARTESIAN_POINT ( 'NONE',  ( 14.92337183194729988, 59.34226448433412315, -8.527530157486177487 ) ) ;
#51811=ORIENTED_EDGE ( 'NONE', *, *, #55220, .F. ) ;
#51812=CARTESIAN_POINT ( 'NONE',  ( 0.1532563361054082862, 56.21726448433411605, 2.638427012816831674 ) ) ;
#51814=CARTESIAN_POINT ( 'NONE',  ( -0.8801773607110991993, 62.85535201082150536, -2.915334737309923874 ) ) ;
#51815=CARTESIAN_POINT ( 'NONE',  ( 2.791683348922237240, 65.38393115100078035, -7.208316651077763204 ) ) ;
#51817=CARTESIAN_POINT ( 'NONE',  ( 3.591859063236761518, 34.95696800326375353, 11.09922568453594849 ) ) ;
#51818=CARTESIAN_POINT ( 'NONE',  ( 12.91533473730993009, 21.60535201082150536, -10.88017736071109987 ) ) ;
#51820=CARTESIAN_POINT ( 'NONE',  ( 19.84674366389459621, 8.508931151000785675, 7.409399052514197653E-17 ) ) ;
#51821=CARTESIAN_POINT ( 'NONE',  ( 2.035157376598824452, 13.68868534415483751, 7.964842623401179544 ) ) ;
#51825=CARTESIAN_POINT ( 'NONE',  ( -1.099225684535947600, 49.54030133659708923, 6.408140936763237150 ) ) ;
#51826=CARTESIAN_POINT ( 'NONE',  ( 0.5774900079438607392, 43.48035201082151247, 5.440088680355550821 ) ) ;
#51827=CARTESIAN_POINT ( 'NONE',  ( -46.94000000000001194, 101.9887809004034267, -6.851115700664164088 ) ) ;
#51828=CARTESIAN_POINT ( 'NONE',  ( 16.40814093676323893, 60.79030133659709634, 11.09922568453595026 ) ) ;
#51829=CARTESIAN_POINT ( 'NONE',  ( 0.5774900079438607392, 43.48035201082151247, 5.440088680355550821 ) ) ;
#51831=CARTESIAN_POINT ( 'NONE',  ( 12.63842701281683034, 62.46726448433410894, 9.846743663894596210 ) ) ;
#51833=CARTESIAN_POINT ( 'NONE',  ( 14.92337183194729988, 24.34226448433411960, -8.527530157486177487 ) ) ;
#51834=CARTESIAN_POINT ( 'NONE',  ( -2.816281873526471635, 8.915301336597083903, -3.434112377981056508 ) ) ;
#51836=CARTESIAN_POINT ( 'NONE',  ( 14.92337183194729633, 62.67559781766745886, 8.527530157486181039 ) ) ;
#51837=CARTESIAN_POINT ( 'NONE',  ( -0.8801773607111008646, 38.27201867748816255, 2.915334737309923430 ) ) ;
#51838=CARTESIAN_POINT ( 'NONE',  ( 18.52753015748618282, 48.92559781766745886, -4.923371831947291888 ) ) ;
#51840=CARTESIAN_POINT ( 'NONE',  ( 0.1532563361054082862, 26.21726448433411605, 2.638427012816831674 ) ) ;
#51841=CARTESIAN_POINT ( 'NONE',  ( 19.84674366389459266, 8.717264484334116048, -2.638427012816827677 ) ) ;
#51842=CARTESIAN_POINT ( 'NONE',  ( 0.6178305044545818747, 8.498634669930421381, -9.382169495545419124 ) ) ;
#51844=CARTESIAN_POINT ( 'NONE',  ( 0.2751277870542910842, 63.21833443783937412, 6.499999999999992006 ) ) ;
#51846=CARTESIAN_POINT ( 'NONE',  ( 21.09922568453594849, 36.20696800326375353, 6.408140936763242479 ) ) ;
#51847=CARTESIAN_POINT ( 'NONE',  ( 14.92337183194729988, 34.34226448433411605, -8.527530157486177487 ) ) ;
#51850=CARTESIAN_POINT ( 'NONE',  ( 15.44008868035555260, 9.730352010821505360, 9.422509992056143702 ) ) ;
#51851=CARTESIAN_POINT ( 'NONE',  ( 7.361572987183169658, 29.96726448433411960, -9.846743663894592657 ) ) ;
#51854=CARTESIAN_POINT ( 'NONE',  ( 1.042145700049383228, 24.74216108172002038, -6.499999999999826805 ) ) ;
#51856=CARTESIAN_POINT ( 'NONE',  ( 15.44008868035555793, 6.397018677488171434, -9.422509992056140149 ) ) ;
#51857=CARTESIAN_POINT ( 'NONE',  ( -42.93999999999999773, 92.00000000000000000, 9.292893218813452094 ) ) ;
#51859=CARTESIAN_POINT ( 'NONE',  ( 2.035157376598824452, 13.68868534415483751, 7.964842623401179544 ) ) ;
#51860=CARTESIAN_POINT ( 'NONE',  ( 13.79529636645030344, 48.26208216824728936, 14.16423886937410614 ) ) ;
#51861=CARTESIAN_POINT ( 'NONE',  ( -2.266590686148945544, 56.38708216824731068, -7.082119434687050408 ) ) ;
#51865=CARTESIAN_POINT ( 'NONE',  ( 10.00000000000000178, 12.25893115100078568, 9.846743663894594434 ) ) ;
#51866=CARTESIAN_POINT ( 'NONE',  ( 13.43411237798105340, 0.5819680032637533085, 12.81628187352647963 ) ) ;
#51869=CARTESIAN_POINT ( 'NONE',  ( 2.791683348922240793, 61.63393115100079456, 7.208316651077764092 ) ) ;
#51872=CARTESIAN_POINT ( 'NONE',  ( 18.52753015748617571, 63.09226448433412315, 4.923371831947298993 ) ) ;
#51873=CARTESIAN_POINT ( 'NONE',  ( 10.00000000000000178, 13.05374883491396787, 14.16423886937410082 ) ) ;
#51874=CARTESIAN_POINT ( 'NONE',  ( 5.076628168052703671, 21.84226448433411960, 8.527530157486179263 ) ) ;
#51878=CARTESIAN_POINT ( 'NONE',  ( 24.16423886937410614, 44.30374883491397497, 8.672049930838204340E-16 ) ) ;
#51879=CARTESIAN_POINT ( 'NONE',  ( 5.076628168052703671, 6.842264484334118713, 8.527530157486179263 ) ) ;
#51881=LINE ( 'NONE', #97900, #53436 ) ;
#51882=CARTESIAN_POINT ( 'NONE',  ( 2.035157376598822676, 37.43868534415484106, -7.964842623401177768 ) ) ;
#51883=CARTESIAN_POINT ( 'NONE',  ( 19.38216949554541557, 37.24863466993041783, -9.382169495545420901 ) ) ;
#51884=CARTESIAN_POINT ( 'NONE',  ( 4.559911319644449179, 3.897018677488170990, 9.422509992056141925 ) ) ;
#51885=CARTESIAN_POINT ( 'NONE',  ( 3.591859063236763294, 33.29030133659708213, -11.09922568453595026 ) ) ;
#51886=CARTESIAN_POINT ( 'NONE',  ( -2.816281873526473856, 64.33196800326376774, 3.434112377981055619 ) ) ;
#51889=CARTESIAN_POINT ( 'NONE',  ( 22.26659068614895176, 39.72041550158063217, -7.082119434687042414 ) ) ;
#51890=FACE_OUTER_BOUND ( 'NONE', #20336, .T. ) ;
#51891=CARTESIAN_POINT ( 'NONE',  ( 20.88017736071110519, 5.563685344154837509, 2.639326808657452039E-16 ) ) ;
#51892=CARTESIAN_POINT ( 'NONE',  ( 17.96484262340118221, 21.18868534415483396, -7.964842623401177768 ) ) ;
#51893=DIRECTION ( 'NONE',  ( -0.000000000000000000, 1.000000000000000000, 0.000000000000000000 ) ) ;
#51895=CARTESIAN_POINT ( 'NONE',  ( 10.00000000000000000, 51.81368534415484106, -10.88017736071110342 ) ) ;
#51896=CARTESIAN_POINT ( 'NONE',  ( 19.42250999205614548, 50.98035201082151247, -5.440088680355545492 ) ) ;
#51897=CARTESIAN_POINT ( 'NONE',  ( 22.81628187352648496, 31.83196800326375353, -3.434112377981050290 ) ) ;
#51900=CARTESIAN_POINT ( 'NONE',  ( 2.791683348922240793, 26.63393115100078745, 7.208316651077764092 ) ) ;
#51902=CARTESIAN_POINT ( 'NONE',  ( 2.035157376598824452, 63.68868534415484106, 7.964842623401179544 ) ) ;
#51903=CARTESIAN_POINT ( 'NONE',  ( -1.099225684535947600, 18.70696800326375353, -6.408140936763238038 ) ) ;
#51905=CARTESIAN_POINT ( 'NONE',  ( 7.084665262690076126, 14.10535201082150358, 10.88017736071109987 ) ) ;
#51906=CARTESIAN_POINT ( 'NONE',  ( 5.076628168052703671, 41.84226448433411605, 8.527530157486179263 ) ) ;
#51907=CARTESIAN_POINT ( 'NONE',  ( -2.816281873526471635, 48.91530133659708213, -3.434112377981056508 ) ) ;
#51908=CARTESIAN_POINT ( 'NONE',  ( 14.92337183194729633, 17.67559781766745175, 8.527530157486181039 ) ) ;
#51909=CARTESIAN_POINT ( 'NONE',  ( 6.204703633549690345, 5.762082168247301794, -14.16423886937410259 ) ) ;
#51910=CARTESIAN_POINT ( 'NONE',  ( 0.1532563361054082862, 36.21726448433410894, 2.638427012816831674 ) ) ;
#51911=CARTESIAN_POINT ( 'NONE',  ( 19.42250999205614193, 15.14701867748817143, 5.440088680355555262 ) ) ;
#51912=DIRECTION ( 'NONE',  ( 0.000000000000000000, -1.000000000000000000, -0.000000000000000000 ) ) ;
#51913=CARTESIAN_POINT ( 'NONE',  ( 14.92337183194729633, 42.67559781766745886, 8.527530157486181039 ) ) ;
#51914=CARTESIAN_POINT ( 'NONE',  ( 2.035157376598822676, 32.43868534415483396, -7.964842623401177768 ) ) ;
#51916=CARTESIAN_POINT ( 'NONE',  ( 19.42250999205614548, 10.98035201082150536, -5.440088680355545492 ) ) ;
#51918=CARTESIAN_POINT ( 'NONE',  ( 7.084665262690076126, 22.02201867748817321, -10.88017736071110164 ) ) ;
#51919=EDGE_CURVE ( 'NONE', #6963, #8562, #21551, .T. ) ;
#51920=CARTESIAN_POINT ( 'NONE',  ( 19.38216949554541202, 45.99863466993041072, 9.382169495545424454 ) ) ;
#51921=CARTESIAN_POINT ( 'NONE',  ( 0.5774900079438607392, 28.48035201082150891, 5.440088680355550821 ) ) ;
#51922=CARTESIAN_POINT ( 'NONE',  ( 1.959929470562281395, 45.51528370094808196, -5.767676674365853629 ) ) ;
#51923=CARTESIAN_POINT ( 'NONE',  ( 2.035157376598824452, 33.68868534415484106, 7.964842623401179544 ) ) ;
#51925=CARTESIAN_POINT ( 'NONE',  ( 2.791683348922237240, 55.38393115100078745, -7.208316651077763204 ) ) ;
#51926=CARTESIAN_POINT ( 'NONE',  ( 4.559911319644449179, 38.89701867748817676, 9.422509992056141925 ) ) ;
#51928=B_SPLINE_CURVE_WITH_KNOTS ( 'NONE', 3,
 ( #10208, #40701, #2727, #16724 ),
 .UNSPECIFIED., .F., .F.,
 ( 4, 4 ),
 ( 5.204893179191170684E-17, 0.002562518741975298216 ),
 .UNSPECIFIED. ) ;
#51931=CARTESIAN_POINT ( 'NONE',  ( 10.00000000000000178, 43.05374883491397497, 14.16423886937410082 ) ) ;
#51932=CARTESIAN_POINT ( 'NONE',  ( 4.559911319644449179, 57.23035201082150536, -9.422509992056141925 ) ) ;
#51936=CARTESIAN_POINT ( 'NONE',  ( 0.1532563361054083140, 66.00893115100079456, 1.131784320476157264E-15 ) ) ;
#51937=PRESENTATION_STYLE_ASSIGNMENT (( #26111 ) ) ;
#51938=CARTESIAN_POINT ( 'NONE',  ( 0.1532563361054083140, 26.00893115100078745, 1.131784320476157264E-15 ) ) ;
#51940=CARTESIAN_POINT ( 'NONE',  ( 12.63842701281683034, 22.46726448433411605, 9.846743663894596210 ) ) ;
#51942=CARTESIAN_POINT ( 'NONE',  ( 12.91533473730993009, 31.60535201082150891, -10.88017736071109987 ) ) ;
#51943=CARTESIAN_POINT ( 'NONE',  ( 19.84674366389459266, 18.71726448433411960, -2.638427012816827677 ) ) ;
#51944=CARTESIAN_POINT ( 'NONE',  ( -1.099225684535947600, 14.54030133659708568, 6.408140936763237150 ) ) ;
#51946=CARTESIAN_POINT ( 'NONE',  ( 4.559911319644449179, 62.23035201082150536, -9.422509992056141925 ) ) ;
#51947=CARTESIAN_POINT ( 'NONE',  ( 2.035157376598822676, 32.43868534415483396, -7.964842623401177768 ) ) ;
#51948=CARTESIAN_POINT ( 'NONE',  ( 16.40814093676323893, 60.79030133659709634, 11.09922568453595026 ) ) ;
#51949=CARTESIAN_POINT ( 'NONE',  ( 6.204703633549690345, 42.84541550158063217, 14.16423886937410082 ) ) ;
#51954=CARTESIAN_POINT ( 'NONE',  ( 6.565887622018943937, 10.16530133659708746, 12.81628187352647430 ) ) ;
#51955=CARTESIAN_POINT ( 'NONE',  ( 19.42250999205614193, 5.147018677488171434, 5.440088680355555262 ) ) ;
#51957=CARTESIAN_POINT ( 'NONE',  ( 15.44008868035555260, 49.73035201082150536, 9.422509992056143702 ) ) ;
#51960=CARTESIAN_POINT ( 'NONE',  ( -0.8801773607111009756, 63.06368534415484106, 1.068504757029289695E-15 ) ) ;
#51962=CARTESIAN_POINT ( 'NONE',  ( 18.52753015748618282, 38.92559781766745175, -4.923371831947291888 ) ) ;
#51963=CARTESIAN_POINT ( 'NONE',  ( 5.076628168052704559, 30.17559781766745175, -8.527530157486179263 ) ) ;
#51964=CARTESIAN_POINT ( 'NONE',  ( 0.1532563361054100626, 20.80059781766744464, -2.638427012816831230 ) ) ;
#51965=VECTOR ( 'NONE', #93789, 1000.000000000000000 ) ;
#51967=CARTESIAN_POINT ( 'NONE',  ( 2.791683348922237240, 5.383931151000785675, -7.208316651077763204 ) ) ;
#51968=CARTESIAN_POINT ( 'NONE',  ( 5.500000000000000000, 11.00000000000000000, 5.000000000000000000 ) ) ;
#51970=CARTESIAN_POINT ( 'NONE',  ( 18.52753015748617571, 38.09226448433412315, 4.923371831947298993 ) ) ;
#51972=CARTESIAN_POINT ( 'NONE',  ( 10.00000000000000000, 57.87363466993042493, -12.81628187352647608 ) ) ;
#51973=CARTESIAN_POINT ( 'NONE',  ( 18.29284471827481440, 55.40189080397284016, -6.499999999999946709 ) ) ;
#51974=CARTESIAN_POINT ( 'NONE',  ( 0.6178305044545818747, 3.498634669930420049, -9.382169495545419124 ) ) ;
#51976=CARTESIAN_POINT ( 'NONE',  ( 4.559911319644449179, 12.23035201082150536, -9.422509992056141925 ) ) ;
#51978=CARTESIAN_POINT ( 'NONE',  ( 17.08211943468705130, 33.47041550158063927, 12.26659068614894998 ) ) ;
#51980=CARTESIAN_POINT ( 'NONE',  ( 24.16423886937410614, 24.51208216824730002, -3.795296366450302550 ) ) ;
#51981=CARTESIAN_POINT ( 'NONE',  ( 10.00000000000000178, 48.05374883491396787, 14.16423886937410082 ) ) ;
#51982=CARTESIAN_POINT ( 'NONE',  ( -4.164238869374099927, 7.012082168247302683, 3.795296366450308767 ) ) ;
#51983=CARTESIAN_POINT ( 'NONE',  ( 17.08211943468705130, 13.47041550158063572, 12.26659068614894998 ) ) ;
#51984=CARTESIAN_POINT ( 'NONE',  ( -0.8801773607111009756, 48.06368534415484817, 1.068504757029289695E-15 ) ) ;
#51987=CARTESIAN_POINT ( 'NONE',  ( 17.20831665107776587, 34.13393115100078745, -7.208316651077762316 ) ) ;
#51988=CARTESIAN_POINT ( 'NONE',  ( 19.42250999205614193, 65.14701867748817676, 5.440088680355555262 ) ) ;
#51989=CARTESIAN_POINT ( 'NONE',  ( 19.84674366389459621, 23.50893115100078390, 7.409399052514197653E-17 ) ) ;
#51990=CARTESIAN_POINT ( 'NONE',  ( 17.96484262340118221, 16.18868534415483396, -7.964842623401177768 ) ) ;
#51991=CARTESIAN_POINT ( 'NONE',  ( 0.6178305044545838731, 59.74863466993041783, 9.382169495545420901 ) ) ;
#51992=CARTESIAN_POINT ( 'NONE',  ( 17.20831665107776587, 54.13393115100079456, -7.208316651077762316 ) ) ;
#51994=CARTESIAN_POINT ( 'NONE',  ( 17.20831665107776587, 29.13393115100078390, -7.208316651077762316 ) ) ;
#51995=CARTESIAN_POINT ( 'NONE',  ( 22.81628187352647785, 46.62363466993041783, 6.195893100308588602E-16 ) ) ;
#51997=CARTESIAN_POINT ( 'NONE',  ( 10.00000000000000000, 36.81368534415484106, -10.88017736071110342 ) ) ;
#51998=CARTESIAN_POINT ( 'NONE',  ( 7.361572987183170547, 37.05059781766744464, 9.846743663894590881 ) ) ;
#51999=CARTESIAN_POINT ( 'NONE',  ( 17.08211943468705840, 30.13708216824730357, -12.26659068614894466 ) ) ;
#52001=CARTESIAN_POINT ( 'NONE',  ( 6.204703633549690345, 5.762082168247301794, -14.16423886937410259 ) ) ;
#52003=CARTESIAN_POINT ( 'NONE',  ( 20.88017736071110519, 65.56368534415483396, 2.639326808657452039E-16 ) ) ;
#52004=CARTESIAN_POINT ( 'NONE',  ( 17.96484262340118221, 59.93868534415484106, 7.964842623401181321 ) ) ;
#52005=CARTESIAN_POINT ( 'NONE',  ( 20.36894250292379738, 54.92874883491396076, -10.36894250292379027 ) ) ;
#52006=CARTESIAN_POINT ( 'NONE',  ( 3.591859063236763294, 3.290301336597087012, -11.09922568453595026 ) ) ;
#52008=CARTESIAN_POINT ( 'NONE',  ( 17.96484262340118221, 61.18868534415482685, -7.964842623401177768 ) ) ;
#52011=CARTESIAN_POINT ( 'NONE',  ( 20.88017736071110164, 10.35535201082150714, 2.915334737309930979 ) ) ;
#52012=CARTESIAN_POINT ( 'NONE',  ( 20.88017736071110519, 15.56368534415483751, 2.639326808657452039E-16 ) ) ;
#52013=CARTESIAN_POINT ( 'NONE',  ( 18.52753015748618282, 48.92559781766745886, -4.923371831947291888 ) ) ;
#52014=CARTESIAN_POINT ( 'NONE',  ( 22.81628187352647785, 56.62363466993042493, 6.195893100308588602E-16 ) ) ;
#52016=ORIENTED_EDGE ( 'NONE', *, *, #30041, .T. ) ;
#52017=CARTESIAN_POINT ( 'NONE',  ( 10.00000000000000000, 16.81368534415483751, -10.88017736071110342 ) ) ;
#52018=CARTESIAN_POINT ( 'NONE',  ( -2.816281873526471635, 3.915301336597087456, -3.434112377981056508 ) ) ;
#52020=CARTESIAN_POINT ( 'NONE',  ( 5.076628168052703671, 16.84226448433411960, 8.527530157486179263 ) ) ;
#52021=CARTESIAN_POINT ( 'NONE',  ( 12.63842701281683922, 44.55059781766745175, -9.846743663894590881 ) ) ;
#52022=CARTESIAN_POINT ( 'NONE',  ( -0.8801773607110991993, 32.85535201082151247, -2.915334737309923874 ) ) ;
#52023=CARTESIAN_POINT ( 'NONE',  ( 3.591859063236761518, 14.95696800326375531, 11.09922568453594849 ) ) ;
#52024=CARTESIAN_POINT ( 'NONE',  ( 15.44008868035555793, 51.39701867748816966, -9.422509992056140149 ) ) ;
#52026=CARTESIAN_POINT ( 'NONE',  ( 0.6178305044545818747, 53.49863466993041072, -9.382169495545419124 ) ) ;
#52028=CARTESIAN_POINT ( 'NONE',  ( 0.5774900079438590739, 67.64701867748817676, -5.440088680355550821 ) ) ;
#52029=CARTESIAN_POINT ( 'NONE',  ( 21.09922568453595559, 37.04030133659708923, -6.408140936763230044 ) ) ;
#52030=CARTESIAN_POINT ( 'NONE',  ( 14.92337183194729633, 7.675597817667451750, 8.527530157486181039 ) ) ;
#52031=CARTESIAN_POINT ( 'NONE',  ( 19.42250999205614193, 35.14701867748816966, 5.440088680355555262 ) ) ;
#52032=CARTESIAN_POINT ( 'NONE',  ( 14.92337183194729988, 64.34226448433412315, -8.527530157486177487 ) ) ;
#52033=CARTESIAN_POINT ( 'NONE',  ( 0.1532563361054083140, 51.00893115100078745, 1.131784320476157264E-15 ) ) ;
#52034=CARTESIAN_POINT ( 'NONE',  ( 7.361572987183170547, 12.05059781766744997, 9.846743663894590881 ) ) ;
#52035=CARTESIAN_POINT ( 'NONE',  ( 19.84674366389459621, 8.508931151000785675, 7.409399052514197653E-17 ) ) ;
#52037=CARTESIAN_POINT ( 'NONE',  ( 10.00000000000000178, 43.05374883491397497, 14.16423886937410082 ) ) ;
#52039=CARTESIAN_POINT ( 'NONE',  ( 20.32896413005680358, 24.74545670184113888, 5.963430220938287007 ) ) ;
#52044=CARTESIAN_POINT ( 'NONE',  ( 10.00000000000000000, 65.55374883491396076, -14.16423886937410082 ) ) ;
#52045=CARTESIAN_POINT ( 'NONE',  ( -0.8801773607110991993, 2.855352010821504471, -2.915334737309923874 ) ) ;
#52046=CARTESIAN_POINT ( 'NONE',  ( 7.361572987183170547, 27.05059781766745175, 9.846743663894590881 ) ) ;
#52047=CARTESIAN_POINT ( 'NONE',  ( 16.40814093676324603, 27.45696800326375708, -11.09922568453594671 ) ) ;
#52050=CARTESIAN_POINT ( 'NONE',  ( 10.00000000000000000, 0.5537488349139675359, -14.16423886937410082 ) ) ;
#52051=CARTESIAN_POINT ( 'NONE',  ( 12.91533473730993009, 11.60535201082150536, -10.88017736071109987 ) ) ;
#52052=CARTESIAN_POINT ( 'NONE',  ( -2.266590686148945544, 62.22041550158063927, 7.082119434687048631 ) ) ;
#52053=CARTESIAN_POINT ( 'NONE',  ( 12.63842701281683922, 29.55059781766745175, -9.846743663894590881 ) ) ;
#52055=CARTESIAN_POINT ( 'NONE',  ( 2.791683348922240793, 16.63393115100078745, 7.208316651077764092 ) ) ;
#52062=CARTESIAN_POINT ( 'NONE',  ( 13.79529636645030344, 18.26208216824730002, 14.16423886937410614 ) ) ;
#52063=CARTESIAN_POINT ( 'NONE',  ( 10.00000000000000178, 19.31368534415484106, 10.88017736071110342 ) ) ;
#52064=CARTESIAN_POINT ( 'NONE',  ( 2.035157376598824452, 43.68868534415484106, 7.964842623401179544 ) ) ;
#52065=CARTESIAN_POINT ( 'NONE',  ( 2.791683348922240793, 66.63393115100079456, 7.208316651077764092 ) ) ;
#52066=CARTESIAN_POINT ( 'NONE',  ( 21.09922568453594849, 21.20696800326375353, 6.408140936763242479 ) ) ;
#52067=CARTESIAN_POINT ( 'NONE',  ( 6.204703633549690345, 2.845415501580634388, 14.16423886937410082 ) ) ;
#52069=CIRCLE ( 'NONE', #69621, 62.00000000000000000 ) ;
#52070=ADVANCED_FACE ( 'NONE', ( #54243 ), #86662, .T. ) ;
#52072=CARTESIAN_POINT ( 'NONE',  ( 22.81628187352648496, 26.83196800326374998, -3.434112377981050290 ) ) ;
#52074=CARTESIAN_POINT ( 'NONE',  ( 12.63842701281683034, 32.46726448433412315, 9.846743663894596210 ) ) ;
#52076=CARTESIAN_POINT ( 'NONE',  ( 19.42250999205614193, 10.14701867748816966, 5.440088680355555262 ) ) ;
#52078=CARTESIAN_POINT ( 'NONE',  ( 24.16423886937409904, 64.09541550158064638, 3.795296366450317205 ) ) ;
#52080=CARTESIAN_POINT ( 'NONE',  ( 17.96484262340118221, 44.93868534415483396, 7.964842623401181321 ) ) ;
#52081=CARTESIAN_POINT ( 'NONE',  ( 19.42250999205614193, 65.14701867748817676, 5.440088680355555262 ) ) ;
#52082=CARTESIAN_POINT ( 'NONE',  ( -0.8801773607111008646, 63.27201867748817676, 2.915334737309923430 ) ) ;
#52083=CARTESIAN_POINT ( 'NONE',  ( 19.42250999205614193, 60.14701867748817676, 5.440088680355555262 ) ) ;
#52087=CARTESIAN_POINT ( 'NONE',  ( 0.1532563361054083140, 31.00893115100078390, 1.131784320476157264E-15 ) ) ;
#52089=CARTESIAN_POINT ( 'NONE',  ( 0.1532563361054100626, 60.80059781766744464, -2.638427012816831230 ) ) ;
#52095=CARTESIAN_POINT ( 'NONE',  ( 20.88017736071110519, 10.56368534415483929, 2.639326808657452039E-16 ) ) ;
#52096=PLANE ( 'NONE',  #69070 ) ;
#52098=CARTESIAN_POINT ( 'NONE',  ( 14.49999999999999822, 60.50000000000000000, -5.000000000000000000 ) ) ;
#52099=CARTESIAN_POINT ( 'NONE',  ( 19.84674366389459621, 43.50893115100078745, 7.409399052514197653E-17 ) ) ;
#52102=CARTESIAN_POINT ( 'NONE',  ( 13.43411237798106583, 17.66530133659708923, -12.81628187352647252 ) ) ;
#52103=CARTESIAN_POINT ( 'NONE',  ( 7.361572987183170547, 17.05059781766745530, 9.846743663894590881 ) ) ;
#52104=EDGE_CURVE ( 'NONE', #31975, #30617, #59193, .T. ) ;
#52106=CARTESIAN_POINT ( 'NONE',  ( -1.099225684535947600, -1.293031996736246469, -6.408140936763238038 ) ) ;
#52107=CARTESIAN_POINT ( 'NONE',  ( 20.15039907845753930, 0.07447313448805115144, 6.262539305110068177 ) ) ;
#52110=CARTESIAN_POINT ( 'NONE',  ( 0.5774900079438607392, 8.480352010821505360, 5.440088680355550821 ) ) ;
#52111=CARTESIAN_POINT ( 'NONE',  ( -4.164238869374099927, 22.01208216824730357, 3.795296366450308767 ) ) ;
#52112=CARTESIAN_POINT ( 'NONE',  ( 1.472469842513823179, 26.42559781766745175, 4.923371831947296329 ) ) ;
#52113=CARTESIAN_POINT ( 'NONE',  ( 2.035157376598824452, 53.68868534415484817, 7.964842623401179544 ) ) ;
#52114=CARTESIAN_POINT ( 'NONE',  ( 22.81628187352648496, 36.83196800326376064, -3.434112377981050290 ) ) ;
#52116=CARTESIAN_POINT ( 'NONE',  ( 0.5774900079438607392, 18.48035201082150536, 5.440088680355550821 ) ) ;
#52119=CARTESIAN_POINT ( 'NONE',  ( 10.00000000000000178, 67.25893115100079456, 9.846743663894594434 ) ) ;
#52120=CARTESIAN_POINT ( 'NONE',  ( 0.1532563361054083140, 21.00893115100078745, 1.131784320476157264E-15 ) ) ;
#52122=CARTESIAN_POINT ( 'NONE',  ( 10.00000000000000000, 32.87363466993042493, -12.81628187352647608 ) ) ;
#52124=CARTESIAN_POINT ( 'NONE',  ( 7.084665262690076126, 37.02201867748817676, -10.88017736071110164 ) ) ;
#52125=PLANE ( 'NONE',  #49589 ) ;
#52127=CARTESIAN_POINT ( 'NONE',  ( 7.084665262690076126, 57.02201867748817676, -10.88017736071110164 ) ) ;
#52128=CARTESIAN_POINT ( 'NONE',  ( 10.00000000000000000, 36.81368534415484106, -10.88017736071110342 ) ) ;
#52129=CARTESIAN_POINT ( 'NONE',  ( 10.00000000000000000, 41.81368534415484106, -10.88017736071110342 ) ) ;
#52130=CARTESIAN_POINT ( 'NONE',  ( 1.472469842513823179, 66.42559781766745175, 4.923371831947296329 ) ) ;
#52131=CARTESIAN_POINT ( 'NONE',  ( -0.8801773607110991993, 52.85535201082151247, -2.915334737309923874 ) ) ;
#52133=UNCERTAINTY_MEASURE_WITH_UNIT (LENGTH_MEASURE( 1.000000000000000082E-05 ), #30053, 'distance_accuracy_value', 'NONE');
#52134=CARTESIAN_POINT ( 'NONE',  ( 2.791683348922240793, 31.63393115100078745, 7.208316651077764092 ) ) ;
#52135=CARTESIAN_POINT ( 'NONE',  ( 15.44008868035555793, 11.39701867748817143, -9.422509992056140149 ) ) ;
#52136=CARTESIAN_POINT ( 'NONE',  ( 0.6178305044545818747, 13.49863466993041783, -9.382169495545419124 ) ) ;
#52138=CARTESIAN_POINT ( 'NONE',  ( 17.96484262340118221, 24.93868534415484461, 7.964842623401181321 ) ) ;
#52140=CARTESIAN_POINT ( 'NONE',  ( 19.42250999205614548, 25.98035201082150891, -5.440088680355545492 ) ) ;
#52141=CARTESIAN_POINT ( 'NONE',  ( 4.559911319644449179, 67.23035201082150536, -9.422509992056141925 ) ) ;
#52142=CARTESIAN_POINT ( 'NONE',  ( 6.204703633549690345, 42.84541550158063217, 14.16423886937410082 ) ) ;
#52143=CARTESIAN_POINT ( 'NONE',  ( 7.361572987183170547, 17.05059781766745530, 9.846743663894590881 ) ) ;
#52144=CARTESIAN_POINT ( 'NONE',  ( 7.084665262690076126, 47.02201867748818387, -10.88017736071110164 ) ) ;
#52146=FILL_AREA_STYLE_COLOUR ( '', #23436 ) ;
#52151=CARTESIAN_POINT ( 'NONE',  ( 18.52753015748618282, 43.92559781766745175, -4.923371831947291888 ) ) ;
#52153=VERTEX_POINT ( 'NONE', #22682 ) ;
#52155=CARTESIAN_POINT ( 'NONE',  ( -2.266590686148945544, 22.22041550158063572, 7.082119434687048631 ) ) ;
#52156=CARTESIAN_POINT ( 'NONE',  ( 17.08211943468705130, 23.47041550158063572, 12.26659068614894998 ) ) ;
#52158=CARTESIAN_POINT ( 'NONE',  ( 10.00000000000000178, 54.31368534415484106, 10.88017736071110342 ) ) ;
#52159=CARTESIAN_POINT ( 'NONE',  ( 4.559911319644449179, 3.897018677488171434, 9.422509992056141925 ) ) ;
#52160=CARTESIAN_POINT ( 'NONE',  ( 16.40814093676323893, 0.7903013365970867898, 11.09922568453595026 ) ) ;
#52161=CARTESIAN_POINT ( 'NONE',  ( 19.84674366389459266, 43.71726448433410894, -2.638427012816827677 ) ) ;
#52163=CARTESIAN_POINT ( 'NONE',  ( 19.42250999205614193, 45.14701867748817676, 5.440088680355555262 ) ) ;
#52164=CARTESIAN_POINT ( 'NONE',  ( -2.816281873526471635, 3.915301336597087456, -3.434112377981056508 ) ) ;
#52165=CARTESIAN_POINT ( 'NONE',  ( 2.917880565312950480, 10.97041550158063572, -12.26659068614894821 ) ) ;
#52166=CARTESIAN_POINT ( 'NONE',  ( -0.8801773607111008646, 8.272018677488171434, 2.915334737309923430 ) ) ;
#52167=CARTESIAN_POINT ( 'NONE',  ( 2.035157376598824452, 13.68868534415483751, 7.964842623401179544 ) ) ;
#52168=CARTESIAN_POINT ( 'NONE',  ( 15.44008868035555793, 46.39701867748817676, -9.422509992056140149 ) ) ;
#52169=CARTESIAN_POINT ( 'NONE',  ( 6.565887622018943937, 45.16530133659708923, 12.81628187352647430 ) ) ;
#52172=CARTESIAN_POINT ( 'NONE',  ( -10.00000000000000000, 82.00000000000000000, -5.000000000000000000 ) ) ;
#52175=MECHANICAL_DESIGN_GEOMETRIC_PRESENTATION_REPRESENTATION('',(#53747),#68097);
#52177=CARTESIAN_POINT ( 'NONE',  ( 10.00000000000000000, 40.55374883491397497, -14.16423886937410082 ) ) ;
#52178=CARTESIAN_POINT ( 'NONE',  ( 20.88017736071110519, 10.56368534415483929, 2.639326808657452039E-16 ) ) ;
#52179=CARTESIAN_POINT ( 'NONE',  ( 0.1532563361054082862, 26.21726448433411605, 2.638427012816831674 ) ) ;
#52180=CARTESIAN_POINT ( 'NONE',  ( 18.52753015748618282, 43.92559781766745175, -4.923371831947291888 ) ) ;
#52181=CARTESIAN_POINT ( 'NONE',  ( 4.559911319644449179, 63.89701867748817676, 9.422509992056141925 ) ) ;
#52182=CARTESIAN_POINT ( 'NONE',  ( 10.00000000000000000, -0.2410688489992152128, -9.846743663894594434 ) ) ;
#52185=ORIENTED_EDGE ( 'NONE', *, *, #72820, .F. ) ;
#52186=CARTESIAN_POINT ( 'NONE',  ( 2.917880565312948704, 37.63708216824731068, 12.26659068614894643 ) ) ;
#52188=CARTESIAN_POINT ( 'NONE',  ( -1.099225684535947600, 28.70696800326375353, -6.408140936763238038 ) ) ;
#52190=CARTESIAN_POINT ( 'NONE',  ( 13.43411237798105340, 60.58196800326376064, 12.81628187352647963 ) ) ;
#52191=CARTESIAN_POINT ( 'NONE',  ( 19.42250999205614193, 25.14701867748817321, 5.440088680355555262 ) ) ;
#52192=CARTESIAN_POINT ( 'NONE',  ( 19.84674366389459621, 38.50893115100078745, 7.409399052514197653E-17 ) ) ;
#52193=CARTESIAN_POINT ( 'NONE',  ( 19.42250999205614548, 30.98035201082150536, -5.440088680355545492 ) ) ;
#52194=( BOUNDED_CURVE ( )  B_SPLINE_CURVE ( 2, ( #62694, #93194, #33663, #9213, #63185, #64159, #79181, #1738, #24721 ),
 .UNSPECIFIED., .F., .T. ) 
 B_SPLINE_CURVE_WITH_KNOTS ( ( 3, 2, 2, 2, 3 ),
 ( 0.8667998787605536437, 0.8690476190476190688, 0.8750000000000000000, 0.8809523809523809312, 0.8832001212394463563 ),
 .UNSPECIFIED. ) 
 CURVE ( )  GEOMETRIC_REPRESENTATION_ITEM ( )  RATIONAL_B_SPLINE_CURVE ( ( 0.9839835555609424134, 0.9871328979762474809, 1.000000000000000000, 0.9659258262890683122, 1.000000000000000000, 0.9659258262890683122, 1.000000000000000000, 0.9871328979762474809, 0.9839835555609424134 ) ) 
 REPRESENTATION_ITEM ( '' )  );
#52196=CARTESIAN_POINT ( 'NONE',  ( 0.1532563361054083140, 46.00893115100079456, 1.131784320476157264E-15 ) ) ;
#52197=CARTESIAN_POINT ( 'NONE',  ( 2.791683348922240793, 46.63393115100077324, 7.208316651077764092 ) ) ;
#52201=CARTESIAN_POINT ( 'NONE',  ( 2.148416515056641440, 32.23726573380442062, 6.499999999999995559 ) ) ;
#52205=CARTESIAN_POINT ( 'NONE',  ( 14.92337183194729633, 22.67559781766745175, 8.527530157486181039 ) ) ;
#52206=CARTESIAN_POINT ( 'NONE',  ( 22.81628187352648496, 31.83196800326375353, -3.434112377981050290 ) ) ;
#52209=CARTESIAN_POINT ( 'NONE',  ( 2.791683348922237240, 55.38393115100078745, -7.208316651077763204 ) ) ;
#52211=CARTESIAN_POINT ( 'NONE',  ( 10.00000000000000000, 44.75893115100078745, -9.846743663894594434 ) ) ;
#52212=CARTESIAN_POINT ( 'NONE',  ( 10.00000000000000000, 40.55374883491397497, -14.16423886937410082 ) ) ;
#52213=CARTESIAN_POINT ( 'NONE',  ( 19.84674366389459621, 48.50893115100078745, 7.409399052514197653E-17 ) ) ;
#52214=CARTESIAN_POINT ( 'NONE',  ( -1.099225684535947600, 48.70696800326375353, -6.408140936763238038 ) ) ;
#52215=DIRECTION ( 'NONE',  ( 0.9970872288863209532, 0.07626964003977952655, 0.000000000000000000 ) ) ;
#52216=CARTESIAN_POINT ( 'NONE',  ( 0.1532563361054082862, 1.217264484334117824, 2.638427012816831674 ) ) ;
#52218=CARTESIAN_POINT ( 'NONE',  ( -0.1503990784575323369, 4.248846992468888750, -6.262539305110070842 ) ) ;
#52219=CARTESIAN_POINT ( 'NONE',  ( 2.791683348922240793, 46.63393115100077324, 7.208316651077764092 ) ) ;
#52220=CARTESIAN_POINT ( 'NONE',  ( 15.44008868035555793, 41.39701867748817676, -9.422509992056140149 ) ) ;
#52221=EDGE_CURVE ( 'NONE', #3044, #96338, #59789, .T. ) ;
#52224=CARTESIAN_POINT ( 'NONE',  ( 19.88701968852526747, 31.79427333184086635, 6.480634945678623637 ) ) ;
#52225=CARTESIAN_POINT ( 'NONE',  ( -0.8801773607110991993, 47.85535201082150536, -2.915334737309923874 ) ) ;
#52228=CARTESIAN_POINT ( 'NONE',  ( 19.42250999205614193, 10.14701867748816966, 5.440088680355555262 ) ) ;
#52229=CARTESIAN_POINT ( 'NONE',  ( 2.791683348922237240, 65.38393115100078035, -7.208316651077763204 ) ) ;
#52230=CARTESIAN_POINT ( 'NONE',  ( 2.035157376598824452, 48.68868534415483396, 7.964842623401179544 ) ) ;
#52232=CARTESIAN_POINT ( 'NONE',  ( 17.96484262340118221, 56.18868534415484817, -7.964842623401177768 ) ) ;
#52233=CARTESIAN_POINT ( 'NONE',  ( 19.72487221294570858, 70.00000000000000000, 6.000000000000000000 ) ) ;
#52234=CARTESIAN_POINT ( 'NONE',  ( 2.035157376598824452, 33.68868534415484106, 7.964842623401179544 ) ) ;
#52236=CARTESIAN_POINT ( 'NONE',  ( 12.63842701281683034, 12.46726448433411782, 9.846743663894596210 ) ) ;
#52237=CARTESIAN_POINT ( 'NONE',  ( 12.63842701281683922, 24.55059781766745175, -9.846743663894590881 ) ) ;
#52240=CARTESIAN_POINT ( 'NONE',  ( -1.099225684535947600, -0.4596986634029132657, 6.408140936763237150 ) ) ;
#52241=CARTESIAN_POINT ( 'NONE',  ( 17.96484262340118221, 6.188685344154837509, -7.964842623401177768 ) ) ;
#52242=CARTESIAN_POINT ( 'NONE',  ( 0.1089645850228810053, 18.16234555792571115, 6.479102184480781013 ) ) ;
#52243=CARTESIAN_POINT ( 'NONE',  ( 2.917880565312948704, 17.63708216824730357, 12.26659068614894643 ) ) ;
#52244=CARTESIAN_POINT ( 'NONE',  ( 24.16423886937410614, 44.51208216824730357, -3.795296366450302550 ) ) ;
#52245=CARTESIAN_POINT ( 'NONE',  ( 15.44008868035555260, 4.730352010821504471, 9.422509992056143702 ) ) ;
#52247=CARTESIAN_POINT ( 'NONE',  ( 17.20831665107776587, 19.13393115100078035, -7.208316651077762316 ) ) ;
#52248=CARTESIAN_POINT ( 'NONE',  ( -0.8801773607110991993, 17.85535201082150536, -2.915334737309923874 ) ) ;
#52249=CARTESIAN_POINT ( 'NONE',  ( 19.84674366389459266, 48.71726448433413026, -2.638427012816827677 ) ) ;
#52253=CARTESIAN_POINT ( 'NONE',  ( 16.40814093676323893, 35.79030133659708923, 11.09922568453595026 ) ) ;
#52254=CARTESIAN_POINT ( 'NONE',  ( 2.791683348922237240, 35.38393115100079456, -7.208316651077763204 ) ) ;
#52255=VERTEX_POINT ( 'NONE', #39655 ) ;
#52256=CARTESIAN_POINT ( 'NONE',  ( 18.52753015748617571, 13.09226448433411960, 4.923371831947298993 ) ) ;
#52259=CARTESIAN_POINT ( 'NONE',  ( 17.96484262340118221, 14.93868534415483751, 7.964842623401181321 ) ) ;
#52260=CARTESIAN_POINT ( 'NONE',  ( -0.3689425029237898834, 46.17874883491397497, -10.36894250292378850 ) ) ;
#52261=CARTESIAN_POINT ( 'NONE',  ( 17.96484262340118221, 46.18868534415484106, -7.964842623401177768 ) ) ;
#52262=CARTESIAN_POINT ( 'NONE',  ( 17.96484262340118221, 66.18868534415483396, -7.964842623401177768 ) ) ;
#52264=CARTESIAN_POINT ( 'NONE',  ( 12.63842701281683922, 19.55059781766745175, -9.846743663894590881 ) ) ;
#52265=CARTESIAN_POINT ( 'NONE',  ( 12.91533473730992121, 9.522018677488171434, 10.88017736071110164 ) ) ;
#52266=CARTESIAN_POINT ( 'NONE',  ( 0.1532563361054082862, 11.21726448433411605, 2.638427012816831674 ) ) ;
#52268=CARTESIAN_POINT ( 'NONE',  ( 0.1532563361054100626, 35.80059781766745175, -2.638427012816831230 ) ) ;
#52269=CARTESIAN_POINT ( 'NONE',  ( 7.084665262690076126, 32.02201867748816966, -10.88017736071110164 ) ) ;
#52272=CARTESIAN_POINT ( 'NONE',  ( 10.00000000000000000, 52.87363466993041783, -12.81628187352647608 ) ) ;
#52274=CARTESIAN_POINT ( 'NONE',  ( 14.92337183194729988, 14.34226448433411782, -8.527530157486177487 ) ) ;
#52275=CARTESIAN_POINT ( 'NONE',  ( 22.81628187352647785, 46.41530133659708213, 3.434112377981063169 ) ) ;
#52276=CARTESIAN_POINT ( 'NONE',  ( 2.035157376598822676, 2.438685344154838397, -7.964842623401177768 ) ) ;
#52277=CARTESIAN_POINT ( 'NONE',  ( 7.361572987183170547, 32.05059781766745175, 9.846743663894590881 ) ) ;
#52278=CARTESIAN_POINT ( 'NONE',  ( 20.00000000000000355, 96.99990787933366221, 4.499999999999999112 ) ) ;
#52280=CARTESIAN_POINT ( 'NONE',  ( 2.791683348922237240, 0.3839311510007847872, -7.208316651077763204 ) ) ;
#52281=CARTESIAN_POINT ( 'NONE',  ( 6.204703633549690345, 32.84541550158063927, 14.16423886937410082 ) ) ;
#52282=CARTESIAN_POINT ( 'NONE',  ( 13.79529636645031943, 50.34541550158064638, -14.16423886937409904 ) ) ;
#52283=CARTESIAN_POINT ( 'NONE',  ( 5.076628168052703671, 51.84226448433412315, 8.527530157486179263 ) ) ;
#52284=CARTESIAN_POINT ( 'NONE',  ( 20.88017736071110519, 40.56368534415484106, 2.639326808657452039E-16 ) ) ;
#52285=CARTESIAN_POINT ( 'NONE',  ( 18.52753015748617571, 8.092264484334117824, 4.923371831947298993 ) ) ;
#52288=ORIENTED_EDGE ( 'NONE', *, *, #26638, .F. ) ;
#52289=CARTESIAN_POINT ( 'NONE',  ( 22.81628187352648496, 51.83196800326376064, -3.434112377981050290 ) ) ;
#52292=CARTESIAN_POINT ( 'NONE',  ( 0.5774900079438607392, 63.48035201082149825, 5.440088680355550821 ) ) ;
#52294=CARTESIAN_POINT ( 'NONE',  ( 6.204703633549690345, 2.845415501580634388, 14.16423886937410082 ) ) ;
#52295=CARTESIAN_POINT ( 'NONE',  ( 12.63842701281683922, 4.550597817667451750, -9.846743663894590881 ) ) ;
#52296=CARTESIAN_POINT ( 'NONE',  ( 17.96484262340118221, 31.18868534415483751, -7.964842623401177768 ) ) ;
#52299=ORIENTED_EDGE ( 'NONE', *, *, #43747, .T. ) ;
#52301=CARTESIAN_POINT ( 'NONE',  ( 20.88017736071110519, 30.56368534415484106, 2.639326808657452039E-16 ) ) ;
#52303=ORIENTED_EDGE ( 'NONE', *, *, #32753, .F. ) ;
#52304=CARTESIAN_POINT ( 'NONE',  ( 12.91533473730993009, 31.60535201082150891, -10.88017736071109987 ) ) ;
#52309=CARTESIAN_POINT ( 'NONE',  ( 7.084665262690076126, 64.10535201082150536, 10.88017736071109987 ) ) ;
#52311=CARTESIAN_POINT ( 'NONE',  ( 20.88017736071110875, 15.77201867748817143, -2.915334737309920765 ) ) ;
#52313=CARTESIAN_POINT ( 'NONE',  ( 18.52753015748618282, 8.925597817667451750, -4.923371831947291888 ) ) ;
#52314=CARTESIAN_POINT ( 'NONE',  ( -0.8801773607111008646, 18.27201867748817321, 2.915334737309923430 ) ) ;
#52316=ORIENTED_EDGE ( 'NONE', *, *, #90582, .F. ) ;
#52317=CARTESIAN_POINT ( 'NONE',  ( -1.099225684535947600, 48.70696800326375353, -6.408140936763238038 ) ) ;
#52318=CARTESIAN_POINT ( 'NONE',  ( 20.88017736071110164, 45.35535201082149115, 2.915334737309930979 ) ) ;
#52319=CARTESIAN_POINT ( 'NONE',  ( -46.88190520701112973, 103.4393505901440875, -6.246661988884179451 ) ) ;
#52320=CARTESIAN_POINT ( 'NONE',  ( 13.43411237798105340, 50.58196800326375353, 12.81628187352647963 ) ) ;
#52321=CARTESIAN_POINT ( 'NONE',  ( -0.8801773607111008646, 48.27201867748816966, 2.915334737309923430 ) ) ;
#52322=CARTESIAN_POINT ( 'NONE',  ( 19.38216949554541202, 5.998634669930420493, 9.382169495545424454 ) ) ;
#52324=CARTESIAN_POINT ( 'NONE',  ( 7.361572987183170547, 17.05059781766745530, 9.846743663894590881 ) ) ;
#52326=CARTESIAN_POINT ( 'NONE',  ( 10.00000000000000000, 7.873634669930421381, -12.81628187352647608 ) ) ;
#52328=CARTESIAN_POINT ( 'NONE',  ( -41.94000000000001194, 93.50000000000000000, 9.500000000000000000 ) ) ;
#52329=CARTESIAN_POINT ( 'NONE',  ( 20.88017736071110519, 40.56368534415484106, 2.639326808657452039E-16 ) ) ;
#52330=CARTESIAN_POINT ( 'NONE',  ( 19.84674366389459621, 43.50893115100078745, 7.409399052514197653E-17 ) ) ;
#52331=FILL_AREA_STYLE_COLOUR ( '', #20013 ) ;
#52332=CARTESIAN_POINT ( 'NONE',  ( 18.52753015748618282, 18.92559781766745175, -4.923371831947291888 ) ) ;
#52333=CARTESIAN_POINT ( 'NONE',  ( 7.361572987183169658, 4.967264484334119601, -9.846743663894592657 ) ) ;
#52335=CARTESIAN_POINT ( 'NONE',  ( 0.6178305044545838731, 9.748634669930416052, 9.382169495545420901 ) ) ;
#52337=SURFACE_STYLE_FILL_AREA ( #46321 ) ;
#52338=CARTESIAN_POINT ( 'NONE',  ( 2.791683348922237240, 60.38393115100078745, -7.208316651077763204 ) ) ;
#52339=CARTESIAN_POINT ( 'NONE',  ( 10.00000000000000178, 32.25893115100078745, 9.846743663894594434 ) ) ;
#52341=CARTESIAN_POINT ( 'NONE',  ( 0.5774900079438590739, 2.647018677488171434, -5.440088680355550821 ) ) ;
#52342=CARTESIAN_POINT ( 'NONE',  ( 17.20831665107776587, 49.13393115100078745, -7.208316651077762316 ) ) ;
#52344=CARTESIAN_POINT ( 'NONE',  ( 17.08211943468705840, 65.13708216824730357, -12.26659068614894466 ) ) ;
#52346=CARTESIAN_POINT ( 'NONE',  ( 20.88017736071110875, 25.77201867748816966, -2.915334737309920765 ) ) ;
#52347=CARTESIAN_POINT ( 'NONE',  ( 20.36894250292379382, 43.67874883491397497, 10.36894250292379205 ) ) ;
#52348=CARTESIAN_POINT ( 'NONE',  ( -0.3689425029237881626, 57.42874883491397497, 10.36894250292379027 ) ) ;
#52350=CARTESIAN_POINT ( 'NONE',  ( 5.076628168052703671, 1.842264484334118047, 8.527530157486179263 ) ) ;
#52351=CARTESIAN_POINT ( 'NONE',  ( 1.472469842513823179, 30.59226448433411960, -4.923371831947296329 ) ) ;
#52352=CARTESIAN_POINT ( 'NONE',  ( 19.38216949554541557, 7.248634669930421381, -9.382169495545420901 ) ) ;
#52359=CARTESIAN_POINT ( 'NONE',  ( -0.3689425029237881626, 7.428748834913967869, 10.36894250292379027 ) ) ;
#52360=CARTESIAN_POINT ( 'NONE',  ( 18.52753015748617571, 23.09226448433411960, 4.923371831947298993 ) ) ;
#52361=CARTESIAN_POINT ( 'NONE',  ( 24.16423886937410614, 39.30374883491396787, 8.672049930838204340E-16 ) ) ;
#52362=CARTESIAN_POINT ( 'NONE',  ( 5.076628168052703671, 11.84226448433411960, 8.527530157486179263 ) ) ;
#52365=CARTESIAN_POINT ( 'NONE',  ( 20.88017736071110164, 30.35535201082151247, 2.915334737309930979 ) ) ;
#52366=CARTESIAN_POINT ( 'NONE',  ( 13.43411237798105340, 40.58196800326375353, 12.81628187352647963 ) ) ;
#52367=CARTESIAN_POINT ( 'NONE',  ( 12.91533473730992121, 4.522018677488169658, 10.88017736071110164 ) ) ;
#52368=CARTESIAN_POINT ( 'NONE',  ( -1.099225684535947600, 39.54030133659708923, 6.408140936763237150 ) ) ;
#52369=CARTESIAN_POINT ( 'NONE',  ( -1.099225684535947600, 58.70696800326375353, -6.408140936763238038 ) ) ;
#52371=DIRECTION ( 'NONE',  ( 0.000000000000000000, -1.000000000000000000, 0.000000000000000000 ) ) ;
#52372=CARTESIAN_POINT ( 'NONE',  ( 20.36894250292379382, 43.67874883491397497, 10.36894250292379205 ) ) ;
#52373=SURFACE_SIDE_STYLE ('',( #57893 ) ) ;
#52374=CARTESIAN_POINT ( 'NONE',  ( 2.035157376598824452, 3.688685344154837953, 7.964842623401179544 ) ) ;
#52375=CARTESIAN_POINT ( 'NONE',  ( 2.035157376598822676, 17.43868534415483751, -7.964842623401177768 ) ) ;
#52378=CARTESIAN_POINT ( 'NONE',  ( 7.084665262690076126, 54.10535201082151247, 10.88017736071109987 ) ) ;
#52379=CARTESIAN_POINT ( 'NONE',  ( 7.084665262690076126, 64.10535201082150536, 10.88017736071109987 ) ) ;
#52380=CARTESIAN_POINT ( 'NONE',  ( 22.81628187352647785, 21.41530133659708923, 3.434112377981063169 ) ) ;
#52381=DIRECTION ( 'NONE',  ( -0.5547001962252290364, -0.8320502943378437211, 0.000000000000000000 ) ) ;
#52383=CARTESIAN_POINT ( 'NONE',  ( 12.63842701281683922, 19.55059781766745175, -9.846743663894590881 ) ) ;
#52385=CARTESIAN_POINT ( 'NONE',  ( 17.96484262340118221, 54.93868534415484106, 7.964842623401181321 ) ) ;
#52389=CARTESIAN_POINT ( 'NONE',  ( 13.43411237798106583, 17.66530133659708923, -12.81628187352647252 ) ) ;
#52390=CARTESIAN_POINT ( 'NONE',  ( 19.42250999205614548, 10.98035201082150358, -5.440088680355545492 ) ) ;
#52393=CARTESIAN_POINT ( 'NONE',  ( 1.472469842513823179, 41.42559781766745886, 4.923371831947296329 ) ) ;
#52394=CARTESIAN_POINT ( 'NONE',  ( -2.816281873526473856, 64.12363466993042493, 9.499525473075851096E-16 ) ) ;
#52395=CARTESIAN_POINT ( 'NONE',  ( 19.84674366389459266, 18.71726448433411960, -2.638427012816827677 ) ) ;
#52396=( NAMED_UNIT ( * ) SI_UNIT ( $, .STERADIAN. ) SOLID_ANGLE_UNIT ( ) );
#52397=CARTESIAN_POINT ( 'NONE',  ( 19.42250999205614548, 30.98035201082150536, -5.440088680355545492 ) ) ;
#52398=CARTESIAN_POINT ( 'NONE',  ( -0.8801773607110991993, 27.85535201082150181, -2.915334737309923874 ) ) ;
#52399=CARTESIAN_POINT ( 'NONE',  ( -0.8801773607111008646, 3.272018677488171434, 2.915334737309923430 ) ) ;
#52400=CARTESIAN_POINT ( 'NONE',  ( 14.92337183194729633, 37.67559781766745175, 8.527530157486181039 ) ) ;
#52401=CARTESIAN_POINT ( 'NONE',  ( 20.88017736071110875, 35.77201867748816966, -2.915334737309920765 ) ) ;
#52402=CARTESIAN_POINT ( 'NONE',  ( 17.96484262340118221, 14.93868534415484106, 7.964842623401181321 ) ) ;
#52404=CARTESIAN_POINT ( 'NONE',  ( 20.88017736071110519, 30.56368534415484106, 2.639326808657452039E-16 ) ) ;
#52405=EDGE_CURVE ( 'NONE', #32248, #13300, #35901, .T. ) ;
#52406=CARTESIAN_POINT ( 'NONE',  ( 6.565887622018943937, 45.16530133659708923, 12.81628187352647430 ) ) ;
#52407=CARTESIAN_POINT ( 'NONE',  ( -0.8801773607110991993, 47.85535201082150536, -2.915334737309923874 ) ) ;
#52409=CARTESIAN_POINT ( 'NONE',  ( 19.42250999205614193, 35.14701867748816966, 5.440088680355555262 ) ) ;
#52410=AXIS2_PLACEMENT_3D ( 'NONE', #41494, #71963, #78973 ) ;
#52412=CARTESIAN_POINT ( 'NONE',  ( 1.472469842513823179, 55.59226448433412315, -4.923371831947296329 ) ) ;
#52413=CARTESIAN_POINT ( 'NONE',  ( 10.00000000000000178, 34.31368534415484106, 10.88017736071110342 ) ) ;
#52414=SURFACE_STYLE_FILL_AREA ( #8878 ) ;
#52417=CARTESIAN_POINT ( 'NONE',  ( 10.00000000000000000, 45.55374883491397497, -14.16423886937410082 ) ) ;
#52418=CARTESIAN_POINT ( 'NONE',  ( 7.084665262690076126, 59.10535201082150536, 10.88017736071109987 ) ) ;
#52419=PRESENTATION_STYLE_ASSIGNMENT (( #21939 ) ) ;
#52421=CARTESIAN_POINT ( 'NONE',  ( 10.00000000000000000, -2.126365330069579951, -12.81628187352647608 ) ) ;
#52422=CARTESIAN_POINT ( 'NONE',  ( 10.00000000000000000, 34.75893115100078745, -9.846743663894594434 ) ) ;
#52425=CARTESIAN_POINT ( 'NONE',  ( 0.1532563361054083140, 31.00893115100078390, 1.131784320476157264E-15 ) ) ;
#52428=CARTESIAN_POINT ( 'NONE',  ( -0.8801773607111009756, 28.06368534415484106, 1.068504757029289695E-15 ) ) ;
#52429=CARTESIAN_POINT ( 'NONE',  ( 10.00000000000000178, 27.25893115100078390, 9.846743663894594434 ) ) ;
#52430=CARTESIAN_POINT ( 'NONE',  ( -2.816281873526473856, 24.12363466993042138, 9.499525473075851096E-16 ) ) ;
#52431=CARTESIAN_POINT ( 'NONE',  ( 0.5774900079438607392, 68.48035201082150536, 5.440088680355550821 ) ) ;
#52432=CARTESIAN_POINT ( 'NONE',  ( 4.559911319644449179, 63.89701867748817676, 9.422509992056141925 ) ) ;
#52433=CARTESIAN_POINT ( 'NONE',  ( 12.91533473730992121, 29.52201867748817321, 10.88017736071110164 ) ) ;
#52434=CARTESIAN_POINT ( 'NONE',  ( 7.084665262690076126, 7.022018677488169658, -10.88017736071110164 ) ) ;
#52435=CARTESIAN_POINT ( 'NONE',  ( 17.08211943468705130, 48.47041550158063927, 12.26659068614894998 ) ) ;
#52436=CIRCLE ( 'NONE', #77983, 0.5000000000000004441 ) ;
#52437=ADVANCED_FACE ( 'NONE', ( #19590 ), #80592, .T. ) ;
#52440=CARTESIAN_POINT ( 'NONE',  ( 13.43411237798106583, 12.66530133659708746, -12.81628187352647252 ) ) ;
#52441=CARTESIAN_POINT ( 'NONE',  ( 20.88017736071110875, 10.77201867748817143, -2.915334737309920765 ) ) ;
#52442=CARTESIAN_POINT ( 'NONE',  ( -0.8801773607110991993, 47.85535201082150536, -2.915334737309923874 ) ) ;
#52443=( LENGTH_UNIT ( ) NAMED_UNIT ( * ) SI_UNIT ( .MILLI., .METRE. ) );
#52445=CARTESIAN_POINT ( 'NONE',  ( 20.88017736071110164, 55.35535201082149825, 2.915334737309930979 ) ) ;
#52446=CARTESIAN_POINT ( 'NONE',  ( 2.791683348922237240, 35.38393115100079456, -7.208316651077763204 ) ) ;
#52447=CARTESIAN_POINT ( 'NONE',  ( 12.63842701281683034, 22.46726448433411605, 9.846743663894596210 ) ) ;
#52448=CARTESIAN_POINT ( 'NONE',  ( 0.1532563361054100626, 15.80059781766745353, -2.638427012816831230 ) ) ;
#52450=CARTESIAN_POINT ( 'NONE',  ( 0.1532563361054083140, 6.008931151000784787, 1.131784320476157264E-15 ) ) ;
#52452=CARTESIAN_POINT ( 'NONE',  ( 20.15039907845753220, 44.72266099184918176, 6.262539305110078836 ) ) ;
#52453=CARTESIAN_POINT ( 'NONE',  ( 10.00000000000000178, 27.25893115100078390, 9.846743663894594434 ) ) ;
#52454=ORIENTED_EDGE ( 'NONE', *, *, #32851, .T. ) ;
#52456=CARTESIAN_POINT ( 'NONE',  ( 19.38216949554541202, 10.99863466993042138, 9.382169495545424454 ) ) ;
#52457=CARTESIAN_POINT ( 'NONE',  ( 20.88017736071110875, 55.77201867748816966, -2.915334737309920765 ) ) ;
#52458=CARTESIAN_POINT ( 'NONE',  ( -4.164238869374099927, 32.01208216824730357, 3.795296366450308767 ) ) ;
#52461=CARTESIAN_POINT ( 'NONE',  ( 20.36894250292379738, 24.92874883491396787, -10.36894250292379027 ) ) ;
#52462=CARTESIAN_POINT ( 'NONE',  ( 6.204703633549690345, 47.84541550158064638, 14.16423886937410082 ) ) ;
#52464=CARTESIAN_POINT ( 'NONE',  ( -4.164238869374099039, 6.803748834913967869, 8.674139862899312516E-16 ) ) ;
#52465=CARTESIAN_POINT ( 'NONE',  ( 13.79529636645030344, 13.26208216824729824, 14.16423886937410614 ) ) ;
#52466=CARTESIAN_POINT ( 'NONE',  ( 15.44008868035555793, 41.39701867748817676, -9.422509992056140149 ) ) ;
#52468=CARTESIAN_POINT ( 'NONE',  ( 5.076628168052704559, 25.17559781766745175, -8.527530157486179263 ) ) ;
#52469=CARTESIAN_POINT ( 'NONE',  ( 13.99999999999999822, 11.50000000000000000, -5.000000000000000000 ) ) ;
#52470=CARTESIAN_POINT ( 'NONE',  ( 17.20831665107776587, 34.13393115100078745, -7.208316651077762316 ) ) ;
#52471=CARTESIAN_POINT ( 'NONE',  ( 21.09922568453595559, 57.04030133659708923, -6.408140936763230044 ) ) ;
#52472=CARTESIAN_POINT ( 'NONE',  ( 10.00000000000000000, 64.75893115100078035, -9.846743663894594434 ) ) ;
#52474=CARTESIAN_POINT ( 'NONE',  ( 7.361572987183169658, 24.96726448433412315, -9.846743663894592657 ) ) ;
#52475=CARTESIAN_POINT ( 'NONE',  ( 3.591859063236763294, 43.29030133659708923, -11.09922568453595026 ) ) ;
#52477=CARTESIAN_POINT ( 'NONE',  ( 7.084665262690076126, 37.02201867748817676, -10.88017736071110164 ) ) ;
#52478=CARTESIAN_POINT ( 'NONE',  ( 12.63842701281683922, 49.55059781766744464, -9.846743663894590881 ) ) ;
#52479=CARTESIAN_POINT ( 'NONE',  ( 20.36894250292379738, 24.92874883491396787, -10.36894250292379027 ) ) ;
#52481=CARTESIAN_POINT ( 'NONE',  ( 2.035157376598822676, 67.43868534415484817, -7.964842623401177768 ) ) ;
#52482=CARTESIAN_POINT ( 'NONE',  ( -0.8801773607111008646, 68.27201867748817676, 2.915334737309923430 ) ) ;
#52483=CARTESIAN_POINT ( 'NONE',  ( -4.164238869374099927, 62.01208216824728936, 3.795296366450308767 ) ) ;
#52484=CARTESIAN_POINT ( 'NONE',  ( -2.816281873526471635, 3.915301336597087456, -3.434112377981056508 ) ) ;
#52485=CARTESIAN_POINT ( 'NONE',  ( 19.72487221294571569, 42.80223176428830811, -6.499999999999990230 ) ) ;
#52486=CARTESIAN_POINT ( 'NONE',  ( 15.44008868035555260, 59.73035201082151247, 9.422509992056143702 ) ) ;
#52489=CARTESIAN_POINT ( 'NONE',  ( 6.565887622018943937, 33.08196800326374643, -12.81628187352647608 ) ) ;
#52490=CARTESIAN_POINT ( 'NONE',  ( 17.08211943468705840, 45.13708216824730357, -12.26659068614894466 ) ) ;
#52492=CARTESIAN_POINT ( 'NONE',  ( 10.00000000000000178, 9.313685344154839285, 10.88017736071110342 ) ) ;
#52493=CARTESIAN_POINT ( 'NONE',  ( 12.91533473730993009, 16.60535201082150891, -10.88017736071109987 ) ) ;
#52494=CARTESIAN_POINT ( 'NONE',  ( 1.472469842513823179, 60.59226448433412315, -4.923371831947296329 ) ) ;
#52495=CARTESIAN_POINT ( 'NONE',  ( -2.816281873526471635, 53.91530133659709634, -3.434112377981056508 ) ) ;
#52497=CARTESIAN_POINT ( 'NONE',  ( 2.035157376598824452, 23.68868534415484461, 7.964842623401179544 ) ) ;
#52498=CARTESIAN_POINT ( 'NONE',  ( -2.816281873526473856, 19.12363466993042138, 9.499525473075851096E-16 ) ) ;
#52502=CARTESIAN_POINT ( 'NONE',  ( 7.361572987183170547, 42.05059781766745886, 9.846743663894590881 ) ) ;
#52503=CARTESIAN_POINT ( 'NONE',  ( -0.8801773607110991993, 37.85535201082151247, -2.915334737309923874 ) ) ;
#52504=EDGE_CURVE ( 'NONE', #56450, #23152, #18615, .T. ) ;
#52505=CARTESIAN_POINT ( 'NONE',  ( 0.6178305044545818747, 18.49863466993041428, -9.382169495545419124 ) ) ;
#52506=CARTESIAN_POINT ( 'NONE',  ( 20.88017736071110875, 45.77201867748816966, -2.915334737309920765 ) ) ;
#52509=CARTESIAN_POINT ( 'NONE',  ( 3.591859063236763294, 53.29030133659708923, -11.09922568453595026 ) ) ;
#52511=CARTESIAN_POINT ( 'NONE',  ( -0.1503990784575328643, 30.12777174578613781, 6.262539305110068177 ) ) ;
#52512=CARTESIAN_POINT ( 'NONE',  ( 0.5774900079438607392, 53.48035201082151247, 5.440088680355550821 ) ) ;
#52513=CARTESIAN_POINT ( 'NONE',  ( 16.40814093676324603, 27.45696800326375708, -11.09922568453594671 ) ) ;
#52514=CARTESIAN_POINT ( 'NONE',  ( 2.917880565312950480, 5.970415501580634832, -12.26659068614894821 ) ) ;
#52515=CARTESIAN_POINT ( 'NONE',  ( 0.1532563361054100626, 5.800597817667452638, -2.638427012816831230 ) ) ;
#52516=CARTESIAN_POINT ( 'NONE',  ( 4.559911319644449179, 37.23035201082150536, -9.422509992056141925 ) ) ;
#52517=CARTESIAN_POINT ( 'NONE',  ( 18.95386800104996183, 3.238109087357262883, -6.500000000000001776 ) ) ;
#52518=CARTESIAN_POINT ( 'NONE',  ( 19.84674366389459266, 63.30059781766745886, 2.638427012816836559 ) ) ;
#52519=CARTESIAN_POINT ( 'NONE',  ( 19.84674366389459266, 18.30059781766745175, 2.638427012816836559 ) ) ;
#52520=CARTESIAN_POINT ( 'NONE',  ( 12.63842701281683034, 12.46726448433411782, 9.846743663894596210 ) ) ;
#52522=CARTESIAN_POINT ( 'NONE',  ( 17.08211943468705130, 43.47041550158063927, 12.26659068614894998 ) ) ;
#52523=DIRECTION ( 'NONE',  ( 0.000000000000000000, 0.000000000000000000, 1.000000000000000000 ) ) ;
#52527=CARTESIAN_POINT ( 'NONE',  ( -4.164238869374098151, 61.59541550158063217, -3.795296366450310543 ) ) ;
#52528=CARTESIAN_POINT ( 'NONE',  ( 2.035157376598822676, 2.438685344154838397, -7.964842623401177768 ) ) ;
#52529=CARTESIAN_POINT ( 'NONE',  ( 1.472469842513823179, 30.59226448433411960, -4.923371831947296329 ) ) ;
#52530=CARTESIAN_POINT ( 'NONE',  ( 0.6178305044545818747, 43.49863466993042493, -9.382169495545419124 ) ) ;
#52533=CARTESIAN_POINT ( 'NONE',  ( 24.16423886937410614, 4.512082168247300906, -3.795296366450302550 ) ) ;
#52534=CARTESIAN_POINT ( 'NONE',  ( -0.8801773607111008646, 13.27201867748817143, 2.915334737309923430 ) ) ;
#52535=CARTESIAN_POINT ( 'NONE',  ( 20.36894250292379738, 59.92874883491397497, -10.36894250292379027 ) ) ;
#52536=CARTESIAN_POINT ( 'NONE',  ( 14.92337183194729988, 39.34226448433412315, -8.527530157486177487 ) ) ;
#52537=CARTESIAN_POINT ( 'NONE',  ( 19.72487221294571569, 40.71833443783938122, -6.499999999999989342 ) ) ;
#52538=CARTESIAN_POINT ( 'NONE',  ( 18.52753015748618282, 18.92559781766745175, -4.923371831947291888 ) ) ;
#52539=EDGE_CURVE ( 'NONE', #53414, #10378, #41629, .T. ) ;
#52547=CARTESIAN_POINT ( 'NONE',  ( 19.84674366389459266, 43.71726448433410894, -2.638427012816827677 ) ) ;
#52548=CARTESIAN_POINT ( 'NONE',  ( 7.084665262690076126, 27.02201867748817676, -10.88017736071110164 ) ) ;
#52549=CARTESIAN_POINT ( 'NONE',  ( 2.035157376598824452, 38.68868534415483396, 7.964842623401179544 ) ) ;
#52550=CARTESIAN_POINT ( 'NONE',  ( 5.076628168052704559, 60.17559781766745175, -8.527530157486179263 ) ) ;
#52551=CARTESIAN_POINT ( 'NONE',  ( 22.81628187352648496, 26.83196800326374998, -3.434112377981050290 ) ) ;
#52552=CARTESIAN_POINT ( 'NONE',  ( 24.16423886937409904, 9.095415501580633943, 3.795296366450317205 ) ) ;
#52553=CARTESIAN_POINT ( 'NONE',  ( 7.084665262690076126, 64.10535201082150536, 10.88017736071109987 ) ) ;
#52554=CARTESIAN_POINT ( 'NONE',  ( 6.565887622018943937, 30.16530133659708568, 12.81628187352647430 ) ) ;
#52555=ORIENTED_EDGE ( 'NONE', *, *, #94873, .T. ) ;
#52556=CARTESIAN_POINT ( 'NONE',  ( 2.791683348922240793, 46.63393115100077324, 7.208316651077764092 ) ) ;
#52557=CARTESIAN_POINT ( 'NONE',  ( 10.00000000000000178, 9.313685344154839285, 10.88017736071110342 ) ) ;
#52559=CARTESIAN_POINT ( 'NONE',  ( 7.084665262690076126, 17.02201867748817676, -10.88017736071110164 ) ) ;
#52560=EDGE_LOOP ( 'NONE', ( #69399, #72102, #11297, #70410, #38289 ) ) ;
#52561=CARTESIAN_POINT ( 'NONE',  ( 20.88017736071110164, 45.35535201082149115, 2.915334737309930979 ) ) ;
#52562=CARTESIAN_POINT ( 'NONE',  ( 15.44008868035555260, 54.73035201082150536, 9.422509992056143702 ) ) ;
#52564=CARTESIAN_POINT ( 'NONE',  ( 12.91533473730992121, 59.52201867748816966, 10.88017736071110164 ) ) ;
#52565=SURFACE_STYLE_USAGE ( .BOTH. , #90068 ) ;
#52566=CARTESIAN_POINT ( 'NONE',  ( -0.8801773607110991993, 52.85535201082151247, -2.915334737309923874 ) ) ;
#52567=CARTESIAN_POINT ( 'NONE',  ( -46.94000000000000483, 100.8832200551196934, 8.297377427102095027 ) ) ;
#52569=CARTESIAN_POINT ( 'NONE',  ( 1.959929470562274068, 11.50257860105348762, 5.767676674365839418 ) ) ;
#52570=( NAMED_UNIT ( * ) PLANE_ANGLE_UNIT ( ) SI_UNIT ( $, .RADIAN. ) );
#52572=CARTESIAN_POINT ( 'NONE',  ( 19.84674366389459621, 28.50893115100078745, 7.409399052514197653E-17 ) ) ;
#52574=CARTESIAN_POINT ( 'NONE',  ( 0.1532563361054083140, 66.00893115100079456, 1.131784320476157264E-15 ) ) ;
#52576=CARTESIAN_POINT ( 'NONE',  ( 10.00000000000000178, 3.053748834913967425, 14.16423886937410082 ) ) ;
#52577=CARTESIAN_POINT ( 'NONE',  ( -0.3289641300567998083, 8.078790035174471029, 5.963430220938281678 ) ) ;
#52578=CARTESIAN_POINT ( 'NONE',  ( -46.68456736488007408, 103.6675473310227034, -5.775421524742654356 ) ) ;
#52579=CARTESIAN_POINT ( 'NONE',  ( 2.791683348922237240, 35.38393115100079456, -7.208316651077763204 ) ) ;
#52580=CARTESIAN_POINT ( 'NONE',  ( 20.88017736071110164, 10.35535201082150714, 2.915334737309930979 ) ) ;
#52584=CARTESIAN_POINT ( 'NONE',  ( 14.92337183194729988, 44.34226448433412315, -8.527530157486177487 ) ) ;
#52586=CARTESIAN_POINT ( 'NONE',  ( -2.816281873526473856, 24.12363466993042138, 9.499525473075851096E-16 ) ) ;
#52587=CARTESIAN_POINT ( 'NONE',  ( 19.84674366389459266, 18.71726448433411960, -2.638427012816827677 ) ) ;
#52588=ADVANCED_FACE ( 'NONE', ( #56128 ), #45186, .T. ) ;
#52591=CARTESIAN_POINT ( 'NONE',  ( -2.816281873526471635, 3.915301336597087456, -3.434112377981056508 ) ) ;
#52593=ORIENTED_EDGE ( 'NONE', *, *, #93798, .T. ) ;
#52595=CARTESIAN_POINT ( 'NONE',  ( 17.96484262340118221, 21.18868534415483396, -7.964842623401177768 ) ) ;
#52596=CARTESIAN_POINT ( 'NONE',  ( 22.26659068614894466, 18.88708216824730002, 7.082119434687054849 ) ) ;
#52597=CARTESIAN_POINT ( 'NONE',  ( 12.63842701281683922, 29.55059781766745175, -9.846743663894590881 ) ) ;
#52598=CARTESIAN_POINT ( 'NONE',  ( -0.8801773607111008646, 58.27201867748816966, 2.915334737309923430 ) ) ;
#52599=CARTESIAN_POINT ( 'NONE',  ( -2.816281873526473856, 34.33196800326376064, 3.434112377981055619 ) ) ;
#52601=CARTESIAN_POINT ( 'NONE',  ( 0.5774900079438590739, 12.64701867748817143, -5.440088680355550821 ) ) ;
#52602=CARTESIAN_POINT ( 'NONE',  ( 1.274849032794231007, 43.57228050351031357, 6.499999999999895195 ) ) ;
#52605=CARTESIAN_POINT ( 'NONE',  ( 3.591859063236761518, 9.956968003263753531, 11.09922568453594849 ) ) ;
#52606=CARTESIAN_POINT ( 'NONE',  ( 22.81628187352647785, 11.62363466993042138, 6.195893100308588602E-16 ) ) ;
#52607=CARTESIAN_POINT ( 'NONE',  ( 2.791683348922237240, 25.38393115100078390, -7.208316651077763204 ) ) ;
#52609=CARTESIAN_POINT ( 'NONE',  ( 6.565887622018943937, 35.16530133659708923, 12.81628187352647430 ) ) ;
#52610=CARTESIAN_POINT ( 'NONE',  ( 18.17829156368507171, 24.16792564121897158, 6.500000000000021316 ) ) ;
#52611=CARTESIAN_POINT ( 'NONE',  ( 17.96484262340118221, 34.93868534415482685, 7.964842623401181321 ) ) ;
#52615=CARTESIAN_POINT ( 'NONE',  ( 18.17829156368507171, 29.16792564121896447, 6.500000000000019540 ) ) ;
#52616=CARTESIAN_POINT ( 'NONE',  ( 17.96484262340118221, 39.93868534415484106, 7.964842623401181321 ) ) ;
#52617=CARTESIAN_POINT ( 'NONE',  ( 4.559911319644449179, 38.89701867748817676, 9.422509992056141925 ) ) ;
#52618=CARTESIAN_POINT ( 'NONE',  ( 5.076628168052704559, 60.17559781766745175, -8.527530157486179263 ) ) ;
#52619=ADVANCED_FACE ( 'NONE', ( #78025 ), #84551, .T. ) ;
#52621=EDGE_CURVE ( 'NONE', #52153, #9012, #11989, .T. ) ;
#52622=CARTESIAN_POINT ( 'NONE',  ( 18.52753015748617571, 38.09226448433412315, 4.923371831947298993 ) ) ;
#52623=CARTESIAN_POINT ( 'NONE',  ( 7.084665262690076126, 14.10535201082150358, 10.88017736071109987 ) ) ;
#52624=CARTESIAN_POINT ( 'NONE',  ( 16.40814093676324603, 12.45696800326375353, -11.09922568453594671 ) ) ;
#52625=VERTEX_POINT ( 'NONE', #1563 ) ;
#52626=CARTESIAN_POINT ( 'NONE',  ( 17.96484262340118221, 21.18868534415483396, -7.964842623401177768 ) ) ;
#52628=CARTESIAN_POINT ( 'NONE',  ( 7.084665262690076126, 32.02201867748816966, -10.88017736071110164 ) ) ;
#52629=CARTESIAN_POINT ( 'NONE',  ( 10.00000000000000000, 4.758931151000784787, -9.846743663894594434 ) ) ;
#52630=CARTESIAN_POINT ( 'NONE',  ( 2.917880565312950480, 40.97041550158063217, -12.26659068614894821 ) ) ;
#52631=CARTESIAN_POINT ( 'NONE',  ( 14.92337183194729988, 24.34226448433411960, -8.527530157486177487 ) ) ;
#52632=CARTESIAN_POINT ( 'NONE',  ( 17.96484262340118221, 46.18868534415484106, -7.964842623401177768 ) ) ;
#52634=CARTESIAN_POINT ( 'NONE',  ( -0.3689425029237881626, 2.428748834913967869, 10.36894250292379027 ) ) ;
#52635=ORIENTED_EDGE ( 'NONE', *, *, #87839, .F. ) ;
#52638=CARTESIAN_POINT ( 'NONE',  ( 19.84674366389459621, 53.50893115100078745, 7.409399052514197653E-17 ) ) ;
#52641=CARTESIAN_POINT ( 'NONE',  ( 2.917880565312950480, 20.97041550158063217, -12.26659068614894821 ) ) ;
#52642=CARTESIAN_POINT ( 'NONE',  ( 24.16423886937410614, 19.51208216824729647, -3.795296366450302550 ) ) ;
#52643=CARTESIAN_POINT ( 'NONE',  ( 17.96484262340118221, 64.93868534415483396, 7.964842623401181321 ) ) ;
#52644=CARTESIAN_POINT ( 'NONE',  ( 6.204703633549690345, 65.76208216824731778, -14.16423886937410259 ) ) ;
#52645=CARTESIAN_POINT ( 'NONE',  ( 10.00000000000000000, 2.873634669930420049, -12.81628187352647608 ) ) ;
#52646=CARTESIAN_POINT ( 'NONE',  ( 5.076628168052704559, 45.17559781766745175, -8.527530157486179263 ) ) ;
#52648=CARTESIAN_POINT ( 'NONE',  ( 7.084665262690076126, 47.02201867748818387, -10.88017736071110164 ) ) ;
#52649=CARTESIAN_POINT ( 'NONE',  ( -2.816281873526473856, 14.33196800326375531, 3.434112377981055619 ) ) ;
#52650=CARTESIAN_POINT ( 'NONE',  ( -2.266590686148945544, 16.38708216824730357, -7.082119434687050408 ) ) ;
#52651=CARTESIAN_POINT ( 'NONE',  ( -0.8801773607110991993, 17.85535201082150536, -2.915334737309923874 ) ) ;
#52652=CARTESIAN_POINT ( 'NONE',  ( 19.42250999205614548, 20.98035201082150891, -5.440088680355545492 ) ) ;
#52654=CARTESIAN_POINT ( 'NONE',  ( 15.44008868035555793, 61.39701867748817676, -9.422509992056140149 ) ) ;
#52655=CARTESIAN_POINT ( 'NONE',  ( 0.6178305044545818747, 48.49863466993042493, -9.382169495545419124 ) ) ;
#52657=ORIENTED_EDGE ( 'NONE', *, *, #73534, .T. ) ;
#52664=CARTESIAN_POINT ( 'NONE',  ( 22.26659068614895176, 64.72041550158064638, -7.082119434687042414 ) ) ;
#52665=CARTESIAN_POINT ( 'NONE',  ( 15.44008868035555260, 4.730352010821505360, 9.422509992056143702 ) ) ;
#52666=CARTESIAN_POINT ( 'NONE',  ( 10.00000000000000000, 24.75893115100078745, -9.846743663894594434 ) ) ;
#52667=CARTESIAN_POINT ( 'NONE',  ( 5.076628168052703671, 41.84226448433411605, 8.527530157486179263 ) ) ;
#52668=CARTESIAN_POINT ( 'NONE',  ( 17.96484262340118221, 64.93868534415483396, 7.964842623401181321 ) ) ;
#52669=ADVANCED_FACE ( 'NONE', ( #62025 ), #89858, .T. ) ;
#52670=CARTESIAN_POINT ( 'NONE',  ( -15.94000000000001371, 93.50000000000000000, 9.500000000000000000 ) ) ;
#52671=CARTESIAN_POINT ( 'NONE',  ( 2.791683348922240793, 1.633931151000784565, 7.208316651077764092 ) ) ;
#52674=CARTESIAN_POINT ( 'NONE',  ( 22.26659068614895176, 39.72041550158063217, -7.082119434687042414 ) ) ;
#52675=ORIENTED_EDGE ( 'NONE', *, *, #83021, .T. ) ;
#52676=CARTESIAN_POINT ( 'NONE',  ( 17.08211943468705840, 40.13708216824731068, -12.26659068614894466 ) ) ;
#52678=CARTESIAN_POINT ( 'NONE',  ( 21.09922568453594849, 56.20696800326375353, 6.408140936763242479 ) ) ;
#52679=CARTESIAN_POINT ( 'NONE',  ( 10.00000000000000000, 26.81368534415484106, -10.88017736071110342 ) ) ;
#52680=CARTESIAN_POINT ( 'NONE',  ( 17.20831665107776587, 39.13393115100079456, -7.208316651077762316 ) ) ;
#52681=CARTESIAN_POINT ( 'NONE',  ( -0.8801773607111009756, 28.06368534415484106, 1.068504757029289695E-15 ) ) ;
#52684=CARTESIAN_POINT ( 'NONE',  ( 2.791683348922240793, 51.63393115100078745, 7.208316651077764092 ) ) ;
#52685=CARTESIAN_POINT ( 'NONE',  ( 0.1532563361054083140, 51.00893115100078745, 1.131784320476157264E-15 ) ) ;
#52690=FACE_OUTER_BOUND ( 'NONE', #91569, .T. ) ;
#52691=ORIENTED_EDGE ( 'NONE', *, *, #76676, .T. ) ;
#52692=CARTESIAN_POINT ( 'NONE',  ( 5.054308323419867577, 70.51564955044841554, -12.00000000000000000 ) ) ;
#52693=CARTESIAN_POINT ( 'NONE',  ( 14.92337183194729633, 37.67559781766745175, 8.527530157486181039 ) ) ;
#52694=DIRECTION ( 'NONE',  ( 0.000000000000000000, 0.000000000000000000, -1.000000000000000000 ) ) ;
#52695=CARTESIAN_POINT ( 'NONE',  ( -1.099225684535947600, 39.54030133659708923, 6.408140936763237150 ) ) ;
#52696=CYLINDRICAL_SURFACE ( 'NONE', #64330, 1.000000000000007772 ) ;
#52697=ORIENTED_EDGE ( 'NONE', *, *, #89650, .T. ) ;
#52698=CARTESIAN_POINT ( 'NONE',  ( 0.1532563361054082862, 61.21726448433412315, 2.638427012816831674 ) ) ;
#52700=CARTESIAN_POINT ( 'NONE',  ( 19.84674366389459266, 38.30059781766745175, 2.638427012816836559 ) ) ;
#52701=CARTESIAN_POINT ( 'NONE',  ( 6.204703633549690345, 35.76208216824729647, -14.16423886937410259 ) ) ;
#52702=CARTESIAN_POINT ( 'NONE',  ( 19.84674366389459266, 43.30059781766744464, 2.638427012816836559 ) ) ;
#52703=CARTESIAN_POINT ( 'NONE',  ( 13.43411237798106583, 47.66530133659709634, -12.81628187352647252 ) ) ;
#52704=FACE_OUTER_BOUND ( 'NONE', #45130, .T. ) ;
#52705=CARTESIAN_POINT ( 'NONE',  ( 10.00000000000000000, 9.758931151000785675, -9.846743663894594434 ) ) ;
#52706=CARTESIAN_POINT ( 'NONE',  ( 10.00000000000000178, 42.25893115100078745, 9.846743663894594434 ) ) ;
#52707=CARTESIAN_POINT ( 'NONE',  ( 10.00000000000000000, 41.81368534415484106, -10.88017736071110342 ) ) ;
#52709=CARTESIAN_POINT ( 'NONE',  ( 17.20831665107776587, 39.13393115100079456, -7.208316651077762316 ) ) ;
#52711=CARTESIAN_POINT ( 'NONE',  ( 4.559911319644449179, 43.89701867748816966, 9.422509992056141925 ) ) ;
#52712=EDGE_LOOP ( 'NONE', ( #90002, #85628, #64688, #57165 ) ) ;
#52714=CARTESIAN_POINT ( 'NONE',  ( 4.559911319644449179, 22.23035201082150536, -9.422509992056141925 ) ) ;
#52715=CARTESIAN_POINT ( 'NONE',  ( 1.472469842513823179, 65.59226448433412315, -4.923371831947296329 ) ) ;
#52716=CARTESIAN_POINT ( 'NONE',  ( 10.00000000000000000, 46.81368534415484106, -10.88017736071110342 ) ) ;
#52720=CARTESIAN_POINT ( 'NONE',  ( 7.084665262690076126, 44.10535201082151247, 10.88017736071109987 ) ) ;
#52722=CARTESIAN_POINT ( 'NONE',  ( 0.1532563361054082862, 16.21726448433411960, 2.638427012816831674 ) ) ;
#52723=CARTESIAN_POINT ( 'NONE',  ( 14.92337183194729633, 27.67559781766745530, 8.527530157486181039 ) ) ;
#52725=CARTESIAN_POINT ( 'NONE',  ( 19.84674366389459621, 63.50893115100078745, 7.409399052514197653E-17 ) ) ;
#52727=CARTESIAN_POINT ( 'NONE',  ( 17.08211943468705840, 65.13708216824730357, -12.26659068614894466 ) ) ;
#52729=CARTESIAN_POINT ( 'NONE',  ( -0.3689425029237881626, 22.42874883491397142, 10.36894250292379027 ) ) ;
#52730=CARTESIAN_POINT ( 'NONE',  ( 13.79529636645031943, 45.34541550158062506, -14.16423886937409904 ) ) ;
#52733=CARTESIAN_POINT ( 'NONE',  ( 1.472469842513823179, 21.42559781766745175, 4.923371831947296329 ) ) ;
#52735=CARTESIAN_POINT ( 'NONE',  ( 17.96484262340118221, 29.93868534415484106, 7.964842623401181321 ) ) ;
#52736=CARTESIAN_POINT ( 'NONE',  ( 19.84674366389459266, 43.30059781766744464, 2.638427012816836559 ) ) ;
#52737=CARTESIAN_POINT ( 'NONE',  ( 10.00000000000000000, 10.55374883491396787, -14.16423886937410082 ) ) ;
#52739=CARTESIAN_POINT ( 'NONE',  ( 10.00000000000000000, 4.758931151000784787, -9.846743663894594434 ) ) ;
#52740=CARTESIAN_POINT ( 'NONE',  ( 22.81628187352648496, 36.83196800326376064, -3.434112377981050290 ) ) ;
#52741=CARTESIAN_POINT ( 'NONE',  ( 17.20831665107776587, 47.88393115100078745, 7.208316651077764980 ) ) ;
#52744=CARTESIAN_POINT ( 'NONE',  ( 7.361572987183169658, 9.967264484334119601, -9.846743663894592657 ) ) ;
#52746=CARTESIAN_POINT ( 'NONE',  ( 17.96484262340118221, 14.93868534415484106, 7.964842623401181321 ) ) ;
#52747=CARTESIAN_POINT ( 'NONE',  ( 17.08211943468705130, 48.47041550158063927, 12.26659068614894998 ) ) ;
#52748=CARTESIAN_POINT ( 'NONE',  ( 15.44008868035555260, 39.73035201082150536, 9.422509992056143702 ) ) ;
#52749=( LENGTH_UNIT ( ) NAMED_UNIT ( * ) SI_UNIT ( .MILLI., .METRE. ) );
#52752=CARTESIAN_POINT ( 'NONE',  ( 17.20831665107776587, 22.88393115100078745, 7.208316651077764980 ) ) ;
#52753=CARTESIAN_POINT ( 'NONE',  ( 4.559911319644449179, 3.897018677488170990, 9.422509992056141925 ) ) ;
#52754=CARTESIAN_POINT ( 'NONE',  ( 7.361572987183170547, 42.05059781766745886, 9.846743663894590881 ) ) ;
#52755=CARTESIAN_POINT ( 'NONE',  ( -46.75578508127857447, 100.8424743063331022, 9.091779743865453511 ) ) ;
#52756=CARTESIAN_POINT ( 'NONE',  ( 1.472469842513823179, 46.42559781766745175, 4.923371831947296329 ) ) ;
#52757=CARTESIAN_POINT ( 'NONE',  ( 4.559911319644449179, 38.89701867748817676, 9.422509992056141925 ) ) ;
#52760=CARTESIAN_POINT ( 'NONE',  ( 21.09922568453595559, 57.04030133659708923, -6.408140936763230044 ) ) ;
#52762=CARTESIAN_POINT ( 'NONE',  ( 7.361572987183169658, 4.967264484334119601, -9.846743663894592657 ) ) ;
#52763=CARTESIAN_POINT ( 'NONE',  ( 16.40814093676323893, 60.79030133659709634, 11.09922568453595026 ) ) ;
#52764=CARTESIAN_POINT ( 'NONE',  ( -0.8801773607111009756, 3.063685344154838397, 1.068504757029289695E-15 ) ) ;
#52765=CARTESIAN_POINT ( 'NONE',  ( 18.52753015748618282, 38.92559781766745175, -4.923371831947291888 ) ) ;
#52767=FACE_OUTER_BOUND ( 'NONE', #44564, .T. ) ;
#52768=CARTESIAN_POINT ( 'NONE',  ( 13.79529636645030344, 28.26208216824729647, 14.16423886937410614 ) ) ;
#52769=CARTESIAN_POINT ( 'NONE',  ( -0.3689425029237898834, 51.17874883491397497, -10.36894250292378850 ) ) ;
#52770=CARTESIAN_POINT ( 'NONE',  ( 7.361572987183170547, 52.05059781766745175, 9.846743663894590881 ) ) ;
#52771=CARTESIAN_POINT ( 'NONE',  ( 2.603489959281591659, 10.43575266056827644, -6.500000000000006217 ) ) ;
#52772=CARTESIAN_POINT ( 'NONE',  ( 15.44008868035555793, 56.39701867748817676, -9.422509992056140149 ) ) ;
#52773=CARTESIAN_POINT ( 'NONE',  ( 1.472469842513823179, 5.592264484334118713, -4.923371831947296329 ) ) ;
#52777=CARTESIAN_POINT ( 'NONE',  ( 22.81628187352647785, 56.41530133659708213, 3.434112377981063169 ) ) ;
#52778=CARTESIAN_POINT ( 'NONE',  ( 2.035157376598824452, 63.68868534415484106, 7.964842623401179544 ) ) ;
#52780=CARTESIAN_POINT ( 'NONE',  ( 24.16423886937410614, 4.303748834913967869, 8.672049930838204340E-16 ) ) ;
#52781=CARTESIAN_POINT ( 'NONE',  ( 7.361572987183169658, 4.967264484334119601, -9.846743663894592657 ) ) ;
#52782=CARTESIAN_POINT ( 'NONE',  ( 4.559911319644449179, 23.89701867748817321, 9.422509992056141925 ) ) ;
#52786=CARTESIAN_POINT ( 'NONE',  ( 15.44008868035555260, 24.73035201082150891, 9.422509992056143702 ) ) ;
#52788=CARTESIAN_POINT ( 'NONE',  ( 4.559911319644449179, 32.23035201082150536, -9.422509992056141925 ) ) ;
#52789=CIRCLE ( 'NONE', #41617, 0.5000000000000004441 ) ;
#52791=EDGE_CURVE ( 'NONE', #57881, #16048, #34956, .T. ) ;
#52794=CARTESIAN_POINT ( 'NONE',  ( 0.6178305044545818747, 18.49863466993041428, -9.382169495545419124 ) ) ;
#52795=CARTESIAN_POINT ( 'NONE',  ( 18.52753015748617571, 3.092264484334118269, 4.923371831947298993 ) ) ;
#52797=CARTESIAN_POINT ( 'NONE',  ( 15.44008868035555260, 14.73035201082150536, 9.422509992056143702 ) ) ;
#52799=CARTESIAN_POINT ( 'NONE',  ( 2.791683348922237240, 0.3839311510007847872, -7.208316651077763204 ) ) ;
#52801=CARTESIAN_POINT ( 'NONE',  ( 17.96484262340118221, 34.93868534415482685, 7.964842623401181321 ) ) ;
#52804=CARTESIAN_POINT ( 'NONE',  ( 10.00000000000000000, 46.81368534415484106, -10.88017736071110342 ) ) ;
#52806=CARTESIAN_POINT ( 'NONE',  ( 16.40814093676324603, 57.45696800326375353, -11.09922568453594671 ) ) ;
#52807=CARTESIAN_POINT ( 'NONE',  ( 7.084665262690076126, 49.10535201082149825, 10.88017736071109987 ) ) ;
#52808=CARTESIAN_POINT ( 'NONE',  ( 10.00000000000000000, 2.873634669930420049, -12.81628187352647608 ) ) ;
#52810=CARTESIAN_POINT ( 'NONE',  ( 2.791683348922240793, 16.63393115100078745, 7.208316651077764092 ) ) ;
#52811=CARTESIAN_POINT ( 'NONE',  ( 16.40814093676323893, 60.79030133659709634, 11.09922568453595026 ) ) ;
#52812=CARTESIAN_POINT ( 'NONE',  ( -0.000000000000000000, 77.49441643560989235, 8.098090826131633335 ) ) ;
#52813=CARTESIAN_POINT ( 'NONE',  ( 17.20831665107776587, 9.133931151000787452, -7.208316651077762316 ) ) ;
#52814=CARTESIAN_POINT ( 'NONE',  ( 22.81628187352648496, 1.831968003263753753, -3.434112377981050290 ) ) ;
#52815=CARTESIAN_POINT ( 'NONE',  ( 14.92337183194729988, 59.34226448433412315, -8.527530157486177487 ) ) ;
#52816=CARTESIAN_POINT ( 'NONE',  ( 2.035157376598822676, 32.43868534415483396, -7.964842623401177768 ) ) ;
#52817=CARTESIAN_POINT ( 'NONE',  ( 19.84674366389459621, 53.50893115100078745, 7.409399052514197653E-17 ) ) ;
#52819=CARTESIAN_POINT ( 'NONE',  ( 0.1532563361054082862, 16.21726448433411960, 2.638427012816831674 ) ) ;
#52820=CARTESIAN_POINT ( 'NONE',  ( 10.00000000000000000, 4.758931151000784787, -9.846743663894594434 ) ) ;
#52822=CARTESIAN_POINT ( 'NONE',  ( 21.09922568453595559, 7.040301336597086568, -6.408140936763230044 ) ) ;
#52823=VERTEX_POINT ( 'NONE', #97373 ) ;
#52825=CARTESIAN_POINT ( 'NONE',  ( 7.361572987183169658, 64.96726448433412315, -9.846743663894592657 ) ) ;
#52828=CARTESIAN_POINT ( 'NONE',  ( 0.5774900079438607392, 3.480352010821504916, 5.440088680355550821 ) ) ;
#52830=CARTESIAN_POINT ( 'NONE',  ( 5.076628168052704559, 45.17559781766745175, -8.527530157486179263 ) ) ;
#52832=CARTESIAN_POINT ( 'NONE',  ( 10.00000000000000178, 4.313685344154837509, 10.88017736071110342 ) ) ;
#52834=CARTESIAN_POINT ( 'NONE',  ( 0.5774900079438607392, 38.48035201082150536, 5.440088680355550821 ) ) ;
#52835=CARTESIAN_POINT ( 'NONE',  ( 2.917880565312948704, 47.63708216824730357, 12.26659068614894643 ) ) ;
#52836=CARTESIAN_POINT ( 'NONE',  ( 10.00000000000000178, 4.313685344154837509, 10.88017736071110342 ) ) ;
#52838=CARTESIAN_POINT ( 'NONE',  ( 5.076628168052704559, 0.1755978176674514724, -8.527530157486179263 ) ) ;
#52839=CARTESIAN_POINT ( 'NONE',  ( 0.1532563361054100626, 30.80059781766744820, -2.638427012816831230 ) ) ;
#52840=CARTESIAN_POINT ( 'NONE',  ( 0.6178305044545818747, 13.49863466993041783, -9.382169495545419124 ) ) ;
#52843=CARTESIAN_POINT ( 'NONE',  ( 19.84674366389459266, 58.71726448433411605, -2.638427012816827677 ) ) ;
#52845=CARTESIAN_POINT ( 'NONE',  ( 2.791683348922237240, 65.38393115100078035, -7.208316651077763204 ) ) ;
#52846=CARTESIAN_POINT ( 'NONE',  ( -4.164238869374099927, 12.01208216824730357, 3.795296366450308767 ) ) ;
#52847=MECHANICAL_DESIGN_GEOMETRIC_PRESENTATION_REPRESENTATION('',(#1786),#12875);
#52848=CARTESIAN_POINT ( 'NONE',  ( 12.63842701281683034, 27.46726448433411250, 9.846743663894596210 ) ) ;
#52849=DIRECTION ( 'NONE',  ( 0.000000000000000000, -1.000000000000000000, -0.000000000000000000 ) ) ;
#52851=EDGE_CURVE ( 'NONE', #37014, #9012, #75880, .T. ) ;
#52852=CARTESIAN_POINT ( 'NONE',  ( -2.266590686148945544, 37.22041550158063217, 7.082119434687048631 ) ) ;
#52853=CARTESIAN_POINT ( 'NONE',  ( 10.00000000000000000, 14.75893115100078568, -9.846743663894594434 ) ) ;
#52854=DIRECTION ( 'NONE',  ( 6.608470384673550777E-17, 1.000000000000000000, -0.000000000000000000 ) ) ;
#52855=CARTESIAN_POINT ( 'NONE',  ( 20.88017736071110875, 35.77201867748816966, -2.915334737309920765 ) ) ;
#52856=CARTESIAN_POINT ( 'NONE',  ( 16.40814093676324603, 57.45696800326375353, -11.09922568453594671 ) ) ;
#52857=CARTESIAN_POINT ( 'NONE',  ( 4.559911319644449179, 2.230352010821504471, -9.422509992056141925 ) ) ;
#52859=CARTESIAN_POINT ( 'NONE',  ( -2.816281873526471635, 28.91530133659708213, -3.434112377981056508 ) ) ;
#52860=SURFACE_STYLE_FILL_AREA ( #68867 ) ;
#52863=CARTESIAN_POINT ( 'NONE',  ( 1.492507162822246602, 12.19955587570480837, -6.500000000000021316 ) ) ;
#52864=CARTESIAN_POINT ( 'NONE',  ( 20.03932841506541962, 35.62161441960502373, -6.397827110478998769 ) ) ;
#52865=CARTESIAN_POINT ( 'NONE',  ( -4.164238869374098151, 41.59541550158061796, -3.795296366450310543 ) ) ;
#52866=CARTESIAN_POINT ( 'NONE',  ( -0.3689425029237898834, 16.17874883491396076, -10.36894250292378850 ) ) ;
#52867=CARTESIAN_POINT ( 'NONE',  ( 12.91533473730993009, 6.605352010821504471, -10.88017736071109987 ) ) ;
#52868=CARTESIAN_POINT ( 'NONE',  ( 2.035157376598824452, 33.68868534415484106, 7.964842623401179544 ) ) ;
#52871=CARTESIAN_POINT ( 'NONE',  ( 10.00000000000000178, 49.31368534415484106, 10.88017736071110342 ) ) ;
#52872=CARTESIAN_POINT ( 'NONE',  ( 4.559911319644449179, 63.89701867748817676, 9.422509992056141925 ) ) ;
#52873=CARTESIAN_POINT ( 'NONE',  ( 16.40814093676324603, 22.45696800326375353, -11.09922568453594671 ) ) ;
#52876=CARTESIAN_POINT ( 'NONE',  ( 10.00000000000000178, 42.25893115100078745, 9.846743663894594434 ) ) ;
#52877=CARTESIAN_POINT ( 'NONE',  ( -2.816281873526473856, 14.12363466993041961, 9.499525473075851096E-16 ) ) ;
#52878=CARTESIAN_POINT ( 'NONE',  ( -0.8801773607110990882, 42.85535201082151247, -2.915334737309924318 ) ) ;
#52879=CARTESIAN_POINT ( 'NONE',  ( 20.88017736071110164, 15.35535201082150358, 2.915334737309930979 ) ) ;
#52880=CARTESIAN_POINT ( 'NONE',  ( 1.472469842513823179, 40.59226448433411605, -4.923371831947296329 ) ) ;
#52882=CARTESIAN_POINT ( 'NONE',  ( 1.472469842513823179, 20.59226448433411960, -4.923371831947296329 ) ) ;
#52883=CARTESIAN_POINT ( 'NONE',  ( 17.08211943468705840, 5.137082168247300906, -12.26659068614894466 ) ) ;
#52885=CARTESIAN_POINT ( 'NONE',  ( 10.00000000000000178, 29.31368534415483751, 10.88017736071110342 ) ) ;
#52887=CARTESIAN_POINT ( 'NONE',  ( 17.96484262340118221, 31.18868534415483751, -7.964842623401177768 ) ) ;
#52888=CARTESIAN_POINT ( 'NONE',  ( 10.00000000000000000, 16.81368534415483751, -10.88017736071110342 ) ) ;
#52891=CARTESIAN_POINT ( 'NONE',  ( 20.88017736071110875, 30.77201867748816966, -2.915334737309920765 ) ) ;
#52893=CARTESIAN_POINT ( 'NONE',  ( 21.09922568453595559, 52.04030133659708923, -6.408140936763230044 ) ) ;
#52894=EDGE_CURVE ( 'NONE', #9521, #27464, #32336, .T. ) ;
#52895=CARTESIAN_POINT ( 'NONE',  ( -0.8801773607111008646, 48.27201867748816966, 2.915334737309923430 ) ) ;
#52896=CARTESIAN_POINT ( 'NONE',  ( 0.5774900079438590739, 47.64701867748817676, -5.440088680355550821 ) ) ;
#52898=CARTESIAN_POINT ( 'NONE',  ( 4.559911319644449179, 32.23035201082150536, -9.422509992056141925 ) ) ;
#52899=SURFACE_SIDE_STYLE ('',( #52414 ) ) ;
#52901=CARTESIAN_POINT ( 'NONE',  ( 17.08211943468705130, 48.47041550158063927, 12.26659068614894998 ) ) ;
#52902=CARTESIAN_POINT ( 'NONE',  ( 7.084665262690076126, 54.10535201082151247, 10.88017736071109987 ) ) ;
#52903=CARTESIAN_POINT ( 'NONE',  ( 1.274849032794292736, 52.55509018479936856, -6.499999999999977796 ) ) ;
#52904=CARTESIAN_POINT ( 'NONE',  ( 7.361572987183170547, 57.05059781766744464, 9.846743663894590881 ) ) ;
#52906=CARTESIAN_POINT ( 'NONE',  ( 2.791683348922240793, 36.63393115100078035, 7.208316651077764092 ) ) ;
#52908=CARTESIAN_POINT ( 'NONE',  ( 14.92337183194729633, 32.67559781766745175, 8.527530157486181039 ) ) ;
#52910=CARTESIAN_POINT ( 'NONE',  ( 19.42250999205614193, 20.14701867748817321, 5.440088680355555262 ) ) ;
#52911=CARTESIAN_POINT ( 'NONE',  ( 7.361572987183170547, 32.05059781766745175, 9.846743663894590881 ) ) ;
#52913=CARTESIAN_POINT ( 'NONE',  ( 22.81628187352647785, 21.41530133659708923, 3.434112377981063169 ) ) ;
#52914=DIRECTION ( 'NONE',  ( 1.000000000000000000, 0.000000000000000000, 0.000000000000000000 ) ) ;
#52915=CARTESIAN_POINT ( 'NONE',  ( 10.00000000000000178, 59.31368534415484106, 10.88017736071110342 ) ) ;
#52916=CARTESIAN_POINT ( 'NONE',  ( 12.91533473730993009, 36.60535201082151247, -10.88017736071109987 ) ) ;
#52917=CARTESIAN_POINT ( 'NONE',  ( -0.8801773607110991993, 2.855352010821504471, -2.915334737309923874 ) ) ;
#52918=CARTESIAN_POINT ( 'NONE',  ( 20.36894250292379382, 48.67874883491396076, 10.36894250292379205 ) ) ;
#52922=CARTESIAN_POINT ( 'NONE',  ( 16.40814093676323893, 20.79030133659708923, 11.09922568453595026 ) ) ;
#52923=CARTESIAN_POINT ( 'NONE',  ( -0.8801773607111009756, 8.063685344154837509, 1.068504757029289695E-15 ) ) ;
#52924=CARTESIAN_POINT ( 'NONE',  ( 15.44008868035555793, 46.39701867748817676, -9.422509992056140149 ) ) ;
#52928=CARTESIAN_POINT ( 'NONE',  ( 2.035157376598822676, 57.43868534415484106, -7.964842623401177768 ) ) ;
#52930=CARTESIAN_POINT ( 'NONE',  ( 12.63842701281683034, 32.46726448433412315, 9.846743663894596210 ) ) ;
#52931=CARTESIAN_POINT ( 'NONE',  ( 2.791683348922240793, 21.63393115100078745, 7.208316651077764092 ) ) ;
#52932=CARTESIAN_POINT ( 'NONE',  ( 12.63842701281683034, 17.46726448433411250, 9.846743663894596210 ) ) ;
#52934=CARTESIAN_POINT ( 'NONE',  ( 0.2751277870542913062, 49.36607318730131055, -6.499999999999992006 ) ) ;
#52935=CARTESIAN_POINT ( 'NONE',  ( 3.591859063236761518, 34.95696800326375353, 11.09922568453594849 ) ) ;
#52936=CARTESIAN_POINT ( 'NONE',  ( 10.00000000000000178, 17.25893115100078745, 9.846743663894594434 ) ) ;
#52939=CARTESIAN_POINT ( 'NONE',  ( 19.84674366389459266, 38.30059781766745175, 2.638427012816836559 ) ) ;
#52942=CARTESIAN_POINT ( 'NONE',  ( 6.565887622018943937, 8.081968003263751754, -12.81628187352647608 ) ) ;
#52943=EDGE_CURVE ( 'NONE', #98205, #13047, #92314, .T. ) ;
#52944=CARTESIAN_POINT ( 'NONE',  ( 4.559911319644449179, 52.23035201082151247, -9.422509992056141925 ) ) ;
#52945=CARTESIAN_POINT ( 'NONE',  ( 24.16423886937409904, 34.09541550158064638, 3.795296366450317205 ) ) ;
#52948=CARTESIAN_POINT ( 'NONE',  ( 13.79529636645030344, 28.26208216824729647, 14.16423886937410614 ) ) ;
#52949=CARTESIAN_POINT ( 'NONE',  ( -2.266590686148945544, 52.22041550158064638, 7.082119434687048631 ) ) ;
#52950=CARTESIAN_POINT ( 'NONE',  ( 22.26659068614895176, 9.720415501580633943, -7.082119434687042414 ) ) ;
#52951=CARTESIAN_POINT ( 'NONE',  ( 17.08211943468705130, 28.47041550158063572, 12.26659068614894998 ) ) ;
#52953=CARTESIAN_POINT ( 'NONE',  ( 4.559911319644449179, 47.23035201082150536, -9.422509992056141925 ) ) ;
#52955=CARTESIAN_POINT ( 'NONE',  ( 19.84674366389459621, 28.50893115100078745, 7.409399052514197653E-17 ) ) ;
#52957=CARTESIAN_POINT ( 'NONE',  ( 2.791683348922240793, 41.63393115100078745, 7.208316651077764092 ) ) ;
#52958=CARTESIAN_POINT ( 'NONE',  ( 15.44008868035555260, 29.73035201082150891, 9.422509992056143702 ) ) ;
#52959=CARTESIAN_POINT ( 'NONE',  ( 3.591859063236763294, 63.29030133659708923, -11.09922568453595026 ) ) ;
#52961=CARTESIAN_POINT ( 'NONE',  ( 19.59242374975066525, 82.55671096202544845, -5.127491817725379875 ) ) ;
#52962=CARTESIAN_POINT ( 'NONE',  ( 12.63842701281683034, 27.46726448433411250, 9.846743663894596210 ) ) ;
#52963=CARTESIAN_POINT ( 'NONE',  ( 3.591859063236761518, 49.95696800326375353, 11.09922568453594849 ) ) ;
#52965=CARTESIAN_POINT ( 'NONE',  ( 20.88017736071110164, 45.35535201082149115, 2.915334737309930979 ) ) ;
#52966=CARTESIAN_POINT ( 'NONE',  ( 19.84674366389459621, 53.50893115100078745, 7.409399052514197653E-17 ) ) ;
#52967=CARTESIAN_POINT ( 'NONE',  ( 13.79529636645031943, 35.34541550158063927, -14.16423886937409904 ) ) ;
#52969=( NAMED_UNIT ( * ) SI_UNIT ( $, .STERADIAN. ) SOLID_ANGLE_UNIT ( ) );
#52970=CARTESIAN_POINT ( 'NONE',  ( 0.5774900079438607392, 58.48035201082151247, 5.440088680355550821 ) ) ;
#52972=CARTESIAN_POINT ( 'NONE',  ( 10.00000000000000178, 58.05374883491397497, 14.16423886937410082 ) ) ;
#52973=CARTESIAN_POINT ( 'NONE',  ( -1.099225684535947600, 8.706968003263753531, -6.408140936763238038 ) ) ;
#52975=CARTESIAN_POINT ( 'NONE',  ( 20.88017736071110875, 55.77201867748816966, -2.915334737309920765 ) ) ;
#52976=EDGE_CURVE ( 'NONE', #62128, #75793, #62400, .T. ) ;
#52978=CARTESIAN_POINT ( 'NONE',  ( -46.61145641952149532, 101.4776089914260950, -8.252540973952291026 ) ) ;
#52979=CARTESIAN_POINT ( 'NONE',  ( 6.204703633549690345, 42.84541550158063217, 14.16423886937410082 ) ) ;
#52981=CARTESIAN_POINT ( 'NONE',  ( -0.8801773607111008646, 13.27201867748817143, 2.915334737309923430 ) ) ;
#52982=CARTESIAN_POINT ( 'NONE',  ( 2.035157376598824452, 23.68868534415484461, 7.964842623401179544 ) ) ;
#52983=CARTESIAN_POINT ( 'NONE',  ( 0.1532563361054083140, 61.00893115100078745, 1.131784320476157264E-15 ) ) ;
#52984=CARTESIAN_POINT ( 'NONE',  ( 0.6178305044545838731, 54.74863466993042493, 9.382169495545420901 ) ) ;
#52986=ORIENTED_EDGE ( 'NONE', *, *, #83788, .T. ) ;
#52987=CARTESIAN_POINT ( 'NONE',  ( 17.96484262340118221, 14.93868534415483751, 7.964842623401181321 ) ) ;
#52988=CARTESIAN_POINT ( 'NONE',  ( 21.09922568453594849, 16.20696800326375353, 6.408140936763242479 ) ) ;
#52989=CARTESIAN_POINT ( 'NONE',  ( 20.10493008474206889, 39.71697413083879269, 6.336235997365759154 ) ) ;
#52991=CARTESIAN_POINT ( 'NONE',  ( 14.92337183194729988, 54.34226448433412315, -8.527530157486177487 ) ) ;
#52992=CARTESIAN_POINT ( 'NONE',  ( 20.88017736071110164, 30.35535201082151247, 2.915334737309930979 ) ) ;
#52993=CARTESIAN_POINT ( 'NONE',  ( 13.43411237798106583, 22.66530133659708923, -12.81628187352647252 ) ) ;
#52994=CARTESIAN_POINT ( 'NONE',  ( 17.96484262340118221, 49.93868534415484106, 7.964842623401181321 ) ) ;
#52995=CARTESIAN_POINT ( 'NONE',  ( 19.10478245763051319, 15.10160829253885950, 5.990408912944332087 ) ) ;
#52997=( GEOMETRIC_REPRESENTATION_CONTEXT ( 3 ) GLOBAL_UNCERTAINTY_ASSIGNED_CONTEXT ( ( #89285 ) ) GLOBAL_UNIT_ASSIGNED_CONTEXT ( ( #10368, #79350, #1903 ) ) REPRESENTATION_CONTEXT ( 'NONE', 'WORKASPACE' ) );
#52998=CARTESIAN_POINT ( 'NONE',  ( 3.591859063236761518, 54.95696800326376064, 11.09922568453594849 ) ) ;
#52999=ORIENTED_EDGE ( 'NONE', *, *, #61604, .T. ) ;
#53000=CARTESIAN_POINT ( 'NONE',  ( 0.5774900079438590739, 47.64701867748817676, -5.440088680355550821 ) ) ;
#53001=CARTESIAN_POINT ( 'NONE',  ( 16.40814093676323893, 30.79030133659708923, 11.09922568453595026 ) ) ;
#53002=CARTESIAN_POINT ( 'NONE',  ( -2.266590686148945544, 2.220415501580634388, 7.082119434687048631 ) ) ;
#53003=CARTESIAN_POINT ( 'NONE',  ( -0.8801773607111009756, 48.06368534415484817, 1.068504757029289695E-15 ) ) ;
#53004=CARTESIAN_POINT ( 'NONE',  ( 13.79529636645030344, 48.26208216824728936, 14.16423886937410614 ) ) ;
#53005=CARTESIAN_POINT ( 'NONE',  ( 7.361572987183169658, 64.96726448433412315, -9.846743663894592657 ) ) ;
#53006=CARTESIAN_POINT ( 'NONE',  ( 2.791683348922240793, 16.63393115100078745, 7.208316651077764092 ) ) ;
#53007=CARTESIAN_POINT ( 'NONE',  ( 1.472469842513823179, 6.425597817667451750, 4.923371831947296329 ) ) ;
#53009=CARTESIAN_POINT ( 'NONE',  ( 20.36894250292379382, 43.67874883491397497, 10.36894250292379205 ) ) ;
#53012=CARTESIAN_POINT ( 'NONE',  ( 17.96484262340118221, 6.188685344154836621, -7.964842623401177768 ) ) ;
#53014=VERTEX_POINT ( 'NONE', #54306 ) ;
#53015=CARTESIAN_POINT ( 'NONE',  ( 0.5774900079438607392, 8.480352010821505360, 5.440088680355550821 ) ) ;
#53016=CARTESIAN_POINT ( 'NONE',  ( 6.204703633549690345, 65.76208216824731778, -14.16423886937410259 ) ) ;
#53017=CARTESIAN_POINT ( 'NONE',  ( 19.84674366389459621, 48.50893115100078745, 7.409399052514197653E-17 ) ) ;
#53018=CARTESIAN_POINT ( 'NONE',  ( 13.43411237798105340, 40.58196800326375353, 12.81628187352647963 ) ) ;
#53021=CARTESIAN_POINT ( 'NONE',  ( -2.266590686148945544, 7.220415501580634832, 7.082119434687048631 ) ) ;
#53022=CARTESIAN_POINT ( 'NONE',  ( 20.88017736071110164, 10.35535201082150714, 2.915334737309930979 ) ) ;
#53023=CARTESIAN_POINT ( 'NONE',  ( 17.96484262340118221, 9.938685344154839285, 7.964842623401181321 ) ) ;
#53024=CARTESIAN_POINT ( 'NONE',  ( 0.1532563361054100626, 45.80059781766745886, -2.638427012816831230 ) ) ;
#53026=CARTESIAN_POINT ( 'NONE',  ( 0.1532563361054083140, 26.00893115100078745, 1.131784320476157264E-15 ) ) ;
#53033=CARTESIAN_POINT ( 'NONE',  ( 5.076628168052704559, 60.17559781766745175, -8.527530157486179263 ) ) ;
#53034=CARTESIAN_POINT ( 'NONE',  ( -0.8801773607111009756, 38.06368534415484106, 1.068504757029289695E-15 ) ) ;
#53035=CARTESIAN_POINT ( 'NONE',  ( -0.8801773607111009756, 33.06368534415484106, 1.068504757029289695E-15 ) ) ;
#53036=CARTESIAN_POINT ( 'NONE',  ( 2.791683348922237240, 65.38393115100078035, -7.208316651077763204 ) ) ;
#53037=CARTESIAN_POINT ( 'NONE',  ( 22.81628187352647785, 26.41530133659708923, 3.434112377981063169 ) ) ;
#53038=CARTESIAN_POINT ( 'NONE',  ( -0.3689425029237898834, 6.178748834913968757, -10.36894250292378850 ) ) ;
#53039=EDGE_CURVE ( 'NONE', #36181, #39274, #41999, .T. ) ;
#53041=CARTESIAN_POINT ( 'NONE',  ( 13.43411237798105340, 45.58196800326374643, 12.81628187352647963 ) ) ;
#53043=CARTESIAN_POINT ( 'NONE',  ( 19.84674366389459621, 48.50893115100078745, 7.409399052514197653E-17 ) ) ;
#53044=CARTESIAN_POINT ( 'NONE',  ( 12.91533473730993009, 6.605352010821504471, -10.88017736071109987 ) ) ;
#53045=ORIENTED_EDGE ( 'NONE', *, *, #73534, .F. ) ;
#53046=CARTESIAN_POINT ( 'NONE',  ( 19.42250999205614548, 15.98035201082150714, -5.440088680355545492 ) ) ;
#53047=VERTEX_POINT ( 'NONE', #45844 ) ;
#53048=CARTESIAN_POINT ( 'NONE',  ( 19.42250999205614548, 60.98035201082151247, -5.440088680355545492 ) ) ;
#53049=CARTESIAN_POINT ( 'NONE',  ( 12.91533473730992121, 59.52201867748816966, 10.88017736071110164 ) ) ;
#53050=CARTESIAN_POINT ( 'NONE',  ( 0.5774900079438607392, 63.48035201082149825, 5.440088680355550821 ) ) ;
#53051=( BOUNDED_SURFACE ( )  B_SPLINE_SURFACE ( 1, 2, ( 
 ( #69250, #14781, #53741, #84259, #61719, #45252, #91242, #69736, #30236, #53246, #1261, #16242, #23761, #31717, #54710, #77713, #67770, #29745, #60254, #83258, #1749, #10704, #55717, #64655, #57169, #86704, #78207, #18701, #32700, #9719, #40218, #87667, #47712, #70727, #49185, #18210, #86212, #19180, #11185, #71696, #93205, #2735, #41219, #3210, #48689, #49660, #79687, #9225, #63684, #2242, #33672, #79192, #64169, #26195, #63196, #32204, #94689, #94187, #48196, #56687, #25717, #87179, #56209, #39735, #62705, #10220, #41705, #17723, #78709, #93701, #95168, #72175, #40709, #24728, #25236, #71214, #26675, #55206, #70230, #3704, #85721, #17234, #33191, #34164, #5173, #97178, #19673, #35658, #43158, #13149, #65651, #50162, #82136, #74132, #13645, #97667, #29133, #12659, #66654, #59637, #21156, #12165, #58651, #42671, #34661, #27161, #73149, #28645, #65157, #73644, #89150, #20661, #51657, #74640, #88654, #88159, #44130, #4690, #20162, #80671, #66143, #90128, #35152, #96676, #50665, #6151, #95675, #27657, #5668, #96174, #51157, #11682, #36150, #59136, #36656, #58145, #81154, #67142, #21658, #28155, #81641, #43648, #89644, #80171, #42192, #72655, #4191, #57661, #23644, #54104, #45123, #61599, #44639, #75133, #90622, #31106, #60622, #69613, #77104, #30116, #22646, #45628, #30611, #658, #76615, #91123, #8132, #39126, #69126, #31597, #61117, #53126, #68632, #92113, #14658, #83634, #15149, #76127, #84617, #91626, #37646, #16121, #8617, #38625, #14155, #84133, #29618, #7653, #38146, #162, #60124, #7142, #46605, #22146, #52630, #1135, #62091, #23142, #53615, #75630, #92600, #15645, #46127, #52142, #82638, #6638, #37156, #98669, #67652, #98162, #83133, #68143, #33560, #47602, #24619, #55085, #72065, #62583, #85605, #64056, #33078, #70603, #34049, #26087, #86588, #9106, #17608, #25603, #18097, #2623, #3590, #94568, #24124, #78591, #17120, #56095, #94083, #63574, #41097, #93088, #56582, #86097, #48078, #48574, #85106, #64545, #93584, #79073, #10103, #9599, #11076, #40600, #3105, #18581, #16617, #54593, #87072, #32589, #71097, #25120, #10586, #41597, #2129, #78096, #49073, #79576, #40102, #71594, #55603, #47093, #77591, #63084, #39620, #70109, #1634, #32085, #72544, #81530, #35034, #50548, #42555, #12054, #43532, #81042, #4077, #96060, #5558, #26561, #66537, #73038, #58533, #27543, #42081, #28537, #34540, #13036, #12550, #65034, #88545, #58037, #4574, #65537, #95561, #35542, #96563, #27050, #20046, #57057, #28038, #36034, #43052, #97064, #73531, #66034, #95052, #74027, #57548, #5058, #88047, #11562, #19559, #50056, #89041, #80560, #20552 ),
 ( #51037, #87559, #19068, #49547, #80059, #2610, #37770, #62573, #71085, #75746, #17106, #67768, #32575, #86085, #33065, #68266, #16605, #94069, #40588, #1124, #9587, #93077, #45250, #47083, #56082, #18084, #85096, #77579, #10089, #63560, #31586, #48064, #29742, #60252, #7268, #17595, #9095, #86576, #25590, #39609, #70098, #32071, #47589, #78579, #63071, #1623, #93572, #48560, #55590, #79060, #78083, #24607, #55074, #37279, #62081, #85592, #40090, #70590, #98288, #2116, #24111, #90745, #22273, #52746, #25106, #83255, #14778, #92588, #54581, #4561, #57537, #89029, #3092, #11550, #50535, #57046, #19059, #3581, #66023, #80546, #49537, #64044, #79567, #11065, #96549, #94557, #71581, #12537, #28025, #18569, #87060, #72531, #34527, #27532, #49063, #65022, #4065, #42542, #95042, #41585, #43037, #35024, #73518, #58521, #72052, #81030, #34038, #80045, #64534, #42070, #20539, #26550, #95550, #27038, #5046, #87548, #88034, #35529, #19547, #50043, #41084, #65525, #58024, #51024, #12043, #73028, #10574, #33548, #96048, #88532, #20034, #26075, #56568, #38, #60985, #29004, #90008, #52992, #83507, #74511, #90989, #74015, #5544, #21033, #60500, #21528, #30486, #7525, #59514, #52022, #75009, #60001, #29993, #7018, #82513, #37523, #68508, #98541, #91497, #90494, #14031, #98037, #22520, #44009, #44510, #6514, #37022, #15024, #22030, #67021, #45496, #38015, #36021, #52503, #67520, #29491, #14529, #83011, #75504, #44999, #23018, #66524, #68014, #75997, #81517, #13024, #6032, #43520, #97051, #28525, #59017, #51523, #82015, #89524, #13526, #36532, #97542, #9972, #61478, #30980, #16493, #77463, #70475, #91984, #8975, #46969, #85474, #38996, #23515, #55470, #47463, #85973, #70974, #2494, #84975, #39974, #32950, #93461, #84494, #31954, #15995, #8006, #533, #46483, #1995, #38504, #39491, #62456, #92958, #24987, #47949, #61972, #92471, #53986, #17483, #76979, #23997, #8492, #69982, #63451, #69490, #1506, #54470, #78459, #1007, #24492, #40477, #31469, #54956, #83998, #77965, #32461, #93957, #16985, #9471, #53486, #15521, #62956, #46003, #76493, #69000, #33916, #42923, #4931, #71938, #64423, #95935, #27417, #18454, #34913, #17964, #48451, #63926, #4448, #94930, #73403, #50413, #3461, #26431, #18948, #3945, #72918, #49922, #56931, #80433, #12416, #42435, #35411, #34417, #87432, #41955, #65410, #86942, #49425, #79928, #11436, #57909, #64908, #10946, #88421, #80923, #78949, #95433, #72419, #26927, #57425, #87918, #19434, #11931, #65903, #10460, #19921, #25482, #55966, #86467, #48938, #40970, #71467, #2980, #33429, #94441, #25953, #56456, #79446, #41470 ) ),
 .UNSPECIFIED., .F., .F., .T. ) 
 B_SPLINE_SURFACE_WITH_KNOTS ( ( 2, 2 ),
 ( 3, 2, 2, 2, 2, 2, 2, 2, 2, 2, 2, 2, 2, 2, 2, 2, 2, 2, 2, 2, 2, 2, 2, 2, 2, 2, 2, 2, 2, 2, 2, 2, 2, 2, 2, 2, 2, 2, 2, 2, 2, 2, 2, 2, 2, 2, 2, 2, 2, 2, 2, 2, 2, 2, 2, 2, 2, 2, 2, 2, 2, 2, 2, 2, 2, 2, 2, 2, 2, 2, 2, 2, 2, 2, 2, 2, 2, 2, 2, 2, 2, 2, 2, 2, 2, 2, 2, 2, 2, 2, 2, 2, 2, 2, 2, 2, 2, 2, 2, 2, 2, 2, 2, 2, 2, 2, 2, 2, 2, 2, 2, 2, 2, 2, 2, 2, 2, 2, 2, 2, 2, 2, 2, 2, 2, 2, 2, 2, 2, 2, 2, 2, 2, 2, 2, 2, 2, 2, 2, 2, 2, 2, 2, 2, 2, 2, 2, 2, 2, 2, 2, 2, 2, 2, 2, 2, 2, 2, 2, 2, 2, 2, 3 ),
 ( 0.000000000000000000, 1.000000000000000000 ),
 ( 0.000000000000000000, 0.005952380952380952051, 0.01190476190476190410, 0.01785714285714285615, 0.02380952380952380820, 0.02976190476190476025, 0.03571428571428571230, 0.04166666666666666435, 0.04761904761904761640, 0.05357142857142856845, 0.05952380952380952051, 0.06547619047619047949, 0.07142857142857142461, 0.07738095238095238360, 0.08333333333333332871, 0.08928571428571428770, 0.09523809523809523281, 0.1011904761904761918, 0.1071428571428571369, 0.1130952380952380959, 0.1190476190476190410, 0.1250000000000000000, 0.1309523809523809590, 0.1369047619047619180, 0.1428571428571428492, 0.1488095238095238082, 0.1547619047619047672, 0.1607142857142857262, 0.1666666666666666574, 0.1726190476190476164, 0.1785714285714285754, 0.1845238095238095344, 0.1904761904761904656, 0.1964285714285714246, 0.2023809523809523836, 0.2083333333333333426, 0.2142857142857142738, 0.2202380952380952328, 0.2261904761904761918, 0.2321428571428571508, 0.2380952380952380820, 0.2440476190476190410, 0.2500000000000000000, 0.2559523809523809312, 0.2619047619047619180, 0.2678571428571428492, 0.2738095238095238360, 0.2797619047619047672, 0.2857142857142856984, 0.2916666666666666852, 0.2976190476190476164, 0.3035714285714285476, 0.3095238095238095344, 0.3154761904761904656, 0.3214285714285714524, 0.3273809523809523836, 0.3333333333333333148, 0.3392857142857143016, 0.3452380952380952328, 0.3511904761904761640, 0.3571428571428571508, 0.3630952380952380820, 0.3690476190476190688, 0.3750000000000000000, 0.3809523809523809312, 0.3869047619047619180, 0.3928571428571428492, 0.3988095238095238360, 0.4047619047619047672, 0.4107142857142856984, 0.4166666666666666852, 0.4226190476190476164, 0.4285714285714285476, 0.4345238095238095344, 0.4404761904761904656, 0.4464285714285714524, 0.4523809523809523836, 0.4583333333333333148, 0.4642857142857143016, 0.4702380952380952328, 0.4761904761904761640, 0.4821428571428571508, 0.4880952380952380820, 0.4940476190476190688, 0.5000000000000000000, 0.5059523809523809312, 0.5119047619047618625, 0.5178571428571429047, 0.5238095238095238360, 0.5297619047619047672, 0.5357142857142856984, 0.5416666666666666297, 0.5476190476190476719, 0.5535714285714286031, 0.5595238095238095344, 0.5654761904761904656, 0.5714285714285713969, 0.5773809523809523281, 0.5833333333333333703, 0.5892857142857143016, 0.5952380952380952328, 0.6011904761904761640, 0.6071428571428570953, 0.6130952380952381375, 0.6190476190476190688, 0.6250000000000000000, 0.6309523809523809312, 0.6369047619047618625, 0.6428571428571429047, 0.6488095238095238360, 0.6547619047619047672, 0.6607142857142856984, 0.6666666666666666297, 0.6726190476190476719, 0.6785714285714286031, 0.6845238095238095344, 0.6904761904761904656, 0.6964285714285713969, 0.7023809523809523281, 0.7083333333333333703, 0.7142857142857143016, 0.7202380952380952328, 0.7261904761904761640, 0.7321428571428570953, 0.7380952380952381375, 0.7440476190476190688, 0.7500000000000000000, 0.7559523809523809312, 0.7619047619047618625, 0.7678571428571429047, 0.7738095238095238360, 0.7797619047619047672, 0.7857142857142856984, 0.7916666666666666297, 0.7976190476190476719, 0.8035714285714286031, 0.8095238095238095344, 0.8154761904761904656, 0.8214285714285713969, 0.8273809523809523281, 0.8333333333333333703, 0.8392857142857143016, 0.8452380952380952328, 0.8511904761904761640, 0.8571428571428570953, 0.8630952380952381375, 0.8690476190476190688, 0.8750000000000000000, 0.8809523809523809312, 0.8869047619047618625, 0.8928571428571429047, 0.8988095238095238360, 0.9047619047619047672, 0.9107142857142856984, 0.9166666666666666297, 0.9226190476190476719, 0.9285714285714286031, 0.9345238095238095344, 0.9404761904761904656, 0.9464285714285713969, 0.9523809523809523281, 0.9583333333333333703, 0.9642857142857143016 ),
 .UNSPECIFIED. ) 
 GEOMETRIC_REPRESENTATION_ITEM ( )  RATIONAL_B_SPLINE_SURFACE ( (
 ( 1.000000000000000000, 0.9659258262890683122, 1.000000000000000000, 0.9659258262890683122, 1.000000000000000000, 0.9659258262890683122, 1.000000000000000000, 0.9659258262890683122, 1.000000000000000000, 0.9659258262890683122, 1.000000000000000000, 0.9659258262890683122, 1.000000000000000000, 0.9659258262890683122, 1.000000000000000000, 0.9659258262890683122, 1.000000000000000000, 0.9659258262890683122, 1.000000000000000000, 0.9659258262890683122, 1.000000000000000000, 0.9659258262890683122, 1.000000000000000000, 0.9659258262890683122, 1.000000000000000000, 0.9659258262890683122, 1.000000000000000000, 0.9659258262890683122, 1.000000000000000000, 0.9659258262890683122, 1.000000000000000000, 0.9659258262890683122, 1.000000000000000000, 0.9659258262890683122, 1.000000000000000000, 0.9659258262890683122, 1.000000000000000000, 0.9659258262890683122, 1.000000000000000000, 0.9659258262890683122, 1.000000000000000000, 0.9659258262890683122, 1.000000000000000000, 0.9659258262890683122, 1.000000000000000000, 0.9659258262890683122, 1.000000000000000000, 0.9659258262890683122, 1.000000000000000000, 0.9659258262890683122, 1.000000000000000000, 0.9659258262890683122, 1.000000000000000000, 0.9659258262890683122, 1.000000000000000000, 0.9659258262890683122, 1.000000000000000000, 0.9659258262890683122, 1.000000000000000000, 0.9659258262890683122, 1.000000000000000000, 0.9659258262890683122, 1.000000000000000000, 0.9659258262890683122, 1.000000000000000000, 0.9659258262890683122, 1.000000000000000000, 0.9659258262890683122, 1.000000000000000000, 0.9659258262890683122, 1.000000000000000000, 0.9659258262890683122, 1.000000000000000000, 0.9659258262890683122, 1.000000000000000000, 0.9659258262890683122, 1.000000000000000000, 0.9659258262890683122, 1.000000000000000000, 0.9659258262890683122, 1.000000000000000000, 0.9659258262890683122, 1.000000000000000000, 0.9659258262890683122, 1.000000000000000000, 0.9659258262890683122, 1.000000000000000000, 0.9659258262890683122, 1.000000000000000000, 0.9659258262890683122, 1.000000000000000000, 0.9659258262890683122, 1.000000000000000000, 0.9659258262890683122, 1.000000000000000000, 0.9659258262890683122, 1.000000000000000000, 0.9659258262890683122, 1.000000000000000000, 0.9659258262890683122, 1.000000000000000000, 0.9659258262890683122, 1.000000000000000000, 0.9659258262890683122, 1.000000000000000000, 0.9659258262890683122, 1.000000000000000000, 0.9659258262890683122, 1.000000000000000000, 0.9659258262890683122, 1.000000000000000000, 0.9659258262890683122, 1.000000000000000000, 0.9659258262890683122, 1.000000000000000000, 0.9659258262890683122, 1.000000000000000000, 0.9659258262890683122, 1.000000000000000000, 0.9659258262890683122, 1.000000000000000000, 0.9659258262890683122, 1.000000000000000000, 0.9659258262890683122, 1.000000000000000000, 0.9659258262890683122, 1.000000000000000000, 0.9659258262890683122, 1.000000000000000000, 0.9659258262890683122, 1.000000000000000000, 0.9659258262890683122, 1.000000000000000000, 0.9659258262890683122, 1.000000000000000000, 0.9659258262890683122, 1.000000000000000000, 0.9659258262890683122, 1.000000000000000000, 0.9659258262890683122, 1.000000000000000000, 0.9659258262890683122, 1.000000000000000000, 0.9659258262890683122, 1.000000000000000000, 0.9659258262890683122, 1.000000000000000000, 0.9659258262890683122, 1.000000000000000000, 0.9659258262890683122, 1.000000000000000000, 0.9659258262890683122, 1.000000000000000000, 0.9659258262890683122, 1.000000000000000000, 0.9659258262890683122, 1.000000000000000000, 0.9659258262890683122, 1.000000000000000000, 0.9659258262890683122, 1.000000000000000000, 0.9659258262890683122, 1.000000000000000000, 0.9659258262890683122, 1.000000000000000000, 0.9659258262890683122, 1.000000000000000000, 0.9659258262890683122, 1.000000000000000000, 0.9659258262890683122, 1.000000000000000000, 0.9659258262890683122, 1.000000000000000000, 0.9659258262890683122, 1.000000000000000000, 0.9659258262890683122, 1.000000000000000000, 0.9659258262890683122, 1.000000000000000000, 0.9659258262890683122, 1.000000000000000000, 0.9659258262890683122, 1.000000000000000000, 0.9659258262890683122, 1.000000000000000000, 0.9659258262890683122, 1.000000000000000000, 0.9659258262890683122, 1.000000000000000000, 0.9659258262890683122, 1.000000000000000000, 0.9659258262890683122, 1.000000000000000000, 0.9659258262890683122, 1.000000000000000000, 0.9659258262890683122, 1.000000000000000000, 0.9659258262890683122, 1.000000000000000000, 0.9659258262890683122, 1.000000000000000000, 0.9659258262890683122, 1.000000000000000000, 0.9659258262890683122, 1.000000000000000000, 0.9659258262890683122, 1.000000000000000000, 0.9659258262890683122, 1.000000000000000000, 0.9659258262890683122, 1.000000000000000000, 0.9659258262890683122, 1.000000000000000000, 0.9659258262890683122, 1.000000000000000000, 0.9659258262890683122, 1.000000000000000000, 0.9659258262890683122, 1.000000000000000000, 0.9659258262890683122, 1.000000000000000000, 0.9659258262890683122, 1.000000000000000000, 0.9659258262890683122, 1.000000000000000000, 0.9659258262890683122, 1.000000000000000000, 0.9659258262890683122, 1.000000000000000000, 0.9659258262890683122, 1.000000000000000000, 0.9659258262890683122, 1.000000000000000000, 0.9659258262890683122, 1.000000000000000000, 0.9659258262890683122, 1.000000000000000000, 0.9659258262890683122, 1.000000000000000000, 0.9659258262890683122, 1.000000000000000000, 0.9659258262890683122, 1.000000000000000000, 0.9659258262890683122, 1.000000000000000000, 0.9659258262890683122, 1.000000000000000000, 0.9659258262890683122, 1.000000000000000000, 0.9659258262890683122, 1.000000000000000000, 0.9659258262890683122, 1.000000000000000000, 0.9659258262890683122, 1.000000000000000000, 0.9659258262890683122, 1.000000000000000000, 0.9659258262890683122, 1.000000000000000000, 0.9659258262890683122, 1.000000000000000000, 0.9659258262890683122, 1.000000000000000000, 0.9659258262890683122, 1.000000000000000000, 0.9659258262890683122, 1.000000000000000000, 0.9659258262890683122, 1.000000000000000000, 0.9659258262890683122, 1.000000000000000000, 0.9659258262890683122, 1.000000000000000000, 0.9659258262890683122, 1.000000000000000000, 0.9659258262890683122, 1.000000000000000000, 0.9659258262890683122, 1.000000000000000000, 0.9659258262890683122, 1.000000000000000000, 0.9659258262890683122, 1.000000000000000000, 0.9659258262890683122, 1.000000000000000000, 0.9659258262890683122, 1.000000000000000000, 0.9659258262890683122, 1.000000000000000000, 0.9659258262890683122, 1.000000000000000000, 0.9659258262890683122, 1.000000000000000000, 0.9659258262890683122, 1.000000000000000000, 0.9659258262890683122, 1.000000000000000000, 0.9659258262890683122, 1.000000000000000000, 0.9659258262890683122, 1.000000000000000000, 0.9659258262890683122, 1.000000000000000000, 0.9659258262890683122, 1.000000000000000000, 0.9659258262890683122, 1.000000000000000000, 0.9659258262890683122, 1.000000000000000000, 0.9659258262890683122, 1.000000000000000000, 0.9659258262890683122, 1.000000000000000000, 0.9659258262890683122, 1.000000000000000000, 0.9659258262890683122, 1.000000000000000000, 0.9659258262890683122, 1.000000000000000000, 0.9659258262890683122, 1.000000000000000000, 0.9659258262890683122, 1.000000000000000000, 0.9659258262890683122, 1.000000000000000000),
 ( 1.000000000000000000, 0.9659258262890683122, 1.000000000000000000, 0.9659258262890683122, 1.000000000000000000, 0.9659258262890683122, 1.000000000000000000, 0.9659258262890683122, 1.000000000000000000, 0.9659258262890683122, 1.000000000000000000, 0.9659258262890683122, 1.000000000000000000, 0.9659258262890683122, 1.000000000000000000, 0.9659258262890683122, 1.000000000000000000, 0.9659258262890683122, 1.000000000000000000, 0.9659258262890683122, 1.000000000000000000, 0.9659258262890683122, 1.000000000000000000, 0.9659258262890683122, 1.000000000000000000, 0.9659258262890683122, 1.000000000000000000, 0.9659258262890683122, 1.000000000000000000, 0.9659258262890683122, 1.000000000000000000, 0.9659258262890683122, 1.000000000000000000, 0.9659258262890683122, 1.000000000000000000, 0.9659258262890683122, 1.000000000000000000, 0.9659258262890683122, 1.000000000000000000, 0.9659258262890683122, 1.000000000000000000, 0.9659258262890683122, 1.000000000000000000, 0.9659258262890683122, 1.000000000000000000, 0.9659258262890683122, 1.000000000000000000, 0.9659258262890683122, 1.000000000000000000, 0.9659258262890683122, 1.000000000000000000, 0.9659258262890683122, 1.000000000000000000, 0.9659258262890683122, 1.000000000000000000, 0.9659258262890683122, 1.000000000000000000, 0.9659258262890683122, 1.000000000000000000, 0.9659258262890683122, 1.000000000000000000, 0.9659258262890683122, 1.000000000000000000, 0.9659258262890683122, 1.000000000000000000, 0.9659258262890683122, 1.000000000000000000, 0.9659258262890683122, 1.000000000000000000, 0.9659258262890683122, 1.000000000000000000, 0.9659258262890683122, 1.000000000000000000, 0.9659258262890683122, 1.000000000000000000, 0.9659258262890683122, 1.000000000000000000, 0.9659258262890683122, 1.000000000000000000, 0.9659258262890683122, 1.000000000000000000, 0.9659258262890683122, 1.000000000000000000, 0.9659258262890683122, 1.000000000000000000, 0.9659258262890683122, 1.000000000000000000, 0.9659258262890683122, 1.000000000000000000, 0.9659258262890683122, 1.000000000000000000, 0.9659258262890683122, 1.000000000000000000, 0.9659258262890683122, 1.000000000000000000, 0.9659258262890683122, 1.000000000000000000, 0.9659258262890683122, 1.000000000000000000, 0.9659258262890683122, 1.000000000000000000, 0.9659258262890683122, 1.000000000000000000, 0.9659258262890683122, 1.000000000000000000, 0.9659258262890683122, 1.000000000000000000, 0.9659258262890683122, 1.000000000000000000, 0.9659258262890683122, 1.000000000000000000, 0.9659258262890683122, 1.000000000000000000, 0.9659258262890683122, 1.000000000000000000, 0.9659258262890683122, 1.000000000000000000, 0.9659258262890683122, 1.000000000000000000, 0.9659258262890683122, 1.000000000000000000, 0.9659258262890683122, 1.000000000000000000, 0.9659258262890683122, 1.000000000000000000, 0.9659258262890683122, 1.000000000000000000, 0.9659258262890683122, 1.000000000000000000, 0.9659258262890683122, 1.000000000000000000, 0.9659258262890683122, 1.000000000000000000, 0.9659258262890683122, 1.000000000000000000, 0.9659258262890683122, 1.000000000000000000, 0.9659258262890683122, 1.000000000000000000, 0.9659258262890683122, 1.000000000000000000, 0.9659258262890683122, 1.000000000000000000, 0.9659258262890683122, 1.000000000000000000, 0.9659258262890683122, 1.000000000000000000, 0.9659258262890683122, 1.000000000000000000, 0.9659258262890683122, 1.000000000000000000, 0.9659258262890683122, 1.000000000000000000, 0.9659258262890683122, 1.000000000000000000, 0.9659258262890683122, 1.000000000000000000, 0.9659258262890683122, 1.000000000000000000, 0.9659258262890683122, 1.000000000000000000, 0.9659258262890683122, 1.000000000000000000, 0.9659258262890683122, 1.000000000000000000, 0.9659258262890683122, 1.000000000000000000, 0.9659258262890683122, 1.000000000000000000, 0.9659258262890683122, 1.000000000000000000, 0.9659258262890683122, 1.000000000000000000, 0.9659258262890683122, 1.000000000000000000, 0.9659258262890683122, 1.000000000000000000, 0.9659258262890683122, 1.000000000000000000, 0.9659258262890683122, 1.000000000000000000, 0.9659258262890683122, 1.000000000000000000, 0.9659258262890683122, 1.000000000000000000, 0.9659258262890683122, 1.000000000000000000, 0.9659258262890683122, 1.000000000000000000, 0.9659258262890683122, 1.000000000000000000, 0.9659258262890683122, 1.000000000000000000, 0.9659258262890683122, 1.000000000000000000, 0.9659258262890683122, 1.000000000000000000, 0.9659258262890683122, 1.000000000000000000, 0.9659258262890683122, 1.000000000000000000, 0.9659258262890683122, 1.000000000000000000, 0.9659258262890683122, 1.000000000000000000, 0.9659258262890683122, 1.000000000000000000, 0.9659258262890683122, 1.000000000000000000, 0.9659258262890683122, 1.000000000000000000, 0.9659258262890683122, 1.000000000000000000, 0.9659258262890683122, 1.000000000000000000, 0.9659258262890683122, 1.000000000000000000, 0.9659258262890683122, 1.000000000000000000, 0.9659258262890683122, 1.000000000000000000, 0.9659258262890683122, 1.000000000000000000, 0.9659258262890683122, 1.000000000000000000, 0.9659258262890683122, 1.000000000000000000, 0.9659258262890683122, 1.000000000000000000, 0.9659258262890683122, 1.000000000000000000, 0.9659258262890683122, 1.000000000000000000, 0.9659258262890683122, 1.000000000000000000, 0.9659258262890683122, 1.000000000000000000, 0.9659258262890683122, 1.000000000000000000, 0.9659258262890683122, 1.000000000000000000, 0.9659258262890683122, 1.000000000000000000, 0.9659258262890683122, 1.000000000000000000, 0.9659258262890683122, 1.000000000000000000, 0.9659258262890683122, 1.000000000000000000, 0.9659258262890683122, 1.000000000000000000, 0.9659258262890683122, 1.000000000000000000, 0.9659258262890683122, 1.000000000000000000, 0.9659258262890683122, 1.000000000000000000, 0.9659258262890683122, 1.000000000000000000, 0.9659258262890683122, 1.000000000000000000, 0.9659258262890683122, 1.000000000000000000, 0.9659258262890683122, 1.000000000000000000, 0.9659258262890683122, 1.000000000000000000, 0.9659258262890683122, 1.000000000000000000, 0.9659258262890683122, 1.000000000000000000, 0.9659258262890683122, 1.000000000000000000, 0.9659258262890683122, 1.000000000000000000, 0.9659258262890683122, 1.000000000000000000, 0.9659258262890683122, 1.000000000000000000, 0.9659258262890683122, 1.000000000000000000, 0.9659258262890683122, 1.000000000000000000, 0.9659258262890683122, 1.000000000000000000, 0.9659258262890683122, 1.000000000000000000, 0.9659258262890683122, 1.000000000000000000, 0.9659258262890683122, 1.000000000000000000, 0.9659258262890683122, 1.000000000000000000, 0.9659258262890683122, 1.000000000000000000, 0.9659258262890683122, 1.000000000000000000, 0.9659258262890683122, 1.000000000000000000, 0.9659258262890683122, 1.000000000000000000, 0.9659258262890683122, 1.000000000000000000, 0.9659258262890683122, 1.000000000000000000, 0.9659258262890683122, 1.000000000000000000, 0.9659258262890683122, 1.000000000000000000, 0.9659258262890683122, 1.000000000000000000, 0.9659258262890683122, 1.000000000000000000, 0.9659258262890683122, 1.000000000000000000, 0.9659258262890683122, 1.000000000000000000, 0.9659258262890683122, 1.000000000000000000, 0.9659258262890683122, 1.000000000000000000, 0.9659258262890683122, 1.000000000000000000, 0.9659258262890683122, 1.000000000000000000) ) ) 
 REPRESENTATION_ITEM ( '' )  SURFACE ( )  );
#53054=CARTESIAN_POINT ( 'NONE',  ( 10.00000000000000000, 56.81368534415484106, -10.88017736071110342 ) ) ;
#53059=EDGE_CURVE ( 'NONE', #44176, #75287, #45547, .T. ) ;
#53060=CARTESIAN_POINT ( 'NONE',  ( 2.791683348922240793, 36.63393115100078035, 7.208316651077764092 ) ) ;
#53067=CARTESIAN_POINT ( 'NONE',  ( 22.26659068614895176, 9.720415501580633943, -7.082119434687042414 ) ) ;
#53069=CARTESIAN_POINT ( 'NONE',  ( -46.83185791578573287, 103.4687159110575010, -5.836295484760862351 ) ) ;
#53070=CARTESIAN_POINT ( 'NONE',  ( 15.44008868035555793, 61.39701867748817676, -9.422509992056140149 ) ) ;
#53071=CARTESIAN_POINT ( 'NONE',  ( 2.035157376598824452, 8.688685344154839285, 7.964842623401179544 ) ) ;
#53072=CARTESIAN_POINT ( 'NONE',  ( 0.9413316022086001267, 48.45508385108958294, 6.499999999999960032 ) ) ;
#53073=CARTESIAN_POINT ( 'NONE',  ( 22.81628187352647785, 41.41530133659708923, 3.434112377981063169 ) ) ;
#53075=DIRECTION ( 'NONE',  ( 0.000000000000000000, 0.000000000000000000, -1.000000000000000000 ) ) ;
#53077=CARTESIAN_POINT ( 'NONE',  ( 19.84674366389459621, 48.50893115100078745, 7.409399052514197653E-17 ) ) ;
#53078=PRESENTATION_STYLE_ASSIGNMENT (( #91074 ) ) ;
#53079=CARTESIAN_POINT ( 'NONE',  ( 19.38216949554541202, 15.99863466993042138, 9.382169495545424454 ) ) ;
#53080=CARTESIAN_POINT ( 'NONE',  ( 10.00000000000000178, 22.25893115100078745, 9.846743663894594434 ) ) ;
#53082=CARTESIAN_POINT ( 'NONE',  ( 1.472469842513823179, 20.59226448433411960, -4.923371831947296329 ) ) ;
#53083=CARTESIAN_POINT ( 'NONE',  ( 0.1532563361054100626, 65.80059781766745175, -2.638427012816831230 ) ) ;
#53088=ORIENTED_EDGE ( 'NONE', *, *, #9284, .F. ) ;
#53089=CARTESIAN_POINT ( 'NONE',  ( 2.035157376598822676, 22.43868534415483396, -7.964842623401177768 ) ) ;
#53090=CARTESIAN_POINT ( 'NONE',  ( 20.36894250292379738, 14.92874883491396432, -10.36894250292379027 ) ) ;
#53091=CARTESIAN_POINT ( 'NONE',  ( 10.00000000000000178, 27.25893115100078390, 9.846743663894594434 ) ) ;
#53092=CARTESIAN_POINT ( 'NONE',  ( 19.84674366389459266, 3.300597817667451750, 2.638427012816836559 ) ) ;
#53093=CARTESIAN_POINT ( 'NONE',  ( 3.591859063236763294, 43.29030133659708923, -11.09922568453595026 ) ) ;
#53094=CARTESIAN_POINT ( 'NONE',  ( 19.72487221294570858, 1.866073187300754110, 6.500000000000000888 ) ) ;
#53095=CARTESIAN_POINT ( 'NONE',  ( -0.8801773607110991993, 17.85535201082150536, -2.915334737309923874 ) ) ;
#53097=CARTESIAN_POINT ( 'NONE',  ( 19.72487221294570858, 70.00000000000000000, 6.500000000000000888 ) ) ;
#53099=CARTESIAN_POINT ( 'NONE',  ( 22.81628187352647785, 11.41530133659708390, 3.434112377981063169 ) ) ;
#53100=CARTESIAN_POINT ( 'NONE',  ( -1.099225684535947600, 8.706968003263753531, -6.408140936763238038 ) ) ;
#53101=CARTESIAN_POINT ( 'NONE',  ( 12.63842701281683034, 22.46726448433411605, 9.846743663894596210 ) ) ;
#53103=CARTESIAN_POINT ( 'NONE',  ( -2.816281873526473856, 39.33196800326374643, 3.434112377981055619 ) ) ;
#53105=CARTESIAN_POINT ( 'NONE',  ( -0.8801773607111008646, 43.27201867748817676, 2.915334737309923430 ) ) ;
#53108=CARTESIAN_POINT ( 'NONE',  ( -0.8801773607111008646, 68.27201867748817676, 2.915334737309923430 ) ) ;
#53110=CARTESIAN_POINT ( 'NONE',  ( 12.91533473730992121, 34.52201867748817676, 10.88017736071110164 ) ) ;
#53112=CARTESIAN_POINT ( 'NONE',  ( 19.42250999205614193, 45.14701867748817676, 5.440088680355555262 ) ) ;
#53113=CARTESIAN_POINT ( 'NONE',  ( 19.80777595082616926, 60.68878173731740588, -6.499999999999965361 ) ) ;
#53114=CARTESIAN_POINT ( 'NONE',  ( 20.15039907845753930, 70.00000000000000000, -6.262539305110068177 ) ) ;
#53116=CARTESIAN_POINT ( 'NONE',  ( 0.1532563361054082862, 56.21726448433411605, 2.638427012816831674 ) ) ;
#53117=CARTESIAN_POINT ( 'NONE',  ( 12.91533473730992121, 4.522018677488169658, 10.88017736071110164 ) ) ;
#53119=CARTESIAN_POINT ( 'NONE',  ( 19.38216949554541202, 10.99863466993042138, 9.382169495545424454 ) ) ;
#53121=CARTESIAN_POINT ( 'NONE',  ( 12.91533473730992121, 44.52201867748816966, 10.88017736071110164 ) ) ;
#53122=CARTESIAN_POINT ( 'NONE',  ( 10.00000000000000000, -2.126365330069579951, -12.81628187352647608 ) ) ;
#53123=CARTESIAN_POINT ( 'NONE',  ( 19.72487221294570858, 6.866073187300758107, 6.500000000000000888 ) ) ;
#53124=CARTESIAN_POINT ( 'NONE',  ( 17.96484262340118221, 29.93868534415484106, 7.964842623401181321 ) ) ;
#53125=CARTESIAN_POINT ( 'NONE',  ( 1.472469842513823179, 16.42559781766745175, 4.923371831947296329 ) ) ;
#53126=CARTESIAN_POINT ( 'NONE',  ( -0.3689425029237898834, 36.17874883491396787, -10.36894250292378850 ) ) ;
#53127=CARTESIAN_POINT ( 'NONE',  ( 18.52753015748618282, 28.92559781766745175, -4.923371831947291888 ) ) ;
#53128=CARTESIAN_POINT ( 'NONE',  ( 19.42250999205614193, 45.14701867748817676, 5.440088680355555262 ) ) ;
#53130=CARTESIAN_POINT ( 'NONE',  ( -4.164238869374099039, 1.803748834913967647, 8.674139862899312516E-16 ) ) ;
#53131=CARTESIAN_POINT ( 'NONE',  ( -46.76825711229114546, 103.5742016582868672, 5.803477452201137865 ) ) ;
#53132=CARTESIAN_POINT ( 'NONE',  ( 14.92337183194729988, 54.34226448433412315, -8.527530157486177487 ) ) ;
#53133=ORIENTED_EDGE ( 'NONE', *, *, #64473, .T. ) ;
#53134=EDGE_LOOP ( 'NONE', ( #50083, #48901, #98171, #80437, #72314 ) ) ;
#53135=CARTESIAN_POINT ( 'NONE',  ( 24.16423886937410614, 34.51208216824731068, -3.795296366450302550 ) ) ;
#53136=CARTESIAN_POINT ( 'NONE',  ( -2.266590686148945544, 27.22041550158063572, 7.082119434687048631 ) ) ;
#53137=CARTESIAN_POINT ( 'NONE',  ( 7.361572987183169658, 9.967264484334119601, -9.846743663894592657 ) ) ;
#53138=CARTESIAN_POINT ( 'NONE',  ( -0.3689425029237881626, 67.42874883491396076, 10.36894250292379027 ) ) ;
#53139=CARTESIAN_POINT ( 'NONE',  ( 10.00000000000000000, 44.75893115100078745, -9.846743663894594434 ) ) ;
#53141=CARTESIAN_POINT ( 'NONE',  ( 17.96484262340118221, 41.18868534415484106, -7.964842623401177768 ) ) ;
#53142=CARTESIAN_POINT ( 'NONE',  ( -2.816281873526471635, 18.91530133659708213, -3.434112377981056508 ) ) ;
#53143=CARTESIAN_POINT ( 'NONE',  ( 2.917880565312948704, 17.63708216824730357, 12.26659068614894643 ) ) ;
#53144=CARTESIAN_POINT ( 'NONE',  ( -0.8801773607111009756, 8.063685344154837509, 1.068504757029289695E-15 ) ) ;
#53146=CARTESIAN_POINT ( 'NONE',  ( 12.91533473730993009, 31.60535201082150891, -10.88017736071109987 ) ) ;
#53148=CARTESIAN_POINT ( 'NONE',  ( 4.559911319644449179, 62.23035201082150536, -9.422509992056141925 ) ) ;
#53150=CARTESIAN_POINT ( 'NONE',  ( 10.00000000000000178, 50.37363466993042493, 12.81628187352647608 ) ) ;
#53153=CARTESIAN_POINT ( 'NONE',  ( 20.15039907845753220, 34.72266099184918176, 6.262539305110077059 ) ) ;
#53159=CARTESIAN_POINT ( 'NONE',  ( -4.164238869374099039, 61.80374883491397497, 8.674139862899312516E-16 ) ) ;
#53160=CARTESIAN_POINT ( 'NONE',  ( 6.204703633549690345, 65.76208216824731778, -14.16423886937410259 ) ) ;
#53161=CARTESIAN_POINT ( 'NONE',  ( 7.361572987183170547, 17.05059781766745530, 9.846743663894590881 ) ) ;
#53162=CARTESIAN_POINT ( 'NONE',  ( 5.076628168052704559, 55.17559781766745175, -8.527530157486179263 ) ) ;
#53163=CARTESIAN_POINT ( 'NONE',  ( 20.24186590665276597, 49.73410085661204505, 6.114288769123062295 ) ) ;
#53165=CARTESIAN_POINT ( 'NONE',  ( 18.72515096720591643, 66.07228050351029935, -6.499999999999699796 ) ) ;
#53166=CARTESIAN_POINT ( 'NONE',  ( 19.84674366389459621, 8.508931151000785675, 7.409399052514197653E-17 ) ) ;
#53168=VERTEX_POINT ( 'NONE', #68348 ) ;
#53169=CARTESIAN_POINT ( 'NONE',  ( 20.36894250292379382, 28.67874883491396787, 10.36894250292379205 ) ) ;
#53170=CARTESIAN_POINT ( 'NONE',  ( 2.917880565312950480, 45.97041550158063927, -12.26659068614894821 ) ) ;
#53173=CARTESIAN_POINT ( 'NONE',  ( 19.38216949554541202, 60.99863466993042493, 9.382169495545424454 ) ) ;
#53174=CARTESIAN_POINT ( 'NONE',  ( 2.791683348922240793, 56.63393115100078035, 7.208316651077764092 ) ) ;
#53175=CARTESIAN_POINT ( 'NONE',  ( -0.8801773607111008646, 23.27201867748817676, 2.915334737309923430 ) ) ;
#53176=CARTESIAN_POINT ( 'NONE',  ( 10.00000000000000178, 65.37363466993042493, 12.81628187352647608 ) ) ;
#53178=CARTESIAN_POINT ( 'NONE',  ( 14.92337183194729988, 59.34226448433412315, -8.527530157486177487 ) ) ;
#53179=CARTESIAN_POINT ( 'NONE',  ( 19.84674366389459621, 48.50893115100078745, 7.409399052514197653E-17 ) ) ;
#53181=DIRECTION ( 'NONE',  ( 0.000000000000000000, -1.000000000000000000, 0.000000000000000000 ) ) ;
#53184=EDGE_CURVE ( 'NONE', #45005, #85332, #9306, .T. ) ;
#53186=CARTESIAN_POINT ( 'NONE',  ( 19.84674366389459266, 8.300597817667451750, 2.638427012816836559 ) ) ;
#53188=ORIENTED_EDGE ( 'NONE', *, *, #89065, .T. ) ;
#53189=CARTESIAN_POINT ( 'NONE',  ( 19.50000000000000355, 79.40087001978915282, 5.000000000000000000 ) ) ;
#53190=CARTESIAN_POINT ( 'NONE',  ( 0.1532563361054083140, 26.00893115100078745, 1.131784320476157264E-15 ) ) ;
#53193=CARTESIAN_POINT ( 'NONE',  ( 10.00000000000000000, 37.87363466993041783, -12.81628187352647608 ) ) ;
#53198=CARTESIAN_POINT ( 'NONE',  ( 0.1532563361054083140, 41.00893115100078745, 1.131784320476157264E-15 ) ) ;
#53199=CARTESIAN_POINT ( 'NONE',  ( -0.3689425029237898834, 31.17874883491396787, -10.36894250292378850 ) ) ;
#53200=CARTESIAN_POINT ( 'NONE',  ( 12.63842701281683922, 44.55059781766745175, -9.846743663894590881 ) ) ;
#53202=CARTESIAN_POINT ( 'NONE',  ( 12.63842701281683034, 7.467264484334118713, 9.846743663894596210 ) ) ;
#53203=CARTESIAN_POINT ( 'NONE',  ( 14.92337183194729633, 47.67559781766745175, 8.527530157486181039 ) ) ;
#53204=CARTESIAN_POINT ( 'NONE',  ( -0.8801773607111009756, 53.06368534415484106, 1.068504757029289695E-15 ) ) ;
#53205=CARTESIAN_POINT ( 'NONE',  ( 1.472469842513823179, 41.42559781766745886, 4.923371831947296329 ) ) ;
#53209=CARTESIAN_POINT ( 'NONE',  ( 19.42250999205614193, 45.14701867748817676, 5.440088680355555262 ) ) ;
#53211=ORIENTED_EDGE ( 'NONE', *, *, #35332, .F. ) ;
#53212=CARTESIAN_POINT ( 'NONE',  ( 2.148416515056625453, 52.23726573380441351, 6.499999999999959144 ) ) ;
#53213=CARTESIAN_POINT ( 'NONE',  ( 17.96484262340118221, 34.93868534415482685, 7.964842623401181321 ) ) ;
#53214=CARTESIAN_POINT ( 'NONE',  ( 0.1532563361054082862, 66.21726448433413736, 2.638427012816831674 ) ) ;
#53215=CARTESIAN_POINT ( 'NONE',  ( 20.88017736071110164, 50.35535201082151247, 2.915334737309930979 ) ) ;
#53219=CARTESIAN_POINT ( 'NONE',  ( 4.559911319644449179, 42.23035201082151247, -9.422509992056141925 ) ) ;
#53221=CARTESIAN_POINT ( 'NONE',  ( 1.472469842513823179, 11.42559781766745175, 4.923371831947296329 ) ) ;
#53222=CARTESIAN_POINT ( 'NONE',  ( 2.791683348922240793, 31.63393115100078745, 7.208316651077764092 ) ) ;
#53225=CARTESIAN_POINT ( 'NONE',  ( -1.099225684535947600, -1.293031996736246469, -6.408140936763238038 ) ) ;
#53226=CARTESIAN_POINT ( 'NONE',  ( -0.3689425029237898834, 66.17874883491396076, -10.36894250292378850 ) ) ;
#53228=CARTESIAN_POINT ( 'NONE',  ( 20.36894250292379382, 18.67874883491397142, 10.36894250292379205 ) ) ;
#53229=CARTESIAN_POINT ( 'NONE',  ( 17.08211943468705840, 50.13708216824730357, -12.26659068614894466 ) ) ;
#53230=CARTESIAN_POINT ( 'NONE',  ( 14.92337183194729633, 12.67559781766745353, 8.527530157486181039 ) ) ;
#53231=VERTEX_POINT ( 'NONE', #31798 ) ;
#53232=CARTESIAN_POINT ( 'NONE',  ( 5.076628168052704559, 30.17559781766745175, -8.527530157486179263 ) ) ;
#53233=CARTESIAN_POINT ( 'NONE',  ( 2.035157376598824452, 28.68868534415484106, 7.964842623401179544 ) ) ;
#53234=CARTESIAN_POINT ( 'NONE',  ( 10.00000000000000000, 44.75893115100078745, -9.846743663894594434 ) ) ;
#53235=CARTESIAN_POINT ( 'NONE',  ( -0.3689425029237881626, 12.42874883491396609, 10.36894250292379027 ) ) ;
#53238=CARTESIAN_POINT ( 'NONE',  ( 12.63842701281683034, 12.46726448433411782, 9.846743663894596210 ) ) ;
#53239=CARTESIAN_POINT ( 'NONE',  ( 10.00000000000000000, 37.87363466993041783, -12.81628187352647608 ) ) ;
#53240=CARTESIAN_POINT ( 'NONE',  ( 10.00000000000000000, 44.75893115100078745, -9.846743663894594434 ) ) ;
#53242=CARTESIAN_POINT ( 'NONE',  ( 2.791683348922240793, 26.63393115100078745, 7.208316651077764092 ) ) ;
#53245=CARTESIAN_POINT ( 'NONE',  ( 10.00000000000000178, 58.05374883491397497, 14.16423886937410082 ) ) ;
#53246=CARTESIAN_POINT ( 'NONE',  ( -0.3689425029237881626, 2.428748834913967869, 10.36894250292379027 ) ) ;
#53247=CARTESIAN_POINT ( 'NONE',  ( 20.15039907845753220, 51.74884699246889852, 6.262539305110077059 ) ) ;
#53248=CARTESIAN_POINT ( 'NONE',  ( 0.1532563361054100626, 40.80059781766745886, -2.638427012816831230 ) ) ;
#53249=CARTESIAN_POINT ( 'NONE',  ( 0.5774900079438607392, 13.48035201082150358, 5.440088680355550821 ) ) ;
#53250=CARTESIAN_POINT ( 'NONE',  ( 2.791683348922237240, 35.38393115100079456, -7.208316651077763204 ) ) ;
#53251=CARTESIAN_POINT ( 'NONE',  ( -1.435044756688069745, 2.551371850025650410E-18, -0.09325026079012421754 ) ) ;
#53252=CARTESIAN_POINT ( 'NONE',  ( 2.791683348922237240, 50.38393115100078035, -7.208316651077763204 ) ) ;
#53254=CARTESIAN_POINT ( 'NONE',  ( 2.035157376598822676, 52.43868534415483396, -7.964842623401177768 ) ) ;
#53257=CARTESIAN_POINT ( 'NONE',  ( 19.38216949554541557, 57.24863466993042493, -9.382169495545420901 ) ) ;
#53259=CARTESIAN_POINT ( 'NONE',  ( 19.84674366389459266, 13.30059781766745353, 2.638427012816836559 ) ) ;
#53260=CARTESIAN_POINT ( 'NONE',  ( 16.40814093676324603, 62.45696800326376064, -11.09922568453594671 ) ) ;
#53261=CARTESIAN_POINT ( 'NONE',  ( 0.5774900079438607392, 8.480352010821505360, 5.440088680355550821 ) ) ;
#53262=CARTESIAN_POINT ( 'NONE',  ( 7.361572987183169658, 49.96726448433410894, -9.846743663894592657 ) ) ;
#53263=PRESENTATION_STYLE_ASSIGNMENT (( #13292 ) ) ;
#53264=CARTESIAN_POINT ( 'NONE',  ( 20.36894250292379382, 28.67874883491396787, 10.36894250292379205 ) ) ;
#53265=CARTESIAN_POINT ( 'NONE',  ( -0.3689425029237881626, 62.42874883491396787, 10.36894250292379027 ) ) ;
#53266=CARTESIAN_POINT ( 'NONE',  ( 5.076628168052704559, 60.17559781766745175, -8.527530157486179263 ) ) ;
#53267=CARTESIAN_POINT ( 'NONE',  ( 17.96484262340118221, 49.93868534415484106, 7.964842623401181321 ) ) ;
#53268=CARTESIAN_POINT ( 'NONE',  ( 19.84674366389459266, 8.717264484334116048, -2.638427012816827677 ) ) ;
#53271=CARTESIAN_POINT ( 'NONE',  ( 21.09922568453595559, 62.04030133659709634, -6.408140936763230044 ) ) ;
#53273=CARTESIAN_POINT ( 'NONE',  ( 5.076628168052703671, 16.84226448433411960, 8.527530157486179263 ) ) ;
#53275=CARTESIAN_POINT ( 'NONE',  ( 10.00000000000000000, 15.55374883491396787, -14.16423886937410082 ) ) ;
#53276=CARTESIAN_POINT ( 'NONE',  ( 7.361572987183170547, 17.05059781766745530, 9.846743663894590881 ) ) ;
#53277=CARTESIAN_POINT ( 'NONE',  ( 17.96484262340118221, 34.93868534415482685, 7.964842623401181321 ) ) ;
#53281=CARTESIAN_POINT ( 'NONE',  ( 20.88017736071110875, 25.77201867748816966, -2.915334737309920765 ) ) ;
#53284=CARTESIAN_POINT ( 'NONE',  ( -0.8801773607110991993, 37.85535201082151247, -2.915334737309923874 ) ) ;
#53285=SURFACE_STYLE_FILL_AREA ( #75296 ) ;
#53286=EDGE_LOOP ( 'NONE', ( #17024, #60, #63941, #42331 ) ) ;
#53289=CARTESIAN_POINT ( 'NONE',  ( 22.81628187352647785, 21.62363466993041783, 6.195893100308588602E-16 ) ) ;
#53290=CARTESIAN_POINT ( 'NONE',  ( 10.00000000000000000, 14.75893115100078568, -9.846743663894594434 ) ) ;
#53293=CARTESIAN_POINT ( 'NONE',  ( 18.52753015748618282, 18.92559781766745175, -4.923371831947291888 ) ) ;
#53294=CARTESIAN_POINT ( 'NONE',  ( 7.084665262690076126, 32.02201867748816966, -10.88017736071110164 ) ) ;
#53295=ORIENTED_EDGE ( 'NONE', *, *, #5537, .T. ) ;
#53297=CARTESIAN_POINT ( 'NONE',  ( 10.00000000000000178, 65.37363466993042493, 12.81628187352647608 ) ) ;
#53298=CARTESIAN_POINT ( 'NONE',  ( 12.91533473730993009, 46.60535201082150536, -10.88017736071109987 ) ) ;
#53300=CARTESIAN_POINT ( 'NONE',  ( 0.6178305044545818747, 53.49863466993041072, -9.382169495545419124 ) ) ;
#53301=CARTESIAN_POINT ( 'NONE',  ( 0.5774900079438590739, 57.64701867748817676, -5.440088680355550821 ) ) ;
#53302=CARTESIAN_POINT ( 'NONE',  ( 3.591859063236761518, -0.04303199673624671928, 11.09922568453594849 ) ) ;
#53303=FILL_AREA_STYLE_COLOUR ( '', #27512 ) ;
#53304=CARTESIAN_POINT ( 'NONE',  ( 12.63842701281683922, 24.55059781766745175, -9.846743663894590881 ) ) ;
#53305=CARTESIAN_POINT ( 'NONE',  ( 10.00000000000000178, 55.37363466993042493, 12.81628187352647608 ) ) ;
#53306=DIRECTION ( 'NONE',  ( -1.000000000000000000, -0.000000000000000000, 0.000000000000000000 ) ) ;
#53307=CARTESIAN_POINT ( 'NONE',  ( 5.076628168052703671, 1.842264484334118047, 8.527530157486179263 ) ) ;
#53308=CARTESIAN_POINT ( 'NONE',  ( 6.565887622018943937, 15.16530133659708568, 12.81628187352647430 ) ) ;
#53309=CARTESIAN_POINT ( 'NONE',  ( -46.68456736488007408, 103.6675473310227034, 5.775421524742653467 ) ) ;
#53311=CARTESIAN_POINT ( 'NONE',  ( 15.44008868035555260, 29.73035201082150891, 9.422509992056143702 ) ) ;
#53312=CARTESIAN_POINT ( 'NONE',  ( -2.816281873526471635, -1.084698663402913210, -3.434112377981056508 ) ) ;
#53314=CARTESIAN_POINT ( 'NONE',  ( 10.00000000000000178, 17.25893115100078745, 9.846743663894594434 ) ) ;
#53315=CARTESIAN_POINT ( 'NONE',  ( 19.84674366389459266, 3.300597817667451750, 2.638427012816836559 ) ) ;
#53316=CARTESIAN_POINT ( 'NONE',  ( 13.43411237798105340, 15.58196800326374998, 12.81628187352647963 ) ) ;
#53319=CARTESIAN_POINT ( 'NONE',  ( 1.472469842513823179, 60.59226448433412315, -4.923371831947296329 ) ) ;
#53321=CARTESIAN_POINT ( 'NONE',  ( 10.00000000000000178, 68.05374883491397497, 14.16423886937410082 ) ) ;
#53322=CARTESIAN_POINT ( 'NONE',  ( 7.361572987183170547, 42.05059781766745886, 9.846743663894590881 ) ) ;
#53323=CARTESIAN_POINT ( 'NONE',  ( 19.72487221294571569, 65.71833443783937412, -6.499999999999983125 ) ) ;
#53324=CARTESIAN_POINT ( 'NONE',  ( 20.88017736071110164, 5.355352010821503583, 2.915334737309930979 ) ) ;
#53326=CARTESIAN_POINT ( 'NONE',  ( 0.5774900079438607392, 28.48035201082150891, 5.440088680355550821 ) ) ;
#53327=CARTESIAN_POINT ( 'NONE',  ( 10.00000000000000178, 63.05374883491396076, 14.16423886937410082 ) ) ;
#53328=CARTESIAN_POINT ( 'NONE',  ( 15.00000000000000000, 11.00000000000000000, 6.000000000000000000 ) ) ;
#53330=CARTESIAN_POINT ( 'NONE',  ( 12.63842701281683034, 22.46726448433411605, 9.846743663894596210 ) ) ;
#53331=CARTESIAN_POINT ( 'NONE',  ( 16.40814093676324603, 7.456968003263754419, -11.09922568453594671 ) ) ;
#53334=EDGE_CURVE ( 'NONE', #14534, #34081, #18292, .T. ) ;
#53337=CARTESIAN_POINT ( 'NONE',  ( 13.79529636645031943, 10.34541550158063394, -14.16423886937409904 ) ) ;
#53338=CARTESIAN_POINT ( 'NONE',  ( 0.1532563361054082862, 31.21726448433412315, 2.638427012816831674 ) ) ;
#53340=ORIENTED_EDGE ( 'NONE', *, *, #82133, .T. ) ;
#53342=CARTESIAN_POINT ( 'NONE',  ( -0.3689425029237881626, 52.42874883491396076, 10.36894250292379027 ) ) ;
#53343=CARTESIAN_POINT ( 'NONE',  ( 18.52753015748618282, 8.925597817667451750, -4.923371831947291888 ) ) ;
#53344=CARTESIAN_POINT ( 'NONE',  ( -39.70923076923077133, 109.3461538461538396, -9.500000000000000000 ) ) ;
#53346=CARTESIAN_POINT ( 'NONE',  ( 19.42250999205614548, 35.98035201082151247, -5.440088680355545492 ) ) ;
#53347=CARTESIAN_POINT ( 'NONE',  ( 3.591859063236761518, 54.95696800326376064, 11.09922568453594849 ) ) ;
#53348=CARTESIAN_POINT ( 'NONE',  ( 7.084665262690076126, 4.105352010821503583, 10.88017736071109987 ) ) ;
#53349=CARTESIAN_POINT ( 'NONE',  ( 6.565887622018943937, 38.08196800326376064, -12.81628187352647608 ) ) ;
#53350=CARTESIAN_POINT ( 'NONE',  ( 12.63842701281683034, 62.46726448433410894, 9.846743663894596210 ) ) ;
#53351=CARTESIAN_POINT ( 'NONE',  ( 5.076628168052704559, 0.1755978176674514724, -8.527530157486179263 ) ) ;
#53356=CARTESIAN_POINT ( 'NONE',  ( 24.16423886937410614, 34.51208216824731068, -3.795296366450302550 ) ) ;
#53357=CARTESIAN_POINT ( 'NONE',  ( 17.08211943468705840, 20.13708216824730357, -12.26659068614894466 ) ) ;
#53358=CARTESIAN_POINT ( 'NONE',  ( -0.8801773607111008646, 3.272018677488171434, 2.915334737309923430 ) ) ;
#53359=CARTESIAN_POINT ( 'NONE',  ( 20.88017736071110875, 30.77201867748816966, -2.915334737309920765 ) ) ;
#53360=CARTESIAN_POINT ( 'NONE',  ( -45.94000000000001194, 107.5383484153110061, 12.00000000000000000 ) ) ;
#53362=CARTESIAN_POINT ( 'NONE',  ( 20.88017736071110519, 65.56368534415483396, 2.639326808657452039E-16 ) ) ;
#53363=CARTESIAN_POINT ( 'NONE',  ( 20.88017736071110164, 60.35535201082151957, 2.915334737309930979 ) ) ;
#53364=CARTESIAN_POINT ( 'NONE',  ( 19.38216949554541202, 30.99863466993042138, 9.382169495545424454 ) ) ;
#53367=CARTESIAN_POINT ( 'NONE',  ( 0.1532563361054083140, 36.00893115100078745, 1.131784320476157264E-15 ) ) ;
#53368=CARTESIAN_POINT ( 'NONE',  ( 2.035157376598822676, 17.43868534415483751, -7.964842623401177768 ) ) ;
#53369=CARTESIAN_POINT ( 'NONE',  ( -1.099225684535947600, 24.54030133659708923, 6.408140936763237150 ) ) ;
#53370=CARTESIAN_POINT ( 'NONE',  ( 5.076628168052703671, 11.84226448433411960, 8.527530157486179263 ) ) ;
#53371=CARTESIAN_POINT ( 'NONE',  ( 0.5774900079438590739, 2.647018677488170990, -5.440088680355550821 ) ) ;
#53372=CARTESIAN_POINT ( 'NONE',  ( 12.63842701281683034, 32.46726448433412315, 9.846743663894596210 ) ) ;
#53373=CARTESIAN_POINT ( 'NONE',  ( 22.81628187352647785, 56.41530133659708213, 3.434112377981063169 ) ) ;
#53374=CARTESIAN_POINT ( 'NONE',  ( 7.361572987183169658, 14.96726448433411960, -9.846743663894592657 ) ) ;
#53375=CARTESIAN_POINT ( 'NONE',  ( 17.08211943468705130, 8.470415501580635720, 12.26659068614894998 ) ) ;
#53376=CARTESIAN_POINT ( 'NONE',  ( 18.18329248733322956, 42.60290668512021028, 6.499999999999960920 ) ) ;
#53377=CARTESIAN_POINT ( 'NONE',  ( 12.91533473730993009, 36.60535201082151247, -10.88017736071109987 ) ) ;
#53378=CARTESIAN_POINT ( 'NONE',  ( 12.91533473730993009, 11.60535201082150536, -10.88017736071109987 ) ) ;
#53379=CARTESIAN_POINT ( 'NONE',  ( 19.42250999205614548, 30.98035201082150536, -5.440088680355545492 ) ) ;
#53380=CARTESIAN_POINT ( 'NONE',  ( 4.559911319644449179, 18.89701867748817321, 9.422509992056141925 ) ) ;
#53382=CARTESIAN_POINT ( 'NONE',  ( 15.44008868035555793, 36.39701867748816966, -9.422509992056140149 ) ) ;
#53384=CARTESIAN_POINT ( 'NONE',  ( 16.40814093676324603, 47.45696800326375353, -11.09922568453594671 ) ) ;
#53385=ADVANCED_FACE ( 'NONE', ( #56296 ), #10791, .F. ) ;
#53386=CARTESIAN_POINT ( 'NONE',  ( 7.084665262690076126, 49.10535201082149825, 10.88017736071109987 ) ) ;
#53388=CARTESIAN_POINT ( 'NONE',  ( -0.8801773607111008646, 53.27201867748816966, 2.915334737309923430 ) ) ;
#53390=CARTESIAN_POINT ( 'NONE',  ( 4.559911319644449179, 47.23035201082150536, -9.422509992056141925 ) ) ;
#53392=CARTESIAN_POINT ( 'NONE',  ( -0.1503990784575328643, 25.12777174578613426, 6.262539305110068177 ) ) ;
#53393=CARTESIAN_POINT ( 'NONE',  ( 22.26659068614895176, 49.72041550158063927, -7.082119434687042414 ) ) ;
#53394=CARTESIAN_POINT ( 'NONE',  ( 12.91533473730993009, 66.60535201082150536, -10.88017736071109987 ) ) ;
#53395=B_SPLINE_CURVE_WITH_KNOTS ( 'NONE', 3,
 ( #13827, #44308, #335, #21330, #74810, #60789 ),
 .UNSPECIFIED., .F., .F.,
 ( 4, 2, 4 ),
 ( 0.000000000000000000, 0.0002605067024380874896, 0.0005210134048761749792 ),
 .UNSPECIFIED. ) ;
#53396=CARTESIAN_POINT ( 'NONE',  ( 19.89103541497712513, 25.66234555792570760, -6.479102184480775684 ) ) ;
#53398=CARTESIAN_POINT ( 'NONE',  ( 10.00000000000000178, 62.25893115100078745, 9.846743663894594434 ) ) ;
#53400=CARTESIAN_POINT ( 'NONE',  ( 14.92337183194729633, 27.67559781766745530, 8.527530157486181039 ) ) ;
#53402=CARTESIAN_POINT ( 'NONE',  ( 17.20831665107776587, 29.13393115100078390, -7.208316651077762316 ) ) ;
#53404=CARTESIAN_POINT ( 'NONE',  ( 12.91533473730993009, 26.60535201082150536, -10.88017736071109987 ) ) ;
#53405=CARTESIAN_POINT ( 'NONE',  ( 18.52753015748617571, 38.09226448433412315, 4.923371831947298993 ) ) ;
#53406=CARTESIAN_POINT ( 'NONE',  ( 0.6178305044545838731, 19.74863466993042138, 9.382169495545420901 ) ) ;
#53407=CARTESIAN_POINT ( 'NONE',  ( 2.035157376598822676, 67.43868534415484817, -7.964842623401177768 ) ) ;
#53408=CARTESIAN_POINT ( 'NONE',  ( 20.88017736071110519, 55.56368534415484817, 2.639326808657452039E-16 ) ) ;
#53409=CARTESIAN_POINT ( 'NONE',  ( 10.00000000000000000, 46.81368534415484106, -10.88017736071110342 ) ) ;
#53410=CARTESIAN_POINT ( 'NONE',  ( 6.204703633549690345, 52.84541550158062506, 14.16423886937410082 ) ) ;
#53412=CARTESIAN_POINT ( 'NONE',  ( 0.6178305044545818747, 28.49863466993041783, -9.382169495545419124 ) ) ;
#53414=VERTEX_POINT ( 'NONE', #19267 ) ;
#53416=CARTESIAN_POINT ( 'NONE',  ( -1.099225684535947600, 8.706968003263753531, -6.408140936763238038 ) ) ;
#53417=CARTESIAN_POINT ( 'NONE',  ( -0.8801773607111009756, 18.06368534415484106, 1.068504757029289695E-15 ) ) ;
#53418=CARTESIAN_POINT ( 'NONE',  ( 20.88017736071110519, 65.56368534415483396, 2.639326808657452039E-16 ) ) ;
#53421=CARTESIAN_POINT ( 'NONE',  ( 0.5774900079438590739, 57.64701867748817676, -5.440088680355550821 ) ) ;
#53422=CARTESIAN_POINT ( 'NONE',  ( 19.84674366389459621, 53.50893115100078745, 7.409399052514197653E-17 ) ) ;
#53423=CARTESIAN_POINT ( 'NONE',  ( 14.92337183194729988, 19.34226448433411960, -8.527530157486177487 ) ) ;
#53424=CARTESIAN_POINT ( 'NONE',  ( 17.20831665107776587, 27.88393115100078390, 7.208316651077764980 ) ) ;
#53425=DIRECTION ( 'NONE',  ( 1.000000000000000000, -0.000000000000000000, 0.000000000000000000 ) ) ;
#53427=CARTESIAN_POINT ( 'NONE',  ( 19.38216949554541557, 42.24863466993041783, -9.382169495545420901 ) ) ;
#53428=CARTESIAN_POINT ( 'NONE',  ( 0.1532563361054082862, 11.21726448433411605, 2.638427012816831674 ) ) ;
#53429=CARTESIAN_POINT ( 'NONE',  ( 19.80777595082616216, 50.68878173731742010, -6.499999999999934275 ) ) ;
#53431=CARTESIAN_POINT ( 'NONE',  ( 19.84674366389459621, 38.50893115100078745, 7.409399052514197653E-17 ) ) ;
#53433=( BOUNDED_SURFACE ( )  B_SPLINE_SURFACE ( 1, 2, ( 
 ( #12494, #42994, #35978, #66479, #97007, #28485, #11024, #58979, #41542, #89482, #3537, #33997, #64495, #14485, #36976, #29950, #98988, #21484, #37481, #21988, #67476, #29451, #90945, #97996, #53442, #30936, #74967, #59958, #89968, #75954, #52464, #51982, #22475, #30442, #44957, #75460, #61435, #7965, #14982, #82469, #7481, #45453, #36486, #6976, #52950, #13485, #38463, #59466, #43963, #51479, #15477, #81973, #28963, #83461, #60455, #68468, #13990, #44465, #6472, #67970, #83951, #68955, #90450, #82966, #98495, #60941, #487, #37978, #91452, #22977, #45960, #91941, #74467, #5991, #66978, #76449, #97499, #9931, #54915, #85429, #31911, #55923, #46924, #62413, #69443, #93418, #24448, #53945, #39449, #84935, #16446, #92428, #63886, #69940, #2940, #47908, #963, #25440, #92918, #86422, #70435, #23953, #70934, #77416, #78413, #47420, #77922, #61927, #32908, #9428, #54426, #2452, #17923, #31423, #8444, #1460, #40435, #63407, #93912, #24941, #55423, #48407, #38951, #8932, #76935, #16938, #39932, #46444, #78910, #17441, #1952, #32416, #10419, #40927, #71424, #33388, #62918, #23472, #85931, #84452, #15951, #88379, #34375, #35864, #80388, #34872, #12375, #56889, #3908, #26887, #49386, #65863, #20378, #64381, #10909, #57380, #86901, #25913, #49876, #64864, #27375, #11891, #94891, #19876, #73861, #42391, #87874, #26389, #19390, #5389, #56415, #87392, #18910, #79887, #71892, #27865, #95896, #3415, #72870, #43361, #42881, #94398, #72379, #95385, #96391, #4404, #50369, #18411, #11394, #41916, #65366, #48894, #79407, #80877, #41431, #58350, #57868, #88872, #73364, #4892, #35372, #50872, #81364, #12863, #33876, #5870, #75838, #52347, #97375, #45338, #60827, #43848, #51363, #44345, #22361, #7358, #90834, #37364, #67857, #37860, #81850, #21365, #20872, #74851, #13363, #89361, #52835, #60340, #66857, #51860, #83344, #85189, #68352, #91328, #97879, #98870, #28843, #74342, #30325, #14866, #6352, #9187, #82844, #6853, #24203, #59346, #36861, #29339, #82345, #54670, #16696, #36361, #89849, #59840, #58855, #96891, #21869, #67353, #98376, #14364, #13866, #47169, #77674, #44834, #90330, #75338, #29832, #66353, #28367, #9682, #70685, #63157, #17200, #72138, #41180, #47677, #25680, #87632, #87139, #19146, #17686, #48158, #11149, #48652, #33636, #32165, #40178, #2204, #32665, #80134, #39702, #56653, #49623, #63646, #40675, #33152, #94650, #26640, #95129, #70189, #1706, #71175, #55164, #26158, #2701, #94154, #78672, #3665, #93665, #10181, #85679, #10666, #56173, #62666, #55677, #25199, #86176, #86666, #93167, #18170, #24692, #78171, #79152, #71661, #41670 ),
 ( #3171, #64132, #18662, #49150, #79651, #34128, #64620, #57136, #12620, #5134, #66617, #97634, #67109, #59601, #11643, #43122, #27125, #97144, #73610, #35625, #20124, #44095, #35115, #50628, #57627, #81608, #66110, #42156, #27623, #73112, #4654, #80636, #52110, #58108, #90097, #36111, #88124, #13615, #81119, #74606, #58616, #12133, #59102, #65614, #28615, #96639, #28116, #50129, #21124, #89117, #42635, #89611, #6119, #19636, #95639, #88617, #51623, #82103, #36625, #13117, #43613, #29099, #96140, #20628, #65120, #51117, #74100, #34622, #21625, #5633, #72621, #4155, #8097, #1100, #23605, #8583, #15115, #16085, #83098, #6606, #54071, #76577, #22612, #24088, #68600, #23108, #625, #45091, #91085, #45591, #37613, #84586, #39089, #52595, #98123, #76089, #75099, #14120, #38111, #53089, #15609, #128, #14626, #38593, #62058, #30577, #7619, #75597, #61082, #92562, #44604, #7109, #68107, #98632, #60086, #37119, #61569, #83601, #91592, #53580, #84093, #31071, #46093, #46572, #30083, #67615, #77071, #92080, #69091, #69580, #31563, #60590, #82602, #29584, #90588, #22115, #25082, #41562, #2587, #41061, #10065, #40065, #40564, #9564, #71062, #93054, #25568, #47563, #48538, #33042, #48041, #79037, #17575, #78553, #62549, #63537, #56060, #86064, #94047, #86554, #18058, #71558, #95019, #33526, #85073, #10550, #3070, #64021, #55565, #94533, #70566, #26052, #56541, #24587, #87035, #18545, #2092, #32551, #49037, #63052, #79541, #34016, #78061, #93549, #55050, #11041, #72029, #85569, #3556, #64513, #54556, #16582, #47058, #77556, #9072, #17083, #39585, #70076, #1596, #32047, #28004, #87525, #81995, #34509, #19039, #26527, #89502, #57024, #4047, #96529, #35507, #43497, #65002, #88015, #19527, #81012, #28506, #13506, #12025, #96027, #50515, #43015, #43988, #49515, #66505, #74490, #66999, #35002, #12513, #97030, #50024, #21013, #73996, #51501, #6014, #80024, #59000, #95529, #20517, #42049, #36506, #57519, #11528, #20014, #58500, #72513, #27019, #80526, #42524, #73008, #4540, #65505, #27509, #89010, #66001, #5522, #58003, #88512, #73497, #5023, #51002, #81497, #13002, #36002, #22499, #15003, #53964, #97521, #38483, #84472, #38972, #6996, #52970, #68977, #90473, #61455, #15498, #23493, #91964, #28983, #511, #37000, #91471, #14008, #46461, #29471, #30957, #59489, #76469, #37501, #45473, #90965, #67993, #45980, #75976, #15971, #22007, #89989, #76955, #7984, #60476, #7504, #8465, #67496, #21505, #98518, #52003, #82492, #29971, #44489, #37995, #83973, #83482, #82989, #68487, #52481, #14, #98017, #30462, #14507, #22996, #60963, #53463, #74989, #6492 ) ),
 .UNSPECIFIED., .F., .F., .F. ) 
 B_SPLINE_SURFACE_WITH_KNOTS ( ( 2, 2 ),
 ( 3, 2, 2, 2, 2, 2, 2, 2, 2, 2, 2, 2, 2, 2, 2, 2, 2, 2, 2, 2, 2, 2, 2, 2, 2, 2, 2, 2, 2, 2, 2, 2, 2, 2, 2, 2, 2, 2, 2, 2, 2, 2, 2, 2, 2, 2, 2, 2, 2, 2, 2, 2, 2, 2, 2, 2, 2, 2, 2, 2, 2, 2, 2, 2, 2, 2, 2, 2, 2, 2, 2, 2, 2, 2, 2, 2, 2, 2, 2, 2, 2, 2, 2, 2, 2, 2, 2, 2, 2, 2, 2, 2, 2, 2, 2, 2, 2, 2, 2, 2, 2, 2, 2, 2, 2, 2, 2, 2, 2, 2, 2, 2, 2, 2, 2, 2, 2, 2, 2, 2, 2, 2, 2, 2, 2, 2, 2, 2, 2, 2, 2, 2, 2, 2, 2, 2, 2, 2, 2, 2, 2, 2, 2, 2, 2, 2, 2, 2, 2, 2, 2, 2, 2, 2, 2, 2, 2, 2, 2, 2, 2, 2, 3 ),
 ( 0.000000000000000000, 1.000000000000000000 ),
 ( 0.000000000000000000, 0.005952380952380952051, 0.01190476190476190410, 0.01785714285714285615, 0.02380952380952380820, 0.02976190476190476025, 0.03571428571428571230, 0.04166666666666666435, 0.04761904761904761640, 0.05357142857142856845, 0.05952380952380952051, 0.06547619047619047949, 0.07142857142857142461, 0.07738095238095238360, 0.08333333333333332871, 0.08928571428571428770, 0.09523809523809523281, 0.1011904761904761918, 0.1071428571428571369, 0.1130952380952380959, 0.1190476190476190410, 0.1250000000000000000, 0.1309523809523809590, 0.1369047619047619180, 0.1428571428571428492, 0.1488095238095238082, 0.1547619047619047672, 0.1607142857142857262, 0.1666666666666666574, 0.1726190476190476164, 0.1785714285714285754, 0.1845238095238095344, 0.1904761904761904656, 0.1964285714285714246, 0.2023809523809523836, 0.2083333333333333426, 0.2142857142857142738, 0.2202380952380952328, 0.2261904761904761918, 0.2321428571428571508, 0.2380952380952380820, 0.2440476190476190410, 0.2500000000000000000, 0.2559523809523809312, 0.2619047619047619180, 0.2678571428571428492, 0.2738095238095238360, 0.2797619047619047672, 0.2857142857142856984, 0.2916666666666666852, 0.2976190476190476164, 0.3035714285714285476, 0.3095238095238095344, 0.3154761904761904656, 0.3214285714285714524, 0.3273809523809523836, 0.3333333333333333148, 0.3392857142857143016, 0.3452380952380952328, 0.3511904761904761640, 0.3571428571428571508, 0.3630952380952380820, 0.3690476190476190688, 0.3750000000000000000, 0.3809523809523809312, 0.3869047619047619180, 0.3928571428571428492, 0.3988095238095238360, 0.4047619047619047672, 0.4107142857142856984, 0.4166666666666666852, 0.4226190476190476164, 0.4285714285714285476, 0.4345238095238095344, 0.4404761904761904656, 0.4464285714285714524, 0.4523809523809523836, 0.4583333333333333148, 0.4642857142857143016, 0.4702380952380952328, 0.4761904761904761640, 0.4821428571428571508, 0.4880952380952380820, 0.4940476190476190688, 0.5000000000000000000, 0.5059523809523809312, 0.5119047619047618625, 0.5178571428571429047, 0.5238095238095238360, 0.5297619047619047672, 0.5357142857142856984, 0.5416666666666666297, 0.5476190476190476719, 0.5535714285714286031, 0.5595238095238095344, 0.5654761904761904656, 0.5714285714285713969, 0.5773809523809523281, 0.5833333333333333703, 0.5892857142857143016, 0.5952380952380952328, 0.6011904761904761640, 0.6071428571428570953, 0.6130952380952381375, 0.6190476190476190688, 0.6250000000000000000, 0.6309523809523809312, 0.6369047619047618625, 0.6428571428571429047, 0.6488095238095238360, 0.6547619047619047672, 0.6607142857142856984, 0.6666666666666666297, 0.6726190476190476719, 0.6785714285714286031, 0.6845238095238095344, 0.6904761904761904656, 0.6964285714285713969, 0.7023809523809523281, 0.7083333333333333703, 0.7142857142857143016, 0.7202380952380952328, 0.7261904761904761640, 0.7321428571428570953, 0.7380952380952381375, 0.7440476190476190688, 0.7500000000000000000, 0.7559523809523809312, 0.7619047619047618625, 0.7678571428571429047, 0.7738095238095238360, 0.7797619047619047672, 0.7857142857142856984, 0.7916666666666666297, 0.7976190476190476719, 0.8035714285714286031, 0.8095238095238095344, 0.8154761904761904656, 0.8214285714285713969, 0.8273809523809523281, 0.8333333333333333703, 0.8392857142857143016, 0.8452380952380952328, 0.8511904761904761640, 0.8571428571428570953, 0.8630952380952381375, 0.8690476190476190688, 0.8750000000000000000, 0.8809523809523809312, 0.8869047619047618625, 0.8928571428571429047, 0.8988095238095238360, 0.9047619047619047672, 0.9107142857142856984, 0.9166666666666666297, 0.9226190476190476719, 0.9285714285714286031, 0.9345238095238095344, 0.9404761904761904656, 0.9464285714285713969, 0.9523809523809523281, 0.9583333333333333703, 0.9642857142857143016 ),
 .UNSPECIFIED. ) 
 GEOMETRIC_REPRESENTATION_ITEM ( )  RATIONAL_B_SPLINE_SURFACE ( (
 ( 1.000000000000000000, 0.9659258262890683122, 1.000000000000000000, 0.9659258262890683122, 1.000000000000000000, 0.9659258262890683122, 1.000000000000000000, 0.9659258262890683122, 1.000000000000000000, 0.9659258262890683122, 1.000000000000000000, 0.9659258262890683122, 1.000000000000000000, 0.9659258262890683122, 1.000000000000000000, 0.9659258262890683122, 1.000000000000000000, 0.9659258262890683122, 1.000000000000000000, 0.9659258262890683122, 1.000000000000000000, 0.9659258262890683122, 1.000000000000000000, 0.9659258262890683122, 1.000000000000000000, 0.9659258262890683122, 1.000000000000000000, 0.9659258262890683122, 1.000000000000000000, 0.9659258262890683122, 1.000000000000000000, 0.9659258262890683122, 1.000000000000000000, 0.9659258262890683122, 1.000000000000000000, 0.9659258262890683122, 1.000000000000000000, 0.9659258262890683122, 1.000000000000000000, 0.9659258262890683122, 1.000000000000000000, 0.9659258262890683122, 1.000000000000000000, 0.9659258262890683122, 1.000000000000000000, 0.9659258262890683122, 1.000000000000000000, 0.9659258262890683122, 1.000000000000000000, 0.9659258262890683122, 1.000000000000000000, 0.9659258262890683122, 1.000000000000000000, 0.9659258262890683122, 1.000000000000000000, 0.9659258262890683122, 1.000000000000000000, 0.9659258262890683122, 1.000000000000000000, 0.9659258262890683122, 1.000000000000000000, 0.9659258262890683122, 1.000000000000000000, 0.9659258262890683122, 1.000000000000000000, 0.9659258262890683122, 1.000000000000000000, 0.9659258262890683122, 1.000000000000000000, 0.9659258262890683122, 1.000000000000000000, 0.9659258262890683122, 1.000000000000000000, 0.9659258262890683122, 1.000000000000000000, 0.9659258262890683122, 1.000000000000000000, 0.9659258262890683122, 1.000000000000000000, 0.9659258262890683122, 1.000000000000000000, 0.9659258262890683122, 1.000000000000000000, 0.9659258262890683122, 1.000000000000000000, 0.9659258262890683122, 1.000000000000000000, 0.9659258262890683122, 1.000000000000000000, 0.9659258262890683122, 1.000000000000000000, 0.9659258262890683122, 1.000000000000000000, 0.9659258262890683122, 1.000000000000000000, 0.9659258262890683122, 1.000000000000000000, 0.9659258262890683122, 1.000000000000000000, 0.9659258262890683122, 1.000000000000000000, 0.9659258262890683122, 1.000000000000000000, 0.9659258262890683122, 1.000000000000000000, 0.9659258262890683122, 1.000000000000000000, 0.9659258262890683122, 1.000000000000000000, 0.9659258262890683122, 1.000000000000000000, 0.9659258262890683122, 1.000000000000000000, 0.9659258262890683122, 1.000000000000000000, 0.9659258262890683122, 1.000000000000000000, 0.9659258262890683122, 1.000000000000000000, 0.9659258262890683122, 1.000000000000000000, 0.9659258262890683122, 1.000000000000000000, 0.9659258262890683122, 1.000000000000000000, 0.9659258262890683122, 1.000000000000000000, 0.9659258262890683122, 1.000000000000000000, 0.9659258262890683122, 1.000000000000000000, 0.9659258262890683122, 1.000000000000000000, 0.9659258262890683122, 1.000000000000000000, 0.9659258262890683122, 1.000000000000000000, 0.9659258262890683122, 1.000000000000000000, 0.9659258262890683122, 1.000000000000000000, 0.9659258262890683122, 1.000000000000000000, 0.9659258262890683122, 1.000000000000000000, 0.9659258262890683122, 1.000000000000000000, 0.9659258262890683122, 1.000000000000000000, 0.9659258262890683122, 1.000000000000000000, 0.9659258262890683122, 1.000000000000000000, 0.9659258262890683122, 1.000000000000000000, 0.9659258262890683122, 1.000000000000000000, 0.9659258262890683122, 1.000000000000000000, 0.9659258262890683122, 1.000000000000000000, 0.9659258262890683122, 1.000000000000000000, 0.9659258262890683122, 1.000000000000000000, 0.9659258262890683122, 1.000000000000000000, 0.9659258262890683122, 1.000000000000000000, 0.9659258262890683122, 1.000000000000000000, 0.9659258262890683122, 1.000000000000000000, 0.9659258262890683122, 1.000000000000000000, 0.9659258262890683122, 1.000000000000000000, 0.9659258262890683122, 1.000000000000000000, 0.9659258262890683122, 1.000000000000000000, 0.9659258262890683122, 1.000000000000000000, 0.9659258262890683122, 1.000000000000000000, 0.9659258262890683122, 1.000000000000000000, 0.9659258262890683122, 1.000000000000000000, 0.9659258262890683122, 1.000000000000000000, 0.9659258262890683122, 1.000000000000000000, 0.9659258262890683122, 1.000000000000000000, 0.9659258262890683122, 1.000000000000000000, 0.9659258262890683122, 1.000000000000000000, 0.9659258262890683122, 1.000000000000000000, 0.9659258262890683122, 1.000000000000000000, 0.9659258262890683122, 1.000000000000000000, 0.9659258262890683122, 1.000000000000000000, 0.9659258262890683122, 1.000000000000000000, 0.9659258262890683122, 1.000000000000000000, 0.9659258262890683122, 1.000000000000000000, 0.9659258262890683122, 1.000000000000000000, 0.9659258262890683122, 1.000000000000000000, 0.9659258262890683122, 1.000000000000000000, 0.9659258262890683122, 1.000000000000000000, 0.9659258262890683122, 1.000000000000000000, 0.9659258262890683122, 1.000000000000000000, 0.9659258262890683122, 1.000000000000000000, 0.9659258262890683122, 1.000000000000000000, 0.9659258262890683122, 1.000000000000000000, 0.9659258262890683122, 1.000000000000000000, 0.9659258262890683122, 1.000000000000000000, 0.9659258262890683122, 1.000000000000000000, 0.9659258262890683122, 1.000000000000000000, 0.9659258262890683122, 1.000000000000000000, 0.9659258262890683122, 1.000000000000000000, 0.9659258262890683122, 1.000000000000000000, 0.9659258262890683122, 1.000000000000000000, 0.9659258262890683122, 1.000000000000000000, 0.9659258262890683122, 1.000000000000000000, 0.9659258262890683122, 1.000000000000000000, 0.9659258262890683122, 1.000000000000000000, 0.9659258262890683122, 1.000000000000000000, 0.9659258262890683122, 1.000000000000000000, 0.9659258262890683122, 1.000000000000000000, 0.9659258262890683122, 1.000000000000000000, 0.9659258262890683122, 1.000000000000000000, 0.9659258262890683122, 1.000000000000000000, 0.9659258262890683122, 1.000000000000000000, 0.9659258262890683122, 1.000000000000000000, 0.9659258262890683122, 1.000000000000000000, 0.9659258262890683122, 1.000000000000000000, 0.9659258262890683122, 1.000000000000000000, 0.9659258262890683122, 1.000000000000000000, 0.9659258262890683122, 1.000000000000000000, 0.9659258262890683122, 1.000000000000000000, 0.9659258262890683122, 1.000000000000000000, 0.9659258262890683122, 1.000000000000000000, 0.9659258262890683122, 1.000000000000000000, 0.9659258262890683122, 1.000000000000000000, 0.9659258262890683122, 1.000000000000000000, 0.9659258262890683122, 1.000000000000000000, 0.9659258262890683122, 1.000000000000000000, 0.9659258262890683122, 1.000000000000000000, 0.9659258262890683122, 1.000000000000000000, 0.9659258262890683122, 1.000000000000000000, 0.9659258262890683122, 1.000000000000000000, 0.9659258262890683122, 1.000000000000000000, 0.9659258262890683122, 1.000000000000000000, 0.9659258262890683122, 1.000000000000000000, 0.9659258262890683122, 1.000000000000000000, 0.9659258262890683122, 1.000000000000000000, 0.9659258262890683122, 1.000000000000000000, 0.9659258262890683122, 1.000000000000000000, 0.9659258262890683122, 1.000000000000000000, 0.9659258262890683122, 1.000000000000000000, 0.9659258262890683122, 1.000000000000000000),
 ( 1.000000000000000000, 0.9659258262890683122, 1.000000000000000000, 0.9659258262890683122, 1.000000000000000000, 0.9659258262890683122, 1.000000000000000000, 0.9659258262890683122, 1.000000000000000000, 0.9659258262890683122, 1.000000000000000000, 0.9659258262890683122, 1.000000000000000000, 0.9659258262890683122, 1.000000000000000000, 0.9659258262890683122, 1.000000000000000000, 0.9659258262890683122, 1.000000000000000000, 0.9659258262890683122, 1.000000000000000000, 0.9659258262890683122, 1.000000000000000000, 0.9659258262890683122, 1.000000000000000000, 0.9659258262890683122, 1.000000000000000000, 0.9659258262890683122, 1.000000000000000000, 0.9659258262890683122, 1.000000000000000000, 0.9659258262890683122, 1.000000000000000000, 0.9659258262890683122, 1.000000000000000000, 0.9659258262890683122, 1.000000000000000000, 0.9659258262890683122, 1.000000000000000000, 0.9659258262890683122, 1.000000000000000000, 0.9659258262890683122, 1.000000000000000000, 0.9659258262890683122, 1.000000000000000000, 0.9659258262890683122, 1.000000000000000000, 0.9659258262890683122, 1.000000000000000000, 0.9659258262890683122, 1.000000000000000000, 0.9659258262890683122, 1.000000000000000000, 0.9659258262890683122, 1.000000000000000000, 0.9659258262890683122, 1.000000000000000000, 0.9659258262890683122, 1.000000000000000000, 0.9659258262890683122, 1.000000000000000000, 0.9659258262890683122, 1.000000000000000000, 0.9659258262890683122, 1.000000000000000000, 0.9659258262890683122, 1.000000000000000000, 0.9659258262890683122, 1.000000000000000000, 0.9659258262890683122, 1.000000000000000000, 0.9659258262890683122, 1.000000000000000000, 0.9659258262890683122, 1.000000000000000000, 0.9659258262890683122, 1.000000000000000000, 0.9659258262890683122, 1.000000000000000000, 0.9659258262890683122, 1.000000000000000000, 0.9659258262890683122, 1.000000000000000000, 0.9659258262890683122, 1.000000000000000000, 0.9659258262890683122, 1.000000000000000000, 0.9659258262890683122, 1.000000000000000000, 0.9659258262890683122, 1.000000000000000000, 0.9659258262890683122, 1.000000000000000000, 0.9659258262890683122, 1.000000000000000000, 0.9659258262890683122, 1.000000000000000000, 0.9659258262890683122, 1.000000000000000000, 0.9659258262890683122, 1.000000000000000000, 0.9659258262890683122, 1.000000000000000000, 0.9659258262890683122, 1.000000000000000000, 0.9659258262890683122, 1.000000000000000000, 0.9659258262890683122, 1.000000000000000000, 0.9659258262890683122, 1.000000000000000000, 0.9659258262890683122, 1.000000000000000000, 0.9659258262890683122, 1.000000000000000000, 0.9659258262890683122, 1.000000000000000000, 0.9659258262890683122, 1.000000000000000000, 0.9659258262890683122, 1.000000000000000000, 0.9659258262890683122, 1.000000000000000000, 0.9659258262890683122, 1.000000000000000000, 0.9659258262890683122, 1.000000000000000000, 0.9659258262890683122, 1.000000000000000000, 0.9659258262890683122, 1.000000000000000000, 0.9659258262890683122, 1.000000000000000000, 0.9659258262890683122, 1.000000000000000000, 0.9659258262890683122, 1.000000000000000000, 0.9659258262890683122, 1.000000000000000000, 0.9659258262890683122, 1.000000000000000000, 0.9659258262890683122, 1.000000000000000000, 0.9659258262890683122, 1.000000000000000000, 0.9659258262890683122, 1.000000000000000000, 0.9659258262890683122, 1.000000000000000000, 0.9659258262890683122, 1.000000000000000000, 0.9659258262890683122, 1.000000000000000000, 0.9659258262890683122, 1.000000000000000000, 0.9659258262890683122, 1.000000000000000000, 0.9659258262890683122, 1.000000000000000000, 0.9659258262890683122, 1.000000000000000000, 0.9659258262890683122, 1.000000000000000000, 0.9659258262890683122, 1.000000000000000000, 0.9659258262890683122, 1.000000000000000000, 0.9659258262890683122, 1.000000000000000000, 0.9659258262890683122, 1.000000000000000000, 0.9659258262890683122, 1.000000000000000000, 0.9659258262890683122, 1.000000000000000000, 0.9659258262890683122, 1.000000000000000000, 0.9659258262890683122, 1.000000000000000000, 0.9659258262890683122, 1.000000000000000000, 0.9659258262890683122, 1.000000000000000000, 0.9659258262890683122, 1.000000000000000000, 0.9659258262890683122, 1.000000000000000000, 0.9659258262890683122, 1.000000000000000000, 0.9659258262890683122, 1.000000000000000000, 0.9659258262890683122, 1.000000000000000000, 0.9659258262890683122, 1.000000000000000000, 0.9659258262890683122, 1.000000000000000000, 0.9659258262890683122, 1.000000000000000000, 0.9659258262890683122, 1.000000000000000000, 0.9659258262890683122, 1.000000000000000000, 0.9659258262890683122, 1.000000000000000000, 0.9659258262890683122, 1.000000000000000000, 0.9659258262890683122, 1.000000000000000000, 0.9659258262890683122, 1.000000000000000000, 0.9659258262890683122, 1.000000000000000000, 0.9659258262890683122, 1.000000000000000000, 0.9659258262890683122, 1.000000000000000000, 0.9659258262890683122, 1.000000000000000000, 0.9659258262890683122, 1.000000000000000000, 0.9659258262890683122, 1.000000000000000000, 0.9659258262890683122, 1.000000000000000000, 0.9659258262890683122, 1.000000000000000000, 0.9659258262890683122, 1.000000000000000000, 0.9659258262890683122, 1.000000000000000000, 0.9659258262890683122, 1.000000000000000000, 0.9659258262890683122, 1.000000000000000000, 0.9659258262890683122, 1.000000000000000000, 0.9659258262890683122, 1.000000000000000000, 0.9659258262890683122, 1.000000000000000000, 0.9659258262890683122, 1.000000000000000000, 0.9659258262890683122, 1.000000000000000000, 0.9659258262890683122, 1.000000000000000000, 0.9659258262890683122, 1.000000000000000000, 0.9659258262890683122, 1.000000000000000000, 0.9659258262890683122, 1.000000000000000000, 0.9659258262890683122, 1.000000000000000000, 0.9659258262890683122, 1.000000000000000000, 0.9659258262890683122, 1.000000000000000000, 0.9659258262890683122, 1.000000000000000000, 0.9659258262890683122, 1.000000000000000000, 0.9659258262890683122, 1.000000000000000000, 0.9659258262890683122, 1.000000000000000000, 0.9659258262890683122, 1.000000000000000000, 0.9659258262890683122, 1.000000000000000000, 0.9659258262890683122, 1.000000000000000000, 0.9659258262890683122, 1.000000000000000000, 0.9659258262890683122, 1.000000000000000000, 0.9659258262890683122, 1.000000000000000000, 0.9659258262890683122, 1.000000000000000000, 0.9659258262890683122, 1.000000000000000000, 0.9659258262890683122, 1.000000000000000000, 0.9659258262890683122, 1.000000000000000000, 0.9659258262890683122, 1.000000000000000000, 0.9659258262890683122, 1.000000000000000000, 0.9659258262890683122, 1.000000000000000000, 0.9659258262890683122, 1.000000000000000000, 0.9659258262890683122, 1.000000000000000000, 0.9659258262890683122, 1.000000000000000000, 0.9659258262890683122, 1.000000000000000000, 0.9659258262890683122, 1.000000000000000000, 0.9659258262890683122, 1.000000000000000000, 0.9659258262890683122, 1.000000000000000000, 0.9659258262890683122, 1.000000000000000000, 0.9659258262890683122, 1.000000000000000000, 0.9659258262890683122, 1.000000000000000000, 0.9659258262890683122, 1.000000000000000000, 0.9659258262890683122, 1.000000000000000000, 0.9659258262890683122, 1.000000000000000000, 0.9659258262890683122, 1.000000000000000000, 0.9659258262890683122, 1.000000000000000000, 0.9659258262890683122, 1.000000000000000000) ) ) 
 REPRESENTATION_ITEM ( '' )  SURFACE ( )  );
#53435=CARTESIAN_POINT ( 'NONE',  ( 10.00000000000000178, 10.37363466993041961, 12.81628187352647608 ) ) ;
#53436=VECTOR ( 'NONE', #27883, 1000.000000000000000 ) ;
#53437=CARTESIAN_POINT ( 'NONE',  ( 2.035157376598824452, 48.68868534415483396, 7.964842623401179544 ) ) ;
#53438=CARTESIAN_POINT ( 'NONE',  ( -4.164238869374099927, 37.01208216824731068, 3.795296366450308767 ) ) ;
#53440=CARTESIAN_POINT ( 'NONE',  ( 20.36894250292379738, 29.92874883491396432, -10.36894250292379027 ) ) ;
#53441=CARTESIAN_POINT ( 'NONE',  ( 17.08211943468705130, 58.47041550158063927, 12.26659068614894998 ) ) ;
#53442=CARTESIAN_POINT ( 'NONE',  ( 10.00000000000000000, 5.553748834913967869, -14.16423886937410082 ) ) ;
#53443=CARTESIAN_POINT ( 'NONE',  ( 17.08211943468705840, 20.13708216824730357, -12.26659068614894466 ) ) ;
#53444=CARTESIAN_POINT ( 'NONE',  ( 19.84674366389459266, 33.30059781766745175, 2.638427012816836559 ) ) ;
#53445=CARTESIAN_POINT ( 'NONE',  ( 20.88017736071110164, 45.35535201082149115, 2.915334737309930979 ) ) ;
#53448=CARTESIAN_POINT ( 'NONE',  ( 18.52753015748618282, 48.92559781766745886, -4.923371831947291888 ) ) ;
#53449=CARTESIAN_POINT ( 'NONE',  ( 12.91533473730992121, 24.52201867748816966, 10.88017736071110164 ) ) ;
#53450=CARTESIAN_POINT ( 'NONE',  ( 21.92686044187657046, 55.16212336850780673, 4.562052436263912550E-16 ) ) ;
#53451=CARTESIAN_POINT ( 'NONE',  ( 14.92337183194729633, 57.67559781766745886, 8.527530157486181039 ) ) ;
#53453=ADVANCED_FACE ( 'NONE', ( #41790 ), #35744, .F. ) ;
#53454=CARTESIAN_POINT ( 'NONE',  ( 18.52753015748617571, 33.09226448433411605, 4.923371831947298993 ) ) ;
#53455=CARTESIAN_POINT ( 'NONE',  ( 19.38216949554541202, 50.99863466993042493, 9.382169495545424454 ) ) ;
#53457=CARTESIAN_POINT ( 'NONE',  ( 19.84674366389459621, 43.50893115100078745, 7.409399052514197653E-17 ) ) ;
#53458=CARTESIAN_POINT ( 'NONE',  ( 0.1532563361054083140, 51.00893115100078745, 1.131784320476157264E-15 ) ) ;
#53459=CARTESIAN_POINT ( 'NONE',  ( 20.36894250292379382, 43.67874883491397497, 10.36894250292379205 ) ) ;
#53461=CARTESIAN_POINT ( 'NONE',  ( 17.08211943468705130, 13.47041550158063572, 12.26659068614894998 ) ) ;
#53462=B_SPLINE_CURVE_WITH_KNOTS ( 'NONE', 3,
 ( #23122, #14133, #82117, #91605, #68612, #52610, #68121, #76592, #59615, #31086 ),
 .UNSPECIFIED., .F., .F.,
 ( 4, 3, 3, 4 ),
 ( 2.368389951639683899E-16, 0.0006253016069560743580, 0.001250604074564920856, 0.002501455912506532226 ),
 .UNSPECIFIED. ) ;
#53463=CARTESIAN_POINT ( 'NONE',  ( 4.559911319644449179, 68.89701867748817676, 9.422509992056141925 ) ) ;
#53465=CARTESIAN_POINT ( 'NONE',  ( 10.00000000000000000, 60.55374883491397497, -14.16423886937410082 ) ) ;
#53466=CARTESIAN_POINT ( 'NONE',  ( 13.43411237798105340, 10.58196800326375353, 12.81628187352647963 ) ) ;
#53467=CARTESIAN_POINT ( 'NONE',  ( 18.17884179759845509, 43.66688879859522388, -6.500000000000054179 ) ) ;
#53468=CARTESIAN_POINT ( 'NONE',  ( -0.8801773607110991993, 67.85535201082151957, -2.915334737309923874 ) ) ;
#53470=CARTESIAN_POINT ( 'NONE',  ( -46.94000000000001194, 101.5930487410390270, -7.918115197747374268 ) ) ;
#53471=CARTESIAN_POINT ( 'NONE',  ( 13.43411237798105340, 30.58196800326374998, 12.81628187352647963 ) ) ;
#53472=CARTESIAN_POINT ( 'NONE',  ( -0.3689425029237881626, 57.42874883491397497, 10.36894250292379027 ) ) ;
#53474=CARTESIAN_POINT ( 'NONE',  ( 4.559911319644449179, 17.23035201082150536, -9.422509992056141925 ) ) ;
#53475=CARTESIAN_POINT ( 'NONE',  ( 19.42250999205614193, 20.14701867748817321, 5.440088680355555262 ) ) ;
#53476=CARTESIAN_POINT ( 'NONE',  ( 19.84674366389459621, 58.50893115100078745, 7.409399052514197653E-17 ) ) ;
#53477=CARTESIAN_POINT ( 'NONE',  ( 0.1532563361054082862, 56.21726448433411605, 2.638427012816831674 ) ) ;
#53478=CARTESIAN_POINT ( 'NONE',  ( 13.43411237798105340, 50.58196800326375353, 12.81628187352647963 ) ) ;
#53479=CARTESIAN_POINT ( 'NONE',  ( 1.472469842513823179, 1.425597817667451528, 4.923371831947296329 ) ) ;
#53480=EDGE_LOOP ( 'NONE', ( #61315, #83283, #34817, #42714 ) ) ;
#53481=CARTESIAN_POINT ( 'NONE',  ( 15.44008868035555793, 11.39701867748817143, -9.422509992056140149 ) ) ;
#53482=CARTESIAN_POINT ( 'NONE',  ( 6.565887622018943937, 25.16530133659708213, 12.81628187352647430 ) ) ;
#53485=CARTESIAN_POINT ( 'NONE',  ( 18.52753015748617571, 43.09226448433412315, 4.923371831947298993 ) ) ;
#53486=CARTESIAN_POINT ( 'NONE',  ( 17.96484262340118221, 54.93868534415484106, 7.964842623401181321 ) ) ;
#53488=CARTESIAN_POINT ( 'NONE',  ( 0.6178305044545818747, 23.49863466993041783, -9.382169495545419124 ) ) ;
#53489=CARTESIAN_POINT ( 'NONE',  ( 2.035157376598822676, 52.43868534415483396, -7.964842623401177768 ) ) ;
#53493=CARTESIAN_POINT ( 'NONE',  ( 22.81628187352647785, 56.41530133659708213, 3.434112377981063169 ) ) ;
#53494=ORIENTED_EDGE ( 'NONE', *, *, #48449, .F. ) ;
#53495=CARTESIAN_POINT ( 'NONE',  ( 1.472469842513823179, 61.42559781766745175, 4.923371831947296329 ) ) ;
#53496=DIRECTION ( 'NONE',  ( 0.000000000000000000, -1.000000000000000000, 0.000000000000000000 ) ) ;
#53497=CARTESIAN_POINT ( 'NONE',  ( -0.8801773607111009756, 53.06368534415484106, 1.068504757029289695E-15 ) ) ;
#53498=CARTESIAN_POINT ( 'NONE',  ( -1.099225684535947600, 44.54030133659708923, 6.408140936763237150 ) ) ;
#53499=CARTESIAN_POINT ( 'NONE',  ( 2.791683348922237240, 10.38393115100078390, -7.208316651077763204 ) ) ;
#53500=CARTESIAN_POINT ( 'NONE',  ( 12.91533473730992121, 54.52201867748816255, 10.88017736071110164 ) ) ;
#53501=CARTESIAN_POINT ( 'NONE',  ( 7.361572987183170547, 67.05059781766746596, 9.846743663894590881 ) ) ;
#53502=CARTESIAN_POINT ( 'NONE',  ( 0.1532563361054082862, 21.21726448433412315, 2.638427012816831674 ) ) ;
#53503=CARTESIAN_POINT ( 'NONE',  ( 17.20831665107776587, 9.133931151000787452, -7.208316651077762316 ) ) ;
#53504=CARTESIAN_POINT ( 'NONE',  ( 6.000000000000000000, 11.50000000000000000, -5.000000000000000000 ) ) ;
#53505=CARTESIAN_POINT ( 'NONE',  ( -2.266590686148945544, 41.38708216824729647, -7.082119434687050408 ) ) ;
#53508=CARTESIAN_POINT ( 'NONE',  ( 12.91533473730992121, 9.522018677488171434, 10.88017736071110164 ) ) ;
#53511=CARTESIAN_POINT ( 'NONE',  ( 0.5774900079438607392, 13.48035201082150358, 5.440088680355550821 ) ) ;
#53512=CARTESIAN_POINT ( 'NONE',  ( 17.96484262340118221, 16.18868534415483396, -7.964842623401177768 ) ) ;
#53513=CARTESIAN_POINT ( 'NONE',  ( 18.52753015748618282, 48.92559781766745886, -4.923371831947291888 ) ) ;
#53514=VECTOR ( 'NONE', #45744, 1000.000000000000000 ) ;
#53515=CARTESIAN_POINT ( 'NONE',  ( 0.6178305044545818747, 33.49863466993042493, -9.382169495545419124 ) ) ;
#53517=CARTESIAN_POINT ( 'NONE',  ( -0.3689425029237898834, 6.178748834913968757, -10.36894250292378850 ) ) ;
#53518=CARTESIAN_POINT ( 'NONE',  ( 17.96484262340118221, 31.18868534415483751, -7.964842623401177768 ) ) ;
#53519=CARTESIAN_POINT ( 'NONE',  ( 7.084665262690076126, 4.105352010821503583, 10.88017736071109987 ) ) ;
#53520=EDGE_CURVE ( 'NONE', #65756, #43512, #69596, .T. ) ;
#53521=CARTESIAN_POINT ( 'NONE',  ( 1.472469842513823179, 46.42559781766745175, 4.923371831947296329 ) ) ;
#53522=DIRECTION ( 'NONE',  ( -1.000000000000000000, -0.000000000000000000, -0.000000000000000000 ) ) ;
#53523=CARTESIAN_POINT ( 'NONE',  ( 1.472469842513823179, 20.59226448433411960, -4.923371831947296329 ) ) ;
#53527=CARTESIAN_POINT ( 'NONE',  ( 2.791683348922237240, 60.38393115100078745, -7.208316651077763204 ) ) ;
#53528=CARTESIAN_POINT ( 'NONE',  ( 4.559911319644449179, 33.89701867748817676, 9.422509992056141925 ) ) ;
#53529=CARTESIAN_POINT ( 'NONE',  ( 20.88017736071110164, 35.35535201082150536, 2.915334737309930979 ) ) ;
#53530=CARTESIAN_POINT ( 'NONE',  ( 10.00000000000000000, 64.75893115100078035, -9.846743663894594434 ) ) ;
#53531=CARTESIAN_POINT ( 'NONE',  ( -1.099225684535947600, 28.70696800326375353, -6.408140936763238038 ) ) ;
#53532=CARTESIAN_POINT ( 'NONE',  ( 24.16423886937409904, 14.09541550158063217, 3.795296366450317205 ) ) ;
#53533=COLOUR_RGB ( '', 0.40784314, 0.44705882, 0.49803922) ;
#53536=CARTESIAN_POINT ( 'NONE',  ( 10.00000000000000178, 40.37363466993042493, 12.81628187352647608 ) ) ;
#53538=CARTESIAN_POINT ( 'NONE',  ( 14.92337183194729988, 49.34226448433411605, -8.527530157486177487 ) ) ;
#53539=CARTESIAN_POINT ( 'NONE',  ( 2.035157376598824452, 13.68868534415483751, 7.964842623401179544 ) ) ;
#53540=ORIENTED_EDGE ( 'NONE', *, *, #33169, .T. ) ;
#53542=CARTESIAN_POINT ( 'NONE',  ( 20.88017736071110519, 10.56368534415483929, 2.639326808657452039E-16 ) ) ;
#53544=CARTESIAN_POINT ( 'NONE',  ( 15.44008868035555793, 61.39701867748817676, -9.422509992056140149 ) ) ;
#53545=CARTESIAN_POINT ( 'NONE',  ( 17.96484262340118221, 54.93868534415484106, 7.964842623401181321 ) ) ;
#53546=CARTESIAN_POINT ( 'NONE',  ( 17.96484262340118221, 61.18868534415482685, -7.964842623401177768 ) ) ;
#53548=CARTESIAN_POINT ( 'NONE',  ( 15.44008868035555793, 56.39701867748817676, -9.422509992056140149 ) ) ;
#53550=VECTOR ( 'NONE', #80665, 1000.000000000000114 ) ;
#53553=CARTESIAN_POINT ( 'NONE',  ( 10.00000000000000000, 39.75893115100078745, -9.846743663894594434 ) ) ;
#53555=CARTESIAN_POINT ( 'NONE',  ( 20.04068437667225666, 19.71974360917720759, 6.396802510829705746 ) ) ;
#53558=CARTESIAN_POINT ( 'NONE',  ( 10.00000000000000178, 18.05374883491396787, 14.16423886937410082 ) ) ;
#53559=ORIENTED_EDGE ( 'NONE', *, *, #16177, .T. ) ;
#53560=CARTESIAN_POINT ( 'NONE',  ( -0.1023957841222410126, 35.13377557478296609, 6.340343622311920058 ) ) ;
#53562=CARTESIAN_POINT ( 'NONE',  ( 7.084665262690076126, 64.10535201082150536, 10.88017736071109987 ) ) ;
#53563=CARTESIAN_POINT ( 'NONE',  ( 0.5774900079438607392, 13.48035201082150358, 5.440088680355550821 ) ) ;
#53564=CARTESIAN_POINT ( 'NONE',  ( 0.1129803114748856863, 59.29427333184092674, -6.480634945678684922 ) ) ;
#53565=CARTESIAN_POINT ( 'NONE',  ( 16.40814093676323893, 40.79030133659708923, 11.09922568453595026 ) ) ;
#53567=CYLINDRICAL_SURFACE ( 'NONE', #35257, 11.92686044187656513 ) ;
#53568=CARTESIAN_POINT ( 'NONE',  ( 14.92337183194729988, 64.34226448433412315, -8.527530157486177487 ) ) ;
#53569=CARTESIAN_POINT ( 'NONE',  ( 1.472469842513823179, 1.425597817667451528, 4.923371831947296329 ) ) ;
#53570=CARTESIAN_POINT ( 'NONE',  ( 0.6178305044545818747, 33.49863466993042493, -9.382169495545419124 ) ) ;
#53571=CARTESIAN_POINT ( 'NONE',  ( 14.92337183194729988, 24.34226448433411960, -8.527530157486177487 ) ) ;
#53573=CARTESIAN_POINT ( 'NONE',  ( 6.565887622018943937, 15.16530133659708568, 12.81628187352647430 ) ) ;
#53576=CARTESIAN_POINT ( 'NONE',  ( 17.20831665107776587, 12.88393115100078390, 7.208316651077764980 ) ) ;
#53580=CARTESIAN_POINT ( 'NONE',  ( 12.91533473730993009, 26.60535201082150536, -10.88017736071109987 ) ) ;
#53581=CARTESIAN_POINT ( 'NONE',  ( 13.79529636645030344, 23.26208216824730002, 14.16423886937410614 ) ) ;
#53582=CARTESIAN_POINT ( 'NONE',  ( 0.1532563361054083140, 36.00893115100078745, 1.131784320476157264E-15 ) ) ;
#53583=CARTESIAN_POINT ( 'NONE',  ( 12.91533473730992121, 64.52201867748817676, 10.88017736071110164 ) ) ;
#53584=CARTESIAN_POINT ( 'NONE',  ( 16.40814093676323893, 45.79030133659708923, 11.09922568453595026 ) ) ;
#53586=CARTESIAN_POINT ( 'NONE',  ( 4.559911319644449179, 18.89701867748817321, 9.422509992056141925 ) ) ;
#53588=CARTESIAN_POINT ( 'NONE',  ( 6.565887622018943937, 8.081968003263751754, -12.81628187352647608 ) ) ;
#53589=CARTESIAN_POINT ( 'NONE',  ( 16.40814093676324603, 12.45696800326375353, -11.09922568453594671 ) ) ;
#53590=CARTESIAN_POINT ( 'NONE',  ( 0.1532563361054083140, 31.00893115100078390, 1.131784320476157264E-15 ) ) ;
#53592=CARTESIAN_POINT ( 'NONE',  ( 6.565887622018943937, 33.08196800326374643, -12.81628187352647608 ) ) ;
#53593=CARTESIAN_POINT ( 'NONE',  ( 14.49999999999999822, 60.50000000000000711, -6.500000000000000888 ) ) ;
#53594=CARTESIAN_POINT ( 'NONE',  ( 0.5774900079438590739, 52.64701867748817676, -5.440088680355550821 ) ) ;
#53599=CARTESIAN_POINT ( 'NONE',  ( 10.00000000000000178, 39.31368534415484106, 10.88017736071110342 ) ) ;
#53601=CARTESIAN_POINT ( 'NONE',  ( 20.88017736071110164, 45.35535201082149115, 2.915334737309930979 ) ) ;
#53605=CARTESIAN_POINT ( 'NONE',  ( 5.076628168052704559, 50.17559781766745886, -8.527530157486179263 ) ) ;
#53606=CARTESIAN_POINT ( 'NONE',  ( 15.44008868035555260, 4.730352010821504471, 9.422509992056143702 ) ) ;
#53608=CARTESIAN_POINT ( 'NONE',  ( -1.099225684535947600, 8.706968003263753531, -6.408140936763238038 ) ) ;
#53610=CARTESIAN_POINT ( 'NONE',  ( 15.44008868035555793, 31.39701867748817676, -9.422509992056140149 ) ) ;
#53611=CARTESIAN_POINT ( 'NONE',  ( 17.20831665107776587, 59.13393115100078745, -7.208316651077762316 ) ) ;
#53613=CARTESIAN_POINT ( 'NONE',  ( 4.559911319644449179, 8.897018677488171434, 9.422509992056141925 ) ) ;
#53614=CARTESIAN_POINT ( 'NONE',  ( 12.91533473730993009, 31.60535201082150891, -10.88017736071109987 ) ) ;
#53615=CARTESIAN_POINT ( 'NONE',  ( -4.164238869374099039, 41.80374883491397497, 8.674139862899312516E-16 ) ) ;
#53616=CARTESIAN_POINT ( 'NONE',  ( 0.1532563361054083140, 31.00893115100078390, 1.131784320476157264E-15 ) ) ;
#53617=CARTESIAN_POINT ( 'NONE',  ( -0.8801773607110991993, 42.85535201082150536, -2.915334737309923874 ) ) ;
#53619=CARTESIAN_POINT ( 'NONE',  ( 6.204703633549690345, 5.762082168247301794, -14.16423886937410259 ) ) ;
#53620=EDGE_CURVE ( 'NONE', #28166, #49358, #93507, .T. ) ;
#53622=CARTESIAN_POINT ( 'NONE',  ( 7.361572987183169658, 54.96726448433413026, -9.846743663894592657 ) ) ;
#53623=( GEOMETRIC_REPRESENTATION_CONTEXT ( 3 ) GLOBAL_UNCERTAINTY_ASSIGNED_CONTEXT ( ( #70221 ) ) GLOBAL_UNIT_ASSIGNED_CONTEXT ( ( #39650, #63113, #55627 ) ) REPRESENTATION_CONTEXT ( 'NONE', 'WORKASPACE' ) );
#53628=CARTESIAN_POINT ( 'NONE',  ( 20.36894250292379382, 33.67874883491396076, 10.36894250292379205 ) ) ;
#53629=CARTESIAN_POINT ( 'NONE',  ( 6.204703633549690345, 17.84541550158063217, 14.16423886937410082 ) ) ;
#53630=CARTESIAN_POINT ( 'NONE',  ( 0.1532563361054083140, 6.008931151000784787, 1.131784320476157264E-15 ) ) ;
#53631=CARTESIAN_POINT ( 'NONE',  ( -1.099225684535947600, 9.540301336597087456, 6.408140936763237150 ) ) ;
#53634=CARTESIAN_POINT ( 'NONE',  ( 7.084665262690076126, 54.10535201082151247, 10.88017736071109987 ) ) ;
#53635=CARTESIAN_POINT ( 'NONE',  ( -2.816281873526473856, 19.12363466993042138, 9.499525473075851096E-16 ) ) ;
#53636=CARTESIAN_POINT ( 'NONE',  ( 24.16423886937409904, 34.09541550158064638, 3.795296366450317205 ) ) ;
#53637=CARTESIAN_POINT ( 'NONE',  ( 4.559911319644449179, 18.89701867748817321, 9.422509992056141925 ) ) ;
#53638=( GEOMETRIC_REPRESENTATION_CONTEXT ( 3 ) GLOBAL_UNCERTAINTY_ASSIGNED_CONTEXT ( ( #72491 ) ) GLOBAL_UNIT_ASSIGNED_CONTEXT ( ( #98428, #5442, #13921 ) ) REPRESENTATION_CONTEXT ( 'NONE', 'WORKASPACE' ) );
#53640=CARTESIAN_POINT ( 'NONE',  ( 20.88017736071110875, 35.77201867748816966, -2.915334737309920765 ) ) ;
#53643=CARTESIAN_POINT ( 'NONE',  ( 0.5774900079438607392, 63.48035201082149825, 5.440088680355550821 ) ) ;
#53644=CARTESIAN_POINT ( 'NONE',  ( 22.81628187352647785, 51.62363466993042493, 6.195893100308588602E-16 ) ) ;
#53647=DIRECTION ( 'NONE',  ( 0.000000000000000000, -1.000000000000000000, 0.000000000000000000 ) ) ;
#53649=CARTESIAN_POINT ( 'NONE',  ( -46.44000000000001194, 92.00000000000000000, 9.500000000000000000 ) ) ;
#53651=CARTESIAN_POINT ( 'NONE',  ( 17.08211943468705130, 58.47041550158063927, 12.26659068614894998 ) ) ;
#53652=CARTESIAN_POINT ( 'NONE',  ( 4.559911319644449179, 3.897018677488171434, 9.422509992056141925 ) ) ;
#53653=CARTESIAN_POINT ( 'NONE',  ( 1.472469842513823179, 20.59226448433411960, -4.923371831947296329 ) ) ;
#53654=CARTESIAN_POINT ( 'NONE',  ( 17.20831665107776587, 59.13393115100078745, -7.208316651077762316 ) ) ;
#53655=CARTESIAN_POINT ( 'NONE',  ( 20.32896413005680714, 60.57879003517448524, -5.963430220938276349 ) ) ;
#53656=CARTESIAN_POINT ( 'NONE',  ( 20.15039907845753220, 49.72266099184918176, 6.262539305110078836 ) ) ;
#53657=CARTESIAN_POINT ( 'NONE',  ( 10.00000000000000000, 9.758931151000785675, -9.846743663894594434 ) ) ;
#53658=CARTESIAN_POINT ( 'NONE',  ( 6.565887622018943937, 10.16530133659708746, 12.81628187352647430 ) ) ;
#53661=CARTESIAN_POINT ( 'NONE',  ( -2.266590686148945544, 32.22041550158063927, 7.082119434687048631 ) ) ;
#53663=CARTESIAN_POINT ( 'NONE',  ( 20.36894250292379738, 44.92874883491396787, -10.36894250292379027 ) ) ;
#53664=ORIENTED_EDGE ( 'NONE', *, *, #4215, .F. ) ;
#53665=CARTESIAN_POINT ( 'NONE',  ( 0.6178305044545818747, 63.49863466993043204, -9.382169495545419124 ) ) ;
#53666=CARTESIAN_POINT ( 'NONE',  ( 1.472469842513823179, 46.42559781766745175, 4.923371831947296329 ) ) ;
#53667=CARTESIAN_POINT ( 'NONE',  ( 20.88017736071110519, 20.56368534415484106, 2.639326808657452039E-16 ) ) ;
#53669=CARTESIAN_POINT ( 'NONE',  ( 12.63842701281683034, 57.46726448433411605, 9.846743663894596210 ) ) ;
#53670=CARTESIAN_POINT ( 'NONE',  ( 5.076628168052704559, 45.17559781766745175, -8.527530157486179263 ) ) ;
#53674=( NAMED_UNIT ( * ) SI_UNIT ( $, .STERADIAN. ) SOLID_ANGLE_UNIT ( ) );
#53676=ORIENTED_EDGE ( 'NONE', *, *, #64231, .F. ) ;
#53678=CARTESIAN_POINT ( 'NONE',  ( 7.361572987183170547, 27.05059781766745175, 9.846743663894590881 ) ) ;
#53680=CARTESIAN_POINT ( 'NONE',  ( 19.38216949554541202, 40.99863466993042493, 9.382169495545424454 ) ) ;
#53684=CARTESIAN_POINT ( 'NONE',  ( 14.49999999999999822, 11.50000000000000000, 6.000000000000000000 ) ) ;
#53685=CARTESIAN_POINT ( 'NONE',  ( 19.84674366389459266, 58.30059781766745886, 2.638427012816836559 ) ) ;
#53686=CARTESIAN_POINT ( 'NONE',  ( 13.79529636645030344, 38.26208216824729647, 14.16423886937410614 ) ) ;
#53687=CARTESIAN_POINT ( 'NONE',  ( 1.472469842513823179, 55.59226448433412315, -4.923371831947296329 ) ) ;
#53689=CARTESIAN_POINT ( 'NONE',  ( 2.791683348922240793, 1.633931151000784565, 7.208316651077764092 ) ) ;
#53690=CARTESIAN_POINT ( 'NONE',  ( -2.816281873526473856, 54.12363466993041783, 9.499525473075851096E-16 ) ) ;
#53691=CARTESIAN_POINT ( 'NONE',  ( 2.917880565312950480, 0.9704155015806342766, -12.26659068614894821 ) ) ;
#53692=CARTESIAN_POINT ( 'NONE',  ( 1.472469842513823179, 51.42559781766745886, 4.923371831947296329 ) ) ;
#53693=CARTESIAN_POINT ( 'NONE',  ( 2.035157376598824452, 58.68868534415482685, 7.964842623401179544 ) ) ;
#53696=CARTESIAN_POINT ( 'NONE',  ( 7.084665262690076126, 59.10535201082150536, 10.88017736071109987 ) ) ;
#53700=CARTESIAN_POINT ( 'NONE',  ( 17.96484262340118221, 31.18868534415483751, -7.964842623401177768 ) ) ;
#53701=CARTESIAN_POINT ( 'NONE',  ( -1.099225684535947600, 3.706968003263753531, -6.408140936763238038 ) ) ;
#53702=CARTESIAN_POINT ( 'NONE',  ( 15.44008868035555793, 51.39701867748816966, -9.422509992056140149 ) ) ;
#53704=CARTESIAN_POINT ( 'NONE',  ( -0.8801773607110991993, 67.85535201082151957, -2.915334737309923874 ) ) ;
#53706=CARTESIAN_POINT ( 'NONE',  ( 20.88017736071110519, 35.56368534415484106, 2.639326808657452039E-16 ) ) ;
#53708=CARTESIAN_POINT ( 'NONE',  ( 17.20831665107776587, 9.133931151000787452, -7.208316651077762316 ) ) ;
#53710=CARTESIAN_POINT ( 'NONE',  ( 19.84674366389459266, 43.30059781766744464, 2.638427012816836559 ) ) ;
#53711=CARTESIAN_POINT ( 'NONE',  ( -32.19000000000001194, 93.50000000000000000, -10.09898361729590199 ) ) ;
#53713=CARTESIAN_POINT ( 'NONE',  ( 19.84674366389459266, 58.71726448433411605, -2.638427012816827677 ) ) ;
#53714=CARTESIAN_POINT ( 'NONE',  ( -4.164238869374099039, 66.80374883491396076, 8.674139862899312516E-16 ) ) ;
#53715=CARTESIAN_POINT ( 'NONE',  ( 19.72487221294571569, 27.80223176428830811, -6.499999999999990230 ) ) ;
#53717=CARTESIAN_POINT ( 'NONE',  ( -0.3689425029237881626, 27.42874883491397142, 10.36894250292379027 ) ) ;
#53718=VECTOR ( 'NONE', #93666, 1000.000000000000000 ) ;
#53720=CARTESIAN_POINT ( 'NONE',  ( -0.3689425029237898834, 51.17874883491397497, -10.36894250292378850 ) ) ;
#53721=CARTESIAN_POINT ( 'NONE',  ( 0.1532563361054083140, 31.00893115100078390, 1.131784320476157264E-15 ) ) ;
#53723=CARTESIAN_POINT ( 'NONE',  ( 18.52753015748617571, 18.09226448433411960, 4.923371831947298993 ) ) ;
#53724=( NAMED_UNIT ( * ) SI_UNIT ( $, .STERADIAN. ) SOLID_ANGLE_UNIT ( ) );
#53725=EDGE_LOOP ( 'NONE', ( #73162, #33830, #74175, #82695, #98616, #91990 ) ) ;
#53726=CARTESIAN_POINT ( 'NONE',  ( 7.361572987183169658, 29.96726448433411960, -9.846743663894592657 ) ) ;
#53727=CARTESIAN_POINT ( 'NONE',  ( 15.44008868035555793, 21.39701867748817321, -9.422509992056140149 ) ) ;
#53728=CARTESIAN_POINT ( 'NONE',  ( 1.472469842513823179, 60.59226448433412315, -4.923371831947296329 ) ) ;
#53729=CARTESIAN_POINT ( 'NONE',  ( -4.164238869374099927, 7.012082168247302683, 3.795296366450308767 ) ) ;
#53732=CARTESIAN_POINT ( 'NONE',  ( 10.00000000000000000, 9.758931151000785675, -9.846743663894594434 ) ) ;
#53733=CARTESIAN_POINT ( 'NONE',  ( 22.81628187352648496, 41.83196800326375353, -3.434112377981050290 ) ) ;
#53734=CARTESIAN_POINT ( 'NONE',  ( 17.20831665107776587, 42.88393115100077324, 7.208316651077764980 ) ) ;
#53736=CARTESIAN_POINT ( 'NONE',  ( 7.361572987183169658, 24.96726448433412315, -9.846743663894592657 ) ) ;
#53738=CARTESIAN_POINT ( 'NONE',  ( -46.67785289142584304, 101.1465011330960948, -8.702494886479120950 ) ) ;
#53739=CARTESIAN_POINT ( 'NONE',  ( 22.26659068614895176, 59.72041550158063927, -7.082119434687042414 ) ) ;
#53740=CARTESIAN_POINT ( 'NONE',  ( 20.88017736071110875, 50.77201867748817676, -2.915334737309920765 ) ) ;
#53741=CARTESIAN_POINT ( 'NONE',  ( 2.917880565312950480, 0.9704155015806342766, -12.26659068614894821 ) ) ;
#53742=CARTESIAN_POINT ( 'NONE',  ( 2.791683348922237240, 40.38393115100078035, -7.208316651077763204 ) ) ;
#53743=CARTESIAN_POINT ( 'NONE',  ( 19.42250999205614548, 10.98035201082150358, -5.440088680355545492 ) ) ;
#53744=CARTESIAN_POINT ( 'NONE',  ( 19.84674366389459621, 33.50893115100078745, 7.409399052514197653E-17 ) ) ;
#53746=CARTESIAN_POINT ( 'NONE',  ( 10.00000000000000000, 49.75893115100078745, -9.846743663894594434 ) ) ;
#53747=STYLED_ITEM ( 'NONE', ( #84137 ), #55465 ) ;
#53748=CARTESIAN_POINT ( 'NONE',  ( 2.035157376598822676, 47.43868534415484817, -7.964842623401177768 ) ) ;
#53755=CARTESIAN_POINT ( 'NONE',  ( 5.076628168052704559, 5.175597817667451750, -8.527530157486179263 ) ) ;
#53756=CARTESIAN_POINT ( 'NONE',  ( 6.565887622018943937, 58.08196800326376064, -12.81628187352647608 ) ) ;
#53757=CARTESIAN_POINT ( 'NONE',  ( 15.44008868035555793, 11.39701867748817143, -9.422509992056140149 ) ) ;
#53758=CARTESIAN_POINT ( 'NONE',  ( 19.84674366389459266, 43.71726448433410894, -2.638427012816827677 ) ) ;
#53760=CARTESIAN_POINT ( 'NONE',  ( -0.3689425029237898834, 26.17874883491396432, -10.36894250292378850 ) ) ;
#53763=CARTESIAN_POINT ( 'NONE',  ( 20.36894250292379382, 53.67874883491397497, 10.36894250292379205 ) ) ;
#53764=CARTESIAN_POINT ( 'NONE',  ( 10.00000000000000178, 57.25893115100078745, 9.846743663894594434 ) ) ;
#53766=CARTESIAN_POINT ( 'NONE',  ( 17.96484262340118221, 54.93868534415484106, 7.964842623401181321 ) ) ;
#53767=CARTESIAN_POINT ( 'NONE',  ( 20.88017736071110875, 65.77201867748817676, -2.915334737309920765 ) ) ;
#53770=CARTESIAN_POINT ( 'NONE',  ( -2.816281873526473856, 54.33196800326376064, 3.434112377981055619 ) ) ;
#53772=CARTESIAN_POINT ( 'NONE',  ( 0.1532563361054082862, 11.21726448433411605, 2.638427012816831674 ) ) ;
#53774=EDGE_LOOP ( 'NONE', ( #68020, #76783, #25287, #38301 ) ) ;
#53775=CARTESIAN_POINT ( 'NONE',  ( 17.08211943468705840, 25.13708216824730357, -12.26659068614894466 ) ) ;
#53776=CARTESIAN_POINT ( 'NONE',  ( 5.076628168052704559, 25.17559781766745175, -8.527530157486179263 ) ) ;
#53777=CARTESIAN_POINT ( 'NONE',  ( 10.00000000000000000, 26.81368534415484106, -10.88017736071110342 ) ) ;
#53778=CARTESIAN_POINT ( 'NONE',  ( -42.16485527613927076, 107.5383484153110061, -4.500000000000000888 ) ) ;
#53780=CARTESIAN_POINT ( 'NONE',  ( 17.96484262340118221, 31.18868534415483751, -7.964842623401177768 ) ) ;
#53782=( BOUNDED_CURVE ( )  B_SPLINE_CURVE ( 2, ( #92982, #24018, #39512, #70004, #86958, #54487, #31487, #71484, #18472 ),
 .UNSPECIFIED., .F., .F. ) 
 B_SPLINE_CURVE_WITH_KNOTS ( ( 3, 2, 2, 2, 3 ),
 ( 0.2239427359034107945, 0.2261904761904761918, 0.2321428571428571508, 0.2380952380952380820, 0.2403429783823026467 ),
 .UNSPECIFIED. ) 
 CURVE ( )  GEOMETRIC_REPRESENTATION_ITEM ( )  RATIONAL_B_SPLINE_CURVE ( ( 0.9839835555609424134, 0.9871328979762477029, 1.000000000000000000, 0.9659258262890683122, 1.000000000000000000, 0.9659258262890683122, 1.000000000000000000, 0.9871328979762523659, 0.9839835555609446338 ) ) 
 REPRESENTATION_ITEM ( '' )  );
#53783=VERTEX_POINT ( 'NONE', #90217 ) ;
#53784=ORIENTED_EDGE ( 'NONE', *, *, #262, .F. ) ;
#53788=CARTESIAN_POINT ( 'NONE',  ( 22.81628187352647785, 16.62363466993042138, 6.195893100308588602E-16 ) ) ;
#53790=CARTESIAN_POINT ( 'NONE',  ( 18.52753015748617571, 13.09226448433411960, 4.923371831947298993 ) ) ;
#53792=CARTESIAN_POINT ( 'NONE',  ( 20.88017736071110164, 10.35535201082150536, 2.915334737309930979 ) ) ;
#53793=CARTESIAN_POINT ( 'NONE',  ( 0.1532563361054083140, 16.00893115100078390, 1.131784320476157264E-15 ) ) ;
#53794=CARTESIAN_POINT ( 'NONE',  ( 4.559911319644449179, 27.23035201082150536, -9.422509992056141925 ) ) ;
#53801=CARTESIAN_POINT ( 'NONE',  ( -2.816281873526471635, 63.91530133659708923, -3.434112377981056508 ) ) ;
#53802=CARTESIAN_POINT ( 'NONE',  ( 0.5774900079438607392, 58.48035201082151247, 5.440088680355550821 ) ) ;
#53804=CARTESIAN_POINT ( 'NONE',  ( 13.43411237798105340, 55.58196800326374643, 12.81628187352647963 ) ) ;
#53805=CARTESIAN_POINT ( 'NONE',  ( 19.42250999205614193, 55.14701867748817676, 5.440088680355555262 ) ) ;
#53806=CARTESIAN_POINT ( 'NONE',  ( 10.00000000000000000, -2.126365330069579951, -12.81628187352647608 ) ) ;
#53808=CARTESIAN_POINT ( 'NONE',  ( 5.076628168052703671, 31.84226448433412315, 8.527530157486179263 ) ) ;
#53809=CARTESIAN_POINT ( 'NONE',  ( 0.6178305044545838731, 49.74863466993041072, 9.382169495545420901 ) ) ;
#53810=CARTESIAN_POINT ( 'NONE',  ( 12.63842701281683922, 24.55059781766745175, -9.846743663894590881 ) ) ;
#53811=CARTESIAN_POINT ( 'NONE',  ( -1.099225684535947600, 18.70696800326375353, -6.408140936763238038 ) ) ;
#53814=CARTESIAN_POINT ( 'NONE',  ( 15.44008868035555260, 39.73035201082150536, 9.422509992056143702 ) ) ;
#53815=CARTESIAN_POINT ( 'NONE',  ( 0.1532563361054083140, 66.00893115100079456, 1.131784320476157264E-15 ) ) ;
#53817=CARTESIAN_POINT ( 'NONE',  ( 7.361572987183170547, 17.05059781766745530, 9.846743663894590881 ) ) ;
#53818=CARTESIAN_POINT ( 'NONE',  ( 0.1532563361054083140, 11.00893115100078568, 1.131784320476157264E-15 ) ) ;
#53819=CARTESIAN_POINT ( 'NONE',  ( 7.084665262690076126, 17.02201867748817676, -10.88017736071110164 ) ) ;
#53820=CARTESIAN_POINT ( 'NONE',  ( 6.565887622018943937, 15.16530133659708568, 12.81628187352647430 ) ) ;
#53822=CARTESIAN_POINT ( 'NONE',  ( 0.5774900079438590739, 2.647018677488170990, -5.440088680355550821 ) ) ;
#53823=CARTESIAN_POINT ( 'NONE',  ( 10.00000000000000178, 57.25893115100078745, 9.846743663894594434 ) ) ;
#53825=CARTESIAN_POINT ( 'NONE',  ( 17.96484262340118221, 11.18868534415484106, -7.964842623401177768 ) ) ;
#53826=CARTESIAN_POINT ( 'NONE',  ( 12.63842701281683034, 47.46726448433412315, 9.846743663894596210 ) ) ;
#53829=CARTESIAN_POINT ( 'NONE',  ( 2.035157376598824452, 18.68868534415484106, 7.964842623401179544 ) ) ;
#53830=CARTESIAN_POINT ( 'NONE',  ( 20.05723567505239302, 69.83236346210667023, -6.413539670616450472 ) ) ;
#53831=CARTESIAN_POINT ( 'NONE',  ( 15.44008868035555793, 36.39701867748816966, -9.422509992056140149 ) ) ;
#53832=CARTESIAN_POINT ( 'NONE',  ( 7.084665262690076126, 4.105352010821503583, 10.88017736071109987 ) ) ;
#53835=CARTESIAN_POINT ( 'NONE',  ( 19.84674366389459621, 23.50893115100078390, 7.409399052514197653E-17 ) ) ;
#53836=CARTESIAN_POINT ( 'NONE',  ( 21.09922568453595559, 12.04030133659708746, -6.408140936763230044 ) ) ;
#53837=CARTESIAN_POINT ( 'NONE',  ( -46.77384778588437086, 103.6211922023598362, 6.142868351312646524 ) ) ;
#53840=CARTESIAN_POINT ( 'NONE',  ( 14.92337183194729633, 62.67559781766745886, 8.527530157486181039 ) ) ;
#53843=CARTESIAN_POINT ( 'NONE',  ( 24.16423886937410614, 14.51208216824730179, -3.795296366450302550 ) ) ;
#53845=CARTESIAN_POINT ( 'NONE',  ( 17.20831665107776587, 37.88393115100078745, 7.208316651077764980 ) ) ;
#53848=CARTESIAN_POINT ( 'NONE',  ( 13.79529636645031943, 60.34541550158063927, -14.16423886937409904 ) ) ;
#53850=CARTESIAN_POINT ( 'NONE',  ( 19.84674366389459266, 3.717264484334118713, -2.638427012816827677 ) ) ;
#53851=CARTESIAN_POINT ( 'NONE',  ( 0.2751277870542910842, 63.21833443783937412, 6.499999999999992006 ) ) ;
#53853=CARTESIAN_POINT ( 'NONE',  ( 10.00000000000000178, 49.31368534415484106, 10.88017736071110342 ) ) ;
#53854=CARTESIAN_POINT ( 'NONE',  ( 22.81628187352648496, 46.83196800326376064, -3.434112377981050290 ) ) ;
#53855=CARTESIAN_POINT ( 'NONE',  ( -0.8801773607110991993, 22.85535201082150181, -2.915334737309923874 ) ) ;
#53856=CARTESIAN_POINT ( 'NONE',  ( 16.40814093676323893, 45.79030133659708923, 11.09922568453595026 ) ) ;
#53857=CARTESIAN_POINT ( 'NONE',  ( 3.591859063236763294, -1.709698663402913210, -11.09922568453595026 ) ) ;
#53858=CARTESIAN_POINT ( 'NONE',  ( 0.2751277870542911952, 53.21833443783938122, 6.499999999999992006 ) ) ;
#53860=CARTESIAN_POINT ( 'NONE',  ( 2.126467202668119061, 1.181022659884616743, -6.500000000000000888 ) ) ;
#53861=CARTESIAN_POINT ( 'NONE',  ( 6.204703633549690345, 37.84541550158063927, 14.16423886937410082 ) ) ;
#53862=CARTESIAN_POINT ( 'NONE',  ( 10.00000000000000178, 13.05374883491396787, 14.16423886937410082 ) ) ;
#53863=CARTESIAN_POINT ( 'NONE',  ( 20.88017736071110875, 25.77201867748816966, -2.915334737309920765 ) ) ;
#53864=( GEOMETRIC_REPRESENTATION_CONTEXT ( 3 ) GLOBAL_UNCERTAINTY_ASSIGNED_CONTEXT ( ( #73142 ) ) GLOBAL_UNIT_ASSIGNED_CONTEXT ( ( #19975, #50967, #10511 ) ) REPRESENTATION_CONTEXT ( 'NONE', 'WORKASPACE' ) );
#53865=CARTESIAN_POINT ( 'NONE',  ( 15.44008868035555793, 31.39701867748817676, -9.422509992056140149 ) ) ;
#53868=CARTESIAN_POINT ( 'NONE',  ( 19.42250999205614548, 65.98035201082151957, -5.440088680355545492 ) ) ;
#53869=CARTESIAN_POINT ( 'NONE',  ( 17.96484262340118221, 59.93868534415484106, 7.964842623401181321 ) ) ;
#53870=CARTESIAN_POINT ( 'NONE',  ( 10.00000000000000178, 25.37363466993041783, 12.81628187352647608 ) ) ;
#53871=CARTESIAN_POINT ( 'NONE',  ( 18.17829156368508237, 19.16792564121896802, 6.499999999999999112 ) ) ;
#53872=CARTESIAN_POINT ( 'NONE',  ( 6.000000000000000000, 11.50000000000000000, 6.000000000000000000 ) ) ;
#53873=CARTESIAN_POINT ( 'NONE',  ( 10.00000000000000178, 7.258931151000785675, 9.846743663894594434 ) ) ;
#53874=CARTESIAN_POINT ( 'NONE',  ( 19.84674366389459266, 33.30059781766744464, 2.638427012816836559 ) ) ;
#53876=CARTESIAN_POINT ( 'NONE',  ( 15.44008868035555793, 11.39701867748817143, -9.422509992056140149 ) ) ;
#53879=EDGE_CURVE ( 'NONE', #65586, #800, #38883, .T. ) ;
#53880=CARTESIAN_POINT ( 'NONE',  ( -2.816281873526471635, 33.91530133659708213, -3.434112377981056508 ) ) ;
#53881=CARTESIAN_POINT ( 'NONE',  ( 5.076628168052703671, 6.842264484334118713, 8.527530157486179263 ) ) ;
#53882=CARTESIAN_POINT ( 'NONE',  ( 20.88017736071110164, 10.35535201082150714, 2.915334737309930979 ) ) ;
#53883=CARTESIAN_POINT ( 'NONE',  ( 12.63842701281683922, 39.55059781766744464, -9.846743663894590881 ) ) ;
#53884=CARTESIAN_POINT ( 'NONE',  ( 19.84674366389459621, 33.50893115100078745, 7.409399052514197653E-17 ) ) ;
#53886=CARTESIAN_POINT ( 'NONE',  ( 10.00000000000000000, 20.55374883491396787, -14.16423886937410082 ) ) ;
#53887=CARTESIAN_POINT ( 'NONE',  ( 0.5774900079438590739, 27.64701867748817676, -5.440088680355550821 ) ) ;
#53888=CARTESIAN_POINT ( 'NONE',  ( 12.91533473730993009, 6.605352010821504471, -10.88017736071109987 ) ) ;
#53889=CARTESIAN_POINT ( 'NONE',  ( 19.42250999205614548, 35.98035201082151247, -5.440088680355545492 ) ) ;
#53890=CARTESIAN_POINT ( 'NONE',  ( 10.00000000000000178, 34.31368534415484106, 10.88017736071110342 ) ) ;
#53892=CARTESIAN_POINT ( 'NONE',  ( 19.42250999205614548, 35.98035201082151247, -5.440088680355545492 ) ) ;
#53893=CARTESIAN_POINT ( 'NONE',  ( 21.09922568453595559, 57.04030133659708923, -6.408140936763230044 ) ) ;
#53894=CARTESIAN_POINT ( 'NONE',  ( 10.00000000000000178, 44.31368534415484106, 10.88017736071110342 ) ) ;
#53895=CARTESIAN_POINT ( 'NONE',  ( 4.559911319644449179, 48.89701867748817676, 9.422509992056141925 ) ) ;
#53896=ORIENTED_EDGE ( 'NONE', *, *, #94873, .F. ) ;
#53897=CARTESIAN_POINT ( 'NONE',  ( 15.44008868035555260, 54.73035201082150536, 9.422509992056143702 ) ) ;
#53899=CARTESIAN_POINT ( 'NONE',  ( -2.266590686148945544, 66.38708216824730357, -7.082119434687050408 ) ) ;
#53900=CARTESIAN_POINT ( 'NONE',  ( 18.52753015748617571, 3.092264484334118269, 4.923371831947298993 ) ) ;
#53901=CARTESIAN_POINT ( 'NONE',  ( 19.10478245763052030, 55.10160829253886305, 5.990408912944319653 ) ) ;
#53902=AXIS2_PLACEMENT_3D ( 'NONE', #14401, #66392, #52381 ) ;
#53904=CARTESIAN_POINT ( 'NONE',  ( 19.84674366389459266, 38.30059781766745175, 2.638427012816836559 ) ) ;
#53906=CARTESIAN_POINT ( 'NONE',  ( 18.52753015748618282, 33.92559781766745886, -4.923371831947291888 ) ) ;
#53907=CARTESIAN_POINT ( 'NONE',  ( 19.42250999205614193, 35.14701867748816966, 5.440088680355555262 ) ) ;
#53908=CARTESIAN_POINT ( 'NONE',  ( 0.1532563361054083140, 36.00893115100078745, 1.131784320476157264E-15 ) ) ;
#53909=CARTESIAN_POINT ( 'NONE',  ( 22.81628187352647785, 16.41530133659708923, 3.434112377981063169 ) ) ;
#53911=CARTESIAN_POINT ( 'NONE',  ( 17.96484262340118221, 61.18868534415482685, -7.964842623401177768 ) ) ;
#53912=CARTESIAN_POINT ( 'NONE',  ( 7.084665262690076126, 49.10535201082149825, 10.88017736071109987 ) ) ;
#53913=( NAMED_UNIT ( * ) PLANE_ANGLE_UNIT ( ) SI_UNIT ( $, .RADIAN. ) );
#53914=CARTESIAN_POINT ( 'NONE',  ( -2.266590686148945544, 62.22041550158063927, 7.082119434687048631 ) ) ;
#53916=CARTESIAN_POINT ( 'NONE',  ( 19.38216949554541202, 15.99863466993042138, 9.382169495545424454 ) ) ;
#53917=CARTESIAN_POINT ( 'NONE',  ( 5.500000000000000000, 11.00000000000000000, -5.000000000000000000 ) ) ;
#53919=CARTESIAN_POINT ( 'NONE',  ( 21.09922568453594849, 11.20696800326375531, 6.408140936763242479 ) ) ;
#53920=CARTESIAN_POINT ( 'NONE',  ( 20.88017736071110519, 15.56368534415483751, 2.639326808657452039E-16 ) ) ;
#53921=CARTESIAN_POINT ( 'NONE',  ( 17.96484262340118221, 61.18868534415482685, -7.964842623401177768 ) ) ;
#53923=CARTESIAN_POINT ( 'NONE',  ( 17.20831665107776587, 2.883931151000785231, 7.208316651077764980 ) ) ;
#53924=CARTESIAN_POINT ( 'NONE',  ( 0.1532563361054082862, 51.21726448433412315, 2.638427012816831674 ) ) ;
#53925=CARTESIAN_POINT ( 'NONE',  ( 19.84674366389459266, 38.30059781766745175, 2.638427012816836559 ) ) ;
#53928=CARTESIAN_POINT ( 'NONE',  ( 1.472469842513823179, 21.42559781766745175, 4.923371831947296329 ) ) ;
#53931=CARTESIAN_POINT ( 'NONE',  ( 14.92337183194729988, 9.342264484334119601, -8.527530157486177487 ) ) ;
#53934=CARTESIAN_POINT ( 'NONE',  ( 20.24186590665276597, 44.73410085661203794, 6.114288769123062295 ) ) ;
#53935=CARTESIAN_POINT ( 'NONE',  ( 17.20831665107776587, 47.88393115100078745, 7.208316651077764980 ) ) ;
#53936=VERTEX_POINT ( 'NONE', #29713 ) ;
#53939=CARTESIAN_POINT ( 'NONE',  ( 16.40814093676324603, 12.45696800326375353, -11.09922568453594671 ) ) ;
#53940=CARTESIAN_POINT ( 'NONE',  ( 7.084665262690076126, 54.10535201082151247, 10.88017736071109987 ) ) ;
#53941=CARTESIAN_POINT ( 'NONE',  ( 24.16423886937409904, 29.09541550158063572, 3.795296366450317205 ) ) ;
#53942=CARTESIAN_POINT ( 'NONE',  ( 1.472469842513823179, 0.5922644843341181575, -4.923371831947296329 ) ) ;
#53943=CARTESIAN_POINT ( 'NONE',  ( 24.16423886937409904, 49.09541550158063217, 3.795296366450317205 ) ) ;
#53944=CARTESIAN_POINT ( 'NONE',  ( 2.917880565312950480, 55.97041550158063217, -12.26659068614894821 ) ) ;
#53945=CARTESIAN_POINT ( 'NONE',  ( 20.36894250292379382, 18.67874883491397142, 10.36894250292379205 ) ) ;
#53946=CARTESIAN_POINT ( 'NONE',  ( 6.204703633549690345, 22.84541550158062861, 14.16423886937410082 ) ) ;
#53947=CARTESIAN_POINT ( 'NONE',  ( -0.2418659066527630297, 38.09014588040356131, 6.114288769123057854 ) ) ;
#53950=CARTESIAN_POINT ( 'NONE',  ( 0.1532563361054082862, 36.21726448433410894, 2.638427012816831674 ) ) ;
#53951=CARTESIAN_POINT ( 'NONE',  ( 17.96484262340118221, 26.18868534415483396, -7.964842623401177768 ) ) ;
#53954=CARTESIAN_POINT ( 'NONE',  ( 19.64201483648641045, 84.95676665491684787, -5.303713241054131444 ) ) ;
#53955=EDGE_CURVE ( 'NONE', #21351, #42200, #68850, .T. ) ;
#53956=CARTESIAN_POINT ( 'NONE',  ( 7.361572987183169658, 44.96726448433412315, -9.846743663894592657 ) ) ;
#53957=CARTESIAN_POINT ( 'NONE',  ( 3.591859063236761518, 54.95696800326376064, 11.09922568453594849 ) ) ;
#53959=CARTESIAN_POINT ( 'NONE',  ( 17.20831665107776587, 37.88393115100078745, 7.208316651077764980 ) ) ;
#53960=CARTESIAN_POINT ( 'NONE',  ( 17.20831665107776587, 47.88393115100078745, 7.208316651077764980 ) ) ;
#53961=CARTESIAN_POINT ( 'NONE',  ( 17.08211943468705130, 43.47041550158063927, 12.26659068614894998 ) ) ;
#53963=CARTESIAN_POINT ( 'NONE',  ( 10.00000000000000178, 13.05374883491396787, 14.16423886937410082 ) ) ;
#53964=CARTESIAN_POINT ( 'NONE',  ( 4.559911319644449179, 57.23035201082150536, -9.422509992056141925 ) ) ;
#53965=CARTESIAN_POINT ( 'NONE',  ( 17.96484262340118221, 9.938685344154839285, 7.964842623401181321 ) ) ;
#53966=CARTESIAN_POINT ( 'NONE',  ( 3.591859063236761518, 4.956968003263753531, 11.09922568453594849 ) ) ;
#53967=CARTESIAN_POINT ( 'NONE',  ( 20.32896413005680714, 2.604976035794174027, -5.963430220938276349 ) ) ;
#53968=CARTESIAN_POINT ( 'NONE',  ( 12.91533473730993009, 66.60535201082150536, -10.88017736071109987 ) ) ;
#53970=CARTESIAN_POINT ( 'NONE',  ( 0.1955144967548973212, 14.32703681773340776, -6.500000000002781775 ) ) ;
#53971=CARTESIAN_POINT ( 'NONE',  ( -4.164238869374099927, 62.01208216824728936, 3.795296366450308767 ) ) ;
#53973=CARTESIAN_POINT ( 'NONE',  ( 15.44008868035555793, 31.39701867748817676, -9.422509992056140149 ) ) ;
#53974=CARTESIAN_POINT ( 'NONE',  ( 4.559911319644449179, 18.89701867748817321, 9.422509992056141925 ) ) ;
#53975=CARTESIAN_POINT ( 'NONE',  ( 14.92337183194729633, 57.67559781766745886, 8.527530157486181039 ) ) ;
#53976=CARTESIAN_POINT ( 'NONE',  ( 19.84674366389459621, 58.50893115100078745, 7.409399052514197653E-17 ) ) ;
#53977=CARTESIAN_POINT ( 'NONE',  ( 3.591859063236761518, 54.95696800326376064, 11.09922568453594849 ) ) ;
#53978=( NAMED_UNIT ( * ) SI_UNIT ( $, .STERADIAN. ) SOLID_ANGLE_UNIT ( ) );
#53979=ORIENTED_EDGE ( 'NONE', *, *, #3531, .T. ) ;
#53980=CARTESIAN_POINT ( 'NONE',  ( 19.42250999205614548, 15.98035201082150714, -5.440088680355545492 ) ) ;
#53981=CARTESIAN_POINT ( 'NONE',  ( 13.43411237798106583, 12.66530133659708746, -12.81628187352647252 ) ) ;
#53985=CARTESIAN_POINT ( 'NONE',  ( 0.1532563361054100626, 45.80059781766745886, -2.638427012816831230 ) ) ;
#53986=CARTESIAN_POINT ( 'NONE',  ( 20.88017736071110164, 50.35535201082151247, 2.915334737309930979 ) ) ;
#53987=CARTESIAN_POINT ( 'NONE',  ( 19.38216949554541202, 20.99863466993042138, 9.382169495545424454 ) ) ;
#53988=CARTESIAN_POINT ( 'NONE',  ( -0.8801773607111008646, 63.27201867748817676, 2.915334737309923430 ) ) ;
#53991=ORIENTED_EDGE ( 'NONE', *, *, #57701, .F. ) ;
#53993=DIRECTION ( 'NONE',  ( 0.000000000000000000, -1.000000000000000000, 0.000000000000000000 ) ) ;
#53994=EDGE_CURVE ( 'NONE', #11431, #18624, #11902, .T. ) ;
#53995=CARTESIAN_POINT ( 'NONE',  ( -0.8801773607110991993, 47.85535201082150536, -2.915334737309923874 ) ) ;
#53996=CARTESIAN_POINT ( 'NONE',  ( 19.38216949554541202, 40.99863466993042493, 9.382169495545424454 ) ) ;
#53997=CARTESIAN_POINT ( 'NONE',  ( 17.08211943468705130, 13.47041550158063572, 12.26659068614894998 ) ) ;
#53999=CARTESIAN_POINT ( 'NONE',  ( 17.20831665107776587, 62.88393115100078745, 7.208316651077764980 ) ) ;
#54000=CARTESIAN_POINT ( 'NONE',  ( 0.1532563361054083140, 1.008931151000784787, 1.131784320476157264E-15 ) ) ;
#54002=CARTESIAN_POINT ( 'NONE',  ( -4.164238869374099927, 42.01208216824728936, 3.795296366450308767 ) ) ;
#54003=FACE_OUTER_BOUND ( 'NONE', #58799, .T. ) ;
#54004=CARTESIAN_POINT ( 'NONE',  ( 7.084665262690076126, 4.105352010821503583, 10.88017736071109987 ) ) ;
#54009=CARTESIAN_POINT ( 'NONE',  ( 0.5774900079438607392, 3.480352010821504916, 5.440088680355550821 ) ) ;
#54010=CARTESIAN_POINT ( 'NONE',  ( -0.8801773607110991993, 7.855352010821506248, -2.915334737309923874 ) ) ;
#54011=CARTESIAN_POINT ( 'NONE',  ( 12.63842701281683034, 42.46726448433412315, 9.846743663894596210 ) ) ;
#54012=CARTESIAN_POINT ( 'NONE',  ( 19.38216949554541557, 37.24863466993041783, -9.382169495545420901 ) ) ;
#54013=PRESENTATION_STYLE_ASSIGNMENT (( #31007 ) ) ;
#54015=CARTESIAN_POINT ( 'NONE',  ( -4.164238869374099927, 7.012082168247302683, 3.795296366450308767 ) ) ;
#54016=CARTESIAN_POINT ( 'NONE',  ( 2.035157376598824452, 28.68868534415484106, 7.964842623401179544 ) ) ;
#54017=CARTESIAN_POINT ( 'NONE',  ( 0.5774900079438590739, 7.647018677488171434, -5.440088680355550821 ) ) ;
#54018=CARTESIAN_POINT ( 'NONE',  ( 18.52753015748618282, 43.92559781766745175, -4.923371831947291888 ) ) ;
#54019=CARTESIAN_POINT ( 'NONE',  ( 17.39651004071838614, 42.93575266056826933, 6.500000000000032863 ) ) ;
#54020=CARTESIAN_POINT ( 'NONE',  ( 5.076628168052704559, 20.17559781766745175, -8.527530157486179263 ) ) ;
#54021=PRESENTATION_STYLE_ASSIGNMENT (( #62006 ) ) ;
#54025=CARTESIAN_POINT ( 'NONE',  ( 14.92337183194729633, 57.67559781766745886, 8.527530157486181039 ) ) ;
#54026=CARTESIAN_POINT ( 'NONE',  ( 7.084665262690076126, 29.10535201082150181, 10.88017736071109987 ) ) ;
#54027=CARTESIAN_POINT ( 'NONE',  ( 4.559911319644449179, 42.23035201082151247, -9.422509992056141925 ) ) ;
#54028=CARTESIAN_POINT ( 'NONE',  ( -2.816281873526473856, 34.12363466993042493, 9.499525473075851096E-16 ) ) ;
#54029=CARTESIAN_POINT ( 'NONE',  ( -0.3689425029237881626, 17.42874883491397142, 10.36894250292379027 ) ) ;
#54031=( BOUNDED_SURFACE ( )  B_SPLINE_SURFACE ( 1, 2, ( 
 ( #51013, #26540, #56554, #94545, #12524, #95540, #42533, #87048, #34029, #18559, #27030, #11054, #95031, #57529, #87538, #80536, #43026, #50033, #49528, #73017, #80035, #35014, #96037, #58012, #97531, #98529, #90481, #98025, #29982, #67505, #29479, #13516, #59988, #75493, #37009, #22018, #52492, #7005, #82999, #6022, #60487, #52011, #14517, #90976, #37510, #6501, #21514, #44986, #7514, #68003, #74499, #22509, #74999, #82500, #14018, #52981, #44498, #38005, #83984, #28990, #83495, #43997, #15014, #45483, #36518, #75985, #68498, #25, #30472, #15509, #60973, #91485, #67010, #23006, #53474, #89513, #45991, #5532, #66514, #36012, #59500, #97041, #28516, #59010, #21023, #82004, #51512, #89998, #93448, #15983, #38984, #69476, #31942, #78443, #77450, #61958, #25471, #46470, #92946, #32936, #9958, #46956, #40464, #24481, #76966, #24973, #31456, #1983, #1489, #62443, #8478, #85961, #54944, #85461, #16973, #7994, #9459, #61466, #54456, #32449, #17470, #47937, #55458, #47453, #62945, #91973, #92457, #30969, #84964, #23502, #522, #70963, #70461, #995, #23985, #2482, #93944, #63437, #55953, #8964, #86453, #16480, #53973, #17951, #76480, #39480, #38492, #77952, #39960, #68987, #69970, #84482, #79916, #3448, #19911, #73394, #18443, #63916, #11425, #40956, #78938, #3935, #87421, #80424, #34404, #48925, #42424, #27897, #64893, #49913, #88411, #96423, #11920, #10448, #79437, #10935, #71927, #26418, #80912, #12406, #95926, #95421, #58386, #27406, #88904, #33417, #18938, #4922, #33905, #72905, #71453, #41459, #64413, #94919, #48437, #2967, #65400, #94427, #72408, #49415, #41945, #4438, #35400, #65893, #25942, #56444, #26917, #86930, #34904, #57414, #87907, #56919, #42913, #19421, #57897, #50402, #90363, #21401, #50901, #36398, #81885, #13397, #89393, #60864, #66891, #98905, #44869, #66389, #52871, #20909, #43395, #60368, #14398, #59379, #20415, #6381, #59875, #37400, #43880, #28877, #51895, #74376, #90865, #45370, #51398, #35894, #82377, #12898, #81396, #74883, #89883, #52378, #36897, #5903, #75372, #30356, #67385, #21901, #22395, #68385, #82882, #73893, #97410, #13899, #44384, #97914, #83377, #14899, #67888, #29374, #5424, #98410, #96922, #28400, #6887, #75874, #29866, #7395, #58895, #37893, #23383, #61356, #32817, #91364, #9343, #40347, #16362, #92351, #84855, #47330, #78325, #47825, #70849, #22890, #23878, #7884, #77831, #54342, #46843, #884, #24852, #15878, #31344, #38376, #62331, #77338, #53362, #8364, #53868, #84378, #91865, #83869, #38872, #2362, #16854, #68877, #93331, #61845, #55334, #39364, #46362, #39846, #76850, #70352, #8850 ),
 ( #92838, #69859, #69363, #1380, #85842, #31835, #24367, #54829, #85342, #1870, #32327, #62831, #17356, #9845, #15393, #45879, #76369, #30859, #407, #64291, #63802, #3823, #79316, #41345, #34278, #10825, #65275, #42798, #86823, #71815, #2854, #87788, #94803, #94308, #64779, #11797, #26305, #56805, #73282, #19788, #26799, #33308, #19304, #57294, #48317, #87301, #95295, #25354, #50277, #71334, #55837, #63314, #27284, #93824, #40833, #49790, #72293, #80298, #25831, #56329, #18327, #18821, #95804, #49302, #48808, #12289, #3321, #79804, #80793, #86331, #4313, #11306, #4805, #33785, #42304, #34787, #41826, #57782, #72776, #88289, #17835, #78825, #10335, #73772, #29261, #50790, #83260, #66267, #6770, #96304, #14282, #74256, #82257, #28768, #5786, #52264, #13775, #67771, #28278, #27780, #37281, #44755, #97294, #44260, #22279, #5301, #75751, #43766, #58265, #35280, #36276, #52752, #74766, #21784, #89762, #20788, #21279, #89276, #51775, #35778, #6274, #58773, #59757, #36780, #59261, #90252, #67271, #97799, #43277, #82760, #75257, #66773, #98292, #29747, #60256, #90750, #96802, #14784, #81762, #45254, #65774, #88781, #20291, #51278, #81280, #12779, #13275, #76253, #92236, #76734, #62215, #69738, #91243, #772, #8730, #68271, #62707, #15277, #98791, #7273, #70232, #37774, #83754, #77225, #16244, #24246, #45758, #68756, #287, #61721, #9228, #8251, #91746, #55208, #7769, #23763, #93207, #30238, #47214, #54225, #47714, #23266, #39248, #77715, #30733, #1751, #54712, #92721, #46726, #60742, #38263, #61240, #1264, #22767, #85723, #53742, #39737, #53248, #85234, #46249, #84740, #31224, #38750, #16737, #31719, #32206, #84261, #15763, #24730, #17236, #69252, #56689, #65160, #48198, #19675, #86706, #70729, #78209, #48691, #95678, #26197, #64657, #33674, #63686, #64171, #33193, #94692, #17725, #49187, #71216, #72177, #87182, #71698, #3706, #41221, #3212, #86214, #18703, #79689, #10706, #11187, #41707, #34167, #95170, #78711, #26677, #25719, #57172, #87669, #19182, #79194, #94189, #49663, #80173, #11684, #10222, #42194, #72658, #56211, #18212, #4193, #34663, #27164, #57664, #2737, #88161, #40711, #9721, #40220, #2244, #32702, #63198, #93703, #25238, #55719, #8013, #13647, #20164, #13151, #58653, #84005, #73646, #89153, #96176, #21158, #51159, #80673, #66145, #12661, #43160, #50668, #91991, #96678, #30986, #74643, #27659, #53495, #20663, #15529, #97180, #81156, #45, #5175, #6153, #74135, #5670, #88656, #60993, #36152, #59138, #89646, #12168, #82138, #35154, #28157, #36658, #91504, #23024, #30494, #28648, #68515, #65653, #35660, #4692, #81643 ) ),
 .UNSPECIFIED., .F., .F., .F. ) 
 B_SPLINE_SURFACE_WITH_KNOTS ( ( 2, 2 ),
 ( 3, 2, 2, 2, 2, 2, 2, 2, 2, 2, 2, 2, 2, 2, 2, 2, 2, 2, 2, 2, 2, 2, 2, 2, 2, 2, 2, 2, 2, 2, 2, 2, 2, 2, 2, 2, 2, 2, 2, 2, 2, 2, 2, 2, 2, 2, 2, 2, 2, 2, 2, 2, 2, 2, 2, 2, 2, 2, 2, 2, 2, 2, 2, 2, 2, 2, 2, 2, 2, 2, 2, 2, 2, 2, 2, 2, 2, 2, 2, 2, 2, 2, 2, 2, 2, 2, 2, 2, 2, 2, 2, 2, 2, 2, 2, 2, 2, 2, 2, 2, 2, 2, 2, 2, 2, 2, 2, 2, 2, 2, 2, 2, 2, 2, 2, 2, 2, 2, 2, 2, 2, 2, 2, 2, 2, 2, 2, 2, 2, 2, 2, 2, 2, 2, 2, 2, 2, 2, 2, 2, 2, 2, 2, 2, 2, 2, 2, 2, 2, 2, 2, 2, 2, 2, 2, 2, 2, 2, 2, 2, 2, 2, 3 ),
 ( 0.000000000000000000, 1.000000000000000000 ),
 ( 0.000000000000000000, 0.005952380952380952051, 0.01190476190476190410, 0.01785714285714285615, 0.02380952380952380820, 0.02976190476190476025, 0.03571428571428571230, 0.04166666666666666435, 0.04761904761904761640, 0.05357142857142856845, 0.05952380952380952051, 0.06547619047619047949, 0.07142857142857142461, 0.07738095238095238360, 0.08333333333333332871, 0.08928571428571428770, 0.09523809523809523281, 0.1011904761904761918, 0.1071428571428571369, 0.1130952380952380959, 0.1190476190476190410, 0.1250000000000000000, 0.1309523809523809590, 0.1369047619047619180, 0.1428571428571428492, 0.1488095238095238082, 0.1547619047619047672, 0.1607142857142857262, 0.1666666666666666574, 0.1726190476190476164, 0.1785714285714285754, 0.1845238095238095344, 0.1904761904761904656, 0.1964285714285714246, 0.2023809523809523836, 0.2083333333333333426, 0.2142857142857142738, 0.2202380952380952328, 0.2261904761904761918, 0.2321428571428571508, 0.2380952380952380820, 0.2440476190476190410, 0.2500000000000000000, 0.2559523809523809312, 0.2619047619047619180, 0.2678571428571428492, 0.2738095238095238360, 0.2797619047619047672, 0.2857142857142856984, 0.2916666666666666852, 0.2976190476190476164, 0.3035714285714285476, 0.3095238095238095344, 0.3154761904761904656, 0.3214285714285714524, 0.3273809523809523836, 0.3333333333333333148, 0.3392857142857143016, 0.3452380952380952328, 0.3511904761904761640, 0.3571428571428571508, 0.3630952380952380820, 0.3690476190476190688, 0.3750000000000000000, 0.3809523809523809312, 0.3869047619047619180, 0.3928571428571428492, 0.3988095238095238360, 0.4047619047619047672, 0.4107142857142856984, 0.4166666666666666852, 0.4226190476190476164, 0.4285714285714285476, 0.4345238095238095344, 0.4404761904761904656, 0.4464285714285714524, 0.4523809523809523836, 0.4583333333333333148, 0.4642857142857143016, 0.4702380952380952328, 0.4761904761904761640, 0.4821428571428571508, 0.4880952380952380820, 0.4940476190476190688, 0.5000000000000000000, 0.5059523809523809312, 0.5119047619047618625, 0.5178571428571429047, 0.5238095238095238360, 0.5297619047619047672, 0.5357142857142856984, 0.5416666666666666297, 0.5476190476190476719, 0.5535714285714286031, 0.5595238095238095344, 0.5654761904761904656, 0.5714285714285713969, 0.5773809523809523281, 0.5833333333333333703, 0.5892857142857143016, 0.5952380952380952328, 0.6011904761904761640, 0.6071428571428570953, 0.6130952380952381375, 0.6190476190476190688, 0.6250000000000000000, 0.6309523809523809312, 0.6369047619047618625, 0.6428571428571429047, 0.6488095238095238360, 0.6547619047619047672, 0.6607142857142856984, 0.6666666666666666297, 0.6726190476190476719, 0.6785714285714286031, 0.6845238095238095344, 0.6904761904761904656, 0.6964285714285713969, 0.7023809523809523281, 0.7083333333333333703, 0.7142857142857143016, 0.7202380952380952328, 0.7261904761904761640, 0.7321428571428570953, 0.7380952380952381375, 0.7440476190476190688, 0.7500000000000000000, 0.7559523809523809312, 0.7619047619047618625, 0.7678571428571429047, 0.7738095238095238360, 0.7797619047619047672, 0.7857142857142856984, 0.7916666666666666297, 0.7976190476190476719, 0.8035714285714286031, 0.8095238095238095344, 0.8154761904761904656, 0.8214285714285713969, 0.8273809523809523281, 0.8333333333333333703, 0.8392857142857143016, 0.8452380952380952328, 0.8511904761904761640, 0.8571428571428570953, 0.8630952380952381375, 0.8690476190476190688, 0.8750000000000000000, 0.8809523809523809312, 0.8869047619047618625, 0.8928571428571429047, 0.8988095238095238360, 0.9047619047619047672, 0.9107142857142856984, 0.9166666666666666297, 0.9226190476190476719, 0.9285714285714286031, 0.9345238095238095344, 0.9404761904761904656, 0.9464285714285713969, 0.9523809523809523281, 0.9583333333333333703, 0.9642857142857143016 ),
 .UNSPECIFIED. ) 
 GEOMETRIC_REPRESENTATION_ITEM ( )  RATIONAL_B_SPLINE_SURFACE ( (
 ( 1.000000000000000000, 0.9659258262890683122, 1.000000000000000000, 0.9659258262890683122, 1.000000000000000000, 0.9659258262890683122, 1.000000000000000000, 0.9659258262890683122, 1.000000000000000000, 0.9659258262890683122, 1.000000000000000000, 0.9659258262890683122, 1.000000000000000000, 0.9659258262890683122, 1.000000000000000000, 0.9659258262890683122, 1.000000000000000000, 0.9659258262890683122, 1.000000000000000000, 0.9659258262890683122, 1.000000000000000000, 0.9659258262890683122, 1.000000000000000000, 0.9659258262890683122, 1.000000000000000000, 0.9659258262890683122, 1.000000000000000000, 0.9659258262890683122, 1.000000000000000000, 0.9659258262890683122, 1.000000000000000000, 0.9659258262890683122, 1.000000000000000000, 0.9659258262890683122, 1.000000000000000000, 0.9659258262890683122, 1.000000000000000000, 0.9659258262890683122, 1.000000000000000000, 0.9659258262890683122, 1.000000000000000000, 0.9659258262890683122, 1.000000000000000000, 0.9659258262890683122, 1.000000000000000000, 0.9659258262890683122, 1.000000000000000000, 0.9659258262890683122, 1.000000000000000000, 0.9659258262890683122, 1.000000000000000000, 0.9659258262890683122, 1.000000000000000000, 0.9659258262890683122, 1.000000000000000000, 0.9659258262890683122, 1.000000000000000000, 0.9659258262890683122, 1.000000000000000000, 0.9659258262890683122, 1.000000000000000000, 0.9659258262890683122, 1.000000000000000000, 0.9659258262890683122, 1.000000000000000000, 0.9659258262890683122, 1.000000000000000000, 0.9659258262890683122, 1.000000000000000000, 0.9659258262890683122, 1.000000000000000000, 0.9659258262890683122, 1.000000000000000000, 0.9659258262890683122, 1.000000000000000000, 0.9659258262890683122, 1.000000000000000000, 0.9659258262890683122, 1.000000000000000000, 0.9659258262890683122, 1.000000000000000000, 0.9659258262890683122, 1.000000000000000000, 0.9659258262890683122, 1.000000000000000000, 0.9659258262890683122, 1.000000000000000000, 0.9659258262890683122, 1.000000000000000000, 0.9659258262890683122, 1.000000000000000000, 0.9659258262890683122, 1.000000000000000000, 0.9659258262890683122, 1.000000000000000000, 0.9659258262890683122, 1.000000000000000000, 0.9659258262890683122, 1.000000000000000000, 0.9659258262890683122, 1.000000000000000000, 0.9659258262890683122, 1.000000000000000000, 0.9659258262890683122, 1.000000000000000000, 0.9659258262890683122, 1.000000000000000000, 0.9659258262890683122, 1.000000000000000000, 0.9659258262890683122, 1.000000000000000000, 0.9659258262890683122, 1.000000000000000000, 0.9659258262890683122, 1.000000000000000000, 0.9659258262890683122, 1.000000000000000000, 0.9659258262890683122, 1.000000000000000000, 0.9659258262890683122, 1.000000000000000000, 0.9659258262890683122, 1.000000000000000000, 0.9659258262890683122, 1.000000000000000000, 0.9659258262890683122, 1.000000000000000000, 0.9659258262890683122, 1.000000000000000000, 0.9659258262890683122, 1.000000000000000000, 0.9659258262890683122, 1.000000000000000000, 0.9659258262890683122, 1.000000000000000000, 0.9659258262890683122, 1.000000000000000000, 0.9659258262890683122, 1.000000000000000000, 0.9659258262890683122, 1.000000000000000000, 0.9659258262890683122, 1.000000000000000000, 0.9659258262890683122, 1.000000000000000000, 0.9659258262890683122, 1.000000000000000000, 0.9659258262890683122, 1.000000000000000000, 0.9659258262890683122, 1.000000000000000000, 0.9659258262890683122, 1.000000000000000000, 0.9659258262890683122, 1.000000000000000000, 0.9659258262890683122, 1.000000000000000000, 0.9659258262890683122, 1.000000000000000000, 0.9659258262890683122, 1.000000000000000000, 0.9659258262890683122, 1.000000000000000000, 0.9659258262890683122, 1.000000000000000000, 0.9659258262890683122, 1.000000000000000000, 0.9659258262890683122, 1.000000000000000000, 0.9659258262890683122, 1.000000000000000000, 0.9659258262890683122, 1.000000000000000000, 0.9659258262890683122, 1.000000000000000000, 0.9659258262890683122, 1.000000000000000000, 0.9659258262890683122, 1.000000000000000000, 0.9659258262890683122, 1.000000000000000000, 0.9659258262890683122, 1.000000000000000000, 0.9659258262890683122, 1.000000000000000000, 0.9659258262890683122, 1.000000000000000000, 0.9659258262890683122, 1.000000000000000000, 0.9659258262890683122, 1.000000000000000000, 0.9659258262890683122, 1.000000000000000000, 0.9659258262890683122, 1.000000000000000000, 0.9659258262890683122, 1.000000000000000000, 0.9659258262890683122, 1.000000000000000000, 0.9659258262890683122, 1.000000000000000000, 0.9659258262890683122, 1.000000000000000000, 0.9659258262890683122, 1.000000000000000000, 0.9659258262890683122, 1.000000000000000000, 0.9659258262890683122, 1.000000000000000000, 0.9659258262890683122, 1.000000000000000000, 0.9659258262890683122, 1.000000000000000000, 0.9659258262890683122, 1.000000000000000000, 0.9659258262890683122, 1.000000000000000000, 0.9659258262890683122, 1.000000000000000000, 0.9659258262890683122, 1.000000000000000000, 0.9659258262890683122, 1.000000000000000000, 0.9659258262890683122, 1.000000000000000000, 0.9659258262890683122, 1.000000000000000000, 0.9659258262890683122, 1.000000000000000000, 0.9659258262890683122, 1.000000000000000000, 0.9659258262890683122, 1.000000000000000000, 0.9659258262890683122, 1.000000000000000000, 0.9659258262890683122, 1.000000000000000000, 0.9659258262890683122, 1.000000000000000000, 0.9659258262890683122, 1.000000000000000000, 0.9659258262890683122, 1.000000000000000000, 0.9659258262890683122, 1.000000000000000000, 0.9659258262890683122, 1.000000000000000000, 0.9659258262890683122, 1.000000000000000000, 0.9659258262890683122, 1.000000000000000000, 0.9659258262890683122, 1.000000000000000000, 0.9659258262890683122, 1.000000000000000000, 0.9659258262890683122, 1.000000000000000000, 0.9659258262890683122, 1.000000000000000000, 0.9659258262890683122, 1.000000000000000000, 0.9659258262890683122, 1.000000000000000000, 0.9659258262890683122, 1.000000000000000000, 0.9659258262890683122, 1.000000000000000000, 0.9659258262890683122, 1.000000000000000000, 0.9659258262890683122, 1.000000000000000000, 0.9659258262890683122, 1.000000000000000000, 0.9659258262890683122, 1.000000000000000000, 0.9659258262890683122, 1.000000000000000000, 0.9659258262890683122, 1.000000000000000000, 0.9659258262890683122, 1.000000000000000000, 0.9659258262890683122, 1.000000000000000000, 0.9659258262890683122, 1.000000000000000000, 0.9659258262890683122, 1.000000000000000000, 0.9659258262890683122, 1.000000000000000000, 0.9659258262890683122, 1.000000000000000000, 0.9659258262890683122, 1.000000000000000000, 0.9659258262890683122, 1.000000000000000000, 0.9659258262890683122, 1.000000000000000000, 0.9659258262890683122, 1.000000000000000000, 0.9659258262890683122, 1.000000000000000000, 0.9659258262890683122, 1.000000000000000000, 0.9659258262890683122, 1.000000000000000000, 0.9659258262890683122, 1.000000000000000000, 0.9659258262890683122, 1.000000000000000000, 0.9659258262890683122, 1.000000000000000000, 0.9659258262890683122, 1.000000000000000000, 0.9659258262890683122, 1.000000000000000000, 0.9659258262890683122, 1.000000000000000000, 0.9659258262890683122, 1.000000000000000000, 0.9659258262890683122, 1.000000000000000000, 0.9659258262890683122, 1.000000000000000000, 0.9659258262890683122, 1.000000000000000000),
 ( 1.000000000000000000, 0.9659258262890683122, 1.000000000000000000, 0.9659258262890683122, 1.000000000000000000, 0.9659258262890683122, 1.000000000000000000, 0.9659258262890683122, 1.000000000000000000, 0.9659258262890683122, 1.000000000000000000, 0.9659258262890683122, 1.000000000000000000, 0.9659258262890683122, 1.000000000000000000, 0.9659258262890683122, 1.000000000000000000, 0.9659258262890683122, 1.000000000000000000, 0.9659258262890683122, 1.000000000000000000, 0.9659258262890683122, 1.000000000000000000, 0.9659258262890683122, 1.000000000000000000, 0.9659258262890683122, 1.000000000000000000, 0.9659258262890683122, 1.000000000000000000, 0.9659258262890683122, 1.000000000000000000, 0.9659258262890683122, 1.000000000000000000, 0.9659258262890683122, 1.000000000000000000, 0.9659258262890683122, 1.000000000000000000, 0.9659258262890683122, 1.000000000000000000, 0.9659258262890683122, 1.000000000000000000, 0.9659258262890683122, 1.000000000000000000, 0.9659258262890683122, 1.000000000000000000, 0.9659258262890683122, 1.000000000000000000, 0.9659258262890683122, 1.000000000000000000, 0.9659258262890683122, 1.000000000000000000, 0.9659258262890683122, 1.000000000000000000, 0.9659258262890683122, 1.000000000000000000, 0.9659258262890683122, 1.000000000000000000, 0.9659258262890683122, 1.000000000000000000, 0.9659258262890683122, 1.000000000000000000, 0.9659258262890683122, 1.000000000000000000, 0.9659258262890683122, 1.000000000000000000, 0.9659258262890683122, 1.000000000000000000, 0.9659258262890683122, 1.000000000000000000, 0.9659258262890683122, 1.000000000000000000, 0.9659258262890683122, 1.000000000000000000, 0.9659258262890683122, 1.000000000000000000, 0.9659258262890683122, 1.000000000000000000, 0.9659258262890683122, 1.000000000000000000, 0.9659258262890683122, 1.000000000000000000, 0.9659258262890683122, 1.000000000000000000, 0.9659258262890683122, 1.000000000000000000, 0.9659258262890683122, 1.000000000000000000, 0.9659258262890683122, 1.000000000000000000, 0.9659258262890683122, 1.000000000000000000, 0.9659258262890683122, 1.000000000000000000, 0.9659258262890683122, 1.000000000000000000, 0.9659258262890683122, 1.000000000000000000, 0.9659258262890683122, 1.000000000000000000, 0.9659258262890683122, 1.000000000000000000, 0.9659258262890683122, 1.000000000000000000, 0.9659258262890683122, 1.000000000000000000, 0.9659258262890683122, 1.000000000000000000, 0.9659258262890683122, 1.000000000000000000, 0.9659258262890683122, 1.000000000000000000, 0.9659258262890683122, 1.000000000000000000, 0.9659258262890683122, 1.000000000000000000, 0.9659258262890683122, 1.000000000000000000, 0.9659258262890683122, 1.000000000000000000, 0.9659258262890683122, 1.000000000000000000, 0.9659258262890683122, 1.000000000000000000, 0.9659258262890683122, 1.000000000000000000, 0.9659258262890683122, 1.000000000000000000, 0.9659258262890683122, 1.000000000000000000, 0.9659258262890683122, 1.000000000000000000, 0.9659258262890683122, 1.000000000000000000, 0.9659258262890683122, 1.000000000000000000, 0.9659258262890683122, 1.000000000000000000, 0.9659258262890683122, 1.000000000000000000, 0.9659258262890683122, 1.000000000000000000, 0.9659258262890683122, 1.000000000000000000, 0.9659258262890683122, 1.000000000000000000, 0.9659258262890683122, 1.000000000000000000, 0.9659258262890683122, 1.000000000000000000, 0.9659258262890683122, 1.000000000000000000, 0.9659258262890683122, 1.000000000000000000, 0.9659258262890683122, 1.000000000000000000, 0.9659258262890683122, 1.000000000000000000, 0.9659258262890683122, 1.000000000000000000, 0.9659258262890683122, 1.000000000000000000, 0.9659258262890683122, 1.000000000000000000, 0.9659258262890683122, 1.000000000000000000, 0.9659258262890683122, 1.000000000000000000, 0.9659258262890683122, 1.000000000000000000, 0.9659258262890683122, 1.000000000000000000, 0.9659258262890683122, 1.000000000000000000, 0.9659258262890683122, 1.000000000000000000, 0.9659258262890683122, 1.000000000000000000, 0.9659258262890683122, 1.000000000000000000, 0.9659258262890683122, 1.000000000000000000, 0.9659258262890683122, 1.000000000000000000, 0.9659258262890683122, 1.000000000000000000, 0.9659258262890683122, 1.000000000000000000, 0.9659258262890683122, 1.000000000000000000, 0.9659258262890683122, 1.000000000000000000, 0.9659258262890683122, 1.000000000000000000, 0.9659258262890683122, 1.000000000000000000, 0.9659258262890683122, 1.000000000000000000, 0.9659258262890683122, 1.000000000000000000, 0.9659258262890683122, 1.000000000000000000, 0.9659258262890683122, 1.000000000000000000, 0.9659258262890683122, 1.000000000000000000, 0.9659258262890683122, 1.000000000000000000, 0.9659258262890683122, 1.000000000000000000, 0.9659258262890683122, 1.000000000000000000, 0.9659258262890683122, 1.000000000000000000, 0.9659258262890683122, 1.000000000000000000, 0.9659258262890683122, 1.000000000000000000, 0.9659258262890683122, 1.000000000000000000, 0.9659258262890683122, 1.000000000000000000, 0.9659258262890683122, 1.000000000000000000, 0.9659258262890683122, 1.000000000000000000, 0.9659258262890683122, 1.000000000000000000, 0.9659258262890683122, 1.000000000000000000, 0.9659258262890683122, 1.000000000000000000, 0.9659258262890683122, 1.000000000000000000, 0.9659258262890683122, 1.000000000000000000, 0.9659258262890683122, 1.000000000000000000, 0.9659258262890683122, 1.000000000000000000, 0.9659258262890683122, 1.000000000000000000, 0.9659258262890683122, 1.000000000000000000, 0.9659258262890683122, 1.000000000000000000, 0.9659258262890683122, 1.000000000000000000, 0.9659258262890683122, 1.000000000000000000, 0.9659258262890683122, 1.000000000000000000, 0.9659258262890683122, 1.000000000000000000, 0.9659258262890683122, 1.000000000000000000, 0.9659258262890683122, 1.000000000000000000, 0.9659258262890683122, 1.000000000000000000, 0.9659258262890683122, 1.000000000000000000, 0.9659258262890683122, 1.000000000000000000, 0.9659258262890683122, 1.000000000000000000, 0.9659258262890683122, 1.000000000000000000, 0.9659258262890683122, 1.000000000000000000, 0.9659258262890683122, 1.000000000000000000, 0.9659258262890683122, 1.000000000000000000, 0.9659258262890683122, 1.000000000000000000, 0.9659258262890683122, 1.000000000000000000, 0.9659258262890683122, 1.000000000000000000, 0.9659258262890683122, 1.000000000000000000, 0.9659258262890683122, 1.000000000000000000, 0.9659258262890683122, 1.000000000000000000, 0.9659258262890683122, 1.000000000000000000, 0.9659258262890683122, 1.000000000000000000, 0.9659258262890683122, 1.000000000000000000, 0.9659258262890683122, 1.000000000000000000, 0.9659258262890683122, 1.000000000000000000, 0.9659258262890683122, 1.000000000000000000, 0.9659258262890683122, 1.000000000000000000, 0.9659258262890683122, 1.000000000000000000, 0.9659258262890683122, 1.000000000000000000, 0.9659258262890683122, 1.000000000000000000, 0.9659258262890683122, 1.000000000000000000, 0.9659258262890683122, 1.000000000000000000, 0.9659258262890683122, 1.000000000000000000, 0.9659258262890683122, 1.000000000000000000, 0.9659258262890683122, 1.000000000000000000, 0.9659258262890683122, 1.000000000000000000, 0.9659258262890683122, 1.000000000000000000, 0.9659258262890683122, 1.000000000000000000, 0.9659258262890683122, 1.000000000000000000, 0.9659258262890683122, 1.000000000000000000) ) ) 
 REPRESENTATION_ITEM ( '' )  SURFACE ( )  );
#54032=CARTESIAN_POINT ( 'NONE',  ( -1.099225684535947600, 44.54030133659708923, 6.408140936763237150 ) ) ;
#54034=CARTESIAN_POINT ( 'NONE',  ( 10.00000000000000178, 47.25893115100078745, 9.846743663894594434 ) ) ;
#54035=CARTESIAN_POINT ( 'NONE',  ( 20.88017736071110875, 20.77201867748816611, -2.915334737309920765 ) ) ;
#54037=CARTESIAN_POINT ( 'NONE',  ( 19.42250999205614548, 10.98035201082150536, -5.440088680355545492 ) ) ;
#54040=CARTESIAN_POINT ( 'NONE',  ( 20.88017736071110164, 55.35535201082149825, 2.915334737309930979 ) ) ;
#54041=CARTESIAN_POINT ( 'NONE',  ( 0.5774900079438607392, 68.48035201082150536, 5.440088680355550821 ) ) ;
#54042=CARTESIAN_POINT ( 'NONE',  ( 0.5774900079438607392, 68.48035201082150536, 5.440088680355550821 ) ) ;
#54043=CARTESIAN_POINT ( 'NONE',  ( 0.1532563361054100626, 15.80059781766745353, -2.638427012816831230 ) ) ;
#54044=CARTESIAN_POINT ( 'NONE',  ( 15.44008868035555793, 61.39701867748817676, -9.422509992056140149 ) ) ;
#54046=CARTESIAN_POINT ( 'NONE',  ( -46.94000000000001194, 102.4380508258080198, 6.413016458746108484 ) ) ;
#54047=CARTESIAN_POINT ( 'NONE',  ( 1.472469842513823179, 0.5922644843341181575, -4.923371831947296329 ) ) ;
#54049=CARTESIAN_POINT ( 'NONE',  ( 2.791683348922237240, 40.38393115100078035, -7.208316651077763204 ) ) ;
#54051=CARTESIAN_POINT ( 'NONE',  ( 10.00000000000000000, 64.75893115100078035, -9.846743663894594434 ) ) ;
#54053=CARTESIAN_POINT ( 'NONE',  ( 13.79529636645031943, 20.34541550158063572, -14.16423886937409904 ) ) ;
#54055=CARTESIAN_POINT ( 'NONE',  ( 20.25388882277768232, 70.00000000000000000, 6.092555545976966691 ) ) ;
#54056=CARTESIAN_POINT ( 'NONE',  ( 20.88017736071110164, 20.35535201082150891, 2.915334737309930979 ) ) ;
#54059=CARTESIAN_POINT ( 'NONE',  ( 0.1532563361054100626, 5.800597817667452638, -2.638427012816831230 ) ) ;
#54060=CARTESIAN_POINT ( 'NONE',  ( 2.791683348922237240, 5.383931151000785675, -7.208316651077763204 ) ) ;
#54061=CARTESIAN_POINT ( 'NONE',  ( 0.6178305044545838731, 29.74863466993042138, 9.382169495545420901 ) ) ;
#54062=CARTESIAN_POINT ( 'NONE',  ( 7.361572987183169658, 19.96726448433411960, -9.846743663894592657 ) ) ;
#54063=EDGE_CURVE ( 'NONE', #61157, #57318, #17760, .T. ) ;
#54064=CARTESIAN_POINT ( 'NONE',  ( 16.40814093676324603, 12.45696800326375353, -11.09922568453594671 ) ) ;
#54066=CARTESIAN_POINT ( 'NONE',  ( 3.640395162852214650, 89.00000000000000000, -12.00000000000000000 ) ) ;
#54067=CARTESIAN_POINT ( 'NONE',  ( 10.00000000000000178, 2.258931151000784787, 9.846743663894594434 ) ) ;
#54070=ORIENTED_EDGE ( 'NONE', *, *, #5113, .T. ) ;
#54071=CARTESIAN_POINT ( 'NONE',  ( 0.5774900079438607392, 18.48035201082150536, 5.440088680355550821 ) ) ;
#54072=CARTESIAN_POINT ( 'NONE',  ( 13.79529636645030344, 13.26208216824729824, 14.16423886937410614 ) ) ;
#54073=CARTESIAN_POINT ( 'NONE',  ( 0.1532563361054082862, 36.21726448433410894, 2.638427012816831674 ) ) ;
#54074=CARTESIAN_POINT ( 'NONE',  ( 0.5774900079438607392, 63.48035201082149825, 5.440088680355550821 ) ) ;
#54075=CARTESIAN_POINT ( 'NONE',  ( 3.591859063236763294, 48.29030133659708923, -11.09922568453595026 ) ) ;
#54077=CARTESIAN_POINT ( 'NONE',  ( 2.035157376598824452, 28.68868534415484106, 7.964842623401179544 ) ) ;
#54079=CARTESIAN_POINT ( 'NONE',  ( 0.6178305044545818747, 13.49863466993041783, -9.382169495545419124 ) ) ;
#54081=CARTESIAN_POINT ( 'NONE',  ( 10.00000000000000000, 7.873634669930421381, -12.81628187352647608 ) ) ;
#54082=CARTESIAN_POINT ( 'NONE',  ( 17.20831665107776587, 37.88393115100078745, 7.208316651077764980 ) ) ;
#54084=CARTESIAN_POINT ( 'NONE',  ( -1.099225684535947600, 54.54030133659708923, 6.408140936763237150 ) ) ;
#54086=CARTESIAN_POINT ( 'NONE',  ( 15.44008868035555260, 54.73035201082150536, 9.422509992056143702 ) ) ;
#54087=CARTESIAN_POINT ( 'NONE',  ( 0.2751277870542909731, 62.28217586085237656, -6.499999999999992006 ) ) ;
#54089=CARTESIAN_POINT ( 'NONE',  ( 19.42250999205614193, 40.14701867748817676, 5.440088680355555262 ) ) ;
#54090=CARTESIAN_POINT ( 'NONE',  ( 19.42250999205614548, 50.98035201082151247, -5.440088680355545492 ) ) ;
#54091=CARTESIAN_POINT ( 'NONE',  ( 19.72487221294571569, 60.71833443783937412, -6.499999999999990230 ) ) ;
#54092=CARTESIAN_POINT ( 'NONE',  ( 12.91533473730992121, 64.52201867748817676, 10.88017736071110164 ) ) ;
#54093=CARTESIAN_POINT ( 'NONE',  ( 12.63842701281683034, 57.46726448433411605, 9.846743663894596210 ) ) ;
#54094=CARTESIAN_POINT ( 'NONE',  ( 12.91533473730993009, 6.605352010821504471, -10.88017736071109987 ) ) ;
#54096=CARTESIAN_POINT ( 'NONE',  ( 16.40814093676323893, 5.790301336597087456, 11.09922568453595026 ) ) ;
#54097=ORIENTED_EDGE ( 'NONE', *, *, #30413, .F. ) ;
#54098=CARTESIAN_POINT ( 'NONE',  ( 4.559911319644449179, 37.23035201082150536, -9.422509992056141925 ) ) ;
#54100=CARTESIAN_POINT ( 'NONE',  ( 13.43411237798105340, 10.58196800326375353, 12.81628187352647963 ) ) ;
#54102=CARTESIAN_POINT ( 'NONE',  ( -0.8801773607110991993, 7.855352010821504471, -2.915334737309923874 ) ) ;
#54103=CARTESIAN_POINT ( 'NONE',  ( 2.035157376598822676, 22.43868534415483396, -7.964842623401177768 ) ) ;
#54104=CARTESIAN_POINT ( 'NONE',  ( -4.164238869374098151, 31.59541550158063927, -3.795296366450310543 ) ) ;
#54105=CARTESIAN_POINT ( 'NONE',  ( 19.84674366389459266, 23.71726448433412315, -2.638427012816827677 ) ) ;
#54106=CARTESIAN_POINT ( 'NONE',  ( 2.035157376598824452, 63.68868534415484106, 7.964842623401179544 ) ) ;
#54108=CARTESIAN_POINT ( 'NONE',  ( 22.26659068614894466, 3.887082168247300906, 7.082119434687054849 ) ) ;
#54110=SURFACE_STYLE_FILL_AREA ( #7659 ) ;
#54111=CARTESIAN_POINT ( 'NONE',  ( 19.84674366389459266, 63.30059781766745886, 2.638427012816836559 ) ) ;
#54114=CARTESIAN_POINT ( 'NONE',  ( -4.164238869374099927, 32.01208216824730357, 3.795296366450308767 ) ) ;
#54115=CARTESIAN_POINT ( 'NONE',  ( -2.266590686148945544, 42.22041550158063217, 7.082119434687048631 ) ) ;
#54116=CARTESIAN_POINT ( 'NONE',  ( 12.63842701281683034, 7.467264484334118713, 9.846743663894596210 ) ) ;
#54117=CARTESIAN_POINT ( 'NONE',  ( 21.09922568453595559, 7.040301336597086568, -6.408140936763230044 ) ) ;
#54118=CARTESIAN_POINT ( 'NONE',  ( 5.076628168052704559, 60.17559781766745175, -8.527530157486179263 ) ) ;
#54120=CARTESIAN_POINT ( 'NONE',  ( 10.00000000000000000, 56.81368534415484106, -10.88017736071110342 ) ) ;
#54121=CARTESIAN_POINT ( 'NONE',  ( 3.591859063236761518, 24.95696800326375353, 11.09922568453594849 ) ) ;
#54122=CARTESIAN_POINT ( 'NONE',  ( 6.204703633549690345, 32.84541550158063927, 14.16423886937410082 ) ) ;
#54123=CARTESIAN_POINT ( 'NONE',  ( 12.91533473730993009, 16.60535201082150891, -10.88017736071109987 ) ) ;
#54124=CARTESIAN_POINT ( 'NONE',  ( 0.5774900079438607392, 33.48035201082150536, 5.440088680355550821 ) ) ;
#54126=CARTESIAN_POINT ( 'NONE',  ( 0.5774900079438590739, 57.64701867748817676, -5.440088680355550821 ) ) ;
#54129=FACE_BOUND ( 'NONE', #3865, .T. ) ;
#54132=EDGE_LOOP ( 'NONE', ( #32455, #14311, #61266, #56966 ) ) ;
#54133=CARTESIAN_POINT ( 'NONE',  ( 2.917880565312950480, 5.970415501580634832, -12.26659068614894821 ) ) ;
#54134=CARTESIAN_POINT ( 'NONE',  ( 22.26659068614894466, 58.88708216824729647, 7.082119434687054849 ) ) ;
#54135=CARTESIAN_POINT ( 'NONE',  ( 10.00000000000000000, 60.55374883491397497, -14.16423886937410082 ) ) ;
#54136=CARTESIAN_POINT ( 'NONE',  ( 19.84674366389459266, 38.71726448433412315, -2.638427012816827677 ) ) ;
#54137=CARTESIAN_POINT ( 'NONE',  ( 19.84674366389459621, 63.50893115100078745, 7.409399052514197653E-17 ) ) ;
#54138=CARTESIAN_POINT ( 'NONE',  ( 21.92686044187657401, 60.37045670184114954, -3.195792623639525765 ) ) ;
#54143=CARTESIAN_POINT ( 'NONE',  ( -1.099225684535947600, 8.706968003263753531, -6.408140936763238038 ) ) ;
#54146=CARTESIAN_POINT ( 'NONE',  ( 13.79529636645031943, 50.34541550158064638, -14.16423886937409904 ) ) ;
#54147=CARTESIAN_POINT ( 'NONE',  ( 10.00000000000000178, 38.05374883491396787, 14.16423886937410082 ) ) ;
#54149=CARTESIAN_POINT ( 'NONE',  ( -1.099225684535947600, 53.70696800326376064, -6.408140936763238038 ) ) ;
#54150=CARTESIAN_POINT ( 'NONE',  ( 7.084665262690076126, 27.02201867748817676, -10.88017736071110164 ) ) ;
#54151=CARTESIAN_POINT ( 'NONE',  ( 0.1532563361054082862, 51.21726448433412315, 2.638427012816831674 ) ) ;
#54152=CARTESIAN_POINT ( 'NONE',  ( 7.084665262690076126, 29.10535201082150181, 10.88017736071109987 ) ) ;
#54154=CARTESIAN_POINT ( 'NONE',  ( 10.00000000000000178, 57.25893115100078745, 9.846743663894594434 ) ) ;
#54159=CARTESIAN_POINT ( 'NONE',  ( 14.92337183194729633, 2.675597817667451750, 8.527530157486181039 ) ) ;
#54160=DIRECTION ( 'NONE',  ( 1.000000000000000000, 0.000000000000000000, 0.000000000000000000 ) ) ;
#54161=ORIENTED_EDGE ( 'NONE', *, *, #65807, .T. ) ;
#54163=CARTESIAN_POINT ( 'NONE',  ( 2.791683348922240793, 26.63393115100078745, 7.208316651077764092 ) ) ;
#54165=CARTESIAN_POINT ( 'NONE',  ( 3.591859063236763294, 43.29030133659708923, -11.09922568453595026 ) ) ;
#54167=ORIENTED_EDGE ( 'NONE', *, *, #4996, .F. ) ;
#54168=AXIS2_PLACEMENT_3D ( 'NONE', #5391, #57382, #20874 ) ;
#54171=CARTESIAN_POINT ( 'NONE',  ( 10.00000000000000000, 59.75893115100078745, -9.846743663894594434 ) ) ;
#54172=CARTESIAN_POINT ( 'NONE',  ( -4.164238869374099039, 36.80374883491396787, 8.674139862899312516E-16 ) ) ;
#54173=CARTESIAN_POINT ( 'NONE',  ( 12.63842701281683034, 57.46726448433411605, 9.846743663894596210 ) ) ;
#54175=CARTESIAN_POINT ( 'NONE',  ( 0.1532563361054100626, 25.80059781766744820, -2.638427012816831230 ) ) ;
#54176=CARTESIAN_POINT ( 'NONE',  ( 13.43411237798106583, 57.66530133659708923, -12.81628187352647252 ) ) ;
#54177=CARTESIAN_POINT ( 'NONE',  ( 6.565887622018943937, -1.918031996736246692, -12.81628187352647608 ) ) ;
#54178=CARTESIAN_POINT ( 'NONE',  ( 4.559911319644449179, 57.23035201082150536, -9.422509992056141925 ) ) ;
#54179=CARTESIAN_POINT ( 'NONE',  ( 0.1532563361054083140, 41.00893115100078745, 1.131784320476157264E-15 ) ) ;
#54182=CARTESIAN_POINT ( 'NONE',  ( 15.44008868035555260, 54.73035201082150536, 9.422509992056143702 ) ) ;
#54187=CARTESIAN_POINT ( 'NONE',  ( -0.8801773607111009756, 28.06368534415484106, 1.068504757029289695E-15 ) ) ;
#54188=CARTESIAN_POINT ( 'NONE',  ( 16.40814093676323893, 5.790301336597087456, 11.09922568453595026 ) ) ;
#54189=CARTESIAN_POINT ( 'NONE',  ( 10.00000000000000000, 51.81368534415484106, -10.88017736071110342 ) ) ;
#54193=CARTESIAN_POINT ( 'NONE',  ( 17.96484262340118221, 39.93868534415484106, 7.964842623401181321 ) ) ;
#54194=CARTESIAN_POINT ( 'NONE',  ( -46.82017113615791004, 100.6079546444643427, 9.324761308090124601 ) ) ;
#54195=CARTESIAN_POINT ( 'NONE',  ( 18.52753015748617571, 43.09226448433412315, 4.923371831947298993 ) ) ;
#54198=CARTESIAN_POINT ( 'NONE',  ( 6.565887622018943937, 8.081968003263751754, -12.81628187352647608 ) ) ;
#54199=CARTESIAN_POINT ( 'NONE',  ( 19.42250999205614193, 20.14701867748817321, 5.440088680355555262 ) ) ;
#54200=CARTESIAN_POINT ( 'NONE',  ( 2.603489959281613420, 60.43575266056826933, -6.500000000000031086 ) ) ;
#54201=CARTESIAN_POINT ( 'NONE',  ( 2.917880565312950480, 20.97041550158063217, -12.26659068614894821 ) ) ;
#54202=CARTESIAN_POINT ( 'NONE',  ( 20.36894250292379738, 59.92874883491397497, -10.36894250292379027 ) ) ;
#54203=CARTESIAN_POINT ( 'NONE',  ( 18.52753015748618282, 28.92559781766745175, -4.923371831947291888 ) ) ;
#54204=CARTESIAN_POINT ( 'NONE',  ( 5.076628168052704559, 15.17559781766745175, -8.527530157486179263 ) ) ;
#54206=CARTESIAN_POINT ( 'NONE',  ( 10.00000000000000000, 19.75893115100078390, -9.846743663894594434 ) ) ;
#54207=CARTESIAN_POINT ( 'NONE',  ( 10.00000000000000000, 21.81368534415484106, -10.88017736071110342 ) ) ;
#54208=CARTESIAN_POINT ( 'NONE',  ( 0.1532563361054082862, 56.21726448433411605, 2.638427012816831674 ) ) ;
#54209=CARTESIAN_POINT ( 'NONE',  ( -0.3689425029237881626, 7.428748834913967869, 10.36894250292379027 ) ) ;
#54212=CARTESIAN_POINT ( 'NONE',  ( 2.791683348922240793, 16.63393115100078745, 7.208316651077764092 ) ) ;
#54213=CARTESIAN_POINT ( 'NONE',  ( -1.099225684535947600, 34.54030133659708923, 6.408140936763237150 ) ) ;
#54214=CARTESIAN_POINT ( 'NONE',  ( 14.92337183194729633, 37.67559781766745175, 8.527530157486181039 ) ) ;
#54216=CARTESIAN_POINT ( 'NONE',  ( 0.1532563361054083140, 16.00893115100078390, 1.131784320476157264E-15 ) ) ;
#54221=CARTESIAN_POINT ( 'NONE',  ( 13.79529636645031943, 50.34541550158064638, -14.16423886937409904 ) ) ;
#54222=CARTESIAN_POINT ( 'NONE',  ( -0.8801773607110991993, 57.85535201082149825, -2.915334737309923874 ) ) ;
#54224=CARTESIAN_POINT ( 'NONE',  ( 15.44008868035555793, 51.39701867748816966, -9.422509992056140149 ) ) ;
#54225=CARTESIAN_POINT ( 'NONE',  ( 7.361572987183170547, 37.05059781766744464, 9.846743663894590881 ) ) ;
#54226=( NAMED_UNIT ( * ) PLANE_ANGLE_UNIT ( ) SI_UNIT ( $, .RADIAN. ) );
#54228=CARTESIAN_POINT ( 'NONE',  ( 5.076628168052704559, 50.17559781766745886, -8.527530157486179263 ) ) ;
#54230=TOROIDAL_SURFACE ( 'NONE', #30243, 9.538348415311009632, 7.000000000000000000 ) ;
#54231=CARTESIAN_POINT ( 'NONE',  ( 15.44008868035555260, 49.73035201082150536, 9.422509992056143702 ) ) ;
#54232=FILL_AREA_STYLE_COLOUR ( '', #13927 ) ;
#54234=ORIENTED_EDGE ( 'NONE', *, *, #53879, .F. ) ;
#54238=CARTESIAN_POINT ( 'NONE',  ( 1.472469842513823179, 41.42559781766745886, 4.923371831947296329 ) ) ;
#54239=CARTESIAN_POINT ( 'NONE',  ( 19.84674366389459266, 28.71726448433411960, -2.638427012816827677 ) ) ;
#54240=CARTESIAN_POINT ( 'NONE',  ( 13.43411237798106583, 52.66530133659708213, -12.81628187352647252 ) ) ;
#54241=CARTESIAN_POINT ( 'NONE',  ( 10.00000000000000000, 21.81368534415484106, -10.88017736071110342 ) ) ;
#54242=CARTESIAN_POINT ( 'NONE',  ( 0.1532563361054100626, 50.80059781766745175, -2.638427012816831230 ) ) ;
#54243=FACE_OUTER_BOUND ( 'NONE', #67660, .T. ) ;
#54244=CARTESIAN_POINT ( 'NONE',  ( 20.36894250292379738, 24.92874883491396787, -10.36894250292379027 ) ) ;
#54245=CARTESIAN_POINT ( 'NONE',  ( 17.08211943468705130, 63.47041550158063927, 12.26659068614894998 ) ) ;
#54246=CARTESIAN_POINT ( 'NONE',  ( 0.1532563361054082862, 51.21726448433412315, 2.638427012816831674 ) ) ;
#54248=CARTESIAN_POINT ( 'NONE',  ( 2.035157376598822676, 47.43868534415484817, -7.964842623401177768 ) ) ;
#54249=CARTESIAN_POINT ( 'NONE',  ( 12.63842701281683922, 19.55059781766745175, -9.846743663894590881 ) ) ;
#54255=CARTESIAN_POINT ( 'NONE',  ( 17.20831665107776587, 4.133931151000785675, -7.208316651077762316 ) ) ;
#54257=CARTESIAN_POINT ( 'NONE',  ( 20.36894250292379382, 23.67874883491397142, 10.36894250292379205 ) ) ;
#54258=CARTESIAN_POINT ( 'NONE',  ( 18.52753015748618282, 13.92559781766745175, -4.923371831947291888 ) ) ;
#54259=CARTESIAN_POINT ( 'NONE',  ( 4.559911319644449179, 42.23035201082151247, -9.422509992056141925 ) ) ;
#54261=CARTESIAN_POINT ( 'NONE',  ( -0.8801773607111008646, 33.27201867748817676, 2.915334737309923430 ) ) ;
#54262=CARTESIAN_POINT ( 'NONE',  ( 17.39651004071841456, 49.08210964143329136, -6.500000000000001776 ) ) ;
#54265=CARTESIAN_POINT ( 'NONE',  ( -1.099225684535947600, 23.70696800326375708, -6.408140936763238038 ) ) ;
#54266=CARTESIAN_POINT ( 'NONE',  ( 10.00000000000000178, 12.25893115100078568, 9.846743663894594434 ) ) ;
#54269=CARTESIAN_POINT ( 'NONE',  ( 19.84674366389459266, 13.71726448433411782, -2.638427012816827677 ) ) ;
#54270=CARTESIAN_POINT ( 'NONE',  ( 19.42250999205614548, 35.98035201082151247, -5.440088680355545492 ) ) ;
#54273=CARTESIAN_POINT ( 'NONE',  ( 21.09922568453595559, 62.04030133659709634, -6.408140936763230044 ) ) ;
#54274=CARTESIAN_POINT ( 'NONE',  ( 2.035157376598822676, 52.43868534415483396, -7.964842623401177768 ) ) ;
#54276=CARTESIAN_POINT ( 'NONE',  ( 20.88017736071110164, 55.35535201082149825, 2.915334737309930979 ) ) ;
#54277=CARTESIAN_POINT ( 'NONE',  ( 3.591859063236763294, 3.290301336597087012, -11.09922568453595026 ) ) ;
#54282=CARTESIAN_POINT ( 'NONE',  ( 1.472469842513823179, 25.59226448433412315, -4.923371831947296329 ) ) ;
#54283=CARTESIAN_POINT ( 'NONE',  ( -2.816281873526473856, 54.33196800326376064, 3.434112377981055619 ) ) ;
#54285=CARTESIAN_POINT ( 'NONE',  ( 19.84674366389459621, 23.50893115100078390, 7.409399052514197653E-17 ) ) ;
#54286=CARTESIAN_POINT ( 'NONE',  ( 21.09922568453595559, 22.04030133659708923, -6.408140936763230044 ) ) ;
#54289=CARTESIAN_POINT ( 'NONE',  ( 15.44008868035555260, 54.73035201082150536, 9.422509992056143702 ) ) ;
#54290=ADVANCED_FACE ( 'NONE', ( #42162 ), #42564, .T. ) ;
#54291=CARTESIAN_POINT ( 'NONE',  ( 17.20831665107776587, 59.13393115100078745, -7.208316651077762316 ) ) ;
#54294=CARTESIAN_POINT ( 'NONE',  ( 0.1532563361054083140, 31.00893115100078390, 1.131784320476157264E-15 ) ) ;
#54295=CARTESIAN_POINT ( 'NONE',  ( 1.472469842513823179, 15.59226448433411960, -4.923371831947296329 ) ) ;
#54296=CARTESIAN_POINT ( 'NONE',  ( 7.084665262690076126, 9.105352010821503583, 10.88017736071109987 ) ) ;
#54297=CARTESIAN_POINT ( 'NONE',  ( 21.09922568453594849, 11.20696800326375531, 6.408140936763242479 ) ) ;
#54298=FILL_AREA_STYLE_COLOUR ( '', #78974 ) ;
#54299=CARTESIAN_POINT ( 'NONE',  ( 0.000000000000000000, 0.000000000000000000, -5.999999999999999112 ) ) ;
#54302=CARTESIAN_POINT ( 'NONE',  ( 20.88017736071110875, 25.77201867748816966, -2.915334737309920765 ) ) ;
#54303=EDGE_CURVE ( 'NONE', #3044, #17262, #30535, .T. ) ;
#54304=CARTESIAN_POINT ( 'NONE',  ( -0.3289641300568005855, 50.10497603579418069, 5.963430220938281678 ) ) ;
#54305=CARTESIAN_POINT ( 'NONE',  ( 10.00000000000000178, 14.31368534415483929, 10.88017736071110342 ) ) ;
#54306=CARTESIAN_POINT ( 'NONE',  ( 0.2751277870542870319, 54.36607318730131055, -6.499999999999985789 ) ) ;
#54307=B_SPLINE_CURVE_WITH_KNOTS ( 'NONE', 3,
 ( #47165, #32662, #93164, #32160 ),
 .UNSPECIFIED., .F., .F.,
 ( 4, 4 ),
 ( 3.291406376790657244E-17, 0.001060528352562001547 ),
 .UNSPECIFIED. ) ;
#54308=CARTESIAN_POINT ( 'NONE',  ( 19.42250999205614548, 35.98035201082151247, -5.440088680355545492 ) ) ;
#54309=CARTESIAN_POINT ( 'NONE',  ( 17.96484262340118221, 6.188685344154837509, -7.964842623401177768 ) ) ;
#54311=CARTESIAN_POINT ( 'NONE',  ( 19.84674366389459266, 3.717264484334118713, -2.638427012816827677 ) ) ;
#54312=CARTESIAN_POINT ( 'NONE',  ( 10.00000000000000000, 19.75893115100078390, -9.846743663894594434 ) ) ;
#54317=CARTESIAN_POINT ( 'NONE',  ( 10.00000000000000178, 18.05374883491396787, 14.16423886937410082 ) ) ;
#54318=CARTESIAN_POINT ( 'NONE',  ( 12.63842701281683922, 39.55059781766744464, -9.846743663894590881 ) ) ;
#54321=CARTESIAN_POINT ( 'NONE',  ( -2.266590686148945544, 47.22041550158063927, 7.082119434687048631 ) ) ;
#54322=CARTESIAN_POINT ( 'NONE',  ( 1.472469842513823179, 16.42559781766745175, 4.923371831947296329 ) ) ;
#54325=CARTESIAN_POINT ( 'NONE',  ( -0.8801773607111008646, 48.27201867748816966, 2.915334737309923430 ) ) ;
#54326=CARTESIAN_POINT ( 'NONE',  ( 19.38216949554541557, 47.24863466993041783, -9.382169495545420901 ) ) ;
#54327=CARTESIAN_POINT ( 'NONE',  ( 2.035157376598824452, 23.68868534415484461, 7.964842623401179544 ) ) ;
#54328=CARTESIAN_POINT ( 'NONE',  ( 0.6178305044545838731, 49.74863466993041072, 9.382169495545420901 ) ) ;
#54329=CARTESIAN_POINT ( 'NONE',  ( 0.1532563361054083140, 66.00893115100079456, 1.131784320476157264E-15 ) ) ;
#54330=CARTESIAN_POINT ( 'NONE',  ( 5.076628168052703671, 6.842264484334118713, 8.527530157486179263 ) ) ;
#54335=CARTESIAN_POINT ( 'NONE',  ( 13.79529636645031943, 55.34541550158062506, -14.16423886937409904 ) ) ;
#54336=CARTESIAN_POINT ( 'NONE',  ( 22.26659068614894466, 18.88708216824730002, 7.082119434687054849 ) ) ;
#54337=CARTESIAN_POINT ( 'NONE',  ( 2.035157376598824452, 13.68868534415483751, 7.964842623401179544 ) ) ;
#54338=CARTESIAN_POINT ( 'NONE',  ( 7.084665262690076126, 42.02201867748816966, -10.88017736071110164 ) ) ;
#54339=CARTESIAN_POINT ( 'NONE',  ( 18.72515096720568906, 15.05509018479935612, 6.500000000000002665 ) ) ;
#54342=CARTESIAN_POINT ( 'NONE',  ( 2.035157376598824452, 63.68868534415484106, 7.964842623401179544 ) ) ;
#54343=CARTESIAN_POINT ( 'NONE',  ( 2.035157376598822676, 67.43868534415484817, -7.964842623401177768 ) ) ;
#54344=CARTESIAN_POINT ( 'NONE',  ( 5.076628168052704559, 25.17559781766745175, -8.527530157486179263 ) ) ;
#54345=CARTESIAN_POINT ( 'NONE',  ( 18.50749283717777161, 19.69955587570480660, 6.499999999999979572 ) ) ;
#54347=CARTESIAN_POINT ( 'NONE',  ( 12.63842701281683034, 12.46726448433411782, 9.846743663894596210 ) ) ;
#54348=CARTESIAN_POINT ( 'NONE',  ( 17.20831665107776587, 37.88393115100078745, 7.208316651077764980 ) ) ;
#54349=CARTESIAN_POINT ( 'NONE',  ( 20.88017736071110164, 20.35535201082150891, 2.915334737309930979 ) ) ;
#54352=CARTESIAN_POINT ( 'NONE',  ( 22.81628187352648496, 36.83196800326376064, -3.434112377981050290 ) ) ;
#54353=CARTESIAN_POINT ( 'NONE',  ( 10.00000000000000178, 7.258931151000785675, 9.846743663894594434 ) ) ;
#54355=CARTESIAN_POINT ( 'NONE',  ( 0.1532563361054082862, 46.21726448433411605, 2.638427012816831674 ) ) ;
#54356=CARTESIAN_POINT ( 'NONE',  ( 17.20831665107776587, 32.88393115100078745, 7.208316651077764980 ) ) ;
#54357=CARTESIAN_POINT ( 'NONE',  ( 10.00000000000000178, 3.053748834913967425, 14.16423886937410082 ) ) ;
#54358=CARTESIAN_POINT ( 'NONE',  ( -2.266590686148945544, 22.22041550158063572, 7.082119434687048631 ) ) ;
#54360=CARTESIAN_POINT ( 'NONE',  ( 15.44008868035555260, 29.73035201082150891, 9.422509992056143702 ) ) ;
#54361=CARTESIAN_POINT ( 'NONE',  ( 12.91533473730992121, 14.52201867748817143, 10.88017736071110164 ) ) ;
#54363=CARTESIAN_POINT ( 'NONE',  ( 20.88017736071110875, 45.77201867748816966, -2.915334737309920765 ) ) ;
#54364=CARTESIAN_POINT ( 'NONE',  ( 20.88017736071110164, 30.35535201082151247, 2.915334737309930979 ) ) ;
#54365=VERTEX_POINT ( 'NONE', #13634 ) ;
#54366=CARTESIAN_POINT ( 'NONE',  ( 22.81628187352648496, 36.83196800326376064, -3.434112377981050290 ) ) ;
#54368=CARTESIAN_POINT ( 'NONE',  ( -0.8801773607111008646, 38.27201867748816255, 2.915334737309923430 ) ) ;
#54369=EDGE_LOOP ( 'NONE', ( #51703, #42719, #5610, #30278 ) ) ;
#54370=CARTESIAN_POINT ( 'NONE',  ( -2.816281873526473856, 59.12363466993042493, 9.499525473075851096E-16 ) ) ;
#54371=CARTESIAN_POINT ( 'NONE',  ( 15.44008868035555260, 54.73035201082150536, 9.422509992056143702 ) ) ;
#54373=CARTESIAN_POINT ( 'NONE',  ( 0.5774900079438607392, 53.48035201082151247, 5.440088680355550821 ) ) ;
#54375=CARTESIAN_POINT ( 'NONE',  ( -0.04068437667222171011, 37.21974360917720759, -6.396802510829769695 ) ) ;
#54376=CARTESIAN_POINT ( 'NONE',  ( 2.917880565312948704, 57.63708216824731068, 12.26659068614894643 ) ) ;
#54377=CARTESIAN_POINT ( 'NONE',  ( 2.035157376598824452, 63.68868534415484106, 7.964842623401179544 ) ) ;
#54380=CARTESIAN_POINT ( 'NONE',  ( 1.472469842513823179, 26.42559781766745175, 4.923371831947296329 ) ) ;
#54382=CARTESIAN_POINT ( 'NONE',  ( 19.84674366389459266, 33.30059781766744464, 2.638427012816836559 ) ) ;
#54384=CARTESIAN_POINT ( 'NONE',  ( 15.44008868035555793, 41.39701867748817676, -9.422509992056140149 ) ) ;
#54385=CARTESIAN_POINT ( 'NONE',  ( 5.076628168052703671, 36.84226448433412315, 8.527530157486179263 ) ) ;
#54386=CARTESIAN_POINT ( 'NONE',  ( 0.6178305044545818747, 18.49863466993041428, -9.382169495545419124 ) ) ;
#54389=CARTESIAN_POINT ( 'NONE',  ( 2.035157376598822676, 52.43868534415483396, -7.964842623401177768 ) ) ;
#54390=CARTESIAN_POINT ( 'NONE',  ( 20.36894250292379382, 63.67874883491396787, 10.36894250292379205 ) ) ;
#54391=EDGE_CURVE ( 'NONE', #62008, #50558, #23355, .T. ) ;
#54394=CARTESIAN_POINT ( 'NONE',  ( 22.81628187352647785, 26.41530133659708923, 3.434112377981063169 ) ) ;
#54395=CARTESIAN_POINT ( 'NONE',  ( 0.1532563361054100626, 50.80059781766745886, -2.638427012816831230 ) ) ;
#54397=CARTESIAN_POINT ( 'NONE',  ( 21.09922568453594849, 31.20696800326375353, 6.408140936763242479 ) ) ;
#54398=CARTESIAN_POINT ( 'NONE',  ( 20.88017736071110519, 25.56368534415483751, 2.639326808657452039E-16 ) ) ;
#54399=CARTESIAN_POINT ( 'NONE',  ( -0.8801773607110991993, 57.85535201082149825, -2.915334737309923874 ) ) ;
#54400=EDGE_LOOP ( 'NONE', ( #5521, #82829, #15192, #43169 ) ) ;
#54402=CARTESIAN_POINT ( 'NONE',  ( 1.472469842513823179, 6.425597817667451750, 4.923371831947296329 ) ) ;
#54403=CARTESIAN_POINT ( 'NONE',  ( 0.1532563361054083140, 56.00893115100078745, 1.131784320476157264E-15 ) ) ;
#54404=CARTESIAN_POINT ( 'NONE',  ( 0.1532563361054082862, 41.21726448433411605, 2.638427012816831674 ) ) ;
#54406=CARTESIAN_POINT ( 'NONE',  ( 14.92337183194729633, 32.67559781766745175, 8.527530157486181039 ) ) ;
#54407=DIRECTION ( 'NONE',  ( 0.000000000000000000, -1.000000000000000000, 0.000000000000000000 ) ) ;
#54409=CARTESIAN_POINT ( 'NONE',  ( 5.076628168052703671, 16.84226448433411960, 8.527530157486179263 ) ) ;
#54410=CARTESIAN_POINT ( 'NONE',  ( 20.03932841506543028, 50.62161441960502373, -6.397827110478998769 ) ) ;
#54412=CARTESIAN_POINT ( 'NONE',  ( 12.63842701281683922, 49.55059781766744464, -9.846743663894590881 ) ) ;
#54415=CARTESIAN_POINT ( 'NONE',  ( 20.32896413005680714, 17.60497603579417358, -5.963430220938276349 ) ) ;
#54417=CARTESIAN_POINT ( 'NONE',  ( -2.816281873526473856, 9.123634669930421381, 9.499525473075851096E-16 ) ) ;
#54418=CARTESIAN_POINT ( 'NONE',  ( -0.8801773607111009756, 58.06368534415484106, 1.068504757029289695E-15 ) ) ;
#54419=CARTESIAN_POINT ( 'NONE',  ( -2.266590686148945544, 51.38708216824730357, -7.082119434687050408 ) ) ;
#54420=EDGE_CURVE ( 'NONE', #74297, #30124, #39330, .T. ) ;
#54421=CIRCLE ( 'NONE', #44857, 0.5000000000000004441 ) ;
#54422=PRESENTATION_STYLE_ASSIGNMENT (( #93413 ) ) ;
#54424=CARTESIAN_POINT ( 'NONE',  ( -0.3689425029237898834, 41.17874883491397497, -10.36894250292378850 ) ) ;
#54425=CARTESIAN_POINT ( 'NONE',  ( 6.204703633549690345, 57.84541550158063927, 14.16423886937410082 ) ) ;
#54426=CARTESIAN_POINT ( 'NONE',  ( 17.08211943468705130, 23.47041550158063572, 12.26659068614894998 ) ) ;
#54427=CARTESIAN_POINT ( 'NONE',  ( 24.16423886937410614, 24.51208216824730002, -3.795296366450302550 ) ) ;
#54431=CARTESIAN_POINT ( 'NONE',  ( 10.00000000000000178, 42.25893115100078745, 9.846743663894594434 ) ) ;
#54432=CARTESIAN_POINT ( 'NONE',  ( 7.084665262690076126, 19.10535201082150181, 10.88017736071109987 ) ) ;
#54433=CARTESIAN_POINT ( 'NONE',  ( 0.2751277870542910842, 67.28217586085239077, -6.499999999999992006 ) ) ;
#54434=CARTESIAN_POINT ( 'NONE',  ( 14.92337183194729633, 62.67559781766745886, 8.527530157486181039 ) ) ;
#54436=CARTESIAN_POINT ( 'NONE',  ( 17.20831665107776587, 44.13393115100078745, -7.208316651077762316 ) ) ;
#54437=CARTESIAN_POINT ( 'NONE',  ( -2.816281873526473856, 49.33196800326374643, 3.434112377981055619 ) ) ;
#54439=CARTESIAN_POINT ( 'NONE',  ( 1.472469842513823179, 41.42559781766745886, 4.923371831947296329 ) ) ;
#54440=CARTESIAN_POINT ( 'NONE',  ( 14.92337183194729988, 59.34226448433412315, -8.527530157486177487 ) ) ;
#54441=CARTESIAN_POINT ( 'NONE',  ( 17.08211943468705130, 33.47041550158063927, 12.26659068614894998 ) ) ;
#54442=CARTESIAN_POINT ( 'NONE',  ( -0.3689425029237881626, 12.42874883491396609, 10.36894250292379027 ) ) ;
#54447=CARTESIAN_POINT ( 'NONE',  ( 10.00000000000000000, 1.813685344154838175, -10.88017736071110342 ) ) ;
#54448=CARTESIAN_POINT ( 'NONE',  ( 0.6178305044545838731, 9.748634669930416052, 9.382169495545420901 ) ) ;
#54450=CARTESIAN_POINT ( 'NONE',  ( 2.791683348922240793, 1.633931151000784565, 7.208316651077764092 ) ) ;
#54454=CARTESIAN_POINT ( 'NONE',  ( 2.917880565312948704, 67.63708216824730357, 12.26659068614894643 ) ) ;
#54456=CARTESIAN_POINT ( 'NONE',  ( 15.44008868035555793, 26.39701867748817321, -9.422509992056140149 ) ) ;
#54457=CARTESIAN_POINT ( 'NONE',  ( 12.91533473730992121, 29.52201867748817321, 10.88017736071110164 ) ) ;
#54458=CARTESIAN_POINT ( 'NONE',  ( 2.791683348922240793, 61.63393115100079456, 7.208316651077764092 ) ) ;
#54459=CARTESIAN_POINT ( 'NONE',  ( 2.791683348922237240, 50.38393115100078035, -7.208316651077763204 ) ) ;
#54460=CARTESIAN_POINT ( 'NONE',  ( -45.94000000000001194, 103.9981609152045507, -5.961202730336931488 ) ) ;
#54461=CARTESIAN_POINT ( 'NONE',  ( -0.1503990784575242878, 64.24884699246891273, -6.262539305110083276 ) ) ;
#54465=CARTESIAN_POINT ( 'NONE',  ( 7.084665262690076126, 34.10535201082151247, 10.88017736071109987 ) ) ;
#54466=CARTESIAN_POINT ( 'NONE',  ( -2.816281873526473856, 24.33196800326375353, 3.434112377981055619 ) ) ;
#54469=CARTESIAN_POINT ( 'NONE',  ( 5.076628168052703671, 56.84226448433412315, 8.527530157486179263 ) ) ;
#54470=CARTESIAN_POINT ( 'NONE',  ( 4.559911319644449179, 52.23035201082151247, -9.422509992056141925 ) ) ;
#54471=CARTESIAN_POINT ( 'NONE',  ( 13.43411237798106583, 17.66530133659708923, -12.81628187352647252 ) ) ;
#54472=CARTESIAN_POINT ( 'NONE',  ( 7.084665262690076126, 57.02201867748817676, -10.88017736071110164 ) ) ;
#54476=CARTESIAN_POINT ( 'NONE',  ( 0.5774900079438590739, 52.64701867748817676, -5.440088680355550821 ) ) ;
#54477=CARTESIAN_POINT ( 'NONE',  ( -2.816281873526473856, 49.12363466993042493, 9.499525473075851096E-16 ) ) ;
#54478=CARTESIAN_POINT ( 'NONE',  ( 20.36894250292379738, 9.928748834913966093, -10.36894250292379027 ) ) ;
#54479=CARTESIAN_POINT ( 'NONE',  ( 5.076628168052704559, 15.17559781766745175, -8.527530157486179263 ) ) ;
#54480=CARTESIAN_POINT ( 'NONE',  ( 19.84674366389459266, 63.71726448433412315, -2.638427012816827677 ) ) ;
#54481=CARTESIAN_POINT ( 'NONE',  ( 2.791683348922240793, 16.63393115100078745, 7.208316651077764092 ) ) ;
#54482=CARTESIAN_POINT ( 'NONE',  ( 19.72487221294571569, 39.78217586085237656, 6.499999999999986677 ) ) ;
#54483=CARTESIAN_POINT ( 'NONE',  ( 22.26659068614894466, 58.88708216824729647, 7.082119434687054849 ) ) ;
#54484=EDGE_LOOP ( 'NONE', ( #84004, #65683, #68531, #70872 ) ) ;
#54486=CARTESIAN_POINT ( 'NONE',  ( -0.8801773607110991993, 7.855352010821504471, -2.915334737309923874 ) ) ;
#54487=CARTESIAN_POINT ( 'NONE',  ( 0.1532563361054082862, 16.21726448433411960, 2.638427012816831674 ) ) ;
#54488=AXIS2_PLACEMENT_3D ( 'NONE', #531, #59509, #91982 ) ;
#54490=CARTESIAN_POINT ( 'NONE',  ( 19.42250999205614548, 5.980352010821504471, -5.440088680355545492 ) ) ;
#54491=CARTESIAN_POINT ( 'NONE',  ( 19.42250999205614193, 10.14701867748816966, 5.440088680355555262 ) ) ;
#54492=CARTESIAN_POINT ( 'NONE',  ( 2.791683348922240793, 41.63393115100078745, 7.208316651077764092 ) ) ;
#54493=CARTESIAN_POINT ( 'NONE',  ( -1.099225684535947600, 43.70696800326375353, -6.408140936763238038 ) ) ;
#54496=CARTESIAN_POINT ( 'NONE',  ( 20.36894250292379382, 23.67874883491397142, 10.36894250292379205 ) ) ;
#54497=CARTESIAN_POINT ( 'NONE',  ( 15.44008868035555260, 29.73035201082150891, 9.422509992056143702 ) ) ;
#54498=CARTESIAN_POINT ( 'NONE',  ( 17.96484262340118221, 4.938685344154837509, 7.964842623401181321 ) ) ;
#54499=CARTESIAN_POINT ( 'NONE',  ( 10.00000000000000178, 47.25893115100078745, 9.846743663894594434 ) ) ;
#54501=CARTESIAN_POINT ( 'NONE',  ( 5.076628168052703671, 31.84226448433412315, 8.527530157486179263 ) ) ;
#54504=LINE ( 'NONE', #70020, #56194 ) ;
#54507=CARTESIAN_POINT ( 'NONE',  ( 2.035157376598824452, 3.688685344154837953, 7.964842623401179544 ) ) ;
#54508=CARTESIAN_POINT ( 'NONE',  ( 19.42250999205614193, 65.14701867748817676, 5.440088680355555262 ) ) ;
#54509=CARTESIAN_POINT ( 'NONE',  ( 7.361572987183170547, 62.05059781766745886, 9.846743663894590881 ) ) ;
#54510=CARTESIAN_POINT ( 'NONE',  ( 2.035157376598822676, 32.43868534415483396, -7.964842623401177768 ) ) ;
#54511=CARTESIAN_POINT ( 'NONE',  ( 2.035157376598822676, 7.438685344154837509, -7.964842623401177768 ) ) ;
#54512=CARTESIAN_POINT ( 'NONE',  ( -1.099225684535947600, 34.54030133659708923, 6.408140936763237150 ) ) ;
#54513=CARTESIAN_POINT ( 'NONE',  ( -4.164238869374099039, 11.80374883491396965, 8.674139862899312516E-16 ) ) ;
#54515=CARTESIAN_POINT ( 'NONE',  ( 6.565887622018943937, 48.08196800326375353, -12.81628187352647608 ) ) ;
#54517=CARTESIAN_POINT ( 'NONE',  ( 12.63842701281683922, 49.55059781766744464, -9.846743663894590881 ) ) ;
#54518=CARTESIAN_POINT ( 'NONE',  ( 7.084665262690076126, 27.02201867748817676, -10.88017736071110164 ) ) ;
#54520=CARTESIAN_POINT ( 'NONE',  ( 20.88017736071110164, 15.35535201082150358, 2.915334737309930979 ) ) ;
#54522=CARTESIAN_POINT ( 'NONE',  ( 12.91533473730993009, 61.60535201082150536, -10.88017736071109987 ) ) ;
#54523=SURFACE_STYLE_FILL_AREA ( #9034 ) ;
#54524=CARTESIAN_POINT ( 'NONE',  ( 18.52753015748618282, 8.925597817667451750, -4.923371831947291888 ) ) ;
#54525=CARTESIAN_POINT ( 'NONE',  ( 0.5774900079438590739, 62.64701867748817676, -5.440088680355550821 ) ) ;
#54526=CARTESIAN_POINT ( 'NONE',  ( 2.791683348922237240, 0.3839311510007847872, -7.208316651077763204 ) ) ;
#54528=( BOUNDED_CURVE ( )  B_SPLINE_CURVE ( 2, ( #11305, #63313, #57293, #80297, #27283, #63800, #10824, #88288, #34786 ),
 .UNSPECIFIED., .F., .F. ) 
 B_SPLINE_CURVE_WITH_KNOTS ( ( 3, 2, 2, 2, 3 ),
 ( 0.6882284501891250406, 0.6904761904761904656, 0.6964285714285713969, 0.7023809523809523281, 0.7046286926680177531 ),
 .UNSPECIFIED. ) 
 CURVE ( )  GEOMETRIC_REPRESENTATION_ITEM ( )  RATIONAL_B_SPLINE_CURVE ( ( 0.9839835555609424134, 0.9871328979762474809, 1.000000000000000000, 0.9659258262890683122, 1.000000000000000000, 0.9659258262890683122, 1.000000000000000000, 0.9871328979762477029, 0.9839835555609425244 ) ) 
 REPRESENTATION_ITEM ( '' )  );
#54531=CARTESIAN_POINT ( 'NONE',  ( 18.52753015748617571, 38.09226448433412315, 4.923371831947298993 ) ) ;
#54534=CARTESIAN_POINT ( 'NONE',  ( 19.72487221294570858, 0.5000000000000000000, -6.500000000000000888 ) ) ;
#54536=CARTESIAN_POINT ( 'NONE',  ( 0.6178305044545818747, 58.49863466993042493, -9.382169495545419124 ) ) ;
#54537=CARTESIAN_POINT ( 'NONE',  ( 22.26659068614894466, 8.887082168247300018, 7.082119434687054849 ) ) ;
#54538=CARTESIAN_POINT ( 'NONE',  ( -0.3689425029237898834, 16.17874883491396076, -10.36894250292378850 ) ) ;
#54539=CARTESIAN_POINT ( 'NONE',  ( 18.18329248733321535, 57.60290668512018897, 6.500000000000005329 ) ) ;
#54540=CARTESIAN_POINT ( 'NONE',  ( 18.72515096720570327, 11.07228050351031712, -6.499999999999992006 ) ) ;
#54541=CARTESIAN_POINT ( 'NONE',  ( 0.5774900079438607392, 23.48035201082150536, 5.440088680355550821 ) ) ;
#54542=CARTESIAN_POINT ( 'NONE',  ( 6.000000000000000000, 61.50000000000000711, -6.500000000000000888 ) ) ;
#54543=VERTEX_POINT ( 'NONE', #64041 ) ;
#54544=CARTESIAN_POINT ( 'NONE',  ( 19.84674366389459621, 8.508931151000785675, 7.409399052514197653E-17 ) ) ;
#54545=CARTESIAN_POINT ( 'NONE',  ( 0.1532563361054083140, 6.008931151000784787, 1.131784320476157264E-15 ) ) ;
#54546=CARTESIAN_POINT ( 'NONE',  ( -1.099225684535947600, 29.54030133659708923, 6.408140936763237150 ) ) ;
#54547=CARTESIAN_POINT ( 'NONE',  ( 10.00000000000000000, 29.75893115100078745, -9.846743663894594434 ) ) ;
#54549=CARTESIAN_POINT ( 'NONE',  ( 22.81628187352648496, 21.83196800326374643, -3.434112377981050290 ) ) ;
#54550=FACE_OUTER_BOUND ( 'NONE', #75585, .T. ) ;
#54552=AXIS2_PLACEMENT_3D ( 'NONE', #1816, #62780, #32768 ) ;
#54553=CARTESIAN_POINT ( 'NONE',  ( 17.20831665107776587, 2.883931151000785231, 7.208316651077764980 ) ) ;
#54556=CARTESIAN_POINT ( 'NONE',  ( 15.44008868035555793, 41.39701867748817676, -9.422509992056140149 ) ) ;
#54557=CARTESIAN_POINT ( 'NONE',  ( 22.26659068614894466, 38.88708216824731068, 7.082119434687054849 ) ) ;
#54558=CARTESIAN_POINT ( 'NONE',  ( 0.1532563361054082862, 41.21726448433411605, 2.638427012816831674 ) ) ;
#54559=CARTESIAN_POINT ( 'NONE',  ( 1.472469842513823179, 1.425597817667451528, 4.923371831947296329 ) ) ;
#54561=CARTESIAN_POINT ( 'NONE',  ( 13.43411237798106583, 52.66530133659708213, -12.81628187352647252 ) ) ;
#54563=CARTESIAN_POINT ( 'NONE',  ( 7.084665262690076126, 27.02201867748817676, -10.88017736071110164 ) ) ;
#54565=EDGE_CURVE ( 'NONE', #70171, #74723, #2608, .T. ) ;
#54566=CARTESIAN_POINT ( 'NONE',  ( 3.591859063236763294, 8.290301336597087456, -11.09922568453595026 ) ) ;
#54567=CARTESIAN_POINT ( 'NONE',  ( 1.472469842513823179, 35.59226448433412315, -4.923371831947296329 ) ) ;
#54569=CARTESIAN_POINT ( 'NONE',  ( 22.81628187352648496, 51.83196800326376064, -3.434112377981050290 ) ) ;
#54570=PRESENTATION_STYLE_ASSIGNMENT (( #39103 ) ) ;
#54571=TOROIDAL_SURFACE ( 'NONE', #51367, 1.000000000000000000, 0.5000000000000000000 ) ;
#54572=CARTESIAN_POINT ( 'NONE',  ( 17.96484262340118221, 49.93868534415484106, 7.964842623401181321 ) ) ;
#54573=CARTESIAN_POINT ( 'NONE',  ( 19.72487221294570858, 46.86607318730077054, 6.500000000000000888 ) ) ;
#54577=CARTESIAN_POINT ( 'NONE',  ( 0.5774900079438607392, 53.48035201082151247, 5.440088680355550821 ) ) ;
#54578=CARTESIAN_POINT ( 'NONE',  ( 12.91533473730992121, 59.52201867748816966, 10.88017736071110164 ) ) ;
#54579=FACE_OUTER_BOUND ( 'NONE', #41902, .T. ) ;
#54580=CARTESIAN_POINT ( 'NONE',  ( 10.00000000000000178, 64.31368534415483396, 10.88017736071110342 ) ) ;
#54581=CARTESIAN_POINT ( 'NONE',  ( 19.42250999205614548, 15.98035201082150714, -5.440088680355545492 ) ) ;
#54582=CARTESIAN_POINT ( 'NONE',  ( 7.361572987183170547, 47.05059781766745175, 9.846743663894590881 ) ) ;
#54583=CARTESIAN_POINT ( 'NONE',  ( 4.559911319644449179, 17.23035201082150536, -9.422509992056141925 ) ) ;
#54585=CARTESIAN_POINT ( 'NONE',  ( 13.43411237798105340, 25.58196800326374998, 12.81628187352647963 ) ) ;
#54587=CARTESIAN_POINT ( 'NONE',  ( 10.00000000000000178, 39.31368534415484106, 10.88017736071110342 ) ) ;
#54588=ADVANCED_FACE ( 'NONE', ( #54579 ), #78081, .T. ) ;
#54589=CARTESIAN_POINT ( 'NONE',  ( 22.81628187352647785, 11.62363466993042138, 6.195893100308588602E-16 ) ) ;
#54590=CARTESIAN_POINT ( 'NONE',  ( 2.603489959281613420, 50.43575266056826933, -6.500000000000031086 ) ) ;
#54591=CARTESIAN_POINT ( 'NONE',  ( -0.8801773607111009756, 13.06368534415483929, 1.068504757029289695E-15 ) ) ;
#54592=CARTESIAN_POINT ( 'NONE',  ( 0.5774900079438607392, 43.48035201082151247, 5.440088680355550821 ) ) ;
#54593=CARTESIAN_POINT ( 'NONE',  ( 20.36894250292379382, 53.67874883491397497, 10.36894250292379205 ) ) ;
#54594=CARTESIAN_POINT ( 'NONE',  ( 10.00000000000000178, 27.25893115100078390, 9.846743663894594434 ) ) ;
#54595=CARTESIAN_POINT ( 'NONE',  ( 20.88017736071110164, 65.35535201082150536, 2.915334737309930979 ) ) ;
#54597=CARTESIAN_POINT ( 'NONE',  ( 17.08211943468705840, 10.13708216824730179, -12.26659068614894466 ) ) ;
#54601=CARTESIAN_POINT ( 'NONE',  ( 17.08211943468705130, 38.47041550158063217, 12.26659068614894998 ) ) ;
#54602=CARTESIAN_POINT ( 'NONE',  ( 22.26659068614894466, 33.88708216824730357, 7.082119434687054849 ) ) ;
#54603=CARTESIAN_POINT ( 'NONE',  ( 7.361572987183169658, -0.03273551566588185635, -9.846743663894592657 ) ) ;
#54604=CARTESIAN_POINT ( 'NONE',  ( 1.472469842513823179, 61.42559781766745175, 4.923371831947296329 ) ) ;
#54606=CARTESIAN_POINT ( 'NONE',  ( 10.00000000000000178, 54.31368534415484106, 10.88017736071110342 ) ) ;
#54607=CARTESIAN_POINT ( 'NONE',  ( 21.09922568453594849, 21.20696800326375353, 6.408140936763242479 ) ) ;
#54608=CARTESIAN_POINT ( 'NONE',  ( -4.164238869374099039, 36.80374883491396787, 8.674139862899312516E-16 ) ) ;
#54609=CARTESIAN_POINT ( 'NONE',  ( 19.42250999205614548, 20.98035201082150891, -5.440088680355545492 ) ) ;
#54610=CARTESIAN_POINT ( 'NONE',  ( 19.42250999205614548, 25.98035201082150891, -5.440088680355545492 ) ) ;
#54611=CARTESIAN_POINT ( 'NONE',  ( 20.32896413005680358, 4.745456701841137992, 5.963430220938287007 ) ) ;
#54612=CARTESIAN_POINT ( 'NONE',  ( 17.96484262340118221, 51.18868534415483396, -7.964842623401177768 ) ) ;
#54616=CARTESIAN_POINT ( 'NONE',  ( 13.99999999999999822, 60.50000000000000000, 6.000000000000000000 ) ) ;
#54618=CARTESIAN_POINT ( 'NONE',  ( 22.26659068614895176, 9.720415501580633943, -7.082119434687042414 ) ) ;
#54619=CARTESIAN_POINT ( 'NONE',  ( -4.164238869374099927, 62.01208216824728936, 3.795296366450308767 ) ) ;
#54620=CARTESIAN_POINT ( 'NONE',  ( -0.3689425029237898834, 66.17874883491396076, -10.36894250292378850 ) ) ;
#54621=CARTESIAN_POINT ( 'NONE',  ( 0.1532563361054083140, 41.00893115100078745, 1.131784320476157264E-15 ) ) ;
#54622=CARTESIAN_POINT ( 'NONE',  ( 10.00000000000000178, 62.25893115100078745, 9.846743663894594434 ) ) ;
#54624=CARTESIAN_POINT ( 'NONE',  ( 14.49999999999999822, 11.50000000000000000, 6.500000000000000888 ) ) ;
#54625=EDGE_CURVE ( 'NONE', #32525, #2388, #16603, .T. ) ;
#54626=AXIS2_PLACEMENT_3D ( 'NONE', #75410, #91897, #22431 ) ;
#54628=CARTESIAN_POINT ( 'NONE',  ( -2.816281873526471635, -1.084698663402913210, -3.434112377981056508 ) ) ;
#54632=CARTESIAN_POINT ( 'NONE',  ( 22.26659068614894466, 48.88708216824730357, 7.082119434687054849 ) ) ;
#54634=CARTESIAN_POINT ( 'NONE',  ( 20.36894250292379382, 43.67874883491397497, 10.36894250292379205 ) ) ;
#54636=CARTESIAN_POINT ( 'NONE',  ( 17.96484262340118221, 21.18868534415483396, -7.964842623401177768 ) ) ;
#54637=CARTESIAN_POINT ( 'NONE',  ( 19.42250999205614193, 40.14701867748817676, 5.440088680355555262 ) ) ;
#54638=CARTESIAN_POINT ( 'NONE',  ( 12.63842701281683922, 54.55059781766745175, -9.846743663894590881 ) ) ;
#54639=CARTESIAN_POINT ( 'NONE',  ( 17.96484262340118221, 34.93868534415482685, 7.964842623401181321 ) ) ;
#54642=CARTESIAN_POINT ( 'NONE',  ( -0.8801773607110991993, 67.85535201082151957, -2.915334737309923874 ) ) ;
#54643=CARTESIAN_POINT ( 'NONE',  ( 10.00000000000000178, 24.31368534415484106, 10.88017736071110342 ) ) ;
#54644=STYLED_ITEM ( 'NONE', ( #4774 ), #73259 ) ;
#54650=CARTESIAN_POINT ( 'NONE',  ( 12.63842701281683922, 29.55059781766745175, -9.846743663894590881 ) ) ;
#54651=CARTESIAN_POINT ( 'NONE',  ( -46.48609177761492361, 103.4075268915744630, 6.315643502655008845 ) ) ;
#54652=CARTESIAN_POINT ( 'NONE',  ( 0.6178305044545818747, 48.49863466993042493, -9.382169495545419124 ) ) ;
#54654=FACE_OUTER_BOUND ( 'NONE', #126, .T. ) ;
#54658=CARTESIAN_POINT ( 'NONE',  ( 1.274849032794292736, 52.55509018479936856, -6.499999999999977796 ) ) ;
#54659=CARTESIAN_POINT ( 'NONE',  ( 1.472469842513823179, 51.42559781766745886, 4.923371831947296329 ) ) ;
#54660=CARTESIAN_POINT ( 'NONE',  ( 10.00000000000000178, 43.05374883491397497, 14.16423886937410082 ) ) ;
#54661=CARTESIAN_POINT ( 'NONE',  ( 14.92337183194729633, 57.67559781766745886, 8.527530157486181039 ) ) ;
#54662=CARTESIAN_POINT ( 'NONE',  ( 19.84674366389459266, 23.71726448433412315, -2.638427012816827677 ) ) ;
#54663=CARTESIAN_POINT ( 'NONE',  ( 13.43411237798106583, 47.66530133659709634, -12.81628187352647252 ) ) ;
#54664=CARTESIAN_POINT ( 'NONE',  ( 1.472469842513823179, 56.42559781766745886, 4.923371831947296329 ) ) ;
#54665=CARTESIAN_POINT ( 'NONE',  ( 0.5774900079438607392, 53.48035201082151247, 5.440088680355550821 ) ) ;
#54666=CARTESIAN_POINT ( 'NONE',  ( 19.84674366389459266, 48.30059781766745175, 2.638427012816836559 ) ) ;
#54668=CARTESIAN_POINT ( 'NONE',  ( 10.00000000000000000, 56.81368534415484106, -10.88017736071110342 ) ) ;
#54669=ORIENTED_EDGE ( 'NONE', *, *, #79343, .F. ) ;
#54670=CARTESIAN_POINT ( 'NONE',  ( -0.3689425029237881626, 52.42874883491396076, 10.36894250292379027 ) ) ;
#54671=FILL_AREA_STYLE_COLOUR ( '', #41667 ) ;
#54672=CARTESIAN_POINT ( 'NONE',  ( 20.88017736071110164, 25.35535201082150891, 2.915334737309930979 ) ) ;
#54673=CARTESIAN_POINT ( 'NONE',  ( 13.43411237798106583, 12.66530133659708746, -12.81628187352647252 ) ) ;
#54674=CARTESIAN_POINT ( 'NONE',  ( 19.42250999205614193, 55.14701867748817676, 5.440088680355555262 ) ) ;
#54676=CARTESIAN_POINT ( 'NONE',  ( 19.72487221294570858, 0.000000000000000000, -6.500000000000000888 ) ) ;
#54678=CARTESIAN_POINT ( 'NONE',  ( -0.8801773607111009756, 48.06368534415484817, 1.068504757029289695E-15 ) ) ;
#54680=CARTESIAN_POINT ( 'NONE',  ( 1.472469842513823179, 40.59226448433411605, -4.923371831947296329 ) ) ;
#54681=DIRECTION ( 'NONE',  ( -0.8320502943378436100, 0.5547001962252291474, -0.000000000000000000 ) ) ;
#54683=CARTESIAN_POINT ( 'NONE',  ( 3.591859063236761518, 4.956968003263753531, 11.09922568453594849 ) ) ;
#54684=CARTESIAN_POINT ( 'NONE',  ( 20.88017736071110519, 15.56368534415483751, 2.639326808657452039E-16 ) ) ;
#54685=CARTESIAN_POINT ( 'NONE',  ( 0.2751277870542967463, 69.50000000000000000, -6.500000000000000888 ) ) ;
#54686=CARTESIAN_POINT ( 'NONE',  ( 24.16423886937410614, 34.30374883491396787, 8.672049930838204340E-16 ) ) ;
#54688=CARTESIAN_POINT ( 'NONE',  ( -4.164238869374099039, 66.80374883491396076, 8.674139862899312516E-16 ) ) ;
#54689=AXIS2_PLACEMENT_3D ( 'NONE', #79920, #95930, #35897 ) ;
#54690=CARTESIAN_POINT ( 'NONE',  ( 2.791683348922237240, 30.38393115100078390, -7.208316651077763204 ) ) ;
#54691=CARTESIAN_POINT ( 'NONE',  ( 19.84674366389459266, 18.30059781766745175, 2.638427012816836559 ) ) ;
#54692=CARTESIAN_POINT ( 'NONE',  ( 20.88017736071110519, 10.56368534415483751, 2.639326808657452039E-16 ) ) ;
#54693=ORIENTED_EDGE ( 'NONE', *, *, #84787, .F. ) ;
#54694=CARTESIAN_POINT ( 'NONE',  ( 17.20831665107776587, 42.88393115100077324, 7.208316651077764980 ) ) ;
#54695=CARTESIAN_POINT ( 'NONE',  ( 4.559911319644449179, 28.89701867748817321, 9.422509992056141925 ) ) ;
#54696=CARTESIAN_POINT ( 'NONE',  ( 5.076628168052703671, 56.84226448433412315, 8.527530157486179263 ) ) ;
#54697=CARTESIAN_POINT ( 'NONE',  ( -2.266590686148945544, 7.220415501580634832, 7.082119434687048631 ) ) ;
#54699=B_SPLINE_CURVE_WITH_KNOTS ( 'NONE', 3,
 ( #84523, #39024, #16020, #46509 ),
 .UNSPECIFIED., .F., .F.,
 ( 4, 4 ),
 ( 3.252606517456513302E-19, 0.001036303429213085783 ),
 .UNSPECIFIED. ) ;
#54702=CARTESIAN_POINT ( 'NONE',  ( 12.63842701281683034, 7.467264484334118713, 9.846743663894596210 ) ) ;
#54703=CARTESIAN_POINT ( 'NONE',  ( 3.591859063236761518, 54.95696800326376064, 11.09922568453594849 ) ) ;
#54704=CARTESIAN_POINT ( 'NONE',  ( 7.361572987183169658, 54.96726448433413026, -9.846743663894592657 ) ) ;
#54706=CARTESIAN_POINT ( 'NONE',  ( 5.076628168052704559, 20.17559781766745175, -8.527530157486179263 ) ) ;
#54708=CARTESIAN_POINT ( 'NONE',  ( -4.164238869374099927, 67.01208216824728936, 3.795296366450308767 ) ) ;
#54709=CARTESIAN_POINT ( 'NONE',  ( 20.88017736071110875, 55.77201867748816966, -2.915334737309920765 ) ) ;
#54710=CARTESIAN_POINT ( 'NONE',  ( 17.08211943468705130, 3.470415501580634388, 12.26659068614894998 ) ) ;
#54711=CARTESIAN_POINT ( 'NONE',  ( 4.559911319644449179, 62.23035201082150536, -9.422509992056141925 ) ) ;
#54712=CARTESIAN_POINT ( 'NONE',  ( 19.84674366389459621, 38.50893115100078745, 7.409399052514197653E-17 ) ) ;
#54713=CARTESIAN_POINT ( 'NONE',  ( 7.084665262690076126, 19.10535201082150181, 10.88017736071109987 ) ) ;
#54715=CARTESIAN_POINT ( 'NONE',  ( 18.06765999051783922, 38.99127512925448968, 6.500000000000047073 ) ) ;
#54716=CARTESIAN_POINT ( 'NONE',  ( 2.791683348922240793, 56.63393115100078035, 7.208316651077764092 ) ) ;
#54718=VERTEX_POINT ( 'NONE', #10086 ) ;
#54719=ORIENTED_EDGE ( 'NONE', *, *, #86910, .T. ) ;
#54722=CARTESIAN_POINT ( 'NONE',  ( 17.20831665107776587, 44.13393115100078745, -7.208316651077762316 ) ) ;
#54723=CARTESIAN_POINT ( 'NONE',  ( 1.472469842513823179, 20.59226448433411960, -4.923371831947296329 ) ) ;
#54724=CARTESIAN_POINT ( 'NONE',  ( 19.38216949554541557, 62.24863466993041072, -9.382169495545420901 ) ) ;
#54725=CARTESIAN_POINT ( 'NONE',  ( 17.96484262340118221, 19.93868534415484106, 7.964842623401181321 ) ) ;
#54726=CARTESIAN_POINT ( 'NONE',  ( 17.20831665107776587, 52.88393115100078035, 7.208316651077764980 ) ) ;
#54728=CARTESIAN_POINT ( 'NONE',  ( -4.164238869374099039, 41.80374883491397497, 8.674139862899312516E-16 ) ) ;
#54729=CARTESIAN_POINT ( 'NONE',  ( 22.26659068614895176, 64.72041550158064638, -7.082119434687042414 ) ) ;
#54730=CARTESIAN_POINT ( 'NONE',  ( 2.791683348922237240, 65.38393115100078035, -7.208316651077763204 ) ) ;
#54733=CARTESIAN_POINT ( 'NONE',  ( 7.084665262690076126, 49.10535201082149825, 10.88017736071109987 ) ) ;
#54734=CARTESIAN_POINT ( 'NONE',  ( 5.076628168052703671, 16.84226448433411960, 8.527530157486179263 ) ) ;
#54739=CARTESIAN_POINT ( 'NONE',  ( 5.076628168052704559, 15.17559781766745175, -8.527530157486179263 ) ) ;
#54741=CARTESIAN_POINT ( 'NONE',  ( 20.36894250292379382, 18.67874883491397142, 10.36894250292379205 ) ) ;
#54742=CARTESIAN_POINT ( 'NONE',  ( 18.52753015748617571, 23.09226448433411960, 4.923371831947298993 ) ) ;
#54743=CARTESIAN_POINT ( 'NONE',  ( 7.084665262690076126, 49.10535201082149825, 10.88017736071109987 ) ) ;
#54746=ORIENTED_EDGE ( 'NONE', *, *, #69115, .F. ) ;
#54747=CARTESIAN_POINT ( 'NONE',  ( 15.44008868035555260, 44.73035201082151247, 9.422509992056143702 ) ) ;
#54751=ORIENTED_EDGE ( 'NONE', *, *, #69799, .T. ) ;
#54752=CARTESIAN_POINT ( 'NONE',  ( -2.266590686148945544, 7.220415501580634832, 7.082119434687048631 ) ) ;
#54754=CARTESIAN_POINT ( 'NONE',  ( 22.81628187352647785, 11.62363466993042138, 6.195893100308588602E-16 ) ) ;
#54756=CARTESIAN_POINT ( 'NONE',  ( 7.361572987183169658, 9.967264484334119601, -9.846743663894592657 ) ) ;
#54758=CARTESIAN_POINT ( 'NONE',  ( 0.6178305044545818747, 43.49863466993042493, -9.382169495545419124 ) ) ;
#54760=CARTESIAN_POINT ( 'NONE',  ( 0.1532563361054083140, 21.00893115100078745, 1.131784320476157264E-15 ) ) ;
#54761=CARTESIAN_POINT ( 'NONE',  ( -0.8801773607111009756, 33.06368534415484106, 1.068504757029289695E-15 ) ) ;
#54762=ORIENTED_EDGE ( 'NONE', *, *, #9284, .T. ) ;
#54764=CARTESIAN_POINT ( 'NONE',  ( 12.91533473730992121, 59.52201867748816966, 10.88017736071110164 ) ) ;
#54767=CARTESIAN_POINT ( 'NONE',  ( 4.559911319644449179, 67.23035201082150536, -9.422509992056141925 ) ) ;
#54768=AXIS2_PLACEMENT_3D ( 'NONE', #49128, #64599, #32646 ) ;
#54769=COLOUR_RGB ( '', 0.09019608, 0.27058824, 0.51372549) ;
#54770=CARTESIAN_POINT ( 'NONE',  ( 3.591859063236763294, 8.290301336597087456, -11.09922568453595026 ) ) ;
#54774=CARTESIAN_POINT ( 'NONE',  ( 7.361572987183169658, 29.96726448433411960, -9.846743663894592657 ) ) ;
#54775=CARTESIAN_POINT ( 'NONE',  ( -2.816281873526471635, 58.91530133659707502, -3.434112377981056508 ) ) ;
#54776=CARTESIAN_POINT ( 'NONE',  ( 6.204703633549690345, 12.84541550158063572, 14.16423886937410082 ) ) ;
#54777=CARTESIAN_POINT ( 'NONE',  ( 12.63842701281683034, 22.46726448433411605, 9.846743663894596210 ) ) ;
#54779=CARTESIAN_POINT ( 'NONE',  ( -1.099225684535947600, 13.70696800326375353, -6.408140936763238038 ) ) ;
#54781=CARTESIAN_POINT ( 'NONE',  ( 0.5774900079438607392, 43.48035201082151247, 5.440088680355550821 ) ) ;
#54782=CARTESIAN_POINT ( 'NONE',  ( 5.076628168052703671, 56.84226448433412315, 8.527530157486179263 ) ) ;
#54783=CARTESIAN_POINT ( 'NONE',  ( 20.15039907845753220, 51.74884699246889852, 6.262539305110077059 ) ) ;
#54784=CARTESIAN_POINT ( 'NONE',  ( 17.20831665107776587, 34.13393115100078745, -7.208316651077762316 ) ) ;
#54785=CARTESIAN_POINT ( 'NONE',  ( 0.1532563361054100626, 25.80059781766744820, -2.638427012816831230 ) ) ;
#54786=CARTESIAN_POINT ( 'NONE',  ( 19.42250999205614548, 15.98035201082150714, -5.440088680355545492 ) ) ;
#54787=CARTESIAN_POINT ( 'NONE',  ( 22.81628187352647785, 21.62363466993041783, 6.195893100308588602E-16 ) ) ;
#54788=CARTESIAN_POINT ( 'NONE',  ( 12.63842701281683034, 27.46726448433411250, 9.846743663894596210 ) ) ;
#54790=CARTESIAN_POINT ( 'NONE',  ( 10.00000000000000000, 16.81368534415483751, -10.88017736071110342 ) ) ;
#54791=CARTESIAN_POINT ( 'NONE',  ( -0.3289641300568005855, 49.27164270246084499, -5.963430220938281678 ) ) ;
#54792=CARTESIAN_POINT ( 'NONE',  ( 0.1532563361054100626, 45.80059781766745886, -2.638427012816831230 ) ) ;
#54793=CARTESIAN_POINT ( 'NONE',  ( 19.42250999205614548, 15.98035201082150714, -5.440088680355545492 ) ) ;
#54794=CARTESIAN_POINT ( 'NONE',  ( 2.035157376598824452, 38.68868534415483396, 7.964842623401179544 ) ) ;
#54795=CARTESIAN_POINT ( 'NONE',  ( 15.44008868035555793, 6.397018677488171434, -9.422509992056140149 ) ) ;
#54797=CARTESIAN_POINT ( 'NONE',  ( 12.63842701281683922, 19.55059781766745175, -9.846743663894590881 ) ) ;
#54798=( BOUNDED_SURFACE ( )  B_SPLINE_SURFACE ( 1, 2, ( 
 ( #68286, #89779, #60759, #52280, #36293, #44769, #91259, #22785, #89294, #20804, #81778, #43780, #74272, #21296, #51788, #82275, #19142, #58610, #88120, #97139, #5628, #57622, #50122, #73107, #58104, #28110, #5130, #12128, #96136, #89607, #27121, #59098, #88610, #19631, #27617, #96634, #42151, #80632, #42629, #4648, #89112, #20120, #65113, #49618, #79647, #35110, #36106, #65609, #50623, #12616, #81114, #73605, #43117, #21117, #72132, #35620, #20624, #66104, #51113, #72616, #66611, #81601, #13112, #34123, #80129, #11636, #28609, #64615, #43608, #11145, #74095, #87628, #57131, #41664, #3659, #95125, #4151, #26633, #34616, #95634, #37113, #82597, #84086, #76082, #46085, #92073, #51616, #7103, #30571, #13611, #91586, #44091, #91079, #38586, #74601, #29094, #44597, #6600, #67610, #22604, #53082, #7610, #90584, #22109, #25562, #86546, #18053, #96020, #18538, #49029, #98009, #45971, #36498, #21999, #28976, #68479, #98508, #66990, #29962, #43977, #14499, #52474, #29463, #59969, #97513, #22489, #83473, #6003, #82979, #28498, #14995, #76461, #60468, #52962, #58992, #90957, #74480, #90463, #74980, #75474, #59479, #51994, #5, #89980, #82483, #7492, #45465, #6484, #6989, #36991, #7976, #75965, #30454, #66494, #60953, #21005, #91462, #67487, #22988, #97021, #53454, #51492, #13498, #61937, #38962, #69455, #93429, #62423, #1960, #499, #47431, #84945, #48416, #40443, #32426, #23483, #31923, #39940, #62927, #16947, #78918, #9940, #38475, #55434, #31435, #70944, #9439, #77931, #85940, #76946, #2462, #1469, #24458, #24951, #30948, #68968, #8941, #70443, #54924, #23962, #25449, #85440, #17451, #32918, #61447, #86432, #92439, #973, #47918, #78423, #63419, #55932, #16456, #54436, #93923, #91953, #46936, #53956, #39459, #84463, #15961, #8456, #46453, #77429, #69950, #41441, #71901, #73372, #95396, #49886, #95904, #65376, #4416, #57392, #3425, #26897, #27875, #63895, #88881, #41925, #19887, #49395, #27385, #87882, #57876, #19400, #50881, #25923, #72387, #42891, #56897, #18918, #33884, #58362, #11900, #79896, #56425, #64389, #94899, #86911, #18421, #88388, #87402, #35380, #89370, #58867, #44355, #67361, #98385, #20882, #29349, #74859, #14374, #66866, #28851, #83351, #37373, #7368, #98879, #60836, #13874, #29840, #22863, #52843, #12871, #59850, #37867, #73869, #59356, #21373, #68360, #35872, #90339, #82854, #44842, #66362, #96898, #51869, #82353, #69833, #84349, #92325, #53840, #84828, #93797, #23357, #1354, #23848, #93304, #7855, #859, #77802, #91841, #31807, #83843, #70328, #1842, #78300, #31318, #16335, #9818, #85815, #54803, #16826, #32300 ),
 ( #38355, #62804, #68848, #24828, #17328, #40319, #381, #70823, #61329, #66626, #50137, #25806, #19645, #13125, #50638, #20637, #86307, #66119, #73121, #36635, #59110, #51126, #40810, #20134, #28127, #43622, #5143, #6129, #97155, #67118, #5642, #80646, #51633, #96648, #58627, #44104, #33281, #74615, #55812, #58117, #17810, #94284, #63774, #12140, #42645, #4663, #35125, #65624, #27632, #53588, #84102, #59610, #15618, #75109, #91093, #75605, #60598, #6615, #52605, #31081, #67624, #37129, #633, #46102, #68116, #53099, #60096, #39097, #83609, #76587, #97643, #15124, #82612, #136, #98642, #54079, #46581, #76097, #98133, #8105, #14635, #29594, #30091, #23615, #45599, #84596, #14128, #44613, #9573, #79551, #18555, #94054, #47066, #25090, #2595, #56068, #48048, #49047, #41069, #11050, #1108, #55058, #92572, #40573, #78562, #77564, #39594, #32055, #32560, #17583, #2101, #34025, #51509, #12032, #20022, #35011, #27027, #28513, #65512, #20525, #36009, #64522, #89510, #57526, #72521, #51010, #13009, #96034, #59007, #50522, #81019, #74004, #97038, #42058, #12521, #43023, #95028, #26537, #80032, #43506, #87535, #73506, #4055, #5030, #5529, #35517, #66008, #28011, #96536, #21020, #19048, #49525, #98526, #30966, #36515, #23499, #29979, #53471, #60484, #37007, #15506, #15011, #14016, #13513, #98023, #91482, #97528, #59986, #22015, #52489, #76477, #22, #83981, #45988, #61463, #67007, #89996, #21512, #33839, #95858, #40403, #57835, #79371, #87841, #64348, #40891, #80353, #79857, #48372, #49355, #55890, #26358, #94856, #10876, #41400, #78876, #34338, #95352, #17889, #56858, #70898, #26851, #27342, #11360, #64833, #2417, #41879, #86387, #71866, #56383, #3377, #10386, #33357, #11851, #71392, #2906, #19360, #57348, #86872, #87359, #63852, #88344, #18873, #72342, #19842, #3875, #32874, #49844, #25884, #34837, #78380, #42361, #94365, #72834, #18382, #48861, #4372, #65332, #9900, #63372, #93877, #25404, #28332, #60309, #52317, #13833, #35335, #43816, #51825, #44314, #28816, #29800, #82810, #90802, #67321, #43330, #14330, #21335, #59315, #97844, #88837, #44803, #13332, #74311, #74815, #12342, #50332, #20840, #89814, #5838, #35834, #37335, #36328, #29309, #75308, #42848, #98342, #5355, #81333, #59805, #90299, #66823, #67825, #58822, #66321, #6819, #80845, #50841, #97345, #51332, #73332, #82312, #81814, #6320, #4859, #12830, #36829, #65828, #96360, #27833, #58319, #20345, #91294, #22329, #91798, #47265, #76785, #61289, #54273, #8302, #16298, #69298, #1803, #14833, #23319, #62264, #68809, #53801, #15330, #77767, #92288, #84312, #75804, #22817, #53297 ) ),
 .UNSPECIFIED., .F., .F., .T. ) 
 B_SPLINE_SURFACE_WITH_KNOTS ( ( 2, 2 ),
 ( 3, 2, 2, 2, 2, 2, 2, 2, 2, 2, 2, 2, 2, 2, 2, 2, 2, 2, 2, 2, 2, 2, 2, 2, 2, 2, 2, 2, 2, 2, 2, 2, 2, 2, 2, 2, 2, 2, 2, 2, 2, 2, 2, 2, 2, 2, 2, 2, 2, 2, 2, 2, 2, 2, 2, 2, 2, 2, 2, 2, 2, 2, 2, 2, 2, 2, 2, 2, 2, 2, 2, 2, 2, 2, 2, 2, 2, 2, 2, 2, 2, 2, 2, 2, 2, 2, 2, 2, 2, 2, 2, 2, 2, 2, 2, 2, 2, 2, 2, 2, 2, 2, 2, 2, 2, 2, 2, 2, 2, 2, 2, 2, 2, 2, 2, 2, 2, 2, 2, 2, 2, 2, 2, 2, 2, 2, 2, 2, 2, 2, 2, 2, 2, 2, 2, 2, 2, 2, 2, 2, 2, 2, 2, 2, 2, 2, 2, 2, 2, 2, 2, 2, 2, 2, 2, 2, 2, 2, 2, 2, 2, 2, 3 ),
 ( 0.000000000000000000, 1.000000000000000000 ),
 ( 0.000000000000000000, 0.005952380952380952051, 0.01190476190476190410, 0.01785714285714285615, 0.02380952380952380820, 0.02976190476190476025, 0.03571428571428571230, 0.04166666666666666435, 0.04761904761904761640, 0.05357142857142856845, 0.05952380952380952051, 0.06547619047619047949, 0.07142857142857142461, 0.07738095238095238360, 0.08333333333333332871, 0.08928571428571428770, 0.09523809523809523281, 0.1011904761904761918, 0.1071428571428571369, 0.1130952380952380959, 0.1190476190476190410, 0.1250000000000000000, 0.1309523809523809590, 0.1369047619047619180, 0.1428571428571428492, 0.1488095238095238082, 0.1547619047619047672, 0.1607142857142857262, 0.1666666666666666574, 0.1726190476190476164, 0.1785714285714285754, 0.1845238095238095344, 0.1904761904761904656, 0.1964285714285714246, 0.2023809523809523836, 0.2083333333333333426, 0.2142857142857142738, 0.2202380952380952328, 0.2261904761904761918, 0.2321428571428571508, 0.2380952380952380820, 0.2440476190476190410, 0.2500000000000000000, 0.2559523809523809312, 0.2619047619047619180, 0.2678571428571428492, 0.2738095238095238360, 0.2797619047619047672, 0.2857142857142856984, 0.2916666666666666852, 0.2976190476190476164, 0.3035714285714285476, 0.3095238095238095344, 0.3154761904761904656, 0.3214285714285714524, 0.3273809523809523836, 0.3333333333333333148, 0.3392857142857143016, 0.3452380952380952328, 0.3511904761904761640, 0.3571428571428571508, 0.3630952380952380820, 0.3690476190476190688, 0.3750000000000000000, 0.3809523809523809312, 0.3869047619047619180, 0.3928571428571428492, 0.3988095238095238360, 0.4047619047619047672, 0.4107142857142856984, 0.4166666666666666852, 0.4226190476190476164, 0.4285714285714285476, 0.4345238095238095344, 0.4404761904761904656, 0.4464285714285714524, 0.4523809523809523836, 0.4583333333333333148, 0.4642857142857143016, 0.4702380952380952328, 0.4761904761904761640, 0.4821428571428571508, 0.4880952380952380820, 0.4940476190476190688, 0.5000000000000000000, 0.5059523809523809312, 0.5119047619047618625, 0.5178571428571429047, 0.5238095238095238360, 0.5297619047619047672, 0.5357142857142856984, 0.5416666666666666297, 0.5476190476190476719, 0.5535714285714286031, 0.5595238095238095344, 0.5654761904761904656, 0.5714285714285713969, 0.5773809523809523281, 0.5833333333333333703, 0.5892857142857143016, 0.5952380952380952328, 0.6011904761904761640, 0.6071428571428570953, 0.6130952380952381375, 0.6190476190476190688, 0.6250000000000000000, 0.6309523809523809312, 0.6369047619047618625, 0.6428571428571429047, 0.6488095238095238360, 0.6547619047619047672, 0.6607142857142856984, 0.6666666666666666297, 0.6726190476190476719, 0.6785714285714286031, 0.6845238095238095344, 0.6904761904761904656, 0.6964285714285713969, 0.7023809523809523281, 0.7083333333333333703, 0.7142857142857143016, 0.7202380952380952328, 0.7261904761904761640, 0.7321428571428570953, 0.7380952380952381375, 0.7440476190476190688, 0.7500000000000000000, 0.7559523809523809312, 0.7619047619047618625, 0.7678571428571429047, 0.7738095238095238360, 0.7797619047619047672, 0.7857142857142856984, 0.7916666666666666297, 0.7976190476190476719, 0.8035714285714286031, 0.8095238095238095344, 0.8154761904761904656, 0.8214285714285713969, 0.8273809523809523281, 0.8333333333333333703, 0.8392857142857143016, 0.8452380952380952328, 0.8511904761904761640, 0.8571428571428570953, 0.8630952380952381375, 0.8690476190476190688, 0.8750000000000000000, 0.8809523809523809312, 0.8869047619047618625, 0.8928571428571429047, 0.8988095238095238360, 0.9047619047619047672, 0.9107142857142856984, 0.9166666666666666297, 0.9226190476190476719, 0.9285714285714286031, 0.9345238095238095344, 0.9404761904761904656, 0.9464285714285713969, 0.9523809523809523281, 0.9583333333333333703, 0.9642857142857143016 ),
 .UNSPECIFIED. ) 
 GEOMETRIC_REPRESENTATION_ITEM ( )  RATIONAL_B_SPLINE_SURFACE ( (
 ( 1.000000000000000000, 0.9659258262890683122, 1.000000000000000000, 0.9659258262890683122, 1.000000000000000000, 0.9659258262890683122, 1.000000000000000000, 0.9659258262890683122, 1.000000000000000000, 0.9659258262890683122, 1.000000000000000000, 0.9659258262890683122, 1.000000000000000000, 0.9659258262890683122, 1.000000000000000000, 0.9659258262890683122, 1.000000000000000000, 0.9659258262890683122, 1.000000000000000000, 0.9659258262890683122, 1.000000000000000000, 0.9659258262890683122, 1.000000000000000000, 0.9659258262890683122, 1.000000000000000000, 0.9659258262890683122, 1.000000000000000000, 0.9659258262890683122, 1.000000000000000000, 0.9659258262890683122, 1.000000000000000000, 0.9659258262890683122, 1.000000000000000000, 0.9659258262890683122, 1.000000000000000000, 0.9659258262890683122, 1.000000000000000000, 0.9659258262890683122, 1.000000000000000000, 0.9659258262890683122, 1.000000000000000000, 0.9659258262890683122, 1.000000000000000000, 0.9659258262890683122, 1.000000000000000000, 0.9659258262890683122, 1.000000000000000000, 0.9659258262890683122, 1.000000000000000000, 0.9659258262890683122, 1.000000000000000000, 0.9659258262890683122, 1.000000000000000000, 0.9659258262890683122, 1.000000000000000000, 0.9659258262890683122, 1.000000000000000000, 0.9659258262890683122, 1.000000000000000000, 0.9659258262890683122, 1.000000000000000000, 0.9659258262890683122, 1.000000000000000000, 0.9659258262890683122, 1.000000000000000000, 0.9659258262890683122, 1.000000000000000000, 0.9659258262890683122, 1.000000000000000000, 0.9659258262890683122, 1.000000000000000000, 0.9659258262890683122, 1.000000000000000000, 0.9659258262890683122, 1.000000000000000000, 0.9659258262890683122, 1.000000000000000000, 0.9659258262890683122, 1.000000000000000000, 0.9659258262890683122, 1.000000000000000000, 0.9659258262890683122, 1.000000000000000000, 0.9659258262890683122, 1.000000000000000000, 0.9659258262890683122, 1.000000000000000000, 0.9659258262890683122, 1.000000000000000000, 0.9659258262890683122, 1.000000000000000000, 0.9659258262890683122, 1.000000000000000000, 0.9659258262890683122, 1.000000000000000000, 0.9659258262890683122, 1.000000000000000000, 0.9659258262890683122, 1.000000000000000000, 0.9659258262890683122, 1.000000000000000000, 0.9659258262890683122, 1.000000000000000000, 0.9659258262890683122, 1.000000000000000000, 0.9659258262890683122, 1.000000000000000000, 0.9659258262890683122, 1.000000000000000000, 0.9659258262890683122, 1.000000000000000000, 0.9659258262890683122, 1.000000000000000000, 0.9659258262890683122, 1.000000000000000000, 0.9659258262890683122, 1.000000000000000000, 0.9659258262890683122, 1.000000000000000000, 0.9659258262890683122, 1.000000000000000000, 0.9659258262890683122, 1.000000000000000000, 0.9659258262890683122, 1.000000000000000000, 0.9659258262890683122, 1.000000000000000000, 0.9659258262890683122, 1.000000000000000000, 0.9659258262890683122, 1.000000000000000000, 0.9659258262890683122, 1.000000000000000000, 0.9659258262890683122, 1.000000000000000000, 0.9659258262890683122, 1.000000000000000000, 0.9659258262890683122, 1.000000000000000000, 0.9659258262890683122, 1.000000000000000000, 0.9659258262890683122, 1.000000000000000000, 0.9659258262890683122, 1.000000000000000000, 0.9659258262890683122, 1.000000000000000000, 0.9659258262890683122, 1.000000000000000000, 0.9659258262890683122, 1.000000000000000000, 0.9659258262890683122, 1.000000000000000000, 0.9659258262890683122, 1.000000000000000000, 0.9659258262890683122, 1.000000000000000000, 0.9659258262890683122, 1.000000000000000000, 0.9659258262890683122, 1.000000000000000000, 0.9659258262890683122, 1.000000000000000000, 0.9659258262890683122, 1.000000000000000000, 0.9659258262890683122, 1.000000000000000000, 0.9659258262890683122, 1.000000000000000000, 0.9659258262890683122, 1.000000000000000000, 0.9659258262890683122, 1.000000000000000000, 0.9659258262890683122, 1.000000000000000000, 0.9659258262890683122, 1.000000000000000000, 0.9659258262890683122, 1.000000000000000000, 0.9659258262890683122, 1.000000000000000000, 0.9659258262890683122, 1.000000000000000000, 0.9659258262890683122, 1.000000000000000000, 0.9659258262890683122, 1.000000000000000000, 0.9659258262890683122, 1.000000000000000000, 0.9659258262890683122, 1.000000000000000000, 0.9659258262890683122, 1.000000000000000000, 0.9659258262890683122, 1.000000000000000000, 0.9659258262890683122, 1.000000000000000000, 0.9659258262890683122, 1.000000000000000000, 0.9659258262890683122, 1.000000000000000000, 0.9659258262890683122, 1.000000000000000000, 0.9659258262890683122, 1.000000000000000000, 0.9659258262890683122, 1.000000000000000000, 0.9659258262890683122, 1.000000000000000000, 0.9659258262890683122, 1.000000000000000000, 0.9659258262890683122, 1.000000000000000000, 0.9659258262890683122, 1.000000000000000000, 0.9659258262890683122, 1.000000000000000000, 0.9659258262890683122, 1.000000000000000000, 0.9659258262890683122, 1.000000000000000000, 0.9659258262890683122, 1.000000000000000000, 0.9659258262890683122, 1.000000000000000000, 0.9659258262890683122, 1.000000000000000000, 0.9659258262890683122, 1.000000000000000000, 0.9659258262890683122, 1.000000000000000000, 0.9659258262890683122, 1.000000000000000000, 0.9659258262890683122, 1.000000000000000000, 0.9659258262890683122, 1.000000000000000000, 0.9659258262890683122, 1.000000000000000000, 0.9659258262890683122, 1.000000000000000000, 0.9659258262890683122, 1.000000000000000000, 0.9659258262890683122, 1.000000000000000000, 0.9659258262890683122, 1.000000000000000000, 0.9659258262890683122, 1.000000000000000000, 0.9659258262890683122, 1.000000000000000000, 0.9659258262890683122, 1.000000000000000000, 0.9659258262890683122, 1.000000000000000000, 0.9659258262890683122, 1.000000000000000000, 0.9659258262890683122, 1.000000000000000000, 0.9659258262890683122, 1.000000000000000000, 0.9659258262890683122, 1.000000000000000000, 0.9659258262890683122, 1.000000000000000000, 0.9659258262890683122, 1.000000000000000000, 0.9659258262890683122, 1.000000000000000000, 0.9659258262890683122, 1.000000000000000000, 0.9659258262890683122, 1.000000000000000000, 0.9659258262890683122, 1.000000000000000000, 0.9659258262890683122, 1.000000000000000000, 0.9659258262890683122, 1.000000000000000000, 0.9659258262890683122, 1.000000000000000000, 0.9659258262890683122, 1.000000000000000000, 0.9659258262890683122, 1.000000000000000000, 0.9659258262890683122, 1.000000000000000000, 0.9659258262890683122, 1.000000000000000000, 0.9659258262890683122, 1.000000000000000000, 0.9659258262890683122, 1.000000000000000000, 0.9659258262890683122, 1.000000000000000000, 0.9659258262890683122, 1.000000000000000000, 0.9659258262890683122, 1.000000000000000000, 0.9659258262890683122, 1.000000000000000000, 0.9659258262890683122, 1.000000000000000000, 0.9659258262890683122, 1.000000000000000000, 0.9659258262890683122, 1.000000000000000000, 0.9659258262890683122, 1.000000000000000000, 0.9659258262890683122, 1.000000000000000000, 0.9659258262890683122, 1.000000000000000000, 0.9659258262890683122, 1.000000000000000000, 0.9659258262890683122, 1.000000000000000000, 0.9659258262890683122, 1.000000000000000000, 0.9659258262890683122, 1.000000000000000000, 0.9659258262890683122, 1.000000000000000000, 0.9659258262890683122, 1.000000000000000000),
 ( 1.000000000000000000, 0.9659258262890683122, 1.000000000000000000, 0.9659258262890683122, 1.000000000000000000, 0.9659258262890683122, 1.000000000000000000, 0.9659258262890683122, 1.000000000000000000, 0.9659258262890683122, 1.000000000000000000, 0.9659258262890683122, 1.000000000000000000, 0.9659258262890683122, 1.000000000000000000, 0.9659258262890683122, 1.000000000000000000, 0.9659258262890683122, 1.000000000000000000, 0.9659258262890683122, 1.000000000000000000, 0.9659258262890683122, 1.000000000000000000, 0.9659258262890683122, 1.000000000000000000, 0.9659258262890683122, 1.000000000000000000, 0.9659258262890683122, 1.000000000000000000, 0.9659258262890683122, 1.000000000000000000, 0.9659258262890683122, 1.000000000000000000, 0.9659258262890683122, 1.000000000000000000, 0.9659258262890683122, 1.000000000000000000, 0.9659258262890683122, 1.000000000000000000, 0.9659258262890683122, 1.000000000000000000, 0.9659258262890683122, 1.000000000000000000, 0.9659258262890683122, 1.000000000000000000, 0.9659258262890683122, 1.000000000000000000, 0.9659258262890683122, 1.000000000000000000, 0.9659258262890683122, 1.000000000000000000, 0.9659258262890683122, 1.000000000000000000, 0.9659258262890683122, 1.000000000000000000, 0.9659258262890683122, 1.000000000000000000, 0.9659258262890683122, 1.000000000000000000, 0.9659258262890683122, 1.000000000000000000, 0.9659258262890683122, 1.000000000000000000, 0.9659258262890683122, 1.000000000000000000, 0.9659258262890683122, 1.000000000000000000, 0.9659258262890683122, 1.000000000000000000, 0.9659258262890683122, 1.000000000000000000, 0.9659258262890683122, 1.000000000000000000, 0.9659258262890683122, 1.000000000000000000, 0.9659258262890683122, 1.000000000000000000, 0.9659258262890683122, 1.000000000000000000, 0.9659258262890683122, 1.000000000000000000, 0.9659258262890683122, 1.000000000000000000, 0.9659258262890683122, 1.000000000000000000, 0.9659258262890683122, 1.000000000000000000, 0.9659258262890683122, 1.000000000000000000, 0.9659258262890683122, 1.000000000000000000, 0.9659258262890683122, 1.000000000000000000, 0.9659258262890683122, 1.000000000000000000, 0.9659258262890683122, 1.000000000000000000, 0.9659258262890683122, 1.000000000000000000, 0.9659258262890683122, 1.000000000000000000, 0.9659258262890683122, 1.000000000000000000, 0.9659258262890683122, 1.000000000000000000, 0.9659258262890683122, 1.000000000000000000, 0.9659258262890683122, 1.000000000000000000, 0.9659258262890683122, 1.000000000000000000, 0.9659258262890683122, 1.000000000000000000, 0.9659258262890683122, 1.000000000000000000, 0.9659258262890683122, 1.000000000000000000, 0.9659258262890683122, 1.000000000000000000, 0.9659258262890683122, 1.000000000000000000, 0.9659258262890683122, 1.000000000000000000, 0.9659258262890683122, 1.000000000000000000, 0.9659258262890683122, 1.000000000000000000, 0.9659258262890683122, 1.000000000000000000, 0.9659258262890683122, 1.000000000000000000, 0.9659258262890683122, 1.000000000000000000, 0.9659258262890683122, 1.000000000000000000, 0.9659258262890683122, 1.000000000000000000, 0.9659258262890683122, 1.000000000000000000, 0.9659258262890683122, 1.000000000000000000, 0.9659258262890683122, 1.000000000000000000, 0.9659258262890683122, 1.000000000000000000, 0.9659258262890683122, 1.000000000000000000, 0.9659258262890683122, 1.000000000000000000, 0.9659258262890683122, 1.000000000000000000, 0.9659258262890683122, 1.000000000000000000, 0.9659258262890683122, 1.000000000000000000, 0.9659258262890683122, 1.000000000000000000, 0.9659258262890683122, 1.000000000000000000, 0.9659258262890683122, 1.000000000000000000, 0.9659258262890683122, 1.000000000000000000, 0.9659258262890683122, 1.000000000000000000, 0.9659258262890683122, 1.000000000000000000, 0.9659258262890683122, 1.000000000000000000, 0.9659258262890683122, 1.000000000000000000, 0.9659258262890683122, 1.000000000000000000, 0.9659258262890683122, 1.000000000000000000, 0.9659258262890683122, 1.000000000000000000, 0.9659258262890683122, 1.000000000000000000, 0.9659258262890683122, 1.000000000000000000, 0.9659258262890683122, 1.000000000000000000, 0.9659258262890683122, 1.000000000000000000, 0.9659258262890683122, 1.000000000000000000, 0.9659258262890683122, 1.000000000000000000, 0.9659258262890683122, 1.000000000000000000, 0.9659258262890683122, 1.000000000000000000, 0.9659258262890683122, 1.000000000000000000, 0.9659258262890683122, 1.000000000000000000, 0.9659258262890683122, 1.000000000000000000, 0.9659258262890683122, 1.000000000000000000, 0.9659258262890683122, 1.000000000000000000, 0.9659258262890683122, 1.000000000000000000, 0.9659258262890683122, 1.000000000000000000, 0.9659258262890683122, 1.000000000000000000, 0.9659258262890683122, 1.000000000000000000, 0.9659258262890683122, 1.000000000000000000, 0.9659258262890683122, 1.000000000000000000, 0.9659258262890683122, 1.000000000000000000, 0.9659258262890683122, 1.000000000000000000, 0.9659258262890683122, 1.000000000000000000, 0.9659258262890683122, 1.000000000000000000, 0.9659258262890683122, 1.000000000000000000, 0.9659258262890683122, 1.000000000000000000, 0.9659258262890683122, 1.000000000000000000, 0.9659258262890683122, 1.000000000000000000, 0.9659258262890683122, 1.000000000000000000, 0.9659258262890683122, 1.000000000000000000, 0.9659258262890683122, 1.000000000000000000, 0.9659258262890683122, 1.000000000000000000, 0.9659258262890683122, 1.000000000000000000, 0.9659258262890683122, 1.000000000000000000, 0.9659258262890683122, 1.000000000000000000, 0.9659258262890683122, 1.000000000000000000, 0.9659258262890683122, 1.000000000000000000, 0.9659258262890683122, 1.000000000000000000, 0.9659258262890683122, 1.000000000000000000, 0.9659258262890683122, 1.000000000000000000, 0.9659258262890683122, 1.000000000000000000, 0.9659258262890683122, 1.000000000000000000, 0.9659258262890683122, 1.000000000000000000, 0.9659258262890683122, 1.000000000000000000, 0.9659258262890683122, 1.000000000000000000, 0.9659258262890683122, 1.000000000000000000, 0.9659258262890683122, 1.000000000000000000, 0.9659258262890683122, 1.000000000000000000, 0.9659258262890683122, 1.000000000000000000, 0.9659258262890683122, 1.000000000000000000, 0.9659258262890683122, 1.000000000000000000, 0.9659258262890683122, 1.000000000000000000, 0.9659258262890683122, 1.000000000000000000, 0.9659258262890683122, 1.000000000000000000, 0.9659258262890683122, 1.000000000000000000, 0.9659258262890683122, 1.000000000000000000, 0.9659258262890683122, 1.000000000000000000, 0.9659258262890683122, 1.000000000000000000, 0.9659258262890683122, 1.000000000000000000, 0.9659258262890683122, 1.000000000000000000, 0.9659258262890683122, 1.000000000000000000, 0.9659258262890683122, 1.000000000000000000, 0.9659258262890683122, 1.000000000000000000, 0.9659258262890683122, 1.000000000000000000, 0.9659258262890683122, 1.000000000000000000, 0.9659258262890683122, 1.000000000000000000, 0.9659258262890683122, 1.000000000000000000, 0.9659258262890683122, 1.000000000000000000, 0.9659258262890683122, 1.000000000000000000, 0.9659258262890683122, 1.000000000000000000, 0.9659258262890683122, 1.000000000000000000, 0.9659258262890683122, 1.000000000000000000, 0.9659258262890683122, 1.000000000000000000, 0.9659258262890683122, 1.000000000000000000, 0.9659258262890683122, 1.000000000000000000) ) ) 
 REPRESENTATION_ITEM ( '' )  SURFACE ( )  );
#54799=CARTESIAN_POINT ( 'NONE',  ( 17.20831665107776587, 44.13393115100078745, -7.208316651077762316 ) ) ;
#54800=CARTESIAN_POINT ( 'NONE',  ( -46.59701958359876528, 103.7651961684614719, 6.068442458532165240 ) ) ;
#54803=CARTESIAN_POINT ( 'NONE',  ( 5.076628168052703671, 66.84226448433412315, 8.527530157486179263 ) ) ;
#54806=CARTESIAN_POINT ( 'NONE',  ( 2.917880565312950480, 20.97041550158063217, -12.26659068614894821 ) ) ;
#54808=CARTESIAN_POINT ( 'NONE',  ( 18.52753015748618282, 38.92559781766745175, -4.923371831947291888 ) ) ;
#54811=CARTESIAN_POINT ( 'NONE',  ( -4.164238869374099039, 56.80374883491397497, 8.674139862899312516E-16 ) ) ;
#54812=CARTESIAN_POINT ( 'NONE',  ( 12.63842701281683922, 19.55059781766745175, -9.846743663894590881 ) ) ;
#54815=CARTESIAN_POINT ( 'NONE',  ( 2.035157376598822676, 52.43868534415483396, -7.964842623401177768 ) ) ;
#54816=CARTESIAN_POINT ( 'NONE',  ( -2.816281873526473856, 49.33196800326374643, 3.434112377981055619 ) ) ;
#54817=CARTESIAN_POINT ( 'NONE',  ( 12.91533473730992121, 14.52201867748817143, 10.88017736071110164 ) ) ;
#54818=CARTESIAN_POINT ( 'NONE',  ( -2.816281873526473856, 54.12363466993041783, 9.499525473075851096E-16 ) ) ;
#54819=CARTESIAN_POINT ( 'NONE',  ( 10.00000000000000000, 64.75893115100078035, -9.846743663894594434 ) ) ;
#54820=CARTESIAN_POINT ( 'NONE',  ( 17.20831665107776587, 19.13393115100078035, -7.208316651077762316 ) ) ;
#54823=CARTESIAN_POINT ( 'NONE',  ( 0.9408516040111585266, 17.46693863883975695, -6.499999999999988454 ) ) ;
#54824=CARTESIAN_POINT ( 'NONE',  ( 13.79529636645030344, 48.26208216824728936, 14.16423886937410614 ) ) ;
#54825=CARTESIAN_POINT ( 'NONE',  ( 17.08211943468705840, 15.13708216824730179, -12.26659068614894466 ) ) ;
#54826=CARTESIAN_POINT ( 'NONE',  ( 10.00000000000000000, 16.81368534415483751, -10.88017736071110342 ) ) ;
#54827=CARTESIAN_POINT ( 'NONE',  ( 19.42250999205614193, 35.14701867748816966, 5.440088680355555262 ) ) ;
#54829=CARTESIAN_POINT ( 'NONE',  ( 0.1532563361054082862, 1.217264484334117824, 2.638427012816831674 ) ) ;
#54831=CARTESIAN_POINT ( 'NONE',  ( 2.791683348922237240, 20.38393115100078745, -7.208316651077763204 ) ) ;
#54833=CARTESIAN_POINT ( 'NONE',  ( 5.500000000000000000, 11.50000000000000000, 6.000000000000000000 ) ) ;
#54834=CARTESIAN_POINT ( 'NONE',  ( 5.076628168052704559, 15.17559781766745175, -8.527530157486179263 ) ) ;
#54835=CARTESIAN_POINT ( 'NONE',  ( 19.84674366389459266, 33.71726448433410894, -2.638427012816827677 ) ) ;
#54837=CARTESIAN_POINT ( 'NONE',  ( 7.084665262690076126, 14.10535201082150358, 10.88017736071109987 ) ) ;
#54838=CARTESIAN_POINT ( 'NONE',  ( 22.81628187352648496, 31.83196800326375353, -3.434112377981050290 ) ) ;
#54840=CARTESIAN_POINT ( 'NONE',  ( 20.36894250292379738, 39.92874883491396787, -10.36894250292379027 ) ) ;
#54841=CARTESIAN_POINT ( 'NONE',  ( 19.84674366389459266, 13.30059781766745353, 2.638427012816836559 ) ) ;
#54843=CARTESIAN_POINT ( 'NONE',  ( 14.92337183194729633, 47.67559781766745175, 8.527530157486181039 ) ) ;
#54845=CARTESIAN_POINT ( 'NONE',  ( 2.791683348922240793, 36.63393115100078035, 7.208316651077764092 ) ) ;
#54846=CARTESIAN_POINT ( 'NONE',  ( 6.204703633549690345, 0.7620821682473009062, -14.16423886937410259 ) ) ;
#54847=CARTESIAN_POINT ( 'NONE',  ( 10.00000000000000000, 15.55374883491396787, -14.16423886937410082 ) ) ;
#54848=CARTESIAN_POINT ( 'NONE',  ( -0.8801773607111009756, 53.06368534415484106, 1.068504757029289695E-15 ) ) ;
#54849=CARTESIAN_POINT ( 'NONE',  ( 2.035157376598824452, 13.68868534415483751, 7.964842623401179544 ) ) ;
#54851=CARTESIAN_POINT ( 'NONE',  ( 15.44008868035555260, 44.73035201082151247, 9.422509992056143702 ) ) ;
#54852=CARTESIAN_POINT ( 'NONE',  ( 20.88017736071110164, 25.35535201082150891, 2.915334737309930979 ) ) ;
#54853=VERTEX_POINT ( 'NONE', #88529 ) ;
#54854=CARTESIAN_POINT ( 'NONE',  ( -2.816281873526473856, 34.33196800326376064, 3.434112377981055619 ) ) ;
#54856=CARTESIAN_POINT ( 'NONE',  ( 2.035157376598824452, 43.68868534415484106, 7.964842623401179544 ) ) ;
#54857=ORIENTED_EDGE ( 'NONE', *, *, #41541, .T. ) ;
#54858=CARTESIAN_POINT ( 'NONE',  ( -1.099225684535947600, 58.70696800326375353, -6.408140936763238038 ) ) ;
#54860=CARTESIAN_POINT ( 'NONE',  ( 12.91533473730993009, 56.60535201082151247, -10.88017736071109987 ) ) ;
#54862=CARTESIAN_POINT ( 'NONE',  ( 12.91533473730993009, 51.60535201082149825, -10.88017736071109987 ) ) ;
#54864=CARTESIAN_POINT ( 'NONE',  ( 4.559911319644449179, 7.230352010821504471, -9.422509992056141925 ) ) ;
#54867=CARTESIAN_POINT ( 'NONE',  ( 13.79529636645030344, 58.26208216824728936, 14.16423886937410614 ) ) ;
#54868=CARTESIAN_POINT ( 'NONE',  ( 4.559911319644449179, 68.89701867748817676, 9.422509992056141925 ) ) ;
#54869=CARTESIAN_POINT ( 'NONE',  ( -4.164238869374099039, 11.80374883491396965, 8.674139862899312516E-16 ) ) ;
#54872=CARTESIAN_POINT ( 'NONE',  ( 20.88017736071110164, 15.35535201082150358, 2.915334737309930979 ) ) ;
#54873=CARTESIAN_POINT ( 'NONE',  ( 14.92337183194729633, 52.67559781766745175, 8.527530157486181039 ) ) ;
#54875=CARTESIAN_POINT ( 'NONE',  ( 10.00000000000000178, 42.25893115100078745, 9.846743663894594434 ) ) ;
#54876=CARTESIAN_POINT ( 'NONE',  ( -0.8801773607111009756, 63.06368534415484106, 1.068504757029289695E-15 ) ) ;
#54877=CARTESIAN_POINT ( 'NONE',  ( 15.44008868035555260, 44.73035201082151247, 9.422509992056143702 ) ) ;
#54878=CARTESIAN_POINT ( 'NONE',  ( 5.076628168052704559, 40.17559781766745175, -8.527530157486179263 ) ) ;
#54879=FILL_AREA_STYLE_COLOUR ( '', #22826 ) ;
#54881=CARTESIAN_POINT ( 'NONE',  ( 15.44008868035555260, 44.73035201082151247, 9.422509992056143702 ) ) ;
#54882=CARTESIAN_POINT ( 'NONE',  ( 13.79529636645030344, 53.26208216824730357, 14.16423886937410614 ) ) ;
#54883=CARTESIAN_POINT ( 'NONE',  ( 22.81628187352647785, 21.41530133659708923, 3.434112377981063169 ) ) ;
#54885=CARTESIAN_POINT ( 'NONE',  ( 3.591859063236761518, 24.95696800326375353, 11.09922568453594849 ) ) ;
#54886=CARTESIAN_POINT ( 'NONE',  ( 0.5774900079438607392, 18.48035201082150536, 5.440088680355550821 ) ) ;
#54888=ORIENTED_EDGE ( 'NONE', *, *, #81084, .T. ) ;
#54889=CARTESIAN_POINT ( 'NONE',  ( 0.5774900079438590739, 67.64701867748817676, -5.440088680355550821 ) ) ;
#54890=ADVANCED_BREP_SHAPE_REPRESENTATION ( '', ( #74133, #27931 ), #40723 ) ;
#54891=CARTESIAN_POINT ( 'NONE',  ( 12.63842701281683922, 49.55059781766744464, -9.846743663894590881 ) ) ;
#54892=CARTESIAN_POINT ( 'NONE',  ( 7.361572987183169658, 14.96726448433411960, -9.846743663894592657 ) ) ;
#54893=CARTESIAN_POINT ( 'NONE',  ( 17.20831665107776587, 39.13393115100079456, -7.208316651077762316 ) ) ;
#54896=CARTESIAN_POINT ( 'NONE',  ( 17.20831665107776587, 24.13393115100078035, -7.208316651077762316 ) ) ;
#54897=CARTESIAN_POINT ( 'NONE',  ( 20.24186590665277308, 56.76028685723173339, 6.114288769123047196 ) ) ;
#54899=CARTESIAN_POINT ( 'NONE',  ( 17.20831665107776587, 29.13393115100078390, -7.208316651077762316 ) ) ;
#54900=CARTESIAN_POINT ( 'NONE',  ( 17.20831665107776587, 2.883931151000785231, 7.208316651077764980 ) ) ;
#54902=CARTESIAN_POINT ( 'NONE',  ( 2.791683348922240793, 46.63393115100077324, 7.208316651077764092 ) ) ;
#54905=CARTESIAN_POINT ( 'NONE',  ( 21.09922568453595559, 27.04030133659708568, -6.408140936763230044 ) ) ;
#54909=CARTESIAN_POINT ( 'NONE',  ( 20.36894250292379738, 49.92874883491396787, -10.36894250292379027 ) ) ;
#54910=CARTESIAN_POINT ( 'NONE',  ( 18.52753015748617571, 3.092264484334118269, 4.923371831947298993 ) ) ;
#54911=CARTESIAN_POINT ( 'NONE',  ( -46.93999999999902428, 100.4992020706143023, 9.114648421618825935 ) ) ;
#54913=CARTESIAN_POINT ( 'NONE',  ( 24.16423886937410614, 49.30374883491396787, 8.672049930838204340E-16 ) ) ;
#54914=CARTESIAN_POINT ( 'NONE',  ( 22.26659068614894466, 63.88708216824730357, 7.082119434687054849 ) ) ;
#54915=CARTESIAN_POINT ( 'NONE',  ( -4.164238869374099039, 16.80374883491396787, 8.674139862899312516E-16 ) ) ;
#54916=CARTESIAN_POINT ( 'NONE',  ( 2.917880565312948704, 32.63708216824730357, 12.26659068614894643 ) ) ;
#54919=CARTESIAN_POINT ( 'NONE',  ( 19.84674366389459266, 38.30059781766745175, 2.638427012816836559 ) ) ;
#54921=CARTESIAN_POINT ( 'NONE',  ( 19.42250999205614193, 35.14701867748816966, 5.440088680355555262 ) ) ;
#54924=CARTESIAN_POINT ( 'NONE',  ( 0.1532563361054083140, 41.00893115100078745, 1.131784320476157264E-15 ) ) ;
#54925=CARTESIAN_POINT ( 'NONE',  ( 3.591859063236761518, 59.95696800326375353, 11.09922568453594849 ) ) ;
#54927=CARTESIAN_POINT ( 'NONE',  ( 19.84674366389459621, 38.50893115100078745, 7.409399052514197653E-17 ) ) ;
#54928=CARTESIAN_POINT ( 'NONE',  ( 7.361572987183170547, 62.05059781766745886, 9.846743663894590881 ) ) ;
#54930=CARTESIAN_POINT ( 'NONE',  ( 13.79529636645030344, 8.262082168247300018, 14.16423886937410614 ) ) ;
#54934=CARTESIAN_POINT ( 'NONE',  ( 19.42250999205614548, 5.980352010821504471, -5.440088680355545492 ) ) ;
#54935=CARTESIAN_POINT ( 'NONE',  ( 0.6178305044545818747, 8.498634669930421381, -9.382169495545419124 ) ) ;
#54937=CARTESIAN_POINT ( 'NONE',  ( 2.035157376598822676, 62.43868534415483396, -7.964842623401177768 ) ) ;
#54938=CARTESIAN_POINT ( 'NONE',  ( 20.32896413005680003, 41.77164270246083788, 5.963430220938287007 ) ) ;
#54939=CARTESIAN_POINT ( 'NONE',  ( 2.603489959281581889, 30.43575266056827999, -6.499999999999995559 ) ) ;
#54942=CARTESIAN_POINT ( 'NONE',  ( 13.79529636645030344, 63.26208216824730357, 14.16423886937410614 ) ) ;
#54944=CARTESIAN_POINT ( 'NONE',  ( 19.42250999205614193, 25.14701867748817321, 5.440088680355555262 ) ) ;
#54945=CARTESIAN_POINT ( 'NONE',  ( 0.5774900079438607392, 43.48035201082151247, 5.440088680355550821 ) ) ;
#54946=CARTESIAN_POINT ( 'NONE',  ( 13.43411237798105340, 0.5819680032637533085, 12.81628187352647963 ) ) ;
#54947=CARTESIAN_POINT ( 'NONE',  ( 7.361572987183170547, 57.05059781766744464, 9.846743663894590881 ) ) ;
#54948=CARTESIAN_POINT ( 'NONE',  ( 6.565887622018943937, 63.08196800326376064, -12.81628187352647608 ) ) ;
#54949=CARTESIAN_POINT ( 'NONE',  ( 14.92337183194729633, 2.675597817667451750, 8.527530157486181039 ) ) ;
#54950=ORIENTED_EDGE ( 'NONE', *, *, #69949, .T. ) ;
#54952=CARTESIAN_POINT ( 'NONE',  ( 17.96484262340118221, 34.93868534415482685, 7.964842623401181321 ) ) ;
#54953=CARTESIAN_POINT ( 'NONE',  ( 6.565887622018943937, 35.16530133659708923, 12.81628187352647430 ) ) ;
#54955=CARTESIAN_POINT ( 'NONE',  ( 0.1532563361054082862, 56.21726448433411605, 2.638427012816831674 ) ) ;
#54956=CARTESIAN_POINT ( 'NONE',  ( 0.5774900079438607392, 53.48035201082151247, 5.440088680355550821 ) ) ;
#54957=CARTESIAN_POINT ( 'NONE',  ( 19.38216949554541557, 32.24863466993041783, -9.382169495545420901 ) ) ;
#54958=CARTESIAN_POINT ( 'NONE',  ( 17.96484262340118221, 56.18868534415484817, -7.964842623401177768 ) ) ;
#54959=CARTESIAN_POINT ( 'NONE',  ( 20.88017736071110164, 15.35535201082150181, 2.915334737309930979 ) ) ;
#54960=CARTESIAN_POINT ( 'NONE',  ( 16.40814093676324603, 62.45696800326376064, -11.09922568453594671 ) ) ;
#54964=CARTESIAN_POINT ( 'NONE',  ( 7.084665262690076126, 2.022018677488170990, -10.88017736071110164 ) ) ;
#54965=CARTESIAN_POINT ( 'NONE',  ( 21.09922568453594849, 51.20696800326375353, 6.408140936763242479 ) ) ;
#54966=CARTESIAN_POINT ( 'NONE',  ( -0.3689425029237881626, 12.42874883491396609, 10.36894250292379027 ) ) ;
#54967=CARTESIAN_POINT ( 'NONE',  ( 10.00000000000000178, 12.25893115100078568, 9.846743663894594434 ) ) ;
#54968=CARTESIAN_POINT ( 'NONE',  ( 7.084665262690076126, 12.02201867748817143, -10.88017736071110164 ) ) ;
#54969=CARTESIAN_POINT ( 'NONE',  ( 18.52753015748618282, 23.92559781766745530, -4.923371831947291888 ) ) ;
#54971=CARTESIAN_POINT ( 'NONE',  ( 6.204703633549690345, 52.84541550158062506, 14.16423886937410082 ) ) ;
#54972=ORIENTED_EDGE ( 'NONE', *, *, #61523, .T. ) ;
#54973=SURFACE_STYLE_USAGE ( .BOTH. , #62974 ) ;
#54974=CARTESIAN_POINT ( 'NONE',  ( 10.00000000000000178, 4.313685344154837509, 10.88017736071110342 ) ) ;
#54978=CARTESIAN_POINT ( 'NONE',  ( 4.559911319644449179, 12.23035201082150714, -9.422509992056141925 ) ) ;
#54979=CARTESIAN_POINT ( 'NONE',  ( 4.559911319644449179, 8.897018677488173211, 9.422509992056141925 ) ) ;
#54980=EDGE_CURVE ( 'NONE', #96981, #76186, #5845, .T. ) ;
#54981=CARTESIAN_POINT ( 'NONE',  ( 14.92337183194729988, 39.34226448433412315, -8.527530157486177487 ) ) ;
#54982=CARTESIAN_POINT ( 'NONE',  ( 13.43411237798106583, 47.66530133659709634, -12.81628187352647252 ) ) ;
#54983=FILL_AREA_STYLE ('',( #62486 ) ) ;
#54985=CARTESIAN_POINT ( 'NONE',  ( 2.917880565312950480, 20.97041550158063217, -12.26659068614894821 ) ) ;
#54986=CARTESIAN_POINT ( 'NONE',  ( 15.44008868035555793, 21.39701867748817321, -9.422509992056140149 ) ) ;
#54987=CARTESIAN_POINT ( 'NONE',  ( 13.79529636645031943, 65.34541550158063217, -14.16423886937409904 ) ) ;
#54988=CARTESIAN_POINT ( 'NONE',  ( 1.472469842513823179, 61.42559781766745175, 4.923371831947296329 ) ) ;
#54991=CARTESIAN_POINT ( 'NONE',  ( 5.076628168052704559, 40.17559781766745175, -8.527530157486179263 ) ) ;
#54993=CARTESIAN_POINT ( 'NONE',  ( -0.8801773607111009756, 33.06368534415484106, 1.068504757029289695E-15 ) ) ;
#54996=SURFACE_STYLE_FILL_AREA ( #69529 ) ;
#54997=CARTESIAN_POINT ( 'NONE',  ( 7.084665262690076126, 64.10535201082150536, 10.88017736071109987 ) ) ;
#54998=CARTESIAN_POINT ( 'NONE',  ( 0.1532563361054100626, 60.80059781766744464, -2.638427012816831230 ) ) ;
#54999=CARTESIAN_POINT ( 'NONE',  ( 2.035157376598822676, 52.43868534415483396, -7.964842623401177768 ) ) ;
#55000=CARTESIAN_POINT ( 'NONE',  ( 19.42250999205614193, 45.14701867748817676, 5.440088680355555262 ) ) ;
#55001=CARTESIAN_POINT ( 'NONE',  ( 10.00000000000000000, 11.81368534415483751, -10.88017736071110342 ) ) ;
#55002=CARTESIAN_POINT ( 'NONE',  ( 22.81628187352648496, 46.83196800326376064, -3.434112377981050290 ) ) ;
#55003=CARTESIAN_POINT ( 'NONE',  ( 17.08211943468705840, 20.13708216824730357, -12.26659068614894466 ) ) ;
#55006=CARTESIAN_POINT ( 'NONE',  ( 22.81628187352647785, 51.62363466993042493, 6.195893100308588602E-16 ) ) ;
#55008=CARTESIAN_POINT ( 'NONE',  ( 5.076628168052703671, 61.84226448433412315, 8.527530157486179263 ) ) ;
#55009=CARTESIAN_POINT ( 'NONE',  ( 12.91533473730992121, 19.52201867748816611, 10.88017736071110164 ) ) ;
#55010=CARTESIAN_POINT ( 'NONE',  ( -0.8801773607111008646, 33.27201867748817676, 2.915334737309923430 ) ) ;
#55011=EDGE_CURVE ( 'NONE', #89108, #36460, #11861, .T. ) ;
#55013=CARTESIAN_POINT ( 'NONE',  ( 10.00000000000000000, 9.758931151000785675, -9.846743663894594434 ) ) ;
#55014=CARTESIAN_POINT ( 'NONE',  ( 2.035157376598822676, 2.438685344154837953, -7.964842623401177768 ) ) ;
#55016=CARTESIAN_POINT ( 'NONE',  ( 17.20831665107776587, 12.88393115100078390, 7.208316651077764980 ) ) ;
#55017=CARTESIAN_POINT ( 'NONE',  ( 10.00000000000000178, 64.31368534415483396, 10.88017736071110342 ) ) ;
#55021=CARTESIAN_POINT ( 'NONE',  ( 7.084665262690076126, 62.02201867748816966, -10.88017736071110164 ) ) ;
#55022=CARTESIAN_POINT ( 'NONE',  ( 0.1532563361054100626, 5.800597817667452638, -2.638427012816831230 ) ) ;
#55024=CARTESIAN_POINT ( 'NONE',  ( 7.361572987183169658, 39.96726448433411605, -9.846743663894592657 ) ) ;
#55028=CARTESIAN_POINT ( 'NONE',  ( -4.164238869374098151, 1.595415501580634388, -3.795296366450310543 ) ) ;
#55029=CARTESIAN_POINT ( 'NONE',  ( -1.099225684535947600, 63.70696800326376774, -6.408140936763238038 ) ) ;
#55030=CARTESIAN_POINT ( 'NONE',  ( 13.79529636645031943, 10.34541550158063394, -14.16423886937409904 ) ) ;
#55031=CARTESIAN_POINT ( 'NONE',  ( -4.164238869374098151, 21.59541550158063217, -3.795296366450310543 ) ) ;
#55033=DIRECTION ( 'NONE',  ( 0.000000000000000000, 0.000000000000000000, -1.000000000000000000 ) ) ;
#55034=CARTESIAN_POINT ( 'NONE',  ( 0.5774900079438590739, 57.64701867748817676, -5.440088680355550821 ) ) ;
#55035=CARTESIAN_POINT ( 'NONE',  ( 4.559911319644449179, 18.89701867748817321, 9.422509992056141925 ) ) ;
#55037=ORIENTED_EDGE ( 'NONE', *, *, #78683, .F. ) ;
#55039=CARTESIAN_POINT ( 'NONE',  ( 17.20831665107776587, 7.883931151000784787, 7.208316651077764980 ) ) ;
#55040=CARTESIAN_POINT ( 'NONE',  ( 6.565887622018943937, 28.08196800326375353, -12.81628187352647608 ) ) ;
#55041=CARTESIAN_POINT ( 'NONE',  ( 12.63842701281683034, 42.46726448433412315, 9.846743663894596210 ) ) ;
#55043=CARTESIAN_POINT ( 'NONE',  ( 19.38216949554541557, 22.24863466993041428, -9.382169495545420901 ) ) ;
#55045=CARTESIAN_POINT ( 'NONE',  ( 14.92337183194729633, 27.67559781766745530, 8.527530157486181039 ) ) ;
#55046=CARTESIAN_POINT ( 'NONE',  ( 1.472469842513823179, 0.5922644843341181575, -4.923371831947296329 ) ) ;
#55050=CARTESIAN_POINT ( 'NONE',  ( 19.42250999205614193, 40.14701867748817676, 5.440088680355555262 ) ) ;
#55051=CARTESIAN_POINT ( 'NONE',  ( -2.266590686148945544, 32.22041550158063927, 7.082119434687048631 ) ) ;
#55052=CARTESIAN_POINT ( 'NONE',  ( 19.84674366389459266, 38.71726448433412315, -2.638427012816827677 ) ) ;
#55053=CARTESIAN_POINT ( 'NONE',  ( -0.8801773607110991993, 67.85535201082151957, -2.915334737309923874 ) ) ;
#55054=CARTESIAN_POINT ( 'NONE',  ( 0.6178305044545818747, 48.49863466993042493, -9.382169495545419124 ) ) ;
#55056=CARTESIAN_POINT ( 'NONE',  ( 0.5774900079438607392, 33.48035201082150536, 5.440088680355550821 ) ) ;
#55058=CARTESIAN_POINT ( 'NONE',  ( -2.816281873526471635, 18.91530133659708213, -3.434112377981056508 ) ) ;
#55059=CARTESIAN_POINT ( 'NONE',  ( 22.81628187352648496, 16.83196800326374998, -3.434112377981050290 ) ) ;
#55060=CARTESIAN_POINT ( 'NONE',  ( 7.361572987183169658, 34.96726448433411605, -9.846743663894592657 ) ) ;
#55062=CARTESIAN_POINT ( 'NONE',  ( -2.816281873526473856, 44.33196800326375353, 3.434112377981055619 ) ) ;
#55064=CARTESIAN_POINT ( 'NONE',  ( 17.96484262340118221, 51.18868534415483396, -7.964842623401177768 ) ) ;
#55066=ADVANCED_FACE ( 'NONE', ( #84721 ), #64848, .F. ) ;
#55068=FACE_OUTER_BOUND ( 'NONE', #79359, .T. ) ;
#55069=CARTESIAN_POINT ( 'NONE',  ( 19.42250999205614548, 50.98035201082151247, -5.440088680355545492 ) ) ;
#55070=CARTESIAN_POINT ( 'NONE',  ( 12.91533473730993009, 61.60535201082150536, -10.88017736071109987 ) ) ;
#55074=CARTESIAN_POINT ( 'NONE',  ( 0.5774900079438590739, 12.64701867748817321, -5.440088680355550821 ) ) ;
#55075=CARTESIAN_POINT ( 'NONE',  ( 19.84674366389459621, 53.50893115100078745, 7.409399052514197653E-17 ) ) ;
#55076=CARTESIAN_POINT ( 'NONE',  ( 10.00000000000000178, 24.31368534415484106, 10.88017736071110342 ) ) ;
#55077=DIRECTION ( 'NONE',  ( 1.000000000000000000, 0.000000000000000000, -0.000000000000000000 ) ) ;
#55078=CARTESIAN_POINT ( 'NONE',  ( 21.09922568453594849, 21.20696800326375353, 6.408140936763242479 ) ) ;
#55080=CARTESIAN_POINT ( 'NONE',  ( 10.00000000000000000, 31.81368534415483751, -10.88017736071110342 ) ) ;
#55081=CARTESIAN_POINT ( 'NONE',  ( 3.591859063236763294, 8.290301336597087456, -11.09922568453595026 ) ) ;
#55083=CARTESIAN_POINT ( 'NONE',  ( 0.5774900079438607392, 18.48035201082150536, 5.440088680355550821 ) ) ;
#55084=CARTESIAN_POINT ( 'NONE',  ( 12.91533473730993009, 41.60535201082149825, -10.88017736071109987 ) ) ;
#55085=CARTESIAN_POINT ( 'NONE',  ( 13.79529636645031943, 45.34541550158062506, -14.16423886937409904 ) ) ;
#55086=CARTESIAN_POINT ( 'NONE',  ( 10.00000000000000178, 42.25893115100078745, 9.846743663894594434 ) ) ;
#55087=CARTESIAN_POINT ( 'NONE',  ( 12.91533473730992121, 59.52201867748816966, 10.88017736071110164 ) ) ;
#55089=CARTESIAN_POINT ( 'NONE',  ( -0.3689425029237881626, 22.42874883491397142, 10.36894250292379027 ) ) ;
#55090=UNCERTAINTY_MEASURE_WITH_UNIT (LENGTH_MEASURE( 1.000000000000000082E-05 ), #4591, 'distance_accuracy_value', 'NONE');
#55094=CARTESIAN_POINT ( 'NONE',  ( 24.16423886937410614, 39.51208216824731068, -3.795296366450302550 ) ) ;
#55095=CARTESIAN_POINT ( 'NONE',  ( -0.3689425029237898834, 41.17874883491397497, -10.36894250292378850 ) ) ;
#55097=CARTESIAN_POINT ( 'NONE',  ( 7.361572987183170547, 2.050597817667451750, 9.846743663894590881 ) ) ;
#55098=CARTESIAN_POINT ( 'NONE',  ( 10.00000000000000000, 59.75893115100078745, -9.846743663894594434 ) ) ;
#55100=CARTESIAN_POINT ( 'NONE',  ( -0.8801773607111009756, 63.06368534415484106, 1.068504757029289695E-15 ) ) ;
#55101=CARTESIAN_POINT ( 'NONE',  ( 13.43411237798105340, 35.58196800326375353, 12.81628187352647963 ) ) ;
#55102=CARTESIAN_POINT ( 'NONE',  ( 10.00000000000000178, 28.05374883491396787, 14.16423886937410082 ) ) ;
#55103=CARTESIAN_POINT ( 'NONE',  ( 7.084665262690076126, 22.02201867748817321, -10.88017736071110164 ) ) ;
#55104=ADVANCED_FACE ( 'NONE', ( #60236 ), #83451, .T. ) ;
#55106=CARTESIAN_POINT ( 'NONE',  ( 0.1532563361054082862, 1.217264484334117824, 2.638427012816831674 ) ) ;
#55110=DIRECTION ( 'NONE',  ( 0.000000000000000000, -1.000000000000000000, 0.000000000000000000 ) ) ;
#55113=CARTESIAN_POINT ( 'NONE',  ( -4.164238869374099039, 6.803748834913967869, 8.674139862899312516E-16 ) ) ;
#55114=CARTESIAN_POINT ( 'NONE',  ( 2.917880565312948704, 67.63708216824730357, 12.26659068614894643 ) ) ;
#55115=CARTESIAN_POINT ( 'NONE',  ( 19.42250999205614548, 15.98035201082150714, -5.440088680355545492 ) ) ;
#55116=CARTESIAN_POINT ( 'NONE',  ( 10.00000000000000178, 37.25893115100078745, 9.846743663894594434 ) ) ;
#55117=CARTESIAN_POINT ( 'NONE',  ( 0.1532563361054100626, 60.80059781766744464, -2.638427012816831230 ) ) ;
#55120=B_SPLINE_CURVE_WITH_KNOTS ( 'NONE', 3,
 ( #40707, #86701, #16240, #71694 ),
 .UNSPECIFIED., .F., .F.,
 ( 4, 4 ),
 ( 5.444379262168902198E-17, 0.002562518741975294313 ),
 .UNSPECIFIED. ) ;
#55122=CARTESIAN_POINT ( 'NONE',  ( 0.6178305044545818747, 8.498634669930421381, -9.382169495545419124 ) ) ;
#55124=CARTESIAN_POINT ( 'NONE',  ( -4.164238869374099039, 41.80374883491397497, 8.674139862899312516E-16 ) ) ;
#55126=CARTESIAN_POINT ( 'NONE',  ( 2.917880565312950480, 50.97041550158064638, -12.26659068614894821 ) ) ;
#55128=CARTESIAN_POINT ( 'NONE',  ( 2.035157376598822676, 22.43868534415483396, -7.964842623401177768 ) ) ;
#55131=CARTESIAN_POINT ( 'NONE',  ( 10.00000000000000000, 31.81368534415483751, -10.88017736071110342 ) ) ;
#55132=CARTESIAN_POINT ( 'NONE',  ( 1.472469842513823179, 55.59226448433412315, -4.923371831947296329 ) ) ;
#55133=CARTESIAN_POINT ( 'NONE',  ( 7.084665262690076126, 39.10535201082150536, 10.88017736071109987 ) ) ;
#55134=CARTESIAN_POINT ( 'NONE',  ( 2.035157376598824452, 68.68868534415484817, 7.964842623401179544 ) ) ;
#55135=CARTESIAN_POINT ( 'NONE',  ( -0.8801773607111008646, 28.27201867748817321, 2.915334737309923430 ) ) ;
#55137=FACE_OUTER_BOUND ( 'NONE', #3846, .T. ) ;
#55139=( NAMED_UNIT ( * ) PLANE_ANGLE_UNIT ( ) SI_UNIT ( $, .RADIAN. ) );
#55143=CARTESIAN_POINT ( 'NONE',  ( 1.472469842513823179, 46.42559781766745175, 4.923371831947296329 ) ) ;
#55145=CARTESIAN_POINT ( 'NONE',  ( 3.591859063236763294, 48.29030133659708923, -11.09922568453595026 ) ) ;
#55146=FILL_AREA_STYLE ('',( #39187 ) ) ;
#55151=CARTESIAN_POINT ( 'NONE',  ( 10.00000000000000000, 49.75893115100078745, -9.846743663894594434 ) ) ;
#55152=CARTESIAN_POINT ( 'NONE',  ( 17.08211943468705130, 43.47041550158063927, 12.26659068614894998 ) ) ;
#55153=CARTESIAN_POINT ( 'NONE',  ( 5.076628168052703671, 61.84226448433412315, 8.527530157486179263 ) ) ;
#55154=ORIENTED_EDGE ( 'NONE', *, *, #76610, .F. ) ;
#55156=CARTESIAN_POINT ( 'NONE',  ( 0.1532563361054100626, 15.80059781766745353, -2.638427012816831230 ) ) ;
#55157=CARTESIAN_POINT ( 'NONE',  ( 6.565887622018943937, 55.16530133659709634, 12.81628187352647430 ) ) ;
#55159=CARTESIAN_POINT ( 'NONE',  ( 10.00000000000000178, 57.25893115100078745, 9.846743663894594434 ) ) ;
#55160=CARTESIAN_POINT ( 'NONE',  ( 12.91533473730992121, 54.52201867748816255, 10.88017736071110164 ) ) ;
#55164=CARTESIAN_POINT ( 'NONE',  ( 17.08211943468705130, 63.47041550158063927, 12.26659068614894998 ) ) ;
#55165=( LENGTH_UNIT ( ) NAMED_UNIT ( * ) SI_UNIT ( .MILLI., .METRE. ) );
#55166=CARTESIAN_POINT ( 'NONE',  ( 7.084665262690076126, 34.10535201082151247, 10.88017736071109987 ) ) ;
#55167=CARTESIAN_POINT ( 'NONE',  ( 21.09922568453594849, 16.20696800326375353, 6.408140936763242479 ) ) ;
#55168=CARTESIAN_POINT ( 'NONE',  ( 10.00000000000000000, 56.81368534415484106, -10.88017736071110342 ) ) ;
#55172=CARTESIAN_POINT ( 'NONE',  ( 2.035157376598822676, 57.43868534415484106, -7.964842623401177768 ) ) ;
#55173=CARTESIAN_POINT ( 'NONE',  ( 1.821158202401517601, 11.16688879859523276, 6.499999999999976019 ) ) ;
#55174=CARTESIAN_POINT ( 'NONE',  ( 5.076628168052704559, 55.17559781766745175, -8.527530157486179263 ) ) ;
#55175=( LENGTH_UNIT ( ) NAMED_UNIT ( * ) SI_UNIT ( .MILLI., .METRE. ) );
#55177=CARTESIAN_POINT ( 'NONE',  ( 22.81628187352647785, 11.62363466993042138, 6.195893100308588602E-16 ) ) ;
#55178=CARTESIAN_POINT ( 'NONE',  ( -0.8801773607111009756, 13.06368534415483929, 1.068504757029289695E-15 ) ) ;
#55180=CARTESIAN_POINT ( 'NONE',  ( -2.266590686148945544, 37.22041550158063217, 7.082119434687048631 ) ) ;
#55181=ADVANCED_FACE ( 'NONE', ( #87185 ), #93706, .T. ) ;
#55182=CARTESIAN_POINT ( 'NONE',  ( 24.16423886937410614, 24.51208216824730002, -3.795296366450302550 ) ) ;
#55183=CARTESIAN_POINT ( 'NONE',  ( 0.5774900079438607392, 3.480352010821504916, 5.440088680355550821 ) ) ;
#55184=VECTOR ( 'NONE', #78597, 1000.000000000000000 ) ;
#55185=CARTESIAN_POINT ( 'NONE',  ( 14.92337183194729988, 29.34226448433411960, -8.527530157486177487 ) ) ;
#55186=CARTESIAN_POINT ( 'NONE',  ( 18.52753015748618282, 18.92559781766745175, -4.923371831947291888 ) ) ;
#55187=CARTESIAN_POINT ( 'NONE',  ( 20.88017736071110519, 15.56368534415483751, 2.639326808657452039E-16 ) ) ;
#55189=ORIENTED_EDGE ( 'NONE', *, *, #41267, .F. ) ;
#55190=CARTESIAN_POINT ( 'NONE',  ( 7.361572987183170547, 37.05059781766744464, 9.846743663894590881 ) ) ;
#55191=CARTESIAN_POINT ( 'NONE',  ( 7.084665262690076126, 34.10535201082151247, 10.88017736071109987 ) ) ;
#55192=CARTESIAN_POINT ( 'NONE',  ( 18.52753015748618282, 58.92559781766745886, -4.923371831947291888 ) ) ;
#55193=CARTESIAN_POINT ( 'NONE',  ( -4.164238869374099927, 22.01208216824730357, 3.795296366450308767 ) ) ;
#55196=COLOUR_RGB ( '', 0.66274510, 0.83137255, 0.94901961) ;
#55197=UNCERTAINTY_MEASURE_WITH_UNIT (LENGTH_MEASURE( 1.000000000000000082E-05 ), #63724, 'distance_accuracy_value', 'NONE');
#55198=( BOUNDED_SURFACE ( )  B_SPLINE_SURFACE ( 1, 2, ( 
 ( #35849, #58841, #95371, #66337, #65351, #95879, #20858, #13348, #27360, #57853, #359, #14347, #90315, #38335, #91817, #75823, #44328, #53315, #98361, #8320, #837, #30311, #21853, #76318, #52820, #52333, #91311, #30808, #14854, #45326, #31297, #38824, #15348, #82827, #7836, #45832, #36846, #7345, #83823, #13849, #69315, #59821, #74832, #51841, #15830, #82328, #29324, #22840, #60812, #68828, #44818, #75325, #6838, #37845, #53818, #67843, #90818, #61306, #83328, #6336, #67336, #37352, #29819, #60328, #22348, #84330, #23338, #68336, #98857, #61797, #46317, #92305, #76803, #97861, #40788, #70803, #54295, #46799, #48761, #62286, #55791, #9297, #92790, #25788, #17794, #69813, #8804, #32773, #78783, #10778, #79268, #71768, #85301, #56283, #32277, #94262, #55285, #85794, #62785, #86779, #41294, #1336, #10290, #3278, #33742, #18282, #84810, #93777, #93284, #16316, #78281, #64243, #24808, #63268, #23832, #33264, #17307, #77292, #2320, #24319, #86286, #48269, #71287, #39317, #9796, #54785, #63756, #40295, #31787, #16808, #25304, #47283, #77785, #47784, #2811, #39807, #70308, #1824, #96253, #73723, #95243, #43724, #74210, #66221, #18778, #34235, #5254, #4264, #13227, #20738, #72731, #65228, #35732, #51231, #27238, #28226, #26750, #49260, #96751, #88730, #34737, #36229, #80744, #35229, #12732, #57245, #95754, #57733, #49739, #58725, #81715, #64731, #11259, #88237, #87253, #26261, #50230, #19745, #27732, #12239, #87742, #20242, #5740, #42749, #42262, #94761, #19254, #56759, #79760, #80246, #73230, #11753, #4758, #89229, #41777, #72247, #50745, #58214, #3781, #65727, #81233, #43229, #82216, #76687, #52706, #60208, #60695, #29699, #44211, #14734, #84213, #91194, #98240, #90703, #22231, #37721, #237, #83213, #83708, #13726, #45210, #30685, #59212, #68225, #75708, #52219, #7222, #15226, #29212, #6231, #53203, #7723, #98745, #89717, #30194, #14231, #23219, #15719, #22720, #36734, #45705, #67726, #67225, #76206, #38220, #68705, #61193, #46204, #53692, #91701, #97748, #8208, #66728, #51734, #97252, #28722, #21231, #74719, #59711, #90207, #21737, #82713, #44710, #75209, #6720, #37236, #55670, #77178, #1217, #31672, #93162, #40670, #54664, #77666, #63153, #39199, #55159, #94146, #38703, #78666, #25673, #79146, #47161, #24687, #10172, #62164, #2692, #86170, #69686, #33144, #93656, #56167, #9180, #92669, #92192, #86659, #39697, #69202, #726, #8685, #32158, #31182, #24197, #85180, #17679, #17192, #71168, #16691, #70185, #40174, #1702, #47672, #78167, #9676, #25191, #18164, #48642, #61672, #62660, #63638, #85673, #23718, #70678, #2199, #32660 ),
 ( #48153, #54177, #84689, #16199, #46681, #26152, #20620, #95631, #4148, #4643, #72613, #87131, #57618, #28107, #35107, #42148, #34613, #65108, #80629, #43113, #27119, #27614, #56646, #88117, #73602, #3164, #12125, #19626, #95122, #50119, #58100, #72129, #49142, #96133, #50620, #42626, #33626, #73104, #57127, #66101, #58607, #65606, #79643, #88607, #11632, #11142, #20117, #81111, #12612, #5127, #89109, #96630, #35615, #41661, #51110, #10658, #94642, #41172, #71655, #64125, #18654, #3656, #34121, #64613, #26629, #87624, #19138, #49615, #80125, #98625, #21113, #44088, #74597, #37110, #83590, #97627, #21616, #7101, #82096, #98113, #38102, #81597, #22602, #68590, #23099, #90089, #67606, #53079, #6111, #45583, #30074, #13607, #76078, #37603, #120, #52102, #36616, #36102, #30567, #82594, #13109, #43604, #51613, #75091, #74091, #67103, #29091, #75589, #45084, #61071, #59590, #68098, #59095, #97136, #91583, #29575, #6597, #60583, #44593, #89604, #60079, #5625, #91075, #14109, #90580, #22106, #52586, #15106, #83089, #7607, #28606, #14618, #66608, #46081, #24579, #16574, #39078, #32037, #2082, #16076, #92069, #40055, #93539, #77545, #76569, #55040, #1092, #10055, #2577, #62540, #23597, #78050, #54546, #54061, #93046, #32542, #47049, #9064, #33033, #40554, #17070, #84575, #9553, #47553, #38583, #39576, #85558, #15598, #71054, #61561, #8087, #53570, #17566, #84083, #31062, #70554, #63042, #25070, #46562, #77063, #8574, #70065, #55553, #69572, #92551, #86054, #31553, #1588, #63529, #69081, #48031, #94037, #616, #62049, #78544, #24079, #85063, #88501, #42514, #26042, #20004, #80517, #81002, #34007, #56533, #79028, #43003, #95009, #65992, #25558, #64011, #19029, #56051, #18534, #49025, #72998, #4036, #57995, #79531, #41551, #27010, #11031, #34499, #64990, #12504, #94523, #86542, #50504, #87022, #57014, #72017, #3547, #65497, #10540, #3059, #96017, #73487, #18049, #64503, #80013, #27500, #26517, #5014, #4528, #87516, #35497, #12015, #48526, #49506, #11516, #41050, #71549, #42040, #33514, #72504, #95517, #57508, #88005, #19516, #50013, #34992, #74977, #29959, #89492, #13495, #98006, #21001, #6482, #36987, #83470, #66491, #37985, #22486, #97018, #28973, #28495, #58988, #37490, #50992, #73987, #90460, #59967, #14991, #35989, #52471, #5512, #12990, #7489, #82480, #89977, #21996, #59476, #51489, #44477, #45462, #82976, #21494, #51991, #13999, #67484, #60465, #29459, #14496, #43486, #44967, #90953, #89000, #75470, #6986, #81984, #67979, #98505, #43974, #74476, #52959, #75961, #96519, #20506, #27992, #6001, #58488, #81487, #36495, #66987, #97509 ) ),
 .UNSPECIFIED., .F., .F., .F. ) 
 B_SPLINE_SURFACE_WITH_KNOTS ( ( 2, 2 ),
 ( 3, 2, 2, 2, 2, 2, 2, 2, 2, 2, 2, 2, 2, 2, 2, 2, 2, 2, 2, 2, 2, 2, 2, 2, 2, 2, 2, 2, 2, 2, 2, 2, 2, 2, 2, 2, 2, 2, 2, 2, 2, 2, 2, 2, 2, 2, 2, 2, 2, 2, 2, 2, 2, 2, 2, 2, 2, 2, 2, 2, 2, 2, 2, 2, 2, 2, 2, 2, 2, 2, 2, 2, 2, 2, 2, 2, 2, 2, 2, 2, 2, 2, 2, 2, 2, 2, 2, 2, 2, 2, 2, 2, 2, 2, 2, 2, 2, 2, 2, 2, 2, 2, 2, 2, 2, 2, 2, 2, 2, 2, 2, 2, 2, 2, 2, 2, 2, 2, 2, 2, 2, 2, 2, 2, 2, 2, 2, 2, 2, 2, 2, 2, 2, 2, 2, 2, 2, 2, 2, 2, 2, 2, 2, 2, 2, 2, 2, 2, 2, 2, 2, 2, 2, 2, 2, 2, 2, 2, 2, 2, 2, 2, 3 ),
 ( 0.000000000000000000, 1.000000000000000000 ),
 ( 0.000000000000000000, 0.005952380952380952051, 0.01190476190476190410, 0.01785714285714285615, 0.02380952380952380820, 0.02976190476190476025, 0.03571428571428571230, 0.04166666666666666435, 0.04761904761904761640, 0.05357142857142856845, 0.05952380952380952051, 0.06547619047619047949, 0.07142857142857142461, 0.07738095238095238360, 0.08333333333333332871, 0.08928571428571428770, 0.09523809523809523281, 0.1011904761904761918, 0.1071428571428571369, 0.1130952380952380959, 0.1190476190476190410, 0.1250000000000000000, 0.1309523809523809590, 0.1369047619047619180, 0.1428571428571428492, 0.1488095238095238082, 0.1547619047619047672, 0.1607142857142857262, 0.1666666666666666574, 0.1726190476190476164, 0.1785714285714285754, 0.1845238095238095344, 0.1904761904761904656, 0.1964285714285714246, 0.2023809523809523836, 0.2083333333333333426, 0.2142857142857142738, 0.2202380952380952328, 0.2261904761904761918, 0.2321428571428571508, 0.2380952380952380820, 0.2440476190476190410, 0.2500000000000000000, 0.2559523809523809312, 0.2619047619047619180, 0.2678571428571428492, 0.2738095238095238360, 0.2797619047619047672, 0.2857142857142856984, 0.2916666666666666852, 0.2976190476190476164, 0.3035714285714285476, 0.3095238095238095344, 0.3154761904761904656, 0.3214285714285714524, 0.3273809523809523836, 0.3333333333333333148, 0.3392857142857143016, 0.3452380952380952328, 0.3511904761904761640, 0.3571428571428571508, 0.3630952380952380820, 0.3690476190476190688, 0.3750000000000000000, 0.3809523809523809312, 0.3869047619047619180, 0.3928571428571428492, 0.3988095238095238360, 0.4047619047619047672, 0.4107142857142856984, 0.4166666666666666852, 0.4226190476190476164, 0.4285714285714285476, 0.4345238095238095344, 0.4404761904761904656, 0.4464285714285714524, 0.4523809523809523836, 0.4583333333333333148, 0.4642857142857143016, 0.4702380952380952328, 0.4761904761904761640, 0.4821428571428571508, 0.4880952380952380820, 0.4940476190476190688, 0.5000000000000000000, 0.5059523809523809312, 0.5119047619047618625, 0.5178571428571429047, 0.5238095238095238360, 0.5297619047619047672, 0.5357142857142856984, 0.5416666666666666297, 0.5476190476190476719, 0.5535714285714286031, 0.5595238095238095344, 0.5654761904761904656, 0.5714285714285713969, 0.5773809523809523281, 0.5833333333333333703, 0.5892857142857143016, 0.5952380952380952328, 0.6011904761904761640, 0.6071428571428570953, 0.6130952380952381375, 0.6190476190476190688, 0.6250000000000000000, 0.6309523809523809312, 0.6369047619047618625, 0.6428571428571429047, 0.6488095238095238360, 0.6547619047619047672, 0.6607142857142856984, 0.6666666666666666297, 0.6726190476190476719, 0.6785714285714286031, 0.6845238095238095344, 0.6904761904761904656, 0.6964285714285713969, 0.7023809523809523281, 0.7083333333333333703, 0.7142857142857143016, 0.7202380952380952328, 0.7261904761904761640, 0.7321428571428570953, 0.7380952380952381375, 0.7440476190476190688, 0.7500000000000000000, 0.7559523809523809312, 0.7619047619047618625, 0.7678571428571429047, 0.7738095238095238360, 0.7797619047619047672, 0.7857142857142856984, 0.7916666666666666297, 0.7976190476190476719, 0.8035714285714286031, 0.8095238095238095344, 0.8154761904761904656, 0.8214285714285713969, 0.8273809523809523281, 0.8333333333333333703, 0.8392857142857143016, 0.8452380952380952328, 0.8511904761904761640, 0.8571428571428570953, 0.8630952380952381375, 0.8690476190476190688, 0.8750000000000000000, 0.8809523809523809312, 0.8869047619047618625, 0.8928571428571429047, 0.8988095238095238360, 0.9047619047619047672, 0.9107142857142856984, 0.9166666666666666297, 0.9226190476190476719, 0.9285714285714286031, 0.9345238095238095344, 0.9404761904761904656, 0.9464285714285713969, 0.9523809523809523281, 0.9583333333333333703, 0.9642857142857143016 ),
 .UNSPECIFIED. ) 
 GEOMETRIC_REPRESENTATION_ITEM ( )  RATIONAL_B_SPLINE_SURFACE ( (
 ( 1.000000000000000000, 0.9659258262890683122, 1.000000000000000000, 0.9659258262890683122, 1.000000000000000000, 0.9659258262890683122, 1.000000000000000000, 0.9659258262890683122, 1.000000000000000000, 0.9659258262890683122, 1.000000000000000000, 0.9659258262890683122, 1.000000000000000000, 0.9659258262890683122, 1.000000000000000000, 0.9659258262890683122, 1.000000000000000000, 0.9659258262890683122, 1.000000000000000000, 0.9659258262890683122, 1.000000000000000000, 0.9659258262890683122, 1.000000000000000000, 0.9659258262890683122, 1.000000000000000000, 0.9659258262890683122, 1.000000000000000000, 0.9659258262890683122, 1.000000000000000000, 0.9659258262890683122, 1.000000000000000000, 0.9659258262890683122, 1.000000000000000000, 0.9659258262890683122, 1.000000000000000000, 0.9659258262890683122, 1.000000000000000000, 0.9659258262890683122, 1.000000000000000000, 0.9659258262890683122, 1.000000000000000000, 0.9659258262890683122, 1.000000000000000000, 0.9659258262890683122, 1.000000000000000000, 0.9659258262890683122, 1.000000000000000000, 0.9659258262890683122, 1.000000000000000000, 0.9659258262890683122, 1.000000000000000000, 0.9659258262890683122, 1.000000000000000000, 0.9659258262890683122, 1.000000000000000000, 0.9659258262890683122, 1.000000000000000000, 0.9659258262890683122, 1.000000000000000000, 0.9659258262890683122, 1.000000000000000000, 0.9659258262890683122, 1.000000000000000000, 0.9659258262890683122, 1.000000000000000000, 0.9659258262890683122, 1.000000000000000000, 0.9659258262890683122, 1.000000000000000000, 0.9659258262890683122, 1.000000000000000000, 0.9659258262890683122, 1.000000000000000000, 0.9659258262890683122, 1.000000000000000000, 0.9659258262890683122, 1.000000000000000000, 0.9659258262890683122, 1.000000000000000000, 0.9659258262890683122, 1.000000000000000000, 0.9659258262890683122, 1.000000000000000000, 0.9659258262890683122, 1.000000000000000000, 0.9659258262890683122, 1.000000000000000000, 0.9659258262890683122, 1.000000000000000000, 0.9659258262890683122, 1.000000000000000000, 0.9659258262890683122, 1.000000000000000000, 0.9659258262890683122, 1.000000000000000000, 0.9659258262890683122, 1.000000000000000000, 0.9659258262890683122, 1.000000000000000000, 0.9659258262890683122, 1.000000000000000000, 0.9659258262890683122, 1.000000000000000000, 0.9659258262890683122, 1.000000000000000000, 0.9659258262890683122, 1.000000000000000000, 0.9659258262890683122, 1.000000000000000000, 0.9659258262890683122, 1.000000000000000000, 0.9659258262890683122, 1.000000000000000000, 0.9659258262890683122, 1.000000000000000000, 0.9659258262890683122, 1.000000000000000000, 0.9659258262890683122, 1.000000000000000000, 0.9659258262890683122, 1.000000000000000000, 0.9659258262890683122, 1.000000000000000000, 0.9659258262890683122, 1.000000000000000000, 0.9659258262890683122, 1.000000000000000000, 0.9659258262890683122, 1.000000000000000000, 0.9659258262890683122, 1.000000000000000000, 0.9659258262890683122, 1.000000000000000000, 0.9659258262890683122, 1.000000000000000000, 0.9659258262890683122, 1.000000000000000000, 0.9659258262890683122, 1.000000000000000000, 0.9659258262890683122, 1.000000000000000000, 0.9659258262890683122, 1.000000000000000000, 0.9659258262890683122, 1.000000000000000000, 0.9659258262890683122, 1.000000000000000000, 0.9659258262890683122, 1.000000000000000000, 0.9659258262890683122, 1.000000000000000000, 0.9659258262890683122, 1.000000000000000000, 0.9659258262890683122, 1.000000000000000000, 0.9659258262890683122, 1.000000000000000000, 0.9659258262890683122, 1.000000000000000000, 0.9659258262890683122, 1.000000000000000000, 0.9659258262890683122, 1.000000000000000000, 0.9659258262890683122, 1.000000000000000000, 0.9659258262890683122, 1.000000000000000000, 0.9659258262890683122, 1.000000000000000000, 0.9659258262890683122, 1.000000000000000000, 0.9659258262890683122, 1.000000000000000000, 0.9659258262890683122, 1.000000000000000000, 0.9659258262890683122, 1.000000000000000000, 0.9659258262890683122, 1.000000000000000000, 0.9659258262890683122, 1.000000000000000000, 0.9659258262890683122, 1.000000000000000000, 0.9659258262890683122, 1.000000000000000000, 0.9659258262890683122, 1.000000000000000000, 0.9659258262890683122, 1.000000000000000000, 0.9659258262890683122, 1.000000000000000000, 0.9659258262890683122, 1.000000000000000000, 0.9659258262890683122, 1.000000000000000000, 0.9659258262890683122, 1.000000000000000000, 0.9659258262890683122, 1.000000000000000000, 0.9659258262890683122, 1.000000000000000000, 0.9659258262890683122, 1.000000000000000000, 0.9659258262890683122, 1.000000000000000000, 0.9659258262890683122, 1.000000000000000000, 0.9659258262890683122, 1.000000000000000000, 0.9659258262890683122, 1.000000000000000000, 0.9659258262890683122, 1.000000000000000000, 0.9659258262890683122, 1.000000000000000000, 0.9659258262890683122, 1.000000000000000000, 0.9659258262890683122, 1.000000000000000000, 0.9659258262890683122, 1.000000000000000000, 0.9659258262890683122, 1.000000000000000000, 0.9659258262890683122, 1.000000000000000000, 0.9659258262890683122, 1.000000000000000000, 0.9659258262890683122, 1.000000000000000000, 0.9659258262890683122, 1.000000000000000000, 0.9659258262890683122, 1.000000000000000000, 0.9659258262890683122, 1.000000000000000000, 0.9659258262890683122, 1.000000000000000000, 0.9659258262890683122, 1.000000000000000000, 0.9659258262890683122, 1.000000000000000000, 0.9659258262890683122, 1.000000000000000000, 0.9659258262890683122, 1.000000000000000000, 0.9659258262890683122, 1.000000000000000000, 0.9659258262890683122, 1.000000000000000000, 0.9659258262890683122, 1.000000000000000000, 0.9659258262890683122, 1.000000000000000000, 0.9659258262890683122, 1.000000000000000000, 0.9659258262890683122, 1.000000000000000000, 0.9659258262890683122, 1.000000000000000000, 0.9659258262890683122, 1.000000000000000000, 0.9659258262890683122, 1.000000000000000000, 0.9659258262890683122, 1.000000000000000000, 0.9659258262890683122, 1.000000000000000000, 0.9659258262890683122, 1.000000000000000000, 0.9659258262890683122, 1.000000000000000000, 0.9659258262890683122, 1.000000000000000000, 0.9659258262890683122, 1.000000000000000000, 0.9659258262890683122, 1.000000000000000000, 0.9659258262890683122, 1.000000000000000000, 0.9659258262890683122, 1.000000000000000000, 0.9659258262890683122, 1.000000000000000000, 0.9659258262890683122, 1.000000000000000000, 0.9659258262890683122, 1.000000000000000000, 0.9659258262890683122, 1.000000000000000000, 0.9659258262890683122, 1.000000000000000000, 0.9659258262890683122, 1.000000000000000000, 0.9659258262890683122, 1.000000000000000000, 0.9659258262890683122, 1.000000000000000000, 0.9659258262890683122, 1.000000000000000000, 0.9659258262890683122, 1.000000000000000000, 0.9659258262890683122, 1.000000000000000000, 0.9659258262890683122, 1.000000000000000000, 0.9659258262890683122, 1.000000000000000000, 0.9659258262890683122, 1.000000000000000000, 0.9659258262890683122, 1.000000000000000000, 0.9659258262890683122, 1.000000000000000000, 0.9659258262890683122, 1.000000000000000000, 0.9659258262890683122, 1.000000000000000000, 0.9659258262890683122, 1.000000000000000000, 0.9659258262890683122, 1.000000000000000000, 0.9659258262890683122, 1.000000000000000000, 0.9659258262890683122, 1.000000000000000000),
 ( 1.000000000000000000, 0.9659258262890683122, 1.000000000000000000, 0.9659258262890683122, 1.000000000000000000, 0.9659258262890683122, 1.000000000000000000, 0.9659258262890683122, 1.000000000000000000, 0.9659258262890683122, 1.000000000000000000, 0.9659258262890683122, 1.000000000000000000, 0.9659258262890683122, 1.000000000000000000, 0.9659258262890683122, 1.000000000000000000, 0.9659258262890683122, 1.000000000000000000, 0.9659258262890683122, 1.000000000000000000, 0.9659258262890683122, 1.000000000000000000, 0.9659258262890683122, 1.000000000000000000, 0.9659258262890683122, 1.000000000000000000, 0.9659258262890683122, 1.000000000000000000, 0.9659258262890683122, 1.000000000000000000, 0.9659258262890683122, 1.000000000000000000, 0.9659258262890683122, 1.000000000000000000, 0.9659258262890683122, 1.000000000000000000, 0.9659258262890683122, 1.000000000000000000, 0.9659258262890683122, 1.000000000000000000, 0.9659258262890683122, 1.000000000000000000, 0.9659258262890683122, 1.000000000000000000, 0.9659258262890683122, 1.000000000000000000, 0.9659258262890683122, 1.000000000000000000, 0.9659258262890683122, 1.000000000000000000, 0.9659258262890683122, 1.000000000000000000, 0.9659258262890683122, 1.000000000000000000, 0.9659258262890683122, 1.000000000000000000, 0.9659258262890683122, 1.000000000000000000, 0.9659258262890683122, 1.000000000000000000, 0.9659258262890683122, 1.000000000000000000, 0.9659258262890683122, 1.000000000000000000, 0.9659258262890683122, 1.000000000000000000, 0.9659258262890683122, 1.000000000000000000, 0.9659258262890683122, 1.000000000000000000, 0.9659258262890683122, 1.000000000000000000, 0.9659258262890683122, 1.000000000000000000, 0.9659258262890683122, 1.000000000000000000, 0.9659258262890683122, 1.000000000000000000, 0.9659258262890683122, 1.000000000000000000, 0.9659258262890683122, 1.000000000000000000, 0.9659258262890683122, 1.000000000000000000, 0.9659258262890683122, 1.000000000000000000, 0.9659258262890683122, 1.000000000000000000, 0.9659258262890683122, 1.000000000000000000, 0.9659258262890683122, 1.000000000000000000, 0.9659258262890683122, 1.000000000000000000, 0.9659258262890683122, 1.000000000000000000, 0.9659258262890683122, 1.000000000000000000, 0.9659258262890683122, 1.000000000000000000, 0.9659258262890683122, 1.000000000000000000, 0.9659258262890683122, 1.000000000000000000, 0.9659258262890683122, 1.000000000000000000, 0.9659258262890683122, 1.000000000000000000, 0.9659258262890683122, 1.000000000000000000, 0.9659258262890683122, 1.000000000000000000, 0.9659258262890683122, 1.000000000000000000, 0.9659258262890683122, 1.000000000000000000, 0.9659258262890683122, 1.000000000000000000, 0.9659258262890683122, 1.000000000000000000, 0.9659258262890683122, 1.000000000000000000, 0.9659258262890683122, 1.000000000000000000, 0.9659258262890683122, 1.000000000000000000, 0.9659258262890683122, 1.000000000000000000, 0.9659258262890683122, 1.000000000000000000, 0.9659258262890683122, 1.000000000000000000, 0.9659258262890683122, 1.000000000000000000, 0.9659258262890683122, 1.000000000000000000, 0.9659258262890683122, 1.000000000000000000, 0.9659258262890683122, 1.000000000000000000, 0.9659258262890683122, 1.000000000000000000, 0.9659258262890683122, 1.000000000000000000, 0.9659258262890683122, 1.000000000000000000, 0.9659258262890683122, 1.000000000000000000, 0.9659258262890683122, 1.000000000000000000, 0.9659258262890683122, 1.000000000000000000, 0.9659258262890683122, 1.000000000000000000, 0.9659258262890683122, 1.000000000000000000, 0.9659258262890683122, 1.000000000000000000, 0.9659258262890683122, 1.000000000000000000, 0.9659258262890683122, 1.000000000000000000, 0.9659258262890683122, 1.000000000000000000, 0.9659258262890683122, 1.000000000000000000, 0.9659258262890683122, 1.000000000000000000, 0.9659258262890683122, 1.000000000000000000, 0.9659258262890683122, 1.000000000000000000, 0.9659258262890683122, 1.000000000000000000, 0.9659258262890683122, 1.000000000000000000, 0.9659258262890683122, 1.000000000000000000, 0.9659258262890683122, 1.000000000000000000, 0.9659258262890683122, 1.000000000000000000, 0.9659258262890683122, 1.000000000000000000, 0.9659258262890683122, 1.000000000000000000, 0.9659258262890683122, 1.000000000000000000, 0.9659258262890683122, 1.000000000000000000, 0.9659258262890683122, 1.000000000000000000, 0.9659258262890683122, 1.000000000000000000, 0.9659258262890683122, 1.000000000000000000, 0.9659258262890683122, 1.000000000000000000, 0.9659258262890683122, 1.000000000000000000, 0.9659258262890683122, 1.000000000000000000, 0.9659258262890683122, 1.000000000000000000, 0.9659258262890683122, 1.000000000000000000, 0.9659258262890683122, 1.000000000000000000, 0.9659258262890683122, 1.000000000000000000, 0.9659258262890683122, 1.000000000000000000, 0.9659258262890683122, 1.000000000000000000, 0.9659258262890683122, 1.000000000000000000, 0.9659258262890683122, 1.000000000000000000, 0.9659258262890683122, 1.000000000000000000, 0.9659258262890683122, 1.000000000000000000, 0.9659258262890683122, 1.000000000000000000, 0.9659258262890683122, 1.000000000000000000, 0.9659258262890683122, 1.000000000000000000, 0.9659258262890683122, 1.000000000000000000, 0.9659258262890683122, 1.000000000000000000, 0.9659258262890683122, 1.000000000000000000, 0.9659258262890683122, 1.000000000000000000, 0.9659258262890683122, 1.000000000000000000, 0.9659258262890683122, 1.000000000000000000, 0.9659258262890683122, 1.000000000000000000, 0.9659258262890683122, 1.000000000000000000, 0.9659258262890683122, 1.000000000000000000, 0.9659258262890683122, 1.000000000000000000, 0.9659258262890683122, 1.000000000000000000, 0.9659258262890683122, 1.000000000000000000, 0.9659258262890683122, 1.000000000000000000, 0.9659258262890683122, 1.000000000000000000, 0.9659258262890683122, 1.000000000000000000, 0.9659258262890683122, 1.000000000000000000, 0.9659258262890683122, 1.000000000000000000, 0.9659258262890683122, 1.000000000000000000, 0.9659258262890683122, 1.000000000000000000, 0.9659258262890683122, 1.000000000000000000, 0.9659258262890683122, 1.000000000000000000, 0.9659258262890683122, 1.000000000000000000, 0.9659258262890683122, 1.000000000000000000, 0.9659258262890683122, 1.000000000000000000, 0.9659258262890683122, 1.000000000000000000, 0.9659258262890683122, 1.000000000000000000, 0.9659258262890683122, 1.000000000000000000, 0.9659258262890683122, 1.000000000000000000, 0.9659258262890683122, 1.000000000000000000, 0.9659258262890683122, 1.000000000000000000, 0.9659258262890683122, 1.000000000000000000, 0.9659258262890683122, 1.000000000000000000, 0.9659258262890683122, 1.000000000000000000, 0.9659258262890683122, 1.000000000000000000, 0.9659258262890683122, 1.000000000000000000, 0.9659258262890683122, 1.000000000000000000, 0.9659258262890683122, 1.000000000000000000, 0.9659258262890683122, 1.000000000000000000, 0.9659258262890683122, 1.000000000000000000, 0.9659258262890683122, 1.000000000000000000, 0.9659258262890683122, 1.000000000000000000, 0.9659258262890683122, 1.000000000000000000, 0.9659258262890683122, 1.000000000000000000, 0.9659258262890683122, 1.000000000000000000, 0.9659258262890683122, 1.000000000000000000, 0.9659258262890683122, 1.000000000000000000, 0.9659258262890683122, 1.000000000000000000, 0.9659258262890683122, 1.000000000000000000) ) ) 
 REPRESENTATION_ITEM ( '' )  SURFACE ( )  );
#55199=CARTESIAN_POINT ( 'NONE',  ( 10.00000000000000000, 14.75893115100078568, -9.846743663894594434 ) ) ;
#55200=CARTESIAN_POINT ( 'NONE',  ( 13.43411237798106583, 47.66530133659709634, -12.81628187352647252 ) ) ;
#55201=CARTESIAN_POINT ( 'NONE',  ( 19.84674366389459621, 58.50893115100078745, 7.409399052514197653E-17 ) ) ;
#55202=ORIENTED_EDGE ( 'NONE', *, *, #13781, .F. ) ;
#55205=CARTESIAN_POINT ( 'NONE',  ( -2.266590686148945544, 66.38708216824730357, -7.082119434687050408 ) ) ;
#55206=CARTESIAN_POINT ( 'NONE',  ( -4.164238869374098151, 16.59541550158063927, -3.795296366450310543 ) ) ;
#55207=CARTESIAN_POINT ( 'NONE',  ( -0.8801773607110991993, 62.85535201082150536, -2.915334737309923874 ) ) ;
#55208=CARTESIAN_POINT ( 'NONE',  ( 0.1532563361054100626, 35.80059781766745175, -2.638427012816831230 ) ) ;
#55209=CARTESIAN_POINT ( 'NONE',  ( -0.8801773607111009756, 18.06368534415484106, 1.068504757029289695E-15 ) ) ;
#55211=CARTESIAN_POINT ( 'NONE',  ( 17.20831665107776587, 62.88393115100078745, 7.208316651077764980 ) ) ;
#55212=CARTESIAN_POINT ( 'NONE',  ( 14.92337183194729633, 2.675597817667451750, 8.527530157486181039 ) ) ;
#55213=CARTESIAN_POINT ( 'NONE',  ( 6.565887622018943937, 60.16530133659707502, 12.81628187352647430 ) ) ;
#55219=SURFACE_STYLE_USAGE ( .BOTH. , #33203 ) ;
#55220=EDGE_CURVE ( 'NONE', #85529, #37825, #82858, .T. ) ;
#55221=CARTESIAN_POINT ( 'NONE',  ( -0.3689425029237898834, 41.17874883491397497, -10.36894250292378850 ) ) ;
#55222=CARTESIAN_POINT ( 'NONE',  ( 17.20831665107776587, 37.88393115100078745, 7.208316651077764980 ) ) ;
#55223=CARTESIAN_POINT ( 'NONE',  ( 18.52753015748617571, 23.09226448433411960, 4.923371831947298993 ) ) ;
#55224=DIRECTION ( 'NONE',  ( 0.000000000000000000, 0.000000000000000000, -1.000000000000000000 ) ) ;
#55225=CARTESIAN_POINT ( 'NONE',  ( -0.8801773607111009756, 18.06368534415484106, 1.068504757029289695E-15 ) ) ;
#55226=CARTESIAN_POINT ( 'NONE',  ( 14.92337183194729633, 62.67559781766745886, 8.527530157486181039 ) ) ;
#55228=CARTESIAN_POINT ( 'NONE',  ( 20.36894250292379382, 43.67874883491397497, 10.36894250292379205 ) ) ;
#55229=CARTESIAN_POINT ( 'NONE',  ( 6.204703633549690345, 52.84541550158062506, 14.16423886937410082 ) ) ;
#55230=DIRECTION ( 'NONE',  ( 1.000000000000000000, 0.000000000000000000, 0.000000000000000000 ) ) ;
#55232=CARTESIAN_POINT ( 'NONE',  ( 12.91533473730993009, 61.60535201082150536, -10.88017736071109987 ) ) ;
#55234=CARTESIAN_POINT ( 'NONE',  ( 7.361572987183169658, 9.967264484334119601, -9.846743663894592657 ) ) ;
#55238=VERTEX_POINT ( 'NONE', #73649 ) ;
#55239=CARTESIAN_POINT ( 'NONE',  ( 18.52753015748617571, 8.092264484334117824, 4.923371831947298993 ) ) ;
#55242=CARTESIAN_POINT ( 'NONE',  ( 24.16423886937410614, 24.30374883491396787, 8.672049930838204340E-16 ) ) ;
#55243=CARTESIAN_POINT ( 'NONE',  ( 7.361572987183169658, 14.96726448433411960, -9.846743663894592657 ) ) ;
#55244=CARTESIAN_POINT ( 'NONE',  ( -0.8801773607111009756, 48.06368534415484817, 1.068504757029289695E-15 ) ) ;
#55247=CARTESIAN_POINT ( 'NONE',  ( 10.00000000000000000, 46.81368534415484106, -10.88017736071110342 ) ) ;
#55251=CARTESIAN_POINT ( 'NONE',  ( 0.5774900079438607392, 43.48035201082151247, 5.440088680355550821 ) ) ;
#55252=CARTESIAN_POINT ( 'NONE',  ( 20.36894250292379738, 4.928748834913967869, -10.36894250292379027 ) ) ;
#55255=CARTESIAN_POINT ( 'NONE',  ( 22.81628187352647785, 31.41530133659709279, 3.434112377981063169 ) ) ;
#55256=CARTESIAN_POINT ( 'NONE',  ( -4.164238869374099039, 1.803748834913967647, 8.674139862899312516E-16 ) ) ;
#55257=CARTESIAN_POINT ( 'NONE',  ( 19.84674366389459266, 13.71726448433411782, -2.638427012816827677 ) ) ;
#55260=CARTESIAN_POINT ( 'NONE',  ( 12.63842701281683922, 14.55059781766744997, -9.846743663894590881 ) ) ;
#55261=CARTESIAN_POINT ( 'NONE',  ( 20.88017736071110164, 45.35535201082149115, 2.915334737309930979 ) ) ;
#55266=CARTESIAN_POINT ( 'NONE',  ( 14.49999999999999822, 11.50000000000000000, -5.000000000000000000 ) ) ;
#55267=CARTESIAN_POINT ( 'NONE',  ( 20.88017736071110875, 50.77201867748817676, -2.915334737309920765 ) ) ;
#55268=CARTESIAN_POINT ( 'NONE',  ( 18.29284471827482150, 40.40189080397284016, -6.499999999999946709 ) ) ;
#55269=VECTOR ( 'NONE', #59793, 1000.000000000000000 ) ;
#55270=CARTESIAN_POINT ( 'NONE',  ( 0.1532563361054083140, 6.008931151000784787, 1.131784320476157264E-15 ) ) ;
#55271=CARTESIAN_POINT ( 'NONE',  ( 21.09922568453594849, 11.20696800326375531, 6.408140936763242479 ) ) ;
#55273=B_SPLINE_CURVE_WITH_KNOTS ( 'NONE', 3,
 ( #30284, #60786, #38306, #332 ),
 .UNSPECIFIED., .F., .F.,
 ( 4, 4 ),
 ( 2.710505431213761085E-19, 0.002657014572710960330 ),
 .UNSPECIFIED. ) ;
#55274=CARTESIAN_POINT ( 'NONE',  ( 1.472469842513823179, 35.59226448433412315, -4.923371831947296329 ) ) ;
#55275=CARTESIAN_POINT ( 'NONE',  ( 21.09922568453595559, 62.04030133659709634, -6.408140936763230044 ) ) ;
#55276=CARTESIAN_POINT ( 'NONE',  ( -4.164238869374099927, 7.012082168247302683, 3.795296366450308767 ) ) ;
#55277=CARTESIAN_POINT ( 'NONE',  ( 1.472469842513823179, 20.59226448433411960, -4.923371831947296329 ) ) ;
#55278=CARTESIAN_POINT ( 'NONE',  ( 6.565887622018943937, 18.08196800326375708, -12.81628187352647608 ) ) ;
#55281=CARTESIAN_POINT ( 'NONE',  ( 19.42250999205614548, 50.98035201082151247, -5.440088680355545492 ) ) ;
#55282=CARTESIAN_POINT ( 'NONE',  ( 3.591859063236763294, -1.709698663402913210, -11.09922568453595026 ) ) ;
#55284=CARTESIAN_POINT ( 'NONE',  ( 5.076628168052704559, 35.17559781766745175, -8.527530157486179263 ) ) ;
#55285=CARTESIAN_POINT ( 'NONE',  ( 10.00000000000000000, 19.75893115100078390, -9.846743663894594434 ) ) ;
#55286=CARTESIAN_POINT ( 'NONE',  ( 17.96484262340118221, 19.93868534415484106, 7.964842623401181321 ) ) ;
#55287=CARTESIAN_POINT ( 'NONE',  ( 19.38216949554541557, 17.24863466993041783, -9.382169495545420901 ) ) ;
#55290=CARTESIAN_POINT ( 'NONE',  ( -0.8801773607110991993, 17.85535201082150536, -2.915334737309923874 ) ) ;
#55292=CARTESIAN_POINT ( 'NONE',  ( -0.8801773607110991993, 67.85535201082151957, -2.915334737309923874 ) ) ;
#55294=CARTESIAN_POINT ( 'NONE',  ( 19.84674366389459621, 43.50893115100078745, 7.409399052514197653E-17 ) ) ;
#55295=CARTESIAN_POINT ( 'NONE',  ( 4.559911319644449179, 17.23035201082150536, -9.422509992056141925 ) ) ;
#55297=CARTESIAN_POINT ( 'NONE',  ( 12.91533473730993009, 51.60535201082149825, -10.88017736071109987 ) ) ;
#55298=CARTESIAN_POINT ( 'NONE',  ( 0.5774900079438607392, 8.480352010821505360, 5.440088680355550821 ) ) ;
#55300=CARTESIAN_POINT ( 'NONE',  ( 7.361572987183170547, 17.05059781766745530, 9.846743663894590881 ) ) ;
#55302=CARTESIAN_POINT ( 'NONE',  ( 17.20831665107776587, 32.88393115100078745, 7.208316651077764980 ) ) ;
#55305=DIRECTION ( 'NONE',  ( 0.000000000000000000, 0.000000000000000000, 1.000000000000000000 ) ) ;
#55306=CARTESIAN_POINT ( 'NONE',  ( -0.3689425029237881626, 2.428748834913967869, 10.36894250292379027 ) ) ;
#55307=ADVANCED_FACE ( 'NONE', ( #43163 ), #87672, .F. ) ;
#55308=CARTESIAN_POINT ( 'NONE',  ( 2.917880565312948704, 17.63708216824730357, 12.26659068614894643 ) ) ;
#55311=CARTESIAN_POINT ( 'NONE',  ( 0.1532563361054100626, 35.80059781766745175, -2.638427012816831230 ) ) ;
#55314=CARTESIAN_POINT ( 'NONE',  ( -2.266590686148945544, 51.38708216824730357, -7.082119434687050408 ) ) ;
#55316=CARTESIAN_POINT ( 'NONE',  ( 19.84674366389459621, 23.50893115100078390, 7.409399052514197653E-17 ) ) ;
#55318=CARTESIAN_POINT ( 'NONE',  ( 10.00000000000000000, 41.81368534415484106, -10.88017736071110342 ) ) ;
#55320=CARTESIAN_POINT ( 'NONE',  ( 3.591859063236761518, 59.95696800326375353, 11.09922568453594849 ) ) ;
#55321=CARTESIAN_POINT ( 'NONE',  ( 4.559911319644449179, 22.23035201082150536, -9.422509992056141925 ) ) ;
#55322=CARTESIAN_POINT ( 'NONE',  ( 3.591859063236761518, 54.95696800326376064, 11.09922568453594849 ) ) ;
#55323=CARTESIAN_POINT ( 'NONE',  ( 3.591859063236761518, 4.956968003263753531, 11.09922568453594849 ) ) ;
#55324=CARTESIAN_POINT ( 'NONE',  ( 5.076628168052704559, 15.17559781766745175, -8.527530157486179263 ) ) ;
#55325=ORIENTED_EDGE ( 'NONE', *, *, #64872, .F. ) ;
#55328=CARTESIAN_POINT ( 'NONE',  ( 17.08211943468705840, 55.13708216824731068, -12.26659068614894466 ) ) ;
#55329=CARTESIAN_POINT ( 'NONE',  ( 22.26659068614894466, 33.88708216824730357, 7.082119434687054849 ) ) ;
#55330=CARTESIAN_POINT ( 'NONE',  ( 7.084665262690076126, 22.02201867748817321, -10.88017736071110164 ) ) ;
#55331=CARTESIAN_POINT ( 'NONE',  ( 2.035157376598822676, 52.43868534415483396, -7.964842623401177768 ) ) ;
#55334=CARTESIAN_POINT ( 'NONE',  ( -0.8801773607111009756, 68.06368534415484817, 1.068504757029289695E-15 ) ) ;
#55336=CARTESIAN_POINT ( 'NONE',  ( 0.1532563361054083140, 16.00893115100078390, 1.131784320476157264E-15 ) ) ;
#55339=CARTESIAN_POINT ( 'NONE',  ( 5.076628168052703671, 21.84226448433411960, 8.527530157486179263 ) ) ;
#55340=CARTESIAN_POINT ( 'NONE',  ( 1.472469842513823179, 45.59226448433412315, -4.923371831947296329 ) ) ;
#55342=CARTESIAN_POINT ( 'NONE',  ( 0.5774900079438590739, 17.64701867748817321, -5.440088680355550821 ) ) ;
#55343=VECTOR ( 'NONE', #54681, 1000.000000000000000 ) ;
#55345=CARTESIAN_POINT ( 'NONE',  ( 21.09922568453595559, 32.04030133659708923, -6.408140936763230044 ) ) ;
#55346=CARTESIAN_POINT ( 'NONE',  ( 2.035157376598822676, 47.43868534415484817, -7.964842623401177768 ) ) ;
#55347=CARTESIAN_POINT ( 'NONE',  ( 13.79529636645031943, 50.34541550158064638, -14.16423886937409904 ) ) ;
#55348=CARTESIAN_POINT ( 'NONE',  ( 7.361572987183170547, 7.050597817667451750, 9.846743663894590881 ) ) ;
#55351=CARTESIAN_POINT ( 'NONE',  ( 12.63842701281683034, 52.46726448433413026, 9.846743663894596210 ) ) ;
#55352=CARTESIAN_POINT ( 'NONE',  ( 17.20831665107776587, 29.13393115100078390, -7.208316651077762316 ) ) ;
#55353=CARTESIAN_POINT ( 'NONE',  ( 24.16423886937410614, 9.303748834913967869, 8.672049930838204340E-16 ) ) ;
#55354=CARTESIAN_POINT ( 'NONE',  ( 20.36894250292379382, 18.67874883491397142, 10.36894250292379205 ) ) ;
#55355=CARTESIAN_POINT ( 'NONE',  ( 19.84674366389459266, 33.71726448433410894, -2.638427012816827677 ) ) ;
#55356=CARTESIAN_POINT ( 'NONE',  ( 20.88017736071110875, 45.77201867748816966, -2.915334737309920765 ) ) ;
#55357=CARTESIAN_POINT ( 'NONE',  ( 4.559911319644449179, 13.89701867748817143, 9.422509992056141925 ) ) ;
#55358=EDGE_CURVE ( 'NONE', #83368, #29627, #95266, .T. ) ;
#55359=CARTESIAN_POINT ( 'NONE',  ( 4.559911319644449179, 43.89701867748816966, 9.422509992056141925 ) ) ;
#55360=CARTESIAN_POINT ( 'NONE',  ( 17.96484262340118221, 24.93868534415484461, 7.964842623401181321 ) ) ;
#55361=ORIENTED_EDGE ( 'NONE', *, *, #50666, .T. ) ;
#55362=CARTESIAN_POINT ( 'NONE',  ( 6.565887622018943937, 30.16530133659708568, 12.81628187352647430 ) ) ;
#55363=( GEOMETRIC_REPRESENTATION_CONTEXT ( 3 ) GLOBAL_UNCERTAINTY_ASSIGNED_CONTEXT ( ( #67132 ) ) GLOBAL_UNIT_ASSIGNED_CONTEXT ( ( #36406, #58904, #58397 ) ) REPRESENTATION_CONTEXT ( 'NONE', 'WORKASPACE' ) );
#55364=CARTESIAN_POINT ( 'NONE',  ( 2.035157376598822676, 42.43868534415483396, -7.964842623401177768 ) ) ;
#55366=CARTESIAN_POINT ( 'NONE',  ( 19.38216949554541202, 60.99863466993042493, 9.382169495545424454 ) ) ;
#55371=CARTESIAN_POINT ( 'NONE',  ( 12.91533473730992121, 44.52201867748816966, 10.88017736071110164 ) ) ;
#55372=CARTESIAN_POINT ( 'NONE',  ( 15.44008868035555260, 4.730352010821504471, 9.422509992056143702 ) ) ;
#55374=CARTESIAN_POINT ( 'NONE',  ( 17.39651004071841456, 7.935752660568278216, 6.500000000000003553 ) ) ;
#55376=CARTESIAN_POINT ( 'NONE',  ( 20.36894250292379738, 54.92874883491396076, -10.36894250292379027 ) ) ;
#55377=CARTESIAN_POINT ( 'NONE',  ( 2.791683348922237240, 10.38393115100078390, -7.208316651077763204 ) ) ;
#55379=CARTESIAN_POINT ( 'NONE',  ( 6.204703633549690345, 7.845415501580634832, 14.16423886937410082 ) ) ;
#55380=CARTESIAN_POINT ( 'NONE',  ( 0.1532563361054100626, 0.8005978176674514168, -2.638427012816831230 ) ) ;
#55381=CARTESIAN_POINT ( 'NONE',  ( 4.559911319644449179, 13.89701867748817143, 9.422509992056141925 ) ) ;
#55382=CARTESIAN_POINT ( 'NONE',  ( 10.00000000000000178, 42.25893115100078745, 9.846743663894594434 ) ) ;
#55384=CARTESIAN_POINT ( 'NONE',  ( 14.92337183194729988, 44.34226448433412315, -8.527530157486177487 ) ) ;
#55385=CARTESIAN_POINT ( 'NONE',  ( -0.8801773607111008646, 38.27201867748816255, 2.915334737309923430 ) ) ;
#55386=CARTESIAN_POINT ( 'NONE',  ( 5.076628168052704559, 50.17559781766745886, -8.527530157486179263 ) ) ;
#55387=CARTESIAN_POINT ( 'NONE',  ( 21.09922568453595559, 32.04030133659708923, -6.408140936763230044 ) ) ;
#55388=CARTESIAN_POINT ( 'NONE',  ( 7.084665262690076126, 69.10535201082151957, 10.88017736071109987 ) ) ;
#55389=CARTESIAN_POINT ( 'NONE',  ( 15.44008868035555793, 51.39701867748816966, -9.422509992056140149 ) ) ;
#55390=CARTESIAN_POINT ( 'NONE',  ( 2.917880565312950480, 60.97041550158063927, -12.26659068614894821 ) ) ;
#55393=CARTESIAN_POINT ( 'NONE',  ( 22.81628187352647785, 16.41530133659708923, 3.434112377981063169 ) ) ;
#55394=DIRECTION ( 'NONE',  ( 0.000000000000000000, 0.000000000000000000, 1.000000000000000000 ) ) ;
#55396=CARTESIAN_POINT ( 'NONE',  ( 19.38216949554541557, 32.24863466993041783, -9.382169495545420901 ) ) ;
#55397=CARTESIAN_POINT ( 'NONE',  ( 4.559911319644449179, 17.23035201082150536, -9.422509992056141925 ) ) ;
#55401=CARTESIAN_POINT ( 'NONE',  ( 14.92337183194729633, 2.675597817667451750, 8.527530157486181039 ) ) ;
#55402=CARTESIAN_POINT ( 'NONE',  ( 19.84674366389459266, 53.71726448433411605, -2.638427012816827677 ) ) ;
#55403=CARTESIAN_POINT ( 'NONE',  ( 10.00000000000000178, 17.25893115100078745, 9.846743663894594434 ) ) ;
#55404=CARTESIAN_POINT ( 'NONE',  ( 19.84674366389459266, 38.71726448433412315, -2.638427012816827677 ) ) ;
#55405=CARTESIAN_POINT ( 'NONE',  ( 0.2751277870542889192, 28.21833443783938122, 6.499999999999990230 ) ) ;
#55408=CARTESIAN_POINT ( 'NONE',  ( 7.361572987183170547, 27.05059781766745175, 9.846743663894590881 ) ) ;
#55409=( NAMED_UNIT ( * ) SI_UNIT ( $, .STERADIAN. ) SOLID_ANGLE_UNIT ( ) );
#55410=CARTESIAN_POINT ( 'NONE',  ( 5.076628168052703671, 51.84226448433412315, 8.527530157486179263 ) ) ;
#55413=CARTESIAN_POINT ( 'NONE',  ( -2.816281873526471635, 28.91530133659708213, -3.434112377981056508 ) ) ;
#55416=CARTESIAN_POINT ( 'NONE',  ( 20.36894250292379382, 43.67874883491397497, 10.36894250292379205 ) ) ;
#55417=CARTESIAN_POINT ( 'NONE',  ( 19.84674366389459621, 13.50893115100078568, 7.409399052514197653E-17 ) ) ;
#55418=( NAMED_UNIT ( * ) SI_UNIT ( $, .STERADIAN. ) SOLID_ANGLE_UNIT ( ) );
#55419=CARTESIAN_POINT ( 'NONE',  ( 20.00000000000137845, 93.04550625941708120, 5.196918121118858203 ) ) ;
#55420=CARTESIAN_POINT ( 'NONE',  ( 22.26659068614895176, 49.72041550158063927, -7.082119434687042414 ) ) ;
#55421=CARTESIAN_POINT ( 'NONE',  ( 10.00000000000000000, 54.75893115100078745, -9.846743663894594434 ) ) ;
#55422=CARTESIAN_POINT ( 'NONE',  ( 13.79529636645030344, 63.26208216824730357, 14.16423886937410614 ) ) ;
#55423=CARTESIAN_POINT ( 'NONE',  ( 10.00000000000000000, 25.55374883491396787, -14.16423886937410082 ) ) ;
#55424=CARTESIAN_POINT ( 'NONE',  ( 6.204703633549690345, 35.76208216824729647, -14.16423886937410259 ) ) ;
#55426=EDGE_CURVE ( 'NONE', #80817, #62008, #9384, .T. ) ;
#55428=CARTESIAN_POINT ( 'NONE',  ( 18.52753015748618282, 58.92559781766745886, -4.923371831947291888 ) ) ;
#55431=CARTESIAN_POINT ( 'NONE',  ( 20.88017736071110519, 35.56368534415484106, 2.639326808657452039E-16 ) ) ;
#55434=CARTESIAN_POINT ( 'NONE',  ( 17.20831665107776587, 37.88393115100078745, 7.208316651077764980 ) ) ;
#55439=CARTESIAN_POINT ( 'NONE',  ( 18.52753015748618282, 48.92559781766745886, -4.923371831947291888 ) ) ;
#55442=ORIENTED_EDGE ( 'NONE', *, *, #56566, .T. ) ;
#55443=CARTESIAN_POINT ( 'NONE',  ( 20.36894250292379738, 19.92874883491396787, -10.36894250292379027 ) ) ;
#55447=CARTESIAN_POINT ( 'NONE',  ( -0.1042174387088628529, 68.10736173766203194, 6.337391062633416894 ) ) ;
#55448=CYLINDRICAL_SURFACE ( 'NONE', #50288, 0.5000000000000004441 ) ;
#55449=CARTESIAN_POINT ( 'NONE',  ( -0.3689425029237881626, 67.42874883491396076, 10.36894250292379027 ) ) ;
#55450=CARTESIAN_POINT ( 'NONE',  ( 22.81628187352647785, 26.62363466993042138, 6.195893100308588602E-16 ) ) ;
#55452=CARTESIAN_POINT ( 'NONE',  ( 19.42250999205614193, 65.14701867748817676, 5.440088680355555262 ) ) ;
#55453=CARTESIAN_POINT ( 'NONE',  ( 21.92686044187656336, 41.97997603579416648, 3.195792623639536423 ) ) ;
#55456=CARTESIAN_POINT ( 'NONE',  ( 10.00000000000000000, 65.55374883491396076, -14.16423886937410082 ) ) ;
#55458=CARTESIAN_POINT ( 'NONE',  ( 4.559911319644449179, 27.23035201082150536, -9.422509992056141925 ) ) ;
#55459=CARTESIAN_POINT ( 'NONE',  ( 12.91533473730993009, 31.60535201082150891, -10.88017736071109987 ) ) ;
#55460=CARTESIAN_POINT ( 'NONE',  ( 21.09922568453594849, 1.206968003263753531, 6.408140936763242479 ) ) ;
#55461=CARTESIAN_POINT ( 'NONE',  ( 17.20831665107776587, 54.13393115100079456, -7.208316651077762316 ) ) ;
#55462=CARTESIAN_POINT ( 'NONE',  ( -42.16485527613927076, 107.5383484153110061, -5.000000000000000888 ) ) ;
#55465=ADVANCED_FACE ( 'NONE', ( #6156 ), #93073, .T. ) ;
#55466=CARTESIAN_POINT ( 'NONE',  ( 2.035157376598824452, 33.68868534415484106, 7.964842623401179544 ) ) ;
#55467=CARTESIAN_POINT ( 'NONE',  ( 6.565887622018943937, 28.08196800326375353, -12.81628187352647608 ) ) ;
#55468=CARTESIAN_POINT ( 'NONE',  ( 0.000000000000000000, 75.98134920320651986, 6.799195827237609180 ) ) ;
#55469=CARTESIAN_POINT ( 'NONE',  ( 14.92337183194729633, 57.67559781766745886, 8.527530157486181039 ) ) ;
#55470=CARTESIAN_POINT ( 'NONE',  ( 20.88017736071110164, 45.35535201082149115, 2.915334737309930979 ) ) ;
#55471=CARTESIAN_POINT ( 'NONE',  ( 0.1532563361054082862, 11.21726448433411605, 2.638427012816831674 ) ) ;
#55473=CARTESIAN_POINT ( 'NONE',  ( -1.099225684535947600, 39.54030133659708923, 6.408140936763237150 ) ) ;
#55474=CARTESIAN_POINT ( 'NONE',  ( 19.42250999205614193, 65.14701867748817676, 5.440088680355555262 ) ) ;
#55475=FACE_OUTER_BOUND ( 'NONE', #87188, .T. ) ;
#55476=CARTESIAN_POINT ( 'NONE',  ( 17.62281668512001076, 53.28593319516823357, 6.500000000000063061 ) ) ;
#55477=CARTESIAN_POINT ( 'NONE',  ( -2.816281873526473856, 64.33196800326376774, 3.434112377981055619 ) ) ;
#55478=ORIENTED_EDGE ( 'NONE', *, *, #96068, .F. ) ;
#55481=CARTESIAN_POINT ( 'NONE',  ( 0.5774900079438590739, 7.647018677488171434, -5.440088680355550821 ) ) ;
#55482=CARTESIAN_POINT ( 'NONE',  ( 21.09922568453595559, 42.04030133659708213, -6.408140936763230044 ) ) ;
#55483=CARTESIAN_POINT ( 'NONE',  ( 22.26659068614894466, 13.88708216824730179, 7.082119434687054849 ) ) ;
#55484=ADVANCED_FACE ( 'NONE', ( #62603 ), #93660, .T. ) ;
#55485=CARTESIAN_POINT ( 'NONE',  ( 17.20831665107776587, 12.88393115100078390, 7.208316651077764980 ) ) ;
#55486=CARTESIAN_POINT ( 'NONE',  ( 4.559911319644449179, 2.230352010821504471, -9.422509992056141925 ) ) ;
#55487=CARTESIAN_POINT ( 'NONE',  ( 5.076628168052703671, 21.84226448433411960, 8.527530157486179263 ) ) ;
#55488=CARTESIAN_POINT ( 'NONE',  ( 17.08211943468705130, 58.47041550158063927, 12.26659068614894998 ) ) ;
#55490=SURFACE_STYLE_FILL_AREA ( #32966 ) ;
#55491=CARTESIAN_POINT ( 'NONE',  ( -0.8801773607111009756, 23.06368534415484106, 1.068504757029289695E-15 ) ) ;
#55495=ORIENTED_EDGE ( 'NONE', *, *, #23445, .F. ) ;
#55496=CARTESIAN_POINT ( 'NONE',  ( 4.559911319644449179, 17.23035201082150536, -9.422509992056141925 ) ) ;
#55497=CARTESIAN_POINT ( 'NONE',  ( 2.035157376598822676, 12.43868534415483751, -7.964842623401177768 ) ) ;
#55498=CARTESIAN_POINT ( 'NONE',  ( 7.361572987183169658, 59.96726448433410894, -9.846743663894592657 ) ) ;
#55499=CARTESIAN_POINT ( 'NONE',  ( 13.43411237798106583, 52.66530133659708213, -12.81628187352647252 ) ) ;
#55502=CARTESIAN_POINT ( 'NONE',  ( 22.26659068614895176, 14.72041550158063572, -7.082119434687042414 ) ) ;
#55503=CARTESIAN_POINT ( 'NONE',  ( 19.42250999205614193, 20.14701867748817321, 5.440088680355555262 ) ) ;
#55504=CARTESIAN_POINT ( 'NONE',  ( 2.035157376598824452, 23.68868534415484461, 7.964842623401179544 ) ) ;
#55505=CARTESIAN_POINT ( 'NONE',  ( 7.361572987183169658, 49.96726448433410894, -9.846743663894592657 ) ) ;
#55507=CARTESIAN_POINT ( 'NONE',  ( 5.076628168052704559, 35.17559781766745175, -8.527530157486179263 ) ) ;
#55508=CARTESIAN_POINT ( 'NONE',  ( 14.92337183194729988, 4.342264484334117824, -8.527530157486177487 ) ) ;
#55513=CARTESIAN_POINT ( 'NONE',  ( 7.361572987183169658, 14.96726448433411960, -9.846743663894592657 ) ) ;
#55514=CARTESIAN_POINT ( 'NONE',  ( 3.591859063236761518, -0.04303199673624671928, 11.09922568453594849 ) ) ;
#55515=CARTESIAN_POINT ( 'NONE',  ( 0.5774900079438590739, 52.64701867748817676, -5.440088680355550821 ) ) ;
#55516=CARTESIAN_POINT ( 'NONE',  ( 19.42250999205614548, 5.980352010821504471, -5.440088680355545492 ) ) ;
#55517=CARTESIAN_POINT ( 'NONE',  ( 3.591859063236763294, 43.29030133659708923, -11.09922568453595026 ) ) ;
#55518=CARTESIAN_POINT ( 'NONE',  ( 6.204703633549690345, 15.76208216824730179, -14.16423886937410259 ) ) ;
#55521=CARTESIAN_POINT ( 'NONE',  ( 6.565887622018943937, 65.16530133659709634, 12.81628187352647430 ) ) ;
#55523=CARTESIAN_POINT ( 'NONE',  ( 14.92337183194729633, 52.67559781766745175, 8.527530157486181039 ) ) ;
#55524=CARTESIAN_POINT ( 'NONE',  ( 4.559911319644449179, 22.23035201082150536, -9.422509992056141925 ) ) ;
#55526=CARTESIAN_POINT ( 'NONE',  ( 7.361572987183170547, 2.050597817667451750, 9.846743663894590881 ) ) ;
#55527=CARTESIAN_POINT ( 'NONE',  ( 20.88017736071110164, 65.35535201082150536, 2.915334737309930979 ) ) ;
#55530=CARTESIAN_POINT ( 'NONE',  ( 12.63842701281683922, 4.550597817667451750, -9.846743663894590881 ) ) ;
#55531=CARTESIAN_POINT ( 'NONE',  ( 12.63842701281683034, 2.467264484334118269, 9.846743663894596210 ) ) ;
#55534=CARTESIAN_POINT ( 'NONE',  ( 12.91533473730992121, 59.52201867748816966, 10.88017736071110164 ) ) ;
#55536=CARTESIAN_POINT ( 'NONE',  ( -0.8801773607111009756, 63.06368534415484106, 1.068504757029289695E-15 ) ) ;
#55537=CARTESIAN_POINT ( 'NONE',  ( 2.791683348922237240, 5.383931151000785675, -7.208316651077763204 ) ) ;
#55540=CARTESIAN_POINT ( 'NONE',  ( 19.84674366389459266, 53.30059781766744464, 2.638427012816836559 ) ) ;
#55542=PLANE ( 'NONE',  #26657 ) ;
#55543=CARTESIAN_POINT ( 'NONE',  ( -4.164238869374099927, 2.012082168247300906, 3.795296366450308767 ) ) ;
#55544=CARTESIAN_POINT ( 'NONE',  ( 3.591859063236763294, 53.29030133659708923, -11.09922568453595026 ) ) ;
#55545=CARTESIAN_POINT ( 'NONE',  ( 17.08211943468705840, 5.137082168247300906, -12.26659068614894466 ) ) ;
#55546=CARTESIAN_POINT ( 'NONE',  ( 24.16423886937410614, 14.30374883491396787, 8.672049930838204340E-16 ) ) ;
#55548=FACE_OUTER_BOUND ( 'NONE', #58272, .T. ) ;
#55549=CARTESIAN_POINT ( 'NONE',  ( 2.035157376598824452, 18.68868534415484106, 7.964842623401179544 ) ) ;
#55552=CARTESIAN_POINT ( 'NONE',  ( 5.076628168052703671, 21.84226448433411960, 8.527530157486179263 ) ) ;
#55553=CARTESIAN_POINT ( 'NONE',  ( 16.40814093676323893, 35.79030133659708923, 11.09922568453595026 ) ) ;
#55554=CARTESIAN_POINT ( 'NONE',  ( 10.00000000000000178, 42.25893115100078745, 9.846743663894594434 ) ) ;
#55555=CARTESIAN_POINT ( 'NONE',  ( 19.84674366389459621, 58.50893115100078745, 7.409399052514197653E-17 ) ) ;
#55556=CARTESIAN_POINT ( 'NONE',  ( 3.591859063236763294, 18.29030133659708568, -11.09922568453595026 ) ) ;
#55559=CARTESIAN_POINT ( 'NONE',  ( 1.472469842513823179, 26.42559781766745175, 4.923371831947296329 ) ) ;
#55561=CARTESIAN_POINT ( 'NONE',  ( 12.63842701281683034, 2.467264484334118269, 9.846743663894596210 ) ) ;
#55563=EDGE_LOOP ( 'NONE', ( #18155, #16165, #88434, #70899 ) ) ;
#55565=CARTESIAN_POINT ( 'NONE',  ( 10.00000000000000000, 36.81368534415484106, -10.88017736071110342 ) ) ;
#55566=CARTESIAN_POINT ( 'NONE',  ( 6.204703633549690345, 32.84541550158063927, 14.16423886937410082 ) ) ;
#55567=CARTESIAN_POINT ( 'NONE',  ( 5.076628168052704559, 45.17559781766745175, -8.527530157486179263 ) ) ;
#55568=CARTESIAN_POINT ( 'NONE',  ( 19.84674366389459266, 18.71726448433411960, -2.638427012816827677 ) ) ;
#55569=CARTESIAN_POINT ( 'NONE',  ( 22.81628187352647785, 51.41530133659708923, 3.434112377981063169 ) ) ;
#55571=CARTESIAN_POINT ( 'NONE',  ( 10.00000000000000178, 29.31368534415483751, 10.88017736071110342 ) ) ;
#55573=TOROIDAL_SURFACE ( 'NONE', #39668, 1.000000000000000000, 0.5000000000000000000 ) ;
#55574=CARTESIAN_POINT ( 'NONE',  ( -1.099225684535947600, 24.54030133659708923, 6.408140936763237150 ) ) ;
#55575=CARTESIAN_POINT ( 'NONE',  ( 18.52753015748618282, 38.92559781766745175, -4.923371831947291888 ) ) ;
#55577=CARTESIAN_POINT ( 'NONE',  ( 21.09922568453595559, 47.04030133659708923, -6.408140936763230044 ) ) ;
#55579=CARTESIAN_POINT ( 'NONE',  ( -0.8801773607111008646, 58.27201867748816966, 2.915334737309923430 ) ) ;
#55580=CARTESIAN_POINT ( 'NONE',  ( 19.72487221294570858, 9.782175860852373006, 6.500000000000000000 ) ) ;
#55585=CARTESIAN_POINT ( 'NONE',  ( 20.88017736071110519, 55.56368534415484817, 2.639326808657452039E-16 ) ) ;
#55586=CARTESIAN_POINT ( 'NONE',  ( 10.00000000000000000, 56.81368534415484106, -10.88017736071110342 ) ) ;
#55587=CARTESIAN_POINT ( 'NONE',  ( 19.88701968852527102, 56.79427333184086280, 6.480634945678608538 ) ) ;
#55590=CARTESIAN_POINT ( 'NONE',  ( 10.00000000000000000, 11.81368534415483751, -10.88017736071110342 ) ) ;
#55591=CARTESIAN_POINT ( 'NONE',  ( 19.84674366389459266, 58.71726448433411605, -2.638427012816827677 ) ) ;
#55592=CARTESIAN_POINT ( 'NONE',  ( 19.42250999205614548, 25.98035201082150891, -5.440088680355545492 ) ) ;
#55594=CARTESIAN_POINT ( 'NONE',  ( 16.40814093676324603, 27.45696800326375708, -11.09922568453594671 ) ) ;
#55595=ORIENTED_EDGE ( 'NONE', *, *, #12529, .T. ) ;
#55596=CARTESIAN_POINT ( 'NONE',  ( 2.035157376598822676, 57.43868534415484106, -7.964842623401177768 ) ) ;
#55597=CARTESIAN_POINT ( 'NONE',  ( 19.84674366389459621, 38.50893115100078745, 7.409399052514197653E-17 ) ) ;
#55598=CARTESIAN_POINT ( 'NONE',  ( -2.816281873526473856, 9.123634669930421381, 9.499525473075851096E-16 ) ) ;
#55601=CARTESIAN_POINT ( 'NONE',  ( 2.035157376598822676, 12.43868534415483751, -7.964842623401177768 ) ) ;
#55602=CARTESIAN_POINT ( 'NONE',  ( -0.8801773607111009756, 38.06368534415484106, 1.068504757029289695E-15 ) ) ;
#55603=CARTESIAN_POINT ( 'NONE',  ( -2.266590686148945544, 56.38708216824731068, -7.082119434687050408 ) ) ;
#55604=CARTESIAN_POINT ( 'NONE',  ( 12.63842701281683922, 39.55059781766744464, -9.846743663894590881 ) ) ;
#55605=CARTESIAN_POINT ( 'NONE',  ( 20.88017736071110519, 55.56368534415484817, 2.639326808657452039E-16 ) ) ;
#55607=CARTESIAN_POINT ( 'NONE',  ( 17.08211943468705840, 15.13708216824730179, -12.26659068614894466 ) ) ;
#55609=CARTESIAN_POINT ( 'NONE',  ( 19.72487221294570858, 11.86607318730075633, 6.500000000000000888 ) ) ;
#55611=CARTESIAN_POINT ( 'NONE',  ( 10.00000000000000178, 53.05374883491396787, 14.16423886937410082 ) ) ;
#55612=CARTESIAN_POINT ( 'NONE',  ( 10.00000000000000178, 33.05374883491396787, 14.16423886937410082 ) ) ;
#55613=CARTESIAN_POINT ( 'NONE',  ( 19.84674366389459266, 18.30059781766745175, 2.638427012816836559 ) ) ;
#55614=CARTESIAN_POINT ( 'NONE',  ( 0.6178305044545818747, 13.49863466993041783, -9.382169495545419124 ) ) ;
#55615=CARTESIAN_POINT ( 'NONE',  ( 0.1532563361054100626, 60.80059781766744464, -2.638427012816831230 ) ) ;
#55616=CARTESIAN_POINT ( 'NONE',  ( 0.000000000000000000, 0.000000000000000000, 5.000000000000000000 ) ) ;
#55617=CARTESIAN_POINT ( 'NONE',  ( 12.91533473730992121, 59.52201867748816966, 10.88017736071110164 ) ) ;
#55618=CARTESIAN_POINT ( 'NONE',  ( 6.565887622018943937, 33.08196800326374643, -12.81628187352647608 ) ) ;
#55619=CARTESIAN_POINT ( 'NONE',  ( 20.36894250292379738, 24.92874883491396787, -10.36894250292379027 ) ) ;
#55620=CARTESIAN_POINT ( 'NONE',  ( 2.035157376598824452, 28.68868534415484106, 7.964842623401179544 ) ) ;
#55621=CARTESIAN_POINT ( 'NONE',  ( 6.000000000000000000, 60.50000000000000711, 6.500000000000000888 ) ) ;
#55622=CARTESIAN_POINT ( 'NONE',  ( 17.20831665107776587, 2.883931151000785231, 7.208316651077764980 ) ) ;
#55624=ORIENTED_EDGE ( 'NONE', *, *, #62283, .F. ) ;
#55626=ORIENTED_EDGE ( 'NONE', *, *, #53039, .T. ) ;
#55627=( NAMED_UNIT ( * ) SI_UNIT ( $, .STERADIAN. ) SOLID_ANGLE_UNIT ( ) );
#55628=CARTESIAN_POINT ( 'NONE',  ( 4.559911319644449179, 3.897018677488171434, 9.422509992056141925 ) ) ;
#55629=CARTESIAN_POINT ( 'NONE',  ( -0.8801773607111008646, 18.27201867748817321, 2.915334737309923430 ) ) ;
#55630=CARTESIAN_POINT ( 'NONE',  ( 19.84674366389459266, 33.71726448433410894, -2.638427012816827677 ) ) ;
#55631=CARTESIAN_POINT ( 'NONE',  ( 3.591859063236763294, -1.709698663402913210, -11.09922568453595026 ) ) ;
#55634=CARTESIAN_POINT ( 'NONE',  ( 0.6178305044545838731, 9.748634669930416052, 9.382169495545420901 ) ) ;
#55637=CARTESIAN_POINT ( 'NONE',  ( 24.16423886937409904, 49.09541550158063217, 3.795296366450317205 ) ) ;
#55639=CARTESIAN_POINT ( 'NONE',  ( 20.36894250292379382, 53.67874883491397497, 10.36894250292379205 ) ) ;
#55640=VERTEX_POINT ( 'NONE', #19482 ) ;
#55641=CARTESIAN_POINT ( 'NONE',  ( 19.42250999205614193, 30.14701867748817321, 5.440088680355555262 ) ) ;
#55642=STYLED_ITEM ( 'NONE', ( #18607 ), #12884 ) ;
#55643=CARTESIAN_POINT ( 'NONE',  ( 10.00000000000000178, 44.31368534415484106, 10.88017736071110342 ) ) ;
#55644=CARTESIAN_POINT ( 'NONE',  ( 0.5774900079438607392, 33.48035201082150536, 5.440088680355550821 ) ) ;
#55645=CARTESIAN_POINT ( 'NONE',  ( 10.00000000000000000, 66.81368534415484817, -10.88017736071110342 ) ) ;
#55646=CARTESIAN_POINT ( 'NONE',  ( 15.44008868035555260, 24.73035201082150891, 9.422509992056143702 ) ) ;
#55653=CARTESIAN_POINT ( 'NONE',  ( 5.076628168052704559, 15.17559781766745175, -8.527530157486179263 ) ) ;
#55657=CARTESIAN_POINT ( 'NONE',  ( 17.20831665107776587, 44.13393115100078745, -7.208316651077762316 ) ) ;
#55659=( NAMED_UNIT ( * ) PLANE_ANGLE_UNIT ( ) SI_UNIT ( $, .RADIAN. ) );
#55662=LINE ( 'NONE', #86161, #58614 ) ;
#55663=CARTESIAN_POINT ( 'NONE',  ( 0.1532563361054083140, 56.00893115100078745, 1.131784320476157264E-15 ) ) ;
#55664=CARTESIAN_POINT ( 'NONE',  ( 10.00000000000000000, 45.55374883491397497, -14.16423886937410082 ) ) ;
#55665=DIRECTION ( 'NONE',  ( 0.000000000000000000, 0.000000000000000000, -1.000000000000000000 ) ) ;
#55666=ORIENTED_EDGE ( 'NONE', *, *, #52621, .F. ) ;
#55667=CARTESIAN_POINT ( 'NONE',  ( 19.88701968852526392, 41.79427333184086280, 6.480634945678624526 ) ) ;
#55668=CARTESIAN_POINT ( 'NONE',  ( 5.076628168052703671, 21.84226448433411960, 8.527530157486179263 ) ) ;
#55669=CARTESIAN_POINT ( 'NONE',  ( 21.09922568453595559, 52.04030133659708923, -6.408140936763230044 ) ) ;
#55670=CARTESIAN_POINT ( 'NONE',  ( 5.076628168052704559, 55.17559781766745175, -8.527530157486179263 ) ) ;
#55671=CARTESIAN_POINT ( 'NONE',  ( 7.084665262690076126, 64.10535201082150536, 10.88017736071109987 ) ) ;
#55672=CARTESIAN_POINT ( 'NONE',  ( 2.791683348922237240, 50.38393115100078035, -7.208316651077763204 ) ) ;
#55673=CARTESIAN_POINT ( 'NONE',  ( 20.24186590665277663, 14.73410085661203972, 6.114288769123037426 ) ) ;
#55674=EDGE_CURVE ( 'NONE', #94197, #51199, #36837, .T. ) ;
#55676=EDGE_CURVE ( 'NONE', #69353, #63612, #4320, .T. ) ;
#55677=CARTESIAN_POINT ( 'NONE',  ( 2.917880565312950480, 65.97041550158063217, -12.26659068614894821 ) ) ;
#55678=CARTESIAN_POINT ( 'NONE',  ( 4.999999999999999112, 0.000000000000000000, -6.500000000000000888 ) ) ;
#55679=CARTESIAN_POINT ( 'NONE',  ( 4.559911319644449179, 42.23035201082151247, -9.422509992056141925 ) ) ;
#55680=CARTESIAN_POINT ( 'NONE',  ( -1.099225684535947600, 8.706968003263753531, -6.408140936763238038 ) ) ;
#55686=AXIS2_PLACEMENT_3D ( 'NONE', #62701, #92231, #48193 ) ;
#55687=CARTESIAN_POINT ( 'NONE',  ( 1.472469842513823179, 45.59226448433412315, -4.923371831947296329 ) ) ;
#55688=SURFACE_STYLE_USAGE ( .BOTH. , #63656 ) ;
#55689=( BOUNDED_CURVE ( )  B_SPLINE_CURVE ( 2, ( #76780, #1315, #62260, #53792, #92766, #93752, #85774, #32254, #85278 ),
 .UNSPECIFIED., .F., .F. ) 
 B_SPLINE_CURVE_WITH_KNOTS ( ( 3, 2, 2, 2, 3 ),
 ( 0.1177146600783225971, 0.1190476190476190410, 0.1250000000000000000, 0.1309523809523809590, 0.1322853399216775416 ),
 .UNSPECIFIED. ) 
 CURVE ( )  GEOMETRIC_REPRESENTATION_ITEM ( )  RATIONAL_B_SPLINE_CURVE ( ( 0.9881565478350731180, 0.9923695281211489805, 1.000000000000000000, 0.9659258262890683122, 1.000000000000000000, 0.9659258262890683122, 1.000000000000000000, 0.9923695281211482033, 0.9881565478350723408 ) ) 
 REPRESENTATION_ITEM ( '' )  );
#55691=CARTESIAN_POINT ( 'NONE',  ( 6.565887622018943937, 10.16530133659708746, 12.81628187352647430 ) ) ;
#55692=CARTESIAN_POINT ( 'NONE',  ( 0.5774900079438590739, 12.64701867748817321, -5.440088680355550821 ) ) ;
#55695=CARTESIAN_POINT ( 'NONE',  ( 22.26659068614895176, 29.72041550158063572, -7.082119434687042414 ) ) ;
#55696=CARTESIAN_POINT ( 'NONE',  ( 22.26659068614895176, 34.72041550158063927, -7.082119434687042414 ) ) ;
#55697=CARTESIAN_POINT ( 'NONE',  ( 2.917880565312950480, 60.97041550158063927, -12.26659068614894821 ) ) ;
#55698=CARTESIAN_POINT ( 'NONE',  ( 5.076628168052704559, 30.17559781766745175, -8.527530157486179263 ) ) ;
#55699=CARTESIAN_POINT ( 'NONE',  ( 10.00000000000000178, 40.37363466993042493, 12.81628187352647608 ) ) ;
#55700=CARTESIAN_POINT ( 'NONE',  ( 15.44008868035555260, 9.730352010821505360, 9.422509992056143702 ) ) ;
#55701=ORIENTED_EDGE ( 'NONE', *, *, #42226, .F. ) ;
#55702=CARTESIAN_POINT ( 'NONE',  ( 1.472469842513823179, 40.59226448433411605, -4.923371831947296329 ) ) ;
#55703=CARTESIAN_POINT ( 'NONE',  ( 4.559911319644449179, 43.89701867748816966, 9.422509992056141925 ) ) ;
#55704=CARTESIAN_POINT ( 'NONE',  ( 18.52753015748618282, 63.92559781766745886, -4.923371831947291888 ) ) ;
#55705=CARTESIAN_POINT ( 'NONE',  ( -2.266590686148945544, 26.38708216824730357, -7.082119434687050408 ) ) ;
#55706=CARTESIAN_POINT ( 'NONE',  ( -0.2418659066527792945, 18.09014588040357197, 6.114288769123030320 ) ) ;
#55707=CARTESIAN_POINT ( 'NONE',  ( 18.61655166652077042, 34.87718327197428891, 6.499999999999981348 ) ) ;
#55708=CARTESIAN_POINT ( 'NONE',  ( 19.84674366389459266, 18.71726448433411960, -2.638427012816827677 ) ) ;
#55709=CARTESIAN_POINT ( 'NONE',  ( 13.43411237798105340, 45.58196800326374643, 12.81628187352647963 ) ) ;
#55710=CARTESIAN_POINT ( 'NONE',  ( 10.00000000000000178, 52.25893115100078745, 9.846743663894594434 ) ) ;
#55711=ORIENTED_EDGE ( 'NONE', *, *, #6012, .F. ) ;
#55714=CARTESIAN_POINT ( 'NONE',  ( 15.44008868035555260, 4.730352010821505360, 9.422509992056143702 ) ) ;
#55715=CARTESIAN_POINT ( 'NONE',  ( 20.88017736071110519, 55.56368534415484817, 2.639326808657452039E-16 ) ) ;
#55717=CARTESIAN_POINT ( 'NONE',  ( 17.08211943468705840, 5.137082168247300906, -12.26659068614894466 ) ) ;
#55718=CARTESIAN_POINT ( 'NONE',  ( 10.00000000000000178, 64.31368534415483396, 10.88017736071110342 ) ) ;
#55719=CARTESIAN_POINT ( 'NONE',  ( 5.076628168052703671, 56.84226448433412315, 8.527530157486179263 ) ) ;
#55720=CARTESIAN_POINT ( 'NONE',  ( 20.88017736071110164, 25.35535201082150891, 2.915334737309930979 ) ) ;
#55722=DIRECTION ( 'NONE',  ( 0.000000000000000000, 0.000000000000000000, -1.000000000000000000 ) ) ;
#55723=ADVANCED_FACE ( 'NONE', ( #50464 ), #14549, .T. ) ;
#55727=CARTESIAN_POINT ( 'NONE',  ( 16.40814093676323893, 60.79030133659709634, 11.09922568453595026 ) ) ;
#55728=VERTEX_POINT ( 'NONE', #1079 ) ;
#55733=CARTESIAN_POINT ( 'NONE',  ( 2.917880565312948704, 47.63708216824730357, 12.26659068614894643 ) ) ;
#55734=CARTESIAN_POINT ( 'NONE',  ( 19.84674366389459266, 63.30059781766745886, 2.638427012816836559 ) ) ;
#55735=CARTESIAN_POINT ( 'NONE',  ( 0.1532563361054083140, 26.00893115100078745, 1.131784320476157264E-15 ) ) ;
#55737=CARTESIAN_POINT ( 'NONE',  ( 19.42250999205614548, 15.98035201082150714, -5.440088680355545492 ) ) ;
#55738=CARTESIAN_POINT ( 'NONE',  ( 18.52753015748617571, 63.09226448433412315, 4.923371831947298993 ) ) ;
#55739=CARTESIAN_POINT ( 'NONE',  ( -0.3289641300568005855, 35.10497603579416648, 5.963430220938281678 ) ) ;
#55740=CARTESIAN_POINT ( 'NONE',  ( -4.164238869374099039, 36.80374883491396787, 8.674139862899312516E-16 ) ) ;
#55741=CARTESIAN_POINT ( 'NONE',  ( 13.79529636645031943, 65.34541550158063217, -14.16423886937409904 ) ) ;
#55744=CARTESIAN_POINT ( 'NONE',  ( 10.00000000000000178, 64.31368534415483396, 10.88017736071110342 ) ) ;
#55745=CARTESIAN_POINT ( 'NONE',  ( 12.63842701281683922, 14.55059781766744997, -9.846743663894590881 ) ) ;
#55747=VERTEX_POINT ( 'NONE', #29562 ) ;
#55750=CARTESIAN_POINT ( 'NONE',  ( 10.00000000000000000, 29.75893115100078745, -9.846743663894594434 ) ) ;
#55751=ORIENTED_EDGE ( 'NONE', *, *, #98842, .F. ) ;
#55752=CARTESIAN_POINT ( 'NONE',  ( 2.917880565312950480, 30.97041550158063572, -12.26659068614894821 ) ) ;
#55753=CARTESIAN_POINT ( 'NONE',  ( 19.84674366389459266, 33.30059781766744464, 2.638427012816836559 ) ) ;
#55754=CARTESIAN_POINT ( 'NONE',  ( 4.559911319644449179, 37.23035201082150536, -9.422509992056141925 ) ) ;
#55757=CARTESIAN_POINT ( 'NONE',  ( 20.88017736071110164, 35.35535201082150536, 2.915334737309930979 ) ) ;
#55760=CARTESIAN_POINT ( 'NONE',  ( 0.5774900079438590739, 42.64701867748816966, -5.440088680355550821 ) ) ;
#55761=CARTESIAN_POINT ( 'NONE',  ( 13.79529636645031943, 10.34541550158063394, -14.16423886937409904 ) ) ;
#55762=ORIENTED_EDGE ( 'NONE', *, *, #30413, .T. ) ;
#55764=CARTESIAN_POINT ( 'NONE',  ( 22.81628187352648496, 36.83196800326376064, -3.434112377981050290 ) ) ;
#55766=CARTESIAN_POINT ( 'NONE',  ( 5.076628168052703671, 26.84226448433411960, 8.527530157486179263 ) ) ;
#55767=LINE ( 'NONE', #86753, #84982 ) ;
#55769=CARTESIAN_POINT ( 'NONE',  ( 7.361572987183169658, 34.96726448433411605, -9.846743663894592657 ) ) ;
#55771=CARTESIAN_POINT ( 'NONE',  ( 21.92686044187657046, 65.16212336850779252, 4.562052436263912550E-16 ) ) ;
#55773=CARTESIAN_POINT ( 'NONE',  ( -43.84463630040269067, 106.6354719102472473, 4.599749066889684990 ) ) ;
#55775=CARTESIAN_POINT ( 'NONE',  ( 0.1532563361054083140, 1.008931151000784787, 1.131784320476157264E-15 ) ) ;
#55776=CARTESIAN_POINT ( 'NONE',  ( -1.099225684535947600, 14.54030133659708568, 6.408140936763237150 ) ) ;
#55777=LINE ( 'NONE', #24308, #96199 ) ;
#55780=CARTESIAN_POINT ( 'NONE',  ( 14.92337183194729988, 44.34226448433412315, -8.527530157486177487 ) ) ;
#55781=CARTESIAN_POINT ( 'NONE',  ( -0.1298530154764001854, 80.39370036920264795, -9.500000000000000000 ) ) ;
#55782=CARTESIAN_POINT ( 'NONE',  ( -2.266590686148945544, 2.220415501580634388, 7.082119434687048631 ) ) ;
#55783=CARTESIAN_POINT ( 'NONE',  ( 0.1532563361054100626, 20.80059781766744464, -2.638427012816831230 ) ) ;
#55784=CARTESIAN_POINT ( 'NONE',  ( -2.816281873526473856, 39.33196800326374643, 3.434112377981055619 ) ) ;
#55787=CARTESIAN_POINT ( 'NONE',  ( 0.5774900079438607392, 48.48035201082150536, 5.440088680355550821 ) ) ;
#55788=CARTESIAN_POINT ( 'NONE',  ( 19.38216949554541557, 12.24863466993041961, -9.382169495545420901 ) ) ;
#55789=CARTESIAN_POINT ( 'NONE',  ( 0.1532563361054082862, 41.21726448433411605, 2.638427012816831674 ) ) ;
#55791=CARTESIAN_POINT ( 'NONE',  ( 1.472469842513823179, 16.42559781766745175, 4.923371831947296329 ) ) ;
#55792=CARTESIAN_POINT ( 'NONE',  ( 15.44008868035555793, 26.39701867748817321, -9.422509992056140149 ) ) ;
#55793=CARTESIAN_POINT ( 'NONE',  ( -2.816281873526473856, 34.12363466993042493, 9.499525473075851096E-16 ) ) ;
#55794=CARTESIAN_POINT ( 'NONE',  ( 5.076628168052703671, 26.84226448433411960, 8.527530157486179263 ) ) ;
#55795=LINE ( 'NONE', #54299, #77394 ) ;
#55796=ADVANCED_FACE ( 'NONE', ( #38572 ), #84562, .T. ) ;
#55797=CARTESIAN_POINT ( 'NONE',  ( 2.035157376598824452, 13.68868534415483751, 7.964842623401179544 ) ) ;
#55800=CARTESIAN_POINT ( 'NONE',  ( 12.91533473730992121, 59.52201867748816966, 10.88017736071110164 ) ) ;
#55803=CARTESIAN_POINT ( 'NONE',  ( 19.84674366389459266, 38.71726448433412315, -2.638427012816827677 ) ) ;
#55804=CARTESIAN_POINT ( 'NONE',  ( 12.91533473730993009, 11.60535201082150714, -10.88017736071109987 ) ) ;
#55805=CARTESIAN_POINT ( 'NONE',  ( 20.88017736071110519, 40.56368534415484106, 2.639326808657452039E-16 ) ) ;
#55807=CARTESIAN_POINT ( 'NONE',  ( -0.8801773607110991993, 17.85535201082150536, -2.915334737309923874 ) ) ;
#55808=CARTESIAN_POINT ( 'NONE',  ( 19.72487221294571569, 59.78217586085237656, 6.499999999999986677 ) ) ;
#55809=CARTESIAN_POINT ( 'NONE',  ( 1.472469842513823179, 40.59226448433411605, -4.923371831947296329 ) ) ;
#55810=CARTESIAN_POINT ( 'NONE',  ( 4.999999999999999112, 11.50000000000000000, -6.500000000000000888 ) ) ;
#55812=CARTESIAN_POINT ( 'NONE',  ( 16.40814093676323893, 5.790301336597087456, 11.09922568453595026 ) ) ;
#55814=CARTESIAN_POINT ( 'NONE',  ( 2.917880565312948704, 2.637082168247300906, 12.26659068614894643 ) ) ;
#55815=CARTESIAN_POINT ( 'NONE',  ( 20.36894250292379382, 18.67874883491397142, 10.36894250292379205 ) ) ;
#55816=CYLINDRICAL_SURFACE ( 'NONE', #6576, 0.5000000000000004441 ) ;
#55818=CARTESIAN_POINT ( 'NONE',  ( 4.559911319644449179, 7.230352010821505360, -9.422509992056141925 ) ) ;
#55819=CARTESIAN_POINT ( 'NONE',  ( 0.1532563361054083140, 16.00893115100078390, 1.131784320476157264E-15 ) ) ;
#55822=CARTESIAN_POINT ( 'NONE',  ( 2.035157376598822676, 42.43868534415483396, -7.964842623401177768 ) ) ;
#55823=CARTESIAN_POINT ( 'NONE',  ( -46.44000000000001194, 93.00000000000000000, 9.500000000000000000 ) ) ;
#55824=CARTESIAN_POINT ( 'NONE',  ( 17.96484262340118221, 29.93868534415484106, 7.964842623401181321 ) ) ;
#55825=CARTESIAN_POINT ( 'NONE',  ( 16.40814093676323893, 50.79030133659708923, 11.09922568453595026 ) ) ;
#55826=CARTESIAN_POINT ( 'NONE',  ( -2.816281873526471635, 8.915301336597083903, -3.434112377981056508 ) ) ;
#55827=CARTESIAN_POINT ( 'NONE',  ( 17.20831665107776587, 9.133931151000787452, -7.208316651077762316 ) ) ;
#55830=DIRECTION ( 'NONE',  ( 0.000000000000000000, 0.000000000000000000, -1.000000000000000000 ) ) ;
#55831=CARTESIAN_POINT ( 'NONE',  ( -4.164238869374099927, 57.01208216824731068, 3.795296366450308767 ) ) ;
#55832=CARTESIAN_POINT ( 'NONE',  ( 20.36894250292379382, 28.67874883491396787, 10.36894250292379205 ) ) ;
#55833=CARTESIAN_POINT ( 'NONE',  ( 17.96484262340118221, 24.93868534415484461, 7.964842623401181321 ) ) ;
#55834=CARTESIAN_POINT ( 'NONE',  ( 20.88017736071110875, 45.77201867748816966, -2.915334737309920765 ) ) ;
#55837=CARTESIAN_POINT ( 'NONE',  ( 5.076628168052704559, 10.17559781766745175, -8.527530157486179263 ) ) ;
#55838=CARTESIAN_POINT ( 'NONE',  ( 18.52753015748617571, 18.09226448433411960, 4.923371831947298993 ) ) ;
#55841=CARTESIAN_POINT ( 'NONE',  ( 7.361572987183170547, 27.05059781766745175, 9.846743663894590881 ) ) ;
#55842=CARTESIAN_POINT ( 'NONE',  ( 19.84674366389459266, 48.71726448433413026, -2.638427012816827677 ) ) ;
#55844=CARTESIAN_POINT ( 'NONE',  ( 20.88017736071110519, 25.56368534415483751, 2.639326808657452039E-16 ) ) ;
#55845=CARTESIAN_POINT ( 'NONE',  ( 21.09922568453594849, 36.20696800326375353, 6.408140936763242479 ) ) ;
#55846=CARTESIAN_POINT ( 'NONE',  ( -0.8801773607110991993, 47.85535201082150536, -2.915334737309923874 ) ) ;
#55847=CARTESIAN_POINT ( 'NONE',  ( 18.52753015748617571, 33.09226448433411605, 4.923371831947298993 ) ) ;
#55848=CARTESIAN_POINT ( 'NONE',  ( 6.204703633549690345, 50.76208216824730357, -14.16423886937410259 ) ) ;
#55849=CARTESIAN_POINT ( 'NONE',  ( 19.84674366389459621, 28.50893115100078745, 7.409399052514197653E-17 ) ) ;
#55851=CARTESIAN_POINT ( 'NONE',  ( 0.1532563361054083140, 56.00893115100078745, 1.131784320476157264E-15 ) ) ;
#55852=CARTESIAN_POINT ( 'NONE',  ( 2.791683348922240793, 26.63393115100078745, 7.208316651077764092 ) ) ;
#55853=CARTESIAN_POINT ( 'NONE',  ( 22.26659068614895176, 4.720415501580633943, -7.082119434687042414 ) ) ;
#55854=CARTESIAN_POINT ( 'NONE',  ( 17.08211943468705840, 20.13708216824730357, -12.26659068614894466 ) ) ;
#55855=CARTESIAN_POINT ( 'NONE',  ( 7.361572987183170547, 37.05059781766744464, 9.846743663894590881 ) ) ;
#55856=CARTESIAN_POINT ( 'NONE',  ( 19.42250999205614548, 40.98035201082150536, -5.440088680355545492 ) ) ;
#55857=CARTESIAN_POINT ( 'NONE',  ( -0.8801773607111008646, 28.27201867748817321, 2.915334737309923430 ) ) ;
#55859=CARTESIAN_POINT ( 'NONE',  ( 17.96484262340118221, 41.18868534415484106, -7.964842623401177768 ) ) ;
#55860=CARTESIAN_POINT ( 'NONE',  ( -0.8801773607111008646, 33.27201867748817676, 2.915334737309923430 ) ) ;
#55862=CARTESIAN_POINT ( 'NONE',  ( 7.084665262690076126, 57.02201867748817676, -10.88017736071110164 ) ) ;
#55863=VERTEX_POINT ( 'NONE', #54534 ) ;
#55864=CARTESIAN_POINT ( 'NONE',  ( 22.81628187352647785, 56.62363466993042493, 6.195893100308588602E-16 ) ) ;
#55865=CARTESIAN_POINT ( 'NONE',  ( 0.5774900079438590739, 62.64701867748817676, -5.440088680355550821 ) ) ;
#55868=DIRECTION ( 'NONE',  ( 0.5547001962252290364, 0.8320502943378437211, 0.000000000000000000 ) ) ;
#55870=CARTESIAN_POINT ( 'NONE',  ( 17.08211943468705130, 63.47041550158063927, 12.26659068614894998 ) ) ;
#55871=CARTESIAN_POINT ( 'NONE',  ( 10.00000000000000178, 12.25893115100078568, 9.846743663894594434 ) ) ;
#55872=CARTESIAN_POINT ( 'NONE',  ( 17.08211943468705840, 10.13708216824730179, -12.26659068614894466 ) ) ;
#55873=CARTESIAN_POINT ( 'NONE',  ( 10.00000000000000000, 4.758931151000784787, -9.846743663894594434 ) ) ;
#55874=CARTESIAN_POINT ( 'NONE',  ( 7.084665262690076126, 7.022018677488169658, -10.88017736071110164 ) ) ;
#55875=CARTESIAN_POINT ( 'NONE',  ( 0.1532563361054082862, 41.21726448433411605, 2.638427012816831674 ) ) ;
#55878=CARTESIAN_POINT ( 'NONE',  ( 0.1532563361054100626, 50.80059781766745175, -2.638427012816831230 ) ) ;
#55880=FACE_OUTER_BOUND ( 'NONE', #51314, .T. ) ;
#55881=CARTESIAN_POINT ( 'NONE',  ( 15.44008868035555260, 34.73035201082151247, 9.422509992056143702 ) ) ;
#55882=CARTESIAN_POINT ( 'NONE',  ( 0.1532563361054100626, 55.80059781766745175, -2.638427012816831230 ) ) ;
#55883=FACE_OUTER_BOUND ( 'NONE', #80478, .T. ) ;
#55885=CARTESIAN_POINT ( 'NONE',  ( 0.5774900079438607392, 53.48035201082151247, 5.440088680355550821 ) ) ;
#55887=CARTESIAN_POINT ( 'NONE',  ( 15.44008868035555793, 11.39701867748817143, -9.422509992056140149 ) ) ;
#55889=EDGE_CURVE ( 'NONE', #17245, #67057, #20245, .T. ) ;
#55890=CARTESIAN_POINT ( 'NONE',  ( 16.40814093676324603, 37.45696800326376064, -11.09922568453594671 ) ) ;
#55894=CARTESIAN_POINT ( 'NONE',  ( -2.816281873526473856, 24.33196800326375353, 3.434112377981055619 ) ) ;
#55895=CARTESIAN_POINT ( 'NONE',  ( 17.96484262340118221, 34.93868534415482685, 7.964842623401181321 ) ) ;
#55897=CARTESIAN_POINT ( 'NONE',  ( -0.8801773607110991993, 67.85535201082151957, -2.915334737309923874 ) ) ;
#55898=CARTESIAN_POINT ( 'NONE',  ( 1.472469842513823179, 61.42559781766745175, 4.923371831947296329 ) ) ;
#55899=CARTESIAN_POINT ( 'NONE',  ( 18.52753015748617571, 13.09226448433411960, 4.923371831947298993 ) ) ;
#55900=CARTESIAN_POINT ( 'NONE',  ( 1.472469842513823179, 36.42559781766745175, 4.923371831947296329 ) ) ;
#55903=CARTESIAN_POINT ( 'NONE',  ( 5.076628168052704559, 40.17559781766745175, -8.527530157486179263 ) ) ;
#55904=CARTESIAN_POINT ( 'NONE',  ( 0.1916775849787266950, 52.25868815902069997, -6.499999999999991118 ) ) ;
#55906=CARTESIAN_POINT ( 'NONE',  ( 2.791683348922237240, 25.38393115100078390, -7.208316651077763204 ) ) ;
#55908=CARTESIAN_POINT ( 'NONE',  ( 0.1532563361054100626, 45.80059781766745886, -2.638427012816831230 ) ) ;
#55911=CARTESIAN_POINT ( 'NONE',  ( 0.6178305044545838731, 24.74863466993042493, 9.382169495545420901 ) ) ;
#55912=EDGE_CURVE ( 'NONE', #75712, #70278, #84014, .T. ) ;
#55913=CARTESIAN_POINT ( 'NONE',  ( 17.20831665107776587, 42.88393115100077324, 7.208316651077764980 ) ) ;
#55914=CARTESIAN_POINT ( 'NONE',  ( 0.1922240491738554657, 8.188781737317407661, 6.500000000000007105 ) ) ;
#55915=CARTESIAN_POINT ( 'NONE',  ( -4.164238869374098151, 46.59541550158063927, -3.795296366450310543 ) ) ;
#55916=CARTESIAN_POINT ( 'NONE',  ( 12.63842701281683034, 22.46726448433411605, 9.846743663894596210 ) ) ;
#55917=FILL_AREA_STYLE_COLOUR ( '', #84415 ) ;
#55920=CARTESIAN_POINT ( 'NONE',  ( -2.266590686148945544, 42.22041550158063217, 7.082119434687048631 ) ) ;
#55921=CARTESIAN_POINT ( 'NONE',  ( 10.00000000000000000, 59.75893115100078745, -9.846743663894594434 ) ) ;
#55922=CARTESIAN_POINT ( 'NONE',  ( 2.917880565312948704, 67.63708216824730357, 12.26659068614894643 ) ) ;
#55923=CARTESIAN_POINT ( 'NONE',  ( -0.3689425029237881626, 17.42874883491397142, 10.36894250292379027 ) ) ;
#55924=CARTESIAN_POINT ( 'NONE',  ( 2.917880565312948704, 37.63708216824731068, 12.26659068614894643 ) ) ;
#55925=CARTESIAN_POINT ( 'NONE',  ( 0.1955144967548975432, 29.32703681773340776, -6.500000000002792433 ) ) ;
#55927=CARTESIAN_POINT ( 'NONE',  ( 17.20831665107776587, 57.88393115100078745, 7.208316651077764980 ) ) ;
#55929=CARTESIAN_POINT ( 'NONE',  ( -0.8801773607111009756, 38.06368534415484106, 1.068504757029289695E-15 ) ) ;
#55932=CARTESIAN_POINT ( 'NONE',  ( 19.84674366389459266, 43.71726448433410894, -2.638427012816827677 ) ) ;
#55933=FACE_OUTER_BOUND ( 'NONE', #27838, .T. ) ;
#55935=CARTESIAN_POINT ( 'NONE',  ( 1.472469842513823179, 55.59226448433412315, -4.923371831947296329 ) ) ;
#55936=CARTESIAN_POINT ( 'NONE',  ( 12.63842701281683922, 59.55059781766744464, -9.846743663894590881 ) ) ;
#55938=ORIENTED_EDGE ( 'NONE', *, *, #82650, .F. ) ;
#55939=CARTESIAN_POINT ( 'NONE',  ( -2.266590686148945544, 31.38708216824730002, -7.082119434687050408 ) ) ;
#55940=DIRECTION ( 'NONE',  ( -1.501154311515388838E-13, 0.8042198116156755727, 0.5943319733994190113 ) ) ;
#55942=CARTESIAN_POINT ( 'NONE',  ( 10.00000000000000178, 70.00000000000000000, 0.000000000000000000 ) ) ;
#55943=CARTESIAN_POINT ( 'NONE',  ( -0.8801773607111008646, 8.272018677488171434, 2.915334737309923430 ) ) ;
#55944=CARTESIAN_POINT ( 'NONE',  ( 21.09922568453595559, 27.04030133659708568, -6.408140936763230044 ) ) ;
#55946=CARTESIAN_POINT ( 'NONE',  ( 0.1532563361054082862, 16.21726448433411960, 2.638427012816831674 ) ) ;
#55949=CARTESIAN_POINT ( 'NONE',  ( -0.3289641300568005855, 9.271642702460841434, -5.963430220938281678 ) ) ;
#55950=CARTESIAN_POINT ( 'NONE',  ( 17.39651004071841456, 14.08210964143329669, -6.500000000000003553 ) ) ;
#55951=CARTESIAN_POINT ( 'NONE',  ( 17.96484262340118221, 14.93868534415484106, 7.964842623401181321 ) ) ;
#55953=CARTESIAN_POINT ( 'NONE',  ( 20.88017736071110519, 30.56368534415484106, 2.639326808657452039E-16 ) ) ;
#55954=CARTESIAN_POINT ( 'NONE',  ( 2.035157376598822676, 42.43868534415483396, -7.964842623401177768 ) ) ;
#55955=CARTESIAN_POINT ( 'NONE',  ( 19.38216949554541557, 2.248634669930420049, -9.382169495545420901 ) ) ;
#55956=CARTESIAN_POINT ( 'NONE',  ( 2.791683348922237240, 65.38393115100078035, -7.208316651077763204 ) ) ;
#55957=CARTESIAN_POINT ( 'NONE',  ( 10.00000000000000000, 62.87363466993042493, -12.81628187352647608 ) ) ;
#55958=CARTESIAN_POINT ( 'NONE',  ( 1.472469842513823179, 15.59226448433411960, -4.923371831947296329 ) ) ;
#55959=AXIS2_PLACEMENT_3D ( 'NONE', #20215, #12712, #5231 ) ;
#55961=CARTESIAN_POINT ( 'NONE',  ( 7.084665262690076126, 29.10535201082150181, 10.88017736071109987 ) ) ;
#55963=CARTESIAN_POINT ( 'NONE',  ( -2.816281873526473856, 29.33196800326376064, 3.434112377981055619 ) ) ;
#55965=CARTESIAN_POINT ( 'NONE',  ( 18.52753015748617571, 58.09226448433411605, 4.923371831947298993 ) ) ;
#55966=CARTESIAN_POINT ( 'NONE',  ( 7.084665262690076126, 67.02201867748817676, -10.88017736071110164 ) ) ;
#55967=B_SPLINE_CURVE_WITH_KNOTS ( 'NONE', 3,
 ( #6433, #36945, #7442, #83426 ),
 .UNSPECIFIED., .F., .F.,
 ( 4, 4 ),
 ( 3.291406376790657244E-17, 0.001060528352562000462 ),
 .UNSPECIFIED. ) ;
#55968=CARTESIAN_POINT ( 'NONE',  ( 19.84674366389459266, 13.71726448433411782, -2.638427012816827677 ) ) ;
#55969=CARTESIAN_POINT ( 'NONE',  ( -2.816281873526471635, 28.91530133659708213, -3.434112377981056508 ) ) ;
#55970=CARTESIAN_POINT ( 'NONE',  ( 15.44008868035555260, 64.73035201082151957, 9.422509992056143702 ) ) ;
#55971=CARTESIAN_POINT ( 'NONE',  ( -46.94000000000001194, 100.4376529975800025, -8.999999999986080468 ) ) ;
#55974=CARTESIAN_POINT ( 'NONE',  ( 19.42250999205614193, 10.14701867748816966, 5.440088680355555262 ) ) ;
#55975=CARTESIAN_POINT ( 'NONE',  ( 3.591859063236763294, 58.29030133659708923, -11.09922568453595026 ) ) ;
#55976=CARTESIAN_POINT ( 'NONE',  ( 13.79529636645031943, 25.34541550158063572, -14.16423886937409904 ) ) ;
#55977=CARTESIAN_POINT ( 'NONE',  ( 5.076628168052703671, 11.84226448433411960, 8.527530157486179263 ) ) ;
#55978=CARTESIAN_POINT ( 'NONE',  ( 17.96484262340118221, 4.938685344154837509, 7.964842623401181321 ) ) ;
#55980=CARTESIAN_POINT ( 'NONE',  ( 0.1532563361054100626, 20.80059781766744464, -2.638427012816831230 ) ) ;
#55981=CARTESIAN_POINT ( 'NONE',  ( -4.164238869374099039, 61.80374883491397497, 8.674139862899312516E-16 ) ) ;
#55982=EDGE_LOOP ( 'NONE', ( #76527, #49461, #5615, #60749 ) ) ;
#55984=CARTESIAN_POINT ( 'NONE',  ( 20.88017736071110519, 25.56368534415483751, 2.639326808657452039E-16 ) ) ;
#55985=CARTESIAN_POINT ( 'NONE',  ( 1.821708436314935620, 31.66792564121895381, -6.500000000000005329 ) ) ;
#55988=CARTESIAN_POINT ( 'NONE',  ( 20.88017736071110875, 25.77201867748816966, -2.915334737309920765 ) ) ;
#55989=CARTESIAN_POINT ( 'NONE',  ( 2.791683348922240793, 51.63393115100078745, 7.208316651077764092 ) ) ;
#55990=VECTOR ( 'NONE', #78163, 1000.000000000000000 ) ;
#55991=CARTESIAN_POINT ( 'NONE',  ( 21.09922568453594849, 51.20696800326375353, 6.408140936763242479 ) ) ;
#55994=CARTESIAN_POINT ( 'NONE',  ( 17.08211943468705130, 23.47041550158063572, 12.26659068614894998 ) ) ;
#55995=CARTESIAN_POINT ( 'NONE',  ( 12.91533473730993009, 36.60535201082151247, -10.88017736071109987 ) ) ;
#55996=CARTESIAN_POINT ( 'NONE',  ( -0.8801773607110991993, 12.85535201082150358, -2.915334737309923874 ) ) ;
#55997=CARTESIAN_POINT ( 'NONE',  ( 2.791683348922240793, 56.63393115100078035, 7.208316651077764092 ) ) ;
#55998=CARTESIAN_POINT ( 'NONE',  ( 1.472469842513823179, 35.59226448433412315, -4.923371831947296329 ) ) ;
#55999=DIRECTION ( 'NONE',  ( 0.000000000000000000, 1.000000000000000000, 0.000000000000000000 ) ) ;
#56000=CARTESIAN_POINT ( 'NONE',  ( 18.52753015748617571, 3.092264484334118269, 4.923371831947298993 ) ) ;
#56003=( BOUNDED_CURVE ( )  B_SPLINE_CURVE ( 3, ( #88625, #80141, #50636, #34135 ),
 .UNSPECIFIED., .F., .T. ) 
 B_SPLINE_CURVE_WITH_KNOTS ( ( 4, 4 ),
 ( 4.712388980384689674, 5.730377828609853452 ),
 .UNSPECIFIED. ) 
 CURVE ( )  GEOMETRIC_REPRESENTATION_ITEM ( )  RATIONAL_B_SPLINE_CURVE ( ( 1.000000000000000000, 0.9154899770527749059, 0.9154899770527749059, 1.000000000000000000 ) ) 
 REPRESENTATION_ITEM ( '' )  );
#56004=CARTESIAN_POINT ( 'NONE',  ( -0.8801773607110991993, 2.855352010821504471, -2.915334737309923874 ) ) ;
#56005=CARTESIAN_POINT ( 'NONE',  ( 18.52753015748618282, 13.92559781766745175, -4.923371831947291888 ) ) ;
#56007=CARTESIAN_POINT ( 'NONE',  ( -1.099225684535947600, -1.293031996736246469, -6.408140936763238038 ) ) ;
#56008=CARTESIAN_POINT ( 'NONE',  ( 0.5774900079438607392, 43.48035201082151247, 5.440088680355550821 ) ) ;
#56009=CARTESIAN_POINT ( 'NONE',  ( -1.099225684535947600, 44.54030133659708923, 6.408140936763237150 ) ) ;
#56010=CARTESIAN_POINT ( 'NONE',  ( 10.00000000000000000, 35.55374883491396787, -14.16423886937410082 ) ) ;
#56011=FACE_OUTER_BOUND ( 'NONE', #74099, .T. ) ;
#56012=( BOUNDED_SURFACE ( )  B_SPLINE_SURFACE ( 1, 2, ( 
 ( #51001, #82987, #59487, #44977, #29969, #60475, #90964, #68486, #81496, #36505, #22497, #21504, #43496, #13001, #58999, #43986, #6011, #66503, #15002, #7503, #97028, #37994, #13, #89988, #30461, #52001, #82491, #36000, #28505, #89501, #66997, #97520, #508, #92933, #46460, #30956, #62933, #54930, #7983, #45979, #69957, #16956, #47924, #17457, #9947, #23492, #93435, #69462, #32432, #47440, #31445, #22995, #8950, #39467, #78429, #62430, #77939, #54442, #68976, #40450, #53963, #982, #53461, #16463, #70950, #60961, #91962, #23970, #61454, #15969, #91470, #24959, #61945, #9445, #84953, #76954, #1476, #39946, #84471, #8464, #70449, #1968, #46943, #83971, #24465, #38970, #2469, #15497, #31930, #92446, #76468, #77437, #85447, #55443, #85947, #38482, #64877, #87407, #88393, #95404, #2954, #87887, #26900, #17938, #26404, #34390, #57397, #11407, #12391, #4421, #32926, #95910, #63426, #10435, #3920, #41930, #49893, #71440, #34887, #94905, #56903, #19405, #48911, #71909, #80404, #33403, #49400, #19892, #93930, #72886, #50385, #73378, #41447, #18924, #11906, #79901, #3432, #42408, #72392, #56431, #65381, #27389, #33891, #63903, #86438, #80894, #64396, #25456, #55939, #94414, #57882, #48422, #25930, #86918, #42896, #78925, #40942, #18429, #79426, #10922, #96904, #13881, #22375, #66370, #44850, #6870, #58875, #36379, #89866, #59858, #43374, #59362, #88887, #73877, #97897, #67367, #52852, #5404, #90345, #20890, #28383, #14882, #66874, #60352, #82864, #83358, #52361, #45351, #36878, #21882, #65877, #29355, #81379, #97391, #81865, #4905, #14381, #75355, #96404, #37381, #12879, #28859, #13378, #21381, #35877, #89377, #35386, #67871, #5884, #98392, #51878, #51378, #82360, #29848, #43863, #74357, #90846, #27879, #44364, #58367, #6364, #74865, #20397, #50885, #54321, #45857, #62812, #30839, #8345, #76348, #76830, #61825, #8831, #31325, #32307, #39345, #7864, #31814, #69839, #60844, #69342, #77316, #1363, #84835, #55314, #47310, #75856, #39827, #7376, #53342, #46825, #16343, #92817, #15376, #77809, #38852, #866, #62311, #91848, #15858, #24348, #38360, #92333, #93310, #37874, #16835, #24833, #17336, #84357, #23856, #54811, #85322, #46343, #9324, #70333, #388, #1849, #85822, #68368, #68857, #30338, #98887, #91344, #22871, #83850, #61337, #23364, #53848, #40816, #71315, #64762, #26284, #80279, #2833, #63781, #49285, #33289, #56785, #65256, #10315, #87769, #49770, #94290, #79297, #33765, #3804, #86313, #3303, #32799, #17816, #41806, #11286, #95784, #48298, #34260, #25813, #56309, #57764, #10806, #4294, #26777, #27265, #95274, #41324, #86805 ),
 ( #18307, #57275, #87280, #11780, #48789, #71796, #79784, #64272, #18801, #88267, #94784, #19284, #42287, #72274, #72759, #34768, #47805, #78805, #78306, #63294, #9825, #40326, #70830, #2343, #93803, #25334, #55818, #81262, #29731, #51259, #75241, #97779, #67755, #67255, #98274, #51758, #74748, #80775, #82243, #96282, #13259, #96783, #81743, #27760, #73753, #19771, #21769, #20769, #6259, #43751, #5284, #97278, #29244, #12761, #58245, #36762, #59741, #74237, #12268, #21261, #66248, #6751, #60239, #28752, #88763, #37268, #35760, #5770, #20274, #36259, #66755, #13757, #59244, #50258, #44243, #50771, #90236, #52248, #4785, #89743, #82742, #14263, #44740, #42778, #73262, #35260, #65757, #43259, #28258, #58754, #89258, #8715, #30222, #92704, #53727, #15748, #54207, #7754, #30716, #16229, #91226, #8239, #47196, #90734, #31703, #77699, #32189, #271, #46234, #92219, #38733, #61225, #61705, #76720, #15260, #84724, #60726, #23747, #76237, #22750, #24229, #46709, #37758, #75735, #758, #77209, #9210, #39723, #70216, #53233, #54695, #91730, #62195, #39233, #23252, #52735, #69234, #31209, #1735, #69721, #1247, #84244, #98774, #22260, #83738, #85217, #83242, #16721, #14765, #45238, #45741, #7254, #68254, #38248, #68739, #55191, #17222, #2228, #41205, #93191, #56675, #11172, #57158, #93689, #40698, #19169, #64644, #25223, #33660, #95155, #64156, #3196, #63671, #87164, #94674, #26183, #41692, #63182, #11667, #42180, #34150, #85708, #32687, #72162, #71201, #80157, #87656, #2724, #33178, #47701, #78695, #25706, #78193, #10693, #3689, #71685, #18195, #94175, #4177, #48675, #18690, #79675, #55703, #56197, #86690, #79178, #26664, #49173, #48183, #9706, #49649, #40204, #24718, #72644, #62691, #70710, #86199, #17711, #10205, #14143, #27149, #81141, #21145, #66132, #88148, #95664, #4677, #65639, #58131, #12156, #67130, #36136, #42661, #59623, #44119, #5159, #5657, #35645, #96662, #58641, #90120, #65144, #57651, #21647, #74629, #52131, #75122, #43142, #89140, #66643, #51141, #73633, #97167, #20650, #88640, #28635, #28142, #81630, #35139, #19660, #82628, #13137, #34648, #50150, #73137, #43635, #80661, #27645, #20148, #51644, #74121, #97657, #50653, #12644, #59124, #89633, #82125, #44627, #96163, #6142, #36645, #13635, #29121, #91613, #61589, #45112, #61104, #90613, #75618, #645, #69113, #24110, #7129, #92101, #22634, #68130, #16604, #38133, #62078, #84607, #54580, #54092, #85095, #38614, #23631, #67638, #31095, #83120, #151, #83622, #68621, #14649, #60612, #6630, #8603, #7643, #16108, #30599, #91108, #84117, #46594, #98658, #37633, #77093, #39113 ) ),
 .UNSPECIFIED., .F., .F., .T. ) 
 B_SPLINE_SURFACE_WITH_KNOTS ( ( 2, 2 ),
 ( 3, 2, 2, 2, 2, 2, 2, 2, 2, 2, 2, 2, 2, 2, 2, 2, 2, 2, 2, 2, 2, 2, 2, 2, 2, 2, 2, 2, 2, 2, 2, 2, 2, 2, 2, 2, 2, 2, 2, 2, 2, 2, 2, 2, 2, 2, 2, 2, 2, 2, 2, 2, 2, 2, 2, 2, 2, 2, 2, 2, 2, 2, 2, 2, 2, 2, 2, 2, 2, 2, 2, 2, 2, 2, 2, 2, 2, 2, 2, 2, 2, 2, 2, 2, 2, 2, 2, 2, 2, 2, 2, 2, 2, 2, 2, 2, 2, 2, 2, 2, 2, 2, 2, 2, 2, 2, 2, 2, 2, 2, 2, 2, 2, 2, 2, 2, 2, 2, 2, 2, 2, 2, 2, 2, 2, 2, 2, 2, 2, 2, 2, 2, 2, 2, 2, 2, 2, 2, 2, 2, 2, 2, 2, 2, 2, 2, 2, 2, 2, 2, 2, 2, 2, 2, 2, 2, 2, 2, 2, 2, 2, 2, 3 ),
 ( 0.000000000000000000, 1.000000000000000000 ),
 ( 0.000000000000000000, 0.005952380952380952051, 0.01190476190476190410, 0.01785714285714285615, 0.02380952380952380820, 0.02976190476190476025, 0.03571428571428571230, 0.04166666666666666435, 0.04761904761904761640, 0.05357142857142856845, 0.05952380952380952051, 0.06547619047619047949, 0.07142857142857142461, 0.07738095238095238360, 0.08333333333333332871, 0.08928571428571428770, 0.09523809523809523281, 0.1011904761904761918, 0.1071428571428571369, 0.1130952380952380959, 0.1190476190476190410, 0.1250000000000000000, 0.1309523809523809590, 0.1369047619047619180, 0.1428571428571428492, 0.1488095238095238082, 0.1547619047619047672, 0.1607142857142857262, 0.1666666666666666574, 0.1726190476190476164, 0.1785714285714285754, 0.1845238095238095344, 0.1904761904761904656, 0.1964285714285714246, 0.2023809523809523836, 0.2083333333333333426, 0.2142857142857142738, 0.2202380952380952328, 0.2261904761904761918, 0.2321428571428571508, 0.2380952380952380820, 0.2440476190476190410, 0.2500000000000000000, 0.2559523809523809312, 0.2619047619047619180, 0.2678571428571428492, 0.2738095238095238360, 0.2797619047619047672, 0.2857142857142856984, 0.2916666666666666852, 0.2976190476190476164, 0.3035714285714285476, 0.3095238095238095344, 0.3154761904761904656, 0.3214285714285714524, 0.3273809523809523836, 0.3333333333333333148, 0.3392857142857143016, 0.3452380952380952328, 0.3511904761904761640, 0.3571428571428571508, 0.3630952380952380820, 0.3690476190476190688, 0.3750000000000000000, 0.3809523809523809312, 0.3869047619047619180, 0.3928571428571428492, 0.3988095238095238360, 0.4047619047619047672, 0.4107142857142856984, 0.4166666666666666852, 0.4226190476190476164, 0.4285714285714285476, 0.4345238095238095344, 0.4404761904761904656, 0.4464285714285714524, 0.4523809523809523836, 0.4583333333333333148, 0.4642857142857143016, 0.4702380952380952328, 0.4761904761904761640, 0.4821428571428571508, 0.4880952380952380820, 0.4940476190476190688, 0.5000000000000000000, 0.5059523809523809312, 0.5119047619047618625, 0.5178571428571429047, 0.5238095238095238360, 0.5297619047619047672, 0.5357142857142856984, 0.5416666666666666297, 0.5476190476190476719, 0.5535714285714286031, 0.5595238095238095344, 0.5654761904761904656, 0.5714285714285713969, 0.5773809523809523281, 0.5833333333333333703, 0.5892857142857143016, 0.5952380952380952328, 0.6011904761904761640, 0.6071428571428570953, 0.6130952380952381375, 0.6190476190476190688, 0.6250000000000000000, 0.6309523809523809312, 0.6369047619047618625, 0.6428571428571429047, 0.6488095238095238360, 0.6547619047619047672, 0.6607142857142856984, 0.6666666666666666297, 0.6726190476190476719, 0.6785714285714286031, 0.6845238095238095344, 0.6904761904761904656, 0.6964285714285713969, 0.7023809523809523281, 0.7083333333333333703, 0.7142857142857143016, 0.7202380952380952328, 0.7261904761904761640, 0.7321428571428570953, 0.7380952380952381375, 0.7440476190476190688, 0.7500000000000000000, 0.7559523809523809312, 0.7619047619047618625, 0.7678571428571429047, 0.7738095238095238360, 0.7797619047619047672, 0.7857142857142856984, 0.7916666666666666297, 0.7976190476190476719, 0.8035714285714286031, 0.8095238095238095344, 0.8154761904761904656, 0.8214285714285713969, 0.8273809523809523281, 0.8333333333333333703, 0.8392857142857143016, 0.8452380952380952328, 0.8511904761904761640, 0.8571428571428570953, 0.8630952380952381375, 0.8690476190476190688, 0.8750000000000000000, 0.8809523809523809312, 0.8869047619047618625, 0.8928571428571429047, 0.8988095238095238360, 0.9047619047619047672, 0.9107142857142856984, 0.9166666666666666297, 0.9226190476190476719, 0.9285714285714286031, 0.9345238095238095344, 0.9404761904761904656, 0.9464285714285713969, 0.9523809523809523281, 0.9583333333333333703, 0.9642857142857143016 ),
 .UNSPECIFIED. ) 
 GEOMETRIC_REPRESENTATION_ITEM ( )  RATIONAL_B_SPLINE_SURFACE ( (
 ( 1.000000000000000000, 0.9659258262890683122, 1.000000000000000000, 0.9659258262890683122, 1.000000000000000000, 0.9659258262890683122, 1.000000000000000000, 0.9659258262890683122, 1.000000000000000000, 0.9659258262890683122, 1.000000000000000000, 0.9659258262890683122, 1.000000000000000000, 0.9659258262890683122, 1.000000000000000000, 0.9659258262890683122, 1.000000000000000000, 0.9659258262890683122, 1.000000000000000000, 0.9659258262890683122, 1.000000000000000000, 0.9659258262890683122, 1.000000000000000000, 0.9659258262890683122, 1.000000000000000000, 0.9659258262890683122, 1.000000000000000000, 0.9659258262890683122, 1.000000000000000000, 0.9659258262890683122, 1.000000000000000000, 0.9659258262890683122, 1.000000000000000000, 0.9659258262890683122, 1.000000000000000000, 0.9659258262890683122, 1.000000000000000000, 0.9659258262890683122, 1.000000000000000000, 0.9659258262890683122, 1.000000000000000000, 0.9659258262890683122, 1.000000000000000000, 0.9659258262890683122, 1.000000000000000000, 0.9659258262890683122, 1.000000000000000000, 0.9659258262890683122, 1.000000000000000000, 0.9659258262890683122, 1.000000000000000000, 0.9659258262890683122, 1.000000000000000000, 0.9659258262890683122, 1.000000000000000000, 0.9659258262890683122, 1.000000000000000000, 0.9659258262890683122, 1.000000000000000000, 0.9659258262890683122, 1.000000000000000000, 0.9659258262890683122, 1.000000000000000000, 0.9659258262890683122, 1.000000000000000000, 0.9659258262890683122, 1.000000000000000000, 0.9659258262890683122, 1.000000000000000000, 0.9659258262890683122, 1.000000000000000000, 0.9659258262890683122, 1.000000000000000000, 0.9659258262890683122, 1.000000000000000000, 0.9659258262890683122, 1.000000000000000000, 0.9659258262890683122, 1.000000000000000000, 0.9659258262890683122, 1.000000000000000000, 0.9659258262890683122, 1.000000000000000000, 0.9659258262890683122, 1.000000000000000000, 0.9659258262890683122, 1.000000000000000000, 0.9659258262890683122, 1.000000000000000000, 0.9659258262890683122, 1.000000000000000000, 0.9659258262890683122, 1.000000000000000000, 0.9659258262890683122, 1.000000000000000000, 0.9659258262890683122, 1.000000000000000000, 0.9659258262890683122, 1.000000000000000000, 0.9659258262890683122, 1.000000000000000000, 0.9659258262890683122, 1.000000000000000000, 0.9659258262890683122, 1.000000000000000000, 0.9659258262890683122, 1.000000000000000000, 0.9659258262890683122, 1.000000000000000000, 0.9659258262890683122, 1.000000000000000000, 0.9659258262890683122, 1.000000000000000000, 0.9659258262890683122, 1.000000000000000000, 0.9659258262890683122, 1.000000000000000000, 0.9659258262890683122, 1.000000000000000000, 0.9659258262890683122, 1.000000000000000000, 0.9659258262890683122, 1.000000000000000000, 0.9659258262890683122, 1.000000000000000000, 0.9659258262890683122, 1.000000000000000000, 0.9659258262890683122, 1.000000000000000000, 0.9659258262890683122, 1.000000000000000000, 0.9659258262890683122, 1.000000000000000000, 0.9659258262890683122, 1.000000000000000000, 0.9659258262890683122, 1.000000000000000000, 0.9659258262890683122, 1.000000000000000000, 0.9659258262890683122, 1.000000000000000000, 0.9659258262890683122, 1.000000000000000000, 0.9659258262890683122, 1.000000000000000000, 0.9659258262890683122, 1.000000000000000000, 0.9659258262890683122, 1.000000000000000000, 0.9659258262890683122, 1.000000000000000000, 0.9659258262890683122, 1.000000000000000000, 0.9659258262890683122, 1.000000000000000000, 0.9659258262890683122, 1.000000000000000000, 0.9659258262890683122, 1.000000000000000000, 0.9659258262890683122, 1.000000000000000000, 0.9659258262890683122, 1.000000000000000000, 0.9659258262890683122, 1.000000000000000000, 0.9659258262890683122, 1.000000000000000000, 0.9659258262890683122, 1.000000000000000000, 0.9659258262890683122, 1.000000000000000000, 0.9659258262890683122, 1.000000000000000000, 0.9659258262890683122, 1.000000000000000000, 0.9659258262890683122, 1.000000000000000000, 0.9659258262890683122, 1.000000000000000000, 0.9659258262890683122, 1.000000000000000000, 0.9659258262890683122, 1.000000000000000000, 0.9659258262890683122, 1.000000000000000000, 0.9659258262890683122, 1.000000000000000000, 0.9659258262890683122, 1.000000000000000000, 0.9659258262890683122, 1.000000000000000000, 0.9659258262890683122, 1.000000000000000000, 0.9659258262890683122, 1.000000000000000000, 0.9659258262890683122, 1.000000000000000000, 0.9659258262890683122, 1.000000000000000000, 0.9659258262890683122, 1.000000000000000000, 0.9659258262890683122, 1.000000000000000000, 0.9659258262890683122, 1.000000000000000000, 0.9659258262890683122, 1.000000000000000000, 0.9659258262890683122, 1.000000000000000000, 0.9659258262890683122, 1.000000000000000000, 0.9659258262890683122, 1.000000000000000000, 0.9659258262890683122, 1.000000000000000000, 0.9659258262890683122, 1.000000000000000000, 0.9659258262890683122, 1.000000000000000000, 0.9659258262890683122, 1.000000000000000000, 0.9659258262890683122, 1.000000000000000000, 0.9659258262890683122, 1.000000000000000000, 0.9659258262890683122, 1.000000000000000000, 0.9659258262890683122, 1.000000000000000000, 0.9659258262890683122, 1.000000000000000000, 0.9659258262890683122, 1.000000000000000000, 0.9659258262890683122, 1.000000000000000000, 0.9659258262890683122, 1.000000000000000000, 0.9659258262890683122, 1.000000000000000000, 0.9659258262890683122, 1.000000000000000000, 0.9659258262890683122, 1.000000000000000000, 0.9659258262890683122, 1.000000000000000000, 0.9659258262890683122, 1.000000000000000000, 0.9659258262890683122, 1.000000000000000000, 0.9659258262890683122, 1.000000000000000000, 0.9659258262890683122, 1.000000000000000000, 0.9659258262890683122, 1.000000000000000000, 0.9659258262890683122, 1.000000000000000000, 0.9659258262890683122, 1.000000000000000000, 0.9659258262890683122, 1.000000000000000000, 0.9659258262890683122, 1.000000000000000000, 0.9659258262890683122, 1.000000000000000000, 0.9659258262890683122, 1.000000000000000000, 0.9659258262890683122, 1.000000000000000000, 0.9659258262890683122, 1.000000000000000000, 0.9659258262890683122, 1.000000000000000000, 0.9659258262890683122, 1.000000000000000000, 0.9659258262890683122, 1.000000000000000000, 0.9659258262890683122, 1.000000000000000000, 0.9659258262890683122, 1.000000000000000000, 0.9659258262890683122, 1.000000000000000000, 0.9659258262890683122, 1.000000000000000000, 0.9659258262890683122, 1.000000000000000000, 0.9659258262890683122, 1.000000000000000000, 0.9659258262890683122, 1.000000000000000000, 0.9659258262890683122, 1.000000000000000000, 0.9659258262890683122, 1.000000000000000000, 0.9659258262890683122, 1.000000000000000000, 0.9659258262890683122, 1.000000000000000000, 0.9659258262890683122, 1.000000000000000000, 0.9659258262890683122, 1.000000000000000000, 0.9659258262890683122, 1.000000000000000000, 0.9659258262890683122, 1.000000000000000000, 0.9659258262890683122, 1.000000000000000000, 0.9659258262890683122, 1.000000000000000000, 0.9659258262890683122, 1.000000000000000000, 0.9659258262890683122, 1.000000000000000000, 0.9659258262890683122, 1.000000000000000000, 0.9659258262890683122, 1.000000000000000000, 0.9659258262890683122, 1.000000000000000000, 0.9659258262890683122, 1.000000000000000000, 0.9659258262890683122, 1.000000000000000000),
 ( 1.000000000000000000, 0.9659258262890683122, 1.000000000000000000, 0.9659258262890683122, 1.000000000000000000, 0.9659258262890683122, 1.000000000000000000, 0.9659258262890683122, 1.000000000000000000, 0.9659258262890683122, 1.000000000000000000, 0.9659258262890683122, 1.000000000000000000, 0.9659258262890683122, 1.000000000000000000, 0.9659258262890683122, 1.000000000000000000, 0.9659258262890683122, 1.000000000000000000, 0.9659258262890683122, 1.000000000000000000, 0.9659258262890683122, 1.000000000000000000, 0.9659258262890683122, 1.000000000000000000, 0.9659258262890683122, 1.000000000000000000, 0.9659258262890683122, 1.000000000000000000, 0.9659258262890683122, 1.000000000000000000, 0.9659258262890683122, 1.000000000000000000, 0.9659258262890683122, 1.000000000000000000, 0.9659258262890683122, 1.000000000000000000, 0.9659258262890683122, 1.000000000000000000, 0.9659258262890683122, 1.000000000000000000, 0.9659258262890683122, 1.000000000000000000, 0.9659258262890683122, 1.000000000000000000, 0.9659258262890683122, 1.000000000000000000, 0.9659258262890683122, 1.000000000000000000, 0.9659258262890683122, 1.000000000000000000, 0.9659258262890683122, 1.000000000000000000, 0.9659258262890683122, 1.000000000000000000, 0.9659258262890683122, 1.000000000000000000, 0.9659258262890683122, 1.000000000000000000, 0.9659258262890683122, 1.000000000000000000, 0.9659258262890683122, 1.000000000000000000, 0.9659258262890683122, 1.000000000000000000, 0.9659258262890683122, 1.000000000000000000, 0.9659258262890683122, 1.000000000000000000, 0.9659258262890683122, 1.000000000000000000, 0.9659258262890683122, 1.000000000000000000, 0.9659258262890683122, 1.000000000000000000, 0.9659258262890683122, 1.000000000000000000, 0.9659258262890683122, 1.000000000000000000, 0.9659258262890683122, 1.000000000000000000, 0.9659258262890683122, 1.000000000000000000, 0.9659258262890683122, 1.000000000000000000, 0.9659258262890683122, 1.000000000000000000, 0.9659258262890683122, 1.000000000000000000, 0.9659258262890683122, 1.000000000000000000, 0.9659258262890683122, 1.000000000000000000, 0.9659258262890683122, 1.000000000000000000, 0.9659258262890683122, 1.000000000000000000, 0.9659258262890683122, 1.000000000000000000, 0.9659258262890683122, 1.000000000000000000, 0.9659258262890683122, 1.000000000000000000, 0.9659258262890683122, 1.000000000000000000, 0.9659258262890683122, 1.000000000000000000, 0.9659258262890683122, 1.000000000000000000, 0.9659258262890683122, 1.000000000000000000, 0.9659258262890683122, 1.000000000000000000, 0.9659258262890683122, 1.000000000000000000, 0.9659258262890683122, 1.000000000000000000, 0.9659258262890683122, 1.000000000000000000, 0.9659258262890683122, 1.000000000000000000, 0.9659258262890683122, 1.000000000000000000, 0.9659258262890683122, 1.000000000000000000, 0.9659258262890683122, 1.000000000000000000, 0.9659258262890683122, 1.000000000000000000, 0.9659258262890683122, 1.000000000000000000, 0.9659258262890683122, 1.000000000000000000, 0.9659258262890683122, 1.000000000000000000, 0.9659258262890683122, 1.000000000000000000, 0.9659258262890683122, 1.000000000000000000, 0.9659258262890683122, 1.000000000000000000, 0.9659258262890683122, 1.000000000000000000, 0.9659258262890683122, 1.000000000000000000, 0.9659258262890683122, 1.000000000000000000, 0.9659258262890683122, 1.000000000000000000, 0.9659258262890683122, 1.000000000000000000, 0.9659258262890683122, 1.000000000000000000, 0.9659258262890683122, 1.000000000000000000, 0.9659258262890683122, 1.000000000000000000, 0.9659258262890683122, 1.000000000000000000, 0.9659258262890683122, 1.000000000000000000, 0.9659258262890683122, 1.000000000000000000, 0.9659258262890683122, 1.000000000000000000, 0.9659258262890683122, 1.000000000000000000, 0.9659258262890683122, 1.000000000000000000, 0.9659258262890683122, 1.000000000000000000, 0.9659258262890683122, 1.000000000000000000, 0.9659258262890683122, 1.000000000000000000, 0.9659258262890683122, 1.000000000000000000, 0.9659258262890683122, 1.000000000000000000, 0.9659258262890683122, 1.000000000000000000, 0.9659258262890683122, 1.000000000000000000, 0.9659258262890683122, 1.000000000000000000, 0.9659258262890683122, 1.000000000000000000, 0.9659258262890683122, 1.000000000000000000, 0.9659258262890683122, 1.000000000000000000, 0.9659258262890683122, 1.000000000000000000, 0.9659258262890683122, 1.000000000000000000, 0.9659258262890683122, 1.000000000000000000, 0.9659258262890683122, 1.000000000000000000, 0.9659258262890683122, 1.000000000000000000, 0.9659258262890683122, 1.000000000000000000, 0.9659258262890683122, 1.000000000000000000, 0.9659258262890683122, 1.000000000000000000, 0.9659258262890683122, 1.000000000000000000, 0.9659258262890683122, 1.000000000000000000, 0.9659258262890683122, 1.000000000000000000, 0.9659258262890683122, 1.000000000000000000, 0.9659258262890683122, 1.000000000000000000, 0.9659258262890683122, 1.000000000000000000, 0.9659258262890683122, 1.000000000000000000, 0.9659258262890683122, 1.000000000000000000, 0.9659258262890683122, 1.000000000000000000, 0.9659258262890683122, 1.000000000000000000, 0.9659258262890683122, 1.000000000000000000, 0.9659258262890683122, 1.000000000000000000, 0.9659258262890683122, 1.000000000000000000, 0.9659258262890683122, 1.000000000000000000, 0.9659258262890683122, 1.000000000000000000, 0.9659258262890683122, 1.000000000000000000, 0.9659258262890683122, 1.000000000000000000, 0.9659258262890683122, 1.000000000000000000, 0.9659258262890683122, 1.000000000000000000, 0.9659258262890683122, 1.000000000000000000, 0.9659258262890683122, 1.000000000000000000, 0.9659258262890683122, 1.000000000000000000, 0.9659258262890683122, 1.000000000000000000, 0.9659258262890683122, 1.000000000000000000, 0.9659258262890683122, 1.000000000000000000, 0.9659258262890683122, 1.000000000000000000, 0.9659258262890683122, 1.000000000000000000, 0.9659258262890683122, 1.000000000000000000, 0.9659258262890683122, 1.000000000000000000, 0.9659258262890683122, 1.000000000000000000, 0.9659258262890683122, 1.000000000000000000, 0.9659258262890683122, 1.000000000000000000, 0.9659258262890683122, 1.000000000000000000, 0.9659258262890683122, 1.000000000000000000, 0.9659258262890683122, 1.000000000000000000, 0.9659258262890683122, 1.000000000000000000, 0.9659258262890683122, 1.000000000000000000, 0.9659258262890683122, 1.000000000000000000, 0.9659258262890683122, 1.000000000000000000, 0.9659258262890683122, 1.000000000000000000, 0.9659258262890683122, 1.000000000000000000, 0.9659258262890683122, 1.000000000000000000, 0.9659258262890683122, 1.000000000000000000, 0.9659258262890683122, 1.000000000000000000, 0.9659258262890683122, 1.000000000000000000, 0.9659258262890683122, 1.000000000000000000, 0.9659258262890683122, 1.000000000000000000, 0.9659258262890683122, 1.000000000000000000, 0.9659258262890683122, 1.000000000000000000, 0.9659258262890683122, 1.000000000000000000, 0.9659258262890683122, 1.000000000000000000, 0.9659258262890683122, 1.000000000000000000, 0.9659258262890683122, 1.000000000000000000, 0.9659258262890683122, 1.000000000000000000, 0.9659258262890683122, 1.000000000000000000, 0.9659258262890683122, 1.000000000000000000, 0.9659258262890683122, 1.000000000000000000, 0.9659258262890683122, 1.000000000000000000, 0.9659258262890683122, 1.000000000000000000) ) ) 
 REPRESENTATION_ITEM ( '' )  SURFACE ( )  );
#56014=ADVANCED_FACE ( 'NONE', ( #2565 ), #55542, .F. ) ;
#56015=CARTESIAN_POINT ( 'NONE',  ( 10.00000000000000000, 57.87363466993042493, -12.81628187352647608 ) ) ;
#56018=CARTESIAN_POINT ( 'NONE',  ( 2.791683348922240793, 56.63393115100078035, 7.208316651077764092 ) ) ;
#56019=CARTESIAN_POINT ( 'NONE',  ( 17.96484262340118221, 16.18868534415483396, -7.964842623401177768 ) ) ;
#56021=ORIENTED_EDGE ( 'NONE', *, *, #26849, .F. ) ;
#56022=CARTESIAN_POINT ( 'NONE',  ( 2.035157376598824452, 68.68868534415484817, 7.964842623401179544 ) ) ;
#56024=CARTESIAN_POINT ( 'NONE',  ( 12.63842701281683034, 12.46726448433411782, 9.846743663894596210 ) ) ;
#56025=CARTESIAN_POINT ( 'NONE',  ( 12.91533473730993009, 66.60535201082150536, -10.88017736071109987 ) ) ;
#56027=CARTESIAN_POINT ( 'NONE',  ( 7.084665262690076126, 57.02201867748817676, -10.88017736071110164 ) ) ;
#56029=CARTESIAN_POINT ( 'NONE',  ( 15.44008868035555260, 64.73035201082151957, 9.422509992056143702 ) ) ;
#56030=CARTESIAN_POINT ( 'NONE',  ( 7.361572987183169658, 9.967264484334119601, -9.846743663894592657 ) ) ;
#56033=CARTESIAN_POINT ( 'NONE',  ( 17.20831665107776587, 57.88393115100078745, 7.208316651077764980 ) ) ;
#56034=ADVANCED_FACE ( 'NONE', ( #70051 ), #64489, .F. ) ;
#56038=CARTESIAN_POINT ( 'NONE',  ( 13.79529636645031943, 5.345415501580634832, -14.16423886937409904 ) ) ;
#56039=CARTESIAN_POINT ( 'NONE',  ( -2.816281873526471635, 63.91530133659708923, -3.434112377981056508 ) ) ;
#56041=CARTESIAN_POINT ( 'NONE',  ( 24.16423886937410614, 4.303748834913967869, 8.672049930838204340E-16 ) ) ;
#56042=CARTESIAN_POINT ( 'NONE',  ( 6.204703633549690345, 35.76208216824729647, -14.16423886937410259 ) ) ;
#56044=CARTESIAN_POINT ( 'NONE',  ( 6.204703633549690345, 5.762082168247301794, -14.16423886937410259 ) ) ;
#56045=CARTESIAN_POINT ( 'NONE',  ( 4.559911319644449179, 23.89701867748817321, 9.422509992056141925 ) ) ;
#56047=ORIENTED_EDGE ( 'NONE', *, *, #84676, .F. ) ;
#56048=CARTESIAN_POINT ( 'NONE',  ( 7.361572987183170547, 2.050597817667451750, 9.846743663894590881 ) ) ;
#56049=CARTESIAN_POINT ( 'NONE',  ( 18.52753015748617571, 18.09226448433411960, 4.923371831947298993 ) ) ;
#56051=CARTESIAN_POINT ( 'NONE',  ( 21.09922568453595559, 42.04030133659708213, -6.408140936763230044 ) ) ;
#56052=CARTESIAN_POINT ( 'NONE',  ( 19.84674366389459266, 33.30059781766744464, 2.638427012816836559 ) ) ;
#56054=CARTESIAN_POINT ( 'NONE',  ( -1.099225684535947600, 24.54030133659708923, 6.408140936763237150 ) ) ;
#56056=CARTESIAN_POINT ( 'NONE',  ( 0.1532563361054083140, 21.00893115100078745, 1.131784320476157264E-15 ) ) ;
#56058=CARTESIAN_POINT ( 'NONE',  ( -4.164238869374099927, 12.01208216824730357, 3.795296366450308767 ) ) ;
#56060=CARTESIAN_POINT ( 'NONE',  ( 10.00000000000000178, 34.31368534415484106, 10.88017736071110342 ) ) ;
#56061=CARTESIAN_POINT ( 'NONE',  ( 22.26659068614894466, 33.88708216824730357, 7.082119434687054849 ) ) ;
#56062=CARTESIAN_POINT ( 'NONE',  ( 1.472469842513823179, 51.42559781766745886, 4.923371831947296329 ) ) ;
#56063=CARTESIAN_POINT ( 'NONE',  ( 18.52753015748617571, 8.092264484334117824, 4.923371831947298993 ) ) ;
#56064=CARTESIAN_POINT ( 'NONE',  ( -1.099225684535947600, 59.54030133659708923, 6.408140936763237150 ) ) ;
#56065=CARTESIAN_POINT ( 'NONE',  ( 0.2751277870542891413, 24.36607318730131411, -6.499999999999989342 ) ) ;
#56066=CARTESIAN_POINT ( 'NONE',  ( -0.8801773607111009756, 28.06368534415484106, 1.068504757029289695E-15 ) ) ;
#56068=CARTESIAN_POINT ( 'NONE',  ( 13.43411237798106583, 17.66530133659708923, -12.81628187352647252 ) ) ;
#56069=CARTESIAN_POINT ( 'NONE',  ( 19.38216949554541202, 15.99863466993042138, 9.382169495545424454 ) ) ;
#56070=CARTESIAN_POINT ( 'NONE',  ( 14.92337183194729988, 39.34226448433412315, -8.527530157486177487 ) ) ;
#56073=CARTESIAN_POINT ( 'NONE',  ( 15.44008868035555260, 64.73035201082151957, 9.422509992056143702 ) ) ;
#56077=CARTESIAN_POINT ( 'NONE',  ( 2.035157376598824452, 58.68868534415482685, 7.964842623401179544 ) ) ;
#56078=VECTOR ( 'NONE', #24490, 1000.000000000000000 ) ;
#56079=CARTESIAN_POINT ( 'NONE',  ( -0.8801773607110991993, 57.85535201082149825, -2.915334737309923874 ) ) ;
#56082=CARTESIAN_POINT ( 'NONE',  ( 10.00000000000000000, 6.813685344154838397, -10.88017736071110342 ) ) ;
#56083=CARTESIAN_POINT ( 'NONE',  ( 10.00000000000000000, 64.75893115100078035, -9.846743663894594434 ) ) ;
#56084=CARTESIAN_POINT ( 'NONE',  ( -0.8801773607111009756, 23.06368534415484106, 1.068504757029289695E-15 ) ) ;
#56087=STYLED_ITEM ( 'NONE', ( #2001 ), #47007 ) ;
#56088=CARTESIAN_POINT ( 'NONE',  ( -1.099225684535947600, 18.70696800326375353, -6.408140936763238038 ) ) ;
#56090=CARTESIAN_POINT ( 'NONE',  ( -0.8801773607110991993, 47.85535201082150536, -2.915334737309923874 ) ) ;
#56091=CARTESIAN_POINT ( 'NONE',  ( 14.92337183194729988, 44.34226448433412315, -8.527530157486177487 ) ) ;
#56092=CARTESIAN_POINT ( 'NONE',  ( 21.09922568453595559, 7.040301336597086568, -6.408140936763230044 ) ) ;
#56093=CARTESIAN_POINT ( 'NONE',  ( 0.5774900079438590739, 32.64701867748816966, -5.440088680355550821 ) ) ;
#56094=CARTESIAN_POINT ( 'NONE',  ( 20.88017736071110875, 40.77201867748818387, -2.915334737309920765 ) ) ;
#56095=CARTESIAN_POINT ( 'NONE',  ( 24.16423886937410614, 49.51208216824730357, -3.795296366450302550 ) ) ;
#56096=CARTESIAN_POINT ( 'NONE',  ( 10.00000000000000000, 34.75893115100078745, -9.846743663894594434 ) ) ;
#56097=CARTESIAN_POINT ( 'NONE',  ( 17.96484262340118221, 54.93868534415484106, 7.964842623401181321 ) ) ;
#56098=CARTESIAN_POINT ( 'NONE',  ( 19.42250999205614548, 55.98035201082150536, -5.440088680355545492 ) ) ;
#56100=CARTESIAN_POINT ( 'NONE',  ( 6.204703633549690345, 20.76208216824730357, -14.16423886937410259 ) ) ;
#56103=CARTESIAN_POINT ( 'NONE',  ( -46.82017113615791004, 100.6079546444643427, 9.324761308090124601 ) ) ;
#56104=EDGE_LOOP ( 'NONE', ( #86528, #39075, #5396, #9747 ) ) ;
#56105=CARTESIAN_POINT ( 'NONE',  ( 24.16423886937410614, 49.51208216824730357, -3.795296366450302550 ) ) ;
#56106=CARTESIAN_POINT ( 'NONE',  ( -0.3689425029237898834, 31.17874883491396787, -10.36894250292378850 ) ) ;
#56107=CARTESIAN_POINT ( 'NONE',  ( 12.63842701281683922, 19.55059781766745175, -9.846743663894590881 ) ) ;
#56108=CARTESIAN_POINT ( 'NONE',  ( 22.81628187352648496, 21.83196800326374643, -3.434112377981050290 ) ) ;
#56110=CYLINDRICAL_SURFACE ( 'NONE', #48224, 0.5000000000000004441 ) ;
#56111=CARTESIAN_POINT ( 'NONE',  ( 12.91533473730993009, 66.60535201082150536, -10.88017736071109987 ) ) ;
#56112=CARTESIAN_POINT ( 'NONE',  ( -2.816281873526473856, 34.12363466993042493, 9.499525473075851096E-16 ) ) ;
#56113=CARTESIAN_POINT ( 'NONE',  ( 20.36894250292379738, 49.92874883491396787, -10.36894250292379027 ) ) ;
#56114=CARTESIAN_POINT ( 'NONE',  ( 15.44008868035555260, 64.73035201082151957, 9.422509992056143702 ) ) ;
#56116=CARTESIAN_POINT ( 'NONE',  ( 0.1532563361054100626, 5.800597817667452638, -2.638427012816831230 ) ) ;
#56118=CARTESIAN_POINT ( 'NONE',  ( 17.20831665107776587, 22.88393115100078745, 7.208316651077764980 ) ) ;
#56123=CARTESIAN_POINT ( 'NONE',  ( -2.266590686148945544, 7.220415501580634832, 7.082119434687048631 ) ) ;
#56124=CARTESIAN_POINT ( 'NONE',  ( 19.42250999205614548, 10.98035201082150536, -5.440088680355545492 ) ) ;
#56125=CARTESIAN_POINT ( 'NONE',  ( 20.88017736071110519, 5.563685344154838397, 2.639326808657452039E-16 ) ) ;
#56126=CARTESIAN_POINT ( 'NONE',  ( 17.20831665107776587, 34.13393115100078745, -7.208316651077762316 ) ) ;
#56127=CARTESIAN_POINT ( 'NONE',  ( 21.09922568453595559, 2.040301336597086568, -6.408140936763230044 ) ) ;
#56128=FACE_OUTER_BOUND ( 'NONE', #53725, .T. ) ;
#56130=DIRECTION ( 'NONE',  ( -0.000000000000000000, -0.000000000000000000, -1.000000000000000000 ) ) ;
#56132=CARTESIAN_POINT ( 'NONE',  ( -2.816281873526473856, 14.33196800326375531, 3.434112377981055619 ) ) ;
#56135=CARTESIAN_POINT ( 'NONE',  ( 10.00000000000000178, 53.05374883491396787, 14.16423886937410082 ) ) ;
#56137=CARTESIAN_POINT ( 'NONE',  ( 24.16423886937410614, 54.30374883491396787, 8.672049930838204340E-16 ) ) ;
#56139=CARTESIAN_POINT ( 'NONE',  ( 17.96484262340118221, 34.93868534415482685, 7.964842623401181321 ) ) ;
#56140=CARTESIAN_POINT ( 'NONE',  ( 19.42250999205614548, 35.98035201082151247, -5.440088680355545492 ) ) ;
#56141=CARTESIAN_POINT ( 'NONE',  ( 20.88017736071110519, 40.56368534415484106, 2.639326808657452039E-16 ) ) ;
#56142=CARTESIAN_POINT ( 'NONE',  ( 4.559911319644449179, 63.89701867748817676, 9.422509992056141925 ) ) ;
#56143=CARTESIAN_POINT ( 'NONE',  ( 10.00000000000000000, 21.81368534415484106, -10.88017736071110342 ) ) ;
#56147=CARTESIAN_POINT ( 'NONE',  ( 14.92337183194729988, 9.342264484334119601, -8.527530157486177487 ) ) ;
#56149=ORIENTED_EDGE ( 'NONE', *, *, #8756, .T. ) ;
#56151=CARTESIAN_POINT ( 'NONE',  ( 5.076628168052704559, 50.17559781766745886, -8.527530157486179263 ) ) ;
#56155=PRESENTATION_STYLE_ASSIGNMENT (( #66089 ) ) ;
#56158=CARTESIAN_POINT ( 'NONE',  ( -45.94000000000000483, 103.9981609152045650, 5.961202730336928823 ) ) ;
#56160=CARTESIAN_POINT ( 'NONE',  ( -2.266590686148945544, 41.38708216824729647, -7.082119434687050408 ) ) ;
#56163=CARTESIAN_POINT ( 'NONE',  ( 20.15039907845753930, 70.00000000000000000, -6.262539305110068177 ) ) ;
#56165=CARTESIAN_POINT ( 'NONE',  ( 0.1532563361054100626, 20.80059781766744464, -2.638427012816831230 ) ) ;
#56167=CARTESIAN_POINT ( 'NONE',  ( 2.791683348922237240, 60.38393115100078745, -7.208316651077763204 ) ) ;
#56168=CARTESIAN_POINT ( 'NONE',  ( -0.8801773607110991993, 67.85535201082151957, -2.915334737309923874 ) ) ;
#56170=CARTESIAN_POINT ( 'NONE',  ( 10.00000000000000178, 62.25893115100078745, 9.846743663894594434 ) ) ;
#56171=CARTESIAN_POINT ( 'NONE',  ( 19.10478245763050964, 20.10160829253885950, 5.990408912944338304 ) ) ;
#56172=VERTEX_POINT ( 'NONE', #85545 ) ;
#56173=CARTESIAN_POINT ( 'NONE',  ( 10.00000000000000000, 65.55374883491396076, -14.16423886937410082 ) ) ;
#56175=CARTESIAN_POINT ( 'NONE',  ( 15.44008868035555793, 46.39701867748817676, -9.422509992056140149 ) ) ;
#56176=CARTESIAN_POINT ( 'NONE',  ( 13.43411237798106583, 17.66530133659708923, -12.81628187352647252 ) ) ;
#56177=CARTESIAN_POINT ( 'NONE',  ( 4.559911319644449179, 68.89701867748817676, 9.422509992056141925 ) ) ;
#56180=CARTESIAN_POINT ( 'NONE',  ( -0.1038446121089069418, 54.24302437010793909, -6.337995344473775106 ) ) ;
#56181=CARTESIAN_POINT ( 'NONE',  ( 2.791683348922240793, 51.63393115100078745, 7.208316651077764092 ) ) ;
#56182=SURFACE_STYLE_FILL_AREA ( #33646 ) ;
#56184=CARTESIAN_POINT ( 'NONE',  ( 22.81628187352647785, 6.415301336597088344, 3.434112377981063169 ) ) ;
#56185=CARTESIAN_POINT ( 'NONE',  ( 2.035157376598824452, 18.68868534415484106, 7.964842623401179544 ) ) ;
#56186=SURFACE_STYLE_FILL_AREA ( #47691 ) ;
#56188=CARTESIAN_POINT ( 'NONE',  ( 10.00000000000000000, 35.55374883491396787, -14.16423886937410082 ) ) ;
#56189=CARTESIAN_POINT ( 'NONE',  ( 6.204703633549690345, 30.76208216824730357, -14.16423886937410259 ) ) ;
#56190=CARTESIAN_POINT ( 'NONE',  ( 24.16423886937409904, 59.09541550158063217, 3.795296366450317205 ) ) ;
#56191=CARTESIAN_POINT ( 'NONE',  ( 17.20831665107776587, 42.88393115100077324, 7.208316651077764980 ) ) ;
#56192=CARTESIAN_POINT ( 'NONE',  ( 13.43411237798105340, 40.58196800326375353, 12.81628187352647963 ) ) ;
#56193=CARTESIAN_POINT ( 'NONE',  ( 17.96484262340118221, 11.18868534415483929, -7.964842623401177768 ) ) ;
#56194=VECTOR ( 'NONE', #84530, 1000.000000000000000 ) ;
#56195=VERTEX_POINT ( 'NONE', #10526 ) ;
#56196=CARTESIAN_POINT ( 'NONE',  ( 2.791683348922240793, 36.63393115100078035, 7.208316651077764092 ) ) ;
#56197=CARTESIAN_POINT ( 'NONE',  ( 7.084665262690076126, 44.10535201082151247, 10.88017736071109987 ) ) ;
#56199=CARTESIAN_POINT ( 'NONE',  ( 0.6178305044545838731, 9.748634669930416052, 9.382169495545420901 ) ) ;
#56200=CARTESIAN_POINT ( 'NONE',  ( 17.08211943468705840, 20.13708216824730357, -12.26659068614894466 ) ) ;
#56203=CARTESIAN_POINT ( 'NONE',  ( 7.361572987183169658, 24.96726448433412315, -9.846743663894592657 ) ) ;
#56204=CARTESIAN_POINT ( 'NONE',  ( 3.591859063236763294, 48.29030133659708923, -11.09922568453595026 ) ) ;
#56205=CARTESIAN_POINT ( 'NONE',  ( 17.20831665107776587, 59.13393115100078745, -7.208316651077762316 ) ) ;
#56208=CARTESIAN_POINT ( 'NONE',  ( -2.266590686148945544, 62.22041550158063927, 7.082119434687048631 ) ) ;
#56209=CARTESIAN_POINT ( 'NONE',  ( 17.08211943468705130, 13.47041550158063572, 12.26659068614894998 ) ) ;
#56210=CARTESIAN_POINT ( 'NONE',  ( 0.1532563361054100626, 0.8005978176674514168, -2.638427012816831230 ) ) ;
#56211=CARTESIAN_POINT ( 'NONE',  ( 19.84674366389459621, 53.50893115100078745, 7.409399052514197653E-17 ) ) ;
#56212=CARTESIAN_POINT ( 'NONE',  ( 15.44008868035555793, 16.39701867748817321, -9.422509992056140149 ) ) ;
#56213=CARTESIAN_POINT ( 'NONE',  ( 20.30776406404415724, 70.00000000000000000, -6.000000000000001776 ) ) ;
#56219=MECHANICAL_DESIGN_GEOMETRIC_PRESENTATION_REPRESENTATION('',(#3484),#44997);
#56220=ORIENTED_EDGE ( 'NONE', *, *, #91567, .T. ) ;
#56222=CARTESIAN_POINT ( 'NONE',  ( 6.204703633549690345, 5.762082168247301794, -14.16423886937410259 ) ) ;
#56223=CARTESIAN_POINT ( 'NONE',  ( -4.164238869374099039, 1.803748834913967647, 8.674139862899312516E-16 ) ) ;
#56224=CARTESIAN_POINT ( 'NONE',  ( -0.3689425029237881626, 42.42874883491396787, 10.36894250292379027 ) ) ;
#56225=CARTESIAN_POINT ( 'NONE',  ( 18.52753015748618282, 63.92559781766745886, -4.923371831947291888 ) ) ;
#56226=CARTESIAN_POINT ( 'NONE',  ( 0.1532563361054083140, 21.00893115100078745, 1.131784320476157264E-15 ) ) ;
#56227=CARTESIAN_POINT ( 'NONE',  ( -2.816281873526473856, 64.12363466993042493, 9.499525473075851096E-16 ) ) ;
#56228=CARTESIAN_POINT ( 'NONE',  ( 4.559911319644449179, 18.89701867748817321, 9.422509992056141925 ) ) ;
#56229=CARTESIAN_POINT ( 'NONE',  ( 0.6178305044545818747, -1.501365330069579951, -9.382169495545419124 ) ) ;
#56230=CARTESIAN_POINT ( 'NONE',  ( 20.36894250292379738, 4.928748834913967869, -10.36894250292379027 ) ) ;
#56231=CARTESIAN_POINT ( 'NONE',  ( -2.266590686148945544, 41.38708216824729647, -7.082119434687050408 ) ) ;
#56232=CARTESIAN_POINT ( 'NONE',  ( 2.035157376598824452, 3.688685344154837953, 7.964842623401179544 ) ) ;
#56236=CARTESIAN_POINT ( 'NONE',  ( 4.559911319644449179, 58.89701867748817676, 9.422509992056141925 ) ) ;
#56238=CARTESIAN_POINT ( 'NONE',  ( 5.076628168052704559, 15.17559781766745175, -8.527530157486179263 ) ) ;
#56244=CARTESIAN_POINT ( 'NONE',  ( 14.92337183194729988, 19.34226448433411960, -8.527530157486177487 ) ) ;
#56245=ORIENTED_EDGE ( 'NONE', *, *, #85954, .F. ) ;
#56246=CARTESIAN_POINT ( 'NONE',  ( 13.79529636645030344, 38.26208216824729647, 14.16423886937410614 ) ) ;
#56247=CARTESIAN_POINT ( 'NONE',  ( 18.52753015748617571, 33.09226448433411605, 4.923371831947298993 ) ) ;
#56248=CARTESIAN_POINT ( 'NONE',  ( 12.91533473730992121, 39.52201867748817676, 10.88017736071110164 ) ) ;
#56249=CARTESIAN_POINT ( 'NONE',  ( 4.559911319644449179, 47.23035201082150536, -9.422509992056141925 ) ) ;
#56251=CARTESIAN_POINT ( 'NONE',  ( -0.1503990784575329198, 2.222660991849184864, -6.262539305110070842 ) ) ;
#56255=CARTESIAN_POINT ( 'NONE',  ( 2.917880565312950480, 0.9704155015806342766, -12.26659068614894821 ) ) ;
#56257=EDGE_LOOP ( 'NONE', ( #59171, #23667, #82143, #42023 ) ) ;
#56258=CARTESIAN_POINT ( 'NONE',  ( 22.81628187352647785, 26.62363466993042138, 6.195893100308588602E-16 ) ) ;
#56259=CARTESIAN_POINT ( 'NONE',  ( 17.20831665107776587, 27.88393115100078390, 7.208316651077764980 ) ) ;
#56261=CARTESIAN_POINT ( 'NONE',  ( 6.565887622018943937, 45.16530133659708923, 12.81628187352647430 ) ) ;
#56262=CARTESIAN_POINT ( 'NONE',  ( -46.34161155552185818, 104.0475784593833737, -5.921604558741679902 ) ) ;
#56263=CARTESIAN_POINT ( 'NONE',  ( 19.84674366389459266, 28.30059781766745886, 2.638427012816836559 ) ) ;
#56264=CARTESIAN_POINT ( 'NONE',  ( 15.44008868035555793, 56.39701867748817676, -9.422509992056140149 ) ) ;
#56265=( GEOMETRIC_REPRESENTATION_CONTEXT ( 3 ) GLOBAL_UNCERTAINTY_ASSIGNED_CONTEXT ( ( #83456 ) ) GLOBAL_UNIT_ASSIGNED_CONTEXT ( ( #22558, #91536, #23052 ) ) REPRESENTATION_CONTEXT ( 'NONE', 'WORKASPACE' ) );
#56266=CARTESIAN_POINT ( 'NONE',  ( 13.99999999999999822, 11.50000000000000000, -6.000000000000000000 ) ) ;
#56270=CARTESIAN_POINT ( 'NONE',  ( 2.035157376598824452, 68.68868534415484817, 7.964842623401179544 ) ) ;
#56271=CARTESIAN_POINT ( 'NONE',  ( -2.816281873526473856, 14.12363466993041961, 9.499525473075851096E-16 ) ) ;
#56272=DIRECTION ( 'NONE',  ( -0.000000000000000000, 1.000000000000000000, -0.000000000000000000 ) ) ;
#56273=CARTESIAN_POINT ( 'NONE',  ( 5.076628168052704559, 40.17559781766745175, -8.527530157486179263 ) ) ;
#56275=CARTESIAN_POINT ( 'NONE',  ( 17.08211943468705130, 3.470415501580634388, 12.26659068614894998 ) ) ;
#56276=CARTESIAN_POINT ( 'NONE',  ( 10.00000000000000178, 37.25893115100078745, 9.846743663894594434 ) ) ;
#56277=CARTESIAN_POINT ( 'NONE',  ( 13.43411237798106583, 37.66530133659708923, -12.81628187352647252 ) ) ;
#56280=CARTESIAN_POINT ( 'NONE',  ( 4.559911319644449179, 52.23035201082151247, -9.422509992056141925 ) ) ;
#56281=CARTESIAN_POINT ( 'NONE',  ( 16.40814093676324603, 12.45696800326375353, -11.09922568453594671 ) ) ;
#56282=CARTESIAN_POINT ( 'NONE',  ( 1.472469842513823179, 40.59226448433411605, -4.923371831947296329 ) ) ;
#56283=CARTESIAN_POINT ( 'NONE',  ( 17.20831665107776587, 19.13393115100078035, -7.208316651077762316 ) ) ;
#56284=CARTESIAN_POINT ( 'NONE',  ( 2.035157376598824452, 33.68868534415484106, 7.964842623401179544 ) ) ;
#56285=CARTESIAN_POINT ( 'NONE',  ( 16.40814093676323893, 35.79030133659708923, 11.09922568453595026 ) ) ;
#56287=CARTESIAN_POINT ( 'NONE',  ( 5.076628168052704559, 20.17559781766745175, -8.527530157486179263 ) ) ;
#56289=CARTESIAN_POINT ( 'NONE',  ( 2.035157376598824452, 23.68868534415484461, 7.964842623401179544 ) ) ;
#56293=CARTESIAN_POINT ( 'NONE',  ( 0.5774900079438607392, 63.48035201082149825, 5.440088680355550821 ) ) ;
#56294=CARTESIAN_POINT ( 'NONE',  ( 14.92337183194729633, 42.67559781766745886, 8.527530157486181039 ) ) ;
#56295=CARTESIAN_POINT ( 'NONE',  ( 12.91533473730993009, 36.60535201082151247, -10.88017736071109987 ) ) ;
#56296=FACE_OUTER_BOUND ( 'NONE', #62310, .T. ) ;
#56298=CARTESIAN_POINT ( 'NONE',  ( -0.8801773607111008646, 43.27201867748817676, 2.915334737309923430 ) ) ;
#56299=CARTESIAN_POINT ( 'NONE',  ( 20.88017736071110164, 10.35535201082150714, 2.915334737309930979 ) ) ;
#56300=CARTESIAN_POINT ( 'NONE',  ( 20.10493008474206889, 59.71697413083878558, 6.336235997365758266 ) ) ;
#56302=( GEOMETRIC_REPRESENTATION_CONTEXT ( 3 ) GLOBAL_UNCERTAINTY_ASSIGNED_CONTEXT ( ( #55090 ) ) GLOBAL_UNIT_ASSIGNED_CONTEXT ( ( #4591, #34067, #35053 ) ) REPRESENTATION_CONTEXT ( 'NONE', 'WORKASPACE' ) );
#56303=CARTESIAN_POINT ( 'NONE',  ( 7.361572987183170547, 37.05059781766744464, 9.846743663894590881 ) ) ;
#56304=CARTESIAN_POINT ( 'NONE',  ( -4.164238869374099927, 37.01208216824731068, 3.795296366450308767 ) ) ;
#56305=CARTESIAN_POINT ( 'NONE',  ( 1.274849032794306947, 7.555090184799359676, -6.499999999999997335 ) ) ;
#56306=CARTESIAN_POINT ( 'NONE',  ( -4.164238869374099039, 21.80374883491396787, 8.674139862899312516E-16 ) ) ;
#56309=CARTESIAN_POINT ( 'NONE',  ( -2.266590686148945544, 66.38708216824730357, -7.082119434687050408 ) ) ;
#56310=CARTESIAN_POINT ( 'NONE',  ( 7.361572987183169658, 29.96726448433411960, -9.846743663894592657 ) ) ;
#56313=CARTESIAN_POINT ( 'NONE',  ( -0.8801773607111009756, 63.06368534415484106, 1.068504757029289695E-15 ) ) ;
#56315=CARTESIAN_POINT ( 'NONE',  ( 17.96484262340118221, 26.18868534415483396, -7.964842623401177768 ) ) ;
#56316=CARTESIAN_POINT ( 'NONE',  ( 16.40814093676323893, 55.79030133659708923, 11.09922568453595026 ) ) ;
#56317=CARTESIAN_POINT ( 'NONE',  ( 22.81628187352647785, 11.62363466993042138, 6.195893100308588602E-16 ) ) ;
#56318=CARTESIAN_POINT ( 'NONE',  ( 5.076628168052704559, 10.17559781766745175, -8.527530157486179263 ) ) ;
#56320=CARTESIAN_POINT ( 'NONE',  ( 7.361572987183169658, -0.03273551566588185635, -9.846743663894592657 ) ) ;
#56322=CARTESIAN_POINT ( 'NONE',  ( 24.16423886937409904, 59.09541550158063217, 3.795296366450317205 ) ) ;
#56324=CARTESIAN_POINT ( 'NONE',  ( 6.204703633549690345, 27.84541550158063217, 14.16423886937410082 ) ) ;
#56325=CARTESIAN_POINT ( 'NONE',  ( 2.035157376598822676, 32.43868534415483396, -7.964842623401177768 ) ) ;
#56326=CARTESIAN_POINT ( 'NONE',  ( 20.88017736071110164, 50.35535201082151247, 2.915334737309930979 ) ) ;
#56327=CARTESIAN_POINT ( 'NONE',  ( 17.39651004071842166, 12.93575266056827822, 6.499999999999998224 ) ) ;
#56329=CARTESIAN_POINT ( 'NONE',  ( 7.361572987183170547, 12.05059781766744997, 9.846743663894590881 ) ) ;
#56330=DIRECTION ( 'NONE',  ( 0.5547001962252290364, 0.8320502943378437211, 0.000000000000000000 ) ) ;
#56331=CARTESIAN_POINT ( 'NONE',  ( 5.076628168052704559, 20.17559781766745175, -8.527530157486179263 ) ) ;
#56333=CARTESIAN_POINT ( 'NONE',  ( 12.63842701281683922, 19.55059781766745175, -9.846743663894590881 ) ) ;
#56334=CARTESIAN_POINT ( 'NONE',  ( 14.92337183194729633, 47.67559781766745175, 8.527530157486181039 ) ) ;
#56336=CARTESIAN_POINT ( 'NONE',  ( 15.44008868035555260, 24.73035201082150891, 9.422509992056143702 ) ) ;
#56338=CARTESIAN_POINT ( 'NONE',  ( 0.6178305044545818747, 48.49863466993042493, -9.382169495545419124 ) ) ;
#56339=CARTESIAN_POINT ( 'NONE',  ( 17.96484262340118221, 54.93868534415484106, 7.964842623401181321 ) ) ;
#56340=CARTESIAN_POINT ( 'NONE',  ( 18.52753015748617571, 28.09226448433411960, 4.923371831947298993 ) ) ;
#56341=CARTESIAN_POINT ( 'NONE',  ( 2.917880565312950480, 50.97041550158064638, -12.26659068614894821 ) ) ;
#56342=CARTESIAN_POINT ( 'NONE',  ( 19.84674366389459266, 23.71726448433412315, -2.638427012816827677 ) ) ;
#56344=CARTESIAN_POINT ( 'NONE',  ( 10.00000000000000178, 57.25893115100078745, 9.846743663894594434 ) ) ;
#56345=CARTESIAN_POINT ( 'NONE',  ( 13.79529636645031943, 5.345415501580634832, -14.16423886937409904 ) ) ;
#56346=CARTESIAN_POINT ( 'NONE',  ( -4.164238869374098151, 26.59541550158063217, -3.795296366450310543 ) ) ;
#56347=CARTESIAN_POINT ( 'NONE',  ( 1.472469842513823179, 30.59226448433411960, -4.923371831947296329 ) ) ;
#56348=CARTESIAN_POINT ( 'NONE',  ( 17.96484262340118221, 29.93868534415484106, 7.964842623401181321 ) ) ;
#56349=CARTESIAN_POINT ( 'NONE',  ( 20.88017736071110164, 50.35535201082151247, 2.915334737309930979 ) ) ;
#56350=CARTESIAN_POINT ( 'NONE',  ( 10.00000000000000178, 49.31368534415484106, 10.88017736071110342 ) ) ;
#56352=CARTESIAN_POINT ( 'NONE',  ( 3.591859063236761518, 34.95696800326375353, 11.09922568453594849 ) ) ;
#56353=CARTESIAN_POINT ( 'NONE',  ( 10.00000000000000000, 56.81368534415484106, -10.88017736071110342 ) ) ;
#56354=ORIENTED_EDGE ( 'NONE', *, *, #90440, .F. ) ;
#56356=CARTESIAN_POINT ( 'NONE',  ( 4.559911319644449179, 63.89701867748817676, 9.422509992056141925 ) ) ;
#56359=CARTESIAN_POINT ( 'NONE',  ( 2.035157376598824452, 58.68868534415482685, 7.964842623401179544 ) ) ;
#56361=EDGE_CURVE ( 'NONE', #53936, #2342, #43958, .T. ) ;
#56362=CARTESIAN_POINT ( 'NONE',  ( 19.72487221294570858, 69.50000000000000000, -6.500000000000000888 ) ) ;
#56364=CARTESIAN_POINT ( 'NONE',  ( -0.3689425029237881626, 67.42874883491396076, 10.36894250292379027 ) ) ;
#56365=CARTESIAN_POINT ( 'NONE',  ( 14.92337183194729633, 7.675597817667451750, 8.527530157486181039 ) ) ;
#56366=CARTESIAN_POINT ( 'NONE',  ( -4.164238869374099927, 2.012082168247300906, 3.795296366450308767 ) ) ;
#56367=CARTESIAN_POINT ( 'NONE',  ( 12.63842701281683034, 7.467264484334118713, 9.846743663894596210 ) ) ;
#56369=CARTESIAN_POINT ( 'NONE',  ( 4.559911319644449179, 8.897018677488171434, 9.422509992056141925 ) ) ;
#56370=CARTESIAN_POINT ( 'NONE',  ( 17.20831665107776587, 49.13393115100078745, -7.208316651077762316 ) ) ;
#56373=CARTESIAN_POINT ( 'NONE',  ( 17.20831665107776587, 54.13393115100079456, -7.208316651077762316 ) ) ;
#56374=VERTEX_POINT ( 'NONE', #88985 ) ;
#56377=CARTESIAN_POINT ( 'NONE',  ( 10.00000000000000178, 49.31368534415484106, 10.88017736071110342 ) ) ;
#56378=CARTESIAN_POINT ( 'NONE',  ( 10.00000000000000178, 57.25893115100078745, 9.846743663894594434 ) ) ;
#56379=PLANE ( 'NONE',  #11602 ) ;
#56380=CARTESIAN_POINT ( 'NONE',  ( 20.03743638938529870, 1.751975280310174465, 6.399506433553883156 ) ) ;
#56381=CARTESIAN_POINT ( 'NONE',  ( 17.96484262340118221, 56.18868534415484817, -7.964842623401177768 ) ) ;
#56382=CARTESIAN_POINT ( 'NONE',  ( 20.88017736071110519, 5.563685344154838397, 2.639326808657452039E-16 ) ) ;
#56383=CARTESIAN_POINT ( 'NONE',  ( 22.81628187352647785, 41.41530133659708923, 3.434112377981063169 ) ) ;
#56384=CARTESIAN_POINT ( 'NONE',  ( -0.1023957841222606496, 10.13377557478296254, 6.340343622311898741 ) ) ;
#56386=CARTESIAN_POINT ( 'NONE',  ( 6.565887622018943937, 35.16530133659708923, 12.81628187352647430 ) ) ;
#56387=CARTESIAN_POINT ( 'NONE',  ( -0.8801773607111009756, 33.06368534415484106, 1.068504757029289695E-15 ) ) ;
#56389=CIRCLE ( 'NONE', #24425, 0.5000000000000004441 ) ;
#56391=CARTESIAN_POINT ( 'NONE',  ( 12.63842701281683034, 62.46726448433410894, 9.846743663894596210 ) ) ;
#56392=CARTESIAN_POINT ( 'NONE',  ( 2.791683348922237240, 10.38393115100078390, -7.208316651077763204 ) ) ;
#56393=CARTESIAN_POINT ( 'NONE',  ( 5.076628168052703671, 56.84226448433412315, 8.527530157486179263 ) ) ;
#56395=PRESENTATION_STYLE_ASSIGNMENT (( #95364 ) ) ;
#56400=CARTESIAN_POINT ( 'NONE',  ( 19.84674366389459266, 23.71726448433412315, -2.638427012816827677 ) ) ;
#56401=CARTESIAN_POINT ( 'NONE',  ( 5.076628168052704559, 60.17559781766745175, -8.527530157486179263 ) ) ;
#56404=CARTESIAN_POINT ( 'NONE',  ( 1.274849032794116210, 8.572280503510292249, 6.499999999999738876 ) ) ;
#56405=CARTESIAN_POINT ( 'NONE',  ( 10.00000000000000178, 20.37363466993042138, 12.81628187352647608 ) ) ;
#56406=CARTESIAN_POINT ( 'NONE',  ( 12.63842701281683034, 42.46726448433412315, 9.846743663894596210 ) ) ;
#56408=CARTESIAN_POINT ( 'NONE',  ( 6.204703633549690345, 50.76208216824730357, -14.16423886937410259 ) ) ;
#56409=CARTESIAN_POINT ( 'NONE',  ( 10.00000000000000178, 12.25893115100078568, 9.846743663894594434 ) ) ;
#56412=CARTESIAN_POINT ( 'NONE',  ( 6.204703633549690345, 62.84541550158063927, 14.16423886937410082 ) ) ;
#56413=CARTESIAN_POINT ( 'NONE',  ( 1.472469842513823179, 56.42559781766745886, 4.923371831947296329 ) ) ;
#56414=CARTESIAN_POINT ( 'NONE',  ( 0.5774900079438590739, 7.647018677488171434, -5.440088680355550821 ) ) ;
#56415=CARTESIAN_POINT ( 'NONE',  ( 2.917880565312950480, 35.97041550158063217, -12.26659068614894821 ) ) ;
#56416=CARTESIAN_POINT ( 'NONE',  ( 17.08211943468705130, 33.47041550158063927, 12.26659068614894998 ) ) ;
#56417=CARTESIAN_POINT ( 'NONE',  ( 18.04007052943794776, 34.00257860105345742, -5.767676674365461942 ) ) ;
#56418=CARTESIAN_POINT ( 'NONE',  ( 0.2751277870542913062, 29.36607318730131411, -6.499999999999992006 ) ) ;
#56420=CARTESIAN_POINT ( 'NONE',  ( 2.791683348922240793, 51.63393115100078745, 7.208316651077764092 ) ) ;
#56422=CARTESIAN_POINT ( 'NONE',  ( 20.88017736071110875, 40.77201867748818387, -2.915334737309920765 ) ) ;
#56425=CARTESIAN_POINT ( 'NONE',  ( 18.52753015748617571, 53.09226448433412315, 4.923371831947298993 ) ) ;
#56426=CARTESIAN_POINT ( 'NONE',  ( 20.15039907845753930, 9.722660991849181755, 6.262539305110064625 ) ) ;
#56428=CARTESIAN_POINT ( 'NONE',  ( 12.63842701281683034, 57.46726448433411605, 9.846743663894596210 ) ) ;
#56431=CARTESIAN_POINT ( 'NONE',  ( 24.16423886937410614, 29.51208216824729647, -3.795296366450302550 ) ) ;
#56433=CARTESIAN_POINT ( 'NONE',  ( 17.96484262340118221, 14.93868534415484106, 7.964842623401181321 ) ) ;
#56435=CARTESIAN_POINT ( 'NONE',  ( 3.591859063236763294, 23.29030133659708568, -11.09922568453595026 ) ) ;
#56437=CARTESIAN_POINT ( 'NONE',  ( 2.791683348922237240, 5.383931151000785675, -7.208316651077763204 ) ) ;
#56438=VECTOR ( 'NONE', #61439, 1000.000000000000000 ) ;
#56439=FACE_OUTER_BOUND ( 'NONE', #88700, .T. ) ;
#56440=CARTESIAN_POINT ( 'NONE',  ( -1.926860441876563801, 9.896642702460841434, 3.195792623639529761 ) ) ;
#56441=CARTESIAN_POINT ( 'NONE',  ( 10.00000000000000178, 70.00000000000000000, 0.000000000000000000 ) ) ;
#56442=CARTESIAN_POINT ( 'NONE',  ( -0.8801773607110991993, 12.85535201082150358, -2.915334737309923874 ) ) ;
#56444=CARTESIAN_POINT ( 'NONE',  ( 12.91533473730992121, 44.52201867748816966, 10.88017736071110164 ) ) ;
#56445=CARTESIAN_POINT ( 'NONE',  ( 7.084665262690076126, 32.02201867748816966, -10.88017736071110164 ) ) ;
#56446=CARTESIAN_POINT ( 'NONE',  ( 7.361572987183169658, 64.96726448433412315, -9.846743663894592657 ) ) ;
#56447=CARTESIAN_POINT ( 'NONE',  ( 2.791683348922240793, 61.63393115100079456, 7.208316651077764092 ) ) ;
#56448=CARTESIAN_POINT ( 'NONE',  ( 6.565887622018943937, 65.16530133659709634, 12.81628187352647430 ) ) ;
#56449=CARTESIAN_POINT ( 'NONE',  ( 0.1532563361054083140, 6.008931151000784787, 1.131784320476157264E-15 ) ) ;
#56450=VERTEX_POINT ( 'NONE', #87502 ) ;
#56451=CARTESIAN_POINT ( 'NONE',  ( 15.44008868035555793, 26.39701867748817321, -9.422509992056140149 ) ) ;
#56452=ADVANCED_FACE ( 'NONE', ( #12487 ), #4900, .T. ) ;
#56453=CARTESIAN_POINT ( 'NONE',  ( 16.40814093676324603, 27.45696800326375708, -11.09922568453594671 ) ) ;
#56455=CARTESIAN_POINT ( 'NONE',  ( 0.1532563361054083140, 66.00893115100079456, 1.131784320476157264E-15 ) ) ;
#56456=CARTESIAN_POINT ( 'NONE',  ( 4.559911319644449179, 68.89701867748817676, 9.422509992056141925 ) ) ;
#56457=CARTESIAN_POINT ( 'NONE',  ( 17.20831665107776587, 14.13393115100078568, -7.208316651077762316 ) ) ;
#56458=CARTESIAN_POINT ( 'NONE',  ( -1.099225684535947600, 33.70696800326375353, -6.408140936763238038 ) ) ;
#56459=CARTESIAN_POINT ( 'NONE',  ( 5.076628168052704559, 5.175597817667451750, -8.527530157486179263 ) ) ;
#56462=CARTESIAN_POINT ( 'NONE',  ( -0.8801773607111009756, 13.06368534415483929, 1.068504757029289695E-15 ) ) ;
#56463=CARTESIAN_POINT ( 'NONE',  ( 16.40814093676323893, 60.79030133659709634, 11.09922568453595026 ) ) ;
#56464=CARTESIAN_POINT ( 'NONE',  ( -4.164238869374099039, 26.80374883491397142, 8.674139862899312516E-16 ) ) ;
#56465=CARTESIAN_POINT ( 'NONE',  ( 2.791683348922240793, 16.63393115100078745, 7.208316651077764092 ) ) ;
#56466=CARTESIAN_POINT ( 'NONE',  ( 15.44008868035555260, 9.730352010821505360, 9.422509992056143702 ) ) ;
#56467=CARTESIAN_POINT ( 'NONE',  ( 14.92337183194729633, 27.67559781766745530, 8.527530157486181039 ) ) ;
#56468=CARTESIAN_POINT ( 'NONE',  ( -0.3689425029237881626, 62.42874883491396787, 10.36894250292379027 ) ) ;
#56470=CARTESIAN_POINT ( 'NONE',  ( 20.88017736071110164, 10.35535201082150714, 2.915334737309930979 ) ) ;
#56471=CARTESIAN_POINT ( 'NONE',  ( 20.88017736071110164, 15.35535201082150358, 2.915334737309930979 ) ) ;
#56473=CARTESIAN_POINT ( 'NONE',  ( 2.791683348922237240, 65.38393115100078035, -7.208316651077763204 ) ) ;
#56474=CARTESIAN_POINT ( 'NONE',  ( 10.00000000000000000, 21.81368534415484106, -10.88017736071110342 ) ) ;
#56475=CARTESIAN_POINT ( 'NONE',  ( 0.1532563361054083140, 51.00893115100078745, 1.131784320476157264E-15 ) ) ;
#56478=CARTESIAN_POINT ( 'NONE',  ( 16.40814093676324603, 47.45696800326375353, -11.09922568453594671 ) ) ;
#56480=CARTESIAN_POINT ( 'NONE',  ( -2.266590686148945544, 16.38708216824730357, -7.082119434687050408 ) ) ;
#56481=CARTESIAN_POINT ( 'NONE',  ( 0.5774900079438607392, 43.48035201082151247, 5.440088680355550821 ) ) ;
#56482=CARTESIAN_POINT ( 'NONE',  ( 17.96484262340118221, 11.18868534415484106, -7.964842623401177768 ) ) ;
#56483=CARTESIAN_POINT ( 'NONE',  ( 12.63842701281683034, 52.46726448433413026, 9.846743663894596210 ) ) ;
#56485=CARTESIAN_POINT ( 'NONE',  ( 2.791683348922240793, 41.63393115100078745, 7.208316651077764092 ) ) ;
#56487=CARTESIAN_POINT ( 'NONE',  ( 10.00000000000000178, 7.258931151000785675, 9.846743663894594434 ) ) ;
#56490=CARTESIAN_POINT ( 'NONE',  ( 10.00000000000000000, 11.81368534415483751, -10.88017736071110342 ) ) ;
#56491=CARTESIAN_POINT ( 'NONE',  ( 18.52753015748617571, 18.09226448433411960, 4.923371831947298993 ) ) ;
#56492=CARTESIAN_POINT ( 'NONE',  ( 1.472469842513823179, 66.42559781766745175, 4.923371831947296329 ) ) ;
#56493=CARTESIAN_POINT ( 'NONE',  ( 7.084665262690076126, 44.10535201082151247, 10.88017736071109987 ) ) ;
#56494=CARTESIAN_POINT ( 'NONE',  ( 7.084665262690076126, 14.10535201082150358, 10.88017736071109987 ) ) ;
#56495=CARTESIAN_POINT ( 'NONE',  ( 6.565887622018943937, 50.16530133659708213, 12.81628187352647430 ) ) ;
#56496=CARTESIAN_POINT ( 'NONE',  ( -4.164238869374099039, 36.80374883491396787, 8.674139862899312516E-16 ) ) ;
#56497=DIRECTION ( 'NONE',  ( 1.000000000000000000, 0.000000000000000000, 0.000000000000000000 ) ) ;
#56498=STYLED_ITEM ( 'NONE', ( #34779 ), #96951 ) ;
#56499=CARTESIAN_POINT ( 'NONE',  ( 22.81628187352648496, 61.83196800326376774, -3.434112377981050290 ) ) ;
#56501=CARTESIAN_POINT ( 'NONE',  ( 19.84674366389459266, 63.30059781766745886, 2.638427012816836559 ) ) ;
#56502=CARTESIAN_POINT ( 'NONE',  ( 10.00000000000000178, 34.31368534415484106, 10.88017736071110342 ) ) ;
#56505=CARTESIAN_POINT ( 'NONE',  ( 0.1532563361054100626, 0.8005978176674514168, -2.638427012816831230 ) ) ;
#56506=CARTESIAN_POINT ( 'NONE',  ( -0.1503990784575328643, 65.12777174578613426, 6.262539305110068177 ) ) ;
#56507=CARTESIAN_POINT ( 'NONE',  ( -46.20903833114419967, 103.7402771300235713, 6.114030023718175499 ) ) ;
#56508=CARTESIAN_POINT ( 'NONE',  ( 2.791683348922237240, 10.38393115100078390, -7.208316651077763204 ) ) ;
#56509=CARTESIAN_POINT ( 'NONE',  ( 17.20831665107776587, 29.13393115100078390, -7.208316651077762316 ) ) ;
#56510=CARTESIAN_POINT ( 'NONE',  ( 0.1532563361054100626, 10.80059781766745175, -2.638427012816831230 ) ) ;
#56511=CARTESIAN_POINT ( 'NONE',  ( 7.361572987183170547, 7.050597817667451750, 9.846743663894590881 ) ) ;
#56512=EDGE_CURVE ( 'NONE', #96626, #64701, #21997, .T. ) ;
#56513=CARTESIAN_POINT ( 'NONE',  ( 15.44008868035555793, 51.39701867748816966, -9.422509992056140149 ) ) ;
#56514=CARTESIAN_POINT ( 'NONE',  ( 10.00000000000000000, 61.81368534415484106, -10.88017736071110342 ) ) ;
#56515=CARTESIAN_POINT ( 'NONE',  ( 12.63842701281683034, 22.46726448433411605, 9.846743663894596210 ) ) ;
#56517=CARTESIAN_POINT ( 'NONE',  ( 1.274849032794294290, 63.57228050351031357, 6.499999999999979572 ) ) ;
#56518=CARTESIAN_POINT ( 'NONE',  ( 18.52753015748617571, 58.09226448433411605, 4.923371831947298993 ) ) ;
#56522=CARTESIAN_POINT ( 'NONE',  ( 2.917880565312950480, 10.97041550158063572, -12.26659068614894821 ) ) ;
#56525=SURFACE_STYLE_FILL_AREA ( #81711 ) ;
#56526=CARTESIAN_POINT ( 'NONE',  ( 22.26659068614894466, 28.88708216824730357, 7.082119434687054849 ) ) ;
#56527=CARTESIAN_POINT ( 'NONE',  ( -2.266590686148945544, 1.387082168247301128, -7.082119434687050408 ) ) ;
#56528=CARTESIAN_POINT ( 'NONE',  ( 0.5774900079438607392, 33.48035201082150536, 5.440088680355550821 ) ) ;
#56530=CARTESIAN_POINT ( 'NONE',  ( 14.92337183194729633, 12.67559781766745353, 8.527530157486181039 ) ) ;
#56531=CARTESIAN_POINT ( 'NONE',  ( 20.88017736071110164, 50.35535201082151247, 2.915334737309930979 ) ) ;
#56532=CARTESIAN_POINT ( 'NONE',  ( 18.52753015748618282, 18.92559781766745175, -4.923371831947291888 ) ) ;
#56533=CARTESIAN_POINT ( 'NONE',  ( 10.00000000000000178, 40.37363466993042493, 12.81628187352647608 ) ) ;
#56534=CARTESIAN_POINT ( 'NONE',  ( 18.52753015748617571, 38.09226448433412315, 4.923371831947298993 ) ) ;
#56536=CARTESIAN_POINT ( 'NONE',  ( 19.42250999205614193, 60.14701867748817676, 5.440088680355555262 ) ) ;
#56537=CARTESIAN_POINT ( 'NONE',  ( 3.591859063236761518, 24.95696800326375353, 11.09922568453594849 ) ) ;
#56539=CARTESIAN_POINT ( 'NONE',  ( 18.52753015748618282, 23.92559781766745530, -4.923371831947291888 ) ) ;
#56540=CARTESIAN_POINT ( 'NONE',  ( 13.79529636645030344, 13.26208216824729824, 14.16423886937410614 ) ) ;
#56541=CARTESIAN_POINT ( 'NONE',  ( 0.5774900079438590739, 37.64701867748817676, -5.440088680355550821 ) ) ;
#56542=CARTESIAN_POINT ( 'NONE',  ( 10.00000000000000178, 38.05374883491396787, 14.16423886937410082 ) ) ;
#56543=CARTESIAN_POINT ( 'NONE',  ( 1.472469842513823179, 55.59226448433412315, -4.923371831947296329 ) ) ;
#56545=CARTESIAN_POINT ( 'NONE',  ( 0.1532563361054083140, 11.00893115100078568, 1.131784320476157264E-15 ) ) ;
#56548=CARTESIAN_POINT ( 'NONE',  ( 20.88017736071110519, 45.56368534415484106, 2.639326808657452039E-16 ) ) ;
#56550=CARTESIAN_POINT ( 'NONE',  ( 22.81628187352648496, 26.83196800326374998, -3.434112377981050290 ) ) ;
#56551=CARTESIAN_POINT ( 'NONE',  ( 0.1532563361054100626, 60.80059781766744464, -2.638427012816831230 ) ) ;
#56554=CARTESIAN_POINT ( 'NONE',  ( 4.559911319644449179, 2.230352010821504471, -9.422509992056141925 ) ) ;
#56555=CARTESIAN_POINT ( 'NONE',  ( 7.084665262690076126, 69.10535201082151957, 10.88017736071109987 ) ) ;
#56559=CARTESIAN_POINT ( 'NONE',  ( 2.603489959281591659, 15.43575266056827999, -6.500000000000006217 ) ) ;
#56560=CARTESIAN_POINT ( 'NONE',  ( 19.84674366389459621, 3.508931151000785231, 7.409399052514197653E-17 ) ) ;
#56561=CARTESIAN_POINT ( 'NONE',  ( 4.559911319644449179, 57.23035201082150536, -9.422509992056141925 ) ) ;
#56565=CARTESIAN_POINT ( 'NONE',  ( 19.84674366389459266, 23.71726448433412315, -2.638427012816827677 ) ) ;
#56566=EDGE_CURVE ( 'NONE', #87620, #95286, #42218, .T. ) ;
#56568=CARTESIAN_POINT ( 'NONE',  ( 10.00000000000000178, 29.31368534415483751, 10.88017736071110342 ) ) ;
#56569=B_SPLINE_CURVE_WITH_KNOTS ( 'NONE', 3,
 ( #45166, #30152, #37684, #16156, #22189, #22683 ),
 .UNSPECIFIED., .F., .F.,
 ( 4, 2, 4 ),
 ( 0.000000000000000000, 0.0002565770811491002636, 0.0005131541622982005273 ),
 .UNSPECIFIED. ) ;
#56570=CARTESIAN_POINT ( 'NONE',  ( 22.81628187352647785, 1.623634669930420271, 6.195893100308588602E-16 ) ) ;
#56571=CARTESIAN_POINT ( 'NONE',  ( 20.88017736071110164, 25.35535201082150891, 2.915334737309930979 ) ) ;
#56574=CARTESIAN_POINT ( 'NONE',  ( 22.81628187352647785, 41.41530133659708923, 3.434112377981063169 ) ) ;
#56576=CARTESIAN_POINT ( 'NONE',  ( 20.88017736071110519, 45.56368534415484106, 2.639326808657452039E-16 ) ) ;
#56577=CARTESIAN_POINT ( 'NONE',  ( 7.361572987183170547, 47.05059781766745175, 9.846743663894590881 ) ) ;
#56579=CARTESIAN_POINT ( 'NONE',  ( 13.43411237798106583, 17.66530133659708923, -12.81628187352647252 ) ) ;
#56581=CARTESIAN_POINT ( 'NONE',  ( -0.8801773607111008646, 33.27201867748817676, 2.915334737309923430 ) ) ;
#56582=CARTESIAN_POINT ( 'NONE',  ( 10.00000000000000000, 50.55374883491396787, -14.16423886937410082 ) ) ;
#56583=CARTESIAN_POINT ( 'NONE',  ( 18.52753015748618282, 43.92559781766745175, -4.923371831947291888 ) ) ;
#56584=CARTESIAN_POINT ( 'NONE',  ( 0.1532563361054082862, 6.217264484334118713, 2.638427012816831674 ) ) ;
#56585=CARTESIAN_POINT ( 'NONE',  ( 0.5774900079438590739, 47.64701867748817676, -5.440088680355550821 ) ) ;
#56587=CARTESIAN_POINT ( 'NONE',  ( -0.3689425029237898834, 11.17874883491396787, -10.36894250292378850 ) ) ;
#56589=CARTESIAN_POINT ( 'NONE',  ( 1.492507162822237943, 22.19955587570480660, -6.499999999999988454 ) ) ;
#56591=CARTESIAN_POINT ( 'NONE',  ( -0.3689425029237881626, 52.42874883491396076, 10.36894250292379027 ) ) ;
#56592=CARTESIAN_POINT ( 'NONE',  ( -4.164238869374098151, 56.59541550158063927, -3.795296366450310543 ) ) ;
#56593=CARTESIAN_POINT ( 'NONE',  ( 10.00000000000000178, 12.25893115100078568, 9.846743663894594434 ) ) ;
#56596=CARTESIAN_POINT ( 'NONE',  ( 1.274849032794317383, 27.55509018479935790, -6.500000000000010658 ) ) ;
#56597=CARTESIAN_POINT ( 'NONE',  ( 10.00000000000000000, 1.813685344154837731, -10.88017736071110342 ) ) ;
#56598=CARTESIAN_POINT ( 'NONE',  ( 16.40814093676323893, 35.79030133659708923, 11.09922568453595026 ) ) ;
#56599=CARTESIAN_POINT ( 'NONE',  ( 10.00000000000000178, 48.05374883491396787, 14.16423886937410082 ) ) ;
#56601=CARTESIAN_POINT ( 'NONE',  ( 0.5774900079438590739, 67.64701867748817676, -5.440088680355550821 ) ) ;
#56606=CARTESIAN_POINT ( 'NONE',  ( 7.361572987183170547, 17.05059781766745530, 9.846743663894590881 ) ) ;
#56608=CARTESIAN_POINT ( 'NONE',  ( -4.164238869374099039, 66.80374883491396076, 8.674139862899312516E-16 ) ) ;
#56609=CARTESIAN_POINT ( 'NONE',  ( 12.91533473730993009, 6.605352010821504471, -10.88017736071109987 ) ) ;
#56610=CARTESIAN_POINT ( 'NONE',  ( 2.791683348922240793, 46.63393115100077324, 7.208316651077764092 ) ) ;
#56611=CARTESIAN_POINT ( 'NONE',  ( 22.81628187352648496, 6.831968003263753531, -3.434112377981050290 ) ) ;
#56612=CARTESIAN_POINT ( 'NONE',  ( 10.00000000000000178, 70.00000000000000000, 0.000000000000000000 ) ) ;
#56615=CARTESIAN_POINT ( 'NONE',  ( 0.6178305044545818747, 23.49863466993041783, -9.382169495545419124 ) ) ;
#56616=ORIENTED_EDGE ( 'NONE', *, *, #10522, .F. ) ;
#56617=CARTESIAN_POINT ( 'NONE',  ( 20.36894250292379382, 63.67874883491396787, 10.36894250292379205 ) ) ;
#56619=CARTESIAN_POINT ( 'NONE',  ( 10.00000000000000000, 60.55374883491397497, -14.16423886937410082 ) ) ;
#56621=CARTESIAN_POINT ( 'NONE',  ( -0.8801773607111009756, 38.06368534415484106, 1.068504757029289695E-15 ) ) ;
#56622=CARTESIAN_POINT ( 'NONE',  ( 7.084665262690076126, 37.02201867748817676, -10.88017736071110164 ) ) ;
#56624=CARTESIAN_POINT ( 'NONE',  ( 10.00000000000000000, 26.81368534415484106, -10.88017736071110342 ) ) ;
#56628=CARTESIAN_POINT ( 'NONE',  ( 2.791683348922237240, 15.38393115100078212, -7.208316651077763204 ) ) ;
#56631=CARTESIAN_POINT ( 'NONE',  ( 17.20831665107776587, 39.13393115100079456, -7.208316651077762316 ) ) ;
#56633=CARTESIAN_POINT ( 'NONE',  ( 18.17884179759845509, 53.66688879859523098, -6.500000000000054179 ) ) ;
#56634=CARTESIAN_POINT ( 'NONE',  ( 0.6178305044545838731, 54.74863466993042493, 9.382169495545420901 ) ) ;
#56635=FILL_AREA_STYLE ('',( #96618 ) ) ;
#56636=ORIENTED_EDGE ( 'NONE', *, *, #35243, .F. ) ;
#56637=CARTESIAN_POINT ( 'NONE',  ( -45.94000000000000483, 93.00000000000000000, 5.000000000000000000 ) ) ;
#56639=CARTESIAN_POINT ( 'NONE',  ( 18.52753015748618282, 63.92559781766745886, -4.923371831947291888 ) ) ;
#56640=CARTESIAN_POINT ( 'NONE',  ( -4.164238869374099927, 42.01208216824728936, 3.795296366450308767 ) ) ;
#56643=LINE ( 'NONE', #72610, #4881 ) ;
#56644=CARTESIAN_POINT ( 'NONE',  ( 0.1532563361054082862, 31.21726448433412315, 2.638427012816831674 ) ) ;
#56645=CARTESIAN_POINT ( 'NONE',  ( 3.591859063236763294, 63.29030133659708923, -11.09922568453595026 ) ) ;
#56646=CARTESIAN_POINT ( 'NONE',  ( 16.40814093676324603, 2.456968003263753531, -11.09922568453594671 ) ) ;
#56647=CARTESIAN_POINT ( 'NONE',  ( 0.5774900079438607392, 63.48035201082149825, 5.440088680355550821 ) ) ;
#56649=CARTESIAN_POINT ( 'NONE',  ( 1.472469842513823179, 55.59226448433412315, -4.923371831947296329 ) ) ;
#56653=CARTESIAN_POINT ( 'NONE',  ( -0.3689425029237898834, 61.17874883491396076, -10.36894250292378850 ) ) ;
#56655=CARTESIAN_POINT ( 'NONE',  ( 19.42250999205614193, 45.14701867748817676, 5.440088680355555262 ) ) ;
#56656=CARTESIAN_POINT ( 'NONE',  ( 3.591859063236761518, 19.95696800326375353, 11.09922568453594849 ) ) ;
#56659=CARTESIAN_POINT ( 'NONE',  ( 10.00000000000000000, 44.75893115100078745, -9.846743663894594434 ) ) ;
#56661=CARTESIAN_POINT ( 'NONE',  ( 22.81628187352647785, 16.41530133659708923, 3.434112377981063169 ) ) ;
#56663=ADVANCED_FACE ( 'NONE', ( #46933 ), #39938, .T. ) ;
#56664=CARTESIAN_POINT ( 'NONE',  ( -0.8801773607110991993, 22.85535201082150181, -2.915334737309923874 ) ) ;
#56667=CARTESIAN_POINT ( 'NONE',  ( 10.00000000000000000, 40.55374883491397497, -14.16423886937410082 ) ) ;
#56668=CARTESIAN_POINT ( 'NONE',  ( 22.26659068614894466, 28.88708216824730357, 7.082119434687054849 ) ) ;
#56669=CARTESIAN_POINT ( 'NONE',  ( 2.035157376598822676, 17.43868534415483751, -7.964842623401177768 ) ) ;
#56670=CARTESIAN_POINT ( 'NONE',  ( 19.84674366389459621, 38.50893115100078745, 7.409399052514197653E-17 ) ) ;
#56671=CARTESIAN_POINT ( 'NONE',  ( 19.38216949554541202, 40.99863466993042493, 9.382169495545424454 ) ) ;
#56672=CARTESIAN_POINT ( 'NONE',  ( 0.5774900079438590739, 7.647018677488171434, -5.440088680355550821 ) ) ;
#56673=EDGE_CURVE ( 'NONE', #9131, #6299, #10683, .T. ) ;
#56674=CARTESIAN_POINT ( 'NONE',  ( 14.92337183194729988, 39.34226448433412315, -8.527530157486177487 ) ) ;
#56675=CARTESIAN_POINT ( 'NONE',  ( 19.42250999205614193, 35.14701867748816966, 5.440088680355555262 ) ) ;
#56676=CARTESIAN_POINT ( 'NONE',  ( -2.816281873526473856, 9.123634669930421381, 9.499525473075851096E-16 ) ) ;
#56677=CARTESIAN_POINT ( 'NONE',  ( 20.36894250292379382, 23.67874883491397142, 10.36894250292379205 ) ) ;
#56680=CARTESIAN_POINT ( 'NONE',  ( 0.1532563361054083140, 26.00893115100078745, 1.131784320476157264E-15 ) ) ;
#56681=CARTESIAN_POINT ( 'NONE',  ( -2.816281873526473856, 54.33196800326376064, 3.434112377981055619 ) ) ;
#56682=CARTESIAN_POINT ( 'NONE',  ( 2.791683348922240793, 51.63393115100078745, 7.208316651077764092 ) ) ;
#56684=DIRECTION ( 'NONE',  ( 0.000000000000000000, -1.000000000000000000, 0.000000000000000000 ) ) ;
#56685=( NAMED_UNIT ( * ) PLANE_ANGLE_UNIT ( ) SI_UNIT ( $, .RADIAN. ) );
#56686=CARTESIAN_POINT ( 'NONE',  ( -2.266590686148945544, 61.38708216824730357, -7.082119434687050408 ) ) ;
#56687=CARTESIAN_POINT ( 'NONE',  ( 6.204703633549690345, 12.84541550158063572, 14.16423886937410082 ) ) ;
#56688=CARTESIAN_POINT ( 'NONE',  ( 0.1532563361054083140, 6.008931151000784787, 1.131784320476157264E-15 ) ) ;
#56689=CARTESIAN_POINT ( 'NONE',  ( 19.84674366389459266, 43.71726448433410894, -2.638427012816827677 ) ) ;
#56690=CARTESIAN_POINT ( 'NONE',  ( 15.44008868035555260, 39.73035201082150536, 9.422509992056143702 ) ) ;
#56692=CARTESIAN_POINT ( 'NONE',  ( 14.92337183194729988, 64.34226448433412315, -8.527530157486177487 ) ) ;
#56693=STYLED_ITEM ( 'NONE', ( #13293 ), #10682 ) ;
#56700=CARTESIAN_POINT ( 'NONE',  ( 24.16423886937410614, 9.303748834913967869, 8.672049930838204340E-16 ) ) ;
#56701=CARTESIAN_POINT ( 'NONE',  ( 20.36894250292379382, 3.678748834913967869, 10.36894250292379205 ) ) ;
#56703=CARTESIAN_POINT ( 'NONE',  ( 13.79529636645030344, 43.26208216824730357, 14.16423886937410614 ) ) ;
#56704=CARTESIAN_POINT ( 'NONE',  ( 19.84674366389459266, 53.30059781766744464, 2.638427012816836559 ) ) ;
#56705=CARTESIAN_POINT ( 'NONE',  ( 1.472469842513823179, 41.42559781766745886, 4.923371831947296329 ) ) ;
#56706=CARTESIAN_POINT ( 'NONE',  ( 12.91533473730992121, 29.52201867748817321, 10.88017736071110164 ) ) ;
#56707=CARTESIAN_POINT ( 'NONE',  ( 7.361572987183170547, 62.05059781766745886, 9.846743663894590881 ) ) ;
#56708=CARTESIAN_POINT ( 'NONE',  ( 10.00000000000000000, 0.5537488349139675359, -14.16423886937410082 ) ) ;
#56709=CARTESIAN_POINT ( 'NONE',  ( 13.79529636645030344, 38.26208216824729647, 14.16423886937410614 ) ) ;
#56710=CARTESIAN_POINT ( 'NONE',  ( 2.035157376598822676, 7.438685344154837509, -7.964842623401177768 ) ) ;
#56711=CARTESIAN_POINT ( 'NONE',  ( 12.63842701281683922, 64.55059781766745175, -9.846743663894590881 ) ) ;
#56713=CARTESIAN_POINT ( 'NONE',  ( 20.88017736071110164, 65.35535201082150536, 2.915334737309930979 ) ) ;
#56715=CARTESIAN_POINT ( 'NONE',  ( 0.1532563361054082862, 26.21726448433411605, 2.638427012816831674 ) ) ;
#56719=CARTESIAN_POINT ( 'NONE',  ( 19.84674366389459266, 18.30059781766745175, 2.638427012816836559 ) ) ;
#56721=CARTESIAN_POINT ( 'NONE',  ( 24.16423886937409904, 39.09541550158062506, 3.795296366450317205 ) ) ;
#56722=CARTESIAN_POINT ( 'NONE',  ( 5.076628168052704559, 30.17559781766745175, -8.527530157486179263 ) ) ;
#56723=CARTESIAN_POINT ( 'NONE',  ( 20.88017736071110519, 60.56368534415484106, 2.639326808657452039E-16 ) ) ;
#56726=CARTESIAN_POINT ( 'NONE',  ( 10.00000000000000178, 39.31368534415484106, 10.88017736071110342 ) ) ;
#56727=CARTESIAN_POINT ( 'NONE',  ( 0.1532563361054100626, 45.80059781766745886, -2.638427012816831230 ) ) ;
#56731=CARTESIAN_POINT ( 'NONE',  ( -4.164238869374099927, 22.01208216824730357, 3.795296366450308767 ) ) ;
#56732=ORIENTED_EDGE ( 'NONE', *, *, #53334, .T. ) ;
#56734=CARTESIAN_POINT ( 'NONE',  ( 22.81628187352648496, 31.83196800326375353, -3.434112377981050290 ) ) ;
#56735=CARTESIAN_POINT ( 'NONE',  ( 5.076628168052703671, 21.84226448433411960, 8.527530157486179263 ) ) ;
#56736=CARTESIAN_POINT ( 'NONE',  ( 16.40814093676324603, 47.45696800326375353, -11.09922568453594671 ) ) ;
#56737=CARTESIAN_POINT ( 'NONE',  ( -46.34323875807880455, 103.6109741468810483, -6.190393423093145664 ) ) ;
#56738=CARTESIAN_POINT ( 'NONE',  ( 18.52753015748618282, 28.92559781766745175, -4.923371831947291888 ) ) ;
#56739=CARTESIAN_POINT ( 'NONE',  ( 17.96484262340118221, 64.93868534415483396, 7.964842623401181321 ) ) ;
#56742=DIRECTION ( 'NONE',  ( -1.000000000000000000, 0.000000000000000000, 0.000000000000000000 ) ) ;
#56743=CARTESIAN_POINT ( 'NONE',  ( -43.18060676906663531, 107.2752179745913708, 4.519309965511820515 ) ) ;
#56744=CARTESIAN_POINT ( 'NONE',  ( -0.1503990784575328643, 45.12777174578613426, 6.262539305110068177 ) ) ;
#56745=CARTESIAN_POINT ( 'NONE',  ( -0.8801773607111008646, 68.27201867748817676, 2.915334737309923430 ) ) ;
#56746=CARTESIAN_POINT ( 'NONE',  ( 22.81628187352647785, 16.41530133659708923, 3.434112377981063169 ) ) ;
#56749=CARTESIAN_POINT ( 'NONE',  ( 19.84674366389459621, 38.50893115100078745, 7.409399052514197653E-17 ) ) ;
#56750=CARTESIAN_POINT ( 'NONE',  ( 3.640395162852214650, 107.5383484153110061, -5.000000000000000000 ) ) ;
#56751=CARTESIAN_POINT ( 'NONE',  ( 17.08211943468705130, 13.47041550158063572, 12.26659068614894998 ) ) ;
#56752=CARTESIAN_POINT ( 'NONE',  ( 5.076628168052703671, 26.84226448433411960, 8.527530157486179263 ) ) ;
#56753=CARTESIAN_POINT ( 'NONE',  ( 6.565887622018943937, 28.08196800326375353, -12.81628187352647608 ) ) ;
#56755=CARTESIAN_POINT ( 'NONE',  ( 7.084665262690076126, 67.02201867748817676, -10.88017736071110164 ) ) ;
#56756=CARTESIAN_POINT ( 'NONE',  ( 13.43411237798105340, 5.581968003263753531, 12.81628187352647963 ) ) ;
#56759=CARTESIAN_POINT ( 'NONE',  ( 19.84674366389459266, 38.71726448433412315, -2.638427012816827677 ) ) ;
#56760=CARTESIAN_POINT ( 'NONE',  ( -0.8801773607110991993, 27.85535201082150181, -2.915334737309923874 ) ) ;
#56761=CARTESIAN_POINT ( 'NONE',  ( -1.099225684535947600, 24.54030133659708923, 6.408140936763237150 ) ) ;
#56762=CIRCLE ( 'NONE', #90295, 0.5000000000000004441 ) ;
#56763=CARTESIAN_POINT ( 'NONE',  ( 2.791683348922240793, 16.63393115100078745, 7.208316651077764092 ) ) ;
#56765=CARTESIAN_POINT ( 'NONE',  ( -0.8801773607111009756, 28.06368534415484106, 1.068504757029289695E-15 ) ) ;
#56768=CARTESIAN_POINT ( 'NONE',  ( -0.8801773607110991993, 57.85535201082149825, -2.915334737309923874 ) ) ;
#56769=CARTESIAN_POINT ( 'NONE',  ( -0.8801773607111008646, 3.272018677488171434, 2.915334737309923430 ) ) ;
#56770=CARTESIAN_POINT ( 'NONE',  ( 14.92337183194729988, 39.34226448433412315, -8.527530157486177487 ) ) ;
#56771=CARTESIAN_POINT ( 'NONE',  ( 20.88017736071110519, 35.56368534415484106, 2.639326808657452039E-16 ) ) ;
#56772=( NAMED_UNIT ( * ) PLANE_ANGLE_UNIT ( ) SI_UNIT ( $, .RADIAN. ) );
#56773=CARTESIAN_POINT ( 'NONE',  ( 15.44008868035555793, 41.39701867748817676, -9.422509992056140149 ) ) ;
#56774=CARTESIAN_POINT ( 'NONE',  ( 4.559911319644449179, 8.897018677488173211, 9.422509992056141925 ) ) ;
#56776=CARTESIAN_POINT ( 'NONE',  ( 6.000000000000000000, 61.00000000000000711, -6.000000000000000000 ) ) ;
#56777=CARTESIAN_POINT ( 'NONE',  ( 18.52753015748618282, 43.92559781766745175, -4.923371831947291888 ) ) ;
#56778=CARTESIAN_POINT ( 'NONE',  ( 17.08211943468705130, 48.47041550158063927, 12.26659068614894998 ) ) ;
#56781=CARTESIAN_POINT ( 'NONE',  ( 2.917880565312950480, 30.97041550158063572, -12.26659068614894821 ) ) ;
#56785=CARTESIAN_POINT ( 'NONE',  ( -0.3689425029237881626, 62.42874883491396787, 10.36894250292379027 ) ) ;
#56786=CARTESIAN_POINT ( 'NONE',  ( 12.63842701281683922, 29.55059781766745175, -9.846743663894590881 ) ) ;
#56789=CARTESIAN_POINT ( 'NONE',  ( 12.91533473730992121, 64.52201867748817676, 10.88017736071110164 ) ) ;
#56790=CARTESIAN_POINT ( 'NONE',  ( 10.00000000000000178, 65.37363466993042493, 12.81628187352647608 ) ) ;
#56791=EDGE_CURVE ( 'NONE', #58660, #10735, #61324, .T. ) ;
#56792=CARTESIAN_POINT ( 'NONE',  ( 19.42250999205614548, 25.98035201082150891, -5.440088680355545492 ) ) ;
#56793=CARTESIAN_POINT ( 'NONE',  ( 21.09922568453594849, 61.20696800326376064, 6.408140936763242479 ) ) ;
#56794=CARTESIAN_POINT ( 'NONE',  ( 22.81628187352648496, 6.831968003263753531, -3.434112377981050290 ) ) ;
#56795=CARTESIAN_POINT ( 'NONE',  ( 7.361572987183169658, 9.967264484334119601, -9.846743663894592657 ) ) ;
#56798=DIRECTION ( 'NONE',  ( 1.000000000000000000, -0.000000000000000000, 0.000000000000000000 ) ) ;
#56799=CARTESIAN_POINT ( 'NONE',  ( 13.79529636645031943, 65.34541550158063217, -14.16423886937409904 ) ) ;
#56800=CARTESIAN_POINT ( 'NONE',  ( 22.26659068614894466, 23.88708216824730357, 7.082119434687054849 ) ) ;
#56801=CARTESIAN_POINT ( 'NONE',  ( 2.035157376598822676, 37.43868534415484106, -7.964842623401177768 ) ) ;
#56802=CARTESIAN_POINT ( 'NONE',  ( 17.96484262340118221, 51.18868534415483396, -7.964842623401177768 ) ) ;
#56805=CARTESIAN_POINT ( 'NONE',  ( 12.63842701281683034, 7.467264484334118713, 9.846743663894596210 ) ) ;
#56807=CARTESIAN_POINT ( 'NONE',  ( 18.52753015748617571, 28.09226448433411960, 4.923371831947298993 ) ) ;
#56809=CARTESIAN_POINT ( 'NONE',  ( 1.472469842513823179, 25.59226448433412315, -4.923371831947296329 ) ) ;
#56810=CARTESIAN_POINT ( 'NONE',  ( 7.361572987183170547, 47.05059781766745175, 9.846743663894590881 ) ) ;
#56811=AXIS2_PLACEMENT_3D ( 'NONE', #3791, #12742, #57256 ) ;
#56812=CARTESIAN_POINT ( 'NONE',  ( 4.559911319644449179, 28.89701867748817321, 9.422509992056141925 ) ) ;
#56813=CARTESIAN_POINT ( 'NONE',  ( 22.81628187352647785, 46.41530133659708213, 3.434112377981063169 ) ) ;
#56815=CARTESIAN_POINT ( 'NONE',  ( 19.84674366389459621, 33.50893115100078745, 7.409399052514197653E-17 ) ) ;
#56816=CARTESIAN_POINT ( 'NONE',  ( 24.16423886937410614, 59.51208216824728936, -3.795296366450302550 ) ) ;
#56817=CARTESIAN_POINT ( 'NONE',  ( 7.361572987183169658, 24.96726448433412315, -9.846743663894592657 ) ) ;
#56820=CARTESIAN_POINT ( 'NONE',  ( 5.076628168052704559, 65.17559781766745175, -8.527530157486179263 ) ) ;
#56821=CARTESIAN_POINT ( 'NONE',  ( 22.26659068614894466, 33.88708216824730357, 7.082119434687054849 ) ) ;
#56822=CARTESIAN_POINT ( 'NONE',  ( 12.63842701281683034, 32.46726448433412315, 9.846743663894596210 ) ) ;
#56824=CARTESIAN_POINT ( 'NONE',  ( -0.8801773607111008646, 23.27201867748817676, 2.915334737309923430 ) ) ;
#56825=B_SPLINE_CURVE_WITH_KNOTS ( 'NONE', 3,
 ( #19317, #41839, #64306, #28293, #49803, #20803 ),
 .UNSPECIFIED., .F., .F.,
 ( 4, 2, 4 ),
 ( 0.000000000000000000, 0.0002701661927229424918, 0.0005403323854458849836 ),
 .UNSPECIFIED. ) ;
#56827=CARTESIAN_POINT ( 'NONE',  ( 17.96484262340118221, 61.18868534415482685, -7.964842623401177768 ) ) ;
#56828=CARTESIAN_POINT ( 'NONE',  ( 0.5774900079438607392, 48.48035201082150536, 5.440088680355550821 ) ) ;
#56830=CARTESIAN_POINT ( 'NONE',  ( 16.40814093676324603, 47.45696800326375353, -11.09922568453594671 ) ) ;
#56831=CARTESIAN_POINT ( 'NONE',  ( 15.44008868035555260, 49.73035201082150536, 9.422509992056143702 ) ) ;
#56832=VERTEX_POINT ( 'NONE', #17423 ) ;
#56833=CARTESIAN_POINT ( 'NONE',  ( 2.791683348922237240, 0.3839311510007847872, -7.208316651077763204 ) ) ;
#56834=CARTESIAN_POINT ( 'NONE',  ( 20.88017736071110875, 65.77201867748817676, -2.915334737309920765 ) ) ;
#56836=ORIENTED_EDGE ( 'NONE', *, *, #61902, .T. ) ;
#56838=CARTESIAN_POINT ( 'NONE',  ( -0.8801773607110991993, 67.85535201082151957, -2.915334737309923874 ) ) ;
#56839=CARTESIAN_POINT ( 'NONE',  ( 17.96484262340118221, 6.188685344154836621, -7.964842623401177768 ) ) ;
#56841=CYLINDRICAL_SURFACE ( 'NONE', #72810, 0.5000000000000004441 ) ;
#56842=CARTESIAN_POINT ( 'NONE',  ( -0.8801773607111008646, 13.27201867748817321, 2.915334737309923430 ) ) ;
#56843=CARTESIAN_POINT ( 'NONE',  ( 0.1532563361054083140, 6.008931151000784787, 1.131784320476157264E-15 ) ) ;
#56844=CARTESIAN_POINT ( 'NONE',  ( 10.00000000000000000, 0.5537488349139675359, -14.16423886937410082 ) ) ;
#56845=CARTESIAN_POINT ( 'NONE',  ( 1.472469842513823179, 6.425597817667451750, 4.923371831947296329 ) ) ;
#56846=CARTESIAN_POINT ( 'NONE',  ( 4.559911319644449179, 7.230352010821504471, -9.422509992056141925 ) ) ;
#56847=CARTESIAN_POINT ( 'NONE',  ( 5.076628168052703671, 51.84226448433412315, 8.527530157486179263 ) ) ;
#56848=ORIENTED_EDGE ( 'NONE', *, *, #16304, .T. ) ;
#56849=CARTESIAN_POINT ( 'NONE',  ( 17.20831665107776587, 47.88393115100078745, 7.208316651077764980 ) ) ;
#56850=ORIENTED_EDGE ( 'NONE', *, *, #2152, .F. ) ;
#56852=CARTESIAN_POINT ( 'NONE',  ( 0.5774900079438607392, 58.48035201082151247, 5.440088680355550821 ) ) ;
#56853=CARTESIAN_POINT ( 'NONE',  ( 5.076628168052704559, 55.17559781766745175, -8.527530157486179263 ) ) ;
#56854=CARTESIAN_POINT ( 'NONE',  ( 0.5774900079438607392, 8.480352010821505360, 5.440088680355550821 ) ) ;
#56856=CARTESIAN_POINT ( 'NONE',  ( 7.084665262690076126, 62.02201867748816966, -10.88017736071110164 ) ) ;
#56857=CARTESIAN_POINT ( 'NONE',  ( 12.91533473730992121, 4.522018677488170546, 10.88017736071110164 ) ) ;
#56858=CARTESIAN_POINT ( 'NONE',  ( -2.816281873526473856, 39.33196800326374643, 3.434112377981055619 ) ) ;
#56859=CARTESIAN_POINT ( 'NONE',  ( 17.96484262340118221, 34.93868534415482685, 7.964842623401181321 ) ) ;
#56861=ORIENTED_EDGE ( 'NONE', *, *, #23089, .F. ) ;
#56862=CARTESIAN_POINT ( 'NONE',  ( 19.38216949554541557, 42.24863466993041783, -9.382169495545420901 ) ) ;
#56863=CARTESIAN_POINT ( 'NONE',  ( 15.44008868035555260, 39.73035201082150536, 9.422509992056143702 ) ) ;
#56864=ORIENTED_EDGE ( 'NONE', *, *, #59229, .T. ) ;
#56865=CARTESIAN_POINT ( 'NONE',  ( 19.84674366389459266, 8.717264484334116048, -2.638427012816827677 ) ) ;
#56866=CARTESIAN_POINT ( 'NONE',  ( 17.20831665107776587, 64.13393115100079456, -7.208316651077762316 ) ) ;
#56867=CARTESIAN_POINT ( 'NONE',  ( 10.00000000000000000, 14.75893115100078568, -9.846743663894594434 ) ) ;
#56868=CARTESIAN_POINT ( 'NONE',  ( 10.00000000000000000, 44.75893115100078745, -9.846743663894594434 ) ) ;
#56874=CARTESIAN_POINT ( 'NONE',  ( 10.00000000000000178, 27.25893115100078390, 9.846743663894594434 ) ) ;
#56875=CARTESIAN_POINT ( 'NONE',  ( 7.361572987183170547, 2.050597817667451750, 9.846743663894590881 ) ) ;
#56876=CARTESIAN_POINT ( 'NONE',  ( 7.361572987183169658, 54.96726448433413026, -9.846743663894592657 ) ) ;
#56879=CARTESIAN_POINT ( 'NONE',  ( 22.81628187352647785, 21.41530133659708923, 3.434112377981063169 ) ) ;
#56880=CARTESIAN_POINT ( 'NONE',  ( 10.00000000000000000, 44.75893115100078745, -9.846743663894594434 ) ) ;
#56882=CARTESIAN_POINT ( 'NONE',  ( -2.266590686148945544, 62.22041550158063927, 7.082119434687048631 ) ) ;
#56883=CARTESIAN_POINT ( 'NONE',  ( 17.20831665107776587, 22.88393115100078745, 7.208316651077764980 ) ) ;
#56885=CARTESIAN_POINT ( 'NONE',  ( -1.926860441876564023, 39.68830936912750929, 1.004413902775740781E-15 ) ) ;
#56886=CARTESIAN_POINT ( 'NONE',  ( -4.164238869374099039, 61.80374883491397497, 8.674139862899312516E-16 ) ) ;
#56887=CARTESIAN_POINT ( 'NONE',  ( 17.20831665107776587, 62.88393115100078745, 7.208316651077764980 ) ) ;
#56888=CARTESIAN_POINT ( 'NONE',  ( 0.5774900079438607392, 3.480352010821504916, 5.440088680355550821 ) ) ;
#56889=CARTESIAN_POINT ( 'NONE',  ( -0.3689425029237898834, 31.17874883491396787, -10.36894250292378850 ) ) ;
#56890=CARTESIAN_POINT ( 'NONE',  ( 17.08211943468705840, 45.13708216824730357, -12.26659068614894466 ) ) ;
#56891=FACE_OUTER_BOUND ( 'NONE', #48992, .T. ) ;
#56893=CARTESIAN_POINT ( 'NONE',  ( 7.361572987183169658, 59.96726448433410894, -9.846743663894592657 ) ) ;
#56895=CARTESIAN_POINT ( 'NONE',  ( 20.88017736071110875, 45.77201867748816966, -2.915334737309920765 ) ) ;
#56896=CARTESIAN_POINT ( 'NONE',  ( 19.65595514172846592, 92.20290667148093178, -5.361975859778444153 ) ) ;
#56897=CARTESIAN_POINT ( 'NONE',  ( 5.076628168052703671, 51.84226448433412315, 8.527530157486179263 ) ) ;
#56898=CARTESIAN_POINT ( 'NONE',  ( -2.816281873526473856, 64.12363466993042493, 9.499525473075851096E-16 ) ) ;
#56899=VECTOR ( 'NONE', #57753, 1000.000000000000000 ) ;
#56900=CARTESIAN_POINT ( 'NONE',  ( 5.076628168052703671, 56.84226448433412315, 8.527530157486179263 ) ) ;
#56901=CARTESIAN_POINT ( 'NONE',  ( 19.84674366389459266, 63.30059781766745886, 2.638427012816836559 ) ) ;
#56903=CARTESIAN_POINT ( 'NONE',  ( 10.00000000000000000, 25.55374883491396787, -14.16423886937410082 ) ) ;
#56908=CARTESIAN_POINT ( 'NONE',  ( 12.91533473730992121, 14.52201867748817143, 10.88017736071110164 ) ) ;
#56909=CARTESIAN_POINT ( 'NONE',  ( 19.38216949554541202, 20.99863466993042138, 9.382169495545424454 ) ) ;
#56912=CARTESIAN_POINT ( 'NONE',  ( 12.63842701281683034, 12.46726448433411782, 9.846743663894596210 ) ) ;
#56914=CARTESIAN_POINT ( 'NONE',  ( 6.204703633549690345, 32.84541550158063927, 14.16423886937410082 ) ) ;
#56915=CARTESIAN_POINT ( 'NONE',  ( 1.472469842513823179, 21.42559781766745175, 4.923371831947296329 ) ) ;
#56916=SURFACE_SIDE_STYLE ('',( #94916 ) ) ;
#56917=CARTESIAN_POINT ( 'NONE',  ( 7.084665262690076126, 4.105352010821503583, 10.88017736071109987 ) ) ;
#56919=CARTESIAN_POINT ( 'NONE',  ( 20.88017736071110875, 45.77201867748816966, -2.915334737309920765 ) ) ;
#56920=CARTESIAN_POINT ( 'NONE',  ( 15.44008868035555260, 39.73035201082150536, 9.422509992056143702 ) ) ;
#56921=CARTESIAN_POINT ( 'NONE',  ( 0.6178305044545838731, -0.2513653300695798953, 9.382169495545420901 ) ) ;
#56923=FACE_OUTER_BOUND ( 'NONE', #38619, .T. ) ;
#56924=CARTESIAN_POINT ( 'NONE',  ( 5.076628168052703671, 11.84226448433411960, 8.527530157486179263 ) ) ;
#56925=DIRECTION ( 'NONE',  ( 0.000000000000000000, 0.000000000000000000, 1.000000000000000000 ) ) ;
#56926=CARTESIAN_POINT ( 'NONE',  ( 0.5774900079438607392, 48.48035201082150536, 5.440088680355550821 ) ) ;
#56927=AXIS2_PLACEMENT_3D ( 'NONE', #82941, #90922, #59441 ) ;
#56930=CARTESIAN_POINT ( 'NONE',  ( 22.81628187352648496, 11.83196800326375531, -3.434112377981050290 ) ) ;
#56931=CARTESIAN_POINT ( 'NONE',  ( 20.88017736071110875, 60.77201867748817676, -2.915334737309920765 ) ) ;
#56932=CARTESIAN_POINT ( 'NONE',  ( 5.076628168052704559, 30.17559781766745175, -8.527530157486179263 ) ) ;
#56933=CARTESIAN_POINT ( 'NONE',  ( 3.591859063236761518, 39.95696800326375353, 11.09922568453594849 ) ) ;
#56934=CARTESIAN_POINT ( 'NONE',  ( 2.791683348922237240, 0.3839311510007847872, -7.208316651077763204 ) ) ;
#56936=FILL_AREA_STYLE ('',( #41961 ) ) ;
#56938=CARTESIAN_POINT ( 'NONE',  ( 4.559911319644449179, 12.23035201082150536, -9.422509992056141925 ) ) ;
#56939=CARTESIAN_POINT ( 'NONE',  ( 19.38216949554541202, 55.99863466993041072, 9.382169495545424454 ) ) ;
#56940=CARTESIAN_POINT ( 'NONE',  ( -0.3689425029237898834, 21.17874883491396432, -10.36894250292378850 ) ) ;
#56941=CARTESIAN_POINT ( 'NONE',  ( 17.20831665107776587, 24.13393115100078035, -7.208316651077762316 ) ) ;
#56942=CARTESIAN_POINT ( 'NONE',  ( 10.00000000000000178, 9.313685344154839285, 10.88017736071110342 ) ) ;
#56943=CARTESIAN_POINT ( 'NONE',  ( -0.8801773607111009756, 8.063685344154837509, 1.068504757029289695E-15 ) ) ;
#56945=AXIS2_PLACEMENT_3D ( 'NONE', #59141, #19679, #35664 ) ;
#56946=CARTESIAN_POINT ( 'NONE',  ( 4.559911319644449179, 18.89701867748817321, 9.422509992056141925 ) ) ;
#56948=CARTESIAN_POINT ( 'NONE',  ( 7.084665262690076126, 19.10535201082150181, 10.88017736071109987 ) ) ;
#56951=CARTESIAN_POINT ( 'NONE',  ( 1.472469842513823179, 66.42559781766745175, 4.923371831947296329 ) ) ;
#56952=CARTESIAN_POINT ( 'NONE',  ( 4.559911319644449179, 23.89701867748817321, 9.422509992056141925 ) ) ;
#56953=CARTESIAN_POINT ( 'NONE',  ( 2.791683348922237240, 60.38393115100078745, -7.208316651077763204 ) ) ;
#56954=CARTESIAN_POINT ( 'NONE',  ( 10.00000000000000000, 52.87363466993041783, -12.81628187352647608 ) ) ;
#56956=CARTESIAN_POINT ( 'NONE',  ( 20.36894250292379382, 33.67874883491396076, 10.36894250292379205 ) ) ;
#56957=CARTESIAN_POINT ( 'NONE',  ( 17.96484262340118221, 41.18868534415484106, -7.964842623401177768 ) ) ;
#56958=CARTESIAN_POINT ( 'NONE',  ( 0.5774900079438607392, 13.48035201082150358, 5.440088680355550821 ) ) ;
#56959=CARTESIAN_POINT ( 'NONE',  ( 18.52753015748618282, 53.92559781766745175, -4.923371831947291888 ) ) ;
#56960=AXIS2_PLACEMENT_3D ( 'NONE', #77982, #86484, #70000 ) ;
#56961=( BOUNDED_SURFACE ( )  B_SPLINE_SURFACE ( 1, 2, ( 
 ( #10471, #9987, #55486, #47478, #1521, #64434, #17498, #87444, #46983, #85490, #70987, #77477, #70490, #2010, #25966, #55978, #79458, #32475, #62970, #48462, #93475, #86480, #94942, #25001, #86952, #48950, #85986, #2509, #32961, #2993, #16999, #63466, #92975, #77978, #71477, #33443, #56942, #47962, #56466, #93968, #17978, #8988, #41482, #18465, #71949, #39505, #24506, #33929, #69995, #54968, #43901, #95945, #34924, #65917, #27428, #80933, #26938, #72929, #18959, #20928, #19931, #73916, #12427, #4458, #96446, #66415, #80444, #57438, #5445, #58915, #42934, #11448, #20434, #65422, #74401, #66911, #27917, #87929, #43416, #50426, #19446, #58409, #96946, #73415, #4942, #97431, #5925, #81418, #49938, #35916, #12919, #3957, #35422, #50922, #28419, #88925, #28896, #89414, #49438, #81906, #79941, #95446, #51417, #13415, #36418, #11941, #42446, #57922, #59401, #41965, #88432, #72431, #34427, #64919, #7418, #46381, #89905, #30878, #76868, #82902, #45387, #91883, #6910, #29886, #15419, #90384, #37915, #8384, #21420, #61374, #38894, #31364, #98431, #75893, #91382, #68402, #60388, #60883, #98923, #14419, #53379, #52887, #90886, #21922, #44402, #69380, #22413, #51914, #82399, #29392, #83399, #13924, #44888, #75391, #7902, #30380, #23405, #37421, #67907, #22912, #14919, #83890, #903, #52401, #53889, #84395, #45901, #76387, #38397, #68899, #59894, #428, #74903, #15894, #6403, #36914, #67406, #97936, #17856, #77854, #24383, #71836, #25852, #70870, #62854, #79337, #39384, #9870, #10847, #55859, #86846, #39867, #9363, #40369, #70375, #24876, #69878, #16877, #61864, #63821, #93351, #48342, #55359, #47352, #2385, #10356, #54851, #1398, #78847, #2877, #85863, #54363, #63341, #1892, #18350, #41368, #32839, #31853, #86355, #17376, #62352, #93847, #40855, #47845, #78349, #3344, #48827, #25373, #92855, #71360, #33327, #46865, #94335, #56349, #92369, #23895, #84872, #16381, #77357, #8867, #85364, #32350, #4827, #42819, #50812, #72312, #95319, #19327, #3844, #35803, #27803, #79825, #18841, #73304, #88804, #20811, #89300, #81784, #26820, #66290, #42325, #5323, #20314, #4338, #94825, #80813, #12311, #51300, #35302, #81303, #27305, #41846, #13298, #57313, #72799, #26328, #88313, #43786, #33807, #64800, #28300, #64313, #50300, #65794, #43299, #56827, #96328, #58286, #12799, #74278, #73792, #96824, #11329, #87324, #49321, #58793, #87806, #34302, #49811, #80318, #11819, #34809, #65297, #95824, #57805, #19811, #6297, #53767, #84283, #76273, #28788, #44285, #83775, #14304, #23289, #30753, #82785, #75281, #45782, #61260, #37305, #38285, #36799, #59288, #7790 ),
 ( #83282, #15782, #68780, #5807, #312, #36298, #82281, #75774, #14806, #22791, #74788, #67293, #97820, #60276, #91768, #21805, #44775, #30262, #29283, #22300, #46271, #66795, #97315, #89786, #21302, #6791, #90775, #7295, #52773, #67794, #37794, #45278, #59779, #68292, #98314, #29768, #90271, #51795, #13798, #98813, #52285, #60766, #91266, #53268, #15298, #8754, #71239, #8274, #93231, #55234, #86236, #38772, #9745, #70755, #32725, #86731, #17747, #40247, #23784, #33217, #63711, #78734, #39272, #47735, #10243, #78232, #17260, #77738, #2269, #63223, #93728, #55745, #77247, #25745, #56238, #48225, #793, #16269, #40736, #85254, #94214, #2763, #54734, #47235, #18234, #76756, #9249, #69273, #69761, #31246, #61742, #25259, #16762, #92260, #62730, #54249, #84761, #1289, #39758, #70258, #1774, #46750, #85748, #62239, #31743, #32230, #92745, #24269, #24756, #89058, #82044, #5579, #18729, #44042, #29525, #36055, #95194, #36562, #81546, #3232, #10729, #49209, #79713, #72202, #26221, #82545, #51558, #56715, #75040, #59546, #20573, #21063, #51056, #13056, #74044, #6546, #79217, #71723, #37058, #87205, #13556, #34191, #11213, #52053, #74545, #94714, #33698, #59051, #6063, #67555, #98066, #60032, #41731, #14062, #58552, #21564, #67051, #43550, #41246, #97085, #28556, #90528, #97576, #29037, #66557, #3730, #48715, #64684, #89553, #90041, #28056, #44544, #64198, #84032, #15553, #1541, #77495, #84527, #91023, #77013, #16024, #7052, #46037, #23546, #46513, #567, #31985, #92501, #22062, #85014, #52536, #98574, #92017, #31013, #39028, #60531, #83539, #15060, #76522, #24031, #38049, #61021, #8527, #22554, #38536, #9007, #83044, #62002, #39523, #62491, #30518, #8038, #54018, #69032, #91533, #69523, #61509, #45531, #1038, #31501, #23048, #53024, #75538, #70017, #53521, #14560, #45029, #76029, #54499, #37556, #7562, #68541, #16527, #47003, #68046, #72, #30025, #94469, #86005, #3011, #11465, #55505, #33947, #94958, #47983, #25510, #78978, #48969, #32493, #48479, #77998, #62988, #86969, #56483, #41983, #93494, #79478, #10006, #17516, #3978, #56959, #33460, #93988, #72447, #70507, #40999, #34446, #18483, #18977, #71004, #40508, #71497, #2527, #55997, #2031, #78492, #92995, #26460, #86499, #10977, #17997, #32980, #63957, #41498, #63484, #25017, #71967, #64452, #10488, #85507, #25987, #3490, #49455, #24529, #87462, #79961, #54988, #17017, #47495, #9504, #40005, #82417, #35440, #6420, #64937, #4476, #58428, #95465, #57940, #88448, #81924, #43432, #97450, #19948, #80949, #66430, #50443, #73933, #13941, #27446, #5945, #66929, #12446, #96464, #50940 ) ),
 .UNSPECIFIED., .F., .F., .F. ) 
 B_SPLINE_SURFACE_WITH_KNOTS ( ( 2, 2 ),
 ( 3, 2, 2, 2, 2, 2, 2, 2, 2, 2, 2, 2, 2, 2, 2, 2, 2, 2, 2, 2, 2, 2, 2, 2, 2, 2, 2, 2, 2, 2, 2, 2, 2, 2, 2, 2, 2, 2, 2, 2, 2, 2, 2, 2, 2, 2, 2, 2, 2, 2, 2, 2, 2, 2, 2, 2, 2, 2, 2, 2, 2, 2, 2, 2, 2, 2, 2, 2, 2, 2, 2, 2, 2, 2, 2, 2, 2, 2, 2, 2, 2, 2, 2, 2, 2, 2, 2, 2, 2, 2, 2, 2, 2, 2, 2, 2, 2, 2, 2, 2, 2, 2, 2, 2, 2, 2, 2, 2, 2, 2, 2, 2, 2, 2, 2, 2, 2, 2, 2, 2, 2, 2, 2, 2, 2, 2, 2, 2, 2, 2, 2, 2, 2, 2, 2, 2, 2, 2, 2, 2, 2, 2, 2, 2, 2, 2, 2, 2, 2, 2, 2, 2, 2, 2, 2, 2, 2, 2, 2, 2, 2, 2, 3 ),
 ( 0.000000000000000000, 1.000000000000000000 ),
 ( 0.000000000000000000, 0.005952380952380952051, 0.01190476190476190410, 0.01785714285714285615, 0.02380952380952380820, 0.02976190476190476025, 0.03571428571428571230, 0.04166666666666666435, 0.04761904761904761640, 0.05357142857142856845, 0.05952380952380952051, 0.06547619047619047949, 0.07142857142857142461, 0.07738095238095238360, 0.08333333333333332871, 0.08928571428571428770, 0.09523809523809523281, 0.1011904761904761918, 0.1071428571428571369, 0.1130952380952380959, 0.1190476190476190410, 0.1250000000000000000, 0.1309523809523809590, 0.1369047619047619180, 0.1428571428571428492, 0.1488095238095238082, 0.1547619047619047672, 0.1607142857142857262, 0.1666666666666666574, 0.1726190476190476164, 0.1785714285714285754, 0.1845238095238095344, 0.1904761904761904656, 0.1964285714285714246, 0.2023809523809523836, 0.2083333333333333426, 0.2142857142857142738, 0.2202380952380952328, 0.2261904761904761918, 0.2321428571428571508, 0.2380952380952380820, 0.2440476190476190410, 0.2500000000000000000, 0.2559523809523809312, 0.2619047619047619180, 0.2678571428571428492, 0.2738095238095238360, 0.2797619047619047672, 0.2857142857142856984, 0.2916666666666666852, 0.2976190476190476164, 0.3035714285714285476, 0.3095238095238095344, 0.3154761904761904656, 0.3214285714285714524, 0.3273809523809523836, 0.3333333333333333148, 0.3392857142857143016, 0.3452380952380952328, 0.3511904761904761640, 0.3571428571428571508, 0.3630952380952380820, 0.3690476190476190688, 0.3750000000000000000, 0.3809523809523809312, 0.3869047619047619180, 0.3928571428571428492, 0.3988095238095238360, 0.4047619047619047672, 0.4107142857142856984, 0.4166666666666666852, 0.4226190476190476164, 0.4285714285714285476, 0.4345238095238095344, 0.4404761904761904656, 0.4464285714285714524, 0.4523809523809523836, 0.4583333333333333148, 0.4642857142857143016, 0.4702380952380952328, 0.4761904761904761640, 0.4821428571428571508, 0.4880952380952380820, 0.4940476190476190688, 0.5000000000000000000, 0.5059523809523809312, 0.5119047619047618625, 0.5178571428571429047, 0.5238095238095238360, 0.5297619047619047672, 0.5357142857142856984, 0.5416666666666666297, 0.5476190476190476719, 0.5535714285714286031, 0.5595238095238095344, 0.5654761904761904656, 0.5714285714285713969, 0.5773809523809523281, 0.5833333333333333703, 0.5892857142857143016, 0.5952380952380952328, 0.6011904761904761640, 0.6071428571428570953, 0.6130952380952381375, 0.6190476190476190688, 0.6250000000000000000, 0.6309523809523809312, 0.6369047619047618625, 0.6428571428571429047, 0.6488095238095238360, 0.6547619047619047672, 0.6607142857142856984, 0.6666666666666666297, 0.6726190476190476719, 0.6785714285714286031, 0.6845238095238095344, 0.6904761904761904656, 0.6964285714285713969, 0.7023809523809523281, 0.7083333333333333703, 0.7142857142857143016, 0.7202380952380952328, 0.7261904761904761640, 0.7321428571428570953, 0.7380952380952381375, 0.7440476190476190688, 0.7500000000000000000, 0.7559523809523809312, 0.7619047619047618625, 0.7678571428571429047, 0.7738095238095238360, 0.7797619047619047672, 0.7857142857142856984, 0.7916666666666666297, 0.7976190476190476719, 0.8035714285714286031, 0.8095238095238095344, 0.8154761904761904656, 0.8214285714285713969, 0.8273809523809523281, 0.8333333333333333703, 0.8392857142857143016, 0.8452380952380952328, 0.8511904761904761640, 0.8571428571428570953, 0.8630952380952381375, 0.8690476190476190688, 0.8750000000000000000, 0.8809523809523809312, 0.8869047619047618625, 0.8928571428571429047, 0.8988095238095238360, 0.9047619047619047672, 0.9107142857142856984, 0.9166666666666666297, 0.9226190476190476719, 0.9285714285714286031, 0.9345238095238095344, 0.9404761904761904656, 0.9464285714285713969, 0.9523809523809523281, 0.9583333333333333703, 0.9642857142857143016 ),
 .UNSPECIFIED. ) 
 GEOMETRIC_REPRESENTATION_ITEM ( )  RATIONAL_B_SPLINE_SURFACE ( (
 ( 1.000000000000000000, 0.9659258262890683122, 1.000000000000000000, 0.9659258262890683122, 1.000000000000000000, 0.9659258262890683122, 1.000000000000000000, 0.9659258262890683122, 1.000000000000000000, 0.9659258262890683122, 1.000000000000000000, 0.9659258262890683122, 1.000000000000000000, 0.9659258262890683122, 1.000000000000000000, 0.9659258262890683122, 1.000000000000000000, 0.9659258262890683122, 1.000000000000000000, 0.9659258262890683122, 1.000000000000000000, 0.9659258262890683122, 1.000000000000000000, 0.9659258262890683122, 1.000000000000000000, 0.9659258262890683122, 1.000000000000000000, 0.9659258262890683122, 1.000000000000000000, 0.9659258262890683122, 1.000000000000000000, 0.9659258262890683122, 1.000000000000000000, 0.9659258262890683122, 1.000000000000000000, 0.9659258262890683122, 1.000000000000000000, 0.9659258262890683122, 1.000000000000000000, 0.9659258262890683122, 1.000000000000000000, 0.9659258262890683122, 1.000000000000000000, 0.9659258262890683122, 1.000000000000000000, 0.9659258262890683122, 1.000000000000000000, 0.9659258262890683122, 1.000000000000000000, 0.9659258262890683122, 1.000000000000000000, 0.9659258262890683122, 1.000000000000000000, 0.9659258262890683122, 1.000000000000000000, 0.9659258262890683122, 1.000000000000000000, 0.9659258262890683122, 1.000000000000000000, 0.9659258262890683122, 1.000000000000000000, 0.9659258262890683122, 1.000000000000000000, 0.9659258262890683122, 1.000000000000000000, 0.9659258262890683122, 1.000000000000000000, 0.9659258262890683122, 1.000000000000000000, 0.9659258262890683122, 1.000000000000000000, 0.9659258262890683122, 1.000000000000000000, 0.9659258262890683122, 1.000000000000000000, 0.9659258262890683122, 1.000000000000000000, 0.9659258262890683122, 1.000000000000000000, 0.9659258262890683122, 1.000000000000000000, 0.9659258262890683122, 1.000000000000000000, 0.9659258262890683122, 1.000000000000000000, 0.9659258262890683122, 1.000000000000000000, 0.9659258262890683122, 1.000000000000000000, 0.9659258262890683122, 1.000000000000000000, 0.9659258262890683122, 1.000000000000000000, 0.9659258262890683122, 1.000000000000000000, 0.9659258262890683122, 1.000000000000000000, 0.9659258262890683122, 1.000000000000000000, 0.9659258262890683122, 1.000000000000000000, 0.9659258262890683122, 1.000000000000000000, 0.9659258262890683122, 1.000000000000000000, 0.9659258262890683122, 1.000000000000000000, 0.9659258262890683122, 1.000000000000000000, 0.9659258262890683122, 1.000000000000000000, 0.9659258262890683122, 1.000000000000000000, 0.9659258262890683122, 1.000000000000000000, 0.9659258262890683122, 1.000000000000000000, 0.9659258262890683122, 1.000000000000000000, 0.9659258262890683122, 1.000000000000000000, 0.9659258262890683122, 1.000000000000000000, 0.9659258262890683122, 1.000000000000000000, 0.9659258262890683122, 1.000000000000000000, 0.9659258262890683122, 1.000000000000000000, 0.9659258262890683122, 1.000000000000000000, 0.9659258262890683122, 1.000000000000000000, 0.9659258262890683122, 1.000000000000000000, 0.9659258262890683122, 1.000000000000000000, 0.9659258262890683122, 1.000000000000000000, 0.9659258262890683122, 1.000000000000000000, 0.9659258262890683122, 1.000000000000000000, 0.9659258262890683122, 1.000000000000000000, 0.9659258262890683122, 1.000000000000000000, 0.9659258262890683122, 1.000000000000000000, 0.9659258262890683122, 1.000000000000000000, 0.9659258262890683122, 1.000000000000000000, 0.9659258262890683122, 1.000000000000000000, 0.9659258262890683122, 1.000000000000000000, 0.9659258262890683122, 1.000000000000000000, 0.9659258262890683122, 1.000000000000000000, 0.9659258262890683122, 1.000000000000000000, 0.9659258262890683122, 1.000000000000000000, 0.9659258262890683122, 1.000000000000000000, 0.9659258262890683122, 1.000000000000000000, 0.9659258262890683122, 1.000000000000000000, 0.9659258262890683122, 1.000000000000000000, 0.9659258262890683122, 1.000000000000000000, 0.9659258262890683122, 1.000000000000000000, 0.9659258262890683122, 1.000000000000000000, 0.9659258262890683122, 1.000000000000000000, 0.9659258262890683122, 1.000000000000000000, 0.9659258262890683122, 1.000000000000000000, 0.9659258262890683122, 1.000000000000000000, 0.9659258262890683122, 1.000000000000000000, 0.9659258262890683122, 1.000000000000000000, 0.9659258262890683122, 1.000000000000000000, 0.9659258262890683122, 1.000000000000000000, 0.9659258262890683122, 1.000000000000000000, 0.9659258262890683122, 1.000000000000000000, 0.9659258262890683122, 1.000000000000000000, 0.9659258262890683122, 1.000000000000000000, 0.9659258262890683122, 1.000000000000000000, 0.9659258262890683122, 1.000000000000000000, 0.9659258262890683122, 1.000000000000000000, 0.9659258262890683122, 1.000000000000000000, 0.9659258262890683122, 1.000000000000000000, 0.9659258262890683122, 1.000000000000000000, 0.9659258262890683122, 1.000000000000000000, 0.9659258262890683122, 1.000000000000000000, 0.9659258262890683122, 1.000000000000000000, 0.9659258262890683122, 1.000000000000000000, 0.9659258262890683122, 1.000000000000000000, 0.9659258262890683122, 1.000000000000000000, 0.9659258262890683122, 1.000000000000000000, 0.9659258262890683122, 1.000000000000000000, 0.9659258262890683122, 1.000000000000000000, 0.9659258262890683122, 1.000000000000000000, 0.9659258262890683122, 1.000000000000000000, 0.9659258262890683122, 1.000000000000000000, 0.9659258262890683122, 1.000000000000000000, 0.9659258262890683122, 1.000000000000000000, 0.9659258262890683122, 1.000000000000000000, 0.9659258262890683122, 1.000000000000000000, 0.9659258262890683122, 1.000000000000000000, 0.9659258262890683122, 1.000000000000000000, 0.9659258262890683122, 1.000000000000000000, 0.9659258262890683122, 1.000000000000000000, 0.9659258262890683122, 1.000000000000000000, 0.9659258262890683122, 1.000000000000000000, 0.9659258262890683122, 1.000000000000000000, 0.9659258262890683122, 1.000000000000000000, 0.9659258262890683122, 1.000000000000000000, 0.9659258262890683122, 1.000000000000000000, 0.9659258262890683122, 1.000000000000000000, 0.9659258262890683122, 1.000000000000000000, 0.9659258262890683122, 1.000000000000000000, 0.9659258262890683122, 1.000000000000000000, 0.9659258262890683122, 1.000000000000000000, 0.9659258262890683122, 1.000000000000000000, 0.9659258262890683122, 1.000000000000000000, 0.9659258262890683122, 1.000000000000000000, 0.9659258262890683122, 1.000000000000000000, 0.9659258262890683122, 1.000000000000000000, 0.9659258262890683122, 1.000000000000000000, 0.9659258262890683122, 1.000000000000000000, 0.9659258262890683122, 1.000000000000000000, 0.9659258262890683122, 1.000000000000000000, 0.9659258262890683122, 1.000000000000000000, 0.9659258262890683122, 1.000000000000000000, 0.9659258262890683122, 1.000000000000000000, 0.9659258262890683122, 1.000000000000000000, 0.9659258262890683122, 1.000000000000000000, 0.9659258262890683122, 1.000000000000000000, 0.9659258262890683122, 1.000000000000000000, 0.9659258262890683122, 1.000000000000000000, 0.9659258262890683122, 1.000000000000000000, 0.9659258262890683122, 1.000000000000000000, 0.9659258262890683122, 1.000000000000000000, 0.9659258262890683122, 1.000000000000000000, 0.9659258262890683122, 1.000000000000000000, 0.9659258262890683122, 1.000000000000000000, 0.9659258262890683122, 1.000000000000000000),
 ( 1.000000000000000000, 0.9659258262890683122, 1.000000000000000000, 0.9659258262890683122, 1.000000000000000000, 0.9659258262890683122, 1.000000000000000000, 0.9659258262890683122, 1.000000000000000000, 0.9659258262890683122, 1.000000000000000000, 0.9659258262890683122, 1.000000000000000000, 0.9659258262890683122, 1.000000000000000000, 0.9659258262890683122, 1.000000000000000000, 0.9659258262890683122, 1.000000000000000000, 0.9659258262890683122, 1.000000000000000000, 0.9659258262890683122, 1.000000000000000000, 0.9659258262890683122, 1.000000000000000000, 0.9659258262890683122, 1.000000000000000000, 0.9659258262890683122, 1.000000000000000000, 0.9659258262890683122, 1.000000000000000000, 0.9659258262890683122, 1.000000000000000000, 0.9659258262890683122, 1.000000000000000000, 0.9659258262890683122, 1.000000000000000000, 0.9659258262890683122, 1.000000000000000000, 0.9659258262890683122, 1.000000000000000000, 0.9659258262890683122, 1.000000000000000000, 0.9659258262890683122, 1.000000000000000000, 0.9659258262890683122, 1.000000000000000000, 0.9659258262890683122, 1.000000000000000000, 0.9659258262890683122, 1.000000000000000000, 0.9659258262890683122, 1.000000000000000000, 0.9659258262890683122, 1.000000000000000000, 0.9659258262890683122, 1.000000000000000000, 0.9659258262890683122, 1.000000000000000000, 0.9659258262890683122, 1.000000000000000000, 0.9659258262890683122, 1.000000000000000000, 0.9659258262890683122, 1.000000000000000000, 0.9659258262890683122, 1.000000000000000000, 0.9659258262890683122, 1.000000000000000000, 0.9659258262890683122, 1.000000000000000000, 0.9659258262890683122, 1.000000000000000000, 0.9659258262890683122, 1.000000000000000000, 0.9659258262890683122, 1.000000000000000000, 0.9659258262890683122, 1.000000000000000000, 0.9659258262890683122, 1.000000000000000000, 0.9659258262890683122, 1.000000000000000000, 0.9659258262890683122, 1.000000000000000000, 0.9659258262890683122, 1.000000000000000000, 0.9659258262890683122, 1.000000000000000000, 0.9659258262890683122, 1.000000000000000000, 0.9659258262890683122, 1.000000000000000000, 0.9659258262890683122, 1.000000000000000000, 0.9659258262890683122, 1.000000000000000000, 0.9659258262890683122, 1.000000000000000000, 0.9659258262890683122, 1.000000000000000000, 0.9659258262890683122, 1.000000000000000000, 0.9659258262890683122, 1.000000000000000000, 0.9659258262890683122, 1.000000000000000000, 0.9659258262890683122, 1.000000000000000000, 0.9659258262890683122, 1.000000000000000000, 0.9659258262890683122, 1.000000000000000000, 0.9659258262890683122, 1.000000000000000000, 0.9659258262890683122, 1.000000000000000000, 0.9659258262890683122, 1.000000000000000000, 0.9659258262890683122, 1.000000000000000000, 0.9659258262890683122, 1.000000000000000000, 0.9659258262890683122, 1.000000000000000000, 0.9659258262890683122, 1.000000000000000000, 0.9659258262890683122, 1.000000000000000000, 0.9659258262890683122, 1.000000000000000000, 0.9659258262890683122, 1.000000000000000000, 0.9659258262890683122, 1.000000000000000000, 0.9659258262890683122, 1.000000000000000000, 0.9659258262890683122, 1.000000000000000000, 0.9659258262890683122, 1.000000000000000000, 0.9659258262890683122, 1.000000000000000000, 0.9659258262890683122, 1.000000000000000000, 0.9659258262890683122, 1.000000000000000000, 0.9659258262890683122, 1.000000000000000000, 0.9659258262890683122, 1.000000000000000000, 0.9659258262890683122, 1.000000000000000000, 0.9659258262890683122, 1.000000000000000000, 0.9659258262890683122, 1.000000000000000000, 0.9659258262890683122, 1.000000000000000000, 0.9659258262890683122, 1.000000000000000000, 0.9659258262890683122, 1.000000000000000000, 0.9659258262890683122, 1.000000000000000000, 0.9659258262890683122, 1.000000000000000000, 0.9659258262890683122, 1.000000000000000000, 0.9659258262890683122, 1.000000000000000000, 0.9659258262890683122, 1.000000000000000000, 0.9659258262890683122, 1.000000000000000000, 0.9659258262890683122, 1.000000000000000000, 0.9659258262890683122, 1.000000000000000000, 0.9659258262890683122, 1.000000000000000000, 0.9659258262890683122, 1.000000000000000000, 0.9659258262890683122, 1.000000000000000000, 0.9659258262890683122, 1.000000000000000000, 0.9659258262890683122, 1.000000000000000000, 0.9659258262890683122, 1.000000000000000000, 0.9659258262890683122, 1.000000000000000000, 0.9659258262890683122, 1.000000000000000000, 0.9659258262890683122, 1.000000000000000000, 0.9659258262890683122, 1.000000000000000000, 0.9659258262890683122, 1.000000000000000000, 0.9659258262890683122, 1.000000000000000000, 0.9659258262890683122, 1.000000000000000000, 0.9659258262890683122, 1.000000000000000000, 0.9659258262890683122, 1.000000000000000000, 0.9659258262890683122, 1.000000000000000000, 0.9659258262890683122, 1.000000000000000000, 0.9659258262890683122, 1.000000000000000000, 0.9659258262890683122, 1.000000000000000000, 0.9659258262890683122, 1.000000000000000000, 0.9659258262890683122, 1.000000000000000000, 0.9659258262890683122, 1.000000000000000000, 0.9659258262890683122, 1.000000000000000000, 0.9659258262890683122, 1.000000000000000000, 0.9659258262890683122, 1.000000000000000000, 0.9659258262890683122, 1.000000000000000000, 0.9659258262890683122, 1.000000000000000000, 0.9659258262890683122, 1.000000000000000000, 0.9659258262890683122, 1.000000000000000000, 0.9659258262890683122, 1.000000000000000000, 0.9659258262890683122, 1.000000000000000000, 0.9659258262890683122, 1.000000000000000000, 0.9659258262890683122, 1.000000000000000000, 0.9659258262890683122, 1.000000000000000000, 0.9659258262890683122, 1.000000000000000000, 0.9659258262890683122, 1.000000000000000000, 0.9659258262890683122, 1.000000000000000000, 0.9659258262890683122, 1.000000000000000000, 0.9659258262890683122, 1.000000000000000000, 0.9659258262890683122, 1.000000000000000000, 0.9659258262890683122, 1.000000000000000000, 0.9659258262890683122, 1.000000000000000000, 0.9659258262890683122, 1.000000000000000000, 0.9659258262890683122, 1.000000000000000000, 0.9659258262890683122, 1.000000000000000000, 0.9659258262890683122, 1.000000000000000000, 0.9659258262890683122, 1.000000000000000000, 0.9659258262890683122, 1.000000000000000000, 0.9659258262890683122, 1.000000000000000000, 0.9659258262890683122, 1.000000000000000000, 0.9659258262890683122, 1.000000000000000000, 0.9659258262890683122, 1.000000000000000000, 0.9659258262890683122, 1.000000000000000000, 0.9659258262890683122, 1.000000000000000000, 0.9659258262890683122, 1.000000000000000000, 0.9659258262890683122, 1.000000000000000000, 0.9659258262890683122, 1.000000000000000000, 0.9659258262890683122, 1.000000000000000000, 0.9659258262890683122, 1.000000000000000000, 0.9659258262890683122, 1.000000000000000000, 0.9659258262890683122, 1.000000000000000000, 0.9659258262890683122, 1.000000000000000000, 0.9659258262890683122, 1.000000000000000000, 0.9659258262890683122, 1.000000000000000000, 0.9659258262890683122, 1.000000000000000000, 0.9659258262890683122, 1.000000000000000000, 0.9659258262890683122, 1.000000000000000000, 0.9659258262890683122, 1.000000000000000000, 0.9659258262890683122, 1.000000000000000000, 0.9659258262890683122, 1.000000000000000000, 0.9659258262890683122, 1.000000000000000000, 0.9659258262890683122, 1.000000000000000000, 0.9659258262890683122, 1.000000000000000000) ) ) 
 REPRESENTATION_ITEM ( '' )  SURFACE ( )  );
#56963=CARTESIAN_POINT ( 'NONE',  ( 14.92337183194729988, 54.34226448433412315, -8.527530157486177487 ) ) ;
#56964=CARTESIAN_POINT ( 'NONE',  ( 1.472469842513823179, 5.592264484334118713, -4.923371831947296329 ) ) ;
#56966=ORIENTED_EDGE ( 'NONE', *, *, #7589, .F. ) ;
#56967=CARTESIAN_POINT ( 'NONE',  ( 15.44008868035555260, 14.73035201082150536, 9.422509992056143702 ) ) ;
#56968=CARTESIAN_POINT ( 'NONE',  ( 17.20831665107776587, 12.88393115100078390, 7.208316651077764980 ) ) ;
#56969=CARTESIAN_POINT ( 'NONE',  ( -2.816281873526473856, 4.123634669930420493, 9.499525473075851096E-16 ) ) ;
#56970=CARTESIAN_POINT ( 'NONE',  ( 4.559911319644449179, 42.23035201082151247, -9.422509992056141925 ) ) ;
#56971=CARTESIAN_POINT ( 'NONE',  ( 19.42250999205614193, 15.14701867748817143, 5.440088680355555262 ) ) ;
#56972=CARTESIAN_POINT ( 'NONE',  ( 3.591859063236763294, 48.29030133659708923, -11.09922568453595026 ) ) ;
#56973=CARTESIAN_POINT ( 'NONE',  ( 13.79529636645030344, 38.26208216824729647, 14.16423886937410614 ) ) ;
#56975=CARTESIAN_POINT ( 'NONE',  ( -1.099225684535947600, 54.54030133659708923, 6.408140936763237150 ) ) ;
#56977=CARTESIAN_POINT ( 'NONE',  ( 0.1532563361054100626, 60.80059781766744464, -2.638427012816831230 ) ) ;
#56978=CARTESIAN_POINT ( 'NONE',  ( 6.565887622018943937, 65.16530133659709634, 12.81628187352647430 ) ) ;
#56979=CARTESIAN_POINT ( 'NONE',  ( -0.8801773607111009756, 28.06368534415484106, 1.068504757029289695E-15 ) ) ;
#56980=CARTESIAN_POINT ( 'NONE',  ( 10.00000000000000000, 59.75893115100078745, -9.846743663894594434 ) ) ;
#56982=CARTESIAN_POINT ( 'NONE',  ( 0.1532563361054100626, 5.800597817667452638, -2.638427012816831230 ) ) ;
#56984=CARTESIAN_POINT ( 'NONE',  ( 14.92337183194729633, 22.67559781766745175, 8.527530157486181039 ) ) ;
#56985=CARTESIAN_POINT ( 'NONE',  ( 19.84674366389459266, 8.717264484334116048, -2.638427012816827677 ) ) ;
#56987=SURFACE_STYLE_FILL_AREA ( #88473 ) ;
#56989=CARTESIAN_POINT ( 'NONE',  ( 2.035157376598824452, 53.68868534415484817, 7.964842623401179544 ) ) ;
#56991=CARTESIAN_POINT ( 'NONE',  ( 1.274849032794292736, 37.55509018479936145, -6.499999999999977796 ) ) ;
#56992=CARTESIAN_POINT ( 'NONE',  ( 17.96484262340118221, 64.93868534415483396, 7.964842623401181321 ) ) ;
#56993=CARTESIAN_POINT ( 'NONE',  ( 18.52753015748618282, 13.92559781766745175, -4.923371831947291888 ) ) ;
#56998=CARTESIAN_POINT ( 'NONE',  ( 7.361572987183169658, 59.96726448433410894, -9.846743663894592657 ) ) ;
#57002=CARTESIAN_POINT ( 'NONE',  ( 20.36894250292379382, 18.67874883491397142, 10.36894250292379205 ) ) ;
#57003=CARTESIAN_POINT ( 'NONE',  ( 0.5600000000000083800, 105.0000000000000000, -4.500000000000001776 ) ) ;
#57004=CARTESIAN_POINT ( 'NONE',  ( 6.204703633549690345, 17.84541550158063217, 14.16423886937410082 ) ) ;
#57005=CARTESIAN_POINT ( 'NONE',  ( -4.164238869374099927, 27.01208216824730357, 3.795296366450308767 ) ) ;
#57006=SURFACE_STYLE_FILL_AREA ( #34491 ) ;
#57007=CARTESIAN_POINT ( 'NONE',  ( 7.084665262690076126, 37.02201867748817676, -10.88017736071110164 ) ) ;
#57010=CARTESIAN_POINT ( 'NONE',  ( 0.1532563361054083140, 21.00893115100078745, 1.131784320476157264E-15 ) ) ;
#57011=( GEOMETRIC_REPRESENTATION_CONTEXT ( 3 ) GLOBAL_UNCERTAINTY_ASSIGNED_CONTEXT ( ( #80161 ) ) GLOBAL_UNIT_ASSIGNED_CONTEXT ( ( #16742, #63691, #77230 ) ) REPRESENTATION_CONTEXT ( 'NONE', 'WORKASPACE' ) );
#57012=CARTESIAN_POINT ( 'NONE',  ( 15.44008868035555260, 54.73035201082150536, 9.422509992056143702 ) ) ;
#57013=CARTESIAN_POINT ( 'NONE',  ( 2.791683348922240793, 16.63393115100078745, 7.208316651077764092 ) ) ;
#57014=CARTESIAN_POINT ( 'NONE',  ( 13.43411237798105340, 45.58196800326374643, 12.81628187352647963 ) ) ;
#57015=CARTESIAN_POINT ( 'NONE',  ( 0.1532563361054082862, 41.21726448433411605, 2.638427012816831674 ) ) ;
#57017=CARTESIAN_POINT ( 'NONE',  ( 0.6178305044545838731, 29.74863466993042138, 9.382169495545420901 ) ) ;
#57019=CARTESIAN_POINT ( 'NONE',  ( 2.791683348922237240, 20.38393115100078745, -7.208316651077763204 ) ) ;
#57020=CARTESIAN_POINT ( 'NONE',  ( 13.79529636645030344, 18.26208216824730002, 14.16423886937410614 ) ) ;
#57024=CARTESIAN_POINT ( 'NONE',  ( 17.96484262340118221, 44.93868534415483396, 7.964842623401181321 ) ) ;
#57025=CARTESIAN_POINT ( 'NONE',  ( 17.96484262340118221, 54.93868534415484106, 7.964842623401181321 ) ) ;
#57026=CARTESIAN_POINT ( 'NONE',  ( 17.08211943468705130, 48.47041550158063927, 12.26659068614894998 ) ) ;
#57027=CARTESIAN_POINT ( 'NONE',  ( 18.52753015748618282, 58.92559781766745886, -4.923371831947291888 ) ) ;
#57028=CARTESIAN_POINT ( 'NONE',  ( 0.1532563361054100626, 10.80059781766745175, -2.638427012816831230 ) ) ;
#57029=CARTESIAN_POINT ( 'NONE',  ( 10.00000000000000178, 60.37363466993041783, 12.81628187352647608 ) ) ;
#57031=CARTESIAN_POINT ( 'NONE',  ( 7.084665262690076126, 47.02201867748818387, -10.88017736071110164 ) ) ;
#57034=CARTESIAN_POINT ( 'NONE',  ( 0.1532563361054100626, 55.80059781766745175, -2.638427012816831230 ) ) ;
#57037=CARTESIAN_POINT ( 'NONE',  ( 0.5774900079438607392, 68.48035201082150536, 5.440088680355550821 ) ) ;
#57038=CARTESIAN_POINT ( 'NONE',  ( 7.084665262690076126, 2.022018677488170990, -10.88017736071110164 ) ) ;
#57040=CARTESIAN_POINT ( 'NONE',  ( 0.5774900079438607392, 68.48035201082150536, 5.440088680355550821 ) ) ;
#57042=CARTESIAN_POINT ( 'NONE',  ( 17.20831665107776587, 4.133931151000785675, -7.208316651077762316 ) ) ;
#57044=CARTESIAN_POINT ( 'NONE',  ( 10.00000000000000178, 37.25893115100078745, 9.846743663894594434 ) ) ;
#57046=CARTESIAN_POINT ( 'NONE',  ( 2.035157376598822676, 17.43868534415483751, -7.964842623401177768 ) ) ;
#57047=CARTESIAN_POINT ( 'NONE',  ( 10.00000000000000178, 0.3736346699304200492, 12.81628187352647608 ) ) ;
#57048=CARTESIAN_POINT ( 'NONE',  ( 17.96484262340118221, 41.18868534415484106, -7.964842623401177768 ) ) ;
#57051=CARTESIAN_POINT ( 'NONE',  ( 6.565887622018943937, 35.16530133659708923, 12.81628187352647430 ) ) ;
#57053=CARTESIAN_POINT ( 'NONE',  ( 10.00000000000000178, 54.31368534415484106, 10.88017736071110342 ) ) ;
#57054=CARTESIAN_POINT ( 'NONE',  ( 13.43411237798106583, 22.66530133659708923, -12.81628187352647252 ) ) ;
#57055=FILL_AREA_STYLE ('',( #89037 ) ) ;
#57056=CARTESIAN_POINT ( 'NONE',  ( 15.44008868035555260, 24.73035201082150891, 9.422509992056143702 ) ) ;
#57057=CARTESIAN_POINT ( 'NONE',  ( 24.16423886937410614, 64.51208216824728936, -3.795296366450302550 ) ) ;
#57059=CARTESIAN_POINT ( 'NONE',  ( 1.472469842513823179, 40.59226448433411605, -4.923371831947296329 ) ) ;
#57060=CARTESIAN_POINT ( 'NONE',  ( 10.00000000000000000, 4.758931151000784787, -9.846743663894594434 ) ) ;
#57061=CARTESIAN_POINT ( 'NONE',  ( -0.8801773607110991993, 62.85535201082150536, -2.915334737309923874 ) ) ;
#57063=CARTESIAN_POINT ( 'NONE',  ( 10.00000000000000178, 33.05374883491396787, 14.16423886937410082 ) ) ;
#57072=VERTEX_POINT ( 'NONE', #24923 ) ;
#57073=CARTESIAN_POINT ( 'NONE',  ( 6.204703633549690345, 42.84541550158063217, 14.16423886937410082 ) ) ;
#57074=CARTESIAN_POINT ( 'NONE',  ( 13.79529636645031943, 45.34541550158062506, -14.16423886937409904 ) ) ;
#57075=CARTESIAN_POINT ( 'NONE',  ( 14.92337183194729633, 12.67559781766745353, 8.527530157486181039 ) ) ;
#57076=CARTESIAN_POINT ( 'NONE',  ( -1.099225684535947600, 13.70696800326375353, -6.408140936763238038 ) ) ;
#57078=FACE_OUTER_BOUND ( 'NONE', #63791, .T. ) ;
#57079=CARTESIAN_POINT ( 'NONE',  ( 20.88017736071110519, 5.563685344154837509, 2.639326808657452039E-16 ) ) ;
#57080=CARTESIAN_POINT ( 'NONE',  ( 10.00000000000000178, 30.37363466993042138, 12.81628187352647608 ) ) ;
#57081=CARTESIAN_POINT ( 'NONE',  ( 6.204703633549690345, 40.76208216824731778, -14.16423886937410259 ) ) ;
#57087=CARTESIAN_POINT ( 'NONE',  ( 1.472469842513823179, 25.59226448433412315, -4.923371831947296329 ) ) ;
#57089=ORIENTED_EDGE ( 'NONE', *, *, #34413, .T. ) ;
#57090=CARTESIAN_POINT ( 'NONE',  ( 10.00000000000000000, 11.81368534415483751, -10.88017736071110342 ) ) ;
#57091=CARTESIAN_POINT ( 'NONE',  ( 2.035157376598824452, 13.68868534415483751, 7.964842623401179544 ) ) ;
#57092=CARTESIAN_POINT ( 'NONE',  ( 5.076628168052703671, 46.84226448433412315, 8.527530157486179263 ) ) ;
#57093=CARTESIAN_POINT ( 'NONE',  ( 10.00000000000000178, 5.373634669930420493, 12.81628187352647608 ) ) ;
#57095=CARTESIAN_POINT ( 'NONE',  ( 13.43411237798106583, 17.66530133659708923, -12.81628187352647252 ) ) ;
#57096=ORIENTED_EDGE ( 'NONE', *, *, #89212, .T. ) ;
#57097=CARTESIAN_POINT ( 'NONE',  ( 22.26659068614895176, 64.72041550158064638, -7.082119434687042414 ) ) ;
#57098=EDGE_LOOP ( 'NONE', ( #60916, #20343, #72113, #68051 ) ) ;
#57099=CARTESIAN_POINT ( 'NONE',  ( -4.164238869374099927, 52.01208216824729647, 3.795296366450308767 ) ) ;
#57100=ORIENTED_EDGE ( 'NONE', *, *, #60095, .T. ) ;
#57101=CARTESIAN_POINT ( 'NONE',  ( 2.035157376598824452, 28.68868534415484106, 7.964842623401179544 ) ) ;
#57102=CARTESIAN_POINT ( 'NONE',  ( 10.00000000000000000, 46.81368534415484106, -10.88017736071110342 ) ) ;
#57104=CARTESIAN_POINT ( 'NONE',  ( 10.00000000000000000, 46.81368534415484106, -10.88017736071110342 ) ) ;
#57105=CARTESIAN_POINT ( 'NONE',  ( 2.035157376598822676, 47.43868534415484817, -7.964842623401177768 ) ) ;
#57107=DIRECTION ( 'NONE',  ( 0.000000000000000000, 0.000000000000000000, -1.000000000000000000 ) ) ;
#57108=CARTESIAN_POINT ( 'NONE',  ( 2.791683348922237240, 10.38393115100078390, -7.208316651077763204 ) ) ;
#57111=CARTESIAN_POINT ( 'NONE',  ( 0.1532563361054100626, 45.80059781766745886, -2.638427012816831230 ) ) ;
#57114=CARTESIAN_POINT ( 'NONE',  ( -2.816281873526473856, 54.12363466993041783, 9.499525473075851096E-16 ) ) ;
#57119=CARTESIAN_POINT ( 'NONE',  ( 0.1532563361054100626, 65.80059781766745175, -2.638427012816831230 ) ) ;
#57120=CARTESIAN_POINT ( 'NONE',  ( 13.79529636645030344, 58.26208216824728936, 14.16423886937410614 ) ) ;
#57122=ORIENTED_EDGE ( 'NONE', *, *, #44244, .T. ) ;
#57124=CARTESIAN_POINT ( 'NONE',  ( 10.00000000000000178, 27.25893115100078390, 9.846743663894594434 ) ) ;
#57127=CARTESIAN_POINT ( 'NONE',  ( 16.40814093676323893, 5.790301336597087456, 11.09922568453595026 ) ) ;
#57128=CARTESIAN_POINT ( 'NONE',  ( 4.559911319644449179, 67.23035201082150536, -9.422509992056141925 ) ) ;
#57131=CARTESIAN_POINT ( 'NONE',  ( 10.00000000000000000, 14.75893115100078568, -9.846743663894594434 ) ) ;
#57132=CARTESIAN_POINT ( 'NONE',  ( 12.63842701281683922, 54.55059781766745175, -9.846743663894590881 ) ) ;
#57135=ORIENTED_EDGE ( 'NONE', *, *, #41014, .T. ) ;
#57136=CARTESIAN_POINT ( 'NONE',  ( -0.8801773607111008646, 3.272018677488171434, 2.915334737309923430 ) ) ;
#57137=CARTESIAN_POINT ( 'NONE',  ( -2.266590686148945544, 11.38708216824730179, -7.082119434687050408 ) ) ;
#57138=CARTESIAN_POINT ( 'NONE',  ( 10.00000000000000178, 12.25893115100078568, 9.846743663894594434 ) ) ;
#57139=CARTESIAN_POINT ( 'NONE',  ( 12.91533473730993009, 46.60535201082150536, -10.88017736071109987 ) ) ;
#57140=CARTESIAN_POINT ( 'NONE',  ( 10.00000000000000000, 27.87363466993042138, -12.81628187352647608 ) ) ;
#57144=CARTESIAN_POINT ( 'NONE',  ( 19.84674366389459621, 53.50893115100078745, 7.409399052514197653E-17 ) ) ;
#57145=CARTESIAN_POINT ( 'NONE',  ( 18.52753015748617571, 8.092264484334117824, 4.923371831947298993 ) ) ;
#57147=CARTESIAN_POINT ( 'NONE',  ( 16.40814093676324603, 22.45696800326375353, -11.09922568453594671 ) ) ;
#57149=CARTESIAN_POINT ( 'NONE',  ( 10.00000000000000178, 29.31368534415483751, 10.88017736071110342 ) ) ;
#57152=CARTESIAN_POINT ( 'NONE',  ( 13.79529636645031943, 55.34541550158062506, -14.16423886937409904 ) ) ;
#57153=CARTESIAN_POINT ( 'NONE',  ( 24.16423886937410614, 29.51208216824729647, -3.795296366450302550 ) ) ;
#57154=CARTESIAN_POINT ( 'NONE',  ( 7.361572987183170547, 37.05059781766744464, 9.846743663894590881 ) ) ;
#57155=CARTESIAN_POINT ( 'NONE',  ( 22.81628187352647785, 31.41530133659709279, 3.434112377981063169 ) ) ;
#57156=CARTESIAN_POINT ( 'NONE',  ( 15.44008868035555260, 29.73035201082150891, 9.422509992056143702 ) ) ;
#57157=CARTESIAN_POINT ( 'NONE',  ( 1.472469842513823179, 55.59226448433412315, -4.923371831947296329 ) ) ;
#57158=CARTESIAN_POINT ( 'NONE',  ( 20.88017736071110519, 35.56368534415484106, 2.639326808657452039E-16 ) ) ;
#57159=CARTESIAN_POINT ( 'NONE',  ( 22.81628187352647785, 6.623634669930420493, 6.195893100308588602E-16 ) ) ;
#57160=CARTESIAN_POINT ( 'NONE',  ( 20.36894250292379738, 19.92874883491396787, -10.36894250292379027 ) ) ;
#57162=CARTESIAN_POINT ( 'NONE',  ( 14.92337183194729633, 27.67559781766745530, 8.527530157486181039 ) ) ;
#57163=( LENGTH_UNIT ( ) NAMED_UNIT ( * ) SI_UNIT ( .MILLI., .METRE. ) );
#57164=CARTESIAN_POINT ( 'NONE',  ( -2.816281873526473856, 4.331968003263754419, 3.434112377981055619 ) ) ;
#57165=ORIENTED_EDGE ( 'NONE', *, *, #53994, .F. ) ;
#57166=DIRECTION ( 'NONE',  ( 0.000000000000000000, -1.000000000000000000, 0.000000000000000000 ) ) ;
#57168=CARTESIAN_POINT ( 'NONE',  ( 0.5774900079438607392, 18.48035201082150536, 5.440088680355550821 ) ) ;
#57169=CARTESIAN_POINT ( 'NONE',  ( 10.00000000000000000, 5.553748834913967869, -14.16423886937410082 ) ) ;
#57171=CARTESIAN_POINT ( 'NONE',  ( 2.791683348922240793, 6.633931151000785675, 7.208316651077764092 ) ) ;
#57172=CARTESIAN_POINT ( 'NONE',  ( 0.1532563361054082862, 51.21726448433412315, 2.638427012816831674 ) ) ;
#57173=CARTESIAN_POINT ( 'NONE',  ( 19.42250999205614548, 30.98035201082150536, -5.440088680355545492 ) ) ;
#57175=CARTESIAN_POINT ( 'NONE',  ( 0.1532563361054083140, 66.00893115100079456, 1.131784320476157264E-15 ) ) ;
#57176=EDGE_CURVE ( 'NONE', #23173, #35624, #70904, .T. ) ;
#57183=CARTESIAN_POINT ( 'NONE',  ( 6.204703633549690345, 12.84541550158063572, 14.16423886937410082 ) ) ;
#57184=CARTESIAN_POINT ( 'NONE',  ( -4.164238869374099927, 7.012082168247302683, 3.795296366450308767 ) ) ;
#57185=CARTESIAN_POINT ( 'NONE',  ( 24.16423886937410614, 59.51208216824728936, -3.795296366450302550 ) ) ;
#57186=CARTESIAN_POINT ( 'NONE',  ( 1.472469842513823179, 51.42559781766745886, 4.923371831947296329 ) ) ;
#57187=CARTESIAN_POINT ( 'NONE',  ( 18.52753015748617571, 38.09226448433412315, 4.923371831947298993 ) ) ;
#57188=CARTESIAN_POINT ( 'NONE',  ( -0.2418659066527493184, 0.1163318810232758099, 6.114288769123083611 ) ) ;
#57189=CARTESIAN_POINT ( 'NONE',  ( 0.5774900079438607392, 38.48035201082150536, 5.440088680355550821 ) ) ;
#57190=CARTESIAN_POINT ( 'NONE',  ( 1.472469842513823179, 65.59226448433412315, -4.923371831947296329 ) ) ;
#57191=CARTESIAN_POINT ( 'NONE',  ( 24.16423886937409904, 49.09541550158063217, 3.795296366450317205 ) ) ;
#57192=CARTESIAN_POINT ( 'NONE',  ( 2.917880565312950480, 65.97041550158063217, -12.26659068614894821 ) ) ;
#57194=CARTESIAN_POINT ( 'NONE',  ( 2.035157376598824452, 58.68868534415482685, 7.964842623401179544 ) ) ;
#57195=VECTOR ( 'NONE', #95587, 1000.000000000000000 ) ;
#57198=DIRECTION ( 'NONE',  ( 0.000000000000000000, 1.000000000000000000, -0.000000000000000000 ) ) ;
#57200=CARTESIAN_POINT ( 'NONE',  ( 5.076628168052703671, 26.84226448433411960, 8.527530157486179263 ) ) ;
#57202=CARTESIAN_POINT ( 'NONE',  ( 2.917880565312950480, 35.97041550158063217, -12.26659068614894821 ) ) ;
#57203=CARTESIAN_POINT ( 'NONE',  ( 19.84674366389459621, 38.50893115100078745, 7.409399052514197653E-17 ) ) ;
#57204=CARTESIAN_POINT ( 'NONE',  ( 0.5774900079438607392, 58.48035201082151247, 5.440088680355550821 ) ) ;
#57208=CARTESIAN_POINT ( 'NONE',  ( 17.96484262340118221, 61.18868534415482685, -7.964842623401177768 ) ) ;
#57209=CARTESIAN_POINT ( 'NONE',  ( 1.472469842513823179, 41.42559781766745886, 4.923371831947296329 ) ) ;
#57210=CARTESIAN_POINT ( 'NONE',  ( 13.43411237798105340, 55.58196800326374643, 12.81628187352647963 ) ) ;
#57213=CARTESIAN_POINT ( 'NONE',  ( 22.26659068614894466, 18.88708216824730002, 7.082119434687054849 ) ) ;
#57216=CARTESIAN_POINT ( 'NONE',  ( 3.591859063236761518, 24.95696800326375353, 11.09922568453594849 ) ) ;
#57217=SURFACE_STYLE_USAGE ( .BOTH. , #49233 ) ;
#57218=CARTESIAN_POINT ( 'NONE',  ( 17.20831665107776587, 17.88393115100078745, 7.208316651077764980 ) ) ;
#57219=CARTESIAN_POINT ( 'NONE',  ( 2.035157376598824452, 18.68868534415484106, 7.964842623401179544 ) ) ;
#57220=CARTESIAN_POINT ( 'NONE',  ( 13.43411237798105340, 55.58196800326374643, 12.81628187352647963 ) ) ;
#57221=CARTESIAN_POINT ( 'NONE',  ( -46.30928139467842186, 104.0823827281712397, -5.529860068218139801 ) ) ;
#57222=CARTESIAN_POINT ( 'NONE',  ( 2.791683348922240793, 26.63393115100078745, 7.208316651077764092 ) ) ;
#57226=CARTESIAN_POINT ( 'NONE',  ( 2.035157376598824452, 68.68868534415484817, 7.964842623401179544 ) ) ;
#57230=CARTESIAN_POINT ( 'NONE',  ( -0.8801773607111009756, 68.06368534415484817, 1.068504757029289695E-15 ) ) ;
#57232=CARTESIAN_POINT ( 'NONE',  ( 6.565887622018943937, 30.16530133659708568, 12.81628187352647430 ) ) ;
#57234=CARTESIAN_POINT ( 'NONE',  ( 18.52753015748618282, 38.92559781766745175, -4.923371831947291888 ) ) ;
#57235=CARTESIAN_POINT ( 'NONE',  ( 19.42250999205614193, 35.14701867748816966, 5.440088680355555262 ) ) ;
#57236=CARTESIAN_POINT ( 'NONE',  ( -4.164238869374099927, 27.01208216824730357, 3.795296366450308767 ) ) ;
#57237=CARTESIAN_POINT ( 'NONE',  ( 14.92337183194729633, 27.67559781766745530, 8.527530157486181039 ) ) ;
#57238=CARTESIAN_POINT ( 'NONE',  ( 19.38216949554541557, 27.24863466993041783, -9.382169495545420901 ) ) ;
#57240=DIRECTION ( 'NONE',  ( -1.000000000000000000, 6.608470384673545847E-17, 0.000000000000000000 ) ) ;
#57241=CARTESIAN_POINT ( 'NONE',  ( 2.035157376598822676, 67.43868534415484817, -7.964842623401177768 ) ) ;
#57242=CARTESIAN_POINT ( 'NONE',  ( -1.099225684535947600, 9.540301336597087456, 6.408140936763237150 ) ) ;
#57245=CARTESIAN_POINT ( 'NONE',  ( 17.20831665107776587, 34.13393115100078745, -7.208316651077762316 ) ) ;
#57246=CARTESIAN_POINT ( 'NONE',  ( 20.88017736071110875, 30.77201867748816966, -2.915334737309920765 ) ) ;
#57247=CARTESIAN_POINT ( 'NONE',  ( -2.816281873526473856, 24.12363466993042138, 9.499525473075851096E-16 ) ) ;
#57248=CARTESIAN_POINT ( 'NONE',  ( 17.20831665107776587, 34.13393115100078745, -7.208316651077762316 ) ) ;
#57251=CARTESIAN_POINT ( 'NONE',  ( 2.035157376598824452, 33.68868534415484106, 7.964842623401179544 ) ) ;
#57252=CARTESIAN_POINT ( 'NONE',  ( 17.96484262340118221, 59.93868534415484106, 7.964842623401181321 ) ) ;
#57253=CARTESIAN_POINT ( 'NONE',  ( 17.96484262340118221, 6.188685344154836621, -7.964842623401177768 ) ) ;
#57254=CARTESIAN_POINT ( 'NONE',  ( 12.63842701281683034, 57.46726448433411605, 9.846743663894596210 ) ) ;
#57255=CARTESIAN_POINT ( 'NONE',  ( 2.035157376598824452, 33.68868534415484106, 7.964842623401179544 ) ) ;
#57256=DIRECTION ( 'NONE',  ( 0.000000000000000000, 0.000000000000000000, 1.000000000000000000 ) ) ;
#57257=EDGE_CURVE ( 'NONE', #36584, #71988, #61183, .T. ) ;
#57258=CARTESIAN_POINT ( 'NONE',  ( 7.084665262690076126, 44.10535201082151247, 10.88017736071109987 ) ) ;
#57260=CARTESIAN_POINT ( 'NONE',  ( 4.559911319644449179, 7.230352010821505360, -9.422509992056141925 ) ) ;
#57261=CARTESIAN_POINT ( 'NONE',  ( 20.00000000000000355, 87.39023020535090325, -4.970182472450021649 ) ) ;
#57262=CARTESIAN_POINT ( 'NONE',  ( 0.1532563361054100626, 0.8005978176674514168, -2.638427012816831230 ) ) ;
#57264=CARTESIAN_POINT ( 'NONE',  ( 17.20831665107776587, 52.88393115100078035, 7.208316651077764980 ) ) ;
#57265=CARTESIAN_POINT ( 'NONE',  ( 24.16423886937410614, 49.51208216824730357, -3.795296366450302550 ) ) ;
#57267=CARTESIAN_POINT ( 'NONE',  ( 19.72487221294571214, 24.78217586085238011, 6.499999999999993783 ) ) ;
#57270=CARTESIAN_POINT ( 'NONE',  ( -4.164238869374099927, 32.01208216824730357, 3.795296366450308767 ) ) ;
#57271=CARTESIAN_POINT ( 'NONE',  ( 0.6178305044545818747, 3.498634669930420049, -9.382169495545419124 ) ) ;
#57274=ORIENTED_EDGE ( 'NONE', *, *, #31556, .T. ) ;
#57275=CARTESIAN_POINT ( 'NONE',  ( 7.084665262690076126, 2.022018677488171434, -10.88017736071110164 ) ) ;
#57276=CARTESIAN_POINT ( 'NONE',  ( 0.1532563361054100626, 30.80059781766744820, -2.638427012816831230 ) ) ;
#57277=CARTESIAN_POINT ( 'NONE',  ( -0.1503990784575279516, 53.10158574516643171, 6.262539305110076171 ) ) ;
#57279=CARTESIAN_POINT ( 'NONE',  ( 20.88017736071110164, 65.35535201082150536, 2.915334737309930979 ) ) ;
#57281=CARTESIAN_POINT ( 'NONE',  ( 12.91533473730992121, 24.52201867748816966, 10.88017736071110164 ) ) ;
#57282=CARTESIAN_POINT ( 'NONE',  ( 10.00000000000000000, 57.87363466993042493, -12.81628187352647608 ) ) ;
#57283=CARTESIAN_POINT ( 'NONE',  ( 16.40814093676324603, 7.456968003263754419, -11.09922568453594671 ) ) ;
#57284=CARTESIAN_POINT ( 'NONE',  ( 0.1532563361054100626, 30.80059781766744820, -2.638427012816831230 ) ) ;
#57285=VERTEX_POINT ( 'NONE', #95875 ) ;
#57286=SURFACE_SIDE_STYLE ('',( #79796 ) ) ;
#57288=CARTESIAN_POINT ( 'NONE',  ( -2.266590686148945544, 62.22041550158063927, 7.082119434687048631 ) ) ;
#57289=CARTESIAN_POINT ( 'NONE',  ( 6.204703633549690345, 32.84541550158063927, 14.16423886937410082 ) ) ;
#57290=CARTESIAN_POINT ( 'NONE',  ( 0.5774900079438590739, 32.64701867748816966, -5.440088680355550821 ) ) ;
#57291=CARTESIAN_POINT ( 'NONE',  ( 4.559911319644449179, 53.89701867748817676, 9.422509992056141925 ) ) ;
#57293=CARTESIAN_POINT ( 'NONE',  ( 18.52753015748617571, 48.09226448433412315, 4.923371831947298993 ) ) ;
#57294=CARTESIAN_POINT ( 'NONE',  ( 19.84674366389459266, 8.717264484334116048, -2.638427012816827677 ) ) ;
#57295=FILL_AREA_STYLE_COLOUR ( '', #35409 ) ;
#57298=CARTESIAN_POINT ( 'NONE',  ( 19.84674366389459266, 18.30059781766745175, 2.638427012816836559 ) ) ;
#57299=CARTESIAN_POINT ( 'NONE',  ( 18.52753015748618282, 53.92559781766745175, -4.923371831947291888 ) ) ;
#57300=COLOUR_RGB ( '', 0.72549020, 0.75294118, 0.79215686) ;
#57301=UNCERTAINTY_MEASURE_WITH_UNIT (LENGTH_MEASURE( 1.000000000000000082E-05 ), #3153, 'distance_accuracy_value', 'NONE');
#57302=CARTESIAN_POINT ( 'NONE',  ( 22.81628187352648496, 46.83196800326376064, -3.434112377981050290 ) ) ;
#57303=CARTESIAN_POINT ( 'NONE',  ( -0.8801773607110991993, 67.85535201082151957, -2.915334737309923874 ) ) ;
#57304=CARTESIAN_POINT ( 'NONE',  ( 10.00000000000000000, 34.75893115100078745, -9.846743663894594434 ) ) ;
#57305=CARTESIAN_POINT ( 'NONE',  ( 20.36894250292379382, 53.67874883491397497, 10.36894250292379205 ) ) ;
#57306=CARTESIAN_POINT ( 'NONE',  ( 2.791683348922240793, 26.63393115100078745, 7.208316651077764092 ) ) ;
#57308=CARTESIAN_POINT ( 'NONE',  ( 17.20831665107776587, 62.88393115100078745, 7.208316651077764980 ) ) ;
#57309=CARTESIAN_POINT ( 'NONE',  ( -0.3689425029237881626, 27.42874883491397142, 10.36894250292379027 ) ) ;
#57310=CARTESIAN_POINT ( 'NONE',  ( 5.076628168052704559, 25.17559781766745175, -8.527530157486179263 ) ) ;
#57311=CARTESIAN_POINT ( 'NONE',  ( 17.39651004071841456, 7.935752660568278216, 6.500000000000003553 ) ) ;
#57312=CARTESIAN_POINT ( 'NONE',  ( 2.035157376598824452, 23.68868534415484461, 7.964842623401179544 ) ) ;
#57313=CARTESIAN_POINT ( 'NONE',  ( 2.035157376598824452, 58.68868534415482685, 7.964842623401179544 ) ) ;
#57314=CARTESIAN_POINT ( 'NONE',  ( 19.42250999205614548, 50.98035201082151247, -5.440088680355545492 ) ) ;
#57315=ORIENTED_EDGE ( 'NONE', *, *, #13416, .T. ) ;
#57316=CARTESIAN_POINT ( 'NONE',  ( 13.43411237798105340, 50.58196800326375353, 12.81628187352647963 ) ) ;
#57317=CARTESIAN_POINT ( 'NONE',  ( 2.035157376598822676, 57.43868534415484106, -7.964842623401177768 ) ) ;
#57318=VERTEX_POINT ( 'NONE', #66335 ) ;
#57321=CARTESIAN_POINT ( 'NONE',  ( 2.035157376598822676, 62.43868534415483396, -7.964842623401177768 ) ) ;
#57323=CARTESIAN_POINT ( 'NONE',  ( -0.8801773607110991993, 57.85535201082149825, -2.915334737309923874 ) ) ;
#57324=CARTESIAN_POINT ( 'NONE',  ( -0.8801773607111008646, 8.272018677488171434, 2.915334737309923430 ) ) ;
#57325=CARTESIAN_POINT ( 'NONE',  ( 2.599899806584774264, 0.4361964623231012195, -6.495912400107028084 ) ) ;
#57327=CARTESIAN_POINT ( 'NONE',  ( 12.91533473730993009, 6.605352010821504471, -10.88017736071109987 ) ) ;
#57328=CARTESIAN_POINT ( 'NONE',  ( 12.63842701281683922, 4.550597817667451750, -9.846743663894590881 ) ) ;
#57329=CARTESIAN_POINT ( 'NONE',  ( 13.79529636645030344, 23.26208216824730002, 14.16423886937410614 ) ) ;
#57330=CARTESIAN_POINT ( 'NONE',  ( 7.084665262690076126, 24.10535201082150181, 10.88017736071109987 ) ) ;
#57331=CARTESIAN_POINT ( 'NONE',  ( 10.00000000000000178, 57.25893115100078745, 9.846743663894594434 ) ) ;
#57333=CARTESIAN_POINT ( 'NONE',  ( 10.00000000000000178, 67.25893115100079456, 9.846743663894594434 ) ) ;
#57334=VERTEX_POINT ( 'NONE', #57850 ) ;
#57336=CARTESIAN_POINT ( 'NONE',  ( 17.39651004071890128, 29.08210964143323096, -6.499999999999448441 ) ) ;
#57337=CARTESIAN_POINT ( 'NONE',  ( 2.035157376598824452, 58.68868534415482685, 7.964842623401179544 ) ) ;
#57338=CARTESIAN_POINT ( 'NONE',  ( 12.63842701281683034, 52.46726448433413026, 9.846743663894596210 ) ) ;
#57340=CARTESIAN_POINT ( 'NONE',  ( 16.40814093676323893, 40.79030133659708923, 11.09922568453595026 ) ) ;
#57341=CARTESIAN_POINT ( 'NONE',  ( 2.035157376598824452, 13.68868534415483751, 7.964842623401179544 ) ) ;
#57343=CARTESIAN_POINT ( 'NONE',  ( -0.8801773607110991993, 62.85535201082150536, -2.915334737309923874 ) ) ;
#57344=CARTESIAN_POINT ( 'NONE',  ( -0.8801773607111009756, 3.063685344154838397, 1.068504757029289695E-15 ) ) ;
#57348=CARTESIAN_POINT ( 'NONE',  ( 6.565887622018943937, 43.08196800326374643, -12.81628187352647608 ) ) ;
#57349=CARTESIAN_POINT ( 'NONE',  ( 17.96484262340118221, 36.18868534415484106, -7.964842623401177768 ) ) ;
#57352=CARTESIAN_POINT ( 'NONE',  ( 22.81628187352647785, 46.62363466993041783, 6.195893100308588602E-16 ) ) ;
#57353=CARTESIAN_POINT ( 'NONE',  ( 20.88017736071110519, 35.56368534415484106, 2.639326808657452039E-16 ) ) ;
#57354=EDGE_CURVE ( 'NONE', #47816, #651, #10161, .T. ) ;
#57355=CARTESIAN_POINT ( 'NONE',  ( 1.472469842513823179, 56.42559781766745886, 4.923371831947296329 ) ) ;
#57357=CARTESIAN_POINT ( 'NONE',  ( 0.1532563361054082862, 61.21726448433412315, 2.638427012816831674 ) ) ;
#57358=DIRECTION ( 'NONE',  ( 0.000000000000000000, -1.000000000000000000, 0.000000000000000000 ) ) ;
#57359=CARTESIAN_POINT ( 'NONE',  ( 5.076628168052704559, 50.17559781766745886, -8.527530157486179263 ) ) ;
#57360=CARTESIAN_POINT ( 'NONE',  ( 15.44008868035555793, 16.39701867748817321, -9.422509992056140149 ) ) ;
#57363=VECTOR ( 'NONE', #96941, 1000.000000000000000 ) ;
#57364=CARTESIAN_POINT ( 'NONE',  ( 2.791683348922237240, 45.38393115100079456, -7.208316651077763204 ) ) ;
#57365=CARTESIAN_POINT ( 'NONE',  ( 7.361572987183169658, 14.96726448433411960, -9.846743663894592657 ) ) ;
#57366=CARTESIAN_POINT ( 'NONE',  ( 19.72487221294571569, 34.78217586085237656, 6.499999999999993783 ) ) ;
#57367=CARTESIAN_POINT ( 'NONE',  ( 0.1532563361054100626, 65.80059781766745175, -2.638427012816831230 ) ) ;
#57370=CARTESIAN_POINT ( 'NONE',  ( 10.00000000000000000, 32.87363466993042493, -12.81628187352647608 ) ) ;
#57371=CARTESIAN_POINT ( 'NONE',  ( 17.20831665107776587, 37.88393115100078745, 7.208316651077764980 ) ) ;
#57373=CARTESIAN_POINT ( 'NONE',  ( 10.00000000000000000, 65.55374883491396076, -14.16423886937410082 ) ) ;
#57374=CARTESIAN_POINT ( 'NONE',  ( 1.472469842513823179, 25.59226448433412315, -4.923371831947296329 ) ) ;
#57376=CARTESIAN_POINT ( 'NONE',  ( 2.917880565312950480, 55.97041550158063217, -12.26659068614894821 ) ) ;
#57379=CARTESIAN_POINT ( 'NONE',  ( 19.42250999205614548, 5.980352010821504471, -5.440088680355545492 ) ) ;
#57380=CARTESIAN_POINT ( 'NONE',  ( 6.204703633549690345, 32.84541550158063927, 14.16423886937410082 ) ) ;
#57381=CARTESIAN_POINT ( 'NONE',  ( 13.79529636645030344, 43.26208216824730357, 14.16423886937410614 ) ) ;
#57382=DIRECTION ( 'NONE',  ( 0.000000000000000000, -1.000000000000000000, 0.000000000000000000 ) ) ;
#57383=DIRECTION ( 'NONE',  ( -1.000000000000000000, -0.000000000000000000, -0.000000000000000000 ) ) ;
#57384=COLOUR_RGB ( '', 0.66274510, 0.83137255, 0.94901961) ;
#57386=CARTESIAN_POINT ( 'NONE',  ( 18.52753015748617571, 13.09226448433411960, 4.923371831947298993 ) ) ;
#57388=CARTESIAN_POINT ( 'NONE',  ( 0.1532563361054100626, 55.80059781766745175, -2.638427012816831230 ) ) ;
#57389=CARTESIAN_POINT ( 'NONE',  ( 4.559911319644449179, 48.89701867748817676, 9.422509992056141925 ) ) ;
#57391=AXIS2_PLACEMENT_3D ( 'NONE', #74876, #52371, #6375 ) ;
#57392=CARTESIAN_POINT ( 'NONE',  ( 19.84674366389459266, 48.30059781766745175, 2.638427012816836559 ) ) ;
#57393=CARTESIAN_POINT ( 'NONE',  ( -3.469446951953614189E-15, 82.00000000000000000, -5.000000000000000000 ) ) ;
#57394=CARTESIAN_POINT ( 'NONE',  ( 12.63842701281683922, 49.55059781766744464, -9.846743663894590881 ) ) ;
#57397=CARTESIAN_POINT ( 'NONE',  ( 2.917880565312948704, 22.63708216824730002, 12.26659068614894643 ) ) ;
#57398=FACE_OUTER_BOUND ( 'NONE', #83691, .T. ) ;
#57401=CARTESIAN_POINT ( 'NONE',  ( 10.00000000000000000, 21.81368534415484106, -10.88017736071110342 ) ) ;
#57402=CARTESIAN_POINT ( 'NONE',  ( 0.6178305044545838731, 29.74863466993042138, 9.382169495545420901 ) ) ;
#57403=CARTESIAN_POINT ( 'NONE',  ( 21.92686044187657046, 62.39664270246084499, -3.195792623639524432 ) ) ;
#57404=CARTESIAN_POINT ( 'NONE',  ( 14.92337183194729633, 7.675597817667451750, 8.527530157486181039 ) ) ;
#57405=CARTESIAN_POINT ( 'NONE',  ( 10.00000000000000000, 52.87363466993041783, -12.81628187352647608 ) ) ;
#57408=CARTESIAN_POINT ( 'NONE',  ( 13.79529636645030344, 23.26208216824730002, 14.16423886937410614 ) ) ;
#57410=DIRECTION ( 'NONE',  ( 0.000000000000000000, 0.000000000000000000, -1.000000000000000000 ) ) ;
#57411=CARTESIAN_POINT ( 'NONE',  ( 4.559911319644449179, 8.897018677488173211, 9.422509992056141925 ) ) ;
#57414=CARTESIAN_POINT ( 'NONE',  ( 20.88017736071110164, 45.35535201082149115, 2.915334737309930979 ) ) ;
#57415=CARTESIAN_POINT ( 'NONE',  ( 12.91533473730992121, 44.52201867748816966, 10.88017736071110164 ) ) ;
#57416=CARTESIAN_POINT ( 'NONE',  ( 0.6178305044545818747, 8.498634669930421381, -9.382169495545419124 ) ) ;
#57417=CARTESIAN_POINT ( 'NONE',  ( 19.84674366389459266, 63.30059781766745886, 2.638427012816836559 ) ) ;
#57418=CARTESIAN_POINT ( 'NONE',  ( -46.30928139467842897, 104.0823827281712255, -5.529860068218140690 ) ) ;
#57419=CARTESIAN_POINT ( 'NONE',  ( 2.791683348922240793, 16.63393115100078745, 7.208316651077764092 ) ) ;
#57420=CARTESIAN_POINT ( 'NONE',  ( 2.603489959281199972, 21.58210964143324873, 6.499999999999559464 ) ) ;
#57421=CARTESIAN_POINT ( 'NONE',  ( -0.8801773607111009756, 43.06368534415484106, 1.068504757029289695E-15 ) ) ;
#57423=CARTESIAN_POINT ( 'NONE',  ( 16.40814093676323893, 5.790301336597087456, 11.09922568453595026 ) ) ;
#57425=CARTESIAN_POINT ( 'NONE',  ( 20.88017736071110164, 65.35535201082150536, 2.915334737309930979 ) ) ;
#57426=CARTESIAN_POINT ( 'NONE',  ( 1.472469842513823179, 31.42559781766745530, 4.923371831947296329 ) ) ;
#57427=CARTESIAN_POINT ( 'NONE',  ( 3.591859063236761518, 44.95696800326376064, 11.09922568453594849 ) ) ;
#57428=CARTESIAN_POINT ( 'NONE',  ( 17.20831665107776587, 2.883931151000785231, 7.208316651077764980 ) ) ;
#57429=LINE ( 'NONE', #70479, #71921 ) ;
#57431=CARTESIAN_POINT ( 'NONE',  ( 1.274849032794280523, 48.57228050351032067, 6.499999999999960032 ) ) ;
#57433=CARTESIAN_POINT ( 'NONE',  ( 10.00000000000000000, 16.81368534415483751, -10.88017736071110342 ) ) ;
#57434=CARTESIAN_POINT ( 'NONE',  ( 22.81628187352648496, 56.83196800326374643, -3.434112377981050290 ) ) ;
#57435=CARTESIAN_POINT ( 'NONE',  ( 22.26659068614894466, 23.88708216824730357, 7.082119434687054849 ) ) ;
#57436=CARTESIAN_POINT ( 'NONE',  ( 10.00000000000000178, 27.25893115100078390, 9.846743663894594434 ) ) ;
#57437=VECTOR ( 'NONE', #51396, 1000.000000000000000 ) ;
#57438=CARTESIAN_POINT ( 'NONE',  ( 20.88017736071110875, 15.77201867748817143, -2.915334737309920765 ) ) ;
#57439=CARTESIAN_POINT ( 'NONE',  ( 0.5774900079438590739, 2.647018677488171434, -5.440088680355550821 ) ) ;
#57442=CARTESIAN_POINT ( 'NONE',  ( -0.8801773607110991993, 12.85535201082150358, -2.915334737309923874 ) ) ;
#57444=CARTESIAN_POINT ( 'NONE',  ( 15.44008868035555260, 19.73035201082150536, 9.422509992056143702 ) ) ;
#57446=CARTESIAN_POINT ( 'NONE',  ( 2.035157376598822676, 27.43868534415483396, -7.964842623401177768 ) ) ;
#57447=ORIENTED_EDGE ( 'NONE', *, *, #64451, .F. ) ;
#57448=CARTESIAN_POINT ( 'NONE',  ( 20.15039907845753220, 26.74884699246889141, 6.262539305110078836 ) ) ;
#57449=CARTESIAN_POINT ( 'NONE',  ( -0.8801773607111008646, 23.27201867748817676, 2.915334737309923430 ) ) ;
#57450=CARTESIAN_POINT ( 'NONE',  ( 7.361572987183170547, 62.05059781766745886, 9.846743663894590881 ) ) ;
#57451=CARTESIAN_POINT ( 'NONE',  ( -0.1503990784575328643, 70.00000000000000000, -6.262539305110068177 ) ) ;
#57453=CARTESIAN_POINT ( 'NONE',  ( 10.00000000000000000, 30.55374883491397142, -14.16423886937410082 ) ) ;
#57454=CARTESIAN_POINT ( 'NONE',  ( -0.8801773607111009756, 38.06368534415484106, 1.068504757029289695E-15 ) ) ;
#57455=CARTESIAN_POINT ( 'NONE',  ( 15.44008868035555793, 21.39701867748817321, -9.422509992056140149 ) ) ;
#57456=CARTESIAN_POINT ( 'NONE',  ( 20.10239578412224404, 42.63377557478297319, -6.340343622311914729 ) ) ;
#57457=CARTESIAN_POINT ( 'NONE',  ( 20.15039907845753575, 62.62777174578612716, -6.262539305110073506 ) ) ;
#57458=CARTESIAN_POINT ( 'NONE',  ( 18.52753015748617571, 43.09226448433412315, 4.923371831947298993 ) ) ;
#57459=CARTESIAN_POINT ( 'NONE',  ( -0.1049300847420624877, 22.21697413083879624, -6.336235997365760042 ) ) ;
#57460=CARTESIAN_POINT ( 'NONE',  ( 19.84674366389459266, 13.71726448433411782, -2.638427012816827677 ) ) ;
#57462=CARTESIAN_POINT ( 'NONE',  ( -0.8801773607110991993, 12.85535201082150358, -2.915334737309923874 ) ) ;
#57463=CARTESIAN_POINT ( 'NONE',  ( 1.472469842513823179, 15.59226448433411960, -4.923371831947296329 ) ) ;
#57464=CARTESIAN_POINT ( 'NONE',  ( 2.791683348922237240, 65.38393115100078035, -7.208316651077763204 ) ) ;
#57465=CARTESIAN_POINT ( 'NONE',  ( 4.559911319644449179, 62.23035201082150536, -9.422509992056141925 ) ) ;
#57466=CARTESIAN_POINT ( 'NONE',  ( -0.8801773607110991993, 17.85535201082150536, -2.915334737309923874 ) ) ;
#57467=CARTESIAN_POINT ( 'NONE',  ( 13.43411237798106583, 57.66530133659708923, -12.81628187352647252 ) ) ;
#57468=CARTESIAN_POINT ( 'NONE',  ( -4.164238869374099039, 31.80374883491396432, 8.674139862899312516E-16 ) ) ;
#57470=EDGE_CURVE ( 'NONE', #75287, #32106, #32650, .T. ) ;
#57471=CARTESIAN_POINT ( 'NONE',  ( 3.591859063236761518, 59.95696800326375353, 11.09922568453594849 ) ) ;
#57473=CARTESIAN_POINT ( 'NONE',  ( 0.1532563361054082862, 66.21726448433413736, 2.638427012816831674 ) ) ;
#57474=CARTESIAN_POINT ( 'NONE',  ( -0.2418659066527510948, 15.11633188102327452, 6.114288769123080058 ) ) ;
#57476=CARTESIAN_POINT ( 'NONE',  ( 2.035157376598822676, 37.43868534415484106, -7.964842623401177768 ) ) ;
#57477=CARTESIAN_POINT ( 'NONE',  ( 0.1532563361054083140, 66.00893115100079456, 1.131784320476157264E-15 ) ) ;
#57479=CARTESIAN_POINT ( 'NONE',  ( 10.00000000000000000, 14.75893115100078568, -9.846743663894594434 ) ) ;
#57481=CARTESIAN_POINT ( 'NONE',  ( 10.00000000000000178, 7.258931151000785675, 9.846743663894594434 ) ) ;
#57482=CARTESIAN_POINT ( 'NONE',  ( 7.361572987183170547, 22.05059781766745530, 9.846743663894590881 ) ) ;
#57483=CARTESIAN_POINT ( 'NONE',  ( 2.791683348922240793, 11.63393115100078568, 7.208316651077764092 ) ) ;
#57484=CARTESIAN_POINT ( 'NONE',  ( 5.076628168052704559, 5.175597817667451750, -8.527530157486179263 ) ) ;
#57485=CARTESIAN_POINT ( 'NONE',  ( 20.88017736071110164, 55.35535201082149825, 2.915334737309930979 ) ) ;
#57487=CARTESIAN_POINT ( 'NONE',  ( 2.791683348922237240, 0.3839311510007847872, -7.208316651077763204 ) ) ;
#57488=CARTESIAN_POINT ( 'NONE',  ( 12.63842701281683034, 17.46726448433411250, 9.846743663894596210 ) ) ;
#57489=ORIENTED_EDGE ( 'NONE', *, *, #3565, .T. ) ;
#57491=CARTESIAN_POINT ( 'NONE',  ( 6.565887622018943937, 0.1653013365970866511, 12.81628187352647430 ) ) ;
#57494=CARTESIAN_POINT ( 'NONE',  ( 20.36894250292379738, 14.92874883491396432, -10.36894250292379027 ) ) ;
#57495=UNCERTAINTY_MEASURE_WITH_UNIT (LENGTH_MEASURE( 1.000000000000000082E-05 ), #94795, 'distance_accuracy_value', 'NONE');
#57497=CARTESIAN_POINT ( 'NONE',  ( 10.00000000000000178, 18.05374883491396787, 14.16423886937410082 ) ) ;
#57498=CARTESIAN_POINT ( 'NONE',  ( -4.164238869374099039, 31.80374883491396432, 8.674139862899312516E-16 ) ) ;
#57500=CARTESIAN_POINT ( 'NONE',  ( 24.16423886937410614, 4.303748834913967869, 8.672049930838204340E-16 ) ) ;
#57501=CARTESIAN_POINT ( 'NONE',  ( 15.44008868035555260, 29.73035201082150891, 9.422509992056143702 ) ) ;
#57502=DIRECTION ( 'NONE',  ( -0.8320502943378436100, 0.5547001962252291474, -0.000000000000000000 ) ) ;
#57503=CARTESIAN_POINT ( 'NONE',  ( 2.791683348922237240, 10.38393115100078390, -7.208316651077763204 ) ) ;
#57504=CARTESIAN_POINT ( 'NONE',  ( -0.8801773607111008646, 53.27201867748816966, 2.915334737309923430 ) ) ;
#57505=CARTESIAN_POINT ( 'NONE',  ( 5.076628168052703671, 16.84226448433411960, 8.527530157486179263 ) ) ;
#57507=CARTESIAN_POINT ( 'NONE',  ( 2.035157376598822676, 17.43868534415483751, -7.964842623401177768 ) ) ;
#57508=CARTESIAN_POINT ( 'NONE',  ( 21.09922568453594849, 51.20696800326375353, 6.408140936763242479 ) ) ;
#57509=CARTESIAN_POINT ( 'NONE',  ( 0.1532563361054082862, 46.21726448433411605, 2.638427012816831674 ) ) ;
#57510=CARTESIAN_POINT ( 'NONE',  ( 19.84674366389459266, 58.30059781766745886, 2.638427012816836559 ) ) ;
#57511=CARTESIAN_POINT ( 'NONE',  ( 0.6178305044545818747, 28.49863466993041783, -9.382169495545419124 ) ) ;
#57514=CARTESIAN_POINT ( 'NONE',  ( 1.472469842513823179, 36.42559781766745175, 4.923371831947296329 ) ) ;
#57515=CARTESIAN_POINT ( 'NONE',  ( 24.16423886937410614, 9.303748834913967869, 8.672049930838204340E-16 ) ) ;
#57519=CARTESIAN_POINT ( 'NONE',  ( 7.084665262690076126, 52.02201867748816255, -10.88017736071110164 ) ) ;
#57520=CARTESIAN_POINT ( 'NONE',  ( 20.88017736071110875, 55.77201867748816966, -2.915334737309920765 ) ) ;
#57521=CARTESIAN_POINT ( 'NONE',  ( -0.3689425029237881626, 42.42874883491396787, 10.36894250292379027 ) ) ;
#57522=CARTESIAN_POINT ( 'NONE',  ( 1.472469842513823179, 56.42559781766745886, 4.923371831947296329 ) ) ;
#57523=CARTESIAN_POINT ( 'NONE',  ( 21.09922568453594849, 61.20696800326376064, 6.408140936763242479 ) ) ;
#57524=CARTESIAN_POINT ( 'NONE',  ( 4.559911319644449179, 47.23035201082150536, -9.422509992056141925 ) ) ;
#57526=CARTESIAN_POINT ( 'NONE',  ( 0.6178305044545818747, 23.49863466993041783, -9.382169495545419124 ) ) ;
#57527=CARTESIAN_POINT ( 'NONE',  ( 12.63842701281683922, 49.55059781766744464, -9.846743663894590881 ) ) ;
#57529=CARTESIAN_POINT ( 'NONE',  ( 12.91533473730992121, 4.522018677488169658, 10.88017736071110164 ) ) ;
#57531=CARTESIAN_POINT ( 'NONE',  ( 4.559911319644449179, 7.230352010821504471, -9.422509992056141925 ) ) ;
#57533=CARTESIAN_POINT ( 'NONE',  ( 18.52753015748618282, 3.925597817667451306, -4.923371831947291888 ) ) ;
#57534=CARTESIAN_POINT ( 'NONE',  ( 15.44008868035555793, 66.39701867748817676, -9.422509992056140149 ) ) ;
#57536=CARTESIAN_POINT ( 'NONE',  ( 17.20831665107776587, 39.13393115100079456, -7.208316651077762316 ) ) ;
#57537=CARTESIAN_POINT ( 'NONE',  ( 15.44008868035555793, 16.39701867748817321, -9.422509992056140149 ) ) ;
#57538=CARTESIAN_POINT ( 'NONE',  ( 2.791683348922237240, 65.38393115100078035, -7.208316651077763204 ) ) ;
#57539=CARTESIAN_POINT ( 'NONE',  ( 0.5774900079438590739, 37.64701867748817676, -5.440088680355550821 ) ) ;
#57541=CARTESIAN_POINT ( 'NONE',  ( 21.09922568453594849, 41.20696800326375353, 6.408140936763242479 ) ) ;
#57543=CARTESIAN_POINT ( 'NONE',  ( 10.00000000000000000, 46.81368534415484106, -10.88017736071110342 ) ) ;
#57544=CARTESIAN_POINT ( 'NONE',  ( -2.816281873526473856, 14.33196800326375531, 3.434112377981055619 ) ) ;
#57546=CARTESIAN_POINT ( 'NONE',  ( 19.84674366389459621, 3.508931151000785231, 7.409399052514197653E-17 ) ) ;
#57547=CARTESIAN_POINT ( 'NONE',  ( 4.559911319644449179, 27.23035201082150536, -9.422509992056141925 ) ) ;
#57548=CARTESIAN_POINT ( 'NONE',  ( -2.266590686148945544, 66.38708216824730357, -7.082119434687050408 ) ) ;
#57549=CARTESIAN_POINT ( 'NONE',  ( 12.63842701281683922, 54.55059781766745175, -9.846743663894590881 ) ) ;
#57550=CARTESIAN_POINT ( 'NONE',  ( 18.52753015748617571, 3.092264484334118269, 4.923371831947298993 ) ) ;
#57551=CARTESIAN_POINT ( 'NONE',  ( 15.44008868035555260, 64.73035201082151957, 9.422509992056143702 ) ) ;
#57553=CARTESIAN_POINT ( 'NONE',  ( 2.917880565312950480, 35.97041550158063217, -12.26659068614894821 ) ) ;
#57558=EDGE_LOOP ( 'NONE', ( #70541, #56836, #81752, #55442 ) ) ;
#57559=CARTESIAN_POINT ( 'NONE',  ( 20.36894250292379738, 44.92874883491396787, -10.36894250292379027 ) ) ;
#57560=CARTESIAN_POINT ( 'NONE',  ( 13.79529636645031943, 55.34541550158062506, -14.16423886937409904 ) ) ;
#57561=CARTESIAN_POINT ( 'NONE',  ( 10.00000000000000000, 19.75893115100078390, -9.846743663894594434 ) ) ;
#57564=CARTESIAN_POINT ( 'NONE',  ( -1.926860441876564023, 42.87045670184114243, 3.195792623639529761 ) ) ;
#57565=CARTESIAN_POINT ( 'NONE',  ( 0.5774900079438590739, 67.64701867748817676, -5.440088680355550821 ) ) ;
#57566=CARTESIAN_POINT ( 'NONE',  ( 24.16423886937410614, 49.51208216824730357, -3.795296366450302550 ) ) ;
#57567=( BOUNDED_CURVE ( )  B_SPLINE_CURVE ( 2, ( #2936, #65362, #50364, #58346, #56885, #49382, #20374, #50868, #87388 ),
 .UNSPECIFIED., .F., .F. ) 
 B_SPLINE_CURVE_WITH_KNOTS ( ( 3, 2, 2, 2, 3 ),
 ( 0.3687123655116599230, 0.3690476190476190688, 0.3750000000000000000, 0.3809523809523809312, 0.3812876344883400770 ),
 .UNSPECIFIED. ) 
 CURVE ( )  GEOMETRIC_REPRESENTATION_ITEM ( )  RATIONAL_B_SPLINE_CURVE ( ( 0.9963778908391760503, 0.9980808541467920403, 1.000000000000000000, 0.9659258262890683122, 1.000000000000000000, 0.9659258262890683122, 1.000000000000000000, 0.9980808541467920403, 0.9963778908391760503 ) ) 
 REPRESENTATION_ITEM ( '' )  );
#57568=CARTESIAN_POINT ( 'NONE',  ( 2.791683348922237240, 10.38393115100078390, -7.208316651077763204 ) ) ;
#57573=LINE ( 'NONE', #41620, #57195 ) ;
#57577=ORIENTED_EDGE ( 'NONE', *, *, #77763, .F. ) ;
#57578=CARTESIAN_POINT ( 'NONE',  ( 15.44008868035555260, 19.73035201082150536, 9.422509992056143702 ) ) ;
#57579=CARTESIAN_POINT ( 'NONE',  ( 20.88017736071110164, 20.35535201082150891, 2.915334737309930979 ) ) ;
#57580=CARTESIAN_POINT ( 'NONE',  ( 12.63842701281683034, 47.46726448433412315, 9.846743663894596210 ) ) ;
#57581=CARTESIAN_POINT ( 'NONE',  ( 16.40814093676324603, 7.456968003263754419, -11.09922568453594671 ) ) ;
#57585=CARTESIAN_POINT ( 'NONE',  ( 19.38216949554541202, 15.99863466993042138, 9.382169495545424454 ) ) ;
#57587=CARTESIAN_POINT ( 'NONE',  ( 1.472469842513823179, 36.42559781766745175, 4.923371831947296329 ) ) ;
#57588=CARTESIAN_POINT ( 'NONE',  ( 22.26659068614894466, 63.88708216824730357, 7.082119434687054849 ) ) ;
#57590=CARTESIAN_POINT ( 'NONE',  ( 7.084665262690076126, 4.105352010821503583, 10.88017736071109987 ) ) ;
#57592=CARTESIAN_POINT ( 'NONE',  ( 10.00000000000000178, 39.31368534415484106, 10.88017736071110342 ) ) ;
#57593=CARTESIAN_POINT ( 'NONE',  ( -0.8801773607110991993, 47.85535201082150536, -2.915334737309923874 ) ) ;
#57594=CARTESIAN_POINT ( 'NONE',  ( 4.559911319644449179, 53.89701867748817676, 9.422509992056141925 ) ) ;
#57596=CARTESIAN_POINT ( 'NONE',  ( 0.5774900079438590739, 42.64701867748816966, -5.440088680355550821 ) ) ;
#57598=CARTESIAN_POINT ( 'NONE',  ( 1.821708436314909640, 46.66792564121895026, -6.499999999999926281 ) ) ;
#57599=LINE ( 'NONE', #59078, #13815 ) ;
#57600=CARTESIAN_POINT ( 'NONE',  ( 17.20831665107776587, 14.13393115100078568, -7.208316651077762316 ) ) ;
#57601=ORIENTED_EDGE ( 'NONE', *, *, #90389, .F. ) ;
#57603=CARTESIAN_POINT ( 'NONE',  ( 12.63842701281683034, 62.46726448433410894, 9.846743663894596210 ) ) ;
#57604=CARTESIAN_POINT ( 'NONE',  ( 10.00000000000000178, 70.00000000000000000, 0.000000000000000000 ) ) ;
#57608=CARTESIAN_POINT ( 'NONE',  ( 19.72487221294570858, 21.86607318730131411, 6.500000000000000888 ) ) ;
#57611=CARTESIAN_POINT ( 'NONE',  ( 0.1532563361054082862, 31.21726448433412315, 2.638427012816831674 ) ) ;
#57612=CARTESIAN_POINT ( 'NONE',  ( 2.917880565312950480, 55.97041550158063217, -12.26659068614894821 ) ) ;
#57616=CARTESIAN_POINT ( 'NONE',  ( 0.1532563361054100626, 30.80059781766744820, -2.638427012816831230 ) ) ;
#57618=CARTESIAN_POINT ( 'NONE',  ( 10.00000000000000178, 0.3736346699304200492, 12.81628187352647608 ) ) ;
#57619=CARTESIAN_POINT ( 'NONE',  ( 0.5774900079438590739, 67.64701867748817676, -5.440088680355550821 ) ) ;
#57622=CARTESIAN_POINT ( 'NONE',  ( 17.20831665107776587, 4.133931151000785675, -7.208316651077762316 ) ) ;
#57623=CARTESIAN_POINT ( 'NONE',  ( 19.84674366389459266, 63.71726448433412315, -2.638427012816827677 ) ) ;
#57627=CARTESIAN_POINT ( 'NONE',  ( 10.00000000000000000, 6.813685344154838397, -10.88017736071110342 ) ) ;
#57628=CARTESIAN_POINT ( 'NONE',  ( -4.164238869374099927, 2.012082168247300906, 3.795296366450308767 ) ) ;
#57629=CARTESIAN_POINT ( 'NONE',  ( 14.92337183194729988, 14.34226448433411782, -8.527530157486177487 ) ) ;
#57630=CARTESIAN_POINT ( 'NONE',  ( 2.035157376598824452, 38.68868534415483396, 7.964842623401179544 ) ) ;
#57632=CARTESIAN_POINT ( 'NONE',  ( 10.00000000000000000, 32.87363466993042493, -12.81628187352647608 ) ) ;
#57638=CARTESIAN_POINT ( 'NONE',  ( -2.816281873526473856, -0.6680319967362464695, 3.434112377981055619 ) ) ;
#57639=CARTESIAN_POINT ( 'NONE',  ( 7.361572987183169658, 19.96726448433411960, -9.846743663894592657 ) ) ;
#57641=CARTESIAN_POINT ( 'NONE',  ( 10.00000000000000178, 20.37363466993042138, 12.81628187352647608 ) ) ;
#57643=CARTESIAN_POINT ( 'NONE',  ( 4.559911319644449179, 32.23035201082150536, -9.422509992056141925 ) ) ;
#57645=CARTESIAN_POINT ( 'NONE',  ( -2.266590686148945544, 47.22041550158063927, 7.082119434687048631 ) ) ;
#57647=CARTESIAN_POINT ( 'NONE',  ( 2.791683348922240793, 46.63393115100077324, 7.208316651077764092 ) ) ;
#57648=CARTESIAN_POINT ( 'NONE',  ( 0.6178305044545818747, 38.49863466993042493, -9.382169495545419124 ) ) ;
#57649=CARTESIAN_POINT ( 'NONE',  ( 15.44008868035555793, 31.39701867748817676, -9.422509992056140149 ) ) ;
#57650=CARTESIAN_POINT ( 'NONE',  ( 5.076628168052703671, 46.84226448433412315, 8.527530157486179263 ) ) ;
#57651=CARTESIAN_POINT ( 'NONE',  ( 4.559911319644449179, 52.23035201082151247, -9.422509992056141925 ) ) ;
#57652=CARTESIAN_POINT ( 'NONE',  ( 21.09922568453594849, 6.206968003263753531, 6.408140936763242479 ) ) ;
#57653=CARTESIAN_POINT ( 'NONE',  ( -2.266590686148945544, 32.22041550158063927, 7.082119434687048631 ) ) ;
#57655=CARTESIAN_POINT ( 'NONE',  ( 17.20831665107776587, 19.13393115100078035, -7.208316651077762316 ) ) ;
#57656=CARTESIAN_POINT ( 'NONE',  ( 19.38216949554541557, 62.24863466993041072, -9.382169495545420901 ) ) ;
#57657=CARTESIAN_POINT ( 'NONE',  ( 5.076628168052704559, 65.17559781766745175, -8.527530157486179263 ) ) ;
#57658=ORIENTED_EDGE ( 'NONE', *, *, #91312, .T. ) ;
#57659=SURFACE_STYLE_FILL_AREA ( #33189 ) ;
#57660=CARTESIAN_POINT ( 'NONE',  ( 12.91533473730992121, 14.52201867748817143, 10.88017736071110164 ) ) ;
#57661=CARTESIAN_POINT ( 'NONE',  ( -0.3689425029237898834, 31.17874883491396787, -10.36894250292378850 ) ) ;
#57663=CARTESIAN_POINT ( 'NONE',  ( 7.084665262690076126, 67.02201867748817676, -10.88017736071110164 ) ) ;
#57664=CARTESIAN_POINT ( 'NONE',  ( 12.63842701281683922, 54.55059781766745175, -9.846743663894590881 ) ) ;
#57665=CARTESIAN_POINT ( 'NONE',  ( 12.91533473730993009, 31.60535201082150891, -10.88017736071109987 ) ) ;
#57673=CARTESIAN_POINT ( 'NONE',  ( 5.076628168052703671, 51.84226448433412315, 8.527530157486179263 ) ) ;
#57677=CARTESIAN_POINT ( 'NONE',  ( -4.164238869374098151, 11.59541550158063217, -3.795296366450310543 ) ) ;
#57678=CARTESIAN_POINT ( 'NONE',  ( 22.26659068614895176, 4.720415501580633943, -7.082119434687042414 ) ) ;
#57679=CARTESIAN_POINT ( 'NONE',  ( 10.00000000000000178, 49.31368534415484106, 10.88017736071110342 ) ) ;
#57680=CARTESIAN_POINT ( 'NONE',  ( -0.3689425029237881626, 52.42874883491396076, 10.36894250292379027 ) ) ;
#57681=CARTESIAN_POINT ( 'NONE',  ( 17.20831665107776587, 52.88393115100078035, 7.208316651077764980 ) ) ;
#57682=CARTESIAN_POINT ( 'NONE',  ( 0.1532563361054082862, 31.21726448433412315, 2.638427012816831674 ) ) ;
#57683=CARTESIAN_POINT ( 'NONE',  ( -0.8801773607110991993, 32.85535201082151247, -2.915334737309923874 ) ) ;
#57684=CARTESIAN_POINT ( 'NONE',  ( 22.81628187352648496, 11.83196800326375531, -3.434112377981050290 ) ) ;
#57685=CARTESIAN_POINT ( 'NONE',  ( 24.16423886937410614, 4.512082168247300906, -3.795296366450302550 ) ) ;
#57687=CARTESIAN_POINT ( 'NONE',  ( 17.08211943468705130, 53.47041550158063217, 12.26659068614894998 ) ) ;
#57688=CARTESIAN_POINT ( 'NONE',  ( 20.88017736071110875, 5.772018677488170546, -2.915334737309920765 ) ) ;
#57694=CARTESIAN_POINT ( 'NONE',  ( 14.92337183194729633, 22.67559781766745175, 8.527530157486181039 ) ) ;
#57696=CARTESIAN_POINT ( 'NONE',  ( 2.917880565312948704, 27.63708216824730357, 12.26659068614894643 ) ) ;
#57697=CARTESIAN_POINT ( 'NONE',  ( 12.63842701281683922, 39.55059781766744464, -9.846743663894590881 ) ) ;
#57698=CARTESIAN_POINT ( 'NONE',  ( -0.8801773607111009756, 63.06368534415484106, 1.068504757029289695E-15 ) ) ;
#57700=CARTESIAN_POINT ( 'NONE',  ( 10.00000000000000000, 51.81368534415484106, -10.88017736071110342 ) ) ;
#57701=EDGE_CURVE ( 'NONE', #44176, #1795, #58636, .T. ) ;
#57702=CARTESIAN_POINT ( 'NONE',  ( 10.00000000000000000, 62.87363466993042493, -12.81628187352647608 ) ) ;
#57705=CARTESIAN_POINT ( 'NONE',  ( 20.36894250292379738, 14.92874883491396432, -10.36894250292379027 ) ) ;
#57708=CARTESIAN_POINT ( 'NONE',  ( 3.591859063236761518, 49.95696800326375353, 11.09922568453594849 ) ) ;
#57709=CARTESIAN_POINT ( 'NONE',  ( -0.8801773607111009756, 18.06368534415484106, 1.068504757029289695E-15 ) ) ;
#57710=CARTESIAN_POINT ( 'NONE',  ( 10.00000000000000178, 17.25893115100078745, 9.846743663894594434 ) ) ;
#57711=CARTESIAN_POINT ( 'NONE',  ( 4.559911319644449179, 17.23035201082150536, -9.422509992056141925 ) ) ;
#57712=CARTESIAN_POINT ( 'NONE',  ( 0.6178305044545838731, 49.74863466993041072, 9.382169495545420901 ) ) ;
#57714=CARTESIAN_POINT ( 'NONE',  ( 2.791683348922237240, 25.38393115100078390, -7.208316651077763204 ) ) ;
#57717=CARTESIAN_POINT ( 'NONE',  ( 15.44008868035555260, 64.73035201082151957, 9.422509992056143702 ) ) ;
#57718=CARTESIAN_POINT ( 'NONE',  ( 19.72487221294570858, 7.802231764288317883, -6.499999999999999112 ) ) ;
#57719=CARTESIAN_POINT ( 'NONE',  ( -0.2418659066527654722, 45.11633188102327807, 6.114288769123054301 ) ) ;
#57720=CARTESIAN_POINT ( 'NONE',  ( 5.076628168052704559, 20.17559781766745175, -8.527530157486179263 ) ) ;
#57721=CARTESIAN_POINT ( 'NONE',  ( -1.099225684535947600, 19.54030133659708568, 6.408140936763237150 ) ) ;
#57723=CARTESIAN_POINT ( 'NONE',  ( 17.20831665107776587, 44.13393115100078745, -7.208316651077762316 ) ) ;
#57725=CARTESIAN_POINT ( 'NONE',  ( 10.00000000000000000, 15.55374883491396787, -14.16423886937410082 ) ) ;
#57726=CARTESIAN_POINT ( 'NONE',  ( 17.20831665107776587, 37.88393115100078745, 7.208316651077764980 ) ) ;
#57727=CARTESIAN_POINT ( 'NONE',  ( 6.565887622018943937, 30.16530133659708568, 12.81628187352647430 ) ) ;
#57730=CARTESIAN_POINT ( 'NONE',  ( 2.035157376598822676, 62.43868534415483396, -7.964842623401177768 ) ) ;
#57731=CARTESIAN_POINT ( 'NONE',  ( 13.43411237798105340, 0.5819680032637533085, 12.81628187352647963 ) ) ;
#57733=CARTESIAN_POINT ( 'NONE',  ( 12.63842701281683922, 34.55059781766745886, -9.846743663894590881 ) ) ;
#57734=CARTESIAN_POINT ( 'NONE',  ( 15.44008868035555793, 21.39701867748817321, -9.422509992056140149 ) ) ;
#57736=CARTESIAN_POINT ( 'NONE',  ( 3.591859063236763294, 33.29030133659708213, -11.09922568453595026 ) ) ;
#57737=CARTESIAN_POINT ( 'NONE',  ( 1.472469842513823179, 30.59226448433411960, -4.923371831947296329 ) ) ;
#57738=( BOUNDED_CURVE ( )  B_SPLINE_CURVE ( 2, ( #18276, #48265, #94257, #25784, #80740, #78778, #10284, #88232, #12235 ),
 .UNSPECIFIED., .F., .F. ) 
 B_SPLINE_CURVE_WITH_KNOTS ( ( 3, 2, 2, 2, 3 ),
 ( 0.2962860886497511448, 0.2976190476190476164, 0.3035714285714285476, 0.3095238095238095344, 0.3108567684931059505 ),
 .UNSPECIFIED. ) 
 CURVE ( )  GEOMETRIC_REPRESENTATION_ITEM ( )  RATIONAL_B_SPLINE_CURVE ( ( 0.9881565478350728959, 0.9923695281211487584, 1.000000000000000000, 0.9659258262890683122, 1.000000000000000000, 0.9659258262890683122, 1.000000000000000000, 0.9923695281211490915, 0.9881565478350733400 ) ) 
 REPRESENTATION_ITEM ( '' )  );
#57741=CARTESIAN_POINT ( 'NONE',  ( 17.96484262340118221, 36.18868534415484106, -7.964842623401177768 ) ) ;
#57744=CARTESIAN_POINT ( 'NONE',  ( 20.88017736071110164, 5.355352010821502695, 2.915334737309930979 ) ) ;
#57745=CARTESIAN_POINT ( 'NONE',  ( 18.52753015748617571, 53.09226448433412315, 4.923371831947298993 ) ) ;
#57746=CARTESIAN_POINT ( 'NONE',  ( 20.88017736071110875, 25.77201867748816966, -2.915334737309920765 ) ) ;
#57748=CARTESIAN_POINT ( 'NONE',  ( -0.8801773607111009756, 53.06368534415484106, 1.068504757029289695E-15 ) ) ;
#57749=B_SPLINE_CURVE_WITH_KNOTS ( 'NONE', 3,
 ( #84985, #8983, #1517, #31962 ),
 .UNSPECIFIED., .F., .F.,
 ( 4, 4 ),
 ( 0.000000000000000000, 0.001036303429213010323 ),
 .UNSPECIFIED. ) ;
#57750=CARTESIAN_POINT ( 'NONE',  ( 17.96484262340118221, 26.18868534415483396, -7.964842623401177768 ) ) ;
#57751=CARTESIAN_POINT ( 'NONE',  ( -0.000000000000000000, 75.99261571001677851, -6.807497417685388186 ) ) ;
#57752=CARTESIAN_POINT ( 'NONE',  ( 18.52753015748617571, 3.092264484334118269, 4.923371831947298993 ) ) ;
#57753=DIRECTION ( 'NONE',  ( -0.000000000000000000, -0.000000000000000000, -1.000000000000000000 ) ) ;
#57754=CARTESIAN_POINT ( 'NONE',  ( 0.1532563361054100626, 55.80059781766745175, -2.638427012816831230 ) ) ;
#57755=CARTESIAN_POINT ( 'NONE',  ( 24.16423886937410614, 54.51208216824730357, -3.795296366450302550 ) ) ;
#57758=CARTESIAN_POINT ( 'NONE',  ( -4.164238869374099039, 6.803748834913967869, 8.674139862899312516E-16 ) ) ;
#57759=CARTESIAN_POINT ( 'NONE',  ( 6.204703633549690345, 40.76208216824731778, -14.16423886937410259 ) ) ;
#57761=CARTESIAN_POINT ( 'NONE',  ( -1.099225684535947600, 4.540301336597087456, 6.408140936763237150 ) ) ;
#57763=ORIENTED_EDGE ( 'NONE', *, *, #9021, .F. ) ;
#57764=CARTESIAN_POINT ( 'NONE',  ( -4.164238869374098151, 66.59541550158060375, -3.795296366450310543 ) ) ;
#57765=CARTESIAN_POINT ( 'NONE',  ( 1.472469842513823179, 40.59226448433411605, -4.923371831947296329 ) ) ;
#57767=CARTESIAN_POINT ( 'NONE',  ( 17.96484262340118221, 59.93868534415484106, 7.964842623401181321 ) ) ;
#57770=CARTESIAN_POINT ( 'NONE',  ( -1.099225684535947600, 59.54030133659708923, 6.408140936763237150 ) ) ;
#57771=CARTESIAN_POINT ( 'NONE',  ( 21.09922568453594849, 31.20696800326375353, 6.408140936763242479 ) ) ;
#57772=CARTESIAN_POINT ( 'NONE',  ( 19.84674366389459266, 33.30059781766744464, 2.638427012816836559 ) ) ;
#57775=CARTESIAN_POINT ( 'NONE',  ( -4.164238869374098151, 61.59541550158063217, -3.795296366450310543 ) ) ;
#57776=CARTESIAN_POINT ( 'NONE',  ( 10.00000000000000000, 11.81368534415483751, -10.88017736071110342 ) ) ;
#57777=CARTESIAN_POINT ( 'NONE',  ( 10.00000000000000000, 45.55374883491397497, -14.16423886937410082 ) ) ;
#57778=CARTESIAN_POINT ( 'NONE',  ( -0.8801773607111009756, 33.06368534415484106, 1.068504757029289695E-15 ) ) ;
#57779=CARTESIAN_POINT ( 'NONE',  ( 12.91533473730993009, 66.60535201082150536, -10.88017736071109987 ) ) ;
#57782=CARTESIAN_POINT ( 'NONE',  ( 0.1532563361054100626, 15.80059781766745353, -2.638427012816831230 ) ) ;
#57784=CARTESIAN_POINT ( 'NONE',  ( 19.84674366389459266, 3.717264484334118713, -2.638427012816827677 ) ) ;
#57786=CARTESIAN_POINT ( 'NONE',  ( 19.84674366389459266, 43.71726448433410894, -2.638427012816827677 ) ) ;
#57787=CARTESIAN_POINT ( 'NONE',  ( 1.472469842513823179, 61.42559781766745175, 4.923371831947296329 ) ) ;
#57788=CARTESIAN_POINT ( 'NONE',  ( 17.96484262340118221, 26.18868534415483396, -7.964842623401177768 ) ) ;
#57791=CARTESIAN_POINT ( 'NONE',  ( -2.816281873526473856, 49.12363466993042493, 9.499525473075851096E-16 ) ) ;
#57793=CARTESIAN_POINT ( 'NONE',  ( -0.8801773607110991993, 62.85535201082150536, -2.915334737309923874 ) ) ;
#57794=CARTESIAN_POINT ( 'NONE',  ( 18.52753015748618282, 23.92559781766745530, -4.923371831947291888 ) ) ;
#57795=CARTESIAN_POINT ( 'NONE',  ( 6.204703633549690345, 52.84541550158062506, 14.16423886937410082 ) ) ;
#57796=CARTESIAN_POINT ( 'NONE',  ( 2.791683348922240793, 21.63393115100078745, 7.208316651077764092 ) ) ;
#57797=DIRECTION ( 'NONE',  ( 0.5547001962252290364, 0.8320502943378437211, 0.000000000000000000 ) ) ;
#57800=CARTESIAN_POINT ( 'NONE',  ( 1.472469842513823179, 61.42559781766745175, 4.923371831947296329 ) ) ;
#57801=CARTESIAN_POINT ( 'NONE',  ( 6.204703633549690345, 27.84541550158063217, 14.16423886937410082 ) ) ;
#57802=CARTESIAN_POINT ( 'NONE',  ( 2.791683348922237240, 45.38393115100079456, -7.208316651077763204 ) ) ;
#57803=CARTESIAN_POINT ( 'NONE',  ( 4.999999999999999112, 11.50000000000000000, -6.000000000000000000 ) ) ;
#57804=CARTESIAN_POINT ( 'NONE',  ( 0.5774900079438607392, 23.48035201082150536, 5.440088680355550821 ) ) ;
#57805=CARTESIAN_POINT ( 'NONE',  ( 19.42250999205614193, 65.14701867748817676, 5.440088680355555262 ) ) ;
#57807=CARTESIAN_POINT ( 'NONE',  ( -1.099225684535947600, 44.54030133659708923, 6.408140936763237150 ) ) ;
#57809=CARTESIAN_POINT ( 'NONE',  ( 0.5774900079438590739, 52.64701867748817676, -5.440088680355550821 ) ) ;
#57811=( NAMED_UNIT ( * ) SI_UNIT ( $, .STERADIAN. ) SOLID_ANGLE_UNIT ( ) );
#57812=LINE ( 'NONE', #97828, #32849 ) ;
#57814=CARTESIAN_POINT ( 'NONE',  ( 12.91533473730992121, 59.52201867748816966, 10.88017736071110164 ) ) ;
#57815=CARTESIAN_POINT ( 'NONE',  ( 15.44008868035555260, 14.73035201082150536, 9.422509992056143702 ) ) ;
#57817=CARTESIAN_POINT ( 'NONE',  ( 18.04007052943773104, 9.002578601053489393, -5.767676674365834977 ) ) ;
#57818=FILL_AREA_STYLE_COLOUR ( '', #8947 ) ;
#57819=CARTESIAN_POINT ( 'NONE',  ( 10.00000000000000000, 6.813685344154838397, -10.88017736071110342 ) ) ;
#57820=CARTESIAN_POINT ( 'NONE',  ( 5.076628168052704559, 25.17559781766745175, -8.527530157486179263 ) ) ;
#57821=CARTESIAN_POINT ( 'NONE',  ( -4.164238869374099927, 17.01208216824730357, 3.795296366450308767 ) ) ;
#57822=CARTESIAN_POINT ( 'NONE',  ( 7.084665262690076126, 17.02201867748817676, -10.88017736071110164 ) ) ;
#57823=CARTESIAN_POINT ( 'NONE',  ( 0.1532563361054100626, 60.80059781766744464, -2.638427012816831230 ) ) ;
#57825=ADVANCED_FACE ( 'NONE', ( #65096 ), #15134, .T. ) ;
#57826=CARTESIAN_POINT ( 'NONE',  ( 14.92337183194729988, 64.34226448433412315, -8.527530157486177487 ) ) ;
#57828=CARTESIAN_POINT ( 'NONE',  ( 20.88017736071110164, 50.35535201082151247, 2.915334737309930979 ) ) ;
#57830=CARTESIAN_POINT ( 'NONE',  ( 13.43411237798106583, 42.66530133659707502, -12.81628187352647252 ) ) ;
#57832=CARTESIAN_POINT ( 'NONE',  ( 19.42250999205614548, 60.98035201082151247, -5.440088680355545492 ) ) ;
#57833=CARTESIAN_POINT ( 'NONE',  ( 7.084665262690076126, 22.02201867748817321, -10.88017736071110164 ) ) ;
#57835=CARTESIAN_POINT ( 'NONE',  ( 13.43411237798105340, 35.58196800326375353, 12.81628187352647963 ) ) ;
#57836=CARTESIAN_POINT ( 'NONE',  ( -0.8801773607110991993, 27.85535201082150181, -2.915334737309923874 ) ) ;
#57837=LINE ( 'NONE', #51334, #57880 ) ;
#57838=CARTESIAN_POINT ( 'NONE',  ( -2.816281873526473856, 44.33196800326375353, 3.434112377981055619 ) ) ;
#57839=CARTESIAN_POINT ( 'NONE',  ( 10.00000000000000178, 34.31368534415484106, 10.88017736071110342 ) ) ;
#57840=CARTESIAN_POINT ( 'NONE',  ( 7.361572987183170547, 52.05059781766745175, 9.846743663894590881 ) ) ;
#57844=CARTESIAN_POINT ( 'NONE',  ( 14.92337183194729988, 64.34226448433412315, -8.527530157486177487 ) ) ;
#57845=DIRECTION ( 'NONE',  ( 0.000000000000000000, 0.000000000000000000, -1.000000000000000000 ) ) ;
#57846=CARTESIAN_POINT ( 'NONE',  ( 19.84674366389459266, 48.71726448433413026, -2.638427012816827677 ) ) ;
#57847=CARTESIAN_POINT ( 'NONE',  ( 4.559911319644449179, 28.89701867748817321, 9.422509992056141925 ) ) ;
#57849=CARTESIAN_POINT ( 'NONE',  ( 10.00000000000000178, 42.25893115100078745, 9.846743663894594434 ) ) ;
#57850=CARTESIAN_POINT ( 'NONE',  ( 19.72487221294570858, 51.86607318730076344, 6.500000000000000888 ) ) ;
#57851=FACE_OUTER_BOUND ( 'NONE', #45660, .T. ) ;
#57852=CARTESIAN_POINT ( 'NONE',  ( 5.076628168052703671, 36.84226448433412315, 8.527530157486179263 ) ) ;
#57853=CARTESIAN_POINT ( 'NONE',  ( 2.791683348922240793, 1.633931151000784565, 7.208316651077764092 ) ) ;
#57854=CARTESIAN_POINT ( 'NONE',  ( 14.92337183194729633, 62.67559781766745886, 8.527530157486181039 ) ) ;
#57856=FILL_AREA_STYLE ('',( #44332 ) ) ;
#57857=LINE ( 'NONE', #12851, #32639 ) ;
#57858=CARTESIAN_POINT ( 'NONE',  ( -2.816281873526473856, 39.33196800326374643, 3.434112377981055619 ) ) ;
#57859=CARTESIAN_POINT ( 'NONE',  ( 17.20831665107776587, 39.13393115100079456, -7.208316651077762316 ) ) ;
#57861=CARTESIAN_POINT ( 'NONE',  ( 6.204703633549690345, 55.76208216824730357, -14.16423886937410259 ) ) ;
#57862=CARTESIAN_POINT ( 'NONE',  ( 14.92337183194729633, 32.67559781766745175, 8.527530157486181039 ) ) ;
#57864=CARTESIAN_POINT ( 'NONE',  ( 24.16423886937410614, 59.30374883491397497, 8.672049930838204340E-16 ) ) ;
#57866=CARTESIAN_POINT ( 'NONE',  ( 19.42250999205614548, 25.98035201082150891, -5.440088680355545492 ) ) ;
#57868=CARTESIAN_POINT ( 'NONE',  ( -2.266590686148945544, 41.38708216824729647, -7.082119434687050408 ) ) ;
#57869=CARTESIAN_POINT ( 'NONE',  ( 6.204703633549690345, 55.76208216824730357, -14.16423886937410259 ) ) ;
#57871=CARTESIAN_POINT ( 'NONE',  ( 1.472469842513823179, 15.59226448433411960, -4.923371831947296329 ) ) ;
#57873=CARTESIAN_POINT ( 'NONE',  ( 2.791683348922237240, 65.38393115100078035, -7.208316651077763204 ) ) ;
#57874=CARTESIAN_POINT ( 'NONE',  ( 12.91533473730992121, 54.52201867748816255, 10.88017736071110164 ) ) ;
#57876=CARTESIAN_POINT ( 'NONE',  ( 1.472469842513823179, 50.59226448433411605, -4.923371831947296329 ) ) ;
#57878=CARTESIAN_POINT ( 'NONE',  ( 5.076628168052704559, 60.17559781766745175, -8.527530157486179263 ) ) ;
#57879=CARTESIAN_POINT ( 'NONE',  ( 2.917880565312948704, 2.637082168247300906, 12.26659068614894643 ) ) ;
#57880=VECTOR ( 'NONE', #43818, 1000.000000000000000 ) ;
#57881=VERTEX_POINT ( 'NONE', #39213 ) ;
#57882=CARTESIAN_POINT ( 'NONE',  ( -4.164238869374099039, 31.80374883491396432, 8.674139862899312516E-16 ) ) ;
#57884=CARTESIAN_POINT ( 'NONE',  ( 2.603489959281601873, 25.43575266056827289, -6.500000000000015987 ) ) ;
#57885=CARTESIAN_POINT ( 'NONE',  ( 19.42250999205614548, 15.98035201082150714, -5.440088680355545492 ) ) ;
#57886=CARTESIAN_POINT ( 'NONE',  ( 21.09922568453594849, 36.20696800326375353, 6.408140936763242479 ) ) ;
#57888=CARTESIAN_POINT ( 'NONE',  ( 2.791683348922240793, 6.633931151000785675, 7.208316651077764092 ) ) ;
#57892=CARTESIAN_POINT ( 'NONE',  ( 24.16423886937410614, 29.51208216824729647, -3.795296366450302550 ) ) ;
#57893=SURFACE_STYLE_FILL_AREA ( #13392 ) ;
#57894=CARTESIAN_POINT ( 'NONE',  ( 10.00000000000000178, 4.313685344154837509, 10.88017736071110342 ) ) ;
#57897=CARTESIAN_POINT ( 'NONE',  ( 15.44008868035555793, 46.39701867748817676, -9.422509992056140149 ) ) ;
#57898=CARTESIAN_POINT ( 'NONE',  ( 2.035157376598822676, 47.43868534415484817, -7.964842623401177768 ) ) ;
#57899=CARTESIAN_POINT ( 'NONE',  ( 16.40814093676324603, 12.45696800326375353, -11.09922568453594671 ) ) ;
#57900=SURFACE_SIDE_STYLE ('',( #93947 ) ) ;
#57901=CARTESIAN_POINT ( 'NONE',  ( 2.271632352219104423, 1.405976953357037207, 6.499999999999993783 ) ) ;
#57902=CARTESIAN_POINT ( 'NONE',  ( 17.20831665107776587, 12.88393115100078390, 7.208316651077764980 ) ) ;
#57905=CARTESIAN_POINT ( 'NONE',  ( 7.084665262690076126, 49.10535201082149825, 10.88017736071109987 ) ) ;
#57907=EDGE_CURVE ( 'NONE', #19780, #10063, #35553, .T. ) ;
#57908=CARTESIAN_POINT ( 'NONE',  ( 10.00000000000000000, 7.873634669930421381, -12.81628187352647608 ) ) ;
#57909=CARTESIAN_POINT ( 'NONE',  ( 0.5774900079438607392, 63.48035201082149825, 5.440088680355550821 ) ) ;
#57910=EDGE_CURVE ( 'NONE', #89108, #39417, #249, .T. ) ;
#57911=CARTESIAN_POINT ( 'NONE',  ( 12.63842701281683034, 22.46726448433411605, 9.846743663894596210 ) ) ;
#57912=CARTESIAN_POINT ( 'NONE',  ( 22.81628187352648496, 46.83196800326376064, -3.434112377981050290 ) ) ;
#57914=CARTESIAN_POINT ( 'NONE',  ( 5.076628168052703671, 1.842264484334118047, 8.527530157486179263 ) ) ;
#57915=EDGE_LOOP ( 'NONE', ( #1674, #21288, #51453, #19795 ) ) ;
#57918=CARTESIAN_POINT ( 'NONE',  ( 12.91533473730992121, 19.52201867748816611, 10.88017736071110164 ) ) ;
#57919=CARTESIAN_POINT ( 'NONE',  ( -2.816281873526473856, 59.33196800326374643, 3.434112377981055619 ) ) ;
#57920=CARTESIAN_POINT ( 'NONE',  ( 22.26659068614895176, 24.72041550158063572, -7.082119434687042414 ) ) ;
#57921=CARTESIAN_POINT ( 'NONE',  ( 5.076628168052704559, 25.17559781766745175, -8.527530157486179263 ) ) ;
#57922=CARTESIAN_POINT ( 'NONE',  ( 7.084665262690076126, 24.10535201082150181, 10.88017736071109987 ) ) ;
#57923=CARTESIAN_POINT ( 'NONE',  ( -0.8801773607111008646, 8.272018677488171434, 2.915334737309923430 ) ) ;
#57926=CARTESIAN_POINT ( 'NONE',  ( 20.88017736071110875, 10.77201867748817143, -2.915334737309920765 ) ) ;
#57927=CARTESIAN_POINT ( 'NONE',  ( -0.8801773607111008646, 38.27201867748816255, 2.915334737309923430 ) ) ;
#57929=CARTESIAN_POINT ( 'NONE',  ( 17.96484262340118221, 31.18868534415483751, -7.964842623401177768 ) ) ;
#57931=CARTESIAN_POINT ( 'NONE',  ( 19.84674366389459266, 63.30059781766745886, 2.638427012816836559 ) ) ;
#57932=CARTESIAN_POINT ( 'NONE',  ( -0.8801773607111009756, 28.06368534415484106, 1.068504757029289695E-15 ) ) ;
#57935=CARTESIAN_POINT ( 'NONE',  ( 6.565887622018943937, 65.16530133659709634, 12.81628187352647430 ) ) ;
#57936=CARTESIAN_POINT ( 'NONE',  ( -0.2418659066527783508, 4.260286857231743163, -6.114288769123032985 ) ) ;
#57937=CARTESIAN_POINT ( 'NONE',  ( 20.36894250292379738, 29.92874883491396432, -10.36894250292379027 ) ) ;
#57938=CARTESIAN_POINT ( 'NONE',  ( 17.96484262340118221, 46.18868534415484106, -7.964842623401177768 ) ) ;
#57939=CARTESIAN_POINT ( 'NONE',  ( 17.96484262340118221, 29.93868534415484106, 7.964842623401181321 ) ) ;
#57940=CARTESIAN_POINT ( 'NONE',  ( 18.52753015748618282, 63.92559781766745886, -4.923371831947291888 ) ) ;
#57942=CARTESIAN_POINT ( 'NONE',  ( 1.472469842513823179, 50.59226448433411605, -4.923371831947296329 ) ) ;
#57943=EDGE_CURVE ( 'NONE', #25434, #85493, #94617, .T. ) ;
#57944=CARTESIAN_POINT ( 'NONE',  ( 19.72487221294570858, 0.000000000000000000, -6.500000000000000888 ) ) ;
#57945=CARTESIAN_POINT ( 'NONE',  ( 2.791683348922237240, 25.38393115100078390, -7.208316651077763204 ) ) ;
#57947=CARTESIAN_POINT ( 'NONE',  ( 10.00000000000000000, 16.81368534415483751, -10.88017736071110342 ) ) ;
#57948=CARTESIAN_POINT ( 'NONE',  ( 17.20831665107776587, 24.13393115100078035, -7.208316651077762316 ) ) ;
#57949=CARTESIAN_POINT ( 'NONE',  ( 6.565887622018943937, 8.081968003263751754, -12.81628187352647608 ) ) ;
#57950=CARTESIAN_POINT ( 'NONE',  ( 20.88017736071110875, 55.77201867748816966, -2.915334737309920765 ) ) ;
#57951=CARTESIAN_POINT ( 'NONE',  ( 17.96484262340118221, 24.93868534415484461, 7.964842623401181321 ) ) ;
#57952=CARTESIAN_POINT ( 'NONE',  ( -2.816281873526471635, 63.91530133659708923, -3.434112377981056508 ) ) ;
#57953=CARTESIAN_POINT ( 'NONE',  ( 24.16423886937410614, 34.30374883491396787, 8.672049930838204340E-16 ) ) ;
#57959=CARTESIAN_POINT ( 'NONE',  ( -1.099225684535947600, -1.293031996736246469, -6.408140936763238038 ) ) ;
#57961=CARTESIAN_POINT ( 'NONE',  ( 19.42250999205614193, 30.14701867748817321, 5.440088680355555262 ) ) ;
#57962=CARTESIAN_POINT ( 'NONE',  ( 17.20831665107776587, 59.13393115100078745, -7.208316651077762316 ) ) ;
#57964=CARTESIAN_POINT ( 'NONE',  ( 14.92337183194729633, 12.67559781766745353, 8.527530157486181039 ) ) ;
#57965=CARTESIAN_POINT ( 'NONE',  ( 12.63842701281683922, 14.55059781766744997, -9.846743663894590881 ) ) ;
#57966=CARTESIAN_POINT ( 'NONE',  ( 1.472469842513823179, 16.42559781766745175, 4.923371831947296329 ) ) ;
#57967=CARTESIAN_POINT ( 'NONE',  ( 0.1532563361054083140, 6.008931151000784787, 1.131784320476157264E-15 ) ) ;
#57970=CARTESIAN_POINT ( 'NONE',  ( 10.00000000000000000, 4.758931151000784787, -9.846743663894594434 ) ) ;
#57972=CARTESIAN_POINT ( 'NONE',  ( 2.791683348922240793, 1.633931151000784565, 7.208316651077764092 ) ) ;
#57973=CARTESIAN_POINT ( 'NONE',  ( 12.63842701281683922, 14.55059781766744997, -9.846743663894590881 ) ) ;
#57976=CARTESIAN_POINT ( 'NONE',  ( 19.84674366389459266, 63.71726448433412315, -2.638427012816827677 ) ) ;
#57979=CARTESIAN_POINT ( 'NONE',  ( 6.204703633549690345, 25.76208216824730712, -14.16423886937410259 ) ) ;
#57981=VECTOR ( 'NONE', #74620, 1000.000000000000000 ) ;
#57982=CARTESIAN_POINT ( 'NONE',  ( 2.917880565312950480, 20.97041550158063217, -12.26659068614894821 ) ) ;
#57983=CARTESIAN_POINT ( 'NONE',  ( -0.3689425029237898834, 36.17874883491396787, -10.36894250292378850 ) ) ;
#57986=CARTESIAN_POINT ( 'NONE',  ( 13.79529636645030344, 18.26208216824730002, 14.16423886937410614 ) ) ;
#57987=CARTESIAN_POINT ( 'NONE',  ( 17.96484262340118221, 34.93868534415482685, 7.964842623401181321 ) ) ;
#57989=CARTESIAN_POINT ( 'NONE',  ( 7.361572987183169658, 9.967264484334119601, -9.846743663894592657 ) ) ;
#57991=CARTESIAN_POINT ( 'NONE',  ( 4.559911319644449179, 58.89701867748817676, 9.422509992056141925 ) ) ;
#57992=CARTESIAN_POINT ( 'NONE',  ( 18.52753015748618282, 33.92559781766745886, -4.923371831947291888 ) ) ;
#57994=CARTESIAN_POINT ( 'NONE',  ( 15.44008868035555793, 16.39701867748817321, -9.422509992056140149 ) ) ;
#57995=CARTESIAN_POINT ( 'NONE',  ( 6.565887622018943937, 43.08196800326374643, -12.81628187352647608 ) ) ;
#57996=CARTESIAN_POINT ( 'NONE',  ( 18.52753015748618282, 53.92559781766745175, -4.923371831947291888 ) ) ;
#57998=CARTESIAN_POINT ( 'NONE',  ( 19.38216949554541557, 32.24863466993041783, -9.382169495545420901 ) ) ;
#58000=CARTESIAN_POINT ( 'NONE',  ( 2.791683348922237240, 40.38393115100078035, -7.208316651077763204 ) ) ;
#58001=CARTESIAN_POINT ( 'NONE',  ( -2.266590686148945544, 22.22041550158063572, 7.082119434687048631 ) ) ;
#58003=CARTESIAN_POINT ( 'NONE',  ( 19.42250999205614193, 55.14701867748817676, 5.440088680355555262 ) ) ;
#58004=CARTESIAN_POINT ( 'NONE',  ( 7.084665262690076126, 49.10535201082149825, 10.88017736071109987 ) ) ;
#58005=CARTESIAN_POINT ( 'NONE',  ( 2.917880565312950480, 50.97041550158064638, -12.26659068614894821 ) ) ;
#58006=CARTESIAN_POINT ( 'NONE',  ( 12.63842701281683034, 57.46726448433411605, 9.846743663894596210 ) ) ;
#58008=CARTESIAN_POINT ( 'NONE',  ( 20.88017736071110164, 35.35535201082150536, 2.915334737309930979 ) ) ;
#58010=CARTESIAN_POINT ( 'NONE',  ( 17.20831665107776587, 59.13393115100078745, -7.208316651077762316 ) ) ;
#58012=CARTESIAN_POINT ( 'NONE',  ( 12.91533473730993009, 6.605352010821504471, -10.88017736071109987 ) ) ;
#58013=CARTESIAN_POINT ( 'NONE',  ( 17.96484262340118221, 66.18868534415483396, -7.964842623401177768 ) ) ;
#58014=ORIENTED_EDGE ( 'NONE', *, *, #35702, .F. ) ;
#58016=CARTESIAN_POINT ( 'NONE',  ( 17.96484262340118221, 9.938685344154837509, 7.964842623401181321 ) ) ;
#58018=CARTESIAN_POINT ( 'NONE',  ( 7.084665262690076126, 62.02201867748816966, -10.88017736071110164 ) ) ;
#58019=AXIS2_PLACEMENT_3D ( 'NONE', #5491, #6453, #81954 ) ;
#58020=CARTESIAN_POINT ( 'NONE',  ( 17.96484262340118221, 66.18868534415483396, -7.964842623401177768 ) ) ;
#58023=CARTESIAN_POINT ( 'NONE',  ( 14.92337183194729988, 34.34226448433411605, -8.527530157486177487 ) ) ;
#58024=CARTESIAN_POINT ( 'NONE',  ( 4.559911319644449179, 27.23035201082150536, -9.422509992056141925 ) ) ;
#58026=CARTESIAN_POINT ( 'NONE',  ( 21.09922568453595559, 2.040301336597086568, -6.408140936763230044 ) ) ;
#58027=CARTESIAN_POINT ( 'NONE',  ( 7.084665262690076126, 29.10535201082150181, 10.88017736071109987 ) ) ;
#58030=CARTESIAN_POINT ( 'NONE',  ( 19.38216949554541202, 40.99863466993042493, 9.382169495545424454 ) ) ;
#58032=CARTESIAN_POINT ( 'NONE',  ( 10.00000000000000178, 70.00000000000000000, 0.000000000000000000 ) ) ;
#58033=CARTESIAN_POINT ( 'NONE',  ( -2.816281873526471635, 13.91530133659708746, -3.434112377981056508 ) ) ;
#58035=LINE ( 'NONE', #36542, #16424 ) ;
#58036=CARTESIAN_POINT ( 'NONE',  ( 12.91533473730993009, 21.60535201082150536, -10.88017736071109987 ) ) ;
#58037=CARTESIAN_POINT ( 'NONE',  ( 6.204703633549690345, 62.84541550158063927, 14.16423886937410082 ) ) ;
#58038=CARTESIAN_POINT ( 'NONE',  ( 0.1532563361054082862, 56.21726448433411605, 2.638427012816831674 ) ) ;
#58039=CARTESIAN_POINT ( 'NONE',  ( 2.791683348922237240, 5.383931151000785675, -7.208316651077763204 ) ) ;
#58040=CARTESIAN_POINT ( 'NONE',  ( 17.96484262340118221, 66.18868534415483396, -7.964842623401177768 ) ) ;
#58042=CARTESIAN_POINT ( 'NONE',  ( 6.204703633549690345, 30.76208216824730357, -14.16423886937410259 ) ) ;
#58045=ORIENTED_EDGE ( 'NONE', *, *, #69562, .F. ) ;
#58047=CARTESIAN_POINT ( 'NONE',  ( 6.204703633549690345, 67.84541550158060375, 14.16423886937410082 ) ) ;
#58048=CARTESIAN_POINT ( 'NONE',  ( 20.36894250292379382, 43.67874883491397497, 10.36894250292379205 ) ) ;
#58049=CARTESIAN_POINT ( 'NONE',  ( 2.791683348922240793, 31.63393115100078745, 7.208316651077764092 ) ) ;
#58052=PRESENTATION_STYLE_ASSIGNMENT (( #20063 ) ) ;
#58053=PRESENTATION_STYLE_ASSIGNMENT (( #12565 ) ) ;
#58054=CARTESIAN_POINT ( 'NONE',  ( 13.79529636645031943, 40.34541550158063217, -14.16423886937409904 ) ) ;
#58056=CARTESIAN_POINT ( 'NONE',  ( 19.84674366389459621, 3.508931151000785231, 7.409399052514197653E-17 ) ) ;
#58066=CARTESIAN_POINT ( 'NONE',  ( 13.79529636645031943, 10.34541550158063394, -14.16423886937409904 ) ) ;
#58067=CARTESIAN_POINT ( 'NONE',  ( 12.91533473730993009, 21.60535201082150536, -10.88017736071109987 ) ) ;
#58068=CARTESIAN_POINT ( 'NONE',  ( 10.00000000000000000, 21.81368534415484106, -10.88017736071110342 ) ) ;
#58069=CARTESIAN_POINT ( 'NONE',  ( 17.20831665107776587, 52.88393115100078035, 7.208316651077764980 ) ) ;
#58070=CARTESIAN_POINT ( 'NONE',  ( -2.816281873526473856, 14.12363466993041961, 9.499525473075851096E-16 ) ) ;
#58071=PRESENTATION_STYLE_ASSIGNMENT (( #96094 ) ) ;
#58072=CARTESIAN_POINT ( 'NONE',  ( 19.38216949554541557, 12.24863466993041961, -9.382169495545420901 ) ) ;
#58074=CARTESIAN_POINT ( 'NONE',  ( 7.361572987183170547, 37.05059781766744464, 9.846743663894590881 ) ) ;
#58075=CARTESIAN_POINT ( 'NONE',  ( 6.204703633549690345, 57.84541550158063927, 14.16423886937410082 ) ) ;
#58077=CARTESIAN_POINT ( 'NONE',  ( 2.035157376598822676, 2.438685344154838397, -7.964842623401177768 ) ) ;
#58079=CARTESIAN_POINT ( 'NONE',  ( 2.035157376598822676, 52.43868534415483396, -7.964842623401177768 ) ) ;
#58080=CARTESIAN_POINT ( 'NONE',  ( 4.559911319644449179, 38.89701867748817676, 9.422509992056141925 ) ) ;
#58081=CARTESIAN_POINT ( 'NONE',  ( -0.8801773607110991993, 47.85535201082150536, -2.915334737309923874 ) ) ;
#58082=CARTESIAN_POINT ( 'NONE',  ( 20.10421743870886147, 5.607361737662019507, -6.337391062633416006 ) ) ;
#58083=CARTESIAN_POINT ( 'NONE',  ( 17.96484262340118221, 34.93868534415482685, 7.964842623401181321 ) ) ;
#58084=CARTESIAN_POINT ( 'NONE',  ( -0.1503990784575279516, 53.10158574516643171, 6.262539305110076171 ) ) ;
#58087=CARTESIAN_POINT ( 'NONE',  ( 2.791683348922237240, 30.38393115100078390, -7.208316651077763204 ) ) ;
#58088=VERTEX_POINT ( 'NONE', #83719 ) ;
#58089=CARTESIAN_POINT ( 'NONE',  ( 19.84674366389459266, 63.30059781766745886, 2.638427012816836559 ) ) ;
#58094=CARTESIAN_POINT ( 'NONE',  ( 5.076628168052704559, 65.17559781766745175, -8.527530157486179263 ) ) ;
#58095=CARTESIAN_POINT ( 'NONE',  ( 24.16423886937410614, 54.51208216824730357, -3.795296366450302550 ) ) ;
#58096=CARTESIAN_POINT ( 'NONE',  ( 18.28836319691949797, 64.34492782695771496, 6.499999999999917399 ) ) ;
#58098=CARTESIAN_POINT ( 'NONE',  ( 1.472469842513823179, 36.42559781766745175, 4.923371831947296329 ) ) ;
#58100=CARTESIAN_POINT ( 'NONE',  ( -2.816281873526473856, 4.123634669930420493, 9.499525473075851096E-16 ) ) ;
#58101=CARTESIAN_POINT ( 'NONE',  ( 2.791683348922240793, 6.633931151000785675, 7.208316651077764092 ) ) ;
#58103=CARTESIAN_POINT ( 'NONE',  ( -0.1503990784575323369, 4.248846992468888750, -6.262539305110070842 ) ) ;
#58104=CARTESIAN_POINT ( 'NONE',  ( 10.00000000000000000, 4.758931151000784787, -9.846743663894594434 ) ) ;
#58105=CARTESIAN_POINT ( 'NONE',  ( 19.84674366389459621, 58.50893115100078745, 7.409399052514197653E-17 ) ) ;
#58106=CARTESIAN_POINT ( 'NONE',  ( 18.72515096720568195, 21.07228050351032422, -6.500000000000018652 ) ) ;
#58108=CARTESIAN_POINT ( 'NONE',  ( 2.035157376598824452, 8.688685344154839285, 7.964842623401179544 ) ) ;
#58109=CARTESIAN_POINT ( 'NONE',  ( -0.3689425029237898834, 1.178748834913967869, -10.36894250292378850 ) ) ;
#58110=CARTESIAN_POINT ( 'NONE',  ( 14.92337183194729988, 9.342264484334119601, -8.527530157486177487 ) ) ;
#58111=CARTESIAN_POINT ( 'NONE',  ( 20.88017736071110519, 50.56368534415484106, 2.639326808657452039E-16 ) ) ;
#58112=CARTESIAN_POINT ( 'NONE',  ( 10.00000000000000178, 25.37363466993041783, 12.81628187352647608 ) ) ;
#58114=CARTESIAN_POINT ( 'NONE',  ( 7.084665262690076126, 4.105352010821503583, 10.88017736071109987 ) ) ;
#58117=CARTESIAN_POINT ( 'NONE',  ( 19.38216949554541202, 5.998634669930420493, 9.382169495545424454 ) ) ;
#58118=CARTESIAN_POINT ( 'NONE',  ( 0.1532563361054083140, 61.00893115100078745, 1.131784320476157264E-15 ) ) ;
#58119=CARTESIAN_POINT ( 'NONE',  ( 5.076628168052703671, 16.84226448433411960, 8.527530157486179263 ) ) ;
#58121=CARTESIAN_POINT ( 'NONE',  ( 22.81628187352647785, 16.62363466993042138, 6.195893100308588602E-16 ) ) ;
#58123=CARTESIAN_POINT ( 'NONE',  ( 20.88017736071110164, 25.35535201082150891, 2.915334737309930979 ) ) ;
#58125=CARTESIAN_POINT ( 'NONE',  ( 17.08211943468705130, 48.47041550158063927, 12.26659068614894998 ) ) ;
#58127=CARTESIAN_POINT ( 'NONE',  ( 4.559911319644449179, 33.89701867748817676, 9.422509992056141925 ) ) ;
#58129=CARTESIAN_POINT ( 'NONE',  ( 14.92337183194729633, 47.67559781766745175, 8.527530157486181039 ) ) ;
#58131=CARTESIAN_POINT ( 'NONE',  ( 10.00000000000000178, 49.31368534415484106, 10.88017736071110342 ) ) ;
#58132=CARTESIAN_POINT ( 'NONE',  ( 22.26659068614894466, 28.88708216824730357, 7.082119434687054849 ) ) ;
#58134=UNCERTAINTY_MEASURE_WITH_UNIT (LENGTH_MEASURE( 1.000000000000000082E-05 ), #61346, 'distance_accuracy_value', 'NONE');
#58136=CARTESIAN_POINT ( 'NONE',  ( 12.63842701281683922, 34.55059781766745886, -9.846743663894590881 ) ) ;
#58137=CARTESIAN_POINT ( 'NONE',  ( 10.00000000000000000, 62.87363466993042493, -12.81628187352647608 ) ) ;
#58138=CARTESIAN_POINT ( 'NONE',  ( 18.52753015748618282, 63.92559781766745886, -4.923371831947291888 ) ) ;
#58139=ORIENTED_EDGE ( 'NONE', *, *, #12731, .F. ) ;
#58140=CARTESIAN_POINT ( 'NONE',  ( 20.88017736071110519, 25.56368534415483751, 2.639326808657452039E-16 ) ) ;
#58143=CARTESIAN_POINT ( 'NONE',  ( 15.44008868035555260, 9.730352010821505360, 9.422509992056143702 ) ) ;
#58144=CARTESIAN_POINT ( 'NONE',  ( 10.00000000000000000, 66.81368534415484817, -10.88017736071110342 ) ) ;
#58145=CARTESIAN_POINT ( 'NONE',  ( 20.36894250292379382, 28.67874883491396787, 10.36894250292379205 ) ) ;
#58146=CARTESIAN_POINT ( 'NONE',  ( 14.92337183194729633, 7.675597817667451750, 8.527530157486181039 ) ) ;
#58148=CARTESIAN_POINT ( 'NONE',  ( 15.44008868035555260, 29.73035201082150891, 9.422509992056143702 ) ) ;
#58149=CARTESIAN_POINT ( 'NONE',  ( 19.39235739573468820, 64.87576471608601025, 6.499999999999992895 ) ) ;
#58153=CARTESIAN_POINT ( 'NONE',  ( 17.20831665107776587, 39.13393115100079456, -7.208316651077762316 ) ) ;
#58155=ORIENTED_EDGE ( 'NONE', *, *, #56673, .T. ) ;
#58157=CARTESIAN_POINT ( 'NONE',  ( 22.26659068614894466, 3.887082168247300906, 7.082119434687054849 ) ) ;
#58158=CARTESIAN_POINT ( 'NONE',  ( -2.266590686148945544, 11.38708216824730179, -7.082119434687050408 ) ) ;
#58159=CARTESIAN_POINT ( 'NONE',  ( 15.44008868035555260, 44.73035201082151247, 9.422509992056143702 ) ) ;
#58160=CARTESIAN_POINT ( 'NONE',  ( 17.08211943468705840, 50.13708216824730357, -12.26659068614894466 ) ) ;
#58161=CARTESIAN_POINT ( 'NONE',  ( 21.09922568453594849, 6.206968003263753531, 6.408140936763242479 ) ) ;
#58162=CARTESIAN_POINT ( 'NONE',  ( 0.1532563361054083140, 36.00893115100078745, 1.131784320476157264E-15 ) ) ;
#58164=CARTESIAN_POINT ( 'NONE',  ( 12.91533473730993009, 36.60535201082151247, -10.88017736071109987 ) ) ;
#58165=CARTESIAN_POINT ( 'NONE',  ( 22.81628187352647785, 11.62363466993042138, 6.195893100308588602E-16 ) ) ;
#58166=CARTESIAN_POINT ( 'NONE',  ( 6.204703633549690345, 2.845415501580634388, 14.16423886937410082 ) ) ;
#58167=CARTESIAN_POINT ( 'NONE',  ( 2.917880565312950480, 55.97041550158063217, -12.26659068614894821 ) ) ;
#58168=CARTESIAN_POINT ( 'NONE',  ( 4.559911319644449179, 22.23035201082150536, -9.422509992056141925 ) ) ;
#58169=CARTESIAN_POINT ( 'NONE',  ( 18.52753015748618282, 38.92559781766745175, -4.923371831947291888 ) ) ;
#58176=CARTESIAN_POINT ( 'NONE',  ( -2.266590686148945544, 46.38708216824730357, -7.082119434687050408 ) ) ;
#58177=CARTESIAN_POINT ( 'NONE',  ( 2.791683348922240793, 51.63393115100078745, 7.208316651077764092 ) ) ;
#58178=CARTESIAN_POINT ( 'NONE',  ( 17.96484262340118221, 61.18868534415482685, -7.964842623401177768 ) ) ;
#58181=CARTESIAN_POINT ( 'NONE',  ( 0.5774900079438590739, 57.64701867748817676, -5.440088680355550821 ) ) ;
#58185=CARTESIAN_POINT ( 'NONE',  ( 22.26659068614895176, 14.72041550158063572, -7.082119434687042414 ) ) ;
#58187=CARTESIAN_POINT ( 'NONE',  ( 13.43411237798105340, 30.58196800326374998, 12.81628187352647963 ) ) ;
#58189=CARTESIAN_POINT ( 'NONE',  ( 21.09922568453594849, 51.20696800326375353, 6.408140936763242479 ) ) ;
#58190=CARTESIAN_POINT ( 'NONE',  ( 2.791683348922237240, 40.38393115100078035, -7.208316651077763204 ) ) ;
#58191=CARTESIAN_POINT ( 'NONE',  ( 20.88017736071110875, 10.77201867748817143, -2.915334737309920765 ) ) ;
#58192=VECTOR ( 'NONE', #40300, 1000.000000000000000 ) ;
#58193=CARTESIAN_POINT ( 'NONE',  ( 16.40814093676323893, 55.79030133659708923, 11.09922568453595026 ) ) ;
#58194=CARTESIAN_POINT ( 'NONE',  ( -46.07360246527855452, 103.8701977390177120, -6.036219926076625164 ) ) ;
#58195=CARTESIAN_POINT ( 'NONE',  ( 19.84674366389459266, 38.71726448433412315, -2.638427012816827677 ) ) ;
#58198=CARTESIAN_POINT ( 'NONE',  ( -45.94000000000000483, 93.00000000000000000, -8.999999999999998224 ) ) ;
#58200=CARTESIAN_POINT ( 'NONE',  ( 0.1532563361054082862, 21.21726448433412315, 2.638427012816831674 ) ) ;
#58201=CARTESIAN_POINT ( 'NONE',  ( 6.565887622018943937, 20.16530133659708213, 12.81628187352647430 ) ) ;
#58203=CARTESIAN_POINT ( 'NONE',  ( 10.00000000000000000, 59.75893115100078745, -9.846743663894594434 ) ) ;
#58205=CARTESIAN_POINT ( 'NONE',  ( 6.204703633549690345, 22.84541550158062861, 14.16423886937410082 ) ) ;
#58206=CARTESIAN_POINT ( 'NONE',  ( 2.791683348922240793, 31.63393115100078745, 7.208316651077764092 ) ) ;
#58207=CARTESIAN_POINT ( 'NONE',  ( 16.40814093676323893, 40.79030133659708923, 11.09922568453595026 ) ) ;
#58210=CARTESIAN_POINT ( 'NONE',  ( 12.91533473730992121, 59.52201867748816966, 10.88017736071110164 ) ) ;
#58211=CARTESIAN_POINT ( 'NONE',  ( -1.099225684535947600, 13.70696800326375353, -6.408140936763238038 ) ) ;
#58214=CARTESIAN_POINT ( 'NONE',  ( 0.1532563361054100626, 40.80059781766745886, -2.638427012816831230 ) ) ;
#58215=CARTESIAN_POINT ( 'NONE',  ( 7.084665262690076126, 44.10535201082151247, 10.88017736071109987 ) ) ;
#58217=CARTESIAN_POINT ( 'NONE',  ( 10.00000000000000000, 42.87363466993042493, -12.81628187352647608 ) ) ;
#58218=CARTESIAN_POINT ( 'NONE',  ( 17.20831665107776587, 37.88393115100078745, 7.208316651077764980 ) ) ;
#58220=CARTESIAN_POINT ( 'NONE',  ( 2.035157376598822676, 32.43868534415483396, -7.964842623401177768 ) ) ;
#58222=CARTESIAN_POINT ( 'NONE',  ( 19.42250999205614193, 20.14701867748817321, 5.440088680355555262 ) ) ;
#58223=CARTESIAN_POINT ( 'NONE',  ( 19.84674366389459621, 53.50893115100078745, 7.409399052514197653E-17 ) ) ;
#58224=CARTESIAN_POINT ( 'NONE',  ( 7.084665262690076126, 24.10535201082150181, 10.88017736071109987 ) ) ;
#58226=B_SPLINE_CURVE_WITH_KNOTS ( 'NONE', 3,
 ( #30940, #61438, #84455, #15954, #55925, #56418 ),
 .UNSPECIFIED., .F., .F.,
 ( 4, 2, 4 ),
 ( 7.805926233243723174E-18, 0.0002626113303185862824, 0.0005252226606371647585 ),
 .UNSPECIFIED. ) ;
#58227=CARTESIAN_POINT ( 'NONE',  ( 12.91533473730992121, 59.52201867748816966, 10.88017736071110164 ) ) ;
#58228=CARTESIAN_POINT ( 'NONE',  ( 2.035157376598822676, 22.43868534415483396, -7.964842623401177768 ) ) ;
#58229=CARTESIAN_POINT ( 'NONE',  ( -2.168404344971008868E-15, 78.76925905125540339, -9.369910658262430303 ) ) ;
#58230=( NAMED_UNIT ( * ) PLANE_ANGLE_UNIT ( ) SI_UNIT ( $, .RADIAN. ) );
#58231=CARTESIAN_POINT ( 'NONE',  ( 7.361572987183169658, 29.96726448433411960, -9.846743663894592657 ) ) ;
#58234=CARTESIAN_POINT ( 'NONE',  ( 1.472469842513823179, 50.59226448433411605, -4.923371831947296329 ) ) ;
#58235=CARTESIAN_POINT ( 'NONE',  ( 17.08211943468705840, 50.13708216824730357, -12.26659068614894466 ) ) ;
#58238=CARTESIAN_POINT ( 'NONE',  ( 13.79529636645031943, 5.345415501580634832, -14.16423886937409904 ) ) ;
#58239=CARTESIAN_POINT ( 'NONE',  ( 6.204703633549690345, 35.76208216824729647, -14.16423886937410259 ) ) ;
#58240=CARTESIAN_POINT ( 'NONE',  ( 6.565887622018943937, 5.165301336597086568, 12.81628187352647430 ) ) ;
#58245=CARTESIAN_POINT ( 'NONE',  ( -0.8801773607111009756, 13.06368534415483929, 1.068504757029289695E-15 ) ) ;
#58246=CARTESIAN_POINT ( 'NONE',  ( 5.076628168052703671, 36.84226448433412315, 8.527530157486179263 ) ) ;
#58248=CARTESIAN_POINT ( 'NONE',  ( 12.91533473730992121, 54.52201867748816255, 10.88017736071110164 ) ) ;
#58251=CARTESIAN_POINT ( 'NONE',  ( 10.00000000000000000, -0.2410688489992152128, -9.846743663894594434 ) ) ;
#58252=CARTESIAN_POINT ( 'NONE',  ( 3.591859063236763294, 23.29030133659708568, -11.09922568453595026 ) ) ;
#58253=CARTESIAN_POINT ( 'NONE',  ( 14.92337183194729988, 29.34226448433411960, -8.527530157486177487 ) ) ;
#58256=DIRECTION ( 'NONE',  ( 0.000000000000000000, 0.000000000000000000, 1.000000000000000000 ) ) ;
#58258=CARTESIAN_POINT ( 'NONE',  ( 24.16423886937410614, 64.51208216824728936, -3.795296366450302550 ) ) ;
#58259=CARTESIAN_POINT ( 'NONE',  ( 15.44008868035555793, 11.39701867748817143, -9.422509992056140149 ) ) ;
#58260=CARTESIAN_POINT ( 'NONE',  ( 10.00000000000000178, 43.05374883491397497, 14.16423886937410082 ) ) ;
#58261=CARTESIAN_POINT ( 'NONE',  ( 4.559911319644449179, 37.23035201082150536, -9.422509992056141925 ) ) ;
#58262=CARTESIAN_POINT ( 'NONE',  ( -0.8801773607111008646, 58.27201867748816966, 2.915334737309923430 ) ) ;
#58264=CARTESIAN_POINT ( 'NONE',  ( 21.92686044187657046, 40.16212336850779963, 4.562052436263912550E-16 ) ) ;
#58265=CARTESIAN_POINT ( 'NONE',  ( 10.00000000000000178, 22.25893115100078745, 9.846743663894594434 ) ) ;
#58267=CARTESIAN_POINT ( 'NONE',  ( 18.52753015748618282, 8.925597817667451750, -4.923371831947291888 ) ) ;
#58269=CARTESIAN_POINT ( 'NONE',  ( 19.84674366389459621, 33.50893115100078745, 7.409399052514197653E-17 ) ) ;
#58270=CARTESIAN_POINT ( 'NONE',  ( 5.076628168052703671, 56.84226448433412315, 8.527530157486179263 ) ) ;
#58271=CARTESIAN_POINT ( 'NONE',  ( 20.88017736071110164, 30.35535201082151247, 2.915334737309930979 ) ) ;
#58272=EDGE_LOOP ( 'NONE', ( #14322, #82505, #11572, #43612 ) ) ;
#58273=CARTESIAN_POINT ( 'NONE',  ( 3.591859063236761518, 44.95696800326376064, 11.09922568453594849 ) ) ;
#58274=CIRCLE ( 'NONE', #4063, 0.5000000000000073275 ) ;
#58276=CARTESIAN_POINT ( 'NONE',  ( 19.42250999205614548, 65.98035201082151957, -5.440088680355545492 ) ) ;
#58277=CARTESIAN_POINT ( 'NONE',  ( 3.591859063236763294, 38.29030133659708923, -11.09922568453595026 ) ) ;
#58278=CARTESIAN_POINT ( 'NONE',  ( 6.204703633549690345, 55.76208216824730357, -14.16423886937410259 ) ) ;
#58279=CARTESIAN_POINT ( 'NONE',  ( 5.076628168052704559, 40.17559781766745175, -8.527530157486179263 ) ) ;
#58281=CARTESIAN_POINT ( 'NONE',  ( 17.20831665107776587, 59.13393115100078745, -7.208316651077762316 ) ) ;
#58282=CARTESIAN_POINT ( 'NONE',  ( 6.204703633549690345, 35.76208216824729647, -14.16423886937410259 ) ) ;
#58283=CARTESIAN_POINT ( 'NONE',  ( 2.791683348922240793, 46.63393115100077324, 7.208316651077764092 ) ) ;
#58284=CARTESIAN_POINT ( 'NONE',  ( 18.17829156368507881, 9.167925641218957367, 6.499999999999990230 ) ) ;
#58285=CARTESIAN_POINT ( 'NONE',  ( 15.44008868035555793, 36.39701867748816966, -9.422509992056140149 ) ) ;
#58286=CARTESIAN_POINT ( 'NONE',  ( 12.91533473730993009, 61.60535201082150536, -10.88017736071109987 ) ) ;
#58289=CARTESIAN_POINT ( 'NONE',  ( -2.816281873526473856, 39.12363466993041783, 9.499525473075851096E-16 ) ) ;
#58291=CARTESIAN_POINT ( 'NONE',  ( 2.035157376598824452, 68.68868534415484817, 7.964842623401179544 ) ) ;
#58292=ORIENTED_EDGE ( 'NONE', *, *, #456, .T. ) ;
#58294=CARTESIAN_POINT ( 'NONE',  ( 17.08211943468705130, 8.470415501580635720, 12.26659068614894998 ) ) ;
#58295=CARTESIAN_POINT ( 'NONE',  ( 14.92337183194729988, 9.342264484334119601, -8.527530157486177487 ) ) ;
#58300=CARTESIAN_POINT ( 'NONE',  ( 10.00000000000000178, 9.313685344154839285, 10.88017736071110342 ) ) ;
#58301=CARTESIAN_POINT ( 'NONE',  ( 19.10478245763058069, 61.02576239577081907, -5.990408912944218400 ) ) ;
#58302=CARTESIAN_POINT ( 'NONE',  ( 10.00000000000000000, 15.55374883491396787, -14.16423886937410082 ) ) ;
#58303=CARTESIAN_POINT ( 'NONE',  ( 12.91533473730992121, 24.52201867748816966, 10.88017736071110164 ) ) ;
#58304=CARTESIAN_POINT ( 'NONE',  ( 17.20831665107776587, 64.13393115100079456, -7.208316651077762316 ) ) ;
#58307=CARTESIAN_POINT ( 'NONE',  ( 14.92337183194729988, 59.34226448433412315, -8.527530157486177487 ) ) ;
#58309=CARTESIAN_POINT ( 'NONE',  ( 20.88017736071110875, 65.77201867748817676, -2.915334737309920765 ) ) ;
#58311=CARTESIAN_POINT ( 'NONE',  ( 16.40814093676324603, 37.45696800326376064, -11.09922568453594671 ) ) ;
#58312=CARTESIAN_POINT ( 'NONE',  ( 15.44008868035555793, 11.39701867748817143, -9.422509992056140149 ) ) ;
#58314=CARTESIAN_POINT ( 'NONE',  ( 7.361572987183169658, -0.03273551566588185635, -9.846743663894592657 ) ) ;
#58315=CARTESIAN_POINT ( 'NONE',  ( 4.559911319644449179, 17.23035201082150536, -9.422509992056141925 ) ) ;
#58317=VERTEX_POINT ( 'NONE', #73496 ) ;
#58318=CARTESIAN_POINT ( 'NONE',  ( 18.52753015748617571, 33.09226448433411605, 4.923371831947298993 ) ) ;
#58319=CARTESIAN_POINT ( 'NONE',  ( 10.00000000000000178, 60.37363466993041783, 12.81628187352647608 ) ) ;
#58320=CARTESIAN_POINT ( 'NONE',  ( 17.96484262340118221, 29.93868534415484106, 7.964842623401181321 ) ) ;
#58321=CARTESIAN_POINT ( 'NONE',  ( -46.94000000000001194, 101.1610691152390586, -7.882642855603069876 ) ) ;
#58323=CARTESIAN_POINT ( 'NONE',  ( 13.43411237798105340, 40.58196800326375353, 12.81628187352647963 ) ) ;
#58324=CARTESIAN_POINT ( 'NONE',  ( 7.084665262690076126, 54.10535201082151247, 10.88017736071109987 ) ) ;
#58325=CARTESIAN_POINT ( 'NONE',  ( 1.472469842513823179, 50.59226448433411605, -4.923371831947296329 ) ) ;
#58326=EDGE_LOOP ( 'NONE', ( #39045, #88165, #15258, #83005, #2882, #63028 ) ) ;
#58328=CARTESIAN_POINT ( 'NONE',  ( 10.00000000000000000, 9.758931151000785675, -9.846743663894594434 ) ) ;
#58329=CARTESIAN_POINT ( 'NONE',  ( 22.81628187352647785, 11.41530133659708390, 3.434112377981063169 ) ) ;
#58331=CARTESIAN_POINT ( 'NONE',  ( 2.791683348922240793, 46.63393115100077324, 7.208316651077764092 ) ) ;
#58332=CARTESIAN_POINT ( 'NONE',  ( 10.00000000000000000, 26.81368534415484106, -10.88017736071110342 ) ) ;
#58333=CARTESIAN_POINT ( 'NONE',  ( 17.20831665107776587, 44.13393115100078745, -7.208316651077762316 ) ) ;
#58335=CARTESIAN_POINT ( 'NONE',  ( 7.361572987183170547, 7.050597817667451750, 9.846743663894590881 ) ) ;
#58337=CARTESIAN_POINT ( 'NONE',  ( 17.20831665107776587, 57.88393115100078745, 7.208316651077764980 ) ) ;
#58339=LINE ( 'NONE', #13351, #83827 ) ;
#58340=CARTESIAN_POINT ( 'NONE',  ( 13.43411237798106583, 42.66530133659707502, -12.81628187352647252 ) ) ;
#58341=CARTESIAN_POINT ( 'NONE',  ( 1.472469842513823179, 36.42559781766745175, 4.923371831947296329 ) ) ;
#58342=CARTESIAN_POINT ( 'NONE',  ( -0.1049300847420783084, 12.21697413083879091, -6.336235997365740502 ) ) ;
#58343=CARTESIAN_POINT ( 'NONE',  ( -4.164238869374099927, 62.01208216824728936, 3.795296366450308767 ) ) ;
#58345=CARTESIAN_POINT ( 'NONE',  ( 0.1532563361054082862, 31.21726448433412315, 2.638427012816831674 ) ) ;
#58346=CARTESIAN_POINT ( 'NONE',  ( -1.926860441876563801, 39.89664270246083788, 3.195792623639529761 ) ) ;
#58347=CARTESIAN_POINT ( 'NONE',  ( -0.3689425029237881626, 57.42874883491397497, 10.36894250292379027 ) ) ;
#58349=CARTESIAN_POINT ( 'NONE',  ( 17.96484262340118221, 19.93868534415484106, 7.964842623401181321 ) ) ;
#58350=CARTESIAN_POINT ( 'NONE',  ( -0.3689425029237898834, 41.17874883491397497, -10.36894250292378850 ) ) ;
#58351=CARTESIAN_POINT ( 'NONE',  ( 10.00000000000000178, 48.05374883491396787, 14.16423886937410082 ) ) ;
#58354=CARTESIAN_POINT ( 'NONE',  ( 7.361572987183170547, 7.050597817667451750, 9.846743663894590881 ) ) ;
#58356=CARTESIAN_POINT ( 'NONE',  ( 2.791683348922240793, 66.63393115100079456, 7.208316651077764092 ) ) ;
#58357=CARTESIAN_POINT ( 'NONE',  ( 18.06765999051784632, 13.99127512925448791, 6.500000000000019540 ) ) ;
#58359=CARTESIAN_POINT ( 'NONE',  ( 15.44008868035555260, 54.73035201082150536, 9.422509992056143702 ) ) ;
#58360=MECHANICAL_DESIGN_GEOMETRIC_PRESENTATION_REPRESENTATION('',(#75938),#69666);
#58362=CARTESIAN_POINT ( 'NONE',  ( 12.63842701281683034, 52.46726448433413026, 9.846743663894596210 ) ) ;
#58364=FILL_AREA_STYLE ('',( #95401 ) ) ;
#58367=CARTESIAN_POINT ( 'NONE',  ( -0.3689425029237898834, 46.17874883491397497, -10.36894250292378850 ) ) ;
#58371=CARTESIAN_POINT ( 'NONE',  ( 0.5774900079438607392, 18.48035201082150536, 5.440088680355550821 ) ) ;
#58372=CARTESIAN_POINT ( 'NONE',  ( 0.6178305044545818747, 43.49863466993042493, -9.382169495545419124 ) ) ;
#58374=CARTESIAN_POINT ( 'NONE',  ( 0.6178305044545838731, 24.74863466993042493, 9.382169495545420901 ) ) ;
#58375=CARTESIAN_POINT ( 'NONE',  ( 22.81628187352647785, 56.41530133659708213, 3.434112377981063169 ) ) ;
#58376=VERTEX_POINT ( 'NONE', #34508 ) ;
#58380=CARTESIAN_POINT ( 'NONE',  ( 13.79529636645031943, 25.34541550158063572, -14.16423886937409904 ) ) ;
#58381=CARTESIAN_POINT ( 'NONE',  ( -4.164238869374098151, 1.595415501580634388, -3.795296366450310543 ) ) ;
#58383=CARTESIAN_POINT ( 'NONE',  ( -0.8801773607111008646, 23.27201867748817676, 2.915334737309923430 ) ) ;
#58386=CARTESIAN_POINT ( 'NONE',  ( 15.44008868035555260, 39.73035201082150536, 9.422509992056143702 ) ) ;
#58387=CARTESIAN_POINT ( 'NONE',  ( 4.559911319644449179, 53.89701867748817676, 9.422509992056141925 ) ) ;
#58388=CARTESIAN_POINT ( 'NONE',  ( 13.43411237798106583, 12.66530133659708746, -12.81628187352647252 ) ) ;
#58390=DIRECTION ( 'NONE',  ( 0.000000000000000000, -1.000000000000000000, 0.000000000000000000 ) ) ;
#58391=CARTESIAN_POINT ( 'NONE',  ( 14.92337183194729633, 27.67559781766745530, 8.527530157486181039 ) ) ;
#58392=CARTESIAN_POINT ( 'NONE',  ( -22.44000000000001194, 93.50000000000000000, 9.500000000000000000 ) ) ;
#58393=CARTESIAN_POINT ( 'NONE',  ( 7.084665262690076126, 44.10535201082151247, 10.88017736071109987 ) ) ;
#58396=CARTESIAN_POINT ( 'NONE',  ( -2.816281873526473856, 9.331968003263753531, 3.434112377981055619 ) ) ;
#58397=( NAMED_UNIT ( * ) SI_UNIT ( $, .STERADIAN. ) SOLID_ANGLE_UNIT ( ) );
#58399=CARTESIAN_POINT ( 'NONE',  ( 7.361572987183169658, 24.96726448433412315, -9.846743663894592657 ) ) ;
#58400=CARTESIAN_POINT ( 'NONE',  ( 13.43411237798106583, 42.66530133659707502, -12.81628187352647252 ) ) ;
#58401=CARTESIAN_POINT ( 'NONE',  ( 2.791683348922237240, 10.38393115100078390, -7.208316651077763204 ) ) ;
#58404=CARTESIAN_POINT ( 'NONE',  ( 0.1532563361054100626, 35.80059781766745175, -2.638427012816831230 ) ) ;
#58405=CARTESIAN_POINT ( 'NONE',  ( 19.42250999205614193, 25.14701867748817321, 5.440088680355555262 ) ) ;
#58407=CARTESIAN_POINT ( 'NONE',  ( -2.266590686148945544, 36.38708216824730357, -7.082119434687050408 ) ) ;
#58408=CARTESIAN_POINT ( 'NONE',  ( 17.20831665107776587, 27.88393115100078390, 7.208316651077764980 ) ) ;
#58409=CARTESIAN_POINT ( 'NONE',  ( 2.035157376598824452, 18.68868534415484106, 7.964842623401179544 ) ) ;
#58410=CARTESIAN_POINT ( 'NONE',  ( 4.559911319644449179, 3.897018677488171434, 9.422509992056141925 ) ) ;
#58412=CARTESIAN_POINT ( 'NONE',  ( 2.035157376598822676, 7.438685344154837509, -7.964842623401177768 ) ) ;
#58414=CARTESIAN_POINT ( 'NONE',  ( 7.084665262690076126, 29.10535201082150181, 10.88017736071109987 ) ) ;
#58416=CARTESIAN_POINT ( 'NONE',  ( 0.5774900079438590739, 42.64701867748816966, -5.440088680355550821 ) ) ;
#58418=CARTESIAN_POINT ( 'NONE',  ( 21.92686044187656691, 27.18830936912750573, 4.562052436263911564E-16 ) ) ;
#58419=CARTESIAN_POINT ( 'NONE',  ( 15.44008868035555793, 36.39701867748816966, -9.422509992056140149 ) ) ;
#58420=CARTESIAN_POINT ( 'NONE',  ( 1.472469842513823179, 66.42559781766745175, 4.923371831947296329 ) ) ;
#58423=CARTESIAN_POINT ( 'NONE',  ( -2.816281873526471635, 63.91530133659708923, -3.434112377981056508 ) ) ;
#58425=CARTESIAN_POINT ( 'NONE',  ( 2.917880565312948704, 27.63708216824730357, 12.26659068614894643 ) ) ;
#58426=CARTESIAN_POINT ( 'NONE',  ( -0.8801773607111008646, 48.27201867748816966, 2.915334737309923430 ) ) ;
#58427=CARTESIAN_POINT ( 'NONE',  ( 19.42250999205614193, 25.14701867748817321, 5.440088680355555262 ) ) ;
#58428=CARTESIAN_POINT ( 'NONE',  ( 19.84674366389459621, 63.50893115100078745, 7.409399052514197653E-17 ) ) ;
#58429=B_SPLINE_CURVE_WITH_KNOTS ( 'NONE', 3,
 ( #70548, #54539, #94030, #2076 ),
 .UNSPECIFIED., .F., .F.,
 ( 4, 4 ),
 ( 0.000000000000000000, 0.002562518741975564930 ),
 .UNSPECIFIED. ) ;
#58430=FACE_OUTER_BOUND ( 'NONE', #64998, .T. ) ;
#58431=CARTESIAN_POINT ( 'NONE',  ( 2.791683348922237240, 55.38393115100078745, -7.208316651077763204 ) ) ;
#58433=CARTESIAN_POINT ( 'NONE',  ( 1.472469842513823179, 15.59226448433411960, -4.923371831947296329 ) ) ;
#58435=CARTESIAN_POINT ( 'NONE',  ( 12.91533473730992121, 19.52201867748816611, 10.88017736071110164 ) ) ;
#58436=CARTESIAN_POINT ( 'NONE',  ( 18.52753015748617571, 28.09226448433411960, 4.923371831947298993 ) ) ;
#58437=CARTESIAN_POINT ( 'NONE',  ( 0.6178305044545818747, 8.498634669930421381, -9.382169495545419124 ) ) ;
#58438=CARTESIAN_POINT ( 'NONE',  ( 12.91533473730992121, 54.52201867748816255, 10.88017736071110164 ) ) ;
#58439=CARTESIAN_POINT ( 'NONE',  ( 20.88017736071110875, 50.77201867748817676, -2.915334737309920765 ) ) ;
#58440=CARTESIAN_POINT ( 'NONE',  ( 17.96484262340118221, 34.93868534415482685, 7.964842623401181321 ) ) ;
#58441=CARTESIAN_POINT ( 'NONE',  ( 6.565887622018943937, 58.08196800326376064, -12.81628187352647608 ) ) ;
#58442=CARTESIAN_POINT ( 'NONE',  ( -2.266590686148945544, 46.38708216824730357, -7.082119434687050408 ) ) ;
#58444=AXIS2_PLACEMENT_3D ( 'NONE', #47674, #24199, #17683 ) ;
#58447=CARTESIAN_POINT ( 'NONE',  ( -2.816281873526473856, -0.6680319967362464695, 3.434112377981055619 ) ) ;
#58448=CARTESIAN_POINT ( 'NONE',  ( 17.96484262340118221, 11.18868534415483929, -7.964842623401177768 ) ) ;
#58449=CARTESIAN_POINT ( 'NONE',  ( 19.42250999205614548, 40.98035201082150536, -5.440088680355545492 ) ) ;
#58450=CARTESIAN_POINT ( 'NONE',  ( 19.84674366389459266, 63.71726448433412315, -2.638427012816827677 ) ) ;
#58452=CARTESIAN_POINT ( 'NONE',  ( 18.52753015748617571, 13.09226448433411960, 4.923371831947298993 ) ) ;
#58453=CARTESIAN_POINT ( 'NONE',  ( 19.84674366389459266, 8.717264484334116048, -2.638427012816827677 ) ) ;
#58454=CARTESIAN_POINT ( 'NONE',  ( 10.00000000000000178, 27.25893115100078390, 9.846743663894594434 ) ) ;
#58456=CARTESIAN_POINT ( 'NONE',  ( 7.361572987183169658, 9.967264484334119601, -9.846743663894592657 ) ) ;
#58458=CARTESIAN_POINT ( 'NONE',  ( 18.17884179759847285, 63.66688879859523809, -6.500000000000002665 ) ) ;
#58459=CARTESIAN_POINT ( 'NONE',  ( 2.791683348922240793, 6.633931151000785675, 7.208316651077764092 ) ) ;
#58461=CARTESIAN_POINT ( 'NONE',  ( 0.1532563361054082862, 6.217264484334118713, 2.638427012816831674 ) ) ;
#58463=CARTESIAN_POINT ( 'NONE',  ( 12.63842701281683922, 24.55059781766745175, -9.846743663894590881 ) ) ;
#58465=ADVANCED_FACE ( 'NONE', ( #67495 ), #56012, .T. ) ;
#58468=CARTESIAN_POINT ( 'NONE',  ( 19.84674366389459621, 63.50893115100078745, 7.409399052514197653E-17 ) ) ;
#58470=( NAMED_UNIT ( * ) PLANE_ANGLE_UNIT ( ) SI_UNIT ( $, .RADIAN. ) );
#58473=CARTESIAN_POINT ( 'NONE',  ( 13.79529636645030344, 13.26208216824729824, 14.16423886937410614 ) ) ;
#58474=EDGE_CURVE ( 'NONE', #31975, #88480, #92587, .T. ) ;
#58475=UNCERTAINTY_MEASURE_WITH_UNIT (LENGTH_MEASURE( 1.000000000000000082E-05 ), #23083, 'distance_accuracy_value', 'NONE');
#58476=DIRECTION ( 'NONE',  ( 0.000000000000000000, 0.000000000000000000, 1.000000000000000000 ) ) ;
#58477=CARTESIAN_POINT ( 'NONE',  ( 13.79529636645030344, 18.26208216824730002, 14.16423886937410614 ) ) ;
#58478=CARTESIAN_POINT ( 'NONE',  ( 2.917880565312948704, 42.63708216824729647, 12.26659068614894643 ) ) ;
#58479=CARTESIAN_POINT ( 'NONE',  ( 24.16423886937410614, 9.512082168247301794, -3.795296366450302550 ) ) ;
#58480=CARTESIAN_POINT ( 'NONE',  ( -0.8801773607111008646, 38.27201867748816255, 2.915334737309923430 ) ) ;
#58483=CARTESIAN_POINT ( 'NONE',  ( 1.472469842513823179, 21.42559781766745175, 4.923371831947296329 ) ) ;
#58484=CARTESIAN_POINT ( 'NONE',  ( 0.5774900079438590739, 57.64701867748817676, -5.440088680355550821 ) ) ;
#58485=CARTESIAN_POINT ( 'NONE',  ( 19.84674366389459266, 33.71726448433410894, -2.638427012816827677 ) ) ;
#58487=CARTESIAN_POINT ( 'NONE',  ( 4.559911319644449179, 7.230352010821505360, -9.422509992056141925 ) ) ;
#58488=CARTESIAN_POINT ( 'NONE',  ( -1.099225684535947600, 64.54030133659709634, 6.408140936763237150 ) ) ;
#58489=CARTESIAN_POINT ( 'NONE',  ( 5.076628168052703671, 56.84226448433412315, 8.527530157486179263 ) ) ;
#58491=MECHANICAL_DESIGN_GEOMETRIC_PRESENTATION_REPRESENTATION('',(#2659),#1070);
#58492=CARTESIAN_POINT ( 'NONE',  ( 6.565887622018943937, 38.08196800326376064, -12.81628187352647608 ) ) ;
#58495=CARTESIAN_POINT ( 'NONE',  ( 0.5774900079438590739, 47.64701867748817676, -5.440088680355550821 ) ) ;
#58496=CARTESIAN_POINT ( 'NONE',  ( 17.20831665107776587, 37.88393115100078745, 7.208316651077764980 ) ) ;
#58497=CARTESIAN_POINT ( 'NONE',  ( 20.36894250292379738, 29.92874883491396432, -10.36894250292379027 ) ) ;
#58500=CARTESIAN_POINT ( 'NONE',  ( 0.5774900079438590739, 52.64701867748817676, -5.440088680355550821 ) ) ;
#58501=CARTESIAN_POINT ( 'NONE',  ( -0.8801773607111009756, 63.06368534415484106, 1.068504757029289695E-15 ) ) ;
#58502=CARTESIAN_POINT ( 'NONE',  ( 6.204703633549690345, 50.76208216824730357, -14.16423886937410259 ) ) ;
#58503=CARTESIAN_POINT ( 'NONE',  ( 0.1532563361054082862, 66.21726448433413736, 2.638427012816831674 ) ) ;
#58504=CARTESIAN_POINT ( 'NONE',  ( 22.81628187352647785, 61.41530133659709634, 3.434112377981063169 ) ) ;
#58505=CARTESIAN_POINT ( 'NONE',  ( 4.559911319644449179, 38.89701867748817676, 9.422509992056141925 ) ) ;
#58506=EDGE_CURVE ( 'NONE', #72124, #30282, #46116, .T. ) ;
#58507=DIRECTION ( 'NONE',  ( 0.000000000000000000, -1.000000000000000000, 0.000000000000000000 ) ) ;
#58508=CARTESIAN_POINT ( 'NONE',  ( 2.791683348922237240, 60.38393115100078745, -7.208316651077763204 ) ) ;
#58510=FILL_AREA_STYLE ('',( #41574 ) ) ;
#58511=CARTESIAN_POINT ( 'NONE',  ( 4.559911319644449179, 7.230352010821505360, -9.422509992056141925 ) ) ;
#58513=ORIENTED_EDGE ( 'NONE', *, *, #43080, .F. ) ;
#58517=CARTESIAN_POINT ( 'NONE',  ( 0.5774900079438590739, 67.64701867748817676, -5.440088680355550821 ) ) ;
#58518=CARTESIAN_POINT ( 'NONE',  ( 19.42250999205614193, 65.14701867748817676, 5.440088680355555262 ) ) ;
#58520=CARTESIAN_POINT ( 'NONE',  ( 19.84674366389459266, 28.71726448433411960, -2.638427012816827677 ) ) ;
#58521=CARTESIAN_POINT ( 'NONE',  ( -0.8801773607111008646, 23.27201867748817676, 2.915334737309923430 ) ) ;
#58522=CARTESIAN_POINT ( 'NONE',  ( 19.38216949554541202, 5.998634669930420493, 9.382169495545424454 ) ) ;
#58523=CARTESIAN_POINT ( 'NONE',  ( 12.91533473730993009, 31.60535201082150891, -10.88017736071109987 ) ) ;
#58525=CARTESIAN_POINT ( 'NONE',  ( -2.816281873526473856, 34.33196800326376064, 3.434112377981055619 ) ) ;
#58527=CARTESIAN_POINT ( 'NONE',  ( 7.084665262690076126, 67.02201867748817676, -10.88017736071110164 ) ) ;
#58528=CARTESIAN_POINT ( 'NONE',  ( 0.6178305044545818747, 23.49863466993041783, -9.382169495545419124 ) ) ;
#58530=CARTESIAN_POINT ( 'NONE',  ( 10.00000000000000000, -0.2410688489992152128, -9.846743663894594434 ) ) ;
#58531=CARTESIAN_POINT ( 'NONE',  ( 7.084665262690076126, 34.10535201082151247, 10.88017736071109987 ) ) ;
#58533=CARTESIAN_POINT ( 'NONE',  ( 2.917880565312950480, 60.97041550158063927, -12.26659068614894821 ) ) ;
#58534=CARTESIAN_POINT ( 'NONE',  ( 14.92337183194729988, 49.34226448433411605, -8.527530157486177487 ) ) ;
#58535=CARTESIAN_POINT ( 'NONE',  ( 0.5774900079438607392, 68.48035201082150536, 5.440088680355550821 ) ) ;
#58536=CARTESIAN_POINT ( 'NONE',  ( -0.8801773607110991993, 57.85535201082149825, -2.915334737309923874 ) ) ;
#58537=CARTESIAN_POINT ( 'NONE',  ( 0.1143410931637199451, 5.216910754863025801, 6.480892540919842126 ) ) ;
#58538=CARTESIAN_POINT ( 'NONE',  ( 24.16423886937409904, 24.09541550158063927, 3.795296366450317205 ) ) ;
#58544=CARTESIAN_POINT ( 'NONE',  ( -4.164238869374098151, 56.59541550158063927, -3.795296366450310543 ) ) ;
#58545=CARTESIAN_POINT ( 'NONE',  ( 6.204703633549690345, 45.76208216824729647, -14.16423886937410259 ) ) ;
#58546=CARTESIAN_POINT ( 'NONE',  ( 19.84674366389459266, 28.71726448433411960, -2.638427012816827677 ) ) ;
#58547=CARTESIAN_POINT ( 'NONE',  ( 13.43411237798106583, 27.66530133659708568, -12.81628187352647252 ) ) ;
#58549=CARTESIAN_POINT ( 'NONE',  ( 7.084665262690076126, 14.10535201082150358, 10.88017736071109987 ) ) ;
#58550=CARTESIAN_POINT ( 'NONE',  ( 2.917880565312948704, 52.63708216824730357, 12.26659068614894643 ) ) ;
#58552=CARTESIAN_POINT ( 'NONE',  ( 5.076628168052703671, 31.84226448433412315, 8.527530157486179263 ) ) ;
#58553=CARTESIAN_POINT ( 'NONE',  ( 1.274849032794305170, 12.55509018479935968, -6.499999999999995559 ) ) ;
#58554=CARTESIAN_POINT ( 'NONE',  ( 0.1532563361054100626, 10.80059781766745175, -2.638427012816831230 ) ) ;
#58555=CARTESIAN_POINT ( 'NONE',  ( 17.62281668512001431, 58.28593319516822646, 6.500000000000010658 ) ) ;
#58562=CARTESIAN_POINT ( 'NONE',  ( 22.26659068614895176, 14.72041550158063572, -7.082119434687042414 ) ) ;
#58563=CARTESIAN_POINT ( 'NONE',  ( 7.084665262690076126, 17.02201867748817676, -10.88017736071110164 ) ) ;
#58564=CARTESIAN_POINT ( 'NONE',  ( 15.44008868035555260, 29.73035201082150891, 9.422509992056143702 ) ) ;
#58565=CARTESIAN_POINT ( 'NONE',  ( 19.84674366389459621, 43.50893115100078745, 7.409399052514197653E-17 ) ) ;
#58566=CARTESIAN_POINT ( 'NONE',  ( -1.099225684535947600, 18.70696800326375353, -6.408140936763238038 ) ) ;
#58567=CARTESIAN_POINT ( 'NONE',  ( 10.00000000000000000, 10.55374883491396787, -14.16423886937410082 ) ) ;
#58573=CARTESIAN_POINT ( 'NONE',  ( 16.40814093676324603, 27.45696800326375708, -11.09922568453594671 ) ) ;
#58574=ORIENTED_EDGE ( 'NONE', *, *, #95864, .T. ) ;
#58575=CARTESIAN_POINT ( 'NONE',  ( 14.92337183194729633, 27.67559781766745530, 8.527530157486181039 ) ) ;
#58576=CARTESIAN_POINT ( 'NONE',  ( -4.164238869374098151, 56.59541550158063927, -3.795296366450310543 ) ) ;
#58577=ORIENTED_EDGE ( 'NONE', *, *, #98768, .F. ) ;
#58578=CARTESIAN_POINT ( 'NONE',  ( 2.917880565312950480, 65.97041550158063217, -12.26659068614894821 ) ) ;
#58580=CARTESIAN_POINT ( 'NONE',  ( 4.559911319644449179, 52.23035201082151247, -9.422509992056141925 ) ) ;
#58581=CARTESIAN_POINT ( 'NONE',  ( 4.559911319644449179, 43.89701867748816966, 9.422509992056141925 ) ) ;
#58582=CARTESIAN_POINT ( 'NONE',  ( 4.559911319644449179, 52.23035201082151247, -9.422509992056141925 ) ) ;
#58584=CARTESIAN_POINT ( 'NONE',  ( 15.44008868035555260, 34.73035201082151247, 9.422509992056143702 ) ) ;
#58589=CARTESIAN_POINT ( 'NONE',  ( 18.52753015748617571, 33.09226448433411605, 4.923371831947298993 ) ) ;
#58591=CARTESIAN_POINT ( 'NONE',  ( 19.84674366389459266, 58.71726448433411605, -2.638427012816827677 ) ) ;
#58592=CARTESIAN_POINT ( 'NONE',  ( -0.1503990784575260087, 24.24884699246888786, -6.262539305110081500 ) ) ;
#58595=B_SPLINE_CURVE_WITH_KNOTS ( 'NONE', 3,
 ( #72412, #96427, #50406, #27410, #87425, #57901, #89397 ),
 .UNSPECIFIED., .F., .F.,
 ( 4, 3, 4 ),
 ( 1.748223473168675632E-18, 0.001126965689051421778, 0.002254079279539391613 ),
 .UNSPECIFIED. ) ;
#58596=CARTESIAN_POINT ( 'NONE',  ( 24.16423886937410614, 4.303748834913967869, 8.672049930838204340E-16 ) ) ;
#58599=CARTESIAN_POINT ( 'NONE',  ( 1.046131998949896280, 25.73810908735718428, 6.499999999999989342 ) ) ;
#58600=CARTESIAN_POINT ( 'NONE',  ( 20.36894250292379738, 64.92874883491397497, -10.36894250292379027 ) ) ;
#58602=VERTEX_POINT ( 'NONE', #78577 ) ;
#58603=( BOUNDED_CURVE ( )  B_SPLINE_CURVE ( 2, ( #70322, #48287, #40313, #41312, #16821, #9811, #94277, #1837, #10306 ),
 .UNSPECIFIED., .F., .F. ) 
 B_SPLINE_CURVE_WITH_KNOTS ( ( 3, 2, 2, 2, 3 ),
 ( 0.6544266512259456769, 0.6547619047619047672, 0.6607142857142858094, 0.6666666666666667407, 0.6670019202026259419 ),
 .UNSPECIFIED. ) 
 CURVE ( )  GEOMETRIC_REPRESENTATION_ITEM ( )  RATIONAL_B_SPLINE_CURVE ( ( 0.9963778908391764944, 0.9980808541467923733, 1.000000000000000000, 0.9659258262890683122, 1.000000000000000000, 0.9659258262890683122, 1.000000000000000000, 0.9980808541467917072, 0.9963778908391753841 ) ) 
 REPRESENTATION_ITEM ( '' )  );
#58605=CARTESIAN_POINT ( 'NONE',  ( 2.791683348922240793, 36.63393115100078035, 7.208316651077764092 ) ) ;
#58607=CARTESIAN_POINT ( 'NONE',  ( 21.09922568453594849, 6.206968003263753531, 6.408140936763242479 ) ) ;
#58608=CARTESIAN_POINT ( 'NONE',  ( 19.84674366389459266, 13.71726448433411782, -2.638427012816827677 ) ) ;
#58609=CARTESIAN_POINT ( 'NONE',  ( 2.603489959281588995, 40.43575266056827644, -6.500000000000003553 ) ) ;
#58610=CARTESIAN_POINT ( 'NONE',  ( 19.84674366389459266, 3.300597817667451750, 2.638427012816836559 ) ) ;
#58611=CARTESIAN_POINT ( 'NONE',  ( 22.81628187352647785, 6.415301336597088344, 3.434112377981063169 ) ) ;
#58614=VECTOR ( 'NONE', #10163, 1000.000000000000000 ) ;
#58616=CARTESIAN_POINT ( 'NONE',  ( 19.42250999205614193, 10.14701867748816966, 5.440088680355555262 ) ) ;
#58617=CARTESIAN_POINT ( 'NONE',  ( 24.16423886937410614, 4.512082168247300906, -3.795296366450302550 ) ) ;
#58618=CARTESIAN_POINT ( 'NONE',  ( 14.92337183194729633, 22.67559781766745175, 8.527530157486181039 ) ) ;
#58619=CARTESIAN_POINT ( 'NONE',  ( 17.96484262340118221, 56.18868534415484817, -7.964842623401177768 ) ) ;
#58620=CARTESIAN_POINT ( 'NONE',  ( 0.6178305044545838731, 24.74863466993042493, 9.382169495545420901 ) ) ;
#58622=CARTESIAN_POINT ( 'NONE',  ( 15.44008868035555793, 6.397018677488170546, -9.422509992056140149 ) ) ;
#58627=CARTESIAN_POINT ( 'NONE',  ( 3.591859063236761518, 4.956968003263753531, 11.09922568453594849 ) ) ;
#58628=CARTESIAN_POINT ( 'NONE',  ( 21.09922568453594849, 1.206968003263753531, 6.408140936763242479 ) ) ;
#58629=CARTESIAN_POINT ( 'NONE',  ( 0.1532563361054082862, 16.21726448433411960, 2.638427012816831674 ) ) ;
#58631=CARTESIAN_POINT ( 'NONE',  ( 10.00000000000000178, 25.37363466993041783, 12.81628187352647608 ) ) ;
#58633=CARTESIAN_POINT ( 'NONE',  ( 20.88017736071110875, 25.77201867748816966, -2.915334737309920765 ) ) ;
#58635=CARTESIAN_POINT ( 'NONE',  ( 13.79529636645031943, 50.34541550158064638, -14.16423886937409904 ) ) ;
#58636=CIRCLE ( 'NONE', #74623, 0.5000000000000004441 ) ;
#58639=CARTESIAN_POINT ( 'NONE',  ( 12.91533473730993009, 26.60535201082150536, -10.88017736071109987 ) ) ;
#58640=CARTESIAN_POINT ( 'NONE',  ( 1.472469842513823179, 45.59226448433412315, -4.923371831947296329 ) ) ;
#58641=CARTESIAN_POINT ( 'NONE',  ( 12.91533473730993009, 51.60535201082149825, -10.88017736071109987 ) ) ;
#58642=CARTESIAN_POINT ( 'NONE',  ( 22.26659068614894466, 33.88708216824730357, 7.082119434687054849 ) ) ;
#58644=CARTESIAN_POINT ( 'NONE',  ( 19.84674366389459621, 33.50893115100078745, 7.409399052514197653E-17 ) ) ;
#58645=CARTESIAN_POINT ( 'NONE',  ( -1.099225684535947600, 59.54030133659708923, 6.408140936763237150 ) ) ;
#58646=CARTESIAN_POINT ( 'NONE',  ( 7.361572987183170547, 62.05059781766745886, 9.846743663894590881 ) ) ;
#58648=CARTESIAN_POINT ( 'NONE',  ( 19.42250999205614193, 25.14701867748817321, 5.440088680355555262 ) ) ;
#58649=CARTESIAN_POINT ( 'NONE',  ( 0.5774900079438590739, 12.64701867748817321, -5.440088680355550821 ) ) ;
#58650=CARTESIAN_POINT ( 'NONE',  ( 5.076628168052703671, 1.842264484334118047, 8.527530157486179263 ) ) ;
#58651=CARTESIAN_POINT ( 'NONE',  ( -4.164238869374099039, 21.80374883491396787, 8.674139862899312516E-16 ) ) ;
#58652=CARTESIAN_POINT ( 'NONE',  ( 0.1532563361054100626, 10.80059781766745175, -2.638427012816831230 ) ) ;
#58653=CARTESIAN_POINT ( 'NONE',  ( 17.20831665107776587, 57.88393115100078745, 7.208316651077764980 ) ) ;
#58654=CARTESIAN_POINT ( 'NONE',  ( -0.8801773607110991993, 37.85535201082151247, -2.915334737309923874 ) ) ;
#58656=CARTESIAN_POINT ( 'NONE',  ( -45.94000000000001194, 103.9981609152045650, -5.961202730336927047 ) ) ;
#58658=DIRECTION ( 'NONE',  ( -0.9970872288863208421, -0.07626964003977952655, 0.000000000000000000 ) ) ;
#58659=CARTESIAN_POINT ( 'NONE',  ( 12.63842701281683922, 44.55059781766745175, -9.846743663894590881 ) ) ;
#58660=VERTEX_POINT ( 'NONE', #79059 ) ;
#58661=VERTEX_POINT ( 'NONE', #85591 ) ;
#58662=CARTESIAN_POINT ( 'NONE',  ( -0.8801773607111009756, 63.06368534415484106, 1.068504757029289695E-15 ) ) ;
#58663=CARTESIAN_POINT ( 'NONE',  ( -0.3689425029237881626, 27.42874883491397142, 10.36894250292379027 ) ) ;
#58664=CARTESIAN_POINT ( 'NONE',  ( 22.26659068614894466, 13.88708216824730179, 7.082119434687054849 ) ) ;
#58665=CARTESIAN_POINT ( 'NONE',  ( 15.44008868035555793, 66.39701867748817676, -9.422509992056140149 ) ) ;
#58666=CARTESIAN_POINT ( 'NONE',  ( 2.917880565312950480, 55.97041550158063217, -12.26659068614894821 ) ) ;
#58667=CARTESIAN_POINT ( 'NONE',  ( 17.20831665107776587, 64.13393115100079456, -7.208316651077762316 ) ) ;
#58668=CARTESIAN_POINT ( 'NONE',  ( 1.472469842513823179, 31.42559781766745530, 4.923371831947296329 ) ) ;
#58670=CARTESIAN_POINT ( 'NONE',  ( 17.96484262340118221, 29.93868534415484106, 7.964842623401181321 ) ) ;
#58671=CARTESIAN_POINT ( 'NONE',  ( 13.43411237798106583, 2.665301336597086568, -12.81628187352647252 ) ) ;
#58672=CARTESIAN_POINT ( 'NONE',  ( 20.36894250292379382, 18.67874883491397142, 10.36894250292379205 ) ) ;
#58673=B_SPLINE_CURVE_WITH_KNOTS ( 'NONE', 3,
 ( #1725, #17702, #32179, #92695, #78685, #40192, #93182, #85694, #70699, #32677 ),
 .UNSPECIFIED., .F., .F.,
 ( 4, 3, 3, 4 ),
 ( 0.000000000000000000, 0.0006253016069560883442, 0.001250604074564952515, 0.002501455912506551308 ),
 .UNSPECIFIED. ) ;
#58674=CARTESIAN_POINT ( 'NONE',  ( -4.164238869374099927, 47.01208216824729647, 3.795296366450308767 ) ) ;
#58676=CARTESIAN_POINT ( 'NONE',  ( 19.42250999205614193, 20.14701867748817321, 5.440088680355555262 ) ) ;
#58677=CARTESIAN_POINT ( 'NONE',  ( -0.2538888227782572504, 0.000000000000000000, 6.092555545977056397 ) ) ;
#58679=CARTESIAN_POINT ( 'NONE',  ( -0.8801773607111009756, 43.06368534415484106, 1.068504757029289695E-15 ) ) ;
#58684=CARTESIAN_POINT ( 'NONE',  ( -4.164238869374099927, 42.01208216824728936, 3.795296366450308767 ) ) ;
#58685=CARTESIAN_POINT ( 'NONE',  ( 17.20831665107776587, 49.13393115100078745, -7.208316651077762316 ) ) ;
#58686=CARTESIAN_POINT ( 'NONE',  ( 0.5774900079438590739, 57.64701867748817676, -5.440088680355550821 ) ) ;
#58690=CARTESIAN_POINT ( 'NONE',  ( 0.5774900079438607392, 53.48035201082151247, 5.440088680355550821 ) ) ;
#58693=CARTESIAN_POINT ( 'NONE',  ( -0.3689425029237881626, 17.42874883491397142, 10.36894250292379027 ) ) ;
#58694=CARTESIAN_POINT ( 'NONE',  ( 16.40814093676323893, 25.79030133659708923, 11.09922568453595026 ) ) ;
#58696=CARTESIAN_POINT ( 'NONE',  ( -2.816281873526471635, 38.91530133659708213, -3.434112377981056508 ) ) ;
#58698=CARTESIAN_POINT ( 'NONE',  ( 19.84674366389459266, 33.30059781766744464, 2.638427012816836559 ) ) ;
#58699=CARTESIAN_POINT ( 'NONE',  ( 4.559911319644449179, 13.89701867748817143, 9.422509992056141925 ) ) ;
#58700=CARTESIAN_POINT ( 'NONE',  ( 22.81628187352647785, 51.41530133659708923, 3.434112377981063169 ) ) ;
#58702=CARTESIAN_POINT ( 'NONE',  ( 17.20831665107776587, 44.13393115100078745, -7.208316651077762316 ) ) ;
#58708=CARTESIAN_POINT ( 'NONE',  ( 0.1922240491738519130, 3.188781737317406328, 6.500000000000000888 ) ) ;
#58711=CARTESIAN_POINT ( 'NONE',  ( -0.1049300847420783223, 17.21697413083878914, -6.336235997365740502 ) ) ;
#58712=CARTESIAN_POINT ( 'NONE',  ( 5.076628168052703671, 21.84226448433411960, 8.527530157486179263 ) ) ;
#58714=CARTESIAN_POINT ( 'NONE',  ( -1.099225684535947600, 18.70696800326375353, -6.408140936763238038 ) ) ;
#58718=CARTESIAN_POINT ( 'NONE',  ( -4.164238869374099927, 22.01208216824730357, 3.795296366450308767 ) ) ;
#58719=CARTESIAN_POINT ( 'NONE',  ( 7.361572987183170547, 52.05059781766745175, 9.846743663894590881 ) ) ;
#58720=CARTESIAN_POINT ( 'NONE',  ( 21.09922568453595559, 47.04030133659708923, -6.408140936763230044 ) ) ;
#58721=CARTESIAN_POINT ( 'NONE',  ( 20.15039907845753220, 37.62777174578614847, -6.262539305110077947 ) ) ;
#58723=CARTESIAN_POINT ( 'NONE',  ( 17.96484262340118221, 66.18868534415483396, -7.964842623401177768 ) ) ;
#58725=CARTESIAN_POINT ( 'NONE',  ( 7.361572987183169658, 34.96726448433411605, -9.846743663894592657 ) ) ;
#58726=CARTESIAN_POINT ( 'NONE',  ( -0.8801773607111008646, 38.27201867748816255, 2.915334737309923430 ) ) ;
#58727=CARTESIAN_POINT ( 'NONE',  ( 19.38216949554541557, 42.24863466993041783, -9.382169495545420901 ) ) ;
#58728=CARTESIAN_POINT ( 'NONE',  ( 18.52753015748617571, 33.09226448433411605, 4.923371831947298993 ) ) ;
#58731=CARTESIAN_POINT ( 'NONE',  ( 19.42250999205614193, 50.14701867748817676, 5.440088680355555262 ) ) ;
#58733=CARTESIAN_POINT ( 'NONE',  ( 7.084665262690076126, 69.10535201082151957, 10.88017736071109987 ) ) ;
#58734=CARTESIAN_POINT ( 'NONE',  ( -0.8801773607110991993, 12.85535201082150358, -2.915334737309923874 ) ) ;
#58735=CARTESIAN_POINT ( 'NONE',  ( 12.63842701281683034, 62.46726448433410894, 9.846743663894596210 ) ) ;
#58736=CARTESIAN_POINT ( 'NONE',  ( 0.5774900079438590739, 47.64701867748817676, -5.440088680355550821 ) ) ;
#58737=DIRECTION ( 'NONE',  ( 0.000000000000000000, 1.000000000000000000, 0.000000000000000000 ) ) ;
#58738=CARTESIAN_POINT ( 'NONE',  ( -0.8801773607111009756, 63.06368534415484106, 1.068504757029289695E-15 ) ) ;
#58739=CARTESIAN_POINT ( 'NONE',  ( 15.44008868035555793, 21.39701867748817321, -9.422509992056140149 ) ) ;
#58741=CARTESIAN_POINT ( 'NONE',  ( 10.00000000000000178, 2.258931151000784787, 9.846743663894594434 ) ) ;
#58742=CARTESIAN_POINT ( 'NONE',  ( 0.1532563361054082862, 31.21726448433412315, 2.638427012816831674 ) ) ;
#58745=CARTESIAN_POINT ( 'NONE',  ( 19.84674366389459621, 53.50893115100078745, 7.409399052514197653E-17 ) ) ;
#58746=CARTESIAN_POINT ( 'NONE',  ( 10.00000000000000000, 50.55374883491396787, -14.16423886937410082 ) ) ;
#58749=CARTESIAN_POINT ( 'NONE',  ( -4.164238869374098151, 11.59541550158063217, -3.795296366450310543 ) ) ;
#58750=CARTESIAN_POINT ( 'NONE',  ( 2.917880565312948704, 32.63708216824730357, 12.26659068614894643 ) ) ;
#58752=CARTESIAN_POINT ( 'NONE',  ( 3.591859063236763294, 3.290301336597087012, -11.09922568453595026 ) ) ;
#58754=CARTESIAN_POINT ( 'NONE',  ( 20.88017736071110164, 20.35535201082150891, 2.915334737309930979 ) ) ;
#58755=CARTESIAN_POINT ( 'NONE',  ( 5.076628168052704559, 50.17559781766745886, -8.527530157486179263 ) ) ;
#58756=CARTESIAN_POINT ( 'NONE',  ( 6.204703633549690345, 0.7620821682473009062, -14.16423886937410259 ) ) ;
#58760=CARTESIAN_POINT ( 'NONE',  ( -2.816281873526473856, 19.12363466993042138, 9.499525473075851096E-16 ) ) ;
#58761=CARTESIAN_POINT ( 'NONE',  ( 14.92337183194729633, 27.67559781766745530, 8.527530157486181039 ) ) ;
#58763=CARTESIAN_POINT ( 'NONE',  ( 5.076628168052703671, 1.842264484334118047, 8.527530157486179263 ) ) ;
#58765=CARTESIAN_POINT ( 'NONE',  ( 15.44008868035555793, 6.397018677488171434, -9.422509992056140149 ) ) ;
#58766=CARTESIAN_POINT ( 'NONE',  ( 2.035157376598824452, 13.68868534415483751, 7.964842623401179544 ) ) ;
#58767=CARTESIAN_POINT ( 'NONE',  ( -4.164238869374098151, 41.59541550158061796, -3.795296366450310543 ) ) ;
#58768=CARTESIAN_POINT ( 'NONE',  ( 4.559911319644449179, 47.23035201082150536, -9.422509992056141925 ) ) ;
#58770=CARTESIAN_POINT ( 'NONE',  ( 17.96484262340118221, 61.18868534415482685, -7.964842623401177768 ) ) ;
#58772=CARTESIAN_POINT ( 'NONE',  ( 18.18329248733323311, 17.60290668512020318, 6.499999999999984901 ) ) ;
#58773=CARTESIAN_POINT ( 'NONE',  ( 7.361572987183169658, 24.96726448433412315, -9.846743663894592657 ) ) ;
#58775=CARTESIAN_POINT ( 'NONE',  ( 10.00000000000000178, 7.258931151000785675, 9.846743663894594434 ) ) ;
#58776=CARTESIAN_POINT ( 'NONE',  ( 2.791683348922240793, 31.63393115100078745, 7.208316651077764092 ) ) ;
#58777=CARTESIAN_POINT ( 'NONE',  ( -2.816281873526471635, -1.084698663402913210, -3.434112377981056508 ) ) ;
#58778=CARTESIAN_POINT ( 'NONE',  ( 19.42250999205614548, 35.98035201082151247, -5.440088680355545492 ) ) ;
#58781=VERTEX_POINT ( 'NONE', #26073 ) ;
#58782=CARTESIAN_POINT ( 'NONE',  ( 0.6178305044545838731, 54.74863466993042493, 9.382169495545420901 ) ) ;
#58783=CARTESIAN_POINT ( 'NONE',  ( 1.472469842513823179, 1.425597817667451528, 4.923371831947296329 ) ) ;
#58784=CARTESIAN_POINT ( 'NONE',  ( 19.38216949554541557, 37.24863466993041783, -9.382169495545420901 ) ) ;
#58785=CARTESIAN_POINT ( 'NONE',  ( 10.00000000000000000, 60.55374883491397497, -14.16423886937410082 ) ) ;
#58786=CARTESIAN_POINT ( 'NONE',  ( 10.00000000000000178, 32.25893115100078745, 9.846743663894594434 ) ) ;
#58787=CARTESIAN_POINT ( 'NONE',  ( 1.046131998950050157, 50.73810908735727310, 6.499999999999992006 ) ) ;
#58789=CARTESIAN_POINT ( 'NONE',  ( 17.08211943468705130, 48.47041550158063927, 12.26659068614894998 ) ) ;
#58790=CARTESIAN_POINT ( 'NONE',  ( 1.472469842513823179, 41.42559781766745886, 4.923371831947296329 ) ) ;
#58792=CARTESIAN_POINT ( 'NONE',  ( 10.00000000000000000, 36.81368534415484106, -10.88017736071110342 ) ) ;
#58793=CARTESIAN_POINT ( 'NONE',  ( -0.8801773607111008646, 63.27201867748817676, 2.915334737309923430 ) ) ;
#58796=CARTESIAN_POINT ( 'NONE',  ( -1.099225684535947600, 48.70696800326375353, -6.408140936763238038 ) ) ;
#58797=ORIENTED_EDGE ( 'NONE', *, *, #68556, .T. ) ;
#58798=CARTESIAN_POINT ( 'NONE',  ( 20.88017736071110875, 65.77201867748817676, -2.915334737309920765 ) ) ;
#58799=EDGE_LOOP ( 'NONE', ( #63695, #79616, #97863, #20327, #40110 ) ) ;
#58800=CARTESIAN_POINT ( 'NONE',  ( -2.266590686148945544, 6.387082168247300906, -7.082119434687050408 ) ) ;
#58801=CARTESIAN_POINT ( 'NONE',  ( 10.00000000000000178, 12.25893115100078568, 9.846743663894594434 ) ) ;
#58805=CARTESIAN_POINT ( 'NONE',  ( 12.91533473730993009, 16.60535201082150891, -10.88017736071109987 ) ) ;
#58806=CARTESIAN_POINT ( 'NONE',  ( 19.10478245763055227, 60.10160829253886305, 5.990408912944262809 ) ) ;
#58807=CARTESIAN_POINT ( 'NONE',  ( -0.3689425029237881626, 22.42874883491397142, 10.36894250292379027 ) ) ;
#58809=CARTESIAN_POINT ( 'NONE',  ( 0.5774900079438590739, 27.64701867748817676, -5.440088680355550821 ) ) ;
#58810=CARTESIAN_POINT ( 'NONE',  ( 7.361572987183169658, 54.96726448433413026, -9.846743663894592657 ) ) ;
#58811=ORIENTED_EDGE ( 'NONE', *, *, #11731, .F. ) ;
#58812=CARTESIAN_POINT ( 'NONE',  ( 17.20831665107776587, 57.88393115100078745, 7.208316651077764980 ) ) ;
#58813=ORIENTED_EDGE ( 'NONE', *, *, #39658, .F. ) ;
#58814=CARTESIAN_POINT ( 'NONE',  ( 4.559911319644449179, 62.23035201082150536, -9.422509992056141925 ) ) ;
#58815=CARTESIAN_POINT ( 'NONE',  ( 10.00000000000000178, 62.25893115100078745, 9.846743663894594434 ) ) ;
#58816=CARTESIAN_POINT ( 'NONE',  ( -1.099225684535947600, 34.54030133659708923, 6.408140936763237150 ) ) ;
#58818=CARTESIAN_POINT ( 'NONE',  ( 1.472469842513823179, 6.425597817667451750, 4.923371831947296329 ) ) ;
#58819=CARTESIAN_POINT ( 'NONE',  ( 2.035157376598824452, 23.68868534415484461, 7.964842623401179544 ) ) ;
#58822=CARTESIAN_POINT ( 'NONE',  ( 22.81628187352648496, 56.83196800326374643, -3.434112377981050290 ) ) ;
#58823=CARTESIAN_POINT ( 'NONE',  ( 2.035157376598824452, 38.68868534415483396, 7.964842623401179544 ) ) ;
#58825=CARTESIAN_POINT ( 'NONE',  ( 19.38216949554541202, 35.99863466993041072, 9.382169495545424454 ) ) ;
#58826=CARTESIAN_POINT ( 'NONE',  ( 4.559911319644449179, 52.23035201082151247, -9.422509992056141925 ) ) ;
#58827=CARTESIAN_POINT ( 'NONE',  ( 12.63842701281683922, 59.55059781766744464, -9.846743663894590881 ) ) ;
#58830=B_SPLINE_CURVE_WITH_KNOTS ( 'NONE', 3,
 ( #23452, #92414, #15935, #47398, #68451, #23938 ),
 .UNSPECIFIED., .F., .F.,
 ( 4, 2, 4 ),
 ( 0.000000000000000000, 0.0002565770811491003721, 0.0005131541622982007441 ),
 .UNSPECIFIED. ) ;
#58831=CARTESIAN_POINT ( 'NONE',  ( 12.63842701281683034, 17.46726448433411250, 9.846743663894596210 ) ) ;
#58832=CARTESIAN_POINT ( 'NONE',  ( 19.38216949554541557, 2.248634669930420049, -9.382169495545420901 ) ) ;
#58834=CARTESIAN_POINT ( 'NONE',  ( 5.054308323419867577, 70.51564955044841554, -5.000000000000000000 ) ) ;
#58835=CARTESIAN_POINT ( 'NONE',  ( -0.8801773607110991993, 22.85535201082150181, -2.915334737309923874 ) ) ;
#58836=CARTESIAN_POINT ( 'NONE',  ( 0.1532563361054100626, 55.80059781766745175, -2.638427012816831230 ) ) ;
#58838=CARTESIAN_POINT ( 'NONE',  ( -45.94000000000001194, 99.99999999999998579, -9.500000000000000000 ) ) ;
#58840=CARTESIAN_POINT ( 'NONE',  ( 19.84674366389459621, 3.508931151000785231, 7.409399052514197653E-17 ) ) ;
#58841=CARTESIAN_POINT ( 'NONE',  ( 7.361572987183169658, -0.03273551566588185635, -9.846743663894592657 ) ) ;
#58842=CARTESIAN_POINT ( 'NONE',  ( 21.09922568453595559, 2.040301336597086568, -6.408140936763230044 ) ) ;
#58843=VERTEX_POINT ( 'NONE', #87057 ) ;
#58846=CARTESIAN_POINT ( 'NONE',  ( -2.816281873526471635, 38.91530133659708213, -3.434112377981056508 ) ) ;
#58847=CARTESIAN_POINT ( 'NONE',  ( 1.472469842513823179, 35.59226448433412315, -4.923371831947296329 ) ) ;
#58849=CARTESIAN_POINT ( 'NONE',  ( 24.16423886937410614, 64.51208216824728936, -3.795296366450302550 ) ) ;
#58850=CARTESIAN_POINT ( 'NONE',  ( 5.076628168052704559, 35.17559781766745175, -8.527530157486179263 ) ) ;
#58851=PLANE ( 'NONE',  #76046 ) ;
#58852=CARTESIAN_POINT ( 'NONE',  ( 15.44008868035555260, 9.730352010821505360, 9.422509992056143702 ) ) ;
#58854=CARTESIAN_POINT ( 'NONE',  ( -0.8801773607110991993, 17.85535201082150536, -2.915334737309923874 ) ) ;
#58855=CARTESIAN_POINT ( 'NONE',  ( 17.08211943468705130, 53.47041550158063217, 12.26659068614894998 ) ) ;
#58856=CARTESIAN_POINT ( 'NONE',  ( 24.16423886937410614, 54.30374883491396787, 8.672049930838204340E-16 ) ) ;
#58858=PRESENTATION_STYLE_ASSIGNMENT (( #94400 ) ) ;
#58859=EDGE_CURVE ( 'NONE', #4978, #79846, #81506, .T. ) ;
#58861=CARTESIAN_POINT ( 'NONE',  ( 12.63842701281683034, 12.46726448433411782, 9.846743663894596210 ) ) ;
#58862=CARTESIAN_POINT ( 'NONE',  ( 17.20831665107776587, 64.13393115100079456, -7.208316651077762316 ) ) ;
#58864=CARTESIAN_POINT ( 'NONE',  ( 0.5774900079438590739, 47.64701867748817676, -5.440088680355550821 ) ) ;
#58865=CARTESIAN_POINT ( 'NONE',  ( 0.2751277870542967463, 70.00000000000000000, -6.000000000000000000 ) ) ;
#58867=CARTESIAN_POINT ( 'NONE',  ( 7.361572987183169658, 54.96726448433413026, -9.846743663894592657 ) ) ;
#58871=ORIENTED_EDGE ( 'NONE', *, *, #75055, .F. ) ;
#58872=CARTESIAN_POINT ( 'NONE',  ( 1.472469842513823179, 16.42559781766745175, 4.923371831947296329 ) ) ;
#58873=LINE ( 'NONE', #86069, #49594 ) ;
#58875=CARTESIAN_POINT ( 'NONE',  ( 17.08211943468705840, 35.13708216824730357, -12.26659068614894466 ) ) ;
#58876=CARTESIAN_POINT ( 'NONE',  ( 0.1532563361054083140, 1.008931151000784787, 1.131784320476157264E-15 ) ) ;
#58878=DIRECTION ( 'NONE',  ( -0.8320502943378437211, 0.5547001962252290364, 0.000000000000000000 ) ) ;
#58879=CARTESIAN_POINT ( 'NONE',  ( -0.8801773607110991993, 32.85535201082151247, -2.915334737309923874 ) ) ;
#58880=CARTESIAN_POINT ( 'NONE',  ( -2.816281873526471635, 38.91530133659708213, -3.434112377981056508 ) ) ;
#58881=CARTESIAN_POINT ( 'NONE',  ( -0.8801773607111008646, 3.272018677488171434, 2.915334737309923430 ) ) ;
#58882=CARTESIAN_POINT ( 'NONE',  ( 10.00000000000000178, 35.37363466993042493, 12.81628187352647608 ) ) ;
#58888=CARTESIAN_POINT ( 'NONE',  ( -4.164238869374098151, 31.59541550158063927, -3.795296366450310543 ) ) ;
#58889=CARTESIAN_POINT ( 'NONE',  ( -4.164238869374098151, 6.595415501580634832, -3.795296366450310543 ) ) ;
#58890=CARTESIAN_POINT ( 'NONE',  ( 4.559911319644449179, 12.23035201082150536, -9.422509992056141925 ) ) ;
#58891=CARTESIAN_POINT ( 'NONE',  ( 20.88017736071110519, 20.56368534415484106, 2.639326808657452039E-16 ) ) ;
#58892=CARTESIAN_POINT ( 'NONE',  ( 0.2751277870542911952, 53.21833443783938122, 6.499999999999992006 ) ) ;
#58895=CARTESIAN_POINT ( 'NONE',  ( 15.44008868035555260, 59.73035201082151247, 9.422509992056143702 ) ) ;
#58896=CARTESIAN_POINT ( 'NONE',  ( 19.42250999205614193, 45.14701867748817676, 5.440088680355555262 ) ) ;
#58897=CARTESIAN_POINT ( 'NONE',  ( -2.816281873526473856, 14.12363466993041961, 9.499525473075851096E-16 ) ) ;
#58898=DIRECTION ( 'NONE',  ( 0.000000000000000000, 0.000000000000000000, -1.000000000000000000 ) ) ;
#58899=CARTESIAN_POINT ( 'NONE',  ( -10.00000000000000000, 82.00000000000000000, 9.500000000000000000 ) ) ;
#58900=CARTESIAN_POINT ( 'NONE',  ( 7.361572987183170547, 22.05059781766745530, 9.846743663894590881 ) ) ;
#58901=CARTESIAN_POINT ( 'NONE',  ( 0.5600000000000083800, 105.0000000000000000, 5.000000000000000000 ) ) ;
#58902=CARTESIAN_POINT ( 'NONE',  ( 20.88017736071110164, 45.35535201082149115, 2.915334737309930979 ) ) ;
#58903=CARTESIAN_POINT ( 'NONE',  ( -1.099225684535947600, 4.540301336597087456, 6.408140936763237150 ) ) ;
#58904=( NAMED_UNIT ( * ) PLANE_ANGLE_UNIT ( ) SI_UNIT ( $, .RADIAN. ) );
#58905=CARTESIAN_POINT ( 'NONE',  ( 19.84674366389459266, 23.30059781766745530, 2.638427012816836559 ) ) ;
#58906=CARTESIAN_POINT ( 'NONE',  ( -2.816281873526473856, 54.33196800326376064, 3.434112377981055619 ) ) ;
#58907=CARTESIAN_POINT ( 'NONE',  ( 5.076628168052704559, 20.17559781766745175, -8.527530157486179263 ) ) ;
#58908=ORIENTED_EDGE ( 'NONE', *, *, #13929, .F. ) ;
#58909=CARTESIAN_POINT ( 'NONE',  ( 2.917880565312950480, 10.97041550158063572, -12.26659068614894821 ) ) ;
#58911=CARTESIAN_POINT ( 'NONE',  ( 7.084665262690076126, 24.10535201082150181, 10.88017736071109987 ) ) ;
#58912=CARTESIAN_POINT ( 'NONE',  ( 22.26659068614895176, 34.72041550158063927, -7.082119434687042414 ) ) ;
#58913=CARTESIAN_POINT ( 'NONE',  ( 5.076628168052704559, 30.17559781766745175, -8.527530157486179263 ) ) ;
#58915=CARTESIAN_POINT ( 'NONE',  ( 17.96484262340118221, 16.18868534415483396, -7.964842623401177768 ) ) ;
#58916=CARTESIAN_POINT ( 'NONE',  ( 10.00000000000000178, 4.313685344154837509, 10.88017736071110342 ) ) ;
#58918=CARTESIAN_POINT ( 'NONE',  ( 19.42250999205614193, 20.14701867748817321, 5.440088680355555262 ) ) ;
#58919=CARTESIAN_POINT ( 'NONE',  ( 16.40814093676324603, 52.45696800326375353, -11.09922568453594671 ) ) ;
#58920=EDGE_CURVE ( 'NONE', #31636, #87937, #58830, .T. ) ;
#58921=CARTESIAN_POINT ( 'NONE',  ( -0.8801773607111008646, 33.27201867748817676, 2.915334737309923430 ) ) ;
#58923=CARTESIAN_POINT ( 'NONE',  ( 2.035157376598822676, 37.43868534415484106, -7.964842623401177768 ) ) ;
#58925=CARTESIAN_POINT ( 'NONE',  ( 10.00000000000000000, 54.75893115100078745, -9.846743663894594434 ) ) ;
#58926=CARTESIAN_POINT ( 'NONE',  ( 19.42250999205614193, 35.14701867748816966, 5.440088680355555262 ) ) ;
#58927=CARTESIAN_POINT ( 'NONE',  ( 5.076628168052704559, 65.17559781766745175, -8.527530157486179263 ) ) ;
#58929=CARTESIAN_POINT ( 'NONE',  ( 3.591859063236761518, 64.95696800326376774, 11.09922568453594849 ) ) ;
#58930=CARTESIAN_POINT ( 'NONE',  ( 19.72487221294570858, 70.00000000000000000, 6.000000000000000000 ) ) ;
#58931=CARTESIAN_POINT ( 'NONE',  ( 24.16423886937410614, 39.51208216824731068, -3.795296366450302550 ) ) ;
#58932=CARTESIAN_POINT ( 'NONE',  ( 0.5774900079438590739, 57.64701867748817676, -5.440088680355550821 ) ) ;
#58933=ADVANCED_FACE ( 'NONE', ( #98972 ), #8429, .T. ) ;
#58934=CARTESIAN_POINT ( 'NONE',  ( 18.72515096720579209, 51.07228050351030646, -6.499999999999869438 ) ) ;
#58936=CARTESIAN_POINT ( 'NONE',  ( 18.52753015748617571, 53.09226448433412315, 4.923371831947298993 ) ) ;
#58937=CARTESIAN_POINT ( 'NONE',  ( 14.92337183194729988, 4.342264484334117824, -8.527530157486177487 ) ) ;
#58938=CARTESIAN_POINT ( 'NONE',  ( 19.84674366389459266, 23.71726448433412315, -2.638427012816827677 ) ) ;
#58940=CARTESIAN_POINT ( 'NONE',  ( 0.1532563361054082862, 16.21726448433411960, 2.638427012816831674 ) ) ;
#58942=CARTESIAN_POINT ( 'NONE',  ( 7.084665262690076126, 32.02201867748816966, -10.88017736071110164 ) ) ;
#58943=CARTESIAN_POINT ( 'NONE',  ( 19.84674366389459621, 18.50893115100078745, 7.409399052514197653E-17 ) ) ;
#58944=CARTESIAN_POINT ( 'NONE',  ( 3.591859063236761518, 9.956968003263753531, 11.09922568453594849 ) ) ;
#58945=CARTESIAN_POINT ( 'NONE',  ( -0.8801773607111008646, 58.27201867748816966, 2.915334737309923430 ) ) ;
#58946=CARTESIAN_POINT ( 'NONE',  ( 4.559911319644449179, 28.89701867748817321, 9.422509992056141925 ) ) ;
#58947=CARTESIAN_POINT ( 'NONE',  ( -2.816281873526473856, 54.12363466993041783, 9.499525473075851096E-16 ) ) ;
#58948=CARTESIAN_POINT ( 'NONE',  ( 10.00000000000000000, 50.55374883491396787, -14.16423886937410082 ) ) ;
#58950=EDGE_CURVE ( 'NONE', #59946, #74297, #83247, .T. ) ;
#58951=CARTESIAN_POINT ( 'NONE',  ( 10.00000000000000178, 65.37363466993042493, 12.81628187352647608 ) ) ;
#58953=CARTESIAN_POINT ( 'NONE',  ( 2.791683348922240793, 66.63393115100079456, 7.208316651077764092 ) ) ;
#58954=CARTESIAN_POINT ( 'NONE',  ( 15.44008868035555793, 6.397018677488170546, -9.422509992056140149 ) ) ;
#58955=CARTESIAN_POINT ( 'NONE',  ( 17.96484262340118221, 51.18868534415483396, -7.964842623401177768 ) ) ;
#58956=CARTESIAN_POINT ( 'NONE',  ( 14.92337183194729988, 64.34226448433412315, -8.527530157486177487 ) ) ;
#58957=EDGE_CURVE ( 'NONE', #1795, #57881, #16922, .T. ) ;
#58959=CARTESIAN_POINT ( 'NONE',  ( 19.84674366389459266, 18.71726448433411960, -2.638427012816827677 ) ) ;
#58963=CARTESIAN_POINT ( 'NONE',  ( -0.8801773607111008646, 58.27201867748816966, 2.915334737309923430 ) ) ;
#58964=CARTESIAN_POINT ( 'NONE',  ( 0.1532563361054100626, 35.80059781766745175, -2.638427012816831230 ) ) ;
#58965=CARTESIAN_POINT ( 'NONE',  ( 19.84674366389459621, 18.50893115100078745, 7.409399052514197653E-17 ) ) ;
#58966=CARTESIAN_POINT ( 'NONE',  ( 7.361572987183170547, 12.05059781766744997, 9.846743663894590881 ) ) ;
#58967=CARTESIAN_POINT ( 'NONE',  ( 17.39651004071841456, 64.08210964143329136, -6.500000000000001776 ) ) ;
#58968=CARTESIAN_POINT ( 'NONE',  ( 7.084665262690076126, 64.10535201082150536, 10.88017736071109987 ) ) ;
#58970=CARTESIAN_POINT ( 'NONE',  ( 2.791683348922240793, 31.63393115100078745, 7.208316651077764092 ) ) ;
#58971=ORIENTED_EDGE ( 'NONE', *, *, #40889, .F. ) ;
#58973=CARTESIAN_POINT ( 'NONE',  ( 7.361572987183170547, 62.05059781766745886, 9.846743663894590881 ) ) ;
#58975=CARTESIAN_POINT ( 'NONE',  ( -4.164238869374099039, 16.80374883491396787, 8.674139862899312516E-16 ) ) ;
#58977=CARTESIAN_POINT ( 'NONE',  ( 2.917880565312950480, 15.97041550158063217, -12.26659068614894821 ) ) ;
#58978=CARTESIAN_POINT ( 'NONE',  ( 13.79529636645031943, 50.34541550158064638, -14.16423886937409904 ) ) ;
#58979=CARTESIAN_POINT ( 'NONE',  ( -4.164238869374099927, 2.012082168247300906, 3.795296366450308767 ) ) ;
#58980=CARTESIAN_POINT ( 'NONE',  ( 20.36894250292379738, 14.92874883491396432, -10.36894250292379027 ) ) ;
#58981=CARTESIAN_POINT ( 'NONE',  ( -0.8801773607111008646, 53.27201867748816966, 2.915334737309923430 ) ) ;
#58984=CARTESIAN_POINT ( 'NONE',  ( 0.1532563361054100626, 25.80059781766744820, -2.638427012816831230 ) ) ;
#58985=CARTESIAN_POINT ( 'NONE',  ( 15.44008868035555793, 66.39701867748817676, -9.422509992056140149 ) ) ;
#58986=CARTESIAN_POINT ( 'NONE',  ( 18.52753015748618282, 28.92559781766745175, -4.923371831947291888 ) ) ;
#58987=CARTESIAN_POINT ( 'NONE',  ( 2.035157376598822676, 12.43868534415483751, -7.964842623401177768 ) ) ;
#58988=CARTESIAN_POINT ( 'NONE',  ( 10.00000000000000178, 55.37363466993042493, 12.81628187352647608 ) ) ;
#58989=CARTESIAN_POINT ( 'NONE',  ( 14.92337183194729633, 52.67559781766745175, 8.527530157486181039 ) ) ;
#58992=CARTESIAN_POINT ( 'NONE',  ( 14.92337183194729633, 27.67559781766745530, 8.527530157486181039 ) ) ;
#58993=CARTESIAN_POINT ( 'NONE',  ( 3.591859063236761518, 44.95696800326376064, 11.09922568453594849 ) ) ;
#58995=CARTESIAN_POINT ( 'NONE',  ( 10.00000000000000178, 39.31368534415484106, 10.88017736071110342 ) ) ;
#58996=CARTESIAN_POINT ( 'NONE',  ( 18.52753015748618282, 38.92559781766745175, -4.923371831947291888 ) ) ;
#58997=CARTESIAN_POINT ( 'NONE',  ( 10.00000000000000000, 20.55374883491396787, -14.16423886937410082 ) ) ;
#58999=CARTESIAN_POINT ( 'NONE',  ( 17.08211943468705130, 3.470415501580634388, 12.26659068614894998 ) ) ;
#59000=CARTESIAN_POINT ( 'NONE',  ( 19.42250999205614548, 50.98035201082151247, -5.440088680355545492 ) ) ;
#59001=CARTESIAN_POINT ( 'NONE',  ( 19.42250999205614193, 65.14701867748817676, 5.440088680355555262 ) ) ;
#59002=CARTESIAN_POINT ( 'NONE',  ( 24.16423886937410614, 49.51208216824730357, -3.795296366450302550 ) ) ;
#59003=CARTESIAN_POINT ( 'NONE',  ( 10.00000000000000178, 62.25893115100078745, 9.846743663894594434 ) ) ;
#59005=CARTESIAN_POINT ( 'NONE',  ( 4.559911319644449179, 53.89701867748817676, 9.422509992056141925 ) ) ;
#59007=CARTESIAN_POINT ( 'NONE',  ( -1.099225684535947600, 24.54030133659708923, 6.408140936763237150 ) ) ;
#59008=CARTESIAN_POINT ( 'NONE',  ( 13.43411237798106583, 2.665301336597086568, -12.81628187352647252 ) ) ;
#59010=CARTESIAN_POINT ( 'NONE',  ( 7.084665262690076126, 19.10535201082150181, 10.88017736071109987 ) ) ;
#59011=CARTESIAN_POINT ( 'NONE',  ( 17.96484262340118221, 11.18868534415484106, -7.964842623401177768 ) ) ;
#59015=CARTESIAN_POINT ( 'NONE',  ( 1.472469842513823179, 15.59226448433411960, -4.923371831947296329 ) ) ;
#59016=CARTESIAN_POINT ( 'NONE',  ( 14.92337183194729633, 37.67559781766745175, 8.527530157486181039 ) ) ;
#59017=CARTESIAN_POINT ( 'NONE',  ( 15.44008868035555793, 41.39701867748817676, -9.422509992056140149 ) ) ;
#59018=CARTESIAN_POINT ( 'NONE',  ( -1.099225684535947600, 13.70696800326375353, -6.408140936763238038 ) ) ;
#59019=CARTESIAN_POINT ( 'NONE',  ( 20.88017736071110519, 30.56368534415484106, 2.639326808657452039E-16 ) ) ;
#59021=EDGE_CURVE ( 'NONE', #68558, #76972, #52436, .T. ) ;
#59023=CARTESIAN_POINT ( 'NONE',  ( 21.09922568453595559, 57.04030133659708923, -6.408140936763230044 ) ) ;
#59025=CARTESIAN_POINT ( 'NONE',  ( 12.91533473730992121, 64.52201867748817676, 10.88017736071110164 ) ) ;
#59026=CARTESIAN_POINT ( 'NONE',  ( 6.565887622018943937, 28.08196800326375353, -12.81628187352647608 ) ) ;
#59027=CARTESIAN_POINT ( 'NONE',  ( 20.36894250292379382, 3.678748834913967869, 10.36894250292379205 ) ) ;
#59028=CARTESIAN_POINT ( 'NONE',  ( 5.076628168052703671, 1.842264484334118047, 8.527530157486179263 ) ) ;
#59029=CARTESIAN_POINT ( 'NONE',  ( 4.559911319644449179, 42.23035201082151247, -9.422509992056141925 ) ) ;
#59030=CARTESIAN_POINT ( 'NONE',  ( 12.63842701281683034, 62.46726448433410894, 9.846743663894596210 ) ) ;
#59031=CARTESIAN_POINT ( 'NONE',  ( 14.92337183194729988, 59.34226448433412315, -8.527530157486177487 ) ) ;
#59033=CARTESIAN_POINT ( 'NONE',  ( 1.472469842513823179, 15.59226448433411960, -4.923371831947296329 ) ) ;
#59034=CARTESIAN_POINT ( 'NONE',  ( 0.5774900079438590739, 57.64701867748817676, -5.440088680355550821 ) ) ;
#59036=CARTESIAN_POINT ( 'NONE',  ( 17.08211943468705130, 23.47041550158063572, 12.26659068614894998 ) ) ;
#59041=CARTESIAN_POINT ( 'NONE',  ( -4.164238869374099927, 62.01208216824728936, 3.795296366450308767 ) ) ;
#59042=CARTESIAN_POINT ( 'NONE',  ( 10.00000000000000178, 63.05374883491396076, 14.16423886937410082 ) ) ;
#59043=CARTESIAN_POINT ( 'NONE',  ( 5.076628168052704559, 30.17559781766745175, -8.527530157486179263 ) ) ;
#59044=CARTESIAN_POINT ( 'NONE',  ( 10.00000000000000178, 30.37363466993042138, 12.81628187352647608 ) ) ;
#59047=CARTESIAN_POINT ( 'NONE',  ( 10.00000000000000178, 9.313685344154839285, 10.88017736071110342 ) ) ;
#59048=CARTESIAN_POINT ( 'NONE',  ( 10.00000000000000178, 53.05374883491396787, 14.16423886937410082 ) ) ;
#59051=CARTESIAN_POINT ( 'NONE',  ( 2.791683348922237240, 30.38393115100078390, -7.208316651077763204 ) ) ;
#59053=CARTESIAN_POINT ( 'NONE',  ( 1.472469842513823179, 5.592264484334118713, -4.923371831947296329 ) ) ;
#59054=CARTESIAN_POINT ( 'NONE',  ( 18.52753015748617571, 3.092264484334118269, 4.923371831947298993 ) ) ;
#59060=CARTESIAN_POINT ( 'NONE',  ( -0.8801773607111008646, 18.27201867748817321, 2.915334737309923430 ) ) ;
#59061=CARTESIAN_POINT ( 'NONE',  ( -0.8801773607110991993, 27.85535201082150181, -2.915334737309923874 ) ) ;
#59062=CARTESIAN_POINT ( 'NONE',  ( 1.472469842513823179, 66.42559781766745175, 4.923371831947296329 ) ) ;
#59063=CARTESIAN_POINT ( 'NONE',  ( 16.40814093676323893, 20.79030133659708923, 11.09922568453595026 ) ) ;
#59064=CARTESIAN_POINT ( 'NONE',  ( 16.40814093676324603, 32.45696800326375353, -11.09922568453594671 ) ) ;
#59066=CARTESIAN_POINT ( 'NONE',  ( 14.92337183194729633, 32.67559781766745175, 8.527530157486181039 ) ) ;
#59067=CARTESIAN_POINT ( 'NONE',  ( -2.266590686148945544, 67.22041550158063217, 7.082119434687048631 ) ) ;
#59070=CARTESIAN_POINT ( 'NONE',  ( -4.164238869374099039, 66.80374883491396076, 8.674139862899312516E-16 ) ) ;
#59072=CARTESIAN_POINT ( 'NONE',  ( 12.91533473730992121, 49.52201867748817676, 10.88017736071110164 ) ) ;
#59073=CARTESIAN_POINT ( 'NONE',  ( 4.559911319644449179, 53.89701867748817676, 9.422509992056141925 ) ) ;
#59074=CARTESIAN_POINT ( 'NONE',  ( 20.88017736071110875, 55.77201867748816966, -2.915334737309920765 ) ) ;
#59075=CARTESIAN_POINT ( 'NONE',  ( 20.88017736071110164, 35.35535201082150536, 2.915334737309930979 ) ) ;
#59076=CARTESIAN_POINT ( 'NONE',  ( -46.94000000000000483, 101.3580217190346389, 7.614242055636530893 ) ) ;
#59078=CARTESIAN_POINT ( 'NONE',  ( -45.94000000000000483, 92.00000000000000000, 5.000000000000000000 ) ) ;
#59080=CARTESIAN_POINT ( 'NONE',  ( 1.472469842513823179, 30.59226448433411960, -4.923371831947296329 ) ) ;
#59082=CARTESIAN_POINT ( 'NONE',  ( 17.20831665107776587, 59.13393115100078745, -7.208316651077762316 ) ) ;
#59084=CARTESIAN_POINT ( 'NONE',  ( 6.204703633549690345, 10.76208216824729824, -14.16423886937410259 ) ) ;
#59088=DIRECTION ( 'NONE',  ( 0.000000000000000000, 0.000000000000000000, -1.000000000000000000 ) ) ;
#59089=CARTESIAN_POINT ( 'NONE',  ( 24.16423886937410614, 59.51208216824728936, -3.795296366450302550 ) ) ;
#59092=FACE_OUTER_BOUND ( 'NONE', #53480, .T. ) ;
#59093=CARTESIAN_POINT ( 'NONE',  ( 0.1532563361054100626, 40.80059781766745886, -2.638427012816831230 ) ) ;
#59095=CARTESIAN_POINT ( 'NONE',  ( 21.09922568453594849, 21.20696800326375353, 6.408140936763242479 ) ) ;
#59096=CARTESIAN_POINT ( 'NONE',  ( 10.00000000000000000, 9.758931151000785675, -9.846743663894594434 ) ) ;
#59097=CARTESIAN_POINT ( 'NONE',  ( 10.00000000000000178, 70.00000000000000000, 0.000000000000000000 ) ) ;
#59098=CARTESIAN_POINT ( 'NONE',  ( 0.1532563361054082862, 6.217264484334118713, 2.638427012816831674 ) ) ;
#59099=CARTESIAN_POINT ( 'NONE',  ( -1.099225684535947600, 8.706968003263753531, -6.408140936763238038 ) ) ;
#59102=CARTESIAN_POINT ( 'NONE',  ( 20.88017736071110519, 10.56368534415483929, 2.639326808657452039E-16 ) ) ;
#59103=CARTESIAN_POINT ( 'NONE',  ( 22.26659068614894466, 8.887082168247300018, 7.082119434687054849 ) ) ;
#59104=CARTESIAN_POINT ( 'NONE',  ( 1.472469842513823179, 30.59226448433411960, -4.923371831947296329 ) ) ;
#59105=CARTESIAN_POINT ( 'NONE',  ( 7.084665262690076126, 59.10535201082150536, 10.88017736071109987 ) ) ;
#59106=CARTESIAN_POINT ( 'NONE',  ( -1.099225684535947600, 24.54030133659708923, 6.408140936763237150 ) ) ;
#59107=CARTESIAN_POINT ( 'NONE',  ( 19.42250999205614193, 20.14701867748817321, 5.440088680355555262 ) ) ;
#59110=CARTESIAN_POINT ( 'NONE',  ( 21.09922568453595559, 2.040301336597086568, -6.408140936763230044 ) ) ;
#59111=CARTESIAN_POINT ( 'NONE',  ( 0.1532563361054082862, 61.21726448433412315, 2.638427012816831674 ) ) ;
#59112=CARTESIAN_POINT ( 'NONE',  ( 10.00000000000000178, 17.25893115100078745, 9.846743663894594434 ) ) ;
#59114=CARTESIAN_POINT ( 'NONE',  ( -2.816281873526471635, 33.91530133659708213, -3.434112377981056508 ) ) ;
#59116=CARTESIAN_POINT ( 'NONE',  ( 10.00000000000000178, 39.31368534415484106, 10.88017736071110342 ) ) ;
#59119=CARTESIAN_POINT ( 'NONE',  ( -45.94000000000000483, 92.00000000000000000, 9.000000000000000000 ) ) ;
#59120=CARTESIAN_POINT ( 'NONE',  ( 20.88017736071110164, 25.35535201082150891, 2.915334737309930979 ) ) ;
#59122=CARTESIAN_POINT ( 'NONE',  ( 4.559911319644449179, 32.23035201082150536, -9.422509992056141925 ) ) ;
#59123=CARTESIAN_POINT ( 'NONE',  ( 7.361572987183169658, 44.96726448433412315, -9.846743663894592657 ) ) ;
#59124=CARTESIAN_POINT ( 'NONE',  ( 4.559911319644449179, 58.89701867748817676, 9.422509992056141925 ) ) ;
#59125=CARTESIAN_POINT ( 'NONE',  ( -4.164238869374099927, 32.01208216824730357, 3.795296366450308767 ) ) ;
#59127=CARTESIAN_POINT ( 'NONE',  ( 12.63842701281683034, 42.46726448433412315, 9.846743663894596210 ) ) ;
#59128=CIRCLE ( 'NONE', #14480, 0.5000000000000004441 ) ;
#59129=CARTESIAN_POINT ( 'NONE',  ( 19.84674366389459621, 63.50893115100078745, 7.409399052514197653E-17 ) ) ;
#59131=CARTESIAN_POINT ( 'NONE',  ( 10.00000000000000178, 24.31368534415484106, 10.88017736071110342 ) ) ;
#59134=CARTESIAN_POINT ( 'NONE',  ( 20.88017736071110519, 10.56368534415483929, 2.639326808657452039E-16 ) ) ;
#59135=CARTESIAN_POINT ( 'NONE',  ( 10.00000000000000000, -0.2410688489992152128, -9.846743663894594434 ) ) ;
#59136=CARTESIAN_POINT ( 'NONE',  ( 13.79529636645030344, 28.26208216824729647, 14.16423886937410614 ) ) ;
#59137=CARTESIAN_POINT ( 'NONE',  ( 17.20831665107776587, 17.88393115100078745, 7.208316651077764980 ) ) ;
#59138=CARTESIAN_POINT ( 'NONE',  ( 17.20831665107776587, 64.13393115100079456, -7.208316651077762316 ) ) ;
#59139=CARTESIAN_POINT ( 'NONE',  ( 4.559911319644449179, 43.89701867748816966, 9.422509992056141925 ) ) ;
#59141=CARTESIAN_POINT ( 'NONE',  ( 3.640395162852214650, 89.00000000000000000, 9.500000000000000000 ) ) ;
#59144=ORIENTED_EDGE ( 'NONE', *, *, #4887, .T. ) ;
#59146=CARTESIAN_POINT ( 'NONE',  ( 2.791683348922240793, 51.63393115100078745, 7.208316651077764092 ) ) ;
#59151=CARTESIAN_POINT ( 'NONE',  ( -4.164238869374099927, 17.01208216824730357, 3.795296366450308767 ) ) ;
#59152=CARTESIAN_POINT ( 'NONE',  ( -2.266590686148945544, 22.22041550158063572, 7.082119434687048631 ) ) ;
#59153=CARTESIAN_POINT ( 'NONE',  ( 0.5774900079438607392, 53.48035201082151247, 5.440088680355550821 ) ) ;
#59154=CARTESIAN_POINT ( 'NONE',  ( 24.16423886937410614, 54.30374883491396787, 8.672049930838204340E-16 ) ) ;
#59155=CARTESIAN_POINT ( 'NONE',  ( 22.81628187352647785, 1.623634669930420271, 6.195893100308588602E-16 ) ) ;
#59156=CARTESIAN_POINT ( 'NONE',  ( 18.52753015748618282, 48.92559781766745886, -4.923371831947291888 ) ) ;
#59158=CARTESIAN_POINT ( 'NONE',  ( -0.8801773607111008646, 48.27201867748816966, 2.915334737309923430 ) ) ;
#59159=CARTESIAN_POINT ( 'NONE',  ( 3.591859063236761518, 4.956968003263753531, 11.09922568453594849 ) ) ;
#59160=CARTESIAN_POINT ( 'NONE',  ( 10.00000000000000000, 20.55374883491396787, -14.16423886937410082 ) ) ;
#59161=CARTESIAN_POINT ( 'NONE',  ( 13.79529636645031943, 55.34541550158062506, -14.16423886937409904 ) ) ;
#59163=CARTESIAN_POINT ( 'NONE',  ( 20.88017736071110519, 20.56368534415484106, 2.639326808657452039E-16 ) ) ;
#59165=CARTESIAN_POINT ( 'NONE',  ( -0.8801773607111008646, 48.27201867748816966, 2.915334737309923430 ) ) ;
#59168=ORIENTED_EDGE ( 'NONE', *, *, #36189, .T. ) ;
#59171=ORIENTED_EDGE ( 'NONE', *, *, #87068, .T. ) ;
#59173=CARTESIAN_POINT ( 'NONE',  ( -0.3689425029237898834, 41.17874883491397497, -10.36894250292378850 ) ) ;
#59174=CARTESIAN_POINT ( 'NONE',  ( 19.84674366389459266, 48.30059781766745175, 2.638427012816836559 ) ) ;
#59175=CARTESIAN_POINT ( 'NONE',  ( 20.15039907845753575, 50.60158574516642460, -6.262539305110073506 ) ) ;
#59177=CARTESIAN_POINT ( 'NONE',  ( -0.8801773607111008646, 53.27201867748816966, 2.915334737309923430 ) ) ;
#59179=CARTESIAN_POINT ( 'NONE',  ( 22.81628187352647785, 56.62363466993042493, 6.195893100308588602E-16 ) ) ;
#59182=CARTESIAN_POINT ( 'NONE',  ( 10.00000000000000178, 38.05374883491396787, 14.16423886937410082 ) ) ;
#59184=CARTESIAN_POINT ( 'NONE',  ( -1.099225684535947600, 18.70696800326375353, -6.408140936763238038 ) ) ;
#59186=CARTESIAN_POINT ( 'NONE',  ( 22.81628187352648496, 41.83196800326375353, -3.434112377981050290 ) ) ;
#59187=CARTESIAN_POINT ( 'NONE',  ( 5.076628168052703671, 31.84226448433412315, 8.527530157486179263 ) ) ;
#59188=CARTESIAN_POINT ( 'NONE',  ( -0.8801773607111008646, 13.27201867748817143, 2.915334737309923430 ) ) ;
#59189=CARTESIAN_POINT ( 'NONE',  ( 13.43411237798106583, 57.66530133659708923, -12.81628187352647252 ) ) ;
#59191=CARTESIAN_POINT ( 'NONE',  ( 18.52753015748617571, 43.09226448433412315, 4.923371831947298993 ) ) ;
#59193=( BOUNDED_CURVE ( )  B_SPLINE_CURVE ( 2, ( #59175, #61151, #45165, #29656, #14191, #75669, #13189, #53163, #68182 ),
 .UNSPECIFIED., .F., .F. ) 
 B_SPLINE_CURVE_WITH_KNOTS ( ( 3, 2, 2, 2, 3 ),
 ( 0.2615695083688028277, 0.2619047619047619735, 0.2678571428571429047, 0.2738095238095238360, 0.2741447773454829817 ),
 .UNSPECIFIED. ) 
 CURVE ( )  GEOMETRIC_REPRESENTATION_ITEM ( )  RATIONAL_B_SPLINE_CURVE ( ( 0.9963778908391760503, 0.9980808541467920403, 1.000000000000000000, 0.9659258262890682012, 1.000000000000000000, 0.9659258262890682012, 1.000000000000000000, 0.9980808541467920403, 0.9963778908391759392 ) ) 
 REPRESENTATION_ITEM ( '' )  );
#59195=CARTESIAN_POINT ( 'NONE',  ( 18.95386800104996539, 18.23810908735726599, -6.499999999999990230 ) ) ;
#59198=CARTESIAN_POINT ( 'NONE',  ( 0.2751277870542910842, 67.28217586085239077, -6.499999999999992006 ) ) ;
#59199=CARTESIAN_POINT ( 'NONE',  ( 1.472469842513823179, 11.42559781766745175, 4.923371831947296329 ) ) ;
#59200=CARTESIAN_POINT ( 'NONE',  ( 22.81628187352647785, 21.62363466993041783, 6.195893100308588602E-16 ) ) ;
#59204=CARTESIAN_POINT ( 'NONE',  ( 7.361572987183170547, 52.05059781766745175, 9.846743663894590881 ) ) ;
#59206=CARTESIAN_POINT ( 'NONE',  ( 6.204703633549690345, 25.76208216824730712, -14.16423886937410259 ) ) ;
#59207=CARTESIAN_POINT ( 'NONE',  ( 0.1532563361054100626, 45.80059781766745886, -2.638427012816831230 ) ) ;
#59208=CARTESIAN_POINT ( 'NONE',  ( 16.40814093676323893, 50.79030133659708923, 11.09922568453595026 ) ) ;
#59210=CARTESIAN_POINT ( 'NONE',  ( 0.1532563361054083140, 11.00893115100078568, 1.131784320476157264E-15 ) ) ;
#59211=CARTESIAN_POINT ( 'NONE',  ( 21.92686044187657046, 47.39664270246085209, -3.195792623639524432 ) ) ;
#59212=CARTESIAN_POINT ( 'NONE',  ( 0.1532563361054083140, 46.00893115100079456, 1.131784320476157264E-15 ) ) ;
#59213=CARTESIAN_POINT ( 'NONE',  ( 20.88017736071110875, 45.77201867748816966, -2.915334737309920765 ) ) ;
#59214=CARTESIAN_POINT ( 'NONE',  ( 10.00000000000000000, 34.75893115100078745, -9.846743663894594434 ) ) ;
#59218=CARTESIAN_POINT ( 'NONE',  ( 7.084665262690076126, 42.02201867748816966, -10.88017736071110164 ) ) ;
#59221=CARTESIAN_POINT ( 'NONE',  ( 12.91533473730992121, 14.52201867748817143, 10.88017736071110164 ) ) ;
#59222=CARTESIAN_POINT ( 'NONE',  ( 2.791683348922240793, 56.63393115100078035, 7.208316651077764092 ) ) ;
#59223=CARTESIAN_POINT ( 'NONE',  ( 12.91533473730992121, 39.52201867748817676, 10.88017736071110164 ) ) ;
#59224=DIRECTION ( 'NONE',  ( -0.8320502943378437211, 0.5547001962252290364, 0.000000000000000000 ) ) ;
#59225=CARTESIAN_POINT ( 'NONE',  ( 12.91533473730993009, 56.60535201082151247, -10.88017736071109987 ) ) ;
#59226=CARTESIAN_POINT ( 'NONE',  ( 17.96484262340118221, 19.93868534415484106, 7.964842623401181321 ) ) ;
#59228=CARTESIAN_POINT ( 'NONE',  ( 2.791683348922237240, 0.3839311510007847872, -7.208316651077763204 ) ) ;
#59229=EDGE_CURVE ( 'NONE', #61453, #26206, #19797, .T. ) ;
#59230=CARTESIAN_POINT ( 'NONE',  ( 10.00000000000000000, 19.75893115100078390, -9.846743663894594434 ) ) ;
#59233=CARTESIAN_POINT ( 'NONE',  ( 1.472469842513823179, 51.42559781766745886, 4.923371831947296329 ) ) ;
#59234=CARTESIAN_POINT ( 'NONE',  ( 22.26659068614894466, 63.88708216824730357, 7.082119434687054849 ) ) ;
#59239=CARTESIAN_POINT ( 'NONE',  ( 6.204703633549690345, 10.76208216824729824, -14.16423886937410259 ) ) ;
#59240=CARTESIAN_POINT ( 'NONE',  ( -0.3689425029237898834, 46.17874883491397497, -10.36894250292378850 ) ) ;
#59241=CARTESIAN_POINT ( 'NONE',  ( 22.81628187352647785, 6.415301336597088344, 3.434112377981063169 ) ) ;
#59243=EDGE_LOOP ( 'NONE', ( #49195, #42222, #45579, #19601, #90963, #20220 ) ) ;
#59244=CARTESIAN_POINT ( 'NONE',  ( 10.00000000000000000, 16.81368534415483751, -10.88017736071110342 ) ) ;
#59245=CARTESIAN_POINT ( 'NONE',  ( 2.791683348922237240, 45.38393115100079456, -7.208316651077763204 ) ) ;
#59246=SURFACE_STYLE_FILL_AREA ( #51760 ) ;
#59250=CARTESIAN_POINT ( 'NONE',  ( 6.565887622018943937, 18.08196800326375708, -12.81628187352647608 ) ) ;
#59251=CARTESIAN_POINT ( 'NONE',  ( 12.63842701281683922, 24.55059781766745175, -9.846743663894590881 ) ) ;
#59253=CARTESIAN_POINT ( 'NONE',  ( 18.52753015748618282, 8.925597817667451750, -4.923371831947291888 ) ) ;
#59254=CARTESIAN_POINT ( 'NONE',  ( 17.84635730667656617, 3.637910973973187190, 6.500000000000000888 ) ) ;
#59255=CARTESIAN_POINT ( 'NONE',  ( -46.82017113615791004, 100.6079546444643569, -9.324761308090124601 ) ) ;
#59256=CARTESIAN_POINT ( 'NONE',  ( 0.5774900079438590739, 7.647018677488171434, -5.440088680355550821 ) ) ;
#59257=CARTESIAN_POINT ( 'NONE',  ( -4.164238869374099039, 36.80374883491396787, 8.674139862899312516E-16 ) ) ;
#59258=CARTESIAN_POINT ( 'NONE',  ( 7.084665262690076126, 42.02201867748816966, -10.88017736071110164 ) ) ;
#59259=CARTESIAN_POINT ( 'NONE',  ( -0.8801773607110991993, 62.85535201082150536, -2.915334737309923874 ) ) ;
#59260=DIRECTION ( 'NONE',  ( 1.000000000000000000, 0.000000000000000000, 0.000000000000000000 ) ) ;
#59261=CARTESIAN_POINT ( 'NONE',  ( 1.472469842513823179, 25.59226448433412315, -4.923371831947296329 ) ) ;
#59263=CARTESIAN_POINT ( 'NONE',  ( 14.92337183194729633, 2.675597817667451750, 8.527530157486181039 ) ) ;
#59264=CARTESIAN_POINT ( 'NONE',  ( -1.419660342300774092, -7.341591041528218084E-16, 2.710667984842351608 ) ) ;
#59265=CARTESIAN_POINT ( 'NONE',  ( 1.472469842513823179, 36.42559781766745175, 4.923371831947296329 ) ) ;
#59266=CARTESIAN_POINT ( 'NONE',  ( 12.63842701281683922, 64.55059781766745175, -9.846743663894590881 ) ) ;
#59267=AXIS2_PLACEMENT_3D ( 'NONE', #4261, #64727, #79264 ) ;
#59268=CARTESIAN_POINT ( 'NONE',  ( 15.44008868035555260, 29.73035201082150891, 9.422509992056143702 ) ) ;
#59273=CARTESIAN_POINT ( 'NONE',  ( 13.43411237798106583, 62.66530133659708923, -12.81628187352647252 ) ) ;
#59275=CARTESIAN_POINT ( 'NONE',  ( 10.00000000000000178, 12.25893115100078568, 9.846743663894594434 ) ) ;
#59276=CARTESIAN_POINT ( 'NONE',  ( 0.6178305044545818747, 43.49863466993042493, -9.382169495545419124 ) ) ;
#59277=CARTESIAN_POINT ( 'NONE',  ( 10.00000000000000000, 1.813685344154838175, -10.88017736071110342 ) ) ;
#59278=CARTESIAN_POINT ( 'NONE',  ( 0.1532563361054082862, 31.21726448433412315, 2.638427012816831674 ) ) ;
#59279=PLANE ( 'NONE',  #31262 ) ;
#59280=CARTESIAN_POINT ( 'NONE',  ( 6.204703633549690345, 20.76208216824730357, -14.16423886937410259 ) ) ;
#59282=CARTESIAN_POINT ( 'NONE',  ( 6.204703633549690345, 42.84541550158063217, 14.16423886937410082 ) ) ;
#59283=CARTESIAN_POINT ( 'NONE',  ( 14.92337183194729988, 49.34226448433411605, -8.527530157486177487 ) ) ;
#59286=CARTESIAN_POINT ( 'NONE',  ( 7.084665262690076126, 44.10535201082151247, 10.88017736071109987 ) ) ;
#59288=CARTESIAN_POINT ( 'NONE',  ( 7.084665262690076126, 69.10535201082151957, 10.88017736071109987 ) ) ;
#59291=CARTESIAN_POINT ( 'NONE',  ( -1.099225684535947600, 59.54030133659708923, 6.408140936763237150 ) ) ;
#59293=CARTESIAN_POINT ( 'NONE',  ( -0.8801773607111009756, 63.06368534415484106, 1.068504757029289695E-15 ) ) ;
#59295=CARTESIAN_POINT ( 'NONE',  ( 13.79529636645030344, 3.262082168247301350, 14.16423886937410614 ) ) ;
#59296=CARTESIAN_POINT ( 'NONE',  ( 2.791683348922237240, 5.383931151000785675, -7.208316651077763204 ) ) ;
#59297=DIRECTION ( 'NONE',  ( -0.7445673648800779088, 0.6675473310227050261, 0.000000000000000000 ) ) ;
#59299=CARTESIAN_POINT ( 'NONE',  ( 15.44008868035555260, 19.73035201082150536, 9.422509992056143702 ) ) ;
#59302=CARTESIAN_POINT ( 'NONE',  ( 4.559911319644449179, 27.23035201082150536, -9.422509992056141925 ) ) ;
#59303=CARTESIAN_POINT ( 'NONE',  ( 1.472469842513823179, 65.59226448433412315, -4.923371831947296329 ) ) ;
#59304=ORIENTED_EDGE ( 'NONE', *, *, #55011, .T. ) ;
#59305=CARTESIAN_POINT ( 'NONE',  ( 1.472469842513823179, 61.42559781766745175, 4.923371831947296329 ) ) ;
#59306=ORIENTED_EDGE ( 'NONE', *, *, #22299, .F. ) ;
#59307=CARTESIAN_POINT ( 'NONE',  ( 7.361572987183169658, -0.03273551566588185635, -9.846743663894592657 ) ) ;
#59308=CARTESIAN_POINT ( 'NONE',  ( 17.20831665107776587, 62.88393115100078745, 7.208316651077764980 ) ) ;
#59309=CARTESIAN_POINT ( 'NONE',  ( -1.099225684535947600, 33.70696800326375353, -6.408140936763238038 ) ) ;
#59310=CARTESIAN_POINT ( 'NONE',  ( -0.8801773607110991993, 22.85535201082150181, -2.915334737309923874 ) ) ;
#59312=CARTESIAN_POINT ( 'NONE',  ( 14.92337183194729633, 2.675597817667451750, 8.527530157486181039 ) ) ;
#59313=CARTESIAN_POINT ( 'NONE',  ( 20.88017736071110875, 20.77201867748816611, -2.915334737309920765 ) ) ;
#59315=CARTESIAN_POINT ( 'NONE',  ( 22.81628187352647785, 51.62363466993042493, 6.195893100308588602E-16 ) ) ;
#59316=CARTESIAN_POINT ( 'NONE',  ( 4.559911319644449179, 48.89701867748817676, 9.422509992056141925 ) ) ;
#59318=CARTESIAN_POINT ( 'NONE',  ( 21.09922568453594849, 51.20696800326375353, 6.408140936763242479 ) ) ;
#59319=CARTESIAN_POINT ( 'NONE',  ( -0.8801773607111009756, 48.06368534415484817, 1.068504757029289695E-15 ) ) ;
#59320=CARTESIAN_POINT ( 'NONE',  ( 10.00000000000000178, 62.25893115100078745, 9.846743663894594434 ) ) ;
#59322=CARTESIAN_POINT ( 'NONE',  ( 17.20831665107776587, 24.13393115100078035, -7.208316651077762316 ) ) ;
#59323=CARTESIAN_POINT ( 'NONE',  ( 13.43411237798106583, 7.665301336597086568, -12.81628187352647252 ) ) ;
#59324=CARTESIAN_POINT ( 'NONE',  ( 6.000000000000000000, 60.50000000000000711, 6.500000000000000888 ) ) ;
#59325=CARTESIAN_POINT ( 'NONE',  ( 18.52753015748618282, 58.92559781766745886, -4.923371831947291888 ) ) ;
#59326=CARTESIAN_POINT ( 'NONE',  ( 0.5774900079438590739, 27.64701867748817676, -5.440088680355550821 ) ) ;
#59327=CARTESIAN_POINT ( 'NONE',  ( 19.84674366389459266, 48.71726448433413026, -2.638427012816827677 ) ) ;
#59329=CARTESIAN_POINT ( 'NONE',  ( 1.472469842513823179, 6.425597817667451750, 4.923371831947296329 ) ) ;
#59330=CARTESIAN_POINT ( 'NONE',  ( 17.39651004071842166, 27.93575266056828355, 6.499999999999998224 ) ) ;
#59331=CARTESIAN_POINT ( 'NONE',  ( 6.565887622018943937, 8.081968003263751754, -12.81628187352647608 ) ) ;
#59333=STYLED_ITEM ( 'NONE', ( #3472 ), #63985 ) ;
#59335=DIRECTION ( 'NONE',  ( 0.000000000000000000, 0.000000000000000000, 1.000000000000000000 ) ) ;
#59336=CARTESIAN_POINT ( 'NONE',  ( -2.816281873526473856, 44.12363466993042493, 9.499525473075851096E-16 ) ) ;
#59337=CARTESIAN_POINT ( 'NONE',  ( 2.791683348922240793, 31.63393115100078745, 7.208316651077764092 ) ) ;
#59339=CARTESIAN_POINT ( 'NONE',  ( 2.035157376598822676, 12.43868534415483751, -7.964842623401177768 ) ) ;
#59340=CARTESIAN_POINT ( 'NONE',  ( 10.00000000000000178, 27.25893115100078390, 9.846743663894594434 ) ) ;
#59343=CARTESIAN_POINT ( 'NONE',  ( 7.084665262690076126, 4.105352010821503583, 10.88017736071109987 ) ) ;
#59345=CARTESIAN_POINT ( 'NONE',  ( 12.91533473730993009, 16.60535201082150891, -10.88017736071109987 ) ) ;
#59346=CARTESIAN_POINT ( 'NONE',  ( -4.164238869374098151, 51.59541550158063217, -3.795296366450310543 ) ) ;
#59347=CARTESIAN_POINT ( 'NONE',  ( 24.16423886937409904, 49.09541550158063217, 3.795296366450317205 ) ) ;
#59350=CARTESIAN_POINT ( 'NONE',  ( 19.84674366389459266, 8.300597817667451750, 2.638427012816836559 ) ) ;
#59351=CARTESIAN_POINT ( 'NONE',  ( 16.40814093676323893, 5.790301336597087456, 11.09922568453595026 ) ) ;
#59354=CYLINDRICAL_SURFACE ( 'NONE', #86460, 0.5000000000000004441 ) ;
#59356=CARTESIAN_POINT ( 'NONE',  ( 10.00000000000000000, 59.75893115100078745, -9.846743663894594434 ) ) ;
#59357=CARTESIAN_POINT ( 'NONE',  ( -46.90022492818602018, 100.5602504341072319, -9.231048971334091746 ) ) ;
#59358=CARTESIAN_POINT ( 'NONE',  ( 18.52753015748618282, 63.92559781766745886, -4.923371831947291888 ) ) ;
#59360=CARTESIAN_POINT ( 'NONE',  ( 14.92337183194729988, 19.34226448433411960, -8.527530157486177487 ) ) ;
#59362=CARTESIAN_POINT ( 'NONE',  ( -0.3689425029237898834, 36.17874883491396787, -10.36894250292378850 ) ) ;
#59364=CARTESIAN_POINT ( 'NONE',  ( 12.63842701281683922, 4.550597817667451750, -9.846743663894590881 ) ) ;
#59365=CARTESIAN_POINT ( 'NONE',  ( 1.152268111383477178, 1.024801820426059406E-17, -6.000000000000281553 ) ) ;
#59366=SURFACE_STYLE_FILL_AREA ( #4424 ) ;
#59367=CARTESIAN_POINT ( 'NONE',  ( -0.8801773607111009756, 28.06368534415484106, 1.068504757029289695E-15 ) ) ;
#59368=CARTESIAN_POINT ( 'NONE',  ( 0.6178305044545838731, 39.74863466993041072, 9.382169495545420901 ) ) ;
#59369=CARTESIAN_POINT ( 'NONE',  ( 7.084665262690076126, 9.105352010821503583, 10.88017736071109987 ) ) ;
#59370=CARTESIAN_POINT ( 'NONE',  ( 22.81628187352647785, 41.62363466993042493, 6.195893100308588602E-16 ) ) ;
#59371=CARTESIAN_POINT ( 'NONE',  ( 3.591859063236761518, 59.95696800326375353, 11.09922568453594849 ) ) ;
#59373=CARTESIAN_POINT ( 'NONE',  ( 1.932340009482149679, 11.49127512925448080, -6.499999999999995559 ) ) ;
#59374=CARTESIAN_POINT ( 'NONE',  ( 22.26659068614895176, 34.72041550158063927, -7.082119434687042414 ) ) ;
#59375=CARTESIAN_POINT ( 'NONE',  ( 20.88017736071110164, 5.355352010821502695, 2.915334737309930979 ) ) ;
#59376=CARTESIAN_POINT ( 'NONE',  ( 12.91533473730992121, 24.52201867748816966, 10.88017736071110164 ) ) ;
#59377=DIRECTION ( 'NONE',  ( -0.07626964003977962370, 0.9970872288863209532, 0.000000000000000000 ) ) ;
#59379=CARTESIAN_POINT ( 'NONE',  ( 20.88017736071110164, 50.35535201082151247, 2.915334737309930979 ) ) ;
#59380=CARTESIAN_POINT ( 'NONE',  ( -0.8801773607111008646, 48.27201867748816966, 2.915334737309923430 ) ) ;
#59381=CARTESIAN_POINT ( 'NONE',  ( 3.591859063236761518, 14.95696800326375531, 11.09922568453594849 ) ) ;
#59384=CARTESIAN_POINT ( 'NONE',  ( 12.63842701281683034, 27.46726448433411250, 9.846743663894596210 ) ) ;
#59385=CARTESIAN_POINT ( 'NONE',  ( -0.8801773607111008646, 63.27201867748817676, 2.915334737309923430 ) ) ;
#59387=CIRCLE ( 'NONE', #14738, 0.5000000000000004441 ) ;
#59389=CARTESIAN_POINT ( 'NONE',  ( 0.6178305044545838731, 14.74863466993041783, 9.382169495545420901 ) ) ;
#59390=CARTESIAN_POINT ( 'NONE',  ( 19.42250999205614193, 10.14701867748816966, 5.440088680355555262 ) ) ;
#59391=CARTESIAN_POINT ( 'NONE',  ( 5.076628168052703671, 36.84226448433412315, 8.527530157486179263 ) ) ;
#59392=CARTESIAN_POINT ( 'NONE',  ( 16.40814093676324603, 52.45696800326375353, -11.09922568453594671 ) ) ;
#59393=CARTESIAN_POINT ( 'NONE',  ( 12.63842701281683034, 22.46726448433411605, 9.846743663894596210 ) ) ;
#59395=CARTESIAN_POINT ( 'NONE',  ( 10.00000000000000000, 10.55374883491396787, -14.16423886937410082 ) ) ;
#59396=CARTESIAN_POINT ( 'NONE',  ( 2.603489959281614308, 36.58210964143329136, 6.500000000000031086 ) ) ;
#59397=CARTESIAN_POINT ( 'NONE',  ( -0.8801773607111008646, 18.27201867748817321, 2.915334737309923430 ) ) ;
#59398=LINE ( 'NONE', #29883, #8951 ) ;
#59399=CARTESIAN_POINT ( 'NONE',  ( -2.266590686148945544, 32.22041550158063927, 7.082119434687048631 ) ) ;
#59400=CARTESIAN_POINT ( 'NONE',  ( 19.84674366389459266, 38.71726448433412315, -2.638427012816827677 ) ) ;
#59401=CARTESIAN_POINT ( 'NONE',  ( 10.00000000000000178, 24.31368534415484106, 10.88017736071110342 ) ) ;
#59402=CARTESIAN_POINT ( 'NONE',  ( -0.8801773607111009756, 13.06368534415483929, 1.068504757029289695E-15 ) ) ;
#59404=CARTESIAN_POINT ( 'NONE',  ( 7.084665262690076126, 29.10535201082150181, 10.88017736071109987 ) ) ;
#59405=CARTESIAN_POINT ( 'NONE',  ( 0.6178305044545818747, 48.49863466993042493, -9.382169495545419124 ) ) ;
#59406=CARTESIAN_POINT ( 'NONE',  ( -0.8801773607110991993, 32.85535201082151247, -2.915334737309923874 ) ) ;
#59407=ORIENTED_EDGE ( 'NONE', *, *, #36355, .T. ) ;
#59408=CARTESIAN_POINT ( 'NONE',  ( 1.472469842513823179, 51.42559781766745886, 4.923371831947296329 ) ) ;
#59409=CARTESIAN_POINT ( 'NONE',  ( 17.96484262340118221, 36.18868534415484106, -7.964842623401177768 ) ) ;
#59410=CARTESIAN_POINT ( 'NONE',  ( 19.84674366389459266, 63.71726448433412315, -2.638427012816827677 ) ) ;
#59412=CARTESIAN_POINT ( 'NONE',  ( 21.09922568453594849, 61.20696800326376064, 6.408140936763242479 ) ) ;
#59414=CARTESIAN_POINT ( 'NONE',  ( 2.917880565312950480, 50.97041550158064638, -12.26659068614894821 ) ) ;
#59415=CARTESIAN_POINT ( 'NONE',  ( -0.8801773607111008646, 58.27201867748816966, 2.915334737309923430 ) ) ;
#59416=DIRECTION ( 'NONE',  ( 0.9970872288863208421, 0.07626964003977952655, -0.000000000000000000 ) ) ;
#59418=CARTESIAN_POINT ( 'NONE',  ( 19.84674366389459621, 63.50893115100078745, 7.409399052514197653E-17 ) ) ;
#59419=AXIS2_PLACEMENT_3D ( 'NONE', #26147, #96128, #55665 ) ;
#59421=CARTESIAN_POINT ( 'NONE',  ( 17.20831665107776587, 14.13393115100078568, -7.208316651077762316 ) ) ;
#59424=CARTESIAN_POINT ( 'NONE',  ( 5.076628168052704559, 15.17559781766745175, -8.527530157486179263 ) ) ;
#59426=EDGE_CURVE ( 'NONE', #79199, #73080, #31235, .T. ) ;
#59427=CARTESIAN_POINT ( 'NONE',  ( 12.91533473730992121, 29.52201867748817321, 10.88017736071110164 ) ) ;
#59428=CARTESIAN_POINT ( 'NONE',  ( 18.52753015748618282, 23.92559781766745530, -4.923371831947291888 ) ) ;
#59429=CARTESIAN_POINT ( 'NONE',  ( 12.91533473730993009, 56.60535201082151247, -10.88017736071109987 ) ) ;
#59430=CARTESIAN_POINT ( 'NONE',  ( 7.084665262690076126, 62.02201867748816966, -10.88017736071110164 ) ) ;
#59431=CARTESIAN_POINT ( 'NONE',  ( -0.8801773607111008646, 33.27201867748817676, 2.915334737309923430 ) ) ;
#59432=CARTESIAN_POINT ( 'NONE',  ( 16.40814093676324603, 57.45696800326375353, -11.09922568453594671 ) ) ;
#59433=CARTESIAN_POINT ( 'NONE',  ( 2.917880565312950480, 45.97041550158063927, -12.26659068614894821 ) ) ;
#59438=CARTESIAN_POINT ( 'NONE',  ( -2.816281873526471635, -1.084698663402913210, -3.434112377981056508 ) ) ;
#59439=CARTESIAN_POINT ( 'NONE',  ( 7.084665262690076126, 4.105352010821503583, 10.88017736071109987 ) ) ;
#59440=CARTESIAN_POINT ( 'NONE',  ( 17.96484262340118221, 49.93868534415484106, 7.964842623401181321 ) ) ;
#59441=DIRECTION ( 'NONE',  ( -1.000000000000000000, 0.000000000000000000, 0.000000000000000000 ) ) ;
#59442=ORIENTED_EDGE ( 'NONE', *, *, #93485, .T. ) ;
#59443=CARTESIAN_POINT ( 'NONE',  ( 1.472469842513823179, 20.59226448433411960, -4.923371831947296329 ) ) ;
#59444=CARTESIAN_POINT ( 'NONE',  ( 15.44008868035555260, 59.73035201082151247, 9.422509992056143702 ) ) ;
#59445=CARTESIAN_POINT ( 'NONE',  ( 12.63842701281683034, 37.46726448433411605, 9.846743663894596210 ) ) ;
#59446=CARTESIAN_POINT ( 'NONE',  ( 19.84674366389459266, 28.30059781766745886, 2.638427012816836559 ) ) ;
#59447=CARTESIAN_POINT ( 'NONE',  ( 0.1532563361054083140, 16.00893115100078390, 1.131784320476157264E-15 ) ) ;
#59449=CARTESIAN_POINT ( 'NONE',  ( 10.00000000000000178, 40.37363466993042493, 12.81628187352647608 ) ) ;
#59450=CARTESIAN_POINT ( 'NONE',  ( 7.084665262690076126, 69.10535201082151957, 10.88017736071109987 ) ) ;
#59454=CARTESIAN_POINT ( 'NONE',  ( 12.63842701281683034, 32.46726448433412315, 9.846743663894596210 ) ) ;
#59456=CARTESIAN_POINT ( 'NONE',  ( 19.38216949554541557, 57.24863466993042493, -9.382169495545420901 ) ) ;
#59459=CARTESIAN_POINT ( 'NONE',  ( 6.565887622018943937, -1.918031996736246692, -12.81628187352647608 ) ) ;
#59460=CARTESIAN_POINT ( 'NONE',  ( 20.88017736071110519, 10.56368534415483751, 2.639326808657452039E-16 ) ) ;
#59461=CARTESIAN_POINT ( 'NONE',  ( -0.3689425029237881626, 37.42874883491396787, 10.36894250292379027 ) ) ;
#59464=CARTESIAN_POINT ( 'NONE',  ( -4.164238869374099927, 37.01208216824731068, 3.795296366450308767 ) ) ;
#59465=CARTESIAN_POINT ( 'NONE',  ( 24.16423886937409904, 44.09541550158063927, 3.795296366450317205 ) ) ;
#59466=CARTESIAN_POINT ( 'NONE',  ( 13.79529636645031943, 10.34541550158063394, -14.16423886937409904 ) ) ;
#59467=CARTESIAN_POINT ( 'NONE',  ( 22.26659068614894466, 8.887082168247300018, 7.082119434687054849 ) ) ;
#59469=CARTESIAN_POINT ( 'NONE',  ( 7.084665262690076126, 44.10535201082151247, 10.88017736071109987 ) ) ;
#59472=CARTESIAN_POINT ( 'NONE',  ( 5.076628168052704559, 35.17559781766745175, -8.527530157486179263 ) ) ;
#59473=DIRECTION ( 'NONE',  ( 1.000000000000000000, 2.799047438454523236E-16, -0.000000000000000000 ) ) ;
#59474=CARTESIAN_POINT ( 'NONE',  ( 7.361572987183169658, 24.96726448433412315, -9.846743663894592657 ) ) ;
#59475=CARTESIAN_POINT ( 'NONE',  ( 15.44008868035555260, 9.730352010821505360, 9.422509992056143702 ) ) ;
#59476=CARTESIAN_POINT ( 'NONE',  ( 0.6178305044545818747, 58.49863466993042493, -9.382169495545419124 ) ) ;
#59477=CARTESIAN_POINT ( 'NONE',  ( 1.472469842513823179, 51.42559781766745886, 4.923371831947296329 ) ) ;
#59479=CARTESIAN_POINT ( 'NONE',  ( 18.52753015748618282, 28.92559781766745175, -4.923371831947291888 ) ) ;
#59480=CARTESIAN_POINT ( 'NONE',  ( 10.00000000000000178, 45.37363466993041783, 12.81628187352647608 ) ) ;
#59483=CARTESIAN_POINT ( 'NONE',  ( 20.88017736071110519, 40.56368534415484106, 2.639326808657452039E-16 ) ) ;
#59484=CARTESIAN_POINT ( 'NONE',  ( 1.472469842513823179, 35.59226448433412315, -4.923371831947296329 ) ) ;
#59485=CARTESIAN_POINT ( 'NONE',  ( 13.79529636645031943, 25.34541550158063572, -14.16423886937409904 ) ) ;
#59487=CARTESIAN_POINT ( 'NONE',  ( 2.917880565312950480, 0.9704155015806342766, -12.26659068614894821 ) ) ;
#59488=B_SPLINE_CURVE_WITH_KNOTS ( 'NONE', 3,
 ( #44429, #6939, #37446, #67937 ),
 .UNSPECIFIED., .F., .F.,
 ( 4, 4 ),
 ( 3.418109631315660599E-17, 0.002392975128318455130 ),
 .UNSPECIFIED. ) ;
#59489=CARTESIAN_POINT ( 'NONE',  ( 12.91533473730993009, 61.60535201082150536, -10.88017736071109987 ) ) ;
#59490=CARTESIAN_POINT ( 'NONE',  ( 15.44008868035555260, 64.73035201082151957, 9.422509992056143702 ) ) ;
#59491=CARTESIAN_POINT ( 'NONE',  ( 17.08211943468705130, 63.47041550158063927, 12.26659068614894998 ) ) ;
#59493=CARTESIAN_POINT ( 'NONE',  ( 1.472469842513823179, 66.42559781766745175, 4.923371831947296329 ) ) ;
#59496=CARTESIAN_POINT ( 'NONE',  ( 10.00000000000000178, 54.31368534415484106, 10.88017736071110342 ) ) ;
#59498=FACE_OUTER_BOUND ( 'NONE', #46518, .T. ) ;
#59500=CARTESIAN_POINT ( 'NONE',  ( 0.5774900079438607392, 18.48035201082150536, 5.440088680355550821 ) ) ;
#59501=CARTESIAN_POINT ( 'NONE',  ( 20.88017736071110519, 5.563685344154838397, 2.639326808657452039E-16 ) ) ;
#59503=CARTESIAN_POINT ( 'NONE',  ( 18.52753015748617571, 48.09226448433412315, 4.923371831947298993 ) ) ;
#59504=CARTESIAN_POINT ( 'NONE',  ( 16.40814093676323893, 55.79030133659708923, 11.09922568453595026 ) ) ;
#59507=CARTESIAN_POINT ( 'NONE',  ( 20.88017736071110519, 20.56368534415484106, 2.639326808657452039E-16 ) ) ;
#59508=CARTESIAN_POINT ( 'NONE',  ( -2.816281873526473856, -0.6680319967362464695, 3.434112377981055619 ) ) ;
#59509=DIRECTION ( 'NONE',  ( -0.000000000000000000, -0.000000000000000000, -1.000000000000000000 ) ) ;
#59511=CARTESIAN_POINT ( 'NONE',  ( 14.92337183194729633, 12.67559781766745353, 8.527530157486181039 ) ) ;
#59513=CARTESIAN_POINT ( 'NONE',  ( 12.63842701281683034, 47.46726448433412315, 9.846743663894596210 ) ) ;
#59514=CARTESIAN_POINT ( 'NONE',  ( 0.5774900079438590739, 32.64701867748816966, -5.440088680355550821 ) ) ;
#59515=CARTESIAN_POINT ( 'NONE',  ( -2.816281873526473856, 4.331968003263754419, 3.434112377981055619 ) ) ;
#59516=CARTESIAN_POINT ( 'NONE',  ( -0.8801773607110991993, 52.85535201082151247, -2.915334737309923874 ) ) ;
#59519=CARTESIAN_POINT ( 'NONE',  ( 19.38216949554541557, 52.24863466993041072, -9.382169495545420901 ) ) ;
#59523=CARTESIAN_POINT ( 'NONE',  ( 6.565887622018943937, 33.08196800326374643, -12.81628187352647608 ) ) ;
#59525=CARTESIAN_POINT ( 'NONE',  ( 10.00000000000000178, 44.31368534415484106, 10.88017736071110342 ) ) ;
#59527=CARTESIAN_POINT ( 'NONE',  ( 12.63842701281683034, 47.46726448433412315, 9.846743663894596210 ) ) ;
#59528=CARTESIAN_POINT ( 'NONE',  ( 2.791683348922240793, 21.63393115100078745, 7.208316651077764092 ) ) ;
#59529=CARTESIAN_POINT ( 'NONE',  ( 0.1532563361054082862, 11.21726448433411605, 2.638427012816831674 ) ) ;
#59530=CARTESIAN_POINT ( 'NONE',  ( 22.26659068614894466, 38.88708216824731068, 7.082119434687054849 ) ) ;
#59531=DIRECTION ( 'NONE',  ( 1.000000000000000000, 0.000000000000000000, 0.000000000000000000 ) ) ;
#59534=ORIENTED_EDGE ( 'NONE', *, *, #84794, .T. ) ;
#59536=AXIS2_PLACEMENT_3D ( 'NONE', #30668, #29195, #54160 ) ;
#59537=CARTESIAN_POINT ( 'NONE',  ( 17.08211943468705840, 65.13708216824730357, -12.26659068614894466 ) ) ;
#59538=CARTESIAN_POINT ( 'NONE',  ( 17.08211943468705130, 63.47041550158063927, 12.26659068614894998 ) ) ;
#59539=CARTESIAN_POINT ( 'NONE',  ( 17.20831665107776587, 34.13393115100078745, -7.208316651077762316 ) ) ;
#59540=CARTESIAN_POINT ( 'NONE',  ( 3.591859063236763294, 23.29030133659708568, -11.09922568453595026 ) ) ;
#59541=DIRECTION ( 'NONE',  ( -1.000000000000000000, -2.799047438454523236E-16, 0.000000000000000000 ) ) ;
#59543=CARTESIAN_POINT ( 'NONE',  ( -2.266590686148945544, 12.22041550158063394, 7.082119434687048631 ) ) ;
#59544=CARTESIAN_POINT ( 'NONE',  ( 15.44008868035555260, 9.730352010821505360, 9.422509992056143702 ) ) ;
#59545=CARTESIAN_POINT ( 'NONE',  ( 17.08211943468705840, 55.13708216824731068, -12.26659068614894466 ) ) ;
#59546=CARTESIAN_POINT ( 'NONE',  ( 2.791683348922240793, 26.63393115100078745, 7.208316651077764092 ) ) ;
#59547=CARTESIAN_POINT ( 'NONE',  ( -0.1079698255113996641, 0.1351729006312037407, 6.323366879845591981 ) ) ;
#59548=CARTESIAN_POINT ( 'NONE',  ( 18.52753015748617571, 8.092264484334117824, 4.923371831947298993 ) ) ;
#59555=CARTESIAN_POINT ( 'NONE',  ( 18.52753015748617571, 48.09226448433412315, 4.923371831947298993 ) ) ;
#59556=CARTESIAN_POINT ( 'NONE',  ( 20.88017736071110164, 25.35535201082150891, 2.915334737309930979 ) ) ;
#59557=CARTESIAN_POINT ( 'NONE',  ( 17.20831665107776587, 62.88393115100078745, 7.208316651077764980 ) ) ;
#59558=CARTESIAN_POINT ( 'NONE',  ( 0.6178305044545818747, 18.49863466993041428, -9.382169495545419124 ) ) ;
#59559=( NAMED_UNIT ( * ) PLANE_ANGLE_UNIT ( ) SI_UNIT ( $, .RADIAN. ) );
#59561=AXIS2_PLACEMENT_3D ( 'NONE', #53872, #39850, #69863 ) ;
#59562=AXIS2_PLACEMENT_3D ( 'NONE', #54066, #70072, #40059 ) ;
#59563=CARTESIAN_POINT ( 'NONE',  ( -2.816281873526471635, 28.91530133659708213, -3.434112377981056508 ) ) ;
#59566=CARTESIAN_POINT ( 'NONE',  ( 10.00000000000000178, 32.25893115100078745, 9.846743663894594434 ) ) ;
#59568=CARTESIAN_POINT ( 'NONE',  ( 12.91533473730993009, 11.60535201082150714, -10.88017736071109987 ) ) ;
#59570=CARTESIAN_POINT ( 'NONE',  ( -0.8801773607110991993, 7.855352010821506248, -2.915334737309923874 ) ) ;
#59572=CARTESIAN_POINT ( 'NONE',  ( 12.91533473730993009, 46.60535201082150536, -10.88017736071109987 ) ) ;
#59573=CARTESIAN_POINT ( 'NONE',  ( 15.44008868035555260, 64.73035201082151957, 9.422509992056143702 ) ) ;
#59574=CARTESIAN_POINT ( 'NONE',  ( 10.00000000000000178, 69.31368534415484817, 10.88017736071110342 ) ) ;
#59576=CARTESIAN_POINT ( 'NONE',  ( -0.8801773607111008646, 48.27201867748816966, 2.915334737309923430 ) ) ;
#59579=CARTESIAN_POINT ( 'NONE',  ( 5.076628168052703671, 31.84226448433412315, 8.527530157486179263 ) ) ;
#59581=CARTESIAN_POINT ( 'NONE',  ( 18.52753015748617571, 58.09226448433411605, 4.923371831947298993 ) ) ;
#59583=CARTESIAN_POINT ( 'NONE',  ( 24.16423886937410614, 9.303748834913967869, 8.672049930838204340E-16 ) ) ;
#59585=FACE_OUTER_BOUND ( 'NONE', #25724, .T. ) ;
#59586=CARTESIAN_POINT ( 'NONE',  ( 1.821158202401655934, 26.16688879859530914, 6.499999999999960920 ) ) ;
#59587=CARTESIAN_POINT ( 'NONE',  ( 19.42250999205614193, 5.147018677488171434, 5.440088680355555262 ) ) ;
#59588=CARTESIAN_POINT ( 'NONE',  ( 5.076628168052704559, 50.17559781766745886, -8.527530157486179263 ) ) ;
#59590=CARTESIAN_POINT ( 'NONE',  ( 16.40814093676323893, 20.79030133659708923, 11.09922568453595026 ) ) ;
#59592=CARTESIAN_POINT ( 'NONE',  ( 10.00000000000000178, 12.25893115100078568, 9.846743663894594434 ) ) ;
#59593=CARTESIAN_POINT ( 'NONE',  ( 2.603489959281581889, 30.43575266056827999, -6.499999999999995559 ) ) ;
#59595=CARTESIAN_POINT ( 'NONE',  ( 6.565887622018943937, 5.165301336597086568, 12.81628187352647430 ) ) ;
#59599=ADVANCED_FACE ( 'NONE', ( #79205 ), #25161, .T. ) ;
#59601=CARTESIAN_POINT ( 'NONE',  ( 12.91533473730992121, 4.522018677488170546, 10.88017736071110164 ) ) ;
#59602=CARTESIAN_POINT ( 'NONE',  ( 2.917880565312948704, 17.63708216824730357, 12.26659068614894643 ) ) ;
#59603=CARTESIAN_POINT ( 'NONE',  ( 17.20831665107776587, 32.88393115100078745, 7.208316651077764980 ) ) ;
#59604=CARTESIAN_POINT ( 'NONE',  ( 12.91533473730993009, 61.60535201082150536, -10.88017736071109987 ) ) ;
#59605=CARTESIAN_POINT ( 'NONE',  ( 16.40814093676324603, 37.45696800326376064, -11.09922568453594671 ) ) ;
#59607=CARTESIAN_POINT ( 'NONE',  ( 4.559911319644449179, 17.23035201082150536, -9.422509992056141925 ) ) ;
#59610=CARTESIAN_POINT ( 'NONE',  ( 0.6178305044545818747, 8.498634669930421381, -9.382169495545419124 ) ) ;
#59611=CARTESIAN_POINT ( 'NONE',  ( 17.20831665107776587, 62.88393115100078745, 7.208316651077764980 ) ) ;
#59612=CARTESIAN_POINT ( 'NONE',  ( 0.1532563361054083140, 26.00893115100078745, 1.131784320476157264E-15 ) ) ;
#59614=CARTESIAN_POINT ( 'NONE',  ( 0.6178305044545838731, 29.74863466993042138, 9.382169495545420901 ) ) ;
#59615=CARTESIAN_POINT ( 'NONE',  ( 17.62281668512003208, 23.28593319516823001, 6.499999999999993783 ) ) ;
#59616=CARTESIAN_POINT ( 'NONE',  ( 2.035157376598824452, 33.68868534415484106, 7.964842623401179544 ) ) ;
#59618=CARTESIAN_POINT ( 'NONE',  ( 19.72487221294570858, 41.86607318730076344, 6.500000000000000888 ) ) ;
#59619=CARTESIAN_POINT ( 'NONE',  ( 20.88017736071110875, 45.77201867748816966, -2.915334737309920765 ) ) ;
#59620=CARTESIAN_POINT ( 'NONE',  ( 7.084665262690076126, 42.02201867748816966, -10.88017736071110164 ) ) ;
#59623=CARTESIAN_POINT ( 'NONE',  ( 20.88017736071110164, 50.35535201082151247, 2.915334737309930979 ) ) ;
#59626=CARTESIAN_POINT ( 'NONE',  ( 1.472469842513823179, 36.42559781766745175, 4.923371831947296329 ) ) ;
#59627=CARTESIAN_POINT ( 'NONE',  ( 12.91533473730993009, 11.60535201082150536, -10.88017736071109987 ) ) ;
#59628=CARTESIAN_POINT ( 'NONE',  ( 0.6178305044545838731, 9.748634669930416052, 9.382169495545420901 ) ) ;
#59630=CARTESIAN_POINT ( 'NONE',  ( 12.91533473730992121, 29.52201867748817321, 10.88017736071110164 ) ) ;
#59632=VECTOR ( 'NONE', #21491, 1000.000000000000000 ) ;
#59633=CARTESIAN_POINT ( 'NONE',  ( 17.39651004071841456, 7.935752660568278216, 6.500000000000003553 ) ) ;
#59634=CARTESIAN_POINT ( 'NONE',  ( 7.084665262690076126, 2.022018677488170990, -10.88017736071110164 ) ) ;
#59635=CARTESIAN_POINT ( 'NONE',  ( 10.00000000000000000, 26.81368534415484106, -10.88017736071110342 ) ) ;
#59636=CARTESIAN_POINT ( 'NONE',  ( -0.8801773607110991993, 67.85535201082151957, -2.915334737309923874 ) ) ;
#59637=CARTESIAN_POINT ( 'NONE',  ( -0.3689425029237898834, 21.17874883491396432, -10.36894250292378850 ) ) ;
#59638=CARTESIAN_POINT ( 'NONE',  ( 2.791683348922237240, 10.38393115100078390, -7.208316651077763204 ) ) ;
#59639=CARTESIAN_POINT ( 'NONE',  ( 19.42250999205614548, 45.98035201082150536, -5.440088680355545492 ) ) ;
#59642=CARTESIAN_POINT ( 'NONE',  ( 17.08211943468705130, 3.470415501580634388, 12.26659068614894998 ) ) ;
#59646=CARTESIAN_POINT ( 'NONE',  ( 12.63842701281683922, 39.55059781766744464, -9.846743663894590881 ) ) ;
#59649=CARTESIAN_POINT ( 'NONE',  ( 2.917880565312948704, 17.63708216824730357, 12.26659068614894643 ) ) ;
#59650=CARTESIAN_POINT ( 'NONE',  ( -0.3689425029237881626, 22.42874883491397142, 10.36894250292379027 ) ) ;
#59651=CARTESIAN_POINT ( 'NONE',  ( 20.88017736071110875, 65.77201867748817676, -2.915334737309920765 ) ) ;
#59652=CARTESIAN_POINT ( 'NONE',  ( 10.00000000000000000, 65.55374883491396076, -14.16423886937410082 ) ) ;
#59653=CARTESIAN_POINT ( 'NONE',  ( 0.1532563361054082862, 66.21726448433413736, 2.638427012816831674 ) ) ;
#59654=CARTESIAN_POINT ( 'NONE',  ( 0.1532563361054082862, 51.21726448433412315, 2.638427012816831674 ) ) ;
#59656=CARTESIAN_POINT ( 'NONE',  ( 7.084665262690076126, 52.02201867748816255, -10.88017736071110164 ) ) ;
#59657=CARTESIAN_POINT ( 'NONE',  ( -2.816281873526473856, 9.123634669930421381, 9.499525473075851096E-16 ) ) ;
#59658=CARTESIAN_POINT ( 'NONE',  ( 6.204703633549690345, 12.84541550158063572, 14.16423886937410082 ) ) ;
#59659=CARTESIAN_POINT ( 'NONE',  ( 0.5774900079438590739, 17.64701867748817321, -5.440088680355550821 ) ) ;
#59660=CARTESIAN_POINT ( 'NONE',  ( -0.8801773607110991993, 22.85535201082150181, -2.915334737309923874 ) ) ;
#59661=CARTESIAN_POINT ( 'NONE',  ( 18.04007052943772038, 54.00257860105348584, -5.767676674365850076 ) ) ;
#59662=CARTESIAN_POINT ( 'NONE',  ( 4.559911319644449179, 48.89701867748817676, 9.422509992056141925 ) ) ;
#59666=ORIENTED_EDGE ( 'NONE', *, *, #93681, .T. ) ;
#59667=ORIENTED_EDGE ( 'NONE', *, *, #92635, .T. ) ;
#59668=DIRECTION ( 'NONE',  ( -1.000000000000000000, 0.000000000000000000, 0.000000000000000000 ) ) ;
#59669=CARTESIAN_POINT ( 'NONE',  ( 6.204703633549690345, 47.84541550158064638, 14.16423886937410082 ) ) ;
#59670=CARTESIAN_POINT ( 'NONE',  ( 17.96484262340118221, 11.18868534415484106, -7.964842623401177768 ) ) ;
#59671=CARTESIAN_POINT ( 'NONE',  ( 7.361572987183169658, 19.96726448433411960, -9.846743663894592657 ) ) ;
#59672=CARTESIAN_POINT ( 'NONE',  ( 0.1532563361054100626, 50.80059781766745175, -2.638427012816831230 ) ) ;
#59674=DIRECTION ( 'NONE',  ( 0.5547001962252290364, 0.8320502943378437211, 0.000000000000000000 ) ) ;
#59676=CARTESIAN_POINT ( 'NONE',  ( 12.63842701281683922, 4.550597817667451750, -9.846743663894590881 ) ) ;
#59679=CARTESIAN_POINT ( 'NONE',  ( -4.164238869374099039, 31.80374883491396432, 8.674139862899312516E-16 ) ) ;
#59680=CARTESIAN_POINT ( 'NONE',  ( 22.81628187352648496, 26.83196800326374998, -3.434112377981050290 ) ) ;
#59682=CARTESIAN_POINT ( 'NONE',  ( 22.81628187352647785, 46.41530133659708213, 3.434112377981063169 ) ) ;
#59683=CARTESIAN_POINT ( 'NONE',  ( 1.472469842513823179, 35.59226448433412315, -4.923371831947296329 ) ) ;
#59684=CARTESIAN_POINT ( 'NONE',  ( 20.88017736071110875, 30.77201867748816966, -2.915334737309920765 ) ) ;
#59685=CARTESIAN_POINT ( 'NONE',  ( 21.09922568453595559, 62.04030133659709634, -6.408140936763230044 ) ) ;
#59686=CARTESIAN_POINT ( 'NONE',  ( -29.94000000000000838, 92.00000000000000000, 9.500000000000000000 ) ) ;
#59687=CARTESIAN_POINT ( 'NONE',  ( 12.63842701281683922, 49.55059781766744464, -9.846743663894590881 ) ) ;
#59688=CARTESIAN_POINT ( 'NONE',  ( 1.472469842513823179, 56.42559781766745886, 4.923371831947296329 ) ) ;
#59693=VECTOR ( 'NONE', #71223, 1000.000000000000000 ) ;
#59695=CARTESIAN_POINT ( 'NONE',  ( 7.361572987183169658, 19.96726448433411960, -9.846743663894592657 ) ) ;
#59696=CARTESIAN_POINT ( 'NONE',  ( -1.099225684535947600, 34.54030133659708923, 6.408140936763237150 ) ) ;
#59699=ORIENTED_EDGE ( 'NONE', *, *, #2579, .F. ) ;
#59700=CARTESIAN_POINT ( 'NONE',  ( 14.92337183194729988, 54.34226448433412315, -8.527530157486177487 ) ) ;
#59702=CARTESIAN_POINT ( 'NONE',  ( 7.361572987183170547, 42.05059781766745886, 9.846743663894590881 ) ) ;
#59703=CARTESIAN_POINT ( 'NONE',  ( 10.00000000000000178, 33.05374883491396787, 14.16423886937410082 ) ) ;
#59704=CARTESIAN_POINT ( 'NONE',  ( 10.00000000000000000, 49.75893115100078745, -9.846743663894594434 ) ) ;
#59705=CARTESIAN_POINT ( 'NONE',  ( -1.099225684535947600, 44.54030133659708923, 6.408140936763237150 ) ) ;
#59706=CARTESIAN_POINT ( 'NONE',  ( 20.24186590665276597, 36.76028685723174760, 6.114288769123060518 ) ) ;
#59708=CARTESIAN_POINT ( 'NONE',  ( 12.63842701281683034, 2.467264484334118269, 9.846743663894596210 ) ) ;
#59711=CARTESIAN_POINT ( 'NONE',  ( 19.84674366389459621, 53.50893115100078745, 7.409399052514197653E-17 ) ) ;
#59712=CARTESIAN_POINT ( 'NONE',  ( 10.00000000000000000, 46.81368534415484106, -10.88017736071110342 ) ) ;
#59713=CARTESIAN_POINT ( 'NONE',  ( 7.361572987183170547, 42.05059781766745886, 9.846743663894590881 ) ) ;
#59716=CARTESIAN_POINT ( 'NONE',  ( 7.084665262690076126, 47.02201867748818387, -10.88017736071110164 ) ) ;
#59720=CARTESIAN_POINT ( 'NONE',  ( 7.084665262690076126, 19.10535201082150181, 10.88017736071109987 ) ) ;
#59721=CARTESIAN_POINT ( 'NONE',  ( 22.81628187352648496, 6.831968003263753531, -3.434112377981050290 ) ) ;
#59722=CARTESIAN_POINT ( 'NONE',  ( 4.559911319644449179, 38.89701867748817676, 9.422509992056141925 ) ) ;
#59724=CARTESIAN_POINT ( 'NONE',  ( 10.00000000000000000, 61.81368534415484106, -10.88017736071110342 ) ) ;
#59725=DIRECTION ( 'NONE',  ( 0.000000000000000000, -1.000000000000000000, 0.000000000000000000 ) ) ;
#59726=CARTESIAN_POINT ( 'NONE',  ( 4.559911319644449179, 37.23035201082150536, -9.422509992056141925 ) ) ;
#59728=CARTESIAN_POINT ( 'NONE',  ( 19.84674366389459266, 8.717264484334116048, -2.638427012816827677 ) ) ;
#59729=CARTESIAN_POINT ( 'NONE',  ( 5.076628168052704559, 30.17559781766745175, -8.527530157486179263 ) ) ;
#59730=FILL_AREA_STYLE_COLOUR ( '', #5816 ) ;
#59732=CARTESIAN_POINT ( 'NONE',  ( 19.84674366389459266, 63.30059781766745886, 2.638427012816836559 ) ) ;
#59733=CARTESIAN_POINT ( 'NONE',  ( 13.79529636645030344, 63.26208216824730357, 14.16423886937410614 ) ) ;
#59736=CARTESIAN_POINT ( 'NONE',  ( 2.917880565312948704, 12.63708216824730179, 12.26659068614894643 ) ) ;
#59737=CARTESIAN_POINT ( 'NONE',  ( 13.79529636645030344, 53.26208216824730357, 14.16423886937410614 ) ) ;
#59738=CARTESIAN_POINT ( 'NONE',  ( 7.084665262690076126, 2.022018677488170990, -10.88017736071110164 ) ) ;
#59739=ORIENTED_EDGE ( 'NONE', *, *, #48327, .F. ) ;
#59740=CARTESIAN_POINT ( 'NONE',  ( 19.84674366389459266, 18.30059781766745175, 2.638427012816836559 ) ) ;
#59741=CARTESIAN_POINT ( 'NONE',  ( 0.5774900079438607392, 13.48035201082150358, 5.440088680355550821 ) ) ;
#59742=CARTESIAN_POINT ( 'NONE',  ( 7.361572987183169658, 44.96726448433412315, -9.846743663894592657 ) ) ;
#59745=LINE ( 'NONE', #19289, #93508 ) ;
#59746=CARTESIAN_POINT ( 'NONE',  ( -1.099225684535947600, 29.54030133659708923, 6.408140936763237150 ) ) ;
#59747=CARTESIAN_POINT ( 'NONE',  ( 14.92337183194729988, 44.34226448433412315, -8.527530157486177487 ) ) ;
#59748=VERTEX_POINT ( 'NONE', #682 ) ;
#59749=CARTESIAN_POINT ( 'NONE',  ( 1.472469842513823179, 6.425597817667451750, 4.923371831947296329 ) ) ;
#59750=EDGE_CURVE ( 'NONE', #12094, #49705, #60651, .T. ) ;
#59753=CARTESIAN_POINT ( 'NONE',  ( -0.8801773607111009756, 8.063685344154837509, 1.068504757029289695E-15 ) ) ;
#59754=CARTESIAN_POINT ( 'NONE',  ( 6.204703633549690345, 40.76208216824731778, -14.16423886937410259 ) ) ;
#59755=CARTESIAN_POINT ( 'NONE',  ( 15.44008868035555260, 59.73035201082151247, 9.422509992056143702 ) ) ;
#59757=CARTESIAN_POINT ( 'NONE',  ( 5.076628168052704559, 25.17559781766745175, -8.527530157486179263 ) ) ;
#59758=( NAMED_UNIT ( * ) SI_UNIT ( $, .STERADIAN. ) SOLID_ANGLE_UNIT ( ) );
#59759=CARTESIAN_POINT ( 'NONE',  ( 5.076628168052703671, 1.842264484334118047, 8.527530157486179263 ) ) ;
#59761=CARTESIAN_POINT ( 'NONE',  ( 0.1532563361054100626, 40.80059781766745886, -2.638427012816831230 ) ) ;
#59762=CARTESIAN_POINT ( 'NONE',  ( 7.084665262690076126, 34.10535201082151247, 10.88017736071109987 ) ) ;
#59764=CARTESIAN_POINT ( 'NONE',  ( 21.09922568453594849, 61.20696800326376064, 6.408140936763242479 ) ) ;
#59767=B_SPLINE_CURVE_WITH_KNOTS ( 'NONE', 3,
 ( #21415, #13919, #5440, #34919 ),
 .UNSPECIFIED., .F., .F.,
 ( 4, 4 ),
 ( 3.469446951953614189E-18, 0.002562518741975320334 ),
 .UNSPECIFIED. ) ;
#59768=CARTESIAN_POINT ( 'NONE',  ( 19.84674366389459266, 13.71726448433411782, -2.638427012816827677 ) ) ;
#59769=CARTESIAN_POINT ( 'NONE',  ( 3.591859063236761518, 49.95696800326375353, 11.09922568453594849 ) ) ;
#59770=CARTESIAN_POINT ( 'NONE',  ( 19.42250999205614548, 10.98035201082150536, -5.440088680355545492 ) ) ;
#59771=CARTESIAN_POINT ( 'NONE',  ( 1.472469842513823179, 40.59226448433411605, -4.923371831947296329 ) ) ;
#59773=SURFACE_STYLE_FILL_AREA ( #6785 ) ;
#59774=CARTESIAN_POINT ( 'NONE',  ( 24.16423886937409904, 49.09541550158063217, 3.795296366450317205 ) ) ;
#59775=CARTESIAN_POINT ( 'NONE',  ( 19.84674366389459621, 63.50893115100078745, 7.409399052514197653E-17 ) ) ;
#59777=CARTESIAN_POINT ( 'NONE',  ( 19.42250999205614548, 35.98035201082151247, -5.440088680355545492 ) ) ;
#59779=CARTESIAN_POINT ( 'NONE',  ( 1.472469842513823179, 6.425597817667451750, 4.923371831947296329 ) ) ;
#59782=CARTESIAN_POINT ( 'NONE',  ( 22.81628187352647785, 61.41530133659709634, 3.434112377981063169 ) ) ;
#59783=CARTESIAN_POINT ( 'NONE',  ( 2.035157376598822676, 62.43868534415483396, -7.964842623401177768 ) ) ;
#59785=CARTESIAN_POINT ( 'NONE',  ( 24.16423886937409904, 9.095415501580633943, 3.795296366450317205 ) ) ;
#59786=CARTESIAN_POINT ( 'NONE',  ( 12.63842701281683034, 12.46726448433411782, 9.846743663894596210 ) ) ;
#59789=( BOUNDED_CURVE ( )  B_SPLINE_CURVE ( 2, ( #98199, #60165, #53655, #54138, #23676, #25155, #47124, #69649, #62615 ),
 .UNSPECIFIED., .F., .T. ) 
 B_SPLINE_CURVE_WITH_KNOTS ( ( 3, 2, 2, 2, 3 ),
 ( 0.1187123655116599508, 0.1190476190476190688, 0.1250000000000000000, 0.1309523809523809312, 0.1312876344883400492 ),
 .UNSPECIFIED. ) 
 CURVE ( )  GEOMETRIC_REPRESENTATION_ITEM ( )  RATIONAL_B_SPLINE_CURVE ( ( 0.9963778908391762723, 0.9980808541467921513, 1.000000000000000000, 0.9659258262890682012, 1.000000000000000000, 0.9659258262890682012, 1.000000000000000000, 0.9980808541467922623, 0.9963778908391763833 ) ) 
 REPRESENTATION_ITEM ( '' )  );
#59790=CARTESIAN_POINT ( 'NONE',  ( 15.44008868035555793, 26.39701867748817321, -9.422509992056140149 ) ) ;
#59791=ORIENTED_EDGE ( 'NONE', *, *, #92673, .F. ) ;
#59792=CARTESIAN_POINT ( 'NONE',  ( 7.084665262690076126, 34.10535201082151247, 10.88017736071109987 ) ) ;
#59793=DIRECTION ( 'NONE',  ( -0.5547001962252291474, -0.8320502943378437211, -0.000000000000000000 ) ) ;
#59796=EDGE_CURVE ( 'NONE', #50559, #80095, #16088, .T. ) ;
#59797=CARTESIAN_POINT ( 'NONE',  ( 20.88017736071110164, 60.35535201082151957, 2.915334737309930979 ) ) ;
#59798=CARTESIAN_POINT ( 'NONE',  ( 5.076628168052704559, 60.17559781766745175, -8.527530157486179263 ) ) ;
#59799=CARTESIAN_POINT ( 'NONE',  ( 15.44008868035555260, 24.73035201082150891, 9.422509992056143702 ) ) ;
#59800=LINE ( 'NONE', #23807, #7999 ) ;
#59801=CARTESIAN_POINT ( 'NONE',  ( 10.00000000000000178, 7.258931151000785675, 9.846743663894594434 ) ) ;
#59802=CARTESIAN_POINT ( 'NONE',  ( 7.084665262690076126, 19.10535201082150181, 10.88017736071109987 ) ) ;
#59805=CARTESIAN_POINT ( 'NONE',  ( 19.38216949554541202, 55.99863466993041072, 9.382169495545424454 ) ) ;
#59806=CARTESIAN_POINT ( 'NONE',  ( 12.91533473730993009, 41.60535201082149825, -10.88017736071109987 ) ) ;
#59807=CARTESIAN_POINT ( 'NONE',  ( -46.94000000000001194, 100.4376529975800025, -8.999999999986080468 ) ) ;
#59808=CARTESIAN_POINT ( 'NONE',  ( 22.81628187352647785, 56.62363466993042493, 6.195893100308588602E-16 ) ) ;
#59809=CARTESIAN_POINT ( 'NONE',  ( 15.44008868035555793, 41.39701867748817676, -9.422509992056140149 ) ) ;
#59810=CARTESIAN_POINT ( 'NONE',  ( 16.40814093676323893, 0.7903013365970867898, 11.09922568453595026 ) ) ;
#59811=DIRECTION ( 'NONE',  ( 0.000000000000000000, -1.000000000000000000, 0.000000000000000000 ) ) ;
#59812=CARTESIAN_POINT ( 'NONE',  ( 2.791683348922237240, 15.38393115100078212, -7.208316651077763204 ) ) ;
#59813=CARTESIAN_POINT ( 'NONE',  ( 13.43411237798105340, 10.58196800326375353, 12.81628187352647963 ) ) ;
#59815=DIRECTION ( 'NONE',  ( -0.000000000000000000, -1.000000000000000000, 0.000000000000000000 ) ) ;
#59816=CARTESIAN_POINT ( 'NONE',  ( 19.84674366389459266, 63.71726448433412315, -2.638427012816827677 ) ) ;
#59817=CARTESIAN_POINT ( 'NONE',  ( 2.035157376598824452, 38.68868534415483396, 7.964842623401179544 ) ) ;
#59818=CARTESIAN_POINT ( 'NONE',  ( 18.52753015748618282, 43.92559781766745175, -4.923371831947291888 ) ) ;
#59820=CARTESIAN_POINT ( 'NONE',  ( 17.20831665107776587, 17.88393115100078745, 7.208316651077764980 ) ) ;
#59821=CARTESIAN_POINT ( 'NONE',  ( 19.84674366389459266, 8.300597817667451750, 2.638427012816836559 ) ) ;
#59822=CARTESIAN_POINT ( 'NONE',  ( -1.099225684535947600, 9.540301336597087456, 6.408140936763237150 ) ) ;
#59825=CARTESIAN_POINT ( 'NONE',  ( 12.63842701281683922, 59.55059781766744464, -9.846743663894590881 ) ) ;
#59827=CARTESIAN_POINT ( 'NONE',  ( -1.099225684535947600, 58.70696800326375353, -6.408140936763238038 ) ) ;
#59828=CARTESIAN_POINT ( 'NONE',  ( 2.791683348922237240, 30.38393115100078390, -7.208316651077763204 ) ) ;
#59830=CARTESIAN_POINT ( 'NONE',  ( 12.91533473730993009, 11.60535201082150714, -10.88017736071109987 ) ) ;
#59831=CARTESIAN_POINT ( 'NONE',  ( 19.84674366389459266, 48.71726448433413026, -2.638427012816827677 ) ) ;
#59837=CARTESIAN_POINT ( 'NONE',  ( 24.16423886937410614, 64.30374883491396076, 8.672049930838204340E-16 ) ) ;
#59838=CARTESIAN_POINT ( 'NONE',  ( 0.1532563361054083140, 6.008931151000784787, 1.131784320476157264E-15 ) ) ;
#59839=CARTESIAN_POINT ( 'NONE',  ( 19.42250999205614193, 20.14701867748817321, 5.440088680355555262 ) ) ;
#59840=CARTESIAN_POINT ( 'NONE',  ( 13.79529636645030344, 53.26208216824730357, 14.16423886937410614 ) ) ;
#59841=CARTESIAN_POINT ( 'NONE',  ( -4.164238869374099039, 51.80374883491396787, 8.674139862899312516E-16 ) ) ;
#59843=CARTESIAN_POINT ( 'NONE',  ( 17.20831665107776587, 4.133931151000785675, -7.208316651077762316 ) ) ;
#59844=AXIS2_PLACEMENT_3D ( 'NONE', #43728, #27243, #66731 ) ;
#59845=CARTESIAN_POINT ( 'NONE',  ( 17.20831665107776587, 24.13393115100078035, -7.208316651077762316 ) ) ;
#59846=CARTESIAN_POINT ( 'NONE',  ( -2.816281873526473856, 4.331968003263754419, 3.434112377981055619 ) ) ;
#59849=DIRECTION ( 'NONE',  ( 0.000000000000000000, 0.000000000000000000, -1.000000000000000000 ) ) ;
#59850=CARTESIAN_POINT ( 'NONE',  ( 17.20831665107776587, 59.13393115100078745, -7.208316651077762316 ) ) ;
#59853=( BOUNDED_CURVE ( )  B_SPLINE_CURVE ( 2, ( #77784, #98359, #83326, #14852, #7342, #23336, #24806, #48268, #93282 ),
 .UNSPECIFIED., .F., .F. ) 
 B_SPLINE_CURVE_WITH_KNOTS ( ( 3, 2, 2, 2, 3 ),
 ( 0.5115695083688026612, 0.5119047619047618625, 0.5178571428571427937, 0.5238095238095238360, 0.5241447773454830372 ),
 .UNSPECIFIED. ) 
 CURVE ( )  GEOMETRIC_REPRESENTATION_ITEM ( )  RATIONAL_B_SPLINE_CURVE ( ( 0.9963778908391753841, 0.9980808541467917072, 1.000000000000000000, 0.9659258262890682012, 1.000000000000000000, 0.9659258262890682012, 1.000000000000000000, 0.9980808541467917072, 0.9963778908391753841 ) ) 
 REPRESENTATION_ITEM ( '' )  );
#59854=CARTESIAN_POINT ( 'NONE',  ( 10.00000000000000000, 10.55374883491396787, -14.16423886937410082 ) ) ;
#59855=CARTESIAN_POINT ( 'NONE',  ( 7.361572987183170547, 27.05059781766745175, 9.846743663894590881 ) ) ;
#59856=LINE ( 'NONE', #45349, #44891 ) ;
#59858=CARTESIAN_POINT ( 'NONE',  ( 6.204703633549690345, 35.76208216824729647, -14.16423886937410259 ) ) ;
#59859=CARTESIAN_POINT ( 'NONE',  ( 18.52753015748618282, 3.925597817667451306, -4.923371831947291888 ) ) ;
#59862=CARTESIAN_POINT ( 'NONE',  ( 15.44008868035555260, 29.73035201082150891, 9.422509992056143702 ) ) ;
#59863=CARTESIAN_POINT ( 'NONE',  ( -2.816281873526473856, 34.33196800326376064, 3.434112377981055619 ) ) ;
#59864=CARTESIAN_POINT ( 'NONE',  ( 20.88017736071110164, 5.355352010821502695, 2.915334737309930979 ) ) ;
#59865=CARTESIAN_POINT ( 'NONE',  ( 22.81628187352647785, 36.41530133659707502, 3.434112377981063169 ) ) ;
#59866=CARTESIAN_POINT ( 'NONE',  ( 0.6178305044545818747, 63.49863466993043204, -9.382169495545419124 ) ) ;
#59867=ORIENTED_EDGE ( 'NONE', *, *, #17104, .F. ) ;
#59869=CARTESIAN_POINT ( 'NONE',  ( 19.80777595082613729, 35.68878173731741299, -6.500000000000036415 ) ) ;
#59870=CARTESIAN_POINT ( 'NONE',  ( 24.16423886937410614, 44.30374883491397497, 8.672049930838204340E-16 ) ) ;
#59871=( LENGTH_UNIT ( ) NAMED_UNIT ( * ) SI_UNIT ( .MILLI., .METRE. ) );
#59872=CARTESIAN_POINT ( 'NONE',  ( 7.084665262690076126, 29.10535201082150181, 10.88017736071109987 ) ) ;
#59875=CARTESIAN_POINT ( 'NONE',  ( 19.42250999205614548, 50.98035201082151247, -5.440088680355545492 ) ) ;
#59877=CARTESIAN_POINT ( 'NONE',  ( 21.09922568453594849, 26.20696800326375353, 6.408140936763242479 ) ) ;
#59880=CARTESIAN_POINT ( 'NONE',  ( 12.63842701281683922, 29.55059781766745175, -9.846743663894590881 ) ) ;
#59882=CARTESIAN_POINT ( 'NONE',  ( -0.8801773607110991993, 52.85535201082151247, -2.915334737309923874 ) ) ;
#59883=CARTESIAN_POINT ( 'NONE',  ( 6.565887622018943937, 23.08196800326375708, -12.81628187352647608 ) ) ;
#59884=CARTESIAN_POINT ( 'NONE',  ( 4.559911319644449179, 7.230352010821504471, -9.422509992056141925 ) ) ;
#59885=CARTESIAN_POINT ( 'NONE',  ( 10.00000000000000000, 34.75893115100078745, -9.846743663894594434 ) ) ;
#59886=CARTESIAN_POINT ( 'NONE',  ( 21.09922568453595559, 62.04030133659709634, -6.408140936763230044 ) ) ;
#59887=CARTESIAN_POINT ( 'NONE',  ( 19.84674366389459266, 13.71726448433411782, -2.638427012816827677 ) ) ;
#59888=CARTESIAN_POINT ( 'NONE',  ( 24.16423886937410614, 9.512082168247301794, -3.795296366450302550 ) ) ;
#59890=CARTESIAN_POINT ( 'NONE',  ( 12.91533473730992121, 39.52201867748817676, 10.88017736071110164 ) ) ;
#59891=CARTESIAN_POINT ( 'NONE',  ( 2.035157376598822676, 2.438685344154837953, -7.964842623401177768 ) ) ;
#59892=CARTESIAN_POINT ( 'NONE',  ( 24.16423886937410614, 34.51208216824731068, -3.795296366450302550 ) ) ;
#59893=CARTESIAN_POINT ( 'NONE',  ( 17.20831665107776587, 42.88393115100077324, 7.208316651077764980 ) ) ;
#59894=CARTESIAN_POINT ( 'NONE',  ( 4.559911319644449179, 37.23035201082150536, -9.422509992056141925 ) ) ;
#59895=CARTESIAN_POINT ( 'NONE',  ( 0.5774900079438590739, 22.64701867748817321, -5.440088680355550821 ) ) ;
#59897=CARTESIAN_POINT ( 'NONE',  ( 19.42250999205614193, 30.14701867748817321, 5.440088680355555262 ) ) ;
#59898=CARTESIAN_POINT ( 'NONE',  ( 19.38216949554541557, 47.24863466993041783, -9.382169495545420901 ) ) ;
#59899=CARTESIAN_POINT ( 'NONE',  ( 20.88017736071110875, 40.77201867748818387, -2.915334737309920765 ) ) ;
#59901=CARTESIAN_POINT ( 'NONE',  ( 10.00000000000000178, 34.31368534415484106, 10.88017736071110342 ) ) ;
#59904=CARTESIAN_POINT ( 'NONE',  ( 2.791683348922237240, 60.38393115100078745, -7.208316651077763204 ) ) ;
#59905=CARTESIAN_POINT ( 'NONE',  ( 17.96484262340118221, 41.18868534415484106, -7.964842623401177768 ) ) ;
#59908=CARTESIAN_POINT ( 'NONE',  ( 13.79529636645031943, 45.34541550158062506, -14.16423886937409904 ) ) ;
#59909=CARTESIAN_POINT ( 'NONE',  ( 4.559911319644449179, 58.89701867748817676, 9.422509992056141925 ) ) ;
#59910=CARTESIAN_POINT ( 'NONE',  ( 20.03932841506544804, 25.62161441960502017, -6.397827110478938373 ) ) ;
#59913=CARTESIAN_POINT ( 'NONE',  ( 5.076628168052703671, 66.84226448433412315, 8.527530157486179263 ) ) ;
#59915=CARTESIAN_POINT ( 'NONE',  ( 0.1532563361054100626, 30.80059781766744820, -2.638427012816831230 ) ) ;
#59917=CARTESIAN_POINT ( 'NONE',  ( 0.1532563361054100626, 15.80059781766745353, -2.638427012816831230 ) ) ;
#59919=CARTESIAN_POINT ( 'NONE',  ( 20.88017736071110164, 30.35535201082151247, 2.915334737309930979 ) ) ;
#59920=CARTESIAN_POINT ( 'NONE',  ( 2.791683348922240793, 26.63393115100078745, 7.208316651077764092 ) ) ;
#59921=CARTESIAN_POINT ( 'NONE',  ( -1.099225684535947600, 18.70696800326375353, -6.408140936763238038 ) ) ;
#59923=CARTESIAN_POINT ( 'NONE',  ( 2.035157376598824452, 63.68868534415484106, 7.964842623401179544 ) ) ;
#59924=CARTESIAN_POINT ( 'NONE',  ( 10.00000000000000000, 36.81368534415484106, -10.88017736071110342 ) ) ;
#59925=CARTESIAN_POINT ( 'NONE',  ( 7.084665262690076126, 2.022018677488170990, -10.88017736071110164 ) ) ;
#59926=CARTESIAN_POINT ( 'NONE',  ( -4.164238869374099039, 41.80374883491397497, 8.674139862899312516E-16 ) ) ;
#59927=EDGE_CURVE ( 'NONE', #6299, #64876, #42938, .T. ) ;
#59929=CARTESIAN_POINT ( 'NONE',  ( -45.94000000000001194, 103.9981609152045507, 5.961202730336935041 ) ) ;
#59931=CARTESIAN_POINT ( 'NONE',  ( -2.816281873526471635, 8.915301336597083903, -3.434112377981056508 ) ) ;
#59932=CARTESIAN_POINT ( 'NONE',  ( 10.00000000000000178, 9.313685344154839285, 10.88017736071110342 ) ) ;
#59933=CARTESIAN_POINT ( 'NONE',  ( 0.5774900079438590739, 52.64701867748817676, -5.440088680355550821 ) ) ;
#59935=CARTESIAN_POINT ( 'NONE',  ( 0.5774900079438590739, 52.64701867748817676, -5.440088680355550821 ) ) ;
#59936=CARTESIAN_POINT ( 'NONE',  ( 2.791683348922237240, 30.38393115100078390, -7.208316651077763204 ) ) ;
#59937=CARTESIAN_POINT ( 'NONE',  ( 19.84674366389459621, 23.50893115100078390, 7.409399052514197653E-17 ) ) ;
#59938=CARTESIAN_POINT ( 'NONE',  ( 10.00000000000000178, 12.25893115100078568, 9.846743663894594434 ) ) ;
#59941=CARTESIAN_POINT ( 'NONE',  ( 0.6178305044545838731, 39.74863466993041072, 9.382169495545420901 ) ) ;
#59942=CARTESIAN_POINT ( 'NONE',  ( 1.472469842513823179, 1.425597817667451528, 4.923371831947296329 ) ) ;
#59945=CARTESIAN_POINT ( 'NONE',  ( 19.84674366389459266, 33.71726448433410894, -2.638427012816827677 ) ) ;
#59946=VERTEX_POINT ( 'NONE', #48107 ) ;
#59947=CARTESIAN_POINT ( 'NONE',  ( 13.43411237798106583, 52.66530133659708213, -12.81628187352647252 ) ) ;
#59950=CARTESIAN_POINT ( 'NONE',  ( 16.40814093676323893, 10.79030133659708923, 11.09922568453595026 ) ) ;
#59952=CARTESIAN_POINT ( 'NONE',  ( 7.084665262690076126, 47.02201867748818387, -10.88017736071110164 ) ) ;
#59953=CARTESIAN_POINT ( 'NONE',  ( 2.917880565312948704, 27.63708216824730357, 12.26659068614894643 ) ) ;
#59956=CARTESIAN_POINT ( 'NONE',  ( -0.3689425029237881626, 27.42874883491397142, 10.36894250292379027 ) ) ;
#59957=CARTESIAN_POINT ( 'NONE',  ( 2.917880565312950480, 40.97041550158063217, -12.26659068614894821 ) ) ;
#59958=CARTESIAN_POINT ( 'NONE',  ( -0.3689425029237898834, 6.178748834913968757, -10.36894250292378850 ) ) ;
#59959=CARTESIAN_POINT ( 'NONE',  ( -4.164238869374099927, 12.01208216824730357, 3.795296366450308767 ) ) ;
#59960=CARTESIAN_POINT ( 'NONE',  ( 7.084665262690076126, 69.10535201082151957, 10.88017736071109987 ) ) ;
#59961=CARTESIAN_POINT ( 'NONE',  ( 7.084665262690076126, 52.02201867748816255, -10.88017736071110164 ) ) ;
#59963=CARTESIAN_POINT ( 'NONE',  ( 10.00000000000000178, 27.25893115100078390, 9.846743663894594434 ) ) ;
#59964=CARTESIAN_POINT ( 'NONE',  ( -0.8801773607110991993, 67.85535201082151957, -2.915334737309923874 ) ) ;
#59965=CARTESIAN_POINT ( 'NONE',  ( 14.92337183194729988, 24.34226448433411960, -8.527530157486177487 ) ) ;
#59966=CARTESIAN_POINT ( 'NONE',  ( -0.8801773607110991993, 27.85535201082150181, -2.915334737309923874 ) ) ;
#59967=CARTESIAN_POINT ( 'NONE',  ( 22.81628187352647785, 56.41530133659708213, 3.434112377981063169 ) ) ;
#59968=CARTESIAN_POINT ( 'NONE',  ( 10.00000000000000178, 67.25893115100079456, 9.846743663894594434 ) ) ;
#59969=CARTESIAN_POINT ( 'NONE',  ( 2.791683348922237240, 25.38393115100078390, -7.208316651077763204 ) ) ;
#59970=CARTESIAN_POINT ( 'NONE',  ( 16.40814093676324603, 42.45696800326375353, -11.09922568453594671 ) ) ;
#59973=CARTESIAN_POINT ( 'NONE',  ( 4.559911319644449179, 38.89701867748817676, 9.422509992056141925 ) ) ;
#59974=CARTESIAN_POINT ( 'NONE',  ( 1.472469842513823179, 46.42559781766745175, 4.923371831947296329 ) ) ;
#59976=CARTESIAN_POINT ( 'NONE',  ( 2.917880565312948704, 32.63708216824730357, 12.26659068614894643 ) ) ;
#59980=CARTESIAN_POINT ( 'NONE',  ( 20.88017736071110875, 60.77201867748817676, -2.915334737309920765 ) ) ;
#59981=CARTESIAN_POINT ( 'NONE',  ( -2.266590686148945544, 57.22041550158063217, 7.082119434687048631 ) ) ;
#59982=CARTESIAN_POINT ( 'NONE',  ( 18.52753015748617571, 63.09226448433412315, 4.923371831947298993 ) ) ;
#59983=CARTESIAN_POINT ( 'NONE',  ( 0.2751277870542911952, 53.21833443783938122, 6.499999999999992006 ) ) ;
#59984=CARTESIAN_POINT ( 'NONE',  ( 15.44008868035555793, 56.39701867748817676, -9.422509992056140149 ) ) ;
#59986=CARTESIAN_POINT ( 'NONE',  ( 13.43411237798106583, 32.66530133659708213, -12.81628187352647252 ) ) ;
#59988=CARTESIAN_POINT ( 'NONE',  ( 0.5774900079438607392, 8.480352010821505360, 5.440088680355550821 ) ) ;
#59989=CARTESIAN_POINT ( 'NONE',  ( 17.96484262340118221, 14.93868534415484106, 7.964842623401181321 ) ) ;
#59990=CARTESIAN_POINT ( 'NONE',  ( 18.52753015748618282, 58.92559781766745886, -4.923371831947291888 ) ) ;
#59991=CARTESIAN_POINT ( 'NONE',  ( 6.565887622018943937, 53.08196800326374643, -12.81628187352647608 ) ) ;
#59992=CARTESIAN_POINT ( 'NONE',  ( -38.70923076923077133, 110.8461538461538396, -9.500000000000000000 ) ) ;
#59995=CARTESIAN_POINT ( 'NONE',  ( 0.5774900079438607392, 23.48035201082150536, 5.440088680355550821 ) ) ;
#59996=CARTESIAN_POINT ( 'NONE',  ( 13.43411237798105340, 15.58196800326374998, 12.81628187352647963 ) ) ;
#59998=CARTESIAN_POINT ( 'NONE',  ( 0.1532563361054083140, 11.00893115100078568, 1.131784320476157264E-15 ) ) ;
#60000=CARTESIAN_POINT ( 'NONE',  ( 10.00000000000000178, 47.25893115100078745, 9.846743663894594434 ) ) ;
#60001=CARTESIAN_POINT ( 'NONE',  ( -0.8801773607111008646, 33.27201867748817676, 2.915334737309923430 ) ) ;
#60002=CARTESIAN_POINT ( 'NONE',  ( 10.00000000000000178, 25.37363466993041783, 12.81628187352647608 ) ) ;
#60003=CARTESIAN_POINT ( 'NONE',  ( 17.96484262340118221, 44.93868534415483396, 7.964842623401181321 ) ) ;
#60005=CYLINDRICAL_SURFACE ( 'NONE', #89615, 0.5000000000000004441 ) ;
#60006=CARTESIAN_POINT ( 'NONE',  ( 0.6178305044545818747, 58.49863466993042493, -9.382169495545419124 ) ) ;
#60007=VERTEX_POINT ( 'NONE', #17147 ) ;
#60008=CARTESIAN_POINT ( 'NONE',  ( 10.00000000000000000, 66.81368534415484817, -10.88017736071110342 ) ) ;
#60009=CARTESIAN_POINT ( 'NONE',  ( -1.099225684535947600, 29.54030133659708923, 6.408140936763237150 ) ) ;
#60010=CARTESIAN_POINT ( 'NONE',  ( 10.00000000000000000, 4.758931151000784787, -9.846743663894594434 ) ) ;
#60011=CARTESIAN_POINT ( 'NONE',  ( -0.8801773607110991993, 37.85535201082151247, -2.915334737309923874 ) ) ;
#60012=CARTESIAN_POINT ( 'NONE',  ( 19.72487221294571214, 2.802231764288312998, -6.500000000000001776 ) ) ;
#60014=CARTESIAN_POINT ( 'NONE',  ( 0.1532563361054100626, 10.80059781766745175, -2.638427012816831230 ) ) ;
#60015=CARTESIAN_POINT ( 'NONE',  ( 5.076628168052703671, 1.842264484334118047, 8.527530157486179263 ) ) ;
#60017=CARTESIAN_POINT ( 'NONE',  ( 24.16423886937410614, 44.30374883491397497, 8.672049930838204340E-16 ) ) ;
#60020=FILL_AREA_STYLE ('',( #29512 ) ) ;
#60022=ORIENTED_EDGE ( 'NONE', *, *, #3166, .T. ) ;
#60023=CARTESIAN_POINT ( 'NONE',  ( -2.266590686148945544, 66.38708216824730357, -7.082119434687050408 ) ) ;
#60024=CARTESIAN_POINT ( 'NONE',  ( 10.00000000000000000, 65.55374883491396076, -14.16423886937410082 ) ) ;
#60025=CARTESIAN_POINT ( 'NONE',  ( 12.63842701281683922, 34.55059781766745886, -9.846743663894590881 ) ) ;
#60026=CARTESIAN_POINT ( 'NONE',  ( -2.816281873526471635, 33.91530133659708213, -3.434112377981056508 ) ) ;
#60029=CARTESIAN_POINT ( 'NONE',  ( 22.26659068614895176, 9.720415501580633943, -7.082119434687042414 ) ) ;
#60030=CARTESIAN_POINT ( 'NONE',  ( -0.8801773607111008646, 18.27201867748817321, 2.915334737309923430 ) ) ;
#60031=CARTESIAN_POINT ( 'NONE',  ( 2.917880565312950480, 50.97041550158064638, -12.26659068614894821 ) ) ;
#60032=CARTESIAN_POINT ( 'NONE',  ( 0.1532563361054082862, 31.21726448433412315, 2.638427012816831674 ) ) ;
#60033=CARTESIAN_POINT ( 'NONE',  ( 0.9408516040111580825, 12.46693863883975872, -6.499999999999988454 ) ) ;
#60034=CARTESIAN_POINT ( 'NONE',  ( 14.92337183194729633, 17.67559781766745175, 8.527530157486181039 ) ) ;
#60036=CARTESIAN_POINT ( 'NONE',  ( 19.84674366389459621, 3.508931151000785231, 7.409399052514197653E-17 ) ) ;
#60042=CARTESIAN_POINT ( 'NONE',  ( 1.472469842513823179, 46.42559781766745175, 4.923371831947296329 ) ) ;
#60043=CARTESIAN_POINT ( 'NONE',  ( 10.00000000000000000, 31.81368534415483751, -10.88017736071110342 ) ) ;
#60044=CARTESIAN_POINT ( 'NONE',  ( 19.42250999205614548, 40.98035201082150536, -5.440088680355545492 ) ) ;
#60045=CARTESIAN_POINT ( 'NONE',  ( 1.472469842513823179, 65.59226448433412315, -4.923371831947296329 ) ) ;
#60046=CARTESIAN_POINT ( 'NONE',  ( 3.591859063236761518, 34.95696800326375353, 11.09922568453594849 ) ) ;
#60047=CARTESIAN_POINT ( 'NONE',  ( 13.79529636645030344, 3.262082168247301350, 14.16423886937410614 ) ) ;
#60048=EDGE_CURVE ( 'NONE', #41390, #68599, #3127, .T. ) ;
#60049=CARTESIAN_POINT ( 'NONE',  ( 10.00000000000000178, 35.37363466993042493, 12.81628187352647608 ) ) ;
#60051=CARTESIAN_POINT ( 'NONE',  ( 12.63842701281683922, 44.55059781766745175, -9.846743663894590881 ) ) ;
#60052=CARTESIAN_POINT ( 'NONE',  ( 7.084665262690076126, 12.02201867748817321, -10.88017736071110164 ) ) ;
#60054=CARTESIAN_POINT ( 'NONE',  ( 7.084665262690076126, 19.10535201082150181, 10.88017736071109987 ) ) ;
#60056=CARTESIAN_POINT ( 'NONE',  ( 4.559911319644449179, 43.89701867748816966, 9.422509992056141925 ) ) ;
#60057=CARTESIAN_POINT ( 'NONE',  ( 4.559911319644449179, 52.23035201082151247, -9.422509992056141925 ) ) ;
#60058=CARTESIAN_POINT ( 'NONE',  ( -0.8801773607110991993, 62.85535201082150536, -2.915334737309923874 ) ) ;
#60060=CARTESIAN_POINT ( 'NONE',  ( 2.791683348922237240, 0.3839311510007847872, -7.208316651077763204 ) ) ;
#60061=CARTESIAN_POINT ( 'NONE',  ( 0.5774900079438590739, 47.64701867748817676, -5.440088680355550821 ) ) ;
#60065=CARTESIAN_POINT ( 'NONE',  ( 5.076628168052704559, 25.17559781766745175, -8.527530157486179263 ) ) ;
#60067=CARTESIAN_POINT ( 'NONE',  ( 19.89220837332776881, 19.74062864464239198, 6.478736007405955455 ) ) ;
#60068=ADVANCED_FACE ( 'NONE', ( #48599 ), #46631, .T. ) ;
#60069=CARTESIAN_POINT ( 'NONE',  ( 2.917880565312950480, 0.9704155015806342766, -12.26659068614894821 ) ) ;
#60071=CARTESIAN_POINT ( 'NONE',  ( -0.1503990784575327533, 7.222660991849186196, -6.262539305110070842 ) ) ;
#60072=CARTESIAN_POINT ( 'NONE',  ( 0.2751277870542893633, 25.30223176428832232, 6.499999999999988454 ) ) ;
#60073=CARTESIAN_POINT ( 'NONE',  ( 15.44008868035555793, 6.397018677488171434, -9.422509992056140149 ) ) ;
#60076=CARTESIAN_POINT ( 'NONE',  ( 2.791683348922240793, 46.63393115100077324, 7.208316651077764092 ) ) ;
#60079=CARTESIAN_POINT ( 'NONE',  ( 10.00000000000000000, 22.87363466993042138, -12.81628187352647608 ) ) ;
#60080=CARTESIAN_POINT ( 'NONE',  ( 19.84674366389459621, 28.50893115100078745, 7.409399052514197653E-17 ) ) ;
#60081=CARTESIAN_POINT ( 'NONE',  ( 0.03258911192389071787, 0.1934760744867406734, 6.401728757118932300 ) ) ;
#60082=CARTESIAN_POINT ( 'NONE',  ( 21.09922568453594849, 6.206968003263753531, 6.408140936763242479 ) ) ;
#60083=ORIENTED_EDGE ( 'NONE', *, *, #28521, .T. ) ;
#60084=B_SPLINE_CURVE_WITH_KNOTS ( 'NONE', 3,
 ( #6674, #29651, #22182, #68663, #22677, #37194 ),
 .UNSPECIFIED., .F., .F.,
 ( 4, 2, 4 ),
 ( 7.874519775189146796E-18, 0.0002626113303185857945, 0.0005252226606371637827 ),
 .UNSPECIFIED. ) ;
#60086=CARTESIAN_POINT ( 'NONE',  ( 20.88017736071110519, 25.56368534415483751, 2.639326808657452039E-16 ) ) ;
#60087=CARTESIAN_POINT ( 'NONE',  ( 6.204703633549690345, 17.84541550158063217, 14.16423886937410082 ) ) ;
#60088=CARTESIAN_POINT ( 'NONE',  ( 0.1532563361054082862, 21.21726448433412315, 2.638427012816831674 ) ) ;
#60089=CARTESIAN_POINT ( 'NONE',  ( 7.084665262690076126, 52.02201867748816255, -10.88017736071110164 ) ) ;
#60090=CARTESIAN_POINT ( 'NONE',  ( 19.38216949554541557, 42.24863466993041783, -9.382169495545420901 ) ) ;
#60092=CARTESIAN_POINT ( 'NONE',  ( 7.084665262690076126, 14.10535201082150358, 10.88017736071109987 ) ) ;
#60095=EDGE_CURVE ( 'NONE', #64921, #25477, #16646, .T. ) ;
#60096=CARTESIAN_POINT ( 'NONE',  ( 22.81628187352647785, 11.62363466993042138, 6.195893100308588602E-16 ) ) ;
#60097=CARTESIAN_POINT ( 'NONE',  ( 10.00000000000000178, 5.373634669930420493, 12.81628187352647608 ) ) ;
#60098=CARTESIAN_POINT ( 'NONE',  ( 19.84674366389459621, 23.50893115100078390, 7.409399052514197653E-17 ) ) ;
#60100=CARTESIAN_POINT ( 'NONE',  ( 13.43411237798106583, 32.66530133659708213, -12.81628187352647252 ) ) ;
#60102=CARTESIAN_POINT ( 'NONE',  ( 10.00000000000000000, 41.81368534415484106, -10.88017736071110342 ) ) ;
#60104=( GEOMETRIC_REPRESENTATION_CONTEXT ( 3 ) GLOBAL_UNCERTAINTY_ASSIGNED_CONTEXT ( ( #51146 ) ) GLOBAL_UNIT_ASSIGNED_CONTEXT ( ( #47184, #63660, #8706 ) ) REPRESENTATION_CONTEXT ( 'NONE', 'WORKASPACE' ) );
#60105=EDGE_CURVE ( 'NONE', #4701, #69569, #70140, .T. ) ;
#60108=CARTESIAN_POINT ( 'NONE',  ( 18.39792806157249672, 29.52224192338640307, 6.499999999999997335 ) ) ;
#60109=CARTESIAN_POINT ( 'NONE',  ( 19.42250999205614548, 45.98035201082150536, -5.440088680355545492 ) ) ;
#60110=CARTESIAN_POINT ( 'NONE',  ( 2.035157376598822676, 42.43868534415483396, -7.964842623401177768 ) ) ;
#60111=CARTESIAN_POINT ( 'NONE',  ( 2.791683348922240793, 61.63393115100079456, 7.208316651077764092 ) ) ;
#60115=CARTESIAN_POINT ( 'NONE',  ( 5.076628168052704559, 35.17559781766745175, -8.527530157486179263 ) ) ;
#60116=CARTESIAN_POINT ( 'NONE',  ( 20.88017736071110164, 10.35535201082150714, 2.915334737309930979 ) ) ;
#60117=CARTESIAN_POINT ( 'NONE',  ( -2.816281873526473856, 14.33196800326375531, 3.434112377981055619 ) ) ;
#60119=CARTESIAN_POINT ( 'NONE',  ( 20.88017736071110164, 20.35535201082150891, 2.915334737309930979 ) ) ;
#60122=CARTESIAN_POINT ( 'NONE',  ( 15.44008868035555260, 29.73035201082150891, 9.422509992056143702 ) ) ;
#60123=CARTESIAN_POINT ( 'NONE',  ( -0.8801773607110991993, 62.85535201082150536, -2.915334737309923874 ) ) ;
#60124=CARTESIAN_POINT ( 'NONE',  ( 17.08211943468705840, 40.13708216824731068, -12.26659068614894466 ) ) ;
#60125=CARTESIAN_POINT ( 'NONE',  ( 5.076628168052704559, 30.17559781766745175, -8.527530157486179263 ) ) ;
#60126=CARTESIAN_POINT ( 'NONE',  ( 4.559911319644449179, 42.23035201082151247, -9.422509992056141925 ) ) ;
#60128=CARTESIAN_POINT ( 'NONE',  ( 17.08211943468705840, 5.137082168247300906, -12.26659068614894466 ) ) ;
#60132=CARTESIAN_POINT ( 'NONE',  ( 17.20831665107776587, 57.88393115100078745, 7.208316651077764980 ) ) ;
#60136=CARTESIAN_POINT ( 'NONE',  ( -0.3689425029237898834, 16.17874883491396076, -10.36894250292378850 ) ) ;
#60137=CARTESIAN_POINT ( 'NONE',  ( -4.164238869374099927, 22.01208216824730357, 3.795296366450308767 ) ) ;
#60139=CARTESIAN_POINT ( 'NONE',  ( 12.91533473730992121, 64.52201867748817676, 10.88017736071110164 ) ) ;
#60140=CARTESIAN_POINT ( 'NONE',  ( 20.36894250292379382, 63.67874883491396787, 10.36894250292379205 ) ) ;
#60141=CARTESIAN_POINT ( 'NONE',  ( 3.591859063236761518, -0.04303199673624671928, 11.09922568453594849 ) ) ;
#60142=CARTESIAN_POINT ( 'NONE',  ( 12.63842701281683922, 49.55059781766744464, -9.846743663894590881 ) ) ;
#60144=CARTESIAN_POINT ( 'NONE',  ( 7.084665262690076126, 49.10535201082149825, 10.88017736071109987 ) ) ;
#60145=CARTESIAN_POINT ( 'NONE',  ( 10.00000000000000178, 25.37363466993041783, 12.81628187352647608 ) ) ;
#60146=CARTESIAN_POINT ( 'NONE',  ( -0.3689425029237881626, 12.42874883491396609, 10.36894250292379027 ) ) ;
#60147=CARTESIAN_POINT ( 'NONE',  ( 20.88017736071110164, 15.35535201082150358, 2.915334737309930979 ) ) ;
#60148=CARTESIAN_POINT ( 'NONE',  ( 2.035157376598824452, 18.68868534415484106, 7.964842623401179544 ) ) ;
#60150=CARTESIAN_POINT ( 'NONE',  ( 12.91533473730993009, 56.60535201082151247, -10.88017736071109987 ) ) ;
#60151=CARTESIAN_POINT ( 'NONE',  ( 6.565887622018943937, 48.08196800326375353, -12.81628187352647608 ) ) ;
#60153=EDGE_LOOP ( 'NONE', ( #44059, #93628, #92624, #66042, #40252, #50190 ) ) ;
#60155=ORIENTED_EDGE ( 'NONE', *, *, #68890, .F. ) ;
#60158=CARTESIAN_POINT ( 'NONE',  ( 14.92337183194729633, 32.67559781766745175, 8.527530157486181039 ) ) ;
#60159=ORIENTED_EDGE ( 'NONE', *, *, #80382, .T. ) ;
#60161=CARTESIAN_POINT ( 'NONE',  ( 6.204703633549690345, 50.76208216824730357, -14.16423886937410259 ) ) ;
#60162=CARTESIAN_POINT ( 'NONE',  ( 7.084665262690076126, 4.105352010821503583, 10.88017736071109987 ) ) ;
#60163=CARTESIAN_POINT ( 'NONE',  ( 0.1532563361054100626, 20.80059781766744464, -2.638427012816831230 ) ) ;
#60164=CARTESIAN_POINT ( 'NONE',  ( 1.472469842513823179, 46.42559781766745175, 4.923371831947296329 ) ) ;
#60165=CARTESIAN_POINT ( 'NONE',  ( 20.24186590665278018, 60.59014588040358262, -6.114288769123040090 ) ) ;
#60166=CARTESIAN_POINT ( 'NONE',  ( -42.60666666666667624, 92.50000000000000000, -9.500000000000000000 ) ) ;
#60168=CARTESIAN_POINT ( 'NONE',  ( 10.00000000000000178, 64.31368534415483396, 10.88017736071110342 ) ) ;
#60171=MECHANICAL_DESIGN_GEOMETRIC_PRESENTATION_REPRESENTATION('',(#39420),#64938);
#60172=ORIENTED_EDGE ( 'NONE', *, *, #5537, .F. ) ;
#60173=CARTESIAN_POINT ( 'NONE',  ( -2.266590686148945544, 37.22041550158063217, 7.082119434687048631 ) ) ;
#60174=CARTESIAN_POINT ( 'NONE',  ( 13.43411237798105340, 20.58196800326374643, 12.81628187352647963 ) ) ;
#60176=CARTESIAN_POINT ( 'NONE',  ( 10.00000000000000000, 52.87363466993041783, -12.81628187352647608 ) ) ;
#60177=CARTESIAN_POINT ( 'NONE',  ( 2.035157376598822676, 22.43868534415483396, -7.964842623401177768 ) ) ;
#60178=CARTESIAN_POINT ( 'NONE',  ( 14.92337183194729633, 37.67559781766745175, 8.527530157486181039 ) ) ;
#60179=CARTESIAN_POINT ( 'NONE',  ( -0.8801773607110991993, 27.85535201082150181, -2.915334737309923874 ) ) ;
#60180=CARTESIAN_POINT ( 'NONE',  ( 3.591859063236763294, 63.29030133659708923, -11.09922568453595026 ) ) ;
#60183=CARTESIAN_POINT ( 'NONE',  ( 18.52753015748618282, 53.92559781766745175, -4.923371831947291888 ) ) ;
#60184=CARTESIAN_POINT ( 'NONE',  ( 18.52753015748618282, 48.92559781766745886, -4.923371831947291888 ) ) ;
#60192=CARTESIAN_POINT ( 'NONE',  ( 1.274849032794278747, 57.55509018479938277, -6.499999999999960032 ) ) ;
#60193=CARTESIAN_POINT ( 'NONE',  ( 0.1532563361054083140, 31.00893115100078390, 1.131784320476157264E-15 ) ) ;
#60194=CARTESIAN_POINT ( 'NONE',  ( -2.816281873526473856, 34.12363466993042493, 9.499525473075851096E-16 ) ) ;
#60198=CARTESIAN_POINT ( 'NONE',  ( 0.1532563361054100626, 60.80059781766744464, -2.638427012816831230 ) ) ;
#60200=CARTESIAN_POINT ( 'NONE',  ( 7.361572987183169658, 34.96726448433411605, -9.846743663894592657 ) ) ;
#60201=CARTESIAN_POINT ( 'NONE',  ( 22.26659068614895176, 34.72041550158063927, -7.082119434687042414 ) ) ;
#60202=CARTESIAN_POINT ( 'NONE',  ( 5.076628168052704559, 40.17559781766745175, -8.527530157486179263 ) ) ;
#60203=CARTESIAN_POINT ( 'NONE',  ( 21.09922568453594849, 51.20696800326375353, 6.408140936763242479 ) ) ;
#60206=CARTESIAN_POINT ( 'NONE',  ( 19.84674366389459266, 3.717264484334118713, -2.638427012816827677 ) ) ;
#60207=CARTESIAN_POINT ( 'NONE',  ( 13.79529636645031943, 5.345415501580634832, -14.16423886937409904 ) ) ;
#60208=CARTESIAN_POINT ( 'NONE',  ( 12.63842701281683034, 42.46726448433412315, 9.846743663894596210 ) ) ;
#60209=CARTESIAN_POINT ( 'NONE',  ( 17.96484262340118221, 39.93868534415484106, 7.964842623401181321 ) ) ;
#60211=CARTESIAN_POINT ( 'NONE',  ( 18.52753015748617571, 43.09226448433412315, 4.923371831947298993 ) ) ;
#60215=CARTESIAN_POINT ( 'NONE',  ( 12.91533473730993009, 51.60535201082149825, -10.88017736071109987 ) ) ;
#60217=CARTESIAN_POINT ( 'NONE',  ( 1.274849032794324932, 22.55509018479936145, -6.500000000000021316 ) ) ;
#60218=CARTESIAN_POINT ( 'NONE',  ( 12.91533473730993009, 16.60535201082150891, -10.88017736071109987 ) ) ;
#60219=CARTESIAN_POINT ( 'NONE',  ( 22.81628187352647785, 1.415301336597087012, 3.434112377981063169 ) ) ;
#60220=CARTESIAN_POINT ( 'NONE',  ( 15.44008868035555793, 46.39701867748817676, -9.422509992056140149 ) ) ;
#60224=CARTESIAN_POINT ( 'NONE',  ( 12.91533473730993009, 41.60535201082149825, -10.88017736071109987 ) ) ;
#60226=CARTESIAN_POINT ( 'NONE',  ( 5.076628168052704559, 10.17559781766745175, -8.527530157486179263 ) ) ;
#60227=CARTESIAN_POINT ( 'NONE',  ( 19.84674366389459621, 23.50893115100078390, 7.409399052514197653E-17 ) ) ;
#60229=CARTESIAN_POINT ( 'NONE',  ( 5.076628168052704559, 60.17559781766745175, -8.527530157486179263 ) ) ;
#60230=CARTESIAN_POINT ( 'NONE',  ( 7.084665262690076126, 4.105352010821503583, 10.88017736071109987 ) ) ;
#60231=CARTESIAN_POINT ( 'NONE',  ( -0.1042174387088690007, 18.10736173766201418, 6.337391062633411565 ) ) ;
#60233=CARTESIAN_POINT ( 'NONE',  ( -4.164238869374099039, 16.80374883491396787, 8.674139862899312516E-16 ) ) ;
#60235=CARTESIAN_POINT ( 'NONE',  ( 20.36894250292379382, 48.67874883491396076, 10.36894250292379205 ) ) ;
#60236=FACE_OUTER_BOUND ( 'NONE', #61196, .T. ) ;
#60237=VERTEX_POINT ( 'NONE', #95590 ) ;
#60238=CARTESIAN_POINT ( 'NONE',  ( 12.63842701281683922, 19.55059781766745175, -9.846743663894590881 ) ) ;
#60239=CARTESIAN_POINT ( 'NONE',  ( 15.44008868035555260, 14.73035201082150536, 9.422509992056143702 ) ) ;
#60240=CARTESIAN_POINT ( 'NONE',  ( 5.076628168052704559, 55.17559781766745175, -8.527530157486179263 ) ) ;
#60241=CARTESIAN_POINT ( 'NONE',  ( 20.36894250292379382, 8.678748834913967869, 10.36894250292379205 ) ) ;
#60244=MECHANICAL_DESIGN_GEOMETRIC_PRESENTATION_REPRESENTATION('',(#4300),#90569);
#60246=CARTESIAN_POINT ( 'NONE',  ( 19.38216949554541202, 35.99863466993041072, 9.382169495545424454 ) ) ;
#60247=CARTESIAN_POINT ( 'NONE',  ( 18.52753015748617571, 38.09226448433412315, 4.923371831947298993 ) ) ;
#60248=ORIENTED_EDGE ( 'NONE', *, *, #37166, .T. ) ;
#60249=CARTESIAN_POINT ( 'NONE',  ( 17.20831665107776587, 7.883931151000784787, 7.208316651077764980 ) ) ;
#60252=CARTESIAN_POINT ( 'NONE',  ( 2.035157376598824452, 8.688685344154839285, 7.964842623401179544 ) ) ;
#60253=CARTESIAN_POINT ( 'NONE',  ( 20.36894250292379382, 53.67874883491397497, 10.36894250292379205 ) ) ;
#60254=CARTESIAN_POINT ( 'NONE',  ( 24.16423886937410614, 4.303748834913967869, 8.672049930838204340E-16 ) ) ;
#60256=CARTESIAN_POINT ( 'NONE',  ( 14.92337183194729633, 27.67559781766745530, 8.527530157486181039 ) ) ;
#60257=CARTESIAN_POINT ( 'NONE',  ( 0.5774900079438590739, 12.64701867748817143, -5.440088680355550821 ) ) ;
#60258=CARTESIAN_POINT ( 'NONE',  ( 14.92337183194729988, 39.34226448433412315, -8.527530157486177487 ) ) ;
#60260=CARTESIAN_POINT ( 'NONE',  ( 7.361572987183169658, 49.96726448433410894, -9.846743663894592657 ) ) ;
#60261=CARTESIAN_POINT ( 'NONE',  ( 20.88017736071110875, 40.77201867748818387, -2.915334737309920765 ) ) ;
#60262=ORIENTED_EDGE ( 'NONE', *, *, #59927, .F. ) ;
#60263=CARTESIAN_POINT ( 'NONE',  ( -1.099225684535947600, 54.54030133659708923, 6.408140936763237150 ) ) ;
#60265=CARTESIAN_POINT ( 'NONE',  ( 18.52753015748617571, 3.092264484334118269, 4.923371831947298993 ) ) ;
#60266=CARTESIAN_POINT ( 'NONE',  ( 19.38216949554541202, 60.99863466993042493, 9.382169495545424454 ) ) ;
#60267=CARTESIAN_POINT ( 'NONE',  ( -0.8801773607111008646, 3.272018677488171434, 2.915334737309923430 ) ) ;
#60268=CARTESIAN_POINT ( 'NONE',  ( 18.52753015748617571, 38.09226448433412315, 4.923371831947298993 ) ) ;
#60269=CARTESIAN_POINT ( 'NONE',  ( 20.00000000000000711, 79.40087001978915282, 4.500000000000000888 ) ) ;
#60271=CARTESIAN_POINT ( 'NONE',  ( 24.16423886937410614, 34.30374883491396787, 8.672049930838204340E-16 ) ) ;
#60272=CARTESIAN_POINT ( 'NONE',  ( 24.16423886937409904, 44.09541550158063927, 3.795296366450317205 ) ) ;
#60273=CARTESIAN_POINT ( 'NONE',  ( 2.791683348922240793, 56.63393115100078035, 7.208316651077764092 ) ) ;
#60275=CARTESIAN_POINT ( 'NONE',  ( 2.035157376598822676, 32.43868534415483396, -7.964842623401177768 ) ) ;
#60276=CARTESIAN_POINT ( 'NONE',  ( 12.63842701281683034, 2.467264484334118269, 9.846743663894596210 ) ) ;
#60280=CARTESIAN_POINT ( 'NONE',  ( 10.00000000000000000, 57.87363466993042493, -12.81628187352647608 ) ) ;
#60283=CARTESIAN_POINT ( 'NONE',  ( 10.00000000000000178, 69.31368534415484817, 10.88017736071110342 ) ) ;
#60285=CARTESIAN_POINT ( 'NONE',  ( -0.3689425029237881626, 12.42874883491396609, 10.36894250292379027 ) ) ;
#60286=CARTESIAN_POINT ( 'NONE',  ( 2.791683348922240793, 1.633931151000784565, 7.208316651077764092 ) ) ;
#60287=CARTESIAN_POINT ( 'NONE',  ( 12.91533473730992121, 29.52201867748817321, 10.88017736071110164 ) ) ;
#60293=CARTESIAN_POINT ( 'NONE',  ( 4.559911319644449179, 28.89701867748817321, 9.422509992056141925 ) ) ;
#60296=ORIENTED_EDGE ( 'NONE', *, *, #42653, .F. ) ;
#60297=CARTESIAN_POINT ( 'NONE',  ( 19.42250999205614548, 30.98035201082150536, -5.440088680355545492 ) ) ;
#60301=CARTESIAN_POINT ( 'NONE',  ( 16.40814093676324603, 17.45696800326375353, -11.09922568453594671 ) ) ;
#60302=CARTESIAN_POINT ( 'NONE',  ( -0.8801773607111009756, 68.06368534415484817, 1.068504757029289695E-15 ) ) ;
#60304=CARTESIAN_POINT ( 'NONE',  ( 17.96484262340118221, 19.93868534415484106, 7.964842623401181321 ) ) ;
#60305=LINE ( 'NONE', #61283, #49441 ) ;
#60306=CARTESIAN_POINT ( 'NONE',  ( 12.63842701281683922, 9.550597817667449974, -9.846743663894590881 ) ) ;
#60307=CARTESIAN_POINT ( 'NONE',  ( 15.44008868035555260, 34.73035201082151247, 9.422509992056143702 ) ) ;
#60309=CARTESIAN_POINT ( 'NONE',  ( 0.6178305044545818747, 48.49863466993042493, -9.382169495545419124 ) ) ;
#60310=CARTESIAN_POINT ( 'NONE',  ( 7.084665262690076126, 47.02201867748818387, -10.88017736071110164 ) ) ;
#60312=CARTESIAN_POINT ( 'NONE',  ( -2.816281873526471635, 48.91530133659708213, -3.434112377981056508 ) ) ;
#60313=CARTESIAN_POINT ( 'NONE',  ( 17.96484262340118221, 44.93868534415483396, 7.964842623401181321 ) ) ;
#60314=CARTESIAN_POINT ( 'NONE',  ( 0.1532563361054083140, 66.00893115100079456, 1.131784320476157264E-15 ) ) ;
#60317=CARTESIAN_POINT ( 'NONE',  ( 5.076628168052704559, 20.17559781766745175, -8.527530157486179263 ) ) ;
#60318=CARTESIAN_POINT ( 'NONE',  ( 10.00000000000000178, 60.37363466993041783, 12.81628187352647608 ) ) ;
#60319=CARTESIAN_POINT ( 'NONE',  ( 1.932340009482190091, 36.49127512925446837, -6.500000000000079936 ) ) ;
#60320=CARTESIAN_POINT ( 'NONE',  ( 5.076628168052703671, 11.84226448433411960, 8.527530157486179263 ) ) ;
#60321=CARTESIAN_POINT ( 'NONE',  ( 10.00000000000000178, 10.37363466993041961, 12.81628187352647608 ) ) ;
#60323=CARTESIAN_POINT ( 'NONE',  ( 10.00000000000000000, 59.75893115100078745, -9.846743663894594434 ) ) ;
#60324=CARTESIAN_POINT ( 'NONE',  ( 4.559911319644449179, 37.23035201082150536, -9.422509992056141925 ) ) ;
#60325=CARTESIAN_POINT ( 'NONE',  ( 19.84674366389459621, 48.50893115100078745, 7.409399052514197653E-17 ) ) ;
#60327=CARTESIAN_POINT ( 'NONE',  ( 18.52753015748617571, 23.09226448433411960, 4.923371831947298993 ) ) ;
#60328=CARTESIAN_POINT ( 'NONE',  ( 17.20831665107776587, 12.88393115100078390, 7.208316651077764980 ) ) ;
#60329=CARTESIAN_POINT ( 'NONE',  ( -1.099225684535947600, 4.540301336597087456, 6.408140936763237150 ) ) ;
#60332=CARTESIAN_POINT ( 'NONE',  ( 14.92337183194729633, 62.67559781766745886, 8.527530157486181039 ) ) ;
#60334=CARTESIAN_POINT ( 'NONE',  ( 7.084665262690076126, 2.022018677488171434, -10.88017736071110164 ) ) ;
#60335=CARTESIAN_POINT ( 'NONE',  ( 2.791683348922237240, 45.38393115100079456, -7.208316651077763204 ) ) ;
#60337=CARTESIAN_POINT ( 'NONE',  ( 4.559911319644449179, 3.897018677488171434, 9.422509992056141925 ) ) ;
#60339=CARTESIAN_POINT ( 'NONE',  ( 20.88017736071110164, 30.35535201082151247, 2.915334737309930979 ) ) ;
#60340=CARTESIAN_POINT ( 'NONE',  ( 6.204703633549690345, 47.84541550158064638, 14.16423886937410082 ) ) ;
#60341=CARTESIAN_POINT ( 'NONE',  ( 24.16423886937410614, 64.30374883491396076, 8.672049930838204340E-16 ) ) ;
#60342=LINE ( 'NONE', #31310, #39905 ) ;
#60343=CARTESIAN_POINT ( 'NONE',  ( 0.1532563361054083140, 6.008931151000784787, 1.131784320476157264E-15 ) ) ;
#60344=CARTESIAN_POINT ( 'NONE',  ( 10.00000000000000178, 27.25893115100078390, 9.846743663894594434 ) ) ;
#60345=CARTESIAN_POINT ( 'NONE',  ( 22.81628187352648496, 6.831968003263753531, -3.434112377981050290 ) ) ;
#60349=CARTESIAN_POINT ( 'NONE',  ( 24.16423886937410614, 4.512082168247300906, -3.795296366450302550 ) ) ;
#60350=CARTESIAN_POINT ( 'NONE',  ( 19.84674366389459621, 23.50893115100078390, 7.409399052514197653E-17 ) ) ;
#60352=CARTESIAN_POINT ( 'NONE',  ( 20.36894250292379382, 38.67874883491396076, 10.36894250292379205 ) ) ;
#60353=CARTESIAN_POINT ( 'NONE',  ( 2.791683348922237240, 5.383931151000785675, -7.208316651077763204 ) ) ;
#60356=CARTESIAN_POINT ( 'NONE',  ( 20.88017736071110519, 35.56368534415484106, 2.639326808657452039E-16 ) ) ;
#60357=CARTESIAN_POINT ( 'NONE',  ( 22.81628187352647785, 51.41530133659708923, 3.434112377981063169 ) ) ;
#60358=CARTESIAN_POINT ( 'NONE',  ( 22.81628187352648496, 36.83196800326376064, -3.434112377981050290 ) ) ;
#60362=CARTESIAN_POINT ( 'NONE',  ( 17.08211943468705130, 38.47041550158063217, 12.26659068614894998 ) ) ;
#60363=CARTESIAN_POINT ( 'NONE',  ( 24.16423886937410614, 9.303748834913967869, 8.672049930838204340E-16 ) ) ;
#60364=CARTESIAN_POINT ( 'NONE',  ( 10.00000000000000000, 6.813685344154838397, -10.88017736071110342 ) ) ;
#60365=CARTESIAN_POINT ( 'NONE',  ( 15.44008868035555793, 26.39701867748817321, -9.422509992056140149 ) ) ;
#60368=CARTESIAN_POINT ( 'NONE',  ( 17.96484262340118221, 49.93868534415484106, 7.964842623401181321 ) ) ;
#60369=CARTESIAN_POINT ( 'NONE',  ( -0.8801773607111008646, 58.27201867748816966, 2.915334737309923430 ) ) ;
#60370=CARTESIAN_POINT ( 'NONE',  ( 22.81628187352647785, 26.41530133659708923, 3.434112377981063169 ) ) ;
#60371=CARTESIAN_POINT ( 'NONE',  ( 19.72487221294570858, 70.00000000000000000, -6.000000000000000000 ) ) ;
#60373=CARTESIAN_POINT ( 'NONE',  ( 10.00000000000000178, 27.25893115100078390, 9.846743663894594434 ) ) ;
#60376=CARTESIAN_POINT ( 'NONE',  ( 10.00000000000000000, 12.87363466993042138, -12.81628187352647608 ) ) ;
#60378=CARTESIAN_POINT ( 'NONE',  ( 7.084665262690076126, 9.105352010821503583, 10.88017736071109987 ) ) ;
#60379=CARTESIAN_POINT ( 'NONE',  ( 17.20831665107776587, 37.88393115100078745, 7.208316651077764980 ) ) ;
#60380=CARTESIAN_POINT ( 'NONE',  ( 21.09922568453594849, 56.20696800326375353, 6.408140936763242479 ) ) ;
#60381=CARTESIAN_POINT ( 'NONE',  ( 12.63842701281683922, 19.55059781766745175, -9.846743663894590881 ) ) ;
#60382=CARTESIAN_POINT ( 'NONE',  ( 17.08211943468705130, 3.470415501580634388, 12.26659068614894998 ) ) ;
#60384=CARTESIAN_POINT ( 'NONE',  ( 19.42250999205614548, 35.98035201082151247, -5.440088680355545492 ) ) ;
#60386=CARTESIAN_POINT ( 'NONE',  ( -0.3689425029237898834, 36.17874883491396787, -10.36894250292378850 ) ) ;
#60387=CARTESIAN_POINT ( 'NONE',  ( 12.63842701281683034, 37.46726448433411605, 9.846743663894596210 ) ) ;
#60388=CARTESIAN_POINT ( 'NONE',  ( 19.42250999205614193, 30.14701867748817321, 5.440088680355555262 ) ) ;
#60390=CARTESIAN_POINT ( 'NONE',  ( 7.084665262690076126, 22.02201867748817321, -10.88017736071110164 ) ) ;
#60393=CARTESIAN_POINT ( 'NONE',  ( -0.8801773607111009756, 28.06368534415484106, 1.068504757029289695E-15 ) ) ;
#60394=CARTESIAN_POINT ( 'NONE',  ( 3.591859063236761518, 39.95696800326375353, 11.09922568453594849 ) ) ;
#60395=CARTESIAN_POINT ( 'NONE',  ( 10.00000000000000000, 46.81368534415484106, -10.88017736071110342 ) ) ;
#60397=CARTESIAN_POINT ( 'NONE',  ( 19.42250999205614193, 55.14701867748817676, 5.440088680355555262 ) ) ;
#60399=CARTESIAN_POINT ( 'NONE',  ( 14.92337183194729988, 54.34226448433412315, -8.527530157486177487 ) ) ;
#60400=CARTESIAN_POINT ( 'NONE',  ( 2.035157376598824452, 43.68868534415484106, 7.964842623401179544 ) ) ;
#60404=FACE_OUTER_BOUND ( 'NONE', #5696, .T. ) ;
#60405=CARTESIAN_POINT ( 'NONE',  ( -0.3689425029237898834, 46.17874883491397497, -10.36894250292378850 ) ) ;
#60406=CARTESIAN_POINT ( 'NONE',  ( 12.91533473730992121, 49.52201867748817676, 10.88017736071110164 ) ) ;
#60407=CARTESIAN_POINT ( 'NONE',  ( 0.2751277870542911397, 55.30223176428831522, 6.499999999999992006 ) ) ;
#60409=( NAMED_UNIT ( * ) PLANE_ANGLE_UNIT ( ) SI_UNIT ( $, .RADIAN. ) );
#60410=CARTESIAN_POINT ( 'NONE',  ( 2.791683348922237240, 65.38393115100078035, -7.208316651077763204 ) ) ;
#60411=CARTESIAN_POINT ( 'NONE',  ( 2.035157376598824452, 3.688685344154837953, 7.964842623401179544 ) ) ;
#60412=CARTESIAN_POINT ( 'NONE',  ( 2.791683348922237240, 35.38393115100079456, -7.208316651077763204 ) ) ;
#60414=CARTESIAN_POINT ( 'NONE',  ( 7.361572987183170547, 37.05059781766744464, 9.846743663894590881 ) ) ;
#60416=CARTESIAN_POINT ( 'NONE',  ( -0.8801773607110991993, 27.85535201082150181, -2.915334737309923874 ) ) ;
#60417=CARTESIAN_POINT ( 'NONE',  ( 1.472469842513823179, 36.42559781766745175, 4.923371831947296329 ) ) ;
#60419=CARTESIAN_POINT ( 'NONE',  ( 2.035157376598822676, 57.43868534415484106, -7.964842623401177768 ) ) ;
#60420=CARTESIAN_POINT ( 'NONE',  ( 12.91533473730993009, 31.60535201082150891, -10.88017736071109987 ) ) ;
#60421=CARTESIAN_POINT ( 'NONE',  ( 20.36894250292379738, 39.92874883491396787, -10.36894250292379027 ) ) ;
#60422=AXIS2_PLACEMENT_3D ( 'NONE', #470, #54407, #31407 ) ;
#60426=CARTESIAN_POINT ( 'NONE',  ( 13.43411237798106583, 17.66530133659708923, -12.81628187352647252 ) ) ;
#60427=CARTESIAN_POINT ( 'NONE',  ( 2.035157376598822676, 12.43868534415483751, -7.964842623401177768 ) ) ;
#60428=CARTESIAN_POINT ( 'NONE',  ( -0.8801773607111008646, 43.27201867748817676, 2.915334737309923430 ) ) ;
#60429=DIRECTION ( 'NONE',  ( 0.000000000000000000, 0.000000000000000000, -1.000000000000000000 ) ) ;
#60430=ADVANCED_FACE ( 'NONE', ( #15559 ), #76036, .F. ) ;
#60432=CARTESIAN_POINT ( 'NONE',  ( 15.44008868035555793, 56.39701867748817676, -9.422509992056140149 ) ) ;
#60433=CARTESIAN_POINT ( 'NONE',  ( 5.076628168052703671, 36.84226448433412315, 8.527530157486179263 ) ) ;
#60434=CARTESIAN_POINT ( 'NONE',  ( 0.1532563361054100626, 20.80059781766744464, -2.638427012816831230 ) ) ;
#60435=CARTESIAN_POINT ( 'NONE',  ( 14.92337183194729633, 7.675597817667451750, 8.527530157486181039 ) ) ;
#60437=CARTESIAN_POINT ( 'NONE',  ( 1.816707512666844604, 50.10290668512023871, -6.499999999999958256 ) ) ;
#60438=CARTESIAN_POINT ( 'NONE',  ( 21.09922568453594849, 41.20696800326375353, 6.408140936763242479 ) ) ;
#60439=CARTESIAN_POINT ( 'NONE',  ( 18.52753015748617571, 8.092264484334117824, 4.923371831947298993 ) ) ;
#60442=CARTESIAN_POINT ( 'NONE',  ( 19.84674366389459266, 33.30059781766744464, 2.638427012816836559 ) ) ;
#60445=( BOUNDED_CURVE ( )  B_SPLINE_CURVE ( 2, ( #79267, #26749, #56282, #95241, #63755, #55789, #48760, #18777, #86285 ),
 .UNSPECIFIED., .F., .T. ) 
 B_SPLINE_CURVE_WITH_KNOTS ( ( 3, 2, 2, 2, 3 ),
 ( 0.5810855930462679453, 0.5833333333333333703, 0.5892857142857143016, 0.5952380952380952328, 0.5974858355251606579 ),
 .UNSPECIFIED. ) 
 CURVE ( )  GEOMETRIC_REPRESENTATION_ITEM ( )  RATIONAL_B_SPLINE_CURVE ( ( 0.9839835555609424134, 0.9871328979762477029, 1.000000000000000000, 0.9659258262890683122, 1.000000000000000000, 0.9659258262890683122, 1.000000000000000000, 0.9871328979762474809, 0.9839835555609424134 ) ) 
 REPRESENTATION_ITEM ( '' )  );
#60447=CARTESIAN_POINT ( 'NONE',  ( 10.00000000000000000, 7.873634669930421381, -12.81628187352647608 ) ) ;
#60448=CARTESIAN_POINT ( 'NONE',  ( 19.42250999205614548, 45.98035201082150536, -5.440088680355545492 ) ) ;
#60449=CARTESIAN_POINT ( 'NONE',  ( 2.917880565312950480, 30.97041550158063572, -12.26659068614894821 ) ) ;
#60450=( BOUNDED_CURVE ( )  B_SPLINE_CURVE ( 2, ( #459, #23438, #38924, #54395, #77885, #16418, #90917, #46414, #92887 ),
 .UNSPECIFIED., .F., .F. ) 
 B_SPLINE_CURVE_WITH_KNOTS ( ( 3, 2, 2, 2, 3 ),
 ( 0.7239427359034107390, 0.7261904761904761640, 0.7321428571428570953, 0.7380952380952381375, 0.7403429783823035626 ),
 .UNSPECIFIED. ) 
 CURVE ( )  GEOMETRIC_REPRESENTATION_ITEM ( )  RATIONAL_B_SPLINE_CURVE ( ( 0.9839835555609424134, 0.9871328979762474809, 1.000000000000000000, 0.9659258262890683122, 1.000000000000000000, 0.9659258262890683122, 1.000000000000000000, 0.9871328979762474809, 0.9839835555609424134 ) ) 
 REPRESENTATION_ITEM ( '' )  );
#60451=UNCERTAINTY_MEASURE_WITH_UNIT (LENGTH_MEASURE( 1.000000000000000082E-05 ), #45703, 'distance_accuracy_value', 'NONE');
#60453=CARTESIAN_POINT ( 'NONE',  ( -0.3689425029237898834, 26.17874883491396432, -10.36894250292378850 ) ) ;
#60454=CARTESIAN_POINT ( 'NONE',  ( -4.164238869374099039, 51.80374883491396787, 8.674139862899312516E-16 ) ) ;
#60455=CARTESIAN_POINT ( 'NONE',  ( -4.164238869374099039, 11.80374883491396965, 8.674139862899312516E-16 ) ) ;
#60456=CARTESIAN_POINT ( 'NONE',  ( 24.16423886937409904, 29.09541550158063572, 3.795296366450317205 ) ) ;
#60458=CARTESIAN_POINT ( 'NONE',  ( 15.44008868035555793, 51.39701867748816966, -9.422509992056140149 ) ) ;
#60461=CARTESIAN_POINT ( 'NONE',  ( 2.791683348922237240, 35.38393115100079456, -7.208316651077763204 ) ) ;
#60462=CARTESIAN_POINT ( 'NONE',  ( 15.44008868035555260, 64.73035201082151957, 9.422509992056143702 ) ) ;
#60463=CARTESIAN_POINT ( 'NONE',  ( 12.63842701281683922, 39.55059781766744464, -9.846743663894590881 ) ) ;
#60464=CARTESIAN_POINT ( 'NONE',  ( 17.96484262340118221, 19.93868534415484106, 7.964842623401181321 ) ) ;
#60465=CARTESIAN_POINT ( 'NONE',  ( 10.00000000000000178, 60.37363466993041783, 12.81628187352647608 ) ) ;
#60466=CARTESIAN_POINT ( 'NONE',  ( 2.791683348922237240, 60.38393115100078745, -7.208316651077763204 ) ) ;
#60467=CARTESIAN_POINT ( 'NONE',  ( 20.00000000000000711, 79.40087001978915282, -5.000000000000000888 ) ) ;
#60468=CARTESIAN_POINT ( 'NONE',  ( 10.00000000000000178, 27.25893115100078390, 9.846743663894594434 ) ) ;
#60469=CARTESIAN_POINT ( 'NONE',  ( 16.40814093676323893, 60.79030133659709634, 11.09922568453595026 ) ) ;
#60471=CARTESIAN_POINT ( 'NONE',  ( 17.96484262340118221, 41.18868534415484106, -7.964842623401177768 ) ) ;
#60472=CARTESIAN_POINT ( 'NONE',  ( 18.52753015748617571, 53.09226448433412315, 4.923371831947298993 ) ) ;
#60473=CARTESIAN_POINT ( 'NONE',  ( -4.164238869374098151, 41.59541550158061796, -3.795296366450310543 ) ) ;
#60475=CARTESIAN_POINT ( 'NONE',  ( -4.164238869374098151, 1.595415501580634388, -3.795296366450310543 ) ) ;
#60476=CARTESIAN_POINT ( 'NONE',  ( 10.00000000000000178, 64.31368534415483396, 10.88017736071110342 ) ) ;
#60477=CARTESIAN_POINT ( 'NONE',  ( 7.084665262690076126, 62.02201867748816966, -10.88017736071110164 ) ) ;
#60478=CARTESIAN_POINT ( 'NONE',  ( 22.26659068614894466, 63.88708216824730357, 7.082119434687054849 ) ) ;
#60479=CARTESIAN_POINT ( 'NONE',  ( 10.00000000000000000, 7.873634669930421381, -12.81628187352647608 ) ) ;
#60481=CARTESIAN_POINT ( 'NONE',  ( 4.559911319644449179, 52.23035201082151247, -9.422509992056141925 ) ) ;
#60484=CARTESIAN_POINT ( 'NONE',  ( 16.40814093676323893, 30.79030133659708923, 11.09922568453595026 ) ) ;
#60485=CARTESIAN_POINT ( 'NONE',  ( 6.204703633549690345, 50.76208216824730357, -14.16423886937410259 ) ) ;
#60487=CARTESIAN_POINT ( 'NONE',  ( 19.42250999205614193, 10.14701867748816966, 5.440088680355555262 ) ) ;
#60488=CARTESIAN_POINT ( 'NONE',  ( 0.5774900079438590739, 27.64701867748817676, -5.440088680355550821 ) ) ;
#60489=CARTESIAN_POINT ( 'NONE',  ( 12.63842701281683034, 52.46726448433413026, 9.846743663894596210 ) ) ;
#60490=CARTESIAN_POINT ( 'NONE',  ( 6.565887622018943937, 50.16530133659708213, 12.81628187352647430 ) ) ;
#60491=CARTESIAN_POINT ( 'NONE',  ( 1.274849032794231007, 43.57228050351031357, 6.499999999999895195 ) ) ;
#60495=CARTESIAN_POINT ( 'NONE',  ( 17.96484262340118221, 16.18868534415483396, -7.964842623401177768 ) ) ;
#60496=CARTESIAN_POINT ( 'NONE',  ( 22.81628187352647785, 21.41530133659708923, 3.434112377981063169 ) ) ;
#60499=CARTESIAN_POINT ( 'NONE',  ( 18.52753015748618282, 53.92559781766745175, -4.923371831947291888 ) ) ;
#60500=CARTESIAN_POINT ( 'NONE',  ( 10.00000000000000000, 31.81368534415483751, -10.88017736071110342 ) ) ;
#60501=CARTESIAN_POINT ( 'NONE',  ( -2.816281873526473856, 19.33196800326375708, 3.434112377981055619 ) ) ;
#60502=CARTESIAN_POINT ( 'NONE',  ( 15.44008868035555260, 44.73035201082151247, 9.422509992056143702 ) ) ;
#60505=CARTESIAN_POINT ( 'NONE',  ( 3.591859063236761518, 49.95696800326375353, 11.09922568453594849 ) ) ;
#60507=CARTESIAN_POINT ( 'NONE',  ( -0.8801773607111008646, 48.27201867748816966, 2.915334737309923430 ) ) ;
#60508=CARTESIAN_POINT ( 'NONE',  ( -2.816281873526471635, 38.91530133659708213, -3.434112377981056508 ) ) ;
#60509=CARTESIAN_POINT ( 'NONE',  ( 12.91533473730992121, 39.52201867748817676, 10.88017736071110164 ) ) ;
#60511=CARTESIAN_POINT ( 'NONE',  ( 5.076628168052703671, 66.84226448433412315, 8.527530157486179263 ) ) ;
#60512=CARTESIAN_POINT ( 'NONE',  ( 18.52753015748617571, 13.09226448433411960, 4.923371831947298993 ) ) ;
#60513=CARTESIAN_POINT ( 'NONE',  ( 10.00000000000000000, 9.758931151000785675, -9.846743663894594434 ) ) ;
#60515=CARTESIAN_POINT ( 'NONE',  ( 10.00000000000000178, 38.05374883491396787, 14.16423886937410082 ) ) ;
#60517=MECHANICAL_DESIGN_GEOMETRIC_PRESENTATION_REPRESENTATION('',(#6280),#66945);
#60518=CARTESIAN_POINT ( 'NONE',  ( 4.559911319644449179, 2.230352010821504471, -9.422509992056141925 ) ) ;
#60521=CARTESIAN_POINT ( 'NONE',  ( 19.42250999205614193, 5.147018677488171434, 5.440088680355555262 ) ) ;
#60522=CARTESIAN_POINT ( 'NONE',  ( -2.266590686148945544, 61.38708216824730357, -7.082119434687050408 ) ) ;
#60524=CARTESIAN_POINT ( 'NONE',  ( 19.84674366389459621, 38.50893115100078745, 7.409399052514197653E-17 ) ) ;
#60525=CARTESIAN_POINT ( 'NONE',  ( 3.591859063236761518, 34.95696800326375353, 11.09922568453594849 ) ) ;
#60528=CARTESIAN_POINT ( 'NONE',  ( 2.917880565312950480, 0.9704155015806342766, -12.26659068614894821 ) ) ;
#60529=CARTESIAN_POINT ( 'NONE',  ( 4.559911319644449179, 13.89701867748817143, 9.422509992056141925 ) ) ;
#60530=CARTESIAN_POINT ( 'NONE',  ( -4.164238869374098151, 51.59541550158063217, -3.795296366450310543 ) ) ;
#60531=CARTESIAN_POINT ( 'NONE',  ( 2.791683348922237240, 40.38393115100078035, -7.208316651077763204 ) ) ;
#60534=CARTESIAN_POINT ( 'NONE',  ( 18.52753015748618282, 23.92559781766745530, -4.923371831947291888 ) ) ;
#60535=FACE_OUTER_BOUND ( 'NONE', #60153, .T. ) ;
#60539=ORIENTED_EDGE ( 'NONE', *, *, #22299, .T. ) ;
#60541=ORIENTED_EDGE ( 'NONE', *, *, #93367, .T. ) ;
#60542=CARTESIAN_POINT ( 'NONE',  ( 2.791683348922240793, 61.63393115100079456, 7.208316651077764092 ) ) ;
#60543=CARTESIAN_POINT ( 'NONE',  ( 12.91533473730992121, 34.52201867748817676, 10.88017736071110164 ) ) ;
#60544=CARTESIAN_POINT ( 'NONE',  ( 19.42250999205614193, 35.14701867748816966, 5.440088680355555262 ) ) ;
#60545=CARTESIAN_POINT ( 'NONE',  ( 2.791683348922237240, 60.38393115100078745, -7.208316651077763204 ) ) ;
#60546=CARTESIAN_POINT ( 'NONE',  ( 22.81628187352648496, 36.83196800326376064, -3.434112377981050290 ) ) ;
#60547=CARTESIAN_POINT ( 'NONE',  ( 20.36894250292379738, 4.928748834913967869, -10.36894250292379027 ) ) ;
#60548=CARTESIAN_POINT ( 'NONE',  ( 10.00000000000000000, 66.81368534415484817, -10.88017736071110342 ) ) ;
#60551=CARTESIAN_POINT ( 'NONE',  ( 6.565887622018943937, 35.16530133659708923, 12.81628187352647430 ) ) ;
#60552=ORIENTED_EDGE ( 'NONE', *, *, #38085, .T. ) ;
#60553=CARTESIAN_POINT ( 'NONE',  ( 14.92337183194729633, 47.67559781766745175, 8.527530157486181039 ) ) ;
#60554=CARTESIAN_POINT ( 'NONE',  ( 0.5774900079438590739, 7.647018677488171434, -5.440088680355550821 ) ) ;
#60556=CARTESIAN_POINT ( 'NONE',  ( 19.42250999205614548, 20.98035201082150891, -5.440088680355545492 ) ) ;
#60559=CARTESIAN_POINT ( 'NONE',  ( 7.084665262690076126, 67.02201867748817676, -10.88017736071110164 ) ) ;
#60560=CARTESIAN_POINT ( 'NONE',  ( 0.5774900079438590739, 57.64701867748817676, -5.440088680355550821 ) ) ;
#60561=CARTESIAN_POINT ( 'NONE',  ( 7.084665262690076126, 59.10535201082150536, 10.88017736071109987 ) ) ;
#60562=( NAMED_UNIT ( * ) PLANE_ANGLE_UNIT ( ) SI_UNIT ( $, .RADIAN. ) );
#60563=CARTESIAN_POINT ( 'NONE',  ( 17.96484262340118221, 56.18868534415484817, -7.964842623401177768 ) ) ;
#60564=CARTESIAN_POINT ( 'NONE',  ( -46.94000000000000483, 100.5295635078712593, 8.861295791683421186 ) ) ;
#60566=CARTESIAN_POINT ( 'NONE',  ( -46.94000000000001194, 103.2691844435154422, 6.361973263950303270 ) ) ;
#60569=CARTESIAN_POINT ( 'NONE',  ( 17.20831665107776587, 47.88393115100078745, 7.208316651077764980 ) ) ;
#60574=CARTESIAN_POINT ( 'NONE',  ( 24.16423886937409904, 9.095415501580633943, 3.795296366450317205 ) ) ;
#60577=CARTESIAN_POINT ( 'NONE',  ( 12.91533473730992121, 9.522018677488171434, 10.88017736071110164 ) ) ;
#60578=CARTESIAN_POINT ( 'NONE',  ( -1.099225684535947600, 43.70696800326375353, -6.408140936763238038 ) ) ;
#60581=CARTESIAN_POINT ( 'NONE',  ( 0.1532563361054082862, 41.21726448433411605, 2.638427012816831674 ) ) ;
#60582=FILL_AREA_STYLE_COLOUR ( '', #6817 ) ;
#60583=CARTESIAN_POINT ( 'NONE',  ( 19.38216949554541557, 22.24863466993041428, -9.382169495545420901 ) ) ;
#60584=CARTESIAN_POINT ( 'NONE',  ( 1.472469842513823179, 25.59226448433412315, -4.923371831947296329 ) ) ;
#60586=CARTESIAN_POINT ( 'NONE',  ( -1.099225684535947600, 4.540301336597087456, 6.408140936763237150 ) ) ;
#60590=CARTESIAN_POINT ( 'NONE',  ( 7.084665262690076126, 29.10535201082150181, 10.88017736071109987 ) ) ;
#60591=CARTESIAN_POINT ( 'NONE',  ( -0.3689425029237881626, 17.42874883491397142, 10.36894250292379027 ) ) ;
#60592=CARTESIAN_POINT ( 'NONE',  ( 1.472469842513823179, 25.59226448433412315, -4.923371831947296329 ) ) ;
#60593=CARTESIAN_POINT ( 'NONE',  ( 12.63842701281683922, 4.550597817667451750, -9.846743663894590881 ) ) ;
#60594=CARTESIAN_POINT ( 'NONE',  ( 0.6178305044545838731, 39.74863466993041072, 9.382169495545420901 ) ) ;
#60596=CARTESIAN_POINT ( 'NONE',  ( 10.00000000000000000, 16.81368534415483751, -10.88017736071110342 ) ) ;
#60598=CARTESIAN_POINT ( 'NONE',  ( -1.099225684535947600, 9.540301336597087456, 6.408140936763237150 ) ) ;
#60599=CARTESIAN_POINT ( 'NONE',  ( 21.09922568453595559, 2.040301336597086568, -6.408140936763230044 ) ) ;
#60600=CARTESIAN_POINT ( 'NONE',  ( 2.791683348922240793, 31.63393115100078745, 7.208316651077764092 ) ) ;
#60602=CARTESIAN_POINT ( 'NONE',  ( -2.816281873526473856, 39.12363466993041783, 9.499525473075851096E-16 ) ) ;
#60604=CARTESIAN_POINT ( 'NONE',  ( 20.88017736071110519, 35.56368534415484106, 2.639326808657452039E-16 ) ) ;
#60609=CARTESIAN_POINT ( 'NONE',  ( 7.084665262690076126, 39.10535201082150536, 10.88017736071109987 ) ) ;
#60610=CARTESIAN_POINT ( 'NONE',  ( 15.44008868035555260, 49.73035201082150536, 9.422509992056143702 ) ) ;
#60611=CARTESIAN_POINT ( 'NONE',  ( 0.1532563361054083140, 61.00893115100078745, 1.131784320476157264E-15 ) ) ;
#60612=CARTESIAN_POINT ( 'NONE',  ( 10.00000000000000000, 66.81368534415484817, -10.88017736071110342 ) ) ;
#60613=CARTESIAN_POINT ( 'NONE',  ( 1.472469842513823179, 51.42559781766745886, 4.923371831947296329 ) ) ;
#60614=CARTESIAN_POINT ( 'NONE',  ( 20.88017736071110519, 5.563685344154837509, 2.639326808657452039E-16 ) ) ;
#60616=CARTESIAN_POINT ( 'NONE',  ( 13.43411237798106583, 7.665301336597086568, -12.81628187352647252 ) ) ;
#60618=CARTESIAN_POINT ( 'NONE',  ( 19.42250999205614193, 40.14701867748817676, 5.440088680355555262 ) ) ;
#60620=CARTESIAN_POINT ( 'NONE',  ( 4.559911319644449179, 28.89701867748817321, 9.422509992056141925 ) ) ;
#60621=CARTESIAN_POINT ( 'NONE',  ( 1.472469842513823179, 11.42559781766745175, 4.923371831947296329 ) ) ;
#60622=CARTESIAN_POINT ( 'NONE',  ( 10.00000000000000178, 33.05374883491396787, 14.16423886937410082 ) ) ;
#60623=CARTESIAN_POINT ( 'NONE',  ( 18.52753015748617571, 23.09226448433411960, 4.923371831947298993 ) ) ;
#60624=CARTESIAN_POINT ( 'NONE',  ( 12.91533473730992121, 44.52201867748816966, 10.88017736071110164 ) ) ;
#60626=CARTESIAN_POINT ( 'NONE',  ( 2.917880565312948704, 2.637082168247300906, 12.26659068614894643 ) ) ;
#60627=LINE ( 'NONE', #5675, #69086 ) ;
#60628=CARTESIAN_POINT ( 'NONE',  ( 5.076628168052703671, 61.84226448433412315, 8.527530157486179263 ) ) ;
#60631=CARTESIAN_POINT ( 'NONE',  ( 24.16423886937409904, 19.09541550158063927, 3.795296366450317205 ) ) ;
#60632=CARTESIAN_POINT ( 'NONE',  ( -2.266590686148945544, 26.38708216824730357, -7.082119434687050408 ) ) ;
#60633=ADVANCED_FACE ( 'NONE', ( #86011 ), #12276, .T. ) ;
#60634=CARTESIAN_POINT ( 'NONE',  ( 7.084665262690076126, 64.10535201082150536, 10.88017736071109987 ) ) ;
#60635=CARTESIAN_POINT ( 'NONE',  ( -4.164238869374099039, 66.80374883491396076, 8.674139862899312516E-16 ) ) ;
#60636=CARTESIAN_POINT ( 'NONE',  ( 18.52753015748618282, 43.92559781766745175, -4.923371831947291888 ) ) ;
#60638=CARTESIAN_POINT ( 'NONE',  ( 17.96484262340118221, 49.93868534415484106, 7.964842623401181321 ) ) ;
#60639=CARTESIAN_POINT ( 'NONE',  ( -2.816281873526473856, 14.12363466993041961, 9.499525473075851096E-16 ) ) ;
#60640=CARTESIAN_POINT ( 'NONE',  ( 17.08211943468705130, 18.47041550158063572, 12.26659068614894998 ) ) ;
#60641=CARTESIAN_POINT ( 'NONE',  ( 15.44008868035555793, 16.39701867748817321, -9.422509992056140149 ) ) ;
#60642=CARTESIAN_POINT ( 'NONE',  ( 17.96484262340118221, 31.18868534415483751, -7.964842623401177768 ) ) ;
#60643=CARTESIAN_POINT ( 'NONE',  ( -0.2418659066527499291, 2.234100856612035724, -6.114288769123083611 ) ) ;
#60644=CARTESIAN_POINT ( 'NONE',  ( 19.42250999205614548, 60.98035201082151247, -5.440088680355545492 ) ) ;
#60646=CARTESIAN_POINT ( 'NONE',  ( -1.099225684535947600, 49.54030133659708923, 6.408140936763237150 ) ) ;
#60649=CARTESIAN_POINT ( 'NONE',  ( 19.80832241502127644, 34.75868815902068576, 6.499999999999991118 ) ) ;
#60651=LINE ( 'NONE', #53649, #4623 ) ;
#60655=CARTESIAN_POINT ( 'NONE',  ( 2.917880565312950480, 55.97041550158063217, -12.26659068614894821 ) ) ;
#60656=CARTESIAN_POINT ( 'NONE',  ( 6.204703633549690345, 67.84541550158060375, 14.16423886937410082 ) ) ;
#60657=CARTESIAN_POINT ( 'NONE',  ( 12.63842701281683034, 17.46726448433411250, 9.846743663894596210 ) ) ;
#60658=CARTESIAN_POINT ( 'NONE',  ( 5.076628168052704559, 65.17559781766745175, -8.527530157486179263 ) ) ;
#60659=CARTESIAN_POINT ( 'NONE',  ( 4.559911319644449179, 67.23035201082150536, -9.422509992056141925 ) ) ;
#60662=CARTESIAN_POINT ( 'NONE',  ( 17.08211943468705840, 30.13708216824730357, -12.26659068614894466 ) ) ;
#60664=CARTESIAN_POINT ( 'NONE',  ( 20.36894250292379382, 38.67874883491396076, 10.36894250292379205 ) ) ;
#60666=CARTESIAN_POINT ( 'NONE',  ( 19.38216949554541557, 62.24863466993041072, -9.382169495545420901 ) ) ;
#60668=CARTESIAN_POINT ( 'NONE',  ( 4.559911319644449179, 23.89701867748817321, 9.422509992056141925 ) ) ;
#60669=CARTESIAN_POINT ( 'NONE',  ( 0.1532563361054083140, 56.00893115100078745, 1.131784320476157264E-15 ) ) ;
#60670=CARTESIAN_POINT ( 'NONE',  ( -0.8801773607111009756, 23.06368534415484106, 1.068504757029289695E-15 ) ) ;
#60673=CARTESIAN_POINT ( 'NONE',  ( 7.361572987183169658, 54.96726448433413026, -9.846743663894592657 ) ) ;
#60674=CARTESIAN_POINT ( 'NONE',  ( 12.63842701281683922, 44.55059781766745175, -9.846743663894590881 ) ) ;
#60676=CARTESIAN_POINT ( 'NONE',  ( 20.15039907845753930, 70.00000000000000000, 6.262539305110068177 ) ) ;
#60679=FILL_AREA_STYLE ('',( #9660 ) ) ;
#60683=CARTESIAN_POINT ( 'NONE',  ( 2.791683348922237240, 25.38393115100078390, -7.208316651077763204 ) ) ;
#60684=CARTESIAN_POINT ( 'NONE',  ( -46.34323875807881166, 103.6109741468810483, 6.190393423093146552 ) ) ;
#60685=CARTESIAN_POINT ( 'NONE',  ( -1.099225684535947600, 38.70696800326375353, -6.408140936763238038 ) ) ;
#60686=CARTESIAN_POINT ( 'NONE',  ( -45.94000000000000483, 103.0000000000000000, 5.000000000000000000 ) ) ;
#60689=CARTESIAN_POINT ( 'NONE',  ( 2.791683348922240793, 36.63393115100078035, 7.208316651077764092 ) ) ;
#60690=CARTESIAN_POINT ( 'NONE',  ( 10.00000000000000178, 28.05374883491396787, 14.16423886937410082 ) ) ;
#60691=CARTESIAN_POINT ( 'NONE',  ( 7.361572987183169658, 39.96726448433411605, -9.846743663894592657 ) ) ;
#60693=CARTESIAN_POINT ( 'NONE',  ( 12.63842701281683922, 4.550597817667451750, -9.846743663894590881 ) ) ;
#60694=CARTESIAN_POINT ( 'NONE',  ( 20.36894250292379738, 4.928748834913967869, -10.36894250292379027 ) ) ;
#60695=CARTESIAN_POINT ( 'NONE',  ( 14.92337183194729633, 42.67559781766745886, 8.527530157486181039 ) ) ;
#60696=CARTESIAN_POINT ( 'NONE',  ( -0.8801773607111008646, 48.27201867748816966, 2.915334737309923430 ) ) ;
#60698=CARTESIAN_POINT ( 'NONE',  ( 2.791683348922240793, 46.63393115100077324, 7.208316651077764092 ) ) ;
#60701=VECTOR ( 'NONE', #27166, 1000.000000000000000 ) ;
#60702=CARTESIAN_POINT ( 'NONE',  ( 19.42250999205614193, 40.14701867748817676, 5.440088680355555262 ) ) ;
#60703=ORIENTED_EDGE ( 'NONE', *, *, #52976, .F. ) ;
#60705=CARTESIAN_POINT ( 'NONE',  ( 15.44008868035555260, 34.73035201082151247, 9.422509992056143702 ) ) ;
#60706=CARTESIAN_POINT ( 'NONE',  ( 1.472469842513823179, 66.42559781766745175, 4.923371831947296329 ) ) ;
#60707=CARTESIAN_POINT ( 'NONE',  ( 19.42250999205614548, 45.98035201082150536, -5.440088680355545492 ) ) ;
#60708=CARTESIAN_POINT ( 'NONE',  ( -1.926860441876564023, 47.87045670184115664, 3.195792623639529761 ) ) ;
#60709=CARTESIAN_POINT ( 'NONE',  ( 10.00000000000000178, 69.31368534415484817, 10.88017736071110342 ) ) ;
#60711=CARTESIAN_POINT ( 'NONE',  ( 2.035157376598822676, 37.43868534415484106, -7.964842623401177768 ) ) ;
#60713=CARTESIAN_POINT ( 'NONE',  ( 5.076628168052703671, 16.84226448433411960, 8.527530157486179263 ) ) ;
#60714=CARTESIAN_POINT ( 'NONE',  ( 17.20831665107776587, 34.13393115100078745, -7.208316651077762316 ) ) ;
#60715=CARTESIAN_POINT ( 'NONE',  ( 19.72487221294571214, 57.80223176428831522, -6.499999999999988454 ) ) ;
#60717=CARTESIAN_POINT ( 'NONE',  ( 16.40814093676323893, 0.7903013365970867898, 11.09922568453595026 ) ) ;
#60718=AXIS2_PLACEMENT_3D ( 'NONE', #22204, #51708, #36205 ) ;
#60719=CARTESIAN_POINT ( 'NONE',  ( 12.91533473730993009, 6.605352010821504471, -10.88017736071109987 ) ) ;
#60721=CARTESIAN_POINT ( 'NONE',  ( 2.917880565312950480, 25.97041550158063572, -12.26659068614894821 ) ) ;
#60723=CARTESIAN_POINT ( 'NONE',  ( 24.16423886937410614, 49.51208216824730357, -3.795296366450302550 ) ) ;
#60725=CARTESIAN_POINT ( 'NONE',  ( 0.1532563361054082862, 26.21726448433411605, 2.638427012816831674 ) ) ;
#60726=CARTESIAN_POINT ( 'NONE',  ( 19.42250999205614548, 25.98035201082150891, -5.440088680355545492 ) ) ;
#60727=EDGE_CURVE ( 'NONE', #80952, #5362, #84064, .T. ) ;
#60728=CARTESIAN_POINT ( 'NONE',  ( 5.076628168052704559, 45.17559781766745175, -8.527530157486179263 ) ) ;
#60729=CARTESIAN_POINT ( 'NONE',  ( 6.204703633549690345, 10.76208216824729824, -14.16423886937410259 ) ) ;
#60731=CARTESIAN_POINT ( 'NONE',  ( 7.361572987183169658, 4.967264484334119601, -9.846743663894592657 ) ) ;
#60732=CARTESIAN_POINT ( 'NONE',  ( 6.565887622018943937, 38.08196800326376064, -12.81628187352647608 ) ) ;
#60733=CARTESIAN_POINT ( 'NONE',  ( 12.63842701281683034, 42.46726448433412315, 9.846743663894596210 ) ) ;
#60735=CARTESIAN_POINT ( 'NONE',  ( 10.00000000000000000, 4.758931151000784787, -9.846743663894594434 ) ) ;
#60738=CARTESIAN_POINT ( 'NONE',  ( 24.16423886937409904, 54.09541550158063217, 3.795296366450317205 ) ) ;
#60739=CARTESIAN_POINT ( 'NONE',  ( 12.91533473730993009, 41.60535201082149825, -10.88017736071109987 ) ) ;
#60740=CARTESIAN_POINT ( 'NONE',  ( -46.48928645636215151, 103.2957187381728232, 6.397878122523974476 ) ) ;
#60742=CARTESIAN_POINT ( 'NONE',  ( 17.20831665107776587, 39.13393115100079456, -7.208316651077762316 ) ) ;
#60743=CARTESIAN_POINT ( 'NONE',  ( -0.8801773607111009756, 8.063685344154837509, 1.068504757029289695E-15 ) ) ;
#60744=CARTESIAN_POINT ( 'NONE',  ( 0.1532563361054100626, 35.80059781766745175, -2.638427012816831230 ) ) ;
#60745=CARTESIAN_POINT ( 'NONE',  ( -0.7670050760944780999, -5.787280142670756450E-16, -2.805511429989595129 ) ) ;
#60746=CARTESIAN_POINT ( 'NONE',  ( 2.791683348922240793, 51.63393115100078745, 7.208316651077764092 ) ) ;
#60747=CARTESIAN_POINT ( 'NONE',  ( 0.5774900079438607392, 48.48035201082150536, 5.440088680355550821 ) ) ;
#60749=ORIENTED_EDGE ( 'NONE', *, *, #12359, .F. ) ;
#60751=CARTESIAN_POINT ( 'NONE',  ( -1.099225684535947600, 63.70696800326376774, -6.408140936763238038 ) ) ;
#60753=EDGE_CURVE ( 'NONE', #40639, #37825, #1601, .T. ) ;
#60754=CARTESIAN_POINT ( 'NONE',  ( 12.63842701281683922, 4.550597817667451750, -9.846743663894590881 ) ) ;
#60755=CARTESIAN_POINT ( 'NONE',  ( 10.00000000000000000, 52.87363466993041783, -12.81628187352647608 ) ) ;
#60756=CARTESIAN_POINT ( 'NONE',  ( 0.5774900079438607392, 3.480352010821504916, 5.440088680355550821 ) ) ;
#60757=CARTESIAN_POINT ( 'NONE',  ( 14.92337183194729988, 54.34226448433412315, -8.527530157486177487 ) ) ;
#60759=CARTESIAN_POINT ( 'NONE',  ( 5.076628168052704559, 0.1755978176674514724, -8.527530157486179263 ) ) ;
#60760=CARTESIAN_POINT ( 'NONE',  ( 2.917880565312948704, 27.63708216824730357, 12.26659068614894643 ) ) ;
#60761=CARTESIAN_POINT ( 'NONE',  ( 6.204703633549690345, 40.76208216824731778, -14.16423886937410259 ) ) ;
#60762=CARTESIAN_POINT ( 'NONE',  ( 2.791683348922237240, 60.38393115100078745, -7.208316651077763204 ) ) ;
#60764=CARTESIAN_POINT ( 'NONE',  ( 2.035157376598822676, 52.43868534415483396, -7.964842623401177768 ) ) ;
#60766=CARTESIAN_POINT ( 'NONE',  ( 19.84674366389459266, 8.300597817667451750, 2.638427012816836559 ) ) ;
#60769=CARTESIAN_POINT ( 'NONE',  ( 6.565887622018943937, 60.16530133659707502, 12.81628187352647430 ) ) ;
#60771=CARTESIAN_POINT ( 'NONE',  ( 2.791683348922237240, 5.383931151000785675, -7.208316651077763204 ) ) ;
#60773=CARTESIAN_POINT ( 'NONE',  ( 17.08211943468705840, 15.13708216824730179, -12.26659068614894466 ) ) ;
#60774=CARTESIAN_POINT ( 'NONE',  ( 5.076628168052703671, 26.84226448433411960, 8.527530157486179263 ) ) ;
#60775=CARTESIAN_POINT ( 'NONE',  ( 7.084665262690076126, 34.10535201082151247, 10.88017736071109987 ) ) ;
#60778=CARTESIAN_POINT ( 'NONE',  ( 0.5774900079438590739, 22.64701867748817321, -5.440088680355550821 ) ) ;
#60780=ORIENTED_EDGE ( 'NONE', *, *, #22369, .F. ) ;
#60781=CARTESIAN_POINT ( 'NONE',  ( 20.88017736071110164, 30.35535201082151247, 2.915334737309930979 ) ) ;
#60783=CARTESIAN_POINT ( 'NONE',  ( 2.603489959281590771, 46.58210964143328425, 6.500000000000003553 ) ) ;
#60784=ORIENTED_EDGE ( 'NONE', *, *, #83927, .T. ) ;
#60785=CARTESIAN_POINT ( 'NONE',  ( 16.40814093676323893, 15.79030133659708746, 11.09922568453595026 ) ) ;
#60786=CARTESIAN_POINT ( 'NONE',  ( 1.046131998949937580, 20.73810908735720560, 6.499999999999992006 ) ) ;
#60787=CARTESIAN_POINT ( 'NONE',  ( 1.472469842513823179, 11.42559781766745175, 4.923371831947296329 ) ) ;
#60789=CARTESIAN_POINT ( 'NONE',  ( 0.2751277870542914172, 58.21833443783938833, 6.499999999999992006 ) ) ;
#60790=CARTESIAN_POINT ( 'NONE',  ( 5.076628168052704559, 15.17559781766745175, -8.527530157486179263 ) ) ;
#60791=CARTESIAN_POINT ( 'NONE',  ( 2.035157376598824452, 28.68868534415484106, 7.964842623401179544 ) ) ;
#60795=CARTESIAN_POINT ( 'NONE',  ( 17.96484262340118221, 39.93868534415484106, 7.964842623401181321 ) ) ;
#60797=CARTESIAN_POINT ( 'NONE',  ( 6.565887622018943937, 58.08196800326376064, -12.81628187352647608 ) ) ;
#60798=CARTESIAN_POINT ( 'NONE',  ( 12.91533473730992121, 54.52201867748816255, 10.88017736071110164 ) ) ;
#60799=CARTESIAN_POINT ( 'NONE',  ( 17.20831665107776587, 64.13393115100079456, -7.208316651077762316 ) ) ;
#60800=FACE_OUTER_BOUND ( 'NONE', #14700, .T. ) ;
#60801=CARTESIAN_POINT ( 'NONE',  ( 0.1532563361054083140, 16.00893115100078390, 1.131784320476157264E-15 ) ) ;
#60802=CARTESIAN_POINT ( 'NONE',  ( 0.6178305044545818747, 48.49863466993042493, -9.382169495545419124 ) ) ;
#60804=CARTESIAN_POINT ( 'NONE',  ( 2.791683348922240793, 11.63393115100078568, 7.208316651077764092 ) ) ;
#60805=CARTESIAN_POINT ( 'NONE',  ( 3.591859063236763294, 13.29030133659708746, -11.09922568453595026 ) ) ;
#60807=DIRECTION ( 'NONE',  ( 1.000000000000000000, 0.000000000000000000, 0.000000000000000000 ) ) ;
#60808=CARTESIAN_POINT ( 'NONE',  ( 15.44008868035555793, 31.39701867748817676, -9.422509992056140149 ) ) ;
#60809=CARTESIAN_POINT ( 'NONE',  ( 7.361572987183169658, 59.96726448433410894, -9.846743663894592657 ) ) ;
#60811=CARTESIAN_POINT ( 'NONE',  ( 18.52753015748618282, 23.92559781766745530, -4.923371831947291888 ) ) ;
#60812=CARTESIAN_POINT ( 'NONE',  ( 10.00000000000000000, 9.758931151000785675, -9.846743663894594434 ) ) ;
#60813=CARTESIAN_POINT ( 'NONE',  ( 3.591859063236761518, 4.956968003263753531, 11.09922568453594849 ) ) ;
#60815=CARTESIAN_POINT ( 'NONE',  ( 7.084665262690076126, 7.022018677488169658, -10.88017736071110164 ) ) ;
#60816=CARTESIAN_POINT ( 'NONE',  ( 1.472469842513823179, 61.42559781766745175, 4.923371831947296329 ) ) ;
#60820=CARTESIAN_POINT ( 'NONE',  ( 4.559911319644449179, 2.230352010821504916, -9.422509992056141925 ) ) ;
#60821=CARTESIAN_POINT ( 'NONE',  ( 5.076628168052703671, 51.84226448433412315, 8.527530157486179263 ) ) ;
#60822=EDGE_CURVE ( 'NONE', #82667, #88856, #13967, .T. ) ;
#60823=CARTESIAN_POINT ( 'NONE',  ( 0.2751277870542981341, 18.21833443783937767, 6.500000000000002665 ) ) ;
#60824=CARTESIAN_POINT ( 'NONE',  ( 20.88017736071110519, 5.563685344154838397, 2.639326808657452039E-16 ) ) ;
#60826=CARTESIAN_POINT ( 'NONE',  ( 20.88017736071110519, 35.56368534415484106, 2.639326808657452039E-16 ) ) ;
#60827=CARTESIAN_POINT ( 'NONE',  ( 24.16423886937410614, 44.30374883491397497, 8.672049930838204340E-16 ) ) ;
#60828=CARTESIAN_POINT ( 'NONE',  ( 12.91533473730992121, 4.522018677488170546, 10.88017736071110164 ) ) ;
#60829=CYLINDRICAL_SURFACE ( 'NONE', #92571, 0.5000000000000004441 ) ;
#60830=FACE_OUTER_BOUND ( 'NONE', #23945, .T. ) ;
#60831=CARTESIAN_POINT ( 'NONE',  ( 18.52753015748617571, 28.09226448433411960, 4.923371831947298993 ) ) ;
#60832=CARTESIAN_POINT ( 'NONE',  ( 19.38216949554541557, 17.24863466993041783, -9.382169495545420901 ) ) ;
#60834=CARTESIAN_POINT ( 'NONE',  ( -46.48928645636214441, 103.2957187381728232, 6.397878122523972699 ) ) ;
#60836=CARTESIAN_POINT ( 'NONE',  ( 17.20831665107776587, 57.88393115100078745, 7.208316651077764980 ) ) ;
#60837=CYLINDRICAL_SURFACE ( 'NONE', #29929, 0.5000000000000004441 ) ;
#60840=CARTESIAN_POINT ( 'NONE',  ( 20.36894250292379382, 13.67874883491396965, 10.36894250292379205 ) ) ;
#60842=CARTESIAN_POINT ( 'NONE',  ( 0.1532563361054082862, 21.21726448433412315, 2.638427012816831674 ) ) ;
#60844=CARTESIAN_POINT ( 'NONE',  ( 13.79529636645031943, 50.34541550158064638, -14.16423886937409904 ) ) ;
#60845=ADVANCED_FACE ( 'NONE', ( #22452 ), #22953, .T. ) ;
#60846=CARTESIAN_POINT ( 'NONE',  ( 0.1532563361054100626, 5.800597817667452638, -2.638427012816831230 ) ) ;
#60849=CARTESIAN_POINT ( 'NONE',  ( -0.8801773607111008646, 38.27201867748816255, 2.915334737309923430 ) ) ;
#60850=CARTESIAN_POINT ( 'NONE',  ( 21.09922568453595559, 47.04030133659708923, -6.408140936763230044 ) ) ;
#60851=CARTESIAN_POINT ( 'NONE',  ( 20.88017736071110875, 10.77201867748817143, -2.915334737309920765 ) ) ;
#60852=CARTESIAN_POINT ( 'NONE',  ( 0.6178305044545818747, 33.49863466993042493, -9.382169495545419124 ) ) ;
#60853=CARTESIAN_POINT ( 'NONE',  ( -2.816281873526473856, 4.331968003263754419, 3.434112377981055619 ) ) ;
#60854=CARTESIAN_POINT ( 'NONE',  ( 1.472469842513823179, 6.425597817667451750, 4.923371831947296329 ) ) ;
#60856=CARTESIAN_POINT ( 'NONE',  ( 2.377183314879979470, 10.78593319516822646, -6.500000000000010658 ) ) ;
#60858=CARTESIAN_POINT ( 'NONE',  ( 2.917880565312948704, 42.63708216824729647, 12.26659068614894643 ) ) ;
#60859=CARTESIAN_POINT ( 'NONE',  ( -0.3689425029237898834, 11.17874883491396787, -10.36894250292378850 ) ) ;
#60860=CARTESIAN_POINT ( 'NONE',  ( -0.8801773607111009756, 3.063685344154837509, 1.068504757029289695E-15 ) ) ;
#60861=CARTESIAN_POINT ( 'NONE',  ( -0.8801773607111008646, 33.27201867748817676, 2.915334737309923430 ) ) ;
#60864=CARTESIAN_POINT ( 'NONE',  ( -0.8801773607111008646, 48.27201867748816966, 2.915334737309923430 ) ) ;
#60865=CARTESIAN_POINT ( 'NONE',  ( 7.084665262690076126, 69.10535201082151957, 10.88017736071109987 ) ) ;
#60866=CARTESIAN_POINT ( 'NONE',  ( 6.565887622018943937, 30.16530133659708568, 12.81628187352647430 ) ) ;
#60867=CARTESIAN_POINT ( 'NONE',  ( 0.5600000000000083800, 105.0000000000000000, -5.000000000000000000 ) ) ;
#60869=CARTESIAN_POINT ( 'NONE',  ( 18.52753015748618282, 38.92559781766745175, -4.923371831947291888 ) ) ;
#60870=CARTESIAN_POINT ( 'NONE',  ( 16.40814093676324603, 17.45696800326375353, -11.09922568453594671 ) ) ;
#60872=CARTESIAN_POINT ( 'NONE',  ( 17.20831665107776587, 7.883931151000784787, 7.208316651077764980 ) ) ;
#60873=CARTESIAN_POINT ( 'NONE',  ( 20.88017736071110875, 15.77201867748817143, -2.915334737309920765 ) ) ;
#60874=CARTESIAN_POINT ( 'NONE',  ( 19.84674366389459266, 38.30059781766745175, 2.638427012816836559 ) ) ;
#60875=CARTESIAN_POINT ( 'NONE',  ( 19.38216949554541557, 62.24863466993041072, -9.382169495545420901 ) ) ;
#60876=CARTESIAN_POINT ( 'NONE',  ( 14.92337183194729988, 24.34226448433411960, -8.527530157486177487 ) ) ;
#60877=CARTESIAN_POINT ( 'NONE',  ( 2.917880565312948704, 7.637082168247301794, 12.26659068614894643 ) ) ;
#60879=CARTESIAN_POINT ( 'NONE',  ( 2.035157376598824452, 28.68868534415484106, 7.964842623401179544 ) ) ;
#60880=CARTESIAN_POINT ( 'NONE',  ( 0.5774900079438590739, 12.64701867748817143, -5.440088680355550821 ) ) ;
#60881=CARTESIAN_POINT ( 'NONE',  ( -2.266590686148945544, 37.22041550158063217, 7.082119434687048631 ) ) ;
#60882=ADVANCED_FACE ( 'NONE', ( #97973 ), #15526, .T. ) ;
#60883=CARTESIAN_POINT ( 'NONE',  ( 20.88017736071110164, 30.35535201082151247, 2.915334737309930979 ) ) ;
#60884=CARTESIAN_POINT ( 'NONE',  ( 15.44008868035555793, 16.39701867748817321, -9.422509992056140149 ) ) ;
#60886=CARTESIAN_POINT ( 'NONE',  ( 10.00000000000000178, 44.31368534415484106, 10.88017736071110342 ) ) ;
#60888=CARTESIAN_POINT ( 'NONE',  ( 21.09922568453595559, 42.04030133659708213, -6.408140936763230044 ) ) ;
#60889=CARTESIAN_POINT ( 'NONE',  ( 10.00000000000000178, 49.31368534415484106, 10.88017736071110342 ) ) ;
#60891=CARTESIAN_POINT ( 'NONE',  ( 15.44008868035555260, 49.73035201082150536, 9.422509992056143702 ) ) ;
#60893=CARTESIAN_POINT ( 'NONE',  ( -0.8801773607111009756, 53.06368534415484106, 1.068504757029289695E-15 ) ) ;
#60897=CARTESIAN_POINT ( 'NONE',  ( 24.16423886937410614, 49.30374883491396787, 8.672049930838204340E-16 ) ) ;
#60898=CARTESIAN_POINT ( 'NONE',  ( 4.559911319644449179, 62.23035201082150536, -9.422509992056141925 ) ) ;
#60899=SURFACE_STYLE_FILL_AREA ( #83905 ) ;
#60900=CARTESIAN_POINT ( 'NONE',  ( -43.70923076923077844, 103.3461538461538396, -9.500000000000000000 ) ) ;
#60901=CARTESIAN_POINT ( 'NONE',  ( 10.00000000000000000, 59.75893115100078745, -9.846743663894594434 ) ) ;
#60903=CARTESIAN_POINT ( 'NONE',  ( 19.84674366389459621, 33.50893115100078745, 7.409399052514197653E-17 ) ) ;
#60905=CARTESIAN_POINT ( 'NONE',  ( 1.472469842513823179, 31.42559781766745530, 4.923371831947296329 ) ) ;
#60907=CARTESIAN_POINT ( 'NONE',  ( 12.91533473730992121, 24.52201867748816966, 10.88017736071110164 ) ) ;
#60908=CARTESIAN_POINT ( 'NONE',  ( 10.00000000000000178, 37.25893115100078745, 9.846743663894594434 ) ) ;
#60910=CARTESIAN_POINT ( 'NONE',  ( 21.09922568453595559, 27.04030133659708568, -6.408140936763230044 ) ) ;
#60912=CARTESIAN_POINT ( 'NONE',  ( 15.44008868035555793, 46.39701867748817676, -9.422509992056140149 ) ) ;
#60913=CARTESIAN_POINT ( 'NONE',  ( 22.26659068614895176, 64.72041550158064638, -7.082119434687042414 ) ) ;
#60914=CARTESIAN_POINT ( 'NONE',  ( 3.591859063236763294, 28.29030133659708568, -11.09922568453595026 ) ) ;
#60915=LINE ( 'NONE', #47384, #5235 ) ;
#60916=ORIENTED_EDGE ( 'NONE', *, *, #46150, .F. ) ;
#60917=CARTESIAN_POINT ( 'NONE',  ( 22.81628187352648496, 11.83196800326375531, -3.434112377981050290 ) ) ;
#60918=CARTESIAN_POINT ( 'NONE',  ( 15.44008868035555793, 21.39701867748817321, -9.422509992056140149 ) ) ;
#60919=CARTESIAN_POINT ( 'NONE',  ( 7.084665262690076126, 59.10535201082150536, 10.88017736071109987 ) ) ;
#60920=CIRCLE ( 'NONE', #81612, 18.93999999999999773 ) ;
#60922=CARTESIAN_POINT ( 'NONE',  ( -0.8801773607111008646, 63.27201867748817676, 2.915334737309923430 ) ) ;
#60924=CARTESIAN_POINT ( 'NONE',  ( 1.472469842513823179, 40.59226448433411605, -4.923371831947296329 ) ) ;
#60925=CARTESIAN_POINT ( 'NONE',  ( 12.63842701281683922, 19.55059781766745175, -9.846743663894590881 ) ) ;
#60926=CARTESIAN_POINT ( 'NONE',  ( 0.1532563361054083140, 11.00893115100078568, 1.131784320476157264E-15 ) ) ;
#60927=CARTESIAN_POINT ( 'NONE',  ( 20.15039907845753220, 57.62777174578613426, -6.262539305110077947 ) ) ;
#60929=CARTESIAN_POINT ( 'NONE',  ( 22.81628187352648496, 41.83196800326375353, -3.434112377981050290 ) ) ;
#60930=CARTESIAN_POINT ( 'NONE',  ( 19.84674366389459266, 18.30059781766745175, 2.638427012816836559 ) ) ;
#60932=CARTESIAN_POINT ( 'NONE',  ( 20.32896413005680358, 44.74545670184113533, 5.963430220938287007 ) ) ;
#60933=CARTESIAN_POINT ( 'NONE',  ( 0.1532563361054083140, 36.00893115100078745, 1.131784320476157264E-15 ) ) ;
#60934=ORIENTED_EDGE ( 'NONE', *, *, #67409, .F. ) ;
#60935=CARTESIAN_POINT ( 'NONE',  ( 21.09922568453595559, 7.040301336597086568, -6.408140936763230044 ) ) ;
#60936=CARTESIAN_POINT ( 'NONE',  ( 7.084665262690076126, 49.10535201082149825, 10.88017736071109987 ) ) ;
#60937=CARTESIAN_POINT ( 'NONE',  ( 10.00000000000000178, 33.05374883491396787, 14.16423886937410082 ) ) ;
#60939=CARTESIAN_POINT ( 'NONE',  ( -2.266590686148945544, 31.38708216824730002, -7.082119434687050408 ) ) ;
#60940=CARTESIAN_POINT ( 'NONE',  ( 24.16423886937410614, 64.30374883491396076, 8.672049930838204340E-16 ) ) ;
#60941=CARTESIAN_POINT ( 'NONE',  ( 24.16423886937409904, 14.09541550158063217, 3.795296366450317205 ) ) ;
#60942=CARTESIAN_POINT ( 'NONE',  ( 20.36894250292379738, 19.92874883491396787, -10.36894250292379027 ) ) ;
#60944=CARTESIAN_POINT ( 'NONE',  ( 4.559911319644449179, 53.89701867748817676, 9.422509992056141925 ) ) ;
#60946=ADVANCED_FACE ( 'NONE', ( #12738 ), #50753, .F. ) ;
#60947=CARTESIAN_POINT ( 'NONE',  ( 18.95785429995052596, 62.24216108172004880, 6.499999999999944933 ) ) ;
#60948=CARTESIAN_POINT ( 'NONE',  ( 7.361572987183170547, 47.05059781766745175, 9.846743663894590881 ) ) ;
#60949=CARTESIAN_POINT ( 'NONE',  ( 7.084665262690076126, 27.02201867748817676, -10.88017736071110164 ) ) ;
#60951=CARTESIAN_POINT ( 'NONE',  ( 19.84674366389459621, 58.50893115100078745, 7.409399052514197653E-17 ) ) ;
#60952=CARTESIAN_POINT ( 'NONE',  ( 19.50000000000000711, 79.40087001978915282, -5.000000000000000888 ) ) ;
#60953=CARTESIAN_POINT ( 'NONE',  ( 5.076628168052703671, 31.84226448433412315, 8.527530157486179263 ) ) ;
#60954=CARTESIAN_POINT ( 'NONE',  ( 19.38216949554541557, 52.24863466993041072, -9.382169495545420901 ) ) ;
#60956=CARTESIAN_POINT ( 'NONE',  ( 19.84674366389459266, 43.71726448433410894, -2.638427012816827677 ) ) ;
#60957=CARTESIAN_POINT ( 'NONE',  ( 12.63842701281683034, 52.46726448433413026, 9.846743663894596210 ) ) ;
#60959=CARTESIAN_POINT ( 'NONE',  ( 2.917880565312948704, 37.63708216824731068, 12.26659068614894643 ) ) ;
#60961=CARTESIAN_POINT ( 'NONE',  ( 24.16423886937409904, 14.09541550158063217, 3.795296366450317205 ) ) ;
#60962=EDGE_CURVE ( 'NONE', #76972, #35320, #97754, .T. ) ;
#60963=CARTESIAN_POINT ( 'NONE',  ( 2.035157376598824452, 68.68868534415484817, 7.964842623401179544 ) ) ;
#60965=CARTESIAN_POINT ( 'NONE',  ( 22.26659068614895176, 59.72041550158063927, -7.082119434687042414 ) ) ;
#60966=CARTESIAN_POINT ( 'NONE',  ( 19.38216949554541202, 10.99863466993042138, 9.382169495545424454 ) ) ;
#60968=CARTESIAN_POINT ( 'NONE',  ( -0.8801773607110991993, 52.85535201082151247, -2.915334737309923874 ) ) ;
#60969=CARTESIAN_POINT ( 'NONE',  ( 1.274849032794294290, 58.57228050351032778, 6.499999999999979572 ) ) ;
#60970=CARTESIAN_POINT ( 'NONE',  ( 0.1532563361054083140, 31.00893115100078390, 1.131784320476157264E-15 ) ) ;
#60971=CARTESIAN_POINT ( 'NONE',  ( -2.266590686148945544, 57.22041550158063217, 7.082119434687048631 ) ) ;
#60973=CARTESIAN_POINT ( 'NONE',  ( 15.44008868035555793, 16.39701867748817321, -9.422509992056140149 ) ) ;
#60974=CARTESIAN_POINT ( 'NONE',  ( 20.88017736071110875, 30.77201867748816966, -2.915334737309920765 ) ) ;
#60975=CARTESIAN_POINT ( 'NONE',  ( 1.472469842513823179, 50.59226448433411605, -4.923371831947296329 ) ) ;
#60976=CARTESIAN_POINT ( 'NONE',  ( 0.1532563361054100626, 50.80059781766745175, -2.638427012816831230 ) ) ;
#60977=CARTESIAN_POINT ( 'NONE',  ( 19.38216949554541557, 47.24863466993041783, -9.382169495545420901 ) ) ;
#60978=CARTESIAN_POINT ( 'NONE',  ( 7.361572987183169658, -0.03273551566588185635, -9.846743663894592657 ) ) ;
#60979=EDGE_LOOP ( 'NONE', ( #43853, #2574, #31794, #62512 ) ) ;
#60980=CARTESIAN_POINT ( 'NONE',  ( 17.96484262340118221, 21.18868534415483396, -7.964842623401177768 ) ) ;
#60981=CARTESIAN_POINT ( 'NONE',  ( 6.565887622018943937, 20.16530133659708213, 12.81628187352647430 ) ) ;
#60984=CARTESIAN_POINT ( 'NONE',  ( 7.361572987183169658, 54.96726448433413026, -9.846743663894592657 ) ) ;
#60985=CARTESIAN_POINT ( 'NONE',  ( 15.44008868035555260, 29.73035201082150891, 9.422509992056143702 ) ) ;
#60986=CARTESIAN_POINT ( 'NONE',  ( 22.81628187352647785, 26.41530133659708923, 3.434112377981063169 ) ) ;
#60987=CARTESIAN_POINT ( 'NONE',  ( 15.44008868035555793, 46.39701867748817676, -9.422509992056140149 ) ) ;
#60991=CARTESIAN_POINT ( 'NONE',  ( 10.00000000000000000, 47.87363466993042493, -12.81628187352647608 ) ) ;
#60993=CARTESIAN_POINT ( 'NONE',  ( 19.84674366389459266, 63.71726448433412315, -2.638427012816827677 ) ) ;
#60994=CARTESIAN_POINT ( 'NONE',  ( 17.96484262340118221, 51.18868534415483396, -7.964842623401177768 ) ) ;
#60995=CARTESIAN_POINT ( 'NONE',  ( 16.40814093676323893, 35.79030133659708923, 11.09922568453595026 ) ) ;
#60996=CARTESIAN_POINT ( 'NONE',  ( 13.79529636645030344, 3.262082168247301350, 14.16423886937410614 ) ) ;
#60998=CARTESIAN_POINT ( 'NONE',  ( 7.084665262690076126, 47.02201867748818387, -10.88017736071110164 ) ) ;
#60999=MECHANICAL_DESIGN_GEOMETRIC_PRESENTATION_REPRESENTATION('',(#97791),#11536);
#61000=CARTESIAN_POINT ( 'NONE',  ( 2.917880565312948704, 47.63708216824730357, 12.26659068614894643 ) ) ;
#61002=CARTESIAN_POINT ( 'NONE',  ( 10.00000000000000000, 14.75893115100078568, -9.846743663894594434 ) ) ;
#61003=CARTESIAN_POINT ( 'NONE',  ( 18.52753015748617571, 8.092264484334117824, 4.923371831947298993 ) ) ;
#61005=CARTESIAN_POINT ( 'NONE',  ( 24.16423886937410614, 39.51208216824731068, -3.795296366450302550 ) ) ;
#61008=CARTESIAN_POINT ( 'NONE',  ( 2.035157376598824452, 13.68868534415483751, 7.964842623401179544 ) ) ;
#61013=CARTESIAN_POINT ( 'NONE',  ( 7.084665262690076126, 14.10535201082150358, 10.88017736071109987 ) ) ;
#61014=CARTESIAN_POINT ( 'NONE',  ( -4.164238869374099927, 62.01208216824728936, 3.795296366450308767 ) ) ;
#61015=CARTESIAN_POINT ( 'NONE',  ( 14.92337183194729633, 47.67559781766745175, 8.527530157486181039 ) ) ;
#61016=CARTESIAN_POINT ( 'NONE',  ( 22.81628187352648496, 36.83196800326376064, -3.434112377981050290 ) ) ;
#61018=CARTESIAN_POINT ( 'NONE',  ( 17.08211943468705130, 3.470415501580634388, 12.26659068614894998 ) ) ;
#61019=CARTESIAN_POINT ( 'NONE',  ( 10.00000000000000178, 24.31368534415484106, 10.88017736071110342 ) ) ;
#61020=CARTESIAN_POINT ( 'NONE',  ( 24.16423886937410614, 64.51208216824728936, -3.795296366450302550 ) ) ;
#61021=CARTESIAN_POINT ( 'NONE',  ( 2.791683348922240793, 41.63393115100078745, 7.208316651077764092 ) ) ;
#61022=CARTESIAN_POINT ( 'NONE',  ( 18.28836319691942336, 44.34492782695770074, 6.500000000000077272 ) ) ;
#61023=CARTESIAN_POINT ( 'NONE',  ( 7.361572987183170547, 17.05059781766745530, 9.846743663894590881 ) ) ;
#61028=ORIENTED_EDGE ( 'NONE', *, *, #21324, .T. ) ;
#61029=CARTESIAN_POINT ( 'NONE',  ( 12.63842701281683034, 62.46726448433410894, 9.846743663894596210 ) ) ;
#61030=CARTESIAN_POINT ( 'NONE',  ( 19.42250999205614193, 35.14701867748816966, 5.440088680355555262 ) ) ;
#61031=CARTESIAN_POINT ( 'NONE',  ( 7.084665262690076126, 39.10535201082150536, 10.88017736071109987 ) ) ;
#61032=CARTESIAN_POINT ( 'NONE',  ( 10.00000000000000178, 62.25893115100078745, 9.846743663894594434 ) ) ;
#61033=CARTESIAN_POINT ( 'NONE',  ( 0.6178305044545818747, 28.49863466993041783, -9.382169495545419124 ) ) ;
#61034=CARTESIAN_POINT ( 'NONE',  ( 24.16423886937410614, 14.30374883491396787, 8.672049930838204340E-16 ) ) ;
#61035=CIRCLE ( 'NONE', #48326, 0.5000000000000004441 ) ;
#61036=CARTESIAN_POINT ( 'NONE',  ( 22.81628187352648496, 41.83196800326375353, -3.434112377981050290 ) ) ;
#61037=ORIENTED_EDGE ( 'NONE', *, *, #93966, .T. ) ;
#61038=CARTESIAN_POINT ( 'NONE',  ( 7.361572987183170547, 42.05059781766745886, 9.846743663894590881 ) ) ;
#61039=CARTESIAN_POINT ( 'NONE',  ( 12.91533473730992121, 9.522018677488171434, 10.88017736071110164 ) ) ;
#61041=CARTESIAN_POINT ( 'NONE',  ( 20.88017736071110875, 20.77201867748816611, -2.915334737309920765 ) ) ;
#61043=CARTESIAN_POINT ( 'NONE',  ( 0.5774900079438590739, 62.64701867748817676, -5.440088680355550821 ) ) ;
#61044=CARTESIAN_POINT ( 'NONE',  ( 4.559911319644449179, 58.89701867748817676, 9.422509992056141925 ) ) ;
#61045=CARTESIAN_POINT ( 'NONE',  ( 19.42250999205614193, 60.14701867748817676, 5.440088680355555262 ) ) ;
#61047=CARTESIAN_POINT ( 'NONE',  ( 0.1532563361054100626, 0.8005978176674514168, -2.638427012816831230 ) ) ;
#61048=CARTESIAN_POINT ( 'NONE',  ( 10.00000000000000000, 51.81368534415484106, -10.88017736071110342 ) ) ;
#61049=FACE_OUTER_BOUND ( 'NONE', #39182, .T. ) ;
#61051=CARTESIAN_POINT ( 'NONE',  ( -46.94000000000247752, 100.6180954154858398, 9.128675877383326309 ) ) ;
#61052=DIRECTION ( 'NONE',  ( 0.000000000000000000, 0.000000000000000000, -1.000000000000000000 ) ) ;
#61055=CARTESIAN_POINT ( 'NONE',  ( 5.076628168052703671, 46.84226448433412315, 8.527530157486179263 ) ) ;
#61058=CIRCLE ( 'NONE', #64250, 0.5000000000000004441 ) ;
#61060=B_SPLINE_CURVE_WITH_KNOTS ( 'NONE', 3,
 ( #56559, #87053, #1616, #78573 ),
 .UNSPECIFIED., .F., .F.,
 ( 4, 4 ),
 ( 1.361094815542225550E-17, 0.002562518741975313395 ),
 .UNSPECIFIED. ) ;
#61062=CARTESIAN_POINT ( 'NONE',  ( 20.36894250292379382, 13.67874883491396965, 10.36894250292379205 ) ) ;
#61066=CARTESIAN_POINT ( 'NONE',  ( 0.5774900079438590739, 7.647018677488171434, -5.440088680355550821 ) ) ;
#61067=CARTESIAN_POINT ( 'NONE',  ( 3.591859063236763294, 38.29030133659708923, -11.09922568453595026 ) ) ;
#61070=CARTESIAN_POINT ( 'NONE',  ( 10.00000000000000000, 49.75893115100078745, -9.846743663894594434 ) ) ;
#61071=CARTESIAN_POINT ( 'NONE',  ( 13.43411237798105340, 20.58196800326374643, 12.81628187352647963 ) ) ;
#61072=CARTESIAN_POINT ( 'NONE',  ( 7.361572987183169658, 29.96726448433411960, -9.846743663894592657 ) ) ;
#61073=CARTESIAN_POINT ( 'NONE',  ( -0.3077640640439943676, 70.00000000000000000, -6.000000000000270894 ) ) ;
#61074=CARTESIAN_POINT ( 'NONE',  ( -1.099225684535947600, 18.70696800326375353, -6.408140936763238038 ) ) ;
#61078=CARTESIAN_POINT ( 'NONE',  ( 14.92337183194729633, 12.67559781766745353, 8.527530157486181039 ) ) ;
#61079=ORIENTED_EDGE ( 'NONE', *, *, #49247, .F. ) ;
#61082=CARTESIAN_POINT ( 'NONE',  ( 10.00000000000000178, 24.31368534415484106, 10.88017736071110342 ) ) ;
#61083=CARTESIAN_POINT ( 'NONE',  ( -0.3689425029237881626, 22.42874883491397142, 10.36894250292379027 ) ) ;
#61084=CARTESIAN_POINT ( 'NONE',  ( 5.076628168052703671, 46.84226448433412315, 8.527530157486179263 ) ) ;
#61085=CARTESIAN_POINT ( 'NONE',  ( 0.1532563361054100626, 5.800597817667452638, -2.638427012816831230 ) ) ;
#61086=CARTESIAN_POINT ( 'NONE',  ( -2.816281873526473856, 44.12363466993042493, 9.499525473075851096E-16 ) ) ;
#61088=CARTESIAN_POINT ( 'NONE',  ( 7.084665262690076126, 19.10535201082150181, 10.88017736071109987 ) ) ;
#61091=CARTESIAN_POINT ( 'NONE',  ( 0.6178305044545838731, 9.748634669930416052, 9.382169495545420901 ) ) ;
#61092=CARTESIAN_POINT ( 'NONE',  ( 18.52753015748617571, 23.09226448433411960, 4.923371831947298993 ) ) ;
#61094=CARTESIAN_POINT ( 'NONE',  ( -1.099225684535947600, 33.70696800326375353, -6.408140936763238038 ) ) ;
#61096=CARTESIAN_POINT ( 'NONE',  ( -0.8801773607110991993, 52.85535201082151247, -2.915334737309923874 ) ) ;
#61100=CARTESIAN_POINT ( 'NONE',  ( 0.5774900079438590739, 42.64701867748816966, -5.440088680355550821 ) ) ;
#61102=CARTESIAN_POINT ( 'NONE',  ( 17.96484262340118221, 49.93868534415484106, 7.964842623401181321 ) ) ;
#61103=CARTESIAN_POINT ( 'NONE',  ( 17.20831665107776587, 59.13393115100078745, -7.208316651077762316 ) ) ;
#61104=CARTESIAN_POINT ( 'NONE',  ( 15.44008868035555793, 61.39701867748817676, -9.422509992056140149 ) ) ;
#61106=CARTESIAN_POINT ( 'NONE',  ( 2.791683348922237240, 55.38393115100078745, -7.208316651077763204 ) ) ;
#61107=CARTESIAN_POINT ( 'NONE',  ( -0.8801773607111009756, 8.063685344154837509, 1.068504757029289695E-15 ) ) ;
#61109=CARTESIAN_POINT ( 'NONE',  ( 6.565887622018943937, 10.16530133659708746, 12.81628187352647430 ) ) ;
#61111=CARTESIAN_POINT ( 'NONE',  ( 2.035157376598824452, 38.68868534415483396, 7.964842623401179544 ) ) ;
#61112=CARTESIAN_POINT ( 'NONE',  ( 0.1532563361054082862, 61.21726448433412315, 2.638427012816831674 ) ) ;
#61115=CARTESIAN_POINT ( 'NONE',  ( 10.00000000000000178, 14.31368534415483751, 10.88017736071110342 ) ) ;
#61116=CARTESIAN_POINT ( 'NONE',  ( 17.96484262340118221, 21.18868534415483396, -7.964842623401177768 ) ) ;
#61117=CARTESIAN_POINT ( 'NONE',  ( 2.917880565312950480, 35.97041550158063217, -12.26659068614894821 ) ) ;
#61118=CARTESIAN_POINT ( 'NONE',  ( 17.20831665107776587, 27.88393115100078390, 7.208316651077764980 ) ) ;
#61119=CARTESIAN_POINT ( 'NONE',  ( 0.5774900079438590739, 47.64701867748817676, -5.440088680355550821 ) ) ;
#61120=( NAMED_UNIT ( * ) PLANE_ANGLE_UNIT ( ) SI_UNIT ( $, .RADIAN. ) );
#61122=CARTESIAN_POINT ( 'NONE',  ( -46.68456736488007408, 103.6675473310227034, 5.775421524742653467 ) ) ;
#61123=CARTESIAN_POINT ( 'NONE',  ( 19.84674366389459266, 58.30059781766745886, 2.638427012816836559 ) ) ;
#61126=CARTESIAN_POINT ( 'NONE',  ( 17.08211943468705840, 40.13708216824731068, -12.26659068614894466 ) ) ;
#61127=CARTESIAN_POINT ( 'NONE',  ( 24.16423886937409904, 29.09541550158063572, 3.795296366450317205 ) ) ;
#61128=CARTESIAN_POINT ( 'NONE',  ( 2.791683348922240793, 1.633931151000784565, 7.208316651077764092 ) ) ;
#61129=CARTESIAN_POINT ( 'NONE',  ( 12.63842701281683922, 44.55059781766745175, -9.846743663894590881 ) ) ;
#61131=CARTESIAN_POINT ( 'NONE',  ( 15.44008868035555260, 39.73035201082150536, 9.422509992056143702 ) ) ;
#61132=CARTESIAN_POINT ( 'NONE',  ( 10.00000000000000178, 15.37363466993042138, 12.81628187352647608 ) ) ;
#61133=CARTESIAN_POINT ( 'NONE',  ( 6.204703633549690345, 35.76208216824729647, -14.16423886937410259 ) ) ;
#61134=CARTESIAN_POINT ( 'NONE',  ( 7.084665262690076126, 9.105352010821503583, 10.88017736071109987 ) ) ;
#61136=CARTESIAN_POINT ( 'NONE',  ( -0.8801773607111009756, 28.06368534415484106, 1.068504757029289695E-15 ) ) ;
#61137=VECTOR ( 'NONE', #32910, 1000.000000000000000 ) ;
#61139=CARTESIAN_POINT ( 'NONE',  ( -0.8801773607111009756, 63.06368534415484106, 1.068504757029289695E-15 ) ) ;
#61140=CARTESIAN_POINT ( 'NONE',  ( 0.6178305044545838731, 49.74863466993041072, 9.382169495545420901 ) ) ;
#61143=CARTESIAN_POINT ( 'NONE',  ( 20.05723567505238947, 0.1676365378933190875, 6.413539670616452248 ) ) ;
#61147=CARTESIAN_POINT ( 'NONE',  ( 2.917880565312948704, 62.63708216824730357, 12.26659068614894643 ) ) ;
#61148=CARTESIAN_POINT ( 'NONE',  ( 17.08211943468705840, 65.13708216824730357, -12.26659068614894466 ) ) ;
#61149=CARTESIAN_POINT ( 'NONE',  ( 0.1532563361054083140, 21.00893115100078745, 1.131784320476157264E-15 ) ) ;
#61150=CARTESIAN_POINT ( 'NONE',  ( 18.52753015748617571, 63.09226448433412315, 4.923371831947298993 ) ) ;
#61151=CARTESIAN_POINT ( 'NONE',  ( 20.24186590665277308, 50.59014588040356841, -6.114288769123048972 ) ) ;
#61153=CARTESIAN_POINT ( 'NONE',  ( 5.076628168052704559, 10.17559781766745175, -8.527530157486179263 ) ) ;
#61155=CARTESIAN_POINT ( 'NONE',  ( -2.816281873526471635, 3.915301336597087456, -3.434112377981056508 ) ) ;
#61157=VERTEX_POINT ( 'NONE', #38226 ) ;
#61158=CARTESIAN_POINT ( 'NONE',  ( 6.204703633549690345, 35.76208216824729647, -14.16423886937410259 ) ) ;
#61159=CARTESIAN_POINT ( 'NONE',  ( 24.16423886937410614, 39.30374883491396787, 8.672049930838204340E-16 ) ) ;
#61162=CARTESIAN_POINT ( 'NONE',  ( 16.40814093676324603, 52.45696800326375353, -11.09922568453594671 ) ) ;
#61163=CARTESIAN_POINT ( 'NONE',  ( 2.035157376598824452, 28.68868534415484106, 7.964842623401179544 ) ) ;
#61164=CARTESIAN_POINT ( 'NONE',  ( 14.92337183194729988, 44.34226448433412315, -8.527530157486177487 ) ) ;
#61165=CARTESIAN_POINT ( 'NONE',  ( 20.88017736071110164, 25.35535201082150891, 2.915334737309930979 ) ) ;
#61166=CARTESIAN_POINT ( 'NONE',  ( 10.00000000000000000, 62.87363466993042493, -12.81628187352647608 ) ) ;
#61168=CARTESIAN_POINT ( 'NONE',  ( 14.92337183194729633, 52.67559781766745175, 8.527530157486181039 ) ) ;
#61169=CARTESIAN_POINT ( 'NONE',  ( 5.076628168052704559, 55.17559781766745175, -8.527530157486179263 ) ) ;
#61176=CARTESIAN_POINT ( 'NONE',  ( 18.52753015748618282, 3.925597817667451306, -4.923371831947291888 ) ) ;
#61179=CARTESIAN_POINT ( 'NONE',  ( 14.92337183194729988, 29.34226448433411960, -8.527530157486177487 ) ) ;
#61180=DIRECTION ( 'NONE',  ( -0.5547001962252291474, -0.8320502943378437211, -0.000000000000000000 ) ) ;
#61181=CARTESIAN_POINT ( 'NONE',  ( -2.816281873526473856, 39.12363466993041783, 9.499525473075851096E-16 ) ) ;
#61183=LINE ( 'NONE', #5369, #2791 ) ;
#61187=CARTESIAN_POINT ( 'NONE',  ( 17.20831665107776587, 49.13393115100078745, -7.208316651077762316 ) ) ;
#61188=CARTESIAN_POINT ( 'NONE',  ( 6.204703633549690345, 37.84541550158063927, 14.16423886937410082 ) ) ;
#61189=CARTESIAN_POINT ( 'NONE',  ( 19.84674366389459621, 63.50893115100078745, 7.409399052514197653E-17 ) ) ;
#61191=CARTESIAN_POINT ( 'NONE',  ( 1.472469842513823179, 1.425597817667451528, 4.923371831947296329 ) ) ;
#61192=CARTESIAN_POINT ( 'NONE',  ( -0.3689425029237881626, 2.428748834913967869, 10.36894250292379027 ) ) ;
#61193=CARTESIAN_POINT ( 'NONE',  ( 0.1532563361054083140, 51.00893115100078745, 1.131784320476157264E-15 ) ) ;
#61194=CARTESIAN_POINT ( 'NONE',  ( 19.42250999205614548, 55.98035201082150536, -5.440088680355545492 ) ) ;
#61195=CARTESIAN_POINT ( 'NONE',  ( 12.63842701281683034, 47.46726448433412315, 9.846743663894596210 ) ) ;
#61196=EDGE_LOOP ( 'NONE', ( #15067, #87812, #59407, #73918 ) ) ;
#61198=CARTESIAN_POINT ( 'NONE',  ( 7.084665262690076126, 62.02201867748816966, -10.88017736071110164 ) ) ;
#61199=AXIS2_PLACEMENT_3D ( 'NONE', #61656, #16184, #52694 ) ;
#61201=EDGE_CURVE ( 'NONE', #50558, #10425, #64903, .T. ) ;
#61202=DIRECTION ( 'NONE',  ( 0.9998643952135762847, -0.01646788341559294114, 0.000000000000000000 ) ) ;
#61203=CARTESIAN_POINT ( 'NONE',  ( 15.44008868035555793, 31.39701867748817676, -9.422509992056140149 ) ) ;
#61204=CARTESIAN_POINT ( 'NONE',  ( 12.63842701281683922, 64.55059781766745175, -9.846743663894590881 ) ) ;
#61205=CARTESIAN_POINT ( 'NONE',  ( 17.96484262340118221, 61.18868534415482685, -7.964842623401177768 ) ) ;
#61206=CARTESIAN_POINT ( 'NONE',  ( -0.3289641300567998083, 48.07879003517447103, 5.963430220938281678 ) ) ;
#61210=CARTESIAN_POINT ( 'NONE',  ( 12.91533473730992121, 39.52201867748817676, 10.88017736071110164 ) ) ;
#61212=CARTESIAN_POINT ( 'NONE',  ( 7.361572987183170547, 12.05059781766744997, 9.846743663894590881 ) ) ;
#61213=CARTESIAN_POINT ( 'NONE',  ( 17.20831665107776587, 42.88393115100077324, 7.208316651077764980 ) ) ;
#61217=CARTESIAN_POINT ( 'NONE',  ( 17.20831665107776587, 59.13393115100078745, -7.208316651077762316 ) ) ;
#61218=CARTESIAN_POINT ( 'NONE',  ( 2.917880565312950480, 65.97041550158063217, -12.26659068614894821 ) ) ;
#61220=CARTESIAN_POINT ( 'NONE',  ( -0.3689425029237898834, 16.17874883491396076, -10.36894250292378850 ) ) ;
#61221=CARTESIAN_POINT ( 'NONE',  ( -4.164238869374099039, 56.80374883491397497, 8.674139862899312516E-16 ) ) ;
#61222=CARTESIAN_POINT ( 'NONE',  ( 17.20831665107776587, 12.88393115100078390, 7.208316651077764980 ) ) ;
#61224=CARTESIAN_POINT ( 'NONE',  ( 18.52753015748618282, 23.92559781766745530, -4.923371831947291888 ) ) ;
#61225=CARTESIAN_POINT ( 'NONE',  ( 17.96484262340118221, 24.93868534415484461, 7.964842623401181321 ) ) ;
#61226=CARTESIAN_POINT ( 'NONE',  ( -2.816281873526473856, -0.8763653300695799508, 9.499525473075851096E-16 ) ) ;
#61227=CARTESIAN_POINT ( 'NONE',  ( 6.204703633549690345, 2.845415501580634388, 14.16423886937410082 ) ) ;
#61230=CARTESIAN_POINT ( 'NONE',  ( 1.472469842513823179, 11.42559781766745175, 4.923371831947296329 ) ) ;
#61231=CARTESIAN_POINT ( 'NONE',  ( 13.43411237798106583, 37.66530133659708923, -12.81628187352647252 ) ) ;
#61232=CARTESIAN_POINT ( 'NONE',  ( 17.20831665107776587, 44.13393115100078745, -7.208316651077762316 ) ) ;
#61234=CARTESIAN_POINT ( 'NONE',  ( 2.791683348922237240, 20.38393115100078745, -7.208316651077763204 ) ) ;
#61236=CARTESIAN_POINT ( 'NONE',  ( 24.16423886937410614, 49.51208216824730357, -3.795296366450302550 ) ) ;
#61237=CARTESIAN_POINT ( 'NONE',  ( 0.5774900079438607392, 58.48035201082151247, 5.440088680355550821 ) ) ;
#61238=CARTESIAN_POINT ( 'NONE',  ( 0.1916775849787264729, 32.25868815902069997, -6.499999999999991118 ) ) ;
#61240=CARTESIAN_POINT ( 'NONE',  ( 12.63842701281683922, 39.55059781766744464, -9.846743663894590881 ) ) ;
#61241=CARTESIAN_POINT ( 'NONE',  ( 4.559911319644449179, 8.897018677488171434, 9.422509992056141925 ) ) ;
#61242=CARTESIAN_POINT ( 'NONE',  ( 0.1532563361054082862, 46.21726448433411605, 2.638427012816831674 ) ) ;
#61243=CARTESIAN_POINT ( 'NONE',  ( 12.63842701281683922, 54.55059781766745175, -9.846743663894590881 ) ) ;
#61246=CARTESIAN_POINT ( 'NONE',  ( 10.00000000000000178, 44.31368534415484106, 10.88017736071110342 ) ) ;
#61248=ORIENTED_EDGE ( 'NONE', *, *, #65480, .F. ) ;
#61249=LINE ( 'NONE', #93711, #13377 ) ;
#61251=CARTESIAN_POINT ( 'NONE',  ( 0.1532563361054083140, 6.008931151000784787, 1.131784320476157264E-15 ) ) ;
#61252=CARTESIAN_POINT ( 'NONE',  ( 21.09922568453595559, 57.04030133659708923, -6.408140936763230044 ) ) ;
#61253=CARTESIAN_POINT ( 'NONE',  ( 12.91533473730993009, 6.605352010821504471, -10.88017736071109987 ) ) ;
#61254=CARTESIAN_POINT ( 'NONE',  ( 1.472469842513823179, 55.59226448433412315, -4.923371831947296329 ) ) ;
#61256=CARTESIAN_POINT ( 'NONE',  ( 2.917880565312950480, 30.97041550158063572, -12.26659068614894821 ) ) ;
#61257=CARTESIAN_POINT ( 'NONE',  ( -4.164238869374098151, 61.59541550158063217, -3.795296366450310543 ) ) ;
#61258=CARTESIAN_POINT ( 'NONE',  ( 17.20831665107776587, 52.88393115100078035, 7.208316651077764980 ) ) ;
#61259=CARTESIAN_POINT ( 'NONE',  ( 20.88017736071110519, 45.56368534415484106, 2.639326808657452039E-16 ) ) ;
#61260=CARTESIAN_POINT ( 'NONE',  ( -0.8801773607111008646, 68.27201867748817676, 2.915334737309923430 ) ) ;
#61262=ORIENTED_EDGE ( 'NONE', *, *, #77311, .F. ) ;
#61263=CARTESIAN_POINT ( 'NONE',  ( 6.565887622018943937, 63.08196800326376064, -12.81628187352647608 ) ) ;
#61265=CARTESIAN_POINT ( 'NONE',  ( 0.1532563361054083140, 11.00893115100078568, 1.131784320476157264E-15 ) ) ;
#61266=ORIENTED_EDGE ( 'NONE', *, *, #61523, .F. ) ;
#61267=CARTESIAN_POINT ( 'NONE',  ( 20.36894250292379738, 14.92874883491396432, -10.36894250292379027 ) ) ;
#61268=CARTESIAN_POINT ( 'NONE',  ( 14.92337183194729633, 22.67559781766745175, 8.527530157486181039 ) ) ;
#61269=CARTESIAN_POINT ( 'NONE',  ( 20.88017736071110875, 35.77201867748816966, -2.915334737309920765 ) ) ;
#61271=ORIENTED_EDGE ( 'NONE', *, *, #20474, .F. ) ;
#61272=CARTESIAN_POINT ( 'NONE',  ( 20.88017736071110164, 30.35535201082151247, 2.915334737309930979 ) ) ;
#61275=CARTESIAN_POINT ( 'NONE',  ( -0.8801773607111008646, 33.27201867748817676, 2.915334737309923430 ) ) ;
#61276=CYLINDRICAL_SURFACE ( 'NONE', #98422, 0.5000000000000004441 ) ;
#61279=ORIENTED_EDGE ( 'NONE', *, *, #19291, .F. ) ;
#61280=CARTESIAN_POINT ( 'NONE',  ( 19.38216949554541202, 20.99863466993042138, 9.382169495545424454 ) ) ;
#61281=CARTESIAN_POINT ( 'NONE',  ( 19.84674366389459266, 13.30059781766745353, 2.638427012816836559 ) ) ;
#61283=CARTESIAN_POINT ( 'NONE',  ( 0.2751277870542967463, 0.000000000000000000, 6.500000000000000888 ) ) ;
#61284=CARTESIAN_POINT ( 'NONE',  ( 10.00000000000000178, 22.25893115100078745, 9.846743663894594434 ) ) ;
#61285=CARTESIAN_POINT ( 'NONE',  ( 7.084665262690076126, 27.02201867748817676, -10.88017736071110164 ) ) ;
#61287=ORIENTED_EDGE ( 'NONE', *, *, #7812, .T. ) ;
#61289=CARTESIAN_POINT ( 'NONE',  ( 22.81628187352648496, 61.83196800326376774, -3.434112377981050290 ) ) ;
#61290=CARTESIAN_POINT ( 'NONE',  ( 20.88017736071110875, 60.77201867748817676, -2.915334737309920765 ) ) ;
#61291=CARTESIAN_POINT ( 'NONE',  ( -0.2418659066527775181, 23.09014588040356841, 6.114288769123032985 ) ) ;
#61292=CARTESIAN_POINT ( 'NONE',  ( 10.00000000000000178, 55.37363466993042493, 12.81628187352647608 ) ) ;
#61293=CARTESIAN_POINT ( 'NONE',  ( 20.88017736071110164, 65.35535201082150536, 2.915334737309930979 ) ) ;
#61294=CARTESIAN_POINT ( 'NONE',  ( 6.565887622018943937, 0.1653013365970866511, 12.81628187352647430 ) ) ;
#61296=CARTESIAN_POINT ( 'NONE',  ( 14.92337183194729633, 27.67559781766745530, 8.527530157486181039 ) ) ;
#61297=CARTESIAN_POINT ( 'NONE',  ( 10.00000000000000000, 47.87363466993042493, -12.81628187352647608 ) ) ;
#61298=CARTESIAN_POINT ( 'NONE',  ( 0.000000000000000000, 77.77738620402351444, 8.380889435745553229 ) ) ;
#61299=CARTESIAN_POINT ( 'NONE',  ( 18.52753015748618282, 23.92559781766745530, -4.923371831947291888 ) ) ;
#61300=CARTESIAN_POINT ( 'NONE',  ( -2.816281873526471635, 18.91530133659708213, -3.434112377981056508 ) ) ;
#61302=CARTESIAN_POINT ( 'NONE',  ( 20.88017736071110164, 30.35535201082151247, 2.915334737309930979 ) ) ;
#61303=CARTESIAN_POINT ( 'NONE',  ( 0.6178305044545838731, -0.2513653300695798953, 9.382169495545420901 ) ) ;
#61305=CARTESIAN_POINT ( 'NONE',  ( 1.472469842513823179, 16.42559781766745175, 4.923371831947296329 ) ) ;
#61306=CARTESIAN_POINT ( 'NONE',  ( 2.791683348922240793, 11.63393115100078568, 7.208316651077764092 ) ) ;
#61307=CARTESIAN_POINT ( 'NONE',  ( 2.035157376598824452, 13.68868534415483751, 7.964842623401179544 ) ) ;
#61308=CARTESIAN_POINT ( 'NONE',  ( 22.81628187352648496, 11.83196800326375531, -3.434112377981050290 ) ) ;
#61310=CARTESIAN_POINT ( 'NONE',  ( 7.361572987183169658, 59.96726448433410894, -9.846743663894592657 ) ) ;
#61313=CARTESIAN_POINT ( 'NONE',  ( 2.035157376598824452, 8.688685344154839285, 7.964842623401179544 ) ) ;
#61314=CARTESIAN_POINT ( 'NONE',  ( 19.84674366389459266, 38.71726448433412315, -2.638427012816827677 ) ) ;
#61315=ORIENTED_EDGE ( 'NONE', *, *, #29174, .F. ) ;
#61318=CARTESIAN_POINT ( 'NONE',  ( 10.00000000000000000, 16.81368534415483751, -10.88017736071110342 ) ) ;
#61319=CARTESIAN_POINT ( 'NONE',  ( -45.94000000000000483, 93.00000000000000000, 9.000000000000000000 ) ) ;
#61320=CARTESIAN_POINT ( 'NONE',  ( 10.00000000000000178, 34.31368534415484106, 10.88017736071110342 ) ) ;
#61321=CARTESIAN_POINT ( 'NONE',  ( 6.204703633549690345, 65.76208216824731778, -14.16423886937410259 ) ) ;
#61323=CARTESIAN_POINT ( 'NONE',  ( 0.1532563361054082862, 6.217264484334118713, 2.638427012816831674 ) ) ;
#61324=B_SPLINE_CURVE_WITH_KNOTS ( 'NONE', 3,
 ( #71876, #55904, #9915, #41895, #63388, #40904 ),
 .UNSPECIFIED., .F., .F.,
 ( 4, 2, 4 ),
 ( 0.000000000000000000, 0.0002565770811490922947, 0.0005131541622981845895 ),
 .UNSPECIFIED. ) ;
#61325=CARTESIAN_POINT ( 'NONE',  ( 19.84674366389459266, 18.71726448433411960, -2.638427012816827677 ) ) ;
#61326=CARTESIAN_POINT ( 'NONE',  ( -1.099225684535947600, 8.706968003263753531, -6.408140936763238038 ) ) ;
#61327=CARTESIAN_POINT ( 'NONE',  ( -46.94000000000001194, 103.2282880252848685, 5.913372230041396449 ) ) ;
#61329=CARTESIAN_POINT ( 'NONE',  ( -1.099225684535947600, -0.4596986634029132657, 6.408140936763237150 ) ) ;
#61331=CARTESIAN_POINT ( 'NONE',  ( -0.3689425029237881626, 17.42874883491397142, 10.36894250292379027 ) ) ;
#61332=B_SPLINE_CURVE_WITH_KNOTS ( 'NONE', 3,
 ( #47970, #63473, #2018, #9491, #46990, #55985, #78479, #48469, #78967, #3478 ),
 .UNSPECIFIED., .F., .F.,
 ( 4, 3, 3, 4 ),
 ( 1.648129954184481677E-17, 0.0006253016069560848747, 0.001250604074564934734, 0.002501455912506530058 ),
 .UNSPECIFIED. ) ;
#61333=CARTESIAN_POINT ( 'NONE',  ( 18.52753015748617571, 43.09226448433412315, 4.923371831947298993 ) ) ;
#61337=CARTESIAN_POINT ( 'NONE',  ( 20.36894250292379738, 59.92874883491397497, -10.36894250292379027 ) ) ;
#61338=CARTESIAN_POINT ( 'NONE',  ( 18.52753015748617571, 13.09226448433411960, 4.923371831947298993 ) ) ;
#61341=CARTESIAN_POINT ( 'NONE',  ( -0.8801773607111009756, 43.06368534415484106, 1.068504757029289695E-15 ) ) ;
#61342=CARTESIAN_POINT ( 'NONE',  ( 6.565887622018943937, 45.16530133659708923, 12.81628187352647430 ) ) ;
#61343=CARTESIAN_POINT ( 'NONE',  ( 17.96484262340118221, 11.18868534415483929, -7.964842623401177768 ) ) ;
#61344=CARTESIAN_POINT ( 'NONE',  ( 21.09922568453595559, 47.04030133659708923, -6.408140936763230044 ) ) ;
#61345=CARTESIAN_POINT ( 'NONE',  ( 6.565887622018943937, 0.1653013365970866511, 12.81628187352647430 ) ) ;
#61346=( LENGTH_UNIT ( ) NAMED_UNIT ( * ) SI_UNIT ( .MILLI., .METRE. ) );
#61350=CARTESIAN_POINT ( 'NONE',  ( -0.3689425029237898834, 46.17874883491397497, -10.36894250292378850 ) ) ;
#61351=CARTESIAN_POINT ( 'NONE',  ( 24.16423886937410614, 14.30374883491396787, 8.672049930838204340E-16 ) ) ;
#61352=CARTESIAN_POINT ( 'NONE',  ( 2.035157376598824452, 18.68868534415484106, 7.964842623401179544 ) ) ;
#61353=CARTESIAN_POINT ( 'NONE',  ( 19.42250999205614548, 30.98035201082150536, -5.440088680355545492 ) ) ;
#61356=CARTESIAN_POINT ( 'NONE',  ( 20.88017736071110164, 60.35535201082151957, 2.915334737309930979 ) ) ;
#61357=CARTESIAN_POINT ( 'NONE',  ( 7.084665262690076126, 62.02201867748816966, -10.88017736071110164 ) ) ;
#61358=CARTESIAN_POINT ( 'NONE',  ( 6.565887622018943937, 28.08196800326375353, -12.81628187352647608 ) ) ;
#61359=DIRECTION ( 'NONE',  ( -1.000000000000000000, 0.000000000000000000, 0.000000000000000000 ) ) ;
#61361=CARTESIAN_POINT ( 'NONE',  ( 19.84674366389459621, 33.50893115100078745, 7.409399052514197653E-17 ) ) ;
#61363=CARTESIAN_POINT ( 'NONE',  ( 20.88017736071110875, 10.77201867748817143, -2.915334737309920765 ) ) ;
#61364=CARTESIAN_POINT ( 'NONE',  ( 16.40814093676324603, 22.45696800326375353, -11.09922568453594671 ) ) ;
#61365=CARTESIAN_POINT ( 'NONE',  ( 7.361572987183170547, 12.05059781766744997, 9.846743663894590881 ) ) ;
#61366=CARTESIAN_POINT ( 'NONE',  ( -0.8801773607111008646, 8.272018677488171434, 2.915334737309923430 ) ) ;
#61367=CARTESIAN_POINT ( 'NONE',  ( 7.361572987183170547, 32.05059781766745175, 9.846743663894590881 ) ) ;
#61368=CARTESIAN_POINT ( 'NONE',  ( 19.38216949554541557, 57.24863466993042493, -9.382169495545420901 ) ) ;
#61369=CARTESIAN_POINT ( 'NONE',  ( 19.84674366389459621, 38.50893115100078745, 7.409399052514197653E-17 ) ) ;
#61370=CARTESIAN_POINT ( 'NONE',  ( 22.26659068614894466, 18.88708216824730002, 7.082119434687054849 ) ) ;
#61371=CARTESIAN_POINT ( 'NONE',  ( 17.96484262340118221, 34.93868534415482685, 7.964842623401181321 ) ) ;
#61372=CARTESIAN_POINT ( 'NONE',  ( -0.8801773607110991993, 7.855352010821504471, -2.915334737309923874 ) ) ;
#61374=CARTESIAN_POINT ( 'NONE',  ( 2.035157376598824452, 28.68868534415484106, 7.964842623401179544 ) ) ;
#61375=CARTESIAN_POINT ( 'NONE',  ( 15.44008868035555260, 29.73035201082150891, 9.422509992056143702 ) ) ;
#61377=CARTESIAN_POINT ( 'NONE',  ( 17.96484262340118221, 46.18868534415484106, -7.964842623401177768 ) ) ;
#61379=CARTESIAN_POINT ( 'NONE',  ( 3.591859063236761518, 64.95696800326376774, 11.09922568453594849 ) ) ;
#61380=CARTESIAN_POINT ( 'NONE',  ( 15.44008868035555260, 44.73035201082151247, 9.422509992056143702 ) ) ;
#61381=CARTESIAN_POINT ( 'NONE',  ( 15.44008868035555793, 46.39701867748817676, -9.422509992056140149 ) ) ;
#61383=CARTESIAN_POINT ( 'NONE',  ( 20.88017736071110519, 50.56368534415484106, 2.639326808657452039E-16 ) ) ;
#61386=CARTESIAN_POINT ( 'NONE',  ( 6.204703633549690345, 65.76208216824731778, -14.16423886937410259 ) ) ;
#61387=CARTESIAN_POINT ( 'NONE',  ( 5.076628168052703671, 1.842264484334118047, 8.527530157486179263 ) ) ;
#61390=CARTESIAN_POINT ( 'NONE',  ( 12.63842701281683922, 39.55059781766744464, -9.846743663894590881 ) ) ;
#61392=CARTESIAN_POINT ( 'NONE',  ( 2.791683348922237240, 30.38393115100078390, -7.208316651077763204 ) ) ;
#61393=CARTESIAN_POINT ( 'NONE',  ( 15.44008868035555793, 46.39701867748817676, -9.422509992056140149 ) ) ;
#61394=CARTESIAN_POINT ( 'NONE',  ( 7.361572987183169658, 39.96726448433411605, -9.846743663894592657 ) ) ;
#61395=CARTESIAN_POINT ( 'NONE',  ( -2.816281873526471635, 23.91530133659708568, -3.434112377981056508 ) ) ;
#61396=CARTESIAN_POINT ( 'NONE',  ( 19.72487221294571214, 2.802231764288312998, -6.500000000000001776 ) ) ;
#61397=CARTESIAN_POINT ( 'NONE',  ( -0.8801773607110991993, 47.85535201082150536, -2.915334737309923874 ) ) ;
#61398=FILL_AREA_STYLE ('',( #45417 ) ) ;
#61399=CARTESIAN_POINT ( 'NONE',  ( 24.16423886937409904, 54.09541550158063217, 3.795296366450317205 ) ) ;
#61402=CARTESIAN_POINT ( 'NONE',  ( 16.40814093676323893, 20.79030133659708923, 11.09922568453595026 ) ) ;
#61403=CARTESIAN_POINT ( 'NONE',  ( 18.17884179759847996, 23.66688879859523453, -6.499999999999984901 ) ) ;
#61406=STYLED_ITEM ( 'NONE', ( #65487 ), #90027 ) ;
#61407=CARTESIAN_POINT ( 'NONE',  ( 19.38216949554541202, 15.99863466993042138, 9.382169495545424454 ) ) ;
#61408=CARTESIAN_POINT ( 'NONE',  ( 19.42250999205614548, 20.98035201082150891, -5.440088680355545492 ) ) ;
#61409=CARTESIAN_POINT ( 'NONE',  ( 19.42250999205614548, 65.98035201082151957, -5.440088680355545492 ) ) ;
#61412=CARTESIAN_POINT ( 'NONE',  ( 10.00000000000000000, 66.81368534415484817, -10.88017736071110342 ) ) ;
#61413=VECTOR ( 'NONE', #34742, 1000.000000000000000 ) ;
#61414=CARTESIAN_POINT ( 'NONE',  ( 5.076628168052703671, 46.84226448433412315, 8.527530157486179263 ) ) ;
#61415=EDGE_CURVE ( 'NONE', #30159, #31207, #47956, .T. ) ;
#61416=CARTESIAN_POINT ( 'NONE',  ( 12.63842701281683034, 32.46726448433412315, 9.846743663894596210 ) ) ;
#61417=CARTESIAN_POINT ( 'NONE',  ( 17.20831665107776587, 32.88393115100078745, 7.208316651077764980 ) ) ;
#61418=CARTESIAN_POINT ( 'NONE',  ( 22.81628187352647785, 36.41530133659707502, 3.434112377981063169 ) ) ;
#61419=CARTESIAN_POINT ( 'NONE',  ( 17.20831665107776587, 14.13393115100078568, -7.208316651077762316 ) ) ;
#61422=CARTESIAN_POINT ( 'NONE',  ( 1.472469842513823179, 51.42559781766745886, 4.923371831947296329 ) ) ;
#61424=CARTESIAN_POINT ( 'NONE',  ( 13.43411237798106583, 62.66530133659708923, -12.81628187352647252 ) ) ;
#61425=CARTESIAN_POINT ( 'NONE',  ( 17.39651004071842166, 32.93575266056827644, 6.499999999999998224 ) ) ;
#61426=CARTESIAN_POINT ( 'NONE',  ( 22.81628187352647785, 11.62363466993042138, 6.195893100308588602E-16 ) ) ;
#61428=CARTESIAN_POINT ( 'NONE',  ( 2.035157376598822676, 52.43868534415483396, -7.964842623401177768 ) ) ;
#61429=CARTESIAN_POINT ( 'NONE',  ( 17.08211943468705840, 35.13708216824730357, -12.26659068614894466 ) ) ;
#61430=CARTESIAN_POINT ( 'NONE',  ( -39.69000000000001194, 92.00000000000000000, -9.500000000000000000 ) ) ;
#61431=CARTESIAN_POINT ( 'NONE',  ( -46.82017113615791004, 100.6079546444643427, 9.324761308090124601 ) ) ;
#61432=EDGE_CURVE ( 'NONE', #49375, #6101, #83744, .T. ) ;
#61433=CARTESIAN_POINT ( 'NONE',  ( 24.16423886937410614, 24.30374883491396787, 8.672049930838204340E-16 ) ) ;
#61434=CARTESIAN_POINT ( 'NONE',  ( 6.204703633549690345, 65.76208216824731778, -14.16423886937410259 ) ) ;
#61435=CARTESIAN_POINT ( 'NONE',  ( 10.00000000000000178, 8.053748834913967869, 14.16423886937410082 ) ) ;
#61436=CARTESIAN_POINT ( 'NONE',  ( 22.26659068614895176, 24.72041550158063572, -7.082119434687042414 ) ) ;
#61438=CARTESIAN_POINT ( 'NONE',  ( -0.1038446121089043744, 29.24302437010794620, -6.337995344473781323 ) ) ;
#61439=DIRECTION ( 'NONE',  ( -0.000000000000000000, -0.000000000000000000, -1.000000000000000000 ) ) ;
#61440=CARTESIAN_POINT ( 'NONE',  ( 0.1532563361054100626, 45.80059781766745886, -2.638427012816831230 ) ) ;
#61441=VERTEX_POINT ( 'NONE', #84698 ) ;
#61442=CARTESIAN_POINT ( 'NONE',  ( 10.00000000000000178, 24.31368534415484106, 10.88017736071110342 ) ) ;
#61443=CARTESIAN_POINT ( 'NONE',  ( 2.602085213965210642E-15, 78.91966277462714174, -9.500000000000000000 ) ) ;
#61444=CARTESIAN_POINT ( 'NONE',  ( 19.84674366389459266, 63.30059781766745886, 2.638427012816836559 ) ) ;
#61447=CARTESIAN_POINT ( 'NONE',  ( 10.00000000000000178, 42.25893115100078745, 9.846743663894594434 ) ) ;
#61448=CARTESIAN_POINT ( 'NONE',  ( 6.565887622018943937, 50.16530133659708213, 12.81628187352647430 ) ) ;
#61450=CARTESIAN_POINT ( 'NONE',  ( 1.472469842513823179, 40.59226448433411605, -4.923371831947296329 ) ) ;
#61451=CARTESIAN_POINT ( 'NONE',  ( 1.472469842513823179, 51.42559781766745886, 4.923371831947296329 ) ) ;
#61452=CARTESIAN_POINT ( 'NONE',  ( -2.266590686148945544, 37.22041550158063217, 7.082119434687048631 ) ) ;
#61453=VERTEX_POINT ( 'NONE', #46687 ) ;
#61454=CARTESIAN_POINT ( 'NONE',  ( 22.26659068614895176, 14.72041550158063572, -7.082119434687042414 ) ) ;
#61455=CARTESIAN_POINT ( 'NONE',  ( 7.084665262690076126, 59.10535201082150536, 10.88017736071109987 ) ) ;
#61457=CARTESIAN_POINT ( 'NONE',  ( 13.79529636645031943, 60.34541550158063927, -14.16423886937409904 ) ) ;
#61458=CARTESIAN_POINT ( 'NONE',  ( 13.43411237798106583, 12.66530133659708746, -12.81628187352647252 ) ) ;
#61459=CARTESIAN_POINT ( 'NONE',  ( 20.15039907845753930, 1.748846992468885198, 6.262539305110068177 ) ) ;
#61460=CARTESIAN_POINT ( 'NONE',  ( 0.1532563361054083140, 1.008931151000784787, 1.131784320476157264E-15 ) ) ;
#61462=CARTESIAN_POINT ( 'NONE',  ( 0.1532563361054082862, 31.21726448433412315, 2.638427012816831674 ) ) ;
#61463=CARTESIAN_POINT ( 'NONE',  ( -2.816281873526473856, 34.12363466993042493, 9.499525473075851096E-16 ) ) ;
#61464=CARTESIAN_POINT ( 'NONE',  ( 20.36894250292379382, 63.67874883491396787, 10.36894250292379205 ) ) ;
#61466=CARTESIAN_POINT ( 'NONE',  ( 17.96484262340118221, 26.18868534415483396, -7.964842623401177768 ) ) ;
#61467=CARTESIAN_POINT ( 'NONE',  ( 10.00000000000000000, 21.81368534415484106, -10.88017736071110342 ) ) ;
#61468=CARTESIAN_POINT ( 'NONE',  ( 1.472469842513823179, 55.59226448433412315, -4.923371831947296329 ) ) ;
#61469=CARTESIAN_POINT ( 'NONE',  ( 19.84674366389459266, 58.30059781766745886, 2.638427012816836559 ) ) ;
#61470=CARTESIAN_POINT ( 'NONE',  ( 22.81628187352648496, 56.83196800326374643, -3.434112377981050290 ) ) ;
#61472=ORIENTED_EDGE ( 'NONE', *, *, #9519, .F. ) ;
#61473=CARTESIAN_POINT ( 'NONE',  ( 15.44008868035555793, 16.39701867748817321, -9.422509992056140149 ) ) ;
#61475=CARTESIAN_POINT ( 'NONE',  ( 13.43411237798106583, 17.66530133659708923, -12.81628187352647252 ) ) ;
#61477=CARTESIAN_POINT ( 'NONE',  ( 0.1532563361054082862, 51.21726448433412315, 2.638427012816831674 ) ) ;
#61478=CARTESIAN_POINT ( 'NONE',  ( -0.8801773607111009756, 43.06368534415484106, 1.068504757029289695E-15 ) ) ;
#61480=CARTESIAN_POINT ( 'NONE',  ( 0.6178305044545838731, 19.74863466993042138, 9.382169495545420901 ) ) ;
#61481=CARTESIAN_POINT ( 'NONE',  ( 7.084665262690076126, 49.10535201082149825, 10.88017736071109987 ) ) ;
#61484=CARTESIAN_POINT ( 'NONE',  ( 10.00000000000000000, 62.87363466993042493, -12.81628187352647608 ) ) ;
#61485=ORIENTED_EDGE ( 'NONE', *, *, #86594, .F. ) ;
#61487=CARTESIAN_POINT ( 'NONE',  ( 0.5774900079438607392, 43.48035201082151247, 5.440088680355550821 ) ) ;
#61488=CARTESIAN_POINT ( 'NONE',  ( 22.81628187352647785, 46.41530133659708213, 3.434112377981063169 ) ) ;
#61489=CARTESIAN_POINT ( 'NONE',  ( 17.08211943468705840, 10.13708216824730179, -12.26659068614894466 ) ) ;
#61490=CARTESIAN_POINT ( 'NONE',  ( 10.00000000000000000, 64.75893115100078035, -9.846743663894594434 ) ) ;
#61491=CARTESIAN_POINT ( 'NONE',  ( 10.00000000000000178, 2.258931151000784787, 9.846743663894594434 ) ) ;
#61493=CARTESIAN_POINT ( 'NONE',  ( 24.16423886937409904, 44.09541550158063927, 3.795296366450317205 ) ) ;
#61494=CARTESIAN_POINT ( 'NONE',  ( 15.44008868035555793, 6.397018677488170546, -9.422509992056140149 ) ) ;
#61495=CARTESIAN_POINT ( 'NONE',  ( 19.42250999205614193, 5.147018677488171434, 5.440088680355555262 ) ) ;
#61497=ORIENTED_EDGE ( 'NONE', *, *, #73376, .F. ) ;
#61499=CARTESIAN_POINT ( 'NONE',  ( 10.00000000000000000, 6.813685344154838397, -10.88017736071110342 ) ) ;
#61500=CARTESIAN_POINT ( 'NONE',  ( 7.084665262690076126, 9.105352010821503583, 10.88017736071109987 ) ) ;
#61501=CARTESIAN_POINT ( 'NONE',  ( 19.84674366389459621, 43.50893115100078745, 7.409399052514197653E-17 ) ) ;
#61503=CARTESIAN_POINT ( 'NONE',  ( -1.099225684535947600, 38.70696800326375353, -6.408140936763238038 ) ) ;
#61504=DIRECTION ( 'NONE',  ( -0.8320502943378437211, 0.5547001962252290364, 0.000000000000000000 ) ) ;
#61506=CARTESIAN_POINT ( 'NONE',  ( 6.204703633549690345, 12.84541550158063572, 14.16423886937410082 ) ) ;
#61507=CARTESIAN_POINT ( 'NONE',  ( 2.035157376598822676, 27.43868534415483396, -7.964842623401177768 ) ) ;
#61508=CARTESIAN_POINT ( 'NONE',  ( -0.8801773607110991993, 2.855352010821504471, -2.915334737309923874 ) ) ;
#61509=CARTESIAN_POINT ( 'NONE',  ( 10.00000000000000000, 44.75893115100078745, -9.846743663894594434 ) ) ;
#61511=CARTESIAN_POINT ( 'NONE',  ( 2.791683348922237240, 25.38393115100078390, -7.208316651077763204 ) ) ;
#61512=CARTESIAN_POINT ( 'NONE',  ( 1.274849032794324932, 32.55509018479936145, -6.500000000000021316 ) ) ;
#61516=CARTESIAN_POINT ( 'NONE',  ( 10.00000000000000000, 54.75893115100078745, -9.846743663894594434 ) ) ;
#61517=CARTESIAN_POINT ( 'NONE',  ( 15.44008868035555260, 34.73035201082151247, 9.422509992056143702 ) ) ;
#61518=CARTESIAN_POINT ( 'NONE',  ( 10.00000000000000000, 36.81368534415484106, -10.88017736071110342 ) ) ;
#61519=CARTESIAN_POINT ( 'NONE',  ( 7.084665262690076126, 9.105352010821503583, 10.88017736071109987 ) ) ;
#61520=CARTESIAN_POINT ( 'NONE',  ( 0.6178305044545818747, 33.49863466993042493, -9.382169495545419124 ) ) ;
#61521=CARTESIAN_POINT ( 'NONE',  ( 10.00000000000000000, 15.55374883491396787, -14.16423886937410082 ) ) ;
#61523=EDGE_CURVE ( 'NONE', #55728, #71988, #48934, .T. ) ;
#61526=CARTESIAN_POINT ( 'NONE',  ( -1.099225684535947600, 49.54030133659708923, 6.408140936763237150 ) ) ;
#61529=CARTESIAN_POINT ( 'NONE',  ( 18.52753015748618282, 48.92559781766745886, -4.923371831947291888 ) ) ;
#61530=CARTESIAN_POINT ( 'NONE',  ( 15.44008868035555793, 26.39701867748817321, -9.422509992056140149 ) ) ;
#61532=CARTESIAN_POINT ( 'NONE',  ( 12.91533473730993009, 16.60535201082150891, -10.88017736071109987 ) ) ;
#61534=CARTESIAN_POINT ( 'NONE',  ( -0.8801773607110991993, 57.85535201082149825, -2.915334737309923874 ) ) ;
#61535=PRESENTATION_STYLE_ASSIGNMENT (( #76546 ) ) ;
#61536=CARTESIAN_POINT ( 'NONE',  ( -0.8801773607110991993, 67.85535201082151957, -2.915334737309923874 ) ) ;
#61537=CIRCLE ( 'NONE', #35982, 19.43999999999999773 ) ;
#61538=CARTESIAN_POINT ( 'NONE',  ( 14.92337183194729988, 14.34226448433411782, -8.527530157486177487 ) ) ;
#61539=CARTESIAN_POINT ( 'NONE',  ( 20.88017736071110519, 55.56368534415484817, 2.639326808657452039E-16 ) ) ;
#61541=CARTESIAN_POINT ( 'NONE',  ( -46.69421152571126044, 101.0768001808267229, 8.798454068542781670 ) ) ;
#61542=CARTESIAN_POINT ( 'NONE',  ( 7.361572987183170547, 2.050597817667451750, 9.846743663894590881 ) ) ;
#61544=( BOUNDED_SURFACE ( )  B_SPLINE_SURFACE ( 1, 2, ( 
 ( #72259, #41305, #34748, #42757, #2820, #3287, #65237, #56769, #65737, #12250, #64254, #87265, #11267, #95255, #95762, #72741, #18786, #57744, #96266, #50240, #27740, #57253, #41787, #3788, #80755, #33752, #34243, #49748, #80258, #86295, #48280, #78792, #33270, #63764, #94271, #29710, #13738, #97261, #90214, #44221, #52228, #6239, #37736, #50754, #5751, #44720, #89725, #12739, #20253, #28239, #89239, #81724, #43238, #58734, #20747, #14744, #83221, #67734, #28730, #29221, #82224, #59221, #68235, #13238, #88743, #81240, #45218, #96764, #21747, #43732, #51238, #60218, #74218, #66229, #98252, #36741, #21242, #75217, #75715, #90712, #36240, #51740, #7229, #59720, #66736, #74725, #98752, #73733, #58222, #67232, #22237, #97755, #82720, #14239, #5263, #6729, #37245, #35741, #52714, #16205, #76696, #62171, #62668, #24205, #61683, #85681, #9189, #78173, #77676, #9683, #92679, #85191, #91202, #54672, #7731, #23724, #8217, #92200, #38227, #84221, #93169, #245, #68713, #70190, #47171, #38711, #54187, #91709, #76218, #84699, #23228, #31679, #46688, #22730, #16698, #69210, #17202, #40180, #8693, #30693, #39703, #53700, #61203, #15730, #70687, #46210, #736, #1708, #39209, #31189, #30202, #32167, #24694, #15235, #77185, #55166, #47679, #69696, #60705, #53213, #83715, #1226, #45716, #87635, #72140, #11151, #19149, #40677, #4157, #64134, #26160, #64622, #18172, #41182, #26643, #2703, #18664, #57630, #2205, #42159, #80136, #95642, #93667, #50132, #3667, #49152, #10668, #34130, #32666, #72624, #95131, #94156, #71663, #33154, #55679, #19639, #3173, #42638, #63159, #71177, #87141, #33637, #34624, #25201, #63648, #65123, #94652, #41671, #56655, #12135, #25682, #86178, #17688, #27128, #56175, #57139, #86668, #48654, #88127, #79154, #10183, #80639, #79653, #49626, #11646, #48160, #78674, #5137, #51626, #35628, #27626, #20127, #66113, #90100, #58111, #5636, #82106, #13617, #44607, #66620, #81122, #60089, #96642, #28119, #13120, #73613, #36114, #50631, #44098, #52113, #4657, #43125, #74609, #65617, #88620, #12623, #6122, #35118, #67112, #21628, #67618, #58619, #51120, #29587, #75102, #89120, #36628, #97147, #20631, #81611, #90591, #52598, #43616, #74103, #6609, #59105, #28618, #82605, #22118, #96143, #89614, #14123, #21127, #83101, #98126, #97637, #29102, #59604, #37122, #14629, #73116, #84097, #69583, #32050, #62062, #24590, #54074, #23111, #61572, #92565, #7622, #53583, #76580, #69094, #24091, #23609, #30580, #8586, #62552, #15612, #16585, #628, #46096, #77074, #31074, #39092, #92083, #55053, #37616, #91595, #31566, #8100, #98635, #7112, #15118 ),
 ( #45094, #85076, #46575, #30086, #83604, #84589, #75600, #1103, #54559, #39588, #76092, #38596, #1600, #47061, #38114, #16089, #77559, #53092, #9075, #93057, #85572, #70079, #68110, #60593, #91088, #68603, #22615, #45594, #131, #61085, #95023, #25571, #34513, #42053, #94050, #86557, #10553, #94536, #64517, #41566, #56063, #72033, #4051, #34020, #95533, #26055, #18062, #33529, #26531, #78557, #48541, #79040, #41064, #57028, #56545, #2590, #79545, #65006, #71561, #87529, #3073, #64024, #49041, #87040, #11045, #18549, #28381, #9567, #63540, #3560, #19043, #70569, #78064, #86067, #48044, #40567, #2095, #17578, #10068, #72517, #58872, #49519, #80028, #11532, #17086, #47566, #40069, #71065, #32554, #63055, #93552, #55568, #25085, #33045, #59360, #91340, #13878, #97389, #30335, #67867, #21880, #75852, #7861, #60842, #21376, #98389, #51874, #43859, #36377, #82357, #7372, #74354, #52360, #29845, #60350, #22868, #82861, #28856, #76344, #44361, #74863, #29351, #89862, #14378, #66871, #90843, #68367, #20888, #6362, #22372, #81863, #59855, #15373, #52848, #36875, #44847, #38359, #51374, #68854, #90344, #98884, #75352, #67365, #6867, #5881, #97893, #83356, #37377, #14880, #45348, #37871, #53338, #83847, #45854, #386, #30835, #89374, #13374, #93307, #2340, #9321, #1846, #23361, #77806, #8342, #1360, #16340, #31811, #38849, #23852, #47803, #69338, #863, #55311, #32304, #46823, #69836, #31322, #76828, #62307, #61822, #47306, #92815, #53845, #39825, #77313, #40323, #32795, #54808, #92330, #24831, #54318, #84833, #8827, #63291, #39342, #24345, #85818, #85319, #16831, #93800, #17333, #70330, #15855, #62809, #78303, #9822, #70827, #61333, #91844, #84355, #46340, #92167, #38197, #22701, #60674, #68684, #90183, #53670, #14711, #75683, #15200, #67704, #90680, #76180, #52197, #68198, #8183, #51710, #91677, #30663, #46179, #44188, #703, #53179, #98719, #60184, #83685, #82194, #23196, #45682, #44690, #22206, #82691, #6208, #69180, #52685, #13703, #74698, #21713, #37700, #83186, #84185, #36710, #14209, #15695, #45185, #91172, #7197, #30170, #7700, #76665, #67201, #75185, #38680, #212, #61169, #31156, #61646, #97727, #29190, #6698, #59688, #37216, #98215, #29674, #53823, #38338, #30812, #75828, #90319, #69321, #75330, #14353, #22351, #82833, #14858, #59825, #22844, #61310, #13854, #52338, #53319, #74839, #36851, #21858, #60816, #44334, #76322, #91822, #76808, #44822, #60332, #38828, #84335, #6843, #83826, #7349, #37356, #90825, #840, #61802, #29822, #52825, #15836, #68341, #67847, #23341, #31301, #6339, #98364, #46322, #83332, #92309, #8324 ) ),
 .UNSPECIFIED., .F., .F., .F. ) 
 B_SPLINE_SURFACE_WITH_KNOTS ( ( 2, 2 ),
 ( 3, 2, 2, 2, 2, 2, 2, 2, 2, 2, 2, 2, 2, 2, 2, 2, 2, 2, 2, 2, 2, 2, 2, 2, 2, 2, 2, 2, 2, 2, 2, 2, 2, 2, 2, 2, 2, 2, 2, 2, 2, 2, 2, 2, 2, 2, 2, 2, 2, 2, 2, 2, 2, 2, 2, 2, 2, 2, 2, 2, 2, 2, 2, 2, 2, 2, 2, 2, 2, 2, 2, 2, 2, 2, 2, 2, 2, 2, 2, 2, 2, 2, 2, 2, 2, 2, 2, 2, 2, 2, 2, 2, 2, 2, 2, 2, 2, 2, 2, 2, 2, 2, 2, 2, 2, 2, 2, 2, 2, 2, 2, 2, 2, 2, 2, 2, 2, 2, 2, 2, 2, 2, 2, 2, 2, 2, 2, 2, 2, 2, 2, 2, 2, 2, 2, 2, 2, 2, 2, 2, 2, 2, 2, 2, 2, 2, 2, 2, 2, 2, 2, 2, 2, 2, 2, 2, 2, 2, 2, 2, 2, 2, 3 ),
 ( 0.000000000000000000, 1.000000000000000000 ),
 ( 0.000000000000000000, 0.005952380952380952051, 0.01190476190476190410, 0.01785714285714285615, 0.02380952380952380820, 0.02976190476190476025, 0.03571428571428571230, 0.04166666666666666435, 0.04761904761904761640, 0.05357142857142856845, 0.05952380952380952051, 0.06547619047619047949, 0.07142857142857142461, 0.07738095238095238360, 0.08333333333333332871, 0.08928571428571428770, 0.09523809523809523281, 0.1011904761904761918, 0.1071428571428571369, 0.1130952380952380959, 0.1190476190476190410, 0.1250000000000000000, 0.1309523809523809590, 0.1369047619047619180, 0.1428571428571428492, 0.1488095238095238082, 0.1547619047619047672, 0.1607142857142857262, 0.1666666666666666574, 0.1726190476190476164, 0.1785714285714285754, 0.1845238095238095344, 0.1904761904761904656, 0.1964285714285714246, 0.2023809523809523836, 0.2083333333333333426, 0.2142857142857142738, 0.2202380952380952328, 0.2261904761904761918, 0.2321428571428571508, 0.2380952380952380820, 0.2440476190476190410, 0.2500000000000000000, 0.2559523809523809312, 0.2619047619047619180, 0.2678571428571428492, 0.2738095238095238360, 0.2797619047619047672, 0.2857142857142856984, 0.2916666666666666852, 0.2976190476190476164, 0.3035714285714285476, 0.3095238095238095344, 0.3154761904761904656, 0.3214285714285714524, 0.3273809523809523836, 0.3333333333333333148, 0.3392857142857143016, 0.3452380952380952328, 0.3511904761904761640, 0.3571428571428571508, 0.3630952380952380820, 0.3690476190476190688, 0.3750000000000000000, 0.3809523809523809312, 0.3869047619047619180, 0.3928571428571428492, 0.3988095238095238360, 0.4047619047619047672, 0.4107142857142856984, 0.4166666666666666852, 0.4226190476190476164, 0.4285714285714285476, 0.4345238095238095344, 0.4404761904761904656, 0.4464285714285714524, 0.4523809523809523836, 0.4583333333333333148, 0.4642857142857143016, 0.4702380952380952328, 0.4761904761904761640, 0.4821428571428571508, 0.4880952380952380820, 0.4940476190476190688, 0.5000000000000000000, 0.5059523809523809312, 0.5119047619047618625, 0.5178571428571429047, 0.5238095238095238360, 0.5297619047619047672, 0.5357142857142856984, 0.5416666666666666297, 0.5476190476190476719, 0.5535714285714286031, 0.5595238095238095344, 0.5654761904761904656, 0.5714285714285713969, 0.5773809523809523281, 0.5833333333333333703, 0.5892857142857143016, 0.5952380952380952328, 0.6011904761904761640, 0.6071428571428570953, 0.6130952380952381375, 0.6190476190476190688, 0.6250000000000000000, 0.6309523809523809312, 0.6369047619047618625, 0.6428571428571429047, 0.6488095238095238360, 0.6547619047619047672, 0.6607142857142856984, 0.6666666666666666297, 0.6726190476190476719, 0.6785714285714286031, 0.6845238095238095344, 0.6904761904761904656, 0.6964285714285713969, 0.7023809523809523281, 0.7083333333333333703, 0.7142857142857143016, 0.7202380952380952328, 0.7261904761904761640, 0.7321428571428570953, 0.7380952380952381375, 0.7440476190476190688, 0.7500000000000000000, 0.7559523809523809312, 0.7619047619047618625, 0.7678571428571429047, 0.7738095238095238360, 0.7797619047619047672, 0.7857142857142856984, 0.7916666666666666297, 0.7976190476190476719, 0.8035714285714286031, 0.8095238095238095344, 0.8154761904761904656, 0.8214285714285713969, 0.8273809523809523281, 0.8333333333333333703, 0.8392857142857143016, 0.8452380952380952328, 0.8511904761904761640, 0.8571428571428570953, 0.8630952380952381375, 0.8690476190476190688, 0.8750000000000000000, 0.8809523809523809312, 0.8869047619047618625, 0.8928571428571429047, 0.8988095238095238360, 0.9047619047619047672, 0.9107142857142856984, 0.9166666666666666297, 0.9226190476190476719, 0.9285714285714286031, 0.9345238095238095344, 0.9404761904761904656, 0.9464285714285713969, 0.9523809523809523281, 0.9583333333333333703, 0.9642857142857143016 ),
 .UNSPECIFIED. ) 
 GEOMETRIC_REPRESENTATION_ITEM ( )  RATIONAL_B_SPLINE_SURFACE ( (
 ( 1.000000000000000000, 0.9659258262890683122, 1.000000000000000000, 0.9659258262890683122, 1.000000000000000000, 0.9659258262890683122, 1.000000000000000000, 0.9659258262890683122, 1.000000000000000000, 0.9659258262890683122, 1.000000000000000000, 0.9659258262890683122, 1.000000000000000000, 0.9659258262890683122, 1.000000000000000000, 0.9659258262890683122, 1.000000000000000000, 0.9659258262890683122, 1.000000000000000000, 0.9659258262890683122, 1.000000000000000000, 0.9659258262890683122, 1.000000000000000000, 0.9659258262890683122, 1.000000000000000000, 0.9659258262890683122, 1.000000000000000000, 0.9659258262890683122, 1.000000000000000000, 0.9659258262890683122, 1.000000000000000000, 0.9659258262890683122, 1.000000000000000000, 0.9659258262890683122, 1.000000000000000000, 0.9659258262890683122, 1.000000000000000000, 0.9659258262890683122, 1.000000000000000000, 0.9659258262890683122, 1.000000000000000000, 0.9659258262890683122, 1.000000000000000000, 0.9659258262890683122, 1.000000000000000000, 0.9659258262890683122, 1.000000000000000000, 0.9659258262890683122, 1.000000000000000000, 0.9659258262890683122, 1.000000000000000000, 0.9659258262890683122, 1.000000000000000000, 0.9659258262890683122, 1.000000000000000000, 0.9659258262890683122, 1.000000000000000000, 0.9659258262890683122, 1.000000000000000000, 0.9659258262890683122, 1.000000000000000000, 0.9659258262890683122, 1.000000000000000000, 0.9659258262890683122, 1.000000000000000000, 0.9659258262890683122, 1.000000000000000000, 0.9659258262890683122, 1.000000000000000000, 0.9659258262890683122, 1.000000000000000000, 0.9659258262890683122, 1.000000000000000000, 0.9659258262890683122, 1.000000000000000000, 0.9659258262890683122, 1.000000000000000000, 0.9659258262890683122, 1.000000000000000000, 0.9659258262890683122, 1.000000000000000000, 0.9659258262890683122, 1.000000000000000000, 0.9659258262890683122, 1.000000000000000000, 0.9659258262890683122, 1.000000000000000000, 0.9659258262890683122, 1.000000000000000000, 0.9659258262890683122, 1.000000000000000000, 0.9659258262890683122, 1.000000000000000000, 0.9659258262890683122, 1.000000000000000000, 0.9659258262890683122, 1.000000000000000000, 0.9659258262890683122, 1.000000000000000000, 0.9659258262890683122, 1.000000000000000000, 0.9659258262890683122, 1.000000000000000000, 0.9659258262890683122, 1.000000000000000000, 0.9659258262890683122, 1.000000000000000000, 0.9659258262890683122, 1.000000000000000000, 0.9659258262890683122, 1.000000000000000000, 0.9659258262890683122, 1.000000000000000000, 0.9659258262890683122, 1.000000000000000000, 0.9659258262890683122, 1.000000000000000000, 0.9659258262890683122, 1.000000000000000000, 0.9659258262890683122, 1.000000000000000000, 0.9659258262890683122, 1.000000000000000000, 0.9659258262890683122, 1.000000000000000000, 0.9659258262890683122, 1.000000000000000000, 0.9659258262890683122, 1.000000000000000000, 0.9659258262890683122, 1.000000000000000000, 0.9659258262890683122, 1.000000000000000000, 0.9659258262890683122, 1.000000000000000000, 0.9659258262890683122, 1.000000000000000000, 0.9659258262890683122, 1.000000000000000000, 0.9659258262890683122, 1.000000000000000000, 0.9659258262890683122, 1.000000000000000000, 0.9659258262890683122, 1.000000000000000000, 0.9659258262890683122, 1.000000000000000000, 0.9659258262890683122, 1.000000000000000000, 0.9659258262890683122, 1.000000000000000000, 0.9659258262890683122, 1.000000000000000000, 0.9659258262890683122, 1.000000000000000000, 0.9659258262890683122, 1.000000000000000000, 0.9659258262890683122, 1.000000000000000000, 0.9659258262890683122, 1.000000000000000000, 0.9659258262890683122, 1.000000000000000000, 0.9659258262890683122, 1.000000000000000000, 0.9659258262890683122, 1.000000000000000000, 0.9659258262890683122, 1.000000000000000000, 0.9659258262890683122, 1.000000000000000000, 0.9659258262890683122, 1.000000000000000000, 0.9659258262890683122, 1.000000000000000000, 0.9659258262890683122, 1.000000000000000000, 0.9659258262890683122, 1.000000000000000000, 0.9659258262890683122, 1.000000000000000000, 0.9659258262890683122, 1.000000000000000000, 0.9659258262890683122, 1.000000000000000000, 0.9659258262890683122, 1.000000000000000000, 0.9659258262890683122, 1.000000000000000000, 0.9659258262890683122, 1.000000000000000000, 0.9659258262890683122, 1.000000000000000000, 0.9659258262890683122, 1.000000000000000000, 0.9659258262890683122, 1.000000000000000000, 0.9659258262890683122, 1.000000000000000000, 0.9659258262890683122, 1.000000000000000000, 0.9659258262890683122, 1.000000000000000000, 0.9659258262890683122, 1.000000000000000000, 0.9659258262890683122, 1.000000000000000000, 0.9659258262890683122, 1.000000000000000000, 0.9659258262890683122, 1.000000000000000000, 0.9659258262890683122, 1.000000000000000000, 0.9659258262890683122, 1.000000000000000000, 0.9659258262890683122, 1.000000000000000000, 0.9659258262890683122, 1.000000000000000000, 0.9659258262890683122, 1.000000000000000000, 0.9659258262890683122, 1.000000000000000000, 0.9659258262890683122, 1.000000000000000000, 0.9659258262890683122, 1.000000000000000000, 0.9659258262890683122, 1.000000000000000000, 0.9659258262890683122, 1.000000000000000000, 0.9659258262890683122, 1.000000000000000000, 0.9659258262890683122, 1.000000000000000000, 0.9659258262890683122, 1.000000000000000000, 0.9659258262890683122, 1.000000000000000000, 0.9659258262890683122, 1.000000000000000000, 0.9659258262890683122, 1.000000000000000000, 0.9659258262890683122, 1.000000000000000000, 0.9659258262890683122, 1.000000000000000000, 0.9659258262890683122, 1.000000000000000000, 0.9659258262890683122, 1.000000000000000000, 0.9659258262890683122, 1.000000000000000000, 0.9659258262890683122, 1.000000000000000000, 0.9659258262890683122, 1.000000000000000000, 0.9659258262890683122, 1.000000000000000000, 0.9659258262890683122, 1.000000000000000000, 0.9659258262890683122, 1.000000000000000000, 0.9659258262890683122, 1.000000000000000000, 0.9659258262890683122, 1.000000000000000000, 0.9659258262890683122, 1.000000000000000000, 0.9659258262890683122, 1.000000000000000000, 0.9659258262890683122, 1.000000000000000000, 0.9659258262890683122, 1.000000000000000000, 0.9659258262890683122, 1.000000000000000000, 0.9659258262890683122, 1.000000000000000000, 0.9659258262890683122, 1.000000000000000000, 0.9659258262890683122, 1.000000000000000000, 0.9659258262890683122, 1.000000000000000000, 0.9659258262890683122, 1.000000000000000000, 0.9659258262890683122, 1.000000000000000000, 0.9659258262890683122, 1.000000000000000000, 0.9659258262890683122, 1.000000000000000000, 0.9659258262890683122, 1.000000000000000000, 0.9659258262890683122, 1.000000000000000000, 0.9659258262890683122, 1.000000000000000000, 0.9659258262890683122, 1.000000000000000000, 0.9659258262890683122, 1.000000000000000000, 0.9659258262890683122, 1.000000000000000000, 0.9659258262890683122, 1.000000000000000000, 0.9659258262890683122, 1.000000000000000000, 0.9659258262890683122, 1.000000000000000000, 0.9659258262890683122, 1.000000000000000000, 0.9659258262890683122, 1.000000000000000000, 0.9659258262890683122, 1.000000000000000000, 0.9659258262890683122, 1.000000000000000000, 0.9659258262890683122, 1.000000000000000000, 0.9659258262890683122, 1.000000000000000000, 0.9659258262890683122, 1.000000000000000000),
 ( 1.000000000000000000, 0.9659258262890683122, 1.000000000000000000, 0.9659258262890683122, 1.000000000000000000, 0.9659258262890683122, 1.000000000000000000, 0.9659258262890683122, 1.000000000000000000, 0.9659258262890683122, 1.000000000000000000, 0.9659258262890683122, 1.000000000000000000, 0.9659258262890683122, 1.000000000000000000, 0.9659258262890683122, 1.000000000000000000, 0.9659258262890683122, 1.000000000000000000, 0.9659258262890683122, 1.000000000000000000, 0.9659258262890683122, 1.000000000000000000, 0.9659258262890683122, 1.000000000000000000, 0.9659258262890683122, 1.000000000000000000, 0.9659258262890683122, 1.000000000000000000, 0.9659258262890683122, 1.000000000000000000, 0.9659258262890683122, 1.000000000000000000, 0.9659258262890683122, 1.000000000000000000, 0.9659258262890683122, 1.000000000000000000, 0.9659258262890683122, 1.000000000000000000, 0.9659258262890683122, 1.000000000000000000, 0.9659258262890683122, 1.000000000000000000, 0.9659258262890683122, 1.000000000000000000, 0.9659258262890683122, 1.000000000000000000, 0.9659258262890683122, 1.000000000000000000, 0.9659258262890683122, 1.000000000000000000, 0.9659258262890683122, 1.000000000000000000, 0.9659258262890683122, 1.000000000000000000, 0.9659258262890683122, 1.000000000000000000, 0.9659258262890683122, 1.000000000000000000, 0.9659258262890683122, 1.000000000000000000, 0.9659258262890683122, 1.000000000000000000, 0.9659258262890683122, 1.000000000000000000, 0.9659258262890683122, 1.000000000000000000, 0.9659258262890683122, 1.000000000000000000, 0.9659258262890683122, 1.000000000000000000, 0.9659258262890683122, 1.000000000000000000, 0.9659258262890683122, 1.000000000000000000, 0.9659258262890683122, 1.000000000000000000, 0.9659258262890683122, 1.000000000000000000, 0.9659258262890683122, 1.000000000000000000, 0.9659258262890683122, 1.000000000000000000, 0.9659258262890683122, 1.000000000000000000, 0.9659258262890683122, 1.000000000000000000, 0.9659258262890683122, 1.000000000000000000, 0.9659258262890683122, 1.000000000000000000, 0.9659258262890683122, 1.000000000000000000, 0.9659258262890683122, 1.000000000000000000, 0.9659258262890683122, 1.000000000000000000, 0.9659258262890683122, 1.000000000000000000, 0.9659258262890683122, 1.000000000000000000, 0.9659258262890683122, 1.000000000000000000, 0.9659258262890683122, 1.000000000000000000, 0.9659258262890683122, 1.000000000000000000, 0.9659258262890683122, 1.000000000000000000, 0.9659258262890683122, 1.000000000000000000, 0.9659258262890683122, 1.000000000000000000, 0.9659258262890683122, 1.000000000000000000, 0.9659258262890683122, 1.000000000000000000, 0.9659258262890683122, 1.000000000000000000, 0.9659258262890683122, 1.000000000000000000, 0.9659258262890683122, 1.000000000000000000, 0.9659258262890683122, 1.000000000000000000, 0.9659258262890683122, 1.000000000000000000, 0.9659258262890683122, 1.000000000000000000, 0.9659258262890683122, 1.000000000000000000, 0.9659258262890683122, 1.000000000000000000, 0.9659258262890683122, 1.000000000000000000, 0.9659258262890683122, 1.000000000000000000, 0.9659258262890683122, 1.000000000000000000, 0.9659258262890683122, 1.000000000000000000, 0.9659258262890683122, 1.000000000000000000, 0.9659258262890683122, 1.000000000000000000, 0.9659258262890683122, 1.000000000000000000, 0.9659258262890683122, 1.000000000000000000, 0.9659258262890683122, 1.000000000000000000, 0.9659258262890683122, 1.000000000000000000, 0.9659258262890683122, 1.000000000000000000, 0.9659258262890683122, 1.000000000000000000, 0.9659258262890683122, 1.000000000000000000, 0.9659258262890683122, 1.000000000000000000, 0.9659258262890683122, 1.000000000000000000, 0.9659258262890683122, 1.000000000000000000, 0.9659258262890683122, 1.000000000000000000, 0.9659258262890683122, 1.000000000000000000, 0.9659258262890683122, 1.000000000000000000, 0.9659258262890683122, 1.000000000000000000, 0.9659258262890683122, 1.000000000000000000, 0.9659258262890683122, 1.000000000000000000, 0.9659258262890683122, 1.000000000000000000, 0.9659258262890683122, 1.000000000000000000, 0.9659258262890683122, 1.000000000000000000, 0.9659258262890683122, 1.000000000000000000, 0.9659258262890683122, 1.000000000000000000, 0.9659258262890683122, 1.000000000000000000, 0.9659258262890683122, 1.000000000000000000, 0.9659258262890683122, 1.000000000000000000, 0.9659258262890683122, 1.000000000000000000, 0.9659258262890683122, 1.000000000000000000, 0.9659258262890683122, 1.000000000000000000, 0.9659258262890683122, 1.000000000000000000, 0.9659258262890683122, 1.000000000000000000, 0.9659258262890683122, 1.000000000000000000, 0.9659258262890683122, 1.000000000000000000, 0.9659258262890683122, 1.000000000000000000, 0.9659258262890683122, 1.000000000000000000, 0.9659258262890683122, 1.000000000000000000, 0.9659258262890683122, 1.000000000000000000, 0.9659258262890683122, 1.000000000000000000, 0.9659258262890683122, 1.000000000000000000, 0.9659258262890683122, 1.000000000000000000, 0.9659258262890683122, 1.000000000000000000, 0.9659258262890683122, 1.000000000000000000, 0.9659258262890683122, 1.000000000000000000, 0.9659258262890683122, 1.000000000000000000, 0.9659258262890683122, 1.000000000000000000, 0.9659258262890683122, 1.000000000000000000, 0.9659258262890683122, 1.000000000000000000, 0.9659258262890683122, 1.000000000000000000, 0.9659258262890683122, 1.000000000000000000, 0.9659258262890683122, 1.000000000000000000, 0.9659258262890683122, 1.000000000000000000, 0.9659258262890683122, 1.000000000000000000, 0.9659258262890683122, 1.000000000000000000, 0.9659258262890683122, 1.000000000000000000, 0.9659258262890683122, 1.000000000000000000, 0.9659258262890683122, 1.000000000000000000, 0.9659258262890683122, 1.000000000000000000, 0.9659258262890683122, 1.000000000000000000, 0.9659258262890683122, 1.000000000000000000, 0.9659258262890683122, 1.000000000000000000, 0.9659258262890683122, 1.000000000000000000, 0.9659258262890683122, 1.000000000000000000, 0.9659258262890683122, 1.000000000000000000, 0.9659258262890683122, 1.000000000000000000, 0.9659258262890683122, 1.000000000000000000, 0.9659258262890683122, 1.000000000000000000, 0.9659258262890683122, 1.000000000000000000, 0.9659258262890683122, 1.000000000000000000, 0.9659258262890683122, 1.000000000000000000, 0.9659258262890683122, 1.000000000000000000, 0.9659258262890683122, 1.000000000000000000, 0.9659258262890683122, 1.000000000000000000, 0.9659258262890683122, 1.000000000000000000, 0.9659258262890683122, 1.000000000000000000, 0.9659258262890683122, 1.000000000000000000, 0.9659258262890683122, 1.000000000000000000, 0.9659258262890683122, 1.000000000000000000, 0.9659258262890683122, 1.000000000000000000, 0.9659258262890683122, 1.000000000000000000, 0.9659258262890683122, 1.000000000000000000, 0.9659258262890683122, 1.000000000000000000, 0.9659258262890683122, 1.000000000000000000, 0.9659258262890683122, 1.000000000000000000, 0.9659258262890683122, 1.000000000000000000, 0.9659258262890683122, 1.000000000000000000, 0.9659258262890683122, 1.000000000000000000, 0.9659258262890683122, 1.000000000000000000, 0.9659258262890683122, 1.000000000000000000, 0.9659258262890683122, 1.000000000000000000, 0.9659258262890683122, 1.000000000000000000, 0.9659258262890683122, 1.000000000000000000, 0.9659258262890683122, 1.000000000000000000) ) ) 
 REPRESENTATION_ITEM ( '' )  SURFACE ( )  );
#61545=CARTESIAN_POINT ( 'NONE',  ( 2.791683348922237240, 45.38393115100079456, -7.208316651077763204 ) ) ;
#61547=ORIENTED_EDGE ( 'NONE', *, *, #34219, .F. ) ;
#61549=VECTOR ( 'NONE', #90486, 1000.000000000000000 ) ;
#61552=CARTESIAN_POINT ( 'NONE',  ( 24.16423886937410614, 19.51208216824729647, -3.795296366450302550 ) ) ;
#61553=DIRECTION ( 'NONE',  ( -0.000000000000000000, -1.000000000000000000, 0.000000000000000000 ) ) ;
#61554=LINE ( 'NONE', #23590, #48229 ) ;
#61555=CARTESIAN_POINT ( 'NONE',  ( 15.44008868035555260, 59.73035201082151247, 9.422509992056143702 ) ) ;
#61556=CARTESIAN_POINT ( 'NONE',  ( -0.8801773607111009756, 8.063685344154837509, 1.068504757029289695E-15 ) ) ;
#61557=CARTESIAN_POINT ( 'NONE',  ( -0.1038446121089037222, 59.24302437010793909, -6.337995344473782211 ) ) ;
#61558=VERTEX_POINT ( 'NONE', #47678 ) ;
#61559=CARTESIAN_POINT ( 'NONE',  ( 19.84674366389459266, 3.717264484334118713, -2.638427012816827677 ) ) ;
#61560=CARTESIAN_POINT ( 'NONE',  ( 19.84674366389459621, 3.508931151000785231, 7.409399052514197653E-17 ) ) ;
#61561=CARTESIAN_POINT ( 'NONE',  ( 6.565887622018943937, 33.08196800326374643, -12.81628187352647608 ) ) ;
#61562=CARTESIAN_POINT ( 'NONE',  ( 14.92337183194729633, 22.67559781766745175, 8.527530157486181039 ) ) ;
#61564=CARTESIAN_POINT ( 'NONE',  ( 21.09922568453595559, 17.04030133659708923, -6.408140936763230044 ) ) ;
#61567=CARTESIAN_POINT ( 'NONE',  ( 19.84674366389459621, 8.508931151000785675, 7.409399052514197653E-17 ) ) ;
#61569=CARTESIAN_POINT ( 'NONE',  ( 19.42250999205614548, 25.98035201082150891, -5.440088680355545492 ) ) ;
#61570=CARTESIAN_POINT ( 'NONE',  ( 17.08211943468705840, 25.13708216824730357, -12.26659068614894466 ) ) ;
#61571=CARTESIAN_POINT ( 'NONE',  ( 10.00000000000000000, 44.75893115100078745, -9.846743663894594434 ) ) ;
#61572=CARTESIAN_POINT ( 'NONE',  ( 4.559911319644449179, 63.89701867748817676, 9.422509992056141925 ) ) ;
#61573=CARTESIAN_POINT ( 'NONE',  ( 10.00000000000000178, 40.37363466993042493, 12.81628187352647608 ) ) ;
#61575=CARTESIAN_POINT ( 'NONE',  ( 20.88017736071110519, 25.56368534415483751, 2.639326808657452039E-16 ) ) ;
#61577=CARTESIAN_POINT ( 'NONE',  ( 0.6178305044545818747, 13.49863466993041783, -9.382169495545419124 ) ) ;
#61578=CARTESIAN_POINT ( 'NONE',  ( 2.791683348922240793, 46.63393115100077324, 7.208316651077764092 ) ) ;
#61580=CARTESIAN_POINT ( 'NONE',  ( -1.099225684535947600, 48.70696800326375353, -6.408140936763238038 ) ) ;
#61582=CARTESIAN_POINT ( 'NONE',  ( 7.084665262690076126, 49.10535201082149825, 10.88017736071109987 ) ) ;
#61586=CARTESIAN_POINT ( 'NONE',  ( 19.42250999205614548, 35.98035201082151247, -5.440088680355545492 ) ) ;
#61587=CARTESIAN_POINT ( 'NONE',  ( 12.91533473730992121, 39.52201867748817676, 10.88017736071110164 ) ) ;
#61589=CARTESIAN_POINT ( 'NONE',  ( 19.42250999205614548, 60.98035201082151247, -5.440088680355545492 ) ) ;
#61590=CARTESIAN_POINT ( 'NONE',  ( 17.20831665107776587, 52.88393115100078035, 7.208316651077764980 ) ) ;
#61591=CARTESIAN_POINT ( 'NONE',  ( 15.44008868035555260, 14.73035201082150536, 9.422509992056143702 ) ) ;
#61592=CARTESIAN_POINT ( 'NONE',  ( 17.39651004071842166, 22.93575266056828355, 6.499999999999998224 ) ) ;
#61593=CARTESIAN_POINT ( 'NONE',  ( -2.816281873526471635, 8.915301336597083903, -3.434112377981056508 ) ) ;
#61595=CARTESIAN_POINT ( 'NONE',  ( 20.88017736071110875, 35.77201867748816966, -2.915334737309920765 ) ) ;
#61596=CARTESIAN_POINT ( 'NONE',  ( -1.099225684535947600, 9.540301336597087456, 6.408140936763237150 ) ) ;
#61598=CARTESIAN_POINT ( 'NONE',  ( -0.8801773607111008646, 28.27201867748817321, 2.915334737309923430 ) ) ;
#61599=CARTESIAN_POINT ( 'NONE',  ( -4.164238869374099927, 32.01208216824730357, 3.795296366450308767 ) ) ;
#61600=CARTESIAN_POINT ( 'NONE',  ( 12.63842701281683034, 27.46726448433411250, 9.846743663894596210 ) ) ;
#61601=CARTESIAN_POINT ( 'NONE',  ( 12.91533473730993009, 56.60535201082151247, -10.88017736071109987 ) ) ;
#61603=CARTESIAN_POINT ( 'NONE',  ( -4.164238869374099927, 7.012082168247302683, 3.795296366450308767 ) ) ;
#61604=EDGE_CURVE ( 'NONE', #88696, #25751, #25681, .T. ) ;
#61606=CARTESIAN_POINT ( 'NONE',  ( 14.92337183194729633, 52.67559781766745175, 8.527530157486181039 ) ) ;
#61610=CARTESIAN_POINT ( 'NONE',  ( -4.164238869374099039, 41.80374883491397497, 8.674139862899312516E-16 ) ) ;
#61611=CARTESIAN_POINT ( 'NONE',  ( 10.00000000000000000, 40.55374883491397497, -14.16423886937410082 ) ) ;
#61612=CARTESIAN_POINT ( 'NONE',  ( 4.559911319644449179, 67.23035201082150536, -9.422509992056141925 ) ) ;
#61613=CARTESIAN_POINT ( 'NONE',  ( 17.20831665107776587, 59.13393115100078745, -7.208316651077762316 ) ) ;
#61615=CARTESIAN_POINT ( 'NONE',  ( 17.96484262340118221, 64.93868534415483396, 7.964842623401181321 ) ) ;
#61616=CARTESIAN_POINT ( 'NONE',  ( -1.099225684535947600, 24.54030133659708923, 6.408140936763237150 ) ) ;
#61617=CARTESIAN_POINT ( 'NONE',  ( 6.204703633549690345, 25.76208216824730712, -14.16423886937410259 ) ) ;
#61618=CARTESIAN_POINT ( 'NONE',  ( 17.96484262340118221, 11.18868534415484106, -7.964842623401177768 ) ) ;
#61619=COLOUR_RGB ( '', 0.31764706, 0.68627451, 0.89019608) ;
#61620=CARTESIAN_POINT ( 'NONE',  ( 2.035157376598822676, 32.43868534415483396, -7.964842623401177768 ) ) ;
#61622=CARTESIAN_POINT ( 'NONE',  ( 12.91533473730992121, 59.52201867748816966, 10.88017736071110164 ) ) ;
#61625=CYLINDRICAL_SURFACE ( 'NONE', #2850, 11.92686044187656513 ) ;
#61626=CARTESIAN_POINT ( 'NONE',  ( -0.3289641300568009741, 12.24545670184113888, -5.963430220938281678 ) ) ;
#61628=CARTESIAN_POINT ( 'NONE',  ( 20.36894250292379382, 58.67874883491396076, 10.36894250292379205 ) ) ;
#61629=CARTESIAN_POINT ( 'NONE',  ( -0.3689425029237898834, 61.17874883491396076, -10.36894250292378850 ) ) ;
#61630=CARTESIAN_POINT ( 'NONE',  ( 0.1532563361054082862, 31.21726448433412315, 2.638427012816831674 ) ) ;
#61631=CARTESIAN_POINT ( 'NONE',  ( 14.92337183194729988, 59.34226448433412315, -8.527530157486177487 ) ) ;
#61634=CARTESIAN_POINT ( 'NONE',  ( -1.099225684535947600, 3.706968003263753531, -6.408140936763238038 ) ) ;
#61638=CARTESIAN_POINT ( 'NONE',  ( 24.16423886937410614, 44.30374883491397497, 8.672049930838204340E-16 ) ) ;
#61639=CARTESIAN_POINT ( 'NONE',  ( -0.3689425029237898834, 41.17874883491397497, -10.36894250292378850 ) ) ;
#61640=VERTEX_POINT ( 'NONE', #18171 ) ;
#61641=CARTESIAN_POINT ( 'NONE',  ( -1.099225684535947600, 58.70696800326375353, -6.408140936763238038 ) ) ;
#61642=CARTESIAN_POINT ( 'NONE',  ( 5.076628168052704559, 45.17559781766745175, -8.527530157486179263 ) ) ;
#61643=CARTESIAN_POINT ( 'NONE',  ( 17.96484262340118221, 29.93868534415484106, 7.964842623401181321 ) ) ;
#61645=CARTESIAN_POINT ( 'NONE',  ( 0.1532563361054100626, 55.80059781766745175, -2.638427012816831230 ) ) ;
#61646=CARTESIAN_POINT ( 'NONE',  ( 1.472469842513823179, 55.59226448433412315, -4.923371831947296329 ) ) ;
#61648=CARTESIAN_POINT ( 'NONE',  ( -1.099225684535947600, 29.54030133659708923, 6.408140936763237150 ) ) ;
#61650=B_SPLINE_CURVE_WITH_KNOTS ( 'NONE', 3,
 ( #84922, #90933, #98480, #84441 ),
 .UNSPECIFIED., .F., .F.,
 ( 4, 4 ),
 ( 6.213755518593340002E-17, 0.001060528352562006968 ),
 .UNSPECIFIED. ) ;
#61652=CARTESIAN_POINT ( 'NONE',  ( 0.2751277870542967463, 70.00000000000000000, 6.000000000000000000 ) ) ;
#61655=CARTESIAN_POINT ( 'NONE',  ( 17.20831665107776587, 27.88393115100078390, 7.208316651077764980 ) ) ;
#61656=CARTESIAN_POINT ( 'NONE',  ( 19.72487221294570858, 70.00000000000000000, -6.000000000000000000 ) ) ;
#61658=CARTESIAN_POINT ( 'NONE',  ( 0.6178305044545818747, 38.49863466993042493, -9.382169495545419124 ) ) ;
#61663=CARTESIAN_POINT ( 'NONE',  ( 0.1532563361054082862, 66.21726448433413736, 2.638427012816831674 ) ) ;
#61664=CARTESIAN_POINT ( 'NONE',  ( 3.640395162852214650, 101.0000000000000000, 9.500000000000000000 ) ) ;
#61665=CARTESIAN_POINT ( 'NONE',  ( 14.92337183194729988, 54.34226448433412315, -8.527530157486177487 ) ) ;
#61666=CARTESIAN_POINT ( 'NONE',  ( 24.16423886937410614, 29.51208216824729647, -3.795296366450302550 ) ) ;
#61667=CARTESIAN_POINT ( 'NONE',  ( 7.361572987183170547, 62.05059781766745886, 9.846743663894590881 ) ) ;
#61669=DIRECTION ( 'NONE',  ( -0.07626964003977962370, 0.9970872288863209532, 0.000000000000000000 ) ) ;
#61670=CARTESIAN_POINT ( 'NONE',  ( 14.92337183194729988, 19.34226448433411960, -8.527530157486177487 ) ) ;
#61671=CARTESIAN_POINT ( 'NONE',  ( -2.816281873526473856, 49.12363466993042493, 9.499525473075851096E-16 ) ) ;
#61672=CARTESIAN_POINT ( 'NONE',  ( 0.1532563361054100626, 65.80059781766745175, -2.638427012816831230 ) ) ;
#61673=CARTESIAN_POINT ( 'NONE',  ( 7.084665262690076126, 54.10535201082151247, 10.88017736071109987 ) ) ;
#61674=CARTESIAN_POINT ( 'NONE',  ( 0.1532563361054100626, 40.80059781766745886, -2.638427012816831230 ) ) ;
#61679=B_SPLINE_CURVE_WITH_KNOTS ( 'NONE', 3,
 ( #75539, #67052, #60033, #58553 ),
 .UNSPECIFIED., .F., .F.,
 ( 4, 4 ),
 ( 4.336808689942017736E-19, 0.001036303429213369844 ),
 .UNSPECIFIED. ) ;
#61680=CARTESIAN_POINT ( 'NONE',  ( 10.00000000000000000, 61.81368534415484106, -10.88017736071110342 ) ) ;
#61681=VERTEX_POINT ( 'NONE', #25200 ) ;
#61683=CARTESIAN_POINT ( 'NONE',  ( 0.5774900079438607392, 23.48035201082150536, 5.440088680355550821 ) ) ;
#61684=CARTESIAN_POINT ( 'NONE',  ( 13.43411237798105340, 5.581968003263753531, 12.81628187352647963 ) ) ;
#61685=CARTESIAN_POINT ( 'NONE',  ( 10.00000000000000178, 54.31368534415484106, 10.88017736071110342 ) ) ;
#61687=CARTESIAN_POINT ( 'NONE',  ( -0.8801773607111009756, 68.06368534415484817, 1.068504757029289695E-15 ) ) ;
#61688=CARTESIAN_POINT ( 'NONE',  ( 20.88017736071110164, 35.35535201082150536, 2.915334737309930979 ) ) ;
#61690=CARTESIAN_POINT ( 'NONE',  ( 19.84674366389459266, 43.71726448433410894, -2.638427012816827677 ) ) ;
#61693=CARTESIAN_POINT ( 'NONE',  ( 18.52753015748618282, 63.92559781766745886, -4.923371831947291888 ) ) ;
#61694=CARTESIAN_POINT ( 'NONE',  ( 2.035157376598822676, 7.438685344154837509, -7.964842623401177768 ) ) ;
#61695=DIRECTION ( 'NONE',  ( -0.8320502943378437211, 0.5547001962252290364, 0.000000000000000000 ) ) ;
#61697=CARTESIAN_POINT ( 'NONE',  ( 22.26659068614895176, 24.72041550158063572, -7.082119434687042414 ) ) ;
#61699=CARTESIAN_POINT ( 'NONE',  ( 20.36894250292379382, 63.67874883491396787, 10.36894250292379205 ) ) ;
#61701=CARTESIAN_POINT ( 'NONE',  ( 19.84674366389459621, 23.50893115100078390, 7.409399052514197653E-17 ) ) ;
#61704=CARTESIAN_POINT ( 'NONE',  ( 17.20831665107776587, 29.13393115100078390, -7.208316651077762316 ) ) ;
#61705=CARTESIAN_POINT ( 'NONE',  ( 19.42250999205614193, 25.14701867748817321, 5.440088680355555262 ) ) ;
#61706=CARTESIAN_POINT ( 'NONE',  ( 5.076628168052703671, 61.84226448433412315, 8.527530157486179263 ) ) ;
#61707=CARTESIAN_POINT ( 'NONE',  ( 13.79529636645031943, 10.34541550158063394, -14.16423886937409904 ) ) ;
#61710=CARTESIAN_POINT ( 'NONE',  ( 1.472469842513823179, 16.42559781766745175, 4.923371831947296329 ) ) ;
#61711=CARTESIAN_POINT ( 'NONE',  ( 22.81628187352648496, 31.83196800326375353, -3.434112377981050290 ) ) ;
#61712=CARTESIAN_POINT ( 'NONE',  ( 1.472469842513823179, 41.42559781766745886, 4.923371831947296329 ) ) ;
#61714=CARTESIAN_POINT ( 'NONE',  ( 0.1532563361054100626, 20.80059781766744464, -2.638427012816831230 ) ) ;
#61715=FACE_OUTER_BOUND ( 'NONE', #57098, .T. ) ;
#61717=CARTESIAN_POINT ( 'NONE',  ( 6.204703633549690345, 55.76208216824730357, -14.16423886937410259 ) ) ;
#61718=CARTESIAN_POINT ( 'NONE',  ( 7.084665262690076126, 57.02201867748817676, -10.88017736071110164 ) ) ;
#61719=CARTESIAN_POINT ( 'NONE',  ( -2.266590686148945544, 1.387082168247301128, -7.082119434687050408 ) ) ;
#61720=CARTESIAN_POINT ( 'NONE',  ( 2.035157376598824452, 53.68868534415484817, 7.964842623401179544 ) ) ;
#61721=CARTESIAN_POINT ( 'NONE',  ( 7.361572987183169658, 34.96726448433411605, -9.846743663894592657 ) ) ;
#61722=CARTESIAN_POINT ( 'NONE',  ( 2.035157376598822676, 2.438685344154837953, -7.964842623401177768 ) ) ;
#61723=CARTESIAN_POINT ( 'NONE',  ( 0.1532563361054083140, 46.00893115100079456, 1.131784320476157264E-15 ) ) ;
#61725=CARTESIAN_POINT ( 'NONE',  ( 4.559911319644449179, 47.23035201082150536, -9.422509992056141925 ) ) ;
#61726=CARTESIAN_POINT ( 'NONE',  ( 12.63842701281683922, 4.550597817667451750, -9.846743663894590881 ) ) ;
#61727=ORIENTED_EDGE ( 'NONE', *, *, #26520, .T. ) ;
#61731=CARTESIAN_POINT ( 'NONE',  ( 19.84674366389459266, 28.30059781766745886, 2.638427012816836559 ) ) ;
#61732=CARTESIAN_POINT ( 'NONE',  ( 16.40814093676323893, 50.79030133659708923, 11.09922568453595026 ) ) ;
#61733=CARTESIAN_POINT ( 'NONE',  ( 0.5774900079438607392, 18.48035201082150536, 5.440088680355550821 ) ) ;
#61734=CARTESIAN_POINT ( 'NONE',  ( 18.52753015748618282, 43.92559781766745175, -4.923371831947291888 ) ) ;
#61735=CARTESIAN_POINT ( 'NONE',  ( -0.2418659066527637791, 35.11633188102327097, 6.114288769123057854 ) ) ;
#61736=CARTESIAN_POINT ( 'NONE',  ( -2.266590686148945544, 32.22041550158063927, 7.082119434687048631 ) ) ;
#61738=CARTESIAN_POINT ( 'NONE',  ( 20.36894250292379382, 58.67874883491396076, 10.36894250292379205 ) ) ;
#61739=CARTESIAN_POINT ( 'NONE',  ( 7.361572987183170547, 57.05059781766744464, 9.846743663894590881 ) ) ;
#61741=CARTESIAN_POINT ( 'NONE',  ( -0.8801773607110991993, 57.85535201082149825, -2.915334737309923874 ) ) ;
#61742=CARTESIAN_POINT ( 'NONE',  ( 19.84674366389459621, 18.50893115100078745, 7.409399052514197653E-17 ) ) ;
#61746=ORIENTED_EDGE ( 'NONE', *, *, #65112, .T. ) ;
#61747=CARTESIAN_POINT ( 'NONE',  ( 19.84674366389459266, 13.30059781766745353, 2.638427012816836559 ) ) ;
#61750=CARTESIAN_POINT ( 'NONE',  ( -2.266590686148945544, 22.22041550158063572, 7.082119434687048631 ) ) ;
#61751=CARTESIAN_POINT ( 'NONE',  ( 14.92337183194729633, 17.67559781766745175, 8.527530157486181039 ) ) ;
#61752=CARTESIAN_POINT ( 'NONE',  ( 19.42250999205614193, 40.14701867748817676, 5.440088680355555262 ) ) ;
#61753=CARTESIAN_POINT ( 'NONE',  ( -46.44000000000001194, 93.00000000000000000, 9.000000000000000000 ) ) ;
#61754=MECHANICAL_DESIGN_GEOMETRIC_PRESENTATION_REPRESENTATION('',(#18657),#69554);
#61756=CARTESIAN_POINT ( 'NONE',  ( -0.8801773607110991993, 32.85535201082151247, -2.915334737309923874 ) ) ;
#61757=EDGE_CURVE ( 'NONE', #85730, #663, #87140, .T. ) ;
#61762=CARTESIAN_POINT ( 'NONE',  ( 17.96484262340118221, 39.93868534415484106, 7.964842623401181321 ) ) ;
#61763=CARTESIAN_POINT ( 'NONE',  ( 19.72487221294571569, 55.71833443783938833, -6.499999999999990230 ) ) ;
#61766=CARTESIAN_POINT ( 'NONE',  ( 22.81628187352648496, 16.83196800326374998, -3.434112377981050290 ) ) ;
#61767=CARTESIAN_POINT ( 'NONE',  ( 18.52753015748617571, 8.092264484334117824, 4.923371831947298993 ) ) ;
#61770=CARTESIAN_POINT ( 'NONE',  ( 7.361572987183170547, 22.05059781766745530, 9.846743663894590881 ) ) ;
#61771=CARTESIAN_POINT ( 'NONE',  ( 10.00000000000000178, 29.31368534415483751, 10.88017736071110342 ) ) ;
#61775=ORIENTED_EDGE ( 'NONE', *, *, #52851, .T. ) ;
#61778=CARTESIAN_POINT ( 'NONE',  ( 4.559911319644449179, 52.23035201082151247, -9.422509992056141925 ) ) ;
#61779=CARTESIAN_POINT ( 'NONE',  ( 1.707155281725207585, 7.901890803972831279, 6.499999999999992006 ) ) ;
#61780=ADVANCED_FACE ( 'NONE', ( #11150 ), #26292, .T. ) ;
#61782=CARTESIAN_POINT ( 'NONE',  ( 2.035157376598824452, 58.68868534415482685, 7.964842623401179544 ) ) ;
#61783=CARTESIAN_POINT ( 'NONE',  ( -2.816281873526473856, -0.8763653300695799508, 9.499525473075851096E-16 ) ) ;
#61785=CARTESIAN_POINT ( 'NONE',  ( 12.63842701281683034, 37.46726448433411605, 9.846743663894596210 ) ) ;
#61786=CARTESIAN_POINT ( 'NONE',  ( 21.09922568453594849, 51.20696800326375353, 6.408140936763242479 ) ) ;
#61788=CARTESIAN_POINT ( 'NONE',  ( 10.00000000000000178, 22.25893115100078745, 9.846743663894594434 ) ) ;
#61789=CARTESIAN_POINT ( 'NONE',  ( 22.81628187352648496, 21.83196800326374643, -3.434112377981050290 ) ) ;
#61793=CARTESIAN_POINT ( 'NONE',  ( 7.084665262690076126, 52.02201867748816255, -10.88017736071110164 ) ) ;
#61794=CARTESIAN_POINT ( 'NONE',  ( 0.1532563361054082862, 61.21726448433412315, 2.638427012816831674 ) ) ;
#61796=CARTESIAN_POINT ( 'NONE',  ( 14.92337183194729988, 24.34226448433411960, -8.527530157486177487 ) ) ;
#61797=CARTESIAN_POINT ( 'NONE',  ( 17.20831665107776587, 14.13393115100078568, -7.208316651077762316 ) ) ;
#61798=CARTESIAN_POINT ( 'NONE',  ( 4.559911319644449179, 8.897018677488171434, 9.422509992056141925 ) ) ;
#61799=CARTESIAN_POINT ( 'NONE',  ( 10.00000000000000000, 12.87363466993042138, -12.81628187352647608 ) ) ;
#61801=( LENGTH_UNIT ( ) NAMED_UNIT ( * ) SI_UNIT ( .MILLI., .METRE. ) );
#61802=CARTESIAN_POINT ( 'NONE',  ( 12.63842701281683922, 64.55059781766745175, -9.846743663894590881 ) ) ;
#61804=CARTESIAN_POINT ( 'NONE',  ( 15.44008868035555260, 14.73035201082150536, 9.422509992056143702 ) ) ;
#61805=CARTESIAN_POINT ( 'NONE',  ( 0.1532563361054100626, 40.80059781766745886, -2.638427012816831230 ) ) ;
#61808=CARTESIAN_POINT ( 'NONE',  ( 7.084665262690076126, 19.10535201082150181, 10.88017736071109987 ) ) ;
#61810=CARTESIAN_POINT ( 'NONE',  ( 0.5774900079438590739, 32.64701867748816966, -5.440088680355550821 ) ) ;
#61811=CARTESIAN_POINT ( 'NONE',  ( 2.917880565312948704, 62.63708216824730357, 12.26659068614894643 ) ) ;
#61814=( BOUNDED_SURFACE ( )  B_SPLINE_SURFACE ( 1, 2, ( 
 ( #39927, #31419, #31907, #23467, #53942, #1455, #62408, #93907, #86417, #46919, #32903, #69439, #958, #77412, #2446, #24443, #54910, #10414, #85424, #70430, #32411, #62911, #70928, #47903, #24936, #85926, #17435, #78408, #9926, #63402, #17918, #95890, #17646, #94983, #42009, #64964, #57481, #12473, #11985, #49480, #3514, #33485, #4009, #58453, #19487, #72476, #65463, #49980, #27472, #80487, #12961, #56508, #34471, #73457, #79988, #95490, #26489, #88969, #34966, #26982, #11006, #33973, #87490, #20478, #41522, #42488, #50964, #42977, #71990, #11490, #72969, #57965, #4985, #88469, #19971, #35466, #96489, #27960, #43456, #73958, #63983, #56763, #72251, #3784, #86289, #41299, #34238, #94764, #85798, #63760, #17310, #9300, #1827, #47787, #71771, #39810, #17797, #94265, #56287, #26264, #9799, #93780, #70806, #79764, #78284, #25309, #40299, #48273, #64735, #24812, #78786, #10293, #16811, #3282, #95247, #86782, #33745, #47287, #18285, #32281, #71291, #32776, #48765, #62788, #2323, #18781, #63273, #93287, #49264, #64247, #55794, #79272, #11262, #54788, #41781, #85305, #77788, #70311, #19258, #28230, #73233, #82218, #36736, #66224, #95757, #66730, #50233, #27241, #57737, #13230, #50748, #89232, #49742, #96756, #4761, #67227, #28724, #20741, #42265, #20246, #58728, #43726, #74213, #26753, #97254, #57248, #5743, #19749, #59214, #13730, #44214, #80251, #88241, #34740, #88734, #73726, #80748, #12243, #42752, #96258, #35232, #65730, #27735, #58218, #22722, #76689, #23720, #14234, #46684, #52709, #29702, #15721, #8211, #91197, #16201, #45212, #14736, #61674, #54179, #98242, #53205, #68227, #29214, #59713, #37239, #38705, #44712, #90706, #60211, #67728, #84691, #83710, #38222, #98747, #37724, #8688, #68708, #75710, #15228, #75211, #6722, #7224, #30197, #69205, #45708, #60698, #7725, #728, #239, #61195, #91703, #23221, #84216, #54666, #85183, #62166, #47164, #9183, #92671, #16693, #1220, #31674, #89821, #65338, #58325, #35342, #64839, #95358, #4378, #43821, #49850, #57840, #95865, #34843, #28821, #88842, #5360, #65834, #4864, #21340, #35839, #27347, #20351, #82318, #26857, #44320, #96365, #74317, #50846, #81338, #74820, #66828, #57355, #66327, #42367, #12835, #43335, #73830, #96862, #88349, #20845, #81820, #19847, #28338, #87847, #13338, #13838, #58827, #51337, #19367, #89335, #72840, #5843, #42854, #36334, #50339, #80850, #97350, #12348, #73337, #59320, #51831, #80359, #11859, #98348, #16303, #98841, #68814, #77278, #60799, #29314, #38318, #83315, #92293, #84795, #15336, #6826, #46304, #60314, #37340, #67830, #91803, #91299, #347, #97850 ),
 ( #53806, #45818, #22334, #29806, #36835, #7331, #61783, #22825, #75809, #30791, #53302, #61294, #83810, #46786, #59810, #37832, #76790, #14840, #45313, #90806, #23816, #7824, #68323, #90305, #52808, #30296, #54277, #21839, #76306, #67326, #84317, #44808, #23325, #15817, #8307, #38809, #69303, #825, #31284, #52322, #82815, #14335, #75314, #94247, #26251, #48747, #39793, #86271, #70293, #24307, #54770, #1808, #25777, #16795, #40280, #17782, #48257, #79256, #62772, #9782, #24795, #33731, #93271, #70788, #55271, #2305, #87240, #77772, #63256, #93764, #10766, #47271, #85783, #2798, #17294, #78768, #39307, #33251, #56271, #3264, #55776, #10276, #94747, #41281, #40775, #63744, #86764, #18268, #71755, #56746, #18766, #49246, #8788, #69800, #31775, #72718, #89215, #72235, #3767, #19242, #58714, #88223, #97241, #5729, #57721, #50218, #73214, #58201, #28215, #5241, #12226, #96240, #89704, #27223, #59200, #88717, #19732, #27720, #96740, #42249, #80732, #42736, #4745, #20728, #20228, #65216, #49724, #79748, #35212, #36216, #65714, #50732, #12721, #81220, #73709, #43213, #21218, #34222, #35719, #51217, #66208, #81703, #4253, #66716, #13216, #43709, #64719, #80233, #11740, #28709, #95228, #74196, #11244, #41764, #87729, #57232, #26737, #34723, #95742, #90194, #21723, #7712, #68693, #52206, #7207, #13714, #224, #713, #83695, #38206, #44197, #15213, #29198, #75695, #60194, #37708, #59696, #6706, #84197, #82700, #14219, #91687, #30673, #90690, #68210, #75196, #31169, #98731, #45692, #92179, #30181, #74708, #53193, #98225, #8194, #61658, #60685, #67711, #61181, #22218, #52695, #83199, #23205, #91184, #76191, #6217, #22710, #53680, #51721, #15706, #46192, #36722, #76675, #38691, #69190, #82203, #67211, #97736, #54165, #33132, #39684, #25661, #25178, #32647, #63627, #62149, #48630, #85659, #40160, #10160, #16185, #46668, #24673, #63142, #17178, #32144, #10645, #94133, #79134, #41159, #77166, #71644, #55145, #54652, #3152, #8674, #39186, #1204, #85170, #49603, #29443, #21980, #95109, #89470, #65094, #37472, #26140, #34108, #74958, #79631, #87611, #26618, #64600, #59947, #20985, #36475, #27105, #34601, #82958, #66968, #57114, #81959, #14473, #56634, #75451, #13474, #6461, #74455, #5983, #6964, #97986, #87121, #97488, #72117, #28954, #59456, #89957, #21473, #51972, #13982, #19122, #90437, #82459, #44456, #36969, #18640, #49129, #67465, #44946, #41650, #80112, #3644, #11619, #42136, #72601, #4137, #75945, #83942, #98980, #16437, #62402, #61424, #23461, #92908, #3400, #64855, #95374, #18897, #41903, #26874, #93406, #11876, #20367, #89837, #95882 ) ),
 .UNSPECIFIED., .F., .F., .F. ) 
 B_SPLINE_SURFACE_WITH_KNOTS ( ( 2, 2 ),
 ( 3, 2, 2, 2, 2, 2, 2, 2, 2, 2, 2, 2, 2, 2, 2, 2, 2, 2, 2, 2, 2, 2, 2, 2, 2, 2, 2, 2, 2, 2, 2, 2, 2, 2, 2, 2, 2, 2, 2, 2, 2, 2, 2, 2, 2, 2, 2, 2, 2, 2, 2, 2, 2, 2, 2, 2, 2, 2, 2, 2, 2, 2, 2, 2, 2, 2, 2, 2, 2, 2, 2, 2, 2, 2, 2, 2, 2, 2, 2, 2, 2, 2, 2, 2, 2, 2, 2, 2, 2, 2, 2, 2, 2, 2, 2, 2, 2, 2, 2, 2, 2, 2, 2, 2, 2, 2, 2, 2, 2, 2, 2, 2, 2, 2, 2, 2, 2, 2, 2, 2, 2, 2, 2, 2, 2, 2, 2, 2, 2, 2, 2, 2, 2, 2, 2, 2, 2, 2, 2, 2, 2, 2, 2, 2, 2, 2, 2, 2, 2, 2, 2, 2, 2, 2, 2, 2, 2, 2, 2, 2, 2, 2, 3 ),
 ( 0.000000000000000000, 1.000000000000000000 ),
 ( 0.000000000000000000, 0.005952380952380952051, 0.01190476190476190410, 0.01785714285714285615, 0.02380952380952380820, 0.02976190476190476025, 0.03571428571428571230, 0.04166666666666666435, 0.04761904761904761640, 0.05357142857142856845, 0.05952380952380952051, 0.06547619047619047949, 0.07142857142857142461, 0.07738095238095238360, 0.08333333333333332871, 0.08928571428571428770, 0.09523809523809523281, 0.1011904761904761918, 0.1071428571428571369, 0.1130952380952380959, 0.1190476190476190410, 0.1250000000000000000, 0.1309523809523809590, 0.1369047619047619180, 0.1428571428571428492, 0.1488095238095238082, 0.1547619047619047672, 0.1607142857142857262, 0.1666666666666666574, 0.1726190476190476164, 0.1785714285714285754, 0.1845238095238095344, 0.1904761904761904656, 0.1964285714285714246, 0.2023809523809523836, 0.2083333333333333426, 0.2142857142857142738, 0.2202380952380952328, 0.2261904761904761918, 0.2321428571428571508, 0.2380952380952380820, 0.2440476190476190410, 0.2500000000000000000, 0.2559523809523809312, 0.2619047619047619180, 0.2678571428571428492, 0.2738095238095238360, 0.2797619047619047672, 0.2857142857142856984, 0.2916666666666666852, 0.2976190476190476164, 0.3035714285714285476, 0.3095238095238095344, 0.3154761904761904656, 0.3214285714285714524, 0.3273809523809523836, 0.3333333333333333148, 0.3392857142857143016, 0.3452380952380952328, 0.3511904761904761640, 0.3571428571428571508, 0.3630952380952380820, 0.3690476190476190688, 0.3750000000000000000, 0.3809523809523809312, 0.3869047619047619180, 0.3928571428571428492, 0.3988095238095238360, 0.4047619047619047672, 0.4107142857142856984, 0.4166666666666666852, 0.4226190476190476164, 0.4285714285714285476, 0.4345238095238095344, 0.4404761904761904656, 0.4464285714285714524, 0.4523809523809523836, 0.4583333333333333148, 0.4642857142857143016, 0.4702380952380952328, 0.4761904761904761640, 0.4821428571428571508, 0.4880952380952380820, 0.4940476190476190688, 0.5000000000000000000, 0.5059523809523809312, 0.5119047619047618625, 0.5178571428571429047, 0.5238095238095238360, 0.5297619047619047672, 0.5357142857142856984, 0.5416666666666666297, 0.5476190476190476719, 0.5535714285714286031, 0.5595238095238095344, 0.5654761904761904656, 0.5714285714285713969, 0.5773809523809523281, 0.5833333333333333703, 0.5892857142857143016, 0.5952380952380952328, 0.6011904761904761640, 0.6071428571428570953, 0.6130952380952381375, 0.6190476190476190688, 0.6250000000000000000, 0.6309523809523809312, 0.6369047619047618625, 0.6428571428571429047, 0.6488095238095238360, 0.6547619047619047672, 0.6607142857142856984, 0.6666666666666666297, 0.6726190476190476719, 0.6785714285714286031, 0.6845238095238095344, 0.6904761904761904656, 0.6964285714285713969, 0.7023809523809523281, 0.7083333333333333703, 0.7142857142857143016, 0.7202380952380952328, 0.7261904761904761640, 0.7321428571428570953, 0.7380952380952381375, 0.7440476190476190688, 0.7500000000000000000, 0.7559523809523809312, 0.7619047619047618625, 0.7678571428571429047, 0.7738095238095238360, 0.7797619047619047672, 0.7857142857142856984, 0.7916666666666666297, 0.7976190476190476719, 0.8035714285714286031, 0.8095238095238095344, 0.8154761904761904656, 0.8214285714285713969, 0.8273809523809523281, 0.8333333333333333703, 0.8392857142857143016, 0.8452380952380952328, 0.8511904761904761640, 0.8571428571428570953, 0.8630952380952381375, 0.8690476190476190688, 0.8750000000000000000, 0.8809523809523809312, 0.8869047619047618625, 0.8928571428571429047, 0.8988095238095238360, 0.9047619047619047672, 0.9107142857142856984, 0.9166666666666666297, 0.9226190476190476719, 0.9285714285714286031, 0.9345238095238095344, 0.9404761904761904656, 0.9464285714285713969, 0.9523809523809523281, 0.9583333333333333703, 0.9642857142857143016 ),
 .UNSPECIFIED. ) 
 GEOMETRIC_REPRESENTATION_ITEM ( )  RATIONAL_B_SPLINE_SURFACE ( (
 ( 1.000000000000000000, 0.9659258262890683122, 1.000000000000000000, 0.9659258262890683122, 1.000000000000000000, 0.9659258262890683122, 1.000000000000000000, 0.9659258262890683122, 1.000000000000000000, 0.9659258262890683122, 1.000000000000000000, 0.9659258262890683122, 1.000000000000000000, 0.9659258262890683122, 1.000000000000000000, 0.9659258262890683122, 1.000000000000000000, 0.9659258262890683122, 1.000000000000000000, 0.9659258262890683122, 1.000000000000000000, 0.9659258262890683122, 1.000000000000000000, 0.9659258262890683122, 1.000000000000000000, 0.9659258262890683122, 1.000000000000000000, 0.9659258262890683122, 1.000000000000000000, 0.9659258262890683122, 1.000000000000000000, 0.9659258262890683122, 1.000000000000000000, 0.9659258262890683122, 1.000000000000000000, 0.9659258262890683122, 1.000000000000000000, 0.9659258262890683122, 1.000000000000000000, 0.9659258262890683122, 1.000000000000000000, 0.9659258262890683122, 1.000000000000000000, 0.9659258262890683122, 1.000000000000000000, 0.9659258262890683122, 1.000000000000000000, 0.9659258262890683122, 1.000000000000000000, 0.9659258262890683122, 1.000000000000000000, 0.9659258262890683122, 1.000000000000000000, 0.9659258262890683122, 1.000000000000000000, 0.9659258262890683122, 1.000000000000000000, 0.9659258262890683122, 1.000000000000000000, 0.9659258262890683122, 1.000000000000000000, 0.9659258262890683122, 1.000000000000000000, 0.9659258262890683122, 1.000000000000000000, 0.9659258262890683122, 1.000000000000000000, 0.9659258262890683122, 1.000000000000000000, 0.9659258262890683122, 1.000000000000000000, 0.9659258262890683122, 1.000000000000000000, 0.9659258262890683122, 1.000000000000000000, 0.9659258262890683122, 1.000000000000000000, 0.9659258262890683122, 1.000000000000000000, 0.9659258262890683122, 1.000000000000000000, 0.9659258262890683122, 1.000000000000000000, 0.9659258262890683122, 1.000000000000000000, 0.9659258262890683122, 1.000000000000000000, 0.9659258262890683122, 1.000000000000000000, 0.9659258262890683122, 1.000000000000000000, 0.9659258262890683122, 1.000000000000000000, 0.9659258262890683122, 1.000000000000000000, 0.9659258262890683122, 1.000000000000000000, 0.9659258262890683122, 1.000000000000000000, 0.9659258262890683122, 1.000000000000000000, 0.9659258262890683122, 1.000000000000000000, 0.9659258262890683122, 1.000000000000000000, 0.9659258262890683122, 1.000000000000000000, 0.9659258262890683122, 1.000000000000000000, 0.9659258262890683122, 1.000000000000000000, 0.9659258262890683122, 1.000000000000000000, 0.9659258262890683122, 1.000000000000000000, 0.9659258262890683122, 1.000000000000000000, 0.9659258262890683122, 1.000000000000000000, 0.9659258262890683122, 1.000000000000000000, 0.9659258262890683122, 1.000000000000000000, 0.9659258262890683122, 1.000000000000000000, 0.9659258262890683122, 1.000000000000000000, 0.9659258262890683122, 1.000000000000000000, 0.9659258262890683122, 1.000000000000000000, 0.9659258262890683122, 1.000000000000000000, 0.9659258262890683122, 1.000000000000000000, 0.9659258262890683122, 1.000000000000000000, 0.9659258262890683122, 1.000000000000000000, 0.9659258262890683122, 1.000000000000000000, 0.9659258262890683122, 1.000000000000000000, 0.9659258262890683122, 1.000000000000000000, 0.9659258262890683122, 1.000000000000000000, 0.9659258262890683122, 1.000000000000000000, 0.9659258262890683122, 1.000000000000000000, 0.9659258262890683122, 1.000000000000000000, 0.9659258262890683122, 1.000000000000000000, 0.9659258262890683122, 1.000000000000000000, 0.9659258262890683122, 1.000000000000000000, 0.9659258262890683122, 1.000000000000000000, 0.9659258262890683122, 1.000000000000000000, 0.9659258262890683122, 1.000000000000000000, 0.9659258262890683122, 1.000000000000000000, 0.9659258262890683122, 1.000000000000000000, 0.9659258262890683122, 1.000000000000000000, 0.9659258262890683122, 1.000000000000000000, 0.9659258262890683122, 1.000000000000000000, 0.9659258262890683122, 1.000000000000000000, 0.9659258262890683122, 1.000000000000000000, 0.9659258262890683122, 1.000000000000000000, 0.9659258262890683122, 1.000000000000000000, 0.9659258262890683122, 1.000000000000000000, 0.9659258262890683122, 1.000000000000000000, 0.9659258262890683122, 1.000000000000000000, 0.9659258262890683122, 1.000000000000000000, 0.9659258262890683122, 1.000000000000000000, 0.9659258262890683122, 1.000000000000000000, 0.9659258262890683122, 1.000000000000000000, 0.9659258262890683122, 1.000000000000000000, 0.9659258262890683122, 1.000000000000000000, 0.9659258262890683122, 1.000000000000000000, 0.9659258262890683122, 1.000000000000000000, 0.9659258262890683122, 1.000000000000000000, 0.9659258262890683122, 1.000000000000000000, 0.9659258262890683122, 1.000000000000000000, 0.9659258262890683122, 1.000000000000000000, 0.9659258262890683122, 1.000000000000000000, 0.9659258262890683122, 1.000000000000000000, 0.9659258262890683122, 1.000000000000000000, 0.9659258262890683122, 1.000000000000000000, 0.9659258262890683122, 1.000000000000000000, 0.9659258262890683122, 1.000000000000000000, 0.9659258262890683122, 1.000000000000000000, 0.9659258262890683122, 1.000000000000000000, 0.9659258262890683122, 1.000000000000000000, 0.9659258262890683122, 1.000000000000000000, 0.9659258262890683122, 1.000000000000000000, 0.9659258262890683122, 1.000000000000000000, 0.9659258262890683122, 1.000000000000000000, 0.9659258262890683122, 1.000000000000000000, 0.9659258262890683122, 1.000000000000000000, 0.9659258262890683122, 1.000000000000000000, 0.9659258262890683122, 1.000000000000000000, 0.9659258262890683122, 1.000000000000000000, 0.9659258262890683122, 1.000000000000000000, 0.9659258262890683122, 1.000000000000000000, 0.9659258262890683122, 1.000000000000000000, 0.9659258262890683122, 1.000000000000000000, 0.9659258262890683122, 1.000000000000000000, 0.9659258262890683122, 1.000000000000000000, 0.9659258262890683122, 1.000000000000000000, 0.9659258262890683122, 1.000000000000000000, 0.9659258262890683122, 1.000000000000000000, 0.9659258262890683122, 1.000000000000000000, 0.9659258262890683122, 1.000000000000000000, 0.9659258262890683122, 1.000000000000000000, 0.9659258262890683122, 1.000000000000000000, 0.9659258262890683122, 1.000000000000000000, 0.9659258262890683122, 1.000000000000000000, 0.9659258262890683122, 1.000000000000000000, 0.9659258262890683122, 1.000000000000000000, 0.9659258262890683122, 1.000000000000000000, 0.9659258262890683122, 1.000000000000000000, 0.9659258262890683122, 1.000000000000000000, 0.9659258262890683122, 1.000000000000000000, 0.9659258262890683122, 1.000000000000000000, 0.9659258262890683122, 1.000000000000000000, 0.9659258262890683122, 1.000000000000000000, 0.9659258262890683122, 1.000000000000000000, 0.9659258262890683122, 1.000000000000000000, 0.9659258262890683122, 1.000000000000000000, 0.9659258262890683122, 1.000000000000000000, 0.9659258262890683122, 1.000000000000000000, 0.9659258262890683122, 1.000000000000000000, 0.9659258262890683122, 1.000000000000000000, 0.9659258262890683122, 1.000000000000000000, 0.9659258262890683122, 1.000000000000000000, 0.9659258262890683122, 1.000000000000000000, 0.9659258262890683122, 1.000000000000000000, 0.9659258262890683122, 1.000000000000000000, 0.9659258262890683122, 1.000000000000000000, 0.9659258262890683122, 1.000000000000000000),
 ( 1.000000000000000000, 0.9659258262890683122, 1.000000000000000000, 0.9659258262890683122, 1.000000000000000000, 0.9659258262890683122, 1.000000000000000000, 0.9659258262890683122, 1.000000000000000000, 0.9659258262890683122, 1.000000000000000000, 0.9659258262890683122, 1.000000000000000000, 0.9659258262890683122, 1.000000000000000000, 0.9659258262890683122, 1.000000000000000000, 0.9659258262890683122, 1.000000000000000000, 0.9659258262890683122, 1.000000000000000000, 0.9659258262890683122, 1.000000000000000000, 0.9659258262890683122, 1.000000000000000000, 0.9659258262890683122, 1.000000000000000000, 0.9659258262890683122, 1.000000000000000000, 0.9659258262890683122, 1.000000000000000000, 0.9659258262890683122, 1.000000000000000000, 0.9659258262890683122, 1.000000000000000000, 0.9659258262890683122, 1.000000000000000000, 0.9659258262890683122, 1.000000000000000000, 0.9659258262890683122, 1.000000000000000000, 0.9659258262890683122, 1.000000000000000000, 0.9659258262890683122, 1.000000000000000000, 0.9659258262890683122, 1.000000000000000000, 0.9659258262890683122, 1.000000000000000000, 0.9659258262890683122, 1.000000000000000000, 0.9659258262890683122, 1.000000000000000000, 0.9659258262890683122, 1.000000000000000000, 0.9659258262890683122, 1.000000000000000000, 0.9659258262890683122, 1.000000000000000000, 0.9659258262890683122, 1.000000000000000000, 0.9659258262890683122, 1.000000000000000000, 0.9659258262890683122, 1.000000000000000000, 0.9659258262890683122, 1.000000000000000000, 0.9659258262890683122, 1.000000000000000000, 0.9659258262890683122, 1.000000000000000000, 0.9659258262890683122, 1.000000000000000000, 0.9659258262890683122, 1.000000000000000000, 0.9659258262890683122, 1.000000000000000000, 0.9659258262890683122, 1.000000000000000000, 0.9659258262890683122, 1.000000000000000000, 0.9659258262890683122, 1.000000000000000000, 0.9659258262890683122, 1.000000000000000000, 0.9659258262890683122, 1.000000000000000000, 0.9659258262890683122, 1.000000000000000000, 0.9659258262890683122, 1.000000000000000000, 0.9659258262890683122, 1.000000000000000000, 0.9659258262890683122, 1.000000000000000000, 0.9659258262890683122, 1.000000000000000000, 0.9659258262890683122, 1.000000000000000000, 0.9659258262890683122, 1.000000000000000000, 0.9659258262890683122, 1.000000000000000000, 0.9659258262890683122, 1.000000000000000000, 0.9659258262890683122, 1.000000000000000000, 0.9659258262890683122, 1.000000000000000000, 0.9659258262890683122, 1.000000000000000000, 0.9659258262890683122, 1.000000000000000000, 0.9659258262890683122, 1.000000000000000000, 0.9659258262890683122, 1.000000000000000000, 0.9659258262890683122, 1.000000000000000000, 0.9659258262890683122, 1.000000000000000000, 0.9659258262890683122, 1.000000000000000000, 0.9659258262890683122, 1.000000000000000000, 0.9659258262890683122, 1.000000000000000000, 0.9659258262890683122, 1.000000000000000000, 0.9659258262890683122, 1.000000000000000000, 0.9659258262890683122, 1.000000000000000000, 0.9659258262890683122, 1.000000000000000000, 0.9659258262890683122, 1.000000000000000000, 0.9659258262890683122, 1.000000000000000000, 0.9659258262890683122, 1.000000000000000000, 0.9659258262890683122, 1.000000000000000000, 0.9659258262890683122, 1.000000000000000000, 0.9659258262890683122, 1.000000000000000000, 0.9659258262890683122, 1.000000000000000000, 0.9659258262890683122, 1.000000000000000000, 0.9659258262890683122, 1.000000000000000000, 0.9659258262890683122, 1.000000000000000000, 0.9659258262890683122, 1.000000000000000000, 0.9659258262890683122, 1.000000000000000000, 0.9659258262890683122, 1.000000000000000000, 0.9659258262890683122, 1.000000000000000000, 0.9659258262890683122, 1.000000000000000000, 0.9659258262890683122, 1.000000000000000000, 0.9659258262890683122, 1.000000000000000000, 0.9659258262890683122, 1.000000000000000000, 0.9659258262890683122, 1.000000000000000000, 0.9659258262890683122, 1.000000000000000000, 0.9659258262890683122, 1.000000000000000000, 0.9659258262890683122, 1.000000000000000000, 0.9659258262890683122, 1.000000000000000000, 0.9659258262890683122, 1.000000000000000000, 0.9659258262890683122, 1.000000000000000000, 0.9659258262890683122, 1.000000000000000000, 0.9659258262890683122, 1.000000000000000000, 0.9659258262890683122, 1.000000000000000000, 0.9659258262890683122, 1.000000000000000000, 0.9659258262890683122, 1.000000000000000000, 0.9659258262890683122, 1.000000000000000000, 0.9659258262890683122, 1.000000000000000000, 0.9659258262890683122, 1.000000000000000000, 0.9659258262890683122, 1.000000000000000000, 0.9659258262890683122, 1.000000000000000000, 0.9659258262890683122, 1.000000000000000000, 0.9659258262890683122, 1.000000000000000000, 0.9659258262890683122, 1.000000000000000000, 0.9659258262890683122, 1.000000000000000000, 0.9659258262890683122, 1.000000000000000000, 0.9659258262890683122, 1.000000000000000000, 0.9659258262890683122, 1.000000000000000000, 0.9659258262890683122, 1.000000000000000000, 0.9659258262890683122, 1.000000000000000000, 0.9659258262890683122, 1.000000000000000000, 0.9659258262890683122, 1.000000000000000000, 0.9659258262890683122, 1.000000000000000000, 0.9659258262890683122, 1.000000000000000000, 0.9659258262890683122, 1.000000000000000000, 0.9659258262890683122, 1.000000000000000000, 0.9659258262890683122, 1.000000000000000000, 0.9659258262890683122, 1.000000000000000000, 0.9659258262890683122, 1.000000000000000000, 0.9659258262890683122, 1.000000000000000000, 0.9659258262890683122, 1.000000000000000000, 0.9659258262890683122, 1.000000000000000000, 0.9659258262890683122, 1.000000000000000000, 0.9659258262890683122, 1.000000000000000000, 0.9659258262890683122, 1.000000000000000000, 0.9659258262890683122, 1.000000000000000000, 0.9659258262890683122, 1.000000000000000000, 0.9659258262890683122, 1.000000000000000000, 0.9659258262890683122, 1.000000000000000000, 0.9659258262890683122, 1.000000000000000000, 0.9659258262890683122, 1.000000000000000000, 0.9659258262890683122, 1.000000000000000000, 0.9659258262890683122, 1.000000000000000000, 0.9659258262890683122, 1.000000000000000000, 0.9659258262890683122, 1.000000000000000000, 0.9659258262890683122, 1.000000000000000000, 0.9659258262890683122, 1.000000000000000000, 0.9659258262890683122, 1.000000000000000000, 0.9659258262890683122, 1.000000000000000000, 0.9659258262890683122, 1.000000000000000000, 0.9659258262890683122, 1.000000000000000000, 0.9659258262890683122, 1.000000000000000000, 0.9659258262890683122, 1.000000000000000000, 0.9659258262890683122, 1.000000000000000000, 0.9659258262890683122, 1.000000000000000000, 0.9659258262890683122, 1.000000000000000000, 0.9659258262890683122, 1.000000000000000000, 0.9659258262890683122, 1.000000000000000000, 0.9659258262890683122, 1.000000000000000000, 0.9659258262890683122, 1.000000000000000000, 0.9659258262890683122, 1.000000000000000000, 0.9659258262890683122, 1.000000000000000000, 0.9659258262890683122, 1.000000000000000000, 0.9659258262890683122, 1.000000000000000000, 0.9659258262890683122, 1.000000000000000000, 0.9659258262890683122, 1.000000000000000000, 0.9659258262890683122, 1.000000000000000000, 0.9659258262890683122, 1.000000000000000000, 0.9659258262890683122, 1.000000000000000000, 0.9659258262890683122, 1.000000000000000000, 0.9659258262890683122, 1.000000000000000000) ) ) 
 REPRESENTATION_ITEM ( '' )  SURFACE ( )  );
#61815=CARTESIAN_POINT ( 'NONE',  ( 18.52753015748618282, 28.92559781766745175, -4.923371831947291888 ) ) ;
#61816=CARTESIAN_POINT ( 'NONE',  ( 3.591859063236761518, 9.956968003263753531, 11.09922568453594849 ) ) ;
#61820=( BOUNDED_CURVE ( )  B_SPLINE_CURVE ( 2, ( #80766, #88756, #41797, #73746, #34759, #95776, #65748, #64265, #81737 ),
 .UNSPECIFIED., .F., .F. ) 
 B_SPLINE_CURVE_WITH_KNOTS ( ( 3, 2, 2, 2, 3 ),
 ( 0.6901409369402313754, 0.6904761904761904656, 0.6964285714285713969, 0.7023809523809523281, 0.7027162059169114183 ),
 .UNSPECIFIED. ) 
 CURVE ( )  GEOMETRIC_REPRESENTATION_ITEM ( )  RATIONAL_B_SPLINE_CURVE ( ( 0.9963778908391764944, 0.9980808541467923733, 1.000000000000000000, 0.9659258262890682012, 1.000000000000000000, 0.9659258262890682012, 1.000000000000000000, 0.9980808541467923733, 0.9963778908391766054 ) ) 
 REPRESENTATION_ITEM ( '' )  );
#61821=CARTESIAN_POINT ( 'NONE',  ( 22.26659068614894466, 8.887082168247300018, 7.082119434687054849 ) ) ;
#61822=CARTESIAN_POINT ( 'NONE',  ( 10.00000000000000178, 37.25893115100078745, 9.846743663894594434 ) ) ;
#61825=CARTESIAN_POINT ( 'NONE',  ( 20.36894250292379382, 48.67874883491396076, 10.36894250292379205 ) ) ;
#61826=CARTESIAN_POINT ( 'NONE',  ( 0.1532563361054082862, 26.21726448433411605, 2.638427012816831674 ) ) ;
#61828=CARTESIAN_POINT ( 'NONE',  ( -0.1491070598754174470, 61.94583914210339515, -4.500000000000001776 ) ) ;
#61829=CARTESIAN_POINT ( 'NONE',  ( 0.5774900079438590739, 42.64701867748816966, -5.440088680355550821 ) ) ;
#61830=CARTESIAN_POINT ( 'NONE',  ( 3.591859063236761518, 49.95696800326375353, 11.09922568453594849 ) ) ;
#61831=CARTESIAN_POINT ( 'NONE',  ( 10.00000000000000178, 24.31368534415484106, 10.88017736071110342 ) ) ;
#61832=CARTESIAN_POINT ( 'NONE',  ( 13.43411237798106583, 52.66530133659708213, -12.81628187352647252 ) ) ;
#61833=CARTESIAN_POINT ( 'NONE',  ( 2.791683348922240793, 66.63393115100079456, 7.208316651077764092 ) ) ;
#61834=CARTESIAN_POINT ( 'NONE',  ( 1.472469842513823179, 1.425597817667451528, 4.923371831947296329 ) ) ;
#61836=CARTESIAN_POINT ( 'NONE',  ( 3.640395162852214650, 89.00000000000000000, 5.000000000000000000 ) ) ;
#61838=CARTESIAN_POINT ( 'NONE',  ( 6.204703633549690345, 60.76208216824730357, -14.16423886937410259 ) ) ;
#61839=CARTESIAN_POINT ( 'NONE',  ( 17.08211943468705130, 18.47041550158063572, 12.26659068614894998 ) ) ;
#61840=CARTESIAN_POINT ( 'NONE',  ( -0.8801773607111009756, 18.06368534415484106, 1.068504757029289695E-15 ) ) ;
#61842=CARTESIAN_POINT ( 'NONE',  ( 20.88017736071110875, 40.77201867748818387, -2.915334737309920765 ) ) ;
#61845=CARTESIAN_POINT ( 'NONE',  ( -0.8801773607110991993, 67.85535201082151957, -2.915334737309923874 ) ) ;
#61846=CARTESIAN_POINT ( 'NONE',  ( 4.559911319644449179, 58.89701867748817676, 9.422509992056141925 ) ) ;
#61847=CARTESIAN_POINT ( 'NONE',  ( 22.81628187352648496, 26.83196800326374998, -3.434112377981050290 ) ) ;
#61848=LINE ( 'NONE', #24370, #15589 ) ;
#61849=CARTESIAN_POINT ( 'NONE',  ( 14.92337183194729988, 4.342264484334117824, -8.527530157486177487 ) ) ;
#61850=CARTESIAN_POINT ( 'NONE',  ( 5.076628168052704559, 30.17559781766745175, -8.527530157486179263 ) ) ;
#61851=CIRCLE ( 'NONE', #76204, 0.5000000000000004441 ) ;
#61853=CARTESIAN_POINT ( 'NONE',  ( 4.559911319644449179, 12.23035201082150536, -9.422509992056141925 ) ) ;
#61856=CARTESIAN_POINT ( 'NONE',  ( -2.816281873526473856, 29.33196800326376064, 3.434112377981055619 ) ) ;
#61857=CARTESIAN_POINT ( 'NONE',  ( 2.791683348922240793, 6.633931151000785675, 7.208316651077764092 ) ) ;
#61859=CARTESIAN_POINT ( 'NONE',  ( 19.84674366389459266, 58.30059781766745886, 2.638427012816836559 ) ) ;
#61860=CARTESIAN_POINT ( 'NONE',  ( 0.1532563361054083140, 31.00893115100078390, 1.131784320476157264E-15 ) ) ;
#61861=CARTESIAN_POINT ( 'NONE',  ( 24.16423886937410614, 14.51208216824730179, -3.795296366450302550 ) ) ;
#61862=CARTESIAN_POINT ( 'NONE',  ( 12.91533473730992121, 29.52201867748817321, 10.88017736071110164 ) ) ;
#61863=CARTESIAN_POINT ( 'NONE',  ( 15.44008868035555260, 9.730352010821505360, 9.422509992056143702 ) ) ;
#61864=CARTESIAN_POINT ( 'NONE',  ( -0.8801773607111009756, 43.06368534415484106, 1.068504757029289695E-15 ) ) ;
#61865=CARTESIAN_POINT ( 'NONE',  ( 20.88017736071110875, 30.77201867748816966, -2.915334737309920765 ) ) ;
#61867=CARTESIAN_POINT ( 'NONE',  ( 22.81628187352647785, 36.41530133659707502, 3.434112377981063169 ) ) ;
#61868=CARTESIAN_POINT ( 'NONE',  ( -0.8801773607111009756, 38.06368534415484106, 1.068504757029289695E-15 ) ) ;
#61870=CARTESIAN_POINT ( 'NONE',  ( 6.565887622018943937, 55.16530133659709634, 12.81628187352647430 ) ) ;
#61871=CARTESIAN_POINT ( 'NONE',  ( -0.8801773607110991993, 47.85535201082150536, -2.915334737309923874 ) ) ;
#61872=ORIENTED_EDGE ( 'NONE', *, *, #26849, .T. ) ;
#61873=CARTESIAN_POINT ( 'NONE',  ( 20.88017736071110875, 45.77201867748816966, -2.915334737309920765 ) ) ;
#61876=CARTESIAN_POINT ( 'NONE',  ( 13.79529636645031943, 60.34541550158063927, -14.16423886937409904 ) ) ;
#61877=CARTESIAN_POINT ( 'NONE',  ( 15.44008868035555260, 64.73035201082151957, 9.422509992056143702 ) ) ;
#61880=CARTESIAN_POINT ( 'NONE',  ( 7.361572987183169658, -0.03273551566588185635, -9.846743663894592657 ) ) ;
#61882=CARTESIAN_POINT ( 'NONE',  ( 19.84674366389459266, 28.30059781766745886, 2.638427012816836559 ) ) ;
#61884=CARTESIAN_POINT ( 'NONE',  ( 17.20831665107776587, 37.88393115100078745, 7.208316651077764980 ) ) ;
#61885=CARTESIAN_POINT ( 'NONE',  ( 2.035157376598824452, 38.68868534415483396, 7.964842623401179544 ) ) ;
#61886=CARTESIAN_POINT ( 'NONE',  ( 0.1532563361054082862, 41.21726448433411605, 2.638427012816831674 ) ) ;
#61887=CARTESIAN_POINT ( 'NONE',  ( 21.09922568453594849, 16.20696800326375353, 6.408140936763242479 ) ) ;
#61888=CARTESIAN_POINT ( 'NONE',  ( 19.80427997160308706, 2.757339608395440678, -6.500000000000000000 ) ) ;
#61890=CARTESIAN_POINT ( 'NONE',  ( -0.8801773607111009756, 43.06368534415484106, 1.068504757029289695E-15 ) ) ;
#61891=CARTESIAN_POINT ( 'NONE',  ( 17.08211943468705130, 63.47041550158063927, 12.26659068614894998 ) ) ;
#61893=CARTESIAN_POINT ( 'NONE',  ( 22.81628187352647785, 21.62363466993041783, 6.195893100308588602E-16 ) ) ;
#61894=CARTESIAN_POINT ( 'NONE',  ( 17.39651004071842522, 24.08210964143329491, -6.499999999999992895 ) ) ;
#61895=ORIENTED_EDGE ( 'NONE', *, *, #16177, .F. ) ;
#61896=CARTESIAN_POINT ( 'NONE',  ( 16.40814093676323893, 30.79030133659708923, 11.09922568453595026 ) ) ;
#61897=CARTESIAN_POINT ( 'NONE',  ( 20.88017736071110164, 20.35535201082150891, 2.915334737309930979 ) ) ;
#61898=CARTESIAN_POINT ( 'NONE',  ( 0.5774900079438590739, 57.64701867748817676, -5.440088680355550821 ) ) ;
#61901=AXIS2_PLACEMENT_3D ( 'NONE', #34194, #57198, #73182 ) ;
#61902=EDGE_CURVE ( 'NONE', #11978, #51199, #88516, .T. ) ;
#61903=CARTESIAN_POINT ( 'NONE',  ( 0.1532563361054083140, 6.008931151000784787, 1.131784320476157264E-15 ) ) ;
#61904=CARTESIAN_POINT ( 'NONE',  ( 19.84674366389459266, 48.30059781766745175, 2.638427012816836559 ) ) ;
#61905=CARTESIAN_POINT ( 'NONE',  ( 5.076628168052704559, 40.17559781766745175, -8.527530157486179263 ) ) ;
#61907=CARTESIAN_POINT ( 'NONE',  ( 2.791683348922240793, 31.63393115100078745, 7.208316651077764092 ) ) ;
#61910=EDGE_CURVE ( 'NONE', #74651, #87105, #25315, .T. ) ;
#61911=CARTESIAN_POINT ( 'NONE',  ( 0.1532563361054083140, 16.00893115100078390, 1.131784320476157264E-15 ) ) ;
#61914=DIRECTION ( 'NONE',  ( 1.000000000000000000, -0.000000000000000000, -0.000000000000000000 ) ) ;
#61915=CARTESIAN_POINT ( 'NONE',  ( 12.63842701281683034, 47.46726448433412315, 9.846743663894596210 ) ) ;
#61919=CARTESIAN_POINT ( 'NONE',  ( 0.6178305044545818747, 8.498634669930421381, -9.382169495545419124 ) ) ;
#61920=CARTESIAN_POINT ( 'NONE',  ( 10.00000000000000000, 56.81368534415484106, -10.88017736071110342 ) ) ;
#61921=CARTESIAN_POINT ( 'NONE',  ( 2.917880565312950480, 45.97041550158063927, -12.26659068614894821 ) ) ;
#61924=CARTESIAN_POINT ( 'NONE',  ( 2.917880565312948704, 42.63708216824729647, 12.26659068614894643 ) ) ;
#61926=CARTESIAN_POINT ( 'NONE',  ( 24.16423886937409904, 54.09541550158063217, 3.795296366450317205 ) ) ;
#61927=CARTESIAN_POINT ( 'NONE',  ( 6.204703633549690345, 22.84541550158062861, 14.16423886937410082 ) ) ;
#61928=CARTESIAN_POINT ( 'NONE',  ( 13.79529636645030344, 23.26208216824730002, 14.16423886937410614 ) ) ;
#61930=LINE ( 'NONE', #75464, #3624 ) ;
#61932=CARTESIAN_POINT ( 'NONE',  ( 7.361572987183170547, 42.05059781766745886, 9.846743663894590881 ) ) ;
#61933=CARTESIAN_POINT ( 'NONE',  ( 20.88017736071110164, 20.35535201082150891, 2.915334737309930979 ) ) ;
#61935=CARTESIAN_POINT ( 'NONE',  ( -0.1503990784575328643, 70.00000000000000000, 6.262539305110068177 ) ) ;
#61936=CARTESIAN_POINT ( 'NONE',  ( 20.00000000000000000, 89.79522682798472033, -5.338983947147861286 ) ) ;
#61937=CARTESIAN_POINT ( 'NONE',  ( 19.84674366389459266, 33.71726448433410894, -2.638427012816827677 ) ) ;
#61938=CARTESIAN_POINT ( 'NONE',  ( 19.38216949554541202, 60.99863466993042493, 9.382169495545424454 ) ) ;
#61941=CARTESIAN_POINT ( 'NONE',  ( 0.1532563361054082862, 46.21726448433411605, 2.638427012816831674 ) ) ;
#61942=CARTESIAN_POINT ( 'NONE',  ( 17.20831665107776587, 49.13393115100078745, -7.208316651077762316 ) ) ;
#61943=CARTESIAN_POINT ( 'NONE',  ( -2.266590686148945544, 42.22041550158063217, 7.082119434687048631 ) ) ;
#61944=ORIENTED_EDGE ( 'NONE', *, *, #7702, .F. ) ;
#61945=CARTESIAN_POINT ( 'NONE',  ( 10.00000000000000000, 15.55374883491396787, -14.16423886937410082 ) ) ;
#61947=CARTESIAN_POINT ( 'NONE',  ( 19.05914839598885635, 44.96693863883977116, 6.499999999999962697 ) ) ;
#61949=CARTESIAN_POINT ( 'NONE',  ( 17.96484262340118221, 4.938685344154837509, 7.964842623401181321 ) ) ;
#61950=CARTESIAN_POINT ( 'NONE',  ( 6.565887622018943937, 5.165301336597086568, 12.81628187352647430 ) ) ;
#61951=CARTESIAN_POINT ( 'NONE',  ( -0.1503990784575282014, 57.22266099184919597, -6.262539305110077947 ) ) ;
#61952=CARTESIAN_POINT ( 'NONE',  ( 0.5774900079438607392, 68.48035201082150536, 5.440088680355550821 ) ) ;
#61953=CARTESIAN_POINT ( 'NONE',  ( 20.32896413005680714, 42.60497603579417358, -5.963430220938276349 ) ) ;
#61954=CARTESIAN_POINT ( 'NONE',  ( -0.1038446121089120627, 14.24302437010793376, -6.337995344473772441 ) ) ;
#61956=CARTESIAN_POINT ( 'NONE',  ( 20.36894250292379738, 64.92874883491397497, -10.36894250292379027 ) ) ;
#61958=CARTESIAN_POINT ( 'NONE',  ( 12.91533473730993009, 21.60535201082150536, -10.88017736071109987 ) ) ;
#61959=CARTESIAN_POINT ( 'NONE',  ( -0.8801773607111008646, 18.27201867748817321, 2.915334737309923430 ) ) ;
#61960=CARTESIAN_POINT ( 'NONE',  ( 5.076628168052703671, 61.84226448433412315, 8.527530157486179263 ) ) ;
#61961=CARTESIAN_POINT ( 'NONE',  ( 5.076628168052703671, 51.84226448433412315, 8.527530157486179263 ) ) ;
#61962=CARTESIAN_POINT ( 'NONE',  ( 0.6178305044545818747, 58.49863466993042493, -9.382169495545419124 ) ) ;
#61965=CARTESIAN_POINT ( 'NONE',  ( 17.96484262340118221, 31.18868534415483751, -7.964842623401177768 ) ) ;
#61967=CARTESIAN_POINT ( 'NONE',  ( 10.00000000000000000, 17.87363466993041783, -12.81628187352647608 ) ) ;
#61968=CARTESIAN_POINT ( 'NONE',  ( -0.2418659066527727997, 54.26028685723174050, -6.114288769123041867 ) ) ;
#61969=AXIS2_PLACEMENT_3D ( 'NONE', #58930, #74413, #66926 ) ;
#61970=CARTESIAN_POINT ( 'NONE',  ( 14.92337183194729633, 62.67559781766745886, 8.527530157486181039 ) ) ;
#61972=CARTESIAN_POINT ( 'NONE',  ( 17.96484262340118221, 49.93868534415484106, 7.964842623401181321 ) ) ;
#61973=CARTESIAN_POINT ( 'NONE',  ( 21.09922568453594849, 26.20696800326375353, 6.408140936763242479 ) ) ;
#61974=CARTESIAN_POINT ( 'NONE',  ( -0.8801773607110991993, 62.85535201082150536, -2.915334737309923874 ) ) ;
#61975=CARTESIAN_POINT ( 'NONE',  ( -0.1503990784575294781, 48.10158574516642460, 6.262539305110072618 ) ) ;
#61976=CARTESIAN_POINT ( 'NONE',  ( 0.1143410931637273975, 50.21691075486305067, 6.480892540919861666 ) ) ;
#61977=CARTESIAN_POINT ( 'NONE',  ( -2.816281873526471635, 63.91530133659708923, -3.434112377981056508 ) ) ;
#61978=ORIENTED_EDGE ( 'NONE', *, *, #51562, .T. ) ;
#61979=CARTESIAN_POINT ( 'NONE',  ( 19.42250999205614548, 50.98035201082151247, -5.440088680355545492 ) ) ;
#61980=CARTESIAN_POINT ( 'NONE',  ( -1.099225684535947600, 53.70696800326376064, -6.408140936763238038 ) ) ;
#61981=CARTESIAN_POINT ( 'NONE',  ( 20.36894250292379738, 19.92874883491396787, -10.36894250292379027 ) ) ;
#61984=CARTESIAN_POINT ( 'NONE',  ( 5.076628168052704559, 25.17559781766745175, -8.527530157486179263 ) ) ;
#61986=CARTESIAN_POINT ( 'NONE',  ( -4.164238869374099927, 62.01208216824728936, 3.795296366450308767 ) ) ;
#61988=CARTESIAN_POINT ( 'NONE',  ( 17.96484262340118221, 4.938685344154837509, 7.964842623401181321 ) ) ;
#61990=CARTESIAN_POINT ( 'NONE',  ( 19.42250999205614193, 10.14701867748816966, 5.440088680355555262 ) ) ;
#61993=CARTESIAN_POINT ( 'NONE',  ( -0.8801773607111008646, 8.272018677488171434, 2.915334737309923430 ) ) ;
#61994=CARTESIAN_POINT ( 'NONE',  ( 20.88017736071110519, 15.56368534415483751, 2.639326808657452039E-16 ) ) ;
#61995=CARTESIAN_POINT ( 'NONE',  ( 0.1532563361054100626, 40.80059781766745886, -2.638427012816831230 ) ) ;
#61997=CARTESIAN_POINT ( 'NONE',  ( 13.43411237798106583, 42.66530133659707502, -12.81628187352647252 ) ) ;
#61999=CARTESIAN_POINT ( 'NONE',  ( -2.266590686148945544, 26.38708216824730357, -7.082119434687050408 ) ) ;
#62000=CARTESIAN_POINT ( 'NONE',  ( 20.88017736071110875, 25.77201867748816966, -2.915334737309920765 ) ) ;
#62001=CARTESIAN_POINT ( 'NONE',  ( 20.88017736071110519, 5.563685344154838397, 2.639326808657452039E-16 ) ) ;
#62002=CARTESIAN_POINT ( 'NONE',  ( 17.20831665107776587, 42.88393115100077324, 7.208316651077764980 ) ) ;
#62004=CARTESIAN_POINT ( 'NONE',  ( 0.1532563361054082862, 26.21726448433411605, 2.638427012816831674 ) ) ;
#62006=SURFACE_STYLE_USAGE ( .BOTH. , #570 ) ;
#62008=VERTEX_POINT ( 'NONE', #85090 ) ;
#62009=CARTESIAN_POINT ( 'NONE',  ( 0.5774900079438590739, 2.647018677488170990, -5.440088680355550821 ) ) ;
#62010=CARTESIAN_POINT ( 'NONE',  ( 2.035157376598824452, 63.68868534415484106, 7.964842623401179544 ) ) ;
#62011=CARTESIAN_POINT ( 'NONE',  ( 17.20831665107776587, 52.88393115100078035, 7.208316651077764980 ) ) ;
#62012=CARTESIAN_POINT ( 'NONE',  ( 4.559911319644449179, 37.23035201082150536, -9.422509992056141925 ) ) ;
#62013=CARTESIAN_POINT ( 'NONE',  ( 0.5774900079438607392, 43.48035201082151247, 5.440088680355550821 ) ) ;
#62014=CARTESIAN_POINT ( 'NONE',  ( 20.88017736071110875, 5.772018677488170546, -2.915334737309920765 ) ) ;
#62015=CARTESIAN_POINT ( 'NONE',  ( 21.09922568453594849, 26.20696800326375353, 6.408140936763242479 ) ) ;
#62016=CARTESIAN_POINT ( 'NONE',  ( -4.164238869374099927, 22.01208216824730357, 3.795296366450308767 ) ) ;
#62018=CARTESIAN_POINT ( 'NONE',  ( 21.09922568453595559, 47.04030133659708923, -6.408140936763230044 ) ) ;
#62020=CARTESIAN_POINT ( 'NONE',  ( 1.472469842513823179, 41.42559781766745886, 4.923371831947296329 ) ) ;
#62021=CARTESIAN_POINT ( 'NONE',  ( 15.44008868035555260, 19.73035201082150536, 9.422509992056143702 ) ) ;
#62022=CARTESIAN_POINT ( 'NONE',  ( -0.8801773607110991993, 22.85535201082150181, -2.915334737309923874 ) ) ;
#62024=CARTESIAN_POINT ( 'NONE',  ( 20.88017736071110519, 60.56368534415484106, 2.639326808657452039E-16 ) ) ;
#62025=FACE_OUTER_BOUND ( 'NONE', #88566, .T. ) ;
#62027=CARTESIAN_POINT ( 'NONE',  ( 18.52753015748617571, 8.092264484334117824, 4.923371831947298993 ) ) ;
#62028=CARTESIAN_POINT ( 'NONE',  ( 12.91533473730993009, 61.60535201082150536, -10.88017736071109987 ) ) ;
#62029=ADVANCED_FACE ( 'NONE', ( #55068 ), #62568, .F. ) ;
#62030=CARTESIAN_POINT ( 'NONE',  ( -46.94000000000001194, 100.5254250115999923, 8.865097534344174690 ) ) ;
#62031=CARTESIAN_POINT ( 'NONE',  ( 0.1532563361054082862, 6.217264484334118713, 2.638427012816831674 ) ) ;
#62033=CARTESIAN_POINT ( 'NONE',  ( 2.791683348922240793, 41.63393115100078745, 7.208316651077764092 ) ) ;
#62035=VERTEX_POINT ( 'NONE', #85586 ) ;
#62038=CARTESIAN_POINT ( 'NONE',  ( 0.6178305044545818747, 53.49863466993041072, -9.382169495545419124 ) ) ;
#62039=CARTESIAN_POINT ( 'NONE',  ( -0.3689425029237898834, 1.178748834913967869, -10.36894250292378850 ) ) ;
#62040=CARTESIAN_POINT ( 'NONE',  ( 22.26659068614895176, 24.72041550158063572, -7.082119434687042414 ) ) ;
#62043=CARTESIAN_POINT ( 'NONE',  ( 20.15039907845753930, 70.00000000000000000, 6.262539305110068177 ) ) ;
#62044=CARTESIAN_POINT ( 'NONE',  ( 7.084665262690076126, 62.02201867748816966, -10.88017736071110164 ) ) ;
#62045=CARTESIAN_POINT ( 'NONE',  ( 17.96484262340118221, 24.93868534415484461, 7.964842623401181321 ) ) ;
#62046=CARTESIAN_POINT ( 'NONE',  ( 1.274849032794280523, 68.57228050351031357, 6.499999999999960032 ) ) ;
#62048=CARTESIAN_POINT ( 'NONE',  ( 10.00000000000000000, 4.758931151000784787, -9.846743663894594434 ) ) ;
#62049=CARTESIAN_POINT ( 'NONE',  ( 6.565887622018943937, 38.08196800326376064, -12.81628187352647608 ) ) ;
#62050=CARTESIAN_POINT ( 'NONE',  ( 18.52753015748618282, 23.92559781766745530, -4.923371831947291888 ) ) ;
#62052=CARTESIAN_POINT ( 'NONE',  ( -0.2538888227776796569, 70.00000000000000000, -6.092555545976966691 ) ) ;
#62053=CARTESIAN_POINT ( 'NONE',  ( 22.81628187352647785, 16.41530133659708923, 3.434112377981063169 ) ) ;
#62056=CARTESIAN_POINT ( 'NONE',  ( 7.361572987183170547, 7.050597817667451750, 9.846743663894590881 ) ) ;
#62058=CARTESIAN_POINT ( 'NONE',  ( 0.5774900079438607392, 23.48035201082150536, 5.440088680355550821 ) ) ;
#62059=CARTESIAN_POINT ( 'NONE',  ( -4.164238869374099039, 36.80374883491396787, 8.674139862899312516E-16 ) ) ;
#62060=CARTESIAN_POINT ( 'NONE',  ( 7.361572987183170547, 42.05059781766745886, 9.846743663894590881 ) ) ;
#62062=CARTESIAN_POINT ( 'NONE',  ( -0.8801773607111009756, 63.06368534415484106, 1.068504757029289695E-15 ) ) ;
#62063=CARTESIAN_POINT ( 'NONE',  ( 3.591859063236763294, 58.29030133659708923, -11.09922568453595026 ) ) ;
#62065=CARTESIAN_POINT ( 'NONE',  ( 0.5774900079438590739, 22.64701867748817321, -5.440088680355550821 ) ) ;
#62066=CARTESIAN_POINT ( 'NONE',  ( -2.816281873526471635, 8.915301336597083903, -3.434112377981056508 ) ) ;
#62067=CARTESIAN_POINT ( 'NONE',  ( 0.1532563361054082862, 36.21726448433410894, 2.638427012816831674 ) ) ;
#62069=CARTESIAN_POINT ( 'NONE',  ( 13.43411237798105340, 50.58196800326375353, 12.81628187352647963 ) ) ;
#62071=CARTESIAN_POINT ( 'NONE',  ( 4.559911319644449179, 48.89701867748817676, 9.422509992056141925 ) ) ;
#62075=CARTESIAN_POINT ( 'NONE',  ( 7.084665262690076126, 54.10535201082151247, 10.88017736071109987 ) ) ;
#62076=CARTESIAN_POINT ( 'NONE',  ( 4.559911319644449179, 58.89701867748817676, 9.422509992056141925 ) ) ;
#62078=CARTESIAN_POINT ( 'NONE',  ( 4.559911319644449179, 63.89701867748817676, 9.422509992056141925 ) ) ;
#62081=CARTESIAN_POINT ( 'NONE',  ( -0.8801773607111009756, 13.06368534415483929, 1.068504757029289695E-15 ) ) ;
#62082=CARTESIAN_POINT ( 'NONE',  ( 10.00000000000000000, 49.75893115100078745, -9.846743663894594434 ) ) ;
#62083=CARTESIAN_POINT ( 'NONE',  ( 7.084665262690076126, 17.02201867748817676, -10.88017736071110164 ) ) ;
#62085=CARTESIAN_POINT ( 'NONE',  ( 19.38216949554541202, 30.99863466993042138, 9.382169495545424454 ) ) ;
#62086=ORIENTED_EDGE ( 'NONE', *, *, #64267, .F. ) ;
#62087=CARTESIAN_POINT ( 'NONE',  ( -0.8801773607111008646, 38.27201867748816255, 2.915334737309923430 ) ) ;
#62088=CARTESIAN_POINT ( 'NONE',  ( 21.09922568453594849, 11.20696800326375531, 6.408140936763242479 ) ) ;
#62089=CARTESIAN_POINT ( 'NONE',  ( 12.91533473730992121, 14.52201867748817143, 10.88017736071110164 ) ) ;
#62090=CARTESIAN_POINT ( 'NONE',  ( -0.8801773607111009756, 43.06368534415484106, 1.068504757029289695E-15 ) ) ;
#62091=CARTESIAN_POINT ( 'NONE',  ( -2.266590686148945544, 41.38708216824729647, -7.082119434687050408 ) ) ;
#62092=CARTESIAN_POINT ( 'NONE',  ( 2.791683348922240793, 26.63393115100078745, 7.208316651077764092 ) ) ;
#62094=CARTESIAN_POINT ( 'NONE',  ( 7.084665262690076126, 59.10535201082150536, 10.88017736071109987 ) ) ;
#62096=CARTESIAN_POINT ( 'NONE',  ( -2.266590686148945544, 22.22041550158063572, 7.082119434687048631 ) ) ;
#62098=CARTESIAN_POINT ( 'NONE',  ( 0.1532563361054083140, 56.00893115100078745, 1.131784320476157264E-15 ) ) ;
#62100=CARTESIAN_POINT ( 'NONE',  ( 2.917880565312948704, 37.63708216824731068, 12.26659068614894643 ) ) ;
#62101=CARTESIAN_POINT ( 'NONE',  ( 6.204703633549690345, 32.84541550158063927, 14.16423886937410082 ) ) ;
#62102=CARTESIAN_POINT ( 'NONE',  ( 17.20831665107776587, 7.883931151000784787, 7.208316651077764980 ) ) ;
#62103=CARTESIAN_POINT ( 'NONE',  ( 0.1532563361054082862, 56.21726448433411605, 2.638427012816831674 ) ) ;
#62105=CARTESIAN_POINT ( 'NONE',  ( 20.88017736071110164, 55.35535201082149825, 2.915334737309930979 ) ) ;
#62106=CARTESIAN_POINT ( 'NONE',  ( -1.099225684535947600, 18.70696800326375353, -6.408140936763238038 ) ) ;
#62107=CARTESIAN_POINT ( 'NONE',  ( 24.16423886937410614, 34.30374883491396787, 8.672049930838204340E-16 ) ) ;
#62108=CARTESIAN_POINT ( 'NONE',  ( -0.8801773607111008646, 33.27201867748817676, 2.915334737309923430 ) ) ;
#62109=CARTESIAN_POINT ( 'NONE',  ( 4.559911319644449179, 33.89701867748817676, 9.422509992056141925 ) ) ;
#62110=LINE ( 'NONE', #69149, #38039 ) ;
#62111=CARTESIAN_POINT ( 'NONE',  ( 7.084665262690076126, 54.10535201082151247, 10.88017736071109987 ) ) ;
#62112=ADVANCED_FACE ( 'NONE', ( #95035 ), #63066, .T. ) ;
#62119=CARTESIAN_POINT ( 'NONE',  ( 13.79529636645030344, 3.262082168247301350, 14.16423886937410614 ) ) ;
#62120=CARTESIAN_POINT ( 'NONE',  ( 2.917880565312950480, 60.97041550158063927, -12.26659068614894821 ) ) ;
#62121=CARTESIAN_POINT ( 'NONE',  ( 2.917880565312950480, 65.97041550158063217, -12.26659068614894821 ) ) ;
#62122=CARTESIAN_POINT ( 'NONE',  ( 2.791683348922237240, 40.38393115100078035, -7.208316651077763204 ) ) ;
#62123=CARTESIAN_POINT ( 'NONE',  ( 0.1532563361054083140, 56.00893115100078745, 1.131784320476157264E-15 ) ) ;
#62127=CARTESIAN_POINT ( 'NONE',  ( 6.565887622018943937, 0.1653013365970866511, 12.81628187352647430 ) ) ;
#62128=VERTEX_POINT ( 'NONE', #26544 ) ;
#62129=CARTESIAN_POINT ( 'NONE',  ( 24.16423886937410614, 44.51208216824730357, -3.795296366450302550 ) ) ;
#62130=B_SPLINE_CURVE_WITH_KNOTS ( 'NONE', 3,
 ( #68418, #29407, #59910, #53396, #7433, #77372 ),
 .UNSPECIFIED., .F., .F.,
 ( 4, 2, 4 ),
 ( 5.553824967135426632E-18, 0.0002605067024380922601, 0.0005210134048761789908 ),
 .UNSPECIFIED. ) ;
#62131=CARTESIAN_POINT ( 'NONE',  ( -2.266590686148945544, 41.38708216824729647, -7.082119434687050408 ) ) ;
#62133=CARTESIAN_POINT ( 'NONE',  ( 10.00000000000000178, 14.31368534415483751, 10.88017736071110342 ) ) ;
#62134=CARTESIAN_POINT ( 'NONE',  ( 21.09922568453595559, 57.04030133659708923, -6.408140936763230044 ) ) ;
#62135=CARTESIAN_POINT ( 'NONE',  ( 0.1532563361054083140, 51.00893115100078745, 1.131784320476157264E-15 ) ) ;
#62136=CARTESIAN_POINT ( 'NONE',  ( -0.8801773607111009756, 38.06368534415484106, 1.068504757029289695E-15 ) ) ;
#62137=CARTESIAN_POINT ( 'NONE',  ( -0.1503990784575242878, 64.24884699246891273, -6.262539305110083276 ) ) ;
#62138=CARTESIAN_POINT ( 'NONE',  ( 19.84674366389459266, 53.30059781766744464, 2.638427012816836559 ) ) ;
#62139=CARTESIAN_POINT ( 'NONE',  ( 19.42250999205614193, 60.14701867748817676, 5.440088680355555262 ) ) ;
#62140=CARTESIAN_POINT ( 'NONE',  ( 0.5774900079438590739, 32.64701867748816966, -5.440088680355550821 ) ) ;
#62141=VECTOR ( 'NONE', #23584, 1000.000000000000000 ) ;
#62143=CARTESIAN_POINT ( 'NONE',  ( 19.84674366389459621, 3.508931151000785231, 7.409399052514197653E-17 ) ) ;
#62147=CARTESIAN_POINT ( 'NONE',  ( 0.1532563361054100626, 35.80059781766745175, -2.638427012816831230 ) ) ;
#62149=CARTESIAN_POINT ( 'NONE',  ( 0.6178305044545838731, 44.74863466993042493, 9.382169495545420901 ) ) ;
#62150=CARTESIAN_POINT ( 'NONE',  ( 19.72487221294570858, 70.00000000000000000, 6.000000000000000000 ) ) ;
#62156=CARTESIAN_POINT ( 'NONE',  ( 7.361572987183169658, 49.96726448433410894, -9.846743663894592657 ) ) ;
#62157=CARTESIAN_POINT ( 'NONE',  ( -0.3689425029237898834, 51.17874883491397497, -10.36894250292378850 ) ) ;
#62158=CARTESIAN_POINT ( 'NONE',  ( 0.1532563361054083140, 61.00893115100078745, 1.131784320476157264E-15 ) ) ;
#62160=CARTESIAN_POINT ( 'NONE',  ( 7.361572987183170547, 22.05059781766745530, 9.846743663894590881 ) ) ;
#62161=CARTESIAN_POINT ( 'NONE',  ( 3.591859063236761518, 49.95696800326375353, 11.09922568453594849 ) ) ;
#62162=EDGE_CURVE ( 'NONE', #53783, #56374, #61060, .T. ) ;
#62164=CARTESIAN_POINT ( 'NONE',  ( 17.20831665107776587, 59.13393115100078745, -7.208316651077762316 ) ) ;
#62165=CARTESIAN_POINT ( 'NONE',  ( 0.5774900079438590739, 47.64701867748817676, -5.440088680355550821 ) ) ;
#62166=CARTESIAN_POINT ( 'NONE',  ( 19.84674366389459266, 48.71726448433413026, -2.638427012816827677 ) ) ;
#62168=CARTESIAN_POINT ( 'NONE',  ( -0.8801773607111009756, 53.06368534415484106, 1.068504757029289695E-15 ) ) ;
#62171=CARTESIAN_POINT ( 'NONE',  ( -0.8801773607110991993, 22.85535201082150181, -2.915334737309923874 ) ) ;
#62172=CARTESIAN_POINT ( 'NONE',  ( 0.6178305044545818747, 13.49863466993041783, -9.382169495545419124 ) ) ;
#62173=CARTESIAN_POINT ( 'NONE',  ( -0.8801773607111009756, 53.06368534415484106, 1.068504757029289695E-15 ) ) ;
#62176=CARTESIAN_POINT ( 'NONE',  ( 20.15039907845753220, 45.60158574516643881, -6.262539305110077947 ) ) ;
#62177=CARTESIAN_POINT ( 'NONE',  ( 12.91533473730992121, 54.52201867748816255, 10.88017736071110164 ) ) ;
#62179=CARTESIAN_POINT ( 'NONE',  ( 0.1532563361054100626, 35.80059781766745175, -2.638427012816831230 ) ) ;
#62180=CARTESIAN_POINT ( 'NONE',  ( 0.1532563361054100626, 5.800597817667452638, -2.638427012816831230 ) ) ;
#62182=CARTESIAN_POINT ( 'NONE',  ( 10.00000000000000000, 7.873634669930421381, -12.81628187352647608 ) ) ;
#62184=CARTESIAN_POINT ( 'NONE',  ( 7.084665262690076126, 14.10535201082150358, 10.88017736071109987 ) ) ;
#62185=SURFACE_SIDE_STYLE ('',( #56186 ) ) ;
#62187=CARTESIAN_POINT ( 'NONE',  ( -0.3689425029237898834, 41.17874883491397497, -10.36894250292378850 ) ) ;
#62188=CARTESIAN_POINT ( 'NONE',  ( 6.204703633549690345, 60.76208216824730357, -14.16423886937410259 ) ) ;
#62189=CARTESIAN_POINT ( 'NONE',  ( 1.472469842513823179, 31.42559781766745530, 4.923371831947296329 ) ) ;
#62190=CARTESIAN_POINT ( 'NONE',  ( 14.92337183194729988, 24.34226448433411960, -8.527530157486177487 ) ) ;
#62191=CARTESIAN_POINT ( 'NONE',  ( -0.8801773607111009756, 18.06368534415484106, 1.068504757029289695E-15 ) ) ;
#62194=CARTESIAN_POINT ( 'NONE',  ( 19.84674366389459266, 38.71726448433412315, -2.638427012816827677 ) ) ;
#62195=CARTESIAN_POINT ( 'NONE',  ( 10.00000000000000178, 29.31368534415483751, 10.88017736071110342 ) ) ;
#62196=B_SPLINE_CURVE_WITH_KNOTS ( 'NONE', 3,
 ( #28745, #60231, #29236, #52242, #90726, #22251 ),
 .UNSPECIFIED., .F., .F.,
 ( 4, 2, 4 ),
 ( 0.000000000000000000, 0.0002605067024380928564, 0.0005210134048761857128 ),
 .UNSPECIFIED. ) ;
#62197=CARTESIAN_POINT ( 'NONE',  ( 0.1532563361054100626, 65.80059781766745175, -2.638427012816831230 ) ) ;
#62198=CARTESIAN_POINT ( 'NONE',  ( 24.16423886937409904, 9.095415501580633943, 3.795296366450317205 ) ) ;
#62199=CARTESIAN_POINT ( 'NONE',  ( -1.926860441876563801, 17.66212336850780673, 1.004413902775740978E-15 ) ) ;
#62202=UNCERTAINTY_MEASURE_WITH_UNIT (LENGTH_MEASURE( 1.000000000000000082E-05 ), #21044, 'distance_accuracy_value', 'NONE');
#62203=CARTESIAN_POINT ( 'NONE',  ( 7.361572987183170547, 17.05059781766745530, 9.846743663894590881 ) ) ;
#62204=CARTESIAN_POINT ( 'NONE',  ( 13.43411237798105340, 35.58196800326375353, 12.81628187352647963 ) ) ;
#62205=CARTESIAN_POINT ( 'NONE',  ( 17.20831665107776587, 49.13393115100078745, -7.208316651077762316 ) ) ;
#62206=EDGE_LOOP ( 'NONE', ( #58574, #30713, #59442, #44932 ) ) ;
#62207=CARTESIAN_POINT ( 'NONE',  ( 5.076628168052703671, 16.84226448433411960, 8.527530157486179263 ) ) ;
#62208=CYLINDRICAL_SURFACE ( 'NONE', #25374, 0.5000000000000004441 ) ;
#62211=CARTESIAN_POINT ( 'NONE',  ( 2.917880565312948704, 52.63708216824730357, 12.26659068614894643 ) ) ;
#62212=CARTESIAN_POINT ( 'NONE',  ( 10.00000000000000178, 49.31368534415484106, 10.88017736071110342 ) ) ;
#62213=FACE_OUTER_BOUND ( 'NONE', #66109, .T. ) ;
#62214=CARTESIAN_POINT ( 'NONE',  ( 12.91533473730993009, 51.60535201082149825, -10.88017736071109987 ) ) ;
#62215=CARTESIAN_POINT ( 'NONE',  ( 0.1532563361054083140, 31.00893115100078390, 1.131784320476157264E-15 ) ) ;
#62216=CARTESIAN_POINT ( 'NONE',  ( 0.5774900079438607392, 23.48035201082150536, 5.440088680355550821 ) ) ;
#62218=CARTESIAN_POINT ( 'NONE',  ( 1.472469842513823179, 50.59226448433411605, -4.923371831947296329 ) ) ;
#62221=CARTESIAN_POINT ( 'NONE',  ( 17.96484262340118221, 46.18868534415484106, -7.964842623401177768 ) ) ;
#62227=CARTESIAN_POINT ( 'NONE',  ( 18.52753015748617571, 48.09226448433412315, 4.923371831947298993 ) ) ;
#62228=CARTESIAN_POINT ( 'NONE',  ( 10.00000000000000178, 17.25893115100078745, 9.846743663894594434 ) ) ;
#62229=CARTESIAN_POINT ( 'NONE',  ( 16.40814093676323893, 55.79030133659708923, 11.09922568453595026 ) ) ;
#62230=CARTESIAN_POINT ( 'NONE',  ( 2.035157376598822676, 17.43868534415483751, -7.964842623401177768 ) ) ;
#62231=CARTESIAN_POINT ( 'NONE',  ( 7.361572987183169658, 44.96726448433412315, -9.846743663894592657 ) ) ;
#62233=CARTESIAN_POINT ( 'NONE',  ( 13.79529636645031943, 45.34541550158062506, -14.16423886937409904 ) ) ;
#62234=CARTESIAN_POINT ( 'NONE',  ( 10.00000000000000000, 55.55374883491396787, -14.16423886937410082 ) ) ;
#62237=CARTESIAN_POINT ( 'NONE',  ( 15.44008868035555793, 51.39701867748816966, -9.422509992056140149 ) ) ;
#62239=CARTESIAN_POINT ( 'NONE',  ( 0.1532563361054082862, 21.21726448433412315, 2.638427012816831674 ) ) ;
#62242=CARTESIAN_POINT ( 'NONE',  ( 20.15039907845753220, 30.60158574516642815, -6.262539305110077947 ) ) ;
#62243=EDGE_LOOP ( 'NONE', ( #57601, #66697, #68082, #29666 ) ) ;
#62244=CARTESIAN_POINT ( 'NONE',  ( 0.1532563361054082862, 16.21726448433411960, 2.638427012816831674 ) ) ;
#62245=ORIENTED_EDGE ( 'NONE', *, *, #38184, .F. ) ;
#62246=CARTESIAN_POINT ( 'NONE',  ( 17.08211943468705130, 13.47041550158063572, 12.26659068614894998 ) ) ;
#62247=CARTESIAN_POINT ( 'NONE',  ( 0.1532563361054083140, 16.00893115100078390, 1.131784320476157264E-15 ) ) ;
#62248=CARTESIAN_POINT ( 'NONE',  ( 15.44008868035555260, 39.73035201082150536, 9.422509992056143702 ) ) ;
#62251=ADVANCED_FACE ( 'NONE', ( #50036 ), #5040, .T. ) ;
#62252=CARTESIAN_POINT ( 'NONE',  ( 19.42250999205614548, 40.98035201082150536, -5.440088680355545492 ) ) ;
#62253=CARTESIAN_POINT ( 'NONE',  ( -0.04068437667224381049, 2.219743609177204036, -6.396802510829708410 ) ) ;
#62255=CARTESIAN_POINT ( 'NONE',  ( 24.16423886937409904, 9.095415501580633943, 3.795296366450317205 ) ) ;
#62257=CARTESIAN_POINT ( 'NONE',  ( -1.099225684535947600, 14.54030133659708568, 6.408140936763237150 ) ) ;
#62258=CARTESIAN_POINT ( 'NONE',  ( 14.92337183194729988, 9.342264484334119601, -8.527530157486177487 ) ) ;
#62260=CARTESIAN_POINT ( 'NONE',  ( 19.42250999205614193, 10.14701867748816966, 5.440088680355555262 ) ) ;
#62261=CARTESIAN_POINT ( 'NONE',  ( 0.1532563361054100626, 20.80059781766744464, -2.638427012816831230 ) ) ;
#62262=CARTESIAN_POINT ( 'NONE',  ( 7.084665262690076126, 37.02201867748817676, -10.88017736071110164 ) ) ;
#62263=EDGE_LOOP ( 'NONE', ( #9729, #67298, #29075, #2586 ) ) ;
#62264=CARTESIAN_POINT ( 'NONE',  ( 0.6178305044545818747, 63.49863466993043204, -9.382169495545419124 ) ) ;
#62265=CARTESIAN_POINT ( 'NONE',  ( 15.44008868035555793, 56.39701867748817676, -9.422509992056140149 ) ) ;
#62267=CARTESIAN_POINT ( 'NONE',  ( 15.44008868035555793, 66.39701867748817676, -9.422509992056140149 ) ) ;
#62270=AXIS2_PLACEMENT_3D ( 'NONE', #94801, #10333, #40345 ) ;
#62272=CARTESIAN_POINT ( 'NONE',  ( 1.472469842513823179, 26.42559781766745175, 4.923371831947296329 ) ) ;
#62273=CARTESIAN_POINT ( 'NONE',  ( 3.591859063236763294, 58.29030133659708923, -11.09922568453595026 ) ) ;
#62274=CARTESIAN_POINT ( 'NONE',  ( 17.08211943468705840, 5.137082168247300906, -12.26659068614894466 ) ) ;
#62275=CARTESIAN_POINT ( 'NONE',  ( 12.63842701281683922, 19.55059781766745175, -9.846743663894590881 ) ) ;
#62276=CARTESIAN_POINT ( 'NONE',  ( 0.6178305044545838731, 24.74863466993042493, 9.382169495545420901 ) ) ;
#62279=CARTESIAN_POINT ( 'NONE',  ( 12.91533473730993009, 51.60535201082149825, -10.88017736071109987 ) ) ;
#62281=CARTESIAN_POINT ( 'NONE',  ( 19.84674366389459266, 63.71726448433412315, -2.638427012816827677 ) ) ;
#62283=EDGE_CURVE ( 'NONE', #16435, #14763, #14960, .T. ) ;
#62285=CARTESIAN_POINT ( 'NONE',  ( 12.63842701281683034, 32.46726448433412315, 9.846743663894596210 ) ) ;
#62286=CARTESIAN_POINT ( 'NONE',  ( 0.1532563361054082862, 16.21726448433411960, 2.638427012816831674 ) ) ;
#62287=CARTESIAN_POINT ( 'NONE',  ( 17.96484262340118221, 11.18868534415483929, -7.964842623401177768 ) ) ;
#62288=CARTESIAN_POINT ( 'NONE',  ( 0.6178305044545818747, 18.49863466993041428, -9.382169495545419124 ) ) ;
#62289=CARTESIAN_POINT ( 'NONE',  ( 7.084665262690076126, 4.105352010821503583, 10.88017736071109987 ) ) ;
#62291=CARTESIAN_POINT ( 'NONE',  ( -0.8801773607111009756, 23.06368534415484106, 1.068504757029289695E-15 ) ) ;
#62294=CARTESIAN_POINT ( 'NONE',  ( 7.361572987183169658, 29.96726448433411960, -9.846743663894592657 ) ) ;
#62295=CARTESIAN_POINT ( 'NONE',  ( 20.88017736071110875, 20.77201867748816611, -2.915334737309920765 ) ) ;
#62297=CARTESIAN_POINT ( 'NONE',  ( 7.084665262690076126, 32.02201867748816966, -10.88017736071110164 ) ) ;
#62298=CARTESIAN_POINT ( 'NONE',  ( -0.8801773607111009756, 3.063685344154838397, 1.068504757029289695E-15 ) ) ;
#62300=CARTESIAN_POINT ( 'NONE',  ( 18.52753015748618282, 18.92559781766745175, -4.923371831947291888 ) ) ;
#62301=CARTESIAN_POINT ( 'NONE',  ( 17.20831665107776587, 42.88393115100077324, 7.208316651077764980 ) ) ;
#62306=CARTESIAN_POINT ( 'NONE',  ( 22.26659068614895176, 24.72041550158063572, -7.082119434687042414 ) ) ;
#62307=CARTESIAN_POINT ( 'NONE',  ( 7.361572987183170547, 37.05059781766744464, 9.846743663894590881 ) ) ;
#62310=EDGE_LOOP ( 'NONE', ( #68626, #48105, #7264, #62623 ) ) ;
#62311=CARTESIAN_POINT ( 'NONE',  ( 24.16423886937409904, 54.09541550158063217, 3.795296366450317205 ) ) ;
#62312=CARTESIAN_POINT ( 'NONE',  ( 0.1532563361054083140, 26.00893115100078745, 1.131784320476157264E-15 ) ) ;
#62315=CARTESIAN_POINT ( 'NONE',  ( 7.084665262690076126, 42.02201867748816966, -10.88017736071110164 ) ) ;
#62316=CARTESIAN_POINT ( 'NONE',  ( 21.09922568453595559, 52.04030133659708923, -6.408140936763230044 ) ) ;
#62318=CARTESIAN_POINT ( 'NONE',  ( 4.559911319644449179, 13.89701867748817143, 9.422509992056141925 ) ) ;
#62319=CARTESIAN_POINT ( 'NONE',  ( -1.099225684535947600, 44.54030133659708923, 6.408140936763237150 ) ) ;
#62320=CARTESIAN_POINT ( 'NONE',  ( 19.38216949554541202, 0.9986346699304200492, 9.382169495545424454 ) ) ;
#62321=CARTESIAN_POINT ( 'NONE',  ( 19.84674366389459266, 3.300597817667451750, 2.638427012816836559 ) ) ;
#62325=CARTESIAN_POINT ( 'NONE',  ( -2.266590686148945544, 57.22041550158063217, 7.082119434687048631 ) ) ;
#62326=CARTESIAN_POINT ( 'NONE',  ( 24.16423886937409904, 9.095415501580633943, 3.795296366450317205 ) ) ;
#62327=CARTESIAN_POINT ( 'NONE',  ( 12.91533473730993009, 21.60535201082150536, -10.88017736071109987 ) ) ;
#62328=CARTESIAN_POINT ( 'NONE',  ( 20.88017736071110519, 30.56368534415484106, 2.639326808657452039E-16 ) ) ;
#62331=CARTESIAN_POINT ( 'NONE',  ( 19.42250999205614193, 65.14701867748817676, 5.440088680355555262 ) ) ;
#62332=FACE_OUTER_BOUND ( 'NONE', #48421, .T. ) ;
#62333=CARTESIAN_POINT ( 'NONE',  ( 7.361572987183170547, 17.05059781766745530, 9.846743663894590881 ) ) ;
#62336=CARTESIAN_POINT ( 'NONE',  ( 18.52753015748618282, 13.92559781766745175, -4.923371831947291888 ) ) ;
#62337=CARTESIAN_POINT ( 'NONE',  ( 12.63842701281683034, 37.46726448433411605, 9.846743663894596210 ) ) ;
#62338=CARTESIAN_POINT ( 'NONE',  ( 7.084665262690076126, 17.02201867748817676, -10.88017736071110164 ) ) ;
#62340=CARTESIAN_POINT ( 'NONE',  ( 6.565887622018943937, 33.08196800326374643, -12.81628187352647608 ) ) ;
#62341=CARTESIAN_POINT ( 'NONE',  ( 1.472469842513823179, 5.592264484334118713, -4.923371831947296329 ) ) ;
#62342=EDGE_CURVE ( 'NONE', #73676, #98326, #84206, .T. ) ;
#62344=CARTESIAN_POINT ( 'NONE',  ( 5.076628168052704559, 55.17559781766745175, -8.527530157486179263 ) ) ;
#62345=B_SPLINE_CURVE_WITH_KNOTS ( 'NONE', 3,
 ( #19235, #49717, #42243, #5721 ),
 .UNSPECIFIED., .F., .F.,
 ( 4, 4 ),
 ( 0.000000000000000000, 0.001036303429213390010 ),
 .UNSPECIFIED. ) ;
#62346=CARTESIAN_POINT ( 'NONE',  ( 5.076628168052703671, 31.84226448433412315, 8.527530157486179263 ) ) ;
#62347=CARTESIAN_POINT ( 'NONE',  ( 24.16423886937409904, 19.09541550158063927, 3.795296366450317205 ) ) ;
#62349=CARTESIAN_POINT ( 'NONE',  ( 12.91533473730993009, 46.60535201082150536, -10.88017736071109987 ) ) ;
#62350=CARTESIAN_POINT ( 'NONE',  ( 0.5774900079438607392, 8.480352010821505360, 5.440088680355550821 ) ) ;
#62352=CARTESIAN_POINT ( 'NONE',  ( 0.5774900079438590739, 47.64701867748817676, -5.440088680355550821 ) ) ;
#62353=CARTESIAN_POINT ( 'NONE',  ( 2.035157376598822676, 32.43868534415483396, -7.964842623401177768 ) ) ;
#62354=ORIENTED_EDGE ( 'NONE', *, *, #28961, .F. ) ;
#62355=CARTESIAN_POINT ( 'NONE',  ( -0.8801773607111009756, 43.06368534415484106, 1.068504757029289695E-15 ) ) ;
#62357=CARTESIAN_POINT ( 'NONE',  ( 3.591859063236761518, 59.95696800326375353, 11.09922568453594849 ) ) ;
#62358=CARTESIAN_POINT ( 'NONE',  ( 2.035157376598822676, 47.43868534415484817, -7.964842623401177768 ) ) ;
#62360=CARTESIAN_POINT ( 'NONE',  ( 7.084665262690076126, 47.02201867748818387, -10.88017736071110164 ) ) ;
#62362=CARTESIAN_POINT ( 'NONE',  ( 19.10478245763049898, 41.02576239577082617, -5.990408912944356956 ) ) ;
#62364=CARTESIAN_POINT ( 'NONE',  ( -2.266590686148945544, 61.38708216824730357, -7.082119434687050408 ) ) ;
#62365=CARTESIAN_POINT ( 'NONE',  ( 0.5774900079438590739, 67.64701867748817676, -5.440088680355550821 ) ) ;
#62366=CARTESIAN_POINT ( 'NONE',  ( -4.164238869374098151, 11.59541550158063217, -3.795296366450310543 ) ) ;
#62368=CARTESIAN_POINT ( 'NONE',  ( 17.96484262340118221, 6.188685344154836621, -7.964842623401177768 ) ) ;
#62369=CARTESIAN_POINT ( 'NONE',  ( 10.00000000000000178, 47.25893115100078745, 9.846743663894594434 ) ) ;
#62371=CARTESIAN_POINT ( 'NONE',  ( 12.63842701281683034, 42.46726448433412315, 9.846743663894596210 ) ) ;
#62372=CARTESIAN_POINT ( 'NONE',  ( 15.44008868035555260, 64.73035201082151957, 9.422509992056143702 ) ) ;
#62373=CARTESIAN_POINT ( 'NONE',  ( 12.91533473730992121, 44.52201867748816966, 10.88017736071110164 ) ) ;
#62374=CARTESIAN_POINT ( 'NONE',  ( 14.92337183194729988, 34.34226448433411605, -8.527530157486177487 ) ) ;
#62376=CARTESIAN_POINT ( 'NONE',  ( 15.44008868035555260, 39.73035201082150536, 9.422509992056143702 ) ) ;
#62377=CARTESIAN_POINT ( 'NONE',  ( -0.3689425029237881626, 52.42874883491396076, 10.36894250292379027 ) ) ;
#62379=B_SPLINE_CURVE_WITH_KNOTS ( 'NONE', 3,
 ( #94408, #34384, #77930, #18917, #56896, #72386, #93428, #26896 ),
 .UNSPECIFIED., .F., .F.,
 ( 4, 2, 2, 4 ),
 ( 0.000000000000000000, 0.004806130321901048823, 0.007209195482851595352, 0.009612260643802141014 ),
 .UNSPECIFIED. ) ;
#62380=CARTESIAN_POINT ( 'NONE',  ( 10.00000000000000000, 17.87363466993041783, -12.81628187352647608 ) ) ;
#62384=CARTESIAN_POINT ( 'NONE',  ( 10.00000000000000000, 22.87363466993042138, -12.81628187352647608 ) ) ;
#62385=CARTESIAN_POINT ( 'NONE',  ( 15.44008868035555793, 26.39701867748817321, -9.422509992056140149 ) ) ;
#62387=CARTESIAN_POINT ( 'NONE',  ( 2.791683348922237240, 0.3839311510007847872, -7.208316651077763204 ) ) ;
#62388=CARTESIAN_POINT ( 'NONE',  ( 10.00000000000000000, 49.75893115100078745, -9.846743663894594434 ) ) ;
#62389=CARTESIAN_POINT ( 'NONE',  ( 7.361572987183170547, 12.05059781766744997, 9.846743663894590881 ) ) ;
#62390=CARTESIAN_POINT ( 'NONE',  ( 1.472469842513823179, 31.42559781766745530, 4.923371831947296329 ) ) ;
#62393=CARTESIAN_POINT ( 'NONE',  ( 14.92337183194729633, 22.67559781766745175, 8.527530157486181039 ) ) ;
#62396=CARTESIAN_POINT ( 'NONE',  ( 2.791683348922237240, 10.38393115100078390, -7.208316651077763204 ) ) ;
#62398=CARTESIAN_POINT ( 'NONE',  ( 2.791683348922240793, 41.63393115100078745, 7.208316651077764092 ) ) ;
#62400=( BOUNDED_CURVE ( )  B_SPLINE_CURVE ( 2, ( #84341, #84819, #68840, #91830, #97877, #372, #14362, #30323, #14864 ),
 .UNSPECIFIED., .F., .F. ) 
 B_SPLINE_CURVE_WITH_KNOTS ( ( 3, 2, 2, 2, 3 ),
 ( 0.1534289457926083233, 0.1547619047619047672, 0.1607142857142857262, 0.1666666666666666574, 0.1679996256359629347 ),
 .UNSPECIFIED. ) 
 CURVE ( )  GEOMETRIC_REPRESENTATION_ITEM ( )  RATIONAL_B_SPLINE_CURVE ( ( 0.9881565478350731180, 0.9923695281211489805, 1.000000000000000000, 0.9659258262890683122, 1.000000000000000000, 0.9659258262890683122, 1.000000000000000000, 0.9923695281211498687, 0.9881565478350742282 ) ) 
 REPRESENTATION_ITEM ( '' )  );
#62402=CARTESIAN_POINT ( 'NONE',  ( 16.40814093676324603, 62.45696800326376064, -11.09922568453594671 ) ) ;
#62404=CARTESIAN_POINT ( 'NONE',  ( 0.6178305044545838731, 19.74863466993042138, 9.382169495545420901 ) ) ;
#62405=DIRECTION ( 'NONE',  ( 0.000000000000000000, 0.000000000000000000, -1.000000000000000000 ) ) ;
#62406=CARTESIAN_POINT ( 'NONE',  ( 10.00000000000000000, 40.55374883491397497, -14.16423886937410082 ) ) ;
#62408=CARTESIAN_POINT ( 'NONE',  ( 0.1532563361054083140, 1.008931151000784787, 1.131784320476157264E-15 ) ) ;
#62410=CARTESIAN_POINT ( 'NONE',  ( -2.266590686148945544, 37.22041550158063217, 7.082119434687048631 ) ) ;
#62411=( GEOMETRIC_REPRESENTATION_CONTEXT ( 3 ) GLOBAL_UNCERTAINTY_ASSIGNED_CONTEXT ( ( #78198 ) ) GLOBAL_UNIT_ASSIGNED_CONTEXT ( ( #36411, #50418, #74895 ) ) REPRESENTATION_CONTEXT ( 'NONE', 'WORKASPACE' ) );
#62412=CARTESIAN_POINT ( 'NONE',  ( 24.16423886937410614, 59.30374883491397497, 8.672049930838204340E-16 ) ) ;
#62413=CARTESIAN_POINT ( 'NONE',  ( 6.204703633549690345, 17.84541550158063217, 14.16423886937410082 ) ) ;
#62414=CARTESIAN_POINT ( 'NONE',  ( 10.00000000000000000, 20.55374883491396787, -14.16423886937410082 ) ) ;
#62418=CARTESIAN_POINT ( 'NONE',  ( 12.63842701281683922, 44.55059781766745175, -9.846743663894590881 ) ) ;
#62420=CARTESIAN_POINT ( 'NONE',  ( 17.96484262340118221, 41.18868534415484106, -7.964842623401177768 ) ) ;
#62423=CARTESIAN_POINT ( 'NONE',  ( 12.63842701281683922, 34.55059781766745886, -9.846743663894590881 ) ) ;
#62424=CARTESIAN_POINT ( 'NONE',  ( 6.565887622018943937, 53.08196800326374643, -12.81628187352647608 ) ) ;
#62426=CARTESIAN_POINT ( 'NONE',  ( 12.63842701281683922, 44.55059781766745175, -9.846743663894590881 ) ) ;
#62427=CARTESIAN_POINT ( 'NONE',  ( 7.361572987183170547, 67.05059781766746596, 9.846743663894590881 ) ) ;
#62429=ORIENTED_EDGE ( 'NONE', *, *, #66244, .F. ) ;
#62430=CARTESIAN_POINT ( 'NONE',  ( -4.164238869374099927, 12.01208216824730357, 3.795296366450308767 ) ) ;
#62433=CARTESIAN_POINT ( 'NONE',  ( 20.88017736071110519, 10.56368534415483929, 2.639326808657452039E-16 ) ) ;
#62434=CARTESIAN_POINT ( 'NONE',  ( 6.565887622018943937, 10.16530133659708746, 12.81628187352647430 ) ) ;
#62437=CARTESIAN_POINT ( 'NONE',  ( 12.91533473730992121, 64.52201867748817676, 10.88017736071110164 ) ) ;
#62439=CARTESIAN_POINT ( 'NONE',  ( -46.58521628013341598, 101.6760492933278215, -7.987317478326372289 ) ) ;
#62440=CARTESIAN_POINT ( 'NONE',  ( 0.1922240491738435031, 43.18878173731741299, 6.499999999999968914 ) ) ;
#62441=CARTESIAN_POINT ( 'NONE',  ( 4.559911319644449179, 2.230352010821504916, -9.422509992056141925 ) ) ;
#62443=CARTESIAN_POINT ( 'NONE',  ( 12.91533473730992121, 24.52201867748816966, 10.88017736071110164 ) ) ;
#62444=CARTESIAN_POINT ( 'NONE',  ( 7.084665262690076126, 27.02201867748817676, -10.88017736071110164 ) ) ;
#62445=CARTESIAN_POINT ( 'NONE',  ( 19.38216949554541202, 5.998634669930420493, 9.382169495545424454 ) ) ;
#62446=CARTESIAN_POINT ( 'NONE',  ( 0.1532563361054100626, 55.80059781766745175, -2.638427012816831230 ) ) ;
#62447=CARTESIAN_POINT ( 'NONE',  ( 21.09922568453594849, 61.20696800326376064, 6.408140936763242479 ) ) ;
#62451=CARTESIAN_POINT ( 'NONE',  ( 17.96484262340118221, 29.93868534415484106, 7.964842623401181321 ) ) ;
#62452=CARTESIAN_POINT ( 'NONE',  ( 21.09922568453595559, 27.04030133659708568, -6.408140936763230044 ) ) ;
#62455=CARTESIAN_POINT ( 'NONE',  ( 19.84674366389459266, 58.30059781766745886, 2.638427012816836559 ) ) ;
#62456=CARTESIAN_POINT ( 'NONE',  ( 7.084665262690076126, 49.10535201082149825, 10.88017736071109987 ) ) ;
#62457=CARTESIAN_POINT ( 'NONE',  ( 1.472469842513823179, 10.59226448433411782, -4.923371831947296329 ) ) ;
#62458=CARTESIAN_POINT ( 'NONE',  ( 3.591859063236763294, 38.29030133659708923, -11.09922568453595026 ) ) ;
#62459=CARTESIAN_POINT ( 'NONE',  ( 20.88017736071110519, 60.56368534415484106, 2.639326808657452039E-16 ) ) ;
#62465=CARTESIAN_POINT ( 'NONE',  ( -0.8801773607111008646, 13.27201867748817143, 2.915334737309923430 ) ) ;
#62466=CARTESIAN_POINT ( 'NONE',  ( -1.099225684535947600, 49.54030133659708923, 6.408140936763237150 ) ) ;
#62467=CARTESIAN_POINT ( 'NONE',  ( 6.204703633549690345, 15.76208216824730179, -14.16423886937410259 ) ) ;
#62468=CARTESIAN_POINT ( 'NONE',  ( 10.00000000000000000, 14.75893115100078568, -9.846743663894594434 ) ) ;
#62470=CARTESIAN_POINT ( 'NONE',  ( 19.84674366389459266, 18.71726448433411960, -2.638427012816827677 ) ) ;
#62472=CARTESIAN_POINT ( 'NONE',  ( 6.204703633549690345, 50.76208216824730357, -14.16423886937410259 ) ) ;
#62477=CARTESIAN_POINT ( 'NONE',  ( 0.5774900079438590739, 2.647018677488170990, -5.440088680355550821 ) ) ;
#62478=DIRECTION ( 'NONE',  ( 0.000000000000000000, 1.000000000000000000, 0.000000000000000000 ) ) ;
#62481=ORIENTED_EDGE ( 'NONE', *, *, #60095, .F. ) ;
#62482=CARTESIAN_POINT ( 'NONE',  ( 12.91533473730993009, 11.60535201082150714, -10.88017736071109987 ) ) ;
#62483=CARTESIAN_POINT ( 'NONE',  ( -0.8801773607111008646, 13.27201867748817321, 2.915334737309923430 ) ) ;
#62484=CARTESIAN_POINT ( 'NONE',  ( 12.63842701281683922, 39.55059781766744464, -9.846743663894590881 ) ) ;
#62485=CARTESIAN_POINT ( 'NONE',  ( 22.81628187352647785, 51.62363466993042493, 6.195893100308588602E-16 ) ) ;
#62486=FILL_AREA_STYLE_COLOUR ( '', #71624 ) ;
#62487=CARTESIAN_POINT ( 'NONE',  ( 17.39651004071841456, 64.08210964143329136, -6.500000000000001776 ) ) ;
#62488=CARTESIAN_POINT ( 'NONE',  ( 10.00000000000000000, 25.55374883491396787, -14.16423886937410082 ) ) ;
#62489=CARTESIAN_POINT ( 'NONE',  ( 10.00000000000000000, 26.81368534415484106, -10.88017736071110342 ) ) ;
#62490=CARTESIAN_POINT ( 'NONE',  ( 10.00000000000000000, 6.813685344154838397, -10.88017736071110342 ) ) ;
#62491=CARTESIAN_POINT ( 'NONE',  ( 19.84674366389459266, 43.30059781766744464, 2.638427012816836559 ) ) ;
#62493=CARTESIAN_POINT ( 'NONE',  ( 7.361572987183170547, 32.05059781766745175, 9.846743663894590881 ) ) ;
#62494=LINE ( 'NONE', #10009, #35086 ) ;
#62500=CARTESIAN_POINT ( 'NONE',  ( 0.5774900079438607392, 68.48035201082150536, 5.440088680355550821 ) ) ;
#62501=CARTESIAN_POINT ( 'NONE',  ( 14.92337183194729988, 54.34226448433412315, -8.527530157486177487 ) ) ;
#62502=CARTESIAN_POINT ( 'NONE',  ( 10.00000000000000000, 46.81368534415484106, -10.88017736071110342 ) ) ;
#62503=CARTESIAN_POINT ( 'NONE',  ( 15.44008868035555793, 11.39701867748817143, -9.422509992056140149 ) ) ;
#62504=CARTESIAN_POINT ( 'NONE',  ( 0.6178305044545818747, 43.49863466993042493, -9.382169495545419124 ) ) ;
#62505=CARTESIAN_POINT ( 'NONE',  ( 17.08211943468705130, 18.47041550158063572, 12.26659068614894998 ) ) ;
#62506=CARTESIAN_POINT ( 'NONE',  ( 13.43411237798105340, 40.58196800326375353, 12.81628187352647963 ) ) ;
#62507=EDGE_LOOP ( 'NONE', ( #97624, #31047, #13437, #3017, #77724, #7323 ) ) ;
#62508=CARTESIAN_POINT ( 'NONE',  ( 1.472469842513823179, 60.59226448433412315, -4.923371831947296329 ) ) ;
#62509=CARTESIAN_POINT ( 'NONE',  ( 12.91533473730992121, 14.52201867748817143, 10.88017736071110164 ) ) ;
#62511=CARTESIAN_POINT ( 'NONE',  ( 7.084665262690076126, 29.10535201082150181, 10.88017736071109987 ) ) ;
#62512=ORIENTED_EDGE ( 'NONE', *, *, #27915, .F. ) ;
#62513=CARTESIAN_POINT ( 'NONE',  ( 12.91533473730992121, 64.52201867748817676, 10.88017736071110164 ) ) ;
#62514=CARTESIAN_POINT ( 'NONE',  ( 7.084665262690076126, 2.022018677488170990, -10.88017736071110164 ) ) ;
#62516=CARTESIAN_POINT ( 'NONE',  ( 1.472469842513823179, 5.592264484334118713, -4.923371831947296329 ) ) ;
#62517=CARTESIAN_POINT ( 'NONE',  ( 17.20831665107776587, 2.883931151000785231, 7.208316651077764980 ) ) ;
#62520=CARTESIAN_POINT ( 'NONE',  ( -46.94000000000000483, 100.7316555907688809, 8.991040189367279112 ) ) ;
#62521=CARTESIAN_POINT ( 'NONE',  ( 0.1532563361054083140, 11.00893115100078568, 1.131784320476157264E-15 ) ) ;
#62524=CARTESIAN_POINT ( 'NONE',  ( 0.1532563361054100626, 35.80059781766745175, -2.638427012816831230 ) ) ;
#62528=CARTESIAN_POINT ( 'NONE',  ( 10.00000000000000000, 5.553748834913967869, -14.16423886937410082 ) ) ;
#62529=CARTESIAN_POINT ( 'NONE',  ( 16.40814093676324603, 57.45696800326375353, -11.09922568453594671 ) ) ;
#62530=CARTESIAN_POINT ( 'NONE',  ( 10.00000000000000000, 5.553748834913967869, -14.16423886937410082 ) ) ;
#62531=CARTESIAN_POINT ( 'NONE',  ( 2.917880565312950480, 20.97041550158063217, -12.26659068614894821 ) ) ;
#62534=CARTESIAN_POINT ( 'NONE',  ( 2.035157376598824452, 63.68868534415484106, 7.964842623401179544 ) ) ;
#62535=CARTESIAN_POINT ( 'NONE',  ( -0.8801773607110991993, 17.85535201082150536, -2.915334737309923874 ) ) ;
#62538=CARTESIAN_POINT ( 'NONE',  ( 1.472469842513823179, 1.425597817667451528, 4.923371831947296329 ) ) ;
#62539=CARTESIAN_POINT ( 'NONE',  ( 0.1532563361054100626, 5.800597817667452638, -2.638427012816831230 ) ) ;
#62540=CARTESIAN_POINT ( 'NONE',  ( -2.816281873526471635, 28.91530133659708213, -3.434112377981056508 ) ) ;
#62541=CARTESIAN_POINT ( 'NONE',  ( 17.20831665107776587, 39.13393115100079456, -7.208316651077762316 ) ) ;
#62542=CARTESIAN_POINT ( 'NONE',  ( 19.38216949554541202, 15.99863466993042138, 9.382169495545424454 ) ) ;
#62544=MECHANICAL_DESIGN_GEOMETRIC_PRESENTATION_REPRESENTATION('',(#49765),#67339);
#62545=CARTESIAN_POINT ( 'NONE',  ( 5.076628168052704559, 10.17559781766745175, -8.527530157486179263 ) ) ;
#62549=CARTESIAN_POINT ( 'NONE',  ( 4.559911319644449179, 33.89701867748817676, 9.422509992056141925 ) ) ;
#62550=CARTESIAN_POINT ( 'NONE',  ( -4.164238869374098151, 36.59541550158063217, -3.795296366450310543 ) ) ;
#62551=CARTESIAN_POINT ( 'NONE',  ( 12.63842701281683034, 42.46726448433412315, 9.846743663894596210 ) ) ;
#62552=CARTESIAN_POINT ( 'NONE',  ( 19.42250999205614548, 65.98035201082151957, -5.440088680355545492 ) ) ;
#62554=CARTESIAN_POINT ( 'NONE',  ( -1.099225684535947600, 49.54030133659708923, 6.408140936763237150 ) ) ;
#62556=CARTESIAN_POINT ( 'NONE',  ( 12.91533473730992121, 24.52201867748816966, 10.88017736071110164 ) ) ;
#62559=CARTESIAN_POINT ( 'NONE',  ( 16.40814093676323893, 25.79030133659708923, 11.09922568453595026 ) ) ;
#62560=CARTESIAN_POINT ( 'NONE',  ( 7.361572987183170547, 42.05059781766745886, 9.846743663894590881 ) ) ;
#62562=CARTESIAN_POINT ( 'NONE',  ( 22.81628187352647785, 51.62363466993042493, 6.195893100308588602E-16 ) ) ;
#62565=CARTESIAN_POINT ( 'NONE',  ( 10.00000000000000000, 51.81368534415484106, -10.88017736071110342 ) ) ;
#62568=PLANE ( 'NONE',  #22542 ) ;
#62569=CARTESIAN_POINT ( 'NONE',  ( -0.8801773607111008646, 58.27201867748816966, 2.915334737309923430 ) ) ;
#62570=CARTESIAN_POINT ( 'NONE',  ( 0.5774900079438590739, 57.64701867748817676, -5.440088680355550821 ) ) ;
#62573=CARTESIAN_POINT ( 'NONE',  ( -0.8801773607111008646, 3.272018677488171434, 2.915334737309923430 ) ) ;
#62574=CARTESIAN_POINT ( 'NONE',  ( 18.52753015748617571, 58.09226448433411605, 4.923371831947298993 ) ) ;
#62575=CARTESIAN_POINT ( 'NONE',  ( 15.44008868035555260, 19.73035201082150536, 9.422509992056143702 ) ) ;
#62577=CARTESIAN_POINT ( 'NONE',  ( 19.38216949554541202, 20.99863466993042138, 9.382169495545424454 ) ) ;
#62579=CARTESIAN_POINT ( 'NONE',  ( 12.91533473730993009, 31.60535201082150891, -10.88017736071109987 ) ) ;
#62580=CARTESIAN_POINT ( 'NONE',  ( 13.43411237798105340, 5.581968003263753531, 12.81628187352647963 ) ) ;
#62581=CARTESIAN_POINT ( 'NONE',  ( 4.559911319644449179, 12.23035201082150536, -9.422509992056141925 ) ) ;
#62582=CARTESIAN_POINT ( 'NONE',  ( 15.44008868035555260, 44.73035201082151247, 9.422509992056143702 ) ) ;
#62583=CARTESIAN_POINT ( 'NONE',  ( 6.204703633549690345, 45.76208216824729647, -14.16423886937410259 ) ) ;
#62584=CARTESIAN_POINT ( 'NONE',  ( 0.1532563361054082862, 36.21726448433410894, 2.638427012816831674 ) ) ;
#62585=CARTESIAN_POINT ( 'NONE',  ( 10.00000000000000178, 54.31368534415484106, 10.88017736071110342 ) ) ;
#62586=CYLINDRICAL_SURFACE ( 'NONE', #5911, 0.5000000000000004441 ) ;
#62587=CARTESIAN_POINT ( 'NONE',  ( -4.164238869374098151, 16.59541550158063927, -3.795296366450310543 ) ) ;
#62590=ORIENTED_EDGE ( 'NONE', *, *, #21380, .T. ) ;
#62593=CARTESIAN_POINT ( 'NONE',  ( 20.36894250292379738, 34.92874883491396076, -10.36894250292379027 ) ) ;
#62594=CARTESIAN_POINT ( 'NONE',  ( 22.26659068614894466, 38.88708216824731068, 7.082119434687054849 ) ) ;
#62595=CARTESIAN_POINT ( 'NONE',  ( 14.92337183194729633, 2.675597817667451750, 8.527530157486181039 ) ) ;
#62596=CARTESIAN_POINT ( 'NONE',  ( 17.20831665107776587, 64.13393115100079456, -7.208316651077762316 ) ) ;
#62597=DIRECTION ( 'NONE',  ( -1.000000000000000000, 0.000000000000000000, 0.000000000000000000 ) ) ;
#62598=CARTESIAN_POINT ( 'NONE',  ( -0.8801773607111009756, 53.06368534415484106, 1.068504757029289695E-15 ) ) ;
#62599=CARTESIAN_POINT ( 'NONE',  ( 19.38216949554541557, 27.24863466993041783, -9.382169495545420901 ) ) ;
#62600=CARTESIAN_POINT ( 'NONE',  ( 2.917880565312950480, 30.97041550158063572, -12.26659068614894821 ) ) ;
#62601=CARTESIAN_POINT ( 'NONE',  ( 10.00000000000000000, 21.81368534415484106, -10.88017736071110342 ) ) ;
#62603=FACE_OUTER_BOUND ( 'NONE', #48346, .T. ) ;
#62605=ORIENTED_EDGE ( 'NONE', *, *, #10297, .F. ) ;
#62607=ORIENTED_EDGE ( 'NONE', *, *, #81288, .T. ) ;
#62610=CARTESIAN_POINT ( 'NONE',  ( 20.36894250292379738, 4.928748834913967869, -10.36894250292379027 ) ) ;
#62611=CARTESIAN_POINT ( 'NONE',  ( 13.79529636645030344, 53.26208216824730357, 14.16423886937410614 ) ) ;
#62612=CARTESIAN_POINT ( 'NONE',  ( 19.42250999205614548, 10.98035201082150536, -5.440088680355545492 ) ) ;
#62613=CARTESIAN_POINT ( 'NONE',  ( 2.791683348922237240, 35.38393115100079456, -7.208316651077763204 ) ) ;
#62614=CARTESIAN_POINT ( 'NONE',  ( 14.92337183194729633, 57.67559781766745886, 8.527530157486181039 ) ) ;
#62615=CARTESIAN_POINT ( 'NONE',  ( 20.15039907845753575, 59.72266099184918176, 6.262539305110074395 ) ) ;
#62617=CARTESIAN_POINT ( 'NONE',  ( 0.6178305044545838731, -0.2513653300695798953, 9.382169495545420901 ) ) ;
#62622=CARTESIAN_POINT ( 'NONE',  ( 22.26659068614894466, 43.88708216824729647, 7.082119434687054849 ) ) ;
#62623=ORIENTED_EDGE ( 'NONE', *, *, #7907, .F. ) ;
#62625=CARTESIAN_POINT ( 'NONE',  ( -0.3689425029237881626, 42.42874883491396787, 10.36894250292379027 ) ) ;
#62627=CARTESIAN_POINT ( 'NONE',  ( 20.88017736071110875, 25.77201867748816966, -2.915334737309920765 ) ) ;
#62629=CARTESIAN_POINT ( 'NONE',  ( 4.559911319644449179, 32.23035201082150536, -9.422509992056141925 ) ) ;
#62630=CARTESIAN_POINT ( 'NONE',  ( 17.20831665107776587, 49.13393115100078745, -7.208316651077762316 ) ) ;
#62631=CARTESIAN_POINT ( 'NONE',  ( 20.88017736071110875, 40.77201867748818387, -2.915334737309920765 ) ) ;
#62633=CARTESIAN_POINT ( 'NONE',  ( 2.035157376598822676, 62.43868534415483396, -7.964842623401177768 ) ) ;
#62634=CARTESIAN_POINT ( 'NONE',  ( 2.035157376598824452, 33.68868534415484106, 7.964842623401179544 ) ) ;
#62638=SURFACE_STYLE_FILL_AREA ( #60679 ) ;
#62643=CARTESIAN_POINT ( 'NONE',  ( 19.84674366389459266, 38.71726448433412315, -2.638427012816827677 ) ) ;
#62644=ADVANCED_FACE ( 'NONE', ( #29990 ), #38994, .F. ) ;
#62650=CARTESIAN_POINT ( 'NONE',  ( 0.5600000000000083800, 105.0000000000000000, 5.000000000000000000 ) ) ;
#62651=CARTESIAN_POINT ( 'NONE',  ( 0.8952175423694801459, 52.60160829253886305, -5.990408912944315212 ) ) ;
#62652=CARTESIAN_POINT ( 'NONE',  ( 18.52753015748618282, 53.92559781766745175, -4.923371831947291888 ) ) ;
#62653=CARTESIAN_POINT ( 'NONE',  ( 13.79529636645031943, 45.34541550158062506, -14.16423886937409904 ) ) ;
#62654=CARTESIAN_POINT ( 'NONE',  ( 14.92337183194729988, 64.34226448433412315, -8.527530157486177487 ) ) ;
#62657=CARTESIAN_POINT ( 'NONE',  ( 10.00000000000000000, 14.75893115100078568, -9.846743663894594434 ) ) ;
#62659=CARTESIAN_POINT ( 'NONE',  ( 10.00000000000000000, 47.87363466993042493, -12.81628187352647608 ) ) ;
#62660=CARTESIAN_POINT ( 'NONE',  ( 0.1532563361054083140, 66.00893115100079456, 1.131784320476157264E-15 ) ) ;
#62661=CARTESIAN_POINT ( 'NONE',  ( -0.8801773607110991993, 57.85535201082149825, -2.915334737309923874 ) ) ;
#62664=EDGE_CURVE ( 'NONE', #66685, #43655, #45937, .T. ) ;
#62666=CARTESIAN_POINT ( 'NONE',  ( 6.204703633549690345, 65.76208216824731778, -14.16423886937410259 ) ) ;
#62667=DIRECTION ( 'NONE',  ( 0.000000000000000000, -1.000000000000000000, 0.000000000000000000 ) ) ;
#62668=CARTESIAN_POINT ( 'NONE',  ( -0.8801773607111009756, 23.06368534415484106, 1.068504757029289695E-15 ) ) ;
#62669=CARTESIAN_POINT ( 'NONE',  ( 10.00000000000000178, 10.37363466993041961, 12.81628187352647608 ) ) ;
#62670=CARTESIAN_POINT ( 'NONE',  ( 2.035157376598824452, 63.68868534415484106, 7.964842623401179544 ) ) ;
#62675=CARTESIAN_POINT ( 'NONE',  ( 20.88017736071110519, 50.56368534415484106, 2.639326808657452039E-16 ) ) ;
#62677=CARTESIAN_POINT ( 'NONE',  ( 7.361572987183170547, 32.05059781766745175, 9.846743663894590881 ) ) ;
#62678=CARTESIAN_POINT ( 'NONE',  ( 10.00000000000000000, -0.2410688489992152128, -9.846743663894594434 ) ) ;
#62680=CARTESIAN_POINT ( 'NONE',  ( 6.565887622018943937, 15.16530133659708568, 12.81628187352647430 ) ) ;
#62681=CARTESIAN_POINT ( 'NONE',  ( 17.96484262340118221, 14.93868534415484106, 7.964842623401181321 ) ) ;
#62683=CARTESIAN_POINT ( 'NONE',  ( 17.08211943468705130, 38.47041550158063217, 12.26659068614894998 ) ) ;
#62684=CARTESIAN_POINT ( 'NONE',  ( 20.36894250292379382, 33.67874883491396076, 10.36894250292379205 ) ) ;
#62685=CARTESIAN_POINT ( 'NONE',  ( 2.035157376598822676, 2.438685344154838397, -7.964842623401177768 ) ) ;
#62687=CARTESIAN_POINT ( 'NONE',  ( 1.472469842513823179, 21.42559781766745175, 4.923371831947296329 ) ) ;
#62688=CARTESIAN_POINT ( 'NONE',  ( 2.035157376598822676, 7.438685344154837509, -7.964842623401177768 ) ) ;
#62690=CARTESIAN_POINT ( 'NONE',  ( 17.20831665107776587, 44.13393115100078745, -7.208316651077762316 ) ) ;
#62691=CARTESIAN_POINT ( 'NONE',  ( 15.44008868035555793, 46.39701867748817676, -9.422509992056140149 ) ) ;
#62692=CARTESIAN_POINT ( 'NONE',  ( 0.6178305044545818747, -1.501365330069579951, -9.382169495545419124 ) ) ;
#62693=CARTESIAN_POINT ( 'NONE',  ( 24.16423886937410614, 24.30374883491396787, 8.672049930838204340E-16 ) ) ;
#62694=CARTESIAN_POINT ( 'NONE',  ( 2.603489959281613420, 60.43575266056826933, -6.500000000000031086 ) ) ;
#62696=CARTESIAN_POINT ( 'NONE',  ( 1.472469842513823179, 10.59226448433411782, -4.923371831947296329 ) ) ;
#62697=CARTESIAN_POINT ( 'NONE',  ( 22.81628187352647785, 46.41530133659708213, 3.434112377981063169 ) ) ;
#62698=CARTESIAN_POINT ( 'NONE',  ( 5.076628168052704559, 50.17559781766745886, -8.527530157486179263 ) ) ;
#62700=COLOUR_RGB ( '', 0.72549020, 0.75294118, 0.79215686) ;
#62701=CARTESIAN_POINT ( 'NONE',  ( 10.00000000000000178, 70.00000000000000000, 0.000000000000000000 ) ) ;
#62703=CARTESIAN_POINT ( 'NONE',  ( 12.91533473730993009, 6.605352010821504471, -10.88017736071109987 ) ) ;
#62704=CARTESIAN_POINT ( 'NONE',  ( 15.44008868035555793, 51.39701867748816966, -9.422509992056140149 ) ) ;
#62705=CARTESIAN_POINT ( 'NONE',  ( 22.26659068614894466, 13.88708216824730179, 7.082119434687054849 ) ) ;
#62706=CARTESIAN_POINT ( 'NONE',  ( 0.5774900079438590739, 57.64701867748817676, -5.440088680355550821 ) ) ;
#62707=CARTESIAN_POINT ( 'NONE',  ( 10.00000000000000178, 32.25893115100078745, 9.846743663894594434 ) ) ;
#62708=CARTESIAN_POINT ( 'NONE',  ( 20.88017736071110875, 25.77201867748816966, -2.915334737309920765 ) ) ;
#62710=CARTESIAN_POINT ( 'NONE',  ( 5.076628168052703671, 66.84226448433412315, 8.527530157486179263 ) ) ;
#62712=CARTESIAN_POINT ( 'NONE',  ( 0.1532563361054100626, 0.8005978176674514168, -2.638427012816831230 ) ) ;
#62713=ORIENTED_EDGE ( 'NONE', *, *, #74082, .F. ) ;
#62718=CARTESIAN_POINT ( 'NONE',  ( -4.164238869374099039, 46.80374883491397497, 8.674139862899312516E-16 ) ) ;
#62719=CARTESIAN_POINT ( 'NONE',  ( 19.84674366389459621, 38.50893115100078745, 7.409399052514197653E-17 ) ) ;
#62720=CARTESIAN_POINT ( 'NONE',  ( 14.92337183194729988, 19.34226448433411960, -8.527530157486177487 ) ) ;
#62721=CARTESIAN_POINT ( 'NONE',  ( 18.18329248733322956, 52.60290668512021739, 6.499999999999960920 ) ) ;
#62722=CARTESIAN_POINT ( 'NONE',  ( -0.8801773607111009756, 23.06368534415484106, 1.068504757029289695E-15 ) ) ;
#62723=CARTESIAN_POINT ( 'NONE',  ( 0.1532563361054082862, 51.21726448433412315, 2.638427012816831674 ) ) ;
#62725=CARTESIAN_POINT ( 'NONE',  ( -2.266590686148945544, 42.22041550158063217, 7.082119434687048631 ) ) ;
#62726=CARTESIAN_POINT ( 'NONE',  ( 17.08211943468705840, 55.13708216824731068, -12.26659068614894466 ) ) ;
#62727=CARTESIAN_POINT ( 'NONE',  ( 18.52753015748618282, 63.92559781766745886, -4.923371831947291888 ) ) ;
#62729=CARTESIAN_POINT ( 'NONE',  ( 20.88017736071110875, 50.77201867748817676, -2.915334737309920765 ) ) ;
#62730=CARTESIAN_POINT ( 'NONE',  ( 14.92337183194729988, 19.34226448433411960, -8.527530157486177487 ) ) ;
#62731=VECTOR ( 'NONE', #31863, 1000.000000000000000 ) ;
#62736=CARTESIAN_POINT ( 'NONE',  ( 18.52753015748618282, 13.92559781766745175, -4.923371831947291888 ) ) ;
#62738=CARTESIAN_POINT ( 'NONE',  ( 2.917880565312950480, 20.97041550158063217, -12.26659068614894821 ) ) ;
#62739=CARTESIAN_POINT ( 'NONE',  ( 5.076628168052704559, 20.17559781766745175, -8.527530157486179263 ) ) ;
#62740=CARTESIAN_POINT ( 'NONE',  ( 7.084665262690076126, 39.10535201082150536, 10.88017736071109987 ) ) ;
#62742=DIRECTION ( 'NONE',  ( 0.000000000000000000, 0.000000000000000000, 1.000000000000000000 ) ) ;
#62744=CARTESIAN_POINT ( 'NONE',  ( 7.084665262690076126, 44.10535201082151247, 10.88017736071109987 ) ) ;
#62749=CARTESIAN_POINT ( 'NONE',  ( 12.91533473730992121, 44.52201867748816966, 10.88017736071110164 ) ) ;
#62750=CARTESIAN_POINT ( 'NONE',  ( 17.08211943468705130, 13.47041550158063572, 12.26659068614894998 ) ) ;
#62752=CARTESIAN_POINT ( 'NONE',  ( 13.43411237798105340, 30.58196800326374998, 12.81628187352647963 ) ) ;
#62753=CARTESIAN_POINT ( 'NONE',  ( 2.791683348922240793, 11.63393115100078568, 7.208316651077764092 ) ) ;
#62754=CARTESIAN_POINT ( 'NONE',  ( 15.44008868035555793, 6.397018677488170546, -9.422509992056140149 ) ) ;
#62757=CARTESIAN_POINT ( 'NONE',  ( 19.84674366389459266, 18.71726448433411960, -2.638427012816827677 ) ) ;
#62758=CARTESIAN_POINT ( 'NONE',  ( 10.00000000000000178, 39.31368534415484106, 10.88017736071110342 ) ) ;
#62765=CARTESIAN_POINT ( 'NONE',  ( 15.44008868035555793, 51.39701867748816966, -9.422509992056140149 ) ) ;
#62767=EDGE_CURVE ( 'NONE', #72922, #27809, #96064, .T. ) ;
#62768=CARTESIAN_POINT ( 'NONE',  ( 6.565887622018943937, 65.16530133659709634, 12.81628187352647430 ) ) ;
#62769=CARTESIAN_POINT ( 'NONE',  ( 19.42250999205614193, 60.14701867748817676, 5.440088680355555262 ) ) ;
#62772=CARTESIAN_POINT ( 'NONE',  ( 3.591859063236761518, 9.956968003263753531, 11.09922568453594849 ) ) ;
#62774=CARTESIAN_POINT ( 'NONE',  ( -0.1503990784575328643, 70.00000000000000000, -6.262539305110068177 ) ) ;
#62775=CARTESIAN_POINT ( 'NONE',  ( 5.076628168052704559, 35.17559781766745175, -8.527530157486179263 ) ) ;
#62777=CARTESIAN_POINT ( 'NONE',  ( -4.164238869374098151, 6.595415501580634832, -3.795296366450310543 ) ) ;
#62778=CARTESIAN_POINT ( 'NONE',  ( 19.84674366389459621, 13.50893115100078568, 7.409399052514197653E-17 ) ) ;
#62779=CARTESIAN_POINT ( 'NONE',  ( 21.09922568453594849, 26.20696800326375353, 6.408140936763242479 ) ) ;
#62780=DIRECTION ( 'NONE',  ( 0.000000000000000000, -1.000000000000000000, 0.000000000000000000 ) ) ;
#62781=CARTESIAN_POINT ( 'NONE',  ( 2.035157376598822676, 52.43868534415483396, -7.964842623401177768 ) ) ;
#62782=CARTESIAN_POINT ( 'NONE',  ( 7.361572987183170547, 67.05059781766746596, 9.846743663894590881 ) ) ;
#62785=CARTESIAN_POINT ( 'NONE',  ( 5.076628168052704559, 20.17559781766745175, -8.527530157486179263 ) ) ;
#62786=CARTESIAN_POINT ( 'NONE',  ( 0.5774900079438590739, 17.64701867748817321, -5.440088680355550821 ) ) ;
#62787=CARTESIAN_POINT ( 'NONE',  ( 10.00000000000000178, 15.37363466993042138, 12.81628187352647608 ) ) ;
#62788=CARTESIAN_POINT ( 'NONE',  ( 2.791683348922237240, 25.38393115100078390, -7.208316651077763204 ) ) ;
#62790=CARTESIAN_POINT ( 'NONE',  ( 17.96484262340118221, 21.18868534415483396, -7.964842623401177768 ) ) ;
#62792=CARTESIAN_POINT ( 'NONE',  ( 17.96484262340118221, 66.18868534415483396, -7.964842623401177768 ) ) ;
#62794=CARTESIAN_POINT ( 'NONE',  ( 10.00000000000000000, 44.75893115100078745, -9.846743663894594434 ) ) ;
#62795=CARTESIAN_POINT ( 'NONE',  ( 17.96484262340118221, 16.18868534415483396, -7.964842623401177768 ) ) ;
#62796=EDGE_CURVE ( 'NONE', #47024, #6299, #31466, .T. ) ;
#62797=CARTESIAN_POINT ( 'NONE',  ( 12.91533473730992121, 49.52201867748817676, 10.88017736071110164 ) ) ;
#62798=CARTESIAN_POINT ( 'NONE',  ( 7.084665262690076126, 19.10535201082150181, 10.88017736071109987 ) ) ;
#62799=CARTESIAN_POINT ( 'NONE',  ( 10.00000000000000000, 9.758931151000785675, -9.846743663894594434 ) ) ;
#62800=CARTESIAN_POINT ( 'NONE',  ( 7.361572987183169658, 44.96726448433412315, -9.846743663894592657 ) ) ;
#62804=CARTESIAN_POINT ( 'NONE',  ( 6.565887622018943937, -1.918031996736246692, -12.81628187352647608 ) ) ;
#62805=CARTESIAN_POINT ( 'NONE',  ( -4.164238869374099039, 1.803748834913967647, 8.674139862899312516E-16 ) ) ;
#62807=CARTESIAN_POINT ( 'NONE',  ( 17.08211943468705130, 18.47041550158063572, 12.26659068614894998 ) ) ;
#62809=CARTESIAN_POINT ( 'NONE',  ( 10.00000000000000178, 42.25893115100078745, 9.846743663894594434 ) ) ;
#62812=CARTESIAN_POINT ( 'NONE',  ( 2.917880565312948704, 47.63708216824730357, 12.26659068614894643 ) ) ;
#62813=CARTESIAN_POINT ( 'NONE',  ( 10.00000000000000178, 22.25893115100078745, 9.846743663894594434 ) ) ;
#62816=CARTESIAN_POINT ( 'NONE',  ( 20.88017736071110519, 45.56368534415484106, 2.639326808657452039E-16 ) ) ;
#62817=CARTESIAN_POINT ( 'NONE',  ( 22.81628187352647785, 61.41530133659709634, 3.434112377981063169 ) ) ;
#62818=CARTESIAN_POINT ( 'NONE',  ( 4.559911319644449179, 12.23035201082150536, -9.422509992056141925 ) ) ;
#62819=CARTESIAN_POINT ( 'NONE',  ( -2.816281873526471635, 43.91530133659708923, -3.434112377981056508 ) ) ;
#62820=CARTESIAN_POINT ( 'NONE',  ( 22.81628187352647785, 16.62363466993042138, 6.195893100308588602E-16 ) ) ;
#62821=CARTESIAN_POINT ( 'NONE',  ( 14.92337183194729988, 14.34226448433411782, -8.527530157486177487 ) ) ;
#62825=CARTESIAN_POINT ( 'NONE',  ( 2.917880565312948704, 47.63708216824730357, 12.26659068614894643 ) ) ;
#62826=CARTESIAN_POINT ( 'NONE',  ( 20.36894250292379382, 33.67874883491396076, 10.36894250292379205 ) ) ;
#62827=CARTESIAN_POINT ( 'NONE',  ( 0.5774900079438590739, 22.64701867748817321, -5.440088680355550821 ) ) ;
#62828=CARTESIAN_POINT ( 'NONE',  ( 15.44008868035555260, 39.73035201082150536, 9.422509992056143702 ) ) ;
#62829=SURFACE_SIDE_STYLE ('',( #93822 ) ) ;
#62831=CARTESIAN_POINT ( 'NONE',  ( 7.361572987183170547, 2.050597817667451750, 9.846743663894590881 ) ) ;
#62833=CARTESIAN_POINT ( 'NONE',  ( 7.361572987183169658, 24.96726448433412315, -9.846743663894592657 ) ) ;
#62834=DIRECTION ( 'NONE',  ( -0.8320502943378436100, 0.5547001962252291474, -0.000000000000000000 ) ) ;
#62836=CARTESIAN_POINT ( 'NONE',  ( 12.63842701281683034, 22.46726448433411605, 9.846743663894596210 ) ) ;
#62837=CARTESIAN_POINT ( 'NONE',  ( 7.361572987183169658, 54.96726448433413026, -9.846743663894592657 ) ) ;
#62838=CARTESIAN_POINT ( 'NONE',  ( 20.88017736071110164, 15.35535201082150358, 2.915334737309930979 ) ) ;
#62839=CARTESIAN_POINT ( 'NONE',  ( 22.81628187352647785, 31.41530133659709279, 3.434112377981063169 ) ) ;
#62841=CARTESIAN_POINT ( 'NONE',  ( 0.5774900079438607392, 48.48035201082150536, 5.440088680355550821 ) ) ;
#62842=CARTESIAN_POINT ( 'NONE',  ( 2.917880565312948704, 52.63708216824730357, 12.26659068614894643 ) ) ;
#62843=CARTESIAN_POINT ( 'NONE',  ( 14.92337183194729633, 7.675597817667451750, 8.527530157486181039 ) ) ;
#62845=CARTESIAN_POINT ( 'NONE',  ( 5.076628168052703671, 51.84226448433412315, 8.527530157486179263 ) ) ;
#62847=CARTESIAN_POINT ( 'NONE',  ( 14.92337183194729988, 34.34226448433411605, -8.527530157486177487 ) ) ;
#62848=CARTESIAN_POINT ( 'NONE',  ( 13.79529636645030344, 8.262082168247300018, 14.16423886937410614 ) ) ;
#62849=CARTESIAN_POINT ( 'NONE',  ( -2.266590686148945544, 17.22041550158063572, 7.082119434687048631 ) ) ;
#62850=CARTESIAN_POINT ( 'NONE',  ( 0.1532563361054100626, 35.80059781766745175, -2.638427012816831230 ) ) ;
#62851=CARTESIAN_POINT ( 'NONE',  ( 20.88017736071110875, 40.77201867748818387, -2.915334737309920765 ) ) ;
#62852=CARTESIAN_POINT ( 'NONE',  ( 10.00000000000000178, 14.31368534415483751, 10.88017736071110342 ) ) ;
#62853=VECTOR ( 'NONE', #7486, 1000.000000000000000 ) ;
#62854=CARTESIAN_POINT ( 'NONE',  ( 19.42250999205614193, 40.14701867748817676, 5.440088680355555262 ) ) ;
#62855=EDGE_CURVE ( 'NONE', #18416, #59748, #28915, .T. ) ;
#62856=CARTESIAN_POINT ( 'NONE',  ( 20.88017736071110519, 25.56368534415483751, 2.639326808657452039E-16 ) ) ;
#62857=VERTEX_POINT ( 'NONE', #2977 ) ;
#62858=CARTESIAN_POINT ( 'NONE',  ( 19.38216949554541557, 37.24863466993041783, -9.382169495545420901 ) ) ;
#62859=CARTESIAN_POINT ( 'NONE',  ( 0.5774900079438607392, 33.48035201082150536, 5.440088680355550821 ) ) ;
#62861=EDGE_CURVE ( 'NONE', #36257, #43815, #26798, .T. ) ;
#62862=CARTESIAN_POINT ( 'NONE',  ( 0.6178305044545838731, 64.74863466993043914, 9.382169495545420901 ) ) ;
#62863=CARTESIAN_POINT ( 'NONE',  ( 20.88017736071110519, 65.56368534415483396, 2.639326808657452039E-16 ) ) ;
#62865=CARTESIAN_POINT ( 'NONE',  ( 19.42250999205614193, 55.14701867748817676, 5.440088680355555262 ) ) ;
#62868=CARTESIAN_POINT ( 'NONE',  ( 22.26659068614895176, 64.72041550158064638, -7.082119434687042414 ) ) ;
#62869=CARTESIAN_POINT ( 'NONE',  ( -0.8801773607111008646, 68.27201867748817676, 2.915334737309923430 ) ) ;
#62870=CARTESIAN_POINT ( 'NONE',  ( -4.164238869374099927, 7.012082168247302683, 3.795296366450308767 ) ) ;
#62871=CARTESIAN_POINT ( 'NONE',  ( 10.00000000000000000, 9.758931151000785675, -9.846743663894594434 ) ) ;
#62872=CARTESIAN_POINT ( 'NONE',  ( 17.96484262340118221, 11.18868534415483929, -7.964842623401177768 ) ) ;
#62873=CARTESIAN_POINT ( 'NONE',  ( 2.791683348922237240, 50.38393115100078035, -7.208316651077763204 ) ) ;
#62875=CARTESIAN_POINT ( 'NONE',  ( 14.92337183194729988, 49.34226448433411605, -8.527530157486177487 ) ) ;
#62876=CARTESIAN_POINT ( 'NONE',  ( 12.91533473730992121, 64.52201867748817676, 10.88017736071110164 ) ) ;
#62877=CARTESIAN_POINT ( 'NONE',  ( -0.8801773607110991993, 42.85535201082150536, -2.915334737309923874 ) ) ;
#62878=CARTESIAN_POINT ( 'NONE',  ( 0.1532563361054083140, 46.00893115100079456, 1.131784320476157264E-15 ) ) ;
#62879=CARTESIAN_POINT ( 'NONE',  ( -2.816281873526471635, 28.91530133659708213, -3.434112377981056508 ) ) ;
#62881=CARTESIAN_POINT ( 'NONE',  ( 15.44008868035555793, 66.39701867748817676, -9.422509992056140149 ) ) ;
#62882=CARTESIAN_POINT ( 'NONE',  ( 2.035157376598824452, 43.68868534415484106, 7.964842623401179544 ) ) ;
#62883=CARTESIAN_POINT ( 'NONE',  ( 24.16423886937410614, 54.51208216824730357, -3.795296366450302550 ) ) ;
#62884=ADVANCED_FACE ( 'NONE', ( #39311 ), #75266, .T. ) ;
#62885=CARTESIAN_POINT ( 'NONE',  ( 21.09922568453594849, 16.20696800326375353, 6.408140936763242479 ) ) ;
#62888=CARTESIAN_POINT ( 'NONE',  ( -1.099225684535947600, 33.70696800326375353, -6.408140936763238038 ) ) ;
#62889=CARTESIAN_POINT ( 'NONE',  ( 2.035157376598822676, 22.43868534415483396, -7.964842623401177768 ) ) ;
#62892=CARTESIAN_POINT ( 'NONE',  ( 2.035157376598822676, 67.43868534415484817, -7.964842623401177768 ) ) ;
#62893=CARTESIAN_POINT ( 'NONE',  ( 1.472469842513823179, 51.42559781766745886, 4.923371831947296329 ) ) ;
#62894=CARTESIAN_POINT ( 'NONE',  ( 0.1532563361054082862, 16.21726448433411960, 2.638427012816831674 ) ) ;
#62895=CARTESIAN_POINT ( 'NONE',  ( 19.84674366389459266, 43.30059781766744464, 2.638427012816836559 ) ) ;
#62897=CARTESIAN_POINT ( 'NONE',  ( 6.565887622018943937, 65.16530133659709634, 12.81628187352647430 ) ) ;
#62900=CARTESIAN_POINT ( 'NONE',  ( 18.52753015748618282, 23.92559781766745530, -4.923371831947291888 ) ) ;
#62903=CARTESIAN_POINT ( 'NONE',  ( 0.1532563361054082862, 51.21726448433412315, 2.638427012816831674 ) ) ;
#62906=CARTESIAN_POINT ( 'NONE',  ( 21.09922568453595559, 22.04030133659708923, -6.408140936763230044 ) ) ;
#62909=CARTESIAN_POINT ( 'NONE',  ( 13.79529636645031943, 45.34541550158062506, -14.16423886937409904 ) ) ;
#62910=CARTESIAN_POINT ( 'NONE',  ( 12.63842701281683034, 12.46726448433411782, 9.846743663894596210 ) ) ;
#62911=CARTESIAN_POINT ( 'NONE',  ( 17.20831665107776587, 4.133931151000785675, -7.208316651077762316 ) ) ;
#62914=CARTESIAN_POINT ( 'NONE',  ( -4.164238869374099039, 46.80374883491397497, 8.674139862899312516E-16 ) ) ;
#62915=CARTESIAN_POINT ( 'NONE',  ( 1.472469842513823179, 65.59226448433412315, -4.923371831947296329 ) ) ;
#62916=EDGE_CURVE ( 'NONE', #1898, #79199, #15340, .T. ) ;
#62917=CARTESIAN_POINT ( 'NONE',  ( 17.08211943468705840, 60.13708216824729647, -12.26659068614894466 ) ) ;
#62918=CARTESIAN_POINT ( 'NONE',  ( 22.26659068614894466, 28.88708216824730357, 7.082119434687054849 ) ) ;
#62919=CARTESIAN_POINT ( 'NONE',  ( 20.36894250292379738, 34.92874883491396076, -10.36894250292379027 ) ) ;
#62922=CARTESIAN_POINT ( 'NONE',  ( 10.00000000000000178, 62.25893115100078745, 9.846743663894594434 ) ) ;
#62924=CARTESIAN_POINT ( 'NONE',  ( 2.035157376598822676, 32.43868534415483396, -7.964842623401177768 ) ) ;
#62926=CARTESIAN_POINT ( 'NONE',  ( 20.00000000000000711, 92.98956734510680633, -4.826711382686650786 ) ) ;
#62927=CARTESIAN_POINT ( 'NONE',  ( 5.076628168052703671, 36.84226448433412315, 8.527530157486179263 ) ) ;
#62928=CARTESIAN_POINT ( 'NONE',  ( -2.816281873526471635, 63.91530133659708923, -3.434112377981056508 ) ) ;
#62930=CARTESIAN_POINT ( 'NONE',  ( 0.1532563361054083140, 46.00893115100079456, 1.131784320476157264E-15 ) ) ;
#62933=CARTESIAN_POINT ( 'NONE',  ( 10.00000000000000178, 8.053748834913967869, 14.16423886937410082 ) ) ;
#62937=CARTESIAN_POINT ( 'NONE',  ( 7.084665262690076126, 9.105352010821503583, 10.88017736071109987 ) ) ;
#62938=CARTESIAN_POINT ( 'NONE',  ( 3.591859063236761518, 29.95696800326375708, 11.09922568453594849 ) ) ;
#62939=CARTESIAN_POINT ( 'NONE',  ( 20.24186590665278018, 2.616331881023272299, -6.114288769123028544 ) ) ;
#62940=CARTESIAN_POINT ( 'NONE',  ( 4.559911319644449179, 63.89701867748817676, 9.422509992056141925 ) ) ;
#62942=CARTESIAN_POINT ( 'NONE',  ( -46.93999999999942219, 101.0602049476338777, -8.583117191026476078 ) ) ;
#62943=CARTESIAN_POINT ( 'NONE',  ( 24.16423886937409904, 64.09541550158064638, 3.795296366450317205 ) ) ;
#62945=CARTESIAN_POINT ( 'NONE',  ( 0.5774900079438590739, 27.64701867748817676, -5.440088680355550821 ) ) ;
#62946=CARTESIAN_POINT ( 'NONE',  ( 20.88017736071110875, 40.77201867748818387, -2.915334737309920765 ) ) ;
#62947=CARTESIAN_POINT ( 'NONE',  ( 22.81628187352647785, 1.415301336597087012, 3.434112377981063169 ) ) ;
#62948=CARTESIAN_POINT ( 'NONE',  ( 19.84674366389459266, 48.71726448433413026, -2.638427012816827677 ) ) ;
#62949=CARTESIAN_POINT ( 'NONE',  ( -2.816281873526473856, 64.12363466993042493, 9.499525473075851096E-16 ) ) ;
#62950=CARTESIAN_POINT ( 'NONE',  ( 2.603489959281588995, 55.43575266056826933, -6.500000000000003553 ) ) ;
#62952=CARTESIAN_POINT ( 'NONE',  ( 19.42250999205614548, 30.98035201082150536, -5.440088680355545492 ) ) ;
#62953=CARTESIAN_POINT ( 'NONE',  ( 21.09922568453594849, 36.20696800326375353, 6.408140936763242479 ) ) ;
#62955=CARTESIAN_POINT ( 'NONE',  ( 18.52753015748618282, 58.92559781766745886, -4.923371831947291888 ) ) ;
#62956=CARTESIAN_POINT ( 'NONE',  ( 20.88017736071110164, 55.35535201082149825, 2.915334737309930979 ) ) ;
#62957=CARTESIAN_POINT ( 'NONE',  ( 1.472469842513823179, 6.425597817667451750, 4.923371831947296329 ) ) ;
#62958=CARTESIAN_POINT ( 'NONE',  ( 16.40814093676323893, 35.79030133659708923, 11.09922568453595026 ) ) ;
#62959=CARTESIAN_POINT ( 'NONE',  ( 7.084665262690076126, 59.10535201082150536, 10.88017736071109987 ) ) ;
#62961=LINE ( 'NONE', #78464, #83279 ) ;
#62962=CARTESIAN_POINT ( 'NONE',  ( -1.099225684535947600, 58.70696800326375353, -6.408140936763238038 ) ) ;
#62965=CARTESIAN_POINT ( 'NONE',  ( 1.932340009482144794, 16.49127512925449324, -6.500000000000007105 ) ) ;
#62966=CARTESIAN_POINT ( 'NONE',  ( 7.084665262690076126, 4.105352010821503583, 10.88017736071109987 ) ) ;
#62967=CARTESIAN_POINT ( 'NONE',  ( 21.09922568453594849, 41.20696800326375353, 6.408140936763242479 ) ) ;
#62968=CARTESIAN_POINT ( 'NONE',  ( 2.917880565312948704, 17.63708216824730357, 12.26659068614894643 ) ) ;
#62969=CARTESIAN_POINT ( 'NONE',  ( 12.63842701281683034, 12.46726448433411782, 9.846743663894596210 ) ) ;
#62970=CARTESIAN_POINT ( 'NONE',  ( 20.88017736071110519, 5.563685344154837509, 2.639326808657452039E-16 ) ) ;
#62971=CARTESIAN_POINT ( 'NONE',  ( 1.472469842513823179, 16.42559781766745175, 4.923371831947296329 ) ) ;
#62972=CARTESIAN_POINT ( 'NONE',  ( -4.164238869374098151, 51.59541550158063217, -3.795296366450310543 ) ) ;
#62974=SURFACE_SIDE_STYLE ('',( #55490 ) ) ;
#62976=CARTESIAN_POINT ( 'NONE',  ( 19.42250999205614548, 20.98035201082150891, -5.440088680355545492 ) ) ;
#62977=CARTESIAN_POINT ( 'NONE',  ( 13.99999999999999822, 11.00000000000000000, -5.000000000000000000 ) ) ;
#62979=CARTESIAN_POINT ( 'NONE',  ( 15.44008868035555793, 16.39701867748817321, -9.422509992056140149 ) ) ;
#62980=CARTESIAN_POINT ( 'NONE',  ( 12.91533473730992121, 9.522018677488171434, 10.88017736071110164 ) ) ;
#62981=CARTESIAN_POINT ( 'NONE',  ( 10.00000000000000178, 52.25893115100078745, 9.846743663894594434 ) ) ;
#62982=CARTESIAN_POINT ( 'NONE',  ( -1.099225684535947600, 49.54030133659708923, 6.408140936763237150 ) ) ;
#62984=CARTESIAN_POINT ( 'NONE',  ( 18.04007052943773459, 64.00257860105350005, -5.767676674365834089 ) ) ;
#62985=CARTESIAN_POINT ( 'NONE',  ( 20.36894250292379382, 18.67874883491397142, 10.36894250292379205 ) ) ;
#62986=CARTESIAN_POINT ( 'NONE',  ( 0.5774900079438607392, 23.48035201082150536, 5.440088680355550821 ) ) ;
#62987=CARTESIAN_POINT ( 'NONE',  ( 12.91533473730992121, 9.522018677488171434, 10.88017736071110164 ) ) ;
#62988=CARTESIAN_POINT ( 'NONE',  ( 7.361572987183170547, 52.05059781766745175, 9.846743663894590881 ) ) ;
#62991=CARTESIAN_POINT ( 'NONE',  ( 18.52753015748618282, 33.92559781766745886, -4.923371831947291888 ) ) ;
#62993=CARTESIAN_POINT ( 'NONE',  ( 0.2751277870542967463, 70.00000000000000000, 6.000000000000000000 ) ) ;
#62994=CARTESIAN_POINT ( 'NONE',  ( 12.63842701281683922, 4.550597817667451750, -9.846743663894590881 ) ) ;
#62998=CARTESIAN_POINT ( 'NONE',  ( 4.559911319644449179, 63.89701867748817676, 9.422509992056141925 ) ) ;
#62999=CARTESIAN_POINT ( 'NONE',  ( -1.099225684535947600, 4.540301336597087456, 6.408140936763237150 ) ) ;
#63000=CARTESIAN_POINT ( 'NONE',  ( 2.035157376598824452, 48.68868534415483396, 7.964842623401179544 ) ) ;
#63001=CARTESIAN_POINT ( 'NONE',  ( 0.5774900079438590739, 47.64701867748817676, -5.440088680355550821 ) ) ;
#63002=CARTESIAN_POINT ( 'NONE',  ( 0.5774900079438607392, 8.480352010821505360, 5.440088680355550821 ) ) ;
#63003=CARTESIAN_POINT ( 'NONE',  ( 13.43411237798105340, 40.58196800326375353, 12.81628187352647963 ) ) ;
#63004=CARTESIAN_POINT ( 'NONE',  ( 22.26659068614895176, 24.72041550158063572, -7.082119434687042414 ) ) ;
#63006=AXIS2_PLACEMENT_3D ( 'NONE', #89380, #67370, #20893 ) ;
#63007=CARTESIAN_POINT ( 'NONE',  ( -2.816281873526473856, 39.33196800326374643, 3.434112377981055619 ) ) ;
#63008=ORIENTED_EDGE ( 'NONE', *, *, #77763, .T. ) ;
#63009=CARTESIAN_POINT ( 'NONE',  ( 0.1532563361054083140, 56.00893115100078745, 1.131784320476157264E-15 ) ) ;
#63010=EDGE_CURVE ( 'NONE', #50375, #50944, #10167, .T. ) ;
#63011=CARTESIAN_POINT ( 'NONE',  ( -0.8801773607111008646, 18.27201867748817321, 2.915334737309923430 ) ) ;
#63013=CARTESIAN_POINT ( 'NONE',  ( 2.791683348922237240, 0.3839311510007847872, -7.208316651077763204 ) ) ;
#63014=( NAMED_UNIT ( * ) SI_UNIT ( $, .STERADIAN. ) SOLID_ANGLE_UNIT ( ) );
#63016=CARTESIAN_POINT ( 'NONE',  ( 0.1532563361054082862, 11.21726448433411605, 2.638427012816831674 ) ) ;
#63017=CARTESIAN_POINT ( 'NONE',  ( 0.1532563361054082862, 1.217264484334117824, 2.638427012816831674 ) ) ;
#63020=CARTESIAN_POINT ( 'NONE',  ( 12.91533473730993009, 56.60535201082151247, -10.88017736071109987 ) ) ;
#63021=DIRECTION ( 'NONE',  ( -0.000000000000000000, 1.000000000000000000, -0.000000000000000000 ) ) ;
#63022=CARTESIAN_POINT ( 'NONE',  ( 0.5774900079438590739, 57.64701867748817676, -5.440088680355550821 ) ) ;
#63023=CARTESIAN_POINT ( 'NONE',  ( 1.472469842513823179, 6.425597817667451750, 4.923371831947296329 ) ) ;
#63026=CARTESIAN_POINT ( 'NONE',  ( 2.791683348922240793, 56.63393115100078035, 7.208316651077764092 ) ) ;
#63027=VERTEX_POINT ( 'NONE', #7828 ) ;
#63028=ORIENTED_EDGE ( 'NONE', *, *, #44760, .F. ) ;
#63030=CARTESIAN_POINT ( 'NONE',  ( 24.16423886937410614, 9.512082168247301794, -3.795296366450302550 ) ) ;
#63031=CARTESIAN_POINT ( 'NONE',  ( -1.099225684535947600, 59.54030133659708923, 6.408140936763237150 ) ) ;
#63032=CARTESIAN_POINT ( 'NONE',  ( 20.36894250292379738, 4.928748834913967869, -10.36894250292379027 ) ) ;
#63033=CARTESIAN_POINT ( 'NONE',  ( 20.36894250292379382, 23.67874883491397142, 10.36894250292379205 ) ) ;
#63035=DIRECTION ( 'NONE',  ( 1.000000000000000000, -0.000000000000000000, 0.000000000000000000 ) ) ;
#63036=CARTESIAN_POINT ( 'NONE',  ( -0.8801773607111009756, 18.06368534415484106, 1.068504757029289695E-15 ) ) ;
#63037=( NAMED_UNIT ( * ) SI_UNIT ( $, .STERADIAN. ) SOLID_ANGLE_UNIT ( ) );
#63039=CARTESIAN_POINT ( 'NONE',  ( 0.1532563361054100626, 0.8005978176674514168, -2.638427012816831230 ) ) ;
#63041=CARTESIAN_POINT ( 'NONE',  ( 1.472469842513823179, 21.42559781766745175, 4.923371831947296329 ) ) ;
#63042=CARTESIAN_POINT ( 'NONE',  ( -1.099225684535947600, 34.54030133659708923, 6.408140936763237150 ) ) ;
#63043=CARTESIAN_POINT ( 'NONE',  ( 7.361572987183170547, 37.05059781766744464, 9.846743663894590881 ) ) ;
#63045=CARTESIAN_POINT ( 'NONE',  ( 17.39651004071841101, 57.93575266056827644, 6.500000000000005329 ) ) ;
#63046=CARTESIAN_POINT ( 'NONE',  ( 3.591859063236761518, 14.95696800326375531, 11.09922568453594849 ) ) ;
#63048=CARTESIAN_POINT ( 'NONE',  ( 5.076628168052703671, 21.84226448433411960, 8.527530157486179263 ) ) ;
#63049=CARTESIAN_POINT ( 'NONE',  ( 7.361572987183169658, 9.967264484334119601, -9.846743663894592657 ) ) ;
#63052=CARTESIAN_POINT ( 'NONE',  ( 7.084665262690076126, 39.10535201082150536, 10.88017736071109987 ) ) ;
#63053=CARTESIAN_POINT ( 'NONE',  ( 13.79529636645030344, 28.26208216824729647, 14.16423886937410614 ) ) ;
#63054=CARTESIAN_POINT ( 'NONE',  ( 1.472469842513823179, 36.42559781766745175, 4.923371831947296329 ) ) ;
#63055=CARTESIAN_POINT ( 'NONE',  ( 19.84674366389459266, 18.30059781766745175, 2.638427012816836559 ) ) ;
#63056=CARTESIAN_POINT ( 'NONE',  ( 19.38216949554541557, 47.24863466993041783, -9.382169495545420901 ) ) ;
#63058=CARTESIAN_POINT ( 'NONE',  ( 2.035157376598822676, 32.43868534415483396, -7.964842623401177768 ) ) ;
#63059=CARTESIAN_POINT ( 'NONE',  ( -2.816281873526471635, 23.91530133659708568, -3.434112377981056508 ) ) ;
#63060=CARTESIAN_POINT ( 'NONE',  ( 1.472469842513823179, 40.59226448433411605, -4.923371831947296329 ) ) ;
#63062=CARTESIAN_POINT ( 'NONE',  ( 3.591859063236763294, 48.29030133659708923, -11.09922568453595026 ) ) ;
#63063=CARTESIAN_POINT ( 'NONE',  ( 0.5774900079438590739, 47.64701867748817676, -5.440088680355550821 ) ) ;
#63066=CYLINDRICAL_SURFACE ( 'NONE', #9758, 11.92686044187656513 ) ;
#63067=CARTESIAN_POINT ( 'NONE',  ( 12.91533473730992121, 49.52201867748817676, 10.88017736071110164 ) ) ;
#63068=CARTESIAN_POINT ( 'NONE',  ( 4.559911319644449179, 52.23035201082151247, -9.422509992056141925 ) ) ;
#63071=CARTESIAN_POINT ( 'NONE',  ( 19.42250999205614548, 10.98035201082150536, -5.440088680355545492 ) ) ;
#63072=CARTESIAN_POINT ( 'NONE',  ( 7.361572987183169658, 59.96726448433410894, -9.846743663894592657 ) ) ;
#63073=CARTESIAN_POINT ( 'NONE',  ( 19.42250999205614548, 20.98035201082150891, -5.440088680355545492 ) ) ;
#63074=PLANE ( 'NONE',  #4845 ) ;
#63076=CARTESIAN_POINT ( 'NONE',  ( 6.565887622018943937, 25.16530133659708213, 12.81628187352647430 ) ) ;
#63078=CARTESIAN_POINT ( 'NONE',  ( 2.035157376598824452, 48.68868534415483396, 7.964842623401179544 ) ) ;
#63079=CARTESIAN_POINT ( 'NONE',  ( 18.52753015748617571, 33.09226448433411605, 4.923371831947298993 ) ) ;
#63080=CARTESIAN_POINT ( 'NONE',  ( 22.81628187352647785, 1.623634669930420271, 6.195893100308588602E-16 ) ) ;
#63081=CARTESIAN_POINT ( 'NONE',  ( 19.72487221294571569, 47.80223176428831522, -6.499999999999982236 ) ) ;
#63082=CARTESIAN_POINT ( 'NONE',  ( 10.00000000000000178, 19.31368534415484106, 10.88017736071110342 ) ) ;
#63083=CARTESIAN_POINT ( 'NONE',  ( 0.5774900079438607392, 38.48035201082150536, 5.440088680355550821 ) ) ;
#63084=CARTESIAN_POINT ( 'NONE',  ( -4.164238869374099927, 57.01208216824731068, 3.795296366450308767 ) ) ;
#63085=CARTESIAN_POINT ( 'NONE',  ( 14.92337183194729988, 39.34226448433412315, -8.527530157486177487 ) ) ;
#63086=CARTESIAN_POINT ( 'NONE',  ( 19.42250999205614193, 55.14701867748817676, 5.440088680355555262 ) ) ;
#63088=CARTESIAN_POINT ( 'NONE',  ( 20.36894250292379738, 14.92874883491396432, -10.36894250292379027 ) ) ;
#63092=CARTESIAN_POINT ( 'NONE',  ( 1.274849032794324932, 22.55509018479936145, -6.500000000000021316 ) ) ;
#63093=EDGE_LOOP ( 'NONE', ( #48241, #26025, #58971, #5208, #34096, #4963 ) ) ;
#63095=CARTESIAN_POINT ( 'NONE',  ( 24.16423886937410614, 29.30374883491396787, 8.672049930838204340E-16 ) ) ;
#63096=CARTESIAN_POINT ( 'NONE',  ( 6.204703633549690345, 40.76208216824731778, -14.16423886937410259 ) ) ;
#63097=CARTESIAN_POINT ( 'NONE',  ( 19.84674366389459266, 8.300597817667451750, 2.638427012816836559 ) ) ;
#63098=CARTESIAN_POINT ( 'NONE',  ( 7.361572987183170547, 62.05059781766745886, 9.846743663894590881 ) ) ;
#63099=CARTESIAN_POINT ( 'NONE',  ( 0.2751277870542967463, 0.000000000000000000, 6.500000000000000888 ) ) ;
#63100=CARTESIAN_POINT ( 'NONE',  ( 20.88017736071110519, 65.56368534415483396, 2.639326808657452039E-16 ) ) ;
#63101=CARTESIAN_POINT ( 'NONE',  ( 22.81628187352648496, 26.83196800326374998, -3.434112377981050290 ) ) ;
#63102=CARTESIAN_POINT ( 'NONE',  ( 20.36894250292379382, 33.67874883491396076, 10.36894250292379205 ) ) ;
#63103=CARTESIAN_POINT ( 'NONE',  ( -0.8801773607111008646, 28.27201867748817321, 2.915334737309923430 ) ) ;
#63105=CARTESIAN_POINT ( 'NONE',  ( 2.035157376598822676, 67.43868534415484817, -7.964842623401177768 ) ) ;
#63108=COLOUR_RGB ( '', 0.72549020, 0.75294118, 0.79215686) ;
#63110=EDGE_CURVE ( 'NONE', #54543, #58661, #16308, .T. ) ;
#63113=( NAMED_UNIT ( * ) PLANE_ANGLE_UNIT ( ) SI_UNIT ( $, .RADIAN. ) );
#63114=CARTESIAN_POINT ( 'NONE',  ( -2.266590686148945544, 66.38708216824730357, -7.082119434687050408 ) ) ;
#63115=CARTESIAN_POINT ( 'NONE',  ( 19.42250999205614548, 5.980352010821504471, -5.440088680355545492 ) ) ;
#63116=CARTESIAN_POINT ( 'NONE',  ( 17.20831665107776587, 42.88393115100077324, 7.208316651077764980 ) ) ;
#63117=CARTESIAN_POINT ( 'NONE',  ( 3.591859063236761518, 9.956968003263753531, 11.09922568453594849 ) ) ;
#63122=CARTESIAN_POINT ( 'NONE',  ( 19.38216949554541557, 7.248634669930421381, -9.382169495545420901 ) ) ;
#63124=CARTESIAN_POINT ( 'NONE',  ( 17.08211943468705130, 48.47041550158063927, 12.26659068614894998 ) ) ;
#63127=CARTESIAN_POINT ( 'NONE',  ( 10.00000000000000000, 50.55374883491396787, -14.16423886937410082 ) ) ;
#63129=CARTESIAN_POINT ( 'NONE',  ( -0.8801773607111009756, 33.06368534415484106, 1.068504757029289695E-15 ) ) ;
#63130=CARTESIAN_POINT ( 'NONE',  ( 20.88017736071110164, 40.35535201082150536, 2.915334737309930979 ) ) ;
#63131=CARTESIAN_POINT ( 'NONE',  ( 7.361572987183170547, 67.05059781766746596, 9.846743663894590881 ) ) ;
#63132=CARTESIAN_POINT ( 'NONE',  ( 4.559911319644449179, 42.23035201082151247, -9.422509992056141925 ) ) ;
#63133=CARTESIAN_POINT ( 'NONE',  ( 0.5774900079438590739, 67.64701867748817676, -5.440088680355550821 ) ) ;
#63134=CARTESIAN_POINT ( 'NONE',  ( 4.559911319644449179, 23.89701867748817321, 9.422509992056141925 ) ) ;
#63137=CARTESIAN_POINT ( 'NONE',  ( 0.1532563361054083140, 11.00893115100078568, 1.131784320476157264E-15 ) ) ;
#63139=VERTEX_POINT ( 'NONE', #59618 ) ;
#63140=CARTESIAN_POINT ( 'NONE',  ( 17.20831665107776587, 49.13393115100078745, -7.208316651077762316 ) ) ;
#63142=CARTESIAN_POINT ( 'NONE',  ( 22.81628187352647785, 46.41530133659708213, 3.434112377981063169 ) ) ;
#63143=( LENGTH_UNIT ( ) NAMED_UNIT ( * ) SI_UNIT ( .MILLI., .METRE. ) );
#63144=CARTESIAN_POINT ( 'NONE',  ( -46.94000000000001194, 93.00000000000000000, 5.000000000000000000 ) ) ;
#63147=CARTESIAN_POINT ( 'NONE',  ( 17.20831665107776587, 52.88393115100078035, 7.208316651077764980 ) ) ;
#63148=CARTESIAN_POINT ( 'NONE',  ( 24.16423886937410614, 49.51208216824730357, -3.795296366450302550 ) ) ;
#63149=CARTESIAN_POINT ( 'NONE',  ( 17.20831665107776587, 54.13393115100079456, -7.208316651077762316 ) ) ;
#63151=CARTESIAN_POINT ( 'NONE',  ( 7.361572987183169658, 19.96726448433411960, -9.846743663894592657 ) ) ;
#63152=CARTESIAN_POINT ( 'NONE',  ( 21.09922568453595559, 57.04030133659708923, -6.408140936763230044 ) ) ;
#63153=CARTESIAN_POINT ( 'NONE',  ( 5.076628168052703671, 56.84226448433412315, 8.527530157486179263 ) ) ;
#63154=CARTESIAN_POINT ( 'NONE',  ( 1.472469842513823179, 1.425597817667451528, 4.923371831947296329 ) ) ;
#63157=CARTESIAN_POINT ( 'NONE',  ( -4.164238869374099927, 57.01208216824731068, 3.795296366450308767 ) ) ;
#63158=( NAMED_UNIT ( * ) PLANE_ANGLE_UNIT ( ) SI_UNIT ( $, .RADIAN. ) );
#63159=CARTESIAN_POINT ( 'NONE',  ( -0.8801773607111009756, 43.06368534415484106, 1.068504757029289695E-15 ) ) ;
#63160=CARTESIAN_POINT ( 'NONE',  ( 22.81628187352647785, 11.41530133659708390, 3.434112377981063169 ) ) ;
#63161=CARTESIAN_POINT ( 'NONE',  ( 17.96484262340118221, 51.18868534415483396, -7.964842623401177768 ) ) ;
#63166=CARTESIAN_POINT ( 'NONE',  ( 5.076628168052704559, 50.17559781766745886, -8.527530157486179263 ) ) ;
#63167=CARTESIAN_POINT ( 'NONE',  ( 1.472469842513823179, 0.5922644843341181575, -4.923371831947296329 ) ) ;
#63169=CARTESIAN_POINT ( 'NONE',  ( -1.099225684535947600, 9.540301336597087456, 6.408140936763237150 ) ) ;
#63170=CARTESIAN_POINT ( 'NONE',  ( 4.559911319644449179, 12.23035201082150714, -9.422509992056141925 ) ) ;
#63171=DIRECTION ( 'NONE',  ( -0.5547001962252290364, -0.8320502943378437211, 0.000000000000000000 ) ) ;
#63173=CARTESIAN_POINT ( 'NONE',  ( 20.36894250292379738, 34.92874883491396076, -10.36894250292379027 ) ) ;
#63174=CARTESIAN_POINT ( 'NONE',  ( 6.204703633549690345, 27.84541550158063217, 14.16423886937410082 ) ) ;
#63175=CARTESIAN_POINT ( 'NONE',  ( 2.917880565312948704, 67.63708216824730357, 12.26659068614894643 ) ) ;
#63176=CARTESIAN_POINT ( 'NONE',  ( -2.816281873526473856, 39.12363466993041783, 9.499525473075851096E-16 ) ) ;
#63177=CARTESIAN_POINT ( 'NONE',  ( 17.96484262340118221, 14.93868534415483751, 7.964842623401181321 ) ) ;
#63181=CARTESIAN_POINT ( 'NONE',  ( 7.361572987183169658, 34.96726448433411605, -9.846743663894592657 ) ) ;
#63182=CARTESIAN_POINT ( 'NONE',  ( 2.035157376598824452, 38.68868534415483396, 7.964842623401179544 ) ) ;
#63183=CARTESIAN_POINT ( 'NONE',  ( 19.84674366389459266, 63.30059781766745886, 2.638427012816836559 ) ) ;
#63184=CARTESIAN_POINT ( 'NONE',  ( 17.08211943468705840, 25.13708216824730357, -12.26659068614894466 ) ) ;
#63185=CARTESIAN_POINT ( 'NONE',  ( 0.1532563361054083140, 61.00893115100078745, 1.131784320476157264E-15 ) ) ;
#63187=( GEOMETRIC_REPRESENTATION_CONTEXT ( 3 ) GLOBAL_UNCERTAINTY_ASSIGNED_CONTEXT ( ( #60451 ) ) GLOBAL_UNIT_ASSIGNED_CONTEXT ( ( #45703, #76205, #15224 ) ) REPRESENTATION_CONTEXT ( 'NONE', 'WORKASPACE' ) );
#63189=CARTESIAN_POINT ( 'NONE',  ( 17.20831665107776587, 29.13393115100078390, -7.208316651077762316 ) ) ;
#63190=CARTESIAN_POINT ( 'NONE',  ( 13.43411237798105340, 55.58196800326374643, 12.81628187352647963 ) ) ;
#63191=CARTESIAN_POINT ( 'NONE',  ( 10.00000000000000000, 54.75893115100078745, -9.846743663894594434 ) ) ;
#63192=ORIENTED_EDGE ( 'NONE', *, *, #82650, .T. ) ;
#63194=CARTESIAN_POINT ( 'NONE',  ( -0.8801773607111008646, 3.272018677488171434, 2.915334737309923430 ) ) ;
#63195=CARTESIAN_POINT ( 'NONE',  ( 12.91533473730993009, 51.60535201082149825, -10.88017736071109987 ) ) ;
#63196=CARTESIAN_POINT ( 'NONE',  ( -4.164238869374099039, 11.80374883491396965, 8.674139862899312516E-16 ) ) ;
#63197=CARTESIAN_POINT ( 'NONE',  ( 2.035157376598822676, 67.43868534415484817, -7.964842623401177768 ) ) ;
#63198=CARTESIAN_POINT ( 'NONE',  ( 0.1532563361054082862, 56.21726448433411605, 2.638427012816831674 ) ) ;
#63199=CARTESIAN_POINT ( 'NONE',  ( 4.559911319644449179, 22.23035201082150536, -9.422509992056141925 ) ) ;
#63201=CARTESIAN_POINT ( 'NONE',  ( 18.52753015748617571, 58.09226448433411605, 4.923371831947298993 ) ) ;
#63203=CARTESIAN_POINT ( 'NONE',  ( 0.1532563361054083140, 1.008931151000784787, 1.131784320476157264E-15 ) ) ;
#63205=CARTESIAN_POINT ( 'NONE',  ( 19.38216949554541202, 60.99863466993042493, 9.382169495545424454 ) ) ;
#63207=VERTEX_POINT ( 'NONE', #34641 ) ;
#63208=DIRECTION ( 'NONE',  ( -0.000000000000000000, 1.000000000000000000, -0.000000000000000000 ) ) ;
#63210=CARTESIAN_POINT ( 'NONE',  ( 24.16423886937409904, 44.09541550158063927, 3.795296366450317205 ) ) ;
#63211=CARTESIAN_POINT ( 'NONE',  ( 0.1532563361054083140, 61.00893115100078745, 1.131784320476157264E-15 ) ) ;
#63212=CARTESIAN_POINT ( 'NONE',  ( 1.472469842513823179, 15.59226448433411960, -4.923371831947296329 ) ) ;
#63214=CARTESIAN_POINT ( 'NONE',  ( 20.88017736071110875, 25.77201867748816966, -2.915334737309920765 ) ) ;
#63215=CARTESIAN_POINT ( 'NONE',  ( 19.84674366389459266, 58.71726448433411605, -2.638427012816827677 ) ) ;
#63218=CARTESIAN_POINT ( 'NONE',  ( 2.917880565312950480, 35.97041550158063217, -12.26659068614894821 ) ) ;
#63219=CARTESIAN_POINT ( 'NONE',  ( -4.164238869374099927, 62.01208216824728936, 3.795296366450308767 ) ) ;
#63220=CARTESIAN_POINT ( 'NONE',  ( 10.00000000000000000, 64.75893115100078035, -9.846743663894594434 ) ) ;
#63221=CARTESIAN_POINT ( 'NONE',  ( 1.274849032794280523, 68.57228050351031357, 6.499999999999960032 ) ) ;
#63222=CARTESIAN_POINT ( 'NONE',  ( 0.5774900079438590739, 62.64701867748817676, -5.440088680355550821 ) ) ;
#63223=CARTESIAN_POINT ( 'NONE',  ( 17.20831665107776587, 14.13393115100078568, -7.208316651077762316 ) ) ;
#63226=DIRECTION ( 'NONE',  ( 0.01646788341559294114, 0.9998643952135761737, 0.000000000000000000 ) ) ;
#63228=EDGE_CURVE ( 'NONE', #16048, #44176, #65138, .T. ) ;
#63229=CARTESIAN_POINT ( 'NONE',  ( 12.63842701281683922, 29.55059781766745175, -9.846743663894590881 ) ) ;
#63230=ORIENTED_EDGE ( 'NONE', *, *, #95160, .F. ) ;
#63232=CARTESIAN_POINT ( 'NONE',  ( 22.26659068614894466, 28.88708216824730357, 7.082119434687054849 ) ) ;
#63233=CARTESIAN_POINT ( 'NONE',  ( 1.472469842513823179, 35.59226448433412315, -4.923371831947296329 ) ) ;
#63234=CARTESIAN_POINT ( 'NONE',  ( -0.8801773607111009756, 43.06368534415484106, 1.068504757029289695E-15 ) ) ;
#63237=CARTESIAN_POINT ( 'NONE',  ( 4.559911319644449179, 42.23035201082151247, -9.422509992056141925 ) ) ;
#63238=ADVANCED_FACE ( 'NONE', ( #21139 ), #51640, .T. ) ;
#63241=CARTESIAN_POINT ( 'NONE',  ( 13.79529636645031943, 5.345415501580634832, -14.16423886937409904 ) ) ;
#63244=CARTESIAN_POINT ( 'NONE',  ( 13.43411237798105340, 35.58196800326375353, 12.81628187352647963 ) ) ;
#63245=CARTESIAN_POINT ( 'NONE',  ( 19.84674366389459621, 23.50893115100078390, 7.409399052514197653E-17 ) ) ;
#63247=CARTESIAN_POINT ( 'NONE',  ( 0.1532563361054100626, 30.80059781766744820, -2.638427012816831230 ) ) ;
#63248=COLOUR_RGB ( '', 0.66274510, 0.83137255, 0.94901961) ;
#63251=CARTESIAN_POINT ( 'NONE',  ( 20.88017736071110519, 50.56368534415484106, 2.639326808657452039E-16 ) ) ;
#63255=CARTESIAN_POINT ( 'NONE',  ( 1.472469842513823179, 5.592264484334118713, -4.923371831947296329 ) ) ;
#63256=CARTESIAN_POINT ( 'NONE',  ( 21.09922568453595559, 12.04030133659708746, -6.408140936763230044 ) ) ;
#63258=CARTESIAN_POINT ( 'NONE',  ( 12.63842701281683034, 47.46726448433412315, 9.846743663894596210 ) ) ;
#63259=CARTESIAN_POINT ( 'NONE',  ( -2.816281873526473856, 64.12363466993042493, 9.499525473075851096E-16 ) ) ;
#63260=CARTESIAN_POINT ( 'NONE',  ( -4.164238869374099039, 11.80374883491396965, 8.674139862899312516E-16 ) ) ;
#63261=CARTESIAN_POINT ( 'NONE',  ( 18.52753015748618282, 13.92559781766745175, -4.923371831947291888 ) ) ;
#63262=CARTESIAN_POINT ( 'NONE',  ( 22.81628187352648496, 36.83196800326376064, -3.434112377981050290 ) ) ;
#63264=LINE ( 'NONE', #45826, #97710 ) ;
#63265=CARTESIAN_POINT ( 'NONE',  ( 12.91533473730992121, 54.52201867748816255, 10.88017736071110164 ) ) ;
#63266=CARTESIAN_POINT ( 'NONE',  ( 6.565887622018943937, 10.16530133659708746, 12.81628187352647430 ) ) ;
#63268=CARTESIAN_POINT ( 'NONE',  ( 19.84674366389459266, 23.30059781766745530, 2.638427012816836559 ) ) ;
#63269=CARTESIAN_POINT ( 'NONE',  ( 4.559911319644449179, 32.23035201082150536, -9.422509992056141925 ) ) ;
#63271=CARTESIAN_POINT ( 'NONE',  ( -2.816281873526473856, 34.33196800326376064, 3.434112377981055619 ) ) ;
#63273=CARTESIAN_POINT ( 'NONE',  ( 0.1532563361054083140, 26.00893115100078745, 1.131784320476157264E-15 ) ) ;
#63276=CARTESIAN_POINT ( 'NONE',  ( 17.85158348494333680, 44.73726573380442773, -6.500000000000027534 ) ) ;
#63278=CARTESIAN_POINT ( 'NONE',  ( 15.44008868035555793, 16.39701867748817321, -9.422509992056140149 ) ) ;
#63279=CARTESIAN_POINT ( 'NONE',  ( 17.96484262340118221, 56.18868534415484817, -7.964842623401177768 ) ) ;
#63281=CARTESIAN_POINT ( 'NONE',  ( 10.00000000000000000, 39.75893115100078745, -9.846743663894594434 ) ) ;
#63282=CARTESIAN_POINT ( 'NONE',  ( -0.8801773607110991993, 22.85535201082150181, -2.915334737309923874 ) ) ;
#63283=DIRECTION ( 'NONE',  ( 6.608470384673550777E-17, 1.000000000000000000, -0.000000000000000000 ) ) ;
#63284=CARTESIAN_POINT ( 'NONE',  ( 2.035157376598822676, 42.43868534415483396, -7.964842623401177768 ) ) ;
#63285=CARTESIAN_POINT ( 'NONE',  ( 15.44008868035555260, 9.730352010821505360, 9.422509992056143702 ) ) ;
#63286=CARTESIAN_POINT ( 'NONE',  ( 10.00000000000000178, 17.25893115100078745, 9.846743663894594434 ) ) ;
#63287=CARTESIAN_POINT ( 'NONE',  ( 12.63842701281683922, 39.55059781766744464, -9.846743663894590881 ) ) ;
#63288=LINE ( 'NONE', #40318, #88003 ) ;
#63289=SURFACE_STYLE_USAGE ( .BOTH. , #71791 ) ;
#63290=CARTESIAN_POINT ( 'NONE',  ( 17.08211943468705840, 25.13708216824730357, -12.26659068614894466 ) ) ;
#63291=CARTESIAN_POINT ( 'NONE',  ( 5.076628168052704559, 40.17559781766745175, -8.527530157486179263 ) ) ;
#63294=CARTESIAN_POINT ( 'NONE',  ( 20.88017736071110875, 5.772018677488170546, -2.915334737309920765 ) ) ;
#63295=CARTESIAN_POINT ( 'NONE',  ( 2.791683348922240793, 26.63393115100078745, 7.208316651077764092 ) ) ;
#63298=CARTESIAN_POINT ( 'NONE',  ( 7.084665262690076126, 44.10535201082151247, 10.88017736071109987 ) ) ;
#63301=CARTESIAN_POINT ( 'NONE',  ( 7.084665262690076126, 12.02201867748817143, -10.88017736071110164 ) ) ;
#63302=CARTESIAN_POINT ( 'NONE',  ( -1.099225684535947600, 43.70696800326375353, -6.408140936763238038 ) ) ;
#63303=CARTESIAN_POINT ( 'NONE',  ( -2.816281873526473856, 14.33196800326375531, 3.434112377981055619 ) ) ;
#63304=CARTESIAN_POINT ( 'NONE',  ( 2.791683348922240793, 16.63393115100078745, 7.208316651077764092 ) ) ;
#63307=CARTESIAN_POINT ( 'NONE',  ( 6.204703633549690345, 47.84541550158064638, 14.16423886937410082 ) ) ;
#63308=CARTESIAN_POINT ( 'NONE',  ( 2.917880565312948704, 27.63708216824730357, 12.26659068614894643 ) ) ;
#63309=CARTESIAN_POINT ( 'NONE',  ( 12.91533473730993009, 16.60535201082150891, -10.88017736071109987 ) ) ;
#63310=CARTESIAN_POINT ( 'NONE',  ( 12.91533473730993009, 51.60535201082149825, -10.88017736071109987 ) ) ;
#63312=FACE_OUTER_BOUND ( 'NONE', #14597, .T. ) ;
#63313=CARTESIAN_POINT ( 'NONE',  ( 18.04007052943771683, 48.01528370094807485, 5.767676674365856293 ) ) ;
#63314=CARTESIAN_POINT ( 'NONE',  ( 2.791683348922237240, 10.38393115100078390, -7.208316651077763204 ) ) ;
#63316=CARTESIAN_POINT ( 'NONE',  ( 7.361572987183170547, 22.05059781766745530, 9.846743663894590881 ) ) ;
#63317=CARTESIAN_POINT ( 'NONE',  ( 5.076628168052704559, 0.1755978176674514724, -8.527530157486179263 ) ) ;
#63318=CARTESIAN_POINT ( 'NONE',  ( 17.20831665107776587, 24.13393115100078035, -7.208316651077762316 ) ) ;
#63319=CARTESIAN_POINT ( 'NONE',  ( 5.076628168052703671, 46.84226448433412315, 8.527530157486179263 ) ) ;
#63322=CARTESIAN_POINT ( 'NONE',  ( 15.44008868035555260, 14.73035201082150536, 9.422509992056143702 ) ) ;
#63324=UNCERTAINTY_MEASURE_WITH_UNIT (LENGTH_MEASURE( 1.000000000000000082E-05 ), #52443, 'distance_accuracy_value', 'NONE');
#63325=CARTESIAN_POINT ( 'NONE',  ( 13.43411237798105340, 35.58196800326375353, 12.81628187352647963 ) ) ;
#63326=CARTESIAN_POINT ( 'NONE',  ( 20.88017736071110164, 55.35535201082149825, 2.915334737309930979 ) ) ;
#63327=CARTESIAN_POINT ( 'NONE',  ( 19.84674366389459266, 28.30059781766745886, 2.638427012816836559 ) ) ;
#63328=CARTESIAN_POINT ( 'NONE',  ( 6.204703633549690345, 40.76208216824731778, -14.16423886937410259 ) ) ;
#63329=CARTESIAN_POINT ( 'NONE',  ( 19.84674366389459621, 23.50893115100078390, 7.409399052514197653E-17 ) ) ;
#63330=CARTESIAN_POINT ( 'NONE',  ( 18.72515096720571037, 55.05509018479936145, 6.499999999999982236 ) ) ;
#63334=CARTESIAN_POINT ( 'NONE',  ( 12.63842701281683034, 47.46726448433412315, 9.846743663894596210 ) ) ;
#63335=CARTESIAN_POINT ( 'NONE',  ( 14.92337183194729633, 37.67559781766745175, 8.527530157486181039 ) ) ;
#63336=CARTESIAN_POINT ( 'NONE',  ( 10.00000000000000000, 15.55374883491396787, -14.16423886937410082 ) ) ;
#63337=CARTESIAN_POINT ( 'NONE',  ( 17.08211943468705130, 23.47041550158063572, 12.26659068614894998 ) ) ;
#63338=CARTESIAN_POINT ( 'NONE',  ( 18.52753015748618282, 28.92559781766745175, -4.923371831947291888 ) ) ;
#63339=CARTESIAN_POINT ( 'NONE',  ( 2.035157376598824452, 48.68868534415483396, 7.964842623401179544 ) ) ;
#63340=CARTESIAN_POINT ( 'NONE',  ( 17.96484262340118221, 26.18868534415483396, -7.964842623401177768 ) ) ;
#63341=CARTESIAN_POINT ( 'NONE',  ( 19.42250999205614548, 45.98035201082150536, -5.440088680355545492 ) ) ;
#63342=CARTESIAN_POINT ( 'NONE',  ( -0.8801773607111008646, 28.27201867748817321, 2.915334737309923430 ) ) ;
#63344=CARTESIAN_POINT ( 'NONE',  ( 20.88017736071110519, 55.56368534415484817, 2.639326808657452039E-16 ) ) ;
#63345=VERTEX_POINT ( 'NONE', #30099 ) ;
#63346=CARTESIAN_POINT ( 'NONE',  ( -1.099225684535947600, 53.70696800326376064, -6.408140936763238038 ) ) ;
#63347=VECTOR ( 'NONE', #67980, 1000.000000000000000 ) ;
#63348=CARTESIAN_POINT ( 'NONE',  ( 10.00000000000000178, 59.31368534415484106, 10.88017736071110342 ) ) ;
#63353=CARTESIAN_POINT ( 'NONE',  ( 20.15039907845753930, 70.00000000000000000, -6.262539305110068177 ) ) ;
#63355=CARTESIAN_POINT ( 'NONE',  ( 22.26659068614895176, 54.72041550158063217, -7.082119434687042414 ) ) ;
#63356=CARTESIAN_POINT ( 'NONE',  ( 0.1532563361054082862, 6.217264484334118713, 2.638427012816831674 ) ) ;
#63358=CARTESIAN_POINT ( 'NONE',  ( 24.16423886937409904, 4.095415501580634832, 3.795296366450317205 ) ) ;
#63359=CARTESIAN_POINT ( 'NONE',  ( 0.1532563361054083140, 1.008931151000784787, 1.131784320476157264E-15 ) ) ;
#63360=CARTESIAN_POINT ( 'NONE',  ( 19.42250999205614548, 10.98035201082150358, -5.440088680355545492 ) ) ;
#63361=CARTESIAN_POINT ( 'NONE',  ( 0.1532563361054100626, 45.80059781766745886, -2.638427012816831230 ) ) ;
#63364=CARTESIAN_POINT ( 'NONE',  ( 5.076628168052704559, 50.17559781766745886, -8.527530157486179263 ) ) ;
#63366=DIRECTION ( 'NONE',  ( -1.000000000000000000, 0.000000000000000000, 0.000000000000000000 ) ) ;
#63367=CARTESIAN_POINT ( 'NONE',  ( -0.8801773607110991993, 37.85535201082151247, -2.915334737309923874 ) ) ;
#63368=CARTESIAN_POINT ( 'NONE',  ( 7.361572987183170547, 52.05059781766745175, 9.846743663894590881 ) ) ;
#63370=CARTESIAN_POINT ( 'NONE',  ( -0.8801773607110991993, 57.85535201082149825, -2.915334737309923874 ) ) ;
#63371=CARTESIAN_POINT ( 'NONE',  ( 10.00000000000000000, 11.81368534415483751, -10.88017736071110342 ) ) ;
#63372=CARTESIAN_POINT ( 'NONE',  ( 13.43411237798106583, 47.66530133659709634, -12.81628187352647252 ) ) ;
#63374=ORIENTED_EDGE ( 'NONE', *, *, #3351, .F. ) ;
#63375=CARTESIAN_POINT ( 'NONE',  ( -1.099225684535947600, 34.54030133659708923, 6.408140936763237150 ) ) ;
#63376=CARTESIAN_POINT ( 'NONE',  ( 12.91533473730993009, 31.60535201082150891, -10.88017736071109987 ) ) ;
#63378=( BOUNDED_SURFACE ( )  B_SPLINE_SURFACE ( 1, 2, ( 
 ( #56844, #86371, #77869, #33342, #9885, #9380, #48355, #56366, #70884, #32858, #87343, #64329, #71379, #39883, #63836, #2892, #24401, #63358, #10373, #94350, #78861, #18858, #79355, #8884, #71850, #39401, #85380, #40874, #25869, #86859, #47371, #62870, #93366, #93861, #41383, #55379, #47860, #18365, #85879, #25389, #94841, #69894, #48844, #26343, #49338, #17391, #55872, #3360, #33824, #78366, #1414, #31867, #40385, #62366, #54869, #16893, #87823, #3859, #89315, #27323, #13313, #79838, #19343, #50315, #11343, #42343, #72818, #43313, #35317, #28315, #4358, #65314, #58302, #34824, #65810, #81796, #95840, #35818, #66304, #57821, #80829, #73318, #81320, #49826, #42834, #95336, #80336, #20331, #88818, #41863, #11835, #12814, #88329, #19827, #72326, #20823, #50826, #12329, #34319, #4841, #73807, #96343, #5337, #27817, #96840, #58807, #51313, #64817, #26835, #57329, #26658, #33654, #40195, #26176, #64149, #55182, #63663, #71678, #94667, #48668, #49643, #41685, #70208, #34145, #1727, #47694, #41198, #79169, #87156, #9699, #32681, #63174, #25699, #72155, #86193, #10198, #56668, #70702, #86683, #57153, #32182, #11166, #87651, #11661, #78687, #56189, #3188, #18187, #40692, #18681, #10684, #93682, #49167, #33170, #71193, #2221, #24711, #19164, #2716, #62684, #93185, #25215, #94168, #85699, #55696, #17705, #79669, #3683, #64639, #48175, #95147, #80150, #17216, #78186, #83177, #45174, #30653, #695, #31148, #9147, #54147, #39166, #46172, #60664, #39664, #45673, #61159, #14702, #8176, #70156, #52676, #83676, #47133, #75675, #69172, #61639, #62131, #7188, #84656, #46648, #8653, #62625, #92639, #16164, #98710, #1673, #32126, #54634, #15191, #23683, #85152, #77144, #92160, #53663, #69655, #1181, #31639, #24163, #53170, #93130, #37691, #16658, #68190, #91164, #77630, #91668, #30161, #23187, #22691, #38670, #76171, #7691, #15686, #84179, #38188, #68675, #202, #76655, #65077, #24657, #63127, #18142, #55126, #17653, #48123, #41635, #3138, #57099, #78638, #40640, #26128, #10145, #33600, #10631, #11116, #55639, #72101, #71138, #56137, #41143, #79615, #93629, #79118, #9647, #25164, #18623, #87108, #42120, #86139, #3628, #2666, #33117, #34583, #87595, #64097, #25644, #72586, #2171, #71628, #4120, #49114, #49585, #63611, #94117, #94613, #86632, #48614, #32628, #56619, #85642, #26602, #34095, #64586, #95094, #19105, #80098, #11603, #17161, #47641, #78137, #40144, #70648, #88087, #97108, #43086, #52078, #44565, #74067, #65576, #21085, #96603, #96103, #36078, #44063, #58578, #89080, #75063, #82571, #59070, #27587, #51583, #89574, #80600, #20594, #28579 ),
 ( #35587, #82069, #51080, #58077, #13579, #6570, #81571, #73571, #74570, #28080, #50095, #57590, #88581, #20089, #50593, #73079, #29062, #6084, #4615, #21587, #36586, #13079, #66581, #67073, #81085, #5096, #43574, #5599, #97601, #59570, #12586, #12098, #90063, #19600, #27087, #14085, #66075, #37082, #95601, #42601, #35076, #47023, #53542, #15085, #54037, #94, #22084, #29548, #37578, #98598, #91047, #45053, #1061, #69053, #75563, #92523, #77037, #38071, #38558, #68563, #30541, #91554, #24050, #98090, #90555, #54520, #7076, #589, #53046, #68071, #69544, #61532, #14584, #52559, #76543, #23569, #85036, #16548, #77514, #30048, #31527, #76053, #39049, #60054, #83063, #45556, #15575, #46056, #9031, #31032, #84548, #61041, #60556, #67581, #22575, #7583, #83565, #23073, #84055, #8061, #92041, #62022, #16047, #46536, #8550, #50333, #1560, #72835, #34838, #95859, #50842, #80846, #4373, #85528, #96361, #27834, #42849, #2051, #11852, #73333, #42362, #80354, #41880, #65333, #27343, #57836, #19843, #40026, #88838, #20346, #12343, #62511, #78022, #4860, #49356, #58320, #65829, #18874, #11361, #35336, #81334, #72343, #39548, #70528, #93016, #70037, #88345, #79858, #32008, #24553, #3876, #55010, #17040, #9525, #32514, #64349, #47519, #94857, #26359, #56859, #87360, #34339, #64834, #95353, #26852, #57349, #87842, #19361, #49845, #35835, #37828, #51333, #44804, #97346, #81815, #14834, #6820, #58823, #96858, #21835, #67826, #98837, #68318, #60795, #74312, #45309, #21336, #83311, #43331, #5356, #89815, #59806, #90300, #30293, #14331, #98343, #6321, #20841, #91295, #5839, #51826, #73823, #67322, #22818, #12831, #43817, #7325, #66322, #29310, #52318, #22330, #28333, #75309, #37336, #29801, #53298, #52804, #60310, #89331, #13333, #36329, #75805, #66824, #82811, #28817, #90803, #59316, #13834, #82313, #44315, #74816, #36830, #97845, #32756, #63251, #55267, #7819, #23320, #62765, #92289, #2299, #9778, #61778, #54274, #24791, #40276, #16299, #17290, #84313, #38314, #85780, #77768, #23812, #25289, #69795, #24302, #1804, #46299, #84790, #46780, #8784, #32261, #62265, #69299, #343, #77274, #76302, #15331, #39303, #1321, #16791, #31772, #53802, #9281, #93760, #92773, #31278, #54764, #68810, #45814, #15813, #76786, #8303, #61290, #47766, #85283, #91799, #70783, #93267, #47266, #39789, #70289, #78264, #83806, #30785, #38802, #822, #80727, #94243, #87725, #41277, #25772, #57717, #49720, #2795, #40769, #64715, #11735, #42732, #12221, #4741, #18264, #88218, #64227, #27219, #86266, #48253, #33727, #3761, #34217, #73210, #57226, #42245, #49242, #63740 ) ),
 .UNSPECIFIED., .F., .F., .F. ) 
 B_SPLINE_SURFACE_WITH_KNOTS ( ( 2, 2 ),
 ( 3, 2, 2, 2, 2, 2, 2, 2, 2, 2, 2, 2, 2, 2, 2, 2, 2, 2, 2, 2, 2, 2, 2, 2, 2, 2, 2, 2, 2, 2, 2, 2, 2, 2, 2, 2, 2, 2, 2, 2, 2, 2, 2, 2, 2, 2, 2, 2, 2, 2, 2, 2, 2, 2, 2, 2, 2, 2, 2, 2, 2, 2, 2, 2, 2, 2, 2, 2, 2, 2, 2, 2, 2, 2, 2, 2, 2, 2, 2, 2, 2, 2, 2, 2, 2, 2, 2, 2, 2, 2, 2, 2, 2, 2, 2, 2, 2, 2, 2, 2, 2, 2, 2, 2, 2, 2, 2, 2, 2, 2, 2, 2, 2, 2, 2, 2, 2, 2, 2, 2, 2, 2, 2, 2, 2, 2, 2, 2, 2, 2, 2, 2, 2, 2, 2, 2, 2, 2, 2, 2, 2, 2, 2, 2, 2, 2, 2, 2, 2, 2, 2, 2, 2, 2, 2, 2, 2, 2, 2, 2, 2, 2, 3 ),
 ( 0.000000000000000000, 1.000000000000000000 ),
 ( 0.000000000000000000, 0.005952380952380952051, 0.01190476190476190410, 0.01785714285714285615, 0.02380952380952380820, 0.02976190476190476025, 0.03571428571428571230, 0.04166666666666666435, 0.04761904761904761640, 0.05357142857142856845, 0.05952380952380952051, 0.06547619047619047949, 0.07142857142857142461, 0.07738095238095238360, 0.08333333333333332871, 0.08928571428571428770, 0.09523809523809523281, 0.1011904761904761918, 0.1071428571428571369, 0.1130952380952380959, 0.1190476190476190410, 0.1250000000000000000, 0.1309523809523809590, 0.1369047619047619180, 0.1428571428571428492, 0.1488095238095238082, 0.1547619047619047672, 0.1607142857142857262, 0.1666666666666666574, 0.1726190476190476164, 0.1785714285714285754, 0.1845238095238095344, 0.1904761904761904656, 0.1964285714285714246, 0.2023809523809523836, 0.2083333333333333426, 0.2142857142857142738, 0.2202380952380952328, 0.2261904761904761918, 0.2321428571428571508, 0.2380952380952380820, 0.2440476190476190410, 0.2500000000000000000, 0.2559523809523809312, 0.2619047619047619180, 0.2678571428571428492, 0.2738095238095238360, 0.2797619047619047672, 0.2857142857142856984, 0.2916666666666666852, 0.2976190476190476164, 0.3035714285714285476, 0.3095238095238095344, 0.3154761904761904656, 0.3214285714285714524, 0.3273809523809523836, 0.3333333333333333148, 0.3392857142857143016, 0.3452380952380952328, 0.3511904761904761640, 0.3571428571428571508, 0.3630952380952380820, 0.3690476190476190688, 0.3750000000000000000, 0.3809523809523809312, 0.3869047619047619180, 0.3928571428571428492, 0.3988095238095238360, 0.4047619047619047672, 0.4107142857142856984, 0.4166666666666666852, 0.4226190476190476164, 0.4285714285714285476, 0.4345238095238095344, 0.4404761904761904656, 0.4464285714285714524, 0.4523809523809523836, 0.4583333333333333148, 0.4642857142857143016, 0.4702380952380952328, 0.4761904761904761640, 0.4821428571428571508, 0.4880952380952380820, 0.4940476190476190688, 0.5000000000000000000, 0.5059523809523809312, 0.5119047619047618625, 0.5178571428571429047, 0.5238095238095238360, 0.5297619047619047672, 0.5357142857142856984, 0.5416666666666666297, 0.5476190476190476719, 0.5535714285714286031, 0.5595238095238095344, 0.5654761904761904656, 0.5714285714285713969, 0.5773809523809523281, 0.5833333333333333703, 0.5892857142857143016, 0.5952380952380952328, 0.6011904761904761640, 0.6071428571428570953, 0.6130952380952381375, 0.6190476190476190688, 0.6250000000000000000, 0.6309523809523809312, 0.6369047619047618625, 0.6428571428571429047, 0.6488095238095238360, 0.6547619047619047672, 0.6607142857142856984, 0.6666666666666666297, 0.6726190476190476719, 0.6785714285714286031, 0.6845238095238095344, 0.6904761904761904656, 0.6964285714285713969, 0.7023809523809523281, 0.7083333333333333703, 0.7142857142857143016, 0.7202380952380952328, 0.7261904761904761640, 0.7321428571428570953, 0.7380952380952381375, 0.7440476190476190688, 0.7500000000000000000, 0.7559523809523809312, 0.7619047619047618625, 0.7678571428571429047, 0.7738095238095238360, 0.7797619047619047672, 0.7857142857142856984, 0.7916666666666666297, 0.7976190476190476719, 0.8035714285714286031, 0.8095238095238095344, 0.8154761904761904656, 0.8214285714285713969, 0.8273809523809523281, 0.8333333333333333703, 0.8392857142857143016, 0.8452380952380952328, 0.8511904761904761640, 0.8571428571428570953, 0.8630952380952381375, 0.8690476190476190688, 0.8750000000000000000, 0.8809523809523809312, 0.8869047619047618625, 0.8928571428571429047, 0.8988095238095238360, 0.9047619047619047672, 0.9107142857142856984, 0.9166666666666666297, 0.9226190476190476719, 0.9285714285714286031, 0.9345238095238095344, 0.9404761904761904656, 0.9464285714285713969, 0.9523809523809523281, 0.9583333333333333703, 0.9642857142857143016 ),
 .UNSPECIFIED. ) 
 GEOMETRIC_REPRESENTATION_ITEM ( )  RATIONAL_B_SPLINE_SURFACE ( (
 ( 1.000000000000000000, 0.9659258262890683122, 1.000000000000000000, 0.9659258262890683122, 1.000000000000000000, 0.9659258262890683122, 1.000000000000000000, 0.9659258262890683122, 1.000000000000000000, 0.9659258262890683122, 1.000000000000000000, 0.9659258262890683122, 1.000000000000000000, 0.9659258262890683122, 1.000000000000000000, 0.9659258262890683122, 1.000000000000000000, 0.9659258262890683122, 1.000000000000000000, 0.9659258262890683122, 1.000000000000000000, 0.9659258262890683122, 1.000000000000000000, 0.9659258262890683122, 1.000000000000000000, 0.9659258262890683122, 1.000000000000000000, 0.9659258262890683122, 1.000000000000000000, 0.9659258262890683122, 1.000000000000000000, 0.9659258262890683122, 1.000000000000000000, 0.9659258262890683122, 1.000000000000000000, 0.9659258262890683122, 1.000000000000000000, 0.9659258262890683122, 1.000000000000000000, 0.9659258262890683122, 1.000000000000000000, 0.9659258262890683122, 1.000000000000000000, 0.9659258262890683122, 1.000000000000000000, 0.9659258262890683122, 1.000000000000000000, 0.9659258262890683122, 1.000000000000000000, 0.9659258262890683122, 1.000000000000000000, 0.9659258262890683122, 1.000000000000000000, 0.9659258262890683122, 1.000000000000000000, 0.9659258262890683122, 1.000000000000000000, 0.9659258262890683122, 1.000000000000000000, 0.9659258262890683122, 1.000000000000000000, 0.9659258262890683122, 1.000000000000000000, 0.9659258262890683122, 1.000000000000000000, 0.9659258262890683122, 1.000000000000000000, 0.9659258262890683122, 1.000000000000000000, 0.9659258262890683122, 1.000000000000000000, 0.9659258262890683122, 1.000000000000000000, 0.9659258262890683122, 1.000000000000000000, 0.9659258262890683122, 1.000000000000000000, 0.9659258262890683122, 1.000000000000000000, 0.9659258262890683122, 1.000000000000000000, 0.9659258262890683122, 1.000000000000000000, 0.9659258262890683122, 1.000000000000000000, 0.9659258262890683122, 1.000000000000000000, 0.9659258262890683122, 1.000000000000000000, 0.9659258262890683122, 1.000000000000000000, 0.9659258262890683122, 1.000000000000000000, 0.9659258262890683122, 1.000000000000000000, 0.9659258262890683122, 1.000000000000000000, 0.9659258262890683122, 1.000000000000000000, 0.9659258262890683122, 1.000000000000000000, 0.9659258262890683122, 1.000000000000000000, 0.9659258262890683122, 1.000000000000000000, 0.9659258262890683122, 1.000000000000000000, 0.9659258262890683122, 1.000000000000000000, 0.9659258262890683122, 1.000000000000000000, 0.9659258262890683122, 1.000000000000000000, 0.9659258262890683122, 1.000000000000000000, 0.9659258262890683122, 1.000000000000000000, 0.9659258262890683122, 1.000000000000000000, 0.9659258262890683122, 1.000000000000000000, 0.9659258262890683122, 1.000000000000000000, 0.9659258262890683122, 1.000000000000000000, 0.9659258262890683122, 1.000000000000000000, 0.9659258262890683122, 1.000000000000000000, 0.9659258262890683122, 1.000000000000000000, 0.9659258262890683122, 1.000000000000000000, 0.9659258262890683122, 1.000000000000000000, 0.9659258262890683122, 1.000000000000000000, 0.9659258262890683122, 1.000000000000000000, 0.9659258262890683122, 1.000000000000000000, 0.9659258262890683122, 1.000000000000000000, 0.9659258262890683122, 1.000000000000000000, 0.9659258262890683122, 1.000000000000000000, 0.9659258262890683122, 1.000000000000000000, 0.9659258262890683122, 1.000000000000000000, 0.9659258262890683122, 1.000000000000000000, 0.9659258262890683122, 1.000000000000000000, 0.9659258262890683122, 1.000000000000000000, 0.9659258262890683122, 1.000000000000000000, 0.9659258262890683122, 1.000000000000000000, 0.9659258262890683122, 1.000000000000000000, 0.9659258262890683122, 1.000000000000000000, 0.9659258262890683122, 1.000000000000000000, 0.9659258262890683122, 1.000000000000000000, 0.9659258262890683122, 1.000000000000000000, 0.9659258262890683122, 1.000000000000000000, 0.9659258262890683122, 1.000000000000000000, 0.9659258262890683122, 1.000000000000000000, 0.9659258262890683122, 1.000000000000000000, 0.9659258262890683122, 1.000000000000000000, 0.9659258262890683122, 1.000000000000000000, 0.9659258262890683122, 1.000000000000000000, 0.9659258262890683122, 1.000000000000000000, 0.9659258262890683122, 1.000000000000000000, 0.9659258262890683122, 1.000000000000000000, 0.9659258262890683122, 1.000000000000000000, 0.9659258262890683122, 1.000000000000000000, 0.9659258262890683122, 1.000000000000000000, 0.9659258262890683122, 1.000000000000000000, 0.9659258262890683122, 1.000000000000000000, 0.9659258262890683122, 1.000000000000000000, 0.9659258262890683122, 1.000000000000000000, 0.9659258262890683122, 1.000000000000000000, 0.9659258262890683122, 1.000000000000000000, 0.9659258262890683122, 1.000000000000000000, 0.9659258262890683122, 1.000000000000000000, 0.9659258262890683122, 1.000000000000000000, 0.9659258262890683122, 1.000000000000000000, 0.9659258262890683122, 1.000000000000000000, 0.9659258262890683122, 1.000000000000000000, 0.9659258262890683122, 1.000000000000000000, 0.9659258262890683122, 1.000000000000000000, 0.9659258262890683122, 1.000000000000000000, 0.9659258262890683122, 1.000000000000000000, 0.9659258262890683122, 1.000000000000000000, 0.9659258262890683122, 1.000000000000000000, 0.9659258262890683122, 1.000000000000000000, 0.9659258262890683122, 1.000000000000000000, 0.9659258262890683122, 1.000000000000000000, 0.9659258262890683122, 1.000000000000000000, 0.9659258262890683122, 1.000000000000000000, 0.9659258262890683122, 1.000000000000000000, 0.9659258262890683122, 1.000000000000000000, 0.9659258262890683122, 1.000000000000000000, 0.9659258262890683122, 1.000000000000000000, 0.9659258262890683122, 1.000000000000000000, 0.9659258262890683122, 1.000000000000000000, 0.9659258262890683122, 1.000000000000000000, 0.9659258262890683122, 1.000000000000000000, 0.9659258262890683122, 1.000000000000000000, 0.9659258262890683122, 1.000000000000000000, 0.9659258262890683122, 1.000000000000000000, 0.9659258262890683122, 1.000000000000000000, 0.9659258262890683122, 1.000000000000000000, 0.9659258262890683122, 1.000000000000000000, 0.9659258262890683122, 1.000000000000000000, 0.9659258262890683122, 1.000000000000000000, 0.9659258262890683122, 1.000000000000000000, 0.9659258262890683122, 1.000000000000000000, 0.9659258262890683122, 1.000000000000000000, 0.9659258262890683122, 1.000000000000000000, 0.9659258262890683122, 1.000000000000000000, 0.9659258262890683122, 1.000000000000000000, 0.9659258262890683122, 1.000000000000000000, 0.9659258262890683122, 1.000000000000000000, 0.9659258262890683122, 1.000000000000000000, 0.9659258262890683122, 1.000000000000000000, 0.9659258262890683122, 1.000000000000000000, 0.9659258262890683122, 1.000000000000000000, 0.9659258262890683122, 1.000000000000000000, 0.9659258262890683122, 1.000000000000000000, 0.9659258262890683122, 1.000000000000000000, 0.9659258262890683122, 1.000000000000000000, 0.9659258262890683122, 1.000000000000000000, 0.9659258262890683122, 1.000000000000000000, 0.9659258262890683122, 1.000000000000000000, 0.9659258262890683122, 1.000000000000000000, 0.9659258262890683122, 1.000000000000000000, 0.9659258262890683122, 1.000000000000000000, 0.9659258262890683122, 1.000000000000000000, 0.9659258262890683122, 1.000000000000000000, 0.9659258262890683122, 1.000000000000000000),
 ( 1.000000000000000000, 0.9659258262890683122, 1.000000000000000000, 0.9659258262890683122, 1.000000000000000000, 0.9659258262890683122, 1.000000000000000000, 0.9659258262890683122, 1.000000000000000000, 0.9659258262890683122, 1.000000000000000000, 0.9659258262890683122, 1.000000000000000000, 0.9659258262890683122, 1.000000000000000000, 0.9659258262890683122, 1.000000000000000000, 0.9659258262890683122, 1.000000000000000000, 0.9659258262890683122, 1.000000000000000000, 0.9659258262890683122, 1.000000000000000000, 0.9659258262890683122, 1.000000000000000000, 0.9659258262890683122, 1.000000000000000000, 0.9659258262890683122, 1.000000000000000000, 0.9659258262890683122, 1.000000000000000000, 0.9659258262890683122, 1.000000000000000000, 0.9659258262890683122, 1.000000000000000000, 0.9659258262890683122, 1.000000000000000000, 0.9659258262890683122, 1.000000000000000000, 0.9659258262890683122, 1.000000000000000000, 0.9659258262890683122, 1.000000000000000000, 0.9659258262890683122, 1.000000000000000000, 0.9659258262890683122, 1.000000000000000000, 0.9659258262890683122, 1.000000000000000000, 0.9659258262890683122, 1.000000000000000000, 0.9659258262890683122, 1.000000000000000000, 0.9659258262890683122, 1.000000000000000000, 0.9659258262890683122, 1.000000000000000000, 0.9659258262890683122, 1.000000000000000000, 0.9659258262890683122, 1.000000000000000000, 0.9659258262890683122, 1.000000000000000000, 0.9659258262890683122, 1.000000000000000000, 0.9659258262890683122, 1.000000000000000000, 0.9659258262890683122, 1.000000000000000000, 0.9659258262890683122, 1.000000000000000000, 0.9659258262890683122, 1.000000000000000000, 0.9659258262890683122, 1.000000000000000000, 0.9659258262890683122, 1.000000000000000000, 0.9659258262890683122, 1.000000000000000000, 0.9659258262890683122, 1.000000000000000000, 0.9659258262890683122, 1.000000000000000000, 0.9659258262890683122, 1.000000000000000000, 0.9659258262890683122, 1.000000000000000000, 0.9659258262890683122, 1.000000000000000000, 0.9659258262890683122, 1.000000000000000000, 0.9659258262890683122, 1.000000000000000000, 0.9659258262890683122, 1.000000000000000000, 0.9659258262890683122, 1.000000000000000000, 0.9659258262890683122, 1.000000000000000000, 0.9659258262890683122, 1.000000000000000000, 0.9659258262890683122, 1.000000000000000000, 0.9659258262890683122, 1.000000000000000000, 0.9659258262890683122, 1.000000000000000000, 0.9659258262890683122, 1.000000000000000000, 0.9659258262890683122, 1.000000000000000000, 0.9659258262890683122, 1.000000000000000000, 0.9659258262890683122, 1.000000000000000000, 0.9659258262890683122, 1.000000000000000000, 0.9659258262890683122, 1.000000000000000000, 0.9659258262890683122, 1.000000000000000000, 0.9659258262890683122, 1.000000000000000000, 0.9659258262890683122, 1.000000000000000000, 0.9659258262890683122, 1.000000000000000000, 0.9659258262890683122, 1.000000000000000000, 0.9659258262890683122, 1.000000000000000000, 0.9659258262890683122, 1.000000000000000000, 0.9659258262890683122, 1.000000000000000000, 0.9659258262890683122, 1.000000000000000000, 0.9659258262890683122, 1.000000000000000000, 0.9659258262890683122, 1.000000000000000000, 0.9659258262890683122, 1.000000000000000000, 0.9659258262890683122, 1.000000000000000000, 0.9659258262890683122, 1.000000000000000000, 0.9659258262890683122, 1.000000000000000000, 0.9659258262890683122, 1.000000000000000000, 0.9659258262890683122, 1.000000000000000000, 0.9659258262890683122, 1.000000000000000000, 0.9659258262890683122, 1.000000000000000000, 0.9659258262890683122, 1.000000000000000000, 0.9659258262890683122, 1.000000000000000000, 0.9659258262890683122, 1.000000000000000000, 0.9659258262890683122, 1.000000000000000000, 0.9659258262890683122, 1.000000000000000000, 0.9659258262890683122, 1.000000000000000000, 0.9659258262890683122, 1.000000000000000000, 0.9659258262890683122, 1.000000000000000000, 0.9659258262890683122, 1.000000000000000000, 0.9659258262890683122, 1.000000000000000000, 0.9659258262890683122, 1.000000000000000000, 0.9659258262890683122, 1.000000000000000000, 0.9659258262890683122, 1.000000000000000000, 0.9659258262890683122, 1.000000000000000000, 0.9659258262890683122, 1.000000000000000000, 0.9659258262890683122, 1.000000000000000000, 0.9659258262890683122, 1.000000000000000000, 0.9659258262890683122, 1.000000000000000000, 0.9659258262890683122, 1.000000000000000000, 0.9659258262890683122, 1.000000000000000000, 0.9659258262890683122, 1.000000000000000000, 0.9659258262890683122, 1.000000000000000000, 0.9659258262890683122, 1.000000000000000000, 0.9659258262890683122, 1.000000000000000000, 0.9659258262890683122, 1.000000000000000000, 0.9659258262890683122, 1.000000000000000000, 0.9659258262890683122, 1.000000000000000000, 0.9659258262890683122, 1.000000000000000000, 0.9659258262890683122, 1.000000000000000000, 0.9659258262890683122, 1.000000000000000000, 0.9659258262890683122, 1.000000000000000000, 0.9659258262890683122, 1.000000000000000000, 0.9659258262890683122, 1.000000000000000000, 0.9659258262890683122, 1.000000000000000000, 0.9659258262890683122, 1.000000000000000000, 0.9659258262890683122, 1.000000000000000000, 0.9659258262890683122, 1.000000000000000000, 0.9659258262890683122, 1.000000000000000000, 0.9659258262890683122, 1.000000000000000000, 0.9659258262890683122, 1.000000000000000000, 0.9659258262890683122, 1.000000000000000000, 0.9659258262890683122, 1.000000000000000000, 0.9659258262890683122, 1.000000000000000000, 0.9659258262890683122, 1.000000000000000000, 0.9659258262890683122, 1.000000000000000000, 0.9659258262890683122, 1.000000000000000000, 0.9659258262890683122, 1.000000000000000000, 0.9659258262890683122, 1.000000000000000000, 0.9659258262890683122, 1.000000000000000000, 0.9659258262890683122, 1.000000000000000000, 0.9659258262890683122, 1.000000000000000000, 0.9659258262890683122, 1.000000000000000000, 0.9659258262890683122, 1.000000000000000000, 0.9659258262890683122, 1.000000000000000000, 0.9659258262890683122, 1.000000000000000000, 0.9659258262890683122, 1.000000000000000000, 0.9659258262890683122, 1.000000000000000000, 0.9659258262890683122, 1.000000000000000000, 0.9659258262890683122, 1.000000000000000000, 0.9659258262890683122, 1.000000000000000000, 0.9659258262890683122, 1.000000000000000000, 0.9659258262890683122, 1.000000000000000000, 0.9659258262890683122, 1.000000000000000000, 0.9659258262890683122, 1.000000000000000000, 0.9659258262890683122, 1.000000000000000000, 0.9659258262890683122, 1.000000000000000000, 0.9659258262890683122, 1.000000000000000000, 0.9659258262890683122, 1.000000000000000000, 0.9659258262890683122, 1.000000000000000000, 0.9659258262890683122, 1.000000000000000000, 0.9659258262890683122, 1.000000000000000000, 0.9659258262890683122, 1.000000000000000000, 0.9659258262890683122, 1.000000000000000000, 0.9659258262890683122, 1.000000000000000000, 0.9659258262890683122, 1.000000000000000000, 0.9659258262890683122, 1.000000000000000000, 0.9659258262890683122, 1.000000000000000000, 0.9659258262890683122, 1.000000000000000000, 0.9659258262890683122, 1.000000000000000000, 0.9659258262890683122, 1.000000000000000000, 0.9659258262890683122, 1.000000000000000000, 0.9659258262890683122, 1.000000000000000000, 0.9659258262890683122, 1.000000000000000000, 0.9659258262890683122, 1.000000000000000000) ) ) 
 REPRESENTATION_ITEM ( '' )  SURFACE ( )  );
#63381=CARTESIAN_POINT ( 'NONE',  ( 17.20831665107776587, 4.133931151000785675, -7.208316651077762316 ) ) ;
#63382=CARTESIAN_POINT ( 'NONE',  ( 0.1532563361054100626, 50.80059781766745175, -2.638427012816831230 ) ) ;
#63383=CARTESIAN_POINT ( 'NONE',  ( 19.84674366389459266, 8.300597817667451750, 2.638427012816836559 ) ) ;
#63384=CARTESIAN_POINT ( 'NONE',  ( 10.00000000000000178, 32.25893115100078745, 9.846743663894594434 ) ) ;
#63385=CARTESIAN_POINT ( 'NONE',  ( -0.1042174387088615761, 28.10736173766202128, 6.337391062633417782 ) ) ;
#63387=CARTESIAN_POINT ( 'NONE',  ( 18.52753015748617571, 23.09226448433411960, 4.923371831947298993 ) ) ;
#63388=CARTESIAN_POINT ( 'NONE',  ( -0.1049300847420622101, 52.21697413083879979, -6.336235997365760930 ) ) ;
#63390=CARTESIAN_POINT ( 'NONE',  ( 2.791683348922240793, 21.63393115100078745, 7.208316651077764092 ) ) ;
#63391=CARTESIAN_POINT ( 'NONE',  ( -0.1503990784575247319, 22.22266099184918886, -6.262539305110083276 ) ) ;
#63393=CARTESIAN_POINT ( 'NONE',  ( 12.63842701281683034, 52.46726448433413026, 9.846743663894596210 ) ) ;
#63396=CARTESIAN_POINT ( 'NONE',  ( 22.81628187352647785, 26.41530133659708923, 3.434112377981063169 ) ) ;
#63397=CARTESIAN_POINT ( 'NONE',  ( 17.20831665107776587, 49.13393115100078745, -7.208316651077762316 ) ) ;
#63399=CARTESIAN_POINT ( 'NONE',  ( -4.164238869374099039, 41.80374883491397497, 8.674139862899312516E-16 ) ) ;
#63400=CARTESIAN_POINT ( 'NONE',  ( 1.472469842513823179, 16.42559781766745175, 4.923371831947296329 ) ) ;
#63402=CARTESIAN_POINT ( 'NONE',  ( 0.1532563361054100626, 5.800597817667452638, -2.638427012816831230 ) ) ;
#63403=CARTESIAN_POINT ( 'NONE',  ( 19.67370888310408716, 90.62786186788183329, 5.438836974231068488 ) ) ;
#63404=CARTESIAN_POINT ( 'NONE',  ( 20.36894250292379738, 49.92874883491396787, -10.36894250292379027 ) ) ;
#63405=CARTESIAN_POINT ( 'NONE',  ( 17.20831665107776587, 59.13393115100078745, -7.208316651077762316 ) ) ;
#63406=CARTESIAN_POINT ( 'NONE',  ( 2.035157376598822676, 12.43868534415483751, -7.964842623401177768 ) ) ;
#63407=CARTESIAN_POINT ( 'NONE',  ( 20.36894250292379738, 24.92874883491396787, -10.36894250292379027 ) ) ;
#63409=CARTESIAN_POINT ( 'NONE',  ( 2.917880565312948704, 42.63708216824729647, 12.26659068614894643 ) ) ;
#63412=CARTESIAN_POINT ( 'NONE',  ( 0.1532563361054083140, 51.00893115100078745, 1.131784320476157264E-15 ) ) ;
#63414=ORIENTED_EDGE ( 'NONE', *, *, #98491, .F. ) ;
#63415=CARTESIAN_POINT ( 'NONE',  ( 15.44008868035555260, 34.73035201082151247, 9.422509992056143702 ) ) ;
#63416=CARTESIAN_POINT ( 'NONE',  ( 20.15039907845753220, 22.62777174578612716, -6.262539305110077947 ) ) ;
#63419=CARTESIAN_POINT ( 'NONE',  ( 19.84674366389459621, 43.50893115100078745, 7.409399052514197653E-17 ) ) ;
#63420=AXIS2_PLACEMENT_3D ( 'NONE', #1467, #18418, #24948 ) ;
#63421=CARTESIAN_POINT ( 'NONE',  ( 0.6178305044545838731, 64.74863466993043914, 9.382169495545420901 ) ) ;
#63423=CARTESIAN_POINT ( 'NONE',  ( 2.791683348922240793, 51.63393115100078745, 7.208316651077764092 ) ) ;
#63424=CARTESIAN_POINT ( 'NONE',  ( 10.00000000000000178, 67.25893115100079456, 9.846743663894594434 ) ) ;
#63426=CARTESIAN_POINT ( 'NONE',  ( 22.26659068614894466, 23.88708216824730357, 7.082119434687054849 ) ) ;
#63427=CARTESIAN_POINT ( 'NONE',  ( 19.67858290521088804, 89.00000000000000000, 5.461713021790605360 ) ) ;
#63429=CARTESIAN_POINT ( 'NONE',  ( 20.88017736071110164, 5.355352010821503583, 2.915334737309930979 ) ) ;
#63430=CARTESIAN_POINT ( 'NONE',  ( -1.099225684535947600, 28.70696800326375353, -6.408140936763238038 ) ) ;
#63432=CARTESIAN_POINT ( 'NONE',  ( 4.559911319644449179, 67.23035201082150536, -9.422509992056141925 ) ) ;
#63433=CARTESIAN_POINT ( 'NONE',  ( -46.94000000000000483, 100.4746355719282320, -9.260812147861324561 ) ) ;
#63435=CARTESIAN_POINT ( 'NONE',  ( -0.8801773607111008646, 3.272018677488171434, 2.915334737309923430 ) ) ;
#63436=CARTESIAN_POINT ( 'NONE',  ( -0.1049300847420659155, 42.21697413083878558, -6.336235997365754713 ) ) ;
#63437=CARTESIAN_POINT ( 'NONE',  ( 20.88017736071110164, 30.35535201082151247, 2.915334737309930979 ) ) ;
#63438=CARTESIAN_POINT ( 'NONE',  ( 2.035157376598824452, 38.68868534415483396, 7.964842623401179544 ) ) ;
#63439=CARTESIAN_POINT ( 'NONE',  ( -2.816281873526471635, -1.084698663402913210, -3.434112377981056508 ) ) ;
#63440=PLANE ( 'NONE',  #53902 ) ;
#63441=CARTESIAN_POINT ( 'NONE',  ( -1.099225684535947600, 63.70696800326376774, -6.408140936763238038 ) ) ;
#63442=CARTESIAN_POINT ( 'NONE',  ( 0.1532563361054100626, 10.80059781766745175, -2.638427012816831230 ) ) ;
#63444=ORIENTED_EDGE ( 'NONE', *, *, #13330, .T. ) ;
#63445=CARTESIAN_POINT ( 'NONE',  ( 7.084665262690076126, 32.02201867748816966, -10.88017736071110164 ) ) ;
#63446=CARTESIAN_POINT ( 'NONE',  ( -2.816281873526471635, 28.91530133659708213, -3.434112377981056508 ) ) ;
#63447=UNCERTAINTY_MEASURE_WITH_UNIT (LENGTH_MEASURE( 1.000000000000000082E-05 ), #16511, 'distance_accuracy_value', 'NONE');
#63449=CARTESIAN_POINT ( 'NONE',  ( 19.84674366389459621, 58.50893115100078745, 7.409399052514197653E-17 ) ) ;
#63451=CARTESIAN_POINT ( 'NONE',  ( 12.91533473730993009, 51.60535201082149825, -10.88017736071109987 ) ) ;
#63453=CARTESIAN_POINT ( 'NONE',  ( 5.076628168052704559, 10.17559781766745175, -8.527530157486179263 ) ) ;
#63455=CARTESIAN_POINT ( 'NONE',  ( 22.81628187352648496, 41.83196800326375353, -3.434112377981050290 ) ) ;
#63456=CARTESIAN_POINT ( 'NONE',  ( 10.00000000000000000, 56.81368534415484106, -10.88017736071110342 ) ) ;
#63457=CARTESIAN_POINT ( 'NONE',  ( 17.39651004071838614, 52.93575266056826933, 6.500000000000032863 ) ) ;
#63458=CARTESIAN_POINT ( 'NONE',  ( 16.40814093676323893, 60.79030133659709634, 11.09922568453595026 ) ) ;
#63462=CARTESIAN_POINT ( 'NONE',  ( 20.88017736071110875, 5.772018677488170546, -2.915334737309920765 ) ) ;
#63463=CARTESIAN_POINT ( 'NONE',  ( -2.816281873526471635, 43.91530133659708923, -3.434112377981056508 ) ) ;
#63464=CARTESIAN_POINT ( 'NONE',  ( 13.79529636645030344, 23.26208216824730002, 14.16423886937410614 ) ) ;
#63465=CARTESIAN_POINT ( 'NONE',  ( 0.1532563361054083140, 11.00893115100078568, 1.131784320476157264E-15 ) ) ;
#63466=CARTESIAN_POINT ( 'NONE',  ( -0.8801773607111008646, 8.272018677488171434, 2.915334737309923430 ) ) ;
#63467=CARTESIAN_POINT ( 'NONE',  ( 7.361572987183170547, 22.05059781766745530, 9.846743663894590881 ) ) ;
#63468=CARTESIAN_POINT ( 'NONE',  ( -0.3689425029237881626, 57.42874883491397497, 10.36894250292379027 ) ) ;
#63470=CARTESIAN_POINT ( 'NONE',  ( 19.42250999205614548, 5.980352010821504471, -5.440088680355545492 ) ) ;
#63472=CARTESIAN_POINT ( 'NONE',  ( 19.42250999205614193, 15.14701867748817143, 5.440088680355555262 ) ) ;
#63473=CARTESIAN_POINT ( 'NONE',  ( 1.383448333479232462, 32.37718327197428181, -6.499999999999977796 ) ) ;
#63475=ORIENTED_EDGE ( 'NONE', *, *, #38200, .F. ) ;
#63477=CARTESIAN_POINT ( 'NONE',  ( 7.084665262690076126, 14.10535201082150358, 10.88017736071109987 ) ) ;
#63478=CARTESIAN_POINT ( 'NONE',  ( 1.472469842513823179, 55.59226448433412315, -4.923371831947296329 ) ) ;
#63480=CARTESIAN_POINT ( 'NONE',  ( 0.000000000000000000, 81.99999999999992895, 5.000000000000000000 ) ) ;
#63481=CARTESIAN_POINT ( 'NONE',  ( 20.36894250292379738, 14.92874883491396432, -10.36894250292379027 ) ) ;
#63482=CARTESIAN_POINT ( 'NONE',  ( 4.559911319644449179, 33.89701867748817676, 9.422509992056141925 ) ) ;
#63483=CARTESIAN_POINT ( 'NONE',  ( 19.42250999205614548, 20.98035201082150891, -5.440088680355545492 ) ) ;
#63484=CARTESIAN_POINT ( 'NONE',  ( 18.52753015748618282, 58.92559781766745886, -4.923371831947291888 ) ) ;
#63486=CARTESIAN_POINT ( 'NONE',  ( 17.20831665107776587, 34.13393115100078745, -7.208316651077762316 ) ) ;
#63488=CARTESIAN_POINT ( 'NONE',  ( 0.1532563361054100626, 10.80059781766745175, -2.638427012816831230 ) ) ;
#63491=CARTESIAN_POINT ( 'NONE',  ( 19.42250999205614548, 5.980352010821504471, -5.440088680355545492 ) ) ;
#63492=CARTESIAN_POINT ( 'NONE',  ( 12.63842701281683922, 9.550597817667449974, -9.846743663894590881 ) ) ;
#63494=CARTESIAN_POINT ( 'NONE',  ( 1.472469842513823179, 65.59226448433412315, -4.923371831947296329 ) ) ;
#63495=CARTESIAN_POINT ( 'NONE',  ( -0.8801773607111009756, 48.06368534415484817, 1.068504757029289695E-15 ) ) ;
#63496=CARTESIAN_POINT ( 'NONE',  ( 2.035157376598824452, 8.688685344154839285, 7.964842623401179544 ) ) ;
#63497=CARTESIAN_POINT ( 'NONE',  ( 0.6178305044545838731, 39.74863466993041072, 9.382169495545420901 ) ) ;
#63498=CARTESIAN_POINT ( 'NONE',  ( -2.266590686148945544, 26.38708216824730357, -7.082119434687050408 ) ) ;
#63502=CARTESIAN_POINT ( 'NONE',  ( 6.565887622018943937, 55.16530133659709634, 12.81628187352647430 ) ) ;
#63503=ORIENTED_EDGE ( 'NONE', *, *, #93485, .F. ) ;
#63504=CARTESIAN_POINT ( 'NONE',  ( 14.92337183194729633, 62.67559781766745886, 8.527530157486181039 ) ) ;
#63505=CARTESIAN_POINT ( 'NONE',  ( 20.88017736071110164, 25.35535201082150891, 2.915334737309930979 ) ) ;
#63507=CARTESIAN_POINT ( 'NONE',  ( -0.8801773607111009756, 68.06368534415484817, 1.068504757029289695E-15 ) ) ;
#63508=CARTESIAN_POINT ( 'NONE',  ( 7.361572987183169658, 14.96726448433411960, -9.846743663894592657 ) ) ;
#63509=CARTESIAN_POINT ( 'NONE',  ( 19.84674366389459621, 3.508931151000785231, 7.409399052514197653E-17 ) ) ;
#63510=CARTESIAN_POINT ( 'NONE',  ( 19.42250999205614548, 50.98035201082151247, -5.440088680355545492 ) ) ;
#63512=CARTESIAN_POINT ( 'NONE',  ( 4.559911319644449179, 58.89701867748817676, 9.422509992056141925 ) ) ;
#63513=CARTESIAN_POINT ( 'NONE',  ( 0.1532563361054100626, 0.8005978176674514168, -2.638427012816831230 ) ) ;
#63516=CARTESIAN_POINT ( 'NONE',  ( 5.076628168052704559, 55.17559781766745175, -8.527530157486179263 ) ) ;
#63517=ORIENTED_EDGE ( 'NONE', *, *, #82866, .T. ) ;
#63520=CARTESIAN_POINT ( 'NONE',  ( -2.266590686148945544, 6.387082168247300906, -7.082119434687050408 ) ) ;
#63521=CARTESIAN_POINT ( 'NONE',  ( 10.00000000000000178, 55.37363466993042493, 12.81628187352647608 ) ) ;
#63522=CARTESIAN_POINT ( 'NONE',  ( 17.08211943468705130, 3.470415501580634388, 12.26659068614894998 ) ) ;
#63523=CARTESIAN_POINT ( 'NONE',  ( 24.16423886937410614, 29.51208216824729647, -3.795296366450302550 ) ) ;
#63525=CARTESIAN_POINT ( 'NONE',  ( 2.035157376598824452, 23.68868534415484461, 7.964842623401179544 ) ) ;
#63528=CARTESIAN_POINT ( 'NONE',  ( 1.472469842513823179, 11.42559781766745175, 4.923371831947296329 ) ) ;
#63529=CARTESIAN_POINT ( 'NONE',  ( 21.09922568453595559, 37.04030133659708923, -6.408140936763230044 ) ) ;
#63530=CARTESIAN_POINT ( 'NONE',  ( 2.791683348922237240, 35.38393115100079456, -7.208316651077763204 ) ) ;
#63532=CARTESIAN_POINT ( 'NONE',  ( -2.816281873526473856, 34.12363466993042493, 9.499525473075851096E-16 ) ) ;
#63535=CARTESIAN_POINT ( 'NONE',  ( 10.00000000000000178, 22.25893115100078745, 9.846743663894594434 ) ) ;
#63536=CARTESIAN_POINT ( 'NONE',  ( -2.266590686148945544, 16.38708216824730357, -7.082119434687050408 ) ) ;
#63537=CARTESIAN_POINT ( 'NONE',  ( 7.084665262690076126, 34.10535201082151247, 10.88017736071109987 ) ) ;
#63538=CARTESIAN_POINT ( 'NONE',  ( 24.16423886937409904, 34.09541550158064638, 3.795296366450317205 ) ) ;
#63539=CARTESIAN_POINT ( 'NONE',  ( 17.20831665107776587, 57.88393115100078745, 7.208316651077764980 ) ) ;
#63540=CARTESIAN_POINT ( 'NONE',  ( 18.52753015748618282, 13.92559781766745175, -4.923371831947291888 ) ) ;
#63541=CARTESIAN_POINT ( 'NONE',  ( 10.00000000000000178, 55.37363466993042493, 12.81628187352647608 ) ) ;
#63543=CARTESIAN_POINT ( 'NONE',  ( 2.035157376598824452, 23.68868534415484461, 7.964842623401179544 ) ) ;
#63546=CARTESIAN_POINT ( 'NONE',  ( 16.40814093676324603, 17.45696800326375353, -11.09922568453594671 ) ) ;
#63547=CARTESIAN_POINT ( 'NONE',  ( 5.076628168052704559, 40.17559781766745175, -8.527530157486179263 ) ) ;
#63549=CARTESIAN_POINT ( 'NONE',  ( 19.72487221294570858, 12.80223176428831167, -6.500000000000000888 ) ) ;
#63550=CARTESIAN_POINT ( 'NONE',  ( 20.88017736071110164, 65.35535201082150536, 2.915334737309930979 ) ) ;
#63551=CARTESIAN_POINT ( 'NONE',  ( 13.99999999999999822, 61.00000000000000711, -5.000000000000000000 ) ) ;
#63555=CARTESIAN_POINT ( 'NONE',  ( 17.96484262340118221, 49.93868534415484106, 7.964842623401181321 ) ) ;
#63556=CARTESIAN_POINT ( 'NONE',  ( 19.42250999205614193, 55.14701867748817676, 5.440088680355555262 ) ) ;
#63560=CARTESIAN_POINT ( 'NONE',  ( -0.8801773607110991993, 7.855352010821506248, -2.915334737309923874 ) ) ;
#63562=CARTESIAN_POINT ( 'NONE',  ( 16.40814093676323893, 0.7903013365970867898, 11.09922568453595026 ) ) ;
#63563=CARTESIAN_POINT ( 'NONE',  ( -0.8801773607110991993, 27.85535201082150181, -2.915334737309923874 ) ) ;
#63566=CARTESIAN_POINT ( 'NONE',  ( 6.565887622018943937, 20.16530133659708213, 12.81628187352647430 ) ) ;
#63568=CARTESIAN_POINT ( 'NONE',  ( 2.035157376598824452, 53.68868534415484817, 7.964842623401179544 ) ) ;
#63569=CARTESIAN_POINT ( 'NONE',  ( 0.1532563361054083140, 41.00893115100078745, 1.131784320476157264E-15 ) ) ;
#63570=CARTESIAN_POINT ( 'NONE',  ( 19.38216949554541202, 0.9986346699304200492, 9.382169495545424454 ) ) ;
#63572=CARTESIAN_POINT ( 'NONE',  ( 10.00000000000000000, 31.81368534415483751, -10.88017736071110342 ) ) ;
#63573=CARTESIAN_POINT ( 'NONE',  ( 20.88017736071110164, 40.35535201082150536, 2.915334737309930979 ) ) ;
#63574=CARTESIAN_POINT ( 'NONE',  ( 20.36894250292379738, 49.92874883491396787, -10.36894250292379027 ) ) ;
#63575=CARTESIAN_POINT ( 'NONE',  ( 12.63842701281683922, 34.55059781766745886, -9.846743663894590881 ) ) ;
#63576=CARTESIAN_POINT ( 'NONE',  ( 0.5774900079438590739, 57.64701867748817676, -5.440088680355550821 ) ) ;
#63578=CARTESIAN_POINT ( 'NONE',  ( 22.26659068614894466, 18.88708216824730002, 7.082119434687054849 ) ) ;
#63581=ORIENTED_EDGE ( 'NONE', *, *, #53955, .T. ) ;
#63582=CARTESIAN_POINT ( 'NONE',  ( 13.79529636645031943, 45.34541550158062506, -14.16423886937409904 ) ) ;
#63583=CARTESIAN_POINT ( 'NONE',  ( 10.00000000000000178, 43.05374883491397497, 14.16423886937410082 ) ) ;
#63584=CARTESIAN_POINT ( 'NONE',  ( 19.84674366389459621, 18.50893115100078745, 7.409399052514197653E-17 ) ) ;
#63585=CARTESIAN_POINT ( 'NONE',  ( 22.81628187352647785, 21.62363466993041783, 6.195893100308588602E-16 ) ) ;
#63587=FACE_OUTER_BOUND ( 'NONE', #50091, .T. ) ;
#63588=CARTESIAN_POINT ( 'NONE',  ( 4.559911319644449179, 62.23035201082150536, -9.422509992056141925 ) ) ;
#63589=CARTESIAN_POINT ( 'NONE',  ( -2.816281873526473856, 29.12363466993041783, 9.499525473075851096E-16 ) ) ;
#63590=EDGE_CURVE ( 'NONE', #49705, #1795, #86488, .T. ) ;
#63591=CARTESIAN_POINT ( 'NONE',  ( 2.917880565312948704, 42.63708216824729647, 12.26659068614894643 ) ) ;
#63593=CARTESIAN_POINT ( 'NONE',  ( 20.15039907845753930, 0.07447313448805115144, -6.262539305110068177 ) ) ;
#63594=CARTESIAN_POINT ( 'NONE',  ( 20.88017736071110519, 65.56368534415483396, 2.639326808657452039E-16 ) ) ;
#63597=SURFACE_STYLE_FILL_AREA ( #80583 ) ;
#63598=CARTESIAN_POINT ( 'NONE',  ( 20.15039907845753930, 70.00000000000000000, -6.262539305110068177 ) ) ;
#63600=CARTESIAN_POINT ( 'NONE',  ( -2.266590686148945544, 2.220415501580634388, 7.082119434687048631 ) ) ;
#63601=CARTESIAN_POINT ( 'NONE',  ( 17.96484262340118221, 6.188685344154837509, -7.964842623401177768 ) ) ;
#63602=CARTESIAN_POINT ( 'NONE',  ( 0.5774900079438590739, 7.647018677488171434, -5.440088680355550821 ) ) ;
#63603=CARTESIAN_POINT ( 'NONE',  ( 17.20831665107776587, 37.88393115100078745, 7.208316651077764980 ) ) ;
#63604=CARTESIAN_POINT ( 'NONE',  ( 22.81628187352648496, 1.831968003263753753, -3.434112377981050290 ) ) ;
#63607=CARTESIAN_POINT ( 'NONE',  ( -2.816281873526471635, 18.91530133659708213, -3.434112377981056508 ) ) ;
#63609=CARTESIAN_POINT ( 'NONE',  ( -4.164238869374098151, 51.59541550158063217, -3.795296366450310543 ) ) ;
#63611=CARTESIAN_POINT ( 'NONE',  ( 24.16423886937410614, 59.30374883491397497, 8.672049930838204340E-16 ) ) ;
#63612=VERTEX_POINT ( 'NONE', #41577 ) ;
#63613=CARTESIAN_POINT ( 'NONE',  ( -0.8801773607110991993, 32.85535201082151247, -2.915334737309923874 ) ) ;
#63614=CARTESIAN_POINT ( 'NONE',  ( 15.44008868035555793, 36.39701867748816966, -9.422509992056140149 ) ) ;
#63615=CARTESIAN_POINT ( 'NONE',  ( 2.035157376598824452, 33.68868534415484106, 7.964842623401179544 ) ) ;
#63616=CARTESIAN_POINT ( 'NONE',  ( 12.91533473730992121, 64.52201867748817676, 10.88017736071110164 ) ) ;
#63617=CARTESIAN_POINT ( 'NONE',  ( 4.559911319644449179, 27.23035201082150536, -9.422509992056141925 ) ) ;
#63621=CARTESIAN_POINT ( 'NONE',  ( 10.00000000000000178, 17.25893115100078745, 9.846743663894594434 ) ) ;
#63625=CARTESIAN_POINT ( 'NONE',  ( 18.52753015748618282, 48.92559781766745886, -4.923371831947291888 ) ) ;
#63627=CARTESIAN_POINT ( 'NONE',  ( -1.099225684535947600, 44.54030133659708923, 6.408140936763237150 ) ) ;
#63629=DIRECTION ( 'NONE',  ( -1.000000000000000000, 0.000000000000000000, 0.000000000000000000 ) ) ;
#63631=CARTESIAN_POINT ( 'NONE',  ( 10.00000000000000178, 67.25893115100079456, 9.846743663894594434 ) ) ;
#63632=CARTESIAN_POINT ( 'NONE',  ( 20.36894250292379738, 44.92874883491396787, -10.36894250292379027 ) ) ;
#63634=VERTEX_POINT ( 'NONE', #25583 ) ;
#63636=CARTESIAN_POINT ( 'NONE',  ( 1.472469842513823179, 16.42559781766745175, 4.923371831947296329 ) ) ;
#63638=CARTESIAN_POINT ( 'NONE',  ( 0.1532563361054082862, 66.21726448433413736, 2.638427012816831674 ) ) ;
#63639=CARTESIAN_POINT ( 'NONE',  ( 17.20831665107776587, 2.883931151000785231, 7.208316651077764980 ) ) ;
#63642=CARTESIAN_POINT ( 'NONE',  ( 1.472469842513823179, 60.59226448433412315, -4.923371831947296329 ) ) ;
#63644=CARTESIAN_POINT ( 'NONE',  ( 18.72515096720568550, 20.05509018479935790, 6.500000000000015099 ) ) ;
#63646=CARTESIAN_POINT ( 'NONE',  ( -4.164238869374098151, 61.59541550158063217, -3.795296366450310543 ) ) ;
#63648=CARTESIAN_POINT ( 'NONE',  ( 10.00000000000000178, 44.31368534415484106, 10.88017736071110342 ) ) ;
#63649=CARTESIAN_POINT ( 'NONE',  ( 22.81628187352648496, 11.83196800326375531, -3.434112377981050290 ) ) ;
#63653=CARTESIAN_POINT ( 'NONE',  ( 0.1916775849787265285, 62.25868815902069286, -6.499999999999991118 ) ) ;
#63655=CARTESIAN_POINT ( 'NONE',  ( 0.1532563361054100626, 55.80059781766745175, -2.638427012816831230 ) ) ;
#63656=SURFACE_SIDE_STYLE ('',( #56182 ) ) ;
#63658=CARTESIAN_POINT ( 'NONE',  ( 6.565887622018943937, 13.08196800326374998, -12.81628187352647608 ) ) ;
#63659=CARTESIAN_POINT ( 'NONE',  ( 15.44008868035555260, 9.730352010821505360, 9.422509992056143702 ) ) ;
#63660=( NAMED_UNIT ( * ) PLANE_ANGLE_UNIT ( ) SI_UNIT ( $, .RADIAN. ) );
#63661=FACE_OUTER_BOUND ( 'NONE', #54484, .T. ) ;
#63662=CARTESIAN_POINT ( 'NONE',  ( -4.164238869374099927, 37.01208216824731068, 3.795296366450308767 ) ) ;
#63663=CARTESIAN_POINT ( 'NONE',  ( 22.26659068614895176, 24.72041550158063572, -7.082119434687042414 ) ) ;
#63664=CARTESIAN_POINT ( 'NONE',  ( 2.035157376598824452, 3.688685344154837953, 7.964842623401179544 ) ) ;
#63665=CARTESIAN_POINT ( 'NONE',  ( 14.92337183194729633, 37.67559781766745175, 8.527530157486181039 ) ) ;
#63666=CARTESIAN_POINT ( 'NONE',  ( 10.00000000000000178, 35.37363466993042493, 12.81628187352647608 ) ) ;
#63667=CARTESIAN_POINT ( 'NONE',  ( 2.035157376598822676, 12.43868534415483751, -7.964842623401177768 ) ) ;
#63669=CARTESIAN_POINT ( 'NONE',  ( 12.63842701281683034, 32.46726448433412315, 9.846743663894596210 ) ) ;
#63671=CARTESIAN_POINT ( 'NONE',  ( 0.5774900079438590739, 37.64701867748817676, -5.440088680355550821 ) ) ;
#63672=CARTESIAN_POINT ( 'NONE',  ( 16.40814093676324603, 2.456968003263753531, -11.09922568453594671 ) ) ;
#63673=CARTESIAN_POINT ( 'NONE',  ( 20.36894250292379382, 18.67874883491397142, 10.36894250292379205 ) ) ;
#63674=CARTESIAN_POINT ( 'NONE',  ( -0.1503990784575359729, 18.10158574516642460, 6.262539305110062848 ) ) ;
#63675=CARTESIAN_POINT ( 'NONE',  ( 1.274849032794292736, 37.55509018479936145, -6.499999999999977796 ) ) ;
#63676=CARTESIAN_POINT ( 'NONE',  ( 14.92337183194729988, 24.34226448433411960, -8.527530157486177487 ) ) ;
#63677=CARTESIAN_POINT ( 'NONE',  ( 10.00000000000000178, 55.37363466993042493, 12.81628187352647608 ) ) ;
#63678=CARTESIAN_POINT ( 'NONE',  ( 19.84674366389459621, 48.50893115100078745, 7.409399052514197653E-17 ) ) ;
#63681=SURFACE_SIDE_STYLE ('',( #57659 ) ) ;
#63682=CARTESIAN_POINT ( 'NONE',  ( 24.16423886937410614, 64.30374883491396076, 8.672049930838204340E-16 ) ) ;
#63683=CARTESIAN_POINT ( 'NONE',  ( 20.88017736071110875, 60.77201867748817676, -2.915334737309920765 ) ) ;
#63684=CARTESIAN_POINT ( 'NONE',  ( 10.00000000000000000, 10.55374883491396787, -14.16423886937410082 ) ) ;
#63685=CARTESIAN_POINT ( 'NONE',  ( 10.00000000000000178, 2.258931151000784787, 9.846743663894594434 ) ) ;
#63686=CARTESIAN_POINT ( 'NONE',  ( 0.1532563361054082862, 46.21726448433411605, 2.638427012816831674 ) ) ;
#63687=CARTESIAN_POINT ( 'NONE',  ( 4.559911319644449179, 13.89701867748817143, 9.422509992056141925 ) ) ;
#63689=CARTESIAN_POINT ( 'NONE',  ( 7.361572987183170547, 67.05059781766746596, 9.846743663894590881 ) ) ;
#63691=( NAMED_UNIT ( * ) PLANE_ANGLE_UNIT ( ) SI_UNIT ( $, .RADIAN. ) );
#63695=ORIENTED_EDGE ( 'NONE', *, *, #59750, .F. ) ;
#63697=CARTESIAN_POINT ( 'NONE',  ( 10.00000000000000000, 5.553748834913967869, -14.16423886937410082 ) ) ;
#63698=CARTESIAN_POINT ( 'NONE',  ( -2.266590686148945544, 1.387082168247301128, -7.082119434687050408 ) ) ;
#63699=CARTESIAN_POINT ( 'NONE',  ( -2.266590686148945544, 42.22041550158063217, 7.082119434687048631 ) ) ;
#63700=CARTESIAN_POINT ( 'NONE',  ( 18.52753015748617571, 58.09226448433411605, 4.923371831947298993 ) ) ;
#63701=CARTESIAN_POINT ( 'NONE',  ( 0.1532563361054100626, 20.80059781766744464, -2.638427012816831230 ) ) ;
#63703=CARTESIAN_POINT ( 'NONE',  ( 20.88017736071110875, 20.77201867748816611, -2.915334737309920765 ) ) ;
#63704=CARTESIAN_POINT ( 'NONE',  ( 5.076628168052704559, 60.17559781766745175, -8.527530157486179263 ) ) ;
#63706=CARTESIAN_POINT ( 'NONE',  ( -2.266590686148945544, 37.22041550158063217, 7.082119434687048631 ) ) ;
#63707=CARTESIAN_POINT ( 'NONE',  ( -0.8801773607110991993, 2.855352010821504471, -2.915334737309923874 ) ) ;
#63708=FACE_OUTER_BOUND ( 'NONE', #68547, .T. ) ;
#63710=CARTESIAN_POINT ( 'NONE',  ( 0.5774900079438607392, 63.48035201082149825, 5.440088680355550821 ) ) ;
#63711=CARTESIAN_POINT ( 'NONE',  ( 10.00000000000000178, 12.25893115100078568, 9.846743663894594434 ) ) ;
#63715=FACE_OUTER_BOUND ( 'NONE', #94021, .T. ) ;
#63716=EDGE_LOOP ( 'NONE', ( #82718, #12322, #41520, #48513, #80569, #5183, #71487, #15300 ) ) ;
#63717=CARTESIAN_POINT ( 'NONE',  ( 5.076628168052704559, 30.17559781766745175, -8.527530157486179263 ) ) ;
#63719=CARTESIAN_POINT ( 'NONE',  ( 10.00000000000000178, 33.05374883491396787, 14.16423886937410082 ) ) ;
#63720=CARTESIAN_POINT ( 'NONE',  ( 18.52753015748617571, 28.09226448433411960, 4.923371831947298993 ) ) ;
#63721=CARTESIAN_POINT ( 'NONE',  ( 0.5774900079438607392, 43.48035201082151247, 5.440088680355550821 ) ) ;
#63724=( LENGTH_UNIT ( ) NAMED_UNIT ( * ) SI_UNIT ( .MILLI., .METRE. ) );
#63725=CARTESIAN_POINT ( 'NONE',  ( 17.96484262340118221, 34.93868534415482685, 7.964842623401181321 ) ) ;
#63728=CARTESIAN_POINT ( 'NONE',  ( 15.44008868035555260, 44.73035201082151247, 9.422509992056143702 ) ) ;
#63729=CARTESIAN_POINT ( 'NONE',  ( 24.16423886937409904, 4.095415501580634832, 3.795296366450317205 ) ) ;
#63730=VERTEX_POINT ( 'NONE', #64527 ) ;
#63732=CARTESIAN_POINT ( 'NONE',  ( 0.1532563361054100626, 0.8005978176674514168, -2.638427012816831230 ) ) ;
#63733=CARTESIAN_POINT ( 'NONE',  ( -2.816281873526471635, 28.91530133659708213, -3.434112377981056508 ) ) ;
#63735=CARTESIAN_POINT ( 'NONE',  ( 1.472469842513823179, 21.42559781766745175, 4.923371831947296329 ) ) ;
#63736=CARTESIAN_POINT ( 'NONE',  ( 4.559911319644449179, 2.230352010821504471, -9.422509992056141925 ) ) ;
#63738=CARTESIAN_POINT ( 'NONE',  ( 1.472469842513823179, 35.59226448433412315, -4.923371831947296329 ) ) ;
#63739=CARTESIAN_POINT ( 'NONE',  ( 19.42250999205614193, 60.14701867748817676, 5.440088680355555262 ) ) ;
#63740=CARTESIAN_POINT ( 'NONE',  ( 10.00000000000000178, 69.31368534415484817, 10.88017736071110342 ) ) ;
#63742=CARTESIAN_POINT ( 'NONE',  ( -1.099225684535947600, 64.54030133659709634, 6.408140936763237150 ) ) ;
#63743=CARTESIAN_POINT ( 'NONE',  ( 2.791683348922237240, 10.38393115100078390, -7.208316651077763204 ) ) ;
#63744=CARTESIAN_POINT ( 'NONE',  ( 13.43411237798105340, 15.58196800326374998, 12.81628187352647963 ) ) ;
#63745=CARTESIAN_POINT ( 'NONE',  ( -0.1503990784575328643, 70.00000000000000000, 6.262539305110068177 ) ) ;
#63746=CARTESIAN_POINT ( 'NONE',  ( 5.076628168052703671, 46.84226448433412315, 8.527530157486179263 ) ) ;
#63747=CARTESIAN_POINT ( 'NONE',  ( 20.88017736071110164, 35.35535201082150536, 2.915334737309930979 ) ) ;
#63748=CARTESIAN_POINT ( 'NONE',  ( 24.16423886937409904, 4.095415501580634832, 3.795296366450317205 ) ) ;
#63749=CARTESIAN_POINT ( 'NONE',  ( 19.84674366389459266, 33.30059781766744464, 2.638427012816836559 ) ) ;
#63750=CARTESIAN_POINT ( 'NONE',  ( -2.816281873526471635, 33.91530133659708213, -3.434112377981056508 ) ) ;
#63753=CARTESIAN_POINT ( 'NONE',  ( 19.42250999205614193, 45.14701867748817676, 5.440088680355555262 ) ) ;
#63754=CARTESIAN_POINT ( 'NONE',  ( -2.816281873526473856, 9.123634669930421381, 9.499525473075851096E-16 ) ) ;
#63755=CARTESIAN_POINT ( 'NONE',  ( 0.1532563361054083140, 41.00893115100078745, 1.131784320476157264E-15 ) ) ;
#63756=CARTESIAN_POINT ( 'NONE',  ( 0.1532563361054083140, 26.00893115100078745, 1.131784320476157264E-15 ) ) ;
#63757=CARTESIAN_POINT ( 'NONE',  ( 10.00000000000000000, 21.81368534415484106, -10.88017736071110342 ) ) ;
#63759=CARTESIAN_POINT ( 'NONE',  ( 13.43411237798105340, 30.58196800326374998, 12.81628187352647963 ) ) ;
#63760=CARTESIAN_POINT ( 'NONE',  ( 19.84674366389459266, 18.30059781766745175, 2.638427012816836559 ) ) ;
#63762=CARTESIAN_POINT ( 'NONE',  ( 19.42250999205614193, 15.14701867748817143, 5.440088680355555262 ) ) ;
#63763=CARTESIAN_POINT ( 'NONE',  ( 4.559911319644449179, 58.89701867748817676, 9.422509992056141925 ) ) ;
#63764=CARTESIAN_POINT ( 'NONE',  ( 2.035157376598824452, 8.688685344154839285, 7.964842623401179544 ) ) ;
#63765=CARTESIAN_POINT ( 'NONE',  ( 2.791683348922240793, 46.63393115100077324, 7.208316651077764092 ) ) ;
#63766=CARTESIAN_POINT ( 'NONE',  ( 15.44008868035555793, 36.39701867748816966, -9.422509992056140149 ) ) ;
#63767=CARTESIAN_POINT ( 'NONE',  ( 19.42250999205614193, 40.14701867748817676, 5.440088680355555262 ) ) ;
#63768=CARTESIAN_POINT ( 'NONE',  ( -0.8801773607111008646, 18.27201867748817321, 2.915334737309923430 ) ) ;
#63769=CARTESIAN_POINT ( 'NONE',  ( 20.32896413005680358, 54.74545670184114243, 5.963430220938287007 ) ) ;
#63770=CARTESIAN_POINT ( 'NONE',  ( 0.1532563361054083140, 36.00893115100078745, 1.131784320476157264E-15 ) ) ;
#63771=CARTESIAN_POINT ( 'NONE',  ( -0.3689425029237881626, 37.42874883491396787, 10.36894250292379027 ) ) ;
#63774=CARTESIAN_POINT ( 'NONE',  ( 22.81628187352647785, 6.623634669930420493, 6.195893100308588602E-16 ) ) ;
#63777=CARTESIAN_POINT ( 'NONE',  ( 17.08211943468705130, 28.47041550158063572, 12.26659068614894998 ) ) ;
#63779=ORIENTED_EDGE ( 'NONE', *, *, #22369, .T. ) ;
#63781=CARTESIAN_POINT ( 'NONE',  ( -4.164238869374099039, 61.80374883491397497, 8.674139862899312516E-16 ) ) ;
#63782=CARTESIAN_POINT ( 'NONE',  ( 19.84674366389459266, 18.71726448433411960, -2.638427012816827677 ) ) ;
#63784=CARTESIAN_POINT ( 'NONE',  ( 15.44008868035555793, 61.39701867748817676, -9.422509992056140149 ) ) ;
#63786=CARTESIAN_POINT ( 'NONE',  ( 17.96484262340118221, 24.93868534415484461, 7.964842623401181321 ) ) ;
#63787=DIRECTION ( 'NONE',  ( 0.000000000000000000, -1.000000000000000000, 0.000000000000000000 ) ) ;
#63788=CARTESIAN_POINT ( 'NONE',  ( 10.00000000000000178, 5.373634669930420493, 12.81628187352647608 ) ) ;
#63789=CARTESIAN_POINT ( 'NONE',  ( 14.92337183194729633, 12.67559781766745353, 8.527530157486181039 ) ) ;
#63790=EDGE_CURVE ( 'NONE', #1898, #79104, #24253, .T. ) ;
#63791=EDGE_LOOP ( 'NONE', ( #15086, #69880, #96710, #71370, #55037, #5097 ) ) ;
#63792=CARTESIAN_POINT ( 'NONE',  ( 2.791683348922237240, 0.3839311510007847872, -7.208316651077763204 ) ) ;
#63794=CARTESIAN_POINT ( 'NONE',  ( 13.79529636645030344, 58.26208216824728936, 14.16423886937410614 ) ) ;
#63795=CARTESIAN_POINT ( 'NONE',  ( 24.16423886937410614, 24.30374883491396787, 8.672049930838204340E-16 ) ) ;
#63796=CARTESIAN_POINT ( 'NONE',  ( -0.8801773607111008646, 28.27201867748817321, 2.915334737309923430 ) ) ;
#63797=CARTESIAN_POINT ( 'NONE',  ( -0.8801773607111008646, 48.27201867748816966, 2.915334737309923430 ) ) ;
#63800=CARTESIAN_POINT ( 'NONE',  ( 19.84674366389459266, 48.71726448433412315, -2.638427012816827677 ) ) ;
#63802=CARTESIAN_POINT ( 'NONE',  ( 18.52753015748618282, 3.925597817667451306, -4.923371831947291888 ) ) ;
#63804=CARTESIAN_POINT ( 'NONE',  ( 0.1532563361054100626, 20.80059781766744464, -2.638427012816831230 ) ) ;
#63805=CARTESIAN_POINT ( 'NONE',  ( 0.1532563361054083140, 26.00893115100078745, 1.131784320476157264E-15 ) ) ;
#63806=CARTESIAN_POINT ( 'NONE',  ( 17.20831665107776587, 52.88393115100078035, 7.208316651077764980 ) ) ;
#63807=CARTESIAN_POINT ( 'NONE',  ( 19.42250999205614548, 20.98035201082150891, -5.440088680355545492 ) ) ;
#63808=B_SPLINE_CURVE_WITH_KNOTS ( 'NONE', 3,
 ( #60715, #91212, #45726, #82730, #22740, #83725 ),
 .UNSPECIFIED., .F., .F.,
 ( 4, 2, 4 ),
 ( 0.000000000000000000, 0.0002701661927229334929, 0.0005403323854458669858 ),
 .UNSPECIFIED. ) ;
#63809=CARTESIAN_POINT ( 'NONE',  ( 3.591859063236761518, 34.95696800326375353, 11.09922568453594849 ) ) ;
#63810=CARTESIAN_POINT ( 'NONE',  ( 4.559911319644449179, 58.89701867748817676, 9.422509992056141925 ) ) ;
#63811=CARTESIAN_POINT ( 'NONE',  ( 5.076628168052704559, 30.17559781766745175, -8.527530157486179263 ) ) ;
#63812=CARTESIAN_POINT ( 'NONE',  ( -2.266590686148945544, 46.38708216824730357, -7.082119434687050408 ) ) ;
#63813=CARTESIAN_POINT ( 'NONE',  ( 1.472469842513823179, 20.59226448433411960, -4.923371831947296329 ) ) ;
#63815=CARTESIAN_POINT ( 'NONE',  ( 10.00000000000000000, 54.75893115100078745, -9.846743663894594434 ) ) ;
#63816=CARTESIAN_POINT ( 'NONE',  ( 0.1532563361054083140, 51.00893115100078745, 1.131784320476157264E-15 ) ) ;
#63817=CARTESIAN_POINT ( 'NONE',  ( 20.36894250292379382, 8.678748834913967869, 10.36894250292379205 ) ) ;
#63818=CARTESIAN_POINT ( 'NONE',  ( -0.3689425029237881626, 32.42874883491395366, 10.36894250292379027 ) ) ;
#63819=CARTESIAN_POINT ( 'NONE',  ( 0.1532563361054083140, 31.00893115100078390, 1.131784320476157264E-15 ) ) ;
#63820=CARTESIAN_POINT ( 'NONE',  ( 20.88017736071110519, 25.56368534415483751, 2.639326808657452039E-16 ) ) ;
#63821=CARTESIAN_POINT ( 'NONE',  ( -0.8801773607111008646, 43.27201867748817676, 2.915334737309923430 ) ) ;
#63822=CARTESIAN_POINT ( 'NONE',  ( -0.8801773607111009756, 48.06368534415484817, 1.068504757029289695E-15 ) ) ;
#63824=CARTESIAN_POINT ( 'NONE',  ( 13.43411237798106583, 32.66530133659708213, -12.81628187352647252 ) ) ;
#63825=CARTESIAN_POINT ( 'NONE',  ( 12.91533473730993009, 56.60535201082151247, -10.88017736071109987 ) ) ;
#63827=CARTESIAN_POINT ( 'NONE',  ( 7.361572987183169658, -0.03273551566588185635, -9.846743663894592657 ) ) ;
#63828=ADVANCED_FACE ( 'NONE', ( #12528 ), #29496, .T. ) ;
#63829=CARTESIAN_POINT ( 'NONE',  ( 0.5774900079438607392, 58.48035201082151247, 5.440088680355550821 ) ) ;
#63831=CARTESIAN_POINT ( 'NONE',  ( 0.5774900079438590739, 57.64701867748817676, -5.440088680355550821 ) ) ;
#63832=DIRECTION ( 'NONE',  ( 0.000000000000000000, 0.000000000000000000, -1.000000000000000000 ) ) ;
#63834=CARTESIAN_POINT ( 'NONE',  ( 10.00000000000000000, 11.81368534415483751, -10.88017736071110342 ) ) ;
#63835=CARTESIAN_POINT ( 'NONE',  ( 17.20831665107776587, 9.133931151000787452, -7.208316651077762316 ) ) ;
#63836=CARTESIAN_POINT ( 'NONE',  ( 17.08211943468705130, 3.470415501580634388, 12.26659068614894998 ) ) ;
#63837=CARTESIAN_POINT ( 'NONE',  ( 19.84674366389459266, 8.300597817667451750, 2.638427012816836559 ) ) ;
#63838=CARTESIAN_POINT ( 'NONE',  ( 0.5774900079438607392, 8.480352010821505360, 5.440088680355550821 ) ) ;
#63839=CARTESIAN_POINT ( 'NONE',  ( 19.84674366389459266, 48.71726448433413026, -2.638427012816827677 ) ) ;
#63840=ORIENTED_EDGE ( 'NONE', *, *, #55676, .F. ) ;
#63842=CARTESIAN_POINT ( 'NONE',  ( 18.52753015748618282, 48.92559781766745886, -4.923371831947291888 ) ) ;
#63844=CARTESIAN_POINT ( 'NONE',  ( 17.96484262340118221, 56.18868534415484817, -7.964842623401177768 ) ) ;
#63845=CARTESIAN_POINT ( 'NONE',  ( 2.791683348922237240, 45.38393115100079456, -7.208316651077763204 ) ) ;
#63848=CARTESIAN_POINT ( 'NONE',  ( 20.88017736071110164, 60.35535201082151957, 2.915334737309930979 ) ) ;
#63850=CARTESIAN_POINT ( 'NONE',  ( 19.42250999205614548, 10.98035201082150536, -5.440088680355545492 ) ) ;
#63852=CARTESIAN_POINT ( 'NONE',  ( -1.099225684535947600, 43.70696800326375353, -6.408140936763238038 ) ) ;
#63855=CARTESIAN_POINT ( 'NONE',  ( -1.099225684535947600, 29.54030133659708923, 6.408140936763237150 ) ) ;
#63856=CARTESIAN_POINT ( 'NONE',  ( 2.035157376598824452, 28.68868534415484106, 7.964842623401179544 ) ) ;
#63859=CARTESIAN_POINT ( 'NONE',  ( 7.361572987183170547, 57.05059781766744464, 9.846743663894590881 ) ) ;
#63860=CARTESIAN_POINT ( 'NONE',  ( 2.791683348922240793, 6.633931151000785675, 7.208316651077764092 ) ) ;
#63861=CARTESIAN_POINT ( 'NONE',  ( 0.1532563361054082862, 56.21726448433411605, 2.638427012816831674 ) ) ;
#63862=CARTESIAN_POINT ( 'NONE',  ( 0.1089645850228758012, 28.16234555792570049, 6.479102184480775684 ) ) ;
#63864=CARTESIAN_POINT ( 'NONE',  ( 14.92337183194729988, 34.34226448433411605, -8.527530157486177487 ) ) ;
#63866=CARTESIAN_POINT ( 'NONE',  ( 1.821158202401482962, 61.16688879859522388, 6.499999999999917399 ) ) ;
#63867=CARTESIAN_POINT ( 'NONE',  ( 18.52753015748617571, 28.09226448433411960, 4.923371831947298993 ) ) ;
#63868=( NAMED_UNIT ( * ) PLANE_ANGLE_UNIT ( ) SI_UNIT ( $, .RADIAN. ) );
#63871=CARTESIAN_POINT ( 'NONE',  ( 17.20831665107776587, 54.13393115100079456, -7.208316651077762316 ) ) ;
#63873=CARTESIAN_POINT ( 'NONE',  ( -0.8801773607110990882, 7.855352010821506248, -2.915334737309924318 ) ) ;
#63874=CARTESIAN_POINT ( 'NONE',  ( 19.38216949554541202, 20.99863466993042138, 9.382169495545424454 ) ) ;
#63875=CARTESIAN_POINT ( 'NONE',  ( 18.52753015748618282, 48.92559781766745886, -4.923371831947291888 ) ) ;
#63877=CARTESIAN_POINT ( 'NONE',  ( -0.03932841506543179738, 8.121614419605014845, 6.397827110478955248 ) ) ;
#63878=CARTESIAN_POINT ( 'NONE',  ( 17.08211943468705840, 50.13708216824730357, -12.26659068614894466 ) ) ;
#63880=CARTESIAN_POINT ( 'NONE',  ( 17.20831665107776587, 19.13393115100078035, -7.208316651077762316 ) ) ;
#63883=CARTESIAN_POINT ( 'NONE',  ( -2.266590686148945544, 46.38708216824730357, -7.082119434687050408 ) ) ;
#63884=CARTESIAN_POINT ( 'NONE',  ( 7.361572987183169658, 54.96726448433413026, -9.846743663894592657 ) ) ;
#63885=CARTESIAN_POINT ( 'NONE',  ( 0.5774900079438590739, 2.647018677488171434, -5.440088680355550821 ) ) ;
#63886=CARTESIAN_POINT ( 'NONE',  ( 22.26659068614895176, 19.72041550158063572, -7.082119434687042414 ) ) ;
#63887=CARTESIAN_POINT ( 'NONE',  ( 24.16423886937410614, 39.30374883491396787, 8.672049930838204340E-16 ) ) ;
#63888=SURFACE_SIDE_STYLE ('',( #33390 ) ) ;
#63889=CARTESIAN_POINT ( 'NONE',  ( -0.8801773607111009756, 28.06368534415484106, 1.068504757029289695E-15 ) ) ;
#63890=CARTESIAN_POINT ( 'NONE',  ( 18.52753015748617571, 53.09226448433412315, 4.923371831947298993 ) ) ;
#63892=CARTESIAN_POINT ( 'NONE',  ( 0.5774900079438607392, 33.48035201082150536, 5.440088680355550821 ) ) ;
#63895=CARTESIAN_POINT ( 'NONE',  ( 17.20831665107776587, 49.13393115100078745, -7.208316651077762316 ) ) ;
#63898=CARTESIAN_POINT ( 'NONE',  ( 17.20831665107776587, 57.88393115100078745, 7.208316651077764980 ) ) ;
#63899=CARTESIAN_POINT ( 'NONE',  ( 14.92337183194729633, 62.67559781766745886, 8.527530157486181039 ) ) ;
#63901=ORIENTED_EDGE ( 'NONE', *, *, #72820, .T. ) ;
#63903=CARTESIAN_POINT ( 'NONE',  ( 13.79529636645031943, 30.34541550158063927, -14.16423886937409904 ) ) ;
#63906=CARTESIAN_POINT ( 'NONE',  ( 4.559911319644449179, 2.230352010821504916, -9.422509992056141925 ) ) ;
#63907=CARTESIAN_POINT ( 'NONE',  ( -2.816281873526473856, 19.12363466993042138, 9.499525473075851096E-16 ) ) ;
#63908=FACE_OUTER_BOUND ( 'NONE', #67814, .T. ) ;
#63909=CARTESIAN_POINT ( 'NONE',  ( 14.92337183194729988, 9.342264484334119601, -8.527530157486177487 ) ) ;
#63913=CARTESIAN_POINT ( 'NONE',  ( 1.959929470562269183, 20.51528370094808196, -5.767676674365832312 ) ) ;
#63914=CARTESIAN_POINT ( 'NONE',  ( -0.8801773607111008646, 8.272018677488171434, 2.915334737309923430 ) ) ;
#63916=CARTESIAN_POINT ( 'NONE',  ( 12.91533473730992121, 34.52201867748817676, 10.88017736071110164 ) ) ;
#63917=CARTESIAN_POINT ( 'NONE',  ( 4.559911319644449179, 43.89701867748816966, 9.422509992056141925 ) ) ;
#63918=CARTESIAN_POINT ( 'NONE',  ( 19.84674366389459621, 63.50893115100078745, 7.409399052514197653E-17 ) ) ;
#63919=CARTESIAN_POINT ( 'NONE',  ( 7.361572987183169658, 64.96726448433412315, -9.846743663894592657 ) ) ;
#63921=CARTESIAN_POINT ( 'NONE',  ( 12.63842701281683922, 14.55059781766744997, -9.846743663894590881 ) ) ;
#63922=ORIENTED_EDGE ( 'NONE', *, *, #82010, .F. ) ;
#63923=CARTESIAN_POINT ( 'NONE',  ( 19.42250999205614193, 30.14701867748817321, 5.440088680355555262 ) ) ;
#63924=CARTESIAN_POINT ( 'NONE',  ( 19.38216949554541202, 35.99863466993041072, 9.382169495545424454 ) ) ;
#63925=CARTESIAN_POINT ( 'NONE',  ( 7.361572987183169658, 64.96726448433412315, -9.846743663894592657 ) ) ;
#63926=CARTESIAN_POINT ( 'NONE',  ( 0.5774900079438607392, 58.48035201082151247, 5.440088680355550821 ) ) ;
#63927=CARTESIAN_POINT ( 'NONE',  ( 10.00000000000000178, 12.25893115100078568, 9.846743663894594434 ) ) ;
#63928=CARTESIAN_POINT ( 'NONE',  ( 22.81628187352648496, 36.83196800326376064, -3.434112377981050290 ) ) ;
#63929=CARTESIAN_POINT ( 'NONE',  ( 19.42250999205614548, 65.98035201082151957, -5.440088680355545492 ) ) ;
#63934=CARTESIAN_POINT ( 'NONE',  ( 2.035157376598822676, 12.43868534415483751, -7.964842623401177768 ) ) ;
#63935=CARTESIAN_POINT ( 'NONE',  ( 21.09922568453595559, 57.04030133659708923, -6.408140936763230044 ) ) ;
#63936=CARTESIAN_POINT ( 'NONE',  ( -4.164238869374098151, 26.59541550158063217, -3.795296366450310543 ) ) ;
#63937=CARTESIAN_POINT ( 'NONE',  ( 1.472469842513823179, 11.42559781766745175, 4.923371831947296329 ) ) ;
#63939=CARTESIAN_POINT ( 'NONE',  ( 14.92337183194729988, 14.34226448433411782, -8.527530157486177487 ) ) ;
#63940=CARTESIAN_POINT ( 'NONE',  ( 10.00000000000000000, 55.55374883491396787, -14.16423886937410082 ) ) ;
#63941=ORIENTED_EDGE ( 'NONE', *, *, #8542, .F. ) ;
#63942=CARTESIAN_POINT ( 'NONE',  ( -0.8801773607111009756, 18.06368534415484106, 1.068504757029289695E-15 ) ) ;
#63943=EDGE_CURVE ( 'NONE', #85865, #51000, #46016, .T. ) ;
#63944=CARTESIAN_POINT ( 'NONE',  ( 17.96484262340118221, 21.18868534415483396, -7.964842623401177768 ) ) ;
#63945=CARTESIAN_POINT ( 'NONE',  ( 19.50000000000000711, 98.59912998021083297, 4.500000000000000888 ) ) ;
#63947=DIRECTION ( 'NONE',  ( -0.000000000000000000, 1.000000000000000000, 0.000000000000000000 ) ) ;
#63948=CARTESIAN_POINT ( 'NONE',  ( 12.91533473730992121, 19.52201867748816611, 10.88017736071110164 ) ) ;
#63949=CARTESIAN_POINT ( 'NONE',  ( 1.472469842513823179, 50.59226448433411605, -4.923371831947296329 ) ) ;
#63951=B_SPLINE_CURVE_WITH_KNOTS ( 'NONE', 3,
 ( #45241, #92222, #37761, #77212 ),
 .UNSPECIFIED., .F., .F.,
 ( 4, 4 ),
 ( 0.000000000000000000, 0.002657014572711323321 ),
 .UNSPECIFIED. ) ;
#63954=CARTESIAN_POINT ( 'NONE',  ( 2.917880565312948704, 22.63708216824730002, 12.26659068614894643 ) ) ;
#63955=CARTESIAN_POINT ( 'NONE',  ( 15.44008868035555793, 41.39701867748817676, -9.422509992056140149 ) ) ;
#63956=CARTESIAN_POINT ( 'NONE',  ( -0.8801773607111008646, 13.27201867748817321, 2.915334737309923430 ) ) ;
#63957=CARTESIAN_POINT ( 'NONE',  ( 19.84674366389459621, 58.50893115100078745, 7.409399052514197653E-17 ) ) ;
#63959=CARTESIAN_POINT ( 'NONE',  ( 14.92337183194729988, 39.34226448433412315, -8.527530157486177487 ) ) ;
#63961=CARTESIAN_POINT ( 'NONE',  ( 19.84674366389459266, 13.30059781766745353, 2.638427012816836559 ) ) ;
#63964=CARTESIAN_POINT ( 'NONE',  ( 20.88017736071110164, 15.35535201082150358, 2.915334737309930979 ) ) ;
#63965=CARTESIAN_POINT ( 'NONE',  ( 18.52753015748617571, 13.09226448433411960, 4.923371831947298993 ) ) ;
#63966=CARTESIAN_POINT ( 'NONE',  ( 5.076628168052704559, 65.17559781766745175, -8.527530157486179263 ) ) ;
#63967=CARTESIAN_POINT ( 'NONE',  ( 20.88017736071110875, 40.77201867748818387, -2.915334737309920765 ) ) ;
#63968=CARTESIAN_POINT ( 'NONE',  ( 15.44008868035555793, 46.39701867748817676, -9.422509992056140149 ) ) ;
#63969=CARTESIAN_POINT ( 'NONE',  ( 19.42250999205614548, 15.98035201082150714, -5.440088680355545492 ) ) ;
#63970=CARTESIAN_POINT ( 'NONE',  ( 0.6178305044545838731, 49.74863466993041072, 9.382169495545420901 ) ) ;
#63971=CARTESIAN_POINT ( 'NONE',  ( 24.16423886937409904, 34.09541550158064638, 3.795296366450317205 ) ) ;
#63972=CARTESIAN_POINT ( 'NONE',  ( 20.24186590665275531, 12.61633188102327630, -6.114288769123077394 ) ) ;
#63973=CARTESIAN_POINT ( 'NONE',  ( 22.81628187352647785, 61.62363466993041783, 6.195893100308588602E-16 ) ) ;
#63975=CARTESIAN_POINT ( 'NONE',  ( 2.791683348922240793, 51.63393115100078745, 7.208316651077764092 ) ) ;
#63976=CARTESIAN_POINT ( 'NONE',  ( 19.42250999205614193, 40.14701867748817676, 5.440088680355555262 ) ) ;
#63979=CARTESIAN_POINT ( 'NONE',  ( 19.84674366389459621, 3.508931151000785231, 7.409399052514197653E-17 ) ) ;
#63982=CARTESIAN_POINT ( 'NONE',  ( 1.274849032794278747, 42.55509018479936856, -6.499999999999960032 ) ) ;
#63983=CARTESIAN_POINT ( 'NONE',  ( 1.472469842513823179, 16.42559781766745175, 4.923371831947296329 ) ) ;
#63984=CARTESIAN_POINT ( 'NONE',  ( 19.84674366389459266, 23.30059781766745530, 2.638427012816836559 ) ) ;
#63985=ADVANCED_FACE ( 'NONE', ( #46494 ), #56961, .T. ) ;
#63986=CARTESIAN_POINT ( 'NONE',  ( 2.791683348922237240, 15.38393115100078212, -7.208316651077763204 ) ) ;
#63987=CARTESIAN_POINT ( 'NONE',  ( 0.1532563361054083140, 6.008931151000784787, 1.131784320476157264E-15 ) ) ;
#63988=CARTESIAN_POINT ( 'NONE',  ( 4.559911319644449179, 62.23035201082150536, -9.422509992056141925 ) ) ;
#63989=CARTESIAN_POINT ( 'NONE',  ( -38.69000000000001194, 93.50000000000000000, 9.500000000000000000 ) ) ;
#63990=CARTESIAN_POINT ( 'NONE',  ( 17.96484262340118221, 56.18868534415484817, -7.964842623401177768 ) ) ;
#63991=CARTESIAN_POINT ( 'NONE',  ( 17.20831665107776587, 19.13393115100078035, -7.208316651077762316 ) ) ;
#63994=CARTESIAN_POINT ( 'NONE',  ( 0.8952175423695086787, 63.52576239577081907, 5.990408912944362285 ) ) ;
#63995=CARTESIAN_POINT ( 'NONE',  ( 5.076628168052704559, 50.17559781766745886, -8.527530157486179263 ) ) ;
#63997=VERTEX_POINT ( 'NONE', #13432 ) ;
#64000=CARTESIAN_POINT ( 'NONE',  ( 19.38216949554541202, 55.99863466993041072, 9.382169495545424454 ) ) ;
#64001=( LENGTH_UNIT ( ) NAMED_UNIT ( * ) SI_UNIT ( .MILLI., .METRE. ) );
#64002=CARTESIAN_POINT ( 'NONE',  ( 2.917880565312948704, 37.63708216824731068, 12.26659068614894643 ) ) ;
#64004=CARTESIAN_POINT ( 'NONE',  ( -0.3689425029237898834, 6.178748834913968757, -10.36894250292378850 ) ) ;
#64005=CARTESIAN_POINT ( 'NONE',  ( 20.88017736071110875, 30.77201867748816966, -2.915334737309920765 ) ) ;
#64007=CARTESIAN_POINT ( 'NONE',  ( 19.84674366389459266, 13.71726448433411782, -2.638427012816827677 ) ) ;
#64008=CARTESIAN_POINT ( 'NONE',  ( 19.42250999205614193, 55.14701867748817676, 5.440088680355555262 ) ) ;
#64009=CARTESIAN_POINT ( 'NONE',  ( 7.361572987183170547, 12.05059781766744997, 9.846743663894590881 ) ) ;
#64011=CARTESIAN_POINT ( 'NONE',  ( 22.81628187352647785, 41.62363466993042493, 6.195893100308588602E-16 ) ) ;
#64012=CARTESIAN_POINT ( 'NONE',  ( 0.1532563361054082862, 36.21726448433410894, 2.638427012816831674 ) ) ;
#64014=CARTESIAN_POINT ( 'NONE',  ( 4.559911319644449179, 58.89701867748817676, 9.422509992056141925 ) ) ;
#64015=CARTESIAN_POINT ( 'NONE',  ( 10.00000000000000000, 22.87363466993042138, -12.81628187352647608 ) ) ;
#64017=CARTESIAN_POINT ( 'NONE',  ( 0.1532563361054100626, 20.80059781766744464, -2.638427012816831230 ) ) ;
#64019=CARTESIAN_POINT ( 'NONE',  ( -0.3689425029237898834, 16.17874883491396076, -10.36894250292378850 ) ) ;
#64021=CARTESIAN_POINT ( 'NONE',  ( 12.91533473730993009, 36.60535201082151247, -10.88017736071109987 ) ) ;
#64022=CARTESIAN_POINT ( 'NONE',  ( -2.266590686148945544, 37.22041550158063217, 7.082119434687048631 ) ) ;
#64023=CARTESIAN_POINT ( 'NONE',  ( 19.84674366389459266, 53.71726448433411605, -2.638427012816827677 ) ) ;
#64024=CARTESIAN_POINT ( 'NONE',  ( 12.63842701281683034, 12.46726448433411782, 9.846743663894596210 ) ) ;
#64025=CARTESIAN_POINT ( 'NONE',  ( 16.40814093676324603, 52.45696800326375353, -11.09922568453594671 ) ) ;
#64026=CARTESIAN_POINT ( 'NONE',  ( 10.00000000000000178, 70.00000000000000000, 0.000000000000000000 ) ) ;
#64027=CARTESIAN_POINT ( 'NONE',  ( 4.559911319644449179, 43.89701867748816966, 9.422509992056141925 ) ) ;
#64030=CARTESIAN_POINT ( 'NONE',  ( 13.43411237798106583, 22.66530133659708923, -12.81628187352647252 ) ) ;
#64031=CARTESIAN_POINT ( 'NONE',  ( 14.92337183194729988, 59.34226448433412315, -8.527530157486177487 ) ) ;
#64033=CARTESIAN_POINT ( 'NONE',  ( -0.1042174387088687926, 13.10736173766201240, 6.337391062633409788 ) ) ;
#64038=CARTESIAN_POINT ( 'NONE',  ( 7.084665262690076126, 52.02201867748816255, -10.88017736071110164 ) ) ;
#64039=VECTOR ( 'NONE', #38324, 1000.000000000000000 ) ;
#64040=CARTESIAN_POINT ( 'NONE',  ( 12.91533473730993009, 51.60535201082149825, -10.88017736071109987 ) ) ;
#64041=CARTESIAN_POINT ( 'NONE',  ( -0.1688089201193209155, 79.91181047996344944, 9.500000000000000000 ) ) ;
#64043=CARTESIAN_POINT ( 'NONE',  ( 19.84674366389459621, 23.50893115100078390, 7.409399052514197653E-17 ) ) ;
#64044=CARTESIAN_POINT ( 'NONE',  ( 2.035157376598824452, 18.68868534415484106, 7.964842623401179544 ) ) ;
#64045=CARTESIAN_POINT ( 'NONE',  ( 5.076628168052703671, 66.84226448433412315, 8.527530157486179263 ) ) ;
#64046=CARTESIAN_POINT ( 'NONE',  ( 4.559911319644449179, 23.89701867748817321, 9.422509992056141925 ) ) ;
#64048=CARTESIAN_POINT ( 'NONE',  ( 20.32896413005680714, 52.60497603579417358, -5.963430220938276349 ) ) ;
#64050=CARTESIAN_POINT ( 'NONE',  ( 6.565887622018943937, 23.08196800326375708, -12.81628187352647608 ) ) ;
#64052=CARTESIAN_POINT ( 'NONE',  ( 0.5774900079438607392, 53.48035201082151247, 5.440088680355550821 ) ) ;
#64053=CARTESIAN_POINT ( 'NONE',  ( 2.791683348922240793, 46.63393115100077324, 7.208316651077764092 ) ) ;
#64054=CARTESIAN_POINT ( 'NONE',  ( 19.38216949554541202, 25.99863466993042138, 9.382169495545424454 ) ) ;
#64055=CARTESIAN_POINT ( 'NONE',  ( -0.8801773607110991993, 32.85535201082151247, -2.915334737309923874 ) ) ;
#64056=CARTESIAN_POINT ( 'NONE',  ( -0.3689425029237898834, 46.17874883491397497, -10.36894250292378850 ) ) ;
#64057=CARTESIAN_POINT ( 'NONE',  ( 5.076628168052703671, 36.84226448433412315, 8.527530157486179263 ) ) ;
#64058=CARTESIAN_POINT ( 'NONE',  ( 2.035157376598822676, 67.43868534415484817, -7.964842623401177768 ) ) ;
#64059=CARTESIAN_POINT ( 'NONE',  ( -0.8801773607111008646, 48.27201867748816966, 2.915334737309923430 ) ) ;
#64061=CARTESIAN_POINT ( 'NONE',  ( 24.16423886937409904, 19.09541550158063927, 3.795296366450317205 ) ) ;
#64062=CARTESIAN_POINT ( 'NONE',  ( 1.711636803080548441, 21.84492782695770430, -6.499999999999988454 ) ) ;
#64064=ORIENTED_EDGE ( 'NONE', *, *, #52539, .F. ) ;
#64065=CARTESIAN_POINT ( 'NONE',  ( 17.08211943468705840, 50.13708216824730357, -12.26659068614894466 ) ) ;
#64066=CARTESIAN_POINT ( 'NONE',  ( 20.36894250292379738, 54.92874883491396076, -10.36894250292379027 ) ) ;
#64067=CARTESIAN_POINT ( 'NONE',  ( 7.361572987183170547, 17.05059781766745530, 9.846743663894590881 ) ) ;
#64068=CARTESIAN_POINT ( 'NONE',  ( 16.40814093676323893, 15.79030133659708746, 11.09922568453595026 ) ) ;
#64071=CARTESIAN_POINT ( 'NONE',  ( 2.035157376598822676, 67.43868534415484817, -7.964842623401177768 ) ) ;
#64072=CARTESIAN_POINT ( 'NONE',  ( 3.591859063236761518, 34.95696800326375353, 11.09922568453594849 ) ) ;
#64073=CARTESIAN_POINT ( 'NONE',  ( -2.266590686148945544, 47.22041550158063927, 7.082119434687048631 ) ) ;
#64075=PRESENTATION_STYLE_ASSIGNMENT (( #33581 ) ) ;
#64077=EDGE_CURVE ( 'NONE', #52255, #81670, #75247, .T. ) ;
#64078=VERTEX_POINT ( 'NONE', #49956 ) ;
#64079=PLANE ( 'NONE',  #49210 ) ;
#64080=CARTESIAN_POINT ( 'NONE',  ( 19.84674366389459266, 18.71726448433411960, -2.638427012816827677 ) ) ;
#64083=CARTESIAN_POINT ( 'NONE',  ( 24.16423886937410614, 14.30374883491396787, 8.672049930838204340E-16 ) ) ;
#64084=CARTESIAN_POINT ( 'NONE',  ( -0.8801773607110991993, 12.85535201082150358, -2.915334737309923874 ) ) ;
#64085=CARTESIAN_POINT ( 'NONE',  ( 17.96484262340118221, 16.18868534415483396, -7.964842623401177768 ) ) ;
#64086=CARTESIAN_POINT ( 'NONE',  ( 14.92337183194729988, 44.34226448433412315, -8.527530157486177487 ) ) ;
#64087=CARTESIAN_POINT ( 'NONE',  ( 10.00000000000000000, 7.873634669930421381, -12.81628187352647608 ) ) ;
#64090=EDGE_CURVE ( 'NONE', #9878, #21520, #45504, .T. ) ;
#64092=STYLED_ITEM ( 'NONE', ( #95907 ), #80374 ) ;
#64093=CARTESIAN_POINT ( 'NONE',  ( 6.565887622018943937, 23.08196800326375708, -12.81628187352647608 ) ) ;
#64095=CARTESIAN_POINT ( 'NONE',  ( 24.16423886937409904, 54.09541550158063217, 3.795296366450317205 ) ) ;
#64097=CARTESIAN_POINT ( 'NONE',  ( 2.917880565312948704, 57.63708216824731068, 12.26659068614894643 ) ) ;
#64098=ORIENTED_EDGE ( 'NONE', *, *, #22288, .F. ) ;
#64099=CARTESIAN_POINT ( 'NONE',  ( 7.084665262690076126, 37.02201867748817676, -10.88017736071110164 ) ) ;
#64100=CARTESIAN_POINT ( 'NONE',  ( 17.96484262340118221, 41.18868534415484106, -7.964842623401177768 ) ) ;
#64101=CARTESIAN_POINT ( 'NONE',  ( 4.559911319644449179, 68.89701867748817676, 9.422509992056141925 ) ) ;
#64102=CARTESIAN_POINT ( 'NONE',  ( 2.035157376598822676, 32.43868534415483396, -7.964842623401177768 ) ) ;
#64107=CARTESIAN_POINT ( 'NONE',  ( 19.84674366389459621, 13.50893115100078568, 7.409399052514197653E-17 ) ) ;
#64111=CARTESIAN_POINT ( 'NONE',  ( 18.52753015748617571, 38.09226448433412315, 4.923371831947298993 ) ) ;
#64112=CYLINDRICAL_SURFACE ( 'NONE', #54768, 11.92686044187656513 ) ;
#64113=EDGE_CURVE ( 'NONE', #43512, #32737, #74416, .T. ) ;
#64117=CARTESIAN_POINT ( 'NONE',  ( -0.1503990784575328643, 65.12777174578613426, 6.262539305110068177 ) ) ;
#64118=CARTESIAN_POINT ( 'NONE',  ( 17.20831665107776587, 62.88393115100078745, 7.208316651077764980 ) ) ;
#64119=CARTESIAN_POINT ( 'NONE',  ( 2.917880565312948704, 47.63708216824730357, 12.26659068614894643 ) ) ;
#64120=DIRECTION ( 'NONE',  ( -0.000000000000000000, -0.000000000000000000, 1.000000000000000000 ) ) ;
#64124=CARTESIAN_POINT ( 'NONE',  ( 14.92337183194729988, 34.34226448433411605, -8.527530157486177487 ) ) ;
#64125=CARTESIAN_POINT ( 'NONE',  ( 6.565887622018943937, 10.16530133659708746, 12.81628187352647430 ) ) ;
#64126=CARTESIAN_POINT ( 'NONE',  ( 18.52753015748617571, 3.092264484334118269, 4.923371831947298993 ) ) ;
#64128=CARTESIAN_POINT ( 'NONE',  ( 7.361572987183169658, 59.96726448433410894, -9.846743663894592657 ) ) ;
#64132=CARTESIAN_POINT ( 'NONE',  ( 7.084665262690076126, 2.022018677488171434, -10.88017736071110164 ) ) ;
#64134=CARTESIAN_POINT ( 'NONE',  ( 7.084665262690076126, 37.02201867748817676, -10.88017736071110164 ) ) ;
#64135=CARTESIAN_POINT ( 'NONE',  ( 10.00000000000000178, 15.37363466993042138, 12.81628187352647608 ) ) ;
#64140=CARTESIAN_POINT ( 'NONE',  ( 18.29284471827484637, 35.40189080397292543, -6.500000000000014211 ) ) ;
#64141=CARTESIAN_POINT ( 'NONE',  ( 14.92337183194729988, 54.34226448433412315, -8.527530157486177487 ) ) ;
#64144=CARTESIAN_POINT ( 'NONE',  ( 16.40814093676324603, 7.456968003263754419, -11.09922568453594671 ) ) ;
#64146=CARTESIAN_POINT ( 'NONE',  ( 15.44008868035555260, 29.73035201082150891, 9.422509992056143702 ) ) ;
#64147=CARTESIAN_POINT ( 'NONE',  ( 6.000000000000000000, 61.50000000000000711, 6.500000000000000888 ) ) ;
#64148=CARTESIAN_POINT ( 'NONE',  ( 22.26659068614894466, 33.88708216824730357, 7.082119434687054849 ) ) ;
#64149=CARTESIAN_POINT ( 'NONE',  ( 24.16423886937410614, 24.30374883491396787, 8.672049930838204340E-16 ) ) ;
#64150=CARTESIAN_POINT ( 'NONE',  ( 17.96484262340118221, 16.18868534415483396, -7.964842623401177768 ) ) ;
#64151=CARTESIAN_POINT ( 'NONE',  ( 5.076628168052703671, 36.84226448433412315, 8.527530157486179263 ) ) ;
#64152=CARTESIAN_POINT ( 'NONE',  ( -2.816281873526473856, 34.33196800326376064, 3.434112377981055619 ) ) ;
#64153=CARTESIAN_POINT ( 'NONE',  ( 17.96484262340118221, 16.18868534415483396, -7.964842623401177768 ) ) ;
#64154=( GEOMETRIC_REPRESENTATION_CONTEXT ( 3 ) GLOBAL_UNCERTAINTY_ASSIGNED_CONTEXT ( ( #45448 ) ) GLOBAL_UNIT_ASSIGNED_CONTEXT ( ( #4806, #54226, #59758 ) ) REPRESENTATION_CONTEXT ( 'NONE', 'WORKASPACE' ) );
#64155=CARTESIAN_POINT ( 'NONE',  ( 7.361572987183170547, 42.05059781766745886, 9.846743663894590881 ) ) ;
#64156=CARTESIAN_POINT ( 'NONE',  ( 4.559911319644449179, 37.23035201082150536, -9.422509992056141925 ) ) ;
#64157=CARTESIAN_POINT ( 'NONE',  ( 10.00000000000000178, 0.3736346699304200492, 12.81628187352647608 ) ) ;
#64158=CARTESIAN_POINT ( 'NONE',  ( 13.79529636645031943, 25.34541550158063572, -14.16423886937409904 ) ) ;
#64159=CARTESIAN_POINT ( 'NONE',  ( 0.1532563361054082862, 61.21726448433412315, 2.638427012816831674 ) ) ;
#64162=CARTESIAN_POINT ( 'NONE',  ( 5.076628168052704559, 20.17559781766745175, -8.527530157486179263 ) ) ;
#64163=CARTESIAN_POINT ( 'NONE',  ( 22.81628187352648496, 51.83196800326376064, -3.434112377981050290 ) ) ;
#64164=CARTESIAN_POINT ( 'NONE',  ( 14.92337183194729988, 59.34226448433412315, -8.527530157486177487 ) ) ;
#64166=DIRECTION ( 'NONE',  ( -6.608470384673550777E-17, -1.000000000000000000, -0.000000000000000000 ) ) ;
#64168=CARTESIAN_POINT ( 'NONE',  ( 13.79529636645030344, 63.26208216824730357, 14.16423886937410614 ) ) ;
#64169=CARTESIAN_POINT ( 'NONE',  ( -2.266590686148945544, 11.38708216824730179, -7.082119434687050408 ) ) ;
#64170=CARTESIAN_POINT ( 'NONE',  ( 15.44008868035555793, 66.39701867748817676, -9.422509992056140149 ) ) ;
#64171=CARTESIAN_POINT ( 'NONE',  ( 1.472469842513823179, 46.42559781766745175, 4.923371831947296329 ) ) ;
#64172=CARTESIAN_POINT ( 'NONE',  ( 17.96484262340118221, 14.93868534415483751, 7.964842623401181321 ) ) ;
#64174=CARTESIAN_POINT ( 'NONE',  ( 1.472469842513823179, 66.42559781766745175, 4.923371831947296329 ) ) ;
#64176=UNCERTAINTY_MEASURE_WITH_UNIT (LENGTH_MEASURE( 1.000000000000000082E-05 ), #83414, 'distance_accuracy_value', 'NONE');
#64179=ORIENTED_EDGE ( 'NONE', *, *, #95864, .F. ) ;
#64182=CARTESIAN_POINT ( 'NONE',  ( -0.3689425029237881626, 7.428748834913967869, 10.36894250292379027 ) ) ;
#64183=CARTESIAN_POINT ( 'NONE',  ( -0.3689425029237881626, 2.428748834913967869, 10.36894250292379027 ) ) ;
#64185=CARTESIAN_POINT ( 'NONE',  ( 10.00000000000000000, 54.75893115100078745, -9.846743663894594434 ) ) ;
#64186=CARTESIAN_POINT ( 'NONE',  ( 2.791683348922237240, 30.38393115100078390, -7.208316651077763204 ) ) ;
#64188=CARTESIAN_POINT ( 'NONE',  ( 0.5774900079438590739, 27.64701867748817676, -5.440088680355550821 ) ) ;
#64189=CARTESIAN_POINT ( 'NONE',  ( 0.1532563361054082862, 56.21726448433411605, 2.638427012816831674 ) ) ;
#64190=SURFACE_STYLE_FILL_AREA ( #94208 ) ;
#64191=CARTESIAN_POINT ( 'NONE',  ( 24.16423886937409904, 44.09541550158063927, 3.795296366450317205 ) ) ;
#64192=CARTESIAN_POINT ( 'NONE',  ( 6.204703633549690345, 65.76208216824731778, -14.16423886937410259 ) ) ;
#64193=CARTESIAN_POINT ( 'NONE',  ( 7.361572987183169658, 64.96726448433412315, -9.846743663894592657 ) ) ;
#64196=CARTESIAN_POINT ( 'NONE',  ( 12.91533473730992121, 64.52201867748817676, 10.88017736071110164 ) ) ;
#64198=CARTESIAN_POINT ( 'NONE',  ( 1.472469842513823179, 35.59226448433412315, -4.923371831947296329 ) ) ;
#64204=CARTESIAN_POINT ( 'NONE',  ( 19.84674366389459266, 18.71726448433411960, -2.638427012816827677 ) ) ;
#64205=ORIENTED_EDGE ( 'NONE', *, *, #69556, .T. ) ;
#64206=CARTESIAN_POINT ( 'NONE',  ( 17.08211943468705840, 35.13708216824730357, -12.26659068614894466 ) ) ;
#64207=CARTESIAN_POINT ( 'NONE',  ( 5.076628168052703671, 31.84226448433412315, 8.527530157486179263 ) ) ;
#64208=CARTESIAN_POINT ( 'NONE',  ( 2.035157376598822676, 57.43868534415484106, -7.964842623401177768 ) ) ;
#64210=CARTESIAN_POINT ( 'NONE',  ( 2.035157376598822676, 42.43868534415483396, -7.964842623401177768 ) ) ;
#64211=CARTESIAN_POINT ( 'NONE',  ( 18.52753015748618282, 43.92559781766745175, -4.923371831947291888 ) ) ;
#64214=CARTESIAN_POINT ( 'NONE',  ( -2.266590686148945544, 12.22041550158063394, 7.082119434687048631 ) ) ;
#64217=CARTESIAN_POINT ( 'NONE',  ( 19.38216949554541202, 25.99863466993042138, 9.382169495545424454 ) ) ;
#64218=FILL_AREA_STYLE ('',( #79239 ) ) ;
#64219=CARTESIAN_POINT ( 'NONE',  ( 0.1532563361054082862, 26.21726448433411605, 2.638427012816831674 ) ) ;
#64220=FILL_AREA_STYLE ('',( #33721 ) ) ;
#64221=CARTESIAN_POINT ( 'NONE',  ( -2.816281873526471635, 43.91530133659708923, -3.434112377981056508 ) ) ;
#64223=CARTESIAN_POINT ( 'NONE',  ( 2.791683348922240793, 31.63393115100078745, 7.208316651077764092 ) ) ;
#64224=CARTESIAN_POINT ( 'NONE',  ( 10.00000000000000178, 64.31368534415483396, 10.88017736071110342 ) ) ;
#64227=CARTESIAN_POINT ( 'NONE',  ( 7.084665262690076126, 67.02201867748817676, -10.88017736071110164 ) ) ;
#64228=CARTESIAN_POINT ( 'NONE',  ( -45.12679085540637658, 105.3517674277019012, 4.910439065983985607 ) ) ;
#64230=CARTESIAN_POINT ( 'NONE',  ( 18.52753015748618282, 3.925597817667451306, -4.923371831947291888 ) ) ;
#64231=EDGE_CURVE ( 'NONE', #58660, #78529, #89591, .T. ) ;
#64233=CARTESIAN_POINT ( 'NONE',  ( 10.00000000000000178, 47.25893115100078745, 9.846743663894594434 ) ) ;
#64235=CARTESIAN_POINT ( 'NONE',  ( -0.3689425029237881626, 7.428748834913967869, 10.36894250292379027 ) ) ;
#64236=CARTESIAN_POINT ( 'NONE',  ( 0.1532563361054083140, 36.00893115100078745, 1.131784320476157264E-15 ) ) ;
#64237=CARTESIAN_POINT ( 'NONE',  ( -2.816281873526473856, 29.12363466993041783, 9.499525473075851096E-16 ) ) ;
#64240=CARTESIAN_POINT ( 'NONE',  ( 15.44008868035555793, 66.39701867748817676, -9.422509992056140149 ) ) ;
#64241=CARTESIAN_POINT ( 'NONE',  ( 22.81628187352648496, 1.831968003263753753, -3.434112377981050290 ) ) ;
#64243=CARTESIAN_POINT ( 'NONE',  ( 17.20831665107776587, 22.88393115100078745, 7.208316651077764980 ) ) ;
#64244=CARTESIAN_POINT ( 'NONE',  ( 10.00000000000000000, 26.81368534415484106, -10.88017736071110342 ) ) ;
#64245=CARTESIAN_POINT ( 'NONE',  ( 22.81628187352647785, 26.62363466993042138, 6.195893100308588602E-16 ) ) ;
#64246=( GEOMETRIC_REPRESENTATION_CONTEXT ( 3 ) GLOBAL_UNCERTAINTY_ASSIGNED_CONTEXT ( ( #37288 ) ) GLOBAL_UNIT_ASSIGNED_CONTEXT ( ( #30566, #8086, #77062 ) ) REPRESENTATION_CONTEXT ( 'NONE', 'WORKASPACE' ) );
#64247=CARTESIAN_POINT ( 'NONE',  ( 2.791683348922240793, 26.63393115100078745, 7.208316651077764092 ) ) ;
#64249=CARTESIAN_POINT ( 'NONE',  ( 12.91533473730992121, 39.52201867748817676, 10.88017736071110164 ) ) ;
#64250=AXIS2_PLACEMENT_3D ( 'NONE', #2306, #8791, #77773 ) ;
#64252=( GEOMETRIC_REPRESENTATION_CONTEXT ( 3 ) GLOBAL_UNCERTAINTY_ASSIGNED_CONTEXT ( ( #20298 ) ) GLOBAL_UNIT_ASSIGNED_CONTEXT ( ( #64498, #72498, #63037 ) ) REPRESENTATION_CONTEXT ( 'NONE', 'WORKASPACE' ) );
#64253=CARTESIAN_POINT ( 'NONE',  ( 7.084665262690076126, 57.02201867748817676, -10.88017736071110164 ) ) ;
#64254=CARTESIAN_POINT ( 'NONE',  ( 4.559911319644449179, 3.897018677488170990, 9.422509992056141925 ) ) ;
#64255=CARTESIAN_POINT ( 'NONE',  ( 12.63842701281683034, 47.46726448433412315, 9.846743663894596210 ) ) ;
#64256=CARTESIAN_POINT ( 'NONE',  ( 4.559911319644449179, 27.23035201082150536, -9.422509992056141925 ) ) ;
#64257=( LENGTH_UNIT ( ) NAMED_UNIT ( * ) SI_UNIT ( .MILLI., .METRE. ) );
#64259=CARTESIAN_POINT ( 'NONE',  ( 10.00000000000000000, 46.81368534415484106, -10.88017736071110342 ) ) ;
#64260=CARTESIAN_POINT ( 'NONE',  ( -0.8801773607111009756, 8.063685344154837509, 1.068504757029289695E-15 ) ) ;
#64263=CARTESIAN_POINT ( 'NONE',  ( 10.00000000000000178, 42.25893115100078745, 9.846743663894594434 ) ) ;
#64264=CARTESIAN_POINT ( 'NONE',  ( 20.36894250292379738, 54.92874883491396076, -10.36894250292379027 ) ) ;
#64265=CARTESIAN_POINT ( 'NONE',  ( 20.24186590665278018, 19.73410085661204150, 6.114288769123035649 ) ) ;
#64267=EDGE_CURVE ( 'NONE', #52153, #71557, #35502, .T. ) ;
#64268=( LENGTH_UNIT ( ) NAMED_UNIT ( * ) SI_UNIT ( .MILLI., .METRE. ) );
#64269=CARTESIAN_POINT ( 'NONE',  ( 10.00000000000000178, 23.05374883491397142, 14.16423886937410082 ) ) ;
#64272=CARTESIAN_POINT ( 'NONE',  ( -0.8801773607111008646, 3.272018677488171434, 2.915334737309923430 ) ) ;
#64273=CARTESIAN_POINT ( 'NONE',  ( 5.076628168052704559, 40.17559781766745175, -8.527530157486179263 ) ) ;
#64276=CARTESIAN_POINT ( 'NONE',  ( 0.5774900079438607392, 58.48035201082151247, 5.440088680355550821 ) ) ;
#64277=CARTESIAN_POINT ( 'NONE',  ( -2.816281873526473856, 64.12363466993042493, 9.499525473075851096E-16 ) ) ;
#64278=CARTESIAN_POINT ( 'NONE',  ( 12.91533473730992121, 34.52201867748817676, 10.88017736071110164 ) ) ;
#64279=CARTESIAN_POINT ( 'NONE',  ( 19.38216949554541202, 60.99863466993042493, 9.382169495545424454 ) ) ;
#64280=CARTESIAN_POINT ( 'NONE',  ( 10.00000000000000000, 7.873634669930421381, -12.81628187352647608 ) ) ;
#64281=CARTESIAN_POINT ( 'NONE',  ( 14.92337183194729988, 9.342264484334119601, -8.527530157486177487 ) ) ;
#64284=CARTESIAN_POINT ( 'NONE',  ( 4.559911319644449179, 7.230352010821505360, -9.422509992056141925 ) ) ;
#64285=VECTOR ( 'NONE', #44452, 1000.000000000000000 ) ;
#64286=CARTESIAN_POINT ( 'NONE',  ( 13.79529636645031943, 30.34541550158063927, -14.16423886937409904 ) ) ;
#64287=CARTESIAN_POINT ( 'NONE',  ( 10.00000000000000178, 34.31368534415484106, 10.88017736071110342 ) ) ;
#64288=CARTESIAN_POINT ( 'NONE',  ( -0.8801773607110991993, 47.85535201082150536, -2.915334737309923874 ) ) ;
#64289=PLANE ( 'NONE',  #89480 ) ;
#64291=CARTESIAN_POINT ( 'NONE',  ( 19.84674366389459266, 3.717264484334118713, -2.638427012816827677 ) ) ;
#64293=CARTESIAN_POINT ( 'NONE',  ( 12.63842701281683034, 22.46726448433411605, 9.846743663894596210 ) ) ;
#64295=DIRECTION ( 'NONE',  ( 0.000000000000000000, 1.000000000000000000, -0.000000000000000000 ) ) ;
#64296=CARTESIAN_POINT ( 'NONE',  ( 5.076628168052704559, 25.17559781766745175, -8.527530157486179263 ) ) ;
#64297=CARTESIAN_POINT ( 'NONE',  ( 10.00000000000000000, 49.75893115100078745, -9.846743663894594434 ) ) ;
#64298=CARTESIAN_POINT ( 'NONE',  ( 2.035157376598822676, 27.43868534415483396, -7.964842623401177768 ) ) ;
#64301=CARTESIAN_POINT ( 'NONE',  ( 13.43411237798106583, 47.66530133659709634, -12.81628187352647252 ) ) ;
#64302=CARTESIAN_POINT ( 'NONE',  ( 2.035157376598822676, 67.43868534415484817, -7.964842623401177768 ) ) ;
#64303=CARTESIAN_POINT ( 'NONE',  ( 2.791683348922240793, 31.63393115100078745, 7.208316651077764092 ) ) ;
#64304=CARTESIAN_POINT ( 'NONE',  ( 17.08211943468705840, 45.13708216824730357, -12.26659068614894466 ) ) ;
#64305=CARTESIAN_POINT ( 'NONE',  ( 10.00000000000000178, 17.25893115100078745, 9.846743663894594434 ) ) ;
#64306=CARTESIAN_POINT ( 'NONE',  ( 0.1143410931637246358, 60.21691075486303646, 6.480892540919863443 ) ) ;
#64307=CARTESIAN_POINT ( 'NONE',  ( 5.076628168052704559, 60.17559781766745175, -8.527530157486179263 ) ) ;
#64308=CARTESIAN_POINT ( 'NONE',  ( -0.3689425029237881626, 12.42874883491396609, 10.36894250292379027 ) ) ;
#64309=CARTESIAN_POINT ( 'NONE',  ( 10.00000000000000178, 28.05374883491396787, 14.16423886937410082 ) ) ;
#64310=CARTESIAN_POINT ( 'NONE',  ( 10.00000000000000178, 27.25893115100078390, 9.846743663894594434 ) ) ;
#64312=CARTESIAN_POINT ( 'NONE',  ( 7.084665262690076126, 19.10535201082150181, 10.88017736071109987 ) ) ;
#64313=CARTESIAN_POINT ( 'NONE',  ( 20.88017736071110164, 60.35535201082151957, 2.915334737309930979 ) ) ;
#64314=CARTESIAN_POINT ( 'NONE',  ( 7.084665262690076126, 47.02201867748818387, -10.88017736071110164 ) ) ;
#64315=ORIENTED_EDGE ( 'NONE', *, *, #6442, .F. ) ;
#64316=CARTESIAN_POINT ( 'NONE',  ( 0.6178305044545838731, 39.74863466993041072, 9.382169495545420901 ) ) ;
#64317=CARTESIAN_POINT ( 'NONE',  ( 19.42250999205614193, 55.14701867748817676, 5.440088680355555262 ) ) ;
#64323=CARTESIAN_POINT ( 'NONE',  ( 15.44008868035555793, 66.39701867748817676, -9.422509992056140149 ) ) ;
#64324=CARTESIAN_POINT ( 'NONE',  ( 20.88017736071110519, 5.563685344154837509, 2.639326808657452039E-16 ) ) ;
#64327=CARTESIAN_POINT ( 'NONE',  ( 0.5774900079438590739, 12.64701867748817321, -5.440088680355550821 ) ) ;
#64328=CARTESIAN_POINT ( 'NONE',  ( 12.63842701281683922, 14.55059781766744997, -9.846743663894590881 ) ) ;
#64329=CARTESIAN_POINT ( 'NONE',  ( 6.204703633549690345, 2.845415501580634388, 14.16423886937410082 ) ) ;
#64330=AXIS2_PLACEMENT_3D ( 'NONE', #60686, #74709, #21725 ) ;
#64331=CARTESIAN_POINT ( 'NONE',  ( 18.52753015748618282, 3.925597817667451306, -4.923371831947291888 ) ) ;
#64333=CARTESIAN_POINT ( 'NONE',  ( 15.44008868035555793, 11.39701867748817143, -9.422509992056140149 ) ) ;
#64334=CARTESIAN_POINT ( 'NONE',  ( 0.1532563361054082862, 51.21726448433412315, 2.638427012816831674 ) ) ;
#64336=CARTESIAN_POINT ( 'NONE',  ( 10.00000000000000000, 44.75893115100078745, -9.846743663894594434 ) ) ;
#64338=CARTESIAN_POINT ( 'NONE',  ( 18.72515096720568195, 31.07228050351032422, -6.500000000000018652 ) ) ;
#64339=CARTESIAN_POINT ( 'NONE',  ( 2.035157376598824452, 53.68868534415484817, 7.964842623401179544 ) ) ;
#64340=CARTESIAN_POINT ( 'NONE',  ( 0.1532563361054100626, 50.80059781766745175, -2.638427012816831230 ) ) ;
#64341=CARTESIAN_POINT ( 'NONE',  ( -1.099225684535947600, 29.54030133659708923, 6.408140936763237150 ) ) ;
#64342=PRESENTATION_STYLE_ASSIGNMENT (( #1424 ) ) ;
#64344=CARTESIAN_POINT ( 'NONE',  ( 7.084665262690076126, 57.02201867748817676, -10.88017736071110164 ) ) ;
#64345=CARTESIAN_POINT ( 'NONE',  ( -4.164238869374099927, 67.01208216824728936, 3.795296366450308767 ) ) ;
#64346=B_SPLINE_CURVE_WITH_KNOTS ( 'NONE', 3,
 ( #49722, #75692, #7708, #76188 ),
 .UNSPECIFIED., .F., .F.,
 ( 4, 4 ),
 ( 6.505213034913026604E-19, 0.001036303429213372230 ),
 .UNSPECIFIED. ) ;
#64347=EDGE_CURVE ( 'NONE', #81215, #91503, #77390, .T. ) ;
#64348=CARTESIAN_POINT ( 'NONE',  ( 21.09922568453594849, 36.20696800326375353, 6.408140936763242479 ) ) ;
#64349=CARTESIAN_POINT ( 'NONE',  ( 7.084665262690076126, 34.10535201082151247, 10.88017736071109987 ) ) ;
#64350=FACE_OUTER_BOUND ( 'NONE', #77033, .T. ) ;
#64351=ORIENTED_EDGE ( 'NONE', *, *, #57701, .T. ) ;
#64352=CARTESIAN_POINT ( 'NONE',  ( 6.565887622018943937, 45.16530133659708923, 12.81628187352647430 ) ) ;
#64353=CARTESIAN_POINT ( 'NONE',  ( 20.88017736071110519, 30.56368534415484106, 2.639326808657452039E-16 ) ) ;
#64355=ORIENTED_EDGE ( 'NONE', *, *, #21603, .T. ) ;
#64356=CARTESIAN_POINT ( 'NONE',  ( 17.20831665107776587, 7.883931151000784787, 7.208316651077764980 ) ) ;
#64357=CARTESIAN_POINT ( 'NONE',  ( 19.84674366389459266, 58.30059781766745886, 2.638427012816836559 ) ) ;
#64358=CARTESIAN_POINT ( 'NONE',  ( 19.84674366389459266, 18.30059781766745175, 2.638427012816836559 ) ) ;
#64359=CARTESIAN_POINT ( 'NONE',  ( 18.52753015748618282, 53.92559781766745175, -4.923371831947291888 ) ) ;
#64361=FILL_AREA_STYLE ('',( #94377 ) ) ;
#64365=CARTESIAN_POINT ( 'NONE',  ( 0.1532563361054082862, 31.21726448433412315, 2.638427012816831674 ) ) ;
#64368=CARTESIAN_POINT ( 'NONE',  ( 14.92337183194729633, 57.67559781766745886, 8.527530157486181039 ) ) ;
#64372=CARTESIAN_POINT ( 'NONE',  ( 21.09922568453594849, 26.20696800326375353, 6.408140936763242479 ) ) ;
#64373=CARTESIAN_POINT ( 'NONE',  ( 14.92337183194729988, 44.34226448433412315, -8.527530157486177487 ) ) ;
#64375=CARTESIAN_POINT ( 'NONE',  ( -4.164238869374099927, 57.01208216824731068, 3.795296366450308767 ) ) ;
#64376=CARTESIAN_POINT ( 'NONE',  ( 18.52753015748617571, 18.09226448433411960, 4.923371831947298993 ) ) ;
#64377=CARTESIAN_POINT ( 'NONE',  ( 19.65571488900285502, 85.77913566376845722, 5.360955758210749877 ) ) ;
#64378=CARTESIAN_POINT ( 'NONE',  ( -0.3689425029237881626, 52.42874883491396076, 10.36894250292379027 ) ) ;
#64379=CARTESIAN_POINT ( 'NONE',  ( 12.63842701281683034, 57.46726448433411605, 9.846743663894596210 ) ) ;
#64380=CARTESIAN_POINT ( 'NONE',  ( -2.266590686148945544, 66.38708216824730357, -7.082119434687050408 ) ) ;
#64381=CARTESIAN_POINT ( 'NONE',  ( -0.3689425029237881626, 32.42874883491395366, 10.36894250292379027 ) ) ;
#64382=CARTESIAN_POINT ( 'NONE',  ( -2.266590686148945544, 42.22041550158063217, 7.082119434687048631 ) ) ;
#64385=CARTESIAN_POINT ( 'NONE',  ( 5.076628168052704559, 50.17559781766745886, -8.527530157486179263 ) ) ;
#64386=CARTESIAN_POINT ( 'NONE',  ( 0.5774900079438590739, 32.64701867748816966, -5.440088680355550821 ) ) ;
#64389=CARTESIAN_POINT ( 'NONE',  ( 19.84674366389459266, 53.30059781766744464, 2.638427012816836559 ) ) ;
#64392=CARTESIAN_POINT ( 'NONE',  ( 14.92337183194729988, 54.34226448433412315, -8.527530157486177487 ) ) ;
#64393=CARTESIAN_POINT ( 'NONE',  ( 18.52753015748617571, 63.09226448433412315, 4.923371831947298993 ) ) ;
#64396=CARTESIAN_POINT ( 'NONE',  ( 2.917880565312950480, 30.97041550158063572, -12.26659068614894821 ) ) ;
#64400=CARTESIAN_POINT ( 'NONE',  ( -0.8801773607111008646, 23.27201867748817676, 2.915334737309923430 ) ) ;
#64402=CARTESIAN_POINT ( 'NONE',  ( 0.6178305044545818747, 18.49863466993041428, -9.382169495545419124 ) ) ;
#64404=CARTESIAN_POINT ( 'NONE',  ( 2.791683348922237240, 10.38393115100078390, -7.208316651077763204 ) ) ;
#64407=EDGE_CURVE ( 'NONE', #84535, #21097, #62130, .T. ) ;
#64408=CARTESIAN_POINT ( 'NONE',  ( 20.36894250292379382, 28.67874883491396787, 10.36894250292379205 ) ) ;
#64409=CARTESIAN_POINT ( 'NONE',  ( 20.15039907845753930, 0.07447313448805115144, -6.262539305110068177 ) ) ;
#64410=FILL_AREA_STYLE ('',( #43391 ) ) ;
#64411=CARTESIAN_POINT ( 'NONE',  ( -0.8801773607111009756, 8.063685344154837509, 1.068504757029289695E-15 ) ) ;
#64413=CARTESIAN_POINT ( 'NONE',  ( 10.00000000000000000, 41.81368534415484106, -10.88017736071110342 ) ) ;
#64414=CARTESIAN_POINT ( 'NONE',  ( 10.00000000000000178, 34.31368534415484106, 10.88017736071110342 ) ) ;
#64415=CARTESIAN_POINT ( 'NONE',  ( 3.591859063236761518, -0.04303199673624671928, 11.09922568453594849 ) ) ;
#64416=CARTESIAN_POINT ( 'NONE',  ( 1.472469842513823179, 65.59226448433412315, -4.923371831947296329 ) ) ;
#64417=CARTESIAN_POINT ( 'NONE',  ( 10.00000000000000000, 4.758931151000784787, -9.846743663894594434 ) ) ;
#64420=CARTESIAN_POINT ( 'NONE',  ( 15.44008868035555260, 44.73035201082151247, 9.422509992056143702 ) ) ;
#64422=CARTESIAN_POINT ( 'NONE',  ( 22.81628187352647785, 11.62363466993042138, 6.195893100308588602E-16 ) ) ;
#64423=CARTESIAN_POINT ( 'NONE',  ( 7.084665262690076126, 57.02201867748817676, -10.88017736071110164 ) ) ;
#64424=CARTESIAN_POINT ( 'NONE',  ( 1.472469842513823179, 25.59226448433412315, -4.923371831947296329 ) ) ;
#64425=CARTESIAN_POINT ( 'NONE',  ( -2.816281873526473856, 39.12363466993041783, 9.499525473075851096E-16 ) ) ;
#64426=CARTESIAN_POINT ( 'NONE',  ( 2.791683348922237240, 5.383931151000785675, -7.208316651077763204 ) ) ;
#64431=CARTESIAN_POINT ( 'NONE',  ( -0.8801773607110991993, 7.855352010821504471, -2.915334737309923874 ) ) ;
#64432=CARTESIAN_POINT ( 'NONE',  ( 21.09922568453595559, 62.04030133659709634, -6.408140936763230044 ) ) ;
#64433=CARTESIAN_POINT ( 'NONE',  ( 1.472469842513823179, 20.59226448433411960, -4.923371831947296329 ) ) ;
#64434=CARTESIAN_POINT ( 'NONE',  ( -0.8801773607110991993, 2.855352010821504471, -2.915334737309923874 ) ) ;
#64435=CARTESIAN_POINT ( 'NONE',  ( 10.00000000000000178, 9.313685344154839285, 10.88017736071110342 ) ) ;
#64436=VERTEX_POINT ( 'NONE', #60407 ) ;
#64437=CARTESIAN_POINT ( 'NONE',  ( -0.8801773607111008646, 8.272018677488171434, 2.915334737309923430 ) ) ;
#64438=ADVANCED_FACE ( 'NONE', ( #14436 ), #63378, .T. ) ;
#64439=CARTESIAN_POINT ( 'NONE',  ( 17.96484262340118221, 16.18868534415483396, -7.964842623401177768 ) ) ;
#64440=FACE_OUTER_BOUND ( 'NONE', #31902, .T. ) ;
#64442=CARTESIAN_POINT ( 'NONE',  ( 14.92337183194729988, 64.34226448433412315, -8.527530157486177487 ) ) ;
#64443=CARTESIAN_POINT ( 'NONE',  ( 0.5774900079438590739, 22.64701867748817321, -5.440088680355550821 ) ) ;
#64444=CARTESIAN_POINT ( 'NONE',  ( 0.1532563361054082862, 61.21726448433412315, 2.638427012816831674 ) ) ;
#64445=DIRECTION ( 'NONE',  ( 0.000000000000000000, -1.000000000000000000, 0.000000000000000000 ) ) ;
#64446=CARTESIAN_POINT ( 'NONE',  ( 16.40814093676323893, 50.79030133659708923, 11.09922568453595026 ) ) ;
#64447=CARTESIAN_POINT ( 'NONE',  ( -0.1503990784575323369, 4.248846992468888750, -6.262539305110070842 ) ) ;
#64448=CARTESIAN_POINT ( 'NONE',  ( 20.36894250292379382, 28.67874883491396787, 10.36894250292379205 ) ) ;
#64449=CARTESIAN_POINT ( 'NONE',  ( 17.96484262340118221, 44.93868534415483396, 7.964842623401181321 ) ) ;
#64450=CARTESIAN_POINT ( 'NONE',  ( 20.88017736071110519, 20.56368534415484106, 2.639326808657452039E-16 ) ) ;
#64451=EDGE_CURVE ( 'NONE', #36584, #49358, #72182, .T. ) ;
#64452=CARTESIAN_POINT ( 'NONE',  ( 12.63842701281683922, 59.55059781766744464, -9.846743663894590881 ) ) ;
#64454=CARTESIAN_POINT ( 'NONE',  ( 2.791683348922240793, 51.63393115100078745, 7.208316651077764092 ) ) ;
#64455=CARTESIAN_POINT ( 'NONE',  ( 7.361572987183170547, 2.050597817667451750, 9.846743663894590881 ) ) ;
#64459=CARTESIAN_POINT ( 'NONE',  ( 0.5774900079438607392, 18.48035201082150536, 5.440088680355550821 ) ) ;
#64460=CARTESIAN_POINT ( 'NONE',  ( 19.84674366389459266, 13.71726448433411782, -2.638427012816827677 ) ) ;
#64462=CARTESIAN_POINT ( 'NONE',  ( 6.565887622018943937, -1.918031996736246692, -12.81628187352647608 ) ) ;
#64463=CARTESIAN_POINT ( 'NONE',  ( 17.96484262340118221, 51.18868534415483396, -7.964842623401177768 ) ) ;
#64464=CARTESIAN_POINT ( 'NONE',  ( 17.96484262340118221, 26.18868534415483396, -7.964842623401177768 ) ) ;
#64465=CARTESIAN_POINT ( 'NONE',  ( 21.09922568453594849, 46.20696800326376064, 6.408140936763242479 ) ) ;
#64466=CARTESIAN_POINT ( 'NONE',  ( 10.00000000000000178, 38.05374883491396787, 14.16423886937410082 ) ) ;
#64468=VECTOR ( 'NONE', #63208, 1000.000000000000000 ) ;
#64469=CARTESIAN_POINT ( 'NONE',  ( 13.43411237798105340, 55.58196800326374643, 12.81628187352647963 ) ) ;
#64471=CARTESIAN_POINT ( 'NONE',  ( 19.84674366389459266, 53.30059781766744464, 2.638427012816836559 ) ) ;
#64472=CARTESIAN_POINT ( 'NONE',  ( 19.42250999205614193, 35.14701867748816966, 5.440088680355555262 ) ) ;
#64473=EDGE_CURVE ( 'NONE', #65586, #27193, #17777, .T. ) ;
#64475=CARTESIAN_POINT ( 'NONE',  ( 1.472469842513823179, 6.425597817667451750, 4.923371831947296329 ) ) ;
#64477=CARTESIAN_POINT ( 'NONE',  ( 2.791683348922240793, 26.63393115100078745, 7.208316651077764092 ) ) ;
#64478=CARTESIAN_POINT ( 'NONE',  ( 1.472469842513823179, 5.592264484334118713, -4.923371831947296329 ) ) ;
#64479=CARTESIAN_POINT ( 'NONE',  ( 14.92337183194729988, 4.342264484334117824, -8.527530157486177487 ) ) ;
#64480=CARTESIAN_POINT ( 'NONE',  ( 0.5774900079438607392, 63.48035201082149825, 5.440088680355550821 ) ) ;
#64482=CARTESIAN_POINT ( 'NONE',  ( 19.42250999205614193, 60.14701867748817676, 5.440088680355555262 ) ) ;
#64483=CARTESIAN_POINT ( 'NONE',  ( 5.076628168052704559, 20.17559781766745175, -8.527530157486179263 ) ) ;
#64484=EDGE_LOOP ( 'NONE', ( #77749, #2663, #55762, #55751 ) ) ;
#64486=CARTESIAN_POINT ( 'NONE',  ( 7.361572987183169658, 54.96726448433413026, -9.846743663894592657 ) ) ;
#64487=ORIENTED_EDGE ( 'NONE', *, *, #4236, .F. ) ;
#64489=CYLINDRICAL_SURFACE ( 'NONE', #95326, 0.5000000000000004441 ) ;
#64490=CARTESIAN_POINT ( 'NONE',  ( -2.266590686148945544, 1.387082168247301128, -7.082119434687050408 ) ) ;
#64491=UNCERTAINTY_MEASURE_WITH_UNIT (LENGTH_MEASURE( 1.000000000000000082E-05 ), #85888, 'distance_accuracy_value', 'NONE');
#64493=CARTESIAN_POINT ( 'NONE',  ( -0.3689425029237898834, 11.17874883491396787, -10.36894250292378850 ) ) ;
#64494=CARTESIAN_POINT ( 'NONE',  ( -4.164238869374099927, 32.01208216824730357, 3.795296366450308767 ) ) ;
#64495=CARTESIAN_POINT ( 'NONE',  ( 10.00000000000000178, 3.053748834913967425, 14.16423886937410082 ) ) ;
#64496=CARTESIAN_POINT ( 'NONE',  ( 10.00000000000000000, 0.5537488349139675359, -14.16423886937410082 ) ) ;
#64497=CARTESIAN_POINT ( 'NONE',  ( 19.42250999205614193, 35.14701867748816966, 5.440088680355555262 ) ) ;
#64498=( LENGTH_UNIT ( ) NAMED_UNIT ( * ) SI_UNIT ( .MILLI., .METRE. ) );
#64500=CARTESIAN_POINT ( 'NONE',  ( 18.52753015748618282, 13.92559781766745175, -4.923371831947291888 ) ) ;
#64501=CARTESIAN_POINT ( 'NONE',  ( 20.88017736071110519, 50.56368534415484106, 2.639326808657452039E-16 ) ) ;
#64502=CARTESIAN_POINT ( 'NONE',  ( 10.00000000000000000, 19.75893115100078390, -9.846743663894594434 ) ) ;
#64503=CARTESIAN_POINT ( 'NONE',  ( 16.40814093676324603, 47.45696800326375353, -11.09922568453594671 ) ) ;
#64504=CARTESIAN_POINT ( 'NONE',  ( 2.791683348922237240, 40.38393115100078035, -7.208316651077763204 ) ) ;
#64506=ADVANCED_FACE ( 'NONE', ( #72712 ), #26734, .F. ) ;
#64507=CARTESIAN_POINT ( 'NONE',  ( 15.44008868035555793, 61.39701867748817676, -9.422509992056140149 ) ) ;
#64508=CARTESIAN_POINT ( 'NONE',  ( 21.09922568453594849, 31.20696800326375353, 6.408140936763242479 ) ) ;
#64510=CARTESIAN_POINT ( 'NONE',  ( 19.84674366389459266, 28.71726448433411960, -2.638427012816827677 ) ) ;
#64511=CARTESIAN_POINT ( 'NONE',  ( 17.08211943468705840, 15.13708216824730179, -12.26659068614894466 ) ) ;
#64513=CARTESIAN_POINT ( 'NONE',  ( 17.96484262340118221, 41.18868534415484106, -7.964842623401177768 ) ) ;
#64514=CARTESIAN_POINT ( 'NONE',  ( 19.42250999205614193, 50.14701867748817676, 5.440088680355555262 ) ) ;
#64515=CARTESIAN_POINT ( 'NONE',  ( 10.00000000000000178, 43.05374883491397497, 14.16423886937410082 ) ) ;
#64516=CARTESIAN_POINT ( 'NONE',  ( 18.52753015748617571, 53.09226448433412315, 4.923371831947298993 ) ) ;
#64517=CARTESIAN_POINT ( 'NONE',  ( 14.92337183194729633, 7.675597817667451750, 8.527530157486181039 ) ) ;
#64520=CARTESIAN_POINT ( 'NONE',  ( 15.44008868035555793, 46.39701867748817676, -9.422509992056140149 ) ) ;
#64521=CARTESIAN_POINT ( 'NONE',  ( 0.5600000000000083800, 105.0000000000000000, 5.000000000000000000 ) ) ;
#64522=CARTESIAN_POINT ( 'NONE',  ( 6.565887622018943937, 23.08196800326375708, -12.81628187352647608 ) ) ;
#64523=CARTESIAN_POINT ( 'NONE',  ( 16.40814093676324603, 22.45696800326375353, -11.09922568453594671 ) ) ;
#64524=CARTESIAN_POINT ( 'NONE',  ( 18.52753015748617571, 53.09226448433412315, 4.923371831947298993 ) ) ;
#64526=CARTESIAN_POINT ( 'NONE',  ( 0.5774900079438590739, 67.64701867748817676, -5.440088680355550821 ) ) ;
#64527=CARTESIAN_POINT ( 'NONE',  ( 19.72487221294570858, 21.86607318730131411, 6.500000000000000888 ) ) ;
#64529=CARTESIAN_POINT ( 'NONE',  ( 0.5774900079438590739, 62.64701867748817676, -5.440088680355550821 ) ) ;
#64530=CARTESIAN_POINT ( 'NONE',  ( 10.00000000000000000, -0.2410688489992152128, -9.846743663894594434 ) ) ;
#64533=CARTESIAN_POINT ( 'NONE',  ( 12.63842701281683034, 37.46726448433411605, 9.846743663894596210 ) ) ;
#64534=CARTESIAN_POINT ( 'NONE',  ( 10.00000000000000178, 24.31368534415484106, 10.88017736071110342 ) ) ;
#64535=CARTESIAN_POINT ( 'NONE',  ( -1.099225684535947600, -0.4596986634029132657, 6.408140936763237150 ) ) ;
#64536=CARTESIAN_POINT ( 'NONE',  ( 10.00000000000000000, 31.81368534415483751, -10.88017736071110342 ) ) ;
#64539=CARTESIAN_POINT ( 'NONE',  ( 3.591859063236761518, 44.95696800326376064, 11.09922568453594849 ) ) ;
#64541=CARTESIAN_POINT ( 'NONE',  ( 2.035157376598822676, 52.43868534415483396, -7.964842623401177768 ) ) ;
#64543=CARTESIAN_POINT ( 'NONE',  ( 21.09922568453594849, 21.20696800326375353, 6.408140936763242479 ) ) ;
#64544=CARTESIAN_POINT ( 'NONE',  ( 7.084665262690076126, 24.10535201082150181, 10.88017736071109987 ) ) ;
#64545=CARTESIAN_POINT ( 'NONE',  ( -4.164238869374098151, 51.59541550158063217, -3.795296366450310543 ) ) ;
#64546=CARTESIAN_POINT ( 'NONE',  ( 7.361572987183169658, 39.96726448433411605, -9.846743663894592657 ) ) ;
#64547=CARTESIAN_POINT ( 'NONE',  ( 4.559911319644449179, 67.23035201082150536, -9.422509992056141925 ) ) ;
#64548=CARTESIAN_POINT ( 'NONE',  ( 10.00000000000000000, -0.2410688489992152128, -9.846743663894594434 ) ) ;
#64550=CARTESIAN_POINT ( 'NONE',  ( 13.79529636645030344, 33.26208216824730357, 14.16423886937410614 ) ) ;
#64554=EDGE_LOOP ( 'NONE', ( #93730, #75834, #24133, #15204, #4233, #41387 ) ) ;
#64555=ORIENTED_EDGE ( 'NONE', *, *, #47389, .T. ) ;
#64556=CARTESIAN_POINT ( 'NONE',  ( 20.36894250292379382, 53.67874883491397497, 10.36894250292379205 ) ) ;
#64557=CARTESIAN_POINT ( 'NONE',  ( -4.164238869374098151, 46.59541550158063927, -3.795296366450310543 ) ) ;
#64558=CARTESIAN_POINT ( 'NONE',  ( 0.1532563361054082862, 11.21726448433411605, 2.638427012816831674 ) ) ;
#64559=CARTESIAN_POINT ( 'NONE',  ( 3.591859063236761518, 14.95696800326375531, 11.09922568453594849 ) ) ;
#64562=CARTESIAN_POINT ( 'NONE',  ( 19.38216949554541202, 35.99863466993041072, 9.382169495545424454 ) ) ;
#64563=CARTESIAN_POINT ( 'NONE',  ( 13.79529636645030344, 48.26208216824728936, 14.16423886937410614 ) ) ;
#64567=SURFACE_STYLE_FILL_AREA ( #71119 ) ;
#64569=ORIENTED_EDGE ( 'NONE', *, *, #60822, .T. ) ;
#64570=CARTESIAN_POINT ( 'NONE',  ( 19.84674366389459621, 13.50893115100078568, 7.409399052514197653E-17 ) ) ;
#64573=CARTESIAN_POINT ( 'NONE',  ( 13.79529636645031943, 15.34541550158063750, -14.16423886937409904 ) ) ;
#64574=CARTESIAN_POINT ( 'NONE',  ( 20.88017736071110875, 10.77201867748817143, -2.915334737309920765 ) ) ;
#64575=CARTESIAN_POINT ( 'NONE',  ( 17.96484262340118221, 6.188685344154837509, -7.964842623401177768 ) ) ;
#64576=CARTESIAN_POINT ( 'NONE',  ( 19.84674366389459621, 53.50893115100078745, 7.409399052514197653E-17 ) ) ;
#64577=CARTESIAN_POINT ( 'NONE',  ( -2.816281873526473856, -0.8763653300695799508, 9.499525473075851096E-16 ) ) ;
#64581=CARTESIAN_POINT ( 'NONE',  ( 16.40814093676324603, 12.45696800326375353, -11.09922568453594671 ) ) ;
#64583=CARTESIAN_POINT ( 'NONE',  ( 10.00000000000000000, 60.55374883491397497, -14.16423886937410082 ) ) ;
#64586=CARTESIAN_POINT ( 'NONE',  ( -2.266590686148945544, 61.38708216824730357, -7.082119434687050408 ) ) ;
#64588=CARTESIAN_POINT ( 'NONE',  ( 10.00000000000000000, 36.81368534415484106, -10.88017736071110342 ) ) ;
#64589=CARTESIAN_POINT ( 'NONE',  ( 2.035157376598824452, 48.68868534415483396, 7.964842623401179544 ) ) ;
#64590=CARTESIAN_POINT ( 'NONE',  ( -0.8801773607111009756, 38.06368534415484106, 1.068504757029289695E-15 ) ) ;
#64592=CARTESIAN_POINT ( 'NONE',  ( 19.42250999205614548, 45.98035201082150536, -5.440088680355545492 ) ) ;
#64594=CARTESIAN_POINT ( 'NONE',  ( 7.361572987183169658, 14.96726448433411960, -9.846743663894592657 ) ) ;
#64597=CARTESIAN_POINT ( 'NONE',  ( 0.1532563361054083140, 51.00893115100078745, 1.131784320476157264E-15 ) ) ;
#64599=DIRECTION ( 'NONE',  ( 0.000000000000000000, -1.000000000000000000, 0.000000000000000000 ) ) ;
#64600=CARTESIAN_POINT ( 'NONE',  ( 16.40814093676324603, 52.45696800326375353, -11.09922568453594671 ) ) ;
#64604=CARTESIAN_POINT ( 'NONE',  ( -46.30928139467843607, 104.0823827281712255, 5.529860068218146019 ) ) ;
#64607=CARTESIAN_POINT ( 'NONE',  ( 13.79529636645031943, 65.34541550158063217, -14.16423886937409904 ) ) ;
#64611=CARTESIAN_POINT ( 'NONE',  ( 19.84674366389459266, 38.71726448433412315, -2.638427012816827677 ) ) ;
#64612=CARTESIAN_POINT ( 'NONE',  ( 22.81628187352647785, 61.41530133659709634, 3.434112377981063169 ) ) ;
#64613=CARTESIAN_POINT ( 'NONE',  ( 19.38216949554541202, 10.99863466993042138, 9.382169495545424454 ) ) ;
#64614=CARTESIAN_POINT ( 'NONE',  ( 17.96484262340118221, 64.93868534415483396, 7.964842623401181321 ) ) ;
#64615=CARTESIAN_POINT ( 'NONE',  ( 19.84674366389459266, 13.71726448433411782, -2.638427012816827677 ) ) ;
#64616=CARTESIAN_POINT ( 'NONE',  ( 17.20831665107776587, 59.13393115100078745, -7.208316651077762316 ) ) ;
#64617=DIRECTION ( 'NONE',  ( -0.000000000000000000, -0.000000000000000000, -1.000000000000000000 ) ) ;
#64618=STYLED_ITEM ( 'NONE', ( #21384 ), #6645 ) ;
#64620=CARTESIAN_POINT ( 'NONE',  ( -0.8801773607111009756, 3.063685344154838397, 1.068504757029289695E-15 ) ) ;
#64622=CARTESIAN_POINT ( 'NONE',  ( 2.035157376598822676, 37.43868534415484106, -7.964842623401177768 ) ) ;
#64623=CARTESIAN_POINT ( 'NONE',  ( -2.816281873526473856, 29.33196800326376064, 3.434112377981055619 ) ) ;
#64624=CARTESIAN_POINT ( 'NONE',  ( 7.084665262690076126, 67.02201867748817676, -10.88017736071110164 ) ) ;
#64628=CARTESIAN_POINT ( 'NONE',  ( 19.84674366389459266, 53.71726448433411605, -2.638427012816827677 ) ) ;
#64629=CARTESIAN_POINT ( 'NONE',  ( 0.1532563361054100626, 20.80059781766744464, -2.638427012816831230 ) ) ;
#64631=CARTESIAN_POINT ( 'NONE',  ( 13.43411237798105340, 20.58196800326374643, 12.81628187352647963 ) ) ;
#64632=DIRECTION ( 'NONE',  ( 1.000000000000000000, 0.000000000000000000, 0.000000000000000000 ) ) ;
#64633=CARTESIAN_POINT ( 'NONE',  ( 19.42250999205614548, 30.98035201082150536, -5.440088680355545492 ) ) ;
#64636=AXIS2_PLACEMENT_3D ( 'NONE', #56612, #65070, #12581 ) ;
#64638=CARTESIAN_POINT ( 'NONE',  ( 17.08211943468705840, 50.13708216824730357, -12.26659068614894466 ) ) ;
#64639=CARTESIAN_POINT ( 'NONE',  ( 10.00000000000000000, 35.55374883491396787, -14.16423886937410082 ) ) ;
#64640=CARTESIAN_POINT ( 'NONE',  ( 10.00000000000000000, 39.75893115100078745, -9.846743663894594434 ) ) ;
#64641=CARTESIAN_POINT ( 'NONE',  ( -2.816281873526471635, 33.91530133659708213, -3.434112377981056508 ) ) ;
#64642=CARTESIAN_POINT ( 'NONE',  ( 0.5774900079438590739, 22.64701867748817321, -5.440088680355550821 ) ) ;
#64643=CARTESIAN_POINT ( 'NONE',  ( 19.84674366389459266, 53.30059781766744464, 2.638427012816836559 ) ) ;
#64644=CARTESIAN_POINT ( 'NONE',  ( 15.44008868035555793, 36.39701867748816966, -9.422509992056140149 ) ) ;
#64645=CARTESIAN_POINT ( 'NONE',  ( -1.099225684535947600, 4.540301336597087456, 6.408140936763237150 ) ) ;
#64646=CARTESIAN_POINT ( 'NONE',  ( -0.3689425029237898834, 16.17874883491396076, -10.36894250292378850 ) ) ;
#64648=CARTESIAN_POINT ( 'NONE',  ( 2.791683348922237240, 30.38393115100078390, -7.208316651077763204 ) ) ;
#64649=CARTESIAN_POINT ( 'NONE',  ( 10.00000000000000000, 1.813685344154837731, -10.88017736071110342 ) ) ;
#64650=CARTESIAN_POINT ( 'NONE',  ( 0.6178305044545838731, 4.748634669930420493, 9.382169495545420901 ) ) ;
#64651=EDGE_LOOP ( 'NONE', ( #40274, #61775, #55666, #83309 ) ) ;
#64652=CARTESIAN_POINT ( 'NONE',  ( 0.2751277870542967463, 0.000000000000000000, 6.500000000000000888 ) ) ;
#64654=CARTESIAN_POINT ( 'NONE',  ( -0.3689425029237898834, 61.17874883491396076, -10.36894250292378850 ) ) ;
#64655=CARTESIAN_POINT ( 'NONE',  ( 13.79529636645031943, 5.345415501580634832, -14.16423886937409904 ) ) ;
#64656=CARTESIAN_POINT ( 'NONE',  ( 1.472469842513823179, 6.425597817667451750, 4.923371831947296329 ) ) ;
#64657=CARTESIAN_POINT ( 'NONE',  ( 0.1532563361054100626, 45.80059781766745886, -2.638427012816831230 ) ) ;
#64658=CARTESIAN_POINT ( 'NONE',  ( -0.8801773607111008646, 38.27201867748816255, 2.915334737309923430 ) ) ;
#64660=CARTESIAN_POINT ( 'NONE',  ( 2.791683348922237240, 65.38393115100078035, -7.208316651077763204 ) ) ;
#64666=ORIENTED_EDGE ( 'NONE', *, *, #92728, .F. ) ;
#64668=CARTESIAN_POINT ( 'NONE',  ( -4.164238869374099927, 2.012082168247300906, 3.795296366450308767 ) ) ;
#64669=CARTESIAN_POINT ( 'NONE',  ( 24.16423886937410614, 9.303748834913967869, 8.672049930838204340E-16 ) ) ;
#64671=CARTESIAN_POINT ( 'NONE',  ( 13.79529636645030344, 53.26208216824730357, 14.16423886937410614 ) ) ;
#64672=CARTESIAN_POINT ( 'NONE',  ( 2.791683348922240793, 56.63393115100078035, 7.208316651077764092 ) ) ;
#64673=CARTESIAN_POINT ( 'NONE',  ( 2.791683348922237240, 35.38393115100079456, -7.208316651077763204 ) ) ;
#64675=CARTESIAN_POINT ( 'NONE',  ( 19.42250999205614193, 35.14701867748816966, 5.440088680355555262 ) ) ;
#64676=CARTESIAN_POINT ( 'NONE',  ( 19.84674366389459266, 63.30059781766745886, 2.638427012816836559 ) ) ;
#64677=CARTESIAN_POINT ( 'NONE',  ( 6.204703633549690345, 7.845415501580634832, 14.16423886937410082 ) ) ;
#64678=CARTESIAN_POINT ( 'NONE',  ( 2.917880565312948704, 57.63708216824731068, 12.26659068614894643 ) ) ;
#64679=VECTOR ( 'NONE', #17306, 1000.000000000000000 ) ;
#64680=EDGE_CURVE ( 'NONE', #93630, #80446, #16814, .T. ) ;
#64681=CARTESIAN_POINT ( 'NONE',  ( 4.559911319644449179, 2.230352010821504916, -9.422509992056141925 ) ) ;
#64683=CARTESIAN_POINT ( 'NONE',  ( 4.559911319644449179, 67.23035201082150536, -9.422509992056141925 ) ) ;
#64684=CARTESIAN_POINT ( 'NONE',  ( 12.63842701281683922, 34.55059781766745886, -9.846743663894590881 ) ) ;
#64688=ORIENTED_EDGE ( 'NONE', *, *, #46498, .T. ) ;
#64689=CARTESIAN_POINT ( 'NONE',  ( 17.20831665107776587, 17.88393115100078745, 7.208316651077764980 ) ) ;
#64691=CARTESIAN_POINT ( 'NONE',  ( -0.3689425029237898834, 36.17874883491396787, -10.36894250292378850 ) ) ;
#64692=CARTESIAN_POINT ( 'NONE',  ( 17.20831665107776587, 37.88393115100078745, 7.208316651077764980 ) ) ;
#64693=CARTESIAN_POINT ( 'NONE',  ( 12.91533473730992121, 54.52201867748816255, 10.88017736071110164 ) ) ;
#64694=CARTESIAN_POINT ( 'NONE',  ( 15.44008868035555793, 51.39701867748816966, -9.422509992056140149 ) ) ;
#64695=CARTESIAN_POINT ( 'NONE',  ( 7.361572987183169658, 44.96726448433412315, -9.846743663894592657 ) ) ;
#64696=CARTESIAN_POINT ( 'NONE',  ( 22.81628187352647785, 61.62363466993041783, 6.195893100308588602E-16 ) ) ;
#64699=CARTESIAN_POINT ( 'NONE',  ( 0.5774900079438607392, 48.48035201082150536, 5.440088680355550821 ) ) ;
#64700=CARTESIAN_POINT ( 'NONE',  ( -4.164238869374099039, 26.80374883491397142, 8.674139862899312516E-16 ) ) ;
#64701=VERTEX_POINT ( 'NONE', #21719 ) ;
#64704=CARTESIAN_POINT ( 'NONE',  ( 0.6178305044545838731, 24.74863466993042493, 9.382169495545420901 ) ) ;
#64705=DIRECTION ( 'NONE',  ( 1.000000000000000000, 0.000000000000000000, 0.000000000000000000 ) ) ;
#64706=CARTESIAN_POINT ( 'NONE',  ( 12.63842701281683034, 17.46726448433411250, 9.846743663894596210 ) ) ;
#64707=CARTESIAN_POINT ( 'NONE',  ( 19.42250999205614193, 5.147018677488171434, 5.440088680355555262 ) ) ;
#64709=CARTESIAN_POINT ( 'NONE',  ( 19.84674366389459266, 33.71726448433410894, -2.638427012816827677 ) ) ;
#64712=CARTESIAN_POINT ( 'NONE',  ( 4.559911319644449179, 67.23035201082150536, -9.422509992056141925 ) ) ;
#64715=CARTESIAN_POINT ( 'NONE',  ( 20.88017736071110519, 65.56368534415483396, 2.639326808657452039E-16 ) ) ;
#64716=CARTESIAN_POINT ( 'NONE',  ( 19.05914839598885280, 29.96693863883976050, 6.499999999999962697 ) ) ;
#64718=CARTESIAN_POINT ( 'NONE',  ( 12.63842701281683922, 4.550597817667451750, -9.846743663894590881 ) ) ;
#64719=CARTESIAN_POINT ( 'NONE',  ( 3.591859063236763294, 28.29030133659708568, -11.09922568453595026 ) ) ;
#64721=CARTESIAN_POINT ( 'NONE',  ( 19.84674366389459266, 38.71726448433412315, -2.638427012816827677 ) ) ;
#64722=CARTESIAN_POINT ( 'NONE',  ( 3.591859063236761518, 64.95696800326376774, 11.09922568453594849 ) ) ;
#64723=CARTESIAN_POINT ( 'NONE',  ( -4.164238869374099039, 26.80374883491397142, 8.674139862899312516E-16 ) ) ;
#64724=CARTESIAN_POINT ( 'NONE',  ( 1.472469842513823179, 26.42559781766745175, 4.923371831947296329 ) ) ;
#64725=CARTESIAN_POINT ( 'NONE',  ( 22.81628187352648496, 26.83196800326374998, -3.434112377981050290 ) ) ;
#64727=DIRECTION ( 'NONE',  ( 0.000000000000000000, -1.000000000000000000, 0.000000000000000000 ) ) ;
#64728=CARTESIAN_POINT ( 'NONE',  ( -0.8801773607111008646, 58.27201867748816966, 2.915334737309923430 ) ) ;
#64729=CARTESIAN_POINT ( 'NONE',  ( 0.6178305044545838731, 4.748634669930420493, 9.382169495545420901 ) ) ;
#64731=CARTESIAN_POINT ( 'NONE',  ( 2.791683348922237240, 35.38393115100079456, -7.208316651077763204 ) ) ;
#64732=CARTESIAN_POINT ( 'NONE',  ( 0.5774900079438607392, 23.48035201082150536, 5.440088680355550821 ) ) ;
#64733=CARTESIAN_POINT ( 'NONE',  ( 22.81628187352647785, 26.41530133659708923, 3.434112377981063169 ) ) ;
#64735=CARTESIAN_POINT ( 'NONE',  ( 10.00000000000000178, 22.25893115100078745, 9.846743663894594434 ) ) ;
#64739=CARTESIAN_POINT ( 'NONE',  ( 20.88017736071110519, 35.56368534415484106, 2.639326808657452039E-16 ) ) ;
#64742=CARTESIAN_POINT ( 'NONE',  ( 15.44008868035555260, 59.73035201082151247, 9.422509992056143702 ) ) ;
#64743=( NAMED_UNIT ( * ) PLANE_ANGLE_UNIT ( ) SI_UNIT ( $, .RADIAN. ) );
#64744=CARTESIAN_POINT ( 'NONE',  ( 14.92337183194729988, 44.34226448433412315, -8.527530157486177487 ) ) ;
#64745=CARTESIAN_POINT ( 'NONE',  ( 7.084665262690076126, 29.10535201082150181, 10.88017736071109987 ) ) ;
#64746=DIRECTION ( 'NONE',  ( 0.000000000000000000, 0.000000000000000000, 1.000000000000000000 ) ) ;
#64747=CARTESIAN_POINT ( 'NONE',  ( 10.00000000000000178, 49.31368534415484106, 10.88017736071110342 ) ) ;
#64748=CARTESIAN_POINT ( 'NONE',  ( 19.42250999205614193, 10.14701867748816966, 5.440088680355555262 ) ) ;
#64749=CARTESIAN_POINT ( 'NONE',  ( 20.00000000000000711, 84.99347556686142013, -4.825407044038334980 ) ) ;
#64750=LINE ( 'NONE', #95262, #51520 ) ;
#64752=CARTESIAN_POINT ( 'NONE',  ( 18.52753015748618282, 53.92559781766745175, -4.923371831947291888 ) ) ;
#64753=CARTESIAN_POINT ( 'NONE',  ( -2.266590686148945544, 57.22041550158063217, 7.082119434687048631 ) ) ;
#64758=CARTESIAN_POINT ( 'NONE',  ( -2.266590686148945544, 36.38708216824730357, -7.082119434687050408 ) ) ;
#64762=CARTESIAN_POINT ( 'NONE',  ( 2.917880565312950480, 60.97041550158063927, -12.26659068614894821 ) ) ;
#64763=CARTESIAN_POINT ( 'NONE',  ( 19.84674366389459266, 33.30059781766744464, 2.638427012816836559 ) ) ;
#64766=CARTESIAN_POINT ( 'NONE',  ( 15.44008868035555260, 64.73035201082151957, 9.422509992056143702 ) ) ;
#64767=CARTESIAN_POINT ( 'NONE',  ( 6.565887622018943937, 65.16530133659709634, 12.81628187352647430 ) ) ;
#64768=CARTESIAN_POINT ( 'NONE',  ( 19.42250999205614548, 30.98035201082150536, -5.440088680355545492 ) ) ;
#64769=CARTESIAN_POINT ( 'NONE',  ( 0.6178305044545818747, 63.49863466993043204, -9.382169495545419124 ) ) ;
#64770=CARTESIAN_POINT ( 'NONE',  ( 6.565887622018943937, 13.08196800326374998, -12.81628187352647608 ) ) ;
#64771=CARTESIAN_POINT ( 'NONE',  ( 10.00000000000000178, 17.25893115100078745, 9.846743663894594434 ) ) ;
#64773=CARTESIAN_POINT ( 'NONE',  ( 20.36894250292379738, 64.92874883491397497, -10.36894250292379027 ) ) ;
#64774=CARTESIAN_POINT ( 'NONE',  ( 2.917880565312948704, 32.63708216824730357, 12.26659068614894643 ) ) ;
#64775=CARTESIAN_POINT ( 'NONE',  ( 2.035157376598822676, 27.43868534415483396, -7.964842623401177768 ) ) ;
#64776=CARTESIAN_POINT ( 'NONE',  ( 2.035157376598824452, 53.68868534415484817, 7.964842623401179544 ) ) ;
#64777=LINE ( 'NONE', #65773, #15978 ) ;
#64779=CARTESIAN_POINT ( 'NONE',  ( 5.076628168052703671, 6.842264484334118713, 8.527530157486179263 ) ) ;
#64780=( LENGTH_UNIT ( ) NAMED_UNIT ( * ) SI_UNIT ( .MILLI., .METRE. ) );
#64781=CARTESIAN_POINT ( 'NONE',  ( -46.61696533502858841, 101.4435428601134959, 8.298995519389800180 ) ) ;
#64782=CARTESIAN_POINT ( 'NONE',  ( 14.92337183194729633, 27.67559781766745530, 8.527530157486181039 ) ) ;
#64783=CARTESIAN_POINT ( 'NONE',  ( 1.472469842513823179, 51.42559781766745886, 4.923371831947296329 ) ) ;
#64786=CARTESIAN_POINT ( 'NONE',  ( 22.81628187352647785, 46.62363466993041783, 6.195893100308588602E-16 ) ) ;
#64788=CARTESIAN_POINT ( 'NONE',  ( 7.084665262690076126, 64.10535201082150536, 10.88017736071109987 ) ) ;
#64789=CARTESIAN_POINT ( 'NONE',  ( 7.361572987183170547, 32.05059781766745175, 9.846743663894590881 ) ) ;
#64790=CARTESIAN_POINT ( 'NONE',  ( 13.79529636645030344, 58.26208216824728936, 14.16423886937410614 ) ) ;
#64791=CARTESIAN_POINT ( 'NONE',  ( 0.1532563361054100626, 25.80059781766744820, -2.638427012816831230 ) ) ;
#64793=CARTESIAN_POINT ( 'NONE',  ( 10.00000000000000000, 64.75893115100078035, -9.846743663894594434 ) ) ;
#64794=CARTESIAN_POINT ( 'NONE',  ( -2.266590686148945544, 6.387082168247300906, -7.082119434687050408 ) ) ;
#64795=EDGE_CURVE ( 'NONE', #39993, #18606, #98220, .T. ) ;
#64796=CARTESIAN_POINT ( 'NONE',  ( 20.36894250292379382, 28.67874883491396787, 10.36894250292379205 ) ) ;
#64797=CARTESIAN_POINT ( 'NONE',  ( 19.84674366389459621, 33.50893115100078745, 7.409399052514197653E-17 ) ) ;
#64798=CARTESIAN_POINT ( 'NONE',  ( 18.28836319691945889, 9.344927826957706074, 6.499999999999995559 ) ) ;
#64799=CARTESIAN_POINT ( 'NONE',  ( 2.035157376598822676, 27.43868534415483396, -7.964842623401177768 ) ) ;
#64800=CARTESIAN_POINT ( 'NONE',  ( 17.96484262340118221, 59.93868534415484106, 7.964842623401181321 ) ) ;
#64801=CARTESIAN_POINT ( 'NONE',  ( 19.10478245763052030, 50.10160829253887727, 5.990408912944319653 ) ) ;
#64803=CARTESIAN_POINT ( 'NONE',  ( -1.099225684535947600, 49.54030133659708923, 6.408140936763237150 ) ) ;
#64804=CARTESIAN_POINT ( 'NONE',  ( -0.8801773607111008646, 48.27201867748816966, 2.915334737309923430 ) ) ;
#64805=ORIENTED_EDGE ( 'NONE', *, *, #9691, .F. ) ;
#64807=CARTESIAN_POINT ( 'NONE',  ( 7.084665262690076126, 67.02201867748817676, -10.88017736071110164 ) ) ;
#64808=AXIS2_PLACEMENT_3D ( 'NONE', #28424, #49444, #18966 ) ;
#64811=CARTESIAN_POINT ( 'NONE',  ( 20.88017736071110519, 65.56368534415483396, 2.639326808657452039E-16 ) ) ;
#64812=CARTESIAN_POINT ( 'NONE',  ( -0.8801773607110991993, 2.855352010821504471, -2.915334737309923874 ) ) ;
#64813=CARTESIAN_POINT ( 'NONE',  ( 1.959929470562272291, 1.502578601053488283, 5.767676674365836753 ) ) ;
#64815=CARTESIAN_POINT ( 'NONE',  ( 2.035157376598824452, 13.68868534415483751, 7.964842623401179544 ) ) ;
#64816=CARTESIAN_POINT ( 'NONE',  ( 7.361572987183169658, 14.96726448433411960, -9.846743663894592657 ) ) ;
#64817=CARTESIAN_POINT ( 'NONE',  ( 6.204703633549690345, 22.84541550158062861, 14.16423886937410082 ) ) ;
#64818=VECTOR ( 'NONE', #51912, 1000.000000000000000 ) ;
#64819=( BOUNDED_SURFACE ( )  B_SPLINE_SURFACE ( 1, 2, ( 
 ( #24515, #45517, #60518, #91519, #62477, #91009, #92003, #552, #1026, #69021, #83526, #54004, #54974, #31486, #38523, #30999, #61495, #76999, #39511, #23532, #24017, #53012, #84514, #70003, #98560, #8511, #16010, #23035, #46499, #54486, #68529, #76017, #92489, #46989, #39014, #30013, #69509, #53508, #92981, #85494, #61990, #7547, #85000, #8026, #38037, #16513, #77483, #1527, #31973, #17004, #47483, #7038, #58, #37543, #68034, #15045, #30505, #61008, #84019, #15540, #46024, #76510, #48956, #40987, #63472, #56471, #26447, #40496, #17504, #64439, #18965, #2999, #70496, #79465, #25498, #34431, #26943, #86957, #47969, #3477, #78965, #78478, #18471, #56948, #71483, #33449, #57444, #64924, #41486, #9994, #33934, #71955, #62976, #63944, #10962, #39991, #95452, #85992, #2017, #77984, #41971, #9490, #55491, #94946, #87449, #49443, #70991, #2515, #32967, #94455, #79948, #93974, #17984, #11452, #55984, #25973, #87934, #32480, #72435, #19450, #93480, #86486, #3963, #25006, #48468, #10476, #66917, #28903, #51921, #11947, #20934, #58414, #50430, #4462, #67412, #20439, #90391, #49943, #88436, #43420, #80449, #42939, #73422, #97439, #28423, #82405, #4946, #42451, #13931, #59406, #12925, #58921, #36922, #19936, #72933, #74910, #80938, #81422, #12431, #35427, #89911, #34930, #27432, #43907, #13422, #97941, #65922, #65427, #96450, #6410, #95951, #35921, #73922, #74407, #5449, #57927, #96952, #29398, #5932, #66419, #89421, #51422, #81912, #44407, #36424, #21425, #27922, #59899, #88929, #50927, #38404, #98436, #15899, #46390, #30884, #82908, #67914, #68905, #14926, #84400, #23410, #83404, #45393, #433, #53894, #75898, #61380, #29893, #14426, #91889, #15425, #7423, #76876, #98931, #22917, #7909, #60395, #37920, #68409, #90892, #21928, #52407, #22420, #52895, #30386, #6916, #75397, #53386, #60889, #44895, #83895, #91388, #37426, #45906, #76393, #33012, #63510, #79991, #56513, #95495, #40036, #11494, #26986, #80492, #48505, #94498, #42015, #94014, #4014, #56989, #19008, #72480, #2059, #11009, #79009, #40535, #93520, #57485, #10512, #70537, #32521, #78520, #33490, #63020, #25536, #56027, #87493, #18510, #34475, #86524, #25047, #64968, #49484, #3039, #48999, #87979, #10033, #55534, #19490, #71033, #71529, #2554, #18024, #49985, #86030, #17544, #33977, #3519, #48011, #41027, #63988, #26017, #87002, #79508, #41526, #71995, #64480, #94989, #26493, #58968, #29438, #5976, #43461, #73963, #66462, #81955, #44451, #35964, #28949, #27477, #28471, #74952, #4505, #13469, #5492, #96494, #89465, #11990, #6455, #42491, #88476, #43950, #20982, #59450, #50475 ),
 ( #80978, #42982, #35471, #19978, #36964, #74449, #12479, #96994, #59942, #89952, #90432, #21468, #51466, #12968, #72975, #34971, #65467, #67460, #73463, #36469, #27967, #4990, #13975, #66963, #57970, #95994, #97482, #51967, #97981, #21972, #52450, #65967, #82452, #58459, #88974, #20482, #50970, #81463, #16431, #69925, #60439, #38938, #8916, #31898, #77402, #44941, #53931, #91436, #75446, #38446, #1447, #62396, #83446, #45438, #84440, #53428, #46909, #30920, #14968, #15937, #76921, #69427, #92904, #68942, #22460, #92416, #473, #39432, #75940, #61419, #67957, #37962, #45946, #76435, #46427, #8431, #948, #31409, #61911, #7465, #24435, #82953, #54409, #6959, #52936, #23941, #22963, #14466, #37467, #60930, #83937, #84921, #98479, #15464, #29934, #68453, #90932, #98975, #30428, #7951, #91929, #23456, #94381, #71878, #17425, #63390, #86404, #9917, #26375, #79873, #24926, #85911, #78396, #32397, #87375, #56400, #62900, #40908, #3891, #3393, #34359, #33856, #2923, #55906, #85414, #16925, #77902, #11377, #93400, #86885, #40420, #55408, #56874, #48876, #1939, #39917, #63867, #10891, #41897, #72359, #64850, #54899, #17907, #70419, #41417, #48390, #78892, #93894, #18890, #95369, #47893, #64365, #47400, #9415, #49372, #70914, #25899, #25422, #2434, #10401, #32892, #71407, #33373, #18395, #79386, #94874, #91189, #75202, #27358, #60200, #22224, #83205, #38214, #82705, #65349, #37714, #14223, #60689, #57852, #44702, #11871, #80862, #90199, #21729, #98230, #52700, #29691, #90695, #7213, #88362, #76198, #7717, #98737, #49861, #95877, #68216, #35353, #45698, #53198, #4875, #96375, #30188, #83702, #59702, #22714, #19857, #80371, #15219, #14727, #65845, #68699, #6712, #67717, #45203, #50351, #29203, #52211, #12360, #26867, #57364, #42865, #42377, #37229, #19377, #87859, #75702, #72853, #4388, #34854, #73350, #93156, #78659, #85175, #24680, #40662, #39690, #2191, #61187, #16685, #92662, #55151, #62156, #76681, #47155, #17672, #85665, #31666, #24190, #54659, #70178, #32653, #77658, #17185, #15711, #9172, #63147, #91693, #1694, #32150, #84682, #62652, #47665, #61665, #38696, #78159, #40166, #9669, #23212, #70671, #46674, #55663, #48145, #93649, #69195, #25183, #1211, #720, #86162, #10164, #231, #30679, #53685, #84203, #46197, #31174, #8201, #92184, #23710, #54171, #16192, #77172, #8680, #39192, #69680, #71160, #35100, #2685, #48635, #42141, #80117, #88109, #10650, #33619, #64118, #26622, #73098, #26145, #94635, #56639, #12116, #87616, #27607, #33136, #42618, #58094, #12605, #79636, #57119, #4635, #87124, #65597, #19618, #50112, #96125, #63631 ) ),
 .UNSPECIFIED., .F., .F., .T. ) 
 B_SPLINE_SURFACE_WITH_KNOTS ( ( 2, 2 ),
 ( 3, 2, 2, 2, 2, 2, 2, 2, 2, 2, 2, 2, 2, 2, 2, 2, 2, 2, 2, 2, 2, 2, 2, 2, 2, 2, 2, 2, 2, 2, 2, 2, 2, 2, 2, 2, 2, 2, 2, 2, 2, 2, 2, 2, 2, 2, 2, 2, 2, 2, 2, 2, 2, 2, 2, 2, 2, 2, 2, 2, 2, 2, 2, 2, 2, 2, 2, 2, 2, 2, 2, 2, 2, 2, 2, 2, 2, 2, 2, 2, 2, 2, 2, 2, 2, 2, 2, 2, 2, 2, 2, 2, 2, 2, 2, 2, 2, 2, 2, 2, 2, 2, 2, 2, 2, 2, 2, 2, 2, 2, 2, 2, 2, 2, 2, 2, 2, 2, 2, 2, 2, 2, 2, 2, 2, 2, 2, 2, 2, 2, 2, 2, 2, 2, 2, 2, 2, 2, 2, 2, 2, 2, 2, 2, 2, 2, 2, 2, 2, 2, 2, 2, 2, 2, 2, 2, 2, 2, 2, 2, 2, 2, 3 ),
 ( 0.000000000000000000, 1.000000000000000000 ),
 ( 0.000000000000000000, 0.005952380952380952051, 0.01190476190476190410, 0.01785714285714285615, 0.02380952380952380820, 0.02976190476190476025, 0.03571428571428571230, 0.04166666666666666435, 0.04761904761904761640, 0.05357142857142856845, 0.05952380952380952051, 0.06547619047619047949, 0.07142857142857142461, 0.07738095238095238360, 0.08333333333333332871, 0.08928571428571428770, 0.09523809523809523281, 0.1011904761904761918, 0.1071428571428571369, 0.1130952380952380959, 0.1190476190476190410, 0.1250000000000000000, 0.1309523809523809590, 0.1369047619047619180, 0.1428571428571428492, 0.1488095238095238082, 0.1547619047619047672, 0.1607142857142857262, 0.1666666666666666574, 0.1726190476190476164, 0.1785714285714285754, 0.1845238095238095344, 0.1904761904761904656, 0.1964285714285714246, 0.2023809523809523836, 0.2083333333333333426, 0.2142857142857142738, 0.2202380952380952328, 0.2261904761904761918, 0.2321428571428571508, 0.2380952380952380820, 0.2440476190476190410, 0.2500000000000000000, 0.2559523809523809312, 0.2619047619047619180, 0.2678571428571428492, 0.2738095238095238360, 0.2797619047619047672, 0.2857142857142856984, 0.2916666666666666852, 0.2976190476190476164, 0.3035714285714285476, 0.3095238095238095344, 0.3154761904761904656, 0.3214285714285714524, 0.3273809523809523836, 0.3333333333333333148, 0.3392857142857143016, 0.3452380952380952328, 0.3511904761904761640, 0.3571428571428571508, 0.3630952380952380820, 0.3690476190476190688, 0.3750000000000000000, 0.3809523809523809312, 0.3869047619047619180, 0.3928571428571428492, 0.3988095238095238360, 0.4047619047619047672, 0.4107142857142856984, 0.4166666666666666852, 0.4226190476190476164, 0.4285714285714285476, 0.4345238095238095344, 0.4404761904761904656, 0.4464285714285714524, 0.4523809523809523836, 0.4583333333333333148, 0.4642857142857143016, 0.4702380952380952328, 0.4761904761904761640, 0.4821428571428571508, 0.4880952380952380820, 0.4940476190476190688, 0.5000000000000000000, 0.5059523809523809312, 0.5119047619047618625, 0.5178571428571429047, 0.5238095238095238360, 0.5297619047619047672, 0.5357142857142856984, 0.5416666666666666297, 0.5476190476190476719, 0.5535714285714286031, 0.5595238095238095344, 0.5654761904761904656, 0.5714285714285713969, 0.5773809523809523281, 0.5833333333333333703, 0.5892857142857143016, 0.5952380952380952328, 0.6011904761904761640, 0.6071428571428570953, 0.6130952380952381375, 0.6190476190476190688, 0.6250000000000000000, 0.6309523809523809312, 0.6369047619047618625, 0.6428571428571429047, 0.6488095238095238360, 0.6547619047619047672, 0.6607142857142856984, 0.6666666666666666297, 0.6726190476190476719, 0.6785714285714286031, 0.6845238095238095344, 0.6904761904761904656, 0.6964285714285713969, 0.7023809523809523281, 0.7083333333333333703, 0.7142857142857143016, 0.7202380952380952328, 0.7261904761904761640, 0.7321428571428570953, 0.7380952380952381375, 0.7440476190476190688, 0.7500000000000000000, 0.7559523809523809312, 0.7619047619047618625, 0.7678571428571429047, 0.7738095238095238360, 0.7797619047619047672, 0.7857142857142856984, 0.7916666666666666297, 0.7976190476190476719, 0.8035714285714286031, 0.8095238095238095344, 0.8154761904761904656, 0.8214285714285713969, 0.8273809523809523281, 0.8333333333333333703, 0.8392857142857143016, 0.8452380952380952328, 0.8511904761904761640, 0.8571428571428570953, 0.8630952380952381375, 0.8690476190476190688, 0.8750000000000000000, 0.8809523809523809312, 0.8869047619047618625, 0.8928571428571429047, 0.8988095238095238360, 0.9047619047619047672, 0.9107142857142856984, 0.9166666666666666297, 0.9226190476190476719, 0.9285714285714286031, 0.9345238095238095344, 0.9404761904761904656, 0.9464285714285713969, 0.9523809523809523281, 0.9583333333333333703, 0.9642857142857143016 ),
 .UNSPECIFIED. ) 
 GEOMETRIC_REPRESENTATION_ITEM ( )  RATIONAL_B_SPLINE_SURFACE ( (
 ( 1.000000000000000000, 0.9659258262890683122, 1.000000000000000000, 0.9659258262890683122, 1.000000000000000000, 0.9659258262890683122, 1.000000000000000000, 0.9659258262890683122, 1.000000000000000000, 0.9659258262890683122, 1.000000000000000000, 0.9659258262890683122, 1.000000000000000000, 0.9659258262890683122, 1.000000000000000000, 0.9659258262890683122, 1.000000000000000000, 0.9659258262890683122, 1.000000000000000000, 0.9659258262890683122, 1.000000000000000000, 0.9659258262890683122, 1.000000000000000000, 0.9659258262890683122, 1.000000000000000000, 0.9659258262890683122, 1.000000000000000000, 0.9659258262890683122, 1.000000000000000000, 0.9659258262890683122, 1.000000000000000000, 0.9659258262890683122, 1.000000000000000000, 0.9659258262890683122, 1.000000000000000000, 0.9659258262890683122, 1.000000000000000000, 0.9659258262890683122, 1.000000000000000000, 0.9659258262890683122, 1.000000000000000000, 0.9659258262890683122, 1.000000000000000000, 0.9659258262890683122, 1.000000000000000000, 0.9659258262890683122, 1.000000000000000000, 0.9659258262890683122, 1.000000000000000000, 0.9659258262890683122, 1.000000000000000000, 0.9659258262890683122, 1.000000000000000000, 0.9659258262890683122, 1.000000000000000000, 0.9659258262890683122, 1.000000000000000000, 0.9659258262890683122, 1.000000000000000000, 0.9659258262890683122, 1.000000000000000000, 0.9659258262890683122, 1.000000000000000000, 0.9659258262890683122, 1.000000000000000000, 0.9659258262890683122, 1.000000000000000000, 0.9659258262890683122, 1.000000000000000000, 0.9659258262890683122, 1.000000000000000000, 0.9659258262890683122, 1.000000000000000000, 0.9659258262890683122, 1.000000000000000000, 0.9659258262890683122, 1.000000000000000000, 0.9659258262890683122, 1.000000000000000000, 0.9659258262890683122, 1.000000000000000000, 0.9659258262890683122, 1.000000000000000000, 0.9659258262890683122, 1.000000000000000000, 0.9659258262890683122, 1.000000000000000000, 0.9659258262890683122, 1.000000000000000000, 0.9659258262890683122, 1.000000000000000000, 0.9659258262890683122, 1.000000000000000000, 0.9659258262890683122, 1.000000000000000000, 0.9659258262890683122, 1.000000000000000000, 0.9659258262890683122, 1.000000000000000000, 0.9659258262890683122, 1.000000000000000000, 0.9659258262890683122, 1.000000000000000000, 0.9659258262890683122, 1.000000000000000000, 0.9659258262890683122, 1.000000000000000000, 0.9659258262890683122, 1.000000000000000000, 0.9659258262890683122, 1.000000000000000000, 0.9659258262890683122, 1.000000000000000000, 0.9659258262890683122, 1.000000000000000000, 0.9659258262890683122, 1.000000000000000000, 0.9659258262890683122, 1.000000000000000000, 0.9659258262890683122, 1.000000000000000000, 0.9659258262890683122, 1.000000000000000000, 0.9659258262890683122, 1.000000000000000000, 0.9659258262890683122, 1.000000000000000000, 0.9659258262890683122, 1.000000000000000000, 0.9659258262890683122, 1.000000000000000000, 0.9659258262890683122, 1.000000000000000000, 0.9659258262890683122, 1.000000000000000000, 0.9659258262890683122, 1.000000000000000000, 0.9659258262890683122, 1.000000000000000000, 0.9659258262890683122, 1.000000000000000000, 0.9659258262890683122, 1.000000000000000000, 0.9659258262890683122, 1.000000000000000000, 0.9659258262890683122, 1.000000000000000000, 0.9659258262890683122, 1.000000000000000000, 0.9659258262890683122, 1.000000000000000000, 0.9659258262890683122, 1.000000000000000000, 0.9659258262890683122, 1.000000000000000000, 0.9659258262890683122, 1.000000000000000000, 0.9659258262890683122, 1.000000000000000000, 0.9659258262890683122, 1.000000000000000000, 0.9659258262890683122, 1.000000000000000000, 0.9659258262890683122, 1.000000000000000000, 0.9659258262890683122, 1.000000000000000000, 0.9659258262890683122, 1.000000000000000000, 0.9659258262890683122, 1.000000000000000000, 0.9659258262890683122, 1.000000000000000000, 0.9659258262890683122, 1.000000000000000000, 0.9659258262890683122, 1.000000000000000000, 0.9659258262890683122, 1.000000000000000000, 0.9659258262890683122, 1.000000000000000000, 0.9659258262890683122, 1.000000000000000000, 0.9659258262890683122, 1.000000000000000000, 0.9659258262890683122, 1.000000000000000000, 0.9659258262890683122, 1.000000000000000000, 0.9659258262890683122, 1.000000000000000000, 0.9659258262890683122, 1.000000000000000000, 0.9659258262890683122, 1.000000000000000000, 0.9659258262890683122, 1.000000000000000000, 0.9659258262890683122, 1.000000000000000000, 0.9659258262890683122, 1.000000000000000000, 0.9659258262890683122, 1.000000000000000000, 0.9659258262890683122, 1.000000000000000000, 0.9659258262890683122, 1.000000000000000000, 0.9659258262890683122, 1.000000000000000000, 0.9659258262890683122, 1.000000000000000000, 0.9659258262890683122, 1.000000000000000000, 0.9659258262890683122, 1.000000000000000000, 0.9659258262890683122, 1.000000000000000000, 0.9659258262890683122, 1.000000000000000000, 0.9659258262890683122, 1.000000000000000000, 0.9659258262890683122, 1.000000000000000000, 0.9659258262890683122, 1.000000000000000000, 0.9659258262890683122, 1.000000000000000000, 0.9659258262890683122, 1.000000000000000000, 0.9659258262890683122, 1.000000000000000000, 0.9659258262890683122, 1.000000000000000000, 0.9659258262890683122, 1.000000000000000000, 0.9659258262890683122, 1.000000000000000000, 0.9659258262890683122, 1.000000000000000000, 0.9659258262890683122, 1.000000000000000000, 0.9659258262890683122, 1.000000000000000000, 0.9659258262890683122, 1.000000000000000000, 0.9659258262890683122, 1.000000000000000000, 0.9659258262890683122, 1.000000000000000000, 0.9659258262890683122, 1.000000000000000000, 0.9659258262890683122, 1.000000000000000000, 0.9659258262890683122, 1.000000000000000000, 0.9659258262890683122, 1.000000000000000000, 0.9659258262890683122, 1.000000000000000000, 0.9659258262890683122, 1.000000000000000000, 0.9659258262890683122, 1.000000000000000000, 0.9659258262890683122, 1.000000000000000000, 0.9659258262890683122, 1.000000000000000000, 0.9659258262890683122, 1.000000000000000000, 0.9659258262890683122, 1.000000000000000000, 0.9659258262890683122, 1.000000000000000000, 0.9659258262890683122, 1.000000000000000000, 0.9659258262890683122, 1.000000000000000000, 0.9659258262890683122, 1.000000000000000000, 0.9659258262890683122, 1.000000000000000000, 0.9659258262890683122, 1.000000000000000000, 0.9659258262890683122, 1.000000000000000000, 0.9659258262890683122, 1.000000000000000000, 0.9659258262890683122, 1.000000000000000000, 0.9659258262890683122, 1.000000000000000000, 0.9659258262890683122, 1.000000000000000000, 0.9659258262890683122, 1.000000000000000000, 0.9659258262890683122, 1.000000000000000000, 0.9659258262890683122, 1.000000000000000000, 0.9659258262890683122, 1.000000000000000000, 0.9659258262890683122, 1.000000000000000000, 0.9659258262890683122, 1.000000000000000000, 0.9659258262890683122, 1.000000000000000000, 0.9659258262890683122, 1.000000000000000000, 0.9659258262890683122, 1.000000000000000000, 0.9659258262890683122, 1.000000000000000000, 0.9659258262890683122, 1.000000000000000000, 0.9659258262890683122, 1.000000000000000000, 0.9659258262890683122, 1.000000000000000000, 0.9659258262890683122, 1.000000000000000000, 0.9659258262890683122, 1.000000000000000000, 0.9659258262890683122, 1.000000000000000000),
 ( 1.000000000000000000, 0.9659258262890683122, 1.000000000000000000, 0.9659258262890683122, 1.000000000000000000, 0.9659258262890683122, 1.000000000000000000, 0.9659258262890683122, 1.000000000000000000, 0.9659258262890683122, 1.000000000000000000, 0.9659258262890683122, 1.000000000000000000, 0.9659258262890683122, 1.000000000000000000, 0.9659258262890683122, 1.000000000000000000, 0.9659258262890683122, 1.000000000000000000, 0.9659258262890683122, 1.000000000000000000, 0.9659258262890683122, 1.000000000000000000, 0.9659258262890683122, 1.000000000000000000, 0.9659258262890683122, 1.000000000000000000, 0.9659258262890683122, 1.000000000000000000, 0.9659258262890683122, 1.000000000000000000, 0.9659258262890683122, 1.000000000000000000, 0.9659258262890683122, 1.000000000000000000, 0.9659258262890683122, 1.000000000000000000, 0.9659258262890683122, 1.000000000000000000, 0.9659258262890683122, 1.000000000000000000, 0.9659258262890683122, 1.000000000000000000, 0.9659258262890683122, 1.000000000000000000, 0.9659258262890683122, 1.000000000000000000, 0.9659258262890683122, 1.000000000000000000, 0.9659258262890683122, 1.000000000000000000, 0.9659258262890683122, 1.000000000000000000, 0.9659258262890683122, 1.000000000000000000, 0.9659258262890683122, 1.000000000000000000, 0.9659258262890683122, 1.000000000000000000, 0.9659258262890683122, 1.000000000000000000, 0.9659258262890683122, 1.000000000000000000, 0.9659258262890683122, 1.000000000000000000, 0.9659258262890683122, 1.000000000000000000, 0.9659258262890683122, 1.000000000000000000, 0.9659258262890683122, 1.000000000000000000, 0.9659258262890683122, 1.000000000000000000, 0.9659258262890683122, 1.000000000000000000, 0.9659258262890683122, 1.000000000000000000, 0.9659258262890683122, 1.000000000000000000, 0.9659258262890683122, 1.000000000000000000, 0.9659258262890683122, 1.000000000000000000, 0.9659258262890683122, 1.000000000000000000, 0.9659258262890683122, 1.000000000000000000, 0.9659258262890683122, 1.000000000000000000, 0.9659258262890683122, 1.000000000000000000, 0.9659258262890683122, 1.000000000000000000, 0.9659258262890683122, 1.000000000000000000, 0.9659258262890683122, 1.000000000000000000, 0.9659258262890683122, 1.000000000000000000, 0.9659258262890683122, 1.000000000000000000, 0.9659258262890683122, 1.000000000000000000, 0.9659258262890683122, 1.000000000000000000, 0.9659258262890683122, 1.000000000000000000, 0.9659258262890683122, 1.000000000000000000, 0.9659258262890683122, 1.000000000000000000, 0.9659258262890683122, 1.000000000000000000, 0.9659258262890683122, 1.000000000000000000, 0.9659258262890683122, 1.000000000000000000, 0.9659258262890683122, 1.000000000000000000, 0.9659258262890683122, 1.000000000000000000, 0.9659258262890683122, 1.000000000000000000, 0.9659258262890683122, 1.000000000000000000, 0.9659258262890683122, 1.000000000000000000, 0.9659258262890683122, 1.000000000000000000, 0.9659258262890683122, 1.000000000000000000, 0.9659258262890683122, 1.000000000000000000, 0.9659258262890683122, 1.000000000000000000, 0.9659258262890683122, 1.000000000000000000, 0.9659258262890683122, 1.000000000000000000, 0.9659258262890683122, 1.000000000000000000, 0.9659258262890683122, 1.000000000000000000, 0.9659258262890683122, 1.000000000000000000, 0.9659258262890683122, 1.000000000000000000, 0.9659258262890683122, 1.000000000000000000, 0.9659258262890683122, 1.000000000000000000, 0.9659258262890683122, 1.000000000000000000, 0.9659258262890683122, 1.000000000000000000, 0.9659258262890683122, 1.000000000000000000, 0.9659258262890683122, 1.000000000000000000, 0.9659258262890683122, 1.000000000000000000, 0.9659258262890683122, 1.000000000000000000, 0.9659258262890683122, 1.000000000000000000, 0.9659258262890683122, 1.000000000000000000, 0.9659258262890683122, 1.000000000000000000, 0.9659258262890683122, 1.000000000000000000, 0.9659258262890683122, 1.000000000000000000, 0.9659258262890683122, 1.000000000000000000, 0.9659258262890683122, 1.000000000000000000, 0.9659258262890683122, 1.000000000000000000, 0.9659258262890683122, 1.000000000000000000, 0.9659258262890683122, 1.000000000000000000, 0.9659258262890683122, 1.000000000000000000, 0.9659258262890683122, 1.000000000000000000, 0.9659258262890683122, 1.000000000000000000, 0.9659258262890683122, 1.000000000000000000, 0.9659258262890683122, 1.000000000000000000, 0.9659258262890683122, 1.000000000000000000, 0.9659258262890683122, 1.000000000000000000, 0.9659258262890683122, 1.000000000000000000, 0.9659258262890683122, 1.000000000000000000, 0.9659258262890683122, 1.000000000000000000, 0.9659258262890683122, 1.000000000000000000, 0.9659258262890683122, 1.000000000000000000, 0.9659258262890683122, 1.000000000000000000, 0.9659258262890683122, 1.000000000000000000, 0.9659258262890683122, 1.000000000000000000, 0.9659258262890683122, 1.000000000000000000, 0.9659258262890683122, 1.000000000000000000, 0.9659258262890683122, 1.000000000000000000, 0.9659258262890683122, 1.000000000000000000, 0.9659258262890683122, 1.000000000000000000, 0.9659258262890683122, 1.000000000000000000, 0.9659258262890683122, 1.000000000000000000, 0.9659258262890683122, 1.000000000000000000, 0.9659258262890683122, 1.000000000000000000, 0.9659258262890683122, 1.000000000000000000, 0.9659258262890683122, 1.000000000000000000, 0.9659258262890683122, 1.000000000000000000, 0.9659258262890683122, 1.000000000000000000, 0.9659258262890683122, 1.000000000000000000, 0.9659258262890683122, 1.000000000000000000, 0.9659258262890683122, 1.000000000000000000, 0.9659258262890683122, 1.000000000000000000, 0.9659258262890683122, 1.000000000000000000, 0.9659258262890683122, 1.000000000000000000, 0.9659258262890683122, 1.000000000000000000, 0.9659258262890683122, 1.000000000000000000, 0.9659258262890683122, 1.000000000000000000, 0.9659258262890683122, 1.000000000000000000, 0.9659258262890683122, 1.000000000000000000, 0.9659258262890683122, 1.000000000000000000, 0.9659258262890683122, 1.000000000000000000, 0.9659258262890683122, 1.000000000000000000, 0.9659258262890683122, 1.000000000000000000, 0.9659258262890683122, 1.000000000000000000, 0.9659258262890683122, 1.000000000000000000, 0.9659258262890683122, 1.000000000000000000, 0.9659258262890683122, 1.000000000000000000, 0.9659258262890683122, 1.000000000000000000, 0.9659258262890683122, 1.000000000000000000, 0.9659258262890683122, 1.000000000000000000, 0.9659258262890683122, 1.000000000000000000, 0.9659258262890683122, 1.000000000000000000, 0.9659258262890683122, 1.000000000000000000, 0.9659258262890683122, 1.000000000000000000, 0.9659258262890683122, 1.000000000000000000, 0.9659258262890683122, 1.000000000000000000, 0.9659258262890683122, 1.000000000000000000, 0.9659258262890683122, 1.000000000000000000, 0.9659258262890683122, 1.000000000000000000, 0.9659258262890683122, 1.000000000000000000, 0.9659258262890683122, 1.000000000000000000, 0.9659258262890683122, 1.000000000000000000, 0.9659258262890683122, 1.000000000000000000, 0.9659258262890683122, 1.000000000000000000, 0.9659258262890683122, 1.000000000000000000, 0.9659258262890683122, 1.000000000000000000, 0.9659258262890683122, 1.000000000000000000, 0.9659258262890683122, 1.000000000000000000, 0.9659258262890683122, 1.000000000000000000, 0.9659258262890683122, 1.000000000000000000, 0.9659258262890683122, 1.000000000000000000) ) ) 
 REPRESENTATION_ITEM ( '' )  SURFACE ( )  );
#64820=CARTESIAN_POINT ( 'NONE',  ( 4.559911319644449179, 28.89701867748817321, 9.422509992056141925 ) ) ;
#64821=CARTESIAN_POINT ( 'NONE',  ( 1.472469842513823179, 60.59226448433412315, -4.923371831947296329 ) ) ;
#64823=CARTESIAN_POINT ( 'NONE',  ( 1.472469842513823179, 60.59226448433412315, -4.923371831947296329 ) ) ;
#64826=CARTESIAN_POINT ( 'NONE',  ( 12.91533473730993009, 46.60535201082150536, -10.88017736071109987 ) ) ;
#64827=CARTESIAN_POINT ( 'NONE',  ( 19.84674366389459266, 53.30059781766744464, 2.638427012816836559 ) ) ;
#64828=CARTESIAN_POINT ( 'NONE',  ( 13.43411237798105340, 40.58196800326375353, 12.81628187352647963 ) ) ;
#64829=CARTESIAN_POINT ( 'NONE',  ( 0.5774900079438590739, 2.647018677488170990, -5.440088680355550821 ) ) ;
#64831=CARTESIAN_POINT ( 'NONE',  ( 17.96484262340118221, 59.93868534415484106, 7.964842623401181321 ) ) ;
#64832=CARTESIAN_POINT ( 'NONE',  ( -0.3689425029237881626, 67.42874883491396076, 10.36894250292379027 ) ) ;
#64833=CARTESIAN_POINT ( 'NONE',  ( 10.00000000000000178, 40.37363466993042493, 12.81628187352647608 ) ) ;
#64834=CARTESIAN_POINT ( 'NONE',  ( 20.88017736071110519, 35.56368534415484106, 2.639326808657452039E-16 ) ) ;
#64835=DIRECTION ( 'NONE',  ( 0.000000000000000000, 0.000000000000000000, 1.000000000000000000 ) ) ;
#64837=CARTESIAN_POINT ( 'NONE',  ( -2.816281873526473856, 39.12363466993041783, 9.499525473075851096E-16 ) ) ;
#64838=CARTESIAN_POINT ( 'NONE',  ( 20.88017736071110164, 40.35535201082150536, 2.915334737309930979 ) ) ;
#64839=CARTESIAN_POINT ( 'NONE',  ( 0.1532563361054083140, 51.00893115100078745, 1.131784320476157264E-15 ) ) ;
#64841=CARTESIAN_POINT ( 'NONE',  ( 1.472469842513823179, 65.59226448433412315, -4.923371831947296329 ) ) ;
#64842=CARTESIAN_POINT ( 'NONE',  ( 19.72487221294570858, 0.000000000000000000, -6.500000000000000888 ) ) ;
#64843=CARTESIAN_POINT ( 'NONE',  ( 17.20831665107776587, 52.88393115100078035, 7.208316651077764980 ) ) ;
#64844=CARTESIAN_POINT ( 'NONE',  ( 2.035157376598824452, 28.68868534415484106, 7.964842623401179544 ) ) ;
#64845=FACE_OUTER_BOUND ( 'NONE', #6071, .T. ) ;
#64846=CARTESIAN_POINT ( 'NONE',  ( 7.361572987183169658, 34.96726448433411605, -9.846743663894592657 ) ) ;
#64848=TOROIDAL_SURFACE ( 'NONE', #76015, 18.53834841531100608, 7.000000000000000000 ) ;
#64850=CARTESIAN_POINT ( 'NONE',  ( 18.52753015748618282, 28.92559781766745175, -4.923371831947291888 ) ) ;
#64851=CARTESIAN_POINT ( 'NONE',  ( 14.92337183194729988, 14.34226448433411782, -8.527530157486177487 ) ) ;
#64853=CARTESIAN_POINT ( 'NONE',  ( 1.472469842513823179, 65.59226448433412315, -4.923371831947296329 ) ) ;
#64854=ORIENTED_EDGE ( 'NONE', *, *, #73972, .T. ) ;
#64855=CARTESIAN_POINT ( 'NONE',  ( 0.6178305044545818747, 63.49863466993043204, -9.382169495545419124 ) ) ;
#64856=CARTESIAN_POINT ( 'NONE',  ( 19.38216949554541202, 40.99863466993042493, 9.382169495545424454 ) ) ;
#64857=CARTESIAN_POINT ( 'NONE',  ( 14.92337183194729633, 47.67559781766745175, 8.527530157486181039 ) ) ;
#64859=CARTESIAN_POINT ( 'NONE',  ( 24.16423886937410614, 64.30374883491396076, 8.672049930838204340E-16 ) ) ;
#64860=CARTESIAN_POINT ( 'NONE',  ( 18.52753015748618282, 18.92559781766745175, -4.923371831947291888 ) ) ;
#64861=CARTESIAN_POINT ( 'NONE',  ( 20.00000000000000711, 81.00835155610852212, 4.500000004094268036 ) ) ;
#64862=CARTESIAN_POINT ( 'NONE',  ( 6.204703633549690345, 52.84541550158062506, 14.16423886937410082 ) ) ;
#64863=CARTESIAN_POINT ( 'NONE',  ( 19.42250999205614193, 5.147018677488171434, 5.440088680355555262 ) ) ;
#64864=CARTESIAN_POINT ( 'NONE',  ( 20.36894250292379382, 33.67874883491396076, 10.36894250292379205 ) ) ;
#64865=CARTESIAN_POINT ( 'NONE',  ( 24.16423886937409904, 34.09541550158064638, 3.795296366450317205 ) ) ;
#64866=DIRECTION ( 'NONE',  ( -0.000000000000000000, -0.000000000000000000, 1.000000000000000000 ) ) ;
#64867=CARTESIAN_POINT ( 'NONE',  ( 0.1532563361054082862, 16.21726448433411960, 2.638427012816831674 ) ) ;
#64869=CARTESIAN_POINT ( 'NONE',  ( 10.00000000000000000, 54.75893115100078745, -9.846743663894594434 ) ) ;
#64870=CARTESIAN_POINT ( 'NONE',  ( 2.035157376598824452, 53.68868534415484817, 7.964842623401179544 ) ) ;
#64872=EDGE_CURVE ( 'NONE', #14724, #86159, #83407, .T. ) ;
#64874=CARTESIAN_POINT ( 'NONE',  ( 14.92337183194729988, 59.34226448433412315, -8.527530157486177487 ) ) ;
#64875=SURFACE_STYLE_USAGE ( .BOTH. , #12389 ) ;
#64876=VERTEX_POINT ( 'NONE', #5725 ) ;
#64877=CARTESIAN_POINT ( 'NONE',  ( 10.00000000000000000, 20.55374883491396787, -14.16423886937410082 ) ) ;
#64878=MECHANICAL_DESIGN_GEOMETRIC_PRESENTATION_REPRESENTATION('',(#12223),#42577);
#64879=CARTESIAN_POINT ( 'NONE',  ( 2.791683348922240793, 1.633931151000784565, 7.208316651077764092 ) ) ;
#64880=CARTESIAN_POINT ( 'NONE',  ( 20.88017736071110519, 45.56368534415484106, 2.639326808657452039E-16 ) ) ;
#64881=CARTESIAN_POINT ( 'NONE',  ( 7.084665262690076126, 24.10535201082150181, 10.88017736071109987 ) ) ;
#64882=CARTESIAN_POINT ( 'NONE',  ( -1.099225684535947600, 18.70696800326375353, -6.408140936763238038 ) ) ;
#64883=CARTESIAN_POINT ( 'NONE',  ( 20.15039907845753220, 61.74884699246888431, 6.262539305110078836 ) ) ;
#64884=CARTESIAN_POINT ( 'NONE',  ( 7.361572987183170547, 7.050597817667451750, 9.846743663894590881 ) ) ;
#64885=CARTESIAN_POINT ( 'NONE',  ( 22.81628187352647785, 46.62363466993041783, 6.195893100308588602E-16 ) ) ;
#64888=CARTESIAN_POINT ( 'NONE',  ( 2.917880565312948704, 22.63708216824730002, 12.26659068614894643 ) ) ;
#64889=CARTESIAN_POINT ( 'NONE',  ( 20.30776406404415724, 0.000000000000000000, -5.999999999999999112 ) ) ;
#64890=FACE_OUTER_BOUND ( 'NONE', #80177, .T. ) ;
#64891=CARTESIAN_POINT ( 'NONE',  ( 7.084665262690076126, 12.02201867748817321, -10.88017736071110164 ) ) ;
#64893=CARTESIAN_POINT ( 'NONE',  ( 10.00000000000000000, 36.81368534415484106, -10.88017736071110342 ) ) ;
#64894=CARTESIAN_POINT ( 'NONE',  ( 2.035157376598824452, 33.68868534415484106, 7.964842623401179544 ) ) ;
#64895=CARTESIAN_POINT ( 'NONE',  ( -2.816281873526473856, 19.12363466993042138, 9.499525473075851096E-16 ) ) ;
#64896=CARTESIAN_POINT ( 'NONE',  ( 10.00000000000000178, 62.25893115100078745, 9.846743663894594434 ) ) ;
#64897=CARTESIAN_POINT ( 'NONE',  ( -0.8801773607110990882, 2.855352010821504471, -2.915334737309924318 ) ) ;
#64898=CARTESIAN_POINT ( 'NONE',  ( 17.20831665107776587, 9.133931151000787452, -7.208316651077762316 ) ) ;
#64902=CARTESIAN_POINT ( 'NONE',  ( 2.035157376598824452, 43.68868534415484106, 7.964842623401179544 ) ) ;
#64903=CIRCLE ( 'NONE', #15426, 0.4999999999999985567 ) ;
#64907=CARTESIAN_POINT ( 'NONE',  ( 3.591859063236761518, -0.04303199673624671928, 11.09922568453594849 ) ) ;
#64908=CARTESIAN_POINT ( 'NONE',  ( 2.035157376598824452, 63.68868534415484106, 7.964842623401179544 ) ) ;
#64909=CARTESIAN_POINT ( 'NONE',  ( 1.472469842513823179, 21.42559781766745175, 4.923371831947296329 ) ) ;
#64910=CARTESIAN_POINT ( 'NONE',  ( -2.816281873526473856, 44.12363466993042493, 9.499525473075851096E-16 ) ) ;
#64911=CARTESIAN_POINT ( 'NONE',  ( 10.00000000000000178, 69.31368534415484817, 10.88017736071110342 ) ) ;
#64916=CARTESIAN_POINT ( 'NONE',  ( 20.88017736071110875, 15.77201867748817143, -2.915334737309920765 ) ) ;
#64917=CARTESIAN_POINT ( 'NONE',  ( 3.591859063236761518, 59.95696800326375353, 11.09922568453594849 ) ) ;
#64918=CARTESIAN_POINT ( 'NONE',  ( 0.1532563361054083140, 26.00893115100078745, 1.131784320476157264E-15 ) ) ;
#64919=CARTESIAN_POINT ( 'NONE',  ( 20.88017736071110164, 25.35535201082150891, 2.915334737309930979 ) ) ;
#64920=CARTESIAN_POINT ( 'NONE',  ( 19.42250999205614193, 10.14701867748816966, 5.440088680355555262 ) ) ;
#64921=VERTEX_POINT ( 'NONE', #66712 ) ;
#64923=CARTESIAN_POINT ( 'NONE',  ( 10.00000000000000000, 16.81368534415483751, -10.88017736071110342 ) ) ;
#64924=CARTESIAN_POINT ( 'NONE',  ( 17.96484262340118221, 19.93868534415484106, 7.964842623401181321 ) ) ;
#64926=CARTESIAN_POINT ( 'NONE',  ( 20.88017736071110164, 25.35535201082150891, 2.915334737309930979 ) ) ;
#64930=CARTESIAN_POINT ( 'NONE',  ( 4.559911319644449179, 17.23035201082150536, -9.422509992056141925 ) ) ;
#64931=CARTESIAN_POINT ( 'NONE',  ( 18.52753015748618282, 53.92559781766745175, -4.923371831947291888 ) ) ;
#64934=CARTESIAN_POINT ( 'NONE',  ( 13.79529636645030344, 33.26208216824730357, 14.16423886937410614 ) ) ;
#64935=CARTESIAN_POINT ( 'NONE',  ( 12.91533473730993009, 41.60535201082149825, -10.88017736071109987 ) ) ;
#64936=CARTESIAN_POINT ( 'NONE',  ( 2.035157376598822676, 17.43868534415483751, -7.964842623401177768 ) ) ;
#64937=CARTESIAN_POINT ( 'NONE',  ( 18.52753015748617571, 63.09226448433412315, 4.923371831947298993 ) ) ;
#64938=( GEOMETRIC_REPRESENTATION_CONTEXT ( 3 ) GLOBAL_UNCERTAINTY_ASSIGNED_CONTEXT ( ( #63447 ) ) GLOBAL_UNIT_ASSIGNED_CONTEXT ( ( #16511, #24512, #69508 ) ) REPRESENTATION_CONTEXT ( 'NONE', 'WORKASPACE' ) );
#64940=CARTESIAN_POINT ( 'NONE',  ( 0.1532563361054082862, 51.21726448433412315, 2.638427012816831674 ) ) ;
#64941=CARTESIAN_POINT ( 'NONE',  ( -0.04068437667224348436, 22.21974360917720404, -6.396802510829702193 ) ) ;
#64942=CARTESIAN_POINT ( 'NONE',  ( 19.84674366389459266, 3.717264484334118713, -2.638427012816827677 ) ) ;
#64945=CARTESIAN_POINT ( 'NONE',  ( 4.559911319644449179, 13.89701867748817143, 9.422509992056141925 ) ) ;
#64946=CARTESIAN_POINT ( 'NONE',  ( 1.472469842513823179, 11.42559781766745175, 4.923371831947296329 ) ) ;
#64947=CARTESIAN_POINT ( 'NONE',  ( 19.42250999205614193, 60.14701867748817676, 5.440088680355555262 ) ) ;
#64948=CARTESIAN_POINT ( 'NONE',  ( 12.91533473730993009, 51.60535201082149825, -10.88017736071109987 ) ) ;
#64949=CARTESIAN_POINT ( 'NONE',  ( 2.035157376598824452, 13.68868534415483751, 7.964842623401179544 ) ) ;
#64950=CARTESIAN_POINT ( 'NONE',  ( 16.40814093676324603, 62.45696800326376064, -11.09922568453594671 ) ) ;
#64951=CARTESIAN_POINT ( 'NONE',  ( -0.3689425029237881626, 27.42874883491397142, 10.36894250292379027 ) ) ;
#64955=CARTESIAN_POINT ( 'NONE',  ( 16.40814093676324603, 57.45696800326375353, -11.09922568453594671 ) ) ;
#64957=CARTESIAN_POINT ( 'NONE',  ( 16.40814093676324603, 7.456968003263754419, -11.09922568453594671 ) ) ;
#64959=CARTESIAN_POINT ( 'NONE',  ( 4.559911319644449179, 33.89701867748817676, 9.422509992056141925 ) ) ;
#64963=CARTESIAN_POINT ( 'NONE',  ( 19.84674366389459266, 8.300597817667451750, 2.638427012816836559 ) ) ;
#64964=CARTESIAN_POINT ( 'NONE',  ( 7.361572987183170547, 7.050597817667451750, 9.846743663894590881 ) ) ;
#64965=CARTESIAN_POINT ( 'NONE',  ( 0.1532563361054083140, 21.00893115100078745, 1.131784320476157264E-15 ) ) ;
#64966=CARTESIAN_POINT ( 'NONE',  ( 12.63842701281683034, 12.46726448433411782, 9.846743663894596210 ) ) ;
#64967=CARTESIAN_POINT ( 'NONE',  ( 1.472469842513823179, 1.425597817667451528, 4.923371831947296329 ) ) ;
#64968=CARTESIAN_POINT ( 'NONE',  ( -0.8801773607111008646, 58.27201867748816966, 2.915334737309923430 ) ) ;
#64970=CARTESIAN_POINT ( 'NONE',  ( -45.94000000000000483, 93.00000000000000000, -9.500000000000000000 ) ) ;
#64971=CARTESIAN_POINT ( 'NONE',  ( 4.559911319644449179, 63.89701867748817676, 9.422509992056141925 ) ) ;
#64972=CARTESIAN_POINT ( 'NONE',  ( 2.791683348922237240, 25.38393115100078390, -7.208316651077763204 ) ) ;
#64974=AXIS2_PLACEMENT_3D ( 'NONE', #17123, #86592, #18101 ) ;
#64976=CARTESIAN_POINT ( 'NONE',  ( 7.361572987183170547, 57.05059781766744464, 9.846743663894590881 ) ) ;
#64979=CARTESIAN_POINT ( 'NONE',  ( 20.88017736071110875, 5.772018677488170546, -2.915334737309920765 ) ) ;
#64980=CARTESIAN_POINT ( 'NONE',  ( 10.00000000000000000, 25.55374883491396787, -14.16423886937410082 ) ) ;
#64982=CARTESIAN_POINT ( 'NONE',  ( -4.164238869374099927, 17.01208216824730357, 3.795296366450308767 ) ) ;
#64983=CARTESIAN_POINT ( 'NONE',  ( 6.204703633549690345, 30.76208216824730357, -14.16423886937410259 ) ) ;
#64984=CARTESIAN_POINT ( 'NONE',  ( 2.917880565312948704, 2.637082168247300906, 12.26659068614894643 ) ) ;
#64985=CARTESIAN_POINT ( 'NONE',  ( 17.96484262340118221, 31.18868534415483751, -7.964842623401177768 ) ) ;
#64986=CARTESIAN_POINT ( 'NONE',  ( 12.63842701281683922, 14.55059781766744997, -9.846743663894590881 ) ) ;
#64987=CARTESIAN_POINT ( 'NONE',  ( 4.559911319644449179, 57.23035201082150536, -9.422509992056141925 ) ) ;
#64988=CARTESIAN_POINT ( 'NONE',  ( 1.472469842513823179, 20.59226448433411960, -4.923371831947296329 ) ) ;
#64989=CARTESIAN_POINT ( 'NONE',  ( 19.42250999205614193, 15.14701867748817143, 5.440088680355555262 ) ) ;
#64990=CARTESIAN_POINT ( 'NONE',  ( -2.816281873526473856, 44.33196800326375353, 3.434112377981055619 ) ) ;
#64991=CARTESIAN_POINT ( 'NONE',  ( 5.076628168052704559, 50.17559781766745886, -8.527530157486179263 ) ) ;
#64994=CARTESIAN_POINT ( 'NONE',  ( 22.81628187352647785, 26.41530133659708923, 3.434112377981063169 ) ) ;
#64996=CARTESIAN_POINT ( 'NONE',  ( 17.20831665107776587, 32.88393115100078745, 7.208316651077764980 ) ) ;
#64997=CARTESIAN_POINT ( 'NONE',  ( 2.917880565312948704, 17.63708216824730357, 12.26659068614894643 ) ) ;
#64998=EDGE_LOOP ( 'NONE', ( #12333, #36044, #35365, #28580, #96826, #27422 ) ) ;
#65002=CARTESIAN_POINT ( 'NONE',  ( 19.42250999205614548, 45.98035201082150536, -5.440088680355545492 ) ) ;
#65003=CARTESIAN_POINT ( 'NONE',  ( 19.42250999205614193, 55.14701867748817676, 5.440088680355555262 ) ) ;
#65004=CARTESIAN_POINT ( 'NONE',  ( 20.36894250292379738, 49.92874883491396787, -10.36894250292379027 ) ) ;
#65005=CARTESIAN_POINT ( 'NONE',  ( 2.791683348922237240, 60.38393115100078745, -7.208316651077763204 ) ) ;
#65006=CARTESIAN_POINT ( 'NONE',  ( 2.791683348922240793, 11.63393115100078568, 7.208316651077764092 ) ) ;
#65007=CARTESIAN_POINT ( 'NONE',  ( 16.40814093676324603, 62.45696800326376064, -11.09922568453594671 ) ) ;
#65008=CARTESIAN_POINT ( 'NONE',  ( -0.8801773607110991993, 47.85535201082150536, -2.915334737309923874 ) ) ;
#65010=CARTESIAN_POINT ( 'NONE',  ( 10.00000000000000178, 52.25893115100078745, 9.846743663894594434 ) ) ;
#65013=ADVANCED_FACE ( 'NONE', ( #7202 ), #86549, .T. ) ;
#65014=CARTESIAN_POINT ( 'NONE',  ( 0.1089645850228953966, 13.16234555792570582, 6.479102184480805882 ) ) ;
#65015=( NAMED_UNIT ( * ) PLANE_ANGLE_UNIT ( ) SI_UNIT ( $, .RADIAN. ) );
#65017=CARTESIAN_POINT ( 'NONE',  ( 19.84674366389459266, 3.717264484334118713, -2.638427012816827677 ) ) ;
#65018=CARTESIAN_POINT ( 'NONE',  ( 0.1532563361054083140, 1.008931151000784787, 1.131784320476157264E-15 ) ) ;
#65021=CARTESIAN_POINT ( 'NONE',  ( 19.84674366389459621, 28.50893115100078745, 7.409399052514197653E-17 ) ) ;
#65022=CARTESIAN_POINT ( 'NONE',  ( 12.91533473730993009, 21.60535201082150536, -10.88017736071109987 ) ) ;
#65023=CARTESIAN_POINT ( 'NONE',  ( 0.1532563361054082862, 61.21726448433412315, 2.638427012816831674 ) ) ;
#65024=CARTESIAN_POINT ( 'NONE',  ( 2.035157376598822676, 37.43868534415484106, -7.964842623401177768 ) ) ;
#65025=CARTESIAN_POINT ( 'NONE',  ( 0.2751277870542909176, 60.30223176428830101, 6.499999999999992006 ) ) ;
#65027=CARTESIAN_POINT ( 'NONE',  ( 10.00000000000000000, 42.87363466993042493, -12.81628187352647608 ) ) ;
#65028=ORIENTED_EDGE ( 'NONE', *, *, #49476, .T. ) ;
#65029=CARTESIAN_POINT ( 'NONE',  ( 4.559911319644449179, 53.89701867748817676, 9.422509992056141925 ) ) ;
#65030=ADVANCED_FACE ( 'NONE', ( #92651 ), #73589, .T. ) ;
#65031=CARTESIAN_POINT ( 'NONE',  ( 22.81628187352648496, 16.83196800326374998, -3.434112377981050290 ) ) ;
#65033=CARTESIAN_POINT ( 'NONE',  ( 17.96484262340118221, 31.18868534415483751, -7.964842623401177768 ) ) ;
#65034=CARTESIAN_POINT ( 'NONE',  ( -0.3689425029237881626, 62.42874883491396787, 10.36894250292379027 ) ) ;
#65036=CARTESIAN_POINT ( 'NONE',  ( 17.20831665107776587, 49.13393115100078745, -7.208316651077762316 ) ) ;
#65037=CARTESIAN_POINT ( 'NONE',  ( 19.84674366389459266, 8.717264484334116048, -2.638427012816827677 ) ) ;
#65038=CARTESIAN_POINT ( 'NONE',  ( -0.8801773607111008646, 63.27201867748817676, 2.915334737309923430 ) ) ;
#65040=CARTESIAN_POINT ( 'NONE',  ( 24.16423886937409904, 34.09541550158064638, 3.795296366450317205 ) ) ;
#65047=CARTESIAN_POINT ( 'NONE',  ( 10.00000000000000000, 45.55374883491397497, -14.16423886937410082 ) ) ;
#65048=CARTESIAN_POINT ( 'NONE',  ( 24.16423886937410614, 49.30374883491396787, 8.672049930838204340E-16 ) ) ;
#65049=CARTESIAN_POINT ( 'NONE',  ( 1.472469842513823179, 16.42559781766745175, 4.923371831947296329 ) ) ;
#65050=CARTESIAN_POINT ( 'NONE',  ( 13.43411237798105340, 15.58196800326374998, 12.81628187352647963 ) ) ;
#65052=CARTESIAN_POINT ( 'NONE',  ( -32.19000000000001194, 93.50000000000000000, 9.500000000000000000 ) ) ;
#65053=FILL_AREA_STYLE_COLOUR ( '', #46728 ) ;
#65054=CARTESIAN_POINT ( 'NONE',  ( 19.38216949554541557, 52.24863466993041072, -9.382169495545420901 ) ) ;
#65055=CARTESIAN_POINT ( 'NONE',  ( -0.3689425029237881626, 47.42874883491396787, 10.36894250292379027 ) ) ;
#65057=CARTESIAN_POINT ( 'NONE',  ( 5.076628168052704559, 5.175597817667451750, -8.527530157486179263 ) ) ;
#65060=CARTESIAN_POINT ( 'NONE',  ( 0.000000000000000000, 0.000000000000000000, 6.500000000000000888 ) ) ;
#65061=CARTESIAN_POINT ( 'NONE',  ( 14.92337183194729988, 19.34226448433411960, -8.527530157486177487 ) ) ;
#65064=ORIENTED_EDGE ( 'NONE', *, *, #93966, .F. ) ;
#65065=CARTESIAN_POINT ( 'NONE',  ( -0.3689425029237898834, 11.17874883491396787, -10.36894250292378850 ) ) ;
#65066=CARTESIAN_POINT ( 'NONE',  ( 17.96484262340118221, 19.93868534415484106, 7.964842623401181321 ) ) ;
#65067=CARTESIAN_POINT ( 'NONE',  ( 15.44008868035555793, 31.39701867748817676, -9.422509992056140149 ) ) ;
#65068=CARTESIAN_POINT ( 'NONE',  ( 14.92337183194729633, 47.67559781766745175, 8.527530157486181039 ) ) ;
#65069=CARTESIAN_POINT ( 'NONE',  ( -2.816281873526473856, 4.123634669930420493, 9.499525473075851096E-16 ) ) ;
#65070=DIRECTION ( 'NONE',  ( 0.000000000000000000, -1.000000000000000000, 0.000000000000000000 ) ) ;
#65072=CARTESIAN_POINT ( 'NONE',  ( 16.40814093676323893, 20.79030133659708923, 11.09922568453595026 ) ) ;
#65073=ORIENTED_EDGE ( 'NONE', *, *, #77356, .T. ) ;
#65074=CARTESIAN_POINT ( 'NONE',  ( 0.1532563361054082862, 36.21726448433410894, 2.638427012816831674 ) ) ;
#65075=CARTESIAN_POINT ( 'NONE',  ( -0.3689425029237898834, 56.17874883491396076, -10.36894250292378850 ) ) ;
#65077=CARTESIAN_POINT ( 'NONE',  ( 17.08211943468705840, 50.13708216824730357, -12.26659068614894466 ) ) ;
#65079=CARTESIAN_POINT ( 'NONE',  ( 20.88017736071110875, 35.77201867748816966, -2.915334737309920765 ) ) ;
#65080=CARTESIAN_POINT ( 'NONE',  ( 15.44008868035555793, 46.39701867748817676, -9.422509992056140149 ) ) ;
#65082=CARTESIAN_POINT ( 'NONE',  ( 17.96484262340118221, 49.93868534415484106, 7.964842623401181321 ) ) ;
#65083=CARTESIAN_POINT ( 'NONE',  ( 19.89103541497711447, 5.662345557925709372, -6.479102184480793447 ) ) ;
#65084=CARTESIAN_POINT ( 'NONE',  ( 17.96484262340118221, 39.93868534415484106, 7.964842623401181321 ) ) ;
#65089=CARTESIAN_POINT ( 'NONE',  ( 7.361572987183169658, 19.96726448433411960, -9.846743663894592657 ) ) ;
#65090=ORIENTED_EDGE ( 'NONE', *, *, #34635, .T. ) ;
#65092=CARTESIAN_POINT ( 'NONE',  ( 10.00000000000000178, 57.25893115100078745, 9.846743663894594434 ) ) ;
#65093=CARTESIAN_POINT ( 'NONE',  ( -39.69000000000001194, 92.00000000000000000, 9.500000000000000000 ) ) ;
#65094=CARTESIAN_POINT ( 'NONE',  ( 16.40814093676323893, 50.79030133659708923, 11.09922568453595026 ) ) ;
#65096=FACE_OUTER_BOUND ( 'NONE', #31100, .T. ) ;
#65102=CARTESIAN_POINT ( 'NONE',  ( 12.63842701281683034, 27.46726448433411250, 9.846743663894596210 ) ) ;
#65103=CARTESIAN_POINT ( 'NONE',  ( -2.266590686148945544, 66.38708216824730357, -7.082119434687050408 ) ) ;
#65106=DIRECTION ( 'NONE',  ( -1.000000000000000000, 0.000000000000000000, 0.000000000000000000 ) ) ;
#65107=CARTESIAN_POINT ( 'NONE',  ( 14.92337183194729633, 32.67559781766745175, 8.527530157486181039 ) ) ;
#65108=CARTESIAN_POINT ( 'NONE',  ( 22.81628187352647785, 1.415301336597087012, 3.434112377981063169 ) ) ;
#65109=CARTESIAN_POINT ( 'NONE',  ( 2.035157376598822676, 67.43868534415484817, -7.964842623401177768 ) ) ;
#65112=EDGE_CURVE ( 'NONE', #16145, #17262, #44086, .T. ) ;
#65113=CARTESIAN_POINT ( 'NONE',  ( 19.84674366389459621, 8.508931151000785675, 7.409399052514197653E-17 ) ) ;
#65114=CARTESIAN_POINT ( 'NONE',  ( 12.63842701281683034, 62.46726448433410894, 9.846743663894596210 ) ) ;
#65116=CARTESIAN_POINT ( 'NONE',  ( 2.602085213965210642E-15, 78.91966277462714174, 9.500000000000000000 ) ) ;
#65120=CARTESIAN_POINT ( 'NONE',  ( 19.42250999205614193, 15.14701867748817143, 5.440088680355555262 ) ) ;
#65121=CARTESIAN_POINT ( 'NONE',  ( -2.266590686148945544, 2.220415501580634388, 7.082119434687048631 ) ) ;
#65122=CARTESIAN_POINT ( 'NONE',  ( 7.361572987183170547, 12.05059781766744997, 9.846743663894590881 ) ) ;
#65123=CARTESIAN_POINT ( 'NONE',  ( 12.91533473730992121, 44.52201867748816966, 10.88017736071110164 ) ) ;
#65124=CARTESIAN_POINT ( 'NONE',  ( 19.38216949554541202, 30.99863466993042138, 9.382169495545424454 ) ) ;
#65126=CARTESIAN_POINT ( 'NONE',  ( -0.8801773607110991993, 7.855352010821504471, -2.915334737309923874 ) ) ;
#65129=CARTESIAN_POINT ( 'NONE',  ( 1.472469842513823179, 46.42559781766745175, 4.923371831947296329 ) ) ;
#65130=CARTESIAN_POINT ( 'NONE',  ( 19.84674366389459266, 18.71726448433411960, -2.638427012816827677 ) ) ;
#65132=CARTESIAN_POINT ( 'NONE',  ( 21.09922568453595559, 27.04030133659708568, -6.408140936763230044 ) ) ;
#65134=CARTESIAN_POINT ( 'NONE',  ( 2.035157376598822676, 32.43868534415483396, -7.964842623401177768 ) ) ;
#65137=CARTESIAN_POINT ( 'NONE',  ( 22.26659068614894466, 43.88708216824729647, 7.082119434687054849 ) ) ;
#65138=LINE ( 'NONE', #59119, #11382 ) ;
#65139=CARTESIAN_POINT ( 'NONE',  ( 18.52753015748617571, 43.09226448433412315, 4.923371831947298993 ) ) ;
#65140=CARTESIAN_POINT ( 'NONE',  ( 6.565887622018943937, 33.08196800326374643, -12.81628187352647608 ) ) ;
#65141=CARTESIAN_POINT ( 'NONE',  ( 4.559911319644449179, 22.23035201082150536, -9.422509992056141925 ) ) ;
#65142=CARTESIAN_POINT ( 'NONE',  ( 14.92337183194729633, 57.67559781766745886, 8.527530157486181039 ) ) ;
#65144=CARTESIAN_POINT ( 'NONE',  ( 7.084665262690076126, 52.02201867748816255, -10.88017736071110164 ) ) ;
#65145=CARTESIAN_POINT ( 'NONE',  ( 19.38216949554541557, 2.248634669930420049, -9.382169495545420901 ) ) ;
#65146=CARTESIAN_POINT ( 'NONE',  ( 20.36894250292379738, 29.92874883491396432, -10.36894250292379027 ) ) ;
#65149=CARTESIAN_POINT ( 'NONE',  ( 5.076628168052704559, 30.17559781766745175, -8.527530157486179263 ) ) ;
#65150=CARTESIAN_POINT ( 'NONE',  ( 3.591859063236761518, 64.95696800326376774, 11.09922568453594849 ) ) ;
#65151=CARTESIAN_POINT ( 'NONE',  ( -2.816281873526471635, -1.084698663402913210, -3.434112377981056508 ) ) ;
#65154=CARTESIAN_POINT ( 'NONE',  ( 21.92686044187656336, 6.979976035794174472, 3.195792623639536423 ) ) ;
#65155=CARTESIAN_POINT ( 'NONE',  ( -0.8801773607110991993, 7.855352010821506248, -2.915334737309923874 ) ) ;
#65156=CARTESIAN_POINT ( 'NONE',  ( 15.44008868035555793, 61.39701867748817676, -9.422509992056140149 ) ) ;
#65157=CARTESIAN_POINT ( 'NONE',  ( 10.00000000000000178, 23.05374883491397142, 14.16423886937410082 ) ) ;
#65159=CARTESIAN_POINT ( 'NONE',  ( 19.42250999205614548, 65.98035201082151957, -5.440088680355545492 ) ) ;
#65160=CARTESIAN_POINT ( 'NONE',  ( 18.52753015748618282, 43.92559781766745175, -4.923371831947291888 ) ) ;
#65161=CARTESIAN_POINT ( 'NONE',  ( -0.8801773607110991993, 27.85535201082150181, -2.915334737309923874 ) ) ;
#65162=CARTESIAN_POINT ( 'NONE',  ( 0.8801356535991349261, 124.4373638429518962, 5.000000000000000000 ) ) ;
#65169=LINE ( 'NONE', #42684, #83689 ) ;
#65170=CARTESIAN_POINT ( 'NONE',  ( -2.266590686148945544, 11.38708216824730179, -7.082119434687050408 ) ) ;
#65171=CARTESIAN_POINT ( 'NONE',  ( -0.3689425029237898834, 16.17874883491396076, -10.36894250292378850 ) ) ;
#65172=CARTESIAN_POINT ( 'NONE',  ( 4.559911319644449179, 48.89701867748817676, 9.422509992056141925 ) ) ;
#65173=CARTESIAN_POINT ( 'NONE',  ( 13.79529636645030344, 58.26208216824728936, 14.16423886937410614 ) ) ;
#65174=CARTESIAN_POINT ( 'NONE',  ( 5.076628168052704559, 60.17559781766745175, -8.527530157486179263 ) ) ;
#65175=CARTESIAN_POINT ( 'NONE',  ( 0.1532563361054100626, 35.80059781766745175, -2.638427012816831230 ) ) ;
#65176=CARTESIAN_POINT ( 'NONE',  ( 17.96484262340118221, 31.18868534415483751, -7.964842623401177768 ) ) ;
#65177=CARTESIAN_POINT ( 'NONE',  ( 0.1532563361054083140, 56.00893115100078745, 1.131784320476157264E-15 ) ) ;
#65178=CARTESIAN_POINT ( 'NONE',  ( 20.36894250292379382, 48.67874883491396076, 10.36894250292379205 ) ) ;
#65179=CARTESIAN_POINT ( 'NONE',  ( -0.3689425029237881626, 67.42874883491396076, 10.36894250292379027 ) ) ;
#65180=CARTESIAN_POINT ( 'NONE',  ( 19.89220837332776171, 14.74062864464239375, 6.478736007405961672 ) ) ;
#65187=CARTESIAN_POINT ( 'NONE',  ( 2.791683348922237240, 25.38393115100078390, -7.208316651077763204 ) ) ;
#65189=CARTESIAN_POINT ( 'NONE',  ( 22.26659068614895176, 29.72041550158063572, -7.082119434687042414 ) ) ;
#65190=CARTESIAN_POINT ( 'NONE',  ( 10.00000000000000000, 29.75893115100078745, -9.846743663894594434 ) ) ;
#65191=CARTESIAN_POINT ( 'NONE',  ( 15.44008868035555793, 56.39701867748817676, -9.422509992056140149 ) ) ;
#65195=CARTESIAN_POINT ( 'NONE',  ( 20.88017736071110875, 55.77201867748816966, -2.915334737309920765 ) ) ;
#65198=CARTESIAN_POINT ( 'NONE',  ( 7.084665262690076126, 49.10535201082149825, 10.88017736071109987 ) ) ;
#65199=CARTESIAN_POINT ( 'NONE',  ( 10.00000000000000178, 18.05374883491396787, 14.16423886937410082 ) ) ;
#65201=EDGE_LOOP ( 'NONE', ( #28920, #25057, #60780, #90470 ) ) ;
#65202=CARTESIAN_POINT ( 'NONE',  ( -1.099225684535947600, 49.54030133659708923, 6.408140936763237150 ) ) ;
#65203=CARTESIAN_POINT ( 'NONE',  ( 20.88017736071110519, 20.56368534415484106, 2.639326808657452039E-16 ) ) ;
#65204=B_SPLINE_CURVE_WITH_KNOTS ( 'NONE', 3,
 ( #57718, #73211, #13211, #13711 ),
 .UNSPECIFIED., .F., .F.,
 ( 4, 4 ),
 ( 0.000000000000000000, 0.002657014572711316816 ),
 .UNSPECIFIED. ) ;
#65205=CARTESIAN_POINT ( 'NONE',  ( 7.361572987183169658, 19.96726448433411960, -9.846743663894592657 ) ) ;
#65206=CARTESIAN_POINT ( 'NONE',  ( 12.91533473730992121, 19.52201867748816611, 10.88017736071110164 ) ) ;
#65207=CARTESIAN_POINT ( 'NONE',  ( 22.81628187352647785, 51.62363466993042493, 6.195893100308588602E-16 ) ) ;
#65208=CARTESIAN_POINT ( 'NONE',  ( -46.43544119129187209, 103.9441758960464028, -5.610234333949387420 ) ) ;
#65209=CARTESIAN_POINT ( 'NONE',  ( 0.1532563361054083140, 36.00893115100078745, 1.131784320476157264E-15 ) ) ;
#65215=CARTESIAN_POINT ( 'NONE',  ( 18.52753015748617571, 8.092264484334117824, 4.923371831947298993 ) ) ;
#65216=CARTESIAN_POINT ( 'NONE',  ( -2.816281873526471635, 23.91530133659708568, -3.434112377981056508 ) ) ;
#65217=CARTESIAN_POINT ( 'NONE',  ( 17.20831665107776587, 37.88393115100078745, 7.208316651077764980 ) ) ;
#65219=CARTESIAN_POINT ( 'NONE',  ( 13.79529636645031943, 25.34541550158063572, -14.16423886937409904 ) ) ;
#65220=CARTESIAN_POINT ( 'NONE',  ( 10.00000000000000178, 27.25893115100078390, 9.846743663894594434 ) ) ;
#65221=CARTESIAN_POINT ( 'NONE',  ( 3.591859063236761518, 34.95696800326375353, 11.09922568453594849 ) ) ;
#65222=CARTESIAN_POINT ( 'NONE',  ( 18.29284471827482150, 15.40189080397285259, -6.499999999999984901 ) ) ;
#65224=CARTESIAN_POINT ( 'NONE',  ( 12.91533473730993009, 56.60535201082151247, -10.88017736071109987 ) ) ;
#65226=CARTESIAN_POINT ( 'NONE',  ( 22.81628187352647785, 1.415301336597087012, 3.434112377981063169 ) ) ;
#65228=CARTESIAN_POINT ( 'NONE',  ( 0.1532563361054082862, 31.21726448433412315, 2.638427012816831674 ) ) ;
#65229=CARTESIAN_POINT ( 'NONE',  ( 17.96484262340118221, 29.93868534415484106, 7.964842623401181321 ) ) ;
#65230=CARTESIAN_POINT ( 'NONE',  ( -2.816281873526473856, 29.12363466993041783, 9.499525473075851096E-16 ) ) ;
#65233=ADVANCED_FACE ( 'NONE', ( #66607 ), #29574, .T. ) ;
#65234=CARTESIAN_POINT ( 'NONE',  ( 20.88017736071110164, 30.35535201082151247, 2.915334737309930979 ) ) ;
#65237=CARTESIAN_POINT ( 'NONE',  ( -0.8801773607111009756, 3.063685344154837509, 1.068504757029289695E-15 ) ) ;
#65238=CARTESIAN_POINT ( 'NONE',  ( 14.92337183194729988, 54.34226448433412315, -8.527530157486177487 ) ) ;
#65239=CARTESIAN_POINT ( 'NONE',  ( 0.5774900079438607392, 33.48035201082150536, 5.440088680355550821 ) ) ;
#65241=CARTESIAN_POINT ( 'NONE',  ( 17.96484262340118221, 61.18868534415482685, -7.964842623401177768 ) ) ;
#65243=CARTESIAN_POINT ( 'NONE',  ( -0.8801773607111009756, 28.06368534415484106, 1.068504757029289695E-15 ) ) ;
#65244=CARTESIAN_POINT ( 'NONE',  ( -0.000000000000000000, 78.34227958332743924, -8.952513576680836138 ) ) ;
#65245=CARTESIAN_POINT ( 'NONE',  ( 1.472469842513823179, 5.592264484334118713, -4.923371831947296329 ) ) ;
#65247=CARTESIAN_POINT ( 'NONE',  ( 1.472469842513823179, 46.42559781766745175, 4.923371831947296329 ) ) ;
#65248=CARTESIAN_POINT ( 'NONE',  ( -4.164238869374099039, 51.80374883491396787, 8.674139862899312516E-16 ) ) ;
#65250=CARTESIAN_POINT ( 'NONE',  ( 20.36894250292379738, 14.92874883491396432, -10.36894250292379027 ) ) ;
#65252=CARTESIAN_POINT ( 'NONE',  ( -0.3689425029237881626, 32.42874883491395366, 10.36894250292379027 ) ) ;
#65253=CARTESIAN_POINT ( 'NONE',  ( -2.816281873526473856, -0.8763653300695799508, 9.499525473075851096E-16 ) ) ;
#65256=CARTESIAN_POINT ( 'NONE',  ( 2.917880565312948704, 62.63708216824730357, 12.26659068614894643 ) ) ;
#65257=CARTESIAN_POINT ( 'NONE',  ( 14.92337183194729988, 39.34226448433412315, -8.527530157486177487 ) ) ;
#65259=CARTESIAN_POINT ( 'NONE',  ( 15.44008868035555260, 59.73035201082151247, 9.422509992056143702 ) ) ;
#65261=CARTESIAN_POINT ( 'NONE',  ( -1.099225684535947600, 58.70696800326375353, -6.408140936763238038 ) ) ;
#65262=CARTESIAN_POINT ( 'NONE',  ( 13.43411237798105340, 30.58196800326374998, 12.81628187352647963 ) ) ;
#65263=CARTESIAN_POINT ( 'NONE',  ( 7.361572987183170547, 27.05059781766745175, 9.846743663894590881 ) ) ;
#65264=ORIENTED_EDGE ( 'NONE', *, *, #69675, .F. ) ;
#65265=CARTESIAN_POINT ( 'NONE',  ( 0.1532563361054082862, 1.217264484334117824, 2.638427012816831674 ) ) ;
#65267=CARTESIAN_POINT ( 'NONE',  ( 18.72515096720569971, 5.055090184799359676, 6.500000000000000000 ) ) ;
#65268=CARTESIAN_POINT ( 'NONE',  ( 10.00000000000000178, 4.313685344154837509, 10.88017736071110342 ) ) ;
#65269=CARTESIAN_POINT ( 'NONE',  ( -0.8801773607110991993, 17.85535201082150536, -2.915334737309923874 ) ) ;
#65270=CARTESIAN_POINT ( 'NONE',  ( 6.204703633549690345, 42.84541550158063217, 14.16423886937410082 ) ) ;
#65271=CARTESIAN_POINT ( 'NONE',  ( 4.559911319644449179, 32.23035201082150536, -9.422509992056141925 ) ) ;
#65272=CARTESIAN_POINT ( 'NONE',  ( 7.084665262690076126, 69.10535201082151957, 10.88017736071109987 ) ) ;
#65275=CARTESIAN_POINT ( 'NONE',  ( 5.076628168052704559, 5.175597817667451750, -8.527530157486179263 ) ) ;
#65278=CARTESIAN_POINT ( 'NONE',  ( 0.1532563361054083140, 36.00893115100078745, 1.131784320476157264E-15 ) ) ;
#65279=CARTESIAN_POINT ( 'NONE',  ( 0.6178305044545818747, -1.501365330069579951, -9.382169495545419124 ) ) ;
#65281=CARTESIAN_POINT ( 'NONE',  ( 19.42250999205614193, 25.14701867748817321, 5.440088680355555262 ) ) ;
#65282=B_SPLINE_CURVE_WITH_KNOTS ( 'NONE', 3,
 ( #51182, #81664, #65180, #5692, #28059, #20576 ),
 .UNSPECIFIED., .F., .F.,
 ( 4, 2, 4 ),
 ( 0.000000000000000000, 0.0002565770811490966858, 0.0005131541622981933715 ),
 .UNSPECIFIED. ) ;
#65285=CARTESIAN_POINT ( 'NONE',  ( 21.09922568453595559, 52.04030133659708923, -6.408140936763230044 ) ) ;
#65287=CARTESIAN_POINT ( 'NONE',  ( 10.00000000000000178, 69.31368534415484817, 10.88017736071110342 ) ) ;
#65288=CARTESIAN_POINT ( 'NONE',  ( 12.63842701281683922, 24.55059781766745175, -9.846743663894590881 ) ) ;
#65289=CARTESIAN_POINT ( 'NONE',  ( 20.36894250292379738, 64.92874883491397497, -10.36894250292379027 ) ) ;
#65290=CARTESIAN_POINT ( 'NONE',  ( 14.92337183194729633, 22.67559781766745175, 8.527530157486181039 ) ) ;
#65292=LINE ( 'NONE', #80808, #15177 ) ;
#65293=CARTESIAN_POINT ( 'NONE',  ( 13.79529636645030344, 28.26208216824729647, 14.16423886937410614 ) ) ;
#65294=CARTESIAN_POINT ( 'NONE',  ( 12.63842701281683034, 37.46726448433411605, 9.846743663894596210 ) ) ;
#65296=CARTESIAN_POINT ( 'NONE',  ( -0.8801773607110991993, 27.85535201082150181, -2.915334737309923874 ) ) ;
#65297=CARTESIAN_POINT ( 'NONE',  ( 15.44008868035555260, 64.73035201082151957, 9.422509992056143702 ) ) ;
#65300=VERTEX_POINT ( 'NONE', #14617 ) ;
#65301=CARTESIAN_POINT ( 'NONE',  ( -2.816281873526473856, 44.33196800326375353, 3.434112377981055619 ) ) ;
#65302=CARTESIAN_POINT ( 'NONE',  ( -0.8801773607110991993, 52.85535201082151247, -2.915334737309923874 ) ) ;
#65304=CARTESIAN_POINT ( 'NONE',  ( 18.04007052943771683, 63.01528370094808196, 5.767676674365856293 ) ) ;
#65308=CARTESIAN_POINT ( 'NONE',  ( 10.00000000000000178, 69.31368534415484817, 10.88017736071110342 ) ) ;
#65309=CARTESIAN_POINT ( 'NONE',  ( 19.42250999205614193, 10.14701867748816966, 5.440088680355555262 ) ) ;
#65310=CARTESIAN_POINT ( 'NONE',  ( 0.2751277870542969683, 2.282175860852373894, -6.500000000000000888 ) ) ;
#65311=CARTESIAN_POINT ( 'NONE',  ( 0.2751277870542967463, 70.00000000000000000, 6.000000000000000000 ) ) ;
#65312=CARTESIAN_POINT ( 'NONE',  ( 19.42250999205614193, 5.147018677488171434, 5.440088680355555262 ) ) ;
#65313=CARTESIAN_POINT ( 'NONE',  ( 7.361572987183170547, 7.050597817667451750, 9.846743663894590881 ) ) ;
#65314=CARTESIAN_POINT ( 'NONE',  ( 13.79529636645031943, 15.34541550158063750, -14.16423886937409904 ) ) ;
#65315=CARTESIAN_POINT ( 'NONE',  ( 19.42250999205614548, 25.98035201082150891, -5.440088680355545492 ) ) ;
#65316=CARTESIAN_POINT ( 'NONE',  ( 19.84674366389459621, 58.50893115100078745, 7.409399052514197653E-17 ) ) ;
#65318=B_SPLINE_CURVE_WITH_KNOTS ( 'NONE', 3,
 ( #45964, #76453, #7969, #38953, #38467, #23955 ),
 .UNSPECIFIED., .F., .F.,
 ( 4, 2, 4 ),
 ( 0.000000000000000000, 0.0002565770811490986915, 0.0005131541622981973831 ),
 .UNSPECIFIED. ) ;
#65319=CARTESIAN_POINT ( 'NONE',  ( 7.361572987183169658, 54.96726448433413026, -9.846743663894592657 ) ) ;
#65320=ORIENTED_EDGE ( 'NONE', *, *, #75170, .T. ) ;
#65322=ADVANCED_FACE ( 'NONE', ( #20619 ), #43112, .T. ) ;
#65323=CARTESIAN_POINT ( 'NONE',  ( 12.91533473730992121, 54.52201867748816255, 10.88017736071110164 ) ) ;
#65325=CARTESIAN_POINT ( 'NONE',  ( 21.09922568453595559, 37.04030133659708923, -6.408140936763230044 ) ) ;
#65326=CARTESIAN_POINT ( 'NONE',  ( 2.035157376598824452, 8.688685344154839285, 7.964842623401179544 ) ) ;
#65328=CARTESIAN_POINT ( 'NONE',  ( 4.559911319644449179, 63.89701867748817676, 9.422509992056141925 ) ) ;
#65329=CARTESIAN_POINT ( 'NONE',  ( 4.559911319644449179, 8.897018677488173211, 9.422509992056141925 ) ) ;
#65330=ADVANCED_FACE ( 'NONE', ( #74090 ), #39164, .T. ) ;
#65331=STYLED_ITEM ( 'NONE', ( #98074 ), #60430 ) ;
#65332=CARTESIAN_POINT ( 'NONE',  ( 19.38216949554541557, 47.24863466993041783, -9.382169495545420901 ) ) ;
#65333=CARTESIAN_POINT ( 'NONE',  ( 2.035157376598822676, 27.43868534415483396, -7.964842623401177768 ) ) ;
#65336=CARTESIAN_POINT ( 'NONE',  ( -1.099225684535947600, 43.70696800326375353, -6.408140936763238038 ) ) ;
#65337=CARTESIAN_POINT ( 'NONE',  ( 15.44008868035555260, 29.73035201082150891, 9.422509992056143702 ) ) ;
#65338=CARTESIAN_POINT ( 'NONE',  ( 2.791683348922237240, 50.38393115100078035, -7.208316651077763204 ) ) ;
#65341=CARTESIAN_POINT ( 'NONE',  ( 12.63842701281683922, 59.55059781766744464, -9.846743663894590881 ) ) ;
#65342=CARTESIAN_POINT ( 'NONE',  ( 19.72487221294570858, 70.00000000000000000, 6.000000000000000000 ) ) ;
#65343=CARTESIAN_POINT ( 'NONE',  ( 2.791683348922237240, 55.38393115100078745, -7.208316651077763204 ) ) ;
#65344=CARTESIAN_POINT ( 'NONE',  ( -0.8801773607111009756, 18.06368534415484106, 1.068504757029289695E-15 ) ) ;
#65345=CARTESIAN_POINT ( 'NONE',  ( 17.20831665107776587, 39.13393115100079456, -7.208316651077762316 ) ) ;
#65348=VECTOR ( 'NONE', #53496, 1000.000000000000000 ) ;
#65349=CARTESIAN_POINT ( 'NONE',  ( 0.1532563361054083140, 36.00893115100078745, 1.131784320476157264E-15 ) ) ;
#65350=CARTESIAN_POINT ( 'NONE',  ( 19.84674366389459266, 8.717264484334116048, -2.638427012816827677 ) ) ;
#65351=CARTESIAN_POINT ( 'NONE',  ( 1.472469842513823179, 0.5922644843341181575, -4.923371831947296329 ) ) ;
#65352=CARTESIAN_POINT ( 'NONE',  ( 7.361572987183169658, 59.96726448433410894, -9.846743663894592657 ) ) ;
#65353=ORIENTED_EDGE ( 'NONE', *, *, #36355, .F. ) ;
#65355=ADVANCED_FACE ( 'NONE', ( #47457 ), #1512, .T. ) ;
#65356=CARTESIAN_POINT ( 'NONE',  ( 3.591859063236761518, 39.95696800326375353, 11.09922568453594849 ) ) ;
#65357=CARTESIAN_POINT ( 'NONE',  ( 7.361572987183169658, 39.96726448433411605, -9.846743663894592657 ) ) ;
#65359=CARTESIAN_POINT ( 'NONE',  ( 10.00000000000000178, 53.05374883491396787, 14.16423886937410082 ) ) ;
#65360=CARTESIAN_POINT ( 'NONE',  ( 19.84674366389459621, 38.50893115100078745, 7.409399052514197653E-17 ) ) ;
#65361=ADVANCED_FACE ( 'NONE', ( #56923 ), #4926, .T. ) ;
#65362=CARTESIAN_POINT ( 'NONE',  ( -0.2418659066527637791, 40.11633188102327097, 6.114288769123057854 ) ) ;
#65363=CARTESIAN_POINT ( 'NONE',  ( 2.917880565312948704, 57.63708216824731068, 12.26659068614894643 ) ) ;
#65365=CARTESIAN_POINT ( 'NONE',  ( 20.88017736071110875, 5.772018677488170546, -2.915334737309920765 ) ) ;
#65366=CARTESIAN_POINT ( 'NONE',  ( 17.08211943468705840, 40.13708216824731068, -12.26659068614894466 ) ) ;
#65367=CARTESIAN_POINT ( 'NONE',  ( -0.3689425029237881626, 47.42874883491396787, 10.36894250292379027 ) ) ;
#65368=CYLINDRICAL_SURFACE ( 'NONE', #54168, 0.5000000000000004441 ) ;
#65370=CARTESIAN_POINT ( 'NONE',  ( 19.84674366389459266, 8.717264484334116048, -2.638427012816827677 ) ) ;
#65371=CARTESIAN_POINT ( 'NONE',  ( 0.8952175423694923584, 28.52576239577082262, 5.990408912944333863 ) ) ;
#65372=CARTESIAN_POINT ( 'NONE',  ( 19.38216949554541202, 0.9986346699304200492, 9.382169495545424454 ) ) ;
#65374=CARTESIAN_POINT ( 'NONE',  ( 4.559911319644449179, 53.89701867748817676, 9.422509992056141925 ) ) ;
#65375=CARTESIAN_POINT ( 'NONE',  ( -0.1038446121089043328, 64.24302437010796041, -6.337995344473781323 ) ) ;
#65376=CARTESIAN_POINT ( 'NONE',  ( 17.20831665107776587, 47.88393115100078745, 7.208316651077764980 ) ) ;
#65377=CARTESIAN_POINT ( 'NONE',  ( -46.93999999999855532, 100.4992147295316585, -9.114672001458391293 ) ) ;
#65378=CARTESIAN_POINT ( 'NONE',  ( 17.20831665107776587, 49.13393115100078745, -7.208316651077762316 ) ) ;
#65379=CARTESIAN_POINT ( 'NONE',  ( -0.3689425029237898834, 1.178748834913967869, -10.36894250292378850 ) ) ;
#65381=CARTESIAN_POINT ( 'NONE',  ( 22.26659068614895176, 29.72041550158063572, -7.082119434687042414 ) ) ;
#65383=SURFACE_SIDE_STYLE ('',( #41931 ) ) ;
#65384=CARTESIAN_POINT ( 'NONE',  ( 19.72487221294571569, 19.78217586085237301, 6.499999999999990230 ) ) ;
#65385=PLANE ( 'NONE',  #91782 ) ;
#65386=CARTESIAN_POINT ( 'NONE',  ( 20.88017736071110164, 15.35535201082150358, 2.915334737309930979 ) ) ;
#65387=CARTESIAN_POINT ( 'NONE',  ( -1.099225684535947600, 34.54030133659708923, 6.408140936763237150 ) ) ;
#65388=CARTESIAN_POINT ( 'NONE',  ( 20.15039907845753575, 62.62777174578612716, -6.262539305110073506 ) ) ;
#65389=CARTESIAN_POINT ( 'NONE',  ( 5.076628168052703671, 11.84226448433411960, 8.527530157486179263 ) ) ;
#65394=CARTESIAN_POINT ( 'NONE',  ( 10.00000000000000178, 28.05374883491396787, 14.16423886937410082 ) ) ;
#65395=CARTESIAN_POINT ( 'NONE',  ( 1.959929470562123965, 21.50257860105346808, 5.767676674365579181 ) ) ;
#65397=CARTESIAN_POINT ( 'NONE',  ( 0.5774900079438607392, 8.480352010821505360, 5.440088680355550821 ) ) ;
#65400=CARTESIAN_POINT ( 'NONE',  ( 0.5774900079438590739, 42.64701867748816966, -5.440088680355550821 ) ) ;
#65401=CARTESIAN_POINT ( 'NONE',  ( 7.084665262690076126, 54.10535201082151247, 10.88017736071109987 ) ) ;
#65402=CARTESIAN_POINT ( 'NONE',  ( 13.43411237798106583, 17.66530133659708923, -12.81628187352647252 ) ) ;
#65403=FACE_OUTER_BOUND ( 'NONE', #64484, .T. ) ;
#65405=CARTESIAN_POINT ( 'NONE',  ( 1.472469842513823179, 5.592264484334118713, -4.923371831947296329 ) ) ;
#65408=CARTESIAN_POINT ( 'NONE',  ( 4.559911319644449179, 47.23035201082150536, -9.422509992056141925 ) ) ;
#65409=CARTESIAN_POINT ( 'NONE',  ( 22.81628187352647785, 1.415301336597087012, 3.434112377981063169 ) ) ;
#65410=CARTESIAN_POINT ( 'NONE',  ( 2.035157376598822676, 62.43868534415483396, -7.964842623401177768 ) ) ;
#65411=CARTESIAN_POINT ( 'NONE',  ( 0.1532563361054082862, 21.21726448433412315, 2.638427012816831674 ) ) ;
#65412=CARTESIAN_POINT ( 'NONE',  ( 6.565887622018943937, 50.16530133659708213, 12.81628187352647430 ) ) ;
#65413=CARTESIAN_POINT ( 'NONE',  ( 18.52753015748618282, 8.925597817667451750, -4.923371831947291888 ) ) ;
#65415=CARTESIAN_POINT ( 'NONE',  ( 1.932340009482164778, 56.49127512925449679, -6.500000000000043521 ) ) ;
#65417=CARTESIAN_POINT ( 'NONE',  ( 2.035157376598824452, 18.68868534415484106, 7.964842623401179544 ) ) ;
#65418=CARTESIAN_POINT ( 'NONE',  ( -2.816281873526473856, 64.12363466993042493, 9.499525473075851096E-16 ) ) ;
#65419=CARTESIAN_POINT ( 'NONE',  ( 13.79529636645031943, 20.34541550158063572, -14.16423886937409904 ) ) ;
#65420=CARTESIAN_POINT ( 'NONE',  ( 5.076628168052703671, 36.84226448433412315, 8.527530157486179263 ) ) ;
#65422=CARTESIAN_POINT ( 'NONE',  ( 7.084665262690076126, 17.02201867748817676, -10.88017736071110164 ) ) ;
#65423=CARTESIAN_POINT ( 'NONE',  ( 19.42250999205614193, 5.147018677488171434, 5.440088680355555262 ) ) ;
#65425=CARTESIAN_POINT ( 'NONE',  ( 20.88017736071110875, 15.77201867748817143, -2.915334737309920765 ) ) ;
#65426=VECTOR ( 'NONE', #98219, 1000.000000000000000 ) ;
#65427=CARTESIAN_POINT ( 'NONE',  ( 12.91533473730993009, 36.60535201082151247, -10.88017736071109987 ) ) ;
#65428=DIRECTION ( 'NONE',  ( 0.000000000000000000, 0.000000000000000000, 1.000000000000000000 ) ) ;
#65429=CARTESIAN_POINT ( 'NONE',  ( 7.084665262690076126, 24.10535201082150181, 10.88017736071109987 ) ) ;
#65431=CARTESIAN_POINT ( 'NONE',  ( 20.24186590665275887, 10.59014588040357374, -6.114288769123074729 ) ) ;
#65432=CARTESIAN_POINT ( 'NONE',  ( 4.559911319644449179, 22.23035201082150536, -9.422509992056141925 ) ) ;
#65433=CARTESIAN_POINT ( 'NONE',  ( 13.99999999999999822, 61.00000000000000711, 5.000000000000000000 ) ) ;
#65435=CARTESIAN_POINT ( 'NONE',  ( 16.40814093676324603, 62.45696800326376064, -11.09922568453594671 ) ) ;
#65436=CARTESIAN_POINT ( 'NONE',  ( 0.5774900079438607392, 68.48035201082150536, 5.440088680355550821 ) ) ;
#65437=CARTESIAN_POINT ( 'NONE',  ( -0.3689425029237881626, 37.42874883491396787, 10.36894250292379027 ) ) ;
#65438=CARTESIAN_POINT ( 'NONE',  ( 20.88017736071110875, 35.77201867748816966, -2.915334737309920765 ) ) ;
#65439=CARTESIAN_POINT ( 'NONE',  ( -0.8801773607111008646, 23.27201867748817676, 2.915334737309923430 ) ) ;
#65441=CARTESIAN_POINT ( 'NONE',  ( 19.39188664607695500, 60.83703382326399378, -6.499999999999968026 ) ) ;
#65442=CARTESIAN_POINT ( 'NONE',  ( 7.361572987183170547, 52.05059781766745175, 9.846743663894590881 ) ) ;
#65444=CARTESIAN_POINT ( 'NONE',  ( 7.361572987183169658, 24.96726448433412315, -9.846743663894592657 ) ) ;
#65447=CARTESIAN_POINT ( 'NONE',  ( 4.559911319644449179, 12.23035201082150536, -9.422509992056141925 ) ) ;
#65448=CARTESIAN_POINT ( 'NONE',  ( 19.84674366389459621, 13.50893115100078568, 7.409399052514197653E-17 ) ) ;
#65449=CARTESIAN_POINT ( 'NONE',  ( 10.00000000000000178, 54.31368534415484106, 10.88017736071110342 ) ) ;
#65450=CARTESIAN_POINT ( 'NONE',  ( -0.8801773607111008646, 13.27201867748817143, 2.915334737309923430 ) ) ;
#65451=CARTESIAN_POINT ( 'NONE',  ( 16.40814093676323893, 55.79030133659708923, 11.09922568453595026 ) ) ;
#65452=CARTESIAN_POINT ( 'NONE',  ( 6.204703633549690345, 27.84541550158063217, 14.16423886937410082 ) ) ;
#65457=CARTESIAN_POINT ( 'NONE',  ( 16.40814093676323893, 5.790301336597087456, 11.09922568453595026 ) ) ;
#65458=CARTESIAN_POINT ( 'NONE',  ( -0.1503990784575403861, 14.24884699246888964, -6.262539305110056631 ) ) ;
#65459=CARTESIAN_POINT ( 'NONE',  ( 0.5774900079438590739, 37.64701867748817676, -5.440088680355550821 ) ) ;
#65462=CARTESIAN_POINT ( 'NONE',  ( 17.20831665107776587, 14.13393115100078568, -7.208316651077762316 ) ) ;
#65463=CARTESIAN_POINT ( 'NONE',  ( 14.92337183194729988, 9.342264484334119601, -8.527530157486177487 ) ) ;
#65464=CARTESIAN_POINT ( 'NONE',  ( 7.361572987183170547, 17.05059781766745530, 9.846743663894590881 ) ) ;
#65465=CARTESIAN_POINT ( 'NONE',  ( 0.1532563361054100626, 15.80059781766745353, -2.638427012816831230 ) ) ;
#65466=CARTESIAN_POINT ( 'NONE',  ( 1.472469842513823179, 5.592264484334118713, -4.923371831947296329 ) ) ;
#65467=CARTESIAN_POINT ( 'NONE',  ( 18.52753015748617571, 3.092264484334118269, 4.923371831947298993 ) ) ;
#65468=CARTESIAN_POINT ( 'NONE',  ( 0.2751277870542914172, 23.21833443783937767, 6.499999999999992006 ) ) ;
#65469=CARTESIAN_POINT ( 'NONE',  ( 1.472469842513823179, 0.5922644843341181575, -4.923371831947296329 ) ) ;
#65471=CARTESIAN_POINT ( 'NONE',  ( 12.63842701281683922, 19.55059781766745175, -9.846743663894590881 ) ) ;
#65472=VERTEX_POINT ( 'NONE', #19425 ) ;
#65475=EDGE_CURVE ( 'NONE', #93851, #72124, #11596, .T. ) ;
#65476=CARTESIAN_POINT ( 'NONE',  ( 3.591859063236761518, 4.956968003263753531, 11.09922568453594849 ) ) ;
#65478=DIRECTION ( 'NONE',  ( 0.000000000000000000, 1.000000000000000000, -0.000000000000000000 ) ) ;
#65479=CARTESIAN_POINT ( 'NONE',  ( 20.36894250292379738, 24.92874883491396787, -10.36894250292379027 ) ) ;
#65480=EDGE_CURVE ( 'NONE', #63345, #93709, #58595, .T. ) ;
#65482=CARTESIAN_POINT ( 'NONE',  ( 19.72487221294570858, 0.000000000000000000, -6.500000000000000888 ) ) ;
#65483=CARTESIAN_POINT ( 'NONE',  ( 24.16423886937409904, 14.09541550158063217, 3.795296366450317205 ) ) ;
#65484=B_SPLINE_CURVE_WITH_KNOTS ( 'NONE', 3,
 ( #22101, #61557, #7601, #53564, #32032, #68584 ),
 .UNSPECIFIED., .F., .F.,
 ( 4, 2, 4 ),
 ( 7.755077673624249124E-18, 0.0002626113303185950102, 0.0005252226606371823226 ),
 .UNSPECIFIED. ) ;
#65485=COLOUR_RGB ( '', 0.31764706, 0.68627451, 0.89019608) ;
#65486=CARTESIAN_POINT ( 'NONE',  ( 13.79529636645030344, 38.26208216824729647, 14.16423886937410614 ) ) ;
#65487=PRESENTATION_STYLE_ASSIGNMENT (( #12980 ) ) ;
#65489=CARTESIAN_POINT ( 'NONE',  ( 2.035157376598824452, 33.68868534415484106, 7.964842623401179544 ) ) ;
#65491=CARTESIAN_POINT ( 'NONE',  ( 7.361572987183170547, 17.05059781766745530, 9.846743663894590881 ) ) ;
#65492=CARTESIAN_POINT ( 'NONE',  ( 17.96484262340118221, 54.93868534415484106, 7.964842623401181321 ) ) ;
#65493=CARTESIAN_POINT ( 'NONE',  ( 1.472469842513823179, 30.59226448433411960, -4.923371831947296329 ) ) ;
#65496=CARTESIAN_POINT ( 'NONE',  ( -0.8801773607111009756, 13.06368534415483929, 1.068504757029289695E-15 ) ) ;
#65497=CARTESIAN_POINT ( 'NONE',  ( 21.09922568453594849, 46.20696800326376064, 6.408140936763242479 ) ) ;
#65498=CARTESIAN_POINT ( 'NONE',  ( 0.1532563361054083140, 51.00893115100078745, 1.131784320476157264E-15 ) ) ;
#65499=CARTESIAN_POINT ( 'NONE',  ( 6.565887622018943937, 25.16530133659708213, 12.81628187352647430 ) ) ;
#65501=CARTESIAN_POINT ( 'NONE',  ( 10.00000000000000178, 37.25893115100078745, 9.846743663894594434 ) ) ;
#65502=CARTESIAN_POINT ( 'NONE',  ( 24.16423886937410614, 14.30374883491396787, 8.672049930838204340E-16 ) ) ;
#65503=ORIENTED_EDGE ( 'NONE', *, *, #97764, .T. ) ;
#65505=CARTESIAN_POINT ( 'NONE',  ( 7.084665262690076126, 54.10535201082151247, 10.88017736071109987 ) ) ;
#65506=CARTESIAN_POINT ( 'NONE',  ( 20.88017736071110164, 50.35535201082151247, 2.915334737309930979 ) ) ;
#65507=CARTESIAN_POINT ( 'NONE',  ( 6.204703633549690345, 40.76208216824731778, -14.16423886937410259 ) ) ;
#65508=CARTESIAN_POINT ( 'NONE',  ( 0.1532563361054082862, 56.21726448433411605, 2.638427012816831674 ) ) ;
#65509=CARTESIAN_POINT ( 'NONE',  ( 6.565887622018943937, 63.08196800326376064, -12.81628187352647608 ) ) ;
#65510=CARTESIAN_POINT ( 'NONE',  ( 10.00000000000000000, 41.81368534415484106, -10.88017736071110342 ) ) ;
#65512=CARTESIAN_POINT ( 'NONE',  ( 16.40814093676324603, 22.45696800326375353, -11.09922568453594671 ) ) ;
#65513=CARTESIAN_POINT ( 'NONE',  ( 1.472469842513823179, 50.59226448433411605, -4.923371831947296329 ) ) ;
#65515=( LENGTH_UNIT ( ) NAMED_UNIT ( * ) SI_UNIT ( .MILLI., .METRE. ) );
#65516=CARTESIAN_POINT ( 'NONE',  ( 12.91533473730993009, 61.60535201082150536, -10.88017736071109987 ) ) ;
#65517=ORIENTED_EDGE ( 'NONE', *, *, #66947, .T. ) ;
#65518=EDGE_CURVE ( 'NONE', #36347, #10365, #3452, .T. ) ;
#65519=CARTESIAN_POINT ( 'NONE',  ( 20.88017736071110875, 5.772018677488170546, -2.915334737309920765 ) ) ;
#65520=CARTESIAN_POINT ( 'NONE',  ( 1.042145700049403656, 59.74216108172000617, -6.499999999999937828 ) ) ;
#65521=CARTESIAN_POINT ( 'NONE',  ( 19.42250999205614548, 65.98035201082151957, -5.440088680355545492 ) ) ;
#65522=CARTESIAN_POINT ( 'NONE',  ( 18.52753015748617571, 3.092264484334118269, 4.923371831947298993 ) ) ;
#65524=CARTESIAN_POINT ( 'NONE',  ( 10.00000000000000000, 29.75893115100078745, -9.846743663894594434 ) ) ;
#65525=CARTESIAN_POINT ( 'NONE',  ( 7.084665262690076126, 27.02201867748817676, -10.88017736071110164 ) ) ;
#65526=CARTESIAN_POINT ( 'NONE',  ( -2.816281873526473856, 9.123634669930421381, 9.499525473075851096E-16 ) ) ;
#65527=CARTESIAN_POINT ( 'NONE',  ( 2.035157376598824452, 38.68868534415483396, 7.964842623401179544 ) ) ;
#65528=CYLINDRICAL_SURFACE ( 'NONE', #25688, 0.5000000000000004441 ) ;
#65530=CARTESIAN_POINT ( 'NONE',  ( 0.6178305044545838731, 34.74863466993042493, 9.382169495545420901 ) ) ;
#65532=CARTESIAN_POINT ( 'NONE',  ( 7.084665262690076126, 64.10535201082150536, 10.88017736071109987 ) ) ;
#65533=CARTESIAN_POINT ( 'NONE',  ( 10.00000000000000178, 20.37363466993042138, 12.81628187352647608 ) ) ;
#65534=CARTESIAN_POINT ( 'NONE',  ( 18.04007052943773459, 19.00257860105348584, -5.767676674365828760 ) ) ;
#65535=CARTESIAN_POINT ( 'NONE',  ( 10.00000000000000178, 2.258931151000784787, 9.846743663894594434 ) ) ;
#65536=CARTESIAN_POINT ( 'NONE',  ( 17.96484262340118221, 24.93868534415484461, 7.964842623401181321 ) ) ;
#65537=CARTESIAN_POINT ( 'NONE',  ( 13.79529636645030344, 63.26208216824730357, 14.16423886937410614 ) ) ;
#65538=CARTESIAN_POINT ( 'NONE',  ( 19.84674366389459621, 58.50893115100078745, 7.409399052514197653E-17 ) ) ;
#65539=CARTESIAN_POINT ( 'NONE',  ( 5.076628168052703671, 1.842264484334118047, 8.527530157486179263 ) ) ;
#65540=CARTESIAN_POINT ( 'NONE',  ( 2.035157376598824452, 58.68868534415482685, 7.964842623401179544 ) ) ;
#65542=CARTESIAN_POINT ( 'NONE',  ( 6.204703633549690345, 27.84541550158063217, 14.16423886937410082 ) ) ;
#65547=CARTESIAN_POINT ( 'NONE',  ( -2.266590686148945544, 47.22041550158063927, 7.082119434687048631 ) ) ;
#65548=CARTESIAN_POINT ( 'NONE',  ( 20.36894250292379382, 48.67874883491396076, 10.36894250292379205 ) ) ;
#65549=CARTESIAN_POINT ( 'NONE',  ( 5.076628168052703671, 36.84226448433412315, 8.527530157486179263 ) ) ;
#65552=CARTESIAN_POINT ( 'NONE',  ( 24.16423886937409904, 39.09541550158062506, 3.795296366450317205 ) ) ;
#65554=CARTESIAN_POINT ( 'NONE',  ( 10.00000000000000000, 4.758931151000784787, -9.846743663894594434 ) ) ;
#65559=EDGE_LOOP ( 'NONE', ( #44762, #66417, #2769, #73936, #38786, #1308 ) ) ;
#65563=CARTESIAN_POINT ( 'NONE',  ( 10.00000000000000178, 13.05374883491396787, 14.16423886937410082 ) ) ;
#65564=CARTESIAN_POINT ( 'NONE',  ( 17.96484262340118221, 16.18868534415483396, -7.964842623401177768 ) ) ;
#65565=CARTESIAN_POINT ( 'NONE',  ( 0.5774900079438607392, 28.48035201082150891, 5.440088680355550821 ) ) ;
#65566=CARTESIAN_POINT ( 'NONE',  ( 0.1532563361054100626, 45.80059781766745886, -2.638427012816831230 ) ) ;
#65567=CARTESIAN_POINT ( 'NONE',  ( -2.816281873526471635, 23.91530133659708568, -3.434112377981056508 ) ) ;
#65568=SURFACE_SIDE_STYLE ('',( #35069 ) ) ;
#65571=CARTESIAN_POINT ( 'NONE',  ( -1.099225684535947600, 19.54030133659708568, 6.408140936763237150 ) ) ;
#65573=CARTESIAN_POINT ( 'NONE',  ( 1.472469842513823179, 30.59226448433411960, -4.923371831947296329 ) ) ;
#65574=CARTESIAN_POINT ( 'NONE',  ( 22.26659068614894466, 53.88708216824731068, 7.082119434687054849 ) ) ;
#65576=CARTESIAN_POINT ( 'NONE',  ( 22.26659068614895176, 64.72041550158064638, -7.082119434687042414 ) ) ;
#65578=CARTESIAN_POINT ( 'NONE',  ( 19.42250999205614548, 50.98035201082151247, -5.440088680355545492 ) ) ;
#65579=CARTESIAN_POINT ( 'NONE',  ( 17.96484262340118221, 44.93868534415483396, 7.964842623401181321 ) ) ;
#65580=CARTESIAN_POINT ( 'NONE',  ( 20.88017736071110164, 45.35535201082149115, 2.915334737309930979 ) ) ;
#65582=CARTESIAN_POINT ( 'NONE',  ( 20.88017736071110875, 40.77201867748818387, -2.915334737309920765 ) ) ;
#65586=VERTEX_POINT ( 'NONE', #11429 ) ;
#65588=EDGE_CURVE ( 'NONE', #46415, #52823, #83831, .T. ) ;
#65589=CARTESIAN_POINT ( 'NONE',  ( 12.63842701281683034, 22.46726448433411605, 9.846743663894596210 ) ) ;
#65591=CARTESIAN_POINT ( 'NONE',  ( 7.361572987183169658, 59.96726448433410894, -9.846743663894592657 ) ) ;
#65595=VERTEX_POINT ( 'NONE', #79441 ) ;
#65597=CARTESIAN_POINT ( 'NONE',  ( 1.472469842513823179, 66.42559781766745175, 4.923371831947296329 ) ) ;
#65598=CARTESIAN_POINT ( 'NONE',  ( 18.52753015748618282, 28.92559781766745175, -4.923371831947291888 ) ) ;
#65599=CARTESIAN_POINT ( 'NONE',  ( 2.917880565312948704, 67.63708216824730357, 12.26659068614894643 ) ) ;
#65602=LINE ( 'NONE', #95627, #81514 ) ;
#65603=CARTESIAN_POINT ( 'NONE',  ( 10.00000000000000000, 29.75893115100078745, -9.846743663894594434 ) ) ;
#65604=CARTESIAN_POINT ( 'NONE',  ( 0.6178305044545838731, 59.74863466993041783, 9.382169495545420901 ) ) ;
#65606=CARTESIAN_POINT ( 'NONE',  ( 22.81628187352647785, 6.415301336597088344, 3.434112377981063169 ) ) ;
#65607=CARTESIAN_POINT ( 'NONE',  ( 0.1532563361054083140, 16.00893115100078390, 1.131784320476157264E-15 ) ) ;
#65609=CARTESIAN_POINT ( 'NONE',  ( 12.63842701281683922, 9.550597817667449974, -9.846743663894590881 ) ) ;
#65610=CARTESIAN_POINT ( 'NONE',  ( 17.20831665107776587, 54.13393115100079456, -7.208316651077762316 ) ) ;
#65611=CARTESIAN_POINT ( 'NONE',  ( 20.88017736071110519, 20.56368534415484106, 2.639326808657452039E-16 ) ) ;
#65614=CARTESIAN_POINT ( 'NONE',  ( 20.88017736071110875, 10.77201867748817143, -2.915334737309920765 ) ) ;
#65615=CARTESIAN_POINT ( 'NONE',  ( 2.917880565312950480, 10.97041550158063572, -12.26659068614894821 ) ) ;
#65616=CARTESIAN_POINT ( 'NONE',  ( 17.20831665107776587, 17.88393115100078745, 7.208316651077764980 ) ) ;
#65617=CARTESIAN_POINT ( 'NONE',  ( 12.91533473730992121, 54.52201867748816255, 10.88017736071110164 ) ) ;
#65619=CARTESIAN_POINT ( 'NONE',  ( 16.40814093676323893, 20.79030133659708923, 11.09922568453595026 ) ) ;
#65621=CARTESIAN_POINT ( 'NONE',  ( -0.8801773607111008646, 3.272018677488171434, 2.915334737309923430 ) ) ;
#65622=CARTESIAN_POINT ( 'NONE',  ( -1.926860441876563801, 57.66212336850780673, 1.004413902775740978E-15 ) ) ;
#65624=CARTESIAN_POINT ( 'NONE',  ( 13.43411237798106583, 7.665301336597086568, -12.81628187352647252 ) ) ;
#65625=CARTESIAN_POINT ( 'NONE',  ( 10.00000000000000178, 62.25893115100078745, 9.846743663894594434 ) ) ;
#65626=CARTESIAN_POINT ( 'NONE',  ( 0.1532563361054083140, 11.00893115100078568, 1.131784320476157264E-15 ) ) ;
#65628=CARTESIAN_POINT ( 'NONE',  ( 21.09922568453594849, 26.20696800326375353, 6.408140936763242479 ) ) ;
#65630=CARTESIAN_POINT ( 'NONE',  ( 7.084665262690076126, 27.02201867748817676, -10.88017736071110164 ) ) ;
#65633=CARTESIAN_POINT ( 'NONE',  ( 10.00000000000000178, 43.05374883491397497, 14.16423886937410082 ) ) ;
#65636=CARTESIAN_POINT ( 'NONE',  ( 22.81628187352648496, 51.83196800326376064, -3.434112377981050290 ) ) ;
#65637=CARTESIAN_POINT ( 'NONE',  ( 12.91533473730993009, 21.60535201082150536, -10.88017736071109987 ) ) ;
#65638=CARTESIAN_POINT ( 'NONE',  ( 1.472469842513823179, 46.42559781766745175, 4.923371831947296329 ) ) ;
#65639=CARTESIAN_POINT ( 'NONE',  ( 7.084665262690076126, 49.10535201082149825, 10.88017736071109987 ) ) ;
#65640=CARTESIAN_POINT ( 'NONE',  ( 22.26659068614895176, 29.72041550158063572, -7.082119434687042414 ) ) ;
#65642=CARTESIAN_POINT ( 'NONE',  ( 19.84674366389459266, 38.71726448433412315, -2.638427012816827677 ) ) ;
#65643=PRESENTATION_STYLE_ASSIGNMENT (( #35144 ) ) ;
#65644=CARTESIAN_POINT ( 'NONE',  ( -2.816281873526473856, -0.6680319967362464695, 3.434112377981055619 ) ) ;
#65645=ORIENTED_EDGE ( 'NONE', *, *, #39553, .F. ) ;
#65646=CARTESIAN_POINT ( 'NONE',  ( 20.88017736071110875, 30.77201867748816966, -2.915334737309920765 ) ) ;
#65650=CARTESIAN_POINT ( 'NONE',  ( 12.91533473730993009, 16.60535201082150891, -10.88017736071109987 ) ) ;
#65651=CARTESIAN_POINT ( 'NONE',  ( 24.16423886937410614, 19.30374883491397142, 8.672049930838204340E-16 ) ) ;
#65652=CARTESIAN_POINT ( 'NONE',  ( 10.00000000000000178, 17.25893115100078745, 9.846743663894594434 ) ) ;
#65653=CARTESIAN_POINT ( 'NONE',  ( 2.791683348922240793, 66.63393115100079456, 7.208316651077764092 ) ) ;
#65654=CARTESIAN_POINT ( 'NONE',  ( 17.96484262340118221, 39.93868534415484106, 7.964842623401181321 ) ) ;
#65659=EDGE_LOOP ( 'NONE', ( #88206, #24510, #57096, #26126, #80360, #14181 ) ) ;
#65661=CARTESIAN_POINT ( 'NONE',  ( 12.63842701281683034, 47.46726448433412315, 9.846743663894596210 ) ) ;
#65666=CARTESIAN_POINT ( 'NONE',  ( -0.3689425029237881626, 12.42874883491396609, 10.36894250292379027 ) ) ;
#65667=CARTESIAN_POINT ( 'NONE',  ( 24.16423886937410614, 14.51208216824730179, -3.795296366450302550 ) ) ;
#65668=CARTESIAN_POINT ( 'NONE',  ( 15.44008868035555793, 51.39701867748816966, -9.422509992056140149 ) ) ;
#65669=CARTESIAN_POINT ( 'NONE',  ( -4.164238869374098151, 56.59541550158063927, -3.795296366450310543 ) ) ;
#65670=CARTESIAN_POINT ( 'NONE',  ( 19.38216949554541202, 5.998634669930420493, 9.382169495545424454 ) ) ;
#65671=CARTESIAN_POINT ( 'NONE',  ( 12.63842701281683034, 37.46726448433411605, 9.846743663894596210 ) ) ;
#65673=CARTESIAN_POINT ( 'NONE',  ( 0.5774900079438607392, 33.48035201082150536, 5.440088680355550821 ) ) ;
#65674=CARTESIAN_POINT ( 'NONE',  ( 13.43411237798105340, 10.58196800326375353, 12.81628187352647963 ) ) ;
#65675=CARTESIAN_POINT ( 'NONE',  ( -2.266590686148945544, 7.220415501580634832, 7.082119434687048631 ) ) ;
#65676=CARTESIAN_POINT ( 'NONE',  ( -4.164238869374098151, 51.59541550158063217, -3.795296366450310543 ) ) ;
#65677=CARTESIAN_POINT ( 'NONE',  ( 2.035157376598824452, 8.688685344154839285, 7.964842623401179544 ) ) ;
#65683=ORIENTED_EDGE ( 'NONE', *, *, #16714, .T. ) ;
#65685=ORIENTED_EDGE ( 'NONE', *, *, #32162, .T. ) ;
#65686=CARTESIAN_POINT ( 'NONE',  ( -2.266590686148945544, 52.22041550158064638, 7.082119434687048631 ) ) ;
#65687=CARTESIAN_POINT ( 'NONE',  ( 19.84674366389459266, 43.30059781766744464, 2.638427012816836559 ) ) ;
#65688=CARTESIAN_POINT ( 'NONE',  ( 2.035157376598824452, 63.68868534415484106, 7.964842623401179544 ) ) ;
#65692=CARTESIAN_POINT ( 'NONE',  ( 2.035157376598824452, 48.68868534415483396, 7.964842623401179544 ) ) ;
#65693=EDGE_CURVE ( 'NONE', #26466, #27072, #48847, .T. ) ;
#65697=CARTESIAN_POINT ( 'NONE',  ( 13.79529636645030344, 23.26208216824730002, 14.16423886937410614 ) ) ;
#65698=CARTESIAN_POINT ( 'NONE',  ( 3.591859063236763294, 28.29030133659708568, -11.09922568453595026 ) ) ;
#65700=CARTESIAN_POINT ( 'NONE',  ( 22.81628187352647785, 41.62363466993042493, 6.195893100308588602E-16 ) ) ;
#65701=CARTESIAN_POINT ( 'NONE',  ( 0.1532563361054082862, 36.21726448433410894, 2.638427012816831674 ) ) ;
#65702=CARTESIAN_POINT ( 'NONE',  ( 0.5774900079438590739, 7.647018677488171434, -5.440088680355550821 ) ) ;
#65704=CARTESIAN_POINT ( 'NONE',  ( 6.565887622018943937, 50.16530133659708213, 12.81628187352647430 ) ) ;
#65707=CARTESIAN_POINT ( 'NONE',  ( 17.20831665107776587, 42.88393115100077324, 7.208316651077764980 ) ) ;
#65708=CARTESIAN_POINT ( 'NONE',  ( 20.15039907845753220, 22.62777174578612716, -6.262539305110077947 ) ) ;
#65712=CARTESIAN_POINT ( 'NONE',  ( 0.2751277870542982451, 17.28217586085238011, -6.500000000000002665 ) ) ;
#65713=CARTESIAN_POINT ( 'NONE',  ( 0.1532563361054100626, 15.80059781766745353, -2.638427012816831230 ) ) ;
#65714=CARTESIAN_POINT ( 'NONE',  ( 3.591859063236761518, 24.95696800326375353, 11.09922568453594849 ) ) ;
#65717=ORIENTED_EDGE ( 'NONE', *, *, #98936, .F. ) ;
#65719=CARTESIAN_POINT ( 'NONE',  ( -4.164238869374099927, 17.01208216824730357, 3.795296366450308767 ) ) ;
#65720=CARTESIAN_POINT ( 'NONE',  ( 10.00000000000000000, 34.75893115100078745, -9.846743663894594434 ) ) ;
#65721=CARTESIAN_POINT ( 'NONE',  ( 13.43411237798105340, 40.58196800326375353, 12.81628187352647963 ) ) ;
#65724=CARTESIAN_POINT ( 'NONE',  ( 2.035157376598822676, 57.43868534415484106, -7.964842623401177768 ) ) ;
#65725=CARTESIAN_POINT ( 'NONE',  ( -2.816281873526473856, 14.12363466993041961, 9.499525473075851096E-16 ) ) ;
#65727=CARTESIAN_POINT ( 'NONE',  ( 0.1532563361054082862, 41.21726448433411605, 2.638427012816831674 ) ) ;
#65728=CARTESIAN_POINT ( 'NONE',  ( 0.5774900079438607392, 43.48035201082151247, 5.440088680355550821 ) ) ;
#65729=CARTESIAN_POINT ( 'NONE',  ( -1.099225684535947600, 38.70696800326375353, -6.408140936763238038 ) ) ;
#65730=CARTESIAN_POINT ( 'NONE',  ( 12.63842701281683034, 37.46726448433411605, 9.846743663894596210 ) ) ;
#65733=CARTESIAN_POINT ( 'NONE',  ( 10.00000000000000000, 36.81368534415484106, -10.88017736071110342 ) ) ;
#65734=B_SPLINE_CURVE_WITH_KNOTS ( 'NONE', 3,
 ( #81431, #36433, #13429, #21936, #35436, #28432 ),
 .UNSPECIFIED., .F., .F.,
 ( 4, 2, 4 ),
 ( 7.788919273297050532E-18, 0.0002626113303185990760, 0.0005252226606371903457 ),
 .UNSPECIFIED. ) ;
#65735=ORIENTED_EDGE ( 'NONE', *, *, #60753, .T. ) ;
#65736=CARTESIAN_POINT ( 'NONE',  ( 4.559911319644449179, 68.89701867748817676, 9.422509992056141925 ) ) ;
#65737=CARTESIAN_POINT ( 'NONE',  ( 0.5774900079438607392, 3.480352010821504027, 5.440088680355550821 ) ) ;
#65738=CARTESIAN_POINT ( 'NONE',  ( 1.472469842513823179, 55.59226448433412315, -4.923371831947296329 ) ) ;
#65739=CARTESIAN_POINT ( 'NONE',  ( 4.559911319644449179, 32.23035201082150536, -9.422509992056141925 ) ) ;
#65741=CARTESIAN_POINT ( 'NONE',  ( 19.42250999205614193, 60.14701867748817676, 5.440088680355555262 ) ) ;
#65742=CARTESIAN_POINT ( 'NONE',  ( 20.88017736071110875, 30.77201867748816966, -2.915334737309920765 ) ) ;
#65743=CARTESIAN_POINT ( 'NONE',  ( 2.602085213965210642E-15, 78.91966277462714174, -9.500000000000000000 ) ) ;
#65744=CARTESIAN_POINT ( 'NONE',  ( 19.84674366389459621, 18.50893115100078745, 7.409399052514197653E-17 ) ) ;
#65745=LINE ( 'NONE', #5760, #56899 ) ;
#65746=CARTESIAN_POINT ( 'NONE',  ( 7.361572987183170547, 47.05059781766745175, 9.846743663894590881 ) ) ;
#65747=CARTESIAN_POINT ( 'NONE',  ( 24.16423886937409904, 54.09541550158063217, 3.795296366450317205 ) ) ;
#65748=CARTESIAN_POINT ( 'NONE',  ( 20.32896413005680358, 19.74545670184113888, 5.963430220938287007 ) ) ;
#65749=CARTESIAN_POINT ( 'NONE',  ( 1.383448333479235126, 62.37718327197428891, -6.499999999999977796 ) ) ;
#65750=CARTESIAN_POINT ( 'NONE',  ( 17.08211943468705840, 5.137082168247300906, -12.26659068614894466 ) ) ;
#65752=CARTESIAN_POINT ( 'NONE',  ( -4.164238869374099039, 36.80374883491396787, 8.674139862899312516E-16 ) ) ;
#65754=CARTESIAN_POINT ( 'NONE',  ( 10.00000000000000178, 0.3736346699304200492, 12.81628187352647608 ) ) ;
#65755=CARTESIAN_POINT ( 'NONE',  ( 19.72487221294571569, 27.80223176428830811, -6.499999999999990230 ) ) ;
#65756=VERTEX_POINT ( 'NONE', #36402 ) ;
#65757=CARTESIAN_POINT ( 'NONE',  ( 15.44008868035555260, 19.73035201082150536, 9.422509992056143702 ) ) ;
#65758=CARTESIAN_POINT ( 'NONE',  ( 17.20831665107776587, 39.13393115100079456, -7.208316651077762316 ) ) ;
#65759=SURFACE_SIDE_STYLE ('',( #59246 ) ) ;
#65761=CARTESIAN_POINT ( 'NONE',  ( 2.035157376598822676, 57.43868534415484106, -7.964842623401177768 ) ) ;
#65763=CARTESIAN_POINT ( 'NONE',  ( -2.816281873526473856, 59.33196800326374643, 3.434112377981055619 ) ) ;
#65764=CARTESIAN_POINT ( 'NONE',  ( 13.43411237798105340, 20.58196800326374643, 12.81628187352647963 ) ) ;
#65765=CARTESIAN_POINT ( 'NONE',  ( 2.791683348922237240, 25.38393115100078390, -7.208316651077763204 ) ) ;
#65766=ORIENTED_EDGE ( 'NONE', *, *, #95193, .F. ) ;
#65768=CARTESIAN_POINT ( 'NONE',  ( -0.3689425029237898834, 66.17874883491396076, -10.36894250292378850 ) ) ;
#65769=CARTESIAN_POINT ( 'NONE',  ( 20.88017736071110164, 20.35535201082150891, 2.915334737309930979 ) ) ;
#65770=CARTESIAN_POINT ( 'NONE',  ( -4.164238869374099927, 47.01208216824729647, 3.795296366450308767 ) ) ;
#65771=CARTESIAN_POINT ( 'NONE',  ( 17.96484262340118221, 36.18868534415484106, -7.964842623401177768 ) ) ;
#65772=CARTESIAN_POINT ( 'NONE',  ( 19.42250999205614548, 60.98035201082151247, -5.440088680355545492 ) ) ;
#65773=CARTESIAN_POINT ( 'NONE',  ( 20.15039907845753930, 70.00000000000000000, 6.262539305110068177 ) ) ;
#65774=CARTESIAN_POINT ( 'NONE',  ( 18.52753015748618282, 28.92559781766745175, -4.923371831947291888 ) ) ;
#65775=CARTESIAN_POINT ( 'NONE',  ( 19.84674366389459621, 13.50893115100078568, 7.409399052514197653E-17 ) ) ;
#65778=CARTESIAN_POINT ( 'NONE',  ( 12.63842701281683034, 37.46726448433411605, 9.846743663894596210 ) ) ;
#65779=CARTESIAN_POINT ( 'NONE',  ( 0.1532563361054083140, 66.00893115100079456, 1.131784320476157264E-15 ) ) ;
#65781=CARTESIAN_POINT ( 'NONE',  ( 10.00000000000000178, 40.37363466993042493, 12.81628187352647608 ) ) ;
#65783=CARTESIAN_POINT ( 'NONE',  ( 10.00000000000000000, 66.81368534415484817, -10.88017736071110342 ) ) ;
#65784=CARTESIAN_POINT ( 'NONE',  ( 16.40814093676323893, 45.79030133659708923, 11.09922568453595026 ) ) ;
#65785=CARTESIAN_POINT ( 'NONE',  ( -0.3689425029237898834, 61.17874883491396076, -10.36894250292378850 ) ) ;
#65786=CARTESIAN_POINT ( 'NONE',  ( 19.84674366389459621, 33.50893115100078745, 7.409399052514197653E-17 ) ) ;
#65787=CARTESIAN_POINT ( 'NONE',  ( 19.50000000000000711, 70.00000000000000000, 5.000000000000000000 ) ) ;
#65788=CARTESIAN_POINT ( 'NONE',  ( 0.1532563361054083140, 66.00893115100079456, 1.131784320476157264E-15 ) ) ;
#65789=CARTESIAN_POINT ( 'NONE',  ( 22.26659068614894466, 18.88708216824730002, 7.082119434687054849 ) ) ;
#65790=CARTESIAN_POINT ( 'NONE',  ( 22.26659068614895176, 34.72041550158063927, -7.082119434687042414 ) ) ;
#65791=CARTESIAN_POINT ( 'NONE',  ( 2.791683348922237240, 50.38393115100078035, -7.208316651077763204 ) ) ;
#65793=CARTESIAN_POINT ( 'NONE',  ( 12.91533473730993009, 36.60535201082151247, -10.88017736071109987 ) ) ;
#65794=CARTESIAN_POINT ( 'NONE',  ( 20.88017736071110875, 60.77201867748817676, -2.915334737309920765 ) ) ;
#65795=CARTESIAN_POINT ( 'NONE',  ( 18.72515096720571037, 50.05509018479936856, 6.499999999999982236 ) ) ;
#65796=ORIENTED_EDGE ( 'NONE', *, *, #17081, .F. ) ;
#65797=CARTESIAN_POINT ( 'NONE',  ( -1.099225684535947600, 39.54030133659708923, 6.408140936763237150 ) ) ;
#65799=CARTESIAN_POINT ( 'NONE',  ( 20.88017736071110875, 60.77201867748817676, -2.915334737309920765 ) ) ;
#65801=CARTESIAN_POINT ( 'NONE',  ( 22.26659068614895176, 4.720415501580633943, -7.082119434687042414 ) ) ;
#65802=CARTESIAN_POINT ( 'NONE',  ( 0.2751277870542871429, 42.28217586085238366, -6.499999999999984901 ) ) ;
#65807=EDGE_CURVE ( 'NONE', #96104, #31762, #10787, .T. ) ;
#65808=CARTESIAN_POINT ( 'NONE',  ( 2.035157376598822676, 17.43868534415483751, -7.964842623401177768 ) ) ;
#65810=CARTESIAN_POINT ( 'NONE',  ( 2.917880565312950480, 15.97041550158063217, -12.26659068614894821 ) ) ;
#65813=CARTESIAN_POINT ( 'NONE',  ( 0.5774900079438607392, 23.48035201082150536, 5.440088680355550821 ) ) ;
#65814=CARTESIAN_POINT ( 'NONE',  ( 2.791683348922237240, 55.38393115100078745, -7.208316651077763204 ) ) ;
#65816=CARTESIAN_POINT ( 'NONE',  ( 17.20831665107776587, 59.13393115100078745, -7.208316651077762316 ) ) ;
#65817=ORIENTED_EDGE ( 'NONE', *, *, #36870, .T. ) ;
#65818=CARTESIAN_POINT ( 'NONE',  ( 10.00000000000000178, 54.31368534415484106, 10.88017736071110342 ) ) ;
#65819=CARTESIAN_POINT ( 'NONE',  ( 1.472469842513823179, 60.59226448433412315, -4.923371831947296329 ) ) ;
#65820=CARTESIAN_POINT ( 'NONE',  ( 22.81628187352647785, 36.41530133659707502, 3.434112377981063169 ) ) ;
#65821=CARTESIAN_POINT ( 'NONE',  ( -0.8801773607110991993, 7.855352010821504471, -2.915334737309923874 ) ) ;
#65823=CARTESIAN_POINT ( 'NONE',  ( 2.035157376598822676, 67.43868534415484817, -7.964842623401177768 ) ) ;
#65824=CARTESIAN_POINT ( 'NONE',  ( 17.96484262340118221, 19.93868534415484106, 7.964842623401181321 ) ) ;
#65826=AXIS2_PLACEMENT_3D ( 'NONE', #56266, #95224, #4247 ) ;
#65827=ORIENTED_EDGE ( 'NONE', *, *, #3881, .F. ) ;
#65828=CARTESIAN_POINT ( 'NONE',  ( 0.6178305044545838731, 59.74863466993041783, 9.382169495545420901 ) ) ;
#65829=CARTESIAN_POINT ( 'NONE',  ( 19.42250999205614193, 30.14701867748817321, 5.440088680355555262 ) ) ;
#65831=CARTESIAN_POINT ( 'NONE',  ( 19.38216949554541557, 37.24863466993041783, -9.382169495545420901 ) ) ;
#65832=CARTESIAN_POINT ( 'NONE',  ( 4.559911319644449179, 47.23035201082150536, -9.422509992056141925 ) ) ;
#65834=CARTESIAN_POINT ( 'NONE',  ( 19.84674366389459266, 53.30059781766744464, 2.638427012816836559 ) ) ;
#65836=ORIENTED_EDGE ( 'NONE', *, *, #46871, .T. ) ;
#65839=CARTESIAN_POINT ( 'NONE',  ( 19.84674366389459266, 63.30059781766745886, 2.638427012816836559 ) ) ;
#65840=FACE_OUTER_BOUND ( 'NONE', #50696, .T. ) ;
#65841=CARTESIAN_POINT ( 'NONE',  ( 0.1532563361054082862, 51.21726448433412315, 2.638427012816831674 ) ) ;
#65842=CARTESIAN_POINT ( 'NONE',  ( 15.44008868035555260, 24.73035201082150891, 9.422509992056143702 ) ) ;
#65845=CARTESIAN_POINT ( 'NONE',  ( 19.84674366389459266, 43.30059781766744464, 2.638427012816836559 ) ) ;
#65846=CARTESIAN_POINT ( 'NONE',  ( 10.00000000000000000, 9.758931151000785675, -9.846743663894594434 ) ) ;
#65847=FACE_OUTER_BOUND ( 'NONE', #22954, .T. ) ;
#65848=CARTESIAN_POINT ( 'NONE',  ( 0.1532563361054100626, 60.80059781766744464, -2.638427012816831230 ) ) ;
#65850=ADVANCED_FACE ( 'NONE', ( #10339 ), #16858, .T. ) ;
#65853=CARTESIAN_POINT ( 'NONE',  ( -2.816281873526473856, 39.12363466993041783, 9.499525473075851096E-16 ) ) ;
#65854=CARTESIAN_POINT ( 'NONE',  ( 14.92337183194729633, 32.67559781766745175, 8.527530157486181039 ) ) ;
#65855=CARTESIAN_POINT ( 'NONE',  ( -0.8801773607111009756, 58.27201867748816966, 2.915334737309923874 ) ) ;
#65856=CARTESIAN_POINT ( 'NONE',  ( 2.917880565312950480, 60.97041550158063927, -12.26659068614894821 ) ) ;
#65857=CARTESIAN_POINT ( 'NONE',  ( 0.1532563361054100626, 30.80059781766744820, -2.638427012816831230 ) ) ;
#65859=CARTESIAN_POINT ( 'NONE',  ( -2.266590686148945544, 56.38708216824731068, -7.082119434687050408 ) ) ;
#65861=CARTESIAN_POINT ( 'NONE',  ( 10.00000000000000000, 16.81368534415483751, -10.88017736071110342 ) ) ;
#65863=CARTESIAN_POINT ( 'NONE',  ( -4.164238869374099927, 32.01208216824730357, 3.795296366450308767 ) ) ;
#65864=CARTESIAN_POINT ( 'NONE',  ( -2.266590686148945544, 52.22041550158064638, 7.082119434687048631 ) ) ;
#65866=LINE ( 'NONE', #27868, #97929 ) ;
#65867=CARTESIAN_POINT ( 'NONE',  ( 0.1532563361054083140, 16.00893115100078390, 1.131784320476157264E-15 ) ) ;
#65868=CARTESIAN_POINT ( 'NONE',  ( 10.00000000000000178, 0.3736346699304200492, 12.81628187352647608 ) ) ;
#65870=CARTESIAN_POINT ( 'NONE',  ( 17.96484262340118221, 51.18868534415483396, -7.964842623401177768 ) ) ;
#65877=CARTESIAN_POINT ( 'NONE',  ( 17.08211943468705840, 40.13708216824731068, -12.26659068614894466 ) ) ;
#65880=CARTESIAN_POINT ( 'NONE',  ( 12.91533473730993009, 21.60535201082150536, -10.88017736071109987 ) ) ;
#65882=CARTESIAN_POINT ( 'NONE',  ( 13.43411237798106583, 37.66530133659708923, -12.81628187352647252 ) ) ;
#65884=CARTESIAN_POINT ( 'NONE',  ( -1.099225684535947600, 63.70696800326376774, -6.408140936763238038 ) ) ;
#65888=SURFACE_STYLE_USAGE ( .BOTH. , #52373 ) ;
#65890=CARTESIAN_POINT ( 'NONE',  ( -0.8801773607111009756, 28.06368534415484106, 1.068504757029289695E-15 ) ) ;
#65891=LINE ( 'NONE', #88903, #6326 ) ;
#65893=CARTESIAN_POINT ( 'NONE',  ( 7.084665262690076126, 44.10535201082151247, 10.88017736071109987 ) ) ;
#65894=CARTESIAN_POINT ( 'NONE',  ( 17.96484262340118221, 44.93868534415483396, 7.964842623401181321 ) ) ;
#65895=CARTESIAN_POINT ( 'NONE',  ( -2.816281873526471635, 8.915301336597083903, -3.434112377981056508 ) ) ;
#65898=CARTESIAN_POINT ( 'NONE',  ( 17.20831665107776587, 22.88393115100078745, 7.208316651077764980 ) ) ;
#65901=CARTESIAN_POINT ( 'NONE',  ( 17.96484262340118221, 44.93868534415483396, 7.964842623401181321 ) ) ;
#65902=CARTESIAN_POINT ( 'NONE',  ( 21.09922568453595559, 7.040301336597086568, -6.408140936763230044 ) ) ;
#65903=CARTESIAN_POINT ( 'NONE',  ( 17.96484262340118221, 66.18868534415483396, -7.964842623401177768 ) ) ;
#65904=CARTESIAN_POINT ( 'NONE',  ( 2.791683348922237240, 25.38393115100078390, -7.208316651077763204 ) ) ;
#65905=CARTESIAN_POINT ( 'NONE',  ( 0.6178305044545818747, 48.49863466993042493, -9.382169495545419124 ) ) ;
#65906=CIRCLE ( 'NONE', #45147, 11.92686044187656513 ) ;
#65907=CARTESIAN_POINT ( 'NONE',  ( 12.63842701281683034, 2.467264484334118269, 9.846743663894596210 ) ) ;
#65911=LINE ( 'NONE', #95941, #9488 ) ;
#65912=CARTESIAN_POINT ( 'NONE',  ( -0.8801773607111009756, 18.06368534415484106, 1.068504757029289695E-15 ) ) ;
#65914=CARTESIAN_POINT ( 'NONE',  ( 13.79529636645031943, 35.34541550158063927, -14.16423886937409904 ) ) ;
#65915=CARTESIAN_POINT ( 'NONE',  ( 19.84674366389459621, 33.50893115100078745, 7.409399052514197653E-17 ) ) ;
#65917=CARTESIAN_POINT ( 'NONE',  ( -0.8801773607110991993, 12.85535201082150358, -2.915334737309923874 ) ) ;
#65918=CARTESIAN_POINT ( 'NONE',  ( 24.16423886937409904, 64.09541550158064638, 3.795296366450317205 ) ) ;
#65921=CARTESIAN_POINT ( 'NONE',  ( 2.035157376598824452, 8.688685344154839285, 7.964842623401179544 ) ) ;
#65922=CARTESIAN_POINT ( 'NONE',  ( 15.44008868035555793, 36.39701867748816966, -9.422509992056140149 ) ) ;
#65925=CARTESIAN_POINT ( 'NONE',  ( 19.72487221294570858, 70.00000000000000000, 6.500000000000000888 ) ) ;
#65926=CARTESIAN_POINT ( 'NONE',  ( -0.8801773607110991993, 22.85535201082150181, -2.915334737309923874 ) ) ;
#65930=CARTESIAN_POINT ( 'NONE',  ( -1.099225684535947600, 59.54030133659708923, 6.408140936763237150 ) ) ;
#65932=CARTESIAN_POINT ( 'NONE',  ( 24.16423886937410614, 34.51208216824731068, -3.795296366450302550 ) ) ;
#65933=CARTESIAN_POINT ( 'NONE',  ( 10.00000000000000178, 54.31368534415484106, 10.88017736071110342 ) ) ;
#65934=CARTESIAN_POINT ( 'NONE',  ( 19.42250999205614193, 30.14701867748817321, 5.440088680355555262 ) ) ;
#65937=EDGE_CURVE ( 'NONE', #35320, #66014, #11662, .T. ) ;
#65939=CARTESIAN_POINT ( 'NONE',  ( 12.63842701281683922, 54.55059781766745175, -9.846743663894590881 ) ) ;
#65942=CARTESIAN_POINT ( 'NONE',  ( 5.076628168052703671, 26.84226448433411960, 8.527530157486179263 ) ) ;
#65944=CARTESIAN_POINT ( 'NONE',  ( -0.8801773607110991993, 17.85535201082150536, -2.915334737309923874 ) ) ;
#65945=CARTESIAN_POINT ( 'NONE',  ( 10.00000000000000000, 19.75893115100078390, -9.846743663894594434 ) ) ;
#65946=CARTESIAN_POINT ( 'NONE',  ( 19.38216949554541202, 5.998634669930420493, 9.382169495545424454 ) ) ;
#65947=CARTESIAN_POINT ( 'NONE',  ( -0.8801773607111008646, 53.27201867748816966, 2.915334737309923430 ) ) ;
#65948=CARTESIAN_POINT ( 'NONE',  ( 12.91533473730992121, 19.52201867748816611, 10.88017736071110164 ) ) ;
#65949=CARTESIAN_POINT ( 'NONE',  ( 21.09922568453594849, 56.20696800326375353, 6.408140936763242479 ) ) ;
#65950=CARTESIAN_POINT ( 'NONE',  ( -4.164238869374098151, 41.59541550158061796, -3.795296366450310543 ) ) ;
#65953=CARTESIAN_POINT ( 'NONE',  ( 21.92686044187656691, 34.95379003517447813, 3.195792623639537755 ) ) ;
#65955=CARTESIAN_POINT ( 'NONE',  ( 10.00000000000000178, 0.3736346699304200492, 12.81628187352647608 ) ) ;
#65956=SURFACE_STYLE_USAGE ( .BOTH. , #35459 ) ;
#65957=CARTESIAN_POINT ( 'NONE',  ( 20.88017736071110875, 35.77201867748816966, -2.915334737309920765 ) ) ;
#65958=CARTESIAN_POINT ( 'NONE',  ( 14.92337183194729633, 57.67559781766745886, 8.527530157486181039 ) ) ;
#65961=CARTESIAN_POINT ( 'NONE',  ( 10.00000000000000178, 17.25893115100078745, 9.846743663894594434 ) ) ;
#65963=CARTESIAN_POINT ( 'NONE',  ( 7.361572987183169658, 24.96726448433412315, -9.846743663894592657 ) ) ;
#65964=CARTESIAN_POINT ( 'NONE',  ( 0.1532563361054100626, 5.800597817667452638, -2.638427012816831230 ) ) ;
#65965=SURFACE_STYLE_USAGE ( .BOTH. , #49483 ) ;
#65967=CARTESIAN_POINT ( 'NONE',  ( 0.1532563361054082862, 6.217264484334118713, 2.638427012816831674 ) ) ;
#65969=CARTESIAN_POINT ( 'NONE',  ( 12.63842701281683034, 2.467264484334118269, 9.846743663894596210 ) ) ;
#65970=CARTESIAN_POINT ( 'NONE',  ( 0.1532563361054083140, 21.00893115100078745, 1.131784320476157264E-15 ) ) ;
#65972=B_SPLINE_CURVE_WITH_KNOTS ( 'NONE', 3,
 ( #52602, #14126, #44610, #14634 ),
 .UNSPECIFIED., .F., .F.,
 ( 4, 4 ),
 ( 6.213755518593340002E-17, 0.001060528352562004582 ),
 .UNSPECIFIED. ) ;
#65973=CARTESIAN_POINT ( 'NONE',  ( -33.42076923076923833, 91.65384615384616041, -9.500000000000000000 ) ) ;
#65974=CARTESIAN_POINT ( 'NONE',  ( -2.816281873526471635, -1.084698663402913210, -3.434112377981056508 ) ) ;
#65976=CARTESIAN_POINT ( 'NONE',  ( 7.084665262690076126, 7.022018677488169658, -10.88017736071110164 ) ) ;
#65977=CARTESIAN_POINT ( 'NONE',  ( -0.3689425029237898834, 16.17874883491396076, -10.36894250292378850 ) ) ;
#65981=CARTESIAN_POINT ( 'NONE',  ( -4.164238869374099927, 22.01208216824730357, 3.795296366450308767 ) ) ;
#65982=CARTESIAN_POINT ( 'NONE',  ( 20.36894250292379738, 44.92874883491396787, -10.36894250292379027 ) ) ;
#65984=CARTESIAN_POINT ( 'NONE',  ( 24.16423886937410614, 19.30374883491397142, 8.672049930838204340E-16 ) ) ;
#65985=CARTESIAN_POINT ( 'NONE',  ( 19.42250999205614548, 30.98035201082150536, -5.440088680355545492 ) ) ;
#65988=CARTESIAN_POINT ( 'NONE',  ( 1.472469842513823179, 10.59226448433411782, -4.923371831947296329 ) ) ;
#65989=CARTESIAN_POINT ( 'NONE',  ( 15.44008868035555260, 59.73035201082151247, 9.422509992056143702 ) ) ;
#65990=CARTESIAN_POINT ( 'NONE',  ( 19.84674366389459621, 28.50893115100078745, 7.409399052514197653E-17 ) ) ;
#65991=CARTESIAN_POINT ( 'NONE',  ( 15.44008868035555260, 4.730352010821505360, 9.422509992056143702 ) ) ;
#65992=CARTESIAN_POINT ( 'NONE',  ( 21.09922568453594849, 41.20696800326375353, 6.408140936763242479 ) ) ;
#65993=CARTESIAN_POINT ( 'NONE',  ( 2.791683348922237240, 55.38393115100078745, -7.208316651077763204 ) ) ;
#65995=CARTESIAN_POINT ( 'NONE',  ( 21.09922568453594849, 36.20696800326375353, 6.408140936763242479 ) ) ;
#65997=CARTESIAN_POINT ( 'NONE',  ( 18.52753015748617571, 33.09226448433411605, 4.923371831947298993 ) ) ;
#65998=CARTESIAN_POINT ( 'NONE',  ( -0.3689425029237881626, 32.42874883491395366, 10.36894250292379027 ) ) ;
#66001=CARTESIAN_POINT ( 'NONE',  ( 15.44008868035555260, 54.73035201082150536, 9.422509992056143702 ) ) ;
#66002=CARTESIAN_POINT ( 'NONE',  ( 20.88017736071110519, 60.56368534415484106, 2.639326808657452039E-16 ) ) ;
#66003=CARTESIAN_POINT ( 'NONE',  ( 24.16423886937409904, 49.09541550158063217, 3.795296366450317205 ) ) ;
#66004=CARTESIAN_POINT ( 'NONE',  ( 2.791683348922237240, 65.38393115100078035, -7.208316651077763204 ) ) ;
#66005=CARTESIAN_POINT ( 'NONE',  ( 16.40814093676323893, 60.79030133659709634, 11.09922568453595026 ) ) ;
#66006=CARTESIAN_POINT ( 'NONE',  ( 17.96484262340118221, 36.18868534415484106, -7.964842623401177768 ) ) ;
#66008=CARTESIAN_POINT ( 'NONE',  ( 3.591859063236763294, 28.29030133659708568, -11.09922568453595026 ) ) ;
#66009=CARTESIAN_POINT ( 'NONE',  ( 0.1532563361054082862, 51.21726448433412315, 2.638427012816831674 ) ) ;
#66012=CARTESIAN_POINT ( 'NONE',  ( 10.00000000000000178, 14.31368534415483929, 10.88017736071110342 ) ) ;
#66014=VERTEX_POINT ( 'NONE', #54833 ) ;
#66017=CARTESIAN_POINT ( 'NONE',  ( 0.5774900079438607392, 3.480352010821504027, 5.440088680355550821 ) ) ;
#66019=CARTESIAN_POINT ( 'NONE',  ( 2.791683348922237240, 0.3839311510007847872, -7.208316651077763204 ) ) ;
#66020=CARTESIAN_POINT ( 'NONE',  ( 4.559911319644449179, 68.89701867748817676, 9.422509992056141925 ) ) ;
#66022=CARTESIAN_POINT ( 'NONE',  ( 12.63842701281683922, 29.55059781766745175, -9.846743663894590881 ) ) ;
#66023=CARTESIAN_POINT ( 'NONE',  ( -0.8801773607111009756, 18.06368534415484106, 1.068504757029289695E-15 ) ) ;
#66024=CARTESIAN_POINT ( 'NONE',  ( 10.00000000000000000, 12.87363466993042138, -12.81628187352647608 ) ) ;
#66025=CARTESIAN_POINT ( 'NONE',  ( 15.44008868035555793, 41.39701867748817676, -9.422509992056140149 ) ) ;
#66027=CARTESIAN_POINT ( 'NONE',  ( 10.00000000000000000, 37.87363466993041783, -12.81628187352647608 ) ) ;
#66029=CARTESIAN_POINT ( 'NONE',  ( 20.88017736071110519, 65.56368534415483396, 2.639326808657452039E-16 ) ) ;
#66030=CARTESIAN_POINT ( 'NONE',  ( -1.099225684535947600, 14.54030133659708568, 6.408140936763237150 ) ) ;
#66032=CARTESIAN_POINT ( 'NONE',  ( 12.91533473730993009, 46.60535201082150536, -10.88017736071109987 ) ) ;
#66033=CARTESIAN_POINT ( 'NONE',  ( 2.791683348922240793, 61.63393115100079456, 7.208316651077764092 ) ) ;
#66034=CARTESIAN_POINT ( 'NONE',  ( 6.204703633549690345, 65.76208216824731778, -14.16423886937410259 ) ) ;
#66035=CARTESIAN_POINT ( 'NONE',  ( 18.52753015748618282, 53.92559781766745175, -4.923371831947291888 ) ) ;
#66036=CARTESIAN_POINT ( 'NONE',  ( 19.84674366389459266, 3.717264484334118713, -2.638427012816827677 ) ) ;
#66037=CARTESIAN_POINT ( 'NONE',  ( 0.5774900079438590739, 67.64701867748817676, -5.440088680355550821 ) ) ;
#66038=CARTESIAN_POINT ( 'NONE',  ( 0.2751277870542967463, 0.000000000000000000, 6.500000000000000888 ) ) ;
#66039=CARTESIAN_POINT ( 'NONE',  ( 20.36894250292379382, 23.67874883491397142, 10.36894250292379205 ) ) ;
#66042=ORIENTED_EDGE ( 'NONE', *, *, #89650, .F. ) ;
#66044=CARTESIAN_POINT ( 'NONE',  ( -0.3689425029237881626, 62.42874883491396787, 10.36894250292379027 ) ) ;
#66045=CARTESIAN_POINT ( 'NONE',  ( 10.00000000000000000, 45.55374883491397497, -14.16423886937410082 ) ) ;
#66046=EDGE_CURVE ( 'NONE', #87620, #51199, #5304, .T. ) ;
#66047=CARTESIAN_POINT ( 'NONE',  ( 2.791683348922237240, 30.38393115100078390, -7.208316651077763204 ) ) ;
#66048=CARTESIAN_POINT ( 'NONE',  ( 3.591859063236761518, 24.95696800326375353, 11.09922568453594849 ) ) ;
#66052=CARTESIAN_POINT ( 'NONE',  ( 6.204703633549690345, 62.84541550158063927, 14.16423886937410082 ) ) ;
#66055=CARTESIAN_POINT ( 'NONE',  ( 5.076628168052704559, 15.17559781766745175, -8.527530157486179263 ) ) ;
#66057=CARTESIAN_POINT ( 'NONE',  ( 17.39651004071841811, 2.935752660568277328, 6.500000000000002665 ) ) ;
#66063=CARTESIAN_POINT ( 'NONE',  ( 19.42250999205614548, 15.98035201082150714, -5.440088680355545492 ) ) ;
#66064=CARTESIAN_POINT ( 'NONE',  ( 4.559911319644449179, 28.89701867748817321, 9.422509992056141925 ) ) ;
#66065=CARTESIAN_POINT ( 'NONE',  ( 7.361572987183169658, 54.96726448433413026, -9.846743663894592657 ) ) ;
#66066=CARTESIAN_POINT ( 'NONE',  ( 13.43411237798105340, 20.58196800326374643, 12.81628187352647963 ) ) ;
#66068=B_SPLINE_CURVE_WITH_KNOTS ( 'NONE', 3,
 ( #82968, #23474, #22979, #76937 ),
 .UNSPECIFIED., .F., .F.,
 ( 4, 4 ),
 ( 3.417008968066607180E-17, 0.001060528352561980947 ),
 .UNSPECIFIED. ) ;
#66069=CARTESIAN_POINT ( 'NONE',  ( 3.591859063236761518, 34.95696800326375353, 11.09922568453594849 ) ) ;
#66070=CARTESIAN_POINT ( 'NONE',  ( 1.472469842513823179, 0.5922644843341181575, -4.923371831947296329 ) ) ;
#66072=CARTESIAN_POINT ( 'NONE',  ( 0.1532563361054082862, 26.21726448433411605, 2.638427012816831674 ) ) ;
#66073=CARTESIAN_POINT ( 'NONE',  ( 20.36894250292379738, 59.92874883491397497, -10.36894250292379027 ) ) ;
#66074=ORIENTED_EDGE ( 'NONE', *, *, #93713, .T. ) ;
#66075=CARTESIAN_POINT ( 'NONE',  ( 10.00000000000000178, 9.313685344154839285, 10.88017736071110342 ) ) ;
#66076=ORIENTED_EDGE ( 'NONE', *, *, #23089, .T. ) ;
#66077=CARTESIAN_POINT ( 'NONE',  ( 0.5774900079438607392, 48.48035201082150536, 5.440088680355550821 ) ) ;
#66078=CARTESIAN_POINT ( 'NONE',  ( 20.88017736071110519, 45.56368534415484106, 2.639326808657452039E-16 ) ) ;
#66079=CARTESIAN_POINT ( 'NONE',  ( 19.42250999205614548, 45.98035201082150536, -5.440088680355545492 ) ) ;
#66081=CARTESIAN_POINT ( 'NONE',  ( 2.035157376598824452, 38.68868534415483396, 7.964842623401179544 ) ) ;
#66085=CARTESIAN_POINT ( 'NONE',  ( 14.92337183194729633, 32.67559781766745175, 8.527530157486181039 ) ) ;
#66087=CARTESIAN_POINT ( 'NONE',  ( 14.92337183194729988, 64.34226448433412315, -8.527530157486177487 ) ) ;
#66088=CYLINDRICAL_SURFACE ( 'NONE', #80409, 11.92686044187656513 ) ;
#66089=SURFACE_STYLE_USAGE ( .BOTH. , #43102 ) ;
#66094=CARTESIAN_POINT ( 'NONE',  ( 12.63842701281683922, 39.55059781766744464, -9.846743663894590881 ) ) ;
#66095=CARTESIAN_POINT ( 'NONE',  ( 6.204703633549690345, 57.84541550158063927, 14.16423886937410082 ) ) ;
#66099=CARTESIAN_POINT ( 'NONE',  ( 17.20831665107776587, 27.88393115100078390, 7.208316651077764980 ) ) ;
#66101=CARTESIAN_POINT ( 'NONE',  ( 19.38216949554541202, 5.998634669930420493, 9.382169495545424454 ) ) ;
#66102=CARTESIAN_POINT ( 'NONE',  ( 18.52753015748618282, 8.925597817667451750, -4.923371831947291888 ) ) ;
#66104=CARTESIAN_POINT ( 'NONE',  ( 2.791683348922240793, 11.63393115100078568, 7.208316651077764092 ) ) ;
#66105=CARTESIAN_POINT ( 'NONE',  ( 3.591859063236763294, 3.290301336597087012, -11.09922568453595026 ) ) ;
#66109=EDGE_LOOP ( 'NONE', ( #24658, #15911, #15421, #28081, #16912, #87698 ) ) ;
#66110=CARTESIAN_POINT ( 'NONE',  ( 4.559911319644449179, 7.230352010821505360, -9.422509992056141925 ) ) ;
#66111=CARTESIAN_POINT ( 'NONE',  ( 24.16423886937410614, 9.512082168247301794, -3.795296366450302550 ) ) ;
#66112=CARTESIAN_POINT ( 'NONE',  ( 19.84674366389459266, 28.71726448433411960, -2.638427012816827677 ) ) ;
#66113=CARTESIAN_POINT ( 'NONE',  ( 19.42250999205614193, 50.14701867748817676, 5.440088680355555262 ) ) ;
#66114=CARTESIAN_POINT ( 'NONE',  ( 0.6178305044545818747, 28.49863466993041783, -9.382169495545419124 ) ) ;
#66118=CARTESIAN_POINT ( 'NONE',  ( 0.000000000000000000, 81.99999999999992895, -5.000000000000000000 ) ) ;
#66119=CARTESIAN_POINT ( 'NONE',  ( 22.81628187352647785, 1.415301336597087012, 3.434112377981063169 ) ) ;
#66120=CARTESIAN_POINT ( 'NONE',  ( 5.076628168052703671, 66.84226448433412315, 8.527530157486179263 ) ) ;
#66121=CARTESIAN_POINT ( 'NONE',  ( 18.52753015748617571, 13.09226448433411960, 4.923371831947298993 ) ) ;
#66123=CARTESIAN_POINT ( 'NONE',  ( 6.565887622018943937, 23.08196800326375708, -12.81628187352647608 ) ) ;
#66125=CARTESIAN_POINT ( 'NONE',  ( 20.88017736071110519, 25.56368534415483751, 2.639326808657452039E-16 ) ) ;
#66127=CARTESIAN_POINT ( 'NONE',  ( 24.16423886937409904, 54.09541550158063217, 3.795296366450317205 ) ) ;
#66130=CARTESIAN_POINT ( 'NONE',  ( 12.91533473730992121, 29.52201867748817321, 10.88017736071110164 ) ) ;
#66131=CARTESIAN_POINT ( 'NONE',  ( 10.00000000000000178, 47.25893115100078745, 9.846743663894594434 ) ) ;
#66132=CARTESIAN_POINT ( 'NONE',  ( -0.8801773607111008646, 48.27201867748816966, 2.915334737309923430 ) ) ;
#66133=CARTESIAN_POINT ( 'NONE',  ( 2.917880565312950480, 30.97041550158063572, -12.26659068614894821 ) ) ;
#66135=CARTESIAN_POINT ( 'NONE',  ( 10.00000000000000178, 42.25893115100078745, 9.846743663894594434 ) ) ;
#66136=SURFACE_SIDE_STYLE ('',( #12160 ) ) ;
#66137=CARTESIAN_POINT ( 'NONE',  ( 10.00000000000000178, 67.25893115100079456, 9.846743663894594434 ) ) ;
#66139=CARTESIAN_POINT ( 'NONE',  ( 4.559911319644449179, 18.89701867748817321, 9.422509992056141925 ) ) ;
#66141=CARTESIAN_POINT ( 'NONE',  ( 15.44008868035555793, 16.39701867748817321, -9.422509992056140149 ) ) ;
#66142=CARTESIAN_POINT ( 'NONE',  ( 18.52753015748617571, 3.092264484334118269, 4.923371831947298993 ) ) ;
#66143=CARTESIAN_POINT ( 'NONE',  ( 10.00000000000000000, 25.55374883491396787, -14.16423886937410082 ) ) ;
#66144=CARTESIAN_POINT ( 'NONE',  ( 12.63842701281683922, 19.55059781766745175, -9.846743663894590881 ) ) ;
#66145=CARTESIAN_POINT ( 'NONE',  ( 12.63842701281683922, 59.55059781766744464, -9.846743663894590881 ) ) ;
#66146=CARTESIAN_POINT ( 'NONE',  ( 2.035157376598824452, 33.68868534415484106, 7.964842623401179544 ) ) ;
#66149=STYLED_ITEM ( 'NONE', ( #53263 ), #51621 ) ;
#66152=CARTESIAN_POINT ( 'NONE',  ( 10.00000000000000000, 49.75893115100078745, -9.846743663894594434 ) ) ;
#66156=CARTESIAN_POINT ( 'NONE',  ( 17.08211943468705840, 25.13708216824730357, -12.26659068614894466 ) ) ;
#66157=CARTESIAN_POINT ( 'NONE',  ( 17.08211943468705130, 13.47041550158063572, 12.26659068614894998 ) ) ;
#66159=CARTESIAN_POINT ( 'NONE',  ( 10.00000000000000000, 61.81368534415484106, -10.88017736071110342 ) ) ;
#66160=CARTESIAN_POINT ( 'NONE',  ( 22.26659068614894466, 53.88708216824731068, 7.082119434687054849 ) ) ;
#66161=CARTESIAN_POINT ( 'NONE',  ( 6.565887622018943937, 0.1653013365970866511, 12.81628187352647430 ) ) ;
#66162=CARTESIAN_POINT ( 'NONE',  ( 1.472469842513823179, 35.59226448433412315, -4.923371831947296329 ) ) ;
#66164=CARTESIAN_POINT ( 'NONE',  ( -0.8801773607111009756, 38.06368534415484106, 1.068504757029289695E-15 ) ) ;
#66165=CARTESIAN_POINT ( 'NONE',  ( 10.00000000000000178, 0.3736346699304200492, 12.81628187352647608 ) ) ;
#66166=CARTESIAN_POINT ( 'NONE',  ( 6.204703633549690345, 17.84541550158063217, 14.16423886937410082 ) ) ;
#66167=CARTESIAN_POINT ( 'NONE',  ( 13.79529636645030344, 53.26208216824730357, 14.16423886937410614 ) ) ;
#66168=CARTESIAN_POINT ( 'NONE',  ( 15.44008868035555793, 21.39701867748817321, -9.422509992056140149 ) ) ;
#66169=CARTESIAN_POINT ( 'NONE',  ( 19.84674366389459266, 38.71726448433412315, -2.638427012816827677 ) ) ;
#66171=CARTESIAN_POINT ( 'NONE',  ( 4.559911319644449179, 38.89701867748817676, 9.422509992056141925 ) ) ;
#66177=CARTESIAN_POINT ( 'NONE',  ( 22.26659068614895176, 49.72041550158063927, -7.082119434687042414 ) ) ;
#66178=CARTESIAN_POINT ( 'NONE',  ( 17.20831665107776587, 42.88393115100077324, 7.208316651077764980 ) ) ;
#66179=CARTESIAN_POINT ( 'NONE',  ( 20.88017736071110519, 55.56368534415484817, 2.639326808657452039E-16 ) ) ;
#66181=CARTESIAN_POINT ( 'NONE',  ( 12.91533473730992121, 49.52201867748817676, 10.88017736071110164 ) ) ;
#66186=CARTESIAN_POINT ( 'NONE',  ( 24.16423886937410614, 19.30374883491397142, 8.672049930838204340E-16 ) ) ;
#66188=CARTESIAN_POINT ( 'NONE',  ( -2.816281873526471635, 18.91530133659708213, -3.434112377981056508 ) ) ;
#66189=ORIENTED_EDGE ( 'NONE', *, *, #27143, .F. ) ;
#66190=CARTESIAN_POINT ( 'NONE',  ( 0.6178305044545838731, 39.74863466993041072, 9.382169495545420901 ) ) ;
#66191=EDGE_CURVE ( 'NONE', #84403, #67137, #18332, .T. ) ;
#66192=CARTESIAN_POINT ( 'NONE',  ( 5.076628168052704559, 30.17559781766745175, -8.527530157486179263 ) ) ;
#66193=CARTESIAN_POINT ( 'NONE',  ( 20.88017736071110519, 10.56368534415483751, 2.639326808657452039E-16 ) ) ;
#66194=CIRCLE ( 'NONE', #59844, 2.999999999999999112 ) ;
#66195=( BOUNDED_CURVE ( )  B_SPLINE_CURVE ( 2, ( #18579, #11559, #12546, #4571, #20043, #35032, #95558, #65534, #71591 ),
 .UNSPECIFIED., .F., .T. ) 
 B_SPLINE_CURVE_WITH_KNOTS ( ( 3, 2, 2, 2, 3 ),
 ( 0.2596570216176965484, 0.2619047619047619180, 0.2678571428571428492, 0.2738095238095238360, 0.2760572640965892055 ),
 .UNSPECIFIED. ) 
 CURVE ( )  GEOMETRIC_REPRESENTATION_ITEM ( )  RATIONAL_B_SPLINE_CURVE ( ( 0.9839835555609426354, 0.9871328979762479250, 1.000000000000000000, 0.9659258262890683122, 1.000000000000000000, 0.9659258262890683122, 1.000000000000000000, 0.9871328979762477029, 0.9839835555609424134 ) ) 
 REPRESENTATION_ITEM ( '' )  );
#66196=CARTESIAN_POINT ( 'NONE',  ( -2.816281873526473856, 54.33196800326376064, 3.434112377981055619 ) ) ;
#66198=CARTESIAN_POINT ( 'NONE',  ( 10.00000000000000000, 49.75893115100078745, -9.846743663894594434 ) ) ;
#66201=CARTESIAN_POINT ( 'NONE',  ( 4.999999999999999112, 60.50000000000000711, 6.500000000000000888 ) ) ;
#66206=CARTESIAN_POINT ( 'NONE',  ( -0.3289641300568005855, 45.10497603579418069, 5.963430220938281678 ) ) ;
#66207=CARTESIAN_POINT ( 'NONE',  ( 7.361572987183170547, 17.05059781766745530, 9.846743663894590881 ) ) ;
#66208=CARTESIAN_POINT ( 'NONE',  ( 21.09922568453595559, 27.04030133659708568, -6.408140936763230044 ) ) ;
#66211=CARTESIAN_POINT ( 'NONE',  ( 2.791683348922240793, 51.63393115100078745, 7.208316651077764092 ) ) ;
#66213=CARTESIAN_POINT ( 'NONE',  ( -2.266590686148945544, 21.38708216824730357, -7.082119434687050408 ) ) ;
#66214=CARTESIAN_POINT ( 'NONE',  ( 0.1532563361054082862, 51.21726448433412315, 2.638427012816831674 ) ) ;
#66215=CARTESIAN_POINT ( 'NONE',  ( 3.591859063236763294, 43.29030133659708923, -11.09922568453595026 ) ) ;
#66218=CARTESIAN_POINT ( 'NONE',  ( 20.88017736071110164, 65.35535201082150536, 2.915334737309930979 ) ) ;
#66221=CARTESIAN_POINT ( 'NONE',  ( 12.63842701281683922, 29.55059781766745175, -9.846743663894590881 ) ) ;
#66222=CARTESIAN_POINT ( 'NONE',  ( 12.91533473730993009, 41.60535201082149825, -10.88017736071109987 ) ) ;
#66223=CARTESIAN_POINT ( 'NONE',  ( 16.40814093676324603, 42.45696800326375353, -11.09922568453594671 ) ) ;
#66224=CARTESIAN_POINT ( 'NONE',  ( 12.63842701281683922, 29.55059781766745175, -9.846743663894590881 ) ) ;
#66226=CARTESIAN_POINT ( 'NONE',  ( 15.44008868035555260, 29.73035201082150891, 9.422509992056143702 ) ) ;
#66229=CARTESIAN_POINT ( 'NONE',  ( 7.084665262690076126, 17.02201867748817676, -10.88017736071110164 ) ) ;
#66230=CARTESIAN_POINT ( 'NONE',  ( 14.92337183194729633, 57.67559781766745886, 8.527530157486181039 ) ) ;
#66231=CARTESIAN_POINT ( 'NONE',  ( 19.42250999205614193, 40.14701867748817676, 5.440088680355555262 ) ) ;
#66233=CARTESIAN_POINT ( 'NONE',  ( 2.035157376598822676, 57.43868534415484106, -7.964842623401177768 ) ) ;
#66234=CARTESIAN_POINT ( 'NONE',  ( 10.00000000000000178, 24.31368534415484106, 10.88017736071110342 ) ) ;
#66235=CARTESIAN_POINT ( 'NONE',  ( -0.000000000000000000, 71.60366622817831228, -5.031467577974828131 ) ) ;
#66236=CARTESIAN_POINT ( 'NONE',  ( 0.1532563361054082862, 1.217264484334117824, 2.638427012816831674 ) ) ;
#66237=CARTESIAN_POINT ( 'NONE',  ( 2.791683348922240793, 21.63393115100078745, 7.208316651077764092 ) ) ;
#66239=CARTESIAN_POINT ( 'NONE',  ( 18.52753015748617571, 48.09226448433412315, 4.923371831947298993 ) ) ;
#66240=CARTESIAN_POINT ( 'NONE',  ( -0.3689425029237881626, 52.42874883491396076, 10.36894250292379027 ) ) ;
#66242=CARTESIAN_POINT ( 'NONE',  ( 1.492507162822264366, 62.19955587570481015, -6.500000000000073719 ) ) ;
#66243=CARTESIAN_POINT ( 'NONE',  ( -2.266590686148945544, 11.38708216824730179, -7.082119434687050408 ) ) ;
#66244=EDGE_CURVE ( 'NONE', #32140, #35669, #16639, .T. ) ;
#66245=CARTESIAN_POINT ( 'NONE',  ( 20.36894250292379382, 38.67874883491396076, 10.36894250292379205 ) ) ;
#66246=CARTESIAN_POINT ( 'NONE',  ( 10.00000000000000000, 7.873634669930421381, -12.81628187352647608 ) ) ;
#66248=CARTESIAN_POINT ( 'NONE',  ( 10.00000000000000178, 14.31368534415483929, 10.88017736071110342 ) ) ;
#66250=CARTESIAN_POINT ( 'NONE',  ( 0.1532563361054082862, 36.21726448433410894, 2.638427012816831674 ) ) ;
#66254=SURFACE_SIDE_STYLE ('',( #89263 ) ) ;
#66255=CARTESIAN_POINT ( 'NONE',  ( 22.81628187352647785, 21.41530133659708923, 3.434112377981063169 ) ) ;
#66256=CARTESIAN_POINT ( 'NONE',  ( 2.791683348922237240, 30.38393115100078390, -7.208316651077763204 ) ) ;
#66257=ORIENTED_EDGE ( 'NONE', *, *, #76586, .T. ) ;
#66258=CARTESIAN_POINT ( 'NONE',  ( 12.63842701281683034, 2.467264484334118269, 9.846743663894596210 ) ) ;
#66260=CARTESIAN_POINT ( 'NONE',  ( -0.8801773607110991993, 2.855352010821504471, -2.915334737309923874 ) ) ;
#66261=CARTESIAN_POINT ( 'NONE',  ( -0.8801773607111008646, 13.27201867748817143, 2.915334737309923430 ) ) ;
#66262=CARTESIAN_POINT ( 'NONE',  ( 2.917880565312950480, 40.97041550158063217, -12.26659068614894821 ) ) ;
#66263=CARTESIAN_POINT ( 'NONE',  ( 19.42250999205614193, 40.14701867748817676, 5.440088680355555262 ) ) ;
#66264=CARTESIAN_POINT ( 'NONE',  ( 4.559911319644449179, 67.23035201082150536, -9.422509992056141925 ) ) ;
#66266=CARTESIAN_POINT ( 'NONE',  ( 21.92686044187657401, 40.37045670184115664, -3.195792623639525765 ) ) ;
#66267=CARTESIAN_POINT ( 'NONE',  ( 17.20831665107776587, 17.88393115100078745, 7.208316651077764980 ) ) ;
#66268=SURFACE_STYLE_FILL_AREA ( #73283 ) ;
#66269=CARTESIAN_POINT ( 'NONE',  ( 14.92337183194729633, 12.67559781766745353, 8.527530157486181039 ) ) ;
#66271=CARTESIAN_POINT ( 'NONE',  ( 10.00000000000000000, 39.75893115100078745, -9.846743663894594434 ) ) ;
#66272=CARTESIAN_POINT ( 'NONE',  ( 19.84674366389459621, 63.50893115100078745, 7.409399052514197653E-17 ) ) ;
#66273=CARTESIAN_POINT ( 'NONE',  ( 10.00000000000000000, 31.81368534415483751, -10.88017736071110342 ) ) ;
#66274=ORIENTED_EDGE ( 'NONE', *, *, #35618, .F. ) ;
#66275=CARTESIAN_POINT ( 'NONE',  ( 10.00000000000000000, 57.87363466993042493, -12.81628187352647608 ) ) ;
#66278=CARTESIAN_POINT ( 'NONE',  ( 1.472469842513823179, 0.5922644843341181575, -4.923371831947296329 ) ) ;
#66279=CARTESIAN_POINT ( 'NONE',  ( 22.81628187352648496, 46.83196800326376064, -3.434112377981050290 ) ) ;
#66280=CARTESIAN_POINT ( 'NONE',  ( 17.08211943468705130, 63.47041550158063927, 12.26659068614894998 ) ) ;
#66281=CARTESIAN_POINT ( 'NONE',  ( 2.791683348922237240, 40.38393115100078035, -7.208316651077763204 ) ) ;
#66283=CARTESIAN_POINT ( 'NONE',  ( 14.92337183194729988, 59.34226448433412315, -8.527530157486177487 ) ) ;
#66284=CARTESIAN_POINT ( 'NONE',  ( 13.79529636645031943, 20.34541550158063572, -14.16423886937409904 ) ) ;
#66285=CARTESIAN_POINT ( 'NONE',  ( 24.16423886937410614, 44.51208216824730357, -3.795296366450302550 ) ) ;
#66286=CARTESIAN_POINT ( 'NONE',  ( 0.1532563361054100626, 40.80059781766745886, -2.638427012816831230 ) ) ;
#66288=CARTESIAN_POINT ( 'NONE',  ( 7.084665262690076126, 39.10535201082150536, 10.88017736071109987 ) ) ;
#66289=EDGE_CURVE ( 'NONE', #78236, #33937, #95439, .T. ) ;
#66290=CARTESIAN_POINT ( 'NONE',  ( 20.88017736071110875, 55.77201867748816966, -2.915334737309920765 ) ) ;
#66291=CARTESIAN_POINT ( 'NONE',  ( 20.88017736071110875, 50.77201867748817676, -2.915334737309920321 ) ) ;
#66293=CARTESIAN_POINT ( 'NONE',  ( -2.816281873526473856, 44.12363466993042493, 9.499525473075851096E-16 ) ) ;
#66294=CARTESIAN_POINT ( 'NONE',  ( 15.44008868035555793, 66.39701867748817676, -9.422509992056140149 ) ) ;
#66296=STYLED_ITEM ( 'NONE', ( #3290 ), #53385 ) ;
#66297=CARTESIAN_POINT ( 'NONE',  ( -4.164238869374099927, 2.012082168247300906, 3.795296366450308767 ) ) ;
#66298=CARTESIAN_POINT ( 'NONE',  ( 2.791683348922240793, 6.633931151000785675, 7.208316651077764092 ) ) ;
#66300=ORIENTED_EDGE ( 'NONE', *, *, #53520, .F. ) ;
#66301=CARTESIAN_POINT ( 'NONE',  ( 0.5774900079438607392, 18.48035201082150536, 5.440088680355550821 ) ) ;
#66304=CARTESIAN_POINT ( 'NONE',  ( -4.164238869374099039, 16.80374883491396787, 8.674139862899312516E-16 ) ) ;
#66306=CARTESIAN_POINT ( 'NONE',  ( 0.5774900079438590739, 17.64701867748817321, -5.440088680355550821 ) ) ;
#66307=CARTESIAN_POINT ( 'NONE',  ( 0.1532563361054082862, 61.21726448433412315, 2.638427012816831674 ) ) ;
#66309=CARTESIAN_POINT ( 'NONE',  ( 19.84674366389459266, 63.30059781766745886, 2.638427012816836559 ) ) ;
#66312=CARTESIAN_POINT ( 'NONE',  ( 19.84674366389459266, 3.300597817667451750, 2.638427012816836559 ) ) ;
#66313=CARTESIAN_POINT ( 'NONE',  ( 0.1532563361054082862, 66.21726448433413736, 2.638427012816831674 ) ) ;
#66314=CARTESIAN_POINT ( 'NONE',  ( 4.559911319644449179, 12.23035201082150536, -9.422509992056141925 ) ) ;
#66316=CARTESIAN_POINT ( 'NONE',  ( 1.472469842513823179, 1.425597817667451528, 4.923371831947296329 ) ) ;
#66317=CARTESIAN_POINT ( 'NONE',  ( 19.42250999205614193, 20.14701867748817321, 5.440088680355555262 ) ) ;
#66321=CARTESIAN_POINT ( 'NONE',  ( 21.09922568453595559, 57.04030133659708923, -6.408140936763230044 ) ) ;
#66322=CARTESIAN_POINT ( 'NONE',  ( 17.96484262340118221, 44.93868534415483396, 7.964842623401181321 ) ) ;
#66324=VECTOR ( 'NONE', #10563, 1000.000000000000000 ) ;
#66325=CARTESIAN_POINT ( 'NONE',  ( -2.816281873526471635, 38.91530133659708213, -3.434112377981056508 ) ) ;
#66326=CARTESIAN_POINT ( 'NONE',  ( 0.5774900079438607392, 53.48035201082151247, 5.440088680355550821 ) ) ;
#66327=CARTESIAN_POINT ( 'NONE',  ( 2.791683348922240793, 56.63393115100078035, 7.208316651077764092 ) ) ;
#66329=CARTESIAN_POINT ( 'NONE',  ( 19.84674366389459266, 23.30059781766745530, 2.638427012816836559 ) ) ;
#66330=CARTESIAN_POINT ( 'NONE',  ( 10.00000000000000178, 5.373634669930420493, 12.81628187352647608 ) ) ;
#66333=CARTESIAN_POINT ( 'NONE',  ( 15.44008868035555260, 19.73035201082150536, 9.422509992056143702 ) ) ;
#66334=CARTESIAN_POINT ( 'NONE',  ( 7.361572987183169658, 54.96726448433413026, -9.846743663894592657 ) ) ;
#66335=CARTESIAN_POINT ( 'NONE',  ( -0.1503990784575247319, 62.22266099184918176, -6.262539305110083276 ) ) ;
#66336=CARTESIAN_POINT ( 'NONE',  ( 7.361572987183169658, 4.967264484334119601, -9.846743663894592657 ) ) ;
#66337=CARTESIAN_POINT ( 'NONE',  ( 2.791683348922237240, 0.3839311510007847872, -7.208316651077763204 ) ) ;
#66338=CARTESIAN_POINT ( 'NONE',  ( 1.472469842513823179, 66.42559781766745175, 4.923371831947296329 ) ) ;
#66342=CARTESIAN_POINT ( 'NONE',  ( 3.591859063236763294, 33.29030133659708213, -11.09922568453595026 ) ) ;
#66343=CARTESIAN_POINT ( 'NONE',  ( 5.076628168052704559, 30.17559781766745175, -8.527530157486179263 ) ) ;
#66344=CARTESIAN_POINT ( 'NONE',  ( 0.8952175423695086787, 58.52576239577082617, 5.990408912944362285 ) ) ;
#66345=CARTESIAN_POINT ( 'NONE',  ( 13.79529636645030344, 63.26208216824730357, 14.16423886937410614 ) ) ;
#66346=CARTESIAN_POINT ( 'NONE',  ( 2.791683348922240793, 26.63393115100078745, 7.208316651077764092 ) ) ;
#66348=CARTESIAN_POINT ( 'NONE',  ( 13.99999999999999822, 61.00000000000000711, -5.000000000000000000 ) ) ;
#66349=CARTESIAN_POINT ( 'NONE',  ( 17.08211943468705840, 60.13708216824729647, -12.26659068614894466 ) ) ;
#66351=B_SPLINE_CURVE_WITH_KNOTS ( 'NONE', 3,
 ( #25311, #63276, #71294, #92795 ),
 .UNSPECIFIED., .F., .F.,
 ( 4, 4 ),
 ( 7.757919228897728493E-18, 0.002392975128318494595 ),
 .UNSPECIFIED. ) ;
#66352=CARTESIAN_POINT ( 'NONE',  ( 2.035157376598822676, 22.43868534415483396, -7.964842623401177768 ) ) ;
#66353=CARTESIAN_POINT ( 'NONE',  ( -0.3689425029237898834, 56.17874883491396076, -10.36894250292378850 ) ) ;
#66354=CARTESIAN_POINT ( 'NONE',  ( -0.3689425029237898834, 56.17874883491396076, -10.36894250292378850 ) ) ;
#66355=CARTESIAN_POINT ( 'NONE',  ( -46.30928139467842897, 104.0823827281712255, -5.529860068218142466 ) ) ;
#66356=( NAMED_UNIT ( * ) PLANE_ANGLE_UNIT ( ) SI_UNIT ( $, .RADIAN. ) );
#66357=CARTESIAN_POINT ( 'NONE',  ( 5.076628168052703671, 11.84226448433411960, 8.527530157486179263 ) ) ;
#66358=CARTESIAN_POINT ( 'NONE',  ( -2.816281873526471635, 3.915301336597087456, -3.434112377981056508 ) ) ;
#66360=CARTESIAN_POINT ( 'NONE',  ( 20.88017736071110519, 55.56368534415484817, 2.639326808657452039E-16 ) ) ;
#66361=AXIS2_PLACEMENT_3D ( 'NONE', #27743, #59224, #72262 ) ;
#66362=CARTESIAN_POINT ( 'NONE',  ( 0.1532563361054082862, 61.21726448433412315, 2.638427012816831674 ) ) ;
#66365=CARTESIAN_POINT ( 'NONE',  ( -4.164238869374099927, 2.012082168247300906, 3.795296366450308767 ) ) ;
#66370=CARTESIAN_POINT ( 'NONE',  ( 24.16423886937410614, 34.51208216824731068, -3.795296366450302550 ) ) ;
#66371=EDGE_CURVE ( 'NONE', #75865, #84653, #33435, .T. ) ;
#66373=CARTESIAN_POINT ( 'NONE',  ( 1.472469842513823179, 0.5922644843341181575, -4.923371831947296329 ) ) ;
#66376=CARTESIAN_POINT ( 'NONE',  ( 7.084665262690076126, 22.02201867748817321, -10.88017736071110164 ) ) ;
#66377=CARTESIAN_POINT ( 'NONE',  ( 13.43411237798106583, 32.66530133659708213, -12.81628187352647252 ) ) ;
#66378=FILL_AREA_STYLE ('',( #82365 ) ) ;
#66379=CARTESIAN_POINT ( 'NONE',  ( 13.43411237798106583, 32.66530133659708213, -12.81628187352647252 ) ) ;
#66380=CARTESIAN_POINT ( 'NONE',  ( 21.09922568453595559, 62.04030133659709634, -6.408140936763230044 ) ) ;
#66384=CARTESIAN_POINT ( 'NONE',  ( 6.204703633549690345, 27.84541550158063217, 14.16423886937410082 ) ) ;
#66386=CARTESIAN_POINT ( 'NONE',  ( 19.42250999205614193, 25.14701867748817321, 5.440088680355555262 ) ) ;
#66389=CARTESIAN_POINT ( 'NONE',  ( 7.084665262690076126, 49.10535201082149825, 10.88017736071109987 ) ) ;
#66390=CARTESIAN_POINT ( 'NONE',  ( 15.44008868035555793, 51.39701867748816966, -9.422509992056140149 ) ) ;
#66391=CARTESIAN_POINT ( 'NONE',  ( 22.81628187352647785, 11.41530133659708390, 3.434112377981063169 ) ) ;
#66392=DIRECTION ( 'NONE',  ( -0.8320502943378437211, 0.5547001962252290364, 0.000000000000000000 ) ) ;
#66393=DIRECTION ( 'NONE',  ( -0.000000000000000000, -0.000000000000000000, -1.000000000000000000 ) ) ;
#66394=CARTESIAN_POINT ( 'NONE',  ( 19.84674366389459266, 18.71726448433411960, -2.638427012816827677 ) ) ;
#66396=CARTESIAN_POINT ( 'NONE',  ( 10.00000000000000178, 44.31368534415484106, 10.88017736071110342 ) ) ;
#66401=CARTESIAN_POINT ( 'NONE',  ( 13.43411237798105340, 10.58196800326375353, 12.81628187352647963 ) ) ;
#66404=CARTESIAN_POINT ( 'NONE',  ( 14.92337183194729988, 29.34226448433411960, -8.527530157486177487 ) ) ;
#66405=CARTESIAN_POINT ( 'NONE',  ( 22.81628187352647785, 51.41530133659708923, 3.434112377981063169 ) ) ;
#66406=CARTESIAN_POINT ( 'NONE',  ( 12.63842701281683922, 24.55059781766745175, -9.846743663894590881 ) ) ;
#66407=EDGE_LOOP ( 'NONE', ( #73078, #52657, #4430, #18784 ) ) ;
#66408=CARTESIAN_POINT ( 'NONE',  ( 17.08211943468705840, 10.13708216824730179, -12.26659068614894466 ) ) ;
#66409=CARTESIAN_POINT ( 'NONE',  ( -47.70923076923077133, 97.34615384615383959, -9.500000000000000000 ) ) ;
#66410=CARTESIAN_POINT ( 'NONE',  ( 0.5774900079438607392, 18.48035201082150536, 5.440088680355550821 ) ) ;
#66412=CARTESIAN_POINT ( 'NONE',  ( 13.79529636645031943, 30.34541550158063927, -14.16423886937409904 ) ) ;
#66414=CARTESIAN_POINT ( 'NONE',  ( 18.52753015748618282, 33.92559781766745886, -4.923371831947291888 ) ) ;
#66415=CARTESIAN_POINT ( 'NONE',  ( 20.88017736071110164, 15.35535201082150358, 2.915334737309930979 ) ) ;
#66416=CARTESIAN_POINT ( 'NONE',  ( 22.26659068614894466, 63.88708216824730357, 7.082119434687054849 ) ) ;
#66417=ORIENTED_EDGE ( 'NONE', *, *, #2197, .F. ) ;
#66418=CARTESIAN_POINT ( 'NONE',  ( 10.00000000000000000, 21.81368534415484106, -10.88017736071110342 ) ) ;
#66419=CARTESIAN_POINT ( 'NONE',  ( 7.084665262690076126, 39.10535201082150536, 10.88017736071109987 ) ) ;
#66422=CARTESIAN_POINT ( 'NONE',  ( 18.52753015748617571, 53.09226448433412315, 4.923371831947298993 ) ) ;
#66423=CARTESIAN_POINT ( 'NONE',  ( -0.8801773607111009756, 33.06368534415484106, 1.068504757029289695E-15 ) ) ;
#66424=VECTOR ( 'NONE', #10438, 1000.000000000000000 ) ;
#66426=CARTESIAN_POINT ( 'NONE',  ( 6.565887622018943937, 60.16530133659707502, 12.81628187352647430 ) ) ;
#66427=CARTESIAN_POINT ( 'NONE',  ( 19.72487221294571569, 30.71833443783938122, -6.499999999999989342 ) ) ;
#66428=CARTESIAN_POINT ( 'NONE',  ( -4.164238869374099039, 36.80374883491396787, 8.674139862899312516E-16 ) ) ;
#66429=CARTESIAN_POINT ( 'NONE',  ( 20.88017736071110164, 55.35535201082149825, 2.915334737309930979 ) ) ;
#66430=CARTESIAN_POINT ( 'NONE',  ( 2.791683348922237240, 65.38393115100078035, -7.208316651077763204 ) ) ;
#66432=CARTESIAN_POINT ( 'NONE',  ( 10.00000000000000000, 44.75893115100078745, -9.846743663894594434 ) ) ;
#66433=CARTESIAN_POINT ( 'NONE',  ( 18.52753015748618282, 3.925597817667451306, -4.923371831947291888 ) ) ;
#66435=CARTESIAN_POINT ( 'NONE',  ( 2.791683348922237240, 20.38393115100078745, -7.208316651077763204 ) ) ;
#66437=CARTESIAN_POINT ( 'NONE',  ( 10.00000000000000000, 21.81368534415484106, -10.88017736071110342 ) ) ;
#66438=CARTESIAN_POINT ( 'NONE',  ( 0.1532563361054083140, 21.00893115100078745, 1.131784320476157264E-15 ) ) ;
#66439=CARTESIAN_POINT ( 'NONE',  ( 13.43411237798106583, 7.665301336597086568, -12.81628187352647252 ) ) ;
#66440=CARTESIAN_POINT ( 'NONE',  ( 15.44008868035555260, 59.73035201082151247, 9.422509992056143702 ) ) ;
#66441=CARTESIAN_POINT ( 'NONE',  ( 7.084665262690076126, 37.02201867748817676, -10.88017736071110164 ) ) ;
#66442=CARTESIAN_POINT ( 'NONE',  ( 6.565887622018943937, 60.16530133659707502, 12.81628187352647430 ) ) ;
#66443=CARTESIAN_POINT ( 'NONE',  ( -0.3689425029237881626, 42.42874883491396787, 10.36894250292379027 ) ) ;
#66447=CARTESIAN_POINT ( 'NONE',  ( 0.1532563361054100626, 65.80059781766745175, -2.638427012816831230 ) ) ;
#66448=CARTESIAN_POINT ( 'NONE',  ( 4.559911319644449179, 2.230352010821504471, -9.422509992056141925 ) ) ;
#66449=CARTESIAN_POINT ( 'NONE',  ( 20.88017736071110519, 40.56368534415484106, 2.639326808657452039E-16 ) ) ;
#66450=CARTESIAN_POINT ( 'NONE',  ( 12.63842701281683034, 57.46726448433411605, 9.846743663894596210 ) ) ;
#66452=CARTESIAN_POINT ( 'NONE',  ( 12.63842701281683034, 17.46726448433411250, 9.846743663894596210 ) ) ;
#66453=CARTESIAN_POINT ( 'NONE',  ( -0.8801773607111009756, 53.06368534415484106, 1.068504757029289695E-15 ) ) ;
#66454=CARTESIAN_POINT ( 'NONE',  ( 2.791683348922240793, 31.63393115100078745, 7.208316651077764092 ) ) ;
#66455=CARTESIAN_POINT ( 'NONE',  ( 0.1532563361054083140, 31.00893115100078390, 1.131784320476157264E-15 ) ) ;
#66456=B_SPLINE_CURVE_WITH_KNOTS ( 'NONE', 3,
 ( #54540, #32029, #610, #31054 ),
 .UNSPECIFIED., .F., .F.,
 ( 4, 4 ),
 ( 1.097135458930219287E-17, 0.001060528352561992873 ),
 .UNSPECIFIED. ) ;
#66458=CARTESIAN_POINT ( 'NONE',  ( 17.20831665107776587, 7.883931151000784787, 7.208316651077764980 ) ) ;
#66461=CARTESIAN_POINT ( 'NONE',  ( -2.816281873526471635, 33.91530133659708213, -3.434112377981056508 ) ) ;
#66462=CARTESIAN_POINT ( 'NONE',  ( 19.42250999205614193, 65.14701867748817676, 5.440088680355555262 ) ) ;
#66464=CARTESIAN_POINT ( 'NONE',  ( 14.92337183194729633, 2.675597817667451750, 8.527530157486181039 ) ) ;
#66466=CARTESIAN_POINT ( 'NONE',  ( 2.791683348922240793, 26.63393115100078745, 7.208316651077764092 ) ) ;
#66467=ORIENTED_EDGE ( 'NONE', *, *, #79732, .F. ) ;
#66469=B_SPLINE_CURVE_WITH_KNOTS ( 'NONE', 3,
 ( #31014, #77999, #70508, #46038, #61022, #9505, #7563, #38050, #32494, #54019 ),
 .UNSPECIFIED., .F., .F.,
 ( 4, 3, 3, 4 ),
 ( 7.757919228897728493E-18, 0.0006253016069561031978, 0.001250604074564932999, 0.002501455912506560415 ),
 .UNSPECIFIED. ) ;
#66471=CARTESIAN_POINT ( 'NONE',  ( 5.076628168052703671, 66.84226448433412315, 8.527530157486179263 ) ) ;
#66472=CARTESIAN_POINT ( 'NONE',  ( 7.084665262690076126, 2.022018677488170990, -10.88017736071110164 ) ) ;
#66474=CARTESIAN_POINT ( 'NONE',  ( 24.16423886937410614, 14.51208216824730179, -3.795296366450302550 ) ) ;
#66476=FACE_OUTER_BOUND ( 'NONE', #82457, .T. ) ;
#66477=CARTESIAN_POINT ( 'NONE',  ( -4.164238869374099039, 11.80374883491396965, 8.674139862899312516E-16 ) ) ;
#66478=CARTESIAN_POINT ( 'NONE',  ( -4.164238869374098151, 46.59541550158063927, -3.795296366450310543 ) ) ;
#66479=CARTESIAN_POINT ( 'NONE',  ( -0.3689425029237898834, 1.178748834913967869, -10.36894250292378850 ) ) ;
#66480=CARTESIAN_POINT ( 'NONE',  ( 2.917880565312950480, 10.97041550158063572, -12.26659068614894821 ) ) ;
#66481=CARTESIAN_POINT ( 'NONE',  ( 19.42250999205614193, 65.14701867748817676, 5.440088680355555262 ) ) ;
#66482=CARTESIAN_POINT ( 'NONE',  ( 20.88017736071110875, 45.77201867748816966, -2.915334737309920765 ) ) ;
#66485=CARTESIAN_POINT ( 'NONE',  ( 14.92337183194729988, 34.34226448433411605, -8.527530157486177487 ) ) ;
#66486=EDGE_CURVE ( 'NONE', #19583, #16885, #90646, .T. ) ;
#66487=CARTESIAN_POINT ( 'NONE',  ( -0.8801773607111008646, 63.27201867748817676, 2.915334737309923430 ) ) ;
#66488=CARTESIAN_POINT ( 'NONE',  ( 19.84674366389459266, 23.71726448433412315, -2.638427012816827677 ) ) ;
#66490=CARTESIAN_POINT ( 'NONE',  ( 2.035157376598824452, 8.688685344154839285, 7.964842623401179544 ) ) ;
#66491=CARTESIAN_POINT ( 'NONE',  ( -2.816281873526473856, 54.12363466993041783, 9.499525473075851096E-16 ) ) ;
#66492=CARTESIAN_POINT ( 'NONE',  ( 7.361572987183170547, 52.05059781766745175, 9.846743663894590881 ) ) ;
#66494=CARTESIAN_POINT ( 'NONE',  ( 2.791683348922240793, 31.63393115100078745, 7.208316651077764092 ) ) ;
#66496=CARTESIAN_POINT ( 'NONE',  ( 13.43411237798105340, 45.58196800326374643, 12.81628187352647963 ) ) ;
#66498=CARTESIAN_POINT ( 'NONE',  ( 0.5774900079438590739, 37.64701867748817676, -5.440088680355550821 ) ) ;
#66499=CARTESIAN_POINT ( 'NONE',  ( 0.1532563361054083140, 36.00893115100078745, 1.131784320476157264E-15 ) ) ;
#66501=CARTESIAN_POINT ( 'NONE',  ( 17.08211943468705130, 23.47041550158063572, 12.26659068614894998 ) ) ;
#66503=CARTESIAN_POINT ( 'NONE',  ( 24.16423886937409904, 4.095415501580634832, 3.795296366450317205 ) ) ;
#66505=CARTESIAN_POINT ( 'NONE',  ( 0.5774900079438607392, 48.48035201082150536, 5.440088680355550821 ) ) ;
#66506=CARTESIAN_POINT ( 'NONE',  ( 10.00000000000000178, 64.31368534415483396, 10.88017736071110342 ) ) ;
#66507=CARTESIAN_POINT ( 'NONE',  ( -2.266590686148945544, 46.38708216824730357, -7.082119434687050408 ) ) ;
#66508=CARTESIAN_POINT ( 'NONE',  ( 13.43411237798106583, 2.665301336597086568, -12.81628187352647252 ) ) ;
#66509=CARTESIAN_POINT ( 'NONE',  ( 13.43411237798106583, 62.66530133659708923, -12.81628187352647252 ) ) ;
#66510=CARTESIAN_POINT ( 'NONE',  ( 15.44008868035555260, 49.73035201082150536, 9.422509992056143702 ) ) ;
#66512=CARTESIAN_POINT ( 'NONE',  ( 21.09922568453595559, 2.040301336597086568, -6.408140936763230044 ) ) ;
#66514=CARTESIAN_POINT ( 'NONE',  ( -0.8801773607111009756, 18.06368534415484106, 1.068504757029289695E-15 ) ) ;
#66515=CARTESIAN_POINT ( 'NONE',  ( 12.91533473730992121, 9.522018677488171434, 10.88017736071110164 ) ) ;
#66519=CARTESIAN_POINT ( 'NONE',  ( 12.91533473730992121, 9.522018677488171434, 10.88017736071110164 ) ) ;
#66520=CARTESIAN_POINT ( 'NONE',  ( 17.20831665107776587, 2.883931151000785231, 7.208316651077764980 ) ) ;
#66523=CARTESIAN_POINT ( 'NONE',  ( 2.791683348922237240, 30.38393115100078390, -7.208316651077763204 ) ) ;
#66524=CARTESIAN_POINT ( 'NONE',  ( 12.91533473730992121, 39.52201867748817676, 10.88017736071110164 ) ) ;
#66525=CARTESIAN_POINT ( 'NONE',  ( 3.591859063236761518, 9.956968003263753531, 11.09922568453594849 ) ) ;
#66526=CARTESIAN_POINT ( 'NONE',  ( 19.42250999205614193, 30.14701867748817321, 5.440088680355555262 ) ) ;
#66529=CARTESIAN_POINT ( 'NONE',  ( 22.81628187352647785, 36.41530133659707502, 3.434112377981063169 ) ) ;
#66531=CARTESIAN_POINT ( 'NONE',  ( 4.559911319644449179, 67.23035201082150536, -9.422509992056141925 ) ) ;
#66532=CARTESIAN_POINT ( 'NONE',  ( 13.43411237798105340, 35.58196800326375353, 12.81628187352647963 ) ) ;
#66534=CARTESIAN_POINT ( 'NONE',  ( 0.1532563361054100626, 0.8005978176674514168, -2.638427012816831230 ) ) ;
#66535=CARTESIAN_POINT ( 'NONE',  ( 20.88017736071110164, 40.35535201082150536, 2.915334737309930979 ) ) ;
#66537=CARTESIAN_POINT ( 'NONE',  ( 10.00000000000000000, 60.55374883491397497, -14.16423886937410082 ) ) ;
#66538=CARTESIAN_POINT ( 'NONE',  ( 19.84674366389459266, 53.71726448433411605, -2.638427012816827677 ) ) ;
#66539=CARTESIAN_POINT ( 'NONE',  ( 18.52753015748618282, 18.92559781766745175, -4.923371831947291888 ) ) ;
#66540=CARTESIAN_POINT ( 'NONE',  ( 20.88017736071110164, 65.35535201082150536, 2.915334737309930979 ) ) ;
#66542=CARTESIAN_POINT ( 'NONE',  ( -2.266590686148945544, 32.22041550158063927, 7.082119434687048631 ) ) ;
#66543=CARTESIAN_POINT ( 'NONE',  ( 20.15039907845753220, 25.60158574516642815, -6.262539305110077947 ) ) ;
#66548=VERTEX_POINT ( 'NONE', #40222 ) ;
#66549=CARTESIAN_POINT ( 'NONE',  ( -0.3689425029237898834, 61.17874883491396076, -10.36894250292378850 ) ) ;
#66550=CARTESIAN_POINT ( 'NONE',  ( 22.26659068614894466, 58.88708216824729647, 7.082119434687054849 ) ) ;
#66551=CARTESIAN_POINT ( 'NONE',  ( 0.1532563361054083140, 31.00893115100078390, 1.131784320476157264E-15 ) ) ;
#66552=CARTESIAN_POINT ( 'NONE',  ( 6.565887622018943937, 30.16530133659708568, 12.81628187352647430 ) ) ;
#66554=CARTESIAN_POINT ( 'NONE',  ( 20.88017736071110519, 10.56368534415483751, 2.639326808657452039E-16 ) ) ;
#66555=CARTESIAN_POINT ( 'NONE',  ( 20.36894250292379738, 54.92874883491396076, -10.36894250292379027 ) ) ;
#66557=CARTESIAN_POINT ( 'NONE',  ( 18.52753015748618282, 33.92559781766745886, -4.923371831947291888 ) ) ;
#66559=CARTESIAN_POINT ( 'NONE',  ( 7.361572987183170547, 7.050597817667451750, 9.846743663894590881 ) ) ;
#66560=CARTESIAN_POINT ( 'NONE',  ( 17.39651004071841101, 57.93575266056827644, 6.500000000000005329 ) ) ;
#66563=EDGE_LOOP ( 'NONE', ( #61497, #8293, #75901, #64854 ) ) ;
#66565=COLOUR_RGB ( '', 0.72549020, 0.75294118, 0.79215686) ;
#66566=CARTESIAN_POINT ( 'NONE',  ( 17.20831665107776587, 44.13393115100078745, -7.208316651077762316 ) ) ;
#66567=CARTESIAN_POINT ( 'NONE',  ( 4.559911319644449179, 18.89701867748817321, 9.422509992056141925 ) ) ;
#66568=CARTESIAN_POINT ( 'NONE',  ( 12.91533473730993009, 21.60535201082150536, -10.88017736071109987 ) ) ;
#66569=FILL_AREA_STYLE_COLOUR ( '', #16408 ) ;
#66570=CARTESIAN_POINT ( 'NONE',  ( 22.81628187352647785, 16.41530133659708923, 3.434112377981063169 ) ) ;
#66571=CARTESIAN_POINT ( 'NONE',  ( 6.204703633549690345, 0.7620821682473009062, -14.16423886937410259 ) ) ;
#66575=CARTESIAN_POINT ( 'NONE',  ( 22.81628187352647785, 36.62363466993041783, 6.195893100308588602E-16 ) ) ;
#66576=CARTESIAN_POINT ( 'NONE',  ( 7.361572987183169658, -0.03273551566588185635, -9.846743663894592657 ) ) ;
#66578=CARTESIAN_POINT ( 'NONE',  ( 5.076628168052703671, 31.84226448433412315, 8.527530157486179263 ) ) ;
#66579=CARTESIAN_POINT ( 'NONE',  ( 15.44008868035555793, 6.397018677488171434, -9.422509992056140149 ) ) ;
#66581=CARTESIAN_POINT ( 'NONE',  ( 15.44008868035555793, 6.397018677488171434, -9.422509992056140149 ) ) ;
#66583=CARTESIAN_POINT ( 'NONE',  ( -0.8801773607111009756, 43.06368534415484106, 1.068504757029289695E-15 ) ) ;
#66584=CARTESIAN_POINT ( 'NONE',  ( 17.96484262340118221, 59.93868534415484106, 7.964842623401181321 ) ) ;
#66585=CARTESIAN_POINT ( 'NONE',  ( 20.88017736071110519, 55.56368534415484817, 2.639326808657452039E-16 ) ) ;
#66586=CARTESIAN_POINT ( 'NONE',  ( 0.1532563361054083140, 1.008931151000784787, 1.131784320476157264E-15 ) ) ;
#66587=CARTESIAN_POINT ( 'NONE',  ( 0.5774900079438607392, 43.48035201082151247, 5.440088680355550821 ) ) ;
#66588=CARTESIAN_POINT ( 'NONE',  ( -46.94000000000001904, 101.9887809003992913, 6.851115700668153785 ) ) ;
#66592=CARTESIAN_POINT ( 'NONE',  ( 7.361572987183169658, 34.96726448433411605, -9.846743663894592657 ) ) ;
#66594=CARTESIAN_POINT ( 'NONE',  ( 1.472469842513823179, 55.59226448433412315, -4.923371831947296329 ) ) ;
#66597=CARTESIAN_POINT ( 'NONE',  ( 13.79529636645031943, 5.345415501580634832, -14.16423886937409904 ) ) ;
#66602=CARTESIAN_POINT ( 'NONE',  ( -0.3689425029237881626, 57.42874883491397497, 10.36894250292379027 ) ) ;
#66605=CARTESIAN_POINT ( 'NONE',  ( 20.10239578412224759, 62.63377557478298741, -6.340343622311902294 ) ) ;
#66606=CARTESIAN_POINT ( 'NONE',  ( 7.361572987183170547, 52.05059781766745175, 9.846743663894590881 ) ) ;
#66607=FACE_OUTER_BOUND ( 'NONE', #97697, .T. ) ;
#66608=CARTESIAN_POINT ( 'NONE',  ( 10.00000000000000178, 25.37363466993041783, 12.81628187352647608 ) ) ;
#66609=CARTESIAN_POINT ( 'NONE',  ( 14.92337183194729633, 7.675597817667451750, 8.527530157486181039 ) ) ;
#66611=CARTESIAN_POINT ( 'NONE',  ( 10.00000000000000178, 12.25893115100078568, 9.846743663894594434 ) ) ;
#66612=CARTESIAN_POINT ( 'NONE',  ( 10.00000000000000000, 2.873634669930420049, -12.81628187352647608 ) ) ;
#66617=CARTESIAN_POINT ( 'NONE',  ( 4.559911319644449179, 3.897018677488171434, 9.422509992056141925 ) ) ;
#66618=CARTESIAN_POINT ( 'NONE',  ( 17.08211943468705130, 8.470415501580635720, 12.26659068614894998 ) ) ;
#66619=CARTESIAN_POINT ( 'NONE',  ( 5.076628168052704559, 30.17559781766745175, -8.527530157486179263 ) ) ;
#66620=CARTESIAN_POINT ( 'NONE',  ( 12.91533473730993009, 51.60535201082149825, -10.88017736071109987 ) ) ;
#66621=CARTESIAN_POINT ( 'NONE',  ( -2.816281873526471635, 28.91530133659708213, -3.434112377981056508 ) ) ;
#66623=CARTESIAN_POINT ( 'NONE',  ( 15.44008868035555793, 16.39701867748817321, -9.422509992056140149 ) ) ;
#66626=CARTESIAN_POINT ( 'NONE',  ( 0.6178305044545838731, -0.2513653300695798953, 9.382169495545420901 ) ) ;
#66627=CARTESIAN_POINT ( 'NONE',  ( 22.81628187352647785, 1.623634669930420271, 6.195893100308588602E-16 ) ) ;
#66628=CARTESIAN_POINT ( 'NONE',  ( 17.20831665107776587, 12.88393115100078390, 7.208316651077764980 ) ) ;
#66630=CARTESIAN_POINT ( 'NONE',  ( 21.09922568453595559, 37.04030133659708923, -6.408140936763230044 ) ) ;
#66633=CARTESIAN_POINT ( 'NONE',  ( 12.91533473730992121, 34.52201867748817676, 10.88017736071110164 ) ) ;
#66634=B_SPLINE_CURVE_WITH_KNOTS ( 'NONE', 3,
 ( #75160, #6671, #68173, #98189 ),
 .UNSPECIFIED., .F., .F.,
 ( 4, 4 ),
 ( 0.000000000000000000, 0.0006041882680322678990 ),
 .UNSPECIFIED. ) ;
#66640=CARTESIAN_POINT ( 'NONE',  ( 20.88017736071110875, 20.77201867748816611, -2.915334737309920765 ) ) ;
#66641=CARTESIAN_POINT ( 'NONE',  ( 20.88017736071110875, 35.77201867748816966, -2.915334737309920765 ) ) ;
#66642=CARTESIAN_POINT ( 'NONE',  ( 18.52753015748617571, 53.09226448433412315, 4.923371831947298993 ) ) ;
#66643=CARTESIAN_POINT ( 'NONE',  ( 2.035157376598824452, 53.68868534415484817, 7.964842623401179544 ) ) ;
#66644=CARTESIAN_POINT ( 'NONE',  ( 10.00000000000000000, 30.55374883491397142, -14.16423886937410082 ) ) ;
#66646=CARTESIAN_POINT ( 'NONE',  ( 5.076628168052703671, 36.84226448433412315, 8.527530157486179263 ) ) ;
#66647=CARTESIAN_POINT ( 'NONE',  ( -2.816281873526473856, 59.33196800326374643, 3.434112377981055619 ) ) ;
#66648=CARTESIAN_POINT ( 'NONE',  ( 6.565887622018943937, 3.081968003263753531, -12.81628187352647608 ) ) ;
#66650=CARTESIAN_POINT ( 'NONE',  ( 7.084665262690076126, 24.10535201082150181, 10.88017736071109987 ) ) ;
#66651=CARTESIAN_POINT ( 'NONE',  ( 4.559911319644449179, 7.230352010821504471, -9.422509992056141925 ) ) ;
#66652=CARTESIAN_POINT ( 'NONE',  ( 17.96484262340118221, 11.18868534415484106, -7.964842623401177768 ) ) ;
#66653=CARTESIAN_POINT ( 'NONE',  ( 2.791683348922237240, 0.3839311510007847872, -7.208316651077763204 ) ) ;
#66654=CARTESIAN_POINT ( 'NONE',  ( 2.917880565312950480, 20.97041550158063217, -12.26659068614894821 ) ) ;
#66655=CARTESIAN_POINT ( 'NONE',  ( 1.472469842513823179, 11.42559781766745175, 4.923371831947296329 ) ) ;
#66657=CARTESIAN_POINT ( 'NONE',  ( -0.8801773607111009756, 33.06368534415484106, 1.068504757029289695E-15 ) ) ;
#66662=CARTESIAN_POINT ( 'NONE',  ( 10.00000000000000178, 47.25893115100078745, 9.846743663894594434 ) ) ;
#66666=CARTESIAN_POINT ( 'NONE',  ( -2.266590686148945544, 21.38708216824730357, -7.082119434687050408 ) ) ;
#66667=CARTESIAN_POINT ( 'NONE',  ( -0.3689425029237881626, 17.42874883491397142, 10.36894250292379027 ) ) ;
#66668=CARTESIAN_POINT ( 'NONE',  ( 20.88017736071110519, 65.56368534415483396, 2.639326808657452039E-16 ) ) ;
#66669=CARTESIAN_POINT ( 'NONE',  ( 17.08211943468705130, 58.47041550158063927, 12.26659068614894998 ) ) ;
#66670=CARTESIAN_POINT ( 'NONE',  ( -2.816281873526473856, -0.8763653300695799508, 9.499525473075851096E-16 ) ) ;
#66671=CARTESIAN_POINT ( 'NONE',  ( 5.076628168052704559, 55.17559781766745175, -8.527530157486179263 ) ) ;
#66673=CARTESIAN_POINT ( 'NONE',  ( 20.88017736071110519, 50.56368534415484106, 2.639326808657452039E-16 ) ) ;
#66674=CARTESIAN_POINT ( 'NONE',  ( 3.591859063236763294, 3.290301336597087012, -11.09922568453595026 ) ) ;
#66675=CARTESIAN_POINT ( 'NONE',  ( 10.00000000000000000, 10.55374883491396787, -14.16423886937410082 ) ) ;
#66676=CARTESIAN_POINT ( 'NONE',  ( 24.16423886937410614, 54.51208216824730357, -3.795296366450302550 ) ) ;
#66678=CARTESIAN_POINT ( 'NONE',  ( 20.88017736071110164, 20.35535201082150891, 2.915334737309930979 ) ) ;
#66680=CARTESIAN_POINT ( 'NONE',  ( 19.42250999205614193, 40.14701867748817676, 5.440088680355555262 ) ) ;
#66684=ORIENTED_EDGE ( 'NONE', *, *, #66820, .T. ) ;
#66685=VERTEX_POINT ( 'NONE', #41223 ) ;
#66686=CARTESIAN_POINT ( 'NONE',  ( 24.16423886937410614, 44.30374883491397497, 8.672049930838204340E-16 ) ) ;
#66687=CARTESIAN_POINT ( 'NONE',  ( 5.076628168052704559, 45.17559781766745175, -8.527530157486179263 ) ) ;
#66688=CARTESIAN_POINT ( 'NONE',  ( 17.96484262340118221, 66.18868534415483396, -7.964842623401177768 ) ) ;
#66691=CARTESIAN_POINT ( 'NONE',  ( -0.8801773607110991993, 52.85535201082151247, -2.915334737309923874 ) ) ;
#66692=CARTESIAN_POINT ( 'NONE',  ( 0.6178305044545838731, 59.74863466993041783, 9.382169495545420901 ) ) ;
#66695=CARTESIAN_POINT ( 'NONE',  ( 20.36894250292379738, 19.92874883491396787, -10.36894250292379027 ) ) ;
#66696=CARTESIAN_POINT ( 'NONE',  ( 10.00000000000000178, 20.37363466993042138, 12.81628187352647608 ) ) ;
#66697=ORIENTED_EDGE ( 'NONE', *, *, #81967, .F. ) ;
#66698=CARTESIAN_POINT ( 'NONE',  ( 16.40814093676324603, 47.45696800326375353, -11.09922568453594671 ) ) ;
#66700=CARTESIAN_POINT ( 'NONE',  ( 12.63842701281683034, 32.46726448433412315, 9.846743663894596210 ) ) ;
#66701=CARTESIAN_POINT ( 'NONE',  ( 17.96484262340118221, 11.18868534415483929, -7.964842623401177768 ) ) ;
#66702=CARTESIAN_POINT ( 'NONE',  ( -2.816281873526473856, 54.12363466993041783, 9.499525473075851096E-16 ) ) ;
#66704=CARTESIAN_POINT ( 'NONE',  ( 0.1532563361054082862, 46.21726448433411605, 2.638427012816831674 ) ) ;
#66709=TOROIDAL_SURFACE ( 'NONE', #49147, 18.53834841531100608, 7.000000000000000000 ) ;
#66711=CARTESIAN_POINT ( 'NONE',  ( -46.34323875807881166, 103.6109741468810483, -6.190393423093146552 ) ) ;
#66712=CARTESIAN_POINT ( 'NONE',  ( 20.15039907845753220, 45.60158574516643881, -6.262539305110077947 ) ) ;
#66715=CARTESIAN_POINT ( 'NONE',  ( 14.92337183194729988, 14.34226448433411782, -8.527530157486177487 ) ) ;
#66716=CARTESIAN_POINT ( 'NONE',  ( 13.43411237798106583, 27.66530133659708568, -12.81628187352647252 ) ) ;
#66719=CARTESIAN_POINT ( 'NONE',  ( 14.92337183194729633, 62.67559781766745886, 8.527530157486181039 ) ) ;
#66722=CARTESIAN_POINT ( 'NONE',  ( 22.26659068614895176, 14.72041550158063572, -7.082119434687042414 ) ) ;
#66723=CARTESIAN_POINT ( 'NONE',  ( 12.63842701281683034, 42.46726448433412315, 9.846743663894596210 ) ) ;
#66724=CARTESIAN_POINT ( 'NONE',  ( 3.591859063236761518, 49.95696800326375353, 11.09922568453594849 ) ) ;
#66726=CARTESIAN_POINT ( 'NONE',  ( 1.472469842513823179, 10.59226448433411782, -4.923371831947296329 ) ) ;
#66728=CARTESIAN_POINT ( 'NONE',  ( 10.00000000000000178, 52.25893115100078745, 9.846743663894594434 ) ) ;
#66729=CARTESIAN_POINT ( 'NONE',  ( 12.91533473730992121, 44.52201867748816966, 10.88017736071110164 ) ) ;
#66730=CARTESIAN_POINT ( 'NONE',  ( 7.361572987183169658, 29.96726448433411960, -9.846743663894592657 ) ) ;
#66731=DIRECTION ( 'NONE',  ( -1.000000000000000000, 0.000000000000000000, 0.000000000000000000 ) ) ;
#66733=CARTESIAN_POINT ( 'NONE',  ( 10.00000000000000000, 46.81368534415484106, -10.88017736071110342 ) ) ;
#66735=DIRECTION ( 'NONE',  ( -0.000000000000000000, -0.000000000000000000, 1.000000000000000000 ) ) ;
#66736=CARTESIAN_POINT ( 'NONE',  ( 10.00000000000000178, 19.31368534415484106, 10.88017736071110342 ) ) ;
#66737=CARTESIAN_POINT ( 'NONE',  ( 2.791683348922240793, 51.63393115100078745, 7.208316651077764092 ) ) ;
#66738=CARTESIAN_POINT ( 'NONE',  ( 7.084665262690076126, 47.02201867748818387, -10.88017736071110164 ) ) ;
#66740=CARTESIAN_POINT ( 'NONE',  ( 0.5774900079438607392, 53.48035201082151247, 5.440088680355550821 ) ) ;
#66741=CARTESIAN_POINT ( 'NONE',  ( 20.88017736071110875, 20.77201867748816611, -2.915334737309920765 ) ) ;
#66743=CARTESIAN_POINT ( 'NONE',  ( 19.72487221294571569, 49.78217586085237656, 6.499999999999993783 ) ) ;
#66744=CARTESIAN_POINT ( 'NONE',  ( 0.1532563361054082862, 21.21726448433412315, 2.638427012816831674 ) ) ;
#66747=CARTESIAN_POINT ( 'NONE',  ( 0.1532563361054082862, 56.21726448433411605, 2.638427012816831674 ) ) ;
#66748=CARTESIAN_POINT ( 'NONE',  ( 6.204703633549690345, 65.76208216824731778, -14.16423886937410259 ) ) ;
#66750=CARTESIAN_POINT ( 'NONE',  ( 20.36894250292379382, 8.678748834913967869, 10.36894250292379205 ) ) ;
#66751=CARTESIAN_POINT ( 'NONE',  ( -4.164238869374099039, 51.80374883491396787, 8.674139862899312516E-16 ) ) ;
#66752=VECTOR ( 'NONE', #20447, 1000.000000000000000 ) ;
#66753=CARTESIAN_POINT ( 'NONE',  ( 22.81628187352647785, 1.623634669930420271, 6.195893100308588602E-16 ) ) ;
#66755=CARTESIAN_POINT ( 'NONE',  ( 15.44008868035555793, 16.39701867748817321, -9.422509992056140149 ) ) ;
#66756=CARTESIAN_POINT ( 'NONE',  ( 10.00000000000000000, 54.75893115100078745, -9.846743663894594434 ) ) ;
#66761=CARTESIAN_POINT ( 'NONE',  ( -2.816281873526473856, 19.33196800326375708, 3.434112377981055619 ) ) ;
#66762=CARTESIAN_POINT ( 'NONE',  ( 7.361572987183169658, 29.96726448433411960, -9.846743663894592657 ) ) ;
#66764=CARTESIAN_POINT ( 'NONE',  ( 7.361572987183169658, 4.967264484334119601, -9.846743663894592657 ) ) ;
#66767=CARTESIAN_POINT ( 'NONE',  ( 2.035157376598822676, 17.43868534415483751, -7.964842623401177768 ) ) ;
#66768=CARTESIAN_POINT ( 'NONE',  ( -0.3689425029237881626, 37.42874883491396787, 10.36894250292379027 ) ) ;
#66769=CARTESIAN_POINT ( 'NONE',  ( 20.88017736071110875, 40.77201867748818387, -2.915334737309920765 ) ) ;
#66770=CARTESIAN_POINT ( 'NONE',  ( 20.88017736071110164, 65.35535201082150536, 2.915334737309930979 ) ) ;
#66772=DIRECTION ( 'NONE',  ( 0.000000000000000000, 0.000000000000000000, 1.000000000000000000 ) ) ;
#66773=CARTESIAN_POINT ( 'NONE',  ( 7.361572987183170547, 27.05059781766745175, 9.846743663894590881 ) ) ;
#66775=CARTESIAN_POINT ( 'NONE',  ( 0.1532563361054082862, 1.217264484334117824, 2.638427012816831674 ) ) ;
#66777=CARTESIAN_POINT ( 'NONE',  ( 2.791683348922237240, 35.38393115100079456, -7.208316651077763204 ) ) ;
#66778=CARTESIAN_POINT ( 'NONE',  ( 0.1532563361054100626, 60.80059781766744464, -2.638427012816831230 ) ) ;
#66779=ADVANCED_FACE ( 'NONE', ( #26679 ), #27662, .T. ) ;
#66780=CARTESIAN_POINT ( 'NONE',  ( 12.91533473730993009, 41.60535201082149825, -10.88017736071109987 ) ) ;
#66784=CARTESIAN_POINT ( 'NONE',  ( 16.40814093676323893, 60.79030133659709634, 11.09922568453595026 ) ) ;
#66786=CARTESIAN_POINT ( 'NONE',  ( 5.076628168052703671, 11.84226448433411960, 8.527530157486179263 ) ) ;
#66787=CARTESIAN_POINT ( 'NONE',  ( 19.38216949554541557, 47.24863466993041783, -9.382169495545420901 ) ) ;
#66788=CARTESIAN_POINT ( 'NONE',  ( 10.00000000000000000, 11.81368534415483751, -10.88017736071110342 ) ) ;
#66789=CARTESIAN_POINT ( 'NONE',  ( 5.076628168052704559, 30.17559781766745175, -8.527530157486179263 ) ) ;
#66791=CARTESIAN_POINT ( 'NONE',  ( 17.08211943468705840, 45.13708216824730357, -12.26659068614894466 ) ) ;
#66792=CARTESIAN_POINT ( 'NONE',  ( 17.20831665107776587, 39.13393115100079456, -7.208316651077762316 ) ) ;
#66794=CARTESIAN_POINT ( 'NONE',  ( 20.88017736071110519, 35.56368534415484106, 2.639326808657452039E-16 ) ) ;
#66795=CARTESIAN_POINT ( 'NONE',  ( 17.20831665107776587, 4.133931151000785675, -7.208316651077762316 ) ) ;
#66796=CARTESIAN_POINT ( 'NONE',  ( 1.472469842513823179, 55.59226448433412315, -4.923371831947296329 ) ) ;
#66798=CARTESIAN_POINT ( 'NONE',  ( 10.00000000000000178, 55.37363466993042493, 12.81628187352647608 ) ) ;
#66800=CARTESIAN_POINT ( 'NONE',  ( 19.42250999205614193, 60.14701867748817676, 5.440088680355555262 ) ) ;
#66802=CARTESIAN_POINT ( 'NONE',  ( 17.08211943468705130, 3.470415501580634388, 12.26659068614894998 ) ) ;
#66803=CARTESIAN_POINT ( 'NONE',  ( 0.1532563361054082862, 1.217264484334117824, 2.638427012816831674 ) ) ;
#66804=CARTESIAN_POINT ( 'NONE',  ( -0.2418659066527711621, 59.26028685723174760, -6.114288769123046308 ) ) ;
#66806=CARTESIAN_POINT ( 'NONE',  ( 20.88017736071110519, 15.56368534415483751, 2.639326808657452039E-16 ) ) ;
#66808=EDGE_LOOP ( 'NONE', ( #19725, #56732, #29646, #12483, #72332, #63008, #20365, #4114 ) ) ;
#66809=CARTESIAN_POINT ( 'NONE',  ( 2.035157376598824452, 23.68868534415484461, 7.964842623401179544 ) ) ;
#66810=CARTESIAN_POINT ( 'NONE',  ( 10.00000000000000000, 64.75893115100078035, -9.846743663894594434 ) ) ;
#66812=CARTESIAN_POINT ( 'NONE',  ( 0.1532563361054083140, 66.00893115100079456, 1.131784320476157264E-15 ) ) ;
#66814=CARTESIAN_POINT ( 'NONE',  ( 7.361572987183170547, 2.050597817667451750, 9.846743663894590881 ) ) ;
#66815=CARTESIAN_POINT ( 'NONE',  ( 0.1532563361054100626, 65.80059781766745175, -2.638427012816831230 ) ) ;
#66816=CARTESIAN_POINT ( 'NONE',  ( 10.00000000000000178, 40.37363466993042493, 12.81628187352647608 ) ) ;
#66817=CARTESIAN_POINT ( 'NONE',  ( -0.8801773607111009756, 23.06368534415484106, 1.068504757029289695E-15 ) ) ;
#66818=CARTESIAN_POINT ( 'NONE',  ( 7.361572987183169658, 4.967264484334119601, -9.846743663894592657 ) ) ;
#66819=CARTESIAN_POINT ( 'NONE',  ( 19.42250999205614193, 25.14701867748817321, 5.440088680355555262 ) ) ;
#66820=EDGE_CURVE ( 'NONE', #92829, #10063, #75062, .T. ) ;
#66823=CARTESIAN_POINT ( 'NONE',  ( 22.81628187352647785, 56.41530133659708213, 3.434112377981063169 ) ) ;
#66824=CARTESIAN_POINT ( 'NONE',  ( -0.8801773607111009756, 48.06368534415484817, 1.068504757029289695E-15 ) ) ;
#66826=CARTESIAN_POINT ( 'NONE',  ( 22.81628187352647785, 51.41530133659708923, 3.434112377981063169 ) ) ;
#66827=CARTESIAN_POINT ( 'NONE',  ( 2.035157376598824452, 48.68868534415483396, 7.964842623401179544 ) ) ;
#66828=CARTESIAN_POINT ( 'NONE',  ( 0.1532563361054082862, 56.21726448433411605, 2.638427012816831674 ) ) ;
#66831=CARTESIAN_POINT ( 'NONE',  ( 19.84674366389459266, 13.71726448433411782, -2.638427012816827677 ) ) ;
#66832=CARTESIAN_POINT ( 'NONE',  ( 16.40814093676323893, 5.790301336597087456, 11.09922568453595026 ) ) ;
#66835=CARTESIAN_POINT ( 'NONE',  ( 12.91533473730992121, 19.52201867748816611, 10.88017736071110164 ) ) ;
#66836=CARTESIAN_POINT ( 'NONE',  ( 10.00000000000000000, 49.75893115100078745, -9.846743663894594434 ) ) ;
#66837=SURFACE_SIDE_STYLE ('',( #4874 ) ) ;
#66839=CARTESIAN_POINT ( 'NONE',  ( 2.791683348922237240, 5.383931151000785675, -7.208316651077763204 ) ) ;
#66841=CARTESIAN_POINT ( 'NONE',  ( 10.00000000000000000, 7.873634669930421381, -12.81628187352647608 ) ) ;
#66845=CARTESIAN_POINT ( 'NONE',  ( -1.099225684535947600, 44.54030133659708923, 6.408140936763237150 ) ) ;
#66847=CARTESIAN_POINT ( 'NONE',  ( 19.84674366389459621, 33.50893115100078745, 7.409399052514197653E-17 ) ) ;
#66848=B_SPLINE_CURVE_WITH_KNOTS ( 'NONE', 3,
 ( #68398, #53376, #25247, #24740 ),
 .UNSPECIFIED., .F., .F.,
 ( 4, 4 ),
 ( 5.284504157781969479E-17, 0.002562518741975526333 ),
 .UNSPECIFIED. ) ;
#66849=CARTESIAN_POINT ( 'NONE',  ( -0.8801773607111009756, 58.06368534415484106, 1.068504757029289695E-15 ) ) ;
#66850=CARTESIAN_POINT ( 'NONE',  ( 10.00000000000000178, 4.313685344154837509, 10.88017736071110342 ) ) ;
#66851=CARTESIAN_POINT ( 'NONE',  ( 18.52753015748618282, 33.92559781766745886, -4.923371831947291888 ) ) ;
#66854=CARTESIAN_POINT ( 'NONE',  ( 2.917880565312950480, 65.97041550158063217, -12.26659068614894821 ) ) ;
#66856=CARTESIAN_POINT ( 'NONE',  ( 19.42250999205614548, 20.98035201082150891, -5.440088680355545492 ) ) ;
#66857=CARTESIAN_POINT ( 'NONE',  ( 10.00000000000000178, 48.05374883491396787, 14.16423886937410082 ) ) ;
#66858=CARTESIAN_POINT ( 'NONE',  ( 17.08211943468705130, 53.47041550158063217, 12.26659068614894998 ) ) ;
#66859=CARTESIAN_POINT ( 'NONE',  ( -0.1503990784575328643, 69.92552686551195507, 6.262539305110068177 ) ) ;
#66861=CARTESIAN_POINT ( 'NONE',  ( 17.20831665107776587, 7.883931151000784787, 7.208316651077764980 ) ) ;
#66862=CARTESIAN_POINT ( 'NONE',  ( 22.81628187352647785, 1.623634669930420271, 6.195893100308588602E-16 ) ) ;
#66864=CARTESIAN_POINT ( 'NONE',  ( 10.00000000000000178, 49.31368534415484106, 10.88017736071110342 ) ) ;
#66866=CARTESIAN_POINT ( 'NONE',  ( 2.791683348922240793, 56.63393115100078035, 7.208316651077764092 ) ) ;
#66867=CARTESIAN_POINT ( 'NONE',  ( 18.72515096720590577, 61.07228050351029935, -6.499999999999718447 ) ) ;
#66869=( BOUNDED_CURVE ( )  B_SPLINE_CURVE ( 2, ( #9499, #65304, #42825, #85503, #77994, #1537, #87813, #62984, #62487 ),
 .UNSPECIFIED., .F., .F. ) 
 B_SPLINE_CURVE_WITH_KNOTS ( ( 3, 2, 2, 2, 3 ),
 ( 0.9025141644748393421, 0.9047619047619047672, 0.9107142857142856984, 0.9166666666666666297, 0.9189144069537320547 ),
 .UNSPECIFIED. ) 
 CURVE ( )  GEOMETRIC_REPRESENTATION_ITEM ( )  RATIONAL_B_SPLINE_CURVE ( ( 0.9839835555609424134, 0.9871328979762474809, 1.000000000000000000, 0.9659258262890683122, 1.000000000000000000, 0.9659258262890683122, 1.000000000000000000, 0.9871328979762477029, 0.9839835555609425244 ) ) 
 REPRESENTATION_ITEM ( '' )  );
#66870=CARTESIAN_POINT ( 'NONE',  ( 22.26659068614894466, 3.887082168247300906, 7.082119434687054849 ) ) ;
#66871=CARTESIAN_POINT ( 'NONE',  ( 1.472469842513823179, 25.59226448433412315, -4.923371831947296329 ) ) ;
#66874=CARTESIAN_POINT ( 'NONE',  ( 17.08211943468705130, 38.47041550158063217, 12.26659068614894998 ) ) ;
#66875=CARTESIAN_POINT ( 'NONE',  ( 2.791683348922237240, 10.38393115100078390, -7.208316651077763204 ) ) ;
#66878=CARTESIAN_POINT ( 'NONE',  ( 17.96484262340118221, 31.18868534415483751, -7.964842623401177768 ) ) ;
#66879=CARTESIAN_POINT ( 'NONE',  ( 6.565887622018943937, 33.08196800326374643, -12.81628187352647608 ) ) ;
#66880=CARTESIAN_POINT ( 'NONE',  ( 20.88017736071110519, 5.563685344154837509, 2.639326808657452039E-16 ) ) ;
#66881=CARTESIAN_POINT ( 'NONE',  ( 6.565887622018943937, 40.16530133659708923, 12.81628187352647430 ) ) ;
#66882=CARTESIAN_POINT ( 'NONE',  ( 19.38216949554541202, 60.99863466993042493, 9.382169495545424454 ) ) ;
#66883=ORIENTED_EDGE ( 'NONE', *, *, #93766, .F. ) ;
#66886=CARTESIAN_POINT ( 'NONE',  ( 24.16423886937410614, 39.30374883491396787, 8.672049930838204340E-16 ) ) ;
#66887=CARTESIAN_POINT ( 'NONE',  ( 10.00000000000000000, 5.553748834913967869, -14.16423886937410082 ) ) ;
#66888=CARTESIAN_POINT ( 'NONE',  ( 4.559911319644449179, 23.89701867748817321, 9.422509992056141925 ) ) ;
#66889=DIRECTION ( 'NONE',  ( 0.5547001962252290364, 0.8320502943378437211, 0.000000000000000000 ) ) ;
#66891=CARTESIAN_POINT ( 'NONE',  ( 0.5774900079438607392, 48.48035201082150536, 5.440088680355550821 ) ) ;
#66892=CARTESIAN_POINT ( 'NONE',  ( 19.42250999205614548, 55.98035201082150536, -5.440088680355545492 ) ) ;
#66893=CARTESIAN_POINT ( 'NONE',  ( -2.816281873526471635, 18.91530133659708213, -3.434112377981056508 ) ) ;
#66895=CARTESIAN_POINT ( 'NONE',  ( 0.2751277870542909176, 30.30223176428831167, 6.499999999999992006 ) ) ;
#66896=CARTESIAN_POINT ( 'NONE',  ( 0.1532563361054100626, 25.80059781766744820, -2.638427012816831230 ) ) ;
#66897=CARTESIAN_POINT ( 'NONE',  ( 4.559911319644449179, 58.89701867748817676, 9.422509992056141925 ) ) ;
#66899=CARTESIAN_POINT ( 'NONE',  ( 19.38216949554541557, 22.24863466993041428, -9.382169495545420901 ) ) ;
#66901=CARTESIAN_POINT ( 'NONE',  ( 17.96484262340118221, 9.938685344154837509, 7.964842623401181321 ) ) ;
#66902=CARTESIAN_POINT ( 'NONE',  ( 17.20831665107776587, 32.88393115100078745, 7.208316651077764980 ) ) ;
#66903=CARTESIAN_POINT ( 'NONE',  ( 3.591859063236763294, 43.29030133659708923, -11.09922568453595026 ) ) ;
#66904=CARTESIAN_POINT ( 'NONE',  ( 10.00000000000000178, 22.25893115100078745, 9.846743663894594434 ) ) ;
#66905=CARTESIAN_POINT ( 'NONE',  ( 10.00000000000000000, 5.553748834913967869, -14.16423886937410082 ) ) ;
#66906=CYLINDRICAL_SURFACE ( 'NONE', #39822, 0.5000000000000004441 ) ;
#66907=CARTESIAN_POINT ( 'NONE',  ( 2.035157376598822676, 22.43868534415483396, -7.964842623401177768 ) ) ;
#66908=DIRECTION ( 'NONE',  ( 0.000000000000000000, 0.000000000000000000, -1.000000000000000000 ) ) ;
#66909=CARTESIAN_POINT ( 'NONE',  ( 7.361572987183170547, 42.05059781766745886, 9.846743663894590881 ) ) ;
#66911=CARTESIAN_POINT ( 'NONE',  ( 2.035157376598822676, 17.43868534415483751, -7.964842623401177768 ) ) ;
#66912=CARTESIAN_POINT ( 'NONE',  ( 7.084665262690076126, 17.02201867748817676, -10.88017736071110164 ) ) ;
#66913=VERTEX_POINT ( 'NONE', #56213 ) ;
#66914=CARTESIAN_POINT ( 'NONE',  ( -0.8801773607111008646, 28.27201867748817321, 2.915334737309923430 ) ) ;
#66916=CARTESIAN_POINT ( 'NONE',  ( 22.81628187352647785, 46.62363466993041783, 6.195893100308588602E-16 ) ) ;
#66917=CARTESIAN_POINT ( 'NONE',  ( -0.8801773607111009756, 28.06368534415484106, 1.068504757029289695E-15 ) ) ;
#66919=CARTESIAN_POINT ( 'NONE',  ( 4.559911319644449179, 33.89701867748817676, 9.422509992056141925 ) ) ;
#66921=CARTESIAN_POINT ( 'NONE',  ( 7.361572987183170547, 52.05059781766745175, 9.846743663894590881 ) ) ;
#66922=CARTESIAN_POINT ( 'NONE',  ( 20.88017736071110519, 30.56368534415484106, 2.639326808657452039E-16 ) ) ;
#66926=DIRECTION ( 'NONE',  ( 0.000000000000000000, 0.000000000000000000, -1.000000000000000000 ) ) ;
#66927=CARTESIAN_POINT ( 'NONE',  ( 2.917880565312948704, 52.63708216824730357, 12.26659068614894643 ) ) ;
#66928=CARTESIAN_POINT ( 'NONE',  ( 0.5774900079438607392, 53.48035201082151247, 5.440088680355550821 ) ) ;
#66929=CARTESIAN_POINT ( 'NONE',  ( 2.791683348922240793, 66.63393115100079456, 7.208316651077764092 ) ) ;
#66931=CARTESIAN_POINT ( 'NONE',  ( 18.52753015748618282, 63.92559781766745886, -4.923371831947291888 ) ) ;
#66932=CARTESIAN_POINT ( 'NONE',  ( 18.52753015748617571, 3.092264484334118269, 4.923371831947298993 ) ) ;
#66933=CARTESIAN_POINT ( 'NONE',  ( 10.00000000000000178, 17.25893115100078745, 9.846743663894594434 ) ) ;
#66935=CARTESIAN_POINT ( 'NONE',  ( 19.84674366389459621, 23.50893115100078390, 7.409399052514197653E-17 ) ) ;
#66937=CARTESIAN_POINT ( 'NONE',  ( 19.42250999205614193, 30.14701867748817321, 5.440088680355555262 ) ) ;
#66938=CARTESIAN_POINT ( 'NONE',  ( 0.1532563361054083140, 26.00893115100078745, 1.131784320476157264E-15 ) ) ;
#66939=CARTESIAN_POINT ( 'NONE',  ( 16.40814093676324603, 7.456968003263754419, -11.09922568453594671 ) ) ;
#66940=CARTESIAN_POINT ( 'NONE',  ( 19.42250999205614548, 60.98035201082151247, -5.440088680355545492 ) ) ;
#66941=CARTESIAN_POINT ( 'NONE',  ( 15.44008868035555793, 61.39701867748817676, -9.422509992056140149 ) ) ;
#66942=CARTESIAN_POINT ( 'NONE',  ( 7.084665262690076126, 27.02201867748817676, -10.88017736071110164 ) ) ;
#66943=CARTESIAN_POINT ( 'NONE',  ( 21.09922568453594849, 61.20696800326376064, 6.408140936763242479 ) ) ;
#66944=CARTESIAN_POINT ( 'NONE',  ( 6.204703633549690345, 50.76208216824730357, -14.16423886937410259 ) ) ;
#66945=( GEOMETRIC_REPRESENTATION_CONTEXT ( 3 ) GLOBAL_UNCERTAINTY_ASSIGNED_CONTEXT ( ( #94180 ) ) GLOBAL_UNIT_ASSIGNED_CONTEXT ( ( #15588, #29564, #78039 ) ) REPRESENTATION_CONTEXT ( 'NONE', 'WORKASPACE' ) );
#66947=EDGE_CURVE ( 'NONE', #14724, #10425, #34665, .T. ) ;
#66948=CARTESIAN_POINT ( 'NONE',  ( 20.15039907845753220, 42.62777174578613426, -6.262539305110077947 ) ) ;
#66951=CARTESIAN_POINT ( 'NONE',  ( 6.565887622018943937, 5.165301336597086568, 12.81628187352647430 ) ) ;
#66952=CARTESIAN_POINT ( 'NONE',  ( 0.5774900079438607392, 3.480352010821504027, 5.440088680355550821 ) ) ;
#66953=CARTESIAN_POINT ( 'NONE',  ( 20.88017736071110519, 45.56368534415484106, 2.639326808657452039E-16 ) ) ;
#66954=CARTESIAN_POINT ( 'NONE',  ( 2.917880565312950480, 0.9704155015806342766, -12.26659068614894821 ) ) ;
#66956=CARTESIAN_POINT ( 'NONE',  ( 18.52753015748618282, 18.92559781766745175, -4.923371831947291888 ) ) ;
#66958=CARTESIAN_POINT ( 'NONE',  ( 19.42250999205614193, 60.14701867748817676, 5.440088680355555262 ) ) ;
#66959=CARTESIAN_POINT ( 'NONE',  ( 14.92337183194729988, 34.34226448433411605, -8.527530157486177487 ) ) ;
#66960=CARTESIAN_POINT ( 'NONE',  ( 18.52753015748617571, 28.09226448433411960, 4.923371831947298993 ) ) ;
#66961=CARTESIAN_POINT ( 'NONE',  ( 7.361572987183170547, 17.05059781766745530, 9.846743663894590881 ) ) ;
#66963=CARTESIAN_POINT ( 'NONE',  ( 12.63842701281683922, 4.550597817667451750, -9.846743663894590881 ) ) ;
#66966=CARTESIAN_POINT ( 'NONE',  ( 0.1532563361054082862, 31.21726448433412315, 2.638427012816831674 ) ) ;
#66968=CARTESIAN_POINT ( 'NONE',  ( -2.816281873526471635, 53.91530133659709634, -3.434112377981056508 ) ) ;
#66970=CARTESIAN_POINT ( 'NONE',  ( 16.40814093676324603, 2.456968003263753531, -11.09922568453594671 ) ) ;
#66971=EDGE_CURVE ( 'NONE', #53047, #11431, #74000, .T. ) ;
#66972=CARTESIAN_POINT ( 'NONE',  ( 4.559911319644449179, 3.897018677488170990, 9.422509992056141925 ) ) ;
#66973=CARTESIAN_POINT ( 'NONE',  ( -4.164238869374098151, 16.59541550158063927, -3.795296366450310543 ) ) ;
#66974=CARTESIAN_POINT ( 'NONE',  ( 2.153642693323453372, 41.13791097397318453, -6.500000000000040856 ) ) ;
#66975=EDGE_CURVE ( 'NONE', #57072, #13800, #28671, .T. ) ;
#66976=CARTESIAN_POINT ( 'NONE',  ( -0.3689425029237898834, 36.17874883491396787, -10.36894250292378850 ) ) ;
#66977=CARTESIAN_POINT ( 'NONE',  ( -4.164238869374099039, 41.80374883491397497, 8.674139862899312516E-16 ) ) ;
#66978=CARTESIAN_POINT ( 'NONE',  ( 2.917880565312950480, 15.97041550158063217, -12.26659068614894821 ) ) ;
#66979=CARTESIAN_POINT ( 'NONE',  ( -2.266590686148945544, 17.22041550158063572, 7.082119434687048631 ) ) ;
#66980=CARTESIAN_POINT ( 'NONE',  ( 17.96484262340118221, 51.18868534415483396, -7.964842623401177768 ) ) ;
#66983=CARTESIAN_POINT ( 'NONE',  ( 7.361572987183170547, 32.05059781766745175, 9.846743663894590881 ) ) ;
#66984=CARTESIAN_POINT ( 'NONE',  ( 0.000000000000000000, 69.50000000000000000, 6.500000000000000888 ) ) ;
#66985=CARTESIAN_POINT ( 'NONE',  ( 12.63842701281683922, 24.55059781766745175, -9.846743663894590881 ) ) ;
#66986=CARTESIAN_POINT ( 'NONE',  ( 20.88017736071110164, 5.355352010821503583, 2.915334737309930979 ) ) ;
#66987=CARTESIAN_POINT ( 'NONE',  ( 6.565887622018943937, 65.16530133659709634, 12.81628187352647430 ) ) ;
#66988=CARTESIAN_POINT ( 'NONE',  ( 10.00000000000000178, 52.25893115100078745, 9.846743663894594434 ) ) ;
#66990=CARTESIAN_POINT ( 'NONE',  ( 17.20831665107776587, 24.13393115100078035, -7.208316651077762316 ) ) ;
#66991=CARTESIAN_POINT ( 'NONE',  ( 10.00000000000000178, 40.37363466993042493, 12.81628187352647608 ) ) ;
#66993=CARTESIAN_POINT ( 'NONE',  ( 2.035157376598822676, 42.43868534415483396, -7.964842623401177768 ) ) ;
#66994=CARTESIAN_POINT ( 'NONE',  ( 17.20831665107776587, 44.13393115100078745, -7.208316651077762316 ) ) ;
#66995=CARTESIAN_POINT ( 'NONE',  ( 24.16423886937409904, 29.09541550158063572, 3.795296366450317205 ) ) ;
#66997=CARTESIAN_POINT ( 'NONE',  ( -4.164238869374099039, 6.803748834913967869, 8.674139862899312516E-16 ) ) ;
#66998=B_SPLINE_CURVE_WITH_KNOTS ( 'NONE', 3,
 ( #79289, #71308, #41316, #2827 ),
 .UNSPECIFIED., .F., .F.,
 ( 4, 4 ),
 ( 0.000000000000000000, 0.002392975128318458166 ),
 .UNSPECIFIED. ) ;
#66999=CARTESIAN_POINT ( 'NONE',  ( 4.559911319644449179, 48.89701867748817676, 9.422509992056141925 ) ) ;
#67001=CARTESIAN_POINT ( 'NONE',  ( -4.164238869374099039, 61.80374883491397497, 8.674139862899312516E-16 ) ) ;
#67002=CARTESIAN_POINT ( 'NONE',  ( 10.00000000000000178, 67.25893115100079456, 9.846743663894594434 ) ) ;
#67004=CARTESIAN_POINT ( 'NONE',  ( 17.96484262340118221, 54.93868534415484106, 7.964842623401181321 ) ) ;
#67005=CARTESIAN_POINT ( 'NONE',  ( 20.15039907845753220, 42.62777174578613426, -6.262539305110077947 ) ) ;
#67007=CARTESIAN_POINT ( 'NONE',  ( -2.816281873526473856, 34.33196800326376064, 3.434112377981055619 ) ) ;
#67008=CARTESIAN_POINT ( 'NONE',  ( 0.1532563361054083140, 61.00893115100078745, 1.131784320476157264E-15 ) ) ;
#67010=CARTESIAN_POINT ( 'NONE',  ( 10.00000000000000000, 16.81368534415483751, -10.88017736071110342 ) ) ;
#67011=CARTESIAN_POINT ( 'NONE',  ( 20.88017736071110519, 10.56368534415483929, 2.639326808657452039E-16 ) ) ;
#67012=CARTESIAN_POINT ( 'NONE',  ( 14.92337183194729633, 42.67559781766745886, 8.527530157486181039 ) ) ;
#67013=CARTESIAN_POINT ( 'NONE',  ( 2.603489959281614308, 41.58210964143329846, 6.500000000000031086 ) ) ;
#67014=ORIENTED_EDGE ( 'NONE', *, *, #22725, .T. ) ;
#67017=CARTESIAN_POINT ( 'NONE',  ( 10.00000000000000178, 10.37363466993041961, 12.81628187352647608 ) ) ;
#67019=CARTESIAN_POINT ( 'NONE',  ( 19.84674366389459266, 8.300597817667451750, 2.638427012816836559 ) ) ;
#67020=CARTESIAN_POINT ( 'NONE',  ( 7.361572987183170547, 52.05059781766745175, 9.846743663894590881 ) ) ;
#67021=CARTESIAN_POINT ( 'NONE',  ( 7.084665262690076126, 37.02201867748817676, -10.88017736071110164 ) ) ;
#67022=CARTESIAN_POINT ( 'NONE',  ( 16.40814093676323893, 10.79030133659708923, 11.09922568453595026 ) ) ;
#67023=CARTESIAN_POINT ( 'NONE',  ( 7.084665262690076126, 52.02201867748816255, -10.88017736071110164 ) ) ;
#67026=CARTESIAN_POINT ( 'NONE',  ( -2.816281873526471635, 48.91530133659708213, -3.434112377981056508 ) ) ;
#67028=CARTESIAN_POINT ( 'NONE',  ( 4.559911319644449179, 63.89701867748817676, 9.422509992056141925 ) ) ;
#67029=CARTESIAN_POINT ( 'NONE',  ( 19.38216949554541202, 35.99863466993041072, 9.382169495545424454 ) ) ;
#67030=CARTESIAN_POINT ( 'NONE',  ( -4.164238869374099039, 1.803748834913967647, 8.674139862899312516E-16 ) ) ;
#67031=SURFACE_STYLE_USAGE ( .BOTH. , #20044 ) ;
#67032=CARTESIAN_POINT ( 'NONE',  ( -0.8801773607110991993, 42.85535201082150536, -2.915334737309923874 ) ) ;
#67034=CARTESIAN_POINT ( 'NONE',  ( 5.076628168052704559, 60.17559781766745175, -8.527530157486179263 ) ) ;
#67035=CARTESIAN_POINT ( 'NONE',  ( 0.1532563361054082862, 16.21726448433411960, 2.638427012816831674 ) ) ;
#67036=CARTESIAN_POINT ( 'NONE',  ( 2.791683348922237240, 10.38393115100078390, -7.208316651077763204 ) ) ;
#67038=CARTESIAN_POINT ( 'NONE',  ( 17.08211943468705130, 48.47041550158063927, 12.26659068614894998 ) ) ;
#67043=CARTESIAN_POINT ( 'NONE',  ( 20.36894250292379382, 58.67874883491396076, 10.36894250292379205 ) ) ;
#67044=CARTESIAN_POINT ( 'NONE',  ( 24.16423886937409904, 64.09541550158064638, 3.795296366450317205 ) ) ;
#67045=CARTESIAN_POINT ( 'NONE',  ( 19.84674366389459266, 33.71726448433410894, -2.638427012816827677 ) ) ;
#67046=CARTESIAN_POINT ( 'NONE',  ( 22.81628187352648496, 26.83196800326374998, -3.434112377981050290 ) ) ;
#67048=FILL_AREA_STYLE_COLOUR ( '', #45073 ) ;
#67049=CARTESIAN_POINT ( 'NONE',  ( 10.00000000000000000, 11.81368534415483751, -10.88017736071110342 ) ) ;
#67050=CARTESIAN_POINT ( 'NONE',  ( 17.08211943468705130, 58.47041550158063927, 12.26659068614894998 ) ) ;
#67051=CARTESIAN_POINT ( 'NONE',  ( 10.00000000000000178, 32.25893115100078745, 9.846743663894594434 ) ) ;
#67052=CARTESIAN_POINT ( 'NONE',  ( 0.6076426042653192416, 12.37576471608601203, -6.500000000000002665 ) ) ;
#67053=CARTESIAN_POINT ( 'NONE',  ( 19.84674366389459266, 3.717264484334118713, -2.638427012816827677 ) ) ;
#67056=ORIENTED_EDGE ( 'NONE', *, *, #74995, .F. ) ;
#67057=VERTEX_POINT ( 'NONE', #98165 ) ;
#67058=( LENGTH_UNIT ( ) NAMED_UNIT ( * ) SI_UNIT ( .MILLI., .METRE. ) );
#67061=CARTESIAN_POINT ( 'NONE',  ( 19.84674366389459266, 43.30059781766744464, 2.638427012816836559 ) ) ;
#67062=CARTESIAN_POINT ( 'NONE',  ( 15.44008868035555260, 14.73035201082150536, 9.422509992056143702 ) ) ;
#67063=CARTESIAN_POINT ( 'NONE',  ( 15.44008868035555793, 26.39701867748817321, -9.422509992056140149 ) ) ;
#67064=CARTESIAN_POINT ( 'NONE',  ( 5.076628168052703671, 61.84226448433412315, 8.527530157486179263 ) ) ;
#67065=CARTESIAN_POINT ( 'NONE',  ( 16.40814093676324603, 17.45696800326375353, -11.09922568453594671 ) ) ;
#67067=CARTESIAN_POINT ( 'NONE',  ( 21.09922568453594849, 31.20696800326375353, 6.408140936763242479 ) ) ;
#67068=EDGE_CURVE ( 'NONE', #8562, #76767, #1176, .T. ) ;
#67070=CARTESIAN_POINT ( 'NONE',  ( 17.20831665107776587, 29.13393115100078390, -7.208316651077762316 ) ) ;
#67071=CARTESIAN_POINT ( 'NONE',  ( 19.42250999205614548, 10.98035201082150536, -5.440088680355545492 ) ) ;
#67073=CARTESIAN_POINT ( 'NONE',  ( 12.91533473730993009, 6.605352010821504471, -10.88017736071109987 ) ) ;
#67075=CARTESIAN_POINT ( 'NONE',  ( 10.00000000000000000, 46.81368534415484106, -10.88017736071110342 ) ) ;
#67076=AXIS2_PLACEMENT_3D ( 'NONE', #70350, #18325, #10823 ) ;
#67077=CARTESIAN_POINT ( 'NONE',  ( 10.00000000000000000, 61.81368534415484106, -10.88017736071110342 ) ) ;
#67078=CARTESIAN_POINT ( 'NONE',  ( 4.559911319644449179, 68.89701867748817676, 9.422509992056141925 ) ) ;
#67080=CARTESIAN_POINT ( 'NONE',  ( 10.00000000000000178, 59.31368534415484106, 10.88017736071110342 ) ) ;
#67086=CARTESIAN_POINT ( 'NONE',  ( 2.791683348922240793, 31.63393115100078745, 7.208316651077764092 ) ) ;
#67087=ORIENTED_EDGE ( 'NONE', *, *, #37685, .T. ) ;
#67088=CARTESIAN_POINT ( 'NONE',  ( 19.84674366389459266, 58.30059781766745886, 2.638427012816836559 ) ) ;
#67090=EDGE_CURVE ( 'NONE', #86126, #3586, #78612, .T. ) ;
#67091=( NAMED_UNIT ( * ) SI_UNIT ( $, .STERADIAN. ) SOLID_ANGLE_UNIT ( ) );
#67094=DIRECTION ( 'NONE',  ( 0.000000000000000000, -1.000000000000000000, 0.000000000000000000 ) ) ;
#67095=CARTESIAN_POINT ( 'NONE',  ( 20.00000000000000711, 98.59912998021083297, -4.500000000000001776 ) ) ;
#67096=CARTESIAN_POINT ( 'NONE',  ( 19.84674366389459621, 38.50893115100078745, 7.409399052514197653E-17 ) ) ;
#67097=CARTESIAN_POINT ( 'NONE',  ( 4.559911319644449179, 12.23035201082150714, -9.422509992056141925 ) ) ;
#67098=CARTESIAN_POINT ( 'NONE',  ( 18.50749283717780003, 64.69955587570481725, 6.499999999999917399 ) ) ;
#67100=DIRECTION ( 'NONE',  ( 0.000000000000000000, -1.000000000000000000, 0.000000000000000000 ) ) ;
#67101=CARTESIAN_POINT ( 'NONE',  ( 7.361572987183170547, 42.05059781766745886, 9.846743663894590881 ) ) ;
#67103=CARTESIAN_POINT ( 'NONE',  ( 0.6178305044545838731, 19.74863466993042138, 9.382169495545420901 ) ) ;
#67104=CARTESIAN_POINT ( 'NONE',  ( 1.472469842513823179, 11.42559781766745175, 4.923371831947296329 ) ) ;
#67106=CARTESIAN_POINT ( 'NONE',  ( 3.591859063236761518, 4.956968003263753531, 11.09922568453594849 ) ) ;
#67107=CARTESIAN_POINT ( 'NONE',  ( 1.959929470562070675, 26.50257860105346452, 5.767676674365487699 ) ) ;
#67108=ORIENTED_EDGE ( 'NONE', *, *, #81967, .T. ) ;
#67109=CARTESIAN_POINT ( 'NONE',  ( 10.00000000000000178, 4.313685344154837509, 10.88017736071110342 ) ) ;
#67110=CARTESIAN_POINT ( 'NONE',  ( 6.204703633549690345, 12.84541550158063572, 14.16423886937410082 ) ) ;
#67111=CARTESIAN_POINT ( 'NONE',  ( 7.361572987183169658, 29.96726448433411960, -9.846743663894592657 ) ) ;
#67112=CARTESIAN_POINT ( 'NONE',  ( 20.88017736071110519, 55.56368534415484817, 2.639326808657452039E-16 ) ) ;
#67113=CARTESIAN_POINT ( 'NONE',  ( 3.591859063236761518, 44.95696800326376064, 11.09922568453594849 ) ) ;
#67115=CARTESIAN_POINT ( 'NONE',  ( -0.8801773607111009756, 8.063685344154837509, 1.068504757029289695E-15 ) ) ;
#67118=CARTESIAN_POINT ( 'NONE',  ( -2.816281873526471635, 3.915301336597087456, -3.434112377981056508 ) ) ;
#67119=CARTESIAN_POINT ( 'NONE',  ( 2.791683348922240793, 66.63393115100079456, 7.208316651077764092 ) ) ;
#67120=CARTESIAN_POINT ( 'NONE',  ( 19.84674366389459621, 28.50893115100078745, 7.409399052514197653E-17 ) ) ;
#67122=CARTESIAN_POINT ( 'NONE',  ( 22.81628187352647785, 36.41530133659707502, 3.434112377981063169 ) ) ;
#67123=CARTESIAN_POINT ( 'NONE',  ( 17.96484262340118221, 46.18868534415484106, -7.964842623401177768 ) ) ;
#67126=CARTESIAN_POINT ( 'NONE',  ( -0.8801773607111008646, 38.27201867748816255, 2.915334737309923430 ) ) ;
#67128=CARTESIAN_POINT ( 'NONE',  ( 0.5774900079438607392, 33.48035201082150536, 5.440088680355550821 ) ) ;
#67129=CARTESIAN_POINT ( 'NONE',  ( 10.00000000000000178, 62.25893115100078745, 9.846743663894594434 ) ) ;
#67130=CARTESIAN_POINT ( 'NONE',  ( 15.44008868035555260, 49.73035201082150536, 9.422509992056143702 ) ) ;
#67131=B_SPLINE_CURVE_WITH_KNOTS ( 'NONE', 3,
 ( #37320, #76775, #30771, #38788 ),
 .UNSPECIFIED., .F., .F.,
 ( 4, 4 ),
 ( 5.421010862427522170E-20, 0.002657014572711328959 ),
 .UNSPECIFIED. ) ;
#67132=UNCERTAINTY_MEASURE_WITH_UNIT (LENGTH_MEASURE( 1.000000000000000082E-05 ), #36406, 'distance_accuracy_value', 'NONE');
#67133=CARTESIAN_POINT ( 'NONE',  ( 17.20831665107776587, 34.13393115100078745, -7.208316651077762316 ) ) ;
#67134=CARTESIAN_POINT ( 'NONE',  ( 19.42250999205614193, 15.14701867748817143, 5.440088680355555262 ) ) ;
#67136=CARTESIAN_POINT ( 'NONE',  ( 10.00000000000000178, 10.37363466993041961, 12.81628187352647608 ) ) ;
#67137=VERTEX_POINT ( 'NONE', #75633 ) ;
#67138=CARTESIAN_POINT ( 'NONE',  ( 17.96484262340118221, 26.18868534415483396, -7.964842623401177768 ) ) ;
#67139=CARTESIAN_POINT ( 'NONE',  ( 0.5774900079438590739, 2.647018677488170990, -5.440088680355550821 ) ) ;
#67140=CARTESIAN_POINT ( 'NONE',  ( -0.8801773607110991993, 12.85535201082150358, -2.915334737309923874 ) ) ;
#67141=CARTESIAN_POINT ( 'NONE',  ( -0.8801773607111008646, 63.27201867748817676, 2.915334737309923430 ) ) ;
#67142=CARTESIAN_POINT ( 'NONE',  ( 24.16423886937409904, 29.09541550158063572, 3.795296366450317205 ) ) ;
#67144=CARTESIAN_POINT ( 'NONE',  ( 19.84674366389459621, 18.50893115100078745, 7.409399052514197653E-17 ) ) ;
#67145=CARTESIAN_POINT ( 'NONE',  ( 20.88017736071110519, 50.56368534415484106, 2.639326808657452039E-16 ) ) ;
#67152=CARTESIAN_POINT ( 'NONE',  ( 14.92337183194729988, 39.34226448433412315, -8.527530157486177487 ) ) ;
#67153=ORIENTED_EDGE ( 'NONE', *, *, #74082, .T. ) ;
#67156=CARTESIAN_POINT ( 'NONE',  ( 2.917880565312948704, 22.63708216824730002, 12.26659068614894643 ) ) ;
#67157=CARTESIAN_POINT ( 'NONE',  ( 10.00000000000000000, 20.55374883491396787, -14.16423886937410082 ) ) ;
#67158=CARTESIAN_POINT ( 'NONE',  ( 20.88017736071110875, 60.77201867748817676, -2.915334737309920765 ) ) ;
#67159=CARTESIAN_POINT ( 'NONE',  ( 2.035157376598824452, 3.688685344154837953, 7.964842623401179544 ) ) ;
#67160=CARTESIAN_POINT ( 'NONE',  ( 0.6178305044545838731, 4.748634669930420493, 9.382169495545420901 ) ) ;
#67161=CARTESIAN_POINT ( 'NONE',  ( 12.63842701281683922, 54.55059781766745175, -9.846743663894590881 ) ) ;
#67163=CARTESIAN_POINT ( 'NONE',  ( -0.8801773607111009756, 48.06368534415484817, 1.068504757029289695E-15 ) ) ;
#67164=CARTESIAN_POINT ( 'NONE',  ( 22.81628187352647785, 6.415301336597088344, 3.434112377981063169 ) ) ;
#67165=CARTESIAN_POINT ( 'NONE',  ( 6.204703633549690345, 10.76208216824729824, -14.16423886937410259 ) ) ;
#67166=CARTESIAN_POINT ( 'NONE',  ( 20.88017736071110164, 20.35535201082150891, 2.915334737309930979 ) ) ;
#67167=CARTESIAN_POINT ( 'NONE',  ( 15.44008868035555260, 19.73035201082150536, 9.422509992056143702 ) ) ;
#67168=CARTESIAN_POINT ( 'NONE',  ( 17.39651004071838614, 52.93575266056826933, 6.500000000000032863 ) ) ;
#67169=CARTESIAN_POINT ( 'NONE',  ( 10.00000000000000178, 44.31368534415484106, 10.88017736071110342 ) ) ;
#67171=CARTESIAN_POINT ( 'NONE',  ( 3.591859063236761518, 49.95696800326375353, 11.09922568453594849 ) ) ;
#67174=CARTESIAN_POINT ( 'NONE',  ( 20.15039907845753930, 4.722660991849187972, 6.262539305110067289 ) ) ;
#67179=CARTESIAN_POINT ( 'NONE',  ( -0.3689425029237881626, 47.42874883491396787, 10.36894250292379027 ) ) ;
#67180=CARTESIAN_POINT ( 'NONE',  ( 17.96484262340118221, 6.188685344154837509, -7.964842623401177768 ) ) ;
#67181=CARTESIAN_POINT ( 'NONE',  ( 18.52753015748618282, 18.92559781766745175, -4.923371831947291888 ) ) ;
#67182=CARTESIAN_POINT ( 'NONE',  ( 1.472469842513823179, 50.59226448433411605, -4.923371831947296329 ) ) ;
#67183=FACE_OUTER_BOUND ( 'NONE', #19283, .T. ) ;
#67184=B_SPLINE_CURVE_WITH_KNOTS ( 'NONE', 3,
 ( #11386, #93904, #63877, #72369, #55914, #24441 ),
 .UNSPECIFIED., .F., .F.,
 ( 4, 2, 4 ),
 ( 0.000000000000000000, 0.0002605067024380913927, 0.0005210134048761827855 ),
 .UNSPECIFIED. ) ;
#67185=CARTESIAN_POINT ( 'NONE',  ( -0.8801773607110991993, 62.85535201082150536, -2.915334737309923874 ) ) ;
#67191=CARTESIAN_POINT ( 'NONE',  ( -0.3689425029237898834, 31.17874883491396787, -10.36894250292378850 ) ) ;
#67192=CARTESIAN_POINT ( 'NONE',  ( 22.81628187352647785, 26.41530133659708923, 3.434112377981063169 ) ) ;
#67194=CARTESIAN_POINT ( 'NONE',  ( 16.40814093676323893, 45.79030133659708923, 11.09922568453595026 ) ) ;
#67195=CARTESIAN_POINT ( 'NONE',  ( 4.559911319644449179, 18.89701867748817321, 9.422509992056141925 ) ) ;
#67196=CARTESIAN_POINT ( 'NONE',  ( 5.076628168052704559, 40.17559781766745175, -8.527530157486179263 ) ) ;
#67197=CARTESIAN_POINT ( 'NONE',  ( 17.96484262340118221, 14.93868534415483751, 7.964842623401181321 ) ) ;
#67198=CARTESIAN_POINT ( 'NONE',  ( -1.099225684535947600, 64.54030133659709634, 6.408140936763237150 ) ) ;
#67199=CARTESIAN_POINT ( 'NONE',  ( -0.1503990784575277295, 39.24884699246889141, -6.262539305110077947 ) ) ;
#67200=CARTESIAN_POINT ( 'NONE',  ( 2.791683348922240793, 36.63393115100078035, 7.208316651077764092 ) ) ;
#67201=CARTESIAN_POINT ( 'NONE',  ( 14.92337183194729988, 54.34226448433412315, -8.527530157486177487 ) ) ;
#67202=CARTESIAN_POINT ( 'NONE',  ( -0.1503990784575328643, 70.00000000000000000, 6.262539305110068177 ) ) ;
#67207=CARTESIAN_POINT ( 'NONE',  ( -45.94000000000000483, 93.00000000000000000, -8.999999999999998224 ) ) ;
#67209=CARTESIAN_POINT ( 'NONE',  ( -41.94000000000001194, 93.50000000000000000, -9.500000000000000000 ) ) ;
#67210=CARTESIAN_POINT ( 'NONE',  ( 19.84674366389459266, 18.30059781766745175, 2.638427012816836559 ) ) ;
#67211=CARTESIAN_POINT ( 'NONE',  ( 10.00000000000000000, 42.87363466993042493, -12.81628187352647608 ) ) ;
#67216=CARTESIAN_POINT ( 'NONE',  ( 19.84674366389459266, 58.30059781766745886, 2.638427012816836559 ) ) ;
#67218=CARTESIAN_POINT ( 'NONE',  ( 22.26659068614894466, 33.88708216824730357, 7.082119434687054849 ) ) ;
#67219=CARTESIAN_POINT ( 'NONE',  ( 14.92337183194729988, 44.34226448433412315, -8.527530157486177487 ) ) ;
#67220=CARTESIAN_POINT ( 'NONE',  ( 22.81628187352648496, 51.83196800326376064, -3.434112377981050290 ) ) ;
#67221=CARTESIAN_POINT ( 'NONE',  ( 5.054308323419911098, 70.51564955044841554, -12.00000000000000000 ) ) ;
#67223=CARTESIAN_POINT ( 'NONE',  ( 10.00000000000000000, -0.2410688489992152128, -9.846743663894594434 ) ) ;
#67225=CARTESIAN_POINT ( 'NONE',  ( 5.076628168052704559, 50.17559781766745886, -8.527530157486179263 ) ) ;
#67226=CARTESIAN_POINT ( 'NONE',  ( 17.96484262340118221, 41.18868534415484106, -7.964842623401177768 ) ) ;
#67227=CARTESIAN_POINT ( 'NONE',  ( 7.361572987183170547, 32.05059781766745175, 9.846743663894590881 ) ) ;
#67229=CARTESIAN_POINT ( 'NONE',  ( 15.44008868035555260, 39.73035201082150536, 9.422509992056143702 ) ) ;
#67232=CARTESIAN_POINT ( 'NONE',  ( 20.88017736071110164, 20.35535201082150891, 2.915334737309930979 ) ) ;
#67233=CARTESIAN_POINT ( 'NONE',  ( 19.84674366389459266, 63.30059781766745886, 2.638427012816836559 ) ) ;
#67234=CARTESIAN_POINT ( 'NONE',  ( -0.8801773607110991993, 37.85535201082151247, -2.915334737309923874 ) ) ;
#67236=CARTESIAN_POINT ( 'NONE',  ( 17.96484262340118221, 64.93868534415483396, 7.964842623401181321 ) ) ;
#67238=CARTESIAN_POINT ( 'NONE',  ( 17.96484262340118221, 31.18868534415483751, -7.964842623401177768 ) ) ;
#67240=CARTESIAN_POINT ( 'NONE',  ( 19.84674366389459266, 13.71726448433411782, -2.638427012816827677 ) ) ;
#67241=CARTESIAN_POINT ( 'NONE',  ( 12.63842701281683034, 22.46726448433411605, 9.846743663894596210 ) ) ;
#67244=CARTESIAN_POINT ( 'NONE',  ( 10.00000000000000000, -2.126365330069579951, -12.81628187352647608 ) ) ;
#67245=CARTESIAN_POINT ( 'NONE',  ( 2.917880565312950480, 60.97041550158063927, -12.26659068614894821 ) ) ;
#67249=CARTESIAN_POINT ( 'NONE',  ( -0.3689425029237881626, 7.428748834913967869, 10.36894250292379027 ) ) ;
#67250=CARTESIAN_POINT ( 'NONE',  ( 10.00000000000000178, 48.05374883491396787, 14.16423886937410082 ) ) ;
#67251=CARTESIAN_POINT ( 'NONE',  ( 21.09922568453595559, 2.040301336597086568, -6.408140936763230044 ) ) ;
#67254=CARTESIAN_POINT ( 'NONE',  ( 14.92337183194729633, 12.67559781766745353, 8.527530157486181039 ) ) ;
#67255=CARTESIAN_POINT ( 'NONE',  ( 2.035157376598824452, 8.688685344154839285, 7.964842623401179544 ) ) ;
#67256=CARTESIAN_POINT ( 'NONE',  ( 0.1532563361054082862, 46.21726448433411605, 2.638427012816831674 ) ) ;
#67259=CARTESIAN_POINT ( 'NONE',  ( 19.84674366389459266, 3.300597817667451750, 2.638427012816836559 ) ) ;
#67260=CARTESIAN_POINT ( 'NONE',  ( -2.816281873526473856, 24.12363466993042138, 9.499525473075851096E-16 ) ) ;
#67261=CARTESIAN_POINT ( 'NONE',  ( 18.52753015748618282, 23.92559781766745530, -4.923371831947291888 ) ) ;
#67263=CARTESIAN_POINT ( 'NONE',  ( 14.92337183194729633, 12.67559781766745353, 8.527530157486181039 ) ) ;
#67266=CARTESIAN_POINT ( 'NONE',  ( 4.559911319644449179, 8.897018677488171434, 9.422509992056141925 ) ) ;
#67267=CARTESIAN_POINT ( 'NONE',  ( 13.79529636645031943, 45.34541550158062506, -14.16423886937409904 ) ) ;
#67268=CARTESIAN_POINT ( 'NONE',  ( 12.91533473730992121, 39.52201867748817676, 10.88017736071110164 ) ) ;
#67269=CARTESIAN_POINT ( 'NONE',  ( 20.88017736071110164, 60.35535201082151957, 2.915334737309930979 ) ) ;
#67271=CARTESIAN_POINT ( 'NONE',  ( 0.1532563361054083140, 26.00893115100078745, 1.131784320476157264E-15 ) ) ;
#67272=CARTESIAN_POINT ( 'NONE',  ( 17.96484262340118221, 11.18868534415483929, -7.964842623401177768 ) ) ;
#67273=CARTESIAN_POINT ( 'NONE',  ( 0.1532563361054083140, 1.008931151000784787, 1.131784320476157264E-15 ) ) ;
#67275=CARTESIAN_POINT ( 'NONE',  ( 17.20831665107776587, 42.88393115100077324, 7.208316651077764980 ) ) ;
#67278=CARTESIAN_POINT ( 'NONE',  ( 20.88017736071110519, 30.56368534415484106, 2.639326808657452039E-16 ) ) ;
#67281=CARTESIAN_POINT ( 'NONE',  ( 6.565887622018943937, 58.08196800326376064, -12.81628187352647608 ) ) ;
#67283=CARTESIAN_POINT ( 'NONE',  ( 18.52753015748617571, 8.092264484334117824, 4.923371831947298993 ) ) ;
#67284=CARTESIAN_POINT ( 'NONE',  ( 16.40814093676324603, 47.45696800326375353, -11.09922568453594671 ) ) ;
#67285=CARTESIAN_POINT ( 'NONE',  ( -2.266590686148945544, 67.22041550158063217, 7.082119434687048631 ) ) ;
#67286=CARTESIAN_POINT ( 'NONE',  ( 1.472469842513823179, 41.42559781766745886, 4.923371831947296329 ) ) ;
#67288=CARTESIAN_POINT ( 'NONE',  ( -2.266590686148945544, 22.22041550158063572, 7.082119434687048631 ) ) ;
#67289=CARTESIAN_POINT ( 'NONE',  ( 17.08211943468705840, 40.13708216824731068, -12.26659068614894466 ) ) ;
#67290=CARTESIAN_POINT ( 'NONE',  ( 18.52753015748618282, 38.92559781766745175, -4.923371831947291888 ) ) ;
#67292=CARTESIAN_POINT ( 'NONE',  ( 7.084665262690076126, 37.02201867748817676, -10.88017736071110164 ) ) ;
#67293=CARTESIAN_POINT ( 'NONE',  ( 7.361572987183170547, 2.050597817667451750, 9.846743663894590881 ) ) ;
#67296=CARTESIAN_POINT ( 'NONE',  ( 16.40814093676324603, 57.45696800326375353, -11.09922568453594671 ) ) ;
#67297=CARTESIAN_POINT ( 'NONE',  ( 12.91533473730992121, 64.52201867748817676, 10.88017736071110164 ) ) ;
#67298=ORIENTED_EDGE ( 'NONE', *, *, #841, .T. ) ;
#67299=CARTESIAN_POINT ( 'NONE',  ( -0.3689425029237898834, 11.17874883491396787, -10.36894250292378850 ) ) ;
#67300=CARTESIAN_POINT ( 'NONE',  ( 0.1532563361054100626, 10.80059781766745175, -2.638427012816831230 ) ) ;
#67301=CARTESIAN_POINT ( 'NONE',  ( -1.926860441876562025, 59.47997603579417358, -3.195792623639529761 ) ) ;
#67303=CARTESIAN_POINT ( 'NONE',  ( 17.96484262340118221, 29.93868534415484106, 7.964842623401181321 ) ) ;
#67306=ORIENTED_EDGE ( 'NONE', *, *, #18762, .F. ) ;
#67307=CARTESIAN_POINT ( 'NONE',  ( 17.96484262340118221, 41.18868534415484106, -7.964842623401177768 ) ) ;
#67308=CARTESIAN_POINT ( 'NONE',  ( 10.00000000000000178, 67.25893115100079456, 9.846743663894594434 ) ) ;
#67310=CARTESIAN_POINT ( 'NONE',  ( 22.81628187352648496, 11.83196800326375531, -3.434112377981050290 ) ) ;
#67312=CARTESIAN_POINT ( 'NONE',  ( 19.42250999205614193, 65.14701867748817676, 5.440088680355555262 ) ) ;
#67313=CARTESIAN_POINT ( 'NONE',  ( 14.92337183194729988, 59.34226448433412315, -8.527530157486177487 ) ) ;
#67314=CARTESIAN_POINT ( 'NONE',  ( 10.00000000000000178, 19.31368534415484106, 10.88017736071110342 ) ) ;
#67315=CARTESIAN_POINT ( 'NONE',  ( 0.000000000000000000, 70.00000000000000000, 5.000000000000000000 ) ) ;
#67316=CARTESIAN_POINT ( 'NONE',  ( 7.361572987183170547, 2.050597817667451750, 9.846743663894590881 ) ) ;
#67317=CARTESIAN_POINT ( 'NONE',  ( -0.8801773607110991993, 17.85535201082150536, -2.915334737309923874 ) ) ;
#67321=CARTESIAN_POINT ( 'NONE',  ( 16.40814093676323893, 50.79030133659708923, 11.09922568453595026 ) ) ;
#67322=CARTESIAN_POINT ( 'NONE',  ( 4.559911319644449179, 43.89701867748816966, 9.422509992056141925 ) ) ;
#67324=CARTESIAN_POINT ( 'NONE',  ( -1.099225684535947600, 53.70696800326376064, -6.408140936763238038 ) ) ;
#67325=CARTESIAN_POINT ( 'NONE',  ( 12.91533473730992121, 49.52201867748817676, 10.88017736071110164 ) ) ;
#67326=CARTESIAN_POINT ( 'NONE',  ( -2.816281873526471635, 3.915301336597087456, -3.434112377981056508 ) ) ;
#67327=CARTESIAN_POINT ( 'NONE',  ( 5.076628168052703671, 21.84226448433411960, 8.527530157486179263 ) ) ;
#67328=CARTESIAN_POINT ( 'NONE',  ( 16.40814093676324603, 2.456968003263753531, -11.09922568453594671 ) ) ;
#67330=CARTESIAN_POINT ( 'NONE',  ( 17.20831665107776587, 64.13393115100079456, -7.208316651077762316 ) ) ;
#67331=CARTESIAN_POINT ( 'NONE',  ( 15.44008868035555793, 41.39701867748817676, -9.422509992056140149 ) ) ;
#67332=CARTESIAN_POINT ( 'NONE',  ( 14.92337183194729633, 47.67559781766745175, 8.527530157486181039 ) ) ;
#67333=SURFACE_STYLE_USAGE ( .BOTH. , #66837 ) ;
#67334=EDGE_CURVE ( 'NONE', #97012, #87349, #9109, .T. ) ;
#67335=CARTESIAN_POINT ( 'NONE',  ( 2.791683348922237240, 25.38393115100078390, -7.208316651077763204 ) ) ;
#67336=CARTESIAN_POINT ( 'NONE',  ( 10.00000000000000178, 12.25893115100078568, 9.846743663894594434 ) ) ;
#67337=CARTESIAN_POINT ( 'NONE',  ( -2.816281873526473856, 9.123634669930421381, 9.499525473075851096E-16 ) ) ;
#67338=ORIENTED_EDGE ( 'NONE', *, *, #87033, .F. ) ;
#67339=( GEOMETRIC_REPRESENTATION_CONTEXT ( 3 ) GLOBAL_UNCERTAINTY_ASSIGNED_CONTEXT ( ( #92242 ) ) GLOBAL_UNIT_ASSIGNED_CONTEXT ( ( #4059, #65015, #28016 ) ) REPRESENTATION_CONTEXT ( 'NONE', 'WORKASPACE' ) );
#67341=CARTESIAN_POINT ( 'NONE',  ( 0.000000000000000000, 0.000000000000000000, 0.000000000000000000 ) ) ;
#67342=CARTESIAN_POINT ( 'NONE',  ( 0.2751277870542967463, 70.00000000000000000, -6.000000000000000000 ) ) ;
#67343=CARTESIAN_POINT ( 'NONE',  ( 22.81628187352647785, 56.62363466993042493, 6.195893100308588602E-16 ) ) ;
#67344=CARTESIAN_POINT ( 'NONE',  ( 18.52753015748617571, 33.09226448433411605, 4.923371831947298993 ) ) ;
#67346=CARTESIAN_POINT ( 'NONE',  ( 10.00000000000000000, 11.81368534415483751, -10.88017736071110342 ) ) ;
#67347=CARTESIAN_POINT ( 'NONE',  ( 19.84674366389459266, 28.30059781766745886, 2.638427012816836559 ) ) ;
#67348=MECHANICAL_DESIGN_GEOMETRIC_PRESENTATION_REPRESENTATION('',(#51358),#52997);
#67349=CARTESIAN_POINT ( 'NONE',  ( 1.274849032794164172, 18.57228050351029935, 6.499999999999802824 ) ) ;
#67350=CARTESIAN_POINT ( 'NONE',  ( 2.035157376598822676, 7.438685344154837509, -7.964842623401177768 ) ) ;
#67352=CARTESIAN_POINT ( 'NONE',  ( 4.559911319644449179, 17.23035201082150536, -9.422509992056141925 ) ) ;
#67353=CARTESIAN_POINT ( 'NONE',  ( 24.16423886937409904, 54.09541550158063217, 3.795296366450317205 ) ) ;
#67354=CARTESIAN_POINT ( 'NONE',  ( 13.79529636645031943, 50.34541550158064638, -14.16423886937409904 ) ) ;
#67356=CARTESIAN_POINT ( 'NONE',  ( -16.94000000000001549, 92.00000000000000000, -10.09898361729590199 ) ) ;
#67358=CARTESIAN_POINT ( 'NONE',  ( 2.791683348922237240, 30.38393115100078390, -7.208316651077763204 ) ) ;
#67359=CARTESIAN_POINT ( 'NONE',  ( 17.20831665107776587, 62.88393115100078745, 7.208316651077764980 ) ) ;
#67360=CARTESIAN_POINT ( 'NONE',  ( 2.603489959281588995, 40.43575266056827644, -6.500000000000003553 ) ) ;
#67361=CARTESIAN_POINT ( 'NONE',  ( 2.791683348922237240, 55.38393115100078745, -7.208316651077763204 ) ) ;
#67364=CARTESIAN_POINT ( 'NONE',  ( 6.204703633549690345, 5.762082168247301794, -14.16423886937410259 ) ) ;
#67365=CARTESIAN_POINT ( 'NONE',  ( 14.92337183194729988, 29.34226448433411960, -8.527530157486177487 ) ) ;
#67367=CARTESIAN_POINT ( 'NONE',  ( -4.164238869374099927, 37.01208216824731068, 3.795296366450308767 ) ) ;
#67368=CARTESIAN_POINT ( 'NONE',  ( 0.1532563361054083140, 6.008931151000784787, 1.131784320476157264E-15 ) ) ;
#67370=DIRECTION ( 'NONE',  ( 0.000000000000000000, -1.000000000000000000, 0.000000000000000000 ) ) ;
#67371=CARTESIAN_POINT ( 'NONE',  ( 20.88017736071110519, 30.56368534415484106, 2.639326808657452039E-16 ) ) ;
#67372=CARTESIAN_POINT ( 'NONE',  ( 22.81628187352648496, 41.83196800326375353, -3.434112377981050290 ) ) ;
#67373=CARTESIAN_POINT ( 'NONE',  ( 0.5774900079438590739, 2.647018677488170990, -5.440088680355550821 ) ) ;
#67374=CARTESIAN_POINT ( 'NONE',  ( 16.40814093676324603, 37.45696800326376064, -11.09922568453594671 ) ) ;
#67375=CARTESIAN_POINT ( 'NONE',  ( 19.50000000000000355, 79.40087001978915282, 5.000000000000000000 ) ) ;
#67378=CARTESIAN_POINT ( 'NONE',  ( 20.10421743870886857, 35.60736173766203194, -6.337391062633418670 ) ) ;
#67379=CARTESIAN_POINT ( 'NONE',  ( 20.36894250292379738, 34.92874883491396076, -10.36894250292379027 ) ) ;
#67380=CARTESIAN_POINT ( 'NONE',  ( 22.26659068614894466, 3.887082168247300906, 7.082119434687054849 ) ) ;
#67381=CARTESIAN_POINT ( 'NONE',  ( 12.91533473730993009, 11.60535201082150536, -10.88017736071109987 ) ) ;
#67382=CARTESIAN_POINT ( 'NONE',  ( 10.00000000000000000, 16.81368534415483751, -10.88017736071110342 ) ) ;
#67385=CARTESIAN_POINT ( 'NONE',  ( 19.42250999205614193, 55.14701867748817676, 5.440088680355555262 ) ) ;
#67386=CARTESIAN_POINT ( 'NONE',  ( 12.91533473730992121, 49.52201867748817676, 10.88017736071110164 ) ) ;
#67387=CARTESIAN_POINT ( 'NONE',  ( 10.00000000000000000, 32.87363466993042493, -12.81628187352647608 ) ) ;
#67389=CARTESIAN_POINT ( 'NONE',  ( 20.10384461210890805, 26.74302437010793554, 6.337995344473785764 ) ) ;
#67390=CARTESIAN_POINT ( 'NONE',  ( 14.92337183194729988, 29.34226448433411960, -8.527530157486177487 ) ) ;
#67391=CARTESIAN_POINT ( 'NONE',  ( 15.44008868035555793, 56.39701867748817676, -9.422509992056140149 ) ) ;
#67393=UNCERTAINTY_MEASURE_WITH_UNIT (LENGTH_MEASURE( 1.000000000000000082E-05 ), #19755, 'distance_accuracy_value', 'NONE');
#67395=CARTESIAN_POINT ( 'NONE',  ( -2.816281873526473856, 19.12363466993042138, 9.499525473075851096E-16 ) ) ;
#67396=SURFACE_SIDE_STYLE ('',( #67897 ) ) ;
#67397=CARTESIAN_POINT ( 'NONE',  ( 4.559911319644449179, 3.897018677488170990, 9.422509992056141925 ) ) ;
#67398=CARTESIAN_POINT ( 'NONE',  ( 7.361572987183170547, 37.05059781766744464, 9.846743663894590881 ) ) ;
#67399=CARTESIAN_POINT ( 'NONE',  ( 13.43411237798105340, 55.58196800326374643, 12.81628187352647963 ) ) ;
#67400=CARTESIAN_POINT ( 'NONE',  ( 0.1532563361054100626, 15.80059781766745353, -2.638427012816831230 ) ) ;
#67401=CARTESIAN_POINT ( 'NONE',  ( -4.164238869374098151, 11.59541550158063217, -3.795296366450310543 ) ) ;
#67402=CARTESIAN_POINT ( 'NONE',  ( 20.88017736071110164, 30.35535201082150891, 2.915334737309930979 ) ) ;
#67403=CARTESIAN_POINT ( 'NONE',  ( 2.035157376598824452, 38.68868534415483396, 7.964842623401179544 ) ) ;
#67404=FILL_AREA_STYLE_COLOUR ( '', #61619 ) ;
#67405=CARTESIAN_POINT ( 'NONE',  ( 0.1532563361054082862, 41.21726448433411605, 2.638427012816831674 ) ) ;
#67406=CARTESIAN_POINT ( 'NONE',  ( 0.5774900079438607392, 38.48035201082150536, 5.440088680355550821 ) ) ;
#67407=CARTESIAN_POINT ( 'NONE',  ( 2.035157376598822676, 17.43868534415483751, -7.964842623401177768 ) ) ;
#67409=EDGE_CURVE ( 'NONE', #97093, #55640, #2415, .T. ) ;
#67410=CARTESIAN_POINT ( 'NONE',  ( 19.42250999205614548, 25.98035201082150891, -5.440088680355545492 ) ) ;
#67411=CARTESIAN_POINT ( 'NONE',  ( 0.6178305044545838731, 39.74863466993041072, 9.382169495545420901 ) ) ;
#67412=CARTESIAN_POINT ( 'NONE',  ( 15.44008868035555260, 29.73035201082150891, 9.422509992056143702 ) ) ;
#67414=CARTESIAN_POINT ( 'NONE',  ( 2.035157376598824452, 38.68868534415483396, 7.964842623401179544 ) ) ;
#67416=ORIENTED_EDGE ( 'NONE', *, *, #56673, .F. ) ;
#67417=CARTESIAN_POINT ( 'NONE',  ( 7.361572987183169658, 59.96726448433410894, -9.846743663894592657 ) ) ;
#67418=CARTESIAN_POINT ( 'NONE',  ( 20.88017736071110875, 30.77201867748816966, -2.915334737309920765 ) ) ;
#67423=CARTESIAN_POINT ( 'NONE',  ( -0.3689425029237881626, 42.42874883491396787, 10.36894250292379027 ) ) ;
#67424=CARTESIAN_POINT ( 'NONE',  ( 4.559911319644449179, 48.89701867748817676, 9.422509992056141925 ) ) ;
#67428=CARTESIAN_POINT ( 'NONE',  ( 0.1532563361054100626, 65.80059781766745175, -2.638427012816831230 ) ) ;
#67431=CARTESIAN_POINT ( 'NONE',  ( 0.1532563361054083140, 16.00893115100078390, 1.131784320476157264E-15 ) ) ;
#67434=AXIS2_PLACEMENT_3D ( 'NONE', #43547, #51053, #81543 ) ;
#67435=CARTESIAN_POINT ( 'NONE',  ( 19.84674366389459266, 23.30059781766745530, 2.638427012816836559 ) ) ;
#67438=CARTESIAN_POINT ( 'NONE',  ( 17.96484262340118221, 21.18868534415483396, -7.964842623401177768 ) ) ;
#67439=CARTESIAN_POINT ( 'NONE',  ( 10.00000000000000178, 22.25893115100078745, 9.846743663894594434 ) ) ;
#67441=CARTESIAN_POINT ( 'NONE',  ( 6.565887622018943937, 10.16530133659708746, 12.81628187352647430 ) ) ;
#67443=CARTESIAN_POINT ( 'NONE',  ( 2.035157376598822676, 62.43868534415483396, -7.964842623401177768 ) ) ;
#67444=CARTESIAN_POINT ( 'NONE',  ( -0.8801773607111008646, 38.27201867748816255, 2.915334737309923430 ) ) ;
#67445=CARTESIAN_POINT ( 'NONE',  ( 10.00000000000000178, 4.313685344154837509, 10.88017736071110342 ) ) ;
#67446=CARTESIAN_POINT ( 'NONE',  ( 24.16423886937410614, 49.51208216824730357, -3.795296366450302550 ) ) ;
#67447=CARTESIAN_POINT ( 'NONE',  ( 20.24186590665275531, 35.59014588040358262, -6.114288769123075618 ) ) ;
#67448=EDGE_LOOP ( 'NONE', ( #62607, #60552, #60784, #64805 ) ) ;
#67449=CARTESIAN_POINT ( 'NONE',  ( 22.81628187352647785, 11.62363466993042138, 6.195893100308588602E-16 ) ) ;
#67450=CARTESIAN_POINT ( 'NONE',  ( 2.035157376598822676, 7.438685344154837509, -7.964842623401177768 ) ) ;
#67451=CARTESIAN_POINT ( 'NONE',  ( 7.084665262690076126, 42.02201867748816966, -10.88017736071110164 ) ) ;
#67454=CARTESIAN_POINT ( 'NONE',  ( 7.084665262690076126, 54.10535201082151247, 10.88017736071109987 ) ) ;
#67455=CARTESIAN_POINT ( 'NONE',  ( 7.361572987183169658, 39.96726448433411605, -9.846743663894592657 ) ) ;
#67456=CARTESIAN_POINT ( 'NONE',  ( 18.52753015748617571, 23.09226448433411960, 4.923371831947298993 ) ) ;
#67457=CARTESIAN_POINT ( 'NONE',  ( 2.791683348922240793, 11.63393115100078568, 7.208316651077764092 ) ) ;
#67460=CARTESIAN_POINT ( 'NONE',  ( 19.84674366389459266, 3.300597817667451750, 2.638427012816836559 ) ) ;
#67463=CARTESIAN_POINT ( 'NONE',  ( 14.92337183194729988, 29.34226448433411960, -8.527530157486177487 ) ) ;
#67465=CARTESIAN_POINT ( 'NONE',  ( 0.6178305044545838731, 59.74863466993041783, 9.382169495545420901 ) ) ;
#67468=CARTESIAN_POINT ( 'NONE',  ( 7.361572987183170547, 67.05059781766746596, 9.846743663894590881 ) ) ;
#67469=CARTESIAN_POINT ( 'NONE',  ( -4.164238869374099039, 26.80374883491397142, 8.674139862899312516E-16 ) ) ;
#67470=( BOUNDED_CURVE ( )  B_SPLINE_CURVE ( 2, ( #80696, #95190, #34188, #4715, #19698, #50690, #35177, #11704, #81183 ),
 .UNSPECIFIED., .F., .T. ) 
 B_SPLINE_CURVE_WITH_KNOTS ( ( 3, 2, 2, 2, 3 ),
 ( 0.01156950836880285202, 0.01190476190476197349, 0.01785714285714290472, 0.02380952380952383596, 0.02414477734548295743 ),
 .UNSPECIFIED. ) 
 CURVE ( )  GEOMETRIC_REPRESENTATION_ITEM ( )  RATIONAL_B_SPLINE_CURVE ( ( 0.9963778908391762723, 0.9980808541467921513, 1.000000000000000000, 0.9659258262890682012, 1.000000000000000000, 0.9659258262890682012, 1.000000000000000000, 0.9980808541467921513, 0.9963778908391762723 ) ) 
 REPRESENTATION_ITEM ( '' )  );
#67473=CARTESIAN_POINT ( 'NONE',  ( 13.79529636645031943, 35.34541550158063927, -14.16423886937409904 ) ) ;
#67475=CARTESIAN_POINT ( 'NONE',  ( 20.36894250292379382, 48.67874883491396076, 10.36894250292379205 ) ) ;
#67476=CARTESIAN_POINT ( 'NONE',  ( 22.26659068614895176, 4.720415501580633943, -7.082119434687042414 ) ) ;
#67477=CARTESIAN_POINT ( 'NONE',  ( -4.164238869374098151, 6.595415501580634832, -3.795296366450310543 ) ) ;
#67478=CARTESIAN_POINT ( 'NONE',  ( 17.96484262340118221, 49.93868534415484106, 7.964842623401181321 ) ) ;
#67480=CARTESIAN_POINT ( 'NONE',  ( 12.63842701281683922, 29.55059781766745175, -9.846743663894590881 ) ) ;
#67482=CARTESIAN_POINT ( 'NONE',  ( 7.361572987183170547, 27.05059781766745175, 9.846743663894590881 ) ) ;
#67483=CARTESIAN_POINT ( 'NONE',  ( 2.035157376598822676, 27.43868534415483396, -7.964842623401177768 ) ) ;
#67484=CARTESIAN_POINT ( 'NONE',  ( 6.565887622018943937, 60.16530133659707502, 12.81628187352647430 ) ) ;
#67485=CARTESIAN_POINT ( 'NONE',  ( 0.1532563361054083140, 61.00893115100078745, 1.131784320476157264E-15 ) ) ;
#67487=CARTESIAN_POINT ( 'NONE',  ( 12.63842701281683034, 32.46726448433412315, 9.846743663894596210 ) ) ;
#67488=CARTESIAN_POINT ( 'NONE',  ( 19.38216949554541202, 45.99863466993041072, 9.382169495545424454 ) ) ;
#67491=CARTESIAN_POINT ( 'NONE',  ( 17.96484262340118221, 39.93868534415484106, 7.964842623401181321 ) ) ;
#67492=CARTESIAN_POINT ( 'NONE',  ( 5.076628168052704559, 50.17559781766745886, -8.527530157486179263 ) ) ;
#67493=CARTESIAN_POINT ( 'NONE',  ( -2.266590686148945544, 31.38708216824730002, -7.082119434687050408 ) ) ;
#67495=FACE_OUTER_BOUND ( 'NONE', #38067, .T. ) ;
#67496=CARTESIAN_POINT ( 'NONE',  ( 17.96484262340118221, 64.93868534415483396, 7.964842623401181321 ) ) ;
#67497=CARTESIAN_POINT ( 'NONE',  ( 19.42250999205614548, 60.98035201082151247, -5.440088680355545492 ) ) ;
#67498=CARTESIAN_POINT ( 'NONE',  ( 20.36894250292379382, 63.67874883491396787, 10.36894250292379205 ) ) ;
#67499=CARTESIAN_POINT ( 'NONE',  ( 0.1532563361054100626, 65.80059781766745175, -2.638427012816831230 ) ) ;
#67502=CARTESIAN_POINT ( 'NONE',  ( 4.559911319644449179, 48.89701867748817676, 9.422509992056141925 ) ) ;
#67505=CARTESIAN_POINT ( 'NONE',  ( -0.8801773607110991993, 7.855352010821504471, -2.915334737309923874 ) ) ;
#67506=CARTESIAN_POINT ( 'NONE',  ( 17.96484262340118221, 9.938685344154839285, 7.964842623401181321 ) ) ;
#67507=( GEOMETRIC_REPRESENTATION_CONTEXT ( 3 ) GLOBAL_UNCERTAINTY_ASSIGNED_CONTEXT ( ( #78102 ) ) GLOBAL_UNIT_ASSIGNED_CONTEXT ( ( #88765, #88270, #29246 ) ) REPRESENTATION_CONTEXT ( 'NONE', 'WORKASPACE' ) );
#67508=CARTESIAN_POINT ( 'NONE',  ( 0.1532563361054083140, 56.00893115100078745, 1.131784320476157264E-15 ) ) ;
#67509=CARTESIAN_POINT ( 'NONE',  ( 16.40814093676323893, 45.79030133659708923, 11.09922568453595026 ) ) ;
#67512=CARTESIAN_POINT ( 'NONE',  ( 10.00000000000000178, 14.31368534415483751, 10.88017736071110342 ) ) ;
#67513=ADVANCED_FACE ( 'NONE', ( #32088 ), #62586, .T. ) ;
#67514=CARTESIAN_POINT ( 'NONE',  ( 22.81628187352647785, 16.62363466993042138, 6.195893100308588602E-16 ) ) ;
#67517=CARTESIAN_POINT ( 'NONE',  ( 10.00000000000000178, 17.25893115100078745, 9.846743663894594434 ) ) ;
#67518=CARTESIAN_POINT ( 'NONE',  ( 19.84674366389459266, 53.71726448433411605, -2.638427012816827677 ) ) ;
#67520=CARTESIAN_POINT ( 'NONE',  ( -0.8801773607111009756, 38.06368534415484106, 1.068504757029289695E-15 ) ) ;
#67521=CARTESIAN_POINT ( 'NONE',  ( 21.09922568453595559, 7.040301336597086568, -6.408140936763230044 ) ) ;
#67522=CARTESIAN_POINT ( 'NONE',  ( 15.44008868035555260, 54.73035201082150536, 9.422509992056143702 ) ) ;
#67525=CARTESIAN_POINT ( 'NONE',  ( 6.565887622018943937, 58.08196800326376064, -12.81628187352647608 ) ) ;
#67527=CARTESIAN_POINT ( 'NONE',  ( 15.44008868035555793, 61.39701867748817676, -9.422509992056140149 ) ) ;
#67528=CARTESIAN_POINT ( 'NONE',  ( 22.81628187352648496, 31.83196800326375353, -3.434112377981050290 ) ) ;
#67529=CARTESIAN_POINT ( 'NONE',  ( 17.08211943468705840, 5.137082168247300906, -12.26659068614894466 ) ) ;
#67530=CARTESIAN_POINT ( 'NONE',  ( 18.52753015748618282, 8.925597817667451750, -4.923371831947291888 ) ) ;
#67531=CARTESIAN_POINT ( 'NONE',  ( 15.44008868035555260, 34.73035201082151247, 9.422509992056143702 ) ) ;
#67533=STYLED_ITEM ( 'NONE', ( #71879 ), #9051 ) ;
#67535=CARTESIAN_POINT ( 'NONE',  ( 1.472469842513823179, 10.59226448433411782, -4.923371831947296329 ) ) ;
#67536=CARTESIAN_POINT ( 'NONE',  ( 12.63842701281683922, 9.550597817667449974, -9.846743663894590881 ) ) ;
#67538=CARTESIAN_POINT ( 'NONE',  ( 10.00000000000000000, 40.55374883491397497, -14.16423886937410082 ) ) ;
#67539=EDGE_CURVE ( 'NONE', #45712, #14534, #47435, .T. ) ;
#67545=CARTESIAN_POINT ( 'NONE',  ( 2.917880565312950480, 65.97041550158063217, -12.26659068614894821 ) ) ;
#67546=CARTESIAN_POINT ( 'NONE',  ( 10.00000000000000178, 58.05374883491397497, 14.16423886937410082 ) ) ;
#67547=CARTESIAN_POINT ( 'NONE',  ( 0.1532563361054100626, 25.80059781766744820, -2.638427012816831230 ) ) ;
#67549=CARTESIAN_POINT ( 'NONE',  ( -2.816281873526473856, 29.33196800326376064, 3.434112377981055619 ) ) ;
#67552=CARTESIAN_POINT ( 'NONE',  ( -4.164238869374099039, 6.803748834913967869, 8.674139862899312516E-16 ) ) ;
#67553=CARTESIAN_POINT ( 'NONE',  ( 2.035157376598824452, 13.68868534415483751, 7.964842623401179544 ) ) ;
#67554=CARTESIAN_POINT ( 'NONE',  ( 17.08211943468705840, 60.13708216824729647, -12.26659068614894466 ) ) ;
#67555=CARTESIAN_POINT ( 'NONE',  ( 0.1532563361054100626, 30.80059781766744820, -2.638427012816831230 ) ) ;
#67557=CARTESIAN_POINT ( 'NONE',  ( 19.84674366389459266, 28.71726448433411960, -2.638427012816827677 ) ) ;
#67562=ORIENTED_EDGE ( 'NONE', *, *, #27998, .T. ) ;
#67563=DIRECTION ( 'NONE',  ( -0.8320502943378437211, 0.5547001962252290364, 0.000000000000000000 ) ) ;
#67565=CARTESIAN_POINT ( 'NONE',  ( 7.361572987183169658, 49.96726448433410894, -9.846743663894592657 ) ) ;
#67566=CARTESIAN_POINT ( 'NONE',  ( 2.917880565312950480, 20.97041550158063217, -12.26659068614894821 ) ) ;
#67567=CARTESIAN_POINT ( 'NONE',  ( 0.5774900079438607392, 38.48035201082150536, 5.440088680355550821 ) ) ;
#67568=CARTESIAN_POINT ( 'NONE',  ( 17.96484262340118221, 44.93868534415483396, 7.964842623401181321 ) ) ;
#67569=CARTESIAN_POINT ( 'NONE',  ( 7.361572987183170547, 67.05059781766746596, 9.846743663894590881 ) ) ;
#67570=CARTESIAN_POINT ( 'NONE',  ( 21.09922568453594849, 11.20696800326375531, 6.408140936763242479 ) ) ;
#67571=( LENGTH_UNIT ( ) NAMED_UNIT ( * ) SI_UNIT ( .MILLI., .METRE. ) );
#67573=CARTESIAN_POINT ( 'NONE',  ( -2.816281873526473856, 29.12363466993041783, 9.499525473075851096E-16 ) ) ;
#67576=CARTESIAN_POINT ( 'NONE',  ( 0.1532563361054100626, 45.80059781766745886, -2.638427012816831230 ) ) ;
#67577=VECTOR ( 'NONE', #74752, 1000.000000000000000 ) ;
#67578=CARTESIAN_POINT ( 'NONE',  ( 7.084665262690076126, 4.105352010821503583, 10.88017736071109987 ) ) ;
#67581=CARTESIAN_POINT ( 'NONE',  ( 17.96484262340118221, 21.18868534415483396, -7.964842623401177768 ) ) ;
#67583=CARTESIAN_POINT ( 'NONE',  ( 12.91533473730992121, 44.52201867748816966, 10.88017736071110164 ) ) ;
#67584=CARTESIAN_POINT ( 'NONE',  ( 7.084665262690076126, 54.10535201082151247, 10.88017736071109987 ) ) ;
#67585=CARTESIAN_POINT ( 'NONE',  ( 15.44008868035555260, 59.73035201082151247, 9.422509992056143702 ) ) ;
#67586=CARTESIAN_POINT ( 'NONE',  ( 14.92337183194729633, 2.675597817667451750, 8.527530157486181039 ) ) ;
#67587=CARTESIAN_POINT ( 'NONE',  ( 20.88017736071110875, 50.77201867748817676, -2.915334737309920765 ) ) ;
#67588=CARTESIAN_POINT ( 'NONE',  ( -0.2418659066527494572, 29.26028685723174050, -6.114288769123083611 ) ) ;
#67591=CARTESIAN_POINT ( 'NONE',  ( 7.361572987183170547, 22.05059781766745530, 9.846743663894590881 ) ) ;
#67592=ORIENTED_EDGE ( 'NONE', *, *, #91159, .F. ) ;
#67593=DIRECTION ( 'NONE',  ( -0.07626964003977962370, 0.9970872288863209532, 0.000000000000000000 ) ) ;
#67595=CARTESIAN_POINT ( 'NONE',  ( 20.36894250292379738, 4.928748834913967869, -10.36894250292379027 ) ) ;
#67598=CARTESIAN_POINT ( 'NONE',  ( 19.72487221294570858, 29.78217586085238366, 6.499999999999992895 ) ) ;
#67600=CARTESIAN_POINT ( 'NONE',  ( -0.8801773607111009756, 13.06368534415483929, 1.068504757029289695E-15 ) ) ;
#67602=ORIENTED_EDGE ( 'NONE', *, *, #19427, .T. ) ;
#67604=CARTESIAN_POINT ( 'NONE',  ( 19.84674366389459266, 48.30059781766745175, 2.638427012816836559 ) ) ;
#67606=CARTESIAN_POINT ( 'NONE',  ( 16.40814093676323893, 15.79030133659708746, 11.09922568453595026 ) ) ;
#67608=CARTESIAN_POINT ( 'NONE',  ( 7.361572987183170547, 12.05059781766744997, 9.846743663894590881 ) ) ;
#67609=CARTESIAN_POINT ( 'NONE',  ( 1.821158202401484294, 36.16688879859522388, 6.499999999999917399 ) ) ;
#67610=CARTESIAN_POINT ( 'NONE',  ( 5.076628168052704559, 20.17559781766745175, -8.527530157486179263 ) ) ;
#67611=CARTESIAN_POINT ( 'NONE',  ( 3.591859063236763294, -1.709698663402913210, -11.09922568453595026 ) ) ;
#67615=CARTESIAN_POINT ( 'NONE',  ( -0.8801773607110991993, 27.85535201082150181, -2.915334737309923874 ) ) ;
#67616=CARTESIAN_POINT ( 'NONE',  ( 2.917880565312950480, 15.97041550158063217, -12.26659068614894821 ) ) ;
#67617=CARTESIAN_POINT ( 'NONE',  ( 18.52753015748618282, 33.92559781766745886, -4.923371831947291888 ) ) ;
#67618=CARTESIAN_POINT ( 'NONE',  ( 19.42250999205614548, 55.98035201082150536, -5.440088680355545492 ) ) ;
#67619=CARTESIAN_POINT ( 'NONE',  ( 19.38216949554541202, 40.99863466993042493, 9.382169495545424454 ) ) ;
#67621=CARTESIAN_POINT ( 'NONE',  ( 0.5774900079438607392, 13.48035201082150358, 5.440088680355550821 ) ) ;
#67624=CARTESIAN_POINT ( 'NONE',  ( 10.00000000000000178, 10.37363466993041961, 12.81628187352647608 ) ) ;
#67625=CARTESIAN_POINT ( 'NONE',  ( 7.361572987183170547, 67.05059781766746596, 9.846743663894590881 ) ) ;
#67626=CARTESIAN_POINT ( 'NONE',  ( 12.63842701281683034, 32.46726448433412315, 9.846743663894596210 ) ) ;
#67628=CARTESIAN_POINT ( 'NONE',  ( 22.81628187352648496, 36.83196800326376064, -3.434112377981050290 ) ) ;
#67630=CARTESIAN_POINT ( 'NONE',  ( 20.88017736071110519, 40.56368534415484106, 2.639326808657452039E-16 ) ) ;
#67634=CARTESIAN_POINT ( 'NONE',  ( 7.084665262690076126, 47.02201867748818387, -10.88017736071110164 ) ) ;
#67636=CARTESIAN_POINT ( 'NONE',  ( 4.559911319644449179, 43.89701867748816966, 9.422509992056141925 ) ) ;
#67637=CARTESIAN_POINT ( 'NONE',  ( 1.472469842513823179, 65.59226448433412315, -4.923371831947296329 ) ) ;
#67638=CARTESIAN_POINT ( 'NONE',  ( 20.88017736071110164, 65.35535201082150536, 2.915334737309930979 ) ) ;
#67642=TOROIDAL_SURFACE ( 'NONE', #11739, 7.538348415311010520, 7.000000000000000000 ) ;
#67643=CARTESIAN_POINT ( 'NONE',  ( 19.84674366389459621, 38.50893115100078745, 7.409399052514197653E-17 ) ) ;
#67644=CARTESIAN_POINT ( 'NONE',  ( 19.42250999205614193, 10.14701867748816966, 5.440088680355555262 ) ) ;
#67645=CARTESIAN_POINT ( 'NONE',  ( 19.38216949554541202, 15.99863466993042138, 9.382169495545424454 ) ) ;
#67646=ORIENTED_EDGE ( 'NONE', *, *, #28961, .T. ) ;
#67647=CARTESIAN_POINT ( 'NONE',  ( -0.8801773607111008646, 28.27201867748817321, 2.915334737309923430 ) ) ;
#67650=CARTESIAN_POINT ( 'NONE',  ( -0.8801773607111009756, 28.06368534415484106, 1.068504757029289695E-15 ) ) ;
#67651=CARTESIAN_POINT ( 'NONE',  ( 18.52753015748618282, 3.925597817667451306, -4.923371831947291888 ) ) ;
#67652=CARTESIAN_POINT ( 'NONE',  ( 22.26659068614894466, 43.88708216824729647, 7.082119434687054849 ) ) ;
#67653=CARTESIAN_POINT ( 'NONE',  ( 14.92337183194729633, 12.67559781766745353, 8.527530157486181039 ) ) ;
#67654=CARTESIAN_POINT ( 'NONE',  ( 20.88017736071110875, 40.77201867748818387, -2.915334737309920765 ) ) ;
#67656=CARTESIAN_POINT ( 'NONE',  ( -4.164238869374099927, 2.012082168247300906, 3.795296366450308767 ) ) ;
#67659=CARTESIAN_POINT ( 'NONE',  ( 17.20831665107776587, 52.88393115100078035, 7.208316651077764980 ) ) ;
#67660=EDGE_LOOP ( 'NONE', ( #20711, #75078, #56149, #32153, #12109, #35567 ) ) ;
#67663=CARTESIAN_POINT ( 'NONE',  ( 10.00000000000000000, 25.55374883491396787, -14.16423886937410082 ) ) ;
#67664=CARTESIAN_POINT ( 'NONE',  ( -0.3689425029237898834, 21.17874883491396432, -10.36894250292378850 ) ) ;
#67665=CARTESIAN_POINT ( 'NONE',  ( 7.084665262690076126, 62.02201867748816966, -10.88017736071110164 ) ) ;
#67666=CARTESIAN_POINT ( 'NONE',  ( 10.00000000000000178, 4.313685344154837509, 10.88017736071110342 ) ) ;
#67667=CARTESIAN_POINT ( 'NONE',  ( 13.43411237798105340, 5.581968003263753531, 12.81628187352647963 ) ) ;
#67668=CARTESIAN_POINT ( 'NONE',  ( 0.1532563361054100626, 45.80059781766745886, -2.638427012816831230 ) ) ;
#67670=CARTESIAN_POINT ( 'NONE',  ( 7.084665262690076126, 42.02201867748816966, -10.88017736071110164 ) ) ;
#67671=CARTESIAN_POINT ( 'NONE',  ( 19.38216949554541202, 10.99863466993042138, 9.382169495545424454 ) ) ;
#67672=CARTESIAN_POINT ( 'NONE',  ( 10.00000000000000178, 13.05374883491396787, 14.16423886937410082 ) ) ;
#67673=CARTESIAN_POINT ( 'NONE',  ( 20.88017736071110875, 15.77201867748817143, -2.915334737309920765 ) ) ;
#67674=CARTESIAN_POINT ( 'NONE',  ( 7.084665262690076126, 14.10535201082150358, 10.88017736071109987 ) ) ;
#67675=CARTESIAN_POINT ( 'NONE',  ( 19.84674366389459266, 53.30059781766744464, 2.638427012816836559 ) ) ;
#67676=CARTESIAN_POINT ( 'NONE',  ( 4.559911319644449179, 57.23035201082150536, -9.422509992056141925 ) ) ;
#67680=DIRECTION ( 'NONE',  ( -0.5547001962252291474, -0.8320502943378437211, -0.000000000000000000 ) ) ;
#67683=CARTESIAN_POINT ( 'NONE',  ( 10.00000000000000178, 32.25893115100078745, 9.846743663894594434 ) ) ;
#67686=CARTESIAN_POINT ( 'NONE',  ( 6.204703633549690345, 42.84541550158063217, 14.16423886937410082 ) ) ;
#67687=CARTESIAN_POINT ( 'NONE',  ( 2.035157376598822676, 2.438685344154838397, -7.964842623401177768 ) ) ;
#67688=CARTESIAN_POINT ( 'NONE',  ( 7.361572987183170547, 22.05059781766745530, 9.846743663894590881 ) ) ;
#67689=CARTESIAN_POINT ( 'NONE',  ( 0.1532563361054083140, 51.00893115100078745, 1.131784320476157264E-15 ) ) ;
#67691=CARTESIAN_POINT ( 'NONE',  ( 17.20831665107776587, 4.133931151000785675, -7.208316651077762316 ) ) ;
#67694=CARTESIAN_POINT ( 'NONE',  ( 17.08211943468705130, 38.47041550158063217, 12.26659068614894998 ) ) ;
#67695=CARTESIAN_POINT ( 'NONE',  ( -1.099225684535947600, 19.54030133659708568, 6.408140936763237150 ) ) ;
#67697=CARTESIAN_POINT ( 'NONE',  ( -2.816281873526473856, 64.33196800326376774, 3.434112377981055619 ) ) ;
#67698=CARTESIAN_POINT ( 'NONE',  ( 20.88017736071110519, 30.56368534415484106, 2.639326808657452039E-16 ) ) ;
#67699=CARTESIAN_POINT ( 'NONE',  ( 0.1532563361054082862, 41.21726448433411605, 2.638427012816831674 ) ) ;
#67700=CARTESIAN_POINT ( 'NONE',  ( 15.44008868035555793, 31.39701867748817676, -9.422509992056140149 ) ) ;
#67701=CARTESIAN_POINT ( 'NONE',  ( 10.00000000000000178, 60.37363466993041783, 12.81628187352647608 ) ) ;
#67702=DIRECTION ( 'NONE',  ( -0.000000000000000000, 1.000000000000000000, -0.000000000000000000 ) ) ;
#67703=CARTESIAN_POINT ( 'NONE',  ( 19.84674366389459266, 43.30059781766744464, 2.638427012816836559 ) ) ;
#67704=CARTESIAN_POINT ( 'NONE',  ( 0.1532563361054083140, 46.00893115100079456, 1.131784320476157264E-15 ) ) ;
#67710=CARTESIAN_POINT ( 'NONE',  ( 19.84674366389459266, 18.71726448433411960, -2.638427012816827677 ) ) ;
#67711=CARTESIAN_POINT ( 'NONE',  ( -2.816281873526471635, 38.91530133659708213, -3.434112377981056508 ) ) ;
#67715=CARTESIAN_POINT ( 'NONE',  ( 0.1532563361054100626, 55.80059781766745175, -2.638427012816831230 ) ) ;
#67717=CARTESIAN_POINT ( 'NONE',  ( 18.52753015748618282, 43.92559781766745175, -4.923371831947291888 ) ) ;
#67718=CARTESIAN_POINT ( 'NONE',  ( -4.164238869374099927, 37.01208216824731068, 3.795296366450308767 ) ) ;
#67719=CARTESIAN_POINT ( 'NONE',  ( 0.1532563361054100626, 40.80059781766745886, -2.638427012816831230 ) ) ;
#67720=B_SPLINE_CURVE_WITH_KNOTS ( 'NONE', 3,
 ( #21337, #27835, #51827, #74817, #58321, #44316, #4374, #88839, #20347, #59807 ),
 .UNSPECIFIED., .F., .F.,
 ( 4, 2, 2, 2, 4 ),
 ( 1.177569344012831190E-16, 0.001974336156922556259, 0.002961504235383763048, 0.003455088274614364924, 0.003948672313844965934 ),
 .UNSPECIFIED. ) ;
#67721=CARTESIAN_POINT ( 'NONE',  ( 10.00000000000000000, 52.87363466993041783, -12.81628187352647608 ) ) ;
#67723=CARTESIAN_POINT ( 'NONE',  ( 19.84674366389459266, 8.300597817667451750, 2.638427012816836559 ) ) ;
#67724=CARTESIAN_POINT ( 'NONE',  ( 17.08211943468705840, 5.137082168247300906, -12.26659068614894466 ) ) ;
#67726=CARTESIAN_POINT ( 'NONE',  ( 7.361572987183169658, 49.96726448433410894, -9.846743663894592657 ) ) ;
#67727=CARTESIAN_POINT ( 'NONE',  ( 19.42250999205614193, 45.14701867748817676, 5.440088680355555262 ) ) ;
#67728=CARTESIAN_POINT ( 'NONE',  ( 19.84674366389459266, 43.30059781766744464, 2.638427012816836559 ) ) ;
#67731=CARTESIAN_POINT ( 'NONE',  ( 20.88017736071110875, 50.77201867748817676, -2.915334737309920765 ) ) ;
#67733=CARTESIAN_POINT ( 'NONE',  ( 1.707155281725172502, 52.90189080397286148, 6.499999999999955591 ) ) ;
#67734=CARTESIAN_POINT ( 'NONE',  ( 2.035157376598824452, 13.68868534415483751, 7.964842623401179544 ) ) ;
#67735=CARTESIAN_POINT ( 'NONE',  ( 6.565887622018943937, 0.1653013365970866511, 12.81628187352647430 ) ) ;
#67736=CARTESIAN_POINT ( 'NONE',  ( 12.91533473730992121, 49.52201867748817676, 10.88017736071110164 ) ) ;
#67739=CYLINDRICAL_SURFACE ( 'NONE', #48569, 0.5000000000000004441 ) ;
#67740=CARTESIAN_POINT ( 'NONE',  ( 15.44008868035555260, 44.73035201082151247, 9.422509992056143702 ) ) ;
#67742=CARTESIAN_POINT ( 'NONE',  ( 2.791683348922237240, 15.38393115100078212, -7.208316651077763204 ) ) ;
#67743=CARTESIAN_POINT ( 'NONE',  ( 19.84674366389459266, 18.30059781766745175, 2.638427012816836559 ) ) ;
#67744=DIRECTION ( 'NONE',  ( 0.000000000000000000, 0.000000000000000000, -1.000000000000000000 ) ) ;
#67746=CARTESIAN_POINT ( 'NONE',  ( 21.09922568453594849, 1.206968003263753531, 6.408140936763242479 ) ) ;
#67748=CARTESIAN_POINT ( 'NONE',  ( 4.559911319644449179, 2.230352010821504916, -9.422509992056141925 ) ) ;
#67750=CARTESIAN_POINT ( 'NONE',  ( 17.08211943468705130, 18.47041550158063572, 12.26659068614894998 ) ) ;
#67751=CARTESIAN_POINT ( 'NONE',  ( 6.204703633549690345, 47.84541550158064638, 14.16423886937410082 ) ) ;
#67754=CARTESIAN_POINT ( 'NONE',  ( 19.84674366389459621, 18.50893115100078745, 7.409399052514197653E-17 ) ) ;
#67755=CARTESIAN_POINT ( 'NONE',  ( 0.5774900079438607392, 8.480352010821505360, 5.440088680355550821 ) ) ;
#67756=CARTESIAN_POINT ( 'NONE',  ( 19.84674366389459266, 53.71726448433411605, -2.638427012816827677 ) ) ;
#67757=CARTESIAN_POINT ( 'NONE',  ( 13.79529636645031943, 5.345415501580634832, -14.16423886937409904 ) ) ;
#67761=CARTESIAN_POINT ( 'NONE',  ( 10.00000000000000178, 2.258931151000784787, 9.846743663894594434 ) ) ;
#67762=CARTESIAN_POINT ( 'NONE',  ( 0.6178305044545818747, 43.49863466993042493, -9.382169495545419124 ) ) ;
#67763=CARTESIAN_POINT ( 'NONE',  ( 0.1532563361054082862, 41.21726448433411605, 2.638427012816831674 ) ) ;
#67765=CARTESIAN_POINT ( 'NONE',  ( 12.63842701281683922, 9.550597817667449974, -9.846743663894590881 ) ) ;
#67768=CARTESIAN_POINT ( 'NONE',  ( 7.084665262690076126, 4.105352010821503583, 10.88017736071109987 ) ) ;
#67769=CARTESIAN_POINT ( 'NONE',  ( -4.164238869374099927, 52.01208216824729647, 3.795296366450308767 ) ) ;
#67770=CARTESIAN_POINT ( 'NONE',  ( 22.26659068614894466, 3.887082168247300906, 7.082119434687054849 ) ) ;
#67771=CARTESIAN_POINT ( 'NONE',  ( 7.361572987183169658, 19.96726448433411960, -9.846743663894592657 ) ) ;
#67772=CARTESIAN_POINT ( 'NONE',  ( 15.44008868035555793, 11.39701867748817143, -9.422509992056140149 ) ) ;
#67773=CARTESIAN_POINT ( 'NONE',  ( 2.791683348922240793, 1.633931151000784565, 7.208316651077764092 ) ) ;
#67775=CARTESIAN_POINT ( 'NONE',  ( 14.92337183194729633, 47.67559781766745175, 8.527530157486181039 ) ) ;
#67776=CARTESIAN_POINT ( 'NONE',  ( 20.88017736071110519, 40.56368534415484106, 2.639326808657452039E-16 ) ) ;
#67778=CARTESIAN_POINT ( 'NONE',  ( 19.38216949554541202, 55.99863466993041072, 9.382169495545424454 ) ) ;
#67781=CARTESIAN_POINT ( 'NONE',  ( 14.92337183194729988, 9.342264484334119601, -8.527530157486177487 ) ) ;
#67782=CARTESIAN_POINT ( 'NONE',  ( 19.38216949554541202, 40.99863466993042493, 9.382169495545424454 ) ) ;
#67783=CARTESIAN_POINT ( 'NONE',  ( 20.88017736071110875, 10.77201867748817143, -2.915334737309920765 ) ) ;
#67784=CARTESIAN_POINT ( 'NONE',  ( 17.20831665107776587, 32.88393115100078745, 7.208316651077764980 ) ) ;
#67785=CARTESIAN_POINT ( 'NONE',  ( 20.00000000000000355, 90.60976979464908254, 4.970182472450021649 ) ) ;
#67786=FACE_OUTER_BOUND ( 'NONE', #33151, .T. ) ;
#67787=CARTESIAN_POINT ( 'NONE',  ( 24.16423886937409904, 24.09541550158063927, 3.795296366450317205 ) ) ;
#67788=CARTESIAN_POINT ( 'NONE',  ( 6.204703633549690345, 50.76208216824730357, -14.16423886937410259 ) ) ;
#67789=CARTESIAN_POINT ( 'NONE',  ( 5.076628168052703671, 56.84226448433412315, 8.527530157486179263 ) ) ;
#67791=CARTESIAN_POINT ( 'NONE',  ( 0.5774900079438607392, 43.48035201082151247, 5.440088680355550821 ) ) ;
#67794=CARTESIAN_POINT ( 'NONE',  ( 0.1532563361054100626, 5.800597817667452638, -2.638427012816831230 ) ) ;
#67796=ORIENTED_EDGE ( 'NONE', *, *, #43800, .F. ) ;
#67797=CARTESIAN_POINT ( 'NONE',  ( -2.816281873526471635, 53.91530133659709634, -3.434112377981056508 ) ) ;
#67799=CARTESIAN_POINT ( 'NONE',  ( 0.1532563361054083140, 1.008931151000784787, 1.131784320476157264E-15 ) ) ;
#67801=CARTESIAN_POINT ( 'NONE',  ( -0.3689425029237898834, 6.178748834913968757, -10.36894250292378850 ) ) ;
#67802=CARTESIAN_POINT ( 'NONE',  ( 7.361572987183170547, 2.050597817667451750, 9.846743663894590881 ) ) ;
#67803=CARTESIAN_POINT ( 'NONE',  ( 0.5774900079438590739, 27.64701867748817676, -5.440088680355550821 ) ) ;
#67805=B_SPLINE_CURVE_WITH_KNOTS ( 'NONE', 3,
 ( #43672, #12683, #72681, #43182 ),
 .UNSPECIFIED., .F., .F.,
 ( 4, 4 ),
 ( 0.000000000000000000, 0.001036303429213370712 ),
 .UNSPECIFIED. ) ;
#67808=CARTESIAN_POINT ( 'NONE',  ( 0.5774900079438590739, 27.64701867748817676, -5.440088680355550821 ) ) ;
#67809=( BOUNDED_CURVE ( )  B_SPLINE_CURVE ( 2, ( #63644, #56171, #19633, #88612, #65611, #80131, #96138, #28112, #58106 ),
 .UNSPECIFIED., .F., .F. ) 
 B_SPLINE_CURVE_WITH_KNOTS ( ( 3, 2, 2, 2, 3 ),
 ( 0.2605718029354654464, 0.2619047619047619180, 0.2678571428571428492, 0.2738095238095238360, 0.2751424827788204741 ),
 .UNSPECIFIED. ) 
 CURVE ( )  GEOMETRIC_REPRESENTATION_ITEM ( )  RATIONAL_B_SPLINE_CURVE ( ( 0.9881565478350731180, 0.9923695281211488695, 1.000000000000000000, 0.9659258262890683122, 1.000000000000000000, 0.9659258262890683122, 1.000000000000000000, 0.9923695281211478703, 0.9881565478350720078 ) ) 
 REPRESENTATION_ITEM ( '' )  );
#67811=CARTESIAN_POINT ( 'NONE',  ( 2.035157376598824452, 33.68868534415484106, 7.964842623401179544 ) ) ;
#67812=CARTESIAN_POINT ( 'NONE',  ( 7.361572987183170547, 67.05059781766746596, 9.846743663894590881 ) ) ;
#67813=VERTEX_POINT ( 'NONE', #4578 ) ;
#67814=EDGE_LOOP ( 'NONE', ( #77325, #71174, #72171, #69530 ) ) ;
#67815=CARTESIAN_POINT ( 'NONE',  ( 16.40814093676324603, 12.45696800326375353, -11.09922568453594671 ) ) ;
#67817=CARTESIAN_POINT ( 'NONE',  ( 2.791683348922240793, 1.633931151000784565, 7.208316651077764092 ) ) ;
#67819=CARTESIAN_POINT ( 'NONE',  ( 20.88017736071110164, 15.35535201082150358, 2.915334737309930979 ) ) ;
#67820=DIRECTION ( 'NONE',  ( 0.000000000000000000, -1.000000000000000000, -0.000000000000000000 ) ) ;
#67821=CARTESIAN_POINT ( 'NONE',  ( 17.20831665107776587, 9.133931151000787452, -7.208316651077762316 ) ) ;
#67822=CARTESIAN_POINT ( 'NONE',  ( 12.91533473730993009, 21.60535201082150536, -10.88017736071109987 ) ) ;
#67825=CARTESIAN_POINT ( 'NONE',  ( 22.81628187352647785, 56.62363466993042493, 6.195893100308588602E-16 ) ) ;
#67826=CARTESIAN_POINT ( 'NONE',  ( 10.00000000000000178, 39.31368534415484106, 10.88017736071110342 ) ) ;
#67827=CARTESIAN_POINT ( 'NONE',  ( -46.68456736488006698, 103.6675473310227176, -5.775421524742654356 ) ) ;
#67828=CARTESIAN_POINT ( 'NONE',  ( 10.00000000000000000, 52.87363466993041783, -12.81628187352647608 ) ) ;
#67829=CARTESIAN_POINT ( 'NONE',  ( 4.559911319644449179, 42.23035201082151247, -9.422509992056141925 ) ) ;
#67830=CARTESIAN_POINT ( 'NONE',  ( 1.472469842513823179, 66.42559781766745175, 4.923371831947296329 ) ) ;
#67832=CARTESIAN_POINT ( 'NONE',  ( 10.00000000000000178, 17.25893115100078745, 9.846743663894594434 ) ) ;
#67833=CARTESIAN_POINT ( 'NONE',  ( -1.099225684535947600, 59.54030133659708923, 6.408140936763237150 ) ) ;
#67835=CARTESIAN_POINT ( 'NONE',  ( -2.816281873526473856, 4.123634669930420493, 9.499525473075851096E-16 ) ) ;
#67838=CARTESIAN_POINT ( 'NONE',  ( 19.84674366389459266, 63.30059781766745886, 2.638427012816836559 ) ) ;
#67839=CARTESIAN_POINT ( 'NONE',  ( 2.035157376598822676, 42.43868534415483396, -7.964842623401177768 ) ) ;
#67840=CARTESIAN_POINT ( 'NONE',  ( 2.791683348922240793, 46.63393115100077324, 7.208316651077764092 ) ) ;
#67843=CARTESIAN_POINT ( 'NONE',  ( 0.1532563361054082862, 11.21726448433411605, 2.638427012816831674 ) ) ;
#67844=CARTESIAN_POINT ( 'NONE',  ( 21.09922568453594849, 6.206968003263753531, 6.408140936763242479 ) ) ;
#67847=CARTESIAN_POINT ( 'NONE',  ( 1.472469842513823179, 65.59226448433412315, -4.923371831947296329 ) ) ;
#67850=CARTESIAN_POINT ( 'NONE',  ( -2.266590686148945544, 66.38708216824730357, -7.082119434687050408 ) ) ;
#67851=CARTESIAN_POINT ( 'NONE',  ( 0.1532563361054082862, 41.21726448433411605, 2.638427012816831674 ) ) ;
#67852=( GEOMETRIC_REPRESENTATION_CONTEXT ( 3 ) GLOBAL_UNCERTAINTY_ASSIGNED_CONTEXT ( ( #97494 ) ) GLOBAL_UNIT_ASSIGNED_CONTEXT ( ( #4906, #3433, #96405 ) ) REPRESENTATION_CONTEXT ( 'NONE', 'WORKASPACE' ) );
#67853=DIRECTION ( 'NONE',  ( 0.000000000000000000, 0.000000000000000000, 1.000000000000000000 ) ) ;
#67854=CARTESIAN_POINT ( 'NONE',  ( 4.559911319644449179, 2.230352010821504916, -9.422509992056141925 ) ) ;
#67855=CARTESIAN_POINT ( 'NONE',  ( 2.603489959281586774, 5.435752660568278216, -6.500000000000001776 ) ) ;
#67856=CARTESIAN_POINT ( 'NONE',  ( 10.00000000000000000, 21.81368534415484106, -10.88017736071110342 ) ) ;
#67857=CARTESIAN_POINT ( 'NONE',  ( 2.917880565312950480, 45.97041550158063927, -12.26659068614894821 ) ) ;
#67858=CARTESIAN_POINT ( 'NONE',  ( -0.3689425029237898834, 61.17874883491396076, -10.36894250292378850 ) ) ;
#67859=CARTESIAN_POINT ( 'NONE',  ( 20.15039907845753575, 15.60158574516642815, -6.262539305110077059 ) ) ;
#67860=CARTESIAN_POINT ( 'NONE',  ( 1.472469842513823179, 26.42559781766745175, 4.923371831947296329 ) ) ;
#67861=CARTESIAN_POINT ( 'NONE',  ( 3.591859063236761518, 14.95696800326375531, 11.09922568453594849 ) ) ;
#67862=ORIENTED_EDGE ( 'NONE', *, *, #69387, .T. ) ;
#67865=DIRECTION ( 'NONE',  ( 0.000000000000000000, 0.000000000000000000, 1.000000000000000000 ) ) ;
#67866=CARTESIAN_POINT ( 'NONE',  ( 24.16423886937409904, 14.09541550158063217, 3.795296366450317205 ) ) ;
#67867=CARTESIAN_POINT ( 'NONE',  ( 2.791683348922237240, 20.38393115100078745, -7.208316651077763204 ) ) ;
#67871=CARTESIAN_POINT ( 'NONE',  ( 20.36894250292379382, 43.67874883491397497, 10.36894250292379205 ) ) ;
#67872=CARTESIAN_POINT ( 'NONE',  ( 2.791683348922240793, 6.633931151000785675, 7.208316651077764092 ) ) ;
#67873=DIRECTION ( 'NONE',  ( -1.000000000000000000, 0.000000000000000000, 0.000000000000000000 ) ) ;
#67875=CARTESIAN_POINT ( 'NONE',  ( 19.42250999205614193, 35.14701867748816966, 5.440088680355555262 ) ) ;
#67876=CARTESIAN_POINT ( 'NONE',  ( -1.099225684535947600, 49.54030133659708923, 6.408140936763237150 ) ) ;
#67878=CARTESIAN_POINT ( 'NONE',  ( 19.38216949554541202, 30.99863466993042138, 9.382169495545424454 ) ) ;
#67879=CARTESIAN_POINT ( 'NONE',  ( 2.791683348922240793, 6.633931151000785675, 7.208316651077764092 ) ) ;
#67880=ORIENTED_EDGE ( 'NONE', *, *, #73972, .F. ) ;
#67881=CARTESIAN_POINT ( 'NONE',  ( 1.912066916745601031, 1.523660046708132265, -6.500000000000000888 ) ) ;
#67882=CARTESIAN_POINT ( 'NONE',  ( 6.204703633549690345, 35.76208216824729647, -14.16423886937410259 ) ) ;
#67883=CARTESIAN_POINT ( 'NONE',  ( 17.08211943468705130, 8.470415501580635720, 12.26659068614894998 ) ) ;
#67884=CARTESIAN_POINT ( 'NONE',  ( 17.96484262340118221, 6.188685344154836621, -7.964842623401177768 ) ) ;
#67885=CARTESIAN_POINT ( 'NONE',  ( -0.8801773607111009756, 23.06368534415484106, 1.068504757029289695E-15 ) ) ;
#67888=CARTESIAN_POINT ( 'NONE',  ( 0.5774900079438590739, 57.64701867748817676, -5.440088680355550821 ) ) ;
#67889=CARTESIAN_POINT ( 'NONE',  ( 0.5774900079438590739, 62.64701867748817676, -5.440088680355550821 ) ) ;
#67890=CARTESIAN_POINT ( 'NONE',  ( 13.43411237798105340, 20.58196800326374643, 12.81628187352647963 ) ) ;
#67893=CARTESIAN_POINT ( 'NONE',  ( 0.1957200283969100785, 30.25733960839543712, 6.499999999999992006 ) ) ;
#67894=CARTESIAN_POINT ( 'NONE',  ( 1.472469842513823179, 20.59226448433411960, -4.923371831947296329 ) ) ;
#67895=COLOUR_RGB ( '', 0.72549020, 0.75294118, 0.79215686) ;
#67896=CARTESIAN_POINT ( 'NONE',  ( 6.565887622018943937, 25.16530133659708213, 12.81628187352647430 ) ) ;
#67897=SURFACE_STYLE_FILL_AREA ( #6389 ) ;
#67898=CARTESIAN_POINT ( 'NONE',  ( 17.96484262340118221, 6.188685344154836621, -7.964842623401177768 ) ) ;
#67899=CARTESIAN_POINT ( 'NONE',  ( 17.20831665107776587, 34.13393115100078745, -7.208316651077762316 ) ) ;
#67900=CARTESIAN_POINT ( 'NONE',  ( 3.591859063236761518, 64.95696800326376774, 11.09922568453594849 ) ) ;
#67901=CARTESIAN_POINT ( 'NONE',  ( 10.00000000000000000, 19.75893115100078390, -9.846743663894594434 ) ) ;
#67902=CARTESIAN_POINT ( 'NONE',  ( 2.917880565312948704, 2.637082168247300906, 12.26659068614894643 ) ) ;
#67904=CARTESIAN_POINT ( 'NONE',  ( 12.91533473730993009, 31.60535201082150891, -10.88017736071109987 ) ) ;
#67905=DIRECTION ( 'NONE',  ( 0.000000000000000000, -1.000000000000000000, 0.000000000000000000 ) ) ;
#67906=CARTESIAN_POINT ( 'NONE',  ( 0.1532563361054083140, 46.00893115100079456, 1.131784320476157264E-15 ) ) ;
#67907=CARTESIAN_POINT ( 'NONE',  ( 15.44008868035555260, 34.73035201082151247, 9.422509992056143702 ) ) ;
#67908=AXIS2_PLACEMENT_3D ( 'NONE', #87013, #18523, #49013 ) ;
#67909=CARTESIAN_POINT ( 'NONE',  ( 7.084665262690076126, 19.10535201082150181, 10.88017736071109987 ) ) ;
#67912=CARTESIAN_POINT ( 'NONE',  ( 7.084665262690076126, 27.02201867748817676, -10.88017736071110164 ) ) ;
#67913=CARTESIAN_POINT ( 'NONE',  ( 0.6178305044545838731, 49.74863466993041072, 9.382169495545420901 ) ) ;
#67914=CARTESIAN_POINT ( 'NONE',  ( 0.5774900079438590739, 42.64701867748816966, -5.440088680355550821 ) ) ;
#67916=CARTESIAN_POINT ( 'NONE',  ( 7.084665262690076126, 34.10535201082151247, 10.88017736071109987 ) ) ;
#67918=CARTESIAN_POINT ( 'NONE',  ( 12.63842701281683034, 52.46726448433413026, 9.846743663894596210 ) ) ;
#67919=CARTESIAN_POINT ( 'NONE',  ( 20.88017736071110875, 35.77201867748816966, -2.915334737309920765 ) ) ;
#67922=CARTESIAN_POINT ( 'NONE',  ( 19.80777595082616926, 30.68878173731741299, -6.499999999999961808 ) ) ;
#67923=CARTESIAN_POINT ( 'NONE',  ( 10.00000000000000000, 40.55374883491397497, -14.16423886937410082 ) ) ;
#67924=CARTESIAN_POINT ( 'NONE',  ( 10.00000000000000178, 49.31368534415484106, 10.88017736071110342 ) ) ;
#67928=CARTESIAN_POINT ( 'NONE',  ( 5.076628168052703671, 56.84226448433412315, 8.527530157486179263 ) ) ;
#67929=CARTESIAN_POINT ( 'NONE',  ( 4.559911319644449179, 3.897018677488170990, 9.422509992056141925 ) ) ;
#67930=CARTESIAN_POINT ( 'NONE',  ( 17.20831665107776587, 34.13393115100078745, -7.208316651077762316 ) ) ;
#67932=CARTESIAN_POINT ( 'NONE',  ( 0.1532563361054082862, 36.21726448433410894, 2.638427012816831674 ) ) ;
#67934=CARTESIAN_POINT ( 'NONE',  ( 20.88017736071110164, 25.35535201082150891, 2.915334737309930979 ) ) ;
#67935=CARTESIAN_POINT ( 'NONE',  ( 17.20831665107776587, 29.13393115100078390, -7.208316651077762316 ) ) ;
#67936=CARTESIAN_POINT ( 'NONE',  ( 19.38216949554541202, 25.99863466993042138, 9.382169495545424454 ) ) ;
#67937=CARTESIAN_POINT ( 'NONE',  ( 1.274849032794231007, 38.57228050351032067, 6.499999999999895195 ) ) ;
#67938=CARTESIAN_POINT ( 'NONE',  ( -0.8801773607111009756, 38.06368534415484106, 1.068504757029289695E-15 ) ) ;
#67939=CARTESIAN_POINT ( 'NONE',  ( 3.591859063236761518, 64.95696800326376774, 11.09922568453594849 ) ) ;
#67940=CARTESIAN_POINT ( 'NONE',  ( 24.16423886937409904, 49.09541550158063217, 3.795296366450317205 ) ) ;
#67941=DIRECTION ( 'NONE',  ( 0.000000000000000000, -1.000000000000000000, 0.000000000000000000 ) ) ;
#67943=CARTESIAN_POINT ( 'NONE',  ( 0.6178305044545838731, 19.74863466993042138, 9.382169495545420901 ) ) ;
#67944=CARTESIAN_POINT ( 'NONE',  ( 10.00000000000000000, 1.813685344154837731, -10.88017736071110342 ) ) ;
#67945=CARTESIAN_POINT ( 'NONE',  ( 19.42250999205614193, 50.14701867748817676, 5.440088680355555262 ) ) ;
#67946=FILL_AREA_STYLE_COLOUR ( '', #85698 ) ;
#67947=VERTEX_POINT ( 'NONE', #96065 ) ;
#67948=CARTESIAN_POINT ( 'NONE',  ( 0.5774900079438607392, 58.48035201082151247, 5.440088680355550821 ) ) ;
#67949=CARTESIAN_POINT ( 'NONE',  ( 12.63842701281683922, 29.55059781766745175, -9.846743663894590881 ) ) ;
#67950=CARTESIAN_POINT ( 'NONE',  ( 1.472469842513823179, 25.59226448433412315, -4.923371831947296329 ) ) ;
#67951=CARTESIAN_POINT ( 'NONE',  ( 14.92337183194729988, 9.342264484334119601, -8.527530157486177487 ) ) ;
#67955=CARTESIAN_POINT ( 'NONE',  ( 16.40814093676323893, 35.79030133659708923, 11.09922568453595026 ) ) ;
#67956=EDGE_CURVE ( 'NONE', #42198, #96185, #34486, .T. ) ;
#67957=CARTESIAN_POINT ( 'NONE',  ( 14.92337183194729988, 14.34226448433411782, -8.527530157486177487 ) ) ;
#67958=CARTESIAN_POINT ( 'NONE',  ( 19.72487221294571569, 50.71833443783938122, -6.499999999999983125 ) ) ;
#67960=CARTESIAN_POINT ( 'NONE',  ( 18.52753015748618282, 38.92559781766745175, -4.923371831947291888 ) ) ;
#67963=CARTESIAN_POINT ( 'NONE',  ( 22.81628187352647785, 11.41530133659708390, 3.434112377981063169 ) ) ;
#67965=CARTESIAN_POINT ( 'NONE',  ( 17.96484262340118221, 56.18868534415484817, -7.964842623401177768 ) ) ;
#67966=CARTESIAN_POINT ( 'NONE',  ( 22.26659068614894466, 28.88708216824730357, 7.082119434687054849 ) ) ;
#67968=CARTESIAN_POINT ( 'NONE',  ( 17.08211943468705130, 28.47041550158063572, 12.26659068614894998 ) ) ;
#67969=CARTESIAN_POINT ( 'NONE',  ( 2.917880565312948704, 47.63708216824730357, 12.26659068614894643 ) ) ;
#67970=CARTESIAN_POINT ( 'NONE',  ( 6.204703633549690345, 12.84541550158063572, 14.16423886937410082 ) ) ;
#67971=CARTESIAN_POINT ( 'NONE',  ( 6.204703633549690345, 15.76208216824730179, -14.16423886937410259 ) ) ;
#67972=CARTESIAN_POINT ( 'NONE',  ( -0.3289641300568009741, 37.24545670184114243, -5.963430220938281678 ) ) ;
#67973=CARTESIAN_POINT ( 'NONE',  ( -0.8801773607111008646, 48.27201867748816966, 2.915334737309923430 ) ) ;
#67975=CARTESIAN_POINT ( 'NONE',  ( 12.63842701281683034, 27.46726448433411250, 9.846743663894596210 ) ) ;
#67976=CARTESIAN_POINT ( 'NONE',  ( 2.603489959281614308, 56.58210964143329846, 6.500000000000031086 ) ) ;
#67977=CARTESIAN_POINT ( 'NONE',  ( 0.1532563361054082862, 46.21726448433411605, 2.638427012816831674 ) ) ;
#67978=CARTESIAN_POINT ( 'NONE',  ( 10.00000000000000178, 29.31368534415483751, 10.88017736071110342 ) ) ;
#67979=CARTESIAN_POINT ( 'NONE',  ( 16.40814093676324603, 62.45696800326376064, -11.09922568453594671 ) ) ;
#67980=DIRECTION ( 'NONE',  ( -0.000000000000000000, 1.000000000000000000, -0.000000000000000000 ) ) ;
#67982=CARTESIAN_POINT ( 'NONE',  ( 0.6178305044545838731, 39.74863466993041072, 9.382169495545420901 ) ) ;
#67985=CARTESIAN_POINT ( 'NONE',  ( 10.00000000000000178, 44.31368534415484106, 10.88017736071110342 ) ) ;
#67986=CARTESIAN_POINT ( 'NONE',  ( 0.1532563361054082862, 51.21726448433412315, 2.638427012816831674 ) ) ;
#67988=CARTESIAN_POINT ( 'NONE',  ( -4.164238869374098151, 26.59541550158063217, -3.795296366450310543 ) ) ;
#67993=CARTESIAN_POINT ( 'NONE',  ( 0.5774900079438590739, 62.64701867748817676, -5.440088680355550821 ) ) ;
#67994=CARTESIAN_POINT ( 'NONE',  ( -0.8801773607110991993, 62.85535201082150536, -2.915334737309923874 ) ) ;
#67995=CARTESIAN_POINT ( 'NONE',  ( 17.08211943468705840, 65.13708216824730357, -12.26659068614894466 ) ) ;
#67996=CARTESIAN_POINT ( 'NONE',  ( 22.81628187352647785, 1.415301336597087012, 3.434112377981063169 ) ) ;
#67999=CARTESIAN_POINT ( 'NONE',  ( 20.88017736071110164, 50.35535201082151247, 2.915334737309930979 ) ) ;
#68001=CARTESIAN_POINT ( 'NONE',  ( 22.26659068614894466, 48.88708216824730357, 7.082119434687054849 ) ) ;
#68003=CARTESIAN_POINT ( 'NONE',  ( 7.084665262690076126, 12.02201867748817143, -10.88017736071110164 ) ) ;
#68004=CARTESIAN_POINT ( 'NONE',  ( 19.42250999205614548, 25.98035201082150891, -5.440088680355545492 ) ) ;
#68005=CARTESIAN_POINT ( 'NONE',  ( 17.20831665107776587, 52.88393115100078035, 7.208316651077764980 ) ) ;
#68006=CARTESIAN_POINT ( 'NONE',  ( 3.591859063236761518, 44.95696800326376064, 11.09922568453594849 ) ) ;
#68009=CARTESIAN_POINT ( 'NONE',  ( 2.035157376598822676, 17.43868534415483751, -7.964842623401177768 ) ) ;
#68010=CARTESIAN_POINT ( 'NONE',  ( -2.816281873526471635, 23.91530133659708568, -3.434112377981056508 ) ) ;
#68013=CARTESIAN_POINT ( 'NONE',  ( 12.63842701281683034, 52.46726448433413026, 9.846743663894596210 ) ) ;
#68014=CARTESIAN_POINT ( 'NONE',  ( 15.44008868035555260, 39.73035201082150536, 9.422509992056143702 ) ) ;
#68015=CARTESIAN_POINT ( 'NONE',  ( 13.43411237798106583, 27.66530133659708568, -12.81628187352647252 ) ) ;
#68016=CARTESIAN_POINT ( 'NONE',  ( 19.42250999205614193, 45.14701867748817676, 5.440088680355555262 ) ) ;
#68019=CARTESIAN_POINT ( 'NONE',  ( -1.099225684535947600, 54.54030133659708923, 6.408140936763237150 ) ) ;
#68020=ORIENTED_EDGE ( 'NONE', *, *, #34546, .F. ) ;
#68021=CARTESIAN_POINT ( 'NONE',  ( 1.492507162822232836, 17.19955587570481370, -6.499999999999984901 ) ) ;
#68022=CARTESIAN_POINT ( 'NONE',  ( 12.91533473730992121, 54.52201867748816255, 10.88017736071110164 ) ) ;
#68023=CARTESIAN_POINT ( 'NONE',  ( 0.6178305044545838731, 29.74863466993042138, 9.382169495545420901 ) ) ;
#68024=CARTESIAN_POINT ( 'NONE',  ( 17.96484262340118221, 34.93868534415482685, 7.964842623401181321 ) ) ;
#68025=CARTESIAN_POINT ( 'NONE',  ( 5.076628168052704559, 65.17559781766745175, -8.527530157486179263 ) ) ;
#68027=CARTESIAN_POINT ( 'NONE',  ( 17.20831665107776587, 22.88393115100078745, 7.208316651077764980 ) ) ;
#68029=CARTESIAN_POINT ( 'NONE',  ( 18.52753015748618282, 3.925597817667451306, -4.923371831947291888 ) ) ;
#68031=CARTESIAN_POINT ( 'NONE',  ( 13.79529636645030344, 43.26208216824730357, 14.16423886937410614 ) ) ;
#68033=EDGE_CURVE ( 'NONE', #20694, #58781, #74528, .T. ) ;
#68034=CARTESIAN_POINT ( 'NONE',  ( -0.8801773607111009756, 13.06368534415483929, 1.068504757029289695E-15 ) ) ;
#68037=CARTESIAN_POINT ( 'NONE',  ( 17.96484262340118221, 9.938685344154839285, 7.964842623401181321 ) ) ;
#68038=CARTESIAN_POINT ( 'NONE',  ( 17.08211943468705840, 60.13708216824729647, -12.26659068614894466 ) ) ;
#68039=CARTESIAN_POINT ( 'NONE',  ( 12.63842701281683034, 47.46726448433412315, 9.846743663894596210 ) ) ;
#68040=CARTESIAN_POINT ( 'NONE',  ( 13.43411237798105340, 35.58196800326375353, 12.81628187352647963 ) ) ;
#68043=CARTESIAN_POINT ( 'NONE',  ( 24.16423886937410614, 4.303748834913967869, 8.672049930838204340E-16 ) ) ;
#68044=CARTESIAN_POINT ( 'NONE',  ( -0.8801773607110991993, 7.855352010821504471, -2.915334737309923874 ) ) ;
#68045=CARTESIAN_POINT ( 'NONE',  ( -2.266590686148945544, 57.22041550158063217, 7.082119434687048631 ) ) ;
#68046=CARTESIAN_POINT ( 'NONE',  ( 19.84674366389459621, 48.50893115100078745, 7.409399052514197653E-17 ) ) ;
#68048=CARTESIAN_POINT ( 'NONE',  ( 12.63842701281683922, 29.55059781766745175, -9.846743663894590881 ) ) ;
#68049=DIRECTION ( 'NONE',  ( 1.000000000000000000, 0.000000000000000000, 0.000000000000000000 ) ) ;
#68051=ORIENTED_EDGE ( 'NONE', *, *, #74995, .T. ) ;
#68055=CARTESIAN_POINT ( 'NONE',  ( -4.164238869374099039, 21.80374883491396787, 8.674139862899312516E-16 ) ) ;
#68056=CARTESIAN_POINT ( 'NONE',  ( 2.035157376598822676, 27.43868534415483396, -7.964842623401177768 ) ) ;
#68057=CARTESIAN_POINT ( 'NONE',  ( 7.084665262690076126, 37.02201867748817676, -10.88017736071110164 ) ) ;
#68058=CARTESIAN_POINT ( 'NONE',  ( 17.20831665107776587, 64.13393115100079456, -7.208316651077762316 ) ) ;
#68059=CARTESIAN_POINT ( 'NONE',  ( 0.6178305044545838731, 24.74863466993042493, 9.382169495545420901 ) ) ;
#68060=CARTESIAN_POINT ( 'NONE',  ( 2.917880565312950480, 0.9704155015806342766, -12.26659068614894821 ) ) ;
#68064=VECTOR ( 'NONE', #74188, 1000.000000000000000 ) ;
#68065=CARTESIAN_POINT ( 'NONE',  ( 10.00000000000000178, 30.37363466993042138, 12.81628187352647608 ) ) ;
#68067=( BOUNDED_CURVE ( )  B_SPLINE_CURVE ( 2, ( #36950, #67447, #50460, #97467, #5476, #65953, #80965, #12465, #13961 ),
 .UNSPECIFIED., .F., .F. ) 
 B_SPLINE_CURVE_WITH_KNOTS ( ( 3, 2, 2, 2, 3 ),
 ( 0.4758552226545170183, 0.4761904761904762196, 0.4821428571428571508, 0.4880952380952381375, 0.4884304916311972833 ),
 .UNSPECIFIED. ) 
 CURVE ( )  GEOMETRIC_REPRESENTATION_ITEM ( )  RATIONAL_B_SPLINE_CURVE ( ( 0.9963778908391753841, 0.9980808541467917072, 1.000000000000000000, 0.9659258262890682012, 1.000000000000000000, 0.9659258262890682012, 1.000000000000000000, 0.9980808541467920403, 0.9963778908391759392 ) ) 
 REPRESENTATION_ITEM ( '' )  );
#68068=CARTESIAN_POINT ( 'NONE',  ( 17.20831665107776587, 39.13393115100079456, -7.208316651077762316 ) ) ;
#68069=CARTESIAN_POINT ( 'NONE',  ( -0.8801773607110991993, 12.85535201082150358, -2.915334737309923874 ) ) ;
#68071=CARTESIAN_POINT ( 'NONE',  ( 17.96484262340118221, 16.18868534415483396, -7.964842623401177768 ) ) ;
#68073=CARTESIAN_POINT ( 'NONE',  ( 7.084665262690076126, 62.02201867748816966, -10.88017736071110164 ) ) ;
#68074=CARTESIAN_POINT ( 'NONE',  ( 2.035157376598824452, 53.68868534415484817, 7.964842623401179544 ) ) ;
#68075=CARTESIAN_POINT ( 'NONE',  ( 12.91533473730993009, 66.60535201082150536, -10.88017736071109987 ) ) ;
#68076=CARTESIAN_POINT ( 'NONE',  ( 19.42250999205614548, 55.98035201082150536, -5.440088680355545492 ) ) ;
#68081=CARTESIAN_POINT ( 'NONE',  ( 17.20831665107776587, 39.13393115100079456, -7.208316651077762316 ) ) ;
#68082=ORIENTED_EDGE ( 'NONE', *, *, #60727, .F. ) ;
#68083=CARTESIAN_POINT ( 'NONE',  ( 5.076628168052704559, 65.17559781766745175, -8.527530157486179263 ) ) ;
#68086=CARTESIAN_POINT ( 'NONE',  ( 6.204703633549690345, 7.845415501580634832, 14.16423886937410082 ) ) ;
#68090=CARTESIAN_POINT ( 'NONE',  ( 4.559911319644449179, 8.897018677488173211, 9.422509992056141925 ) ) ;
#68092=CARTESIAN_POINT ( 'NONE',  ( 22.81628187352648496, 46.83196800326376064, -3.434112377981050290 ) ) ;
#68095=CARTESIAN_POINT ( 'NONE',  ( 2.791683348922237240, 40.38393115100078035, -7.208316651077763204 ) ) ;
#68096=CARTESIAN_POINT ( 'NONE',  ( 19.72487221294570858, 0.000000000000000000, -6.500000000000000888 ) ) ;
#68097=( GEOMETRIC_REPRESENTATION_CONTEXT ( 3 ) GLOBAL_UNCERTAINTY_ASSIGNED_CONTEXT ( ( #72300 ) ) GLOBAL_UNIT_ASSIGNED_CONTEXT ( ( #46609, #61120, #91630 ) ) REPRESENTATION_CONTEXT ( 'NONE', 'WORKASPACE' ) );
#68098=CARTESIAN_POINT ( 'NONE',  ( 19.38216949554541202, 20.99863466993042138, 9.382169495545424454 ) ) ;
#68099=CARTESIAN_POINT ( 'NONE',  ( 2.791683348922237240, 30.38393115100078390, -7.208316651077763204 ) ) ;
#68101=CARTESIAN_POINT ( 'NONE',  ( 10.00000000000000178, 67.25893115100079456, 9.846743663894594434 ) ) ;
#68107=CARTESIAN_POINT ( 'NONE',  ( 19.42250999205614193, 25.14701867748817321, 5.440088680355555262 ) ) ;
#68108=CARTESIAN_POINT ( 'NONE',  ( -4.164238869374098151, 16.59541550158063927, -3.795296366450310543 ) ) ;
#68109=CARTESIAN_POINT ( 'NONE',  ( 14.92337183194729988, 34.34226448433411605, -8.527530157486177487 ) ) ;
#68110=CARTESIAN_POINT ( 'NONE',  ( 14.92337183194729988, 4.342264484334117824, -8.527530157486177487 ) ) ;
#68111=CARTESIAN_POINT ( 'NONE',  ( 22.81628187352647785, 36.62363466993041783, 6.195893100308588602E-16 ) ) ;
#68113=CARTESIAN_POINT ( 'NONE',  ( 19.42250999205614548, 15.98035201082150714, -5.440088680355545492 ) ) ;
#68114=EDGE_CURVE ( 'NONE', #45674, #35045, #44296, .T. ) ;
#68116=CARTESIAN_POINT ( 'NONE',  ( 21.09922568453594849, 11.20696800326375531, 6.408140936763242479 ) ) ;
#68117=CARTESIAN_POINT ( 'NONE',  ( 19.38216949554541557, 2.248634669930420049, -9.382169495545420901 ) ) ;
#68118=CARTESIAN_POINT ( 'NONE',  ( 7.361572987183170547, 22.05059781766745530, 9.846743663894590881 ) ) ;
#68120=CARTESIAN_POINT ( 'NONE',  ( 10.00000000000000000, 37.87363466993041783, -12.81628187352647608 ) ) ;
#68121=CARTESIAN_POINT ( 'NONE',  ( 18.06765999051784988, 23.99127512925449679, 6.500000000000021316 ) ) ;
#68122=CARTESIAN_POINT ( 'NONE',  ( 0.5774900079438590739, 42.64701867748816966, -5.440088680355550821 ) ) ;
#68127=CARTESIAN_POINT ( 'NONE',  ( 15.44008868035555260, 39.73035201082150536, 9.422509992056143702 ) ) ;
#68128=CARTESIAN_POINT ( 'NONE',  ( 4.559911319644449179, 48.89701867748817676, 9.422509992056141925 ) ) ;
#68129=CARTESIAN_POINT ( 'NONE',  ( 7.361572987183169658, 59.96726448433410894, -9.846743663894592657 ) ) ;
#68130=CARTESIAN_POINT ( 'NONE',  ( -0.8801773607111008646, 63.27201867748817676, 2.915334737309923430 ) ) ;
#68132=CARTESIAN_POINT ( 'NONE',  ( 2.791683348922240793, 46.63393115100077324, 7.208316651077764092 ) ) ;
#68133=CARTESIAN_POINT ( 'NONE',  ( 0.5774900079438590739, 2.647018677488170990, -5.440088680355550821 ) ) ;
#68135=CARTESIAN_POINT ( 'NONE',  ( 10.00000000000000000, 12.87363466993042138, -12.81628187352647608 ) ) ;
#68138=CARTESIAN_POINT ( 'NONE',  ( 17.96484262340118221, 34.93868534415482685, 7.964842623401181321 ) ) ;
#68139=CARTESIAN_POINT ( 'NONE',  ( 19.39188664607694434, 15.83703382326399911, -6.500000000000004441 ) ) ;
#68140=CARTESIAN_POINT ( 'NONE',  ( 20.88017736071110164, 5.355352010821502695, 2.915334737309930979 ) ) ;
#68141=CARTESIAN_POINT ( 'NONE',  ( 20.88017736071110519, 25.56368534415483751, 2.639326808657452039E-16 ) ) ;
#68142=CARTESIAN_POINT ( 'NONE',  ( 17.96484262340118221, 64.93868534415483396, 7.964842623401181321 ) ) ;
#68143=CARTESIAN_POINT ( 'NONE',  ( 24.16423886937410614, 44.51208216824730357, -3.795296366450302550 ) ) ;
#68144=CARTESIAN_POINT ( 'NONE',  ( 7.361572987183170547, 32.05059781766745175, 9.846743663894590881 ) ) ;
#68145=CARTESIAN_POINT ( 'NONE',  ( 15.44008868035555793, 41.39701867748817676, -9.422509992056140149 ) ) ;
#68151=CARTESIAN_POINT ( 'NONE',  ( 10.00000000000000178, 62.25893115100078745, 9.846743663894594434 ) ) ;
#68155=CARTESIAN_POINT ( 'NONE',  ( 20.36894250292379382, 18.67874883491397142, 10.36894250292379205 ) ) ;
#68156=CARTESIAN_POINT ( 'NONE',  ( 20.36894250292379382, 18.67874883491397142, 10.36894250292379205 ) ) ;
#68158=CARTESIAN_POINT ( 'NONE',  ( 20.88017736071110164, 55.35535201082149825, 2.915334737309930979 ) ) ;
#68159=CARTESIAN_POINT ( 'NONE',  ( 2.917880565312948704, 67.63708216824730357, 12.26659068614894643 ) ) ;
#68160=CARTESIAN_POINT ( 'NONE',  ( 10.00000000000000000, 7.873634669930421381, -12.81628187352647608 ) ) ;
#68161=CARTESIAN_POINT ( 'NONE',  ( 5.076628168052703671, 46.84226448433412315, 8.527530157486179263 ) ) ;
#68163=CARTESIAN_POINT ( 'NONE',  ( 2.035157376598822676, 52.43868534415483396, -7.964842623401177768 ) ) ;
#68164=CARTESIAN_POINT ( 'NONE',  ( 6.565887622018943937, 18.08196800326375708, -12.81628187352647608 ) ) ;
#68165=CARTESIAN_POINT ( 'NONE',  ( 6.204703633549690345, 15.76208216824730179, -14.16423886937410259 ) ) ;
#68166=CARTESIAN_POINT ( 'NONE',  ( 4.559911319644449179, 8.897018677488173211, 9.422509992056141925 ) ) ;
#68167=CARTESIAN_POINT ( 'NONE',  ( 12.91533473730992121, 29.52201867748817321, 10.88017736071110164 ) ) ;
#68169=CARTESIAN_POINT ( 'NONE',  ( 10.00000000000000000, 56.81368534415484106, -10.88017736071110342 ) ) ;
#68170=CARTESIAN_POINT ( 'NONE',  ( 22.81628187352647785, 46.62363466993041783, 6.195893100308588602E-16 ) ) ;
#68173=CARTESIAN_POINT ( 'NONE',  ( -46.07478503777810630, 103.8690650836416722, -6.036883934524842843 ) ) ;
#68178=CARTESIAN_POINT ( 'NONE',  ( 2.917880565312950480, 65.97041550158063217, -12.26659068614894821 ) ) ;
#68179=CARTESIAN_POINT ( 'NONE',  ( 6.204703633549690345, 62.84541550158063927, 14.16423886937410082 ) ) ;
#68180=CARTESIAN_POINT ( 'NONE',  ( 14.92337183194729633, 22.67559781766745175, 8.527530157486181039 ) ) ;
#68181=CARTESIAN_POINT ( 'NONE',  ( 14.92337183194729988, 64.34226448433412315, -8.527530157486177487 ) ) ;
#68182=CARTESIAN_POINT ( 'NONE',  ( 20.15039907845753220, 49.72266099184918176, 6.262539305110078836 ) ) ;
#68184=CARTESIAN_POINT ( 'NONE',  ( 7.361572987183169658, -0.03273551566588185635, -9.846743663894592657 ) ) ;
#68188=CARTESIAN_POINT ( 'NONE',  ( 24.16423886937409904, 39.09541550158062506, 3.795296366450317205 ) ) ;
#68190=CARTESIAN_POINT ( 'NONE',  ( -4.164238869374099039, 46.80374883491397497, 8.674139862899312516E-16 ) ) ;
#68192=CARTESIAN_POINT ( 'NONE',  ( 22.81628187352647785, 56.62363466993042493, 6.195893100308588602E-16 ) ) ;
#68193=CARTESIAN_POINT ( 'NONE',  ( 0.1532563361054100626, 55.80059781766745175, -2.638427012816831230 ) ) ;
#68194=CARTESIAN_POINT ( 'NONE',  ( 20.88017736071110875, 20.77201867748816611, -2.915334737309920765 ) ) ;
#68195=CARTESIAN_POINT ( 'NONE',  ( -2.816281873526473856, 64.33196800326376774, 3.434112377981055619 ) ) ;
#68197=CARTESIAN_POINT ( 'NONE',  ( 17.20831665107776587, 52.88393115100078035, 7.208316651077764980 ) ) ;
#68198=CARTESIAN_POINT ( 'NONE',  ( 5.076628168052703671, 46.84226448433412315, 8.527530157486179263 ) ) ;
#68203=VERTEX_POINT ( 'NONE', #46985 ) ;
#68207=CARTESIAN_POINT ( 'NONE',  ( 12.63842701281683034, 27.46726448433411250, 9.846743663894596210 ) ) ;
#68210=CARTESIAN_POINT ( 'NONE',  ( 21.09922568453594849, 36.20696800326375353, 6.408140936763242479 ) ) ;
#68213=ORIENTED_EDGE ( 'NONE', *, *, #74721, .T. ) ;
#68214=CARTESIAN_POINT ( 'NONE',  ( 2.791683348922240793, 66.63393115100079456, 7.208316651077764092 ) ) ;
#68215=CARTESIAN_POINT ( 'NONE',  ( -0.1023957841222447179, 65.13377557478294477, 6.340343622311912952 ) ) ;
#68216=CARTESIAN_POINT ( 'NONE',  ( 2.791683348922237240, 40.38393115100078035, -7.208316651077763204 ) ) ;
#68217=CARTESIAN_POINT ( 'NONE',  ( -0.3689425029237881626, 32.42874883491395366, 10.36894250292379027 ) ) ;
#68218=CARTESIAN_POINT ( 'NONE',  ( 0.1532563361054083140, 46.00893115100079456, 1.131784320476157264E-15 ) ) ;
#68219=CARTESIAN_POINT ( 'NONE',  ( 6.565887622018943937, 65.16530133659709634, 12.81628187352647430 ) ) ;
#68222=CARTESIAN_POINT ( 'NONE',  ( 17.20831665107776587, 4.133931151000785675, -7.208316651077762316 ) ) ;
#68224=CARTESIAN_POINT ( 'NONE',  ( -2.266590686148945544, 6.387082168247300906, -7.082119434687050408 ) ) ;
#68225=CARTESIAN_POINT ( 'NONE',  ( 0.1532563361054082862, 46.21726448433411605, 2.638427012816831674 ) ) ;
#68226=CARTESIAN_POINT ( 'NONE',  ( 20.88017736071110519, 50.56368534415484106, 2.639326808657452039E-16 ) ) ;
#68227=CARTESIAN_POINT ( 'NONE',  ( 2.791683348922240793, 41.63393115100078745, 7.208316651077764092 ) ) ;
#68232=CARTESIAN_POINT ( 'NONE',  ( 20.88017736071110519, 40.56368534415484106, 2.639326808657452039E-16 ) ) ;
#68235=CARTESIAN_POINT ( 'NONE',  ( 15.44008868035555260, 14.73035201082150536, 9.422509992056143702 ) ) ;
#68236=CARTESIAN_POINT ( 'NONE',  ( 3.591859063236763294, 3.290301336597087012, -11.09922568453595026 ) ) ;
#68237=CARTESIAN_POINT ( 'NONE',  ( 10.00000000000000000, 41.81368534415484106, -10.88017736071110342 ) ) ;
#68241=CARTESIAN_POINT ( 'NONE',  ( 0.5774900079438607392, 38.48035201082150536, 5.440088680355550821 ) ) ;
#68242=DIRECTION ( 'NONE',  ( 0.9970872288863210642, 0.07626964003977958206, 2.765979555393854277E-17 ) ) ;
#68243=CARTESIAN_POINT ( 'NONE',  ( 7.361572987183170547, 17.05059781766745530, 9.846743663894590881 ) ) ;
#68244=CARTESIAN_POINT ( 'NONE',  ( 19.84674366389459266, 38.71726448433412315, -2.638427012816827677 ) ) ;
#68246=CARTESIAN_POINT ( 'NONE',  ( 2.791683348922240793, 61.63393115100079456, 7.208316651077764092 ) ) ;
#68247=CARTESIAN_POINT ( 'NONE',  ( 2.917880565312948704, 62.63708216824730357, 12.26659068614894643 ) ) ;
#68249=CARTESIAN_POINT ( 'NONE',  ( -0.3689425029237898834, 26.17874883491396432, -10.36894250292378850 ) ) ;
#68250=CARTESIAN_POINT ( 'NONE',  ( -2.266590686148945544, 46.38708216824730357, -7.082119434687050408 ) ) ;
#68251=CARTESIAN_POINT ( 'NONE',  ( -0.8801773607111009756, 3.063685344154837509, 1.068504757029289695E-15 ) ) ;
#68253=CARTESIAN_POINT ( 'NONE',  ( 2.791683348922237240, 20.38393115100078745, -7.208316651077763204 ) ) ;
#68254=CARTESIAN_POINT ( 'NONE',  ( 0.5774900079438607392, 33.48035201082150536, 5.440088680355550821 ) ) ;
#68255=CARTESIAN_POINT ( 'NONE',  ( 12.63842701281683922, 44.55059781766745175, -9.846743663894590881 ) ) ;
#68256=CARTESIAN_POINT ( 'NONE',  ( 6.204703633549690345, 5.762082168247301794, -14.16423886937410259 ) ) ;
#68259=( NAMED_UNIT ( * ) PLANE_ANGLE_UNIT ( ) SI_UNIT ( $, .RADIAN. ) );
#68260=CARTESIAN_POINT ( 'NONE',  ( -2.816281873526473856, 34.12363466993042493, 9.499525473075851096E-16 ) ) ;
#68261=CARTESIAN_POINT ( 'NONE',  ( 10.00000000000000000, 39.75893115100078745, -9.846743663894594434 ) ) ;
#68263=CARTESIAN_POINT ( 'NONE',  ( 19.84674366389459266, 3.300597817667451750, 2.638427012816836559 ) ) ;
#68265=CARTESIAN_POINT ( 'NONE',  ( 18.72515096720578853, 60.05509018479938277, 6.499999999999877431 ) ) ;
#68266=CARTESIAN_POINT ( 'NONE',  ( 17.96484262340118221, 4.938685344154837509, 7.964842623401181321 ) ) ;
#68267=CARTESIAN_POINT ( 'NONE',  ( 13.79529636645030344, 48.26208216824728936, 14.16423886937410614 ) ) ;
#68268=CARTESIAN_POINT ( 'NONE',  ( 2.035157376598822676, 42.43868534415483396, -7.964842623401177768 ) ) ;
#68269=CARTESIAN_POINT ( 'NONE',  ( -46.94000000000001194, 93.00000000000000000, -8.999999999999998224 ) ) ;
#68270=CARTESIAN_POINT ( 'NONE',  ( 20.24186590665277308, 51.76028685723174760, 6.114288769123050749 ) ) ;
#68271=CARTESIAN_POINT ( 'NONE',  ( 7.361572987183170547, 32.05059781766745175, 9.846743663894590881 ) ) ;
#68272=CARTESIAN_POINT ( 'NONE',  ( 15.44008868035555793, 6.397018677488170546, -9.422509992056140149 ) ) ;
#68273=CARTESIAN_POINT ( 'NONE',  ( 0.1532563361054082862, 36.21726448433410894, 2.638427012816831674 ) ) ;
#68274=CARTESIAN_POINT ( 'NONE',  ( 0.05299164502591494075, 8.154255672638641206E-15, -4.488953749917677705 ) ) ;
#68275=CARTESIAN_POINT ( 'NONE',  ( 7.361572987183170547, 57.05059781766744464, 9.846743663894590881 ) ) ;
#68276=CARTESIAN_POINT ( 'NONE',  ( 12.91533473730993009, 51.60535201082149825, -10.88017736071109987 ) ) ;
#68277=ORIENTED_EDGE ( 'NONE', *, *, #86509, .F. ) ;
#68278=VERTEX_POINT ( 'NONE', #8022 ) ;
#68279=CARTESIAN_POINT ( 'NONE',  ( 10.00000000000000178, 60.37363466993041783, 12.81628187352647608 ) ) ;
#68281=CARTESIAN_POINT ( 'NONE',  ( 1.472469842513823179, 11.42559781766745175, 4.923371831947296329 ) ) ;
#68282=CARTESIAN_POINT ( 'NONE',  ( 13.43411237798105340, 60.58196800326376064, 12.81628187352647963 ) ) ;
#68283=CARTESIAN_POINT ( 'NONE',  ( 20.88017736071110164, 5.355352010821503583, 2.915334737309930979 ) ) ;
#68284=CARTESIAN_POINT ( 'NONE',  ( 14.92337183194729988, 49.34226448433411605, -8.527530157486177487 ) ) ;
#68285=( NAMED_UNIT ( * ) PLANE_ANGLE_UNIT ( ) SI_UNIT ( $, .RADIAN. ) );
#68286=CARTESIAN_POINT ( 'NONE',  ( 10.00000000000000000, -0.2410688489992152128, -9.846743663894594434 ) ) ;
#68287=CARTESIAN_POINT ( 'NONE',  ( -2.266590686148945544, 26.38708216824730357, -7.082119434687050408 ) ) ;
#68288=CARTESIAN_POINT ( 'NONE',  ( 10.00000000000000178, 48.05374883491396787, 14.16423886937410082 ) ) ;
#68289=CARTESIAN_POINT ( 'NONE',  ( 10.00000000000000000, 54.75893115100078745, -9.846743663894594434 ) ) ;
#68291=CARTESIAN_POINT ( 'NONE',  ( 10.00000000000000178, 54.31368534415484106, 10.88017736071110342 ) ) ;
#68292=CARTESIAN_POINT ( 'NONE',  ( 2.791683348922240793, 6.633931151000785675, 7.208316651077764092 ) ) ;
#68295=CARTESIAN_POINT ( 'NONE',  ( -2.816281873526473856, 59.33196800326374643, 3.434112377981055619 ) ) ;
#68297=CARTESIAN_POINT ( 'NONE',  ( 12.63842701281683922, 14.55059781766744997, -9.846743663894590881 ) ) ;
#68299=CARTESIAN_POINT ( 'NONE',  ( 22.26659068614895176, 24.72041550158063572, -7.082119434687042414 ) ) ;
#68300=CARTESIAN_POINT ( 'NONE',  ( 7.361572987183170547, 7.050597817667451750, 9.846743663894590881 ) ) ;
#68301=CARTESIAN_POINT ( 'NONE',  ( 4.559911319644449179, 32.23035201082150536, -9.422509992056141925 ) ) ;
#68304=CARTESIAN_POINT ( 'NONE',  ( 12.91533473730992121, 34.52201867748817676, 10.88017736071110164 ) ) ;
#68305=ORIENTED_EDGE ( 'NONE', *, *, #16957, .T. ) ;
#68306=FILL_AREA_STYLE_COLOUR ( '', #88819 ) ;
#68308=CARTESIAN_POINT ( 'NONE',  ( 21.09922568453595559, 12.04030133659708746, -6.408140936763230044 ) ) ;
#68309=CARTESIAN_POINT ( 'NONE',  ( 20.88017736071110164, 65.35535201082150536, 2.915334737309930979 ) ) ;
#68313=CARTESIAN_POINT ( 'NONE',  ( 2.791683348922240793, 11.63393115100078568, 7.208316651077764092 ) ) ;
#68314=CARTESIAN_POINT ( 'NONE',  ( 20.88017736071110164, 35.35535201082150536, 2.915334737309930979 ) ) ;
#68318=CARTESIAN_POINT ( 'NONE',  ( 15.44008868035555260, 39.73035201082150536, 9.422509992056143702 ) ) ;
#68320=CARTESIAN_POINT ( 'NONE',  ( 3.591859063236761518, 54.95696800326376064, 11.09922568453594849 ) ) ;
#68321=CARTESIAN_POINT ( 'NONE',  ( 17.96484262340118221, 59.93868534415484106, 7.964842623401181321 ) ) ;
#68323=CARTESIAN_POINT ( 'NONE',  ( 16.40814093676324603, 2.456968003263753531, -11.09922568453594671 ) ) ;
#68325=CARTESIAN_POINT ( 'NONE',  ( 0.1532563361054082862, 11.21726448433411605, 2.638427012816831674 ) ) ;
#68326=CARTESIAN_POINT ( 'NONE',  ( -2.816281873526473856, 59.33196800326374643, 3.434112377981055619 ) ) ;
#68327=CARTESIAN_POINT ( 'NONE',  ( 5.500000000000000000, 61.00000000000000711, -5.000000000000000000 ) ) ;
#68328=CARTESIAN_POINT ( 'NONE',  ( 5.076628168052703671, 6.842264484334118713, 8.527530157486179263 ) ) ;
#68329=CARTESIAN_POINT ( 'NONE',  ( 3.591859063236761518, 24.95696800326375353, 11.09922568453594849 ) ) ;
#68330=DIRECTION ( 'NONE',  ( -0.000000000000000000, -0.000000000000000000, 1.000000000000000000 ) ) ;
#68331=CARTESIAN_POINT ( 'NONE',  ( 0.1532563361054083140, 61.00893115100078745, 1.131784320476157264E-15 ) ) ;
#68332=CARTESIAN_POINT ( 'NONE',  ( 17.96484262340118221, 29.93868534415484106, 7.964842623401181321 ) ) ;
#68333=CARTESIAN_POINT ( 'NONE',  ( 1.472469842513823179, 66.42559781766745175, 4.923371831947296329 ) ) ;
#68335=CARTESIAN_POINT ( 'NONE',  ( 19.84674366389459266, 18.30059781766745175, 2.638427012816836559 ) ) ;
#68336=CARTESIAN_POINT ( 'NONE',  ( 19.84674366389459266, 13.71726448433411782, -2.638427012816827677 ) ) ;
#68337=CARTESIAN_POINT ( 'NONE',  ( -2.816281873526473856, 4.123634669930420493, 9.499525473075851096E-16 ) ) ;
#68338=EDGE_LOOP ( 'NONE', ( #98072, #16181, #12196, #45395, #47481 ) ) ;
#68339=AXIS2_PLACEMENT_3D ( 'NONE', #94584, #72560, #25616 ) ;
#68340=CARTESIAN_POINT ( 'NONE',  ( 15.44008868035555793, 6.397018677488170546, -9.422509992056140149 ) ) ;
#68341=CARTESIAN_POINT ( 'NONE',  ( 2.791683348922237240, 65.38393115100078035, -7.208316651077763204 ) ) ;
#68343=CARTESIAN_POINT ( 'NONE',  ( 4.559911319644449179, 8.897018677488173211, 9.422509992056141925 ) ) ;
#68344=CARTESIAN_POINT ( 'NONE',  ( 5.076628168052703671, 46.84226448433412315, 8.527530157486179263 ) ) ;
#68347=CARTESIAN_POINT ( 'NONE',  ( 0.5774900079438590739, 7.647018677488171434, -5.440088680355550821 ) ) ;
#68348=CARTESIAN_POINT ( 'NONE',  ( 0.2751277870542909731, 47.28217586085238366, -6.499999999999992006 ) ) ;
#68349=EDGE_CURVE ( 'NONE', #66685, #19583, #11836, .T. ) ;
#68351=CARTESIAN_POINT ( 'NONE',  ( 20.88017736071110519, 30.56368534415484106, 2.639326808657452039E-16 ) ) ;
#68352=CARTESIAN_POINT ( 'NONE',  ( 22.26659068614894466, 48.88708216824730357, 7.082119434687054849 ) ) ;
#68353=CARTESIAN_POINT ( 'NONE',  ( 10.00000000000000178, 68.05374883491397497, 14.16423886937410082 ) ) ;
#68355=CARTESIAN_POINT ( 'NONE',  ( 19.84674366389459621, 3.508931151000785231, 7.409399052514197653E-17 ) ) ;
#68356=CARTESIAN_POINT ( 'NONE',  ( 2.791683348922240793, 31.63393115100078745, 7.208316651077764092 ) ) ;
#68357=CARTESIAN_POINT ( 'NONE',  ( 22.81628187352647785, 11.41530133659708390, 3.434112377981063169 ) ) ;
#68360=CARTESIAN_POINT ( 'NONE',  ( 5.076628168052704559, 60.17559781766745175, -8.527530157486179263 ) ) ;
#68361=COLOUR_RGB ( '', 0.66274510, 0.83137255, 0.94901961) ;
#68366=CARTESIAN_POINT ( 'NONE',  ( 10.00000000000000178, 8.053748834913967869, 14.16423886937410082 ) ) ;
#68367=CARTESIAN_POINT ( 'NONE',  ( 0.1532563361054083140, 26.00893115100078745, 1.131784320476157264E-15 ) ) ;
#68368=CARTESIAN_POINT ( 'NONE',  ( 17.08211943468705130, 58.47041550158063927, 12.26659068614894998 ) ) ;
#68369=CARTESIAN_POINT ( 'NONE',  ( 0.1532563361054082862, 6.217264484334118713, 2.638427012816831674 ) ) ;
#68372=CARTESIAN_POINT ( 'NONE',  ( -0.8801773607110991993, 37.85535201082151247, -2.915334737309923874 ) ) ;
#68373=CARTESIAN_POINT ( 'NONE',  ( 19.38216949554541202, 50.99863466993042493, 9.382169495545424454 ) ) ;
#68374=CARTESIAN_POINT ( 'NONE',  ( 2.035157376598822676, 2.438685344154837953, -7.964842623401177768 ) ) ;
#68375=CARTESIAN_POINT ( 'NONE',  ( -1.099225684535947600, 33.70696800326375353, -6.408140936763238038 ) ) ;
#68376=CARTESIAN_POINT ( 'NONE',  ( 0.1532563361054100626, 0.8005978176674514168, -2.638427012816831230 ) ) ;
#68377=ORIENTED_EDGE ( 'NONE', *, *, #13215, .T. ) ;
#68380=CARTESIAN_POINT ( 'NONE',  ( 22.26659068614894466, 43.88708216824729647, 7.082119434687054849 ) ) ;
#68381=CARTESIAN_POINT ( 'NONE',  ( 6.204703633549690345, 7.845415501580634832, 14.16423886937410082 ) ) ;
#68382=CARTESIAN_POINT ( 'NONE',  ( 15.44008868035555793, 41.39701867748817676, -9.422509992056140149 ) ) ;
#68385=CARTESIAN_POINT ( 'NONE',  ( 20.88017736071110875, 55.77201867748816966, -2.915334737309920765 ) ) ;
#68386=CARTESIAN_POINT ( 'NONE',  ( 2.035157376598824452, 58.68868534415482685, 7.964842623401179544 ) ) ;
#68387=CARTESIAN_POINT ( 'NONE',  ( 0.6178305044545838731, 29.74863466993042138, 9.382169495545420901 ) ) ;
#68390=CARTESIAN_POINT ( 'NONE',  ( 2.791683348922240793, 36.63393115100078035, 7.208316651077764092 ) ) ;
#68391=CARTESIAN_POINT ( 'NONE',  ( 22.81628187352647785, 16.41530133659708923, 3.434112377981063169 ) ) ;
#68392=CARTESIAN_POINT ( 'NONE',  ( 19.84674366389459266, 3.300597817667451750, 2.638427012816836559 ) ) ;
#68393=CARTESIAN_POINT ( 'NONE',  ( 12.91533473730992121, 4.522018677488169658, 10.88017736071110164 ) ) ;
#68394=CARTESIAN_POINT ( 'NONE',  ( 19.84674366389459266, 43.71726448433410894, -2.638427012816827677 ) ) ;
#68395=CARTESIAN_POINT ( 'NONE',  ( 10.00000000000000178, 60.37363466993041783, 12.81628187352647608 ) ) ;
#68396=CARTESIAN_POINT ( 'NONE',  ( 0.1532563361054100626, 20.80059781766744464, -2.638427012816831230 ) ) ;
#68397=CARTESIAN_POINT ( 'NONE',  ( 10.00000000000000178, 3.053748834913967425, 14.16423886937410082 ) ) ;
#68398=CARTESIAN_POINT ( 'NONE',  ( 17.39651004071838614, 42.93575266056826933, 6.500000000000032863 ) ) ;
#68399=CARTESIAN_POINT ( 'NONE',  ( 7.084665262690076126, 27.02201867748817676, -10.88017736071110164 ) ) ;
#68400=CARTESIAN_POINT ( 'NONE',  ( 4.559911319644449179, 17.23035201082150536, -9.422509992056141925 ) ) ;
#68401=CARTESIAN_POINT ( 'NONE',  ( 6.204703633549690345, 45.76208216824729647, -14.16423886937410259 ) ) ;
#68402=CARTESIAN_POINT ( 'NONE',  ( 17.96484262340118221, 29.93868534415484106, 7.964842623401181321 ) ) ;
#68403=EDGE_CURVE ( 'NONE', #21055, #92145, #88154, .T. ) ;
#68404=CARTESIAN_POINT ( 'NONE',  ( 20.88017736071110164, 15.35535201082150358, 2.915334737309930979 ) ) ;
#68406=CARTESIAN_POINT ( 'NONE',  ( 20.88017736071110164, 25.35535201082150891, 2.915334737309930979 ) ) ;
#68408=CARTESIAN_POINT ( 'NONE',  ( 3.591859063236763294, 48.29030133659708923, -11.09922568453595026 ) ) ;
#68409=CARTESIAN_POINT ( 'NONE',  ( 4.559911319644449179, 47.23035201082150536, -9.422509992056141925 ) ) ;
#68410=CARTESIAN_POINT ( 'NONE',  ( 1.472469842513823179, 45.59226448433412315, -4.923371831947296329 ) ) ;
#68411=CARTESIAN_POINT ( 'NONE',  ( 12.91533473730993009, 51.60535201082149825, -10.88017736071109987 ) ) ;
#68413=CARTESIAN_POINT ( 'NONE',  ( 2.035157376598824452, 48.68868534415483396, 7.964842623401179544 ) ) ;
#68416=CARTESIAN_POINT ( 'NONE',  ( 6.204703633549690345, 42.84541550158063217, 14.16423886937410082 ) ) ;
#68417=CARTESIAN_POINT ( 'NONE',  ( 17.96484262340118221, 61.18868534415482685, -7.964842623401177768 ) ) ;
#68418=CARTESIAN_POINT ( 'NONE',  ( 20.15039907845753220, 25.60158574516642815, -6.262539305110077947 ) ) ;
#68420=CARTESIAN_POINT ( 'NONE',  ( 1.472469842513823179, 61.42559781766745175, 4.923371831947296329 ) ) ;
#68422=CARTESIAN_POINT ( 'NONE',  ( 5.076628168052703671, 31.84226448433412315, 8.527530157486179263 ) ) ;
#68424=CARTESIAN_POINT ( 'NONE',  ( 19.84674366389459266, 38.71726448433412315, -2.638427012816827677 ) ) ;
#68427=CARTESIAN_POINT ( 'NONE',  ( 17.96484262340118221, 19.93868534415484106, 7.964842623401181321 ) ) ;
#68428=CARTESIAN_POINT ( 'NONE',  ( 17.20831665107776587, 34.13393115100078745, -7.208316651077762316 ) ) ;
#68429=CARTESIAN_POINT ( 'NONE',  ( 21.09922568453594849, 26.20696800326375353, 6.408140936763242479 ) ) ;
#68430=CYLINDRICAL_SURFACE ( 'NONE', #80262, 0.5000000000000004441 ) ;
#68431=CARTESIAN_POINT ( 'NONE',  ( 19.42250999205614548, 60.98035201082151247, -5.440088680355545492 ) ) ;
#68432=CARTESIAN_POINT ( 'NONE',  ( 10.00000000000000178, 34.31368534415484106, 10.88017736071110342 ) ) ;
#68433=CARTESIAN_POINT ( 'NONE',  ( -0.8801773607111009756, 3.063685344154837509, 1.068504757029289695E-15 ) ) ;
#68434=CARTESIAN_POINT ( 'NONE',  ( 13.79529636645030344, 63.26208216824730357, 14.16423886937410614 ) ) ;
#68438=CARTESIAN_POINT ( 'NONE',  ( 0.6178305044545818747, 18.49863466993041428, -9.382169495545419124 ) ) ;
#68439=CARTESIAN_POINT ( 'NONE',  ( 6.000000000000000000, 10.49999999999999822, -6.000000000000000000 ) ) ;
#68441=CARTESIAN_POINT ( 'NONE',  ( 10.00000000000000178, 20.37363466993042138, 12.81628187352647608 ) ) ;
#68442=CARTESIAN_POINT ( 'NONE',  ( 7.084665262690076126, 22.02201867748817321, -10.88017736071110164 ) ) ;
#68444=CARTESIAN_POINT ( 'NONE',  ( 2.035157376598824452, 48.68868534415483396, 7.964842623401179544 ) ) ;
#68445=CARTESIAN_POINT ( 'NONE',  ( -33.19000000000001194, 92.00000000000000000, -10.09898361729590199 ) ) ;
#68447=CARTESIAN_POINT ( 'NONE',  ( 2.035157376598822676, 62.43868534415483396, -7.964842623401177768 ) ) ;
#68448=CARTESIAN_POINT ( 'NONE',  ( 18.52753015748617571, 33.09226448433411605, 4.923371831947298993 ) ) ;
#68449=CARTESIAN_POINT ( 'NONE',  ( 10.00000000000000000, 29.75893115100078745, -9.846743663894594434 ) ) ;
#68450=CARTESIAN_POINT ( 'NONE',  ( 14.92337183194729988, 19.34226448433411960, -8.527530157486177487 ) ) ;
#68451=CARTESIAN_POINT ( 'NONE',  ( 20.10493008474206178, 54.71697413083881401, 6.336235997365760042 ) ) ;
#68452=CARTESIAN_POINT ( 'NONE',  ( 6.565887622018943937, 38.08196800326376064, -12.81628187352647608 ) ) ;
#68453=CARTESIAN_POINT ( 'NONE',  ( 12.63842701281683922, 19.55059781766745175, -9.846743663894590881 ) ) ;
#68455=CARTESIAN_POINT ( 'NONE',  ( 20.24186590665277308, 45.59014588040356841, -6.114288769123051637 ) ) ;
#68456=CARTESIAN_POINT ( 'NONE',  ( 17.20831665107776587, 34.13393115100078745, -7.208316651077762316 ) ) ;
#68459=CARTESIAN_POINT ( 'NONE',  ( 16.40814093676324603, 17.45696800326375353, -11.09922568453594671 ) ) ;
#68461=CARTESIAN_POINT ( 'NONE',  ( 20.88017736071110875, 45.77201867748816966, -2.915334737309920765 ) ) ;
#68462=CARTESIAN_POINT ( 'NONE',  ( 17.08211943468705130, 28.47041550158063572, 12.26659068614894998 ) ) ;
#68465=CARTESIAN_POINT ( 'NONE',  ( 6.204703633549690345, 35.76208216824729647, -14.16423886937410259 ) ) ;
#68466=EDGE_CURVE ( 'NONE', #663, #55728, #10759, .T. ) ;
#68467=CARTESIAN_POINT ( 'NONE',  ( 13.79529636645030344, 58.26208216824728936, 14.16423886937410614 ) ) ;
#68468=CARTESIAN_POINT ( 'NONE',  ( -4.164238869374099927, 12.01208216824730357, 3.795296366450308767 ) ) ;
#68469=CARTESIAN_POINT ( 'NONE',  ( 13.79529636645030344, 28.26208216824729647, 14.16423886937410614 ) ) ;
#68470=CARTESIAN_POINT ( 'NONE',  ( 18.04007052943773104, 33.01528370094807485, 5.767676674365834977 ) ) ;
#68471=CARTESIAN_POINT ( 'NONE',  ( 0.5774900079438590739, 47.64701867748817676, -5.440088680355550821 ) ) ;
#68473=CARTESIAN_POINT ( 'NONE',  ( 19.42250999205614548, 65.98035201082151957, -5.440088680355545492 ) ) ;
#68474=CARTESIAN_POINT ( 'NONE',  ( 2.791683348922240793, 36.63393115100078035, 7.208316651077764092 ) ) ;
#68475=CARTESIAN_POINT ( 'NONE',  ( 19.42250999205614548, 20.98035201082150891, -5.440088680355545492 ) ) ;
#68477=CARTESIAN_POINT ( 'NONE',  ( 19.84674366389459621, 63.50893115100078745, 7.409399052514197653E-17 ) ) ;
#68478=CARTESIAN_POINT ( 'NONE',  ( 20.00000000000000711, 82.59735310505368489, -4.636598378016183908 ) ) ;
#68479=CARTESIAN_POINT ( 'NONE',  ( 19.84674366389459266, 23.71726448433412315, -2.638427012816827677 ) ) ;
#68480=CARTESIAN_POINT ( 'NONE',  ( 0.6178305044545818747, 53.49863466993041072, -9.382169495545419124 ) ) ;
#68482=CARTESIAN_POINT ( 'NONE',  ( 20.88017736071110519, 45.56368534415484106, 2.639326808657452039E-16 ) ) ;
#68483=CARTESIAN_POINT ( 'NONE',  ( 19.84674366389459621, 48.50893115100078745, 7.409399052514197653E-17 ) ) ;
#68484=CARTESIAN_POINT ( 'NONE',  ( 6.204703633549690345, 45.76208216824729647, -14.16423886937410259 ) ) ;
#68486=CARTESIAN_POINT ( 'NONE',  ( -4.164238869374099927, 2.012082168247300906, 3.795296366450308767 ) ) ;
#68487=CARTESIAN_POINT ( 'NONE',  ( 4.559911319644449179, 67.23035201082150536, -9.422509992056141925 ) ) ;
#68489=CARTESIAN_POINT ( 'NONE',  ( 24.16423886937410614, 59.30374883491397497, 8.672049930838204340E-16 ) ) ;
#68490=CARTESIAN_POINT ( 'NONE',  ( 0.6178305044545838731, 14.74863466993041783, 9.382169495545420901 ) ) ;
#68492=CARTESIAN_POINT ( 'NONE',  ( 2.035157376598822676, 57.43868534415484106, -7.964842623401177768 ) ) ;
#68493=DIRECTION ( 'NONE',  ( 0.000000000000000000, 0.000000000000000000, -1.000000000000000000 ) ) ;
#68495=CARTESIAN_POINT ( 'NONE',  ( -46.75138744620058873, 100.8579332310653598, -9.074091037931069081 ) ) ;
#68496=CARTESIAN_POINT ( 'NONE',  ( 0.5774900079438590739, 2.647018677488171434, -5.440088680355550821 ) ) ;
#68498=CARTESIAN_POINT ( 'NONE',  ( 20.88017736071110519, 15.56368534415483751, 2.639326808657452039E-16 ) ) ;
#68499=CARTESIAN_POINT ( 'NONE',  ( 4.559911319644449179, 28.89701867748817321, 9.422509992056141925 ) ) ;
#68500=CARTESIAN_POINT ( 'NONE',  ( 17.20831665107776587, 62.88393115100078745, 7.208316651077764980 ) ) ;
#68501=CARTESIAN_POINT ( 'NONE',  ( 10.00000000000000178, 50.37363466993042493, 12.81628187352647608 ) ) ;
#68503=CARTESIAN_POINT ( 'NONE',  ( -0.8801773607111009756, 18.06368534415484106, 1.068504757029289695E-15 ) ) ;
#68504=CARTESIAN_POINT ( 'NONE',  ( 0.6178305044545838731, 24.74863466993042493, 9.382169495545420901 ) ) ;
#68507=CARTESIAN_POINT ( 'NONE',  ( 12.63842701281683922, 54.55059781766745175, -9.846743663894590881 ) ) ;
#68508=CARTESIAN_POINT ( 'NONE',  ( 10.00000000000000178, 34.31368534415484106, 10.88017736071110342 ) ) ;
#68509=CARTESIAN_POINT ( 'NONE',  ( 21.09922568453594849, 16.20696800326375353, 6.408140936763242479 ) ) ;
#68510=CARTESIAN_POINT ( 'NONE',  ( 10.00000000000000178, 44.31368534415484106, 10.88017736071110342 ) ) ;
#68512=DIRECTION ( 'NONE',  ( -0.000000000000000000, -0.000000000000000000, -1.000000000000000000 ) ) ;
#68513=CARTESIAN_POINT ( 'NONE',  ( 13.43411237798106583, 52.66530133659708213, -12.81628187352647252 ) ) ;
#68515=CARTESIAN_POINT ( 'NONE',  ( 1.472469842513823179, 66.42559781766745175, 4.923371831947296329 ) ) ;
#68517=CARTESIAN_POINT ( 'NONE',  ( 7.084665262690076126, 47.02201867748818387, -10.88017736071110164 ) ) ;
#68518=CARTESIAN_POINT ( 'NONE',  ( 21.09922568453595559, 32.04030133659708923, -6.408140936763230044 ) ) ;
#68519=CARTESIAN_POINT ( 'NONE',  ( 17.20831665107776587, 9.133931151000787452, -7.208316651077762316 ) ) ;
#68520=CARTESIAN_POINT ( 'NONE',  ( 17.08211943468705130, 48.47041550158063927, 12.26659068614894998 ) ) ;
#68521=CARTESIAN_POINT ( 'NONE',  ( 2.791683348922240793, 66.63393115100079456, 7.208316651077764092 ) ) ;
#68522=CARTESIAN_POINT ( 'NONE',  ( 17.20831665107776587, 17.88393115100078745, 7.208316651077764980 ) ) ;
#68523=CARTESIAN_POINT ( 'NONE',  ( 19.84674366389459266, 3.717264484334118713, -2.638427012816827677 ) ) ;
#68525=CARTESIAN_POINT ( 'NONE',  ( 13.79529636645031943, 45.34541550158062506, -14.16423886937409904 ) ) ;
#68529=CARTESIAN_POINT ( 'NONE',  ( -0.8801773607111009756, 8.063685344154837509, 1.068504757029289695E-15 ) ) ;
#68531=ORIENTED_EDGE ( 'NONE', *, *, #69799, .F. ) ;
#68532=CARTESIAN_POINT ( 'NONE',  ( 2.035157376598822676, 7.438685344154837509, -7.964842623401177768 ) ) ;
#68533=CARTESIAN_POINT ( 'NONE',  ( 2.917880565312948704, 67.63708216824730357, 12.26659068614894643 ) ) ;
#68534=CARTESIAN_POINT ( 'NONE',  ( 7.361572987183169658, 49.96726448433410894, -9.846743663894592657 ) ) ;
#68535=CARTESIAN_POINT ( 'NONE',  ( 13.43411237798105340, 45.58196800326374643, 12.81628187352647963 ) ) ;
#68536=FACE_OUTER_BOUND ( 'NONE', #82131, .T. ) ;
#68538=CARTESIAN_POINT ( 'NONE',  ( -0.3689425029237881626, 7.428748834913967869, 10.36894250292379027 ) ) ;
#68539=CARTESIAN_POINT ( 'NONE',  ( 20.88017736071110875, 20.77201867748816611, -2.915334737309920765 ) ) ;
#68540=CARTESIAN_POINT ( 'NONE',  ( 15.44008868035555793, 6.397018677488171434, -9.422509992056140149 ) ) ;
#68541=CARTESIAN_POINT ( 'NONE',  ( 17.20831665107776587, 47.88393115100078745, 7.208316651077764980 ) ) ;
#68543=CARTESIAN_POINT ( 'NONE',  ( 5.076628168052704559, 25.17559781766745175, -8.527530157486179263 ) ) ;
#68546=VECTOR ( 'NONE', #25117, 1000.000000000000000 ) ;
#68547=EDGE_LOOP ( 'NONE', ( #10051, #52288, #30056, #83566 ) ) ;
#68549=ORIENTED_EDGE ( 'NONE', *, *, #7812, .F. ) ;
#68550=CARTESIAN_POINT ( 'NONE',  ( 19.84674366389459266, 58.71726448433411605, -2.638427012816827677 ) ) ;
#68551=CARTESIAN_POINT ( 'NONE',  ( 12.91533473730993009, 36.60535201082151247, -10.88017736071109987 ) ) ;
#68552=CARTESIAN_POINT ( 'NONE',  ( 19.42250999205614548, 35.98035201082151247, -5.440088680355545492 ) ) ;
#68553=CARTESIAN_POINT ( 'NONE',  ( 3.591859063236761518, 24.95696800326375353, 11.09922568453594849 ) ) ;
#68554=CARTESIAN_POINT ( 'NONE',  ( 20.36894250292379382, 8.678748834913967869, 10.36894250292379205 ) ) ;
#68555=CARTESIAN_POINT ( 'NONE',  ( 17.96484262340118221, 66.18868534415483396, -7.964842623401177768 ) ) ;
#68556=EDGE_CURVE ( 'NONE', #13373, #107, #20082, .T. ) ;
#68557=CARTESIAN_POINT ( 'NONE',  ( 0.6178305044545838731, 49.74863466993041072, 9.382169495545420901 ) ) ;
#68558=VERTEX_POINT ( 'NONE', #41844 ) ;
#68559=CARTESIAN_POINT ( 'NONE',  ( 10.00000000000000000, 44.75893115100078745, -9.846743663894594434 ) ) ;
#68561=CARTESIAN_POINT ( 'NONE',  ( -0.8801773607111008646, 13.27201867748817321, 2.915334737309923430 ) ) ;
#68563=CARTESIAN_POINT ( 'NONE',  ( 7.084665262690076126, 14.10535201082150358, 10.88017736071109987 ) ) ;
#68565=CARTESIAN_POINT ( 'NONE',  ( 10.00000000000000178, 54.31368534415484106, 10.88017736071110342 ) ) ;
#68566=CARTESIAN_POINT ( 'NONE',  ( 15.44008868035555260, 59.73035201082151247, 9.422509992056143702 ) ) ;
#68568=FACE_OUTER_BOUND ( 'NONE', #4513, .T. ) ;
#68569=CARTESIAN_POINT ( 'NONE',  ( 10.00000000000000178, 54.31368534415484106, 10.88017736071110342 ) ) ;
#68570=CARTESIAN_POINT ( 'NONE',  ( -0.2418659066527703572, 53.09014588040358262, 6.114288769123046308 ) ) ;
#68574=CARTESIAN_POINT ( 'NONE',  ( 18.52753015748618282, 43.92559781766745175, -4.923371831947291888 ) ) ;
#68576=CARTESIAN_POINT ( 'NONE',  ( 0.1532563361054082862, 66.21726448433413736, 2.638427012816831674 ) ) ;
#68577=CARTESIAN_POINT ( 'NONE',  ( 20.15039907845753930, 69.92552686551195507, -6.262539305110068177 ) ) ;
#68579=CARTESIAN_POINT ( 'NONE',  ( 13.79529636645030344, 8.262082168247300018, 14.16423886937410614 ) ) ;
#68581=CARTESIAN_POINT ( 'NONE',  ( 20.15039907845753930, 69.92552686551195507, 6.262539305110068177 ) ) ;
#68582=CARTESIAN_POINT ( 'NONE',  ( 4.559911319644449179, 63.89701867748817676, 9.422509992056141925 ) ) ;
#68583=CARTESIAN_POINT ( 'NONE',  ( 17.96484262340118221, 9.938685344154839285, 7.964842623401181321 ) ) ;
#68584=CARTESIAN_POINT ( 'NONE',  ( 0.2751277870542909176, 59.36607318730130345, -6.499999999999992006 ) ) ;
#68585=CARTESIAN_POINT ( 'NONE',  ( 3.591859063236761518, 39.95696800326375353, 11.09922568453594849 ) ) ;
#68586=ORIENTED_EDGE ( 'NONE', *, *, #9939, .T. ) ;
#68588=CARTESIAN_POINT ( 'NONE',  ( 12.63842701281683034, 42.46726448433412315, 9.846743663894596210 ) ) ;
#68589=CARTESIAN_POINT ( 'NONE',  ( 5.076628168052703671, 1.842264484334118047, 8.527530157486179263 ) ) ;
#68590=CARTESIAN_POINT ( 'NONE',  ( 6.565887622018943937, 15.16530133659708568, 12.81628187352647430 ) ) ;
#68591=CARTESIAN_POINT ( 'NONE',  ( 5.076628168052703671, 26.84226448433411960, 8.527530157486179263 ) ) ;
#68594=CARTESIAN_POINT ( 'NONE',  ( -0.2002127540270186579, 69.97534054108130874, -6.181800700215005939 ) ) ;
#68595=CARTESIAN_POINT ( 'NONE',  ( 22.81628187352647785, 11.62363466993042138, 6.195893100308588602E-16 ) ) ;
#68597=CARTESIAN_POINT ( 'NONE',  ( 2.791683348922240793, 11.63393115100078568, 7.208316651077764092 ) ) ;
#68599=VERTEX_POINT ( 'NONE', #49808 ) ;
#68600=CARTESIAN_POINT ( 'NONE',  ( 10.00000000000000178, 19.31368534415484106, 10.88017736071110342 ) ) ;
#68601=CARTESIAN_POINT ( 'NONE',  ( 24.16423886937409904, 14.09541550158063217, 3.795296366450317205 ) ) ;
#68602=CARTESIAN_POINT ( 'NONE',  ( 19.84674366389459266, 38.30059781766745175, 2.638427012816836559 ) ) ;
#68603=CARTESIAN_POINT ( 'NONE',  ( 7.361572987183169658, 4.967264484334119601, -9.846743663894592657 ) ) ;
#68604=CARTESIAN_POINT ( 'NONE',  ( 10.00000000000000000, 42.87363466993042493, -12.81628187352647608 ) ) ;
#68606=CARTESIAN_POINT ( 'NONE',  ( -0.8801773607111009756, 18.06368534415484106, 1.068504757029289695E-15 ) ) ;
#68608=CARTESIAN_POINT ( 'NONE',  ( 21.09922568453595559, 12.04030133659708746, -6.408140936763230044 ) ) ;
#68609=CARTESIAN_POINT ( 'NONE',  ( 5.076628168052703671, 31.84226448433412315, 8.527530157486179263 ) ) ;
#68611=CARTESIAN_POINT ( 'NONE',  ( 3.591859063236761518, 29.95696800326375708, 11.09922568453594849 ) ) ;
#68612=CARTESIAN_POINT ( 'NONE',  ( 18.28836319691945889, 24.34492782695771140, 6.499999999999999112 ) ) ;
#68613=CARTESIAN_POINT ( 'NONE',  ( 17.96484262340118221, 39.93868534415484106, 7.964842623401181321 ) ) ;
#68615=VECTOR ( 'NONE', #31337, 1000.000000000000000 ) ;
#68617=CARTESIAN_POINT ( 'NONE',  ( -0.8801773607111009756, 68.06368534415484817, 1.068504757029289695E-15 ) ) ;
#68618=CARTESIAN_POINT ( 'NONE',  ( 7.084665262690076126, 42.02201867748816966, -10.88017736071110164 ) ) ;
#68619=CARTESIAN_POINT ( 'NONE',  ( -0.8801773607111008646, 48.27201867748816966, 2.915334737309923430 ) ) ;
#68620=CARTESIAN_POINT ( 'NONE',  ( 19.89103541497709671, 60.66234555792570404, -6.479102184480829862 ) ) ;
#68621=CARTESIAN_POINT ( 'NONE',  ( 15.44008868035555793, 66.39701867748817676, -9.422509992056140149 ) ) ;
#68622=CARTESIAN_POINT ( 'NONE',  ( 7.361572987183169658, 54.96726448433413026, -9.846743663894592657 ) ) ;
#68623=CARTESIAN_POINT ( 'NONE',  ( 4.559911319644449179, 3.897018677488170990, 9.422509992056141925 ) ) ;
#68625=CARTESIAN_POINT ( 'NONE',  ( 0.6178305044545818747, 18.49863466993041428, -9.382169495545419124 ) ) ;
#68626=ORIENTED_EDGE ( 'NONE', *, *, #24209, .T. ) ;
#68627=CARTESIAN_POINT ( 'NONE',  ( 2.035157376598824452, 33.68868534415484106, 7.964842623401179544 ) ) ;
#68628=CARTESIAN_POINT ( 'NONE',  ( 7.361572987183169658, 59.96726448433410894, -9.846743663894592657 ) ) ;
#68629=CARTESIAN_POINT ( 'NONE',  ( 19.72487221294571214, 15.71833443783937589, -6.500000000000001776 ) ) ;
#68630=CARTESIAN_POINT ( 'NONE',  ( 19.42250999205614193, 20.14701867748817321, 5.440088680355555262 ) ) ;
#68631=CARTESIAN_POINT ( 'NONE',  ( 12.91533473730992121, 24.52201867748816966, 10.88017736071110164 ) ) ;
#68632=CARTESIAN_POINT ( 'NONE',  ( -2.266590686148945544, 36.38708216824730357, -7.082119434687050408 ) ) ;
#68633=CARTESIAN_POINT ( 'NONE',  ( 0.1532563361054082862, 21.21726448433412315, 2.638427012816831674 ) ) ;
#68634=CARTESIAN_POINT ( 'NONE',  ( 20.88017736071110164, 40.35535201082150536, 2.915334737309930979 ) ) ;
#68636=CARTESIAN_POINT ( 'NONE',  ( 13.79529636645031943, 5.345415501580634832, -14.16423886937409904 ) ) ;
#68638=CARTESIAN_POINT ( 'NONE',  ( 2.791683348922240793, 56.63393115100078035, 7.208316651077764092 ) ) ;
#68641=CARTESIAN_POINT ( 'NONE',  ( 24.16423886937410614, 39.30374883491396787, 8.672049930838204340E-16 ) ) ;
#68642=CARTESIAN_POINT ( 'NONE',  ( 17.08211943468705840, 25.13708216824730357, -12.26659068614894466 ) ) ;
#68643=CARTESIAN_POINT ( 'NONE',  ( 19.84674366389459266, 3.717264484334118713, -2.638427012816827677 ) ) ;
#68644=CARTESIAN_POINT ( 'NONE',  ( 18.52753015748617571, 43.09226448433412315, 4.923371831947298993 ) ) ;
#68646=CARTESIAN_POINT ( 'NONE',  ( 17.96484262340118221, 51.18868534415483396, -7.964842623401177768 ) ) ;
#68647=CARTESIAN_POINT ( 'NONE',  ( 0.6178305044545818747, 18.49863466993041428, -9.382169495545419124 ) ) ;
#68648=CARTESIAN_POINT ( 'NONE',  ( 17.08211943468705840, 35.13708216824730357, -12.26659068614894466 ) ) ;
#68649=CARTESIAN_POINT ( 'NONE',  ( -0.8801773607111009756, 18.06368534415484106, 1.068504757029289695E-15 ) ) ;
#68650=CARTESIAN_POINT ( 'NONE',  ( 4.559911319644449179, 28.89701867748817321, 9.422509992056141925 ) ) ;
#68651=( BOUNDED_SURFACE ( )  B_SPLINE_SURFACE ( 1, 2, ( 
 ( #7434, #61880, #37930, #70885, #2893, #55380, #63359, #10374, #40875, #86860, #10863, #18366, #48846, #33825, #40387, #41864, #72327, #26344, #93368, #78367, #64331, #86372, #11344, #49340, #55873, #48356, #94842, #79839, #78863, #87344, #2403, #24895, #56845, #79356, #17874, #34320, #33343, #56367, #71851, #32861, #71381, #63837, #93862, #18859, #3860, #9886, #85880, #94351, #62871, #32365, #25870, #41384, #3361, #1908, #25390, #17392, #47861, #77205, #38729, #77694, #23742, #45736, #53230, #61222, #23248, #15745, #68735, #24714, #92700, #266, #8710, #40198, #39719, #70706, #54204, #15257, #9206, #39228, #22747, #76235, #17218, #30711, #24224, #76716, #91726, #93187, #85213, #47697, #53723, #54691, #8234, #84239, #55186, #16717, #38244, #7750, #1243, #47190, #78189, #9702, #2223, #46230, #85702, #754, #62687, #84720, #16224, #31205, #32683, #91220, #69229, #70211, #83734, #46705, #61701, #92216, #69717, #31699, #62190, #1730, #32184, #80597, #19595, #14082, #89077, #96600, #97105, #66072, #12095, #51077, #21584, #28576, #35582, #28077, #58575, #74064, #36582, #20590, #21082, #50092, #81568, #67070, #95599, #5596, #13076, #88578, #43569, #51578, #65573, #42597, #89571, #44060, #36075, #27085, #66578, #50590, #59566, #52074, #59066, #73076, #82067, #5093, #4612, #13575, #74567, #6081, #97597, #82568, #90060, #29059, #35073, #44562, #4116, #88084, #34580, #65074, #57587, #96100, #27582, #58074, #20087, #81081, #12584, #43083, #73569, #84052, #92037, #14581, #37575, #68068, #30538, #77034, #91044, #15081, #585, #75559, #91551, #31524, #75060, #16043, #62020, #16545, #83560, #61038, #46531, #98595, #39046, #23566, #7073, #69541, #31029, #92521, #45552, #30044, #38555, #60051, #68559, #76540, #37078, #24046, #83060, #67576, #6567, #1058, #98087, #52556, #46053, #15572, #54034, #45050, #60553, #22572, #23070, #8547, #53043, #76050, #61529, #7580, #53538, #54517, #29545, #85031, #90551, #22081, #38068, #8056, #91, #69050, #84544, #63975, #47517, #41517, #3030, #3508, #55523, #78019, #1557, #64471, #17535, #87482, #47020, #85525, #40525, #77511, #40023, #70526, #94489, #25527, #79498, #2049, #63009, #48497, #32511, #56018, #86517, #33968, #17038, #9028, #71984, #9522, #78510, #93512, #25038, #2546, #32004, #86020, #41018, #10504, #94978, #48002, #33479, #24549, #62508, #56977, #33003, #71024, #71520, #10025, #55008, #94004, #26481, #26007, #63504, #18015, #78999, #56501, #10997, #86992, #18499, #93013, #48990, #39545, #70033, #88962, #80967, #4494, #96482, #66447, #80479, #57473, #5478, #58953, #42971, #11483, #20470 ),
 ( #19481, #42003, #89453, #12954, #57959, #59438, #4979, #58447, #12467, #43450, #73451, #95484, #65955, #36457, #73951, #50463, #35458, #27954, #50957, #51454, #81453, #35952, #34465, #96982, #81943, #72469, #28459, #20969, #34959, #13452, #43938, #11979, #87967, #74437, #5962, #66951, #4001, #97469, #65457, #28933, #18996, #49473, #49973, #79980, #19965, #42480, #64957, #26975, #72963, #95983, #27465, #88463, #53416, #59931, #45932, #83923, #74940, #83435, #91422, #51954, #46416, #97970, #82439, #89940, #53919, #21457, #67449, #60917, #98961, #7937, #29426, #52440, #82938, #45422, #91916, #6948, #29920, #15453, #90419, #7452, #76906, #13963, #30909, #8419, #31396, #98467, #75927, #61407, #14455, #84428, #38433, #21959, #15925, #76423, #38926, #60426, #44927, #44438, #69413, #90919, #6444, #36952, #75434, #14955, #37455, #67943, #22449, #68931, #68441, #23440, #52922, #37949, #22950, #30417, #461, #936, #48864, #31886, #3380, #86875, #62384, #93387, #92889, #1433, #17413, #46897, #24421, #55894, #25407, #79374, #54885, #17891, #39418, #77388, #71869, #47879, #69913, #78383, #10879, #10390, #41403, #24912, #84908, #78879, #9903, #92403, #16420, #18385, #85401, #93880, #47386, #16913, #63855, #86390, #8901, #77888, #70900, #48375, #61896, #23926, #54397, #9400, #94369, #70407, #33360, #55396, #85896, #1925, #25887, #39901, #32383, #40894, #62888, #40406, #2420, #32877, #63375, #71395, #2909, #56386, #51335, #4376, #73335, #58825, #43333, #34841, #96860, #80848, #34343, #65831, #27836, #88840, #43819, #88347, #72347, #73825, #19845, #66325, #64837, #50337, #18877, #87845, #95862, #27345, #4862, #58323, #35338, #96363, #12833, #95356, #81817, #13335, #5358, #56862, #3879, #35837, #42365, #74315, #89333, #11857, #65336, #28335, #20843, #57838, #33843, #26855, #87363, #64352, #20348, #72838, #94860, #12345, #50844, #81336, #57352, #42852, #26363, #19365, #49359, #79861, #49848, #11364, #41883, #80357, #36331, #60312, #44806, #37830, #90804, #74818, #98839, #84315, #22332, #52320, #91297, #37338, #59318, #66826, #6323, #36833, #29312, #82316, #38316, #7329, #67828, #90302, #83313, #53300, #67324, #44317, #22821, #45816, #29803, #97348, #68320, #82813, #61292, #53804, #14837, #97847, #30294, #6822, #59808, #45311, #83808, #98346, #52806, #15815, #91801, #60797, #21837, #15334, #76304, #89817, #75807, #7821, #28819, #23323, #13836, #21338, #5841, #68812, #51828, #14333, #345, #30787, #46301, #75312, #39305, #69797, #32263, #78765, #92775, #16793, #2302, #77276, #93269, #33249, #76788, #17780, #63742, #18266, #85285, #62768, #48255 ) ),
 .UNSPECIFIED., .F., .F., .F. ) 
 B_SPLINE_SURFACE_WITH_KNOTS ( ( 2, 2 ),
 ( 3, 2, 2, 2, 2, 2, 2, 2, 2, 2, 2, 2, 2, 2, 2, 2, 2, 2, 2, 2, 2, 2, 2, 2, 2, 2, 2, 2, 2, 2, 2, 2, 2, 2, 2, 2, 2, 2, 2, 2, 2, 2, 2, 2, 2, 2, 2, 2, 2, 2, 2, 2, 2, 2, 2, 2, 2, 2, 2, 2, 2, 2, 2, 2, 2, 2, 2, 2, 2, 2, 2, 2, 2, 2, 2, 2, 2, 2, 2, 2, 2, 2, 2, 2, 2, 2, 2, 2, 2, 2, 2, 2, 2, 2, 2, 2, 2, 2, 2, 2, 2, 2, 2, 2, 2, 2, 2, 2, 2, 2, 2, 2, 2, 2, 2, 2, 2, 2, 2, 2, 2, 2, 2, 2, 2, 2, 2, 2, 2, 2, 2, 2, 2, 2, 2, 2, 2, 2, 2, 2, 2, 2, 2, 2, 2, 2, 2, 2, 2, 2, 2, 2, 2, 2, 2, 2, 2, 2, 2, 2, 2, 2, 3 ),
 ( 0.000000000000000000, 1.000000000000000000 ),
 ( 0.000000000000000000, 0.005952380952380952051, 0.01190476190476190410, 0.01785714285714285615, 0.02380952380952380820, 0.02976190476190476025, 0.03571428571428571230, 0.04166666666666666435, 0.04761904761904761640, 0.05357142857142856845, 0.05952380952380952051, 0.06547619047619047949, 0.07142857142857142461, 0.07738095238095238360, 0.08333333333333332871, 0.08928571428571428770, 0.09523809523809523281, 0.1011904761904761918, 0.1071428571428571369, 0.1130952380952380959, 0.1190476190476190410, 0.1250000000000000000, 0.1309523809523809590, 0.1369047619047619180, 0.1428571428571428492, 0.1488095238095238082, 0.1547619047619047672, 0.1607142857142857262, 0.1666666666666666574, 0.1726190476190476164, 0.1785714285714285754, 0.1845238095238095344, 0.1904761904761904656, 0.1964285714285714246, 0.2023809523809523836, 0.2083333333333333426, 0.2142857142857142738, 0.2202380952380952328, 0.2261904761904761918, 0.2321428571428571508, 0.2380952380952380820, 0.2440476190476190410, 0.2500000000000000000, 0.2559523809523809312, 0.2619047619047619180, 0.2678571428571428492, 0.2738095238095238360, 0.2797619047619047672, 0.2857142857142856984, 0.2916666666666666852, 0.2976190476190476164, 0.3035714285714285476, 0.3095238095238095344, 0.3154761904761904656, 0.3214285714285714524, 0.3273809523809523836, 0.3333333333333333148, 0.3392857142857143016, 0.3452380952380952328, 0.3511904761904761640, 0.3571428571428571508, 0.3630952380952380820, 0.3690476190476190688, 0.3750000000000000000, 0.3809523809523809312, 0.3869047619047619180, 0.3928571428571428492, 0.3988095238095238360, 0.4047619047619047672, 0.4107142857142856984, 0.4166666666666666852, 0.4226190476190476164, 0.4285714285714285476, 0.4345238095238095344, 0.4404761904761904656, 0.4464285714285714524, 0.4523809523809523836, 0.4583333333333333148, 0.4642857142857143016, 0.4702380952380952328, 0.4761904761904761640, 0.4821428571428571508, 0.4880952380952380820, 0.4940476190476190688, 0.5000000000000000000, 0.5059523809523809312, 0.5119047619047618625, 0.5178571428571429047, 0.5238095238095238360, 0.5297619047619047672, 0.5357142857142856984, 0.5416666666666666297, 0.5476190476190476719, 0.5535714285714286031, 0.5595238095238095344, 0.5654761904761904656, 0.5714285714285713969, 0.5773809523809523281, 0.5833333333333333703, 0.5892857142857143016, 0.5952380952380952328, 0.6011904761904761640, 0.6071428571428570953, 0.6130952380952381375, 0.6190476190476190688, 0.6250000000000000000, 0.6309523809523809312, 0.6369047619047618625, 0.6428571428571429047, 0.6488095238095238360, 0.6547619047619047672, 0.6607142857142856984, 0.6666666666666666297, 0.6726190476190476719, 0.6785714285714286031, 0.6845238095238095344, 0.6904761904761904656, 0.6964285714285713969, 0.7023809523809523281, 0.7083333333333333703, 0.7142857142857143016, 0.7202380952380952328, 0.7261904761904761640, 0.7321428571428570953, 0.7380952380952381375, 0.7440476190476190688, 0.7500000000000000000, 0.7559523809523809312, 0.7619047619047618625, 0.7678571428571429047, 0.7738095238095238360, 0.7797619047619047672, 0.7857142857142856984, 0.7916666666666666297, 0.7976190476190476719, 0.8035714285714286031, 0.8095238095238095344, 0.8154761904761904656, 0.8214285714285713969, 0.8273809523809523281, 0.8333333333333333703, 0.8392857142857143016, 0.8452380952380952328, 0.8511904761904761640, 0.8571428571428570953, 0.8630952380952381375, 0.8690476190476190688, 0.8750000000000000000, 0.8809523809523809312, 0.8869047619047618625, 0.8928571428571429047, 0.8988095238095238360, 0.9047619047619047672, 0.9107142857142856984, 0.9166666666666666297, 0.9226190476190476719, 0.9285714285714286031, 0.9345238095238095344, 0.9404761904761904656, 0.9464285714285713969, 0.9523809523809523281, 0.9583333333333333703, 0.9642857142857143016 ),
 .UNSPECIFIED. ) 
 GEOMETRIC_REPRESENTATION_ITEM ( )  RATIONAL_B_SPLINE_SURFACE ( (
 ( 1.000000000000000000, 0.9659258262890683122, 1.000000000000000000, 0.9659258262890683122, 1.000000000000000000, 0.9659258262890683122, 1.000000000000000000, 0.9659258262890683122, 1.000000000000000000, 0.9659258262890683122, 1.000000000000000000, 0.9659258262890683122, 1.000000000000000000, 0.9659258262890683122, 1.000000000000000000, 0.9659258262890683122, 1.000000000000000000, 0.9659258262890683122, 1.000000000000000000, 0.9659258262890683122, 1.000000000000000000, 0.9659258262890683122, 1.000000000000000000, 0.9659258262890683122, 1.000000000000000000, 0.9659258262890683122, 1.000000000000000000, 0.9659258262890683122, 1.000000000000000000, 0.9659258262890683122, 1.000000000000000000, 0.9659258262890683122, 1.000000000000000000, 0.9659258262890683122, 1.000000000000000000, 0.9659258262890683122, 1.000000000000000000, 0.9659258262890683122, 1.000000000000000000, 0.9659258262890683122, 1.000000000000000000, 0.9659258262890683122, 1.000000000000000000, 0.9659258262890683122, 1.000000000000000000, 0.9659258262890683122, 1.000000000000000000, 0.9659258262890683122, 1.000000000000000000, 0.9659258262890683122, 1.000000000000000000, 0.9659258262890683122, 1.000000000000000000, 0.9659258262890683122, 1.000000000000000000, 0.9659258262890683122, 1.000000000000000000, 0.9659258262890683122, 1.000000000000000000, 0.9659258262890683122, 1.000000000000000000, 0.9659258262890683122, 1.000000000000000000, 0.9659258262890683122, 1.000000000000000000, 0.9659258262890683122, 1.000000000000000000, 0.9659258262890683122, 1.000000000000000000, 0.9659258262890683122, 1.000000000000000000, 0.9659258262890683122, 1.000000000000000000, 0.9659258262890683122, 1.000000000000000000, 0.9659258262890683122, 1.000000000000000000, 0.9659258262890683122, 1.000000000000000000, 0.9659258262890683122, 1.000000000000000000, 0.9659258262890683122, 1.000000000000000000, 0.9659258262890683122, 1.000000000000000000, 0.9659258262890683122, 1.000000000000000000, 0.9659258262890683122, 1.000000000000000000, 0.9659258262890683122, 1.000000000000000000, 0.9659258262890683122, 1.000000000000000000, 0.9659258262890683122, 1.000000000000000000, 0.9659258262890683122, 1.000000000000000000, 0.9659258262890683122, 1.000000000000000000, 0.9659258262890683122, 1.000000000000000000, 0.9659258262890683122, 1.000000000000000000, 0.9659258262890683122, 1.000000000000000000, 0.9659258262890683122, 1.000000000000000000, 0.9659258262890683122, 1.000000000000000000, 0.9659258262890683122, 1.000000000000000000, 0.9659258262890683122, 1.000000000000000000, 0.9659258262890683122, 1.000000000000000000, 0.9659258262890683122, 1.000000000000000000, 0.9659258262890683122, 1.000000000000000000, 0.9659258262890683122, 1.000000000000000000, 0.9659258262890683122, 1.000000000000000000, 0.9659258262890683122, 1.000000000000000000, 0.9659258262890683122, 1.000000000000000000, 0.9659258262890683122, 1.000000000000000000, 0.9659258262890683122, 1.000000000000000000, 0.9659258262890683122, 1.000000000000000000, 0.9659258262890683122, 1.000000000000000000, 0.9659258262890683122, 1.000000000000000000, 0.9659258262890683122, 1.000000000000000000, 0.9659258262890683122, 1.000000000000000000, 0.9659258262890683122, 1.000000000000000000, 0.9659258262890683122, 1.000000000000000000, 0.9659258262890683122, 1.000000000000000000, 0.9659258262890683122, 1.000000000000000000, 0.9659258262890683122, 1.000000000000000000, 0.9659258262890683122, 1.000000000000000000, 0.9659258262890683122, 1.000000000000000000, 0.9659258262890683122, 1.000000000000000000, 0.9659258262890683122, 1.000000000000000000, 0.9659258262890683122, 1.000000000000000000, 0.9659258262890683122, 1.000000000000000000, 0.9659258262890683122, 1.000000000000000000, 0.9659258262890683122, 1.000000000000000000, 0.9659258262890683122, 1.000000000000000000, 0.9659258262890683122, 1.000000000000000000, 0.9659258262890683122, 1.000000000000000000, 0.9659258262890683122, 1.000000000000000000, 0.9659258262890683122, 1.000000000000000000, 0.9659258262890683122, 1.000000000000000000, 0.9659258262890683122, 1.000000000000000000, 0.9659258262890683122, 1.000000000000000000, 0.9659258262890683122, 1.000000000000000000, 0.9659258262890683122, 1.000000000000000000, 0.9659258262890683122, 1.000000000000000000, 0.9659258262890683122, 1.000000000000000000, 0.9659258262890683122, 1.000000000000000000, 0.9659258262890683122, 1.000000000000000000, 0.9659258262890683122, 1.000000000000000000, 0.9659258262890683122, 1.000000000000000000, 0.9659258262890683122, 1.000000000000000000, 0.9659258262890683122, 1.000000000000000000, 0.9659258262890683122, 1.000000000000000000, 0.9659258262890683122, 1.000000000000000000, 0.9659258262890683122, 1.000000000000000000, 0.9659258262890683122, 1.000000000000000000, 0.9659258262890683122, 1.000000000000000000, 0.9659258262890683122, 1.000000000000000000, 0.9659258262890683122, 1.000000000000000000, 0.9659258262890683122, 1.000000000000000000, 0.9659258262890683122, 1.000000000000000000, 0.9659258262890683122, 1.000000000000000000, 0.9659258262890683122, 1.000000000000000000, 0.9659258262890683122, 1.000000000000000000, 0.9659258262890683122, 1.000000000000000000, 0.9659258262890683122, 1.000000000000000000, 0.9659258262890683122, 1.000000000000000000, 0.9659258262890683122, 1.000000000000000000, 0.9659258262890683122, 1.000000000000000000, 0.9659258262890683122, 1.000000000000000000, 0.9659258262890683122, 1.000000000000000000, 0.9659258262890683122, 1.000000000000000000, 0.9659258262890683122, 1.000000000000000000, 0.9659258262890683122, 1.000000000000000000, 0.9659258262890683122, 1.000000000000000000, 0.9659258262890683122, 1.000000000000000000, 0.9659258262890683122, 1.000000000000000000, 0.9659258262890683122, 1.000000000000000000, 0.9659258262890683122, 1.000000000000000000, 0.9659258262890683122, 1.000000000000000000, 0.9659258262890683122, 1.000000000000000000, 0.9659258262890683122, 1.000000000000000000, 0.9659258262890683122, 1.000000000000000000, 0.9659258262890683122, 1.000000000000000000, 0.9659258262890683122, 1.000000000000000000, 0.9659258262890683122, 1.000000000000000000, 0.9659258262890683122, 1.000000000000000000, 0.9659258262890683122, 1.000000000000000000, 0.9659258262890683122, 1.000000000000000000, 0.9659258262890683122, 1.000000000000000000, 0.9659258262890683122, 1.000000000000000000, 0.9659258262890683122, 1.000000000000000000, 0.9659258262890683122, 1.000000000000000000, 0.9659258262890683122, 1.000000000000000000, 0.9659258262890683122, 1.000000000000000000, 0.9659258262890683122, 1.000000000000000000, 0.9659258262890683122, 1.000000000000000000, 0.9659258262890683122, 1.000000000000000000, 0.9659258262890683122, 1.000000000000000000, 0.9659258262890683122, 1.000000000000000000, 0.9659258262890683122, 1.000000000000000000, 0.9659258262890683122, 1.000000000000000000, 0.9659258262890683122, 1.000000000000000000, 0.9659258262890683122, 1.000000000000000000, 0.9659258262890683122, 1.000000000000000000, 0.9659258262890683122, 1.000000000000000000, 0.9659258262890683122, 1.000000000000000000, 0.9659258262890683122, 1.000000000000000000, 0.9659258262890683122, 1.000000000000000000, 0.9659258262890683122, 1.000000000000000000, 0.9659258262890683122, 1.000000000000000000, 0.9659258262890683122, 1.000000000000000000, 0.9659258262890683122, 1.000000000000000000),
 ( 1.000000000000000000, 0.9659258262890683122, 1.000000000000000000, 0.9659258262890683122, 1.000000000000000000, 0.9659258262890683122, 1.000000000000000000, 0.9659258262890683122, 1.000000000000000000, 0.9659258262890683122, 1.000000000000000000, 0.9659258262890683122, 1.000000000000000000, 0.9659258262890683122, 1.000000000000000000, 0.9659258262890683122, 1.000000000000000000, 0.9659258262890683122, 1.000000000000000000, 0.9659258262890683122, 1.000000000000000000, 0.9659258262890683122, 1.000000000000000000, 0.9659258262890683122, 1.000000000000000000, 0.9659258262890683122, 1.000000000000000000, 0.9659258262890683122, 1.000000000000000000, 0.9659258262890683122, 1.000000000000000000, 0.9659258262890683122, 1.000000000000000000, 0.9659258262890683122, 1.000000000000000000, 0.9659258262890683122, 1.000000000000000000, 0.9659258262890683122, 1.000000000000000000, 0.9659258262890683122, 1.000000000000000000, 0.9659258262890683122, 1.000000000000000000, 0.9659258262890683122, 1.000000000000000000, 0.9659258262890683122, 1.000000000000000000, 0.9659258262890683122, 1.000000000000000000, 0.9659258262890683122, 1.000000000000000000, 0.9659258262890683122, 1.000000000000000000, 0.9659258262890683122, 1.000000000000000000, 0.9659258262890683122, 1.000000000000000000, 0.9659258262890683122, 1.000000000000000000, 0.9659258262890683122, 1.000000000000000000, 0.9659258262890683122, 1.000000000000000000, 0.9659258262890683122, 1.000000000000000000, 0.9659258262890683122, 1.000000000000000000, 0.9659258262890683122, 1.000000000000000000, 0.9659258262890683122, 1.000000000000000000, 0.9659258262890683122, 1.000000000000000000, 0.9659258262890683122, 1.000000000000000000, 0.9659258262890683122, 1.000000000000000000, 0.9659258262890683122, 1.000000000000000000, 0.9659258262890683122, 1.000000000000000000, 0.9659258262890683122, 1.000000000000000000, 0.9659258262890683122, 1.000000000000000000, 0.9659258262890683122, 1.000000000000000000, 0.9659258262890683122, 1.000000000000000000, 0.9659258262890683122, 1.000000000000000000, 0.9659258262890683122, 1.000000000000000000, 0.9659258262890683122, 1.000000000000000000, 0.9659258262890683122, 1.000000000000000000, 0.9659258262890683122, 1.000000000000000000, 0.9659258262890683122, 1.000000000000000000, 0.9659258262890683122, 1.000000000000000000, 0.9659258262890683122, 1.000000000000000000, 0.9659258262890683122, 1.000000000000000000, 0.9659258262890683122, 1.000000000000000000, 0.9659258262890683122, 1.000000000000000000, 0.9659258262890683122, 1.000000000000000000, 0.9659258262890683122, 1.000000000000000000, 0.9659258262890683122, 1.000000000000000000, 0.9659258262890683122, 1.000000000000000000, 0.9659258262890683122, 1.000000000000000000, 0.9659258262890683122, 1.000000000000000000, 0.9659258262890683122, 1.000000000000000000, 0.9659258262890683122, 1.000000000000000000, 0.9659258262890683122, 1.000000000000000000, 0.9659258262890683122, 1.000000000000000000, 0.9659258262890683122, 1.000000000000000000, 0.9659258262890683122, 1.000000000000000000, 0.9659258262890683122, 1.000000000000000000, 0.9659258262890683122, 1.000000000000000000, 0.9659258262890683122, 1.000000000000000000, 0.9659258262890683122, 1.000000000000000000, 0.9659258262890683122, 1.000000000000000000, 0.9659258262890683122, 1.000000000000000000, 0.9659258262890683122, 1.000000000000000000, 0.9659258262890683122, 1.000000000000000000, 0.9659258262890683122, 1.000000000000000000, 0.9659258262890683122, 1.000000000000000000, 0.9659258262890683122, 1.000000000000000000, 0.9659258262890683122, 1.000000000000000000, 0.9659258262890683122, 1.000000000000000000, 0.9659258262890683122, 1.000000000000000000, 0.9659258262890683122, 1.000000000000000000, 0.9659258262890683122, 1.000000000000000000, 0.9659258262890683122, 1.000000000000000000, 0.9659258262890683122, 1.000000000000000000, 0.9659258262890683122, 1.000000000000000000, 0.9659258262890683122, 1.000000000000000000, 0.9659258262890683122, 1.000000000000000000, 0.9659258262890683122, 1.000000000000000000, 0.9659258262890683122, 1.000000000000000000, 0.9659258262890683122, 1.000000000000000000, 0.9659258262890683122, 1.000000000000000000, 0.9659258262890683122, 1.000000000000000000, 0.9659258262890683122, 1.000000000000000000, 0.9659258262890683122, 1.000000000000000000, 0.9659258262890683122, 1.000000000000000000, 0.9659258262890683122, 1.000000000000000000, 0.9659258262890683122, 1.000000000000000000, 0.9659258262890683122, 1.000000000000000000, 0.9659258262890683122, 1.000000000000000000, 0.9659258262890683122, 1.000000000000000000, 0.9659258262890683122, 1.000000000000000000, 0.9659258262890683122, 1.000000000000000000, 0.9659258262890683122, 1.000000000000000000, 0.9659258262890683122, 1.000000000000000000, 0.9659258262890683122, 1.000000000000000000, 0.9659258262890683122, 1.000000000000000000, 0.9659258262890683122, 1.000000000000000000, 0.9659258262890683122, 1.000000000000000000, 0.9659258262890683122, 1.000000000000000000, 0.9659258262890683122, 1.000000000000000000, 0.9659258262890683122, 1.000000000000000000, 0.9659258262890683122, 1.000000000000000000, 0.9659258262890683122, 1.000000000000000000, 0.9659258262890683122, 1.000000000000000000, 0.9659258262890683122, 1.000000000000000000, 0.9659258262890683122, 1.000000000000000000, 0.9659258262890683122, 1.000000000000000000, 0.9659258262890683122, 1.000000000000000000, 0.9659258262890683122, 1.000000000000000000, 0.9659258262890683122, 1.000000000000000000, 0.9659258262890683122, 1.000000000000000000, 0.9659258262890683122, 1.000000000000000000, 0.9659258262890683122, 1.000000000000000000, 0.9659258262890683122, 1.000000000000000000, 0.9659258262890683122, 1.000000000000000000, 0.9659258262890683122, 1.000000000000000000, 0.9659258262890683122, 1.000000000000000000, 0.9659258262890683122, 1.000000000000000000, 0.9659258262890683122, 1.000000000000000000, 0.9659258262890683122, 1.000000000000000000, 0.9659258262890683122, 1.000000000000000000, 0.9659258262890683122, 1.000000000000000000, 0.9659258262890683122, 1.000000000000000000, 0.9659258262890683122, 1.000000000000000000, 0.9659258262890683122, 1.000000000000000000, 0.9659258262890683122, 1.000000000000000000, 0.9659258262890683122, 1.000000000000000000, 0.9659258262890683122, 1.000000000000000000, 0.9659258262890683122, 1.000000000000000000, 0.9659258262890683122, 1.000000000000000000, 0.9659258262890683122, 1.000000000000000000, 0.9659258262890683122, 1.000000000000000000, 0.9659258262890683122, 1.000000000000000000, 0.9659258262890683122, 1.000000000000000000, 0.9659258262890683122, 1.000000000000000000, 0.9659258262890683122, 1.000000000000000000, 0.9659258262890683122, 1.000000000000000000, 0.9659258262890683122, 1.000000000000000000, 0.9659258262890683122, 1.000000000000000000, 0.9659258262890683122, 1.000000000000000000, 0.9659258262890683122, 1.000000000000000000, 0.9659258262890683122, 1.000000000000000000, 0.9659258262890683122, 1.000000000000000000, 0.9659258262890683122, 1.000000000000000000, 0.9659258262890683122, 1.000000000000000000, 0.9659258262890683122, 1.000000000000000000, 0.9659258262890683122, 1.000000000000000000, 0.9659258262890683122, 1.000000000000000000, 0.9659258262890683122, 1.000000000000000000, 0.9659258262890683122, 1.000000000000000000, 0.9659258262890683122, 1.000000000000000000) ) ) 
 REPRESENTATION_ITEM ( '' )  SURFACE ( )  );
#68652=CARTESIAN_POINT ( 'NONE',  ( 18.04007052943771683, 53.01528370094807485, 5.767676674365856293 ) ) ;
#68653=CARTESIAN_POINT ( 'NONE',  ( 2.035157376598822676, 52.43868534415483396, -7.964842623401177768 ) ) ;
#68659=CARTESIAN_POINT ( 'NONE',  ( -0.2418659066527775181, 13.09014588040356841, 6.114288769123032985 ) ) ;
#68660=DIRECTION ( 'NONE',  ( 0.000000000000000000, -0.000000000000000000, 1.000000000000000000 ) ) ;
#68663=CARTESIAN_POINT ( 'NONE',  ( 0.1129803114748898080, 19.29427333184091609, -6.480634945678687586 ) ) ;
#68664=CARTESIAN_POINT ( 'NONE',  ( 20.36894250292379738, 59.92874883491397497, -10.36894250292379027 ) ) ;
#68665=CARTESIAN_POINT ( 'NONE',  ( 13.79529636645030344, 63.26208216824730357, 14.16423886937410614 ) ) ;
#68666=CARTESIAN_POINT ( 'NONE',  ( 2.791683348922237240, 20.38393115100078745, -7.208316651077763204 ) ) ;
#68667=CARTESIAN_POINT ( 'NONE',  ( 17.20831665107776587, 62.88393115100078745, 7.208316651077764980 ) ) ;
#68668=CARTESIAN_POINT ( 'NONE',  ( -0.8801773607111009756, 68.06368534415484817, 1.068504757029289695E-15 ) ) ;
#68670=EDGE_CURVE ( 'NONE', #92829, #98109, #35671, .T. ) ;
#68673=CARTESIAN_POINT ( 'NONE',  ( 13.79529636645030344, 33.26208216824730357, 14.16423886937410614 ) ) ;
#68674=EDGE_CURVE ( 'NONE', #17007, #39149, #2225, .T. ) ;
#68675=CARTESIAN_POINT ( 'NONE',  ( 24.16423886937410614, 49.51208216824730357, -3.795296366450302550 ) ) ;
#68677=CARTESIAN_POINT ( 'NONE',  ( 22.81628187352647785, 61.41530133659709634, 3.434112377981063169 ) ) ;
#68678=CARTESIAN_POINT ( 'NONE',  ( -0.8801773607111009756, 28.06368534415484106, 1.068504757029289695E-15 ) ) ;
#68679=CARTESIAN_POINT ( 'NONE',  ( 17.20831665107776587, 47.88393115100078745, 7.208316651077764980 ) ) ;
#68680=CARTESIAN_POINT ( 'NONE',  ( 2.035157376598824452, 23.68868534415484461, 7.964842623401179544 ) ) ;
#68683=CARTESIAN_POINT ( 'NONE',  ( 0.1532563361054083140, 61.00893115100078745, 1.131784320476157264E-15 ) ) ;
#68684=CARTESIAN_POINT ( 'NONE',  ( 10.00000000000000000, 44.75893115100078745, -9.846743663894594434 ) ) ;
#68685=LINE ( 'NONE', #67202, #36072 ) ;
#68686=CARTESIAN_POINT ( 'NONE',  ( 0.2751277870542965243, 3.218334437839379891, 6.500000000000000888 ) ) ;
#68687=CARTESIAN_POINT ( 'NONE',  ( 12.63842701281683034, 2.467264484334118269, 9.846743663894596210 ) ) ;
#68688=CARTESIAN_POINT ( 'NONE',  ( 18.29284471827479663, 20.40189080397285437, -6.500000000000035527 ) ) ;
#68689=ORIENTED_EDGE ( 'NONE', *, *, #97764, .F. ) ;
#68690=CARTESIAN_POINT ( 'NONE',  ( 19.65595514172846947, 85.79709332851908243, 5.361975859778444153 ) ) ;
#68691=CARTESIAN_POINT ( 'NONE',  ( 7.361572987183170547, 32.05059781766745175, 9.846743663894590881 ) ) ;
#68693=CARTESIAN_POINT ( 'NONE',  ( 22.81628187352647785, 31.62363466993042138, 6.195893100308588602E-16 ) ) ;
#68697=DIRECTION ( 'NONE',  ( 0.000000000000000000, 0.000000000000000000, 1.000000000000000000 ) ) ;
#68699=CARTESIAN_POINT ( 'NONE',  ( 19.84674366389459621, 43.50893115100078745, 7.409399052514197653E-17 ) ) ;
#68700=CARTESIAN_POINT ( 'NONE',  ( -2.266590686148945544, 32.22041550158063927, 7.082119434687048631 ) ) ;
#68701=CARTESIAN_POINT ( 'NONE',  ( 0.1532563361054082862, 56.21726448433411605, 2.638427012816831674 ) ) ;
#68702=CARTESIAN_POINT ( 'NONE',  ( 17.39651004071841811, 2.935752660568277328, 6.500000000000002665 ) ) ;
#68703=CARTESIAN_POINT ( 'NONE',  ( 19.84674366389459266, 8.717264484334116048, -2.638427012816827677 ) ) ;
#68704=CARTESIAN_POINT ( 'NONE',  ( -4.164238869374098151, 1.595415501580634388, -3.795296366450310543 ) ) ;
#68705=CARTESIAN_POINT ( 'NONE',  ( 0.1532563361054100626, 50.80059781766745175, -2.638427012816831230 ) ) ;
#68706=CARTESIAN_POINT ( 'NONE',  ( 4.559911319644449179, 52.23035201082151247, -9.422509992056141925 ) ) ;
#68708=CARTESIAN_POINT ( 'NONE',  ( 10.00000000000000000, 44.75893115100078745, -9.846743663894594434 ) ) ;
#68710=CARTESIAN_POINT ( 'NONE',  ( 2.035157376598822676, 47.43868534415484817, -7.964842623401177768 ) ) ;
#68713=CARTESIAN_POINT ( 'NONE',  ( 4.559911319644449179, 27.23035201082150536, -9.422509992056141925 ) ) ;
#68715=CARTESIAN_POINT ( 'NONE',  ( -2.816281873526473856, -0.8763653300695799508, 9.499525473075851096E-16 ) ) ;
#68716=CARTESIAN_POINT ( 'NONE',  ( 10.00000000000000178, 59.31368534415484106, 10.88017736071110342 ) ) ;
#68719=CARTESIAN_POINT ( 'NONE',  ( 4.559911319644449179, 68.89701867748817676, 9.422509992056141925 ) ) ;
#68722=CARTESIAN_POINT ( 'NONE',  ( 17.96484262340118221, 36.18868534415484106, -7.964842623401177768 ) ) ;
#68723=CARTESIAN_POINT ( 'NONE',  ( -46.44000000000001194, 100.8660254037844339, 9.500000000000000000 ) ) ;
#68724=CARTESIAN_POINT ( 'NONE',  ( 5.076628168052704559, 15.17559781766745175, -8.527530157486179263 ) ) ;
#68725=CARTESIAN_POINT ( 'NONE',  ( 14.92337183194729633, 37.67559781766745175, 8.527530157486181039 ) ) ;
#68726=( NAMED_UNIT ( * ) PLANE_ANGLE_UNIT ( ) SI_UNIT ( $, .RADIAN. ) );
#68728=CARTESIAN_POINT ( 'NONE',  ( 3.591859063236761518, -0.04303199673624671928, 11.09922568453594849 ) ) ;
#68729=VECTOR ( 'NONE', #92165, 1000.000000000000000 ) ;
#68730=CARTESIAN_POINT ( 'NONE',  ( -4.164238869374099039, 61.80374883491397497, 8.674139862899312516E-16 ) ) ;
#68733=CARTESIAN_POINT ( 'NONE',  ( 2.917880565312948704, 22.63708216824730002, 12.26659068614894643 ) ) ;
#68734=CARTESIAN_POINT ( 'NONE',  ( 24.16423886937409904, 54.09541550158063217, 3.795296366450317205 ) ) ;
#68735=CARTESIAN_POINT ( 'NONE',  ( 19.84674366389459621, 13.50893115100078568, 7.409399052514197653E-17 ) ) ;
#68736=CARTESIAN_POINT ( 'NONE',  ( -0.8801773607111008646, 3.272018677488171434, 2.915334737309923430 ) ) ;
#68738=CARTESIAN_POINT ( 'NONE',  ( 1.472469842513823179, 20.59226448433411960, -4.923371831947296329 ) ) ;
#68739=CARTESIAN_POINT ( 'NONE',  ( 4.559911319644449179, 33.89701867748817676, 9.422509992056141925 ) ) ;
#68740=CARTESIAN_POINT ( 'NONE',  ( 17.20831665107776587, 47.88393115100078745, 7.208316651077764980 ) ) ;
#68741=CARTESIAN_POINT ( 'NONE',  ( -2.266590686148945544, 12.22041550158063394, 7.082119434687048631 ) ) ;
#68744=CARTESIAN_POINT ( 'NONE',  ( 0.1532563361054083140, 6.008931151000784787, 1.131784320476157264E-15 ) ) ;
#68745=CARTESIAN_POINT ( 'NONE',  ( 6.565887622018943937, 40.16530133659708923, 12.81628187352647430 ) ) ;
#68746=CARTESIAN_POINT ( 'NONE',  ( 19.84674366389459266, 38.30059781766745175, 2.638427012816836559 ) ) ;
#68748=CARTESIAN_POINT ( 'NONE',  ( 19.84674366389459266, 28.30059781766745886, 2.638427012816836559 ) ) ;
#68751=CARTESIAN_POINT ( 'NONE',  ( -0.3689425029237881626, 57.42874883491397497, 10.36894250292379027 ) ) ;
#68752=CARTESIAN_POINT ( 'NONE',  ( 12.91533473730993009, 56.60535201082151247, -10.88017736071109987 ) ) ;
#68753=FILL_AREA_STYLE_COLOUR ( '', #72911 ) ;
#68755=CARTESIAN_POINT ( 'NONE',  ( 21.92686044187657046, 52.39664270246083788, -3.195792623639524432 ) ) ;
#68756=CARTESIAN_POINT ( 'NONE',  ( 12.63842701281683922, 34.55059781766745886, -9.846743663894590881 ) ) ;
#68757=CARTESIAN_POINT ( 'NONE',  ( 10.00000000000000000, 1.813685344154837731, -10.88017736071110342 ) ) ;
#68758=CARTESIAN_POINT ( 'NONE',  ( 0.1532563361054083140, 46.00893115100079456, 1.131784320476157264E-15 ) ) ;
#68760=CARTESIAN_POINT ( 'NONE',  ( 14.92337183194729988, 54.34226448433412315, -8.527530157486177487 ) ) ;
#68761=CARTESIAN_POINT ( 'NONE',  ( 19.42250999205614548, 50.98035201082151247, -5.440088680355545492 ) ) ;
#68768=CARTESIAN_POINT ( 'NONE',  ( 0.1532563361054100626, 5.800597817667452638, -2.638427012816831230 ) ) ;
#68769=CARTESIAN_POINT ( 'NONE',  ( 6.565887622018943937, 55.16530133659709634, 12.81628187352647430 ) ) ;
#68770=CARTESIAN_POINT ( 'NONE',  ( -2.266590686148945544, 66.38708216824730357, -7.082119434687050408 ) ) ;
#68771=CARTESIAN_POINT ( 'NONE',  ( 14.92337183194729988, 44.34226448433412315, -8.527530157486177487 ) ) ;
#68772=CARTESIAN_POINT ( 'NONE',  ( 20.00000000000000355, 88.21129152568919096, 4.994901225422943902 ) ) ;
#68775=CARTESIAN_POINT ( 'NONE',  ( 24.16423886937410614, 29.30374883491396787, 8.672049930838204340E-16 ) ) ;
#68776=CARTESIAN_POINT ( 'NONE',  ( 10.00000000000000178, 58.05374883491397497, 14.16423886937410082 ) ) ;
#68777=CARTESIAN_POINT ( 'NONE',  ( 10.00000000000000178, 62.25893115100078745, 9.846743663894594434 ) ) ;
#68779=CARTESIAN_POINT ( 'NONE',  ( -0.8801773607111008646, 48.27201867748816966, 2.915334737309923430 ) ) ;
#68780=CARTESIAN_POINT ( 'NONE',  ( 5.076628168052704559, 0.1755978176674514724, -8.527530157486179263 ) ) ;
#68782=CARTESIAN_POINT ( 'NONE',  ( 19.38216949554541557, 62.24863466993041072, -9.382169495545420901 ) ) ;
#68785=CARTESIAN_POINT ( 'NONE',  ( 7.361572987183169658, 4.967264484334119601, -9.846743663894592657 ) ) ;
#68786=ORIENTED_EDGE ( 'NONE', *, *, #27348, .F. ) ;
#68787=CARTESIAN_POINT ( 'NONE',  ( 20.36894250292379738, 19.92874883491396787, -10.36894250292379027 ) ) ;
#68788=CARTESIAN_POINT ( 'NONE',  ( 2.791683348922240793, 21.63393115100078745, 7.208316651077764092 ) ) ;
#68789=CARTESIAN_POINT ( 'NONE',  ( 20.88017736071110164, 35.35535201082150536, 2.915334737309930979 ) ) ;
#68793=CARTESIAN_POINT ( 'NONE',  ( 12.91533473730993009, 26.60535201082150536, -10.88017736071109987 ) ) ;
#68795=AXIS2_PLACEMENT_3D ( 'NONE', #45878, #40346, #31343 ) ;
#68796=FACE_OUTER_BOUND ( 'NONE', #64554, .T. ) ;
#68797=VERTEX_POINT ( 'NONE', #52771 ) ;
#68801=CARTESIAN_POINT ( 'NONE',  ( 6.565887622018943937, 18.08196800326375708, -12.81628187352647608 ) ) ;
#68802=CARTESIAN_POINT ( 'NONE',  ( 1.472469842513823179, 5.592264484334118713, -4.923371831947296329 ) ) ;
#68805=CARTESIAN_POINT ( 'NONE',  ( 1.472469842513823179, 16.42559781766745175, 4.923371831947296329 ) ) ;
#68807=CARTESIAN_POINT ( 'NONE',  ( 20.88017736071110519, 25.56368534415483751, 2.639326808657452039E-16 ) ) ;
#68809=CARTESIAN_POINT ( 'NONE',  ( -1.099225684535947600, 63.70696800326376774, -6.408140936763238038 ) ) ;
#68810=CARTESIAN_POINT ( 'NONE',  ( 15.44008868035555260, 59.73035201082151247, 9.422509992056143702 ) ) ;
#68812=CARTESIAN_POINT ( 'NONE',  ( 13.43411237798105340, 60.58196800326376064, 12.81628187352647963 ) ) ;
#68813=CARTESIAN_POINT ( 'NONE',  ( 2.035157376598822676, 57.43868534415484106, -7.964842623401177768 ) ) ;
#68814=CARTESIAN_POINT ( 'NONE',  ( 19.84674366389459266, 63.71726448433412315, -2.638427012816827677 ) ) ;
#68816=CARTESIAN_POINT ( 'NONE',  ( 2.791683348922240793, 26.63393115100078745, 7.208316651077764092 ) ) ;
#68817=CARTESIAN_POINT ( 'NONE',  ( 10.00000000000000178, 50.37363466993042493, 12.81628187352647608 ) ) ;
#68818=CARTESIAN_POINT ( 'NONE',  ( -0.1688089201193209155, 79.91181047996344944, 9.500000000000000000 ) ) ;
#68819=CARTESIAN_POINT ( 'NONE',  ( 19.84674366389459266, 23.30059781766745530, 2.638427012816836559 ) ) ;
#68820=CARTESIAN_POINT ( 'NONE',  ( 10.00000000000000178, 15.37363466993042138, 12.81628187352647608 ) ) ;
#68823=CARTESIAN_POINT ( 'NONE',  ( 15.44008868035555260, 34.73035201082151247, 9.422509992056143702 ) ) ;
#68824=CARTESIAN_POINT ( 'NONE',  ( 7.361572987183170547, 62.05059781766745886, 9.846743663894590881 ) ) ;
#68827=CARTESIAN_POINT ( 'NONE',  ( 14.92337183194729988, 19.34226448433411960, -8.527530157486177487 ) ) ;
#68828=CARTESIAN_POINT ( 'NONE',  ( 7.361572987183169658, 9.967264484334119601, -9.846743663894592657 ) ) ;
#68829=CARTESIAN_POINT ( 'NONE',  ( 10.00000000000000178, 19.31368534415484106, 10.88017736071110342 ) ) ;
#68831=CARTESIAN_POINT ( 'NONE',  ( -1.099225684535947600, 13.70696800326375353, -6.408140936763238038 ) ) ;
#68835=CARTESIAN_POINT ( 'NONE',  ( 7.084665262690076126, 4.105352010821503583, 10.88017736071109987 ) ) ;
#68836=CARTESIAN_POINT ( 'NONE',  ( 19.84674366389459621, 48.50893115100078745, 7.409399052514197653E-17 ) ) ;
#68839=CARTESIAN_POINT ( 'NONE',  ( 0.5774900079438607392, 23.48035201082150536, 5.440088680355550821 ) ) ;
#68840=CARTESIAN_POINT ( 'NONE',  ( 0.5774900079438590739, 12.64701867748817321, -5.440088680355550821 ) ) ;
#68841=CARTESIAN_POINT ( 'NONE',  ( -0.8801773607110991993, 27.85535201082150181, -2.915334737309923874 ) ) ;
#68842=CARTESIAN_POINT ( 'NONE',  ( 2.035157376598822676, 2.438685344154838397, -7.964842623401177768 ) ) ;
#68844=CARTESIAN_POINT ( 'NONE',  ( 19.84674366389459266, 3.300597817667451750, 2.638427012816836559 ) ) ;
#68845=CARTESIAN_POINT ( 'NONE',  ( 18.52753015748618282, 18.92559781766745175, -4.923371831947291888 ) ) ;
#68846=CARTESIAN_POINT ( 'NONE',  ( 3.591859063236763294, 8.290301336597087456, -11.09922568453595026 ) ) ;
#68848=CARTESIAN_POINT ( 'NONE',  ( 3.591859063236763294, -1.709698663402913210, -11.09922568453595026 ) ) ;
#68850=( BOUNDED_CURVE ( )  B_SPLINE_CURVE ( 2, ( #97758, #30205, #61206, #60708, #7232, #90715, #92203, #37739, #38230 ),
 .UNSPECIFIED., .F., .F. ) 
 B_SPLINE_CURVE_WITH_KNOTS ( ( 3, 2, 2, 2, 3 ),
 ( 0.2972837940830885262, 0.2976190476190476719, 0.3035714285714286031, 0.3095238095238095344, 0.3098590630597686801 ),
 .UNSPECIFIED. ) 
 CURVE ( )  GEOMETRIC_REPRESENTATION_ITEM ( )  RATIONAL_B_SPLINE_CURVE ( ( 0.9963778908391760503, 0.9980808541467920403, 1.000000000000000000, 0.9659258262890682012, 1.000000000000000000, 0.9659258262890682012, 1.000000000000000000, 0.9980808541467920403, 0.9963778908391759392 ) ) 
 REPRESENTATION_ITEM ( '' )  );
#68852=CARTESIAN_POINT ( 'NONE',  ( 6.204703633549690345, 15.76208216824730179, -14.16423886937410259 ) ) ;
#68854=CARTESIAN_POINT ( 'NONE',  ( 19.84674366389459621, 28.50893115100078745, 7.409399052514197653E-17 ) ) ;
#68857=CARTESIAN_POINT ( 'NONE',  ( 20.36894250292379382, 58.67874883491396076, 10.36894250292379205 ) ) ;
#68858=CARTESIAN_POINT ( 'NONE',  ( 12.63842701281683034, 12.46726448433411782, 9.846743663894596210 ) ) ;
#68859=CARTESIAN_POINT ( 'NONE',  ( 0.2751277870542978565, 12.28217586085238011, -6.500000000000002665 ) ) ;
#68861=CARTESIAN_POINT ( 'NONE',  ( 2.035157376598824452, 43.68868534415484106, 7.964842623401179544 ) ) ;
#68862=CARTESIAN_POINT ( 'NONE',  ( 6.565887622018943937, 55.16530133659709634, 12.81628187352647430 ) ) ;
#68863=CARTESIAN_POINT ( 'NONE',  ( 19.42250999205614193, 15.14701867748817143, 5.440088680355555262 ) ) ;
#68864=TOROIDAL_SURFACE ( 'NONE', #30581, 9.538348415311009632, 7.000000000000000000 ) ;
#68865=CARTESIAN_POINT ( 'NONE',  ( 21.09922568453594849, 51.20696800326375353, 6.408140936763242479 ) ) ;
#68866=CARTESIAN_POINT ( 'NONE',  ( 3.591859063236761518, -0.04303199673624671928, 11.09922568453594849 ) ) ;
#68867=FILL_AREA_STYLE ('',( #30848 ) ) ;
#68870=CARTESIAN_POINT ( 'NONE',  ( 1.485411327523655789, 2.210147928482776969, -6.499999999999963585 ) ) ;
#68871=CARTESIAN_POINT ( 'NONE',  ( 6.204703633549690345, 45.76208216824729647, -14.16423886937410259 ) ) ;
#68872=CARTESIAN_POINT ( 'NONE',  ( 13.79529636645031943, 10.34541550158063394, -14.16423886937409904 ) ) ;
#68873=CARTESIAN_POINT ( 'NONE',  ( 7.084665262690076126, 4.105352010821503583, 10.88017736071109987 ) ) ;
#68874=CARTESIAN_POINT ( 'NONE',  ( -0.8801773607110991993, 32.85535201082151247, -2.915334737309923874 ) ) ;
#68877=CARTESIAN_POINT ( 'NONE',  ( 2.035157376598822676, 67.43868534415484817, -7.964842623401177768 ) ) ;
#68878=CARTESIAN_POINT ( 'NONE',  ( -0.8801773607111009756, 63.06368534415484106, 1.068504757029289695E-15 ) ) ;
#68879=CARTESIAN_POINT ( 'NONE',  ( 22.81628187352647785, 31.62363466993042138, 6.195893100308588602E-16 ) ) ;
#68880=DIRECTION ( 'NONE',  ( 0.000000000000000000, 0.000000000000000000, 1.000000000000000000 ) ) ;
#68882=CARTESIAN_POINT ( 'NONE',  ( 1.472469842513823179, 31.42559781766745530, 4.923371831947296329 ) ) ;
#68883=CARTESIAN_POINT ( 'NONE',  ( 12.91533473730992121, 19.52201867748816611, 10.88017736071110164 ) ) ;
#68886=CARTESIAN_POINT ( 'NONE',  ( 0.6178305044545818747, 23.49863466993041783, -9.382169495545419124 ) ) ;
#68887=CARTESIAN_POINT ( 'NONE',  ( 2.791683348922237240, 10.38393115100078390, -7.208316651077763204 ) ) ;
#68888=CARTESIAN_POINT ( 'NONE',  ( -0.8801773607111008646, 13.27201867748817143, 2.915334737309923430 ) ) ;
#68890=EDGE_CURVE ( 'NONE', #45005, #85730, #31519, .T. ) ;
#68891=CARTESIAN_POINT ( 'NONE',  ( 14.92337183194729633, 32.67559781766745175, 8.527530157486181039 ) ) ;
#68892=CARTESIAN_POINT ( 'NONE',  ( 22.81628187352648496, 61.83196800326376774, -3.434112377981050290 ) ) ;
#68893=CARTESIAN_POINT ( 'NONE',  ( 17.20831665107776587, 34.13393115100078745, -7.208316651077762316 ) ) ;
#68894=CARTESIAN_POINT ( 'NONE',  ( -4.164238869374099927, 2.012082168247300906, 3.795296366450308767 ) ) ;
#68895=CARTESIAN_POINT ( 'NONE',  ( 17.08211943468705130, 18.47041550158063572, 12.26659068614894998 ) ) ;
#68896=CARTESIAN_POINT ( 'NONE',  ( -0.8801773607110991993, 32.85535201082151247, -2.915334737309923874 ) ) ;
#68897=CARTESIAN_POINT ( 'NONE',  ( 20.88017736071110519, 10.56368534415483751, 2.639326808657452039E-16 ) ) ;
#68898=CARTESIAN_POINT ( 'NONE',  ( 6.204703633549690345, 42.84541550158063217, 14.16423886937410082 ) ) ;
#68899=CARTESIAN_POINT ( 'NONE',  ( 7.084665262690076126, 37.02201867748817676, -10.88017736071110164 ) ) ;
#68900=CARTESIAN_POINT ( 'NONE',  ( 19.42250999205614548, 15.98035201082150714, -5.440088680355545492 ) ) ;
#68902=CARTESIAN_POINT ( 'NONE',  ( 10.00000000000000178, 34.31368534415484106, 10.88017736071110342 ) ) ;
#68904=CARTESIAN_POINT ( 'NONE',  ( -2.816281873526473856, 64.12363466993042493, 9.499525473075851096E-16 ) ) ;
#68905=CARTESIAN_POINT ( 'NONE',  ( -0.8801773607110991993, 42.85535201082150536, -2.915334737309923874 ) ) ;
#68906=CARTESIAN_POINT ( 'NONE',  ( 4.559911319644449179, 53.89701867748817676, 9.422509992056141925 ) ) ;
#68907=ORIENTED_EDGE ( 'NONE', *, *, #90582, .T. ) ;
#68908=CARTESIAN_POINT ( 'NONE',  ( 19.42250999205614193, 45.14701867748817676, 5.440088680355555262 ) ) ;
#68911=CARTESIAN_POINT ( 'NONE',  ( -4.164238869374099927, 42.01208216824728936, 3.795296366450308767 ) ) ;
#68912=CARTESIAN_POINT ( 'NONE',  ( 20.88017736071110875, 60.77201867748817676, -2.915334737309920765 ) ) ;
#68914=CARTESIAN_POINT ( 'NONE',  ( 18.52753015748617571, 63.09226448433412315, 4.923371831947298993 ) ) ;
#68916=CARTESIAN_POINT ( 'NONE',  ( 10.00000000000000178, 37.25893115100078745, 9.846743663894594434 ) ) ;
#68917=ORIENTED_EDGE ( 'NONE', *, *, #51664, .F. ) ;
#68919=CARTESIAN_POINT ( 'NONE',  ( 7.361572987183169658, 39.96726448433411605, -9.846743663894592657 ) ) ;
#68920=CARTESIAN_POINT ( 'NONE',  ( 7.084665262690076126, 34.10535201082151247, 10.88017736071109987 ) ) ;
#68921=CARTESIAN_POINT ( 'NONE',  ( 12.63842701281683034, 32.46726448433412315, 9.846743663894596210 ) ) ;
#68922=CARTESIAN_POINT ( 'NONE',  ( -1.099225684535947600, 23.70696800326375708, -6.408140936763238038 ) ) ;
#68923=DIRECTION ( 'NONE',  ( 0.000000000000000000, -0.000000000000000000, 1.000000000000000000 ) ) ;
#68924=CARTESIAN_POINT ( 'NONE',  ( 7.084665262690076126, 47.02201867748818387, -10.88017736071110164 ) ) ;
#68925=CARTESIAN_POINT ( 'NONE',  ( 15.44008868035555793, 6.397018677488170546, -9.422509992056140149 ) ) ;
#68926=CARTESIAN_POINT ( 'NONE',  ( 13.79529636645031943, 55.34541550158062506, -14.16423886937409904 ) ) ;
#68927=VECTOR ( 'NONE', #59416, 1000.000000000000114 ) ;
#68928=CARTESIAN_POINT ( 'NONE',  ( 19.38216949554541202, 20.99863466993042138, 9.382169495545424454 ) ) ;
#68929=CYLINDRICAL_SURFACE ( 'NONE', #5157, 0.5000000000000004441 ) ;
#68931=CARTESIAN_POINT ( 'NONE',  ( 6.565887622018943937, 20.16530133659708213, 12.81628187352647430 ) ) ;
#68932=CARTESIAN_POINT ( 'NONE',  ( 20.88017736071110519, 20.56368534415484106, 2.639326808657452039E-16 ) ) ;
#68933=CARTESIAN_POINT ( 'NONE',  ( 19.42250999205614193, 55.14701867748817676, 5.440088680355555262 ) ) ;
#68935=ORIENTED_EDGE ( 'NONE', *, *, #88268, .T. ) ;
#68936=CARTESIAN_POINT ( 'NONE',  ( 0.1532563361054100626, 0.8005978176674514168, -2.638427012816831230 ) ) ;
#68937=CARTESIAN_POINT ( 'NONE',  ( 0.1532563361054100626, 55.80059781766745175, -2.638427012816831230 ) ) ;
#68938=CARTESIAN_POINT ( 'NONE',  ( 14.92337183194729633, 32.67559781766745175, 8.527530157486181039 ) ) ;
#68939=CARTESIAN_POINT ( 'NONE',  ( 5.076628168052703671, 31.84226448433412315, 8.527530157486179263 ) ) ;
#68942=CARTESIAN_POINT ( 'NONE',  ( 17.20831665107776587, 12.88393115100078390, 7.208316651077764980 ) ) ;
#68945=CARTESIAN_POINT ( 'NONE',  ( 17.20831665107776587, 44.13393115100078745, -7.208316651077762316 ) ) ;
#68946=ORIENTED_EDGE ( 'NONE', *, *, #43284, .F. ) ;
#68947=CARTESIAN_POINT ( 'NONE',  ( 19.72487221294571569, 65.71833443783937412, -6.499999999999983125 ) ) ;
#68948=CARTESIAN_POINT ( 'NONE',  ( 6.565887622018943937, 18.08196800326375708, -12.81628187352647608 ) ) ;
#68950=CARTESIAN_POINT ( 'NONE',  ( -0.8801773607111009756, 53.06368534415484106, 1.068504757029289695E-15 ) ) ;
#68951=CARTESIAN_POINT ( 'NONE',  ( 6.204703633549690345, 35.76208216824729647, -14.16423886937410259 ) ) ;
#68953=CARTESIAN_POINT ( 'NONE',  ( -4.164238869374099927, 32.01208216824730357, 3.795296366450308767 ) ) ;
#68954=CARTESIAN_POINT ( 'NONE',  ( 20.36894250292379382, 63.67874883491396787, 10.36894250292379205 ) ) ;
#68955=CARTESIAN_POINT ( 'NONE',  ( 13.79529636645030344, 13.26208216824729824, 14.16423886937410614 ) ) ;
#68956=CARTESIAN_POINT ( 'NONE',  ( -2.266590686148945544, 31.38708216824730002, -7.082119434687050408 ) ) ;
#68958=CARTESIAN_POINT ( 'NONE',  ( 15.44008868035555260, 54.73035201082150536, 9.422509992056143702 ) ) ;
#68962=CARTESIAN_POINT ( 'NONE',  ( 18.52753015748617571, 38.09226448433412315, 4.923371831947298993 ) ) ;
#68963=CARTESIAN_POINT ( 'NONE',  ( 10.00000000000000000, 21.81368534415484106, -10.88017736071110342 ) ) ;
#68964=CARTESIAN_POINT ( 'NONE',  ( 21.92686044187656691, 54.95379003517447813, 3.195792623639537755 ) ) ;
#68965=CARTESIAN_POINT ( 'NONE',  ( 10.00000000000000178, 62.25893115100078745, 9.846743663894594434 ) ) ;
#68968=CARTESIAN_POINT ( 'NONE',  ( 2.791683348922237240, 40.38393115100078035, -7.208316651077763204 ) ) ;
#68969=CARTESIAN_POINT ( 'NONE',  ( 16.40814093676323893, 50.79030133659708923, 11.09922568453595026 ) ) ;
#68971=CARTESIAN_POINT ( 'NONE',  ( 19.84674366389459266, 38.30059781766745175, 2.638427012816836559 ) ) ;
#68972=CARTESIAN_POINT ( 'NONE',  ( 0.1532563361054100626, 50.80059781766745175, -2.638427012816831230 ) ) ;
#68974=CARTESIAN_POINT ( 'NONE',  ( 17.08211943468705130, 38.47041550158063217, 12.26659068614894998 ) ) ;
#68976=CARTESIAN_POINT ( 'NONE',  ( 2.917880565312948704, 12.63708216824730179, 12.26659068614894643 ) ) ;
#68977=CARTESIAN_POINT ( 'NONE',  ( 2.035157376598824452, 58.68868534415482685, 7.964842623401179544 ) ) ;
#68979=CARTESIAN_POINT ( 'NONE',  ( 6.204703633549690345, 52.84541550158062506, 14.16423886937410082 ) ) ;
#68980=CARTESIAN_POINT ( 'NONE',  ( -1.099225684535947600, 9.540301336597087456, 6.408140936763237150 ) ) ;
#68981=CARTESIAN_POINT ( 'NONE',  ( -0.1023957841222405962, 55.13377557478295898, 6.340343622311920058 ) ) ;
#68982=CARTESIAN_POINT ( 'NONE',  ( 18.52753015748617571, 3.092264484334118269, 4.923371831947298993 ) ) ;
#68984=CARTESIAN_POINT ( 'NONE',  ( -46.94000000000001194, 101.9444105523804893, -6.894162316358291243 ) ) ;
#68985=CARTESIAN_POINT ( 'NONE',  ( -4.164238869374099927, 57.01208216824731068, 3.795296366450308767 ) ) ;
#68987=CARTESIAN_POINT ( 'NONE',  ( -0.8801773607110991993, 32.85535201082151247, -2.915334737309923874 ) ) ;
#68988=CARTESIAN_POINT ( 'NONE',  ( 7.084665262690076126, 29.10535201082150181, 10.88017736071109987 ) ) ;
#68989=CARTESIAN_POINT ( 'NONE',  ( 5.076628168052704559, 50.17559781766745886, -8.527530157486179263 ) ) ;
#68990=CARTESIAN_POINT ( 'NONE',  ( 5.076628168052704559, 50.17559781766745886, -8.527530157486179263 ) ) ;
#68991=CARTESIAN_POINT ( 'NONE',  ( 10.00000000000000178, 55.37363466993042493, 12.81628187352647608 ) ) ;
#68992=( NAMED_UNIT ( * ) PLANE_ANGLE_UNIT ( ) SI_UNIT ( $, .RADIAN. ) );
#68993=EDGE_LOOP ( 'NONE', ( #5343, #75973, #51370, #62713 ) ) ;
#68994=CARTESIAN_POINT ( 'NONE',  ( 15.44008868035555260, 14.73035201082150536, 9.422509992056143702 ) ) ;
#68995=CARTESIAN_POINT ( 'NONE',  ( 0.6178305044545838731, 14.74863466993041783, 9.382169495545420901 ) ) ;
#68999=CARTESIAN_POINT ( 'NONE',  ( 7.361572987183170547, 47.05059781766745175, 9.846743663894590881 ) ) ;
#69000=CARTESIAN_POINT ( 'NONE',  ( 19.42250999205614548, 55.98035201082150536, -5.440088680355545492 ) ) ;
#69002=CARTESIAN_POINT ( 'NONE',  ( 19.38216949554541557, 27.24863466993041783, -9.382169495545420901 ) ) ;
#69003=CARTESIAN_POINT ( 'NONE',  ( 4.559911319644449179, 47.23035201082150536, -9.422509992056141925 ) ) ;
#69005=CARTESIAN_POINT ( 'NONE',  ( 0.5600000000000083800, 105.0000000000000000, -5.000000000000000000 ) ) ;
#69007=CARTESIAN_POINT ( 'NONE',  ( -2.816281873526473856, 54.33196800326376064, 3.434112377981055619 ) ) ;
#69010=CARTESIAN_POINT ( 'NONE',  ( 20.88017736071110875, 45.77201867748816966, -2.915334737309920765 ) ) ;
#69011=CARTESIAN_POINT ( 'NONE',  ( 13.43411237798105340, 50.58196800326375353, 12.81628187352647963 ) ) ;
#69012=CARTESIAN_POINT ( 'NONE',  ( 12.63842701281683922, 4.550597817667451750, -9.846743663894590881 ) ) ;
#69014=CARTESIAN_POINT ( 'NONE',  ( 0.1532563361054100626, 60.80059781766744464, -2.638427012816831230 ) ) ;
#69015=CARTESIAN_POINT ( 'NONE',  ( 12.63842701281683922, 34.55059781766745886, -9.846743663894590881 ) ) ;
#69016=CARTESIAN_POINT ( 'NONE',  ( 7.361572987183170547, 2.050597817667451750, 9.846743663894590881 ) ) ;
#69018=CARTESIAN_POINT ( 'NONE',  ( -0.3689425029237881626, 47.42874883491396787, 10.36894250292379027 ) ) ;
#69019=VECTOR ( 'NONE', #52854, 1000.000000000000000 ) ;
#69020=CARTESIAN_POINT ( 'NONE',  ( 2.035157376598822676, 2.438685344154837953, -7.964842623401177768 ) ) ;
#69021=CARTESIAN_POINT ( 'NONE',  ( 2.035157376598824452, 3.688685344154837953, 7.964842623401179544 ) ) ;
#69024=CARTESIAN_POINT ( 'NONE',  ( 20.88017736071110164, 15.35535201082150358, 2.915334737309930979 ) ) ;
#69025=CARTESIAN_POINT ( 'NONE',  ( 10.00000000000000178, 4.313685344154837509, 10.88017736071110342 ) ) ;
#69026=CARTESIAN_POINT ( 'NONE',  ( 18.52753015748617571, 43.09226448433412315, 4.923371831947298993 ) ) ;
#69027=CARTESIAN_POINT ( 'NONE',  ( 16.40814093676323893, 35.79030133659708923, 11.09922568453595026 ) ) ;
#69029=CARTESIAN_POINT ( 'NONE',  ( -0.3689425029237881626, 12.42874883491396609, 10.36894250292379027 ) ) ;
#69030=CARTESIAN_POINT ( 'NONE',  ( 19.42250999205614193, 25.14701867748817321, 5.440088680355555262 ) ) ;
#69031=CARTESIAN_POINT ( 'NONE',  ( 12.91533473730993009, 6.605352010821504471, -10.88017736071109987 ) ) ;
#69032=CARTESIAN_POINT ( 'NONE',  ( 17.20831665107776587, 44.13393115100078745, -7.208316651077762316 ) ) ;
#69034=CARTESIAN_POINT ( 'NONE',  ( 19.84674366389459621, 18.50893115100078745, 7.409399052514197653E-17 ) ) ;
#69036=CARTESIAN_POINT ( 'NONE',  ( 0.8952175423694934686, 32.60160829253884884, -5.990408912944337416 ) ) ;
#69039=( NAMED_UNIT ( * ) PLANE_ANGLE_UNIT ( ) SI_UNIT ( $, .RADIAN. ) );
#69041=CARTESIAN_POINT ( 'NONE',  ( 1.472469842513823179, 55.59226448433412315, -4.923371831947296329 ) ) ;
#69042=CARTESIAN_POINT ( 'NONE',  ( 20.88017736071110519, 35.56368534415484106, 2.639326808657452039E-16 ) ) ;
#69043=CARTESIAN_POINT ( 'NONE',  ( 0.5774900079438607392, 33.48035201082150536, 5.440088680355550821 ) ) ;
#69044=CARTESIAN_POINT ( 'NONE',  ( -0.8801773607111008646, 3.272018677488171434, 2.915334737309923430 ) ) ;
#69045=CARTESIAN_POINT ( 'NONE',  ( 13.43411237798105340, 30.58196800326374998, 12.81628187352647963 ) ) ;
#69046=CARTESIAN_POINT ( 'NONE',  ( 24.16423886937410614, 14.51208216824730179, -3.795296366450302550 ) ) ;
#69048=CARTESIAN_POINT ( 'NONE',  ( 0.6178305044545818747, 48.49863466993042493, -9.382169495545419124 ) ) ;
#69050=CARTESIAN_POINT ( 'NONE',  ( 0.1532563361054082862, 51.21726448433412315, 2.638427012816831674 ) ) ;
#69051=CARTESIAN_POINT ( 'NONE',  ( 19.42250999205614548, 25.98035201082150891, -5.440088680355545492 ) ) ;
#69053=CARTESIAN_POINT ( 'NONE',  ( -0.8801773607110991993, 12.85535201082150358, -2.915334737309923874 ) ) ;
#69055=CARTESIAN_POINT ( 'NONE',  ( 12.91533473730992121, 54.52201867748816255, 10.88017736071110164 ) ) ;
#69056=CARTESIAN_POINT ( 'NONE',  ( 7.084665262690076126, 69.10535201082151957, 10.88017736071109987 ) ) ;
#69057=CARTESIAN_POINT ( 'NONE',  ( 17.96484262340118221, 59.93868534415484106, 7.964842623401181321 ) ) ;
#69058=CARTESIAN_POINT ( 'NONE',  ( 5.076628168052704559, 15.17559781766745175, -8.527530157486179263 ) ) ;
#69059=CARTESIAN_POINT ( 'NONE',  ( -0.8801773607111009756, 53.06368534415484106, 1.068504757029289695E-15 ) ) ;
#69061=CARTESIAN_POINT ( 'NONE',  ( 0.1532563361054082862, 11.21726448433411782, 2.638427012816831674 ) ) ;
#69064=ORIENTED_EDGE ( 'NONE', *, *, #19988, .T. ) ;
#69065=CARTESIAN_POINT ( 'NONE',  ( 17.20831665107776587, 42.88393115100077324, 7.208316651077764980 ) ) ;
#69068=CARTESIAN_POINT ( 'NONE',  ( 0.1532563361054100626, 65.80059781766745175, -2.638427012816831230 ) ) ;
#69070=AXIS2_PLACEMENT_3D ( 'NONE', #97131, #14104, #14611 ) ;
#69072=CARTESIAN_POINT ( 'NONE',  ( -0.3689425029237881626, 17.42874883491397142, 10.36894250292379027 ) ) ;
#69073=CARTESIAN_POINT ( 'NONE',  ( 20.04068437667225311, 29.71974360917721114, 6.396802510829709298 ) ) ;
#69075=CARTESIAN_POINT ( 'NONE',  ( 10.00000000000000178, 14.31368534415483929, 10.88017736071110342 ) ) ;
#69076=CARTESIAN_POINT ( 'NONE',  ( 6.565887622018943937, 43.08196800326374643, -12.81628187352647608 ) ) ;
#69077=ORIENTED_EDGE ( 'NONE', *, *, #19004, .T. ) ;
#69078=( NAMED_UNIT ( * ) PLANE_ANGLE_UNIT ( ) SI_UNIT ( $, .RADIAN. ) );
#69079=CIRCLE ( 'NONE', #25970, 11.99999999999999645 ) ;
#69080=CARTESIAN_POINT ( 'NONE',  ( 18.52753015748617571, 3.092264484334118269, 4.923371831947298993 ) ) ;
#69081=CARTESIAN_POINT ( 'NONE',  ( 19.38216949554541557, 37.24863466993041783, -9.382169495545420901 ) ) ;
#69082=CARTESIAN_POINT ( 'NONE',  ( 18.52753015748617571, 23.09226448433411960, 4.923371831947298993 ) ) ;
#69085=CARTESIAN_POINT ( 'NONE',  ( 13.43411237798105340, 20.58196800326374643, 12.81628187352647963 ) ) ;
#69086=VECTOR ( 'NONE', #58658, 1000.000000000000114 ) ;
#69088=CARTESIAN_POINT ( 'NONE',  ( 18.52753015748618282, 3.925597817667451306, -4.923371831947291888 ) ) ;
#69091=CARTESIAN_POINT ( 'NONE',  ( 0.5774900079438607392, 28.48035201082150891, 5.440088680355550821 ) ) ;
#69092=CARTESIAN_POINT ( 'NONE',  ( 10.00000000000000000, 20.55374883491396787, -14.16423886937410082 ) ) ;
#69093=CARTESIAN_POINT ( 'NONE',  ( 1.472469842513823179, 40.59226448433411605, -4.923371831947296329 ) ) ;
#69094=CARTESIAN_POINT ( 'NONE',  ( 17.96484262340118221, 64.93868534415483396, 7.964842623401181321 ) ) ;
#69095=CARTESIAN_POINT ( 'NONE',  ( 22.81628187352647785, 46.62363466993041783, 6.195893100308588602E-16 ) ) ;
#69097=CARTESIAN_POINT ( 'NONE',  ( 20.88017736071110164, 25.35535201082150891, 2.915334737309930979 ) ) ;
#69100=CARTESIAN_POINT ( 'NONE',  ( 22.81628187352648496, 11.83196800326375531, -3.434112377981050290 ) ) ;
#69101=CARTESIAN_POINT ( 'NONE',  ( 12.63842701281683922, 24.55059781766745175, -9.846743663894590881 ) ) ;
#69103=CARTESIAN_POINT ( 'NONE',  ( -2.816281873526471635, 53.91530133659709634, -3.434112377981056508 ) ) ;
#69105=CARTESIAN_POINT ( 'NONE',  ( 2.035157376598822676, 52.43868534415483396, -7.964842623401177768 ) ) ;
#69108=CARTESIAN_POINT ( 'NONE',  ( 12.91533473730992121, 44.52201867748816966, 10.88017736071110164 ) ) ;
#69110=CARTESIAN_POINT ( 'NONE',  ( 0.5774900079438590739, 42.64701867748816966, -5.440088680355550821 ) ) ;
#69111=CARTESIAN_POINT ( 'NONE',  ( 14.92337183194729988, 59.34226448433412315, -8.527530157486177487 ) ) ;
#69113=CARTESIAN_POINT ( 'NONE',  ( 4.559911319644449179, 62.23035201082150536, -9.422509992056141925 ) ) ;
#69115=EDGE_CURVE ( 'NONE', #76088, #6068, #43983, .T. ) ;
#69116=CARTESIAN_POINT ( 'NONE',  ( 14.92337183194729988, 54.34226448433412315, -8.527530157486177487 ) ) ;
#69117=CARTESIAN_POINT ( 'NONE',  ( 2.035157376598824452, 13.68868534415483751, 7.964842623401179544 ) ) ;
#69119=CARTESIAN_POINT ( 'NONE',  ( 22.81628187352647785, 11.41530133659708390, 3.434112377981063169 ) ) ;
#69121=CARTESIAN_POINT ( 'NONE',  ( 19.42250999205614548, 35.98035201082151247, -5.440088680355545492 ) ) ;
#69122=CARTESIAN_POINT ( 'NONE',  ( 13.43411237798106583, 2.665301336597086568, -12.81628187352647252 ) ) ;
#69124=CARTESIAN_POINT ( 'NONE',  ( 4.559911319644449179, 13.89701867748817143, 9.422509992056141925 ) ) ;
#69125=CARTESIAN_POINT ( 'NONE',  ( 17.96484262340118221, 24.93868534415484461, 7.964842623401181321 ) ) ;
#69126=CARTESIAN_POINT ( 'NONE',  ( 10.00000000000000000, 35.55374883491396787, -14.16423886937410082 ) ) ;
#69127=CARTESIAN_POINT ( 'NONE',  ( 18.52753015748618282, 33.92559781766745886, -4.923371831947291888 ) ) ;
#69128=CARTESIAN_POINT ( 'NONE',  ( 19.42250999205614548, 40.98035201082150536, -5.440088680355545492 ) ) ;
#69130=CARTESIAN_POINT ( 'NONE',  ( 6.204703633549690345, 7.845415501580634832, 14.16423886937410082 ) ) ;
#69131=UNCERTAINTY_MEASURE_WITH_UNIT (LENGTH_MEASURE( 1.000000000000000082E-05 ), #47099, 'distance_accuracy_value', 'NONE');
#69134=CARTESIAN_POINT ( 'NONE',  ( 0.1532563361054100626, 60.80059781766744464, -2.638427012816831230 ) ) ;
#69137=CARTESIAN_POINT ( 'NONE',  ( -2.266590686148945544, 41.38708216824729647, -7.082119434687050408 ) ) ;
#69138=CARTESIAN_POINT ( 'NONE',  ( -0.3689425029237881626, 32.42874883491395366, 10.36894250292379027 ) ) ;
#69139=CARTESIAN_POINT ( 'NONE',  ( 5.076628168052704559, 5.175597817667451750, -8.527530157486179263 ) ) ;
#69140=CARTESIAN_POINT ( 'NONE',  ( 18.52753015748617571, 63.09226448433412315, 4.923371831947298993 ) ) ;
#69142=CARTESIAN_POINT ( 'NONE',  ( 12.91533473730992121, 54.52201867748816255, 10.88017736071110164 ) ) ;
#69143=CARTESIAN_POINT ( 'NONE',  ( 0.6178305044545838731, 19.74863466993042138, 9.382169495545420901 ) ) ;
#69144=CARTESIAN_POINT ( 'NONE',  ( 2.917880565312948704, 32.63708216824730357, 12.26659068614894643 ) ) ;
#69145=CARTESIAN_POINT ( 'NONE',  ( 20.88017736071110519, 15.56368534415483751, 2.639326808657452039E-16 ) ) ;
#69147=CARTESIAN_POINT ( 'NONE',  ( 19.42250999205614193, 30.14701867748817321, 5.440088680355555262 ) ) ;
#69149=CARTESIAN_POINT ( 'NONE',  ( -35.44000000000001194, 93.50000000000000000, -10.09898361729590199 ) ) ;
#69150=CARTESIAN_POINT ( 'NONE',  ( -0.8801773607110991993, 52.85535201082151247, -2.915334737309923874 ) ) ;
#69151=MECHANICAL_DESIGN_GEOMETRIC_PRESENTATION_REPRESENTATION('',(#86700),#80416);
#69152=CARTESIAN_POINT ( 'NONE',  ( -2.816281873526471635, 48.91530133659708213, -3.434112377981056508 ) ) ;
#69154=EDGE_LOOP ( 'NONE', ( #83191, #96939, #69064, #43061, #77423, #38665 ) ) ;
#69155=SURFACE_STYLE_FILL_AREA ( #38650 ) ;
#69158=ORIENTED_EDGE ( 'NONE', *, *, #66244, .T. ) ;
#69159=CARTESIAN_POINT ( 'NONE',  ( 20.36894250292379382, 8.678748834913967869, 10.36894250292379205 ) ) ;
#69160=CARTESIAN_POINT ( 'NONE',  ( 24.16423886937410614, 54.51208216824730357, -3.795296366450302550 ) ) ;
#69161=CARTESIAN_POINT ( 'NONE',  ( 10.00000000000000000, 1.813685344154838175, -10.88017736071110342 ) ) ;
#69162=CARTESIAN_POINT ( 'NONE',  ( 10.00000000000000178, 22.25893115100078745, 9.846743663894594434 ) ) ;
#69163=CARTESIAN_POINT ( 'NONE',  ( 0.1532563361054100626, 55.80059781766745175, -2.638427012816831230 ) ) ;
#69165=CARTESIAN_POINT ( 'NONE',  ( 20.04068437667227798, 49.71974360917720048, 6.396802510829645350 ) ) ;
#69166=CARTESIAN_POINT ( 'NONE',  ( -1.099225684535947600, 4.540301336597087456, 6.408140936763237150 ) ) ;
#69167=CARTESIAN_POINT ( 'NONE',  ( -1.099225684535947600, 33.70696800326375353, -6.408140936763238038 ) ) ;
#69170=CARTESIAN_POINT ( 'NONE',  ( 10.00000000000000178, 28.05374883491396787, 14.16423886937410082 ) ) ;
#69172=CARTESIAN_POINT ( 'NONE',  ( 2.917880565312950480, 40.97041550158063217, -12.26659068614894821 ) ) ;
#69174=CARTESIAN_POINT ( 'NONE',  ( 22.81628187352647785, 51.41530133659708923, 3.434112377981063169 ) ) ;
#69175=CARTESIAN_POINT ( 'NONE',  ( 2.035157376598824452, 23.68868534415484461, 7.964842623401179544 ) ) ;
#69176=CARTESIAN_POINT ( 'NONE',  ( 10.00000000000000178, 52.25893115100078745, 9.846743663894594434 ) ) ;
#69177=CARTESIAN_POINT ( 'NONE',  ( 12.91533473730992121, 24.52201867748816966, 10.88017736071110164 ) ) ;
#69179=CARTESIAN_POINT ( 'NONE',  ( 7.361572987183169658, 49.96726448433410894, -9.846743663894592657 ) ) ;
#69180=CARTESIAN_POINT ( 'NONE',  ( 0.1532563361054100626, 50.80059781766745175, -2.638427012816831230 ) ) ;
#69185=CARTESIAN_POINT ( 'NONE',  ( 7.361572987183170547, 7.050597817667451750, 9.846743663894590881 ) ) ;
#69186=CARTESIAN_POINT ( 'NONE',  ( 17.39651004071838969, 59.08210964143329846, -6.500000000000027534 ) ) ;
#69188=CARTESIAN_POINT ( 'NONE',  ( 12.63842701281683922, 34.55059781766745886, -9.846743663894590881 ) ) ;
#69190=CARTESIAN_POINT ( 'NONE',  ( 16.40814093676324603, 42.45696800326375353, -11.09922568453594671 ) ) ;
#69191=( NAMED_UNIT ( * ) SI_UNIT ( $, .STERADIAN. ) SOLID_ANGLE_UNIT ( ) );
#69193=ORIENTED_EDGE ( 'NONE', *, *, #64795, .T. ) ;
#69195=CARTESIAN_POINT ( 'NONE',  ( 2.791683348922240793, 56.63393115100078035, 7.208316651077764092 ) ) ;
#69196=CARTESIAN_POINT ( 'NONE',  ( -0.3689425029237881626, 37.42874883491396787, 10.36894250292379027 ) ) ;
#69197=CARTESIAN_POINT ( 'NONE',  ( 10.00000000000000000, 59.75893115100078745, -9.846743663894594434 ) ) ;
#69199=CARTESIAN_POINT ( 'NONE',  ( 5.076628168052704559, 25.17559781766745175, -8.527530157486179263 ) ) ;
#69200=CARTESIAN_POINT ( 'NONE',  ( -1.099225684535947600, 53.70696800326376064, -6.408140936763238038 ) ) ;
#69201=CARTESIAN_POINT ( 'NONE',  ( 22.26659068614894466, 3.887082168247300906, 7.082119434687054849 ) ) ;
#69202=CARTESIAN_POINT ( 'NONE',  ( 2.791683348922240793, 61.63393115100079456, 7.208316651077764092 ) ) ;
#69203=CARTESIAN_POINT ( 'NONE',  ( 2.035157376598822676, 47.43868534415484817, -7.964842623401177768 ) ) ;
#69205=CARTESIAN_POINT ( 'NONE',  ( 0.1532563361054082862, 46.21726448433411605, 2.638427012816831674 ) ) ;
#69207=CARTESIAN_POINT ( 'NONE',  ( 12.91533473730992121, 59.52201867748816966, 10.88017736071110164 ) ) ;
#69210=CARTESIAN_POINT ( 'NONE',  ( 17.96484262340118221, 29.93868534415484106, 7.964842623401181321 ) ) ;
#69211=CARTESIAN_POINT ( 'NONE',  ( 0.6178305044545818747, 3.498634669930420049, -9.382169495545419124 ) ) ;
#69212=CARTESIAN_POINT ( 'NONE',  ( 2.035157376598824452, 58.68868534415482685, 7.964842623401179544 ) ) ;
#69216=CARTESIAN_POINT ( 'NONE',  ( 10.00000000000000178, 44.31368534415484106, 10.88017736071110342 ) ) ;
#69218=CARTESIAN_POINT ( 'NONE',  ( 10.00000000000000178, 32.25893115100078745, 9.846743663894594434 ) ) ;
#69219=DIRECTION ( 'NONE',  ( 0.5547001962252290364, 0.8320502943378437211, 0.000000000000000000 ) ) ;
#69222=CARTESIAN_POINT ( 'NONE',  ( 2.791683348922237240, 60.38393115100078745, -7.208316651077763204 ) ) ;
#69223=CARTESIAN_POINT ( 'NONE',  ( 0.5774900079438607392, 8.480352010821505360, 5.440088680355550821 ) ) ;
#69225=CARTESIAN_POINT ( 'NONE',  ( 17.08211943468705130, 28.47041550158063572, 12.26659068614894998 ) ) ;
#69227=CARTESIAN_POINT ( 'NONE',  ( 22.26659068614894466, 63.88708216824730357, 7.082119434687054849 ) ) ;
#69228=CARTESIAN_POINT ( 'NONE',  ( 14.92337183194729988, 34.34226448433411605, -8.527530157486177487 ) ) ;
#69229=CARTESIAN_POINT ( 'NONE',  ( 14.92337183194729633, 22.67559781766745175, 8.527530157486181039 ) ) ;
#69230=CARTESIAN_POINT ( 'NONE',  ( 15.44008868035555793, 6.397018677488170546, -9.422509992056140149 ) ) ;
#69232=CARTESIAN_POINT ( 'NONE',  ( 1.472469842513823179, 26.42559781766745175, 4.923371831947296329 ) ) ;
#69234=CARTESIAN_POINT ( 'NONE',  ( 19.42250999205614193, 30.14701867748817321, 5.440088680355555262 ) ) ;
#69235=CARTESIAN_POINT ( 'NONE',  ( 2.791683348922240793, 66.63393115100079456, 7.208316651077764092 ) ) ;
#69236=CARTESIAN_POINT ( 'NONE',  ( 24.16423886937410614, 9.512082168247301794, -3.795296366450302550 ) ) ;
#69239=( BOUNDED_CURVE ( )  B_SPLINE_CURVE ( 2, ( #56744, #57719, #66206, #42734, #80231, #42246, #4251, #19730, #5239 ),
 .UNSPECIFIED., .F., .F. ) 
 B_SPLINE_CURVE_WITH_KNOTS ( ( 3, 2, 2, 2, 3 ),
 ( 0.2972837940830885262, 0.2976190476190476719, 0.3035714285714286031, 0.3095238095238095344, 0.3098590630597686801 ),
 .UNSPECIFIED. ) 
 CURVE ( )  GEOMETRIC_REPRESENTATION_ITEM ( )  RATIONAL_B_SPLINE_CURVE ( ( 0.9963778908391760503, 0.9980808541467920403, 1.000000000000000000, 0.9659258262890683122, 1.000000000000000000, 0.9659258262890683122, 1.000000000000000000, 0.9980808541467920403, 0.9963778908391759392 ) ) 
 REPRESENTATION_ITEM ( '' )  );
#69240=CARTESIAN_POINT ( 'NONE',  ( 10.00000000000000178, 7.258931151000785675, 9.846743663894594434 ) ) ;
#69241=CARTESIAN_POINT ( 'NONE',  ( -1.099225684535947600, 43.70696800326375353, -6.408140936763238038 ) ) ;
#69243=CARTESIAN_POINT ( 'NONE',  ( 7.361572987183169658, 39.96726448433411605, -9.846743663894592657 ) ) ;
#69245=CARTESIAN_POINT ( 'NONE',  ( 0.1532563361054083140, 21.00893115100078745, 1.131784320476157264E-15 ) ) ;
#69248=CARTESIAN_POINT ( 'NONE',  ( 20.36894250292379738, 49.92874883491396787, -10.36894250292379027 ) ) ;
#69249=CARTESIAN_POINT ( 'NONE',  ( 2.035157376598824452, 53.68868534415484817, 7.964842623401179544 ) ) ;
#69250=CARTESIAN_POINT ( 'NONE',  ( 10.00000000000000000, 0.5537488349139675359, -14.16423886937410082 ) ) ;
#69251=CARTESIAN_POINT ( 'NONE',  ( 20.88017736071110875, 60.77201867748817676, -2.915334737309920765 ) ) ;
#69252=CARTESIAN_POINT ( 'NONE',  ( 19.84674366389459621, 43.50893115100078745, 7.409399052514197653E-17 ) ) ;
#69253=CARTESIAN_POINT ( 'NONE',  ( 4.559911319644449179, 2.230352010821504471, -9.422509992056141925 ) ) ;
#69254=CARTESIAN_POINT ( 'NONE',  ( 18.17829156368506105, 39.16792564121896447, 6.500000000000047073 ) ) ;
#69255=CARTESIAN_POINT ( 'NONE',  ( 12.63842701281683034, 47.46726448433412315, 9.846743663894596210 ) ) ;
#69256=CARTESIAN_POINT ( 'NONE',  ( 15.44008868035555793, 51.39701867748816966, -9.422509992056140149 ) ) ;
#69257=CARTESIAN_POINT ( 'NONE',  ( 19.84674366389459621, 3.508931151000785231, 7.409399052514197653E-17 ) ) ;
#69259=ORIENTED_EDGE ( 'NONE', *, *, #67956, .F. ) ;
#69261=DIRECTION ( 'NONE',  ( -0.000000000000000000, 1.000000000000000000, -0.000000000000000000 ) ) ;
#69263=CARTESIAN_POINT ( 'NONE',  ( 0.1532563361054100626, 15.80059781766745353, -2.638427012816831230 ) ) ;
#69264=CARTESIAN_POINT ( 'NONE',  ( 21.09922568453595559, 62.04030133659709634, -6.408140936763230044 ) ) ;
#69265=CARTESIAN_POINT ( 'NONE',  ( 19.42250999205614193, 15.14701867748817143, 5.440088680355555262 ) ) ;
#69266=CARTESIAN_POINT ( 'NONE',  ( 0.1532563361054082862, 46.21726448433411605, 2.638427012816831674 ) ) ;
#69268=CARTESIAN_POINT ( 'NONE',  ( 2.917880565312950480, 25.97041550158063572, -12.26659068614894821 ) ) ;
#69269=CARTESIAN_POINT ( 'NONE',  ( -4.164238869374099927, 52.01208216824729647, 3.795296366450308767 ) ) ;
#69270=CARTESIAN_POINT ( 'NONE',  ( 18.52753015748617571, 53.09226448433412315, 4.923371831947298993 ) ) ;
#69272=CARTESIAN_POINT ( 'NONE',  ( 2.035157376598822676, 57.43868534415484106, -7.964842623401177768 ) ) ;
#69273=CARTESIAN_POINT ( 'NONE',  ( 17.20831665107776587, 17.88393115100078745, 7.208316651077764980 ) ) ;
#69277=CARTESIAN_POINT ( 'NONE',  ( 14.92337183194729633, 12.67559781766745353, 8.527530157486181039 ) ) ;
#69278=ORIENTED_EDGE ( 'NONE', *, *, #29241, .F. ) ;
#69279=CARTESIAN_POINT ( 'NONE',  ( 13.79529636645031943, 20.34541550158063572, -14.16423886937409904 ) ) ;
#69280=CARTESIAN_POINT ( 'NONE',  ( 0.1532563361054100626, 15.80059781766745353, -2.638427012816831230 ) ) ;
#69281=CARTESIAN_POINT ( 'NONE',  ( 19.42250999205614193, 50.14701867748817676, 5.440088680355555262 ) ) ;
#69285=CARTESIAN_POINT ( 'NONE',  ( 19.42250999205614193, 30.14701867748817321, 5.440088680355555262 ) ) ;
#69288=CARTESIAN_POINT ( 'NONE',  ( 12.91533473730992121, 39.52201867748817676, 10.88017736071110164 ) ) ;
#69289=VECTOR ( 'NONE', #21131, 1000.000000000000114 ) ;
#69292=CARTESIAN_POINT ( 'NONE',  ( 22.81628187352647785, 16.41530133659708923, 3.434112377981063169 ) ) ;
#69293=CARTESIAN_POINT ( 'NONE',  ( 2.791683348922237240, 15.38393115100078212, -7.208316651077763204 ) ) ;
#69295=CARTESIAN_POINT ( 'NONE',  ( 10.00000000000000000, 19.75893115100078390, -9.846743663894594434 ) ) ;
#69296=CARTESIAN_POINT ( 'NONE',  ( 17.96484262340118221, 26.18868534415483396, -7.964842623401177768 ) ) ;
#69298=CARTESIAN_POINT ( 'NONE',  ( 13.43411237798106583, 62.66530133659708923, -12.81628187352647252 ) ) ;
#69299=CARTESIAN_POINT ( 'NONE',  ( 12.91533473730993009, 56.60535201082151247, -10.88017736071109987 ) ) ;
#69300=CARTESIAN_POINT ( 'NONE',  ( -46.48928645636215151, 103.2957187381725248, -6.397878122524185862 ) ) ;
#69302=CARTESIAN_POINT ( 'NONE',  ( 12.91533473730993009, 66.60535201082150536, -10.88017736071109987 ) ) ;
#69303=CARTESIAN_POINT ( 'NONE',  ( 10.00000000000000178, 5.373634669930420493, 12.81628187352647608 ) ) ;
#69305=CARTESIAN_POINT ( 'NONE',  ( 1.472469842513823179, 30.59226448433411960, -4.923371831947296329 ) ) ;
#69306=CARTESIAN_POINT ( 'NONE',  ( -2.816281873526471635, 53.91530133659709634, -3.434112377981056508 ) ) ;
#69307=CARTESIAN_POINT ( 'NONE',  ( 1.711636803080583080, 36.84492782695769364, -6.500000000000066613 ) ) ;
#69308=CARTESIAN_POINT ( 'NONE',  ( 1.472469842513823179, 25.59226448433412315, -4.923371831947296329 ) ) ;
#69309=CARTESIAN_POINT ( 'NONE',  ( 21.09922568453595559, 17.04030133659708923, -6.408140936763230044 ) ) ;
#69312=CARTESIAN_POINT ( 'NONE',  ( 19.42250999205614193, 30.14701867748817321, 5.440088680355555262 ) ) ;
#69313=CARTESIAN_POINT ( 'NONE',  ( 19.84674366389459266, 58.71726448433411605, -2.638427012816827677 ) ) ;
#69314=CARTESIAN_POINT ( 'NONE',  ( 1.472469842513823179, 15.59226448433411960, -4.923371831947296329 ) ) ;
#69315=CARTESIAN_POINT ( 'NONE',  ( 18.52753015748617571, 8.092264484334117824, 4.923371831947298993 ) ) ;
#69316=CARTESIAN_POINT ( 'NONE',  ( 2.035157376598822676, 7.438685344154837509, -7.964842623401177768 ) ) ;
#69317=EDGE_CURVE ( 'NONE', #32549, #8076, #42215, .T. ) ;
#69318=CARTESIAN_POINT ( 'NONE',  ( 19.38216949554541202, 20.99863466993042138, 9.382169495545424454 ) ) ;
#69319=CARTESIAN_POINT ( 'NONE',  ( 4.559911319644449179, 3.897018677488170990, 9.422509992056141925 ) ) ;
#69320=SURFACE_STYLE_USAGE ( .BOTH. , #82832 ) ;
#69321=CARTESIAN_POINT ( 'NONE',  ( 19.84674366389459266, 58.30059781766745886, 2.638427012816836559 ) ) ;
#69323=CARTESIAN_POINT ( 'NONE',  ( 12.91533473730992121, 14.52201867748817143, 10.88017736071110164 ) ) ;
#69325=CARTESIAN_POINT ( 'NONE',  ( 1.472469842513823179, 41.42559781766745886, 4.923371831947296329 ) ) ;
#69327=CARTESIAN_POINT ( 'NONE',  ( 4.559911319644449179, 18.89701867748817321, 9.422509992056141925 ) ) ;
#69329=CARTESIAN_POINT ( 'NONE',  ( 19.42250999205614193, 35.14701867748816966, 5.440088680355555262 ) ) ;
#69330=CARTESIAN_POINT ( 'NONE',  ( -0.3689425029237898834, 66.17874883491396076, -10.36894250292378850 ) ) ;
#69331=CARTESIAN_POINT ( 'NONE',  ( 14.92337183194729633, 22.67559781766745175, 8.527530157486181039 ) ) ;
#69332=CARTESIAN_POINT ( 'NONE',  ( 6.565887622018943937, 13.08196800326374998, -12.81628187352647608 ) ) ;
#69333=CARTESIAN_POINT ( 'NONE',  ( -46.86082856188268408, 103.4709495335575156, 5.834510888469651491 ) ) ;
#69335=DIRECTION ( 'NONE',  ( -1.000000000000000000, 0.000000000000000000, 0.000000000000000000 ) ) ;
#69337=CARTESIAN_POINT ( 'NONE',  ( -4.164238869374099927, 17.01208216824730357, 3.795296366450308767 ) ) ;
#69338=CARTESIAN_POINT ( 'NONE',  ( 2.791683348922237240, 35.38393115100079456, -7.208316651077763204 ) ) ;
#69342=CARTESIAN_POINT ( 'NONE',  ( 10.00000000000000000, 50.55374883491396787, -14.16423886937410082 ) ) ;
#69343=CARTESIAN_POINT ( 'NONE',  ( 14.92337183194729633, 27.67559781766745530, 8.527530157486181039 ) ) ;
#69345=DIRECTION ( 'NONE',  ( 0.000000000000000000, 0.000000000000000000, -1.000000000000000000 ) ) ;
#69346=CARTESIAN_POINT ( 'NONE',  ( 0.5774900079438607392, 48.48035201082150536, 5.440088680355550821 ) ) ;
#69347=CARTESIAN_POINT ( 'NONE',  ( -2.816281873526471635, 48.91530133659708213, -3.434112377981056508 ) ) ;
#69348=CARTESIAN_POINT ( 'NONE',  ( 0.5774900079438590739, 22.64701867748817321, -5.440088680355550821 ) ) ;
#69349=CARTESIAN_POINT ( 'NONE',  ( 21.09922568453595559, 52.04030133659708923, -6.408140936763230044 ) ) ;
#69350=CARTESIAN_POINT ( 'NONE',  ( 10.00000000000000178, 0.3736346699304200492, 12.81628187352647608 ) ) ;
#69351=CARTESIAN_POINT ( 'NONE',  ( 0.1532563361054082862, 6.217264484334118713, 2.638427012816831674 ) ) ;
#69353=VERTEX_POINT ( 'NONE', #27187 ) ;
#69357=CARTESIAN_POINT ( 'NONE',  ( 10.00000000000000000, 60.55374883491397497, -14.16423886937410082 ) ) ;
#69358=CARTESIAN_POINT ( 'NONE',  ( 2.917880565312950480, 10.97041550158063572, -12.26659068614894821 ) ) ;
#69359=CARTESIAN_POINT ( 'NONE',  ( 15.44008868035555793, 16.39701867748817321, -9.422509992056140149 ) ) ;
#69360=CARTESIAN_POINT ( 'NONE',  ( 17.96484262340118221, 39.93868534415484106, 7.964842623401181321 ) ) ;
#69362=CARTESIAN_POINT ( 'NONE',  ( -46.51339001641208881, 100.8236536580530895, -9.499999999999998224 ) ) ;
#69363=CARTESIAN_POINT ( 'NONE',  ( 5.076628168052704559, 0.1755978176674514724, -8.527530157486179263 ) ) ;
#69364=CARTESIAN_POINT ( 'NONE',  ( 17.96484262340118221, 64.93868534415483396, 7.964842623401181321 ) ) ;
#69365=CARTESIAN_POINT ( 'NONE',  ( 22.81628187352647785, 26.62363466993042138, 6.195893100308588602E-16 ) ) ;
#69366=CARTESIAN_POINT ( 'NONE',  ( 17.84635730667657683, 18.63791097397319874, 6.499999999999999112 ) ) ;
#69368=CARTESIAN_POINT ( 'NONE',  ( 19.84674366389459621, 13.50893115100078568, 7.409399052514197653E-17 ) ) ;
#69369=CARTESIAN_POINT ( 'NONE',  ( 17.20831665107776587, 42.88393115100077324, 7.208316651077764980 ) ) ;
#69370=B_SPLINE_CURVE_WITH_KNOTS ( 'NONE', 3,
 ( #19121, #2680, #56633, #80111 ),
 .UNSPECIFIED., .F., .F.,
 ( 4, 4 ),
 ( 0.000000000000000000, 0.002657014572711344572 ),
 .UNSPECIFIED. ) ;
#69371=CARTESIAN_POINT ( 'NONE',  ( 19.42250999205614548, 15.98035201082150714, -5.440088680355545492 ) ) ;
#69372=CARTESIAN_POINT ( 'NONE',  ( 3.591859063236763294, 33.29030133659708213, -11.09922568453595026 ) ) ;
#69373=CARTESIAN_POINT ( 'NONE',  ( 18.52753015748618282, 8.925597817667451750, -4.923371831947291888 ) ) ;
#69375=CARTESIAN_POINT ( 'NONE',  ( 18.52753015748617571, 58.09226448433411605, 4.923371831947298993 ) ) ;
#69376=CARTESIAN_POINT ( 'NONE',  ( 17.20831665107776587, 27.88393115100078390, 7.208316651077764980 ) ) ;
#69377=CARTESIAN_POINT ( 'NONE',  ( 24.16423886937410614, 14.30374883491396787, 8.672049930838204340E-16 ) ) ;
#69378=CARTESIAN_POINT ( 'NONE',  ( 17.96484262340118221, 36.18868534415484106, -7.964842623401177768 ) ) ;
#69379=CARTESIAN_POINT ( 'NONE',  ( 2.035157376598824452, 8.688685344154839285, 7.964842623401179544 ) ) ;
#69380=CARTESIAN_POINT ( 'NONE',  ( 7.084665262690076126, 32.02201867748816966, -10.88017736071110164 ) ) ;
#69381=CARTESIAN_POINT ( 'NONE',  ( 12.91533473730992121, 34.52201867748817676, 10.88017736071110164 ) ) ;
#69383=CARTESIAN_POINT ( 'NONE',  ( 12.91533473730992121, 34.52201867748817676, 10.88017736071110164 ) ) ;
#69386=CARTESIAN_POINT ( 'NONE',  ( 10.00000000000000178, 55.37363466993042493, 12.81628187352647608 ) ) ;
#69387=EDGE_CURVE ( 'NONE', #47240, #81206, #96202, .T. ) ;
#69388=CARTESIAN_POINT ( 'NONE',  ( 4.559911319644449179, 52.23035201082151247, -9.422509992056141925 ) ) ;
#69390=CARTESIAN_POINT ( 'NONE',  ( 20.88017736071110164, 55.35535201082149825, 2.915334737309930979 ) ) ;
#69393=CARTESIAN_POINT ( 'NONE',  ( 17.08211943468705840, 65.13708216824730357, -12.26659068614894466 ) ) ;
#69394=CARTESIAN_POINT ( 'NONE',  ( 15.44008868035555793, 61.39701867748817676, -9.422509992056140149 ) ) ;
#69395=CARTESIAN_POINT ( 'NONE',  ( 0.6076426042653105819, 52.37576471608601736, -6.499999999999992006 ) ) ;
#69397=CARTESIAN_POINT ( 'NONE',  ( 4.559911319644449179, 2.230352010821504471, -9.422509992056141925 ) ) ;
#69398=CARTESIAN_POINT ( 'NONE',  ( 17.20831665107776587, 27.88393115100078390, 7.208316651077764980 ) ) ;
#69399=ORIENTED_EDGE ( 'NONE', *, *, #76676, .F. ) ;
#69400=CARTESIAN_POINT ( 'NONE',  ( 0.1532563361054100626, 35.80059781766745175, -2.638427012816831230 ) ) ;
#69401=MECHANICAL_DESIGN_GEOMETRIC_PRESENTATION_REPRESENTATION('',(#7171),#32706);
#69402=CARTESIAN_POINT ( 'NONE',  ( 10.00000000000000000, 36.81368534415484106, -10.88017736071110342 ) ) ;
#69403=CARTESIAN_POINT ( 'NONE',  ( 1.472469842513823179, 35.59226448433412315, -4.923371831947296329 ) ) ;
#69404=CARTESIAN_POINT ( 'NONE',  ( 22.81628187352647785, 26.41530133659708923, 3.434112377981063169 ) ) ;
#69405=CARTESIAN_POINT ( 'NONE',  ( 20.15039907845753930, 2.627771745786128044, -6.262539305110069954 ) ) ;
#69406=CARTESIAN_POINT ( 'NONE',  ( 10.00000000000000000, 66.81368534415484817, -10.88017736071110342 ) ) ;
#69407=CARTESIAN_POINT ( 'NONE',  ( 19.42250999205614548, 50.98035201082151247, -5.440088680355545492 ) ) ;
#69408=CARTESIAN_POINT ( 'NONE',  ( -4.164238869374098151, 56.59541550158063927, -3.795296366450310543 ) ) ;
#69409=CARTESIAN_POINT ( 'NONE',  ( 13.43411237798106583, 27.66530133659708568, -12.81628187352647252 ) ) ;
#69413=CARTESIAN_POINT ( 'NONE',  ( 3.591859063236763294, 18.29030133659708568, -11.09922568453595026 ) ) ;
#69414=CARTESIAN_POINT ( 'NONE',  ( 7.084665262690076126, 27.02201867748817676, -10.88017736071110164 ) ) ;
#69415=CARTESIAN_POINT ( 'NONE',  ( 10.00000000000000000, 66.81368534415484817, -10.88017736071110342 ) ) ;
#69416=EDGE_CURVE ( 'NONE', #51568, #22305, #95704, .T. ) ;
#69419=CARTESIAN_POINT ( 'NONE',  ( 2.035157376598824452, 68.68868534415484817, 7.964842623401179544 ) ) ;
#69420=( BOUNDED_CURVE ( )  B_SPLINE_CURVE ( 2, ( #3435, #18432, #48915, #40453, #64880, #41450, #71914, #49403, #26407 ),
 .UNSPECIFIED., .F., .T. ) 
 B_SPLINE_CURVE_WITH_KNOTS ( ( 3, 2, 2, 2, 3 ),
 ( 0.6177146600783226527, 0.6190476190476190688, 0.6250000000000000000, 0.6309523809523809312, 0.6322853399216773473 ),
 .UNSPECIFIED. ) 
 CURVE ( )  GEOMETRIC_REPRESENTATION_ITEM ( )  RATIONAL_B_SPLINE_CURVE ( ( 0.9881565478350733400, 0.9923695281211490915, 1.000000000000000000, 0.9659258262890683122, 1.000000000000000000, 0.9659258262890683122, 1.000000000000000000, 0.9923695281211490915, 0.9881565478350733400 ) ) 
 REPRESENTATION_ITEM ( '' )  );
#69421=CARTESIAN_POINT ( 'NONE',  ( 12.63842701281683034, 52.46726448433413026, 9.846743663894596210 ) ) ;
#69422=CARTESIAN_POINT ( 'NONE',  ( 12.63842701281683034, 37.46726448433411605, 9.846743663894596210 ) ) ;
#69424=CARTESIAN_POINT ( 'NONE',  ( 2.791683348922237240, 30.38393115100078390, -7.208316651077763204 ) ) ;
#69425=CARTESIAN_POINT ( 'NONE',  ( 0.2751277870542911397, 40.30223176428831522, 6.499999999999992006 ) ) ;
#69427=CARTESIAN_POINT ( 'NONE',  ( 12.63842701281683034, 12.46726448433411782, 9.846743663894596210 ) ) ;
#69428=CARTESIAN_POINT ( 'NONE',  ( 20.10421743870887212, 50.60736173766202484, -6.337391062633415117 ) ) ;
#69429=CARTESIAN_POINT ( 'NONE',  ( 21.92686044187656691, 44.95379003517448524, 3.195792623639537755 ) ) ;
#69430=CARTESIAN_POINT ( 'NONE',  ( 1.472469842513823179, 46.42559781766745175, 4.923371831947296329 ) ) ;
#69433=CARTESIAN_POINT ( 'NONE',  ( -2.816281873526471635, 18.91530133659708213, -3.434112377981056508 ) ) ;
#69436=CARTESIAN_POINT ( 'NONE',  ( 17.96484262340118221, 51.18868534415483396, -7.964842623401177768 ) ) ;
#69437=CARTESIAN_POINT ( 'NONE',  ( -2.266590686148945544, 26.38708216824730357, -7.082119434687050408 ) ) ;
#69439=CARTESIAN_POINT ( 'NONE',  ( 7.361572987183170547, 2.050597817667451750, 9.846743663894590881 ) ) ;
#69441=CARTESIAN_POINT ( 'NONE',  ( -4.164238869374099039, 41.80374883491397497, 8.674139862899312516E-16 ) ) ;
#69442=CARTESIAN_POINT ( 'NONE',  ( -2.266590686148945544, 56.38708216824731068, -7.082119434687050408 ) ) ;
#69443=CARTESIAN_POINT ( 'NONE',  ( 10.00000000000000178, 18.05374883491396787, 14.16423886937410082 ) ) ;
#69444=CARTESIAN_POINT ( 'NONE',  ( 17.08211943468705840, 25.13708216824730357, -12.26659068614894466 ) ) ;
#69448=CARTESIAN_POINT ( 'NONE',  ( 14.92337183194729988, 39.34226448433412315, -8.527530157486177487 ) ) ;
#69450=CARTESIAN_POINT ( 'NONE',  ( 19.42250999205614193, 20.14701867748817321, 5.440088680355555262 ) ) ;
#69455=CARTESIAN_POINT ( 'NONE',  ( 17.20831665107776587, 34.13393115100078745, -7.208316651077762316 ) ) ;
#69456=CARTESIAN_POINT ( 'NONE',  ( -1.099225684535947600, 59.54030133659708923, 6.408140936763237150 ) ) ;
#69458=CARTESIAN_POINT ( 'NONE',  ( 1.472469842513823179, 46.42559781766745175, 4.923371831947296329 ) ) ;
#69459=CARTESIAN_POINT ( 'NONE',  ( 18.52753015748618282, 53.92559781766745175, -4.923371831947291888 ) ) ;
#69460=CARTESIAN_POINT ( 'NONE',  ( 24.16423886937409904, 39.09541550158062506, 3.795296366450317205 ) ) ;
#69462=CARTESIAN_POINT ( 'NONE',  ( 13.79529636645031943, 10.34541550158063394, -14.16423886937409904 ) ) ;
#69466=CARTESIAN_POINT ( 'NONE',  ( 4.559911319644449179, 8.897018677488173211, 9.422509992056141925 ) ) ;
#69467=CARTESIAN_POINT ( 'NONE',  ( 19.38216949554541557, 7.248634669930421381, -9.382169495545420901 ) ) ;
#69469=CARTESIAN_POINT ( 'NONE',  ( 19.42250999205614548, 65.98035201082151957, -5.440088680355545492 ) ) ;
#69472=CARTESIAN_POINT ( 'NONE',  ( -0.1503990784575403861, 14.24884699246888964, -6.262539305110056631 ) ) ;
#69474=CARTESIAN_POINT ( 'NONE',  ( 10.00000000000000000, 60.55374883491397497, -14.16423886937410082 ) ) ;
#69476=CARTESIAN_POINT ( 'NONE',  ( 20.88017736071110875, 20.77201867748816611, -2.915334737309920765 ) ) ;
#69477=CARTESIAN_POINT ( 'NONE',  ( -0.8801773607110991993, 27.85535201082150181, -2.915334737309923874 ) ) ;
#69478=MECHANICAL_DESIGN_GEOMETRIC_PRESENTATION_REPRESENTATION('',(#56693),#93374);
#69479=CARTESIAN_POINT ( 'NONE',  ( 18.52753015748617571, 58.09226448433411605, 4.923371831947298993 ) ) ;
#69480=CARTESIAN_POINT ( 'NONE',  ( 14.92337183194729988, 49.34226448433411605, -8.527530157486177487 ) ) ;
#69481=CARTESIAN_POINT ( 'NONE',  ( -44.73376486625691939, 105.7482819899384197, -5.219775981216077554 ) ) ;
#69482=SURFACE_STYLE_USAGE ( .BOTH. , #17474 ) ;
#69484=CARTESIAN_POINT ( 'NONE',  ( 0.5774900079438590739, 17.64701867748817321, -5.440088680355550821 ) ) ;
#69485=CARTESIAN_POINT ( 'NONE',  ( 3.591859063236763294, 18.29030133659708568, -11.09922568453595026 ) ) ;
#69487=B_SPLINE_CURVE_WITH_KNOTS ( 'NONE', 3,
 ( #61073, #62052, #68594, #69574 ),
 .UNSPECIFIED., .F., .F.,
 ( 4, 4 ),
 ( 5.143108168158485451E-18, 0.0003153927346766731811 ),
 .UNSPECIFIED. ) ;
#69488=CARTESIAN_POINT ( 'NONE',  ( 7.361572987183170547, 67.05059781766746596, 9.846743663894590881 ) ) ;
#69490=CARTESIAN_POINT ( 'NONE',  ( 10.00000000000000000, 51.81368534415484106, -10.88017736071110342 ) ) ;
#69492=CARTESIAN_POINT ( 'NONE',  ( 21.09922568453595559, 22.04030133659708923, -6.408140936763230044 ) ) ;
#69493=CARTESIAN_POINT ( 'NONE',  ( -0.8801773607110991993, 57.85535201082149825, -2.915334737309923874 ) ) ;
#69495=( LENGTH_UNIT ( ) NAMED_UNIT ( * ) SI_UNIT ( .MILLI., .METRE. ) );
#69496=CARTESIAN_POINT ( 'NONE',  ( 19.38216949554541557, 62.24863466993041072, -9.382169495545420901 ) ) ;
#69498=CARTESIAN_POINT ( 'NONE',  ( 0.5774900079438590739, 47.64701867748817676, -5.440088680355550821 ) ) ;
#69500=CARTESIAN_POINT ( 'NONE',  ( 4.559911319644449179, 43.89701867748816966, 9.422509992056141925 ) ) ;
#69501=CARTESIAN_POINT ( 'NONE',  ( 0.6178305044545818747, 53.49863466993041072, -9.382169495545419124 ) ) ;
#69502=CARTESIAN_POINT ( 'NONE',  ( 14.92337183194729988, 4.342264484334117824, -8.527530157486177487 ) ) ;
#69503=FILL_AREA_STYLE ('',( #90508 ) ) ;
#69504=CARTESIAN_POINT ( 'NONE',  ( 12.63842701281683922, 19.55059781766745175, -9.846743663894590881 ) ) ;
#69505=CARTESIAN_POINT ( 'NONE',  ( 18.72515096720572458, 40.05509018479936145, 6.499999999999964473 ) ) ;
#69506=CARTESIAN_POINT ( 'NONE',  ( -2.266590686148945544, 57.22041550158063217, 7.082119434687048631 ) ) ;
#69507=ORIENTED_EDGE ( 'NONE', *, *, #17117, .F. ) ;
#69508=( NAMED_UNIT ( * ) SI_UNIT ( $, .STERADIAN. ) SOLID_ANGLE_UNIT ( ) );
#69509=CARTESIAN_POINT ( 'NONE',  ( 10.00000000000000178, 9.313685344154839285, 10.88017736071110342 ) ) ;
#69510=CARTESIAN_POINT ( 'NONE',  ( -0.1049300847420697458, 7.216974130838790913, -6.336235997365749384 ) ) ;
#69513=CARTESIAN_POINT ( 'NONE',  ( 4.559911319644449179, 8.897018677488173211, 9.422509992056141925 ) ) ;
#69514=CARTESIAN_POINT ( 'NONE',  ( 7.084665262690076126, 12.02201867748817321, -10.88017736071110164 ) ) ;
#69515=CARTESIAN_POINT ( 'NONE',  ( 2.791683348922237240, 45.38393115100079456, -7.208316651077763204 ) ) ;
#69517=CARTESIAN_POINT ( 'NONE',  ( 22.81628187352647785, 41.62363466993042493, 6.195893100308588602E-16 ) ) ;
#69520=CARTESIAN_POINT ( 'NONE',  ( 17.08211943468705840, 20.13708216824730357, -12.26659068614894466 ) ) ;
#69521=CARTESIAN_POINT ( 'NONE',  ( 19.42250999205614548, 20.98035201082150891, -5.440088680355545492 ) ) ;
#69522=CARTESIAN_POINT ( 'NONE',  ( 0.5774900079438607392, 8.480352010821505360, 5.440088680355550821 ) ) ;
#69523=CARTESIAN_POINT ( 'NONE',  ( 12.63842701281683922, 44.55059781766745175, -9.846743663894590881 ) ) ;
#69525=CARTESIAN_POINT ( 'NONE',  ( 7.361572987183170547, 22.05059781766745530, 9.846743663894590881 ) ) ;
#69526=CARTESIAN_POINT ( 'NONE',  ( 0.1532563361054082862, 1.217264484334117824, 2.638427012816831674 ) ) ;
#69528=ORIENTED_EDGE ( 'NONE', *, *, #43388, .F. ) ;
#69529=FILL_AREA_STYLE ('',( #17524 ) ) ;
#69530=ORIENTED_EDGE ( 'NONE', *, *, #36721, .T. ) ;
#69531=CARTESIAN_POINT ( 'NONE',  ( 18.52753015748617571, 58.09226448433411605, 4.923371831947298993 ) ) ;
#69532=CARTESIAN_POINT ( 'NONE',  ( 12.91533473730992121, 29.52201867748817321, 10.88017736071110164 ) ) ;
#69533=CARTESIAN_POINT ( 'NONE',  ( -0.8801773607111009756, 43.06368534415484106, 1.068504757029289695E-15 ) ) ;
#69534=CARTESIAN_POINT ( 'NONE',  ( 20.88017736071110164, 5.355352010821502695, 2.915334737309930979 ) ) ;
#69535=CARTESIAN_POINT ( 'NONE',  ( 22.81628187352647785, 26.62363466993042138, 6.195893100308588602E-16 ) ) ;
#69536=CARTESIAN_POINT ( 'NONE',  ( -2.266590686148945544, 16.38708216824730357, -7.082119434687050408 ) ) ;
#69539=CARTESIAN_POINT ( 'NONE',  ( -2.816281873526471635, 43.91530133659708923, -3.434112377981056508 ) ) ;
#69541=CARTESIAN_POINT ( 'NONE',  ( 19.84674366389459266, 43.30059781766744464, 2.638427012816836559 ) ) ;
#69542=CARTESIAN_POINT ( 'NONE',  ( 10.00000000000000000, 26.81368534415484106, -10.88017736071110342 ) ) ;
#69543=ORIENTED_EDGE ( 'NONE', *, *, #30955, .T. ) ;
#69544=CARTESIAN_POINT ( 'NONE',  ( 15.44008868035555793, 16.39701867748817321, -9.422509992056140149 ) ) ;
#69546=CARTESIAN_POINT ( 'NONE',  ( 12.91533473730992121, 59.52201867748816966, 10.88017736071110164 ) ) ;
#69547=FILL_AREA_STYLE_COLOUR ( '', #67895 ) ;
#69550=CARTESIAN_POINT ( 'NONE',  ( 19.84674366389459266, 8.300597817667451750, 2.638427012816836559 ) ) ;
#69552=CARTESIAN_POINT ( 'NONE',  ( 7.084665262690076126, 64.10535201082150536, 10.88017736071109987 ) ) ;
#69554=( GEOMETRIC_REPRESENTATION_CONTEXT ( 3 ) GLOBAL_UNCERTAINTY_ASSIGNED_CONTEXT ( ( #86464 ) ) GLOBAL_UNIT_ASSIGNED_CONTEXT ( ( #55175, #25209, #87148 ) ) REPRESENTATION_CONTEXT ( 'NONE', 'WORKASPACE' ) );
#69555=CARTESIAN_POINT ( 'NONE',  ( 17.20831665107776587, 7.883931151000784787, 7.208316651077764980 ) ) ;
#69556=EDGE_CURVE ( 'NONE', #56832, #51000, #4115, .T. ) ;
#69557=CARTESIAN_POINT ( 'NONE',  ( 2.791683348922240793, 46.63393115100077324, 7.208316651077764092 ) ) ;
#69561=CARTESIAN_POINT ( 'NONE',  ( 0.2751277870542909176, 30.30223176428831167, 6.499999999999992006 ) ) ;
#69562=EDGE_CURVE ( 'NONE', #91132, #12692, #34155, .T. ) ;
#69563=CARTESIAN_POINT ( 'NONE',  ( 17.08211943468705130, 13.47041550158063572, 12.26659068614894998 ) ) ;
#69564=CARTESIAN_POINT ( 'NONE',  ( 19.50000000000000355, 70.00000000000000000, 4.500000000000000888 ) ) ;
#69566=CARTESIAN_POINT ( 'NONE',  ( 12.91533473730993009, 61.60535201082150536, -10.88017736071109987 ) ) ;
#69567=CARTESIAN_POINT ( 'NONE',  ( 0.5774900079438590739, 27.64701867748817676, -5.440088680355550821 ) ) ;
#69568=CARTESIAN_POINT ( 'NONE',  ( 0.1532563361054082862, 66.21726448433412315, 2.638427012816831674 ) ) ;
#69569=VERTEX_POINT ( 'NONE', #44661 ) ;
#69570=CARTESIAN_POINT ( 'NONE',  ( 14.92337183194729633, 7.675597817667451750, 8.527530157486181039 ) ) ;
#69571=CARTESIAN_POINT ( 'NONE',  ( 0.1532563361054082862, 6.217264484334118713, 2.638427012816831674 ) ) ;
#69572=CARTESIAN_POINT ( 'NONE',  ( 19.38216949554541202, 35.99863466993041072, 9.382169495545424454 ) ) ;
#69573=CARTESIAN_POINT ( 'NONE',  ( 19.84674366389459266, 28.30059781766745886, 2.638427012816836559 ) ) ;
#69574=CARTESIAN_POINT ( 'NONE',  ( -0.1503990784575328643, 69.92552686551195507, -6.262539305110068177 ) ) ;
#69575=CARTESIAN_POINT ( 'NONE',  ( 16.40814093676323893, 15.79030133659708746, 11.09922568453595026 ) ) ;
#69578=CARTESIAN_POINT ( 'NONE',  ( 1.472469842513823179, 5.592264484334118713, -4.923371831947296329 ) ) ;
#69580=CARTESIAN_POINT ( 'NONE',  ( 2.035157376598824452, 28.68868534415484106, 7.964842623401179544 ) ) ;
#69581=CARTESIAN_POINT ( 'NONE',  ( 6.204703633549690345, 35.76208216824729647, -14.16423886937410259 ) ) ;
#69582=CARTESIAN_POINT ( 'NONE',  ( 0.1532563361054100626, 35.80059781766745175, -2.638427012816831230 ) ) ;
#69583=CARTESIAN_POINT ( 'NONE',  ( 0.5774900079438590739, 62.64701867748817676, -5.440088680355550821 ) ) ;
#69584=CARTESIAN_POINT ( 'NONE',  ( -1.099225684535947600, 48.70696800326375353, -6.408140936763238038 ) ) ;
#69586=CARTESIAN_POINT ( 'NONE',  ( 2.035157376598822676, 22.43868534415483396, -7.964842623401177768 ) ) ;
#69589=CARTESIAN_POINT ( 'NONE',  ( -2.816281873526473856, 9.331968003263753531, 3.434112377981055619 ) ) ;
#69590=CARTESIAN_POINT ( 'NONE',  ( 5.076628168052704559, 35.17559781766745175, -8.527530157486179263 ) ) ;
#69592=CARTESIAN_POINT ( 'NONE',  ( -2.816281873526473856, 49.12363466993042493, 9.499525473075851096E-16 ) ) ;
#69594=CARTESIAN_POINT ( 'NONE',  ( 2.035157376598822676, 57.43868534415484106, -7.964842623401177768 ) ) ;
#69595=CARTESIAN_POINT ( 'NONE',  ( 0.6076426042653108039, 62.37576471608601025, -6.499999999999992006 ) ) ;
#69596=CIRCLE ( 'NONE', #74349, 9.538348415311009632 ) ;
#69597=CARTESIAN_POINT ( 'NONE',  ( 18.28836319691945889, 29.34492782695770785, 6.499999999999997335 ) ) ;
#69599=CARTESIAN_POINT ( 'NONE',  ( 17.96484262340118221, 59.93868534415484106, 7.964842623401181321 ) ) ;
#69600=CARTESIAN_POINT ( 'NONE',  ( 15.44008868035555793, 41.39701867748817676, -9.422509992056140149 ) ) ;
#69602=DIRECTION ( 'NONE',  ( -0.000000000000000000, -0.000000000000000000, -1.000000000000000000 ) ) ;
#69604=CARTESIAN_POINT ( 'NONE',  ( 7.361572987183169658, 44.96726448433412315, -9.846743663894592657 ) ) ;
#69605=CARTESIAN_POINT ( 'NONE',  ( 2.035157376598824452, 28.68868534415484106, 7.964842623401179544 ) ) ;
#69606=DIRECTION ( 'NONE',  ( 0.000000000000000000, 0.000000000000000000, 1.000000000000000000 ) ) ;
#69607=CARTESIAN_POINT ( 'NONE',  ( 0.6178305044545838731, 29.74863466993042138, 9.382169495545420901 ) ) ;
#69609=CARTESIAN_POINT ( 'NONE',  ( 20.88017736071110164, 40.35535201082150536, 2.915334737309930979 ) ) ;
#69610=CARTESIAN_POINT ( 'NONE',  ( 6.565887622018943937, 5.165301336597086568, 12.81628187352647430 ) ) ;
#69611=CARTESIAN_POINT ( 'NONE',  ( 19.42250999205614193, 10.14701867748816966, 5.440088680355555262 ) ) ;
#69612=CARTESIAN_POINT ( 'NONE',  ( 12.91533473730992121, 39.52201867748817676, 10.88017736071110164 ) ) ;
#69613=CARTESIAN_POINT ( 'NONE',  ( 13.79529636645030344, 33.26208216824730357, 14.16423886937410614 ) ) ;
#69614=CARTESIAN_POINT ( 'NONE',  ( 19.84674366389459266, 28.71726448433411960, -2.638427012816827677 ) ) ;
#69615=CARTESIAN_POINT ( 'NONE',  ( 20.88017736071110164, 55.35535201082149825, 2.915334737309930979 ) ) ;
#69616=DIRECTION ( 'NONE',  ( -6.608470384673550777E-17, -1.000000000000000000, 0.000000000000000000 ) ) ;
#69617=CARTESIAN_POINT ( 'NONE',  ( 22.26659068614894466, 8.887082168247300018, 7.082119434687054849 ) ) ;
#69619=SURFACE_STYLE_USAGE ( .BOTH. , #9112 ) ;
#69620=CARTESIAN_POINT ( 'NONE',  ( 12.63842701281683922, 64.55059781766745175, -9.846743663894590881 ) ) ;
#69621=AXIS2_PLACEMENT_3D ( 'NONE', #7175, #6186, #74675 ) ;
#69622=ORIENTED_EDGE ( 'NONE', *, *, #17077, .F. ) ;
#69624=CARTESIAN_POINT ( 'NONE',  ( 22.26659068614894466, 33.88708216824730357, 7.082119434687054849 ) ) ;
#69625=CARTESIAN_POINT ( 'NONE',  ( -4.164238869374099927, 37.01208216824731068, 3.795296366450308767 ) ) ;
#69626=CARTESIAN_POINT ( 'NONE',  ( 18.52753015748617571, 8.092264484334117824, 4.923371831947298993 ) ) ;
#69627=B_SPLINE_CURVE_WITH_KNOTS ( 'NONE', 3,
 ( #59633, #36652, #22642, #53123 ),
 .UNSPECIFIED., .F., .F.,
 ( 4, 4 ),
 ( 7.152448122690996019E-18, 0.002562518741975553654 ),
 .UNSPECIFIED. ) ;
#69628=CARTESIAN_POINT ( 'NONE',  ( 5.076628168052704559, 65.17559781766745175, -8.527530157486179263 ) ) ;
#69630=CARTESIAN_POINT ( 'NONE',  ( 7.084665262690076126, 64.10535201082150536, 10.88017736071109987 ) ) ;
#69631=CARTESIAN_POINT ( 'NONE',  ( 19.38216949554541202, 15.99863466993042138, 9.382169495545424454 ) ) ;
#69632=CARTESIAN_POINT ( 'NONE',  ( 24.16423886937409904, 29.09541550158063572, 3.795296366450317205 ) ) ;
#69633=CARTESIAN_POINT ( 'NONE',  ( 0.5774900079438590739, 32.64701867748816966, -5.440088680355550821 ) ) ;
#69634=CARTESIAN_POINT ( 'NONE',  ( 7.084665262690076126, 27.02201867748817676, -10.88017736071110164 ) ) ;
#69636=CARTESIAN_POINT ( 'NONE',  ( 10.00000000000000178, 59.31368534415484106, 10.88017736071110342 ) ) ;
#69644=CARTESIAN_POINT ( 'NONE',  ( 24.16423886937410614, 9.303748834913967869, 8.672049930838204340E-16 ) ) ;
#69645=CARTESIAN_POINT ( 'NONE',  ( 17.08211943468705840, 60.13708216824729647, -12.26659068614894466 ) ) ;
#69646=CARTESIAN_POINT ( 'NONE',  ( -0.8801773607111009756, 3.063685344154838397, 1.068504757029289695E-15 ) ) ;
#69647=CARTESIAN_POINT ( 'NONE',  ( 12.63842701281683034, 32.46726448433412315, 9.846743663894596210 ) ) ;
#69648=CARTESIAN_POINT ( 'NONE',  ( 0.1532563361054082862, 66.21726448433413736, 2.638427012816831674 ) ) ;
#69649=CARTESIAN_POINT ( 'NONE',  ( 20.24186590665277663, 59.73410085661204505, 6.114288769123047196 ) ) ;
#69652=CARTESIAN_POINT ( 'NONE',  ( -2.816281873526473856, 9.123634669930421381, 9.499525473075851096E-16 ) ) ;
#69654=CARTESIAN_POINT ( 'NONE',  ( 6.204703633549690345, 40.76208216824731778, -14.16423886937410259 ) ) ;
#69655=CARTESIAN_POINT ( 'NONE',  ( 17.08211943468705840, 45.13708216824730357, -12.26659068614894466 ) ) ;
#69657=CARTESIAN_POINT ( 'NONE',  ( 19.42250999205614193, 15.14701867748817143, 5.440088680355555262 ) ) ;
#69658=CARTESIAN_POINT ( 'NONE',  ( 6.565887622018943937, 53.08196800326374643, -12.81628187352647608 ) ) ;
#69659=CARTESIAN_POINT ( 'NONE',  ( 19.42250999205614548, 30.98035201082150536, -5.440088680355545492 ) ) ;
#69660=CARTESIAN_POINT ( 'NONE',  ( 10.00000000000000000, 44.75893115100078745, -9.846743663894594434 ) ) ;
#69661=CARTESIAN_POINT ( 'NONE',  ( 20.88017736071110164, 30.35535201082151247, 2.915334737309930979 ) ) ;
#69663=CARTESIAN_POINT ( 'NONE',  ( 5.076628168052704559, 60.17559781766745175, -8.527530157486179263 ) ) ;
#69664=CARTESIAN_POINT ( 'NONE',  ( 20.88017736071110519, 65.56368534415483396, 2.639326808657452039E-16 ) ) ;
#69665=CARTESIAN_POINT ( 'NONE',  ( 4.559911319644449179, 22.23035201082150536, -9.422509992056141925 ) ) ;
#69666=( GEOMETRIC_REPRESENTATION_CONTEXT ( 3 ) GLOBAL_UNCERTAINTY_ASSIGNED_CONTEXT ( ( #27289 ) ) GLOBAL_UNIT_ASSIGNED_CONTEXT ( ( #80642, #4160, #74106 ) ) REPRESENTATION_CONTEXT ( 'NONE', 'WORKASPACE' ) );
#69673=CARTESIAN_POINT ( 'NONE',  ( 10.00000000000000000, 34.75893115100078745, -9.846743663894594434 ) ) ;
#69674=CARTESIAN_POINT ( 'NONE',  ( -23.44000000000001194, 92.00000000000000000, 9.500000000000000000 ) ) ;
#69675=EDGE_CURVE ( 'NONE', #30783, #39614, #48188, .T. ) ;
#69678=CARTESIAN_POINT ( 'NONE',  ( -0.1503990784575328643, 70.00000000000000000, -6.262539305110068177 ) ) ;
#69680=CARTESIAN_POINT ( 'NONE',  ( 0.1532563361054100626, 60.80059781766744464, -2.638427012816831230 ) ) ;
#69681=CARTESIAN_POINT ( 'NONE',  ( -4.164238869374099927, 47.01208216824729647, 3.795296366450308767 ) ) ;
#69682=CARTESIAN_POINT ( 'NONE',  ( 19.84674366389459266, 63.71726448433412315, -2.638427012816827677 ) ) ;
#69683=CARTESIAN_POINT ( 'NONE',  ( 20.10384461210892582, 41.74302437010792488, 6.337995344473752901 ) ) ;
#69684=CARTESIAN_POINT ( 'NONE',  ( 17.20831665107776587, 12.88393115100078390, 7.208316651077764980 ) ) ;
#69685=CARTESIAN_POINT ( 'NONE',  ( 21.09922568453594849, 56.20696800326375353, 6.408140936763242479 ) ) ;
#69686=CARTESIAN_POINT ( 'NONE',  ( 10.00000000000000000, 59.75893115100078745, -9.846743663894594434 ) ) ;
#69687=CARTESIAN_POINT ( 'NONE',  ( 12.91533473730992121, 59.52201867748816966, 10.88017736071110164 ) ) ;
#69689=AXIS2_PLACEMENT_3D ( 'NONE', #53778, #7306, #29778 ) ;
#69691=CARTESIAN_POINT ( 'NONE',  ( 19.42250999205614548, 55.98035201082150536, -5.440088680355545492 ) ) ;
#69692=EDGE_CURVE ( 'NONE', #84535, #71042, #92139, .T. ) ;
#69696=CARTESIAN_POINT ( 'NONE',  ( 12.91533473730992121, 34.52201867748817676, 10.88017736071110164 ) ) ;
#69697=CARTESIAN_POINT ( 'NONE',  ( 21.09922568453595559, 7.040301336597086568, -6.408140936763230044 ) ) ;
#69698=CARTESIAN_POINT ( 'NONE',  ( 20.88017736071110164, 55.35535201082149825, 2.915334737309930979 ) ) ;
#69702=CARTESIAN_POINT ( 'NONE',  ( 15.44008868035555793, 41.39701867748817676, -9.422509992056140149 ) ) ;
#69704=CARTESIAN_POINT ( 'NONE',  ( 14.92337183194729633, 32.67559781766745175, 8.527530157486181039 ) ) ;
#69705=CARTESIAN_POINT ( 'NONE',  ( 17.20831665107776587, 4.133931151000785675, -7.208316651077762316 ) ) ;
#69707=CARTESIAN_POINT ( 'NONE',  ( -2.816281873526473856, 14.33196800326375531, 3.434112377981055619 ) ) ;
#69708=CARTESIAN_POINT ( 'NONE',  ( 12.91533473730993009, 16.60535201082150891, -10.88017736071109987 ) ) ;
#69709=PLANE ( 'NONE',  #84045 ) ;
#69712=CARTESIAN_POINT ( 'NONE',  ( -4.164238869374099927, 22.01208216824730357, 3.795296366450308767 ) ) ;
#69714=CARTESIAN_POINT ( 'NONE',  ( 24.16423886937410614, 64.30374883491396076, 8.672049930838204340E-16 ) ) ;
#69715=CARTESIAN_POINT ( 'NONE',  ( 7.361572987183169658, 34.96726448433411605, -9.846743663894592657 ) ) ;
#69717=CARTESIAN_POINT ( 'NONE',  ( 18.52753015748618282, 23.92559781766745530, -4.923371831947291888 ) ) ;
#69718=CARTESIAN_POINT ( 'NONE',  ( -0.8801773607110991993, 17.85535201082150536, -2.915334737309923874 ) ) ;
#69720=CARTESIAN_POINT ( 'NONE',  ( 0.1532563361054083140, 36.00893115100078745, 1.131784320476157264E-15 ) ) ;
#69721=CARTESIAN_POINT ( 'NONE',  ( 20.88017736071110875, 30.77201867748816966, -2.915334737309920765 ) ) ;
#69722=CARTESIAN_POINT ( 'NONE',  ( 1.472469842513823179, 65.59226448433412315, -4.923371831947296329 ) ) ;
#69723=CARTESIAN_POINT ( 'NONE',  ( 17.08211943468705840, 10.13708216824730179, -12.26659068614894466 ) ) ;
#69725=CARTESIAN_POINT ( 'NONE',  ( 1.274849032794278747, 42.55509018479936856, -6.499999999999960032 ) ) ;
#69726=CARTESIAN_POINT ( 'NONE',  ( 2.791683348922237240, 15.38393115100078212, -7.208316651077763204 ) ) ;
#69727=CARTESIAN_POINT ( 'NONE',  ( 13.43411237798106583, 32.66530133659708213, -12.81628187352647252 ) ) ;
#69728=CARTESIAN_POINT ( 'NONE',  ( 2.791683348922237240, 60.38393115100078745, -7.208316651077763204 ) ) ;
#69730=CARTESIAN_POINT ( 'NONE',  ( 17.20831665107776587, 17.88393115100078745, 7.208316651077764980 ) ) ;
#69733=CARTESIAN_POINT ( 'NONE',  ( -46.53118954259812057, 102.2886238795329490, -7.275463144368016444 ) ) ;
#69734=CARTESIAN_POINT ( 'NONE',  ( 13.79529636645031943, 60.34541550158063927, -14.16423886937409904 ) ) ;
#69735=CARTESIAN_POINT ( 'NONE',  ( 19.42250999205614548, 50.98035201082151247, -5.440088680355545492 ) ) ;
#69736=CARTESIAN_POINT ( 'NONE',  ( -4.164238869374099927, 2.012082168247300906, 3.795296366450308767 ) ) ;
#69737=CARTESIAN_POINT ( 'NONE',  ( -0.8801773607111008646, 53.27201867748816966, 2.915334737309923430 ) ) ;
#69738=CARTESIAN_POINT ( 'NONE',  ( 0.1532563361054082862, 31.21726448433412315, 2.638427012816831674 ) ) ;
#69739=CARTESIAN_POINT ( 'NONE',  ( 17.96484262340118221, 16.18868534415483396, -7.964842623401177768 ) ) ;
#69741=CARTESIAN_POINT ( 'NONE',  ( 0.1532563361054100626, 50.80059781766745175, -2.638427012816831230 ) ) ;
#69743=CARTESIAN_POINT ( 'NONE',  ( 2.035157376598824452, 53.68868534415484817, 7.964842623401179544 ) ) ;
#69744=CARTESIAN_POINT ( 'NONE',  ( 19.84674366389459266, 3.300597817667451750, 2.638427012816836559 ) ) ;
#69748=CARTESIAN_POINT ( 'NONE',  ( -0.1503990784575294781, 68.10158574516643171, 6.262539305110072618 ) ) ;
#69750=CARTESIAN_POINT ( 'NONE',  ( 7.361572987183170547, 47.05059781766745175, 9.846743663894590881 ) ) ;
#69751=CARTESIAN_POINT ( 'NONE',  ( 18.52753015748618282, 18.92559781766745175, -4.923371831947291888 ) ) ;
#69752=CARTESIAN_POINT ( 'NONE',  ( -2.816281873526473856, 59.33196800326374643, 3.434112377981055619 ) ) ;
#69753=CARTESIAN_POINT ( 'NONE',  ( -0.8801773607110991993, 22.85535201082150181, -2.915334737309923874 ) ) ;
#69754=CARTESIAN_POINT ( 'NONE',  ( 12.63842701281683922, 54.55059781766745175, -9.846743663894590881 ) ) ;
#69755=CARTESIAN_POINT ( 'NONE',  ( 2.917880565312948704, 32.63708216824730357, 12.26659068614894643 ) ) ;
#69757=CARTESIAN_POINT ( 'NONE',  ( 2.917880565312948704, 62.63708216824730357, 12.26659068614894643 ) ) ;
#69758=CARTESIAN_POINT ( 'NONE',  ( 7.361572987183170547, 62.05059781766745886, 9.846743663894590881 ) ) ;
#69760=CARTESIAN_POINT ( 'NONE',  ( -0.8801773607111009756, 53.06368534415484106, 1.068504757029289695E-15 ) ) ;
#69761=CARTESIAN_POINT ( 'NONE',  ( 18.52753015748617571, 18.09226448433411960, 4.923371831947298993 ) ) ;
#69762=DIRECTION ( 'NONE',  ( -0.8320502943378436100, 0.5547001962252291474, -0.000000000000000000 ) ) ;
#69766=CARTESIAN_POINT ( 'NONE',  ( 12.63842701281683922, 9.550597817667449974, -9.846743663894590881 ) ) ;
#69767=VERTEX_POINT ( 'NONE', #16140 ) ;
#69768=CARTESIAN_POINT ( 'NONE',  ( 22.26659068614894466, 23.88708216824730357, 7.082119434687054849 ) ) ;
#69769=CARTESIAN_POINT ( 'NONE',  ( 18.52753015748618282, 23.92559781766745530, -4.923371831947291888 ) ) ;
#69770=CARTESIAN_POINT ( 'NONE',  ( 17.96484262340118221, 44.93868534415483396, 7.964842623401181321 ) ) ;
#69774=CARTESIAN_POINT ( 'NONE',  ( -0.8801773607110991993, 37.85535201082151247, -2.915334737309923874 ) ) ;
#69775=CARTESIAN_POINT ( 'NONE',  ( -0.1503990784575279516, 43.10158574516643171, 6.262539305110076171 ) ) ;
#69776=EDGE_CURVE ( 'NONE', #86034, #5496, #62110, .T. ) ;
#69779=CARTESIAN_POINT ( 'NONE',  ( 17.96484262340118221, 46.18868534415484106, -7.964842623401177768 ) ) ;
#69780=CARTESIAN_POINT ( 'NONE',  ( 6.204703633549690345, 12.84541550158063572, 14.16423886937410082 ) ) ;
#69781=ORIENTED_EDGE ( 'NONE', *, *, #1621, .T. ) ;
#69782=CARTESIAN_POINT ( 'NONE',  ( -1.099225684535947600, 19.54030133659708568, 6.408140936763237150 ) ) ;
#69784=CARTESIAN_POINT ( 'NONE',  ( 0.1532563361054082862, 16.21726448433411960, 2.638427012816831674 ) ) ;
#69787=CARTESIAN_POINT ( 'NONE',  ( 1.472469842513823179, 20.59226448433411960, -4.923371831947296329 ) ) ;
#69788=CARTESIAN_POINT ( 'NONE',  ( -0.8801773607111008646, 33.27201867748817676, 2.915334737309923430 ) ) ;
#69789=MECHANICAL_DESIGN_GEOMETRIC_PRESENTATION_REPRESENTATION('',(#36227),#84138);
#69795=CARTESIAN_POINT ( 'NONE',  ( 15.44008868035555260, 54.73035201082150536, 9.422509992056143702 ) ) ;
#69797=CARTESIAN_POINT ( 'NONE',  ( 19.38216949554541557, 62.24863466993041072, -9.382169495545420901 ) ) ;
#69798=CARTESIAN_POINT ( 'NONE',  ( 20.88017736071110164, 60.35535201082151957, 2.915334737309930979 ) ) ;
#69799=EDGE_CURVE ( 'NONE', #23173, #87694, #46148, .T. ) ;
#69800=CARTESIAN_POINT ( 'NONE',  ( 19.38216949554541557, 17.24863466993041783, -9.382169495545420901 ) ) ;
#69802=CARTESIAN_POINT ( 'NONE',  ( 0.1532563361054100626, 30.80059781766744820, -2.638427012816831230 ) ) ;
#69803=CARTESIAN_POINT ( 'NONE',  ( 16.40814093676324603, 57.45696800326375353, -11.09922568453594671 ) ) ;
#69805=CARTESIAN_POINT ( 'NONE',  ( 14.92337183194729988, 19.34226448433411960, -8.527530157486177487 ) ) ;
#69806=CARTESIAN_POINT ( 'NONE',  ( 22.81628187352647785, 21.41530133659708923, 3.434112377981063169 ) ) ;
#69808=LINE ( 'NONE', #15824, #94462 ) ;
#69809=STYLED_ITEM ( 'NONE', ( #46834 ), #299 ) ;
#69810=CARTESIAN_POINT ( 'NONE',  ( 10.00000000000000178, 44.31368534415484106, 10.88017736071110342 ) ) ;
#69811=CARTESIAN_POINT ( 'NONE',  ( 12.63842701281683922, 64.55059781766745175, -9.846743663894590881 ) ) ;
#69813=CARTESIAN_POINT ( 'NONE',  ( 12.63842701281683034, 17.46726448433411250, 9.846743663894596210 ) ) ;
#69814=CARTESIAN_POINT ( 'NONE',  ( -0.8801773607111009756, 8.063685344154837509, 1.068504757029289695E-15 ) ) ;
#69815=CARTESIAN_POINT ( 'NONE',  ( 3.591859063236761518, 9.956968003263753531, 11.09922568453594849 ) ) ;
#69816=CARTESIAN_POINT ( 'NONE',  ( 15.44008868035555260, 4.730352010821504471, 9.422509992056143702 ) ) ;
#69818=CARTESIAN_POINT ( 'NONE',  ( 19.42250999205614548, 25.98035201082150891, -5.440088680355545492 ) ) ;
#69822=CARTESIAN_POINT ( 'NONE',  ( 19.84674366389459266, 28.71726448433411960, -2.638427012816827677 ) ) ;
#69823=CARTESIAN_POINT ( 'NONE',  ( 20.88017736071110519, 15.56368534415483751, 2.639326808657452039E-16 ) ) ;
#69825=CARTESIAN_POINT ( 'NONE',  ( 15.44008868035555793, 26.39701867748817321, -9.422509992056140149 ) ) ;
#69826=CARTESIAN_POINT ( 'NONE',  ( 13.79529636645031943, 60.34541550158063927, -14.16423886937409904 ) ) ;
#69828=CARTESIAN_POINT ( 'NONE',  ( 10.00000000000000178, 2.258931151000784787, 9.846743663894594434 ) ) ;
#69830=CARTESIAN_POINT ( 'NONE',  ( 18.52753015748618282, 38.92559781766745175, -4.923371831947291888 ) ) ;
#69833=CARTESIAN_POINT ( 'NONE',  ( 7.361572987183170547, 62.05059781766745886, 9.846743663894590881 ) ) ;
#69835=CARTESIAN_POINT ( 'NONE',  ( 2.917880565312950480, 25.97041550158063572, -12.26659068614894821 ) ) ;
#69836=CARTESIAN_POINT ( 'NONE',  ( 1.472469842513823179, 36.42559781766745175, 4.923371831947296329 ) ) ;
#69839=CARTESIAN_POINT ( 'NONE',  ( 17.08211943468705840, 50.13708216824730357, -12.26659068614894466 ) ) ;
#69840=CARTESIAN_POINT ( 'NONE',  ( 0.1532563361054082862, 21.21726448433412315, 2.638427012816831674 ) ) ;
#69843=CARTESIAN_POINT ( 'NONE',  ( 19.42250999205614548, 50.98035201082151247, -5.440088680355545492 ) ) ;
#69844=CARTESIAN_POINT ( 'NONE',  ( 6.565887622018943937, 58.08196800326376064, -12.81628187352647608 ) ) ;
#69845=CARTESIAN_POINT ( 'NONE',  ( 15.44008868035555793, 11.39701867748817143, -9.422509992056140149 ) ) ;
#69846=CARTESIAN_POINT ( 'NONE',  ( 19.38216949554541557, 52.24863466993041072, -9.382169495545420901 ) ) ;
#69847=CARTESIAN_POINT ( 'NONE',  ( -2.816281873526473856, -0.6680319967362464695, 3.434112377981055619 ) ) ;
#69848=CARTESIAN_POINT ( 'NONE',  ( 0.1532563361054083140, 1.008931151000784787, 1.131784320476157264E-15 ) ) ;
#69852=CARTESIAN_POINT ( 'NONE',  ( -0.3689425029237881626, 57.42874883491397497, 10.36894250292379027 ) ) ;
#69853=CARTESIAN_POINT ( 'NONE',  ( 17.08211943468705130, 13.47041550158063572, 12.26659068614894998 ) ) ;
#69854=CARTESIAN_POINT ( 'NONE',  ( 15.44008868035555260, 14.73035201082150536, 9.422509992056143702 ) ) ;
#69855=AXIS2_PLACEMENT_3D ( 'NONE', #51592, #82076, #97610 ) ;
#69856=CARTESIAN_POINT ( 'NONE',  ( 7.084665262690076126, 34.10535201082151247, 10.88017736071109987 ) ) ;
#69857=LINE ( 'NONE', #1379, #23980 ) ;
#69859=CARTESIAN_POINT ( 'NONE',  ( 7.361572987183169658, -0.03273551566588185635, -9.846743663894592657 ) ) ;
#69861=CARTESIAN_POINT ( 'NONE',  ( 5.076628168052703671, 26.84226448433411960, 8.527530157486179263 ) ) ;
#69863=DIRECTION ( 'NONE',  ( -1.000000000000000000, 0.000000000000000000, 0.000000000000000000 ) ) ;
#69864=CARTESIAN_POINT ( 'NONE',  ( 19.84674366389459266, 8.717264484334116048, -2.638427012816827677 ) ) ;
#69865=CARTESIAN_POINT ( 'NONE',  ( 1.472469842513823179, 30.59226448433411960, -4.923371831947296329 ) ) ;
#69866=CARTESIAN_POINT ( 'NONE',  ( 2.035157376598824452, 13.68868534415483751, 7.964842623401179544 ) ) ;
#69869=CARTESIAN_POINT ( 'NONE',  ( -2.816281873526473856, 34.12363466993042493, 9.499525473075851096E-16 ) ) ;
#69870=CARTESIAN_POINT ( 'NONE',  ( 1.472469842513823179, 10.59226448433411782, -4.923371831947296329 ) ) ;
#69872=CARTESIAN_POINT ( 'NONE',  ( 18.52753015748618282, 53.92559781766745175, -4.923371831947291888 ) ) ;
#69873=CARTESIAN_POINT ( 'NONE',  ( 7.361572987183170547, 27.05059781766745175, 9.846743663894590881 ) ) ;
#69874=CARTESIAN_POINT ( 'NONE',  ( -4.164238869374098151, 1.595415501580634388, -3.795296366450310543 ) ) ;
#69875=CARTESIAN_POINT ( 'NONE',  ( 6.204703633549690345, 20.76208216824730357, -14.16423886937410259 ) ) ;
#69876=CARTESIAN_POINT ( 'NONE',  ( 2.035157376598822676, 42.43868534415483396, -7.964842623401177768 ) ) ;
#69877=CARTESIAN_POINT ( 'NONE',  ( 17.96484262340118221, 11.18868534415483929, -7.964842623401177768 ) ) ;
#69878=CARTESIAN_POINT ( 'NONE',  ( 0.5774900079438590739, 42.64701867748816966, -5.440088680355550821 ) ) ;
#69879=CARTESIAN_POINT ( 'NONE',  ( 10.00000000000000178, 29.31368534415483751, 10.88017736071110342 ) ) ;
#69880=ORIENTED_EDGE ( 'NONE', *, *, #72374, .F. ) ;
#69881=CARTESIAN_POINT ( 'NONE',  ( 19.38216949554541202, 30.99863466993042138, 9.382169495545424454 ) ) ;
#69882=CARTESIAN_POINT ( 'NONE',  ( 19.42250999205614193, 40.14701867748817676, 5.440088680355555262 ) ) ;
#69883=ORIENTED_EDGE ( 'NONE', *, *, #37217, .T. ) ;
#69884=CARTESIAN_POINT ( 'NONE',  ( -2.816281873526473856, 54.33196800326376064, 3.434112377981055619 ) ) ;
#69885=ADVANCED_FACE ( 'NONE', ( #47620 ), #66709, .F. ) ;
#69886=CARTESIAN_POINT ( 'NONE',  ( 12.91533473730993009, 46.60535201082150536, -10.88017736071109987 ) ) ;
#69888=CARTESIAN_POINT ( 'NONE',  ( 0.5774900079438590739, 47.64701867748817676, -5.440088680355550821 ) ) ;
#69890=CARTESIAN_POINT ( 'NONE',  ( 19.72487221294571214, 57.80223176428831522, -6.499999999999988454 ) ) ;
#69892=CARTESIAN_POINT ( 'NONE',  ( 20.36894250292379382, 63.67874883491396787, 10.36894250292379205 ) ) ;
#69893=CARTESIAN_POINT ( 'NONE',  ( 10.00000000000000000, 66.81368534415484817, -10.88017736071110342 ) ) ;
#69894=CARTESIAN_POINT ( 'NONE',  ( 24.16423886937409904, 9.095415501580633943, 3.795296366450317205 ) ) ;
#69895=SURFACE_SIDE_STYLE ('',( #39402 ) ) ;
#69896=CARTESIAN_POINT ( 'NONE',  ( 19.42250999205614193, 10.14701867748816966, 5.440088680355555262 ) ) ;
#69897=CARTESIAN_POINT ( 'NONE',  ( 7.361572987183169658, 49.96726448433410894, -9.846743663894592657 ) ) ;
#69899=CARTESIAN_POINT ( 'NONE',  ( 1.472469842513823179, 40.59226448433411605, -4.923371831947296329 ) ) ;
#69901=CARTESIAN_POINT ( 'NONE',  ( 15.44008868035555260, 39.73035201082150536, 9.422509992056143702 ) ) ;
#69902=CARTESIAN_POINT ( 'NONE',  ( 18.52753015748618282, 43.92559781766745175, -4.923371831947291888 ) ) ;
#69903=CARTESIAN_POINT ( 'NONE',  ( 6.565887622018943937, 18.08196800326375708, -12.81628187352647608 ) ) ;
#69904=DIRECTION ( 'NONE',  ( -0.8320502943378437211, 0.5547001962252290364, 0.000000000000000000 ) ) ;
#69906=CARTESIAN_POINT ( 'NONE',  ( 2.035157376598822676, 47.43868534415484817, -7.964842623401177768 ) ) ;
#69907=CARTESIAN_POINT ( 'NONE',  ( -0.3689425029237881626, 57.42874883491397497, 10.36894250292379027 ) ) ;
#69910=CARTESIAN_POINT ( 'NONE',  ( 3.591859063236763294, 18.29030133659708568, -11.09922568453595026 ) ) ;
#69912=ORIENTED_EDGE ( 'NONE', *, *, #2414, .F. ) ;
#69913=CARTESIAN_POINT ( 'NONE',  ( 21.09922568453594849, 26.20696800326375353, 6.408140936763242479 ) ) ;
#69914=CARTESIAN_POINT ( 'NONE',  ( 17.96484262340118221, 19.93868534415484106, 7.964842623401181321 ) ) ;
#69918=CARTESIAN_POINT ( 'NONE',  ( 2.791683348922240793, 46.63393115100077324, 7.208316651077764092 ) ) ;
#69919=CARTESIAN_POINT ( 'NONE',  ( 2.791683348922240793, 31.63393115100078745, 7.208316651077764092 ) ) ;
#69922=CARTESIAN_POINT ( 'NONE',  ( 17.20831665107776587, 29.13393115100078390, -7.208316651077762316 ) ) ;
#69923=CARTESIAN_POINT ( 'NONE',  ( 20.24186590665278018, 57.61633188102329228, -6.114288769123040090 ) ) ;
#69924=CARTESIAN_POINT ( 'NONE',  ( 0.000000000000000000, 81.99999999999992895, 5.000000000000000000 ) ) ;
#69925=CARTESIAN_POINT ( 'NONE',  ( 17.20831665107776587, 7.883931151000784787, 7.208316651077764980 ) ) ;
#69926=MECHANICAL_DESIGN_GEOMETRIC_PRESENTATION_REPRESENTATION('',(#25273),#76284);
#69929=CARTESIAN_POINT ( 'NONE',  ( 18.52753015748618282, 43.92559781766745175, -4.923371831947291888 ) ) ;
#69930=ORIENTED_EDGE ( 'NONE', *, *, #84695, .T. ) ;
#69933=CARTESIAN_POINT ( 'NONE',  ( 19.38216949554541202, 15.99863466993042138, 9.382169495545424454 ) ) ;
#69934=CARTESIAN_POINT ( 'NONE',  ( 15.44008868035555260, 54.73035201082150536, 9.422509992056143702 ) ) ;
#69935=CARTESIAN_POINT ( 'NONE',  ( 20.36894250292379738, 44.92874883491396787, -10.36894250292379027 ) ) ;
#69936=( NAMED_UNIT ( * ) PLANE_ANGLE_UNIT ( ) SI_UNIT ( $, .RADIAN. ) );
#69938=CARTESIAN_POINT ( 'NONE',  ( -2.266590686148945544, 47.22041550158063927, 7.082119434687048631 ) ) ;
#69939=CARTESIAN_POINT ( 'NONE',  ( 17.08211943468705130, 53.47041550158063217, 12.26659068614894998 ) ) ;
#69940=CARTESIAN_POINT ( 'NONE',  ( 20.36894250292379738, 19.92874883491396787, -10.36894250292379027 ) ) ;
#69941=CARTESIAN_POINT ( 'NONE',  ( 2.917880565312948704, 22.63708216824730002, 12.26659068614894643 ) ) ;
#69945=CARTESIAN_POINT ( 'NONE',  ( 1.472469842513823179, 46.42559781766745175, 4.923371831947296329 ) ) ;
#69946=CARTESIAN_POINT ( 'NONE',  ( 19.42250999205614193, 40.14701867748817676, 5.440088680355555262 ) ) ;
#69948=CARTESIAN_POINT ( 'NONE',  ( 20.00000000000000711, 88.18274230950564174, -5.338627755225069826 ) ) ;
#69949=EDGE_CURVE ( 'NONE', #39693, #40991, #8153, .T. ) ;
#69950=CARTESIAN_POINT ( 'NONE',  ( 1.472469842513823179, 46.42559781766745175, 4.923371831947296329 ) ) ;
#69951=CARTESIAN_POINT ( 'NONE',  ( 21.09922568453595559, 62.04030133659709634, -6.408140936763230044 ) ) ;
#69953=CARTESIAN_POINT ( 'NONE',  ( 7.361572987183170547, 37.05059781766744464, 9.846743663894590881 ) ) ;
#69954=CARTESIAN_POINT ( 'NONE',  ( 5.076628168052704559, 60.17559781766745175, -8.527530157486179263 ) ) ;
#69955=CARTESIAN_POINT ( 'NONE',  ( -4.164238869374099039, 36.80374883491396787, 8.674139862899312516E-16 ) ) ;
#69957=CARTESIAN_POINT ( 'NONE',  ( 22.26659068614894466, 8.887082168247300018, 7.082119434687054849 ) ) ;
#69961=CARTESIAN_POINT ( 'NONE',  ( 7.084665262690076126, 12.02201867748817321, -10.88017736071110164 ) ) ;
#69962=CARTESIAN_POINT ( 'NONE',  ( 22.81628187352647785, 6.623634669930420493, 6.195893100308588602E-16 ) ) ;
#69964=CARTESIAN_POINT ( 'NONE',  ( 10.00000000000000000, 66.81368534415484817, -10.88017736071110342 ) ) ;
#69965=CARTESIAN_POINT ( 'NONE',  ( 20.24186590665276597, 41.76028685723173339, 6.114288769123062295 ) ) ;
#69968=CARTESIAN_POINT ( 'NONE',  ( 10.00000000000000000, 1.813685344154838175, -10.88017736071110342 ) ) ;
#69970=CARTESIAN_POINT ( 'NONE',  ( -0.8801773607111009756, 33.06368534415484106, 1.068504757029289695E-15 ) ) ;
#69971=CARTESIAN_POINT ( 'NONE',  ( 0.5774900079438607392, 23.48035201082150536, 5.440088680355550821 ) ) ;
#69972=CARTESIAN_POINT ( 'NONE',  ( 10.00000000000000178, 5.373634669930420493, 12.81628187352647608 ) ) ;
#69973=CARTESIAN_POINT ( 'NONE',  ( 7.361572987183169658, 49.96726448433410894, -9.846743663894592657 ) ) ;
#69974=CARTESIAN_POINT ( 'NONE',  ( -1.099225684535947600, 64.54030133659709634, 6.408140936763237150 ) ) ;
#69975=CARTESIAN_POINT ( 'NONE',  ( 10.00000000000000000, -0.2410688489992152128, -9.846743663894594434 ) ) ;
#69977=CARTESIAN_POINT ( 'NONE',  ( -0.8801773607110991993, 27.85535201082150181, -2.915334737309923874 ) ) ;
#69978=CARTESIAN_POINT ( 'NONE',  ( 0.6178305044545838731, 29.74863466993042138, 9.382169495545420901 ) ) ;
#69979=CARTESIAN_POINT ( 'NONE',  ( 13.99999999999999822, 61.00000000000000711, 6.500000000000000888 ) ) ;
#69980=AXIS2_PLACEMENT_3D ( 'NONE', #562, #61504, #95960 ) ;
#69981=CARTESIAN_POINT ( 'NONE',  ( 2.791683348922237240, 55.38393115100078745, -7.208316651077763204 ) ) ;
#69982=CARTESIAN_POINT ( 'NONE',  ( 15.44008868035555793, 51.39701867748816966, -9.422509992056140149 ) ) ;
#69983=CARTESIAN_POINT ( 'NONE',  ( 18.52753015748617571, 13.09226448433411960, 4.923371831947298993 ) ) ;
#69984=CARTESIAN_POINT ( 'NONE',  ( 22.81628187352647785, 21.41530133659708923, 3.434112377981063169 ) ) ;
#69985=CARTESIAN_POINT ( 'NONE',  ( 17.96484262340118221, 64.93868534415483396, 7.964842623401181321 ) ) ;
#69990=CARTESIAN_POINT ( 'NONE',  ( 2.035157376598824452, 48.68868534415483396, 7.964842623401179544 ) ) ;
#69991=CARTESIAN_POINT ( 'NONE',  ( 0.6178305044545818747, 48.49863466993042493, -9.382169495545419124 ) ) ;
#69992=CARTESIAN_POINT ( 'NONE',  ( 17.08211943468705840, 15.13708216824730179, -12.26659068614894466 ) ) ;
#69993=CARTESIAN_POINT ( 'NONE',  ( 19.84674366389459621, 23.50893115100078390, 7.409399052514197653E-17 ) ) ;
#69995=CARTESIAN_POINT ( 'NONE',  ( 10.00000000000000000, 11.81368534415483751, -10.88017736071110342 ) ) ;
#69996=CARTESIAN_POINT ( 'NONE',  ( 12.63842701281683922, 24.55059781766745175, -9.846743663894590881 ) ) ;
#69998=CARTESIAN_POINT ( 'NONE',  ( 10.00000000000000178, 58.05374883491397497, 14.16423886937410082 ) ) ;
#70000=DIRECTION ( 'NONE',  ( 0.000000000000000000, 0.000000000000000000, 1.000000000000000000 ) ) ;
#70002=EDGE_CURVE ( 'NONE', #1078, #87032, #95481, .T. ) ;
#70003=CARTESIAN_POINT ( 'NONE',  ( 12.91533473730993009, 6.605352010821504471, -10.88017736071109987 ) ) ;
#70004=CARTESIAN_POINT ( 'NONE',  ( 0.1532563361054100626, 15.80059781766745353, -2.638427012816831230 ) ) ;
#70005=AXIS2_PLACEMENT_3D ( 'NONE', #1039, #53522, #24530 ) ;
#70007=CARTESIAN_POINT ( 'NONE',  ( 2.035157376598822676, 2.438685344154838397, -7.964842623401177768 ) ) ;
#70008=CARTESIAN_POINT ( 'NONE',  ( 12.91533473730993009, 6.605352010821504471, -10.88017736071109987 ) ) ;
#70009=CARTESIAN_POINT ( 'NONE',  ( 14.92337183194729988, 44.34226448433412315, -8.527530157486177487 ) ) ;
#70010=CARTESIAN_POINT ( 'NONE',  ( -2.816281873526473856, 49.12363466993042493, 9.499525473075851096E-16 ) ) ;
#70011=CARTESIAN_POINT ( 'NONE',  ( -42.94000000000001194, 92.00000000000000000, 9.000000000000000000 ) ) ;
#70012=CARTESIAN_POINT ( 'NONE',  ( 6.204703633549690345, 25.76208216824730712, -14.16423886937410259 ) ) ;
#70013=CARTESIAN_POINT ( 'NONE',  ( 4.559911319644449179, 23.89701867748817321, 9.422509992056141925 ) ) ;
#70014=CARTESIAN_POINT ( 'NONE',  ( 6.204703633549690345, 67.84541550158060375, 14.16423886937410082 ) ) ;
#70017=CARTESIAN_POINT ( 'NONE',  ( 0.1532563361054082862, 46.21726448433411605, 2.638427012816831674 ) ) ;
#70019=CARTESIAN_POINT ( 'NONE',  ( 14.92337183194729633, 32.67559781766745175, 8.527530157486181039 ) ) ;
#70020=CARTESIAN_POINT ( 'NONE',  ( -46.44000000000001194, 93.00000000000000000, -9.500000000000000000 ) ) ;
#70023=CARTESIAN_POINT ( 'NONE',  ( 4.559911319644449179, 67.23035201082150536, -9.422509992056141925 ) ) ;
#70025=CARTESIAN_POINT ( 'NONE',  ( 19.84674366389459621, 58.50893115100078745, 7.409399052514197653E-17 ) ) ;
#70026=CARTESIAN_POINT ( 'NONE',  ( -0.8801773607110991993, 42.85535201082150536, -2.915334737309923874 ) ) ;
#70027=CARTESIAN_POINT ( 'NONE',  ( 17.96484262340118221, 4.938685344154837509, 7.964842623401181321 ) ) ;
#70028=CARTESIAN_POINT ( 'NONE',  ( 10.00000000000000178, 30.37363466993042138, 12.81628187352647608 ) ) ;
#70029=CARTESIAN_POINT ( 'NONE',  ( -4.164238869374098151, 16.59541550158063927, -3.795296366450310543 ) ) ;
#70031=CARTESIAN_POINT ( 'NONE',  ( 13.43411237798106583, 47.66530133659709634, -12.81628187352647252 ) ) ;
#70033=CARTESIAN_POINT ( 'NONE',  ( 10.00000000000000000, 64.75893115100078035, -9.846743663894594434 ) ) ;
#70034=CARTESIAN_POINT ( 'NONE',  ( 20.88017736071110519, 15.56368534415483751, 2.639326808657452039E-16 ) ) ;
#70035=ORIENTED_EDGE ( 'NONE', *, *, #12967, .F. ) ;
#70037=CARTESIAN_POINT ( 'NONE',  ( 7.084665262690076126, 32.02201867748816966, -10.88017736071110164 ) ) ;
#70039=CARTESIAN_POINT ( 'NONE',  ( 19.42250999205614193, 65.14701867748817676, 5.440088680355555262 ) ) ;
#70040=CARTESIAN_POINT ( 'NONE',  ( 20.88017736071110875, 65.77201867748817676, -2.915334737309920765 ) ) ;
#70042=CARTESIAN_POINT ( 'NONE',  ( 10.00000000000000178, 12.25893115100078568, 9.846743663894594434 ) ) ;
#70043=CARTESIAN_POINT ( 'NONE',  ( 7.084665262690076126, 69.10535201082151957, 10.88017736071109987 ) ) ;
#70044=CARTESIAN_POINT ( 'NONE',  ( -46.52365679472261206, 102.3054413859459828, 7.234551493516248932 ) ) ;
#70045=CARTESIAN_POINT ( 'NONE',  ( 10.00000000000000178, 2.258931151000784787, 9.846743663894594434 ) ) ;
#70048=CARTESIAN_POINT ( 'NONE',  ( 19.84674366389459266, 38.30059781766745175, 2.638427012816836559 ) ) ;
#70051=FACE_OUTER_BOUND ( 'NONE', #54132, .T. ) ;
#70052=CARTESIAN_POINT ( 'NONE',  ( 20.36894250292379382, 8.678748834913967869, 10.36894250292379205 ) ) ;
#70053=CARTESIAN_POINT ( 'NONE',  ( 10.00000000000000000, 62.87363466993042493, -12.81628187352647608 ) ) ;
#70054=SURFACE_SIDE_STYLE ('',( #56525 ) ) ;
#70055=CARTESIAN_POINT ( 'NONE',  ( 17.08211943468705130, 18.47041550158063572, 12.26659068614894998 ) ) ;
#70057=DIRECTION ( 'NONE',  ( 0.000000000000000000, -1.000000000000000000, 0.000000000000000000 ) ) ;
#70058=DIRECTION ( 'NONE',  ( 0.000000000000000000, -1.000000000000000000, 0.000000000000000000 ) ) ;
#70059=CARTESIAN_POINT ( 'NONE',  ( -0.8801773607111009756, 63.06368534415484106, 1.068504757029289695E-15 ) ) ;
#70060=CARTESIAN_POINT ( 'NONE',  ( -0.8801773607110991993, 22.85535201082150181, -2.915334737309923874 ) ) ;
#70063=CARTESIAN_POINT ( 'NONE',  ( 14.92337183194729988, 9.342264484334119601, -8.527530157486177487 ) ) ;
#70064=CARTESIAN_POINT ( 'NONE',  ( 19.84674366389459266, 8.717264484334116048, -2.638427012816827677 ) ) ;
#70065=CARTESIAN_POINT ( 'NONE',  ( 13.43411237798105340, 35.58196800326375353, 12.81628187352647963 ) ) ;
#70066=CARTESIAN_POINT ( 'NONE',  ( 10.00000000000000178, 27.25893115100078390, 9.846743663894594434 ) ) ;
#70070=CARTESIAN_POINT ( 'NONE',  ( 13.43411237798106583, 17.66530133659708923, -12.81628187352647252 ) ) ;
#70072=DIRECTION ( 'NONE',  ( 0.000000000000000000, 0.000000000000000000, 1.000000000000000000 ) ) ;
#70073=CARTESIAN_POINT ( 'NONE',  ( 2.791683348922240793, 6.633931151000785675, 7.208316651077764092 ) ) ;
#70074=ORIENTED_EDGE ( 'NONE', *, *, #49530, .T. ) ;
#70076=CARTESIAN_POINT ( 'NONE',  ( -0.8801773607110991993, 42.85535201082150536, -2.915334737309923874 ) ) ;
#70077=CARTESIAN_POINT ( 'NONE',  ( -4.164238869374099927, 32.01208216824730357, 3.795296366450308767 ) ) ;
#70078=CARTESIAN_POINT ( 'NONE',  ( 2.791683348922240793, 36.63393115100078035, 7.208316651077764092 ) ) ;
#70079=CARTESIAN_POINT ( 'NONE',  ( 17.20831665107776587, 4.133931151000785675, -7.208316651077762316 ) ) ;
#70080=CARTESIAN_POINT ( 'NONE',  ( 3.591859063236761518, 59.95696800326375353, 11.09922568453594849 ) ) ;
#70082=CARTESIAN_POINT ( 'NONE',  ( 12.91533473730993009, 21.60535201082150536, -10.88017736071109987 ) ) ;
#70083=CARTESIAN_POINT ( 'NONE',  ( 3.591859063236761518, 24.95696800326375353, 11.09922568453594849 ) ) ;
#70084=CARTESIAN_POINT ( 'NONE',  ( 0.1532563361054082862, 41.21726448433411605, 2.638427012816831674 ) ) ;
#70086=CARTESIAN_POINT ( 'NONE',  ( 10.00000000000000178, 55.37363466993042493, 12.81628187352647608 ) ) ;
#70088=CARTESIAN_POINT ( 'NONE',  ( 4.559911319644449179, 53.89701867748817676, 9.422509992056141925 ) ) ;
#70093=( BOUNDED_SURFACE ( )  B_SPLINE_SURFACE ( 1, 2, ( 
 ( #89378, #41448, #5406, #18925, #66373, #96907, #58876, #51380, #33892, #64879, #79902, #26902, #83360, #14382, #43864, #29356, #74866, #6365, #82361, #53850, #59859, #91849, #37876, #59364, #15377, #82867, #76350, #60353, #13883, #60846, #67368, #68369, #37382, #67872, #51879, #22872, #98393, #44367, #91345, #7865, #89867, #97392, #90346, #98888, #53343, #30339, #14883, #45352, #83851, #28860, #97898, #66875, #21884, #21382, #36380, #45859, #7377, #36879, #52362, #38361, #30840, #68858, #390, #44851, #61338, #75357, #6871, #23365, #13380, #29850, #74359, #90847, #52853, #5888, #22378, #75857, #16838, #39346, #55819, #10316, #54322, #867, #47311, #76831, #15859, #39828, #24349, #17337, #70334, #84836, #78307, #63782, #1850, #77810, #9826, #54812, #25814, #32308, #24834, #2344, #46826, #92819, #9325, #69840, #86314, #40817, #16344, #31326, #62813, #8346, #46344, #93311, #85323, #47806, #55316, #77318, #40327, #94291, #85823, #70831, #8832, #32800, #84358, #38854, #1364, #31815, #62312, #61826, #17817, #63295, #92334, #93806, #33291, #25335, #69343, #48299, #78806, #71316, #2834, #23857, #48790, #26285, #87281, #56786, #96784, #56310, #73263, #5285, #80280, #57276, #49772, #12269, #43260, #12762, #35761, #86806, #87770, #71798, #42779, #19285, #11781, #64763, #88764, #79785, #95275, #3304, #27266, #42288, #18308, #72275, #18802, #49286, #11288, #79298, #3805, #66250, #80776, #33766, #58246, #26778, #20275, #4295, #41807, #4786, #34261, #35261, #72760, #34769, #94785, #65758, #65257, #95785, #96283, #50772, #64273, #41325, #57765, #27762, #81263, #73754, #88269, #19772, #10807, #50259, #82244, #81744, #6260, #74239, #51260, #52736, #22262, #28753, #13758, #83243, #45742, #68255, #53234, #59742, #60728, #59245, #13260, #98775, #36763, #67256, #30223, #37269, #14766, #20770, #97279, #89744, #21262, #68740, #28259, #45239, #76238, #52249, #29245, #21770, #75736, #15261, #83739, #7755, #58755, #90237, #43752, #7255, #82744, #14264, #97780, #91227, #51759, #44741, #5772, #98275, #75242, #89259, #44245, #74749, #6752, #67756, #36260, #29732, #38249, #37759, #66756, #22751, #60240, #90735, #47197, #759, #47702, #54208, #24719, #24230, #54696, #38734, #9707, #85218, #31210, #78194, #93690, #76721, #84245, #77210, #55192, #40205, #85709, #70217, #1736, #70711, #15749, #84725, #53728, #8716, #46235, #23253, #17223, #93192, #61706, #16230, #2229, #17712, #32688, #25224, #31704, #63183, #92220, #8240, #55704, #86200, #39234, #40699, #16722, #39724, #48184, #23748, #69722, #62197, #46710, #78696, #10206, #69235, #1248, #92705, #91731 ),
 ( #77700, #9211, #32190, #62692, #272, #30717, #61226, #59508, #14025, #79676, #26665, #44004, #64157, #36525, #88149, #19661, #21524, #49174, #11173, #74506, #80158, #65145, #63672, #41206, #3197, #71686, #71202, #2725, #51518, #52018, #95156, #72163, #64645, #27150, #90004, #28998, #82509, #33179, #3690, #86691, #57652, #34151, #57159, #41693, #6028, #94675, #87657, #18196, #42181, #19170, #94176, #87165, #33661, #26184, #56676, #25707, #18691, #56199, #95665, #48676, #67017, #49650, #97538, #11668, #72645, #82012, #4178, #13522, #34649, #79179, #10694, #53981, #30481, #75501, #23511, #38993, #22026, #29487, #22516, #530, #84490, #68995, #15517, #45999, #15992, #59996, #98537, #98032, #52988, #90489, #67514, #30977, #38501, #44994, #29989, #61475, #61967, #46480, #69485, #75992, #76975, #7013, #52498, #8488, #91981, #83504, #84971, #60981, #83993, #1004, #37518, #15021, #7521, #60496, #31465, #92466, #14525, #83008, #38012, #37016, #75005, #35, #45491, #76489, #91494, #68010, #23994, #54466, #23015, #68504, #90985, #53482, #44505, #6510, #8003, #85470, #47460, #31950, #2976, #2491, #62452, #47946, #56453, #70971, #17960, #55467, #85969, #86939, #94437, #63446, #24489, #55963, #93953, #69978, #17479, #32945, #77459, #25950, #92954, #8972, #16490, #33426, #46965, #16982, #25479, #86462, #10456, #77961, #39970, #70471, #40473, #18451, #48933, #32457, #78453, #9967, #48446, #39489, #1500, #54953, #9468, #1991, #78946, #63924, #62953, #40964, #93457, #24982, #71463, #58784, #44766, #73783, #82271, #80804, #58277, #20303, #88795, #29758, #88302, #6287, #37295, #13289, #89290, #81774, #44273, #75271, #6781, #67782, #19800, #20800, #4817, #74778, #51289, #43777, #96814, #21795, #12788, #28290, #35291, #59276, #74268, #50291, #5313, #50803, #81292, #43288, #12301, #35791, #98304, #13786, #65784, #90262, #5799, #52275, #36289, #66279, #36790, #66787, #67284, #97306, #28778, #27792, #97812, #89775, #21292, #29273, #82774, #96317, #73293, #51785, #59769, #14294, #42809, #31237, #61732, #39263, #75763, #15289, #14795, #38276, #7284, #83271, #84753, #54240, #60755, #45771, #16258, #77728, #1280, #85244, #91757, #30251, #46262, #30745, #76264, #68769, #784, #7781, #62229, #39751, #83766, #301, #98803, #46740, #61252, #91255, #92250, #8742, #23280, #53756, #70248, #16750, #23775, #22781, #77238, #69752, #45268, #84274, #31733, #22290, #47225, #68282, #52763, #60266, #24260, #90765, #37785, #92736, #69264, #54724, #53260, #15773, #76747, #8264, #9240, #1764, #38764, #2752, #56227, #48705, #87685, #32220, #72192, #19199, #72675 ) ),
 .UNSPECIFIED., .F., .F., .F. ) 
 B_SPLINE_SURFACE_WITH_KNOTS ( ( 2, 2 ),
 ( 3, 2, 2, 2, 2, 2, 2, 2, 2, 2, 2, 2, 2, 2, 2, 2, 2, 2, 2, 2, 2, 2, 2, 2, 2, 2, 2, 2, 2, 2, 2, 2, 2, 2, 2, 2, 2, 2, 2, 2, 2, 2, 2, 2, 2, 2, 2, 2, 2, 2, 2, 2, 2, 2, 2, 2, 2, 2, 2, 2, 2, 2, 2, 2, 2, 2, 2, 2, 2, 2, 2, 2, 2, 2, 2, 2, 2, 2, 2, 2, 2, 2, 2, 2, 2, 2, 2, 2, 2, 2, 2, 2, 2, 2, 2, 2, 2, 2, 2, 2, 2, 2, 2, 2, 2, 2, 2, 2, 2, 2, 2, 2, 2, 2, 2, 2, 2, 2, 2, 2, 2, 2, 2, 2, 2, 2, 2, 2, 2, 2, 2, 2, 2, 2, 2, 2, 2, 2, 2, 2, 2, 2, 2, 2, 2, 2, 2, 2, 2, 2, 2, 2, 2, 2, 2, 2, 2, 2, 2, 2, 2, 2, 3 ),
 ( 0.000000000000000000, 1.000000000000000000 ),
 ( 0.000000000000000000, 0.005952380952380952051, 0.01190476190476190410, 0.01785714285714285615, 0.02380952380952380820, 0.02976190476190476025, 0.03571428571428571230, 0.04166666666666666435, 0.04761904761904761640, 0.05357142857142856845, 0.05952380952380952051, 0.06547619047619047949, 0.07142857142857142461, 0.07738095238095238360, 0.08333333333333332871, 0.08928571428571428770, 0.09523809523809523281, 0.1011904761904761918, 0.1071428571428571369, 0.1130952380952380959, 0.1190476190476190410, 0.1250000000000000000, 0.1309523809523809590, 0.1369047619047619180, 0.1428571428571428492, 0.1488095238095238082, 0.1547619047619047672, 0.1607142857142857262, 0.1666666666666666574, 0.1726190476190476164, 0.1785714285714285754, 0.1845238095238095344, 0.1904761904761904656, 0.1964285714285714246, 0.2023809523809523836, 0.2083333333333333426, 0.2142857142857142738, 0.2202380952380952328, 0.2261904761904761918, 0.2321428571428571508, 0.2380952380952380820, 0.2440476190476190410, 0.2500000000000000000, 0.2559523809523809312, 0.2619047619047619180, 0.2678571428571428492, 0.2738095238095238360, 0.2797619047619047672, 0.2857142857142856984, 0.2916666666666666852, 0.2976190476190476164, 0.3035714285714285476, 0.3095238095238095344, 0.3154761904761904656, 0.3214285714285714524, 0.3273809523809523836, 0.3333333333333333148, 0.3392857142857143016, 0.3452380952380952328, 0.3511904761904761640, 0.3571428571428571508, 0.3630952380952380820, 0.3690476190476190688, 0.3750000000000000000, 0.3809523809523809312, 0.3869047619047619180, 0.3928571428571428492, 0.3988095238095238360, 0.4047619047619047672, 0.4107142857142856984, 0.4166666666666666852, 0.4226190476190476164, 0.4285714285714285476, 0.4345238095238095344, 0.4404761904761904656, 0.4464285714285714524, 0.4523809523809523836, 0.4583333333333333148, 0.4642857142857143016, 0.4702380952380952328, 0.4761904761904761640, 0.4821428571428571508, 0.4880952380952380820, 0.4940476190476190688, 0.5000000000000000000, 0.5059523809523809312, 0.5119047619047618625, 0.5178571428571429047, 0.5238095238095238360, 0.5297619047619047672, 0.5357142857142856984, 0.5416666666666666297, 0.5476190476190476719, 0.5535714285714286031, 0.5595238095238095344, 0.5654761904761904656, 0.5714285714285713969, 0.5773809523809523281, 0.5833333333333333703, 0.5892857142857143016, 0.5952380952380952328, 0.6011904761904761640, 0.6071428571428570953, 0.6130952380952381375, 0.6190476190476190688, 0.6250000000000000000, 0.6309523809523809312, 0.6369047619047618625, 0.6428571428571429047, 0.6488095238095238360, 0.6547619047619047672, 0.6607142857142856984, 0.6666666666666666297, 0.6726190476190476719, 0.6785714285714286031, 0.6845238095238095344, 0.6904761904761904656, 0.6964285714285713969, 0.7023809523809523281, 0.7083333333333333703, 0.7142857142857143016, 0.7202380952380952328, 0.7261904761904761640, 0.7321428571428570953, 0.7380952380952381375, 0.7440476190476190688, 0.7500000000000000000, 0.7559523809523809312, 0.7619047619047618625, 0.7678571428571429047, 0.7738095238095238360, 0.7797619047619047672, 0.7857142857142856984, 0.7916666666666666297, 0.7976190476190476719, 0.8035714285714286031, 0.8095238095238095344, 0.8154761904761904656, 0.8214285714285713969, 0.8273809523809523281, 0.8333333333333333703, 0.8392857142857143016, 0.8452380952380952328, 0.8511904761904761640, 0.8571428571428570953, 0.8630952380952381375, 0.8690476190476190688, 0.8750000000000000000, 0.8809523809523809312, 0.8869047619047618625, 0.8928571428571429047, 0.8988095238095238360, 0.9047619047619047672, 0.9107142857142856984, 0.9166666666666666297, 0.9226190476190476719, 0.9285714285714286031, 0.9345238095238095344, 0.9404761904761904656, 0.9464285714285713969, 0.9523809523809523281, 0.9583333333333333703, 0.9642857142857143016 ),
 .UNSPECIFIED. ) 
 GEOMETRIC_REPRESENTATION_ITEM ( )  RATIONAL_B_SPLINE_SURFACE ( (
 ( 1.000000000000000000, 0.9659258262890683122, 1.000000000000000000, 0.9659258262890683122, 1.000000000000000000, 0.9659258262890683122, 1.000000000000000000, 0.9659258262890683122, 1.000000000000000000, 0.9659258262890683122, 1.000000000000000000, 0.9659258262890683122, 1.000000000000000000, 0.9659258262890683122, 1.000000000000000000, 0.9659258262890683122, 1.000000000000000000, 0.9659258262890683122, 1.000000000000000000, 0.9659258262890683122, 1.000000000000000000, 0.9659258262890683122, 1.000000000000000000, 0.9659258262890683122, 1.000000000000000000, 0.9659258262890683122, 1.000000000000000000, 0.9659258262890683122, 1.000000000000000000, 0.9659258262890683122, 1.000000000000000000, 0.9659258262890683122, 1.000000000000000000, 0.9659258262890683122, 1.000000000000000000, 0.9659258262890683122, 1.000000000000000000, 0.9659258262890683122, 1.000000000000000000, 0.9659258262890683122, 1.000000000000000000, 0.9659258262890683122, 1.000000000000000000, 0.9659258262890683122, 1.000000000000000000, 0.9659258262890683122, 1.000000000000000000, 0.9659258262890683122, 1.000000000000000000, 0.9659258262890683122, 1.000000000000000000, 0.9659258262890683122, 1.000000000000000000, 0.9659258262890683122, 1.000000000000000000, 0.9659258262890683122, 1.000000000000000000, 0.9659258262890683122, 1.000000000000000000, 0.9659258262890683122, 1.000000000000000000, 0.9659258262890683122, 1.000000000000000000, 0.9659258262890683122, 1.000000000000000000, 0.9659258262890683122, 1.000000000000000000, 0.9659258262890683122, 1.000000000000000000, 0.9659258262890683122, 1.000000000000000000, 0.9659258262890683122, 1.000000000000000000, 0.9659258262890683122, 1.000000000000000000, 0.9659258262890683122, 1.000000000000000000, 0.9659258262890683122, 1.000000000000000000, 0.9659258262890683122, 1.000000000000000000, 0.9659258262890683122, 1.000000000000000000, 0.9659258262890683122, 1.000000000000000000, 0.9659258262890683122, 1.000000000000000000, 0.9659258262890683122, 1.000000000000000000, 0.9659258262890683122, 1.000000000000000000, 0.9659258262890683122, 1.000000000000000000, 0.9659258262890683122, 1.000000000000000000, 0.9659258262890683122, 1.000000000000000000, 0.9659258262890683122, 1.000000000000000000, 0.9659258262890683122, 1.000000000000000000, 0.9659258262890683122, 1.000000000000000000, 0.9659258262890683122, 1.000000000000000000, 0.9659258262890683122, 1.000000000000000000, 0.9659258262890683122, 1.000000000000000000, 0.9659258262890683122, 1.000000000000000000, 0.9659258262890683122, 1.000000000000000000, 0.9659258262890683122, 1.000000000000000000, 0.9659258262890683122, 1.000000000000000000, 0.9659258262890683122, 1.000000000000000000, 0.9659258262890683122, 1.000000000000000000, 0.9659258262890683122, 1.000000000000000000, 0.9659258262890683122, 1.000000000000000000, 0.9659258262890683122, 1.000000000000000000, 0.9659258262890683122, 1.000000000000000000, 0.9659258262890683122, 1.000000000000000000, 0.9659258262890683122, 1.000000000000000000, 0.9659258262890683122, 1.000000000000000000, 0.9659258262890683122, 1.000000000000000000, 0.9659258262890683122, 1.000000000000000000, 0.9659258262890683122, 1.000000000000000000, 0.9659258262890683122, 1.000000000000000000, 0.9659258262890683122, 1.000000000000000000, 0.9659258262890683122, 1.000000000000000000, 0.9659258262890683122, 1.000000000000000000, 0.9659258262890683122, 1.000000000000000000, 0.9659258262890683122, 1.000000000000000000, 0.9659258262890683122, 1.000000000000000000, 0.9659258262890683122, 1.000000000000000000, 0.9659258262890683122, 1.000000000000000000, 0.9659258262890683122, 1.000000000000000000, 0.9659258262890683122, 1.000000000000000000, 0.9659258262890683122, 1.000000000000000000, 0.9659258262890683122, 1.000000000000000000, 0.9659258262890683122, 1.000000000000000000, 0.9659258262890683122, 1.000000000000000000, 0.9659258262890683122, 1.000000000000000000, 0.9659258262890683122, 1.000000000000000000, 0.9659258262890683122, 1.000000000000000000, 0.9659258262890683122, 1.000000000000000000, 0.9659258262890683122, 1.000000000000000000, 0.9659258262890683122, 1.000000000000000000, 0.9659258262890683122, 1.000000000000000000, 0.9659258262890683122, 1.000000000000000000, 0.9659258262890683122, 1.000000000000000000, 0.9659258262890683122, 1.000000000000000000, 0.9659258262890683122, 1.000000000000000000, 0.9659258262890683122, 1.000000000000000000, 0.9659258262890683122, 1.000000000000000000, 0.9659258262890683122, 1.000000000000000000, 0.9659258262890683122, 1.000000000000000000, 0.9659258262890683122, 1.000000000000000000, 0.9659258262890683122, 1.000000000000000000, 0.9659258262890683122, 1.000000000000000000, 0.9659258262890683122, 1.000000000000000000, 0.9659258262890683122, 1.000000000000000000, 0.9659258262890683122, 1.000000000000000000, 0.9659258262890683122, 1.000000000000000000, 0.9659258262890683122, 1.000000000000000000, 0.9659258262890683122, 1.000000000000000000, 0.9659258262890683122, 1.000000000000000000, 0.9659258262890683122, 1.000000000000000000, 0.9659258262890683122, 1.000000000000000000, 0.9659258262890683122, 1.000000000000000000, 0.9659258262890683122, 1.000000000000000000, 0.9659258262890683122, 1.000000000000000000, 0.9659258262890683122, 1.000000000000000000, 0.9659258262890683122, 1.000000000000000000, 0.9659258262890683122, 1.000000000000000000, 0.9659258262890683122, 1.000000000000000000, 0.9659258262890683122, 1.000000000000000000, 0.9659258262890683122, 1.000000000000000000, 0.9659258262890683122, 1.000000000000000000, 0.9659258262890683122, 1.000000000000000000, 0.9659258262890683122, 1.000000000000000000, 0.9659258262890683122, 1.000000000000000000, 0.9659258262890683122, 1.000000000000000000, 0.9659258262890683122, 1.000000000000000000, 0.9659258262890683122, 1.000000000000000000, 0.9659258262890683122, 1.000000000000000000, 0.9659258262890683122, 1.000000000000000000, 0.9659258262890683122, 1.000000000000000000, 0.9659258262890683122, 1.000000000000000000, 0.9659258262890683122, 1.000000000000000000, 0.9659258262890683122, 1.000000000000000000, 0.9659258262890683122, 1.000000000000000000, 0.9659258262890683122, 1.000000000000000000, 0.9659258262890683122, 1.000000000000000000, 0.9659258262890683122, 1.000000000000000000, 0.9659258262890683122, 1.000000000000000000, 0.9659258262890683122, 1.000000000000000000, 0.9659258262890683122, 1.000000000000000000, 0.9659258262890683122, 1.000000000000000000, 0.9659258262890683122, 1.000000000000000000, 0.9659258262890683122, 1.000000000000000000, 0.9659258262890683122, 1.000000000000000000, 0.9659258262890683122, 1.000000000000000000, 0.9659258262890683122, 1.000000000000000000, 0.9659258262890683122, 1.000000000000000000, 0.9659258262890683122, 1.000000000000000000, 0.9659258262890683122, 1.000000000000000000, 0.9659258262890683122, 1.000000000000000000, 0.9659258262890683122, 1.000000000000000000, 0.9659258262890683122, 1.000000000000000000, 0.9659258262890683122, 1.000000000000000000, 0.9659258262890683122, 1.000000000000000000, 0.9659258262890683122, 1.000000000000000000, 0.9659258262890683122, 1.000000000000000000, 0.9659258262890683122, 1.000000000000000000, 0.9659258262890683122, 1.000000000000000000, 0.9659258262890683122, 1.000000000000000000, 0.9659258262890683122, 1.000000000000000000, 0.9659258262890683122, 1.000000000000000000),
 ( 1.000000000000000000, 0.9659258262890683122, 1.000000000000000000, 0.9659258262890683122, 1.000000000000000000, 0.9659258262890683122, 1.000000000000000000, 0.9659258262890683122, 1.000000000000000000, 0.9659258262890683122, 1.000000000000000000, 0.9659258262890683122, 1.000000000000000000, 0.9659258262890683122, 1.000000000000000000, 0.9659258262890683122, 1.000000000000000000, 0.9659258262890683122, 1.000000000000000000, 0.9659258262890683122, 1.000000000000000000, 0.9659258262890683122, 1.000000000000000000, 0.9659258262890683122, 1.000000000000000000, 0.9659258262890683122, 1.000000000000000000, 0.9659258262890683122, 1.000000000000000000, 0.9659258262890683122, 1.000000000000000000, 0.9659258262890683122, 1.000000000000000000, 0.9659258262890683122, 1.000000000000000000, 0.9659258262890683122, 1.000000000000000000, 0.9659258262890683122, 1.000000000000000000, 0.9659258262890683122, 1.000000000000000000, 0.9659258262890683122, 1.000000000000000000, 0.9659258262890683122, 1.000000000000000000, 0.9659258262890683122, 1.000000000000000000, 0.9659258262890683122, 1.000000000000000000, 0.9659258262890683122, 1.000000000000000000, 0.9659258262890683122, 1.000000000000000000, 0.9659258262890683122, 1.000000000000000000, 0.9659258262890683122, 1.000000000000000000, 0.9659258262890683122, 1.000000000000000000, 0.9659258262890683122, 1.000000000000000000, 0.9659258262890683122, 1.000000000000000000, 0.9659258262890683122, 1.000000000000000000, 0.9659258262890683122, 1.000000000000000000, 0.9659258262890683122, 1.000000000000000000, 0.9659258262890683122, 1.000000000000000000, 0.9659258262890683122, 1.000000000000000000, 0.9659258262890683122, 1.000000000000000000, 0.9659258262890683122, 1.000000000000000000, 0.9659258262890683122, 1.000000000000000000, 0.9659258262890683122, 1.000000000000000000, 0.9659258262890683122, 1.000000000000000000, 0.9659258262890683122, 1.000000000000000000, 0.9659258262890683122, 1.000000000000000000, 0.9659258262890683122, 1.000000000000000000, 0.9659258262890683122, 1.000000000000000000, 0.9659258262890683122, 1.000000000000000000, 0.9659258262890683122, 1.000000000000000000, 0.9659258262890683122, 1.000000000000000000, 0.9659258262890683122, 1.000000000000000000, 0.9659258262890683122, 1.000000000000000000, 0.9659258262890683122, 1.000000000000000000, 0.9659258262890683122, 1.000000000000000000, 0.9659258262890683122, 1.000000000000000000, 0.9659258262890683122, 1.000000000000000000, 0.9659258262890683122, 1.000000000000000000, 0.9659258262890683122, 1.000000000000000000, 0.9659258262890683122, 1.000000000000000000, 0.9659258262890683122, 1.000000000000000000, 0.9659258262890683122, 1.000000000000000000, 0.9659258262890683122, 1.000000000000000000, 0.9659258262890683122, 1.000000000000000000, 0.9659258262890683122, 1.000000000000000000, 0.9659258262890683122, 1.000000000000000000, 0.9659258262890683122, 1.000000000000000000, 0.9659258262890683122, 1.000000000000000000, 0.9659258262890683122, 1.000000000000000000, 0.9659258262890683122, 1.000000000000000000, 0.9659258262890683122, 1.000000000000000000, 0.9659258262890683122, 1.000000000000000000, 0.9659258262890683122, 1.000000000000000000, 0.9659258262890683122, 1.000000000000000000, 0.9659258262890683122, 1.000000000000000000, 0.9659258262890683122, 1.000000000000000000, 0.9659258262890683122, 1.000000000000000000, 0.9659258262890683122, 1.000000000000000000, 0.9659258262890683122, 1.000000000000000000, 0.9659258262890683122, 1.000000000000000000, 0.9659258262890683122, 1.000000000000000000, 0.9659258262890683122, 1.000000000000000000, 0.9659258262890683122, 1.000000000000000000, 0.9659258262890683122, 1.000000000000000000, 0.9659258262890683122, 1.000000000000000000, 0.9659258262890683122, 1.000000000000000000, 0.9659258262890683122, 1.000000000000000000, 0.9659258262890683122, 1.000000000000000000, 0.9659258262890683122, 1.000000000000000000, 0.9659258262890683122, 1.000000000000000000, 0.9659258262890683122, 1.000000000000000000, 0.9659258262890683122, 1.000000000000000000, 0.9659258262890683122, 1.000000000000000000, 0.9659258262890683122, 1.000000000000000000, 0.9659258262890683122, 1.000000000000000000, 0.9659258262890683122, 1.000000000000000000, 0.9659258262890683122, 1.000000000000000000, 0.9659258262890683122, 1.000000000000000000, 0.9659258262890683122, 1.000000000000000000, 0.9659258262890683122, 1.000000000000000000, 0.9659258262890683122, 1.000000000000000000, 0.9659258262890683122, 1.000000000000000000, 0.9659258262890683122, 1.000000000000000000, 0.9659258262890683122, 1.000000000000000000, 0.9659258262890683122, 1.000000000000000000, 0.9659258262890683122, 1.000000000000000000, 0.9659258262890683122, 1.000000000000000000, 0.9659258262890683122, 1.000000000000000000, 0.9659258262890683122, 1.000000000000000000, 0.9659258262890683122, 1.000000000000000000, 0.9659258262890683122, 1.000000000000000000, 0.9659258262890683122, 1.000000000000000000, 0.9659258262890683122, 1.000000000000000000, 0.9659258262890683122, 1.000000000000000000, 0.9659258262890683122, 1.000000000000000000, 0.9659258262890683122, 1.000000000000000000, 0.9659258262890683122, 1.000000000000000000, 0.9659258262890683122, 1.000000000000000000, 0.9659258262890683122, 1.000000000000000000, 0.9659258262890683122, 1.000000000000000000, 0.9659258262890683122, 1.000000000000000000, 0.9659258262890683122, 1.000000000000000000, 0.9659258262890683122, 1.000000000000000000, 0.9659258262890683122, 1.000000000000000000, 0.9659258262890683122, 1.000000000000000000, 0.9659258262890683122, 1.000000000000000000, 0.9659258262890683122, 1.000000000000000000, 0.9659258262890683122, 1.000000000000000000, 0.9659258262890683122, 1.000000000000000000, 0.9659258262890683122, 1.000000000000000000, 0.9659258262890683122, 1.000000000000000000, 0.9659258262890683122, 1.000000000000000000, 0.9659258262890683122, 1.000000000000000000, 0.9659258262890683122, 1.000000000000000000, 0.9659258262890683122, 1.000000000000000000, 0.9659258262890683122, 1.000000000000000000, 0.9659258262890683122, 1.000000000000000000, 0.9659258262890683122, 1.000000000000000000, 0.9659258262890683122, 1.000000000000000000, 0.9659258262890683122, 1.000000000000000000, 0.9659258262890683122, 1.000000000000000000, 0.9659258262890683122, 1.000000000000000000, 0.9659258262890683122, 1.000000000000000000, 0.9659258262890683122, 1.000000000000000000, 0.9659258262890683122, 1.000000000000000000, 0.9659258262890683122, 1.000000000000000000, 0.9659258262890683122, 1.000000000000000000, 0.9659258262890683122, 1.000000000000000000, 0.9659258262890683122, 1.000000000000000000, 0.9659258262890683122, 1.000000000000000000, 0.9659258262890683122, 1.000000000000000000, 0.9659258262890683122, 1.000000000000000000, 0.9659258262890683122, 1.000000000000000000, 0.9659258262890683122, 1.000000000000000000, 0.9659258262890683122, 1.000000000000000000, 0.9659258262890683122, 1.000000000000000000, 0.9659258262890683122, 1.000000000000000000, 0.9659258262890683122, 1.000000000000000000, 0.9659258262890683122, 1.000000000000000000, 0.9659258262890683122, 1.000000000000000000, 0.9659258262890683122, 1.000000000000000000, 0.9659258262890683122, 1.000000000000000000, 0.9659258262890683122, 1.000000000000000000, 0.9659258262890683122, 1.000000000000000000, 0.9659258262890683122, 1.000000000000000000) ) ) 
 REPRESENTATION_ITEM ( '' )  SURFACE ( )  );
#70094=CARTESIAN_POINT ( 'NONE',  ( 15.44008868035555260, 49.73035201082150536, 9.422509992056143702 ) ) ;
#70095=CARTESIAN_POINT ( 'NONE',  ( -0.8801773607111009756, 53.06368534415484106, 1.068504757029289695E-15 ) ) ;
#70098=CARTESIAN_POINT ( 'NONE',  ( 19.42250999205614193, 10.14701867748816966, 5.440088680355555262 ) ) ;
#70099=CARTESIAN_POINT ( 'NONE',  ( 12.63842701281683034, 47.46726448433412315, 9.846743663894596210 ) ) ;
#70100=CARTESIAN_POINT ( 'NONE',  ( 10.00000000000000000, 16.81368534415483751, -10.88017736071110342 ) ) ;
#70101=CARTESIAN_POINT ( 'NONE',  ( 19.84674366389459266, 23.71726448433412315, -2.638427012816827677 ) ) ;
#70102=CARTESIAN_POINT ( 'NONE',  ( 10.00000000000000178, 25.37363466993041783, 12.81628187352647608 ) ) ;
#70104=CARTESIAN_POINT ( 'NONE',  ( 2.035157376598822676, 42.43868534415483396, -7.964842623401177768 ) ) ;
#70105=CARTESIAN_POINT ( 'NONE',  ( 16.40814093676324603, 12.45696800326375353, -11.09922568453594671 ) ) ;
#70107=CARTESIAN_POINT ( 'NONE',  ( 17.96484262340118221, 11.18868534415483929, -7.964842623401177768 ) ) ;
#70108=CARTESIAN_POINT ( 'NONE',  ( 7.084665262690076126, 44.10535201082151247, 10.88017736071109987 ) ) ;
#70109=CARTESIAN_POINT ( 'NONE',  ( -0.3689425029237881626, 57.42874883491397497, 10.36894250292379027 ) ) ;
#70110=CARTESIAN_POINT ( 'NONE',  ( 2.791683348922237240, 25.38393115100078390, -7.208316651077763204 ) ) ;
#70111=CARTESIAN_POINT ( 'NONE',  ( 20.88017736071110164, 60.35535201082151957, 2.915334737309930979 ) ) ;
#70113=CARTESIAN_POINT ( 'NONE',  ( 13.79529636645031943, 10.34541550158063394, -14.16423886937409904 ) ) ;
#70116=FILL_AREA_STYLE_COLOUR ( '', #33936 ) ;
#70120=CARTESIAN_POINT ( 'NONE',  ( 6.204703633549690345, 40.76208216824731778, -14.16423886937410259 ) ) ;
#70121=CARTESIAN_POINT ( 'NONE',  ( 6.204703633549690345, 35.76208216824729647, -14.16423886937410259 ) ) ;
#70122=CARTESIAN_POINT ( 'NONE',  ( -0.8801773607110991993, 67.85535201082151957, -2.915334737309923874 ) ) ;
#70123=CARTESIAN_POINT ( 'NONE',  ( 0.1532563361054082862, 66.21726448433413736, 2.638427012816831674 ) ) ;
#70124=CYLINDRICAL_SURFACE ( 'NONE', #84990, 0.5000000000000004441 ) ;
#70125=CARTESIAN_POINT ( 'NONE',  ( 19.42250999205614548, 60.98035201082151247, -5.440088680355545492 ) ) ;
#70126=CARTESIAN_POINT ( 'NONE',  ( 21.09922568453595559, 37.04030133659708923, -6.408140936763230044 ) ) ;
#70127=CARTESIAN_POINT ( 'NONE',  ( 17.08211943468705130, 28.47041550158063572, 12.26659068614894998 ) ) ;
#70130=CARTESIAN_POINT ( 'NONE',  ( 19.42250999205614548, 30.98035201082150536, -5.440088680355545492 ) ) ;
#70132=CARTESIAN_POINT ( 'NONE',  ( 17.96484262340118221, 29.93868534415484106, 7.964842623401181321 ) ) ;
#70133=DIRECTION ( 'NONE',  ( -0.000000000000000000, -0.000000000000000000, 1.000000000000000000 ) ) ;
#70134=CARTESIAN_POINT ( 'NONE',  ( 2.791683348922237240, 0.3839311510007847872, -7.208316651077763204 ) ) ;
#70140=LINE ( 'NONE', #63598, #33282 ) ;
#70142=CARTESIAN_POINT ( 'NONE',  ( 2.917880565312948704, 2.637082168247300906, 12.26659068614894643 ) ) ;
#70143=CARTESIAN_POINT ( 'NONE',  ( 24.16423886937410614, 64.30374883491396076, 8.672049930838204340E-16 ) ) ;
#70144=CARTESIAN_POINT ( 'NONE',  ( 7.084665262690076126, 7.022018677488170546, -10.88017736071110164 ) ) ;
#70145=CARTESIAN_POINT ( 'NONE',  ( 7.361572987183169658, 39.96726448433411605, -9.846743663894592657 ) ) ;
#70146=CARTESIAN_POINT ( 'NONE',  ( 1.472469842513823179, 60.59226448433412315, -4.923371831947296329 ) ) ;
#70151=CARTESIAN_POINT ( 'NONE',  ( 22.81628187352648496, 1.831968003263753753, -3.434112377981050290 ) ) ;
#70152=ORIENTED_EDGE ( 'NONE', *, *, #2197, .T. ) ;
#70153=CARTESIAN_POINT ( 'NONE',  ( 13.79529636645030344, 48.26208216824728936, 14.16423886937410614 ) ) ;
#70155=EDGE_CURVE ( 'NONE', #31263, #24281, #3259, .T. ) ;
#70156=CARTESIAN_POINT ( 'NONE',  ( 20.36894250292379738, 39.92874883491396787, -10.36894250292379027 ) ) ;
#70158=CARTESIAN_POINT ( 'NONE',  ( -0.8801773607110991993, 17.85535201082150536, -2.915334737309923874 ) ) ;
#70159=CARTESIAN_POINT ( 'NONE',  ( 18.72515096720568195, 21.07228050351032422, -6.500000000000018652 ) ) ;
#70160=CARTESIAN_POINT ( 'NONE',  ( 4.559911319644449179, 43.89701867748816966, 9.422509992056141925 ) ) ;
#70161=CARTESIAN_POINT ( 'NONE',  ( 5.076628168052704559, 55.17559781766745175, -8.527530157486179263 ) ) ;
#70162=CARTESIAN_POINT ( 'NONE',  ( 4.559911319644449179, 37.23035201082150536, -9.422509992056141925 ) ) ;
#70163=CARTESIAN_POINT ( 'NONE',  ( -0.3289641300568005855, 64.27164270246085209, -5.963430220938281678 ) ) ;
#70164=CARTESIAN_POINT ( 'NONE',  ( 7.084665262690076126, 67.02201867748817676, -10.88017736071110164 ) ) ;
#70165=CARTESIAN_POINT ( 'NONE',  ( -0.8801773607111009756, 33.06368534415484106, 1.068504757029289695E-15 ) ) ;
#70169=CARTESIAN_POINT ( 'NONE',  ( 0.1532563361054083140, 6.008931151000784787, 1.131784320476157264E-15 ) ) ;
#70171=VERTEX_POINT ( 'NONE', #63593 ) ;
#70172=CARTESIAN_POINT ( 'NONE',  ( 19.84674366389459266, 48.30059781766745175, 2.638427012816836559 ) ) ;
#70175=VECTOR ( 'NONE', #93085, 1000.000000000000000 ) ;
#70176=CARTESIAN_POINT ( 'NONE',  ( 12.63842701281683922, 64.55059781766745175, -9.846743663894590881 ) ) ;
#70177=CARTESIAN_POINT ( 'NONE',  ( -0.8801773607111009756, 53.06368534415484106, 1.068504757029289695E-15 ) ) ;
#70178=CARTESIAN_POINT ( 'NONE',  ( 2.791683348922240793, 51.63393115100078745, 7.208316651077764092 ) ) ;
#70179=CARTESIAN_POINT ( 'NONE',  ( 10.00000000000000000, 50.55374883491396787, -14.16423886937410082 ) ) ;
#70180=CARTESIAN_POINT ( 'NONE',  ( 10.00000000000000000, 54.75893115100078745, -9.846743663894594434 ) ) ;
#70182=CARTESIAN_POINT ( 'NONE',  ( 1.816707512666851931, 5.102906685120229824, -6.499999999999991118 ) ) ;
#70183=CARTESIAN_POINT ( 'NONE',  ( 0.1532563361054083140, 26.00893115100078745, 1.131784320476157264E-15 ) ) ;
#70184=CARTESIAN_POINT ( 'NONE',  ( -1.099225684535947600, 49.54030133659708923, 6.408140936763237150 ) ) ;
#70185=CARTESIAN_POINT ( 'NONE',  ( 18.52753015748618282, 63.92559781766745886, -4.923371831947291888 ) ) ;
#70186=CARTESIAN_POINT ( 'NONE',  ( -0.8801773607111008646, 53.27201867748816966, 2.915334737309923430 ) ) ;
#70188=ORIENTED_EDGE ( 'NONE', *, *, #34546, .T. ) ;
#70189=CARTESIAN_POINT ( 'NONE',  ( 6.204703633549690345, 62.84541550158063927, 14.16423886937410082 ) ) ;
#70190=CARTESIAN_POINT ( 'NONE',  ( 2.035157376598822676, 27.43868534415483396, -7.964842623401177768 ) ) ;
#70191=CARTESIAN_POINT ( 'NONE',  ( 3.591859063236761518, 9.956968003263753531, 11.09922568453594849 ) ) ;
#70192=CARTESIAN_POINT ( 'NONE',  ( 0.5774900079438607392, 63.48035201082149825, 5.440088680355550821 ) ) ;
#70195=CARTESIAN_POINT ( 'NONE',  ( 19.72487221294571569, 45.71833443783938122, -6.499999999999989342 ) ) ;
#70196=CARTESIAN_POINT ( 'NONE',  ( -0.8801773607111008646, 48.27201867748816966, 2.915334737309923430 ) ) ;
#70199=CARTESIAN_POINT ( 'NONE',  ( 14.92337183194729988, 39.34226448433412315, -8.527530157486177487 ) ) ;
#70200=CARTESIAN_POINT ( 'NONE',  ( 14.92337183194729988, 4.342264484334117824, -8.527530157486177487 ) ) ;
#70202=CARTESIAN_POINT ( 'NONE',  ( 19.38216949554541202, 5.998634669930420493, 9.382169495545424454 ) ) ;
#70203=CARTESIAN_POINT ( 'NONE',  ( 2.035157376598822676, 17.43868534415483751, -7.964842623401177768 ) ) ;
#70204=CARTESIAN_POINT ( 'NONE',  ( -20.19000000000001194, 92.00000000000000000, -10.09898361729590199 ) ) ;
#70206=EDGE_CURVE ( 'NONE', #76154, #62128, #61679, .T. ) ;
#70207=CARTESIAN_POINT ( 'NONE',  ( 22.26659068614895176, 39.72041550158063217, -7.082119434687042414 ) ) ;
#70208=CARTESIAN_POINT ( 'NONE',  ( 2.917880565312950480, 25.97041550158063572, -12.26659068614894821 ) ) ;
#70209=CARTESIAN_POINT ( 'NONE',  ( -4.164238869374098151, 66.59541550158060375, -3.795296366450310543 ) ) ;
#70210=CARTESIAN_POINT ( 'NONE',  ( 2.791683348922240793, 31.63393115100078745, 7.208316651077764092 ) ) ;
#70211=CARTESIAN_POINT ( 'NONE',  ( 17.20831665107776587, 22.88393115100078745, 7.208316651077764980 ) ) ;
#70212=CARTESIAN_POINT ( 'NONE',  ( 10.00000000000000178, 19.31368534415484106, 10.88017736071110342 ) ) ;
#70215=CARTESIAN_POINT ( 'NONE',  ( 0.1532563361054100626, 40.80059781766745886, -2.638427012816831230 ) ) ;
#70216=CARTESIAN_POINT ( 'NONE',  ( 0.5774900079438607392, 28.48035201082150891, 5.440088680355550821 ) ) ;
#70217=CARTESIAN_POINT ( 'NONE',  ( 12.63842701281683922, 59.55059781766744464, -9.846743663894590881 ) ) ;
#70218=CARTESIAN_POINT ( 'NONE',  ( 10.00000000000000000, 15.55374883491396787, -14.16423886937410082 ) ) ;
#70219=CARTESIAN_POINT ( 'NONE',  ( -1.926860441876564023, 17.87045670184113533, 3.195792623639529761 ) ) ;
#70221=UNCERTAINTY_MEASURE_WITH_UNIT (LENGTH_MEASURE( 1.000000000000000082E-05 ), #39650, 'distance_accuracy_value', 'NONE');
#70222=CARTESIAN_POINT ( 'NONE',  ( 19.84674366389459621, 8.508931151000785675, 7.409399052514197653E-17 ) ) ;
#70223=CARTESIAN_POINT ( 'NONE',  ( 3.591859063236761518, 44.95696800326376064, 11.09922568453594849 ) ) ;
#70224=CARTESIAN_POINT ( 'NONE',  ( 1.472469842513823179, 51.42559781766745886, 4.923371831947296329 ) ) ;
#70228=CARTESIAN_POINT ( 'NONE',  ( 19.42250999205614548, 5.980352010821504471, -5.440088680355545492 ) ) ;
#70229=CARTESIAN_POINT ( 'NONE',  ( 20.88017736071110164, 50.35535201082151247, 2.915334737309930979 ) ) ;
#70230=CARTESIAN_POINT ( 'NONE',  ( -4.164238869374099039, 16.80374883491396787, 8.674139862899312516E-16 ) ) ;
#70231=CARTESIAN_POINT ( 'NONE',  ( 2.035157376598822676, 62.43868534415483396, -7.964842623401177768 ) ) ;
#70232=CARTESIAN_POINT ( 'NONE',  ( 18.52753015748617571, 33.09226448433411605, 4.923371831947298993 ) ) ;
#70233=CARTESIAN_POINT ( 'NONE',  ( -0.8801773607110991993, 22.85535201082150181, -2.915334737309923874 ) ) ;
#70235=CARTESIAN_POINT ( 'NONE',  ( 19.84674366389459266, 58.71726448433411605, -2.638427012816827677 ) ) ;
#70238=CARTESIAN_POINT ( 'NONE',  ( 17.39651004071841456, 7.935752660568278216, 6.500000000000003553 ) ) ;
#70241=ORIENTED_EDGE ( 'NONE', *, *, #44876, .T. ) ;
#70243=CARTESIAN_POINT ( 'NONE',  ( 0.2751277870542909731, 62.28217586085237656, -6.499999999999992006 ) ) ;
#70245=CARTESIAN_POINT ( 'NONE',  ( 2.917880565312950480, 0.9704155015806342766, -12.26659068614894821 ) ) ;
#70246=CARTESIAN_POINT ( 'NONE',  ( 5.076628168052703671, 46.84226448433412315, 8.527530157486179263 ) ) ;
#70247=CARTESIAN_POINT ( 'NONE',  ( 5.076628168052703671, 16.84226448433411960, 8.527530157486179263 ) ) ;
#70248=CARTESIAN_POINT ( 'NONE',  ( 3.591859063236763294, 58.29030133659708923, -11.09922568453595026 ) ) ;
#70249=CARTESIAN_POINT ( 'NONE',  ( 12.91533473730992121, 24.52201867748816966, 10.88017736071110164 ) ) ;
#70250=CARTESIAN_POINT ( 'NONE',  ( 12.63842701281683922, 44.55059781766745175, -9.846743663894590881 ) ) ;
#70252=CARTESIAN_POINT ( 'NONE',  ( -4.164238869374098151, 36.59541550158063217, -3.795296366450310543 ) ) ;
#70254=CARTESIAN_POINT ( 'NONE',  ( 6.204703633549690345, 57.84541550158063927, 14.16423886937410082 ) ) ;
#70257=CARTESIAN_POINT ( 'NONE',  ( 20.88017736071110875, 55.77201867748816966, -2.915334737309920765 ) ) ;
#70258=CARTESIAN_POINT ( 'NONE',  ( 2.791683348922237240, 20.38393115100078745, -7.208316651077763204 ) ) ;
#70261=DIRECTION ( 'NONE',  ( 0.9998643952135762847, -0.01646788341559294114, 2.168110298962930704E-16 ) ) ;
#70262=ORIENTED_EDGE ( 'NONE', *, *, #13781, .T. ) ;
#70263=CARTESIAN_POINT ( 'NONE',  ( 0.1532563361054100626, 10.80059781766745175, -2.638427012816831230 ) ) ;
#70265=CARTESIAN_POINT ( 'NONE',  ( 6.204703633549690345, 20.76208216824730357, -14.16423886937410259 ) ) ;
#70266=CARTESIAN_POINT ( 'NONE',  ( 12.63842701281683922, 24.55059781766745175, -9.846743663894590881 ) ) ;
#70267=CARTESIAN_POINT ( 'NONE',  ( 17.96484262340118221, 39.93868534415484106, 7.964842623401181321 ) ) ;
#70270=CARTESIAN_POINT ( 'NONE',  ( 4.559911319644449179, 38.89701867748817676, 9.422509992056141925 ) ) ;
#70274=CARTESIAN_POINT ( 'NONE',  ( 4.559911319644449179, 42.23035201082151247, -9.422509992056141925 ) ) ;
#70275=CARTESIAN_POINT ( 'NONE',  ( 24.16423886937410614, 9.303748834913967869, 8.672049930838204340E-16 ) ) ;
#70278=VERTEX_POINT ( 'NONE', #13057 ) ;
#70279=CARTESIAN_POINT ( 'NONE',  ( 22.81628187352647785, 26.41530133659708923, 3.434112377981063169 ) ) ;
#70280=CARTESIAN_POINT ( 'NONE',  ( 7.361572987183170547, 12.05059781766744997, 9.846743663894590881 ) ) ;
#70281=CARTESIAN_POINT ( 'NONE',  ( 10.00000000000000000, 1.813685344154837731, -10.88017736071110342 ) ) ;
#70282=CARTESIAN_POINT ( 'NONE',  ( 6.565887622018943937, 43.08196800326374643, -12.81628187352647608 ) ) ;
#70283=DIRECTION ( 'NONE',  ( -0.000000000000000000, 1.000000000000000000, -0.000000000000000000 ) ) ;
#70284=CARTESIAN_POINT ( 'NONE',  ( 5.076628168052703671, 11.84226448433411960, 8.527530157486179263 ) ) ;
#70285=CARTESIAN_POINT ( 'NONE',  ( 20.88017736071110875, 25.77201867748816966, -2.915334737309920765 ) ) ;
#70286=B_SPLINE_CURVE_WITH_KNOTS ( 'NONE', 3,
 ( #52485, #18, #53467, #82496 ),
 .UNSPECIFIED., .F., .F.,
 ( 4, 4 ),
 ( 0.000000000000000000, 0.002657014572711347607 ),
 .UNSPECIFIED. ) ;
#70289=CARTESIAN_POINT ( 'NONE',  ( 2.035157376598822676, 62.43868534415483396, -7.964842623401177768 ) ) ;
#70292=CARTESIAN_POINT ( 'NONE',  ( 7.084665262690076126, 59.10535201082150536, 10.88017736071109987 ) ) ;
#70293=CARTESIAN_POINT ( 'NONE',  ( 10.00000000000000000, 7.873634669930421381, -12.81628187352647608 ) ) ;
#70296=CARTESIAN_POINT ( 'NONE',  ( 10.00000000000000178, 32.25893115100078745, 9.846743663894594434 ) ) ;
#70297=CARTESIAN_POINT ( 'NONE',  ( 21.09922568453594849, 61.20696800326376064, 6.408140936763242479 ) ) ;
#70298=CARTESIAN_POINT ( 'NONE',  ( -2.266590686148945544, 1.387082168247301128, -7.082119434687050408 ) ) ;
#70299=CARTESIAN_POINT ( 'NONE',  ( 1.472469842513823179, 16.42559781766745175, 4.923371831947296329 ) ) ;
#70301=CARTESIAN_POINT ( 'NONE',  ( -2.816281873526473856, 19.12363466993042138, 9.499525473075851096E-16 ) ) ;
#70303=CARTESIAN_POINT ( 'NONE',  ( 19.42250999205614193, 55.14701867748817676, 5.440088680355555262 ) ) ;
#70305=CARTESIAN_POINT ( 'NONE',  ( 10.00000000000000000, 59.75893115100078745, -9.846743663894594434 ) ) ;
#70306=CARTESIAN_POINT ( 'NONE',  ( -0.1503990784575242878, 29.24884699246888786, -6.262539305110083276 ) ) ;
#70307=CARTESIAN_POINT ( 'NONE',  ( 19.84674366389459266, 28.71726448433411960, -2.638427012816827677 ) ) ;
#70308=CARTESIAN_POINT ( 'NONE',  ( 18.52753015748617571, 28.09226448433411960, 4.923371831947298993 ) ) ;
#70309=CARTESIAN_POINT ( 'NONE',  ( 4.559911319644449179, 17.23035201082150536, -9.422509992056141925 ) ) ;
#70310=CARTESIAN_POINT ( 'NONE',  ( 19.38216949554541202, 10.99863466993042138, 9.382169495545424454 ) ) ;
#70311=CARTESIAN_POINT ( 'NONE',  ( 19.84674366389459266, 28.30059781766745886, 2.638427012816836559 ) ) ;
#70314=CARTESIAN_POINT ( 'NONE',  ( 10.00000000000000178, 19.31368534415484106, 10.88017736071110342 ) ) ;
#70316=CARTESIAN_POINT ( 'NONE',  ( 7.361572987183169658, 39.96726448433411605, -9.846743663894592657 ) ) ;
#70317=CARTESIAN_POINT ( 'NONE',  ( 10.00000000000000000, 21.81368534415484106, -10.88017736071110342 ) ) ;
#70320=CARTESIAN_POINT ( 'NONE',  ( 10.00000000000000000, 26.81368534415484106, -10.88017736071110342 ) ) ;
#70321=CARTESIAN_POINT ( 'NONE',  ( 0.5774900079438607392, 18.48035201082150536, 5.440088680355550821 ) ) ;
#70322=CARTESIAN_POINT ( 'NONE',  ( -0.1503990784575328643, 20.12777174578613071, 6.262539305110068177 ) ) ;
#70323=CARTESIAN_POINT ( 'NONE',  ( 1.472469842513823179, 20.59226448433411960, -4.923371831947296329 ) ) ;
#70324=CARTESIAN_POINT ( 'NONE',  ( 10.00000000000000178, 37.25893115100078745, 9.846743663894594434 ) ) ;
#70326=CARTESIAN_POINT ( 'NONE',  ( 1.383448333479223358, 7.377183271974286249, -6.499999999999965361 ) ) ;
#70327=EDGE_CURVE ( 'NONE', #50256, #47024, #47651, .T. ) ;
#70328=CARTESIAN_POINT ( 'NONE',  ( 2.791683348922237240, 65.38393115100078035, -7.208316651077763204 ) ) ;
#70329=CARTESIAN_POINT ( 'NONE',  ( 20.36894250292379738, 29.92874883491396432, -10.36894250292379027 ) ) ;
#70330=CARTESIAN_POINT ( 'NONE',  ( 5.076628168052703671, 41.84226448433411605, 8.527530157486179263 ) ) ;
#70333=CARTESIAN_POINT ( 'NONE',  ( 2.917880565312948704, 57.63708216824731068, 12.26659068614894643 ) ) ;
#70334=CARTESIAN_POINT ( 'NONE',  ( 18.52753015748617571, 18.09226448433411960, 4.923371831947298993 ) ) ;
#70335=CARTESIAN_POINT ( 'NONE',  ( 2.603489959281590771, 66.58210964143327715, 6.500000000000003553 ) ) ;
#70337=CARTESIAN_POINT ( 'NONE',  ( 12.91533473730993009, 41.60535201082149825, -10.88017736071109987 ) ) ;
#70339=CARTESIAN_POINT ( 'NONE',  ( 7.084665262690076126, 17.02201867748817676, -10.88017736071110164 ) ) ;
#70340=CARTESIAN_POINT ( 'NONE',  ( 13.43411237798106583, 47.66530133659709634, -12.81628187352647252 ) ) ;
#70341=CARTESIAN_POINT ( 'NONE',  ( 16.40814093676324603, 12.45696800326375353, -11.09922568453594671 ) ) ;
#70342=CARTESIAN_POINT ( 'NONE',  ( 2.791683348922237240, 20.38393115100078745, -7.208316651077763204 ) ) ;
#70345=CARTESIAN_POINT ( 'NONE',  ( 1.274849032794305170, 17.55509018479936145, -6.499999999999995559 ) ) ;
#70346=CARTESIAN_POINT ( 'NONE',  ( 20.36894250292379382, 48.67874883491396076, 10.36894250292379205 ) ) ;
#70347=CARTESIAN_POINT ( 'NONE',  ( 17.08211943468705840, 30.13708216824730357, -12.26659068614894466 ) ) ;
#70348=CARTESIAN_POINT ( 'NONE',  ( 20.88017736071110519, 20.56368534415484106, 2.639326808657452039E-16 ) ) ;
#70349=CARTESIAN_POINT ( 'NONE',  ( 12.91533473730992121, 39.52201867748817676, 10.88017736071110164 ) ) ;
#70350=CARTESIAN_POINT ( 'NONE',  ( 10.00000000000000178, 70.00000000000000000, 0.000000000000000000 ) ) ;
#70352=CARTESIAN_POINT ( 'NONE',  ( 7.084665262690076126, 69.10535201082151957, 10.88017736071109987 ) ) ;
#70353=CARTESIAN_POINT ( 'NONE',  ( 19.84674366389459266, 23.30059781766745530, 2.638427012816836559 ) ) ;
#70354=CARTESIAN_POINT ( 'NONE',  ( -41.94000000000001194, 93.50000000000000000, 9.500000000000000000 ) ) ;
#70356=CARTESIAN_POINT ( 'NONE',  ( 2.791683348922237240, 15.38393115100078212, -7.208316651077763204 ) ) ;
#70357=CARTESIAN_POINT ( 'NONE',  ( 0.1532563361054100626, 40.80059781766745886, -2.638427012816831230 ) ) ;
#70358=CARTESIAN_POINT ( 'NONE',  ( -0.8801773607110991993, 7.855352010821504471, -2.915334737309923874 ) ) ;
#70362=CARTESIAN_POINT ( 'NONE',  ( 10.00000000000000000, 27.87363466993042138, -12.81628187352647608 ) ) ;
#70363=CARTESIAN_POINT ( 'NONE',  ( 7.084665262690076126, 59.10535201082150536, 10.88017736071109987 ) ) ;
#70364=CARTESIAN_POINT ( 'NONE',  ( -2.266590686148945544, 52.22041550158064638, 7.082119434687048631 ) ) ;
#70365=CARTESIAN_POINT ( 'NONE',  ( 7.361572987183169658, 4.967264484334119601, -9.846743663894592657 ) ) ;
#70367=CARTESIAN_POINT ( 'NONE',  ( 19.84674366389459621, 48.50893115100078745, 7.409399052514197653E-17 ) ) ;
#70368=CARTESIAN_POINT ( 'NONE',  ( 0.1532563361054083140, 36.00893115100078745, 1.131784320476157264E-15 ) ) ;
#70370=CARTESIAN_POINT ( 'NONE',  ( -4.164238869374099039, 11.80374883491396965, 8.674139862899312516E-16 ) ) ;
#70372=CARTESIAN_POINT ( 'NONE',  ( 10.00000000000000000, 41.81368534415484106, -10.88017736071110342 ) ) ;
#70373=CARTESIAN_POINT ( 'NONE',  ( 15.44008868035555260, 14.73035201082150536, 9.422509992056143702 ) ) ;
#70375=CARTESIAN_POINT ( 'NONE',  ( 4.559911319644449179, 42.23035201082151247, -9.422509992056141925 ) ) ;
#70376=CARTESIAN_POINT ( 'NONE',  ( 0.5774900079438590739, 27.64701867748817676, -5.440088680355550821 ) ) ;
#70378=CARTESIAN_POINT ( 'NONE',  ( 17.96484262340118221, 36.18868534415484106, -7.964842623401177768 ) ) ;
#70380=CARTESIAN_POINT ( 'NONE',  ( -1.099225684535947600, 63.70696800326376774, -6.408140936763238038 ) ) ;
#70381=CARTESIAN_POINT ( 'NONE',  ( 4.559911319644449179, 47.23035201082150536, -9.422509992056141925 ) ) ;
#70383=CARTESIAN_POINT ( 'NONE',  ( 19.42250999205614548, 50.98035201082151247, -5.440088680355545492 ) ) ;
#70384=FILL_AREA_STYLE_COLOUR ( '', #40243 ) ;
#70385=CYLINDRICAL_SURFACE ( 'NONE', #86732, 11.92686044187656513 ) ;
#70387=CARTESIAN_POINT ( 'NONE',  ( 17.08211943468705130, 58.47041550158063927, 12.26659068614894998 ) ) ;
#70388=CARTESIAN_POINT ( 'NONE',  ( 0.1532563361054083140, 1.008931151000784787, 1.131784320476157264E-15 ) ) ;
#70390=CARTESIAN_POINT ( 'NONE',  ( -0.8801773607111009756, 8.063685344154837509, 1.068504757029289695E-15 ) ) ;
#70391=CARTESIAN_POINT ( 'NONE',  ( 2.791683348922240793, 46.63393115100077324, 7.208316651077764092 ) ) ;
#70393=CARTESIAN_POINT ( 'NONE',  ( 7.361572987183170547, 42.05059781766745886, 9.846743663894590881 ) ) ;
#70394=CARTESIAN_POINT ( 'NONE',  ( 4.559911319644449179, 63.89701867748817676, 9.422509992056141925 ) ) ;
#70395=CARTESIAN_POINT ( 'NONE',  ( 10.00000000000000178, 39.31368534415484106, 10.88017736071110342 ) ) ;
#70396=CARTESIAN_POINT ( 'NONE',  ( 0.1532563361054082862, 51.21726448433412315, 2.638427012816831674 ) ) ;
#70397=SURFACE_STYLE_FILL_AREA ( #33833 ) ;
#70398=CARTESIAN_POINT ( 'NONE',  ( -0.8801773607110991993, 67.85535201082151957, -2.915334737309923874 ) ) ;
#70399=CARTESIAN_POINT ( 'NONE',  ( 12.91533473730992121, 49.52201867748817676, 10.88017736071110164 ) ) ;
#70400=CARTESIAN_POINT ( 'NONE',  ( 24.16423886937410614, 54.30374883491396787, 8.672049930838204340E-16 ) ) ;
#70404=CARTESIAN_POINT ( 'NONE',  ( 6.565887622018943937, 25.16530133659708213, 12.81628187352647430 ) ) ;
#70405=DIRECTION ( 'NONE',  ( -1.000000000000000000, 0.000000000000000000, 0.000000000000000000 ) ) ;
#70407=CARTESIAN_POINT ( 'NONE',  ( 22.81628187352648496, 31.83196800326375353, -3.434112377981050290 ) ) ;
#70408=CARTESIAN_POINT ( 'NONE',  ( 19.42250999205614548, 15.98035201082150714, -5.440088680355545492 ) ) ;
#70410=ORIENTED_EDGE ( 'NONE', *, *, #29805, .F. ) ;
#70411=CARTESIAN_POINT ( 'NONE',  ( 18.52753015748617571, 48.09226448433412315, 4.923371831947298993 ) ) ;
#70412=CARTESIAN_POINT ( 'NONE',  ( 5.076628168052703671, 6.842264484334118713, 8.527530157486179263 ) ) ;
#70413=CARTESIAN_POINT ( 'NONE',  ( 7.361572987183169658, 34.96726448433411605, -9.846743663894592657 ) ) ;
#70416=CARTESIAN_POINT ( 'NONE',  ( 2.791683348922237240, 25.38393115100078390, -7.208316651077763204 ) ) ;
#70419=CARTESIAN_POINT ( 'NONE',  ( 12.63842701281683922, 29.55059781766745175, -9.846743663894590881 ) ) ;
#70420=SURFACE_SIDE_STYLE ('',( #41418 ) ) ;
#70422=CARTESIAN_POINT ( 'NONE',  ( 0.1532563361054083140, 41.00893115100078745, 1.131784320476157264E-15 ) ) ;
#70425=CARTESIAN_POINT ( 'NONE',  ( 19.38216949554541557, 32.24863466993041783, -9.382169495545420901 ) ) ;
#70427=CARTESIAN_POINT ( 'NONE',  ( -2.266590686148945544, 46.38708216824730357, -7.082119434687050408 ) ) ;
#70428=CARTESIAN_POINT ( 'NONE',  ( 17.20831665107776587, 24.13393115100078035, -7.208316651077762316 ) ) ;
#70430=CARTESIAN_POINT ( 'NONE',  ( 19.84674366389459266, 3.717264484334118713, -2.638427012816827677 ) ) ;
#70432=CARTESIAN_POINT ( 'NONE',  ( 22.26659068614894466, 43.88708216824729647, 7.082119434687054849 ) ) ;
#70433=CARTESIAN_POINT ( 'NONE',  ( 5.076628168052704559, 65.17559781766745175, -8.527530157486179263 ) ) ;
#70434=CARTESIAN_POINT ( 'NONE',  ( 24.16423886937410614, 54.51208216824730357, -3.795296366450302550 ) ) ;
#70435=CARTESIAN_POINT ( 'NONE',  ( -2.266590686148945544, 21.38708216824730357, -7.082119434687050408 ) ) ;
#70436=CARTESIAN_POINT ( 'NONE',  ( 2.917880565312950480, 25.97041550158063572, -12.26659068614894821 ) ) ;
#70438=CARTESIAN_POINT ( 'NONE',  ( 5.076628168052703671, 61.84226448433412315, 8.527530157486179263 ) ) ;
#70439=CARTESIAN_POINT ( 'NONE',  ( 17.96484262340118221, 34.93868534415482685, 7.964842623401181321 ) ) ;
#70440=CARTESIAN_POINT ( 'NONE',  ( 13.99999999999999822, 61.50000000000000711, 6.000000000000000000 ) ) ;
#70441=CARTESIAN_POINT ( 'NONE',  ( 20.00000000000000711, 98.59912998021081876, -4.500000000000000000 ) ) ;
#70443=CARTESIAN_POINT ( 'NONE',  ( 0.1532563361054100626, 40.80059781766745886, -2.638427012816831230 ) ) ;
#70444=CARTESIAN_POINT ( 'NONE',  ( 22.81628187352647785, 56.62363466993042493, 6.195893100308588602E-16 ) ) ;
#70446=CARTESIAN_POINT ( 'NONE',  ( 14.92337183194729633, 47.67559781766745175, 8.527530157486181039 ) ) ;
#70449=CARTESIAN_POINT ( 'NONE',  ( -2.266590686148945544, 17.22041550158063572, 7.082119434687048631 ) ) ;
#70453=CARTESIAN_POINT ( 'NONE',  ( 0.5774900079438590739, 12.64701867748817321, -5.440088680355550821 ) ) ;
#70454=CARTESIAN_POINT ( 'NONE',  ( -2.816281873526471635, 8.915301336597083903, -3.434112377981056508 ) ) ;
#70455=CARTESIAN_POINT ( 'NONE',  ( 21.92686044187656691, 2.188309369127507953, 4.562052436263911564E-16 ) ) ;
#70456=CARTESIAN_POINT ( 'NONE',  ( 15.44008868035555260, 64.73035201082151957, 9.422509992056143702 ) ) ;
#70457=DIRECTION ( 'NONE',  ( 1.000000000000000000, 0.000000000000000000, 0.000000000000000000 ) ) ;
#70458=CARTESIAN_POINT ( 'NONE',  ( 1.472469842513823179, 31.42559781766745530, 4.923371831947296329 ) ) ;
#70459=CARTESIAN_POINT ( 'NONE',  ( 24.16423886937410614, 64.30374883491396076, 8.672049930838204340E-16 ) ) ;
#70461=CARTESIAN_POINT ( 'NONE',  ( 10.00000000000000178, 29.31368534415483751, 10.88017736071110342 ) ) ;
#70462=CARTESIAN_POINT ( 'NONE',  ( 4.559911319644449179, 37.23035201082150536, -9.422509992056141925 ) ) ;
#70463=CARTESIAN_POINT ( 'NONE',  ( 5.076628168052704559, 65.17559781766745175, -8.527530157486179263 ) ) ;
#70464=CARTESIAN_POINT ( 'NONE',  ( 14.92337183194729988, 59.34226448433412315, -8.527530157486177487 ) ) ;
#70465=CARTESIAN_POINT ( 'NONE',  ( 10.00000000000000000, 57.87363466993042493, -12.81628187352647608 ) ) ;
#70466=CARTESIAN_POINT ( 'NONE',  ( 2.791683348922240793, 1.633931151000784565, 7.208316651077764092 ) ) ;
#70470=CARTESIAN_POINT ( 'NONE',  ( 20.88017736071110164, 25.35535201082150891, 2.915334737309930979 ) ) ;
#70471=CARTESIAN_POINT ( 'NONE',  ( 6.565887622018943937, 33.08196800326374643, -12.81628187352647608 ) ) ;
#70474=CARTESIAN_POINT ( 'NONE',  ( 10.00000000000000000, -2.126365330069579951, -12.81628187352647608 ) ) ;
#70475=CARTESIAN_POINT ( 'NONE',  ( 4.559911319644449179, 43.89701867748816966, 9.422509992056141925 ) ) ;
#70476=CARTESIAN_POINT ( 'NONE',  ( 0.1532563361054100626, 10.80059781766745175, -2.638427012816831230 ) ) ;
#70477=CARTESIAN_POINT ( 'NONE',  ( 22.81628187352647785, 31.41530133659709279, 3.434112377981063169 ) ) ;
#70478=CARTESIAN_POINT ( 'NONE',  ( 12.91533473730993009, 66.60535201082150536, -10.88017736071109987 ) ) ;
#70479=CARTESIAN_POINT ( 'NONE',  ( -20.19000000000001194, 92.00000000000000000, 9.500000000000000000 ) ) ;
#70480=CARTESIAN_POINT ( 'NONE',  ( 18.39792806157253224, 54.52224192338642439, 6.499999999999920952 ) ) ;
#70481=CARTESIAN_POINT ( 'NONE',  ( 0.6178305044545838731, 64.74863466993043914, 9.382169495545420901 ) ) ;
#70486=CARTESIAN_POINT ( 'NONE',  ( -0.8801773607111008646, 8.272018677488171434, 2.915334737309923430 ) ) ;
#70487=CARTESIAN_POINT ( 'NONE',  ( 22.81628187352647785, 51.41530133659708923, 3.434112377981063169 ) ) ;
#70488=CARTESIAN_POINT ( 'NONE',  ( 22.26659068614895176, 14.72041550158063572, -7.082119434687042414 ) ) ;
#70489=CARTESIAN_POINT ( 'NONE',  ( 14.92337183194729988, 14.34226448433411782, -8.527530157486177487 ) ) ;
#70490=CARTESIAN_POINT ( 'NONE',  ( 10.00000000000000178, 4.313685344154837509, 10.88017736071110342 ) ) ;
#70491=CARTESIAN_POINT ( 'NONE',  ( 10.00000000000000000, 19.75893115100078390, -9.846743663894594434 ) ) ;
#70492=CARTESIAN_POINT ( 'NONE',  ( 13.79529636645031943, 50.34541550158064638, -14.16423886937409904 ) ) ;
#70495=CARTESIAN_POINT ( 'NONE',  ( -0.8801773607111009756, 3.063685344154837509, 1.068504757029289695E-15 ) ) ;
#70496=CARTESIAN_POINT ( 'NONE',  ( 10.00000000000000000, 16.81368534415483751, -10.88017736071110342 ) ) ;
#70500=CARTESIAN_POINT ( 'NONE',  ( 20.88017736071110519, 15.56368534415483751, 2.639326808657452039E-16 ) ) ;
#70501=CARTESIAN_POINT ( 'NONE',  ( 17.96484262340118221, 14.93868534415484106, 7.964842623401181321 ) ) ;
#70502=CARTESIAN_POINT ( 'NONE',  ( 12.63842701281683034, 52.46726448433413026, 9.846743663894596210 ) ) ;
#70504=CARTESIAN_POINT ( 'NONE',  ( 6.204703633549690345, 15.76208216824730179, -14.16423886937410259 ) ) ;
#70505=CARTESIAN_POINT ( 'NONE',  ( 10.00000000000000000, 31.81368534415483751, -10.88017736071110342 ) ) ;
#70506=CARTESIAN_POINT ( 'NONE',  ( 22.26659068614895176, 64.72041550158064638, -7.082119434687042414 ) ) ;
#70507=CARTESIAN_POINT ( 'NONE',  ( 10.00000000000000000, 54.75893115100078745, -9.846743663894594434 ) ) ;
#70508=CARTESIAN_POINT ( 'NONE',  ( 18.50749283717773253, 44.69955587570481015, 6.500000000000077272 ) ) ;
#70509=CARTESIAN_POINT ( 'NONE',  ( 17.20831665107776587, 42.88393115100077324, 7.208316651077764980 ) ) ;
#70511=CARTESIAN_POINT ( 'NONE',  ( 19.84674366389459266, 8.300597817667451750, 2.638427012816836559 ) ) ;
#70514=EDGE_CURVE ( 'NONE', #72554, #5105, #51073, .T. ) ;
#70516=CARTESIAN_POINT ( 'NONE',  ( 10.00000000000000178, 4.313685344154837509, 10.88017736071110342 ) ) ;
#70517=CARTESIAN_POINT ( 'NONE',  ( 7.361572987183170547, 2.050597817667451750, 9.846743663894590881 ) ) ;
#70518=CARTESIAN_POINT ( 'NONE',  ( 7.084665262690076126, 49.10535201082149825, 10.88017736071109987 ) ) ;
#70519=CARTESIAN_POINT ( 'NONE',  ( 12.91533473730993009, 46.60535201082150536, -10.88017736071109987 ) ) ;
#70520=CARTESIAN_POINT ( 'NONE',  ( 0.5774900079438590739, 12.64701867748817143, -5.440088680355550821 ) ) ;
#70521=CARTESIAN_POINT ( 'NONE',  ( 22.81628187352647785, 46.41530133659708213, 3.434112377981063169 ) ) ;
#70522=CARTESIAN_POINT ( 'NONE',  ( 6.204703633549690345, 22.84541550158062861, 14.16423886937410082 ) ) ;
#70524=CARTESIAN_POINT ( 'NONE',  ( -2.816281873526473856, 44.12363466993042493, 9.499525473075851096E-16 ) ) ;
#70526=CARTESIAN_POINT ( 'NONE',  ( 7.361572987183169658, 54.96726448433413026, -9.846743663894592657 ) ) ;
#70527=CARTESIAN_POINT ( 'NONE',  ( 7.084665262690076126, 17.02201867748817676, -10.88017736071110164 ) ) ;
#70528=CARTESIAN_POINT ( 'NONE',  ( 12.91533473730993009, 31.60535201082150891, -10.88017736071109987 ) ) ;
#70531=CARTESIAN_POINT ( 'NONE',  ( 0.1532563361054100626, 10.80059781766745175, -2.638427012816831230 ) ) ;
#70532=CARTESIAN_POINT ( 'NONE',  ( 10.00000000000000000, 66.81368534415484817, -10.88017736071110342 ) ) ;
#70534=CARTESIAN_POINT ( 'NONE',  ( 2.791683348922240793, 6.633931151000785675, 7.208316651077764092 ) ) ;
#70535=CARTESIAN_POINT ( 'NONE',  ( -0.8801773607111008646, 68.27201867748817676, 2.915334737309923430 ) ) ;
#70537=CARTESIAN_POINT ( 'NONE',  ( 20.88017736071110875, 55.77201867748816966, -2.915334737309920765 ) ) ;
#70539=CARTESIAN_POINT ( 'NONE',  ( 4.559911319644449179, 68.89701867748817676, 9.422509992056141925 ) ) ;
#70540=CARTESIAN_POINT ( 'NONE',  ( 1.472469842513823179, 1.425597817667451528, 4.923371831947296329 ) ) ;
#70541=ORIENTED_EDGE ( 'NONE', *, *, #28143, .F. ) ;
#70542=CARTESIAN_POINT ( 'NONE',  ( 19.84674366389459266, 53.71726448433411605, -2.638427012816827677 ) ) ;
#70543=ORIENTED_EDGE ( 'NONE', *, *, #53059, .F. ) ;
#70544=ORIENTED_EDGE ( 'NONE', *, *, #74961, .F. ) ;
#70545=CARTESIAN_POINT ( 'NONE',  ( 17.08211943468705840, 10.13708216824730179, -12.26659068614894466 ) ) ;
#70546=CARTESIAN_POINT ( 'NONE',  ( -2.816281873526471635, 53.91530133659709634, -3.434112377981056508 ) ) ;
#70547=CARTESIAN_POINT ( 'NONE',  ( 10.00000000000000178, 23.05374883491397142, 14.16423886937410082 ) ) ;
#70548=CARTESIAN_POINT ( 'NONE',  ( 17.39651004071841101, 57.93575266056827644, 6.500000000000005329 ) ) ;
#70550=CARTESIAN_POINT ( 'NONE',  ( 10.00000000000000000, 21.81368534415484106, -10.88017736071110342 ) ) ;
#70552=CARTESIAN_POINT ( 'NONE',  ( 2.791683348922237240, 0.3839311510007847872, -7.208316651077763204 ) ) ;
#70553=CARTESIAN_POINT ( 'NONE',  ( 17.20831665107776587, 9.133931151000787452, -7.208316651077762316 ) ) ;
#70554=CARTESIAN_POINT ( 'NONE',  ( -2.816281873526473856, 34.33196800326376064, 3.434112377981055619 ) ) ;
#70555=CARTESIAN_POINT ( 'NONE',  ( 14.92337183194729633, 32.67559781766745175, 8.527530157486181039 ) ) ;
#70558=CARTESIAN_POINT ( 'NONE',  ( -1.099225684535947600, 9.540301336597087456, 6.408140936763237150 ) ) ;
#70560=AXIS2_PLACEMENT_3D ( 'NONE', #93071, #19539, #97046 ) ;
#70561=CARTESIAN_POINT ( 'NONE',  ( 1.472469842513823179, 31.42559781766745530, 4.923371831947296329 ) ) ;
#70562=CARTESIAN_POINT ( 'NONE',  ( 14.92337183194729988, 4.342264484334117824, -8.527530157486177487 ) ) ;
#70566=CARTESIAN_POINT ( 'NONE',  ( 4.559911319644449179, 37.23035201082150536, -9.422509992056141925 ) ) ;
#70567=CARTESIAN_POINT ( 'NONE',  ( 20.36894250292379382, 38.67874883491396076, 10.36894250292379205 ) ) ;
#70568=CARTESIAN_POINT ( 'NONE',  ( 14.92337183194729988, 39.34226448433412315, -8.527530157486177487 ) ) ;
#70569=CARTESIAN_POINT ( 'NONE',  ( 12.63842701281683922, 14.55059781766744997, -9.846743663894590881 ) ) ;
#70571=CARTESIAN_POINT ( 'NONE',  ( 13.43411237798105340, 55.58196800326374643, 12.81628187352647963 ) ) ;
#70573=CARTESIAN_POINT ( 'NONE',  ( 17.96484262340118221, 26.18868534415483396, -7.964842623401177768 ) ) ;
#70575=CARTESIAN_POINT ( 'NONE',  ( -1.099225684535947600, 18.70696800326375353, -6.408140936763238038 ) ) ;
#70576=CARTESIAN_POINT ( 'NONE',  ( 19.84674366389459621, 38.50893115100078745, 7.409399052514197653E-17 ) ) ;
#70578=CARTESIAN_POINT ( 'NONE',  ( 3.591859063236761518, 44.95696800326376064, 11.09922568453594849 ) ) ;
#70581=CARTESIAN_POINT ( 'NONE',  ( 19.42250999205614193, 60.14701867748817676, 5.440088680355555262 ) ) ;
#70585=CARTESIAN_POINT ( 'NONE',  ( -0.8801773607110991993, 47.85535201082150536, -2.915334737309923874 ) ) ;
#70586=CARTESIAN_POINT ( 'NONE',  ( 0.5774900079438607392, 53.48035201082151247, 5.440088680355550821 ) ) ;
#70587=CARTESIAN_POINT ( 'NONE',  ( -45.94000000000001194, 92.50000000000000000, 9.000000000000000000 ) ) ;
#70590=CARTESIAN_POINT ( 'NONE',  ( 2.035157376598824452, 13.68868534415483751, 7.964842623401179544 ) ) ;
#70591=CARTESIAN_POINT ( 'NONE',  ( 3.591859063236763294, -1.709698663402913210, -11.09922568453595026 ) ) ;
#70592=CARTESIAN_POINT ( 'NONE',  ( -0.8801773607111009756, 18.06368534415484106, 1.068504757029289695E-15 ) ) ;
#70595=CARTESIAN_POINT ( 'NONE',  ( 22.81628187352647785, 26.62363466993042138, 6.195893100308588602E-16 ) ) ;
#70597=CARTESIAN_POINT ( 'NONE',  ( 15.44008868035555260, 54.73035201082150536, 9.422509992056143702 ) ) ;
#70599=CARTESIAN_POINT ( 'NONE',  ( 19.84674366389459266, 38.71726448433412315, -2.638427012816827677 ) ) ;
#70600=CARTESIAN_POINT ( 'NONE',  ( 21.09922568453594849, 1.206968003263753531, 6.408140936763242479 ) ) ;
#70601=CARTESIAN_POINT ( 'NONE',  ( 4.559911319644449179, 18.89701867748817321, 9.422509992056141925 ) ) ;
#70602=CARTESIAN_POINT ( 'NONE',  ( -0.8801773607110991993, 37.85535201082151247, -2.915334737309923874 ) ) ;
#70603=CARTESIAN_POINT ( 'NONE',  ( -4.164238869374098151, 46.59541550158063927, -3.795296366450310543 ) ) ;
#70604=CARTESIAN_POINT ( 'NONE',  ( 17.20831665107776587, 42.88393115100077324, 7.208316651077764980 ) ) ;
#70605=CARTESIAN_POINT ( 'NONE',  ( -0.8801773607111008646, 58.27201867748816966, 2.915334737309923430 ) ) ;
#70607=CARTESIAN_POINT ( 'NONE',  ( 17.08211943468705130, 13.47041550158063572, 12.26659068614894998 ) ) ;
#70613=CARTESIAN_POINT ( 'NONE',  ( 2.917880565312948704, 32.63708216824730357, 12.26659068614894643 ) ) ;
#70614=CARTESIAN_POINT ( 'NONE',  ( 17.08211943468705840, 40.13708216824731068, -12.26659068614894466 ) ) ;
#70615=CARTESIAN_POINT ( 'NONE',  ( 10.00000000000000000, -0.2410688489992152128, -9.846743663894594434 ) ) ;
#70616=CARTESIAN_POINT ( 'NONE',  ( 21.09922568453594849, 21.20696800326375353, 6.408140936763242479 ) ) ;
#70617=CARTESIAN_POINT ( 'NONE',  ( 19.84674366389459621, 63.50893115100078745, 7.409399052514197653E-17 ) ) ;
#70619=CARTESIAN_POINT ( 'NONE',  ( 0.5774900079438607392, 58.48035201082151247, 5.440088680355550821 ) ) ;
#70620=CARTESIAN_POINT ( 'NONE',  ( 10.00000000000000000, 37.87363466993041783, -12.81628187352647608 ) ) ;
#70621=CARTESIAN_POINT ( 'NONE',  ( 20.36894250292379382, 23.67874883491397142, 10.36894250292379205 ) ) ;
#70622=CARTESIAN_POINT ( 'NONE',  ( -0.8801773607110991993, 27.85535201082150181, -2.915334737309923874 ) ) ;
#70623=DIRECTION ( 'NONE',  ( 1.000000000000000000, 0.000000000000000000, 0.000000000000000000 ) ) ;
#70624=CARTESIAN_POINT ( 'NONE',  ( 7.361572987183169658, -0.03273551566588185635, -9.846743663894592657 ) ) ;
#70626=CARTESIAN_POINT ( 'NONE',  ( 18.52753015748617571, 8.092264484334117824, 4.923371831947298993 ) ) ;
#70629=ORIENTED_EDGE ( 'NONE', *, *, #47660, .F. ) ;
#70632=CARTESIAN_POINT ( 'NONE',  ( 10.00000000000000178, 8.053748834913967869, 14.16423886937410082 ) ) ;
#70633=CARTESIAN_POINT ( 'NONE',  ( 10.00000000000000178, 4.313685344154837509, 10.88017736071110342 ) ) ;
#70634=CARTESIAN_POINT ( 'NONE',  ( 17.96484262340118221, 11.18868534415484106, -7.964842623401177768 ) ) ;
#70635=CARTESIAN_POINT ( 'NONE',  ( 18.52753015748618282, 38.92559781766745175, -4.923371831947291888 ) ) ;
#70636=CARTESIAN_POINT ( 'NONE',  ( -2.816281873526473856, 9.331968003263753531, 3.434112377981055619 ) ) ;
#70639=EDGE_CURVE ( 'NONE', #8299, #93746, #89190, .T. ) ;
#70641=CARTESIAN_POINT ( 'NONE',  ( -1.099225684535947600, -1.293031996736246469, -6.408140936763238038 ) ) ;
#70645=CARTESIAN_POINT ( 'NONE',  ( 24.16423886937410614, 49.51208216824730357, -3.795296366450302550 ) ) ;
#70648=CARTESIAN_POINT ( 'NONE',  ( 13.79529636645030344, 63.26208216824730357, 14.16423886937410614 ) ) ;
#70650=CARTESIAN_POINT ( 'NONE',  ( 17.96484262340118221, 39.93868534415484106, 7.964842623401181321 ) ) ;
#70651=CARTESIAN_POINT ( 'NONE',  ( -0.8801773607111009756, 33.06368534415484106, 1.068504757029289695E-15 ) ) ;
#70652=CARTESIAN_POINT ( 'NONE',  ( 12.63842701281683922, 59.55059781766744464, -9.846743663894590881 ) ) ;
#70653=CARTESIAN_POINT ( 'NONE',  ( 10.00000000000000000, 41.81368534415484106, -10.88017736071110342 ) ) ;
#70654=AXIS2_PLACEMENT_3D ( 'NONE', #29357, #50886, #67873 ) ;
#70655=CARTESIAN_POINT ( 'NONE',  ( 10.00000000000000178, 69.31368534415484817, 10.88017736071110342 ) ) ;
#70656=CARTESIAN_POINT ( 'NONE',  ( 0.5774900079438607392, 23.48035201082150536, 5.440088680355550821 ) ) ;
#70660=CARTESIAN_POINT ( 'NONE',  ( 0.1532563361054082862, 21.21726448433412315, 2.638427012816831674 ) ) ;
#70664=CARTESIAN_POINT ( 'NONE',  ( 14.92337183194729988, 44.34226448433412315, -8.527530157486177487 ) ) ;
#70665=CARTESIAN_POINT ( 'NONE',  ( 13.99999999999999822, 11.50000000000000000, 5.000000000000000000 ) ) ;
#70666=SURFACE_STYLE_USAGE ( .BOTH. , #85171 ) ;
#70667=VECTOR ( 'NONE', #93401, 1000.000000000000000 ) ;
#70669=CARTESIAN_POINT ( 'NONE',  ( -46.46849503609698218, 103.9079590269317066, 5.994465626573347805 ) ) ;
#70671=CARTESIAN_POINT ( 'NONE',  ( 1.472469842513823179, 55.59226448433412315, -4.923371831947296329 ) ) ;
#70672=CARTESIAN_POINT ( 'NONE',  ( 13.79529636645030344, 43.26208216824730357, 14.16423886937410614 ) ) ;
#70673=CARTESIAN_POINT ( 'NONE',  ( 17.20831665107776587, 59.13393115100078745, -7.208316651077762316 ) ) ;
#70676=CARTESIAN_POINT ( 'NONE',  ( 1.472469842513823179, 25.59226448433412315, -4.923371831947296329 ) ) ;
#70677=CARTESIAN_POINT ( 'NONE',  ( 3.591859063236761518, 54.95696800326376064, 11.09922568453594849 ) ) ;
#70678=CARTESIAN_POINT ( 'NONE',  ( 5.076628168052703671, 66.84226448433412315, 8.527530157486179263 ) ) ;
#70679=CARTESIAN_POINT ( 'NONE',  ( 4.559911319644449179, 63.89701867748817676, 9.422509992056141925 ) ) ;
#70685=CARTESIAN_POINT ( 'NONE',  ( -4.164238869374099039, 56.80374883491397497, 8.674139862899312516E-16 ) ) ;
#70686=SURFACE_STYLE_USAGE ( .BOTH. , #40179 ) ;
#70687=CARTESIAN_POINT ( 'NONE',  ( 10.00000000000000000, 31.81368534415483751, -10.88017736071110342 ) ) ;
#70688=CARTESIAN_POINT ( 'NONE',  ( 13.43411237798105340, 15.58196800326374998, 12.81628187352647963 ) ) ;
#70689=CARTESIAN_POINT ( 'NONE',  ( 17.96484262340118221, 59.93868534415484106, 7.964842623401181321 ) ) ;
#70690=CARTESIAN_POINT ( 'NONE',  ( -1.926860441876563801, 62.66212336850780673, 1.004413902775740978E-15 ) ) ;
#70694=CARTESIAN_POINT ( 'NONE',  ( 7.361572987183170547, 57.05059781766744464, 9.846743663894590881 ) ) ;
#70695=CARTESIAN_POINT ( 'NONE',  ( 14.92337183194729633, 2.675597817667451750, 8.527530157486181039 ) ) ;
#70697=CARTESIAN_POINT ( 'NONE',  ( -1.099225684535947600, 8.706968003263753531, -6.408140936763238038 ) ) ;
#70698=CARTESIAN_POINT ( 'NONE',  ( 2.035157376598824452, 8.688685344154839285, 7.964842623401179544 ) ) ;
#70699=CARTESIAN_POINT ( 'NONE',  ( 2.377183314880000786, 65.78593319516822646, -6.500000000000057732 ) ) ;
#70701=CARTESIAN_POINT ( 'NONE',  ( 2.917880565312948704, 32.63708216824730357, 12.26659068614894643 ) ) ;
#70702=CARTESIAN_POINT ( 'NONE',  ( 24.16423886937409904, 29.09541550158063572, 3.795296366450317205 ) ) ;
#70703=CARTESIAN_POINT ( 'NONE',  ( 7.084665262690076126, 4.105352010821503583, 10.88017736071109987 ) ) ;
#70705=CARTESIAN_POINT ( 'NONE',  ( 14.92337183194729633, 32.67559781766745175, 8.527530157486181039 ) ) ;
#70706=CARTESIAN_POINT ( 'NONE',  ( 7.361572987183169658, 14.96726448433411960, -9.846743663894592657 ) ) ;
#70707=CARTESIAN_POINT ( 'NONE',  ( 20.88017736071110519, 20.56368534415484106, 2.639326808657452039E-16 ) ) ;
#70709=CARTESIAN_POINT ( 'NONE',  ( 1.472469842513823179, 36.42559781766745175, 4.923371831947296329 ) ) ;
#70710=CARTESIAN_POINT ( 'NONE',  ( 12.91533473730993009, 46.60535201082150536, -10.88017736071109987 ) ) ;
#70711=CARTESIAN_POINT ( 'NONE',  ( 7.361572987183169658, 59.96726448433410894, -9.846743663894592657 ) ) ;
#70712=CARTESIAN_POINT ( 'NONE',  ( -2.266590686148945544, 21.38708216824730357, -7.082119434687050408 ) ) ;
#70717=STYLED_ITEM ( 'NONE', ( #50005 ), #48558 ) ;
#70718=CARTESIAN_POINT ( 'NONE',  ( 18.52753015748618282, 8.925597817667451750, -4.923371831947291888 ) ) ;
#70719=CARTESIAN_POINT ( 'NONE',  ( 10.00000000000000178, 45.37363466993041783, 12.81628187352647608 ) ) ;
#70720=CARTESIAN_POINT ( 'NONE',  ( 14.92337183194729988, 49.34226448433411605, -8.527530157486177487 ) ) ;
#70722=EDGE_CURVE ( 'NONE', #1078, #9131, #9008, .T. ) ;
#70723=MECHANICAL_DESIGN_GEOMETRIC_PRESENTATION_REPRESENTATION('',(#73832),#2073);
#70725=CARTESIAN_POINT ( 'NONE',  ( -46.54653926366209760, 102.0639713352970404, -7.520849704105015299 ) ) ;
#70726=CARTESIAN_POINT ( 'NONE',  ( 6.204703633549690345, 65.76208216824731778, -14.16423886937410259 ) ) ;
#70727=CARTESIAN_POINT ( 'NONE',  ( -0.3689425029237881626, 7.428748834913967869, 10.36894250292379027 ) ) ;
#70728=CARTESIAN_POINT ( 'NONE',  ( 17.20831665107776587, 2.883931151000785231, 7.208316651077764980 ) ) ;
#70729=CARTESIAN_POINT ( 'NONE',  ( 10.00000000000000000, 44.75893115100078745, -9.846743663894594434 ) ) ;
#70730=CARTESIAN_POINT ( 'NONE',  ( 4.559911319644449179, 17.23035201082150536, -9.422509992056141925 ) ) ;
#70731=AXIS2_PLACEMENT_3D ( 'NONE', #89260, #6261, #27763 ) ;
#70733=CARTESIAN_POINT ( 'NONE',  ( 7.361572987183170547, 62.05059781766745886, 9.846743663894590881 ) ) ;
#70734=FILL_AREA_STYLE ('',( #54232 ) ) ;
#70740=( NAMED_UNIT ( * ) SI_UNIT ( $, .STERADIAN. ) SOLID_ANGLE_UNIT ( ) );
#70741=CARTESIAN_POINT ( 'NONE',  ( 22.26659068614895176, 39.72041550158063217, -7.082119434687042414 ) ) ;
#70742=CARTESIAN_POINT ( 'NONE',  ( 1.472469842513823179, 56.42559781766745886, 4.923371831947296329 ) ) ;
#70743=CARTESIAN_POINT ( 'NONE',  ( 12.63842701281683922, 19.55059781766745175, -9.846743663894590881 ) ) ;
#70745=CARTESIAN_POINT ( 'NONE',  ( 17.96484262340118221, 21.18868534415483396, -7.964842623401177768 ) ) ;
#70746=CARTESIAN_POINT ( 'NONE',  ( 7.361572987183170547, 67.05059781766746596, 9.846743663894590881 ) ) ;
#70747=CARTESIAN_POINT ( 'NONE',  ( -1.926860441876562025, 34.47997603579417358, -3.195792623639529761 ) ) ;
#70749=B_SPLINE_CURVE_WITH_KNOTS ( 'NONE', 3,
 ( #83669, #15679, #77140, #69165, #1174, #53656 ),
 .UNSPECIFIED., .F., .F.,
 ( 4, 2, 4 ),
 ( 0.000000000000000000, 0.0002565770811490990710, 0.0005131541622981981420 ),
 .UNSPECIFIED. ) ;
#70750=CARTESIAN_POINT ( 'NONE',  ( 10.00000000000000178, 38.05374883491396787, 14.16423886937410082 ) ) ;
#70751=CARTESIAN_POINT ( 'NONE',  ( 13.79529636645031943, 60.34541550158063927, -14.16423886937409904 ) ) ;
#70752=CARTESIAN_POINT ( 'NONE',  ( 0.1532563361054083140, 66.00893115100079456, 1.131784320476157264E-15 ) ) ;
#70754=CARTESIAN_POINT ( 'NONE',  ( 20.88017736071110519, 65.56368534415483396, 2.639326808657452039E-16 ) ) ;
#70755=CARTESIAN_POINT ( 'NONE',  ( 0.1532563361054100626, 10.80059781766745175, -2.638427012816831230 ) ) ;
#70760=CARTESIAN_POINT ( 'NONE',  ( 17.20831665107776587, 22.88393115100078745, 7.208316651077764980 ) ) ;
#70761=ORIENTED_EDGE ( 'NONE', *, *, #13694, .F. ) ;
#70762=CARTESIAN_POINT ( 'NONE',  ( 17.08211943468705840, 30.13708216824730357, -12.26659068614894466 ) ) ;
#70763=CARTESIAN_POINT ( 'NONE',  ( 14.92337183194729988, 24.34226448433411960, -8.527530157486177487 ) ) ;
#70764=CARTESIAN_POINT ( 'NONE',  ( 0.5774900079438590739, 47.64701867748817676, -5.440088680355550821 ) ) ;
#70767=CARTESIAN_POINT ( 'NONE',  ( 20.88017736071110519, 40.56368534415484106, 2.639326808657452039E-16 ) ) ;
#70771=CARTESIAN_POINT ( 'NONE',  ( 24.16423886937410614, 9.512082168247301794, -3.795296366450302550 ) ) ;
#70774=CARTESIAN_POINT ( 'NONE',  ( 19.38216949554541557, 32.24863466993041783, -9.382169495545420901 ) ) ;
#70775=CARTESIAN_POINT ( 'NONE',  ( -45.94000000000000483, 92.00000000000000000, -9.500000000000000000 ) ) ;
#70776=CARTESIAN_POINT ( 'NONE',  ( 19.84674366389459266, 8.717264484334116048, -2.638427012816827677 ) ) ;
#70777=( NAMED_UNIT ( * ) SI_UNIT ( $, .STERADIAN. ) SOLID_ANGLE_UNIT ( ) );
#70779=CARTESIAN_POINT ( 'NONE',  ( 0.1532563361054100626, 25.80059781766744820, -2.638427012816831230 ) ) ;
#70782=CARTESIAN_POINT ( 'NONE',  ( 2.153642693323417845, 46.13791097397317742, -6.499999999999926281 ) ) ;
#70783=CARTESIAN_POINT ( 'NONE',  ( 12.91533473730993009, 61.60535201082150536, -10.88017736071109987 ) ) ;
#70786=CARTESIAN_POINT ( 'NONE',  ( 10.00000000000000000, 9.758931151000785675, -9.846743663894594434 ) ) ;
#70788=CARTESIAN_POINT ( 'NONE',  ( 19.38216949554541202, 10.99863466993042138, 9.382169495545424454 ) ) ;
#70791=CARTESIAN_POINT ( 'NONE',  ( 10.00000000000000000, 24.75893115100078745, -9.846743663894594434 ) ) ;
#70792=CARTESIAN_POINT ( 'NONE',  ( 3.591859063236763294, 63.29030133659708923, -11.09922568453595026 ) ) ;
#70793=CARTESIAN_POINT ( 'NONE',  ( 22.26659068614895176, 9.720415501580633943, -7.082119434687042414 ) ) ;
#70794=CARTESIAN_POINT ( 'NONE',  ( 10.00000000000000000, 14.75893115100078568, -9.846743663894594434 ) ) ;
#70795=CARTESIAN_POINT ( 'NONE',  ( 22.81628187352647785, 36.62363466993041783, 6.195893100308588602E-16 ) ) ;
#70797=DIRECTION ( 'NONE',  ( 0.7353630527936759753, 0.6776733583268310657, -0.000000000000000000 ) ) ;
#70798=CARTESIAN_POINT ( 'NONE',  ( 4.559911319644449179, 43.89701867748816966, 9.422509992056141925 ) ) ;
#70799=EDGE_CURVE ( 'NONE', #97286, #13047, #15554, .T. ) ;
#70800=CARTESIAN_POINT ( 'NONE',  ( 13.43411237798105340, 10.58196800326375353, 12.81628187352647963 ) ) ;
#70802=CARTESIAN_POINT ( 'NONE',  ( 17.20831665107776587, 32.88393115100078745, 7.208316651077764980 ) ) ;
#70803=CARTESIAN_POINT ( 'NONE',  ( 2.791683348922237240, 15.38393115100078212, -7.208316651077763204 ) ) ;
#70804=CARTESIAN_POINT ( 'NONE',  ( 0.5774900079438590739, 7.647018677488171434, -5.440088680355550821 ) ) ;
#70805=CARTESIAN_POINT ( 'NONE',  ( 10.00000000000000000, 22.87363466993042138, -12.81628187352647608 ) ) ;
#70806=CARTESIAN_POINT ( 'NONE',  ( 0.1532563361054083140, 21.00893115100078745, 1.131784320476157264E-15 ) ) ;
#70808=EDGE_CURVE ( 'NONE', #89305, #74710, #66469, .T. ) ;
#70809=CARTESIAN_POINT ( 'NONE',  ( 7.084665262690076126, 17.02201867748817676, -10.88017736071110164 ) ) ;
#70811=CARTESIAN_POINT ( 'NONE',  ( -0.8801773607111009756, 58.06368534415484106, 1.068504757029289695E-15 ) ) ;
#70813=CARTESIAN_POINT ( 'NONE',  ( 10.00000000000000000, 49.75893115100078745, -9.846743663894594434 ) ) ;
#70814=CARTESIAN_POINT ( 'NONE',  ( 17.96484262340118221, 19.93868534415484106, 7.964842623401181321 ) ) ;
#70815=SURFACE_STYLE_USAGE ( .BOTH. , #71781 ) ;
#70816=CARTESIAN_POINT ( 'NONE',  ( 15.44008868035555260, 44.73035201082151247, 9.422509992056143702 ) ) ;
#70817=CARTESIAN_POINT ( 'NONE',  ( 12.91533473730993009, 16.60535201082150891, -10.88017736071109987 ) ) ;
#70819=CARTESIAN_POINT ( 'NONE',  ( 18.52753015748618282, 13.92559781766745175, -4.923371831947291888 ) ) ;
#70820=CARTESIAN_POINT ( 'NONE',  ( 2.791683348922240793, 41.63393115100078745, 7.208316651077764092 ) ) ;
#70822=DIRECTION ( 'NONE',  ( 0.000000000000000000, -1.000000000000000000, 0.000000000000000000 ) ) ;
#70823=CARTESIAN_POINT ( 'NONE',  ( -2.816281873526473856, -0.6680319967362464695, 3.434112377981055619 ) ) ;
#70825=CARTESIAN_POINT ( 'NONE',  ( -0.3689425029237881626, 22.42874883491397142, 10.36894250292379027 ) ) ;
#70827=CARTESIAN_POINT ( 'NONE',  ( 17.20831665107776587, 42.88393115100077324, 7.208316651077764980 ) ) ;
#70830=CARTESIAN_POINT ( 'NONE',  ( 15.44008868035555793, 6.397018677488171434, -9.422509992056140149 ) ) ;
#70831=CARTESIAN_POINT ( 'NONE',  ( 12.63842701281683922, 24.55059781766745175, -9.846743663894590881 ) ) ;
#70834=CARTESIAN_POINT ( 'NONE',  ( 15.44008868035555260, 39.73035201082150536, 9.422509992056143702 ) ) ;
#70835=CARTESIAN_POINT ( 'NONE',  ( 21.09922568453594849, 61.20696800326376064, 6.408140936763242479 ) ) ;
#70836=CARTESIAN_POINT ( 'NONE',  ( 20.88017736071110875, 15.77201867748817143, -2.915334737309920765 ) ) ;
#70837=CARTESIAN_POINT ( 'NONE',  ( 6.565887622018943937, 48.08196800326375353, -12.81628187352647608 ) ) ;
#70838=CARTESIAN_POINT ( 'NONE',  ( -1.099225684535947600, 13.70696800326375353, -6.408140936763238038 ) ) ;
#70839=CARTESIAN_POINT ( 'NONE',  ( 0.1532563361054100626, 20.80059781766744464, -2.638427012816831230 ) ) ;
#70842=EDGE_CURVE ( 'NONE', #31369, #17262, #23652, .T. ) ;
#70843=CARTESIAN_POINT ( 'NONE',  ( -4.164238869374098151, 56.59541550158063927, -3.795296366450310543 ) ) ;
#70844=CARTESIAN_POINT ( 'NONE',  ( -2.266590686148945544, 27.22041550158063572, 7.082119434687048631 ) ) ;
#70845=CARTESIAN_POINT ( 'NONE',  ( 7.084665262690076126, 24.10535201082150181, 10.88017736071109987 ) ) ;
#70846=CARTESIAN_POINT ( 'NONE',  ( -0.8801773607111008646, 53.27201867748816966, 2.915334737309923430 ) ) ;
#70847=( NAMED_UNIT ( * ) SI_UNIT ( $, .STERADIAN. ) SOLID_ANGLE_UNIT ( ) );
#70849=CARTESIAN_POINT ( 'NONE',  ( 0.5774900079438590739, 62.64701867748817676, -5.440088680355550821 ) ) ;
#70850=PLANE ( 'NONE',  #32186 ) ;
#70851=CARTESIAN_POINT ( 'NONE',  ( 1.472469842513823179, 15.59226448433411960, -4.923371831947296329 ) ) ;
#70852=CARTESIAN_POINT ( 'NONE',  ( 18.52753015748617571, 28.09226448433411960, 4.923371831947298993 ) ) ;
#70853=CARTESIAN_POINT ( 'NONE',  ( 7.361572987183169658, 49.96726448433410894, -9.846743663894592657 ) ) ;
#70854=CARTESIAN_POINT ( 'NONE',  ( 15.44008868035555260, 19.73035201082150536, 9.422509992056143702 ) ) ;
#70855=CARTESIAN_POINT ( 'NONE',  ( -1.099225684535947600, 33.70696800326375353, -6.408140936763238038 ) ) ;
#70857=CARTESIAN_POINT ( 'NONE',  ( 2.035157376598824452, 48.68868534415483396, 7.964842623401179544 ) ) ;
#70858=CARTESIAN_POINT ( 'NONE',  ( 17.20831665107776587, 34.13393115100078745, -7.208316651077762316 ) ) ;
#70859=CARTESIAN_POINT ( 'NONE',  ( 24.16423886937410614, 49.30374883491396787, 8.672049930838204340E-16 ) ) ;
#70860=CARTESIAN_POINT ( 'NONE',  ( 18.52753015748618282, 18.92559781766745175, -4.923371831947291888 ) ) ;
#70862=CARTESIAN_POINT ( 'NONE',  ( 1.472469842513823179, 55.59226448433412315, -4.923371831947296329 ) ) ;
#70863=CARTESIAN_POINT ( 'NONE',  ( 1.472469842513823179, 26.42559781766745175, 4.923371831947296329 ) ) ;
#70864=CARTESIAN_POINT ( 'NONE',  ( 20.36894250292379738, 14.92874883491396432, -10.36894250292379027 ) ) ;
#70865=CARTESIAN_POINT ( 'NONE',  ( 20.36894250292379738, 14.92874883491396432, -10.36894250292379027 ) ) ;
#70866=CARTESIAN_POINT ( 'NONE',  ( 1.472469842513823179, 36.42559781766745175, 4.923371831947296329 ) ) ;
#70867=CARTESIAN_POINT ( 'NONE',  ( 10.00000000000000000, 46.81368534415484106, -10.88017736071110342 ) ) ;
#70868=CARTESIAN_POINT ( 'NONE',  ( 12.91533473730993009, 21.60535201082150536, -10.88017736071109987 ) ) ;
#70870=CARTESIAN_POINT ( 'NONE',  ( 17.96484262340118221, 39.93868534415484106, 7.964842623401181321 ) ) ;
#70871=CARTESIAN_POINT ( 'NONE',  ( 7.084665262690076126, 27.02201867748817676, -10.88017736071110164 ) ) ;
#70872=ORIENTED_EDGE ( 'NONE', *, *, #57176, .T. ) ;
#70873=CARTESIAN_POINT ( 'NONE',  ( 22.81628187352647785, 36.62363466993041783, 6.195893100308588602E-16 ) ) ;
#70874=CARTESIAN_POINT ( 'NONE',  ( 17.96484262340118221, 39.93868534415484106, 7.964842623401181321 ) ) ;
#70876=CARTESIAN_POINT ( 'NONE',  ( 3.591859063236763294, 58.29030133659708923, -11.09922568453595026 ) ) ;
#70877=CARTESIAN_POINT ( 'NONE',  ( 19.42250999205614193, 65.14701867748817676, 5.440088680355555262 ) ) ;
#70879=CARTESIAN_POINT ( 'NONE',  ( 7.084665262690076126, 67.02201867748817676, -10.88017736071110164 ) ) ;
#70881=B_SPLINE_CURVE_WITH_KNOTS ( 'NONE', 3,
 ( #91118, #159, #21655, #8614 ),
 .UNSPECIFIED., .F., .F.,
 ( 4, 4 ),
 ( 9.320633277890009387E-17, 0.001060528352562005667 ),
 .UNSPECIFIED. ) ;
#70882=CARTESIAN_POINT ( 'NONE',  ( 2.917880565312950480, 65.97041550158063217, -12.26659068614894821 ) ) ;
#70883=CARTESIAN_POINT ( 'NONE',  ( 14.92337183194729988, 14.34226448433411782, -8.527530157486177487 ) ) ;
#70884=CARTESIAN_POINT ( 'NONE',  ( -2.266590686148945544, 2.220415501580634388, 7.082119434687048631 ) ) ;
#70885=CARTESIAN_POINT ( 'NONE',  ( 2.791683348922237240, 0.3839311510007847872, -7.208316651077763204 ) ) ;
#70886=CARTESIAN_POINT ( 'NONE',  ( 15.44008868035555793, 6.397018677488170546, -9.422509992056140149 ) ) ;
#70887=CARTESIAN_POINT ( 'NONE',  ( 5.076628168052703671, 41.84226448433411605, 8.527530157486179263 ) ) ;
#70889=CARTESIAN_POINT ( 'NONE',  ( 7.361572987183170547, 47.05059781766745175, 9.846743663894590881 ) ) ;
#70890=DIRECTION ( 'NONE',  ( 0.000000000000000000, 0.000000000000000000, 1.000000000000000000 ) ) ;
#70891=CARTESIAN_POINT ( 'NONE',  ( 4.559911319644449179, 42.23035201082151247, -9.422509992056141925 ) ) ;
#70892=CARTESIAN_POINT ( 'NONE',  ( 17.20831665107776587, 47.88393115100078745, 7.208316651077764980 ) ) ;
#70893=CARTESIAN_POINT ( 'NONE',  ( 13.43411237798105340, 30.58196800326374998, 12.81628187352647963 ) ) ;
#70895=CARTESIAN_POINT ( 'NONE',  ( 20.88017736071110519, 50.56368534415484106, 2.639326808657452039E-16 ) ) ;
#70896=CARTESIAN_POINT ( 'NONE',  ( -0.8801773607110991993, 7.855352010821506248, -2.915334737309923874 ) ) ;
#70898=CARTESIAN_POINT ( 'NONE',  ( -1.099225684535947600, 39.54030133659708923, 6.408140936763237150 ) ) ;
#70899=ORIENTED_EDGE ( 'NONE', *, *, #55426, .F. ) ;
#70900=CARTESIAN_POINT ( 'NONE',  ( 10.00000000000000178, 30.37363466993042138, 12.81628187352647608 ) ) ;
#70901=CARTESIAN_POINT ( 'NONE',  ( 15.44008868035555793, 31.39701867748817676, -9.422509992056140149 ) ) ;
#70904=B_SPLINE_CURVE_WITH_KNOTS ( 'NONE', 3,
 ( #35351, #88359, #45694, #37710, #19855, #38209 ),
 .UNSPECIFIED., .F., .F.,
 ( 4, 2, 4 ),
 ( 5.870982294470536311E-18, 0.0002626113303185901855, 0.0005252226606371745163 ),
 .UNSPECIFIED. ) ;
#70905=CARTESIAN_POINT ( 'NONE',  ( 10.00000000000000178, 2.258931151000784787, 9.846743663894594434 ) ) ;
#70906=CARTESIAN_POINT ( 'NONE',  ( 7.361572987183169658, 54.96726448433413026, -9.846743663894592657 ) ) ;
#70907=CARTESIAN_POINT ( 'NONE',  ( 19.84674366389459266, 13.30059781766745353, 2.638427012816836559 ) ) ;
#70908=CARTESIAN_POINT ( 'NONE',  ( 0.1532563361054083140, 36.00893115100078745, 1.131784320476157264E-15 ) ) ;
#70911=CARTESIAN_POINT ( 'NONE',  ( 1.472469842513823179, 30.59226448433411960, -4.923371831947296329 ) ) ;
#70913=CARTESIAN_POINT ( 'NONE',  ( 17.39651004071838969, 59.08210964143329846, -6.500000000000027534 ) ) ;
#70914=CARTESIAN_POINT ( 'NONE',  ( 7.361572987183170547, 32.05059781766745175, 9.846743663894590881 ) ) ;
#70917=CARTESIAN_POINT ( 'NONE',  ( 7.361572987183169658, 49.96726448433410894, -9.846743663894592657 ) ) ;
#70919=B_SPLINE_CURVE_WITH_KNOTS ( 'NONE', 3,
 ( #97563, #21550, #6534, #25974, #69510, #10477 ),
 .UNSPECIFIED., .F., .F.,
 ( 4, 2, 4 ),
 ( 0.000000000000000000, 0.0002565770811490999926, 0.0005131541622981999852 ),
 .UNSPECIFIED. ) ;
#70920=CARTESIAN_POINT ( 'NONE',  ( -0.8801773607111009756, 8.063685344154837509, 1.068504757029289695E-15 ) ) ;
#70922=CARTESIAN_POINT ( 'NONE',  ( 22.81628187352647785, 26.62363466993042138, 6.195893100308588602E-16 ) ) ;
#70924=CARTESIAN_POINT ( 'NONE',  ( 24.16423886937410614, 44.30374883491397497, 8.672049930838204340E-16 ) ) ;
#70925=CARTESIAN_POINT ( 'NONE',  ( 2.791683348922240793, 21.63393115100078745, 7.208316651077764092 ) ) ;
#70927=EDGE_CURVE ( 'NONE', #98371, #28728, #18853, .T. ) ;
#70928=CARTESIAN_POINT ( 'NONE',  ( 14.92337183194729988, 4.342264484334117824, -8.527530157486177487 ) ) ;
#70931=CARTESIAN_POINT ( 'NONE',  ( 17.08211943468705130, 43.47041550158063927, 12.26659068614894998 ) ) ;
#70932=CARTESIAN_POINT ( 'NONE',  ( 17.20831665107776587, 54.13393115100079456, -7.208316651077762316 ) ) ;
#70933=CARTESIAN_POINT ( 'NONE',  ( 4.559911319644449179, 12.23035201082150714, -9.422509992056141925 ) ) ;
#70934=CARTESIAN_POINT ( 'NONE',  ( -4.164238869374099039, 21.80374883491396787, 8.674139862899312516E-16 ) ) ;
#70935=CARTESIAN_POINT ( 'NONE',  ( 20.36894250292379738, 39.92874883491396787, -10.36894250292379027 ) ) ;
#70936=CYLINDRICAL_SURFACE ( 'NONE', #10045, 2.999999999999999112 ) ;
#70937=PRODUCT_DEFINITION ( 'UNKNOWN', '', #77461, #88487 ) ;
#70939=CARTESIAN_POINT ( 'NONE',  ( 7.361572987183169658, 49.96726448433410894, -9.846743663894592657 ) ) ;
#70941=CARTESIAN_POINT ( 'NONE',  ( 12.91533473730993009, 36.60535201082151247, -10.88017736071109987 ) ) ;
#70943=CARTESIAN_POINT ( 'NONE',  ( 1.816707512666846824, 65.10290668512024581, -6.499999999999958256 ) ) ;
#70944=CARTESIAN_POINT ( 'NONE',  ( 19.84674366389459266, 38.30059781766745175, 2.638427012816836559 ) ) ;
#70945=CARTESIAN_POINT ( 'NONE',  ( 0.6178305044545818747, 63.49863466993043204, -9.382169495545419124 ) ) ;
#70947=CARTESIAN_POINT ( 'NONE',  ( 10.00000000000000178, 47.25893115100078745, 9.846743663894594434 ) ) ;
#70948=CARTESIAN_POINT ( 'NONE',  ( 14.92337183194729988, 64.34226448433412315, -8.527530157486177487 ) ) ;
#70950=CARTESIAN_POINT ( 'NONE',  ( 22.26659068614894466, 13.88708216824730179, 7.082119434687054849 ) ) ;
#70953=CARTESIAN_POINT ( 'NONE',  ( -0.8801773607110991993, 2.855352010821504471, -2.915334737309923874 ) ) ;
#70954=CARTESIAN_POINT ( 'NONE',  ( 10.00000000000000000, 22.87363466993042138, -12.81628187352647608 ) ) ;
#70956=CARTESIAN_POINT ( 'NONE',  ( 2.035157376598824452, 63.68868534415484106, 7.964842623401179544 ) ) ;
#70960=CARTESIAN_POINT ( 'NONE',  ( 10.00000000000000178, 9.313685344154839285, 10.88017736071110342 ) ) ;
#70962=CARTESIAN_POINT ( 'NONE',  ( 5.500000000000000000, 60.50000000000000000, -6.000000000000000000 ) ) ;
#70963=CARTESIAN_POINT ( 'NONE',  ( 7.084665262690076126, 29.10535201082150181, 10.88017736071109987 ) ) ;
#70964=CARTESIAN_POINT ( 'NONE',  ( 10.00000000000000178, 39.31368534415484106, 10.88017736071110342 ) ) ;
#70965=CARTESIAN_POINT ( 'NONE',  ( 16.40814093676324603, 2.456968003263753531, -11.09922568453594671 ) ) ;
#70967=CARTESIAN_POINT ( 'NONE',  ( 13.43411237798106583, 57.66530133659708923, -12.81628187352647252 ) ) ;
#70968=CARTESIAN_POINT ( 'NONE',  ( 14.92337183194729633, 7.675597817667451750, 8.527530157486181039 ) ) ;
#70969=ORIENTED_EDGE ( 'NONE', *, *, #19427, .F. ) ;
#70970=CARTESIAN_POINT ( 'NONE',  ( 20.88017736071110519, 25.56368534415483751, 2.639326808657452039E-16 ) ) ;
#70971=CARTESIAN_POINT ( 'NONE',  ( 13.43411237798106583, 27.66530133659708568, -12.81628187352647252 ) ) ;
#70973=CARTESIAN_POINT ( 'NONE',  ( -1.099225684535947600, -1.293031996736246469, -6.408140936763238038 ) ) ;
#70974=CARTESIAN_POINT ( 'NONE',  ( 19.42250999205614548, 45.98035201082150536, -5.440088680355545492 ) ) ;
#70975=CARTESIAN_POINT ( 'NONE',  ( 14.92337183194729988, 9.342264484334119601, -8.527530157486177487 ) ) ;
#70976=CARTESIAN_POINT ( 'NONE',  ( 13.43411237798105340, 40.58196800326375353, 12.81628187352647963 ) ) ;
#70977=CARTESIAN_POINT ( 'NONE',  ( 2.035157376598824452, 63.68868534415484106, 7.964842623401179544 ) ) ;
#70979=CARTESIAN_POINT ( 'NONE',  ( 18.17829156368510723, 54.16792564121899289, 6.499999999999959144 ) ) ;
#70980=CARTESIAN_POINT ( 'NONE',  ( 6.565887622018943937, 60.16530133659707502, 12.81628187352647430 ) ) ;
#70983=CARTESIAN_POINT ( 'NONE',  ( 15.44008868035555260, 9.730352010821505360, 9.422509992056143702 ) ) ;
#70984=CARTESIAN_POINT ( 'NONE',  ( -1.099225684535947600, 48.70696800326375353, -6.408140936763238038 ) ) ;
#70985=CARTESIAN_POINT ( 'NONE',  ( 10.00000000000000000, 15.55374883491396787, -14.16423886937410082 ) ) ;
#70986=CARTESIAN_POINT ( 'NONE',  ( 0.1532563361054082862, 21.21726448433412315, 2.638427012816831674 ) ) ;
#70987=CARTESIAN_POINT ( 'NONE',  ( 4.559911319644449179, 3.897018677488170990, 9.422509992056141925 ) ) ;
#70988=CARTESIAN_POINT ( 'NONE',  ( 5.076628168052704559, 20.17559781766745175, -8.527530157486179263 ) ) ;
#70989=CARTESIAN_POINT ( 'NONE',  ( -0.3689425029237898834, 51.17874883491397497, -10.36894250292378850 ) ) ;
#70991=CARTESIAN_POINT ( 'NONE',  ( 4.559911319644449179, 23.89701867748817321, 9.422509992056141925 ) ) ;
#70995=CARTESIAN_POINT ( 'NONE',  ( 2.035157376598824452, 13.68868534415483751, 7.964842623401179544 ) ) ;
#70996=CARTESIAN_POINT ( 'NONE',  ( 19.84674366389459266, 53.71726448433411605, -2.638427012816827677 ) ) ;
#70997=CARTESIAN_POINT ( 'NONE',  ( 21.09922568453595559, 52.04030133659708923, -6.408140936763230044 ) ) ;
#70998=CARTESIAN_POINT ( 'NONE',  ( -0.2418659066527782397, 5.116331881023271855, 6.114288769123032985 ) ) ;
#71001=CARTESIAN_POINT ( 'NONE',  ( 24.16423886937410614, 19.51208216824729647, -3.795296366450302550 ) ) ;
#71002=CARTESIAN_POINT ( 'NONE',  ( 20.88017736071110164, 40.35535201082150536, 2.915334737309930979 ) ) ;
#71003=CARTESIAN_POINT ( 'NONE',  ( 2.035157376598822676, 22.43868534415483396, -7.964842623401177768 ) ) ;
#71004=CARTESIAN_POINT ( 'NONE',  ( 0.1532563361054100626, 55.80059781766745175, -2.638427012816831230 ) ) ;
#71005=COLOUR_RGB ( '', 0.31764706, 0.68627451, 0.89019608) ;
#71006=DIRECTION ( 'NONE',  ( -0.000000000000000000, 0.000000000000000000, 1.000000000000000000 ) ) ;
#71007=CARTESIAN_POINT ( 'NONE',  ( 19.84674366389459621, 38.50893115100078745, 7.409399052514197653E-17 ) ) ;
#71009=CARTESIAN_POINT ( 'NONE',  ( 5.076628168052704559, 5.175597817667451750, -8.527530157486179263 ) ) ;
#71011=VERTEX_POINT ( 'NONE', #57457 ) ;
#71013=CARTESIAN_POINT ( 'NONE',  ( 12.63842701281683034, 17.46726448433411250, 9.846743663894596210 ) ) ;
#71014=CARTESIAN_POINT ( 'NONE',  ( 10.00000000000000178, 5.373634669930420493, 12.81628187352647608 ) ) ;
#71015=CARTESIAN_POINT ( 'NONE',  ( 20.88017736071110519, 45.56368534415484106, 2.639326808657452039E-16 ) ) ;
#71016=CARTESIAN_POINT ( 'NONE',  ( 4.559911319644449179, 2.230352010821504471, -9.422509992056141925 ) ) ;
#71017=CARTESIAN_POINT ( 'NONE',  ( -2.816281873526473856, 44.12363466993042493, 9.499525473075851096E-16 ) ) ;
#71018=CARTESIAN_POINT ( 'NONE',  ( 13.79529636645030344, 33.26208216824730357, 14.16423886937410614 ) ) ;
#71019=EDGE_CURVE ( 'NONE', #76182, #80952, #41984, .T. ) ;
#71021=CARTESIAN_POINT ( 'NONE',  ( -2.816281873526473856, 54.33196800326376064, 3.434112377981055619 ) ) ;
#71023=( BOUNDED_CURVE ( )  B_SPLINE_CURVE ( 2, ( #4898, #19886, #89369, #72879, #4414, #50378, #28376, #80397, #43855 ),
 .UNSPECIFIED., .F., .F. ) 
 B_SPLINE_CURVE_WITH_KNOTS ( ( 3, 2, 2, 2, 3 ),
 ( 0.2248575172211797479, 0.2261904761904761918, 0.2321428571428571508, 0.2380952380952380820, 0.2394281970645344149 ),
 .UNSPECIFIED. ) 
 CURVE ( )  GEOMETRIC_REPRESENTATION_ITEM ( )  RATIONAL_B_SPLINE_CURVE ( ( 0.9881565478350731180, 0.9923695281211489805, 1.000000000000000000, 0.9659258262890683122, 1.000000000000000000, 0.9659258262890683122, 1.000000000000000000, 0.9923695281211495356, 0.9881565478350737841 ) ) 
 REPRESENTATION_ITEM ( '' )  );
#71024=CARTESIAN_POINT ( 'NONE',  ( 0.1532563361054082862, 61.21726448433412315, 2.638427012816831674 ) ) ;
#71025=CARTESIAN_POINT ( 'NONE',  ( 0.5774900079438590739, 22.64701867748817321, -5.440088680355550821 ) ) ;
#71027=CARTESIAN_POINT ( 'NONE',  ( 7.084665262690076126, 69.10535201082151957, 10.88017736071109987 ) ) ;
#71028=DIRECTION ( 'NONE',  ( 0.000000000000000000, 0.000000000000000000, 1.000000000000000000 ) ) ;
#71029=CARTESIAN_POINT ( 'NONE',  ( 19.84674366389459266, 3.717264484334118713, -2.638427012816827677 ) ) ;
#71030=CARTESIAN_POINT ( 'NONE',  ( 7.361572987183170547, 2.050597817667451750, 9.846743663894590881 ) ) ;
#71032=COLOUR_RGB ( '', 0.09019608, 0.27058824, 0.51372549) ;
#71033=CARTESIAN_POINT ( 'NONE',  ( 17.96484262340118221, 59.93868534415484106, 7.964842623401181321 ) ) ;
#71035=CARTESIAN_POINT ( 'NONE',  ( 2.035157376598824452, 68.68868534415484817, 7.964842623401179544 ) ) ;
#71036=CARTESIAN_POINT ( 'NONE',  ( 17.20831665107776587, 9.133931151000787452, -7.208316651077762316 ) ) ;
#71040=CARTESIAN_POINT ( 'NONE',  ( 0.1532563361054082862, 51.21726448433412315, 2.638427012816831674 ) ) ;
#71041=ORIENTED_EDGE ( 'NONE', *, *, #73190, .T. ) ;
#71042=VERTEX_POINT ( 'NONE', #88943 ) ;
#71044=CARTESIAN_POINT ( 'NONE',  ( 2.917880565312950480, 5.970415501580634832, -12.26659068614894821 ) ) ;
#71045=CARTESIAN_POINT ( 'NONE',  ( -2.816281873526473856, 54.33196800326376064, 3.434112377981055619 ) ) ;
#71046=CARTESIAN_POINT ( 'NONE',  ( 2.917880565312950480, 5.970415501580634832, -12.26659068614894821 ) ) ;
#71047=CARTESIAN_POINT ( 'NONE',  ( 24.16423886937410614, 39.30374883491396787, 8.672049930838204340E-16 ) ) ;
#71048=LINE ( 'NONE', #3538, #29022 ) ;
#71049=CARTESIAN_POINT ( 'NONE',  ( 20.88017736071110875, 25.77201867748816966, -2.915334737309920765 ) ) ;
#71050=DIRECTION ( 'NONE',  ( 1.000000000000000000, 0.000000000000000000, -0.000000000000000000 ) ) ;
#71052=CARTESIAN_POINT ( 'NONE',  ( 17.20831665107776587, 2.883931151000785231, 7.208316651077764980 ) ) ;
#71053=CARTESIAN_POINT ( 'NONE',  ( 14.92337183194729633, 12.67559781766745353, 8.527530157486181039 ) ) ;
#71054=CARTESIAN_POINT ( 'NONE',  ( 10.00000000000000000, 32.87363466993042493, -12.81628187352647608 ) ) ;
#71055=CARTESIAN_POINT ( 'NONE',  ( 5.076628168052703671, 41.84226448433411605, 8.527530157486179263 ) ) ;
#71057=CARTESIAN_POINT ( 'NONE',  ( 13.43411237798105340, 30.58196800326374998, 12.81628187352647963 ) ) ;
#71058=CARTESIAN_POINT ( 'NONE',  ( 20.03932841506541251, 40.62161441960500952, -6.397827110479001433 ) ) ;
#71059=CARTESIAN_POINT ( 'NONE',  ( 10.00000000000000178, 32.25893115100078745, 9.846743663894594434 ) ) ;
#71060=CARTESIAN_POINT ( 'NONE',  ( 24.16423886937410614, 19.51208216824729647, -3.795296366450302550 ) ) ;
#71061=ORIENTED_EDGE ( 'NONE', *, *, #9519, .T. ) ;
#71062=CARTESIAN_POINT ( 'NONE',  ( 10.00000000000000000, 31.81368534415483751, -10.88017736071110342 ) ) ;
#71063=CARTESIAN_POINT ( 'NONE',  ( 2.917880565312950480, 25.97041550158063572, -12.26659068614894821 ) ) ;
#71064=CARTESIAN_POINT ( 'NONE',  ( 19.84674366389459266, 48.30059781766745175, 2.638427012816836559 ) ) ;
#71065=CARTESIAN_POINT ( 'NONE',  ( 17.20831665107776587, 17.88393115100078745, 7.208316651077764980 ) ) ;
#71066=CARTESIAN_POINT ( 'NONE',  ( -1.099225684535947600, 54.54030133659708923, 6.408140936763237150 ) ) ;
#71067=CYLINDRICAL_SURFACE ( 'NONE', #95948, 11.92686044187656513 ) ;
#71068=CARTESIAN_POINT ( 'NONE',  ( 7.084665262690076126, 34.10535201082151247, 10.88017736071109987 ) ) ;
#71069=CARTESIAN_POINT ( 'NONE',  ( 20.15039907845753220, 22.62777174578612716, -6.262539305110077947 ) ) ;
#71071=CARTESIAN_POINT ( 'NONE',  ( -2.816281873526473856, 24.12363466993042138, 9.499525473075851096E-16 ) ) ;
#71072=CARTESIAN_POINT ( 'NONE',  ( 17.20831665107776587, 42.88393115100077324, 7.208316651077764980 ) ) ;
#71074=CARTESIAN_POINT ( 'NONE',  ( 0.6178305044545818747, 43.49863466993042493, -9.382169495545419124 ) ) ;
#71075=CARTESIAN_POINT ( 'NONE',  ( 19.42250999205614193, 50.14701867748817676, 5.440088680355555262 ) ) ;
#71080=CARTESIAN_POINT ( 'NONE',  ( 0.5774900079438590739, 52.64701867748817676, -5.440088680355550821 ) ) ;
#71081=CARTESIAN_POINT ( 'NONE',  ( 7.084665262690076126, 52.02201867748816255, -10.88017736071110164 ) ) ;
#71085=CARTESIAN_POINT ( 'NONE',  ( 0.5774900079438607392, 3.480352010821504916, 5.440088680355550821 ) ) ;
#71086=CARTESIAN_POINT ( 'NONE',  ( 3.591859063236761518, -0.04303199673624671928, 11.09922568453594849 ) ) ;
#71087=CARTESIAN_POINT ( 'NONE',  ( 12.91533473730993009, 26.60535201082150536, -10.88017736071109987 ) ) ;
#71089=CARTESIAN_POINT ( 'NONE',  ( -2.816281873526473856, 29.33196800326376064, 3.434112377981055619 ) ) ;
#71090=ORIENTED_EDGE ( 'NONE', *, *, #90955, .F. ) ;
#71091=CARTESIAN_POINT ( 'NONE',  ( 20.88017736071110519, 50.56368534415484106, 2.639326808657452039E-16 ) ) ;
#71092=CARTESIAN_POINT ( 'NONE',  ( 2.791683348922240793, 36.63393115100078035, 7.208316651077764092 ) ) ;
#71093=CARTESIAN_POINT ( 'NONE',  ( -1.099225684535947600, 3.706968003263753531, -6.408140936763238038 ) ) ;
#71095=CARTESIAN_POINT ( 'NONE',  ( 20.88017736071110164, 30.35535201082151247, 2.915334737309930979 ) ) ;
#71096=CARTESIAN_POINT ( 'NONE',  ( 15.44008868035555260, 39.73035201082150536, 9.422509992056143702 ) ) ;
#71097=CARTESIAN_POINT ( 'NONE',  ( 24.16423886937410614, 54.30374883491396787, 8.672049930838204340E-16 ) ) ;
#71098=CARTESIAN_POINT ( 'NONE',  ( 2.791683348922240793, 36.63393115100078035, 7.208316651077764092 ) ) ;
#71099=CARTESIAN_POINT ( 'NONE',  ( 2.035157376598822676, 62.43868534415483396, -7.964842623401177768 ) ) ;
#71101=CARTESIAN_POINT ( 'NONE',  ( 24.16423886937409904, 14.09541550158063217, 3.795296366450317205 ) ) ;
#71105=B_SPLINE_CURVE_WITH_KNOTS ( 'NONE', 3,
 ( #42257, #94757, #79756, #48756, #35224, #41772 ),
 .UNSPECIFIED., .F., .F.,
 ( 4, 2, 4 ),
 ( 5.553824967135426632E-18, 0.0002605067024380912301, 0.0005210134048761769308 ),
 .UNSPECIFIED. ) ;
#71107=CARTESIAN_POINT ( 'NONE',  ( 17.08211943468705840, 55.13708216824731068, -12.26659068614894466 ) ) ;
#71108=CARTESIAN_POINT ( 'NONE',  ( 17.08211943468705130, 33.47041550158063927, 12.26659068614894998 ) ) ;
#71109=CARTESIAN_POINT ( 'NONE',  ( 19.84674366389459266, 23.30059781766745530, 2.638427012816836559 ) ) ;
#71111=CARTESIAN_POINT ( 'NONE',  ( 3.591859063236763294, 13.29030133659708746, -11.09922568453595026 ) ) ;
#71112=CARTESIAN_POINT ( 'NONE',  ( 0.1532563361054082862, 61.21726448433412315, 2.638427012816831674 ) ) ;
#71113=DIRECTION ( 'NONE',  ( 0.000000000000000000, 0.000000000000000000, -1.000000000000000000 ) ) ;
#71114=CARTESIAN_POINT ( 'NONE',  ( 15.44008868035555260, 59.73035201082151247, 9.422509992056143702 ) ) ;
#71115=CARTESIAN_POINT ( 'NONE',  ( 3.591859063236761518, 29.95696800326375708, 11.09922568453594849 ) ) ;
#71116=CARTESIAN_POINT ( 'NONE',  ( 17.08211943468705130, 43.47041550158063927, 12.26659068614894998 ) ) ;
#71117=CARTESIAN_POINT ( 'NONE',  ( 19.42250999205614548, 25.98035201082150891, -5.440088680355545492 ) ) ;
#71119=FILL_AREA_STYLE ('',( #41122 ) ) ;
#71121=CARTESIAN_POINT ( 'NONE',  ( 10.00000000000000178, 7.258931151000785675, 9.846743663894594434 ) ) ;
#71122=ORIENTED_EDGE ( 'NONE', *, *, #17117, .T. ) ;
#71125=DIRECTION ( 'NONE',  ( 0.9970872288863208421, 0.07626964003977952655, 0.000000000000000000 ) ) ;
#71127=CARTESIAN_POINT ( 'NONE',  ( 19.42250999205614193, 10.14701867748816966, 5.440088680355555262 ) ) ;
#71128=CARTESIAN_POINT ( 'NONE',  ( 20.88017736071110875, 5.772018677488170546, -2.915334737309920765 ) ) ;
#71129=CARTESIAN_POINT ( 'NONE',  ( 1.472469842513823179, 36.42559781766745175, 4.923371831947296329 ) ) ;
#71130=CARTESIAN_POINT ( 'NONE',  ( 13.43411237798105340, 10.58196800326375353, 12.81628187352647963 ) ) ;
#71132=ADVANCED_FACE ( 'NONE', ( #28437 ), #88449, .T. ) ;
#71134=CARTESIAN_POINT ( 'NONE',  ( 22.81628187352648496, 16.83196800326374998, -3.434112377981050290 ) ) ;
#71136=CARTESIAN_POINT ( 'NONE',  ( 13.79529636645031943, 40.34541550158063217, -14.16423886937409904 ) ) ;
#71138=CARTESIAN_POINT ( 'NONE',  ( 24.16423886937409904, 54.09541550158063217, 3.795296366450317205 ) ) ;
#71140=CARTESIAN_POINT ( 'NONE',  ( 20.88017736071110519, 30.56368534415484106, 2.639326808657452039E-16 ) ) ;
#71141=CARTESIAN_POINT ( 'NONE',  ( 20.88017736071110519, 40.56368534415484106, 2.639326808657452039E-16 ) ) ;
#71142=CARTESIAN_POINT ( 'NONE',  ( 10.00000000000000178, 39.31368534415484106, 10.88017736071110342 ) ) ;
#71143=CARTESIAN_POINT ( 'NONE',  ( 12.91533473730992121, 59.52201867748816966, 10.88017736071110164 ) ) ;
#71144=CARTESIAN_POINT ( 'NONE',  ( 20.88017736071110164, 30.35535201082151247, 2.915334737309930979 ) ) ;
#71149=CARTESIAN_POINT ( 'NONE',  ( 17.20831665107776587, 12.88393115100078390, 7.208316651077764980 ) ) ;
#71153=CARTESIAN_POINT ( 'NONE',  ( 12.63842701281683034, 42.46726448433412315, 9.846743663894596210 ) ) ;
#71159=FACE_OUTER_BOUND ( 'NONE', #85003, .T. ) ;
#71160=CARTESIAN_POINT ( 'NONE',  ( 0.1532563361054083140, 61.00893115100078745, 1.131784320476157264E-15 ) ) ;
#71161=CARTESIAN_POINT ( 'NONE',  ( 17.08211943468705130, 48.47041550158063927, 12.26659068614894998 ) ) ;
#71165=CARTESIAN_POINT ( 'NONE',  ( 12.63842701281683922, 24.55059781766745175, -9.846743663894590881 ) ) ;
#71167=MECHANICAL_DESIGN_GEOMETRIC_PRESENTATION_REPRESENTATION('',(#66296),#12060);
#71168=CARTESIAN_POINT ( 'NONE',  ( 19.84674366389459621, 63.50893115100078745, 7.409399052514197653E-17 ) ) ;
#71169=CARTESIAN_POINT ( 'NONE',  ( 7.361572987183169658, -0.03273551566588185635, -9.846743663894592657 ) ) ;
#71171=CARTESIAN_POINT ( 'NONE',  ( 18.52753015748617571, 43.09226448433412315, 4.923371831947298993 ) ) ;
#71172=PLANE ( 'NONE',  #58444 ) ;
#71174=ORIENTED_EDGE ( 'NONE', *, *, #93367, .F. ) ;
#71175=CARTESIAN_POINT ( 'NONE',  ( 13.79529636645030344, 63.26208216824730357, 14.16423886937410614 ) ) ;
#71177=CARTESIAN_POINT ( 'NONE',  ( -0.8801773607111008646, 43.27201867748817676, 2.915334737309923430 ) ) ;
#71178=CARTESIAN_POINT ( 'NONE',  ( 13.43411237798106583, 7.665301336597086568, -12.81628187352647252 ) ) ;
#71180=CARTESIAN_POINT ( 'NONE',  ( -0.1503990784575247319, 62.22266099184918176, -6.262539305110083276 ) ) ;
#71183=CARTESIAN_POINT ( 'NONE',  ( -0.1049300847420627930, 62.21697413083880690, -6.336235997365760042 ) ) ;
#71184=CARTESIAN_POINT ( 'NONE',  ( 2.791683348922237240, 55.38393115100078745, -7.208316651077763204 ) ) ;
#71185=CARTESIAN_POINT ( 'NONE',  ( 5.076628168052704559, 0.1755978176674514724, -8.527530157486179263 ) ) ;
#71187=CARTESIAN_POINT ( 'NONE',  ( 10.00000000000000178, 5.373634669930420493, 12.81628187352647608 ) ) ;
#71188=CARTESIAN_POINT ( 'NONE',  ( 19.42250999205614193, 10.14701867748816966, 5.440088680355555262 ) ) ;
#71191=CARTESIAN_POINT ( 'NONE',  ( -4.164238869374098151, 31.59541550158063927, -3.795296366450310543 ) ) ;
#71192=ADVANCED_FACE ( 'NONE', ( #58430 ), #44907, .T. ) ;
#71193=CARTESIAN_POINT ( 'NONE',  ( 2.917880565312948704, 32.63708216824730357, 12.26659068614894643 ) ) ;
#71194=CARTESIAN_POINT ( 'NONE',  ( -2.266590686148945544, 61.38708216824730357, -7.082119434687050408 ) ) ;
#71195=CARTESIAN_POINT ( 'NONE',  ( 19.84674366389459266, 33.30059781766744464, 2.638427012816836559 ) ) ;
#71196=CARTESIAN_POINT ( 'NONE',  ( 13.43411237798106583, 42.66530133659707502, -12.81628187352647252 ) ) ;
#71197=CARTESIAN_POINT ( 'NONE',  ( 0.5774900079438590739, 17.64701867748817321, -5.440088680355550821 ) ) ;
#71200=CARTESIAN_POINT ( 'NONE',  ( 18.52753015748618282, 38.92559781766745175, -4.923371831947291888 ) ) ;
#71201=CARTESIAN_POINT ( 'NONE',  ( 19.42250999205614193, 40.14701867748817676, 5.440088680355555262 ) ) ;
#71202=CARTESIAN_POINT ( 'NONE',  ( 3.591859063236763294, 3.290301336597087012, -11.09922568453595026 ) ) ;
#71203=CARTESIAN_POINT ( 'NONE',  ( 2.917880565312948704, 27.63708216824730357, 12.26659068614894643 ) ) ;
#71207=CARTESIAN_POINT ( 'NONE',  ( 1.472469842513823179, 25.59226448433412315, -4.923371831947296329 ) ) ;
#71208=CARTESIAN_POINT ( 'NONE',  ( 3.591859063236761518, 49.95696800326375353, 11.09922568453594849 ) ) ;
#71209=CARTESIAN_POINT ( 'NONE',  ( 12.63842701281683922, 54.55059781766745175, -9.846743663894590881 ) ) ;
#71211=CARTESIAN_POINT ( 'NONE',  ( 1.274849032794131976, 13.57228050351029403, 6.499999999999760192 ) ) ;
#71213=CARTESIAN_POINT ( 'NONE',  ( -4.164238869374098151, 66.59541550158060375, -3.795296366450310543 ) ) ;
#71214=CARTESIAN_POINT ( 'NONE',  ( -0.3689425029237898834, 16.17874883491396076, -10.36894250292378850 ) ) ;
#71215=CARTESIAN_POINT ( 'NONE',  ( 0.5774900079438607392, 68.48035201082150536, 5.440088680355550821 ) ) ;
#71216=CARTESIAN_POINT ( 'NONE',  ( 12.63842701281683034, 47.46726448433412315, 9.846743663894596210 ) ) ;
#71217=CARTESIAN_POINT ( 'NONE',  ( 17.96484262340118221, 26.18868534415483396, -7.964842623401177768 ) ) ;
#71220=DIRECTION ( 'NONE',  ( 0.000000000000000000, -1.000000000000000000, 0.000000000000000000 ) ) ;
#71221=ORIENTED_EDGE ( 'NONE', *, *, #88945, .T. ) ;
#71222=ORIENTED_EDGE ( 'NONE', *, *, #45945, .T. ) ;
#71223=DIRECTION ( 'NONE',  ( 0.8320502943378436100, -0.5547001962252291474, 0.000000000000000000 ) ) ;
#71224=CARTESIAN_POINT ( 'NONE',  ( 24.16423886937410614, 14.51208216824730179, -3.795296366450302550 ) ) ;
#71226=CARTESIAN_POINT ( 'NONE',  ( 22.26659068614894466, 43.88708216824729647, 7.082119434687054849 ) ) ;
#71227=CARTESIAN_POINT ( 'NONE',  ( 19.84674366389459621, 53.50893115100078745, 7.409399052514197653E-17 ) ) ;
#71228=CARTESIAN_POINT ( 'NONE',  ( 1.472469842513823179, 26.42559781766745175, 4.923371831947296329 ) ) ;
#71230=CARTESIAN_POINT ( 'NONE',  ( 15.44008868035555260, 19.73035201082150536, 9.422509992056143702 ) ) ;
#71231=CARTESIAN_POINT ( 'NONE',  ( 12.63842701281683922, 64.55059781766745175, -9.846743663894590881 ) ) ;
#71233=CARTESIAN_POINT ( 'NONE',  ( 17.08211943468705840, 35.13708216824730357, -12.26659068614894466 ) ) ;
#71234=CARTESIAN_POINT ( 'NONE',  ( 0.5774900079438590739, 7.647018677488171434, -5.440088680355550821 ) ) ;
#71235=CARTESIAN_POINT ( 'NONE',  ( 2.791683348922240793, 66.63393115100079456, 7.208316651077764092 ) ) ;
#71238=CARTESIAN_POINT ( 'NONE',  ( 7.084665262690076126, 62.02201867748816966, -10.88017736071110164 ) ) ;
#71239=CARTESIAN_POINT ( 'NONE',  ( 14.92337183194729988, 9.342264484334119601, -8.527530157486177487 ) ) ;
#71240=CARTESIAN_POINT ( 'NONE',  ( 20.00000000000000355, 70.00000000000000000, -4.500000000000002665 ) ) ;
#71243=ORIENTED_EDGE ( 'NONE', *, *, #89428, .F. ) ;
#71244=CARTESIAN_POINT ( 'NONE',  ( 0.1532563361054100626, 25.80059781766744820, -2.638427012816831230 ) ) ;
#71245=ORIENTED_EDGE ( 'NONE', *, *, #83698, .F. ) ;
#71247=CARTESIAN_POINT ( 'NONE',  ( -2.266590686148945544, 32.22041550158063927, 7.082119434687048631 ) ) ;
#71248=CARTESIAN_POINT ( 'NONE',  ( 17.20831665107776587, 29.13393115100078390, -7.208316651077762316 ) ) ;
#71249=CARTESIAN_POINT ( 'NONE',  ( 10.00000000000000178, 44.31368534415484106, 10.88017736071110342 ) ) ;
#71252=ORIENTED_EDGE ( 'NONE', *, *, #16957, .F. ) ;
#71253=CARTESIAN_POINT ( 'NONE',  ( -0.8801773607111008646, 38.27201867748816255, 2.915334737309923430 ) ) ;
#71257=CARTESIAN_POINT ( 'NONE',  ( -2.266590686148945544, 11.38708216824730179, -7.082119434687050408 ) ) ;
#71260=CARTESIAN_POINT ( 'NONE',  ( 19.38216949554541557, 37.24863466993041783, -9.382169495545420901 ) ) ;
#71261=CARTESIAN_POINT ( 'NONE',  ( 2.917880565312950480, 0.9704155015806342766, -12.26659068614894821 ) ) ;
#71262=CARTESIAN_POINT ( 'NONE',  ( 14.92337183194729633, 17.67559781766745175, 8.527530157486181039 ) ) ;
#71264=CARTESIAN_POINT ( 'NONE',  ( 7.361572987183169658, 29.96726448433411960, -9.846743663894592657 ) ) ;
#71266=CARTESIAN_POINT ( 'NONE',  ( 20.88017736071110164, 60.35535201082151957, 2.915334737309930979 ) ) ;
#71269=CARTESIAN_POINT ( 'NONE',  ( 20.32896413005680714, 65.57879003517447813, -5.963430220938276349 ) ) ;
#71272=CARTESIAN_POINT ( 'NONE',  ( 2.603489959281581889, 20.43575266056827999, -6.499999999999995559 ) ) ;
#71275=CARTESIAN_POINT ( 'NONE',  ( 7.361572987183170547, 7.050597817667451750, 9.846743663894590881 ) ) ;
#71277=DIRECTION ( 'NONE',  ( 0.5547001962252290364, 0.8320502943378437211, 0.000000000000000000 ) ) ;
#71278=CARTESIAN_POINT ( 'NONE',  ( 0.1532563361054083140, 51.00893115100078745, 1.131784320476157264E-15 ) ) ;
#71279=CARTESIAN_POINT ( 'NONE',  ( 20.88017736071110519, 35.56368534415484106, 2.639326808657452039E-16 ) ) ;
#71280=CARTESIAN_POINT ( 'NONE',  ( -0.3689425029237898834, 6.178748834913968757, -10.36894250292378850 ) ) ;
#71281=CARTESIAN_POINT ( 'NONE',  ( 5.076628168052704559, 30.17559781766745175, -8.527530157486179263 ) ) ;
#71282=CARTESIAN_POINT ( 'NONE',  ( -1.099225684535947600, 33.70696800326375353, -6.408140936763238038 ) ) ;
#71284=CARTESIAN_POINT ( 'NONE',  ( 12.91533473730992121, 49.52201867748817676, 10.88017736071110164 ) ) ;
#71285=CARTESIAN_POINT ( 'NONE',  ( 0.6178305044545818747, 3.498634669930420049, -9.382169495545419124 ) ) ;
#71287=CARTESIAN_POINT ( 'NONE',  ( 5.076628168052704559, 25.17559781766745175, -8.527530157486179263 ) ) ;
#71288=CARTESIAN_POINT ( 'NONE',  ( -0.8801773607111008646, 33.27201867748817676, 2.915334737309923430 ) ) ;
#71289=CARTESIAN_POINT ( 'NONE',  ( -2.816281873526471635, 33.91530133659708213, -3.434112377981056508 ) ) ;
#71291=CARTESIAN_POINT ( 'NONE',  ( 10.00000000000000000, 24.75893115100078745, -9.846743663894594434 ) ) ;
#71294=CARTESIAN_POINT ( 'NONE',  ( 18.29284471827481795, 45.40189080397284016, -6.499999999999946709 ) ) ;
#71297=CARTESIAN_POINT ( 'NONE',  ( 20.88017736071110164, 20.35535201082150891, 2.915334737309930979 ) ) ;
#71299=CARTESIAN_POINT ( 'NONE',  ( 20.88017736071110875, 55.77201867748816966, -2.915334737309920765 ) ) ;
#71300=CARTESIAN_POINT ( 'NONE',  ( 19.84674366389459266, 43.30059781766744464, 2.638427012816836559 ) ) ;
#71301=CARTESIAN_POINT ( 'NONE',  ( 2.035157376598822676, 27.43868534415483396, -7.964842623401177768 ) ) ;
#71303=CARTESIAN_POINT ( 'NONE',  ( -0.8801773607110991993, 52.85535201082151247, -2.915334737309923874 ) ) ;
#71304=CARTESIAN_POINT ( 'NONE',  ( 7.084665262690076126, 12.02201867748817321, -10.88017736071110164 ) ) ;
#71307=CARTESIAN_POINT ( 'NONE',  ( 19.84674366389459621, 33.50893115100078745, 7.409399052514197653E-17 ) ) ;
#71308=CARTESIAN_POINT ( 'NONE',  ( 2.148416515056650766, 47.23726573380441351, 6.500000000000004441 ) ) ;
#71312=CARTESIAN_POINT ( 'NONE',  ( 6.204703633549690345, 22.84541550158062861, 14.16423886937410082 ) ) ;
#71315=CARTESIAN_POINT ( 'NONE',  ( 6.204703633549690345, 60.76208216824730357, -14.16423886937410259 ) ) ;
#71316=CARTESIAN_POINT ( 'NONE',  ( 19.84674366389459266, 28.30059781766745886, 2.638427012816836559 ) ) ;
#71319=CARTESIAN_POINT ( 'NONE',  ( 20.88017736071110164, 55.35535201082149825, 2.915334737309930979 ) ) ;
#71320=CARTESIAN_POINT ( 'NONE',  ( -1.099225684535947600, 63.70696800326376774, -6.408140936763238038 ) ) ;
#71322=CARTESIAN_POINT ( 'NONE',  ( 17.96484262340118221, 36.18868534415484106, -7.964842623401177768 ) ) ;
#71323=CARTESIAN_POINT ( 'NONE',  ( 21.09922568453595559, 57.04030133659708923, -6.408140936763230044 ) ) ;
#71324=CARTESIAN_POINT ( 'NONE',  ( 22.81628187352647785, 6.415301336597088344, 3.434112377981063169 ) ) ;
#71325=CARTESIAN_POINT ( 'NONE',  ( 0.1532563361054082862, 11.21726448433411605, 2.638427012816831674 ) ) ;
#71327=CARTESIAN_POINT ( 'NONE',  ( 10.00000000000000000, -0.2410688489992152128, -9.846743663894594434 ) ) ;
#71328=CARTESIAN_POINT ( 'NONE',  ( 0.2751277870542912507, 20.30223176428831167, 6.499999999999992006 ) ) ;
#71329=CARTESIAN_POINT ( 'NONE',  ( 17.08211943468705840, 50.13708216824730357, -12.26659068614894466 ) ) ;
#71330=CARTESIAN_POINT ( 'NONE',  ( 10.00000000000000000, 25.55374883491396787, -14.16423886937410082 ) ) ;
#71331=CARTESIAN_POINT ( 'NONE',  ( 19.42250999205614193, 45.14701867748817676, 5.440088680355555262 ) ) ;
#71332=CARTESIAN_POINT ( 'NONE',  ( 0.2751277870542965243, 3.218334437839379891, 6.500000000000000888 ) ) ;
#71334=CARTESIAN_POINT ( 'NONE',  ( 7.361572987183169658, 9.967264484334119601, -9.846743663894592657 ) ) ;
#71336=CARTESIAN_POINT ( 'NONE',  ( 14.92337183194729633, 17.67559781766745175, 8.527530157486181039 ) ) ;
#71339=CARTESIAN_POINT ( 'NONE',  ( 1.472469842513823179, 21.42559781766745175, 4.923371831947296329 ) ) ;
#71340=CARTESIAN_POINT ( 'NONE',  ( 18.52753015748618282, 43.92559781766745175, -4.923371831947291888 ) ) ;
#71341=CARTESIAN_POINT ( 'NONE',  ( 0.5774900079438607392, 28.48035201082150891, 5.440088680355550821 ) ) ;
#71344=UNCERTAINTY_MEASURE_WITH_UNIT (LENGTH_MEASURE( 1.000000000000000082E-05 ), #38409, 'distance_accuracy_value', 'NONE');
#71345=CARTESIAN_POINT ( 'NONE',  ( 13.43411237798106583, 32.66530133659708213, -12.81628187352647252 ) ) ;
#71346=CARTESIAN_POINT ( 'NONE',  ( 15.44008868035555260, 49.73035201082150536, 9.422509992056143702 ) ) ;
#71347=CARTESIAN_POINT ( 'NONE',  ( 10.00000000000000000, 29.75893115100078745, -9.846743663894594434 ) ) ;
#71348=CARTESIAN_POINT ( 'NONE',  ( 2.917880565312950480, 40.97041550158063217, -12.26659068614894821 ) ) ;
#71349=CARTESIAN_POINT ( 'NONE',  ( 0.1532563361054083140, 16.00893115100078390, 1.131784320476157264E-15 ) ) ;
#71352=CARTESIAN_POINT ( 'NONE',  ( 7.361572987183169658, 49.96726448433410894, -9.846743663894592657 ) ) ;
#71353=CARTESIAN_POINT ( 'NONE',  ( 17.20831665107776587, 49.13393115100078745, -7.208316651077762316 ) ) ;
#71354=CARTESIAN_POINT ( 'NONE',  ( 6.204703633549690345, 5.762082168247301794, -14.16423886937410259 ) ) ;
#71355=CARTESIAN_POINT ( 'NONE',  ( -4.164238869374099927, 37.01208216824731068, 3.795296366450308767 ) ) ;
#71356=CARTESIAN_POINT ( 'NONE',  ( 12.63842701281683922, 24.55059781766745175, -9.846743663894590881 ) ) ;
#71357=CARTESIAN_POINT ( 'NONE',  ( 7.084665262690076126, 47.02201867748818387, -10.88017736071110164 ) ) ;
#71358=CARTESIAN_POINT ( 'NONE',  ( 7.084665262690076126, 22.02201867748817321, -10.88017736071110164 ) ) ;
#71360=CARTESIAN_POINT ( 'NONE',  ( 12.91533473730992121, 49.52201867748817676, 10.88017736071110164 ) ) ;
#71361=CARTESIAN_POINT ( 'NONE',  ( 17.96484262340118221, 31.18868534415483751, -7.964842623401177768 ) ) ;
#71362=ORIENTED_EDGE ( 'NONE', *, *, #80532, .F. ) ;
#71363=CARTESIAN_POINT ( 'NONE',  ( 22.81628187352647785, 31.62363466993042138, 6.195893100308588602E-16 ) ) ;
#71365=CARTESIAN_POINT ( 'NONE',  ( 7.084665262690076126, 49.10535201082149825, 10.88017736071109987 ) ) ;
#71369=CARTESIAN_POINT ( 'NONE',  ( 7.084665262690076126, 62.02201867748816966, -10.88017736071110164 ) ) ;
#71370=ORIENTED_EDGE ( 'NONE', *, *, #37885, .F. ) ;
#71372=CARTESIAN_POINT ( 'NONE',  ( -0.8801773607111008646, 68.27201867748817676, 2.915334737309923430 ) ) ;
#71375=CARTESIAN_POINT ( 'NONE',  ( 18.72515096720572458, 40.05509018479936145, 6.499999999999964473 ) ) ;
#71376=LINE ( 'NONE', #25866, #87162 ) ;
#71377=CARTESIAN_POINT ( 'NONE',  ( 6.204703633549690345, 60.76208216824730357, -14.16423886937410259 ) ) ;
#71378=CARTESIAN_POINT ( 'NONE',  ( 2.791683348922237240, 15.38393115100078212, -7.208316651077763204 ) ) ;
#71379=CARTESIAN_POINT ( 'NONE',  ( 10.00000000000000178, 3.053748834913967425, 14.16423886937410082 ) ) ;
#71381=CARTESIAN_POINT ( 'NONE',  ( 18.52753015748617571, 8.092264484334117824, 4.923371831947298993 ) ) ;
#71382=CARTESIAN_POINT ( 'NONE',  ( 19.42250999205614548, 5.980352010821504471, -5.440088680355545492 ) ) ;
#71383=CARTESIAN_POINT ( 'NONE',  ( 2.791683348922240793, 41.63393115100078745, 7.208316651077764092 ) ) ;
#71385=CARTESIAN_POINT ( 'NONE',  ( 19.84674366389459621, 43.50893115100078745, 7.409399052514197653E-17 ) ) ;
#71387=CARTESIAN_POINT ( 'NONE',  ( 7.084665262690076126, 52.02201867748816255, -10.88017736071110164 ) ) ;
#71388=CARTESIAN_POINT ( 'NONE',  ( 1.472469842513823179, 56.42559781766745886, 4.923371831947296329 ) ) ;
#71389=CARTESIAN_POINT ( 'NONE',  ( 15.44008868035555260, 64.73035201082151957, 9.422509992056143702 ) ) ;
#71390=CARTESIAN_POINT ( 'NONE',  ( 0.5774900079438590739, 57.64701867748817676, -5.440088680355550821 ) ) ;
#71391=CARTESIAN_POINT ( 'NONE',  ( -2.266590686148945544, 67.22041550158063217, 7.082119434687048631 ) ) ;
#71392=CARTESIAN_POINT ( 'NONE',  ( 16.40814093676324603, 42.45696800326375353, -11.09922568453594671 ) ) ;
#71395=CARTESIAN_POINT ( 'NONE',  ( 0.6178305044545838731, 34.74863466993042493, 9.382169495545420901 ) ) ;
#71396=CARTESIAN_POINT ( 'NONE',  ( 0.5774900079438607392, 28.48035201082150891, 5.440088680355550821 ) ) ;
#71398=ORIENTED_EDGE ( 'NONE', *, *, #16746, .T. ) ;
#71399=CARTESIAN_POINT ( 'NONE',  ( -2.816281873526471635, -1.084698663402913210, -3.434112377981056508 ) ) ;
#71400=CARTESIAN_POINT ( 'NONE',  ( 0.1532563361054083140, 11.00893115100078568, 1.131784320476157264E-15 ) ) ;
#71401=CARTESIAN_POINT ( 'NONE',  ( 18.52753015748617571, 48.09226448433412315, 4.923371831947298993 ) ) ;
#71403=CARTESIAN_POINT ( 'NONE',  ( 0.6178305044545818747, 63.49863466993043204, -9.382169495545419124 ) ) ;
#71404=CARTESIAN_POINT ( 'NONE',  ( 18.52753015748617571, 43.09226448433412315, 4.923371831947298993 ) ) ;
#71407=CARTESIAN_POINT ( 'NONE',  ( 19.84674366389459266, 33.30059781766744464, 2.638427012816836559 ) ) ;
#71408=DIRECTION ( 'NONE',  ( 0.000000000000000000, 0.000000000000000000, -1.000000000000000000 ) ) ;
#71410=CARTESIAN_POINT ( 'NONE',  ( 19.84674366389459621, 63.50893115100078745, 7.409399052514197653E-17 ) ) ;
#71412=EDGE_CURVE ( 'NONE', #40991, #85047, #84892, .T. ) ;
#71414=CARTESIAN_POINT ( 'NONE',  ( 19.38216949554541557, 22.24863466993041428, -9.382169495545420901 ) ) ;
#71415=CARTESIAN_POINT ( 'NONE',  ( 0.1532563361054100626, 40.80059781766745886, -2.638427012816831230 ) ) ;
#71416=CARTESIAN_POINT ( 'NONE',  ( 0.000000000000000000, 10.49999999999999822, -6.000000000000000000 ) ) ;
#71418=CARTESIAN_POINT ( 'NONE',  ( 13.79529636645030344, 43.26208216824730357, 14.16423886937410614 ) ) ;
#71419=CARTESIAN_POINT ( 'NONE',  ( 17.20831665107776587, 12.88393115100078390, 7.208316651077764980 ) ) ;
#71420=CARTESIAN_POINT ( 'NONE',  ( 19.99999999999862510, 87.39268192868374285, 5.318367326097882319 ) ) ;
#71421=CARTESIAN_POINT ( 'NONE',  ( 10.00000000000000000, 45.55374883491397497, -14.16423886937410082 ) ) ;
#71422=CARTESIAN_POINT ( 'NONE',  ( 17.20831665107776587, 52.88393115100078035, 7.208316651077764980 ) ) ;
#71423=CARTESIAN_POINT ( 'NONE',  ( 10.00000000000000000, 11.81368534415483751, -10.88017736071110342 ) ) ;
#71424=CARTESIAN_POINT ( 'NONE',  ( 17.08211943468705130, 28.47041550158063572, 12.26659068614894998 ) ) ;
#71426=CARTESIAN_POINT ( 'NONE',  ( -0.3689425029237898834, 36.17874883491396787, -10.36894250292378850 ) ) ;
#71429=CARTESIAN_POINT ( 'NONE',  ( 17.20831665107776587, 59.13393115100078745, -7.208316651077762316 ) ) ;
#71430=MECHANICAL_DESIGN_GEOMETRIC_PRESENTATION_REPRESENTATION('',(#2790),#84209);
#71431=CARTESIAN_POINT ( 'NONE',  ( 15.44008868035555793, 41.39701867748817676, -9.422509992056140149 ) ) ;
#71434=DIRECTION ( 'NONE',  ( -0.000000000000000000, -1.000000000000000000, 0.000000000000000000 ) ) ;
#71437=CARTESIAN_POINT ( 'NONE',  ( 5.076628168052704559, 50.17559781766745886, -8.527530157486179263 ) ) ;
#71438=CARTESIAN_POINT ( 'NONE',  ( 2.791683348922240793, 66.63393115100079456, 7.208316651077764092 ) ) ;
#71440=CARTESIAN_POINT ( 'NONE',  ( 20.36894250292379738, 24.92874883491396787, -10.36894250292379027 ) ) ;
#71444=CARTESIAN_POINT ( 'NONE',  ( 4.559911319644449179, 7.230352010821505360, -9.422509992056141925 ) ) ;
#71445=CARTESIAN_POINT ( 'NONE',  ( 21.09922568453594849, 31.20696800326375353, 6.408140936763242479 ) ) ;
#71447=CARTESIAN_POINT ( 'NONE',  ( 7.361572987183170547, 17.05059781766745530, 9.846743663894590881 ) ) ;
#71448=CARTESIAN_POINT ( 'NONE',  ( -0.2418659066527782397, 10.11633188102327274, 6.114288769123032985 ) ) ;
#71450=CARTESIAN_POINT ( 'NONE',  ( 0.2751277870542914172, 43.21833443783938122, 6.499999999999992006 ) ) ;
#71451=CARTESIAN_POINT ( 'NONE',  ( 20.88017736071110875, 15.77201867748817143, -2.915334737309920765 ) ) ;
#71452=CARTESIAN_POINT ( 'NONE',  ( -0.1503990784575247319, 32.22266099184917465, -6.262539305110083276 ) ) ;
#71453=CARTESIAN_POINT ( 'NONE',  ( 15.44008868035555793, 41.39701867748817676, -9.422509992056140149 ) ) ;
#71454=CARTESIAN_POINT ( 'NONE',  ( 10.00000000000000000, 41.81368534415484106, -10.88017736071110342 ) ) ;
#71455=CARTESIAN_POINT ( 'NONE',  ( 3.591859063236761518, 4.956968003263753531, 11.09922568453594849 ) ) ;
#71457=CARTESIAN_POINT ( 'NONE',  ( -42.50369195530268485, 107.9060299417078426, -4.500000000000000888 ) ) ;
#71458=CARTESIAN_POINT ( 'NONE',  ( 14.92337183194729988, 14.34226448433411782, -8.527530157486177487 ) ) ;
#71462=CARTESIAN_POINT ( 'NONE',  ( 20.88017736071110519, 30.56368534415484106, 2.639326808657452039E-16 ) ) ;
#71463=CARTESIAN_POINT ( 'NONE',  ( 21.09922568453595559, 37.04030133659708923, -6.408140936763230044 ) ) ;
#71464=CARTESIAN_POINT ( 'NONE',  ( -0.1503990784575277295, 54.24884699246889852, -6.262539305110077947 ) ) ;
#71466=CARTESIAN_POINT ( 'NONE',  ( 12.63842701281683034, 57.46726448433411605, 9.846743663894596210 ) ) ;
#71467=CARTESIAN_POINT ( 'NONE',  ( -0.8801773607110991993, 67.85535201082151957, -2.915334737309923874 ) ) ;
#71468=CARTESIAN_POINT ( 'NONE',  ( 7.361572987183170547, 7.050597817667451750, 9.846743663894590881 ) ) ;
#71470=CARTESIAN_POINT ( 'NONE',  ( -2.816281873526473856, 34.33196800326376064, 3.434112377981055619 ) ) ;
#71471=CARTESIAN_POINT ( 'NONE',  ( 19.42250999205614548, 55.98035201082150536, -5.440088680355545492 ) ) ;
#71472=DIRECTION ( 'NONE',  ( -0.5547001962252291474, -0.8320502943378437211, -0.000000000000000000 ) ) ;
#71475=CARTESIAN_POINT ( 'NONE',  ( 0.6178305044545838731, 59.74863466993041783, 9.382169495545420901 ) ) ;
#71476=CARTESIAN_POINT ( 'NONE',  ( 1.472469842513823179, 15.59226448433411960, -4.923371831947296329 ) ) ;
#71477=CARTESIAN_POINT ( 'NONE',  ( 4.559911319644449179, 8.897018677488171434, 9.422509992056141925 ) ) ;
#71478=CARTESIAN_POINT ( 'NONE',  ( 17.20831665107776587, 24.13393115100078035, -7.208316651077762316 ) ) ;
#71479=CARTESIAN_POINT ( 'NONE',  ( -2.266590686148945544, 62.22041550158063927, 7.082119434687048631 ) ) ;
#71481=CARTESIAN_POINT ( 'NONE',  ( 17.96484262340118221, 16.18868534415483396, -7.964842623401177768 ) ) ;
#71483=CARTESIAN_POINT ( 'NONE',  ( 10.00000000000000178, 19.31368534415484106, 10.88017736071110342 ) ) ;
#71484=CARTESIAN_POINT ( 'NONE',  ( 1.959929470562091547, 16.50257860105346097, 5.767676674365524114 ) ) ;
#71485=VECTOR ( 'NONE', #81151, 1000.000000000000000 ) ;
#71487=ORIENTED_EDGE ( 'NONE', *, *, #18758, .F. ) ;
#71488=CARTESIAN_POINT ( 'NONE',  ( 20.32896413005680714, 27.60497603579417714, -5.963430220938276349 ) ) ;
#71489=CARTESIAN_POINT ( 'NONE',  ( 19.42250999205614193, 25.14701867748817321, 5.440088680355555262 ) ) ;
#71491=CARTESIAN_POINT ( 'NONE',  ( 19.84674366389459266, 58.30059781766745886, 2.638427012816836559 ) ) ;
#71492=CARTESIAN_POINT ( 'NONE',  ( 1.274849032794280523, 68.57228050351031357, 6.499999999999960032 ) ) ;
#71493=CARTESIAN_POINT ( 'NONE',  ( 20.36894250292379738, 24.92874883491396787, -10.36894250292379027 ) ) ;
#71494=CARTESIAN_POINT ( 'NONE',  ( 19.42250999205614193, 35.14701867748816966, 5.440088680355555262 ) ) ;
#71496=CARTESIAN_POINT ( 'NONE',  ( 15.44008868035555260, 14.73035201082150536, 9.422509992056143702 ) ) ;
#71497=CARTESIAN_POINT ( 'NONE',  ( 0.1532563361054082862, 56.21726448433411605, 2.638427012816831674 ) ) ;
#71500=CARTESIAN_POINT ( 'NONE',  ( 12.63842701281683922, 39.55059781766744464, -9.846743663894590881 ) ) ;
#71502=CARTESIAN_POINT ( 'NONE',  ( 2.791683348922240793, 11.63393115100078568, 7.208316651077764092 ) ) ;
#71506=CARTESIAN_POINT ( 'NONE',  ( 15.44008868035555260, 19.73035201082150536, 9.422509992056143702 ) ) ;
#71507=CARTESIAN_POINT ( 'NONE',  ( 2.791683348922237240, 15.38393115100078212, -7.208316651077763204 ) ) ;
#71508=CARTESIAN_POINT ( 'NONE',  ( 16.40814093676323893, 0.7903013365970867898, 11.09922568453595026 ) ) ;
#71509=CARTESIAN_POINT ( 'NONE',  ( 20.88017736071110519, 50.56368534415484106, 2.639326808657452039E-16 ) ) ;
#71510=CARTESIAN_POINT ( 'NONE',  ( 7.084665262690076126, 17.02201867748817676, -10.88017736071110164 ) ) ;
#71511=CARTESIAN_POINT ( 'NONE',  ( 13.43411237798106583, 42.66530133659707502, -12.81628187352647252 ) ) ;
#71512=CARTESIAN_POINT ( 'NONE',  ( 2.917880565312950480, 30.97041550158063572, -12.26659068614894821 ) ) ;
#71514=CARTESIAN_POINT ( 'NONE',  ( 20.15039907845753575, 12.62777174578613071, -6.262539305110077059 ) ) ;
#71516=ADVANCED_FACE ( 'NONE', ( #16401 ), #68651, .T. ) ;
#71518=CARTESIAN_POINT ( 'NONE',  ( 22.81628187352648496, 56.83196800326374643, -3.434112377981050290 ) ) ;
#71520=CARTESIAN_POINT ( 'NONE',  ( 1.472469842513823179, 61.42559781766745175, 4.923371831947296329 ) ) ;
#71521=CARTESIAN_POINT ( 'NONE',  ( 12.91533473730992121, 39.52201867748817676, 10.88017736071110164 ) ) ;
#71524=CARTESIAN_POINT ( 'NONE',  ( 5.076628168052703671, 1.842264484334118047, 8.527530157486179263 ) ) ;
#71525=CARTESIAN_POINT ( 'NONE',  ( 0.9408516040111367662, 42.46693863883976405, -6.499999999999915623 ) ) ;
#71526=CARTESIAN_POINT ( 'NONE',  ( 19.84674366389459621, 23.50893115100078390, 7.409399052514197653E-17 ) ) ;
#71527=CARTESIAN_POINT ( 'NONE',  ( 0.5774900079438590739, 67.64701867748817676, -5.440088680355550821 ) ) ;
#71528=CARTESIAN_POINT ( 'NONE',  ( 5.076628168052703671, 1.842264484334118047, 8.527530157486179263 ) ) ;
#71529=CARTESIAN_POINT ( 'NONE',  ( 19.42250999205614193, 60.14701867748817676, 5.440088680355555262 ) ) ;
#71531=CARTESIAN_POINT ( 'NONE',  ( 15.44008868035555793, 61.39701867748817676, -9.422509992056140149 ) ) ;
#71532=CARTESIAN_POINT ( 'NONE',  ( 2.791683348922240793, 11.63393115100078568, 7.208316651077764092 ) ) ;
#71535=CARTESIAN_POINT ( 'NONE',  ( 2.791683348922240793, 51.63393115100078745, 7.208316651077764092 ) ) ;
#71539=CARTESIAN_POINT ( 'NONE',  ( 17.08211943468705130, 8.470415501580635720, 12.26659068614894998 ) ) ;
#71540=CARTESIAN_POINT ( 'NONE',  ( 22.81628187352647785, 61.62363466993041783, 6.195893100308588602E-16 ) ) ;
#71541=CARTESIAN_POINT ( 'NONE',  ( 2.917880565312948704, 7.637082168247301794, 12.26659068614894643 ) ) ;
#71542=CARTESIAN_POINT ( 'NONE',  ( -4.164238869374099927, 37.01208216824731068, 3.795296366450308767 ) ) ;
#71544=CARTESIAN_POINT ( 'NONE',  ( 17.96484262340118221, 26.18868534415483396, -7.964842623401177768 ) ) ;
#71546=CARTESIAN_POINT ( 'NONE',  ( 1.472469842513823179, 11.42559781766745175, 4.923371831947296329 ) ) ;
#71547=CARTESIAN_POINT ( 'NONE',  ( 19.42250999205614548, 55.98035201082150536, -5.440088680355545492 ) ) ;
#71548=CARTESIAN_POINT ( 'NONE',  ( 12.63842701281683922, 19.55059781766745175, -9.846743663894590881 ) ) ;
#71549=CARTESIAN_POINT ( 'NONE',  ( 6.565887622018943937, 50.16530133659708213, 12.81628187352647430 ) ) ;
#71550=CARTESIAN_POINT ( 'NONE',  ( 19.84674366389459621, 38.50893115100078745, 7.409399052514197653E-17 ) ) ;
#71551=CARTESIAN_POINT ( 'NONE',  ( 18.04007052943772038, 59.00257860105349295, -5.767676674365850076 ) ) ;
#71552=CARTESIAN_POINT ( 'NONE',  ( 2.035157376598824452, 58.68868534415482685, 7.964842623401179544 ) ) ;
#71553=CARTESIAN_POINT ( 'NONE',  ( 10.00000000000000178, 35.37363466993042493, 12.81628187352647608 ) ) ;
#71555=CARTESIAN_POINT ( 'NONE',  ( 1.472469842513823179, 21.42559781766745175, 4.923371831947296329 ) ) ;
#71556=CARTESIAN_POINT ( 'NONE',  ( -0.3689425029237881626, 7.428748834913967869, 10.36894250292379027 ) ) ;
#71557=VERTEX_POINT ( 'NONE', #24793 ) ;
#71558=CARTESIAN_POINT ( 'NONE',  ( 20.88017736071110164, 35.35535201082150536, 2.915334737309930979 ) ) ;
#71559=CARTESIAN_POINT ( 'NONE',  ( 10.00000000000000000, 35.55374883491396787, -14.16423886937410082 ) ) ;
#71560=CARTESIAN_POINT ( 'NONE',  ( 1.472469842513823179, 50.59226448433411605, -4.923371831947296329 ) ) ;
#71561=CARTESIAN_POINT ( 'NONE',  ( 5.076628168052703671, 11.84226448433411960, 8.527530157486179263 ) ) ;
#71562=CARTESIAN_POINT ( 'NONE',  ( 19.38216949554541557, 52.24863466993041072, -9.382169495545420901 ) ) ;
#71563=CARTESIAN_POINT ( 'NONE',  ( 0.5774900079438590739, 42.64701867748816966, -5.440088680355550821 ) ) ;
#71565=CARTESIAN_POINT ( 'NONE',  ( 6.565887622018943937, 18.08196800326375708, -12.81628187352647608 ) ) ;
#71566=CARTESIAN_POINT ( 'NONE',  ( 2.791683348922240793, 41.63393115100078745, 7.208316651077764092 ) ) ;
#71569=CARTESIAN_POINT ( 'NONE',  ( 20.88017736071110519, 60.56368534415484106, 2.639326808657452039E-16 ) ) ;
#71576=CARTESIAN_POINT ( 'NONE',  ( 7.084665262690076126, 57.02201867748817676, -10.88017736071110164 ) ) ;
#71577=CARTESIAN_POINT ( 'NONE',  ( -0.8801773607110991993, 62.85535201082150536, -2.915334737309923874 ) ) ;
#71580=CARTESIAN_POINT ( 'NONE',  ( 12.63842701281683034, 22.46726448433411605, 9.846743663894596210 ) ) ;
#71581=CARTESIAN_POINT ( 'NONE',  ( 15.44008868035555260, 19.73035201082150536, 9.422509992056143702 ) ) ;
#71582=CARTESIAN_POINT ( 'NONE',  ( 5.076628168052704559, 65.17559781766745175, -8.527530157486179263 ) ) ;
#71583=CARTESIAN_POINT ( 'NONE',  ( 15.44008868035555793, 26.39701867748817321, -9.422509992056140149 ) ) ;
#71586=CARTESIAN_POINT ( 'NONE',  ( 21.09922568453595559, 22.04030133659708923, -6.408140936763230044 ) ) ;
#71588=CARTESIAN_POINT ( 'NONE',  ( 4.559911319644449179, 48.89701867748817676, 9.422509992056141925 ) ) ;
#71589=CARTESIAN_POINT ( 'NONE',  ( 19.84674366389459266, 33.30059781766744464, 2.638427012816836559 ) ) ;
#71590=CARTESIAN_POINT ( 'NONE',  ( 10.00000000000000178, 25.37363466993041783, 12.81628187352647608 ) ) ;
#71591=CARTESIAN_POINT ( 'NONE',  ( 17.39651004071842522, 19.08210964143329491, -6.499999999999992895 ) ) ;
#71592=CARTESIAN_POINT ( 'NONE',  ( 15.44008868035555260, 29.73035201082150891, 9.422509992056143702 ) ) ;
#71593=CARTESIAN_POINT ( 'NONE',  ( 7.084665262690076126, 37.02201867748817676, -10.88017736071110164 ) ) ;
#71594=CARTESIAN_POINT ( 'NONE',  ( -0.3689425029237898834, 56.17874883491396076, -10.36894250292378850 ) ) ;
#71595=CARTESIAN_POINT ( 'NONE',  ( 12.63842701281683922, 44.55059781766745175, -9.846743663894590881 ) ) ;
#71596=CARTESIAN_POINT ( 'NONE',  ( 19.84674366389459621, 8.508931151000785675, 7.409399052514197653E-17 ) ) ;
#71597=CARTESIAN_POINT ( 'NONE',  ( 12.91533473730992121, 44.52201867748816966, 10.88017736071110164 ) ) ;
#71599=CARTESIAN_POINT ( 'NONE',  ( 2.917880565312950480, 15.97041550158063217, -12.26659068614894821 ) ) ;
#71602=CARTESIAN_POINT ( 'NONE',  ( 10.00000000000000178, 48.05374883491396787, 14.16423886937410082 ) ) ;
#71603=CARTESIAN_POINT ( 'NONE',  ( 24.16423886937410614, 54.30374883491396787, 8.672049930838204340E-16 ) ) ;
#71605=CARTESIAN_POINT ( 'NONE',  ( 7.361572987183170547, 22.05059781766745530, 9.846743663894590881 ) ) ;
#71607=CARTESIAN_POINT ( 'NONE',  ( 0.2751277870542914172, 58.21833443783938833, 6.499999999999992006 ) ) ;
#71608=CARTESIAN_POINT ( 'NONE',  ( 2.035157376598824452, 68.68868534415484817, 7.964842623401179544 ) ) ;
#71609=CARTESIAN_POINT ( 'NONE',  ( 0.6178305044545838731, 34.74863466993042493, 9.382169495545420901 ) ) ;
#71610=CARTESIAN_POINT ( 'NONE',  ( -4.164238869374098151, 46.59541550158063927, -3.795296366450310543 ) ) ;
#71612=CARTESIAN_POINT ( 'NONE',  ( 10.00000000000000178, 69.31368534415484817, 10.88017736071110342 ) ) ;
#71615=CARTESIAN_POINT ( 'NONE',  ( 19.84674366389459266, 23.30059781766745530, 2.638427012816836559 ) ) ;
#71616=DIRECTION ( 'NONE',  ( 0.000000000000000000, 0.000000000000000000, -1.000000000000000000 ) ) ;
#71618=CARTESIAN_POINT ( 'NONE',  ( 4.559911319644449179, 12.23035201082150714, -9.422509992056141925 ) ) ;
#71619=CARTESIAN_POINT ( 'NONE',  ( 17.96484262340118221, 14.93868534415484106, 7.964842623401181321 ) ) ;
#71620=CARTESIAN_POINT ( 'NONE',  ( 12.63842701281683922, 44.55059781766745175, -9.846743663894590881 ) ) ;
#71621=CARTESIAN_POINT ( 'NONE',  ( 16.40814093676323893, 0.7903013365970867898, 11.09922568453595026 ) ) ;
#71622=FILL_AREA_STYLE ('',( #73072 ) ) ;
#71624=COLOUR_RGB ( '', 0.40784314, 0.44705882, 0.49803922) ;
#71625=CARTESIAN_POINT ( 'NONE',  ( 10.00000000000000000, 22.87363466993042138, -12.81628187352647608 ) ) ;
#71627=CARTESIAN_POINT ( 'NONE',  ( 17.08211943468705840, 55.13708216824731068, -12.26659068614894466 ) ) ;
#71628=CARTESIAN_POINT ( 'NONE',  ( 17.08211943468705130, 58.47041550158063927, 12.26659068614894998 ) ) ;
#71629=VERTEX_POINT ( 'NONE', #84792 ) ;
#71630=CARTESIAN_POINT ( 'NONE',  ( 15.44008868035555793, 36.39701867748816966, -9.422509992056140149 ) ) ;
#71631=CARTESIAN_POINT ( 'NONE',  ( 19.42250999205614548, 40.98035201082150536, -5.440088680355545492 ) ) ;
#71632=CARTESIAN_POINT ( 'NONE',  ( 4.559911319644449179, 67.23035201082150536, -9.422509992056141925 ) ) ;
#71633=CARTESIAN_POINT ( 'NONE',  ( 7.084665262690076126, 22.02201867748817321, -10.88017736071110164 ) ) ;
#71638=CARTESIAN_POINT ( 'NONE',  ( 19.84674366389459266, 8.717264484334116048, -2.638427012816827677 ) ) ;
#71642=CARTESIAN_POINT ( 'NONE',  ( 0.1532563361054083140, 41.00893115100078745, 1.131784320476157264E-15 ) ) ;
#71643=CARTESIAN_POINT ( 'NONE',  ( 17.39651004071841456, 9.082109641433294911, -6.500000000000003553 ) ) ;
#71644=CARTESIAN_POINT ( 'NONE',  ( 6.565887622018943937, 48.08196800326375353, -12.81628187352647608 ) ) ;
#71646=ORIENTED_EDGE ( 'NONE', *, *, #55011, .F. ) ;
#71647=DIRECTION ( 'NONE',  ( -0.000000000000000000, -0.000000000000000000, -1.000000000000000000 ) ) ;
#71648=CARTESIAN_POINT ( 'NONE',  ( -45.64141537884788846, 104.8111512546448125, 5.509330541965931971 ) ) ;
#71649=CARTESIAN_POINT ( 'NONE',  ( 1.274849032794280523, 48.57228050351032067, 6.499999999999960032 ) ) ;
#71650=CARTESIAN_POINT ( 'NONE',  ( -4.164238869374098151, 51.59541550158063217, -3.795296366450310543 ) ) ;
#71654=CARTESIAN_POINT ( 'NONE',  ( 12.63842701281683922, 29.55059781766745175, -9.846743663894590881 ) ) ;
#71655=CARTESIAN_POINT ( 'NONE',  ( 3.591859063236761518, 9.956968003263753531, 11.09922568453594849 ) ) ;
#71656=CARTESIAN_POINT ( 'NONE',  ( 7.084665262690076126, 62.02201867748816966, -10.88017736071110164 ) ) ;
#71658=CARTESIAN_POINT ( 'NONE',  ( 19.84674366389459266, 58.30059781766745886, 2.638427012816836559 ) ) ;
#71660=ORIENTED_EDGE ( 'NONE', *, *, #35122, .T. ) ;
#71661=CARTESIAN_POINT ( 'NONE',  ( 6.204703633549690345, 67.84541550158060375, 14.16423886937410082 ) ) ;
#71662=PRESENTATION_STYLE_ASSIGNMENT (( #70686 ) ) ;
#71663=CARTESIAN_POINT ( 'NONE',  ( 10.00000000000000000, 41.81368534415484106, -10.88017736071110342 ) ) ;
#71664=CARTESIAN_POINT ( 'NONE',  ( 16.40814093676323893, 10.79030133659708923, 11.09922568453595026 ) ) ;
#71669=CARTESIAN_POINT ( 'NONE',  ( 2.791683348922237240, 50.38393115100078035, -7.208316651077763204 ) ) ;
#71670=CARTESIAN_POINT ( 'NONE',  ( 18.52753015748618282, 3.925597817667451306, -4.923371831947291888 ) ) ;
#71672=CARTESIAN_POINT ( 'NONE',  ( -1.099225684535947600, 4.540301336597087456, 6.408140936763237150 ) ) ;
#71674=CARTESIAN_POINT ( 'NONE',  ( 0.5774900079438590739, 27.64701867748817676, -5.440088680355550821 ) ) ;
#71676=CARTESIAN_POINT ( 'NONE',  ( 13.79529636645030344, 33.26208216824730357, 14.16423886937410614 ) ) ;
#71678=CARTESIAN_POINT ( 'NONE',  ( 20.36894250292379738, 24.92874883491396787, -10.36894250292379027 ) ) ;
#71679=CARTESIAN_POINT ( 'NONE',  ( 12.91533473730993009, 11.60535201082150714, -10.88017736071109987 ) ) ;
#71680=CARTESIAN_POINT ( 'NONE',  ( 5.076628168052703671, 46.84226448433412315, 8.527530157486179263 ) ) ;
#71681=CARTESIAN_POINT ( 'NONE',  ( 22.81628187352648496, 36.83196800326376064, -3.434112377981050290 ) ) ;
#71682=CARTESIAN_POINT ( 'NONE',  ( 7.084665262690076126, 9.105352010821503583, 10.88017736071109987 ) ) ;
#71684=CARTESIAN_POINT ( 'NONE',  ( 0.1532563361054082862, 36.21726448433410894, 2.638427012816831674 ) ) ;
#71685=CARTESIAN_POINT ( 'NONE',  ( 2.035157376598822676, 42.43868534415483396, -7.964842623401177768 ) ) ;
#71686=CARTESIAN_POINT ( 'NONE',  ( 6.565887622018943937, 3.081968003263753531, -12.81628187352647608 ) ) ;
#71687=CARTESIAN_POINT ( 'NONE',  ( 22.26659068614895176, 19.72041550158063572, -7.082119434687042414 ) ) ;
#71690=CARTESIAN_POINT ( 'NONE',  ( 1.472469842513823179, 21.42559781766745175, 4.923371831947296329 ) ) ;
#71691=CARTESIAN_POINT ( 'NONE',  ( 16.40814093676324603, 57.45696800326375353, -11.09922568453594671 ) ) ;
#71692=CARTESIAN_POINT ( 'NONE',  ( 18.52753015748618282, 58.92559781766745886, -4.923371831947291888 ) ) ;
#71693=ORIENTED_EDGE ( 'NONE', *, *, #28330, .T. ) ;
#71694=CARTESIAN_POINT ( 'NONE',  ( 0.2751277870542911952, 34.36607318730131055, -6.499999999999992006 ) ) ;
#71695=CARTESIAN_POINT ( 'NONE',  ( 24.16423886937410614, 64.51208216824728936, -3.795296366450302550 ) ) ;
#71696=CARTESIAN_POINT ( 'NONE',  ( 20.36894250292379382, 8.678748834913967869, 10.36894250292379205 ) ) ;
#71697=CARTESIAN_POINT ( 'NONE',  ( 1.472469842513823179, 0.5922644843341181575, -4.923371831947296329 ) ) ;
#71698=CARTESIAN_POINT ( 'NONE',  ( 18.52753015748617571, 48.09226448433412315, 4.923371831947298993 ) ) ;
#71699=CARTESIAN_POINT ( 'NONE',  ( 15.44008868035555793, 26.39701867748817321, -9.422509992056140149 ) ) ;
#71701=CARTESIAN_POINT ( 'NONE',  ( 10.00000000000000000, 64.75893115100078035, -9.846743663894594434 ) ) ;
#71702=COLOUR_RGB ( '', 0.40784314, 0.44705882, 0.49803922) ;
#71709=CARTESIAN_POINT ( 'NONE',  ( 13.79529636645031943, 5.345415501580634832, -14.16423886937409904 ) ) ;
#71712=CARTESIAN_POINT ( 'NONE',  ( 5.076628168052703671, 51.84226448433412315, 8.527530157486179263 ) ) ;
#71713=CARTESIAN_POINT ( 'NONE',  ( 1.472469842513823179, 36.42559781766745175, 4.923371831947296329 ) ) ;
#71714=CARTESIAN_POINT ( 'NONE',  ( 20.88017736071110164, 30.35535201082151247, 2.915334737309930979 ) ) ;
#71715=CARTESIAN_POINT ( 'NONE',  ( 2.791683348922240793, 61.63393115100079456, 7.208316651077764092 ) ) ;
#71716=CARTESIAN_POINT ( 'NONE',  ( 13.79529636645031943, 5.345415501580634832, -14.16423886937409904 ) ) ;
#71717=CARTESIAN_POINT ( 'NONE',  ( 13.79529636645030344, 43.26208216824730357, 14.16423886937410614 ) ) ;
#71718=CARTESIAN_POINT ( 'NONE',  ( 4.559911319644449179, 8.897018677488173211, 9.422509992056141925 ) ) ;
#71719=CARTESIAN_POINT ( 'NONE',  ( 14.92337183194729988, 64.34226448433412315, -8.527530157486177487 ) ) ;
#71721=CARTESIAN_POINT ( 'NONE',  ( 4.559911319644449179, 62.23035201082150536, -9.422509992056141925 ) ) ;
#71723=CARTESIAN_POINT ( 'NONE',  ( 19.84674366389459266, 28.30059781766745886, 2.638427012816836559 ) ) ;
#71727=ORIENTED_EDGE ( 'NONE', *, *, #28521, .F. ) ;
#71728=CARTESIAN_POINT ( 'NONE',  ( 10.00000000000000000, 19.75893115100078390, -9.846743663894594434 ) ) ;
#71730=CARTESIAN_POINT ( 'NONE',  ( -0.3689425029237881626, 27.42874883491397142, 10.36894250292379027 ) ) ;
#71731=CARTESIAN_POINT ( 'NONE',  ( 10.00000000000000178, 27.25893115100078390, 9.846743663894594434 ) ) ;
#71732=CARTESIAN_POINT ( 'NONE',  ( 4.559911319644449179, 57.23035201082150536, -9.422509992056141925 ) ) ;
#71733=DIRECTION ( 'NONE',  ( -1.000000000000000000, 0.000000000000000000, 0.000000000000000000 ) ) ;
#71734=CARTESIAN_POINT ( 'NONE',  ( 2.035157376598824452, 43.68868534415484106, 7.964842623401179544 ) ) ;
#71735=CARTESIAN_POINT ( 'NONE',  ( 5.076628168052703671, 41.84226448433411605, 8.527530157486179263 ) ) ;
#71739=CARTESIAN_POINT ( 'NONE',  ( 2.035157376598822676, 42.43868534415483396, -7.964842623401177768 ) ) ;
#71740=CARTESIAN_POINT ( 'NONE',  ( -0.3689425029237898834, 6.178748834913968757, -10.36894250292378850 ) ) ;
#71741=ORIENTED_EDGE ( 'NONE', *, *, #3531, .F. ) ;
#71743=CARTESIAN_POINT ( 'NONE',  ( -2.816281873526471635, 33.91530133659708213, -3.434112377981056508 ) ) ;
#71745=LINE ( 'NONE', #94234, #41416 ) ;
#71746=CARTESIAN_POINT ( 'NONE',  ( 5.076628168052704559, 25.17559781766745175, -8.527530157486179263 ) ) ;
#71747=CARTESIAN_POINT ( 'NONE',  ( 12.91533473730992121, 4.522018677488169658, 10.88017736071110164 ) ) ;
#71748=CARTESIAN_POINT ( 'NONE',  ( 10.00000000000000000, 29.75893115100078745, -9.846743663894594434 ) ) ;
#71749=EDGE_CURVE ( 'NONE', #38758, #23770, #69239, .T. ) ;
#71750=CARTESIAN_POINT ( 'NONE',  ( -0.8801773607111008646, 63.27201867748817676, 2.915334737309923430 ) ) ;
#71753=CARTESIAN_POINT ( 'NONE',  ( -0.04068437667225256044, 17.21974360917720404, -6.396802510829700417 ) ) ;
#71754=CARTESIAN_POINT ( 'NONE',  ( 1.472469842513823179, 6.425597817667451750, 4.923371831947296329 ) ) ;
#71755=CARTESIAN_POINT ( 'NONE',  ( 21.09922568453594849, 16.20696800326375353, 6.408140936763242479 ) ) ;
#71758=CARTESIAN_POINT ( 'NONE',  ( 1.472469842513823179, 50.59226448433411605, -4.923371831947296329 ) ) ;
#71759=CARTESIAN_POINT ( 'NONE',  ( 19.10478245763053451, 35.10160829253886305, 5.990408912944295672 ) ) ;
#71760=CARTESIAN_POINT ( 'NONE',  ( -2.266590686148945544, 11.38708216824730179, -7.082119434687050408 ) ) ;
#71761=CARTESIAN_POINT ( 'NONE',  ( 0.1532563361054082862, 31.21726448433412315, 2.638427012816831674 ) ) ;
#71762=CARTESIAN_POINT ( 'NONE',  ( -2.816281873526471635, 28.91530133659708213, -3.434112377981056508 ) ) ;
#71765=CARTESIAN_POINT ( 'NONE',  ( 0.5774900079438607392, 53.48035201082151247, 5.440088680355550821 ) ) ;
#71766=CARTESIAN_POINT ( 'NONE',  ( -1.099225684535947600, 8.706968003263753531, -6.408140936763238038 ) ) ;
#71767=LINE ( 'NONE', #79759, #64679 ) ;
#71768=CARTESIAN_POINT ( 'NONE',  ( 19.84674366389459266, 18.71726448433411960, -2.638427012816827677 ) ) ;
#71769=CARTESIAN_POINT ( 'NONE',  ( 17.96484262340118221, 26.18868534415483396, -7.964842623401177768 ) ) ;
#71770=CARTESIAN_POINT ( 'NONE',  ( 0.6178305044545838731, 29.74863466993042138, 9.382169495545420901 ) ) ;
#71771=CARTESIAN_POINT ( 'NONE',  ( 14.92337183194729988, 19.34226448433411960, -8.527530157486177487 ) ) ;
#71773=( NAMED_UNIT ( * ) SI_UNIT ( $, .STERADIAN. ) SOLID_ANGLE_UNIT ( ) );
#71775=CARTESIAN_POINT ( 'NONE',  ( 12.91533473730993009, 31.60535201082150891, -10.88017736071109987 ) ) ;
#71776=VERTEX_POINT ( 'NONE', #34721 ) ;
#71777=CARTESIAN_POINT ( 'NONE',  ( 20.88017736071110519, 60.56368534415484106, 2.639326808657452039E-16 ) ) ;
#71779=CARTESIAN_POINT ( 'NONE',  ( 7.361572987183170547, 47.05059781766745175, 9.846743663894590881 ) ) ;
#71780=CARTESIAN_POINT ( 'NONE',  ( 12.91533473730992121, 24.52201867748816966, 10.88017736071110164 ) ) ;
#71781=SURFACE_SIDE_STYLE ('',( #41308 ) ) ;
#71782=CARTESIAN_POINT ( 'NONE',  ( 0.5774900079438607392, 48.48035201082150536, 5.440088680355550821 ) ) ;
#71783=CARTESIAN_POINT ( 'NONE',  ( -0.8801773607111009756, 13.06368534415483929, 1.068504757029289695E-15 ) ) ;
#71786=CARTESIAN_POINT ( 'NONE',  ( 5.076628168052703671, 41.84226448433411605, 8.527530157486179263 ) ) ;
#71787=CARTESIAN_POINT ( 'NONE',  ( 20.36894250292379382, 38.67874883491396076, 10.36894250292379205 ) ) ;
#71789=CARTESIAN_POINT ( 'NONE',  ( 2.603489959281586774, 5.435752660568278216, -6.500000000000001776 ) ) ;
#71791=SURFACE_SIDE_STYLE ('',( #32793 ) ) ;
#71793=CARTESIAN_POINT ( 'NONE',  ( 2.917880565312948704, 22.63708216824730002, 12.26659068614894643 ) ) ;
#71796=CARTESIAN_POINT ( 'NONE',  ( -0.8801773607110991993, 2.855352010821504471, -2.915334737309923874 ) ) ;
#71798=CARTESIAN_POINT ( 'NONE',  ( 12.63842701281683034, 32.46726448433412315, 9.846743663894596210 ) ) ;
#71801=CARTESIAN_POINT ( 'NONE',  ( 17.96484262340118221, 54.93868534415484106, 7.964842623401181321 ) ) ;
#71802=CARTESIAN_POINT ( 'NONE',  ( 19.38216949554541202, 60.99863466993042493, 9.382169495545424454 ) ) ;
#71803=CARTESIAN_POINT ( 'NONE',  ( 10.00000000000000000, 36.81368534415484106, -10.88017736071110342 ) ) ;
#71804=CARTESIAN_POINT ( 'NONE',  ( 0.6178305044545838731, 64.74863466993043914, 9.382169495545420901 ) ) ;
#71805=CARTESIAN_POINT ( 'NONE',  ( 22.81628187352648496, 11.83196800326375531, -3.434112377981050290 ) ) ;
#71806=CARTESIAN_POINT ( 'NONE',  ( 10.00000000000000178, 12.25893115100078568, 9.846743663894594434 ) ) ;
#71809=CARTESIAN_POINT ( 'NONE',  ( 2.917880565312950480, 60.97041550158063927, -12.26659068614894821 ) ) ;
#71810=CARTESIAN_POINT ( 'NONE',  ( 2.917880565312950480, 20.97041550158063217, -12.26659068614894821 ) ) ;
#71811=CARTESIAN_POINT ( 'NONE',  ( 19.42250999205614193, 30.14701867748817321, 5.440088680355555262 ) ) ;
#71812=CARTESIAN_POINT ( 'NONE',  ( -0.8801773607111008646, 43.27201867748817676, 2.915334737309923430 ) ) ;
#71815=CARTESIAN_POINT ( 'NONE',  ( 0.1532563361054100626, 5.800597817667452638, -2.638427012816831230 ) ) ;
#71817=CARTESIAN_POINT ( 'NONE',  ( 17.20831665107776587, 17.88393115100078745, 7.208316651077764980 ) ) ;
#71819=CARTESIAN_POINT ( 'NONE',  ( 2.791683348922237240, 20.38393115100078745, -7.208316651077763204 ) ) ;
#71820=CARTESIAN_POINT ( 'NONE',  ( 2.791683348922240793, 51.63393115100078745, 7.208316651077764092 ) ) ;
#71822=CARTESIAN_POINT ( 'NONE',  ( 20.88017736071110875, 25.77201867748816966, -2.915334737309920765 ) ) ;
#71823=CARTESIAN_POINT ( 'NONE',  ( 0.6178305044545838731, 44.74863466993042493, 9.382169495545420901 ) ) ;
#71824=CARTESIAN_POINT ( 'NONE',  ( 10.00000000000000000, 56.81368534415484106, -10.88017736071110342 ) ) ;
#71825=CARTESIAN_POINT ( 'NONE',  ( 10.00000000000000178, 27.25893115100078390, 9.846743663894594434 ) ) ;
#71826=CARTESIAN_POINT ( 'NONE',  ( 22.26659068614895176, 44.72041550158063927, -7.082119434687042414 ) ) ;
#71827=CARTESIAN_POINT ( 'NONE',  ( 2.791683348922240793, 16.63393115100078745, 7.208316651077764092 ) ) ;
#71828=CARTESIAN_POINT ( 'NONE',  ( 1.821158202401483850, 51.16688879859522388, 6.499999999999917399 ) ) ;
#71829=CARTESIAN_POINT ( 'NONE',  ( 0.1532563361054100626, 60.80059781766744464, -2.638427012816831230 ) ) ;
#71830=CARTESIAN_POINT ( 'NONE',  ( -0.3689425029237898834, 11.17874883491396787, -10.36894250292378850 ) ) ;
#71831=CARTESIAN_POINT ( 'NONE',  ( 17.08211943468705840, 25.13708216824730357, -12.26659068614894466 ) ) ;
#71832=CARTESIAN_POINT ( 'NONE',  ( 5.076628168052703671, 31.84226448433412315, 8.527530157486179263 ) ) ;
#71834=CARTESIAN_POINT ( 'NONE',  ( 17.96484262340118221, 21.18868534415483396, -7.964842623401177768 ) ) ;
#71835=EDGE_CURVE ( 'NONE', #84403, #10365, #26114, .T. ) ;
#71836=CARTESIAN_POINT ( 'NONE',  ( 12.91533473730992121, 39.52201867748817676, 10.88017736071110164 ) ) ;
#71837=CARTESIAN_POINT ( 'NONE',  ( 7.084665262690076126, 37.02201867748817676, -10.88017736071110164 ) ) ;
#71839=CARTESIAN_POINT ( 'NONE',  ( -0.8801773607110991993, 57.85535201082149825, -2.915334737309923874 ) ) ;
#71842=CARTESIAN_POINT ( 'NONE',  ( 15.44008868035555793, 61.39701867748817676, -9.422509992056140149 ) ) ;
#71844=CARTESIAN_POINT ( 'NONE',  ( 20.88017736071110519, 60.56368534415484106, 2.639326808657452039E-16 ) ) ;
#71845=SURFACE_STYLE_USAGE ( .BOTH. , #41857 ) ;
#71848=CARTESIAN_POINT ( 'NONE',  ( 2.917880565312948704, 67.63708216824730357, 12.26659068614894643 ) ) ;
#71849=CARTESIAN_POINT ( 'NONE',  ( 1.472469842513823179, 6.425597817667451750, 4.923371831947296329 ) ) ;
#71850=CARTESIAN_POINT ( 'NONE',  ( 10.00000000000000000, 5.553748834913967869, -14.16423886937410082 ) ) ;
#71851=CARTESIAN_POINT ( 'NONE',  ( 14.92337183194729633, 7.675597817667451750, 8.527530157486181039 ) ) ;
#71852=CARTESIAN_POINT ( 'NONE',  ( 10.00000000000000000, 11.81368534415483751, -10.88017736071110342 ) ) ;
#71853=CARTESIAN_POINT ( 'NONE',  ( 14.92337183194729988, 44.34226448433412315, -8.527530157486177487 ) ) ;
#71856=CARTESIAN_POINT ( 'NONE',  ( 7.361572987183169658, 49.96726448433410894, -9.846743663894592657 ) ) ;
#71857=ORIENTED_EDGE ( 'NONE', *, *, #62162, .T. ) ;
#71859=CARTESIAN_POINT ( 'NONE',  ( 20.88017736071110875, 50.77201867748817676, -2.915334737309920765 ) ) ;
#71860=CARTESIAN_POINT ( 'NONE',  ( 0.1532563361054082862, 46.21726448433411605, 2.638427012816831674 ) ) ;
#71862=CARTESIAN_POINT ( 'NONE',  ( 4.559911319644449179, 53.89701867748817676, 9.422509992056141925 ) ) ;
#71863=CARTESIAN_POINT ( 'NONE',  ( 13.79529636645031943, 65.34541550158063217, -14.16423886937409904 ) ) ;
#71864=AXIS2_PLACEMENT_3D ( 'NONE', #62993, #47498, #17021 ) ;
#71866=CARTESIAN_POINT ( 'NONE',  ( 21.09922568453594849, 41.20696800326375353, 6.408140936763242479 ) ) ;
#71868=ORIENTED_EDGE ( 'NONE', *, *, #53039, .F. ) ;
#71869=CARTESIAN_POINT ( 'NONE',  ( 16.40814093676323893, 25.79030133659708923, 11.09922568453595026 ) ) ;
#71870=CARTESIAN_POINT ( 'NONE',  ( 20.88017736071110875, 35.77201867748816966, -2.915334737309920765 ) ) ;
#71872=CARTESIAN_POINT ( 'NONE',  ( -2.816281873526473856, -0.8763653300695799508, 9.499525473075851096E-16 ) ) ;
#71873=CARTESIAN_POINT ( 'NONE',  ( 12.63842701281683034, 17.46726448433411250, 9.846743663894596210 ) ) ;
#71874=CARTESIAN_POINT ( 'NONE',  ( 14.92337183194729633, 47.67559781766745175, 8.527530157486181039 ) ) ;
#71876=CARTESIAN_POINT ( 'NONE',  ( 0.2751277870542910842, 52.28217586085238366, -6.499999999999992006 ) ) ;
#71878=CARTESIAN_POINT ( 'NONE',  ( 0.1532563361054082862, 21.21726448433412315, 2.638427012816831674 ) ) ;
#71879=PRESENTATION_STYLE_ASSIGNMENT (( #48877 ) ) ;
#71881=CARTESIAN_POINT ( 'NONE',  ( 2.791683348922237240, 55.38393115100078745, -7.208316651077763204 ) ) ;
#71883=CARTESIAN_POINT ( 'NONE',  ( 13.43411237798105340, 25.58196800326374998, 12.81628187352647963 ) ) ;
#71884=CARTESIAN_POINT ( 'NONE',  ( 0.1532563361054083140, 41.00893115100078745, 1.131784320476157264E-15 ) ) ;
#71886=CARTESIAN_POINT ( 'NONE',  ( 13.79529636645030344, 58.26208216824728936, 14.16423886937410614 ) ) ;
#71887=CARTESIAN_POINT ( 'NONE',  ( 2.791683348922237240, 15.38393115100078212, -7.208316651077763204 ) ) ;
#71888=CARTESIAN_POINT ( 'NONE',  ( 20.00000000000000711, 85.81090550035371223, 4.886738312952367380 ) ) ;
#71889=CARTESIAN_POINT ( 'NONE',  ( 10.00000000000000178, 63.05374883491396076, 14.16423886937410082 ) ) ;
#71890=CARTESIAN_POINT ( 'NONE',  ( 2.791683348922240793, 56.63393115100078035, 7.208316651077764092 ) ) ;
#71891=CARTESIAN_POINT ( 'NONE',  ( 10.00000000000000178, 9.313685344154839285, 10.88017736071110342 ) ) ;
#71892=CARTESIAN_POINT ( 'NONE',  ( -4.164238869374099039, 36.80374883491396787, 8.674139862899312516E-16 ) ) ;
#71893=CARTESIAN_POINT ( 'NONE',  ( 17.08211943468705840, 35.13708216824730357, -12.26659068614894466 ) ) ;
#71894=CARTESIAN_POINT ( 'NONE',  ( 18.52753015748618282, 33.92559781766745886, -4.923371831947291888 ) ) ;
#71897=CARTESIAN_POINT ( 'NONE',  ( 12.63842701281683034, 57.46726448433411605, 9.846743663894596210 ) ) ;
#71899=CARTESIAN_POINT ( 'NONE',  ( 17.96484262340118221, 39.93868534415484106, 7.964842623401181321 ) ) ;
#71901=CARTESIAN_POINT ( 'NONE',  ( 5.076628168052703671, 46.84226448433412315, 8.527530157486179263 ) ) ;
#71902=LINE ( 'NONE', #95398, #12316 ) ;
#71904=CARTESIAN_POINT ( 'NONE',  ( 14.92337183194729633, 52.67559781766745175, 8.527530157486181039 ) ) ;
#71905=CARTESIAN_POINT ( 'NONE',  ( -0.1503990784575407469, 12.22266099184918531, -6.262539305110056631 ) ) ;
#71906=AXIS2_PLACEMENT_3D ( 'NONE', #79691, #10708, #94191 ) ;
#71909=CARTESIAN_POINT ( 'NONE',  ( -0.3689425029237898834, 26.17874883491396432, -10.36894250292378850 ) ) ;
#71910=EDGE_CURVE ( 'NONE', #93709, #52823, #27338, .T. ) ;
#71911=EDGE_CURVE ( 'NONE', #98100, #35821, #64346, .T. ) ;
#71914=CARTESIAN_POINT ( 'NONE',  ( 19.42250999205614548, 45.98035201082150536, -5.440088680355545492 ) ) ;
#71915=CARTESIAN_POINT ( 'NONE',  ( 0.5774900079438590739, 22.64701867748817321, -5.440088680355550821 ) ) ;
#71916=CARTESIAN_POINT ( 'NONE',  ( 6.565887622018943937, 28.08196800326375353, -12.81628187352647608 ) ) ;
#71918=CARTESIAN_POINT ( 'NONE',  ( 12.63842701281683034, 17.46726448433411250, 9.846743663894596210 ) ) ;
#71921=VECTOR ( 'NONE', #71472, 1000.000000000000000 ) ;
#71924=CARTESIAN_POINT ( 'NONE',  ( 0.5774900079438607392, 3.480352010821504916, 5.440088680355550821 ) ) ;
#71925=CARTESIAN_POINT ( 'NONE',  ( 0.2751277870542912507, 20.30223176428831167, 6.499999999999992006 ) ) ;
#71927=CARTESIAN_POINT ( 'NONE',  ( 0.5774900079438607392, 38.48035201082150536, 5.440088680355550821 ) ) ;
#71928=CARTESIAN_POINT ( 'NONE',  ( 17.96484262340118221, 41.18868534415484106, -7.964842623401177768 ) ) ;
#71929=CARTESIAN_POINT ( 'NONE',  ( -2.816281873526473856, 4.331968003263754419, 3.434112377981055619 ) ) ;
#71931=CARTESIAN_POINT ( 'NONE',  ( -0.1503990784575328643, 70.00000000000000000, -6.262539305110068177 ) ) ;
#71932=CARTESIAN_POINT ( 'NONE',  ( 12.63842701281683922, 4.550597817667451750, -9.846743663894590881 ) ) ;
#71936=CARTESIAN_POINT ( 'NONE',  ( 7.084665262690076126, 47.02201867748818387, -10.88017736071110164 ) ) ;
#71937=CARTESIAN_POINT ( 'NONE',  ( 0.6178305044545818747, 3.498634669930420049, -9.382169495545419124 ) ) ;
#71938=CARTESIAN_POINT ( 'NONE',  ( 10.00000000000000000, 56.81368534415484106, -10.88017736071110342 ) ) ;
#71939=CARTESIAN_POINT ( 'NONE',  ( 7.361572987183169658, 9.967264484334119601, -9.846743663894592657 ) ) ;
#71940=CARTESIAN_POINT ( 'NONE',  ( -1.099225684535947600, 28.70696800326375353, -6.408140936763238038 ) ) ;
#71941=CARTESIAN_POINT ( 'NONE',  ( 17.20831665107776587, 7.883931151000784787, 7.208316651077764980 ) ) ;
#71943=VERTEX_POINT ( 'NONE', #67209 ) ;
#71945=CARTESIAN_POINT ( 'NONE',  ( 17.96484262340118221, 4.938685344154837509, 7.964842623401181321 ) ) ;
#71946=CYLINDRICAL_SURFACE ( 'NONE', #24960, 0.5000000000000004441 ) ;
#71948=CARTESIAN_POINT ( 'NONE',  ( 17.20831665107776587, 17.88393115100078745, 7.208316651077764980 ) ) ;
#71949=CARTESIAN_POINT ( 'NONE',  ( 19.42250999205614548, 10.98035201082150358, -5.440088680355545492 ) ) ;
#71951=CARTESIAN_POINT ( 'NONE',  ( 7.084665262690076126, 7.022018677488170546, -10.88017736071110164 ) ) ;
#71953=AXIS2_PLACEMENT_3D ( 'NONE', #1603, #40071, #98637 ) ;
#71954=CARTESIAN_POINT ( 'NONE',  ( 17.96484262340118221, 14.93868534415483751, 7.964842623401181321 ) ) ;
#71955=CARTESIAN_POINT ( 'NONE',  ( 20.88017736071110875, 20.77201867748816611, -2.915334737309920765 ) ) ;
#71957=ORIENTED_EDGE ( 'NONE', *, *, #8714, .F. ) ;
#71959=CARTESIAN_POINT ( 'NONE',  ( 0.5774900079438590739, 27.64701867748817676, -5.440088680355550821 ) ) ;
#71960=CARTESIAN_POINT ( 'NONE',  ( 2.791683348922240793, 56.63393115100078035, 7.208316651077764092 ) ) ;
#71962=CARTESIAN_POINT ( 'NONE',  ( 19.38216949554541557, 47.24863466993041783, -9.382169495545420901 ) ) ;
#71963=DIRECTION ( 'NONE',  ( -0.000000000000000000, -0.000000000000000000, 1.000000000000000000 ) ) ;
#71964=CARTESIAN_POINT ( 'NONE',  ( 17.08211943468705130, 28.47041550158063572, 12.26659068614894998 ) ) ;
#71965=CARTESIAN_POINT ( 'NONE',  ( 19.42250999205614548, 35.98035201082151247, -5.440088680355545492 ) ) ;
#71966=CARTESIAN_POINT ( 'NONE',  ( 7.084665262690076126, 14.10535201082150358, 10.88017736071109987 ) ) ;
#71967=CARTESIAN_POINT ( 'NONE',  ( 14.92337183194729988, 59.34226448433412315, -8.527530157486177487 ) ) ;
#71969=CARTESIAN_POINT ( 'NONE',  ( 1.472469842513823179, 30.59226448433411960, -4.923371831947296329 ) ) ;
#71971=CARTESIAN_POINT ( 'NONE',  ( 5.076628168052703671, 11.84226448433411960, 8.527530157486179263 ) ) ;
#71974=CARTESIAN_POINT ( 'NONE',  ( -0.8801773607111008646, 8.272018677488171434, 2.915334737309923430 ) ) ;
#71975=CARTESIAN_POINT ( 'NONE',  ( 7.361572987183170547, 12.05059781766744997, 9.846743663894590881 ) ) ;
#71976=CARTESIAN_POINT ( 'NONE',  ( 20.88017736071110164, 40.35535201082150536, 2.915334737309930979 ) ) ;
#71977=CARTESIAN_POINT ( 'NONE',  ( -0.8801773607111008646, 23.27201867748817676, 2.915334737309923430 ) ) ;
#71978=CARTESIAN_POINT ( 'NONE',  ( 10.00000000000000178, 40.37363466993042493, 12.81628187352647608 ) ) ;
#71979=CARTESIAN_POINT ( 'NONE',  ( -0.3689425029237881626, 37.42874883491396787, 10.36894250292379027 ) ) ;
#71982=CARTESIAN_POINT ( 'NONE',  ( -2.816281873526473856, 64.33196800326376774, 3.434112377981055619 ) ) ;
#71983=ORIENTED_EDGE ( 'NONE', *, *, #25103, .F. ) ;
#71984=CARTESIAN_POINT ( 'NONE',  ( 14.92337183194729633, 57.67559781766745886, 8.527530157486181039 ) ) ;
#71986=CARTESIAN_POINT ( 'NONE',  ( -0.8801773607110991993, 27.85535201082150181, -2.915334737309923874 ) ) ;
#71988=VERTEX_POINT ( 'NONE', #29683 ) ;
#71989=CARTESIAN_POINT ( 'NONE',  ( 2.791683348922237240, 5.383931151000785675, -7.208316651077763204 ) ) ;
#71990=CARTESIAN_POINT ( 'NONE',  ( 18.52753015748618282, 13.92559781766745175, -4.923371831947291888 ) ) ;
#71991=CARTESIAN_POINT ( 'NONE',  ( 19.84674366389459266, 18.71726448433411960, -2.638427012816827677 ) ) ;
#71992=CARTESIAN_POINT ( 'NONE',  ( 0.1532563361054082862, 16.21726448433411960, 2.638427012816831674 ) ) ;
#71993=FACE_OUTER_BOUND ( 'NONE', #39486, .T. ) ;
#71995=CARTESIAN_POINT ( 'NONE',  ( -0.8801773607111008646, 63.27201867748817676, 2.915334737309923430 ) ) ;
#71996=CARTESIAN_POINT ( 'NONE',  ( 4.559911319644449179, 67.23035201082150536, -9.422509992056141925 ) ) ;
#71997=CARTESIAN_POINT ( 'NONE',  ( 14.92337183194729988, 14.34226448433411782, -8.527530157486177487 ) ) ;
#72000=CARTESIAN_POINT ( 'NONE',  ( 5.076628168052703671, 51.84226448433412315, 8.527530157486179263 ) ) ;
#72003=CARTESIAN_POINT ( 'NONE',  ( -4.164238869374099039, 11.80374883491396965, 8.674139862899312516E-16 ) ) ;
#72005=CARTESIAN_POINT ( 'NONE',  ( -45.94000000000001194, 99.99999999999998579, -9.500000000000000000 ) ) ;
#72006=CARTESIAN_POINT ( 'NONE',  ( -2.266590686148945544, 12.22041550158063394, 7.082119434687048631 ) ) ;
#72007=CARTESIAN_POINT ( 'NONE',  ( 24.16423886937410614, 34.51208216824731068, -3.795296366450302550 ) ) ;
#72008=CARTESIAN_POINT ( 'NONE',  ( 20.88017736071110164, 30.35535201082151247, 2.915334737309930979 ) ) ;
#72010=ORIENTED_EDGE ( 'NONE', *, *, #11212, .F. ) ;
#72011=CARTESIAN_POINT ( 'NONE',  ( 12.63842701281683034, 17.46726448433411250, 9.846743663894596210 ) ) ;
#72012=EDGE_CURVE ( 'NONE', #73005, #80852, #51249, .T. ) ;
#72013=CARTESIAN_POINT ( 'NONE',  ( 10.00000000000000000, 51.81368534415484106, -10.88017736071110342 ) ) ;
#72014=CARTESIAN_POINT ( 'NONE',  ( 12.63842701281683034, 17.46726448433411250, 9.846743663894596210 ) ) ;
#72017=CARTESIAN_POINT ( 'NONE',  ( 16.40814093676323893, 45.79030133659708923, 11.09922568453595026 ) ) ;
#72018=CARTESIAN_POINT ( 'NONE',  ( 18.52753015748617571, 33.09226448433411605, 4.923371831947298993 ) ) ;
#72019=CARTESIAN_POINT ( 'NONE',  ( 17.39651004071841811, 4.082109641433293135, -6.499999999999999112 ) ) ;
#72020=CARTESIAN_POINT ( 'NONE',  ( 17.96484262340118221, 61.18868534415482685, -7.964842623401177768 ) ) ;
#72021=CARTESIAN_POINT ( 'NONE',  ( -2.816281873526473856, 29.33196800326376064, 3.434112377981055619 ) ) ;
#72023=CARTESIAN_POINT ( 'NONE',  ( 10.00000000000000000, 19.75893115100078390, -9.846743663894594434 ) ) ;
#72026=CARTESIAN_POINT ( 'NONE',  ( 17.08211943468705840, 10.13708216824730179, -12.26659068614894466 ) ) ;
#72028=EDGE_CURVE ( 'NONE', #13314, #47944, #81000, .T. ) ;
#72029=CARTESIAN_POINT ( 'NONE',  ( 20.88017736071110519, 40.56368534415484106, 2.639326808657452039E-16 ) ) ;
#72030=CARTESIAN_POINT ( 'NONE',  ( 15.44008868035555793, 51.39701867748816966, -9.422509992056140149 ) ) ;
#72031=CARTESIAN_POINT ( 'NONE',  ( 13.79529636645030344, 43.26208216824730357, 14.16423886937410614 ) ) ;
#72032=CARTESIAN_POINT ( 'NONE',  ( 14.92337183194729633, 52.67559781766745175, 8.527530157486181039 ) ) ;
#72033=CARTESIAN_POINT ( 'NONE',  ( 19.84674366389459266, 8.300597817667451750, 2.638427012816836559 ) ) ;
#72036=CARTESIAN_POINT ( 'NONE',  ( 12.91533473730993009, 36.60535201082151247, -10.88017736071109987 ) ) ;
#72037=CYLINDRICAL_SURFACE ( 'NONE', #27861, 19.43999999999999773 ) ;
#72038=CARTESIAN_POINT ( 'NONE',  ( 21.09922568453594849, 21.20696800326375353, 6.408140936763242479 ) ) ;
#72039=CARTESIAN_POINT ( 'NONE',  ( 7.361572987183169658, 49.96726448433410894, -9.846743663894592657 ) ) ;
#72041=( BOUNDED_SURFACE ( )  B_SPLINE_SURFACE ( 1, 2, ( 
 ( #45366, #75870, #21897, #76365, #74878, #82373, #60860, #53358, #28873, #52374, #97910, #68873, #28396, #97406, #7391, #43876, #21397, #59375, #51891, #22886, #14394, #67884, #37889, #52867, #60364, #75368, #13895, #44865, #7879, #20905, #38372, #29370, #98901, #6883, #44380, #30353, #29861, #6378, #98406, #5899, #37396, #90860, #90359, #22391, #36893, #83373, #83865, #67381, #15389, #51394, #58890, #81881, #74372, #36394, #92835, #17831, #46839, #54337, #32813, #25350, #880, #24363, #69854, #40830, #403, #38868, #78321, #84374, #92347, #31340, #69359, #63309, #54826, #39842, #85837, #24848, #32324, #47326, #61840, #85338, #48313, #61352, #78821, #1377, #9841, #16851, #23873, #2358, #1866, #84851, #70348, #76846, #77825, #9340, #31831, #62327, #16358, #55330, #17351, #77334, #62827, #91861, #47821, #10331, #93327, #40342, #23379, #70845, #8360, #93819, #8846, #55833, #39360, #86327, #30855, #53863, #15873, #46358, #88285, #79800, #34274, #33780, #50785, #64775, #4309, #12776, #95291, #63796, #72772, #18816, #27776, #20287, #49786, #41340, #80789, #94799, #71811, #3317, #27280, #26793, #34783, #33304, #80294, #49298, #81276, #73278, #65271, #56325, #57290, #95799, #57778, #11792, #25827, #42793, #86820, #19784, #64287, #4800, #42300, #50272, #12286, #10820, #35276, #87784, #19300, #65771, #18323, #48804, #41822, #96300, #58261, #56801, #88776, #79313, #26301, #87297, #11302, #72288, #3819, #74253, #22276, #67268, #52748, #37772, #66263, #91241, #97292, #66769, #83257, #14780, #36776, #60739, #89759, #59258, #75748, #68268, #43764, #97796, #13772, #83751, #43273, #21276, #7270, #28273, #51772, #29258, #90250, #98787, #21782, #82756, #29744, #30235, #22765, #52261, #14279, #44752, #73768, #96798, #58768, #89272, #20783, #51274, #76732, #47711, #16734, #84258, #85231, #91744, #62212, #1260, #8727, #39245, #15761, #70229, #32203, #53740, #69735, #7766, #62704, #63195, #47211, #1748, #38261, #77712, #23264, #31716, #92233, #92717, #46247, #69249, #78206, #38748, #770, #85720, #93204, #23759, #24243, #31222, #55715, #54709, #9224, #15274, #9718, #68752, #40217, #61718, #2241, #284, #32699, #54222, #30731, #84737, #61237, #18209, #42191, #41704, #80170, #10219, #87666, #94688, #17722, #4688, #4190, #63683, #79686, #34660, #65156, #25716, #49184, #72174, #3703, #34163, #51156, #60123, #29132, #67141, #75132, #96675, #90621, #21155, #82135, #21657, #20161, #68142, #28644, #36655, #51656, #43647, #45122, #50664, #97666, #5667, #58144, #22145, #52141, #43157, #13644, #59636, #82637, #90127, #37645, #29617, #88653, #6637, #81640 ),
 ( #59135, #98161, #36149, #66653, #13148, #14657, #14154, #97177, #12657, #28154, #58650, #75629, #73643, #89643, #7141, #37155, #66142, #35657, #44129, #74639, #67651, #89149, #6150, #44638, #52629, #74131, #20660, #83132, #81153, #5172, #48939, #79447, #62957, #17965, #10947, #71468, #41472, #93463, #25954, #30115, #77465, #92959, #48452, #84976, #24989, #9973, #70975, #2982, #33430, #71939, #63453, #47950, #62457, #70476, #31955, #55471, #60621, #1508, #85974, #1996, #63927, #16494, #9472, #25483, #69983, #40478, #91122, #55968, #78950, #56457, #24493, #39975, #86943, #94442, #85477, #2496, #17484, #39492, #32462, #22645, #53125, #78460, #93958, #18456, #46971, #16986, #40971, #8976, #47464, #86468, #10461, #11932, #20919, #28410, #80434, #72919, #95936, #80924, #50911, #27906, #34914, #19922, #13406, #65411, #64909, #81895, #27418, #35412, #43891, #57911, #94931, #4932, #49923, #58905, #51408, #12417, #72420, #12909, #26928, #3946, #34419, #58399, #88422, #65904, #64424, #42924, #42437, #3462, #5435, #96436, #87433, #50415, #88917, #20424, #73404, #33917, #73904, #26434, #81407, #95434, #35907, #43406, #66404, #96935, #41956, #89403, #56932, #18949, #49426, #79930, #11437, #4449, #57426, #87919, #19436, #61367, #98423, #53372, #68891, #66902, #23399, #29384, #6391, #91374, #22900, #67899, #91877, #21915, #59885, #7894, #419, #74892, #29877, #44880, #15889, #74391, #13915, #83882, #59391, #67398, #36906, #44393, #38388, #60379, #14908, #60874, #98915, #7409, #22405, #97924, #90877, #53883, #36408, #84390, #75382, #15409, #52880, #90376, #76379, #75886, #52393, #45380, #51906, #83390, #37905, #6898, #37412, #82893, #30370, #45892, #14409, #68394, #97421, #30870, #5915, #28887, #89893, #21411, #82391, #23890, #39861, #24378, #9356, #54355, #1392, #78838, #16376, #84867, #86346, #63334, #54843, #8862, #85358, #77847, #70367, #93839, #24869, #31847, #46857, #46374, #16870, #71352, #1885, #47344, #78341, #32343, #40361, #93345, #25846, #38886, #62845, #17849, #92850, #55351, #39378, #2871, #17369, #85857, #897, #77351, #69872, #33320, #31359, #47838, #63815, #25365, #62344, #9862, #70862, #2377, #55851, #32832, #48334, #10349, #40849, #94325, #56344, #86838, #76863, #8378, #69375, #61859, #92363, #4821, #35796, #58281, #66283, #49804, #12792, #18343, #64307, #79819, #35295, #71829, #80312, #95819, #57800, #88799, #20308, #96818, #50295, #34802, #49315, #57308, #18835, #11812, #28295, #87318, #42320, #87800, #50807, #3338, #64793, #12306, #56820, #27299, #48822, #42813, #65788, #43292, #11321, #95312, #73787, #81296, #41840 ) ),
 .UNSPECIFIED., .F., .F., .F. ) 
 B_SPLINE_SURFACE_WITH_KNOTS ( ( 2, 2 ),
 ( 3, 2, 2, 2, 2, 2, 2, 2, 2, 2, 2, 2, 2, 2, 2, 2, 2, 2, 2, 2, 2, 2, 2, 2, 2, 2, 2, 2, 2, 2, 2, 2, 2, 2, 2, 2, 2, 2, 2, 2, 2, 2, 2, 2, 2, 2, 2, 2, 2, 2, 2, 2, 2, 2, 2, 2, 2, 2, 2, 2, 2, 2, 2, 2, 2, 2, 2, 2, 2, 2, 2, 2, 2, 2, 2, 2, 2, 2, 2, 2, 2, 2, 2, 2, 2, 2, 2, 2, 2, 2, 2, 2, 2, 2, 2, 2, 2, 2, 2, 2, 2, 2, 2, 2, 2, 2, 2, 2, 2, 2, 2, 2, 2, 2, 2, 2, 2, 2, 2, 2, 2, 2, 2, 2, 2, 2, 2, 2, 2, 2, 2, 2, 2, 2, 2, 2, 2, 2, 2, 2, 2, 2, 2, 2, 2, 2, 2, 2, 2, 2, 2, 2, 2, 2, 2, 2, 2, 2, 2, 2, 2, 2, 3 ),
 ( 0.000000000000000000, 1.000000000000000000 ),
 ( 0.000000000000000000, 0.005952380952380952051, 0.01190476190476190410, 0.01785714285714285615, 0.02380952380952380820, 0.02976190476190476025, 0.03571428571428571230, 0.04166666666666666435, 0.04761904761904761640, 0.05357142857142856845, 0.05952380952380952051, 0.06547619047619047949, 0.07142857142857142461, 0.07738095238095238360, 0.08333333333333332871, 0.08928571428571428770, 0.09523809523809523281, 0.1011904761904761918, 0.1071428571428571369, 0.1130952380952380959, 0.1190476190476190410, 0.1250000000000000000, 0.1309523809523809590, 0.1369047619047619180, 0.1428571428571428492, 0.1488095238095238082, 0.1547619047619047672, 0.1607142857142857262, 0.1666666666666666574, 0.1726190476190476164, 0.1785714285714285754, 0.1845238095238095344, 0.1904761904761904656, 0.1964285714285714246, 0.2023809523809523836, 0.2083333333333333426, 0.2142857142857142738, 0.2202380952380952328, 0.2261904761904761918, 0.2321428571428571508, 0.2380952380952380820, 0.2440476190476190410, 0.2500000000000000000, 0.2559523809523809312, 0.2619047619047619180, 0.2678571428571428492, 0.2738095238095238360, 0.2797619047619047672, 0.2857142857142856984, 0.2916666666666666852, 0.2976190476190476164, 0.3035714285714285476, 0.3095238095238095344, 0.3154761904761904656, 0.3214285714285714524, 0.3273809523809523836, 0.3333333333333333148, 0.3392857142857143016, 0.3452380952380952328, 0.3511904761904761640, 0.3571428571428571508, 0.3630952380952380820, 0.3690476190476190688, 0.3750000000000000000, 0.3809523809523809312, 0.3869047619047619180, 0.3928571428571428492, 0.3988095238095238360, 0.4047619047619047672, 0.4107142857142856984, 0.4166666666666666852, 0.4226190476190476164, 0.4285714285714285476, 0.4345238095238095344, 0.4404761904761904656, 0.4464285714285714524, 0.4523809523809523836, 0.4583333333333333148, 0.4642857142857143016, 0.4702380952380952328, 0.4761904761904761640, 0.4821428571428571508, 0.4880952380952380820, 0.4940476190476190688, 0.5000000000000000000, 0.5059523809523809312, 0.5119047619047618625, 0.5178571428571429047, 0.5238095238095238360, 0.5297619047619047672, 0.5357142857142856984, 0.5416666666666666297, 0.5476190476190476719, 0.5535714285714286031, 0.5595238095238095344, 0.5654761904761904656, 0.5714285714285713969, 0.5773809523809523281, 0.5833333333333333703, 0.5892857142857143016, 0.5952380952380952328, 0.6011904761904761640, 0.6071428571428570953, 0.6130952380952381375, 0.6190476190476190688, 0.6250000000000000000, 0.6309523809523809312, 0.6369047619047618625, 0.6428571428571429047, 0.6488095238095238360, 0.6547619047619047672, 0.6607142857142856984, 0.6666666666666666297, 0.6726190476190476719, 0.6785714285714286031, 0.6845238095238095344, 0.6904761904761904656, 0.6964285714285713969, 0.7023809523809523281, 0.7083333333333333703, 0.7142857142857143016, 0.7202380952380952328, 0.7261904761904761640, 0.7321428571428570953, 0.7380952380952381375, 0.7440476190476190688, 0.7500000000000000000, 0.7559523809523809312, 0.7619047619047618625, 0.7678571428571429047, 0.7738095238095238360, 0.7797619047619047672, 0.7857142857142856984, 0.7916666666666666297, 0.7976190476190476719, 0.8035714285714286031, 0.8095238095238095344, 0.8154761904761904656, 0.8214285714285713969, 0.8273809523809523281, 0.8333333333333333703, 0.8392857142857143016, 0.8452380952380952328, 0.8511904761904761640, 0.8571428571428570953, 0.8630952380952381375, 0.8690476190476190688, 0.8750000000000000000, 0.8809523809523809312, 0.8869047619047618625, 0.8928571428571429047, 0.8988095238095238360, 0.9047619047619047672, 0.9107142857142856984, 0.9166666666666666297, 0.9226190476190476719, 0.9285714285714286031, 0.9345238095238095344, 0.9404761904761904656, 0.9464285714285713969, 0.9523809523809523281, 0.9583333333333333703, 0.9642857142857143016 ),
 .UNSPECIFIED. ) 
 GEOMETRIC_REPRESENTATION_ITEM ( )  RATIONAL_B_SPLINE_SURFACE ( (
 ( 1.000000000000000000, 0.9659258262890683122, 1.000000000000000000, 0.9659258262890683122, 1.000000000000000000, 0.9659258262890683122, 1.000000000000000000, 0.9659258262890683122, 1.000000000000000000, 0.9659258262890683122, 1.000000000000000000, 0.9659258262890683122, 1.000000000000000000, 0.9659258262890683122, 1.000000000000000000, 0.9659258262890683122, 1.000000000000000000, 0.9659258262890683122, 1.000000000000000000, 0.9659258262890683122, 1.000000000000000000, 0.9659258262890683122, 1.000000000000000000, 0.9659258262890683122, 1.000000000000000000, 0.9659258262890683122, 1.000000000000000000, 0.9659258262890683122, 1.000000000000000000, 0.9659258262890683122, 1.000000000000000000, 0.9659258262890683122, 1.000000000000000000, 0.9659258262890683122, 1.000000000000000000, 0.9659258262890683122, 1.000000000000000000, 0.9659258262890683122, 1.000000000000000000, 0.9659258262890683122, 1.000000000000000000, 0.9659258262890683122, 1.000000000000000000, 0.9659258262890683122, 1.000000000000000000, 0.9659258262890683122, 1.000000000000000000, 0.9659258262890683122, 1.000000000000000000, 0.9659258262890683122, 1.000000000000000000, 0.9659258262890683122, 1.000000000000000000, 0.9659258262890683122, 1.000000000000000000, 0.9659258262890683122, 1.000000000000000000, 0.9659258262890683122, 1.000000000000000000, 0.9659258262890683122, 1.000000000000000000, 0.9659258262890683122, 1.000000000000000000, 0.9659258262890683122, 1.000000000000000000, 0.9659258262890683122, 1.000000000000000000, 0.9659258262890683122, 1.000000000000000000, 0.9659258262890683122, 1.000000000000000000, 0.9659258262890683122, 1.000000000000000000, 0.9659258262890683122, 1.000000000000000000, 0.9659258262890683122, 1.000000000000000000, 0.9659258262890683122, 1.000000000000000000, 0.9659258262890683122, 1.000000000000000000, 0.9659258262890683122, 1.000000000000000000, 0.9659258262890683122, 1.000000000000000000, 0.9659258262890683122, 1.000000000000000000, 0.9659258262890683122, 1.000000000000000000, 0.9659258262890683122, 1.000000000000000000, 0.9659258262890683122, 1.000000000000000000, 0.9659258262890683122, 1.000000000000000000, 0.9659258262890683122, 1.000000000000000000, 0.9659258262890683122, 1.000000000000000000, 0.9659258262890683122, 1.000000000000000000, 0.9659258262890683122, 1.000000000000000000, 0.9659258262890683122, 1.000000000000000000, 0.9659258262890683122, 1.000000000000000000, 0.9659258262890683122, 1.000000000000000000, 0.9659258262890683122, 1.000000000000000000, 0.9659258262890683122, 1.000000000000000000, 0.9659258262890683122, 1.000000000000000000, 0.9659258262890683122, 1.000000000000000000, 0.9659258262890683122, 1.000000000000000000, 0.9659258262890683122, 1.000000000000000000, 0.9659258262890683122, 1.000000000000000000, 0.9659258262890683122, 1.000000000000000000, 0.9659258262890683122, 1.000000000000000000, 0.9659258262890683122, 1.000000000000000000, 0.9659258262890683122, 1.000000000000000000, 0.9659258262890683122, 1.000000000000000000, 0.9659258262890683122, 1.000000000000000000, 0.9659258262890683122, 1.000000000000000000, 0.9659258262890683122, 1.000000000000000000, 0.9659258262890683122, 1.000000000000000000, 0.9659258262890683122, 1.000000000000000000, 0.9659258262890683122, 1.000000000000000000, 0.9659258262890683122, 1.000000000000000000, 0.9659258262890683122, 1.000000000000000000, 0.9659258262890683122, 1.000000000000000000, 0.9659258262890683122, 1.000000000000000000, 0.9659258262890683122, 1.000000000000000000, 0.9659258262890683122, 1.000000000000000000, 0.9659258262890683122, 1.000000000000000000, 0.9659258262890683122, 1.000000000000000000, 0.9659258262890683122, 1.000000000000000000, 0.9659258262890683122, 1.000000000000000000, 0.9659258262890683122, 1.000000000000000000, 0.9659258262890683122, 1.000000000000000000, 0.9659258262890683122, 1.000000000000000000, 0.9659258262890683122, 1.000000000000000000, 0.9659258262890683122, 1.000000000000000000, 0.9659258262890683122, 1.000000000000000000, 0.9659258262890683122, 1.000000000000000000, 0.9659258262890683122, 1.000000000000000000, 0.9659258262890683122, 1.000000000000000000, 0.9659258262890683122, 1.000000000000000000, 0.9659258262890683122, 1.000000000000000000, 0.9659258262890683122, 1.000000000000000000, 0.9659258262890683122, 1.000000000000000000, 0.9659258262890683122, 1.000000000000000000, 0.9659258262890683122, 1.000000000000000000, 0.9659258262890683122, 1.000000000000000000, 0.9659258262890683122, 1.000000000000000000, 0.9659258262890683122, 1.000000000000000000, 0.9659258262890683122, 1.000000000000000000, 0.9659258262890683122, 1.000000000000000000, 0.9659258262890683122, 1.000000000000000000, 0.9659258262890683122, 1.000000000000000000, 0.9659258262890683122, 1.000000000000000000, 0.9659258262890683122, 1.000000000000000000, 0.9659258262890683122, 1.000000000000000000, 0.9659258262890683122, 1.000000000000000000, 0.9659258262890683122, 1.000000000000000000, 0.9659258262890683122, 1.000000000000000000, 0.9659258262890683122, 1.000000000000000000, 0.9659258262890683122, 1.000000000000000000, 0.9659258262890683122, 1.000000000000000000, 0.9659258262890683122, 1.000000000000000000, 0.9659258262890683122, 1.000000000000000000, 0.9659258262890683122, 1.000000000000000000, 0.9659258262890683122, 1.000000000000000000, 0.9659258262890683122, 1.000000000000000000, 0.9659258262890683122, 1.000000000000000000, 0.9659258262890683122, 1.000000000000000000, 0.9659258262890683122, 1.000000000000000000, 0.9659258262890683122, 1.000000000000000000, 0.9659258262890683122, 1.000000000000000000, 0.9659258262890683122, 1.000000000000000000, 0.9659258262890683122, 1.000000000000000000, 0.9659258262890683122, 1.000000000000000000, 0.9659258262890683122, 1.000000000000000000, 0.9659258262890683122, 1.000000000000000000, 0.9659258262890683122, 1.000000000000000000, 0.9659258262890683122, 1.000000000000000000, 0.9659258262890683122, 1.000000000000000000, 0.9659258262890683122, 1.000000000000000000, 0.9659258262890683122, 1.000000000000000000, 0.9659258262890683122, 1.000000000000000000, 0.9659258262890683122, 1.000000000000000000, 0.9659258262890683122, 1.000000000000000000, 0.9659258262890683122, 1.000000000000000000, 0.9659258262890683122, 1.000000000000000000, 0.9659258262890683122, 1.000000000000000000, 0.9659258262890683122, 1.000000000000000000, 0.9659258262890683122, 1.000000000000000000, 0.9659258262890683122, 1.000000000000000000, 0.9659258262890683122, 1.000000000000000000, 0.9659258262890683122, 1.000000000000000000, 0.9659258262890683122, 1.000000000000000000, 0.9659258262890683122, 1.000000000000000000, 0.9659258262890683122, 1.000000000000000000, 0.9659258262890683122, 1.000000000000000000, 0.9659258262890683122, 1.000000000000000000, 0.9659258262890683122, 1.000000000000000000, 0.9659258262890683122, 1.000000000000000000, 0.9659258262890683122, 1.000000000000000000, 0.9659258262890683122, 1.000000000000000000, 0.9659258262890683122, 1.000000000000000000, 0.9659258262890683122, 1.000000000000000000, 0.9659258262890683122, 1.000000000000000000, 0.9659258262890683122, 1.000000000000000000, 0.9659258262890683122, 1.000000000000000000, 0.9659258262890683122, 1.000000000000000000, 0.9659258262890683122, 1.000000000000000000, 0.9659258262890683122, 1.000000000000000000, 0.9659258262890683122, 1.000000000000000000),
 ( 1.000000000000000000, 0.9659258262890683122, 1.000000000000000000, 0.9659258262890683122, 1.000000000000000000, 0.9659258262890683122, 1.000000000000000000, 0.9659258262890683122, 1.000000000000000000, 0.9659258262890683122, 1.000000000000000000, 0.9659258262890683122, 1.000000000000000000, 0.9659258262890683122, 1.000000000000000000, 0.9659258262890683122, 1.000000000000000000, 0.9659258262890683122, 1.000000000000000000, 0.9659258262890683122, 1.000000000000000000, 0.9659258262890683122, 1.000000000000000000, 0.9659258262890683122, 1.000000000000000000, 0.9659258262890683122, 1.000000000000000000, 0.9659258262890683122, 1.000000000000000000, 0.9659258262890683122, 1.000000000000000000, 0.9659258262890683122, 1.000000000000000000, 0.9659258262890683122, 1.000000000000000000, 0.9659258262890683122, 1.000000000000000000, 0.9659258262890683122, 1.000000000000000000, 0.9659258262890683122, 1.000000000000000000, 0.9659258262890683122, 1.000000000000000000, 0.9659258262890683122, 1.000000000000000000, 0.9659258262890683122, 1.000000000000000000, 0.9659258262890683122, 1.000000000000000000, 0.9659258262890683122, 1.000000000000000000, 0.9659258262890683122, 1.000000000000000000, 0.9659258262890683122, 1.000000000000000000, 0.9659258262890683122, 1.000000000000000000, 0.9659258262890683122, 1.000000000000000000, 0.9659258262890683122, 1.000000000000000000, 0.9659258262890683122, 1.000000000000000000, 0.9659258262890683122, 1.000000000000000000, 0.9659258262890683122, 1.000000000000000000, 0.9659258262890683122, 1.000000000000000000, 0.9659258262890683122, 1.000000000000000000, 0.9659258262890683122, 1.000000000000000000, 0.9659258262890683122, 1.000000000000000000, 0.9659258262890683122, 1.000000000000000000, 0.9659258262890683122, 1.000000000000000000, 0.9659258262890683122, 1.000000000000000000, 0.9659258262890683122, 1.000000000000000000, 0.9659258262890683122, 1.000000000000000000, 0.9659258262890683122, 1.000000000000000000, 0.9659258262890683122, 1.000000000000000000, 0.9659258262890683122, 1.000000000000000000, 0.9659258262890683122, 1.000000000000000000, 0.9659258262890683122, 1.000000000000000000, 0.9659258262890683122, 1.000000000000000000, 0.9659258262890683122, 1.000000000000000000, 0.9659258262890683122, 1.000000000000000000, 0.9659258262890683122, 1.000000000000000000, 0.9659258262890683122, 1.000000000000000000, 0.9659258262890683122, 1.000000000000000000, 0.9659258262890683122, 1.000000000000000000, 0.9659258262890683122, 1.000000000000000000, 0.9659258262890683122, 1.000000000000000000, 0.9659258262890683122, 1.000000000000000000, 0.9659258262890683122, 1.000000000000000000, 0.9659258262890683122, 1.000000000000000000, 0.9659258262890683122, 1.000000000000000000, 0.9659258262890683122, 1.000000000000000000, 0.9659258262890683122, 1.000000000000000000, 0.9659258262890683122, 1.000000000000000000, 0.9659258262890683122, 1.000000000000000000, 0.9659258262890683122, 1.000000000000000000, 0.9659258262890683122, 1.000000000000000000, 0.9659258262890683122, 1.000000000000000000, 0.9659258262890683122, 1.000000000000000000, 0.9659258262890683122, 1.000000000000000000, 0.9659258262890683122, 1.000000000000000000, 0.9659258262890683122, 1.000000000000000000, 0.9659258262890683122, 1.000000000000000000, 0.9659258262890683122, 1.000000000000000000, 0.9659258262890683122, 1.000000000000000000, 0.9659258262890683122, 1.000000000000000000, 0.9659258262890683122, 1.000000000000000000, 0.9659258262890683122, 1.000000000000000000, 0.9659258262890683122, 1.000000000000000000, 0.9659258262890683122, 1.000000000000000000, 0.9659258262890683122, 1.000000000000000000, 0.9659258262890683122, 1.000000000000000000, 0.9659258262890683122, 1.000000000000000000, 0.9659258262890683122, 1.000000000000000000, 0.9659258262890683122, 1.000000000000000000, 0.9659258262890683122, 1.000000000000000000, 0.9659258262890683122, 1.000000000000000000, 0.9659258262890683122, 1.000000000000000000, 0.9659258262890683122, 1.000000000000000000, 0.9659258262890683122, 1.000000000000000000, 0.9659258262890683122, 1.000000000000000000, 0.9659258262890683122, 1.000000000000000000, 0.9659258262890683122, 1.000000000000000000, 0.9659258262890683122, 1.000000000000000000, 0.9659258262890683122, 1.000000000000000000, 0.9659258262890683122, 1.000000000000000000, 0.9659258262890683122, 1.000000000000000000, 0.9659258262890683122, 1.000000000000000000, 0.9659258262890683122, 1.000000000000000000, 0.9659258262890683122, 1.000000000000000000, 0.9659258262890683122, 1.000000000000000000, 0.9659258262890683122, 1.000000000000000000, 0.9659258262890683122, 1.000000000000000000, 0.9659258262890683122, 1.000000000000000000, 0.9659258262890683122, 1.000000000000000000, 0.9659258262890683122, 1.000000000000000000, 0.9659258262890683122, 1.000000000000000000, 0.9659258262890683122, 1.000000000000000000, 0.9659258262890683122, 1.000000000000000000, 0.9659258262890683122, 1.000000000000000000, 0.9659258262890683122, 1.000000000000000000, 0.9659258262890683122, 1.000000000000000000, 0.9659258262890683122, 1.000000000000000000, 0.9659258262890683122, 1.000000000000000000, 0.9659258262890683122, 1.000000000000000000, 0.9659258262890683122, 1.000000000000000000, 0.9659258262890683122, 1.000000000000000000, 0.9659258262890683122, 1.000000000000000000, 0.9659258262890683122, 1.000000000000000000, 0.9659258262890683122, 1.000000000000000000, 0.9659258262890683122, 1.000000000000000000, 0.9659258262890683122, 1.000000000000000000, 0.9659258262890683122, 1.000000000000000000, 0.9659258262890683122, 1.000000000000000000, 0.9659258262890683122, 1.000000000000000000, 0.9659258262890683122, 1.000000000000000000, 0.9659258262890683122, 1.000000000000000000, 0.9659258262890683122, 1.000000000000000000, 0.9659258262890683122, 1.000000000000000000, 0.9659258262890683122, 1.000000000000000000, 0.9659258262890683122, 1.000000000000000000, 0.9659258262890683122, 1.000000000000000000, 0.9659258262890683122, 1.000000000000000000, 0.9659258262890683122, 1.000000000000000000, 0.9659258262890683122, 1.000000000000000000, 0.9659258262890683122, 1.000000000000000000, 0.9659258262890683122, 1.000000000000000000, 0.9659258262890683122, 1.000000000000000000, 0.9659258262890683122, 1.000000000000000000, 0.9659258262890683122, 1.000000000000000000, 0.9659258262890683122, 1.000000000000000000, 0.9659258262890683122, 1.000000000000000000, 0.9659258262890683122, 1.000000000000000000, 0.9659258262890683122, 1.000000000000000000, 0.9659258262890683122, 1.000000000000000000, 0.9659258262890683122, 1.000000000000000000, 0.9659258262890683122, 1.000000000000000000, 0.9659258262890683122, 1.000000000000000000, 0.9659258262890683122, 1.000000000000000000, 0.9659258262890683122, 1.000000000000000000, 0.9659258262890683122, 1.000000000000000000, 0.9659258262890683122, 1.000000000000000000, 0.9659258262890683122, 1.000000000000000000, 0.9659258262890683122, 1.000000000000000000, 0.9659258262890683122, 1.000000000000000000, 0.9659258262890683122, 1.000000000000000000, 0.9659258262890683122, 1.000000000000000000, 0.9659258262890683122, 1.000000000000000000, 0.9659258262890683122, 1.000000000000000000, 0.9659258262890683122, 1.000000000000000000, 0.9659258262890683122, 1.000000000000000000, 0.9659258262890683122, 1.000000000000000000, 0.9659258262890683122, 1.000000000000000000) ) ) 
 REPRESENTATION_ITEM ( '' )  SURFACE ( )  );
#72043=CARTESIAN_POINT ( 'NONE',  ( 20.88017736071110875, 60.77201867748817676, -2.915334737309920765 ) ) ;
#72047=CARTESIAN_POINT ( 'NONE',  ( 17.96484262340118221, 66.18868534415483396, -7.964842623401177768 ) ) ;
#72049=CARTESIAN_POINT ( 'NONE',  ( -0.8801773607111008646, 68.27201867748817676, 2.915334737309923430 ) ) ;
#72051=CARTESIAN_POINT ( 'NONE',  ( 7.361572987183170547, 22.05059781766745530, 9.846743663894590881 ) ) ;
#72052=CARTESIAN_POINT ( 'NONE',  ( 0.5774900079438607392, 23.48035201082150536, 5.440088680355550821 ) ) ;
#72053=CARTESIAN_POINT ( 'NONE',  ( 1.472469842513823179, 60.59226448433412315, -4.923371831947296329 ) ) ;
#72054=CARTESIAN_POINT ( 'NONE',  ( 20.88017736071110875, 35.77201867748816966, -2.915334737309920765 ) ) ;
#72055=CARTESIAN_POINT ( 'NONE',  ( 0.9413316022086168910, 13.45508385108958826, 6.499999999999973355 ) ) ;
#72056=CARTESIAN_POINT ( 'NONE',  ( 17.39651004071841456, 64.08210964143329136, -6.500000000000001776 ) ) ;
#72058=CARTESIAN_POINT ( 'NONE',  ( -2.816281873526473856, 44.12363466993042493, 9.499525473075851096E-16 ) ) ;
#72060=CARTESIAN_POINT ( 'NONE',  ( 10.00000000000000178, 49.31368534415484106, 10.88017736071110342 ) ) ;
#72061=CARTESIAN_POINT ( 'NONE',  ( 22.81628187352647785, 26.41530133659708923, 3.434112377981063169 ) ) ;
#72062=CARTESIAN_POINT ( 'NONE',  ( -13.69000000000001194, 92.00000000000000000, 9.500000000000000000 ) ) ;
#72064=CARTESIAN_POINT ( 'NONE',  ( 19.42250999205614548, 20.98035201082150891, -5.440088680355545492 ) ) ;
#72065=CARTESIAN_POINT ( 'NONE',  ( 10.00000000000000000, 45.55374883491397497, -14.16423886937410082 ) ) ;
#72066=CARTESIAN_POINT ( 'NONE',  ( 2.791683348922240793, 46.63393115100077324, 7.208316651077764092 ) ) ;
#72067=CARTESIAN_POINT ( 'NONE',  ( 5.076628168052704559, 0.1755978176674514724, -8.527530157486179263 ) ) ;
#72068=CARTESIAN_POINT ( 'NONE',  ( 0.5774900079438607392, 68.48035201082150536, 5.440088680355550821 ) ) ;
#72070=CARTESIAN_POINT ( 'NONE',  ( 20.36894250292379382, 13.67874883491396965, 10.36894250292379205 ) ) ;
#72073=CARTESIAN_POINT ( 'NONE',  ( 17.39651004071842166, 12.93575266056827822, 6.499999999999998224 ) ) ;
#72075=CARTESIAN_POINT ( 'NONE',  ( 6.204703633549690345, 52.84541550158062506, 14.16423886937410082 ) ) ;
#72076=CARTESIAN_POINT ( 'NONE',  ( 22.26659068614894466, 43.88708216824729647, 7.082119434687054849 ) ) ;
#72077=CARTESIAN_POINT ( 'NONE',  ( 7.361572987183169658, 19.96726448433411960, -9.846743663894592657 ) ) ;
#72080=CARTESIAN_POINT ( 'NONE',  ( 20.88017736071110875, 5.772018677488170546, -2.915334737309920765 ) ) ;
#72081=CARTESIAN_POINT ( 'NONE',  ( 22.81628187352647785, 26.62363466993042138, 6.195893100308588602E-16 ) ) ;
#72082=CARTESIAN_POINT ( 'NONE',  ( -0.3689425029237881626, 37.42874883491396787, 10.36894250292379027 ) ) ;
#72086=( LENGTH_UNIT ( ) NAMED_UNIT ( * ) SI_UNIT ( .MILLI., .METRE. ) );
#72087=CARTESIAN_POINT ( 'NONE',  ( 12.63842701281683922, 24.55059781766745175, -9.846743663894590881 ) ) ;
#72090=CARTESIAN_POINT ( 'NONE',  ( -0.8801773607111008646, 8.272018677488171434, 2.915334737309923430 ) ) ;
#72091=CARTESIAN_POINT ( 'NONE',  ( 10.00000000000000000, 6.813685344154838397, -10.88017736071110342 ) ) ;
#72092=CARTESIAN_POINT ( 'NONE',  ( 14.92337183194729633, 52.67559781766745175, 8.527530157486181039 ) ) ;
#72093=CARTESIAN_POINT ( 'NONE',  ( 19.38216949554541202, 5.998634669930420493, 9.382169495545424454 ) ) ;
#72094=DIRECTION ( 'NONE',  ( -0.000000000000000000, -1.000000000000000000, 0.000000000000000000 ) ) ;
#72097=CARTESIAN_POINT ( 'NONE',  ( 13.43411237798106583, 12.66530133659708746, -12.81628187352647252 ) ) ;
#72099=CARTESIAN_POINT ( 'NONE',  ( 22.26659068614895176, 54.72041550158063217, -7.082119434687042414 ) ) ;
#72101=CARTESIAN_POINT ( 'NONE',  ( 22.26659068614894466, 53.88708216824731068, 7.082119434687054849 ) ) ;
#72102=ORIENTED_EDGE ( 'NONE', *, *, #55358, .F. ) ;
#72103=CARTESIAN_POINT ( 'NONE',  ( 4.559911319644449179, 38.89701867748817676, 9.422509992056141925 ) ) ;
#72104=CARTESIAN_POINT ( 'NONE',  ( 12.91533473730993009, 46.60535201082150536, -10.88017736071109987 ) ) ;
#72105=CARTESIAN_POINT ( 'NONE',  ( 7.084665262690076126, 32.02201867748816966, -10.88017736071110164 ) ) ;
#72106=CARTESIAN_POINT ( 'NONE',  ( 20.88017736071110875, 45.77201867748816966, -2.915334737309920765 ) ) ;
#72107=EDGE_CURVE ( 'NONE', #68599, #32737, #41399, .T. ) ;
#72108=EDGE_CURVE ( 'NONE', #156, #90281, #3455, .T. ) ;
#72112=CARTESIAN_POINT ( 'NONE',  ( 0.1532563361054082862, 11.21726448433411605, 2.638427012816831674 ) ) ;
#72113=ORIENTED_EDGE ( 'NONE', *, *, #96068, .T. ) ;
#72115=CARTESIAN_POINT ( 'NONE',  ( 12.63842701281683922, 44.55059781766745175, -9.846743663894590881 ) ) ;
#72117=CARTESIAN_POINT ( 'NONE',  ( 22.81628187352648496, 56.83196800326374643, -3.434112377981050290 ) ) ;
#72119=DIRECTION ( 'NONE',  ( 0.000000000000000000, 0.000000000000000000, -1.000000000000000000 ) ) ;
#72120=CARTESIAN_POINT ( 'NONE',  ( -43.50402400080862009, 106.3600696521562412, 5.072649039476010202 ) ) ;
#72122=CARTESIAN_POINT ( 'NONE',  ( 2.917880565312950480, 60.97041550158063927, -12.26659068614894821 ) ) ;
#72124=VERTEX_POINT ( 'NONE', #83692 ) ;
#72127=CARTESIAN_POINT ( 'NONE',  ( 2.791683348922237240, 30.38393115100078390, -7.208316651077763204 ) ) ;
#72128=CARTESIAN_POINT ( 'NONE',  ( -1.099225684535947600, 63.70696800326376774, -6.408140936763238038 ) ) ;
#72129=CARTESIAN_POINT ( 'NONE',  ( -2.816281873526473856, 4.331968003263754419, 3.434112377981055619 ) ) ;
#72130=CARTESIAN_POINT ( 'NONE',  ( 0.1532563361054100626, 0.8005978176674514168, -2.638427012816831230 ) ) ;
#72132=CARTESIAN_POINT ( 'NONE',  ( 0.1532563361054083140, 11.00893115100078568, 1.131784320476157264E-15 ) ) ;
#72133=CARTESIAN_POINT ( 'NONE',  ( 7.361572987183170547, 52.05059781766745175, 9.846743663894590881 ) ) ;
#72138=CARTESIAN_POINT ( 'NONE',  ( -0.3689425029237881626, 57.42874883491397497, 10.36894250292379027 ) ) ;
#72140=CARTESIAN_POINT ( 'NONE',  ( 19.42250999205614548, 35.98035201082151247, -5.440088680355545492 ) ) ;
#72141=CARTESIAN_POINT ( 'NONE',  ( 13.43411237798106583, 22.66530133659708923, -12.81628187352647252 ) ) ;
#72143=CARTESIAN_POINT ( 'NONE',  ( 4.559911319644449179, 2.230352010821504471, -9.422509992056141925 ) ) ;
#72145=CARTESIAN_POINT ( 'NONE',  ( 1.274849032794280523, 68.57228050351031357, 6.499999999999960032 ) ) ;
#72146=CARTESIAN_POINT ( 'NONE',  ( 17.20831665107776587, 52.88393115100078035, 7.208316651077764980 ) ) ;
#72147=CARTESIAN_POINT ( 'NONE',  ( 2.791683348922237240, 20.38393115100078745, -7.208316651077763204 ) ) ;
#72149=CARTESIAN_POINT ( 'NONE',  ( 22.81628187352648496, 16.83196800326374998, -3.434112377981050290 ) ) ;
#72150=CARTESIAN_POINT ( 'NONE',  ( -45.94000000000001194, 99.99999999999998579, -5.000000000000000000 ) ) ;
#72151=CARTESIAN_POINT ( 'NONE',  ( 20.88017736071110164, 30.35535201082151247, 2.915334737309930979 ) ) ;
#72154=CARTESIAN_POINT ( 'NONE',  ( 2.917880565312950480, 35.97041550158063217, -12.26659068614894821 ) ) ;
#72155=CARTESIAN_POINT ( 'NONE',  ( 13.79529636645030344, 28.26208216824729647, 14.16423886937410614 ) ) ;
#72156=CARTESIAN_POINT ( 'NONE',  ( 20.88017736071110164, 10.35535201082150714, 2.915334737309930979 ) ) ;
#72157=CARTESIAN_POINT ( 'NONE',  ( 19.84674366389459621, 48.50893115100078745, 7.409399052514197653E-17 ) ) ;
#72158=CARTESIAN_POINT ( 'NONE',  ( 0.6178305044545818747, 43.49863466993042493, -9.382169495545419124 ) ) ;
#72159=CARTESIAN_POINT ( 'NONE',  ( 2.035157376598822676, 22.43868534415483396, -7.964842623401177768 ) ) ;
#72161=CARTESIAN_POINT ( 'NONE',  ( 19.84674366389459266, 48.71726448433413026, -2.638427012816827677 ) ) ;
#72162=CARTESIAN_POINT ( 'NONE',  ( 17.96484262340118221, 39.93868534415484106, 7.964842623401181321 ) ) ;
#72163=CARTESIAN_POINT ( 'NONE',  ( -2.816281873526473856, 4.331968003263754419, 3.434112377981055619 ) ) ;
#72164=CARTESIAN_POINT ( 'NONE',  ( 2.917880565312950480, 25.97041550158063572, -12.26659068614894821 ) ) ;
#72167=UNCERTAINTY_MEASURE_WITH_UNIT (LENGTH_MEASURE( 1.000000000000000082E-05 ), #72086, 'distance_accuracy_value', 'NONE');
#72168=CARTESIAN_POINT ( 'NONE',  ( 18.52753015748617571, 28.09226448433411960, 4.923371831947298993 ) ) ;
#72169=CARTESIAN_POINT ( 'NONE',  ( 10.00000000000000000, 47.87363466993042493, -12.81628187352647608 ) ) ;
#72170=CARTESIAN_POINT ( 'NONE',  ( 7.361572987183170547, 67.05059781766746596, 9.846743663894590881 ) ) ;
#72171=ORIENTED_EDGE ( 'NONE', *, *, #11124, .T. ) ;
#72172=CARTESIAN_POINT ( 'NONE',  ( 20.03743638938528804, 11.75197528031017136, 6.399506433553904472 ) ) ;
#72173=CARTESIAN_POINT ( 'NONE',  ( 7.084665262690076126, 2.022018677488171434, -10.88017736071110164 ) ) ;
#72174=CARTESIAN_POINT ( 'NONE',  ( 7.084665262690076126, 62.02201867748816966, -10.88017736071110164 ) ) ;
#72175=CARTESIAN_POINT ( 'NONE',  ( 13.79529636645031943, 15.34541550158063750, -14.16423886937409904 ) ) ;
#72176=CARTESIAN_POINT ( 'NONE',  ( 12.91533473730992121, 64.52201867748817676, 10.88017736071110164 ) ) ;
#72177=CARTESIAN_POINT ( 'NONE',  ( 14.92337183194729633, 47.67559781766745175, 8.527530157486181039 ) ) ;
#72178=CARTESIAN_POINT ( 'NONE',  ( 12.91533473730993009, 36.60535201082151247, -10.88017736071109987 ) ) ;
#72180=CARTESIAN_POINT ( 'NONE',  ( 14.92337183194729633, 62.67559781766745886, 8.527530157486181039 ) ) ;
#72182=CIRCLE ( 'NONE', #65826, 0.5000000000000004441 ) ;
#72185=ORIENTED_EDGE ( 'NONE', *, *, #90571, .F. ) ;
#72187=CARTESIAN_POINT ( 'NONE',  ( -2.266590686148945544, 2.220415501580634388, 7.082119434687048631 ) ) ;
#72188=CARTESIAN_POINT ( 'NONE',  ( 24.16423886937409904, 4.095415501580634832, 3.795296366450317205 ) ) ;
#72189=CARTESIAN_POINT ( 'NONE',  ( 24.16423886937409904, 49.09541550158063217, 3.795296366450317205 ) ) ;
#72190=CARTESIAN_POINT ( 'NONE',  ( 18.52753015748617571, 53.09226448433412315, 4.923371831947298993 ) ) ;
#72191=CARTESIAN_POINT ( 'NONE',  ( 10.00000000000000178, 32.25893115100078745, 9.846743663894594434 ) ) ;
#72192=CARTESIAN_POINT ( 'NONE',  ( 3.591859063236761518, 64.95696800326376774, 11.09922568453594849 ) ) ;
#72193=CARTESIAN_POINT ( 'NONE',  ( 7.084665262690076126, 32.02201867748816966, -10.88017736071110164 ) ) ;
#72194=CARTESIAN_POINT ( 'NONE',  ( 7.361572987183169658, 59.96726448433410894, -9.846743663894592657 ) ) ;
#72195=CARTESIAN_POINT ( 'NONE',  ( 6.204703633549690345, 5.762082168247301794, -14.16423886937410259 ) ) ;
#72196=CARTESIAN_POINT ( 'NONE',  ( -4.164238869374099039, 56.80374883491397497, 8.674139862899312516E-16 ) ) ;
#72197=CARTESIAN_POINT ( 'NONE',  ( 15.44008868035555260, 4.730352010821505360, 9.422509992056143702 ) ) ;
#72198=CARTESIAN_POINT ( 'NONE',  ( 0.1532563361054082862, 66.21726448433413736, 2.638427012816831674 ) ) ;
#72200=CARTESIAN_POINT ( 'NONE',  ( -38.69000000000001194, 93.50000000000000000, 9.500000000000000000 ) ) ;
#72201=CARTESIAN_POINT ( 'NONE',  ( 20.88017736071110519, 60.56368534415484106, 2.639326808657452039E-16 ) ) ;
#72202=CARTESIAN_POINT ( 'NONE',  ( 2.791683348922237240, 25.38393115100078390, -7.208316651077763204 ) ) ;
#72208=CARTESIAN_POINT ( 'NONE',  ( 7.361572987183170547, 17.05059781766745530, 9.846743663894590881 ) ) ;
#72210=CARTESIAN_POINT ( 'NONE',  ( 20.36894250292379382, 28.67874883491396787, 10.36894250292379205 ) ) ;
#72211=CARTESIAN_POINT ( 'NONE',  ( 10.00000000000000000, 34.75893115100078745, -9.846743663894594434 ) ) ;
#72212=CARTESIAN_POINT ( 'NONE',  ( 17.96484262340118221, 51.18868534415483396, -7.964842623401177768 ) ) ;
#72214=CARTESIAN_POINT ( 'NONE',  ( 7.084665262690076126, 49.10535201082149825, 10.88017736071109987 ) ) ;
#72215=CARTESIAN_POINT ( 'NONE',  ( 0.1532563361054083140, 46.00893115100079456, 1.131784320476157264E-15 ) ) ;
#72218=CARTESIAN_POINT ( 'NONE',  ( -0.8801773607111008646, 48.27201867748816966, 2.915334737309923430 ) ) ;
#72219=CARTESIAN_POINT ( 'NONE',  ( 22.26659068614895176, 24.72041550158063572, -7.082119434687042414 ) ) ;
#72222=CARTESIAN_POINT ( 'NONE',  ( 22.81628187352647785, 36.41530133659707502, 3.434112377981063169 ) ) ;
#72223=CARTESIAN_POINT ( 'NONE',  ( 1.472469842513823179, 20.59226448433411960, -4.923371831947296329 ) ) ;
#72224=CARTESIAN_POINT ( 'NONE',  ( 2.035157376598824452, 3.688685344154837953, 7.964842623401179544 ) ) ;
#72225=CARTESIAN_POINT ( 'NONE',  ( 10.00000000000000000, 52.87363466993041783, -12.81628187352647608 ) ) ;
#72226=CYLINDRICAL_SURFACE ( 'NONE', #55959, 0.5000000000000004441 ) ;
#72227=CARTESIAN_POINT ( 'NONE',  ( 14.92337183194729633, 32.67559781766745175, 8.527530157486181039 ) ) ;
#72228=EDGE_CURVE ( 'NONE', #13314, #14763, #85656, .T. ) ;
#72229=CARTESIAN_POINT ( 'NONE',  ( 2.035157376598824452, 58.68868534415482685, 7.964842623401179544 ) ) ;
#72230=ORIENTED_EDGE ( 'NONE', *, *, #5652, .F. ) ;
#72234=CARTESIAN_POINT ( 'NONE',  ( 17.20831665107776587, 2.883931151000785231, 7.208316651077764980 ) ) ;
#72235=CARTESIAN_POINT ( 'NONE',  ( 6.565887622018943937, 18.08196800326375708, -12.81628187352647608 ) ) ;
#72237=CARTESIAN_POINT ( 'NONE',  ( 0.1532563361054100626, 40.80059781766745886, -2.638427012816831230 ) ) ;
#72239=CARTESIAN_POINT ( 'NONE',  ( 22.26659068614895176, 4.720415501580633943, -7.082119434687042414 ) ) ;
#72240=CARTESIAN_POINT ( 'NONE',  ( 17.20831665107776587, 32.88393115100078745, 7.208316651077764980 ) ) ;
#72241=CARTESIAN_POINT ( 'NONE',  ( 21.09922568453594849, 31.20696800326375353, 6.408140936763242479 ) ) ;
#72244=CARTESIAN_POINT ( 'NONE',  ( 10.00000000000000000, 61.81368534415484106, -10.88017736071110342 ) ) ;
#72245=CARTESIAN_POINT ( 'NONE',  ( 3.591859063236761518, 4.956968003263753531, 11.09922568453594849 ) ) ;
#72247=CARTESIAN_POINT ( 'NONE',  ( 2.791683348922237240, 40.38393115100078035, -7.208316651077763204 ) ) ;
#72248=CARTESIAN_POINT ( 'NONE',  ( 7.084665262690076126, 22.02201867748817321, -10.88017736071110164 ) ) ;
#72249=CARTESIAN_POINT ( 'NONE',  ( 10.00000000000000178, 30.37363466993042138, 12.81628187352647608 ) ) ;
#72250=MECHANICAL_DESIGN_GEOMETRIC_PRESENTATION_REPRESENTATION('',(#81812),#64246);
#72251=CARTESIAN_POINT ( 'NONE',  ( 5.076628168052703671, 16.84226448433411960, 8.527530157486179263 ) ) ;
#72253=CARTESIAN_POINT ( 'NONE',  ( 3.035766082959412415E-15, 78.91966277462714174, -5.000000000000000000 ) ) ;
#72255=CARTESIAN_POINT ( 'NONE',  ( -0.8801773607110991993, 27.85535201082150181, -2.915334737309923874 ) ) ;
#72256=ORIENTED_EDGE ( 'NONE', *, *, #24195, .T. ) ;
#72258=CARTESIAN_POINT ( 'NONE',  ( 17.96484262340118221, 64.93868534415483396, 7.964842623401181321 ) ) ;
#72259=CARTESIAN_POINT ( 'NONE',  ( 10.00000000000000000, 1.813685344154837731, -10.88017736071110342 ) ) ;
#72260=CARTESIAN_POINT ( 'NONE',  ( 14.92337183194729633, 37.67559781766745175, 8.527530157486181039 ) ) ;
#72261=CARTESIAN_POINT ( 'NONE',  ( 17.96484262340118221, 26.18868534415483396, -7.964842623401177768 ) ) ;
#72262=DIRECTION ( 'NONE',  ( -0.5547001962252290364, -0.8320502943378437211, 0.000000000000000000 ) ) ;
#72264=CARTESIAN_POINT ( 'NONE',  ( 4.559911319644449179, 48.89701867748817676, 9.422509992056141925 ) ) ;
#72265=CARTESIAN_POINT ( 'NONE',  ( 17.96484262340118221, 9.938685344154839285, 7.964842623401181321 ) ) ;
#72267=CARTESIAN_POINT ( 'NONE',  ( 12.63842701281683922, 4.550597817667451750, -9.846743663894590881 ) ) ;
#72268=CARTESIAN_POINT ( 'NONE',  ( 17.20831665107776587, 57.88393115100078745, 7.208316651077764980 ) ) ;
#72269=CARTESIAN_POINT ( 'NONE',  ( 10.00000000000000178, 48.05374883491396787, 14.16423886937410082 ) ) ;
#72271=CARTESIAN_POINT ( 'NONE',  ( 10.00000000000000000, 35.55374883491396787, -14.16423886937410082 ) ) ;
#72274=CARTESIAN_POINT ( 'NONE',  ( 12.91533473730992121, 4.522018677488170546, 10.88017736071110164 ) ) ;
#72275=CARTESIAN_POINT ( 'NONE',  ( 7.361572987183169658, 34.96726448433411605, -9.846743663894592657 ) ) ;
#72277=PLANE ( 'NONE',  #86989 ) ;
#72278=CARTESIAN_POINT ( 'NONE',  ( -0.8801773607110991993, 62.85535201082150536, -2.915334737309923874 ) ) ;
#72280=CARTESIAN_POINT ( 'NONE',  ( -0.8801773607111008646, 33.27201867748817676, 2.915334737309923430 ) ) ;
#72281=CARTESIAN_POINT ( 'NONE',  ( 13.43411237798105340, 55.58196800326374643, 12.81628187352647963 ) ) ;
#72282=CARTESIAN_POINT ( 'NONE',  ( 22.81628187352648496, 16.83196800326374998, -3.434112377981050290 ) ) ;
#72283=CARTESIAN_POINT ( 'NONE',  ( 19.84674366389459621, 8.508931151000785675, 7.409399052514197653E-17 ) ) ;
#72285=CARTESIAN_POINT ( 'NONE',  ( -4.164238869374099927, 62.01208216824728936, 3.795296366450308767 ) ) ;
#72287=CARTESIAN_POINT ( 'NONE',  ( 10.00000000000000178, 23.05374883491397142, 14.16423886937410082 ) ) ;
#72288=CARTESIAN_POINT ( 'NONE',  ( 2.035157376598824452, 38.68868534415483396, 7.964842623401179544 ) ) ;
#72289=CARTESIAN_POINT ( 'NONE',  ( 20.88017736071110519, 45.56368534415484106, 2.639326808657452039E-16 ) ) ;
#72293=CARTESIAN_POINT ( 'NONE',  ( 1.472469842513823179, 11.42559781766745175, 4.923371831947296329 ) ) ;
#72294=CARTESIAN_POINT ( 'NONE',  ( 20.03743638938523830, 21.75197528031017669, 6.399506433553980855 ) ) ;
#72295=CARTESIAN_POINT ( 'NONE',  ( -46.50477113700967635, 102.7537820721726831, 6.796471197945592735 ) ) ;
#72296=CARTESIAN_POINT ( 'NONE',  ( 0.1532563361054100626, 20.80059781766744464, -2.638427012816831230 ) ) ;
#72297=CARTESIAN_POINT ( 'NONE',  ( 0.1532563361054083140, 56.00893115100078745, 1.131784320476157264E-15 ) ) ;
#72299=CARTESIAN_POINT ( 'NONE',  ( 10.00000000000000000, 26.81368534415484106, -10.88017736071110342 ) ) ;
#72300=UNCERTAINTY_MEASURE_WITH_UNIT (LENGTH_MEASURE( 1.000000000000000082E-05 ), #46609, 'distance_accuracy_value', 'NONE');
#72301=CARTESIAN_POINT ( 'NONE',  ( 0.6178305044545838731, 39.74863466993041072, 9.382169495545420901 ) ) ;
#72302=CARTESIAN_POINT ( 'NONE',  ( 0.5774900079438607392, 63.48035201082149825, 5.440088680355550821 ) ) ;
#72303=CARTESIAN_POINT ( 'NONE',  ( 2.791683348922237240, 25.38393115100078390, -7.208316651077763204 ) ) ;
#72304=CARTESIAN_POINT ( 'NONE',  ( 2.917880565312950480, 60.97041550158063927, -12.26659068614894821 ) ) ;
#72305=CARTESIAN_POINT ( 'NONE',  ( 10.00000000000000178, 27.25893115100078390, 9.846743663894594434 ) ) ;
#72307=CARTESIAN_POINT ( 'NONE',  ( 22.26659068614895176, 14.72041550158063572, -7.082119434687042414 ) ) ;
#72308=CARTESIAN_POINT ( 'NONE',  ( -0.3689425029237881626, 37.42874883491396787, 10.36894250292379027 ) ) ;
#72309=CARTESIAN_POINT ( 'NONE',  ( 0.1532563361054083140, 26.00893115100078745, 1.131784320476157264E-15 ) ) ;
#72310=CARTESIAN_POINT ( 'NONE',  ( -0.3077640640441539621, 70.00000000000000000, 5.999999999999999112 ) ) ;
#72311=CARTESIAN_POINT ( 'NONE',  ( 19.42250999205614193, 30.14701867748817321, 5.440088680355555262 ) ) ;
#72312=CARTESIAN_POINT ( 'NONE',  ( -0.8801773607110991993, 52.85535201082151247, -2.915334737309923874 ) ) ;
#72313=CARTESIAN_POINT ( 'NONE',  ( 1.472469842513823179, 56.42559781766745886, 4.923371831947296329 ) ) ;
#72314=ORIENTED_EDGE ( 'NONE', *, *, #23539, .T. ) ;
#72315=CARTESIAN_POINT ( 'NONE',  ( -2.816281873526471635, 48.91530133659708213, -3.434112377981056508 ) ) ;
#72316=CARTESIAN_POINT ( 'NONE',  ( 20.88017736071110875, 50.77201867748817676, -2.915334737309920765 ) ) ;
#72317=ORIENTED_EDGE ( 'NONE', *, *, #16399, .T. ) ;
#72318=CARTESIAN_POINT ( 'NONE',  ( 7.084665262690076126, 59.10535201082150536, 10.88017736071109987 ) ) ;
#72321=CARTESIAN_POINT ( 'NONE',  ( 17.96484262340118221, 64.93868534415483396, 7.964842623401181321 ) ) ;
#72322=CARTESIAN_POINT ( 'NONE',  ( 20.88017736071110875, 60.77201867748817676, -2.915334737309920321 ) ) ;
#72323=CARTESIAN_POINT ( 'NONE',  ( 19.72487221294570858, 0.000000000000000000, -6.500000000000000888 ) ) ;
#72324=CARTESIAN_POINT ( 'NONE',  ( 12.91533473730992121, 9.522018677488171434, 10.88017736071110164 ) ) ;
#72325=CARTESIAN_POINT ( 'NONE',  ( 17.20831665107776587, 14.13393115100078568, -7.208316651077762316 ) ) ;
#72326=CARTESIAN_POINT ( 'NONE',  ( 17.08211943468705840, 20.13708216824730357, -12.26659068614894466 ) ) ;
#72327=CARTESIAN_POINT ( 'NONE',  ( 18.52753015748617571, 3.092264484334118269, 4.923371831947298993 ) ) ;
#72328=CARTESIAN_POINT ( 'NONE',  ( 19.42250999205614193, 30.14701867748817321, 5.440088680355555262 ) ) ;
#72329=CARTESIAN_POINT ( 'NONE',  ( 5.076628168052703671, 56.84226448433412315, 8.527530157486179263 ) ) ;
#72331=CARTESIAN_POINT ( 'NONE',  ( 7.361572987183170547, 52.05059781766745175, 9.846743663894590881 ) ) ;
#72332=ORIENTED_EDGE ( 'NONE', *, *, #93915, .F. ) ;
#72333=CYLINDRICAL_SURFACE ( 'NONE', #82855, 0.5000000000000004441 ) ;
#72335=CARTESIAN_POINT ( 'NONE',  ( 17.96484262340118221, 51.18868534415483396, -7.964842623401177768 ) ) ;
#72336=CARTESIAN_POINT ( 'NONE',  ( 10.00000000000000000, 49.75893115100078745, -9.846743663894594434 ) ) ;
#72337=CARTESIAN_POINT ( 'NONE',  ( 0.5774900079438607392, 13.48035201082150358, 5.440088680355550821 ) ) ;
#72339=CARTESIAN_POINT ( 'NONE',  ( 2.035157376598824452, 63.68868534415484106, 7.964842623401179544 ) ) ;
#72340=CARTESIAN_POINT ( 'NONE',  ( 20.88017736071110875, 10.77201867748817143, -2.915334737309920765 ) ) ;
#72342=CARTESIAN_POINT ( 'NONE',  ( -2.816281873526473856, 44.33196800326375353, 3.434112377981055619 ) ) ;
#72343=CARTESIAN_POINT ( 'NONE',  ( 17.96484262340118221, 31.18868534415483751, -7.964842623401177768 ) ) ;
#72344=DIRECTION ( 'NONE',  ( 0.000000000000000000, -1.000000000000000000, 0.000000000000000000 ) ) ;
#72345=EDGE_CURVE ( 'NONE', #64921, #20501, #75654, .T. ) ;
#72347=CARTESIAN_POINT ( 'NONE',  ( 3.591859063236763294, 38.29030133659708923, -11.09922568453595026 ) ) ;
#72348=CARTESIAN_POINT ( 'NONE',  ( 4.559911319644449179, 32.23035201082150536, -9.422509992056141925 ) ) ;
#72350=CARTESIAN_POINT ( 'NONE',  ( 0.1532563361054100626, 60.80059781766744464, -2.638427012816831230 ) ) ;
#72352=CARTESIAN_POINT ( 'NONE',  ( 5.076628168052703671, 11.84226448433411960, 8.527530157486179263 ) ) ;
#72353=CARTESIAN_POINT ( 'NONE',  ( 7.361572987183169658, 49.96726448433410894, -9.846743663894592657 ) ) ;
#72354=CARTESIAN_POINT ( 'NONE',  ( 0.5774900079438590739, 17.64701867748817321, -5.440088680355550821 ) ) ;
#72355=CARTESIAN_POINT ( 'NONE',  ( 0.1532563361054100626, 35.80059781766745175, -2.638427012816831230 ) ) ;
#72359=CARTESIAN_POINT ( 'NONE',  ( 19.84674366389459266, 28.71726448433411960, -2.638427012816827677 ) ) ;
#72360=CARTESIAN_POINT ( 'NONE',  ( 0.1532563361054082862, 11.21726448433411605, 2.638427012816831674 ) ) ;
#72361=CARTESIAN_POINT ( 'NONE',  ( 0.6081133539230624274, 8.337033823263999111, 6.500000000000005329 ) ) ;
#72362=CARTESIAN_POINT ( 'NONE',  ( 2.791683348922237240, 65.38393115100078035, -7.208316651077763204 ) ) ;
#72363=ORIENTED_EDGE ( 'NONE', *, *, #32933, .F. ) ;
#72365=CARTESIAN_POINT ( 'NONE',  ( 19.88565890683628368, 7.716910754863025801, -6.480892540919851008 ) ) ;
#72366=CARTESIAN_POINT ( 'NONE',  ( 3.591859063236763294, 38.29030133659708923, -11.09922568453595026 ) ) ;
#72368=CARTESIAN_POINT ( 'NONE',  ( 7.361572987183169658, 44.96726448433412315, -9.846743663894592657 ) ) ;
#72369=CARTESIAN_POINT ( 'NONE',  ( 0.1089645850228881108, 8.162345557925705819, 6.479102184480789894 ) ) ;
#72370=CARTESIAN_POINT ( 'NONE',  ( 6.204703633549690345, 60.76208216824730357, -14.16423886937410259 ) ) ;
#72371=CARTESIAN_POINT ( 'NONE',  ( 14.92337183194729988, 24.34226448433411960, -8.527530157486177487 ) ) ;
#72373=CARTESIAN_POINT ( 'NONE',  ( 19.50000000000000711, 79.40087001978916703, 4.999999999999999112 ) ) ;
#72374=EDGE_CURVE ( 'NONE', #90157, #9521, #90934, .T. ) ;
#72375=CARTESIAN_POINT ( 'NONE',  ( 6.204703633549690345, 50.76208216824730357, -14.16423886937410259 ) ) ;
#72376=CARTESIAN_POINT ( 'NONE',  ( 10.00000000000000178, 57.25893115100078745, 9.846743663894594434 ) ) ;
#72378=CARTESIAN_POINT ( 'NONE',  ( 12.91533473730992121, 4.522018677488170546, 10.88017736071110164 ) ) ;
#72379=CARTESIAN_POINT ( 'NONE',  ( 17.08211943468705130, 38.47041550158063217, 12.26659068614894998 ) ) ;
#72380=CARTESIAN_POINT ( 'NONE',  ( 20.36894250292379382, 33.67874883491396076, 10.36894250292379205 ) ) ;
#72383=CARTESIAN_POINT ( 'NONE',  ( 14.92337183194729633, 57.67559781766745886, 8.527530157486181039 ) ) ;
#72385=CARTESIAN_POINT ( 'NONE',  ( 20.88017736071110875, 55.77201867748816966, -2.915334737309920765 ) ) ;
#72386=CARTESIAN_POINT ( 'NONE',  ( 19.67388484268946058, 90.60256703073459050, -5.439657303569386926 ) ) ;
#72387=CARTESIAN_POINT ( 'NONE',  ( 1.472469842513823179, 51.42559781766745886, 4.923371831947296329 ) ) ;
#72388=CARTESIAN_POINT ( 'NONE',  ( 13.43411237798106583, 62.66530133659708923, -12.81628187352647252 ) ) ;
#72389=CARTESIAN_POINT ( 'NONE',  ( 1.472469842513823179, 56.42559781766745886, 4.923371831947296329 ) ) ;
#72390=FACE_OUTER_BOUND ( 'NONE', #96481, .T. ) ;
#72392=CARTESIAN_POINT ( 'NONE',  ( 24.16423886937410614, 29.30374883491396787, 8.672049930838204340E-16 ) ) ;
#72394=DIRECTION ( 'NONE',  ( 0.000000000000000000, 0.000000000000000000, -1.000000000000000000 ) ) ;
#72395=CARTESIAN_POINT ( 'NONE',  ( 4.559911319644449179, 23.89701867748817321, 9.422509992056141925 ) ) ;
#72397=CARTESIAN_POINT ( 'NONE',  ( 6.565887622018943937, 23.08196800326375708, -12.81628187352647608 ) ) ;
#72399=CARTESIAN_POINT ( 'NONE',  ( 2.791683348922240793, 11.63393115100078568, 7.208316651077764092 ) ) ;
#72403=B_SPLINE_CURVE_WITH_KNOTS ( 'NONE', 3,
 ( #98394, #36381, #89868, #21383, #82362, #53851 ),
 .UNSPECIFIED., .F., .F.,
 ( 4, 2, 4 ),
 ( 0.000000000000000000, 0.0002605067024380873812, 0.0005210134048761747624 ),
 .UNSPECIFIED. ) ;
#72404=CARTESIAN_POINT ( 'NONE',  ( 2.917880565312948704, 27.63708216824730357, 12.26659068614894643 ) ) ;
#72406=CARTESIAN_POINT ( 'NONE',  ( 4.559911319644449179, 3.897018677488171434, 9.422509992056141925 ) ) ;
#72408=CARTESIAN_POINT ( 'NONE',  ( -0.8801773607111009756, 43.06368534415484106, 1.068504757029289695E-15 ) ) ;
#72409=CARTESIAN_POINT ( 'NONE',  ( 17.96484262340118221, 31.18868534415483751, -7.964842623401177768 ) ) ;
#72410=VECTOR ( 'NONE', #80739, 1000.000000000000000 ) ;
#72411=CARTESIAN_POINT ( 'NONE',  ( 13.43411237798105340, 10.58196800326375353, 12.81628187352647963 ) ) ;
#72412=CARTESIAN_POINT ( 'NONE',  ( 0.6261916924966959286, 0.5000000000000002220, 6.500000000000003553 ) ) ;
#72413=CARTESIAN_POINT ( 'NONE',  ( 14.92337183194729633, 12.67559781766745353, 8.527530157486181039 ) ) ;
#72415=CARTESIAN_POINT ( 'NONE',  ( 17.96484262340118221, 39.93868534415484106, 7.964842623401181321 ) ) ;
#72417=UNCERTAINTY_MEASURE_WITH_UNIT (LENGTH_MEASURE( 1.000000000000000082E-05 ), #64780, 'distance_accuracy_value', 'NONE');
#72418=CARTESIAN_POINT ( 'NONE',  ( 16.40814093676324603, 2.456968003263753531, -11.09922568453594671 ) ) ;
#72419=CARTESIAN_POINT ( 'NONE',  ( 17.96484262340118221, 64.93868534415483396, 7.964842623401181321 ) ) ;
#72420=CARTESIAN_POINT ( 'NONE',  ( 18.52753015748618282, 23.92559781766745530, -4.923371831947291888 ) ) ;
#72421=CARTESIAN_POINT ( 'NONE',  ( 16.40814093676323893, 40.79030133659708923, 11.09922568453595026 ) ) ;
#72422=CARTESIAN_POINT ( 'NONE',  ( 7.084665262690076126, 69.10535201082151957, 10.88017736071109987 ) ) ;
#72425=PRESENTATION_STYLE_ASSIGNMENT (( #41477 ) ) ;
#72427=CARTESIAN_POINT ( 'NONE',  ( 10.00000000000000000, 1.813685344154837731, -10.88017736071110342 ) ) ;
#72428=FACE_OUTER_BOUND ( 'NONE', #79892, .T. ) ;
#72429=CARTESIAN_POINT ( 'NONE',  ( 2.917880565312948704, 22.63708216824730002, 12.26659068614894643 ) ) ;
#72430=CARTESIAN_POINT ( 'NONE',  ( 12.63842701281683922, 24.55059781766745175, -9.846743663894590881 ) ) ;
#72431=CARTESIAN_POINT ( 'NONE',  ( 17.96484262340118221, 24.93868534415484461, 7.964842623401181321 ) ) ;
#72432=CARTESIAN_POINT ( 'NONE',  ( -2.266590686148945544, 66.38708216824730357, -7.082119434687050408 ) ) ;
#72434=CARTESIAN_POINT ( 'NONE',  ( 2.035157376598824452, 13.68868534415483751, 7.964842623401179544 ) ) ;
#72435=CARTESIAN_POINT ( 'NONE',  ( 15.44008868035555793, 26.39701867748817321, -9.422509992056140149 ) ) ;
#72437=ORIENTED_EDGE ( 'NONE', *, *, #59750, .T. ) ;
#72438=CARTESIAN_POINT ( 'NONE',  ( 21.92686044187657046, 27.39664270246083788, -3.195792623639524432 ) ) ;
#72439=CARTESIAN_POINT ( 'NONE',  ( 17.96484262340118221, 26.18868534415483396, -7.964842623401177768 ) ) ;
#72440=CARTESIAN_POINT ( 'NONE',  ( 17.20831665107776587, 62.88393115100078745, 7.208316651077764980 ) ) ;
#72442=CARTESIAN_POINT ( 'NONE',  ( 13.43411237798106583, 57.66530133659708923, -12.81628187352647252 ) ) ;
#72443=CARTESIAN_POINT ( 'NONE',  ( -0.1503990784575328643, 5.127771745786130708, 6.262539305110068177 ) ) ;
#72444=CARTESIAN_POINT ( 'NONE',  ( 13.79529636645031943, 30.34541550158063927, -14.16423886937409904 ) ) ;
#72445=CARTESIAN_POINT ( 'NONE',  ( 19.42250999205614548, 40.98035201082150536, -5.440088680355545492 ) ) ;
#72446=CARTESIAN_POINT ( 'NONE',  ( 12.91533473730993009, 11.60535201082150714, -10.88017736071109987 ) ) ;
#72447=CARTESIAN_POINT ( 'NONE',  ( 12.63842701281683922, 54.55059781766745175, -9.846743663894590881 ) ) ;
#72449=CARTESIAN_POINT ( 'NONE',  ( 18.52753015748618282, 43.92559781766745175, -4.923371831947291888 ) ) ;
#72451=LINE ( 'NONE', #11469, #38333 ) ;
#72452=CARTESIAN_POINT ( 'NONE',  ( 18.52753015748618282, 13.92559781766745175, -4.923371831947291888 ) ) ;
#72455=CARTESIAN_POINT ( 'NONE',  ( 4.559911319644449179, 7.230352010821504471, -9.422509992056141925 ) ) ;
#72456=CARTESIAN_POINT ( 'NONE',  ( 1.472469842513823179, 5.592264484334118713, -4.923371831947296329 ) ) ;
#72457=CARTESIAN_POINT ( 'NONE',  ( 17.20831665107776587, 64.13393115100079456, -7.208316651077762316 ) ) ;
#72458=CARTESIAN_POINT ( 'NONE',  ( 15.44008868035555793, 61.39701867748817676, -9.422509992056140149 ) ) ;
#72459=CARTESIAN_POINT ( 'NONE',  ( 4.559911319644449179, 22.23035201082150536, -9.422509992056141925 ) ) ;
#72460=CARTESIAN_POINT ( 'NONE',  ( 6.565887622018943937, 48.08196800326375353, -12.81628187352647608 ) ) ;
#72461=CARTESIAN_POINT ( 'NONE',  ( 24.16423886937409904, 29.09541550158063572, 3.795296366450317205 ) ) ;
#72466=CARTESIAN_POINT ( 'NONE',  ( -2.816281873526471635, 53.91530133659709634, -3.434112377981056508 ) ) ;
#72468=EDGE_LOOP ( 'NONE', ( #29999, #57100, #14007, #22676 ) ) ;
#72469=CARTESIAN_POINT ( 'NONE',  ( 6.565887622018943937, 3.081968003263753531, -12.81628187352647608 ) ) ;
#72470=FILL_AREA_STYLE_COLOUR ( '', #36185 ) ;
#72471=CARTESIAN_POINT ( 'NONE',  ( 17.96484262340118221, 29.93868534415484106, 7.964842623401181321 ) ) ;
#72475=CARTESIAN_POINT ( 'NONE',  ( 19.84674366389459266, 8.717264484334116048, -2.638427012816827677 ) ) ;
#72476=CARTESIAN_POINT ( 'NONE',  ( 17.20831665107776587, 9.133931151000787452, -7.208316651077762316 ) ) ;
#72477=CARTESIAN_POINT ( 'NONE',  ( 18.52753015748617571, 23.09226448433411960, 4.923371831947298993 ) ) ;
#72478=CARTESIAN_POINT ( 'NONE',  ( 19.84674366389459621, 13.50893115100078568, 7.409399052514197653E-17 ) ) ;
#72479=CARTESIAN_POINT ( 'NONE',  ( 0.1532563361054082862, 1.217264484334117824, 2.638427012816831674 ) ) ;
#72480=CARTESIAN_POINT ( 'NONE',  ( 7.084665262690076126, 54.10535201082151247, 10.88017736071109987 ) ) ;
#72482=CARTESIAN_POINT ( 'NONE',  ( 10.00000000000000000, 56.81368534415484106, -10.88017736071110342 ) ) ;
#72483=CARTESIAN_POINT ( 'NONE',  ( 5.076628168052704559, 25.17559781766745175, -8.527530157486179263 ) ) ;
#72486=CARTESIAN_POINT ( 'NONE',  ( 1.472469842513823179, 60.59226448433412315, -4.923371831947296329 ) ) ;
#72488=ORIENTED_EDGE ( 'NONE', *, *, #17104, .T. ) ;
#72489=CARTESIAN_POINT ( 'NONE',  ( 17.96484262340118221, 4.938685344154837509, 7.964842623401181321 ) ) ;
#72490=CARTESIAN_POINT ( 'NONE',  ( 24.16423886937410614, 24.51208216824730002, -3.795296366450302550 ) ) ;
#72491=UNCERTAINTY_MEASURE_WITH_UNIT (LENGTH_MEASURE( 1.000000000000000082E-05 ), #98428, 'distance_accuracy_value', 'NONE');
#72492=CYLINDRICAL_SURFACE ( 'NONE', #67908, 0.5000000000000004441 ) ;
#72494=CARTESIAN_POINT ( 'NONE',  ( -4.164238869374098151, 11.59541550158063217, -3.795296366450310543 ) ) ;
#72495=CARTESIAN_POINT ( 'NONE',  ( 20.36894250292379382, 33.67874883491396076, 10.36894250292379205 ) ) ;
#72497=CARTESIAN_POINT ( 'NONE',  ( 15.44008868035555260, 39.73035201082150536, 9.422509992056143702 ) ) ;
#72498=( NAMED_UNIT ( * ) PLANE_ANGLE_UNIT ( ) SI_UNIT ( $, .RADIAN. ) );
#72500=CARTESIAN_POINT ( 'NONE',  ( 10.00000000000000000, 14.75893115100078568, -9.846743663894594434 ) ) ;
#72501=CARTESIAN_POINT ( 'NONE',  ( 7.084665262690076126, 57.02201867748817676, -10.88017736071110164 ) ) ;
#72502=CARTESIAN_POINT ( 'NONE',  ( 7.361572987183169658, 19.96726448433411960, -9.846743663894592657 ) ) ;
#72503=CARTESIAN_POINT ( 'NONE',  ( 10.00000000000000000, 6.813685344154838397, -10.88017736071110342 ) ) ;
#72504=CARTESIAN_POINT ( 'NONE',  ( 16.40814093676323893, 50.79030133659708923, 11.09922568453595026 ) ) ;
#72505=CARTESIAN_POINT ( 'NONE',  ( 7.361572987183170547, 42.05059781766745886, 9.846743663894590881 ) ) ;
#72507=CARTESIAN_POINT ( 'NONE',  ( 21.09922568453595559, 27.04030133659708568, -6.408140936763230044 ) ) ;
#72509=CARTESIAN_POINT ( 'NONE',  ( 0.1532563361054100626, 25.80059781766744820, -2.638427012816831230 ) ) ;
#72510=CARTESIAN_POINT ( 'NONE',  ( 24.16423886937410614, 9.512082168247301794, -3.795296366450302550 ) ) ;
#72513=CARTESIAN_POINT ( 'NONE',  ( -0.8801773607110991993, 52.85535201082151247, -2.915334737309923874 ) ) ;
#72514=CARTESIAN_POINT ( 'NONE',  ( 7.084665262690076126, 52.02201867748816255, -10.88017736071110164 ) ) ;
#72515=CARTESIAN_POINT ( 'NONE',  ( 6.204703633549690345, 47.84541550158064638, 14.16423886937410082 ) ) ;
#72516=CARTESIAN_POINT ( 'NONE',  ( 12.63842701281683922, 59.55059781766744464, -9.846743663894590881 ) ) ;
#72517=CARTESIAN_POINT ( 'NONE',  ( 0.1532563361054082862, 16.21726448433411960, 2.638427012816831674 ) ) ;
#72518=DIRECTION ( 'NONE',  ( 0.000000000000000000, 0.000000000000000000, -1.000000000000000000 ) ) ;
#72519=CARTESIAN_POINT ( 'NONE',  ( 20.88017736071110164, 45.35535201082149115, 2.915334737309930979 ) ) ;
#72521=CARTESIAN_POINT ( 'NONE',  ( -1.099225684535947600, 23.70696800326375708, -6.408140936763238038 ) ) ;
#72522=CARTESIAN_POINT ( 'NONE',  ( 2.791683348922240793, 56.63393115100078035, 7.208316651077764092 ) ) ;
#72524=CARTESIAN_POINT ( 'NONE',  ( 20.88017736071110519, 65.56368534415483396, 2.639326808657452039E-16 ) ) ;
#72525=CARTESIAN_POINT ( 'NONE',  ( 7.084665262690076126, 7.022018677488169658, -10.88017736071110164 ) ) ;
#72526=CARTESIAN_POINT ( 'NONE',  ( 5.076628168052703671, 1.842264484334118047, 8.527530157486179263 ) ) ;
#72527=CARTESIAN_POINT ( 'NONE',  ( 17.96484262340118221, 64.93868534415483396, 7.964842623401181321 ) ) ;
#72530=CARTESIAN_POINT ( 'NONE',  ( 7.361572987183170547, 37.05059781766744464, 9.846743663894590881 ) ) ;
#72531=CARTESIAN_POINT ( 'NONE',  ( 20.88017736071110875, 20.77201867748816611, -2.915334737309920765 ) ) ;
#72532=CARTESIAN_POINT ( 'NONE',  ( 0.1532563361054083140, 61.00893115100078745, 1.131784320476157264E-15 ) ) ;
#72533=CARTESIAN_POINT ( 'NONE',  ( 0.5774900079438607392, 33.48035201082150536, 5.440088680355550821 ) ) ;
#72536=CARTESIAN_POINT ( 'NONE',  ( 19.38216949554541557, 37.24863466993041783, -9.382169495545420901 ) ) ;
#72538=CARTESIAN_POINT ( 'NONE',  ( 12.91533473730992121, 54.52201867748816255, 10.88017736071110164 ) ) ;
#72540=CARTESIAN_POINT ( 'NONE',  ( 21.09922568453595559, 17.04030133659708923, -6.408140936763230044 ) ) ;
#72542=CARTESIAN_POINT ( 'NONE',  ( 0.1532563361054082862, 1.217264484334117824, 2.638427012816831674 ) ) ;
#72543=CARTESIAN_POINT ( 'NONE',  ( 10.00000000000000178, 24.31368534415484106, 10.88017736071110342 ) ) ;
#72544=CARTESIAN_POINT ( 'NONE',  ( 10.00000000000000178, 58.05374883491397497, 14.16423886937410082 ) ) ;
#72545=CARTESIAN_POINT ( 'NONE',  ( 7.361572987183170547, 47.05059781766745175, 9.846743663894590881 ) ) ;
#72546=CARTESIAN_POINT ( 'NONE',  ( 14.92337183194729633, 7.675597817667451750, 8.527530157486181039 ) ) ;
#72547=CARTESIAN_POINT ( 'NONE',  ( 19.42250999205614193, 60.14701867748817676, 5.440088680355555262 ) ) ;
#72549=CARTESIAN_POINT ( 'NONE',  ( 22.26659068614894466, 23.88708216824730357, 7.082119434687054849 ) ) ;
#72554=VERTEX_POINT ( 'NONE', #16433 ) ;
#72556=CARTESIAN_POINT ( 'NONE',  ( -0.3689425029237881626, 42.42874883491396787, 10.36894250292379027 ) ) ;
#72557=CARTESIAN_POINT ( 'NONE',  ( -0.3689425029237881626, 47.42874883491396787, 10.36894250292379027 ) ) ;
#72558=CARTESIAN_POINT ( 'NONE',  ( 12.63842701281683922, 14.55059781766744997, -9.846743663894590881 ) ) ;
#72559=CARTESIAN_POINT ( 'NONE',  ( -2.816281873526473856, 14.33196800326375531, 3.434112377981055619 ) ) ;
#72560=DIRECTION ( 'NONE',  ( 0.000000000000000000, 0.8042198116157012189, -0.5943319733993840392 ) ) ;
#72561=CARTESIAN_POINT ( 'NONE',  ( 17.96484262340118221, 6.188685344154836621, -7.964842623401177768 ) ) ;
#72562=CARTESIAN_POINT ( 'NONE',  ( -1.099225684535947600, 49.54030133659708923, 6.408140936763237150 ) ) ;
#72563=CARTESIAN_POINT ( 'NONE',  ( 6.204703633549690345, 37.84541550158063927, 14.16423886937410082 ) ) ;
#72564=CARTESIAN_POINT ( 'NONE',  ( 12.63842701281683922, 4.550597817667451750, -9.846743663894590881 ) ) ;
#72567=SURFACE_SIDE_STYLE ('',( #63597 ) ) ;
#72568=CARTESIAN_POINT ( 'NONE',  ( 18.52753015748617571, 13.09226448433411960, 4.923371831947298993 ) ) ;
#72572=CARTESIAN_POINT ( 'NONE',  ( 2.917880565312950480, 10.97041550158063572, -12.26659068614894821 ) ) ;
#72573=CARTESIAN_POINT ( 'NONE',  ( 4.559911319644449179, 2.230352010821504916, -9.422509992056141925 ) ) ;
#72574=CARTESIAN_POINT ( 'NONE',  ( -0.8801773607111008646, 28.27201867748817321, 2.915334737309923430 ) ) ;
#72575=CARTESIAN_POINT ( 'NONE',  ( 5.076628168052704559, 55.17559781766745175, -8.527530157486179263 ) ) ;
#72576=CARTESIAN_POINT ( 'NONE',  ( 3.591859063236761518, -0.04303199673624671928, 11.09922568453594849 ) ) ;
#72581=CARTESIAN_POINT ( 'NONE',  ( 21.09922568453595559, 12.04030133659708746, -6.408140936763230044 ) ) ;
#72584=CARTESIAN_POINT ( 'NONE',  ( 2.917880565312950480, 55.97041550158063217, -12.26659068614894821 ) ) ;
#72585=EDGE_LOOP ( 'NONE', ( #73217, #1098, #79639, #89416 ) ) ;
#72586=CARTESIAN_POINT ( 'NONE',  ( 10.00000000000000178, 58.05374883491397497, 14.16423886937410082 ) ) ;
#72588=CARTESIAN_POINT ( 'NONE',  ( 0.5774900079438590739, 32.64701867748816966, -5.440088680355550821 ) ) ;
#72589=CARTESIAN_POINT ( 'NONE',  ( 7.084665262690076126, 39.10535201082150536, 10.88017736071109987 ) ) ;
#72590=CARTESIAN_POINT ( 'NONE',  ( 4.559911319644449179, 48.89701867748817676, 9.422509992056141925 ) ) ;
#72592=CARTESIAN_POINT ( 'NONE',  ( 20.88017736071110519, 45.56368534415484106, 2.639326808657452039E-16 ) ) ;
#72593=DIRECTION ( 'NONE',  ( -0.000000000000000000, -0.000000000000000000, -1.000000000000000000 ) ) ;
#72596=CARTESIAN_POINT ( 'NONE',  ( 17.20831665107776587, 17.88393115100078745, 7.208316651077764980 ) ) ;
#72599=CARTESIAN_POINT ( 'NONE',  ( 14.92337183194729633, 52.67559781766745175, 8.527530157486181039 ) ) ;
#72600=MECHANICAL_DESIGN_GEOMETRIC_PRESENTATION_REPRESENTATION('',(#78979),#67852);
#72601=CARTESIAN_POINT ( 'NONE',  ( 21.09922568453594849, 61.20696800326376064, 6.408140936763242479 ) ) ;
#72607=CARTESIAN_POINT ( 'NONE',  ( 2.917880565312948704, 62.63708216824730357, 12.26659068614894643 ) ) ;
#72608=LINE ( 'NONE', #40664, #75414 ) ;
#72610=CARTESIAN_POINT ( 'NONE',  ( 0.000000000000000000, 70.00000000000000000, -6.000000000000000000 ) ) ;
#72611=CARTESIAN_POINT ( 'NONE',  ( 19.84674366389459266, 38.30059781766745175, 2.638427012816836559 ) ) ;
#72612=CARTESIAN_POINT ( 'NONE',  ( -2.816281873526473856, 59.12363466993042493, 9.499525473075851096E-16 ) ) ;
#72613=CARTESIAN_POINT ( 'NONE',  ( 3.591859063236761518, -0.04303199673624671928, 11.09922568453594849 ) ) ;
#72614=CARTESIAN_POINT ( 'NONE',  ( 20.88017736071110875, 65.77201867748817676, -2.915334737309920765 ) ) ;
#72616=CARTESIAN_POINT ( 'NONE',  ( 7.361572987183170547, 12.05059781766744997, 9.846743663894590881 ) ) ;
#72617=CARTESIAN_POINT ( 'NONE',  ( 10.00000000000000000, 59.75893115100078745, -9.846743663894594434 ) ) ;
#72620=ORIENTED_EDGE ( 'NONE', *, *, #17361, .T. ) ;
#72621=CARTESIAN_POINT ( 'NONE',  ( 15.44008868035555793, 16.39701867748817321, -9.422509992056140149 ) ) ;
#72622=CARTESIAN_POINT ( 'NONE',  ( 22.26659068614895176, 4.720415501580633943, -7.082119434687042414 ) ) ;
#72623=CARTESIAN_POINT ( 'NONE',  ( 7.361572987183169658, 9.967264484334119601, -9.846743663894592657 ) ) ;
#72624=CARTESIAN_POINT ( 'NONE',  ( 17.96484262340118221, 41.18868534415484106, -7.964842623401177768 ) ) ;
#72625=CARTESIAN_POINT ( 'NONE',  ( 6.565887622018943937, 23.08196800326375708, -12.81628187352647608 ) ) ;
#72626=CARTESIAN_POINT ( 'NONE',  ( 15.44008868035555793, 66.39701867748817676, -9.422509992056140149 ) ) ;
#72628=CARTESIAN_POINT ( 'NONE',  ( -24.42076923076924189, 85.65384615384614619, -9.500000000000000000 ) ) ;
#72630=CARTESIAN_POINT ( 'NONE',  ( 5.076628168052703671, 56.84226448433412315, 8.527530157486179263 ) ) ;
#72631=CARTESIAN_POINT ( 'NONE',  ( 2.791683348922237240, 15.38393115100078212, -7.208316651077763204 ) ) ;
#72633=CARTESIAN_POINT ( 'NONE',  ( 19.38216949554541557, 17.24863466993041783, -9.382169495545420901 ) ) ;
#72635=CARTESIAN_POINT ( 'NONE',  ( 0.5774900079438607392, 23.48035201082150536, 5.440088680355550821 ) ) ;
#72637=AXIS2_PLACEMENT_3D ( 'NONE', #8553, #39052, #31035 ) ;
#72638=CARTESIAN_POINT ( 'NONE',  ( 22.26659068614895176, 49.72041550158063927, -7.082119434687042414 ) ) ;
#72640=CARTESIAN_POINT ( 'NONE',  ( 17.20831665107776587, 44.13393115100078745, -7.208316651077762316 ) ) ;
#72641=CARTESIAN_POINT ( 'NONE',  ( 22.81628187352647785, 36.62363466993041783, 6.195893100308588602E-16 ) ) ;
#72642=CARTESIAN_POINT ( 'NONE',  ( 20.88017736071110875, 30.77201867748816966, -2.915334737309920765 ) ) ;
#72643=CARTESIAN_POINT ( 'NONE',  ( 12.63842701281683922, 49.55059781766744464, -9.846743663894590881 ) ) ;
#72644=CARTESIAN_POINT ( 'NONE',  ( 17.96484262340118221, 46.18868534415484106, -7.964842623401177768 ) ) ;
#72645=CARTESIAN_POINT ( 'NONE',  ( 21.09922568453594849, 11.20696800326375531, 6.408140936763242479 ) ) ;
#72646=CARTESIAN_POINT ( 'NONE',  ( 24.16423886937409904, 39.09541550158062506, 3.795296366450317205 ) ) ;
#72647=CARTESIAN_POINT ( 'NONE',  ( 5.500000000000000000, 11.00000000000000000, -5.000000000000000000 ) ) ;
#72648=CARTESIAN_POINT ( 'NONE',  ( 17.20831665107776587, 22.88393115100078745, 7.208316651077764980 ) ) ;
#72649=CARTESIAN_POINT ( 'NONE',  ( -2.816281873526471635, 63.91530133659708923, -3.434112377981056508 ) ) ;
#72650=CARTESIAN_POINT ( 'NONE',  ( 17.20831665107776587, 64.13393115100079456, -7.208316651077762316 ) ) ;
#72652=LINE ( 'NONE', #64652, #3035 ) ;
#72654=CARTESIAN_POINT ( 'NONE',  ( 20.88017736071110519, 20.56368534415484106, 2.639326808657452039E-16 ) ) ;
#72655=CARTESIAN_POINT ( 'NONE',  ( 6.204703633549690345, 30.76208216824730357, -14.16423886937410259 ) ) ;
#72657=CARTESIAN_POINT ( 'NONE',  ( 20.88017736071110519, 65.56368534415483396, 2.639326808657452039E-16 ) ) ;
#72658=CARTESIAN_POINT ( 'NONE',  ( 19.84674366389459266, 53.30059781766744464, 2.638427012816836559 ) ) ;
#72659=CARTESIAN_POINT ( 'NONE',  ( 0.5774900079438590739, 37.64701867748817676, -5.440088680355550821 ) ) ;
#72668=LINE ( 'NONE', #80682, #37380 ) ;
#72669=CARTESIAN_POINT ( 'NONE',  ( 13.79529636645030344, 13.26208216824729824, 14.16423886937410614 ) ) ;
#72670=CARTESIAN_POINT ( 'NONE',  ( 24.16423886937410614, 4.512082168247300906, -3.795296366450302550 ) ) ;
#72672=CARTESIAN_POINT ( 'NONE',  ( 17.08211943468705840, 55.13708216824731068, -12.26659068614894466 ) ) ;
#72673=CARTESIAN_POINT ( 'NONE',  ( 17.20831665107776587, 57.88393115100078745, 7.208316651077764980 ) ) ;
#72674=CARTESIAN_POINT ( 'NONE',  ( 1.472469842513823179, 30.59226448433411960, -4.923371831947296329 ) ) ;
#72675=CARTESIAN_POINT ( 'NONE',  ( 10.00000000000000178, 65.37363466993042493, 12.81628187352647608 ) ) ;
#72676=CARTESIAN_POINT ( 'NONE',  ( 19.42250999205614548, 35.98035201082151247, -5.440088680355545492 ) ) ;
#72677=CARTESIAN_POINT ( 'NONE',  ( -1.099225684535947600, -1.293031996736246469, -6.408140936763238038 ) ) ;
#72678=CARTESIAN_POINT ( 'NONE',  ( -2.266590686148945544, 51.38708216824730357, -7.082119434687050408 ) ) ;
#72680=CARTESIAN_POINT ( 'NONE',  ( 20.88017736071110164, 5.355352010821503583, 2.915334737309930979 ) ) ;
#72681=CARTESIAN_POINT ( 'NONE',  ( 19.05914839598884924, 4.966938638839758724, 6.499999999999964473 ) ) ;
#72684=ORIENTED_EDGE ( 'NONE', *, *, #27998, .F. ) ;
#72687=CARTESIAN_POINT ( 'NONE',  ( 0.1532563361054100626, 20.80059781766744464, -2.638427012816831230 ) ) ;
#72689=CARTESIAN_POINT ( 'NONE',  ( 6.204703633549690345, 35.76208216824729647, -14.16423886937410259 ) ) ;
#72690=CARTESIAN_POINT ( 'NONE',  ( 7.361572987183169658, 34.96726448433411605, -9.846743663894592657 ) ) ;
#72691=CARTESIAN_POINT ( 'NONE',  ( 0.5774900079438607392, 53.48035201082151247, 5.440088680355550821 ) ) ;
#72692=CARTESIAN_POINT ( 'NONE',  ( 20.03743638938529159, 36.75197528031017669, 6.399506433553890261 ) ) ;
#72693=CARTESIAN_POINT ( 'NONE',  ( 17.96484262340118221, 49.93868534415484106, 7.964842623401181321 ) ) ;
#72696=CARTESIAN_POINT ( 'NONE',  ( 16.40814093676323893, 55.79030133659708923, 11.09922568453595026 ) ) ;
#72700=CARTESIAN_POINT ( 'NONE',  ( -4.164238869374098151, 16.59541550158063927, -3.795296366450310543 ) ) ;
#72702=CARTESIAN_POINT ( 'NONE',  ( 0.6178305044545818747, 48.49863466993042493, -9.382169495545419124 ) ) ;
#72703=CARTESIAN_POINT ( 'NONE',  ( 0.5774900079438590739, 17.64701867748817321, -5.440088680355550821 ) ) ;
#72704=CARTESIAN_POINT ( 'NONE',  ( 12.63842701281683922, 19.55059781766745175, -9.846743663894590881 ) ) ;
#72705=CARTESIAN_POINT ( 'NONE',  ( -0.8801773607111008646, 18.27201867748817321, 2.915334737309923430 ) ) ;
#72706=CARTESIAN_POINT ( 'NONE',  ( 0.6178305044545838731, 59.74863466993041783, 9.382169495545420901 ) ) ;
#72708=CARTESIAN_POINT ( 'NONE',  ( 2.791683348922237240, 30.38393115100078390, -7.208316651077763204 ) ) ;
#72710=CARTESIAN_POINT ( 'NONE',  ( 21.92686044187657046, 22.39664270246083788, -3.195792623639524432 ) ) ;
#72712=FACE_OUTER_BOUND ( 'NONE', #74798, .T. ) ;
#72717=CARTESIAN_POINT ( 'NONE',  ( 10.00000000000000000, 4.758931151000784787, -9.846743663894594434 ) ) ;
#72718=CARTESIAN_POINT ( 'NONE',  ( 13.43411237798106583, 17.66530133659708923, -12.81628187352647252 ) ) ;
#72721=CARTESIAN_POINT ( 'NONE',  ( 5.076628168052704559, 45.17559781766745175, -8.527530157486179263 ) ) ;
#72723=CARTESIAN_POINT ( 'NONE',  ( 2.917880565312948704, 17.63708216824730357, 12.26659068614894643 ) ) ;
#72724=CARTESIAN_POINT ( 'NONE',  ( 1.472469842513823179, 30.59226448433411960, -4.923371831947296329 ) ) ;
#72725=CARTESIAN_POINT ( 'NONE',  ( 3.591859063236763294, 38.29030133659708923, -11.09922568453595026 ) ) ;
#72728=CARTESIAN_POINT ( 'NONE',  ( -0.8801773607111009756, 63.06368534415484106, 1.068504757029289695E-15 ) ) ;
#72729=CARTESIAN_POINT ( 'NONE',  ( 21.09922568453594849, 1.206968003263753531, 6.408140936763242479 ) ) ;
#72731=CARTESIAN_POINT ( 'NONE',  ( 0.1532563361054083140, 31.00893115100078390, 1.131784320476157264E-15 ) ) ;
#72732=CARTESIAN_POINT ( 'NONE',  ( 12.91533473730992121, 24.52201867748816966, 10.88017736071110164 ) ) ;
#72733=CARTESIAN_POINT ( 'NONE',  ( 19.38216949554541202, 30.99863466993042138, 9.382169495545424454 ) ) ;
#72737=CARTESIAN_POINT ( 'NONE',  ( 10.00000000000000000, 31.81368534415483751, -10.88017736071110342 ) ) ;
#72741=CARTESIAN_POINT ( 'NONE',  ( 17.96484262340118221, 4.938685344154837509, 7.964842623401181321 ) ) ;
#72742=CARTESIAN_POINT ( 'NONE',  ( 2.791683348922240793, 61.63393115100079456, 7.208316651077764092 ) ) ;
#72743=CARTESIAN_POINT ( 'NONE',  ( 15.44008868035555260, 34.73035201082151247, 9.422509992056143702 ) ) ;
#72745=CARTESIAN_POINT ( 'NONE',  ( 0.5774900079438607392, 58.48035201082151247, 5.440088680355550821 ) ) ;
#72746=CARTESIAN_POINT ( 'NONE',  ( 10.00000000000000000, 26.81368534415484106, -10.88017736071110342 ) ) ;
#72748=CARTESIAN_POINT ( 'NONE',  ( 1.472469842513823179, 0.5922644843341181575, -4.923371831947296329 ) ) ;
#72750=CARTESIAN_POINT ( 'NONE',  ( 12.63842701281683034, 52.46726448433413026, 9.846743663894596210 ) ) ;
#72751=CARTESIAN_POINT ( 'NONE',  ( -2.266590686148945544, 52.22041550158064638, 7.082119434687048631 ) ) ;
#72754=CARTESIAN_POINT ( 'NONE',  ( 6.204703633549690345, 12.84541550158063572, 14.16423886937410082 ) ) ;
#72755=CARTESIAN_POINT ( 'NONE',  ( 10.00000000000000178, 38.05374883491396787, 14.16423886937410082 ) ) ;
#72756=CARTESIAN_POINT ( 'NONE',  ( 13.43411237798105340, 10.58196800326375353, 12.81628187352647963 ) ) ;
#72759=CARTESIAN_POINT ( 'NONE',  ( 15.44008868035555260, 4.730352010821505360, 9.422509992056143702 ) ) ;
#72760=CARTESIAN_POINT ( 'NONE',  ( 19.84674366389459621, 38.50893115100078745, 7.409399052514197653E-17 ) ) ;
#72762=DIRECTION ( 'NONE',  ( -0.000000000000000000, 1.000000000000000000, 0.000000000000000000 ) ) ;
#72763=CARTESIAN_POINT ( 'NONE',  ( 15.44008868035555793, 56.39701867748817676, -9.422509992056140149 ) ) ;
#72766=CARTESIAN_POINT ( 'NONE',  ( 3.591859063236761518, 29.95696800326375708, 11.09922568453594849 ) ) ;
#72767=CARTESIAN_POINT ( 'NONE',  ( 0.1532563361054083140, 31.00893115100078390, 1.131784320476157264E-15 ) ) ;
#72769=CARTESIAN_POINT ( 'NONE',  ( 18.61655166652078464, 4.877183271974287138, 6.499999999999961808 ) ) ;
#72770=CARTESIAN_POINT ( 'NONE',  ( 6.204703633549690345, 67.84541550158060375, 14.16423886937410082 ) ) ;
#72771=CARTESIAN_POINT ( 'NONE',  ( 22.26659068614894466, 43.88708216824729647, 7.082119434687054849 ) ) ;
#72772=CARTESIAN_POINT ( 'NONE',  ( 0.5774900079438607392, 28.48035201082150891, 5.440088680355550821 ) ) ;
#72773=CARTESIAN_POINT ( 'NONE',  ( 15.44008868035555260, 44.73035201082151247, 9.422509992056143702 ) ) ;
#72776=CARTESIAN_POINT ( 'NONE',  ( 0.1532563361054083140, 16.00893115100078390, 1.131784320476157264E-15 ) ) ;
#72780=CARTESIAN_POINT ( 'NONE',  ( 19.84674366389459621, 43.50893115100078745, 7.409399052514197653E-17 ) ) ;
#72781=CARTESIAN_POINT ( 'NONE',  ( 19.84674366389459266, 48.30059781766745175, 2.638427012816836559 ) ) ;
#72784=CARTESIAN_POINT ( 'NONE',  ( 10.00000000000000000, 21.81368534415484106, -10.88017736071110342 ) ) ;
#72785=VERTEX_POINT ( 'NONE', #50353 ) ;
#72786=CARTESIAN_POINT ( 'NONE',  ( 22.81628187352647785, 51.62363466993042493, 6.195893100308588602E-16 ) ) ;
#72788=CARTESIAN_POINT ( 'NONE',  ( 17.96484262340118221, 64.93868534415483396, 7.964842623401181321 ) ) ;
#72789=CARTESIAN_POINT ( 'NONE',  ( 12.63842701281683034, 22.46726448433411605, 9.846743663894596210 ) ) ;
#72790=CARTESIAN_POINT ( 'NONE',  ( 6.204703633549690345, 62.84541550158063927, 14.16423886937410082 ) ) ;
#72791=CARTESIAN_POINT ( 'NONE',  ( 19.84674366389459266, 18.30059781766745175, 2.638427012816836559 ) ) ;
#72794=CARTESIAN_POINT ( 'NONE',  ( 17.08211943468705130, 23.47041550158063572, 12.26659068614894998 ) ) ;
#72795=CARTESIAN_POINT ( 'NONE',  ( 13.79529636645030344, 38.26208216824729647, 14.16423886937410614 ) ) ;
#72796=CARTESIAN_POINT ( 'NONE',  ( 7.361572987183170547, 42.05059781766745886, 9.846743663894590881 ) ) ;
#72798=CARTESIAN_POINT ( 'NONE',  ( 7.084665262690076126, 27.02201867748817676, -10.88017736071110164 ) ) ;
#72799=CARTESIAN_POINT ( 'NONE',  ( 4.559911319644449179, 58.89701867748817676, 9.422509992056141925 ) ) ;
#72800=CARTESIAN_POINT ( 'NONE',  ( 1.959929470562282283, 56.50257860105349295, 5.767676674365853629 ) ) ;
#72802=CARTESIAN_POINT ( 'NONE',  ( 10.00000000000000178, 45.37363466993041783, 12.81628187352647608 ) ) ;
#72803=CARTESIAN_POINT ( 'NONE',  ( 12.91533473730992121, 59.52201867748816966, 10.88017736071110164 ) ) ;
#72804=ORIENTED_EDGE ( 'NONE', *, *, #14357, .F. ) ;
#72806=PRESENTATION_STYLE_ASSIGNMENT (( #79830 ) ) ;
#72807=CARTESIAN_POINT ( 'NONE',  ( -0.8801773607111008646, 68.27201867748817676, 2.915334737309923430 ) ) ;
#72810=AXIS2_PLACEMENT_3D ( 'NONE', #65311, #79352, #17388 ) ;
#72811=CARTESIAN_POINT ( 'NONE',  ( -0.8801773607111008646, 58.27201867748816966, 2.915334737309923430 ) ) ;
#72812=CARTESIAN_POINT ( 'NONE',  ( 2.035157376598824452, 8.688685344154839285, 7.964842623401179544 ) ) ;
#72815=CARTESIAN_POINT ( 'NONE',  ( 17.39651004071841101, 37.93575266056827644, 6.500000000000005329 ) ) ;
#72816=CARTESIAN_POINT ( 'NONE',  ( 20.88017736071110519, 5.563685344154838397, 2.639326808657452039E-16 ) ) ;
#72817=CARTESIAN_POINT ( 'NONE',  ( 5.076628168052703671, 11.84226448433411960, 8.527530157486179263 ) ) ;
#72818=CARTESIAN_POINT ( 'NONE',  ( 24.16423886937410614, 14.30374883491396787, 8.672049930838204340E-16 ) ) ;
#72820=EDGE_CURVE ( 'NONE', #4466, #67947, #31918, .T. ) ;
#72821=CARTESIAN_POINT ( 'NONE',  ( -0.8801773607111008646, 28.27201867748817321, 2.915334737309923430 ) ) ;
#72822=CARTESIAN_POINT ( 'NONE',  ( 17.20831665107776587, 54.13393115100079456, -7.208316651077762316 ) ) ;
#72824=CARTESIAN_POINT ( 'NONE',  ( 1.472469842513823179, 56.42559781766745886, 4.923371831947296329 ) ) ;
#72827=CARTESIAN_POINT ( 'NONE',  ( 2.035157376598822676, 47.43868534415484817, -7.964842623401177768 ) ) ;
#72829=CARTESIAN_POINT ( 'NONE',  ( 0.6178305044545818747, 38.49863466993042493, -9.382169495545419124 ) ) ;
#72830=CARTESIAN_POINT ( 'NONE',  ( 7.084665262690076126, 14.10535201082150358, 10.88017736071109987 ) ) ;
#72832=CARTESIAN_POINT ( 'NONE',  ( 20.88017736071110875, 65.77201867748817676, -2.915334737309920765 ) ) ;
#72833=CARTESIAN_POINT ( 'NONE',  ( 2.035157376598822676, 2.438685344154838397, -7.964842623401177768 ) ) ;
#72834=CARTESIAN_POINT ( 'NONE',  ( 22.81628187352647785, 46.41530133659708213, 3.434112377981063169 ) ) ;
#72835=CARTESIAN_POINT ( 'NONE',  ( 7.084665262690076126, 24.10535201082150181, 10.88017736071109987 ) ) ;
#72838=CARTESIAN_POINT ( 'NONE',  ( 13.43411237798105340, 45.58196800326374643, 12.81628187352647963 ) ) ;
#72839=CARTESIAN_POINT ( 'NONE',  ( 7.084665262690076126, 29.10535201082150181, 10.88017736071109987 ) ) ;
#72840=CARTESIAN_POINT ( 'NONE',  ( 2.791683348922237240, 60.38393115100078745, -7.208316651077763204 ) ) ;
#72841=ORIENTED_EDGE ( 'NONE', *, *, #57907, .T. ) ;
#72844=CARTESIAN_POINT ( 'NONE',  ( 1.472469842513823179, 66.42559781766745175, 4.923371831947296329 ) ) ;
#72846=CARTESIAN_POINT ( 'NONE',  ( 5.076628168052704559, 55.17559781766745175, -8.527530157486179263 ) ) ;
#72847=CARTESIAN_POINT ( 'NONE',  ( 7.084665262690076126, 22.02201867748817321, -10.88017736071110164 ) ) ;
#72848=CARTESIAN_POINT ( 'NONE',  ( 5.076628168052703671, 11.84226448433411960, 8.527530157486179263 ) ) ;
#72851=CARTESIAN_POINT ( 'NONE',  ( 19.72487221294571214, 57.80223176428831522, -6.499999999999988454 ) ) ;
#72852=EDGE_CURVE ( 'NONE', #87105, #65300, #24568, .T. ) ;
#72853=CARTESIAN_POINT ( 'NONE',  ( 5.076628168052703671, 46.84226448433412315, 8.527530157486179263 ) ) ;
#72854=CARTESIAN_POINT ( 'NONE',  ( 10.00000000000000178, 12.25893115100078568, 9.846743663894594434 ) ) ;
#72855=CARTESIAN_POINT ( 'NONE',  ( 19.84674366389459266, 28.71726448433411960, -2.638427012816827677 ) ) ;
#72856=CARTESIAN_POINT ( 'NONE',  ( 18.52753015748617571, 58.09226448433411605, 4.923371831947298993 ) ) ;
#72858=DIRECTION ( 'NONE',  ( -0.000000000000000000, -0.000000000000000000, 1.000000000000000000 ) ) ;
#72859=CARTESIAN_POINT ( 'NONE',  ( -2.816281873526471635, 33.91530133659708213, -3.434112377981056508 ) ) ;
#72860=CARTESIAN_POINT ( 'NONE',  ( 14.92337183194729633, 42.67559781766745886, 8.527530157486181039 ) ) ;
#72862=CARTESIAN_POINT ( 'NONE',  ( 13.79529636645031943, 55.34541550158062506, -14.16423886937409904 ) ) ;
#72863=CARTESIAN_POINT ( 'NONE',  ( 17.20831665107776587, 37.88393115100078745, 7.208316651077764980 ) ) ;
#72865=ORIENTED_EDGE ( 'NONE', *, *, #86681, .T. ) ;
#72867=CARTESIAN_POINT ( 'NONE',  ( 22.26659068614894466, 58.88708216824729647, 7.082119434687054849 ) ) ;
#72869=CARTESIAN_POINT ( 'NONE',  ( 19.42250999205614193, 10.14701867748816966, 5.440088680355555262 ) ) ;
#72870=CARTESIAN_POINT ( 'NONE',  ( 2.917880565312948704, 37.63708216824731068, 12.26659068614894643 ) ) ;
#72871=CARTESIAN_POINT ( 'NONE',  ( 10.00000000000000178, 58.05374883491397497, 14.16423886937410082 ) ) ;
#72873=CARTESIAN_POINT ( 'NONE',  ( 19.10478245763051319, 5.101608292538858613, 5.990408912944327646 ) ) ;
#72874=CARTESIAN_POINT ( 'NONE',  ( 1.472469842513823179, 5.592264484334118713, -4.923371831947296329 ) ) ;
#72876=CARTESIAN_POINT ( 'NONE',  ( 0.6178305044545818747, 3.498634669930420049, -9.382169495545419124 ) ) ;
#72878=CARTESIAN_POINT ( 'NONE',  ( 17.96484262340118221, 56.18868534415484817, -7.964842623401177768 ) ) ;
#72879=CARTESIAN_POINT ( 'NONE',  ( -0.8801773607110990882, 17.85535201082150536, -2.915334737309924318 ) ) ;
#72882=CARTESIAN_POINT ( 'NONE',  ( 1.472469842513823179, 51.42559781766745886, 4.923371831947296329 ) ) ;
#72886=CARTESIAN_POINT ( 'NONE',  ( -0.3689425029237881626, 27.42874883491397142, 10.36894250292379027 ) ) ;
#72890=DIRECTION ( 'NONE',  ( -0.5547001962252290364, -0.8320502943378437211, 0.000000000000000000 ) ) ;
#72891=CARTESIAN_POINT ( 'NONE',  ( 20.88017736071110519, 25.56368534415483751, 2.639326808657452039E-16 ) ) ;
#72892=CARTESIAN_POINT ( 'NONE',  ( -2.816281873526473856, 24.33196800326375353, 3.434112377981055619 ) ) ;
#72894=CARTESIAN_POINT ( 'NONE',  ( 7.361572987183169658, 4.967264484334119601, -9.846743663894592657 ) ) ;
#72895=CARTESIAN_POINT ( 'NONE',  ( 21.09922568453594849, 61.20696800326376064, 6.408140936763242479 ) ) ;
#72898=CARTESIAN_POINT ( 'NONE',  ( 24.16423886937409904, 29.09541550158063572, 3.795296366450317205 ) ) ;
#72900=CARTESIAN_POINT ( 'NONE',  ( 20.10384461210892582, 61.74302437010793909, 6.337995344473753789 ) ) ;
#72901=CARTESIAN_POINT ( 'NONE',  ( 7.084665262690076126, 9.105352010821503583, 10.88017736071109987 ) ) ;
#72905=CARTESIAN_POINT ( 'NONE',  ( 17.96484262340118221, 41.18868534415484106, -7.964842623401177768 ) ) ;
#72906=CARTESIAN_POINT ( 'NONE',  ( 4.559911319644449179, 52.23035201082151247, -9.422509992056141925 ) ) ;
#72907=CARTESIAN_POINT ( 'NONE',  ( 0.6178305044545838731, 14.74863466993041783, 9.382169495545420901 ) ) ;
#72908=CARTESIAN_POINT ( 'NONE',  ( 7.361572987183170547, 62.05059781766745886, 9.846743663894590881 ) ) ;
#72909=CARTESIAN_POINT ( 'NONE',  ( 0.5774900079438590739, 2.647018677488171434, -5.440088680355550821 ) ) ;
#72910=CARTESIAN_POINT ( 'NONE',  ( 5.076628168052703671, 6.842264484334118713, 8.527530157486179263 ) ) ;
#72911=COLOUR_RGB ( '', 0.31764706, 0.68627451, 0.89019608) ;
#72912=DIRECTION ( 'NONE',  ( 1.000000000000000000, 0.000000000000000000, 0.000000000000000000 ) ) ;
#72913=CARTESIAN_POINT ( 'NONE',  ( 4.559911319644449179, 38.89701867748817676, 9.422509992056141925 ) ) ;
#72917=CARTESIAN_POINT ( 'NONE',  ( 0.6178305044545818747, 8.498634669930421381, -9.382169495545419124 ) ) ;
#72918=CARTESIAN_POINT ( 'NONE',  ( 20.88017736071110164, 60.35535201082151957, 2.915334737309930979 ) ) ;
#72919=CARTESIAN_POINT ( 'NONE',  ( 12.63842701281683922, 19.55059781766745175, -9.846743663894590881 ) ) ;
#72920=CARTESIAN_POINT ( 'NONE',  ( -2.816281873526473856, 49.12363466993042493, 9.499525473075851096E-16 ) ) ;
#72921=CARTESIAN_POINT ( 'NONE',  ( 1.472469842513823179, 1.425597817667451528, 4.923371831947296329 ) ) ;
#72922=VERTEX_POINT ( 'NONE', #57366 ) ;
#72923=CARTESIAN_POINT ( 'NONE',  ( 2.603489959281588995, 55.43575266056826933, -6.500000000000003553 ) ) ;
#72925=CARTESIAN_POINT ( 'NONE',  ( 19.42250999205614548, 15.98035201082150714, -5.440088680355545492 ) ) ;
#72926=CARTESIAN_POINT ( 'NONE',  ( 0.6178305044545838731, 64.74863466993043914, 9.382169495545420901 ) ) ;
#72927=CARTESIAN_POINT ( 'NONE',  ( 24.16423886937410614, 24.51208216824730002, -3.795296366450302550 ) ) ;
#72928=CARTESIAN_POINT ( 'NONE',  ( 7.361572987183169658, 24.96726448433412315, -9.846743663894592657 ) ) ;
#72929=CARTESIAN_POINT ( 'NONE',  ( 2.035157376598824452, 13.68868534415483751, 7.964842623401179544 ) ) ;
#72930=CARTESIAN_POINT ( 'NONE',  ( 7.084665262690076126, 2.022018677488171434, -10.88017736071110164 ) ) ;
#72932=CARTESIAN_POINT ( 'NONE',  ( 7.084665262690076126, 14.10535201082150358, 10.88017736071109987 ) ) ;
#72933=CARTESIAN_POINT ( 'NONE',  ( 4.559911319644449179, 33.89701867748817676, 9.422509992056141925 ) ) ;
#72935=CARTESIAN_POINT ( 'NONE',  ( 15.44008868035555260, 29.73035201082150891, 9.422509992056143702 ) ) ;
#72936=ORIENTED_EDGE ( 'NONE', *, *, #67334, .F. ) ;
#72937=CARTESIAN_POINT ( 'NONE',  ( 12.91533473730992121, 24.52201867748816966, 10.88017736071110164 ) ) ;
#72938=CARTESIAN_POINT ( 'NONE',  ( 12.63842701281683922, 64.55059781766745175, -9.846743663894590881 ) ) ;
#72940=ADVANCED_FACE ( 'NONE', ( #65847 ), #55198, .T. ) ;
#72941=CARTESIAN_POINT ( 'NONE',  ( -2.816281873526471635, 58.91530133659707502, -3.434112377981056508 ) ) ;
#72943=CARTESIAN_POINT ( 'NONE',  ( -0.3689425029237898834, 36.17874883491396787, -10.36894250292378850 ) ) ;
#72944=CARTESIAN_POINT ( 'NONE',  ( 17.96484262340118221, 36.18868534415484106, -7.964842623401177768 ) ) ;
#72945=CARTESIAN_POINT ( 'NONE',  ( 12.91533473730993009, 21.60535201082150536, -10.88017736071109987 ) ) ;
#72947=AXIS2_PLACEMENT_3D ( 'NONE', #76183, #52523, #59531 ) ;
#72948=CARTESIAN_POINT ( 'NONE',  ( 19.84674366389459266, 53.30059781766744464, 2.638427012816836559 ) ) ;
#72949=EDGE_CURVE ( 'NONE', #92829, #85493, #26274, .T. ) ;
#72950=CARTESIAN_POINT ( 'NONE',  ( 12.63842701281683922, 24.55059781766745175, -9.846743663894590881 ) ) ;
#72952=CARTESIAN_POINT ( 'NONE',  ( 0.5774900079438590739, 7.647018677488171434, -5.440088680355550821 ) ) ;
#72953=CARTESIAN_POINT ( 'NONE',  ( 10.00000000000000178, 12.25893115100078568, 9.846743663894594434 ) ) ;
#72954=CARTESIAN_POINT ( 'NONE',  ( 19.38216949554541557, 12.24863466993041961, -9.382169495545420901 ) ) ;
#72955=CARTESIAN_POINT ( 'NONE',  ( -0.8801773607111008646, 63.27201867748817676, 2.915334737309923430 ) ) ;
#72956=CARTESIAN_POINT ( 'NONE',  ( 10.00000000000000000, 21.81368534415484106, -10.88017736071110342 ) ) ;
#72957=CARTESIAN_POINT ( 'NONE',  ( 22.81628187352647785, 61.62363466993041783, 6.195893100308588602E-16 ) ) ;
#72958=CARTESIAN_POINT ( 'NONE',  ( 20.36894250292379382, 28.67874883491396787, 10.36894250292379205 ) ) ;
#72961=CARTESIAN_POINT ( 'NONE',  ( 0.6178305044545838731, 64.74863466993043914, 9.382169495545420901 ) ) ;
#72963=CARTESIAN_POINT ( 'NONE',  ( 10.00000000000000000, 7.873634669930421381, -12.81628187352647608 ) ) ;
#72965=CARTESIAN_POINT ( 'NONE',  ( 2.035157376598824452, 38.68868534415483396, 7.964842623401179544 ) ) ;
#72967=VERTEX_POINT ( 'NONE', #38472 ) ;
#72968=CARTESIAN_POINT ( 'NONE',  ( 12.63842701281683922, 19.55059781766745175, -9.846743663894590881 ) ) ;
#72969=CARTESIAN_POINT ( 'NONE',  ( 14.92337183194729988, 14.34226448433411782, -8.527530157486177487 ) ) ;
#72971=CARTESIAN_POINT ( 'NONE',  ( 5.076628168052704559, 20.17559781766745175, -8.527530157486179263 ) ) ;
#72972=CARTESIAN_POINT ( 'NONE',  ( 12.63842701281683922, 9.550597817667449974, -9.846743663894590881 ) ) ;
#72974=EDGE_CURVE ( 'NONE', #51686, #651, #30450, .T. ) ;
#72975=CARTESIAN_POINT ( 'NONE',  ( 14.92337183194729633, 2.675597817667451750, 8.527530157486181039 ) ) ;
#72978=CARTESIAN_POINT ( 'NONE',  ( 19.84674366389459621, 8.508931151000785675, 7.409399052514197653E-17 ) ) ;
#72979=CARTESIAN_POINT ( 'NONE',  ( 18.52753015748617571, 13.09226448433411960, 4.923371831947298993 ) ) ;
#72980=VERTEX_POINT ( 'NONE', #61443 ) ;
#72982=DIRECTION ( 'NONE',  ( 0.5547001962252290364, 0.8320502943378437211, 0.000000000000000000 ) ) ;
#72983=CARTESIAN_POINT ( 'NONE',  ( -2.816281873526473856, 4.123634669930420493, 9.499525473075851096E-16 ) ) ;
#72984=ORIENTED_EDGE ( 'NONE', *, *, #91919, .T. ) ;
#72985=FILL_AREA_STYLE ('',( #79998 ) ) ;
#72986=CARTESIAN_POINT ( 'NONE',  ( 17.08211943468705840, 25.13708216824730357, -12.26659068614894466 ) ) ;
#72988=CARTESIAN_POINT ( 'NONE',  ( 13.79529636645030344, 13.26208216824729824, 14.16423886937410614 ) ) ;
#72989=CARTESIAN_POINT ( 'NONE',  ( -2.266590686148945544, 37.22041550158063217, 7.082119434687048631 ) ) ;
#72991=CARTESIAN_POINT ( 'NONE',  ( -2.266590686148945544, 2.220415501580634388, 7.082119434687048631 ) ) ;
#72992=CARTESIAN_POINT ( 'NONE',  ( 12.91533473730992121, 34.52201867748817676, 10.88017736071110164 ) ) ;
#72994=CARTESIAN_POINT ( 'NONE',  ( 17.20831665107776587, 12.88393115100078390, 7.208316651077764980 ) ) ;
#72995=CARTESIAN_POINT ( 'NONE',  ( 20.88017736071110875, 50.77201867748817676, -2.915334737309920765 ) ) ;
#72996=CARTESIAN_POINT ( 'NONE',  ( 0.1532563361054083140, 21.00893115100078745, 1.131784320476157264E-15 ) ) ;
#72997=CARTESIAN_POINT ( 'NONE',  ( 10.00000000000000178, 9.313685344154839285, 10.88017736071110342 ) ) ;
#72998=CARTESIAN_POINT ( 'NONE',  ( 13.43411237798106583, 42.66530133659707502, -12.81628187352647252 ) ) ;
#72999=CARTESIAN_POINT ( 'NONE',  ( 18.52753015748618282, 48.92559781766745886, -4.923371831947291888 ) ) ;
#73001=CARTESIAN_POINT ( 'NONE',  ( 10.00000000000000178, 30.37363466993042138, 12.81628187352647608 ) ) ;
#73003=CARTESIAN_POINT ( 'NONE',  ( 17.20831665107776587, 42.88393115100077324, 7.208316651077764980 ) ) ;
#73004=CARTESIAN_POINT ( 'NONE',  ( 24.16423886937410614, 19.30374883491397142, 8.672049930838204340E-16 ) ) ;
#73005=VERTEX_POINT ( 'NONE', #54433 ) ;
#73007=CIRCLE ( 'NONE', #85802, 18.53834841531100608 ) ;
#73008=CARTESIAN_POINT ( 'NONE',  ( 2.035157376598824452, 53.68868534415484817, 7.964842623401179544 ) ) ;
#73009=CARTESIAN_POINT ( 'NONE',  ( 15.44008868035555260, 49.73035201082150536, 9.422509992056143702 ) ) ;
#73010=CARTESIAN_POINT ( 'NONE',  ( 6.204703633549690345, 42.84541550158063217, 14.16423886937410082 ) ) ;
#73011=CARTESIAN_POINT ( 'NONE',  ( 18.52753015748618282, 48.92559781766745886, -4.923371831947291888 ) ) ;
#73013=CARTESIAN_POINT ( 'NONE',  ( -0.8801773607111008646, 38.27201867748816255, 2.915334737309923430 ) ) ;
#73014=CARTESIAN_POINT ( 'NONE',  ( 0.1916775849787346053, 27.25868815902070352, -6.500000000000015099 ) ) ;
#73015=CARTESIAN_POINT ( 'NONE',  ( 5.076628168052704559, 55.17559781766745175, -8.527530157486179263 ) ) ;
#73017=CARTESIAN_POINT ( 'NONE',  ( 20.88017736071110875, 5.772018677488170546, -2.915334737309920765 ) ) ;
#73018=CARTESIAN_POINT ( 'NONE',  ( -0.03932841506543007654, 13.12161441960500952, 6.397827110478970347 ) ) ;
#73019=CARTESIAN_POINT ( 'NONE',  ( 7.084665262690076126, 4.105352010821503583, 10.88017736071109987 ) ) ;
#73022=CARTESIAN_POINT ( 'NONE',  ( 1.472469842513823179, 1.425597817667451528, 4.923371831947296329 ) ) ;
#73023=CARTESIAN_POINT ( 'NONE',  ( 12.91533473730992121, 64.52201867748817676, 10.88017736071110164 ) ) ;
#73025=CARTESIAN_POINT ( 'NONE',  ( 2.791683348922240793, 31.63393115100078745, 7.208316651077764092 ) ) ;
#73028=CARTESIAN_POINT ( 'NONE',  ( -0.8801773607110991993, 27.85535201082150181, -2.915334737309923874 ) ) ;
#73029=CARTESIAN_POINT ( 'NONE',  ( 22.81628187352647785, 11.62363466993042138, 6.195893100308588602E-16 ) ) ;
#73030=CARTESIAN_POINT ( 'NONE',  ( 4.559911319644449179, 28.89701867748817321, 9.422509992056141925 ) ) ;
#73032=CARTESIAN_POINT ( 'NONE',  ( 21.09922568453595559, 37.04030133659708923, -6.408140936763230044 ) ) ;
#73034=CYLINDRICAL_SURFACE ( 'NONE', #38268, 11.92686044187656513 ) ;
#73035=CARTESIAN_POINT ( 'NONE',  ( 6.565887622018943937, 15.16530133659708568, 12.81628187352647430 ) ) ;
#73037=CARTESIAN_POINT ( 'NONE',  ( 20.88017736071110875, 25.77201867748816966, -2.915334737309920765 ) ) ;
#73038=CARTESIAN_POINT ( 'NONE',  ( 6.204703633549690345, 60.76208216824730357, -14.16423886937410259 ) ) ;
#73040=CARTESIAN_POINT ( 'NONE',  ( 1.472469842513823179, 50.59226448433411605, -4.923371831947296329 ) ) ;
#73041=CARTESIAN_POINT ( 'NONE',  ( 1.472469842513823179, 0.5922644843341181575, -4.923371831947296329 ) ) ;
#73042=CARTESIAN_POINT ( 'NONE',  ( 15.44008868035555793, 61.39701867748817676, -9.422509992056140149 ) ) ;
#73044=CARTESIAN_POINT ( 'NONE',  ( -2.266590686148945544, 31.38708216824730002, -7.082119434687050408 ) ) ;
#73047=AXIS2_PLACEMENT_3D ( 'NONE', #70440, #25447, #48903 ) ;
#73052=CARTESIAN_POINT ( 'NONE',  ( 2.917880565312948704, 42.63708216824729647, 12.26659068614894643 ) ) ;
#73053=CARTESIAN_POINT ( 'NONE',  ( 13.79529636645030344, 48.26208216824728936, 14.16423886937410614 ) ) ;
#73054=CARTESIAN_POINT ( 'NONE',  ( 17.20831665107776587, 22.88393115100078745, 7.208316651077764980 ) ) ;
#73055=CARTESIAN_POINT ( 'NONE',  ( 22.81628187352648496, 31.83196800326375353, -3.434112377981050290 ) ) ;
#73057=PLANE ( 'NONE',  #67434 ) ;
#73058=CARTESIAN_POINT ( 'NONE',  ( 17.08211943468705840, 45.13708216824730357, -12.26659068614894466 ) ) ;
#73060=CARTESIAN_POINT ( 'NONE',  ( 19.84674366389459266, 8.300597817667451750, 2.638427012816836559 ) ) ;
#73062=CARTESIAN_POINT ( 'NONE',  ( 3.591859063236763294, 53.29030133659708923, -11.09922568453595026 ) ) ;
#73067=CARTESIAN_POINT ( 'NONE',  ( -0.3689425029237881626, 12.42874883491396609, 10.36894250292379027 ) ) ;
#73068=CARTESIAN_POINT ( 'NONE',  ( 12.91533473730992121, 19.52201867748816611, 10.88017736071110164 ) ) ;
#73069=CARTESIAN_POINT ( 'NONE',  ( 19.42250999205614548, 25.98035201082150891, -5.440088680355545492 ) ) ;
#73070=CARTESIAN_POINT ( 'NONE',  ( 1.472469842513823179, 51.42559781766745886, 4.923371831947296329 ) ) ;
#73071=CARTESIAN_POINT ( 'NONE',  ( 22.81628187352648496, 16.83196800326374998, -3.434112377981050290 ) ) ;
#73072=FILL_AREA_STYLE_COLOUR ( '', #2460 ) ;
#73073=CARTESIAN_POINT ( 'NONE',  ( 17.39651004071838614, 42.93575266056826933, 6.500000000000032863 ) ) ;
#73074=CARTESIAN_POINT ( 'NONE',  ( 0.6178305044545838731, 24.74863466993042493, 9.382169495545420901 ) ) ;
#73076=CARTESIAN_POINT ( 'NONE',  ( 17.20831665107776587, 32.88393115100078745, 7.208316651077764980 ) ) ;
#73077=CARTESIAN_POINT ( 'NONE',  ( 13.79529636645031943, 60.34541550158063927, -14.16423886937409904 ) ) ;
#73078=ORIENTED_EDGE ( 'NONE', *, *, #26882, .T. ) ;
#73079=CARTESIAN_POINT ( 'NONE',  ( 17.96484262340118221, 4.938685344154837509, 7.964842623401181321 ) ) ;
#73080=VERTEX_POINT ( 'NONE', #56776 ) ;
#73081=CARTESIAN_POINT ( 'NONE',  ( 15.44008868035555260, 44.73035201082151247, 9.422509992056143702 ) ) ;
#73082=CARTESIAN_POINT ( 'NONE',  ( 10.00000000000000000, 51.81368534415484106, -10.88017736071110342 ) ) ;
#73083=CARTESIAN_POINT ( 'NONE',  ( -0.8801773607110991993, 52.85535201082151247, -2.915334737309923874 ) ) ;
#73085=CARTESIAN_POINT ( 'NONE',  ( 12.91533473730992121, 39.52201867748817676, 10.88017736071110164 ) ) ;
#73089=CARTESIAN_POINT ( 'NONE',  ( 10.00000000000000178, 22.25893115100078745, 9.846743663894594434 ) ) ;
#73090=ORIENTED_EDGE ( 'NONE', *, *, #26789, .T. ) ;
#73091=CARTESIAN_POINT ( 'NONE',  ( 19.84674366389459621, 53.50893115100078745, 7.409399052514197653E-17 ) ) ;
#73098=CARTESIAN_POINT ( 'NONE',  ( 19.84674366389459266, 63.30059781766745886, 2.638427012816836559 ) ) ;
#73099=CARTESIAN_POINT ( 'NONE',  ( -2.266590686148945544, 67.22041550158063217, 7.082119434687048631 ) ) ;
#73101=ORIENTED_EDGE ( 'NONE', *, *, #7589, .T. ) ;
#73102=CARTESIAN_POINT ( 'NONE',  ( 12.63842701281683034, 37.46726448433411605, 9.846743663894596210 ) ) ;
#73103=CARTESIAN_POINT ( 'NONE',  ( -1.099225684535947600, 59.54030133659708923, 6.408140936763237150 ) ) ;
#73104=CARTESIAN_POINT ( 'NONE',  ( 13.43411237798105340, 5.581968003263753531, 12.81628187352647963 ) ) ;
#73105=CARTESIAN_POINT ( 'NONE',  ( 12.63842701281683034, 12.46726448433411782, 9.846743663894596210 ) ) ;
#73107=CARTESIAN_POINT ( 'NONE',  ( 12.63842701281683922, 4.550597817667451750, -9.846743663894590881 ) ) ;
#73108=CARTESIAN_POINT ( 'NONE',  ( 10.00000000000000000, 64.75893115100078035, -9.846743663894594434 ) ) ;
#73112=CARTESIAN_POINT ( 'NONE',  ( -0.8801773607110991993, 7.855352010821506248, -2.915334737309923874 ) ) ;
#73113=CARTESIAN_POINT ( 'NONE',  ( 17.08211943468705840, 5.137082168247300906, -12.26659068614894466 ) ) ;
#73114=CARTESIAN_POINT ( 'NONE',  ( 14.92337183194729633, 17.67559781766745175, 8.527530157486181039 ) ) ;
#73115=B_SPLINE_CURVE_WITH_KNOTS ( 'NONE', 3,
 ( #28703, #59195, #75190, #75687 ),
 .UNSPECIFIED., .F., .F.,
 ( 4, 4 ),
 ( 0.000000000000000000, 0.002657014572711316816 ),
 .UNSPECIFIED. ) ;
#73116=CARTESIAN_POINT ( 'NONE',  ( 4.559911319644449179, 62.23035201082150536, -9.422509992056141925 ) ) ;
#73117=CARTESIAN_POINT ( 'NONE',  ( 19.38216949554541557, 22.24863466993041428, -9.382169495545420901 ) ) ;
#73118=CARTESIAN_POINT ( 'NONE',  ( 7.084665262690076126, 64.10535201082150536, 10.88017736071109987 ) ) ;
#73121=CARTESIAN_POINT ( 'NONE',  ( 22.81628187352647785, 1.623634669930420271, 6.195893100308588602E-16 ) ) ;
#73122=CARTESIAN_POINT ( 'NONE',  ( 0.6178305044545838731, -0.2513653300695798953, 9.382169495545420901 ) ) ;
#73123=CARTESIAN_POINT ( 'NONE',  ( 19.84674366389459266, 8.300597817667451750, 2.638427012816836559 ) ) ;
#73125=CARTESIAN_POINT ( 'NONE',  ( 0.6178305044545838731, 24.74863466993042493, 9.382169495545420901 ) ) ;
#73128=CARTESIAN_POINT ( 'NONE',  ( -0.8801773607111008646, 33.27201867748817676, 2.915334737309923430 ) ) ;
#73130=CARTESIAN_POINT ( 'NONE',  ( -0.3689425029237881626, 47.42874883491396787, 10.36894250292379027 ) ) ;
#73132=EDGE_CURVE ( 'NONE', #75285, #87937, #78862, .T. ) ;
#73133=CARTESIAN_POINT ( 'NONE',  ( 22.81628187352648496, 31.83196800326375353, -3.434112377981050290 ) ) ;
#73134=CARTESIAN_POINT ( 'NONE',  ( 10.00000000000000000, 26.81368534415484106, -10.88017736071110342 ) ) ;
#73136=CARTESIAN_POINT ( 'NONE',  ( 10.00000000000000000, 54.75893115100078745, -9.846743663894594434 ) ) ;
#73137=CARTESIAN_POINT ( 'NONE',  ( 10.00000000000000000, 56.81368534415484106, -10.88017736071110342 ) ) ;
#73138=CARTESIAN_POINT ( 'NONE',  ( 22.26659068614894466, 38.88708216824731068, 7.082119434687054849 ) ) ;
#73142=UNCERTAINTY_MEASURE_WITH_UNIT (LENGTH_MEASURE( 1.000000000000000082E-05 ), #19975, 'distance_accuracy_value', 'NONE');
#73143=CARTESIAN_POINT ( 'NONE',  ( 0.1532563361054100626, 35.80059781766745175, -2.638427012816831230 ) ) ;
#73144=FILL_AREA_STYLE ('',( #95162 ) ) ;
#73145=CARTESIAN_POINT ( 'NONE',  ( 12.63842701281683034, 62.46726448433410894, 9.846743663894596210 ) ) ;
#73147=CARTESIAN_POINT ( 'NONE',  ( 19.72487221294570858, 11.86607318730075633, 6.500000000000000888 ) ) ;
#73148=CARTESIAN_POINT ( 'NONE',  ( 2.035157376598824452, 13.68868534415483751, 7.964842623401179544 ) ) ;
#73149=CARTESIAN_POINT ( 'NONE',  ( 2.917880565312948704, 22.63708216824730002, 12.26659068614894643 ) ) ;
#73150=CARTESIAN_POINT ( 'NONE',  ( 19.84674366389459621, 8.508931151000785675, 7.409399052514197653E-17 ) ) ;
#73153=CARTESIAN_POINT ( 'NONE',  ( 4.559911319644449179, 33.89701867748817676, 9.422509992056141925 ) ) ;
#73160=CARTESIAN_POINT ( 'NONE',  ( 1.472469842513823179, 41.42559781766745886, 4.923371831947296329 ) ) ;
#73162=ORIENTED_EDGE ( 'NONE', *, *, #70206, .T. ) ;
#73164=CARTESIAN_POINT ( 'NONE',  ( 20.36894250292379738, 9.928748834913966093, -10.36894250292379027 ) ) ;
#73165=CARTESIAN_POINT ( 'NONE',  ( -4.164238869374098151, 6.595415501580634832, -3.795296366450310543 ) ) ;
#73166=CARTESIAN_POINT ( 'NONE',  ( 20.88017736071110164, 50.35535201082151247, 2.915334737309930979 ) ) ;
#73167=CARTESIAN_POINT ( 'NONE',  ( 17.08211943468705130, 53.47041550158063217, 12.26659068614894998 ) ) ;
#73168=CARTESIAN_POINT ( 'NONE',  ( 16.40814093676323893, 5.790301336597087456, 11.09922568453595026 ) ) ;
#73169=CARTESIAN_POINT ( 'NONE',  ( 0.1532563361054083140, 31.00893115100078390, 1.131784320476157264E-15 ) ) ;
#73171=CARTESIAN_POINT ( 'NONE',  ( -0.8801773607111008646, 28.27201867748817321, 2.915334737309923430 ) ) ;
#73172=CARTESIAN_POINT ( 'NONE',  ( 19.38216949554541557, 12.24863466993041961, -9.382169495545420901 ) ) ;
#73173=CARTESIAN_POINT ( 'NONE',  ( 20.36894250292379382, 3.678748834913967869, 10.36894250292379205 ) ) ;
#73174=CARTESIAN_POINT ( 'NONE',  ( -0.3689425029237881626, 52.42874883491396076, 10.36894250292379027 ) ) ;
#73175=CARTESIAN_POINT ( 'NONE',  ( 2.917880565312948704, 67.63708216824730357, 12.26659068614894643 ) ) ;
#73179=( GEOMETRIC_REPRESENTATION_CONTEXT ( 3 ) GLOBAL_UNCERTAINTY_ASSIGNED_CONTEXT ( ( #72167 ) ) GLOBAL_UNIT_ASSIGNED_CONTEXT ( ( #72086, #80083, #48597 ) ) REPRESENTATION_CONTEXT ( 'NONE', 'WORKASPACE' ) );
#73182=DIRECTION ( 'NONE',  ( 0.000000000000000000, 0.000000000000000000, 1.000000000000000000 ) ) ;
#73184=ORIENTED_EDGE ( 'NONE', *, *, #58950, .T. ) ;
#73185=CARTESIAN_POINT ( 'NONE',  ( -2.266590686148945544, 42.22041550158063217, 7.082119434687048631 ) ) ;
#73186=CARTESIAN_POINT ( 'NONE',  ( 1.472469842513823179, 51.42559781766745886, 4.923371831947296329 ) ) ;
#73187=CARTESIAN_POINT ( 'NONE',  ( 10.00000000000000000, 51.81368534415484106, -10.88017736071110342 ) ) ;
#73190=EDGE_CURVE ( 'NONE', #11556, #6265, #98743, .T. ) ;
#73193=CARTESIAN_POINT ( 'NONE',  ( 20.88017736071110164, 55.35535201082149825, 2.915334737309930979 ) ) ;
#73194=CARTESIAN_POINT ( 'NONE',  ( -2.816281873526473856, 54.33196800326376064, 3.434112377981055619 ) ) ;
#73197=CARTESIAN_POINT ( 'NONE',  ( 4.559911319644449179, 48.89701867748817676, 9.422509992056141925 ) ) ;
#73198=CARTESIAN_POINT ( 'NONE',  ( -0.3689425029237898834, 16.17874883491396076, -10.36894250292378850 ) ) ;
#73199=CARTESIAN_POINT ( 'NONE',  ( 3.591859063236761518, 29.95696800326375708, 11.09922568453594849 ) ) ;
#73201=CARTESIAN_POINT ( 'NONE',  ( -1.099225684535947600, 48.70696800326375353, -6.408140936763238038 ) ) ;
#73202=CARTESIAN_POINT ( 'NONE',  ( 7.084665262690076126, 19.10535201082150181, 10.88017736071109987 ) ) ;
#73203=CARTESIAN_POINT ( 'NONE',  ( 19.84674366389459621, 33.50893115100078745, 7.409399052514197653E-17 ) ) ;
#73204=CARTESIAN_POINT ( 'NONE',  ( 15.44008868035555260, 19.73035201082150536, 9.422509992056143702 ) ) ;
#73206=CARTESIAN_POINT ( 'NONE',  ( 12.63842701281683922, 39.55059781766744464, -9.846743663894590881 ) ) ;
#73207=CARTESIAN_POINT ( 'NONE',  ( -0.8801773607111008646, 68.27201867748817676, 2.915334737309923430 ) ) ;
#73210=CARTESIAN_POINT ( 'NONE',  ( 0.5774900079438607392, 68.48035201082150536, 5.440088680355550821 ) ) ;
#73211=CARTESIAN_POINT ( 'NONE',  ( 18.95386800104995828, 8.238109087357269544, -6.499999999999999112 ) ) ;
#73213=CARTESIAN_POINT ( 'NONE',  ( 18.52753015748617571, 23.09226448433411960, 4.923371831947298993 ) ) ;
#73214=CARTESIAN_POINT ( 'NONE',  ( 3.591859063236761518, 19.95696800326375353, 11.09922568453594849 ) ) ;
#73216=EDGE_CURVE ( 'NONE', #65756, #55747, #64750, .T. ) ;
#73217=ORIENTED_EDGE ( 'NONE', *, *, #52104, .F. ) ;
#73219=CARTESIAN_POINT ( 'NONE',  ( 12.63842701281683034, 42.46726448433412315, 9.846743663894596210 ) ) ;
#73221=CARTESIAN_POINT ( 'NONE',  ( 24.16423886937410614, 24.51208216824730002, -3.795296366450302550 ) ) ;
#73222=CARTESIAN_POINT ( 'NONE',  ( 19.84674366389459266, 38.71726448433412315, -2.638427012816827677 ) ) ;
#73223=CARTESIAN_POINT ( 'NONE',  ( 22.81628187352647785, 51.41530133659708923, 3.434112377981063169 ) ) ;
#73226=CARTESIAN_POINT ( 'NONE',  ( 20.88017736071110164, 60.35535201082151957, 2.915334737309930979 ) ) ;
#73227=CARTESIAN_POINT ( 'NONE',  ( 3.591859063236763294, 13.29030133659708746, -11.09922568453595026 ) ) ;
#73228=CARTESIAN_POINT ( 'NONE',  ( -0.04068437667222076642, 67.21974360917720048, -6.396802510829771471 ) ) ;
#73230=CARTESIAN_POINT ( 'NONE',  ( 14.92337183194729988, 39.34226448433412315, -8.527530157486177487 ) ) ;
#73231=CARTESIAN_POINT ( 'NONE',  ( -0.8801773607111008646, 43.27201867748817676, 2.915334737309923430 ) ) ;
#73232=CARTESIAN_POINT ( 'NONE',  ( 22.81628187352647785, 31.62363466993042138, 6.195893100308588602E-16 ) ) ;
#73233=CARTESIAN_POINT ( 'NONE',  ( 18.52753015748618282, 28.92559781766745175, -4.923371831947291888 ) ) ;
#73236=CARTESIAN_POINT ( 'NONE',  ( 12.91533473730992121, 29.52201867748817321, 10.88017736071110164 ) ) ;
#73240=CARTESIAN_POINT ( 'NONE',  ( 0.1532563361054083140, 61.00893115100078745, 1.131784320476157264E-15 ) ) ;
#73241=CARTESIAN_POINT ( 'NONE',  ( 19.42250999205614193, 30.14701867748817321, 5.440088680355555262 ) ) ;
#73242=DIRECTION ( 'NONE',  ( 1.000000000000000000, 0.000000000000000000, 0.000000000000000000 ) ) ;
#73243=CARTESIAN_POINT ( 'NONE',  ( 20.88017736071110164, 60.35535201082151957, 2.915334737309930979 ) ) ;
#73245=CARTESIAN_POINT ( 'NONE',  ( 15.44008868035555260, 24.73035201082150891, 9.422509992056143702 ) ) ;
#73248=CARTESIAN_POINT ( 'NONE',  ( 1.472469842513823179, 30.59226448433411960, -4.923371831947296329 ) ) ;
#73249=CARTESIAN_POINT ( 'NONE',  ( 18.52753015748618282, 48.92559781766745886, -4.923371831947291888 ) ) ;
#73251=CARTESIAN_POINT ( 'NONE',  ( 13.79529636645030344, 53.26208216824730357, 14.16423886937410614 ) ) ;
#73255=CARTESIAN_POINT ( 'NONE',  ( 6.204703633549690345, 15.76208216824730179, -14.16423886937410259 ) ) ;
#73257=CARTESIAN_POINT ( 'NONE',  ( 17.08211943468705840, 40.13708216824731068, -12.26659068614894466 ) ) ;
#73258=CARTESIAN_POINT ( 'NONE',  ( 16.40814093676323893, 10.79030133659708923, 11.09922568453595026 ) ) ;
#73259=ADVANCED_FACE ( 'NONE', ( #3794 ), #86472, .T. ) ;
#73262=CARTESIAN_POINT ( 'NONE',  ( 10.00000000000000178, 19.31368534415484106, 10.88017736071110342 ) ) ;
#73263=CARTESIAN_POINT ( 'NONE',  ( 5.076628168052704559, 30.17559781766745175, -8.527530157486179263 ) ) ;
#73266=CARTESIAN_POINT ( 'NONE',  ( 4.559911319644449179, 58.89701867748817676, 9.422509992056141925 ) ) ;
#73268=ADVANCED_FACE ( 'NONE', ( #95283 ), #86319, .T. ) ;
#73269=CARTESIAN_POINT ( 'NONE',  ( 3.591859063236761518, 64.95696800326376774, 11.09922568453594849 ) ) ;
#73270=CARTESIAN_POINT ( 'NONE',  ( 19.38216949554541557, 27.24863466993041783, -9.382169495545420901 ) ) ;
#73271=CARTESIAN_POINT ( 'NONE',  ( 2.791683348922240793, 21.63393115100078745, 7.208316651077764092 ) ) ;
#73275=CARTESIAN_POINT ( 'NONE',  ( 7.084665262690076126, 4.105352010821503583, 10.88017736071109987 ) ) ;
#73276=CARTESIAN_POINT ( 'NONE',  ( 15.44008868035555260, 9.730352010821505360, 9.422509992056143702 ) ) ;
#73277=CARTESIAN_POINT ( 'NONE',  ( 24.16423886937409904, 39.09541550158062506, 3.795296366450317205 ) ) ;
#73278=CARTESIAN_POINT ( 'NONE',  ( 7.084665262690076126, 32.02201867748816966, -10.88017736071110164 ) ) ;
#73279=CARTESIAN_POINT ( 'NONE',  ( 19.42250999205614193, 60.14701867748817676, 5.440088680355555262 ) ) ;
#73282=CARTESIAN_POINT ( 'NONE',  ( 14.92337183194729633, 7.675597817667451750, 8.527530157486181039 ) ) ;
#73283=FILL_AREA_STYLE ('',( #57295 ) ) ;
#73284=CARTESIAN_POINT ( 'NONE',  ( 2.791683348922237240, 10.38393115100078390, -7.208316651077763204 ) ) ;
#73285=CARTESIAN_POINT ( 'NONE',  ( 2.791683348922240793, 41.63393115100078745, 7.208316651077764092 ) ) ;
#73286=CARTESIAN_POINT ( 'NONE',  ( 2.791683348922237240, 65.38393115100078035, -7.208316651077763204 ) ) ;
#73287=( GEOMETRIC_REPRESENTATION_CONTEXT ( 3 ) GLOBAL_UNCERTAINTY_ASSIGNED_CONTEXT ( ( #49177 ) ) GLOBAL_UNIT_ASSIGNED_CONTEXT ( ( #49709, #10752, #93749 ) ) REPRESENTATION_CONTEXT ( 'NONE', 'WORKASPACE' ) );
#73288=CARTESIAN_POINT ( 'NONE',  ( -0.8801773607111008646, 23.27201867748817676, 2.915334737309923430 ) ) ;
#73290=CARTESIAN_POINT ( 'NONE',  ( 6.565887622018943937, 45.16530133659708923, 12.81628187352647430 ) ) ;
#73292=CARTESIAN_POINT ( 'NONE',  ( 0.5774900079438590739, 67.64701867748817676, -5.440088680355550821 ) ) ;
#73293=CARTESIAN_POINT ( 'NONE',  ( -1.099225684535947600, 49.54030133659708923, 6.408140936763237150 ) ) ;
#73294=CARTESIAN_POINT ( 'NONE',  ( 13.79529636645030344, 53.26208216824730357, 14.16423886937410614 ) ) ;
#73295=CARTESIAN_POINT ( 'NONE',  ( 12.63842701281683922, 34.55059781766745886, -9.846743663894590881 ) ) ;
#73296=CARTESIAN_POINT ( 'NONE',  ( -0.1503990784575247319, 47.22266099184918886, -6.262539305110083276 ) ) ;
#73298=CARTESIAN_POINT ( 'NONE',  ( 2.917880565312950480, 15.97041550158063217, -12.26659068614894821 ) ) ;
#73299=CARTESIAN_POINT ( 'NONE',  ( -2.266590686148945544, 27.22041550158063572, 7.082119434687048631 ) ) ;
#73300=CARTESIAN_POINT ( 'NONE',  ( 18.52753015748618282, 48.92559781766745886, -4.923371831947291888 ) ) ;
#73302=CARTESIAN_POINT ( 'NONE',  ( 17.96484262340118221, 41.18868534415484106, -7.964842623401177768 ) ) ;
#73304=CARTESIAN_POINT ( 'NONE',  ( 12.91533473730992121, 54.52201867748816255, 10.88017736071110164 ) ) ;
#73305=MECHANICAL_DESIGN_GEOMETRIC_PRESENTATION_REPRESENTATION('',(#90863),#39845);
#73307=CARTESIAN_POINT ( 'NONE',  ( 3.591859063236763294, 43.29030133659708923, -11.09922568453595026 ) ) ;
#73308=CARTESIAN_POINT ( 'NONE',  ( 20.88017736071110164, 55.35535201082149825, 2.915334737309930979 ) ) ;
#73310=( NAMED_UNIT ( * ) PLANE_ANGLE_UNIT ( ) SI_UNIT ( $, .RADIAN. ) );
#73314=CARTESIAN_POINT ( 'NONE',  ( -0.1503990784575359729, 13.10158574516642105, 6.262539305110062848 ) ) ;
#73315=CARTESIAN_POINT ( 'NONE',  ( 7.084665262690076126, 9.105352010821503583, 10.88017736071109987 ) ) ;
#73317=CARTESIAN_POINT ( 'NONE',  ( 7.084665262690076126, 2.022018677488171434, -10.88017736071110164 ) ) ;
#73318=CARTESIAN_POINT ( 'NONE',  ( -0.3689425029237881626, 17.42874883491397142, 10.36894250292379027 ) ) ;
#73319=CARTESIAN_POINT ( 'NONE',  ( 2.035157376598822676, 17.43868534415483751, -7.964842623401177768 ) ) ;
#73320=CARTESIAN_POINT ( 'NONE',  ( 7.361572987183170547, 57.05059781766744464, 9.846743663894590881 ) ) ;
#73321=ORIENTED_EDGE ( 'NONE', *, *, #20672, .F. ) ;
#73322=CARTESIAN_POINT ( 'NONE',  ( 0.6178305044545818747, -1.501365330069579951, -9.382169495545419124 ) ) ;
#73324=CARTESIAN_POINT ( 'NONE',  ( 12.91533473730992121, 49.52201867748817676, 10.88017736071110164 ) ) ;
#73326=CARTESIAN_POINT ( 'NONE',  ( -2.816281873526471635, 33.91530133659708213, -3.434112377981056508 ) ) ;
#73327=CARTESIAN_POINT ( 'NONE',  ( 7.084665262690076126, 9.105352010821503583, 10.88017736071109987 ) ) ;
#73329=CARTESIAN_POINT ( 'NONE',  ( 7.084665262690076126, 67.02201867748817676, -10.88017736071110164 ) ) ;
#73330=CARTESIAN_POINT ( 'NONE',  ( 0.5774900079438590739, 22.64701867748817321, -5.440088680355550821 ) ) ;
#73331=COLOUR_RGB ( '', 0.09019608, 0.27058824, 0.51372549) ;
#73332=CARTESIAN_POINT ( 'NONE',  ( 3.591859063236763294, 58.29030133659708923, -11.09922568453595026 ) ) ;
#73333=CARTESIAN_POINT ( 'NONE',  ( 12.91533473730993009, 26.60535201082150536, -10.88017736071109987 ) ) ;
#73335=CARTESIAN_POINT ( 'NONE',  ( 16.40814093676323893, 35.79030133659708923, 11.09922568453595026 ) ) ;
#73336=CARTESIAN_POINT ( 'NONE',  ( -0.8801773607111009756, 53.06368534415484106, 1.068504757029289695E-15 ) ) ;
#73337=CARTESIAN_POINT ( 'NONE',  ( 7.361572987183170547, 62.05059781766745886, 9.846743663894590881 ) ) ;
#73338=EDGE_LOOP ( 'NONE', ( #59667, #46767, #65735, #51811 ) ) ;
#73340=CARTESIAN_POINT ( 'NONE',  ( 14.92337183194729633, 7.675597817667451750, 8.527530157486181039 ) ) ;
#73341=CARTESIAN_POINT ( 'NONE',  ( 2.791683348922237240, 60.38393115100078745, -7.208316651077763204 ) ) ;
#73343=CARTESIAN_POINT ( 'NONE',  ( 17.20831665107776587, 54.13393115100079456, -7.208316651077762316 ) ) ;
#73344=CARTESIAN_POINT ( 'NONE',  ( 12.91533473730993009, 16.60535201082150891, -10.88017736071109987 ) ) ;
#73345=CARTESIAN_POINT ( 'NONE',  ( 7.361572987183170547, 42.05059781766745886, 9.846743663894590881 ) ) ;
#73347=( NAMED_UNIT ( * ) SI_UNIT ( $, .STERADIAN. ) SOLID_ANGLE_UNIT ( ) );
#73350=CARTESIAN_POINT ( 'NONE',  ( 12.63842701281683034, 47.46726448433412315, 9.846743663894596210 ) ) ;
#73351=CARTESIAN_POINT ( 'NONE',  ( 17.20831665107776587, 7.883931151000784787, 7.208316651077764980 ) ) ;
#73352=SURFACE_STYLE_USAGE ( .BOTH. , #96377 ) ;
#73353=CARTESIAN_POINT ( 'NONE',  ( 2.791683348922237240, 60.38393115100078745, -7.208316651077763204 ) ) ;
#73355=CARTESIAN_POINT ( 'NONE',  ( 10.00000000000000178, 35.37363466993042493, 12.81628187352647608 ) ) ;
#73356=CARTESIAN_POINT ( 'NONE',  ( 0.1532563361054083140, 46.00893115100079456, 1.131784320476157264E-15 ) ) ;
#73358=CARTESIAN_POINT ( 'NONE',  ( 22.26659068614894466, 58.88708216824729647, 7.082119434687054849 ) ) ;
#73359=CARTESIAN_POINT ( 'NONE',  ( 1.472469842513823179, 36.42559781766745175, 4.923371831947296329 ) ) ;
#73360=CARTESIAN_POINT ( 'NONE',  ( 19.59274024544212978, 82.56817434445966342, 5.128398454507835602 ) ) ;
#73361=CARTESIAN_POINT ( 'NONE',  ( 24.16423886937410614, 54.30374883491396787, 8.672049930838204340E-16 ) ) ;
#73363=CARTESIAN_POINT ( 'NONE',  ( -0.8801773607111008646, 23.27201867748817676, 2.915334737309923430 ) ) ;
#73364=CARTESIAN_POINT ( 'NONE',  ( -4.164238869374099039, 41.80374883491397497, 8.674139862899312516E-16 ) ) ;
#73365=CARTESIAN_POINT ( 'NONE',  ( -4.164238869374099927, 52.01208216824729647, 3.795296366450308767 ) ) ;
#73367=CARTESIAN_POINT ( 'NONE',  ( 20.88017736071110164, 5.355352010821504471, 2.915334737309930979 ) ) ;
#73368=CARTESIAN_POINT ( 'NONE',  ( 14.92337183194729633, 17.67559781766745175, 8.527530157486181039 ) ) ;
#73369=CARTESIAN_POINT ( 'NONE',  ( 0.6178305044545838731, -0.2513653300695798953, 9.382169495545420901 ) ) ;
#73370=CARTESIAN_POINT ( 'NONE',  ( -0.8801773607111008646, 48.27201867748816966, 2.915334737309923430 ) ) ;
#73371=CARTESIAN_POINT ( 'NONE',  ( 1.042145700049421198, 39.74216108172002748, -6.499999999999917399 ) ) ;
#73372=CARTESIAN_POINT ( 'NONE',  ( 7.361572987183170547, 47.05059781766745175, 9.846743663894590881 ) ) ;
#73376=EDGE_CURVE ( 'NONE', #76972, #40989, #34775, .T. ) ;
#73377=ORIENTED_EDGE ( 'NONE', *, *, #74320, .F. ) ;
#73378=CARTESIAN_POINT ( 'NONE',  ( 6.204703633549690345, 27.84541550158063217, 14.16423886937410082 ) ) ;
#73382=CARTESIAN_POINT ( 'NONE',  ( 10.00000000000000000, 16.81368534415483751, -10.88017736071110342 ) ) ;
#73383=CARTESIAN_POINT ( 'NONE',  ( 13.43411237798105340, 35.58196800326375353, 12.81628187352647963 ) ) ;
#73389=CARTESIAN_POINT ( 'NONE',  ( -4.164238869374099927, 27.01208216824730357, 3.795296366450308767 ) ) ;
#73390=CARTESIAN_POINT ( 'NONE',  ( 6.204703633549690345, 5.762082168247301794, -14.16423886937410259 ) ) ;
#73391=CARTESIAN_POINT ( 'NONE',  ( 15.44008868035555260, 19.73035201082150536, 9.422509992056143702 ) ) ;
#73394=CARTESIAN_POINT ( 'NONE',  ( 7.084665262690076126, 34.10535201082151247, 10.88017736071109987 ) ) ;
#73395=CARTESIAN_POINT ( 'NONE',  ( 4.559911319644449179, 57.23035201082150536, -9.422509992056141925 ) ) ;
#73396=CARTESIAN_POINT ( 'NONE',  ( -2.816281873526473856, 9.331968003263753531, 3.434112377981055619 ) ) ;
#73399=CARTESIAN_POINT ( 'NONE',  ( 19.84674366389459266, 18.30059781766745175, 2.638427012816836559 ) ) ;
#73401=CARTESIAN_POINT ( 'NONE',  ( 0.5774900079438607392, 38.48035201082150536, 5.440088680355550821 ) ) ;
#73402=CARTESIAN_POINT ( 'NONE',  ( -2.816281873526473856, 4.123634669930420493, 9.499525473075851096E-16 ) ) ;
#73403=CARTESIAN_POINT ( 'NONE',  ( 7.084665262690076126, 59.10535201082150536, 10.88017736071109987 ) ) ;
#73404=CARTESIAN_POINT ( 'NONE',  ( 14.92337183194729633, 27.67559781766745530, 8.527530157486181039 ) ) ;
#73405=CARTESIAN_POINT ( 'NONE',  ( 10.00000000000000178, 45.37363466993041783, 12.81628187352647608 ) ) ;
#73406=CARTESIAN_POINT ( 'NONE',  ( 19.84674366389459621, 8.508931151000785675, 7.409399052514197653E-17 ) ) ;
#73409=FACE_OUTER_BOUND ( 'NONE', #19568, .T. ) ;
#73410=CARTESIAN_POINT ( 'NONE',  ( 15.44008868035555793, 16.39701867748817321, -9.422509992056140149 ) ) ;
#73411=CARTESIAN_POINT ( 'NONE',  ( -2.816281873526473856, 54.12363466993041783, 9.499525473075851096E-16 ) ) ;
#73412=CARTESIAN_POINT ( 'NONE',  ( -2.266590686148945544, 22.22041550158063572, 7.082119434687048631 ) ) ;
#73413=CARTESIAN_POINT ( 'NONE',  ( 12.63842701281683922, 29.55059781766745175, -9.846743663894590881 ) ) ;
#73415=CARTESIAN_POINT ( 'NONE',  ( 7.084665262690076126, 19.10535201082150181, 10.88017736071109987 ) ) ;
#73416=CARTESIAN_POINT ( 'NONE',  ( 22.26659068614895176, 64.72041550158064638, -7.082119434687042414 ) ) ;
#73419=CARTESIAN_POINT ( 'NONE',  ( 0.5774900079438607392, 8.480352010821505360, 5.440088680355550821 ) ) ;
#73422=CARTESIAN_POINT ( 'NONE',  ( 15.44008868035555793, 31.39701867748817676, -9.422509992056140149 ) ) ;
#73424=CARTESIAN_POINT ( 'NONE',  ( -0.8801773607111009756, 43.06368534415484106, 1.068504757029289695E-15 ) ) ;
#73425=ORIENTED_EDGE ( 'NONE', *, *, #97574, .T. ) ;
#73426=CARTESIAN_POINT ( 'NONE',  ( 12.63842701281683034, 62.46726448433410894, 9.846743663894596210 ) ) ;
#73427=CARTESIAN_POINT ( 'NONE',  ( 2.035157376598824452, 18.68868534415484106, 7.964842623401179544 ) ) ;
#73428=CARTESIAN_POINT ( 'NONE',  ( 22.81628187352648496, 61.83196800326376774, -3.434112377981050290 ) ) ;
#73430=CARTESIAN_POINT ( 'NONE',  ( 24.16423886937410614, 39.30374883491396787, 8.672049930838204340E-16 ) ) ;
#73431=CARTESIAN_POINT ( 'NONE',  ( 0.5774900079438590739, 52.64701867748817676, -5.440088680355550821 ) ) ;
#73432=CARTESIAN_POINT ( 'NONE',  ( 10.00000000000000000, 36.81368534415484106, -10.88017736071110342 ) ) ;
#73434=DIRECTION ( 'NONE',  ( 0.000000000000000000, 0.000000000000000000, -1.000000000000000000 ) ) ;
#73435=CARTESIAN_POINT ( 'NONE',  ( 12.63842701281683034, 52.46726448433413026, 9.846743663894596210 ) ) ;
#73438=CARTESIAN_POINT ( 'NONE',  ( 0.2751277870542909731, 22.28217586085237656, -6.499999999999992006 ) ) ;
#73439=CARTESIAN_POINT ( 'NONE',  ( 10.00000000000000178, 17.25893115100078745, 9.846743663894594434 ) ) ;
#73442=CARTESIAN_POINT ( 'NONE',  ( 12.91533473730993009, 6.605352010821504471, -10.88017736071109987 ) ) ;
#73443=CARTESIAN_POINT ( 'NONE',  ( 5.076628168052704559, 30.17559781766745175, -8.527530157486179263 ) ) ;
#73444=CARTESIAN_POINT ( 'NONE',  ( 10.00000000000000000, 7.873634669930421381, -12.81628187352647608 ) ) ;
#73445=CARTESIAN_POINT ( 'NONE',  ( 0.5774900079438607392, 58.48035201082151247, 5.440088680355550821 ) ) ;
#73446=CARTESIAN_POINT ( 'NONE',  ( 4.559911319644449179, 13.89701867748817143, 9.422509992056141925 ) ) ;
#73447=CARTESIAN_POINT ( 'NONE',  ( 10.00000000000000000, 52.87363466993041783, -12.81628187352647608 ) ) ;
#73448=CARTESIAN_POINT ( 'NONE',  ( 10.00000000000000000, 40.55374883491397497, -14.16423886937410082 ) ) ;
#73451=CARTESIAN_POINT ( 'NONE',  ( 3.591859063236761518, -0.04303199673624671928, 11.09922568453594849 ) ) ;
#73453=CARTESIAN_POINT ( 'NONE',  ( 2.035157376598824452, 28.68868534415484106, 7.964842623401179544 ) ) ;
#73454=CARTESIAN_POINT ( 'NONE',  ( 19.84674366389459266, 58.30059781766745886, 2.638427012816836559 ) ) ;
#73455=ORIENTED_EDGE ( 'NONE', *, *, #10286, .F. ) ;
#73456=CARTESIAN_POINT ( 'NONE',  ( 5.076628168052704559, 20.17559781766745175, -8.527530157486179263 ) ) ;
#73457=CARTESIAN_POINT ( 'NONE',  ( 0.1532563361054100626, 10.80059781766745175, -2.638427012816831230 ) ) ;
#73458=CARTESIAN_POINT ( 'NONE',  ( 18.52753015748617571, 28.09226448433411960, 4.923371831947298993 ) ) ;
#73459=CARTESIAN_POINT ( 'NONE',  ( 14.92337183194729633, 17.67559781766745175, 8.527530157486181039 ) ) ;
#73460=CARTESIAN_POINT ( 'NONE',  ( 10.00000000000000000, 4.758931151000784787, -9.846743663894594434 ) ) ;
#73463=CARTESIAN_POINT ( 'NONE',  ( 19.84674366389459621, 3.508931151000785231, 7.409399052514197653E-17 ) ) ;
#73465=CARTESIAN_POINT ( 'NONE',  ( 12.63842701281683034, 7.467264484334118713, 9.846743663894596210 ) ) ;
#73466=CARTESIAN_POINT ( 'NONE',  ( 14.92337183194729633, 22.67559781766745175, 8.527530157486181039 ) ) ;
#73467=ORIENTED_EDGE ( 'NONE', *, *, #14425, .F. ) ;
#73470=CARTESIAN_POINT ( 'NONE',  ( 13.43411237798105340, 5.581968003263753531, 12.81628187352647963 ) ) ;
#73471=CARTESIAN_POINT ( 'NONE',  ( -4.164238869374099927, 22.01208216824730357, 3.795296366450308767 ) ) ;
#73474=CARTESIAN_POINT ( 'NONE',  ( -4.164238869374098151, 21.59541550158063217, -3.795296366450310543 ) ) ;
#73475=CARTESIAN_POINT ( 'NONE',  ( 13.79529636645030344, 43.26208216824730357, 14.16423886937410614 ) ) ;
#73477=CARTESIAN_POINT ( 'NONE',  ( -0.3689425029237898834, 16.17874883491396076, -10.36894250292378850 ) ) ;
#73478=CARTESIAN_POINT ( 'NONE',  ( 20.88017736071110875, 35.77201867748816966, -2.915334737309920765 ) ) ;
#73481=( BOUNDED_CURVE ( )  B_SPLINE_CURVE ( 2, ( #73073, #96095, #80092, #81564, #27577, #51072, #13071, #32447, #1981 ),
 .UNSPECIFIED., .F., .T. ) 
 B_SPLINE_CURVE_WITH_KNOTS ( ( 3, 2, 2, 2, 3 ),
 ( 0.6167998787605536437, 0.6190476190476190688, 0.6250000000000000000, 0.6309523809523809312, 0.6332001212394463563 ),
 .UNSPECIFIED. ) 
 CURVE ( )  GEOMETRIC_REPRESENTATION_ITEM ( )  RATIONAL_B_SPLINE_CURVE ( ( 0.9839835555609424134, 0.9871328979762474809, 1.000000000000000000, 0.9659258262890683122, 1.000000000000000000, 0.9659258262890683122, 1.000000000000000000, 0.9871328979762474809, 0.9839835555609424134 ) ) 
 REPRESENTATION_ITEM ( '' )  );
#73482=CARTESIAN_POINT ( 'NONE',  ( 14.92337183194729633, 17.67559781766745175, 8.527530157486181039 ) ) ;
#73483=CARTESIAN_POINT ( 'NONE',  ( 4.559911319644449179, 62.23035201082150536, -9.422509992056141925 ) ) ;
#73484=CARTESIAN_POINT ( 'NONE',  ( 10.00000000000000000, 24.75893115100078745, -9.846743663894594434 ) ) ;
#73486=CARTESIAN_POINT ( 'NONE',  ( 0.5774900079438590739, 12.64701867748817321, -5.440088680355550821 ) ) ;
#73487=CARTESIAN_POINT ( 'NONE',  ( 21.09922568453595559, 47.04030133659708923, -6.408140936763230044 ) ) ;
#73488=CARTESIAN_POINT ( 'NONE',  ( 2.791683348922240793, 46.63393115100077324, 7.208316651077764092 ) ) ;
#73490=CARTESIAN_POINT ( 'NONE',  ( 22.81628187352647785, 41.62363466993042493, 6.195893100308588602E-16 ) ) ;
#73492=CARTESIAN_POINT ( 'NONE',  ( 17.20831665107776587, 34.13393115100078745, -7.208316651077762316 ) ) ;
#73493=CARTESIAN_POINT ( 'NONE',  ( 2.917880565312948704, 22.63708216824730002, 12.26659068614894643 ) ) ;
#73496=CARTESIAN_POINT ( 'NONE',  ( 0.2751277870542910842, 63.21833443783937412, 6.499999999999992006 ) ) ;
#73497=CARTESIAN_POINT ( 'NONE',  ( 20.88017736071110519, 55.56368534415484817, 2.639326808657452039E-16 ) ) ;
#73498=CARTESIAN_POINT ( 'NONE',  ( 12.91533473730993009, 51.60535201082149825, -10.88017736071109987 ) ) ;
#73499=CARTESIAN_POINT ( 'NONE',  ( -0.3689425029237881626, 47.42874883491396787, 10.36894250292379027 ) ) ;
#73500=CARTESIAN_POINT ( 'NONE',  ( 1.472469842513823179, 61.42559781766745175, 4.923371831947296329 ) ) ;
#73502=CARTESIAN_POINT ( 'NONE',  ( 19.42250999205614548, 40.98035201082150536, -5.440088680355545492 ) ) ;
#73503=ADVANCED_FACE ( 'NONE', ( #90738 ), #18139, .T. ) ;
#73506=CARTESIAN_POINT ( 'NONE',  ( 19.38216949554541557, 27.24863466993041783, -9.382169495545420901 ) ) ;
#73507=CARTESIAN_POINT ( 'NONE',  ( 17.20831665107776587, 52.88393115100078035, 7.208316651077764980 ) ) ;
#73510=CARTESIAN_POINT ( 'NONE',  ( 10.00000000000000178, 64.31368534415483396, 10.88017736071110342 ) ) ;
#73513=CARTESIAN_POINT ( 'NONE',  ( 7.084665262690076126, 69.10535201082151957, 10.88017736071109987 ) ) ;
#73514=CARTESIAN_POINT ( 'NONE',  ( 0.1532563361054100626, 5.800597817667452638, -2.638427012816831230 ) ) ;
#73517=CARTESIAN_POINT ( 'NONE',  ( 1.472469842513823179, 30.59226448433411960, -4.923371831947296329 ) ) ;
#73518=CARTESIAN_POINT ( 'NONE',  ( -0.8801773607111009756, 23.06368534415484106, 1.068504757029289695E-15 ) ) ;
#73519=CARTESIAN_POINT ( 'NONE',  ( -2.816281873526471635, 8.915301336597083903, -3.434112377981056508 ) ) ;
#73520=CARTESIAN_POINT ( 'NONE',  ( 10.00000000000000000, 36.81368534415484106, -10.88017736071110342 ) ) ;
#73523=CARTESIAN_POINT ( 'NONE',  ( 19.38216949554541557, 32.24863466993041783, -9.382169495545420901 ) ) ;
#73525=CARTESIAN_POINT ( 'NONE',  ( -0.8801773607111009756, 63.06368534415484106, 1.068504757029289695E-15 ) ) ;
#73526=CARTESIAN_POINT ( 'NONE',  ( -2.816281873526473856, 24.33196800326375353, 3.434112377981055619 ) ) ;
#73527=FACE_OUTER_BOUND ( 'NONE', #27191, .T. ) ;
#73529=CARTESIAN_POINT ( 'NONE',  ( 20.88017736071110519, 45.56368534415484106, 2.639326808657452039E-16 ) ) ;
#73531=CARTESIAN_POINT ( 'NONE',  ( 10.00000000000000000, 65.55374883491396076, -14.16423886937410082 ) ) ;
#73532=CARTESIAN_POINT ( 'NONE',  ( 17.20831665107776587, 52.88393115100078035, 7.208316651077764980 ) ) ;
#73533=CARTESIAN_POINT ( 'NONE',  ( 0.5774900079438590739, 67.64701867748817676, -5.440088680355550821 ) ) ;
#73534=EDGE_CURVE ( 'NONE', #24048, #98205, #90878, .T. ) ;
#73535=CARTESIAN_POINT ( 'NONE',  ( 15.44008868035555260, 59.73035201082151247, 9.422509992056143702 ) ) ;
#73537=CARTESIAN_POINT ( 'NONE',  ( -4.164238869374099039, 26.80374883491397142, 8.674139862899312516E-16 ) ) ;
#73543=CARTESIAN_POINT ( 'NONE',  ( 24.16423886937409904, 64.09541550158064638, 3.795296366450317205 ) ) ;
#73544=CARTESIAN_POINT ( 'NONE',  ( 6.204703633549690345, 50.76208216824730357, -14.16423886937410259 ) ) ;
#73545=CARTESIAN_POINT ( 'NONE',  ( 0.1532563361054082862, 26.21726448433411605, 2.638427012816831674 ) ) ;
#73548=CARTESIAN_POINT ( 'NONE',  ( -0.8801773607111008646, 3.272018677488171434, 2.915334737309923430 ) ) ;
#73549=CARTESIAN_POINT ( 'NONE',  ( -4.164238869374098151, 56.59541550158063927, -3.795296366450310543 ) ) ;
#73551=CARTESIAN_POINT ( 'NONE',  ( 14.92337183194729633, 7.675597817667451750, 8.527530157486181039 ) ) ;
#73557=ORIENTED_EDGE ( 'NONE', *, *, #53994, .T. ) ;
#73561=CARTESIAN_POINT ( 'NONE',  ( 20.88017736071110164, 15.35535201082150358, 2.915334737309930979 ) ) ;
#73562=CARTESIAN_POINT ( 'NONE',  ( 7.084665262690076126, 22.02201867748817321, -10.88017736071110164 ) ) ;
#73563=CARTESIAN_POINT ( 'NONE',  ( 12.63842701281683922, 54.55059781766745175, -9.846743663894590881 ) ) ;
#73564=CARTESIAN_POINT ( 'NONE',  ( -2.816281873526471635, 13.91530133659708746, -3.434112377981056508 ) ) ;
#73566=CARTESIAN_POINT ( 'NONE',  ( 22.81628187352647785, 31.62363466993042138, 6.195893100308588602E-16 ) ) ;
#73567=CARTESIAN_POINT ( 'NONE',  ( 2.791683348922237240, 0.3839311510007847872, -7.208316651077763204 ) ) ;
#73569=CARTESIAN_POINT ( 'NONE',  ( 18.52753015748617571, 38.09226448433412315, 4.923371831947298993 ) ) ;
#73570=CARTESIAN_POINT ( 'NONE',  ( -4.164238869374099927, 62.01208216824728936, 3.795296366450308767 ) ) ;
#73571=CARTESIAN_POINT ( 'NONE',  ( -0.8801773607111008646, 3.272018677488171434, 2.915334737309923430 ) ) ;
#73573=CARTESIAN_POINT ( 'NONE',  ( 0.5774900079438590739, 42.64701867748816966, -5.440088680355550821 ) ) ;
#73574=CARTESIAN_POINT ( 'NONE',  ( 17.96484262340118221, 39.93868534415484106, 7.964842623401181321 ) ) ;
#73575=CARTESIAN_POINT ( 'NONE',  ( 20.88017736071110875, 50.77201867748817676, -2.915334737309920765 ) ) ;
#73577=CARTESIAN_POINT ( 'NONE',  ( 15.44008868035555260, 39.73035201082150536, 9.422509992056143702 ) ) ;
#73579=CARTESIAN_POINT ( 'NONE',  ( 20.24186590665277663, 64.73410085661204505, 6.114288769123050749 ) ) ;
#73583=AXIS2_PLACEMENT_3D ( 'NONE', #79546, #11046, #72518 ) ;
#73584=CARTESIAN_POINT ( 'NONE',  ( 7.361572987183169658, 29.96726448433411960, -9.846743663894592657 ) ) ;
#73585=ORIENTED_EDGE ( 'NONE', *, *, #18762, .T. ) ;
#73586=CARTESIAN_POINT ( 'NONE',  ( 0.1532563361054083140, 61.00893115100078745, 1.131784320476157264E-15 ) ) ;
#73589=( BOUNDED_SURFACE ( )  B_SPLINE_SURFACE ( 1, 2, ( 
 ( #23199, #15700, #1196, #84190, #39180, #84670, #85164, #30667, #47145, #46185, #31161, #31656, #16673, #68687, #54159, #83690, #218, #77646, #62143, #17172, #61176, #9160, #76670, #8188, #98725, #93144, #39678, #92172, #47654, #76184, #70169, #78147, #1685, #24669, #38684, #69185, #32138, #23699, #85653, #91178, #22705, #53186, #15207, #71638, #26612, #33611, #56147, #49124, #19117, #33128, #10155, #57108, #11614, #94623, #63137, #72112, #18149, #27100, #19609, #79626, #40650, #95104, #3147, #71149, #11127, #49598, #64107, #26135, #50105, #57600, #34103, #2676, #87606, #64594, #55653, #56628, #3638, #87116, #93639, #2181, #18634, #10639, #80107, #41645, #63621, #42130, #80613, #72596, #48623, #4132, #34595, #25174, #32640, #94127, #25655, #86641, #48134, #65089, #95613, #78649, #88100, #12108, #41153, #70660, #86152, #17662, #79127, #67591, #73089, #65589, #98099, #81095, #74580, #28091, #12597, #44577, #36599, #88591, #27599, #51596, #97614, #29560, #60065, #90565, #5108, #75077, #51093, #14093, #4627, #35090, #20605, #89587, #21096, #22094, #44072, #29074, #36087, #50603, #52572, #35597, #81582, #96115, #97119, #83076, #42610, #73584, #37092, #58087, #59080, #82080, #52087, #20099, #6095, #67086, #59579, #43097, #82580, #90072, #66085, #96614, #58589, #6582, #89091, #13590, #13091, #21598, #43587, #74076, #5609, #66592, #28590, #92533, #15094, #62524, #93028, #85045, #37587, #53060, #24063, #23085, #32020, #39558, #91568, #84070, #54531, #70048, #46069, #47033, #45567, #68081, #16559, #8561, #53553, #55024, #603, #54049, #31537, #76063, #15585, #76554, #38570, #62033, #92055, #106, #30057, #7592, #38086, #69065, #77528, #30553, #8072, #39064, #68574, #31046, #1571, #14600, #9047, #24563, #45066, #61545, #23580, #16061, #84559, #46549, #77047, #69557, #61055, #1076, #75574, #7087, #98609, #60569, #91060, #22588, #83575, #85542, #25056, #79014, #17055, #78528, #10039, #3527, #63995, #19014, #40541, #2562, #87008, #71040, #94505, #71535, #72000, #17549, #33984, #33019, #18031, #3043, #41533, #55540, #41035, #70542, #86037, #79513, #49009, #4020, #48017, #64486, #63516, #94020, #95501, #49490, #26024, #86531, #34482, #63026, #33496, #64976, #11015, #11501, #25543, #56033, #56518, #48511, #10523, #93525, #18518, #47536, #87500, #94995, #26500, #56998, #79996, #42022, #72486, #26993, #78035, #9537, #40041, #2066, #32528, #58973, #4997, #13984, #6463, #35970, #27484, #81962, #58468, #57976, #97001, #5985, #20488, #50976, #36971, #44458, #20987, #88482, #13476, #51472, #42498, #81470, #89472, #43956, #66471, #67468, #28956 ),
 ( #97988, #59459, #80499, #96000, #36477, #65974, #74960, #82461, #35478, #27973, #97490, #57491, #88982, #89959, #19985, #11996, #21476, #74457, #96500, #87985, #43469, #28476, #66970, #50483, #12974, #73969, #5498, #51974, #19497, #42988, #72983, #49992, #4511, #34976, #65476, #80986, #12485, #73470, #98487, #23463, #8923, #15471, #75947, #15943, #60935, #82960, #90439, #29942, #60447, #52942, #6966, #61919, #30926, #37474, #54417, #38944, #98982, #480, #30434, #91443, #53435, #84927, #59950, #52456, #16440, #67963, #61426, #14974, #90938, #31415, #53939, #75453, #14475, #38454, #84446, #46915, #77408, #39439, #22466, #92422, #37971, #954, #21982, #44948, #7473, #76442, #7957, #69933, #91935, #46434, #22968, #83453, #29445, #45444, #68459, #83944, #45954, #68948, #76928, #8438, #23947, #69433, #17912, #78898, #10900, #62404, #33378, #94386, #56405, #11384, #41422, #63874, #47407, #56879, #87381, #3402, #62906, #71414, #33864, #2931, #40914, #2440, #25903, #86890, #18400, #79393, #18900, #41905, #9922, #55911, #48883, #48396, #40426, #71883, #86411, #24932, #64372, #63396, #70922, #1944, #54905, #49377, #32899, #1452, #31904, #39923, #93902, #92911, #93408, #55413, #94880, #10408, #26380, #85920, #17430, #79878, #47899, #24440, #85419, #16930, #32406, #77910, #78403, #25428, #9420, #70425, #11877, #27852, #57370, #42382, #66342, #35853, #89839, #72859, #28356, #88369, #34863, #82334, #36351, #81355, #73355, #21355, #49865, #20369, #51846, #96880, #97366, #50357, #19863, #50863, #80868, #35360, #80378, #27365, #72366, #74332, #4882, #58846, #65853, #57858, #12853, #20862, #65356, #4394, #89352, #13352, #96381, #64856, #73849, #12366, #28834, #13855, #43352, #95885, #51354, #58340, #42872, #5379, #81838, #88859, #43837, #3897, #59336, #5858, #66845, #34365, #95376, #87865, #26877, #19382, #9179, #24196, #25190, #17191, #44335, #9675, #74840, #23217, #16690, #54663, #62659, #84210, #8206, #38701, #1216, #47671, #61671, #84687, #70184, #46202, #62161, #2198, #6340, #85671, #31671, #16198, #77664, #92668, #15717, #39696, #55669, #85179, #92190, #32157, #77177, #97869, #36852, #76686, #69200, #725, #53690, #78165, #47160, #31179, #70677, #55157, #46679, #1700, #8684, #39197, #69685, #32659, #67343, #29329, #63152, #23715, #93161, #54176, #24686, #40173, #93655, #91699, #59827, #86168, #72612, #4642, #73103, #65604, #79144, #19625, #26151, #88116, #48152, #10171, #94641, #64612, #95120, #35106, #19137, #4147, #11141, #25672, #96132, #10656, #56645, #78665, #72128, #27613, #17678, #48641, #12123, #40669, #34120, #26628, #27118 ) ),
 .UNSPECIFIED., .F., .F., .F. ) 
 B_SPLINE_SURFACE_WITH_KNOTS ( ( 2, 2 ),
 ( 3, 2, 2, 2, 2, 2, 2, 2, 2, 2, 2, 2, 2, 2, 2, 2, 2, 2, 2, 2, 2, 2, 2, 2, 2, 2, 2, 2, 2, 2, 2, 2, 2, 2, 2, 2, 2, 2, 2, 2, 2, 2, 2, 2, 2, 2, 2, 2, 2, 2, 2, 2, 2, 2, 2, 2, 2, 2, 2, 2, 2, 2, 2, 2, 2, 2, 2, 2, 2, 2, 2, 2, 2, 2, 2, 2, 2, 2, 2, 2, 2, 2, 2, 2, 2, 2, 2, 2, 2, 2, 2, 2, 2, 2, 2, 2, 2, 2, 2, 2, 2, 2, 2, 2, 2, 2, 2, 2, 2, 2, 2, 2, 2, 2, 2, 2, 2, 2, 2, 2, 2, 2, 2, 2, 2, 2, 2, 2, 2, 2, 2, 2, 2, 2, 2, 2, 2, 2, 2, 2, 2, 2, 2, 2, 2, 2, 2, 2, 2, 2, 2, 2, 2, 2, 2, 2, 2, 2, 2, 2, 2, 2, 3 ),
 ( 0.000000000000000000, 1.000000000000000000 ),
 ( 0.000000000000000000, 0.005952380952380952051, 0.01190476190476190410, 0.01785714285714285615, 0.02380952380952380820, 0.02976190476190476025, 0.03571428571428571230, 0.04166666666666666435, 0.04761904761904761640, 0.05357142857142856845, 0.05952380952380952051, 0.06547619047619047949, 0.07142857142857142461, 0.07738095238095238360, 0.08333333333333332871, 0.08928571428571428770, 0.09523809523809523281, 0.1011904761904761918, 0.1071428571428571369, 0.1130952380952380959, 0.1190476190476190410, 0.1250000000000000000, 0.1309523809523809590, 0.1369047619047619180, 0.1428571428571428492, 0.1488095238095238082, 0.1547619047619047672, 0.1607142857142857262, 0.1666666666666666574, 0.1726190476190476164, 0.1785714285714285754, 0.1845238095238095344, 0.1904761904761904656, 0.1964285714285714246, 0.2023809523809523836, 0.2083333333333333426, 0.2142857142857142738, 0.2202380952380952328, 0.2261904761904761918, 0.2321428571428571508, 0.2380952380952380820, 0.2440476190476190410, 0.2500000000000000000, 0.2559523809523809312, 0.2619047619047619180, 0.2678571428571428492, 0.2738095238095238360, 0.2797619047619047672, 0.2857142857142856984, 0.2916666666666666852, 0.2976190476190476164, 0.3035714285714285476, 0.3095238095238095344, 0.3154761904761904656, 0.3214285714285714524, 0.3273809523809523836, 0.3333333333333333148, 0.3392857142857143016, 0.3452380952380952328, 0.3511904761904761640, 0.3571428571428571508, 0.3630952380952380820, 0.3690476190476190688, 0.3750000000000000000, 0.3809523809523809312, 0.3869047619047619180, 0.3928571428571428492, 0.3988095238095238360, 0.4047619047619047672, 0.4107142857142856984, 0.4166666666666666852, 0.4226190476190476164, 0.4285714285714285476, 0.4345238095238095344, 0.4404761904761904656, 0.4464285714285714524, 0.4523809523809523836, 0.4583333333333333148, 0.4642857142857143016, 0.4702380952380952328, 0.4761904761904761640, 0.4821428571428571508, 0.4880952380952380820, 0.4940476190476190688, 0.5000000000000000000, 0.5059523809523809312, 0.5119047619047618625, 0.5178571428571429047, 0.5238095238095238360, 0.5297619047619047672, 0.5357142857142856984, 0.5416666666666666297, 0.5476190476190476719, 0.5535714285714286031, 0.5595238095238095344, 0.5654761904761904656, 0.5714285714285713969, 0.5773809523809523281, 0.5833333333333333703, 0.5892857142857143016, 0.5952380952380952328, 0.6011904761904761640, 0.6071428571428570953, 0.6130952380952381375, 0.6190476190476190688, 0.6250000000000000000, 0.6309523809523809312, 0.6369047619047618625, 0.6428571428571429047, 0.6488095238095238360, 0.6547619047619047672, 0.6607142857142856984, 0.6666666666666666297, 0.6726190476190476719, 0.6785714285714286031, 0.6845238095238095344, 0.6904761904761904656, 0.6964285714285713969, 0.7023809523809523281, 0.7083333333333333703, 0.7142857142857143016, 0.7202380952380952328, 0.7261904761904761640, 0.7321428571428570953, 0.7380952380952381375, 0.7440476190476190688, 0.7500000000000000000, 0.7559523809523809312, 0.7619047619047618625, 0.7678571428571429047, 0.7738095238095238360, 0.7797619047619047672, 0.7857142857142856984, 0.7916666666666666297, 0.7976190476190476719, 0.8035714285714286031, 0.8095238095238095344, 0.8154761904761904656, 0.8214285714285713969, 0.8273809523809523281, 0.8333333333333333703, 0.8392857142857143016, 0.8452380952380952328, 0.8511904761904761640, 0.8571428571428570953, 0.8630952380952381375, 0.8690476190476190688, 0.8750000000000000000, 0.8809523809523809312, 0.8869047619047618625, 0.8928571428571429047, 0.8988095238095238360, 0.9047619047619047672, 0.9107142857142856984, 0.9166666666666666297, 0.9226190476190476719, 0.9285714285714286031, 0.9345238095238095344, 0.9404761904761904656, 0.9464285714285713969, 0.9523809523809523281, 0.9583333333333333703, 0.9642857142857143016 ),
 .UNSPECIFIED. ) 
 GEOMETRIC_REPRESENTATION_ITEM ( )  RATIONAL_B_SPLINE_SURFACE ( (
 ( 1.000000000000000000, 0.9659258262890683122, 1.000000000000000000, 0.9659258262890683122, 1.000000000000000000, 0.9659258262890683122, 1.000000000000000000, 0.9659258262890683122, 1.000000000000000000, 0.9659258262890683122, 1.000000000000000000, 0.9659258262890683122, 1.000000000000000000, 0.9659258262890683122, 1.000000000000000000, 0.9659258262890683122, 1.000000000000000000, 0.9659258262890683122, 1.000000000000000000, 0.9659258262890683122, 1.000000000000000000, 0.9659258262890683122, 1.000000000000000000, 0.9659258262890683122, 1.000000000000000000, 0.9659258262890683122, 1.000000000000000000, 0.9659258262890683122, 1.000000000000000000, 0.9659258262890683122, 1.000000000000000000, 0.9659258262890683122, 1.000000000000000000, 0.9659258262890683122, 1.000000000000000000, 0.9659258262890683122, 1.000000000000000000, 0.9659258262890683122, 1.000000000000000000, 0.9659258262890683122, 1.000000000000000000, 0.9659258262890683122, 1.000000000000000000, 0.9659258262890683122, 1.000000000000000000, 0.9659258262890683122, 1.000000000000000000, 0.9659258262890683122, 1.000000000000000000, 0.9659258262890683122, 1.000000000000000000, 0.9659258262890683122, 1.000000000000000000, 0.9659258262890683122, 1.000000000000000000, 0.9659258262890683122, 1.000000000000000000, 0.9659258262890683122, 1.000000000000000000, 0.9659258262890683122, 1.000000000000000000, 0.9659258262890683122, 1.000000000000000000, 0.9659258262890683122, 1.000000000000000000, 0.9659258262890683122, 1.000000000000000000, 0.9659258262890683122, 1.000000000000000000, 0.9659258262890683122, 1.000000000000000000, 0.9659258262890683122, 1.000000000000000000, 0.9659258262890683122, 1.000000000000000000, 0.9659258262890683122, 1.000000000000000000, 0.9659258262890683122, 1.000000000000000000, 0.9659258262890683122, 1.000000000000000000, 0.9659258262890683122, 1.000000000000000000, 0.9659258262890683122, 1.000000000000000000, 0.9659258262890683122, 1.000000000000000000, 0.9659258262890683122, 1.000000000000000000, 0.9659258262890683122, 1.000000000000000000, 0.9659258262890683122, 1.000000000000000000, 0.9659258262890683122, 1.000000000000000000, 0.9659258262890683122, 1.000000000000000000, 0.9659258262890683122, 1.000000000000000000, 0.9659258262890683122, 1.000000000000000000, 0.9659258262890683122, 1.000000000000000000, 0.9659258262890683122, 1.000000000000000000, 0.9659258262890683122, 1.000000000000000000, 0.9659258262890683122, 1.000000000000000000, 0.9659258262890683122, 1.000000000000000000, 0.9659258262890683122, 1.000000000000000000, 0.9659258262890683122, 1.000000000000000000, 0.9659258262890683122, 1.000000000000000000, 0.9659258262890683122, 1.000000000000000000, 0.9659258262890683122, 1.000000000000000000, 0.9659258262890683122, 1.000000000000000000, 0.9659258262890683122, 1.000000000000000000, 0.9659258262890683122, 1.000000000000000000, 0.9659258262890683122, 1.000000000000000000, 0.9659258262890683122, 1.000000000000000000, 0.9659258262890683122, 1.000000000000000000, 0.9659258262890683122, 1.000000000000000000, 0.9659258262890683122, 1.000000000000000000, 0.9659258262890683122, 1.000000000000000000, 0.9659258262890683122, 1.000000000000000000, 0.9659258262890683122, 1.000000000000000000, 0.9659258262890683122, 1.000000000000000000, 0.9659258262890683122, 1.000000000000000000, 0.9659258262890683122, 1.000000000000000000, 0.9659258262890683122, 1.000000000000000000, 0.9659258262890683122, 1.000000000000000000, 0.9659258262890683122, 1.000000000000000000, 0.9659258262890683122, 1.000000000000000000, 0.9659258262890683122, 1.000000000000000000, 0.9659258262890683122, 1.000000000000000000, 0.9659258262890683122, 1.000000000000000000, 0.9659258262890683122, 1.000000000000000000, 0.9659258262890683122, 1.000000000000000000, 0.9659258262890683122, 1.000000000000000000, 0.9659258262890683122, 1.000000000000000000, 0.9659258262890683122, 1.000000000000000000, 0.9659258262890683122, 1.000000000000000000, 0.9659258262890683122, 1.000000000000000000, 0.9659258262890683122, 1.000000000000000000, 0.9659258262890683122, 1.000000000000000000, 0.9659258262890683122, 1.000000000000000000, 0.9659258262890683122, 1.000000000000000000, 0.9659258262890683122, 1.000000000000000000, 0.9659258262890683122, 1.000000000000000000, 0.9659258262890683122, 1.000000000000000000, 0.9659258262890683122, 1.000000000000000000, 0.9659258262890683122, 1.000000000000000000, 0.9659258262890683122, 1.000000000000000000, 0.9659258262890683122, 1.000000000000000000, 0.9659258262890683122, 1.000000000000000000, 0.9659258262890683122, 1.000000000000000000, 0.9659258262890683122, 1.000000000000000000, 0.9659258262890683122, 1.000000000000000000, 0.9659258262890683122, 1.000000000000000000, 0.9659258262890683122, 1.000000000000000000, 0.9659258262890683122, 1.000000000000000000, 0.9659258262890683122, 1.000000000000000000, 0.9659258262890683122, 1.000000000000000000, 0.9659258262890683122, 1.000000000000000000, 0.9659258262890683122, 1.000000000000000000, 0.9659258262890683122, 1.000000000000000000, 0.9659258262890683122, 1.000000000000000000, 0.9659258262890683122, 1.000000000000000000, 0.9659258262890683122, 1.000000000000000000, 0.9659258262890683122, 1.000000000000000000, 0.9659258262890683122, 1.000000000000000000, 0.9659258262890683122, 1.000000000000000000, 0.9659258262890683122, 1.000000000000000000, 0.9659258262890683122, 1.000000000000000000, 0.9659258262890683122, 1.000000000000000000, 0.9659258262890683122, 1.000000000000000000, 0.9659258262890683122, 1.000000000000000000, 0.9659258262890683122, 1.000000000000000000, 0.9659258262890683122, 1.000000000000000000, 0.9659258262890683122, 1.000000000000000000, 0.9659258262890683122, 1.000000000000000000, 0.9659258262890683122, 1.000000000000000000, 0.9659258262890683122, 1.000000000000000000, 0.9659258262890683122, 1.000000000000000000, 0.9659258262890683122, 1.000000000000000000, 0.9659258262890683122, 1.000000000000000000, 0.9659258262890683122, 1.000000000000000000, 0.9659258262890683122, 1.000000000000000000, 0.9659258262890683122, 1.000000000000000000, 0.9659258262890683122, 1.000000000000000000, 0.9659258262890683122, 1.000000000000000000, 0.9659258262890683122, 1.000000000000000000, 0.9659258262890683122, 1.000000000000000000, 0.9659258262890683122, 1.000000000000000000, 0.9659258262890683122, 1.000000000000000000, 0.9659258262890683122, 1.000000000000000000, 0.9659258262890683122, 1.000000000000000000, 0.9659258262890683122, 1.000000000000000000, 0.9659258262890683122, 1.000000000000000000, 0.9659258262890683122, 1.000000000000000000, 0.9659258262890683122, 1.000000000000000000, 0.9659258262890683122, 1.000000000000000000, 0.9659258262890683122, 1.000000000000000000, 0.9659258262890683122, 1.000000000000000000, 0.9659258262890683122, 1.000000000000000000, 0.9659258262890683122, 1.000000000000000000, 0.9659258262890683122, 1.000000000000000000, 0.9659258262890683122, 1.000000000000000000, 0.9659258262890683122, 1.000000000000000000, 0.9659258262890683122, 1.000000000000000000, 0.9659258262890683122, 1.000000000000000000, 0.9659258262890683122, 1.000000000000000000, 0.9659258262890683122, 1.000000000000000000, 0.9659258262890683122, 1.000000000000000000, 0.9659258262890683122, 1.000000000000000000, 0.9659258262890683122, 1.000000000000000000, 0.9659258262890683122, 1.000000000000000000),
 ( 1.000000000000000000, 0.9659258262890683122, 1.000000000000000000, 0.9659258262890683122, 1.000000000000000000, 0.9659258262890683122, 1.000000000000000000, 0.9659258262890683122, 1.000000000000000000, 0.9659258262890683122, 1.000000000000000000, 0.9659258262890683122, 1.000000000000000000, 0.9659258262890683122, 1.000000000000000000, 0.9659258262890683122, 1.000000000000000000, 0.9659258262890683122, 1.000000000000000000, 0.9659258262890683122, 1.000000000000000000, 0.9659258262890683122, 1.000000000000000000, 0.9659258262890683122, 1.000000000000000000, 0.9659258262890683122, 1.000000000000000000, 0.9659258262890683122, 1.000000000000000000, 0.9659258262890683122, 1.000000000000000000, 0.9659258262890683122, 1.000000000000000000, 0.9659258262890683122, 1.000000000000000000, 0.9659258262890683122, 1.000000000000000000, 0.9659258262890683122, 1.000000000000000000, 0.9659258262890683122, 1.000000000000000000, 0.9659258262890683122, 1.000000000000000000, 0.9659258262890683122, 1.000000000000000000, 0.9659258262890683122, 1.000000000000000000, 0.9659258262890683122, 1.000000000000000000, 0.9659258262890683122, 1.000000000000000000, 0.9659258262890683122, 1.000000000000000000, 0.9659258262890683122, 1.000000000000000000, 0.9659258262890683122, 1.000000000000000000, 0.9659258262890683122, 1.000000000000000000, 0.9659258262890683122, 1.000000000000000000, 0.9659258262890683122, 1.000000000000000000, 0.9659258262890683122, 1.000000000000000000, 0.9659258262890683122, 1.000000000000000000, 0.9659258262890683122, 1.000000000000000000, 0.9659258262890683122, 1.000000000000000000, 0.9659258262890683122, 1.000000000000000000, 0.9659258262890683122, 1.000000000000000000, 0.9659258262890683122, 1.000000000000000000, 0.9659258262890683122, 1.000000000000000000, 0.9659258262890683122, 1.000000000000000000, 0.9659258262890683122, 1.000000000000000000, 0.9659258262890683122, 1.000000000000000000, 0.9659258262890683122, 1.000000000000000000, 0.9659258262890683122, 1.000000000000000000, 0.9659258262890683122, 1.000000000000000000, 0.9659258262890683122, 1.000000000000000000, 0.9659258262890683122, 1.000000000000000000, 0.9659258262890683122, 1.000000000000000000, 0.9659258262890683122, 1.000000000000000000, 0.9659258262890683122, 1.000000000000000000, 0.9659258262890683122, 1.000000000000000000, 0.9659258262890683122, 1.000000000000000000, 0.9659258262890683122, 1.000000000000000000, 0.9659258262890683122, 1.000000000000000000, 0.9659258262890683122, 1.000000000000000000, 0.9659258262890683122, 1.000000000000000000, 0.9659258262890683122, 1.000000000000000000, 0.9659258262890683122, 1.000000000000000000, 0.9659258262890683122, 1.000000000000000000, 0.9659258262890683122, 1.000000000000000000, 0.9659258262890683122, 1.000000000000000000, 0.9659258262890683122, 1.000000000000000000, 0.9659258262890683122, 1.000000000000000000, 0.9659258262890683122, 1.000000000000000000, 0.9659258262890683122, 1.000000000000000000, 0.9659258262890683122, 1.000000000000000000, 0.9659258262890683122, 1.000000000000000000, 0.9659258262890683122, 1.000000000000000000, 0.9659258262890683122, 1.000000000000000000, 0.9659258262890683122, 1.000000000000000000, 0.9659258262890683122, 1.000000000000000000, 0.9659258262890683122, 1.000000000000000000, 0.9659258262890683122, 1.000000000000000000, 0.9659258262890683122, 1.000000000000000000, 0.9659258262890683122, 1.000000000000000000, 0.9659258262890683122, 1.000000000000000000, 0.9659258262890683122, 1.000000000000000000, 0.9659258262890683122, 1.000000000000000000, 0.9659258262890683122, 1.000000000000000000, 0.9659258262890683122, 1.000000000000000000, 0.9659258262890683122, 1.000000000000000000, 0.9659258262890683122, 1.000000000000000000, 0.9659258262890683122, 1.000000000000000000, 0.9659258262890683122, 1.000000000000000000, 0.9659258262890683122, 1.000000000000000000, 0.9659258262890683122, 1.000000000000000000, 0.9659258262890683122, 1.000000000000000000, 0.9659258262890683122, 1.000000000000000000, 0.9659258262890683122, 1.000000000000000000, 0.9659258262890683122, 1.000000000000000000, 0.9659258262890683122, 1.000000000000000000, 0.9659258262890683122, 1.000000000000000000, 0.9659258262890683122, 1.000000000000000000, 0.9659258262890683122, 1.000000000000000000, 0.9659258262890683122, 1.000000000000000000, 0.9659258262890683122, 1.000000000000000000, 0.9659258262890683122, 1.000000000000000000, 0.9659258262890683122, 1.000000000000000000, 0.9659258262890683122, 1.000000000000000000, 0.9659258262890683122, 1.000000000000000000, 0.9659258262890683122, 1.000000000000000000, 0.9659258262890683122, 1.000000000000000000, 0.9659258262890683122, 1.000000000000000000, 0.9659258262890683122, 1.000000000000000000, 0.9659258262890683122, 1.000000000000000000, 0.9659258262890683122, 1.000000000000000000, 0.9659258262890683122, 1.000000000000000000, 0.9659258262890683122, 1.000000000000000000, 0.9659258262890683122, 1.000000000000000000, 0.9659258262890683122, 1.000000000000000000, 0.9659258262890683122, 1.000000000000000000, 0.9659258262890683122, 1.000000000000000000, 0.9659258262890683122, 1.000000000000000000, 0.9659258262890683122, 1.000000000000000000, 0.9659258262890683122, 1.000000000000000000, 0.9659258262890683122, 1.000000000000000000, 0.9659258262890683122, 1.000000000000000000, 0.9659258262890683122, 1.000000000000000000, 0.9659258262890683122, 1.000000000000000000, 0.9659258262890683122, 1.000000000000000000, 0.9659258262890683122, 1.000000000000000000, 0.9659258262890683122, 1.000000000000000000, 0.9659258262890683122, 1.000000000000000000, 0.9659258262890683122, 1.000000000000000000, 0.9659258262890683122, 1.000000000000000000, 0.9659258262890683122, 1.000000000000000000, 0.9659258262890683122, 1.000000000000000000, 0.9659258262890683122, 1.000000000000000000, 0.9659258262890683122, 1.000000000000000000, 0.9659258262890683122, 1.000000000000000000, 0.9659258262890683122, 1.000000000000000000, 0.9659258262890683122, 1.000000000000000000, 0.9659258262890683122, 1.000000000000000000, 0.9659258262890683122, 1.000000000000000000, 0.9659258262890683122, 1.000000000000000000, 0.9659258262890683122, 1.000000000000000000, 0.9659258262890683122, 1.000000000000000000, 0.9659258262890683122, 1.000000000000000000, 0.9659258262890683122, 1.000000000000000000, 0.9659258262890683122, 1.000000000000000000, 0.9659258262890683122, 1.000000000000000000, 0.9659258262890683122, 1.000000000000000000, 0.9659258262890683122, 1.000000000000000000, 0.9659258262890683122, 1.000000000000000000, 0.9659258262890683122, 1.000000000000000000, 0.9659258262890683122, 1.000000000000000000, 0.9659258262890683122, 1.000000000000000000, 0.9659258262890683122, 1.000000000000000000, 0.9659258262890683122, 1.000000000000000000, 0.9659258262890683122, 1.000000000000000000, 0.9659258262890683122, 1.000000000000000000, 0.9659258262890683122, 1.000000000000000000, 0.9659258262890683122, 1.000000000000000000, 0.9659258262890683122, 1.000000000000000000, 0.9659258262890683122, 1.000000000000000000, 0.9659258262890683122, 1.000000000000000000, 0.9659258262890683122, 1.000000000000000000, 0.9659258262890683122, 1.000000000000000000, 0.9659258262890683122, 1.000000000000000000, 0.9659258262890683122, 1.000000000000000000, 0.9659258262890683122, 1.000000000000000000, 0.9659258262890683122, 1.000000000000000000) ) ) 
 REPRESENTATION_ITEM ( '' )  SURFACE ( )  );
#73591=LINE ( 'NONE', #20612, #49273 ) ;
#73592=CARTESIAN_POINT ( 'NONE',  ( 18.95785429995052240, 47.24216108172004880, 6.499999999999941380 ) ) ;
#73593=CARTESIAN_POINT ( 'NONE',  ( 14.92337183194729988, 39.34226448433412315, -8.527530157486177487 ) ) ;
#73594=CARTESIAN_POINT ( 'NONE',  ( 24.16423886937410614, 64.30374883491396076, 8.672049930838204340E-16 ) ) ;
#73595=CARTESIAN_POINT ( 'NONE',  ( 17.62281668512001076, 63.28593319516823357, 6.500000000000063061 ) ) ;
#73598=CARTESIAN_POINT ( 'NONE',  ( 7.361572987183170547, 37.05059781766744464, 9.846743663894590881 ) ) ;
#73601=DIRECTION ( 'NONE',  ( 0.000000000000000000, -1.000000000000000000, 0.000000000000000000 ) ) ;
#73602=CARTESIAN_POINT ( 'NONE',  ( 10.00000000000000000, 2.873634669930420049, -12.81628187352647608 ) ) ;
#73603=CARTESIAN_POINT ( 'NONE',  ( 5.076628168052703671, 16.84226448433411960, 8.527530157486179263 ) ) ;
#73605=CARTESIAN_POINT ( 'NONE',  ( 2.791683348922237240, 10.38393115100078390, -7.208316651077763204 ) ) ;
#73606=CARTESIAN_POINT ( 'NONE',  ( -2.816281873526473856, 4.331968003263754419, 3.434112377981055619 ) ) ;
#73609=ORIENTED_EDGE ( 'NONE', *, *, #35042, .T. ) ;
#73610=CARTESIAN_POINT ( 'NONE',  ( 20.88017736071110519, 5.563685344154838397, 2.639326808657452039E-16 ) ) ;
#73611=CARTESIAN_POINT ( 'NONE',  ( -4.164238869374098151, 1.595415501580634388, -3.795296366450310543 ) ) ;
#73612=CARTESIAN_POINT ( 'NONE',  ( 2.791683348922237240, 30.38393115100078390, -7.208316651077763204 ) ) ;
#73613=CARTESIAN_POINT ( 'NONE',  ( -0.8801773607110991993, 52.85535201082151247, -2.915334737309923874 ) ) ;
#73615=CARTESIAN_POINT ( 'NONE',  ( 19.38216949554541557, 27.24863466993041783, -9.382169495545420901 ) ) ;
#73618=B_SPLINE_CURVE_WITH_KNOTS ( 'NONE', 3,
 ( #64889, #78934, #25467, #64409 ),
 .UNSPECIFIED., .F., .F.,
 ( 4, 4 ),
 ( 0.000000000000000000, 0.0003153927346769886298 ),
 .UNSPECIFIED. ) ;
#73621=CARTESIAN_POINT ( 'NONE',  ( 13.43411237798105340, 0.5819680032637533085, 12.81628187352647963 ) ) ;
#73622=CARTESIAN_POINT ( 'NONE',  ( 7.361572987183170547, 12.05059781766744997, 9.846743663894590881 ) ) ;
#73624=CARTESIAN_POINT ( 'NONE',  ( 0.6178305044545818747, 18.49863466993041428, -9.382169495545419124 ) ) ;
#73626=CARTESIAN_POINT ( 'NONE',  ( 20.88017736071110875, 20.77201867748816611, -2.915334737309920765 ) ) ;
#73629=CARTESIAN_POINT ( 'NONE',  ( 2.917880565312950480, 45.97041550158063927, -12.26659068614894821 ) ) ;
#73631=CARTESIAN_POINT ( 'NONE',  ( -0.8801773607111008646, 23.27201867748817676, 2.915334737309923430 ) ) ;
#73632=CARTESIAN_POINT ( 'NONE',  ( 0.1532563361054083140, 51.00893115100078745, 1.131784320476157264E-15 ) ) ;
#73633=CARTESIAN_POINT ( 'NONE',  ( 7.084665262690076126, 54.10535201082151247, 10.88017736071109987 ) ) ;
#73634=CARTESIAN_POINT ( 'NONE',  ( 6.204703633549690345, 35.76208216824729647, -14.16423886937410259 ) ) ;
#73635=CARTESIAN_POINT ( 'NONE',  ( 5.076628168052704559, 40.17559781766745175, -8.527530157486179263 ) ) ;
#73636=CARTESIAN_POINT ( 'NONE',  ( 6.565887622018943937, 63.08196800326376064, -12.81628187352647608 ) ) ;
#73637=CARTESIAN_POINT ( 'NONE',  ( 19.84674366389459266, 63.71726448433412315, -2.638427012816827677 ) ) ;
#73639=CARTESIAN_POINT ( 'NONE',  ( -0.8801773607111009756, 18.06368534415484106, 1.068504757029289695E-15 ) ) ;
#73642=CARTESIAN_POINT ( 'NONE',  ( 0.5774900079438607392, 8.480352010821505360, 5.440088680355550821 ) ) ;
#73643=CARTESIAN_POINT ( 'NONE',  ( 10.00000000000000178, 2.258931151000784787, 9.846743663894594434 ) ) ;
#73644=CARTESIAN_POINT ( 'NONE',  ( 13.79529636645030344, 23.26208216824730002, 14.16423886937410614 ) ) ;
#73645=CARTESIAN_POINT ( 'NONE',  ( 12.63842701281683034, 7.467264484334118713, 9.846743663894596210 ) ) ;
#73646=CARTESIAN_POINT ( 'NONE',  ( 19.84674366389459266, 58.30059781766745886, 2.638427012816836559 ) ) ;
#73647=CARTESIAN_POINT ( 'NONE',  ( 20.88017736071110875, 35.77201867748816966, -2.915334737309920765 ) ) ;
#73649=CARTESIAN_POINT ( 'NONE',  ( 19.72487221294570858, 0.5000000000000000000, 6.500000000000000888 ) ) ;
#73654=CARTESIAN_POINT ( 'NONE',  ( 0.1532563361054082862, 46.21726448433411605, 2.638427012816831674 ) ) ;
#73658=CARTESIAN_POINT ( 'NONE',  ( 0.5774900079438590739, 62.64701867748817676, -5.440088680355550821 ) ) ;
#73659=CARTESIAN_POINT ( 'NONE',  ( 10.00000000000000000, 15.55374883491396787, -14.16423886937410082 ) ) ;
#73660=CARTESIAN_POINT ( 'NONE',  ( 13.79529636645031943, 10.34541550158063394, -14.16423886937409904 ) ) ;
#73661=CARTESIAN_POINT ( 'NONE',  ( 7.084665262690076126, 57.02201867748817676, -10.88017736071110164 ) ) ;
#73662=CARTESIAN_POINT ( 'NONE',  ( 10.00000000000000178, 53.05374883491396787, 14.16423886937410082 ) ) ;
#73663=CARTESIAN_POINT ( 'NONE',  ( 0.1532563361054082862, 36.21726448433410894, 2.638427012816831674 ) ) ;
#73665=CARTESIAN_POINT ( 'NONE',  ( 0.5774900079438590739, 32.64701867748816966, -5.440088680355550821 ) ) ;
#73666=CARTESIAN_POINT ( 'NONE',  ( 22.81628187352647785, 6.623634669930420493, 6.195893100308588602E-16 ) ) ;
#73667=CARTESIAN_POINT ( 'NONE',  ( 24.16423886937410614, 4.303748834913967869, 8.672049930838204340E-16 ) ) ;
#73668=CARTESIAN_POINT ( 'NONE',  ( 20.36894250292379382, 53.67874883491397497, 10.36894250292379205 ) ) ;
#73669=CARTESIAN_POINT ( 'NONE',  ( 0.5774900079438607392, 18.48035201082150536, 5.440088680355550821 ) ) ;
#73671=CARTESIAN_POINT ( 'NONE',  ( 17.96484262340118221, 49.93868534415484106, 7.964842623401181321 ) ) ;
#73675=ORIENTED_EDGE ( 'NONE', *, *, #902, .F. ) ;
#73676=VERTEX_POINT ( 'NONE', #11690 ) ;
#73677=CARTESIAN_POINT ( 'NONE',  ( 20.36894250292379738, 44.92874883491396787, -10.36894250292379027 ) ) ;
#73678=CARTESIAN_POINT ( 'NONE',  ( 19.84674366389459266, 53.30059781766744464, 2.638427012816836559 ) ) ;
#73679=CARTESIAN_POINT ( 'NONE',  ( 2.035157376598822676, 62.43868534415483396, -7.964842623401177768 ) ) ;
#73681=CARTESIAN_POINT ( 'NONE',  ( 4.559911319644449179, 53.89701867748817676, 9.422509992056141925 ) ) ;
#73682=CARTESIAN_POINT ( 'NONE',  ( 6.565887622018943937, 60.16530133659707502, 12.81628187352647430 ) ) ;
#73684=EDGE_LOOP ( 'NONE', ( #36666, #19925, #8889, #14319, #46661, #8876, #49829, #15158 ) ) ;
#73685=CARTESIAN_POINT ( 'NONE',  ( 17.96484262340118221, 49.93868534415484106, 7.964842623401181321 ) ) ;
#73686=CIRCLE ( 'NONE', #88039, 2.999999999999999112 ) ;
#73687=CARTESIAN_POINT ( 'NONE',  ( -0.3689425029237881626, 22.42874883491397142, 10.36894250292379027 ) ) ;
#73689=CARTESIAN_POINT ( 'NONE',  ( -2.816281873526473856, 24.12363466993042138, 9.499525473075851096E-16 ) ) ;
#73691=CARTESIAN_POINT ( 'NONE',  ( -2.816281873526473856, 44.12363466993042493, 9.499525473075851096E-16 ) ) ;
#73692=CARTESIAN_POINT ( 'NONE',  ( 7.084665262690076126, 14.10535201082150358, 10.88017736071109987 ) ) ;
#73693=CARTESIAN_POINT ( 'NONE',  ( 19.84674366389459266, 38.30059781766745175, 2.638427012816836559 ) ) ;
#73694=CARTESIAN_POINT ( 'NONE',  ( 19.42250999205614548, 10.98035201082150358, -5.440088680355545492 ) ) ;
#73695=MECHANICAL_DESIGN_GEOMETRIC_PRESENTATION_REPRESENTATION('',(#92895),#46587);
#73696=CARTESIAN_POINT ( 'NONE',  ( 10.00000000000000000, 57.87363466993042493, -12.81628187352647608 ) ) ;
#73698=CARTESIAN_POINT ( 'NONE',  ( 19.84674366389459621, 38.50893115100078745, 7.409399052514197653E-17 ) ) ;
#73705=ADVANCED_FACE ( 'NONE', ( #48204 ), #26683, .T. ) ;
#73707=CARTESIAN_POINT ( 'NONE',  ( 14.92337183194729988, 24.34226448433411960, -8.527530157486177487 ) ) ;
#73709=CARTESIAN_POINT ( 'NONE',  ( 16.40814093676323893, 25.79030133659708923, 11.09922568453595026 ) ) ;
#73711=EDGE_LOOP ( 'NONE', ( #21150, #8545, #90554, #95866 ) ) ;
#73712=CARTESIAN_POINT ( 'NONE',  ( 2.791683348922240793, 56.63393115100078035, 7.208316651077764092 ) ) ;
#73714=CARTESIAN_POINT ( 'NONE',  ( 22.26659068614895176, 24.72041550158063572, -7.082119434687042414 ) ) ;
#73715=CARTESIAN_POINT ( 'NONE',  ( 0.1532563361054083140, 41.00893115100078745, 1.131784320476157264E-15 ) ) ;
#73717=CARTESIAN_POINT ( 'NONE',  ( 10.00000000000000178, 40.37363466993042493, 12.81628187352647608 ) ) ;
#73719=FILL_AREA_STYLE_COLOUR ( '', #17753 ) ;
#73720=CARTESIAN_POINT ( 'NONE',  ( 10.00000000000000178, 64.31368534415483396, 10.88017736071110342 ) ) ;
#73721=B_SPLINE_CURVE_WITH_KNOTS ( 'NONE', 3,
 ( #44645, #77597, #23649, #45633, #53131, #61122 ),
 .UNSPECIFIED., .F., .F.,
 ( 4, 2, 4 ),
 ( 0.000000000000000000, 0.0003798359240359669084, 0.0007596718480719338168 ),
 .UNSPECIFIED. ) ;
#73723=CARTESIAN_POINT ( 'NONE',  ( 19.84674366389459266, 28.71726448433411960, -2.638427012816827677 ) ) ;
#73724=CARTESIAN_POINT ( 'NONE',  ( 0.5774900079438607392, 38.48035201082150536, 5.440088680355550821 ) ) ;
#73725=CARTESIAN_POINT ( 'NONE',  ( 3.591859063236761518, 44.95696800326376064, 11.09922568453594849 ) ) ;
#73726=CARTESIAN_POINT ( 'NONE',  ( 0.1532563361054082862, 36.21726448433410894, 2.638427012816831674 ) ) ;
#73730=CARTESIAN_POINT ( 'NONE',  ( -0.8801773607110991993, 37.85535201082151247, -2.915334737309923874 ) ) ;
#73733=CARTESIAN_POINT ( 'NONE',  ( 17.96484262340118221, 19.93868534415484106, 7.964842623401181321 ) ) ;
#73734=CARTESIAN_POINT ( 'NONE',  ( 1.472469842513823179, 60.59226448433412315, -4.923371831947296329 ) ) ;
#73735=CARTESIAN_POINT ( 'NONE',  ( 20.88017736071110164, 40.35535201082150536, 2.915334737309930979 ) ) ;
#73736=CARTESIAN_POINT ( 'NONE',  ( 2.831191079880678085, 79.91181047996344944, -5.000000000000000000 ) ) ;
#73737=EDGE_CURVE ( 'NONE', #11511, #17245, #60627, .T. ) ;
#73738=CARTESIAN_POINT ( 'NONE',  ( 4.559911319644449179, 58.89701867748817676, 9.422509992056141925 ) ) ;
#73739=CARTESIAN_POINT ( 'NONE',  ( 17.96484262340118221, 29.93868534415484106, 7.964842623401181321 ) ) ;
#73740=CARTESIAN_POINT ( 'NONE',  ( 19.72487221294571569, 40.71833443783938122, -6.499999999999989342 ) ) ;
#73741=CARTESIAN_POINT ( 'NONE',  ( 7.361572987183170547, 2.050597817667451750, 9.846743663894590881 ) ) ;
#73742=CARTESIAN_POINT ( 'NONE',  ( 2.791683348922240793, 26.63393115100078745, 7.208316651077764092 ) ) ;
#73744=CARTESIAN_POINT ( 'NONE',  ( 14.92337183194729988, 54.34226448433412315, -8.527530157486177487 ) ) ;
#73745=CARTESIAN_POINT ( 'NONE',  ( -2.266590686148945544, 47.22041550158063927, 7.082119434687048631 ) ) ;
#73746=CARTESIAN_POINT ( 'NONE',  ( 21.92686044187657401, 20.37045670184114243, -3.195792623639525765 ) ) ;
#73748=CARTESIAN_POINT ( 'NONE',  ( 13.79529636645031943, 10.34541550158063394, -14.16423886937409904 ) ) ;
#73749=CARTESIAN_POINT ( 'NONE',  ( 17.08211943468705840, 35.13708216824730357, -12.26659068614894466 ) ) ;
#73751=CARTESIAN_POINT ( 'NONE',  ( 10.00000000000000000, 2.873634669930420049, -12.81628187352647608 ) ) ;
#73753=CARTESIAN_POINT ( 'NONE',  ( 19.42250999205614548, 10.98035201082150536, -5.440088680355545492 ) ) ;
#73754=CARTESIAN_POINT ( 'NONE',  ( 0.1532563361054082862, 41.21726448433411605, 2.638427012816831674 ) ) ;
#73755=DIRECTION ( 'NONE',  ( 0.000000000000000000, -1.000000000000000000, 0.000000000000000000 ) ) ;
#73759=CARTESIAN_POINT ( 'NONE',  ( 6.565887622018943937, 20.16530133659708213, 12.81628187352647430 ) ) ;
#73760=CARTESIAN_POINT ( 'NONE',  ( 18.52753015748618282, 28.92559781766745175, -4.923371831947291888 ) ) ;
#73762=CARTESIAN_POINT ( 'NONE',  ( 10.00000000000000178, 12.25893115100078568, 9.846743663894594434 ) ) ;
#73765=CARTESIAN_POINT ( 'NONE',  ( -4.164238869374099927, 67.01208216824728936, 3.795296366450308767 ) ) ;
#73766=CARTESIAN_POINT ( 'NONE',  ( 17.96484262340118221, 9.938685344154837509, 7.964842623401181321 ) ) ;
#73767=CARTESIAN_POINT ( 'NONE',  ( 24.16423886937410614, 39.51208216824731068, -3.795296366450302550 ) ) ;
#73768=CARTESIAN_POINT ( 'NONE',  ( 10.00000000000000000, 46.81368534415484106, -10.88017736071110342 ) ) ;
#73769=CARTESIAN_POINT ( 'NONE',  ( 17.96484262340118221, 59.93868534415484106, 7.964842623401181321 ) ) ;
#73772=CARTESIAN_POINT ( 'NONE',  ( 7.361572987183170547, 17.05059781766745530, 9.846743663894590881 ) ) ;
#73774=CARTESIAN_POINT ( 'NONE',  ( 0.1532563361054083140, 11.00893115100078568, 1.131784320476157264E-15 ) ) ;
#73776=CARTESIAN_POINT ( 'NONE',  ( 17.20831665107776587, 39.13393115100079456, -7.208316651077762316 ) ) ;
#73777=CARTESIAN_POINT ( 'NONE',  ( 19.84674366389459621, 58.50893115100078745, 7.409399052514197653E-17 ) ) ;
#73778=CARTESIAN_POINT ( 'NONE',  ( 20.88017736071110875, 30.77201867748816966, -2.915334737309920765 ) ) ;
#73780=CARTESIAN_POINT ( 'NONE',  ( 19.38216949554541202, 45.99863466993041072, 9.382169495545424454 ) ) ;
#73782=CARTESIAN_POINT ( 'NONE',  ( -0.8801773607111009756, 68.06368534415484817, 1.068504757029289695E-15 ) ) ;
#73783=CARTESIAN_POINT ( 'NONE',  ( 13.43411237798106583, 37.66530133659708923, -12.81628187352647252 ) ) ;
#73784=CARTESIAN_POINT ( 'NONE',  ( -4.164238869374099927, 57.01208216824731068, 3.795296366450308767 ) ) ;
#73785=CARTESIAN_POINT ( 'NONE',  ( 14.92337183194729988, 39.34226448433412315, -8.527530157486177487 ) ) ;
#73787=CARTESIAN_POINT ( 'NONE',  ( 5.076628168052703671, 66.84226448433412315, 8.527530157486179263 ) ) ;
#73788=CARTESIAN_POINT ( 'NONE',  ( 24.16423886937409904, 39.09541550158062506, 3.795296366450317205 ) ) ;
#73789=CARTESIAN_POINT ( 'NONE',  ( 19.84674366389459266, 38.30059781766745175, 2.638427012816836559 ) ) ;
#73790=CARTESIAN_POINT ( 'NONE',  ( 17.84635730667657327, 8.637910973973182749, 6.499999999999990230 ) ) ;
#73791=CARTESIAN_POINT ( 'NONE',  ( 12.91533473730993009, 31.60535201082150891, -10.88017736071109987 ) ) ;
#73792=CARTESIAN_POINT ( 'NONE',  ( 4.559911319644449179, 62.23035201082150536, -9.422509992056141925 ) ) ;
#73795=CARTESIAN_POINT ( 'NONE',  ( 19.38216949554541557, 42.24863466993041783, -9.382169495545420901 ) ) ;
#73796=CARTESIAN_POINT ( 'NONE',  ( 4.559911319644449179, 62.23035201082150536, -9.422509992056141925 ) ) ;
#73799=( NAMED_UNIT ( * ) SI_UNIT ( $, .STERADIAN. ) SOLID_ANGLE_UNIT ( ) );
#73800=CARTESIAN_POINT ( 'NONE',  ( 7.361572987183169658, 9.967264484334119601, -9.846743663894592657 ) ) ;
#73801=CARTESIAN_POINT ( 'NONE',  ( -0.2418659066527710233, 60.11633188102327807, 6.114288769123046308 ) ) ;
#73803=CARTESIAN_POINT ( 'NONE',  ( -1.926860441876563801, 12.66212336850780495, 1.004413902775740978E-15 ) ) ;
#73804=CARTESIAN_POINT ( 'NONE',  ( 17.96484262340118221, 11.18868534415483929, -7.964842623401177768 ) ) ;
#73805=VECTOR ( 'NONE', #72344, 1000.000000000000000 ) ;
#73806=CARTESIAN_POINT ( 'NONE',  ( 1.472469842513823179, 1.425597817667451528, 4.923371831947296329 ) ) ;
#73807=CARTESIAN_POINT ( 'NONE',  ( -2.266590686148945544, 21.38708216824730357, -7.082119434687050408 ) ) ;
#73808=CARTESIAN_POINT ( 'NONE',  ( 20.88017736071110875, 25.77201867748816966, -2.915334737309920765 ) ) ;
#73809=CARTESIAN_POINT ( 'NONE',  ( 14.92337183194729633, 62.67559781766745886, 8.527530157486181039 ) ) ;
#73810=ORIENTED_EDGE ( 'NONE', *, *, #902, .T. ) ;
#73811=CARTESIAN_POINT ( 'NONE',  ( 7.361572987183170547, 62.05059781766745886, 9.846743663894590881 ) ) ;
#73813=CARTESIAN_POINT ( 'NONE',  ( 17.20831665107776587, 2.883931151000785231, 7.208316651077764980 ) ) ;
#73814=CARTESIAN_POINT ( 'NONE',  ( 18.52753015748618282, 63.92559781766745886, -4.923371831947291888 ) ) ;
#73816=CARTESIAN_POINT ( 'NONE',  ( 12.91533473730993009, 11.60535201082150536, -10.88017736071109987 ) ) ;
#73818=CARTESIAN_POINT ( 'NONE',  ( 10.00000000000000178, 69.31368534415484817, 10.88017736071110342 ) ) ;
#73819=CARTESIAN_POINT ( 'NONE',  ( 7.084665262690076126, 24.10535201082150181, 10.88017736071109987 ) ) ;
#73823=CARTESIAN_POINT ( 'NONE',  ( 2.035157376598824452, 43.68868534415484106, 7.964842623401179544 ) ) ;
#73825=CARTESIAN_POINT ( 'NONE',  ( 0.6178305044545818747, 38.49863466993042493, -9.382169495545419124 ) ) ;
#73826=CARTESIAN_POINT ( 'NONE',  ( 0.5774900079438590739, 42.64701867748816966, -5.440088680355550821 ) ) ;
#73828=AXIS2_PLACEMENT_3D ( 'NONE', #38811, #97351, #36836 ) ;
#73830=CARTESIAN_POINT ( 'NONE',  ( 12.63842701281683034, 57.46726448433411605, 9.846743663894596210 ) ) ;
#73832=STYLED_ITEM ( 'NONE', ( #93872 ), #92244 ) ;
#73834=CARTESIAN_POINT ( 'NONE',  ( 14.92337183194729633, 22.67559781766745175, 8.527530157486181039 ) ) ;
#73836=CARTESIAN_POINT ( 'NONE',  ( 16.40814093676324603, 12.45696800326375353, -11.09922568453594671 ) ) ;
#73838=CARTESIAN_POINT ( 'NONE',  ( 5.076628168052704559, 60.17559781766745175, -8.527530157486179263 ) ) ;
#73839=CARTESIAN_POINT ( 'NONE',  ( 17.96484262340118221, 16.18868534415483396, -7.964842623401177768 ) ) ;
#73840=CARTESIAN_POINT ( 'NONE',  ( 5.076628168052704559, 55.17559781766745175, -8.527530157486179263 ) ) ;
#73843=CARTESIAN_POINT ( 'NONE',  ( 1.472469842513823179, 10.59226448433411782, -4.923371831947296329 ) ) ;
#73845=CARTESIAN_POINT ( 'NONE',  ( -2.816281873526473856, 4.331968003263754419, 3.434112377981055619 ) ) ;
#73849=CARTESIAN_POINT ( 'NONE',  ( 21.09922568453594849, 41.20696800326375353, 6.408140936763242479 ) ) ;
#73850=CARTESIAN_POINT ( 'NONE',  ( 18.52753015748617571, 28.09226448433411960, 4.923371831947298993 ) ) ;
#73852=CARTESIAN_POINT ( 'NONE',  ( -2.266590686148945544, 56.38708216824731068, -7.082119434687050408 ) ) ;
#73853=CARTESIAN_POINT ( 'NONE',  ( 0.1532563361054083140, 31.00893115100078390, 1.131784320476157264E-15 ) ) ;
#73856=CARTESIAN_POINT ( 'NONE',  ( 13.79529636645030344, 58.26208216824728936, 14.16423886937410614 ) ) ;
#73859=CARTESIAN_POINT ( 'NONE',  ( 17.96484262340118221, 24.93868534415484461, 7.964842623401181321 ) ) ;
#73860=( GEOMETRIC_REPRESENTATION_CONTEXT ( 3 ) GLOBAL_UNCERTAINTY_ASSIGNED_CONTEXT ( ( #93196 ) ) GLOBAL_UNIT_ASSIGNED_CONTEXT ( ( #25423, #63868, #55409 ) ) REPRESENTATION_CONTEXT ( 'NONE', 'WORKASPACE' ) );
#73861=CARTESIAN_POINT ( 'NONE',  ( 22.26659068614895176, 34.72041550158063927, -7.082119434687042414 ) ) ;
#73862=CARTESIAN_POINT ( 'NONE',  ( 24.16423886937409904, 59.09541550158063217, 3.795296366450317205 ) ) ;
#73863=CARTESIAN_POINT ( 'NONE',  ( 0.2751277870542909731, 22.28217586085237656, -6.499999999999992006 ) ) ;
#73864=CARTESIAN_POINT ( 'NONE',  ( 12.63842701281683922, 9.550597817667449974, -9.846743663894590881 ) ) ;
#73865=CARTESIAN_POINT ( 'NONE',  ( 0.1532563361054083140, 66.00893115100079456, 1.131784320476157264E-15 ) ) ;
#73867=CARTESIAN_POINT ( 'NONE',  ( 15.44008868035555793, 46.39701867748817676, -9.422509992056140149 ) ) ;
#73869=CARTESIAN_POINT ( 'NONE',  ( 12.63842701281683922, 59.55059781766744464, -9.846743663894590881 ) ) ;
#73871=CARTESIAN_POINT ( 'NONE',  ( 2.791683348922240793, 66.63393115100079456, 7.208316651077764092 ) ) ;
#73874=CIRCLE ( 'NONE', #33963, 1.000000000000007772 ) ;
#73875=CARTESIAN_POINT ( 'NONE',  ( 19.72487221294571569, 14.78217586085237656, 6.499999999999995559 ) ) ;
#73877=CARTESIAN_POINT ( 'NONE',  ( -4.164238869374098151, 36.59541550158063217, -3.795296366450310543 ) ) ;
#73879=CARTESIAN_POINT ( 'NONE',  ( 20.88017736071110164, 20.35535201082150891, 2.915334737309930979 ) ) ;
#73880=CARTESIAN_POINT ( 'NONE',  ( 21.09922568453595559, 42.04030133659708213, -6.408140936763230044 ) ) ;
#73881=CARTESIAN_POINT ( 'NONE',  ( 15.44008868035555260, 9.730352010821505360, 9.422509992056143702 ) ) ;
#73882=CARTESIAN_POINT ( 'NONE',  ( -2.816281873526473856, 39.12363466993041783, 9.499525473075851096E-16 ) ) ;
#73883=CARTESIAN_POINT ( 'NONE',  ( 13.43411237798105340, 60.58196800326376064, 12.81628187352647963 ) ) ;
#73887=CARTESIAN_POINT ( 'NONE',  ( 2.917880565312950480, 25.97041550158063572, -12.26659068614894821 ) ) ;
#73888=CARTESIAN_POINT ( 'NONE',  ( -0.3689425029237881626, 2.428748834913967869, 10.36894250292379027 ) ) ;
#73889=DIRECTION ( 'NONE',  ( -0.000000000000000000, 1.000000000000000000, -0.000000000000000000 ) ) ;
#73890=CARTESIAN_POINT ( 'NONE',  ( -0.8801773607110991993, 27.85535201082150181, -2.915334737309923874 ) ) ;
#73892=CARTESIAN_POINT ( 'NONE',  ( 20.15039907845753220, 34.72266099184918176, 6.262539305110077059 ) ) ;
#73893=CARTESIAN_POINT ( 'NONE',  ( 17.96484262340118221, 56.18868534415484817, -7.964842623401177768 ) ) ;
#73894=CARTESIAN_POINT ( 'NONE',  ( 4.559911319644449179, 48.89701867748817676, 9.422509992056141925 ) ) ;
#73895=CARTESIAN_POINT ( 'NONE',  ( 10.00000000000000178, 15.37363466993042138, 12.81628187352647608 ) ) ;
#73898=CARTESIAN_POINT ( 'NONE',  ( 14.92337183194729988, 19.34226448433411960, -8.527530157486177487 ) ) ;
#73899=CARTESIAN_POINT ( 'NONE',  ( 0.5774900079438590739, 37.64701867748817676, -5.440088680355550821 ) ) ;
#73901=CARTESIAN_POINT ( 'NONE',  ( 0.6178305044545838731, 9.748634669930416052, 9.382169495545420901 ) ) ;
#73904=CARTESIAN_POINT ( 'NONE',  ( 18.52753015748617571, 28.09226448433411960, 4.923371831947298993 ) ) ;
#73905=CARTESIAN_POINT ( 'NONE',  ( -2.816281873526473856, 44.33196800326375353, 3.434112377981055619 ) ) ;
#73907=CARTESIAN_POINT ( 'NONE',  ( 18.52753015748618282, 3.925597817667451306, -4.923371831947291888 ) ) ;
#73910=CYLINDRICAL_SURFACE ( 'NONE', #588, 0.5000000000000004441 ) ;
#73911=CARTESIAN_POINT ( 'NONE',  ( 1.472469842513823179, 35.59226448433412315, -4.923371831947296329 ) ) ;
#73912=CARTESIAN_POINT ( 'NONE',  ( 0.5774900079438590739, 17.64701867748817321, -5.440088680355550821 ) ) ;
#73913=SURFACE_STYLE_USAGE ( .BOTH. , #28416 ) ;
#73914=CARTESIAN_POINT ( 'NONE',  ( 2.917880565312948704, 32.63708216824730357, 12.26659068614894643 ) ) ;
#73915=CARTESIAN_POINT ( 'NONE',  ( 19.84674366389459266, 33.30059781766744464, 2.638427012816836559 ) ) ;
#73916=CARTESIAN_POINT ( 'NONE',  ( 12.91533473730992121, 14.52201867748817143, 10.88017736071110164 ) ) ;
#73917=CARTESIAN_POINT ( 'NONE',  ( 17.08211943468705130, 63.47041550158063927, 12.26659068614894998 ) ) ;
#73918=ORIENTED_EDGE ( 'NONE', *, *, #40647, .T. ) ;
#73920=CARTESIAN_POINT ( 'NONE',  ( 4.559911319644449179, 27.23035201082150536, -9.422509992056141925 ) ) ;
#73922=CARTESIAN_POINT ( 'NONE',  ( 0.5774900079438590739, 37.64701867748817676, -5.440088680355550821 ) ) ;
#73923=CYLINDRICAL_SURFACE ( 'NONE', #64808, 0.5000000000000004441 ) ;
#73924=CARTESIAN_POINT ( 'NONE',  ( -0.8801773607111009756, 38.06368534415484106, 1.068504757029289695E-15 ) ) ;
#73925=VERTEX_POINT ( 'NONE', #74142 ) ;
#73926=CARTESIAN_POINT ( 'NONE',  ( 0.1532563361054100626, 60.80059781766744464, -2.638427012816831230 ) ) ;
#73927=CARTESIAN_POINT ( 'NONE',  ( 20.88017736071110875, 40.77201867748818387, -2.915334737309920765 ) ) ;
#73929=CARTESIAN_POINT ( 'NONE',  ( 10.00000000000000178, 60.37363466993041783, 12.81628187352647608 ) ) ;
#73930=LINE ( 'NONE', #98443, #66752 ) ;
#73931=CARTESIAN_POINT ( 'NONE',  ( 13.79529636645031943, 35.34541550158063927, -14.16423886937409904 ) ) ;
#73932=CARTESIAN_POINT ( 'NONE',  ( 2.035157376598822676, 57.43868534415484106, -7.964842623401177768 ) ) ;
#73933=CARTESIAN_POINT ( 'NONE',  ( 0.1532563361054100626, 65.80059781766745175, -2.638427012816831230 ) ) ;
#73935=CARTESIAN_POINT ( 'NONE',  ( 17.20831665107776587, 49.13393115100078745, -7.208316651077762316 ) ) ;
#73936=ORIENTED_EDGE ( 'NONE', *, *, #12478, .F. ) ;
#73937=LINE ( 'NONE', #3982, #90983 ) ;
#73939=CARTESIAN_POINT ( 'NONE',  ( 18.52753015748618282, 18.92559781766745175, -4.923371831947291888 ) ) ;
#73941=CARTESIAN_POINT ( 'NONE',  ( 12.91533473730993009, 21.60535201082150536, -10.88017736071109987 ) ) ;
#73942=CARTESIAN_POINT ( 'NONE',  ( 19.84674366389459266, 18.30059781766745175, 2.638427012816836559 ) ) ;
#73943=CARTESIAN_POINT ( 'NONE',  ( 17.96484262340118221, 59.93868534415484106, 7.964842623401181321 ) ) ;
#73944=CARTESIAN_POINT ( 'NONE',  ( 7.084665262690076126, 29.10535201082150181, 10.88017736071109987 ) ) ;
#73945=CARTESIAN_POINT ( 'NONE',  ( 10.00000000000000000, 57.87363466993042493, -12.81628187352647608 ) ) ;
#73946=CARTESIAN_POINT ( 'NONE',  ( 6.204703633549690345, 45.76208216824729647, -14.16423886937410259 ) ) ;
#73951=CARTESIAN_POINT ( 'NONE',  ( 16.40814093676323893, 0.7903013365970867898, 11.09922568453595026 ) ) ;
#73952=CARTESIAN_POINT ( 'NONE',  ( 7.084665262690076126, 12.02201867748817143, -10.88017736071110164 ) ) ;
#73954=CARTESIAN_POINT ( 'NONE',  ( -0.8801773607111009756, 48.06368534415484817, 1.068504757029289695E-15 ) ) ;
#73955=CARTESIAN_POINT ( 'NONE',  ( 7.361572987183170547, 57.05059781766744464, 9.846743663894590881 ) ) ;
#73957=CARTESIAN_POINT ( 'NONE',  ( 14.92337183194729633, 17.67559781766745175, 8.527530157486181039 ) ) ;
#73958=CARTESIAN_POINT ( 'NONE',  ( 0.1532563361054082862, 16.21726448433411960, 2.638427012816831674 ) ) ;
#73959=CARTESIAN_POINT ( 'NONE',  ( 1.472469842513823179, 35.59226448433412315, -4.923371831947296329 ) ) ;
#73960=CARTESIAN_POINT ( 'NONE',  ( 5.076628168052703671, 11.84226448433411960, 8.527530157486179263 ) ) ;
#73961=CARTESIAN_POINT ( 'NONE',  ( 17.20831665107776587, 14.13393115100078568, -7.208316651077762316 ) ) ;
#73963=CARTESIAN_POINT ( 'NONE',  ( 17.96484262340118221, 64.93868534415483396, 7.964842623401181321 ) ) ;
#73965=CARTESIAN_POINT ( 'NONE',  ( 0.1532563361054083140, 6.008931151000784787, 1.131784320476157264E-15 ) ) ;
#73966=CARTESIAN_POINT ( 'NONE',  ( 17.20831665107776587, 22.88393115100078745, 7.208316651077764980 ) ) ;
#73969=CARTESIAN_POINT ( 'NONE',  ( 6.565887622018943937, 3.081968003263753531, -12.81628187352647608 ) ) ;
#73972=EDGE_CURVE ( 'NONE', #20878, #40989, #36159, .T. ) ;
#73973=CARTESIAN_POINT ( 'NONE',  ( 20.36894250292379738, 19.92874883491396787, -10.36894250292379027 ) ) ;
#73976=CARTESIAN_POINT ( 'NONE',  ( 10.00000000000000000, 15.55374883491396787, -14.16423886937410082 ) ) ;
#73977=CARTESIAN_POINT ( 'NONE',  ( -2.266590686148945544, 46.38708216824730357, -7.082119434687050408 ) ) ;
#73979=CARTESIAN_POINT ( 'NONE',  ( 6.204703633549690345, 17.84541550158063217, 14.16423886937410082 ) ) ;
#73980=CARTESIAN_POINT ( 'NONE',  ( 2.035157376598822676, 67.43868534415484817, -7.964842623401177768 ) ) ;
#73981=CARTESIAN_POINT ( 'NONE',  ( 10.00000000000000178, 34.31368534415484106, 10.88017736071110342 ) ) ;
#73983=CARTESIAN_POINT ( 'NONE',  ( 0.1532563361054082862, 31.21726448433412315, 2.638427012816831674 ) ) ;
#73984=CARTESIAN_POINT ( 'NONE',  ( 7.084665262690076126, 67.02201867748817676, -10.88017736071110164 ) ) ;
#73985=CARTESIAN_POINT ( 'NONE',  ( 19.84674366389459621, 33.50893115100078745, 7.409399052514197653E-17 ) ) ;
#73986=CARTESIAN_POINT ( 'NONE',  ( 4.559911319644449179, 8.897018677488173211, 9.422509992056141925 ) ) ;
#73987=CARTESIAN_POINT ( 'NONE',  ( 19.38216949554541202, 55.99863466993041072, 9.382169495545424454 ) ) ;
#73988=CARTESIAN_POINT ( 'NONE',  ( 10.00000000000000000, 44.75893115100078745, -9.846743663894594434 ) ) ;
#73989=CARTESIAN_POINT ( 'NONE',  ( 10.00000000000000000, 37.87363466993041783, -12.81628187352647608 ) ) ;
#73992=CARTESIAN_POINT ( 'NONE',  ( 7.084665262690076126, 49.10535201082149825, 10.88017736071109987 ) ) ;
#73993=CARTESIAN_POINT ( 'NONE',  ( 14.92337183194729988, 44.34226448433412315, -8.527530157486177487 ) ) ;
#73994=CARTESIAN_POINT ( 'NONE',  ( 17.08211943468705130, 28.47041550158063572, 12.26659068614894998 ) ) ;
#73996=CARTESIAN_POINT ( 'NONE',  ( 19.42250999205614193, 50.14701867748817676, 5.440088680355555262 ) ) ;
#73998=CARTESIAN_POINT ( 'NONE',  ( 17.08211943468705840, 50.13708216824730357, -12.26659068614894466 ) ) ;
#73999=CARTESIAN_POINT ( 'NONE',  ( -2.816281873526471635, -1.084698663402913210, -3.434112377981056508 ) ) ;
#74000=B_SPLINE_CURVE_WITH_KNOTS ( 'NONE', 3,
 ( #35156, #58149, #50670, #18214 ),
 .UNSPECIFIED., .F., .F.,
 ( 4, 4 ),
 ( 0.000000000000000000, 0.001036303429213241475 ),
 .UNSPECIFIED. ) ;
#74002=CARTESIAN_POINT ( 'NONE',  ( -0.8801773607110991993, 57.85535201082149825, -2.915334737309923874 ) ) ;
#74003=CARTESIAN_POINT ( 'NONE',  ( -46.30928139467842897, 104.0823827281712255, 5.529860068218143354 ) ) ;
#74004=CARTESIAN_POINT ( 'NONE',  ( 6.565887622018943937, 25.16530133659708213, 12.81628187352647430 ) ) ;
#74005=CARTESIAN_POINT ( 'NONE',  ( 10.00000000000000178, 57.25893115100078745, 9.846743663894594434 ) ) ;
#74007=CARTESIAN_POINT ( 'NONE',  ( 17.96484262340118221, 4.938685344154837509, 7.964842623401181321 ) ) ;
#74010=CARTESIAN_POINT ( 'NONE',  ( -0.8801773607111008646, 3.272018677488171434, 2.915334737309923430 ) ) ;
#74011=CARTESIAN_POINT ( 'NONE',  ( 20.10421743870887212, 65.60736173766201773, -6.337391062633413341 ) ) ;
#74012=CARTESIAN_POINT ( 'NONE',  ( 2.035157376598822676, 67.43868534415484817, -7.964842623401177768 ) ) ;
#74013=CARTESIAN_POINT ( 'NONE',  ( 14.92337183194729988, 4.342264484334117824, -8.527530157486177487 ) ) ;
#74014=CARTESIAN_POINT ( 'NONE',  ( 19.84674366389459266, 38.71726448433412315, -2.638427012816827677 ) ) ;
#74015=CARTESIAN_POINT ( 'NONE',  ( 17.96484262340118221, 31.18868534415483751, -7.964842623401177768 ) ) ;
#74016=CARTESIAN_POINT ( 'NONE',  ( 10.00000000000000000, 2.873634669930420049, -12.81628187352647608 ) ) ;
#74017=CARTESIAN_POINT ( 'NONE',  ( 4.559911319644449179, 37.23035201082150536, -9.422509992056141925 ) ) ;
#74019=CARTESIAN_POINT ( 'NONE',  ( 17.85158348494336877, 64.73726573380444904, -6.500000000000001776 ) ) ;
#74020=CARTESIAN_POINT ( 'NONE',  ( 0.6178305044545838731, 39.74863466993041072, 9.382169495545420901 ) ) ;
#74021=ORIENTED_EDGE ( 'NONE', *, *, #45654, .F. ) ;
#74022=CARTESIAN_POINT ( 'NONE',  ( 17.96484262340118221, 66.18868534415483396, -7.964842623401177768 ) ) ;
#74023=CARTESIAN_POINT ( 'NONE',  ( 19.38216949554541557, 32.24863466993041783, -9.382169495545420901 ) ) ;
#74024=FACE_OUTER_BOUND ( 'NONE', #51186, .T. ) ;
#74025=CARTESIAN_POINT ( 'NONE',  ( 7.084665262690076126, 37.02201867748817676, -10.88017736071110164 ) ) ;
#74026=CARTESIAN_POINT ( 'NONE',  ( 17.20831665107776587, 62.88393115100078745, 7.208316651077764980 ) ) ;
#74027=CARTESIAN_POINT ( 'NONE',  ( -0.3689425029237898834, 66.17874883491396076, -10.36894250292378850 ) ) ;
#74028=CARTESIAN_POINT ( 'NONE',  ( 18.52753015748617571, 53.09226448433412315, 4.923371831947298993 ) ) ;
#74029=CARTESIAN_POINT ( 'NONE',  ( 0.1532563361054083140, 16.00893115100078390, 1.131784320476157264E-15 ) ) ;
#74030=CARTESIAN_POINT ( 'NONE',  ( 20.88017736071110875, 60.77201867748817676, -2.915334737309920765 ) ) ;
#74032=CARTESIAN_POINT ( 'NONE',  ( 6.204703633549690345, 25.76208216824730712, -14.16423886937410259 ) ) ;
#74037=CARTESIAN_POINT ( 'NONE',  ( 2.917880565312950480, 55.97041550158063217, -12.26659068614894821 ) ) ;
#74038=CARTESIAN_POINT ( 'NONE',  ( -4.164238869374099927, 67.01208216824728936, 3.795296366450308767 ) ) ;
#74039=CARTESIAN_POINT ( 'NONE',  ( 19.84674366389459266, 33.30059781766744464, 2.638427012816836559 ) ) ;
#74041=DIRECTION ( 'NONE',  ( -0.8320502943378436100, 0.5547001962252291474, -0.000000000000000000 ) ) ;
#74042=CARTESIAN_POINT ( 'NONE',  ( 17.96484262340118221, 14.93868534415483751, 7.964842623401181321 ) ) ;
#74043=CARTESIAN_POINT ( 'NONE',  ( 13.79529636645031943, 60.34541550158063927, -14.16423886937409904 ) ) ;
#74044=CARTESIAN_POINT ( 'NONE',  ( 14.92337183194729633, 27.67559781766745530, 8.527530157486181039 ) ) ;
#74045=DIRECTION ( 'NONE',  ( 0.000000000000000000, 0.000000000000000000, 1.000000000000000000 ) ) ;
#74046=CARTESIAN_POINT ( 'NONE',  ( 1.472469842513823179, 15.59226448433411960, -4.923371831947296329 ) ) ;
#74048=CARTESIAN_POINT ( 'NONE',  ( 18.52753015748618282, 3.925597817667451306, -4.923371831947291888 ) ) ;
#74054=CARTESIAN_POINT ( 'NONE',  ( 14.92337183194729633, 42.67559781766745886, 8.527530157486181039 ) ) ;
#74055=CARTESIAN_POINT ( 'NONE',  ( -0.3689425029237898834, 21.17874883491396432, -10.36894250292378850 ) ) ;
#74056=CARTESIAN_POINT ( 'NONE',  ( 19.42250999205614548, 20.98035201082150891, -5.440088680355545492 ) ) ;
#74057=CARTESIAN_POINT ( 'NONE',  ( 4.559911319644449179, 23.89701867748817321, 9.422509992056141925 ) ) ;
#74058=CARTESIAN_POINT ( 'NONE',  ( 12.63842701281683922, 59.55059781766744464, -9.846743663894590881 ) ) ;
#74059=CARTESIAN_POINT ( 'NONE',  ( 10.00000000000000000, 17.87363466993041783, -12.81628187352647608 ) ) ;
#74060=CARTESIAN_POINT ( 'NONE',  ( -0.3689425029237898834, 11.17874883491396787, -10.36894250292378850 ) ) ;
#74062=CARTESIAN_POINT ( 'NONE',  ( 6.565887622018943937, 33.08196800326374643, -12.81628187352647608 ) ) ;
#74064=CARTESIAN_POINT ( 'NONE',  ( 17.20831665107776587, 27.88393115100078390, 7.208316651077764980 ) ) ;
#74065=CARTESIAN_POINT ( 'NONE',  ( 20.88017736071110875, 5.772018677488170546, -2.915334737309920765 ) ) ;
#74067=CARTESIAN_POINT ( 'NONE',  ( 24.16423886937410614, 64.51208216824728936, -3.795296366450302550 ) ) ;
#74068=ORIENTED_EDGE ( 'NONE', *, *, #65937, .T. ) ;
#74069=CARTESIAN_POINT ( 'NONE',  ( 12.91533473730993009, 51.60535201082149825, -10.88017736071109987 ) ) ;
#74070=CARTESIAN_POINT ( 'NONE',  ( 7.084665262690076126, 59.10535201082150536, 10.88017736071109987 ) ) ;
#74071=CARTESIAN_POINT ( 'NONE',  ( 12.91533473730992121, 54.52201867748816255, 10.88017736071110164 ) ) ;
#74073=CARTESIAN_POINT ( 'NONE',  ( 7.084665262690076126, 44.10535201082151247, 10.88017736071109987 ) ) ;
#74076=CARTESIAN_POINT ( 'NONE',  ( 12.63842701281683922, 34.55059781766745886, -9.846743663894590881 ) ) ;
#74078=CARTESIAN_POINT ( 'NONE',  ( 5.076628168052704559, 55.17559781766745175, -8.527530157486179263 ) ) ;
#74080=CARTESIAN_POINT ( 'NONE',  ( -2.266590686148945544, 11.38708216824730179, -7.082119434687050408 ) ) ;
#74082=EDGE_CURVE ( 'NONE', #27101, #6459, #73721, .T. ) ;
#74086=CARTESIAN_POINT ( 'NONE',  ( -0.3689425029237881626, 62.42874883491396787, 10.36894250292379027 ) ) ;
#74089=CARTESIAN_POINT ( 'NONE',  ( 0.1532563361054100626, 50.80059781766745175, -2.638427012816831230 ) ) ;
#74090=FACE_OUTER_BOUND ( 'NONE', #12803, .T. ) ;
#74091=CARTESIAN_POINT ( 'NONE',  ( -1.099225684535947600, 19.54030133659708568, 6.408140936763237150 ) ) ;
#74092=CARTESIAN_POINT ( 'NONE',  ( 1.472469842513823179, 15.59226448433411960, -4.923371831947296329 ) ) ;
#74095=CARTESIAN_POINT ( 'NONE',  ( 14.92337183194729988, 14.34226448433411782, -8.527530157486177487 ) ) ;
#74096=CARTESIAN_POINT ( 'NONE',  ( 21.09922568453594849, 1.206968003263753531, 6.408140936763242479 ) ) ;
#74097=CARTESIAN_POINT ( 'NONE',  ( 2.603489959281601873, 25.43575266056827289, -6.500000000000015987 ) ) ;
#74099=EDGE_LOOP ( 'NONE', ( #98391, #61271, #57315, #20273, #9133, #82444 ) ) ;
#74100=CARTESIAN_POINT ( 'NONE',  ( 20.88017736071110519, 15.56368534415483751, 2.639326808657452039E-16 ) ) ;
#74101=CARTESIAN_POINT ( 'NONE',  ( 13.79529636645031943, 5.345415501580634832, -14.16423886937409904 ) ) ;
#74102=CARTESIAN_POINT ( 'NONE',  ( 17.20831665107776587, 22.88393115100078745, 7.208316651077764980 ) ) ;
#74103=CARTESIAN_POINT ( 'NONE',  ( 2.035157376598824452, 58.68868534415482685, 7.964842623401179544 ) ) ;
#74104=CARTESIAN_POINT ( 'NONE',  ( 16.40814093676323893, 30.79030133659708923, 11.09922568453595026 ) ) ;
#74106=( NAMED_UNIT ( * ) SI_UNIT ( $, .STERADIAN. ) SOLID_ANGLE_UNIT ( ) );
#74109=CARTESIAN_POINT ( 'NONE',  ( 0.1532563361054100626, 60.80059781766744464, -2.638427012816831230 ) ) ;
#74110=CARTESIAN_POINT ( 'NONE',  ( 12.63842701281683034, 12.46726448433411782, 9.846743663894596210 ) ) ;
#74112=CARTESIAN_POINT ( 'NONE',  ( -1.099225684535947600, 18.70696800326375353, -6.408140936763238038 ) ) ;
#74113=CARTESIAN_POINT ( 'NONE',  ( 1.932340009482121035, 51.49127512925449679, -6.499999999999929834 ) ) ;
#74114=CARTESIAN_POINT ( 'NONE',  ( 7.084665262690076126, 39.10535201082150536, 10.88017736071109987 ) ) ;
#74118=CARTESIAN_POINT ( 'NONE',  ( 2.035157376598822676, 32.43868534415483396, -7.964842623401177768 ) ) ;
#74119=CARTESIAN_POINT ( 'NONE',  ( 17.96484262340118221, 31.18868534415483751, -7.964842623401177768 ) ) ;
#74120=CARTESIAN_POINT ( 'NONE',  ( 5.076628168052704559, 50.17559781766745886, -8.527530157486179263 ) ) ;
#74121=CARTESIAN_POINT ( 'NONE',  ( -0.8801773607111009756, 58.06368534415484106, 1.068504757029289695E-15 ) ) ;
#74122=CARTESIAN_POINT ( 'NONE',  ( -0.3689425029237881626, 37.42874883491396787, 10.36894250292379027 ) ) ;
#74124=CARTESIAN_POINT ( 'NONE',  ( 7.361572987183170547, 32.05059781766745175, 9.846743663894590881 ) ) ;
#74125=CARTESIAN_POINT ( 'NONE',  ( 6.565887622018943937, -1.918031996736246692, -12.81628187352647608 ) ) ;
#74127=CARTESIAN_POINT ( 'NONE',  ( 19.42250999205614193, 20.14701867748817321, 5.440088680355555262 ) ) ;
#74128=CARTESIAN_POINT ( 'NONE',  ( 20.24186590665277663, 6.760286857231743163, 6.114288769123037426 ) ) ;
#74129=CARTESIAN_POINT ( 'NONE',  ( -0.8801773607110991993, 2.855352010821504471, -2.915334737309923874 ) ) ;
#74130=CARTESIAN_POINT ( 'NONE',  ( -0.8801773607111008646, 18.27201867748817321, 2.915334737309923430 ) ) ;
#74131=CARTESIAN_POINT ( 'NONE',  ( 7.361572987183169658, 4.967264484334119601, -9.846743663894592657 ) ) ;
#74132=CARTESIAN_POINT ( 'NONE',  ( 20.36894250292379738, 19.92874883491396787, -10.36894250292379027 ) ) ;
#74133=MANIFOLD_SOLID_BREP ( 'Fillet3', #76155 ) ;
#74134=CARTESIAN_POINT ( 'NONE',  ( 2.791683348922237240, 20.38393115100078745, -7.208316651077763204 ) ) ;
#74135=CARTESIAN_POINT ( 'NONE',  ( 18.52753015748617571, 63.09226448433412315, 4.923371831947298993 ) ) ;
#74136=CARTESIAN_POINT ( 'NONE',  ( 20.88017736071110519, 30.56368534415484106, 2.639326808657452039E-16 ) ) ;
#74138=CARTESIAN_POINT ( 'NONE',  ( -45.65232842522237178, 104.2922929041766338, -5.788770647549307924 ) ) ;
#74142=CARTESIAN_POINT ( 'NONE',  ( -0.1503990784575263973, 27.22266099184919241, -6.262539305110081500 ) ) ;
#74143=CARTESIAN_POINT ( 'NONE',  ( 14.92337183194729633, 42.67559781766745886, 8.527530157486181039 ) ) ;
#74144=EDGE_LOOP ( 'NONE', ( #43834, #92056, #91061, #28217, #22796, #16084 ) ) ;
#74147=CARTESIAN_POINT ( 'NONE',  ( 20.36894250292379382, 23.67874883491397142, 10.36894250292379205 ) ) ;
#74148=CARTESIAN_POINT ( 'NONE',  ( 2.917880565312950480, 10.97041550158063572, -12.26659068614894821 ) ) ;
#74149=CARTESIAN_POINT ( 'NONE',  ( 15.44008868035555260, 59.73035201082151247, 9.422509992056143702 ) ) ;
#74150=CARTESIAN_POINT ( 'NONE',  ( -2.266590686148945544, 56.38708216824731068, -7.082119434687050408 ) ) ;
#74151=CARTESIAN_POINT ( 'NONE',  ( 22.81628187352647785, 1.415301336597087012, 3.434112377981063169 ) ) ;
#74152=CARTESIAN_POINT ( 'NONE',  ( 12.63842701281683034, 47.46726448433412315, 9.846743663894596210 ) ) ;
#74154=CARTESIAN_POINT ( 'NONE',  ( 12.91533473730992121, 44.52201867748816966, 10.88017736071110164 ) ) ;
#74155=CARTESIAN_POINT ( 'NONE',  ( 13.43411237798105340, 5.581968003263753531, 12.81628187352647963 ) ) ;
#74156=CARTESIAN_POINT ( 'NONE',  ( 2.917880565312948704, 22.63708216824730002, 12.26659068614894643 ) ) ;
#74157=CARTESIAN_POINT ( 'NONE',  ( 0.5774900079438607392, 13.48035201082150358, 5.440088680355550821 ) ) ;
#74160=CARTESIAN_POINT ( 'NONE',  ( 2.035157376598822676, 47.43868534415484817, -7.964842623401177768 ) ) ;
#74166=CARTESIAN_POINT ( 'NONE',  ( 2.917880565312950480, 45.97041550158063927, -12.26659068614894821 ) ) ;
#74167=CARTESIAN_POINT ( 'NONE',  ( 7.361572987183169658, 44.96726448433412315, -9.846743663894592657 ) ) ;
#74168=CARTESIAN_POINT ( 'NONE',  ( 7.084665262690076126, 64.10535201082150536, 10.88017736071109987 ) ) ;
#74170=CARTESIAN_POINT ( 'NONE',  ( 19.42250999205614548, 55.98035201082150536, -5.440088680355545492 ) ) ;
#74172=MECHANICAL_DESIGN_GEOMETRIC_PRESENTATION_REPRESENTATION('',(#5542),#45493);
#74175=ORIENTED_EDGE ( 'NONE', *, *, #20672, .T. ) ;
#74177=CARTESIAN_POINT ( 'NONE',  ( 22.26659068614894466, 23.88708216824730357, 7.082119434687054849 ) ) ;
#74180=CARTESIAN_POINT ( 'NONE',  ( -1.099225684535947600, 23.70696800326375708, -6.408140936763238038 ) ) ;
#74181=ORIENTED_EDGE ( 'NONE', *, *, #73190, .F. ) ;
#74182=CARTESIAN_POINT ( 'NONE',  ( 21.09922568453595559, 47.04030133659708923, -6.408140936763230044 ) ) ;
#74183=CARTESIAN_POINT ( 'NONE',  ( 18.52753015748618282, 33.92559781766745886, -4.923371831947291888 ) ) ;
#74184=CARTESIAN_POINT ( 'NONE',  ( 19.42250999205614193, 10.14701867748816966, 5.440088680355555262 ) ) ;
#74185=CARTESIAN_POINT ( 'NONE',  ( 19.38216949554541557, 52.24863466993041072, -9.382169495545420901 ) ) ;
#74186=CARTESIAN_POINT ( 'NONE',  ( -45.94000000000001194, 103.7452903794826682, 5.529860068218143354 ) ) ;
#74187=CARTESIAN_POINT ( 'NONE',  ( 12.63842701281683034, 47.46726448433412315, 9.846743663894596210 ) ) ;
#74188=DIRECTION ( 'NONE',  ( 0.000000000000000000, 1.000000000000000000, 0.000000000000000000 ) ) ;
#74192=CARTESIAN_POINT ( 'NONE',  ( 0.5600000000000083800, 105.0000000000000000, 4.500000000000000888 ) ) ;
#74195=CARTESIAN_POINT ( 'NONE',  ( 12.63842701281683922, 19.55059781766745175, -9.846743663894590881 ) ) ;
#74196=CARTESIAN_POINT ( 'NONE',  ( -2.816281873526473856, 29.33196800326376064, 3.434112377981055619 ) ) ;
#74197=DIRECTION ( 'NONE',  ( 0.000000000000000000, 0.000000000000000000, 1.000000000000000000 ) ) ;
#74199=CARTESIAN_POINT ( 'NONE',  ( 2.791683348922240793, 61.63393115100079456, 7.208316651077764092 ) ) ;
#74201=CARTESIAN_POINT ( 'NONE',  ( -2.266590686148945544, 16.38708216824730357, -7.082119434687050408 ) ) ;
#74202=CARTESIAN_POINT ( 'NONE',  ( 12.63842701281683034, 47.46726448433412315, 9.846743663894596210 ) ) ;
#74203=CARTESIAN_POINT ( 'NONE',  ( -2.816281873526471635, 43.91530133659708923, -3.434112377981056508 ) ) ;
#74205=CARTESIAN_POINT ( 'NONE',  ( 21.92686044187656691, 37.18830936912750929, 4.562052436263911564E-16 ) ) ;
#74207=CARTESIAN_POINT ( 'NONE',  ( 19.42250999205614193, 65.14701867748817676, 5.440088680355555262 ) ) ;
#74210=CARTESIAN_POINT ( 'NONE',  ( 14.92337183194729988, 29.34226448433411960, -8.527530157486177487 ) ) ;
#74211=CARTESIAN_POINT ( 'NONE',  ( 12.91533473730993009, 36.60535201082151247, -10.88017736071109987 ) ) ;
#74213=CARTESIAN_POINT ( 'NONE',  ( 19.84674366389459621, 33.50893115100078745, 7.409399052514197653E-17 ) ) ;
#74214=DIRECTION ( 'NONE',  ( 0.000000000000000000, 0.000000000000000000, -1.000000000000000000 ) ) ;
#74215=CARTESIAN_POINT ( 'NONE',  ( 7.084665262690076126, 49.10535201082149825, 10.88017736071109987 ) ) ;
#74216=ORIENTED_EDGE ( 'NONE', *, *, #73737, .F. ) ;
#74218=CARTESIAN_POINT ( 'NONE',  ( 10.00000000000000000, 16.81368534415483751, -10.88017736071110342 ) ) ;
#74219=CARTESIAN_POINT ( 'NONE',  ( 7.361572987183170547, 57.05059781766744464, 9.846743663894590881 ) ) ;
#74220=CARTESIAN_POINT ( 'NONE',  ( 12.91533473730993009, 41.60535201082149825, -10.88017736071109987 ) ) ;
#74222=CARTESIAN_POINT ( 'NONE',  ( 15.44008868035555793, 61.39701867748817676, -9.422509992056140149 ) ) ;
#74223=CARTESIAN_POINT ( 'NONE',  ( -0.8801773607111009756, 33.06368534415484106, 1.068504757029289695E-15 ) ) ;
#74225=CARTESIAN_POINT ( 'NONE',  ( 14.92337183194729988, 19.34226448433411960, -8.527530157486177487 ) ) ;
#74228=CARTESIAN_POINT ( 'NONE',  ( 10.00000000000000178, 47.25893115100078745, 9.846743663894594434 ) ) ;
#74230=CARTESIAN_POINT ( 'NONE',  ( -2.266590686148945544, 67.22041550158063217, 7.082119434687048631 ) ) ;
#74231=CARTESIAN_POINT ( 'NONE',  ( 20.15039907845753930, 70.00000000000000000, 6.262539305110068177 ) ) ;
#74232=CARTESIAN_POINT ( 'NONE',  ( 24.16423886937410614, 9.303748834913967869, 8.672049930838204340E-16 ) ) ;
#74233=CARTESIAN_POINT ( 'NONE',  ( 17.08211943468705130, 43.47041550158063927, 12.26659068614894998 ) ) ;
#74234=B_SPLINE_CURVE_WITH_KNOTS ( 'NONE', 3,
 ( #32917, #70943, #48904, #1959 ),
 .UNSPECIFIED., .F., .F.,
 ( 4, 4 ),
 ( 5.974731160962075775E-17, 0.002562518741975290844 ),
 .UNSPECIFIED. ) ;
#74235=CARTESIAN_POINT ( 'NONE',  ( 22.81628187352648496, 6.831968003263753531, -3.434112377981050290 ) ) ;
#74237=CARTESIAN_POINT ( 'NONE',  ( 2.035157376598824452, 13.68868534415483751, 7.964842623401179544 ) ) ;
#74238=B_SPLINE_CURVE_WITH_KNOTS ( 'NONE', 3,
 ( #36890, #67378, #52864, #97907, #59869, #90857 ),
 .UNSPECIFIED., .F., .F.,
 ( 4, 2, 4 ),
 ( 4.906538933386797396E-18, 0.0002605067024380966511, 0.0005210134048761883149 ),
 .UNSPECIFIED. ) ;
#74239=CARTESIAN_POINT ( 'NONE',  ( 17.20831665107776587, 42.88393115100077324, 7.208316651077764980 ) ) ;
#74245=CARTESIAN_POINT ( 'NONE',  ( 19.38216949554541202, 20.99863466993042138, 9.382169495545424454 ) ) ;
#74246=CARTESIAN_POINT ( 'NONE',  ( 0.1532563361054100626, 25.80059781766744820, -2.638427012816831230 ) ) ;
#74248=CARTESIAN_POINT ( 'NONE',  ( 7.361572987183170547, 7.050597817667451750, 9.846743663894590881 ) ) ;
#74251=CARTESIAN_POINT ( 'NONE',  ( 20.88017736071110519, 15.56368534415483751, 2.639326808657452039E-16 ) ) ;
#74252=CARTESIAN_POINT ( 'NONE',  ( 10.00000000000000000, 40.55374883491397497, -14.16423886937410082 ) ) ;
#74253=CARTESIAN_POINT ( 'NONE',  ( 7.084665262690076126, 39.10535201082150536, 10.88017736071109987 ) ) ;
#74254=CARTESIAN_POINT ( 'NONE',  ( 7.084665262690076126, 59.10535201082150536, 10.88017736071109987 ) ) ;
#74256=CARTESIAN_POINT ( 'NONE',  ( 19.84674366389459266, 18.71726448433411960, -2.638427012816827677 ) ) ;
#74258=CARTESIAN_POINT ( 'NONE',  ( 14.92337183194729633, 7.675597817667451750, 8.527530157486181039 ) ) ;
#74259=CARTESIAN_POINT ( 'NONE',  ( -1.511515493404499644, 5.397528278722328023E-15, 1.315623007559852509 ) ) ;
#74260=CARTESIAN_POINT ( 'NONE',  ( 19.84674366389459266, 38.30059781766745175, 2.638427012816836559 ) ) ;
#74261=CARTESIAN_POINT ( 'NONE',  ( 0.1532563361054100626, 65.80059781766745175, -2.638427012816831230 ) ) ;
#74262=CARTESIAN_POINT ( 'NONE',  ( 15.44008868035555260, 34.73035201082151247, 9.422509992056143702 ) ) ;
#74266=CARTESIAN_POINT ( 'NONE',  ( 6.565887622018943937, 63.08196800326376064, -12.81628187352647608 ) ) ;
#74268=CARTESIAN_POINT ( 'NONE',  ( -1.099225684535947600, 43.70696800326375353, -6.408140936763238038 ) ) ;
#74269=CARTESIAN_POINT ( 'NONE',  ( 2.917880565312948704, 57.63708216824731068, 12.26659068614894643 ) ) ;
#74270=CARTESIAN_POINT ( 'NONE',  ( 1.472469842513823179, 35.59226448433412315, -4.923371831947296329 ) ) ;
#74272=CARTESIAN_POINT ( 'NONE',  ( 10.00000000000000178, 2.258931151000784787, 9.846743663894594434 ) ) ;
#74273=CARTESIAN_POINT ( 'NONE',  ( -4.164238869374098151, 21.59541550158063217, -3.795296366450310543 ) ) ;
#74274=CARTESIAN_POINT ( 'NONE',  ( 6.204703633549690345, 45.76208216824729647, -14.16423886937410259 ) ) ;
#74275=CARTESIAN_POINT ( 'NONE',  ( 18.52753015748618282, 43.92559781766745175, -4.923371831947291888 ) ) ;
#74277=CARTESIAN_POINT ( 'NONE',  ( -0.8801773607110991993, 42.85535201082150536, -2.915334737309923874 ) ) ;
#74278=CARTESIAN_POINT ( 'NONE',  ( 7.084665262690076126, 62.02201867748816966, -10.88017736071110164 ) ) ;
#74281=CARTESIAN_POINT ( 'NONE',  ( 13.43411237798105340, 60.58196800326376064, 12.81628187352647963 ) ) ;
#74283=CARTESIAN_POINT ( 'NONE',  ( 5.076628168052703671, 1.842264484334118047, 8.527530157486179263 ) ) ;
#74285=AXIS2_PLACEMENT_3D ( 'NONE', #20376, #88870, #96889 ) ;
#74286=CARTESIAN_POINT ( 'NONE',  ( -4.164238869374098151, 6.595415501580634832, -3.795296366450310543 ) ) ;
#74287=CARTESIAN_POINT ( 'NONE',  ( 19.84674366389459266, 13.71726448433411782, -2.638427012816827677 ) ) ;
#74290=CARTESIAN_POINT ( 'NONE',  ( 10.00000000000000178, 19.31368534415484106, 10.88017736071110342 ) ) ;
#74291=CARTESIAN_POINT ( 'NONE',  ( 0.1532563361054082862, 1.217264484334118047, 2.638427012816831674 ) ) ;
#74295=CARTESIAN_POINT ( 'NONE',  ( 4.559911319644449179, 18.89701867748817321, 9.422509992056141925 ) ) ;
#74296=CARTESIAN_POINT ( 'NONE',  ( 19.84674366389459266, 58.30059781766745886, 2.638427012816836559 ) ) ;
#74297=VERTEX_POINT ( 'NONE', #79585 ) ;
#74299=CARTESIAN_POINT ( 'NONE',  ( 5.076628168052704559, 55.17559781766745175, -8.527530157486179263 ) ) ;
#74300=ORIENTED_EDGE ( 'NONE', *, *, #85356, .F. ) ;
#74301=MECHANICAL_DESIGN_GEOMETRIC_PRESENTATION_REPRESENTATION('',(#27985),#39217);
#74302=CARTESIAN_POINT ( 'NONE',  ( -0.8801773607111008646, 68.27201867748817676, 2.915334737309923430 ) ) ;
#74303=CARTESIAN_POINT ( 'NONE',  ( 19.84674366389459266, 63.30059781766745886, 2.638427012816836559 ) ) ;
#74304=CARTESIAN_POINT ( 'NONE',  ( 0.6178305044545838731, 39.74863466993041072, 9.382169495545420901 ) ) ;
#74305=( NAMED_UNIT ( * ) SI_UNIT ( $, .STERADIAN. ) SOLID_ANGLE_UNIT ( ) );
#74307=CARTESIAN_POINT ( 'NONE',  ( 7.084665262690076126, 69.10535201082151957, 10.88017736071109987 ) ) ;
#74308=CARTESIAN_POINT ( 'NONE',  ( 17.96484262340118221, 24.93868534415484461, 7.964842623401181321 ) ) ;
#74310=ORIENTED_EDGE ( 'NONE', *, *, #69675, .T. ) ;
#74311=CARTESIAN_POINT ( 'NONE',  ( 13.43411237798106583, 52.66530133659708213, -12.81628187352647252 ) ) ;
#74312=CARTESIAN_POINT ( 'NONE',  ( 19.42250999205614193, 40.14701867748817676, 5.440088680355555262 ) ) ;
#74315=CARTESIAN_POINT ( 'NONE',  ( 6.565887622018943937, 43.08196800326374643, -12.81628187352647608 ) ) ;
#74316=CARTESIAN_POINT ( 'NONE',  ( 0.5774900079438590739, 47.64701867748817676, -5.440088680355550821 ) ) ;
#74317=CARTESIAN_POINT ( 'NONE',  ( 2.791683348922237240, 55.38393115100078745, -7.208316651077763204 ) ) ;
#74319=CARTESIAN_POINT ( 'NONE',  ( 0.1532563361054083140, 21.00893115100078745, 1.131784320476157264E-15 ) ) ;
#74320=EDGE_CURVE ( 'NONE', #19684, #80817, #85068, .T. ) ;
#74321=CARTESIAN_POINT ( 'NONE',  ( 22.81628187352647785, 1.623634669930420271, 6.195893100308588602E-16 ) ) ;
#74322=DIRECTION ( 'NONE',  ( 0.000000000000000000, 0.000000000000000000, -1.000000000000000000 ) ) ;
#74323=CARTESIAN_POINT ( 'NONE',  ( 18.52753015748617571, 58.09226448433411605, 4.923371831947298993 ) ) ;
#74324=CARTESIAN_POINT ( 'NONE',  ( 7.084665262690076126, 19.10535201082150181, 10.88017736071109987 ) ) ;
#74325=CARTESIAN_POINT ( 'NONE',  ( 18.52753015748617571, 53.09226448433412315, 4.923371831947298993 ) ) ;
#74327=CARTESIAN_POINT ( 'NONE',  ( 18.52753015748618282, 13.92559781766745175, -4.923371831947291888 ) ) ;
#74329=CARTESIAN_POINT ( 'NONE',  ( 19.38216949554541557, 7.248634669930421381, -9.382169495545420901 ) ) ;
#74332=CARTESIAN_POINT ( 'NONE',  ( 0.6178305044545818747, 38.49863466993042493, -9.382169495545419124 ) ) ;
#74334=CARTESIAN_POINT ( 'NONE',  ( 17.20831665107776587, 32.88393115100078745, 7.208316651077764980 ) ) ;
#74336=CARTESIAN_POINT ( 'NONE',  ( 7.084665262690076126, 12.02201867748817321, -10.88017736071110164 ) ) ;
#74337=CARTESIAN_POINT ( 'NONE',  ( 5.076628168052703671, 26.84226448433411960, 8.527530157486179263 ) ) ;
#74339=CARTESIAN_POINT ( 'NONE',  ( 24.16423886937409904, 64.09541550158064638, 3.795296366450317205 ) ) ;
#74340=CARTESIAN_POINT ( 'NONE',  ( -42.94000000000001194, 92.00000000000000000, 9.000000000000000000 ) ) ;
#74341=CARTESIAN_POINT ( 'NONE',  ( 19.42250999205614193, 25.14701867748817321, 5.440088680355555262 ) ) ;
#74342=CARTESIAN_POINT ( 'NONE',  ( 20.36894250292379738, 49.92874883491396787, -10.36894250292379027 ) ) ;
#74343=CARTESIAN_POINT ( 'NONE',  ( 20.36894250292379738, 49.92874883491396787, -10.36894250292379027 ) ) ;
#74345=CARTESIAN_POINT ( 'NONE',  ( 14.92337183194729633, 12.67559781766745353, 8.527530157486181039 ) ) ;
#74346=CARTESIAN_POINT ( 'NONE',  ( 5.076628168052703671, 66.84226448433412315, 8.527530157486179263 ) ) ;
#74348=CARTESIAN_POINT ( 'NONE',  ( 15.44008868035555260, 44.73035201082151247, 9.422509992056143702 ) ) ;
#74349=AXIS2_PLACEMENT_3D ( 'NONE', #73736, #64746, #73242 ) ;
#74352=CARTESIAN_POINT ( 'NONE',  ( 14.92337183194729633, 62.67559781766745886, 8.527530157486181039 ) ) ;
#74353=CARTESIAN_POINT ( 'NONE',  ( -2.266590686148945544, 2.220415501580634388, 7.082119434687048631 ) ) ;
#74354=CARTESIAN_POINT ( 'NONE',  ( 17.20831665107776587, 22.88393115100078745, 7.208316651077764980 ) ) ;
#74356=( GEOMETRIC_REPRESENTATION_CONTEXT ( 3 ) GLOBAL_UNCERTAINTY_ASSIGNED_CONTEXT ( ( #86338 ) ) GLOBAL_UNIT_ASSIGNED_CONTEXT ( ( #6784, #68285, #28781 ) ) REPRESENTATION_CONTEXT ( 'NONE', 'WORKASPACE' ) );
#74357=CARTESIAN_POINT ( 'NONE',  ( 13.79529636645031943, 45.34541550158062506, -14.16423886937409904 ) ) ;
#74359=CARTESIAN_POINT ( 'NONE',  ( 14.92337183194729988, 14.34226448433411782, -8.527530157486177487 ) ) ;
#74362=CARTESIAN_POINT ( 'NONE',  ( 2.035157376598824452, 33.68868534415484106, 7.964842623401179544 ) ) ;
#74363=CARTESIAN_POINT ( 'NONE',  ( 22.81628187352647785, 31.62363466993042138, 6.195893100308588602E-16 ) ) ;
#74364=CARTESIAN_POINT ( 'NONE',  ( 10.00000000000000000, 1.813685344154837731, -10.88017736071110342 ) ) ;
#74365=CARTESIAN_POINT ( 'NONE',  ( -1.099225684535947600, 29.54030133659708923, 6.408140936763237150 ) ) ;
#74366=CARTESIAN_POINT ( 'NONE',  ( 21.09922568453595559, 57.04030133659708923, -6.408140936763230044 ) ) ;
#74370=CARTESIAN_POINT ( 'NONE',  ( -4.164238869374098151, 46.59541550158063927, -3.795296366450310543 ) ) ;
#74371=CARTESIAN_POINT ( 'NONE',  ( 24.16423886937409904, 4.095415501580634832, 3.795296366450317205 ) ) ;
#74372=CARTESIAN_POINT ( 'NONE',  ( 0.5774900079438590739, 12.64701867748817143, -5.440088680355550821 ) ) ;
#74373=CARTESIAN_POINT ( 'NONE',  ( 12.91533473730993009, 16.60535201082150891, -10.88017736071109987 ) ) ;
#74376=CARTESIAN_POINT ( 'NONE',  ( 7.084665262690076126, 52.02201867748816255, -10.88017736071110164 ) ) ;
#74377=CARTESIAN_POINT ( 'NONE',  ( 10.00000000000000178, 49.31368534415484106, 10.88017736071110342 ) ) ;
#74378=CARTESIAN_POINT ( 'NONE',  ( 21.09922568453594849, 16.20696800326375353, 6.408140936763242479 ) ) ;
#74381=CARTESIAN_POINT ( 'NONE',  ( 12.63842701281683922, 24.55059781766745175, -9.846743663894590881 ) ) ;
#74383=CARTESIAN_POINT ( 'NONE',  ( 20.88017736071110875, 50.77201867748817676, -2.915334737309920765 ) ) ;
#74385=AXIS2_PLACEMENT_3D ( 'NONE', #29167, #75664, #59668 ) ;
#74387=CARTESIAN_POINT ( 'NONE',  ( -2.816281873526471635, 18.91530133659708213, -3.434112377981056508 ) ) ;
#74388=CARTESIAN_POINT ( 'NONE',  ( 2.603489959281060973, 26.58210964143323096, 6.499999999999401368 ) ) ;
#74391=CARTESIAN_POINT ( 'NONE',  ( 0.1532563361054082862, 36.21726448433410894, 2.638427012816831674 ) ) ;
#74392=CARTESIAN_POINT ( 'NONE',  ( 10.00000000000000000, 42.87363466993042493, -12.81628187352647608 ) ) ;
#74393=CARTESIAN_POINT ( 'NONE',  ( 19.84674366389459266, 23.71726448433412315, -2.638427012816827677 ) ) ;
#74395=CARTESIAN_POINT ( 'NONE',  ( -0.3689425029237881626, 7.428748834913967869, 10.36894250292379027 ) ) ;
#74396=CARTESIAN_POINT ( 'NONE',  ( 20.15039907845753930, 69.92552686551195507, -6.262539305110068177 ) ) ;
#74397=CARTESIAN_POINT ( 'NONE',  ( 4.559911319644449179, 13.89701867748817143, 9.422509992056141925 ) ) ;
#74399=CARTESIAN_POINT ( 'NONE',  ( 22.26659068614894466, 28.88708216824730357, 7.082119434687054849 ) ) ;
#74400=CARTESIAN_POINT ( 'NONE',  ( 12.63842701281683034, 27.46726448433411250, 9.846743663894596210 ) ) ;
#74401=CARTESIAN_POINT ( 'NONE',  ( 4.559911319644449179, 17.23035201082150536, -9.422509992056141925 ) ) ;
#74402=CARTESIAN_POINT ( 'NONE',  ( -0.8801773607110991993, 12.85535201082150358, -2.915334737309923874 ) ) ;
#74404=CARTESIAN_POINT ( 'NONE',  ( 0.5774900079438607392, 23.48035201082150536, 5.440088680355550821 ) ) ;
#74406=CARTESIAN_POINT ( 'NONE',  ( 3.591859063236763294, 43.29030133659708923, -11.09922568453595026 ) ) ;
#74407=CARTESIAN_POINT ( 'NONE',  ( -0.8801773607110991993, 37.85535201082151247, -2.915334737309923874 ) ) ;
#74409=CARTESIAN_POINT ( 'NONE',  ( 2.791683348922240793, 56.63393115100078035, 7.208316651077764092 ) ) ;
#74410=CARTESIAN_POINT ( 'NONE',  ( -0.8801773607111009756, 43.06368534415484106, 1.068504757029289695E-15 ) ) ;
#74411=CARTESIAN_POINT ( 'NONE',  ( 1.472469842513823179, 65.59226448433412315, -4.923371831947296329 ) ) ;
#74413=DIRECTION ( 'NONE',  ( 0.000000000000000000, -1.000000000000000000, 0.000000000000000000 ) ) ;
#74414=CARTESIAN_POINT ( 'NONE',  ( 6.204703633549690345, 50.76208216824730357, -14.16423886937410259 ) ) ;
#74415=CARTESIAN_POINT ( 'NONE',  ( 20.88017736071110875, 50.77201867748817676, -2.915334737309920765 ) ) ;
#74416=LINE ( 'NONE', #11959, #68927 ) ;
#74418=CARTESIAN_POINT ( 'NONE',  ( 18.52753015748617571, 48.09226448433412315, 4.923371831947298993 ) ) ;
#74419=CARTESIAN_POINT ( 'NONE',  ( 12.63842701281683034, 2.467264484334118269, 9.846743663894596210 ) ) ;
#74420=CARTESIAN_POINT ( 'NONE',  ( 12.63842701281683922, 19.55059781766745175, -9.846743663894590881 ) ) ;
#74423=CARTESIAN_POINT ( 'NONE',  ( 0.1532563361054083140, 26.00893115100078745, 1.131784320476157264E-15 ) ) ;
#74425=CARTESIAN_POINT ( 'NONE',  ( 0.5774900079438607392, 28.48035201082150891, 5.440088680355550821 ) ) ;
#74426=CARTESIAN_POINT ( 'NONE',  ( 19.84674366389459621, 23.50893115100078390, 7.409399052514197653E-17 ) ) ;
#74427=CARTESIAN_POINT ( 'NONE',  ( -2.816281873526473856, 14.33196800326375531, 3.434112377981055619 ) ) ;
#74428=CARTESIAN_POINT ( 'NONE',  ( 19.42250999205614193, 65.14701867748817676, 5.440088680355555262 ) ) ;
#74429=CARTESIAN_POINT ( 'NONE',  ( 17.96484262340118221, 36.18868534415484106, -7.964842623401177768 ) ) ;
#74430=CARTESIAN_POINT ( 'NONE',  ( 22.81628187352647785, 56.62363466993042493, 6.195893100308588602E-16 ) ) ;
#74431=CARTESIAN_POINT ( 'NONE',  ( 2.917880565312948704, 47.63708216824730357, 12.26659068614894643 ) ) ;
#74432=AXIS2_PLACEMENT_3D ( 'NONE', #70587, #48062, #40086 ) ;
#74436=ORIENTED_EDGE ( 'NONE', *, *, #82079, .F. ) ;
#74437=CARTESIAN_POINT ( 'NONE',  ( 0.6178305044545838731, 4.748634669930420493, 9.382169495545420901 ) ) ;
#74438=CARTESIAN_POINT ( 'NONE',  ( -0.8801773607111008646, 3.272018677488171434, 2.915334737309923430 ) ) ;
#74439=CARTESIAN_POINT ( 'NONE',  ( 15.44008868035555793, 51.39701867748816966, -9.422509992056140149 ) ) ;
#74440=VERTEX_POINT ( 'NONE', #86595 ) ;
#74441=CARTESIAN_POINT ( 'NONE',  ( 0.1532563361054083140, 16.00893115100078390, 1.131784320476157264E-15 ) ) ;
#74442=CARTESIAN_POINT ( 'NONE',  ( 17.96484262340118221, 56.18868534415484817, -7.964842623401177768 ) ) ;
#74443=CARTESIAN_POINT ( 'NONE',  ( 0.1532563361054082862, 31.21726448433412315, 2.638427012816831674 ) ) ;
#74444=CARTESIAN_POINT ( 'NONE',  ( 19.84674366389459266, 18.71726448433411960, -2.638427012816827677 ) ) ;
#74446=CARTESIAN_POINT ( 'NONE',  ( 18.52753015748617571, 8.092264484334117824, 4.923371831947298993 ) ) ;
#74448=CARTESIAN_POINT ( 'NONE',  ( 0.6178305044545838731, 34.74863466993042493, 9.382169495545420901 ) ) ;
#74449=CARTESIAN_POINT ( 'NONE',  ( 0.1532563361054100626, 0.8005978176674514168, -2.638427012816831230 ) ) ;
#74452=CARTESIAN_POINT ( 'NONE',  ( 7.361572987183169658, 29.96726448433411960, -9.846743663894592657 ) ) ;
#74454=( BOUNDED_CURVE ( )  B_SPLINE_CURVE ( 2, ( #16500, #39003, #69498, #1014, #31475, #46977, #8982, #3467, #57431 ),
 .UNSPECIFIED., .F., .T. ) 
 B_SPLINE_CURVE_WITH_KNOTS ( ( 3, 2, 2, 2, 3 ),
 ( 0.6534289457926083511, 0.6547619047619047672, 0.6607142857142856984, 0.6666666666666666297, 0.6679996256359631568 ),
 .UNSPECIFIED. ) 
 CURVE ( )  GEOMETRIC_REPRESENTATION_ITEM ( )  RATIONAL_B_SPLINE_CURVE ( ( 0.9881565478350733400, 0.9923695281211490915, 1.000000000000000000, 0.9659258262890683122, 1.000000000000000000, 0.9659258262890683122, 1.000000000000000000, 0.9923695281211485364, 0.9881565478350726739 ) ) 
 REPRESENTATION_ITEM ( '' )  );
#74455=CARTESIAN_POINT ( 'NONE',  ( 13.43411237798105340, 55.58196800326374643, 12.81628187352647963 ) ) ;
#74456=CARTESIAN_POINT ( 'NONE',  ( 20.15039907845753575, 12.62777174578613071, -6.262539305110077059 ) ) ;
#74457=CARTESIAN_POINT ( 'NONE',  ( 22.81628187352647785, 1.415301336597087012, 3.434112377981063169 ) ) ;
#74458=( LENGTH_UNIT ( ) NAMED_UNIT ( * ) SI_UNIT ( .MILLI., .METRE. ) );
#74460=CARTESIAN_POINT ( 'NONE',  ( 24.16423886937410614, 24.30374883491396787, 8.672049930838204340E-16 ) ) ;
#74463=CARTESIAN_POINT ( 'NONE',  ( 6.204703633549690345, 30.76208216824730357, -14.16423886937410259 ) ) ;
#74464=CARTESIAN_POINT ( 'NONE',  ( -4.164238869374098151, 41.59541550158061796, -3.795296366450310543 ) ) ;
#74467=CARTESIAN_POINT ( 'NONE',  ( 10.00000000000000000, 15.55374883491396787, -14.16423886937410082 ) ) ;
#74468=CARTESIAN_POINT ( 'NONE',  ( 24.16423886937409904, 14.09541550158063217, 3.795296366450317205 ) ) ;
#74470=CARTESIAN_POINT ( 'NONE',  ( 17.96484262340118221, 46.18868534415484106, -7.964842623401177768 ) ) ;
#74472=CARTESIAN_POINT ( 'NONE',  ( 2.791683348922240793, 31.63393115100078745, 7.208316651077764092 ) ) ;
#74473=LINE ( 'NONE', #28970, #6972 ) ;
#74474=CARTESIAN_POINT ( 'NONE',  ( 14.92337183194729633, 27.67559781766745530, 8.527530157486181039 ) ) ;
#74475=CARTESIAN_POINT ( 'NONE',  ( 15.44008868035555260, 14.73035201082150536, 9.422509992056143702 ) ) ;
#74476=CARTESIAN_POINT ( 'NONE',  ( 6.565887622018943937, 63.08196800326376064, -12.81628187352647608 ) ) ;
#74477=CARTESIAN_POINT ( 'NONE',  ( 17.20831665107776587, 47.88393115100078745, 7.208316651077764980 ) ) ;
#74480=CARTESIAN_POINT ( 'NONE',  ( 18.52753015748617571, 28.09226448433411960, 4.923371831947298993 ) ) ;
#74482=CARTESIAN_POINT ( 'NONE',  ( 22.81628187352648496, 41.83196800326375353, -3.434112377981050290 ) ) ;
#74484=CARTESIAN_POINT ( 'NONE',  ( 20.88017736071110875, 40.77201867748818387, -2.915334737309920765 ) ) ;
#74485=CARTESIAN_POINT ( 'NONE',  ( 7.361572987183169658, 39.96726448433411605, -9.846743663894592657 ) ) ;
#74486=CARTESIAN_POINT ( 'NONE',  ( -4.164238869374099039, 26.80374883491397142, 8.674139862899312516E-16 ) ) ;
#74488=VERTEX_POINT ( 'NONE', #35043 ) ;
#74490=CARTESIAN_POINT ( 'NONE',  ( 2.035157376598824452, 48.68868534415483396, 7.964842623401179544 ) ) ;
#74492=CARTESIAN_POINT ( 'NONE',  ( 13.79529636645031943, 55.34541550158062506, -14.16423886937409904 ) ) ;
#74493=CARTESIAN_POINT ( 'NONE',  ( 10.00000000000000178, 0.3736346699304200492, 12.81628187352647608 ) ) ;
#74495=CARTESIAN_POINT ( 'NONE',  ( 17.96484262340118221, 59.93868534415484106, 7.964842623401181321 ) ) ;
#74497=CARTESIAN_POINT ( 'NONE',  ( -1.099225684535947600, -0.4596986634029132657, 6.408140936763237150 ) ) ;
#74499=CARTESIAN_POINT ( 'NONE',  ( 4.559911319644449179, 12.23035201082150536, -9.422509992056141925 ) ) ;
#74500=CARTESIAN_POINT ( 'NONE',  ( -0.8801773607110991993, 7.855352010821506248, -2.915334737309923874 ) ) ;
#74501=CARTESIAN_POINT ( 'NONE',  ( 5.076628168052703671, 41.84226448433411605, 8.527530157486179263 ) ) ;
#74505=CARTESIAN_POINT ( 'NONE',  ( 17.96484262340118221, 4.938685344154837509, 7.964842623401181321 ) ) ;
#74506=CARTESIAN_POINT ( 'NONE',  ( 22.81628187352648496, 1.831968003263753753, -3.434112377981050290 ) ) ;
#74508=CARTESIAN_POINT ( 'NONE',  ( 2.791683348922240793, 16.63393115100078745, 7.208316651077764092 ) ) ;
#74510=CARTESIAN_POINT ( 'NONE',  ( 10.00000000000000000, 34.75893115100078745, -9.846743663894594434 ) ) ;
#74511=CARTESIAN_POINT ( 'NONE',  ( 20.88017736071110875, 30.77201867748816966, -2.915334737309920765 ) ) ;
#74512=ADVANCED_FACE ( 'NONE', ( #20053 ), #64819, .T. ) ;
#74514=CARTESIAN_POINT ( 'NONE',  ( 13.43411237798106583, 7.665301336597086568, -12.81628187352647252 ) ) ;
#74515=CARTESIAN_POINT ( 'NONE',  ( 4.559911319644449179, 52.23035201082151247, -9.422509992056141925 ) ) ;
#74517=CARTESIAN_POINT ( 'NONE',  ( 10.00000000000000000, 57.87363466993042493, -12.81628187352647608 ) ) ;
#74519=CARTESIAN_POINT ( 'NONE',  ( 2.035157376598824452, 68.68868534415484817, 7.964842623401179544 ) ) ;
#74520=CARTESIAN_POINT ( 'NONE',  ( -1.099225684535947600, 33.70696800326375353, -6.408140936763238038 ) ) ;
#74521=CARTESIAN_POINT ( 'NONE',  ( 10.00000000000000000, 0.5537488349139675359, -14.16423886937410082 ) ) ;
#74523=CARTESIAN_POINT ( 'NONE',  ( 10.00000000000000178, 34.31368534415484106, 10.88017736071110342 ) ) ;
#74525=CARTESIAN_POINT ( 'NONE',  ( 19.84674366389459266, 58.71726448433411605, -2.638427012816827677 ) ) ;
#74526=CARTESIAN_POINT ( 'NONE',  ( 7.361572987183169658, 19.96726448433411960, -9.846743663894592657 ) ) ;
#74527=CARTESIAN_POINT ( 'NONE',  ( 14.92337183194729988, 4.342264484334117824, -8.527530157486177487 ) ) ;
#74528=LINE ( 'NONE', #66038, #47513 ) ;
#74529=CARTESIAN_POINT ( 'NONE',  ( 6.204703633549690345, 47.84541550158064638, 14.16423886937410082 ) ) ;
#74530=CARTESIAN_POINT ( 'NONE',  ( 1.821158202401483406, 56.16688879859522388, 6.499999999999917399 ) ) ;
#74534=CARTESIAN_POINT ( 'NONE',  ( 2.917880565312948704, 57.63708216824731068, 12.26659068614894643 ) ) ;
#74535=CARTESIAN_POINT ( 'NONE',  ( 10.00000000000000000, 60.55374883491397497, -14.16423886937410082 ) ) ;
#74536=CARTESIAN_POINT ( 'NONE',  ( 17.20831665107776587, 27.88393115100078390, 7.208316651077764980 ) ) ;
#74537=CARTESIAN_POINT ( 'NONE',  ( 19.38216949554541557, 22.24863466993041428, -9.382169495545420901 ) ) ;
#74540=CARTESIAN_POINT ( 'NONE',  ( 13.79529636645031943, 10.34541550158063394, -14.16423886937409904 ) ) ;
#74541=CARTESIAN_POINT ( 'NONE',  ( 2.035157376598824452, 18.68868534415484106, 7.964842623401179544 ) ) ;
#74542=CARTESIAN_POINT ( 'NONE',  ( 6.204703633549690345, 52.84541550158062506, 14.16423886937410082 ) ) ;
#74545=CARTESIAN_POINT ( 'NONE',  ( 10.00000000000000000, 29.75893115100078745, -9.846743663894594434 ) ) ;
#74547=CARTESIAN_POINT ( 'NONE',  ( 18.52753015748618282, 3.925597817667451306, -4.923371831947291888 ) ) ;
#74552=VERTEX_POINT ( 'NONE', #71649 ) ;
#74555=CARTESIAN_POINT ( 'NONE',  ( 2.791683348922237240, 45.38393115100079456, -7.208316651077763204 ) ) ;
#74556=CARTESIAN_POINT ( 'NONE',  ( 24.16423886937410614, 19.30374883491397142, 8.672049930838204340E-16 ) ) ;
#74557=CARTESIAN_POINT ( 'NONE',  ( 20.88017736071110875, 25.77201867748816966, -2.915334737309920765 ) ) ;
#74558=CARTESIAN_POINT ( 'NONE',  ( 10.00000000000000178, 29.31368534415483751, 10.88017736071110342 ) ) ;
#74559=CARTESIAN_POINT ( 'NONE',  ( 18.52753015748618282, 63.92559781766745886, -4.923371831947291888 ) ) ;
#74560=CARTESIAN_POINT ( 'NONE',  ( 22.81628187352648496, 11.83196800326375531, -3.434112377981050290 ) ) ;
#74561=CARTESIAN_POINT ( 'NONE',  ( 17.08211943468705130, 3.470415501580634388, 12.26659068614894998 ) ) ;
#74565=CARTESIAN_POINT ( 'NONE',  ( 19.38216949554541202, 30.99863466993042138, 9.382169495545424454 ) ) ;
#74567=CARTESIAN_POINT ( 'NONE',  ( 18.52753015748618282, 33.92559781766745886, -4.923371831947291888 ) ) ;
#74568=CARTESIAN_POINT ( 'NONE',  ( 20.88017736071110164, 10.35535201082150714, 2.915334737309930979 ) ) ;
#74570=CARTESIAN_POINT ( 'NONE',  ( 0.5774900079438607392, 3.480352010821504916, 5.440088680355550821 ) ) ;
#74571=ORIENTED_EDGE ( 'NONE', *, *, #68670, .T. ) ;
#74572=CARTESIAN_POINT ( 'NONE',  ( 2.035157376598824452, 53.68868534415484817, 7.964842623401179544 ) ) ;
#74573=CARTESIAN_POINT ( 'NONE',  ( 0.5774900079438607392, 58.48035201082151247, 5.440088680355550821 ) ) ;
#74574=CARTESIAN_POINT ( 'NONE',  ( 7.084665262690076126, 47.02201867748818387, -10.88017736071110164 ) ) ;
#74575=CARTESIAN_POINT ( 'NONE',  ( 0.5774900079438607392, 58.48035201082151247, 5.440088680355550821 ) ) ;
#74576=CARTESIAN_POINT ( 'NONE',  ( -1.926860441876562247, 52.45379003517449235, -3.195792623639530650 ) ) ;
#74580=CARTESIAN_POINT ( 'NONE',  ( 18.52753015748617571, 23.09226448433411960, 4.923371831947298993 ) ) ;
#74582=CARTESIAN_POINT ( 'NONE',  ( 10.00000000000000000, 54.75893115100078745, -9.846743663894594434 ) ) ;
#74584=AXIS2_PLACEMENT_3D ( 'NONE', #32329, #61359, #68880 ) ;
#74585=CARTESIAN_POINT ( 'NONE',  ( -2.266590686148945544, 6.387082168247300906, -7.082119434687050408 ) ) ;
#74590=CARTESIAN_POINT ( 'NONE',  ( 12.63842701281683034, 37.46726448433411605, 9.846743663894596210 ) ) ;
#74591=CARTESIAN_POINT ( 'NONE',  ( 20.88017736071110875, 10.77201867748817143, -2.915334737309920765 ) ) ;
#74594=FACE_OUTER_BOUND ( 'NONE', #82852, .T. ) ;
#74595=CARTESIAN_POINT ( 'NONE',  ( 19.84674366389459266, 43.30059781766744464, 2.638427012816836559 ) ) ;
#74597=CARTESIAN_POINT ( 'NONE',  ( 10.00000000000000000, 12.87363466993042138, -12.81628187352647608 ) ) ;
#74598=CARTESIAN_POINT ( 'NONE',  ( 1.472469842513823179, 16.42559781766745175, 4.923371831947296329 ) ) ;
#74600=DIRECTION ( 'NONE',  ( -0.5547001962252291474, -0.8320502943378437211, -0.000000000000000000 ) ) ;
#74601=CARTESIAN_POINT ( 'NONE',  ( 14.92337183194729988, 19.34226448433411960, -8.527530157486177487 ) ) ;
#74602=CARTESIAN_POINT ( 'NONE',  ( 0.1532563361054083140, 66.00893115100079456, 1.131784320476157264E-15 ) ) ;
#74606=CARTESIAN_POINT ( 'NONE',  ( 17.96484262340118221, 9.938685344154839285, 7.964842623401181321 ) ) ;
#74607=CARTESIAN_POINT ( 'NONE',  ( 2.917880565312950480, 5.970415501580634832, -12.26659068614894821 ) ) ;
#74608=CARTESIAN_POINT ( 'NONE',  ( 12.63842701281683922, 24.55059781766745175, -9.846743663894590881 ) ) ;
#74609=CARTESIAN_POINT ( 'NONE',  ( 10.00000000000000178, 54.31368534415484106, 10.88017736071110342 ) ) ;
#74610=CARTESIAN_POINT ( 'NONE',  ( -1.099225684535947600, 38.70696800326375353, -6.408140936763238038 ) ) ;
#74611=CARTESIAN_POINT ( 'NONE',  ( 20.88017736071110519, 20.56368534415484106, 2.639326808657452039E-16 ) ) ;
#74615=CARTESIAN_POINT ( 'NONE',  ( 13.43411237798105340, 5.581968003263753531, 12.81628187352647963 ) ) ;
#74616=CARTESIAN_POINT ( 'NONE',  ( 6.565887622018943937, -1.918031996736246692, -12.81628187352647608 ) ) ;
#74617=CARTESIAN_POINT ( 'NONE',  ( 2.791683348922240793, 26.63393115100078745, 7.208316651077764092 ) ) ;
#74619=CARTESIAN_POINT ( 'NONE',  ( 22.81628187352647785, 41.41530133659708923, 3.434112377981063169 ) ) ;
#74620=DIRECTION ( 'NONE',  ( -0.000000000000000000, 1.000000000000000000, -0.000000000000000000 ) ) ;
#74621=CARTESIAN_POINT ( 'NONE',  ( 20.88017736071110875, 40.77201867748818387, -2.915334737309920765 ) ) ;
#74623=AXIS2_PLACEMENT_3D ( 'NONE', #31662, #77654, #716 ) ;
#74625=CARTESIAN_POINT ( 'NONE',  ( 20.88017736071110164, 45.35535201082149115, 2.915334737309930979 ) ) ;
#74626=CARTESIAN_POINT ( 'NONE',  ( 19.42250999205614193, 25.14701867748817321, 5.440088680355555262 ) ) ;
#74627=CARTESIAN_POINT ( 'NONE',  ( 12.63842701281683034, 62.46726448433410894, 9.846743663894596210 ) ) ;
#74629=CARTESIAN_POINT ( 'NONE',  ( 0.5774900079438590739, 52.64701867748817676, -5.440088680355550821 ) ) ;
#74631=ADVANCED_FACE ( 'NONE', ( #19129 ), #41654, .T. ) ;
#74632=CARTESIAN_POINT ( 'NONE',  ( 1.472469842513823179, 40.59226448433411605, -4.923371831947296329 ) ) ;
#74633=CARTESIAN_POINT ( 'NONE',  ( 10.00000000000000178, 65.37363466993042493, 12.81628187352647608 ) ) ;
#74634=CARTESIAN_POINT ( 'NONE',  ( 16.40814093676323893, 15.79030133659708746, 11.09922568453595026 ) ) ;
#74635=ORIENTED_EDGE ( 'NONE', *, *, #72374, .T. ) ;
#74636=CARTESIAN_POINT ( 'NONE',  ( 15.44008868035555260, 19.73035201082150536, 9.422509992056143702 ) ) ;
#74638=CARTESIAN_POINT ( 'NONE',  ( 7.084665262690076126, 14.10535201082150358, 10.88017736071109987 ) ) ;
#74639=CARTESIAN_POINT ( 'NONE',  ( 19.84674366389459266, 3.717264484334118713, -2.638427012816827677 ) ) ;
#74640=CARTESIAN_POINT ( 'NONE',  ( 24.16423886937409904, 24.09541550158063927, 3.795296366450317205 ) ) ;
#74642=CARTESIAN_POINT ( 'NONE',  ( 1.472469842513823179, 10.59226448433411782, -4.923371831947296329 ) ) ;
#74643=CARTESIAN_POINT ( 'NONE',  ( 0.1532563361054083140, 61.00893115100078745, 1.131784320476157264E-15 ) ) ;
#74644=CARTESIAN_POINT ( 'NONE',  ( 10.00000000000000000, 51.81368534415484106, -10.88017736071110342 ) ) ;
#74645=CARTESIAN_POINT ( 'NONE',  ( 0.1955144967548735624, 34.32703681773342197, -6.500000000002695622 ) ) ;
#74646=DIRECTION ( 'NONE',  ( -1.000000000000000000, 6.608470384673550777E-17, 0.000000000000000000 ) ) ;
#74649=CARTESIAN_POINT ( 'NONE',  ( 0.1532563361054083140, 46.00893115100079456, 1.131784320476157264E-15 ) ) ;
#74651=VERTEX_POINT ( 'NONE', #83582 ) ;
#74653=CARTESIAN_POINT ( 'NONE',  ( -0.3689425029237881626, 17.42874883491397142, 10.36894250292379027 ) ) ;
#74654=CARTESIAN_POINT ( 'NONE',  ( 17.08211943468705840, 30.13708216824730357, -12.26659068614894466 ) ) ;
#74655=CARTESIAN_POINT ( 'NONE',  ( -0.8801773607111009756, 63.06368534415484106, 1.068504757029289695E-15 ) ) ;
#74656=CARTESIAN_POINT ( 'NONE',  ( 0.5774900079438590739, 2.647018677488171434, -5.440088680355550821 ) ) ;
#74657=CARTESIAN_POINT ( 'NONE',  ( -2.816281873526473856, 4.123634669930420493, 9.499525473075851096E-16 ) ) ;
#74658=CARTESIAN_POINT ( 'NONE',  ( 2.791683348922240793, 51.63393115100078745, 7.208316651077764092 ) ) ;
#74660=CARTESIAN_POINT ( 'NONE',  ( 0.5774900079438590739, 47.64701867748817676, -5.440088680355550821 ) ) ;
#74661=CARTESIAN_POINT ( 'NONE',  ( 3.591859063236761518, -0.04303199673624671928, 11.09922568453594849 ) ) ;
#74662=CARTESIAN_POINT ( 'NONE',  ( 24.16423886937410614, 19.51208216824729647, -3.795296366450302550 ) ) ;
#74663=CARTESIAN_POINT ( 'NONE',  ( 2.035157376598824452, 18.68868534415484106, 7.964842623401179544 ) ) ;
#74664=COLOUR_RGB ( '', 0.72549020, 0.75294118, 0.79215686) ;
#74665=CARTESIAN_POINT ( 'NONE',  ( -0.8801773607111009756, 23.06368534415484106, 1.068504757029289695E-15 ) ) ;
#74667=CARTESIAN_POINT ( 'NONE',  ( -0.8801773607110991993, 42.85535201082150536, -2.915334737309923874 ) ) ;
#74669=CARTESIAN_POINT ( 'NONE',  ( 21.09922568453594849, 46.20696800326376064, 6.408140936763242479 ) ) ;
#74672=CARTESIAN_POINT ( 'NONE',  ( 20.04068437667225666, 4.719743609177204924, 6.396802510829709298 ) ) ;
#74675=DIRECTION ( 'NONE',  ( 1.000000000000000000, 0.000000000000000000, 0.000000000000000000 ) ) ;
#74676=CARTESIAN_POINT ( 'NONE',  ( 6.204703633549690345, 45.76208216824729647, -14.16423886937410259 ) ) ;
#74677=CARTESIAN_POINT ( 'NONE',  ( 12.63842701281683922, 24.55059781766745175, -9.846743663894590881 ) ) ;
#74678=CARTESIAN_POINT ( 'NONE',  ( 7.361572987183169658, 49.96726448433410894, -9.846743663894592657 ) ) ;
#74679=CARTESIAN_POINT ( 'NONE',  ( 0.5774900079438607392, 68.48035201082150536, 5.440088680355550821 ) ) ;
#74682=STYLED_ITEM ( 'NONE', ( #94686 ), #15201 ) ;
#74683=CARTESIAN_POINT ( 'NONE',  ( 4.559911319644449179, 68.89701867748817676, 9.422509992056141925 ) ) ;
#74686=CARTESIAN_POINT ( 'NONE',  ( 22.26659068614894466, 28.88708216824730357, 7.082119434687054849 ) ) ;
#74688=CARTESIAN_POINT ( 'NONE',  ( 16.40814093676324603, 27.45696800326375708, -11.09922568453594671 ) ) ;
#74690=CARTESIAN_POINT ( 'NONE',  ( 13.43411237798106583, 47.66530133659709634, -12.81628187352647252 ) ) ;
#74692=CARTESIAN_POINT ( 'NONE',  ( 4.559911319644449179, 13.89701867748817321, 9.422509992056141925 ) ) ;
#74693=CARTESIAN_POINT ( 'NONE',  ( 1.472469842513823179, 36.42559781766745175, 4.923371831947296329 ) ) ;
#74694=CARTESIAN_POINT ( 'NONE',  ( -0.8801773607110991993, 7.855352010821504471, -2.915334737309923874 ) ) ;
#74697=CARTESIAN_POINT ( 'NONE',  ( 1.472469842513823179, 41.42559781766745886, 4.923371831947296329 ) ) ;
#74698=CARTESIAN_POINT ( 'NONE',  ( 1.472469842513823179, 51.42559781766745886, 4.923371831947296329 ) ) ;
#74706=CARTESIAN_POINT ( 'NONE',  ( 10.00000000000000178, 17.25893115100078745, 9.846743663894594434 ) ) ;
#74708=CARTESIAN_POINT ( 'NONE',  ( 13.43411237798106583, 37.66530133659708923, -12.81628187352647252 ) ) ;
#74709=DIRECTION ( 'NONE',  ( -0.000000000000000000, -0.000000000000000000, -1.000000000000000000 ) ) ;
#74710=VERTEX_POINT ( 'NONE', #7093 ) ;
#74711=CARTESIAN_POINT ( 'NONE',  ( 0.1532563361054082862, 56.21726448433411605, 2.638427012816831674 ) ) ;
#74713=CARTESIAN_POINT ( 'NONE',  ( -0.3689425029237898834, 21.17874883491396432, -10.36894250292378850 ) ) ;
#74714=CARTESIAN_POINT ( 'NONE',  ( 7.361572987183170547, 42.05059781766745886, 9.846743663894590881 ) ) ;
#74715=CARTESIAN_POINT ( 'NONE',  ( 13.43411237798105340, 50.58196800326375353, 12.81628187352647963 ) ) ;
#74716=CYLINDRICAL_SURFACE ( 'NONE', #27262, 6.999999999999995559 ) ;
#74717=CARTESIAN_POINT ( 'NONE',  ( 7.361572987183170547, 2.050597817667451750, 9.846743663894590881 ) ) ;
#74719=CARTESIAN_POINT ( 'NONE',  ( 19.84674366389459266, 53.30059781766744464, 2.638427012816836559 ) ) ;
#74720=CARTESIAN_POINT ( 'NONE',  ( 19.42250999205614193, 35.14701867748816966, 5.440088680355555262 ) ) ;
#74721=EDGE_CURVE ( 'NONE', #31822, #1572, #43789, .T. ) ;
#74722=CARTESIAN_POINT ( 'NONE',  ( 10.00000000000000178, 49.31368534415484106, 10.88017736071110342 ) ) ;
#74723=VERTEX_POINT ( 'NONE', #35607 ) ;
#74725=CARTESIAN_POINT ( 'NONE',  ( 12.91533473730992121, 19.52201867748816611, 10.88017736071110164 ) ) ;
#74726=CARTESIAN_POINT ( 'NONE',  ( 5.076628168052704559, 50.17559781766745886, -8.527530157486179263 ) ) ;
#74727=CARTESIAN_POINT ( 'NONE',  ( -0.8801773607111008646, 43.27201867748817676, 2.915334737309923430 ) ) ;
#74729=CARTESIAN_POINT ( 'NONE',  ( 2.035157376598824452, 58.68868534415482685, 7.964842623401179544 ) ) ;
#74731=CARTESIAN_POINT ( 'NONE',  ( 19.42250999205614548, 25.98035201082150891, -5.440088680355545492 ) ) ;
#74733=CARTESIAN_POINT ( 'NONE',  ( 1.472469842513823179, 10.59226448433411782, -4.923371831947296329 ) ) ;
#74734=CARTESIAN_POINT ( 'NONE',  ( 18.52753015748618282, 28.92559781766745175, -4.923371831947291888 ) ) ;
#74735=( NAMED_UNIT ( * ) SI_UNIT ( $, .STERADIAN. ) SOLID_ANGLE_UNIT ( ) );
#74737=CARTESIAN_POINT ( 'NONE',  ( 12.63842701281683922, 59.55059781766744464, -9.846743663894590881 ) ) ;
#74738=CARTESIAN_POINT ( 'NONE',  ( -4.164238869374099927, 67.01208216824728936, 3.795296366450308767 ) ) ;
#74741=CARTESIAN_POINT ( 'NONE',  ( 13.79529636645030344, 3.262082168247301350, 14.16423886937410614 ) ) ;
#74742=CARTESIAN_POINT ( 'NONE',  ( -4.164238869374099039, 46.80374883491397497, 8.674139862899312516E-16 ) ) ;
#74744=CARTESIAN_POINT ( 'NONE',  ( 3.591859063236761518, 4.956968003263753531, 11.09922568453594849 ) ) ;
#74745=ORIENTED_EDGE ( 'NONE', *, *, #96468, .T. ) ;
#74746=CARTESIAN_POINT ( 'NONE',  ( 19.84674366389459621, 8.508931151000785675, 7.409399052514197653E-17 ) ) ;
#74748=CARTESIAN_POINT ( 'NONE',  ( 10.00000000000000178, 9.313685344154839285, 10.88017736071110342 ) ) ;
#74749=CARTESIAN_POINT ( 'NONE',  ( 19.84674366389459266, 53.30059781766744464, 2.638427012816836559 ) ) ;
#74752=DIRECTION ( 'NONE',  ( 0.000000000000000000, 1.000000000000000000, -0.000000000000000000 ) ) ;
#74754=CARTESIAN_POINT ( 'NONE',  ( 3.591859063236761518, 24.95696800326375353, 11.09922568453594849 ) ) ;
#74755=CARTESIAN_POINT ( 'NONE',  ( 10.00000000000000000, 29.75893115100078745, -9.846743663894594434 ) ) ;
#74758=CARTESIAN_POINT ( 'NONE',  ( 5.076628168052703671, 11.84226448433411960, 8.527530157486179263 ) ) ;
#74760=CARTESIAN_POINT ( 'NONE',  ( -46.75594628505023564, 100.8419086298434877, -9.092420010817928500 ) ) ;
#74761=CARTESIAN_POINT ( 'NONE',  ( 12.91533473730993009, 11.60535201082150536, -10.88017736071109987 ) ) ;
#74762=CARTESIAN_POINT ( 'NONE',  ( 2.917880565312950480, 45.97041550158063927, -12.26659068614894821 ) ) ;
#74763=AXIS2_PLACEMENT_3D ( 'NONE', #65060, #88070, #25627 ) ;
#74764=CARTESIAN_POINT ( 'NONE',  ( -0.8801773607110991993, 67.85535201082151957, -2.915334737309923874 ) ) ;
#74766=CARTESIAN_POINT ( 'NONE',  ( 18.52753015748617571, 23.09226448433411960, 4.923371831947298993 ) ) ;
#74767=CARTESIAN_POINT ( 'NONE',  ( 20.88017736071110519, 5.563685344154837509, 2.639326808657452039E-16 ) ) ;
#74768=CARTESIAN_POINT ( 'NONE',  ( 7.361572987183169658, 4.967264484334119601, -9.846743663894592657 ) ) ;
#74770=CARTESIAN_POINT ( 'NONE',  ( 5.076628168052703671, 41.84226448433411605, 8.527530157486179263 ) ) ;
#74771=CARTESIAN_POINT ( 'NONE',  ( 10.00000000000000000, 36.81368534415484106, -10.88017736071110342 ) ) ;
#74774=ORIENTED_EDGE ( 'NONE', *, *, #77311, .T. ) ;
#74775=CARTESIAN_POINT ( 'NONE',  ( 0.6178305044545838731, 59.74863466993041783, 9.382169495545420901 ) ) ;
#74777=CARTESIAN_POINT ( 'NONE',  ( 10.00000000000000178, 7.258931151000785675, 9.846743663894594434 ) ) ;
#74778=CARTESIAN_POINT ( 'NONE',  ( 22.81628187352648496, 41.83196800326375353, -3.434112377981050290 ) ) ;
#74779=CARTESIAN_POINT ( 'NONE',  ( 7.084665262690076126, 9.105352010821503583, 10.88017736071109987 ) ) ;
#74780=CARTESIAN_POINT ( 'NONE',  ( 5.076628168052703671, 36.84226448433412315, 8.527530157486179263 ) ) ;
#74783=CARTESIAN_POINT ( 'NONE',  ( -4.164238869374099927, 22.01208216824730357, 3.795296366450308767 ) ) ;
#74784=CARTESIAN_POINT ( 'NONE',  ( 2.917880565312948704, 47.63708216824730357, 12.26659068614894643 ) ) ;
#74785=CARTESIAN_POINT ( 'NONE',  ( 14.92337183194729633, 42.67559781766745886, 8.527530157486181039 ) ) ;
#74787=CARTESIAN_POINT ( 'NONE',  ( 10.00000000000000178, 34.31368534415484106, 10.88017736071110342 ) ) ;
#74788=CARTESIAN_POINT ( 'NONE',  ( 5.076628168052703671, 1.842264484334118047, 8.527530157486179263 ) ) ;
#74791=CARTESIAN_POINT ( 'NONE',  ( 22.81628187352647785, 56.62363466993042493, 6.195893100308588602E-16 ) ) ;
#74792=EDGE_LOOP ( 'NONE', ( #26378, #94340, #71122, #54070, #85598 ) ) ;
#74793=CARTESIAN_POINT ( 'NONE',  ( 19.42250999205614548, 60.98035201082151247, -5.440088680355545492 ) ) ;
#74795=CARTESIAN_POINT ( 'NONE',  ( 17.08211943468705840, 10.13708216824730179, -12.26659068614894466 ) ) ;
#74796=CARTESIAN_POINT ( 'NONE',  ( 5.076628168052704559, 10.17559781766745175, -8.527530157486179263 ) ) ;
#74798=EDGE_LOOP ( 'NONE', ( #4493, #21855, #57447, #56245 ) ) ;
#74799=CARTESIAN_POINT ( 'NONE',  ( 17.96484262340118221, 14.93868534415483751, 7.964842623401181321 ) ) ;
#74801=CARTESIAN_POINT ( 'NONE',  ( 0.5774900079438607392, 33.48035201082150536, 5.440088680355550821 ) ) ;
#74802=( NAMED_UNIT ( * ) SI_UNIT ( $, .STERADIAN. ) SOLID_ANGLE_UNIT ( ) );
#74805=CARTESIAN_POINT ( 'NONE',  ( 5.076628168052704559, 60.17559781766745175, -8.527530157486179263 ) ) ;
#74807=CARTESIAN_POINT ( 'NONE',  ( 7.084665262690076126, 69.10535201082151957, 10.88017736071109987 ) ) ;
#74808=CARTESIAN_POINT ( 'NONE',  ( 19.84674366389459621, 63.50893115100078745, 7.409399052514197653E-17 ) ) ;
#74809=CARTESIAN_POINT ( 'NONE',  ( 0.5774900079438590739, 22.64701867748817321, -5.440088680355550821 ) ) ;
#74810=CARTESIAN_POINT ( 'NONE',  ( 0.1922240491738455570, 58.18878173731742010, 6.499999999999968914 ) ) ;
#74811=CARTESIAN_POINT ( 'NONE',  ( 0.5774900079438590739, 67.64701867748817676, -5.440088680355550821 ) ) ;
#74812=CARTESIAN_POINT ( 'NONE',  ( -0.8801773607110991993, 12.85535201082150358, -2.915334737309923874 ) ) ;
#74815=CARTESIAN_POINT ( 'NONE',  ( 10.00000000000000000, 52.87363466993041783, -12.81628187352647608 ) ) ;
#74816=CARTESIAN_POINT ( 'NONE',  ( 15.44008868035555260, 49.73035201082150536, 9.422509992056143702 ) ) ;
#74817=CARTESIAN_POINT ( 'NONE',  ( -46.94000000000000483, 101.3580217190410337, -7.614242055628325012 ) ) ;
#74818=CARTESIAN_POINT ( 'NONE',  ( 0.6178305044545838731, 49.74863466993041072, 9.382169495545420901 ) ) ;
#74819=CARTESIAN_POINT ( 'NONE',  ( 10.00000000000000178, 44.31368534415484106, 10.88017736071110342 ) ) ;
#74820=CARTESIAN_POINT ( 'NONE',  ( 0.1532563361054083140, 56.00893115100078745, 1.131784320476157264E-15 ) ) ;
#74821=CARTESIAN_POINT ( 'NONE',  ( 19.50000000000000711, 105.0000000000000000, -4.500000000000000888 ) ) ;
#74823=CARTESIAN_POINT ( 'NONE',  ( 18.52753015748617571, 18.09226448433411960, 4.923371831947298993 ) ) ;
#74824=CARTESIAN_POINT ( 'NONE',  ( 10.00000000000000178, 0.3736346699304200492, 12.81628187352647608 ) ) ;
#74825=DIRECTION ( 'NONE',  ( 1.000000000000000000, 0.000000000000000000, 0.000000000000000000 ) ) ;
#74826=CARTESIAN_POINT ( 'NONE',  ( 7.361572987183169658, 64.96726448433412315, -9.846743663894592657 ) ) ;
#74827=CARTESIAN_POINT ( 'NONE',  ( 12.91533473730992121, 39.52201867748817676, 10.88017736071110164 ) ) ;
#74828=CARTESIAN_POINT ( 'NONE',  ( 0.1532563361054082862, 46.21726448433411605, 2.638427012816831674 ) ) ;
#74830=( GEOMETRIC_REPRESENTATION_CONTEXT ( 3 ) GLOBAL_UNCERTAINTY_ASSIGNED_CONTEXT ( ( #41353 ) ) GLOBAL_UNIT_ASSIGNED_CONTEXT ( ( #84750, #17736, #70740 ) ) REPRESENTATION_CONTEXT ( 'NONE', 'WORKASPACE' ) );
#74831=CARTESIAN_POINT ( 'NONE',  ( 7.361572987183169658, 19.96726448433411960, -9.846743663894592657 ) ) ;
#74832=CARTESIAN_POINT ( 'NONE',  ( 19.84674366389459621, 8.508931151000785675, 7.409399052514197653E-17 ) ) ;
#74833=EDGE_CURVE ( 'NONE', #87186, #14534, #37101, .T. ) ;
#74834=CARTESIAN_POINT ( 'NONE',  ( 13.43411237798106583, 2.665301336597086568, -12.81628187352647252 ) ) ;
#74837=SURFACE_STYLE_FILL_AREA ( #57856 ) ;
#74839=CARTESIAN_POINT ( 'NONE',  ( 0.1532563361054100626, 60.80059781766744464, -2.638427012816831230 ) ) ;
#74840=CARTESIAN_POINT ( 'NONE',  ( 21.09922568453595559, 47.04030133659708923, -6.408140936763230044 ) ) ;
#74841=CARTESIAN_POINT ( 'NONE',  ( 2.791683348922240793, 36.63393115100078035, 7.208316651077764092 ) ) ;
#74843=CARTESIAN_POINT ( 'NONE',  ( 0.5774900079438607392, 8.480352010821505360, 5.440088680355550821 ) ) ;
#74845=CARTESIAN_POINT ( 'NONE',  ( 2.791683348922240793, 31.63393115100078745, 7.208316651077764092 ) ) ;
#74846=ORIENTED_EDGE ( 'NONE', *, *, #8053, .T. ) ;
#74848=CARTESIAN_POINT ( 'NONE',  ( 19.42250999205614193, 5.147018677488171434, 5.440088680355555262 ) ) ;
#74850=CARTESIAN_POINT ( 'NONE',  ( -0.8801773607110991993, 22.85535201082150181, -2.915334737309923874 ) ) ;
#74851=CARTESIAN_POINT ( 'NONE',  ( -4.164238869374099927, 47.01208216824729647, 3.795296366450308767 ) ) ;
#74852=CARTESIAN_POINT ( 'NONE',  ( -4.164238869374099927, 57.01208216824731068, 3.795296366450308767 ) ) ;
#74854=( LENGTH_UNIT ( ) NAMED_UNIT ( * ) SI_UNIT ( .MILLI., .METRE. ) );
#74855=CARTESIAN_POINT ( 'NONE',  ( 0.1532563361054082862, 11.21726448433411605, 2.638427012816831674 ) ) ;
#74856=CARTESIAN_POINT ( 'NONE',  ( 14.92337183194729633, 62.67559781766745886, 8.527530157486181039 ) ) ;
#74857=VERTEX_POINT ( 'NONE', #67095 ) ;
#74859=CARTESIAN_POINT ( 'NONE',  ( 0.1532563361054082862, 56.21726448433411605, 2.638427012816831674 ) ) ;
#74861=CARTESIAN_POINT ( 'NONE',  ( 12.63842701281683034, 62.46726448433410894, 9.846743663894596210 ) ) ;
#74862=CARTESIAN_POINT ( 'NONE',  ( -2.266590686148945544, 12.22041550158063394, 7.082119434687048631 ) ) ;
#74863=CARTESIAN_POINT ( 'NONE',  ( 10.00000000000000000, 24.75893115100078745, -9.846743663894594434 ) ) ;
#74865=CARTESIAN_POINT ( 'NONE',  ( -4.164238869374098151, 46.59541550158063927, -3.795296366450310543 ) ) ;
#74866=CARTESIAN_POINT ( 'NONE',  ( 18.52753015748617571, 3.092264484334118269, 4.923371831947298993 ) ) ;
#74869=CARTESIAN_POINT ( 'NONE',  ( -0.8801773607111009756, 38.06368534415484106, 1.068504757029289695E-15 ) ) ;
#74870=CARTESIAN_POINT ( 'NONE',  ( 16.40814093676323893, 40.79030133659708923, 11.09922568453595026 ) ) ;
#74871=CARTESIAN_POINT ( 'NONE',  ( 0.6178305044545838731, 34.74863466993042493, 9.382169495545420901 ) ) ;
#74872=CARTESIAN_POINT ( 'NONE',  ( 10.00000000000000178, 60.37363466993041783, 12.81628187352647608 ) ) ;
#74876=CARTESIAN_POINT ( 'NONE',  ( 4.999999999999999112, 0.000000000000000000, -6.000000000000000000 ) ) ;
#74877=CARTESIAN_POINT ( 'NONE',  ( -4.164238869374099927, 37.01208216824731068, 3.795296366450308767 ) ) ;
#74878=CARTESIAN_POINT ( 'NONE',  ( 0.5774900079438590739, 2.647018677488170990, -5.440088680355550821 ) ) ;
#74879=CARTESIAN_POINT ( 'NONE',  ( 20.88017736071110875, 25.77201867748816966, -2.915334737309920765 ) ) ;
#74883=CARTESIAN_POINT ( 'NONE',  ( 2.035157376598824452, 53.68868534415484817, 7.964842623401179544 ) ) ;
#74884=CARTESIAN_POINT ( 'NONE',  ( 7.084665262690076126, 49.10535201082149825, 10.88017736071109987 ) ) ;
#74885=CARTESIAN_POINT ( 'NONE',  ( 0.6178305044545818747, 28.49863466993041783, -9.382169495545419124 ) ) ;
#74887=CARTESIAN_POINT ( 'NONE',  ( 7.361572987183169658, 19.96726448433411960, -9.846743663894592657 ) ) ;
#74888=CARTESIAN_POINT ( 'NONE',  ( 4.559911319644449179, 57.23035201082150536, -9.422509992056141925 ) ) ;
#74889=CARTESIAN_POINT ( 'NONE',  ( 0.6178305044545818747, 18.49863466993041428, -9.382169495545419124 ) ) ;
#74890=CARTESIAN_POINT ( 'NONE',  ( -0.8801773607111009756, 43.27201867748816966, 2.915334737309923874 ) ) ;
#74891=CARTESIAN_POINT ( 'NONE',  ( 20.88017736071110519, 10.56368534415483751, 2.639326808657452039E-16 ) ) ;
#74892=CARTESIAN_POINT ( 'NONE',  ( 2.791683348922237240, 35.38393115100079456, -7.208316651077763204 ) ) ;
#74893=CARTESIAN_POINT ( 'NONE',  ( 0.6178305044545818747, 63.49863466993043204, -9.382169495545419124 ) ) ;
#74894=CARTESIAN_POINT ( 'NONE',  ( 14.92337183194729633, 12.67559781766745353, 8.527530157486181039 ) ) ;
#74895=( NAMED_UNIT ( * ) SI_UNIT ( $, .STERADIAN. ) SOLID_ANGLE_UNIT ( ) );
#74896=CARTESIAN_POINT ( 'NONE',  ( 24.16423886937410614, 4.512082168247300906, -3.795296366450302550 ) ) ;
#74897=CARTESIAN_POINT ( 'NONE',  ( 2.603489959281613420, 35.43575266056827644, -6.500000000000031086 ) ) ;
#74898=CARTESIAN_POINT ( 'NONE',  ( 20.88017736071110519, 15.56368534415483751, 2.639326808657452039E-16 ) ) ;
#74899=CARTESIAN_POINT ( 'NONE',  ( 7.084665262690076126, 2.022018677488170990, -10.88017736071110164 ) ) ;
#74900=CARTESIAN_POINT ( 'NONE',  ( 1.472469842513823179, 50.59226448433411605, -4.923371831947296329 ) ) ;
#74903=CARTESIAN_POINT ( 'NONE',  ( 0.5774900079438590739, 37.64701867748817676, -5.440088680355550821 ) ) ;
#74904=CARTESIAN_POINT ( 'NONE',  ( -0.8801773607111009756, 18.06368534415484106, 1.068504757029289695E-15 ) ) ;
#74906=CARTESIAN_POINT ( 'NONE',  ( 2.035157376598822676, 27.43868534415483396, -7.964842623401177768 ) ) ;
#74908=CARTESIAN_POINT ( 'NONE',  ( 16.40814093676324603, 42.45696800326375353, -11.09922568453594671 ) ) ;
#74909=EDGE_CURVE ( 'NONE', #56172, #17129, #39147, .T. ) ;
#74910=CARTESIAN_POINT ( 'NONE',  ( 7.084665262690076126, 34.10535201082151247, 10.88017736071109987 ) ) ;
#74911=CARTESIAN_POINT ( 'NONE',  ( 0.1532563361054100626, 45.80059781766745175, -2.638427012816831230 ) ) ;
#74912=CARTESIAN_POINT ( 'NONE',  ( 10.00000000000000000, 41.81368534415484106, -10.88017736071110342 ) ) ;
#74914=ORIENTED_EDGE ( 'NONE', *, *, #85954, .T. ) ;
#74915=CARTESIAN_POINT ( 'NONE',  ( 10.00000000000000000, 59.75893115100078745, -9.846743663894594434 ) ) ;
#74916=CARTESIAN_POINT ( 'NONE',  ( 10.00000000000000000, 36.81368534415484106, -10.88017736071110342 ) ) ;
#74917=CARTESIAN_POINT ( 'NONE',  ( 0.1532563361054083140, 66.00893115100079456, 1.131784320476157264E-15 ) ) ;
#74920=CARTESIAN_POINT ( 'NONE',  ( 24.16423886937410614, 44.30374883491397497, 8.672049930838204340E-16 ) ) ;
#74921=CARTESIAN_POINT ( 'NONE',  ( 0.5774900079438607392, 58.48035201082151247, 5.440088680355550821 ) ) ;
#74923=DIRECTION ( 'NONE',  ( 1.000000000000000000, 0.000000000000000000, 0.000000000000000000 ) ) ;
#74924=CARTESIAN_POINT ( 'NONE',  ( 1.472469842513823179, 56.42559781766745886, 4.923371831947296329 ) ) ;
#74926=CARTESIAN_POINT ( 'NONE',  ( 2.791683348922237240, 25.38393115100078390, -7.208316651077763204 ) ) ;
#74928=CARTESIAN_POINT ( 'NONE',  ( 5.076628168052704559, 25.17559781766745175, -8.527530157486179263 ) ) ;
#74930=CARTESIAN_POINT ( 'NONE',  ( 19.42250999205614548, 20.98035201082150891, -5.440088680355545492 ) ) ;
#74931=CARTESIAN_POINT ( 'NONE',  ( 0.1532563361054100626, 25.80059781766744820, -2.638427012816831230 ) ) ;
#74932=CARTESIAN_POINT ( 'NONE',  ( 10.00000000000000000, 12.87363466993042138, -12.81628187352647608 ) ) ;
#74934=CARTESIAN_POINT ( 'NONE',  ( 2.035157376598824452, 33.68868534415484106, 7.964842623401179544 ) ) ;
#74935=CARTESIAN_POINT ( 'NONE',  ( 4.559911319644449179, 7.230352010821504471, -9.422509992056141925 ) ) ;
#74936=CARTESIAN_POINT ( 'NONE',  ( -4.164238869374099927, 47.01208216824729647, 3.795296366450308767 ) ) ;
#74938=CARTESIAN_POINT ( 'NONE',  ( -43.49071039140426365, 106.3659493636330069, 5.092460419850055153 ) ) ;
#74940=CARTESIAN_POINT ( 'NONE',  ( -1.099225684535947600, 9.540301336597087456, 6.408140936763237150 ) ) ;
#74941=CARTESIAN_POINT ( 'NONE',  ( 17.96484262340118221, 4.938685344154837509, 7.964842623401181321 ) ) ;
#74942=CARTESIAN_POINT ( 'NONE',  ( 10.00000000000000178, 44.31368534415484106, 10.88017736071110342 ) ) ;
#74944=VERTEX_POINT ( 'NONE', #51102 ) ;
#74946=CARTESIAN_POINT ( 'NONE',  ( 12.91533473730993009, 51.60535201082149825, -10.88017736071109987 ) ) ;
#74947=CARTESIAN_POINT ( 'NONE',  ( 14.92337183194729633, 32.67559781766745175, 8.527530157486181039 ) ) ;
#74948=CARTESIAN_POINT ( 'NONE',  ( 0.1532563361054083140, 21.00893115100078745, 1.131784320476157264E-15 ) ) ;
#74949=CARTESIAN_POINT ( 'NONE',  ( 18.52753015748618282, 8.925597817667451750, -4.923371831947291888 ) ) ;
#74951=CARTESIAN_POINT ( 'NONE',  ( 13.43411237798106583, 37.66530133659708923, -12.81628187352647252 ) ) ;
#74952=CARTESIAN_POINT ( 'NONE',  ( 12.91533473730993009, 66.60535201082150536, -10.88017736071109987 ) ) ;
#74953=CARTESIAN_POINT ( 'NONE',  ( -0.1503990784575242878, 34.24884699246889141, -6.262539305110083276 ) ) ;
#74955=CARTESIAN_POINT ( 'NONE',  ( 14.92337183194729633, 27.67559781766745530, 8.527530157486181039 ) ) ;
#74956=ORIENTED_EDGE ( 'NONE', *, *, #49763, .T. ) ;
#74958=CARTESIAN_POINT ( 'NONE',  ( 22.81628187352647785, 51.62363466993042493, 6.195893100308588602E-16 ) ) ;
#74960=CARTESIAN_POINT ( 'NONE',  ( -2.816281873526473856, -0.8763653300695799508, 9.499525473075851096E-16 ) ) ;
#74961=EDGE_CURVE ( 'NONE', #17245, #36257, #8278, .T. ) ;
#74962=CARTESIAN_POINT ( 'NONE',  ( 24.16423886937410614, 39.30374883491396787, 8.672049930838204340E-16 ) ) ;
#74965=CARTESIAN_POINT ( 'NONE',  ( 10.00000000000000178, 28.05374883491396787, 14.16423886937410082 ) ) ;
#74966=CARTESIAN_POINT ( 'NONE',  ( 22.26659068614894466, 43.88708216824729647, 7.082119434687054849 ) ) ;
#74967=CARTESIAN_POINT ( 'NONE',  ( 2.917880565312950480, 5.970415501580634832, -12.26659068614894821 ) ) ;
#74968=CARTESIAN_POINT ( 'NONE',  ( 24.16423886937410614, 14.51208216824730179, -3.795296366450302550 ) ) ;
#74970=CARTESIAN_POINT ( 'NONE',  ( 0.5774900079438607392, 43.48035201082151247, 5.440088680355550821 ) ) ;
#74972=CARTESIAN_POINT ( 'NONE',  ( 7.361572987183169658, 24.96726448433412315, -9.846743663894592657 ) ) ;
#74973=CARTESIAN_POINT ( 'NONE',  ( 20.88017736071110164, 65.35535201082150536, 2.915334737309930979 ) ) ;
#74974=CARTESIAN_POINT ( 'NONE',  ( 2.791683348922240793, 26.63393115100078745, 7.208316651077764092 ) ) ;
#74976=CARTESIAN_POINT ( 'NONE',  ( 2.035157376598822676, 22.43868534415483396, -7.964842623401177768 ) ) ;
#74977=CARTESIAN_POINT ( 'NONE',  ( 19.38216949554541557, 52.24863466993041072, -9.382169495545420901 ) ) ;
#74980=CARTESIAN_POINT ( 'NONE',  ( 19.84674366389459621, 28.50893115100078745, 7.409399052514197653E-17 ) ) ;
#74981=CARTESIAN_POINT ( 'NONE',  ( -1.099225684535947600, 39.54030133659708923, 6.408140936763237150 ) ) ;
#74984=CARTESIAN_POINT ( 'NONE',  ( 0.5774900079438607392, 38.48035201082150536, 5.440088680355550821 ) ) ;
#74985=CARTESIAN_POINT ( 'NONE',  ( 14.92337183194729988, 39.34226448433412315, -8.527530157486177487 ) ) ;
#74986=CARTESIAN_POINT ( 'NONE',  ( 10.00000000000000000, 30.55374883491397142, -14.16423886937410082 ) ) ;
#74988=FILL_AREA_STYLE_COLOUR ( '', #28377 ) ;
#74989=CARTESIAN_POINT ( 'NONE',  ( 7.084665262690076126, 69.10535201082151957, 10.88017736071109987 ) ) ;
#74990=CARTESIAN_POINT ( 'NONE',  ( 0.5774900079438607392, 63.48035201082149825, 5.440088680355550821 ) ) ;
#74991=CARTESIAN_POINT ( 'NONE',  ( 10.00000000000000178, 53.05374883491396787, 14.16423886937410082 ) ) ;
#74992=CARTESIAN_POINT ( 'NONE',  ( 5.076628168052703671, 61.84226448433412315, 8.527530157486179263 ) ) ;
#74993=CARTESIAN_POINT ( 'NONE',  ( -0.03932841506541361054, 53.12161441960503794, 6.397827110479011203 ) ) ;
#74994=CARTESIAN_POINT ( 'NONE',  ( 7.084665262690076126, 54.10535201082151247, 10.88017736071109987 ) ) ;
#74995=EDGE_CURVE ( 'NONE', #93612, #43655, #47042, .T. ) ;
#74999=CARTESIAN_POINT ( 'NONE',  ( 0.5774900079438590739, 12.64701867748817143, -5.440088680355550821 ) ) ;
#75000=CARTESIAN_POINT ( 'NONE',  ( 0.5774900079438590739, 12.64701867748817321, -5.440088680355550821 ) ) ;
#75001=CARTESIAN_POINT ( 'NONE',  ( 12.63842701281683034, 42.46726448433412315, 9.846743663894596210 ) ) ;
#75002=CARTESIAN_POINT ( 'NONE',  ( 10.00000000000000000, 52.87363466993041783, -12.81628187352647608 ) ) ;
#75003=ORIENTED_EDGE ( 'NONE', *, *, #75431, .T. ) ;
#75004=CARTESIAN_POINT ( 'NONE',  ( 17.96484262340118221, 11.18868534415483929, -7.964842623401177768 ) ) ;
#75005=CARTESIAN_POINT ( 'NONE',  ( 10.00000000000000000, 22.87363466993042138, -12.81628187352647608 ) ) ;
#75007=CARTESIAN_POINT ( 'NONE',  ( 12.63842701281683922, 9.550597817667449974, -9.846743663894590881 ) ) ;
#75008=CARTESIAN_POINT ( 'NONE',  ( 17.20831665107776587, 44.13393115100078745, -7.208316651077762316 ) ) ;
#75009=CARTESIAN_POINT ( 'NONE',  ( -0.8801773607111009756, 33.06368534415484106, 1.068504757029289695E-15 ) ) ;
#75010=CARTESIAN_POINT ( 'NONE',  ( -2.816281873526473856, 14.33196800326375531, 3.434112377981055619 ) ) ;
#75011=CARTESIAN_POINT ( 'NONE',  ( 19.42250999205614548, 50.98035201082151247, -5.440088680355545492 ) ) ;
#75013=CARTESIAN_POINT ( 'NONE',  ( 2.831191079880678085, 79.91181047996344944, 12.00000000000000000 ) ) ;
#75014=CARTESIAN_POINT ( 'NONE',  ( 6.565887622018943937, 55.16530133659709634, 12.81628187352647430 ) ) ;
#75016=CARTESIAN_POINT ( 'NONE',  ( 20.88017736071110519, 60.56368534415484106, 2.639326808657452039E-16 ) ) ;
#75017=CARTESIAN_POINT ( 'NONE',  ( 22.81628187352647785, 31.62363466993042138, 6.195893100308588602E-16 ) ) ;
#75018=CARTESIAN_POINT ( 'NONE',  ( 6.204703633549690345, 2.845415501580634388, 14.16423886937410082 ) ) ;
#75019=CARTESIAN_POINT ( 'NONE',  ( 19.84674366389459621, 8.508931151000785675, 7.409399052514197653E-17 ) ) ;
#75020=CARTESIAN_POINT ( 'NONE',  ( 2.035157376598824452, 33.68868534415484106, 7.964842623401179544 ) ) ;
#75022=CARTESIAN_POINT ( 'NONE',  ( 14.92337183194729988, 64.34226448433412315, -8.527530157486177487 ) ) ;
#75023=CARTESIAN_POINT ( 'NONE',  ( 10.00000000000000000, 19.75893115100078390, -9.846743663894594434 ) ) ;
#75024=CARTESIAN_POINT ( 'NONE',  ( 5.076628168052704559, 0.1755978176674514724, -8.527530157486179263 ) ) ;
#75026=CARTESIAN_POINT ( 'NONE',  ( 22.26659068614894466, 43.88708216824729647, 7.082119434687054849 ) ) ;
#75031=CARTESIAN_POINT ( 'NONE',  ( -0.3689425029237881626, 57.42874883491397497, 10.36894250292379027 ) ) ;
#75032=CARTESIAN_POINT ( 'NONE',  ( 13.79529636645030344, 63.26208216824730357, 14.16423886937410614 ) ) ;
#75033=CARTESIAN_POINT ( 'NONE',  ( 14.92337183194729988, 34.34226448433411605, -8.527530157486177487 ) ) ;
#75034=CARTESIAN_POINT ( 'NONE',  ( 19.38216949554541557, 27.24863466993041783, -9.382169495545420901 ) ) ;
#75037=CARTESIAN_POINT ( 'NONE',  ( 20.36894250292379738, 4.928748834913967869, -10.36894250292379027 ) ) ;
#75038=CARTESIAN_POINT ( 'NONE',  ( 20.88017736071110875, 15.77201867748817143, -2.915334737309920765 ) ) ;
#75039=CARTESIAN_POINT ( 'NONE',  ( 13.79529636645031943, 50.34541550158064638, -14.16423886937409904 ) ) ;
#75040=CARTESIAN_POINT ( 'NONE',  ( 1.472469842513823179, 26.42559781766745175, 4.923371831947296329 ) ) ;
#75042=CARTESIAN_POINT ( 'NONE',  ( 12.63842701281683034, 17.46726448433411250, 9.846743663894596210 ) ) ;
#75045=ORIENTED_EDGE ( 'NONE', *, *, #40802, .F. ) ;
#75048=CARTESIAN_POINT ( 'NONE',  ( 18.52753015748618282, 48.92559781766745886, -4.923371831947291888 ) ) ;
#75049=CARTESIAN_POINT ( 'NONE',  ( 22.26659068614895176, 19.72041550158063572, -7.082119434687042414 ) ) ;
#75050=CARTESIAN_POINT ( 'NONE',  ( 4.559911319644449179, 17.23035201082150536, -9.422509992056141925 ) ) ;
#75051=CARTESIAN_POINT ( 'NONE',  ( -0.8801773607111008646, 38.27201867748816255, 2.915334737309923430 ) ) ;
#75052=SURFACE_STYLE_USAGE ( .BOTH. , #97098 ) ;
#75053=CARTESIAN_POINT ( 'NONE',  ( 0.6178305044545818747, 23.49863466993041783, -9.382169495545419124 ) ) ;
#75054=CARTESIAN_POINT ( 'NONE',  ( 2.917880565312948704, 7.637082168247301794, 12.26659068614894643 ) ) ;
#75055=EDGE_CURVE ( 'NONE', #63345, #55238, #61554, .T. ) ;
#75056=CARTESIAN_POINT ( 'NONE',  ( 2.035157376598822676, 67.43868534415484817, -7.964842623401177768 ) ) ;
#75058=CARTESIAN_POINT ( 'NONE',  ( 3.591859063236763294, 38.29030133659708923, -11.09922568453595026 ) ) ;
#75059=ORIENTED_EDGE ( 'NONE', *, *, #81167, .F. ) ;
#75060=CARTESIAN_POINT ( 'NONE',  ( 0.1532563361054083140, 41.00893115100078745, 1.131784320476157264E-15 ) ) ;
#75061=CARTESIAN_POINT ( 'NONE',  ( 4.559911319644449179, 12.23035201082150714, -9.422509992056141925 ) ) ;
#75062=B_SPLINE_CURVE_WITH_KNOTS ( 'NONE', 3,
 ( #19678, #87671, #42675, #26199 ),
 .UNSPECIFIED., .F., .F.,
 ( 4, 4 ),
 ( 0.000000000000000000, 0.002657014572711318551 ),
 .UNSPECIFIED. ) ;
#75063=CARTESIAN_POINT ( 'NONE',  ( -2.266590686148945544, 66.38708216824730357, -7.082119434687050408 ) ) ;
#75065=CARTESIAN_POINT ( 'NONE',  ( 17.96484262340118221, 41.18868534415484106, -7.964842623401177768 ) ) ;
#75067=CARTESIAN_POINT ( 'NONE',  ( 7.084665262690076126, 52.02201867748816255, -10.88017736071110164 ) ) ;
#75068=FACE_OUTER_BOUND ( 'NONE', #36145, .T. ) ;
#75069=CARTESIAN_POINT ( 'NONE',  ( 12.63842701281683034, 2.467264484334118269, 9.846743663894596210 ) ) ;
#75070=ADVANCED_FACE ( 'NONE', ( #55548 ), #77056, .T. ) ;
#75071=CARTESIAN_POINT ( 'NONE',  ( 20.88017736071110519, 60.56368534415484106, 2.639326808657452039E-16 ) ) ;
#75072=CIRCLE ( 'NONE', #92693, 0.5000000000000009992 ) ;
#75073=CARTESIAN_POINT ( 'NONE',  ( -0.3289641300568009741, 52.24545670184113533, -5.963430220938281678 ) ) ;
#75074=DIRECTION ( 'NONE',  ( 0.000000000000000000, -1.000000000000000000, 0.000000000000000000 ) ) ;
#75077=CARTESIAN_POINT ( 'NONE',  ( 0.1532563361054100626, 25.80059781766744820, -2.638427012816831230 ) ) ;
#75078=ORIENTED_EDGE ( 'NONE', *, *, #81442, .T. ) ;
#75081=CARTESIAN_POINT ( 'NONE',  ( -2.266590686148945544, 7.220415501580634832, 7.082119434687048631 ) ) ;
#75083=CARTESIAN_POINT ( 'NONE',  ( -0.03447792253739101476, 35.15514106990691090, 6.401564815979742917 ) ) ;
#75085=CARTESIAN_POINT ( 'NONE',  ( 2.035157376598822676, 12.43868534415483751, -7.964842623401177768 ) ) ;
#75089=CARTESIAN_POINT ( 'NONE',  ( 12.63842701281683922, 44.55059781766745175, -9.846743663894590881 ) ) ;
#75090=DIRECTION ( 'NONE',  ( 0.000000000000000000, 0.000000000000000000, -1.000000000000000000 ) ) ;
#75091=CARTESIAN_POINT ( 'NONE',  ( -2.816281873526473856, 19.33196800326375708, 3.434112377981055619 ) ) ;
#75092=CARTESIAN_POINT ( 'NONE',  ( 12.63842701281683922, 4.550597817667451750, -9.846743663894590881 ) ) ;
#75094=CARTESIAN_POINT ( 'NONE',  ( 16.40814093676324603, 7.456968003263754419, -11.09922568453594671 ) ) ;
#75095=CARTESIAN_POINT ( 'NONE',  ( 0.1532563361054082862, 26.21726448433411960, 2.638427012816831674 ) ) ;
#75097=EDGE_CURVE ( 'NONE', #64078, #13373, #79583, .T. ) ;
#75098=EDGE_LOOP ( 'NONE', ( #71243, #90245, #36684, #42019 ) ) ;
#75099=CARTESIAN_POINT ( 'NONE',  ( 10.00000000000000000, 21.81368534415484106, -10.88017736071110342 ) ) ;
#75100=CARTESIAN_POINT ( 'NONE',  ( 6.204703633549690345, 25.76208216824730712, -14.16423886937410259 ) ) ;
#75101=CARTESIAN_POINT ( 'NONE',  ( 14.92337183194729633, 32.67559781766745175, 8.527530157486181039 ) ) ;
#75102=CARTESIAN_POINT ( 'NONE',  ( 10.00000000000000000, 56.81368534415484106, -10.88017736071110342 ) ) ;
#75103=CARTESIAN_POINT ( 'NONE',  ( 6.565887622018943937, 38.08196800326376064, -12.81628187352647608 ) ) ;
#75105=CARTESIAN_POINT ( 'NONE',  ( 12.91533473730992121, 9.522018677488171434, 10.88017736071110164 ) ) ;
#75109=CARTESIAN_POINT ( 'NONE',  ( -2.816281873526471635, 8.915301336597083903, -3.434112377981056508 ) ) ;
#75110=CARTESIAN_POINT ( 'NONE',  ( 1.472469842513823179, 65.59226448433412315, -4.923371831947296329 ) ) ;
#75111=CARTESIAN_POINT ( 'NONE',  ( 10.00000000000000178, 22.25893115100078745, 9.846743663894594434 ) ) ;
#75113=CARTESIAN_POINT ( 'NONE',  ( 22.81628187352648496, 41.83196800326375353, -3.434112377981050290 ) ) ;
#75115=CARTESIAN_POINT ( 'NONE',  ( 15.44008868035555793, 36.39701867748816966, -9.422509992056140149 ) ) ;
#75118=CARTESIAN_POINT ( 'NONE',  ( 19.80777595082616926, 20.68878173731740944, -6.499999999999961808 ) ) ;
#75119=CARTESIAN_POINT ( 'NONE',  ( 19.42250999205614548, 40.98035201082150536, -5.440088680355545492 ) ) ;
#75120=CARTESIAN_POINT ( 'NONE',  ( 15.44008868035555260, 44.73035201082151247, 9.422509992056143702 ) ) ;
#75121=CARTESIAN_POINT ( 'NONE',  ( 17.20831665107776587, 62.88393115100078745, 7.208316651077764980 ) ) ;
#75122=CARTESIAN_POINT ( 'NONE',  ( -0.8801773607111009756, 53.06368534415484106, 1.068504757029289695E-15 ) ) ;
#75124=CARTESIAN_POINT ( 'NONE',  ( 18.52753015748618282, 33.92559781766745886, -4.923371831947291888 ) ) ;
#75125=CARTESIAN_POINT ( 'NONE',  ( -0.8801773607111008646, 13.27201867748817143, 2.915334737309923430 ) ) ;
#75127=CARTESIAN_POINT ( 'NONE',  ( 3.591859063236761518, 9.956968003263753531, 11.09922568453594849 ) ) ;
#75129=CARTESIAN_POINT ( 'NONE',  ( 4.559911319644449179, 28.89701867748817321, 9.422509992056141925 ) ) ;
#75131=CARTESIAN_POINT ( 'NONE',  ( 2.035157376598822676, 32.43868534415483396, -7.964842623401177768 ) ) ;
#75132=CARTESIAN_POINT ( 'NONE',  ( 0.5774900079438607392, 63.48035201082149825, 5.440088680355550821 ) ) ;
#75133=CARTESIAN_POINT ( 'NONE',  ( -0.3689425029237881626, 32.42874883491395366, 10.36894250292379027 ) ) ;
#75134=CARTESIAN_POINT ( 'NONE',  ( 17.20831665107776587, 9.133931151000787452, -7.208316651077762316 ) ) ;
#75135=CARTESIAN_POINT ( 'NONE',  ( -0.8801773607111009756, 53.06368534415484106, 1.068504757029289695E-15 ) ) ;
#75136=CARTESIAN_POINT ( 'NONE',  ( 19.39188664607695500, 45.83703382326400799, -6.499999999999968026 ) ) ;
#75137=CARTESIAN_POINT ( 'NONE',  ( 24.16423886937409904, 4.095415501580634832, 3.795296366450317205 ) ) ;
#75140=CARTESIAN_POINT ( 'NONE',  ( 0.1532563361054083140, 61.00893115100078745, 1.131784320476157264E-15 ) ) ;
#75141=ORIENTED_EDGE ( 'NONE', *, *, #55889, .F. ) ;
#75144=CARTESIAN_POINT ( 'NONE',  ( 13.79529636645031943, 25.34541550158063572, -14.16423886937409904 ) ) ;
#75145=CARTESIAN_POINT ( 'NONE',  ( 13.79529636645030344, 18.26208216824730002, 14.16423886937410614 ) ) ;
#75146=CARTESIAN_POINT ( 'NONE',  ( 10.00000000000000178, 64.31368534415483396, 10.88017736071110342 ) ) ;
#75147=CARTESIAN_POINT ( 'NONE',  ( -2.266590686148945544, 62.22041550158063927, 7.082119434687048631 ) ) ;
#75148=CARTESIAN_POINT ( 'NONE',  ( 10.00000000000000178, 5.373634669930420493, 12.81628187352647608 ) ) ;
#75149=CARTESIAN_POINT ( 'NONE',  ( 17.20831665107776587, 49.13393115100078745, -7.208316651077762316 ) ) ;
#75151=CARTESIAN_POINT ( 'NONE',  ( 10.00000000000000178, 44.31368534415484106, 10.88017736071110342 ) ) ;
#75152=CARTESIAN_POINT ( 'NONE',  ( -2.816281873526473856, 9.331968003263753531, 3.434112377981055619 ) ) ;
#75153=CARTESIAN_POINT ( 'NONE',  ( 17.08211943468705840, 15.13708216824730179, -12.26659068614894466 ) ) ;
#75154=CARTESIAN_POINT ( 'NONE',  ( 2.035157376598822676, 12.43868534415483751, -7.964842623401177768 ) ) ;
#75155=CARTESIAN_POINT ( 'NONE',  ( 4.559911319644449179, 18.89701867748817321, 9.422509992056141925 ) ) ;
#75156=CARTESIAN_POINT ( 'NONE',  ( 20.88017736071110875, 45.77201867748816966, -2.915334737309920765 ) ) ;
#75157=CARTESIAN_POINT ( 'NONE',  ( 16.40814093676323893, 45.79030133659708923, 11.09922568453595026 ) ) ;
#75160=CARTESIAN_POINT ( 'NONE',  ( -46.34323875807881166, 103.6109741468810483, -6.190393423093146552 ) ) ;
#75161=CARTESIAN_POINT ( 'NONE',  ( 7.361572987183170547, 32.05059781766745175, 9.846743663894590881 ) ) ;
#75162=ORIENTED_EDGE ( 'NONE', *, *, #66486, .T. ) ;
#75164=CARTESIAN_POINT ( 'NONE',  ( 19.72487221294571569, 60.71833443783937412, -6.499999999999990230 ) ) ;
#75165=CARTESIAN_POINT ( 'NONE',  ( 24.16423886937410614, 49.51208216824730357, -3.795296366450302550 ) ) ;
#75166=CARTESIAN_POINT ( 'NONE',  ( 4.559911319644449179, 7.230352010821505360, -9.422509992056141925 ) ) ;
#75167=CARTESIAN_POINT ( 'NONE',  ( 19.84674366389459621, 28.50893115100078745, 7.409399052514197653E-17 ) ) ;
#75168=CARTESIAN_POINT ( 'NONE',  ( 14.92337183194729633, 42.67559781766745886, 8.527530157486181039 ) ) ;
#75170=EDGE_CURVE ( 'NONE', #91555, #85493, #66456, .T. ) ;
#75171=CARTESIAN_POINT ( 'NONE',  ( 12.63842701281683034, 2.467264484334118269, 9.846743663894596210 ) ) ;
#75175=CARTESIAN_POINT ( 'NONE',  ( 6.204703633549690345, 37.84541550158063927, 14.16423886937410082 ) ) ;
#75177=CARTESIAN_POINT ( 'NONE',  ( -2.816281873526473856, 29.33196800326376064, 3.434112377981055619 ) ) ;
#75179=CARTESIAN_POINT ( 'NONE',  ( -2.816281873526471635, 63.91530133659708923, -3.434112377981056508 ) ) ;
#75180=CARTESIAN_POINT ( 'NONE',  ( 0.1532563361054082862, 31.21726448433412315, 2.638427012816831674 ) ) ;
#75181=CARTESIAN_POINT ( 'NONE',  ( -0.8801773607110991993, 32.85535201082151247, -2.915334737309923874 ) ) ;
#75182=CARTESIAN_POINT ( 'NONE',  ( 20.24186590665275531, 32.61633188102328518, -6.114288769123075618 ) ) ;
#75183=LINE ( 'NONE', #91170, #89490 ) ;
#75184=CARTESIAN_POINT ( 'NONE',  ( 5.076628168052704559, 40.17559781766745175, -8.527530157486179263 ) ) ;
#75185=CARTESIAN_POINT ( 'NONE',  ( 12.63842701281683922, 54.55059781766745175, -9.846743663894590881 ) ) ;
#75188=ORIENTED_EDGE ( 'NONE', *, *, #61432, .F. ) ;
#75189=EDGE_CURVE ( 'NONE', #69767, #89063, #39035, .T. ) ;
#75190=CARTESIAN_POINT ( 'NONE',  ( 18.17884179759847996, 18.66688879859523453, -6.499999999999984901 ) ) ;
#75191=DIRECTION ( 'NONE',  ( 1.000000000000000000, -7.138779736530071317E-16, 0.000000000000000000 ) ) ;
#75192=CARTESIAN_POINT ( 'NONE',  ( 18.72515096720568195, 21.07228050351032422, -6.500000000000018652 ) ) ;
#75194=CARTESIAN_POINT ( 'NONE',  ( 7.361572987183169658, 14.96726448433411960, -9.846743663894592657 ) ) ;
#75195=ADVANCED_FACE ( 'NONE', ( #84568 ), #54571, .T. ) ;
#75196=CARTESIAN_POINT ( 'NONE',  ( 22.81628187352647785, 36.41530133659707502, 3.434112377981063169 ) ) ;
#75200=CARTESIAN_POINT ( 'NONE',  ( 1.472469842513823179, 60.59226448433412315, -4.923371831947296329 ) ) ;
#75202=CARTESIAN_POINT ( 'NONE',  ( 12.63842701281683922, 34.55059781766745886, -9.846743663894590881 ) ) ;
#75203=CARTESIAN_POINT ( 'NONE',  ( 17.08211943468705130, 38.47041550158063217, 12.26659068614894998 ) ) ;
#75204=CARTESIAN_POINT ( 'NONE',  ( 0.1532563361054082862, 41.21726448433411605, 2.638427012816831674 ) ) ;
#75205=CARTESIAN_POINT ( 'NONE',  ( -2.816281873526473856, 49.33196800326374643, 3.434112377981055619 ) ) ;
#75206=DIRECTION ( 'NONE',  ( 0.000000000000000000, -1.000000000000000000, 0.000000000000000000 ) ) ;
#75207=CARTESIAN_POINT ( 'NONE',  ( 14.92337183194729633, 12.67559781766745353, 8.527530157486181039 ) ) ;
#75208=FILL_AREA_STYLE_COLOUR ( '', #55196 ) ;
#75209=CARTESIAN_POINT ( 'NONE',  ( 12.63842701281683922, 54.55059781766745175, -9.846743663894590881 ) ) ;
#75210=CARTESIAN_POINT ( 'NONE',  ( 2.035157376598824452, 38.68868534415483396, 7.964842623401179544 ) ) ;
#75211=CARTESIAN_POINT ( 'NONE',  ( 2.791683348922237240, 45.38393115100079456, -7.208316651077763204 ) ) ;
#75214=CARTESIAN_POINT ( 'NONE',  ( 20.88017736071110164, 50.35535201082151247, 2.915334737309930979 ) ) ;
#75217=CARTESIAN_POINT ( 'NONE',  ( -0.8801773607110991993, 17.85535201082150536, -2.915334737309923874 ) ) ;
#75218=CARTESIAN_POINT ( 'NONE',  ( 7.361572987183170547, 67.05059781766746596, 9.846743663894590881 ) ) ;
#75219=CARTESIAN_POINT ( 'NONE',  ( 12.91533473730992121, 44.52201867748816966, 10.88017736071110164 ) ) ;
#75221=CARTESIAN_POINT ( 'NONE',  ( 4.559911319644449179, 67.23035201082150536, -9.422509992056141925 ) ) ;
#75223=CARTESIAN_POINT ( 'NONE',  ( 0.5774900079438590739, 37.64701867748817676, -5.440088680355550821 ) ) ;
#75225=CARTESIAN_POINT ( 'NONE',  ( 5.076628168052703671, 11.84226448433411960, 8.527530157486179263 ) ) ;
#75226=CARTESIAN_POINT ( 'NONE',  ( 1.472469842513823179, 26.42559781766745175, 4.923371831947296329 ) ) ;
#75229=CARTESIAN_POINT ( 'NONE',  ( 7.361572987183169658, 64.96726448433412315, -9.846743663894592657 ) ) ;
#75230=CARTESIAN_POINT ( 'NONE',  ( -0.3689425029237881626, 67.42874883491396076, 10.36894250292379027 ) ) ;
#75233=CARTESIAN_POINT ( 'NONE',  ( 19.80427997160309417, 27.75733960839543712, -6.499999999999987566 ) ) ;
#75235=CARTESIAN_POINT ( 'NONE',  ( -0.3689425029237881626, 17.42874883491397142, 10.36894250292379027 ) ) ;
#75236=CARTESIAN_POINT ( 'NONE',  ( -2.266590686148945544, 56.38708216824731068, -7.082119434687050408 ) ) ;
#75237=CARTESIAN_POINT ( 'NONE',  ( 20.03447792253739124, 32.65514106990688958, -6.401564815979717160 ) ) ;
#75240=CARTESIAN_POINT ( 'NONE',  ( 1.472469842513823179, 30.59226448433411960, -4.923371831947296329 ) ) ;
#75241=CARTESIAN_POINT ( 'NONE',  ( -0.8801773607111009756, 8.063685344154837509, 1.068504757029289695E-15 ) ) ;
#75242=CARTESIAN_POINT ( 'NONE',  ( 14.92337183194729633, 52.67559781766745175, 8.527530157486181039 ) ) ;
#75246=CARTESIAN_POINT ( 'NONE',  ( 6.565887622018943937, 43.08196800326374643, -12.81628187352647608 ) ) ;
#75247=B_SPLINE_CURVE_WITH_KNOTS ( 'NONE', 3,
 ( #27935, #20451, #26956, #81434, #57456, #19464 ),
 .UNSPECIFIED., .F., .F.,
 ( 4, 2, 4 ),
 ( 0.000000000000000000, 0.0002701661927229340350, 0.0005403323854458680700 ),
 .UNSPECIFIED. ) ;
#75248=CARTESIAN_POINT ( 'NONE',  ( 14.92337183194729633, 47.67559781766745175, 8.527530157486181039 ) ) ;
#75250=CARTESIAN_POINT ( 'NONE',  ( 0.1532563361054082862, 6.217264484334118713, 2.638427012816831674 ) ) ;
#75253=CARTESIAN_POINT ( 'NONE',  ( 20.88017736071110164, 15.35535201082150358, 2.915334737309930979 ) ) ;
#75254=CARTESIAN_POINT ( 'NONE',  ( 2.917880565312948704, 57.63708216824731068, 12.26659068614894643 ) ) ;
#75255=CARTESIAN_POINT ( 'NONE',  ( -0.8801773607111008646, 68.27201867748817676, 2.915334737309923430 ) ) ;
#75257=CARTESIAN_POINT ( 'NONE',  ( 5.076628168052703671, 26.84226448433411960, 8.527530157486179263 ) ) ;
#75258=CARTESIAN_POINT ( 'NONE',  ( 4.559911319644449179, 7.230352010821504471, -9.422509992056141925 ) ) ;
#75259=CARTESIAN_POINT ( 'NONE',  ( 17.20831665107776587, 7.883931151000784787, 7.208316651077764980 ) ) ;
#75260=( BOUNDED_SURFACE ( )  B_SPLINE_SURFACE ( 1, 2, ( 
 ( #58530, #20549, #43529, #81527, #5555, #66534, #42079, #72542, #28534, #51533, #59028, #6042, #65535, #4075, #34538, #95559, #27048, #96058, #57546, #8505, #6524, #91000, #69502, #69012, #60010, #29502, #15035, #7535, #30991, #52515, #38026, #45508, #84010, #37534, #7028, #84505, #76504, #46493, #52030, #82523, #83516, #38515, #75019, #91995, #67530, #68519, #76992, #98551, #49, #30497, #23526, #53499, #8018, #2508, #63465, #94450, #63937, #41481, #55977, #40488, #54967, #62969, #24505, #55485, #3471, #92973, #47961, #93474, #25964, #77476, #70489, #17976, #62468, #32960, #54479, #48461, #71476, #18464, #85489, #2009, #79457, #56465, #16998, #93967, #78471, #31966, #32474, #71948, #33927, #25000, #85985, #86951, #48949, #47477, #33441, #16505, #46982, #77977, #2991, #17496, #64433, #10956, #9985, #70986, #24007, #78959, #25492, #84989, #10470, #40979, #9484, #86478, #8987, #39504, #69993, #1520, #39987, #56941, #27916, #72430, #88431, #72928, #57921, #3956, #49936, #28418, #64918, #34426, #35915, #12918, #4457, #19930, #57436, #74400, #50425, #58408, #36417, #80932, #87443, #96445, #42445, #51416, #43900, #73413, #95445, #12426, #58913, #88924, #5444, #50920, #42932, #20433, #18958, #4941, #34922, #5924, #96945, #81416, #79940, #35421, #43415, #73915, #65915, #94941, #66414, #26442, #89412, #87928, #20927, #81905, #13414, #49436, #26937, #11447, #41964, #19445, #80443, #11940, #65420, #95944, #27427, #60387, #52400, #55222, #90885, #47223, #62719, #59400, #17249, #21921, #97934, #85242, #16748, #23773, #85736, #14418, #82900, #1762, #93219, #67405, #54238, #37420, #9734, #66909, #6399, #77726, #51913, #59893, #29391, #36913, #32218, #84751, #8740, #54722, #92734, #1278, #16256, #90383, #46738, #47725, #28895, #78223, #67906, #9238, #77236, #44887, #70246, #69750, #75390, #39261, #44401, #31731, #62227, #98430, #29885, #6908, #97429, #89903, #24258, #39749, #21419, #24743, #82398, #13923, #74900, #40234, #86226, #2750, #57186, #93715, #71712, #18717, #79703, #11697, #80184, #57681, #72190, #56704, #71227, #79207, #40725, #3223, #19690, #10232, #64185, #10717, #42206, #25250, #86719, #34180, #78722, #49199, #70742, #64672, #87683, #34678, #33206, #18223, #95694, #72673, #63700, #11201, #94705, #48212, #48703, #88177, #50177, #41234, #33687, #4208, #65174, #94203, #49680, #32713, #63211, #25733, #19197, #26211, #80687, #27178, #87194, #41721, #2258, #95182, #3719, #55734, #26690, #17737, #56225, #58667, #90638, #21172, #89169, #28663, #29147, #35677, #20680, #43665, #36170, #59653, #89662, #96694, #81175, #12183, #81658 ),
 ( #22163, #13167, #51675, #5685, #51174, #98177, #66670, #90144, #6658, #4707, #60141, #66161, #43175, #21674, #52160, #97195, #29633, #74151, #59155, #44653, #37174, #12675, #82153, #13665, #52645, #42689, #50683, #82653, #27676, #44149, #74657, #6168, #36672, #67160, #14169, #97685, #75148, #67667, #73168, #65670, #58161, #88672, #20180, #77116, #54117, #1151, #84630, #7157, #68160, #84151, #16630, #91638, #23156, #76140, #39633, #31611, #53631, #22662, #7666, #38157, #15657, #46140, #76626, #92612, #77605, #93599, #32601, #18111, #79089, #34063, #25136, #10601, #41115, #87085, #71111, #55614, #57076, #49088, #87572, #72559, #4092, #33574, #64559, #34556, #95069, #65050, #64068, #49560, #85617, #86111, #17622, #26573, #9614, #94583, #18595, #79591, #19084, #80072, #95576, #11092, #11578, #48092, #94094, #78605, #42092, #17134, #10114, #47613, #25615, #78108, #40115, #2638, #70616, #33092, #63585, #56108, #21059, #74537, #21558, #88558, #5071, #82538, #59540, #20061, #97080, #51051, #35050, #35558, #44538, #6541, #66048, #96575, #97568, #90034, #50563, #36556, #19572, #80573, #96076, #67046, #28052, #75034, #52047, #58547, #20566, #14056, #82040, #43545, #37050, #81541, #5574, #67549, #13051, #27063, #36049, #66552, #59044, #44037, #12069, #42571, #81058, #12562, #51553, #73055, #13551, #4588, #84521, #23540, #31006, #46032, #37550, #53515, #16521, #60026, #77489, #66, #8519, #84026, #60525, #1032, #561, #68040, #69027, #75531, #76517, #15547, #30513, #61016, #98566, #54012, #16018, #30020, #8032, #90521, #46507, #46995, #61503, #77007, #22057, #92010, #7045, #91527, #76023, #23041, #91015, #53018, #31493, #22548, #83533, #39021, #69517, #7554, #38531, #15051, #9001, #61997, #92496, #39517, #24025, #52530, #54493, #45525, #85008, #98061, #29519, #38044, #83038, #14555, #45024, #68535, #25981, #93982, #94464, #31979, #78972, #17511, #79956, #71962, #56478, #54982, #25504, #3006, #48963, #48474, #11460, #41493, #70010, #79473, #62982, #33942, #40994, #10483, #10972, #9497, #64446, #32974, #55991, #94953, #62485, #1535, #70997, #26455, #86492, #55499, #56954, #17992, #87457, #18972, #92989, #24523, #86000, #2025, #85501, #17011, #47489, #77992, #78486, #10000, #39999, #93488, #2521, #35435, #12441, #82413, #41979, #80456, #42949, #72442, #3971, #11955, #20943, #26951, #34937, #72941, #42459, #5941, #65930, #81430, #28431, #66426, #73929, #88937, #4471, #96458, #59412, #34441, #21432, #73428, #51430, #27929, #65435, #43914, #43428, #95959, #12934, #19459, #20446, #58423, #4955, #50936, #27441, #96959, #58929, #57935, #5457 ) ),
 .UNSPECIFIED., .F., .F., .F. ) 
 B_SPLINE_SURFACE_WITH_KNOTS ( ( 2, 2 ),
 ( 3, 2, 2, 2, 2, 2, 2, 2, 2, 2, 2, 2, 2, 2, 2, 2, 2, 2, 2, 2, 2, 2, 2, 2, 2, 2, 2, 2, 2, 2, 2, 2, 2, 2, 2, 2, 2, 2, 2, 2, 2, 2, 2, 2, 2, 2, 2, 2, 2, 2, 2, 2, 2, 2, 2, 2, 2, 2, 2, 2, 2, 2, 2, 2, 2, 2, 2, 2, 2, 2, 2, 2, 2, 2, 2, 2, 2, 2, 2, 2, 2, 2, 2, 2, 2, 2, 2, 2, 2, 2, 2, 2, 2, 2, 2, 2, 2, 2, 2, 2, 2, 2, 2, 2, 2, 2, 2, 2, 2, 2, 2, 2, 2, 2, 2, 2, 2, 2, 2, 2, 2, 2, 2, 2, 2, 2, 2, 2, 2, 2, 2, 2, 2, 2, 2, 2, 2, 2, 2, 2, 2, 2, 2, 2, 2, 2, 2, 2, 2, 2, 2, 2, 2, 2, 2, 2, 2, 2, 2, 2, 2, 2, 3 ),
 ( 0.000000000000000000, 1.000000000000000000 ),
 ( 0.000000000000000000, 0.005952380952380952051, 0.01190476190476190410, 0.01785714285714285615, 0.02380952380952380820, 0.02976190476190476025, 0.03571428571428571230, 0.04166666666666666435, 0.04761904761904761640, 0.05357142857142856845, 0.05952380952380952051, 0.06547619047619047949, 0.07142857142857142461, 0.07738095238095238360, 0.08333333333333332871, 0.08928571428571428770, 0.09523809523809523281, 0.1011904761904761918, 0.1071428571428571369, 0.1130952380952380959, 0.1190476190476190410, 0.1250000000000000000, 0.1309523809523809590, 0.1369047619047619180, 0.1428571428571428492, 0.1488095238095238082, 0.1547619047619047672, 0.1607142857142857262, 0.1666666666666666574, 0.1726190476190476164, 0.1785714285714285754, 0.1845238095238095344, 0.1904761904761904656, 0.1964285714285714246, 0.2023809523809523836, 0.2083333333333333426, 0.2142857142857142738, 0.2202380952380952328, 0.2261904761904761918, 0.2321428571428571508, 0.2380952380952380820, 0.2440476190476190410, 0.2500000000000000000, 0.2559523809523809312, 0.2619047619047619180, 0.2678571428571428492, 0.2738095238095238360, 0.2797619047619047672, 0.2857142857142856984, 0.2916666666666666852, 0.2976190476190476164, 0.3035714285714285476, 0.3095238095238095344, 0.3154761904761904656, 0.3214285714285714524, 0.3273809523809523836, 0.3333333333333333148, 0.3392857142857143016, 0.3452380952380952328, 0.3511904761904761640, 0.3571428571428571508, 0.3630952380952380820, 0.3690476190476190688, 0.3750000000000000000, 0.3809523809523809312, 0.3869047619047619180, 0.3928571428571428492, 0.3988095238095238360, 0.4047619047619047672, 0.4107142857142856984, 0.4166666666666666852, 0.4226190476190476164, 0.4285714285714285476, 0.4345238095238095344, 0.4404761904761904656, 0.4464285714285714524, 0.4523809523809523836, 0.4583333333333333148, 0.4642857142857143016, 0.4702380952380952328, 0.4761904761904761640, 0.4821428571428571508, 0.4880952380952380820, 0.4940476190476190688, 0.5000000000000000000, 0.5059523809523809312, 0.5119047619047618625, 0.5178571428571429047, 0.5238095238095238360, 0.5297619047619047672, 0.5357142857142856984, 0.5416666666666666297, 0.5476190476190476719, 0.5535714285714286031, 0.5595238095238095344, 0.5654761904761904656, 0.5714285714285713969, 0.5773809523809523281, 0.5833333333333333703, 0.5892857142857143016, 0.5952380952380952328, 0.6011904761904761640, 0.6071428571428570953, 0.6130952380952381375, 0.6190476190476190688, 0.6250000000000000000, 0.6309523809523809312, 0.6369047619047618625, 0.6428571428571429047, 0.6488095238095238360, 0.6547619047619047672, 0.6607142857142856984, 0.6666666666666666297, 0.6726190476190476719, 0.6785714285714286031, 0.6845238095238095344, 0.6904761904761904656, 0.6964285714285713969, 0.7023809523809523281, 0.7083333333333333703, 0.7142857142857143016, 0.7202380952380952328, 0.7261904761904761640, 0.7321428571428570953, 0.7380952380952381375, 0.7440476190476190688, 0.7500000000000000000, 0.7559523809523809312, 0.7619047619047618625, 0.7678571428571429047, 0.7738095238095238360, 0.7797619047619047672, 0.7857142857142856984, 0.7916666666666666297, 0.7976190476190476719, 0.8035714285714286031, 0.8095238095238095344, 0.8154761904761904656, 0.8214285714285713969, 0.8273809523809523281, 0.8333333333333333703, 0.8392857142857143016, 0.8452380952380952328, 0.8511904761904761640, 0.8571428571428570953, 0.8630952380952381375, 0.8690476190476190688, 0.8750000000000000000, 0.8809523809523809312, 0.8869047619047618625, 0.8928571428571429047, 0.8988095238095238360, 0.9047619047619047672, 0.9107142857142856984, 0.9166666666666666297, 0.9226190476190476719, 0.9285714285714286031, 0.9345238095238095344, 0.9404761904761904656, 0.9464285714285713969, 0.9523809523809523281, 0.9583333333333333703, 0.9642857142857143016 ),
 .UNSPECIFIED. ) 
 GEOMETRIC_REPRESENTATION_ITEM ( )  RATIONAL_B_SPLINE_SURFACE ( (
 ( 1.000000000000000000, 0.9659258262890683122, 1.000000000000000000, 0.9659258262890683122, 1.000000000000000000, 0.9659258262890683122, 1.000000000000000000, 0.9659258262890683122, 1.000000000000000000, 0.9659258262890683122, 1.000000000000000000, 0.9659258262890683122, 1.000000000000000000, 0.9659258262890683122, 1.000000000000000000, 0.9659258262890683122, 1.000000000000000000, 0.9659258262890683122, 1.000000000000000000, 0.9659258262890683122, 1.000000000000000000, 0.9659258262890683122, 1.000000000000000000, 0.9659258262890683122, 1.000000000000000000, 0.9659258262890683122, 1.000000000000000000, 0.9659258262890683122, 1.000000000000000000, 0.9659258262890683122, 1.000000000000000000, 0.9659258262890683122, 1.000000000000000000, 0.9659258262890683122, 1.000000000000000000, 0.9659258262890683122, 1.000000000000000000, 0.9659258262890683122, 1.000000000000000000, 0.9659258262890683122, 1.000000000000000000, 0.9659258262890683122, 1.000000000000000000, 0.9659258262890683122, 1.000000000000000000, 0.9659258262890683122, 1.000000000000000000, 0.9659258262890683122, 1.000000000000000000, 0.9659258262890683122, 1.000000000000000000, 0.9659258262890683122, 1.000000000000000000, 0.9659258262890683122, 1.000000000000000000, 0.9659258262890683122, 1.000000000000000000, 0.9659258262890683122, 1.000000000000000000, 0.9659258262890683122, 1.000000000000000000, 0.9659258262890683122, 1.000000000000000000, 0.9659258262890683122, 1.000000000000000000, 0.9659258262890683122, 1.000000000000000000, 0.9659258262890683122, 1.000000000000000000, 0.9659258262890683122, 1.000000000000000000, 0.9659258262890683122, 1.000000000000000000, 0.9659258262890683122, 1.000000000000000000, 0.9659258262890683122, 1.000000000000000000, 0.9659258262890683122, 1.000000000000000000, 0.9659258262890683122, 1.000000000000000000, 0.9659258262890683122, 1.000000000000000000, 0.9659258262890683122, 1.000000000000000000, 0.9659258262890683122, 1.000000000000000000, 0.9659258262890683122, 1.000000000000000000, 0.9659258262890683122, 1.000000000000000000, 0.9659258262890683122, 1.000000000000000000, 0.9659258262890683122, 1.000000000000000000, 0.9659258262890683122, 1.000000000000000000, 0.9659258262890683122, 1.000000000000000000, 0.9659258262890683122, 1.000000000000000000, 0.9659258262890683122, 1.000000000000000000, 0.9659258262890683122, 1.000000000000000000, 0.9659258262890683122, 1.000000000000000000, 0.9659258262890683122, 1.000000000000000000, 0.9659258262890683122, 1.000000000000000000, 0.9659258262890683122, 1.000000000000000000, 0.9659258262890683122, 1.000000000000000000, 0.9659258262890683122, 1.000000000000000000, 0.9659258262890683122, 1.000000000000000000, 0.9659258262890683122, 1.000000000000000000, 0.9659258262890683122, 1.000000000000000000, 0.9659258262890683122, 1.000000000000000000, 0.9659258262890683122, 1.000000000000000000, 0.9659258262890683122, 1.000000000000000000, 0.9659258262890683122, 1.000000000000000000, 0.9659258262890683122, 1.000000000000000000, 0.9659258262890683122, 1.000000000000000000, 0.9659258262890683122, 1.000000000000000000, 0.9659258262890683122, 1.000000000000000000, 0.9659258262890683122, 1.000000000000000000, 0.9659258262890683122, 1.000000000000000000, 0.9659258262890683122, 1.000000000000000000, 0.9659258262890683122, 1.000000000000000000, 0.9659258262890683122, 1.000000000000000000, 0.9659258262890683122, 1.000000000000000000, 0.9659258262890683122, 1.000000000000000000, 0.9659258262890683122, 1.000000000000000000, 0.9659258262890683122, 1.000000000000000000, 0.9659258262890683122, 1.000000000000000000, 0.9659258262890683122, 1.000000000000000000, 0.9659258262890683122, 1.000000000000000000, 0.9659258262890683122, 1.000000000000000000, 0.9659258262890683122, 1.000000000000000000, 0.9659258262890683122, 1.000000000000000000, 0.9659258262890683122, 1.000000000000000000, 0.9659258262890683122, 1.000000000000000000, 0.9659258262890683122, 1.000000000000000000, 0.9659258262890683122, 1.000000000000000000, 0.9659258262890683122, 1.000000000000000000, 0.9659258262890683122, 1.000000000000000000, 0.9659258262890683122, 1.000000000000000000, 0.9659258262890683122, 1.000000000000000000, 0.9659258262890683122, 1.000000000000000000, 0.9659258262890683122, 1.000000000000000000, 0.9659258262890683122, 1.000000000000000000, 0.9659258262890683122, 1.000000000000000000, 0.9659258262890683122, 1.000000000000000000, 0.9659258262890683122, 1.000000000000000000, 0.9659258262890683122, 1.000000000000000000, 0.9659258262890683122, 1.000000000000000000, 0.9659258262890683122, 1.000000000000000000, 0.9659258262890683122, 1.000000000000000000, 0.9659258262890683122, 1.000000000000000000, 0.9659258262890683122, 1.000000000000000000, 0.9659258262890683122, 1.000000000000000000, 0.9659258262890683122, 1.000000000000000000, 0.9659258262890683122, 1.000000000000000000, 0.9659258262890683122, 1.000000000000000000, 0.9659258262890683122, 1.000000000000000000, 0.9659258262890683122, 1.000000000000000000, 0.9659258262890683122, 1.000000000000000000, 0.9659258262890683122, 1.000000000000000000, 0.9659258262890683122, 1.000000000000000000, 0.9659258262890683122, 1.000000000000000000, 0.9659258262890683122, 1.000000000000000000, 0.9659258262890683122, 1.000000000000000000, 0.9659258262890683122, 1.000000000000000000, 0.9659258262890683122, 1.000000000000000000, 0.9659258262890683122, 1.000000000000000000, 0.9659258262890683122, 1.000000000000000000, 0.9659258262890683122, 1.000000000000000000, 0.9659258262890683122, 1.000000000000000000, 0.9659258262890683122, 1.000000000000000000, 0.9659258262890683122, 1.000000000000000000, 0.9659258262890683122, 1.000000000000000000, 0.9659258262890683122, 1.000000000000000000, 0.9659258262890683122, 1.000000000000000000, 0.9659258262890683122, 1.000000000000000000, 0.9659258262890683122, 1.000000000000000000, 0.9659258262890683122, 1.000000000000000000, 0.9659258262890683122, 1.000000000000000000, 0.9659258262890683122, 1.000000000000000000, 0.9659258262890683122, 1.000000000000000000, 0.9659258262890683122, 1.000000000000000000, 0.9659258262890683122, 1.000000000000000000, 0.9659258262890683122, 1.000000000000000000, 0.9659258262890683122, 1.000000000000000000, 0.9659258262890683122, 1.000000000000000000, 0.9659258262890683122, 1.000000000000000000, 0.9659258262890683122, 1.000000000000000000, 0.9659258262890683122, 1.000000000000000000, 0.9659258262890683122, 1.000000000000000000, 0.9659258262890683122, 1.000000000000000000, 0.9659258262890683122, 1.000000000000000000, 0.9659258262890683122, 1.000000000000000000, 0.9659258262890683122, 1.000000000000000000, 0.9659258262890683122, 1.000000000000000000, 0.9659258262890683122, 1.000000000000000000, 0.9659258262890683122, 1.000000000000000000, 0.9659258262890683122, 1.000000000000000000, 0.9659258262890683122, 1.000000000000000000, 0.9659258262890683122, 1.000000000000000000, 0.9659258262890683122, 1.000000000000000000, 0.9659258262890683122, 1.000000000000000000, 0.9659258262890683122, 1.000000000000000000, 0.9659258262890683122, 1.000000000000000000, 0.9659258262890683122, 1.000000000000000000, 0.9659258262890683122, 1.000000000000000000, 0.9659258262890683122, 1.000000000000000000, 0.9659258262890683122, 1.000000000000000000, 0.9659258262890683122, 1.000000000000000000, 0.9659258262890683122, 1.000000000000000000),
 ( 1.000000000000000000, 0.9659258262890683122, 1.000000000000000000, 0.9659258262890683122, 1.000000000000000000, 0.9659258262890683122, 1.000000000000000000, 0.9659258262890683122, 1.000000000000000000, 0.9659258262890683122, 1.000000000000000000, 0.9659258262890683122, 1.000000000000000000, 0.9659258262890683122, 1.000000000000000000, 0.9659258262890683122, 1.000000000000000000, 0.9659258262890683122, 1.000000000000000000, 0.9659258262890683122, 1.000000000000000000, 0.9659258262890683122, 1.000000000000000000, 0.9659258262890683122, 1.000000000000000000, 0.9659258262890683122, 1.000000000000000000, 0.9659258262890683122, 1.000000000000000000, 0.9659258262890683122, 1.000000000000000000, 0.9659258262890683122, 1.000000000000000000, 0.9659258262890683122, 1.000000000000000000, 0.9659258262890683122, 1.000000000000000000, 0.9659258262890683122, 1.000000000000000000, 0.9659258262890683122, 1.000000000000000000, 0.9659258262890683122, 1.000000000000000000, 0.9659258262890683122, 1.000000000000000000, 0.9659258262890683122, 1.000000000000000000, 0.9659258262890683122, 1.000000000000000000, 0.9659258262890683122, 1.000000000000000000, 0.9659258262890683122, 1.000000000000000000, 0.9659258262890683122, 1.000000000000000000, 0.9659258262890683122, 1.000000000000000000, 0.9659258262890683122, 1.000000000000000000, 0.9659258262890683122, 1.000000000000000000, 0.9659258262890683122, 1.000000000000000000, 0.9659258262890683122, 1.000000000000000000, 0.9659258262890683122, 1.000000000000000000, 0.9659258262890683122, 1.000000000000000000, 0.9659258262890683122, 1.000000000000000000, 0.9659258262890683122, 1.000000000000000000, 0.9659258262890683122, 1.000000000000000000, 0.9659258262890683122, 1.000000000000000000, 0.9659258262890683122, 1.000000000000000000, 0.9659258262890683122, 1.000000000000000000, 0.9659258262890683122, 1.000000000000000000, 0.9659258262890683122, 1.000000000000000000, 0.9659258262890683122, 1.000000000000000000, 0.9659258262890683122, 1.000000000000000000, 0.9659258262890683122, 1.000000000000000000, 0.9659258262890683122, 1.000000000000000000, 0.9659258262890683122, 1.000000000000000000, 0.9659258262890683122, 1.000000000000000000, 0.9659258262890683122, 1.000000000000000000, 0.9659258262890683122, 1.000000000000000000, 0.9659258262890683122, 1.000000000000000000, 0.9659258262890683122, 1.000000000000000000, 0.9659258262890683122, 1.000000000000000000, 0.9659258262890683122, 1.000000000000000000, 0.9659258262890683122, 1.000000000000000000, 0.9659258262890683122, 1.000000000000000000, 0.9659258262890683122, 1.000000000000000000, 0.9659258262890683122, 1.000000000000000000, 0.9659258262890683122, 1.000000000000000000, 0.9659258262890683122, 1.000000000000000000, 0.9659258262890683122, 1.000000000000000000, 0.9659258262890683122, 1.000000000000000000, 0.9659258262890683122, 1.000000000000000000, 0.9659258262890683122, 1.000000000000000000, 0.9659258262890683122, 1.000000000000000000, 0.9659258262890683122, 1.000000000000000000, 0.9659258262890683122, 1.000000000000000000, 0.9659258262890683122, 1.000000000000000000, 0.9659258262890683122, 1.000000000000000000, 0.9659258262890683122, 1.000000000000000000, 0.9659258262890683122, 1.000000000000000000, 0.9659258262890683122, 1.000000000000000000, 0.9659258262890683122, 1.000000000000000000, 0.9659258262890683122, 1.000000000000000000, 0.9659258262890683122, 1.000000000000000000, 0.9659258262890683122, 1.000000000000000000, 0.9659258262890683122, 1.000000000000000000, 0.9659258262890683122, 1.000000000000000000, 0.9659258262890683122, 1.000000000000000000, 0.9659258262890683122, 1.000000000000000000, 0.9659258262890683122, 1.000000000000000000, 0.9659258262890683122, 1.000000000000000000, 0.9659258262890683122, 1.000000000000000000, 0.9659258262890683122, 1.000000000000000000, 0.9659258262890683122, 1.000000000000000000, 0.9659258262890683122, 1.000000000000000000, 0.9659258262890683122, 1.000000000000000000, 0.9659258262890683122, 1.000000000000000000, 0.9659258262890683122, 1.000000000000000000, 0.9659258262890683122, 1.000000000000000000, 0.9659258262890683122, 1.000000000000000000, 0.9659258262890683122, 1.000000000000000000, 0.9659258262890683122, 1.000000000000000000, 0.9659258262890683122, 1.000000000000000000, 0.9659258262890683122, 1.000000000000000000, 0.9659258262890683122, 1.000000000000000000, 0.9659258262890683122, 1.000000000000000000, 0.9659258262890683122, 1.000000000000000000, 0.9659258262890683122, 1.000000000000000000, 0.9659258262890683122, 1.000000000000000000, 0.9659258262890683122, 1.000000000000000000, 0.9659258262890683122, 1.000000000000000000, 0.9659258262890683122, 1.000000000000000000, 0.9659258262890683122, 1.000000000000000000, 0.9659258262890683122, 1.000000000000000000, 0.9659258262890683122, 1.000000000000000000, 0.9659258262890683122, 1.000000000000000000, 0.9659258262890683122, 1.000000000000000000, 0.9659258262890683122, 1.000000000000000000, 0.9659258262890683122, 1.000000000000000000, 0.9659258262890683122, 1.000000000000000000, 0.9659258262890683122, 1.000000000000000000, 0.9659258262890683122, 1.000000000000000000, 0.9659258262890683122, 1.000000000000000000, 0.9659258262890683122, 1.000000000000000000, 0.9659258262890683122, 1.000000000000000000, 0.9659258262890683122, 1.000000000000000000, 0.9659258262890683122, 1.000000000000000000, 0.9659258262890683122, 1.000000000000000000, 0.9659258262890683122, 1.000000000000000000, 0.9659258262890683122, 1.000000000000000000, 0.9659258262890683122, 1.000000000000000000, 0.9659258262890683122, 1.000000000000000000, 0.9659258262890683122, 1.000000000000000000, 0.9659258262890683122, 1.000000000000000000, 0.9659258262890683122, 1.000000000000000000, 0.9659258262890683122, 1.000000000000000000, 0.9659258262890683122, 1.000000000000000000, 0.9659258262890683122, 1.000000000000000000, 0.9659258262890683122, 1.000000000000000000, 0.9659258262890683122, 1.000000000000000000, 0.9659258262890683122, 1.000000000000000000, 0.9659258262890683122, 1.000000000000000000, 0.9659258262890683122, 1.000000000000000000, 0.9659258262890683122, 1.000000000000000000, 0.9659258262890683122, 1.000000000000000000, 0.9659258262890683122, 1.000000000000000000, 0.9659258262890683122, 1.000000000000000000, 0.9659258262890683122, 1.000000000000000000, 0.9659258262890683122, 1.000000000000000000, 0.9659258262890683122, 1.000000000000000000, 0.9659258262890683122, 1.000000000000000000, 0.9659258262890683122, 1.000000000000000000, 0.9659258262890683122, 1.000000000000000000, 0.9659258262890683122, 1.000000000000000000, 0.9659258262890683122, 1.000000000000000000, 0.9659258262890683122, 1.000000000000000000, 0.9659258262890683122, 1.000000000000000000, 0.9659258262890683122, 1.000000000000000000, 0.9659258262890683122, 1.000000000000000000, 0.9659258262890683122, 1.000000000000000000, 0.9659258262890683122, 1.000000000000000000, 0.9659258262890683122, 1.000000000000000000, 0.9659258262890683122, 1.000000000000000000, 0.9659258262890683122, 1.000000000000000000, 0.9659258262890683122, 1.000000000000000000, 0.9659258262890683122, 1.000000000000000000, 0.9659258262890683122, 1.000000000000000000, 0.9659258262890683122, 1.000000000000000000, 0.9659258262890683122, 1.000000000000000000, 0.9659258262890683122, 1.000000000000000000, 0.9659258262890683122, 1.000000000000000000) ) ) 
 REPRESENTATION_ITEM ( '' )  SURFACE ( )  );
#75262=CARTESIAN_POINT ( 'NONE',  ( 19.84674366389459621, 48.50893115100078745, 7.409399052514197653E-17 ) ) ;
#75264=CARTESIAN_POINT ( 'NONE',  ( 15.44008868035555793, 36.39701867748816966, -9.422509992056140149 ) ) ;
#75265=UNCERTAINTY_MEASURE_WITH_UNIT (LENGTH_MEASURE( 1.000000000000000082E-05 ), #40154, 'distance_accuracy_value', 'NONE');
#75266=TOROIDAL_SURFACE ( 'NONE', #24176, 1.000000000000000000, 0.5000000000000000000 ) ;
#75268=CARTESIAN_POINT ( 'NONE',  ( 6.565887622018943937, 65.16530133659709634, 12.81628187352647430 ) ) ;
#75270=CARTESIAN_POINT ( 'NONE',  ( 17.20831665107776587, 4.133931151000785675, -7.208316651077762316 ) ) ;
#75271=CARTESIAN_POINT ( 'NONE',  ( 13.43411237798105340, 40.58196800326375353, 12.81628187352647963 ) ) ;
#75272=CARTESIAN_POINT ( 'NONE',  ( -4.164238869374099927, 67.01208216824728936, 3.795296366450308767 ) ) ;
#75273=CARTESIAN_POINT ( 'NONE',  ( 12.63842701281683034, 37.46726448433411605, 9.846743663894596210 ) ) ;
#75274=CARTESIAN_POINT ( 'NONE',  ( -35.44000000000001194, 93.50000000000000000, -10.09898361729590199 ) ) ;
#75275=CARTESIAN_POINT ( 'NONE',  ( 22.26659068614894466, 33.88708216824730357, 7.082119434687054849 ) ) ;
#75276=CARTESIAN_POINT ( 'NONE',  ( 10.00000000000000000, 40.55374883491397497, -14.16423886937410082 ) ) ;
#75277=CARTESIAN_POINT ( 'NONE',  ( 19.84674366389459266, 53.30059781766744464, 2.638427012816836559 ) ) ;
#75280=CARTESIAN_POINT ( 'NONE',  ( 17.96484262340118221, 36.18868534415484106, -7.964842623401177768 ) ) ;
#75281=CARTESIAN_POINT ( 'NONE',  ( -0.8801773607110991993, 67.85535201082151957, -2.915334737309923874 ) ) ;
#75283=CARTESIAN_POINT ( 'NONE',  ( -1.099225684535947600, 64.54030133659709634, 6.408140936763237150 ) ) ;
#75285=VERTEX_POINT ( 'NONE', #39569 ) ;
#75286=CARTESIAN_POINT ( 'NONE',  ( 1.472469842513823179, 0.5922644843341181575, -4.923371831947296329 ) ) ;
#75287=VERTEX_POINT ( 'NONE', #45575 ) ;
#75288=CARTESIAN_POINT ( 'NONE',  ( -4.164238869374099039, 11.80374883491396965, 8.674139862899312516E-16 ) ) ;
#75289=CARTESIAN_POINT ( 'NONE',  ( 7.361572987183170547, 12.05059781766744997, 9.846743663894590881 ) ) ;
#75290=CARTESIAN_POINT ( 'NONE',  ( 10.00000000000000178, 34.31368534415484106, 10.88017736071110342 ) ) ;
#75293=CARTESIAN_POINT ( 'NONE',  ( -0.8801773607111008646, 23.27201867748817676, 2.915334737309923430 ) ) ;
#75295=CARTESIAN_POINT ( 'NONE',  ( 20.88017736071110875, 30.77201867748816966, -2.915334737309920765 ) ) ;
#75296=FILL_AREA_STYLE ('',( #68306 ) ) ;
#75299=CARTESIAN_POINT ( 'NONE',  ( 7.084665262690076126, 67.02201867748817676, -10.88017736071110164 ) ) ;
#75301=CARTESIAN_POINT ( 'NONE',  ( 0.5774900079438590739, 17.64701867748817321, -5.440088680355550821 ) ) ;
#75303=CARTESIAN_POINT ( 'NONE',  ( 17.20831665107776587, 4.133931151000785675, -7.208316651077762316 ) ) ;
#75304=CARTESIAN_POINT ( 'NONE',  ( 20.88017736071110164, 20.35535201082150891, 2.915334737309930979 ) ) ;
#75305=COLOUR_RGB ( '', 0.72549020, 0.75294118, 0.79215686) ;
#75308=CARTESIAN_POINT ( 'NONE',  ( 3.591859063236761518, 54.95696800326376064, 11.09922568453594849 ) ) ;
#75309=CARTESIAN_POINT ( 'NONE',  ( 19.42250999205614548, 45.98035201082150536, -5.440088680355545492 ) ) ;
#75310=CARTESIAN_POINT ( 'NONE',  ( -1.926860441876564023, 22.87045670184114599, 3.195792623639529761 ) ) ;
#75312=CARTESIAN_POINT ( 'NONE',  ( 22.81628187352648496, 61.83196800326376774, -3.434112377981050290 ) ) ;
#75313=CARTESIAN_POINT ( 'NONE',  ( 15.44008868035555793, 51.39701867748816966, -9.422509992056140149 ) ) ;
#75314=CARTESIAN_POINT ( 'NONE',  ( 22.81628187352647785, 6.623634669930420493, 6.195893100308588602E-16 ) ) ;
#75316=CARTESIAN_POINT ( 'NONE',  ( 14.92337183194729633, 12.67559781766745353, 8.527530157486181039 ) ) ;
#75317=DIRECTION ( 'NONE',  ( 0.000000000000000000, 0.000000000000000000, 1.000000000000000000 ) ) ;
#75318=CARTESIAN_POINT ( 'NONE',  ( 0.6178305044545838731, 4.748634669930420493, 9.382169495545420901 ) ) ;
#75320=CARTESIAN_POINT ( 'NONE',  ( 12.63842701281683034, 62.46726448433410894, 9.846743663894596210 ) ) ;
#75321=CARTESIAN_POINT ( 'NONE',  ( 7.084665262690076126, 42.02201867748816966, -10.88017736071110164 ) ) ;
#75322=CARTESIAN_POINT ( 'NONE',  ( 7.361572987183169658, 49.96726448433410894, -9.846743663894592657 ) ) ;
#75323=CYLINDRICAL_SURFACE ( 'NONE', #85475, 0.5000000000000004441 ) ;
#75324=CARTESIAN_POINT ( 'NONE',  ( 10.00000000000000178, 22.25893115100078745, 9.846743663894594434 ) ) ;
#75325=CARTESIAN_POINT ( 'NONE',  ( 2.791683348922237240, 10.38393115100078390, -7.208316651077763204 ) ) ;
#75326=CARTESIAN_POINT ( 'NONE',  ( -1.099225684535947600, -1.293031996736246469, -6.408140936763238038 ) ) ;
#75329=CARTESIAN_POINT ( 'NONE',  ( 10.00000000000000178, 4.313685344154837509, 10.88017736071110342 ) ) ;
#75330=CARTESIAN_POINT ( 'NONE',  ( 19.84674366389459621, 58.50893115100078745, 7.409399052514197653E-17 ) ) ;
#75332=CARTESIAN_POINT ( 'NONE',  ( -0.8801773607110991993, 2.855352010821504471, -2.915334737309923874 ) ) ;
#75333=CARTESIAN_POINT ( 'NONE',  ( 2.791683348922240793, 51.63393115100078745, 7.208316651077764092 ) ) ;
#75335=CARTESIAN_POINT ( 'NONE',  ( -0.8801773607111008646, 3.272018677488171434, 2.915334737309923430 ) ) ;
#75337=CARTESIAN_POINT ( 'NONE',  ( 15.44008868035555793, 21.39701867748817321, -9.422509992056140149 ) ) ;
#75338=CARTESIAN_POINT ( 'NONE',  ( 6.204703633549690345, 55.76208216824730357, -14.16423886937410259 ) ) ;
#75339=CARTESIAN_POINT ( 'NONE',  ( 20.36894250292379738, 64.92874883491397497, -10.36894250292379027 ) ) ;
#75341=CARTESIAN_POINT ( 'NONE',  ( 1.472469842513823179, 5.592264484334118713, -4.923371831947296329 ) ) ;
#75344=CARTESIAN_POINT ( 'NONE',  ( 14.92337183194729988, 19.34226448433411960, -8.527530157486177487 ) ) ;
#75345=CARTESIAN_POINT ( 'NONE',  ( -2.816281873526473856, 14.33196800326375531, 3.434112377981055619 ) ) ;
#75350=CARTESIAN_POINT ( 'NONE',  ( 19.84674366389459266, 63.30059781766745886, 2.638427012816836559 ) ) ;
#75351=CARTESIAN_POINT ( 'NONE',  ( 24.16423886937410614, 9.512082168247301794, -3.795296366450302550 ) ) ;
#75352=CARTESIAN_POINT ( 'NONE',  ( 17.20831665107776587, 29.13393115100078390, -7.208316651077762316 ) ) ;
#75354=VERTEX_POINT ( 'NONE', #26511 ) ;
#75355=CARTESIAN_POINT ( 'NONE',  ( -4.164238869374098151, 41.59541550158061796, -3.795296366450310543 ) ) ;
#75357=CARTESIAN_POINT ( 'NONE',  ( 19.84674366389459266, 13.30059781766745353, 2.638427012816836559 ) ) ;
#75360=CARTESIAN_POINT ( 'NONE',  ( 7.084665262690076126, 29.10535201082150181, 10.88017736071109987 ) ) ;
#75361=CARTESIAN_POINT ( 'NONE',  ( 22.81628187352648496, 56.83196800326374643, -3.434112377981050290 ) ) ;
#75362=CARTESIAN_POINT ( 'NONE',  ( 22.81628187352647785, 31.41530133659709279, 3.434112377981063169 ) ) ;
#75363=CARTESIAN_POINT ( 'NONE',  ( 10.00000000000000000, -0.2410688489992152128, -9.846743663894594434 ) ) ;
#75367=CARTESIAN_POINT ( 'NONE',  ( 10.00000000000000178, 38.05374883491396787, 14.16423886937410082 ) ) ;
#75368=CARTESIAN_POINT ( 'NONE',  ( 7.084665262690076126, 7.022018677488169658, -10.88017736071110164 ) ) ;
#75369=CARTESIAN_POINT ( 'NONE',  ( 0.5774900079438590739, 17.64701867748817321, -5.440088680355550821 ) ) ;
#75372=CARTESIAN_POINT ( 'NONE',  ( 15.44008868035555260, 54.73035201082150536, 9.422509992056143702 ) ) ;
#75373=CARTESIAN_POINT ( 'NONE',  ( 10.00000000000000000, 61.81368534415484106, -10.88017736071110342 ) ) ;
#75374=CARTESIAN_POINT ( 'NONE',  ( 10.00000000000000000, 27.87363466993042138, -12.81628187352647608 ) ) ;
#75375=CARTESIAN_POINT ( 'NONE',  ( 15.64039516285221154, 89.00000000000000000, 9.500000000000000000 ) ) ;
#75377=CARTESIAN_POINT ( 'NONE',  ( 2.791683348922237240, 20.38393115100078745, -7.208316651077763204 ) ) ;
#75378=CARTESIAN_POINT ( 'NONE',  ( -0.8801773607110991993, 57.85535201082149825, -2.915334737309923874 ) ) ;
#75379=CARTESIAN_POINT ( 'NONE',  ( -2.816281873526471635, 13.91530133659708746, -3.434112377981056508 ) ) ;
#75380=CARTESIAN_POINT ( 'NONE',  ( 7.361572987183170547, 2.050597817667451750, 9.846743663894590881 ) ) ;
#75381=CARTESIAN_POINT ( 'NONE',  ( 10.00000000000000178, 4.313685344154837509, 10.88017736071110342 ) ) ;
#75382=CARTESIAN_POINT ( 'NONE',  ( 5.076628168052704559, 40.17559781766745175, -8.527530157486179263 ) ) ;
#75383=CARTESIAN_POINT ( 'NONE',  ( 0.6178305044545838731, 59.74863466993041783, 9.382169495545420901 ) ) ;
#75384=CARTESIAN_POINT ( 'NONE',  ( 1.472469842513823179, 15.59226448433411960, -4.923371831947296329 ) ) ;
#75385=CARTESIAN_POINT ( 'NONE',  ( -2.266590686148945544, 1.387082168247301128, -7.082119434687050408 ) ) ;
#75387=CARTESIAN_POINT ( 'NONE',  ( 19.42250999205614193, 30.14701867748817321, 5.440088680355555262 ) ) ;
#75388=CARTESIAN_POINT ( 'NONE',  ( 0.5774900079438607392, 3.480352010821504027, 5.440088680355550821 ) ) ;
#75389=CARTESIAN_POINT ( 'NONE',  ( 17.08211943468705130, 28.47041550158063572, 12.26659068614894998 ) ) ;
#75390=CARTESIAN_POINT ( 'NONE',  ( 10.00000000000000178, 47.25893115100078745, 9.846743663894594434 ) ) ;
#75391=CARTESIAN_POINT ( 'NONE',  ( 2.035157376598824452, 33.68868534415484106, 7.964842623401179544 ) ) ;
#75392=CARTESIAN_POINT ( 'NONE',  ( 7.084665262690076126, 12.02201867748817321, -10.88017736071110164 ) ) ;
#75394=CARTESIAN_POINT ( 'NONE',  ( 15.44008868035555793, 21.39701867748817321, -9.422509992056140149 ) ) ;
#75395=CARTESIAN_POINT ( 'NONE',  ( 16.40814093676323893, 40.79030133659708923, 11.09922568453595026 ) ) ;
#75397=CARTESIAN_POINT ( 'NONE',  ( 4.559911319644449179, 48.89701867748817676, 9.422509992056141925 ) ) ;
#75399=CARTESIAN_POINT ( 'NONE',  ( -0.8801773607111008646, 38.27201867748816255, 2.915334737309923430 ) ) ;
#75401=EDGE_LOOP ( 'NONE', ( #67646, #52454, #82222, #4597, #39163, #11115 ) ) ;
#75402=CARTESIAN_POINT ( 'NONE',  ( 7.361572987183170547, 57.05059781766744464, 9.846743663894590881 ) ) ;
#75403=CARTESIAN_POINT ( 'NONE',  ( 2.035157376598822676, 42.43868534415483396, -7.964842623401177768 ) ) ;
#75406=CARTESIAN_POINT ( 'NONE',  ( 20.03932841506543383, 30.62161441960502373, -6.397827110478934820 ) ) ;
#75407=CARTESIAN_POINT ( 'NONE',  ( -0.3689425029237881626, 47.42874883491396787, 10.36894250292379027 ) ) ;
#75408=CARTESIAN_POINT ( 'NONE',  ( 19.42250999205614548, 55.98035201082150536, -5.440088680355545492 ) ) ;
#75409=EDGE_CURVE ( 'NONE', #67057, #83368, #71048, .T. ) ;
#75410=CARTESIAN_POINT ( 'NONE',  ( 13.99999999999999822, 60.50000000000000711, -6.000000000000000000 ) ) ;
#75413=CARTESIAN_POINT ( 'NONE',  ( 19.84674366389459266, 58.71726448433411605, -2.638427012816827677 ) ) ;
#75414=VECTOR ( 'NONE', #64120, 1000.000000000000000 ) ;
#75415=( NAMED_UNIT ( * ) PLANE_ANGLE_UNIT ( ) SI_UNIT ( $, .RADIAN. ) );
#75416=CARTESIAN_POINT ( 'NONE',  ( 0.1532563361054100626, 35.80059781766745175, -2.638427012816831230 ) ) ;
#75419=CARTESIAN_POINT ( 'NONE',  ( 18.52753015748618282, 38.92559781766745175, -4.923371831947291888 ) ) ;
#75421=CARTESIAN_POINT ( 'NONE',  ( 2.035157376598822676, 22.43868534415483396, -7.964842623401177768 ) ) ;
#75422=CARTESIAN_POINT ( 'NONE',  ( 18.52753015748617571, 23.09226448433411960, 4.923371831947298993 ) ) ;
#75423=ADVANCED_FACE ( 'NONE', ( #78538 ), #10529, .T. ) ;
#75424=CARTESIAN_POINT ( 'NONE',  ( -1.099225684535947600, 24.54030133659708923, 6.408140936763237150 ) ) ;
#75425=CARTESIAN_POINT ( 'NONE',  ( 4.559911319644449179, 68.89701867748817676, 9.422509992056141925 ) ) ;
#75426=CARTESIAN_POINT ( 'NONE',  ( 20.88017736071110164, 60.35535201082151957, 2.915334737309930979 ) ) ;
#75427=CARTESIAN_POINT ( 'NONE',  ( 20.88017736071110519, 30.56368534415484106, 2.639326808657452039E-16 ) ) ;
#75428=CARTESIAN_POINT ( 'NONE',  ( 4.559911319644449179, 2.230352010821504471, -9.422509992056141925 ) ) ;
#75429=CARTESIAN_POINT ( 'NONE',  ( -2.266590686148945544, 42.22041550158063217, 7.082119434687048631 ) ) ;
#75431=EDGE_CURVE ( 'NONE', #80833, #14724, #84996, .T. ) ;
#75432=CARTESIAN_POINT ( 'NONE',  ( -42.16485527613927076, 107.5383484153110061, 5.000000000000000000 ) ) ;
#75434=CARTESIAN_POINT ( 'NONE',  ( -2.816281873526473856, 19.12363466993042138, 9.499525473075851096E-16 ) ) ;
#75435=CARTESIAN_POINT ( 'NONE',  ( 2.035157376598822676, 2.438685344154837953, -7.964842623401177768 ) ) ;
#75436=CARTESIAN_POINT ( 'NONE',  ( 4.559911319644449179, 42.23035201082151247, -9.422509992056141925 ) ) ;
#75437=DIRECTION ( 'NONE',  ( 0.000000000000000000, -1.000000000000000000, 0.000000000000000000 ) ) ;
#75441=CARTESIAN_POINT ( 'NONE',  ( 4.559911319644449179, 52.23035201082151247, -9.422509992056141925 ) ) ;
#75442=CARTESIAN_POINT ( 'NONE',  ( 2.791683348922240793, 36.63393115100078035, 7.208316651077764092 ) ) ;
#75443=CARTESIAN_POINT ( 'NONE',  ( 18.52753015748618282, 23.92559781766745530, -4.923371831947291888 ) ) ;
#75444=CARTESIAN_POINT ( 'NONE',  ( 2.791683348922237240, 15.38393115100078212, -7.208316651077763204 ) ) ;
#75446=CARTESIAN_POINT ( 'NONE',  ( 10.00000000000000000, 9.758931151000785675, -9.846743663894594434 ) ) ;
#75449=CARTESIAN_POINT ( 'NONE',  ( 1.472469842513823179, 36.42559781766745175, 4.923371831947296329 ) ) ;
#75451=CARTESIAN_POINT ( 'NONE',  ( 3.591859063236761518, 54.95696800326376064, 11.09922568453594849 ) ) ;
#75453=CARTESIAN_POINT ( 'NONE',  ( 13.43411237798106583, 12.66530133659708746, -12.81628187352647252 ) ) ;
#75454=CARTESIAN_POINT ( 'NONE',  ( 0.5774900079438607392, 58.48035201082151247, 5.440088680355550821 ) ) ;
#75455=CARTESIAN_POINT ( 'NONE',  ( 10.00000000000000000, 35.55374883491396787, -14.16423886937410082 ) ) ;
#75458=CARTESIAN_POINT ( 'NONE',  ( -0.3689425029237881626, 32.42874883491395366, 10.36894250292379027 ) ) ;
#75459=CARTESIAN_POINT ( 'NONE',  ( -4.164238869374099927, 47.01208216824729647, 3.795296366450308767 ) ) ;
#75460=CARTESIAN_POINT ( 'NONE',  ( 6.204703633549690345, 7.845415501580634832, 14.16423886937410082 ) ) ;
#75461=CARTESIAN_POINT ( 'NONE',  ( -0.3689425029237898834, 11.17874883491396787, -10.36894250292378850 ) ) ;
#75462=CARTESIAN_POINT ( 'NONE',  ( -1.926860441876563801, 37.66212336850780673, 1.004413902775740978E-15 ) ) ;
#75463=CARTESIAN_POINT ( 'NONE',  ( 19.42250999205614193, 50.14701867748817676, 5.440088680355555262 ) ) ;
#75464=CARTESIAN_POINT ( 'NONE',  ( 0.2751277870542967463, 0.000000000000000000, 6.500000000000000888 ) ) ;
#75465=CARTESIAN_POINT ( 'NONE',  ( 10.00000000000000000, 29.75893115100078745, -9.846743663894594434 ) ) ;
#75466=B_SPLINE_CURVE_WITH_KNOTS ( 'NONE', 3,
 ( #91356, #15385, #52863, #97401, #44376, #21893, #59373, #75866, #60856, #6374 ),
 .UNSPECIFIED., .F., .F.,
 ( 4, 3, 3, 4 ),
 ( 1.011508913927958987E-17, 0.0006253016069560887779, 0.001250604074564930397, 0.002501455912506543935 ),
 .UNSPECIFIED. ) ;
#75467=CARTESIAN_POINT ( 'NONE',  ( 0.5774900079438590739, 67.64701867748817676, -5.440088680355550821 ) ) ;
#75468=CARTESIAN_POINT ( 'NONE',  ( 0.1532563361054083140, 41.00893115100078745, 1.131784320476157264E-15 ) ) ;
#75469=CARTESIAN_POINT ( 'NONE',  ( -0.8801773607111008646, 18.27201867748817321, 2.915334737309923430 ) ) ;
#75470=CARTESIAN_POINT ( 'NONE',  ( 22.81628187352648496, 61.83196800326376774, -3.434112377981050290 ) ) ;
#75472=PLANE ( 'NONE',  #18689 ) ;
#75474=CARTESIAN_POINT ( 'NONE',  ( 19.84674366389459266, 28.71726448433411960, -2.638427012816827677 ) ) ;
#75475=CARTESIAN_POINT ( 'NONE',  ( 13.43411237798106583, 47.66530133659709634, -12.81628187352647252 ) ) ;
#75477=VECTOR ( 'NONE', #58390, 1000.000000000000000 ) ;
#75478=CARTESIAN_POINT ( 'NONE',  ( 0.5774900079438590739, 42.64701867748816966, -5.440088680355550821 ) ) ;
#75479=CARTESIAN_POINT ( 'NONE',  ( 14.92337183194729633, 57.67559781766745886, 8.527530157486181039 ) ) ;
#75480=CARTESIAN_POINT ( 'NONE',  ( -0.3689425029237898834, 26.17874883491396432, -10.36894250292378850 ) ) ;
#75484=CARTESIAN_POINT ( 'NONE',  ( 12.91533473730993009, 66.60535201082150536, -10.88017736071109987 ) ) ;
#75485=CARTESIAN_POINT ( 'NONE',  ( 22.26659068614895176, 64.72041550158064638, -7.082119434687042414 ) ) ;
#75487=CARTESIAN_POINT ( 'NONE',  ( 17.20831665107776587, 64.13393115100079456, -7.208316651077762316 ) ) ;
#75489=CARTESIAN_POINT ( 'NONE',  ( 12.91533473730993009, 51.60535201082149825, -10.88017736071109987 ) ) ;
#75490=CARTESIAN_POINT ( 'NONE',  ( 19.72487221294570858, 70.00000000000000000, 6.000000000000000000 ) ) ;
#75491=CARTESIAN_POINT ( 'NONE',  ( 20.36894250292379382, 43.67874883491397497, 10.36894250292379205 ) ) ;
#75493=CARTESIAN_POINT ( 'NONE',  ( 2.035157376598824452, 8.688685344154839285, 7.964842623401179544 ) ) ;
#75494=CARTESIAN_POINT ( 'NONE',  ( 2.035157376598822676, 22.43868534415483396, -7.964842623401177768 ) ) ;
#75496=CARTESIAN_POINT ( 'NONE',  ( 19.84674366389459266, 53.30059781766744464, 2.638427012816836559 ) ) ;
#75497=CARTESIAN_POINT ( 'NONE',  ( -2.816281873526473856, 54.12363466993041783, 9.499525473075851096E-16 ) ) ;
#75500=CARTESIAN_POINT ( 'NONE',  ( 20.88017736071110519, 15.56368534415483751, 2.639326808657452039E-16 ) ) ;
#75501=CARTESIAN_POINT ( 'NONE',  ( 6.565887622018943937, 13.08196800326374998, -12.81628187352647608 ) ) ;
#75503=CARTESIAN_POINT ( 'NONE',  ( 17.20831665107776587, 49.13393115100078745, -7.208316651077762316 ) ) ;
#75504=CARTESIAN_POINT ( 'NONE',  ( 4.559911319644449179, 38.89701867748817676, 9.422509992056141925 ) ) ;
#75505=CARTESIAN_POINT ( 'NONE',  ( 10.00000000000000178, 15.37363466993042138, 12.81628187352647608 ) ) ;
#75506=CARTESIAN_POINT ( 'NONE',  ( 17.96484262340118221, 46.18868534415484106, -7.964842623401177768 ) ) ;
#75509=CARTESIAN_POINT ( 'NONE',  ( 16.40814093676324603, 47.45696800326375353, -11.09922568453594671 ) ) ;
#75511=CARTESIAN_POINT ( 'NONE',  ( 1.383448333479226466, 17.37718327197429247, -6.499999999999972466 ) ) ;
#75512=CARTESIAN_POINT ( 'NONE',  ( 2.035157376598824452, 53.68868534415484817, 7.964842623401179544 ) ) ;
#75513=CARTESIAN_POINT ( 'NONE',  ( 3.591859063236761518, 39.95696800326375353, 11.09922568453594849 ) ) ;
#75514=CARTESIAN_POINT ( 'NONE',  ( -4.164238869374098151, 6.595415501580634832, -3.795296366450310543 ) ) ;
#75515=CARTESIAN_POINT ( 'NONE',  ( 20.88017736071110519, 40.56368534415484106, 2.639326808657452039E-16 ) ) ;
#75517=CARTESIAN_POINT ( 'NONE',  ( 19.84674366389459266, 23.30059781766745530, 2.638427012816836559 ) ) ;
#75518=CARTESIAN_POINT ( 'NONE',  ( 7.361572987183169658, -0.03273551566588185635, -9.846743663894592657 ) ) ;
#75519=CARTESIAN_POINT ( 'NONE',  ( 20.36894250292379738, 44.92874883491396787, -10.36894250292379027 ) ) ;
#75526=ORIENTED_EDGE ( 'NONE', *, *, #64113, .F. ) ;
#75528=CARTESIAN_POINT ( 'NONE',  ( 10.00000000000000000, 55.55374883491396787, -14.16423886937410082 ) ) ;
#75529=CARTESIAN_POINT ( 'NONE',  ( 24.16423886937410614, 59.30374883491397497, 8.672049930838204340E-16 ) ) ;
#75530=CARTESIAN_POINT ( 'NONE',  ( 18.52753015748618282, 23.92559781766745530, -4.923371831947291888 ) ) ;
#75531=CARTESIAN_POINT ( 'NONE',  ( 19.38216949554541202, 35.99863466993041072, 9.382169495545424454 ) ) ;
#75533=CARTESIAN_POINT ( 'NONE',  ( 6.204703633549690345, 10.76208216824729824, -14.16423886937410259 ) ) ;
#75534=CARTESIAN_POINT ( 'NONE',  ( 12.91533473730993009, 16.60535201082150891, -10.88017736071109987 ) ) ;
#75535=CARTESIAN_POINT ( 'NONE',  ( 6.204703633549690345, 55.76208216824730357, -14.16423886937410259 ) ) ;
#75538=CARTESIAN_POINT ( 'NONE',  ( 0.1532563361054083140, 46.00893115100079456, 1.131784320476157264E-15 ) ) ;
#75539=CARTESIAN_POINT ( 'NONE',  ( 0.2751277870542978565, 12.28217586085238011, -6.500000000000002665 ) ) ;
#75540=CARTESIAN_POINT ( 'NONE',  ( 17.20831665107776587, 29.13393115100078390, -7.208316651077762316 ) ) ;
#75543=ORIENTED_EDGE ( 'NONE', *, *, #24173, .T. ) ;
#75545=SURFACE_SIDE_STYLE ('',( #45036 ) ) ;
#75547=CARTESIAN_POINT ( 'NONE',  ( 10.00000000000000178, 52.25893115100078745, 9.846743663894594434 ) ) ;
#75548=CARTESIAN_POINT ( 'NONE',  ( -2.266590686148945544, 21.38708216824730357, -7.082119434687050408 ) ) ;
#75549=CARTESIAN_POINT ( 'NONE',  ( 12.91533473730993009, 26.60535201082150536, -10.88017736071109987 ) ) ;
#75550=CARTESIAN_POINT ( 'NONE',  ( 7.084665262690076126, 44.10535201082151247, 10.88017736071109987 ) ) ;
#75551=CARTESIAN_POINT ( 'NONE',  ( 18.52753015748617571, 63.09226448433412315, 4.923371831947298993 ) ) ;
#75552=CARTESIAN_POINT ( 'NONE',  ( 16.40814093676323893, 35.79030133659708923, 11.09922568453595026 ) ) ;
#75553=CARTESIAN_POINT ( 'NONE',  ( -4.164238869374099039, 1.803748834913967647, 8.674139862899312516E-16 ) ) ;
#75554=CARTESIAN_POINT ( 'NONE',  ( 0.5774900079438607392, 68.48035201082150536, 5.440088680355550821 ) ) ;
#75557=CARTESIAN_POINT ( 'NONE',  ( 21.09922568453595559, 37.04030133659708923, -6.408140936763230044 ) ) ;
#75559=CARTESIAN_POINT ( 'NONE',  ( 2.791683348922237240, 40.38393115100078035, -7.208316651077763204 ) ) ;
#75560=CARTESIAN_POINT ( 'NONE',  ( 0.5774900079438590739, 12.64701867748817321, -5.440088680355550821 ) ) ;
#75563=CARTESIAN_POINT ( 'NONE',  ( -0.8801773607111009756, 13.06368534415483929, 1.068504757029289695E-15 ) ) ;
#75565=CARTESIAN_POINT ( 'NONE',  ( -0.8801773607111009756, 63.06368534415484106, 1.068504757029289695E-15 ) ) ;
#75566=CARTESIAN_POINT ( 'NONE',  ( 10.00000000000000178, 54.31368534415484106, 10.88017736071110342 ) ) ;
#75567=CARTESIAN_POINT ( 'NONE',  ( 4.559911319644449179, 67.23035201082150536, -9.422509992056141925 ) ) ;
#75568=SURFACE_STYLE_FILL_AREA ( #6574 ) ;
#75569=CARTESIAN_POINT ( 'NONE',  ( 0.5774900079438607392, 48.48035201082150536, 5.440088680355550821 ) ) ;
#75574=CARTESIAN_POINT ( 'NONE',  ( 10.00000000000000178, 47.25893115100078745, 9.846743663894594434 ) ) ;
#75578=CARTESIAN_POINT ( 'NONE',  ( -4.164238869374099039, 6.803748834913967869, 8.674139862899312516E-16 ) ) ;
#75581=CARTESIAN_POINT ( 'NONE',  ( 0.1532563361054100626, 35.80059781766745175, -2.638427012816831230 ) ) ;
#75582=CARTESIAN_POINT ( 'NONE',  ( 20.88017736071110875, 5.772018677488170546, -2.915334737309920765 ) ) ;
#75584=CARTESIAN_POINT ( 'NONE',  ( 10.00000000000000178, 45.37363466993041783, 12.81628187352647608 ) ) ;
#75585=EDGE_LOOP ( 'NONE', ( #42201, #89081, #62354, #23274, #66257 ) ) ;
#75587=CARTESIAN_POINT ( 'NONE',  ( 12.63842701281683922, 39.55059781766744464, -9.846743663894590881 ) ) ;
#75589=CARTESIAN_POINT ( 'NONE',  ( 6.565887622018943937, 20.16530133659708213, 12.81628187352647430 ) ) ;
#75590=CARTESIAN_POINT ( 'NONE',  ( 19.84674366389459266, 18.30059781766745175, 2.638427012816836559 ) ) ;
#75591=CARTESIAN_POINT ( 'NONE',  ( 0.3881751172101555181, 0.3700748648336783519, 6.487123156197995399 ) ) ;
#75592=CARTESIAN_POINT ( 'NONE',  ( 10.00000000000000178, 0.3736346699304200492, 12.81628187352647608 ) ) ;
#75593=CARTESIAN_POINT ( 'NONE',  ( 1.959929470562276732, 25.51528370094808551, -5.767676674365845635 ) ) ;
#75597=CARTESIAN_POINT ( 'NONE',  ( 7.084665262690076126, 24.10535201082150181, 10.88017736071109987 ) ) ;
#75598=CARTESIAN_POINT ( 'NONE',  ( 20.36894250292379382, 13.67874883491396965, 10.36894250292379205 ) ) ;
#75599=CARTESIAN_POINT ( 'NONE',  ( 10.00000000000000000, 29.75893115100078745, -9.846743663894594434 ) ) ;
#75600=CARTESIAN_POINT ( 'NONE',  ( 0.1532563361054083140, 1.008931151000784787, 1.131784320476157264E-15 ) ) ;
#75601=CARTESIAN_POINT ( 'NONE',  ( 0.6178305044545818747, 38.49863466993042493, -9.382169495545419124 ) ) ;
#75603=CARTESIAN_POINT ( 'NONE',  ( 20.88017736071110164, 15.35535201082150358, 2.915334737309930979 ) ) ;
#75605=CARTESIAN_POINT ( 'NONE',  ( -2.816281873526473856, 9.331968003263753531, 3.434112377981055619 ) ) ;
#75606=CARTESIAN_POINT ( 'NONE',  ( 10.00000000000000000, 2.873634669930420049, -12.81628187352647608 ) ) ;
#75607=CARTESIAN_POINT ( 'NONE',  ( 18.52753015748618282, 23.92559781766745530, -4.923371831947291888 ) ) ;
#75609=CARTESIAN_POINT ( 'NONE',  ( 10.00000000000000178, 30.37363466993042138, 12.81628187352647608 ) ) ;
#75611=CARTESIAN_POINT ( 'NONE',  ( 12.91533473730992121, 39.52201867748817676, 10.88017736071110164 ) ) ;
#75612=FACE_OUTER_BOUND ( 'NONE', #28319, .T. ) ;
#75614=CARTESIAN_POINT ( 'NONE',  ( 17.62281668512002852, 28.28593319516823001, 6.499999999999993783 ) ) ;
#75615=CARTESIAN_POINT ( 'NONE',  ( 2.035157376598824452, 38.68868534415483396, 7.964842623401179544 ) ) ;
#75616=CARTESIAN_POINT ( 'NONE',  ( 2.035157376598822676, 47.43868534415484817, -7.964842623401177768 ) ) ;
#75617=CARTESIAN_POINT ( 'NONE',  ( 20.15039907845753220, 60.60158574516643881, -6.262539305110077947 ) ) ;
#75618=CARTESIAN_POINT ( 'NONE',  ( 10.00000000000000000, 61.81368534415484106, -10.88017736071110342 ) ) ;
#75621=CARTESIAN_POINT ( 'NONE',  ( 7.361572987183170547, 52.05059781766745175, 9.846743663894590881 ) ) ;
#75622=CARTESIAN_POINT ( 'NONE',  ( 10.00000000000000000, 6.813685344154838397, -10.88017736071110342 ) ) ;
#75624=CARTESIAN_POINT ( 'NONE',  ( -2.816281873526473856, 9.123634669930421381, 9.499525473075851096E-16 ) ) ;
#75625=ORIENTED_EDGE ( 'NONE', *, *, #56361, .F. ) ;
#75626=CARTESIAN_POINT ( 'NONE',  ( 17.96484262340118221, 29.93868534415484106, 7.964842623401181321 ) ) ;
#75628=CARTESIAN_POINT ( 'NONE',  ( 10.00000000000000178, 34.31368534415484106, 10.88017736071110342 ) ) ;
#75629=CARTESIAN_POINT ( 'NONE',  ( 7.361572987183170547, 2.050597817667451750, 9.846743663894590881 ) ) ;
#75630=CARTESIAN_POINT ( 'NONE',  ( -4.164238869374099927, 42.01208216824728936, 3.795296366450308767 ) ) ;
#75631=CARTESIAN_POINT ( 'NONE',  ( 10.00000000000000000, 29.75893115100078745, -9.846743663894594434 ) ) ;
#75632=CARTESIAN_POINT ( 'NONE',  ( 20.88017736071110519, 45.56368534415484106, 2.639326808657452039E-16 ) ) ;
#75633=CARTESIAN_POINT ( 'NONE',  ( 0.2751277870542911952, 19.36607318730131055, -6.499999999999992006 ) ) ;
#75634=FILL_AREA_STYLE ('',( #52146 ) ) ;
#75635=EDGE_CURVE ( 'NONE', #13640, #89305, #29553, .T. ) ;
#75638=CARTESIAN_POINT ( 'NONE',  ( 18.52753015748617571, 53.09226448433412315, 4.923371831947298993 ) ) ;
#75641=ORIENTED_EDGE ( 'NONE', *, *, #30643, .T. ) ;
#75642=CARTESIAN_POINT ( 'NONE',  ( 6.204703633549690345, 25.76208216824730712, -14.16423886937410259 ) ) ;
#75643=CARTESIAN_POINT ( 'NONE',  ( 24.16423886937410614, 24.30374883491396787, 8.672049930838204340E-16 ) ) ;
#75644=CARTESIAN_POINT ( 'NONE',  ( 0.5774900079438607392, 58.48035201082151247, 5.440088680355550821 ) ) ;
#75645=CARTESIAN_POINT ( 'NONE',  ( 20.36894250292379738, 64.92874883491397497, -10.36894250292379027 ) ) ;
#75646=CARTESIAN_POINT ( 'NONE',  ( 10.00000000000000178, 52.25893115100078745, 9.846743663894594434 ) ) ;
#75648=CARTESIAN_POINT ( 'NONE',  ( 15.44008868035555793, 41.39701867748817676, -9.422509992056140149 ) ) ;
#75649=CARTESIAN_POINT ( 'NONE',  ( 19.38216949554541202, 25.99863466993042138, 9.382169495545424454 ) ) ;
#75650=CARTESIAN_POINT ( 'NONE',  ( 24.16423886937410614, 14.51208216824730179, -3.795296366450302550 ) ) ;
#75651=CARTESIAN_POINT ( 'NONE',  ( 12.91533473730993009, 11.60535201082150714, -10.88017736071109987 ) ) ;
#75653=CARTESIAN_POINT ( 'NONE',  ( 2.035157376598824452, 23.68868534415484461, 7.964842623401179544 ) ) ;
#75654=( BOUNDED_CURVE ( )  B_SPLINE_CURVE ( 2, ( #30922, #68455, #98977, #91438, #7953, #69429, #60932, #53934, #52452 ),
 .UNSPECIFIED., .F., .F. ) 
 B_SPLINE_CURVE_WITH_KNOTS ( ( 3, 2, 2, 2, 3 ),
 ( 0.3329980797973742246, 0.3333333333333333703, 0.3392857142857143016, 0.3452380952380952328, 0.3455733487740543786 ),
 .UNSPECIFIED. ) 
 CURVE ( )  GEOMETRIC_REPRESENTATION_ITEM ( )  RATIONAL_B_SPLINE_CURVE ( ( 0.9963778908391760503, 0.9980808541467920403, 1.000000000000000000, 0.9659258262890682012, 1.000000000000000000, 0.9659258262890682012, 1.000000000000000000, 0.9980808541467920403, 0.9963778908391759392 ) ) 
 REPRESENTATION_ITEM ( '' )  );
#75655=CARTESIAN_POINT ( 'NONE',  ( 19.84674366389459621, 53.50893115100078745, 7.409399052514197653E-17 ) ) ;
#75656=CARTESIAN_POINT ( 'NONE',  ( 19.42250999205614548, 55.98035201082150536, -5.440088680355545492 ) ) ;
#75659=DIRECTION ( 'NONE',  ( -0.000000000000000000, -0.000000000000000000, 1.000000000000000000 ) ) ;
#75662=FACE_OUTER_BOUND ( 'NONE', #24499, .T. ) ;
#75664=DIRECTION ( 'NONE',  ( -0.000000000000000000, -0.000000000000000000, 1.000000000000000000 ) ) ;
#75665=CARTESIAN_POINT ( 'NONE',  ( 13.79529636645031943, 65.34541550158063217, -14.16423886937409904 ) ) ;
#75666=CARTESIAN_POINT ( 'NONE',  ( 24.16423886937410614, 64.30374883491396076, 8.672049930838204340E-16 ) ) ;
#75667=CARTESIAN_POINT ( 'NONE',  ( 5.076628168052703671, 26.84226448433411960, 8.527530157486179263 ) ) ;
#75668=CARTESIAN_POINT ( 'NONE',  ( 19.84674366389459266, 63.30059781766745886, 2.638427012816836559 ) ) ;
#75669=CARTESIAN_POINT ( 'NONE',  ( 21.92686044187656691, 49.95379003517448524, 3.195792623639537755 ) ) ;
#75670=CARTESIAN_POINT ( 'NONE',  ( -0.8801773607111009756, 63.06368534415484106, 1.068504757029289695E-15 ) ) ;
#75673=CARTESIAN_POINT ( 'NONE',  ( 22.26659068614895176, 29.72041550158063572, -7.082119434687042414 ) ) ;
#75675=CARTESIAN_POINT ( 'NONE',  ( 6.204703633549690345, 40.76208216824731778, -14.16423886937410259 ) ) ;
#75677=CARTESIAN_POINT ( 'NONE',  ( 22.81628187352648496, 56.83196800326374643, -3.434112377981050290 ) ) ;
#75678=CARTESIAN_POINT ( 'NONE',  ( 12.63842701281683922, 49.55059781766744464, -9.846743663894590881 ) ) ;
#75679=CARTESIAN_POINT ( 'NONE',  ( 15.44008868035555260, 24.73035201082150891, 9.422509992056143702 ) ) ;
#75682=CARTESIAN_POINT ( 'NONE',  ( 17.20831665107776587, 57.88393115100078745, 7.208316651077764980 ) ) ;
#75683=CARTESIAN_POINT ( 'NONE',  ( 1.472469842513823179, 45.59226448433412315, -4.923371831947296329 ) ) ;
#75684=EDGE_CURVE ( 'NONE', #97143, #58843, #78438, .T. ) ;
#75687=CARTESIAN_POINT ( 'NONE',  ( 17.39651004071842522, 19.08210964143329491, -6.499999999999992895 ) ) ;
#75692=CARTESIAN_POINT ( 'NONE',  ( 0.6076426042653185755, 7.375764716086007589, -6.500000000000003553 ) ) ;
#75693=CARTESIAN_POINT ( 'NONE',  ( 1.472469842513823179, 31.42559781766745530, 4.923371831947296329 ) ) ;
#75694=CARTESIAN_POINT ( 'NONE',  ( 0.2751277870542906956, 37.28217586085238366, -6.499999999999992006 ) ) ;
#75695=CARTESIAN_POINT ( 'NONE',  ( -2.816281873526471635, 33.91530133659708213, -3.434112377981056508 ) ) ;
#75696=AXIS2_PLACEMENT_3D ( 'NONE', #49881, #94894, #41435 ) ;
#75700=CARTESIAN_POINT ( 'NONE',  ( 5.076628168052704559, 55.17559781766745175, -8.527530157486179263 ) ) ;
#75701=CARTESIAN_POINT ( 'NONE',  ( 0.1957200283969084964, 65.25733960839544068, 6.499999999999983125 ) ) ;
#75702=CARTESIAN_POINT ( 'NONE',  ( 2.791683348922240793, 46.63393115100077324, 7.208316651077764092 ) ) ;
#75703=CARTESIAN_POINT ( 'NONE',  ( -2.266590686148945544, 31.38708216824730002, -7.082119434687050408 ) ) ;
#75704=CARTESIAN_POINT ( 'NONE',  ( 17.20831665107776587, 49.13393115100078745, -7.208316651077762316 ) ) ;
#75705=CARTESIAN_POINT ( 'NONE',  ( 19.38216949554541202, 60.99863466993042493, 9.382169495545424454 ) ) ;
#75706=CARTESIAN_POINT ( 'NONE',  ( 20.32896413005680003, 36.77164270246084499, 5.963430220938287007 ) ) ;
#75707=CARTESIAN_POINT ( 'NONE',  ( 10.00000000000000178, 7.258931151000785675, 9.846743663894594434 ) ) ;
#75708=CARTESIAN_POINT ( 'NONE',  ( 1.472469842513823179, 46.42559781766745175, 4.923371831947296329 ) ) ;
#75709=CARTESIAN_POINT ( 'NONE',  ( 4.559911319644449179, 48.89701867748817676, 9.422509992056141925 ) ) ;
#75710=CARTESIAN_POINT ( 'NONE',  ( 7.361572987183169658, 44.96726448433412315, -9.846743663894592657 ) ) ;
#75712=VERTEX_POINT ( 'NONE', #65384 ) ;
#75713=CARTESIAN_POINT ( 'NONE',  ( 4.559911319644449179, 52.23035201082151247, -9.422509992056141925 ) ) ;
#75714=ORIENTED_EDGE ( 'NONE', *, *, #28284, .F. ) ;
#75715=CARTESIAN_POINT ( 'NONE',  ( -0.8801773607111009756, 18.06368534415484106, 1.068504757029289695E-15 ) ) ;
#75716=CARTESIAN_POINT ( 'NONE',  ( 21.09922568453594849, 1.206968003263753531, 6.408140936763242479 ) ) ;
#75717=CARTESIAN_POINT ( 'NONE',  ( 20.88017736071110519, 45.56368534415484106, 2.639326808657452039E-16 ) ) ;
#75720=CARTESIAN_POINT ( 'NONE',  ( 20.88017736071110164, 45.35535201082149115, 2.915334737309930979 ) ) ;
#75721=DIRECTION ( 'NONE',  ( -0.07626964003977962370, 0.9970872288863209532, 0.000000000000000000 ) ) ;
#75722=CARTESIAN_POINT ( 'NONE',  ( 7.361572987183169658, 9.967264484334119601, -9.846743663894592657 ) ) ;
#75724=CARTESIAN_POINT ( 'NONE',  ( 2.791683348922240793, 36.63393115100078035, 7.208316651077764092 ) ) ;
#75725=CARTESIAN_POINT ( 'NONE',  ( 6.000000000000000000, 11.00000000000000000, 6.000000000000000000 ) ) ;
#75727=CARTESIAN_POINT ( 'NONE',  ( 18.52753015748617571, 63.09226448433412315, 4.923371831947298993 ) ) ;
#75728=CARTESIAN_POINT ( 'NONE',  ( 10.00000000000000000, 6.813685344154838397, -10.88017736071110342 ) ) ;
#75730=EDGE_CURVE ( 'NONE', #72124, #54543, #88192, .T. ) ;
#75731=CARTESIAN_POINT ( 'NONE',  ( 17.08211943468705840, 20.13708216824730357, -12.26659068614894466 ) ) ;
#75732=CARTESIAN_POINT ( 'NONE',  ( 6.204703633549690345, 52.84541550158062506, 14.16423886937410082 ) ) ;
#75733=CARTESIAN_POINT ( 'NONE',  ( 4.559911319644449179, 7.230352010821504471, -9.422509992056141925 ) ) ;
#75734=CARTESIAN_POINT ( 'NONE',  ( 14.92337183194729988, 29.34226448433411960, -8.527530157486177487 ) ) ;
#75735=CARTESIAN_POINT ( 'NONE',  ( 2.035157376598822676, 27.43868534415483396, -7.964842623401177768 ) ) ;
#75736=CARTESIAN_POINT ( 'NONE',  ( 14.92337183194729988, 49.34226448433411605, -8.527530157486177487 ) ) ;
#75737=CARTESIAN_POINT ( 'NONE',  ( -4.164238869374099039, 1.803748834913967647, 8.674139862899312516E-16 ) ) ;
#75740=CARTESIAN_POINT ( 'NONE',  ( -2.816281873526473856, 34.33196800326376064, 3.434112377981055619 ) ) ;
#75741=CARTESIAN_POINT ( 'NONE',  ( 12.63842701281683034, 37.46726448433411605, 9.846743663894596210 ) ) ;
#75743=CARTESIAN_POINT ( 'NONE',  ( 17.20831665107776587, 14.13393115100078568, -7.208316651077762316 ) ) ;
#75745=CARTESIAN_POINT ( 'NONE',  ( 19.72487221294570858, 16.86607318730074567, 6.500000000000000888 ) ) ;
#75746=CARTESIAN_POINT ( 'NONE',  ( 2.035157376598824452, 3.688685344154837953, 7.964842623401179544 ) ) ;
#75747=CARTESIAN_POINT ( 'NONE',  ( -4.164238869374098151, 51.59541550158063217, -3.795296366450310543 ) ) ;
#75748=CARTESIAN_POINT ( 'NONE',  ( 4.559911319644449179, 42.23035201082151247, -9.422509992056141925 ) ) ;
#75749=FILL_AREA_STYLE ('',( #68753 ) ) ;
#75750=CARTESIAN_POINT ( 'NONE',  ( 1.274849032793998305, 2.555090184799397424, -6.499999999999581668 ) ) ;
#75751=CARTESIAN_POINT ( 'NONE',  ( 5.076628168052703671, 21.84226448433411960, 8.527530157486179263 ) ) ;
#75752=CARTESIAN_POINT ( 'NONE',  ( 2.035157376598824452, 3.688685344154837953, 7.964842623401179544 ) ) ;
#75753=CARTESIAN_POINT ( 'NONE',  ( 7.361572987183169658, 44.96726448433412315, -9.846743663894592657 ) ) ;
#75755=CARTESIAN_POINT ( 'NONE',  ( 0.1532563361054082862, 56.21726448433411605, 2.638427012816831674 ) ) ;
#75756=CARTESIAN_POINT ( 'NONE',  ( 4.559911319644449179, 37.23035201082150536, -9.422509992056141925 ) ) ;
#75759=CARTESIAN_POINT ( 'NONE',  ( 21.09922568453594849, 56.20696800326375353, 6.408140936763242479 ) ) ;
#75762=CARTESIAN_POINT ( 'NONE',  ( 18.52753015748618282, 8.925597817667451750, -4.923371831947291888 ) ) ;
#75763=CARTESIAN_POINT ( 'NONE',  ( 21.09922568453594849, 51.20696800326375353, 6.408140936763242479 ) ) ;
#75764=CARTESIAN_POINT ( 'NONE',  ( 4.559911319644449179, 7.230352010821505360, -9.422509992056141925 ) ) ;
#75765=CARTESIAN_POINT ( 'NONE',  ( 2.791683348922237240, 45.38393115100079456, -7.208316651077763204 ) ) ;
#75767=AXIS2_PLACEMENT_3D ( 'NONE', #25457, #55940, #86439 ) ;
#75769=CARTESIAN_POINT ( 'NONE',  ( 24.16423886937410614, 49.51208216824730357, -3.795296366450302550 ) ) ;
#75770=CARTESIAN_POINT ( 'NONE',  ( 10.00000000000000000, 59.75893115100078745, -9.846743663894594434 ) ) ;
#75772=CARTESIAN_POINT ( 'NONE',  ( 20.88017736071110164, 55.35535201082149825, 2.915334737309930979 ) ) ;
#75774=CARTESIAN_POINT ( 'NONE',  ( 0.1532563361054082862, 1.217264484334117824, 2.638427012816831674 ) ) ;
#75777=CARTESIAN_POINT ( 'NONE',  ( 13.43411237798105340, 55.58196800326374643, 12.81628187352647963 ) ) ;
#75778=CARTESIAN_POINT ( 'NONE',  ( 1.472469842513823179, 16.42559781766745175, 4.923371831947296329 ) ) ;
#75780=CARTESIAN_POINT ( 'NONE',  ( -0.3689425029237881626, 2.428748834913967869, 10.36894250292379027 ) ) ;
#75781=CARTESIAN_POINT ( 'NONE',  ( 1.472469842513823179, 0.5922644843341181575, -4.923371831947296329 ) ) ;
#75782=CARTESIAN_POINT ( 'NONE',  ( 17.96484262340118221, 26.18868534415483396, -7.964842623401177768 ) ) ;
#75785=CARTESIAN_POINT ( 'NONE',  ( 15.44008868035555260, 29.73035201082150891, 9.422509992056143702 ) ) ;
#75786=AXIS2_PLACEMENT_3D ( 'NONE', #31328, #37384, #69345 ) ;
#75789=CARTESIAN_POINT ( 'NONE',  ( 12.91533473730993009, 36.60535201082151247, -10.88017736071109987 ) ) ;
#75793=VERTEX_POINT ( 'NONE', #6366 ) ;
#75794=CARTESIAN_POINT ( 'NONE',  ( 0.6178305044545818747, 13.49863466993041783, -9.382169495545419124 ) ) ;
#75796=CARTESIAN_POINT ( 'NONE',  ( -0.8801773607111008646, 63.27201867748817676, 2.915334737309923430 ) ) ;
#75799=CARTESIAN_POINT ( 'NONE',  ( 0.1532563361054082862, 11.21726448433411605, 2.638427012816831674 ) ) ;
#75800=CARTESIAN_POINT ( 'NONE',  ( -0.8801773607111009756, 38.06368534415484106, 1.068504757029289695E-15 ) ) ;
#75801=STYLED_ITEM ( 'NONE', ( #80189 ), #52070 ) ;
#75804=CARTESIAN_POINT ( 'NONE',  ( 3.591859063236761518, 64.95696800326376774, 11.09922568453594849 ) ) ;
#75805=CARTESIAN_POINT ( 'NONE',  ( -0.8801773607110991993, 47.85535201082150536, -2.915334737309923874 ) ) ;
#75806=CARTESIAN_POINT ( 'NONE',  ( 2.148416515056634335, 7.237265733804436607, 6.499999999999997335 ) ) ;
#75807=CARTESIAN_POINT ( 'NONE',  ( -2.816281873526473856, 59.12363466993042493, 9.499525473075851096E-16 ) ) ;
#75808=CARTESIAN_POINT ( 'NONE',  ( -0.8801773607111008646, 63.27201867748817676, 2.915334737309923430 ) ) ;
#75809=CARTESIAN_POINT ( 'NONE',  ( -1.099225684535947600, -0.4596986634029132657, 6.408140936763237150 ) ) ;
#75811=CARTESIAN_POINT ( 'NONE',  ( 2.791683348922240793, 21.63393115100078745, 7.208316651077764092 ) ) ;
#75812=CARTESIAN_POINT ( 'NONE',  ( 0.6178305044545838731, 54.74863466993042493, 9.382169495545420901 ) ) ;
#75814=CARTESIAN_POINT ( 'NONE',  ( 14.92337183194729988, 9.342264484334119601, -8.527530157486177487 ) ) ;
#75815=CARTESIAN_POINT ( 'NONE',  ( 0.6178305044545818747, 3.498634669930420049, -9.382169495545419124 ) ) ;
#75816=AXIS2_PLACEMENT_3D ( 'NONE', #56441, #48922, #57410 ) ;
#75818=CARTESIAN_POINT ( 'NONE',  ( 0.1532563361054082862, 61.21726448433412315, 2.638427012816831674 ) ) ;
#75819=CARTESIAN_POINT ( 'NONE',  ( 4.559911319644449179, 38.89701867748817676, 9.422509992056141925 ) ) ;
#75820=CARTESIAN_POINT ( 'NONE',  ( 1.472469842513823179, 46.42559781766745175, 4.923371831947296329 ) ) ;
#75822=CARTESIAN_POINT ( 'NONE',  ( 7.361572987183170547, 22.05059781766745530, 9.846743663894590881 ) ) ;
#75823=CARTESIAN_POINT ( 'NONE',  ( 17.20831665107776587, 2.883931151000785231, 7.208316651077764980 ) ) ;
#75824=CARTESIAN_POINT ( 'NONE',  ( 6.565887622018943937, -1.918031996736246692, -12.81628187352647608 ) ) ;
#75826=CARTESIAN_POINT ( 'NONE',  ( 7.084665262690076126, 2.022018677488170990, -10.88017736071110164 ) ) ;
#75827=( LENGTH_UNIT ( ) NAMED_UNIT ( * ) SI_UNIT ( .MILLI., .METRE. ) );
#75828=CARTESIAN_POINT ( 'NONE',  ( 17.20831665107776587, 57.88393115100078745, 7.208316651077764980 ) ) ;
#75831=CARTESIAN_POINT ( 'NONE',  ( 19.42250999205614193, 5.147018677488171434, 5.440088680355555262 ) ) ;
#75832=CARTESIAN_POINT ( 'NONE',  ( 18.52753015748618282, 43.92559781766745175, -4.923371831947291888 ) ) ;
#75834=ORIENTED_EDGE ( 'NONE', *, *, #61902, .F. ) ;
#75835=CARTESIAN_POINT ( 'NONE',  ( 17.96484262340118221, 6.188685344154837509, -7.964842623401177768 ) ) ;
#75837=CARTESIAN_POINT ( 'NONE',  ( 7.084665262690076126, 39.10535201082150536, 10.88017736071109987 ) ) ;
#75838=CARTESIAN_POINT ( 'NONE',  ( 17.08211943468705130, 43.47041550158063927, 12.26659068614894998 ) ) ;
#75839=CARTESIAN_POINT ( 'NONE',  ( 2.917880565312950480, 65.97041550158063217, -12.26659068614894821 ) ) ;
#75841=CARTESIAN_POINT ( 'NONE',  ( 19.10478245763048832, 6.025762395770821733, -5.990408912944375608 ) ) ;
#75842=( BOUNDED_CURVE ( )  B_SPLINE_CURVE ( 2, ( #71375, #3356, #25865, #94837, #17387, #41379, #84887, #62362, #47367 ),
 .UNSPECIFIED., .F., .T. ) 
 B_SPLINE_CURVE_WITH_KNOTS ( ( 3, 2, 2, 2, 3 ),
 ( 0.5462860886497512558, 0.5476190476190476719, 0.5535714285714286031, 0.5595238095238095344, 0.5608567684931060615 ),
 .UNSPECIFIED. ) 
 CURVE ( )  GEOMETRIC_REPRESENTATION_ITEM ( )  RATIONAL_B_SPLINE_CURVE ( ( 0.9881565478350734510, 0.9923695281211492025, 1.000000000000000000, 0.9659258262890683122, 1.000000000000000000, 0.9659258262890683122, 1.000000000000000000, 0.9923695281211484254, 0.9881565478350726739 ) ) 
 REPRESENTATION_ITEM ( '' )  );
#75843=CARTESIAN_POINT ( 'NONE',  ( 0.1532563361054082862, 31.21726448433412315, 2.638427012816831674 ) ) ;
#75844=CARTESIAN_POINT ( 'NONE',  ( 22.81628187352647785, 16.62363466993042138, 6.195893100308588602E-16 ) ) ;
#75851=CARTESIAN_POINT ( 'NONE',  ( 20.36894250292379382, 8.678748834913967869, 10.36894250292379205 ) ) ;
#75852=CARTESIAN_POINT ( 'NONE',  ( 0.1532563361054100626, 20.80059781766744464, -2.638427012816831230 ) ) ;
#75855=VECTOR ( 'NONE', #63021, 1000.000000000000000 ) ;
#75856=CARTESIAN_POINT ( 'NONE',  ( -4.164238869374099039, 51.80374883491396787, 8.674139862899312516E-16 ) ) ;
#75857=CARTESIAN_POINT ( 'NONE',  ( 2.791683348922237240, 15.38393115100078212, -7.208316651077763204 ) ) ;
#75860=CARTESIAN_POINT ( 'NONE',  ( 7.084665262690076126, 37.02201867748817676, -10.88017736071110164 ) ) ;
#75861=CARTESIAN_POINT ( 'NONE',  ( 22.81628187352647785, 51.62363466993042493, 6.195893100308588602E-16 ) ) ;
#75862=CARTESIAN_POINT ( 'NONE',  ( 17.96484262340118221, 9.938685344154837509, 7.964842623401181321 ) ) ;
#75863=CARTESIAN_POINT ( 'NONE',  ( -2.816281873526473856, 29.33196800326376064, 3.434112377981055619 ) ) ;
#75864=CARTESIAN_POINT ( 'NONE',  ( 0.9413316022086137824, 53.45508385108959004, 6.499999999999978684 ) ) ;
#75865=VERTEX_POINT ( 'NONE', #59365 ) ;
#75866=CARTESIAN_POINT ( 'NONE',  ( 2.153642693323437385, 11.13791097397318275, -6.499999999999995559 ) ) ;
#75868=CARTESIAN_POINT ( 'NONE',  ( 24.16423886937410614, 39.51208216824731068, -3.795296366450302550 ) ) ;
#75869=CARTESIAN_POINT ( 'NONE',  ( 20.36894250292379738, 19.92874883491396787, -10.36894250292379027 ) ) ;
#75870=CARTESIAN_POINT ( 'NONE',  ( 7.084665262690076126, 2.022018677488170990, -10.88017736071110164 ) ) ;
#75871=CARTESIAN_POINT ( 'NONE',  ( 0.5774900079438590739, 32.64701867748816966, -5.440088680355550821 ) ) ;
#75874=CARTESIAN_POINT ( 'NONE',  ( 7.084665262690076126, 59.10535201082150536, 10.88017736071109987 ) ) ;
#75875=CARTESIAN_POINT ( 'NONE',  ( 10.00000000000000178, 64.31368534415483396, 10.88017736071110342 ) ) ;
#75876=CARTESIAN_POINT ( 'NONE',  ( 19.38216949554541557, 22.24863466993041428, -9.382169495545420901 ) ) ;
#75879=CARTESIAN_POINT ( 'NONE',  ( 5.076628168052703671, 36.84226448433412315, 8.527530157486179263 ) ) ;
#75880=CIRCLE ( 'NONE', #74285, 1.000000000000000888 ) ;
#75883=CARTESIAN_POINT ( 'NONE',  ( 21.09922568453595559, 22.04030133659708923, -6.408140936763230044 ) ) ;
#75885=CARTESIAN_POINT ( 'NONE',  ( -0.8801773607111009756, 13.06368534415483929, 1.068504757029289695E-15 ) ) ;
#75886=CARTESIAN_POINT ( 'NONE',  ( 0.1532563361054082862, 41.21726448433411605, 2.638427012816831674 ) ) ;
#75887=CARTESIAN_POINT ( 'NONE',  ( -1.099225684535947600, 59.54030133659708923, 6.408140936763237150 ) ) ;
#75888=CARTESIAN_POINT ( 'NONE',  ( 0.1532563361054082862, 16.21726448433411960, 2.638427012816831674 ) ) ;
#75891=CARTESIAN_POINT ( 'NONE',  ( 0.5774900079438590739, 37.64701867748817676, -5.440088680355550821 ) ) ;
#75892=CARTESIAN_POINT ( 'NONE',  ( 15.44008868035555260, 4.730352010821504471, 9.422509992056143702 ) ) ;
#75893=CARTESIAN_POINT ( 'NONE',  ( 12.91533473730992121, 29.52201867748817321, 10.88017736071110164 ) ) ;
#75894=CARTESIAN_POINT ( 'NONE',  ( 0.5774900079438607392, 13.48035201082150358, 5.440088680355550821 ) ) ;
#75896=CARTESIAN_POINT ( 'NONE',  ( 4.559911319644449179, 32.23035201082150536, -9.422509992056141925 ) ) ;
#75897=CARTESIAN_POINT ( 'NONE',  ( 22.81628187352648496, 41.83196800326375353, -3.434112377981050290 ) ) ;
#75898=CARTESIAN_POINT ( 'NONE',  ( 12.91533473730992121, 44.52201867748816966, 10.88017736071110164 ) ) ;
#75899=CARTESIAN_POINT ( 'NONE',  ( 2.603489959281613420, 45.43575266056827644, -6.500000000000031086 ) ) ;
#75900=CARTESIAN_POINT ( 'NONE',  ( 2.035157376598822676, 57.43868534415484106, -7.964842623401177768 ) ) ;
#75901=ORIENTED_EDGE ( 'NONE', *, *, #85467, .T. ) ;
#75902=CARTESIAN_POINT ( 'NONE',  ( 7.084665262690076126, 37.02201867748817676, -10.88017736071110164 ) ) ;
#75906=CARTESIAN_POINT ( 'NONE',  ( 24.16423886937409904, 49.09541550158063217, 3.795296366450317205 ) ) ;
#75907=CARTESIAN_POINT ( 'NONE',  ( 19.42250999205614193, 65.14701867748817676, 5.440088680355555262 ) ) ;
#75910=CARTESIAN_POINT ( 'NONE',  ( 18.52753015748617571, 58.09226448433411605, 4.923371831947298993 ) ) ;
#75912=CARTESIAN_POINT ( 'NONE',  ( 17.20831665107776587, 39.13393115100079456, -7.208316651077762316 ) ) ;
#75913=ORIENTED_EDGE ( 'NONE', *, *, #98121, .F. ) ;
#75914=CARTESIAN_POINT ( 'NONE',  ( 19.84674366389459266, 38.30059781766745175, 2.638427012816836559 ) ) ;
#75916=CARTESIAN_POINT ( 'NONE',  ( 10.00000000000000178, 29.31368534415483751, 10.88017736071110342 ) ) ;
#75917=CARTESIAN_POINT ( 'NONE',  ( 7.361572987183170547, 42.05059781766745886, 9.846743663894590881 ) ) ;
#75918=CARTESIAN_POINT ( 'NONE',  ( 6.565887622018943937, 25.16530133659708213, 12.81628187352647430 ) ) ;
#75919=CARTESIAN_POINT ( 'NONE',  ( 0.5774900079438607392, 58.48035201082151247, 5.440088680355550821 ) ) ;
#75920=CARTESIAN_POINT ( 'NONE',  ( 12.91533473730992121, 39.52201867748817676, 10.88017736071110164 ) ) ;
#75921=CARTESIAN_POINT ( 'NONE',  ( -2.816281873526473856, 64.33196800326376774, 3.434112377981055619 ) ) ;
#75922=CARTESIAN_POINT ( 'NONE',  ( 24.16423886937410614, 64.51208216824728936, -3.795296366450302550 ) ) ;
#75923=EDGE_CURVE ( 'NONE', #61157, #58317, #72403, .T. ) ;
#75927=CARTESIAN_POINT ( 'NONE',  ( 16.40814093676323893, 15.79030133659708746, 11.09922568453595026 ) ) ;
#75928=CARTESIAN_POINT ( 'NONE',  ( 17.96484262340118221, 9.938685344154837509, 7.964842623401181321 ) ) ;
#75929=CARTESIAN_POINT ( 'NONE',  ( 19.42250999205614193, 45.14701867748817676, 5.440088680355555262 ) ) ;
#75933=CARTESIAN_POINT ( 'NONE',  ( 7.084665262690076126, 62.02201867748816966, -10.88017736071110164 ) ) ;
#75934=CARTESIAN_POINT ( 'NONE',  ( 7.361572987183170547, 37.05059781766744464, 9.846743663894590881 ) ) ;
#75935=CARTESIAN_POINT ( 'NONE',  ( 14.92337183194729633, 22.67559781766745175, 8.527530157486181039 ) ) ;
#75936=CARTESIAN_POINT ( 'NONE',  ( 18.52753015748617571, 18.09226448433411960, 4.923371831947298993 ) ) ;
#75938=STYLED_ITEM ( 'NONE', ( #42641 ), #54290 ) ;
#75940=CARTESIAN_POINT ( 'NONE',  ( 18.52753015748618282, 13.92559781766745175, -4.923371831947291888 ) ) ;
#75943=CARTESIAN_POINT ( 'NONE',  ( 1.472469842513823179, 26.42559781766745175, 4.923371831947296329 ) ) ;
#75945=CARTESIAN_POINT ( 'NONE',  ( 22.81628187352647785, 61.62363466993041783, 6.195893100308588602E-16 ) ) ;
#75947=CARTESIAN_POINT ( 'NONE',  ( 22.81628187352647785, 6.623634669930420493, 6.195893100308588602E-16 ) ) ;
#75949=CARTESIAN_POINT ( 'NONE',  ( -0.8801773607110991993, 57.85535201082149825, -2.915334737309923874 ) ) ;
#75950=CARTESIAN_POINT ( 'NONE',  ( 10.00000000000000000, 30.55374883491397142, -14.16423886937410082 ) ) ;
#75952=CARTESIAN_POINT ( 'NONE',  ( -4.164238869374098151, 26.59541550158063217, -3.795296366450310543 ) ) ;
#75953=CARTESIAN_POINT ( 'NONE',  ( 22.26659068614894466, 53.88708216824731068, 7.082119434687054849 ) ) ;
#75954=CARTESIAN_POINT ( 'NONE',  ( -4.164238869374098151, 6.595415501580634832, -3.795296366450310543 ) ) ;
#75955=CARTESIAN_POINT ( 'NONE',  ( 6.204703633549690345, 32.84541550158063927, 14.16423886937410082 ) ) ;
#75956=CARTESIAN_POINT ( 'NONE',  ( 7.084665262690076126, 42.02201867748816966, -10.88017736071110164 ) ) ;
#75958=DIRECTION ( 'NONE',  ( -0.000000000000000000, -0.000000000000000000, -1.000000000000000000 ) ) ;
#75959=CARTESIAN_POINT ( 'NONE',  ( 17.20831665107776587, 44.13393115100078745, -7.208316651077762316 ) ) ;
#75960=CARTESIAN_POINT ( 'NONE',  ( -0.8801773607111009756, 18.06368534415484106, 1.068504757029289695E-15 ) ) ;
#75961=CARTESIAN_POINT ( 'NONE',  ( 0.6178305044545818747, 63.49863466993043204, -9.382169495545419124 ) ) ;
#75962=CARTESIAN_POINT ( 'NONE',  ( 0.1532563361054083140, 66.00893115100079456, 1.131784320476157264E-15 ) ) ;
#75965=CARTESIAN_POINT ( 'NONE',  ( 0.1532563361054082862, 31.21726448433412315, 2.638427012816831674 ) ) ;
#75966=CARTESIAN_POINT ( 'NONE',  ( 3.591859063236763294, 58.29030133659708923, -11.09922568453595026 ) ) ;
#75968=( GEOMETRIC_REPRESENTATION_CONTEXT ( 3 ) GLOBAL_UNCERTAINTY_ASSIGNED_CONTEXT ( ( #11434 ) ) GLOBAL_UNIT_ASSIGNED_CONTEXT ( ( #57163, #80164, #20654 ) ) REPRESENTATION_CONTEXT ( 'NONE', 'WORKASPACE' ) );
#75969=CARTESIAN_POINT ( 'NONE',  ( 12.91533473730993009, 46.60535201082150536, -10.88017736071109987 ) ) ;
#75970=CARTESIAN_POINT ( 'NONE',  ( 7.361572987183170547, 47.05059781766745175, 9.846743663894590881 ) ) ;
#75972=CARTESIAN_POINT ( 'NONE',  ( 17.08211943468705840, 35.13708216824730357, -12.26659068614894466 ) ) ;
#75973=ORIENTED_EDGE ( 'NONE', *, *, #25547, .F. ) ;
#75976=CARTESIAN_POINT ( 'NONE',  ( -0.8801773607111009756, 63.06368534415484106, 1.068504757029289695E-15 ) ) ;
#75977=CARTESIAN_POINT ( 'NONE',  ( 2.917880565312950480, 55.97041550158063217, -12.26659068614894821 ) ) ;
#75978=CARTESIAN_POINT ( 'NONE',  ( 3.591859063236761518, 14.95696800326375531, 11.09922568453594849 ) ) ;
#75980=CARTESIAN_POINT ( 'NONE',  ( 12.91533473730993009, 56.60535201082151247, -10.88017736071109987 ) ) ;
#75982=CARTESIAN_POINT ( 'NONE',  ( -46.67091953292581508, 101.1773697441846736, -8.660634561519810148 ) ) ;
#75983=CARTESIAN_POINT ( 'NONE',  ( 10.00000000000000178, 53.05374883491396787, 14.16423886937410082 ) ) ;
#75985=CARTESIAN_POINT ( 'NONE',  ( 20.88017736071110164, 15.35535201082150358, 2.915334737309930979 ) ) ;
#75986=CARTESIAN_POINT ( 'NONE',  ( 17.96484262340118221, 21.18868534415483396, -7.964842623401177768 ) ) ;
#75987=CARTESIAN_POINT ( 'NONE',  ( 7.361572987183170547, 62.05059781766745886, 9.846743663894590881 ) ) ;
#75988=CARTESIAN_POINT ( 'NONE',  ( 10.00000000000000000, 47.87363466993042493, -12.81628187352647608 ) ) ;
#75989=CARTESIAN_POINT ( 'NONE',  ( 0.2751277870542870319, 54.36607318730131055, -6.499999999999985789 ) ) ;
#75991=CARTESIAN_POINT ( 'NONE',  ( 19.42250999205614193, 20.14701867748817321, 5.440088680355555262 ) ) ;
#75992=CARTESIAN_POINT ( 'NONE',  ( 0.6178305044545818747, 18.49863466993041428, -9.382169495545419124 ) ) ;
#75995=EDGE_CURVE ( 'NONE', #39993, #24774, #46345, .T. ) ;
#75996=CARTESIAN_POINT ( 'NONE',  ( 19.84674366389459621, 43.50893115100078745, 7.409399052514197653E-17 ) ) ;
#75997=CARTESIAN_POINT ( 'NONE',  ( 17.96484262340118221, 39.93868534415484106, 7.964842623401181321 ) ) ;
#75998=CARTESIAN_POINT ( 'NONE',  ( 3.591859063236763294, 28.29030133659708568, -11.09922568453595026 ) ) ;
#75999=CARTESIAN_POINT ( 'NONE',  ( 0.5774900079438607392, 43.48035201082151247, 5.440088680355550821 ) ) ;
#76002=CARTESIAN_POINT ( 'NONE',  ( -1.099225684535947600, 49.54030133659708923, 6.408140936763237150 ) ) ;
#76005=CARTESIAN_POINT ( 'NONE',  ( 20.88017736071110164, 55.35535201082149825, 2.915334737309930979 ) ) ;
#76006=CARTESIAN_POINT ( 'NONE',  ( -2.816281873526473856, 34.33196800326376064, 3.434112377981055619 ) ) ;
#76007=CARTESIAN_POINT ( 'NONE',  ( -0.3689425029237881626, 7.428748834913967869, 10.36894250292379027 ) ) ;
#76008=CARTESIAN_POINT ( 'NONE',  ( 7.084665262690076126, 54.10535201082151247, 10.88017736071109987 ) ) ;
#76009=CARTESIAN_POINT ( 'NONE',  ( -4.164238869374098151, 46.59541550158063927, -3.795296366450310543 ) ) ;
#76010=CARTESIAN_POINT ( 'NONE',  ( 0.1532563361054082862, 66.21726448433413736, 2.638427012816831674 ) ) ;
#76011=CARTESIAN_POINT ( 'NONE',  ( 7.361572987183170547, 17.05059781766745530, 9.846743663894590881 ) ) ;
#76012=CARTESIAN_POINT ( 'NONE',  ( 17.20831665107776587, 4.133931151000785675, -7.208316651077762316 ) ) ;
#76014=CARTESIAN_POINT ( 'NONE',  ( -2.266590686148945544, 47.22041550158063927, 7.082119434687048631 ) ) ;
#76015=AXIS2_PLACEMENT_3D ( 'NONE', #91221, #6748, #16225 ) ;
#76017=CARTESIAN_POINT ( 'NONE',  ( -0.8801773607111008646, 8.272018677488171434, 2.915334737309923430 ) ) ;
#76020=CARTESIAN_POINT ( 'NONE',  ( 12.91533473730993009, 6.605352010821504471, -10.88017736071109987 ) ) ;
#76021=CARTESIAN_POINT ( 'NONE',  ( -4.164238869374098151, 66.59541550158060375, -3.795296366450310543 ) ) ;
#76022=CARTESIAN_POINT ( 'NONE',  ( 19.84674366389459266, 38.71726448433412315, -2.638427012816827677 ) ) ;
#76023=CARTESIAN_POINT ( 'NONE',  ( 3.591859063236761518, 39.95696800326375353, 11.09922568453594849 ) ) ;
#76026=CARTESIAN_POINT ( 'NONE',  ( 13.79529636645030344, 8.262082168247300018, 14.16423886937410614 ) ) ;
#76027=CARTESIAN_POINT ( 'NONE',  ( 15.44008868035555793, 6.397018677488170546, -9.422509992056140149 ) ) ;
#76028=CARTESIAN_POINT ( 'NONE',  ( 20.88017736071110875, 5.772018677488170546, -2.915334737309920765 ) ) ;
#76029=CARTESIAN_POINT ( 'NONE',  ( 7.361572987183170547, 47.05059781766745175, 9.846743663894590881 ) ) ;
#76031=CARTESIAN_POINT ( 'NONE',  ( 0.1532563361054100626, 25.80059781766744820, -2.638427012816831230 ) ) ;
#76032=CARTESIAN_POINT ( 'NONE',  ( 0.5774900079438607392, 33.48035201082150536, 5.440088680355550821 ) ) ;
#76036=PLANE ( 'NONE',  #90890 ) ;
#76038=CARTESIAN_POINT ( 'NONE',  ( 7.361572987183169658, 54.96726448433413026, -9.846743663894592657 ) ) ;
#76039=CARTESIAN_POINT ( 'NONE',  ( -0.8801773607111008646, 28.27201867748817321, 2.915334737309923430 ) ) ;
#76040=CARTESIAN_POINT ( 'NONE',  ( 17.96484262340118221, 34.93868534415482685, 7.964842623401181321 ) ) ;
#76041=CARTESIAN_POINT ( 'NONE',  ( 0.1532563361054100626, 65.80059781766745175, -2.638427012816831230 ) ) ;
#76042=CARTESIAN_POINT ( 'NONE',  ( 16.40814093676324603, 37.45696800326376064, -11.09922568453594671 ) ) ;
#76043=CARTESIAN_POINT ( 'NONE',  ( 22.26659068614894466, 3.887082168247300906, 7.082119434687054849 ) ) ;
#76046=AXIS2_PLACEMENT_3D ( 'NONE', #89844, #37360, #67853 ) ;
#76048=CARTESIAN_POINT ( 'NONE',  ( 16.40814093676323893, 40.79030133659708923, 11.09922568453595026 ) ) ;
#76050=CARTESIAN_POINT ( 'NONE',  ( 19.84674366389459266, 48.71726448433413026, -2.638427012816827677 ) ) ;
#76051=CARTESIAN_POINT ( 'NONE',  ( -0.8801773607111009756, 8.063685344154837509, 1.068504757029289695E-15 ) ) ;
#76053=CARTESIAN_POINT ( 'NONE',  ( 2.035157376598824452, 18.68868534415484106, 7.964842623401179544 ) ) ;
#76055=ORIENTED_EDGE ( 'NONE', *, *, #97449, .T. ) ;
#76056=CARTESIAN_POINT ( 'NONE',  ( 20.88017736071110519, 55.56368534415484817, 2.639326808657452039E-16 ) ) ;
#76057=CARTESIAN_POINT ( 'NONE',  ( 7.084665262690076126, 57.02201867748817676, -10.88017736071110164 ) ) ;
#76058=CARTESIAN_POINT ( 'NONE',  ( 17.96484262340118221, 54.93868534415484106, 7.964842623401181321 ) ) ;
#76059=CARTESIAN_POINT ( 'NONE',  ( -0.1503990784575242878, 29.24884699246888786, -6.262539305110083276 ) ) ;
#76060=( GEOMETRIC_REPRESENTATION_CONTEXT ( 3 ) GLOBAL_UNCERTAINTY_ASSIGNED_CONTEXT ( ( #96312 ) ) GLOBAL_UNIT_ASSIGNED_CONTEXT ( ( #47990, #78005, #46520 ) ) REPRESENTATION_CONTEXT ( 'NONE', 'WORKASPACE' ) );
#76063=CARTESIAN_POINT ( 'NONE',  ( 0.1532563361054100626, 40.80059781766745886, -2.638427012816831230 ) ) ;
#76066=PRESENTATION_STYLE_ASSIGNMENT (( #91063 ) ) ;
#76067=CARTESIAN_POINT ( 'NONE',  ( 17.08211943468705840, 10.13708216824730179, -12.26659068614894466 ) ) ;
#76068=CARTESIAN_POINT ( 'NONE',  ( -1.926860441876563801, 7.662123368507804066, 1.004413902775740978E-15 ) ) ;
#76070=CARTESIAN_POINT ( 'NONE',  ( 10.00000000000000000, 1.813685344154838175, -10.88017736071110342 ) ) ;
#76072=CARTESIAN_POINT ( 'NONE',  ( 13.43411237798106583, 47.66530133659709634, -12.81628187352647252 ) ) ;
#76075=CARTESIAN_POINT ( 'NONE',  ( 10.00000000000000178, 42.25893115100078745, 9.846743663894594434 ) ) ;
#76076=FILL_AREA_STYLE ('',( #60582 ) ) ;
#76078=CARTESIAN_POINT ( 'NONE',  ( 21.09922568453595559, 17.04030133659708923, -6.408140936763230044 ) ) ;
#76079=CARTESIAN_POINT ( 'NONE',  ( 12.63842701281683034, 22.46726448433411605, 9.846743663894596210 ) ) ;
#76081=EDGE_CURVE ( 'NONE', #74857, #48470, #39829, .T. ) ;
#76082=CARTESIAN_POINT ( 'NONE',  ( 7.361572987183170547, 17.05059781766745530, 9.846743663894590881 ) ) ;
#76083=CARTESIAN_POINT ( 'NONE',  ( 0.6178305044545838731, 19.74863466993042138, 9.382169495545420901 ) ) ;
#76085=CARTESIAN_POINT ( 'NONE',  ( 18.52753015748617571, 8.092264484334117824, 4.923371831947298993 ) ) ;
#76088=VERTEX_POINT ( 'NONE', #70335 ) ;
#76089=CARTESIAN_POINT ( 'NONE',  ( 12.91533473730993009, 21.60535201082150536, -10.88017736071109987 ) ) ;
#76090=CARTESIAN_POINT ( 'NONE',  ( 22.26659068614895176, 19.72041550158063572, -7.082119434687042414 ) ) ;
#76091=CARTESIAN_POINT ( 'NONE',  ( 1.472469842513823179, 45.59226448433412315, -4.923371831947296329 ) ) ;
#76092=CARTESIAN_POINT ( 'NONE',  ( 5.076628168052703671, 1.842264484334118047, 8.527530157486179263 ) ) ;
#76093=CARTESIAN_POINT ( 'NONE',  ( 10.00000000000000178, 35.37363466993042493, 12.81628187352647608 ) ) ;
#76095=CARTESIAN_POINT ( 'NONE',  ( 12.91533473730993009, 11.60535201082150536, -10.88017736071109987 ) ) ;
#76097=CARTESIAN_POINT ( 'NONE',  ( -2.816281873526471635, 13.91530133659708746, -3.434112377981056508 ) ) ;
#76098=CARTESIAN_POINT ( 'NONE',  ( 10.00000000000000000, 12.87363466993042138, -12.81628187352647608 ) ) ;
#76099=CARTESIAN_POINT ( 'NONE',  ( 5.076628168052704559, 25.17559781766745175, -8.527530157486179263 ) ) ;
#76101=CARTESIAN_POINT ( 'NONE',  ( 0.6178305044545838731, 34.74863466993042493, 9.382169495545420901 ) ) ;
#76104=CARTESIAN_POINT ( 'NONE',  ( 12.91533473730992121, 44.52201867748816966, 10.88017736071110164 ) ) ;
#76106=AXIS2_PLACEMENT_3D ( 'NONE', #18299, #17808, #8822 ) ;
#76108=CARTESIAN_POINT ( 'NONE',  ( 2.035157376598822676, 67.43868534415484817, -7.964842623401177768 ) ) ;
#76109=CARTESIAN_POINT ( 'NONE',  ( 20.88017736071110519, 40.56368534415484106, 2.639326808657452039E-16 ) ) ;
#76110=CARTESIAN_POINT ( 'NONE',  ( 19.42250999205614548, 45.98035201082150536, -5.440088680355545492 ) ) ;
#76111=CARTESIAN_POINT ( 'NONE',  ( 2.791683348922240793, 66.63393115100079456, 7.208316651077764092 ) ) ;
#76115=CARTESIAN_POINT ( 'NONE',  ( 18.52753015748617571, 48.09226448433412315, 4.923371831947298993 ) ) ;
#76116=CARTESIAN_POINT ( 'NONE',  ( 0.5774900079438590739, 12.64701867748817143, -5.440088680355550821 ) ) ;
#76117=CARTESIAN_POINT ( 'NONE',  ( 0.5600000000000083800, 105.0000000000000000, -5.000000000000000000 ) ) ;
#76118=CARTESIAN_POINT ( 'NONE',  ( 21.09922568453595559, 17.04030133659708923, -6.408140936763230044 ) ) ;
#76120=CARTESIAN_POINT ( 'NONE',  ( 4.559911319644449179, 32.23035201082150536, -9.422509992056141925 ) ) ;
#76123=CARTESIAN_POINT ( 'NONE',  ( -1.099225684535947600, -0.4596986634029132657, 6.408140936763237150 ) ) ;
#76125=CARTESIAN_POINT ( 'NONE',  ( 15.44008868035555260, 19.73035201082150536, 9.422509992056143702 ) ) ;
#76126=CARTESIAN_POINT ( 'NONE',  ( 20.88017736071110875, 30.77201867748816966, -2.915334737309920765 ) ) ;
#76127=CARTESIAN_POINT ( 'NONE',  ( -0.3689425029237881626, 37.42874883491396787, 10.36894250292379027 ) ) ;
#76128=CARTESIAN_POINT ( 'NONE',  ( 17.20831665107776587, 32.88393115100078745, 7.208316651077764980 ) ) ;
#76129=CARTESIAN_POINT ( 'NONE',  ( 2.035157376598824452, 48.68868534415483396, 7.964842623401179544 ) ) ;
#76130=CARTESIAN_POINT ( 'NONE',  ( 20.36894250292379738, 9.928748834913966093, -10.36894250292379027 ) ) ;
#76132=CARTESIAN_POINT ( 'NONE',  ( 18.52753015748618282, 53.92559781766745175, -4.923371831947291888 ) ) ;
#76136=CARTESIAN_POINT ( 'NONE',  ( 10.00000000000000178, 38.05374883491396787, 14.16423886937410082 ) ) ;
#76137=CARTESIAN_POINT ( 'NONE',  ( 13.79529636645030344, 28.26208216824729647, 14.16423886937410614 ) ) ;
#76139=CARTESIAN_POINT ( 'NONE',  ( 7.084665262690076126, 67.02201867748817676, -10.88017736071110164 ) ) ;
#76140=CARTESIAN_POINT ( 'NONE',  ( -2.816281873526471635, 8.915301336597083903, -3.434112377981056508 ) ) ;
#76141=CARTESIAN_POINT ( 'NONE',  ( 10.00000000000000178, 42.25893115100078745, 9.846743663894594434 ) ) ;
#76143=CARTESIAN_POINT ( 'NONE',  ( 0.5774900079438607392, 48.48035201082150536, 5.440088680355550821 ) ) ;
#76144=CARTESIAN_POINT ( 'NONE',  ( 19.38216949554541202, 20.99863466993042138, 9.382169495545424454 ) ) ;
#76145=CARTESIAN_POINT ( 'NONE',  ( 22.26659068614894466, 18.88708216824730002, 7.082119434687054849 ) ) ;
#76146=B_SPLINE_CURVE_WITH_KNOTS ( 'NONE', 3,
 ( #61396, #61888, #8410, #46407, #76895, #69405 ),
 .UNSPECIFIED., .F., .F.,
 ( 4, 2, 4 ),
 ( 0.000000000000000000, 0.0002701661927229353360, 0.0005403323854458706721 ),
 .UNSPECIFIED. ) ;
#76147=CARTESIAN_POINT ( 'NONE',  ( 17.96484262340118221, 9.938685344154839285, 7.964842623401181321 ) ) ;
#76148=CARTESIAN_POINT ( 'NONE',  ( 2.035157376598824452, 28.68868534415484106, 7.964842623401179544 ) ) ;
#76149=CARTESIAN_POINT ( 'NONE',  ( 2.035157376598822676, 62.43868534415483396, -7.964842623401177768 ) ) ;
#76150=CARTESIAN_POINT ( 'NONE',  ( 19.38216949554541202, 45.99863466993041072, 9.382169495545424454 ) ) ;
#76152=ORIENTED_EDGE ( 'NONE', *, *, #42696, .F. ) ;
#76154=VERTEX_POINT ( 'NONE', #68859 ) ;
#76155=CLOSED_SHELL ( 'NONE', ( #69885, #81404, #21909, #90987, #12766, #18110, #23830, #37728, #62112, #32897, #2897, #12595, #26279, #78964, #10269, #73268, #34091, #6469, #41742, #60845, #25972, #52619, #7036, #77148, #9556, #78148, #3093, #26969, #89630, #65233, #12759, #52437, #19868, #74631, #36423, #4321, #8958, #81803, #65322, #77087, #40246, #2978, #42968, #86630, #15153, #38971, #31283, #67513, #30755, #43327, #27462, #90875, #15841, #46683, #11327, #29676, #91020, #49566, #41691, #60068, #25660, #71132, #11854, #24979, #33216, #23180, #95738, #87950, #16422, #34592, #77031, #26728, #75070, #95609, #65850, #94268, #45324, #20079, #58933, #23014, #19100, #20572, #93975, #83901, #28088, #73705, #16864, #84997, #93564, #55796, #65361, #55181, #91661, #71192, #28035, #62251, #20450, #55307, #95683, #44043, #24749, #48086, #13371, #36135, #62644, #62029, #7130, #49240, #48558, #66779, #85111, #92555, #26233, #15640, #44448, #78122, #27339, #82120, #60946, #55066, #19431, #46801, #56014, #18183, #53385, #19831, #16060, #47247, #848, #80415, #6645, #93062, #12884, #35455, #29558, #51621, #23940, #30487, #91278, #60430, #49361, #92159, #19881, #38414, #43699, #42677, #87504, #13196, #53453, #1175, #2331, #38090, #30045, #63238, #56663, #91107, #56034, #2186, #31806, #62884, #10638, #64506, #36956, #86485, #35340, #75195, #36527, #12080, #77280, #96123, #79158, #13448, #90133, #16393, #80643, #92016, #4651, #40861, #4200, #29830, #82383, #33405, #144, #54290, #21696, #79132, #15201, #26911, #72940, #76824, #93637, #30196, #32648, #40986, #81586, #80046, #61780, #49642, #55723, #60882, #65330, #13909, #52070, #41388, #55104, #58465, #73259, #86608, #85915, #71516, #63828, #25021, #73503, #74512, #52588, #96951, #80618, #90027, #32638, #76858, #91888, #9315, #47653, #10682, #80374, #35604, #299, #32075, #13115, #32379, #26594, #92244, #86447, #64438, #60633, #55484, #59599, #47007, #65030, #32199, #63985, #88026, #76770, #42960, #90548, #55465, #29361, #31045, #75423, #47285, #13803, #86830, #93125, #11640, #3977, #10384, #35550, #57825, #52669, #56452, #17407, #9051, #32760, #65013, #10140, #40761, #82807, #22944, #65355, #6924, #92275, #46692, #38771, #32981, #54588, #96321, #29352, #7963, #383, #13572, #89114, #25072, #90277, #32722, #42135, #6563 ) ) ;
#76159=CARTESIAN_POINT ( 'NONE',  ( 10.00000000000000000, 55.55374883491396787, -14.16423886937410082 ) ) ;
#76160=CARTESIAN_POINT ( 'NONE',  ( 20.36894250292379738, 59.92874883491397497, -10.36894250292379027 ) ) ;
#76161=CARTESIAN_POINT ( 'NONE',  ( 12.63842701281683034, 27.46726448433411250, 9.846743663894596210 ) ) ;
#76162=CARTESIAN_POINT ( 'NONE',  ( 0.1532563361054083140, 61.00893115100078745, 1.131784320476157264E-15 ) ) ;
#76165=CARTESIAN_POINT ( 'NONE',  ( 2.791683348922237240, 10.38393115100078390, -7.208316651077763204 ) ) ;
#76166=CARTESIAN_POINT ( 'NONE',  ( 0.6178305044545818747, 33.49863466993042493, -9.382169495545419124 ) ) ;
#76170=CARTESIAN_POINT ( 'NONE',  ( 10.00000000000000000, 35.55374883491396787, -14.16423886937410082 ) ) ;
#76171=CARTESIAN_POINT ( 'NONE',  ( 17.08211943468705130, 48.47041550158063927, 12.26659068614894998 ) ) ;
#76173=CARTESIAN_POINT ( 'NONE',  ( 3.591859063236761518, 59.95696800326375353, 11.09922568453594849 ) ) ;
#76174=CARTESIAN_POINT ( 'NONE',  ( 7.084665262690076126, 24.10535201082150181, 10.88017736071109987 ) ) ;
#76175=CARTESIAN_POINT ( 'NONE',  ( 19.84674366389459266, 48.71726448433413026, -2.638427012816827677 ) ) ;
#76176=CARTESIAN_POINT ( 'NONE',  ( 10.00000000000000178, 24.31368534415484106, 10.88017736071110342 ) ) ;
#76179=CARTESIAN_POINT ( 'NONE',  ( 10.00000000000000178, 52.25893115100078745, 9.846743663894594434 ) ) ;
#76180=CARTESIAN_POINT ( 'NONE',  ( 1.472469842513823179, 46.42559781766745175, 4.923371831947296329 ) ) ;
#76182=VERTEX_POINT ( 'NONE', #45860 ) ;
#76183=CARTESIAN_POINT ( 'NONE',  ( 3.640395162852214650, 89.00000000000000000, -5.000000000000000000 ) ) ;
#76184=CARTESIAN_POINT ( 'NONE',  ( 0.1532563361054100626, 5.800597817667452638, -2.638427012816831230 ) ) ;
#76186=VERTEX_POINT ( 'NONE', #32309 ) ;
#76188=CARTESIAN_POINT ( 'NONE',  ( 1.274849032794306947, 7.555090184799359676, -6.499999999999997335 ) ) ;
#76189=CARTESIAN_POINT ( 'NONE',  ( 5.076628168052703671, 31.84226448433412315, 8.527530157486179263 ) ) ;
#76190=CARTESIAN_POINT ( 'NONE',  ( -46.43582398220812024, 103.5217676819815580, 6.243076731245754019 ) ) ;
#76191=CARTESIAN_POINT ( 'NONE',  ( 10.00000000000000178, 40.37363466993042493, 12.81628187352647608 ) ) ;
#76196=CARTESIAN_POINT ( 'NONE',  ( 0.1532563361054083140, 66.00893115100079456, 1.131784320476157264E-15 ) ) ;
#76198=CARTESIAN_POINT ( 'NONE',  ( 14.92337183194729988, 39.34226448433412315, -8.527530157486177487 ) ) ;
#76199=CARTESIAN_POINT ( 'NONE',  ( -4.164238869374098151, 31.59541550158063927, -3.795296366450310543 ) ) ;
#76200=CARTESIAN_POINT ( 'NONE',  ( 14.92337183194729988, 54.34226448433412315, -8.527530157486177487 ) ) ;
#76202=CARTESIAN_POINT ( 'NONE',  ( 0.1532563361054082862, 6.217264484334118713, 2.638427012816831674 ) ) ;
#76204=AXIS2_PLACEMENT_3D ( 'NONE', #26003, #79493, #56497 ) ;
#76205=( NAMED_UNIT ( * ) PLANE_ANGLE_UNIT ( ) SI_UNIT ( $, .RADIAN. ) );
#76206=CARTESIAN_POINT ( 'NONE',  ( 2.791683348922237240, 50.38393115100078035, -7.208316651077763204 ) ) ;
#76207=CARTESIAN_POINT ( 'NONE',  ( 7.084665262690076126, 52.02201867748816255, -10.88017736071110164 ) ) ;
#76213=CARTESIAN_POINT ( 'NONE',  ( 4.559911319644449179, 47.23035201082150536, -9.422509992056141925 ) ) ;
#76216=ORIENTED_EDGE ( 'NONE', *, *, #43822, .F. ) ;
#76218=CARTESIAN_POINT ( 'NONE',  ( 0.5774900079438607392, 28.48035201082150891, 5.440088680355550821 ) ) ;
#76219=CARTESIAN_POINT ( 'NONE',  ( 3.591859063236761518, 4.956968003263753531, 11.09922568453594849 ) ) ;
#76220=CARTESIAN_POINT ( 'NONE',  ( 0.5774900079438590739, 57.64701867748817676, -5.440088680355550821 ) ) ;
#76222=CARTESIAN_POINT ( 'NONE',  ( 19.84674366389459621, 13.50893115100078568, 7.409399052514197653E-17 ) ) ;
#76224=CARTESIAN_POINT ( 'NONE',  ( -0.8801773607111008646, 33.27201867748817676, 2.915334737309923430 ) ) ;
#76226=CARTESIAN_POINT ( 'NONE',  ( 18.52753015748617571, 13.09226448433411960, 4.923371831947298993 ) ) ;
#76227=CARTESIAN_POINT ( 'NONE',  ( 7.361572987183169658, 39.96726448433411605, -9.846743663894592657 ) ) ;
#76230=CARTESIAN_POINT ( 'NONE',  ( 22.81628187352648496, 1.831968003263753753, -3.434112377981050290 ) ) ;
#76231=CARTESIAN_POINT ( 'NONE',  ( -2.266590686148945544, 62.22041550158063927, 7.082119434687048631 ) ) ;
#76232=CARTESIAN_POINT ( 'NONE',  ( -15.94000000000001371, 93.50000000000000000, -9.500000000000000000 ) ) ;
#76233=CARTESIAN_POINT ( 'NONE',  ( 24.16423886937409904, 24.09541550158063927, 3.795296366450317205 ) ) ;
#76234=CARTESIAN_POINT ( 'NONE',  ( 20.36894250292379738, 54.92874883491396076, -10.36894250292379027 ) ) ;
#76235=CARTESIAN_POINT ( 'NONE',  ( 0.1532563361054082862, 16.21726448433411960, 2.638427012816831674 ) ) ;
#76236=CARTESIAN_POINT ( 'NONE',  ( 7.361572987183170547, 27.05059781766745175, 9.846743663894590881 ) ) ;
#76237=CARTESIAN_POINT ( 'NONE',  ( 15.44008868035555793, 26.39701867748817321, -9.422509992056140149 ) ) ;
#76238=CARTESIAN_POINT ( 'NONE',  ( 19.84674366389459621, 48.50893115100078745, 7.409399052514197653E-17 ) ) ;
#76239=CARTESIAN_POINT ( 'NONE',  ( 22.26659068614894466, 13.88708216824730179, 7.082119434687054849 ) ) ;
#76243=CARTESIAN_POINT ( 'NONE',  ( 0.1532563361054083140, 16.00893115100078390, 1.131784320476157264E-15 ) ) ;
#76244=CARTESIAN_POINT ( 'NONE',  ( 6.565887622018943937, 35.16530133659708923, 12.81628187352647430 ) ) ;
#76245=CARTESIAN_POINT ( 'NONE',  ( 0.1532563361054082862, 36.21726448433410894, 2.638427012816831674 ) ) ;
#76246=ORIENTED_EDGE ( 'NONE', *, *, #82418, .T. ) ;
#76247=CARTESIAN_POINT ( 'NONE',  ( 14.92337183194729633, 27.67559781766745530, 8.527530157486181039 ) ) ;
#76251=CARTESIAN_POINT ( 'NONE',  ( 22.26659068614894466, 53.88708216824731068, 7.082119434687054849 ) ) ;
#76253=CARTESIAN_POINT ( 'NONE',  ( 2.791683348922237240, 30.38393115100078390, -7.208316651077763204 ) ) ;
#76254=CARTESIAN_POINT ( 'NONE',  ( 17.20831665107776587, 34.13393115100078745, -7.208316651077762316 ) ) ;
#76255=CARTESIAN_POINT ( 'NONE',  ( 18.95785429995052951, 2.242161081720065230, 6.499999999999868550 ) ) ;
#76256=CARTESIAN_POINT ( 'NONE',  ( 18.52753015748617571, 53.09226448433412315, 4.923371831947298993 ) ) ;
#76257=CARTESIAN_POINT ( 'NONE',  ( 17.96484262340118221, 56.18868534415484817, -7.964842623401177768 ) ) ;
#76261=CARTESIAN_POINT ( 'NONE',  ( 13.43411237798106583, 57.66530133659708923, -12.81628187352647252 ) ) ;
#76263=CARTESIAN_POINT ( 'NONE',  ( 0.1532563361054082862, 11.21726448433411605, 2.638427012816831674 ) ) ;
#76264=CARTESIAN_POINT ( 'NONE',  ( 3.591859063236761518, 54.95696800326376064, 11.09922568453594849 ) ) ;
#76265=CARTESIAN_POINT ( 'NONE',  ( 19.42250999205614193, 10.14701867748816966, 5.440088680355555262 ) ) ;
#76266=CARTESIAN_POINT ( 'NONE',  ( 12.63842701281683922, 49.55059781766744464, -9.846743663894590881 ) ) ;
#76267=CARTESIAN_POINT ( 'NONE',  ( 17.39651004071842522, 19.08210964143329491, -6.499999999999992895 ) ) ;
#76268=CARTESIAN_POINT ( 'NONE',  ( 10.00000000000000000, 30.55374883491397142, -14.16423886937410082 ) ) ;
#76269=CARTESIAN_POINT ( 'NONE',  ( 24.16423886937409904, 59.09541550158063217, 3.795296366450317205 ) ) ;
#76270=CARTESIAN_POINT ( 'NONE',  ( 17.20831665107776587, 57.88393115100078745, 7.208316651077764980 ) ) ;
#76272=CARTESIAN_POINT ( 'NONE',  ( 19.42250999205614548, 45.98035201082150536, -5.440088680355545492 ) ) ;
#76273=CARTESIAN_POINT ( 'NONE',  ( 17.96484262340118221, 66.18868534415483396, -7.964842623401177768 ) ) ;
#76277=CARTESIAN_POINT ( 'NONE',  ( -2.816281873526473856, 59.12363466993042493, 9.499525473075851096E-16 ) ) ;
#76278=ORIENTED_EDGE ( 'NONE', *, *, #83822, .T. ) ;
#76279=CARTESIAN_POINT ( 'NONE',  ( 14.92337183194729633, 7.675597817667451750, 8.527530157486181039 ) ) ;
#76281=CARTESIAN_POINT ( 'NONE',  ( -0.3689425029237898834, 21.17874883491396432, -10.36894250292378850 ) ) ;
#76282=CARTESIAN_POINT ( 'NONE',  ( 2.791683348922237240, 25.38393115100078390, -7.208316651077763204 ) ) ;
#76283=CARTESIAN_POINT ( 'NONE',  ( 12.91533473730993009, 26.60535201082150536, -10.88017736071109987 ) ) ;
#76284=( GEOMETRIC_REPRESENTATION_CONTEXT ( 3 ) GLOBAL_UNCERTAINTY_ASSIGNED_CONTEXT ( ( #2368 ) ) GLOBAL_UNIT_ASSIGNED_CONTEXT ( ( #13505, #37500, #52969 ) ) REPRESENTATION_CONTEXT ( 'NONE', 'WORKASPACE' ) );
#76287=CARTESIAN_POINT ( 'NONE',  ( 2.035157376598822676, 27.43868534415483396, -7.964842623401177768 ) ) ;
#76289=CARTESIAN_POINT ( 'NONE',  ( 10.00000000000000178, 39.31368534415484106, 10.88017736071110342 ) ) ;
#76290=SURFACE_STYLE_USAGE ( .BOTH. , #23308 ) ;
#76291=ORIENTED_EDGE ( 'NONE', *, *, #90758, .F. ) ;
#76293=CARTESIAN_POINT ( 'NONE',  ( 21.09922568453594849, 16.20696800326375353, 6.408140936763242479 ) ) ;
#76294=CARTESIAN_POINT ( 'NONE',  ( 1.472469842513823179, 16.42559781766745175, 4.923371831947296329 ) ) ;
#76297=CARTESIAN_POINT ( 'NONE',  ( 2.791683348922237240, 20.38393115100078745, -7.208316651077763204 ) ) ;
#76298=CARTESIAN_POINT ( 'NONE',  ( 20.88017736071110519, 30.56368534415484106, 2.639326808657452039E-16 ) ) ;
#76302=CARTESIAN_POINT ( 'NONE',  ( 4.559911319644449179, 57.23035201082150536, -9.422509992056141925 ) ) ;
#76303=FACE_OUTER_BOUND ( 'NONE', #54369, .T. ) ;
#76304=CARTESIAN_POINT ( 'NONE',  ( -1.099225684535947600, 58.70696800326375353, -6.408140936763238038 ) ) ;
#76305=CARTESIAN_POINT ( 'NONE',  ( -0.8801773607110991993, 62.85535201082150536, -2.915334737309923874 ) ) ;
#76306=CARTESIAN_POINT ( 'NONE',  ( -1.099225684535947600, 3.706968003263753531, -6.408140936763238038 ) ) ;
#76308=CARTESIAN_POINT ( 'NONE',  ( 17.20831665107776587, 34.13393115100078745, -7.208316651077762316 ) ) ;
#76309=CARTESIAN_POINT ( 'NONE',  ( 6.565887622018943937, 55.16530133659709634, 12.81628187352647430 ) ) ;
#76310=CARTESIAN_POINT ( 'NONE',  ( 1.274849032794292736, 37.55509018479936145, -6.499999999999977796 ) ) ;
#76311=CARTESIAN_POINT ( 'NONE',  ( 12.63842701281683034, 12.46726448433411782, 9.846743663894596210 ) ) ;
#76312=CARTESIAN_POINT ( 'NONE',  ( -1.099225684535947600, 19.54030133659708568, 6.408140936763237150 ) ) ;
#76313=CARTESIAN_POINT ( 'NONE',  ( -46.43542959741873943, 103.9441885970218351, 5.610226944091865953 ) ) ;
#76315=CARTESIAN_POINT ( 'NONE',  ( 10.00000000000000000, 36.81368534415484106, -10.88017736071110342 ) ) ;
#76316=CARTESIAN_POINT ( 'NONE',  ( 18.52753015748618282, 63.92559781766745886, -4.923371831947291888 ) ) ;
#76317=CARTESIAN_POINT ( 'NONE',  ( 10.00000000000000000, 24.75893115100078745, -9.846743663894594434 ) ) ;
#76318=CARTESIAN_POINT ( 'NONE',  ( 12.63842701281683922, 4.550597817667451750, -9.846743663894590881 ) ) ;
#76319=CARTESIAN_POINT ( 'NONE',  ( 2.035157376598822676, 17.43868534415483751, -7.964842623401177768 ) ) ;
#76320=CARTESIAN_POINT ( 'NONE',  ( 13.43411237798106583, 17.66530133659708923, -12.81628187352647252 ) ) ;
#76322=CARTESIAN_POINT ( 'NONE',  ( 5.076628168052703671, 61.84226448433412315, 8.527530157486179263 ) ) ;
#76324=CARTESIAN_POINT ( 'NONE',  ( 20.88017736071110164, 10.35535201082150714, 2.915334737309930979 ) ) ;
#76325=CARTESIAN_POINT ( 'NONE',  ( 14.92337183194729988, 49.34226448433411605, -8.527530157486177487 ) ) ;
#76327=ORIENTED_EDGE ( 'NONE', *, *, #97574, .F. ) ;
#76329=CARTESIAN_POINT ( 'NONE',  ( 2.917880565312948704, 67.63708216824730357, 12.26659068614894643 ) ) ;
#76330=CARTESIAN_POINT ( 'NONE',  ( 19.90229974777923161, 69.67742753483354079, -6.500000000000000000 ) ) ;
#76331=CARTESIAN_POINT ( 'NONE',  ( -0.8801773607110991993, 32.85535201082151247, -2.915334737309923874 ) ) ;
#76333=CARTESIAN_POINT ( 'NONE',  ( 10.00000000000000000, 60.55374883491397497, -14.16423886937410082 ) ) ;
#76335=CARTESIAN_POINT ( 'NONE',  ( 18.52753015748618282, 23.92559781766745530, -4.923371831947291888 ) ) ;
#76336=CARTESIAN_POINT ( 'NONE',  ( 21.09922568453594849, 11.20696800326375531, 6.408140936763242479 ) ) ;
#76343=CARTESIAN_POINT ( 'NONE',  ( 22.26659068614895176, 14.72041550158063572, -7.082119434687042414 ) ) ;
#76344=CARTESIAN_POINT ( 'NONE',  ( 14.92337183194729988, 24.34226448433411960, -8.527530157486177487 ) ) ;
#76348=CARTESIAN_POINT ( 'NONE',  ( 13.79529636645030344, 48.26208216824728936, 14.16423886937410614 ) ) ;
#76350=CARTESIAN_POINT ( 'NONE',  ( 5.076628168052704559, 5.175597817667451750, -8.527530157486179263 ) ) ;
#76353=CARTESIAN_POINT ( 'NONE',  ( 12.91533473730993009, 31.60535201082150891, -10.88017736071109987 ) ) ;
#76354=CARTESIAN_POINT ( 'NONE',  ( 3.591859063236763294, 53.29030133659708923, -11.09922568453595026 ) ) ;
#76355=CARTESIAN_POINT ( 'NONE',  ( 10.00000000000000178, 19.31368534415484106, 10.88017736071110342 ) ) ;
#76356=CARTESIAN_POINT ( 'NONE',  ( 22.81628187352648496, 41.83196800326375353, -3.434112377981050290 ) ) ;
#76357=CARTESIAN_POINT ( 'NONE',  ( 12.63842701281683922, 64.55059781766745175, -9.846743663894590881 ) ) ;
#76358=CARTESIAN_POINT ( 'NONE',  ( 1.472469842513823179, 0.5922644843341181575, -4.923371831947296329 ) ) ;
#76363=CARTESIAN_POINT ( 'NONE',  ( 24.16423886937409904, 39.09541550158062506, 3.795296366450317205 ) ) ;
#76364=CARTESIAN_POINT ( 'NONE',  ( 20.36894250292379738, 9.928748834913966093, -10.36894250292379027 ) ) ;
#76365=CARTESIAN_POINT ( 'NONE',  ( 2.035157376598822676, 2.438685344154837953, -7.964842623401177768 ) ) ;
#76366=CARTESIAN_POINT ( 'NONE',  ( 0.5774900079438590739, 37.64701867748817676, -5.440088680355550821 ) ) ;
#76369=CARTESIAN_POINT ( 'NONE',  ( 18.52753015748617571, 3.092264484334118269, 4.923371831947298993 ) ) ;
#76371=CARTESIAN_POINT ( 'NONE',  ( -2.816281873526473856, 24.12363466993042138, 9.499525473075851096E-16 ) ) ;
#76372=CARTESIAN_POINT ( 'NONE',  ( 1.707155281725170726, 62.90189080397286148, 6.499999999999955591 ) ) ;
#76374=CARTESIAN_POINT ( 'NONE',  ( 14.92337183194729633, 32.67559781766745175, 8.527530157486181039 ) ) ;
#76375=CARTESIAN_POINT ( 'NONE',  ( 4.559911319644449179, 13.89701867748817143, 9.422509992056141925 ) ) ;
#76376=CARTESIAN_POINT ( 'NONE',  ( 0.6178305044545838731, 24.74863466993042493, 9.382169495545420901 ) ) ;
#76377=CARTESIAN_POINT ( 'NONE',  ( 2.791683348922237240, 15.38393115100078212, -7.208316651077763204 ) ) ;
#76378=CARTESIAN_POINT ( 'NONE',  ( 7.084665262690076126, 12.02201867748817143, -10.88017736071110164 ) ) ;
#76379=CARTESIAN_POINT ( 'NONE',  ( 0.1532563361054083140, 41.00893115100078745, 1.131784320476157264E-15 ) ) ;
#76380=CARTESIAN_POINT ( 'NONE',  ( 6.565887622018943937, 58.08196800326376064, -12.81628187352647608 ) ) ;
#76381=CARTESIAN_POINT ( 'NONE',  ( 7.361572987183169658, 19.96726448433411960, -9.846743663894592657 ) ) ;
#76382=CARTESIAN_POINT ( 'NONE',  ( 20.36894250292379738, 9.928748834913966093, -10.36894250292379027 ) ) ;
#76384=CARTESIAN_POINT ( 'NONE',  ( 4.559911319644449179, 33.89701867748817676, 9.422509992056141925 ) ) ;
#76385=CARTESIAN_POINT ( 'NONE',  ( -0.8801773607111008646, 8.272018677488171434, 2.915334737309923430 ) ) ;
#76386=CARTESIAN_POINT ( 'NONE',  ( 17.08211943468705840, 40.13708216824731068, -12.26659068614894466 ) ) ;
#76387=CARTESIAN_POINT ( 'NONE',  ( 12.91533473730993009, 36.60535201082151247, -10.88017736071109987 ) ) ;
#76389=CARTESIAN_POINT ( 'NONE',  ( 20.88017736071110519, 20.56368534415484106, 2.639326808657452039E-16 ) ) ;
#76391=CARTESIAN_POINT ( 'NONE',  ( 20.88017736071110519, 45.56368534415484106, 2.639326808657452039E-16 ) ) ;
#76392=CARTESIAN_POINT ( 'NONE',  ( 10.00000000000000178, 60.37363466993041783, 12.81628187352647608 ) ) ;
#76393=CARTESIAN_POINT ( 'NONE',  ( 20.88017736071110519, 50.56368534415484106, 2.639326808657452039E-16 ) ) ;
#76394=CARTESIAN_POINT ( 'NONE',  ( 4.559911319644449179, 57.23035201082150536, -9.422509992056141925 ) ) ;
#76395=AXIS2_PLACEMENT_3D ( 'NONE', #97947, #43429, #81921 ) ;
#76397=CARTESIAN_POINT ( 'NONE',  ( 7.084665262690076126, 57.02201867748817676, -10.88017736071110164 ) ) ;
#76400=CARTESIAN_POINT ( 'NONE',  ( -4.164238869374098151, 41.59541550158061796, -3.795296366450310543 ) ) ;
#76401=CARTESIAN_POINT ( 'NONE',  ( 7.361572987183169658, -0.03273551566588185635, -9.846743663894592657 ) ) ;
#76404=CARTESIAN_POINT ( 'NONE',  ( 1.472469842513823179, 60.59226448433412315, -4.923371831947296329 ) ) ;
#76405=CARTESIAN_POINT ( 'NONE',  ( 10.00000000000000178, 32.25893115100078745, 9.846743663894594434 ) ) ;
#76407=CARTESIAN_POINT ( 'NONE',  ( 10.00000000000000000, 34.75893115100078745, -9.846743663894594434 ) ) ;
#76410=CARTESIAN_POINT ( 'NONE',  ( 0.5774900079438590739, 42.64701867748816966, -5.440088680355550821 ) ) ;
#76411=CARTESIAN_POINT ( 'NONE',  ( 7.361572987183170547, 37.05059781766744464, 9.846743663894590881 ) ) ;
#76412=CARTESIAN_POINT ( 'NONE',  ( 21.09922568453594849, 21.20696800326375353, 6.408140936763242479 ) ) ;
#76414=CARTESIAN_POINT ( 'NONE',  ( 12.91533473730992121, 59.52201867748816966, 10.88017736071110164 ) ) ;
#76415=CARTESIAN_POINT ( 'NONE',  ( 20.88017736071110875, 40.77201867748818387, -2.915334737309920765 ) ) ;
#76416=CARTESIAN_POINT ( 'NONE',  ( 2.035157376598822676, 2.438685344154837953, -7.964842623401177768 ) ) ;
#76417=CARTESIAN_POINT ( 'NONE',  ( 2.917880565312948704, 52.63708216824730357, 12.26659068614894643 ) ) ;
#76418=EDGE_CURVE ( 'NONE', #21351, #32629, #26286, .T. ) ;
#76420=CARTESIAN_POINT ( 'NONE',  ( 22.81628187352648496, 16.83196800326374998, -3.434112377981050290 ) ) ;
#76422=ORIENTED_EDGE ( 'NONE', *, *, #81515, .F. ) ;
#76423=CARTESIAN_POINT ( 'NONE',  ( 19.38216949554541557, 17.24863466993041783, -9.382169495545420901 ) ) ;
#76424=CARTESIAN_POINT ( 'NONE',  ( 15.44008868035555793, 16.39701867748817321, -9.422509992056140149 ) ) ;
#76425=CARTESIAN_POINT ( 'NONE',  ( 15.44008868035555793, 66.39701867748817676, -9.422509992056140149 ) ) ;
#76427=CARTESIAN_POINT ( 'NONE',  ( -0.8801773607111008646, 68.27201867748817676, 2.915334737309923430 ) ) ;
#76428=( BOUNDED_CURVE ( )  B_SPLINE_CURVE ( 2, ( #4187, #89147, #88650, #50159, #51153, #65154, #80668, #74128, #80167 ),
 .UNSPECIFIED., .F., .T. ) 
 B_SPLINE_CURVE_WITH_KNOTS ( ( 3, 2, 2, 2, 3 ),
 ( 0.8329980797973741691, 0.8333333333333333703, 0.8392857142857143016, 0.8452380952380952328, 0.8455733487740543231 ),
 .UNSPECIFIED. ) 
 CURVE ( )  GEOMETRIC_REPRESENTATION_ITEM ( )  RATIONAL_B_SPLINE_CURVE ( ( 0.9963778908391753841, 0.9980808541467917072, 1.000000000000000000, 0.9659258262890683122, 1.000000000000000000, 0.9659258262890683122, 1.000000000000000000, 0.9980808541467922623, 0.9963778908391764944 ) ) 
 REPRESENTATION_ITEM ( '' )  );
#76429=CARTESIAN_POINT ( 'NONE',  ( 2.791683348922237240, 55.38393115100078745, -7.208316651077763204 ) ) ;
#76430=CARTESIAN_POINT ( 'NONE',  ( 7.361572987183169658, 29.96726448433411960, -9.846743663894592657 ) ) ;
#76431=CARTESIAN_POINT ( 'NONE',  ( 10.00000000000000000, 29.75893115100078745, -9.846743663894594434 ) ) ;
#76432=DIRECTION ( 'NONE',  ( 1.000000000000000000, 0.000000000000000000, 0.000000000000000000 ) ) ;
#76434=CARTESIAN_POINT ( 'NONE',  ( 10.00000000000000000, 42.87363466993042493, -12.81628187352647608 ) ) ;
#76435=CARTESIAN_POINT ( 'NONE',  ( 7.361572987183169658, 14.96726448433411960, -9.846743663894592657 ) ) ;
#76438=CARTESIAN_POINT ( 'NONE',  ( 14.92337183194729988, 49.34226448433411605, -8.527530157486177487 ) ) ;
#76439=ORIENTED_EDGE ( 'NONE', *, *, #60822, .F. ) ;
#76442=CARTESIAN_POINT ( 'NONE',  ( 13.43411237798105340, 15.58196800326374998, 12.81628187352647963 ) ) ;
#76443=CARTESIAN_POINT ( 'NONE',  ( 15.44008868035555793, 51.39701867748816966, -9.422509992056140149 ) ) ;
#76444=CARTESIAN_POINT ( 'NONE',  ( 2.917880565312948704, 32.63708216824730357, 12.26659068614894643 ) ) ;
#76446=DIRECTION ( 'NONE',  ( 0.000000000000000000, -1.000000000000000000, 0.000000000000000000 ) ) ;
#76447=CARTESIAN_POINT ( 'NONE',  ( -4.164238869374099927, 27.01208216824730357, 3.795296366450308767 ) ) ;
#76448=CARTESIAN_POINT ( 'NONE',  ( 22.26659068614895176, 59.72041550158063927, -7.082119434687042414 ) ) ;
#76449=CARTESIAN_POINT ( 'NONE',  ( -0.3689425029237898834, 16.17874883491396076, -10.36894250292378850 ) ) ;
#76450=CARTESIAN_POINT ( 'NONE',  ( 17.08211943468705130, 23.47041550158063572, 12.26659068614894998 ) ) ;
#76452=CARTESIAN_POINT ( 'NONE',  ( 2.035157376598822676, 42.43868534415483396, -7.964842623401177768 ) ) ;
#76453=CARTESIAN_POINT ( 'NONE',  ( 19.80832241502128355, 24.75868815902069997, 6.499999999999992895 ) ) ;
#76456=CARTESIAN_POINT ( 'NONE',  ( 19.84674366389459621, 48.50893115100078745, 7.409399052514197653E-17 ) ) ;
#76457=CARTESIAN_POINT ( 'NONE',  ( 15.44008868035555260, 19.73035201082150536, 9.422509992056143702 ) ) ;
#76458=DIRECTION ( 'NONE',  ( -0.000000000000000000, -0.000000000000000000, 1.000000000000000000 ) ) ;
#76459=CARTESIAN_POINT ( 'NONE',  ( 5.076628168052704559, 65.17559781766745175, -8.527530157486179263 ) ) ;
#76460=CARTESIAN_POINT ( 'NONE',  ( 19.65543155966253153, 85.76032626422811234, -5.359767647080686537 ) ) ;
#76461=CARTESIAN_POINT ( 'NONE',  ( 7.361572987183170547, 27.05059781766745175, 9.846743663894590881 ) ) ;
#76462=CARTESIAN_POINT ( 'NONE',  ( -2.816281873526473856, 59.12363466993042493, 9.499525473075851096E-16 ) ) ;
#76464=CARTESIAN_POINT ( 'NONE',  ( 17.20831665107776587, 47.88393115100078745, 7.208316651077764980 ) ) ;
#76465=CARTESIAN_POINT ( 'NONE',  ( 14.92337183194729633, 47.67559781766745175, 8.527530157486181039 ) ) ;
#76466=CARTESIAN_POINT ( 'NONE',  ( 24.16423886937410614, 44.51208216824730357, -3.795296366450302550 ) ) ;
#76468=CARTESIAN_POINT ( 'NONE',  ( 24.16423886937410614, 19.30374883491397142, 8.672049930838204340E-16 ) ) ;
#76469=CARTESIAN_POINT ( 'NONE',  ( 10.00000000000000000, 61.81368534415484106, -10.88017736071110342 ) ) ;
#76471=CARTESIAN_POINT ( 'NONE',  ( 24.16423886937410614, 54.51208216824730357, -3.795296366450302550 ) ) ;
#76472=CARTESIAN_POINT ( 'NONE',  ( 19.38216949554541557, 17.24863466993041783, -9.382169495545420901 ) ) ;
#76474=CARTESIAN_POINT ( 'NONE',  ( 4.559911319644449179, 68.89701867748817676, 9.422509992056141925 ) ) ;
#76477=CARTESIAN_POINT ( 'NONE',  ( 3.591859063236763294, 33.29030133659708213, -11.09922568453595026 ) ) ;
#76478=CARTESIAN_POINT ( 'NONE',  ( 2.917880565312950480, 60.97041550158063927, -12.26659068614894821 ) ) ;
#76480=CARTESIAN_POINT ( 'NONE',  ( 10.00000000000000000, 31.81368534415483751, -10.88017736071110342 ) ) ;
#76481=CARTESIAN_POINT ( 'NONE',  ( 20.88017736071110875, 20.77201867748816611, -2.915334737309920765 ) ) ;
#76482=CARTESIAN_POINT ( 'NONE',  ( 0.1532563361054100626, 55.80059781766745175, -2.638427012816831230 ) ) ;
#76483=CARTESIAN_POINT ( 'NONE',  ( 7.361572987183169658, 59.96726448433410894, -9.846743663894592657 ) ) ;
#76484=CARTESIAN_POINT ( 'NONE',  ( -2.816281873526473856, 54.33196800326376064, 3.434112377981055619 ) ) ;
#76487=AXIS2_PLACEMENT_3D ( 'NONE', #25149, #33103, #33586 ) ;
#76488=CARTESIAN_POINT ( 'NONE',  ( 4.559911319644449179, 13.89701867748817143, 9.422509992056141925 ) ) ;
#76489=CARTESIAN_POINT ( 'NONE',  ( 0.6178305044545818747, 23.49863466993041783, -9.382169495545419124 ) ) ;
#76490=CARTESIAN_POINT ( 'NONE',  ( 20.15039907845753575, 39.72266099184919597, 6.262539305110075283 ) ) ;
#76492=CARTESIAN_POINT ( 'NONE',  ( 1.472469842513823179, 51.42559781766745886, 4.923371831947296329 ) ) ;
#76493=CARTESIAN_POINT ( 'NONE',  ( 20.88017736071110875, 55.77201867748816966, -2.915334737309920765 ) ) ;
#76494=CARTESIAN_POINT ( 'NONE',  ( 19.38216949554541557, 22.24863466993041428, -9.382169495545420901 ) ) ;
#76495=CARTESIAN_POINT ( 'NONE',  ( 4.559911319644449179, 42.23035201082151247, -9.422509992056141925 ) ) ;
#76498=CARTESIAN_POINT ( 'NONE',  ( 0.6178305044545838731, 49.74863466993041072, 9.382169495545420901 ) ) ;
#76501=CARTESIAN_POINT ( 'NONE',  ( 19.42250999205614193, 50.14701867748817676, 5.440088680355555262 ) ) ;
#76502=CARTESIAN_POINT ( 'NONE',  ( 22.81628187352647785, 41.41530133659708923, 3.434112377981063169 ) ) ;
#76503=CARTESIAN_POINT ( 'NONE',  ( 24.16423886937410614, 19.30374883491397142, 8.672049930838204340E-16 ) ) ;
#76504=CARTESIAN_POINT ( 'NONE',  ( 10.00000000000000178, 7.258931151000785675, 9.846743663894594434 ) ) ;
#76505=CARTESIAN_POINT ( 'NONE',  ( -0.1503990784575328643, 70.00000000000000000, -6.262539305110068177 ) ) ;
#76506=CARTESIAN_POINT ( 'NONE',  ( 19.84674366389459266, 33.30059781766744464, 2.638427012816836559 ) ) ;
#76507=CARTESIAN_POINT ( 'NONE',  ( 19.84674366389459266, 8.717264484334116048, -2.638427012816827677 ) ) ;
#76509=CARTESIAN_POINT ( 'NONE',  ( -0.3689425029237881626, 37.42874883491396787, 10.36894250292379027 ) ) ;
#76510=CARTESIAN_POINT ( 'NONE',  ( 12.91533473730992121, 14.52201867748817143, 10.88017736071110164 ) ) ;
#76513=CARTESIAN_POINT ( 'NONE',  ( 17.96484262340118221, 14.93868534415484106, 7.964842623401181321 ) ) ;
#76514=CARTESIAN_POINT ( 'NONE',  ( 19.42250999205614548, 10.98035201082150536, -5.440088680355545492 ) ) ;
#76515=CARTESIAN_POINT ( 'NONE',  ( 0.1532563361054083140, 41.00893115100078745, 1.131784320476157264E-15 ) ) ;
#76517=CARTESIAN_POINT ( 'NONE',  ( 21.09922568453594849, 36.20696800326375353, 6.408140936763242479 ) ) ;
#76519=CARTESIAN_POINT ( 'NONE',  ( -4.164238869374099039, 11.80374883491396965, 8.674139862899312516E-16 ) ) ;
#76520=CARTESIAN_POINT ( 'NONE',  ( 2.035157376598822676, 32.43868534415483396, -7.964842623401177768 ) ) ;
#76521=CARTESIAN_POINT ( 'NONE',  ( 10.00000000000000000, 65.55374883491396076, -14.16423886937410082 ) ) ;
#76522=CARTESIAN_POINT ( 'NONE',  ( 0.1532563361054083140, 41.00893115100078745, 1.131784320476157264E-15 ) ) ;
#76524=CARTESIAN_POINT ( 'NONE',  ( 1.472469842513823179, 21.42559781766745175, 4.923371831947296329 ) ) ;
#76525=DIRECTION ( 'NONE',  ( 0.000000000000000000, 0.000000000000000000, -1.000000000000000000 ) ) ;
#76527=ORIENTED_EDGE ( 'NONE', *, *, #17730, .T. ) ;
#76531=CARTESIAN_POINT ( 'NONE',  ( 5.076628168052703671, 51.84226448433412315, 8.527530157486179263 ) ) ;
#76532=CARTESIAN_POINT ( 'NONE',  ( 0.5774900079438590739, 32.64701867748816966, -5.440088680355550821 ) ) ;
#76533=CARTESIAN_POINT ( 'NONE',  ( 10.00000000000000178, 39.31368534415484106, 10.88017736071110342 ) ) ;
#76534=( NAMED_UNIT ( * ) SI_UNIT ( $, .STERADIAN. ) SOLID_ANGLE_UNIT ( ) );
#76535=CARTESIAN_POINT ( 'NONE',  ( 19.38216949554541202, 30.99863466993042138, 9.382169495545424454 ) ) ;
#76536=CARTESIAN_POINT ( 'NONE',  ( -2.266590686148945544, 22.22041550158063572, 7.082119434687048631 ) ) ;
#76538=CARTESIAN_POINT ( 'NONE',  ( 16.40814093676323893, 50.79030133659708923, 11.09922568453595026 ) ) ;
#76540=CARTESIAN_POINT ( 'NONE',  ( 7.361572987183169658, 44.96726448433412315, -9.846743663894592657 ) ) ;
#76541=CARTESIAN_POINT ( 'NONE',  ( 10.00000000000000178, 24.31368534415484106, 10.88017736071110342 ) ) ;
#76543=CARTESIAN_POINT ( 'NONE',  ( 4.559911319644449179, 17.23035201082150536, -9.422509992056141925 ) ) ;
#76545=CARTESIAN_POINT ( 'NONE',  ( 17.96484262340118221, 56.18868534415484817, -7.964842623401177768 ) ) ;
#76546=SURFACE_STYLE_USAGE ( .BOTH. , #9528 ) ;
#76547=CARTESIAN_POINT ( 'NONE',  ( 18.72515096720570327, 6.072280503510315341, -6.499999999999985789 ) ) ;
#76548=CARTESIAN_POINT ( 'NONE',  ( -0.8801773607111008646, 53.27201867748816966, 2.915334737309923430 ) ) ;
#76549=CARTESIAN_POINT ( 'NONE',  ( -0.3289641300568005855, 29.27164270246084143, -5.963430220938281678 ) ) ;
#76550=CARTESIAN_POINT ( 'NONE',  ( -46.48928645636214441, 103.2957187381728232, 6.397878122523972699 ) ) ;
#76554=CARTESIAN_POINT ( 'NONE',  ( 0.1532563361054082862, 41.21726448433411605, 2.638427012816831674 ) ) ;
#76556=CARTESIAN_POINT ( 'NONE',  ( 7.361572987183170547, 67.05059781766746596, 9.846743663894590881 ) ) ;
#76558=B_SPLINE_CURVE_WITH_KNOTS ( 'NONE', 3,
 ( #6765, #7267, #82253, #37278, #45249, #75745 ),
 .UNSPECIFIED., .F., .F.,
 ( 4, 2, 4 ),
 ( 0.000000000000000000, 0.0002626113303184730917, 0.0005252226606369461833 ),
 .UNSPECIFIED. ) ;
#76560=CARTESIAN_POINT ( 'NONE',  ( 20.36894250292379738, 24.92874883491396787, -10.36894250292379027 ) ) ;
#76563=DIRECTION ( 'NONE',  ( 0.000000000000000000, -1.000000000000000000, 0.000000000000000000 ) ) ;
#76564=CARTESIAN_POINT ( 'NONE',  ( 4.559911319644449179, 57.23035201082150536, -9.422509992056141925 ) ) ;
#76565=CARTESIAN_POINT ( 'NONE',  ( 4.559911319644449179, 7.230352010821505360, -9.422509992056141925 ) ) ;
#76566=CARTESIAN_POINT ( 'NONE',  ( 0.6178305044545818747, 38.49863466993042493, -9.382169495545419124 ) ) ;
#76568=DIRECTION ( 'NONE',  ( 0.000000000000000000, 0.000000000000000000, 1.000000000000000000 ) ) ;
#76569=CARTESIAN_POINT ( 'NONE',  ( 10.00000000000000000, 27.87363466993042138, -12.81628187352647608 ) ) ;
#76570=CARTESIAN_POINT ( 'NONE',  ( 12.63842701281683922, 24.55059781766745175, -9.846743663894590881 ) ) ;
#76572=CARTESIAN_POINT ( 'NONE',  ( 19.38216949554541557, 17.24863466993041783, -9.382169495545420901 ) ) ;
#76574=CARTESIAN_POINT ( 'NONE',  ( 19.84674366389459266, 3.300597817667451750, 2.638427012816836559 ) ) ;
#76576=VERTEX_POINT ( 'NONE', #57277 ) ;
#76577=CARTESIAN_POINT ( 'NONE',  ( 2.035157376598824452, 18.68868534415484106, 7.964842623401179544 ) ) ;
#76578=CARTESIAN_POINT ( 'NONE',  ( 24.16423886937409904, 24.09541550158063927, 3.795296366450317205 ) ) ;
#76579=CARTESIAN_POINT ( 'NONE',  ( 12.63842701281683922, 34.55059781766745886, -9.846743663894590881 ) ) ;
#76580=CARTESIAN_POINT ( 'NONE',  ( 15.44008868035555260, 64.73035201082151957, 9.422509992056143702 ) ) ;
#76581=CARTESIAN_POINT ( 'NONE',  ( 21.09922568453594849, 46.20696800326376064, 6.408140936763242479 ) ) ;
#76583=CARTESIAN_POINT ( 'NONE',  ( 12.91533473730992121, 19.52201867748816611, 10.88017736071110164 ) ) ;
#76586=EDGE_CURVE ( 'NONE', #68599, #35522, #69079, .T. ) ;
#76587=CARTESIAN_POINT ( 'NONE',  ( 19.38216949554541557, 12.24863466993041961, -9.382169495545420901 ) ) ;
#76588=CARTESIAN_POINT ( 'NONE',  ( -2.816281873526471635, 13.91530133659708746, -3.434112377981056508 ) ) ;
#76589=CARTESIAN_POINT ( 'NONE',  ( 18.52753015748617571, 28.09226448433411960, 4.923371831947298993 ) ) ;
#76591=CARTESIAN_POINT ( 'NONE',  ( 21.09922568453595559, 32.04030133659708923, -6.408140936763230044 ) ) ;
#76592=CARTESIAN_POINT ( 'NONE',  ( 17.84635730667656262, 23.63791097397319518, 6.500000000000021316 ) ) ;
#76593=CARTESIAN_POINT ( 'NONE',  ( 4.559911319644449179, 58.89701867748817676, 9.422509992056141925 ) ) ;
#76598=CARTESIAN_POINT ( 'NONE',  ( 18.06765999051784988, 28.99127512925449324, 6.500000000000019540 ) ) ;
#76599=CARTESIAN_POINT ( 'NONE',  ( -0.8801773607111009756, 43.06368534415484106, 1.068504757029289695E-15 ) ) ;
#76600=CARTESIAN_POINT ( 'NONE',  ( 0.5774900079438607392, 48.48035201082150536, 5.440088680355550821 ) ) ;
#76603=CARTESIAN_POINT ( 'NONE',  ( -0.1298530154764001854, 80.39370036920264795, 9.500000000000000000 ) ) ;
#76604=CARTESIAN_POINT ( 'NONE',  ( 14.92337183194729633, 47.67559781766745175, 8.527530157486181039 ) ) ;
#76605=CARTESIAN_POINT ( 'NONE',  ( -0.8801773607111009756, 13.06368534415483929, 1.068504757029289695E-15 ) ) ;
#76606=CARTESIAN_POINT ( 'NONE',  ( 19.84674366389459266, 23.30059781766745530, 2.638427012816836559 ) ) ;
#76607=CARTESIAN_POINT ( 'NONE',  ( 21.09922568453594849, 11.20696800326375531, 6.408140936763242479 ) ) ;
#76609=CARTESIAN_POINT ( 'NONE',  ( 4.559911319644449179, 42.23035201082151247, -9.422509992056141925 ) ) ;
#76610=EDGE_CURVE ( 'NONE', #72980, #41390, #41968, .T. ) ;
#76611=CARTESIAN_POINT ( 'NONE',  ( 7.361572987183169658, 64.96726448433412315, -9.846743663894592657 ) ) ;
#76612=LINE ( 'NONE', #8128, #34965 ) ;
#76613=CARTESIAN_POINT ( 'NONE',  ( 2.035157376598822676, 7.438685344154837509, -7.964842623401177768 ) ) ;
#76614=CARTESIAN_POINT ( 'NONE',  ( -0.8801773607111009756, 23.06368534415484106, 1.068504757029289695E-15 ) ) ;
#76615=CARTESIAN_POINT ( 'NONE',  ( 22.26659068614895176, 34.72041550158063927, -7.082119434687042414 ) ) ;
#76616=CARTESIAN_POINT ( 'NONE',  ( 19.84674366389459266, 33.30059781766744464, 2.638427012816836559 ) ) ;
#76617=CARTESIAN_POINT ( 'NONE',  ( 0.5774900079438607392, 48.48035201082150536, 5.440088680355550821 ) ) ;
#76618=CARTESIAN_POINT ( 'NONE',  ( -4.164238869374098151, 1.595415501580634388, -3.795296366450310543 ) ) ;
#76620=CARTESIAN_POINT ( 'NONE',  ( 7.361572987183170547, 62.05059781766745886, 9.846743663894590881 ) ) ;
#76623=CARTESIAN_POINT ( 'NONE',  ( -0.3689425029237898834, 41.17874883491397497, -10.36894250292378850 ) ) ;
#76624=CARTESIAN_POINT ( 'NONE',  ( 17.08211943468705130, 28.47041550158063572, 12.26659068614894998 ) ) ;
#76625=CARTESIAN_POINT ( 'NONE',  ( 5.076628168052703671, 1.842264484334118047, 8.527530157486179263 ) ) ;
#76626=CARTESIAN_POINT ( 'NONE',  ( 16.40814093676323893, 10.79030133659708923, 11.09922568453595026 ) ) ;
#76627=CARTESIAN_POINT ( 'NONE',  ( 1.472469842513823179, 56.42559781766745886, 4.923371831947296329 ) ) ;
#76629=CARTESIAN_POINT ( 'NONE',  ( 7.084665262690076126, 57.02201867748817676, -10.88017736071110164 ) ) ;
#76630=CARTESIAN_POINT ( 'NONE',  ( -2.816281873526471635, 13.91530133659708746, -3.434112377981056508 ) ) ;
#76631=CARTESIAN_POINT ( 'NONE',  ( -4.164238869374098151, 26.59541550158063217, -3.795296366450310543 ) ) ;
#76632=CARTESIAN_POINT ( 'NONE',  ( 19.42250999205614548, 10.98035201082150536, -5.440088680355545492 ) ) ;
#76633=CARTESIAN_POINT ( 'NONE',  ( 20.88017736071110164, 30.35535201082151247, 2.915334737309930979 ) ) ;
#76635=CARTESIAN_POINT ( 'NONE',  ( 15.44008868035555793, 51.39701867748816966, -9.422509992056140149 ) ) ;
#76636=CARTESIAN_POINT ( 'NONE',  ( 16.40814093676324603, 52.45696800326375353, -11.09922568453594671 ) ) ;
#76639=PLANE ( 'NONE',  #74763 ) ;
#76643=CARTESIAN_POINT ( 'NONE',  ( 20.36894250292379738, 54.92874883491396076, -10.36894250292379027 ) ) ;
#76644=CARTESIAN_POINT ( 'NONE',  ( -2.266590686148945544, 66.38708216824730357, -7.082119434687050408 ) ) ;
#76645=CARTESIAN_POINT ( 'NONE',  ( 18.52753015748617571, 18.09226448433411960, 4.923371831947298993 ) ) ;
#76646=CARTESIAN_POINT ( 'NONE',  ( 18.52753015748618282, 63.92559781766745886, -4.923371831947291888 ) ) ;
#76651=CARTESIAN_POINT ( 'NONE',  ( 16.40814093676324603, 2.456968003263753531, -11.09922568453594671 ) ) ;
#76654=CARTESIAN_POINT ( 'NONE',  ( -4.164238869374099927, 37.01208216824731068, 3.795296366450308767 ) ) ;
#76655=CARTESIAN_POINT ( 'NONE',  ( 20.36894250292379738, 49.92874883491396787, -10.36894250292379027 ) ) ;
#76657=CARTESIAN_POINT ( 'NONE',  ( -2.816281873526473856, 59.12363466993042493, 9.499525473075851096E-16 ) ) ;
#76659=CARTESIAN_POINT ( 'NONE',  ( 12.91533473730992121, 29.52201867748817321, 10.88017736071110164 ) ) ;
#76660=CARTESIAN_POINT ( 'NONE',  ( 14.92337183194729988, 49.34226448433411605, -8.527530157486177487 ) ) ;
#76661=CARTESIAN_POINT ( 'NONE',  ( 20.88017736071110164, 20.35535201082150891, 2.915334737309930979 ) ) ;
#76664=CARTESIAN_POINT ( 'NONE',  ( 2.791683348922237240, 50.38393115100078035, -7.208316651077763204 ) ) ;
#76665=CARTESIAN_POINT ( 'NONE',  ( 17.20831665107776587, 54.13393115100079456, -7.208316651077762316 ) ) ;
#76670=CARTESIAN_POINT ( 'NONE',  ( 14.92337183194729988, 4.342264484334117824, -8.527530157486177487 ) ) ;
#76671=CARTESIAN_POINT ( 'NONE',  ( 18.29284471827480729, 60.40189080397281884, -6.499999999999946709 ) ) ;
#76673=CARTESIAN_POINT ( 'NONE',  ( 18.52753015748617571, 33.09226448433411605, 4.923371831947298993 ) ) ;
#76675=CARTESIAN_POINT ( 'NONE',  ( 21.09922568453595559, 42.04030133659708213, -6.408140936763230044 ) ) ;
#76676=EDGE_CURVE ( 'NONE', #29627, #90281, #86636, .T. ) ;
#76679=CARTESIAN_POINT ( 'NONE',  ( 5.076628168052704559, 65.17559781766745175, -8.527530157486179263 ) ) ;
#76681=CARTESIAN_POINT ( 'NONE',  ( 5.076628168052704559, 50.17559781766745886, -8.527530157486179263 ) ) ;
#76682=CARTESIAN_POINT ( 'NONE',  ( -2.266590686148945544, 37.22041550158063217, 7.082119434687048631 ) ) ;
#76683=CARTESIAN_POINT ( 'NONE',  ( 7.361572987183169658, 59.96726448433410894, -9.846743663894592657 ) ) ;
#76685=CARTESIAN_POINT ( 'NONE',  ( 14.92337183194729988, 14.34226448433411782, -8.527530157486177487 ) ) ;
#76686=CARTESIAN_POINT ( 'NONE',  ( 0.6178305044545818747, 53.49863466993041072, -9.382169495545419124 ) ) ;
#76687=CARTESIAN_POINT ( 'NONE',  ( 7.361572987183170547, 42.05059781766745886, 9.846743663894590881 ) ) ;
#76688=CARTESIAN_POINT ( 'NONE',  ( 4.559911319644449179, 47.23035201082150536, -9.422509992056141925 ) ) ;
#76689=CARTESIAN_POINT ( 'NONE',  ( 19.84674366389459266, 38.30059781766745175, 2.638427012816836559 ) ) ;
#76693=CARTESIAN_POINT ( 'NONE',  ( 20.88017736071110875, 60.77201867748817676, -2.915334737309920765 ) ) ;
#76696=CARTESIAN_POINT ( 'NONE',  ( 0.5774900079438590739, 22.64701867748817321, -5.440088680355550821 ) ) ;
#76698=CARTESIAN_POINT ( 'NONE',  ( 19.38216949554541202, 0.9986346699304200492, 9.382169495545424454 ) ) ;
#76699=CARTESIAN_POINT ( 'NONE',  ( 17.96484262340118221, 54.93868534415484106, 7.964842623401181321 ) ) ;
#76701=CARTESIAN_POINT ( 'NONE',  ( 17.39651004071841456, 14.08210964143329669, -6.500000000000003553 ) ) ;
#76702=CARTESIAN_POINT ( 'NONE',  ( 20.15039907845753220, 24.72266099184919241, 6.262539305110077947 ) ) ;
#76703=CARTESIAN_POINT ( 'NONE',  ( -0.8801773607111009756, 43.06368534415484106, 1.068504757029289695E-15 ) ) ;
#76705=CARTESIAN_POINT ( 'NONE',  ( 0.1532563361054083140, 41.00893115100078745, 1.131784320476157264E-15 ) ) ;
#76706=CARTESIAN_POINT ( 'NONE',  ( 13.99999999999999822, 60.50000000000000711, -6.500000000000000888 ) ) ;
#76708=CARTESIAN_POINT ( 'NONE',  ( 1.472469842513823179, 60.59226448433412315, -4.923371831947296329 ) ) ;
#76710=CARTESIAN_POINT ( 'NONE',  ( -0.8801773607110991993, 12.85535201082150358, -2.915334737309923874 ) ) ;
#76712=CARTESIAN_POINT ( 'NONE',  ( -4.164238869374099039, 21.80374883491396787, 8.674139862899312516E-16 ) ) ;
#76714=CARTESIAN_POINT ( 'NONE',  ( 13.79529636645031943, 55.34541550158062506, -14.16423886937409904 ) ) ;
#76715=CARTESIAN_POINT ( 'NONE',  ( 18.52753015748618282, 33.92559781766745886, -4.923371831947291888 ) ) ;
#76716=CARTESIAN_POINT ( 'NONE',  ( 7.361572987183170547, 17.05059781766745530, 9.846743663894590881 ) ) ;
#76717=CARTESIAN_POINT ( 'NONE',  ( 10.00000000000000000, 6.813685344154838397, -10.88017736071110342 ) ) ;
#76718=ORIENTED_EDGE ( 'NONE', *, *, #55889, .T. ) ;
#76719=CARTESIAN_POINT ( 'NONE',  ( 1.472469842513823179, 31.42559781766745530, 4.923371831947296329 ) ) ;
#76720=CARTESIAN_POINT ( 'NONE',  ( 20.88017736071110164, 25.35535201082150891, 2.915334737309930979 ) ) ;
#76721=CARTESIAN_POINT ( 'NONE',  ( 19.84674366389459266, 58.30059781766745886, 2.638427012816836559 ) ) ;
#76722=CARTESIAN_POINT ( 'NONE',  ( 24.16423886937409904, 14.09541550158063217, 3.795296366450317205 ) ) ;
#76724=CARTESIAN_POINT ( 'NONE',  ( 14.92337183194729988, 14.34226448433411782, -8.527530157486177487 ) ) ;
#76725=CARTESIAN_POINT ( 'NONE',  ( 13.43411237798106583, 42.66530133659707502, -12.81628187352647252 ) ) ;
#76726=CARTESIAN_POINT ( 'NONE',  ( 7.361572987183169658, 34.96726448433411605, -9.846743663894592657 ) ) ;
#76727=VERTEX_POINT ( 'NONE', #44246 ) ;
#76728=CARTESIAN_POINT ( 'NONE',  ( 5.076628168052703671, 26.84226448433411960, 8.527530157486179263 ) ) ;
#76730=DIRECTION ( 'NONE',  ( -0.000000000000000000, 1.000000000000000000, 0.000000000000000000 ) ) ;
#76731=CARTESIAN_POINT ( 'NONE',  ( 17.08211943468705130, 53.47041550158063217, 12.26659068614894998 ) ) ;
#76732=CARTESIAN_POINT ( 'NONE',  ( -0.8801773607111009756, 48.06368534415484817, 1.068504757029289695E-15 ) ) ;
#76734=CARTESIAN_POINT ( 'NONE',  ( 0.1532563361054100626, 30.80059781766744820, -2.638427012816831230 ) ) ;
#76735=CARTESIAN_POINT ( 'NONE',  ( -0.8801773607110991993, 7.855352010821504471, -2.915334737309923874 ) ) ;
#76736=CARTESIAN_POINT ( 'NONE',  ( 18.61655166652078108, 39.87718327197428891, 6.499999999999962697 ) ) ;
#76737=CARTESIAN_POINT ( 'NONE',  ( 10.00000000000000178, 52.25893115100078745, 9.846743663894594434 ) ) ;
#76739=CARTESIAN_POINT ( 'NONE',  ( 19.42250999205614193, 55.14701867748817676, 5.440088680355555262 ) ) ;
#76740=CARTESIAN_POINT ( 'NONE',  ( 1.472469842513823179, 1.425597817667451528, 4.923371831947296329 ) ) ;
#76746=CARTESIAN_POINT ( 'NONE',  ( 5.076628168052703671, 6.842264484334118713, 8.527530157486179263 ) ) ;
#76747=CARTESIAN_POINT ( 'NONE',  ( 10.00000000000000000, 62.87363466993042493, -12.81628187352647608 ) ) ;
#76748=CARTESIAN_POINT ( 'NONE',  ( 12.91533473730993009, 11.60535201082150714, -10.88017736071109987 ) ) ;
#76749=CARTESIAN_POINT ( 'NONE',  ( 17.20831665107776587, 44.13393115100078745, -7.208316651077762316 ) ) ;
#76751=CARTESIAN_POINT ( 'NONE',  ( 24.16423886937410614, 64.51208216824728936, -3.795296366450302550 ) ) ;
#76752=CARTESIAN_POINT ( 'NONE',  ( 19.84674366389459266, 58.30059781766745886, 2.638427012816836559 ) ) ;
#76755=CARTESIAN_POINT ( 'NONE',  ( 4.559911319644449179, 57.23035201082150536, -9.422509992056141925 ) ) ;
#76756=CARTESIAN_POINT ( 'NONE',  ( 12.63842701281683034, 17.46726448433411250, 9.846743663894596210 ) ) ;
#76759=CARTESIAN_POINT ( 'NONE',  ( 20.24186590665275531, 30.59014588040357197, -6.114288769123077394 ) ) ;
#76761=CARTESIAN_POINT ( 'NONE',  ( 19.84674366389459266, 8.717264484334116048, -2.638427012816827677 ) ) ;
#76763=CARTESIAN_POINT ( 'NONE',  ( 17.08211943468705840, 20.13708216824730357, -12.26659068614894466 ) ) ;
#76764=CARTESIAN_POINT ( 'NONE',  ( 10.00000000000000178, 17.25893115100078745, 9.846743663894594434 ) ) ;
#76765=CARTESIAN_POINT ( 'NONE',  ( 2.035157376598824452, 28.68868534415484106, 7.964842623401179544 ) ) ;
#76767=VERTEX_POINT ( 'NONE', #97781 ) ;
#76769=CARTESIAN_POINT ( 'NONE',  ( -0.8801773607110991993, 27.85535201082150181, -2.915334737309923874 ) ) ;
#76770=ADVANCED_FACE ( 'NONE', ( #14265 ), #3532, .T. ) ;
#76773=CARTESIAN_POINT ( 'NONE',  ( 20.88017736071110875, 35.77201867748816966, -2.915334737309920765 ) ) ;
#76774=CIRCLE ( 'NONE', #68795, 0.5000000000000004441 ) ;
#76775=CARTESIAN_POINT ( 'NONE',  ( 1.046131998950040387, 65.73810908735725889, 6.499999999999984901 ) ) ;
#76777=CARTESIAN_POINT ( 'NONE',  ( 10.00000000000000000, 12.87363466993042138, -12.81628187352647608 ) ) ;
#76778=CARTESIAN_POINT ( 'NONE',  ( 12.63842701281683922, 14.55059781766744997, -9.846743663894590881 ) ) ;
#76780=CARTESIAN_POINT ( 'NONE',  ( 18.72515096720569616, 10.05509018479935968, 6.500000000000001776 ) ) ;
#76781=CARTESIAN_POINT ( 'NONE',  ( 7.361572987183169658, 14.96726448433411960, -9.846743663894592657 ) ) ;
#76782=CARTESIAN_POINT ( 'NONE',  ( 12.91533473730992121, 29.52201867748817321, 10.88017736071110164 ) ) ;
#76783=ORIENTED_EDGE ( 'NONE', *, *, #28711, .T. ) ;
#76785=CARTESIAN_POINT ( 'NONE',  ( 22.81628187352647785, 61.62363466993041783, 6.195893100308588602E-16 ) ) ;
#76786=CARTESIAN_POINT ( 'NONE',  ( 20.88017736071110164, 60.35535201082151957, 2.915334737309930979 ) ) ;
#76787=CARTESIAN_POINT ( 'NONE',  ( -0.3289641300567998083, 23.07879003517447103, 5.963430220938281678 ) ) ;
#76788=CARTESIAN_POINT ( 'NONE',  ( -2.816281873526473856, 64.12363466993042493, 9.499525473075851096E-16 ) ) ;
#76789=CARTESIAN_POINT ( 'NONE',  ( 4.559911319644449179, 62.23035201082150536, -9.422509992056141925 ) ) ;
#76790=CARTESIAN_POINT ( 'NONE',  ( 21.09922568453594849, 1.206968003263753531, 6.408140936763242479 ) ) ;
#76793=CARTESIAN_POINT ( 'NONE',  ( 0.1532563361054100626, 35.80059781766745175, -2.638427012816831230 ) ) ;
#76794=CARTESIAN_POINT ( 'NONE',  ( -2.816281873526473856, 49.12363466993042493, 9.499525473075851096E-16 ) ) ;
#76796=CARTESIAN_POINT ( 'NONE',  ( 1.472469842513823179, 15.59226448433411960, -4.923371831947296329 ) ) ;
#76797=CARTESIAN_POINT ( 'NONE',  ( 13.43411237798105340, 20.58196800326374643, 12.81628187352647963 ) ) ;
#76800=CARTESIAN_POINT ( 'NONE',  ( 17.96484262340118221, 41.18868534415484106, -7.964842623401177768 ) ) ;
#76801=CARTESIAN_POINT ( 'NONE',  ( 6.565887622018943937, 0.1653013365970866511, 12.81628187352647430 ) ) ;
#76802=CARTESIAN_POINT ( 'NONE',  ( 1.472469842513823179, 25.59226448433412315, -4.923371831947296329 ) ) ;
#76803=CARTESIAN_POINT ( 'NONE',  ( 10.00000000000000000, 14.75893115100078568, -9.846743663894594434 ) ) ;
#76804=CARTESIAN_POINT ( 'NONE',  ( 2.035157376598822676, 12.43868534415483751, -7.964842623401177768 ) ) ;
#76805=CARTESIAN_POINT ( 'NONE',  ( -2.816281873526471635, 13.91530133659708746, -3.434112377981056508 ) ) ;
#76806=CARTESIAN_POINT ( 'NONE',  ( 0.5774900079438607392, 3.480352010821504027, 5.440088680355550821 ) ) ;
#76808=CARTESIAN_POINT ( 'NONE',  ( 10.00000000000000178, 62.25893115100078745, 9.846743663894594434 ) ) ;
#76809=( GEOMETRIC_REPRESENTATION_CONTEXT ( 3 ) GLOBAL_UNCERTAINTY_ASSIGNED_CONTEXT ( ( #91231 ) ) GLOBAL_UNIT_ASSIGNED_CONTEXT ( ( #1585, #69078, #94035 ) ) REPRESENTATION_CONTEXT ( 'NONE', 'WORKASPACE' ) );
#76811=CARTESIAN_POINT ( 'NONE',  ( 17.96484262340118221, 24.93868534415484461, 7.964842623401181321 ) ) ;
#76812=CARTESIAN_POINT ( 'NONE',  ( 19.84674366389459266, 48.30059781766745175, 2.638427012816836559 ) ) ;
#76813=CARTESIAN_POINT ( 'NONE',  ( 20.88017736071110164, 20.35535201082150891, 2.915334737309930979 ) ) ;
#76815=CARTESIAN_POINT ( 'NONE',  ( 12.91533473730992121, 34.52201867748817676, 10.88017736071110164 ) ) ;
#76816=CARTESIAN_POINT ( 'NONE',  ( 10.00000000000000000, 65.55374883491396076, -14.16423886937410082 ) ) ;
#76818=SURFACE_SIDE_STYLE ('',( #90333 ) ) ;
#76819=CARTESIAN_POINT ( 'NONE',  ( 12.63842701281683034, 27.46726448433411250, 9.846743663894596210 ) ) ;
#76820=CARTESIAN_POINT ( 'NONE',  ( 6.565887622018943937, 10.16530133659708746, 12.81628187352647430 ) ) ;
#76824=ADVANCED_FACE ( 'NONE', ( #88063 ), #45572, .T. ) ;
#76826=CARTESIAN_POINT ( 'NONE',  ( 13.79529636645031943, 5.345415501580634832, -14.16423886937409904 ) ) ;
#76828=CARTESIAN_POINT ( 'NONE',  ( 5.076628168052703671, 36.84226448433412315, 8.527530157486179263 ) ) ;
#76830=CARTESIAN_POINT ( 'NONE',  ( 17.08211943468705130, 48.47041550158063927, 12.26659068614894998 ) ) ;
#76831=CARTESIAN_POINT ( 'NONE',  ( 7.361572987183170547, 17.05059781766745530, 9.846743663894590881 ) ) ;
#76834=CARTESIAN_POINT ( 'NONE',  ( 4.559911319644449179, 42.23035201082151247, -9.422509992056141925 ) ) ;
#76835=CARTESIAN_POINT ( 'NONE',  ( 13.43411237798105340, 55.58196800326374643, 12.81628187352647963 ) ) ;
#76836=CARTESIAN_POINT ( 'NONE',  ( 17.96484262340118221, 21.18868534415483396, -7.964842623401177768 ) ) ;
#76838=CARTESIAN_POINT ( 'NONE',  ( 0.6178305044545818747, 48.49863466993042493, -9.382169495545419124 ) ) ;
#76839=CARTESIAN_POINT ( 'NONE',  ( 0.1532563361054082862, 61.21726448433412315, 2.638427012816831674 ) ) ;
#76840=CARTESIAN_POINT ( 'NONE',  ( 12.63842701281683922, 4.550597817667451750, -9.846743663894590881 ) ) ;
#76843=CARTESIAN_POINT ( 'NONE',  ( 2.562013731377108972, 0.5000000000000000000, -6.499999999999999112 ) ) ;
#76844=CARTESIAN_POINT ( 'NONE',  ( 22.26659068614895176, 59.72041550158063927, -7.082119434687042414 ) ) ;
#76845=CARTESIAN_POINT ( 'NONE',  ( -4.164238869374099927, 17.01208216824730357, 3.795296366450308767 ) ) ;
#76846=CARTESIAN_POINT ( 'NONE',  ( 20.88017736071110875, 20.77201867748816611, -2.915334737309920765 ) ) ;
#76847=CARTESIAN_POINT ( 'NONE',  ( 20.88017736071110875, 35.77201867748816966, -2.915334737309920765 ) ) ;
#76850=CARTESIAN_POINT ( 'NONE',  ( 4.559911319644449179, 68.89701867748817676, 9.422509992056141925 ) ) ;
#76851=CARTESIAN_POINT ( 'NONE',  ( 15.44008868035555793, 61.39701867748817676, -9.422509992056140149 ) ) ;
#76852=CARTESIAN_POINT ( 'NONE',  ( 16.40814093676323893, 20.79030133659708923, 11.09922568453595026 ) ) ;
#76853=CARTESIAN_POINT ( 'NONE',  ( 18.06765999051786409, 18.99127512925449679, 6.499999999999999112 ) ) ;
#76856=CARTESIAN_POINT ( 'NONE',  ( 7.361572987183170547, 12.05059781766744997, 9.846743663894590881 ) ) ;
#76857=CARTESIAN_POINT ( 'NONE',  ( 0.1532563361054100626, 35.80059781766745175, -2.638427012816831230 ) ) ;
#76858=ADVANCED_FACE ( 'NONE', ( #15075 ), #85287, .T. ) ;
#76859=CARTESIAN_POINT ( 'NONE',  ( 20.88017736071110519, 15.56368534415483751, 2.639326808657452039E-16 ) ) ;
#76860=CARTESIAN_POINT ( 'NONE',  ( 3.591859063236763294, 38.29030133659708923, -11.09922568453595026 ) ) ;
#76861=CARTESIAN_POINT ( 'NONE',  ( 19.84674366389459621, 8.508931151000785675, 7.409399052514197653E-17 ) ) ;
#76862=CARTESIAN_POINT ( 'NONE',  ( 2.035157376598824452, 13.68868534415483751, 7.964842623401179544 ) ) ;
#76863=CARTESIAN_POINT ( 'NONE',  ( 14.92337183194729633, 57.67559781766745886, 8.527530157486181039 ) ) ;
#76864=CARTESIAN_POINT ( 'NONE',  ( 19.84674366389459266, 33.71726448433410894, -2.638427012816827677 ) ) ;
#76865=CARTESIAN_POINT ( 'NONE',  ( 22.26659068614895176, 24.72041550158063572, -7.082119434687042414 ) ) ;
#76866=CARTESIAN_POINT ( 'NONE',  ( 10.00000000000000000, 31.81368534415483751, -10.88017736071110342 ) ) ;
#76867=CARTESIAN_POINT ( 'NONE',  ( 4.559911319644449179, 12.23035201082150536, -9.422509992056141925 ) ) ;
#76868=CARTESIAN_POINT ( 'NONE',  ( 15.44008868035555793, 26.39701867748817321, -9.422509992056140149 ) ) ;
#76869=CARTESIAN_POINT ( 'NONE',  ( 15.44008868035555260, 34.73035201082151247, 9.422509992056143702 ) ) ;
#76871=EDGE_CURVE ( 'NONE', #65586, #69353, #28320, .T. ) ;
#76872=CARTESIAN_POINT ( 'NONE',  ( 12.91533473730993009, 46.60535201082150536, -10.88017736071109987 ) ) ;
#76874=ORIENTED_EDGE ( 'NONE', *, *, #38798, .F. ) ;
#76875=CARTESIAN_POINT ( 'NONE',  ( 0.6178305044545838731, 59.74863466993041783, 9.382169495545420901 ) ) ;
#76876=CARTESIAN_POINT ( 'NONE',  ( 19.42250999205614548, 45.98035201082150536, -5.440088680355545492 ) ) ;
#76877=CARTESIAN_POINT ( 'NONE',  ( 0.5774900079438607392, 48.48035201082150536, 5.440088680355550821 ) ) ;
#76879=CARTESIAN_POINT ( 'NONE',  ( -0.8801773607111008646, 53.27201867748816966, 2.915334737309923430 ) ) ;
#76884=CARTESIAN_POINT ( 'NONE',  ( -4.164238869374099039, 61.80374883491397497, 8.674139862899312516E-16 ) ) ;
#76885=CARTESIAN_POINT ( 'NONE',  ( 12.91533473730993009, 61.60535201082150536, -10.88017736071109987 ) ) ;
#76886=CARTESIAN_POINT ( 'NONE',  ( 20.88017736071110164, 55.35535201082149825, 2.915334737309930979 ) ) ;
#76890=CARTESIAN_POINT ( 'NONE',  ( 0.1532563361054083140, 31.00893115100078390, 1.131784320476157264E-15 ) ) ;
#76892=CARTESIAN_POINT ( 'NONE',  ( 19.84674366389459266, 28.71726448433411960, -2.638427012816827677 ) ) ;
#76893=CARTESIAN_POINT ( 'NONE',  ( -0.8801773607111009756, 38.06368534415484106, 1.068504757029289695E-15 ) ) ;
#76894=CARTESIAN_POINT ( 'NONE',  ( 12.63842701281683034, 42.46726448433412315, 9.846743663894596210 ) ) ;
#76895=CARTESIAN_POINT ( 'NONE',  ( 20.10239578412226891, 2.633775574782959428, -6.340343622311910288 ) ) ;
#76896=CARTESIAN_POINT ( 'NONE',  ( 20.88017736071110164, 55.35535201082149825, 2.915334737309930979 ) ) ;
#76897=CARTESIAN_POINT ( 'NONE',  ( 20.88017736071110875, 50.77201867748817676, -2.915334737309920765 ) ) ;
#76898=SURFACE_STYLE_FILL_AREA ( #61398 ) ;
#76899=CARTESIAN_POINT ( 'NONE',  ( -4.164238869374099039, 51.80374883491396787, 8.674139862899312516E-16 ) ) ;
#76901=AXIS2_PLACEMENT_3D ( 'NONE', #5849, #98851, #60807 ) ;
#76903=CARTESIAN_POINT ( 'NONE',  ( 3.591859063236763294, 23.29030133659708568, -11.09922568453595026 ) ) ;
#76905=ORIENTED_EDGE ( 'NONE', *, *, #46967, .T. ) ;
#76906=CARTESIAN_POINT ( 'NONE',  ( -1.099225684535947600, 14.54030133659708568, 6.408140936763237150 ) ) ;
#76907=CARTESIAN_POINT ( 'NONE',  ( 17.96484262340118221, 21.18868534415483396, -7.964842623401177768 ) ) ;
#76908=CARTESIAN_POINT ( 'NONE',  ( 12.91533473730992121, 64.52201867748817676, 10.88017736071110164 ) ) ;
#76911=ORIENTED_EDGE ( 'NONE', *, *, #63010, .F. ) ;
#76913=CARTESIAN_POINT ( 'NONE',  ( 12.63842701281683922, 4.550597817667451750, -9.846743663894590881 ) ) ;
#76915=CARTESIAN_POINT ( 'NONE',  ( 2.791683348922240793, 51.63393115100078745, 7.208316651077764092 ) ) ;
#76916=CARTESIAN_POINT ( 'NONE',  ( 14.92337183194729988, 34.34226448433411605, -8.527530157486177487 ) ) ;
#76918=CARTESIAN_POINT ( 'NONE',  ( 0.1532563361054082862, 21.21726448433412315, 2.638427012816831674 ) ) ;
#76919=CARTESIAN_POINT ( 'NONE',  ( 21.92686044187656336, 56.97997603579417358, 3.195792623639536423 ) ) ;
#76921=CARTESIAN_POINT ( 'NONE',  ( 10.00000000000000178, 12.25893115100078568, 9.846743663894594434 ) ) ;
#76924=CARTESIAN_POINT ( 'NONE',  ( 2.791683348922237240, 40.38393115100078035, -7.208316651077763204 ) ) ;
#76925=EDGE_LOOP ( 'NONE', ( #8418, #18468, #60262, #8177 ) ) ;
#76926=B_SPLINE_CURVE_WITH_KNOTS ( 'NONE', 3,
 ( #63092, #26093, #56589, #9606, #64062, #47100, #9113, #24626, #33567, #86105 ),
 .UNSPECIFIED., .F., .F.,
 ( 4, 3, 3, 4 ),
 ( 2.023017827855918282E-17, 0.0006253016069560817305, 0.001250604074564927361, 0.002501455912506536129 ),
 .UNSPECIFIED. ) ;
#76928=CARTESIAN_POINT ( 'NONE',  ( 3.591859063236763294, 18.29030133659708568, -11.09922568453595026 ) ) ;
#76929=CARTESIAN_POINT ( 'NONE',  ( 19.42250999205614548, 55.98035201082150536, -5.440088680355545492 ) ) ;
#76930=CARTESIAN_POINT ( 'NONE',  ( 6.204703633549690345, 32.84541550158063927, 14.16423886937410082 ) ) ;
#76931=B_SPLINE_CURVE_WITH_KNOTS ( 'NONE', 3,
 ( #14316, #36808, #88812, #5815, #51309, #20326, #12808, #44785, #4349, #50820 ),
 .UNSPECIFIED., .F., .F.,
 ( 4, 2, 2, 2, 4 ),
 ( 3.632321844000487879E-16, 0.0002035700444593245724, 0.0004071400889182858829, 0.0008142801778362085581, 0.001628560355672053908 ),
 .UNSPECIFIED. ) ;
#76933=CARTESIAN_POINT ( 'NONE',  ( -4.164238869374099927, 42.01208216824728936, 3.795296366450308767 ) ) ;
#76934=CARTESIAN_POINT ( 'NONE',  ( 22.26659068614895176, 64.72041550158064638, -7.082119434687042414 ) ) ;
#76935=CARTESIAN_POINT ( 'NONE',  ( -2.266590686148945544, 26.38708216824730357, -7.082119434687050408 ) ) ;
#76936=CARTESIAN_POINT ( 'NONE',  ( -2.266590686148945544, 22.22041550158063572, 7.082119434687048631 ) ) ;
#76937=CARTESIAN_POINT ( 'NONE',  ( 19.72487221294570148, 35.71833443783938833, -6.500000000000010658 ) ) ;
#76938=DIRECTION ( 'NONE',  ( 0.000000000000000000, -1.000000000000000000, -0.000000000000000000 ) ) ;
#76939=LINE ( 'NONE', #39935, #56438 ) ;
#76940=CARTESIAN_POINT ( 'NONE',  ( 7.361572987183170547, 37.05059781766744464, 9.846743663894590881 ) ) ;
#76942=CARTESIAN_POINT ( 'NONE',  ( 17.96484262340118221, 21.18868534415483396, -7.964842623401177768 ) ) ;
#76945=CARTESIAN_POINT ( 'NONE',  ( 20.00000000000000711, 87.39023020535609021, -4.970182471799478918 ) ) ;
#76946=CARTESIAN_POINT ( 'NONE',  ( 17.20831665107776587, 39.13393115100079456, -7.208316651077762316 ) ) ;
#76947=CARTESIAN_POINT ( 'NONE',  ( -2.816281873526473856, 59.33196800326374643, 3.434112377981055619 ) ) ;
#76949=CARTESIAN_POINT ( 'NONE',  ( 10.00000000000000178, 37.25893115100078745, 9.846743663894594434 ) ) ;
#76950=CARTESIAN_POINT ( 'NONE',  ( 2.791683348922240793, 46.63393115100077324, 7.208316651077764092 ) ) ;
#76952=CARTESIAN_POINT ( 'NONE',  ( 13.79529636645030344, 43.26208216824730357, 14.16423886937410614 ) ) ;
#76953=ORIENTED_EDGE ( 'NONE', *, *, #36104, .T. ) ;
#76954=CARTESIAN_POINT ( 'NONE',  ( -0.3689425029237898834, 16.17874883491396076, -10.36894250292378850 ) ) ;
#76955=CARTESIAN_POINT ( 'NONE',  ( 4.559911319644449179, 63.89701867748817676, 9.422509992056141925 ) ) ;
#76957=CARTESIAN_POINT ( 'NONE',  ( 7.084665262690076126, 7.022018677488170546, -10.88017736071110164 ) ) ;
#76958=CARTESIAN_POINT ( 'NONE',  ( -2.816281873526473856, 9.331968003263753531, 3.434112377981055619 ) ) ;
#76960=CARTESIAN_POINT ( 'NONE',  ( 19.84674366389459266, 3.717264484334118713, -2.638427012816827677 ) ) ;
#76962=CARTESIAN_POINT ( 'NONE',  ( 0.1532563361054100626, 30.80059781766745175, -2.638427012816831230 ) ) ;
#76964=CARTESIAN_POINT ( 'NONE',  ( -2.266590686148945544, 61.38708216824730357, -7.082119434687050408 ) ) ;
#76966=CARTESIAN_POINT ( 'NONE',  ( 0.5774900079438607392, 23.48035201082150536, 5.440088680355550821 ) ) ;
#76967=CARTESIAN_POINT ( 'NONE',  ( 20.88017736071110519, 25.56368534415483751, 2.639326808657452039E-16 ) ) ;
#76968=CARTESIAN_POINT ( 'NONE',  ( 19.84674366389459266, 53.71726448433411605, -2.638427012816827677 ) ) ;
#76969=CARTESIAN_POINT ( 'NONE',  ( 17.20831665107776587, 59.13393115100078745, -7.208316651077762316 ) ) ;
#76970=CARTESIAN_POINT ( 'NONE',  ( 13.43411237798105340, 55.58196800326374643, 12.81628187352647963 ) ) ;
#76971=CARTESIAN_POINT ( 'NONE',  ( 7.361572987183170547, 2.050597817667451750, 9.846743663894590881 ) ) ;
#76972=VERTEX_POINT ( 'NONE', #97063 ) ;
#76974=CARTESIAN_POINT ( 'NONE',  ( 0.5774900079438590739, 22.64701867748817321, -5.440088680355550821 ) ) ;
#76975=CARTESIAN_POINT ( 'NONE',  ( -1.099225684535947600, 18.70696800326375353, -6.408140936763238038 ) ) ;
#76978=CARTESIAN_POINT ( 'NONE',  ( 5.076628168052703671, 41.84226448433411605, 8.527530157486179263 ) ) ;
#76979=CARTESIAN_POINT ( 'NONE',  ( 20.88017736071110875, 50.77201867748817676, -2.915334737309920765 ) ) ;
#76980=CARTESIAN_POINT ( 'NONE',  ( 21.09922568453594849, 21.20696800326375353, 6.408140936763242479 ) ) ;
#76981=CARTESIAN_POINT ( 'NONE',  ( 0.5774900079438590739, 57.64701867748817676, -5.440088680355550821 ) ) ;
#76983=CARTESIAN_POINT ( 'NONE',  ( -0.1023957841222410819, 50.13377557478298030, 6.340343622311920058 ) ) ;
#76984=AXIS2_PLACEMENT_3D ( 'NONE', #16072, #31550, #46559 ) ;
#76985=CARTESIAN_POINT ( 'NONE',  ( 3.591859063236761518, 64.95696800326376774, 11.09922568453594849 ) ) ;
#76989=CARTESIAN_POINT ( 'NONE',  ( 7.084665262690076126, 49.10535201082149825, 10.88017736071109987 ) ) ;
#76990=CARTESIAN_POINT ( 'NONE',  ( 21.09922568453595559, 47.04030133659708923, -6.408140936763230044 ) ) ;
#76991=CARTESIAN_POINT ( 'NONE',  ( 13.79529636645031943, 15.34541550158063750, -14.16423886937409904 ) ) ;
#76992=CARTESIAN_POINT ( 'NONE',  ( 14.92337183194729988, 9.342264484334119601, -8.527530157486177487 ) ) ;
#76994=CARTESIAN_POINT ( 'NONE',  ( 0.1532563361054083140, 66.00893115100079456, 1.131784320476157264E-15 ) ) ;
#76995=CARTESIAN_POINT ( 'NONE',  ( 2.791683348922237240, 15.38393115100078212, -7.208316651077763204 ) ) ;
#76997=CARTESIAN_POINT ( 'NONE',  ( 24.16423886937409904, 54.09541550158063217, 3.795296366450317205 ) ) ;
#76999=CARTESIAN_POINT ( 'NONE',  ( 20.88017736071110164, 5.355352010821502695, 2.915334737309930979 ) ) ;
#77002=ORIENTED_EDGE ( 'NONE', *, *, #63590, .F. ) ;
#77003=CARTESIAN_POINT ( 'NONE',  ( 19.42250999205614193, 10.14701867748816966, 5.440088680355555262 ) ) ;
#77004=CARTESIAN_POINT ( 'NONE',  ( -0.8801773607111008646, 8.272018677488171434, 2.915334737309923430 ) ) ;
#77006=CARTESIAN_POINT ( 'NONE',  ( 18.52753015748618282, 43.92559781766745175, -4.923371831947291888 ) ) ;
#77007=CARTESIAN_POINT ( 'NONE',  ( -2.816281873526471635, 38.91530133659708213, -3.434112377981056508 ) ) ;
#77010=CARTESIAN_POINT ( 'NONE',  ( 2.917880565312950480, 25.97041550158063572, -12.26659068614894821 ) ) ;
#77011=CARTESIAN_POINT ( 'NONE',  ( 7.084665262690076126, 22.02201867748817321, -10.88017736071110164 ) ) ;
#77012=CARTESIAN_POINT ( 'NONE',  ( 4.559911319644449179, 3.897018677488171434, 9.422509992056141925 ) ) ;
#77013=CARTESIAN_POINT ( 'NONE',  ( 7.361572987183170547, 37.05059781766744464, 9.846743663894590881 ) ) ;
#77014=EDGE_CURVE ( 'NONE', #84056, #38312, #86767, .T. ) ;
#77016=CARTESIAN_POINT ( 'NONE',  ( 14.92337183194729988, 19.34226448433411960, -8.527530157486177487 ) ) ;
#77017=CARTESIAN_POINT ( 'NONE',  ( 0.1532563361054100626, 0.8005978176674514168, -2.638427012816831230 ) ) ;
#77022=CARTESIAN_POINT ( 'NONE',  ( 12.63842701281683922, 54.55059781766745175, -9.846743663894590881 ) ) ;
#77023=CARTESIAN_POINT ( 'NONE',  ( 15.44008868035555793, 36.39701867748816966, -9.422509992056140149 ) ) ;
#77024=CARTESIAN_POINT ( 'NONE',  ( 0.5774900079438590739, 37.64701867748817676, -5.440088680355550821 ) ) ;
#77025=CARTESIAN_POINT ( 'NONE',  ( 12.91533473730992121, 4.522018677488169658, 10.88017736071110164 ) ) ;
#77026=CARTESIAN_POINT ( 'NONE',  ( 6.565887622018943937, 30.16530133659708568, 12.81628187352647430 ) ) ;
#77027=CARTESIAN_POINT ( 'NONE',  ( 20.36894250292379382, 23.67874883491397142, 10.36894250292379205 ) ) ;
#77028=ORIENTED_EDGE ( 'NONE', *, *, #72974, .F. ) ;
#77031=ADVANCED_FACE ( 'NONE', ( #49855 ), #97355, .T. ) ;
#77032=CARTESIAN_POINT ( 'NONE',  ( 3.591859063236761518, 44.95696800326376064, 11.09922568453594849 ) ) ;
#77033=EDGE_LOOP ( 'NONE', ( #9633, #911, #86848, #45471, #90791, #34879 ) ) ;
#77034=CARTESIAN_POINT ( 'NONE',  ( 12.63842701281683922, 39.55059781766744464, -9.846743663894590881 ) ) ;
#77035=CARTESIAN_POINT ( 'NONE',  ( 20.88017736071110875, 25.77201867748816966, -2.915334737309920765 ) ) ;
#77037=CARTESIAN_POINT ( 'NONE',  ( 0.5774900079438607392, 13.48035201082150358, 5.440088680355550821 ) ) ;
#77039=CARTESIAN_POINT ( 'NONE',  ( 20.88017736071110875, 55.77201867748816966, -2.915334737309920765 ) ) ;
#77040=CARTESIAN_POINT ( 'NONE',  ( 7.084665262690076126, 67.02201867748817676, -10.88017736071110164 ) ) ;
#77041=CARTESIAN_POINT ( 'NONE',  ( 19.42250999205614548, 65.98035201082151957, -5.440088680355545492 ) ) ;
#77042=CARTESIAN_POINT ( 'NONE',  ( 17.20831665107776587, 4.133931151000785675, -7.208316651077762316 ) ) ;
#77043=CARTESIAN_POINT ( 'NONE',  ( 4.559911319644449179, 62.23035201082150536, -9.422509992056141925 ) ) ;
#77045=CARTESIAN_POINT ( 'NONE',  ( 1.472469842513823179, 11.42559781766745175, 4.923371831947296329 ) ) ;
#77046=CARTESIAN_POINT ( 'NONE',  ( 5.076628168052703671, 11.84226448433411960, 8.527530157486179263 ) ) ;
#77047=CARTESIAN_POINT ( 'NONE',  ( 1.472469842513823179, 46.42559781766745175, 4.923371831947296329 ) ) ;
#77054=CARTESIAN_POINT ( 'NONE',  ( 22.26659068614895176, 19.72041550158063572, -7.082119434687042414 ) ) ;
#77055=CARTESIAN_POINT ( 'NONE',  ( 10.00000000000000178, 70.00000000000000000, 0.000000000000000000 ) ) ;
#77056=CYLINDRICAL_SURFACE ( 'NONE', #32235, 0.5000000000000004441 ) ;
#77057=CARTESIAN_POINT ( 'NONE',  ( 20.88017736071110164, 25.35535201082150891, 2.915334737309930979 ) ) ;
#77058=CARTESIAN_POINT ( 'NONE',  ( 0.2751277870542876980, 48.21833443783936701, 6.499999999999984901 ) ) ;
#77060=CARTESIAN_POINT ( 'NONE',  ( 1.472469842513823179, 0.5922644843341181575, -4.923371831947296329 ) ) ;
#77062=( NAMED_UNIT ( * ) SI_UNIT ( $, .STERADIAN. ) SOLID_ANGLE_UNIT ( ) );
#77063=CARTESIAN_POINT ( 'NONE',  ( 6.565887622018943937, 35.16530133659708923, 12.81628187352647430 ) ) ;
#77064=CARTESIAN_POINT ( 'NONE',  ( 14.92337183194729633, 17.67559781766745175, 8.527530157486181039 ) ) ;
#77065=CARTESIAN_POINT ( 'NONE',  ( 16.40814093676323893, 20.79030133659708923, 11.09922568453595026 ) ) ;
#77068=CARTESIAN_POINT ( 'NONE',  ( 19.84674366389459266, 3.717264484334118713, -2.638427012816827677 ) ) ;
#77071=CARTESIAN_POINT ( 'NONE',  ( -0.8801773607111009756, 28.06368534415484106, 1.068504757029289695E-15 ) ) ;
#77072=CARTESIAN_POINT ( 'NONE',  ( 22.26659068614894466, 23.88708216824730357, 7.082119434687054849 ) ) ;
#77073=CARTESIAN_POINT ( 'NONE',  ( 2.791683348922240793, 41.63393115100078745, 7.208316651077764092 ) ) ;
#77074=CARTESIAN_POINT ( 'NONE',  ( 7.084665262690076126, 67.02201867748817676, -10.88017736071110164 ) ) ;
#77075=CARTESIAN_POINT ( 'NONE',  ( -2.816281873526473856, 59.12363466993042493, 9.499525473075851096E-16 ) ) ;
#77077=CARTESIAN_POINT ( 'NONE',  ( 19.42250999205614548, 25.98035201082150891, -5.440088680355545492 ) ) ;
#77079=COLOUR_RGB ( '', 0.72549020, 0.75294118, 0.79215686) ;
#77080=CARTESIAN_POINT ( 'NONE',  ( -1.099225684535947600, 4.540301336597087456, 6.408140936763237150 ) ) ;
#77081=CARTESIAN_POINT ( 'NONE',  ( 7.361572987183170547, 47.05059781766745175, 9.846743663894590881 ) ) ;
#77083=CARTESIAN_POINT ( 'NONE',  ( 19.38216949554541557, 47.24863466993041783, -9.382169495545420901 ) ) ;
#77085=CARTESIAN_POINT ( 'NONE',  ( -0.8801773607111008646, 48.27201867748816966, 2.915334737309923430 ) ) ;
#77087=ADVANCED_FACE ( 'NONE', ( #65840 ), #26861, .T. ) ;
#77089=CARTESIAN_POINT ( 'NONE',  ( 4.559911319644449179, 52.23035201082151247, -9.422509992056141925 ) ) ;
#77091=CARTESIAN_POINT ( 'NONE',  ( 17.96484262340118221, 46.18868534415484106, -7.964842623401177768 ) ) ;
#77093=CARTESIAN_POINT ( 'NONE',  ( 7.084665262690076126, 69.10535201082151957, 10.88017736071109987 ) ) ;
#77094=CARTESIAN_POINT ( 'NONE',  ( 14.92337183194729633, 52.67559781766745175, 8.527530157486181039 ) ) ;
#77095=CARTESIAN_POINT ( 'NONE',  ( 7.084665262690076126, 12.02201867748817143, -10.88017736071110164 ) ) ;
#77097=CARTESIAN_POINT ( 'NONE',  ( -1.099225684535947600, 19.54030133659708568, 6.408140936763237150 ) ) ;
#77099=CARTESIAN_POINT ( 'NONE',  ( 10.00000000000000000, 36.81368534415484106, -10.88017736071110342 ) ) ;
#77100=CARTESIAN_POINT ( 'NONE',  ( 22.81628187352647785, 1.415301336597087012, 3.434112377981063169 ) ) ;
#77101=CARTESIAN_POINT ( 'NONE',  ( 20.10239578412226180, 47.63377557478296609, -6.340343622311913840 ) ) ;
#77102=CARTESIAN_POINT ( 'NONE',  ( 4.559911319644449179, 17.23035201082150536, -9.422509992056141925 ) ) ;
#77103=CARTESIAN_POINT ( 'NONE',  ( 19.42250999205614193, 30.14701867748817321, 5.440088680355555262 ) ) ;
#77104=CARTESIAN_POINT ( 'NONE',  ( 17.08211943468705130, 33.47041550158063927, 12.26659068614894998 ) ) ;
#77105=CARTESIAN_POINT ( 'NONE',  ( 19.84674366389459266, 28.30059781766745886, 2.638427012816836559 ) ) ;
#77106=CARTESIAN_POINT ( 'NONE',  ( -0.8801773607111009756, 58.06368534415484106, 1.068504757029289695E-15 ) ) ;
#77108=CARTESIAN_POINT ( 'NONE',  ( -2.266590686148945544, 2.220415501580634388, 7.082119434687048631 ) ) ;
#77110=CARTESIAN_POINT ( 'NONE',  ( 17.20831665107776587, 64.13393115100079456, -7.208316651077762316 ) ) ;
#77112=CARTESIAN_POINT ( 'NONE',  ( 20.36894250292379382, 28.67874883491396787, 10.36894250292379205 ) ) ;
#77113=CARTESIAN_POINT ( 'NONE',  ( -4.164238869374099927, 32.01208216824730357, 3.795296366450308767 ) ) ;
#77115=CARTESIAN_POINT ( 'NONE',  ( 17.20831665107776587, 2.883931151000785231, 7.208316651077764980 ) ) ;
#77116=CARTESIAN_POINT ( 'NONE',  ( 22.81628187352648496, 6.831968003263753531, -3.434112377981050290 ) ) ;
#77117=CARTESIAN_POINT ( 'NONE',  ( 19.84674366389459266, 63.30059781766745886, 2.638427012816836559 ) ) ;
#77119=CARTESIAN_POINT ( 'NONE',  ( 2.035157376598824452, 63.68868534415484106, 7.964842623401179544 ) ) ;
#77120=CARTESIAN_POINT ( 'NONE',  ( 6.565887622018943937, 25.16530133659708213, 12.81628187352647430 ) ) ;
#77121=CARTESIAN_POINT ( 'NONE',  ( 17.08211943468705130, 33.47041550158063927, 12.26659068614894998 ) ) ;
#77122=CARTESIAN_POINT ( 'NONE',  ( 2.035157376598822676, 32.43868534415483396, -7.964842623401177768 ) ) ;
#77124=CARTESIAN_POINT ( 'NONE',  ( 15.44008868035555260, 34.73035201082151247, 9.422509992056143702 ) ) ;
#77127=CARTESIAN_POINT ( 'NONE',  ( 20.88017736071110164, 50.35535201082151247, 2.915334737309930979 ) ) ;
#77131=CARTESIAN_POINT ( 'NONE',  ( 17.39651004071838969, 54.08210964143329846, -6.500000000000027534 ) ) ;
#77133=DIRECTION ( 'NONE',  ( -0.000000000000000000, 1.000000000000000000, -0.000000000000000000 ) ) ;
#77135=CARTESIAN_POINT ( 'NONE',  ( 22.26659068614894466, 3.887082168247300906, 7.082119434687054849 ) ) ;
#77136=CARTESIAN_POINT ( 'NONE',  ( 24.16423886937410614, 59.30374883491397497, 8.672049930838204340E-16 ) ) ;
#77137=CARTESIAN_POINT ( 'NONE',  ( -4.164238869374099039, 66.80374883491396076, 8.674139862899312516E-16 ) ) ;
#77138=CARTESIAN_POINT ( 'NONE',  ( 12.63842701281683922, 39.55059781766744464, -9.846743663894590881 ) ) ;
#77139=CARTESIAN_POINT ( 'NONE',  ( 5.076628168052703671, 56.84226448433412315, 8.527530157486179263 ) ) ;
#77140=CARTESIAN_POINT ( 'NONE',  ( 19.89220837332778657, 49.74062864464239908, 6.478736007405907493 ) ) ;
#77141=CARTESIAN_POINT ( 'NONE',  ( -2.816281873526471635, 8.915301336597083903, -3.434112377981056508 ) ) ;
#77143=CARTESIAN_POINT ( 'NONE',  ( 17.08211943468705840, 45.13708216824730357, -12.26659068614894466 ) ) ;
#77144=CARTESIAN_POINT ( 'NONE',  ( 24.16423886937410614, 44.51208216824730357, -3.795296366450302550 ) ) ;
#77146=CARTESIAN_POINT ( 'NONE',  ( 7.084665262690076126, 24.10535201082150181, 10.88017736071109987 ) ) ;
#77147=CARTESIAN_POINT ( 'NONE',  ( 13.43411237798106583, 62.66530133659708923, -12.81628187352647252 ) ) ;
#77148=ADVANCED_FACE ( 'NONE', ( #80855 ), #21344, .T. ) ;
#77149=CARTESIAN_POINT ( 'NONE',  ( 7.361572987183170547, 52.05059781766745175, 9.846743663894590881 ) ) ;
#77150=CARTESIAN_POINT ( 'NONE',  ( 7.084665262690076126, 32.02201867748816966, -10.88017736071110164 ) ) ;
#77152=CARTESIAN_POINT ( 'NONE',  ( 1.472469842513823179, 55.59226448433412315, -4.923371831947296329 ) ) ;
#77154=CARTESIAN_POINT ( 'NONE',  ( 15.44008868035555793, 21.39701867748817321, -9.422509992056140149 ) ) ;
#77160=PRESENTATION_STYLE_ASSIGNMENT (( #8668 ) ) ;
#77164=CARTESIAN_POINT ( 'NONE',  ( 10.00000000000000000, 29.75893115100078745, -9.846743663894594434 ) ) ;
#77166=CARTESIAN_POINT ( 'NONE',  ( 10.00000000000000000, 47.87363466993042493, -12.81628187352647608 ) ) ;
#77167=B_SPLINE_CURVE_WITH_KNOTS ( 'NONE', 3,
 ( #79420, #59357, #65377, #36372 ),
 .UNSPECIFIED., .F., .F.,
 ( 4, 4 ),
 ( 1.110764993427085326E-17, 0.0003904528506838490006 ),
 .UNSPECIFIED. ) ;
#77170=CARTESIAN_POINT ( 'NONE',  ( 0.1532563361054100626, 65.80059781766745175, -2.638427012816831230 ) ) ;
#77172=CARTESIAN_POINT ( 'NONE',  ( 5.076628168052704559, 60.17559781766745175, -8.527530157486179263 ) ) ;
#77173=CARTESIAN_POINT ( 'NONE',  ( 24.16423886937410614, 44.30374883491397497, 8.672049930838204340E-16 ) ) ;
#77174=CARTESIAN_POINT ( 'NONE',  ( 18.52753015748617571, 63.09226448433412315, 4.923371831947298993 ) ) ;
#77176=CARTESIAN_POINT ( 'NONE',  ( 19.84674366389459266, 13.30059781766745353, 2.638427012816836559 ) ) ;
#77177=CARTESIAN_POINT ( 'NONE',  ( 10.00000000000000000, 52.87363466993041783, -12.81628187352647608 ) ) ;
#77178=CARTESIAN_POINT ( 'NONE',  ( 2.791683348922237240, 55.38393115100078745, -7.208316651077763204 ) ) ;
#77179=CARTESIAN_POINT ( 'NONE',  ( 12.91533473730992121, 49.52201867748817676, 10.88017736071110164 ) ) ;
#77180=CARTESIAN_POINT ( 'NONE',  ( 20.15039907845753575, 39.72266099184919597, 6.262539305110075283 ) ) ;
#77185=CARTESIAN_POINT ( 'NONE',  ( 4.559911319644449179, 33.89701867748817676, 9.422509992056141925 ) ) ;
#77186=CARTESIAN_POINT ( 'NONE',  ( 21.09922568453594849, 6.206968003263753531, 6.408140936763242479 ) ) ;
#77187=CARTESIAN_POINT ( 'NONE',  ( 15.44008868035555260, 59.73035201082151247, 9.422509992056143702 ) ) ;
#77193=CARTESIAN_POINT ( 'NONE',  ( 17.96484262340118221, 41.18868534415484106, -7.964842623401177768 ) ) ;
#77195=CARTESIAN_POINT ( 'NONE',  ( 5.076628168052703671, 31.84226448433412315, 8.527530157486179263 ) ) ;
#77196=CARTESIAN_POINT ( 'NONE',  ( 7.361572987183170547, 2.050597817667451750, 9.846743663894590881 ) ) ;
#77199=CARTESIAN_POINT ( 'NONE',  ( 22.81628187352647785, 11.41530133659708390, 3.434112377981063169 ) ) ;
#77200=CARTESIAN_POINT ( 'NONE',  ( 20.88017736071110875, 10.77201867748817143, -2.915334737309920765 ) ) ;
#77202=CARTESIAN_POINT ( 'NONE',  ( 10.00000000000000178, 18.05374883491396787, 14.16423886937410082 ) ) ;
#77204=CARTESIAN_POINT ( 'NONE',  ( 6.204703633549690345, 65.76208216824731778, -14.16423886937410259 ) ) ;
#77205=CARTESIAN_POINT ( 'NONE',  ( 2.791683348922240793, 11.63393115100078568, 7.208316651077764092 ) ) ;
#77206=SURFACE_SIDE_STYLE ('',( #46706 ) ) ;
#77208=CARTESIAN_POINT ( 'NONE',  ( 19.84674366389459621, 28.50893115100078745, 7.409399052514197653E-17 ) ) ;
#77209=CARTESIAN_POINT ( 'NONE',  ( -0.8801773607110991993, 27.85535201082150181, -2.915334737309923874 ) ) ;
#77210=CARTESIAN_POINT ( 'NONE',  ( 19.84674366389459266, 58.71726448433411605, -2.638427012816827677 ) ) ;
#77211=CARTESIAN_POINT ( 'NONE',  ( 22.26659068614895176, 14.72041550158063572, -7.082119434687042414 ) ) ;
#77212=CARTESIAN_POINT ( 'NONE',  ( 17.39651004071841456, 49.08210964143329136, -6.500000000000001776 ) ) ;
#77215=CARTESIAN_POINT ( 'NONE',  ( 5.076628168052703671, 16.84226448433411960, 8.527530157486179263 ) ) ;
#77216=CARTESIAN_POINT ( 'NONE',  ( 22.81628187352647785, 31.41530133659709279, 3.434112377981063169 ) ) ;
#77217=CARTESIAN_POINT ( 'NONE',  ( 14.92337183194729988, 39.34226448433412315, -8.527530157486177487 ) ) ;
#77219=CARTESIAN_POINT ( 'NONE',  ( 2.791683348922237240, 15.38393115100078212, -7.208316651077763204 ) ) ;
#77220=CARTESIAN_POINT ( 'NONE',  ( 19.50000000000000355, 79.40087001978915282, -5.000000000000000000 ) ) ;
#77222=CARTESIAN_POINT ( 'NONE',  ( 17.08211943468705840, 60.13708216824729647, -12.26659068614894466 ) ) ;
#77224=CARTESIAN_POINT ( 'NONE',  ( 19.42250999205614548, 55.98035201082150536, -5.440088680355545492 ) ) ;
#77225=CARTESIAN_POINT ( 'NONE',  ( 19.84674366389459266, 33.71726448433410894, -2.638427012816827677 ) ) ;
#77226=CARTESIAN_POINT ( 'NONE',  ( 15.44008868035555260, 19.73035201082150536, 9.422509992056143702 ) ) ;
#77228=CARTESIAN_POINT ( 'NONE',  ( 5.076628168052704559, 55.17559781766745175, -8.527530157486179263 ) ) ;
#77229=CARTESIAN_POINT ( 'NONE',  ( 17.96484262340118221, 44.93868534415483396, 7.964842623401181321 ) ) ;
#77230=( NAMED_UNIT ( * ) SI_UNIT ( $, .STERADIAN. ) SOLID_ANGLE_UNIT ( ) );
#77232=ORIENTED_EDGE ( 'NONE', *, *, #59426, .F. ) ;
#77233=CARTESIAN_POINT ( 'NONE',  ( 19.50000000000000711, 105.0000000000000000, -5.000000000000000000 ) ) ;
#77236=CARTESIAN_POINT ( 'NONE',  ( 1.472469842513823179, 46.42559781766745175, 4.923371831947296329 ) ) ;
#77237=CARTESIAN_POINT ( 'NONE',  ( 14.92337183194729633, 17.67559781766745175, 8.527530157486181039 ) ) ;
#77238=CARTESIAN_POINT ( 'NONE',  ( -2.816281873526473856, 59.12363466993042493, 9.499525473075851096E-16 ) ) ;
#77239=CARTESIAN_POINT ( 'NONE',  ( 17.96484262340118221, 16.18868534415483396, -7.964842623401177768 ) ) ;
#77240=CARTESIAN_POINT ( 'NONE',  ( 14.92337183194729633, 52.67559781766745175, 8.527530157486181039 ) ) ;
#77242=CARTESIAN_POINT ( 'NONE',  ( 24.16423886937410614, 54.51208216824730357, -3.795296366450302550 ) ) ;
#77243=CARTESIAN_POINT ( 'NONE',  ( 18.52753015748617571, 63.09226448433412315, 4.923371831947298993 ) ) ;
#77245=CARTESIAN_POINT ( 'NONE',  ( 2.035157376598824452, 48.68868534415483396, 7.964842623401179544 ) ) ;
#77247=CARTESIAN_POINT ( 'NONE',  ( 10.00000000000000000, 14.75893115100078568, -9.846743663894594434 ) ) ;
#77248=LINE ( 'NONE', #39273, #82901 ) ;
#77250=CARTESIAN_POINT ( 'NONE',  ( 0.000000000000000000, 0.5000000000000000000, 6.000000000000000000 ) ) ;
#77252=CARTESIAN_POINT ( 'NONE',  ( 7.361572987183170547, 12.05059781766744997, 9.846743663894590881 ) ) ;
#77254=CARTESIAN_POINT ( 'NONE',  ( 24.16423886937409904, 14.09541550158063217, 3.795296366450317205 ) ) ;
#77255=CARTESIAN_POINT ( 'NONE',  ( 2.791683348922240793, 16.63393115100078745, 7.208316651077764092 ) ) ;
#77256=CARTESIAN_POINT ( 'NONE',  ( 10.00000000000000178, 39.31368534415484106, 10.88017736071110342 ) ) ;
#77258=CARTESIAN_POINT ( 'NONE',  ( 2.035157376598824452, 28.68868534415484106, 7.964842623401179544 ) ) ;
#77260=ORIENTED_EDGE ( 'NONE', *, *, #14357, .T. ) ;
#77261=CARTESIAN_POINT ( 'NONE',  ( 2.917880565312950480, 5.970415501580634832, -12.26659068614894821 ) ) ;
#77264=CARTESIAN_POINT ( 'NONE',  ( -2.816281873526471635, 23.91530133659708568, -3.434112377981056508 ) ) ;
#77265=CARTESIAN_POINT ( 'NONE',  ( 0.1532563361054083140, 16.00893115100078390, 1.131784320476157264E-15 ) ) ;
#77268=CARTESIAN_POINT ( 'NONE',  ( 10.00000000000000178, 12.25893115100078568, 9.846743663894594434 ) ) ;
#77269=CARTESIAN_POINT ( 'NONE',  ( 2.035157376598822676, 27.43868534415483396, -7.964842623401177768 ) ) ;
#77271=ORIENTED_EDGE ( 'NONE', *, *, #456, .F. ) ;
#77274=CARTESIAN_POINT ( 'NONE',  ( 7.084665262690076126, 57.02201867748817676, -10.88017736071110164 ) ) ;
#77275=CARTESIAN_POINT ( 'NONE',  ( 1.274849032794116210, 8.572280503510292249, 6.499999999999738876 ) ) ;
#77276=CARTESIAN_POINT ( 'NONE',  ( 0.6178305044545818747, 63.49863466993043204, -9.382169495545419124 ) ) ;
#77277=CARTESIAN_POINT ( 'NONE',  ( 17.96484262340118221, 66.18868534415483396, -7.964842623401177768 ) ) ;
#77278=CARTESIAN_POINT ( 'NONE',  ( 18.52753015748618282, 63.92559781766745886, -4.923371831947291888 ) ) ;
#77279=CARTESIAN_POINT ( 'NONE',  ( 20.15039907845753930, 70.00000000000000000, 6.262539305110068177 ) ) ;
#77280=ADVANCED_FACE ( 'NONE', ( #5848 ), #36339, .F. ) ;
#77281=CARTESIAN_POINT ( 'NONE',  ( 7.361572987183170547, 27.05059781766745175, 9.846743663894590881 ) ) ;
#77282=CARTESIAN_POINT ( 'NONE',  ( 16.40814093676323893, 55.79030133659708923, 11.09922568453595026 ) ) ;
#77284=CARTESIAN_POINT ( 'NONE',  ( 0.1532563361054100626, 15.80059781766745353, -2.638427012816831230 ) ) ;
#77285=( BOUNDED_SURFACE ( )  B_SPLINE_SURFACE ( 1, 2, ( 
 ( #17059, #25059, #85547, #17554, #64490, #55028, #10043, #55543, #26029, #39562, #32532, #79018, #24567, #3530, #47037, #94998, #86041, #94509, #40544, #78532, #26505, #87012, #77533, #56038, #62528, #33023, #71044, #2567, #63520, #47540, #41039, #3046, #9541, #94024, #9050, #33500, #33989, #18036, #71539, #70052, #48515, #93032, #25546, #63030, #10528, #40045, #70545, #18521, #2070, #93528, #56522, #49012, #79518, #11019, #72003, #85049, #16563, #1575, #32024, #80988, #49494, #58473, #4515, #13479, #5987, #35482, #26996, #66474, #80503, #57494, #87989, #36480, #95504, #19501, #97003, #65977, #34980, #66973, #58975, #20491, #42025, #50489, #88986, #50978, #96503, #97492, #28479, #57002, #12488, #49996, #81473, #27977, #12976, #73973, #12000, #89474, #19989, #42989, #43471, #19017, #87503, #27486, #5499, #73471, #42503, #43959, #5000, #35973, #51474, #79999, #11503, #96004, #20989, #81965, #74460, #72490, #4023, #65479, #72986, #34485, #64980, #57979, #88486, #98489, #69437, #28958, #67469, #7960, #13985, #21984, #59953, #97990, #91937, #22468, #68462, #29945, #67966, #53941, #98984, #29446, #83455, #89962, #30436, #6465, #75950, #14977, #60449, #90940, #90444, #83947, #45956, #52458, #45447, #21478, #76444, #76930, #60937, #15473, #51978, #91446, #36972, #52945, #6969, #7476, #82962, #14478, #61429, #44951, #75455, #68951, #38456, #37476, #37973, #22971, #8440, #53438, #482, #59461, #30929, #82464, #23466, #84448, #15945, #38946, #46437, #44459, #74962, #24442, #1454, #31906, #48886, #39442, #62406, #10411, #9924, #47411, #10903, #2934, #63399, #84930, #93411, #2444, #93905, #78405, #79398, #71418, #957, #55416, #92913, #32900, #70924, #40428, #17915, #69935, #33381, #62909, #24934, #25431, #61921, #41425, #70427, #55915, #85923, #85422, #86894, #17433, #78902, #94390, #92424, #31418, #39925, #47901, #86414, #48399, #40918, #18404, #77913, #54909, #63878, #25906, #16932, #56408, #1946, #23949, #54419, #9422, #16442, #46918, #32408, #77411, #8926, #35856, #65359, #12369, #42385, #11882, #96883, #42875, #11387, #27368, #89355, #33868, #51356, #72862, #81358, #57861, #34866, #81841, #73852, #88372, #20865, #64375, #13355, #4397, #12856, #19867, #95888, #71886, #5382, #94884, #73358, #49380, #50362, #80871, #4885, #35363, #41908, #27856, #88863, #72370, #65856, #26383, #20372, #3406, #96384, #58343, #56882, #50866, #79881, #43354, #49868, #66345, #3901, #26880, #28360, #34369, #64859, #58849, #87385, #80381, #18903, #95379, #57373, #87868, #19384, #84337, #67850, #36354, #45332, #90323, #366, #91825, #22353, #13858, #53321 ),
 ( #21861, #60334, #60820, #6344, #52341, #75332, #98368, #91319, #52828, #29332, #45840, #68835, #66850, #14859, #29824, #82836, #75831, #90827, #37853, #83335, #23343, #97369, #44826, #83828, #14356, #6845, #36855, #30814, #7352, #37357, #28837, #44338, #74843, #61313, #68343, #98864, #30318, #22847, #51850, #21357, #15355, #76324, #7843, #82338, #38340, #53825, #43840, #59830, #67346, #74336, #5861, #59339, #89842, #97872, #47290, #2325, #33268, #55797, #46806, #93290, #77298, #69323, #61804, #24326, #63762, #40795, #92798, #85307, #9302, #24814, #63278, #40301, #54790, #70809, #2816, #32779, #94269, #55290, #16813, #32284, #93782, #8811, #77792, #39812, #70314, #25312, #85800, #1342, #17800, #71297, #8326, #17313, #1831, #62790, #47789, #78287, #9802, #86292, #25792, #38830, #48276, #78789, #62291, #10296, #39323, #56289, #15839, #46324, #844, #84816, #16322, #76811, #31303, #92311, #23837, #54302, #69818, #31793, #49745, #11759, #4765, #26266, #42267, #80254, #19752, #72255, #56765, #88739, #80752, #20250, #5259, #35738, #19261, #73236, #66226, #27738, #18783, #65234, #49266, #41302, #33749, #79766, #35236, #71775, #72737, #95759, #27244, #58220, #41783, #26757, #3786, #12736, #11264, #57251, #87261, #4271, #96760, #34241, #34743, #87747, #50751, #3285, #64739, #12247, #95252, #57741, #18287, #42754, #65733, #81237, #88243, #50237, #43234, #73730, #96260, #28236, #86785, #94766, #48769, #79276, #10783, #64249, #67229, #30199, #60702, #51738, #68232, #51235, #81720, #97257, #37730, #89722, #97752, #59218, #90211, #38224, #28727, #82717, #29216, #98749, #13233, #6235, #52711, #21237, #37241, #89235, #83217, #7226, #53209, #82221, #36737, #15232, #91199, #13734, #29706, #14236, #66733, #59716, #76213, #68710, #21743, #52225, #22726, #83712, #44218, #45713, #43729, #74215, #74722, #7728, #44716, #242, #58731, #75214, #6726, #67731, #98247, #20744, #14740, #60215, #45214, #5747, #75713, #36237, #90709, #22234, #62168, #3064, #732, #8690, #39205, #1223, #33518, #24201, #54182, #87025, #79534, #91706, #18052, #31676, #69691, #10543, #92674, #41053, #54668, #34010, #23225, #85186, #26046, #84696, #48529, #31186, #11034, #71552, #64014, #53696, #38708, #69207, #41556, #94526, #56536, #18537, #49028, #76693, #8214, #72020, #64507, #30690, #61680, #61198, #15725, #92197, #37074, #90057, #54876, #45548, #16900, #39891, #70394, #52553, #38063, #62876, #62372, #82563, #30040, #14079, #36579, #97593, #44559, #68555, #29054, #83057, #60548, #91041, #92876, #75056, #22078, #98084, #9387, #29542, #75554, #21580, #7070, #82062, #37572 ) ),
 .UNSPECIFIED., .F., .F., .F. ) 
 B_SPLINE_SURFACE_WITH_KNOTS ( ( 2, 2 ),
 ( 3, 2, 2, 2, 2, 2, 2, 2, 2, 2, 2, 2, 2, 2, 2, 2, 2, 2, 2, 2, 2, 2, 2, 2, 2, 2, 2, 2, 2, 2, 2, 2, 2, 2, 2, 2, 2, 2, 2, 2, 2, 2, 2, 2, 2, 2, 2, 2, 2, 2, 2, 2, 2, 2, 2, 2, 2, 2, 2, 2, 2, 2, 2, 2, 2, 2, 2, 2, 2, 2, 2, 2, 2, 2, 2, 2, 2, 2, 2, 2, 2, 2, 2, 2, 2, 2, 2, 2, 2, 2, 2, 2, 2, 2, 2, 2, 2, 2, 2, 2, 2, 2, 2, 2, 2, 2, 2, 2, 2, 2, 2, 2, 2, 2, 2, 2, 2, 2, 2, 2, 2, 2, 2, 2, 2, 2, 2, 2, 2, 2, 2, 2, 2, 2, 2, 2, 2, 2, 2, 2, 2, 2, 2, 2, 2, 2, 2, 2, 2, 2, 2, 2, 2, 2, 2, 2, 2, 2, 2, 2, 2, 2, 3 ),
 ( 0.000000000000000000, 1.000000000000000000 ),
 ( 0.000000000000000000, 0.005952380952380952051, 0.01190476190476190410, 0.01785714285714285615, 0.02380952380952380820, 0.02976190476190476025, 0.03571428571428571230, 0.04166666666666666435, 0.04761904761904761640, 0.05357142857142856845, 0.05952380952380952051, 0.06547619047619047949, 0.07142857142857142461, 0.07738095238095238360, 0.08333333333333332871, 0.08928571428571428770, 0.09523809523809523281, 0.1011904761904761918, 0.1071428571428571369, 0.1130952380952380959, 0.1190476190476190410, 0.1250000000000000000, 0.1309523809523809590, 0.1369047619047619180, 0.1428571428571428492, 0.1488095238095238082, 0.1547619047619047672, 0.1607142857142857262, 0.1666666666666666574, 0.1726190476190476164, 0.1785714285714285754, 0.1845238095238095344, 0.1904761904761904656, 0.1964285714285714246, 0.2023809523809523836, 0.2083333333333333426, 0.2142857142857142738, 0.2202380952380952328, 0.2261904761904761918, 0.2321428571428571508, 0.2380952380952380820, 0.2440476190476190410, 0.2500000000000000000, 0.2559523809523809312, 0.2619047619047619180, 0.2678571428571428492, 0.2738095238095238360, 0.2797619047619047672, 0.2857142857142856984, 0.2916666666666666852, 0.2976190476190476164, 0.3035714285714285476, 0.3095238095238095344, 0.3154761904761904656, 0.3214285714285714524, 0.3273809523809523836, 0.3333333333333333148, 0.3392857142857143016, 0.3452380952380952328, 0.3511904761904761640, 0.3571428571428571508, 0.3630952380952380820, 0.3690476190476190688, 0.3750000000000000000, 0.3809523809523809312, 0.3869047619047619180, 0.3928571428571428492, 0.3988095238095238360, 0.4047619047619047672, 0.4107142857142856984, 0.4166666666666666852, 0.4226190476190476164, 0.4285714285714285476, 0.4345238095238095344, 0.4404761904761904656, 0.4464285714285714524, 0.4523809523809523836, 0.4583333333333333148, 0.4642857142857143016, 0.4702380952380952328, 0.4761904761904761640, 0.4821428571428571508, 0.4880952380952380820, 0.4940476190476190688, 0.5000000000000000000, 0.5059523809523809312, 0.5119047619047618625, 0.5178571428571429047, 0.5238095238095238360, 0.5297619047619047672, 0.5357142857142856984, 0.5416666666666666297, 0.5476190476190476719, 0.5535714285714286031, 0.5595238095238095344, 0.5654761904761904656, 0.5714285714285713969, 0.5773809523809523281, 0.5833333333333333703, 0.5892857142857143016, 0.5952380952380952328, 0.6011904761904761640, 0.6071428571428570953, 0.6130952380952381375, 0.6190476190476190688, 0.6250000000000000000, 0.6309523809523809312, 0.6369047619047618625, 0.6428571428571429047, 0.6488095238095238360, 0.6547619047619047672, 0.6607142857142856984, 0.6666666666666666297, 0.6726190476190476719, 0.6785714285714286031, 0.6845238095238095344, 0.6904761904761904656, 0.6964285714285713969, 0.7023809523809523281, 0.7083333333333333703, 0.7142857142857143016, 0.7202380952380952328, 0.7261904761904761640, 0.7321428571428570953, 0.7380952380952381375, 0.7440476190476190688, 0.7500000000000000000, 0.7559523809523809312, 0.7619047619047618625, 0.7678571428571429047, 0.7738095238095238360, 0.7797619047619047672, 0.7857142857142856984, 0.7916666666666666297, 0.7976190476190476719, 0.8035714285714286031, 0.8095238095238095344, 0.8154761904761904656, 0.8214285714285713969, 0.8273809523809523281, 0.8333333333333333703, 0.8392857142857143016, 0.8452380952380952328, 0.8511904761904761640, 0.8571428571428570953, 0.8630952380952381375, 0.8690476190476190688, 0.8750000000000000000, 0.8809523809523809312, 0.8869047619047618625, 0.8928571428571429047, 0.8988095238095238360, 0.9047619047619047672, 0.9107142857142856984, 0.9166666666666666297, 0.9226190476190476719, 0.9285714285714286031, 0.9345238095238095344, 0.9404761904761904656, 0.9464285714285713969, 0.9523809523809523281, 0.9583333333333333703, 0.9642857142857143016 ),
 .UNSPECIFIED. ) 
 GEOMETRIC_REPRESENTATION_ITEM ( )  RATIONAL_B_SPLINE_SURFACE ( (
 ( 1.000000000000000000, 0.9659258262890683122, 1.000000000000000000, 0.9659258262890683122, 1.000000000000000000, 0.9659258262890683122, 1.000000000000000000, 0.9659258262890683122, 1.000000000000000000, 0.9659258262890683122, 1.000000000000000000, 0.9659258262890683122, 1.000000000000000000, 0.9659258262890683122, 1.000000000000000000, 0.9659258262890683122, 1.000000000000000000, 0.9659258262890683122, 1.000000000000000000, 0.9659258262890683122, 1.000000000000000000, 0.9659258262890683122, 1.000000000000000000, 0.9659258262890683122, 1.000000000000000000, 0.9659258262890683122, 1.000000000000000000, 0.9659258262890683122, 1.000000000000000000, 0.9659258262890683122, 1.000000000000000000, 0.9659258262890683122, 1.000000000000000000, 0.9659258262890683122, 1.000000000000000000, 0.9659258262890683122, 1.000000000000000000, 0.9659258262890683122, 1.000000000000000000, 0.9659258262890683122, 1.000000000000000000, 0.9659258262890683122, 1.000000000000000000, 0.9659258262890683122, 1.000000000000000000, 0.9659258262890683122, 1.000000000000000000, 0.9659258262890683122, 1.000000000000000000, 0.9659258262890683122, 1.000000000000000000, 0.9659258262890683122, 1.000000000000000000, 0.9659258262890683122, 1.000000000000000000, 0.9659258262890683122, 1.000000000000000000, 0.9659258262890683122, 1.000000000000000000, 0.9659258262890683122, 1.000000000000000000, 0.9659258262890683122, 1.000000000000000000, 0.9659258262890683122, 1.000000000000000000, 0.9659258262890683122, 1.000000000000000000, 0.9659258262890683122, 1.000000000000000000, 0.9659258262890683122, 1.000000000000000000, 0.9659258262890683122, 1.000000000000000000, 0.9659258262890683122, 1.000000000000000000, 0.9659258262890683122, 1.000000000000000000, 0.9659258262890683122, 1.000000000000000000, 0.9659258262890683122, 1.000000000000000000, 0.9659258262890683122, 1.000000000000000000, 0.9659258262890683122, 1.000000000000000000, 0.9659258262890683122, 1.000000000000000000, 0.9659258262890683122, 1.000000000000000000, 0.9659258262890683122, 1.000000000000000000, 0.9659258262890683122, 1.000000000000000000, 0.9659258262890683122, 1.000000000000000000, 0.9659258262890683122, 1.000000000000000000, 0.9659258262890683122, 1.000000000000000000, 0.9659258262890683122, 1.000000000000000000, 0.9659258262890683122, 1.000000000000000000, 0.9659258262890683122, 1.000000000000000000, 0.9659258262890683122, 1.000000000000000000, 0.9659258262890683122, 1.000000000000000000, 0.9659258262890683122, 1.000000000000000000, 0.9659258262890683122, 1.000000000000000000, 0.9659258262890683122, 1.000000000000000000, 0.9659258262890683122, 1.000000000000000000, 0.9659258262890683122, 1.000000000000000000, 0.9659258262890683122, 1.000000000000000000, 0.9659258262890683122, 1.000000000000000000, 0.9659258262890683122, 1.000000000000000000, 0.9659258262890683122, 1.000000000000000000, 0.9659258262890683122, 1.000000000000000000, 0.9659258262890683122, 1.000000000000000000, 0.9659258262890683122, 1.000000000000000000, 0.9659258262890683122, 1.000000000000000000, 0.9659258262890683122, 1.000000000000000000, 0.9659258262890683122, 1.000000000000000000, 0.9659258262890683122, 1.000000000000000000, 0.9659258262890683122, 1.000000000000000000, 0.9659258262890683122, 1.000000000000000000, 0.9659258262890683122, 1.000000000000000000, 0.9659258262890683122, 1.000000000000000000, 0.9659258262890683122, 1.000000000000000000, 0.9659258262890683122, 1.000000000000000000, 0.9659258262890683122, 1.000000000000000000, 0.9659258262890683122, 1.000000000000000000, 0.9659258262890683122, 1.000000000000000000, 0.9659258262890683122, 1.000000000000000000, 0.9659258262890683122, 1.000000000000000000, 0.9659258262890683122, 1.000000000000000000, 0.9659258262890683122, 1.000000000000000000, 0.9659258262890683122, 1.000000000000000000, 0.9659258262890683122, 1.000000000000000000, 0.9659258262890683122, 1.000000000000000000, 0.9659258262890683122, 1.000000000000000000, 0.9659258262890683122, 1.000000000000000000, 0.9659258262890683122, 1.000000000000000000, 0.9659258262890683122, 1.000000000000000000, 0.9659258262890683122, 1.000000000000000000, 0.9659258262890683122, 1.000000000000000000, 0.9659258262890683122, 1.000000000000000000, 0.9659258262890683122, 1.000000000000000000, 0.9659258262890683122, 1.000000000000000000, 0.9659258262890683122, 1.000000000000000000, 0.9659258262890683122, 1.000000000000000000, 0.9659258262890683122, 1.000000000000000000, 0.9659258262890683122, 1.000000000000000000, 0.9659258262890683122, 1.000000000000000000, 0.9659258262890683122, 1.000000000000000000, 0.9659258262890683122, 1.000000000000000000, 0.9659258262890683122, 1.000000000000000000, 0.9659258262890683122, 1.000000000000000000, 0.9659258262890683122, 1.000000000000000000, 0.9659258262890683122, 1.000000000000000000, 0.9659258262890683122, 1.000000000000000000, 0.9659258262890683122, 1.000000000000000000, 0.9659258262890683122, 1.000000000000000000, 0.9659258262890683122, 1.000000000000000000, 0.9659258262890683122, 1.000000000000000000, 0.9659258262890683122, 1.000000000000000000, 0.9659258262890683122, 1.000000000000000000, 0.9659258262890683122, 1.000000000000000000, 0.9659258262890683122, 1.000000000000000000, 0.9659258262890683122, 1.000000000000000000, 0.9659258262890683122, 1.000000000000000000, 0.9659258262890683122, 1.000000000000000000, 0.9659258262890683122, 1.000000000000000000, 0.9659258262890683122, 1.000000000000000000, 0.9659258262890683122, 1.000000000000000000, 0.9659258262890683122, 1.000000000000000000, 0.9659258262890683122, 1.000000000000000000, 0.9659258262890683122, 1.000000000000000000, 0.9659258262890683122, 1.000000000000000000, 0.9659258262890683122, 1.000000000000000000, 0.9659258262890683122, 1.000000000000000000, 0.9659258262890683122, 1.000000000000000000, 0.9659258262890683122, 1.000000000000000000, 0.9659258262890683122, 1.000000000000000000, 0.9659258262890683122, 1.000000000000000000, 0.9659258262890683122, 1.000000000000000000, 0.9659258262890683122, 1.000000000000000000, 0.9659258262890683122, 1.000000000000000000, 0.9659258262890683122, 1.000000000000000000, 0.9659258262890683122, 1.000000000000000000, 0.9659258262890683122, 1.000000000000000000, 0.9659258262890683122, 1.000000000000000000, 0.9659258262890683122, 1.000000000000000000, 0.9659258262890683122, 1.000000000000000000, 0.9659258262890683122, 1.000000000000000000, 0.9659258262890683122, 1.000000000000000000, 0.9659258262890683122, 1.000000000000000000, 0.9659258262890683122, 1.000000000000000000, 0.9659258262890683122, 1.000000000000000000, 0.9659258262890683122, 1.000000000000000000, 0.9659258262890683122, 1.000000000000000000, 0.9659258262890683122, 1.000000000000000000, 0.9659258262890683122, 1.000000000000000000, 0.9659258262890683122, 1.000000000000000000, 0.9659258262890683122, 1.000000000000000000, 0.9659258262890683122, 1.000000000000000000, 0.9659258262890683122, 1.000000000000000000, 0.9659258262890683122, 1.000000000000000000, 0.9659258262890683122, 1.000000000000000000, 0.9659258262890683122, 1.000000000000000000, 0.9659258262890683122, 1.000000000000000000, 0.9659258262890683122, 1.000000000000000000, 0.9659258262890683122, 1.000000000000000000, 0.9659258262890683122, 1.000000000000000000, 0.9659258262890683122, 1.000000000000000000, 0.9659258262890683122, 1.000000000000000000),
 ( 1.000000000000000000, 0.9659258262890683122, 1.000000000000000000, 0.9659258262890683122, 1.000000000000000000, 0.9659258262890683122, 1.000000000000000000, 0.9659258262890683122, 1.000000000000000000, 0.9659258262890683122, 1.000000000000000000, 0.9659258262890683122, 1.000000000000000000, 0.9659258262890683122, 1.000000000000000000, 0.9659258262890683122, 1.000000000000000000, 0.9659258262890683122, 1.000000000000000000, 0.9659258262890683122, 1.000000000000000000, 0.9659258262890683122, 1.000000000000000000, 0.9659258262890683122, 1.000000000000000000, 0.9659258262890683122, 1.000000000000000000, 0.9659258262890683122, 1.000000000000000000, 0.9659258262890683122, 1.000000000000000000, 0.9659258262890683122, 1.000000000000000000, 0.9659258262890683122, 1.000000000000000000, 0.9659258262890683122, 1.000000000000000000, 0.9659258262890683122, 1.000000000000000000, 0.9659258262890683122, 1.000000000000000000, 0.9659258262890683122, 1.000000000000000000, 0.9659258262890683122, 1.000000000000000000, 0.9659258262890683122, 1.000000000000000000, 0.9659258262890683122, 1.000000000000000000, 0.9659258262890683122, 1.000000000000000000, 0.9659258262890683122, 1.000000000000000000, 0.9659258262890683122, 1.000000000000000000, 0.9659258262890683122, 1.000000000000000000, 0.9659258262890683122, 1.000000000000000000, 0.9659258262890683122, 1.000000000000000000, 0.9659258262890683122, 1.000000000000000000, 0.9659258262890683122, 1.000000000000000000, 0.9659258262890683122, 1.000000000000000000, 0.9659258262890683122, 1.000000000000000000, 0.9659258262890683122, 1.000000000000000000, 0.9659258262890683122, 1.000000000000000000, 0.9659258262890683122, 1.000000000000000000, 0.9659258262890683122, 1.000000000000000000, 0.9659258262890683122, 1.000000000000000000, 0.9659258262890683122, 1.000000000000000000, 0.9659258262890683122, 1.000000000000000000, 0.9659258262890683122, 1.000000000000000000, 0.9659258262890683122, 1.000000000000000000, 0.9659258262890683122, 1.000000000000000000, 0.9659258262890683122, 1.000000000000000000, 0.9659258262890683122, 1.000000000000000000, 0.9659258262890683122, 1.000000000000000000, 0.9659258262890683122, 1.000000000000000000, 0.9659258262890683122, 1.000000000000000000, 0.9659258262890683122, 1.000000000000000000, 0.9659258262890683122, 1.000000000000000000, 0.9659258262890683122, 1.000000000000000000, 0.9659258262890683122, 1.000000000000000000, 0.9659258262890683122, 1.000000000000000000, 0.9659258262890683122, 1.000000000000000000, 0.9659258262890683122, 1.000000000000000000, 0.9659258262890683122, 1.000000000000000000, 0.9659258262890683122, 1.000000000000000000, 0.9659258262890683122, 1.000000000000000000, 0.9659258262890683122, 1.000000000000000000, 0.9659258262890683122, 1.000000000000000000, 0.9659258262890683122, 1.000000000000000000, 0.9659258262890683122, 1.000000000000000000, 0.9659258262890683122, 1.000000000000000000, 0.9659258262890683122, 1.000000000000000000, 0.9659258262890683122, 1.000000000000000000, 0.9659258262890683122, 1.000000000000000000, 0.9659258262890683122, 1.000000000000000000, 0.9659258262890683122, 1.000000000000000000, 0.9659258262890683122, 1.000000000000000000, 0.9659258262890683122, 1.000000000000000000, 0.9659258262890683122, 1.000000000000000000, 0.9659258262890683122, 1.000000000000000000, 0.9659258262890683122, 1.000000000000000000, 0.9659258262890683122, 1.000000000000000000, 0.9659258262890683122, 1.000000000000000000, 0.9659258262890683122, 1.000000000000000000, 0.9659258262890683122, 1.000000000000000000, 0.9659258262890683122, 1.000000000000000000, 0.9659258262890683122, 1.000000000000000000, 0.9659258262890683122, 1.000000000000000000, 0.9659258262890683122, 1.000000000000000000, 0.9659258262890683122, 1.000000000000000000, 0.9659258262890683122, 1.000000000000000000, 0.9659258262890683122, 1.000000000000000000, 0.9659258262890683122, 1.000000000000000000, 0.9659258262890683122, 1.000000000000000000, 0.9659258262890683122, 1.000000000000000000, 0.9659258262890683122, 1.000000000000000000, 0.9659258262890683122, 1.000000000000000000, 0.9659258262890683122, 1.000000000000000000, 0.9659258262890683122, 1.000000000000000000, 0.9659258262890683122, 1.000000000000000000, 0.9659258262890683122, 1.000000000000000000, 0.9659258262890683122, 1.000000000000000000, 0.9659258262890683122, 1.000000000000000000, 0.9659258262890683122, 1.000000000000000000, 0.9659258262890683122, 1.000000000000000000, 0.9659258262890683122, 1.000000000000000000, 0.9659258262890683122, 1.000000000000000000, 0.9659258262890683122, 1.000000000000000000, 0.9659258262890683122, 1.000000000000000000, 0.9659258262890683122, 1.000000000000000000, 0.9659258262890683122, 1.000000000000000000, 0.9659258262890683122, 1.000000000000000000, 0.9659258262890683122, 1.000000000000000000, 0.9659258262890683122, 1.000000000000000000, 0.9659258262890683122, 1.000000000000000000, 0.9659258262890683122, 1.000000000000000000, 0.9659258262890683122, 1.000000000000000000, 0.9659258262890683122, 1.000000000000000000, 0.9659258262890683122, 1.000000000000000000, 0.9659258262890683122, 1.000000000000000000, 0.9659258262890683122, 1.000000000000000000, 0.9659258262890683122, 1.000000000000000000, 0.9659258262890683122, 1.000000000000000000, 0.9659258262890683122, 1.000000000000000000, 0.9659258262890683122, 1.000000000000000000, 0.9659258262890683122, 1.000000000000000000, 0.9659258262890683122, 1.000000000000000000, 0.9659258262890683122, 1.000000000000000000, 0.9659258262890683122, 1.000000000000000000, 0.9659258262890683122, 1.000000000000000000, 0.9659258262890683122, 1.000000000000000000, 0.9659258262890683122, 1.000000000000000000, 0.9659258262890683122, 1.000000000000000000, 0.9659258262890683122, 1.000000000000000000, 0.9659258262890683122, 1.000000000000000000, 0.9659258262890683122, 1.000000000000000000, 0.9659258262890683122, 1.000000000000000000, 0.9659258262890683122, 1.000000000000000000, 0.9659258262890683122, 1.000000000000000000, 0.9659258262890683122, 1.000000000000000000, 0.9659258262890683122, 1.000000000000000000, 0.9659258262890683122, 1.000000000000000000, 0.9659258262890683122, 1.000000000000000000, 0.9659258262890683122, 1.000000000000000000, 0.9659258262890683122, 1.000000000000000000, 0.9659258262890683122, 1.000000000000000000, 0.9659258262890683122, 1.000000000000000000, 0.9659258262890683122, 1.000000000000000000, 0.9659258262890683122, 1.000000000000000000, 0.9659258262890683122, 1.000000000000000000, 0.9659258262890683122, 1.000000000000000000, 0.9659258262890683122, 1.000000000000000000, 0.9659258262890683122, 1.000000000000000000, 0.9659258262890683122, 1.000000000000000000, 0.9659258262890683122, 1.000000000000000000, 0.9659258262890683122, 1.000000000000000000, 0.9659258262890683122, 1.000000000000000000, 0.9659258262890683122, 1.000000000000000000, 0.9659258262890683122, 1.000000000000000000, 0.9659258262890683122, 1.000000000000000000, 0.9659258262890683122, 1.000000000000000000, 0.9659258262890683122, 1.000000000000000000, 0.9659258262890683122, 1.000000000000000000, 0.9659258262890683122, 1.000000000000000000, 0.9659258262890683122, 1.000000000000000000, 0.9659258262890683122, 1.000000000000000000, 0.9659258262890683122, 1.000000000000000000, 0.9659258262890683122, 1.000000000000000000, 0.9659258262890683122, 1.000000000000000000) ) ) 
 REPRESENTATION_ITEM ( '' )  SURFACE ( )  );
#77286=CARTESIAN_POINT ( 'NONE',  ( 3.591859063236763294, 23.29030133659708568, -11.09922568453595026 ) ) ;
#77288=DIRECTION ( 'NONE',  ( 0.000000000000000000, 1.000000000000000000, 0.000000000000000000 ) ) ;
#77289=CARTESIAN_POINT ( 'NONE',  ( 17.96484262340118221, 54.93868534415484106, 7.964842623401181321 ) ) ;
#77290=CARTESIAN_POINT ( 'NONE',  ( 10.00000000000000178, 62.25893115100078745, 9.846743663894594434 ) ) ;
#77291=CARTESIAN_POINT ( 'NONE',  ( 19.84674366389459266, 33.30059781766744464, 2.638427012816836559 ) ) ;
#77292=CARTESIAN_POINT ( 'NONE',  ( 17.20831665107776587, 24.13393115100078035, -7.208316651077762316 ) ) ;
#77293=CARTESIAN_POINT ( 'NONE',  ( 15.44008868035555793, 11.39701867748817143, -9.422509992056140149 ) ) ;
#77294=CARTESIAN_POINT ( 'NONE',  ( -2.816281873526473856, 14.12363466993041961, 9.499525473075851096E-16 ) ) ;
#77295=CARTESIAN_POINT ( 'NONE',  ( 4.559911319644449179, 2.230352010821504471, -9.422509992056141925 ) ) ;
#77298=CARTESIAN_POINT ( 'NONE',  ( 10.00000000000000178, 14.31368534415483929, 10.88017736071110342 ) ) ;
#77300=CARTESIAN_POINT ( 'NONE',  ( 7.361572987183169658, 34.96726448433411605, -9.846743663894592657 ) ) ;
#77301=CARTESIAN_POINT ( 'NONE',  ( -0.8801773607111008646, 13.27201867748817321, 2.915334737309923430 ) ) ;
#77302=CARTESIAN_POINT ( 'NONE',  ( 1.472469842513823179, 5.592264484334118713, -4.923371831947296329 ) ) ;
#77303=CARTESIAN_POINT ( 'NONE',  ( 10.00000000000000000, 36.81368534415484106, -10.88017736071110342 ) ) ;
#77304=CARTESIAN_POINT ( 'NONE',  ( 6.204703633549690345, 60.76208216824730357, -14.16423886937410259 ) ) ;
#77305=CARTESIAN_POINT ( 'NONE',  ( 0.2751277870542911397, 40.30223176428831522, 6.499999999999992006 ) ) ;
#77306=CARTESIAN_POINT ( 'NONE',  ( 0.1532563361054082862, 1.217264484334117824, 2.638427012816831674 ) ) ;
#77307=CARTESIAN_POINT ( 'NONE',  ( 17.20831665107776587, 29.13393115100078390, -7.208316651077762316 ) ) ;
#77311=EDGE_CURVE ( 'NONE', #21166, #68203, #34351, .T. ) ;
#77312=CARTESIAN_POINT ( 'NONE',  ( 24.16423886937409904, 24.09541550158063927, 3.795296366450317205 ) ) ;
#77313=CARTESIAN_POINT ( 'NONE',  ( 19.84674366389459266, 38.30059781766745175, 2.638427012816836559 ) ) ;
#77314=DIRECTION ( 'NONE',  ( 0.000000000000000000, -1.000000000000000000, 0.000000000000000000 ) ) ;
#77316=CARTESIAN_POINT ( 'NONE',  ( 6.204703633549690345, 50.76208216824730357, -14.16423886937410259 ) ) ;
#77318=CARTESIAN_POINT ( 'NONE',  ( 19.84674366389459266, 23.71726448433412315, -2.638427012816827677 ) ) ;
#77321=CARTESIAN_POINT ( 'NONE',  ( 17.96484262340118221, 39.93868534415484106, 7.964842623401181321 ) ) ;
#77322=CARTESIAN_POINT ( 'NONE',  ( 10.00000000000000178, 55.37363466993042493, 12.81628187352647608 ) ) ;
#77323=CARTESIAN_POINT ( 'NONE',  ( 2.035157376598822676, 17.43868534415483751, -7.964842623401177768 ) ) ;
#77324=CARTESIAN_POINT ( 'NONE',  ( -1.099225684535947600, 49.54030133659708923, 6.408140936763237150 ) ) ;
#77325=ORIENTED_EDGE ( 'NONE', *, *, #510, .T. ) ;
#77326=CARTESIAN_POINT ( 'NONE',  ( 17.20831665107776587, 62.88393115100078745, 7.208316651077764980 ) ) ;
#77327=CARTESIAN_POINT ( 'NONE',  ( 2.791683348922240793, 1.633931151000784565, 7.208316651077764092 ) ) ;
#77329=VECTOR ( 'NONE', #90106, 1000.000000000000000 ) ;
#77331=DIRECTION ( 'NONE',  ( -1.000000000000000000, 0.000000000000000000, 0.000000000000000000 ) ) ;
#77332=CARTESIAN_POINT ( 'NONE',  ( 24.16423886937409904, 54.09541550158063217, 3.795296366450317205 ) ) ;
#77333=CARTESIAN_POINT ( 'NONE',  ( -4.164238869374099039, 16.80374883491396787, 8.674139862899312516E-16 ) ) ;
#77334=CARTESIAN_POINT ( 'NONE',  ( 2.035157376598822676, 22.43868534415483396, -7.964842623401177768 ) ) ;
#77335=CARTESIAN_POINT ( 'NONE',  ( 2.035157376598822676, 42.43868534415483396, -7.964842623401177768 ) ) ;
#77338=CARTESIAN_POINT ( 'NONE',  ( 20.88017736071110164, 65.35535201082150536, 2.915334737309930979 ) ) ;
#77339=CARTESIAN_POINT ( 'NONE',  ( 19.42250999205614548, 65.98035201082151957, -5.440088680355545492 ) ) ;
#77340=CARTESIAN_POINT ( 'NONE',  ( 17.20831665107776587, 22.88393115100078745, 7.208316651077764980 ) ) ;
#77343=CARTESIAN_POINT ( 'NONE',  ( 17.20831665107776587, 7.883931151000784787, 7.208316651077764980 ) ) ;
#77344=CARTESIAN_POINT ( 'NONE',  ( 12.63842701281683922, 34.55059781766745886, -9.846743663894590881 ) ) ;
#77345=CARTESIAN_POINT ( 'NONE',  ( 2.035157376598822676, 12.43868534415483751, -7.964842623401177768 ) ) ;
#77346=B_SPLINE_CURVE_WITH_KNOTS ( 'NONE', 3,
 ( #23000, #6018, #74993, #37004, #29475, #59983 ),
 .UNSPECIFIED., .F., .F.,
 ( 4, 2, 4 ),
 ( 0.000000000000000000, 0.0002605067024380876522, 0.0005210134048761753045 ),
 .UNSPECIFIED. ) ;
#77347=CARTESIAN_POINT ( 'NONE',  ( 22.81628187352647785, 26.62363466993042138, 6.195893100308588602E-16 ) ) ;
#77349=CARTESIAN_POINT ( 'NONE',  ( 14.92337183194729988, 4.342264484334117824, -8.527530157486177487 ) ) ;
#77351=CARTESIAN_POINT ( 'NONE',  ( 19.84674366389459266, 53.71726448433411605, -2.638427012816827677 ) ) ;
#77352=CARTESIAN_POINT ( 'NONE',  ( 1.472469842513823179, 31.42559781766745530, 4.923371831947296329 ) ) ;
#77353=CARTESIAN_POINT ( 'NONE',  ( 13.79529636645030344, 23.26208216824730002, 14.16423886937410614 ) ) ;
#77354=CARTESIAN_POINT ( 'NONE',  ( 10.00000000000000000, 51.81368534415484106, -10.88017736071110342 ) ) ;
#77355=CARTESIAN_POINT ( 'NONE',  ( 7.084665262690076126, 7.022018677488169658, -10.88017736071110164 ) ) ;
#77356=EDGE_CURVE ( 'NONE', #74440, #78790, #91811, .T. ) ;
#77357=CARTESIAN_POINT ( 'NONE',  ( 15.44008868035555793, 51.39701867748816966, -9.422509992056140149 ) ) ;
#77358=CARTESIAN_POINT ( 'NONE',  ( 17.96484262340118221, 36.18868534415484106, -7.964842623401177768 ) ) ;
#77360=CARTESIAN_POINT ( 'NONE',  ( 20.88017736071110519, 40.56368534415484106, 2.639326808657452039E-16 ) ) ;
#77363=CARTESIAN_POINT ( 'NONE',  ( 16.40814093676323893, 60.79030133659709634, 11.09922568453595026 ) ) ;
#77364=CARTESIAN_POINT ( 'NONE',  ( 12.91533473730992121, 49.52201867748817676, 10.88017736071110164 ) ) ;
#77366=CARTESIAN_POINT ( 'NONE',  ( -0.8801773607111009756, 48.06368534415484817, 1.068504757029289695E-15 ) ) ;
#77370=CARTESIAN_POINT ( 'NONE',  ( 24.16423886937410614, 59.51208216824728936, -3.795296366450302550 ) ) ;
#77371=CARTESIAN_POINT ( 'NONE',  ( 15.44008868035555260, 59.73035201082151247, 9.422509992056143702 ) ) ;
#77372=CARTESIAN_POINT ( 'NONE',  ( 19.72487221294571569, 25.71833443783938478, -6.499999999999989342 ) ) ;
#77374=CARTESIAN_POINT ( 'NONE',  ( 20.88017736071110164, 10.35535201082150714, 2.915334737309930979 ) ) ;
#77375=CARTESIAN_POINT ( 'NONE',  ( 18.52753015748617571, 33.09226448433411605, 4.923371831947298993 ) ) ;
#77377=CARTESIAN_POINT ( 'NONE',  ( 10.00000000000000178, 32.25893115100078745, 9.846743663894594434 ) ) ;
#77378=CARTESIAN_POINT ( 'NONE',  ( 0.5774900079438607392, 33.48035201082150536, 5.440088680355550821 ) ) ;
#77379=CARTESIAN_POINT ( 'NONE',  ( 2.791683348922237240, 40.38393115100078035, -7.208316651077763204 ) ) ;
#77380=CARTESIAN_POINT ( 'NONE',  ( 22.81628187352648496, 16.83196800326374998, -3.434112377981050290 ) ) ;
#77381=CARTESIAN_POINT ( 'NONE',  ( 17.96484262340118221, 66.18868534415483396, -7.964842623401177768 ) ) ;
#77382=CARTESIAN_POINT ( 'NONE',  ( 0.5774900079438590739, 52.64701867748817676, -5.440088680355550821 ) ) ;
#77383=CARTESIAN_POINT ( 'NONE',  ( -4.164238869374099927, 57.01208216824731068, 3.795296366450308767 ) ) ;
#77385=CARTESIAN_POINT ( 'NONE',  ( 22.81628187352648496, 26.83196800326374998, -3.434112377981050290 ) ) ;
#77386=DIRECTION ( 'NONE',  ( -0.000000000000000000, 1.000000000000000000, 0.000000000000000000 ) ) ;
#77388=CARTESIAN_POINT ( 'NONE',  ( 13.43411237798105340, 25.58196800326374998, 12.81628187352647963 ) ) ;
#77389=CARTESIAN_POINT ( 'NONE',  ( 12.91533473730992121, 19.52201867748816611, 10.88017736071110164 ) ) ;
#77390=( BOUNDED_CURVE ( )  B_SPLINE_CURVE ( 2, ( #30894, #53901, #46880, #76886, #46398, #82918, #23909, #16398, #38908 ),
 .UNSPECIFIED., .F., .F. ) 
 B_SPLINE_CURVE_WITH_KNOTS ( ( 3, 2, 2, 2, 3 ),
 ( 0.7605718029354654464, 0.7619047619047618625, 0.7678571428571429047, 0.7738095238095238360, 0.7751424827788201410 ),
 .UNSPECIFIED. ) 
 CURVE ( )  GEOMETRIC_REPRESENTATION_ITEM ( )  RATIONAL_B_SPLINE_CURVE ( ( 0.9881565478350733400, 0.9923695281211490915, 1.000000000000000000, 0.9659258262890683122, 1.000000000000000000, 0.9659258262890683122, 1.000000000000000000, 0.9923695281211497576, 0.9881565478350740062 ) ) 
 REPRESENTATION_ITEM ( '' )  );
#77391=VECTOR ( 'NONE', #58256, 1000.000000000000000 ) ;
#77393=CARTESIAN_POINT ( 'NONE',  ( 0.1532563361054082862, 1.217264484334117824, 2.638427012816831674 ) ) ;
#77394=VECTOR ( 'NONE', #24813, 1000.000000000000000 ) ;
#77395=CARTESIAN_POINT ( 'NONE',  ( 19.84674366389459621, 43.50893115100078745, 7.409399052514197653E-17 ) ) ;
#77396=CARTESIAN_POINT ( 'NONE',  ( 7.361572987183169658, 39.96726448433411605, -9.846743663894592657 ) ) ;
#77399=CARTESIAN_POINT ( 'NONE',  ( 7.361572987183170547, 22.05059781766745530, 9.846743663894590881 ) ) ;
#77400=CARTESIAN_POINT ( 'NONE',  ( -0.03447792253739219437, 40.15514106990689669, 6.401564815979744694 ) ) ;
#77402=CARTESIAN_POINT ( 'NONE',  ( 18.52753015748618282, 8.925597817667451750, -4.923371831947291888 ) ) ;
#77405=CARTESIAN_POINT ( 'NONE',  ( 10.00000000000000000, 49.75893115100078745, -9.846743663894594434 ) ) ;
#77407=DIRECTION ( 'NONE',  ( 0.000000000000000000, -1.000000000000000000, -0.000000000000000000 ) ) ;
#77408=CARTESIAN_POINT ( 'NONE',  ( -1.099225684535947600, 13.70696800326375353, -6.408140936763238038 ) ) ;
#77410=CARTESIAN_POINT ( 'NONE',  ( 15.44008868035555793, 46.39701867748817676, -9.422509992056140149 ) ) ;
#77411=CARTESIAN_POINT ( 'NONE',  ( -0.3689425029237881626, 52.42874883491396076, 10.36894250292379027 ) ) ;
#77412=CARTESIAN_POINT ( 'NONE',  ( 12.63842701281683034, 2.467264484334118269, 9.846743663894596210 ) ) ;
#77414=CARTESIAN_POINT ( 'NONE',  ( 6.204703633549690345, 40.76208216824731778, -14.16423886937410259 ) ) ;
#77415=CARTESIAN_POINT ( 'NONE',  ( -2.266590686148945544, 61.38708216824730357, -7.082119434687050408 ) ) ;
#77416=CARTESIAN_POINT ( 'NONE',  ( -4.164238869374099927, 22.01208216824730357, 3.795296366450308767 ) ) ;
#77417=CARTESIAN_POINT ( 'NONE',  ( -4.164238869374098151, 21.59541550158063217, -3.795296366450310543 ) ) ;
#77422=CARTESIAN_POINT ( 'NONE',  ( 19.84674366389459266, 43.30059781766744464, 2.638427012816836559 ) ) ;
#77423=ORIENTED_EDGE ( 'NONE', *, *, #24581, .F. ) ;
#77424=CARTESIAN_POINT ( 'NONE',  ( 2.035157376598822676, 37.43868534415484106, -7.964842623401177768 ) ) ;
#77429=CARTESIAN_POINT ( 'NONE',  ( 0.1532563361054082862, 46.21726448433411605, 2.638427012816831674 ) ) ;
#77430=CARTESIAN_POINT ( 'NONE',  ( -2.816281873526473856, 54.33196800326376064, 3.434112377981055619 ) ) ;
#77432=CARTESIAN_POINT ( 'NONE',  ( 7.361572987183170547, 47.05059781766745175, 9.846743663894590881 ) ) ;
#77433=CARTESIAN_POINT ( 'NONE',  ( 10.00000000000000178, 47.25893115100078745, 9.846743663894594434 ) ) ;
#77435=CARTESIAN_POINT ( 'NONE',  ( 24.16423886937410614, 39.30374883491396787, 8.672049930838204340E-16 ) ) ;
#77437=CARTESIAN_POINT ( 'NONE',  ( 24.16423886937410614, 19.51208216824729647, -3.795296366450302550 ) ) ;
#77438=EDGE_CURVE ( 'NONE', #6459, #95671, #21521, .T. ) ;
#77439=DIRECTION ( 'NONE',  ( -0.000000000000000000, 1.000000000000000000, 0.000000000000000000 ) ) ;
#77442=CARTESIAN_POINT ( 'NONE',  ( 7.084665262690076126, 4.105352010821503583, 10.88017736071109987 ) ) ;
#77443=CARTESIAN_POINT ( 'NONE',  ( 16.40814093676324603, 7.456968003263754419, -11.09922568453594671 ) ) ;
#77444=CARTESIAN_POINT ( 'NONE',  ( 20.88017736071110519, 65.56368534415483396, 2.639326808657452039E-16 ) ) ;
#77446=CARTESIAN_POINT ( 'NONE',  ( 0.1129803114748713505, 14.29427333184090720, -6.480634945678661829 ) ) ;
#77447=DIRECTION ( 'NONE',  ( 0.000000000000000000, 1.000000000000000000, 0.000000000000000000 ) ) ;
#77448=CARTESIAN_POINT ( 'NONE',  ( 2.917880565312948704, 62.63708216824730357, 12.26659068614894643 ) ) ;
#77449=CARTESIAN_POINT ( 'NONE',  ( 0.1077916266722676458, 42.24062864464241329, -6.478736007405996311 ) ) ;
#77450=CARTESIAN_POINT ( 'NONE',  ( 15.44008868035555793, 21.39701867748817321, -9.422509992056140149 ) ) ;
#77451=CARTESIAN_POINT ( 'NONE',  ( 0.5774900079438590739, 22.64701867748817321, -5.440088680355550821 ) ) ;
#77452=CARTESIAN_POINT ( 'NONE',  ( 2.791683348922237240, 50.38393115100078035, -7.208316651077763204 ) ) ;
#77453=CARTESIAN_POINT ( 'NONE',  ( 19.84674366389459621, 53.50893115100078745, 7.409399052514197653E-17 ) ) ;
#77454=CARTESIAN_POINT ( 'NONE',  ( -2.816281873526471635, 63.91530133659708923, -3.434112377981056508 ) ) ;
#77455=CARTESIAN_POINT ( 'NONE',  ( 0.000000000000000000, 70.00000000000000000, -5.000000000000000000 ) ) ;
#77458=CARTESIAN_POINT ( 'NONE',  ( 7.084665262690076126, 24.10535201082150181, 10.88017736071109987 ) ) ;
#77459=CARTESIAN_POINT ( 'NONE',  ( 10.00000000000000178, 30.37363466993042138, 12.81628187352647608 ) ) ;
#77461=PRODUCT_DEFINITION_FORMATION_WITH_SPECIFIED_SOURCE ( 'ANY', '', #98603, .NOT_KNOWN. ) ;
#77462=CARTESIAN_POINT ( 'NONE',  ( 0.1532563361054100626, 55.80059781766745175, -2.638427012816831230 ) ) ;
#77463=CARTESIAN_POINT ( 'NONE',  ( 2.035157376598824452, 43.68868534415484106, 7.964842623401179544 ) ) ;
#77465=CARTESIAN_POINT ( 'NONE',  ( 18.52753015748617571, 8.092264484334117824, 4.923371831947298993 ) ) ;
#77466=CARTESIAN_POINT ( 'NONE',  ( -2.816281873526471635, 18.91530133659708213, -3.434112377981056508 ) ) ;
#77467=CARTESIAN_POINT ( 'NONE',  ( 20.88017736071110164, 60.35535201082151957, 2.915334737309930979 ) ) ;
#77469=FACE_OUTER_BOUND ( 'NONE', #89330, .T. ) ;
#77470=ORIENTED_EDGE ( 'NONE', *, *, #54063, .T. ) ;
#77472=LINE ( 'NONE', #84006, #65348 ) ;
#77473=CARTESIAN_POINT ( 'NONE',  ( -0.8801773607110991993, 52.85535201082151247, -2.915334737309923874 ) ) ;
#77474=CARTESIAN_POINT ( 'NONE',  ( -2.816281873526473856, 49.33196800326374643, 3.434112377981055619 ) ) ;
#77476=CARTESIAN_POINT ( 'NONE',  ( 17.20831665107776587, 14.13393115100078568, -7.208316651077762316 ) ) ;
#77477=CARTESIAN_POINT ( 'NONE',  ( 7.084665262690076126, 4.105352010821503583, 10.88017736071109987 ) ) ;
#77478=CARTESIAN_POINT ( 'NONE',  ( 1.472469842513823179, 21.42559781766745175, 4.923371831947296329 ) ) ;
#77480=CARTESIAN_POINT ( 'NONE',  ( 17.08211943468705840, 55.13708216824731068, -12.26659068614894466 ) ) ;
#77482=CARTESIAN_POINT ( 'NONE',  ( 20.88017736071110519, 5.563685344154837509, 2.639326808657452039E-16 ) ) ;
#77483=CARTESIAN_POINT ( 'NONE',  ( 15.44008868035555793, 11.39701867748817143, -9.422509992056140149 ) ) ;
#77484=PLANE ( 'NONE',  #23246 ) ;
#77486=CARTESIAN_POINT ( 'NONE',  ( 20.88017736071110875, 10.77201867748817143, -2.915334737309920765 ) ) ;
#77487=CARTESIAN_POINT ( 'NONE',  ( 20.88017736071110519, 10.56368534415483929, 2.639326808657452039E-16 ) ) ;
#77488=CARTESIAN_POINT ( 'NONE',  ( 1.472469842513823179, 40.59226448433411605, -4.923371831947296329 ) ) ;
#77489=CARTESIAN_POINT ( 'NONE',  ( -2.816281873526473856, 34.12363466993042493, 9.499525473075851096E-16 ) ) ;
#77492=CARTESIAN_POINT ( 'NONE',  ( 22.26659068614895176, 24.72041550158063572, -7.082119434687042414 ) ) ;
#77493=CARTESIAN_POINT ( 'NONE',  ( 15.44008868035555260, 19.73035201082150536, 9.422509992056143702 ) ) ;
#77494=CARTESIAN_POINT ( 'NONE',  ( 15.44008868035555260, 4.730352010821505360, 9.422509992056143702 ) ) ;
#77495=CARTESIAN_POINT ( 'NONE',  ( 1.472469842513823179, 36.42559781766745175, 4.923371831947296329 ) ) ;
#77497=CARTESIAN_POINT ( 'NONE',  ( 2.791683348922237240, 40.38393115100078035, -7.208316651077763204 ) ) ;
#77501=CARTESIAN_POINT ( 'NONE',  ( 12.91533473730992121, 4.522018677488169658, 10.88017736071110164 ) ) ;
#77502=CARTESIAN_POINT ( 'NONE',  ( 0.5774900079438607392, 63.48035201082149825, 5.440088680355550821 ) ) ;
#77503=CARTESIAN_POINT ( 'NONE',  ( 15.44008868035555793, 31.39701867748817676, -9.422509992056140149 ) ) ;
#77504=CARTESIAN_POINT ( 'NONE',  ( 20.88017736071110875, 10.77201867748817143, -2.915334737309920765 ) ) ;
#77505=CARTESIAN_POINT ( 'NONE',  ( 6.565887622018943937, 25.16530133659708213, 12.81628187352647430 ) ) ;
#77506=CARTESIAN_POINT ( 'NONE',  ( 20.36894250292379738, 19.92874883491396787, -10.36894250292379027 ) ) ;
#77509=CARTESIAN_POINT ( 'NONE',  ( -2.816281873526473856, 44.33196800326375353, 3.434112377981055619 ) ) ;
#77511=CARTESIAN_POINT ( 'NONE',  ( 12.63842701281683922, 54.55059781766745175, -9.846743663894590881 ) ) ;
#77512=CARTESIAN_POINT ( 'NONE',  ( 7.084665262690076126, 14.10535201082150358, 10.88017736071109987 ) ) ;
#77513=ORIENTED_EDGE ( 'NONE', *, *, #8268, .F. ) ;
#77514=CARTESIAN_POINT ( 'NONE',  ( -0.8801773607111009756, 18.06368534415484106, 1.068504757029289695E-15 ) ) ;
#77516=CARTESIAN_POINT ( 'NONE',  ( 15.44008868035555260, 64.73035201082151957, 9.422509992056143702 ) ) ;
#77517=CARTESIAN_POINT ( 'NONE',  ( 2.035157376598824452, 68.68868534415484817, 7.964842623401179544 ) ) ;
#77519=CARTESIAN_POINT ( 'NONE',  ( 17.20831665107776587, 9.133931151000787452, -7.208316651077762316 ) ) ;
#77520=CARTESIAN_POINT ( 'NONE',  ( 20.88017736071110875, 65.77201867748817676, -2.915334737309920765 ) ) ;
#77523=CARTESIAN_POINT ( 'NONE',  ( -46.61145641952149532, 101.4776089914260950, 8.252540973952291026 ) ) ;
#77525=CARTESIAN_POINT ( 'NONE',  ( 2.791683348922240793, 6.633931151000785675, 7.208316651077764092 ) ) ;
#77528=CARTESIAN_POINT ( 'NONE',  ( 18.52753015748617571, 43.09226448433412315, 4.923371831947298993 ) ) ;
#77530=ORIENTED_EDGE ( 'NONE', *, *, #94607, .F. ) ;
#77533=CARTESIAN_POINT ( 'NONE',  ( 17.08211943468705840, 5.137082168247300906, -12.26659068614894466 ) ) ;
#77534=CARTESIAN_POINT ( 'NONE',  ( 10.00000000000000178, 60.37363466993041783, 12.81628187352647608 ) ) ;
#77535=PRESENTATION_STYLE_ASSIGNMENT (( #87014 ) ) ;
#77536=CARTESIAN_POINT ( 'NONE',  ( 13.79529636645030344, 13.26208216824729824, 14.16423886937410614 ) ) ;
#77539=CARTESIAN_POINT ( 'NONE',  ( 4.559911319644449179, 58.89701867748817676, 9.422509992056141925 ) ) ;
#77540=CARTESIAN_POINT ( 'NONE',  ( 4.559911319644449179, 22.23035201082150536, -9.422509992056141925 ) ) ;
#77541=CARTESIAN_POINT ( 'NONE',  ( 1.959929470562281395, 65.51528370094808906, -5.767676674365853629 ) ) ;
#77542=ORIENTED_EDGE ( 'NONE', *, *, #14315, .F. ) ;
#77543=CARTESIAN_POINT ( 'NONE',  ( 0.1532563361054082862, 6.217264484334118713, 2.638427012816831674 ) ) ;
#77544=CARTESIAN_POINT ( 'NONE',  ( 19.84674366389459266, 3.300597817667451750, 2.638427012816836559 ) ) ;
#77545=CARTESIAN_POINT ( 'NONE',  ( 13.43411237798106583, 27.66530133659708568, -12.81628187352647252 ) ) ;
#77546=CARTESIAN_POINT ( 'NONE',  ( 19.84674366389459266, 23.30059781766745530, 2.638427012816836559 ) ) ;
#77548=CARTESIAN_POINT ( 'NONE',  ( 13.43411237798105340, 10.58196800326375353, 12.81628187352647963 ) ) ;
#77552=CARTESIAN_POINT ( 'NONE',  ( 0.1532563361054082862, 11.21726448433411605, 2.638427012816831674 ) ) ;
#77553=ORIENTED_EDGE ( 'NONE', *, *, #26104, .F. ) ;
#77556=CARTESIAN_POINT ( 'NONE',  ( 7.084665262690076126, 42.02201867748816966, -10.88017736071110164 ) ) ;
#77557=CARTESIAN_POINT ( 'NONE',  ( 24.16423886937410614, 29.30374883491396787, 8.672049930838204340E-16 ) ) ;
#77558=CARTESIAN_POINT ( 'NONE',  ( 7.361572987183170547, 37.05059781766744464, 9.846743663894590881 ) ) ;
#77559=CARTESIAN_POINT ( 'NONE',  ( 18.52753015748617571, 3.092264484334118269, 4.923371831947298993 ) ) ;
#77560=CARTESIAN_POINT ( 'NONE',  ( 3.591859063236761518, 49.95696800326375353, 11.09922568453594849 ) ) ;
#77562=CARTESIAN_POINT ( 'NONE',  ( 7.084665262690076126, 32.02201867748816966, -10.88017736071110164 ) ) ;
#77564=CARTESIAN_POINT ( 'NONE',  ( 0.6178305044545838731, 19.74863466993042138, 9.382169495545420901 ) ) ;
#77565=CARTESIAN_POINT ( 'NONE',  ( -2.816281873526473856, 4.331968003263754419, 3.434112377981055619 ) ) ;
#77566=CARTESIAN_POINT ( 'NONE',  ( 14.92337183194729633, 42.67559781766745886, 8.527530157486181039 ) ) ;
#77568=CARTESIAN_POINT ( 'NONE',  ( -2.816281873526473856, 54.33196800326376064, 3.434112377981055619 ) ) ;
#77570=CARTESIAN_POINT ( 'NONE',  ( 17.96484262340118221, 56.18868534415484817, -7.964842623401177768 ) ) ;
#77573=DIRECTION ( 'NONE',  ( 0.000000000000000000, 0.000000000000000000, 1.000000000000000000 ) ) ;
#77575=CARTESIAN_POINT ( 'NONE',  ( 2.035157376598824452, 53.68868534415484817, 7.964842623401179544 ) ) ;
#77576=CARTESIAN_POINT ( 'NONE',  ( 20.88017736071110164, 60.35535201082151957, 2.915334737309930979 ) ) ;
#77579=CARTESIAN_POINT ( 'NONE',  ( 2.035157376598822676, 7.438685344154837509, -7.964842623401177768 ) ) ;
#77580=CARTESIAN_POINT ( 'NONE',  ( 17.20831665107776587, 47.88393115100078745, 7.208316651077764980 ) ) ;
#77581=CARTESIAN_POINT ( 'NONE',  ( 20.88017736071110875, 20.77201867748816611, -2.915334737309920765 ) ) ;
#77582=CARTESIAN_POINT ( 'NONE',  ( 18.04007052943773104, 23.01528370094808551, 5.767676674365834977 ) ) ;
#77583=CARTESIAN_POINT ( 'NONE',  ( -2.816281873526473856, 19.12363466993042138, 9.499525473075851096E-16 ) ) ;
#77585=CARTESIAN_POINT ( 'NONE',  ( 20.88017736071110519, 35.56368534415484106, 2.639326808657452039E-16 ) ) ;
#77586=CARTESIAN_POINT ( 'NONE',  ( 22.81628187352647785, 6.415301336597088344, 3.434112377981063169 ) ) ;
#77589=CARTESIAN_POINT ( 'NONE',  ( 17.96484262340118221, 14.93868534415483751, 7.964842623401181321 ) ) ;
#77590=CARTESIAN_POINT ( 'NONE',  ( 20.88017736071110519, 40.56368534415484106, 2.639326808657452039E-16 ) ) ;
#77591=CARTESIAN_POINT ( 'NONE',  ( -4.164238869374099039, 56.80374883491397497, 8.674139862899312516E-16 ) ) ;
#77592=CARTESIAN_POINT ( 'NONE',  ( 1.472469842513823179, 21.42559781766745175, 4.923371831947296329 ) ) ;
#77593=CARTESIAN_POINT ( 'NONE',  ( 17.96484262340118221, 66.18868534415483396, -7.964842623401177768 ) ) ;
#77595=CARTESIAN_POINT ( 'NONE',  ( 10.00000000000000178, 23.05374883491397142, 14.16423886937410082 ) ) ;
#77597=CARTESIAN_POINT ( 'NONE',  ( -46.94000000000000483, 103.1204114943229939, 5.953233499612015756 ) ) ;
#77599=STYLED_ITEM ( 'NONE', ( #13681 ), #17407 ) ;
#77602=CARTESIAN_POINT ( 'NONE',  ( 20.36894250292379738, 39.92874883491396787, -10.36894250292379027 ) ) ;
#77603=CARTESIAN_POINT ( 'NONE',  ( 13.79529636645030344, 38.26208216824729647, 14.16423886937410614 ) ) ;
#77604=CARTESIAN_POINT ( 'NONE',  ( 0.5774900079438590739, 67.64701867748817676, -5.440088680355550821 ) ) ;
#77605=CARTESIAN_POINT ( 'NONE',  ( 21.09922568453594849, 11.20696800326375531, 6.408140936763242479 ) ) ;
#77606=CARTESIAN_POINT ( 'NONE',  ( 14.92337183194729988, 59.34226448433412315, -8.527530157486177487 ) ) ;
#77607=PLANE ( 'NONE',  #40310 ) ;
#77608=CARTESIAN_POINT ( 'NONE',  ( 7.084665262690076126, 59.10535201082150536, 10.88017736071109987 ) ) ;
#77609=CARTESIAN_POINT ( 'NONE',  ( 10.00000000000000000, 17.87363466993041783, -12.81628187352647608 ) ) ;
#77610=CARTESIAN_POINT ( 'NONE',  ( 10.00000000000000000, 35.55374883491396787, -14.16423886937410082 ) ) ;
#77611=CARTESIAN_POINT ( 'NONE',  ( 0.5774900079438590739, 27.64701867748817676, -5.440088680355550821 ) ) ;
#77613=CARTESIAN_POINT ( 'NONE',  ( 20.88017736071110519, 35.56368534415484106, 2.639326808657452039E-16 ) ) ;
#77616=ORIENTED_EDGE ( 'NONE', *, *, #81167, .T. ) ;
#77620=CARTESIAN_POINT ( 'NONE',  ( 13.79529636645030344, 63.26208216824730357, 14.16423886937410614 ) ) ;
#77621=CARTESIAN_POINT ( 'NONE',  ( 20.88017736071110164, 10.35535201082150714, 2.915334737309930979 ) ) ;
#77622=CARTESIAN_POINT ( 'NONE',  ( 2.791683348922240793, 41.63393115100078745, 7.208316651077764092 ) ) ;
#77623=CARTESIAN_POINT ( 'NONE',  ( 12.63842701281683034, 57.46726448433411605, 9.846743663894596210 ) ) ;
#77626=CARTESIAN_POINT ( 'NONE',  ( 10.00000000000000000, 2.873634669930420049, -12.81628187352647608 ) ) ;
#77628=CARTESIAN_POINT ( 'NONE',  ( -4.164238869374099039, 46.80374883491397497, 8.674139862899312516E-16 ) ) ;
#77629=ORIENTED_EDGE ( 'NONE', *, *, #41733, .F. ) ;
#77630=CARTESIAN_POINT ( 'NONE',  ( -2.266590686148945544, 47.22041550158063927, 7.082119434687048631 ) ) ;
#77632=CARTESIAN_POINT ( 'NONE',  ( 4.559911319644449179, 23.89701867748817321, 9.422509992056141925 ) ) ;
#77634=CARTESIAN_POINT ( 'NONE',  ( -0.8801773607111008646, 43.27201867748817676, 2.915334737309923430 ) ) ;
#77635=CARTESIAN_POINT ( 'NONE',  ( 1.472469842513823179, 51.42559781766745886, 4.923371831947296329 ) ) ;
#77636=CARTESIAN_POINT ( 'NONE',  ( 7.084665262690076126, 34.10535201082151247, 10.88017736071109987 ) ) ;
#77638=CARTESIAN_POINT ( 'NONE',  ( 2.035157376598824452, 63.68868534415484106, 7.964842623401179544 ) ) ;
#77639=CARTESIAN_POINT ( 'NONE',  ( 10.00000000000000178, 29.31368534415483751, 10.88017736071110342 ) ) ;
#77642=EDGE_CURVE ( 'NONE', #800, #11760, #9655, .T. ) ;
#77644=PLANE ( 'NONE',  #92034 ) ;
#77646=CARTESIAN_POINT ( 'NONE',  ( 19.84674366389459266, 3.300597817667451750, 2.638427012816836559 ) ) ;
#77649=DIRECTION ( 'NONE',  ( 0.000000000000000000, 1.000000000000000000, -0.000000000000000000 ) ) ;
#77650=CARTESIAN_POINT ( 'NONE',  ( 7.361572987183169658, 29.96726448433411960, -9.846743663894592657 ) ) ;
#77652=AXIS2_PLACEMENT_3D ( 'NONE', #87855, #42862, #19373 ) ;
#77654=DIRECTION ( 'NONE',  ( -1.000000000000000000, 0.000000000000000000, 0.000000000000000000 ) ) ;
#77658=CARTESIAN_POINT ( 'NONE',  ( 7.361572987183170547, 52.05059781766745175, 9.846743663894590881 ) ) ;
#77659=CARTESIAN_POINT ( 'NONE',  ( 20.36894250292379382, 48.67874883491396076, 10.36894250292379205 ) ) ;
#77660=CARTESIAN_POINT ( 'NONE',  ( 19.84674366389459266, 53.71726448433411605, -2.638427012816827677 ) ) ;
#77663=CARTESIAN_POINT ( 'NONE',  ( 19.84674366389459266, 23.30059781766745530, 2.638427012816836559 ) ) ;
#77664=CARTESIAN_POINT ( 'NONE',  ( 21.09922568453594849, 51.20696800326375353, 6.408140936763242479 ) ) ;
#77666=CARTESIAN_POINT ( 'NONE',  ( 2.791683348922240793, 56.63393115100078035, 7.208316651077764092 ) ) ;
#77667=CARTESIAN_POINT ( 'NONE',  ( 0.5774900079438590739, 52.64701867748817676, -5.440088680355550821 ) ) ;
#77674=CARTESIAN_POINT ( 'NONE',  ( 17.08211943468705840, 55.13708216824731068, -12.26659068614894466 ) ) ;
#77676=CARTESIAN_POINT ( 'NONE',  ( 10.00000000000000178, 24.31368534415484106, 10.88017736071110342 ) ) ;
#77677=CARTESIAN_POINT ( 'NONE',  ( -1.099225684535947600, 13.70696800326375353, -6.408140936763238038 ) ) ;
#77678=CARTESIAN_POINT ( 'NONE',  ( 0.5774900079438607392, 53.48035201082151247, 5.440088680355550821 ) ) ;
#77679=CARTESIAN_POINT ( 'NONE',  ( 20.88017736071110164, 65.35535201082151957, 2.915334737309930979 ) ) ;
#77682=CARTESIAN_POINT ( 'NONE',  ( 7.084665262690076126, 59.10535201082150536, 10.88017736071109987 ) ) ;
#77684=CARTESIAN_POINT ( 'NONE',  ( 1.472469842513823179, 41.42559781766745886, 4.923371831947296329 ) ) ;
#77686=CARTESIAN_POINT ( 'NONE',  ( 0.6178305044545838731, 4.748634669930420493, 9.382169495545420901 ) ) ;
#77687=CARTESIAN_POINT ( 'NONE',  ( 20.88017736071110164, 10.35535201082150714, 2.915334737309930979 ) ) ;
#77689=CARTESIAN_POINT ( 'NONE',  ( -4.164238869374099927, 42.01208216824728936, 3.795296366450308767 ) ) ;
#77690=VECTOR ( 'NONE', #81946, 1000.000000000000000 ) ;
#77691=CARTESIAN_POINT ( 'NONE',  ( 17.08211943468705130, 63.47041550158063927, 12.26659068614894998 ) ) ;
#77692=CARTESIAN_POINT ( 'NONE',  ( 12.63842701281683034, 32.46726448433412315, 9.846743663894596210 ) ) ;
#77694=CARTESIAN_POINT ( 'NONE',  ( 7.361572987183170547, 12.05059781766744997, 9.846743663894590881 ) ) ;
#77695=CARTESIAN_POINT ( 'NONE',  ( -0.8801773607111008646, 8.272018677488171434, 2.915334737309923430 ) ) ;
#77697=CARTESIAN_POINT ( 'NONE',  ( 1.472469842513823179, 35.59226448433412315, -4.923371831947296329 ) ) ;
#77699=CARTESIAN_POINT ( 'NONE',  ( 2.035157376598824452, 23.68868534415484461, 7.964842623401179544 ) ) ;
#77700=CARTESIAN_POINT ( 'NONE',  ( 10.00000000000000000, -2.126365330069579951, -12.81628187352647608 ) ) ;
#77701=CARTESIAN_POINT ( 'NONE',  ( -2.266590686148945544, 27.22041550158063572, 7.082119434687048631 ) ) ;
#77704=CARTESIAN_POINT ( 'NONE',  ( 5.076628168052704559, 10.17559781766745175, -8.527530157486179263 ) ) ;
#77705=CARTESIAN_POINT ( 'NONE',  ( 6.565887622018943937, 53.08196800326374643, -12.81628187352647608 ) ) ;
#77706=CARTESIAN_POINT ( 'NONE',  ( 2.791683348922240793, 56.63393115100078035, 7.208316651077764092 ) ) ;
#77708=CARTESIAN_POINT ( 'NONE',  ( 18.52753015748618282, 18.92559781766745175, -4.923371831947291888 ) ) ;
#77709=DIRECTION ( 'NONE',  ( 0.000000000000000000, -1.000000000000000000, 0.000000000000000000 ) ) ;
#77711=CARTESIAN_POINT ( 'NONE',  ( 2.035157376598824452, 3.688685344154837953, 7.964842623401179544 ) ) ;
#77712=CARTESIAN_POINT ( 'NONE',  ( 2.035157376598822676, 52.43868534415483396, -7.964842623401177768 ) ) ;
#77713=CARTESIAN_POINT ( 'NONE',  ( 20.36894250292379382, 3.678748834913967869, 10.36894250292379205 ) ) ;
#77714=CARTESIAN_POINT ( 'NONE',  ( 17.96484262340118221, 59.93868534415484106, 7.964842623401181321 ) ) ;
#77715=CARTESIAN_POINT ( 'NONE',  ( 17.20831665107776587, 37.88393115100078745, 7.208316651077764980 ) ) ;
#77716=CARTESIAN_POINT ( 'NONE',  ( 19.42250999205614548, 20.98035201082150891, -5.440088680355545492 ) ) ;
#77718=CARTESIAN_POINT ( 'NONE',  ( 18.52753015748618282, 58.92559781766745886, -4.923371831947291888 ) ) ;
#77722=( GEOMETRIC_REPRESENTATION_CONTEXT ( 3 ) GLOBAL_UNCERTAINTY_ASSIGNED_CONTEXT ( ( #29124 ) ) GLOBAL_UNIT_ASSIGNED_CONTEXT ( ( #59871, #27401, #20410 ) ) REPRESENTATION_CONTEXT ( 'NONE', 'WORKASPACE' ) );
#77724=ORIENTED_EDGE ( 'NONE', *, *, #77960, .F. ) ;
#77726=CARTESIAN_POINT ( 'NONE',  ( 12.63842701281683034, 42.46726448433412315, 9.846743663894596210 ) ) ;
#77727=CARTESIAN_POINT ( 'NONE',  ( 19.84674366389459621, 23.50893115100078390, 7.409399052514197653E-17 ) ) ;
#77728=CARTESIAN_POINT ( 'NONE',  ( 0.6178305044545818747, 53.49863466993041072, -9.382169495545419124 ) ) ;
#77729=CARTESIAN_POINT ( 'NONE',  ( 15.44008868035555793, 21.39701867748817321, -9.422509992056140149 ) ) ;
#77730=CARTESIAN_POINT ( 'NONE',  ( 5.076628168052704559, 45.17559781766745175, -8.527530157486179263 ) ) ;
#77732=CARTESIAN_POINT ( 'NONE',  ( 6.204703633549690345, 35.76208216824729647, -14.16423886937410259 ) ) ;
#77734=CARTESIAN_POINT ( 'NONE',  ( -0.3689425029237881626, 52.42874883491396076, 10.36894250292379027 ) ) ;
#77737=CARTESIAN_POINT ( 'NONE',  ( 4.559911319644449179, 52.23035201082151247, -9.422509992056141925 ) ) ;
#77738=CARTESIAN_POINT ( 'NONE',  ( 19.84674366389459266, 13.71726448433411782, -2.638427012816827677 ) ) ;
#77741=CARTESIAN_POINT ( 'NONE',  ( 21.92686044187656691, 29.95379003517447458, 3.195792623639537755 ) ) ;
#77742=ORIENTED_EDGE ( 'NONE', *, *, #89863, .T. ) ;
#77743=CARTESIAN_POINT ( 'NONE',  ( 18.52753015748618282, 8.925597817667451750, -4.923371831947291888 ) ) ;
#77745=CARTESIAN_POINT ( 'NONE',  ( -2.266590686148945544, 17.22041550158063572, 7.082119434687048631 ) ) ;
#77746=CARTESIAN_POINT ( 'NONE',  ( 1.472469842513823179, 21.42559781766745175, 4.923371831947296329 ) ) ;
#77747=CARTESIAN_POINT ( 'NONE',  ( 20.88017736071110164, 45.35535201082149115, 2.915334737309930979 ) ) ;
#77748=CARTESIAN_POINT ( 'NONE',  ( -46.44000000000001194, 100.8660254037844339, -9.500000000000000000 ) ) ;
#77749=ORIENTED_EDGE ( 'NONE', *, *, #45376, .T. ) ;
#77750=CARTESIAN_POINT ( 'NONE',  ( 19.42250999205614193, 40.14701867748817676, 5.440088680355555262 ) ) ;
#77751=CARTESIAN_POINT ( 'NONE',  ( -0.1049300847420728683, 2.216974130838790469, -6.336235997365750272 ) ) ;
#77753=CARTESIAN_POINT ( 'NONE',  ( 19.42250999205614193, 45.14701867748817676, 5.440088680355555262 ) ) ;
#77754=CARTESIAN_POINT ( 'NONE',  ( -0.3689425029237898834, 1.178748834913967869, -10.36894250292378850 ) ) ;
#77756=CARTESIAN_POINT ( 'NONE',  ( -1.099225684535947600, 24.54030133659708923, 6.408140936763237150 ) ) ;
#77758=CARTESIAN_POINT ( 'NONE',  ( 18.52753015748618282, 8.925597817667451750, -4.923371831947291888 ) ) ;
#77760=CARTESIAN_POINT ( 'NONE',  ( 0.1532563361054082862, 16.21726448433411960, 2.638427012816831674 ) ) ;
#77761=CARTESIAN_POINT ( 'NONE',  ( 2.035157376598822676, 37.43868534415484106, -7.964842623401177768 ) ) ;
#77762=AXIS2_PLACEMENT_3D ( 'NONE', #41926, #17932, #48905 ) ;
#77763=EDGE_CURVE ( 'NONE', #86159, #43937, #49733, .T. ) ;
#77767=CARTESIAN_POINT ( 'NONE',  ( -2.816281873526473856, 64.33196800326376774, 3.434112377981055619 ) ) ;
#77768=CARTESIAN_POINT ( 'NONE',  ( 7.084665262690076126, 54.10535201082151247, 10.88017736071109987 ) ) ;
#77771=CARTESIAN_POINT ( 'NONE',  ( 10.00000000000000178, 64.31368534415483396, 10.88017736071110342 ) ) ;
#77772=CARTESIAN_POINT ( 'NONE',  ( 22.81628187352648496, 11.83196800326375531, -3.434112377981050290 ) ) ;
#77773=DIRECTION ( 'NONE',  ( 0.000000000000000000, 0.000000000000000000, 1.000000000000000000 ) ) ;
#77774=CARTESIAN_POINT ( 'NONE',  ( 12.63842701281683922, 29.55059781766745175, -9.846743663894590881 ) ) ;
#77775=CARTESIAN_POINT ( 'NONE',  ( 22.81628187352647785, 61.41530133659709634, 3.434112377981063169 ) ) ;
#77776=CARTESIAN_POINT ( 'NONE',  ( 20.36894250292379382, 13.67874883491396965, 10.36894250292379205 ) ) ;
#77777=CARTESIAN_POINT ( 'NONE',  ( 10.00000000000000000, 19.75893115100078390, -9.846743663894594434 ) ) ;
#77778=CARTESIAN_POINT ( 'NONE',  ( 21.09922568453594849, 16.20696800326375353, 6.408140936763242479 ) ) ;
#77780=FACE_OUTER_BOUND ( 'NONE', #72468, .T. ) ;
#77782=CARTESIAN_POINT ( 'NONE',  ( -0.8801773607111009756, 53.06368534415484106, 1.068504757029289695E-15 ) ) ;
#77783=CARTESIAN_POINT ( 'NONE',  ( 18.52753015748618282, 58.92559781766745886, -4.923371831947291888 ) ) ;
#77784=CARTESIAN_POINT ( 'NONE',  ( -0.1503990784575277573, 33.10158574516643171, 6.262539305110076171 ) ) ;
#77785=CARTESIAN_POINT ( 'NONE',  ( 10.00000000000000178, 27.25893115100078390, 9.846743663894594434 ) ) ;
#77786=CARTESIAN_POINT ( 'NONE',  ( 10.00000000000000178, 9.313685344154839285, 10.88017736071110342 ) ) ;
#77787=CARTESIAN_POINT ( 'NONE',  ( 16.40814093676324603, 22.45696800326375353, -11.09922568453594671 ) ) ;
#77788=CARTESIAN_POINT ( 'NONE',  ( 18.52753015748617571, 28.09226448433411960, 4.923371831947298993 ) ) ;
#77789=( NAMED_UNIT ( * ) PLANE_ANGLE_UNIT ( ) SI_UNIT ( $, .RADIAN. ) );
#77792=CARTESIAN_POINT ( 'NONE',  ( 4.559911319644449179, 18.89701867748817321, 9.422509992056141925 ) ) ;
#77794=CARTESIAN_POINT ( 'NONE',  ( 19.84674366389459266, 48.30059781766745175, 2.638427012816836559 ) ) ;
#77795=CARTESIAN_POINT ( 'NONE',  ( 4.559911319644449179, 12.23035201082150714, -9.422509992056141925 ) ) ;
#77797=CARTESIAN_POINT ( 'NONE',  ( -0.8801773607111008646, 33.27201867748817676, 2.915334737309923430 ) ) ;
#77798=CARTESIAN_POINT ( 'NONE',  ( 7.084665262690076126, 14.10535201082150358, 10.88017736071109987 ) ) ;
#77799=CARTESIAN_POINT ( 'NONE',  ( 2.791683348922237240, 20.38393115100078745, -7.208316651077763204 ) ) ;
#77800=CARTESIAN_POINT ( 'NONE',  ( 19.84674366389459266, 38.71726448433412315, -2.638427012816827677 ) ) ;
#77802=CARTESIAN_POINT ( 'NONE',  ( 12.63842701281683922, 64.55059781766745175, -9.846743663894590881 ) ) ;
#77803=( NAMED_UNIT ( * ) SI_UNIT ( $, .STERADIAN. ) SOLID_ANGLE_UNIT ( ) );
#77805=CARTESIAN_POINT ( 'NONE',  ( 6.204703633549690345, 27.84541550158063217, 14.16423886937410082 ) ) ;
#77806=CARTESIAN_POINT ( 'NONE',  ( 19.84674366389459266, 33.71726448433410894, -2.638427012816827677 ) ) ;
#77807=DIRECTION ( 'NONE',  ( -0.000000000000000000, 1.000000000000000000, -0.000000000000000000 ) ) ;
#77809=CARTESIAN_POINT ( 'NONE',  ( 17.08211943468705130, 53.47041550158063217, 12.26659068614894998 ) ) ;
#77810=CARTESIAN_POINT ( 'NONE',  ( 17.20831665107776587, 19.13393115100078035, -7.208316651077762316 ) ) ;
#77813=CARTESIAN_POINT ( 'NONE',  ( 12.91533473730992121, 49.52201867748817676, 10.88017736071110164 ) ) ;
#77816=CARTESIAN_POINT ( 'NONE',  ( 15.44008868035555260, 14.73035201082150536, 9.422509992056143702 ) ) ;
#77817=CARTESIAN_POINT ( 'NONE',  ( 3.591859063236763294, 53.29030133659708923, -11.09922568453595026 ) ) ;
#77818=CARTESIAN_POINT ( 'NONE',  ( 3.591859063236763294, 13.29030133659708746, -11.09922568453595026 ) ) ;
#77819=CARTESIAN_POINT ( 'NONE',  ( 17.20831665107776587, 12.88393115100078390, 7.208316651077764980 ) ) ;
#77822=CARTESIAN_POINT ( 'NONE',  ( -0.03447792253739259682, 20.15514106990689669, 6.401564815979746470 ) ) ;
#77823=CARTESIAN_POINT ( 'NONE',  ( 17.08211943468705130, 48.47041550158063927, 12.26659068614894998 ) ) ;
#77824=CARTESIAN_POINT ( 'NONE',  ( -2.266590686148945544, 16.38708216824730357, -7.082119434687050408 ) ) ;
#77825=CARTESIAN_POINT ( 'NONE',  ( 19.42250999205614548, 20.98035201082150891, -5.440088680355545492 ) ) ;
#77827=CARTESIAN_POINT ( 'NONE',  ( 17.96484262340118221, 34.93868534415482685, 7.964842623401181321 ) ) ;
#77831=CARTESIAN_POINT ( 'NONE',  ( 0.5774900079438607392, 63.48035201082149825, 5.440088680355550821 ) ) ;
#77832=CARTESIAN_POINT ( 'NONE',  ( 7.361572987183169658, 19.96726448433411960, -9.846743663894592657 ) ) ;
#77835=CARTESIAN_POINT ( 'NONE',  ( 7.361572987183169658, 9.967264484334119601, -9.846743663894592657 ) ) ;
#77836=CARTESIAN_POINT ( 'NONE',  ( 7.361572987183169658, 39.96726448433411605, -9.846743663894592657 ) ) ;
#77839=CARTESIAN_POINT ( 'NONE',  ( 12.91533473730993009, 16.60535201082150891, -10.88017736071109987 ) ) ;
#77842=CARTESIAN_POINT ( 'NONE',  ( 3.591859063236763294, 28.29030133659708568, -11.09922568453595026 ) ) ;
#77843=CARTESIAN_POINT ( 'NONE',  ( 7.084665262690076126, 49.10535201082149825, 10.88017736071109987 ) ) ;
#77844=CARTESIAN_POINT ( 'NONE',  ( -4.164238869374099039, 51.80374883491396787, 8.674139862899312516E-16 ) ) ;
#77845=CARTESIAN_POINT ( 'NONE',  ( 2.791683348922240793, 11.63393115100078568, 7.208316651077764092 ) ) ;
#77847=CARTESIAN_POINT ( 'NONE',  ( 19.84674366389459266, 48.30059781766745175, 2.638427012816836559 ) ) ;
#77848=CARTESIAN_POINT ( 'NONE',  ( 7.361572987183169658, 29.96726448433411960, -9.846743663894592657 ) ) ;
#77849=CARTESIAN_POINT ( 'NONE',  ( 6.204703633549690345, 7.845415501580634832, 14.16423886937410082 ) ) ;
#77850=CARTESIAN_POINT ( 'NONE',  ( 22.26659068614894466, 23.88708216824730357, 7.082119434687054849 ) ) ;
#77851=CARTESIAN_POINT ( 'NONE',  ( 10.00000000000000178, 44.31368534415484106, 10.88017736071110342 ) ) ;
#77852=CARTESIAN_POINT ( 'NONE',  ( 7.084665262690076126, 14.10535201082150358, 10.88017736071109987 ) ) ;
#77854=CARTESIAN_POINT ( 'NONE',  ( 7.084665262690076126, 39.10535201082150536, 10.88017736071109987 ) ) ;
#77855=CARTESIAN_POINT ( 'NONE',  ( 7.084665262690076126, 29.10535201082150181, 10.88017736071109987 ) ) ;
#77857=CARTESIAN_POINT ( 'NONE',  ( -1.099225684535947600, 34.54030133659708923, 6.408140936763237150 ) ) ;
#77858=CARTESIAN_POINT ( 'NONE',  ( 15.44008868035555260, 39.73035201082150536, 9.422509992056143702 ) ) ;
#77860=CARTESIAN_POINT ( 'NONE',  ( 6.565887622018943937, 63.08196800326376064, -12.81628187352647608 ) ) ;
#77861=CARTESIAN_POINT ( 'NONE',  ( 20.88017736071110875, 45.77201867748816966, -2.915334737309920765 ) ) ;
#77863=CARTESIAN_POINT ( 'NONE',  ( 12.91533473730992121, 54.52201867748816255, 10.88017736071110164 ) ) ;
#77864=DIRECTION ( 'NONE',  ( -0.8320502943378437211, 0.5547001962252290364, 0.000000000000000000 ) ) ;
#77867=CARTESIAN_POINT ( 'NONE',  ( 22.26659068614894466, 63.88708216824730357, 7.082119434687054849 ) ) ;
#77868=CARTESIAN_POINT ( 'NONE',  ( 2.791683348922237240, 0.3839311510007847872, -7.208316651077763204 ) ) ;
#77869=CARTESIAN_POINT ( 'NONE',  ( 2.917880565312950480, 0.9704155015806342766, -12.26659068614894821 ) ) ;
#77871=CARTESIAN_POINT ( 'NONE',  ( 15.44008868035555260, 14.73035201082150536, 9.422509992056143702 ) ) ;
#77872=CARTESIAN_POINT ( 'NONE',  ( 2.791683348922240793, 51.63393115100078745, 7.208316651077764092 ) ) ;
#77874=CARTESIAN_POINT ( 'NONE',  ( 1.472469842513823179, 50.59226448433411605, -4.923371831947296329 ) ) ;
#77876=CARTESIAN_POINT ( 'NONE',  ( -0.8801773607111008646, 33.27201867748817676, 2.915334737309923430 ) ) ;
#77877=CARTESIAN_POINT ( 'NONE',  ( 1.472469842513823179, 40.59226448433411605, -4.923371831947296329 ) ) ;
#77878=CARTESIAN_POINT ( 'NONE',  ( -15.94000000000001371, 93.50000000000000000, -10.09898361729590199 ) ) ;
#77879=CARTESIAN_POINT ( 'NONE',  ( 20.88017736071110164, 65.35535201082150536, 2.915334737309930979 ) ) ;
#77880=CARTESIAN_POINT ( 'NONE',  ( 0.5774900079438590739, 47.64701867748817676, -5.440088680355550821 ) ) ;
#77881=CARTESIAN_POINT ( 'NONE',  ( 24.16423886937409904, 64.09541550158064638, 3.795296366450317205 ) ) ;
#77882=EDGE_CURVE ( 'NONE', #10063, #29181, #22773, .T. ) ;
#77884=CARTESIAN_POINT ( 'NONE',  ( 21.09922568453594849, 26.20696800326375353, 6.408140936763242479 ) ) ;
#77885=CARTESIAN_POINT ( 'NONE',  ( 0.1532563361054083140, 51.00893115100078745, 1.131784320476157264E-15 ) ) ;
#77888=CARTESIAN_POINT ( 'NONE',  ( 6.565887622018943937, 30.16530133659708568, 12.81628187352647430 ) ) ;
#77889=CARTESIAN_POINT ( 'NONE',  ( 15.44008868035555260, 24.73035201082150891, 9.422509992056143702 ) ) ;
#77892=CARTESIAN_POINT ( 'NONE',  ( 4.559911319644449179, 67.23035201082150536, -9.422509992056141925 ) ) ;
#77893=CARTESIAN_POINT ( 'NONE',  ( 18.52753015748618282, 53.92559781766745175, -4.923371831947291888 ) ) ;
#77895=CARTESIAN_POINT ( 'NONE',  ( 12.63842701281683034, 12.46726448433411782, 9.846743663894596210 ) ) ;
#77896=CARTESIAN_POINT ( 'NONE',  ( 1.472469842513823179, 41.42559781766745886, 4.923371831947296329 ) ) ;
#77899=CARTESIAN_POINT ( 'NONE',  ( 14.92337183194729988, 24.34226448433411960, -8.527530157486177487 ) ) ;
#77900=CARTESIAN_POINT ( 'NONE',  ( -42.94000000000001194, 92.50000000000000000, 9.500000000000000000 ) ) ;
#77902=CARTESIAN_POINT ( 'NONE',  ( 0.1532563361054083140, 26.00893115100078745, 1.131784320476157264E-15 ) ) ;
#77906=CARTESIAN_POINT ( 'NONE',  ( 19.84674366389459266, 48.30059781766745175, 2.638427012816836559 ) ) ;
#77910=CARTESIAN_POINT ( 'NONE',  ( 22.81628187352647785, 31.41530133659709279, 3.434112377981063169 ) ) ;
#77913=CARTESIAN_POINT ( 'NONE',  ( 22.26659068614895176, 49.72041550158063927, -7.082119434687042414 ) ) ;
#77914=CARTESIAN_POINT ( 'NONE',  ( 1.472469842513823179, 15.59226448433411960, -4.923371831947296329 ) ) ;
#77916=CARTESIAN_POINT ( 'NONE',  ( 19.72487221294571569, 45.71833443783938122, -6.499999999999989342 ) ) ;
#77919=CARTESIAN_POINT ( 'NONE',  ( 13.79529636645030344, 43.26208216824730357, 14.16423886937410614 ) ) ;
#77920=CARTESIAN_POINT ( 'NONE',  ( 10.00000000000000000, 64.75893115100078035, -9.846743663894594434 ) ) ;
#77921=CARTESIAN_POINT ( 'NONE',  ( 2.917880565312950480, 60.97041550158063927, -12.26659068614894821 ) ) ;
#77922=CARTESIAN_POINT ( 'NONE',  ( 2.917880565312948704, 22.63708216824730002, 12.26659068614894643 ) ) ;
#77923=CARTESIAN_POINT ( 'NONE',  ( -2.266590686148945544, 21.38708216824730357, -7.082119434687050408 ) ) ;
#77924=LINE ( 'NONE', #17443, #61137 ) ;
#77926=CARTESIAN_POINT ( 'NONE',  ( 14.92337183194729988, 59.34226448433412315, -8.527530157486177487 ) ) ;
#77928=CARTESIAN_POINT ( 'NONE',  ( 0.5774900079438607392, 38.48035201082150536, 5.440088680355550821 ) ) ;
#77930=CARTESIAN_POINT ( 'NONE',  ( 19.59355889808634643, 95.39896427371951404, -5.130931023488903620 ) ) ;
#77931=CARTESIAN_POINT ( 'NONE',  ( 19.84674366389459266, 38.71726448433412315, -2.638427012816827677 ) ) ;
#77932=CARTESIAN_POINT ( 'NONE',  ( 3.591859063236763294, 53.29030133659708923, -11.09922568453595026 ) ) ;
#77934=CARTESIAN_POINT ( 'NONE',  ( 14.92337183194729988, 39.34226448433412315, -8.527530157486177487 ) ) ;
#77936=B_SPLINE_CURVE_WITH_KNOTS ( 'NONE', 3,
 ( #85431, #34377, #95387, #47422, #93420, #1954, #78415, #66355 ),
 .UNSPECIFIED., .F., .F.,
 ( 4, 2, 2, 4 ),
 ( 0.000000000000000000, 0.002747544437249704527, 0.004121316655874556791, 0.005495088874499409054 ),
 .UNSPECIFIED. ) ;
#77937=ORIENTED_EDGE ( 'NONE', *, *, #39969, .T. ) ;
#77939=CARTESIAN_POINT ( 'NONE',  ( -2.266590686148945544, 12.22041550158063394, 7.082119434687048631 ) ) ;
#77940=CARTESIAN_POINT ( 'NONE',  ( 19.72487221294570858, 70.00000000000000000, 6.500000000000000888 ) ) ;
#77943=CARTESIAN_POINT ( 'NONE',  ( 15.44008868035555793, 6.397018677488171434, -9.422509992056140149 ) ) ;
#77944=CARTESIAN_POINT ( 'NONE',  ( 22.81628187352647785, 6.415301336597088344, 3.434112377981063169 ) ) ;
#77945=CARTESIAN_POINT ( 'NONE',  ( 21.92686044187657046, 2.396642702460841434, -3.195792623639524432 ) ) ;
#77946=CARTESIAN_POINT ( 'NONE',  ( 20.88017736071110875, 65.77201867748817676, -2.915334737309920765 ) ) ;
#77948=CARTESIAN_POINT ( 'NONE',  ( -46.94000000000126960, 101.3832071409885884, -8.175121524388728744 ) ) ;
#77950=CARTESIAN_POINT ( 'NONE',  ( 22.26659068614894466, 58.88708216824729647, 7.082119434687054849 ) ) ;
#77951=DIRECTION ( 'NONE',  ( -0.000000000000000000, 1.000000000000000000, 0.000000000000000000 ) ) ;
#77952=CARTESIAN_POINT ( 'NONE',  ( 2.035157376598822676, 32.43868534415483396, -7.964842623401177768 ) ) ;
#77953=CARTESIAN_POINT ( 'NONE',  ( -0.8801773607111009756, 38.06368534415484106, 1.068504757029289695E-15 ) ) ;
#77954=CARTESIAN_POINT ( 'NONE',  ( -2.816281873526473856, 4.123634669930420493, 9.499525473075851096E-16 ) ) ;
#77955=CARTESIAN_POINT ( 'NONE',  ( 14.92337183194729633, 47.67559781766745175, 8.527530157486181039 ) ) ;
#77956=CARTESIAN_POINT ( 'NONE',  ( -2.816281873526471635, 58.91530133659707502, -3.434112377981056508 ) ) ;
#77957=FILL_AREA_STYLE ('',( #85966 ) ) ;
#77959=CARTESIAN_POINT ( 'NONE',  ( 15.44008868035555793, 36.39701867748816966, -9.422509992056140149 ) ) ;
#77960=EDGE_CURVE ( 'NONE', #63027, #54853, #35341, .T. ) ;
#77961=CARTESIAN_POINT ( 'NONE',  ( 13.43411237798106583, 32.66530133659708213, -12.81628187352647252 ) ) ;
#77962=CARTESIAN_POINT ( 'NONE',  ( -0.1503990784575328643, 55.12777174578612716, 6.262539305110068177 ) ) ;
#77963=( GEOMETRIC_REPRESENTATION_CONTEXT ( 3 ) GLOBAL_UNCERTAINTY_ASSIGNED_CONTEXT ( ( #47202 ) ) GLOBAL_UNIT_ASSIGNED_CONTEXT ( ( #78487, #23042, #84027 ) ) REPRESENTATION_CONTEXT ( 'NONE', 'WORKASPACE' ) );
#77964=CARTESIAN_POINT ( 'NONE',  ( 10.00000000000000178, 57.25893115100078745, 9.846743663894594434 ) ) ;
#77965=CARTESIAN_POINT ( 'NONE',  ( 4.559911319644449179, 53.89701867748817676, 9.422509992056141925 ) ) ;
#77966=CARTESIAN_POINT ( 'NONE',  ( 21.09922568453594849, 41.20696800326375353, 6.408140936763242479 ) ) ;
#77967=CARTESIAN_POINT ( 'NONE',  ( 12.91533473730993009, 61.60535201082150536, -10.88017736071109987 ) ) ;
#77970=CARTESIAN_POINT ( 'NONE',  ( 0.6178305044545838731, 59.74863466993041783, 9.382169495545420901 ) ) ;
#77974=CARTESIAN_POINT ( 'NONE',  ( 20.88017736071110164, 10.35535201082150714, 2.915334737309930979 ) ) ;
#77975=CARTESIAN_POINT ( 'NONE',  ( -2.816281873526471635, 48.91530133659708213, -3.434112377981056508 ) ) ;
#77976=CARTESIAN_POINT ( 'NONE',  ( -4.164238869374099927, 12.01208216824730357, 3.795296366450308767 ) ) ;
#77977=CARTESIAN_POINT ( 'NONE',  ( 7.361572987183169658, 19.96726448433411960, -9.846743663894592657 ) ) ;
#77978=CARTESIAN_POINT ( 'NONE',  ( 2.035157376598824452, 8.688685344154839285, 7.964842623401179544 ) ) ;
#77979=CARTESIAN_POINT ( 'NONE',  ( 12.63842701281683922, 14.55059781766744997, -9.846743663894590881 ) ) ;
#77980=CARTESIAN_POINT ( 'NONE',  ( 6.204703633549690345, 55.76208216824730357, -14.16423886937410259 ) ) ;
#77982=CARTESIAN_POINT ( 'NONE',  ( -46.44000000000001194, 99.99999999999998579, 9.000000000000000000 ) ) ;
#77983=AXIS2_PLACEMENT_3D ( 'NONE', #15461, #45942, #76432 ) ;
#77984=CARTESIAN_POINT ( 'NONE',  ( 2.035157376598822676, 22.43868534415483396, -7.964842623401177768 ) ) ;
#77985=CARTESIAN_POINT ( 'NONE',  ( 19.88701968852524615, 46.79427333184086280, 6.480634945678618308 ) ) ;
#77989=CARTESIAN_POINT ( 'NONE',  ( 4.559911319644449179, 2.230352010821504916, -9.422509992056141925 ) ) ;
#77990=CARTESIAN_POINT ( 'NONE',  ( 0.5774900079438590739, 12.64701867748817321, -5.440088680355550821 ) ) ;
#77991=CARTESIAN_POINT ( 'NONE',  ( 7.361572987183170547, 47.05059781766745175, 9.846743663894590881 ) ) ;
#77992=CARTESIAN_POINT ( 'NONE',  ( 6.565887622018943937, 55.16530133659709634, 12.81628187352647430 ) ) ;
#77994=CARTESIAN_POINT ( 'NONE',  ( 19.84674366389459621, 63.50893115100078745, 7.409399052514197653E-17 ) ) ;
#77995=CARTESIAN_POINT ( 'NONE',  ( -4.164238869374099039, 21.80374883491396787, 8.674139862899312516E-16 ) ) ;
#77996=CARTESIAN_POINT ( 'NONE',  ( 10.00000000000000178, 29.31368534415483751, 10.88017736071110342 ) ) ;
#77997=CARTESIAN_POINT ( 'NONE',  ( 2.035157376598822676, 7.438685344154837509, -7.964842623401177768 ) ) ;
#77998=CARTESIAN_POINT ( 'NONE',  ( 5.076628168052703671, 51.84226448433412315, 8.527530157486179263 ) ) ;
#77999=CARTESIAN_POINT ( 'NONE',  ( 18.61655166652076687, 44.87718327197428181, 6.499999999999981348 ) ) ;
#78000=CARTESIAN_POINT ( 'NONE',  ( 14.92337183194729633, 42.67559781766745886, 8.527530157486181039 ) ) ;
#78002=CARTESIAN_POINT ( 'NONE',  ( 19.84674366389459621, 8.508931151000785675, 7.409399052514197653E-17 ) ) ;
#78004=ORIENTED_EDGE ( 'NONE', *, *, #32334, .T. ) ;
#78005=( NAMED_UNIT ( * ) PLANE_ANGLE_UNIT ( ) SI_UNIT ( $, .RADIAN. ) );
#78006=CARTESIAN_POINT ( 'NONE',  ( 2.035157376598824452, 68.68868534415484817, 7.964842623401179544 ) ) ;
#78007=CARTESIAN_POINT ( 'NONE',  ( 6.565887622018943937, 3.081968003263753531, -12.81628187352647608 ) ) ;
#78008=CARTESIAN_POINT ( 'NONE',  ( 15.44008868035555793, 41.39701867748817676, -9.422509992056140149 ) ) ;
#78009=CARTESIAN_POINT ( 'NONE',  ( 7.084665262690076126, 12.02201867748817143, -10.88017736071110164 ) ) ;
#78010=CARTESIAN_POINT ( 'NONE',  ( 22.81628187352647785, 41.41530133659708923, 3.434112377981063169 ) ) ;
#78011=CARTESIAN_POINT ( 'NONE',  ( 10.00000000000000178, 23.05374883491397142, 14.16423886937410082 ) ) ;
#78015=CARTESIAN_POINT ( 'NONE',  ( 16.40814093676324603, 42.45696800326375353, -11.09922568453594671 ) ) ;
#78018=( BOUNDED_CURVE ( )  B_SPLINE_CURVE ( 2, ( #74097, #75593, #89609, #6602, #90093, #75095, #21120, #67107, #45587 ),
 .UNSPECIFIED., .F., .T. ) 
 B_SPLINE_CURVE_WITH_KNOTS ( ( 3, 2, 2, 2, 3 ),
 ( 0.3667998787605536437, 0.3690476190476190688, 0.3750000000000000000, 0.3809523809523809312, 0.3832001212394454126 ),
 .UNSPECIFIED. ) 
 CURVE ( )  GEOMETRIC_REPRESENTATION_ITEM ( )  RATIONAL_B_SPLINE_CURVE ( ( 0.9839835555609424134, 0.9871328979762475919, 1.000000000000000000, 0.9659258262890683122, 1.000000000000000000, 0.9659258262890683122, 1.000000000000000000, 0.9871328979762530320, 0.9839835555609450779 ) ) 
 REPRESENTATION_ITEM ( '' )  );
#78019=CARTESIAN_POINT ( 'NONE',  ( 17.20831665107776587, 52.88393115100078035, 7.208316651077764980 ) ) ;
#78020=CARTESIAN_POINT ( 'NONE',  ( 7.084665262690076126, 22.02201867748817321, -10.88017736071110164 ) ) ;
#78021=ORIENTED_EDGE ( 'NONE', *, *, #70002, .T. ) ;
#78022=CARTESIAN_POINT ( 'NONE',  ( 10.00000000000000178, 29.31368534415483751, 10.88017736071110342 ) ) ;
#78024=CARTESIAN_POINT ( 'NONE',  ( 2.791683348922237240, 10.38393115100078390, -7.208316651077763204 ) ) ;
#78025=FACE_OUTER_BOUND ( 'NONE', #26639, .T. ) ;
#78027=VECTOR ( 'NONE', #57166, 1000.000000000000000 ) ;
#78028=CARTESIAN_POINT ( 'NONE',  ( 1.472469842513823179, 11.42559781766745175, 4.923371831947296329 ) ) ;
#78029=CARTESIAN_POINT ( 'NONE',  ( 4.559911319644449179, 67.23035201082150536, -9.422509992056141925 ) ) ;
#78031=CARTESIAN_POINT ( 'NONE',  ( 0.8952175423694819223, 38.52576239577081907, 5.990408912944316100 ) ) ;
#78032=CARTESIAN_POINT ( 'NONE',  ( -0.8801773607111008646, 63.27201867748817676, 2.915334737309923430 ) ) ;
#78033=CARTESIAN_POINT ( 'NONE',  ( 12.63842701281683922, 4.550597817667451750, -9.846743663894590881 ) ) ;
#78035=CARTESIAN_POINT ( 'NONE',  ( 0.1532563361054083140, 61.00893115100078745, 1.131784320476157264E-15 ) ) ;
#78039=( NAMED_UNIT ( * ) SI_UNIT ( $, .STERADIAN. ) SOLID_ANGLE_UNIT ( ) );
#78040=CARTESIAN_POINT ( 'NONE',  ( 19.38216949554541557, 57.24863466993042493, -9.382169495545420901 ) ) ;
#78042=CARTESIAN_POINT ( 'NONE',  ( -4.164238869374099039, 21.80374883491396787, 8.674139862899312516E-16 ) ) ;
#78045=CARTESIAN_POINT ( 'NONE',  ( 12.91533473730992121, 59.52201867748816966, 10.88017736071110164 ) ) ;
#78046=CARTESIAN_POINT ( 'NONE',  ( -0.8801773607111008646, 18.27201867748817321, 2.915334737309923430 ) ) ;
#78048=CARTESIAN_POINT ( 'NONE',  ( 0.1532563361054083140, 6.008931151000784787, 1.131784320476157264E-15 ) ) ;
#78049=CARTESIAN_POINT ( 'NONE',  ( 10.00000000000000178, 7.258931151000785675, 9.846743663894594434 ) ) ;
#78050=CARTESIAN_POINT ( 'NONE',  ( -2.816281873526473856, 29.33196800326376064, 3.434112377981055619 ) ) ;
#78051=CARTESIAN_POINT ( 'NONE',  ( 18.52753015748617571, 43.09226448433412315, 4.923371831947298993 ) ) ;
#78054=CARTESIAN_POINT ( 'NONE',  ( 0.6178305044545838731, 14.74863466993041783, 9.382169495545420901 ) ) ;
#78057=CARTESIAN_POINT ( 'NONE',  ( 7.361572987183170547, 27.05059781766745175, 9.846743663894590881 ) ) ;
#78058=CARTESIAN_POINT ( 'NONE',  ( 17.20831665107776587, 9.133931151000787452, -7.208316651077762316 ) ) ;
#78059=ORIENTED_EDGE ( 'NONE', *, *, #57257, .F. ) ;
#78061=CARTESIAN_POINT ( 'NONE',  ( 15.44008868035555260, 39.73035201082150536, 9.422509992056143702 ) ) ;
#78062=CARTESIAN_POINT ( 'NONE',  ( -0.3689425029237881626, 37.42874883491396787, 10.36894250292379027 ) ) ;
#78063=CARTESIAN_POINT ( 'NONE',  ( 5.076628168052704559, 40.17559781766745175, -8.527530157486179263 ) ) ;
#78064=CARTESIAN_POINT ( 'NONE',  ( 10.00000000000000000, 14.75893115100078568, -9.846743663894594434 ) ) ;
#78065=CARTESIAN_POINT ( 'NONE',  ( 19.38216949554541202, 55.99863466993041072, 9.382169495545424454 ) ) ;
#78067=CARTESIAN_POINT ( 'NONE',  ( -0.8801773607111009756, 33.06368534415484106, 1.068504757029289695E-15 ) ) ;
#78069=CARTESIAN_POINT ( 'NONE',  ( 3.591859063236763294, 28.29030133659708568, -11.09922568453595026 ) ) ;
#78070=CARTESIAN_POINT ( 'NONE',  ( 12.63842701281683922, 44.55059781766745175, -9.846743663894590881 ) ) ;
#78072=CARTESIAN_POINT ( 'NONE',  ( 22.81628187352647785, 46.41530133659708213, 3.434112377981063169 ) ) ;
#78074=CARTESIAN_POINT ( 'NONE',  ( 7.084665262690076126, 54.10535201082151247, 10.88017736071109987 ) ) ;
#78079=CARTESIAN_POINT ( 'NONE',  ( 19.42250999205614548, 55.98035201082150536, -5.440088680355545492 ) ) ;
#78080=CARTESIAN_POINT ( 'NONE',  ( 2.035157376598822676, 62.43868534415483396, -7.964842623401177768 ) ) ;
#78081=CYLINDRICAL_SURFACE ( 'NONE', #74432, 0.5000000000000004441 ) ;
#78083=CARTESIAN_POINT ( 'NONE',  ( 4.559911319644449179, 12.23035201082150714, -9.422509992056141925 ) ) ;
#78084=CARTESIAN_POINT ( 'NONE',  ( 14.92337183194729988, 64.34226448433412315, -8.527530157486177487 ) ) ;
#78085=CARTESIAN_POINT ( 'NONE',  ( 17.96484262340118221, 21.18868534415483396, -7.964842623401177768 ) ) ;
#78088=CARTESIAN_POINT ( 'NONE',  ( 19.38216949554541202, 25.99863466993042138, 9.382169495545424454 ) ) ;
#78090=CARTESIAN_POINT ( 'NONE',  ( 19.42250999205614193, 50.14701867748817676, 5.440088680355555262 ) ) ;
#78091=CARTESIAN_POINT ( 'NONE',  ( 19.84674366389459266, 43.30059781766744464, 2.638427012816836559 ) ) ;
#78092=CARTESIAN_POINT ( 'NONE',  ( -2.816281873526473856, 4.331968003263754419, 3.434112377981055619 ) ) ;
#78093=CARTESIAN_POINT ( 'NONE',  ( 20.15039907845753575, 47.62777174578613426, -6.262539305110073506 ) ) ;
#78094=CARTESIAN_POINT ( 'NONE',  ( 19.42250999205614548, 10.98035201082150358, -5.440088680355545492 ) ) ;
#78095=CARTESIAN_POINT ( 'NONE',  ( 20.88017736071110519, 45.56368534415484106, 2.639326808657452039E-16 ) ) ;
#78096=CARTESIAN_POINT ( 'NONE',  ( 13.79529636645031943, 55.34541550158062506, -14.16423886937409904 ) ) ;
#78097=CARTESIAN_POINT ( 'NONE',  ( 17.20831665107776587, 44.13393115100078745, -7.208316651077762316 ) ) ;
#78099=CARTESIAN_POINT ( 'NONE',  ( 20.88017736071110875, 65.77201867748817676, -2.915334737309920765 ) ) ;
#78100=CARTESIAN_POINT ( 'NONE',  ( 20.36894250292379382, 18.67874883491397142, 10.36894250292379205 ) ) ;
#78102=UNCERTAINTY_MEASURE_WITH_UNIT (LENGTH_MEASURE( 1.000000000000000082E-05 ), #88765, 'distance_accuracy_value', 'NONE');
#78105=CARTESIAN_POINT ( 'NONE',  ( -4.164238869374098151, 31.59541550158063927, -3.795296366450310543 ) ) ;
#78106=CARTESIAN_POINT ( 'NONE',  ( -4.164238869374098151, 41.59541550158061796, -3.795296366450310543 ) ) ;
#78107=CARTESIAN_POINT ( 'NONE',  ( 2.791683348922237240, 5.383931151000785675, -7.208316651077763204 ) ) ;
#78108=CARTESIAN_POINT ( 'NONE',  ( 13.43411237798105340, 20.58196800326374643, 12.81628187352647963 ) ) ;
#78109=CARTESIAN_POINT ( 'NONE',  ( 12.63842701281683034, 57.46726448433411605, 9.846743663894596210 ) ) ;
#78111=CARTESIAN_POINT ( 'NONE',  ( 7.084665262690076126, 62.02201867748816966, -10.88017736071110164 ) ) ;
#78112=CARTESIAN_POINT ( 'NONE',  ( -1.099225684535947600, 38.70696800326375353, -6.408140936763238038 ) ) ;
#78113=CARTESIAN_POINT ( 'NONE',  ( 13.79529636645031943, 25.34541550158063572, -14.16423886937409904 ) ) ;
#78114=CARTESIAN_POINT ( 'NONE',  ( 7.084665262690076126, 27.02201867748817676, -10.88017736071110164 ) ) ;
#78115=CARTESIAN_POINT ( 'NONE',  ( 3.640395162852214650, 89.00000000000000000, 12.00000000000000000 ) ) ;
#78116=CARTESIAN_POINT ( 'NONE',  ( 7.361572987183170547, 2.050597817667451750, 9.846743663894590881 ) ) ;
#78122=ADVANCED_FACE ( 'NONE', ( #45207 ), #74716, .F. ) ;
#78123=ORIENTED_EDGE ( 'NONE', *, *, #77014, .F. ) ;
#78124=CARTESIAN_POINT ( 'NONE',  ( 2.917880565312948704, 7.637082168247301794, 12.26659068614894643 ) ) ;
#78125=CARTESIAN_POINT ( 'NONE',  ( -4.164238869374099927, 67.01208216824728936, 3.795296366450308767 ) ) ;
#78126=CARTESIAN_POINT ( 'NONE',  ( 12.91533473730992121, 9.522018677488171434, 10.88017736071110164 ) ) ;
#78127=CARTESIAN_POINT ( 'NONE',  ( 5.076628168052703671, 41.84226448433411605, 8.527530157486179263 ) ) ;
#78128=CARTESIAN_POINT ( 'NONE',  ( -2.816281873526473856, 9.123634669930421381, 9.499525473075851096E-16 ) ) ;
#78132=CARTESIAN_POINT ( 'NONE',  ( 0.6178305044545838731, 4.748634669930420493, 9.382169495545420901 ) ) ;
#78135=CARTESIAN_POINT ( 'NONE',  ( 10.00000000000000178, 48.05374883491396787, 14.16423886937410082 ) ) ;
#78137=CARTESIAN_POINT ( 'NONE',  ( 6.204703633549690345, 62.84541550158063927, 14.16423886937410082 ) ) ;
#78139=CARTESIAN_POINT ( 'NONE',  ( 20.88017736071110164, 20.35535201082150891, 2.915334737309930979 ) ) ;
#78140=CARTESIAN_POINT ( 'NONE',  ( 10.00000000000000000, 41.81368534415484106, -10.88017736071110342 ) ) ;
#78141=CARTESIAN_POINT ( 'NONE',  ( 19.84674366389459621, 58.50893115100078745, 7.409399052514197653E-17 ) ) ;
#78142=CARTESIAN_POINT ( 'NONE',  ( 19.42250999205614548, 40.98035201082150536, -5.440088680355545492 ) ) ;
#78143=CARTESIAN_POINT ( 'NONE',  ( 15.44008868035555793, 66.39701867748817676, -9.422509992056140149 ) ) ;
#78144=CARTESIAN_POINT ( 'NONE',  ( -0.8801773607111008646, 23.27201867748817676, 2.915334737309923430 ) ) ;
#78147=CARTESIAN_POINT ( 'NONE',  ( 0.1532563361054082862, 6.217264484334118713, 2.638427012816831674 ) ) ;
#78148=ADVANCED_FACE ( 'NONE', ( #52704 ), #14227, .T. ) ;
#78152=CARTESIAN_POINT ( 'NONE',  ( 0.1532563361054082862, 41.21726448433411605, 2.638427012816831674 ) ) ;
#78154=DIRECTION ( 'NONE',  ( 0.000000000000000000, -1.000000000000000000, 0.000000000000000000 ) ) ;
#78159=CARTESIAN_POINT ( 'NONE',  ( 10.00000000000000000, 54.75893115100078745, -9.846743663894594434 ) ) ;
#78160=CARTESIAN_POINT ( 'NONE',  ( 22.26659068614895176, 44.72041550158063927, -7.082119434687042414 ) ) ;
#78161=CARTESIAN_POINT ( 'NONE',  ( 0.1532563361054100626, 65.80059781766745175, -2.638427012816831230 ) ) ;
#78163=DIRECTION ( 'NONE',  ( -0.000000000000000000, 1.000000000000000000, -0.000000000000000000 ) ) ;
#78164=CARTESIAN_POINT ( 'NONE',  ( 2.791683348922240793, 21.63393115100078745, 7.208316651077764092 ) ) ;
#78165=CARTESIAN_POINT ( 'NONE',  ( -2.816281873526473856, 54.33196800326376064, 3.434112377981055619 ) ) ;
#78167=CARTESIAN_POINT ( 'NONE',  ( 10.00000000000000000, 64.75893115100078035, -9.846743663894594434 ) ) ;
#78168=CARTESIAN_POINT ( 'NONE',  ( 10.00000000000000000, 61.81368534415484106, -10.88017736071110342 ) ) ;
#78171=CARTESIAN_POINT ( 'NONE',  ( -0.3689425029237881626, 67.42874883491396076, 10.36894250292379027 ) ) ;
#78172=DIRECTION ( 'NONE',  ( 0.000000000000000000, 0.000000000000000000, 1.000000000000000000 ) ) ;
#78173=CARTESIAN_POINT ( 'NONE',  ( 7.084665262690076126, 24.10535201082150181, 10.88017736071109987 ) ) ;
#78174=CARTESIAN_POINT ( 'NONE',  ( 16.40814093676324603, 7.456968003263754419, -11.09922568453594671 ) ) ;
#78175=CARTESIAN_POINT ( 'NONE',  ( 4.559911319644449179, 53.89701867748817676, 9.422509992056141925 ) ) ;
#78179=CARTESIAN_POINT ( 'NONE',  ( 10.00000000000000178, 52.25893115100078745, 9.846743663894594434 ) ) ;
#78180=CARTESIAN_POINT ( 'NONE',  ( 10.00000000000000000, 4.758931151000784787, -9.846743663894594434 ) ) ;
#78182=CARTESIAN_POINT ( 'NONE',  ( 13.43411237798105340, 5.581968003263753531, 12.81628187352647963 ) ) ;
#78183=CARTESIAN_POINT ( 'NONE',  ( -0.8801773607110991993, 17.85535201082150536, -2.915334737309923874 ) ) ;
#78184=CARTESIAN_POINT ( 'NONE',  ( -0.1503990784575328643, 69.92552686551195507, -6.262539305110068177 ) ) ;
#78185=CARTESIAN_POINT ( 'NONE',  ( -4.164238869374098151, 41.59541550158061796, -3.795296366450310543 ) ) ;
#78186=CARTESIAN_POINT ( 'NONE',  ( -4.164238869374098151, 36.59541550158063217, -3.795296366450310543 ) ) ;
#78187=CARTESIAN_POINT ( 'NONE',  ( 4.559911319644449179, 3.897018677488171434, 9.422509992056141925 ) ) ;
#78188=CARTESIAN_POINT ( 'NONE',  ( 1.472469842513823179, 35.59226448433412315, -4.923371831947296329 ) ) ;
#78189=CARTESIAN_POINT ( 'NONE',  ( 5.076628168052704559, 20.17559781766745175, -8.527530157486179263 ) ) ;
#78190=CARTESIAN_POINT ( 'NONE',  ( 17.96484262340118221, 19.93868534415484106, 7.964842623401181321 ) ) ;
#78192=CARTESIAN_POINT ( 'NONE',  ( 17.20831665107776587, 39.13393115100079456, -7.208316651077762316 ) ) ;
#78193=CARTESIAN_POINT ( 'NONE',  ( 10.00000000000000000, 41.81368534415484106, -10.88017736071110342 ) ) ;
#78194=CARTESIAN_POINT ( 'NONE',  ( 17.20831665107776587, 57.88393115100078745, 7.208316651077764980 ) ) ;
#78195=CARTESIAN_POINT ( 'NONE',  ( -2.266590686148945544, 16.38708216824730357, -7.082119434687050408 ) ) ;
#78196=LINE ( 'NONE', #17714, #7281 ) ;
#78198=UNCERTAINTY_MEASURE_WITH_UNIT (LENGTH_MEASURE( 1.000000000000000082E-05 ), #36411, 'distance_accuracy_value', 'NONE');
#78199=CARTESIAN_POINT ( 'NONE',  ( 7.361572987183169658, 14.96726448433411960, -9.846743663894592657 ) ) ;
#78200=CARTESIAN_POINT ( 'NONE',  ( 22.81628187352647785, 51.41530133659708923, 3.434112377981063169 ) ) ;
#78201=CARTESIAN_POINT ( 'NONE',  ( 7.361572987183169658, 49.96726448433410894, -9.846743663894592657 ) ) ;
#78205=CARTESIAN_POINT ( 'NONE',  ( 7.084665262690076126, 7.022018677488170546, -10.88017736071110164 ) ) ;
#78206=CARTESIAN_POINT ( 'NONE',  ( 4.559911319644449179, 53.89701867748817676, 9.422509992056141925 ) ) ;
#78207=CARTESIAN_POINT ( 'NONE',  ( 2.917880565312950480, 5.970415501580634832, -12.26659068614894821 ) ) ;
#78208=CARTESIAN_POINT ( 'NONE',  ( 2.791683348922237240, 0.3839311510007847872, -7.208316651077763204 ) ) ;
#78209=CARTESIAN_POINT ( 'NONE',  ( 7.361572987183169658, 44.96726448433412315, -9.846743663894592657 ) ) ;
#78210=CARTESIAN_POINT ( 'NONE',  ( 12.91533473730992121, 19.52201867748816611, 10.88017736071110164 ) ) ;
#78212=CARTESIAN_POINT ( 'NONE',  ( 17.20831665107776587, 64.13393115100079456, -7.208316651077762316 ) ) ;
#78214=CARTESIAN_POINT ( 'NONE',  ( 18.52753015748617571, 3.092264484334118269, 4.923371831947298993 ) ) ;
#78221=CARTESIAN_POINT ( 'NONE',  ( -0.3689425029237898834, 1.178748834913967869, -10.36894250292378850 ) ) ;
#78222=CARTESIAN_POINT ( 'NONE',  ( 10.00000000000000000, 40.55374883491397497, -14.16423886937410082 ) ) ;
#78223=CARTESIAN_POINT ( 'NONE',  ( 0.1532563361054100626, 45.80059781766745886, -2.638427012816831230 ) ) ;
#78224=CARTESIAN_POINT ( 'NONE',  ( 2.791683348922240793, 26.63393115100078745, 7.208316651077764092 ) ) ;
#78225=CARTESIAN_POINT ( 'NONE',  ( 20.88017736071110164, 25.35535201082150891, 2.915334737309930979 ) ) ;
#78226=CARTESIAN_POINT ( 'NONE',  ( 5.076628168052703671, 61.84226448433412315, 8.527530157486179263 ) ) ;
#78228=CARTESIAN_POINT ( 'NONE',  ( 10.00000000000000000, 60.55374883491397497, -14.16423886937410082 ) ) ;
#78230=DIRECTION ( 'NONE',  ( -0.000000000000000000, 1.000000000000000000, 0.000000000000000000 ) ) ;
#78231=CARTESIAN_POINT ( 'NONE',  ( -0.8801773607111008646, 68.27201867748817676, 2.915334737309923430 ) ) ;
#78232=CARTESIAN_POINT ( 'NONE',  ( 19.84674366389459266, 13.30059781766745353, 2.638427012816836559 ) ) ;
#78235=CARTESIAN_POINT ( 'NONE',  ( 20.32896413005680358, 29.74545670184113888, 5.963430220938287007 ) ) ;
#78236=VERTEX_POINT ( 'NONE', #68702 ) ;
#78237=CARTESIAN_POINT ( 'NONE',  ( 17.20831665107776587, 29.13393115100078390, -7.208316651077762316 ) ) ;
#78238=ORIENTED_EDGE ( 'NONE', *, *, #21581, .F. ) ;
#78239=CARTESIAN_POINT ( 'NONE',  ( 13.79529636645031943, 30.34541550158063927, -14.16423886937409904 ) ) ;
#78240=CARTESIAN_POINT ( 'NONE',  ( 19.84674366389459621, 23.50893115100078390, 7.409399052514197653E-17 ) ) ;
#78241=CARTESIAN_POINT ( 'NONE',  ( 4.559911319644449179, 47.23035201082150536, -9.422509992056141925 ) ) ;
#78243=EDGE_LOOP ( 'NONE', ( #63517, #20595, #86506, #55626 ) ) ;
#78244=CARTESIAN_POINT ( 'NONE',  ( 15.44008868035555260, 34.73035201082151247, 9.422509992056143702 ) ) ;
#78250=CARTESIAN_POINT ( 'NONE',  ( 22.26659068614895176, 4.720415501580633943, -7.082119434687042414 ) ) ;
#78254=CARTESIAN_POINT ( 'NONE',  ( 6.565887622018943937, 30.16530133659708568, 12.81628187352647430 ) ) ;
#78255=CARTESIAN_POINT ( 'NONE',  ( 6.204703633549690345, 0.7620821682473009062, -14.16423886937410259 ) ) ;
#78256=CARTESIAN_POINT ( 'NONE',  ( 18.52753015748618282, 3.925597817667451306, -4.923371831947291888 ) ) ;
#78258=CARTESIAN_POINT ( 'NONE',  ( 22.81628187352647785, 46.41530133659708213, 3.434112377981063169 ) ) ;
#78259=DIRECTION ( 'NONE',  ( -0.000000000000000000, -0.000000000000000000, 1.000000000000000000 ) ) ;
#78260=CARTESIAN_POINT ( 'NONE',  ( 17.20831665107776587, 32.88393115100078745, 7.208316651077764980 ) ) ;
#78263=CARTESIAN_POINT ( 'NONE',  ( 20.24186590665278018, 65.59014588040358262, -6.114288769123040090 ) ) ;
#78264=CARTESIAN_POINT ( 'NONE',  ( 0.5774900079438590739, 62.64701867748817676, -5.440088680355550821 ) ) ;
#78267=CARTESIAN_POINT ( 'NONE',  ( 14.92337183194729988, 9.342264484334119601, -8.527530157486177487 ) ) ;
#78270=CARTESIAN_POINT ( 'NONE',  ( 5.076628168052703671, 36.84226448433412315, 8.527530157486179263 ) ) ;
#78271=CARTESIAN_POINT ( 'NONE',  ( 20.88017736071110875, 35.77201867748816966, -2.915334737309920321 ) ) ;
#78272=CARTESIAN_POINT ( 'NONE',  ( -4.164238869374098151, 1.595415501580634388, -3.795296366450310543 ) ) ;
#78273=CARTESIAN_POINT ( 'NONE',  ( 19.84674366389459266, 18.30059781766745175, 2.638427012816836559 ) ) ;
#78274=CARTESIAN_POINT ( 'NONE',  ( 19.38216949554541557, 17.24863466993041783, -9.382169495545420901 ) ) ;
#78277=CARTESIAN_POINT ( 'NONE',  ( 7.084665262690076126, 47.02201867748818387, -10.88017736071110164 ) ) ;
#78279=CARTESIAN_POINT ( 'NONE',  ( 12.63842701281683922, 59.55059781766744464, -9.846743663894590881 ) ) ;
#78281=CARTESIAN_POINT ( 'NONE',  ( 14.92337183194729633, 22.67559781766745175, 8.527530157486181039 ) ) ;
#78282=CARTESIAN_POINT ( 'NONE',  ( 19.42250999205614193, 20.14701867748817321, 5.440088680355555262 ) ) ;
#78283=CARTESIAN_POINT ( 'NONE',  ( 22.81628187352647785, 11.62363466993042138, 6.195893100308588602E-16 ) ) ;
#78284=CARTESIAN_POINT ( 'NONE',  ( 1.472469842513823179, 21.42559781766745175, 4.923371831947296329 ) ) ;
#78287=CARTESIAN_POINT ( 'NONE',  ( 12.91533473730993009, 21.60535201082150536, -10.88017736071109987 ) ) ;
#78288=CARTESIAN_POINT ( 'NONE',  ( 20.88017736071110164, 60.35535201082151957, 2.915334737309930979 ) ) ;
#78290=CARTESIAN_POINT ( 'NONE',  ( 0.1532563361054082862, 46.21726448433411605, 2.638427012816831674 ) ) ;
#78291=CARTESIAN_POINT ( 'NONE',  ( 4.559911319644449179, 13.89701867748817321, 9.422509992056141925 ) ) ;
#78293=CARTESIAN_POINT ( 'NONE',  ( 15.44008868035555260, 49.73035201082150536, 9.422509992056143702 ) ) ;
#78294=CARTESIAN_POINT ( 'NONE',  ( -0.8801773607111008646, 8.272018677488171434, 2.915334737309923430 ) ) ;
#78295=CARTESIAN_POINT ( 'NONE',  ( 17.20831665107776587, 9.133931151000787452, -7.208316651077762316 ) ) ;
#78297=CARTESIAN_POINT ( 'NONE',  ( 17.20831665107776587, 39.13393115100079456, -7.208316651077762316 ) ) ;
#78299=CARTESIAN_POINT ( 'NONE',  ( 1.274849032794294290, 58.57228050351032778, 6.499999999999979572 ) ) ;
#78300=CARTESIAN_POINT ( 'NONE',  ( 0.1532563361054100626, 65.80059781766745175, -2.638427012816831230 ) ) ;
#78302=CARTESIAN_POINT ( 'NONE',  ( 13.79529636645030344, 18.26208216824730002, 14.16423886937410614 ) ) ;
#78303=CARTESIAN_POINT ( 'NONE',  ( 12.63842701281683034, 42.46726448433412315, 9.846743663894596210 ) ) ;
#78305=LINE ( 'NONE', #32796, #41711 ) ;
#78306=CARTESIAN_POINT ( 'NONE',  ( 20.88017736071110519, 5.563685344154838397, 2.639326808657452039E-16 ) ) ;
#78307=CARTESIAN_POINT ( 'NONE',  ( 19.84674366389459621, 18.50893115100078745, 7.409399052514197653E-17 ) ) ;
#78309=DIRECTION ( 'NONE',  ( 0.000000000000000000, 0.000000000000000000, 1.000000000000000000 ) ) ;
#78310=CARTESIAN_POINT ( 'NONE',  ( 15.44008868035555793, 51.39701867748816966, -9.422509992056140149 ) ) ;
#78312=CARTESIAN_POINT ( 'NONE',  ( 7.084665262690076126, 19.10535201082150181, 10.88017736071109987 ) ) ;
#78313=CARTESIAN_POINT ( 'NONE',  ( -1.099225684535947600, 48.70696800326375353, -6.408140936763238038 ) ) ;
#78314=CARTESIAN_POINT ( 'NONE',  ( 3.591859063236761518, 9.956968003263753531, 11.09922568453594849 ) ) ;
#78315=CARTESIAN_POINT ( 'NONE',  ( 7.361572987183170547, 17.05059781766745530, 9.846743663894590881 ) ) ;
#78316=ORIENTED_EDGE ( 'NONE', *, *, #25547, .T. ) ;
#78319=CARTESIAN_POINT ( 'NONE',  ( 6.204703633549690345, 50.76208216824730357, -14.16423886937410259 ) ) ;
#78320=CARTESIAN_POINT ( 'NONE',  ( 17.08211943468705130, 23.47041550158063572, 12.26659068614894998 ) ) ;
#78321=CARTESIAN_POINT ( 'NONE',  ( 20.88017736071110519, 15.56368534415483751, 2.639326808657452039E-16 ) ) ;
#78322=CARTESIAN_POINT ( 'NONE',  ( 4.559911319644449179, 52.23035201082151247, -9.422509992056141925 ) ) ;
#78325=CARTESIAN_POINT ( 'NONE',  ( 4.559911319644449179, 62.23035201082150536, -9.422509992056141925 ) ) ;
#78326=SURFACE_STYLE_FILL_AREA ( #3322 ) ;
#78327=CARTESIAN_POINT ( 'NONE',  ( 17.20831665107776587, 14.13393115100078568, -7.208316651077762316 ) ) ;
#78329=CARTESIAN_POINT ( 'NONE',  ( 5.076628168052704559, 30.17559781766745175, -8.527530157486179263 ) ) ;
#78330=CARTESIAN_POINT ( 'NONE',  ( 5.076628168052704559, 45.17559781766745175, -8.527530157486179263 ) ) ;
#78331=EDGE_CURVE ( 'NONE', #36181, #2342, #16741, .T. ) ;
#78332=CARTESIAN_POINT ( 'NONE',  ( 2.035157376598824452, 18.68868534415484106, 7.964842623401179544 ) ) ;
#78333=UNCERTAINTY_MEASURE_WITH_UNIT (LENGTH_MEASURE( 1.000000000000000082E-05 ), #14258, 'distance_accuracy_value', 'NONE');
#78335=CARTESIAN_POINT ( 'NONE',  ( 16.40814093676324603, 32.45696800326375353, -11.09922568453594671 ) ) ;
#78336=CARTESIAN_POINT ( 'NONE',  ( 20.88017736071110875, 50.77201867748817676, -2.915334737309920765 ) ) ;
#78337=CARTESIAN_POINT ( 'NONE',  ( 18.52753015748618282, 28.92559781766745175, -4.923371831947291888 ) ) ;
#78338=CARTESIAN_POINT ( 'NONE',  ( 24.16423886937410614, 44.30374883491397497, 8.672049930838204340E-16 ) ) ;
#78339=CARTESIAN_POINT ( 'NONE',  ( 0.1532563361054083140, 6.008931151000784787, 1.131784320476157264E-15 ) ) ;
#78341=CARTESIAN_POINT ( 'NONE',  ( 1.472469842513823179, 50.59226448433411605, -4.923371831947296329 ) ) ;
#78342=CARTESIAN_POINT ( 'NONE',  ( 14.92337183194729633, 27.67559781766745530, 8.527530157486181039 ) ) ;
#78343=CARTESIAN_POINT ( 'NONE',  ( 10.00000000000000178, 13.05374883491396787, 14.16423886937410082 ) ) ;
#78344=CARTESIAN_POINT ( 'NONE',  ( 13.79529636645030344, 13.26208216824729824, 14.16423886937410614 ) ) ;
#78345=CARTESIAN_POINT ( 'NONE',  ( 7.361572987183170547, 32.05059781766745175, 9.846743663894590881 ) ) ;
#78347=CARTESIAN_POINT ( 'NONE',  ( 17.96484262340118221, 51.18868534415483396, -7.964842623401177768 ) ) ;
#78348=CARTESIAN_POINT ( 'NONE',  ( 19.42250999205614548, 15.98035201082150714, -5.440088680355545492 ) ) ;
#78349=CARTESIAN_POINT ( 'NONE',  ( 0.5774900079438607392, 48.48035201082150536, 5.440088680355550821 ) ) ;
#78350=CARTESIAN_POINT ( 'NONE',  ( -0.8801773607110991993, 27.85535201082150181, -2.915334737309923874 ) ) ;
#78352=CARTESIAN_POINT ( 'NONE',  ( 0.6178305044545818747, 33.49863466993042493, -9.382169495545419124 ) ) ;
#78354=CARTESIAN_POINT ( 'NONE',  ( 15.44008868035555260, 34.73035201082151247, 9.422509992056143702 ) ) ;
#78356=CARTESIAN_POINT ( 'NONE',  ( -2.816281873526471635, 53.91530133659709634, -3.434112377981056508 ) ) ;
#78357=CARTESIAN_POINT ( 'NONE',  ( 19.42250999205614193, 60.14701867748817676, 5.440088680355555262 ) ) ;
#78358=ORIENTED_EDGE ( 'NONE', *, *, #37415, .F. ) ;
#78359=CARTESIAN_POINT ( 'NONE',  ( -0.8801773607111008646, 48.27201867748816966, 2.915334737309923430 ) ) ;
#78360=CARTESIAN_POINT ( 'NONE',  ( 0.5774900079438590739, 7.647018677488171434, -5.440088680355550821 ) ) ;
#78362=CARTESIAN_POINT ( 'NONE',  ( 19.84674366389459266, 8.717264484334116048, -2.638427012816827677 ) ) ;
#78364=CARTESIAN_POINT ( 'NONE',  ( 6.204703633549690345, 57.84541550158063927, 14.16423886937410082 ) ) ;
#78365=CARTESIAN_POINT ( 'NONE',  ( 19.84674366389459266, 8.300597817667451750, 2.638427012816836559 ) ) ;
#78366=CARTESIAN_POINT ( 'NONE',  ( 6.204703633549690345, 10.76208216824729824, -14.16423886937410259 ) ) ;
#78367=CARTESIAN_POINT ( 'NONE',  ( 19.84674366389459266, 3.717264484334118713, -2.638427012816827677 ) ) ;
#78368=CARTESIAN_POINT ( 'NONE',  ( 19.42250999205614193, 15.14701867748817143, 5.440088680355555262 ) ) ;
#78369=CARTESIAN_POINT ( 'NONE',  ( 7.361572987183169658, 44.96726448433412315, -9.846743663894592657 ) ) ;
#78371=CARTESIAN_POINT ( 'NONE',  ( 1.472469842513823179, 51.42559781766745886, 4.923371831947296329 ) ) ;
#78373=CARTESIAN_POINT ( 'NONE',  ( 20.88017736071110519, 45.56368534415484106, 2.639326808657452039E-16 ) ) ;
#78374=CARTESIAN_POINT ( 'NONE',  ( 5.076628168052703671, 56.84226448433412315, 8.527530157486179263 ) ) ;
#78375=CARTESIAN_POINT ( 'NONE',  ( 19.42250999205614548, 65.98035201082151957, -5.440088680355545492 ) ) ;
#78376=CARTESIAN_POINT ( 'NONE',  ( 7.084665262690076126, 42.02201867748816966, -10.88017736071110164 ) ) ;
#78377=CARTESIAN_POINT ( 'NONE',  ( 0.5774900079438607392, 3.480352010821504916, 5.440088680355550821 ) ) ;
#78379=COLOUR_RGB ( '', 0.09019608, 0.27058824, 0.51372549) ;
#78380=CARTESIAN_POINT ( 'NONE',  ( 16.40814093676323893, 45.79030133659708923, 11.09922568453595026 ) ) ;
#78383=CARTESIAN_POINT ( 'NONE',  ( 22.81628187352647785, 26.41530133659708923, 3.434112377981063169 ) ) ;
#78384=CARTESIAN_POINT ( 'NONE',  ( 20.88017736071110875, 20.77201867748816611, -2.915334737309920765 ) ) ;
#78385=ORIENTED_EDGE ( 'NONE', *, *, #80080, .F. ) ;
#78387=CARTESIAN_POINT ( 'NONE',  ( 15.44008868035555793, 66.39701867748817676, -9.422509992056140149 ) ) ;
#78388=CARTESIAN_POINT ( 'NONE',  ( 10.00000000000000000, 54.75893115100078745, -9.846743663894594434 ) ) ;
#78389=CARTESIAN_POINT ( 'NONE',  ( 19.84674366389459621, 18.50893115100078745, 7.409399052514197653E-17 ) ) ;
#78390=CARTESIAN_POINT ( 'NONE',  ( 10.00000000000000000, 39.75893115100078745, -9.846743663894594434 ) ) ;
#78392=CARTESIAN_POINT ( 'NONE',  ( 14.92337183194729988, 29.34226448433411960, -8.527530157486177487 ) ) ;
#78395=EDGE_CURVE ( 'NONE', #3044, #71011, #32657, .T. ) ;
#78396=CARTESIAN_POINT ( 'NONE',  ( 18.52753015748617571, 23.09226448433411960, 4.923371831947298993 ) ) ;
#78399=CARTESIAN_POINT ( 'NONE',  ( 18.52753015748617571, 43.09226448433412315, 4.923371831947298993 ) ) ;
#78400=ORIENTED_EDGE ( 'NONE', *, *, #35618, .T. ) ;
#78403=CARTESIAN_POINT ( 'NONE',  ( 22.81628187352647785, 31.62363466993042138, 6.195893100308588602E-16 ) ) ;
#78404=CARTESIAN_POINT ( 'NONE',  ( -0.1491070598754174470, 61.94583914210339515, -4.500000000000001776 ) ) ;
#78405=CARTESIAN_POINT ( 'NONE',  ( 6.204703633549690345, 42.84541550158063217, 14.16423886937410082 ) ) ;
#78406=CARTESIAN_POINT ( 'NONE',  ( 19.84674366389459266, 18.71726448433411960, -2.638427012816827677 ) ) ;
#78408=CARTESIAN_POINT ( 'NONE',  ( 2.791683348922237240, 5.383931151000785675, -7.208316651077763204 ) ) ;
#78409=CARTESIAN_POINT ( 'NONE',  ( 20.00000000000000711, 95.40264689493518802, 4.636598378017573907 ) ) ;
#78410=CARTESIAN_POINT ( 'NONE',  ( 17.08211943468705840, 45.13708216824730357, -12.26659068614894466 ) ) ;
#78411=CARTESIAN_POINT ( 'NONE',  ( 19.84674366389459266, 63.30059781766745886, 2.638427012816836559 ) ) ;
#78412=CARTESIAN_POINT ( 'NONE',  ( 12.91533473730993009, 11.60535201082150714, -10.88017736071109987 ) ) ;
#78413=CARTESIAN_POINT ( 'NONE',  ( -2.266590686148945544, 22.22041550158063572, 7.082119434687048631 ) ) ;
#78414=CARTESIAN_POINT ( 'NONE',  ( -4.164238869374098151, 41.59541550158061796, -3.795296366450310543 ) ) ;
#78415=CARTESIAN_POINT ( 'NONE',  ( -46.02077283339401248, 104.3984410555176510, -5.346056167492045041 ) ) ;
#78418=CARTESIAN_POINT ( 'NONE',  ( 10.00000000000000178, 52.25893115100078745, 9.846743663894594434 ) ) ;
#78420=CARTESIAN_POINT ( 'NONE',  ( 19.42250999205614548, 30.98035201082150536, -5.440088680355545492 ) ) ;
#78422=CARTESIAN_POINT ( 'NONE',  ( 20.00000000000000711, 95.39111596591838804, -4.637569774571024261 ) ) ;
#78423=CARTESIAN_POINT ( 'NONE',  ( 19.84674366389459266, 43.30059781766744464, 2.638427012816836559 ) ) ;
#78426=CARTESIAN_POINT ( 'NONE',  ( 2.791683348922240793, 46.63393115100077324, 7.208316651077764092 ) ) ;
#78427=CARTESIAN_POINT ( 'NONE',  ( 5.076628168052703671, 66.84226448433412315, 8.527530157486179263 ) ) ;
#78429=CARTESIAN_POINT ( 'NONE',  ( -4.164238869374099039, 11.80374883491396965, 8.674139862899312516E-16 ) ) ;
#78430=B_SPLINE_CURVE_WITH_KNOTS ( 'NONE', 3,
 ( #37982, #30446, #60947, #89488 ),
 .UNSPECIFIED., .F., .F.,
 ( 4, 4 ),
 ( 6.206335383118182794E-17, 0.002562518741975522863 ),
 .UNSPECIFIED. ) ;
#78434=CARTESIAN_POINT ( 'NONE',  ( 2.917880565312948704, 67.63708216824730357, 12.26659068614894643 ) ) ;
#78435=CARTESIAN_POINT ( 'NONE',  ( 10.00000000000000178, 30.37363466993042138, 12.81628187352647608 ) ) ;
#78437=CARTESIAN_POINT ( 'NONE',  ( 14.92337183194729633, 2.675597817667451750, 8.527530157486181039 ) ) ;
#78438=B_SPLINE_CURVE_WITH_KNOTS ( 'NONE', 3,
 ( #16465, #55447, #46945, #85949, #8952, #39469 ),
 .UNSPECIFIED., .F., .F.,
 ( 4, 2, 4 ),
 ( 0.000000000000000000, 0.0002605067024380860801, 0.0005210134048761721603 ),
 .UNSPECIFIED. ) ;
#78439=CARTESIAN_POINT ( 'NONE',  ( -1.926860441876564023, 9.688309369127509285, 1.004413902775740781E-15 ) ) ;
#78440=CARTESIAN_POINT ( 'NONE',  ( 15.44008868035555260, 4.730352010821505360, 9.422509992056143702 ) ) ;
#78442=CARTESIAN_POINT ( 'NONE',  ( 19.72487221294570858, 70.00000000000000000, 6.500000000000000888 ) ) ;
#78443=CARTESIAN_POINT ( 'NONE',  ( 17.96484262340118221, 21.18868534415483396, -7.964842623401177768 ) ) ;
#78444=CARTESIAN_POINT ( 'NONE',  ( 19.42250999205614548, 35.98035201082151247, -5.440088680355545492 ) ) ;
#78445=CARTESIAN_POINT ( 'NONE',  ( 10.00000000000000000, -2.126365330069579951, -12.81628187352647608 ) ) ;
#78446=CARTESIAN_POINT ( 'NONE',  ( 0.1532563361054083140, 51.00893115100078745, 1.131784320476157264E-15 ) ) ;
#78447=CARTESIAN_POINT ( 'NONE',  ( -43.79232545471665361, 106.6932607868292706, -5.013557994010066743 ) ) ;
#78448=CARTESIAN_POINT ( 'NONE',  ( 19.84674366389459621, 8.508931151000785675, 7.409399052514197653E-17 ) ) ;
#78451=CARTESIAN_POINT ( 'NONE',  ( 12.91533473730993009, 31.60535201082150891, -10.88017736071109987 ) ) ;
#78453=CARTESIAN_POINT ( 'NONE',  ( -2.816281873526473856, 34.12363466993042493, 9.499525473075851096E-16 ) ) ;
#78457=CARTESIAN_POINT ( 'NONE',  ( 6.565887622018943937, -1.918031996736246692, -12.81628187352647608 ) ) ;
#78458=EDGE_CURVE ( 'NONE', #93612, #63139, #11945, .T. ) ;
#78459=CARTESIAN_POINT ( 'NONE',  ( 2.035157376598822676, 52.43868534415483396, -7.964842623401177768 ) ) ;
#78460=CARTESIAN_POINT ( 'NONE',  ( 2.791683348922240793, 16.63393115100078745, 7.208316651077764092 ) ) ;
#78461=CARTESIAN_POINT ( 'NONE',  ( 13.43411237798106583, 32.66530133659708213, -12.81628187352647252 ) ) ;
#78462=CARTESIAN_POINT ( 'NONE',  ( 0.5774900079438607392, 68.48035201082150536, 5.440088680355550821 ) ) ;
#78463=SURFACE_STYLE_FILL_AREA ( #47953 ) ;
#78464=CARTESIAN_POINT ( 'NONE',  ( 19.50000000000000711, 80.28026998469363207, 5.000000000000000000 ) ) ;
#78468=CARTESIAN_POINT ( 'NONE',  ( -0.8801773607111009756, 8.063685344154837509, 1.068504757029289695E-15 ) ) ;
#78469=CARTESIAN_POINT ( 'NONE',  ( 19.38216949554541557, 52.24863466993041072, -9.382169495545420901 ) ) ;
#78470=CARTESIAN_POINT ( 'NONE',  ( 20.36894250292379382, 18.67874883491397142, 10.36894250292379205 ) ) ;
#78471=CARTESIAN_POINT ( 'NONE',  ( 10.00000000000000178, 17.25893115100078745, 9.846743663894594434 ) ) ;
#78472=( NAMED_UNIT ( * ) SI_UNIT ( $, .STERADIAN. ) SOLID_ANGLE_UNIT ( ) );
#78473=CARTESIAN_POINT ( 'NONE',  ( 14.92337183194729988, 19.34226448433411960, -8.527530157486177487 ) ) ;
#78474=CARTESIAN_POINT ( 'NONE',  ( 24.16423886937410614, 54.51208216824730357, -3.795296366450302550 ) ) ;
#78476=( GEOMETRIC_REPRESENTATION_CONTEXT ( 3 ) GLOBAL_UNCERTAINTY_ASSIGNED_CONTEXT ( ( #26427 ) ) GLOBAL_UNIT_ASSIGNED_CONTEXT ( ( #64001, #18524, #48022 ) ) REPRESENTATION_CONTEXT ( 'NONE', 'WORKASPACE' ) );
#78477=CARTESIAN_POINT ( 'NONE',  ( 7.084665262690076126, 4.105352010821503583, 10.88017736071109987 ) ) ;
#78478=CARTESIAN_POINT ( 'NONE',  ( 2.035157376598824452, 18.68868534415484106, 7.964842623401179544 ) ) ;
#78479=CARTESIAN_POINT ( 'NONE',  ( 1.932340009482155896, 31.49127512925447547, -6.500000000000005329 ) ) ;
#78481=EDGE_LOOP ( 'NONE', ( #7922, #3353, #7151, #51302, #61287, #20611 ) ) ;
#78482=CARTESIAN_POINT ( 'NONE',  ( 19.42250999205614548, 15.98035201082150714, -5.440088680355545492 ) ) ;
#78483=CARTESIAN_POINT ( 'NONE',  ( 10.00000000000000178, 9.313685344154839285, 10.88017736071110342 ) ) ;
#78484=CARTESIAN_POINT ( 'NONE',  ( 14.92337183194729633, 52.67559781766745175, 8.527530157486181039 ) ) ;
#78486=CARTESIAN_POINT ( 'NONE',  ( 10.00000000000000178, 55.37363466993042493, 12.81628187352647608 ) ) ;
#78487=( LENGTH_UNIT ( ) NAMED_UNIT ( * ) SI_UNIT ( .MILLI., .METRE. ) );
#78488=SURFACE_SIDE_STYLE ('',( #50306 ) ) ;
#78489=CARTESIAN_POINT ( 'NONE',  ( 24.16423886937410614, 14.30374883491396787, 8.672049930838204340E-16 ) ) ;
#78490=CARTESIAN_POINT ( 'NONE',  ( 17.96484262340118221, 24.93868534415484461, 7.964842623401181321 ) ) ;
#78491=CARTESIAN_POINT ( 'NONE',  ( 20.88017736071110164, 15.35535201082150358, 2.915334737309930979 ) ) ;
#78492=CARTESIAN_POINT ( 'NONE',  ( 7.361572987183170547, 57.05059781766744464, 9.846743663894590881 ) ) ;
#78494=CARTESIAN_POINT ( 'NONE',  ( 18.52753015748617571, 38.09226448433412315, 4.923371831947298993 ) ) ;
#78496=FACE_OUTER_BOUND ( 'NONE', #31149, .T. ) ;
#78497=CARTESIAN_POINT ( 'NONE',  ( 18.52753015748618282, 8.925597817667451750, -4.923371831947291888 ) ) ;
#78502=CARTESIAN_POINT ( 'NONE',  ( 10.00000000000000178, 17.25893115100078745, 9.846743663894594434 ) ) ;
#78503=CARTESIAN_POINT ( 'NONE',  ( -2.816281873526473856, -0.6680319967362464695, 3.434112377981055619 ) ) ;
#78504=CARTESIAN_POINT ( 'NONE',  ( 4.559911319644449179, 43.89701867748816966, 9.422509992056141925 ) ) ;
#78505=CARTESIAN_POINT ( 'NONE',  ( -0.8801773607111009756, 3.063685344154837509, 1.068504757029289695E-15 ) ) ;
#78506=CARTESIAN_POINT ( 'NONE',  ( 0.6178305044545818747, 48.49863466993042493, -9.382169495545419124 ) ) ;
#78507=CARTESIAN_POINT ( 'NONE',  ( 10.00000000000000178, 13.05374883491396787, 14.16423886937410082 ) ) ;
#78508=CARTESIAN_POINT ( 'NONE',  ( 0.6178305044545838731, 59.74863466993041783, 9.382169495545420901 ) ) ;
#78510=CARTESIAN_POINT ( 'NONE',  ( 18.52753015748617571, 58.09226448433411605, 4.923371831947298993 ) ) ;
#78511=CARTESIAN_POINT ( 'NONE',  ( 0.5774900079438607392, 23.48035201082150536, 5.440088680355550821 ) ) ;
#78513=CARTESIAN_POINT ( 'NONE',  ( -0.8801773607110991993, 67.85535201082151957, -2.915334737309923874 ) ) ;
#78514=DIRECTION ( 'NONE',  ( 0.000000000000000000, 0.000000000000000000, 1.000000000000000000 ) ) ;
#78516=CARTESIAN_POINT ( 'NONE',  ( 14.92337183194729988, 4.342264484334117824, -8.527530157486177487 ) ) ;
#78517=CARTESIAN_POINT ( 'NONE',  ( 2.035157376598822676, 67.43868534415484817, -7.964842623401177768 ) ) ;
#78520=CARTESIAN_POINT ( 'NONE',  ( 17.96484262340118221, 56.18868534415484817, -7.964842623401177768 ) ) ;
#78522=CARTESIAN_POINT ( 'NONE',  ( -0.8801773607110991993, 67.85535201082151957, -2.915334737309923874 ) ) ;
#78523=CARTESIAN_POINT ( 'NONE',  ( 10.00000000000000000, -0.2410688489992152128, -9.846743663894594434 ) ) ;
#78527=CARTESIAN_POINT ( 'NONE',  ( -0.1298530154764001854, 80.39370036920264795, -5.000000000000000000 ) ) ;
#78528=CARTESIAN_POINT ( 'NONE',  ( 12.63842701281683922, 49.55059781766744464, -9.846743663894590881 ) ) ;
#78529=VERTEX_POINT ( 'NONE', #87621 ) ;
#78532=CARTESIAN_POINT ( 'NONE',  ( 24.16423886937410614, 4.512082168247300906, -3.795296366450302550 ) ) ;
#78533=CARTESIAN_POINT ( 'NONE',  ( 21.09922568453594849, 61.20696800326376064, 6.408140936763242479 ) ) ;
#78534=CARTESIAN_POINT ( 'NONE',  ( 10.00000000000000178, 3.053748834913967425, 14.16423886937410082 ) ) ;
#78536=CARTESIAN_POINT ( 'NONE',  ( 2.917880565312948704, 22.63708216824730002, 12.26659068614894643 ) ) ;
#78538=FACE_OUTER_BOUND ( 'NONE', #34195, .T. ) ;
#78539=CARTESIAN_POINT ( 'NONE',  ( 19.42250999205614193, 25.14701867748817321, 5.440088680355555262 ) ) ;
#78542=CARTESIAN_POINT ( 'NONE',  ( 19.84674366389459621, 3.508931151000785231, 7.409399052514197653E-17 ) ) ;
#78543=CARTESIAN_POINT ( 'NONE',  ( 12.63842701281683034, 22.46726448433411605, 9.846743663894596210 ) ) ;
#78544=CARTESIAN_POINT ( 'NONE',  ( 3.591859063236763294, 38.29030133659708923, -11.09922568453595026 ) ) ;
#78545=CARTESIAN_POINT ( 'NONE',  ( 18.52753015748618282, 33.92559781766745886, -4.923371831947291888 ) ) ;
#78547=CARTESIAN_POINT ( 'NONE',  ( -1.099225684535947600, 33.70696800326375353, -6.408140936763238038 ) ) ;
#78548=CARTESIAN_POINT ( 'NONE',  ( 19.80777595082616216, 40.68878173731739878, -6.499999999999961808 ) ) ;
#78550=CARTESIAN_POINT ( 'NONE',  ( 0.1532563361054082862, 21.21726448433412315, 2.638427012816831674 ) ) ;
#78551=CARTESIAN_POINT ( 'NONE',  ( 2.917880565312948704, 12.63708216824730179, 12.26659068614894643 ) ) ;
#78553=CARTESIAN_POINT ( 'NONE',  ( 2.035157376598824452, 33.68868534415484106, 7.964842623401179544 ) ) ;
#78554=CARTESIAN_POINT ( 'NONE',  ( 17.08211943468705840, 35.13708216824730357, -12.26659068614894466 ) ) ;
#78555=CARTESIAN_POINT ( 'NONE',  ( 12.63842701281683922, 54.55059781766745175, -9.846743663894590881 ) ) ;
#78557=CARTESIAN_POINT ( 'NONE',  ( 7.361572987183169658, 9.967264484334119601, -9.846743663894592657 ) ) ;
#78559=CARTESIAN_POINT ( 'NONE',  ( 19.38216949554541557, 57.24863466993042493, -9.382169495545420901 ) ) ;
#78561=CARTESIAN_POINT ( 'NONE',  ( 2.035157376598822676, 27.43868534415483396, -7.964842623401177768 ) ) ;
#78562=CARTESIAN_POINT ( 'NONE',  ( -1.099225684535947600, 19.54030133659708568, 6.408140936763237150 ) ) ;
#78563=CARTESIAN_POINT ( 'NONE',  ( 6.565887622018943937, 20.16530133659708213, 12.81628187352647430 ) ) ;
#78564=CARTESIAN_POINT ( 'NONE',  ( 1.472469842513823179, 46.42559781766745175, 4.923371831947296329 ) ) ;
#78566=CARTESIAN_POINT ( 'NONE',  ( 19.38216949554541202, 50.99863466993042493, 9.382169495545424454 ) ) ;
#78567=SURFACE_SIDE_STYLE ('',( #25095 ) ) ;
#78569=CARTESIAN_POINT ( 'NONE',  ( 20.88017736071110164, 55.35535201082149825, 2.915334737309930979 ) ) ;
#78573=CARTESIAN_POINT ( 'NONE',  ( 0.2751277870542980231, 14.36607318730130878, -6.500000000000002665 ) ) ;
#78574=CARTESIAN_POINT ( 'NONE',  ( 12.91533473730993009, 51.60535201082149825, -10.88017736071109987 ) ) ;
#78575=CARTESIAN_POINT ( 'NONE',  ( 0.5774900079438590739, 52.64701867748817676, -5.440088680355550821 ) ) ;
#78576=CARTESIAN_POINT ( 'NONE',  ( 0.2751277870542967463, 70.00000000000000000, -6.500000000000000888 ) ) ;
#78577=CARTESIAN_POINT ( 'NONE',  ( -46.48928645636213730, 103.2957187381727238, -6.397878122524045530 ) ) ;
#78578=EDGE_CURVE ( 'NONE', #58660, #53014, #65602, .T. ) ;
#78579=CARTESIAN_POINT ( 'NONE',  ( 20.88017736071110875, 10.77201867748817143, -2.915334737309920765 ) ) ;
#78580=CARTESIAN_POINT ( 'NONE',  ( 0.1532563361054083140, 66.00893115100079456, 1.131784320476157264E-15 ) ) ;
#78581=CARTESIAN_POINT ( 'NONE',  ( 12.91533473730993009, 21.60535201082150536, -10.88017736071109987 ) ) ;
#78583=CARTESIAN_POINT ( 'NONE',  ( 19.38216949554541557, 27.24863466993041783, -9.382169495545420901 ) ) ;
#78585=CARTESIAN_POINT ( 'NONE',  ( 15.44008868035555793, 46.39701867748817676, -9.422509992056140149 ) ) ;
#78586=CARTESIAN_POINT ( 'NONE',  ( 2.791683348922240793, 41.63393115100078745, 7.208316651077764092 ) ) ;
#78587=CARTESIAN_POINT ( 'NONE',  ( 0.6178305044545818747, 8.498634669930421381, -9.382169495545419124 ) ) ;
#78589=CARTESIAN_POINT ( 'NONE',  ( 20.88017736071110519, 30.56368534415484106, 2.639326808657452039E-16 ) ) ;
#78590=CARTESIAN_POINT ( 'NONE',  ( -0.8801773607111008646, 38.27201867748816255, 2.915334737309923430 ) ) ;
#78591=CARTESIAN_POINT ( 'NONE',  ( 24.16423886937409904, 49.09541550158063217, 3.795296366450317205 ) ) ;
#78592=CARTESIAN_POINT ( 'NONE',  ( 18.52753015748617571, 38.09226448433412315, 4.923371831947298993 ) ) ;
#78593=CARTESIAN_POINT ( 'NONE',  ( -0.8801773607111009756, 63.06368534415484106, 1.068504757029289695E-15 ) ) ;
#78595=CARTESIAN_POINT ( 'NONE',  ( 2.917880565312948704, 12.63708216824730179, 12.26659068614894643 ) ) ;
#78597=DIRECTION ( 'NONE',  ( 0.000000000000000000, -1.000000000000000000, 0.000000000000000000 ) ) ;
#78601=CARTESIAN_POINT ( 'NONE',  ( -4.164238869374099927, 52.01208216824729647, 3.795296366450308767 ) ) ;
#78602=CARTESIAN_POINT ( 'NONE',  ( 17.08211943468705840, 35.13708216824730357, -12.26659068614894466 ) ) ;
#78603=CARTESIAN_POINT ( 'NONE',  ( 0.1532563361054100626, 20.80059781766744464, -2.638427012816831230 ) ) ;
#78605=CARTESIAN_POINT ( 'NONE',  ( -2.816281873526473856, 19.33196800326375708, 3.434112377981055619 ) ) ;
#78606=CARTESIAN_POINT ( 'NONE',  ( 0.1532563361054100626, 55.80059781766745175, -2.638427012816831230 ) ) ;
#78608=CARTESIAN_POINT ( 'NONE',  ( 17.96484262340118221, 56.18868534415484817, -7.964842623401177768 ) ) ;
#78609=CARTESIAN_POINT ( 'NONE',  ( 21.09922568453594849, 26.20696800326375353, 6.408140936763242479 ) ) ;
#78610=CARTESIAN_POINT ( 'NONE',  ( 22.26659068614894466, 33.88708216824730357, 7.082119434687054849 ) ) ;
#78611=CARTESIAN_POINT ( 'NONE',  ( 19.42250999205614193, 30.14701867748817321, 5.440088680355555262 ) ) ;
#78612=B_SPLINE_CURVE_WITH_KNOTS ( 'NONE', 3,
 ( #29621, #37649, #89648, #43653 ),
 .UNSPECIFIED., .F., .F.,
 ( 4, 4 ),
 ( 0.000000000000000000, 0.002657014572711344572 ),
 .UNSPECIFIED. ) ;
#78615=B_SPLINE_CURVE_WITH_KNOTS ( 'NONE', 3,
 ( #35392, #75864, #39354, #53858 ),
 .UNSPECIFIED., .F., .F.,
 ( 4, 4 ),
 ( 2.168404344971008868E-18, 0.001060528352562004799 ),
 .UNSPECIFIED. ) ;
#78617=CARTESIAN_POINT ( 'NONE',  ( 0.1532563361054083140, 6.008931151000784787, 1.131784320476157264E-15 ) ) ;
#78621=EDGE_LOOP ( 'NONE', ( #55202, #5204, #46899, #46521, #32003, #22563 ) ) ;
#78622=CARTESIAN_POINT ( 'NONE',  ( 6.204703633549690345, 5.762082168247301794, -14.16423886937410259 ) ) ;
#78623=CARTESIAN_POINT ( 'NONE',  ( 12.91533473730993009, 6.605352010821504471, -10.88017736071109987 ) ) ;
#78624=CARTESIAN_POINT ( 'NONE',  ( 17.96484262340118221, 9.938685344154839285, 7.964842623401181321 ) ) ;
#78625=CARTESIAN_POINT ( 'NONE',  ( 2.791683348922237240, 30.38393115100078390, -7.208316651077763204 ) ) ;
#78626=CARTESIAN_POINT ( 'NONE',  ( 10.00000000000000178, 0.3736346699304200492, 12.81628187352647608 ) ) ;
#78630=B_SPLINE_CURVE_WITH_KNOTS ( 'NONE', 3,
 ( #98062, #14057, #46033, #8034 ),
 .UNSPECIFIED., .F., .F.,
 ( 4, 4 ),
 ( 1.758547849261791993E-16, 0.002392975128318475080 ),
 .UNSPECIFIED. ) ;
#78631=CARTESIAN_POINT ( 'NONE',  ( 3.591859063236761518, 19.95696800326375353, 11.09922568453594849 ) ) ;
#78636=CARTESIAN_POINT ( 'NONE',  ( -4.164238869374099927, 52.01208216824729647, 3.795296366450308767 ) ) ;
#78638=CARTESIAN_POINT ( 'NONE',  ( -2.266590686148945544, 52.22041550158064638, 7.082119434687048631 ) ) ;
#78640=CARTESIAN_POINT ( 'NONE',  ( 15.44008868035555260, 29.73035201082150891, 9.422509992056143702 ) ) ;
#78641=CARTESIAN_POINT ( 'NONE',  ( 20.88017736071110519, 35.56368534415484106, 2.639326808657452039E-16 ) ) ;
#78642=CARTESIAN_POINT ( 'NONE',  ( 4.559911319644449179, 33.89701867748817676, 9.422509992056141925 ) ) ;
#78644=CARTESIAN_POINT ( 'NONE',  ( 0.5774900079438590739, 62.64701867748817676, -5.440088680355550821 ) ) ;
#78645=CARTESIAN_POINT ( 'NONE',  ( 0.5774900079438607392, 28.48035201082150891, 5.440088680355550821 ) ) ;
#78648=ORIENTED_EDGE ( 'NONE', *, *, #64680, .F. ) ;
#78649=CARTESIAN_POINT ( 'NONE',  ( 2.791683348922237240, 20.38393115100078745, -7.208316651077763204 ) ) ;
#78653=CARTESIAN_POINT ( 'NONE',  ( 12.63842701281683922, 49.55059781766744464, -9.846743663894590881 ) ) ;
#78654=LINE ( 'NONE', #79630, #43638 ) ;
#78655=COLOUR_RGB ( '', 0.09019608, 0.27058824, 0.51372549) ;
#78657=CARTESIAN_POINT ( 'NONE',  ( 18.18329248733315140, 22.60290668512023871, 6.499999999999997335 ) ) ;
#78658=CARTESIAN_POINT ( 'NONE',  ( 1.274849032794294290, 53.57228050351032067, 6.499999999999979572 ) ) ;
#78659=CARTESIAN_POINT ( 'NONE',  ( 17.20831665107776587, 47.88393115100078745, 7.208316651077764980 ) ) ;
#78660=CARTESIAN_POINT ( 'NONE',  ( -2.266590686148945544, 47.22041550158063927, 7.082119434687048631 ) ) ;
#78661=CARTESIAN_POINT ( 'NONE',  ( -10.44000000000001194, 92.00000000000000000, 9.500000000000000000 ) ) ;
#78664=CARTESIAN_POINT ( 'NONE',  ( 17.20831665107776587, 17.88393115100078745, 7.208316651077764980 ) ) ;
#78665=CARTESIAN_POINT ( 'NONE',  ( 0.6178305044545818747, 63.49863466993043204, -9.382169495545419124 ) ) ;
#78666=CARTESIAN_POINT ( 'NONE',  ( 17.20831665107776587, 57.88393115100078745, 7.208316651077764980 ) ) ;
#78667=CARTESIAN_POINT ( 'NONE',  ( 20.88017736071110164, 65.35535201082150536, 2.915334737309930979 ) ) ;
#78668=CARTESIAN_POINT ( 'NONE',  ( 14.92337183194729988, 44.34226448433412315, -8.527530157486177487 ) ) ;
#78672=CARTESIAN_POINT ( 'NONE',  ( 24.16423886937410614, 64.30374883491396076, 8.672049930838204340E-16 ) ) ;
#78674=CARTESIAN_POINT ( 'NONE',  ( 4.559911319644449179, 48.89701867748817676, 9.422509992056141925 ) ) ;
#78675=CARTESIAN_POINT ( 'NONE',  ( 16.40814093676324603, 17.45696800326375353, -11.09922568453594671 ) ) ;
#78677=CARTESIAN_POINT ( 'NONE',  ( 19.10478245763058780, 66.02576239577082617, -5.990408912944208630 ) ) ;
#78679=CARTESIAN_POINT ( 'NONE',  ( 0.2751277870542909176, 30.30223176428831167, 6.499999999999992006 ) ) ;
#78680=CARTESIAN_POINT ( 'NONE',  ( 14.92337183194729988, 49.34226448433411605, -8.527530157486177487 ) ) ;
#78682=CARTESIAN_POINT ( 'NONE',  ( 13.43411237798106583, 12.66530133659708746, -12.81628187352647252 ) ) ;
#78683=EDGE_CURVE ( 'NONE', #66913, #47405, #56643, .T. ) ;
#78684=CARTESIAN_POINT ( 'NONE',  ( 20.88017736071110519, 10.56368534415483929, 2.639326808657452039E-16 ) ) ;
#78685=CARTESIAN_POINT ( 'NONE',  ( 1.711636803080581304, 66.84492782695771496, -6.500000000000075495 ) ) ;
#78686=CARTESIAN_POINT ( 'NONE',  ( -4.164238869374099927, 32.01208216824730357, 3.795296366450308767 ) ) ;
#78687=CARTESIAN_POINT ( 'NONE',  ( 10.00000000000000000, 30.55374883491397142, -14.16423886937410082 ) ) ;
#78688=CARTESIAN_POINT ( 'NONE',  ( 24.16423886937410614, 64.51208216824728936, -3.795296366450302550 ) ) ;
#78690=CARTESIAN_POINT ( 'NONE',  ( 21.09922568453595559, 42.04030133659708213, -6.408140936763230044 ) ) ;
#78691=CARTESIAN_POINT ( 'NONE',  ( 20.88017736071110164, 15.35535201082150358, 2.915334737309930979 ) ) ;
#78693=ORIENTED_EDGE ( 'NONE', *, *, #81843, .F. ) ;
#78694=CARTESIAN_POINT ( 'NONE',  ( 10.00000000000000000, 39.75893115100078745, -9.846743663894594434 ) ) ;
#78695=CARTESIAN_POINT ( 'NONE',  ( 15.44008868035555793, 41.39701867748817676, -9.422509992056140149 ) ) ;
#78696=CARTESIAN_POINT ( 'NONE',  ( 0.1532563361054082862, 66.21726448433413736, 2.638427012816831674 ) ) ;
#78697=CARTESIAN_POINT ( 'NONE',  ( 24.16423886937409904, 24.09541550158063927, 3.795296366450317205 ) ) ;
#78702=CARTESIAN_POINT ( 'NONE',  ( 2.791683348922237240, 20.38393115100078745, -7.208316651077763204 ) ) ;
#78703=CARTESIAN_POINT ( 'NONE',  ( -1.099225684535947600, 48.70696800326375353, -6.408140936763238038 ) ) ;
#78704=CARTESIAN_POINT ( 'NONE',  ( 10.00000000000000178, 57.25893115100078745, 9.846743663894594434 ) ) ;
#78705=ORIENTED_EDGE ( 'NONE', *, *, #23183, .T. ) ;
#78708=CARTESIAN_POINT ( 'NONE',  ( 13.79529636645031943, 65.34541550158063217, -14.16423886937409904 ) ) ;
#78709=CARTESIAN_POINT ( 'NONE',  ( 22.26659068614895176, 14.72041550158063572, -7.082119434687042414 ) ) ;
#78710=CARTESIAN_POINT ( 'NONE',  ( 17.96484262340118221, 64.93868534415483396, 7.964842623401181321 ) ) ;
#78711=CARTESIAN_POINT ( 'NONE',  ( 1.472469842513823179, 50.59226448433411605, -4.923371831947296329 ) ) ;
#78712=CARTESIAN_POINT ( 'NONE',  ( 12.91533473730993009, 16.60535201082150891, -10.88017736071109987 ) ) ;
#78713=COLOUR_RGB ( '', 0.40784314, 0.44705882, 0.49803922) ;
#78714=CARTESIAN_POINT ( 'NONE',  ( 2.791683348922240793, 66.63393115100079456, 7.208316651077764092 ) ) ;
#78719=CARTESIAN_POINT ( 'NONE',  ( -25.69000000000001194, 93.50000000000000000, -9.500000000000000000 ) ) ;
#78721=CARTESIAN_POINT ( 'NONE',  ( 6.204703633549690345, 37.84541550158063927, 14.16423886937410082 ) ) ;
#78722=CARTESIAN_POINT ( 'NONE',  ( 0.1532563361054083140, 56.00893115100078745, 1.131784320476157264E-15 ) ) ;
#78723=CARTESIAN_POINT ( 'NONE',  ( 1.472469842513823179, 25.59226448433412315, -4.923371831947296329 ) ) ;
#78724=CARTESIAN_POINT ( 'NONE',  ( 18.95785429995052240, 52.24216108172004880, 6.499999999999943157 ) ) ;
#78725=CARTESIAN_POINT ( 'NONE',  ( -0.8801773607110991993, 17.85535201082150536, -2.915334737309923874 ) ) ;
#78726=CARTESIAN_POINT ( 'NONE',  ( 19.84674366389459621, 63.50893115100078745, 7.409399052514197653E-17 ) ) ;
#78728=CARTESIAN_POINT ( 'NONE',  ( 24.16423886937410614, 39.51208216824731068, -3.795296366450302550 ) ) ;
#78729=CARTESIAN_POINT ( 'NONE',  ( 7.084665262690076126, 4.105352010821503583, 10.88017736071109987 ) ) ;
#78732=CARTESIAN_POINT ( 'NONE',  ( 10.00000000000000178, 69.31368534415484817, 10.88017736071110342 ) ) ;
#78734=CARTESIAN_POINT ( 'NONE',  ( 12.63842701281683034, 12.46726448433411782, 9.846743663894596210 ) ) ;
#78740=CARTESIAN_POINT ( 'NONE',  ( 1.472469842513823179, 25.59226448433412315, -4.923371831947296329 ) ) ;
#78742=CARTESIAN_POINT ( 'NONE',  ( -4.164238869374098151, 26.59541550158063217, -3.795296366450310543 ) ) ;
#78743=CARTESIAN_POINT ( 'NONE',  ( 5.076628168052704559, 40.17559781766745175, -8.527530157486179263 ) ) ;
#78744=CARTESIAN_POINT ( 'NONE',  ( -0.8801773607111008646, 43.27201867748817676, 2.915334737309923430 ) ) ;
#78746=SURFACE_SIDE_STYLE ('',( #47248 ) ) ;
#78749=CARTESIAN_POINT ( 'NONE',  ( 10.00000000000000000, 41.81368534415484106, -10.88017736071110342 ) ) ;
#78751=CARTESIAN_POINT ( 'NONE',  ( 0.1916775849787280273, 2.258688159020693753, -6.500000000000000888 ) ) ;
#78753=ORIENTED_EDGE ( 'NONE', *, *, #46962, .F. ) ;
#78756=CARTESIAN_POINT ( 'NONE',  ( 21.09922568453594849, 26.20696800326375353, 6.408140936763242479 ) ) ;
#78757=LINE ( 'NONE', #70775, #79723 ) ;
#78758=CARTESIAN_POINT ( 'NONE',  ( 2.791683348922237240, 20.38393115100078745, -7.208316651077763204 ) ) ;
#78759=SURFACE_STYLE_FILL_AREA ( #64220 ) ;
#78761=CARTESIAN_POINT ( 'NONE',  ( 14.92337183194729988, 29.34226448433411960, -8.527530157486177487 ) ) ;
#78762=CARTESIAN_POINT ( 'NONE',  ( 19.42250999205614548, 55.98035201082150536, -5.440088680355545492 ) ) ;
#78765=CARTESIAN_POINT ( 'NONE',  ( 13.43411237798106583, 62.66530133659708923, -12.81628187352647252 ) ) ;
#78766=CARTESIAN_POINT ( 'NONE',  ( 0.1532563361054100626, 10.80059781766745175, -2.638427012816831230 ) ) ;
#78768=CARTESIAN_POINT ( 'NONE',  ( 0.6178305044545818747, 13.49863466993041783, -9.382169495545419124 ) ) ;
#78770=CARTESIAN_POINT ( 'NONE',  ( 20.30776406404415724, 0.000000000000000000, -5.999999999999999112 ) ) ;
#78772=CARTESIAN_POINT ( 'NONE',  ( 19.84674366389459266, 48.30059781766745175, 2.638427012816836559 ) ) ;
#78774=CARTESIAN_POINT ( 'NONE',  ( 17.08211943468705130, 8.470415501580635720, 12.26659068614894998 ) ) ;
#78775=CARTESIAN_POINT ( 'NONE',  ( 0.1532563361054082862, 21.21726448433412315, 2.638427012816831674 ) ) ;
#78777=CARTESIAN_POINT ( 'NONE',  ( 19.38216949554541557, 37.24863466993041783, -9.382169495545420901 ) ) ;
#78778=CARTESIAN_POINT ( 'NONE',  ( -0.8801773607111009756, 23.27201867748817676, 2.915334737309923874 ) ) ;
#78779=CARTESIAN_POINT ( 'NONE',  ( -0.8801773607110991993, 42.85535201082150536, -2.915334737309923874 ) ) ;
#78780=CARTESIAN_POINT ( 'NONE',  ( 13.43411237798106583, 2.665301336597086568, -12.81628187352647252 ) ) ;
#78781=LINE ( 'NONE', #11752, #31143 ) ;
#78783=CARTESIAN_POINT ( 'NONE',  ( 18.52753015748617571, 18.09226448433411960, 4.923371831947298993 ) ) ;
#78784=CARTESIAN_POINT ( 'NONE',  ( 0.5774900079438590739, 32.64701867748816966, -5.440088680355550821 ) ) ;
#78785=CARTESIAN_POINT ( 'NONE',  ( 13.43411237798105340, 35.58196800326375353, 12.81628187352647963 ) ) ;
#78786=CARTESIAN_POINT ( 'NONE',  ( 14.92337183194729633, 22.67559781766745175, 8.527530157486181039 ) ) ;
#78787=( BOUNDED_SURFACE ( )  B_SPLINE_SURFACE ( 3, 2, ( 
 ( #60952, #60467, #7491 ),
 ( #92926, #90956, #22488 ),
 ( #52961, #37987, #68478 ),
 ( #53954, #91461, #22987 ),
 ( #76460, #38474, #498 ),
 ( #84944, #46452, #76945 ),
 ( #8455, #69948, #972 ),
 ( #31433, #61936, #31921 ),
 ( #92437, #23961, #46935 ),
 ( #39458, #1468, #87401 ),
 ( #17450, #33396, #62926 ),
 ( #9938, #17931, #78422 ),
 ( #40442, #32425, #26396 ),
 ( #47916, #18420, #70441 ) ),
 .UNSPECIFIED., .F., .F., .F. ) 
 B_SPLINE_SURFACE_WITH_KNOTS ( ( 4, 2, 2, 2, 2, 2, 4 ),
 ( 3, 3 ),
 ( 0.000000000000000000, 0.004797171936611956643, 0.007195757904917934530, 0.009594343873223913285, 0.01199292984152989031, 0.01439151580983586906, 0.01918868774644782657 ),
 ( 0.000000000000000000, 1.000000000000000000 ),
 .UNSPECIFIED. ) 
 GEOMETRIC_REPRESENTATION_ITEM ( )  RATIONAL_B_SPLINE_SURFACE ( (
 ( 1.000000000000000000, 0.7071067811865475727, 1.000000000000000000),
 ( 1.000000000000000000, 0.7404680669573554530, 1.000000000000000000),
 ( 1.000000000000000000, 0.7699744256204830162, 1.000000000000000000),
 ( 1.000000000000000000, 0.8013264333401337591, 1.000000000000000000),
 ( 1.000000000000000000, 0.8096066803150596680, 1.000000000000000000),
 ( 1.000000000000000000, 0.8208168491805714062, 1.000000000000000000),
 ( 1.000000000000000000, 0.8237352673350482046, 1.000000000000000000),
 ( 1.000000000000000000, 0.8237872525054150685, 1.000000000000000000),
 ( 1.000000000000000000, 0.8209201555335595701, 1.000000000000000000),
 ( 1.000000000000000000, 0.8097813946840403121, 1.000000000000000000),
 ( 1.000000000000000000, 0.8015207097676279036, 1.000000000000000000),
 ( 1.000000000000000000, 0.7701797223629573974, 1.000000000000000000),
 ( 1.000000000000000000, 0.7406378784107900959, 1.000000000000000000),
 ( 1.000000000000000000, 0.7071067811865475727, 1.000000000000000000) ) ) 
 REPRESENTATION_ITEM ( '' )  SURFACE ( )  );
#78789=CARTESIAN_POINT ( 'NONE',  ( -0.8801773607110991993, 22.85535201082150181, -2.915334737309923874 ) ) ;
#78790=VERTEX_POINT ( 'NONE', #51107 ) ;
#78791=CARTESIAN_POINT ( 'NONE',  ( 2.035157376598822676, 67.43868534415484817, -7.964842623401177768 ) ) ;
#78792=CARTESIAN_POINT ( 'NONE',  ( -0.8801773607111008646, 8.272018677488171434, 2.915334737309923430 ) ) ;
#78793=CARTESIAN_POINT ( 'NONE',  ( 2.791683348922240793, 41.63393115100078745, 7.208316651077764092 ) ) ;
#78794=CARTESIAN_POINT ( 'NONE',  ( 12.91533473730993009, 16.60535201082150891, -10.88017736071109987 ) ) ;
#78796=CARTESIAN_POINT ( 'NONE',  ( 17.96484262340118221, 39.93868534415484106, 7.964842623401181321 ) ) ;
#78797=CARTESIAN_POINT ( 'NONE',  ( 2.035157376598822676, 7.438685344154837509, -7.964842623401177768 ) ) ;
#78798=CARTESIAN_POINT ( 'NONE',  ( 12.63842701281683922, 34.55059781766745886, -9.846743663894590881 ) ) ;
#78801=CARTESIAN_POINT ( 'NONE',  ( -2.266590686148945544, 26.38708216824730357, -7.082119434687050408 ) ) ;
#78805=CARTESIAN_POINT ( 'NONE',  ( 20.88017736071110164, 5.355352010821503583, 2.915334737309930979 ) ) ;
#78806=CARTESIAN_POINT ( 'NONE',  ( 18.52753015748617571, 28.09226448433411960, 4.923371831947298993 ) ) ;
#78809=CARTESIAN_POINT ( 'NONE',  ( 19.42250999205614548, 45.98035201082150536, -5.440088680355545492 ) ) ;
#78810=CARTESIAN_POINT ( 'NONE',  ( 22.81628187352647785, 61.62363466993041783, 6.195893100308588602E-16 ) ) ;
#78812=CARTESIAN_POINT ( 'NONE',  ( 2.035157376598824452, 33.68868534415484106, 7.964842623401179544 ) ) ;
#78814=CARTESIAN_POINT ( 'NONE',  ( 16.40814093676323893, 15.79030133659708746, 11.09922568453595026 ) ) ;
#78815=CARTESIAN_POINT ( 'NONE',  ( 5.076628168052703671, 16.84226448433411960, 8.527530157486179263 ) ) ;
#78817=FILL_AREA_STYLE ('',( #19296 ) ) ;
#78819=CARTESIAN_POINT ( 'NONE',  ( 10.00000000000000178, 58.05374883491397497, 14.16423886937410082 ) ) ;
#78820=CARTESIAN_POINT ( 'NONE',  ( -0.3689425029237881626, 27.42874883491397142, 10.36894250292379027 ) ) ;
#78821=CARTESIAN_POINT ( 'NONE',  ( 4.559911319644449179, 18.89701867748817321, 9.422509992056141925 ) ) ;
#78822=CARTESIAN_POINT ( 'NONE',  ( 7.084665262690076126, 47.02201867748818387, -10.88017736071110164 ) ) ;
#78825=CARTESIAN_POINT ( 'NONE',  ( 2.791683348922240793, 16.63393115100078745, 7.208316651077764092 ) ) ;
#78827=CARTESIAN_POINT ( 'NONE',  ( 2.791683348922240793, 16.63393115100078745, 7.208316651077764092 ) ) ;
#78830=CARTESIAN_POINT ( 'NONE',  ( 14.92337183194729988, 24.34226448433411960, -8.527530157486177487 ) ) ;
#78831=CARTESIAN_POINT ( 'NONE',  ( 10.00000000000000178, 52.25893115100078745, 9.846743663894594434 ) ) ;
#78832=CARTESIAN_POINT ( 'NONE',  ( 19.38216949554541557, 37.24863466993041783, -9.382169495545420901 ) ) ;
#78833=CARTESIAN_POINT ( 'NONE',  ( -0.8801773607110991993, 57.85535201082149825, -2.915334737309923874 ) ) ;
#78834=CARTESIAN_POINT ( 'NONE',  ( 14.92337183194729988, 29.34226448433411960, -8.527530157486177487 ) ) ;
#78835=CARTESIAN_POINT ( 'NONE',  ( -0.3689425029237881626, 42.42874883491396787, 10.36894250292379027 ) ) ;
#78836=CARTESIAN_POINT ( 'NONE',  ( 19.84674366389459621, 18.50893115100078745, 7.409399052514197653E-17 ) ) ;
#78838=CARTESIAN_POINT ( 'NONE',  ( 2.791683348922240793, 46.63393115100077324, 7.208316651077764092 ) ) ;
#78839=CARTESIAN_POINT ( 'NONE',  ( 5.076628168052703671, 36.84226448433412315, 8.527530157486179263 ) ) ;
#78840=CARTESIAN_POINT ( 'NONE',  ( 24.16423886937410614, 4.303748834913967869, 8.672049930838204340E-16 ) ) ;
#78841=CARTESIAN_POINT ( 'NONE',  ( -0.3689425029237898834, 16.17874883491396076, -10.36894250292378850 ) ) ;
#78842=CARTESIAN_POINT ( 'NONE',  ( 14.92337183194729988, 24.34226448433411960, -8.527530157486177487 ) ) ;
#78843=CARTESIAN_POINT ( 'NONE',  ( 7.084665262690076126, 42.02201867748816966, -10.88017736071110164 ) ) ;
#78844=CARTESIAN_POINT ( 'NONE',  ( 17.96484262340118221, 19.93868534415484106, 7.964842623401181321 ) ) ;
#78847=CARTESIAN_POINT ( 'NONE',  ( 19.42250999205614193, 45.14701867748817676, 5.440088680355555262 ) ) ;
#78848=CARTESIAN_POINT ( 'NONE',  ( 10.00000000000000000, 26.81368534415484106, -10.88017736071110342 ) ) ;
#78850=CARTESIAN_POINT ( 'NONE',  ( -0.8801773607111008646, 53.27201867748816966, 2.915334737309923430 ) ) ;
#78853=CARTESIAN_POINT ( 'NONE',  ( 15.44008868035555260, 64.73035201082151957, 9.422509992056143702 ) ) ;
#78855=CARTESIAN_POINT ( 'NONE',  ( 17.96484262340118221, 61.18868534415482685, -7.964842623401177768 ) ) ;
#78856=FILL_AREA_STYLE ('',( #70384 ) ) ;
#78858=DIRECTION ( 'NONE',  ( -0.000000000000000000, 1.000000000000000000, 0.000000000000000000 ) ) ;
#78859=CARTESIAN_POINT ( 'NONE',  ( 13.79529636645031943, 55.34541550158062506, -14.16423886937409904 ) ) ;
#78860=CARTESIAN_POINT ( 'NONE',  ( 2.791683348922237240, 5.383931151000785675, -7.208316651077763204 ) ) ;
#78861=CARTESIAN_POINT ( 'NONE',  ( 22.26659068614895176, 4.720415501580633943, -7.082119434687042414 ) ) ;
#78862=( BOUNDED_CURVE ( )  B_SPLINE_CURVE ( 2, ( #31431, #496, #30945, #10795, #53450, #68964, #63769, #33278, #79775 ),
 .UNSPECIFIED., .F., .T. ) 
 B_SPLINE_CURVE_WITH_KNOTS ( ( 3, 2, 2, 2, 3 ),
 ( 0.1901409369402313476, 0.1904761904761904656, 0.1964285714285713969, 0.2023809523809524391, 0.2027162059169115571 ),
 .UNSPECIFIED. ) 
 CURVE ( )  GEOMETRIC_REPRESENTATION_ITEM ( )  RATIONAL_B_SPLINE_CURVE ( ( 0.9963778908391762723, 0.9980808541467921513, 1.000000000000000000, 0.9659258262890682012, 1.000000000000000000, 0.9659258262890682012, 1.000000000000000000, 0.9980808541467921513, 0.9963778908391762723 ) ) 
 REPRESENTATION_ITEM ( '' )  );
#78863=CARTESIAN_POINT ( 'NONE',  ( 1.472469842513823179, 5.592264484334118713, -4.923371831947296329 ) ) ;
#78864=CARTESIAN_POINT ( 'NONE',  ( 12.91533473730993009, 6.605352010821504471, -10.88017736071109987 ) ) ;
#78865=CARTESIAN_POINT ( 'NONE',  ( 17.20831665107776587, 47.88393115100078745, 7.208316651077764980 ) ) ;
#78866=ORIENTED_EDGE ( 'NONE', *, *, #54063, .F. ) ;
#78867=CARTESIAN_POINT ( 'NONE',  ( 0.1532563361054100626, 45.80059781766745886, -2.638427012816831230 ) ) ;
#78870=CARTESIAN_POINT ( 'NONE',  ( -0.8801773607111009756, 48.06368534415484817, 1.068504757029289695E-15 ) ) ;
#78871=CARTESIAN_POINT ( 'NONE',  ( 2.791683348922240793, 51.63393115100078745, 7.208316651077764092 ) ) ;
#78872=( NAMED_UNIT ( * ) PLANE_ANGLE_UNIT ( ) SI_UNIT ( $, .RADIAN. ) );
#78874=CARTESIAN_POINT ( 'NONE',  ( 12.91533473730992121, 59.52201867748816966, 10.88017736071110164 ) ) ;
#78875=CARTESIAN_POINT ( 'NONE',  ( 20.88017736071110164, 5.355352010821503583, 2.915334737309930979 ) ) ;
#78876=CARTESIAN_POINT ( 'NONE',  ( 0.6178305044545818747, 38.49863466993042493, -9.382169495545419124 ) ) ;
#78879=CARTESIAN_POINT ( 'NONE',  ( 13.43411237798106583, 27.66530133659708568, -12.81628187352647252 ) ) ;
#78880=CARTESIAN_POINT ( 'NONE',  ( 7.084665262690076126, 32.02201867748816966, -10.88017736071110164 ) ) ;
#78882=CARTESIAN_POINT ( 'NONE',  ( 1.472469842513823179, 10.59226448433411782, -4.923371831947296329 ) ) ;
#78883=CARTESIAN_POINT ( 'NONE',  ( 14.92337183194729633, 62.67559781766745886, 8.527530157486181039 ) ) ;
#78884=CARTESIAN_POINT ( 'NONE',  ( 19.84674366389459266, 18.71726448433411960, -2.638427012816827677 ) ) ;
#78885=CARTESIAN_POINT ( 'NONE',  ( 1.472469842513823179, 55.59226448433412315, -4.923371831947296329 ) ) ;
#78888=CARTESIAN_POINT ( 'NONE',  ( 0.1532563361054082862, 41.21726448433411605, 2.638427012816831674 ) ) ;
#78890=CARTESIAN_POINT ( 'NONE',  ( 1.046131998950050379, 60.73810908735726599, 6.499999999999992006 ) ) ;
#78892=CARTESIAN_POINT ( 'NONE',  ( 5.076628168052704559, 30.17559781766745175, -8.527530157486179263 ) ) ;
#78893=CARTESIAN_POINT ( 'NONE',  ( 2.791683348922237240, 0.3839311510007847872, -7.208316651077763204 ) ) ;
#78895=CARTESIAN_POINT ( 'NONE',  ( 10.00000000000000000, 59.75893115100078745, -9.846743663894594434 ) ) ;
#78898=CARTESIAN_POINT ( 'NONE',  ( -2.816281873526473856, 19.33196800326375708, 3.434112377981055619 ) ) ;
#78899=CARTESIAN_POINT ( 'NONE',  ( 5.076628168052704559, 50.17559781766745886, -8.527530157486179263 ) ) ;
#78902=CARTESIAN_POINT ( 'NONE',  ( 2.917880565312948704, 47.63708216824730357, 12.26659068614894643 ) ) ;
#78903=CARTESIAN_POINT ( 'NONE',  ( 0.1532563361054082862, 16.21726448433411960, 2.638427012816831674 ) ) ;
#78907=CARTESIAN_POINT ( 'NONE',  ( 13.79529636645030344, 48.26208216824728936, 14.16423886937410614 ) ) ;
#78908=CARTESIAN_POINT ( 'NONE',  ( 1.472469842513823179, 61.42559781766745175, 4.923371831947296329 ) ) ;
#78909=CARTESIAN_POINT ( 'NONE',  ( 15.44008868035555793, 6.397018677488171434, -9.422509992056140149 ) ) ;
#78910=CARTESIAN_POINT ( 'NONE',  ( -2.266590686148945544, 27.22041550158063572, 7.082119434687048631 ) ) ;
#78911=CARTESIAN_POINT ( 'NONE',  ( 17.08211943468705130, 43.47041550158063927, 12.26659068614894998 ) ) ;
#78913=DIRECTION ( 'NONE',  ( 0.000000000000000000, -1.000000000000000000, -0.000000000000000000 ) ) ;
#78914=CARTESIAN_POINT ( 'NONE',  ( 17.20831665107776587, 52.88393115100078035, 7.208316651077764980 ) ) ;
#78915=CARTESIAN_POINT ( 'NONE',  ( 10.00000000000000000, 36.81368534415484106, -10.88017736071110342 ) ) ;
#78918=CARTESIAN_POINT ( 'NONE',  ( 10.00000000000000178, 37.25893115100078745, 9.846743663894594434 ) ) ;
#78919=CARTESIAN_POINT ( 'NONE',  ( 6.565887622018943937, 63.08196800326376064, -12.81628187352647608 ) ) ;
#78921=CARTESIAN_POINT ( 'NONE',  ( 7.361572987183170547, 62.05059781766745886, 9.846743663894590881 ) ) ;
#78922=CARTESIAN_POINT ( 'NONE',  ( 2.791683348922240793, 61.63393115100079456, 7.208316651077764092 ) ) ;
#78925=CARTESIAN_POINT ( 'NONE',  ( 6.204703633549690345, 32.84541550158063927, 14.16423886937410082 ) ) ;
#78929=CARTESIAN_POINT ( 'NONE',  ( 19.42250999205614193, 5.147018677488171434, 5.440088680355555262 ) ) ;
#78930=CARTESIAN_POINT ( 'NONE',  ( 3.591859063236763294, 18.29030133659708568, -11.09922568453595026 ) ) ;
#78932=CARTESIAN_POINT ( 'NONE',  ( 0.1532563361054100626, 10.80059781766745175, -2.638427012816831230 ) ) ;
#78934=CARTESIAN_POINT ( 'NONE',  ( 20.25388882277826141, 0.000000000000000000, -6.092555545977055509 ) ) ;
#78935=CARTESIAN_POINT ( 'NONE',  ( -0.03932841506541493587, 43.12161441960501662, 6.397827110479010315 ) ) ;
#78936=CARTESIAN_POINT ( 'NONE',  ( 10.00000000000000000, 11.81368534415483751, -10.88017736071110342 ) ) ;
#78938=CARTESIAN_POINT ( 'NONE',  ( 19.42250999205614193, 35.14701867748816966, 5.440088680355555262 ) ) ;
#78939=CARTESIAN_POINT ( 'NONE',  ( -0.8801773607111009756, 43.06368534415484106, 1.068504757029289695E-15 ) ) ;
#78940=CARTESIAN_POINT ( 'NONE',  ( 10.00000000000000178, 67.25893115100079456, 9.846743663894594434 ) ) ;
#78941=CARTESIAN_POINT ( 'NONE',  ( -45.35639774302337912, 104.5887517005673004, -5.643674680800299548 ) ) ;
#78942=CARTESIAN_POINT ( 'NONE',  ( 12.63842701281683034, 12.46726448433411782, 9.846743663894596210 ) ) ;
#78945=CARTESIAN_POINT ( 'NONE',  ( 17.96484262340118221, 36.18868534415484106, -7.964842623401177768 ) ) ;
#78946=CARTESIAN_POINT ( 'NONE',  ( 16.40814093676323893, 35.79030133659708923, 11.09922568453595026 ) ) ;
#78947=CARTESIAN_POINT ( 'NONE',  ( 19.72487221294571569, 34.78217586085237656, 6.499999999999993783 ) ) ;
#78948=CARTESIAN_POINT ( 'NONE',  ( 1.472469842513823179, 61.42559781766745175, 4.923371831947296329 ) ) ;
#78949=CARTESIAN_POINT ( 'NONE',  ( 12.91533473730992121, 64.52201867748817676, 10.88017736071110164 ) ) ;
#78950=CARTESIAN_POINT ( 'NONE',  ( 18.52753015748618282, 13.92559781766745175, -4.923371831947291888 ) ) ;
#78951=CARTESIAN_POINT ( 'NONE',  ( 22.81628187352647785, 36.62363466993041783, 6.195893100308588602E-16 ) ) ;
#78952=CARTESIAN_POINT ( 'NONE',  ( 12.91533473730992121, 64.52201867748817676, 10.88017736071110164 ) ) ;
#78954=CARTESIAN_POINT ( 'NONE',  ( 3.591859063236761518, 59.95696800326375353, 11.09922568453594849 ) ) ;
#78955=ORIENTED_EDGE ( 'NONE', *, *, #14144, .F. ) ;
#78957=CARTESIAN_POINT ( 'NONE',  ( 20.88017736071110875, 10.77201867748817143, -2.915334737309920765 ) ) ;
#78958=CARTESIAN_POINT ( 'NONE',  ( 13.43411237798106583, 57.66530133659708923, -12.81628187352647252 ) ) ;
#78959=CARTESIAN_POINT ( 'NONE',  ( 2.791683348922240793, 21.63393115100078745, 7.208316651077764092 ) ) ;
#78960=CARTESIAN_POINT ( 'NONE',  ( 14.92337183194729633, 22.67559781766745175, 8.527530157486181039 ) ) ;
#78961=CARTESIAN_POINT ( 'NONE',  ( 6.204703633549690345, 57.84541550158063927, 14.16423886937410082 ) ) ;
#78962=ORIENTED_EDGE ( 'NONE', *, *, #95741, .T. ) ;
#78963=CARTESIAN_POINT ( 'NONE',  ( 0.5774900079438607392, 13.48035201082150358, 5.440088680355550821 ) ) ;
#78964=ADVANCED_FACE ( 'NONE', ( #59092 ), #53567, .T. ) ;
#78965=CARTESIAN_POINT ( 'NONE',  ( 0.5774900079438607392, 18.48035201082150536, 5.440088680355550821 ) ) ;
#78966=B_SPLINE_CURVE_WITH_KNOTS ( 'NONE', 3,
 ( #91528, #1033, #16522, #9002, #2026, #92011 ),
 .UNSPECIFIED., .F., .F.,
 ( 4, 2, 4 ),
 ( 0.000000000000000000, 0.0002565770811490979868, 0.0005131541622981959736 ),
 .UNSPECIFIED. ) ;
#78967=CARTESIAN_POINT ( 'NONE',  ( 2.377183314879972809, 30.78593319516822291, -6.499999999999988454 ) ) ;
#78968=ORIENTED_EDGE ( 'NONE', *, *, #64451, .T. ) ;
#78970=CARTESIAN_POINT ( 'NONE',  ( 19.42250999205614548, 20.98035201082150891, -5.440088680355545492 ) ) ;
#78971=CARTESIAN_POINT ( 'NONE',  ( 12.63842701281683922, 54.55059781766745175, -9.846743663894590881 ) ) ;
#78972=CARTESIAN_POINT ( 'NONE',  ( 22.81628187352647785, 46.62363466993041783, 6.195893100308588602E-16 ) ) ;
#78973=DIRECTION ( 'NONE',  ( -1.000000000000000000, 0.000000000000000000, 0.000000000000000000 ) ) ;
#78974=COLOUR_RGB ( '', 0.08235294, 0.09019608, 0.10196078) ;
#78975=CARTESIAN_POINT ( 'NONE',  ( 24.16423886937410614, 24.30374883491396787, 8.672049930838204340E-16 ) ) ;
#78976=CARTESIAN_POINT ( 'NONE',  ( 7.084665262690076126, 34.10535201082151247, 10.88017736071109987 ) ) ;
#78977=CARTESIAN_POINT ( 'NONE',  ( 10.00000000000000000, 16.81368534415483751, -10.88017736071110342 ) ) ;
#78978=CARTESIAN_POINT ( 'NONE',  ( 0.1532563361054083140, 51.00893115100078745, 1.131784320476157264E-15 ) ) ;
#78979=STYLED_ITEM ( 'NONE', ( #49401 ), #90548 ) ;
#78981=CARTESIAN_POINT ( 'NONE',  ( 0.1532563361054082862, 31.21726448433412315, 2.638427012816831674 ) ) ;
#78982=AXIS2_PLACEMENT_3D ( 'NONE', #75490, #38489, #68493 ) ;
#78984=CARTESIAN_POINT ( 'NONE',  ( 18.52753015748617571, 13.09226448433411960, 4.923371831947298993 ) ) ;
#78988=CARTESIAN_POINT ( 'NONE',  ( 14.92337183194729988, 14.34226448433411782, -8.527530157486177487 ) ) ;
#78989=CARTESIAN_POINT ( 'NONE',  ( 7.361572987183170547, 67.05059781766746596, 9.846743663894590881 ) ) ;
#78990=CARTESIAN_POINT ( 'NONE',  ( 0.5774900079438590739, 47.64701867748817676, -5.440088680355550821 ) ) ;
#78991=CARTESIAN_POINT ( 'NONE',  ( 0.5774900079438607392, 48.48035201082150536, 5.440088680355550821 ) ) ;
#78992=CARTESIAN_POINT ( 'NONE',  ( 15.44008868035555260, 14.73035201082150536, 9.422509992056143702 ) ) ;
#78993=CARTESIAN_POINT ( 'NONE',  ( -2.816281873526473856, 49.33196800326374643, 3.434112377981055619 ) ) ;
#78994=CARTESIAN_POINT ( 'NONE',  ( 24.16423886937410614, 29.51208216824729647, -3.795296366450302550 ) ) ;
#78995=CARTESIAN_POINT ( 'NONE',  ( 20.24186590665277663, 11.76028685723174227, 6.114288769123037426 ) ) ;
#78997=CARTESIAN_POINT ( 'NONE',  ( 6.565887622018943937, 58.08196800326376064, -12.81628187352647608 ) ) ;
#78999=CARTESIAN_POINT ( 'NONE',  ( 18.52753015748617571, 63.09226448433412315, 4.923371831947298993 ) ) ;
#79000=CARTESIAN_POINT ( 'NONE',  ( 0.5774900079438607392, 38.48035201082150536, 5.440088680355550821 ) ) ;
#79002=CARTESIAN_POINT ( 'NONE',  ( 5.076628168052704559, 0.1755978176674514724, -8.527530157486179263 ) ) ;
#79004=B_SPLINE_CURVE_WITH_KNOTS ( 'NONE', 3,
 ( #29477, #37507, #44495, #60969 ),
 .UNSPECIFIED., .F., .F.,
 ( 4, 4 ),
 ( 2.478060227011367871E-17, 0.002392975128318431711 ),
 .UNSPECIFIED. ) ;
#79005=CARTESIAN_POINT ( 'NONE',  ( 2.791683348922240793, 11.63393115100078568, 7.208316651077764092 ) ) ;
#79006=CARTESIAN_POINT ( 'NONE',  ( 2.035157376598824452, 63.68868534415484106, 7.964842623401179544 ) ) ;
#79009=CARTESIAN_POINT ( 'NONE',  ( 15.44008868035555260, 54.73035201082150536, 9.422509992056143702 ) ) ;
#79010=CARTESIAN_POINT ( 'NONE',  ( 17.96484262340118221, 66.18868534415483396, -7.964842623401177768 ) ) ;
#79011=CARTESIAN_POINT ( 'NONE',  ( 19.84674366389459266, 8.300597817667451750, 2.638427012816836559 ) ) ;
#79014=CARTESIAN_POINT ( 'NONE',  ( 17.20831665107776587, 49.13393115100078745, -7.208316651077762316 ) ) ;
#79018=CARTESIAN_POINT ( 'NONE',  ( 6.204703633549690345, 2.845415501580634388, 14.16423886937410082 ) ) ;
#79019=CARTESIAN_POINT ( 'NONE',  ( 3.591859063236761518, 64.95696800326376774, 11.09922568453594849 ) ) ;
#79020=CARTESIAN_POINT ( 'NONE',  ( 13.79529636645031943, 5.345415501580634832, -14.16423886937409904 ) ) ;
#79021=CARTESIAN_POINT ( 'NONE',  ( 22.26659068614894466, 33.88708216824730357, 7.082119434687054849 ) ) ;
#79023=CARTESIAN_POINT ( 'NONE',  ( 12.91533473730993009, 16.60535201082150891, -10.88017736071109987 ) ) ;
#79025=CARTESIAN_POINT ( 'NONE',  ( 2.791683348922240793, 11.63393115100078568, 7.208316651077764092 ) ) ;
#79027=CARTESIAN_POINT ( 'NONE',  ( 10.00000000000000178, 17.25893115100078745, 9.846743663894594434 ) ) ;
#79028=CARTESIAN_POINT ( 'NONE',  ( 13.43411237798105340, 40.58196800326375353, 12.81628187352647963 ) ) ;
#79029=CARTESIAN_POINT ( 'NONE',  ( 0.1532563361054083140, 41.00893115100078745, 1.131784320476157264E-15 ) ) ;
#79030=CARTESIAN_POINT ( 'NONE',  ( 0.2751277870542893633, 25.30223176428832232, 6.499999999999988454 ) ) ;
#79031=CARTESIAN_POINT ( 'NONE',  ( -1.099225684535947600, 28.70696800326375353, -6.408140936763238038 ) ) ;
#79033=CARTESIAN_POINT ( 'NONE',  ( 7.361572987183170547, 22.05059781766745530, 9.846743663894590881 ) ) ;
#79034=CARTESIAN_POINT ( 'NONE',  ( 22.26659068614894466, 13.88708216824730179, 7.082119434687054849 ) ) ;
#79037=CARTESIAN_POINT ( 'NONE',  ( -0.8801773607111008646, 33.27201867748817676, 2.915334737309923430 ) ) ;
#79038=CARTESIAN_POINT ( 'NONE',  ( 22.26659068614895176, 29.72041550158063572, -7.082119434687042414 ) ) ;
#79039=CARTESIAN_POINT ( 'NONE',  ( 7.361572987183170547, 52.05059781766745175, 9.846743663894590881 ) ) ;
#79040=CARTESIAN_POINT ( 'NONE',  ( 2.791683348922237240, 10.38393115100078390, -7.208316651077763204 ) ) ;
#79041=CARTESIAN_POINT ( 'NONE',  ( 0.6178305044545838731, 59.74863466993041783, 9.382169495545420901 ) ) ;
#79043=CARTESIAN_POINT ( 'NONE',  ( 7.084665262690076126, 29.10535201082150181, 10.88017736071109987 ) ) ;
#79046=CARTESIAN_POINT ( 'NONE',  ( 21.09922568453594849, 26.20696800326375353, 6.408140936763242479 ) ) ;
#79047=CARTESIAN_POINT ( 'NONE',  ( 1.472469842513823179, 41.42559781766745886, 4.923371831947296329 ) ) ;
#79049=( BOUNDED_CURVE ( )  B_SPLINE_CURVE ( 2, ( #96610, #78263, #71269, #20096, #55771, #35085, #24790, #73579, #5102 ),
 .UNSPECIFIED., .F., .F. ) 
 B_SPLINE_CURVE_WITH_KNOTS ( ( 3, 2, 2, 2, 3 ),
 ( 0.04728379408308854698, 0.04761904761904767192, 0.05357142857142860315, 0.05952380952380953438, 0.05985906305976865238 ),
 .UNSPECIFIED. ) 
 CURVE ( )  GEOMETRIC_REPRESENTATION_ITEM ( )  RATIONAL_B_SPLINE_CURVE ( ( 0.9963778908391762723, 0.9980808541467921513, 1.000000000000000000, 0.9659258262890682012, 1.000000000000000000, 0.9659258262890682012, 1.000000000000000000, 0.9980808541467921513, 0.9963778908391762723 ) ) 
 REPRESENTATION_ITEM ( '' )  );
#79051=CARTESIAN_POINT ( 'NONE',  ( 13.99999999999999822, 11.00000000000000000, -6.500000000000000888 ) ) ;
#79055=CARTESIAN_POINT ( 'NONE',  ( 20.88017736071110519, 60.56368534415484106, 2.639326808657452039E-16 ) ) ;
#79056=CARTESIAN_POINT ( 'NONE',  ( 15.44008868035555793, 56.39701867748817676, -9.422509992056140149 ) ) ;
#79059=CARTESIAN_POINT ( 'NONE',  ( 0.2751277870542910842, 52.28217586085238366, -6.499999999999992006 ) ) ;
#79060=CARTESIAN_POINT ( 'NONE',  ( 7.084665262690076126, 12.02201867748817321, -10.88017736071110164 ) ) ;
#79061=CARTESIAN_POINT ( 'NONE',  ( 12.63842701281683034, 62.46726448433410894, 9.846743663894596210 ) ) ;
#79062=CARTESIAN_POINT ( 'NONE',  ( 2.035157376598824452, 18.68868534415484106, 7.964842623401179544 ) ) ;
#79063=CARTESIAN_POINT ( 'NONE',  ( 18.18329248733321535, 37.60290668512019607, 6.500000000000005329 ) ) ;
#79065=CARTESIAN_POINT ( 'NONE',  ( 21.09922568453594849, 31.20696800326375353, 6.408140936763242479 ) ) ;
#79067=CARTESIAN_POINT ( 'NONE',  ( 20.88017736071110519, 55.56368534415484817, 2.639326808657452039E-16 ) ) ;
#79068=CARTESIAN_POINT ( 'NONE',  ( 12.63842701281683922, 34.55059781766745886, -9.846743663894590881 ) ) ;
#79069=CARTESIAN_POINT ( 'NONE',  ( -1.099225684535947600, 19.54030133659708568, 6.408140936763237150 ) ) ;
#79070=PRESENTATION_STYLE_ASSIGNMENT (( #34047 ) ) ;
#79071=CARTESIAN_POINT ( 'NONE',  ( -0.8801773607110991993, 27.85535201082150181, -2.915334737309923874 ) ) ;
#79072=CARTESIAN_POINT ( 'NONE',  ( 0.5774900079438590739, 42.64701867748816966, -5.440088680355550821 ) ) ;
#79073=CARTESIAN_POINT ( 'NONE',  ( -4.164238869374099927, 52.01208216824729647, 3.795296366450308767 ) ) ;
#79074=CARTESIAN_POINT ( 'NONE',  ( 2.791683348922240793, 41.63393115100078745, 7.208316651077764092 ) ) ;
#79075=CARTESIAN_POINT ( 'NONE',  ( 15.44008868035555260, 54.73035201082150536, 9.422509992056143702 ) ) ;
#79076=CARTESIAN_POINT ( 'NONE',  ( 10.00000000000000178, 49.31368534415484106, 10.88017736071110342 ) ) ;
#79078=CARTESIAN_POINT ( 'NONE',  ( 13.79529636645031943, 15.34541550158063750, -14.16423886937409904 ) ) ;
#79080=EDGE_CURVE ( 'NONE', #16145, #71011, #83384, .T. ) ;
#79082=CARTESIAN_POINT ( 'NONE',  ( 2.791683348922240793, 66.63393115100079456, 7.208316651077764092 ) ) ;
#79083=ORIENTED_EDGE ( 'NONE', *, *, #42578, .T. ) ;
#79085=CARTESIAN_POINT ( 'NONE',  ( 22.26659068614895176, 44.72041550158063927, -7.082119434687042414 ) ) ;
#79086=CARTESIAN_POINT ( 'NONE',  ( -4.164238869374098151, 31.59541550158063927, -3.795296366450310543 ) ) ;
#79087=CARTESIAN_POINT ( 'NONE',  ( 2.791683348922240793, 21.63393115100078745, 7.208316651077764092 ) ) ;
#79089=CARTESIAN_POINT ( 'NONE',  ( 21.09922568453595559, 12.04030133659708746, -6.408140936763230044 ) ) ;
#79092=CARTESIAN_POINT ( 'NONE',  ( 12.91533473730992121, 4.522018677488169658, 10.88017736071110164 ) ) ;
#79093=CARTESIAN_POINT ( 'NONE',  ( 19.38216949554541202, 30.99863466993042138, 9.382169495545424454 ) ) ;
#79094=CARTESIAN_POINT ( 'NONE',  ( 20.36894250292379382, 43.67874883491397497, 10.36894250292379205 ) ) ;
#79096=CARTESIAN_POINT ( 'NONE',  ( 5.076628168052704559, 0.1755978176674514724, -8.527530157486179263 ) ) ;
#79097=EDGE_CURVE ( 'NONE', #54543, #43815, #83239, .T. ) ;
#79099=CARTESIAN_POINT ( 'NONE',  ( 2.791683348922240793, 6.633931151000785675, 7.208316651077764092 ) ) ;
#79100=ORIENTED_EDGE ( 'NONE', *, *, #2450, .F. ) ;
#79101=( NAMED_UNIT ( * ) PLANE_ANGLE_UNIT ( ) SI_UNIT ( $, .RADIAN. ) );
#79102=CARTESIAN_POINT ( 'NONE',  ( 12.63842701281683034, 17.46726448433411250, 9.846743663894596210 ) ) ;
#79104=VERTEX_POINT ( 'NONE', #52098 ) ;
#79105=CARTESIAN_POINT ( 'NONE',  ( 13.79529636645030344, 8.262082168247300018, 14.16423886937410614 ) ) ;
#79106=CARTESIAN_POINT ( 'NONE',  ( 2.035157376598822676, 2.438685344154838397, -7.964842623401177768 ) ) ;
#79107=CARTESIAN_POINT ( 'NONE',  ( 0.5774900079438607392, 13.48035201082150358, 5.440088680355550821 ) ) ;
#79108=CARTESIAN_POINT ( 'NONE',  ( 14.92337183194729988, 34.34226448433411605, -8.527530157486177487 ) ) ;
#79109=CARTESIAN_POINT ( 'NONE',  ( 16.40814093676323893, 5.790301336597087456, 11.09922568453595026 ) ) ;
#79113=CARTESIAN_POINT ( 'NONE',  ( -1.099225684535947600, 13.70696800326375353, -6.408140936763238038 ) ) ;
#79116=CARTESIAN_POINT ( 'NONE',  ( 10.00000000000000178, 43.05374883491397497, 14.16423886937410082 ) ) ;
#79118=CARTESIAN_POINT ( 'NONE',  ( 17.08211943468705840, 55.13708216824731068, -12.26659068614894466 ) ) ;
#79120=CARTESIAN_POINT ( 'NONE',  ( 15.44008868035555793, 31.39701867748817676, -9.422509992056140149 ) ) ;
#79121=CARTESIAN_POINT ( 'NONE',  ( 0.5774900079438607392, 38.48035201082150536, 5.440088680355550821 ) ) ;
#79122=CARTESIAN_POINT ( 'NONE',  ( 15.44008868035555260, 59.73035201082151247, 9.422509992056143702 ) ) ;
#79123=CARTESIAN_POINT ( 'NONE',  ( 12.91533473730993009, 31.60535201082150891, -10.88017736071109987 ) ) ;
#79125=CARTESIAN_POINT ( 'NONE',  ( 0.1089645850228809637, 33.16234555792569694, 6.479102184480781013 ) ) ;
#79127=CARTESIAN_POINT ( 'NONE',  ( 5.076628168052703671, 21.84226448433411960, 8.527530157486179263 ) ) ;
#79131=CARTESIAN_POINT ( 'NONE',  ( 17.20831665107776587, 47.88393115100078745, 7.208316651077764980 ) ) ;
#79132=ADVANCED_FACE ( 'NONE', ( #74594 ), #2380, .T. ) ;
#79134=CARTESIAN_POINT ( 'NONE',  ( 16.40814093676324603, 47.45696800326375353, -11.09922568453594671 ) ) ;
#79136=ORIENTED_EDGE ( 'NONE', *, *, #89747, .F. ) ;
#79137=CARTESIAN_POINT ( 'NONE',  ( 17.39651004071842166, 22.93575266056828355, 6.499999999999998224 ) ) ;
#79140=CARTESIAN_POINT ( 'NONE',  ( 24.16423886937410614, 44.51208216824730357, -3.795296366450302550 ) ) ;
#79143=CARTESIAN_POINT ( 'NONE',  ( 19.84674366389459621, 28.50893115100078745, 7.409399052514197653E-17 ) ) ;
#79144=CARTESIAN_POINT ( 'NONE',  ( 3.591859063236761518, 59.95696800326375353, 11.09922568453594849 ) ) ;
#79146=CARTESIAN_POINT ( 'NONE',  ( 19.84674366389459266, 58.30059781766745886, 2.638427012816836559 ) ) ;
#79147=CARTESIAN_POINT ( 'NONE',  ( 19.84674366389459621, 3.508931151000785231, 7.409399052514197653E-17 ) ) ;
#79149=CARTESIAN_POINT ( 'NONE',  ( 14.92337183194729633, 62.67559781766745886, 8.527530157486181039 ) ) ;
#79152=CARTESIAN_POINT ( 'NONE',  ( 2.917880565312948704, 67.63708216824730357, 12.26659068614894643 ) ) ;
#79154=CARTESIAN_POINT ( 'NONE',  ( 2.035157376598822676, 47.43868534415484817, -7.964842623401177768 ) ) ;
#79155=CARTESIAN_POINT ( 'NONE',  ( 6.565887622018943937, 15.16530133659708568, 12.81628187352647430 ) ) ;
#79156=CARTESIAN_POINT ( 'NONE',  ( -0.8801773607110991993, 67.85535201082151957, -2.915334737309923874 ) ) ;
#79157=CARTESIAN_POINT ( 'NONE',  ( -0.3289641300568009741, 62.24545670184114243, -5.963430220938281678 ) ) ;
#79158=ADVANCED_FACE ( 'NONE', ( #42054 ), #95534, .T. ) ;
#79161=CARTESIAN_POINT ( 'NONE',  ( 12.63842701281683034, 57.46726448433411605, 9.846743663894596210 ) ) ;
#79162=CARTESIAN_POINT ( 'NONE',  ( -22.44000000000001194, 93.50000000000000000, 9.500000000000000000 ) ) ;
#79164=CARTESIAN_POINT ( 'NONE',  ( -1.099225684535947600, 13.70696800326375353, -6.408140936763238038 ) ) ;
#79165=CARTESIAN_POINT ( 'NONE',  ( 20.88017736071110519, 20.56368534415484106, 2.639326808657452039E-16 ) ) ;
#79168=CARTESIAN_POINT ( 'NONE',  ( -0.3689425029237898834, 31.17874883491396787, -10.36894250292378850 ) ) ;
#79169=CARTESIAN_POINT ( 'NONE',  ( -4.164238869374099927, 27.01208216824730357, 3.795296366450308767 ) ) ;
#79170=CARTESIAN_POINT ( 'NONE',  ( 13.79529636645030344, 63.26208216824730357, 14.16423886937410614 ) ) ;
#79171=CARTESIAN_POINT ( 'NONE',  ( 14.92337183194729988, 49.34226448433411605, -8.527530157486177487 ) ) ;
#79172=CARTESIAN_POINT ( 'NONE',  ( 19.38216949554541202, 30.99863466993042138, 9.382169495545424454 ) ) ;
#79173=CARTESIAN_POINT ( 'NONE',  ( 7.084665262690076126, 14.10535201082150358, 10.88017736071109987 ) ) ;
#79176=CARTESIAN_POINT ( 'NONE',  ( 12.63842701281683034, 37.46726448433411605, 9.846743663894596210 ) ) ;
#79177=B_SPLINE_CURVE_WITH_KNOTS ( 'NONE', 3,
 ( #63081, #2126, #32586, #24616, #77101, #78093 ),
 .UNSPECIFIED., .F., .F.,
 ( 4, 2, 4 ),
 ( 0.000000000000000000, 0.0002701661927229306740, 0.0005403323854458613480 ),
 .UNSPECIFIED. ) ;
#79178=CARTESIAN_POINT ( 'NONE',  ( 12.91533473730992121, 44.52201867748816966, 10.88017736071110164 ) ) ;
#79179=CARTESIAN_POINT ( 'NONE',  ( 19.38216949554541557, 12.24863466993041961, -9.382169495545420901 ) ) ;
#79180=CARTESIAN_POINT ( 'NONE',  ( -4.164238869374099039, 16.80374883491396787, 8.674139862899312516E-16 ) ) ;
#79181=CARTESIAN_POINT ( 'NONE',  ( 1.472469842513823179, 61.42559781766745175, 4.923371831947296329 ) ) ;
#79184=CARTESIAN_POINT ( 'NONE',  ( 0.1532563361054082862, 21.21726448433412315, 2.638427012816831674 ) ) ;
#79185=CARTESIAN_POINT ( 'NONE',  ( 6.565887622018943937, 55.16530133659709634, 12.81628187352647430 ) ) ;
#79186=CARTESIAN_POINT ( 'NONE',  ( 7.361572987183169658, 59.96726448433410894, -9.846743663894592657 ) ) ;
#79189=( LENGTH_UNIT ( ) NAMED_UNIT ( * ) SI_UNIT ( .MILLI., .METRE. ) );
#79190=CARTESIAN_POINT ( 'NONE',  ( 10.00000000000000000, 65.55374883491396076, -14.16423886937410082 ) ) ;
#79191=B_SPLINE_CURVE_WITH_KNOTS ( 'NONE', 3,
 ( #68577, #92059, #8564, #6585 ),
 .UNSPECIFIED., .F., .F.,
 ( 4, 4 ),
 ( 0.000000000000000000, 0.0003153491572467357934 ),
 .UNSPECIFIED. ) ;
#79192=CARTESIAN_POINT ( 'NONE',  ( -0.3689425029237898834, 11.17874883491396787, -10.36894250292378850 ) ) ;
#79193=CARTESIAN_POINT ( 'NONE',  ( -0.8801773607111009756, 68.06368534415484817, 1.068504757029289695E-15 ) ) ;
#79194=CARTESIAN_POINT ( 'NONE',  ( 5.076628168052703671, 51.84226448433412315, 8.527530157486179263 ) ) ;
#79195=CARTESIAN_POINT ( 'NONE',  ( 12.91533473730993009, 26.60535201082150536, -10.88017736071109987 ) ) ;
#79199=VERTEX_POINT ( 'NONE', #89014 ) ;
#79201=ORIENTED_EDGE ( 'NONE', *, *, #89523, .F. ) ;
#79204=CARTESIAN_POINT ( 'NONE',  ( 6.204703633549690345, 2.845415501580634388, 14.16423886937410082 ) ) ;
#79205=FACE_OUTER_BOUND ( 'NONE', #41713, .T. ) ;
#79206=CARTESIAN_POINT ( 'NONE',  ( 10.00000000000000178, 38.05374883491396787, 14.16423886937410082 ) ) ;
#79207=CARTESIAN_POINT ( 'NONE',  ( 19.84674366389459266, 53.71726448433411605, -2.638427012816827677 ) ) ;
#79208=CARTESIAN_POINT ( 'NONE',  ( 12.63842701281683922, 34.55059781766745886, -9.846743663894590881 ) ) ;
#79209=CARTESIAN_POINT ( 'NONE',  ( 7.084665262690076126, 19.10535201082150181, 10.88017736071109987 ) ) ;
#79210=CARTESIAN_POINT ( 'NONE',  ( 0.1532563361054100626, 55.80059781766745175, -2.638427012816831230 ) ) ;
#79211=CARTESIAN_POINT ( 'NONE',  ( -0.3689425029237898834, 1.178748834913967869, -10.36894250292378850 ) ) ;
#79212=CARTESIAN_POINT ( 'NONE',  ( 6.204703633549690345, 42.84541550158063217, 14.16423886937410082 ) ) ;
#79213=CARTESIAN_POINT ( 'NONE',  ( 0.5774900079438607392, 8.480352010821505360, 5.440088680355550821 ) ) ;
#79215=DIRECTION ( 'NONE',  ( -0.000000000000000000, -0.000000000000000000, 1.000000000000000000 ) ) ;
#79216=CARTESIAN_POINT ( 'NONE',  ( 7.084665262690076126, 59.10535201082150536, 10.88017736071109987 ) ) ;
#79217=CARTESIAN_POINT ( 'NONE',  ( 18.52753015748617571, 28.09226448433411960, 4.923371831947298993 ) ) ;
#79219=ORIENTED_EDGE ( 'NONE', *, *, #64077, .T. ) ;
#79222=ORIENTED_EDGE ( 'NONE', *, *, #33355, .F. ) ;
#79223=CARTESIAN_POINT ( 'NONE',  ( 12.63842701281683922, 19.55059781766745175, -9.846743663894590881 ) ) ;
#79225=CARTESIAN_POINT ( 'NONE',  ( -2.266590686148945544, 26.38708216824730357, -7.082119434687050408 ) ) ;
#79227=CARTESIAN_POINT ( 'NONE',  ( 1.472469842513823179, 36.42559781766745175, 4.923371831947296329 ) ) ;
#79228=CARTESIAN_POINT ( 'NONE',  ( 17.96484262340118221, 49.93868534415484106, 7.964842623401181321 ) ) ;
#79229=CARTESIAN_POINT ( 'NONE',  ( 0.000000000000000000, 0.000000000000000000, -6.500000000000000888 ) ) ;
#79230=CARTESIAN_POINT ( 'NONE',  ( 19.42250999205614548, 35.98035201082151247, -5.440088680355545492 ) ) ;
#79234=CARTESIAN_POINT ( 'NONE',  ( 20.88017736071110164, 45.35535201082149115, 2.915334737309930979 ) ) ;
#79235=CARTESIAN_POINT ( 'NONE',  ( -4.164238869374099927, 2.012082168247300906, 3.795296366450308767 ) ) ;
#79237=ORIENTED_EDGE ( 'NONE', *, *, #10500, .F. ) ;
#79238=CARTESIAN_POINT ( 'NONE',  ( 3.591859063236763294, 33.29030133659708213, -11.09922568453595026 ) ) ;
#79239=FILL_AREA_STYLE_COLOUR ( '', #36618 ) ;
#79240=CARTESIAN_POINT ( 'NONE',  ( 12.63842701281683922, 29.55059781766745175, -9.846743663894590881 ) ) ;
#79241=CARTESIAN_POINT ( 'NONE',  ( 0.5774900079438590739, 2.647018677488170990, -5.440088680355550821 ) ) ;
#79242=CARTESIAN_POINT ( 'NONE',  ( 22.81628187352648496, 46.83196800326376064, -3.434112377981050290 ) ) ;
#79244=CARTESIAN_POINT ( 'NONE',  ( 19.84674366389459266, 23.30059781766745530, 2.638427012816836559 ) ) ;
#79245=AXIS2_PLACEMENT_3D ( 'NONE', #76706, #67744, #84230 ) ;
#79246=CARTESIAN_POINT ( 'NONE',  ( 20.88017736071110519, 60.56368534415484106, 2.639326808657452039E-16 ) ) ;
#79252=COLOUR_RGB ( '', 0.08235294, 0.09019608, 0.10196078) ;
#79253=CARTESIAN_POINT ( 'NONE',  ( 0.1077916266722445948, 17.24062864464239198, -6.478736007405951902 ) ) ;
#79254=CARTESIAN_POINT ( 'NONE',  ( 2.791683348922237240, 5.383931151000785675, -7.208316651077763204 ) ) ;
#79256=CARTESIAN_POINT ( 'NONE',  ( 0.6178305044545838731, 9.748634669930416052, 9.382169495545420901 ) ) ;
#79257=CARTESIAN_POINT ( 'NONE',  ( 2.603489959281614308, 41.58210964143329846, 6.500000000000031086 ) ) ;
#79258=CARTESIAN_POINT ( 'NONE',  ( 0.1532563361054082862, 46.21726448433411605, 2.638427012816831674 ) ) ;
#79260=CARTESIAN_POINT ( 'NONE',  ( -2.266590686148945544, 6.387082168247300906, -7.082119434687050408 ) ) ;
#79261=CARTESIAN_POINT ( 'NONE',  ( 12.63842701281683034, 32.46726448433412315, 9.846743663894596210 ) ) ;
#79262=CARTESIAN_POINT ( 'NONE',  ( 22.81628187352647785, 26.62363466993042138, 6.195893100308588602E-16 ) ) ;
#79264=DIRECTION ( 'NONE',  ( 0.000000000000000000, 0.000000000000000000, -1.000000000000000000 ) ) ;
#79265=CARTESIAN_POINT ( 'NONE',  ( 12.91533473730992121, 44.52201867748816966, 10.88017736071110164 ) ) ;
#79266=CARTESIAN_POINT ( 'NONE',  ( 6.565887622018943937, 13.08196800326374998, -12.81628187352647608 ) ) ;
#79267=CARTESIAN_POINT ( 'NONE',  ( 2.603489959281588995, 40.43575266056827644, -6.500000000000003553 ) ) ;
#79268=CARTESIAN_POINT ( 'NONE',  ( 19.84674366389459621, 18.50893115100078745, 7.409399052514197653E-17 ) ) ;
#79269=CARTESIAN_POINT ( 'NONE',  ( 17.96484262340118221, 21.18868534415483396, -7.964842623401177768 ) ) ;
#79270=CARTESIAN_POINT ( 'NONE',  ( 3.591859063236763294, 28.29030133659708568, -11.09922568453595026 ) ) ;
#79272=CARTESIAN_POINT ( 'NONE',  ( 7.361572987183170547, 27.05059781766745175, 9.846743663894590881 ) ) ;
#79273=( GEOMETRIC_REPRESENTATION_CONTEXT ( 3 ) GLOBAL_UNCERTAINTY_ASSIGNED_CONTEXT ( ( #81162 ) ) GLOBAL_UNIT_ASSIGNED_CONTEXT ( ( #4389, #12847, #28351 ) ) REPRESENTATION_CONTEXT ( 'NONE', 'WORKASPACE' ) );
#79276=CARTESIAN_POINT ( 'NONE',  ( 7.084665262690076126, 39.10535201082150536, 10.88017736071109987 ) ) ;
#79277=CARTESIAN_POINT ( 'NONE',  ( 20.88017736071110519, 65.56368534415483396, 2.639326808657452039E-16 ) ) ;
#79278=FILL_AREA_STYLE_COLOUR ( '', #63248 ) ;
#79279=CARTESIAN_POINT ( 'NONE',  ( 7.361572987183170547, 37.05059781766744464, 9.846743663894590881 ) ) ;
#79280=CARTESIAN_POINT ( 'NONE',  ( 20.88017736071110164, 30.35535201082151247, 2.915334737309930979 ) ) ;
#79283=CARTESIAN_POINT ( 'NONE',  ( 7.084665262690076126, 42.02201867748816966, -10.88017736071110164 ) ) ;
#79284=CARTESIAN_POINT ( 'NONE',  ( 0.5774900079438590739, 12.64701867748817321, -5.440088680355550821 ) ) ;
#79287=CARTESIAN_POINT ( 'NONE',  ( 7.361572987183169658, 34.96726448433411605, -9.846743663894592657 ) ) ;
#79288=CARTESIAN_POINT ( 'NONE',  ( -0.3689425029237898834, 46.17874883491397497, -10.36894250292378850 ) ) ;
#79289=CARTESIAN_POINT ( 'NONE',  ( 2.603489959281590771, 46.58210964143328425, 6.500000000000003553 ) ) ;
#79291=CARTESIAN_POINT ( 'NONE',  ( 1.932340009482151011, 6.491275129254484355, -6.500000000000002665 ) ) ;
#79293=CARTESIAN_POINT ( 'NONE',  ( -4.164238869374099927, 27.01208216824730357, 3.795296366450308767 ) ) ;
#79297=CARTESIAN_POINT ( 'NONE',  ( 20.36894250292379382, 63.67874883491396787, 10.36894250292379205 ) ) ;
#79298=CARTESIAN_POINT ( 'NONE',  ( 0.1532563361054100626, 35.80059781766745175, -2.638427012816831230 ) ) ;
#79301=CARTESIAN_POINT ( 'NONE',  ( 12.91533473730993009, 61.60535201082150536, -10.88017736071109987 ) ) ;
#79302=CARTESIAN_POINT ( 'NONE',  ( 21.09922568453595559, 62.04030133659709634, -6.408140936763230044 ) ) ;
#79304=CARTESIAN_POINT ( 'NONE',  ( 10.00000000000000000, 31.81368534415483751, -10.88017736071110342 ) ) ;
#79305=CARTESIAN_POINT ( 'NONE',  ( 19.38216949554541557, 62.24863466993041072, -9.382169495545420901 ) ) ;
#79306=CARTESIAN_POINT ( 'NONE',  ( 13.43411237798106583, 12.66530133659708746, -12.81628187352647252 ) ) ;
#79307=CARTESIAN_POINT ( 'NONE',  ( 18.52753015748617571, 18.09226448433411960, 4.923371831947298993 ) ) ;
#79311=CARTESIAN_POINT ( 'NONE',  ( 7.084665262690076126, 7.022018677488170546, -10.88017736071110164 ) ) ;
#79312=CARTESIAN_POINT ( 'NONE',  ( 2.917880565312950480, 25.97041550158063572, -12.26659068614894821 ) ) ;
#79313=CARTESIAN_POINT ( 'NONE',  ( -0.8801773607110991993, 37.85535201082151247, -2.915334737309923874 ) ) ;
#79314=CARTESIAN_POINT ( 'NONE',  ( 2.035157376598824452, 48.68868534415483396, 7.964842623401179544 ) ) ;
#79316=CARTESIAN_POINT ( 'NONE',  ( 14.92337183194729988, 4.342264484334117824, -8.527530157486177487 ) ) ;
#79318=CARTESIAN_POINT ( 'NONE',  ( 19.84674366389459621, 23.50893115100078390, 7.409399052514197653E-17 ) ) ;
#79320=CARTESIAN_POINT ( 'NONE',  ( 14.92337183194729988, 29.34226448433411960, -8.527530157486177487 ) ) ;
#79321=CARTESIAN_POINT ( 'NONE',  ( 12.63842701281683034, 47.46726448433412315, 9.846743663894596210 ) ) ;
#79322=CIRCLE ( 'NONE', #76106, 7.000000000000006217 ) ;
#79323=CARTESIAN_POINT ( 'NONE',  ( 12.91533473730992121, 24.52201867748816966, 10.88017736071110164 ) ) ;
#79324=UNCERTAINTY_MEASURE_WITH_UNIT (LENGTH_MEASURE( 1.000000000000000082E-05 ), #79597, 'distance_accuracy_value', 'NONE');
#79325=CARTESIAN_POINT ( 'NONE',  ( -1.099225684535947600, 39.54030133659708923, 6.408140936763237150 ) ) ;
#79326=CARTESIAN_POINT ( 'NONE',  ( 10.00000000000000178, 49.31368534415484106, 10.88017736071110342 ) ) ;
#79327=CARTESIAN_POINT ( 'NONE',  ( 7.361572987183170547, 27.05059781766745175, 9.846743663894590881 ) ) ;
#79328=CARTESIAN_POINT ( 'NONE',  ( -4.164238869374099039, 41.80374883491397497, 8.674139862899312516E-16 ) ) ;
#79329=CARTESIAN_POINT ( 'NONE',  ( 0.1532563361054082862, 16.21726448433411960, 2.638427012816831674 ) ) ;
#79330=CARTESIAN_POINT ( 'NONE',  ( 0.1916775849787265562, 47.25868815902069997, -6.499999999999990230 ) ) ;
#79333=CARTESIAN_POINT ( 'NONE',  ( -2.266590686148945544, 11.38708216824730179, -7.082119434687050408 ) ) ;
#79334=CARTESIAN_POINT ( 'NONE',  ( 10.00000000000000000, 25.55374883491396787, -14.16423886937410082 ) ) ;
#79335=CARTESIAN_POINT ( 'NONE',  ( 12.63842701281683922, 29.55059781766745175, -9.846743663894590881 ) ) ;
#79336=CARTESIAN_POINT ( 'NONE',  ( 4.559911319644449179, 27.23035201082150536, -9.422509992056141925 ) ) ;
#79337=CARTESIAN_POINT ( 'NONE',  ( 20.88017736071110164, 40.35535201082150536, 2.915334737309930979 ) ) ;
#79338=CARTESIAN_POINT ( 'NONE',  ( 15.44008868035555260, 49.73035201082150536, 9.422509992056143702 ) ) ;
#79339=ORIENTED_EDGE ( 'NONE', *, *, #29437, .T. ) ;
#79340=STYLED_ITEM ( 'NONE', ( #34255 ), #32075 ) ;
#79341=CARTESIAN_POINT ( 'NONE',  ( 4.559911319644449179, 53.89701867748817676, 9.422509992056141925 ) ) ;
#79343=EDGE_CURVE ( 'NONE', #13314, #79733, #47607, .T. ) ;
#79346=CARTESIAN_POINT ( 'NONE',  ( 4.559911319644449179, 68.89701867748817676, 9.422509992056141925 ) ) ;
#79347=ORIENTED_EDGE ( 'NONE', *, *, #14935, .F. ) ;
#79349=CARTESIAN_POINT ( 'NONE',  ( 17.96484262340118221, 66.18868534415483396, -7.964842623401177768 ) ) ;
#79350=( NAMED_UNIT ( * ) PLANE_ANGLE_UNIT ( ) SI_UNIT ( $, .RADIAN. ) );
#79351=LINE ( 'NONE', #63353, #62731 ) ;
#79352=DIRECTION ( 'NONE',  ( 0.000000000000000000, -1.000000000000000000, 0.000000000000000000 ) ) ;
#79353=CARTESIAN_POINT ( 'NONE',  ( 2.035157376598822676, 12.43868534415483751, -7.964842623401177768 ) ) ;
#79354=CARTESIAN_POINT ( 'NONE',  ( 1.472469842513823179, 16.42559781766745175, 4.923371831947296329 ) ) ;
#79355=CARTESIAN_POINT ( 'NONE',  ( 17.08211943468705840, 5.137082168247300906, -12.26659068614894466 ) ) ;
#79356=CARTESIAN_POINT ( 'NONE',  ( 2.791683348922240793, 6.633931151000785675, 7.208316651077764092 ) ) ;
#79357=CARTESIAN_POINT ( 'NONE',  ( 20.88017736071110875, 5.772018677488170546, -2.915334737309920765 ) ) ;
#79358=CARTESIAN_POINT ( 'NONE',  ( 14.92337183194729988, 49.34226448433411605, -8.527530157486177487 ) ) ;
#79359=EDGE_LOOP ( 'NONE', ( #90732, #36819, #52986, #6054, #34840 ) ) ;
#79360=CARTESIAN_POINT ( 'NONE',  ( 19.84674366389459266, 43.71726448433410894, -2.638427012816827677 ) ) ;
#79362=CARTESIAN_POINT ( 'NONE',  ( 4.559911319644449179, 52.23035201082151247, -9.422509992056141925 ) ) ;
#79363=CARTESIAN_POINT ( 'NONE',  ( 17.20831665107776587, 49.13393115100078745, -7.208316651077762316 ) ) ;
#79364=CARTESIAN_POINT ( 'NONE',  ( 0.6178305044545818747, 28.49863466993041783, -9.382169495545419124 ) ) ;
#79365=CARTESIAN_POINT ( 'NONE',  ( 2.562013731377108972, 0.5000000000000000000, -6.499999999999999112 ) ) ;
#79367=CARTESIAN_POINT ( 'NONE',  ( 19.42250999205614193, 65.14701867748817676, 5.440088680355555262 ) ) ;
#79368=CARTESIAN_POINT ( 'NONE',  ( 17.96484262340118221, 11.18868534415484106, -7.964842623401177768 ) ) ;
#79370=EDGE_CURVE ( 'NONE', #52255, #72967, #70286, .T. ) ;
#79371=CARTESIAN_POINT ( 'NONE',  ( 16.40814093676323893, 35.79030133659708923, 11.09922568453595026 ) ) ;
#79374=CARTESIAN_POINT ( 'NONE',  ( 0.6178305044545838731, 24.74863466993042493, 9.382169495545420901 ) ) ;
#79375=CARTESIAN_POINT ( 'NONE',  ( 4.559911319644449179, 38.89701867748817676, 9.422509992056141925 ) ) ;
#79379=CARTESIAN_POINT ( 'NONE',  ( 6.565887622018943937, -1.918031996736246692, -12.81628187352647608 ) ) ;
#79380=CARTESIAN_POINT ( 'NONE',  ( 5.076628168052703671, 16.84226448433411960, 8.527530157486179263 ) ) ;
#79381=CARTESIAN_POINT ( 'NONE',  ( 10.00000000000000178, 57.25893115100078745, 9.846743663894594434 ) ) ;
#79383=CARTESIAN_POINT ( 'NONE',  ( 18.52753015748618282, 38.92559781766745175, -4.923371831947291888 ) ) ;
#79386=CARTESIAN_POINT ( 'NONE',  ( 18.52753015748618282, 33.92559781766745886, -4.923371831947291888 ) ) ;
#79389=CARTESIAN_POINT ( 'NONE',  ( 0.1532563361054082862, 61.21726448433412315, 2.638427012816831674 ) ) ;
#79390=ORIENTED_EDGE ( 'NONE', *, *, #84787, .T. ) ;
#79393=CARTESIAN_POINT ( 'NONE',  ( -2.816281873526471635, 23.91530133659708568, -3.434112377981056508 ) ) ;
#79394=CARTESIAN_POINT ( 'NONE',  ( 0.1532563361054083140, 51.00893115100078745, 1.131784320476157264E-15 ) ) ;
#79398=CARTESIAN_POINT ( 'NONE',  ( 10.00000000000000178, 43.05374883491397497, 14.16423886937410082 ) ) ;
#79399=CARTESIAN_POINT ( 'NONE',  ( 14.92337183194729988, 19.34226448433411960, -8.527530157486177487 ) ) ;
#79401=CARTESIAN_POINT ( 'NONE',  ( 20.00000000000000711, 82.60888403408161196, 4.637569774571720593 ) ) ;
#79402=CARTESIAN_POINT ( 'NONE',  ( 13.79529636645031943, 60.34541550158063927, -14.16423886937409904 ) ) ;
#79403=CARTESIAN_POINT ( 'NONE',  ( 18.52753015748617571, 63.09226448433412315, 4.923371831947298993 ) ) ;
#79406=CARTESIAN_POINT ( 'NONE',  ( 20.88017736071110875, 10.77201867748817143, -2.915334737309920765 ) ) ;
#79407=CARTESIAN_POINT ( 'NONE',  ( 10.00000000000000000, 40.55374883491397497, -14.16423886937410082 ) ) ;
#79409=CARTESIAN_POINT ( 'NONE',  ( 10.00000000000000178, 38.05374883491396787, 14.16423886937410082 ) ) ;
#79413=CARTESIAN_POINT ( 'NONE',  ( 10.00000000000000000, 59.75893115100078745, -9.846743663894594434 ) ) ;
#79416=CARTESIAN_POINT ( 'NONE',  ( 4.559911319644449179, 42.23035201082151247, -9.422509992056141925 ) ) ;
#79420=CARTESIAN_POINT ( 'NONE',  ( -46.82017113615791004, 100.6079546444643569, -9.324761308090124601 ) ) ;
#79423=CARTESIAN_POINT ( 'NONE',  ( 10.00000000000000178, 62.25893115100078745, 9.846743663894594434 ) ) ;
#79426=CARTESIAN_POINT ( 'NONE',  ( 17.08211943468705130, 33.47041550158063927, 12.26659068614894998 ) ) ;
#79429=CARTESIAN_POINT ( 'NONE',  ( 20.88017736071110875, 15.77201867748817143, -2.915334737309920765 ) ) ;
#79430=CARTESIAN_POINT ( 'NONE',  ( 13.43411237798106583, 27.66530133659708568, -12.81628187352647252 ) ) ;
#79431=CARTESIAN_POINT ( 'NONE',  ( -0.1503990784575328643, 40.12777174578613426, 6.262539305110068177 ) ) ;
#79432=CARTESIAN_POINT ( 'NONE',  ( 18.52753015748617571, 18.09226448433411960, 4.923371831947298993 ) ) ;
#79435=CARTESIAN_POINT ( 'NONE',  ( 20.88017736071110164, 10.35535201082150714, 2.915334737309930979 ) ) ;
#79437=CARTESIAN_POINT ( 'NONE',  ( -0.8801773607111009756, 38.06368534415484106, 1.068504757029289695E-15 ) ) ;
#79438=CARTESIAN_POINT ( 'NONE',  ( 15.44008868035555793, 36.39701867748816966, -9.422509992056140149 ) ) ;
#79439=CARTESIAN_POINT ( 'NONE',  ( 6.565887622018943937, 0.1653013365970866511, 12.81628187352647430 ) ) ;
#79441=CARTESIAN_POINT ( 'NONE',  ( 17.39651004071841101, 57.93575266056827644, 6.500000000000005329 ) ) ;
#79442=CARTESIAN_POINT ( 'NONE',  ( 7.361572987183170547, 7.050597817667451750, 9.846743663894590881 ) ) ;
#79443=ORIENTED_EDGE ( 'NONE', *, *, #27348, .T. ) ;
#79444=CARTESIAN_POINT ( 'NONE',  ( 15.44008868035555260, 29.73035201082150891, 9.422509992056143702 ) ) ;
#79445=CARTESIAN_POINT ( 'NONE',  ( 16.40814093676323893, 10.79030133659708923, 11.09922568453595026 ) ) ;
#79446=CARTESIAN_POINT ( 'NONE',  ( 7.084665262690076126, 69.10535201082151957, 10.88017736071109987 ) ) ;
#79447=CARTESIAN_POINT ( 'NONE',  ( 0.1532563361054082862, 6.217264484334118713, 2.638427012816831674 ) ) ;
#79448=VECTOR ( 'NONE', #80858, 1000.000000000000000 ) ;
#79449=CARTESIAN_POINT ( 'NONE',  ( 19.38216949554541202, 30.99863466993042138, 9.382169495545424454 ) ) ;
#79450=CARTESIAN_POINT ( 'NONE',  ( 0.1532563361054083140, 6.008931151000784787, 1.131784320476157264E-15 ) ) ;
#79452=SURFACE_SIDE_STYLE ('',( #48944 ) ) ;
#79454=CARTESIAN_POINT ( 'NONE',  ( 7.084665262690076126, 9.105352010821503583, 10.88017736071109987 ) ) ;
#79455=CARTESIAN_POINT ( 'NONE',  ( 22.81628187352648496, 61.83196800326376774, -3.434112377981050290 ) ) ;
#79456=CARTESIAN_POINT ( 'NONE',  ( -0.3689425029237881626, 27.42874883491397142, 10.36894250292379027 ) ) ;
#79457=CARTESIAN_POINT ( 'NONE',  ( 1.472469842513823179, 16.42559781766745175, 4.923371831947296329 ) ) ;
#79458=CARTESIAN_POINT ( 'NONE',  ( 19.42250999205614193, 5.147018677488171434, 5.440088680355555262 ) ) ;
#79460=CARTESIAN_POINT ( 'NONE',  ( 2.791683348922240793, 26.63393115100078745, 7.208316651077764092 ) ) ;
#79461=CARTESIAN_POINT ( 'NONE',  ( 20.36894250292379738, 64.92874883491397497, -10.36894250292379027 ) ) ;
#79463=CARTESIAN_POINT ( 'NONE',  ( 20.88017736071110519, 10.56368534415483751, 2.639326808657452039E-16 ) ) ;
#79465=CARTESIAN_POINT ( 'NONE',  ( 7.084665262690076126, 17.02201867748817676, -10.88017736071110164 ) ) ;
#79466=CARTESIAN_POINT ( 'NONE',  ( 2.603489959281586774, 5.435752660568278216, -6.500000000000001776 ) ) ;
#79470=CARTESIAN_POINT ( 'NONE',  ( 7.084665262690076126, 29.10535201082150181, 10.88017736071109987 ) ) ;
#79471=CARTESIAN_POINT ( 'NONE',  ( 10.00000000000000000, 54.75893115100078745, -9.846743663894594434 ) ) ;
#79473=CARTESIAN_POINT ( 'NONE',  ( -2.816281873526473856, 49.33196800326374643, 3.434112377981055619 ) ) ;
#79474=CARTESIAN_POINT ( 'NONE',  ( -1.926860441876563801, 4.896642702460841434, 3.195792623639529761 ) ) ;
#79475=CARTESIAN_POINT ( 'NONE',  ( 20.36894250292379738, 39.92874883491396787, -10.36894250292379027 ) ) ;
#79476=CARTESIAN_POINT ( 'NONE',  ( 4.559911319644449179, 37.23035201082150536, -9.422509992056141925 ) ) ;
#79477=CARTESIAN_POINT ( 'NONE',  ( -0.8801773607111009756, 13.06368534415483929, 1.068504757029289695E-15 ) ) ;
#79478=CARTESIAN_POINT ( 'NONE',  ( 18.52753015748617571, 53.09226448433412315, 4.923371831947298993 ) ) ;
#79479=CARTESIAN_POINT ( 'NONE',  ( 19.05866839779139710, 60.95508385108959715, -6.499999999999974243 ) ) ;
#79480=CARTESIAN_POINT ( 'NONE',  ( 12.63842701281683034, 37.46726448433411605, 9.846743663894596210 ) ) ;
#79482=CARTESIAN_POINT ( 'NONE',  ( 12.63842701281683922, 14.55059781766744997, -9.846743663894590881 ) ) ;
#79485=ORIENTED_EDGE ( 'NONE', *, *, #15942, .T. ) ;
#79486=CARTESIAN_POINT ( 'NONE',  ( 7.084665262690076126, 19.10535201082150181, 10.88017736071109987 ) ) ;
#79487=CARTESIAN_POINT ( 'NONE',  ( 0.1532563361054100626, 10.80059781766745175, -2.638427012816831230 ) ) ;
#79488=CARTESIAN_POINT ( 'NONE',  ( 10.00000000000000000, 2.873634669930420049, -12.81628187352647608 ) ) ;
#79489=CARTESIAN_POINT ( 'NONE',  ( 17.96484262340118221, 39.93868534415484106, 7.964842623401181321 ) ) ;
#79490=CARTESIAN_POINT ( 'NONE',  ( 17.96484262340118221, 21.18868534415483396, -7.964842623401177768 ) ) ;
#79491=CARTESIAN_POINT ( 'NONE',  ( 19.38216949554541557, 47.24863466993041783, -9.382169495545420901 ) ) ;
#79492=CARTESIAN_POINT ( 'NONE',  ( 22.26659068614895176, 29.72041550158063572, -7.082119434687042414 ) ) ;
#79493=DIRECTION ( 'NONE',  ( 0.000000000000000000, 0.000000000000000000, 1.000000000000000000 ) ) ;
#79496=CARTESIAN_POINT ( 'NONE',  ( 0.6178305044545818747, 53.49863466993041072, -9.382169495545419124 ) ) ;
#79498=CARTESIAN_POINT ( 'NONE',  ( 1.472469842513823179, 55.59226448433412315, -4.923371831947296329 ) ) ;
#79499=CARTESIAN_POINT ( 'NONE',  ( 3.591859063236761518, 64.95696800326376774, 11.09922568453594849 ) ) ;
#79501=CARTESIAN_POINT ( 'NONE',  ( 20.88017736071110164, 30.35535201082151247, 2.915334737309930979 ) ) ;
#79503=CARTESIAN_POINT ( 'NONE',  ( 10.00000000000000178, 2.258931151000784787, 9.846743663894594434 ) ) ;
#79505=CARTESIAN_POINT ( 'NONE',  ( 19.84674366389459266, 23.71726448433412315, -2.638427012816827677 ) ) ;
#79506=CARTESIAN_POINT ( 'NONE',  ( 5.076628168052703671, 16.84226448433411960, 8.527530157486179263 ) ) ;
#79507=CARTESIAN_POINT ( 'NONE',  ( 12.63842701281683034, 7.467264484334118713, 9.846743663894596210 ) ) ;
#79508=CARTESIAN_POINT ( 'NONE',  ( -0.8801773607110991993, 62.85535201082150536, -2.915334737309923874 ) ) ;
#79509=CARTESIAN_POINT ( 'NONE',  ( 19.42250999205614548, 65.98035201082151957, -5.440088680355545492 ) ) ;
#79510=CARTESIAN_POINT ( 'NONE',  ( 7.361572987183169658, 24.96726448433412315, -9.846743663894592657 ) ) ;
#79513=CARTESIAN_POINT ( 'NONE',  ( 17.20831665107776587, 54.13393115100079456, -7.208316651077762316 ) ) ;
#79518=CARTESIAN_POINT ( 'NONE',  ( -2.266590686148945544, 11.38708216824730179, -7.082119434687050408 ) ) ;
#79521=CARTESIAN_POINT ( 'NONE',  ( 24.16423886937410614, 4.512082168247300906, -3.795296366450302550 ) ) ;
#79522=CARTESIAN_POINT ( 'NONE',  ( 6.204703633549690345, 27.84541550158063217, 14.16423886937410082 ) ) ;
#79525=CARTESIAN_POINT ( 'NONE',  ( 19.42250999205614548, 40.98035201082150536, -5.440088680355545492 ) ) ;
#79528=CARTESIAN_POINT ( 'NONE',  ( 12.63842701281683922, 19.55059781766745175, -9.846743663894590881 ) ) ;
#79529=CARTESIAN_POINT ( 'NONE',  ( 20.88017736071110164, 60.35535201082151957, 2.915334737309930979 ) ) ;
#79530=CARTESIAN_POINT ( 'NONE',  ( 14.92337183194729988, 9.342264484334119601, -8.527530157486177487 ) ) ;
#79531=CARTESIAN_POINT ( 'NONE',  ( 3.591859063236763294, 43.29030133659708923, -11.09922568453595026 ) ) ;
#79532=CARTESIAN_POINT ( 'NONE',  ( 10.00000000000000178, 32.25893115100078745, 9.846743663894594434 ) ) ;
#79533=CARTESIAN_POINT ( 'NONE',  ( -0.1023957841222422477, 25.13377557478296964, 6.340343622311917393 ) ) ;
#79534=CARTESIAN_POINT ( 'NONE',  ( 19.42250999205614193, 55.14701867748817676, 5.440088680355555262 ) ) ;
#79535=CARTESIAN_POINT ( 'NONE',  ( -2.816281873526471635, 28.91530133659708213, -3.434112377981056508 ) ) ;
#79538=CARTESIAN_POINT ( 'NONE',  ( 5.076628168052703671, 26.84226448433411960, 8.527530157486179263 ) ) ;
#79539=CARTESIAN_POINT ( 'NONE',  ( -0.3689425029237881626, 12.42874883491396609, 10.36894250292379027 ) ) ;
#79541=CARTESIAN_POINT ( 'NONE',  ( 10.00000000000000178, 39.31368534415484106, 10.88017736071110342 ) ) ;
#79542=CARTESIAN_POINT ( 'NONE',  ( 12.91533473730992121, 59.52201867748816966, 10.88017736071110164 ) ) ;
#79543=CARTESIAN_POINT ( 'NONE',  ( 2.917880565312948704, 37.63708216824731068, 12.26659068614894643 ) ) ;
#79544=CARTESIAN_POINT ( 'NONE',  ( 0.1532563361054100626, 55.80059781766745175, -2.638427012816831230 ) ) ;
#79545=CARTESIAN_POINT ( 'NONE',  ( 1.472469842513823179, 11.42559781766745175, 4.923371831947296329 ) ) ;
#79546=CARTESIAN_POINT ( 'NONE',  ( 5.500000000000000000, 61.50000000000000711, 6.000000000000000000 ) ) ;
#79548=CARTESIAN_POINT ( 'NONE',  ( 17.96484262340118221, 44.93868534415483396, 7.964842623401181321 ) ) ;
#79549=CARTESIAN_POINT ( 'NONE',  ( 19.72487221294570858, 70.00000000000000000, 6.000000000000000000 ) ) ;
#79551=CARTESIAN_POINT ( 'NONE',  ( 22.81628187352647785, 16.41530133659708923, 3.434112377981063169 ) ) ;
#79552=CARTESIAN_POINT ( 'NONE',  ( 16.40814093676323893, 15.79030133659708746, 11.09922568453595026 ) ) ;
#79553=CARTESIAN_POINT ( 'NONE',  ( 18.52753015748618282, 53.92559781766745175, -4.923371831947291888 ) ) ;
#79555=CARTESIAN_POINT ( 'NONE',  ( -0.8801773607110991993, 67.85535201082151957, -2.915334737309923874 ) ) ;
#79556=CARTESIAN_POINT ( 'NONE',  ( 18.17884179759833074, 33.66688879859532335, -6.499999999999955591 ) ) ;
#79561=CARTESIAN_POINT ( 'NONE',  ( 4.559911319644449179, 63.89701867748817676, 9.422509992056141925 ) ) ;
#79562=CARTESIAN_POINT ( 'NONE',  ( 7.084665262690076126, 57.02201867748817676, -10.88017736071110164 ) ) ;
#79566=CARTESIAN_POINT ( 'NONE',  ( 10.00000000000000000, 24.75893115100078745, -9.846743663894594434 ) ) ;
#79567=CARTESIAN_POINT ( 'NONE',  ( 4.559911319644449179, 18.89701867748817321, 9.422509992056141925 ) ) ;
#79568=CARTESIAN_POINT ( 'NONE',  ( 10.00000000000000178, 67.25893115100079456, 9.846743663894594434 ) ) ;
#79569=CARTESIAN_POINT ( 'NONE',  ( 10.00000000000000000, 41.81368534415484106, -10.88017736071110342 ) ) ;
#79571=CARTESIAN_POINT ( 'NONE',  ( 21.09922568453595559, 42.04030133659708213, -6.408140936763230044 ) ) ;
#79573=CARTESIAN_POINT ( 'NONE',  ( 15.44008868035555260, 44.73035201082151247, 9.422509992056143702 ) ) ;
#79574=CARTESIAN_POINT ( 'NONE',  ( 22.81628187352648496, 21.83196800326374643, -3.434112377981050290 ) ) ;
#79575=CARTESIAN_POINT ( 'NONE',  ( 4.559911319644449179, 28.89701867748817321, 9.422509992056141925 ) ) ;
#79576=CARTESIAN_POINT ( 'NONE',  ( 6.204703633549690345, 55.76208216824730357, -14.16423886937410259 ) ) ;
#79577=CARTESIAN_POINT ( 'NONE',  ( 0.1532563361054083140, 46.00893115100079456, 1.131784320476157264E-15 ) ) ;
#79578=CARTESIAN_POINT ( 'NONE',  ( 12.63842701281683034, 7.467264484334118713, 9.846743663894596210 ) ) ;
#79579=CARTESIAN_POINT ( 'NONE',  ( 12.91533473730993009, 46.60535201082150536, -10.88017736071109987 ) ) ;
#79580=B_SPLINE_CURVE_WITH_KNOTS ( 'NONE', 3,
 ( #51716, #11736, #82200, #44193 ),
 .UNSPECIFIED., .F., .F.,
 ( 4, 4 ),
 ( 8.673617379884035472E-19, 0.001036303429213374615 ),
 .UNSPECIFIED. ) ;
#79582=CARTESIAN_POINT ( 'NONE',  ( -0.3689425029237898834, 21.17874883491396432, -10.36894250292378850 ) ) ;
#79583=B_SPLINE_CURVE_WITH_KNOTS ( 'NONE', 3,
 ( #8079, #38576, #85552, #31548 ),
 .UNSPECIFIED., .F., .F.,
 ( 4, 4 ),
 ( 0.000000000000000000, 0.001036303429213373964 ),
 .UNSPECIFIED. ) ;
#79585=CARTESIAN_POINT ( 'NONE',  ( 20.15039907845753220, 56.74884699246889141, 6.262539305110074395 ) ) ;
#79588=CARTESIAN_POINT ( 'NONE',  ( -4.164238869374099927, 42.01208216824728936, 3.795296366450308767 ) ) ;
#79589=CARTESIAN_POINT ( 'NONE',  ( -0.3689425029237898834, 46.17874883491397497, -10.36894250292378850 ) ) ;
#79590=CARTESIAN_POINT ( 'NONE',  ( 19.84674366389459266, 18.71726448433411960, -2.638427012816827677 ) ) ;
#79591=CARTESIAN_POINT ( 'NONE',  ( 13.43411237798106583, 17.66530133659708923, -12.81628187352647252 ) ) ;
#79593=DIRECTION ( 'NONE',  ( 0.000000000000000000, -1.000000000000000000, 0.000000000000000000 ) ) ;
#79594=CARTESIAN_POINT ( 'NONE',  ( 2.035157376598822676, 2.438685344154837953, -7.964842623401177768 ) ) ;
#79595=CARTESIAN_POINT ( 'NONE',  ( 21.09922568453595559, 27.04030133659708568, -6.408140936763230044 ) ) ;
#79596=CARTESIAN_POINT ( 'NONE',  ( -2.266590686148945544, 42.22041550158063217, 7.082119434687048631 ) ) ;
#79597=( LENGTH_UNIT ( ) NAMED_UNIT ( * ) SI_UNIT ( .MILLI., .METRE. ) );
#79601=CARTESIAN_POINT ( 'NONE',  ( 19.84674366389459266, 18.30059781766745175, 2.638427012816836559 ) ) ;
#79603=CARTESIAN_POINT ( 'NONE',  ( 15.44008868035555260, 4.730352010821505360, 9.422509992056143702 ) ) ;
#79604=CARTESIAN_POINT ( 'NONE',  ( 20.88017736071110164, 15.35535201082150358, 2.915334737309930979 ) ) ;
#79605=CARTESIAN_POINT ( 'NONE',  ( 19.84674366389459266, 48.30059781766745175, 2.638427012816836559 ) ) ;
#79606=CARTESIAN_POINT ( 'NONE',  ( 3.591859063236763294, 8.290301336597087456, -11.09922568453595026 ) ) ;
#79611=CARTESIAN_POINT ( 'NONE',  ( 22.81628187352647785, 16.41530133659708923, 3.434112377981063169 ) ) ;
#79613=CARTESIAN_POINT ( 'NONE',  ( 13.79529636645031943, 65.34541550158063217, -14.16423886937409904 ) ) ;
#79615=CARTESIAN_POINT ( 'NONE',  ( 22.26659068614895176, 54.72041550158063217, -7.082119434687042414 ) ) ;
#79616=ORIENTED_EDGE ( 'NONE', *, *, #5483, .F. ) ;
#79617=CARTESIAN_POINT ( 'NONE',  ( 7.084665262690076126, 29.10535201082150181, 10.88017736071109987 ) ) ;
#79618=CARTESIAN_POINT ( 'NONE',  ( 4.559911319644449179, 42.23035201082151247, -9.422509992056141925 ) ) ;
#79619=VECTOR ( 'NONE', #63947, 1000.000000000000000 ) ;
#79620=CARTESIAN_POINT ( 'NONE',  ( 0.5774900079438590739, 42.64701867748816966, -5.440088680355550821 ) ) ;
#79622=CARTESIAN_POINT ( 'NONE',  ( 17.96484262340118221, 41.18868534415484106, -7.964842623401177768 ) ) ;
#79626=CARTESIAN_POINT ( 'NONE',  ( 7.361572987183170547, 12.05059781766744997, 9.846743663894590881 ) ) ;
#79629=CARTESIAN_POINT ( 'NONE',  ( 2.791683348922240793, 41.63393115100078745, 7.208316651077764092 ) ) ;
#79630=CARTESIAN_POINT ( 'NONE',  ( 0.2751277870542967463, 0.000000000000000000, 6.500000000000000888 ) ) ;
#79631=CARTESIAN_POINT ( 'NONE',  ( 22.81628187352648496, 51.83196800326376064, -3.434112377981050290 ) ) ;
#79633=CARTESIAN_POINT ( 'NONE',  ( 0.2751277870542868098, 57.28217586085237656, -6.499999999999985789 ) ) ;
#79635=CARTESIAN_POINT ( 'NONE',  ( -45.04367043435856743, 105.4369522167675086, 5.288592931995918178 ) ) ;
#79636=CARTESIAN_POINT ( 'NONE',  ( 1.472469842513823179, 65.59226448433412315, -4.923371831947296329 ) ) ;
#79637=CARTESIAN_POINT ( 'NONE',  ( 13.79529636645031943, 60.34541550158063927, -14.16423886937409904 ) ) ;
#79639=ORIENTED_EDGE ( 'NONE', *, *, #46291, .T. ) ;
#79641=CARTESIAN_POINT ( 'NONE',  ( 19.84674366389459266, 33.71726448433410894, -2.638427012816827677 ) ) ;
#79643=CARTESIAN_POINT ( 'NONE',  ( 22.81628187352647785, 6.623634669930420493, 6.195893100308588602E-16 ) ) ;
#79644=CARTESIAN_POINT ( 'NONE',  ( -0.8801773607111008646, 68.27201867748817676, 2.915334737309923430 ) ) ;
#79647=CARTESIAN_POINT ( 'NONE',  ( 18.52753015748618282, 8.925597817667451750, -4.923371831947291888 ) ) ;
#79648=CARTESIAN_POINT ( 'NONE',  ( 7.361572987183169658, 64.96726448433412315, -9.846743663894592657 ) ) ;
#79649=FACE_OUTER_BOUND ( 'NONE', #44077, .T. ) ;
#79651=CARTESIAN_POINT ( 'NONE',  ( 0.5774900079438590739, 2.647018677488171434, -5.440088680355550821 ) ) ;
#79653=CARTESIAN_POINT ( 'NONE',  ( -0.8801773607111009756, 48.06368534415484817, 1.068504757029289695E-15 ) ) ;
#79654=CARTESIAN_POINT ( 'NONE',  ( 3.591859063236761518, 14.95696800326375531, 11.09922568453594849 ) ) ;
#79656=CARTESIAN_POINT ( 'NONE',  ( 10.00000000000000178, 4.313685344154837509, 10.88017736071110342 ) ) ;
#79657=B_SPLINE_CURVE_WITH_KNOTS ( 'NONE', 3,
 ( #959, #54911, #10415, #61431 ),
 .UNSPECIFIED., .F., .F.,
 ( 4, 4 ),
 ( -4.898238651910869251E-06, 0.0003854743236894886405 ),
 .UNSPECIFIED. ) ;
#79658=EDGE_CURVE ( 'NONE', #76576, #19224, #77346, .T. ) ;
#79660=CARTESIAN_POINT ( 'NONE',  ( 19.05914839598886346, 59.96693863883976405, 6.499999999999922728 ) ) ;
#79661=CARTESIAN_POINT ( 'NONE',  ( 10.00000000000000178, 47.25893115100078745, 9.846743663894594434 ) ) ;
#79662=CARTESIAN_POINT ( 'NONE',  ( 19.84674366389459266, 8.717264484334116048, -2.638427012816827677 ) ) ;
#79664=CARTESIAN_POINT ( 'NONE',  ( -1.099225684535947600, 23.70696800326375708, -6.408140936763238038 ) ) ;
#79666=CARTESIAN_POINT ( 'NONE',  ( -0.8801773607111009756, 23.06368534415484106, 1.068504757029289695E-15 ) ) ;
#79668=CARTESIAN_POINT ( 'NONE',  ( 20.36894250292379382, 38.67874883491396076, 10.36894250292379205 ) ) ;
#79669=CARTESIAN_POINT ( 'NONE',  ( 17.08211943468705840, 35.13708216824730357, -12.26659068614894466 ) ) ;
#79670=CARTESIAN_POINT ( 'NONE',  ( 20.88017736071110875, 5.772018677488170546, -2.915334737309920765 ) ) ;
#79671=CARTESIAN_POINT ( 'NONE',  ( 17.20831665107776587, 47.88393115100078745, 7.208316651077764980 ) ) ;
#79672=CARTESIAN_POINT ( 'NONE',  ( 10.00000000000000000, 42.87363466993042493, -12.81628187352647608 ) ) ;
#79673=CARTESIAN_POINT ( 'NONE',  ( 19.42250999205614548, 15.98035201082150714, -5.440088680355545492 ) ) ;
#79674=CARTESIAN_POINT ( 'NONE',  ( 12.63842701281683922, 39.55059781766744464, -9.846743663894590881 ) ) ;
#79675=CARTESIAN_POINT ( 'NONE',  ( 2.035157376598824452, 43.68868534415484106, 7.964842623401179544 ) ) ;
#79676=CARTESIAN_POINT ( 'NONE',  ( 0.6178305044545838731, -0.2513653300695798953, 9.382169495545420901 ) ) ;
#79677=CARTESIAN_POINT ( 'NONE',  ( 2.917880565312950480, 20.97041550158063217, -12.26659068614894821 ) ) ;
#79679=CARTESIAN_POINT ( 'NONE',  ( 5.076628168052703671, 26.84226448433411960, 8.527530157486179263 ) ) ;
#79680=CARTESIAN_POINT ( 'NONE',  ( 19.38216949554541202, 55.99863466993041072, 9.382169495545424454 ) ) ;
#79681=CARTESIAN_POINT ( 'NONE',  ( 17.20831665107776587, 52.88393115100078035, 7.208316651077764980 ) ) ;
#79685=CARTESIAN_POINT ( 'NONE',  ( 7.084665262690076126, 4.105352010821503583, 10.88017736071109987 ) ) ;
#79686=CARTESIAN_POINT ( 'NONE',  ( 19.42250999205614548, 60.98035201082151247, -5.440088680355545492 ) ) ;
#79687=CARTESIAN_POINT ( 'NONE',  ( 17.08211943468705840, 10.13708216824730179, -12.26659068614894466 ) ) ;
#79688=CARTESIAN_POINT ( 'NONE',  ( 4.559911319644449179, 63.89701867748817676, 9.422509992056141925 ) ) ;
#79689=CARTESIAN_POINT ( 'NONE',  ( 14.92337183194729988, 49.34226448433411605, -8.527530157486177487 ) ) ;
#79690=CARTESIAN_POINT ( 'NONE',  ( 19.42250999205614193, 35.14701867748816966, 5.440088680355555262 ) ) ;
#79691=CARTESIAN_POINT ( 'NONE',  ( 2.831191079880678085, 79.91181047996344944, -9.500000000000000000 ) ) ;
#79692=CARTESIAN_POINT ( 'NONE',  ( 19.42250999205614193, 25.14701867748817321, 5.440088680355555262 ) ) ;
#79696=AXIS2_PLACEMENT_3D ( 'NONE', #52692, #21216, #51718 ) ;
#79698=ORIENTED_EDGE ( 'NONE', *, *, #22584, .T. ) ;
#79700=CARTESIAN_POINT ( 'NONE',  ( 17.08211943468705130, 8.470415501580635720, 12.26659068614894998 ) ) ;
#79701=CARTESIAN_POINT ( 'NONE',  ( -2.266590686148945544, 12.22041550158063394, 7.082119434687048631 ) ) ;
#79702=CARTESIAN_POINT ( 'NONE',  ( 22.26659068614895176, 54.72041550158063217, -7.082119434687042414 ) ) ;
#79703=CARTESIAN_POINT ( 'NONE',  ( 10.00000000000000178, 52.25893115100078745, 9.846743663894594434 ) ) ;
#79704=CARTESIAN_POINT ( 'NONE',  ( 18.52753015748618282, 38.92559781766745175, -4.923371831947291888 ) ) ;
#79706=CARTESIAN_POINT ( 'NONE',  ( 10.00000000000000178, 34.31368534415484106, 10.88017736071110342 ) ) ;
#79707=CARTESIAN_POINT ( 'NONE',  ( 0.1532563361054100626, 65.80059781766745175, -2.638427012816831230 ) ) ;
#79709=CARTESIAN_POINT ( 'NONE',  ( 10.00000000000000000, 65.55374883491396076, -14.16423886937410082 ) ) ;
#79712=CARTESIAN_POINT ( 'NONE',  ( 15.44008868035555793, 66.39701867748817676, -9.422509992056140149 ) ) ;
#79713=CARTESIAN_POINT ( 'NONE',  ( 5.076628168052704559, 25.17559781766745175, -8.527530157486179263 ) ) ;
#79718=CARTESIAN_POINT ( 'NONE',  ( 5.076628168052703671, 21.84226448433411960, 8.527530157486179263 ) ) ;
#79720=CARTESIAN_POINT ( 'NONE',  ( 24.16423886937410614, 29.30374883491396787, 8.672049930838204340E-16 ) ) ;
#79721=CARTESIAN_POINT ( 'NONE',  ( 0.1532563361054100626, 30.80059781766744820, -2.638427012816831230 ) ) ;
#79722=CARTESIAN_POINT ( 'NONE',  ( -0.8801773607110991993, 57.85535201082149825, -2.915334737309923874 ) ) ;
#79723=VECTOR ( 'NONE', #64705, 1000.000000000000000 ) ;
#79725=CARTESIAN_POINT ( 'NONE',  ( 15.44008868035555260, 39.73035201082150536, 9.422509992056143702 ) ) ;
#79726=CARTESIAN_POINT ( 'NONE',  ( 12.63842701281683034, 47.46726448433412315, 9.846743663894596210 ) ) ;
#79730=CARTESIAN_POINT ( 'NONE',  ( 24.16423886937409904, 24.09541550158063927, 3.795296366450317205 ) ) ;
#79732=EDGE_CURVE ( 'NONE', #74723, #18712, #13141, .T. ) ;
#79733=VERTEX_POINT ( 'NONE', #61951 ) ;
#79734=CARTESIAN_POINT ( 'NONE',  ( 16.40814093676323893, 35.79030133659708923, 11.09922568453595026 ) ) ;
#79736=CARTESIAN_POINT ( 'NONE',  ( 17.20831665107776587, 19.13393115100078035, -7.208316651077762316 ) ) ;
#79737=CARTESIAN_POINT ( 'NONE',  ( -0.8801773607111009756, 3.063685344154837509, 1.068504757029289695E-15 ) ) ;
#79738=CARTESIAN_POINT ( 'NONE',  ( -1.099225684535947600, 58.70696800326375353, -6.408140936763238038 ) ) ;
#79740=CARTESIAN_POINT ( 'NONE',  ( 7.361572987183170547, 32.05059781766745175, 9.846743663894590881 ) ) ;
#79742=CARTESIAN_POINT ( 'NONE',  ( 0.5774900079438607392, 63.48035201082149825, 5.440088680355550821 ) ) ;
#79745=CARTESIAN_POINT ( 'NONE',  ( 19.72487221294570858, 61.86607318730076344, 6.500000000000000888 ) ) ;
#79747=CARTESIAN_POINT ( 'NONE',  ( 4.559911319644449179, 68.89701867748817676, 9.422509992056141925 ) ) ;
#79748=CARTESIAN_POINT ( 'NONE',  ( -2.816281873526473856, 24.33196800326375353, 3.434112377981055619 ) ) ;
#79750=CARTESIAN_POINT ( 'NONE',  ( 1.472469842513823179, 45.59226448433412315, -4.923371831947296329 ) ) ;
#79751=CARTESIAN_POINT ( 'NONE',  ( -1.099225684535947600, 63.70696800326376774, -6.408140936763238038 ) ) ;
#79752=CARTESIAN_POINT ( 'NONE',  ( 24.16423886937410614, 9.303748834913967869, 8.672049930838204340E-16 ) ) ;
#79753=CARTESIAN_POINT ( 'NONE',  ( 7.361572987183170547, 27.05059781766745175, 9.846743663894590881 ) ) ;
#79754=CARTESIAN_POINT ( 'NONE',  ( 16.40814093676323893, 35.79030133659708923, 11.09922568453595026 ) ) ;
#79756=CARTESIAN_POINT ( 'NONE',  ( 20.03932841506543028, 15.62161441960501485, -6.397827110478962354 ) ) ;
#79757=CARTESIAN_POINT ( 'NONE',  ( -0.8801773607110991993, 67.85535201082151957, -2.915334737309923874 ) ) ;
#79759=CARTESIAN_POINT ( 'NONE',  ( 14.49999999999999822, 11.00000000000000000, 6.000000000000000000 ) ) ;
#79760=CARTESIAN_POINT ( 'NONE',  ( 18.52753015748618282, 38.92559781766745175, -4.923371831947291888 ) ) ;
#79761=CARTESIAN_POINT ( 'NONE',  ( 0.5774900079438590739, 27.64701867748817676, -5.440088680355550821 ) ) ;
#79763=CARTESIAN_POINT ( 'NONE',  ( 10.00000000000000000, 27.87363466993042138, -12.81628187352647608 ) ) ;
#79764=CARTESIAN_POINT ( 'NONE',  ( 0.1532563361054082862, 21.21726448433412315, 2.638427012816831674 ) ) ;
#79766=CARTESIAN_POINT ( 'NONE',  ( 17.96484262340118221, 31.18868534415483751, -7.964842623401177768 ) ) ;
#79768=CARTESIAN_POINT ( 'NONE',  ( 4.559911319644449179, 63.89701867748817676, 9.422509992056141925 ) ) ;
#79769=CARTESIAN_POINT ( 'NONE',  ( 12.63842701281683034, 37.46726448433411605, 9.846743663894596210 ) ) ;
#79770=CARTESIAN_POINT ( 'NONE',  ( -0.8801773607111009756, 28.06368534415484106, 1.068504757029289695E-15 ) ) ;
#79771=CARTESIAN_POINT ( 'NONE',  ( -0.8801773607111008646, 48.27201867748816966, 2.915334737309923430 ) ) ;
#79772=AXIS2_PLACEMENT_3D ( 'NONE', #11423, #85458, #20413 ) ;
#79773=CARTESIAN_POINT ( 'NONE',  ( 19.42250999205614193, 15.14701867748817143, 5.440088680355555262 ) ) ;
#79774=CARTESIAN_POINT ( 'NONE',  ( 0.2751277870542911397, 40.30223176428831522, 6.499999999999992006 ) ) ;
#79775=CARTESIAN_POINT ( 'NONE',  ( 20.15039907845753220, 54.72266099184918886, 6.262539305110078836 ) ) ;
#79776=CARTESIAN_POINT ( 'NONE',  ( 14.92337183194729988, 49.34226448433411605, -8.527530157486177487 ) ) ;
#79777=CARTESIAN_POINT ( 'NONE',  ( -0.3689425029237898834, 56.17874883491396076, -10.36894250292378850 ) ) ;
#79781=CARTESIAN_POINT ( 'NONE',  ( 24.16423886937409904, 39.09541550158062506, 3.795296366450317205 ) ) ;
#79784=CARTESIAN_POINT ( 'NONE',  ( -0.8801773607111009756, 3.063685344154838397, 1.068504757029289695E-15 ) ) ;
#79785=CARTESIAN_POINT ( 'NONE',  ( 19.84674366389459266, 33.71726448433410894, -2.638427012816827677 ) ) ;
#79786=DIRECTION ( 'NONE',  ( -0.000000000000000000, 1.000000000000000000, -0.000000000000000000 ) ) ;
#79788=CARTESIAN_POINT ( 'NONE',  ( 7.084665262690076126, 62.02201867748816966, -10.88017736071110164 ) ) ;
#79790=CARTESIAN_POINT ( 'NONE',  ( 2.035157376598824452, 28.68868534415484106, 7.964842623401179544 ) ) ;
#79792=CARTESIAN_POINT ( 'NONE',  ( 13.43411237798106583, 57.66530133659708923, -12.81628187352647252 ) ) ;
#79793=CARTESIAN_POINT ( 'NONE',  ( 21.09922568453594849, 16.20696800326375353, 6.408140936763242479 ) ) ;
#79794=CARTESIAN_POINT ( 'NONE',  ( 10.00000000000000000, 19.75893115100078390, -9.846743663894594434 ) ) ;
#79796=SURFACE_STYLE_FILL_AREA ( #78817 ) ;
#79798=CARTESIAN_POINT ( 'NONE',  ( -4.164238869374098151, 66.59541550158060375, -3.795296366450310543 ) ) ;
#79799=CARTESIAN_POINT ( 'NONE',  ( 20.36894250292379382, 23.67874883491397142, 10.36894250292379205 ) ) ;
#79800=CARTESIAN_POINT ( 'NONE',  ( 12.91533473730993009, 26.60535201082150536, -10.88017736071109987 ) ) ;
#79801=CARTESIAN_POINT ( 'NONE',  ( 0.5774900079438607392, 53.48035201082151247, 5.440088680355550821 ) ) ;
#79804=CARTESIAN_POINT ( 'NONE',  ( 19.84674366389459266, 13.71726448433411782, -2.638427012816827677 ) ) ;
#79807=CARTESIAN_POINT ( 'NONE',  ( 2.791683348922240793, 26.63393115100078745, 7.208316651077764092 ) ) ;
#79808=CARTESIAN_POINT ( 'NONE',  ( 19.84674366389459621, 43.50893115100078745, 7.409399052514197653E-17 ) ) ;
#79809=CARTESIAN_POINT ( 'NONE',  ( 0.5774900079438607392, 23.48035201082150536, 5.440088680355550821 ) ) ;
#79810=CARTESIAN_POINT ( 'NONE',  ( 6.565887622018943937, 43.08196800326374643, -12.81628187352647608 ) ) ;
#79812=CARTESIAN_POINT ( 'NONE',  ( 5.076628168052703671, 1.842264484334118047, 8.527530157486179263 ) ) ;
#79813=CARTESIAN_POINT ( 'NONE',  ( 14.92337183194729988, 34.34226448433411605, -8.527530157486177487 ) ) ;
#79814=CARTESIAN_POINT ( 'NONE',  ( 22.26659068614894466, 58.88708216824729647, 7.082119434687054849 ) ) ;
#79815=CARTESIAN_POINT ( 'NONE',  ( 0.1532563361054083140, 26.00893115100078745, 1.131784320476157264E-15 ) ) ;
#79816=CARTESIAN_POINT ( 'NONE',  ( 0.2751277870542909731, 44.36607318730131055, -6.499999999999992006 ) ) ;
#79817=EDGE_CURVE ( 'NONE', #64436, #18416, #26177, .T. ) ;
#79819=CARTESIAN_POINT ( 'NONE',  ( 2.791683348922237240, 60.38393115100078745, -7.208316651077763204 ) ) ;
#79820=CARTESIAN_POINT ( 'NONE',  ( 13.79529636645030344, 13.26208216824729824, 14.16423886937410614 ) ) ;
#79821=CARTESIAN_POINT ( 'NONE',  ( -4.164238869374099927, 27.01208216824730357, 3.795296366450308767 ) ) ;
#79822=CARTESIAN_POINT ( 'NONE',  ( 14.92337183194729988, 34.34226448433411605, -8.527530157486177487 ) ) ;
#79823=CARTESIAN_POINT ( 'NONE',  ( 18.72515096720569616, 10.05509018479935968, 6.500000000000001776 ) ) ;
#79824=CARTESIAN_POINT ( 'NONE',  ( 12.91533473730992121, 29.52201867748817321, 10.88017736071110164 ) ) ;
#79825=CARTESIAN_POINT ( 'NONE',  ( 7.084665262690076126, 54.10535201082151247, 10.88017736071109987 ) ) ;
#79826=EDGE_LOOP ( 'NONE', ( #15684, #75526, #85945, #25747 ) ) ;
#79827=CARTESIAN_POINT ( 'NONE',  ( 10.00000000000000000, 47.87363466993042493, -12.81628187352647608 ) ) ;
#79828=CARTESIAN_POINT ( 'NONE',  ( 17.96484262340118221, 54.93868534415484106, 7.964842623401181321 ) ) ;
#79830=SURFACE_STYLE_USAGE ( .BOTH. , #18848 ) ;
#79831=CARTESIAN_POINT ( 'NONE',  ( 19.42250999205614548, 65.98035201082151957, -5.440088680355545492 ) ) ;
#79833=CARTESIAN_POINT ( 'NONE',  ( 4.559911319644449179, 68.89701867748817676, 9.422509992056141925 ) ) ;
#79835=LINE ( 'NONE', #72323, #979 ) ;
#79836=CARTESIAN_POINT ( 'NONE',  ( 2.035157376598822676, 2.438685344154838397, -7.964842623401177768 ) ) ;
#79837=CARTESIAN_POINT ( 'NONE',  ( 18.52753015748618282, 3.925597817667451306, -4.923371831947291888 ) ) ;
#79838=CARTESIAN_POINT ( 'NONE',  ( 13.79529636645030344, 13.26208216824729824, 14.16423886937410614 ) ) ;
#79839=CARTESIAN_POINT ( 'NONE',  ( 2.791683348922237240, 5.383931151000785675, -7.208316651077763204 ) ) ;
#79840=CARTESIAN_POINT ( 'NONE',  ( 15.44008868035555260, 29.73035201082150891, 9.422509992056143702 ) ) ;
#79841=CARTESIAN_POINT ( 'NONE',  ( 18.52753015748618282, 48.92559781766745886, -4.923371831947291888 ) ) ;
#79843=EDGE_CURVE ( 'NONE', #21583, #32106, #27886, .T. ) ;
#79845=CARTESIAN_POINT ( 'NONE',  ( 0.1532563361054083140, 46.00893115100079456, 1.131784320476157264E-15 ) ) ;
#79846=VERTEX_POINT ( 'NONE', #79431 ) ;
#79848=CARTESIAN_POINT ( 'NONE',  ( 7.084665262690076126, 54.10535201082151247, 10.88017736071109987 ) ) ;
#79849=CARTESIAN_POINT ( 'NONE',  ( 12.63842701281683034, 47.46726448433412315, 9.846743663894596210 ) ) ;
#79850=CARTESIAN_POINT ( 'NONE',  ( -2.816281873526473856, 29.33196800326376064, 3.434112377981055619 ) ) ;
#79851=CARTESIAN_POINT ( 'NONE',  ( -0.8801773607111008646, 13.27201867748817143, 2.915334737309923430 ) ) ;
#79853=CARTESIAN_POINT ( 'NONE',  ( 20.88017736071110875, 55.77201867748816966, -2.915334737309920765 ) ) ;
#79855=CARTESIAN_POINT ( 'NONE',  ( 7.084665262690076126, 9.105352010821503583, 10.88017736071109987 ) ) ;
#79857=CARTESIAN_POINT ( 'NONE',  ( 22.81628187352648496, 36.83196800326376064, -3.434112377981050290 ) ) ;
#79858=CARTESIAN_POINT ( 'NONE',  ( 2.035157376598822676, 32.43868534415483396, -7.964842623401177768 ) ) ;
#79859=LINE ( 'NONE', #94366, #73805 ) ;
#79861=CARTESIAN_POINT ( 'NONE',  ( 13.43411237798106583, 47.66530133659709634, -12.81628187352647252 ) ) ;
#79862=CARTESIAN_POINT ( 'NONE',  ( 17.96484262340118221, 39.93868534415484106, 7.964842623401181321 ) ) ;
#79864=CIRCLE ( 'NONE', #36778, 7.000000000000006217 ) ;
#79865=CARTESIAN_POINT ( 'NONE',  ( 2.791683348922237240, 65.38393115100078035, -7.208316651077763204 ) ) ;
#79866=CARTESIAN_POINT ( 'NONE',  ( 0.1532563361054083140, 16.00893115100078390, 1.131784320476157264E-15 ) ) ;
#79867=CARTESIAN_POINT ( 'NONE',  ( 12.63842701281683922, 49.55059781766744464, -9.846743663894590881 ) ) ;
#79868=CARTESIAN_POINT ( 'NONE',  ( 20.88017736071110519, 20.56368534415484106, 2.639326808657452039E-16 ) ) ;
#79869=CARTESIAN_POINT ( 'NONE',  ( -36.44000000000001194, 92.00000000000000000, 9.500000000000000000 ) ) ;
#79870=CARTESIAN_POINT ( 'NONE',  ( 0.1532563361054082862, 36.21726448433410894, 2.638427012816831674 ) ) ;
#79873=CARTESIAN_POINT ( 'NONE',  ( 12.63842701281683034, 22.46726448433411605, 9.846743663894596210 ) ) ;
#79874=CARTESIAN_POINT ( 'NONE',  ( 17.20831665107776587, 9.133931151000787452, -7.208316651077762316 ) ) ;
#79875=CARTESIAN_POINT ( 'NONE',  ( 0.2751277870542981341, 8.218334437839383000, 6.500000000000002665 ) ) ;
#79876=CARTESIAN_POINT ( 'NONE',  ( 12.63842701281683922, 54.55059781766745175, -9.846743663894590881 ) ) ;
#79878=CARTESIAN_POINT ( 'NONE',  ( 6.565887622018943937, 30.16530133659708568, 12.81628187352647430 ) ) ;
#79879=CARTESIAN_POINT ( 'NONE',  ( 0.1532563361054100626, 45.80059781766745886, -2.638427012816831230 ) ) ;
#79881=CARTESIAN_POINT ( 'NONE',  ( 2.917880565312948704, 62.63708216824730357, 12.26659068614894643 ) ) ;
#79882=CARTESIAN_POINT ( 'NONE',  ( 7.361572987183170547, 12.05059781766744997, 9.846743663894590881 ) ) ;
#79883=CARTESIAN_POINT ( 'NONE',  ( 20.00000000000141043, 85.78121477524163652, 5.248003389972544674 ) ) ;
#79884=CARTESIAN_POINT ( 'NONE',  ( 2.917880565312948704, 62.63708216824730357, 12.26659068614894643 ) ) ;
#79885=CARTESIAN_POINT ( 'NONE',  ( 19.84674366389459621, 63.50893115100078745, 7.409399052514197653E-17 ) ) ;
#79886=CARTESIAN_POINT ( 'NONE',  ( -4.164238869374099927, 67.01208216824728936, 3.795296366450308767 ) ) ;
#79887=CARTESIAN_POINT ( 'NONE',  ( -4.164238869374098151, 36.59541550158063217, -3.795296366450310543 ) ) ;
#79888=CARTESIAN_POINT ( 'NONE',  ( 24.16423886937410614, 34.51208216824731068, -3.795296366450302550 ) ) ;
#79890=CARTESIAN_POINT ( 'NONE',  ( -0.8801773607110990882, 27.85535201082150181, -2.915334737309924318 ) ) ;
#79891=CARTESIAN_POINT ( 'NONE',  ( 1.472469842513823179, 50.59226448433411605, -4.923371831947296329 ) ) ;
#79892=EDGE_LOOP ( 'NONE', ( #3652, #69912, #5477, #63475 ) ) ;
#79893=CARTESIAN_POINT ( 'NONE',  ( 19.42250999205614193, 55.14701867748817676, 5.440088680355555262 ) ) ;
#79896=CARTESIAN_POINT ( 'NONE',  ( 17.20831665107776587, 52.88393115100078035, 7.208316651077764980 ) ) ;
#79897=CARTESIAN_POINT ( 'NONE',  ( -2.816281873526473856, 64.33196800326376774, 3.434112377981055619 ) ) ;
#79898=CARTESIAN_POINT ( 'NONE',  ( 18.52753015748617571, 53.09226448433412315, 4.923371831947298993 ) ) ;
#79901=CARTESIAN_POINT ( 'NONE',  ( 20.36894250292379382, 28.67874883491396787, 10.36894250292379205 ) ) ;
#79902=CARTESIAN_POINT ( 'NONE',  ( 5.076628168052703671, 1.842264484334118047, 8.527530157486179263 ) ) ;
#79904=CARTESIAN_POINT ( 'NONE',  ( -0.8801773607110991993, 22.85535201082150181, -2.915334737309923874 ) ) ;
#79905=CARTESIAN_POINT ( 'NONE',  ( 3.591859063236761518, 19.95696800326375353, 11.09922568453594849 ) ) ;
#79906=CARTESIAN_POINT ( 'NONE',  ( 20.24186590665278018, 62.61633188102329228, -6.114288769123040090 ) ) ;
#79907=CARTESIAN_POINT ( 'NONE',  ( 10.00000000000000178, 12.25893115100078568, 9.846743663894594434 ) ) ;
#79909=EDGE_LOOP ( 'NONE', ( #32581, #69883, #39086, #82408 ) ) ;
#79911=CARTESIAN_POINT ( 'NONE',  ( 22.26659068614894466, 33.88708216824730357, 7.082119434687054849 ) ) ;
#79914=CARTESIAN_POINT ( 'NONE',  ( 2.035157376598824452, 3.688685344154837953, 7.964842623401179544 ) ) ;
#79916=CARTESIAN_POINT ( 'NONE',  ( 0.5774900079438607392, 33.48035201082150536, 5.440088680355550821 ) ) ;
#79917=CARTESIAN_POINT ( 'NONE',  ( 17.96484262340118221, 39.93868534415484106, 7.964842623401181321 ) ) ;
#79918=CARTESIAN_POINT ( 'NONE',  ( 19.38216949554541557, 17.24863466993041783, -9.382169495545420901 ) ) ;
#79919=CARTESIAN_POINT ( 'NONE',  ( 0.1532563361054100626, 65.80059781766745175, -2.638427012816831230 ) ) ;
#79920=CARTESIAN_POINT ( 'NONE',  ( 0.2751277870542967463, 70.00000000000000000, 6.000000000000000000 ) ) ;
#79921=CARTESIAN_POINT ( 'NONE',  ( 7.361572987183170547, 12.05059781766744997, 9.846743663894590881 ) ) ;
#79924=CARTESIAN_POINT ( 'NONE',  ( 18.28836319691943046, 49.34492782695771496, 6.500000000000079936 ) ) ;
#79925=CARTESIAN_POINT ( 'NONE',  ( 12.91533473730992121, 49.52201867748817676, 10.88017736071110164 ) ) ;
#79927=CARTESIAN_POINT ( 'NONE',  ( 16.40814093676323893, 0.7903013365970867898, 11.09922568453595026 ) ) ;
#79928=CARTESIAN_POINT ( 'NONE',  ( -0.8801773607111009756, 63.06368534415484106, 1.068504757029289695E-15 ) ) ;
#79930=CARTESIAN_POINT ( 'NONE',  ( 0.1532563361054100626, 30.80059781766744820, -2.638427012816831230 ) ) ;
#79931=CARTESIAN_POINT ( 'NONE',  ( 6.565887622018943937, 33.08196800326374643, -12.81628187352647608 ) ) ;
#79932=CARTESIAN_POINT ( 'NONE',  ( 2.791683348922240793, 1.633931151000784565, 7.208316651077764092 ) ) ;
#79937=CARTESIAN_POINT ( 'NONE',  ( 10.00000000000000178, 9.313685344154839285, 10.88017736071110342 ) ) ;
#79938=CARTESIAN_POINT ( 'NONE',  ( 19.38216949554541557, 62.24863466993041072, -9.382169495545420901 ) ) ;
#79939=CARTESIAN_POINT ( 'NONE',  ( -4.164238869374099927, 22.01208216824730357, 3.795296366450308767 ) ) ;
#79940=CARTESIAN_POINT ( 'NONE',  ( 14.92337183194729633, 32.67559781766745175, 8.527530157486181039 ) ) ;
#79941=CARTESIAN_POINT ( 'NONE',  ( 0.5774900079438590739, 22.64701867748817321, -5.440088680355550821 ) ) ;
#79943=CARTESIAN_POINT ( 'NONE',  ( 17.96484262340118221, 9.938685344154839285, 7.964842623401181321 ) ) ;
#79947=CARTESIAN_POINT ( 'NONE',  ( 7.084665262690076126, 7.022018677488169658, -10.88017736071110164 ) ) ;
#79948=CARTESIAN_POINT ( 'NONE',  ( 15.44008868035555260, 24.73035201082150891, 9.422509992056143702 ) ) ;
#79949=CARTESIAN_POINT ( 'NONE',  ( 20.15039907845753575, 32.62777174578613426, -6.262539305110076171 ) ) ;
#79951=CARTESIAN_POINT ( 'NONE',  ( 20.15039907845753220, 27.62777174578613071, -6.262539305110077947 ) ) ;
#79952=CARTESIAN_POINT ( 'NONE',  ( 20.88017736071110164, 25.35535201082150891, 2.915334737309930979 ) ) ;
#79953=CARTESIAN_POINT ( 'NONE',  ( 18.52753015748618282, 58.92559781766745886, -4.923371831947291888 ) ) ;
#79955=FACE_OUTER_BOUND ( 'NONE', #87863, .T. ) ;
#79956=CARTESIAN_POINT ( 'NONE',  ( 21.09922568453595559, 47.04030133659708923, -6.408140936763230044 ) ) ;
#79958=CARTESIAN_POINT ( 'NONE',  ( 13.79529636645030344, 28.26208216824729647, 14.16423886937410614 ) ) ;
#79959=CARTESIAN_POINT ( 'NONE',  ( -0.8801773607110991993, 37.85535201082151247, -2.915334737309923874 ) ) ;
#79960=CARTESIAN_POINT ( 'NONE',  ( 12.91533473730992121, 19.52201867748816611, 10.88017736071110164 ) ) ;
#79961=CARTESIAN_POINT ( 'NONE',  ( 0.1532563361054082862, 61.21726448433412315, 2.638427012816831674 ) ) ;
#79963=CARTESIAN_POINT ( 'NONE',  ( 0.1532563361054100626, 55.80059781766745175, -2.638427012816831230 ) ) ;
#79965=CARTESIAN_POINT ( 'NONE',  ( 0.1532563361054083140, 6.008931151000784787, 1.131784320476157264E-15 ) ) ;
#79968=CARTESIAN_POINT ( 'NONE',  ( 15.44008868035555260, 9.730352010821505360, 9.422509992056143702 ) ) ;
#79969=CARTESIAN_POINT ( 'NONE',  ( 19.84674366389459621, 8.508931151000785675, 7.409399052514197653E-17 ) ) ;
#79970=CARTESIAN_POINT ( 'NONE',  ( -2.816281873526473856, 4.331968003263754419, 3.434112377981055619 ) ) ;
#79971=CARTESIAN_POINT ( 'NONE',  ( 12.91533473730993009, 61.60535201082150536, -10.88017736071109987 ) ) ;
#79972=CARTESIAN_POINT ( 'NONE',  ( 7.084665262690076126, 24.10535201082150181, 10.88017736071109987 ) ) ;
#79973=CARTESIAN_POINT ( 'NONE',  ( -1.099225684535947600, 39.54030133659708923, 6.408140936763237150 ) ) ;
#79974=CARTESIAN_POINT ( 'NONE',  ( -4.164238869374099927, 32.01208216824730357, 3.795296366450308767 ) ) ;
#79978=CARTESIAN_POINT ( 'NONE',  ( 3.591859063236763294, 58.29030133659708923, -11.09922568453595026 ) ) ;
#79980=CARTESIAN_POINT ( 'NONE',  ( 22.81628187352648496, 6.831968003263753531, -3.434112377981050290 ) ) ;
#79981=PRESENTATION_STYLE_ASSIGNMENT (( #65956 ) ) ;
#79982=CARTESIAN_POINT ( 'NONE',  ( 15.44008868035555793, 36.39701867748816966, -9.422509992056140149 ) ) ;
#79984=CARTESIAN_POINT ( 'NONE',  ( 5.076628168052703671, 61.84226448433412315, 8.527530157486179263 ) ) ;
#79986=CARTESIAN_POINT ( 'NONE',  ( 17.20831665107776587, 7.883931151000784787, 7.208316651077764980 ) ) ;
#79987=CARTESIAN_POINT ( 'NONE',  ( -0.2418659066527703017, 64.26028685723176181, -6.114288769123047196 ) ) ;
#79988=CARTESIAN_POINT ( 'NONE',  ( 0.1532563361054083140, 11.00893115100078568, 1.131784320476157264E-15 ) ) ;
#79989=CARTESIAN_POINT ( 'NONE',  ( 1.472469842513823179, 20.59226448433411960, -4.923371831947296329 ) ) ;
#79990=CARTESIAN_POINT ( 'NONE',  ( 1.472469842513823179, 11.42559781766745175, 4.923371831947296329 ) ) ;
#79991=CARTESIAN_POINT ( 'NONE',  ( 17.96484262340118221, 51.18868534415483396, -7.964842623401177768 ) ) ;
#79992=CARTESIAN_POINT ( 'NONE',  ( -0.8801773607111009756, 38.06368534415484106, 1.068504757029289695E-15 ) ) ;
#79993=CARTESIAN_POINT ( 'NONE',  ( 15.44008868035555260, 59.73035201082151247, 9.422509992056143702 ) ) ;
#79994=CARTESIAN_POINT ( 'NONE',  ( 19.84674366389459266, 13.30059781766745353, 2.638427012816836559 ) ) ;
#79996=CARTESIAN_POINT ( 'NONE',  ( 5.076628168052704559, 60.17559781766745175, -8.527530157486179263 ) ) ;
#79998=FILL_AREA_STYLE_COLOUR ( '', #80920 ) ;
#79999=CARTESIAN_POINT ( 'NONE',  ( 13.79529636645030344, 23.26208216824730002, 14.16423886937410614 ) ) ;
#80001=CARTESIAN_POINT ( 'NONE',  ( 10.00000000000000000, 10.55374883491396787, -14.16423886937410082 ) ) ;
#80002=CARTESIAN_POINT ( 'NONE',  ( 20.36894250292379382, 28.67874883491396787, 10.36894250292379205 ) ) ;
#80003=EDGE_CURVE ( 'NONE', #71011, #14567, #16965, .T. ) ;
#80005=CARTESIAN_POINT ( 'NONE',  ( 20.88017736071110519, 35.56368534415484106, 2.639326808657452039E-16 ) ) ;
#80008=CARTESIAN_POINT ( 'NONE',  ( 7.361572987183169658, 19.96726448433411960, -9.846743663894592657 ) ) ;
#80009=CARTESIAN_POINT ( 'NONE',  ( 12.91533473730992121, 59.52201867748816966, 10.88017736071110164 ) ) ;
#80010=CARTESIAN_POINT ( 'NONE',  ( 2.791683348922240793, 11.63393115100078568, 7.208316651077764092 ) ) ;
#80011=VECTOR ( 'NONE', #52849, 1000.000000000000000 ) ;
#80013=CARTESIAN_POINT ( 'NONE',  ( 13.43411237798106583, 47.66530133659709634, -12.81628187352647252 ) ) ;
#80014=CARTESIAN_POINT ( 'NONE',  ( 14.92337183194729988, 34.34226448433411605, -8.527530157486177487 ) ) ;
#80017=CARTESIAN_POINT ( 'NONE',  ( 21.09922568453595559, 32.04030133659708923, -6.408140936763230044 ) ) ;
#80019=CARTESIAN_POINT ( 'NONE',  ( 0.1532563361054083140, 31.00893115100078390, 1.131784320476157264E-15 ) ) ;
#80020=MECHANICAL_DESIGN_GEOMETRIC_PRESENTATION_REPRESENTATION('',(#30484),#76809);
#80021=CARTESIAN_POINT ( 'NONE',  ( -4.164238869374099927, 7.012082168247302683, 3.795296366450308767 ) ) ;
#80024=CARTESIAN_POINT ( 'NONE',  ( 20.88017736071110875, 50.77201867748817676, -2.915334737309920765 ) ) ;
#80025=CARTESIAN_POINT ( 'NONE',  ( 17.96484262340118221, 56.18868534415484817, -7.964842623401177768 ) ) ;
#80026=CARTESIAN_POINT ( 'NONE',  ( -4.164238869374098151, 41.59541550158061796, -3.795296366450310543 ) ) ;
#80027=CARTESIAN_POINT ( 'NONE',  ( 19.84674366389459266, 58.71726448433411605, -2.638427012816827677 ) ) ;
#80028=CARTESIAN_POINT ( 'NONE',  ( 5.076628168052703671, 16.84226448433411960, 8.527530157486179263 ) ) ;
#80029=CARTESIAN_POINT ( 'NONE',  ( -2.816281873526473856, 64.12363466993042493, 9.499525473075851096E-16 ) ) ;
#80030=CARTESIAN_POINT ( 'NONE',  ( 0.5774900079438607392, 43.48035201082151247, 5.440088680355550821 ) ) ;
#80031=CARTESIAN_POINT ( 'NONE',  ( 0.2751277870543045734, 27.28217586085238011, -6.500000000000012434 ) ) ;
#80032=CARTESIAN_POINT ( 'NONE',  ( 22.81628187352647785, 26.62363466993042138, 6.195893100308588602E-16 ) ) ;
#80033=CARTESIAN_POINT ( 'NONE',  ( 5.076628168052703671, 56.84226448433412315, 8.527530157486179263 ) ) ;
#80035=CARTESIAN_POINT ( 'NONE',  ( 19.42250999205614548, 5.980352010821504471, -5.440088680355545492 ) ) ;
#80036=CARTESIAN_POINT ( 'NONE',  ( -0.1503990784575359729, 13.10158574516642105, 6.262539305110062848 ) ) ;
#80037=CARTESIAN_POINT ( 'NONE',  ( 15.44008868035555260, 9.730352010821505360, 9.422509992056143702 ) ) ;
#80039=CARTESIAN_POINT ( 'NONE',  ( 1.472469842513823179, 0.5922644843341181575, -4.923371831947296329 ) ) ;
#80041=CARTESIAN_POINT ( 'NONE',  ( 12.91533473730993009, 66.60535201082150536, -10.88017736071109987 ) ) ;
#80044=CARTESIAN_POINT ( 'NONE',  ( 2.791683348922240793, 41.63393115100078745, 7.208316651077764092 ) ) ;
#80045=CARTESIAN_POINT ( 'NONE',  ( 7.084665262690076126, 24.10535201082150181, 10.88017736071109987 ) ) ;
#80046=ADVANCED_FACE ( 'NONE', ( #63908 ), #26581, .T. ) ;
#80047=CARTESIAN_POINT ( 'NONE',  ( 2.791683348922240793, 66.63393115100079456, 7.208316651077764092 ) ) ;
#80048=CARTESIAN_POINT ( 'NONE',  ( 7.084665262690076126, 34.10535201082151247, 10.88017736071109987 ) ) ;
#80052=CARTESIAN_POINT ( 'NONE',  ( 22.81628187352648496, 41.83196800326375353, -3.434112377981050290 ) ) ;
#80054=CARTESIAN_POINT ( 'NONE',  ( -0.8801773607111008646, 48.27201867748816966, 2.915334737309923430 ) ) ;
#80055=CARTESIAN_POINT ( 'NONE',  ( 16.40814093676323893, 20.79030133659708923, 11.09922568453595026 ) ) ;
#80058=CARTESIAN_POINT ( 'NONE',  ( 7.084665262690076126, 29.10535201082150181, 10.88017736071109987 ) ) ;
#80059=CARTESIAN_POINT ( 'NONE',  ( 0.5774900079438590739, 2.647018677488171434, -5.440088680355550821 ) ) ;
#80060=CARTESIAN_POINT ( 'NONE',  ( 5.076628168052704559, 45.17559781766745175, -8.527530157486179263 ) ) ;
#80061=CARTESIAN_POINT ( 'NONE',  ( 7.084665262690076126, 69.10535201082151957, 10.88017736071109987 ) ) ;
#80062=CARTESIAN_POINT ( 'NONE',  ( 7.084665262690076126, 59.10535201082150536, 10.88017736071109987 ) ) ;
#80064=CARTESIAN_POINT ( 'NONE',  ( 13.79529636645031943, 35.34541550158063927, -14.16423886937409904 ) ) ;
#80069=CARTESIAN_POINT ( 'NONE',  ( 10.00000000000000178, 43.05374883491397497, 14.16423886937410082 ) ) ;
#80070=CARTESIAN_POINT ( 'NONE',  ( 2.917880565312950480, 55.97041550158063217, -12.26659068614894821 ) ) ;
#80071=CARTESIAN_POINT ( 'NONE',  ( 2.791683348922237240, 20.38393115100078745, -7.208316651077763204 ) ) ;
#80072=CARTESIAN_POINT ( 'NONE',  ( 6.565887622018943937, 18.08196800326375708, -12.81628187352647608 ) ) ;
#80075=CARTESIAN_POINT ( 'NONE',  ( 7.084665262690076126, 2.022018677488170990, -10.88017736071110164 ) ) ;
#80076=CARTESIAN_POINT ( 'NONE',  ( 10.00000000000000178, 35.37363466993042493, 12.81628187352647608 ) ) ;
#80077=CARTESIAN_POINT ( 'NONE',  ( -0.3689425029237898834, 41.17874883491397497, -10.36894250292378850 ) ) ;
#80079=CARTESIAN_POINT ( 'NONE',  ( 19.84674366389459621, 8.508931151000785675, 7.409399052514197653E-17 ) ) ;
#80080=EDGE_CURVE ( 'NONE', #71943, #32664, #32922, .T. ) ;
#80082=ORIENTED_EDGE ( 'NONE', *, *, #1701, .F. ) ;
#80083=( NAMED_UNIT ( * ) PLANE_ANGLE_UNIT ( ) SI_UNIT ( $, .RADIAN. ) );
#80084=CARTESIAN_POINT ( 'NONE',  ( 7.361572987183169658, 19.96726448433411960, -9.846743663894592657 ) ) ;
#80087=CARTESIAN_POINT ( 'NONE',  ( 15.44008868035555793, 6.397018677488171434, -9.422509992056140149 ) ) ;
#80088=CARTESIAN_POINT ( 'NONE',  ( 2.035157376598824452, 23.68868534415484461, 7.964842623401179544 ) ) ;
#80089=CARTESIAN_POINT ( 'NONE',  ( 17.20831665107776587, 44.13393115100078745, -7.208316651077762316 ) ) ;
#80090=CARTESIAN_POINT ( 'NONE',  ( 16.40814093676324603, 2.456968003263753531, -11.09922568453594671 ) ) ;
#80092=CARTESIAN_POINT ( 'NONE',  ( 18.52753015748617571, 43.09226448433412315, 4.923371831947298993 ) ) ;
#80093=( GEOMETRIC_REPRESENTATION_CONTEXT ( 3 ) GLOBAL_UNCERTAINTY_ASSIGNED_CONTEXT ( ( #29447 ) ) GLOBAL_UNIT_ASSIGNED_CONTEXT ( ( #97388, #88885, #4420 ) ) REPRESENTATION_CONTEXT ( 'NONE', 'WORKASPACE' ) );
#80094=CARTESIAN_POINT ( 'NONE',  ( 0.6178305044545838731, 14.74863466993041783, 9.382169495545420901 ) ) ;
#80095=VERTEX_POINT ( 'NONE', #71905 ) ;
#80096=CARTESIAN_POINT ( 'NONE',  ( 17.08211943468705130, 58.47041550158063927, 12.26659068614894998 ) ) ;
#80098=CARTESIAN_POINT ( 'NONE',  ( -4.164238869374099927, 62.01208216824728936, 3.795296366450308767 ) ) ;
#80100=CARTESIAN_POINT ( 'NONE',  ( 0.5774900079438590739, 37.64701867748817676, -5.440088680355550821 ) ) ;
#80101=CARTESIAN_POINT ( 'NONE',  ( 17.96484262340118221, 46.18868534415484106, -7.964842623401177768 ) ) ;
#80102=CARTESIAN_POINT ( 'NONE',  ( 15.44008868035555793, 56.39701867748817676, -9.422509992056140149 ) ) ;
#80104=CARTESIAN_POINT ( 'NONE',  ( 12.91533473730992121, 44.52201867748816966, 10.88017736071110164 ) ) ;
#80107=CARTESIAN_POINT ( 'NONE',  ( 5.076628168052703671, 16.84226448433411960, 8.527530157486179263 ) ) ;
#80110=CARTESIAN_POINT ( 'NONE',  ( 14.92337183194729633, 42.67559781766745886, 8.527530157486181039 ) ) ;
#80111=CARTESIAN_POINT ( 'NONE',  ( 17.39651004071838969, 54.08210964143329846, -6.500000000000027534 ) ) ;
#80112=CARTESIAN_POINT ( 'NONE',  ( 10.00000000000000178, 60.37363466993041783, 12.81628187352647608 ) ) ;
#80113=AXIS2_PLACEMENT_3D ( 'NONE', #10858, #55868, #77864 ) ;
#80115=CARTESIAN_POINT ( 'NONE',  ( 6.000000000000000000, 60.50000000000000711, 6.000000000000000000 ) ) ;
#80117=CARTESIAN_POINT ( 'NONE',  ( 7.361572987183170547, 62.05059781766745886, 9.846743663894590881 ) ) ;
#80118=CARTESIAN_POINT ( 'NONE',  ( 14.92337183194729633, 27.67559781766745530, 8.527530157486181039 ) ) ;
#80119=CARTESIAN_POINT ( 'NONE',  ( 20.36894250292379738, 59.92874883491397497, -10.36894250292379027 ) ) ;
#80124=CARTESIAN_POINT ( 'NONE',  ( 12.63842701281683034, 32.46726448433412315, 9.846743663894596210 ) ) ;
#80125=CARTESIAN_POINT ( 'NONE',  ( 21.09922568453595559, 12.04030133659708746, -6.408140936763230044 ) ) ;
#80126=CARTESIAN_POINT ( 'NONE',  ( 10.00000000000000000, -0.2410688489992152128, -9.846743663894594434 ) ) ;
#80129=CARTESIAN_POINT ( 'NONE',  ( 18.52753015748617571, 13.09226448433411960, 4.923371831947298993 ) ) ;
#80130=CARTESIAN_POINT ( 'NONE',  ( 10.00000000000000178, 52.25893115100078745, 9.846743663894594434 ) ) ;
#80131=CARTESIAN_POINT ( 'NONE',  ( 20.88017736071110875, 20.77201867748816966, -2.915334737309920321 ) ) ;
#80134=CARTESIAN_POINT ( 'NONE',  ( 6.204703633549690345, 60.76208216824730357, -14.16423886937410259 ) ) ;
#80135=CARTESIAN_POINT ( 'NONE',  ( 17.20831665107776587, 7.883931151000784787, 7.208316651077764980 ) ) ;
#80136=CARTESIAN_POINT ( 'NONE',  ( 10.00000000000000178, 39.31368534415484106, 10.88017736071110342 ) ) ;
#80137=CARTESIAN_POINT ( 'NONE',  ( 19.38216949554541202, 20.99863466993042138, 9.382169495545424454 ) ) ;
#80139=CARTESIAN_POINT ( 'NONE',  ( 19.42250999205614548, 5.980352010821504471, -5.440088680355545492 ) ) ;
#80141=CARTESIAN_POINT ( 'NONE',  ( 19.90229974777923161, 0.3225724651664713671, -6.500000000000000000 ) ) ;
#80142=CARTESIAN_POINT ( 'NONE',  ( 12.63842701281683034, 52.46726448433413026, 9.846743663894596210 ) ) ;
#80143=CARTESIAN_POINT ( 'NONE',  ( 5.076628168052704559, 15.17559781766745175, -8.527530157486179263 ) ) ;
#80145=CARTESIAN_POINT ( 'NONE',  ( 22.81628187352647785, 26.41530133659708923, 3.434112377981063169 ) ) ;
#80147=CARTESIAN_POINT ( 'NONE',  ( 12.91533473730993009, 31.60535201082150891, -10.88017736071109987 ) ) ;
#80149=CARTESIAN_POINT ( 'NONE',  ( 22.26659068614895176, 44.72041550158063927, -7.082119434687042414 ) ) ;
#80150=CARTESIAN_POINT ( 'NONE',  ( -0.3689425029237898834, 36.17874883491396787, -10.36894250292378850 ) ) ;
#80151=CARTESIAN_POINT ( 'NONE',  ( 19.84674366389459266, 43.71726448433410894, -2.638427012816827677 ) ) ;
#80152=CARTESIAN_POINT ( 'NONE',  ( 3.591859063236761518, 34.95696800326375353, 11.09922568453594849 ) ) ;
#80153=CARTESIAN_POINT ( 'NONE',  ( -0.8801773607111009756, 23.06368534415484106, 1.068504757029289695E-15 ) ) ;
#80155=CARTESIAN_POINT ( 'NONE',  ( 0.1532563361054100626, 45.80059781766745886, -2.638427012816831230 ) ) ;
#80156=EDGE_CURVE ( 'NONE', #97107, #63207, #33400, .T. ) ;
#80157=CARTESIAN_POINT ( 'NONE',  ( 20.88017736071110164, 40.35535201082150536, 2.915334737309930979 ) ) ;
#80158=CARTESIAN_POINT ( 'NONE',  ( 21.09922568453595559, 2.040301336597086568, -6.408140936763230044 ) ) ;
#80159=CARTESIAN_POINT ( 'NONE',  ( 17.08211943468705130, 38.47041550158063217, 12.26659068614894998 ) ) ;
#80161=UNCERTAINTY_MEASURE_WITH_UNIT (LENGTH_MEASURE( 1.000000000000000082E-05 ), #16742, 'distance_accuracy_value', 'NONE');
#80163=CARTESIAN_POINT ( 'NONE',  ( 0.1532563361054100626, 30.80059781766744820, -2.638427012816831230 ) ) ;
#80164=( NAMED_UNIT ( * ) PLANE_ANGLE_UNIT ( ) SI_UNIT ( $, .RADIAN. ) );
#80165=CARTESIAN_POINT ( 'NONE',  ( 2.791683348922237240, 65.38393115100078035, -7.208316651077763204 ) ) ;
#80167=CARTESIAN_POINT ( 'NONE',  ( 20.15039907845753575, 6.748846992468889638, 6.262539305110063736 ) ) ;
#80169=CARTESIAN_POINT ( 'NONE',  ( 17.96484262340118221, 19.93868534415484106, 7.964842623401181321 ) ) ;
#80170=CARTESIAN_POINT ( 'NONE',  ( 10.00000000000000178, 59.31368534415484106, 10.88017736071110342 ) ) ;
#80171=CARTESIAN_POINT ( 'NONE',  ( 13.79529636645031943, 30.34541550158063927, -14.16423886937409904 ) ) ;
#80172=CARTESIAN_POINT ( 'NONE',  ( 7.361572987183170547, 7.050597817667451750, 9.846743663894590881 ) ) ;
#80173=CARTESIAN_POINT ( 'NONE',  ( 12.63842701281683034, 52.46726448433413026, 9.846743663894596210 ) ) ;
#80174=CARTESIAN_POINT ( 'NONE',  ( -0.8801773607111008646, 28.27201867748817321, 2.915334737309923430 ) ) ;
#80176=CARTESIAN_POINT ( 'NONE',  ( -44.43653038997627647, 105.4840905893460672, -5.301235023115286715 ) ) ;
#80177=EDGE_LOOP ( 'NONE', ( #10711, #17827, #96514, #15188 ) ) ;
#80181=CARTESIAN_POINT ( 'NONE',  ( 2.917880565312950480, 10.97041550158063572, -12.26659068614894821 ) ) ;
#80182=CARTESIAN_POINT ( 'NONE',  ( -2.266590686148945544, 6.387082168247300906, -7.082119434687050408 ) ) ;
#80183=CARTESIAN_POINT ( 'NONE',  ( 13.79529636645031943, 60.34541550158063927, -14.16423886937409904 ) ) ;
#80184=CARTESIAN_POINT ( 'NONE',  ( 14.92337183194729633, 52.67559781766745175, 8.527530157486181039 ) ) ;
#80185=CARTESIAN_POINT ( 'NONE',  ( 14.92337183194729988, 39.34226448433412315, -8.527530157486177487 ) ) ;
#80186=CARTESIAN_POINT ( 'NONE',  ( -0.3289641300568005855, 0.1049760357941743188, 5.963430220938281678 ) ) ;
#80187=CARTESIAN_POINT ( 'NONE',  ( 7.084665262690076126, 27.02201867748817676, -10.88017736071110164 ) ) ;
#80188=CARTESIAN_POINT ( 'NONE',  ( -2.816281873526471635, -1.084698663402913210, -3.434112377981056508 ) ) ;
#80189=PRESENTATION_STYLE_ASSIGNMENT (( #96196 ) ) ;
#80190=CARTESIAN_POINT ( 'NONE',  ( -0.3689425029237898834, 56.17874883491396076, -10.36894250292378850 ) ) ;
#80191=STYLED_ITEM ( 'NONE', ( #22335 ), #23940 ) ;
#80192=CARTESIAN_POINT ( 'NONE',  ( 7.084665262690076126, 2.022018677488171434, -10.88017736071110164 ) ) ;
#80193=CARTESIAN_POINT ( 'NONE',  ( 19.84674366389459266, 38.30059781766745175, 2.638427012816836559 ) ) ;
#80197=LINE ( 'NONE', #36180, #17465 ) ;
#80199=ORIENTED_EDGE ( 'NONE', *, *, #77014, .T. ) ;
#80203=CARTESIAN_POINT ( 'NONE',  ( 12.63842701281683034, 27.46726448433411250, 9.846743663894596210 ) ) ;
#80204=ORIENTED_EDGE ( 'NONE', *, *, #21324, .F. ) ;
#80205=CARTESIAN_POINT ( 'NONE',  ( 2.917880565312948704, 32.63708216824730357, 12.26659068614894643 ) ) ;
#80206=CARTESIAN_POINT ( 'NONE',  ( 17.20831665107776587, 39.13393115100079456, -7.208316651077762316 ) ) ;
#80207=CARTESIAN_POINT ( 'NONE',  ( 12.91533473730993009, 51.60535201082149825, -10.88017736071109987 ) ) ;
#80209=CARTESIAN_POINT ( 'NONE',  ( 20.10384461210893292, 36.74302437010793909, 6.337995344473749348 ) ) ;
#80210=VECTOR ( 'NONE', #2251, 1000.000000000000000 ) ;
#80211=CARTESIAN_POINT ( 'NONE',  ( 19.42250999205614193, 50.14701867748817676, 5.440088680355555262 ) ) ;
#80214=CARTESIAN_POINT ( 'NONE',  ( 2.035157376598824452, 48.68868534415483396, 7.964842623401179544 ) ) ;
#80215=CARTESIAN_POINT ( 'NONE',  ( 6.204703633549690345, 17.84541550158063217, 14.16423886937410082 ) ) ;
#80218=( GEOMETRIC_REPRESENTATION_CONTEXT ( 3 ) GLOBAL_UNCERTAINTY_ASSIGNED_CONTEXT ( ( #62202 ) ) GLOBAL_UNIT_ASSIGNED_CONTEXT ( ( #21044, #4572, #89534 ) ) REPRESENTATION_CONTEXT ( 'NONE', 'WORKASPACE' ) );
#80219=CARTESIAN_POINT ( 'NONE',  ( 19.38216949554541202, 45.99863466993041072, 9.382169495545424454 ) ) ;
#80220=CARTESIAN_POINT ( 'NONE',  ( 12.91533473730992121, 19.52201867748816611, 10.88017736071110164 ) ) ;
#80221=CARTESIAN_POINT ( 'NONE',  ( 0.1532563361054083140, 26.00893115100078745, 1.131784320476157264E-15 ) ) ;
#80222=CARTESIAN_POINT ( 'NONE',  ( 7.084665262690076126, 7.022018677488169658, -10.88017736071110164 ) ) ;
#80223=CARTESIAN_POINT ( 'NONE',  ( 22.81628187352647785, 56.62363466993042493, 6.195893100308588602E-16 ) ) ;
#80224=CARTESIAN_POINT ( 'NONE',  ( -46.46849503609894327, 103.9079590269318629, -5.994465626570869787 ) ) ;
#80225=CARTESIAN_POINT ( 'NONE',  ( 18.52753015748618282, 33.92559781766745886, -4.923371831947291888 ) ) ;
#80226=CARTESIAN_POINT ( 'NONE',  ( 20.32896413005680003, 21.77164270246084143, 5.963430220938287007 ) ) ;
#80227=ORIENTED_EDGE ( 'NONE', *, *, #54391, .F. ) ;
#80229=DIRECTION ( 'NONE',  ( 0.000000000000000000, -1.000000000000000000, -0.000000000000000000 ) ) ;
#80231=CARTESIAN_POINT ( 'NONE',  ( -1.926860441876564023, 44.68830936912751639, 1.004413902775740781E-15 ) ) ;
#80232=CARTESIAN_POINT ( 'NONE',  ( 12.63842701281683034, 7.467264484334118713, 9.846743663894596210 ) ) ;
#80233=CARTESIAN_POINT ( 'NONE',  ( 0.6178305044545818747, 28.49863466993041783, -9.382169495545419124 ) ) ;
#80235=CARTESIAN_POINT ( 'NONE',  ( 7.361572987183169658, 39.96726448433411605, -9.846743663894592657 ) ) ;
#80237=CARTESIAN_POINT ( 'NONE',  ( 2.917880565312948704, 27.63708216824730357, 12.26659068614894643 ) ) ;
#80238=CARTESIAN_POINT ( 'NONE',  ( 17.20831665107776587, 34.13393115100078745, -7.208316651077762316 ) ) ;
#80239=CARTESIAN_POINT ( 'NONE',  ( 10.00000000000000000, 37.87363466993041783, -12.81628187352647608 ) ) ;
#80240=B_SPLINE_CURVE_WITH_KNOTS ( 'NONE', 3,
 ( #80031, #73014, #90971, #51508, #45986, #97526 ),
 .UNSPECIFIED., .F., .F.,
 ( 4, 2, 4 ),
 ( 0.000000000000000000, 0.0002565770811490962521, 0.0005131541622981925042 ),
 .UNSPECIFIED. ) ;
#80243=CARTESIAN_POINT ( 'NONE',  ( 0.5774900079438607392, 68.48035201082150536, 5.440088680355550821 ) ) ;
#80244=CARTESIAN_POINT ( 'NONE',  ( 10.00000000000000178, 10.37363466993041961, 12.81628187352647608 ) ) ;
#80245=CARTESIAN_POINT ( 'NONE',  ( 18.72515096720609051, 25.05509018479941119, 6.499999999999470646 ) ) ;
#80246=CARTESIAN_POINT ( 'NONE',  ( 17.20831665107776587, 39.13393115100079456, -7.208316651077762316 ) ) ;
#80247=CARTESIAN_POINT ( 'NONE',  ( 2.035157376598824452, 23.68868534415484461, 7.964842623401179544 ) ) ;
#80249=CARTESIAN_POINT ( 'NONE',  ( 6.565887622018943937, 25.16530133659708213, 12.81628187352647430 ) ) ;
#80251=CARTESIAN_POINT ( 'NONE',  ( 2.791683348922237240, 35.38393115100079456, -7.208316651077763204 ) ) ;
#80252=PRODUCT_CONTEXT ( 'NONE', #21905, 'mechanical' ) ;
#80253=LINE ( 'NONE', #5258, #61413 ) ;
#80254=CARTESIAN_POINT ( 'NONE',  ( 2.035157376598822676, 27.43868534415483396, -7.964842623401177768 ) ) ;
#80255=VERTEX_POINT ( 'NONE', #4902 ) ;
#80258=CARTESIAN_POINT ( 'NONE',  ( 0.5774900079438590739, 7.647018677488171434, -5.440088680355550821 ) ) ;
#80259=CARTESIAN_POINT ( 'NONE',  ( 0.1532563361054082862, 61.21726448433412315, 2.638427012816831674 ) ) ;
#80260=CARTESIAN_POINT ( 'NONE',  ( 12.91533473730993009, 26.60535201082150536, -10.88017736071109987 ) ) ;
#80262=AXIS2_PLACEMENT_3D ( 'NONE', #22442, #68923, #52914 ) ;
#80263=CARTESIAN_POINT ( 'NONE',  ( 2.035157376598824452, 48.68868534415483396, 7.964842623401179544 ) ) ;
#80264=CARTESIAN_POINT ( 'NONE',  ( 17.96484262340118221, 24.93868534415484461, 7.964842623401181321 ) ) ;
#80266=DIRECTION ( 'NONE',  ( 0.000000000000000000, -1.000000000000000000, 0.000000000000000000 ) ) ;
#80268=DIRECTION ( 'NONE',  ( -1.000000000000000000, 0.000000000000000000, 0.000000000000000000 ) ) ;
#80270=CARTESIAN_POINT ( 'NONE',  ( 14.92337183194729633, 47.67559781766745175, 8.527530157486181039 ) ) ;
#80271=CARTESIAN_POINT ( 'NONE',  ( -4.164238869374099039, 46.80374883491397497, 8.674139862899312516E-16 ) ) ;
#80272=CARTESIAN_POINT ( 'NONE',  ( 0.8719017118913388043, 123.9374316453451286, 5.000000000000000000 ) ) ;
#80273=CARTESIAN_POINT ( 'NONE',  ( 24.16423886937410614, 14.30374883491396787, 8.672049930838204340E-16 ) ) ;
#80274=CARTESIAN_POINT ( 'NONE',  ( 17.08211943468705130, 38.47041550158063217, 12.26659068614894998 ) ) ;
#80275=CARTESIAN_POINT ( 'NONE',  ( 0.6178305044545838731, 4.748634669930420493, 9.382169495545420901 ) ) ;
#80277=ORIENTED_EDGE ( 'NONE', *, *, #91447, .F. ) ;
#80279=CARTESIAN_POINT ( 'NONE',  ( -2.266590686148945544, 61.38708216824730357, -7.082119434687050408 ) ) ;
#80280=CARTESIAN_POINT ( 'NONE',  ( 1.472469842513823179, 30.59226448433411960, -4.923371831947296329 ) ) ;
#80282=CARTESIAN_POINT ( 'NONE',  ( 20.88017736071110875, 55.77201867748816966, -2.915334737309920765 ) ) ;
#80283=CARTESIAN_POINT ( 'NONE',  ( 0.000000000000000000, 81.99999999999992895, 5.000000000000000000 ) ) ;
#80284=CARTESIAN_POINT ( 'NONE',  ( 20.88017736071110875, 25.77201867748816966, -2.915334737309920765 ) ) ;
#80285=CARTESIAN_POINT ( 'NONE',  ( 10.00000000000000000, 62.87363466993042493, -12.81628187352647608 ) ) ;
#80286=CARTESIAN_POINT ( 'NONE',  ( 16.40814093676323893, 25.79030133659708923, 11.09922568453595026 ) ) ;
#80287=CARTESIAN_POINT ( 'NONE',  ( 5.076628168052704559, 25.17559781766745175, -8.527530157486179263 ) ) ;
#80291=CARTESIAN_POINT ( 'NONE',  ( 17.08211943468705130, 63.47041550158063927, 12.26659068614894998 ) ) ;
#80293=CARTESIAN_POINT ( 'NONE',  ( 13.79529636645031943, 25.34541550158063572, -14.16423886937409904 ) ) ;
#80294=CARTESIAN_POINT ( 'NONE',  ( 15.44008868035555793, 31.39701867748817676, -9.422509992056140149 ) ) ;
#80295=CARTESIAN_POINT ( 'NONE',  ( 10.00000000000000178, 44.31368534415484106, 10.88017736071110342 ) ) ;
#80297=CARTESIAN_POINT ( 'NONE',  ( 19.84674366389459266, 48.30059781766745175, 2.638427012816836559 ) ) ;
#80298=CARTESIAN_POINT ( 'NONE',  ( 2.791683348922240793, 11.63393115100078568, 7.208316651077764092 ) ) ;
#80301=CARTESIAN_POINT ( 'NONE',  ( 10.00000000000000178, 27.25893115100078390, 9.846743663894594434 ) ) ;
#80302=CARTESIAN_POINT ( 'NONE',  ( 1.472469842513823179, 56.42559781766745886, 4.923371831947296329 ) ) ;
#80305=CARTESIAN_POINT ( 'NONE',  ( -2.816281873526473856, 49.33196800326374643, 3.434112377981055619 ) ) ;
#80307=CARTESIAN_POINT ( 'NONE',  ( 2.035157376598824452, 68.68868534415484817, 7.964842623401179544 ) ) ;
#80308=CARTESIAN_POINT ( 'NONE',  ( 1.472469842513823179, 31.42559781766745530, 4.923371831947296329 ) ) ;
#80309=CARTESIAN_POINT ( 'NONE',  ( 10.00000000000000178, 53.05374883491396787, 14.16423886937410082 ) ) ;
#80310=CARTESIAN_POINT ( 'NONE',  ( 1.472469842513823179, 25.59226448433412315, -4.923371831947296329 ) ) ;
#80312=CARTESIAN_POINT ( 'NONE',  ( 0.1532563361054083140, 61.00893115100078745, 1.131784320476157264E-15 ) ) ;
#80313=CARTESIAN_POINT ( 'NONE',  ( 13.79529636645030344, 23.26208216824730002, 14.16423886937410614 ) ) ;
#80314=CARTESIAN_POINT ( 'NONE',  ( -4.164238869374099039, 36.80374883491396787, 8.674139862899312516E-16 ) ) ;
#80315=CARTESIAN_POINT ( 'NONE',  ( 0.1532563361054082862, 46.21726448433411605, 2.638427012816831674 ) ) ;
#80316=CARTESIAN_POINT ( 'NONE',  ( 20.15039907845753575, 12.62777174578613071, -6.262539305110077059 ) ) ;
#80317=CARTESIAN_POINT ( 'NONE',  ( 12.91533473730992121, 24.52201867748816966, 10.88017736071110164 ) ) ;
#80318=CARTESIAN_POINT ( 'NONE',  ( 7.084665262690076126, 64.10535201082150536, 10.88017736071109987 ) ) ;
#80319=CARTESIAN_POINT ( 'NONE',  ( 18.72515096720579209, 51.07228050351030646, -6.499999999999869438 ) ) ;
#80321=CARTESIAN_POINT ( 'NONE',  ( 19.38216949554541202, 50.99863466993042493, 9.382169495545424454 ) ) ;
#80322=CARTESIAN_POINT ( 'NONE',  ( 2.035157376598824452, 58.68868534415482685, 7.964842623401179544 ) ) ;
#80323=EDGE_LOOP ( 'NONE', ( #92907, #72841, #84363, #2273 ) ) ;
#80327=CARTESIAN_POINT ( 'NONE',  ( -0.8801773607111008646, 58.27201867748816966, 2.915334737309923430 ) ) ;
#80330=CARTESIAN_POINT ( 'NONE',  ( 17.96484262340118221, 59.93868534415484106, 7.964842623401181321 ) ) ;
#80331=CARTESIAN_POINT ( 'NONE',  ( 10.00000000000000000, 16.81368534415483751, -10.88017736071110342 ) ) ;
#80333=CARTESIAN_POINT ( 'NONE',  ( 20.15039907845753930, 0.07447313448805115144, 6.262539305110068177 ) ) ;
#80334=CARTESIAN_POINT ( 'NONE',  ( 19.42250999205614193, 10.14701867748816966, 5.440088680355555262 ) ) ;
#80335=CARTESIAN_POINT ( 'NONE',  ( 19.84674366389459621, 8.508931151000785675, 7.409399052514197653E-17 ) ) ;
#80336=CARTESIAN_POINT ( 'NONE',  ( 17.08211943468705130, 18.47041550158063572, 12.26659068614894998 ) ) ;
#80339=CARTESIAN_POINT ( 'NONE',  ( -0.8801773607110991993, 22.85535201082150181, -2.915334737309923874 ) ) ;
#80340=CARTESIAN_POINT ( 'NONE',  ( 19.84674366389459266, 63.71726448433412315, -2.638427012816827677 ) ) ;
#80342=CARTESIAN_POINT ( 'NONE',  ( 3.591859063236763294, -1.709698663402913210, -11.09922568453595026 ) ) ;
#80344=DIRECTION ( 'NONE',  ( 0.000000000000000000, -1.000000000000000000, 0.000000000000000000 ) ) ;
#80346=CARTESIAN_POINT ( 'NONE',  ( 2.035157376598822676, 52.43868534415483396, -7.964842623401177768 ) ) ;
#80347=CARTESIAN_POINT ( 'NONE',  ( 12.63842701281683922, 49.55059781766744464, -9.846743663894590881 ) ) ;
#80348=CARTESIAN_POINT ( 'NONE',  ( 22.81628187352647785, 41.62363466993042493, 6.195893100308588602E-16 ) ) ;
#80349=CARTESIAN_POINT ( 'NONE',  ( 7.084665262690076126, 2.022018677488170990, -10.88017736071110164 ) ) ;
#80351=CARTESIAN_POINT ( 'NONE',  ( 10.00000000000000000, 56.81368534415484106, -10.88017736071110342 ) ) ;
#80352=CARTESIAN_POINT ( 'NONE',  ( -0.8801773607111008646, 3.272018677488171434, 2.915334737309923430 ) ) ;
#80353=CARTESIAN_POINT ( 'NONE',  ( 22.81628187352647785, 36.62363466993041783, 6.195893100308588602E-16 ) ) ;
#80354=CARTESIAN_POINT ( 'NONE',  ( 7.084665262690076126, 27.02201867748817676, -10.88017736071110164 ) ) ;
#80357=CARTESIAN_POINT ( 'NONE',  ( 0.6178305044545818747, 48.49863466993042493, -9.382169495545419124 ) ) ;
#80358=CARTESIAN_POINT ( 'NONE',  ( 0.5774900079438607392, 33.48035201082150536, 5.440088680355550821 ) ) ;
#80359=CARTESIAN_POINT ( 'NONE',  ( 14.92337183194729633, 62.67559781766745886, 8.527530157486181039 ) ) ;
#80360=ORIENTED_EDGE ( 'NONE', *, *, #85898, .F. ) ;
#80363=CARTESIAN_POINT ( 'NONE',  ( 0.1532563361054083140, 66.00893115100079456, 1.131784320476157264E-15 ) ) ;
#80365=CARTESIAN_POINT ( 'NONE',  ( 19.84674366389459266, 53.71726448433411605, -2.638427012816827677 ) ) ;
#80366=CARTESIAN_POINT ( 'NONE',  ( 4.559911319644449179, 23.89701867748817321, 9.422509992056141925 ) ) ;
#80371=CARTESIAN_POINT ( 'NONE',  ( 14.92337183194729633, 42.67559781766745886, 8.527530157486181039 ) ) ;
#80372=CARTESIAN_POINT ( 'NONE',  ( 19.84674366389459266, 3.300597817667451750, 2.638427012816836559 ) ) ;
#80373=CARTESIAN_POINT ( 'NONE',  ( 17.39651004071890128, 29.08210964143323096, -6.499999999999448441 ) ) ;
#80374=ADVANCED_FACE ( 'NONE', ( #72390 ), #84121, .T. ) ;
#80375=CARTESIAN_POINT ( 'NONE',  ( 1.472469842513823179, 61.42559781766745175, 4.923371831947296329 ) ) ;
#80376=ORIENTED_EDGE ( 'NONE', *, *, #94068, .T. ) ;
#80378=CARTESIAN_POINT ( 'NONE',  ( 10.00000000000000000, 37.87363466993041783, -12.81628187352647608 ) ) ;
#80379=CARTESIAN_POINT ( 'NONE',  ( 10.00000000000000178, 47.25893115100078745, 9.846743663894594434 ) ) ;
#80381=CARTESIAN_POINT ( 'NONE',  ( 20.36894250292379738, 64.92874883491397497, -10.36894250292379027 ) ) ;
#80382=EDGE_CURVE ( 'NONE', #54853, #45554, #97915, .T. ) ;
#80383=CARTESIAN_POINT ( 'NONE',  ( 12.63842701281683034, 37.46726448433411605, 9.846743663894596210 ) ) ;
#80385=CARTESIAN_POINT ( 'NONE',  ( -2.266590686148945544, 57.22041550158063217, 7.082119434687048631 ) ) ;
#80387=CARTESIAN_POINT ( 'NONE',  ( 4.559911319644449179, 2.230352010821504916, -9.422509992056141925 ) ) ;
#80388=CARTESIAN_POINT ( 'NONE',  ( 10.00000000000000000, 30.55374883491397142, -14.16423886937410082 ) ) ;
#80389=CARTESIAN_POINT ( 'NONE',  ( 20.36894250292379738, 44.92874883491396787, -10.36894250292379027 ) ) ;
#80391=CARTESIAN_POINT ( 'NONE',  ( 17.20831665107776587, 17.88393115100078745, 7.208316651077764980 ) ) ;
#80394=CARTESIAN_POINT ( 'NONE',  ( -2.816281873526473856, -0.8763653300695799508, 9.499525473075851096E-16 ) ) ;
#80395=ORIENTED_EDGE ( 'NONE', *, *, #57910, .F. ) ;
#80396=CARTESIAN_POINT ( 'NONE',  ( 4.559911319644449179, 52.23035201082151247, -9.422509992056141925 ) ) ;
#80397=CARTESIAN_POINT ( 'NONE',  ( 0.8952175423694606060, 18.52576239577081196, 5.990408912944278796 ) ) ;
#80399=CARTESIAN_POINT ( 'NONE',  ( 5.076628168052703671, 51.84226448433412315, 8.527530157486179263 ) ) ;
#80401=ORIENTED_EDGE ( 'NONE', *, *, #91159, .T. ) ;
#80404=CARTESIAN_POINT ( 'NONE',  ( -2.266590686148945544, 26.38708216824730357, -7.082119434687050408 ) ) ;
#80405=CARTESIAN_POINT ( 'NONE',  ( 0.6076426042653101378, 37.37576471608601736, -6.499999999999992006 ) ) ;
#80408=CARTESIAN_POINT ( 'NONE',  ( 4.559911319644449179, 13.89701867748817321, 9.422509992056141925 ) ) ;
#80409=AXIS2_PLACEMENT_3D ( 'NONE', #57604, #43590, #88594 ) ;
#80410=CARTESIAN_POINT ( 'NONE',  ( 0.6178305044545838731, 19.74863466993042138, 9.382169495545420901 ) ) ;
#80411=CARTESIAN_POINT ( 'NONE',  ( 21.92686044187656691, 62.18830936912750218, 4.562052436263911564E-16 ) ) ;
#80412=CARTESIAN_POINT ( 'NONE',  ( 0.1532563361054100626, 15.80059781766745353, -2.638427012816831230 ) ) ;
#80413=CARTESIAN_POINT ( 'NONE',  ( 13.43411237798106583, 52.66530133659708213, -12.81628187352647252 ) ) ;
#80415=ADVANCED_FACE ( 'NONE', ( #62332 ), #70850, .F. ) ;
#80416=( GEOMETRIC_REPRESENTATION_CONTEXT ( 3 ) GLOBAL_UNCERTAINTY_ASSIGNED_CONTEXT ( ( #81474 ) ) GLOBAL_UNIT_ASSIGNED_CONTEXT ( ( #65515, #13012, #43509 ) ) REPRESENTATION_CONTEXT ( 'NONE', 'WORKASPACE' ) );
#80418=CARTESIAN_POINT ( 'NONE',  ( -0.3689425029237881626, 32.42874883491395366, 10.36894250292379027 ) ) ;
#80421=CARTESIAN_POINT ( 'NONE',  ( 15.44008868035555793, 6.397018677488171434, -9.422509992056140149 ) ) ;
#80424=CARTESIAN_POINT ( 'NONE',  ( 20.88017736071110875, 35.77201867748816966, -2.915334737309920765 ) ) ;
#80425=CARTESIAN_POINT ( 'NONE',  ( 20.88017736071110875, 50.77201867748817676, -2.915334737309920765 ) ) ;
#80426=CARTESIAN_POINT ( 'NONE',  ( 10.00000000000000000, 12.87363466993042138, -12.81628187352647608 ) ) ;
#80428=CARTESIAN_POINT ( 'NONE',  ( 0.8952175423694350709, 3.525762395770809743, 5.990408912944235276 ) ) ;
#80429=CARTESIAN_POINT ( 'NONE',  ( 2.791683348922240793, 6.633931151000785675, 7.208316651077764092 ) ) ;
#80430=CARTESIAN_POINT ( 'NONE',  ( 15.44008868035555793, 41.39701867748817676, -9.422509992056140149 ) ) ;
#80432=CARTESIAN_POINT ( 'NONE',  ( 0.6178305044545838731, -0.2513653300695798953, 9.382169495545420901 ) ) ;
#80433=CARTESIAN_POINT ( 'NONE',  ( 19.42250999205614548, 60.98035201082151247, -5.440088680355545492 ) ) ;
#80434=CARTESIAN_POINT ( 'NONE',  ( 14.92337183194729988, 19.34226448433411960, -8.527530157486177487 ) ) ;
#80435=CARTESIAN_POINT ( 'NONE',  ( 19.38216949554541202, 50.99863466993042493, 9.382169495545424454 ) ) ;
#80436=CARTESIAN_POINT ( 'NONE',  ( 19.84674366389459266, 3.300597817667451750, 2.638427012816836559 ) ) ;
#80437=ORIENTED_EDGE ( 'NONE', *, *, #5113, .F. ) ;
#80439=CARTESIAN_POINT ( 'NONE',  ( 0.6081133539230469953, 28.33703382326400444, 6.499999999999966249 ) ) ;
#80440=CARTESIAN_POINT ( 'NONE',  ( 12.91533473730993009, 26.60535201082150536, -10.88017736071109987 ) ) ;
#80441=DIRECTION ( 'NONE',  ( -1.000000000000000000, 0.000000000000000000, 0.000000000000000000 ) ) ;
#80442=CARTESIAN_POINT ( 'NONE',  ( 24.16423886937409904, 24.09541550158063927, 3.795296366450317205 ) ) ;
#80443=CARTESIAN_POINT ( 'NONE',  ( 1.472469842513823179, 36.42559781766745175, 4.923371831947296329 ) ) ;
#80444=CARTESIAN_POINT ( 'NONE',  ( 20.88017736071110519, 15.56368534415483751, 2.639326808657452039E-16 ) ) ;
#80445=CARTESIAN_POINT ( 'NONE',  ( 2.917880565312950480, 65.97041550158063217, -12.26659068614894821 ) ) ;
#80446=VERTEX_POINT ( 'NONE', #1871 ) ;
#80447=CARTESIAN_POINT ( 'NONE',  ( 10.00000000000000000, 11.81368534415483751, -10.88017736071110342 ) ) ;
#80449=CARTESIAN_POINT ( 'NONE',  ( 19.42250999205614548, 30.98035201082150536, -5.440088680355545492 ) ) ;
#80451=CARTESIAN_POINT ( 'NONE',  ( 10.00000000000000000, 31.81368534415483751, -10.88017736071110342 ) ) ;
#80452=ORIENTED_EDGE ( 'NONE', *, *, #34219, .T. ) ;
#80453=CARTESIAN_POINT ( 'NONE',  ( 0.1532563361054100626, 65.80059781766745175, -2.638427012816831230 ) ) ;
#80454=CARTESIAN_POINT ( 'NONE',  ( 7.084665262690076126, 27.02201867748817676, -10.88017736071110164 ) ) ;
#80456=CARTESIAN_POINT ( 'NONE',  ( 19.38216949554541557, 57.24863466993042493, -9.382169495545420901 ) ) ;
#80458=CARTESIAN_POINT ( 'NONE',  ( 24.16423886937410614, 29.51208216824729647, -3.795296366450302550 ) ) ;
#80459=CARTESIAN_POINT ( 'NONE',  ( 20.88017736071110519, 35.56368534415484106, 2.639326808657452039E-16 ) ) ;
#80460=CARTESIAN_POINT ( 'NONE',  ( 2.035157376598822676, 12.43868534415483751, -7.964842623401177768 ) ) ;
#80463=CARTESIAN_POINT ( 'NONE',  ( 14.92337183194729633, 47.67559781766745175, 8.527530157486181039 ) ) ;
#80464=CARTESIAN_POINT ( 'NONE',  ( 1.472469842513823179, 21.42559781766745175, 4.923371831947296329 ) ) ;
#80466=CARTESIAN_POINT ( 'NONE',  ( 15.44008868035555793, 16.39701867748817321, -9.422509992056140149 ) ) ;
#80467=CARTESIAN_POINT ( 'NONE',  ( 2.791683348922240793, 16.63393115100078745, 7.208316651077764092 ) ) ;
#80468=CARTESIAN_POINT ( 'NONE',  ( 10.00000000000000178, 10.37363466993041961, 12.81628187352647608 ) ) ;
#80469=CARTESIAN_POINT ( 'NONE',  ( -0.8801773607110991993, 57.85535201082149825, -2.915334737309923874 ) ) ;
#80470=CARTESIAN_POINT ( 'NONE',  ( 15.44008868035555793, 51.39701867748816966, -9.422509992056140149 ) ) ;
#80471=CARTESIAN_POINT ( 'NONE',  ( 17.96484262340118221, 16.18868534415483396, -7.964842623401177768 ) ) ;
#80472=CARTESIAN_POINT ( 'NONE',  ( 19.38216949554541557, 62.24863466993041072, -9.382169495545420901 ) ) ;
#80473=CARTESIAN_POINT ( 'NONE',  ( 6.204703633549690345, 30.76208216824730357, -14.16423886937410259 ) ) ;
#80474=FILL_AREA_STYLE ('',( #87963 ) ) ;
#80475=B_SPLINE_CURVE_WITH_KNOTS ( 'NONE', 3,
 ( #72073, #47608, #85611, #55609 ),
 .UNSPECIFIED., .F., .F.,
 ( 4, 4 ),
 ( 3.878959614448864246E-18, 0.002562518741975557991 ),
 .UNSPECIFIED. ) ;
#80477=CARTESIAN_POINT ( 'NONE',  ( 16.40814093676324603, 62.45696800326376064, -11.09922568453594671 ) ) ;
#80478=EDGE_LOOP ( 'NONE', ( #65836, #43448, #28114, #83628 ) ) ;
#80479=CARTESIAN_POINT ( 'NONE',  ( 0.1532563361054083140, 66.00893115100079456, 1.131784320476157264E-15 ) ) ;
#80480=CARTESIAN_POINT ( 'NONE',  ( 19.72487221294571569, 20.71833443783938122, -6.499999999999990230 ) ) ;
#80481=CARTESIAN_POINT ( 'NONE',  ( 7.084665262690076126, 32.02201867748816966, -10.88017736071110164 ) ) ;
#80482=CARTESIAN_POINT ( 'NONE',  ( 5.076628168052703671, 66.84226448433412315, 8.527530157486179263 ) ) ;
#80485=CARTESIAN_POINT ( 'NONE',  ( 2.791683348922240793, 16.63393115100078745, 7.208316651077764092 ) ) ;
#80487=CARTESIAN_POINT ( 'NONE',  ( 7.361572987183169658, 9.967264484334119601, -9.846743663894592657 ) ) ;
#80488=CARTESIAN_POINT ( 'NONE',  ( 0.1532563361054100626, 25.80059781766744820, -2.638427012816831230 ) ) ;
#80490=CARTESIAN_POINT ( 'NONE',  ( 7.361572987183169658, 14.96726448433411960, -9.846743663894592657 ) ) ;
#80491=CARTESIAN_POINT ( 'NONE',  ( 5.076628168052704559, 0.1755978176674514724, -8.527530157486179263 ) ) ;
#80492=CARTESIAN_POINT ( 'NONE',  ( 2.035157376598822676, 52.43868534415483396, -7.964842623401177768 ) ) ;
#80494=CARTESIAN_POINT ( 'NONE',  ( 0.1532563361054082862, 1.217264484334117824, 2.638427012816831674 ) ) ;
#80495=CARTESIAN_POINT ( 'NONE',  ( 19.84674366389459621, 23.50893115100078390, 7.409399052514197653E-17 ) ) ;
#80499=CARTESIAN_POINT ( 'NONE',  ( 3.591859063236763294, -1.709698663402913210, -11.09922568453595026 ) ) ;
#80503=CARTESIAN_POINT ( 'NONE',  ( 22.26659068614895176, 14.72041550158063572, -7.082119434687042414 ) ) ;
#80505=UNCERTAINTY_MEASURE_WITH_UNIT (LENGTH_MEASURE( 1.000000000000000082E-05 ), #8290, 'distance_accuracy_value', 'NONE');
#80506=DIRECTION ( 'NONE',  ( 1.000000000000000000, 0.000000000000000000, 0.000000000000000000 ) ) ;
#80507=CARTESIAN_POINT ( 'NONE',  ( 24.16423886937410614, 19.51208216824729647, -3.795296366450302550 ) ) ;
#80508=CARTESIAN_POINT ( 'NONE',  ( 24.16423886937410614, 34.30374883491396787, 8.672049930838204340E-16 ) ) ;
#80510=CARTESIAN_POINT ( 'NONE',  ( 17.96484262340118221, 36.18868534415484106, -7.964842623401177768 ) ) ;
#80512=CARTESIAN_POINT ( 'NONE',  ( 19.84674366389459621, 18.50893115100078745, 7.409399052514197653E-17 ) ) ;
#80513=CARTESIAN_POINT ( 'NONE',  ( 7.084665262690076126, 62.02201867748816966, -10.88017736071110164 ) ) ;
#80514=CARTESIAN_POINT ( 'NONE',  ( 0.1532563361054100626, 15.80059781766745353, -2.638427012816831230 ) ) ;
#80516=CARTESIAN_POINT ( 'NONE',  ( 12.91533473730993009, 6.605352010821504471, -10.88017736071109987 ) ) ;
#80517=CARTESIAN_POINT ( 'NONE',  ( 0.6178305044545838731, 39.74863466993041072, 9.382169495545420901 ) ) ;
#80518=CARTESIAN_POINT ( 'NONE',  ( 0.1532563361054100626, 55.80059781766745175, -2.638427012816831230 ) ) ;
#80520=CARTESIAN_POINT ( 'NONE',  ( 6.565887622018943937, 30.16530133659708568, 12.81628187352647430 ) ) ;
#80522=CARTESIAN_POINT ( 'NONE',  ( 19.84674366389459266, 33.30059781766744464, 2.638427012816836559 ) ) ;
#80523=CARTESIAN_POINT ( 'NONE',  ( 17.08211943468705130, 18.47041550158063572, 12.26659068614894998 ) ) ;
#80524=VERTEX_POINT ( 'NONE', #95296 ) ;
#80526=CARTESIAN_POINT ( 'NONE',  ( -0.8801773607111008646, 53.27201867748816966, 2.915334737309923430 ) ) ;
#80527=CARTESIAN_POINT ( 'NONE',  ( 10.00000000000000178, 59.31368534415484106, 10.88017736071110342 ) ) ;
#80528=CARTESIAN_POINT ( 'NONE',  ( 13.79529636645031943, 45.34541550158062506, -14.16423886937409904 ) ) ;
#80529=CARTESIAN_POINT ( 'NONE',  ( 0.1532563361054100626, 60.80059781766744464, -2.638427012816831230 ) ) ;
#80531=CARTESIAN_POINT ( 'NONE',  ( 10.00000000000000000, 36.81368534415484106, -10.88017736071110342 ) ) ;
#80532=EDGE_CURVE ( 'NONE', #84166, #58317, #27781, .T. ) ;
#80534=CARTESIAN_POINT ( 'NONE',  ( 7.361572987183170547, 57.05059781766744464, 9.846743663894590881 ) ) ;
#80536=CARTESIAN_POINT ( 'NONE',  ( 17.96484262340118221, 4.938685344154837509, 7.964842623401181321 ) ) ;
#80537=CARTESIAN_POINT ( 'NONE',  ( 7.084665262690076126, 67.02201867748817676, -10.88017736071110164 ) ) ;
#80538=CARTESIAN_POINT ( 'NONE',  ( -0.8801773607110991993, 2.855352010821504471, -2.915334737309923874 ) ) ;
#80541=CARTESIAN_POINT ( 'NONE',  ( 17.20831665107776587, 4.133931151000785675, -7.208316651077762316 ) ) ;
#80542=CARTESIAN_POINT ( 'NONE',  ( 12.63842701281683922, 4.550597817667451750, -9.846743663894590881 ) ) ;
#80545=CARTESIAN_POINT ( 'NONE',  ( 7.361572987183169658, 29.96726448433411960, -9.846743663894592657 ) ) ;
#80546=CARTESIAN_POINT ( 'NONE',  ( -0.8801773607111008646, 18.27201867748817321, 2.915334737309923430 ) ) ;
#80547=CARTESIAN_POINT ( 'NONE',  ( 10.00000000000000178, 5.373634669930420493, 12.81628187352647608 ) ) ;
#80548=CARTESIAN_POINT ( 'NONE',  ( 19.42250999205614193, 35.14701867748816966, 5.440088680355555262 ) ) ;
#80549=CARTESIAN_POINT ( 'NONE',  ( 19.72487221294570858, 36.86607318730075633, 6.500000000000000888 ) ) ;
#80551=CARTESIAN_POINT ( 'NONE',  ( 21.09922568453595559, 32.04030133659708923, -6.408140936763230044 ) ) ;
#80553=CARTESIAN_POINT ( 'NONE',  ( 4.559911319644449179, 68.89701867748817676, 9.422509992056141925 ) ) ;
#80556=CARTESIAN_POINT ( 'NONE',  ( 13.43411237798105340, 20.58196800326374643, 12.81628187352647963 ) ) ;
#80557=CARTESIAN_POINT ( 'NONE',  ( 19.72487221294570858, 51.86607318730076344, 6.500000000000000888 ) ) ;
#80559=CARTESIAN_POINT ( 'NONE',  ( 20.88017736071110519, 25.56368534415483751, 2.639326808657452039E-16 ) ) ;
#80560=CARTESIAN_POINT ( 'NONE',  ( 6.204703633549690345, 67.84541550158060375, 14.16423886937410082 ) ) ;
#80561=CARTESIAN_POINT ( 'NONE',  ( 2.791683348922237240, 60.38393115100078745, -7.208316651077763204 ) ) ;
#80562=CARTESIAN_POINT ( 'NONE',  ( 14.92337183194729988, 9.342264484334119601, -8.527530157486177487 ) ) ;
#80563=CARTESIAN_POINT ( 'NONE',  ( 2.035157376598822676, 57.43868534415484106, -7.964842623401177768 ) ) ;
#80565=CARTESIAN_POINT ( 'NONE',  ( -4.164238869374098151, 36.59541550158063217, -3.795296366450310543 ) ) ;
#80569=ORIENTED_EDGE ( 'NONE', *, *, #52851, .F. ) ;
#80570=CARTESIAN_POINT ( 'NONE',  ( 13.79529636645030344, 48.26208216824728936, 14.16423886937410614 ) ) ;
#80571=CARTESIAN_POINT ( 'NONE',  ( -2.266590686148945544, 51.38708216824730357, -7.082119434687050408 ) ) ;
#80572=CARTESIAN_POINT ( 'NONE',  ( 12.63842701281683034, 22.46726448433411605, 9.846743663894596210 ) ) ;
#80573=CARTESIAN_POINT ( 'NONE',  ( 22.81628187352647785, 26.41530133659708923, 3.434112377981063169 ) ) ;
#80576=CARTESIAN_POINT ( 'NONE',  ( 10.00000000000000178, 69.31368534415484817, 10.88017736071110342 ) ) ;
#80577=CARTESIAN_POINT ( 'NONE',  ( -4.164238869374098151, 41.59541550158061796, -3.795296366450310543 ) ) ;
#80579=CARTESIAN_POINT ( 'NONE',  ( 12.63842701281683922, 14.55059781766744997, -9.846743663894590881 ) ) ;
#80583=FILL_AREA_STYLE ('',( #42105 ) ) ;
#80587=CARTESIAN_POINT ( 'NONE',  ( 17.08211943468705840, 10.13708216824730179, -12.26659068614894466 ) ) ;
#80588=CARTESIAN_POINT ( 'NONE',  ( 17.96484262340118221, 26.18868534415483396, -7.964842623401177768 ) ) ;
#80589=CARTESIAN_POINT ( 'NONE',  ( 12.91533473730992121, 24.52201867748816966, 10.88017736071110164 ) ) ;
#80590=CARTESIAN_POINT ( 'NONE',  ( 0.1532563361054100626, 50.80059781766745175, -2.638427012816831230 ) ) ;
#80591=CARTESIAN_POINT ( 'NONE',  ( 22.81628187352647785, 11.41530133659708390, 3.434112377981063169 ) ) ;
#80592=CYLINDRICAL_SURFACE ( 'NONE', #64636, 11.92686044187656513 ) ;
#80595=CARTESIAN_POINT ( 'NONE',  ( -1.099225684535947600, 24.54030133659708923, 6.408140936763237150 ) ) ;
#80597=CARTESIAN_POINT ( 'NONE',  ( 7.361572987183169658, 24.96726448433412315, -9.846743663894592657 ) ) ;
#80598=CARTESIAN_POINT ( 'NONE',  ( 20.36894250292379382, 53.67874883491397497, 10.36894250292379205 ) ) ;
#80600=CARTESIAN_POINT ( 'NONE',  ( 2.917880565312948704, 67.63708216824730357, 12.26659068614894643 ) ) ;
#80602=CARTESIAN_POINT ( 'NONE',  ( 12.91533473730992121, 34.52201867748817676, 10.88017736071110164 ) ) ;
#80603=CARTESIAN_POINT ( 'NONE',  ( -0.8801773607111008646, 48.27201867748816966, 2.915334737309923430 ) ) ;
#80604=CARTESIAN_POINT ( 'NONE',  ( 0.5774900079438590739, 57.64701867748817676, -5.440088680355550821 ) ) ;
#80607=CARTESIAN_POINT ( 'NONE',  ( 15.44008868035555793, 46.39701867748817676, -9.422509992056140149 ) ) ;
#80611=EDGE_CURVE ( 'NONE', #45739, #63730, #3330, .T. ) ;
#80613=CARTESIAN_POINT ( 'NONE',  ( 14.92337183194729633, 17.67559781766745175, 8.527530157486181039 ) ) ;
#80615=CARTESIAN_POINT ( 'NONE',  ( 10.00000000000000178, 52.25893115100078745, 9.846743663894594434 ) ) ;
#80618=ADVANCED_FACE ( 'NONE', ( #19789 ), #47019, .T. ) ;
#80623=CARTESIAN_POINT ( 'NONE',  ( 7.361572987183170547, 32.05059781766745175, 9.846743663894590881 ) ) ;
#80624=CARTESIAN_POINT ( 'NONE',  ( -4.164238869374099039, 66.80374883491396076, 8.674139862899312516E-16 ) ) ;
#80626=ORIENTED_EDGE ( 'NONE', *, *, #70722, .F. ) ;
#80628=CARTESIAN_POINT ( 'NONE',  ( 7.361572987183169658, 34.96726448433411605, -9.846743663894592657 ) ) ;
#80629=CARTESIAN_POINT ( 'NONE',  ( 22.81628187352647785, 1.623634669930420271, 6.195893100308588602E-16 ) ) ;
#80630=CARTESIAN_POINT ( 'NONE',  ( 7.361572987183170547, 7.050597817667451750, 9.846743663894590881 ) ) ;
#80632=CARTESIAN_POINT ( 'NONE',  ( 12.63842701281683034, 7.467264484334118713, 9.846743663894596210 ) ) ;
#80633=CARTESIAN_POINT ( 'NONE',  ( 19.84674366389459266, 53.30059781766744464, 2.638427012816836559 ) ) ;
#80634=CARTESIAN_POINT ( 'NONE',  ( 1.816707512666850599, 20.10290668512022805, -6.499999999999995559 ) ) ;
#80635=ORIENTED_EDGE ( 'NONE', *, *, #49476, .F. ) ;
#80636=CARTESIAN_POINT ( 'NONE',  ( -0.8801773607111008646, 8.272018677488171434, 2.915334737309923430 ) ) ;
#80637=CARTESIAN_POINT ( 'NONE',  ( -2.266590686148945544, 1.387082168247301128, -7.082119434687050408 ) ) ;
#80638=CARTESIAN_POINT ( 'NONE',  ( 2.791683348922240793, 11.63393115100078568, 7.208316651077764092 ) ) ;
#80639=CARTESIAN_POINT ( 'NONE',  ( -0.8801773607110991993, 47.85535201082150536, -2.915334737309923874 ) ) ;
#80640=CARTESIAN_POINT ( 'NONE',  ( 21.09922568453594849, 31.20696800326375353, 6.408140936763242479 ) ) ;
#80642=( LENGTH_UNIT ( ) NAMED_UNIT ( * ) SI_UNIT ( .MILLI., .METRE. ) );
#80643=ADVANCED_FACE ( 'NONE', ( #63708 ), #93724, .F. ) ;
#80646=CARTESIAN_POINT ( 'NONE',  ( -2.816281873526473856, 4.331968003263754419, 3.434112377981055619 ) ) ;
#80647=CARTESIAN_POINT ( 'NONE',  ( -1.099225684535947600, -0.4596986634029132657, 6.408140936763237150 ) ) ;
#80648=CARTESIAN_POINT ( 'NONE',  ( 2.791683348922240793, 11.63393115100078568, 7.208316651077764092 ) ) ;
#80650=CARTESIAN_POINT ( 'NONE',  ( 19.38216949554541557, 22.24863466993041428, -9.382169495545420901 ) ) ;
#80651=CARTESIAN_POINT ( 'NONE',  ( 1.602071938427535924, 52.02224192338640307, -6.500000000000077272 ) ) ;
#80652=CARTESIAN_POINT ( 'NONE',  ( -0.8801773607110991993, 32.85535201082151247, -2.915334737309923874 ) ) ;
#80655=CARTESIAN_POINT ( 'NONE',  ( 24.16423886937410614, 49.30374883491396787, 8.672049930838204340E-16 ) ) ;
#80657=CARTESIAN_POINT ( 'NONE',  ( 21.09922568453595559, 37.04030133659708923, -6.408140936763230044 ) ) ;
#80658=CARTESIAN_POINT ( 'NONE',  ( 7.084665262690076126, 29.10535201082150181, 10.88017736071109987 ) ) ;
#80660=CARTESIAN_POINT ( 'NONE',  ( 7.361572987183170547, 47.05059781766745175, 9.846743663894590881 ) ) ;
#80661=CARTESIAN_POINT ( 'NONE',  ( 4.559911319644449179, 57.23035201082150536, -9.422509992056141925 ) ) ;
#80662=CARTESIAN_POINT ( 'NONE',  ( 24.16423886937410614, 29.51208216824729647, -3.795296366450302550 ) ) ;
#80664=CARTESIAN_POINT ( 'NONE',  ( 2.791683348922237240, 25.38393115100078390, -7.208316651077763204 ) ) ;
#80665=DIRECTION ( 'NONE',  ( 0.5547001962252290364, 0.8320502943378437211, 0.000000000000000000 ) ) ;
#80666=CARTESIAN_POINT ( 'NONE',  ( 14.92337183194729988, 64.34226448433412315, -8.527530157486177487 ) ) ;
#80668=CARTESIAN_POINT ( 'NONE',  ( 20.32896413005680003, 6.771642702460840546, 5.963430220938287007 ) ) ;
#80670=CARTESIAN_POINT ( 'NONE',  ( 20.88017736071110164, 10.35535201082150714, 2.915334737309930979 ) ) ;
#80671=CARTESIAN_POINT ( 'NONE',  ( 13.79529636645031943, 25.34541550158063572, -14.16423886937409904 ) ) ;
#80672=CARTESIAN_POINT ( 'NONE',  ( 19.84674366389459266, 13.30059781766745353, 2.638427012816836559 ) ) ;
#80673=CARTESIAN_POINT ( 'NONE',  ( 14.92337183194729988, 59.34226448433412315, -8.527530157486177487 ) ) ;
#80674=CARTESIAN_POINT ( 'NONE',  ( 2.035157376598824452, 38.68868534415483396, 7.964842623401179544 ) ) ;
#80677=ORIENTED_EDGE ( 'NONE', *, *, #66947, .F. ) ;
#80679=CARTESIAN_POINT ( 'NONE',  ( 7.361572987183169658, 39.96726448433411605, -9.846743663894592657 ) ) ;
#80682=CARTESIAN_POINT ( 'NONE',  ( 19.72487221294570858, 70.00000000000000000, 6.500000000000000888 ) ) ;
#80683=CARTESIAN_POINT ( 'NONE',  ( -2.266590686148945544, 7.220415501580634832, 7.082119434687048631 ) ) ;
#80684=CARTESIAN_POINT ( 'NONE',  ( 10.00000000000000000, 10.55374883491396787, -14.16423886937410082 ) ) ;
#80685=CARTESIAN_POINT ( 'NONE',  ( 17.96484262340118221, 46.18868534415484106, -7.964842623401177768 ) ) ;
#80686=CARTESIAN_POINT ( 'NONE',  ( -4.164238869374098151, 61.59541550158063217, -3.795296366450310543 ) ) ;
#80687=CARTESIAN_POINT ( 'NONE',  ( 5.076628168052703671, 61.84226448433412315, 8.527530157486179263 ) ) ;
#80688=CARTESIAN_POINT ( 'NONE',  ( 0.1532563361054100626, 30.80059781766744820, -2.638427012816831230 ) ) ;
#80690=CARTESIAN_POINT ( 'NONE',  ( 15.44008868035555260, 29.73035201082150891, 9.422509992056143702 ) ) ;
#80691=CARTESIAN_POINT ( 'NONE',  ( 10.00000000000000000, 7.873634669930421381, -12.81628187352647608 ) ) ;
#80692=CARTESIAN_POINT ( 'NONE',  ( 22.26659068614895176, 4.720415501580633943, -7.082119434687042414 ) ) ;
#80693=CARTESIAN_POINT ( 'NONE',  ( 20.36894250292379738, 54.92874883491396076, -10.36894250292379027 ) ) ;
#80695=CARTESIAN_POINT ( 'NONE',  ( 17.96484262340118221, 11.18868534415484106, -7.964842623401177768 ) ) ;
#80696=CARTESIAN_POINT ( 'NONE',  ( -0.1503990784575294781, 68.10158574516643171, 6.262539305110072618 ) ) ;
#80699=ORIENTED_EDGE ( 'NONE', *, *, #36828, .F. ) ;
#80700=ORIENTED_EDGE ( 'NONE', *, *, #79097, .F. ) ;
#80703=CARTESIAN_POINT ( 'NONE',  ( -2.266590686148945544, 51.38708216824730357, -7.082119434687050408 ) ) ;
#80704=CARTESIAN_POINT ( 'NONE',  ( 18.52753015748618282, 28.92559781766745175, -4.923371831947291888 ) ) ;
#80705=CARTESIAN_POINT ( 'NONE',  ( -0.8801773607111008646, 63.27201867748817676, 2.915334737309923430 ) ) ;
#80708=CARTESIAN_POINT ( 'NONE',  ( 20.88017736071110164, 60.35535201082151957, 2.915334737309930979 ) ) ;
#80710=CARTESIAN_POINT ( 'NONE',  ( -2.816281873526473856, 54.12363466993041783, 9.499525473075851096E-16 ) ) ;
#80712=ORIENTED_EDGE ( 'NONE', *, *, #89464, .T. ) ;
#80713=CARTESIAN_POINT ( 'NONE',  ( 2.035157376598822676, 47.43868534415484817, -7.964842623401177768 ) ) ;
#80714=CARTESIAN_POINT ( 'NONE',  ( 22.26659068614895176, 19.72041550158063572, -7.082119434687042414 ) ) ;
#80715=CARTESIAN_POINT ( 'NONE',  ( 6.565887622018943937, 23.08196800326375708, -12.81628187352647608 ) ) ;
#80717=CARTESIAN_POINT ( 'NONE',  ( 10.00000000000000178, 45.37363466993041783, 12.81628187352647608 ) ) ;
#80718=CARTESIAN_POINT ( 'NONE',  ( 7.361572987183170547, 17.05059781766745530, 9.846743663894590881 ) ) ;
#80719=CARTESIAN_POINT ( 'NONE',  ( 10.00000000000000000, 16.81368534415483751, -10.88017736071110342 ) ) ;
#80720=CARTESIAN_POINT ( 'NONE',  ( -2.816281873526471635, 53.91530133659709634, -3.434112377981056508 ) ) ;
#80722=CARTESIAN_POINT ( 'NONE',  ( 19.84674366389459266, 43.71726448433410894, -2.638427012816827677 ) ) ;
#80724=CARTESIAN_POINT ( 'NONE',  ( 14.49999999999999822, 11.00000000000000000, -5.000000000000000000 ) ) ;
#80727=CARTESIAN_POINT ( 'NONE',  ( 2.035157376598824452, 63.68868534415484106, 7.964842623401179544 ) ) ;
#80728=LINE ( 'NONE', #49721, #51548 ) ;
#80730=CARTESIAN_POINT ( 'NONE',  ( 1.472469842513823179, 21.42559781766745175, 4.923371831947296329 ) ) ;
#80732=CARTESIAN_POINT ( 'NONE',  ( 10.00000000000000000, 22.87363466993042138, -12.81628187352647608 ) ) ;
#80734=CARTESIAN_POINT ( 'NONE',  ( 0.1532563361054100626, 45.80059781766745886, -2.638427012816831230 ) ) ;
#80736=CARTESIAN_POINT ( 'NONE',  ( 24.16423886937410614, 19.51208216824729647, -3.795296366450302550 ) ) ;
#80737=CARTESIAN_POINT ( 'NONE',  ( 19.84674366389459266, 28.30059781766745886, 2.638427012816836559 ) ) ;
#80738=CARTESIAN_POINT ( 'NONE',  ( 21.09922568453594849, 36.20696800326375353, 6.408140936763242479 ) ) ;
#80739=DIRECTION ( 'NONE',  ( -6.608470384673550777E-17, -1.000000000000000000, -0.000000000000000000 ) ) ;
#80740=CARTESIAN_POINT ( 'NONE',  ( -0.8801773607111009756, 23.06368534415484106, 1.068504757029289695E-15 ) ) ;
#80741=CARTESIAN_POINT ( 'NONE',  ( 20.88017736071110519, 65.56368534415483396, 2.639326808657452039E-16 ) ) ;
#80742=CARTESIAN_POINT ( 'NONE',  ( 19.38216949554541557, 2.248634669930420049, -9.382169495545420901 ) ) ;
#80743=CARTESIAN_POINT ( 'NONE',  ( 0.2751277870542910842, 67.28217586085239077, -6.499999999999992006 ) ) ;
#80744=CARTESIAN_POINT ( 'NONE',  ( 19.84674366389459621, 33.50893115100078745, 7.409399052514197653E-17 ) ) ;
#80745=CARTESIAN_POINT ( 'NONE',  ( 10.00000000000000178, 24.31368534415484106, 10.88017736071110342 ) ) ;
#80746=CARTESIAN_POINT ( 'NONE',  ( -2.816281873526471635, 23.91530133659708568, -3.434112377981056508 ) ) ;
#80748=CARTESIAN_POINT ( 'NONE',  ( 1.472469842513823179, 36.42559781766745175, 4.923371831947296329 ) ) ;
#80752=CARTESIAN_POINT ( 'NONE',  ( 0.5774900079438607392, 28.48035201082150891, 5.440088680355550821 ) ) ;
#80753=EDGE_LOOP ( 'NONE', ( #96997, #49572, #43060, #74300 ) ) ;
#80755=CARTESIAN_POINT ( 'NONE',  ( 10.00000000000000000, 6.813685344154838397, -10.88017736071110342 ) ) ;
#80756=CARTESIAN_POINT ( 'NONE',  ( 18.52753015748617571, 58.09226448433411605, 4.923371831947298993 ) ) ;
#80757=CARTESIAN_POINT ( 'NONE',  ( 10.00000000000000178, 24.31368534415484106, 10.88017736071110342 ) ) ;
#80759=CARTESIAN_POINT ( 'NONE',  ( -0.8801773607111009756, 58.06368534415484106, 1.068504757029289695E-15 ) ) ;
#80760=CARTESIAN_POINT ( 'NONE',  ( 19.42250999205614193, 20.14701867748817321, 5.440088680355555262 ) ) ;
#80762=CARTESIAN_POINT ( 'NONE',  ( 1.472469842513823179, 1.425597817667451528, 4.923371831947296329 ) ) ;
#80763=CARTESIAN_POINT ( 'NONE',  ( -46.68456736488007408, 103.6675473310227034, -5.775421524742654356 ) ) ;
#80764=CARTESIAN_POINT ( 'NONE',  ( 12.63842701281683034, 57.46726448433411605, 9.846743663894596210 ) ) ;
#80765=CARTESIAN_POINT ( 'NONE',  ( 24.16423886937409904, 59.09541550158063217, 3.795296366450317205 ) ) ;
#80766=CARTESIAN_POINT ( 'NONE',  ( 20.15039907845753220, 20.60158574516643171, -6.262539305110077947 ) ) ;
#80769=CARTESIAN_POINT ( 'NONE',  ( 20.36894250292379382, 3.678748834913967869, 10.36894250292379205 ) ) ;
#80770=CARTESIAN_POINT ( 'NONE',  ( 24.16423886937409904, 34.09541550158064638, 3.795296366450317205 ) ) ;
#80771=CARTESIAN_POINT ( 'NONE',  ( -2.816281873526473856, 9.331968003263753531, 3.434112377981055619 ) ) ;
#80775=CARTESIAN_POINT ( 'NONE',  ( 12.91533473730992121, 9.522018677488171434, 10.88017736071110164 ) ) ;
#80776=CARTESIAN_POINT ( 'NONE',  ( 1.472469842513823179, 36.42559781766745175, 4.923371831947296329 ) ) ;
#80778=CARTESIAN_POINT ( 'NONE',  ( 10.00000000000000000, 61.81368534415484106, -10.88017736071110342 ) ) ;
#80780=CARTESIAN_POINT ( 'NONE',  ( 13.43411237798106583, 62.66530133659708923, -12.81628187352647252 ) ) ;
#80781=CARTESIAN_POINT ( 'NONE',  ( 6.565887622018943937, 25.16530133659708213, 12.81628187352647430 ) ) ;
#80782=CARTESIAN_POINT ( 'NONE',  ( 18.52753015748618282, 33.92559781766745886, -4.923371831947291888 ) ) ;
#80786=CARTESIAN_POINT ( 'NONE',  ( 17.96484262340118221, 4.938685344154837509, 7.964842623401181321 ) ) ;
#80787=CARTESIAN_POINT ( 'NONE',  ( 12.91533473730992121, 19.52201867748816611, 10.88017736071110164 ) ) ;
#80788=CARTESIAN_POINT ( 'NONE',  ( 24.16423886937409904, 44.09541550158063927, 3.795296366450317205 ) ) ;
#80789=CARTESIAN_POINT ( 'NONE',  ( 15.44008868035555260, 29.73035201082150891, 9.422509992056143702 ) ) ;
#80790=CARTESIAN_POINT ( 'NONE',  ( 2.035157376598822676, 62.43868534415483396, -7.964842623401177768 ) ) ;
#80793=CARTESIAN_POINT ( 'NONE',  ( 18.52753015748618282, 13.92559781766745175, -4.923371831947291888 ) ) ;
#80795=CARTESIAN_POINT ( 'NONE',  ( 17.20831665107776587, 12.88393115100078390, 7.208316651077764980 ) ) ;
#80797=CARTESIAN_POINT ( 'NONE',  ( 19.84674366389459621, 38.50893115100078745, 7.409399052514197653E-17 ) ) ;
#80798=CARTESIAN_POINT ( 'NONE',  ( 10.00000000000000178, 57.25893115100078745, 9.846743663894594434 ) ) ;
#80801=CARTESIAN_POINT ( 'NONE',  ( 16.40814093676324603, 42.45696800326375353, -11.09922568453594671 ) ) ;
#80803=CARTESIAN_POINT ( 'NONE',  ( 19.42250999205614193, 65.14701867748817676, 5.440088680355555262 ) ) ;
#80804=CARTESIAN_POINT ( 'NONE',  ( 6.565887622018943937, 38.08196800326376064, -12.81628187352647608 ) ) ;
#80805=CARTESIAN_POINT ( 'NONE',  ( 24.16423886937409904, 59.09541550158063217, 3.795296366450317205 ) ) ;
#80806=CARTESIAN_POINT ( 'NONE',  ( 1.472469842513823179, 26.42559781766745175, 4.923371831947296329 ) ) ;
#80807=CARTESIAN_POINT ( 'NONE',  ( 0.1077916266722762639, 47.24062864464239908, -6.478736007406001640 ) ) ;
#80808=CARTESIAN_POINT ( 'NONE',  ( -0.1503990784575328643, 70.00000000000000000, -6.262539305110068177 ) ) ;
#80809=CARTESIAN_POINT ( 'NONE',  ( -0.3689425029237898834, 31.17874883491396787, -10.36894250292378850 ) ) ;
#80810=CARTESIAN_POINT ( 'NONE',  ( 19.84674366389459621, 48.50893115100078745, 7.409399052514197653E-17 ) ) ;
#80811=CARTESIAN_POINT ( 'NONE',  ( 20.03447792253738768, 12.65514106990690024, -6.401564815979734036 ) ) ;
#80812=CARTESIAN_POINT ( 'NONE',  ( 2.035157376598822676, 37.43868534415484106, -7.964842623401177768 ) ) ;
#80813=CARTESIAN_POINT ( 'NONE',  ( 7.084665262690076126, 57.02201867748817676, -10.88017736071110164 ) ) ;
#80815=CARTESIAN_POINT ( 'NONE',  ( 22.81628187352648496, 41.83196800326375353, -3.434112377981050290 ) ) ;
#80816=CARTESIAN_POINT ( 'NONE',  ( 2.035157376598822676, 52.43868534415483396, -7.964842623401177768 ) ) ;
#80817=VERTEX_POINT ( 'NONE', #47231 ) ;
#80825=CARTESIAN_POINT ( 'NONE',  ( 15.44008868035555260, 64.73035201082151957, 9.422509992056143702 ) ) ;
#80826=CARTESIAN_POINT ( 'NONE',  ( 19.42250999205614548, 10.98035201082150358, -5.440088680355545492 ) ) ;
#80827=SURFACE_STYLE_USAGE ( .BOTH. , #98194 ) ;
#80828=CARTESIAN_POINT ( 'NONE',  ( 20.88017736071110164, 10.35535201082150714, 2.915334737309930979 ) ) ;
#80829=CARTESIAN_POINT ( 'NONE',  ( -2.266590686148945544, 17.22041550158063572, 7.082119434687048631 ) ) ;
#80831=CARTESIAN_POINT ( 'NONE',  ( 4.559911319644449179, 17.23035201082150536, -9.422509992056141925 ) ) ;
#80832=CARTESIAN_POINT ( 'NONE',  ( 19.84674366389459266, 58.71726448433411605, -2.638427012816827677 ) ) ;
#80833=VERTEX_POINT ( 'NONE', #86233 ) ;
#80834=CARTESIAN_POINT ( 'NONE',  ( 18.52753015748617571, 63.09226448433412315, 4.923371831947298993 ) ) ;
#80835=EDGE_LOOP ( 'NONE', ( #39278, #53540, #53979, #21189, #33238, #95829 ) ) ;
#80836=CARTESIAN_POINT ( 'NONE',  ( -0.8801773607111009756, 58.06368534415484106, 1.068504757029289695E-15 ) ) ;
#80837=CARTESIAN_POINT ( 'NONE',  ( 10.00000000000000000, 59.75893115100078745, -9.846743663894594434 ) ) ;
#80838=CARTESIAN_POINT ( 'NONE',  ( 15.44008868035555793, 6.397018677488170546, -9.422509992056140149 ) ) ;
#80839=CARTESIAN_POINT ( 'NONE',  ( 2.831191079880678085, 79.91181047996344944, 9.500000000000000000 ) ) ;
#80840=CARTESIAN_POINT ( 'NONE',  ( 0.5774900079438590739, 62.64701867748817676, -5.440088680355550821 ) ) ;
#80841=CARTESIAN_POINT ( 'NONE',  ( 4.559911319644449179, 22.23035201082150536, -9.422509992056141925 ) ) ;
#80845=CARTESIAN_POINT ( 'NONE',  ( 16.40814093676324603, 57.45696800326375353, -11.09922568453594671 ) ) ;
#80846=CARTESIAN_POINT ( 'NONE',  ( 17.96484262340118221, 24.93868534415484461, 7.964842623401181321 ) ) ;
#80847=CARTESIAN_POINT ( 'NONE',  ( 0.6076426042653101378, 47.37576471608601736, -6.499999999999992006 ) ) ;
#80848=CARTESIAN_POINT ( 'NONE',  ( 22.81628187352648496, 36.83196800326376064, -3.434112377981050290 ) ) ;
#80849=CARTESIAN_POINT ( 'NONE',  ( 12.91533473730993009, 36.60535201082151247, -10.88017736071109987 ) ) ;
#80850=CARTESIAN_POINT ( 'NONE',  ( 1.472469842513823179, 61.42559781766745175, 4.923371831947296329 ) ) ;
#80852=VERTEX_POINT ( 'NONE', #31740 ) ;
#80854=CARTESIAN_POINT ( 'NONE',  ( 17.20831665107776587, 59.13393115100078745, -7.208316651077762316 ) ) ;
#80855=FACE_OUTER_BOUND ( 'NONE', #26157, .T. ) ;
#80856=CARTESIAN_POINT ( 'NONE',  ( 5.076628168052704559, 45.17559781766745175, -8.527530157486179263 ) ) ;
#80857=CARTESIAN_POINT ( 'NONE',  ( 12.91533473730993009, 21.60535201082150536, -10.88017736071109987 ) ) ;
#80858=DIRECTION ( 'NONE',  ( -0.5547001962252291474, -0.8320502943378437211, -0.000000000000000000 ) ) ;
#80859=CARTESIAN_POINT ( 'NONE',  ( 5.076628168052703671, 41.84226448433411605, 8.527530157486179263 ) ) ;
#80862=CARTESIAN_POINT ( 'NONE',  ( 12.63842701281683034, 37.46726448433411605, 9.846743663894596210 ) ) ;
#80863=CARTESIAN_POINT ( 'NONE',  ( 5.076628168052703671, 6.842264484334118713, 8.527530157486179263 ) ) ;
#80865=CARTESIAN_POINT ( 'NONE',  ( 5.076628168052704559, 55.17559781766745175, -8.527530157486179263 ) ) ;
#80868=CARTESIAN_POINT ( 'NONE',  ( 16.40814093676324603, 37.45696800326376064, -11.09922568453594671 ) ) ;
#80869=CARTESIAN_POINT ( 'NONE',  ( 0.1532563361054082862, 41.21726448433411605, 2.638427012816831674 ) ) ;
#80871=CARTESIAN_POINT ( 'NONE',  ( 24.16423886937410614, 59.51208216824728936, -3.795296366450302550 ) ) ;
#80872=CARTESIAN_POINT ( 'NONE',  ( 10.00000000000000000, 34.75893115100078745, -9.846743663894594434 ) ) ;
#80874=CARTESIAN_POINT ( 'NONE',  ( 20.36894250292379738, 54.92874883491396076, -10.36894250292379027 ) ) ;
#80876=CARTESIAN_POINT ( 'NONE',  ( 4.559911319644449179, 18.89701867748817321, 9.422509992056141925 ) ) ;
#80877=CARTESIAN_POINT ( 'NONE',  ( 6.204703633549690345, 40.76208216824731778, -14.16423886937410259 ) ) ;
#80878=CARTESIAN_POINT ( 'NONE',  ( 24.16423886937410614, 59.30374883491397497, 8.672049930838204340E-16 ) ) ;
#80879=DIRECTION ( 'NONE',  ( -0.8320502943378437211, 0.5547001962252290364, 0.000000000000000000 ) ) ;
#80881=CARTESIAN_POINT ( 'NONE',  ( 7.361572987183170547, 12.05059781766744997, 9.846743663894590881 ) ) ;
#80883=CARTESIAN_POINT ( 'NONE',  ( 1.472469842513823179, 65.59226448433412315, -4.923371831947296329 ) ) ;
#80885=CARTESIAN_POINT ( 'NONE',  ( 7.084665262690076126, 49.10535201082149825, 10.88017736071109987 ) ) ;
#80886=CARTESIAN_POINT ( 'NONE',  ( 0.1129803114748867132, 64.29427333184091253, -6.480634945678686698 ) ) ;
#80890=CARTESIAN_POINT ( 'NONE',  ( 1.472469842513823179, 60.59226448433412315, -4.923371831947296329 ) ) ;
#80892=AXIS2_PLACEMENT_3D ( 'NONE', #61753, #92755, #16280 ) ;
#80894=CARTESIAN_POINT ( 'NONE',  ( 6.204703633549690345, 30.76208216824730357, -14.16423886937410259 ) ) ;
#80898=CARTESIAN_POINT ( 'NONE',  ( 15.44008868035555793, 16.39701867748817321, -9.422509992056140149 ) ) ;
#80899=CARTESIAN_POINT ( 'NONE',  ( 0.6178305044545838731, 34.74863466993042493, 9.382169495545420901 ) ) ;
#80901=CARTESIAN_POINT ( 'NONE',  ( 0.1532563361054100626, 5.800597817667452638, -2.638427012816831230 ) ) ;
#80905=EDGE_CURVE ( 'NONE', #97143, #5600, #67470, .T. ) ;
#80906=CARTESIAN_POINT ( 'NONE',  ( 10.00000000000000000, 25.55374883491396787, -14.16423886937410082 ) ) ;
#80907=CARTESIAN_POINT ( 'NONE',  ( 13.79529636645030344, 3.262082168247301350, 14.16423886937410614 ) ) ;
#80909=CARTESIAN_POINT ( 'NONE',  ( 12.91533473730992121, 29.52201867748817321, 10.88017736071110164 ) ) ;
#80912=CARTESIAN_POINT ( 'NONE',  ( 4.559911319644449179, 38.89701867748817676, 9.422509992056141925 ) ) ;
#80913=CARTESIAN_POINT ( 'NONE',  ( 20.88017736071110164, 55.35535201082149825, 2.915334737309930979 ) ) ;
#80914=CARTESIAN_POINT ( 'NONE',  ( 22.81628187352648496, 6.831968003263753531, -3.434112377981050290 ) ) ;
#80916=CARTESIAN_POINT ( 'NONE',  ( 19.84674366389459266, 23.71726448433412315, -2.638427012816827677 ) ) ;
#80919=CARTESIAN_POINT ( 'NONE',  ( 20.88017736071110875, 45.77201867748816966, -2.915334737309920765 ) ) ;
#80920=COLOUR_RGB ( '', 0.40784314, 0.44705882, 0.49803922) ;
#80922=CARTESIAN_POINT ( 'NONE',  ( 21.09922568453595559, 2.040301336597086568, -6.408140936763230044 ) ) ;
#80923=CARTESIAN_POINT ( 'NONE',  ( 10.00000000000000178, 64.31368534415483396, 10.88017736071110342 ) ) ;
#80924=CARTESIAN_POINT ( 'NONE',  ( 7.361572987183169658, 19.96726448433411960, -9.846743663894592657 ) ) ;
#80925=CARTESIAN_POINT ( 'NONE',  ( 19.38216949554541557, 52.24863466993041072, -9.382169495545420901 ) ) ;
#80926=CARTESIAN_POINT ( 'NONE',  ( 12.63842701281683922, 4.550597817667451750, -9.846743663894590881 ) ) ;
#80928=CARTESIAN_POINT ( 'NONE',  ( 1.383448333479217141, 57.37718327197430312, -6.499999999999959144 ) ) ;
#80930=CARTESIAN_POINT ( 'NONE',  ( 7.084665262690076126, 22.02201867748817321, -10.88017736071110164 ) ) ;
#80931=CARTESIAN_POINT ( 'NONE',  ( 0.6178305044545818747, 58.49863466993042493, -9.382169495545419124 ) ) ;
#80932=CARTESIAN_POINT ( 'NONE',  ( 19.84674366389459266, 28.30059781766745886, 2.638427012816836559 ) ) ;
#80933=CARTESIAN_POINT ( 'NONE',  ( -0.8801773607111008646, 13.27201867748817143, 2.915334737309923430 ) ) ;
#80934=CARTESIAN_POINT ( 'NONE',  ( 17.08211943468705840, 65.13708216824730357, -12.26659068614894466 ) ) ;
#80935=ORIENTED_EDGE ( 'NONE', *, *, #75635, .T. ) ;
#80936=CARTESIAN_POINT ( 'NONE',  ( 2.035157376598822676, 17.43868534415483751, -7.964842623401177768 ) ) ;
#80938=CARTESIAN_POINT ( 'NONE',  ( 10.00000000000000178, 34.31368534415484106, 10.88017736071110342 ) ) ;
#80940=CARTESIAN_POINT ( 'NONE',  ( 7.084665262690076126, 39.10535201082150536, 10.88017736071109987 ) ) ;
#80942=CARTESIAN_POINT ( 'NONE',  ( 20.24186590665277663, 9.734100856612039721, 6.114288769123037426 ) ) ;
#80943=CARTESIAN_POINT ( 'NONE',  ( 17.96484262340118221, 29.93868534415484106, 7.964842623401181321 ) ) ;
#80945=CARTESIAN_POINT ( 'NONE',  ( 22.26659068614894466, 38.88708216824731068, 7.082119434687054849 ) ) ;
#80946=CARTESIAN_POINT ( 'NONE',  ( 2.035157376598822676, 37.43868534415484106, -7.964842623401177768 ) ) ;
#80947=CARTESIAN_POINT ( 'NONE',  ( 20.88017736071110875, 30.77201867748816966, -2.915334737309920765 ) ) ;
#80949=CARTESIAN_POINT ( 'NONE',  ( 5.076628168052704559, 65.17559781766745175, -8.527530157486179263 ) ) ;
#80951=CARTESIAN_POINT ( 'NONE',  ( 2.791683348922240793, 46.63393115100077324, 7.208316651077764092 ) ) ;
#80952=VERTEX_POINT ( 'NONE', #95703 ) ;
#80953=DIRECTION ( 'NONE',  ( -0.000000000000000000, -1.000000000000000000, 0.000000000000000000 ) ) ;
#80954=CARTESIAN_POINT ( 'NONE',  ( 2.791683348922240793, 16.63393115100078745, 7.208316651077764092 ) ) ;
#80956=CARTESIAN_POINT ( 'NONE',  ( 12.91533473730992121, 9.522018677488171434, 10.88017736071110164 ) ) ;
#80957=CARTESIAN_POINT ( 'NONE',  ( 12.63842701281683922, 29.55059781766745175, -9.846743663894590881 ) ) ;
#80958=CARTESIAN_POINT ( 'NONE',  ( 22.81628187352647785, 11.41530133659708390, 3.434112377981063169 ) ) ;
#80959=CARTESIAN_POINT ( 'NONE',  ( 4.559911319644449179, 53.89701867748817676, 9.422509992056141925 ) ) ;
#80960=CARTESIAN_POINT ( 'NONE',  ( -0.8801773607111008646, 18.27201867748817321, 2.915334737309923430 ) ) ;
#80961=CARTESIAN_POINT ( 'NONE',  ( 13.43411237798106583, 52.66530133659708213, -12.81628187352647252 ) ) ;
#80962=CARTESIAN_POINT ( 'NONE',  ( -2.266590686148945544, 32.22041550158063927, 7.082119434687048631 ) ) ;
#80963=EDGE_CURVE ( 'NONE', #58088, #91901, #67805, .T. ) ;
#80965=CARTESIAN_POINT ( 'NONE',  ( 20.32896413005680358, 34.74545670184113533, 5.963430220938287007 ) ) ;
#80966=ORIENTED_EDGE ( 'NONE', *, *, #71910, .T. ) ;
#80967=CARTESIAN_POINT ( 'NONE',  ( 5.076628168052704559, 65.17559781766745175, -8.527530157486179263 ) ) ;
#80969=CARTESIAN_POINT ( 'NONE',  ( 17.96484262340118221, 31.18868534415483751, -7.964842623401177768 ) ) ;
#80970=CARTESIAN_POINT ( 'NONE',  ( 14.92337183194729633, 62.67559781766745886, 8.527530157486181039 ) ) ;
#80973=CARTESIAN_POINT ( 'NONE',  ( 10.00000000000000000, 19.75893115100078390, -9.846743663894594434 ) ) ;
#80974=CIRCLE ( 'NONE', #10751, 0.4999999999999985567 ) ;
#80975=CARTESIAN_POINT ( 'NONE',  ( 0.1532563361054100626, 20.80059781766744464, -2.638427012816831230 ) ) ;
#80976=CARTESIAN_POINT ( 'NONE',  ( 18.52753015748618282, 8.925597817667451750, -4.923371831947291888 ) ) ;
#80978=CARTESIAN_POINT ( 'NONE',  ( 10.00000000000000000, -0.2410688489992152128, -9.846743663894594434 ) ) ;
#80981=CARTESIAN_POINT ( 'NONE',  ( 10.00000000000000000, 4.758931151000784787, -9.846743663894594434 ) ) ;
#80982=CARTESIAN_POINT ( 'NONE',  ( 2.791683348922237240, 15.38393115100078212, -7.208316651077763204 ) ) ;
#80986=CARTESIAN_POINT ( 'NONE',  ( 6.565887622018943937, 5.165301336597086568, 12.81628187352647430 ) ) ;
#80987=CARTESIAN_POINT ( 'NONE',  ( 19.42250999205614548, 5.980352010821504471, -5.440088680355545492 ) ) ;
#80988=CARTESIAN_POINT ( 'NONE',  ( 6.204703633549690345, 12.84541550158063572, 14.16423886937410082 ) ) ;
#80990=CARTESIAN_POINT ( 'NONE',  ( 13.79529636645031943, 20.34541550158063572, -14.16423886937409904 ) ) ;
#80991=CARTESIAN_POINT ( 'NONE',  ( 22.26659068614894466, 38.88708216824731068, 7.082119434687054849 ) ) ;
#80992=CARTESIAN_POINT ( 'NONE',  ( 13.79529636645031943, 10.34541550158063394, -14.16423886937409904 ) ) ;
#80993=CARTESIAN_POINT ( 'NONE',  ( 2.035157376598824452, 68.68868534415484817, 7.964842623401179544 ) ) ;
#80994=CARTESIAN_POINT ( 'NONE',  ( -0.8801773607110991993, 32.85535201082151247, -2.915334737309923874 ) ) ;
#80997=CARTESIAN_POINT ( 'NONE',  ( 2.791683348922240793, 21.63393115100078745, 7.208316651077764092 ) ) ;
#80998=CARTESIAN_POINT ( 'NONE',  ( 17.96484262340118221, 61.18868534415482685, -7.964842623401177768 ) ) ;
#80999=CARTESIAN_POINT ( 'NONE',  ( 12.63842701281683034, 27.46726448433411250, 9.846743663894596210 ) ) ;
#81000=B_SPLINE_CURVE_WITH_KNOTS ( 'NONE', 3,
 ( #89702, #14720, #221, #60192 ),
 .UNSPECIFIED., .F., .F.,
 ( 4, 4 ),
 ( 0.000000000000000000, 0.001036303429213360086 ),
 .UNSPECIFIED. ) ;
#81001=CARTESIAN_POINT ( 'NONE',  ( 7.084665262690076126, 17.02201867748817676, -10.88017736071110164 ) ) ;
#81002=CARTESIAN_POINT ( 'NONE',  ( 3.591859063236761518, 39.95696800326375353, 11.09922568453594849 ) ) ;
#81003=CARTESIAN_POINT ( 'NONE',  ( 0.1532563361054082862, 51.21726448433412315, 2.638427012816831674 ) ) ;
#81006=CARTESIAN_POINT ( 'NONE',  ( 6.565887622018943937, 48.08196800326375353, -12.81628187352647608 ) ) ;
#81008=CARTESIAN_POINT ( 'NONE',  ( 10.00000000000000000, 44.75893115100078745, -9.846743663894594434 ) ) ;
#81009=CARTESIAN_POINT ( 'NONE',  ( -2.266590686148945544, 27.22041550158063572, 7.082119434687048631 ) ) ;
#81012=CARTESIAN_POINT ( 'NONE',  ( 12.91533473730993009, 46.60535201082150536, -10.88017736071109987 ) ) ;
#81013=CARTESIAN_POINT ( 'NONE',  ( 2.035157376598822676, 47.43868534415484817, -7.964842623401177768 ) ) ;
#81014=CARTESIAN_POINT ( 'NONE',  ( 10.00000000000000000, 45.55374883491397497, -14.16423886937410082 ) ) ;
#81015=CARTESIAN_POINT ( 'NONE',  ( 10.00000000000000000, 64.75893115100078035, -9.846743663894594434 ) ) ;
#81016=CARTESIAN_POINT ( 'NONE',  ( 0.1916775849787232255, 57.25868815902070708, -6.499999999999983125 ) ) ;
#81017=CARTESIAN_POINT ( 'NONE',  ( 10.00000000000000178, 39.31368534415484106, 10.88017736071110342 ) ) ;
#81019=CARTESIAN_POINT ( 'NONE',  ( 3.591859063236761518, 24.95696800326375353, 11.09922568453594849 ) ) ;
#81020=CARTESIAN_POINT ( 'NONE',  ( 14.92337183194729988, 54.34226448433412315, -8.527530157486177487 ) ) ;
#81024=CARTESIAN_POINT ( 'NONE',  ( 7.084665262690076126, 9.105352010821503583, 10.88017736071109987 ) ) ;
#81025=CARTESIAN_POINT ( 'NONE',  ( 19.72487221294571569, 65.71833443783937412, -6.499999999999983125 ) ) ;
#81026=CARTESIAN_POINT ( 'NONE',  ( 2.035157376598824452, 63.68868534415484106, 7.964842623401179544 ) ) ;
#81027=CARTESIAN_POINT ( 'NONE',  ( 1.472469842513823179, 5.592264484334118713, -4.923371831947296329 ) ) ;
#81029=CARTESIAN_POINT ( 'NONE',  ( 0.1532563361054083140, 31.00893115100078390, 1.131784320476157264E-15 ) ) ;
#81030=CARTESIAN_POINT ( 'NONE',  ( 2.035157376598824452, 23.68868534415484461, 7.964842623401179544 ) ) ;
#81031=CARTESIAN_POINT ( 'NONE',  ( 0.6178305044545818747, 8.498634669930421381, -9.382169495545419124 ) ) ;
#81032=CARTESIAN_POINT ( 'NONE',  ( 15.44008868035555793, 36.39701867748816966, -9.422509992056140149 ) ) ;
#81034=CARTESIAN_POINT ( 'NONE',  ( 18.72515096720591643, 66.07228050351029935, -6.499999999999699796 ) ) ;
#81035=CARTESIAN_POINT ( 'NONE',  ( 16.40814093676324603, 42.45696800326375353, -11.09922568453594671 ) ) ;
#81036=ORIENTED_EDGE ( 'NONE', *, *, #83558, .T. ) ;
#81037=CARTESIAN_POINT ( 'NONE',  ( 7.084665262690076126, 59.10535201082150536, 10.88017736071109987 ) ) ;
#81038=CARTESIAN_POINT ( 'NONE',  ( 21.09922568453595559, 22.04030133659708923, -6.408140936763230044 ) ) ;
#81040=CARTESIAN_POINT ( 'NONE',  ( 12.91533473730992121, 34.52201867748817676, 10.88017736071110164 ) ) ;
#81042=CARTESIAN_POINT ( 'NONE',  ( 24.16423886937410614, 59.51208216824728936, -3.795296366450302550 ) ) ;
#81043=AXIS2_PLACEMENT_3D ( 'NONE', #23169, #53647, #15670 ) ;
#81044=CARTESIAN_POINT ( 'NONE',  ( 17.20831665107776587, 57.88393115100078745, 7.208316651077764980 ) ) ;
#81045=CARTESIAN_POINT ( 'NONE',  ( 17.20831665107776587, 2.883931151000785231, 7.208316651077764980 ) ) ;
#81046=CARTESIAN_POINT ( 'NONE',  ( 10.00000000000000178, 64.31368534415483396, 10.88017736071110342 ) ) ;
#81048=CARTESIAN_POINT ( 'NONE',  ( 13.79529636645031943, 25.34541550158063572, -14.16423886937409904 ) ) ;
#81050=SURFACE_STYLE_USAGE ( .BOTH. , #44029 ) ;
#81053=ORIENTED_EDGE ( 'NONE', *, *, #6012, .T. ) ;
#81055=CARTESIAN_POINT ( 'NONE',  ( 10.00000000000000178, 68.05374883491397497, 14.16423886937410082 ) ) ;
#81056=CARTESIAN_POINT ( 'NONE',  ( 13.79529636645031943, 50.34541550158064638, -14.16423886937409904 ) ) ;
#81057=CARTESIAN_POINT ( 'NONE',  ( 12.63842701281683034, 32.46726448433412315, 9.846743663894596210 ) ) ;
#81058=CARTESIAN_POINT ( 'NONE',  ( 21.09922568453594849, 31.20696800326375353, 6.408140936763242479 ) ) ;
#81061=CARTESIAN_POINT ( 'NONE',  ( -0.8801773607111009756, 3.063685344154837509, 1.068504757029289695E-15 ) ) ;
#81062=CARTESIAN_POINT ( 'NONE',  ( 22.26659068614895176, 59.72041550158063927, -7.082119434687042414 ) ) ;
#81063=EDGE_CURVE ( 'NONE', #22152, #61681, #4580, .T. ) ;
#81064=EDGE_CURVE ( 'NONE', #16885, #3586, #98151, .T. ) ;
#81066=CARTESIAN_POINT ( 'NONE',  ( 17.20831665107776587, 12.88393115100078390, 7.208316651077764980 ) ) ;
#81072=ORIENTED_EDGE ( 'NONE', *, *, #92033, .T. ) ;
#81073=CARTESIAN_POINT ( 'NONE',  ( 17.08211943468705130, 13.47041550158063572, 12.26659068614894998 ) ) ;
#81074=CARTESIAN_POINT ( 'NONE',  ( 4.559911319644449179, 13.89701867748817321, 9.422509992056141925 ) ) ;
#81075=CARTESIAN_POINT ( 'NONE',  ( 7.084665262690076126, 27.02201867748817676, -10.88017736071110164 ) ) ;
#81076=CARTESIAN_POINT ( 'NONE',  ( 19.84674366389459266, 53.71726448433411605, -2.638427012816827677 ) ) ;
#81077=CARTESIAN_POINT ( 'NONE',  ( 16.40814093676324603, 12.45696800326375353, -11.09922568453594671 ) ) ;
#81079=CARTESIAN_POINT ( 'NONE',  ( 3.591859063236763294, 28.29030133659708568, -11.09922568453595026 ) ) ;
#81081=CARTESIAN_POINT ( 'NONE',  ( 12.63842701281683034, 37.46726448433411605, 9.846743663894596210 ) ) ;
#81082=CARTESIAN_POINT ( 'NONE',  ( 24.16423886937410614, 64.30374883491396076, 8.672049930838204340E-16 ) ) ;
#81084=EDGE_CURVE ( 'NONE', #34211, #88366, #65282, .T. ) ;
#81085=CARTESIAN_POINT ( 'NONE',  ( 10.00000000000000000, 6.813685344154838397, -10.88017736071110342 ) ) ;
#81086=ORIENTED_EDGE ( 'NONE', *, *, #26747, .F. ) ;
#81087=CARTESIAN_POINT ( 'NONE',  ( 7.084665262690076126, 44.10535201082151247, 10.88017736071109987 ) ) ;
#81088=CARTESIAN_POINT ( 'NONE',  ( 0.5774900079438590739, 42.64701867748816966, -5.440088680355550821 ) ) ;
#81089=CARTESIAN_POINT ( 'NONE',  ( 0.5774900079438590739, 47.64701867748817676, -5.440088680355550821 ) ) ;
#81091=CARTESIAN_POINT ( 'NONE',  ( -0.8801773607111009756, 38.06368534415484106, 1.068504757029289695E-15 ) ) ;
#81095=CARTESIAN_POINT ( 'NONE',  ( 17.20831665107776587, 22.88393115100078745, 7.208316651077764980 ) ) ;
#81096=ORIENTED_EDGE ( 'NONE', *, *, #21818, .T. ) ;
#81097=CARTESIAN_POINT ( 'NONE',  ( 18.52753015748618282, 58.92559781766745886, -4.923371831947291888 ) ) ;
#81099=SURFACE_STYLE_FILL_AREA ( #56635 ) ;
#81105=CARTESIAN_POINT ( 'NONE',  ( 20.36894250292379382, 63.67874883491396787, 10.36894250292379205 ) ) ;
#81106=CARTESIAN_POINT ( 'NONE',  ( -0.1503990784575275907, 58.10158574516644592, 6.262539305110076171 ) ) ;
#81109=CARTESIAN_POINT ( 'NONE',  ( 5.076628168052704559, 30.17559781766745175, -8.527530157486179263 ) ) ;
#81110=DIRECTION ( 'NONE',  ( 0.000000000000000000, -1.000000000000000000, 0.000000000000000000 ) ) ;
#81111=CARTESIAN_POINT ( 'NONE',  ( 13.43411237798106583, 7.665301336597086568, -12.81628187352647252 ) ) ;
#81112=CARTESIAN_POINT ( 'NONE',  ( 10.00000000000000000, 4.758931151000784787, -9.846743663894594434 ) ) ;
#81114=CARTESIAN_POINT ( 'NONE',  ( 5.076628168052704559, 10.17559781766745175, -8.527530157486179263 ) ) ;
#81115=CARTESIAN_POINT ( 'NONE',  ( 12.63842701281683922, 59.55059781766744464, -9.846743663894590881 ) ) ;
#81119=CARTESIAN_POINT ( 'NONE',  ( 15.44008868035555260, 9.730352010821505360, 9.422509992056143702 ) ) ;
#81120=CARTESIAN_POINT ( 'NONE',  ( -0.3689425029237881626, 7.428748834913967869, 10.36894250292379027 ) ) ;
#81121=CARTESIAN_POINT ( 'NONE',  ( 19.84674366389459621, 13.50893115100078568, 7.409399052514197653E-17 ) ) ;
#81122=CARTESIAN_POINT ( 'NONE',  ( 10.00000000000000000, 51.81368534415484106, -10.88017736071110342 ) ) ;
#81123=CARTESIAN_POINT ( 'NONE',  ( 16.40814093676324603, 27.45696800326375708, -11.09922568453594671 ) ) ;
#81128=CARTESIAN_POINT ( 'NONE',  ( 19.84674366389459266, 63.71726448433412315, -2.638427012816827677 ) ) ;
#81129=CARTESIAN_POINT ( 'NONE',  ( 17.20831665107776587, 14.13393115100078568, -7.208316651077762316 ) ) ;
#81131=CARTESIAN_POINT ( 'NONE',  ( -2.816281873526473856, 19.12363466993042138, 9.499525473075851096E-16 ) ) ;
#81132=CARTESIAN_POINT ( 'NONE',  ( 2.153642693323417845, 51.13791097397318453, -6.499999999999929834 ) ) ;
#81133=CARTESIAN_POINT ( 'NONE',  ( 12.91533473730993009, 21.60535201082150536, -10.88017736071109987 ) ) ;
#81137=CARTESIAN_POINT ( 'NONE',  ( 24.16423886937410614, 54.30374883491396787, 8.672049930838204340E-16 ) ) ;
#81139=CARTESIAN_POINT ( 'NONE',  ( 19.42250999205614193, 30.14701867748817321, 5.440088680355555262 ) ) ;
#81140=CARTESIAN_POINT ( 'NONE',  ( 0.1532563361054082862, 51.21726448433412315, 2.638427012816831674 ) ) ;
#81141=CARTESIAN_POINT ( 'NONE',  ( -0.8801773607110991993, 47.85535201082150536, -2.915334737309923874 ) ) ;
#81142=CARTESIAN_POINT ( 'NONE',  ( 24.16423886937410614, 34.51208216824731068, -3.795296366450302550 ) ) ;
#81143=LINE ( 'NONE', #72647, #48742 ) ;
#81144=UNCERTAINTY_MEASURE_WITH_UNIT (LENGTH_MEASURE( 1.000000000000000082E-05 ), #82421, 'distance_accuracy_value', 'NONE');
#81145=CARTESIAN_POINT ( 'NONE',  ( 7.361572987183169658, 39.96726448433411605, -9.846743663894592657 ) ) ;
#81147=CARTESIAN_POINT ( 'NONE',  ( 17.20831665107776587, 62.88393115100078745, 7.208316651077764980 ) ) ;
#81149=CARTESIAN_POINT ( 'NONE',  ( 17.96484262340118221, 31.18868534415483751, -7.964842623401177768 ) ) ;
#81151=DIRECTION ( 'NONE',  ( -0.000000000000000000, 0.000000000000000000, 1.000000000000000000 ) ) ;
#81152=CARTESIAN_POINT ( 'NONE',  ( 12.91533473730992121, 9.522018677488171434, 10.88017736071110164 ) ) ;
#81153=CARTESIAN_POINT ( 'NONE',  ( 1.472469842513823179, 5.592264484334118713, -4.923371831947296329 ) ) ;
#81154=CARTESIAN_POINT ( 'NONE',  ( 22.26659068614894466, 28.88708216824730357, 7.082119434687054849 ) ) ;
#81155=CARTESIAN_POINT ( 'NONE',  ( 17.20831665107776587, 12.88393115100078390, 7.208316651077764980 ) ) ;
#81156=CARTESIAN_POINT ( 'NONE',  ( 10.00000000000000178, 62.25893115100078745, 9.846743663894594434 ) ) ;
#81157=CARTESIAN_POINT ( 'NONE',  ( 0.5774900079438590739, 32.64701867748816966, -5.440088680355550821 ) ) ;
#81158=CARTESIAN_POINT ( 'NONE',  ( -0.03743638938522143161, 34.25197528031020511, -6.399506433553973750 ) ) ;
#81162=UNCERTAINTY_MEASURE_WITH_UNIT (LENGTH_MEASURE( 1.000000000000000082E-05 ), #4389, 'distance_accuracy_value', 'NONE');
#81164=MECHANICAL_DESIGN_GEOMETRIC_PRESENTATION_REPRESENTATION('',(#89159),#77963);
#81166=CARTESIAN_POINT ( 'NONE',  ( 1.472469842513823179, 50.59226448433411605, -4.923371831947296329 ) ) ;
#81167=EDGE_CURVE ( 'NONE', #78236, #38312, #94328, .T. ) ;
#81171=CARTESIAN_POINT ( 'NONE',  ( -0.3689425029237898834, 26.17874883491396432, -10.36894250292378850 ) ) ;
#81172=CARTESIAN_POINT ( 'NONE',  ( -0.3689425029237881626, 7.428748834913967869, 10.36894250292379027 ) ) ;
#81173=CARTESIAN_POINT ( 'NONE',  ( 19.42250999205614548, 55.98035201082150536, -5.440088680355545492 ) ) ;
#81174=CARTESIAN_POINT ( 'NONE',  ( 24.16423886937410614, 49.30374883491396787, 8.672049930838204340E-16 ) ) ;
#81175=CARTESIAN_POINT ( 'NONE',  ( 5.076628168052703671, 66.84226448433412315, 8.527530157486179263 ) ) ;
#81176=CARTESIAN_POINT ( 'NONE',  ( 7.361572987183169658, 29.96726448433411960, -9.846743663894592657 ) ) ;
#81178=CARTESIAN_POINT ( 'NONE',  ( 7.084665262690076126, 37.02201867748817676, -10.88017736071110164 ) ) ;
#81179=CARTESIAN_POINT ( 'NONE',  ( 13.43411237798106583, 12.66530133659708746, -12.81628187352647252 ) ) ;
#81180=CARTESIAN_POINT ( 'NONE',  ( 6.204703633549690345, 47.84541550158064638, 14.16423886937410082 ) ) ;
#81182=CARTESIAN_POINT ( 'NONE',  ( -0.8801773607111008646, 13.27201867748817321, 2.915334737309923430 ) ) ;
#81183=CARTESIAN_POINT ( 'NONE',  ( -0.1503990784575247319, 67.22266099184919597, -6.262539305110083276 ) ) ;
#81185=CARTESIAN_POINT ( 'NONE',  ( 20.88017736071110164, 45.35535201082149115, 2.915334737309930979 ) ) ;
#81192=CARTESIAN_POINT ( 'NONE',  ( 13.79529636645031943, 50.34541550158064638, -14.16423886937409904 ) ) ;
#81193=CARTESIAN_POINT ( 'NONE',  ( 0.1532563361054082862, 41.21726448433411605, 2.638427012816831674 ) ) ;
#81194=CARTESIAN_POINT ( 'NONE',  ( 10.00000000000000178, 59.31368534415484106, 10.88017736071110342 ) ) ;
#81197=CARTESIAN_POINT ( 'NONE',  ( -0.8801773607111008646, 48.27201867748816966, 2.915334737309923430 ) ) ;
#81199=CARTESIAN_POINT ( 'NONE',  ( -1.099225684535947600, 59.54030133659708923, 6.408140936763237150 ) ) ;
#81202=CARTESIAN_POINT ( 'NONE',  ( 7.084665262690076126, 47.02201867748818387, -10.88017736071110164 ) ) ;
#81203=CARTESIAN_POINT ( 'NONE',  ( 24.16423886937410614, 14.51208216824730179, -3.795296366450302550 ) ) ;
#81205=CARTESIAN_POINT ( 'NONE',  ( 19.38216949554541557, 22.24863466993041428, -9.382169495545420901 ) ) ;
#81206=VERTEX_POINT ( 'NONE', #27565 ) ;
#81207=CARTESIAN_POINT ( 'NONE',  ( 22.81628187352648496, 46.83196800326376064, -3.434112377981050290 ) ) ;
#81208=CARTESIAN_POINT ( 'NONE',  ( 12.91533473730992121, 14.52201867748817143, 10.88017736071110164 ) ) ;
#81209=CARTESIAN_POINT ( 'NONE',  ( 18.52753015748617571, 33.09226448433411605, 4.923371831947298993 ) ) ;
#81210=CARTESIAN_POINT ( 'NONE',  ( 7.084665262690076126, 12.02201867748817143, -10.88017736071110164 ) ) ;
#81211=CARTESIAN_POINT ( 'NONE',  ( 21.09922568453594849, 56.20696800326375353, 6.408140936763242479 ) ) ;
#81213=CARTESIAN_POINT ( 'NONE',  ( 14.92337183194729633, 47.67559781766745175, 8.527530157486181039 ) ) ;
#81214=CARTESIAN_POINT ( 'NONE',  ( 2.035157376598824452, 68.68868534415484817, 7.964842623401179544 ) ) ;
#81215=VERTEX_POINT ( 'NONE', #6066 ) ;
#81219=CARTESIAN_POINT ( 'NONE',  ( 18.52753015748618282, 23.92559781766745530, -4.923371831947291888 ) ) ;
#81220=CARTESIAN_POINT ( 'NONE',  ( 13.43411237798105340, 25.58196800326374998, 12.81628187352647963 ) ) ;
#81221=DIRECTION ( 'NONE',  ( -0.07626964003977219908, 0.9970872288863213972, 0.000000000000000000 ) ) ;
#81222=ORIENTED_EDGE ( 'NONE', *, *, #88059, .F. ) ;
#81224=CARTESIAN_POINT ( 'NONE',  ( 12.63842701281683034, 62.46726448433410894, 9.846743663894596210 ) ) ;
#81226=CARTESIAN_POINT ( 'NONE',  ( 2.917880565312950480, 25.97041550158063572, -12.26659068614894821 ) ) ;
#81227=CARTESIAN_POINT ( 'NONE',  ( 7.361572987183170547, 32.05059781766745175, 9.846743663894590881 ) ) ;
#81228=CARTESIAN_POINT ( 'NONE',  ( 3.591859063236761518, 44.95696800326376064, 11.09922568453594849 ) ) ;
#81231=CARTESIAN_POINT ( 'NONE',  ( -0.8801773607111008646, 63.27201867748817676, 2.915334737309923430 ) ) ;
#81233=CARTESIAN_POINT ( 'NONE',  ( 1.472469842513823179, 41.42559781766745886, 4.923371831947296329 ) ) ;
#81234=CARTESIAN_POINT ( 'NONE',  ( 20.88017736071110164, 35.35535201082150536, 2.915334737309930979 ) ) ;
#81235=CARTESIAN_POINT ( 'NONE',  ( -2.816281873526473856, 44.33196800326375353, 3.434112377981055619 ) ) ;
#81236=CYLINDRICAL_SURFACE ( 'NONE', #95447, 0.5000000000000004441 ) ;
#81237=CARTESIAN_POINT ( 'NONE',  ( 7.084665262690076126, 37.02201867748817676, -10.88017736071110164 ) ) ;
#81239=CARTESIAN_POINT ( 'NONE',  ( -0.8801773607111008646, 68.27201867748817676, 2.915334737309923430 ) ) ;
#81240=CARTESIAN_POINT ( 'NONE',  ( 20.88017736071110164, 15.35535201082150358, 2.915334737309930979 ) ) ;
#81241=CARTESIAN_POINT ( 'NONE',  ( 12.63842701281683034, 52.46726448433413026, 9.846743663894596210 ) ) ;
#81242=CARTESIAN_POINT ( 'NONE',  ( 19.42250999205614548, 35.98035201082151247, -5.440088680355545492 ) ) ;
#81244=CARTESIAN_POINT ( 'NONE',  ( -0.8801773607110991993, 62.85535201082150536, -2.915334737309923874 ) ) ;
#81246=CARTESIAN_POINT ( 'NONE',  ( -0.8801773607111008646, 23.27201867748817676, 2.915334737309923430 ) ) ;
#81247=CARTESIAN_POINT ( 'NONE',  ( 0.000000000000000000, 76.61857121896082390, -7.300603792374249501 ) ) ;
#81248=CARTESIAN_POINT ( 'NONE',  ( 5.076628168052704559, 0.1755978176674514724, -8.527530157486179263 ) ) ;
#81249=CARTESIAN_POINT ( 'NONE',  ( 10.00000000000000000, 29.75893115100078745, -9.846743663894594434 ) ) ;
#81252=CARTESIAN_POINT ( 'NONE',  ( 10.00000000000000000, 54.75893115100078745, -9.846743663894594434 ) ) ;
#81253=CARTESIAN_POINT ( 'NONE',  ( 24.16423886937410614, 59.51208216824728936, -3.795296366450302550 ) ) ;
#81257=VECTOR ( 'NONE', #77133, 1000.000000000000000 ) ;
#81258=CARTESIAN_POINT ( 'NONE',  ( 24.16423886937409904, 9.095415501580633943, 3.795296366450317205 ) ) ;
#81259=CARTESIAN_POINT ( 'NONE',  ( -4.164238869374099927, 37.01208216824731068, 3.795296366450308767 ) ) ;
#81260=CARTESIAN_POINT ( 'NONE',  ( 16.40814093676324603, 2.456968003263753531, -11.09922568453594671 ) ) ;
#81262=CARTESIAN_POINT ( 'NONE',  ( 2.035157376598822676, 7.438685344154837509, -7.964842623401177768 ) ) ;
#81263=CARTESIAN_POINT ( 'NONE',  ( 0.1532563361054083140, 41.00893115100078745, 1.131784320476157264E-15 ) ) ;
#81264=CARTESIAN_POINT ( 'NONE',  ( 10.00000000000000000, 0.5537488349139675359, -14.16423886937410082 ) ) ;
#81267=CARTESIAN_POINT ( 'NONE',  ( 19.84674366389459266, 3.717264484334118713, -2.638427012816827677 ) ) ;
#81268=CARTESIAN_POINT ( 'NONE',  ( 6.565887622018943937, 28.08196800326375353, -12.81628187352647608 ) ) ;
#81269=CARTESIAN_POINT ( 'NONE',  ( 10.00000000000000178, 27.25893115100078390, 9.846743663894594434 ) ) ;
#81271=CARTESIAN_POINT ( 'NONE',  ( 14.92337183194729988, 14.34226448433411782, -8.527530157486177487 ) ) ;
#81273=CARTESIAN_POINT ( 'NONE',  ( 17.96484262340118221, 6.188685344154837509, -7.964842623401177768 ) ) ;
#81274=CARTESIAN_POINT ( 'NONE',  ( 20.88017736071110875, 20.77201867748816611, -2.915334737309920765 ) ) ;
#81275=CARTESIAN_POINT ( 'NONE',  ( -0.3689425029237898834, 36.17874883491396787, -10.36894250292378850 ) ) ;
#81276=CARTESIAN_POINT ( 'NONE',  ( 10.00000000000000000, 31.81368534415483751, -10.88017736071110342 ) ) ;
#81277=CARTESIAN_POINT ( 'NONE',  ( 19.42250999205614548, 65.98035201082151957, -5.440088680355545492 ) ) ;
#81279=CARTESIAN_POINT ( 'NONE',  ( 21.92686044187656691, 39.95379003517447813, 3.195792623639537755 ) ) ;
#81280=CARTESIAN_POINT ( 'NONE',  ( 10.00000000000000000, 29.75893115100078745, -9.846743663894594434 ) ) ;
#81282=CARTESIAN_POINT ( 'NONE',  ( 1.472469842513823179, 10.59226448433411782, -4.923371831947296329 ) ) ;
#81284=CARTESIAN_POINT ( 'NONE',  ( 12.63842701281683034, 32.46726448433412315, 9.846743663894596210 ) ) ;
#81285=CARTESIAN_POINT ( 'NONE',  ( 6.565887622018943937, -1.918031996736246692, -12.81628187352647608 ) ) ;
#81286=CARTESIAN_POINT ( 'NONE',  ( 17.96484262340118221, 41.18868534415484106, -7.964842623401177768 ) ) ;
#81288=EDGE_CURVE ( 'NONE', #14954, #65595, #87962, .T. ) ;
#81290=CARTESIAN_POINT ( 'NONE',  ( 16.40814093676323893, 45.79030133659708923, 11.09922568453595026 ) ) ;
#81291=CARTESIAN_POINT ( 'NONE',  ( 20.88017736071110519, 60.56368534415484106, 2.639326808657452039E-16 ) ) ;
#81292=CARTESIAN_POINT ( 'NONE',  ( -1.099225684535947600, 44.54030133659708923, 6.408140936763237150 ) ) ;
#81293=CARTESIAN_POINT ( 'NONE',  ( 24.16423886937409904, 54.09541550158063217, 3.795296366450317205 ) ) ;
#81294=CARTESIAN_POINT ( 'NONE',  ( 19.84674366389459266, 33.71726448433410894, -2.638427012816827677 ) ) ;
#81296=CARTESIAN_POINT ( 'NONE',  ( 7.361572987183170547, 67.05059781766746596, 9.846743663894590881 ) ) ;
#81299=CARTESIAN_POINT ( 'NONE',  ( -2.266590686148945544, 46.38708216824730357, -7.082119434687050408 ) ) ;
#81300=CARTESIAN_POINT ( 'NONE',  ( 14.92337183194729988, 44.34226448433412315, -8.527530157486177487 ) ) ;
#81302=CARTESIAN_POINT ( 'NONE',  ( 4.559911319644449179, 33.89701867748817676, 9.422509992056141925 ) ) ;
#81303=CARTESIAN_POINT ( 'NONE',  ( -0.8801773607110991993, 57.85535201082149825, -2.915334737309923874 ) ) ;
#81305=CARTESIAN_POINT ( 'NONE',  ( 2.603489959281614308, 56.58210964143329846, 6.500000000000031086 ) ) ;
#81307=CARTESIAN_POINT ( 'NONE',  ( 22.81628187352647785, 46.62363466993041783, 6.195893100308588602E-16 ) ) ;
#81308=ORIENTED_EDGE ( 'NONE', *, *, #84118, .T. ) ;
#81309=CARTESIAN_POINT ( 'NONE',  ( 17.96484262340118221, 61.18868534415482685, -7.964842623401177768 ) ) ;
#81311=CARTESIAN_POINT ( 'NONE',  ( -4.164238869374099039, 6.803748834913967869, 8.674139862899312516E-16 ) ) ;
#81312=CARTESIAN_POINT ( 'NONE',  ( 12.63842701281683034, 2.467264484334118269, 9.846743663894596210 ) ) ;
#81316=CARTESIAN_POINT ( 'NONE',  ( 7.084665262690076126, 12.02201867748817143, -10.88017736071110164 ) ) ;
#81320=CARTESIAN_POINT ( 'NONE',  ( 2.917880565312948704, 17.63708216824730357, 12.26659068614894643 ) ) ;
#81321=CARTESIAN_POINT ( 'NONE',  ( 12.91533473730992121, 19.52201867748816611, 10.88017736071110164 ) ) ;
#81322=CARTESIAN_POINT ( 'NONE',  ( 0.1532563361054083140, 66.00893115100079456, 1.131784320476157264E-15 ) ) ;
#81324=CARTESIAN_POINT ( 'NONE',  ( 19.84674366389459621, 58.50893115100078745, 7.409399052514197653E-17 ) ) ;
#81326=CARTESIAN_POINT ( 'NONE',  ( 0.1532563361054083140, 1.008931151000784787, 1.131784320476157264E-15 ) ) ;
#81327=CARTESIAN_POINT ( 'NONE',  ( 17.20831665107776587, 59.13393115100078745, -7.208316651077762316 ) ) ;
#81328=CARTESIAN_POINT ( 'NONE',  ( 10.00000000000000178, 35.37363466993042493, 12.81628187352647608 ) ) ;
#81329=CARTESIAN_POINT ( 'NONE',  ( 17.96484262340118221, 6.188685344154836621, -7.964842623401177768 ) ) ;
#81331=CARTESIAN_POINT ( 'NONE',  ( -0.8801773607111009756, 68.06368534415484817, 1.068504757029289695E-15 ) ) ;
#81332=CARTESIAN_POINT ( 'NONE',  ( 2.035157376598822676, 22.43868534415483396, -7.964842623401177768 ) ) ;
#81333=CARTESIAN_POINT ( 'NONE',  ( 16.40814093676323893, 55.79030133659708923, 11.09922568453595026 ) ) ;
#81334=CARTESIAN_POINT ( 'NONE',  ( 19.42250999205614548, 30.98035201082150536, -5.440088680355545492 ) ) ;
#81336=CARTESIAN_POINT ( 'NONE',  ( 22.81628187352647785, 46.41530133659708213, 3.434112377981063169 ) ) ;
#81337=CARTESIAN_POINT ( 'NONE',  ( -0.8801773607111008646, 53.27201867748816966, 2.915334737309923430 ) ) ;
#81338=CARTESIAN_POINT ( 'NONE',  ( 0.1532563361054100626, 55.80059781766745175, -2.638427012816831230 ) ) ;
#81342=CARTESIAN_POINT ( 'NONE',  ( 19.84674366389459266, 13.30059781766745353, 2.638427012816836559 ) ) ;
#81343=CARTESIAN_POINT ( 'NONE',  ( 22.81628187352648496, 11.83196800326375531, -3.434112377981050290 ) ) ;
#81346=CARTESIAN_POINT ( 'NONE',  ( 19.42250999205614193, 20.14701867748817321, 5.440088680355555262 ) ) ;
#81347=CARTESIAN_POINT ( 'NONE',  ( 2.791683348922237240, 45.38393115100079456, -7.208316651077763204 ) ) ;
#81350=CARTESIAN_POINT ( 'NONE',  ( 2.791683348922237240, 10.38393115100078390, -7.208316651077763204 ) ) ;
#81352=CARTESIAN_POINT ( 'NONE',  ( 0.6178305044545838731, -0.2513653300695798953, 9.382169495545420901 ) ) ;
#81355=CARTESIAN_POINT ( 'NONE',  ( 6.565887622018943937, 35.16530133659708923, 12.81628187352647430 ) ) ;
#81356=CARTESIAN_POINT ( 'NONE',  ( 14.92337183194729633, 37.67559781766745175, 8.527530157486181039 ) ) ;
#81358=CARTESIAN_POINT ( 'NONE',  ( 10.00000000000000000, 55.55374883491396787, -14.16423886937410082 ) ) ;
#81359=CARTESIAN_POINT ( 'NONE',  ( 14.92337183194729633, 27.67559781766745530, 8.527530157486181039 ) ) ;
#81361=CARTESIAN_POINT ( 'NONE',  ( 6.204703633549690345, 60.76208216824730357, -14.16423886937410259 ) ) ;
#81363=CARTESIAN_POINT ( 'NONE',  ( 19.42250999205614548, 15.98035201082150714, -5.440088680355545492 ) ) ;
#81364=CARTESIAN_POINT ( 'NONE',  ( 2.917880565312948704, 42.63708216824729647, 12.26659068614894643 ) ) ;
#81365=CARTESIAN_POINT ( 'NONE',  ( 24.16423886937410614, 49.51208216824730357, -3.795296366450302550 ) ) ;
#81368=CARTESIAN_POINT ( 'NONE',  ( 2.791683348922237240, 10.38393115100078390, -7.208316651077763204 ) ) ;
#81369=CARTESIAN_POINT ( 'NONE',  ( -1.099225684535947600, 3.706968003263753531, -6.408140936763238038 ) ) ;
#81370=CARTESIAN_POINT ( 'NONE',  ( 18.61655166652078464, 14.87718327197428714, 6.499999999999960920 ) ) ;
#81372=CARTESIAN_POINT ( 'NONE',  ( 12.91533473730993009, 51.60535201082149825, -10.88017736071109987 ) ) ;
#81379=CARTESIAN_POINT ( 'NONE',  ( 10.00000000000000000, 40.55374883491397497, -14.16423886937410082 ) ) ;
#81381=( NAMED_UNIT ( * ) PLANE_ANGLE_UNIT ( ) SI_UNIT ( $, .RADIAN. ) );
#81382=CARTESIAN_POINT ( 'NONE',  ( 0.5774900079438590739, 17.64701867748817321, -5.440088680355550821 ) ) ;
#81383=CARTESIAN_POINT ( 'NONE',  ( 10.00000000000000000, 37.87363466993041783, -12.81628187352647608 ) ) ;
#81384=CARTESIAN_POINT ( 'NONE',  ( 20.32896413005680714, 62.60497603579418069, -5.963430220938276349 ) ) ;
#81385=CARTESIAN_POINT ( 'NONE',  ( 6.565887622018943937, 15.16530133659708568, 12.81628187352647430 ) ) ;
#81386=CARTESIAN_POINT ( 'NONE',  ( 22.81628187352647785, 61.62363466993041783, 6.195893100308588602E-16 ) ) ;
#81390=CARTESIAN_POINT ( 'NONE',  ( 24.16423886937410614, 29.30374883491396787, 8.672049930838204340E-16 ) ) ;
#81391=CARTESIAN_POINT ( 'NONE',  ( -4.164238869374099039, 1.803748834913967647, 8.674139862899312516E-16 ) ) ;
#81393=CARTESIAN_POINT ( 'NONE',  ( 20.88017736071110164, 25.35535201082150891, 2.915334737309930979 ) ) ;
#81394=LINE ( 'NONE', #12896, #57437 ) ;
#81395=CARTESIAN_POINT ( 'NONE',  ( -35.67076923076924544, 93.15384615384616041, -9.500000000000000000 ) ) ;
#81396=CARTESIAN_POINT ( 'NONE',  ( 0.5774900079438607392, 53.48035201082151247, 5.440088680355550821 ) ) ;
#81397=CARTESIAN_POINT ( 'NONE',  ( 15.44008868035555260, 44.73035201082151247, 9.422509992056143702 ) ) ;
#81398=CARTESIAN_POINT ( 'NONE',  ( 22.81628187352648496, 16.83196800326374998, -3.434112377981050290 ) ) ;
#81399=CARTESIAN_POINT ( 'NONE',  ( 0.1922240491738349266, 48.18878173731740588, 6.499999999999949374 ) ) ;
#81401=CARTESIAN_POINT ( 'NONE',  ( 1.472469842513823179, 26.42559781766745175, 4.923371831947296329 ) ) ;
#81403=CARTESIAN_POINT ( 'NONE',  ( 17.96484262340118221, 41.18868534415484106, -7.964842623401177768 ) ) ;
#81404=ADVANCED_FACE ( 'NONE', ( #14565 ), #30618, .F. ) ;
#81405=CARTESIAN_POINT ( 'NONE',  ( 6.565887622018943937, 8.081968003263751754, -12.81628187352647608 ) ) ;
#81406=CARTESIAN_POINT ( 'NONE',  ( 1.472469842513823179, 1.425597817667451528, 4.923371831947296329 ) ) ;
#81407=CARTESIAN_POINT ( 'NONE',  ( 19.84674366389459621, 28.50893115100078745, 7.409399052514197653E-17 ) ) ;
#81408=CARTESIAN_POINT ( 'NONE',  ( 19.38216949554541557, 47.24863466993041783, -9.382169495545420901 ) ) ;
#81409=CARTESIAN_POINT ( 'NONE',  ( 12.63842701281683034, 7.467264484334118713, 9.846743663894596210 ) ) ;
#81412=LINE ( 'NONE', #66409, #57363 ) ;
#81413=CARTESIAN_POINT ( 'NONE',  ( 17.96484262340118221, 21.18868534415483396, -7.964842623401177768 ) ) ;
#81414=LINE ( 'NONE', #21417, #64818 ) ;
#81415=CARTESIAN_POINT ( 'NONE',  ( -4.164238869374098151, 36.59541550158063217, -3.795296366450310543 ) ) ;
#81416=CARTESIAN_POINT ( 'NONE',  ( 12.63842701281683034, 32.46726448433412315, 9.846743663894596210 ) ) ;
#81418=CARTESIAN_POINT ( 'NONE',  ( 17.96484262340118221, 19.93868534415484106, 7.964842623401181321 ) ) ;
#81419=CARTESIAN_POINT ( 'NONE',  ( 2.035157376598824452, 8.688685344154839285, 7.964842623401179544 ) ) ;
#81421=CARTESIAN_POINT ( 'NONE',  ( -0.8801773607111009756, 33.06368534415484106, 1.068504757029289695E-15 ) ) ;
#81422=CARTESIAN_POINT ( 'NONE',  ( 12.91533473730992121, 34.52201867748817676, 10.88017736071110164 ) ) ;
#81424=CARTESIAN_POINT ( 'NONE',  ( 17.96484262340118221, 34.93868534415482685, 7.964842623401181321 ) ) ;
#81425=ORIENTED_EDGE ( 'NONE', *, *, #18638, .F. ) ;
#81427=CARTESIAN_POINT ( 'NONE',  ( 4.559911319644449179, 33.89701867748817676, 9.422509992056141925 ) ) ;
#81430=CARTESIAN_POINT ( 'NONE',  ( 0.6178305044545838731, 59.74863466993041783, 9.382169495545420901 ) ) ;
#81431=CARTESIAN_POINT ( 'NONE',  ( -0.1503990784575403861, 9.248846992468887862, -6.262539305110056631 ) ) ;
#81432=CARTESIAN_POINT ( 'NONE',  ( 2.917880565312948704, 37.63708216824731068, 12.26659068614894643 ) ) ;
#81433=CARTESIAN_POINT ( 'NONE',  ( 0.5774900079438590739, 47.64701867748817676, -5.440088680355550821 ) ) ;
#81434=CARTESIAN_POINT ( 'NONE',  ( 20.03447792253738768, 42.65514106990691090, -6.401564815979734036 ) ) ;
#81436=CARTESIAN_POINT ( 'NONE',  ( 10.00000000000000178, 47.25893115100078745, 9.846743663894594434 ) ) ;
#81440=CARTESIAN_POINT ( 'NONE',  ( 19.84674366389459266, 18.30059781766745175, 2.638427012816836559 ) ) ;
#81442=EDGE_CURVE ( 'NONE', #55640, #80446, #29784, .T. ) ;
#81443=CARTESIAN_POINT ( 'NONE',  ( 7.084665262690076126, 17.02201867748817676, -10.88017736071110164 ) ) ;
#81444=CARTESIAN_POINT ( 'NONE',  ( 0.1532563361054082862, 31.21726448433412315, 2.638427012816831674 ) ) ;
#81445=CARTESIAN_POINT ( 'NONE',  ( 21.09922568453594849, 11.20696800326375531, 6.408140936763242479 ) ) ;
#81446=CARTESIAN_POINT ( 'NONE',  ( 2.035157376598824452, 53.68868534415484817, 7.964842623401179544 ) ) ;
#81447=CARTESIAN_POINT ( 'NONE',  ( 15.44008868035555793, 26.39701867748817321, -9.422509992056140149 ) ) ;
#81448=CARTESIAN_POINT ( 'NONE',  ( 3.591859063236763294, 53.29030133659708923, -11.09922568453595026 ) ) ;
#81449=CARTESIAN_POINT ( 'NONE',  ( 6.204703633549690345, 40.76208216824731778, -14.16423886937410259 ) ) ;
#81453=CARTESIAN_POINT ( 'NONE',  ( 21.09922568453595559, 2.040301336597086568, -6.408140936763230044 ) ) ;
#81454=CARTESIAN_POINT ( 'NONE',  ( 19.42250999205614548, 10.98035201082150358, -5.440088680355545492 ) ) ;
#81455=CARTESIAN_POINT ( 'NONE',  ( 4.559911319644449179, 47.23035201082150536, -9.422509992056141925 ) ) ;
#81456=CARTESIAN_POINT ( 'NONE',  ( 5.076628168052704559, 65.17559781766745175, -8.527530157486179263 ) ) ;
#81458=CARTESIAN_POINT ( 'NONE',  ( 7.361572987183170547, 12.05059781766744997, 9.846743663894590881 ) ) ;
#81459=CARTESIAN_POINT ( 'NONE',  ( 12.63842701281683034, 42.46726448433412315, 9.846743663894596210 ) ) ;
#81460=CARTESIAN_POINT ( 'NONE',  ( 1.472469842513823179, 6.425597817667451750, 4.923371831947296329 ) ) ;
#81461=CARTESIAN_POINT ( 'NONE',  ( 10.00000000000000000, 19.75893115100078390, -9.846743663894594434 ) ) ;
#81463=CARTESIAN_POINT ( 'NONE',  ( 12.63842701281683034, 7.467264484334118713, 9.846743663894596210 ) ) ;
#81465=CARTESIAN_POINT ( 'NONE',  ( 5.076628168052704559, 10.17559781766745175, -8.527530157486179263 ) ) ;
#81466=CARTESIAN_POINT ( 'NONE',  ( 10.00000000000000178, 22.25893115100078745, 9.846743663894594434 ) ) ;
#81470=CARTESIAN_POINT ( 'NONE',  ( 0.1532563361054082862, 66.21726448433413736, 2.638427012816831674 ) ) ;
#81471=ORIENTED_EDGE ( 'NONE', *, *, #49595, .T. ) ;
#81472=PRESENTATION_STYLE_ASSIGNMENT (( #43470 ) ) ;
#81473=CARTESIAN_POINT ( 'NONE',  ( 24.16423886937410614, 19.30374883491397142, 8.672049930838204340E-16 ) ) ;
#81474=UNCERTAINTY_MEASURE_WITH_UNIT (LENGTH_MEASURE( 1.000000000000000082E-05 ), #65515, 'distance_accuracy_value', 'NONE');
#81476=CARTESIAN_POINT ( 'NONE',  ( 24.16423886937410614, 19.30374883491397142, 8.672049930838204340E-16 ) ) ;
#81477=CARTESIAN_POINT ( 'NONE',  ( 20.36894250292379738, 49.92874883491396787, -10.36894250292379027 ) ) ;
#81479=CARTESIAN_POINT ( 'NONE',  ( 2.917880565312950480, 15.97041550158063217, -12.26659068614894821 ) ) ;
#81480=CARTESIAN_POINT ( 'NONE',  ( 10.00000000000000178, 39.31368534415484106, 10.88017736071110342 ) ) ;
#81482=CARTESIAN_POINT ( 'NONE',  ( 2.791683348922240793, 26.63393115100078745, 7.208316651077764092 ) ) ;
#81483=CARTESIAN_POINT ( 'NONE',  ( 0.5774900079438607392, 53.48035201082151247, 5.440088680355550821 ) ) ;
#81484=CARTESIAN_POINT ( 'NONE',  ( 0.1532563361054100626, 35.80059781766745175, -2.638427012816831230 ) ) ;
#81486=CARTESIAN_POINT ( 'NONE',  ( -0.8801773607111008646, 8.272018677488171434, 2.915334737309923430 ) ) ;
#81487=CARTESIAN_POINT ( 'NONE',  ( 0.6178305044545838731, 64.74863466993043914, 9.382169495545420901 ) ) ;
#81488=CARTESIAN_POINT ( 'NONE',  ( 19.84674366389459621, 48.50893115100078745, 7.409399052514197653E-17 ) ) ;
#81490=CARTESIAN_POINT ( 'NONE',  ( 21.09922568453594849, 41.20696800326375353, 6.408140936763242479 ) ) ;
#81492=CARTESIAN_POINT ( 'NONE',  ( 0.5774900079438607392, 48.48035201082150536, 5.440088680355550821 ) ) ;
#81493=CARTESIAN_POINT ( 'NONE',  ( 5.076628168052704559, 40.17559781766745175, -8.527530157486179263 ) ) ;
#81494=CARTESIAN_POINT ( 'NONE',  ( 22.26659068614894466, 23.88708216824730357, 7.082119434687054849 ) ) ;
#81496=CARTESIAN_POINT ( 'NONE',  ( -2.266590686148945544, 2.220415501580634388, 7.082119434687048631 ) ) ;
#81497=CARTESIAN_POINT ( 'NONE',  ( 17.96484262340118221, 56.18868534415484817, -7.964842623401177768 ) ) ;
#81498=CARTESIAN_POINT ( 'NONE',  ( -0.8801773607111008646, 63.27201867748817676, 2.915334737309923430 ) ) ;
#81499=CARTESIAN_POINT ( 'NONE',  ( 10.00000000000000000, 50.55374883491396787, -14.16423886937410082 ) ) ;
#81500=CARTESIAN_POINT ( 'NONE',  ( 14.92337183194729988, 64.34226448433412315, -8.527530157486177487 ) ) ;
#81501=CARTESIAN_POINT ( 'NONE',  ( -1.099225684535947600, 64.54030133659709634, 6.408140936763237150 ) ) ;
#81502=CARTESIAN_POINT ( 'NONE',  ( 19.42250999205614193, 55.14701867748817676, 5.440088680355555262 ) ) ;
#81503=DIRECTION ( 'NONE',  ( 0.000000000000000000, 0.000000000000000000, 1.000000000000000000 ) ) ;
#81505=CARTESIAN_POINT ( 'NONE',  ( 7.361572987183170547, 52.05059781766745175, 9.846743663894590881 ) ) ;
#81506=B_SPLINE_CURVE_WITH_KNOTS ( 'NONE', 3,
 ( #69425, #45435, #92902, #77400, #38443, #38936 ),
 .UNSPECIFIED., .F., .F.,
 ( 4, 2, 4 ),
 ( 0.000000000000000000, 0.0002701661927229432507, 0.0005403323854458865014 ),
 .UNSPECIFIED. ) ;
#81508=CARTESIAN_POINT ( 'NONE',  ( 17.96484262340118221, 6.188685344154837509, -7.964842623401177768 ) ) ;
#81511=CARTESIAN_POINT ( 'NONE',  ( 0.5774900079438590739, 7.647018677488171434, -5.440088680355550821 ) ) ;
#81512=CARTESIAN_POINT ( 'NONE',  ( 12.63842701281683034, 2.467264484334118269, 9.846743663894596210 ) ) ;
#81513=CARTESIAN_POINT ( 'NONE',  ( 7.084665262690076126, 67.02201867748817676, -10.88017736071110164 ) ) ;
#81514=VECTOR ( 'NONE', #20617, 1000.000000000000000 ) ;
#81515=EDGE_CURVE ( 'NONE', #93646, #18045, #54504, .T. ) ;
#81516=CARTESIAN_POINT ( 'NONE',  ( 19.84674366389459266, 38.30059781766745175, 2.638427012816836559 ) ) ;
#81517=CARTESIAN_POINT ( 'NONE',  ( 19.42250999205614193, 40.14701867748817676, 5.440088680355555262 ) ) ;
#81518=CARTESIAN_POINT ( 'NONE',  ( 10.00000000000000000, 7.873634669930421381, -12.81628187352647608 ) ) ;
#81519=CARTESIAN_POINT ( 'NONE',  ( -0.8801773607111009756, 38.06368534415484106, 1.068504757029289695E-15 ) ) ;
#81522=CARTESIAN_POINT ( 'NONE',  ( 13.43411237798105340, 40.58196800326375353, 12.81628187352647963 ) ) ;
#81524=CARTESIAN_POINT ( 'NONE',  ( 10.00000000000000000, 61.81368534415484106, -10.88017736071110342 ) ) ;
#81525=EDGE_CURVE ( 'NONE', #86159, #43572, #59387, .T. ) ;
#81526=CARTESIAN_POINT ( 'NONE',  ( -2.816281873526471635, 28.91530133659708213, -3.434112377981056508 ) ) ;
#81527=CARTESIAN_POINT ( 'NONE',  ( 2.791683348922237240, 0.3839311510007847872, -7.208316651077763204 ) ) ;
#81528=CARTESIAN_POINT ( 'NONE',  ( 2.035157376598824452, 38.68868534415483396, 7.964842623401179544 ) ) ;
#81529=CARTESIAN_POINT ( 'NONE',  ( 5.076628168052703671, 66.84226448433412315, 8.527530157486179263 ) ) ;
#81530=CARTESIAN_POINT ( 'NONE',  ( 13.79529636645030344, 58.26208216824728936, 14.16423886937410614 ) ) ;
#81531=CARTESIAN_POINT ( 'NONE',  ( 19.84674366389459266, 53.30059781766744464, 2.638427012816836559 ) ) ;
#81532=CARTESIAN_POINT ( 'NONE',  ( 10.00000000000000178, 2.258931151000784787, 9.846743663894594434 ) ) ;
#81533=CARTESIAN_POINT ( 'NONE',  ( 7.084665262690076126, 62.02201867748816966, -10.88017736071110164 ) ) ;
#81535=CARTESIAN_POINT ( 'NONE',  ( -4.164238869374098151, 31.59541550158063927, -3.795296366450310543 ) ) ;
#81538=CARTESIAN_POINT ( 'NONE',  ( 6.204703633549690345, 57.84541550158063927, 14.16423886937410082 ) ) ;
#81539=CARTESIAN_POINT ( 'NONE',  ( 24.16423886937410614, 64.30374883491396076, 8.672049930838204340E-16 ) ) ;
#81540=CARTESIAN_POINT ( 'NONE',  ( 0.1532563361054100626, 30.80059781766744820, -2.638427012816831230 ) ) ;
#81541=CARTESIAN_POINT ( 'NONE',  ( -2.816281873526471635, 28.91530133659708213, -3.434112377981056508 ) ) ;
#81543=DIRECTION ( 'NONE',  ( -0.5547001962252290364, -0.8320502943378437211, 0.000000000000000000 ) ) ;
#81544=CARTESIAN_POINT ( 'NONE',  ( 4.559911319644449179, 17.23035201082150536, -9.422509992056141925 ) ) ;
#81545=CARTESIAN_POINT ( 'NONE',  ( 6.204703633549690345, 57.84541550158063927, 14.16423886937410082 ) ) ;
#81546=CARTESIAN_POINT ( 'NONE',  ( 14.92337183194729988, 24.34226448433411960, -8.527530157486177487 ) ) ;
#81548=CARTESIAN_POINT ( 'NONE',  ( 14.92337183194729988, 9.342264484334119601, -8.527530157486177487 ) ) ;
#81551=CARTESIAN_POINT ( 'NONE',  ( 18.50749283717775029, 59.69955587570481725, 6.500000000000035527 ) ) ;
#81553=ORIENTED_EDGE ( 'NONE', *, *, #66371, .F. ) ;
#81558=CARTESIAN_POINT ( 'NONE',  ( 2.791683348922237240, 40.38393115100078035, -7.208316651077763204 ) ) ;
#81559=CARTESIAN_POINT ( 'NONE',  ( -0.8801773607111008646, 23.27201867748817676, 2.915334737309923430 ) ) ;
#81560=CARTESIAN_POINT ( 'NONE',  ( 2.035157376598824452, 18.68868534415484106, 7.964842623401179544 ) ) ;
#81561=CARTESIAN_POINT ( 'NONE',  ( 0.1532563361054100626, 55.80059781766745175, -2.638427012816831230 ) ) ;
#81562=CARTESIAN_POINT ( 'NONE',  ( 10.00000000000000178, 15.37363466993042138, 12.81628187352647608 ) ) ;
#81563=CARTESIAN_POINT ( 'NONE',  ( -4.164238869374099039, 6.803748834913967869, 8.674139862899312516E-16 ) ) ;
#81564=CARTESIAN_POINT ( 'NONE',  ( 19.84674366389459266, 43.30059781766744464, 2.638427012816836559 ) ) ;
#81566=CARTESIAN_POINT ( 'NONE',  ( 16.40814093676323893, 35.79030133659708923, 11.09922568453595026 ) ) ;
#81568=CARTESIAN_POINT ( 'NONE',  ( 18.52753015748618282, 28.92559781766745175, -4.923371831947291888 ) ) ;
#81569=CARTESIAN_POINT ( 'NONE',  ( 22.26659068614895176, 59.72041550158063927, -7.082119434687042414 ) ) ;
#81571=CARTESIAN_POINT ( 'NONE',  ( -0.8801773607111009756, 3.063685344154838397, 1.068504757029289695E-15 ) ) ;
#81574=CARTESIAN_POINT ( 'NONE',  ( 17.96484262340118221, 49.93868534415484106, 7.964842623401181321 ) ) ;
#81575=CARTESIAN_POINT ( 'NONE',  ( 15.44008868035555260, 44.73035201082151247, 9.422509992056143702 ) ) ;
#81576=CARTESIAN_POINT ( 'NONE',  ( 10.00000000000000000, 51.81368534415484106, -10.88017736071110342 ) ) ;
#81578=CARTESIAN_POINT ( 'NONE',  ( 7.084665262690076126, 39.10535201082150536, 10.88017736071109987 ) ) ;
#81579=CARTESIAN_POINT ( 'NONE',  ( 1.602071938427535702, 47.02224192338641018, -6.500000000000077272 ) ) ;
#81582=CARTESIAN_POINT ( 'NONE',  ( 18.52753015748618282, 28.92559781766745175, -4.923371831947291888 ) ) ;
#81583=ORIENTED_EDGE ( 'NONE', *, *, #40324, .T. ) ;
#81584=CARTESIAN_POINT ( 'NONE',  ( 2.791683348922240793, 51.63393115100078745, 7.208316651077764092 ) ) ;
#81586=ADVANCED_FACE ( 'NONE', ( #60535 ), #40022, .T. ) ;
#81587=CARTESIAN_POINT ( 'NONE',  ( 2.917880565312950480, 10.97041550158063572, -12.26659068614894821 ) ) ;
#81591=CARTESIAN_POINT ( 'NONE',  ( 13.79529636645030344, 63.26208216824730357, 14.16423886937410614 ) ) ;
#81595=CARTESIAN_POINT ( 'NONE',  ( 18.52753015748617571, 48.09226448433412315, 4.923371831947298993 ) ) ;
#81597=CARTESIAN_POINT ( 'NONE',  ( 0.6178305044545838731, 14.74863466993041783, 9.382169495545420901 ) ) ;
#81598=CARTESIAN_POINT ( 'NONE',  ( 17.20831665107776587, 4.133931151000785675, -7.208316651077762316 ) ) ;
#81601=CARTESIAN_POINT ( 'NONE',  ( 12.63842701281683034, 12.46726448433411782, 9.846743663894596210 ) ) ;
#81602=CARTESIAN_POINT ( 'NONE',  ( 2.791683348922240793, 66.63393115100079456, 7.208316651077764092 ) ) ;
#81606=EDGE_CURVE ( 'NONE', #68278, #83096, #11635, .T. ) ;
#81608=CARTESIAN_POINT ( 'NONE',  ( 7.084665262690076126, 7.022018677488170546, -10.88017736071110164 ) ) ;
#81609=CARTESIAN_POINT ( 'NONE',  ( -0.3689425029237881626, 2.428748834913967869, 10.36894250292379027 ) ) ;
#81610=CARTESIAN_POINT ( 'NONE',  ( 0.1532563361054083140, 26.00893115100078745, 1.131784320476157264E-15 ) ) ;
#81611=CARTESIAN_POINT ( 'NONE',  ( -0.8801773607110991993, 57.85535201082149825, -2.915334737309923874 ) ) ;
#81612=AXIS2_PLACEMENT_3D ( 'NONE', #69005, #68512, #30984 ) ;
#81613=CARTESIAN_POINT ( 'NONE',  ( 13.43411237798106583, 32.66530133659708213, -12.81628187352647252 ) ) ;
#81615=CARTESIAN_POINT ( 'NONE',  ( 10.00000000000000000, 6.813685344154838397, -10.88017736071110342 ) ) ;
#81617=CARTESIAN_POINT ( 'NONE',  ( 17.20831665107776587, 59.13393115100078745, -7.208316651077762316 ) ) ;
#81618=CARTESIAN_POINT ( 'NONE',  ( 14.92337183194729988, 19.34226448433411960, -8.527530157486177487 ) ) ;
#81620=CARTESIAN_POINT ( 'NONE',  ( 22.81628187352648496, 26.83196800326374998, -3.434112377981050290 ) ) ;
#81623=CARTESIAN_POINT ( 'NONE',  ( 19.42250999205614548, 40.98035201082150536, -5.440088680355545492 ) ) ;
#81627=CARTESIAN_POINT ( 'NONE',  ( 12.91533473730992121, 24.52201867748816966, 10.88017736071110164 ) ) ;
#81628=CARTESIAN_POINT ( 'NONE',  ( 19.84674366389459266, 48.30059781766745175, 2.638427012816836559 ) ) ;
#81630=CARTESIAN_POINT ( 'NONE',  ( 20.88017736071110164, 55.35535201082149825, 2.915334737309930979 ) ) ;
#81631=CARTESIAN_POINT ( 'NONE',  ( -4.164238869374099927, 37.01208216824731068, 3.795296366450308767 ) ) ;
#81633=CARTESIAN_POINT ( 'NONE',  ( 7.361572987183170547, 37.05059781766744464, 9.846743663894590881 ) ) ;
#81634=CARTESIAN_POINT ( 'NONE',  ( 16.40814093676324603, 62.45696800326376064, -11.09922568453594671 ) ) ;
#81635=CARTESIAN_POINT ( 'NONE',  ( 19.84674366389459266, 63.30059781766745886, 2.638427012816836559 ) ) ;
#81637=CARTESIAN_POINT ( 'NONE',  ( 2.035157376598824452, 28.68868534415484106, 7.964842623401179544 ) ) ;
#81639=CARTESIAN_POINT ( 'NONE',  ( -0.8801773607111009756, 18.06368534415484106, 1.068504757029289695E-15 ) ) ;
#81640=CARTESIAN_POINT ( 'NONE',  ( 10.00000000000000178, 69.31368534415484817, 10.88017736071110342 ) ) ;
#81641=CARTESIAN_POINT ( 'NONE',  ( 22.26659068614895176, 29.72041550158063572, -7.082119434687042414 ) ) ;
#81642=CARTESIAN_POINT ( 'NONE',  ( 10.00000000000000178, 12.25893115100078568, 9.846743663894594434 ) ) ;
#81643=CARTESIAN_POINT ( 'NONE',  ( 10.00000000000000178, 67.25893115100079456, 9.846743663894594434 ) ) ;
#81644=CARTESIAN_POINT ( 'NONE',  ( 12.91533473730992121, 34.52201867748817676, 10.88017736071110164 ) ) ;
#81649=CARTESIAN_POINT ( 'NONE',  ( 5.076628168052704559, 45.17559781766745175, -8.527530157486179263 ) ) ;
#81652=( GEOMETRIC_REPRESENTATION_CONTEXT ( 3 ) GLOBAL_UNCERTAINTY_ASSIGNED_CONTEXT ( ( #35483 ) ) GLOBAL_UNIT_ASSIGNED_CONTEXT ( ( #40834, #87302, #24368 ) ) REPRESENTATION_CONTEXT ( 'NONE', 'WORKASPACE' ) );
#81654=CARTESIAN_POINT ( 'NONE',  ( 6.204703633549690345, 27.84541550158063217, 14.16423886937410082 ) ) ;
#81655=CARTESIAN_POINT ( 'NONE',  ( 24.16423886937410614, 9.512082168247301794, -3.795296366450302550 ) ) ;
#81656=CARTESIAN_POINT ( 'NONE',  ( 4.559911319644449179, 58.89701867748817676, 9.422509992056141925 ) ) ;
#81657=CARTESIAN_POINT ( 'NONE',  ( 6.204703633549690345, 52.84541550158062506, 14.16423886937410082 ) ) ;
#81658=CARTESIAN_POINT ( 'NONE',  ( 10.00000000000000178, 67.25893115100079456, 9.846743663894594434 ) ) ;
#81659=CARTESIAN_POINT ( 'NONE',  ( 19.84674366389459266, 53.71726448433411605, -2.638427012816827677 ) ) ;
#81660=CARTESIAN_POINT ( 'NONE',  ( 10.00000000000000000, 46.81368534415484106, -10.88017736071110342 ) ) ;
#81661=CARTESIAN_POINT ( 'NONE',  ( -1.099225684535947600, 4.540301336597087456, 6.408140936763237150 ) ) ;
#81662=CARTESIAN_POINT ( 'NONE',  ( -4.164238869374099039, 21.80374883491396787, 8.674139862899312516E-16 ) ) ;
#81663=CARTESIAN_POINT ( 'NONE',  ( 10.00000000000000000, 16.81368534415483751, -10.88017736071110342 ) ) ;
#81664=CARTESIAN_POINT ( 'NONE',  ( 19.80832241502128355, 14.75868815902069997, 6.499999999999992895 ) ) ;
#81666=CARTESIAN_POINT ( 'NONE',  ( 4.559911319644449179, 47.23035201082150536, -9.422509992056141925 ) ) ;
#81668=ORIENTED_EDGE ( 'NONE', *, *, #10500, .T. ) ;
#81670=VERTEX_POINT ( 'NONE', #66948 ) ;
#81672=CARTESIAN_POINT ( 'NONE',  ( -4.164238869374099927, 47.01208216824729647, 3.795296366450308767 ) ) ;
#81673=CARTESIAN_POINT ( 'NONE',  ( 1.472469842513823179, 41.42559781766745886, 4.923371831947296329 ) ) ;
#81674=CARTESIAN_POINT ( 'NONE',  ( 19.42250999205614193, 60.14701867748817676, 5.440088680355555262 ) ) ;
#81676=EDGE_CURVE ( 'NONE', #39981, #45554, #68067, .T. ) ;
#81677=CARTESIAN_POINT ( 'NONE',  ( 2.035157376598822676, 57.43868534415484106, -7.964842623401177768 ) ) ;
#81678=CARTESIAN_POINT ( 'NONE',  ( 13.43411237798106583, 57.66530133659708923, -12.81628187352647252 ) ) ;
#81681=CARTESIAN_POINT ( 'NONE',  ( 0.5774900079438590739, 47.64701867748817676, -5.440088680355550821 ) ) ;
#81682=( GEOMETRIC_REPRESENTATION_CONTEXT ( 3 ) GLOBAL_UNCERTAINTY_ASSIGNED_CONTEXT ( ( #22400 ) ) GLOBAL_UNIT_ASSIGNED_CONTEXT ( ( #69495, #86948, #2505 ) ) REPRESENTATION_CONTEXT ( 'NONE', 'WORKASPACE' ) );
#81683=CARTESIAN_POINT ( 'NONE',  ( 2.917880565312950480, 25.97041550158063572, -12.26659068614894821 ) ) ;
#81685=CARTESIAN_POINT ( 'NONE',  ( 10.00000000000000000, 22.87363466993042138, -12.81628187352647608 ) ) ;
#81687=CARTESIAN_POINT ( 'NONE',  ( 3.591859063236763294, 43.29030133659708923, -11.09922568453595026 ) ) ;
#81688=CARTESIAN_POINT ( 'NONE',  ( -0.8801773607110991993, 17.85535201082150536, -2.915334737309923874 ) ) ;
#81689=CARTESIAN_POINT ( 'NONE',  ( 17.20831665107776587, 37.88393115100078745, 7.208316651077764980 ) ) ;
#81690=CARTESIAN_POINT ( 'NONE',  ( 10.00000000000000178, 9.313685344154839285, 10.88017736071110342 ) ) ;
#81692=CARTESIAN_POINT ( 'NONE',  ( -2.816281873526471635, 58.91530133659707502, -3.434112377981056508 ) ) ;
#81694=CARTESIAN_POINT ( 'NONE',  ( 5.076628168052703671, 41.84226448433411605, 8.527530157486179263 ) ) ;
#81696=CARTESIAN_POINT ( 'NONE',  ( 2.035157376598822676, 67.43868534415484817, -7.964842623401177768 ) ) ;
#81698=CARTESIAN_POINT ( 'NONE',  ( -13.69000000000001549, 92.00000000000000000, -10.09898361729590199 ) ) ;
#81700=CARTESIAN_POINT ( 'NONE',  ( 4.555630843329481650, 77.03495325336413657, 9.500000000000000000 ) ) ;
#81702=CARTESIAN_POINT ( 'NONE',  ( 2.791683348922240793, 11.63393115100078568, 7.208316651077764092 ) ) ;
#81703=CARTESIAN_POINT ( 'NONE',  ( 19.38216949554541557, 27.24863466993041783, -9.382169495545420901 ) ) ;
#81705=CARTESIAN_POINT ( 'NONE',  ( 17.20831665107776587, 52.88393115100078035, 7.208316651077764980 ) ) ;
#81707=CARTESIAN_POINT ( 'NONE',  ( 2.917880565312950480, 20.97041550158063217, -12.26659068614894821 ) ) ;
#81708=CARTESIAN_POINT ( 'NONE',  ( 17.20831665107776587, 42.88393115100077324, 7.208316651077764980 ) ) ;
#81709=CARTESIAN_POINT ( 'NONE',  ( 16.40814093676324603, 47.45696800326375353, -11.09922568453594671 ) ) ;
#81711=FILL_AREA_STYLE ('',( #73719 ) ) ;
#81712=CARTESIAN_POINT ( 'NONE',  ( 19.42250999205614548, 60.98035201082151247, -5.440088680355545492 ) ) ;
#81714=CARTESIAN_POINT ( 'NONE',  ( 20.24186590665277308, 47.61633188102327097, -6.114288769123048972 ) ) ;
#81715=CARTESIAN_POINT ( 'NONE',  ( 5.076628168052704559, 35.17559781766745175, -8.527530157486179263 ) ) ;
#81716=CARTESIAN_POINT ( 'NONE',  ( -0.8801773607111009756, 43.06368534415484106, 1.068504757029289695E-15 ) ) ;
#81717=CARTESIAN_POINT ( 'NONE',  ( 19.38216949554541557, 37.24863466993041783, -9.382169495545420901 ) ) ;
#81720=CARTESIAN_POINT ( 'NONE',  ( 19.42250999205614548, 40.98035201082150536, -5.440088680355545492 ) ) ;
#81724=CARTESIAN_POINT ( 'NONE',  ( 2.035157376598822676, 12.43868534415483751, -7.964842623401177768 ) ) ;
#81725=CARTESIAN_POINT ( 'NONE',  ( 18.52753015748617571, 63.09226448433412315, 4.923371831947298993 ) ) ;
#81726=CARTESIAN_POINT ( 'NONE',  ( 20.88017736071110519, 40.56368534415484106, 2.639326808657452039E-16 ) ) ;
#81728=CARTESIAN_POINT ( 'NONE',  ( 4.559911319644449179, 62.23035201082150536, -9.422509992056141925 ) ) ;
#81729=CARTESIAN_POINT ( 'NONE',  ( -0.8801773607111008646, 28.27201867748817321, 2.915334737309923430 ) ) ;
#81730=CARTESIAN_POINT ( 'NONE',  ( -0.000000000000000000, 71.20572488941321865, -5.000000000000000888 ) ) ;
#81731=CARTESIAN_POINT ( 'NONE',  ( 10.00000000000000000, -0.2410688489992152128, -9.846743663894594434 ) ) ;
#81732=CARTESIAN_POINT ( 'NONE',  ( 1.472469842513823179, 25.59226448433412315, -4.923371831947296329 ) ) ;
#81735=CARTESIAN_POINT ( 'NONE',  ( 5.076628168052703671, 46.84226448433412315, 8.527530157486179263 ) ) ;
#81736=CARTESIAN_POINT ( 'NONE',  ( 17.08211943468705130, 53.47041550158063217, 12.26659068614894998 ) ) ;
#81737=CARTESIAN_POINT ( 'NONE',  ( 20.15039907845753220, 19.72266099184918886, 6.262539305110075283 ) ) ;
#81739=CARTESIAN_POINT ( 'NONE',  ( 13.79529636645030344, 13.26208216824729824, 14.16423886937410614 ) ) ;
#81740=CARTESIAN_POINT ( 'NONE',  ( -4.164238869374098151, 31.59541550158063927, -3.795296366450310543 ) ) ;
#81741=CARTESIAN_POINT ( 'NONE',  ( 6.565887622018943937, 8.081968003263751754, -12.81628187352647608 ) ) ;
#81743=CARTESIAN_POINT ( 'NONE',  ( 20.88017736071110519, 10.56368534415483929, 2.639326808657452039E-16 ) ) ;
#81744=CARTESIAN_POINT ( 'NONE',  ( 12.63842701281683034, 42.46726448433412315, 9.846743663894596210 ) ) ;
#81749=CARTESIAN_POINT ( 'NONE',  ( 12.63842701281683034, 2.467264484334118269, 9.846743663894596210 ) ) ;
#81750=CARTESIAN_POINT ( 'NONE',  ( -1.099225684535947600, 28.70696800326375353, -6.408140936763238038 ) ) ;
#81751=CARTESIAN_POINT ( 'NONE',  ( 7.361572987183170547, 32.05059781766745175, 9.846743663894590881 ) ) ;
#81752=ORIENTED_EDGE ( 'NONE', *, *, #66046, .F. ) ;
#81753=CARTESIAN_POINT ( 'NONE',  ( 5.076628168052703671, 6.842264484334118713, 8.527530157486179263 ) ) ;
#81756=CARTESIAN_POINT ( 'NONE',  ( 18.50749283717776805, 4.699555875704811925, 6.500000000000004441 ) ) ;
#81758=CARTESIAN_POINT ( 'NONE',  ( 19.42250999205614548, 15.98035201082150714, -5.440088680355545492 ) ) ;
#81759=CARTESIAN_POINT ( 'NONE',  ( -4.164238869374099927, 42.01208216824728936, 3.795296366450308767 ) ) ;
#81760=CARTESIAN_POINT ( 'NONE',  ( 2.035157376598824452, 68.68868534415484817, 7.964842623401179544 ) ) ;
#81761=CARTESIAN_POINT ( 'NONE',  ( -0.1503990784575242878, 49.24884699246889141, -6.262539305110083276 ) ) ;
#81762=CARTESIAN_POINT ( 'NONE',  ( 19.84674366389459621, 28.50893115100078745, 7.409399052514197653E-17 ) ) ;
#81763=CARTESIAN_POINT ( 'NONE',  ( 20.15039907845753220, 21.74884699246888786, 6.262539305110078836 ) ) ;
#81764=CARTESIAN_POINT ( 'NONE',  ( 0.1532563361054100626, 5.800597817667452638, -2.638427012816831230 ) ) ;
#81765=( GEOMETRIC_REPRESENTATION_CONTEXT ( 3 ) GLOBAL_UNCERTAINTY_ASSIGNED_CONTEXT ( ( #93093 ) ) GLOBAL_UNIT_ASSIGNED_CONTEXT ( ( #26035, #4029, #48025 ) ) REPRESENTATION_CONTEXT ( 'NONE', 'WORKASPACE' ) );
#81766=CARTESIAN_POINT ( 'NONE',  ( 1.152268111383477178, 1.024801820426059406E-17, -6.000000000000281553 ) ) ;
#81767=CARTESIAN_POINT ( 'NONE',  ( 1.472469842513823179, 35.59226448433412315, -4.923371831947296329 ) ) ;
#81768=CARTESIAN_POINT ( 'NONE',  ( 18.52753015748617571, 63.09226448433412315, 4.923371831947298993 ) ) ;
#81769=CARTESIAN_POINT ( 'NONE',  ( 17.96484262340118221, 39.93868534415484106, 7.964842623401181321 ) ) ;
#81771=ORIENTED_EDGE ( 'NONE', *, *, #90440, .T. ) ;
#81772=CARTESIAN_POINT ( 'NONE',  ( 3.591859063236763294, 58.29030133659708923, -11.09922568453595026 ) ) ;
#81773=CARTESIAN_POINT ( 'NONE',  ( 2.791683348922240793, 1.633931151000784565, 7.208316651077764092 ) ) ;
#81774=CARTESIAN_POINT ( 'NONE',  ( 6.565887622018943937, 40.16530133659708923, 12.81628187352647430 ) ) ;
#81775=CARTESIAN_POINT ( 'NONE',  ( 22.26659068614895176, 59.72041550158063927, -7.082119434687042414 ) ) ;
#81776=CARTESIAN_POINT ( 'NONE',  ( 19.84674366389459266, 33.30059781766744464, 2.638427012816836559 ) ) ;
#81778=CARTESIAN_POINT ( 'NONE',  ( 5.076628168052703671, 1.842264484334118047, 8.527530157486179263 ) ) ;
#81779=CARTESIAN_POINT ( 'NONE',  ( 20.36894250292379382, 18.67874883491397142, 10.36894250292379205 ) ) ;
#81780=CARTESIAN_POINT ( 'NONE',  ( 13.79529636645031943, 40.34541550158063217, -14.16423886937409904 ) ) ;
#81781=CARTESIAN_POINT ( 'NONE',  ( 2.791683348922240793, 41.63393115100078745, 7.208316651077764092 ) ) ;
#81783=CARTESIAN_POINT ( 'NONE',  ( 12.91533473730993009, 41.60535201082149825, -10.88017736071109987 ) ) ;
#81784=CARTESIAN_POINT ( 'NONE',  ( 20.88017736071110164, 55.35535201082149825, 2.915334737309930979 ) ) ;
#81786=CARTESIAN_POINT ( 'NONE',  ( 21.09922568453595559, 42.04030133659708213, -6.408140936763230044 ) ) ;
#81787=CARTESIAN_POINT ( 'NONE',  ( 19.42250999205614193, 65.14701867748817676, 5.440088680355555262 ) ) ;
#81789=CARTESIAN_POINT ( 'NONE',  ( 20.36894250292379382, 8.678748834913967869, 10.36894250292379205 ) ) ;
#81790=CARTESIAN_POINT ( 'NONE',  ( 19.84674366389459266, 8.300597817667451750, 2.638427012816836559 ) ) ;
#81791=CARTESIAN_POINT ( 'NONE',  ( -0.1503990784575328643, 60.12777174578613426, 6.262539305110068177 ) ) ;
#81793=CARTESIAN_POINT ( 'NONE',  ( 4.559911319644449179, 17.23035201082150536, -9.422509992056141925 ) ) ;
#81796=CARTESIAN_POINT ( 'NONE',  ( -0.3689425029237898834, 16.17874883491396076, -10.36894250292378850 ) ) ;
#81798=CARTESIAN_POINT ( 'NONE',  ( 10.00000000000000000, 26.81368534415484106, -10.88017736071110342 ) ) ;
#81799=CARTESIAN_POINT ( 'NONE',  ( 12.63842701281683922, 64.55059781766745175, -9.846743663894590881 ) ) ;
#81800=ORIENTED_EDGE ( 'NONE', *, *, #19747, .F. ) ;
#81801=CARTESIAN_POINT ( 'NONE',  ( 10.00000000000000178, 62.25893115100078745, 9.846743663894594434 ) ) ;
#81802=ORIENTED_EDGE ( 'NONE', *, *, #15942, .F. ) ;
#81803=ADVANCED_FACE ( 'NONE', ( #43447 ), #68929, .T. ) ;
#81804=CARTESIAN_POINT ( 'NONE',  ( 4.559911319644449179, 68.89701867748817676, 9.422509992056141925 ) ) ;
#81805=CARTESIAN_POINT ( 'NONE',  ( 19.84674366389459266, 58.71726448433411605, -2.638427012816827677 ) ) ;
#81806=CARTESIAN_POINT ( 'NONE',  ( 6.565887622018943937, 33.08196800326374643, -12.81628187352647608 ) ) ;
#81807=CARTESIAN_POINT ( 'NONE',  ( 17.96484262340118221, 4.938685344154837509, 7.964842623401181321 ) ) ;
#81809=CARTESIAN_POINT ( 'NONE',  ( 19.84674366389459621, 3.508931151000785231, 7.409399052514197653E-17 ) ) ;
#81810=CARTESIAN_POINT ( 'NONE',  ( 15.44008868035555260, 19.73035201082150536, 9.422509992056143702 ) ) ;
#81811=EDGE_CURVE ( 'NONE', #85332, #35045, #16911, .T. ) ;
#81812=STYLED_ITEM ( 'NONE', ( #53078 ), #65330 ) ;
#81814=CARTESIAN_POINT ( 'NONE',  ( -1.099225684535947600, 58.70696800326375353, -6.408140936763238038 ) ) ;
#81815=CARTESIAN_POINT ( 'NONE',  ( -0.8801773607111009756, 38.06368534415484106, 1.068504757029289695E-15 ) ) ;
#81817=CARTESIAN_POINT ( 'NONE',  ( 22.81628187352647785, 41.62363466993042493, 6.195893100308588602E-16 ) ) ;
#81818=CARTESIAN_POINT ( 'NONE',  ( 7.084665262690076126, 47.02201867748818387, -10.88017736071110164 ) ) ;
#81820=CARTESIAN_POINT ( 'NONE',  ( 19.84674366389459266, 58.30059781766745886, 2.638427012816836559 ) ) ;
#81823=CARTESIAN_POINT ( 'NONE',  ( 0.1532563361054082862, 21.21726448433412315, 2.638427012816831674 ) ) ;
#81825=CARTESIAN_POINT ( 'NONE',  ( 16.40814093676323893, 10.79030133659708923, 11.09922568453595026 ) ) ;
#81827=CARTESIAN_POINT ( 'NONE',  ( 17.20831665107776587, 57.88393115100078745, 7.208316651077764980 ) ) ;
#81828=CARTESIAN_POINT ( 'NONE',  ( 10.00000000000000178, 24.31368534415484106, 10.88017736071110342 ) ) ;
#81829=CARTESIAN_POINT ( 'NONE',  ( 2.791683348922237240, 50.38393115100078035, -7.208316651077763204 ) ) ;
#81831=DIRECTION ( 'NONE',  ( 0.000000000000000000, 0.000000000000000000, -1.000000000000000000 ) ) ;
#81832=CARTESIAN_POINT ( 'NONE',  ( 14.92337183194729633, 12.67559781766745353, 8.527530157486181039 ) ) ;
#81833=CARTESIAN_POINT ( 'NONE',  ( 19.38216949554541557, 2.248634669930420049, -9.382169495545420901 ) ) ;
#81834=ORIENTED_EDGE ( 'NONE', *, *, #91599, .F. ) ;
#81835=AXIS2_PLACEMENT_3D ( 'NONE', #17824, #63787, #42293 ) ;
#81838=CARTESIAN_POINT ( 'NONE',  ( 3.591859063236763294, 43.29030133659708923, -11.09922568453595026 ) ) ;
#81839=CARTESIAN_POINT ( 'NONE',  ( 0.1532563361054082862, 31.21726448433412315, 2.638427012816831674 ) ) ;
#81841=CARTESIAN_POINT ( 'NONE',  ( -0.3689425029237898834, 56.17874883491396076, -10.36894250292378850 ) ) ;
#81842=CARTESIAN_POINT ( 'NONE',  ( 1.472469842513823179, 35.59226448433412315, -4.923371831947296329 ) ) ;
#81843=EDGE_CURVE ( 'NONE', #58088, #61640, #7935, .T. ) ;
#81845=CARTESIAN_POINT ( 'NONE',  ( 2.603489959281601873, 25.43575266056827289, -6.500000000000015987 ) ) ;
#81846=CARTESIAN_POINT ( 'NONE',  ( 19.42250999205614193, 10.14701867748816966, 5.440088680355555262 ) ) ;
#81848=CARTESIAN_POINT ( 'NONE',  ( -0.8801773607111008646, 18.27201867748817321, 2.915334737309923430 ) ) ;
#81850=CARTESIAN_POINT ( 'NONE',  ( -2.266590686148945544, 46.38708216824730357, -7.082119434687050408 ) ) ;
#81851=CARTESIAN_POINT ( 'NONE',  ( 20.36894250292379738, 54.92874883491396076, -10.36894250292379027 ) ) ;
#81854=B_SPLINE_CURVE_WITH_KNOTS ( 'NONE', 3,
 ( #97480, #60437, #21970, #52934 ),
 .UNSPECIFIED., .F., .F.,
 ( 4, 4 ),
 ( 5.204893179191169451E-17, 0.002562518741975293446 ),
 .UNSPECIFIED. ) ;
#81855=CARTESIAN_POINT ( 'NONE',  ( 2.791683348922237240, 5.383931151000785675, -7.208316651077763204 ) ) ;
#81856=CARTESIAN_POINT ( 'NONE',  ( -2.816281873526473856, 4.123634669930420493, 9.499525473075851096E-16 ) ) ;
#81858=CARTESIAN_POINT ( 'NONE',  ( 20.88017736071110519, 45.56368534415484106, 2.639326808657452039E-16 ) ) ;
#81860=CARTESIAN_POINT ( 'NONE',  ( 7.361572987183169658, 64.96726448433412315, -9.846743663894592657 ) ) ;
#81861=CARTESIAN_POINT ( 'NONE',  ( -4.164238869374098151, 1.595415501580634388, -3.795296366450310543 ) ) ;
#81863=CARTESIAN_POINT ( 'NONE',  ( 5.076628168052703671, 26.84226448433411960, 8.527530157486179263 ) ) ;
#81865=CARTESIAN_POINT ( 'NONE',  ( 2.917880565312950480, 40.97041550158063217, -12.26659068614894821 ) ) ;
#81866=EDGE_CURVE ( 'NONE', #3611, #30159, #60450, .T. ) ;
#81869=CARTESIAN_POINT ( 'NONE',  ( -26.69000000000001194, 92.00000000000000000, -10.09898361729590199 ) ) ;
#81870=CARTESIAN_POINT ( 'NONE',  ( 17.96484262340118221, 36.18868534415484106, -7.964842623401177768 ) ) ;
#81871=CARTESIAN_POINT ( 'NONE',  ( 22.81628187352647785, 36.62363466993041783, 6.195893100308588602E-16 ) ) ;
#81872=CARTESIAN_POINT ( 'NONE',  ( 17.96484262340118221, 6.188685344154836621, -7.964842623401177768 ) ) ;
#81873=CARTESIAN_POINT ( 'NONE',  ( 10.00000000000000000, 32.87363466993042493, -12.81628187352647608 ) ) ;
#81874=CARTESIAN_POINT ( 'NONE',  ( -1.099225684535947600, 59.54030133659708923, 6.408140936763237150 ) ) ;
#81878=CARTESIAN_POINT ( 'NONE',  ( 17.39651004071897589, 34.08210964143323451, -6.499999999999361400 ) ) ;
#81879=CARTESIAN_POINT ( 'NONE',  ( 6.204703633549690345, 25.76208216824730712, -14.16423886937410259 ) ) ;
#81880=CARTESIAN_POINT ( 'NONE',  ( -0.3689425029237881626, 7.428748834913967869, 10.36894250292379027 ) ) ;
#81881=CARTESIAN_POINT ( 'NONE',  ( 2.035157376598822676, 12.43868534415483751, -7.964842623401177768 ) ) ;
#81882=CARTESIAN_POINT ( 'NONE',  ( 15.44008868035555793, 16.39701867748817321, -9.422509992056140149 ) ) ;
#81884=CYLINDRICAL_SURFACE ( 'NONE', #92680, 0.5000000000000004441 ) ;
#81885=CARTESIAN_POINT ( 'NONE',  ( 0.5774900079438590739, 47.64701867748817676, -5.440088680355550821 ) ) ;
#81886=CARTESIAN_POINT ( 'NONE',  ( 0.5774900079438590739, 52.64701867748817676, -5.440088680355550821 ) ) ;
#81887=CARTESIAN_POINT ( 'NONE',  ( 10.00000000000000000, 7.873634669930421381, -12.81628187352647608 ) ) ;
#81890=CARTESIAN_POINT ( 'NONE',  ( 2.791683348922240793, 21.63393115100078745, 7.208316651077764092 ) ) ;
#81891=CARTESIAN_POINT ( 'NONE',  ( 20.88017736071110519, 45.56368534415484106, 2.639326808657452039E-16 ) ) ;
#81893=CARTESIAN_POINT ( 'NONE',  ( 13.43411237798105340, 15.58196800326374998, 12.81628187352647963 ) ) ;
#81894=CARTESIAN_POINT ( 'NONE',  ( 5.076628168052704559, 0.1755978176674514724, -8.527530157486179263 ) ) ;
#81895=CARTESIAN_POINT ( 'NONE',  ( 2.791683348922240793, 21.63393115100078745, 7.208316651077764092 ) ) ;
#81896=CARTESIAN_POINT ( 'NONE',  ( -1.099225684535947600, 43.70696800326375353, -6.408140936763238038 ) ) ;
#81898=CARTESIAN_POINT ( 'NONE',  ( 17.20831665107776587, 22.88393115100078745, 7.208316651077764980 ) ) ;
#81899=VECTOR ( 'NONE', #57502, 1000.000000000000000 ) ;
#81901=CARTESIAN_POINT ( 'NONE',  ( -2.266590686148945544, 2.220415501580634388, 7.082119434687048631 ) ) ;
#81902=FACE_OUTER_BOUND ( 'NONE', #57558, .T. ) ;
#81903=CARTESIAN_POINT ( 'NONE',  ( 2.035157376598824452, 23.68868534415484461, 7.964842623401179544 ) ) ;
#81904=CARTESIAN_POINT ( 'NONE',  ( 20.36894250292379382, 28.67874883491396787, 10.36894250292379205 ) ) ;
#81905=CARTESIAN_POINT ( 'NONE',  ( 7.361572987183169658, 34.96726448433411605, -9.846743663894592657 ) ) ;
#81906=CARTESIAN_POINT ( 'NONE',  ( 2.035157376598822676, 22.43868534415483396, -7.964842623401177768 ) ) ;
#81907=CARTESIAN_POINT ( 'NONE',  ( 19.42250999205614548, 20.98035201082150891, -5.440088680355545492 ) ) ;
#81909=VECTOR ( 'NONE', #68330, 1000.000000000000000 ) ;
#81910=CARTESIAN_POINT ( 'NONE',  ( 17.96484262340118221, 21.18868534415483396, -7.964842623401177768 ) ) ;
#81911=CARTESIAN_POINT ( 'NONE',  ( 6.565887622018943937, 40.16530133659708923, 12.81628187352647430 ) ) ;
#81912=CARTESIAN_POINT ( 'NONE',  ( 15.44008868035555260, 39.73035201082150536, 9.422509992056143702 ) ) ;
#81914=CARTESIAN_POINT ( 'NONE',  ( -0.8801773607110991993, 37.85535201082151247, -2.915334737309923874 ) ) ;
#81916=CARTESIAN_POINT ( 'NONE',  ( 5.076628168052703671, 56.84226448433412315, 8.527530157486179263 ) ) ;
#81917=CARTESIAN_POINT ( 'NONE',  ( -0.8801773607110991993, 32.85535201082151247, -2.915334737309923874 ) ) ;
#81921=DIRECTION ( 'NONE',  ( 0.000000000000000000, 0.000000000000000000, 1.000000000000000000 ) ) ;
#81922=CARTESIAN_POINT ( 'NONE',  ( 20.36894250292379738, 44.92874883491396787, -10.36894250292379027 ) ) ;
#81923=CARTESIAN_POINT ( 'NONE',  ( -0.8801773607111009756, 53.06368534415484106, 1.068504757029289695E-15 ) ) ;
#81924=CARTESIAN_POINT ( 'NONE',  ( 14.92337183194729988, 64.34226448433412315, -8.527530157486177487 ) ) ;
#81926=CARTESIAN_POINT ( 'NONE',  ( 17.20831665107776587, 44.13393115100078745, -7.208316651077762316 ) ) ;
#81927=CARTESIAN_POINT ( 'NONE',  ( 7.361572987183169658, 4.967264484334119601, -9.846743663894592657 ) ) ;
#81928=CARTESIAN_POINT ( 'NONE',  ( 0.1532563361054083140, 21.00893115100078745, 1.131784320476157264E-15 ) ) ;
#81930=CARTESIAN_POINT ( 'NONE',  ( 0.1532563361054100626, 25.80059781766744820, -2.638427012816831230 ) ) ;
#81932=CARTESIAN_POINT ( 'NONE',  ( 4.559911319644449179, 22.23035201082150536, -9.422509992056141925 ) ) ;
#81933=CARTESIAN_POINT ( 'NONE',  ( 2.791683348922237240, 20.38393115100078745, -7.208316651077763204 ) ) ;
#81934=CARTESIAN_POINT ( 'NONE',  ( 15.44008868035555793, 56.39701867748817676, -9.422509992056140149 ) ) ;
#81935=CARTESIAN_POINT ( 'NONE',  ( 20.88017736071110875, 35.77201867748816966, -2.915334737309920765 ) ) ;
#81936=CARTESIAN_POINT ( 'NONE',  ( 22.81628187352648496, 51.83196800326376064, -3.434112377981050290 ) ) ;
#81937=CARTESIAN_POINT ( 'NONE',  ( -0.3689425029237898834, 41.17874883491397497, -10.36894250292378850 ) ) ;
#81943=CARTESIAN_POINT ( 'NONE',  ( 10.00000000000000000, 2.873634669930420049, -12.81628187352647608 ) ) ;
#81944=CARTESIAN_POINT ( 'NONE',  ( 0.5774900079438590739, 7.647018677488171434, -5.440088680355550821 ) ) ;
#81945=CARTESIAN_POINT ( 'NONE',  ( 17.96484262340118221, 46.18868534415484106, -7.964842623401177768 ) ) ;
#81946=DIRECTION ( 'NONE',  ( -0.000000000000000000, -0.000000000000000000, 1.000000000000000000 ) ) ;
#81947=ORIENTED_EDGE ( 'NONE', *, *, #42696, .T. ) ;
#81948=CARTESIAN_POINT ( 'NONE',  ( 7.361572987183169658, 14.96726448433411960, -9.846743663894592657 ) ) ;
#81950=CARTESIAN_POINT ( 'NONE',  ( 19.42250999205614193, 55.14701867748817676, 5.440088680355555262 ) ) ;
#81951=CARTESIAN_POINT ( 'NONE',  ( 18.52753015748618282, 33.92559781766745886, -4.923371831947291888 ) ) ;
#81952=CARTESIAN_POINT ( 'NONE',  ( 19.84674366389459621, 28.50893115100078745, 7.409399052514197653E-17 ) ) ;
#81953=CARTESIAN_POINT ( 'NONE',  ( 18.52753015748617571, 13.09226448433411960, 4.923371831947298993 ) ) ;
#81954=DIRECTION ( 'NONE',  ( 0.000000000000000000, 0.000000000000000000, -1.000000000000000000 ) ) ;
#81955=CARTESIAN_POINT ( 'NONE',  ( 20.88017736071110164, 65.35535201082150536, 2.915334737309930979 ) ) ;
#81958=CARTESIAN_POINT ( 'NONE',  ( 5.076628168052703671, 31.84226448433412315, 8.527530157486179263 ) ) ;
#81959=CARTESIAN_POINT ( 'NONE',  ( -2.816281873526473856, 54.33196800326376064, 3.434112377981055619 ) ) ;
#81962=CARTESIAN_POINT ( 'NONE',  ( 19.84674366389459266, 63.30059781766745886, 2.638427012816836559 ) ) ;
#81963=CIRCLE ( 'NONE', #51645, 18.53834841531100608 ) ;
#81964=CARTESIAN_POINT ( 'NONE',  ( -0.8801773607111009756, 3.063685344154837509, 1.068504757029289695E-15 ) ) ;
#81965=CARTESIAN_POINT ( 'NONE',  ( 24.16423886937409904, 24.09541550158063927, 3.795296366450317205 ) ) ;
#81966=CIRCLE ( 'NONE', #46858, 0.5000000000000004441 ) ;
#81967=EDGE_CURVE ( 'NONE', #5362, #58376, #60915, .T. ) ;
#81968=CARTESIAN_POINT ( 'NONE',  ( 10.00000000000000178, 70.00000000000000000, 0.000000000000000000 ) ) ;
#81970=CARTESIAN_POINT ( 'NONE',  ( 24.16423886937410614, 34.30374883491396787, 8.672049930838204340E-16 ) ) ;
#81972=CARTESIAN_POINT ( 'NONE',  ( 17.08211943468705840, 40.13708216824731068, -12.26659068614894466 ) ) ;
#81973=CARTESIAN_POINT ( 'NONE',  ( -0.3689425029237898834, 11.17874883491396787, -10.36894250292378850 ) ) ;
#81974=CARTESIAN_POINT ( 'NONE',  ( 17.08211943468705840, 15.13708216824730179, -12.26659068614894466 ) ) ;
#81975=CARTESIAN_POINT ( 'NONE',  ( -0.8801773607111009756, 68.06368534415484817, 1.068504757029289695E-15 ) ) ;
#81976=CARTESIAN_POINT ( 'NONE',  ( 7.084665262690076126, 54.10535201082151247, 10.88017736071109987 ) ) ;
#81979=CARTESIAN_POINT ( 'NONE',  ( 1.472469842513823179, 31.42559781766745530, 4.923371831947296329 ) ) ;
#81982=CARTESIAN_POINT ( 'NONE',  ( 0.1532563361054082862, 26.21726448433411605, 2.638427012816831674 ) ) ;
#81983=CARTESIAN_POINT ( 'NONE',  ( 4.559911319644449179, 13.89701867748817321, 9.422509992056141925 ) ) ;
#81984=CARTESIAN_POINT ( 'NONE',  ( 19.38216949554541557, 62.24863466993041072, -9.382169495545420901 ) ) ;
#81985=CARTESIAN_POINT ( 'NONE',  ( 19.84674366389459266, 53.30059781766744464, 2.638427012816836559 ) ) ;
#81987=CARTESIAN_POINT ( 'NONE',  ( 16.40814093676324603, 37.45696800326376064, -11.09922568453594671 ) ) ;
#81989=( BOUNDED_SURFACE ( )  B_SPLINE_SURFACE ( 1, 2, ( 
 ( #32026, #48517, #31544, #62039, #9053, #18040, #47543, #49014, #94513, #17061, #9543, #32534, #78534, #86535, #63522, #2074, #94026, #26032, #56041, #79521, #40546, #63032, #55545, #79020, #62530, #86044, #71046, #2569, #10531, #33025, #24570, #25549, #39069, #41041, #71541, #3048, #33503, #1083, #92539, #24069, #54537, #85053, #16565, #85549, #47039, #39565, #93037, #55030, #80001, #42030, #34489, #64493, #11506, #72494, #66477, #95000, #72006, #12978, #97005, #19019, #87507, #72988, #34982, #27979, #49497, #65483, #4518, #42991, #95507, #4026, #43475, #5003, #73976, #28483, #58977, #42506, #96506, #89478, #50980, #64982, #88489, #26999, #26508, #57004, #57497, #58477, #87991, #96006, #19991, #50493, #81476, #80507, #19504, #5502, #50001, #80990, #12003, #27489, #57982, #12491, #88989, #73474, #35485, #65981, #20493, #35975, #20991, #51477, #41538, #3535, #11021, #33995, #82467, #14483, #61433, #51980, #6973, #52461, #45958, #13987, #37479, #15475, #21482, #60453, #13483, #75952, #30439, #76447, #44463, #59956, #38460, #83949, #74965, #52948, #67968, #89966, #90447, #485, #91939, #29449, #21986, #53440, #7962, #6470, #91450, #74463, #5989, #36974, #60939, #82964, #30934, #68953, #44954, #75458, #98493, #90942, #22975, #7479, #29947, #37976, #23469, #98986, #81970, #22472, #83459, #14980, #43961, #67473, #45450, #68465, #36484, #66976, #97496, #97994, #28960, #59464, #62410, #25437, #9425, #92916, #85928, #39929, #47905, #1949, #33385, #46441, #1457, #40432, #85426, #8442, #15949, #23951, #84932, #77414, #38949, #54424, #16444, #10416, #69441, #76933, #55920, #40923, #61924, #31421, #16935, #77919, #70931, #92426, #70432, #47416, #17438, #39447, #46922, #86419, #78410, #17920, #71421, #2937, #32413, #2448, #63883, #8930, #62914, #48404, #69938, #93415, #84450, #9928, #32905, #78907, #31909, #24445, #94395, #53943, #54913, #24938, #55420, #63404, #93909, #961, #5386, #72375, #34372, #96388, #27862, #18906, #35368, #18408, #48891, #64378, #4889, #64862, #43359, #50869, #3905, #95382, #19387, #4401, #73361, #50366, #26884, #80874, #12860, #42878, #35861, #34869, #57376, #42388, #65859, #87389, #87871, #49872, #80385, #58347, #65363, #11391, #88376, #73856, #11888, #88869, #72867, #95892, #57864, #27372, #19873, #12372, #66349, #79402, #20375, #81361, #25910, #10906, #86898, #94888, #56886, #49383, #41428, #26386, #79884, #56412, #71889, #3412, #33873, #41913, #5867, #74339, #59837, #21866, #14863, #36358, #52344, #90326, #29828, #82342, #66854, #98868, #90831, #30322, #15359, #45843, #29336, #83341, #76329, #37857, #28840 ),
 ( #82841, #36858, #67854, #14361, #44830, #98373, #97372, #75335, #6849, #37361, #60337, #59343, #52832, #22358, #7846, #89845, #74848, #53324, #60824, #21362, #45335, #75835, #51856, #6349, #38344, #96888, #44342, #67350, #68347, #91324, #13863, #7355, #89358, #20869, #97876, #22851, #83833, #28364, #58852, #51360, #81846, #13359, #43845, #17318, #93295, #8816, #24819, #55804, #85806, #48282, #77795, #46809, #85309, #47793, #31306, #77301, #1345, #92803, #78291, #47294, #54305, #32290, #86297, #39328, #40308, #24330, #69823, #1834, #54793, #62795, #16817, #78794, #61318, #16326, #55295, #31797, #23346, #30819, #38833, #849, #92313, #53829, #69327, #61808, #25317, #84340, #91829, #70814, #17804, #76813, #46326, #62295, #9305, #9807, #8329, #39814, #70317, #2329, #84818, #23839, #32785, #63282, #93788, #10302, #68839, #371, #15843, #58224, #80757, #71780, #19266, #3289, #94273, #86790, #33754, #57746, #25796, #72261, #49750, #80260, #12252, #11269, #64256, #71301, #33272, #94771, #79770, #41307, #3790, #20255, #10790, #64745, #41789, #4769, #26270, #95257, #73241, #79280, #11764, #2822, #34750, #88249, #35241, #19757, #49270, #88745, #65739, #18788, #34245, #26763, #42272, #50242, #65239, #57255, #95764, #27742, #42759, #50756, #72743, #87752, #4276, #96268, #56771, #27248, #81242, #40800, #63766, #56295, #87267, #18291, #48774, #21244, #83223, #67234, #51742, #44722, #97757, #6731, #59722, #91204, #5265, #59223, #98254, #44223, #66231, #73735, #81726, #43734, #36242, #96766, #13240, #74220, #68237, #28241, #35743, #14746, #98754, #20749, #89241, #74727, #36743, #29712, #51240, #29223, #6241, #75219, #97263, #5753, #45220, #37247, #75717, #30204, #60707, #90216, #60220, #22732, #52716, #66738, #21749, #28732, #58736, #89727, #82226, #90714, #13740, #52230, #82722, #14241, #7231, #67736, #22239, #43240, #37738, #53215, #12741, #84223, #16207, #63161, #53702, #8695, #54189, #47681, #15732, #39211, #17204, #23230, #62173, #15237, #77678, #32169, #78175, #46212, #61685, #40182, #85683, #76699, #54674, #69698, #91711, #92202, #2207, #93669, #31191, #23726, #55168, #9686, #8219, #93171, #76220, #7733, #38713, #38229, #45718, #69212, #738, #84702, #68716, #46690, #77187, #70689, #247, #30695, #32668, #25203, #1228, #61205, #31681, #92682, #1711, #24207, #85193, #16700, #47173, #9191, #39705, #83717, #70192, #62670, #24696, #73118, #87143, #42161, #4659, #95644, #86670, #34132, #18174, #10185, #2705, #48656, #72626, #40679, #18666, #64624, #95133, #27130, #26162, #79156, #86180, #48162, #10670, #94654, #56177, #49154, #35120 ) ),
 .UNSPECIFIED., .F., .F., .T. ) 
 B_SPLINE_SURFACE_WITH_KNOTS ( ( 2, 2 ),
 ( 3, 2, 2, 2, 2, 2, 2, 2, 2, 2, 2, 2, 2, 2, 2, 2, 2, 2, 2, 2, 2, 2, 2, 2, 2, 2, 2, 2, 2, 2, 2, 2, 2, 2, 2, 2, 2, 2, 2, 2, 2, 2, 2, 2, 2, 2, 2, 2, 2, 2, 2, 2, 2, 2, 2, 2, 2, 2, 2, 2, 2, 2, 2, 2, 2, 2, 2, 2, 2, 2, 2, 2, 2, 2, 2, 2, 2, 2, 2, 2, 2, 2, 2, 2, 2, 2, 2, 2, 2, 2, 2, 2, 2, 2, 2, 2, 2, 2, 2, 2, 2, 2, 2, 2, 2, 2, 2, 2, 2, 2, 2, 2, 2, 2, 2, 2, 2, 2, 2, 2, 2, 2, 2, 2, 2, 2, 2, 2, 2, 2, 2, 2, 2, 2, 2, 2, 2, 2, 2, 2, 2, 2, 2, 2, 2, 2, 2, 2, 2, 2, 2, 2, 2, 2, 2, 2, 2, 2, 2, 2, 2, 2, 3 ),
 ( 0.000000000000000000, 1.000000000000000000 ),
 ( 0.000000000000000000, 0.005952380952380952051, 0.01190476190476190410, 0.01785714285714285615, 0.02380952380952380820, 0.02976190476190476025, 0.03571428571428571230, 0.04166666666666666435, 0.04761904761904761640, 0.05357142857142856845, 0.05952380952380952051, 0.06547619047619047949, 0.07142857142857142461, 0.07738095238095238360, 0.08333333333333332871, 0.08928571428571428770, 0.09523809523809523281, 0.1011904761904761918, 0.1071428571428571369, 0.1130952380952380959, 0.1190476190476190410, 0.1250000000000000000, 0.1309523809523809590, 0.1369047619047619180, 0.1428571428571428492, 0.1488095238095238082, 0.1547619047619047672, 0.1607142857142857262, 0.1666666666666666574, 0.1726190476190476164, 0.1785714285714285754, 0.1845238095238095344, 0.1904761904761904656, 0.1964285714285714246, 0.2023809523809523836, 0.2083333333333333426, 0.2142857142857142738, 0.2202380952380952328, 0.2261904761904761918, 0.2321428571428571508, 0.2380952380952380820, 0.2440476190476190410, 0.2500000000000000000, 0.2559523809523809312, 0.2619047619047619180, 0.2678571428571428492, 0.2738095238095238360, 0.2797619047619047672, 0.2857142857142856984, 0.2916666666666666852, 0.2976190476190476164, 0.3035714285714285476, 0.3095238095238095344, 0.3154761904761904656, 0.3214285714285714524, 0.3273809523809523836, 0.3333333333333333148, 0.3392857142857143016, 0.3452380952380952328, 0.3511904761904761640, 0.3571428571428571508, 0.3630952380952380820, 0.3690476190476190688, 0.3750000000000000000, 0.3809523809523809312, 0.3869047619047619180, 0.3928571428571428492, 0.3988095238095238360, 0.4047619047619047672, 0.4107142857142856984, 0.4166666666666666852, 0.4226190476190476164, 0.4285714285714285476, 0.4345238095238095344, 0.4404761904761904656, 0.4464285714285714524, 0.4523809523809523836, 0.4583333333333333148, 0.4642857142857143016, 0.4702380952380952328, 0.4761904761904761640, 0.4821428571428571508, 0.4880952380952380820, 0.4940476190476190688, 0.5000000000000000000, 0.5059523809523809312, 0.5119047619047618625, 0.5178571428571429047, 0.5238095238095238360, 0.5297619047619047672, 0.5357142857142856984, 0.5416666666666666297, 0.5476190476190476719, 0.5535714285714286031, 0.5595238095238095344, 0.5654761904761904656, 0.5714285714285713969, 0.5773809523809523281, 0.5833333333333333703, 0.5892857142857143016, 0.5952380952380952328, 0.6011904761904761640, 0.6071428571428570953, 0.6130952380952381375, 0.6190476190476190688, 0.6250000000000000000, 0.6309523809523809312, 0.6369047619047618625, 0.6428571428571429047, 0.6488095238095238360, 0.6547619047619047672, 0.6607142857142856984, 0.6666666666666666297, 0.6726190476190476719, 0.6785714285714286031, 0.6845238095238095344, 0.6904761904761904656, 0.6964285714285713969, 0.7023809523809523281, 0.7083333333333333703, 0.7142857142857143016, 0.7202380952380952328, 0.7261904761904761640, 0.7321428571428570953, 0.7380952380952381375, 0.7440476190476190688, 0.7500000000000000000, 0.7559523809523809312, 0.7619047619047618625, 0.7678571428571429047, 0.7738095238095238360, 0.7797619047619047672, 0.7857142857142856984, 0.7916666666666666297, 0.7976190476190476719, 0.8035714285714286031, 0.8095238095238095344, 0.8154761904761904656, 0.8214285714285713969, 0.8273809523809523281, 0.8333333333333333703, 0.8392857142857143016, 0.8452380952380952328, 0.8511904761904761640, 0.8571428571428570953, 0.8630952380952381375, 0.8690476190476190688, 0.8750000000000000000, 0.8809523809523809312, 0.8869047619047618625, 0.8928571428571429047, 0.8988095238095238360, 0.9047619047619047672, 0.9107142857142856984, 0.9166666666666666297, 0.9226190476190476719, 0.9285714285714286031, 0.9345238095238095344, 0.9404761904761904656, 0.9464285714285713969, 0.9523809523809523281, 0.9583333333333333703, 0.9642857142857143016 ),
 .UNSPECIFIED. ) 
 GEOMETRIC_REPRESENTATION_ITEM ( )  RATIONAL_B_SPLINE_SURFACE ( (
 ( 1.000000000000000000, 0.9659258262890683122, 1.000000000000000000, 0.9659258262890683122, 1.000000000000000000, 0.9659258262890683122, 1.000000000000000000, 0.9659258262890683122, 1.000000000000000000, 0.9659258262890683122, 1.000000000000000000, 0.9659258262890683122, 1.000000000000000000, 0.9659258262890683122, 1.000000000000000000, 0.9659258262890683122, 1.000000000000000000, 0.9659258262890683122, 1.000000000000000000, 0.9659258262890683122, 1.000000000000000000, 0.9659258262890683122, 1.000000000000000000, 0.9659258262890683122, 1.000000000000000000, 0.9659258262890683122, 1.000000000000000000, 0.9659258262890683122, 1.000000000000000000, 0.9659258262890683122, 1.000000000000000000, 0.9659258262890683122, 1.000000000000000000, 0.9659258262890683122, 1.000000000000000000, 0.9659258262890683122, 1.000000000000000000, 0.9659258262890683122, 1.000000000000000000, 0.9659258262890683122, 1.000000000000000000, 0.9659258262890683122, 1.000000000000000000, 0.9659258262890683122, 1.000000000000000000, 0.9659258262890683122, 1.000000000000000000, 0.9659258262890683122, 1.000000000000000000, 0.9659258262890683122, 1.000000000000000000, 0.9659258262890683122, 1.000000000000000000, 0.9659258262890683122, 1.000000000000000000, 0.9659258262890683122, 1.000000000000000000, 0.9659258262890683122, 1.000000000000000000, 0.9659258262890683122, 1.000000000000000000, 0.9659258262890683122, 1.000000000000000000, 0.9659258262890683122, 1.000000000000000000, 0.9659258262890683122, 1.000000000000000000, 0.9659258262890683122, 1.000000000000000000, 0.9659258262890683122, 1.000000000000000000, 0.9659258262890683122, 1.000000000000000000, 0.9659258262890683122, 1.000000000000000000, 0.9659258262890683122, 1.000000000000000000, 0.9659258262890683122, 1.000000000000000000, 0.9659258262890683122, 1.000000000000000000, 0.9659258262890683122, 1.000000000000000000, 0.9659258262890683122, 1.000000000000000000, 0.9659258262890683122, 1.000000000000000000, 0.9659258262890683122, 1.000000000000000000, 0.9659258262890683122, 1.000000000000000000, 0.9659258262890683122, 1.000000000000000000, 0.9659258262890683122, 1.000000000000000000, 0.9659258262890683122, 1.000000000000000000, 0.9659258262890683122, 1.000000000000000000, 0.9659258262890683122, 1.000000000000000000, 0.9659258262890683122, 1.000000000000000000, 0.9659258262890683122, 1.000000000000000000, 0.9659258262890683122, 1.000000000000000000, 0.9659258262890683122, 1.000000000000000000, 0.9659258262890683122, 1.000000000000000000, 0.9659258262890683122, 1.000000000000000000, 0.9659258262890683122, 1.000000000000000000, 0.9659258262890683122, 1.000000000000000000, 0.9659258262890683122, 1.000000000000000000, 0.9659258262890683122, 1.000000000000000000, 0.9659258262890683122, 1.000000000000000000, 0.9659258262890683122, 1.000000000000000000, 0.9659258262890683122, 1.000000000000000000, 0.9659258262890683122, 1.000000000000000000, 0.9659258262890683122, 1.000000000000000000, 0.9659258262890683122, 1.000000000000000000, 0.9659258262890683122, 1.000000000000000000, 0.9659258262890683122, 1.000000000000000000, 0.9659258262890683122, 1.000000000000000000, 0.9659258262890683122, 1.000000000000000000, 0.9659258262890683122, 1.000000000000000000, 0.9659258262890683122, 1.000000000000000000, 0.9659258262890683122, 1.000000000000000000, 0.9659258262890683122, 1.000000000000000000, 0.9659258262890683122, 1.000000000000000000, 0.9659258262890683122, 1.000000000000000000, 0.9659258262890683122, 1.000000000000000000, 0.9659258262890683122, 1.000000000000000000, 0.9659258262890683122, 1.000000000000000000, 0.9659258262890683122, 1.000000000000000000, 0.9659258262890683122, 1.000000000000000000, 0.9659258262890683122, 1.000000000000000000, 0.9659258262890683122, 1.000000000000000000, 0.9659258262890683122, 1.000000000000000000, 0.9659258262890683122, 1.000000000000000000, 0.9659258262890683122, 1.000000000000000000, 0.9659258262890683122, 1.000000000000000000, 0.9659258262890683122, 1.000000000000000000, 0.9659258262890683122, 1.000000000000000000, 0.9659258262890683122, 1.000000000000000000, 0.9659258262890683122, 1.000000000000000000, 0.9659258262890683122, 1.000000000000000000, 0.9659258262890683122, 1.000000000000000000, 0.9659258262890683122, 1.000000000000000000, 0.9659258262890683122, 1.000000000000000000, 0.9659258262890683122, 1.000000000000000000, 0.9659258262890683122, 1.000000000000000000, 0.9659258262890683122, 1.000000000000000000, 0.9659258262890683122, 1.000000000000000000, 0.9659258262890683122, 1.000000000000000000, 0.9659258262890683122, 1.000000000000000000, 0.9659258262890683122, 1.000000000000000000, 0.9659258262890683122, 1.000000000000000000, 0.9659258262890683122, 1.000000000000000000, 0.9659258262890683122, 1.000000000000000000, 0.9659258262890683122, 1.000000000000000000, 0.9659258262890683122, 1.000000000000000000, 0.9659258262890683122, 1.000000000000000000, 0.9659258262890683122, 1.000000000000000000, 0.9659258262890683122, 1.000000000000000000, 0.9659258262890683122, 1.000000000000000000, 0.9659258262890683122, 1.000000000000000000, 0.9659258262890683122, 1.000000000000000000, 0.9659258262890683122, 1.000000000000000000, 0.9659258262890683122, 1.000000000000000000, 0.9659258262890683122, 1.000000000000000000, 0.9659258262890683122, 1.000000000000000000, 0.9659258262890683122, 1.000000000000000000, 0.9659258262890683122, 1.000000000000000000, 0.9659258262890683122, 1.000000000000000000, 0.9659258262890683122, 1.000000000000000000, 0.9659258262890683122, 1.000000000000000000, 0.9659258262890683122, 1.000000000000000000, 0.9659258262890683122, 1.000000000000000000, 0.9659258262890683122, 1.000000000000000000, 0.9659258262890683122, 1.000000000000000000, 0.9659258262890683122, 1.000000000000000000, 0.9659258262890683122, 1.000000000000000000, 0.9659258262890683122, 1.000000000000000000, 0.9659258262890683122, 1.000000000000000000, 0.9659258262890683122, 1.000000000000000000, 0.9659258262890683122, 1.000000000000000000, 0.9659258262890683122, 1.000000000000000000, 0.9659258262890683122, 1.000000000000000000, 0.9659258262890683122, 1.000000000000000000, 0.9659258262890683122, 1.000000000000000000, 0.9659258262890683122, 1.000000000000000000, 0.9659258262890683122, 1.000000000000000000, 0.9659258262890683122, 1.000000000000000000, 0.9659258262890683122, 1.000000000000000000, 0.9659258262890683122, 1.000000000000000000, 0.9659258262890683122, 1.000000000000000000, 0.9659258262890683122, 1.000000000000000000, 0.9659258262890683122, 1.000000000000000000, 0.9659258262890683122, 1.000000000000000000, 0.9659258262890683122, 1.000000000000000000, 0.9659258262890683122, 1.000000000000000000, 0.9659258262890683122, 1.000000000000000000, 0.9659258262890683122, 1.000000000000000000, 0.9659258262890683122, 1.000000000000000000, 0.9659258262890683122, 1.000000000000000000, 0.9659258262890683122, 1.000000000000000000, 0.9659258262890683122, 1.000000000000000000, 0.9659258262890683122, 1.000000000000000000, 0.9659258262890683122, 1.000000000000000000, 0.9659258262890683122, 1.000000000000000000, 0.9659258262890683122, 1.000000000000000000, 0.9659258262890683122, 1.000000000000000000, 0.9659258262890683122, 1.000000000000000000, 0.9659258262890683122, 1.000000000000000000, 0.9659258262890683122, 1.000000000000000000, 0.9659258262890683122, 1.000000000000000000),
 ( 1.000000000000000000, 0.9659258262890683122, 1.000000000000000000, 0.9659258262890683122, 1.000000000000000000, 0.9659258262890683122, 1.000000000000000000, 0.9659258262890683122, 1.000000000000000000, 0.9659258262890683122, 1.000000000000000000, 0.9659258262890683122, 1.000000000000000000, 0.9659258262890683122, 1.000000000000000000, 0.9659258262890683122, 1.000000000000000000, 0.9659258262890683122, 1.000000000000000000, 0.9659258262890683122, 1.000000000000000000, 0.9659258262890683122, 1.000000000000000000, 0.9659258262890683122, 1.000000000000000000, 0.9659258262890683122, 1.000000000000000000, 0.9659258262890683122, 1.000000000000000000, 0.9659258262890683122, 1.000000000000000000, 0.9659258262890683122, 1.000000000000000000, 0.9659258262890683122, 1.000000000000000000, 0.9659258262890683122, 1.000000000000000000, 0.9659258262890683122, 1.000000000000000000, 0.9659258262890683122, 1.000000000000000000, 0.9659258262890683122, 1.000000000000000000, 0.9659258262890683122, 1.000000000000000000, 0.9659258262890683122, 1.000000000000000000, 0.9659258262890683122, 1.000000000000000000, 0.9659258262890683122, 1.000000000000000000, 0.9659258262890683122, 1.000000000000000000, 0.9659258262890683122, 1.000000000000000000, 0.9659258262890683122, 1.000000000000000000, 0.9659258262890683122, 1.000000000000000000, 0.9659258262890683122, 1.000000000000000000, 0.9659258262890683122, 1.000000000000000000, 0.9659258262890683122, 1.000000000000000000, 0.9659258262890683122, 1.000000000000000000, 0.9659258262890683122, 1.000000000000000000, 0.9659258262890683122, 1.000000000000000000, 0.9659258262890683122, 1.000000000000000000, 0.9659258262890683122, 1.000000000000000000, 0.9659258262890683122, 1.000000000000000000, 0.9659258262890683122, 1.000000000000000000, 0.9659258262890683122, 1.000000000000000000, 0.9659258262890683122, 1.000000000000000000, 0.9659258262890683122, 1.000000000000000000, 0.9659258262890683122, 1.000000000000000000, 0.9659258262890683122, 1.000000000000000000, 0.9659258262890683122, 1.000000000000000000, 0.9659258262890683122, 1.000000000000000000, 0.9659258262890683122, 1.000000000000000000, 0.9659258262890683122, 1.000000000000000000, 0.9659258262890683122, 1.000000000000000000, 0.9659258262890683122, 1.000000000000000000, 0.9659258262890683122, 1.000000000000000000, 0.9659258262890683122, 1.000000000000000000, 0.9659258262890683122, 1.000000000000000000, 0.9659258262890683122, 1.000000000000000000, 0.9659258262890683122, 1.000000000000000000, 0.9659258262890683122, 1.000000000000000000, 0.9659258262890683122, 1.000000000000000000, 0.9659258262890683122, 1.000000000000000000, 0.9659258262890683122, 1.000000000000000000, 0.9659258262890683122, 1.000000000000000000, 0.9659258262890683122, 1.000000000000000000, 0.9659258262890683122, 1.000000000000000000, 0.9659258262890683122, 1.000000000000000000, 0.9659258262890683122, 1.000000000000000000, 0.9659258262890683122, 1.000000000000000000, 0.9659258262890683122, 1.000000000000000000, 0.9659258262890683122, 1.000000000000000000, 0.9659258262890683122, 1.000000000000000000, 0.9659258262890683122, 1.000000000000000000, 0.9659258262890683122, 1.000000000000000000, 0.9659258262890683122, 1.000000000000000000, 0.9659258262890683122, 1.000000000000000000, 0.9659258262890683122, 1.000000000000000000, 0.9659258262890683122, 1.000000000000000000, 0.9659258262890683122, 1.000000000000000000, 0.9659258262890683122, 1.000000000000000000, 0.9659258262890683122, 1.000000000000000000, 0.9659258262890683122, 1.000000000000000000, 0.9659258262890683122, 1.000000000000000000, 0.9659258262890683122, 1.000000000000000000, 0.9659258262890683122, 1.000000000000000000, 0.9659258262890683122, 1.000000000000000000, 0.9659258262890683122, 1.000000000000000000, 0.9659258262890683122, 1.000000000000000000, 0.9659258262890683122, 1.000000000000000000, 0.9659258262890683122, 1.000000000000000000, 0.9659258262890683122, 1.000000000000000000, 0.9659258262890683122, 1.000000000000000000, 0.9659258262890683122, 1.000000000000000000, 0.9659258262890683122, 1.000000000000000000, 0.9659258262890683122, 1.000000000000000000, 0.9659258262890683122, 1.000000000000000000, 0.9659258262890683122, 1.000000000000000000, 0.9659258262890683122, 1.000000000000000000, 0.9659258262890683122, 1.000000000000000000, 0.9659258262890683122, 1.000000000000000000, 0.9659258262890683122, 1.000000000000000000, 0.9659258262890683122, 1.000000000000000000, 0.9659258262890683122, 1.000000000000000000, 0.9659258262890683122, 1.000000000000000000, 0.9659258262890683122, 1.000000000000000000, 0.9659258262890683122, 1.000000000000000000, 0.9659258262890683122, 1.000000000000000000, 0.9659258262890683122, 1.000000000000000000, 0.9659258262890683122, 1.000000000000000000, 0.9659258262890683122, 1.000000000000000000, 0.9659258262890683122, 1.000000000000000000, 0.9659258262890683122, 1.000000000000000000, 0.9659258262890683122, 1.000000000000000000, 0.9659258262890683122, 1.000000000000000000, 0.9659258262890683122, 1.000000000000000000, 0.9659258262890683122, 1.000000000000000000, 0.9659258262890683122, 1.000000000000000000, 0.9659258262890683122, 1.000000000000000000, 0.9659258262890683122, 1.000000000000000000, 0.9659258262890683122, 1.000000000000000000, 0.9659258262890683122, 1.000000000000000000, 0.9659258262890683122, 1.000000000000000000, 0.9659258262890683122, 1.000000000000000000, 0.9659258262890683122, 1.000000000000000000, 0.9659258262890683122, 1.000000000000000000, 0.9659258262890683122, 1.000000000000000000, 0.9659258262890683122, 1.000000000000000000, 0.9659258262890683122, 1.000000000000000000, 0.9659258262890683122, 1.000000000000000000, 0.9659258262890683122, 1.000000000000000000, 0.9659258262890683122, 1.000000000000000000, 0.9659258262890683122, 1.000000000000000000, 0.9659258262890683122, 1.000000000000000000, 0.9659258262890683122, 1.000000000000000000, 0.9659258262890683122, 1.000000000000000000, 0.9659258262890683122, 1.000000000000000000, 0.9659258262890683122, 1.000000000000000000, 0.9659258262890683122, 1.000000000000000000, 0.9659258262890683122, 1.000000000000000000, 0.9659258262890683122, 1.000000000000000000, 0.9659258262890683122, 1.000000000000000000, 0.9659258262890683122, 1.000000000000000000, 0.9659258262890683122, 1.000000000000000000, 0.9659258262890683122, 1.000000000000000000, 0.9659258262890683122, 1.000000000000000000, 0.9659258262890683122, 1.000000000000000000, 0.9659258262890683122, 1.000000000000000000, 0.9659258262890683122, 1.000000000000000000, 0.9659258262890683122, 1.000000000000000000, 0.9659258262890683122, 1.000000000000000000, 0.9659258262890683122, 1.000000000000000000, 0.9659258262890683122, 1.000000000000000000, 0.9659258262890683122, 1.000000000000000000, 0.9659258262890683122, 1.000000000000000000, 0.9659258262890683122, 1.000000000000000000, 0.9659258262890683122, 1.000000000000000000, 0.9659258262890683122, 1.000000000000000000, 0.9659258262890683122, 1.000000000000000000, 0.9659258262890683122, 1.000000000000000000, 0.9659258262890683122, 1.000000000000000000, 0.9659258262890683122, 1.000000000000000000, 0.9659258262890683122, 1.000000000000000000, 0.9659258262890683122, 1.000000000000000000, 0.9659258262890683122, 1.000000000000000000, 0.9659258262890683122, 1.000000000000000000, 0.9659258262890683122, 1.000000000000000000) ) ) 
 REPRESENTATION_ITEM ( '' )  SURFACE ( )  );
#81990=CARTESIAN_POINT ( 'NONE',  ( 0.5774900079438607392, 43.48035201082151247, 5.440088680355550821 ) ) ;
#81991=CARTESIAN_POINT ( 'NONE',  ( 7.361572987183170547, 42.05059781766745886, 9.846743663894590881 ) ) ;
#81992=CARTESIAN_POINT ( 'NONE',  ( -4.164238869374099927, 27.01208216824730357, 3.795296366450308767 ) ) ;
#81993=ORIENTED_EDGE ( 'NONE', *, *, #17478, .T. ) ;
#81995=CARTESIAN_POINT ( 'NONE',  ( 4.559911319644449179, 43.89701867748816966, 9.422509992056141925 ) ) ;
#81997=CARTESIAN_POINT ( 'NONE',  ( 24.16423886937409904, 54.09541550158063217, 3.795296366450317205 ) ) ;
#81998=CARTESIAN_POINT ( 'NONE',  ( 19.84674366389459266, 63.71726448433412315, -2.638427012816827677 ) ) ;
#82000=CARTESIAN_POINT ( 'NONE',  ( 7.084665262690076126, 57.02201867748817676, -10.88017736071110164 ) ) ;
#82002=CARTESIAN_POINT ( 'NONE',  ( -2.816281873526473856, 4.123634669930420493, 9.499525473075851096E-16 ) ) ;
#82004=CARTESIAN_POINT ( 'NONE',  ( 12.91533473730992121, 19.52201867748816611, 10.88017736071110164 ) ) ;
#82005=CARTESIAN_POINT ( 'NONE',  ( -0.8801773607111008646, 13.27201867748817321, 2.915334737309923430 ) ) ;
#82006=CARTESIAN_POINT ( 'NONE',  ( 10.00000000000000000, 44.75893115100078745, -9.846743663894594434 ) ) ;
#82010=EDGE_CURVE ( 'NONE', #80524, #71988, #61035, .T. ) ;
#82011=CARTESIAN_POINT ( 'NONE',  ( 20.88017736071110519, 5.563685344154837509, 2.639326808657452039E-16 ) ) ;
#82012=CARTESIAN_POINT ( 'NONE',  ( 22.81628187352647785, 11.41530133659708390, 3.434112377981063169 ) ) ;
#82013=CARTESIAN_POINT ( 'NONE',  ( 0.1532563361054083140, 16.00893115100078390, 1.131784320476157264E-15 ) ) ;
#82014=CARTESIAN_POINT ( 'NONE',  ( 0.1532563361054100626, 40.80059781766745886, -2.638427012816831230 ) ) ;
#82015=CARTESIAN_POINT ( 'NONE',  ( 10.00000000000000000, 41.81368534415484106, -10.88017736071110342 ) ) ;
#82016=CARTESIAN_POINT ( 'NONE',  ( 19.38216949554541557, 2.248634669930420049, -9.382169495545420901 ) ) ;
#82017=CARTESIAN_POINT ( 'NONE',  ( 19.42250999205614193, 55.14701867748817676, 5.440088680355555262 ) ) ;
#82020=CARTESIAN_POINT ( 'NONE',  ( 0.6178305044545838731, 54.74863466993042493, 9.382169495545420901 ) ) ;
#82022=CARTESIAN_POINT ( 'NONE',  ( -0.8801773607111009756, 68.06368534415484817, 1.068504757029289695E-15 ) ) ;
#82023=CARTESIAN_POINT ( 'NONE',  ( 19.38216949554541557, 37.24863466993041783, -9.382169495545420901 ) ) ;
#82024=CARTESIAN_POINT ( 'NONE',  ( -2.266590686148945544, 6.387082168247300906, -7.082119434687050408 ) ) ;
#82025=CARTESIAN_POINT ( 'NONE',  ( 20.32896413005680714, 32.60497603579418069, -5.963430220938276349 ) ) ;
#82026=CARTESIAN_POINT ( 'NONE',  ( 12.91533473730993009, 36.60535201082151247, -10.88017736071109987 ) ) ;
#82027=CARTESIAN_POINT ( 'NONE',  ( 7.361572987183170547, 62.05059781766745886, 9.846743663894590881 ) ) ;
#82028=CARTESIAN_POINT ( 'NONE',  ( 10.00000000000000000, 59.75893115100078745, -9.846743663894594434 ) ) ;
#82029=CARTESIAN_POINT ( 'NONE',  ( 1.472469842513823179, 20.59226448433411960, -4.923371831947296329 ) ) ;
#82030=CARTESIAN_POINT ( 'NONE',  ( 15.44008868035555793, 66.39701867748817676, -9.422509992056140149 ) ) ;
#82032=CARTESIAN_POINT ( 'NONE',  ( 10.00000000000000000, 25.55374883491396787, -14.16423886937410082 ) ) ;
#82033=B_SPLINE_CURVE_WITH_KNOTS ( 'NONE', 3,
 ( #27095, #89087, #5607, #81579, #93266, #57598, #40275, #70782, #17776, #95607 ),
 .UNSPECIFIED., .F., .F.,
 ( 4, 3, 3, 4 ),
 ( 7.573910767901059648E-18, 0.0006253016069560931147, 0.001250604074564911532, 0.002501455912506553476 ),
 .UNSPECIFIED. ) ;
#82036=ORIENTED_EDGE ( 'NONE', *, *, #17361, .F. ) ;
#82037=CARTESIAN_POINT ( 'NONE',  ( 24.16423886937410614, 59.51208216824728936, -3.795296366450302550 ) ) ;
#82038=CARTESIAN_POINT ( 'NONE',  ( 20.36894250292379738, 59.92874883491397497, -10.36894250292379027 ) ) ;
#82039=CARTESIAN_POINT ( 'NONE',  ( 1.472469842513823179, 35.59226448433412315, -4.923371831947296329 ) ) ;
#82040=CARTESIAN_POINT ( 'NONE',  ( 3.591859063236763294, 28.29030133659708568, -11.09922568453595026 ) ) ;
#82042=CARTESIAN_POINT ( 'NONE',  ( 15.44008868035555260, 14.73035201082150536, 9.422509992056143702 ) ) ;
#82043=CARTESIAN_POINT ( 'NONE',  ( 22.26659068614894466, 58.88708216824729647, 7.082119434687054849 ) ) ;
#82044=CARTESIAN_POINT ( 'NONE',  ( 14.92337183194729633, 22.67559781766745175, 8.527530157486181039 ) ) ;
#82046=CARTESIAN_POINT ( 'NONE',  ( 0.1532563361054100626, 15.80059781766745353, -2.638427012816831230 ) ) ;
#82051=B_SPLINE_CURVE_WITH_KNOTS ( 'NONE', 3,
 ( #6322, #80847, #95860, #12832 ),
 .UNSPECIFIED., .F., .F.,
 ( 4, 4 ),
 ( 0.000000000000000000, 0.001036303429213365724 ),
 .UNSPECIFIED. ) ;
#82055=CARTESIAN_POINT ( 'NONE',  ( 19.84674366389459621, 43.50893115100078745, 7.409399052514197653E-17 ) ) ;
#82056=CARTESIAN_POINT ( 'NONE',  ( 6.204703633549690345, 17.84541550158063217, 14.16423886937410082 ) ) ;
#82057=CARTESIAN_POINT ( 'NONE',  ( 17.96484262340118221, 21.18868534415483396, -7.964842623401177768 ) ) ;
#82058=CARTESIAN_POINT ( 'NONE',  ( 20.88017736071110875, 20.77201867748816611, -2.915334737309920765 ) ) ;
#82059=CARTESIAN_POINT ( 'NONE',  ( 1.472469842513823179, 60.59226448433412315, -4.923371831947296329 ) ) ;
#82060=CARTESIAN_POINT ( 'NONE',  ( -1.099225684535947600, 14.54030133659708568, 6.408140936763237150 ) ) ;
#82061=CARTESIAN_POINT ( 'NONE',  ( 22.26659068614895176, 4.720415501580633943, -7.082119434687042414 ) ) ;
#82062=CARTESIAN_POINT ( 'NONE',  ( 7.084665262690076126, 69.10535201082151957, 10.88017736071109987 ) ) ;
#82065=CARTESIAN_POINT ( 'NONE',  ( 13.43411237798106583, 37.66530133659708923, -12.81628187352647252 ) ) ;
#82067=CARTESIAN_POINT ( 'NONE',  ( 18.52753015748617571, 33.09226448433411605, 4.923371831947298993 ) ) ;
#82068=CARTESIAN_POINT ( 'NONE',  ( 0.5774900079438607392, 8.480352010821505360, 5.440088680355550821 ) ) ;
#82069=CARTESIAN_POINT ( 'NONE',  ( 7.084665262690076126, 2.022018677488171434, -10.88017736071110164 ) ) ;
#82071=CARTESIAN_POINT ( 'NONE',  ( 10.00000000000000000, 41.81368534415484106, -10.88017736071110342 ) ) ;
#82072=CARTESIAN_POINT ( 'NONE',  ( 7.084665262690076126, 64.10535201082150536, 10.88017736071109987 ) ) ;
#82073=CARTESIAN_POINT ( 'NONE',  ( 10.00000000000000000, 56.81368534415484106, -10.88017736071110342 ) ) ;
#82075=CARTESIAN_POINT ( 'NONE',  ( 4.559911319644449179, 48.89701867748817676, 9.422509992056141925 ) ) ;
#82076=DIRECTION ( 'NONE',  ( 0.000000000000000000, -1.000000000000000000, 0.000000000000000000 ) ) ;
#82079=EDGE_CURVE ( 'NONE', #87620, #40639, #24879, .T. ) ;
#82080=CARTESIAN_POINT ( 'NONE',  ( 0.1532563361054100626, 30.80059781766744820, -2.638427012816831230 ) ) ;
#82082=CARTESIAN_POINT ( 'NONE',  ( 12.63842701281683922, 59.55059781766744464, -9.846743663894590881 ) ) ;
#82085=CARTESIAN_POINT ( 'NONE',  ( -2.266590686148945544, 12.22041550158063394, 7.082119434687048631 ) ) ;
#82086=ORIENTED_EDGE ( 'NONE', *, *, #30643, .F. ) ;
#82090=CARTESIAN_POINT ( 'NONE',  ( 7.084665262690076126, 4.105352010821503583, 10.88017736071109987 ) ) ;
#82094=CARTESIAN_POINT ( 'NONE',  ( 1.472469842513823179, 40.59226448433411605, -4.923371831947296329 ) ) ;
#82096=CARTESIAN_POINT ( 'NONE',  ( -2.816281873526473856, 14.12363466993041961, 9.499525473075851096E-16 ) ) ;
#82097=CARTESIAN_POINT ( 'NONE',  ( 18.52753015748617571, 8.092264484334117824, 4.923371831947298993 ) ) ;
#82099=CARTESIAN_POINT ( 'NONE',  ( 22.81628187352647785, 1.415301336597087012, 3.434112377981063169 ) ) ;
#82103=CARTESIAN_POINT ( 'NONE',  ( 2.035157376598824452, 13.68868534415483751, 7.964842623401179544 ) ) ;
#82104=( NAMED_UNIT ( * ) SI_UNIT ( $, .STERADIAN. ) SOLID_ANGLE_UNIT ( ) );
#82105=CARTESIAN_POINT ( 'NONE',  ( 12.63842701281683034, 32.46726448433412315, 9.846743663894596210 ) ) ;
#82106=CARTESIAN_POINT ( 'NONE',  ( 19.42250999205614548, 50.98035201082151247, -5.440088680355545492 ) ) ;
#82107=CARTESIAN_POINT ( 'NONE',  ( -2.816281873526471635, 43.91530133659708923, -3.434112377981056508 ) ) ;
#82109=CARTESIAN_POINT ( 'NONE',  ( 17.96484262340118221, 11.18868534415483929, -7.964842623401177768 ) ) ;
#82111=CARTESIAN_POINT ( 'NONE',  ( -0.3289641300568009741, 57.24545670184114954, -5.963430220938281678 ) ) ;
#82113=CARTESIAN_POINT ( 'NONE',  ( 2.791683348922240793, 61.63393115100079456, 7.208316651077764092 ) ) ;
#82114=CARTESIAN_POINT ( 'NONE',  ( 10.00000000000000000, 24.75893115100078745, -9.846743663894594434 ) ) ;
#82116=CARTESIAN_POINT ( 'NONE',  ( 13.43411237798105340, 40.58196800326375353, 12.81628187352647963 ) ) ;
#82117=CARTESIAN_POINT ( 'NONE',  ( 18.50749283717776805, 24.69955587570481725, 6.499999999999999112 ) ) ;
#82118=CARTESIAN_POINT ( 'NONE',  ( 7.084665262690076126, 42.02201867748816966, -10.88017736071110164 ) ) ;
#82120=ADVANCED_FACE ( 'NONE', ( #23924 ), #11574, .F. ) ;
#82121=DIRECTION ( 'NONE',  ( -1.000000000000000000, 0.000000000000000000, -0.000000000000000000 ) ) ;
#82122=CARTESIAN_POINT ( 'NONE',  ( 0.5774900079438590739, 27.64701867748817676, -5.440088680355550821 ) ) ;
#82123=CARTESIAN_POINT ( 'NONE',  ( 15.44008868035555793, 36.39701867748816966, -9.422509992056140149 ) ) ;
#82124=CARTESIAN_POINT ( 'NONE',  ( 17.20831665107776587, 54.13393115100079456, -7.208316651077762316 ) ) ;
#82125=CARTESIAN_POINT ( 'NONE',  ( 10.00000000000000178, 59.31368534415484106, 10.88017736071110342 ) ) ;
#82126=CARTESIAN_POINT ( 'NONE',  ( 10.00000000000000178, 38.05374883491396787, 14.16423886937410082 ) ) ;
#82128=CARTESIAN_POINT ( 'NONE',  ( 10.00000000000000000, 34.75893115100078745, -9.846743663894594434 ) ) ;
#82129=CARTESIAN_POINT ( 'NONE',  ( 3.591859063236761518, 59.95696800326375353, 11.09922568453594849 ) ) ;
#82130=CARTESIAN_POINT ( 'NONE',  ( 0.6178305044545838731, -0.2513653300695798953, 9.382169495545420901 ) ) ;
#82131=EDGE_LOOP ( 'NONE', ( #73455, #41303, #80395, #59304 ) ) ;
#82132=CARTESIAN_POINT ( 'NONE',  ( 2.035157376598824452, 23.68868534415484461, 7.964842623401179544 ) ) ;
#82133=EDGE_CURVE ( 'NONE', #66548, #31259, #79859, .T. ) ;
#82134=CARTESIAN_POINT ( 'NONE',  ( 17.96484262340118221, 9.938685344154839285, 7.964842623401181321 ) ) ;
#82135=CARTESIAN_POINT ( 'NONE',  ( 10.00000000000000178, 64.31368534415483396, 10.88017736071110342 ) ) ;
#82136=CARTESIAN_POINT ( 'NONE',  ( 22.26659068614895176, 19.72041550158063572, -7.082119434687042414 ) ) ;
#82137=CARTESIAN_POINT ( 'NONE',  ( 18.52753015748617571, 8.092264484334117824, 4.923371831947298993 ) ) ;
#82138=CARTESIAN_POINT ( 'NONE',  ( 10.00000000000000000, 64.75893115100078035, -9.846743663894594434 ) ) ;
#82139=CARTESIAN_POINT ( 'NONE',  ( 17.96484262340118221, 49.93868534415484106, 7.964842623401181321 ) ) ;
#82143=ORIENTED_EDGE ( 'NONE', *, *, #34635, .F. ) ;
#82145=CARTESIAN_POINT ( 'NONE',  ( 17.20831665107776587, 44.13393115100078745, -7.208316651077762316 ) ) ;
#82147=EDGE_LOOP ( 'NONE', ( #68946, #43871, #6083, #30030 ) ) ;
#82149=CARTESIAN_POINT ( 'NONE',  ( 24.16423886937410614, 19.51208216824729647, -3.795296366450302550 ) ) ;
#82150=CARTESIAN_POINT ( 'NONE',  ( 24.16423886937410614, 29.30374883491396787, 8.672049930838204340E-16 ) ) ;
#82151=CARTESIAN_POINT ( 'NONE',  ( -0.8801773607111009756, 58.06368534415484106, 1.068504757029289695E-15 ) ) ;
#82152=CARTESIAN_POINT ( 'NONE',  ( 10.00000000000000178, 63.05374883491396076, 14.16423886937410082 ) ) ;
#82153=CARTESIAN_POINT ( 'NONE',  ( 16.40814093676324603, 2.456968003263753531, -11.09922568453594671 ) ) ;
#82154=CARTESIAN_POINT ( 'NONE',  ( 10.00000000000000000, 49.75893115100078745, -9.846743663894594434 ) ) ;
#82156=CARTESIAN_POINT ( 'NONE',  ( 20.88017736071110875, 40.77201867748818387, -2.915334737309920765 ) ) ;
#82157=CARTESIAN_POINT ( 'NONE',  ( 13.43411237798105340, 0.5819680032637533085, 12.81628187352647963 ) ) ;
#82158=CARTESIAN_POINT ( 'NONE',  ( -4.164238869374098151, 16.59541550158063927, -3.795296366450310543 ) ) ;
#82159=CARTESIAN_POINT ( 'NONE',  ( -4.164238869374099039, 51.80374883491396787, 8.674139862899312516E-16 ) ) ;
#82160=CARTESIAN_POINT ( 'NONE',  ( 4.559911319644449179, 12.23035201082150714, -9.422509992056141925 ) ) ;
#82161=CARTESIAN_POINT ( 'NONE',  ( -0.1503990784575329198, 2.222660991849184864, -6.262539305110070842 ) ) ;
#82162=CARTESIAN_POINT ( 'NONE',  ( 15.44008868035555260, 39.73035201082150536, 9.422509992056143702 ) ) ;
#82165=CARTESIAN_POINT ( 'NONE',  ( -38.69000000000001194, 93.50000000000000000, -10.09898361729590199 ) ) ;
#82166=ORIENTED_EDGE ( 'NONE', *, *, #20593, .T. ) ;
#82167=CARTESIAN_POINT ( 'NONE',  ( 2.791683348922237240, 30.38393115100078390, -7.208316651077763204 ) ) ;
#82168=ORIENTED_EDGE ( 'NONE', *, *, #15190, .T. ) ;
#82169=CARTESIAN_POINT ( 'NONE',  ( -4.164238869374098151, 46.59541550158063927, -3.795296366450310543 ) ) ;
#82170=CARTESIAN_POINT ( 'NONE',  ( 12.63842701281683922, 19.55059781766745175, -9.846743663894590881 ) ) ;
#82171=CARTESIAN_POINT ( 'NONE',  ( 7.361572987183170547, 47.05059781766745175, 9.846743663894590881 ) ) ;
#82172=CARTESIAN_POINT ( 'NONE',  ( 20.88017736071110519, 65.56368534415483396, 2.639326808657452039E-16 ) ) ;
#82175=CARTESIAN_POINT ( 'NONE',  ( -0.8801773607111009756, 68.06368534415484817, 1.068504757029289695E-15 ) ) ;
#82179=CARTESIAN_POINT ( 'NONE',  ( 22.81628187352647785, 56.41530133659708213, 3.434112377981063169 ) ) ;
#82181=ORIENTED_EDGE ( 'NONE', *, *, #87706, .T. ) ;
#82182=CARTESIAN_POINT ( 'NONE',  ( 22.26659068614895176, 34.72041550158063927, -7.082119434687042414 ) ) ;
#82184=CARTESIAN_POINT ( 'NONE',  ( 13.43411237798105340, 25.58196800326374998, 12.81628187352647963 ) ) ;
#82186=CARTESIAN_POINT ( 'NONE',  ( 0.6178305044545818747, 43.49863466993042493, -9.382169495545419124 ) ) ;
#82187=CARTESIAN_POINT ( 'NONE',  ( 2.035157376598822676, 17.43868534415483751, -7.964842623401177768 ) ) ;
#82188=CARTESIAN_POINT ( 'NONE',  ( 2.791683348922237240, 30.38393115100078390, -7.208316651077763204 ) ) ;
#82189=CARTESIAN_POINT ( 'NONE',  ( -0.8801773607111009756, 8.063685344154837509, 1.068504757029289695E-15 ) ) ;
#82190=( GEOMETRIC_REPRESENTATION_CONTEXT ( 3 ) GLOBAL_UNCERTAINTY_ASSIGNED_CONTEXT ( ( #67393 ) ) GLOBAL_UNIT_ASSIGNED_CONTEXT ( ( #19755, #64743, #26761 ) ) REPRESENTATION_CONTEXT ( 'NONE', 'WORKASPACE' ) );
#82193=CARTESIAN_POINT ( 'NONE',  ( 17.20831665107776587, 39.13393115100079456, -7.208316651077762316 ) ) ;
#82194=CARTESIAN_POINT ( 'NONE',  ( 14.92337183194729988, 49.34226448433411605, -8.527530157486177487 ) ) ;
#82195=CARTESIAN_POINT ( 'NONE',  ( 20.24186590665278018, 22.61633188102327097, -6.114288769123028544 ) ) ;
#82200=CARTESIAN_POINT ( 'NONE',  ( 0.9408516040111464251, 27.46693863883976405, -6.499999999999936051 ) ) ;
#82201=CARTESIAN_POINT ( 'NONE',  ( 19.59355889808634288, 82.60103572628047175, 5.130931023488903620 ) ) ;
#82202=CARTESIAN_POINT ( 'NONE',  ( 12.63842701281683034, 12.46726448433411782, 9.846743663894596210 ) ) ;
#82203=CARTESIAN_POINT ( 'NONE',  ( 13.43411237798106583, 42.66530133659707502, -12.81628187352647252 ) ) ;
#82207=CARTESIAN_POINT ( 'NONE',  ( 0.1532563361054083140, 61.00893115100078745, 1.131784320476157264E-15 ) ) ;
#82209=CARTESIAN_POINT ( 'NONE',  ( 22.26659068614894466, 18.88708216824730002, 7.082119434687054849 ) ) ;
#82210=CARTESIAN_POINT ( 'NONE',  ( 12.63842701281683034, 52.46726448433413026, 9.846743663894596210 ) ) ;
#82211=CARTESIAN_POINT ( 'NONE',  ( 6.565887622018943937, 45.16530133659708923, 12.81628187352647430 ) ) ;
#82213=CARTESIAN_POINT ( 'NONE',  ( 2.791683348922240793, 11.63393115100078568, 7.208316651077764092 ) ) ;
#82216=CARTESIAN_POINT ( 'NONE',  ( 5.076628168052703671, 41.84226448433411605, 8.527530157486179263 ) ) ;
#82217=CARTESIAN_POINT ( 'NONE',  ( 20.88017736071110164, 45.35535201082149115, 2.915334737309930979 ) ) ;
#82218=CARTESIAN_POINT ( 'NONE',  ( 17.20831665107776587, 29.13393115100078390, -7.208316651077762316 ) ) ;
#82220=CARTESIAN_POINT ( 'NONE',  ( 3.558677480090427725, 70.40124509038875544, -5.000000000000000000 ) ) ;
#82221=CARTESIAN_POINT ( 'NONE',  ( 20.88017736071110164, 45.35535201082149115, 2.915334737309930979 ) ) ;
#82222=ORIENTED_EDGE ( 'NONE', *, *, #86270, .T. ) ;
#82223=CARTESIAN_POINT ( 'NONE',  ( -0.8801773607111009756, 68.06368534415484817, 1.068504757029289695E-15 ) ) ;
#82224=CARTESIAN_POINT ( 'NONE',  ( 10.00000000000000178, 14.31368534415483751, 10.88017736071110342 ) ) ;
#82225=CARTESIAN_POINT ( 'NONE',  ( 2.791683348922237240, 60.38393115100078745, -7.208316651077763204 ) ) ;
#82226=CARTESIAN_POINT ( 'NONE',  ( -0.8801773607111009756, 48.06368534415484817, 1.068504757029289695E-15 ) ) ;
#82228=CARTESIAN_POINT ( 'NONE',  ( 17.96484262340118221, 59.93868534415484106, 7.964842623401181321 ) ) ;
#82229=CARTESIAN_POINT ( 'NONE',  ( 19.42250999205614193, 25.14701867748817321, 5.440088680355555262 ) ) ;
#82230=CARTESIAN_POINT ( 'NONE',  ( 20.00000000000000355, 82.59735310507680595, -4.636598376030807600 ) ) ;
#82231=CARTESIAN_POINT ( 'NONE',  ( 2.791683348922240793, 1.633931151000784565, 7.208316651077764092 ) ) ;
#82232=CARTESIAN_POINT ( 'NONE',  ( 10.00000000000000178, 22.25893115100078745, 9.846743663894594434 ) ) ;
#82235=CARTESIAN_POINT ( 'NONE',  ( 2.791683348922240793, 66.63393115100079456, 7.208316651077764092 ) ) ;
#82236=CARTESIAN_POINT ( 'NONE',  ( 20.88017736071110164, 5.355352010821503583, 2.915334737309930979 ) ) ;
#82238=CARTESIAN_POINT ( 'NONE',  ( -4.164238869374099039, 11.80374883491396965, 8.674139862899312516E-16 ) ) ;
#82240=CARTESIAN_POINT ( 'NONE',  ( -0.3689425029237898834, 56.17874883491396076, -10.36894250292378850 ) ) ;
#82241=CARTESIAN_POINT ( 'NONE',  ( 21.09922568453594849, 1.206968003263753531, 6.408140936763242479 ) ) ;
#82243=CARTESIAN_POINT ( 'NONE',  ( 15.44008868035555260, 9.730352010821505360, 9.422509992056143702 ) ) ;
#82244=CARTESIAN_POINT ( 'NONE',  ( 10.00000000000000178, 42.25893115100078745, 9.846743663894594434 ) ) ;
#82247=CARTESIAN_POINT ( 'NONE',  ( 1.472469842513823179, 1.425597817667451528, 4.923371831947296329 ) ) ;
#82248=CARTESIAN_POINT ( 'NONE',  ( 0.6178305044545838731, 24.74863466993042493, 9.382169495545420901 ) ) ;
#82249=CARTESIAN_POINT ( 'NONE',  ( 10.00000000000000178, 32.25893115100078745, 9.846743663894594434 ) ) ;
#82251=CARTESIAN_POINT ( 'NONE',  ( 0.1532563361054083140, 11.00893115100078568, 1.131784320476157264E-15 ) ) ;
#82253=CARTESIAN_POINT ( 'NONE',  ( 20.03743638938529159, 16.75197528031016603, 6.399506433553905360 ) ) ;
#82254=CARTESIAN_POINT ( 'NONE',  ( 19.42250999205614193, 15.14701867748817143, 5.440088680355555262 ) ) ;
#82255=CARTESIAN_POINT ( 'NONE',  ( 20.36894250292379738, 39.92874883491396787, -10.36894250292379027 ) ) ;
#82256=CARTESIAN_POINT ( 'NONE',  ( 0.5774900079438607392, 58.48035201082151247, 5.440088680355550821 ) ) ;
#82257=CARTESIAN_POINT ( 'NONE',  ( 18.52753015748618282, 18.92559781766745175, -4.923371831947291888 ) ) ;
#82258=CARTESIAN_POINT ( 'NONE',  ( 20.10384461210890450, 21.74302437010793199, 6.337995344473785764 ) ) ;
#82259=CARTESIAN_POINT ( 'NONE',  ( 0.1532563361054083140, 6.008931151000784787, 1.131784320476157264E-15 ) ) ;
#82260=( BOUNDED_SURFACE ( )  B_SPLINE_SURFACE ( 1, 2, ( 
 ( #45329, #75826, #77295, #91820, #53822, #84333, #22843, #8808, #76806, #7348, #69319, #62289, #75329, #92793, #69816, #24323, #82831, #14351, #6841, #37355, #90823, #37849, #68340, #98861, #30315, #60815, #91316, #23391, #9349, #70358, #91872, #8857, #15399, #1877, #2367, #85349, #39855, #45886, #16862, #30865, #46850, #31351, #16370, #61363, #8371, #85849, #53876, #84386, #93338, #32333, #61853, #77345, #15885, #32824, #39372, #47336, #93830, #69866, #76375, #54837, #892, #9853, #63322, #31842, #46369, #62838, #76859, #38879, #69371, #24860, #1388, #77839, #7890, #62338, #92358, #53368, #55342, #17362, #38383, #92846, #47831, #78332, #24373, #83877, #40353, #68883, #70854, #23885, #413, #54349, #84863, #42309, #63807, #27288, #87308, #49308, #72784, #86337, #35284, #94810, #3829, #18827, #41352, #73288, #79809, #4318, #19794, #17842, #4811, #79323, #56336, #34792, #65281, #41832, #55844, #71822, #3329, #57788, #50284, #25839, #72299, #26311, #48324, #64298, #40841, #95301, #86829, #34285, #71341, #2860, #56812, #26805, #95810, #88294, #59268, #7277, #98296, #58271, #67278, #73778, #44266, #82263, #28773, #89769, #66273, #52269, #14288, #35784, #51779, #88790, #44761, #45262, #29267, #82765, #20297, #59762, #5308, #21285, #74262, #13780, #96809, #51283, #29753, #28285, #58778, #37287, #75264, #5793, #74771, #89284, #75756, #6281, #90256, #37779, #36785, #50796, #97805, #43772, #52757, #96310, #21790, #20794, #6777, #81769, #13282, #36282, #67776, #60261, #90756, #81286, #22284, #66780, #27785, #83265, #14789, #12784, #43283, #97300, #31722, #46731, #49077, #41101, #11080, #86591, #61246, #71597, #39253, #77229, #18100, #7774, #3109, #31228, #92240, #62221, #30244, #79579, #38755, #8734, #61725, #53748, #56585, #23766, #48577, #64059, #60747, #18584, #23272, #292, #79076, #10589, #54231, #87075, #15766, #84265, #33563, #94571, #68761, #84745, #69256, #68276, #98796, #38269, #26090, #53254, #91751, #30738, #46254, #91248, #16248, #69743, #777, #1269, #22775, #83759, #92726, #15282, #76739, #8254, #24250, #45764, #56098, #76257, #95055, #11566, #42084, #97068, #26564, #80563, #59034, #58536, #49550, #19072, #4577, #65540, #89044, #80062, #96063, #35039, #73535, #27053, #72547, #43536, #35546, #74030, #89539, #21049, #73042, #28041, #51540, #81533, #4080, #20049, #34543, #57061, #87562, #65038, #20555, #95564, #27546, #50551, #81046, #13040, #57551, #12057, #88050, #66540, #19563, #42558, #50059, #58040, #82030, #88548, #12553, #43056, #5561, #5061, #66037, #96566, #51040, #36037, #72068, #28541, #41600, #3593, #34052 ),
 ( #64548, #75518, #75024, #91997, #7033, #45512, #54000, #37539, #6048, #15040, #60015, #69016, #61491, #91005, #82528, #23031, #37038, #14044, #44525, #68523, #68029, #76012, #74527, #22536, #90510, #23528, #15536, #7541, #97558, #98556, #38032, #54, #53007, #13540, #84013, #44024, #30501, #6529, #46019, #83522, #61003, #91514, #52035, #76507, #30007, #53503, #8021, #67536, #60513, #36547, #38518, #67036, #547, #30993, #29019, #59529, #90023, #21544, #22045, #98051, #29508, #52520, #83027, #14543, #45013, #25493, #2510, #92976, #47479, #46984, #63939, #77979, #17499, #25967, #9485, #76995, #85987, #31968, #40981, #33444, #62971, #54481, #93969, #8989, #84992, #16507, #40490, #39988, #47964, #46495, #93476, #62470, #94451, #86481, #78473, #69504, #70491, #9988, #70988, #25002, #84508, #55980, #16006, #32962, #77478, #17979, #55487, #63467, #48463, #24011, #78960, #2011, #32476, #10472, #8507, #39010, #54969, #71478, #2994, #69996, #1020, #31480, #61984, #92483, #39506, #1522, #24507, #85491, #17000, #79460, #18466, #10958, #86953, #48951, #56467, #29330, #73850, #13353, #20863, #14354, #35361, #12854, #6342, #88861, #35854, #5380, #66343, #59828, #43838, #28835, #51355, #81839, #90321, #59337, #96881, #5859, #52339, #96382, #65854, #74334, #67344, #36352, #66847, #27853, #21859, #20370, #51847, #28358, #89840, #97367, #21356, #82336, #58847, #13856, #89353, #44336, #58341, #74841, #36853, #97870, #82834, #50864, #81356, #57371, #2932, #41906, #93903, #87866, #11879, #57859, #94388, #41423, #19864, #65357, #25904, #34367, #87382, #71415, #71884, #80869, #42873, #10901, #3403, #34864, #95886, #56406, #72860, #55913, #86412, #33379, #42383, #33866, #12367, #88370, #64373, #94881, #56880, #72368, #4395, #19383, #26381, #79879, #73356, #18901, #4883, #3898, #49378, #11385, #80379, #86891, #64857, #95377, #26878, #27366, #49866, #48884, #63875, #63397, #50360, #25429, #17913, #48397, #78899, #10409, #40915, #18402, #79394, #5452, #59408, #14430, #36429, #66921, #13426, #67918, #36926, #97442, #66422, #20938, #51427, #29896, #35925, #28906, #60399, #21931, #58925, #28427, #89914, #51925, #52412, #89425, #82409, #21428, #97944, #74409, #81916, #75402, #29402, #6920, #90896, #22424, #13935, #90394, #43425, #44899, #5937, #6414, #44412, #96955, #74915, #67417, #82912, #59904, #37429, #73926, #11951, #42944, #26450, #11457, #87453, #96454, #3481, #73426, #88933, #20443, #3967, #57931, #50932, #12436, #33938, #49948, #64442, #25977, #18474, #94949, #88440, #56473, #34435, #80453, #42455, #4950, #56951, #41975, #18968, #27926, #49446 ) ),
 .UNSPECIFIED., .F., .F., .F. ) 
 B_SPLINE_SURFACE_WITH_KNOTS ( ( 2, 2 ),
 ( 3, 2, 2, 2, 2, 2, 2, 2, 2, 2, 2, 2, 2, 2, 2, 2, 2, 2, 2, 2, 2, 2, 2, 2, 2, 2, 2, 2, 2, 2, 2, 2, 2, 2, 2, 2, 2, 2, 2, 2, 2, 2, 2, 2, 2, 2, 2, 2, 2, 2, 2, 2, 2, 2, 2, 2, 2, 2, 2, 2, 2, 2, 2, 2, 2, 2, 2, 2, 2, 2, 2, 2, 2, 2, 2, 2, 2, 2, 2, 2, 2, 2, 2, 2, 2, 2, 2, 2, 2, 2, 2, 2, 2, 2, 2, 2, 2, 2, 2, 2, 2, 2, 2, 2, 2, 2, 2, 2, 2, 2, 2, 2, 2, 2, 2, 2, 2, 2, 2, 2, 2, 2, 2, 2, 2, 2, 2, 2, 2, 2, 2, 2, 2, 2, 2, 2, 2, 2, 2, 2, 2, 2, 2, 2, 2, 2, 2, 2, 2, 2, 2, 2, 2, 2, 2, 2, 2, 2, 2, 2, 2, 2, 3 ),
 ( 0.000000000000000000, 1.000000000000000000 ),
 ( 0.000000000000000000, 0.005952380952380952051, 0.01190476190476190410, 0.01785714285714285615, 0.02380952380952380820, 0.02976190476190476025, 0.03571428571428571230, 0.04166666666666666435, 0.04761904761904761640, 0.05357142857142856845, 0.05952380952380952051, 0.06547619047619047949, 0.07142857142857142461, 0.07738095238095238360, 0.08333333333333332871, 0.08928571428571428770, 0.09523809523809523281, 0.1011904761904761918, 0.1071428571428571369, 0.1130952380952380959, 0.1190476190476190410, 0.1250000000000000000, 0.1309523809523809590, 0.1369047619047619180, 0.1428571428571428492, 0.1488095238095238082, 0.1547619047619047672, 0.1607142857142857262, 0.1666666666666666574, 0.1726190476190476164, 0.1785714285714285754, 0.1845238095238095344, 0.1904761904761904656, 0.1964285714285714246, 0.2023809523809523836, 0.2083333333333333426, 0.2142857142857142738, 0.2202380952380952328, 0.2261904761904761918, 0.2321428571428571508, 0.2380952380952380820, 0.2440476190476190410, 0.2500000000000000000, 0.2559523809523809312, 0.2619047619047619180, 0.2678571428571428492, 0.2738095238095238360, 0.2797619047619047672, 0.2857142857142856984, 0.2916666666666666852, 0.2976190476190476164, 0.3035714285714285476, 0.3095238095238095344, 0.3154761904761904656, 0.3214285714285714524, 0.3273809523809523836, 0.3333333333333333148, 0.3392857142857143016, 0.3452380952380952328, 0.3511904761904761640, 0.3571428571428571508, 0.3630952380952380820, 0.3690476190476190688, 0.3750000000000000000, 0.3809523809523809312, 0.3869047619047619180, 0.3928571428571428492, 0.3988095238095238360, 0.4047619047619047672, 0.4107142857142856984, 0.4166666666666666852, 0.4226190476190476164, 0.4285714285714285476, 0.4345238095238095344, 0.4404761904761904656, 0.4464285714285714524, 0.4523809523809523836, 0.4583333333333333148, 0.4642857142857143016, 0.4702380952380952328, 0.4761904761904761640, 0.4821428571428571508, 0.4880952380952380820, 0.4940476190476190688, 0.5000000000000000000, 0.5059523809523809312, 0.5119047619047618625, 0.5178571428571429047, 0.5238095238095238360, 0.5297619047619047672, 0.5357142857142856984, 0.5416666666666666297, 0.5476190476190476719, 0.5535714285714286031, 0.5595238095238095344, 0.5654761904761904656, 0.5714285714285713969, 0.5773809523809523281, 0.5833333333333333703, 0.5892857142857143016, 0.5952380952380952328, 0.6011904761904761640, 0.6071428571428570953, 0.6130952380952381375, 0.6190476190476190688, 0.6250000000000000000, 0.6309523809523809312, 0.6369047619047618625, 0.6428571428571429047, 0.6488095238095238360, 0.6547619047619047672, 0.6607142857142856984, 0.6666666666666666297, 0.6726190476190476719, 0.6785714285714286031, 0.6845238095238095344, 0.6904761904761904656, 0.6964285714285713969, 0.7023809523809523281, 0.7083333333333333703, 0.7142857142857143016, 0.7202380952380952328, 0.7261904761904761640, 0.7321428571428570953, 0.7380952380952381375, 0.7440476190476190688, 0.7500000000000000000, 0.7559523809523809312, 0.7619047619047618625, 0.7678571428571429047, 0.7738095238095238360, 0.7797619047619047672, 0.7857142857142856984, 0.7916666666666666297, 0.7976190476190476719, 0.8035714285714286031, 0.8095238095238095344, 0.8154761904761904656, 0.8214285714285713969, 0.8273809523809523281, 0.8333333333333333703, 0.8392857142857143016, 0.8452380952380952328, 0.8511904761904761640, 0.8571428571428570953, 0.8630952380952381375, 0.8690476190476190688, 0.8750000000000000000, 0.8809523809523809312, 0.8869047619047618625, 0.8928571428571429047, 0.8988095238095238360, 0.9047619047619047672, 0.9107142857142856984, 0.9166666666666666297, 0.9226190476190476719, 0.9285714285714286031, 0.9345238095238095344, 0.9404761904761904656, 0.9464285714285713969, 0.9523809523809523281, 0.9583333333333333703, 0.9642857142857143016 ),
 .UNSPECIFIED. ) 
 GEOMETRIC_REPRESENTATION_ITEM ( )  RATIONAL_B_SPLINE_SURFACE ( (
 ( 1.000000000000000000, 0.9659258262890683122, 1.000000000000000000, 0.9659258262890683122, 1.000000000000000000, 0.9659258262890683122, 1.000000000000000000, 0.9659258262890683122, 1.000000000000000000, 0.9659258262890683122, 1.000000000000000000, 0.9659258262890683122, 1.000000000000000000, 0.9659258262890683122, 1.000000000000000000, 0.9659258262890683122, 1.000000000000000000, 0.9659258262890683122, 1.000000000000000000, 0.9659258262890683122, 1.000000000000000000, 0.9659258262890683122, 1.000000000000000000, 0.9659258262890683122, 1.000000000000000000, 0.9659258262890683122, 1.000000000000000000, 0.9659258262890683122, 1.000000000000000000, 0.9659258262890683122, 1.000000000000000000, 0.9659258262890683122, 1.000000000000000000, 0.9659258262890683122, 1.000000000000000000, 0.9659258262890683122, 1.000000000000000000, 0.9659258262890683122, 1.000000000000000000, 0.9659258262890683122, 1.000000000000000000, 0.9659258262890683122, 1.000000000000000000, 0.9659258262890683122, 1.000000000000000000, 0.9659258262890683122, 1.000000000000000000, 0.9659258262890683122, 1.000000000000000000, 0.9659258262890683122, 1.000000000000000000, 0.9659258262890683122, 1.000000000000000000, 0.9659258262890683122, 1.000000000000000000, 0.9659258262890683122, 1.000000000000000000, 0.9659258262890683122, 1.000000000000000000, 0.9659258262890683122, 1.000000000000000000, 0.9659258262890683122, 1.000000000000000000, 0.9659258262890683122, 1.000000000000000000, 0.9659258262890683122, 1.000000000000000000, 0.9659258262890683122, 1.000000000000000000, 0.9659258262890683122, 1.000000000000000000, 0.9659258262890683122, 1.000000000000000000, 0.9659258262890683122, 1.000000000000000000, 0.9659258262890683122, 1.000000000000000000, 0.9659258262890683122, 1.000000000000000000, 0.9659258262890683122, 1.000000000000000000, 0.9659258262890683122, 1.000000000000000000, 0.9659258262890683122, 1.000000000000000000, 0.9659258262890683122, 1.000000000000000000, 0.9659258262890683122, 1.000000000000000000, 0.9659258262890683122, 1.000000000000000000, 0.9659258262890683122, 1.000000000000000000, 0.9659258262890683122, 1.000000000000000000, 0.9659258262890683122, 1.000000000000000000, 0.9659258262890683122, 1.000000000000000000, 0.9659258262890683122, 1.000000000000000000, 0.9659258262890683122, 1.000000000000000000, 0.9659258262890683122, 1.000000000000000000, 0.9659258262890683122, 1.000000000000000000, 0.9659258262890683122, 1.000000000000000000, 0.9659258262890683122, 1.000000000000000000, 0.9659258262890683122, 1.000000000000000000, 0.9659258262890683122, 1.000000000000000000, 0.9659258262890683122, 1.000000000000000000, 0.9659258262890683122, 1.000000000000000000, 0.9659258262890683122, 1.000000000000000000, 0.9659258262890683122, 1.000000000000000000, 0.9659258262890683122, 1.000000000000000000, 0.9659258262890683122, 1.000000000000000000, 0.9659258262890683122, 1.000000000000000000, 0.9659258262890683122, 1.000000000000000000, 0.9659258262890683122, 1.000000000000000000, 0.9659258262890683122, 1.000000000000000000, 0.9659258262890683122, 1.000000000000000000, 0.9659258262890683122, 1.000000000000000000, 0.9659258262890683122, 1.000000000000000000, 0.9659258262890683122, 1.000000000000000000, 0.9659258262890683122, 1.000000000000000000, 0.9659258262890683122, 1.000000000000000000, 0.9659258262890683122, 1.000000000000000000, 0.9659258262890683122, 1.000000000000000000, 0.9659258262890683122, 1.000000000000000000, 0.9659258262890683122, 1.000000000000000000, 0.9659258262890683122, 1.000000000000000000, 0.9659258262890683122, 1.000000000000000000, 0.9659258262890683122, 1.000000000000000000, 0.9659258262890683122, 1.000000000000000000, 0.9659258262890683122, 1.000000000000000000, 0.9659258262890683122, 1.000000000000000000, 0.9659258262890683122, 1.000000000000000000, 0.9659258262890683122, 1.000000000000000000, 0.9659258262890683122, 1.000000000000000000, 0.9659258262890683122, 1.000000000000000000, 0.9659258262890683122, 1.000000000000000000, 0.9659258262890683122, 1.000000000000000000, 0.9659258262890683122, 1.000000000000000000, 0.9659258262890683122, 1.000000000000000000, 0.9659258262890683122, 1.000000000000000000, 0.9659258262890683122, 1.000000000000000000, 0.9659258262890683122, 1.000000000000000000, 0.9659258262890683122, 1.000000000000000000, 0.9659258262890683122, 1.000000000000000000, 0.9659258262890683122, 1.000000000000000000, 0.9659258262890683122, 1.000000000000000000, 0.9659258262890683122, 1.000000000000000000, 0.9659258262890683122, 1.000000000000000000, 0.9659258262890683122, 1.000000000000000000, 0.9659258262890683122, 1.000000000000000000, 0.9659258262890683122, 1.000000000000000000, 0.9659258262890683122, 1.000000000000000000, 0.9659258262890683122, 1.000000000000000000, 0.9659258262890683122, 1.000000000000000000, 0.9659258262890683122, 1.000000000000000000, 0.9659258262890683122, 1.000000000000000000, 0.9659258262890683122, 1.000000000000000000, 0.9659258262890683122, 1.000000000000000000, 0.9659258262890683122, 1.000000000000000000, 0.9659258262890683122, 1.000000000000000000, 0.9659258262890683122, 1.000000000000000000, 0.9659258262890683122, 1.000000000000000000, 0.9659258262890683122, 1.000000000000000000, 0.9659258262890683122, 1.000000000000000000, 0.9659258262890683122, 1.000000000000000000, 0.9659258262890683122, 1.000000000000000000, 0.9659258262890683122, 1.000000000000000000, 0.9659258262890683122, 1.000000000000000000, 0.9659258262890683122, 1.000000000000000000, 0.9659258262890683122, 1.000000000000000000, 0.9659258262890683122, 1.000000000000000000, 0.9659258262890683122, 1.000000000000000000, 0.9659258262890683122, 1.000000000000000000, 0.9659258262890683122, 1.000000000000000000, 0.9659258262890683122, 1.000000000000000000, 0.9659258262890683122, 1.000000000000000000, 0.9659258262890683122, 1.000000000000000000, 0.9659258262890683122, 1.000000000000000000, 0.9659258262890683122, 1.000000000000000000, 0.9659258262890683122, 1.000000000000000000, 0.9659258262890683122, 1.000000000000000000, 0.9659258262890683122, 1.000000000000000000, 0.9659258262890683122, 1.000000000000000000, 0.9659258262890683122, 1.000000000000000000, 0.9659258262890683122, 1.000000000000000000, 0.9659258262890683122, 1.000000000000000000, 0.9659258262890683122, 1.000000000000000000, 0.9659258262890683122, 1.000000000000000000, 0.9659258262890683122, 1.000000000000000000, 0.9659258262890683122, 1.000000000000000000, 0.9659258262890683122, 1.000000000000000000, 0.9659258262890683122, 1.000000000000000000, 0.9659258262890683122, 1.000000000000000000, 0.9659258262890683122, 1.000000000000000000, 0.9659258262890683122, 1.000000000000000000, 0.9659258262890683122, 1.000000000000000000, 0.9659258262890683122, 1.000000000000000000, 0.9659258262890683122, 1.000000000000000000, 0.9659258262890683122, 1.000000000000000000, 0.9659258262890683122, 1.000000000000000000, 0.9659258262890683122, 1.000000000000000000, 0.9659258262890683122, 1.000000000000000000, 0.9659258262890683122, 1.000000000000000000, 0.9659258262890683122, 1.000000000000000000, 0.9659258262890683122, 1.000000000000000000, 0.9659258262890683122, 1.000000000000000000, 0.9659258262890683122, 1.000000000000000000, 0.9659258262890683122, 1.000000000000000000, 0.9659258262890683122, 1.000000000000000000, 0.9659258262890683122, 1.000000000000000000),
 ( 1.000000000000000000, 0.9659258262890683122, 1.000000000000000000, 0.9659258262890683122, 1.000000000000000000, 0.9659258262890683122, 1.000000000000000000, 0.9659258262890683122, 1.000000000000000000, 0.9659258262890683122, 1.000000000000000000, 0.9659258262890683122, 1.000000000000000000, 0.9659258262890683122, 1.000000000000000000, 0.9659258262890683122, 1.000000000000000000, 0.9659258262890683122, 1.000000000000000000, 0.9659258262890683122, 1.000000000000000000, 0.9659258262890683122, 1.000000000000000000, 0.9659258262890683122, 1.000000000000000000, 0.9659258262890683122, 1.000000000000000000, 0.9659258262890683122, 1.000000000000000000, 0.9659258262890683122, 1.000000000000000000, 0.9659258262890683122, 1.000000000000000000, 0.9659258262890683122, 1.000000000000000000, 0.9659258262890683122, 1.000000000000000000, 0.9659258262890683122, 1.000000000000000000, 0.9659258262890683122, 1.000000000000000000, 0.9659258262890683122, 1.000000000000000000, 0.9659258262890683122, 1.000000000000000000, 0.9659258262890683122, 1.000000000000000000, 0.9659258262890683122, 1.000000000000000000, 0.9659258262890683122, 1.000000000000000000, 0.9659258262890683122, 1.000000000000000000, 0.9659258262890683122, 1.000000000000000000, 0.9659258262890683122, 1.000000000000000000, 0.9659258262890683122, 1.000000000000000000, 0.9659258262890683122, 1.000000000000000000, 0.9659258262890683122, 1.000000000000000000, 0.9659258262890683122, 1.000000000000000000, 0.9659258262890683122, 1.000000000000000000, 0.9659258262890683122, 1.000000000000000000, 0.9659258262890683122, 1.000000000000000000, 0.9659258262890683122, 1.000000000000000000, 0.9659258262890683122, 1.000000000000000000, 0.9659258262890683122, 1.000000000000000000, 0.9659258262890683122, 1.000000000000000000, 0.9659258262890683122, 1.000000000000000000, 0.9659258262890683122, 1.000000000000000000, 0.9659258262890683122, 1.000000000000000000, 0.9659258262890683122, 1.000000000000000000, 0.9659258262890683122, 1.000000000000000000, 0.9659258262890683122, 1.000000000000000000, 0.9659258262890683122, 1.000000000000000000, 0.9659258262890683122, 1.000000000000000000, 0.9659258262890683122, 1.000000000000000000, 0.9659258262890683122, 1.000000000000000000, 0.9659258262890683122, 1.000000000000000000, 0.9659258262890683122, 1.000000000000000000, 0.9659258262890683122, 1.000000000000000000, 0.9659258262890683122, 1.000000000000000000, 0.9659258262890683122, 1.000000000000000000, 0.9659258262890683122, 1.000000000000000000, 0.9659258262890683122, 1.000000000000000000, 0.9659258262890683122, 1.000000000000000000, 0.9659258262890683122, 1.000000000000000000, 0.9659258262890683122, 1.000000000000000000, 0.9659258262890683122, 1.000000000000000000, 0.9659258262890683122, 1.000000000000000000, 0.9659258262890683122, 1.000000000000000000, 0.9659258262890683122, 1.000000000000000000, 0.9659258262890683122, 1.000000000000000000, 0.9659258262890683122, 1.000000000000000000, 0.9659258262890683122, 1.000000000000000000, 0.9659258262890683122, 1.000000000000000000, 0.9659258262890683122, 1.000000000000000000, 0.9659258262890683122, 1.000000000000000000, 0.9659258262890683122, 1.000000000000000000, 0.9659258262890683122, 1.000000000000000000, 0.9659258262890683122, 1.000000000000000000, 0.9659258262890683122, 1.000000000000000000, 0.9659258262890683122, 1.000000000000000000, 0.9659258262890683122, 1.000000000000000000, 0.9659258262890683122, 1.000000000000000000, 0.9659258262890683122, 1.000000000000000000, 0.9659258262890683122, 1.000000000000000000, 0.9659258262890683122, 1.000000000000000000, 0.9659258262890683122, 1.000000000000000000, 0.9659258262890683122, 1.000000000000000000, 0.9659258262890683122, 1.000000000000000000, 0.9659258262890683122, 1.000000000000000000, 0.9659258262890683122, 1.000000000000000000, 0.9659258262890683122, 1.000000000000000000, 0.9659258262890683122, 1.000000000000000000, 0.9659258262890683122, 1.000000000000000000, 0.9659258262890683122, 1.000000000000000000, 0.9659258262890683122, 1.000000000000000000, 0.9659258262890683122, 1.000000000000000000, 0.9659258262890683122, 1.000000000000000000, 0.9659258262890683122, 1.000000000000000000, 0.9659258262890683122, 1.000000000000000000, 0.9659258262890683122, 1.000000000000000000, 0.9659258262890683122, 1.000000000000000000, 0.9659258262890683122, 1.000000000000000000, 0.9659258262890683122, 1.000000000000000000, 0.9659258262890683122, 1.000000000000000000, 0.9659258262890683122, 1.000000000000000000, 0.9659258262890683122, 1.000000000000000000, 0.9659258262890683122, 1.000000000000000000, 0.9659258262890683122, 1.000000000000000000, 0.9659258262890683122, 1.000000000000000000, 0.9659258262890683122, 1.000000000000000000, 0.9659258262890683122, 1.000000000000000000, 0.9659258262890683122, 1.000000000000000000, 0.9659258262890683122, 1.000000000000000000, 0.9659258262890683122, 1.000000000000000000, 0.9659258262890683122, 1.000000000000000000, 0.9659258262890683122, 1.000000000000000000, 0.9659258262890683122, 1.000000000000000000, 0.9659258262890683122, 1.000000000000000000, 0.9659258262890683122, 1.000000000000000000, 0.9659258262890683122, 1.000000000000000000, 0.9659258262890683122, 1.000000000000000000, 0.9659258262890683122, 1.000000000000000000, 0.9659258262890683122, 1.000000000000000000, 0.9659258262890683122, 1.000000000000000000, 0.9659258262890683122, 1.000000000000000000, 0.9659258262890683122, 1.000000000000000000, 0.9659258262890683122, 1.000000000000000000, 0.9659258262890683122, 1.000000000000000000, 0.9659258262890683122, 1.000000000000000000, 0.9659258262890683122, 1.000000000000000000, 0.9659258262890683122, 1.000000000000000000, 0.9659258262890683122, 1.000000000000000000, 0.9659258262890683122, 1.000000000000000000, 0.9659258262890683122, 1.000000000000000000, 0.9659258262890683122, 1.000000000000000000, 0.9659258262890683122, 1.000000000000000000, 0.9659258262890683122, 1.000000000000000000, 0.9659258262890683122, 1.000000000000000000, 0.9659258262890683122, 1.000000000000000000, 0.9659258262890683122, 1.000000000000000000, 0.9659258262890683122, 1.000000000000000000, 0.9659258262890683122, 1.000000000000000000, 0.9659258262890683122, 1.000000000000000000, 0.9659258262890683122, 1.000000000000000000, 0.9659258262890683122, 1.000000000000000000, 0.9659258262890683122, 1.000000000000000000, 0.9659258262890683122, 1.000000000000000000, 0.9659258262890683122, 1.000000000000000000, 0.9659258262890683122, 1.000000000000000000, 0.9659258262890683122, 1.000000000000000000, 0.9659258262890683122, 1.000000000000000000, 0.9659258262890683122, 1.000000000000000000, 0.9659258262890683122, 1.000000000000000000, 0.9659258262890683122, 1.000000000000000000, 0.9659258262890683122, 1.000000000000000000, 0.9659258262890683122, 1.000000000000000000, 0.9659258262890683122, 1.000000000000000000, 0.9659258262890683122, 1.000000000000000000, 0.9659258262890683122, 1.000000000000000000, 0.9659258262890683122, 1.000000000000000000, 0.9659258262890683122, 1.000000000000000000, 0.9659258262890683122, 1.000000000000000000, 0.9659258262890683122, 1.000000000000000000, 0.9659258262890683122, 1.000000000000000000, 0.9659258262890683122, 1.000000000000000000, 0.9659258262890683122, 1.000000000000000000, 0.9659258262890683122, 1.000000000000000000, 0.9659258262890683122, 1.000000000000000000) ) ) 
 REPRESENTATION_ITEM ( '' )  SURFACE ( )  );
#82261=CARTESIAN_POINT ( 'NONE',  ( -1.161435516476850394, -2.368486780965353193E-16, 4.088522901378193630 ) ) ;
#82262=CARTESIAN_POINT ( 'NONE',  ( 17.20831665107776587, 34.13393115100078745, -7.208316651077762316 ) ) ;
#82263=CARTESIAN_POINT ( 'NONE',  ( 17.96484262340118221, 31.18868534415483751, -7.964842623401177768 ) ) ;
#82264=UNCERTAINTY_MEASURE_WITH_UNIT (LENGTH_MEASURE( 1.000000000000000082E-05 ), #67571, 'distance_accuracy_value', 'NONE');
#82265=( BOUNDED_CURVE ( )  B_SPLINE_CURVE ( 3, ( #78184, #24219, #39715, #54685 ),
 .UNSPECIFIED., .F., .T. ) 
 B_SPLINE_CURVE_WITH_KNOTS ( ( 4, 4 ),
 ( 3.694400132159526340, 4.712388980384689674 ),
 .UNSPECIFIED. ) 
 CURVE ( )  GEOMETRIC_REPRESENTATION_ITEM ( )  RATIONAL_B_SPLINE_CURVE ( ( 1.000000000000000000, 0.9154899770527751279, 0.9154899770527751279, 1.000000000000000000 ) ) 
 REPRESENTATION_ITEM ( '' )  );
#82267=CARTESIAN_POINT ( 'NONE',  ( 3.591859063236763294, 63.29030133659708923, -11.09922568453595026 ) ) ;
#82270=CARTESIAN_POINT ( 'NONE',  ( 10.00000000000000000, 14.75893115100078568, -9.846743663894594434 ) ) ;
#82271=CARTESIAN_POINT ( 'NONE',  ( 10.00000000000000000, 37.87363466993041783, -12.81628187352647608 ) ) ;
#82272=CARTESIAN_POINT ( 'NONE',  ( -0.8801773607110991993, 2.855352010821504471, -2.915334737309923874 ) ) ;
#82273=CARTESIAN_POINT ( 'NONE',  ( 7.361572987183169658, 29.96726448433411960, -9.846743663894592657 ) ) ;
#82274=CARTESIAN_POINT ( 'NONE',  ( 20.00000000000000711, 89.81050759285248830, 4.994480956901625746 ) ) ;
#82275=CARTESIAN_POINT ( 'NONE',  ( 17.20831665107776587, 2.883931151000785231, 7.208316651077764980 ) ) ;
#82276=CARTESIAN_POINT ( 'NONE',  ( -0.3689425029237898834, 16.17874883491396076, -10.36894250292378850 ) ) ;
#82277=CARTESIAN_POINT ( 'NONE',  ( -0.3689425029237881626, 47.42874883491396787, 10.36894250292379027 ) ) ;
#82278=CARTESIAN_POINT ( 'NONE',  ( 0.1532563361054083140, 46.00893115100079456, 1.131784320476157264E-15 ) ) ;
#82280=CARTESIAN_POINT ( 'NONE',  ( 4.559911319644449179, 38.89701867748817676, 9.422509992056141925 ) ) ;
#82281=CARTESIAN_POINT ( 'NONE',  ( 0.1532563361054083140, 1.008931151000784787, 1.131784320476157264E-15 ) ) ;
#82283=CARTESIAN_POINT ( 'NONE',  ( 19.38216949554541557, 52.24863466993041072, -9.382169495545420901 ) ) ;
#82285=CARTESIAN_POINT ( 'NONE',  ( 4.559911319644449179, 67.23035201082150536, -9.422509992056141925 ) ) ;
#82288=CARTESIAN_POINT ( 'NONE',  ( 1.472469842513823179, 6.425597817667451750, 4.923371831947296329 ) ) ;
#82291=CARTESIAN_POINT ( 'NONE',  ( 20.88017736071110164, 20.35535201082150891, 2.915334737309930979 ) ) ;
#82294=EDGE_CURVE ( 'NONE', #4379, #64701, #31915, .T. ) ;
#82296=CARTESIAN_POINT ( 'NONE',  ( 20.88017736071110519, 40.56368534415484106, 2.639326808657452039E-16 ) ) ;
#82297=CARTESIAN_POINT ( 'NONE',  ( 12.63842701281683922, 54.55059781766745175, -9.846743663894590881 ) ) ;
#82299=CARTESIAN_POINT ( 'NONE',  ( 19.84674366389459266, 58.71726448433411605, -2.638427012816827677 ) ) ;
#82301=CARTESIAN_POINT ( 'NONE',  ( 17.96484262340118221, 59.93868534415484106, 7.964842623401181321 ) ) ;
#82303=CARTESIAN_POINT ( 'NONE',  ( 19.38216949554541202, 35.99863466993041072, 9.382169495545424454 ) ) ;
#82304=CARTESIAN_POINT ( 'NONE',  ( 4.559911319644449179, 27.23035201082150536, -9.422509992056141925 ) ) ;
#82305=CARTESIAN_POINT ( 'NONE',  ( 20.15039907845753575, 6.748846992468889638, 6.262539305110063736 ) ) ;
#82306=CARTESIAN_POINT ( 'NONE',  ( 19.84674366389459266, 8.717264484334116048, -2.638427012816827677 ) ) ;
#82307=CARTESIAN_POINT ( 'NONE',  ( 20.88017736071110875, 15.77201867748817143, -2.915334737309920765 ) ) ;
#82309=B_SPLINE_CURVE_WITH_KNOTS ( 'NONE', 3,
 ( #80743, #51733, #28225, #73228, #21230, #36733 ),
 .UNSPECIFIED., .F., .F.,
 ( 4, 2, 4 ),
 ( 0.000000000000000000, 0.0002565770811490928911, 0.0005131541622981857821 ),
 .UNSPECIFIED. ) ;
#82311=ORIENTED_EDGE ( 'NONE', *, *, #90341, .F. ) ;
#82312=CARTESIAN_POINT ( 'NONE',  ( 0.6178305044545818747, 58.49863466993042493, -9.382169495545419124 ) ) ;
#82313=CARTESIAN_POINT ( 'NONE',  ( 10.00000000000000178, 49.31368534415484106, 10.88017736071110342 ) ) ;
#82315=MECHANICAL_DESIGN_GEOMETRIC_PRESENTATION_REPRESENTATION('',(#32780),#63187);
#82316=CARTESIAN_POINT ( 'NONE',  ( 19.38216949554541557, 52.24863466993041072, -9.382169495545420901 ) ) ;
#82317=CARTESIAN_POINT ( 'NONE',  ( -0.8801773607110991993, 42.85535201082150536, -2.915334737309923874 ) ) ;
#82318=CARTESIAN_POINT ( 'NONE',  ( 12.63842701281683922, 54.55059781766745175, -9.846743663894590881 ) ) ;
#82320=CARTESIAN_POINT ( 'NONE',  ( 17.20831665107776587, 17.88393115100078745, 7.208316651077764980 ) ) ;
#82321=CARTESIAN_POINT ( 'NONE',  ( -2.816281873526473856, 4.331968003263754419, 3.434112377981055619 ) ) ;
#82323=CARTESIAN_POINT ( 'NONE',  ( 18.52753015748618282, 63.92559781766745886, -4.923371831947291888 ) ) ;
#82324=CARTESIAN_POINT ( 'NONE',  ( 19.42250999205614193, 35.14701867748816966, 5.440088680355555262 ) ) ;
#82325=CARTESIAN_POINT ( 'NONE',  ( 5.076628168052704559, 50.17559781766745886, -8.527530157486179263 ) ) ;
#82327=CARTESIAN_POINT ( 'NONE',  ( 1.472469842513823179, 26.42559781766745175, 4.923371831947296329 ) ) ;
#82328=CARTESIAN_POINT ( 'NONE',  ( 17.20831665107776587, 9.133931151000787452, -7.208316651077762316 ) ) ;
#82329=CARTESIAN_POINT ( 'NONE',  ( -2.816281873526471635, 8.915301336597083903, -3.434112377981056508 ) ) ;
#82332=FACE_OUTER_BOUND ( 'NONE', #96040, .T. ) ;
#82333=FACE_OUTER_BOUND ( 'NONE', #48596, .T. ) ;
#82334=CARTESIAN_POINT ( 'NONE',  ( 0.6178305044545838731, 34.74863466993042493, 9.382169495545420901 ) ) ;
#82336=CARTESIAN_POINT ( 'NONE',  ( 2.791683348922237240, 35.38393115100079456, -7.208316651077763204 ) ) ;
#82338=CARTESIAN_POINT ( 'NONE',  ( 20.88017736071110875, 10.77201867748817143, -2.915334737309920765 ) ) ;
#82339=CARTESIAN_POINT ( 'NONE',  ( 12.63842701281683034, 32.46726448433412315, 9.846743663894596210 ) ) ;
#82340=ORIENTED_EDGE ( 'NONE', *, *, #24209, .F. ) ;
#82342=CARTESIAN_POINT ( 'NONE',  ( 6.204703633549690345, 65.76208216824731778, -14.16423886937410259 ) ) ;
#82344=CARTESIAN_POINT ( 'NONE',  ( 20.88017736071110164, 20.35535201082150891, 2.915334737309930979 ) ) ;
#82345=CARTESIAN_POINT ( 'NONE',  ( -2.266590686148945544, 52.22041550158064638, 7.082119434687048631 ) ) ;
#82346=CARTESIAN_POINT ( 'NONE',  ( 22.26659068614895176, 54.72041550158063217, -7.082119434687042414 ) ) ;
#82349=CARTESIAN_POINT ( 'NONE',  ( 5.076628168052704559, 5.175597817667451750, -8.527530157486179263 ) ) ;
#82350=CARTESIAN_POINT ( 'NONE',  ( 13.43411237798106583, 2.665301336597086568, -12.81628187352647252 ) ) ;
#82353=CARTESIAN_POINT ( 'NONE',  ( 5.076628168052703671, 61.84226448433412315, 8.527530157486179263 ) ) ;
#82355=CARTESIAN_POINT ( 'NONE',  ( 19.84674366389459621, 63.50893115100078745, 7.409399052514197653E-17 ) ) ;
#82356=CARTESIAN_POINT ( 'NONE',  ( -2.266590686148945544, 6.387082168247300906, -7.082119434687050408 ) ) ;
#82357=CARTESIAN_POINT ( 'NONE',  ( 12.63842701281683034, 22.46726448433411605, 9.846743663894596210 ) ) ;
#82360=CARTESIAN_POINT ( 'NONE',  ( 22.26659068614895176, 44.72041550158063927, -7.082119434687042414 ) ) ;
#82361=CARTESIAN_POINT ( 'NONE',  ( 19.84674366389459621, 3.508931151000785231, 7.409399052514197653E-17 ) ) ;
#82362=CARTESIAN_POINT ( 'NONE',  ( 0.1922240491738418933, 63.18878173731739878, 6.499999999999971578 ) ) ;
#82363=CARTESIAN_POINT ( 'NONE',  ( 10.00000000000000178, 29.31368534415483751, 10.88017736071110342 ) ) ;
#82364=CARTESIAN_POINT ( 'NONE',  ( 6.565887622018943937, 35.16530133659708923, 12.81628187352647430 ) ) ;
#82365=FILL_AREA_STYLE_COLOUR ( '', #4953 ) ;
#82366=CARTESIAN_POINT ( 'NONE',  ( 19.38216949554541202, 35.99863466993041072, 9.382169495545424454 ) ) ;
#82367=CARTESIAN_POINT ( 'NONE',  ( 0.6178305044545818747, 58.49863466993042493, -9.382169495545419124 ) ) ;
#82371=CARTESIAN_POINT ( 'NONE',  ( 13.79529636645030344, 43.26208216824730357, 14.16423886937410614 ) ) ;
#82372=CARTESIAN_POINT ( 'NONE',  ( 10.00000000000000178, 3.053748834913967425, 14.16423886937410082 ) ) ;
#82373=CARTESIAN_POINT ( 'NONE',  ( -0.8801773607110991993, 2.855352010821504471, -2.915334737309923874 ) ) ;
#82374=CARTESIAN_POINT ( 'NONE',  ( 2.035157376598824452, 18.68868534415484106, 7.964842623401179544 ) ) ;
#82375=CARTESIAN_POINT ( 'NONE',  ( 5.054308323419911098, 70.51564955044841554, 12.00000000000000000 ) ) ;
#82377=CARTESIAN_POINT ( 'NONE',  ( -0.8801773607111009756, 53.06368534415484106, 1.068504757029289695E-15 ) ) ;
#82378=CARTESIAN_POINT ( 'NONE',  ( -0.8801773607111008646, 53.27201867748816966, 2.915334737309923430 ) ) ;
#82379=CARTESIAN_POINT ( 'NONE',  ( -2.816281873526471635, 23.91530133659708568, -3.434112377981056508 ) ) ;
#82382=CARTESIAN_POINT ( 'NONE',  ( 18.52753015748617571, 28.09226448433411960, 4.923371831947298993 ) ) ;
#82383=ADVANCED_FACE ( 'NONE', ( #64350 ), #9398, .T. ) ;
#82384=CARTESIAN_POINT ( 'NONE',  ( 10.00000000000000000, 51.81368534415484106, -10.88017736071110342 ) ) ;
#82387=CARTESIAN_POINT ( 'NONE',  ( 22.81628187352648496, 16.83196800326374998, -3.434112377981050290 ) ) ;
#82389=CARTESIAN_POINT ( 'NONE',  ( 10.00000000000000178, 14.31368534415483751, 10.88017736071110342 ) ) ;
#82391=CARTESIAN_POINT ( 'NONE',  ( 5.076628168052704559, 45.17559781766745175, -8.527530157486179263 ) ) ;
#82392=CARTESIAN_POINT ( 'NONE',  ( 22.81628187352647785, 51.62363466993042493, 6.195893100308588602E-16 ) ) ;
#82393=CARTESIAN_POINT ( 'NONE',  ( 1.472469842513823179, 25.59226448433412315, -4.923371831947296329 ) ) ;
#82394=CARTESIAN_POINT ( 'NONE',  ( 22.26659068614895176, 9.720415501580633943, -7.082119434687042414 ) ) ;
#82396=CARTESIAN_POINT ( 'NONE',  ( 7.084665262690076126, 19.10535201082150181, 10.88017736071109987 ) ) ;
#82397=PRESENTATION_STYLE_ASSIGNMENT (( #73913 ) ) ;
#82398=CARTESIAN_POINT ( 'NONE',  ( 5.076628168052704559, 50.17559781766745886, -8.527530157486179263 ) ) ;
#82399=CARTESIAN_POINT ( 'NONE',  ( 0.5774900079438590739, 32.64701867748816966, -5.440088680355550821 ) ) ;
#82400=CARTESIAN_POINT ( 'NONE',  ( 12.91533473730992121, 14.52201867748817143, 10.88017736071110164 ) ) ;
#82401=ORIENTED_EDGE ( 'NONE', *, *, #63590, .T. ) ;
#82403=CARTESIAN_POINT ( 'NONE',  ( -0.8801773607111009756, 23.06368534415484106, 1.068504757029289695E-15 ) ) ;
#82404=CARTESIAN_POINT ( 'NONE',  ( 22.81628187352648496, 46.83196800326376064, -3.434112377981050290 ) ) ;
#82405=CARTESIAN_POINT ( 'NONE',  ( 7.084665262690076126, 32.02201867748816966, -10.88017736071110164 ) ) ;
#82407=CARTESIAN_POINT ( 'NONE',  ( 10.00000000000000000, 36.81368534415484106, -10.88017736071110342 ) ) ;
#82408=ORIENTED_EDGE ( 'NONE', *, *, #40716, .T. ) ;
#82409=CARTESIAN_POINT ( 'NONE',  ( 0.1532563361054083140, 56.00893115100078745, 1.131784320476157264E-15 ) ) ;
#82410=CARTESIAN_POINT ( 'NONE',  ( -0.8801773607110991993, 42.85535201082150536, -2.915334737309923874 ) ) ;
#82412=CARTESIAN_POINT ( 'NONE',  ( 5.076628168052703671, 66.84226448433412315, 8.527530157486179263 ) ) ;
#82413=CARTESIAN_POINT ( 'NONE',  ( 22.81628187352648496, 56.83196800326374643, -3.434112377981050290 ) ) ;
#82415=CARTESIAN_POINT ( 'NONE',  ( 17.08211943468705840, 45.13708216824730357, -12.26659068614894466 ) ) ;
#82416=CARTESIAN_POINT ( 'NONE',  ( 7.084665262690076126, 52.02201867748816255, -10.88017736071110164 ) ) ;
#82417=CARTESIAN_POINT ( 'NONE',  ( 12.63842701281683034, 62.46726448433410894, 9.846743663894596210 ) ) ;
#82418=EDGE_CURVE ( 'NONE', #86252, #57318, #57837, .T. ) ;
#82420=CARTESIAN_POINT ( 'NONE',  ( 0.1532563361054082862, 66.21726448433413736, 2.638427012816831674 ) ) ;
#82421=( LENGTH_UNIT ( ) NAMED_UNIT ( * ) SI_UNIT ( .MILLI., .METRE. ) );
#82422=CARTESIAN_POINT ( 'NONE',  ( 2.791683348922237240, 20.38393115100078745, -7.208316651077763204 ) ) ;
#82424=CARTESIAN_POINT ( 'NONE',  ( 10.00000000000000178, 27.25893115100078390, 9.846743663894594434 ) ) ;
#82426=CARTESIAN_POINT ( 'NONE',  ( 15.44008868035555260, 29.73035201082150891, 9.422509992056143702 ) ) ;
#82427=CARTESIAN_POINT ( 'NONE',  ( 0.1532563361054082862, 21.21726448433412315, 2.638427012816831674 ) ) ;
#82429=CARTESIAN_POINT ( 'NONE',  ( 0.6178305044545838731, 14.74863466993041783, 9.382169495545420901 ) ) ;
#82431=CARTESIAN_POINT ( 'NONE',  ( 0.5774900079438590739, 62.64701867748817676, -5.440088680355550821 ) ) ;
#82432=CARTESIAN_POINT ( 'NONE',  ( 0.5774900079438607392, 38.48035201082150536, 5.440088680355550821 ) ) ;
#82433=CARTESIAN_POINT ( 'NONE',  ( 0.6178305044545838731, 54.74863466993042493, 9.382169495545420901 ) ) ;
#82434=CARTESIAN_POINT ( 'NONE',  ( -0.3689425029237898834, 51.17874883491397497, -10.36894250292378850 ) ) ;
#82438=ORIENTED_EDGE ( 'NONE', *, *, #58859, .F. ) ;
#82439=CARTESIAN_POINT ( 'NONE',  ( 16.40814093676323893, 10.79030133659708923, 11.09922568453595026 ) ) ;
#82440=CARTESIAN_POINT ( 'NONE',  ( 20.88017736071110875, 5.772018677488170546, -2.915334737309920765 ) ) ;
#82441=CARTESIAN_POINT ( 'NONE',  ( 7.084665262690076126, 44.10535201082151247, 10.88017736071109987 ) ) ;
#82443=EDGE_CURVE ( 'NONE', #53168, #26718, #82051, .T. ) ;
#82444=ORIENTED_EDGE ( 'NONE', *, *, #56566, .F. ) ;
#82445=CARTESIAN_POINT ( 'NONE',  ( 7.084665262690076126, 59.10535201082150536, 10.88017736071109987 ) ) ;
#82446=CARTESIAN_POINT ( 'NONE',  ( 17.20831665107776587, 39.13393115100079456, -7.208316651077762316 ) ) ;
#82447=CARTESIAN_POINT ( 'NONE',  ( 5.076628168052703671, 26.84226448433411960, 8.527530157486179263 ) ) ;
#82448=B_SPLINE_CURVE_WITH_KNOTS ( 'NONE', 3,
 ( #60684, #76190, #54651, #92656 ),
 .UNSPECIFIED., .F., .F.,
 ( 4, 4 ),
 ( 0.000000000000000000, 0.0004119852744258499034 ),
 .UNSPECIFIED. ) ;
#82449=CARTESIAN_POINT ( 'NONE',  ( 0.1532563361054082862, 11.21726448433411605, 2.638427012816831674 ) ) ;
#82451=CARTESIAN_POINT ( 'NONE',  ( -1.099225684535947600, 38.70696800326375353, -6.408140936763238038 ) ) ;
#82452=CARTESIAN_POINT ( 'NONE',  ( 1.472469842513823179, 6.425597817667451750, 4.923371831947296329 ) ) ;
#82455=MECHANICAL_DESIGN_GEOMETRIC_PRESENTATION_REPRESENTATION('',(#34547),#42562);
#82456=CARTESIAN_POINT ( 'NONE',  ( 1.472469842513823179, 35.59226448433412315, -4.923371831947296329 ) ) ;
#82457=EDGE_LOOP ( 'NONE', ( #12689, #96828, #94519, #40483 ) ) ;
#82459=CARTESIAN_POINT ( 'NONE',  ( -1.099225684535947600, 58.70696800326375353, -6.408140936763238038 ) ) ;
#82460=CARTESIAN_POINT ( 'NONE',  ( 17.85158348494334035, 54.73726573380444194, -6.500000000000027534 ) ) ;
#82461=CARTESIAN_POINT ( 'NONE',  ( -2.816281873526473856, -0.6680319967362464695, 3.434112377981055619 ) ) ;
#82462=CARTESIAN_POINT ( 'NONE',  ( -0.8801773607111009756, 13.06368534415483929, 1.068504757029289695E-15 ) ) ;
#82464=CARTESIAN_POINT ( 'NONE',  ( 6.204703633549690345, 37.84541550158063927, 14.16423886937410082 ) ) ;
#82467=CARTESIAN_POINT ( 'NONE',  ( 22.26659068614894466, 23.88708216824730357, 7.082119434687054849 ) ) ;
#82468=CARTESIAN_POINT ( 'NONE',  ( 6.204703633549690345, 40.76208216824731778, -14.16423886937410259 ) ) ;
#82469=CARTESIAN_POINT ( 'NONE',  ( 20.36894250292379382, 8.678748834913967869, 10.36894250292379205 ) ) ;
#82470=CARTESIAN_POINT ( 'NONE',  ( 20.36894250292379382, 8.678748834913967869, 10.36894250292379205 ) ) ;
#82471=CARTESIAN_POINT ( 'NONE',  ( 7.084665262690076126, 67.02201867748817676, -10.88017736071110164 ) ) ;
#82472=CARTESIAN_POINT ( 'NONE',  ( 0.5774900079438607392, 48.48035201082150536, 5.440088680355550821 ) ) ;
#82474=ORIENTED_EDGE ( 'NONE', *, *, #37685, .F. ) ;
#82475=CARTESIAN_POINT ( 'NONE',  ( 1.472469842513823179, 36.42559781766745175, 4.923371831947296329 ) ) ;
#82476=CARTESIAN_POINT ( 'NONE',  ( 4.559911319644449179, 63.89701867748817676, 9.422509992056141925 ) ) ;
#82477=CARTESIAN_POINT ( 'NONE',  ( 10.00000000000000000, 29.75893115100078745, -9.846743663894594434 ) ) ;
#82479=CARTESIAN_POINT ( 'NONE',  ( 17.96484262340118221, 6.188685344154837509, -7.964842623401177768 ) ) ;
#82480=CARTESIAN_POINT ( 'NONE',  ( 10.00000000000000000, 57.87363466993042493, -12.81628187352647608 ) ) ;
#82481=CARTESIAN_POINT ( 'NONE',  ( 14.92337183194729988, 54.34226448433412315, -8.527530157486177487 ) ) ;
#82483=CARTESIAN_POINT ( 'NONE',  ( 10.00000000000000000, 29.75893115100078745, -9.846743663894594434 ) ) ;
#82484=CARTESIAN_POINT ( 'NONE',  ( 0.6178305044545818747, 38.49863466993042493, -9.382169495545419124 ) ) ;
#82487=CARTESIAN_POINT ( 'NONE',  ( 2.035157376598822676, 37.43868534415484106, -7.964842623401177768 ) ) ;
#82488=CARTESIAN_POINT ( 'NONE',  ( 5.076628168052703671, 36.84226448433412315, 8.527530157486179263 ) ) ;
#82489=CARTESIAN_POINT ( 'NONE',  ( 13.79529636645031943, 30.34541550158063927, -14.16423886937409904 ) ) ;
#82491=CARTESIAN_POINT ( 'NONE',  ( 2.917880565312950480, 5.970415501580634832, -12.26659068614894821 ) ) ;
#82492=CARTESIAN_POINT ( 'NONE',  ( 20.88017736071110875, 65.77201867748817676, -2.915334737309920765 ) ) ;
#82493=DIRECTION ( 'NONE',  ( -0.000000000000000000, -0.000000000000000000, -1.000000000000000000 ) ) ;
#82494=CARTESIAN_POINT ( 'NONE',  ( 20.36894250292379738, 59.92874883491397497, -10.36894250292379027 ) ) ;
#82495=CARTESIAN_POINT ( 'NONE',  ( 0.6178305044545818747, 3.498634669930420049, -9.382169495545419124 ) ) ;
#82496=CARTESIAN_POINT ( 'NONE',  ( 17.39651004071838969, 44.08210964143329846, -6.500000000000027534 ) ) ;
#82497=CARTESIAN_POINT ( 'NONE',  ( 20.88017736071110519, 55.56368534415484817, 2.639326808657452039E-16 ) ) ;
#82500=CARTESIAN_POINT ( 'NONE',  ( -0.8801773607110991993, 12.85535201082150358, -2.915334737309923874 ) ) ;
#82501=CARTESIAN_POINT ( 'NONE',  ( 20.88017736071110875, 15.77201867748817143, -2.915334737309920765 ) ) ;
#82502=CARTESIAN_POINT ( 'NONE',  ( 0.1532563361054083140, 41.00893115100078745, 1.131784320476157264E-15 ) ) ;
#82503=CARTESIAN_POINT ( 'NONE',  ( 21.09922568453595559, 57.04030133659708923, -6.408140936763230044 ) ) ;
#82505=ORIENTED_EDGE ( 'NONE', *, *, #18638, .T. ) ;
#82508=CARTESIAN_POINT ( 'NONE',  ( 20.88017736071110164, 20.35535201082150891, 2.915334737309930979 ) ) ;
#82509=CARTESIAN_POINT ( 'NONE',  ( 10.00000000000000178, 5.373634669930420493, 12.81628187352647608 ) ) ;
#82511=CARTESIAN_POINT ( 'NONE',  ( 0.1532563361054082862, 6.217264484334118713, 2.638427012816831674 ) ) ;
#82512=CARTESIAN_POINT ( 'NONE',  ( 14.92337183194729633, 52.67559781766745175, 8.527530157486181039 ) ) ;
#82513=CARTESIAN_POINT ( 'NONE',  ( 4.559911319644449179, 33.89701867748817676, 9.422509992056141925 ) ) ;
#82515=CARTESIAN_POINT ( 'NONE',  ( 6.565887622018943937, 15.16530133659708568, 12.81628187352647430 ) ) ;
#82516=CARTESIAN_POINT ( 'NONE',  ( 20.88017736071110875, 50.77201867748817676, -2.915334737309920765 ) ) ;
#82518=FACE_OUTER_BOUND ( 'NONE', #15671, .T. ) ;
#82519=CARTESIAN_POINT ( 'NONE',  ( 22.81628187352648496, 51.83196800326376064, -3.434112377981050290 ) ) ;
#82522=CARTESIAN_POINT ( 'NONE',  ( 0.6178305044545818747, 38.49863466993042493, -9.382169495545419124 ) ) ;
#82523=CARTESIAN_POINT ( 'NONE',  ( 17.20831665107776587, 7.883931151000784787, 7.208316651077764980 ) ) ;
#82524=CARTESIAN_POINT ( 'NONE',  ( 20.88017736071110875, 35.77201867748816966, -2.915334737309920765 ) ) ;
#82525=CARTESIAN_POINT ( 'NONE',  ( 0.1532563361054083140, 66.00893115100079456, 1.131784320476157264E-15 ) ) ;
#82526=CARTESIAN_POINT ( 'NONE',  ( 2.791683348922240793, 51.63393115100078745, 7.208316651077764092 ) ) ;
#82527=CARTESIAN_POINT ( 'NONE',  ( 17.20831665107776587, 14.13393115100078568, -7.208316651077762316 ) ) ;
#82528=CARTESIAN_POINT ( 'NONE',  ( 14.92337183194729633, 2.675597817667451750, 8.527530157486181039 ) ) ;
#82529=CARTESIAN_POINT ( 'NONE',  ( 24.16423886937409904, 49.09541550158063217, 3.795296366450317205 ) ) ;
#82534=CARTESIAN_POINT ( 'NONE',  ( 20.36894250292379382, 63.67874883491396787, 10.36894250292379205 ) ) ;
#82535=CARTESIAN_POINT ( 'NONE',  ( 22.26659068614895176, 64.72041550158064638, -7.082119434687042414 ) ) ;
#82537=CARTESIAN_POINT ( 'NONE',  ( 18.52753015748618282, 28.92559781766745175, -4.923371831947291888 ) ) ;
#82538=CARTESIAN_POINT ( 'NONE',  ( 6.565887622018943937, 23.08196800326375708, -12.81628187352647608 ) ) ;
#82541=CARTESIAN_POINT ( 'NONE',  ( 24.16423886937409904, 4.095415501580634832, 3.795296366450317205 ) ) ;
#82542=CARTESIAN_POINT ( 'NONE',  ( 2.035157376598824452, 8.688685344154839285, 7.964842623401179544 ) ) ;
#82543=CARTESIAN_POINT ( 'NONE',  ( -4.164238869374099039, 56.80374883491397497, 8.674139862899312516E-16 ) ) ;
#82545=CARTESIAN_POINT ( 'NONE',  ( 0.1532563361054100626, 25.80059781766744820, -2.638427012816831230 ) ) ;
#82548=CARTESIAN_POINT ( 'NONE',  ( 18.52753015748617571, 18.09226448433411960, 4.923371831947298993 ) ) ;
#82556=CARTESIAN_POINT ( 'NONE',  ( 19.84674366389459266, 48.30059781766745175, 2.638427012816836559 ) ) ;
#82557=CARTESIAN_POINT ( 'NONE',  ( 17.08211943468705130, 18.47041550158063572, 12.26659068614894998 ) ) ;
#82558=CARTESIAN_POINT ( 'NONE',  ( 0.5774900079438607392, 23.48035201082150536, 5.440088680355550821 ) ) ;
#82559=CARTESIAN_POINT ( 'NONE',  ( 4.559911319644449179, 43.89701867748816966, 9.422509992056141925 ) ) ;
#82561=CARTESIAN_POINT ( 'NONE',  ( 22.81628187352648496, 21.83196800326374643, -3.434112377981050290 ) ) ;
#82562=CARTESIAN_POINT ( 'NONE',  ( 13.79529636645030344, 8.262082168247300018, 14.16423886937410614 ) ) ;
#82563=CARTESIAN_POINT ( 'NONE',  ( 17.96484262340118221, 64.93868534415483396, 7.964842623401181321 ) ) ;
#82566=CARTESIAN_POINT ( 'NONE',  ( -2.816281873526473856, 34.33196800326376064, 3.434112377981055619 ) ) ;
#82568=CARTESIAN_POINT ( 'NONE',  ( 12.63842701281683922, 34.55059781766745886, -9.846743663894590881 ) ) ;
#82569=CARTESIAN_POINT ( 'NONE',  ( 10.00000000000000000, 6.813685344154838397, -10.88017736071110342 ) ) ;
#82571=CARTESIAN_POINT ( 'NONE',  ( -4.164238869374098151, 66.59541550158060375, -3.795296366450310543 ) ) ;
#82572=ORIENTED_EDGE ( 'NONE', *, *, #49123, .T. ) ;
#82573=CARTESIAN_POINT ( 'NONE',  ( 19.42250999205614548, 45.98035201082150536, -5.440088680355545492 ) ) ;
#82574=CARTESIAN_POINT ( 'NONE',  ( 20.88017736071110875, 60.77201867748817676, -2.915334737309920765 ) ) ;
#82575=CARTESIAN_POINT ( 'NONE',  ( 7.084665262690076126, 67.02201867748817676, -10.88017736071110164 ) ) ;
#82576=CARTESIAN_POINT ( 'NONE',  ( 12.91533473730993009, 56.60535201082151247, -10.88017736071109987 ) ) ;
#82580=CARTESIAN_POINT ( 'NONE',  ( 10.00000000000000178, 32.25893115100078745, 9.846743663894594434 ) ) ;
#82582=CARTESIAN_POINT ( 'NONE',  ( 0.1532563361054082862, 61.21726448433412315, 2.638427012816831674 ) ) ;
#82583=DIRECTION ( 'NONE',  ( 0.000000000000000000, 0.000000000000000000, 1.000000000000000000 ) ) ;
#82584=CARTESIAN_POINT ( 'NONE',  ( -0.3689425029237898834, 1.178748834913967869, -10.36894250292378850 ) ) ;
#82588=CARTESIAN_POINT ( 'NONE',  ( 20.00000000000000355, 70.00000000000000000, 6.500000000000000888 ) ) ;
#82589=CARTESIAN_POINT ( 'NONE',  ( 20.88017736071110164, 5.355352010821503583, 2.915334737309930979 ) ) ;
#82592=CARTESIAN_POINT ( 'NONE',  ( 10.00000000000000000, 39.75893115100078745, -9.846743663894594434 ) ) ;
#82594=CARTESIAN_POINT ( 'NONE',  ( 0.6178305044545818747, 18.49863466993041428, -9.382169495545419124 ) ) ;
#82595=CARTESIAN_POINT ( 'NONE',  ( 0.1532563361054082862, 6.217264484334118713, 2.638427012816831674 ) ) ;
#82597=CARTESIAN_POINT ( 'NONE',  ( 2.791683348922240793, 16.63393115100078745, 7.208316651077764092 ) ) ;
#82598=CARTESIAN_POINT ( 'NONE',  ( 10.00000000000000178, 5.373634669930420493, 12.81628187352647608 ) ) ;
#82600=ORIENTED_EDGE ( 'NONE', *, *, #45704, .F. ) ;
#82602=CARTESIAN_POINT ( 'NONE',  ( 10.00000000000000178, 29.31368534415483751, 10.88017736071110342 ) ) ;
#82603=CARTESIAN_POINT ( 'NONE',  ( 22.26659068614895176, 24.72041550158063572, -7.082119434687042414 ) ) ;
#82604=CARTESIAN_POINT ( 'NONE',  ( 19.84674366389459266, 33.30059781766744464, 2.638427012816836559 ) ) ;
#82605=CARTESIAN_POINT ( 'NONE',  ( 12.91533473730992121, 59.52201867748816966, 10.88017736071110164 ) ) ;
#82606=CARTESIAN_POINT ( 'NONE',  ( -1.099225684535947600, 33.70696800326375353, -6.408140936763238038 ) ) ;
#82608=CARTESIAN_POINT ( 'NONE',  ( 20.88017736071110875, 10.77201867748817143, -2.915334737309920765 ) ) ;
#82612=CARTESIAN_POINT ( 'NONE',  ( 10.00000000000000000, 12.87363466993042138, -12.81628187352647608 ) ) ;
#82613=CARTESIAN_POINT ( 'NONE',  ( 10.00000000000000000, -2.126365330069579951, -12.81628187352647608 ) ) ;
#82614=CARTESIAN_POINT ( 'NONE',  ( 7.361572987183170547, 27.05059781766745175, 9.846743663894590881 ) ) ;
#82616=CARTESIAN_POINT ( 'NONE',  ( 16.40814093676323893, 35.79030133659708923, 11.09922568453595026 ) ) ;
#82618=CARTESIAN_POINT ( 'NONE',  ( 12.91533473730993009, 36.60535201082151247, -10.88017736071109987 ) ) ;
#82623=CARTESIAN_POINT ( 'NONE',  ( 4.559911319644449179, 62.23035201082150536, -9.422509992056141925 ) ) ;
#82625=CARTESIAN_POINT ( 'NONE',  ( 10.00000000000000178, 44.31368534415484106, 10.88017736071110342 ) ) ;
#82626=CARTESIAN_POINT ( 'NONE',  ( -0.8801773607110991993, 42.85535201082150536, -2.915334737309923874 ) ) ;
#82627=CARTESIAN_POINT ( 'NONE',  ( 14.92337183194729633, 62.67559781766745886, 8.527530157486181039 ) ) ;
#82628=CARTESIAN_POINT ( 'NONE',  ( 19.42250999205614548, 55.98035201082150536, -5.440088680355545492 ) ) ;
#82629=CARTESIAN_POINT ( 'NONE',  ( 17.20831665107776587, 42.88393115100077324, 7.208316651077764980 ) ) ;
#82630=CARTESIAN_POINT ( 'NONE',  ( 20.88017736071110164, 15.35535201082150358, 2.915334737309930979 ) ) ;
#82631=CARTESIAN_POINT ( 'NONE',  ( 10.00000000000000000, 7.873634669930421381, -12.81628187352647608 ) ) ;
#82632=ORIENTED_EDGE ( 'NONE', *, *, #72028, .T. ) ;
#82633=CARTESIAN_POINT ( 'NONE',  ( 20.88017736071110875, 25.77201867748816966, -2.915334737309920765 ) ) ;
#82635=CARTESIAN_POINT ( 'NONE',  ( 2.035157376598822676, 2.438685344154837953, -7.964842623401177768 ) ) ;
#82636=CARTESIAN_POINT ( 'NONE',  ( 20.88017736071110164, 30.35535201082151247, 2.915334737309930979 ) ) ;
#82637=CARTESIAN_POINT ( 'NONE',  ( -0.8801773607111009756, 68.06368534415484817, 1.068504757029289695E-15 ) ) ;
#82638=CARTESIAN_POINT ( 'NONE',  ( 10.00000000000000178, 43.05374883491397497, 14.16423886937410082 ) ) ;
#82639=CARTESIAN_POINT ( 'NONE',  ( 14.92337183194729988, 14.34226448433411782, -8.527530157486177487 ) ) ;
#82640=CARTESIAN_POINT ( 'NONE',  ( 2.035157376598822676, 42.43868534415483396, -7.964842623401177768 ) ) ;
#82642=CARTESIAN_POINT ( 'NONE',  ( 6.204703633549690345, 2.845415501580634388, 14.16423886937410082 ) ) ;
#82643=ORIENTED_EDGE ( 'NONE', *, *, #62342, .F. ) ;
#82645=CARTESIAN_POINT ( 'NONE',  ( 10.00000000000000000, 64.75893115100078035, -9.846743663894594434 ) ) ;
#82648=CARTESIAN_POINT ( 'NONE',  ( 24.16423886937409904, 24.09541550158063927, 3.795296366450317205 ) ) ;
#82649=CARTESIAN_POINT ( 'NONE',  ( 20.36894250292379382, 23.67874883491397142, 10.36894250292379205 ) ) ;
#82650=EDGE_CURVE ( 'NONE', #90281, #31231, #96424, .T. ) ;
#82651=CARTESIAN_POINT ( 'NONE',  ( 2.035157376598824452, 58.68868534415482685, 7.964842623401179544 ) ) ;
#82652=CARTESIAN_POINT ( 'NONE',  ( -2.266590686148945544, 67.22041550158063217, 7.082119434687048631 ) ) ;
#82653=CARTESIAN_POINT ( 'NONE',  ( 0.6178305044545818747, 3.498634669930420049, -9.382169495545419124 ) ) ;
#82654=CARTESIAN_POINT ( 'NONE',  ( 0.1532563361054083140, 46.00893115100079456, 1.131784320476157264E-15 ) ) ;
#82656=CARTESIAN_POINT ( 'NONE',  ( 20.88017736071110164, 50.35535201082151247, 2.915334737309930979 ) ) ;
#82657=CARTESIAN_POINT ( 'NONE',  ( 19.38216949554541557, 7.248634669930421381, -9.382169495545420901 ) ) ;
#82658=CARTESIAN_POINT ( 'NONE',  ( -0.3689425029237881626, 17.42874883491397142, 10.36894250292379027 ) ) ;
#82659=CARTESIAN_POINT ( 'NONE',  ( 0.5774900079438607392, 8.480352010821505360, 5.440088680355550821 ) ) ;
#82660=CARTESIAN_POINT ( 'NONE',  ( 17.96484262340118221, 16.18868534415483396, -7.964842623401177768 ) ) ;
#82662=CARTESIAN_POINT ( 'NONE',  ( 12.91533473730992121, 39.52201867748817676, 10.88017736071110164 ) ) ;
#82667=VERTEX_POINT ( 'NONE', #42363 ) ;
#82668=CARTESIAN_POINT ( 'NONE',  ( 0.1532563361054083140, 31.00893115100078390, 1.131784320476157264E-15 ) ) ;
#82671=CARTESIAN_POINT ( 'NONE',  ( 20.36894250292379738, 39.92874883491396787, -10.36894250292379027 ) ) ;
#82672=CARTESIAN_POINT ( 'NONE',  ( 10.00000000000000178, 9.313685344154839285, 10.88017736071110342 ) ) ;
#82673=CARTESIAN_POINT ( 'NONE',  ( 19.84674366389459266, 23.71726448433412315, -2.638427012816827677 ) ) ;
#82674=CARTESIAN_POINT ( 'NONE',  ( 18.52753015748617571, 43.09226448433412315, 4.923371831947298993 ) ) ;
#82677=CARTESIAN_POINT ( 'NONE',  ( 2.035157376598822676, 67.43868534415484817, -7.964842623401177768 ) ) ;
#82680=CARTESIAN_POINT ( 'NONE',  ( 24.16423886937410614, 34.51208216824731068, -3.795296366450302550 ) ) ;
#82682=CARTESIAN_POINT ( 'NONE',  ( -2.816281873526471635, 28.91530133659708213, -3.434112377981056508 ) ) ;
#82684=CARTESIAN_POINT ( 'NONE',  ( 10.00000000000000000, 62.87363466993042493, -12.81628187352647608 ) ) ;
#82687=CARTESIAN_POINT ( 'NONE',  ( 0.1532563361054100626, 40.80059781766745886, -2.638427012816831230 ) ) ;
#82688=CARTESIAN_POINT ( 'NONE',  ( 4.559911319644449179, 27.23035201082150536, -9.422509992056141925 ) ) ;
#82689=LINE ( 'NONE', #89205, #27168 ) ;
#82690=CARTESIAN_POINT ( 'NONE',  ( 19.84674366389459621, 43.50893115100078745, 7.409399052514197653E-17 ) ) ;
#82691=CARTESIAN_POINT ( 'NONE',  ( 2.791683348922237240, 50.38393115100078035, -7.208316651077763204 ) ) ;
#82695=ORIENTED_EDGE ( 'NONE', *, *, #85924, .F. ) ;
#82699=CARTESIAN_POINT ( 'NONE',  ( 5.076628168052703671, 11.84226448433411960, 8.527530157486179263 ) ) ;
#82700=CARTESIAN_POINT ( 'NONE',  ( 6.565887622018943937, 35.16530133659708923, 12.81628187352647430 ) ) ;
#82703=CARTESIAN_POINT ( 'NONE',  ( 1.472469842513823179, 56.42559781766745886, 4.923371831947296329 ) ) ;
#82705=CARTESIAN_POINT ( 'NONE',  ( 0.1532563361054100626, 35.80059781766745175, -2.638427012816831230 ) ) ;
#82706=CARTESIAN_POINT ( 'NONE',  ( 6.204703633549690345, 40.76208216824731778, -14.16423886937410259 ) ) ;
#82707=CARTESIAN_POINT ( 'NONE',  ( 2.791683348922237240, 50.38393115100078035, -7.208316651077763204 ) ) ;
#82708=CARTESIAN_POINT ( 'NONE',  ( 19.38216949554541557, 42.24863466993041783, -9.382169495545420901 ) ) ;
#82711=CARTESIAN_POINT ( 'NONE',  ( 12.63842701281683034, 12.46726448433411782, 9.846743663894596210 ) ) ;
#82713=CARTESIAN_POINT ( 'NONE',  ( 17.20831665107776587, 54.13393115100079456, -7.208316651077762316 ) ) ;
#82714=CARTESIAN_POINT ( 'NONE',  ( 20.88017736071110875, 35.77201867748816966, -2.915334737309920765 ) ) ;
#82717=CARTESIAN_POINT ( 'NONE',  ( -0.8801773607110991993, 42.85535201082150536, -2.915334737309923874 ) ) ;
#82718=ORIENTED_EDGE ( 'NONE', *, *, #39741, .F. ) ;
#82720=CARTESIAN_POINT ( 'NONE',  ( 19.42250999205614548, 20.98035201082150891, -5.440088680355545492 ) ) ;
#82721=CARTESIAN_POINT ( 'NONE',  ( 0.1532563361054083140, 66.00893115100079456, 1.131784320476157264E-15 ) ) ;
#82722=CARTESIAN_POINT ( 'NONE',  ( 4.559911319644449179, 48.89701867748817676, 9.422509992056141925 ) ) ;
#82724=CARTESIAN_POINT ( 'NONE',  ( 17.96484262340118221, 54.93868534415484106, 7.964842623401181321 ) ) ;
#82726=CARTESIAN_POINT ( 'NONE',  ( 7.084665262690076126, 34.10535201082151247, 10.88017736071109987 ) ) ;
#82727=CARTESIAN_POINT ( 'NONE',  ( 3.558677480090426837, 70.40124509038876965, -12.00000000000000000 ) ) ;
#82728=CARTESIAN_POINT ( 'NONE',  ( 14.92337183194729633, 7.675597817667451750, 8.527530157486181039 ) ) ;
#82729=CARTESIAN_POINT ( 'NONE',  ( 18.52753015748618282, 23.92559781766745530, -4.923371831947291888 ) ) ;
#82730=CARTESIAN_POINT ( 'NONE',  ( 20.03447792253738768, 57.65514106990691090, -6.401564815979734924 ) ) ;
#82732=CARTESIAN_POINT ( 'NONE',  ( 0.6178305044545838731, -0.2513653300695798953, 9.382169495545420901 ) ) ;
#82733=B_SPLINE_CURVE_WITH_KNOTS ( 'NONE', 3,
 ( #62176, #9195, #2707, #40682, #48658, #70195 ),
 .UNSPECIFIED., .F., .F.,
 ( 4, 2, 4 ),
 ( 6.254634441385501517E-18, 0.0002605067024380970848, 0.0005210134048761879896 ),
 .UNSPECIFIED. ) ;
#82734=CARTESIAN_POINT ( 'NONE',  ( 13.79529636645031943, 60.34541550158063927, -14.16423886937409904 ) ) ;
#82736=CARTESIAN_POINT ( 'NONE',  ( 6.204703633549690345, 27.84541550158063217, 14.16423886937410082 ) ) ;
#82738=CARTESIAN_POINT ( 'NONE',  ( 6.204703633549690345, 45.76208216824729647, -14.16423886937410259 ) ) ;
#82739=CARTESIAN_POINT ( 'NONE',  ( 20.88017736071110164, 5.355352010821502695, 2.915334737309930979 ) ) ;
#82741=CARTESIAN_POINT ( 'NONE',  ( 10.00000000000000000, 24.75893115100078745, -9.846743663894594434 ) ) ;
#82742=CARTESIAN_POINT ( 'NONE',  ( 0.5774900079438607392, 18.48035201082150536, 5.440088680355550821 ) ) ;
#82743=EDGE_CURVE ( 'NONE', #17129, #21583, #67720, .T. ) ;
#82744=CARTESIAN_POINT ( 'NONE',  ( 0.1532563361054083140, 51.00893115100078745, 1.131784320476157264E-15 ) ) ;
#82749=CARTESIAN_POINT ( 'NONE',  ( -2.816281873526473856, 39.33196800326374643, 3.434112377981055619 ) ) ;
#82750=CARTESIAN_POINT ( 'NONE',  ( 0.1532563361054082862, 46.21726448433411605, 2.638427012816831674 ) ) ;
#82752=CARTESIAN_POINT ( 'NONE',  ( 19.84674366389459621, 13.50893115100078568, 7.409399052514197653E-17 ) ) ;
#82754=CARTESIAN_POINT ( 'NONE',  ( 19.42250999205614193, 10.14701867748816966, 5.440088680355555262 ) ) ;
#82755=CARTESIAN_POINT ( 'NONE',  ( 17.08211943468705130, 58.47041550158063927, 12.26659068614894998 ) ) ;
#82756=CARTESIAN_POINT ( 'NONE',  ( 20.88017736071110164, 45.35535201082149115, 2.915334737309930979 ) ) ;
#82758=CARTESIAN_POINT ( 'NONE',  ( 10.00000000000000000, 56.81368534415484106, -10.88017736071110342 ) ) ;
#82759=CARTESIAN_POINT ( 'NONE',  ( 20.24186590665276952, 39.73410085661203794, 6.114288769123060518 ) ) ;
#82760=CARTESIAN_POINT ( 'NONE',  ( 2.791683348922240793, 26.63393115100078745, 7.208316651077764092 ) ) ;
#82761=CARTESIAN_POINT ( 'NONE',  ( 20.88017736071110875, 10.77201867748817143, -2.915334737309920765 ) ) ;
#82762=CARTESIAN_POINT ( 'NONE',  ( 19.84674366389459266, 8.717264484334116048, -2.638427012816827677 ) ) ;
#82764=CARTESIAN_POINT ( 'NONE',  ( 7.361572987183169658, 39.96726448433411605, -9.846743663894592657 ) ) ;
#82765=CARTESIAN_POINT ( 'NONE',  ( 2.035157376598824452, 33.68868534415484106, 7.964842623401179544 ) ) ;
#82770=CARTESIAN_POINT ( 'NONE',  ( 16.40814093676324603, 62.45696800326376064, -11.09922568453594671 ) ) ;
#82773=CARTESIAN_POINT ( 'NONE',  ( 2.791683348922237240, 5.383931151000785675, -7.208316651077763204 ) ) ;
#82774=CARTESIAN_POINT ( 'NONE',  ( -2.816281873526473856, 49.12363466993042493, 9.499525473075851096E-16 ) ) ;
#82775=CARTESIAN_POINT ( 'NONE',  ( 2.035157376598822676, 7.438685344154837509, -7.964842623401177768 ) ) ;
#82776=CARTESIAN_POINT ( 'NONE',  ( 17.20831665107776587, 39.13393115100079456, -7.208316651077762316 ) ) ;
#82778=CARTESIAN_POINT ( 'NONE',  ( 6.000000000000000000, 60.50000000000000000, -6.000000000000000000 ) ) ;
#82779=CARTESIAN_POINT ( 'NONE',  ( 13.79529636645030344, 33.26208216824730357, 14.16423886937410614 ) ) ;
#82780=CARTESIAN_POINT ( 'NONE',  ( -0.3689425029237898834, 41.17874883491397497, -10.36894250292378850 ) ) ;
#82781=CARTESIAN_POINT ( 'NONE',  ( 17.20831665107776587, 54.13393115100079456, -7.208316651077762316 ) ) ;
#82783=CARTESIAN_POINT ( 'NONE',  ( -0.8801773607111009756, 33.06368534415484106, 1.068504757029289695E-15 ) ) ;
#82785=CARTESIAN_POINT ( 'NONE',  ( 0.5774900079438590739, 67.64701867748817676, -5.440088680355550821 ) ) ;
#82787=CARTESIAN_POINT ( 'NONE',  ( -1.099225684535947600, 53.70696800326376064, -6.408140936763238038 ) ) ;
#82788=CARTESIAN_POINT ( 'NONE',  ( 10.00000000000000000, 66.81368534415484817, -10.88017736071110342 ) ) ;
#82790=CARTESIAN_POINT ( 'NONE',  ( 10.00000000000000000, 10.55374883491396787, -14.16423886937410082 ) ) ;
#82791=CARTESIAN_POINT ( 'NONE',  ( 0.1532563361054082862, 11.21726448433411605, 2.638427012816831674 ) ) ;
#82792=CARTESIAN_POINT ( 'NONE',  ( 15.44008868035555793, 26.39701867748817321, -9.422509992056140149 ) ) ;
#82795=CARTESIAN_POINT ( 'NONE',  ( 7.084665262690076126, 34.10535201082151247, 10.88017736071109987 ) ) ;
#82797=CARTESIAN_POINT ( 'NONE',  ( 20.88017736071110164, 35.35535201082150536, 2.915334737309930979 ) ) ;
#82798=CARTESIAN_POINT ( 'NONE',  ( 0.2751277870542967463, 70.00000000000000000, -6.000000000000000000 ) ) ;
#82801=CARTESIAN_POINT ( 'NONE',  ( 17.96484262340118221, 64.93868534415483396, 7.964842623401181321 ) ) ;
#82803=CARTESIAN_POINT ( 'NONE',  ( 7.084665262690076126, 17.02201867748817676, -10.88017736071110164 ) ) ;
#82804=DIRECTION ( 'NONE',  ( 0.000000000000000000, -1.000000000000000000, 0.000000000000000000 ) ) ;
#82805=CARTESIAN_POINT ( 'NONE',  ( 14.92337183194729988, 9.342264484334119601, -8.527530157486177487 ) ) ;
#82806=CARTESIAN_POINT ( 'NONE',  ( 17.96484262340118221, 21.18868534415483396, -7.964842623401177768 ) ) ;
#82807=ADVANCED_FACE ( 'NONE', ( #76303 ), #15797, .T. ) ;
#82810=CARTESIAN_POINT ( 'NONE',  ( 10.00000000000000178, 50.37363466993042493, 12.81628187352647608 ) ) ;
#82811=CARTESIAN_POINT ( 'NONE',  ( -0.8801773607111008646, 48.27201867748816966, 2.915334737309923430 ) ) ;
#82813=CARTESIAN_POINT ( 'NONE',  ( 6.565887622018943937, 55.16530133659709634, 12.81628187352647430 ) ) ;
#82814=CARTESIAN_POINT ( 'NONE',  ( 20.88017736071110164, 45.35535201082149115, 2.915334737309930979 ) ) ;
#82815=CARTESIAN_POINT ( 'NONE',  ( 21.09922568453594849, 6.206968003263753531, 6.408140936763242479 ) ) ;
#82817=CARTESIAN_POINT ( 'NONE',  ( 18.52753015748617571, 13.09226448433411960, 4.923371831947298993 ) ) ;
#82819=CARTESIAN_POINT ( 'NONE',  ( 19.38216949554541202, 10.99863466993042138, 9.382169495545424454 ) ) ;
#82821=CARTESIAN_POINT ( 'NONE',  ( 10.00000000000000178, 67.25893115100079456, 9.846743663894594434 ) ) ;
#82822=CARTESIAN_POINT ( 'NONE',  ( 7.084665262690076126, 37.02201867748817676, -10.88017736071110164 ) ) ;
#82823=CARTESIAN_POINT ( 'NONE',  ( 17.20831665107776587, 49.13393115100078745, -7.208316651077762316 ) ) ;
#82826=CARTESIAN_POINT ( 'NONE',  ( 1.472469842513823179, 21.42559781766745175, 4.923371831947296329 ) ) ;
#82827=CARTESIAN_POINT ( 'NONE',  ( 2.791683348922240793, 6.633931151000785675, 7.208316651077764092 ) ) ;
#82828=CARTESIAN_POINT ( 'NONE',  ( 3.591859063236763294, -1.709698663402913210, -11.09922568453595026 ) ) ;
#82829=ORIENTED_EDGE ( 'NONE', *, *, #78395, .T. ) ;
#82831=CARTESIAN_POINT ( 'NONE',  ( 19.42250999205614193, 5.147018677488171434, 5.440088680355555262 ) ) ;
#82832=SURFACE_SIDE_STYLE ('',( #52337 ) ) ;
#82833=CARTESIAN_POINT ( 'NONE',  ( 17.20831665107776587, 59.13393115100078745, -7.208316651077762316 ) ) ;
#82834=CARTESIAN_POINT ( 'NONE',  ( 10.00000000000000178, 37.25893115100078745, 9.846743663894594434 ) ) ;
#82836=CARTESIAN_POINT ( 'NONE',  ( 17.96484262340118221, 4.938685344154837509, 7.964842623401181321 ) ) ;
#82837=CARTESIAN_POINT ( 'NONE',  ( 0.1532563361054082862, 51.21726448433412315, 2.638427012816831674 ) ) ;
#82838=ORIENTED_EDGE ( 'NONE', *, *, #92728, .T. ) ;
#82841=CARTESIAN_POINT ( 'NONE',  ( 10.00000000000000000, 1.813685344154838175, -10.88017736071110342 ) ) ;
#82843=CARTESIAN_POINT ( 'NONE',  ( 7.084665262690076126, 17.02201867748817676, -10.88017736071110164 ) ) ;
#82844=CARTESIAN_POINT ( 'NONE',  ( 2.917880565312950480, 50.97041550158064638, -12.26659068614894821 ) ) ;
#82845=CARTESIAN_POINT ( 'NONE',  ( 24.16423886937409904, 54.09541550158063217, 3.795296366450317205 ) ) ;
#82847=CARTESIAN_POINT ( 'NONE',  ( 10.00000000000000000, 4.758931151000784787, -9.846743663894594434 ) ) ;
#82848=( BOUNDED_CURVE ( )  B_SPLINE_CURVE ( 2, ( #63674, #55706, #17225, #70219, #62199, #40207, #41208, #93692, #2231 ),
 .UNSPECIFIED., .F., .T. ) 
 B_SPLINE_CURVE_WITH_KNOTS ( ( 3, 2, 2, 2, 3 ),
 ( 0.7258552226545171848, 0.7261904761904762751, 0.7321428571428572063, 0.7380952380952381375, 0.7384304916311973388 ),
 .UNSPECIFIED. ) 
 CURVE ( )  GEOMETRIC_REPRESENTATION_ITEM ( )  RATIONAL_B_SPLINE_CURVE ( ( 0.9963778908391764944, 0.9980808541467923733, 1.000000000000000000, 0.9659258262890682012, 1.000000000000000000, 0.9659258262890682012, 1.000000000000000000, 0.9980808541467917072, 0.9963778908391753841 ) ) 
 REPRESENTATION_ITEM ( '' )  );
#82849=CARTESIAN_POINT ( 'NONE',  ( 0.1532563361054083140, 31.00893115100078390, 1.131784320476157264E-15 ) ) ;
#82850=CARTESIAN_POINT ( 'NONE',  ( 6.565887622018943937, 8.081968003263751754, -12.81628187352647608 ) ) ;
#82851=ORIENTED_EDGE ( 'NONE', *, *, #33204, .T. ) ;
#82852=EDGE_LOOP ( 'NONE', ( #8403, #83687, #96330, #7955, #29583, #39778 ) ) ;
#82854=CARTESIAN_POINT ( 'NONE',  ( 0.1532563361054100626, 60.80059781766744464, -2.638427012816831230 ) ) ;
#82855=AXIS2_PLACEMENT_3D ( 'NONE', #3866, #80344, #86378 ) ;
#82858=( BOUNDED_CURVE ( )  B_SPLINE_CURVE ( 2, ( #10709, #41224, #79692, #11190, #36155, #36661, #20666, #43654, #49666 ),
 .UNSPECIFIED., .F., .F. ) 
 B_SPLINE_CURVE_WITH_KNOTS ( ( 3, 2, 2, 2, 3 ),
 ( 0.3320003743640375649, 0.3333333333333333148, 0.3392857142857143016, 0.3452380952380952328, 0.3465710542073918710 ),
 .UNSPECIFIED. ) 
 CURVE ( )  GEOMETRIC_REPRESENTATION_ITEM ( )  RATIONAL_B_SPLINE_CURVE ( ( 0.9881565478350775589, 0.9923695281211528663, 1.000000000000000000, 0.9659258262890683122, 1.000000000000000000, 0.9659258262890683122, 1.000000000000000000, 0.9923695281211478703, 0.9881565478350720078 ) ) 
 REPRESENTATION_ITEM ( '' )  );
#82860=CARTESIAN_POINT ( 'NONE',  ( 17.08211943468705130, 8.470415501580635720, 12.26659068614894998 ) ) ;
#82861=CARTESIAN_POINT ( 'NONE',  ( 18.52753015748618282, 23.92559781766745530, -4.923371831947291888 ) ) ;
#82864=CARTESIAN_POINT ( 'NONE',  ( 22.26659068614894466, 38.88708216824731068, 7.082119434687054849 ) ) ;
#82866=EDGE_CURVE ( 'NONE', #39274, #4466, #90364, .T. ) ;
#82867=CARTESIAN_POINT ( 'NONE',  ( 7.361572987183169658, 4.967264484334119601, -9.846743663894592657 ) ) ;
#82870=CARTESIAN_POINT ( 'NONE',  ( 2.035157376598822676, 27.43868534415483396, -7.964842623401177768 ) ) ;
#82871=CARTESIAN_POINT ( 'NONE',  ( 19.38216949554541557, 42.24863466993041783, -9.382169495545420901 ) ) ;
#82872=CARTESIAN_POINT ( 'NONE',  ( -0.8801773607110991993, 7.855352010821504471, -2.915334737309923874 ) ) ;
#82873=CARTESIAN_POINT ( 'NONE',  ( 22.81628187352647785, 36.62363466993041783, 6.195893100308588602E-16 ) ) ;
#82874=CARTESIAN_POINT ( 'NONE',  ( 7.361572987183169658, 4.967264484334119601, -9.846743663894592657 ) ) ;
#82878=CARTESIAN_POINT ( 'NONE',  ( -0.3689425029237881626, 47.42874883491396787, 10.36894250292379027 ) ) ;
#82879=CARTESIAN_POINT ( 'NONE',  ( -0.8801773607110991993, 22.85535201082150181, -2.915334737309923874 ) ) ;
#82881=LINE ( 'NONE', #81395, #1709 ) ;
#82882=CARTESIAN_POINT ( 'NONE',  ( 19.42250999205614548, 55.98035201082150536, -5.440088680355545492 ) ) ;
#82883=CARTESIAN_POINT ( 'NONE',  ( 20.88017736071110164, 65.35535201082150536, 2.915334737309930979 ) ) ;
#82884=CARTESIAN_POINT ( 'NONE',  ( 19.38216949554541202, 20.99863466993042138, 9.382169495545424454 ) ) ;
#82885=DIRECTION ( 'NONE',  ( 0.000000000000000000, -1.000000000000000000, 0.000000000000000000 ) ) ;
#82887=CARTESIAN_POINT ( 'NONE',  ( 10.00000000000000178, 22.25893115100078745, 9.846743663894594434 ) ) ;
#82888=CARTESIAN_POINT ( 'NONE',  ( -0.8801773607111009756, 53.06368534415484106, 1.068504757029289695E-15 ) ) ;
#82889=CARTESIAN_POINT ( 'NONE',  ( -2.816281873526473856, 24.12363466993042138, 9.499525473075851096E-16 ) ) ;
#82890=EDGE_CURVE ( 'NONE', #38545, #9043, #90529, .T. ) ;
#82892=CARTESIAN_POINT ( 'NONE',  ( 20.88017736071110875, 5.772018677488170546, -2.915334737309920765 ) ) ;
#82893=CARTESIAN_POINT ( 'NONE',  ( 17.20831665107776587, 42.88393115100077324, 7.208316651077764980 ) ) ;
#82894=CARTESIAN_POINT ( 'NONE',  ( 6.565887622018943937, 63.08196800326376064, -12.81628187352647608 ) ) ;
#82895=CARTESIAN_POINT ( 'NONE',  ( 0.1532563361054083140, 16.00893115100078390, 1.131784320476157264E-15 ) ) ;
#82896=CARTESIAN_POINT ( 'NONE',  ( 19.10478245763047056, 31.02576239577081907, -5.990408912944402253 ) ) ;
#82897=CARTESIAN_POINT ( 'NONE',  ( 17.96484262340118221, 39.93868534415484106, 7.964842623401181321 ) ) ;
#82898=CARTESIAN_POINT ( 'NONE',  ( -2.266590686148945544, 31.38708216824730002, -7.082119434687050408 ) ) ;
#82900=CARTESIAN_POINT ( 'NONE',  ( 1.472469842513823179, 40.59226448433411605, -4.923371831947296329 ) ) ;
#82901=VECTOR ( 'NONE', #69762, 1000.000000000000000 ) ;
#82902=CARTESIAN_POINT ( 'NONE',  ( 12.91533473730993009, 26.60535201082150536, -10.88017736071109987 ) ) ;
#82903=CARTESIAN_POINT ( 'NONE',  ( 4.559911319644449179, 17.23035201082150536, -9.422509992056141925 ) ) ;
#82905=CARTESIAN_POINT ( 'NONE',  ( 7.084665262690076126, 24.10535201082150181, 10.88017736071109987 ) ) ;
#82907=CARTESIAN_POINT ( 'NONE',  ( 10.00000000000000178, 45.37363466993041783, 12.81628187352647608 ) ) ;
#82908=CARTESIAN_POINT ( 'NONE',  ( 2.035157376598822676, 42.43868534415483396, -7.964842623401177768 ) ) ;
#82910=CARTESIAN_POINT ( 'NONE',  ( 17.96484262340118221, 36.18868534415484106, -7.964842623401177768 ) ) ;
#82912=CARTESIAN_POINT ( 'NONE',  ( 5.076628168052704559, 60.17559781766745175, -8.527530157486179263 ) ) ;
#82913=CARTESIAN_POINT ( 'NONE',  ( 19.42250999205614548, 35.98035201082151247, -5.440088680355545492 ) ) ;
#82916=CARTESIAN_POINT ( 'NONE',  ( 13.79529636645031943, 40.34541550158063217, -14.16423886937409904 ) ) ;
#82917=CARTESIAN_POINT ( 'NONE',  ( 12.91533473730992121, 59.52201867748816966, 10.88017736071110164 ) ) ;
#82918=CARTESIAN_POINT ( 'NONE',  ( 20.88017736071110875, 55.77201867748816966, -2.915334737309920321 ) ) ;
#82920=CARTESIAN_POINT ( 'NONE',  ( 2.791683348922240793, 56.63393115100078035, 7.208316651077764092 ) ) ;
#82921=CARTESIAN_POINT ( 'NONE',  ( -0.8801773607111009756, 3.063685344154837509, 1.068504757029289695E-15 ) ) ;
#82922=CARTESIAN_POINT ( 'NONE',  ( 7.361572987183169658, 34.96726448433411605, -9.846743663894592657 ) ) ;
#82923=ORIENTED_EDGE ( 'NONE', *, *, #95271, .F. ) ;
#82924=CARTESIAN_POINT ( 'NONE',  ( 2.791683348922240793, 31.63393115100078745, 7.208316651077764092 ) ) ;
#82926=CARTESIAN_POINT ( 'NONE',  ( 4.559911319644449179, 32.23035201082150536, -9.422509992056141925 ) ) ;
#82927=CARTESIAN_POINT ( 'NONE',  ( 5.076628168052703671, 21.84226448433411960, 8.527530157486179263 ) ) ;
#82928=CARTESIAN_POINT ( 'NONE',  ( -2.816281873526473856, 24.33196800326375353, 3.434112377981055619 ) ) ;
#82929=CARTESIAN_POINT ( 'NONE',  ( 2.035157376598824452, 68.68868534415484817, 7.964842623401179544 ) ) ;
#82930=CARTESIAN_POINT ( 'NONE',  ( -0.8801773607111009756, 53.06368534415484106, 1.068504757029289695E-15 ) ) ;
#82931=CARTESIAN_POINT ( 'NONE',  ( 7.084665262690076126, 34.10535201082151247, 10.88017736071109987 ) ) ;
#82932=CARTESIAN_POINT ( 'NONE',  ( 6.565887622018943937, 65.16530133659709634, 12.81628187352647430 ) ) ;
#82933=CARTESIAN_POINT ( 'NONE',  ( 20.36894250292379382, 38.67874883491396076, 10.36894250292379205 ) ) ;
#82938=CARTESIAN_POINT ( 'NONE',  ( 10.00000000000000000, 12.87363466993042138, -12.81628187352647608 ) ) ;
#82939=CARTESIAN_POINT ( 'NONE',  ( 20.88017736071110519, 10.56368534415483751, 2.639326808657452039E-16 ) ) ;
#82940=CARTESIAN_POINT ( 'NONE',  ( -0.8801773607111008646, 53.27201867748816966, 2.915334737309923430 ) ) ;
#82941=CARTESIAN_POINT ( 'NONE',  ( 6.000000000000000000, 60.50000000000000711, 6.000000000000000000 ) ) ;
#82945=CARTESIAN_POINT ( 'NONE',  ( 7.084665262690076126, 57.02201867748817676, -10.88017736071110164 ) ) ;
#82946=CARTESIAN_POINT ( 'NONE',  ( 0.1532563361054082862, 36.21726448433410894, 2.638427012816831674 ) ) ;
#82947=CARTESIAN_POINT ( 'NONE',  ( 0.1532563361054100626, 25.80059781766744820, -2.638427012816831230 ) ) ;
#82948=CARTESIAN_POINT ( 'NONE',  ( 0.1532563361054082862, 16.21726448433411960, 2.638427012816831674 ) ) ;
#82951=CARTESIAN_POINT ( 'NONE',  ( 18.95386800104996539, 63.23810908735725889, -6.499999999999984901 ) ) ;
#82952=CARTESIAN_POINT ( 'NONE',  ( 22.81628187352648496, 36.83196800326376064, -3.434112377981050290 ) ) ;
#82953=CARTESIAN_POINT ( 'NONE',  ( 2.791683348922240793, 16.63393115100078745, 7.208316651077764092 ) ) ;
#82956=CARTESIAN_POINT ( 'NONE',  ( 18.52753015748617571, 28.09226448433411960, 4.923371831947298993 ) ) ;
#82957=EDGE_LOOP ( 'NONE', ( #71857, #16766, #63840, #83746, #16879, #33346 ) ) ;
#82958=CARTESIAN_POINT ( 'NONE',  ( -1.099225684535947600, 53.70696800326376064, -6.408140936763238038 ) ) ;
#82960=CARTESIAN_POINT ( 'NONE',  ( 19.38216949554541557, 7.248634669930421381, -9.382169495545420901 ) ) ;
#82961=CARTESIAN_POINT ( 'NONE',  ( -0.8801773607111009756, 48.06368534415484817, 1.068504757029289695E-15 ) ) ;
#82962=CARTESIAN_POINT ( 'NONE',  ( 22.26659068614895176, 34.72041550158063927, -7.082119434687042414 ) ) ;
#82963=CARTESIAN_POINT ( 'NONE',  ( 1.274849032794278747, 42.55509018479936856, -6.499999999999960032 ) ) ;
#82964=CARTESIAN_POINT ( 'NONE',  ( -4.164238869374098151, 31.59541550158063927, -3.795296366450310543 ) ) ;
#82965=CARTESIAN_POINT ( 'NONE',  ( 17.08211943468705840, 50.13708216824730357, -12.26659068614894466 ) ) ;
#82966=CARTESIAN_POINT ( 'NONE',  ( 20.36894250292379382, 13.67874883491396965, 10.36894250292379205 ) ) ;
#82967=CARTESIAN_POINT ( 'NONE',  ( -2.266590686148945544, 11.38708216824730179, -7.082119434687050408 ) ) ;
#82968=CARTESIAN_POINT ( 'NONE',  ( 18.72515096720568906, 36.07228050351032778, -6.500000000000007105 ) ) ;
#82969=CARTESIAN_POINT ( 'NONE',  ( -0.8801773607111008646, 43.27201867748817676, 2.915334737309923430 ) ) ;
#82971=CARTESIAN_POINT ( 'NONE',  ( 12.63842701281683034, 32.46726448433412315, 9.846743663894596210 ) ) ;
#82973=CARTESIAN_POINT ( 'NONE',  ( 12.91533473730992121, 64.52201867748817676, 10.88017736071110164 ) ) ;
#82974=CARTESIAN_POINT ( 'NONE',  ( 17.20831665107776587, 24.13393115100078035, -7.208316651077762316 ) ) ;
#82975=CARTESIAN_POINT ( 'NONE',  ( 20.88017736071110875, 20.77201867748816611, -2.915334737309920765 ) ) ;
#82976=CARTESIAN_POINT ( 'NONE',  ( -2.816281873526473856, 59.33196800326374643, 3.434112377981055619 ) ) ;
#82977=CARTESIAN_POINT ( 'NONE',  ( 2.791683348922237240, 65.38393115100078035, -7.208316651077763204 ) ) ;
#82978=DIRECTION ( 'NONE',  ( 0.000000000000000000, 0.000000000000000000, -1.000000000000000000 ) ) ;
#82979=CARTESIAN_POINT ( 'NONE',  ( 1.472469842513823179, 26.42559781766745175, 4.923371831947296329 ) ) ;
#82980=CARTESIAN_POINT ( 'NONE',  ( 13.43411237798106583, 42.66530133659707502, -12.81628187352647252 ) ) ;
#82982=CARTESIAN_POINT ( 'NONE',  ( 12.91533473730992121, 39.52201867748817676, 10.88017736071110164 ) ) ;
#82983=CARTESIAN_POINT ( 'NONE',  ( 17.20831665107776587, 59.13393115100078745, -7.208316651077762316 ) ) ;
#82985=CARTESIAN_POINT ( 'NONE',  ( 24.16423886937410614, 29.51208216824729647, -3.795296366450302550 ) ) ;
#82987=CARTESIAN_POINT ( 'NONE',  ( 6.204703633549690345, 0.7620821682473009062, -14.16423886937410259 ) ) ;
#82989=CARTESIAN_POINT ( 'NONE',  ( 7.084665262690076126, 67.02201867748817676, -10.88017736071110164 ) ) ;
#82990=CARTESIAN_POINT ( 'NONE',  ( 0.5774900079438607392, 68.48035201082150536, 5.440088680355550821 ) ) ;
#82991=CARTESIAN_POINT ( 'NONE',  ( 22.26659068614894466, 58.88708216824729647, 7.082119434687054849 ) ) ;
#82992=CARTESIAN_POINT ( 'NONE',  ( -2.816281873526473856, 4.331968003263754419, 3.434112377981055619 ) ) ;
#82994=CARTESIAN_POINT ( 'NONE',  ( -0.8801773607111009756, 58.06368534415484106, 1.068504757029289695E-15 ) ) ;
#82995=CARTESIAN_POINT ( 'NONE',  ( -0.2418659066527515111, 27.23410085661203439, -6.114288769123079170 ) ) ;
#82996=VECTOR ( 'NONE', #66889, 1000.000000000000114 ) ;
#82997=CARTESIAN_POINT ( 'NONE',  ( 10.00000000000000000, 50.55374883491396787, -14.16423886937410082 ) ) ;
#82999=CARTESIAN_POINT ( 'NONE',  ( 15.44008868035555260, 9.730352010821505360, 9.422509992056143702 ) ) ;
#83000=CARTESIAN_POINT ( 'NONE',  ( 19.42250999205614548, 20.98035201082150891, -5.440088680355545492 ) ) ;
#83001=CARTESIAN_POINT ( 'NONE',  ( 0.1532563361054100626, 60.80059781766744464, -2.638427012816831230 ) ) ;
#83002=CARTESIAN_POINT ( 'NONE',  ( -1.099225684535947600, 44.54030133659708923, 6.408140936763237150 ) ) ;
#83005=ORIENTED_EDGE ( 'NONE', *, *, #9939, .F. ) ;
#83007=CARTESIAN_POINT ( 'NONE',  ( 4.559911319644449179, 12.23035201082150536, -9.422509992056141925 ) ) ;
#83008=CARTESIAN_POINT ( 'NONE',  ( 19.38216949554541557, 22.24863466993041428, -9.382169495545420901 ) ) ;
#83010=CARTESIAN_POINT ( 'NONE',  ( 0.1532563361054083140, 46.00893115100079456, 1.131784320476157264E-15 ) ) ;
#83011=CARTESIAN_POINT ( 'NONE',  ( 2.035157376598824452, 38.68868534415483396, 7.964842623401179544 ) ) ;
#83012=CARTESIAN_POINT ( 'NONE',  ( 16.40814093676323893, 25.79030133659708923, 11.09922568453595026 ) ) ;
#83013=CARTESIAN_POINT ( 'NONE',  ( 19.42250999205614548, 45.98035201082150536, -5.440088680355545492 ) ) ;
#83015=FACE_OUTER_BOUND ( 'NONE', #16251, .T. ) ;
#83016=CARTESIAN_POINT ( 'NONE',  ( 19.38216949554541202, 45.99863466993041072, 9.382169495545424454 ) ) ;
#83019=CARTESIAN_POINT ( 'NONE',  ( 19.42250999205614193, 45.14701867748817676, 5.440088680355555262 ) ) ;
#83020=CARTESIAN_POINT ( 'NONE',  ( -1.099225684535947600, 39.54030133659708923, 6.408140936763237150 ) ) ;
#83021=EDGE_CURVE ( 'NONE', #95671, #80833, #14069, .T. ) ;
#83022=CARTESIAN_POINT ( 'NONE',  ( 15.44008868035555260, 44.73035201082151247, 9.422509992056143702 ) ) ;
#83023=CARTESIAN_POINT ( 'NONE',  ( 14.92337183194729633, 62.67559781766745886, 8.527530157486181039 ) ) ;
#83024=CARTESIAN_POINT ( 'NONE',  ( 2.791683348922237240, 65.38393115100078035, -7.208316651077763204 ) ) ;
#83026=CARTESIAN_POINT ( 'NONE',  ( 14.92337183194729633, 22.67559781766745175, 8.527530157486181039 ) ) ;
#83027=CARTESIAN_POINT ( 'NONE',  ( 14.92337183194729633, 12.67559781766745353, 8.527530157486181039 ) ) ;
#83028=CARTESIAN_POINT ( 'NONE',  ( 24.16423886937410614, 49.51208216824730357, -3.795296366450302550 ) ) ;
#83029=CARTESIAN_POINT ( 'NONE',  ( 21.92686044187656691, 24.95379003517448169, 3.195792623639537755 ) ) ;
#83035=CARTESIAN_POINT ( 'NONE',  ( 6.204703633549690345, 62.84541550158063927, 14.16423886937410082 ) ) ;
#83036=CARTESIAN_POINT ( 'NONE',  ( -2.266590686148945544, 67.22041550158063217, 7.082119434687048631 ) ) ;
#83037=CARTESIAN_POINT ( 'NONE',  ( 10.00000000000000178, 27.25893115100078390, 9.846743663894594434 ) ) ;
#83038=CARTESIAN_POINT ( 'NONE',  ( 3.591859063236761518, 44.95696800326376064, 11.09922568453594849 ) ) ;
#83041=CARTESIAN_POINT ( 'NONE',  ( -2.266590686148945544, 6.387082168247300906, -7.082119434687050408 ) ) ;
#83042=CARTESIAN_POINT ( 'NONE',  ( 7.084665262690076126, 19.10535201082150181, 10.88017736071109987 ) ) ;
#83043=CARTESIAN_POINT ( 'NONE',  ( -0.3689425029237881626, 62.42874883491396787, 10.36894250292379027 ) ) ;
#83044=CARTESIAN_POINT ( 'NONE',  ( 14.92337183194729633, 42.67559781766745886, 8.527530157486181039 ) ) ;
#83045=CARTESIAN_POINT ( 'NONE',  ( 10.00000000000000000, 19.75893115100078390, -9.846743663894594434 ) ) ;
#83046=CARTESIAN_POINT ( 'NONE',  ( 17.84635730667654840, 58.63791097397317742, 6.500000000000043521 ) ) ;
#83048=ORIENTED_EDGE ( 'NONE', *, *, #26429, .T. ) ;
#83052=CARTESIAN_POINT ( 'NONE',  ( -2.266590686148945544, 17.22041550158063572, 7.082119434687048631 ) ) ;
#83053=CARTESIAN_POINT ( 'NONE',  ( 7.084665262690076126, 39.10535201082150536, 10.88017736071109987 ) ) ;
#83054=CARTESIAN_POINT ( 'NONE',  ( 0.5774900079438590739, 32.64701867748816966, -5.440088680355550821 ) ) ;
#83055=CARTESIAN_POINT ( 'NONE',  ( 21.09922568453595559, 27.04030133659708568, -6.408140936763230044 ) ) ;
#83056=CARTESIAN_POINT ( 'NONE',  ( 24.16423886937410614, 9.512082168247301794, -3.795296366450302550 ) ) ;
#83057=CARTESIAN_POINT ( 'NONE',  ( 12.91533473730993009, 66.60535201082150536, -10.88017736071109987 ) ) ;
#83058=CARTESIAN_POINT ( 'NONE',  ( -2.816281873526471635, 33.91530133659708213, -3.434112377981056508 ) ) ;
#83060=CARTESIAN_POINT ( 'NONE',  ( 1.472469842513823179, 45.59226448433412315, -4.923371831947296329 ) ) ;
#83061=CARTESIAN_POINT ( 'NONE',  ( 10.00000000000000000, 1.813685344154838175, -10.88017736071110342 ) ) ;
#83063=CARTESIAN_POINT ( 'NONE',  ( 10.00000000000000178, 19.31368534415484106, 10.88017736071110342 ) ) ;
#83065=CARTESIAN_POINT ( 'NONE',  ( 7.084665262690076126, 64.10535201082150536, 10.88017736071109987 ) ) ;
#83066=AXIS2_PLACEMENT_3D ( 'NONE', #20289, #19302, #87786 ) ;
#83067=CARTESIAN_POINT ( 'NONE',  ( 15.44008868035555793, 56.39701867748817676, -9.422509992056140149 ) ) ;
#83068=CARTESIAN_POINT ( 'NONE',  ( 15.44008868035555260, 64.73035201082151957, 9.422509992056143702 ) ) ;
#83070=CARTESIAN_POINT ( 'NONE',  ( 5.076628168052704559, 0.1755978176674514724, -8.527530157486179263 ) ) ;
#83071=CARTESIAN_POINT ( 'NONE',  ( 2.035157376598824452, 53.68868534415484817, 7.964842623401179544 ) ) ;
#83073=EDGE_CURVE ( 'NONE', #3586, #72554, #40267, .T. ) ;
#83076=CARTESIAN_POINT ( 'NONE',  ( 12.63842701281683922, 29.55059781766745175, -9.846743663894590881 ) ) ;
#83078=CARTESIAN_POINT ( 'NONE',  ( 2.791683348922240793, 66.63393115100079456, 7.208316651077764092 ) ) ;
#83079=CARTESIAN_POINT ( 'NONE',  ( 0.1955144967548914092, 24.32703681773340421, -6.500000000002779998 ) ) ;
#83080=CARTESIAN_POINT ( 'NONE',  ( -4.164238869374099927, 2.012082168247300906, 3.795296366450308767 ) ) ;
#83081=CARTESIAN_POINT ( 'NONE',  ( -1.926860441876562247, 7.453790035174473694, -3.195792623639530650 ) ) ;
#83083=CARTESIAN_POINT ( 'NONE',  ( 19.42250999205614193, 10.14701867748816966, 5.440088680355555262 ) ) ;
#83087=CARTESIAN_POINT ( 'NONE',  ( 7.361572987183169658, 44.96726448433412315, -9.846743663894592657 ) ) ;
#83089=CARTESIAN_POINT ( 'NONE',  ( -1.099225684535947600, 24.54030133659708923, 6.408140936763237150 ) ) ;
#83090=CARTESIAN_POINT ( 'NONE',  ( 1.472469842513823179, 20.59226448433411960, -4.923371831947296329 ) ) ;
#83092=CARTESIAN_POINT ( 'NONE',  ( 0.1532563361054082862, 66.21726448433413736, 2.638427012816831674 ) ) ;
#83095=ORIENTED_EDGE ( 'NONE', *, *, #8322, .T. ) ;
#83096=VERTEX_POINT ( 'NONE', #34218 ) ;
#83098=CARTESIAN_POINT ( 'NONE',  ( -0.8801773607111009756, 18.06368534415484106, 1.068504757029289695E-15 ) ) ;
#83099=CARTESIAN_POINT ( 'NONE',  ( 24.16423886937409904, 19.09541550158063927, 3.795296366450317205 ) ) ;
#83100=CARTESIAN_POINT ( 'NONE',  ( 19.84674366389459266, 23.71726448433412315, -2.638427012816827677 ) ) ;
#83101=CARTESIAN_POINT ( 'NONE',  ( 20.88017736071110875, 60.77201867748817676, -2.915334737309920765 ) ) ;
#83102=CARTESIAN_POINT ( 'NONE',  ( -1.099225684535947600, 44.54030133659708923, 6.408140936763237150 ) ) ;
#83104=CARTESIAN_POINT ( 'NONE',  ( 17.96484262340118221, 14.93868534415483751, 7.964842623401181321 ) ) ;
#83107=CARTESIAN_POINT ( 'NONE',  ( 16.40814093676324603, 7.456968003263754419, -11.09922568453594671 ) ) ;
#83108=CARTESIAN_POINT ( 'NONE',  ( 19.84674366389459266, 28.71726448433411960, -2.638427012816827677 ) ) ;
#83110=CARTESIAN_POINT ( 'NONE',  ( 22.81628187352647785, 36.62363466993041783, 6.195893100308588602E-16 ) ) ;
#83111=LINE ( 'NONE', #21637, #14918 ) ;
#83112=CARTESIAN_POINT ( 'NONE',  ( 15.44008868035555260, 34.73035201082151247, 9.422509992056143702 ) ) ;
#83113=DIRECTION ( 'NONE',  ( 0.000000000000000000, -0.000000000000000000, 1.000000000000000000 ) ) ;
#83115=CARTESIAN_POINT ( 'NONE',  ( 4.559911319644449179, 68.89701867748817676, 9.422509992056141925 ) ) ;
#83116=CARTESIAN_POINT ( 'NONE',  ( -0.8801773607111009756, 38.06368534415484106, 1.068504757029289695E-15 ) ) ;
#83118=CARTESIAN_POINT ( 'NONE',  ( 15.44008868035555260, 39.73035201082150536, 9.422509992056143702 ) ) ;
#83119=CARTESIAN_POINT ( 'NONE',  ( 12.63842701281683922, 64.55059781766745175, -9.846743663894590881 ) ) ;
#83120=CARTESIAN_POINT ( 'NONE',  ( 20.88017736071110875, 65.77201867748817676, -2.915334737309920765 ) ) ;
#83121=UNCERTAINTY_MEASURE_WITH_UNIT (LENGTH_MEASURE( 1.000000000000000082E-05 ), #64268, 'distance_accuracy_value', 'NONE');
#83122=CARTESIAN_POINT ( 'NONE',  ( 19.84674366389459266, 38.30059781766745175, 2.638427012816836559 ) ) ;
#83123=CARTESIAN_POINT ( 'NONE',  ( 4.559911319644449179, 8.897018677488171434, 9.422509992056141925 ) ) ;
#83125=CARTESIAN_POINT ( 'NONE',  ( 6.565887622018943937, 18.08196800326375708, -12.81628187352647608 ) ) ;
#83127=CARTESIAN_POINT ( 'NONE',  ( 19.42250999205614548, 25.98035201082150891, -5.440088680355545492 ) ) ;
#83130=CARTESIAN_POINT ( 'NONE',  ( 4.559911319644449179, 2.230352010821504471, -9.422509992056141925 ) ) ;
#83131=CARTESIAN_POINT ( 'NONE',  ( 4.559911319644449179, 33.89701867748817676, 9.422509992056141925 ) ) ;
#83132=CARTESIAN_POINT ( 'NONE',  ( 2.791683348922237240, 5.383931151000785675, -7.208316651077763204 ) ) ;
#83133=CARTESIAN_POINT ( 'NONE',  ( 24.16423886937410614, 44.30374883491397497, 8.672049930838204340E-16 ) ) ;
#83134=CARTESIAN_POINT ( 'NONE',  ( 19.84674366389459266, 23.30059781766745530, 2.638427012816836559 ) ) ;
#83135=CARTESIAN_POINT ( 'NONE',  ( 7.084665262690076126, 44.10535201082151247, 10.88017736071109987 ) ) ;
#83136=( BOUNDED_CURVE ( )  B_SPLINE_CURVE ( 2, ( #53392, #84888, #38905, #39398, #92868, #15432, #24398, #16889, #7914 ),
 .UNSPECIFIED., .F., .F. ) 
 B_SPLINE_CURVE_WITH_KNOTS ( ( 3, 2, 2, 2, 3 ),
 ( 0.5829980797973742801, 0.5833333333333333703, 0.5892857142857143016, 0.5952380952380952328, 0.5955733487740544341 ),
 .UNSPECIFIED. ) 
 CURVE ( )  GEOMETRIC_REPRESENTATION_ITEM ( )  RATIONAL_B_SPLINE_CURVE ( ( 0.9963778908391764944, 0.9980808541467923733, 1.000000000000000000, 0.9659258262890683122, 1.000000000000000000, 0.9659258262890683122, 1.000000000000000000, 0.9980808541467918182, 0.9963778908391756062 ) ) 
 REPRESENTATION_ITEM ( '' )  );
#83139=ORIENTED_EDGE ( 'NONE', *, *, #54625, .T. ) ;
#83141=CARTESIAN_POINT ( 'NONE',  ( 5.076628168052704559, 55.17559781766745175, -8.527530157486179263 ) ) ;
#83145=CARTESIAN_POINT ( 'NONE',  ( -4.164238869374098151, 21.59541550158063217, -3.795296366450310543 ) ) ;
#83146=CARTESIAN_POINT ( 'NONE',  ( -4.164238869374099927, 17.01208216824730357, 3.795296366450308767 ) ) ;
#83147=CARTESIAN_POINT ( 'NONE',  ( 0.5774900079438590739, 62.64701867748817676, -5.440088680355550821 ) ) ;
#83148=CARTESIAN_POINT ( 'NONE',  ( 24.16423886937410614, 64.51208216824728936, -3.795296366450302550 ) ) ;
#83149=CARTESIAN_POINT ( 'NONE',  ( 18.52753015748617571, 48.09226448433412315, 4.923371831947298993 ) ) ;
#83151=CARTESIAN_POINT ( 'NONE',  ( 2.035157376598824452, 48.68868534415483396, 7.964842623401179544 ) ) ;
#83152=CARTESIAN_POINT ( 'NONE',  ( 6.565887622018943937, 15.16530133659708568, 12.81628187352647430 ) ) ;
#83153=CARTESIAN_POINT ( 'NONE',  ( 13.79529636645031943, 15.34541550158063750, -14.16423886937409904 ) ) ;
#83154=CARTESIAN_POINT ( 'NONE',  ( 19.42250999205614193, 15.14701867748817143, 5.440088680355555262 ) ) ;
#83155=CARTESIAN_POINT ( 'NONE',  ( 17.96484262340118221, 21.18868534415483396, -7.964842623401177768 ) ) ;
#83157=CARTESIAN_POINT ( 'NONE',  ( 12.91533473730993009, 61.60535201082150536, -10.88017736071109987 ) ) ;
#83158=CARTESIAN_POINT ( 'NONE',  ( -1.099225684535947600, 48.70696800326375353, -6.408140936763238038 ) ) ;
#83166=CARTESIAN_POINT ( 'NONE',  ( 20.36894250292379738, 64.92874883491397497, -10.36894250292379027 ) ) ;
#83167=CARTESIAN_POINT ( 'NONE',  ( 17.96484262340118221, 4.938685344154837509, 7.964842623401181321 ) ) ;
#83168=CARTESIAN_POINT ( 'NONE',  ( 2.791683348922237240, 25.38393115100078390, -7.208316651077763204 ) ) ;
#83169=CARTESIAN_POINT ( 'NONE',  ( 5.076628168052703671, 46.84226448433412315, 8.527530157486179263 ) ) ;
#83170=CARTESIAN_POINT ( 'NONE',  ( 20.88017736071110875, 65.77201867748817676, -2.915334737309920765 ) ) ;
#83172=CARTESIAN_POINT ( 'NONE',  ( 5.076628168052703671, 1.842264484334118047, 8.527530157486179263 ) ) ;
#83176=CARTESIAN_POINT ( 'NONE',  ( 2.917880565312950480, 30.97041550158063572, -12.26659068614894821 ) ) ;
#83177=CARTESIAN_POINT ( 'NONE',  ( -4.164238869374099039, 36.80374883491396787, 8.674139862899312516E-16 ) ) ;
#83178=VERTEX_POINT ( 'NONE', #79745 ) ;
#83179=CARTESIAN_POINT ( 'NONE',  ( 6.565887622018943937, 60.16530133659707502, 12.81628187352647430 ) ) ;
#83180=CARTESIAN_POINT ( 'NONE',  ( 2.035157376598822676, 27.43868534415483396, -7.964842623401177768 ) ) ;
#83181=CARTESIAN_POINT ( 'NONE',  ( 14.92337183194729988, 39.34226448433412315, -8.527530157486177487 ) ) ;
#83182=CARTESIAN_POINT ( 'NONE',  ( 20.88017736071110519, 30.56368534415484106, 2.639326808657452039E-16 ) ) ;
#83183=CARTESIAN_POINT ( 'NONE',  ( 13.43411237798105340, 60.58196800326376064, 12.81628187352647963 ) ) ;
#83185=CARTESIAN_POINT ( 'NONE',  ( 5.076628168052703671, 56.84226448433412315, 8.527530157486179263 ) ) ;
#83186=CARTESIAN_POINT ( 'NONE',  ( 7.361572987183170547, 52.05059781766745175, 9.846743663894590881 ) ) ;
#83189=CARTESIAN_POINT ( 'NONE',  ( 2.603489959281613420, 45.43575266056827644, -6.500000000000031086 ) ) ;
#83191=ORIENTED_EDGE ( 'NONE', *, *, #54565, .T. ) ;
#83196=CARTESIAN_POINT ( 'NONE',  ( 19.54820696779682976, 81.00406362210809164, 5.000000000000000000 ) ) ;
#83197=CARTESIAN_POINT ( 'NONE',  ( 10.00000000000000178, 27.25893115100078390, 9.846743663894594434 ) ) ;
#83198=CARTESIAN_POINT ( 'NONE',  ( 20.15039907845753575, 10.60158574516642460, -6.262539305110077059 ) ) ;
#83199=CARTESIAN_POINT ( 'NONE',  ( 0.6178305044545838731, 39.74863466993041072, 9.382169495545420901 ) ) ;
#83200=VECTOR ( 'NONE', #91745, 1000.000000000000000 ) ;
#83202=ORIENTED_EDGE ( 'NONE', *, *, #43046, .T. ) ;
#83203=CARTESIAN_POINT ( 'NONE',  ( 7.361572987183169658, 59.96726448433410894, -9.846743663894592657 ) ) ;
#83205=CARTESIAN_POINT ( 'NONE',  ( 2.791683348922237240, 35.38393115100079456, -7.208316651077763204 ) ) ;
#83206=CARTESIAN_POINT ( 'NONE',  ( 2.917880565312950480, 35.97041550158063217, -12.26659068614894821 ) ) ;
#83207=CARTESIAN_POINT ( 'NONE',  ( 5.076628168052703671, 46.84226448433412315, 8.527530157486179263 ) ) ;
#83208=CARTESIAN_POINT ( 'NONE',  ( -1.099225684535947600, 64.54030133659709634, 6.408140936763237150 ) ) ;
#83209=APPLICATION_CONTEXT ( 'automotive_design' ) ;
#83211=CARTESIAN_POINT ( 'NONE',  ( 5.076628168052703671, 1.842264484334118047, 8.527530157486179263 ) ) ;
#83212=CARTESIAN_POINT ( 'NONE',  ( 10.00000000000000000, 5.553748834913967869, -14.16423886937410082 ) ) ;
#83213=CARTESIAN_POINT ( 'NONE',  ( 7.361572987183169658, 44.96726448433412315, -9.846743663894592657 ) ) ;
#83214=CARTESIAN_POINT ( 'NONE',  ( 10.00000000000000000, 36.81368534415484106, -10.88017736071110342 ) ) ;
#83216=EDGE_CURVE ( 'NONE', #92463, #74651, #4501, .T. ) ;
#83217=CARTESIAN_POINT ( 'NONE',  ( 15.44008868035555260, 44.73035201082151247, 9.422509992056143702 ) ) ;
#83218=VERTEX_POINT ( 'NONE', #71272 ) ;
#83221=CARTESIAN_POINT ( 'NONE',  ( 0.5774900079438607392, 13.48035201082150358, 5.440088680355550821 ) ) ;
#83222=CARTESIAN_POINT ( 'NONE',  ( 3.591859063236761518, -0.04303199673624671928, 11.09922568453594849 ) ) ;
#83223=CARTESIAN_POINT ( 'NONE',  ( 0.5774900079438590739, 37.64701867748817676, -5.440088680355550821 ) ) ;
#83224=CARTESIAN_POINT ( 'NONE',  ( -0.8801773607111008646, 68.27201867748817676, 2.915334737309923430 ) ) ;
#83225=CARTESIAN_POINT ( 'NONE',  ( 4.559911319644449179, 38.89701867748817676, 9.422509992056141925 ) ) ;
#83227=CARTESIAN_POINT ( 'NONE',  ( 1.472469842513823179, 16.42559781766745175, 4.923371831947296329 ) ) ;
#83228=CARTESIAN_POINT ( 'NONE',  ( 10.00000000000000178, 42.25893115100078745, 9.846743663894594434 ) ) ;
#83231=CARTESIAN_POINT ( 'NONE',  ( 14.92337183194729988, 64.34226448433412315, -8.527530157486177487 ) ) ;
#83232=CARTESIAN_POINT ( 'NONE',  ( -4.164238869374098151, 66.59541550158060375, -3.795296366450310543 ) ) ;
#83233=AXIS2_PLACEMENT_3D ( 'NONE', #44362, #6363, #43860 ) ;
#83236=CARTESIAN_POINT ( 'NONE',  ( 6.204703633549690345, 22.84541550158062861, 14.16423886937410082 ) ) ;
#83237=CARTESIAN_POINT ( 'NONE',  ( 10.00000000000000000, 50.55374883491396787, -14.16423886937410082 ) ) ;
#83239=CIRCLE ( 'NONE', #89586, 2.999999999999999112 ) ;
#83240=ORIENTED_EDGE ( 'NONE', *, *, #49046, .T. ) ;
#83241=CARTESIAN_POINT ( 'NONE',  ( 12.63842701281683922, 24.55059781766745175, -9.846743663894590881 ) ) ;
#83242=CARTESIAN_POINT ( 'NONE',  ( 4.559911319644449179, 32.23035201082150536, -9.422509992056141925 ) ) ;
#83243=CARTESIAN_POINT ( 'NONE',  ( 17.20831665107776587, 44.13393115100078745, -7.208316651077762316 ) ) ;
#83244=CARTESIAN_POINT ( 'NONE',  ( -0.3689425029237898834, 6.178748834913968757, -10.36894250292378850 ) ) ;
#83245=CARTESIAN_POINT ( 'NONE',  ( 2.603489959281584998, 6.582109641433292246, 6.499999999999998224 ) ) ;
#83247=( BOUNDED_CURVE ( )  B_SPLINE_CURVE ( 2, ( #60927, #69923, #84919, #91433, #22960, #76919, #31896, #54897, #85412 ),
 .UNSPECIFIED., .F., .F. ) 
 B_SPLINE_CURVE_WITH_KNOTS ( ( 3, 2, 2, 2, 3 ),
 ( 0.1187123655116599508, 0.1190476190476190688, 0.1250000000000000000, 0.1309523809523809312, 0.1312876344883400492 ),
 .UNSPECIFIED. ) 
 CURVE ( )  GEOMETRIC_REPRESENTATION_ITEM ( )  RATIONAL_B_SPLINE_CURVE ( ( 0.9963778908391762723, 0.9980808541467921513, 1.000000000000000000, 0.9659258262890683122, 1.000000000000000000, 0.9659258262890683122, 1.000000000000000000, 0.9980808541467922623, 0.9963778908391764944 ) ) 
 REPRESENTATION_ITEM ( '' )  );
#83249=CARTESIAN_POINT ( 'NONE',  ( -1.099225684535947600, 38.70696800326375353, -6.408140936763238038 ) ) ;
#83250=CARTESIAN_POINT ( 'NONE',  ( 2.791683348922240793, 46.63393115100077324, 7.208316651077764092 ) ) ;
#83252=CARTESIAN_POINT ( 'NONE',  ( 0.1532563361054100626, 5.800597817667452638, -2.638427012816831230 ) ) ;
#83255=CARTESIAN_POINT ( 'NONE',  ( 20.88017736071110164, 15.35535201082150358, 2.915334737309930979 ) ) ;
#83256=CARTESIAN_POINT ( 'NONE',  ( 24.16423886937410614, 54.51208216824730357, -3.795296366450302550 ) ) ;
#83257=CARTESIAN_POINT ( 'NONE',  ( 19.42250999205614548, 40.98035201082150536, -5.440088680355545492 ) ) ;
#83258=CARTESIAN_POINT ( 'NONE',  ( 24.16423886937410614, 4.512082168247300906, -3.795296366450302550 ) ) ;
#83259=CARTESIAN_POINT ( 'NONE',  ( 6.000000000000000000, 61.50000000000000711, -6.000000000000000000 ) ) ;
#83260=CARTESIAN_POINT ( 'NONE',  ( 14.92337183194729633, 17.67559781766745175, 8.527530157486181039 ) ) ;
#83261=CARTESIAN_POINT ( 'NONE',  ( 12.91533473730992121, 4.522018677488169658, 10.88017736071110164 ) ) ;
#83262=CARTESIAN_POINT ( 'NONE',  ( 18.52753015748618282, 43.92559781766745175, -4.923371831947291888 ) ) ;
#83263=CARTESIAN_POINT ( 'NONE',  ( 12.63842701281683922, 49.55059781766744464, -9.846743663894590881 ) ) ;
#83265=CARTESIAN_POINT ( 'NONE',  ( 7.084665262690076126, 42.02201867748816966, -10.88017736071110164 ) ) ;
#83268=CARTESIAN_POINT ( 'NONE',  ( 0.6178305044545818747, 58.49863466993042493, -9.382169495545419124 ) ) ;
#83270=CARTESIAN_POINT ( 'NONE',  ( 1.472469842513823179, 6.425597817667451750, 4.923371831947296329 ) ) ;
#83271=CARTESIAN_POINT ( 'NONE',  ( 19.38216949554541557, 52.24863466993041072, -9.382169495545420901 ) ) ;
#83272=CARTESIAN_POINT ( 'NONE',  ( 20.88017736071110875, 5.772018677488170546, -2.915334737309920765 ) ) ;
#83273=CARTESIAN_POINT ( 'NONE',  ( 19.84674366389459266, 48.71726448433413026, -2.638427012816827677 ) ) ;
#83275=SURFACE_STYLE_USAGE ( .BOTH. , #6291 ) ;
#83276=CARTESIAN_POINT ( 'NONE',  ( 10.00000000000000178, 33.05374883491396787, 14.16423886937410082 ) ) ;
#83277=CARTESIAN_POINT ( 'NONE',  ( -2.266590686148945544, 51.38708216824730357, -7.082119434687050408 ) ) ;
#83278=CARTESIAN_POINT ( 'NONE',  ( 19.84674366389459621, 58.50893115100078745, 7.409399052514197653E-17 ) ) ;
#83279=VECTOR ( 'NONE', #47469, 1000.000000000000000 ) ;
#83281=CARTESIAN_POINT ( 'NONE',  ( 12.91533473730993009, 56.60535201082151247, -10.88017736071109987 ) ) ;
#83282=CARTESIAN_POINT ( 'NONE',  ( 10.00000000000000000, -0.2410688489992152128, -9.846743663894594434 ) ) ;
#83283=ORIENTED_EDGE ( 'NONE', *, *, #69692, .T. ) ;
#83284=CARTESIAN_POINT ( 'NONE',  ( 0.6178305044545818747, 58.49863466993042493, -9.382169495545419124 ) ) ;
#83287=CARTESIAN_POINT ( 'NONE',  ( 0.5774900079438590739, 67.64701867748817676, -5.440088680355550821 ) ) ;
#83288=EDGE_LOOP ( 'NONE', ( #19176, #18591, #71957, #23209 ) ) ;
#83289=CARTESIAN_POINT ( 'NONE',  ( 10.00000000000000178, 3.053748834913967425, 14.16423886937410082 ) ) ;
#83290=CARTESIAN_POINT ( 'NONE',  ( 19.84674366389459621, 3.508931151000785231, 7.409399052514197653E-17 ) ) ;
#83291=CARTESIAN_POINT ( 'NONE',  ( 12.91533473730992121, 24.52201867748816966, 10.88017736071110164 ) ) ;
#83294=CARTESIAN_POINT ( 'NONE',  ( 7.084665262690076126, 29.10535201082150181, 10.88017736071109987 ) ) ;
#83296=DIRECTION ( 'NONE',  ( 0.000000000000000000, 0.000000000000000000, -1.000000000000000000 ) ) ;
#83299=CARTESIAN_POINT ( 'NONE',  ( 22.81628187352648496, 21.83196800326374643, -3.434112377981050290 ) ) ;
#83300=CARTESIAN_POINT ( 'NONE',  ( 1.472469842513823179, 0.5922644843341181575, -4.923371831947296329 ) ) ;
#83301=CARTESIAN_POINT ( 'NONE',  ( 12.91533473730993009, 16.60535201082150891, -10.88017736071109987 ) ) ;
#83303=CARTESIAN_POINT ( 'NONE',  ( 5.076628168052703671, 6.842264484334118713, 8.527530157486179263 ) ) ;
#83304=CARTESIAN_POINT ( 'NONE',  ( 17.96484262340118221, 31.18868534415483751, -7.964842623401177768 ) ) ;
#83309=ORIENTED_EDGE ( 'NONE', *, *, #64267, .T. ) ;
#83311=CARTESIAN_POINT ( 'NONE',  ( 20.88017736071110875, 40.77201867748818387, -2.915334737309920765 ) ) ;
#83313=CARTESIAN_POINT ( 'NONE',  ( 3.591859063236763294, 53.29030133659708923, -11.09922568453595026 ) ) ;
#83314=CARTESIAN_POINT ( 'NONE',  ( 0.5774900079438590739, 62.64701867748817676, -5.440088680355550821 ) ) ;
#83315=CARTESIAN_POINT ( 'NONE',  ( 10.00000000000000000, 64.75893115100078035, -9.846743663894594434 ) ) ;
#83317=CARTESIAN_POINT ( 'NONE',  ( 14.92337183194729633, 17.67559781766745175, 8.527530157486181039 ) ) ;
#83318=CARTESIAN_POINT ( 'NONE',  ( 13.43411237798105340, 50.58196800326375353, 12.81628187352647963 ) ) ;
#83320=CARTESIAN_POINT ( 'NONE',  ( 10.00000000000000000, -0.2410688489992152128, -9.846743663894594434 ) ) ;
#83321=CARTESIAN_POINT ( 'NONE',  ( 3.591859063236761518, 4.956968003263753531, 11.09922568453594849 ) ) ;
#83323=CARTESIAN_POINT ( 'NONE',  ( 2.791683348922237240, 65.38393115100078035, -7.208316651077763204 ) ) ;
#83324=CARTESIAN_POINT ( 'NONE',  ( 10.00000000000000178, 29.31368534415483751, 10.88017736071110342 ) ) ;
#83325=CARTESIAN_POINT ( 'NONE',  ( 1.472469842513823179, 50.59226448433411605, -4.923371831947296329 ) ) ;
#83326=CARTESIAN_POINT ( 'NONE',  ( -0.3289641300567998083, 33.07879003517447813, 5.963430220938281678 ) ) ;
#83327=CARTESIAN_POINT ( 'NONE',  ( 19.84674366389459621, 18.50893115100078745, 7.409399052514197653E-17 ) ) ;
#83328=CARTESIAN_POINT ( 'NONE',  ( 5.076628168052703671, 11.84226448433411960, 8.527530157486179263 ) ) ;
#83329=CARTESIAN_POINT ( 'NONE',  ( 16.40814093676323893, 0.7903013365970867898, 11.09922568453595026 ) ) ;
#83332=CARTESIAN_POINT ( 'NONE',  ( 5.076628168052703671, 66.84226448433412315, 8.527530157486179263 ) ) ;
#83335=CARTESIAN_POINT ( 'NONE',  ( 20.88017736071110875, 5.772018677488170546, -2.915334737309920765 ) ) ;
#83336=CARTESIAN_POINT ( 'NONE',  ( 1.472469842513823179, 40.59226448433411605, -4.923371831947296329 ) ) ;
#83338=COLOUR_RGB ( '', 0.40784314, 0.44705882, 0.49803922) ;
#83339=CARTESIAN_POINT ( 'NONE',  ( 0.2751277870542891413, 24.36607318730131411, -6.499999999999989342 ) ) ;
#83340=EDGE_CURVE ( 'NONE', #85384, #73925, #80728, .T. ) ;
#83341=CARTESIAN_POINT ( 'NONE',  ( -0.3689425029237881626, 67.42874883491396076, 10.36894250292379027 ) ) ;
#83343=CARTESIAN_POINT ( 'NONE',  ( 12.91533473730992121, 29.52201867748817321, 10.88017736071110164 ) ) ;
#83344=CARTESIAN_POINT ( 'NONE',  ( 17.08211943468705130, 48.47041550158063927, 12.26659068614894998 ) ) ;
#83345=CARTESIAN_POINT ( 'NONE',  ( 4.559911319644449179, 3.897018677488171434, 9.422509992056141925 ) ) ;
#83348=CARTESIAN_POINT ( 'NONE',  ( 7.361572987183169658, 29.96726448433411960, -9.846743663894592657 ) ) ;
#83349=CARTESIAN_POINT ( 'NONE',  ( 13.43411237798105340, 15.58196800326374998, 12.81628187352647963 ) ) ;
#83351=CARTESIAN_POINT ( 'NONE',  ( 7.361572987183170547, 57.05059781766744464, 9.846743663894590881 ) ) ;
#83354=CARTESIAN_POINT ( 'NONE',  ( 22.26659068614895176, 4.720415501580633943, -7.082119434687042414 ) ) ;
#83356=CARTESIAN_POINT ( 'NONE',  ( 5.076628168052704559, 30.17559781766745175, -8.527530157486179263 ) ) ;
#83358=CARTESIAN_POINT ( 'NONE',  ( 24.16423886937409904, 39.09541550158062506, 3.795296366450317205 ) ) ;
#83360=CARTESIAN_POINT ( 'NONE',  ( 10.00000000000000178, 2.258931151000784787, 9.846743663894594434 ) ) ;
#83362=CARTESIAN_POINT ( 'NONE',  ( -0.1503990784575328643, 35.12777174578612716, 6.262539305110068177 ) ) ;
#83363=CARTESIAN_POINT ( 'NONE',  ( 4.559911319644449179, 32.23035201082150536, -9.422509992056141925 ) ) ;
#83364=CARTESIAN_POINT ( 'NONE',  ( 16.40814093676323893, 55.79030133659708923, 11.09922568453595026 ) ) ;
#83365=CARTESIAN_POINT ( 'NONE',  ( 0.5774900079438607392, 3.480352010821504027, 5.440088680355550821 ) ) ;
#83366=CARTESIAN_POINT ( 'NONE',  ( 6.565887622018943937, 33.08196800326374643, -12.81628187352647608 ) ) ;
#83368=VERTEX_POINT ( 'NONE', #81700 ) ;
#83371=CARTESIAN_POINT ( 'NONE',  ( 17.08211943468705130, 43.47041550158063927, 12.26659068614894998 ) ) ;
#83372=CARTESIAN_POINT ( 'NONE',  ( 2.917880565312948704, 17.63708216824730357, 12.26659068614894643 ) ) ;
#83373=CARTESIAN_POINT ( 'NONE',  ( 17.96484262340118221, 11.18868534415483929, -7.964842623401177768 ) ) ;
#83374=CARTESIAN_POINT ( 'NONE',  ( 20.88017736071110519, 40.56368534415484106, 2.639326808657452039E-16 ) ) ;
#83376=DIRECTION ( 'NONE',  ( 0.5547001962252290364, 0.8320502943378437211, 0.000000000000000000 ) ) ;
#83377=CARTESIAN_POINT ( 'NONE',  ( 4.559911319644449179, 57.23035201082150536, -9.422509992056141925 ) ) ;
#83378=CARTESIAN_POINT ( 'NONE',  ( 15.44008868035555260, 64.73035201082151957, 9.422509992056143702 ) ) ;
#83379=CARTESIAN_POINT ( 'NONE',  ( 22.81628187352647785, 21.62363466993041783, 6.195893100308588602E-16 ) ) ;
#83381=CARTESIAN_POINT ( 'NONE',  ( 20.03743638938523119, 26.75197528031018734, 6.399506433553979079 ) ) ;
#83382=CARTESIAN_POINT ( 'NONE',  ( 12.63842701281683034, 42.46726448433412315, 9.846743663894596210 ) ) ;
#83384=B_SPLINE_CURVE_WITH_KNOTS ( 'NONE', 3,
 ( #84081, #15596, #45081, #37106, #66605, #89601 ),
 .UNSPECIFIED., .F., .F.,
 ( 4, 2, 4 ),
 ( 0.000000000000000000, 0.0002701661927229330050, 0.0005403323854458660100 ),
 .UNSPECIFIED. ) ;
#83387=CARTESIAN_POINT ( 'NONE',  ( 3.591859063236761518, 19.95696800326375353, 11.09922568453594849 ) ) ;
#83388=FACE_OUTER_BOUND ( 'NONE', #20627, .T. ) ;
#83389=CARTESIAN_POINT ( 'NONE',  ( 19.42250999205614193, 5.147018677488171434, 5.440088680355555262 ) ) ;
#83390=CARTESIAN_POINT ( 'NONE',  ( 7.361572987183170547, 42.05059781766745886, 9.846743663894590881 ) ) ;
#83392=CARTESIAN_POINT ( 'NONE',  ( 5.076628168052704559, 15.17559781766745175, -8.527530157486179263 ) ) ;
#83393=CARTESIAN_POINT ( 'NONE',  ( 13.79529636645031943, 5.345415501580634832, -14.16423886937409904 ) ) ;
#83395=CARTESIAN_POINT ( 'NONE',  ( 4.559911319644449179, 32.23035201082150536, -9.422509992056141925 ) ) ;
#83396=CARTESIAN_POINT ( 'NONE',  ( 4.559911319644449179, 2.230352010821504471, -9.422509992056141925 ) ) ;
#83397=CARTESIAN_POINT ( 'NONE',  ( 10.00000000000000000, 30.55374883491397142, -14.16423886937410082 ) ) ;
#83399=CARTESIAN_POINT ( 'NONE',  ( -0.8801773607111009756, 33.06368534415484106, 1.068504757029289695E-15 ) ) ;
#83400=CARTESIAN_POINT ( 'NONE',  ( -0.8801773607110991993, 22.85535201082150181, -2.915334737309923874 ) ) ;
#83402=CARTESIAN_POINT ( 'NONE',  ( 10.00000000000000000, 31.81368534415483751, -10.88017736071110342 ) ) ;
#83403=CARTESIAN_POINT ( 'NONE',  ( 6.565887622018943937, 43.08196800326374643, -12.81628187352647608 ) ) ;
#83404=CARTESIAN_POINT ( 'NONE',  ( 2.035157376598824452, 43.68868534415484106, 7.964842623401179544 ) ) ;
#83406=CARTESIAN_POINT ( 'NONE',  ( 19.42250999205614193, 50.14701867748817676, 5.440088680355555262 ) ) ;
#83407=CIRCLE ( 'NONE', #40298, 19.43999999999999773 ) ;
#83409=CARTESIAN_POINT ( 'NONE',  ( 12.91533473730992121, 34.52201867748817676, 10.88017736071110164 ) ) ;
#83412=CARTESIAN_POINT ( 'NONE',  ( 13.79529636645030344, 48.26208216824728936, 14.16423886937410614 ) ) ;
#83413=CARTESIAN_POINT ( 'NONE',  ( 14.92337183194729633, 2.675597817667451750, 8.527530157486181039 ) ) ;
#83414=( LENGTH_UNIT ( ) NAMED_UNIT ( * ) SI_UNIT ( .MILLI., .METRE. ) );
#83415=CARTESIAN_POINT ( 'NONE',  ( 14.92337183194729633, 57.67559781766745886, 8.527530157486181039 ) ) ;
#83418=CARTESIAN_POINT ( 'NONE',  ( 0.1532563361054082862, 36.21726448433410894, 2.638427012816831674 ) ) ;
#83420=AXIS2_PLACEMENT_3D ( 'NONE', #41117, #10116, #71113 ) ;
#83421=CARTESIAN_POINT ( 'NONE',  ( 1.472469842513823179, 35.59226448433412315, -4.923371831947296329 ) ) ;
#83424=CARTESIAN_POINT ( 'NONE',  ( 17.96484262340118221, 29.93868534415484106, 7.964842623401181321 ) ) ;
#83425=CARTESIAN_POINT ( 'NONE',  ( 17.20831665107776587, 37.88393115100078745, 7.208316651077764980 ) ) ;
#83426=CARTESIAN_POINT ( 'NONE',  ( 19.72487221294571569, 25.71833443783938478, -6.499999999999989342 ) ) ;
#83427=CARTESIAN_POINT ( 'NONE',  ( 20.88017736071110519, 60.56368534415484106, 2.639326808657452039E-16 ) ) ;
#83428=CARTESIAN_POINT ( 'NONE',  ( -0.8801773607111008646, 28.27201867748817321, 2.915334737309923430 ) ) ;
#83429=CARTESIAN_POINT ( 'NONE',  ( -1.099225684535947600, 64.54030133659709634, 6.408140936763237150 ) ) ;
#83430=CARTESIAN_POINT ( 'NONE',  ( 13.79529636645031943, 40.34541550158063217, -14.16423886937409904 ) ) ;
#83431=EDGE_CURVE ( 'NONE', #62035, #89063, #39443, .T. ) ;
#83435=CARTESIAN_POINT ( 'NONE',  ( 0.6178305044545838731, 9.748634669930416052, 9.382169495545420901 ) ) ;
#83436=CARTESIAN_POINT ( 'NONE',  ( -0.8801773607110991993, 12.85535201082150358, -2.915334737309923874 ) ) ;
#83437=CARTESIAN_POINT ( 'NONE',  ( 10.00000000000000000, 46.81368534415484106, -10.88017736071110342 ) ) ;
#83440=CARTESIAN_POINT ( 'NONE',  ( 20.88017736071110875, 60.77201867748817676, -2.915334737309920765 ) ) ;
#83441=CARTESIAN_POINT ( 'NONE',  ( 17.20831665107776587, 37.88393115100078745, 7.208316651077764980 ) ) ;
#83442=CARTESIAN_POINT ( 'NONE',  ( 1.472469842513823179, 20.59226448433411960, -4.923371831947296329 ) ) ;
#83443=CARTESIAN_POINT ( 'NONE',  ( 14.92337183194729633, 17.67559781766745175, 8.527530157486181039 ) ) ;
#83446=CARTESIAN_POINT ( 'NONE',  ( 1.472469842513823179, 10.59226448433411782, -4.923371831947296329 ) ) ;
#83449=CARTESIAN_POINT ( 'NONE',  ( 5.076628168052703671, 26.84226448433411960, 8.527530157486179263 ) ) ;
#83451=( BOUNDED_SURFACE ( )  B_SPLINE_SURFACE ( 1, 2, ( 
 ( #29240, #59738, #37754, #45737, #30712, #7751, #68251, #68736, #90233, #38730, #91727, #90731, #38245, #29728, #52245, #21766, #23249, #82739, #44737, #37265, #84240, #46231, #69230, #22257, #76717, #14762, #75733, #62688, #56672, #48179, #17708, #77695, #87161, #32185, #10689, #71682, #24715, #2224, #55700, #25703, #9207, #25219, #54692, #39720, #86196, #56193, #24225, #86687, #17219, #2721, #3192, #63667, #32684, #26181, #48672, #18686, #18191, #49171, #33174, #79173, #31700, #94172, #47191, #63177, #41202, #78691, #55187, #33658, #79673, #64153, #1731, #10202, #9703, #94672, #40695, #11170, #71197, #69718, #62191, #47698, #1244, #93686, #85214, #92701, #70212, #93188, #85703, #78190, #16718, #40199, #70707, #66640, #51137, #12152, #12641, #65637, #42659, #51641, #65141, #72159, #64642, #97164, #80153, #73631, #27147, #11665, #43633, #95662, #49646, #81627, #20145, #96659, #28632, #59120, #89629, #95152, #26662, #21140, #28139, #58639, #73134, #3687, #88638, #50651, #82122, #43138, #89138, #35136, #42178, #41689, #34645, #80658, #34148, #66130, #57156, #19167, #81139, #20648, #87654, #72642, #5156, #4175, #57649, #88145, #35643, #19657, #13134, #74118, #36130, #50148, #4675, #96160, #5654, #27643, #58127, #15630, #83619, #53110, #14646, #38130, #15135, #45611, #91610, #14139, #61586, #92097, #84114, #36642, #52128, #23126, #22134, #31091, #38611, #90610, #83116, #67126, #29605, #75615, #29116, #60609, #53599, #91103, #68127, #52616, #54089, #98655, #76109, #30595, #75119, #45108, #7125, #37630, #7640, #68618, #30101, #147, #61100, #46113, #76599, #44624, #23628, #13632, #8115, #97654, #82625, #69108, #22631, #44115, #642, #74625, #6139, #59619, #60109, #90117, #21644, #6626, #37140, #67634, #98144, #24603, #26069, #70585, #25100, #2606, #47077, #93074, #17100, #9583, #33059, #63067, #70094, #63555, #41078, #94064, #16600, #40084, #55069, #17592, #2111, #78574, #32570, #64038, #77089, #32065, #71080, #47585, #39109, #46591, #54577, #77575, #9090, #62075, #18076, #86081, #92583, #10570, #25586, #85587, #55585, #93567, #78079, #94552, #39606, #16105, #8599, #71576, #24106, #48059, #1617, #85091, #86572, #62569, #10083, #56077, #40583, #48554, #3086, #33543, #84604, #69599, #1120, #31582, #79055, #12532, #27034, #18565, #4555, #35020, #13018, #58018, #43032, #50037, #64529, #43517, #49533, #95546, #49057, #81026, #79561, #34033, #96043, #35524, #87054, #26545, #27528, #11060, #41579, #95036, #65521, #72047, #50531, #5041, #51020, #87544, #34523, #74012, #58517, #19055, #88527, #89025, #57040, #96543, #20029, #73513, #5540 ),
 ( #11546, #88029, #42538, #66019, #80039, #12038, #3577, #42065, #73022, #28019, #72526, #20536, #4060, #81512, #36017, #66520, #19542, #97048, #56560, #65017, #57533, #80541, #61849, #84861, #89520, #92356, #6030, #23388, #6512, #90491, #36529, #82511, #28523, #31839, #29489, #16367, #53873, #14027, #8369, #77343, #90006, #67019, #46848, #69864, #84383, #21029, #31349, #75007, #85347, #77835, #38877, #97539, #16859, #44507, #59998, #29000, #15883, #46367, #23883, #76856, #47334, #54347, #59511, #8854, #39369, #13524, #69368, #1385, #62336, #888, #9347, #92844, #24371, #39851, #54834, #70356, #59015, #51521, #82013, #21526, #44006, #74508, #52020, #37018, #67517, #98034, #26309, #2365, #18333, #57298, #1875, #41830, #87791, #42307, #10340, #56333, #3326, #48813, #40838, #71819, #32331, #72296, #33791, #93827, #71339, #32821, #55339, #19306, #2857, #62836, #93336, #40351, #86827, #33311, #94807, #49306, #95299, #63318, #78830, #49794, #3827, #25356, #64296, #34282, #56809, #41350, #63805, #87306, #18825, #79807, #11310, #55841, #80301, #11800, #64782, #24856, #70852, #26802, #94312, #85846, #17359, #25837, #79320, #47829, #17839, #10830, #78329, #9851, #86335, #48322, #28282, #12782, #14286, #58776, #13279, #89767, #35282, #81284, #5305, #96805, #21283, #51281, #58269, #51778, #29265, #82262, #4809, #89281, #43281, #5789, #20792, #66777, #81767, #52268, #65278, #20295, #59265, #35782, #27286, #34789, #42801, #65778, #96307, #50281, #6278, #74260, #80797, #97804, #13778, #73776, #43770, #36280, #66271, #82764, #27783, #4316, #95808, #59761, #12293, #97298, #88785, #73285, #74770, #50793, #28770, #44264, #36784, #67275, #90255, #21788, #72780, #57786, #88292, #19792, #31227, #775, #15281, #6775, #91750, #23270, #1267, #46252, #61723, #38267, #52756, #31721, #37778, #83757, #37285, #69255, #67775, #22282, #84264, #23765, #75262, #14788, #15765, #98295, #29751, #83263, #53746, #60260, #54228, #53252, #62218, #69741, #22772, #45762, #90754, #60746, #7773, #45258, #76737, #84743, #8253, #291, #76256, #85237, #30737, #38754, #92239, #7276, #68760, #61243, #16247, #46730, #77228, #30242, #8733, #92724, #39251, #75755, #24249, #54716, #44759, #68275, #98795, #91247, #95173, #9231, #63201, #3215, #48201, #70235, #77718, #85726, #47717, #40223, #93210, #49190, #18215, #24733, #41710, #26200, #86216, #86710, #40714, #17728, #26680, #70733, #47217, #39740, #72180, #55211, #48694, #2247, #17239, #18706, #32705, #78212, #56692, #94192, #71701, #3710, #34170, #64660, #1754, #32209, #57175, #33677, #64174, #78714, #62710, #63689, #25722 ) ),
 .UNSPECIFIED., .F., .F., .F. ) 
 B_SPLINE_SURFACE_WITH_KNOTS ( ( 2, 2 ),
 ( 3, 2, 2, 2, 2, 2, 2, 2, 2, 2, 2, 2, 2, 2, 2, 2, 2, 2, 2, 2, 2, 2, 2, 2, 2, 2, 2, 2, 2, 2, 2, 2, 2, 2, 2, 2, 2, 2, 2, 2, 2, 2, 2, 2, 2, 2, 2, 2, 2, 2, 2, 2, 2, 2, 2, 2, 2, 2, 2, 2, 2, 2, 2, 2, 2, 2, 2, 2, 2, 2, 2, 2, 2, 2, 2, 2, 2, 2, 2, 2, 2, 2, 2, 2, 2, 2, 2, 2, 2, 2, 2, 2, 2, 2, 2, 2, 2, 2, 2, 2, 2, 2, 2, 2, 2, 2, 2, 2, 2, 2, 2, 2, 2, 2, 2, 2, 2, 2, 2, 2, 2, 2, 2, 2, 2, 2, 2, 2, 2, 2, 2, 2, 2, 2, 2, 2, 2, 2, 2, 2, 2, 2, 2, 2, 2, 2, 2, 2, 2, 2, 2, 2, 2, 2, 2, 2, 2, 2, 2, 2, 2, 2, 3 ),
 ( 0.000000000000000000, 1.000000000000000000 ),
 ( 0.000000000000000000, 0.005952380952380952051, 0.01190476190476190410, 0.01785714285714285615, 0.02380952380952380820, 0.02976190476190476025, 0.03571428571428571230, 0.04166666666666666435, 0.04761904761904761640, 0.05357142857142856845, 0.05952380952380952051, 0.06547619047619047949, 0.07142857142857142461, 0.07738095238095238360, 0.08333333333333332871, 0.08928571428571428770, 0.09523809523809523281, 0.1011904761904761918, 0.1071428571428571369, 0.1130952380952380959, 0.1190476190476190410, 0.1250000000000000000, 0.1309523809523809590, 0.1369047619047619180, 0.1428571428571428492, 0.1488095238095238082, 0.1547619047619047672, 0.1607142857142857262, 0.1666666666666666574, 0.1726190476190476164, 0.1785714285714285754, 0.1845238095238095344, 0.1904761904761904656, 0.1964285714285714246, 0.2023809523809523836, 0.2083333333333333426, 0.2142857142857142738, 0.2202380952380952328, 0.2261904761904761918, 0.2321428571428571508, 0.2380952380952380820, 0.2440476190476190410, 0.2500000000000000000, 0.2559523809523809312, 0.2619047619047619180, 0.2678571428571428492, 0.2738095238095238360, 0.2797619047619047672, 0.2857142857142856984, 0.2916666666666666852, 0.2976190476190476164, 0.3035714285714285476, 0.3095238095238095344, 0.3154761904761904656, 0.3214285714285714524, 0.3273809523809523836, 0.3333333333333333148, 0.3392857142857143016, 0.3452380952380952328, 0.3511904761904761640, 0.3571428571428571508, 0.3630952380952380820, 0.3690476190476190688, 0.3750000000000000000, 0.3809523809523809312, 0.3869047619047619180, 0.3928571428571428492, 0.3988095238095238360, 0.4047619047619047672, 0.4107142857142856984, 0.4166666666666666852, 0.4226190476190476164, 0.4285714285714285476, 0.4345238095238095344, 0.4404761904761904656, 0.4464285714285714524, 0.4523809523809523836, 0.4583333333333333148, 0.4642857142857143016, 0.4702380952380952328, 0.4761904761904761640, 0.4821428571428571508, 0.4880952380952380820, 0.4940476190476190688, 0.5000000000000000000, 0.5059523809523809312, 0.5119047619047618625, 0.5178571428571429047, 0.5238095238095238360, 0.5297619047619047672, 0.5357142857142856984, 0.5416666666666666297, 0.5476190476190476719, 0.5535714285714286031, 0.5595238095238095344, 0.5654761904761904656, 0.5714285714285713969, 0.5773809523809523281, 0.5833333333333333703, 0.5892857142857143016, 0.5952380952380952328, 0.6011904761904761640, 0.6071428571428570953, 0.6130952380952381375, 0.6190476190476190688, 0.6250000000000000000, 0.6309523809523809312, 0.6369047619047618625, 0.6428571428571429047, 0.6488095238095238360, 0.6547619047619047672, 0.6607142857142856984, 0.6666666666666666297, 0.6726190476190476719, 0.6785714285714286031, 0.6845238095238095344, 0.6904761904761904656, 0.6964285714285713969, 0.7023809523809523281, 0.7083333333333333703, 0.7142857142857143016, 0.7202380952380952328, 0.7261904761904761640, 0.7321428571428570953, 0.7380952380952381375, 0.7440476190476190688, 0.7500000000000000000, 0.7559523809523809312, 0.7619047619047618625, 0.7678571428571429047, 0.7738095238095238360, 0.7797619047619047672, 0.7857142857142856984, 0.7916666666666666297, 0.7976190476190476719, 0.8035714285714286031, 0.8095238095238095344, 0.8154761904761904656, 0.8214285714285713969, 0.8273809523809523281, 0.8333333333333333703, 0.8392857142857143016, 0.8452380952380952328, 0.8511904761904761640, 0.8571428571428570953, 0.8630952380952381375, 0.8690476190476190688, 0.8750000000000000000, 0.8809523809523809312, 0.8869047619047618625, 0.8928571428571429047, 0.8988095238095238360, 0.9047619047619047672, 0.9107142857142856984, 0.9166666666666666297, 0.9226190476190476719, 0.9285714285714286031, 0.9345238095238095344, 0.9404761904761904656, 0.9464285714285713969, 0.9523809523809523281, 0.9583333333333333703, 0.9642857142857143016 ),
 .UNSPECIFIED. ) 
 GEOMETRIC_REPRESENTATION_ITEM ( )  RATIONAL_B_SPLINE_SURFACE ( (
 ( 1.000000000000000000, 0.9659258262890683122, 1.000000000000000000, 0.9659258262890683122, 1.000000000000000000, 0.9659258262890683122, 1.000000000000000000, 0.9659258262890683122, 1.000000000000000000, 0.9659258262890683122, 1.000000000000000000, 0.9659258262890683122, 1.000000000000000000, 0.9659258262890683122, 1.000000000000000000, 0.9659258262890683122, 1.000000000000000000, 0.9659258262890683122, 1.000000000000000000, 0.9659258262890683122, 1.000000000000000000, 0.9659258262890683122, 1.000000000000000000, 0.9659258262890683122, 1.000000000000000000, 0.9659258262890683122, 1.000000000000000000, 0.9659258262890683122, 1.000000000000000000, 0.9659258262890683122, 1.000000000000000000, 0.9659258262890683122, 1.000000000000000000, 0.9659258262890683122, 1.000000000000000000, 0.9659258262890683122, 1.000000000000000000, 0.9659258262890683122, 1.000000000000000000, 0.9659258262890683122, 1.000000000000000000, 0.9659258262890683122, 1.000000000000000000, 0.9659258262890683122, 1.000000000000000000, 0.9659258262890683122, 1.000000000000000000, 0.9659258262890683122, 1.000000000000000000, 0.9659258262890683122, 1.000000000000000000, 0.9659258262890683122, 1.000000000000000000, 0.9659258262890683122, 1.000000000000000000, 0.9659258262890683122, 1.000000000000000000, 0.9659258262890683122, 1.000000000000000000, 0.9659258262890683122, 1.000000000000000000, 0.9659258262890683122, 1.000000000000000000, 0.9659258262890683122, 1.000000000000000000, 0.9659258262890683122, 1.000000000000000000, 0.9659258262890683122, 1.000000000000000000, 0.9659258262890683122, 1.000000000000000000, 0.9659258262890683122, 1.000000000000000000, 0.9659258262890683122, 1.000000000000000000, 0.9659258262890683122, 1.000000000000000000, 0.9659258262890683122, 1.000000000000000000, 0.9659258262890683122, 1.000000000000000000, 0.9659258262890683122, 1.000000000000000000, 0.9659258262890683122, 1.000000000000000000, 0.9659258262890683122, 1.000000000000000000, 0.9659258262890683122, 1.000000000000000000, 0.9659258262890683122, 1.000000000000000000, 0.9659258262890683122, 1.000000000000000000, 0.9659258262890683122, 1.000000000000000000, 0.9659258262890683122, 1.000000000000000000, 0.9659258262890683122, 1.000000000000000000, 0.9659258262890683122, 1.000000000000000000, 0.9659258262890683122, 1.000000000000000000, 0.9659258262890683122, 1.000000000000000000, 0.9659258262890683122, 1.000000000000000000, 0.9659258262890683122, 1.000000000000000000, 0.9659258262890683122, 1.000000000000000000, 0.9659258262890683122, 1.000000000000000000, 0.9659258262890683122, 1.000000000000000000, 0.9659258262890683122, 1.000000000000000000, 0.9659258262890683122, 1.000000000000000000, 0.9659258262890683122, 1.000000000000000000, 0.9659258262890683122, 1.000000000000000000, 0.9659258262890683122, 1.000000000000000000, 0.9659258262890683122, 1.000000000000000000, 0.9659258262890683122, 1.000000000000000000, 0.9659258262890683122, 1.000000000000000000, 0.9659258262890683122, 1.000000000000000000, 0.9659258262890683122, 1.000000000000000000, 0.9659258262890683122, 1.000000000000000000, 0.9659258262890683122, 1.000000000000000000, 0.9659258262890683122, 1.000000000000000000, 0.9659258262890683122, 1.000000000000000000, 0.9659258262890683122, 1.000000000000000000, 0.9659258262890683122, 1.000000000000000000, 0.9659258262890683122, 1.000000000000000000, 0.9659258262890683122, 1.000000000000000000, 0.9659258262890683122, 1.000000000000000000, 0.9659258262890683122, 1.000000000000000000, 0.9659258262890683122, 1.000000000000000000, 0.9659258262890683122, 1.000000000000000000, 0.9659258262890683122, 1.000000000000000000, 0.9659258262890683122, 1.000000000000000000, 0.9659258262890683122, 1.000000000000000000, 0.9659258262890683122, 1.000000000000000000, 0.9659258262890683122, 1.000000000000000000, 0.9659258262890683122, 1.000000000000000000, 0.9659258262890683122, 1.000000000000000000, 0.9659258262890683122, 1.000000000000000000, 0.9659258262890683122, 1.000000000000000000, 0.9659258262890683122, 1.000000000000000000, 0.9659258262890683122, 1.000000000000000000, 0.9659258262890683122, 1.000000000000000000, 0.9659258262890683122, 1.000000000000000000, 0.9659258262890683122, 1.000000000000000000, 0.9659258262890683122, 1.000000000000000000, 0.9659258262890683122, 1.000000000000000000, 0.9659258262890683122, 1.000000000000000000, 0.9659258262890683122, 1.000000000000000000, 0.9659258262890683122, 1.000000000000000000, 0.9659258262890683122, 1.000000000000000000, 0.9659258262890683122, 1.000000000000000000, 0.9659258262890683122, 1.000000000000000000, 0.9659258262890683122, 1.000000000000000000, 0.9659258262890683122, 1.000000000000000000, 0.9659258262890683122, 1.000000000000000000, 0.9659258262890683122, 1.000000000000000000, 0.9659258262890683122, 1.000000000000000000, 0.9659258262890683122, 1.000000000000000000, 0.9659258262890683122, 1.000000000000000000, 0.9659258262890683122, 1.000000000000000000, 0.9659258262890683122, 1.000000000000000000, 0.9659258262890683122, 1.000000000000000000, 0.9659258262890683122, 1.000000000000000000, 0.9659258262890683122, 1.000000000000000000, 0.9659258262890683122, 1.000000000000000000, 0.9659258262890683122, 1.000000000000000000, 0.9659258262890683122, 1.000000000000000000, 0.9659258262890683122, 1.000000000000000000, 0.9659258262890683122, 1.000000000000000000, 0.9659258262890683122, 1.000000000000000000, 0.9659258262890683122, 1.000000000000000000, 0.9659258262890683122, 1.000000000000000000, 0.9659258262890683122, 1.000000000000000000, 0.9659258262890683122, 1.000000000000000000, 0.9659258262890683122, 1.000000000000000000, 0.9659258262890683122, 1.000000000000000000, 0.9659258262890683122, 1.000000000000000000, 0.9659258262890683122, 1.000000000000000000, 0.9659258262890683122, 1.000000000000000000, 0.9659258262890683122, 1.000000000000000000, 0.9659258262890683122, 1.000000000000000000, 0.9659258262890683122, 1.000000000000000000, 0.9659258262890683122, 1.000000000000000000, 0.9659258262890683122, 1.000000000000000000, 0.9659258262890683122, 1.000000000000000000, 0.9659258262890683122, 1.000000000000000000, 0.9659258262890683122, 1.000000000000000000, 0.9659258262890683122, 1.000000000000000000, 0.9659258262890683122, 1.000000000000000000, 0.9659258262890683122, 1.000000000000000000, 0.9659258262890683122, 1.000000000000000000, 0.9659258262890683122, 1.000000000000000000, 0.9659258262890683122, 1.000000000000000000, 0.9659258262890683122, 1.000000000000000000, 0.9659258262890683122, 1.000000000000000000, 0.9659258262890683122, 1.000000000000000000, 0.9659258262890683122, 1.000000000000000000, 0.9659258262890683122, 1.000000000000000000, 0.9659258262890683122, 1.000000000000000000, 0.9659258262890683122, 1.000000000000000000, 0.9659258262890683122, 1.000000000000000000, 0.9659258262890683122, 1.000000000000000000, 0.9659258262890683122, 1.000000000000000000, 0.9659258262890683122, 1.000000000000000000, 0.9659258262890683122, 1.000000000000000000, 0.9659258262890683122, 1.000000000000000000, 0.9659258262890683122, 1.000000000000000000, 0.9659258262890683122, 1.000000000000000000, 0.9659258262890683122, 1.000000000000000000, 0.9659258262890683122, 1.000000000000000000, 0.9659258262890683122, 1.000000000000000000, 0.9659258262890683122, 1.000000000000000000, 0.9659258262890683122, 1.000000000000000000),
 ( 1.000000000000000000, 0.9659258262890683122, 1.000000000000000000, 0.9659258262890683122, 1.000000000000000000, 0.9659258262890683122, 1.000000000000000000, 0.9659258262890683122, 1.000000000000000000, 0.9659258262890683122, 1.000000000000000000, 0.9659258262890683122, 1.000000000000000000, 0.9659258262890683122, 1.000000000000000000, 0.9659258262890683122, 1.000000000000000000, 0.9659258262890683122, 1.000000000000000000, 0.9659258262890683122, 1.000000000000000000, 0.9659258262890683122, 1.000000000000000000, 0.9659258262890683122, 1.000000000000000000, 0.9659258262890683122, 1.000000000000000000, 0.9659258262890683122, 1.000000000000000000, 0.9659258262890683122, 1.000000000000000000, 0.9659258262890683122, 1.000000000000000000, 0.9659258262890683122, 1.000000000000000000, 0.9659258262890683122, 1.000000000000000000, 0.9659258262890683122, 1.000000000000000000, 0.9659258262890683122, 1.000000000000000000, 0.9659258262890683122, 1.000000000000000000, 0.9659258262890683122, 1.000000000000000000, 0.9659258262890683122, 1.000000000000000000, 0.9659258262890683122, 1.000000000000000000, 0.9659258262890683122, 1.000000000000000000, 0.9659258262890683122, 1.000000000000000000, 0.9659258262890683122, 1.000000000000000000, 0.9659258262890683122, 1.000000000000000000, 0.9659258262890683122, 1.000000000000000000, 0.9659258262890683122, 1.000000000000000000, 0.9659258262890683122, 1.000000000000000000, 0.9659258262890683122, 1.000000000000000000, 0.9659258262890683122, 1.000000000000000000, 0.9659258262890683122, 1.000000000000000000, 0.9659258262890683122, 1.000000000000000000, 0.9659258262890683122, 1.000000000000000000, 0.9659258262890683122, 1.000000000000000000, 0.9659258262890683122, 1.000000000000000000, 0.9659258262890683122, 1.000000000000000000, 0.9659258262890683122, 1.000000000000000000, 0.9659258262890683122, 1.000000000000000000, 0.9659258262890683122, 1.000000000000000000, 0.9659258262890683122, 1.000000000000000000, 0.9659258262890683122, 1.000000000000000000, 0.9659258262890683122, 1.000000000000000000, 0.9659258262890683122, 1.000000000000000000, 0.9659258262890683122, 1.000000000000000000, 0.9659258262890683122, 1.000000000000000000, 0.9659258262890683122, 1.000000000000000000, 0.9659258262890683122, 1.000000000000000000, 0.9659258262890683122, 1.000000000000000000, 0.9659258262890683122, 1.000000000000000000, 0.9659258262890683122, 1.000000000000000000, 0.9659258262890683122, 1.000000000000000000, 0.9659258262890683122, 1.000000000000000000, 0.9659258262890683122, 1.000000000000000000, 0.9659258262890683122, 1.000000000000000000, 0.9659258262890683122, 1.000000000000000000, 0.9659258262890683122, 1.000000000000000000, 0.9659258262890683122, 1.000000000000000000, 0.9659258262890683122, 1.000000000000000000, 0.9659258262890683122, 1.000000000000000000, 0.9659258262890683122, 1.000000000000000000, 0.9659258262890683122, 1.000000000000000000, 0.9659258262890683122, 1.000000000000000000, 0.9659258262890683122, 1.000000000000000000, 0.9659258262890683122, 1.000000000000000000, 0.9659258262890683122, 1.000000000000000000, 0.9659258262890683122, 1.000000000000000000, 0.9659258262890683122, 1.000000000000000000, 0.9659258262890683122, 1.000000000000000000, 0.9659258262890683122, 1.000000000000000000, 0.9659258262890683122, 1.000000000000000000, 0.9659258262890683122, 1.000000000000000000, 0.9659258262890683122, 1.000000000000000000, 0.9659258262890683122, 1.000000000000000000, 0.9659258262890683122, 1.000000000000000000, 0.9659258262890683122, 1.000000000000000000, 0.9659258262890683122, 1.000000000000000000, 0.9659258262890683122, 1.000000000000000000, 0.9659258262890683122, 1.000000000000000000, 0.9659258262890683122, 1.000000000000000000, 0.9659258262890683122, 1.000000000000000000, 0.9659258262890683122, 1.000000000000000000, 0.9659258262890683122, 1.000000000000000000, 0.9659258262890683122, 1.000000000000000000, 0.9659258262890683122, 1.000000000000000000, 0.9659258262890683122, 1.000000000000000000, 0.9659258262890683122, 1.000000000000000000, 0.9659258262890683122, 1.000000000000000000, 0.9659258262890683122, 1.000000000000000000, 0.9659258262890683122, 1.000000000000000000, 0.9659258262890683122, 1.000000000000000000, 0.9659258262890683122, 1.000000000000000000, 0.9659258262890683122, 1.000000000000000000, 0.9659258262890683122, 1.000000000000000000, 0.9659258262890683122, 1.000000000000000000, 0.9659258262890683122, 1.000000000000000000, 0.9659258262890683122, 1.000000000000000000, 0.9659258262890683122, 1.000000000000000000, 0.9659258262890683122, 1.000000000000000000, 0.9659258262890683122, 1.000000000000000000, 0.9659258262890683122, 1.000000000000000000, 0.9659258262890683122, 1.000000000000000000, 0.9659258262890683122, 1.000000000000000000, 0.9659258262890683122, 1.000000000000000000, 0.9659258262890683122, 1.000000000000000000, 0.9659258262890683122, 1.000000000000000000, 0.9659258262890683122, 1.000000000000000000, 0.9659258262890683122, 1.000000000000000000, 0.9659258262890683122, 1.000000000000000000, 0.9659258262890683122, 1.000000000000000000, 0.9659258262890683122, 1.000000000000000000, 0.9659258262890683122, 1.000000000000000000, 0.9659258262890683122, 1.000000000000000000, 0.9659258262890683122, 1.000000000000000000, 0.9659258262890683122, 1.000000000000000000, 0.9659258262890683122, 1.000000000000000000, 0.9659258262890683122, 1.000000000000000000, 0.9659258262890683122, 1.000000000000000000, 0.9659258262890683122, 1.000000000000000000, 0.9659258262890683122, 1.000000000000000000, 0.9659258262890683122, 1.000000000000000000, 0.9659258262890683122, 1.000000000000000000, 0.9659258262890683122, 1.000000000000000000, 0.9659258262890683122, 1.000000000000000000, 0.9659258262890683122, 1.000000000000000000, 0.9659258262890683122, 1.000000000000000000, 0.9659258262890683122, 1.000000000000000000, 0.9659258262890683122, 1.000000000000000000, 0.9659258262890683122, 1.000000000000000000, 0.9659258262890683122, 1.000000000000000000, 0.9659258262890683122, 1.000000000000000000, 0.9659258262890683122, 1.000000000000000000, 0.9659258262890683122, 1.000000000000000000, 0.9659258262890683122, 1.000000000000000000, 0.9659258262890683122, 1.000000000000000000, 0.9659258262890683122, 1.000000000000000000, 0.9659258262890683122, 1.000000000000000000, 0.9659258262890683122, 1.000000000000000000, 0.9659258262890683122, 1.000000000000000000, 0.9659258262890683122, 1.000000000000000000, 0.9659258262890683122, 1.000000000000000000, 0.9659258262890683122, 1.000000000000000000, 0.9659258262890683122, 1.000000000000000000, 0.9659258262890683122, 1.000000000000000000, 0.9659258262890683122, 1.000000000000000000, 0.9659258262890683122, 1.000000000000000000, 0.9659258262890683122, 1.000000000000000000, 0.9659258262890683122, 1.000000000000000000, 0.9659258262890683122, 1.000000000000000000, 0.9659258262890683122, 1.000000000000000000, 0.9659258262890683122, 1.000000000000000000, 0.9659258262890683122, 1.000000000000000000, 0.9659258262890683122, 1.000000000000000000, 0.9659258262890683122, 1.000000000000000000, 0.9659258262890683122, 1.000000000000000000, 0.9659258262890683122, 1.000000000000000000, 0.9659258262890683122, 1.000000000000000000, 0.9659258262890683122, 1.000000000000000000, 0.9659258262890683122, 1.000000000000000000, 0.9659258262890683122, 1.000000000000000000) ) ) 
 REPRESENTATION_ITEM ( '' )  SURFACE ( )  );
#83453=CARTESIAN_POINT ( 'NONE',  ( 22.81628187352648496, 16.83196800326374998, -3.434112377981050290 ) ) ;
#83454=CARTESIAN_POINT ( 'NONE',  ( 7.084665262690076126, 57.02201867748817676, -10.88017736071110164 ) ) ;
#83455=CARTESIAN_POINT ( 'NONE',  ( 22.26659068614895176, 29.72041550158063572, -7.082119434687042414 ) ) ;
#83456=UNCERTAINTY_MEASURE_WITH_UNIT (LENGTH_MEASURE( 1.000000000000000082E-05 ), #22558, 'distance_accuracy_value', 'NONE');
#83459=CARTESIAN_POINT ( 'NONE',  ( 22.26659068614895176, 34.72041550158063927, -7.082119434687042414 ) ) ;
#83460=CARTESIAN_POINT ( 'NONE',  ( 13.79529636645031943, 40.34541550158063217, -14.16423886937409904 ) ) ;
#83461=CARTESIAN_POINT ( 'NONE',  ( -4.164238869374098151, 11.59541550158063217, -3.795296366450310543 ) ) ;
#83462=CARTESIAN_POINT ( 'NONE',  ( -2.266590686148945544, 32.22041550158063927, 7.082119434687048631 ) ) ;
#83464=CARTESIAN_POINT ( 'NONE',  ( 4.559911319644449179, 52.23035201082151247, -9.422509992056141925 ) ) ;
#83466=CARTESIAN_POINT ( 'NONE',  ( 10.00000000000000178, 32.25893115100078745, 9.846743663894594434 ) ) ;
#83467=CARTESIAN_POINT ( 'NONE',  ( 0.5774900079438607392, 63.48035201082149825, 5.440088680355550821 ) ) ;
#83468=CARTESIAN_POINT ( 'NONE',  ( 19.84674366389459266, 48.71726448433413026, -2.638427012816827677 ) ) ;
#83469=CARTESIAN_POINT ( 'NONE',  ( -0.8801773607111009756, 28.06368534415484106, 1.068504757029289695E-15 ) ) ;
#83470=CARTESIAN_POINT ( 'NONE',  ( -2.816281873526471635, 53.91530133659709634, -3.434112377981056508 ) ) ;
#83471=CARTESIAN_POINT ( 'NONE',  ( 14.92337183194729988, 59.34226448433412315, -8.527530157486177487 ) ) ;
#83473=CARTESIAN_POINT ( 'NONE',  ( 0.1532563361054083140, 26.00893115100078745, 1.131784320476157264E-15 ) ) ;
#83474=CARTESIAN_POINT ( 'NONE',  ( 19.38216949554541557, 62.24863466993041072, -9.382169495545420901 ) ) ;
#83477=CARTESIAN_POINT ( 'NONE',  ( 19.42250999205614548, 45.98035201082150536, -5.440088680355545492 ) ) ;
#83478=CARTESIAN_POINT ( 'NONE',  ( 5.076628168052704559, 55.17559781766745175, -8.527530157486179263 ) ) ;
#83479=CARTESIAN_POINT ( 'NONE',  ( 22.26659068614895176, 34.72041550158063927, -7.082119434687042414 ) ) ;
#83482=CARTESIAN_POINT ( 'NONE',  ( 10.00000000000000000, 66.81368534415484817, -10.88017736071110342 ) ) ;
#83484=CARTESIAN_POINT ( 'NONE',  ( 17.08211943468705130, 58.47041550158063927, 12.26659068614894998 ) ) ;
#83486=CARTESIAN_POINT ( 'NONE',  ( 21.09922568453595559, 12.04030133659708746, -6.408140936763230044 ) ) ;
#83489=CARTESIAN_POINT ( 'NONE',  ( -0.8801773607111008646, 48.27201867748816966, 2.915334737309923430 ) ) ;
#83490=MECHANICAL_DESIGN_GEOMETRIC_PRESENTATION_REPRESENTATION('',(#96270),#24408);
#83491=CARTESIAN_POINT ( 'NONE',  ( -0.3289641300568009741, 27.24545670184114243, -5.963430220938281678 ) ) ;
#83493=CARTESIAN_POINT ( 'NONE',  ( 17.08211943468705130, 43.47041550158063927, 12.26659068614894998 ) ) ;
#83495=CARTESIAN_POINT ( 'NONE',  ( 10.00000000000000178, 14.31368534415483751, 10.88017736071110342 ) ) ;
#83496=CARTESIAN_POINT ( 'NONE',  ( 10.00000000000000178, 19.31368534415484106, 10.88017736071110342 ) ) ;
#83498=CARTESIAN_POINT ( 'NONE',  ( 0.1532563361054082862, 51.21726448433412315, 2.638427012816831674 ) ) ;
#83499=CARTESIAN_POINT ( 'NONE',  ( 21.09922568453594849, 56.20696800326375353, 6.408140936763242479 ) ) ;
#83500=CARTESIAN_POINT ( 'NONE',  ( 1.707155281725178941, 42.90189080397286148, 6.499999999999955591 ) ) ;
#83502=CARTESIAN_POINT ( 'NONE',  ( 4.559911319644449179, 18.89701867748817321, 9.422509992056141925 ) ) ;
#83504=CARTESIAN_POINT ( 'NONE',  ( 0.6178305044545838731, 19.74863466993042138, 9.382169495545420901 ) ) ;
#83506=CARTESIAN_POINT ( 'NONE',  ( 5.076628168052704559, 50.17559781766745886, -8.527530157486179263 ) ) ;
#83507=CARTESIAN_POINT ( 'NONE',  ( 20.88017736071110519, 30.56368534415484106, 2.639326808657452039E-16 ) ) ;
#83508=CARTESIAN_POINT ( 'NONE',  ( 3.591859063236761518, 24.95696800326375353, 11.09922568453594849 ) ) ;
#83509=CARTESIAN_POINT ( 'NONE',  ( -0.8801773607111008646, 48.27201867748816966, 2.915334737309923430 ) ) ;
#83511=CARTESIAN_POINT ( 'NONE',  ( 18.61655166652077753, 54.87718327197430312, 6.499999999999981348 ) ) ;
#83512=CARTESIAN_POINT ( 'NONE',  ( 6.565887622018943937, 50.16530133659708213, 12.81628187352647430 ) ) ;
#83514=CARTESIAN_POINT ( 'NONE',  ( 15.44008868035555260, 54.73035201082150536, 9.422509992056143702 ) ) ;
#83515=CARTESIAN_POINT ( 'NONE',  ( 3.591859063236761518, 34.95696800326375353, 11.09922568453594849 ) ) ;
#83516=CARTESIAN_POINT ( 'NONE',  ( 18.52753015748617571, 8.092264484334117824, 4.923371831947298993 ) ) ;
#83517=CARTESIAN_POINT ( 'NONE',  ( 19.42250999205614193, 50.14701867748817676, 5.440088680355555262 ) ) ;
#83518=CARTESIAN_POINT ( 'NONE',  ( 17.08211943468705130, 43.47041550158063927, 12.26659068614894998 ) ) ;
#83521=CARTESIAN_POINT ( 'NONE',  ( 1.472469842513823179, 11.42559781766745175, 4.923371831947296329 ) ) ;
#83522=CARTESIAN_POINT ( 'NONE',  ( 17.20831665107776587, 7.883931151000784787, 7.208316651077764980 ) ) ;
#83524=CARTESIAN_POINT ( 'NONE',  ( 10.00000000000000000, 45.55374883491397497, -14.16423886937410082 ) ) ;
#83526=CARTESIAN_POINT ( 'NONE',  ( 4.559911319644449179, 3.897018677488170990, 9.422509992056141925 ) ) ;
#83529=AXIS2_PLACEMENT_3D ( 'NONE', #14717, #46663, #90686 ) ;
#83530=CARTESIAN_POINT ( 'NONE',  ( 2.035157376598824452, 13.68868534415483751, 7.964842623401179544 ) ) ;
#83531=CARTESIAN_POINT ( 'NONE',  ( -0.3689425029237881626, 57.42874883491397497, 10.36894250292379027 ) ) ;
#83532=CARTESIAN_POINT ( 'NONE',  ( 19.84674366389459266, 48.71726448433413026, -2.638427012816827677 ) ) ;
#83533=CARTESIAN_POINT ( 'NONE',  ( 21.09922568453594849, 41.20696800326375353, 6.408140936763242479 ) ) ;
#83534=CYLINDRICAL_SURFACE ( 'NONE', #87451, 7.000000000000006217 ) ;
#83536=CARTESIAN_POINT ( 'NONE',  ( 6.204703633549690345, 7.845415501580634832, 14.16423886937410082 ) ) ;
#83537=CARTESIAN_POINT ( 'NONE',  ( -0.8801773607110991993, 17.85535201082150536, -2.915334737309923874 ) ) ;
#83538=CARTESIAN_POINT ( 'NONE',  ( 10.00000000000000000, 1.813685344154838175, -10.88017736071110342 ) ) ;
#83539=CARTESIAN_POINT ( 'NONE',  ( 1.472469842513823179, 40.59226448433411605, -4.923371831947296329 ) ) ;
#83541=CARTESIAN_POINT ( 'NONE',  ( 10.00000000000000000, 24.75893115100078745, -9.846743663894594434 ) ) ;
#83542=DIRECTION ( 'NONE',  ( 0.000000000000000000, 0.000000000000000000, 1.000000000000000000 ) ) ;
#83547=EDGE_CURVE ( 'NONE', #87897, #91043, #65204, .T. ) ;
#83549=CARTESIAN_POINT ( 'NONE',  ( 12.63842701281683034, 57.46726448433411605, 9.846743663894596210 ) ) ;
#83550=CARTESIAN_POINT ( 'NONE',  ( 12.91533473730992121, 39.52201867748817676, 10.88017736071110164 ) ) ;
#83551=CARTESIAN_POINT ( 'NONE',  ( 4.559911319644449179, 37.23035201082150536, -9.422509992056141925 ) ) ;
#83553=CARTESIAN_POINT ( 'NONE',  ( 21.09922568453594849, 36.20696800326375353, 6.408140936763242479 ) ) ;
#83554=CARTESIAN_POINT ( 'NONE',  ( 20.36894250292379382, 3.678748834913967869, 10.36894250292379205 ) ) ;
#83557=CARTESIAN_POINT ( 'NONE',  ( 19.38216949554541202, 45.99863466993041072, 9.382169495545424454 ) ) ;
#83558=EDGE_CURVE ( 'NONE', #22423, #91046, #79580, .T. ) ;
#83560=CARTESIAN_POINT ( 'NONE',  ( 5.076628168052703671, 41.84226448433411605, 8.527530157486179263 ) ) ;
#83561=CARTESIAN_POINT ( 'NONE',  ( 4.559911319644449179, 8.897018677488173211, 9.422509992056141925 ) ) ;
#83562=VERTEX_POINT ( 'NONE', #19239 ) ;
#83565=CARTESIAN_POINT ( 'NONE',  ( 10.00000000000000000, 21.81368534415484106, -10.88017736071110342 ) ) ;
#83566=ORIENTED_EDGE ( 'NONE', *, *, #60962, .F. ) ;
#83567=CARTESIAN_POINT ( 'NONE',  ( 2.035157376598824452, 58.68868534415482685, 7.964842623401179544 ) ) ;
#83568=CARTESIAN_POINT ( 'NONE',  ( 20.88017736071110875, 55.77201867748816966, -2.915334737309920765 ) ) ;
#83569=CARTESIAN_POINT ( 'NONE',  ( 20.88017736071110875, 65.77201867748817676, -2.915334737309920765 ) ) ;
#83571=CARTESIAN_POINT ( 'NONE',  ( 7.084665262690076126, 57.02201867748817676, -10.88017736071110164 ) ) ;
#83575=CARTESIAN_POINT ( 'NONE',  ( 19.84674366389459621, 48.50893115100078745, 7.409399052514197653E-17 ) ) ;
#83577=CARTESIAN_POINT ( 'NONE',  ( 19.80832241502127644, 19.75868815902069642, 6.499999999999986677 ) ) ;
#83579=CARTESIAN_POINT ( 'NONE',  ( -2.266590686148945544, 1.387082168247301128, -7.082119434687050408 ) ) ;
#83580=ORIENTED_EDGE ( 'NONE', *, *, #11165, .F. ) ;
#83582=CARTESIAN_POINT ( 'NONE',  ( 18.72515096720583827, 30.05509018479937566, 6.499999999999810818 ) ) ;
#83583=CARTESIAN_POINT ( 'NONE',  ( 7.084665262690076126, 2.022018677488171434, -10.88017736071110164 ) ) ;
#83584=CARTESIAN_POINT ( 'NONE',  ( 0.1532563361054100626, 65.80059781766745175, -2.638427012816831230 ) ) ;
#83585=CARTESIAN_POINT ( 'NONE',  ( 21.09922568453595559, 47.04030133659708923, -6.408140936763230044 ) ) ;
#83588=CARTESIAN_POINT ( 'NONE',  ( 18.52753015748618282, 48.92559781766745886, -4.923371831947291888 ) ) ;
#83589=CARTESIAN_POINT ( 'NONE',  ( 14.92337183194729988, 4.342264484334117824, -8.527530157486177487 ) ) ;
#83590=CARTESIAN_POINT ( 'NONE',  ( 3.591859063236763294, 13.29030133659708746, -11.09922568453595026 ) ) ;
#83592=CARTESIAN_POINT ( 'NONE',  ( 17.20831665107776587, 22.88393115100078745, 7.208316651077764980 ) ) ;
#83594=CARTESIAN_POINT ( 'NONE',  ( 22.81628187352648496, 1.831968003263753753, -3.434112377981050290 ) ) ;
#83599=B_SPLINE_CURVE_WITH_KNOTS ( 'NONE', 3,
 ( #42617, #36094, #73592, #51101 ),
 .UNSPECIFIED., .F., .F.,
 ( 4, 4 ),
 ( 5.284504157781969479E-17, 0.002562518741975523297 ),
 .UNSPECIFIED. ) ;
#83601=CARTESIAN_POINT ( 'NONE',  ( 17.96484262340118221, 26.18868534415483396, -7.964842623401177768 ) ) ;
#83602=CARTESIAN_POINT ( 'NONE',  ( 24.16423886937410614, 14.30374883491396787, 8.672049930838204340E-16 ) ) ;
#83603=CARTESIAN_POINT ( 'NONE',  ( 10.00000000000000000, 24.75893115100078745, -9.846743663894594434 ) ) ;
#83604=CARTESIAN_POINT ( 'NONE',  ( 1.472469842513823179, 0.5922644843341181575, -4.923371831947296329 ) ) ;
#83605=CARTESIAN_POINT ( 'NONE',  ( -2.816281873526473856, 34.12363466993042493, 9.499525473075851096E-16 ) ) ;
#83607=CARTESIAN_POINT ( 'NONE',  ( -0.8801773607111009756, 13.06368534415483929, 1.068504757029289695E-15 ) ) ;
#83609=CARTESIAN_POINT ( 'NONE',  ( 21.09922568453595559, 12.04030133659708746, -6.408140936763230044 ) ) ;
#83610=CARTESIAN_POINT ( 'NONE',  ( 22.81628187352647785, 6.415301336597088344, 3.434112377981063169 ) ) ;
#83611=CARTESIAN_POINT ( 'NONE',  ( 17.20831665107776587, 24.13393115100078035, -7.208316651077762316 ) ) ;
#83613=CARTESIAN_POINT ( 'NONE',  ( -1.099225684535947600, 29.54030133659708923, 6.408140936763237150 ) ) ;
#83615=CARTESIAN_POINT ( 'NONE',  ( 0.5774900079438607392, 43.48035201082151247, 5.440088680355550821 ) ) ;
#83619=CARTESIAN_POINT ( 'NONE',  ( 10.00000000000000178, 34.31368534415484106, 10.88017736071110342 ) ) ;
#83620=CARTESIAN_POINT ( 'NONE',  ( 20.88017736071110519, 45.56368534415484106, 2.639326808657452039E-16 ) ) ;
#83621=CARTESIAN_POINT ( 'NONE',  ( 10.00000000000000000, 64.75893115100078035, -9.846743663894594434 ) ) ;
#83622=CARTESIAN_POINT ( 'NONE',  ( 17.96484262340118221, 66.18868534415483396, -7.964842623401177768 ) ) ;
#83623=COLOUR_RGB ( '', 0.08235294, 0.09019608, 0.10196078) ;
#83624=CARTESIAN_POINT ( 'NONE',  ( 5.076628168052703671, 46.84226448433412315, 8.527530157486179263 ) ) ;
#83625=CARTESIAN_POINT ( 'NONE',  ( -0.8801773607111008646, 8.272018677488171434, 2.915334737309923430 ) ) ;
#83627=CARTESIAN_POINT ( 'NONE',  ( 22.81628187352647785, 6.623634669930420493, 6.195893100308588602E-16 ) ) ;
#83628=ORIENTED_EDGE ( 'NONE', *, *, #64347, .F. ) ;
#83629=CARTESIAN_POINT ( 'NONE',  ( 7.084665262690076126, 37.02201867748817676, -10.88017736071110164 ) ) ;
#83631=CARTESIAN_POINT ( 'NONE',  ( -2.816281873526473856, -0.6680319967362464695, 3.434112377981055619 ) ) ;
#83633=CARTESIAN_POINT ( 'NONE',  ( 4.559911319644449179, 27.23035201082150536, -9.422509992056141925 ) ) ;
#83634=CARTESIAN_POINT ( 'NONE',  ( -4.164238869374099927, 37.01208216824731068, 3.795296366450308767 ) ) ;
#83635=CARTESIAN_POINT ( 'NONE',  ( 10.00000000000000178, 32.25893115100078745, 9.846743663894594434 ) ) ;
#83636=CARTESIAN_POINT ( 'NONE',  ( 17.96484262340118221, 51.18868534415483396, -7.964842623401177768 ) ) ;
#83638=CARTESIAN_POINT ( 'NONE',  ( 24.16423886937410614, 9.512082168247301794, -3.795296366450302550 ) ) ;
#83640=( NAMED_UNIT ( * ) PLANE_ANGLE_UNIT ( ) SI_UNIT ( $, .RADIAN. ) );
#83641=CARTESIAN_POINT ( 'NONE',  ( 0.1532563361054082862, 56.21726448433411605, 2.638427012816831674 ) ) ;
#83642=ORIENTED_EDGE ( 'NONE', *, *, #17668, .T. ) ;
#83644=CARTESIAN_POINT ( 'NONE',  ( 6.204703633549690345, 37.84541550158063927, 14.16423886937410082 ) ) ;
#83645=CARTESIAN_POINT ( 'NONE',  ( 6.204703633549690345, 22.84541550158062861, 14.16423886937410082 ) ) ;
#83646=CARTESIAN_POINT ( 'NONE',  ( 7.084665262690076126, 69.10535201082151957, 10.88017736071109987 ) ) ;
#83647=CARTESIAN_POINT ( 'NONE',  ( -0.8801773607110991993, 2.855352010821504471, -2.915334737309923874 ) ) ;
#83648=CARTESIAN_POINT ( 'NONE',  ( 5.076628168052704559, 50.17559781766745886, -8.527530157486179263 ) ) ;
#83650=CARTESIAN_POINT ( 'NONE',  ( 0.5774900079438607392, 43.48035201082151247, 5.440088680355550821 ) ) ;
#83651=CARTESIAN_POINT ( 'NONE',  ( 16.40814093676323893, 20.79030133659708923, 11.09922568453595026 ) ) ;
#83652=CARTESIAN_POINT ( 'NONE',  ( 24.16423886937410614, 14.30374883491396787, 8.672049930838204340E-16 ) ) ;
#83653=CARTESIAN_POINT ( 'NONE',  ( 10.00000000000000178, 14.31368534415483929, 10.88017736071110342 ) ) ;
#83654=CARTESIAN_POINT ( 'NONE',  ( -0.8801773607111009756, 33.06368534415484106, 1.068504757029289695E-15 ) ) ;
#83656=CARTESIAN_POINT ( 'NONE',  ( -0.8801773607111008646, 58.27201867748816966, 2.915334737309923430 ) ) ;
#83658=ORIENTED_EDGE ( 'NONE', *, *, #90304, .T. ) ;
#83664=CARTESIAN_POINT ( 'NONE',  ( 24.16423886937409904, 64.09541550158064638, 3.795296366450317205 ) ) ;
#83665=CARTESIAN_POINT ( 'NONE',  ( 22.26659068614895176, 59.72041550158063927, -7.082119434687042414 ) ) ;
#83666=CARTESIAN_POINT ( 'NONE',  ( 1.472469842513823179, 26.42559781766745175, 4.923371831947296329 ) ) ;
#83667=CARTESIAN_POINT ( 'NONE',  ( 0.1532563361054082862, 56.21726448433411605, 2.638427012816831674 ) ) ;
#83669=CARTESIAN_POINT ( 'NONE',  ( 19.72487221294571569, 49.78217586085237656, 6.499999999999993783 ) ) ;
#83670=CARTESIAN_POINT ( 'NONE',  ( 12.63842701281683922, 9.550597817667449974, -9.846743663894590881 ) ) ;
#83675=CARTESIAN_POINT ( 'NONE',  ( 10.00000000000000000, 30.55374883491397142, -14.16423886937410082 ) ) ;
#83676=CARTESIAN_POINT ( 'NONE',  ( 13.79529636645031943, 40.34541550158063217, -14.16423886937409904 ) ) ;
#83678=CARTESIAN_POINT ( 'NONE',  ( -2.816281873526473856, 54.12363466993041783, 9.499525473075851096E-16 ) ) ;
#83679=CARTESIAN_POINT ( 'NONE',  ( 0.5774900079438590739, 27.64701867748817676, -5.440088680355550821 ) ) ;
#83680=CARTESIAN_POINT ( 'NONE',  ( 7.361572987183169658, 49.96726448433410894, -9.846743663894592657 ) ) ;
#83681=CARTESIAN_POINT ( 'NONE',  ( 17.96484262340118221, 24.93868534415484461, 7.964842623401181321 ) ) ;
#83682=CARTESIAN_POINT ( 'NONE',  ( 21.09922568453594849, 61.20696800326376064, 6.408140936763242479 ) ) ;
#83684=CARTESIAN_POINT ( 'NONE',  ( 18.52753015748617571, 58.09226448433411605, 4.923371831947298993 ) ) ;
#83685=CARTESIAN_POINT ( 'NONE',  ( 17.20831665107776587, 49.13393115100078745, -7.208316651077762316 ) ) ;
#83687=ORIENTED_EDGE ( 'NONE', *, *, #48244, .F. ) ;
#83689=VECTOR ( 'NONE', #33684, 1000.000000000000000 ) ;
#83690=CARTESIAN_POINT ( 'NONE',  ( 17.20831665107776587, 2.883931151000785231, 7.208316651077764980 ) ) ;
#83691=EDGE_LOOP ( 'NONE', ( #26081, #820, #96116, #16533, #58908, #28490 ) ) ;
#83692=CARTESIAN_POINT ( 'NONE',  ( -0.1298530154764001854, 80.39370036920264795, 9.500000000000000000 ) ) ;
#83693=CARTESIAN_POINT ( 'NONE',  ( 0.1532563361054082862, 36.21726448433410894, 2.638427012816831674 ) ) ;
#83695=CARTESIAN_POINT ( 'NONE',  ( 10.00000000000000000, 32.87363466993042493, -12.81628187352647608 ) ) ;
#83698=EDGE_CURVE ( 'NONE', #51739, #94197, #796, .T. ) ;
#83702=CARTESIAN_POINT ( 'NONE',  ( 5.076628168052703671, 41.84226448433411605, 8.527530157486179263 ) ) ;
#83703=CARTESIAN_POINT ( 'NONE',  ( -4.164238869374099039, 31.80374883491396432, 8.674139862899312516E-16 ) ) ;
#83704=CARTESIAN_POINT ( 'NONE',  ( 0.1532563361054082862, 66.21726448433413736, 2.638427012816831674 ) ) ;
#83706=CARTESIAN_POINT ( 'NONE',  ( 14.92337183194729633, 7.675597817667451750, 8.527530157486181039 ) ) ;
#83707=CARTESIAN_POINT ( 'NONE',  ( 6.204703633549690345, 0.7620821682473009062, -14.16423886937410259 ) ) ;
#83708=CARTESIAN_POINT ( 'NONE',  ( 5.076628168052704559, 45.17559781766745175, -8.527530157486179263 ) ) ;
#83709=CARTESIAN_POINT ( 'NONE',  ( 20.88017736071110519, 55.56368534415484817, 2.639326808657452039E-16 ) ) ;
#83710=CARTESIAN_POINT ( 'NONE',  ( 19.84674366389459266, 43.71726448433410894, -2.638427012816827677 ) ) ;
#83712=CARTESIAN_POINT ( 'NONE',  ( -0.8801773607111008646, 48.27201867748816966, 2.915334737309923430 ) ) ;
#83714=CARTESIAN_POINT ( 'NONE',  ( 0.9408516040111469803, 22.46693863883976050, -6.499999999999953815 ) ) ;
#83715=CARTESIAN_POINT ( 'NONE',  ( 19.42250999205614193, 35.14701867748816966, 5.440088680355555262 ) ) ;
#83716=CARTESIAN_POINT ( 'NONE',  ( -2.816281873526471635, 3.915301336597087456, -3.434112377981056508 ) ) ;
#83717=CARTESIAN_POINT ( 'NONE',  ( -0.8801773607111008646, 63.27201867748817676, 2.915334737309923430 ) ) ;
#83719=CARTESIAN_POINT ( 'NONE',  ( 19.72487221294570858, 4.782175860852374782, 6.500000000000002665 ) ) ;
#83721=CARTESIAN_POINT ( 'NONE',  ( 20.88017736071110875, 45.77201867748816966, -2.915334737309920765 ) ) ;
#83722=CARTESIAN_POINT ( 'NONE',  ( 20.00000000000001066, 95.39111596594167963, -4.637569772578755689 ) ) ;
#83723=CARTESIAN_POINT ( 'NONE',  ( 10.00000000000000178, 12.25893115100078568, 9.846743663894594434 ) ) ;
#83724=CARTESIAN_POINT ( 'NONE',  ( 19.84674366389459621, 33.50893115100078745, 7.409399052514197653E-17 ) ) ;
#83725=CARTESIAN_POINT ( 'NONE',  ( 20.15039907845753220, 57.62777174578613426, -6.262539305110077947 ) ) ;
#83726=( BOUNDED_CURVE ( )  B_SPLINE_CURVE ( 2, ( #71514, #63972, #4490, #86988, #87479, #18992, #34462, #78995, #10501 ),
 .UNSPECIFIED., .F., .T. ) 
 B_SPLINE_CURVE_WITH_KNOTS ( ( 3, 2, 2, 2, 3 ),
 ( 0.7615695083688026612, 0.7619047619047618625, 0.7678571428571429047, 0.7738095238095238360, 0.7741447773454829262 ),
 .UNSPECIFIED. ) 
 CURVE ( )  GEOMETRIC_REPRESENTATION_ITEM ( )  RATIONAL_B_SPLINE_CURVE ( ( 0.9963778908391753841, 0.9980808541467917072, 1.000000000000000000, 0.9659258262890683122, 1.000000000000000000, 0.9659258262890683122, 1.000000000000000000, 0.9980808541467922623, 0.9963778908391764944 ) ) 
 REPRESENTATION_ITEM ( '' )  );
#83728=CARTESIAN_POINT ( 'NONE',  ( 13.43411237798105340, 0.5819680032637533085, 12.81628187352647963 ) ) ;
#83729=CARTESIAN_POINT ( 'NONE',  ( 12.91533473730992121, 4.522018677488170546, 10.88017736071110164 ) ) ;
#83732=CARTESIAN_POINT ( 'NONE',  ( 22.26659068614895176, 19.72041550158063572, -7.082119434687042414 ) ) ;
#83733=CARTESIAN_POINT ( 'NONE',  ( 10.00000000000000178, 53.05374883491396787, 14.16423886937410082 ) ) ;
#83734=CARTESIAN_POINT ( 'NONE',  ( 18.52753015748617571, 23.09226448433411960, 4.923371831947298993 ) ) ;
#83735=( NAMED_UNIT ( * ) PLANE_ANGLE_UNIT ( ) SI_UNIT ( $, .RADIAN. ) );
#83737=CARTESIAN_POINT ( 'NONE',  ( 0.1532563361054083140, 26.00893115100078745, 1.131784320476157264E-15 ) ) ;
#83738=CARTESIAN_POINT ( 'NONE',  ( 10.00000000000000000, 31.81368534415483751, -10.88017736071110342 ) ) ;
#83739=CARTESIAN_POINT ( 'NONE',  ( 10.00000000000000000, 49.75893115100078745, -9.846743663894594434 ) ) ;
#83740=CARTESIAN_POINT ( 'NONE',  ( 20.36894250292379382, 13.67874883491396965, 10.36894250292379205 ) ) ;
#83742=CARTESIAN_POINT ( 'NONE',  ( 2.791683348922240793, 11.63393115100078568, 7.208316651077764092 ) ) ;
#83743=CARTESIAN_POINT ( 'NONE',  ( 0.6178305044545838731, 39.74863466993041072, 9.382169495545420901 ) ) ;
#83744=B_SPLINE_CURVE_WITH_KNOTS ( 'NONE', 3,
 ( #98251, #29709, #83714, #60217 ),
 .UNSPECIFIED., .F., .F.,
 ( 4, 4 ),
 ( 0.000000000000000000, 0.001036303429213395648 ),
 .UNSPECIFIED. ) ;
#83745=CARTESIAN_POINT ( 'NONE',  ( 1.472469842513823179, 45.59226448433412315, -4.923371831947296329 ) ) ;
#83746=ORIENTED_EDGE ( 'NONE', *, *, #76871, .F. ) ;
#83747=CARTESIAN_POINT ( 'NONE',  ( 7.361572987183170547, 27.05059781766745175, 9.846743663894590881 ) ) ;
#83749=LINE ( 'NONE', #44256, #1193 ) ;
#83750=CARTESIAN_POINT ( 'NONE',  ( 22.26659068614894466, 58.88708216824729647, 7.082119434687054849 ) ) ;
#83751=CARTESIAN_POINT ( 'NONE',  ( -0.8801773607111008646, 43.27201867748817676, 2.915334737309923430 ) ) ;
#83752=CARTESIAN_POINT ( 'NONE',  ( -0.1503990784575247319, 32.22266099184917465, -6.262539305110083276 ) ) ;
#83754=CARTESIAN_POINT ( 'NONE',  ( 19.84674366389459621, 33.50893115100078745, 7.409399052514197653E-17 ) ) ;
#83755=CARTESIAN_POINT ( 'NONE',  ( 0.1532563361054100626, 40.80059781766745886, -2.638427012816831230 ) ) ;
#83757=CARTESIAN_POINT ( 'NONE',  ( 7.361572987183170547, 47.05059781766745175, 9.846743663894590881 ) ) ;
#83759=CARTESIAN_POINT ( 'NONE',  ( 12.91533473730992121, 54.52201867748816255, 10.88017736071110164 ) ) ;
#83763=CARTESIAN_POINT ( 'NONE',  ( 16.40814093676324603, 57.45696800326375353, -11.09922568453594671 ) ) ;
#83765=CARTESIAN_POINT ( 'NONE',  ( 19.84674366389459621, 13.50893115100078568, 7.409399052514197653E-17 ) ) ;
#83766=CARTESIAN_POINT ( 'NONE',  ( 21.09922568453594849, 56.20696800326375353, 6.408140936763242479 ) ) ;
#83767=CARTESIAN_POINT ( 'NONE',  ( 19.42250999205614548, 5.980352010821504471, -5.440088680355545492 ) ) ;
#83768=CARTESIAN_POINT ( 'NONE',  ( 17.20831665107776587, 47.88393115100078745, 7.208316651077764980 ) ) ;
#83769=CARTESIAN_POINT ( 'NONE',  ( 20.00000000000000711, 85.01043265490480394, 4.826711383682784628 ) ) ;
#83770=CARTESIAN_POINT ( 'NONE',  ( 22.26659068614894466, 28.88708216824730357, 7.082119434687054849 ) ) ;
#83771=CARTESIAN_POINT ( 'NONE',  ( 2.917880565312950480, 55.97041550158063217, -12.26659068614894821 ) ) ;
#83772=CARTESIAN_POINT ( 'NONE',  ( 0.1532563361054083140, 61.00893115100078745, 1.131784320476157264E-15 ) ) ;
#83773=CARTESIAN_POINT ( 'NONE',  ( 10.00000000000000000, 51.81368534415484106, -10.88017736071110342 ) ) ;
#83774=CIRCLE ( 'NONE', #45426, 1.000000000000000888 ) ;
#83775=CARTESIAN_POINT ( 'NONE',  ( 10.00000000000000000, 66.81368534415484817, -10.88017736071110342 ) ) ;
#83778=CARTESIAN_POINT ( 'NONE',  ( 22.81628187352648496, 56.83196800326374643, -3.434112377981050290 ) ) ;
#83779=ORIENTED_EDGE ( 'NONE', *, *, #3166, .F. ) ;
#83780=CARTESIAN_POINT ( 'NONE',  ( 12.63842701281683034, 12.46726448433411782, 9.846743663894596210 ) ) ;
#83782=CARTESIAN_POINT ( 'NONE',  ( 13.79529636645030344, 18.26208216824730002, 14.16423886937410614 ) ) ;
#83783=CARTESIAN_POINT ( 'NONE',  ( 17.20831665107776587, 17.88393115100078745, 7.208316651077764980 ) ) ;
#83784=CARTESIAN_POINT ( 'NONE',  ( 10.00000000000000178, 29.31368534415483751, 10.88017736071110342 ) ) ;
#83787=CARTESIAN_POINT ( 'NONE',  ( 17.96484262340118221, 26.18868534415483396, -7.964842623401177768 ) ) ;
#83788=EDGE_CURVE ( 'NONE', #87349, #88123, #27620, .T. ) ;
#83789=COLOUR_RGB ( '', 0.66274510, 0.83137255, 0.94901961) ;
#83791=EDGE_CURVE ( 'NONE', #54718, #88041, #37220, .T. ) ;
#83793=CARTESIAN_POINT ( 'NONE',  ( 0.5774900079438607392, 38.48035201082150536, 5.440088680355550821 ) ) ;
#83796=EDGE_LOOP ( 'NONE', ( #43495, #2996, #25268, #72936 ) ) ;
#83797=CARTESIAN_POINT ( 'NONE',  ( 13.43411237798106583, 17.66530133659708923, -12.81628187352647252 ) ) ;
#83799=CARTESIAN_POINT ( 'NONE',  ( 7.361572987183169658, 14.96726448433411960, -9.846743663894592657 ) ) ;
#83801=CARTESIAN_POINT ( 'NONE',  ( 7.361572987183170547, 12.05059781766744997, 9.846743663894590881 ) ) ;
#83802=CARTESIAN_POINT ( 'NONE',  ( 0.5774900079438590739, 32.64701867748816966, -5.440088680355550821 ) ) ;
#83806=CARTESIAN_POINT ( 'NONE',  ( -0.8801773607110991993, 62.85535201082150536, -2.915334737309923874 ) ) ;
#83807=CARTESIAN_POINT ( 'NONE',  ( -0.1503990784575247319, 22.22266099184918886, -6.262539305110083276 ) ) ;
#83808=CARTESIAN_POINT ( 'NONE',  ( 21.09922568453595559, 57.04030133659708923, -6.408140936763230044 ) ) ;
#83809=CARTESIAN_POINT ( 'NONE',  ( 2.035157376598822676, 62.43868534415483396, -7.964842623401177768 ) ) ;
#83810=CARTESIAN_POINT ( 'NONE',  ( 10.00000000000000178, 0.3736346699304200492, 12.81628187352647608 ) ) ;
#83811=SURFACE_STYLE_USAGE ( .BOTH. , #90807 ) ;
#83812=CARTESIAN_POINT ( 'NONE',  ( 0.1532563361054082862, 26.21726448433411605, 2.638427012816831674 ) ) ;
#83813=CARTESIAN_POINT ( 'NONE',  ( 13.43411237798105340, 55.58196800326374643, 12.81628187352647963 ) ) ;
#83814=DIRECTION ( 'NONE',  ( 1.000000000000000000, 0.000000000000000000, 0.000000000000000000 ) ) ;
#83815=CARTESIAN_POINT ( 'NONE',  ( 17.20831665107776587, 4.133931151000785675, -7.208316651077762316 ) ) ;
#83816=CARTESIAN_POINT ( 'NONE',  ( -2.816281873526473856, 24.12363466993042138, 9.499525473075851096E-16 ) ) ;
#83817=CARTESIAN_POINT ( 'NONE',  ( -16.94000000000001194, 92.00000000000000000, -10.09898361729590199 ) ) ;
#83818=DIRECTION ( 'NONE',  ( -6.608470384673550777E-17, -1.000000000000000000, 0.000000000000000000 ) ) ;
#83819=CARTESIAN_POINT ( 'NONE',  ( -0.8801773607110991993, 32.85535201082151247, -2.915334737309923874 ) ) ;
#83820=CARTESIAN_POINT ( 'NONE',  ( -2.816281873526473856, -0.8763653300695799508, 9.499525473075851096E-16 ) ) ;
#83822=EDGE_CURVE ( 'NONE', #32106, #93746, #73874, .T. ) ;
#83823=CARTESIAN_POINT ( 'NONE',  ( 14.92337183194729633, 7.675597817667451750, 8.527530157486181039 ) ) ;
#83824=CARTESIAN_POINT ( 'NONE',  ( 13.43411237798105340, 10.58196800326375353, 12.81628187352647963 ) ) ;
#83826=CARTESIAN_POINT ( 'NONE',  ( 19.84674366389459621, 63.50893115100078745, 7.409399052514197653E-17 ) ) ;
#83827=VECTOR ( 'NONE', #43836, 1000.000000000000000 ) ;
#83828=CARTESIAN_POINT ( 'NONE',  ( 12.91533473730993009, 6.605352010821504471, -10.88017736071109987 ) ) ;
#83829=CARTESIAN_POINT ( 'NONE',  ( 14.92337183194729633, 42.67559781766745886, 8.527530157486181039 ) ) ;
#83831=( BOUNDED_CURVE ( )  B_SPLINE_CURVE ( 2, ( #33909, #12410, #72909, #64897, #88415, #20419, #49917, #80428, #50905 ),
 .UNSPECIFIED., .F., .F. ) 
 B_SPLINE_CURVE_WITH_KNOTS ( ( 3, 2, 2, 2, 3 ),
 ( 0.01057180293546599974, 0.01190476190476190410, 0.01785714285714285615, 0.02380952380952380820, 0.02514248277882003349 ),
 .UNSPECIFIED. ) 
 CURVE ( )  GEOMETRIC_REPRESENTATION_ITEM ( )  RATIONAL_B_SPLINE_CURVE ( ( 0.9881565478350764486, 0.9923695281211519781, 1.000000000000000000, 0.9659258262890683122, 1.000000000000000000, 0.9659258262890683122, 1.000000000000000000, 0.9923695281211502017, 0.9881565478350745613 ) ) 
 REPRESENTATION_ITEM ( '' )  );
#83833=CARTESIAN_POINT ( 'NONE',  ( 10.00000000000000178, 9.313685344154839285, 10.88017736071110342 ) ) ;
#83835=CARTESIAN_POINT ( 'NONE',  ( 15.44008868035555793, 31.39701867748817676, -9.422509992056140149 ) ) ;
#83836=CARTESIAN_POINT ( 'NONE',  ( -4.164238869374099039, 61.80374883491397497, 8.674139862899312516E-16 ) ) ;
#83838=CARTESIAN_POINT ( 'NONE',  ( 10.00000000000000178, 7.258931151000785675, 9.846743663894594434 ) ) ;
#83839=CARTESIAN_POINT ( 'NONE',  ( 17.20831665107776587, 19.13393115100078035, -7.208316651077762316 ) ) ;
#83840=CARTESIAN_POINT ( 'NONE',  ( 16.40814093676323893, 15.79030133659708746, 11.09922568453595026 ) ) ;
#83841=CARTESIAN_POINT ( 'NONE',  ( -46.94000000000001194, 103.2691844435154422, 6.361973263950303270 ) ) ;
#83843=CARTESIAN_POINT ( 'NONE',  ( 5.076628168052704559, 65.17559781766745175, -8.527530157486179263 ) ) ;
#83846=CARTESIAN_POINT ( 'NONE',  ( -4.164238869374099927, 7.012082168247302683, 3.795296366450308767 ) ) ;
#83847=CARTESIAN_POINT ( 'NONE',  ( 1.472469842513823179, 31.42559781766745530, 4.923371831947296329 ) ) ;
#83850=CARTESIAN_POINT ( 'NONE',  ( 22.26659068614895176, 59.72041550158063927, -7.082119434687042414 ) ) ;
#83851=CARTESIAN_POINT ( 'NONE',  ( 10.00000000000000000, 9.758931151000785675, -9.846743663894594434 ) ) ;
#83854=CARTESIAN_POINT ( 'NONE',  ( 12.91533473730993009, 36.60535201082151247, -10.88017736071109987 ) ) ;
#83855=CARTESIAN_POINT ( 'NONE',  ( 19.38216949554541202, 45.99863466993041072, 9.382169495545424454 ) ) ;
#83856=CARTESIAN_POINT ( 'NONE',  ( 15.44008868035555793, 16.39701867748817321, -9.422509992056140149 ) ) ;
#83857=CARTESIAN_POINT ( 'NONE',  ( 21.09922568453594849, 36.20696800326375353, 6.408140936763242479 ) ) ;
#83858=CARTESIAN_POINT ( 'NONE',  ( 5.076628168052704559, 65.17559781766745175, -8.527530157486179263 ) ) ;
#83859=CARTESIAN_POINT ( 'NONE',  ( 10.00000000000000000, 4.758931151000784787, -9.846743663894594434 ) ) ;
#83863=CARTESIAN_POINT ( 'NONE',  ( 13.79529636645030344, 38.26208216824729647, 14.16423886937410614 ) ) ;
#83864=CARTESIAN_POINT ( 'NONE',  ( 13.79529636645031943, 20.34541550158063572, -14.16423886937409904 ) ) ;
#83865=CARTESIAN_POINT ( 'NONE',  ( 15.44008868035555793, 11.39701867748817143, -9.422509992056140149 ) ) ;
#83866=CARTESIAN_POINT ( 'NONE',  ( 12.91533473730992121, 34.52201867748817676, 10.88017736071110164 ) ) ;
#83867=DIRECTION ( 'NONE',  ( -1.000000000000000000, -0.000000000000000000, -0.000000000000000000 ) ) ;
#83869=CARTESIAN_POINT ( 'NONE',  ( 12.91533473730993009, 66.60535201082150536, -10.88017736071109987 ) ) ;
#83870=CARTESIAN_POINT ( 'NONE',  ( 19.42250999205614548, 60.98035201082151247, -5.440088680355545492 ) ) ;
#83871=CARTESIAN_POINT ( 'NONE',  ( 21.09922568453595559, 32.04030133659708923, -6.408140936763230044 ) ) ;
#83874=CARTESIAN_POINT ( 'NONE',  ( 14.92337183194729988, 39.34226448433412315, -8.527530157486177487 ) ) ;
#83877=CARTESIAN_POINT ( 'NONE',  ( 7.084665262690076126, 19.10535201082150181, 10.88017736071109987 ) ) ;
#83878=CARTESIAN_POINT ( 'NONE',  ( 6.565887622018943937, 13.08196800326374998, -12.81628187352647608 ) ) ;
#83880=CARTESIAN_POINT ( 'NONE',  ( 10.00000000000000000, 14.75893115100078568, -9.846743663894594434 ) ) ;
#83881=CARTESIAN_POINT ( 'NONE',  ( -0.8801773607111008646, 3.272018677488171434, 2.915334737309923430 ) ) ;
#83882=CARTESIAN_POINT ( 'NONE',  ( 2.791683348922240793, 36.63393115100078035, 7.208316651077764092 ) ) ;
#83883=CARTESIAN_POINT ( 'NONE',  ( -2.816281873526471635, 58.91530133659707502, -3.434112377981056508 ) ) ;
#83884=CARTESIAN_POINT ( 'NONE',  ( 17.20831665107776587, 12.88393115100078390, 7.208316651077764980 ) ) ;
#83885=CARTESIAN_POINT ( 'NONE',  ( -0.3689425029237898834, 6.178748834913968757, -10.36894250292378850 ) ) ;
#83887=CARTESIAN_POINT ( 'NONE',  ( 2.035157376598822676, 27.43868534415483396, -7.964842623401177768 ) ) ;
#83888=CARTESIAN_POINT ( 'NONE',  ( 2.035157376598822676, 12.43868534415483751, -7.964842623401177768 ) ) ;
#83889=CARTESIAN_POINT ( 'NONE',  ( 10.00000000000000178, 48.05374883491396787, 14.16423886937410082 ) ) ;
#83890=CARTESIAN_POINT ( 'NONE',  ( 20.88017736071110164, 35.35535201082150536, 2.915334737309930979 ) ) ;
#83891=CARTESIAN_POINT ( 'NONE',  ( 15.44008868035555260, 19.73035201082150536, 9.422509992056143702 ) ) ;
#83893=CARTESIAN_POINT ( 'NONE',  ( 12.91533473730993009, 36.60535201082151247, -10.88017736071109987 ) ) ;
#83894=CARTESIAN_POINT ( 'NONE',  ( 16.40814093676323893, 50.79030133659708923, 11.09922568453595026 ) ) ;
#83895=CARTESIAN_POINT ( 'NONE',  ( 15.44008868035555260, 49.73035201082150536, 9.422509992056143702 ) ) ;
#83896=CARTESIAN_POINT ( 'NONE',  ( 10.00000000000000178, 54.31368534415484106, 10.88017736071110342 ) ) ;
#83899=CARTESIAN_POINT ( 'NONE',  ( 15.44008868035555793, 56.39701867748817676, -9.422509992056140149 ) ) ;
#83901=ADVANCED_FACE ( 'NONE', ( #52690 ), #30176, .T. ) ;
#83903=CARTESIAN_POINT ( 'NONE',  ( 13.79529636645031943, 50.34541550158064638, -14.16423886937409904 ) ) ;
#83904=CARTESIAN_POINT ( 'NONE',  ( 10.00000000000000178, 69.31368534415484817, 10.88017736071110342 ) ) ;
#83905=FILL_AREA_STYLE ('',( #90400 ) ) ;
#83907=CARTESIAN_POINT ( 'NONE',  ( 12.63842701281683034, 62.46726448433410894, 9.846743663894596210 ) ) ;
#83909=CARTESIAN_POINT ( 'NONE',  ( 1.472469842513823179, 36.42559781766745175, 4.923371831947296329 ) ) ;
#83911=CARTESIAN_POINT ( 'NONE',  ( 18.52753015748617571, 33.09226448433411605, 4.923371831947298993 ) ) ;
#83913=CARTESIAN_POINT ( 'NONE',  ( 17.96484262340118221, 31.18868534415483751, -7.964842623401177768 ) ) ;
#83914=CARTESIAN_POINT ( 'NONE',  ( 18.52753015748617571, 43.09226448433412315, 4.923371831947298993 ) ) ;
#83915=CARTESIAN_POINT ( 'NONE',  ( -0.8801773607111009756, 68.06368534415484817, 1.068504757029289695E-15 ) ) ;
#83916=CARTESIAN_POINT ( 'NONE',  ( 19.42250999205614193, 50.14701867748817676, 5.440088680355555262 ) ) ;
#83917=CARTESIAN_POINT ( 'NONE',  ( 20.88017736071110519, 5.563685344154837509, 2.639326808657452039E-16 ) ) ;
#83918=CARTESIAN_POINT ( 'NONE',  ( 20.36894250292379738, 54.92874883491396076, -10.36894250292379027 ) ) ;
#83920=CARTESIAN_POINT ( 'NONE',  ( -1.099225684535947600, 28.70696800326375353, -6.408140936763238038 ) ) ;
#83922=ORIENTED_EDGE ( 'NONE', *, *, #66971, .F. ) ;
#83923=CARTESIAN_POINT ( 'NONE',  ( -2.816281873526473856, 9.331968003263753531, 3.434112377981055619 ) ) ;
#83924=CARTESIAN_POINT ( 'NONE',  ( 0.5774900079438590739, 22.64701867748817321, -5.440088680355550821 ) ) ;
#83925=CARTESIAN_POINT ( 'NONE',  ( 4.559911319644449179, 53.89701867748817676, 9.422509992056141925 ) ) ;
#83927=EDGE_CURVE ( 'NONE', #94683, #31369, #91427, .T. ) ;
#83928=CARTESIAN_POINT ( 'NONE',  ( -0.8801773607111008646, 53.27201867748816966, 2.915334737309923430 ) ) ;
#83929=CARTESIAN_POINT ( 'NONE',  ( 5.076628168052704559, 55.17559781766745175, -8.527530157486179263 ) ) ;
#83930=CARTESIAN_POINT ( 'NONE',  ( 17.20831665107776587, 29.13393115100078390, -7.208316651077762316 ) ) ;
#83931=CARTESIAN_POINT ( 'NONE',  ( 0.1532563361054100626, 30.80059781766744820, -2.638427012816831230 ) ) ;
#83935=CARTESIAN_POINT ( 'NONE',  ( -2.816281873526473856, 34.33196800326376064, 3.434112377981055619 ) ) ;
#83937=CARTESIAN_POINT ( 'NONE',  ( 19.84674366389459621, 18.50893115100078745, 7.409399052514197653E-17 ) ) ;
#83940=CARTESIAN_POINT ( 'NONE',  ( 17.20831665107776587, 39.13393115100079456, -7.208316651077762316 ) ) ;
#83942=CARTESIAN_POINT ( 'NONE',  ( 22.81628187352648496, 61.83196800326376774, -3.434112377981050290 ) ) ;
#83944=CARTESIAN_POINT ( 'NONE',  ( 13.43411237798106583, 17.66530133659708923, -12.81628187352647252 ) ) ;
#83946=CARTESIAN_POINT ( 'NONE',  ( -0.8801773607111008646, 53.27201867748816966, 2.915334737309923430 ) ) ;
#83947=CARTESIAN_POINT ( 'NONE',  ( -4.164238869374098151, 31.59541550158063927, -3.795296366450310543 ) ) ;
#83949=CARTESIAN_POINT ( 'NONE',  ( 6.204703633549690345, 27.84541550158063217, 14.16423886937410082 ) ) ;
#83950=CARTESIAN_POINT ( 'NONE',  ( 2.917880565312948704, 57.63708216824731068, 12.26659068614894643 ) ) ;
#83951=CARTESIAN_POINT ( 'NONE',  ( 10.00000000000000178, 13.05374883491396787, 14.16423886937410082 ) ) ;
#83952=CARTESIAN_POINT ( 'NONE',  ( 24.16423886937410614, 29.30374883491396787, 8.672049930838204340E-16 ) ) ;
#83954=CARTESIAN_POINT ( 'NONE',  ( 4.559911319644449179, 48.89701867748817676, 9.422509992056141925 ) ) ;
#83956=CARTESIAN_POINT ( 'NONE',  ( 7.084665262690076126, 64.10535201082150536, 10.88017736071109987 ) ) ;
#83957=CARTESIAN_POINT ( 'NONE',  ( 1.472469842513823179, 45.59226448433412315, -4.923371831947296329 ) ) ;
#83958=CARTESIAN_POINT ( 'NONE',  ( 19.42250999205614548, 25.98035201082150891, -5.440088680355545492 ) ) ;
#83960=CARTESIAN_POINT ( 'NONE',  ( 5.076628168052704559, 60.17559781766745175, -8.527530157486179263 ) ) ;
#83962=CARTESIAN_POINT ( 'NONE',  ( 6.565887622018943937, 58.08196800326376064, -12.81628187352647608 ) ) ;
#83965=CARTESIAN_POINT ( 'NONE',  ( 17.20831665107776587, 44.13393115100078745, -7.208316651077762316 ) ) ;
#83966=CARTESIAN_POINT ( 'NONE',  ( 5.076628168052703671, 51.84226448433412315, 8.527530157486179263 ) ) ;
#83968=VECTOR ( 'NONE', #97875, 1000.000000000000000 ) ;
#83969=CARTESIAN_POINT ( 'NONE',  ( 24.16423886937410614, 34.51208216824731068, -3.795296366450302550 ) ) ;
#83971=CARTESIAN_POINT ( 'NONE',  ( 6.204703633549690345, 17.84541550158063217, 14.16423886937410082 ) ) ;
#83973=CARTESIAN_POINT ( 'NONE',  ( 12.91533473730993009, 66.60535201082150536, -10.88017736071109987 ) ) ;
#83975=CARTESIAN_POINT ( 'NONE',  ( 2.917880565312948704, 57.63708216824731068, 12.26659068614894643 ) ) ;
#83976=CARTESIAN_POINT ( 'NONE',  ( -2.816281873526471635, 13.91530133659708746, -3.434112377981056508 ) ) ;
#83978=CARTESIAN_POINT ( 'NONE',  ( 0.1532563361054082862, 1.217264484334117824, 2.638427012816831674 ) ) ;
#83981=CARTESIAN_POINT ( 'NONE',  ( -1.099225684535947600, 33.70696800326375353, -6.408140936763238038 ) ) ;
#83982=CARTESIAN_POINT ( 'NONE',  ( -0.8801773607110991993, 2.855352010821504471, -2.915334737309923874 ) ) ;
#83984=CARTESIAN_POINT ( 'NONE',  ( 4.559911319644449179, 13.89701867748817143, 9.422509992056141925 ) ) ;
#83985=CARTESIAN_POINT ( 'NONE',  ( 2.035157376598822676, 27.43868534415483396, -7.964842623401177768 ) ) ;
#83986=CARTESIAN_POINT ( 'NONE',  ( 10.00000000000000000, 59.75893115100078745, -9.846743663894594434 ) ) ;
#83987=CARTESIAN_POINT ( 'NONE',  ( 17.20831665107776587, 47.88393115100078745, 7.208316651077764980 ) ) ;
#83988=CARTESIAN_POINT ( 'NONE',  ( 6.565887622018943937, 48.08196800326375353, -12.81628187352647608 ) ) ;
#83989=CARTESIAN_POINT ( 'NONE',  ( 0.1532563361054083140, 1.008931151000784787, 1.131784320476157264E-15 ) ) ;
#83991=CARTESIAN_POINT ( 'NONE',  ( -0.8801773607111009756, 13.06368534415483929, 1.068504757029289695E-15 ) ) ;
#83993=CARTESIAN_POINT ( 'NONE',  ( 10.00000000000000178, 20.37363466993042138, 12.81628187352647608 ) ) ;
#83994=CARTESIAN_POINT ( 'NONE',  ( 19.80832241502127289, 39.75868815902069997, 6.499999999999984901 ) ) ;
#83996=CARTESIAN_POINT ( 'NONE',  ( 2.791683348922240793, 46.63393115100077324, 7.208316651077764092 ) ) ;
#83998=CARTESIAN_POINT ( 'NONE',  ( 2.035157376598824452, 53.68868534415484817, 7.964842623401179544 ) ) ;
#83999=CARTESIAN_POINT ( 'NONE',  ( -1.099225684535947600, 23.70696800326375708, -6.408140936763238038 ) ) ;
#84000=CARTESIAN_POINT ( 'NONE',  ( 0.5774900079438607392, 53.48035201082151247, 5.440088680355550821 ) ) ;
#84003=CARTESIAN_POINT ( 'NONE',  ( 10.00000000000000178, 55.37363466993042493, 12.81628187352647608 ) ) ;
#84004=ORIENTED_EDGE ( 'NONE', *, *, #49763, .F. ) ;
#84005=CARTESIAN_POINT ( 'NONE',  ( 18.52753015748617571, 58.09226448433411605, 4.923371831947298993 ) ) ;
#84006=CARTESIAN_POINT ( 'NONE',  ( -0.1503990784575328643, 70.00000000000000000, -6.262539305110068177 ) ) ;
#84007=CARTESIAN_POINT ( 'NONE',  ( 4.559911319644449179, 52.23035201082151247, -9.422509992056141925 ) ) ;
#84008=CARTESIAN_POINT ( 'NONE',  ( 19.38216949554541557, 47.24863466993041783, -9.382169495545420901 ) ) ;
#84009=CARTESIAN_POINT ( 'NONE',  ( -0.3689425029237898834, 11.17874883491396787, -10.36894250292378850 ) ) ;
#84010=CARTESIAN_POINT ( 'NONE',  ( 1.472469842513823179, 6.425597817667451750, 4.923371831947296329 ) ) ;
#84012=CARTESIAN_POINT ( 'NONE',  ( 5.076628168052703671, 11.84226448433411960, 8.527530157486179263 ) ) ;
#84013=CARTESIAN_POINT ( 'NONE',  ( 5.076628168052703671, 6.842264484334118713, 8.527530157486179263 ) ) ;
#84014=B_SPLINE_CURVE_WITH_KNOTS ( 'NONE', 3,
 ( #8563, #83577, #60067, #53555, #84072, #14095 ),
 .UNSPECIFIED., .F., .F.,
 ( 4, 2, 4 ),
 ( 0.000000000000000000, 0.0002565770811490952221, 0.0005131541622981904442 ),
 .UNSPECIFIED. ) ;
#84016=CARTESIAN_POINT ( 'NONE',  ( -4.164238869374099039, 41.80374883491397497, 8.674139862899312516E-16 ) ) ;
#84018=CARTESIAN_POINT ( 'NONE',  ( 1.046131998950050379, 55.73810908735726599, 6.499999999999992006 ) ) ;
#84019=CARTESIAN_POINT ( 'NONE',  ( 4.559911319644449179, 13.89701867748817143, 9.422509992056141925 ) ) ;
#84021=ORIENTED_EDGE ( 'NONE', *, *, #95734, .F. ) ;
#84022=CARTESIAN_POINT ( 'NONE',  ( 12.91533473730992121, 14.52201867748817143, 10.88017736071110164 ) ) ;
#84023=CARTESIAN_POINT ( 'NONE',  ( 17.96484262340118221, 4.938685344154837509, 7.964842623401181321 ) ) ;
#84024=CARTESIAN_POINT ( 'NONE',  ( 7.361572987183169658, 44.96726448433412315, -9.846743663894592657 ) ) ;
#84026=CARTESIAN_POINT ( 'NONE',  ( 0.6178305044545838731, 34.74863466993042493, 9.382169495545420901 ) ) ;
#84027=( NAMED_UNIT ( * ) SI_UNIT ( $, .STERADIAN. ) SOLID_ANGLE_UNIT ( ) );
#84029=CARTESIAN_POINT ( 'NONE',  ( 24.16423886937410614, 9.512082168247301794, -3.795296366450302550 ) ) ;
#84030=CARTESIAN_POINT ( 'NONE',  ( 17.96484262340118221, 21.18868534415483396, -7.964842623401177768 ) ) ;
#84031=CARTESIAN_POINT ( 'NONE',  ( 0.5774900079438590739, 2.647018677488171434, -5.440088680355550821 ) ) ;
#84032=CARTESIAN_POINT ( 'NONE',  ( 0.1532563361054100626, 35.80059781766745175, -2.638427012816831230 ) ) ;
#84034=CARTESIAN_POINT ( 'NONE',  ( 0.1532563361054082862, 21.21726448433412315, 2.638427012816831674 ) ) ;
#84040=CARTESIAN_POINT ( 'NONE',  ( 5.076628168052704559, 55.17559781766745175, -8.527530157486179263 ) ) ;
#84041=CARTESIAN_POINT ( 'NONE',  ( 0.5774900079438607392, 28.48035201082150891, 5.440088680355550821 ) ) ;
#84042=CARTESIAN_POINT ( 'NONE',  ( 15.44008868035555260, 39.73035201082150536, 9.422509992056143702 ) ) ;
#84043=PRESENTATION_STYLE_ASSIGNMENT (( #75052 ) ) ;
#84044=CARTESIAN_POINT ( 'NONE',  ( -1.099225684535947600, 24.54030133659708923, 6.408140936763237150 ) ) ;
#84045=AXIS2_PLACEMENT_3D ( 'NONE', #70204, #61695, #63171 ) ;
#84046=CARTESIAN_POINT ( 'NONE',  ( 17.08211943468705840, 15.13708216824730179, -12.26659068614894466 ) ) ;
#84048=VECTOR ( 'NONE', #98821, 1000.000000000000000 ) ;
#84050=CARTESIAN_POINT ( 'NONE',  ( 6.565887622018943937, 50.16530133659708213, 12.81628187352647430 ) ) ;
#84051=EDGE_LOOP ( 'NONE', ( #82181, #23855, #28678, #74068 ) ) ;
#84052=CARTESIAN_POINT ( 'NONE',  ( 19.84674366389459266, 38.30059781766745175, 2.638427012816836559 ) ) ;
#84053=CARTESIAN_POINT ( 'NONE',  ( 17.96484262340118221, 9.938685344154839285, 7.964842623401181321 ) ) ;
#84055=CARTESIAN_POINT ( 'NONE',  ( 4.559911319644449179, 22.23035201082150536, -9.422509992056141925 ) ) ;
#84056=VERTEX_POINT ( 'NONE', #48135 ) ;
#84057=CARTESIAN_POINT ( 'NONE',  ( 17.96484262340118221, 59.93868534415484106, 7.964842623401181321 ) ) ;
#84058=CARTESIAN_POINT ( 'NONE',  ( 19.42250999205614193, 60.14701867748817676, 5.440088680355555262 ) ) ;
#84059=CARTESIAN_POINT ( 'NONE',  ( 0.5774900079438607392, 58.48035201082151247, 5.440088680355550821 ) ) ;
#84061=CARTESIAN_POINT ( 'NONE',  ( 2.035157376598822676, 57.43868534415484106, -7.964842623401177768 ) ) ;
#84062=CARTESIAN_POINT ( 'NONE',  ( -0.2418659066527716062, 52.23410085661203794, -6.114288769123046308 ) ) ;
#84064=CIRCLE ( 'NONE', #56927, 0.5000000000000004441 ) ;
#84065=CARTESIAN_POINT ( 'NONE',  ( -46.94000000000001194, 101.2919103424992358, 7.700697297268528807 ) ) ;
#84070=CARTESIAN_POINT ( 'NONE',  ( 17.20831665107776587, 37.88393115100078745, 7.208316651077764980 ) ) ;
#84072=CARTESIAN_POINT ( 'NONE',  ( 20.10493008474206533, 19.71697413083879269, 6.336235997365759154 ) ) ;
#84073=CARTESIAN_POINT ( 'NONE',  ( 20.36894250292379382, 18.67874883491397142, 10.36894250292379205 ) ) ;
#84076=CARTESIAN_POINT ( 'NONE',  ( 12.91533473730992121, 64.52201867748817676, 10.88017736071110164 ) ) ;
#84077=CARTESIAN_POINT ( 'NONE',  ( 4.559911319644449179, 3.897018677488171434, 9.422509992056141925 ) ) ;
#84079=CARTESIAN_POINT ( 'NONE',  ( 0.6178305044545838731, 39.74863466993041072, 9.382169495545420901 ) ) ;
#84081=CARTESIAN_POINT ( 'NONE',  ( 19.72487221294571924, 62.80223176428831522, -6.499999999999984901 ) ) ;
#84082=CARTESIAN_POINT ( 'NONE',  ( 2.791683348922240793, 1.633931151000784565, 7.208316651077764092 ) ) ;
#84083=CARTESIAN_POINT ( 'NONE',  ( -2.816281873526471635, 33.91530133659708213, -3.434112377981056508 ) ) ;
#84084=CARTESIAN_POINT ( 'NONE',  ( 12.63842701281683034, 17.46726448433411250, 9.846743663894596210 ) ) ;
#84086=CARTESIAN_POINT ( 'NONE',  ( 5.076628168052703671, 16.84226448433411960, 8.527530157486179263 ) ) ;
#84087=CARTESIAN_POINT ( 'NONE',  ( 21.09922568453594849, 16.20696800326375353, 6.408140936763242479 ) ) ;
#84088=CARTESIAN_POINT ( 'NONE',  ( 19.89103541497709315, 40.66234555792571825, -6.479102184480824533 ) ) ;
#84090=CARTESIAN_POINT ( 'NONE',  ( 12.63842701281683922, 4.550597817667451750, -9.846743663894590881 ) ) ;
#84091=ORIENTED_EDGE ( 'NONE', *, *, #52539, .T. ) ;
#84093=CARTESIAN_POINT ( 'NONE',  ( 10.00000000000000000, 26.81368534415484106, -10.88017736071110342 ) ) ;
#84094=CARTESIAN_POINT ( 'NONE',  ( 13.79529636645030344, 18.26208216824730002, 14.16423886937410614 ) ) ;
#84095=CARTESIAN_POINT ( 'NONE',  ( 19.84674366389459621, 38.50893115100078745, 7.409399052514197653E-17 ) ) ;
#84097=CARTESIAN_POINT ( 'NONE',  ( 2.035157376598822676, 62.43868534415483396, -7.964842623401177768 ) ) ;
#84098=CARTESIAN_POINT ( 'NONE',  ( 19.38216949554541202, 45.99863466993041072, 9.382169495545424454 ) ) ;
#84100=CARTESIAN_POINT ( 'NONE',  ( 15.44008868035555260, 9.730352010821505360, 9.422509992056143702 ) ) ;
#84102=CARTESIAN_POINT ( 'NONE',  ( 3.591859063236763294, 8.290301336597087456, -11.09922568453595026 ) ) ;
#84103=CARTESIAN_POINT ( 'NONE',  ( -1.099225684535947600, 3.706968003263753531, -6.408140936763238038 ) ) ;
#84104=CARTESIAN_POINT ( 'NONE',  ( 19.84674366389459621, 33.50893115100078745, 7.409399052514197653E-17 ) ) ;
#84106=CARTESIAN_POINT ( 'NONE',  ( 10.00000000000000178, 35.37363466993042493, 12.81628187352647608 ) ) ;
#84108=CARTESIAN_POINT ( 'NONE',  ( 12.91533473730993009, 56.60535201082151247, -10.88017736071109987 ) ) ;
#84109=CARTESIAN_POINT ( 'NONE',  ( 0.9408516040111470913, 62.46693863883975695, -6.499999999999953815 ) ) ;
#84113=( BOUNDED_CURVE ( )  B_SPLINE_CURVE ( 2, ( #22593, #37593, #52577, #14608, #76068, #83081, #38575, #16068, #60071 ),
 .UNSPECIFIED., .F., .F. ) 
 B_SPLINE_CURVE_WITH_KNOTS ( ( 3, 2, 2, 2, 3 ),
 ( 0.8687123655116599785, 0.8690476190476190688, 0.8750000000000000000, 0.8809523809523809312, 0.8812876344883400215 ),
 .UNSPECIFIED. ) 
 CURVE ( )  GEOMETRIC_REPRESENTATION_ITEM ( )  RATIONAL_B_SPLINE_CURVE ( ( 0.9963778908391764944, 0.9980808541467923733, 1.000000000000000000, 0.9659258262890682012, 1.000000000000000000, 0.9659258262890682012, 1.000000000000000000, 0.9980808541467922623, 0.9963778908391764944 ) ) 
 REPRESENTATION_ITEM ( '' )  );
#84114=CARTESIAN_POINT ( 'NONE',  ( 15.44008868035555793, 36.39701867748816966, -9.422509992056140149 ) ) ;
#84115=CARTESIAN_POINT ( 'NONE',  ( 15.44008868035555793, 46.39701867748817676, -9.422509992056140149 ) ) ;
#84116=DIRECTION ( 'NONE',  ( -0.000000000000000000, -0.000000000000000000, -1.000000000000000000 ) ) ;
#84117=CARTESIAN_POINT ( 'NONE',  ( -0.8801773607111008646, 68.27201867748817676, 2.915334737309923430 ) ) ;
#84118=EDGE_CURVE ( 'NONE', #3611, #89098, #81854, .T. ) ;
#84121=( BOUNDED_SURFACE ( )  B_SPLINE_SURFACE ( 1, 2, ( 
 ( #88391, #19403, #3918, #65379, #89860, #81861, #5879, #66365, #74353, #27388, #57879, #36375, #96902, #19890, #41928, #89373, #66870, #28854, #14377, #60349, #83354, #6865, #23360, #76826, #21879, #67364, #14878, #44360, #82356, #7371, #90842, #83846, #37870, #52359, #45853, #31321, #68366, #45347, #82860, #75851, #61821, #13877, #44845, #75351, #37376, #29350, #84354, #53337, #59854, #98883, #862, #385, #92328, #30833, #30334, #52846, #74862, #6361, #36873, #8341, #51873, #91843, #38847, #60840, #15854, #67866, #97891, #53843, #76343, #22371, #90343, #91339, #22866, #68852, #98388, #15372, #7860, #29844, #46339, #69337, #38358, #61331, #55308, #16338, #54317, #78302, #62807, #55815, #9820, #92814, #17813, #3298, #40321, #17332, #24344, #85817, #33762, #84831, #54806, #85318, #47305, #1359, #56306, #25330, #31810, #70825, #71793, #71312, #64269, #2830, #2339, #24830, #46821, #77312, #8826, #48785, #62306, #32794, #63290, #86309, #93799, #48294, #69835, #39341, #78801, #10311, #10803, #79293, #23851, #16830, #47802, #77805, #40813, #33286, #63777, #32302, #86803, #9320, #93306, #39824, #94286, #70329, #18302, #1844, #25808, #41321, #56781, #50253, #13256, #81740, #95269, #57270, #96279, #65252, #58750, #42774, #26772, #27756, #88758, #50767, #5767, #80770, #34256, #5281, #12264, #87765, #73749, #89255, #72271, #58239, #87277, #19279, #64758, #20270, #65752, #81259, #35757, #11282, #49764, #49282, #72755, #18797, #80274, #66245, #4289, #79781, #41800, #11775, #51254, #3801, #73257, #88263, #12757, #57759, #42283, #4782, #43748, #43255, #27260, #19767, #35255, #96779, #28255, #36255, #20766, #26281, #74233, #94781, #34762, #95780, #29727, #52244, #45233, #15256, #36758, #52730, #37264, #82738, #90729, #59240, #68250, #14257, #74742, #84237, #30218, #97774, #91219, #67751, #67250, #7248, #45734, #60235, #22256, #46228, #23245, #60723, #29239, #22746, #53229, #51755, #83237, #98769, #28749, #53720, #6255, #89739, #66751, #30709, #97276, #44239, #37753, #75732, #83733, #59737, #90232, #21765, #14760, #68734, #15744, #44736, #98271, #76234, #7748, #76714, #21258, #38243, #8233, #82240, #75236, #263, #61221, #6746, #91725, #13753, #17706, #40693, #752, #9700, #47187, #39225, #92214, #56190, #86194, #9205, #46704, #54202, #32183, #38727, #31697, #62188, #55697, #17217, #71194, #92698, #31204, #2717, #48176, #1728, #47695, #25700, #8709, #79170, #77691, #61699, #69227, #39718, #69714, #78688, #23740, #16222, #32682, #2222, #86684, #77204, #84718, #24222, #1241, #70209, #54688, #10199, #85210, #16715, #63175, #93683, #18188 ),
 ( #85700, #48669, #25216, #62685, #93186, #24712, #40196, #33171, #55183, #63664, #78187, #70703, #94169, #97042, #37010, #74007, #96539, #89514, #59501, #79670, #28517, #81508, #28014, #36013, #3189, #13517, #58511, #18682, #29480, #74500, #41686, #36519, #13013, #11167, #51513, #89999, #5533, #66515, #90482, #67506, #6023, #72156, #67011, #97532, #94668, #59011, #43998, #71679, #98026, #49168, #33655, #10685, #75000, #41199, #87157, #82005, #21024, #28991, #5034, #35520, #66012, #21515, #14019, #59989, #89020, #43510, #52012, #82501, #22019, #64150, #44499, #52493, #26178, #20529, #6502, #56669, #51014, #46957, #996, #61959, #84965, #44987, #53974, #91486, #83496, #37511, #1490, #31457, #53475, #90977, #98530, #76481, #83000, #75986, #7515, #92458, #61467, #16481, #38006, #75494, #77451, #23986, #45992, #91974, #69971, #52982, #24482, #23007, #7006, #22510, #23503, #84483, #15984, #46471, #76967, #29983, #68004, #8479, #38985, #31943, #39481, #62444, #14518, #83985, #60488, #69477, #15510, #7995, #38493, #8965, #68499, #68988, #15015, #54457, #92947, #45484, #26, #30473, #523, #60974, #30970, #72409, #41946, #55459, #17471, #56445, #25472, #18939, #2968, #85962, #86931, #48926, #10936, #64894, #10449, #93449, #64414, #40957, #47938, #33906, #49416, #32450, #18444, #47454, #78444, #24974, #79438, #25943, #41460, #94920, #70462, #9959, #9460, #32937, #77953, #40465, #26419, #63438, #39961, #1984, #70964, #34405, #56920, #79917, #86454, #87422, #2483, #62946, #11426, #71928, #93945, #95422, #71454, #94428, #3449, #55954, #17952, #48438, #78939, #3936, #54945, #33418, #63917, #85462, #16974, #57415, #81397, #65894, #58896, #12899, #95927, #20910, #6382, #43396, #20416, #27407, #88905, #36898, #87908, #57898, #88412, #50403, #4439, #59380, #28401, #34905, #73894, #74884, #74377, #67386, #5904, #5425, #27898, #19422, #49914, #80425, #51896, #35895, #66390, #89394, #96923, #51399, #72906, #11921, #81886, #13398, #13900, #82378, #26918, #42425, #58387, #65401, #43881, #50902, #36399, #35401, #89884, #80913, #96425, #19912, #66892, #12407, #21402, #42914, #97411, #28878, #73395, #44385, #4923, #84856, #98411, #60369, #408, #68386, #61846, #45880, #29867, #30860, #91866, #53869, #8851, #53363, #37401, #8365, #83870, #90866, #76851, #92352, #75373, #61357, #90365, #22396, #67889, #23384, #68878, #84379, #38873, #14399, #52872, #52379, #75875, #21902, #83378, #69364, #7396, #82883, #44870, #14900, #77339, #885, #23879, #30357, #31345, #45371, #6888, #54343, #15879, #37894, #39365, #15394, #38377, #46363, #98906, #60865, #91365 ) ),
 .UNSPECIFIED., .F., .F., .F. ) 
 B_SPLINE_SURFACE_WITH_KNOTS ( ( 2, 2 ),
 ( 3, 2, 2, 2, 2, 2, 2, 2, 2, 2, 2, 2, 2, 2, 2, 2, 2, 2, 2, 2, 2, 2, 2, 2, 2, 2, 2, 2, 2, 2, 2, 2, 2, 2, 2, 2, 2, 2, 2, 2, 2, 2, 2, 2, 2, 2, 2, 2, 2, 2, 2, 2, 2, 2, 2, 2, 2, 2, 2, 2, 2, 2, 2, 2, 2, 2, 2, 2, 2, 2, 2, 2, 2, 2, 2, 2, 2, 2, 2, 2, 2, 2, 2, 2, 2, 2, 2, 2, 2, 2, 2, 2, 2, 2, 2, 2, 2, 2, 2, 2, 2, 2, 2, 2, 2, 2, 2, 2, 2, 2, 2, 2, 2, 2, 2, 2, 2, 2, 2, 2, 2, 2, 2, 2, 2, 2, 2, 2, 2, 2, 2, 2, 2, 2, 2, 2, 2, 2, 2, 2, 2, 2, 2, 2, 2, 2, 2, 2, 2, 2, 2, 2, 2, 2, 2, 2, 2, 2, 2, 2, 2, 2, 3 ),
 ( 0.000000000000000000, 1.000000000000000000 ),
 ( 0.000000000000000000, 0.005952380952380952051, 0.01190476190476190410, 0.01785714285714285615, 0.02380952380952380820, 0.02976190476190476025, 0.03571428571428571230, 0.04166666666666666435, 0.04761904761904761640, 0.05357142857142856845, 0.05952380952380952051, 0.06547619047619047949, 0.07142857142857142461, 0.07738095238095238360, 0.08333333333333332871, 0.08928571428571428770, 0.09523809523809523281, 0.1011904761904761918, 0.1071428571428571369, 0.1130952380952380959, 0.1190476190476190410, 0.1250000000000000000, 0.1309523809523809590, 0.1369047619047619180, 0.1428571428571428492, 0.1488095238095238082, 0.1547619047619047672, 0.1607142857142857262, 0.1666666666666666574, 0.1726190476190476164, 0.1785714285714285754, 0.1845238095238095344, 0.1904761904761904656, 0.1964285714285714246, 0.2023809523809523836, 0.2083333333333333426, 0.2142857142857142738, 0.2202380952380952328, 0.2261904761904761918, 0.2321428571428571508, 0.2380952380952380820, 0.2440476190476190410, 0.2500000000000000000, 0.2559523809523809312, 0.2619047619047619180, 0.2678571428571428492, 0.2738095238095238360, 0.2797619047619047672, 0.2857142857142856984, 0.2916666666666666852, 0.2976190476190476164, 0.3035714285714285476, 0.3095238095238095344, 0.3154761904761904656, 0.3214285714285714524, 0.3273809523809523836, 0.3333333333333333148, 0.3392857142857143016, 0.3452380952380952328, 0.3511904761904761640, 0.3571428571428571508, 0.3630952380952380820, 0.3690476190476190688, 0.3750000000000000000, 0.3809523809523809312, 0.3869047619047619180, 0.3928571428571428492, 0.3988095238095238360, 0.4047619047619047672, 0.4107142857142856984, 0.4166666666666666852, 0.4226190476190476164, 0.4285714285714285476, 0.4345238095238095344, 0.4404761904761904656, 0.4464285714285714524, 0.4523809523809523836, 0.4583333333333333148, 0.4642857142857143016, 0.4702380952380952328, 0.4761904761904761640, 0.4821428571428571508, 0.4880952380952380820, 0.4940476190476190688, 0.5000000000000000000, 0.5059523809523809312, 0.5119047619047618625, 0.5178571428571429047, 0.5238095238095238360, 0.5297619047619047672, 0.5357142857142856984, 0.5416666666666666297, 0.5476190476190476719, 0.5535714285714286031, 0.5595238095238095344, 0.5654761904761904656, 0.5714285714285713969, 0.5773809523809523281, 0.5833333333333333703, 0.5892857142857143016, 0.5952380952380952328, 0.6011904761904761640, 0.6071428571428570953, 0.6130952380952381375, 0.6190476190476190688, 0.6250000000000000000, 0.6309523809523809312, 0.6369047619047618625, 0.6428571428571429047, 0.6488095238095238360, 0.6547619047619047672, 0.6607142857142856984, 0.6666666666666666297, 0.6726190476190476719, 0.6785714285714286031, 0.6845238095238095344, 0.6904761904761904656, 0.6964285714285713969, 0.7023809523809523281, 0.7083333333333333703, 0.7142857142857143016, 0.7202380952380952328, 0.7261904761904761640, 0.7321428571428570953, 0.7380952380952381375, 0.7440476190476190688, 0.7500000000000000000, 0.7559523809523809312, 0.7619047619047618625, 0.7678571428571429047, 0.7738095238095238360, 0.7797619047619047672, 0.7857142857142856984, 0.7916666666666666297, 0.7976190476190476719, 0.8035714285714286031, 0.8095238095238095344, 0.8154761904761904656, 0.8214285714285713969, 0.8273809523809523281, 0.8333333333333333703, 0.8392857142857143016, 0.8452380952380952328, 0.8511904761904761640, 0.8571428571428570953, 0.8630952380952381375, 0.8690476190476190688, 0.8750000000000000000, 0.8809523809523809312, 0.8869047619047618625, 0.8928571428571429047, 0.8988095238095238360, 0.9047619047619047672, 0.9107142857142856984, 0.9166666666666666297, 0.9226190476190476719, 0.9285714285714286031, 0.9345238095238095344, 0.9404761904761904656, 0.9464285714285713969, 0.9523809523809523281, 0.9583333333333333703, 0.9642857142857143016 ),
 .UNSPECIFIED. ) 
 GEOMETRIC_REPRESENTATION_ITEM ( )  RATIONAL_B_SPLINE_SURFACE ( (
 ( 1.000000000000000000, 0.9659258262890683122, 1.000000000000000000, 0.9659258262890683122, 1.000000000000000000, 0.9659258262890683122, 1.000000000000000000, 0.9659258262890683122, 1.000000000000000000, 0.9659258262890683122, 1.000000000000000000, 0.9659258262890683122, 1.000000000000000000, 0.9659258262890683122, 1.000000000000000000, 0.9659258262890683122, 1.000000000000000000, 0.9659258262890683122, 1.000000000000000000, 0.9659258262890683122, 1.000000000000000000, 0.9659258262890683122, 1.000000000000000000, 0.9659258262890683122, 1.000000000000000000, 0.9659258262890683122, 1.000000000000000000, 0.9659258262890683122, 1.000000000000000000, 0.9659258262890683122, 1.000000000000000000, 0.9659258262890683122, 1.000000000000000000, 0.9659258262890683122, 1.000000000000000000, 0.9659258262890683122, 1.000000000000000000, 0.9659258262890683122, 1.000000000000000000, 0.9659258262890683122, 1.000000000000000000, 0.9659258262890683122, 1.000000000000000000, 0.9659258262890683122, 1.000000000000000000, 0.9659258262890683122, 1.000000000000000000, 0.9659258262890683122, 1.000000000000000000, 0.9659258262890683122, 1.000000000000000000, 0.9659258262890683122, 1.000000000000000000, 0.9659258262890683122, 1.000000000000000000, 0.9659258262890683122, 1.000000000000000000, 0.9659258262890683122, 1.000000000000000000, 0.9659258262890683122, 1.000000000000000000, 0.9659258262890683122, 1.000000000000000000, 0.9659258262890683122, 1.000000000000000000, 0.9659258262890683122, 1.000000000000000000, 0.9659258262890683122, 1.000000000000000000, 0.9659258262890683122, 1.000000000000000000, 0.9659258262890683122, 1.000000000000000000, 0.9659258262890683122, 1.000000000000000000, 0.9659258262890683122, 1.000000000000000000, 0.9659258262890683122, 1.000000000000000000, 0.9659258262890683122, 1.000000000000000000, 0.9659258262890683122, 1.000000000000000000, 0.9659258262890683122, 1.000000000000000000, 0.9659258262890683122, 1.000000000000000000, 0.9659258262890683122, 1.000000000000000000, 0.9659258262890683122, 1.000000000000000000, 0.9659258262890683122, 1.000000000000000000, 0.9659258262890683122, 1.000000000000000000, 0.9659258262890683122, 1.000000000000000000, 0.9659258262890683122, 1.000000000000000000, 0.9659258262890683122, 1.000000000000000000, 0.9659258262890683122, 1.000000000000000000, 0.9659258262890683122, 1.000000000000000000, 0.9659258262890683122, 1.000000000000000000, 0.9659258262890683122, 1.000000000000000000, 0.9659258262890683122, 1.000000000000000000, 0.9659258262890683122, 1.000000000000000000, 0.9659258262890683122, 1.000000000000000000, 0.9659258262890683122, 1.000000000000000000, 0.9659258262890683122, 1.000000000000000000, 0.9659258262890683122, 1.000000000000000000, 0.9659258262890683122, 1.000000000000000000, 0.9659258262890683122, 1.000000000000000000, 0.9659258262890683122, 1.000000000000000000, 0.9659258262890683122, 1.000000000000000000, 0.9659258262890683122, 1.000000000000000000, 0.9659258262890683122, 1.000000000000000000, 0.9659258262890683122, 1.000000000000000000, 0.9659258262890683122, 1.000000000000000000, 0.9659258262890683122, 1.000000000000000000, 0.9659258262890683122, 1.000000000000000000, 0.9659258262890683122, 1.000000000000000000, 0.9659258262890683122, 1.000000000000000000, 0.9659258262890683122, 1.000000000000000000, 0.9659258262890683122, 1.000000000000000000, 0.9659258262890683122, 1.000000000000000000, 0.9659258262890683122, 1.000000000000000000, 0.9659258262890683122, 1.000000000000000000, 0.9659258262890683122, 1.000000000000000000, 0.9659258262890683122, 1.000000000000000000, 0.9659258262890683122, 1.000000000000000000, 0.9659258262890683122, 1.000000000000000000, 0.9659258262890683122, 1.000000000000000000, 0.9659258262890683122, 1.000000000000000000, 0.9659258262890683122, 1.000000000000000000, 0.9659258262890683122, 1.000000000000000000, 0.9659258262890683122, 1.000000000000000000, 0.9659258262890683122, 1.000000000000000000, 0.9659258262890683122, 1.000000000000000000, 0.9659258262890683122, 1.000000000000000000, 0.9659258262890683122, 1.000000000000000000, 0.9659258262890683122, 1.000000000000000000, 0.9659258262890683122, 1.000000000000000000, 0.9659258262890683122, 1.000000000000000000, 0.9659258262890683122, 1.000000000000000000, 0.9659258262890683122, 1.000000000000000000, 0.9659258262890683122, 1.000000000000000000, 0.9659258262890683122, 1.000000000000000000, 0.9659258262890683122, 1.000000000000000000, 0.9659258262890683122, 1.000000000000000000, 0.9659258262890683122, 1.000000000000000000, 0.9659258262890683122, 1.000000000000000000, 0.9659258262890683122, 1.000000000000000000, 0.9659258262890683122, 1.000000000000000000, 0.9659258262890683122, 1.000000000000000000, 0.9659258262890683122, 1.000000000000000000, 0.9659258262890683122, 1.000000000000000000, 0.9659258262890683122, 1.000000000000000000, 0.9659258262890683122, 1.000000000000000000, 0.9659258262890683122, 1.000000000000000000, 0.9659258262890683122, 1.000000000000000000, 0.9659258262890683122, 1.000000000000000000, 0.9659258262890683122, 1.000000000000000000, 0.9659258262890683122, 1.000000000000000000, 0.9659258262890683122, 1.000000000000000000, 0.9659258262890683122, 1.000000000000000000, 0.9659258262890683122, 1.000000000000000000, 0.9659258262890683122, 1.000000000000000000, 0.9659258262890683122, 1.000000000000000000, 0.9659258262890683122, 1.000000000000000000, 0.9659258262890683122, 1.000000000000000000, 0.9659258262890683122, 1.000000000000000000, 0.9659258262890683122, 1.000000000000000000, 0.9659258262890683122, 1.000000000000000000, 0.9659258262890683122, 1.000000000000000000, 0.9659258262890683122, 1.000000000000000000, 0.9659258262890683122, 1.000000000000000000, 0.9659258262890683122, 1.000000000000000000, 0.9659258262890683122, 1.000000000000000000, 0.9659258262890683122, 1.000000000000000000, 0.9659258262890683122, 1.000000000000000000, 0.9659258262890683122, 1.000000000000000000, 0.9659258262890683122, 1.000000000000000000, 0.9659258262890683122, 1.000000000000000000, 0.9659258262890683122, 1.000000000000000000, 0.9659258262890683122, 1.000000000000000000, 0.9659258262890683122, 1.000000000000000000, 0.9659258262890683122, 1.000000000000000000, 0.9659258262890683122, 1.000000000000000000, 0.9659258262890683122, 1.000000000000000000, 0.9659258262890683122, 1.000000000000000000, 0.9659258262890683122, 1.000000000000000000, 0.9659258262890683122, 1.000000000000000000, 0.9659258262890683122, 1.000000000000000000, 0.9659258262890683122, 1.000000000000000000, 0.9659258262890683122, 1.000000000000000000, 0.9659258262890683122, 1.000000000000000000, 0.9659258262890683122, 1.000000000000000000, 0.9659258262890683122, 1.000000000000000000, 0.9659258262890683122, 1.000000000000000000, 0.9659258262890683122, 1.000000000000000000, 0.9659258262890683122, 1.000000000000000000, 0.9659258262890683122, 1.000000000000000000, 0.9659258262890683122, 1.000000000000000000, 0.9659258262890683122, 1.000000000000000000, 0.9659258262890683122, 1.000000000000000000, 0.9659258262890683122, 1.000000000000000000, 0.9659258262890683122, 1.000000000000000000, 0.9659258262890683122, 1.000000000000000000, 0.9659258262890683122, 1.000000000000000000, 0.9659258262890683122, 1.000000000000000000, 0.9659258262890683122, 1.000000000000000000, 0.9659258262890683122, 1.000000000000000000),
 ( 1.000000000000000000, 0.9659258262890683122, 1.000000000000000000, 0.9659258262890683122, 1.000000000000000000, 0.9659258262890683122, 1.000000000000000000, 0.9659258262890683122, 1.000000000000000000, 0.9659258262890683122, 1.000000000000000000, 0.9659258262890683122, 1.000000000000000000, 0.9659258262890683122, 1.000000000000000000, 0.9659258262890683122, 1.000000000000000000, 0.9659258262890683122, 1.000000000000000000, 0.9659258262890683122, 1.000000000000000000, 0.9659258262890683122, 1.000000000000000000, 0.9659258262890683122, 1.000000000000000000, 0.9659258262890683122, 1.000000000000000000, 0.9659258262890683122, 1.000000000000000000, 0.9659258262890683122, 1.000000000000000000, 0.9659258262890683122, 1.000000000000000000, 0.9659258262890683122, 1.000000000000000000, 0.9659258262890683122, 1.000000000000000000, 0.9659258262890683122, 1.000000000000000000, 0.9659258262890683122, 1.000000000000000000, 0.9659258262890683122, 1.000000000000000000, 0.9659258262890683122, 1.000000000000000000, 0.9659258262890683122, 1.000000000000000000, 0.9659258262890683122, 1.000000000000000000, 0.9659258262890683122, 1.000000000000000000, 0.9659258262890683122, 1.000000000000000000, 0.9659258262890683122, 1.000000000000000000, 0.9659258262890683122, 1.000000000000000000, 0.9659258262890683122, 1.000000000000000000, 0.9659258262890683122, 1.000000000000000000, 0.9659258262890683122, 1.000000000000000000, 0.9659258262890683122, 1.000000000000000000, 0.9659258262890683122, 1.000000000000000000, 0.9659258262890683122, 1.000000000000000000, 0.9659258262890683122, 1.000000000000000000, 0.9659258262890683122, 1.000000000000000000, 0.9659258262890683122, 1.000000000000000000, 0.9659258262890683122, 1.000000000000000000, 0.9659258262890683122, 1.000000000000000000, 0.9659258262890683122, 1.000000000000000000, 0.9659258262890683122, 1.000000000000000000, 0.9659258262890683122, 1.000000000000000000, 0.9659258262890683122, 1.000000000000000000, 0.9659258262890683122, 1.000000000000000000, 0.9659258262890683122, 1.000000000000000000, 0.9659258262890683122, 1.000000000000000000, 0.9659258262890683122, 1.000000000000000000, 0.9659258262890683122, 1.000000000000000000, 0.9659258262890683122, 1.000000000000000000, 0.9659258262890683122, 1.000000000000000000, 0.9659258262890683122, 1.000000000000000000, 0.9659258262890683122, 1.000000000000000000, 0.9659258262890683122, 1.000000000000000000, 0.9659258262890683122, 1.000000000000000000, 0.9659258262890683122, 1.000000000000000000, 0.9659258262890683122, 1.000000000000000000, 0.9659258262890683122, 1.000000000000000000, 0.9659258262890683122, 1.000000000000000000, 0.9659258262890683122, 1.000000000000000000, 0.9659258262890683122, 1.000000000000000000, 0.9659258262890683122, 1.000000000000000000, 0.9659258262890683122, 1.000000000000000000, 0.9659258262890683122, 1.000000000000000000, 0.9659258262890683122, 1.000000000000000000, 0.9659258262890683122, 1.000000000000000000, 0.9659258262890683122, 1.000000000000000000, 0.9659258262890683122, 1.000000000000000000, 0.9659258262890683122, 1.000000000000000000, 0.9659258262890683122, 1.000000000000000000, 0.9659258262890683122, 1.000000000000000000, 0.9659258262890683122, 1.000000000000000000, 0.9659258262890683122, 1.000000000000000000, 0.9659258262890683122, 1.000000000000000000, 0.9659258262890683122, 1.000000000000000000, 0.9659258262890683122, 1.000000000000000000, 0.9659258262890683122, 1.000000000000000000, 0.9659258262890683122, 1.000000000000000000, 0.9659258262890683122, 1.000000000000000000, 0.9659258262890683122, 1.000000000000000000, 0.9659258262890683122, 1.000000000000000000, 0.9659258262890683122, 1.000000000000000000, 0.9659258262890683122, 1.000000000000000000, 0.9659258262890683122, 1.000000000000000000, 0.9659258262890683122, 1.000000000000000000, 0.9659258262890683122, 1.000000000000000000, 0.9659258262890683122, 1.000000000000000000, 0.9659258262890683122, 1.000000000000000000, 0.9659258262890683122, 1.000000000000000000, 0.9659258262890683122, 1.000000000000000000, 0.9659258262890683122, 1.000000000000000000, 0.9659258262890683122, 1.000000000000000000, 0.9659258262890683122, 1.000000000000000000, 0.9659258262890683122, 1.000000000000000000, 0.9659258262890683122, 1.000000000000000000, 0.9659258262890683122, 1.000000000000000000, 0.9659258262890683122, 1.000000000000000000, 0.9659258262890683122, 1.000000000000000000, 0.9659258262890683122, 1.000000000000000000, 0.9659258262890683122, 1.000000000000000000, 0.9659258262890683122, 1.000000000000000000, 0.9659258262890683122, 1.000000000000000000, 0.9659258262890683122, 1.000000000000000000, 0.9659258262890683122, 1.000000000000000000, 0.9659258262890683122, 1.000000000000000000, 0.9659258262890683122, 1.000000000000000000, 0.9659258262890683122, 1.000000000000000000, 0.9659258262890683122, 1.000000000000000000, 0.9659258262890683122, 1.000000000000000000, 0.9659258262890683122, 1.000000000000000000, 0.9659258262890683122, 1.000000000000000000, 0.9659258262890683122, 1.000000000000000000, 0.9659258262890683122, 1.000000000000000000, 0.9659258262890683122, 1.000000000000000000, 0.9659258262890683122, 1.000000000000000000, 0.9659258262890683122, 1.000000000000000000, 0.9659258262890683122, 1.000000000000000000, 0.9659258262890683122, 1.000000000000000000, 0.9659258262890683122, 1.000000000000000000, 0.9659258262890683122, 1.000000000000000000, 0.9659258262890683122, 1.000000000000000000, 0.9659258262890683122, 1.000000000000000000, 0.9659258262890683122, 1.000000000000000000, 0.9659258262890683122, 1.000000000000000000, 0.9659258262890683122, 1.000000000000000000, 0.9659258262890683122, 1.000000000000000000, 0.9659258262890683122, 1.000000000000000000, 0.9659258262890683122, 1.000000000000000000, 0.9659258262890683122, 1.000000000000000000, 0.9659258262890683122, 1.000000000000000000, 0.9659258262890683122, 1.000000000000000000, 0.9659258262890683122, 1.000000000000000000, 0.9659258262890683122, 1.000000000000000000, 0.9659258262890683122, 1.000000000000000000, 0.9659258262890683122, 1.000000000000000000, 0.9659258262890683122, 1.000000000000000000, 0.9659258262890683122, 1.000000000000000000, 0.9659258262890683122, 1.000000000000000000, 0.9659258262890683122, 1.000000000000000000, 0.9659258262890683122, 1.000000000000000000, 0.9659258262890683122, 1.000000000000000000, 0.9659258262890683122, 1.000000000000000000, 0.9659258262890683122, 1.000000000000000000, 0.9659258262890683122, 1.000000000000000000, 0.9659258262890683122, 1.000000000000000000, 0.9659258262890683122, 1.000000000000000000, 0.9659258262890683122, 1.000000000000000000, 0.9659258262890683122, 1.000000000000000000, 0.9659258262890683122, 1.000000000000000000, 0.9659258262890683122, 1.000000000000000000, 0.9659258262890683122, 1.000000000000000000, 0.9659258262890683122, 1.000000000000000000, 0.9659258262890683122, 1.000000000000000000, 0.9659258262890683122, 1.000000000000000000, 0.9659258262890683122, 1.000000000000000000, 0.9659258262890683122, 1.000000000000000000, 0.9659258262890683122, 1.000000000000000000, 0.9659258262890683122, 1.000000000000000000, 0.9659258262890683122, 1.000000000000000000, 0.9659258262890683122, 1.000000000000000000, 0.9659258262890683122, 1.000000000000000000, 0.9659258262890683122, 1.000000000000000000, 0.9659258262890683122, 1.000000000000000000) ) ) 
 REPRESENTATION_ITEM ( '' )  SURFACE ( )  );
#84122=CARTESIAN_POINT ( 'NONE',  ( 18.52753015748618282, 48.92559781766745886, -4.923371831947291888 ) ) ;
#84123=CARTESIAN_POINT ( 'NONE',  ( 0.5774900079438607392, 3.480352010821504027, 5.440088680355550821 ) ) ;
#84125=CARTESIAN_POINT ( 'NONE',  ( 13.43411237798105340, 5.581968003263753531, 12.81628187352647963 ) ) ;
#84128=CARTESIAN_POINT ( 'NONE',  ( 10.00000000000000178, 34.31368534415484106, 10.88017736071110342 ) ) ;
#84129=CARTESIAN_POINT ( 'NONE',  ( 14.92337183194729633, 57.67559781766745886, 8.527530157486181039 ) ) ;
#84131=CARTESIAN_POINT ( 'NONE',  ( 2.035157376598824452, 8.688685344154839285, 7.964842623401179544 ) ) ;
#84132=CARTESIAN_POINT ( 'NONE',  ( 4.559911319644449179, 32.23035201082150536, -9.422509992056141925 ) ) ;
#84133=CARTESIAN_POINT ( 'NONE',  ( 24.16423886937409904, 39.09541550158062506, 3.795296366450317205 ) ) ;
#84134=CARTESIAN_POINT ( 'NONE',  ( 0.1532563361054082862, 31.21726448433412315, 2.638427012816831674 ) ) ;
#84135=CARTESIAN_POINT ( 'NONE',  ( 20.88017736071110164, 50.35535201082151247, 2.915334737309930979 ) ) ;
#84137=PRESENTATION_STYLE_ASSIGNMENT (( #46131 ) ) ;
#84138=( GEOMETRIC_REPRESENTATION_CONTEXT ( 3 ) GLOBAL_UNCERTAINTY_ASSIGNED_CONTEXT ( ( #44121 ) ) GLOBAL_UNIT_ASSIGNED_CONTEXT ( ( #52749, #46248, #39246 ) ) REPRESENTATION_CONTEXT ( 'NONE', 'WORKASPACE' ) );
#84140=UNCERTAINTY_MEASURE_WITH_UNIT (LENGTH_MEASURE( 1.000000000000000082E-05 ), #21266, 'distance_accuracy_value', 'NONE');
#84142=CARTESIAN_POINT ( 'NONE',  ( 14.92337183194729633, 57.67559781766745886, 8.527530157486181039 ) ) ;
#84145=ORIENTED_EDGE ( 'NONE', *, *, #13820, .F. ) ;
#84146=CARTESIAN_POINT ( 'NONE',  ( 10.00000000000000000, 35.55374883491396787, -14.16423886937410082 ) ) ;
#84147=CARTESIAN_POINT ( 'NONE',  ( 2.917880565312950480, 20.97041550158063217, -12.26659068614894821 ) ) ;
#84148=VECTOR ( 'NONE', #95011, 1000.000000000000000 ) ;
#84149=CARTESIAN_POINT ( 'NONE',  ( 2.791683348922240793, 6.633931151000785675, 7.208316651077764092 ) ) ;
#84150=EDGE_CURVE ( 'NONE', #29028, #156, #94725, .T. ) ;
#84151=CARTESIAN_POINT ( 'NONE',  ( 6.565887622018943937, 8.081968003263751754, -12.81628187352647608 ) ) ;
#84154=CARTESIAN_POINT ( 'NONE',  ( 20.88017736071110875, 60.77201867748817676, -2.915334737309920765 ) ) ;
#84155=CARTESIAN_POINT ( 'NONE',  ( 21.09922568453595559, 22.04030133659708923, -6.408140936763230044 ) ) ;
#84156=CARTESIAN_POINT ( 'NONE',  ( 2.917880565312950480, 35.97041550158063217, -12.26659068614894821 ) ) ;
#84157=CARTESIAN_POINT ( 'NONE',  ( 4.559911319644449179, 12.23035201082150714, -9.422509992056141925 ) ) ;
#84158=CARTESIAN_POINT ( 'NONE',  ( 15.44008868035555793, 36.39701867748816966, -9.422509992056140149 ) ) ;
#84160=CARTESIAN_POINT ( 'NONE',  ( 7.084665262690076126, 57.02201867748817676, -10.88017736071110164 ) ) ;
#84162=CARTESIAN_POINT ( 'NONE',  ( 10.00000000000000000, 47.87363466993042493, -12.81628187352647608 ) ) ;
#84165=CARTESIAN_POINT ( 'NONE',  ( 19.90229974777923161, 0.3225724651664713671, 6.500000000000000000 ) ) ;
#84166=VERTEX_POINT ( 'NONE', #28470 ) ;
#84169=FILL_AREA_STYLE ('',( #57818 ) ) ;
#84170=CARTESIAN_POINT ( 'NONE',  ( -0.3689425029237881626, 57.42874883491397497, 10.36894250292379027 ) ) ;
#84171=CARTESIAN_POINT ( 'NONE',  ( 13.79529636645031943, 60.34541550158063927, -14.16423886937409904 ) ) ;
#84172=CARTESIAN_POINT ( 'NONE',  ( 17.20831665107776587, 24.13393115100078035, -7.208316651077762316 ) ) ;
#84173=CARTESIAN_POINT ( 'NONE',  ( 17.20831665107776587, 64.13393115100079456, -7.208316651077762316 ) ) ;
#84175=CARTESIAN_POINT ( 'NONE',  ( 22.81628187352647785, 1.623634669930420271, 6.195893100308588602E-16 ) ) ;
#84178=CARTESIAN_POINT ( 'NONE',  ( -2.266590686148945544, 36.38708216824730357, -7.082119434687050408 ) ) ;
#84179=CARTESIAN_POINT ( 'NONE',  ( 24.16423886937409904, 49.09541550158063217, 3.795296366450317205 ) ) ;
#84181=CARTESIAN_POINT ( 'NONE',  ( 0.6178305044545818747, 58.49863466993042493, -9.382169495545419124 ) ) ;
#84182=CARTESIAN_POINT ( 'NONE',  ( 12.63842701281683922, 44.55059781766745175, -9.846743663894590881 ) ) ;
#84183=CARTESIAN_POINT ( 'NONE',  ( 19.42250999205614548, 20.98035201082150891, -5.440088680355545492 ) ) ;
#84184=CARTESIAN_POINT ( 'NONE',  ( 17.20831665107776587, 59.13393115100078745, -7.208316651077762316 ) ) ;
#84185=CARTESIAN_POINT ( 'NONE',  ( 10.00000000000000178, 52.25893115100078745, 9.846743663894594434 ) ) ;
#84186=CARTESIAN_POINT ( 'NONE',  ( -2.816281873526473856, 29.12363466993041783, 9.499525473075851096E-16 ) ) ;
#84190=CARTESIAN_POINT ( 'NONE',  ( 2.791683348922237240, 0.3839311510007847872, -7.208316651077763204 ) ) ;
#84192=ORIENTED_EDGE ( 'NONE', *, *, #22725, .F. ) ;
#84195=CARTESIAN_POINT ( 'NONE',  ( 1.472469842513823179, 26.42559781766745175, 4.923371831947296329 ) ) ;
#84197=CARTESIAN_POINT ( 'NONE',  ( 3.591859063236761518, 34.95696800326375353, 11.09922568453594849 ) ) ;
#84203=CARTESIAN_POINT ( 'NONE',  ( 19.84674366389459621, 58.50893115100078745, 7.409399052514197653E-17 ) ) ;
#84204=CARTESIAN_POINT ( 'NONE',  ( 20.36894250292379382, 38.67874883491396076, 10.36894250292379205 ) ) ;
#84205=CARTESIAN_POINT ( 'NONE',  ( 1.472469842513823179, 56.42559781766745886, 4.923371831947296329 ) ) ;
#84206=B_SPLINE_CURVE_WITH_KNOTS ( 'NONE', 3,
 ( #96542, #74011, #35019, #27526, #88526, #81025 ),
 .UNSPECIFIED., .F., .F.,
 ( 4, 2, 4 ),
 ( 4.336808689942017736E-18, 0.0002605067024380912301, 0.0005210134048761781234 ),
 .UNSPECIFIED. ) ;
#84208=CARTESIAN_POINT ( 'NONE',  ( 0.1532563361054083140, 6.008931151000784787, 1.131784320476157264E-15 ) ) ;
#84209=( GEOMETRIC_REPRESENTATION_CONTEXT ( 3 ) GLOBAL_UNCERTAINTY_ASSIGNED_CONTEXT ( ( #93459 ) ) GLOBAL_UNIT_ASSIGNED_CONTEXT ( ( #2289, #87225, #20588 ) ) REPRESENTATION_CONTEXT ( 'NONE', 'WORKASPACE' ) );
#84210=CARTESIAN_POINT ( 'NONE',  ( 6.565887622018943937, 48.08196800326375353, -12.81628187352647608 ) ) ;
#84211=CARTESIAN_POINT ( 'NONE',  ( -4.164238869374099927, 2.012082168247300906, 3.795296366450308767 ) ) ;
#84212=EDGE_CURVE ( 'NONE', #16145, #42399, #89128, .T. ) ;
#84213=CARTESIAN_POINT ( 'NONE',  ( 19.84674366389459621, 43.50893115100078745, 7.409399052514197653E-17 ) ) ;
#84214=CARTESIAN_POINT ( 'NONE',  ( 10.00000000000000178, 49.31368534415484106, 10.88017736071110342 ) ) ;
#84216=CARTESIAN_POINT ( 'NONE',  ( 18.52753015748617571, 48.09226448433412315, 4.923371831947298993 ) ) ;
#84220=CARTESIAN_POINT ( 'NONE',  ( 1.274849032794294290, 53.57228050351032067, 6.499999999999979572 ) ) ;
#84221=CARTESIAN_POINT ( 'NONE',  ( 12.91533473730993009, 26.60535201082150536, -10.88017736071109987 ) ) ;
#84222=CARTESIAN_POINT ( 'NONE',  ( 0.6178305044545838731, 4.748634669930420493, 9.382169495545420901 ) ) ;
#84223=CARTESIAN_POINT ( 'NONE',  ( 20.88017736071110875, 50.77201867748817676, -2.915334737309920765 ) ) ;
#84226=CARTESIAN_POINT ( 'NONE',  ( 7.084665262690076126, 42.02201867748816966, -10.88017736071110164 ) ) ;
#84228=CARTESIAN_POINT ( 'NONE',  ( 12.63842701281683922, 9.550597817667449974, -9.846743663894590881 ) ) ;
#84229=CARTESIAN_POINT ( 'NONE',  ( 0.1532563361054082862, 36.21726448433410894, 2.638427012816831674 ) ) ;
#84230=DIRECTION ( 'NONE',  ( -1.000000000000000000, 0.000000000000000000, 0.000000000000000000 ) ) ;
#84232=CARTESIAN_POINT ( 'NONE',  ( 12.63842701281683034, 62.46726448433410894, 9.846743663894596210 ) ) ;
#84234=CARTESIAN_POINT ( 'NONE',  ( 10.00000000000000000, 1.813685344154838175, -10.88017736071110342 ) ) ;
#84236=CARTESIAN_POINT ( 'NONE',  ( 6.204703633549690345, 20.76208216824730357, -14.16423886937410259 ) ) ;
#84237=CARTESIAN_POINT ( 'NONE',  ( -4.164238869374099927, 47.01208216824729647, 3.795296366450308767 ) ) ;
#84238=CARTESIAN_POINT ( 'NONE',  ( 18.52753015748617571, 33.09226448433411605, 4.923371831947298993 ) ) ;
#84239=CARTESIAN_POINT ( 'NONE',  ( 19.84674366389459266, 18.71726448433411960, -2.638427012816827677 ) ) ;
#84240=CARTESIAN_POINT ( 'NONE',  ( 19.42250999205614548, 5.980352010821504471, -5.440088680355545492 ) ) ;
#84243=CARTESIAN_POINT ( 'NONE',  ( 0.1532563361054083140, 31.00893115100078390, 1.131784320476157264E-15 ) ) ;
#84244=CARTESIAN_POINT ( 'NONE',  ( 17.96484262340118221, 31.18868534415483751, -7.964842623401177768 ) ) ;
#84245=CARTESIAN_POINT ( 'NONE',  ( 19.84674366389459621, 58.50893115100078745, 7.409399052514197653E-17 ) ) ;
#84246=CARTESIAN_POINT ( 'NONE',  ( 10.00000000000000178, 8.053748834913967869, 14.16423886937410082 ) ) ;
#84251=CARTESIAN_POINT ( 'NONE',  ( 19.84674366389459266, 13.30059781766745353, 2.638427012816836559 ) ) ;
#84252=CARTESIAN_POINT ( 'NONE',  ( 21.09922568453595559, 42.04030133659708213, -6.408140936763230044 ) ) ;
#84253=CARTESIAN_POINT ( 'NONE',  ( 10.00000000000000178, 47.25893115100078745, 9.846743663894594434 ) ) ;
#84255=CARTESIAN_POINT ( 'NONE',  ( 2.791683348922237240, 25.38393115100078390, -7.208316651077763204 ) ) ;
#84257=CARTESIAN_POINT ( 'NONE',  ( 6.204703633549690345, 57.84541550158063927, 14.16423886937410082 ) ) ;
#84258=CARTESIAN_POINT ( 'NONE',  ( 2.035157376598824452, 48.68868534415483396, 7.964842623401179544 ) ) ;
#84259=CARTESIAN_POINT ( 'NONE',  ( -0.3689425029237898834, 1.178748834913967869, -10.36894250292378850 ) ) ;
#84261=CARTESIAN_POINT ( 'NONE',  ( 14.92337183194729633, 42.67559781766745886, 8.527530157486181039 ) ) ;
#84262=CARTESIAN_POINT ( 'NONE',  ( 10.00000000000000000, 11.81368534415483751, -10.88017736071110342 ) ) ;
#84264=CARTESIAN_POINT ( 'NONE',  ( 18.52753015748617571, 48.09226448433412315, 4.923371831947298993 ) ) ;
#84265=CARTESIAN_POINT ( 'NONE',  ( 20.88017736071110164, 50.35535201082151247, 2.915334737309930979 ) ) ;
#84266=SURFACE_STYLE_FILL_AREA ( #70734 ) ;
#84268=ORIENTED_EDGE ( 'NONE', *, *, #43796, .F. ) ;
#84269=ORIENTED_EDGE ( 'NONE', *, *, #97258, .F. ) ;
#84270=LINE ( 'NONE', #15770, #90036 ) ;
#84273=CARTESIAN_POINT ( 'NONE',  ( 18.52753015748618282, 3.925597817667451306, -4.923371831947291888 ) ) ;
#84274=CARTESIAN_POINT ( 'NONE',  ( 0.6178305044545838731, 59.74863466993041783, 9.382169495545420901 ) ) ;
#84275=CARTESIAN_POINT ( 'NONE',  ( 2.917880565312948704, 67.63708216824730357, 12.26659068614894643 ) ) ;
#84276=CARTESIAN_POINT ( 'NONE',  ( 1.472469842513823179, 46.42559781766745175, 4.923371831947296329 ) ) ;
#84278=CARTESIAN_POINT ( 'NONE',  ( 22.26659068614895176, 59.72041550158063927, -7.082119434687042414 ) ) ;
#84279=CARTESIAN_POINT ( 'NONE',  ( 12.63842701281683034, 52.46726448433413026, 9.846743663894596210 ) ) ;
#84281=CARTESIAN_POINT ( 'NONE',  ( 19.42250999205614193, 45.14701867748817676, 5.440088680355555262 ) ) ;
#84283=CARTESIAN_POINT ( 'NONE',  ( 19.42250999205614548, 65.98035201082151957, -5.440088680355545492 ) ) ;
#84286=CARTESIAN_POINT ( 'NONE',  ( -2.816281873526471635, 58.91530133659707502, -3.434112377981056508 ) ) ;
#84289=CARTESIAN_POINT ( 'NONE',  ( 5.076628168052703671, 11.84226448433411960, 8.527530157486179263 ) ) ;
#84290=ORIENTED_EDGE ( 'NONE', *, *, #61910, .F. ) ;
#84291=CARTESIAN_POINT ( 'NONE',  ( 13.79529636645030344, 13.26208216824729824, 14.16423886937410614 ) ) ;
#84292=CARTESIAN_POINT ( 'NONE',  ( 1.472469842513823179, 25.59226448433412315, -4.923371831947296329 ) ) ;
#84293=CARTESIAN_POINT ( 'NONE',  ( 15.44008868035555793, 31.39701867748817676, -9.422509992056140149 ) ) ;
#84297=VECTOR ( 'NONE', #85625, 1000.000000000000000 ) ;
#84298=CARTESIAN_POINT ( 'NONE',  ( 2.035157376598822676, 32.43868534415483396, -7.964842623401177768 ) ) ;
#84300=CARTESIAN_POINT ( 'NONE',  ( -0.8801773607111009756, 38.06368534415484106, 1.068504757029289695E-15 ) ) ;
#84301=CARTESIAN_POINT ( 'NONE',  ( 20.10421743870887568, 55.60736173766201773, -6.337391062633416894 ) ) ;
#84304=CARTESIAN_POINT ( 'NONE',  ( 21.09922568453595559, 17.04030133659708923, -6.408140936763230044 ) ) ;
#84305=CARTESIAN_POINT ( 'NONE',  ( 0.1532563361054082862, 11.21726448433411605, 2.638427012816831674 ) ) ;
#84308=CARTESIAN_POINT ( 'NONE',  ( 2.791683348922240793, 16.63393115100078745, 7.208316651077764092 ) ) ;
#84309=CARTESIAN_POINT ( 'NONE',  ( 20.88017736071110164, 25.35535201082150891, 2.915334737309930979 ) ) ;
#84310=ORIENTED_EDGE ( 'NONE', *, *, #12967, .T. ) ;
#84312=CARTESIAN_POINT ( 'NONE',  ( 0.6178305044545838731, 64.74863466993043914, 9.382169495545420901 ) ) ;
#84313=CARTESIAN_POINT ( 'NONE',  ( 0.5774900079438607392, 53.48035201082151247, 5.440088680355550821 ) ) ;
#84315=CARTESIAN_POINT ( 'NONE',  ( 6.565887622018943937, 50.16530133659708213, 12.81628187352647430 ) ) ;
#84316=CARTESIAN_POINT ( 'NONE',  ( 20.88017736071110875, 55.77201867748816966, -2.915334737309920765 ) ) ;
#84317=CARTESIAN_POINT ( 'NONE',  ( -2.816281873526473856, 4.123634669930420493, 9.499525473075851096E-16 ) ) ;
#84318=CARTESIAN_POINT ( 'NONE',  ( 17.20831665107776587, 32.88393115100078745, 7.208316651077764980 ) ) ;
#84319=CARTESIAN_POINT ( 'NONE',  ( 16.40814093676323893, 50.79030133659708923, 11.09922568453595026 ) ) ;
#84320=CARTESIAN_POINT ( 'NONE',  ( 6.000000000000000000, 11.50000000000000000, -6.000000000000000000 ) ) ;
#84321=CARTESIAN_POINT ( 'NONE',  ( 10.00000000000000000, 24.75893115100078745, -9.846743663894594434 ) ) ;
#84322=CARTESIAN_POINT ( 'NONE',  ( -2.816281873526473856, 19.33196800326375708, 3.434112377981055619 ) ) ;
#84325=CARTESIAN_POINT ( 'NONE',  ( 17.96484262340118221, 34.93868534415482685, 7.964842623401181321 ) ) ;
#84326=CARTESIAN_POINT ( 'NONE',  ( 6.565887622018943937, -1.918031996736246692, -12.81628187352647608 ) ) ;
#84329=CARTESIAN_POINT ( 'NONE',  ( 14.92337183194729633, 22.67559781766745175, 8.527530157486181039 ) ) ;
#84330=CARTESIAN_POINT ( 'NONE',  ( 19.84674366389459266, 13.30059781766745353, 2.638427012816836559 ) ) ;
#84331=CARTESIAN_POINT ( 'NONE',  ( -0.8801773607111008646, 18.27201867748817321, 2.915334737309923430 ) ) ;
#84332=CARTESIAN_POINT ( 'NONE',  ( 10.00000000000000178, 10.37363466993041961, 12.81628187352647608 ) ) ;
#84333=CARTESIAN_POINT ( 'NONE',  ( -0.8801773607110991993, 2.855352010821504471, -2.915334737309923874 ) ) ;
#84335=CARTESIAN_POINT ( 'NONE',  ( 18.52753015748617571, 63.09226448433412315, 4.923371831947298993 ) ) ;
#84337=CARTESIAN_POINT ( 'NONE',  ( -0.3689425029237898834, 66.17874883491396076, -10.36894250292378850 ) ) ;
#84338=CARTESIAN_POINT ( 'NONE',  ( 18.52753015748618282, 38.92559781766745175, -4.923371831947291888 ) ) ;
#84340=CARTESIAN_POINT ( 'NONE',  ( 12.91533473730992121, 19.52201867748816611, 10.88017736071110164 ) ) ;
#84341=CARTESIAN_POINT ( 'NONE',  ( 1.274849032794305170, 12.55509018479935968, -6.499999999999995559 ) ) ;
#84342=CARTESIAN_POINT ( 'NONE',  ( 4.559911319644449179, 27.23035201082150536, -9.422509992056141925 ) ) ;
#84344=CARTESIAN_POINT ( 'NONE',  ( -0.3689425029237881626, 62.42874883491396787, 10.36894250292379027 ) ) ;
#84346=FILL_AREA_STYLE_COLOUR ( '', #54769 ) ;
#84347=CARTESIAN_POINT ( 'NONE',  ( 14.92337183194729988, 24.34226448433411960, -8.527530157486177487 ) ) ;
#84348=CARTESIAN_POINT ( 'NONE',  ( 10.00000000000000000, 7.873634669930421381, -12.81628187352647608 ) ) ;
#84349=CARTESIAN_POINT ( 'NONE',  ( 10.00000000000000178, 62.25893115100078745, 9.846743663894594434 ) ) ;
#84354=CARTESIAN_POINT ( 'NONE',  ( 17.08211943468705840, 10.13708216824730179, -12.26659068614894466 ) ) ;
#84355=CARTESIAN_POINT ( 'NONE',  ( 19.84674366389459621, 43.50893115100078745, 7.409399052514197653E-17 ) ) ;
#84357=CARTESIAN_POINT ( 'NONE',  ( -2.266590686148945544, 56.38708216824731068, -7.082119434687050408 ) ) ;
#84358=CARTESIAN_POINT ( 'NONE',  ( 5.076628168052704559, 25.17559781766745175, -8.527530157486179263 ) ) ;
#84361=CARTESIAN_POINT ( 'NONE',  ( 20.88017736071110164, 50.35535201082151247, 2.915334737309930979 ) ) ;
#84362=CARTESIAN_POINT ( 'NONE',  ( 6.565887622018943937, 53.08196800326374643, -12.81628187352647608 ) ) ;
#84363=ORIENTED_EDGE ( 'NONE', *, *, #77882, .T. ) ;
#84365=CARTESIAN_POINT ( 'NONE',  ( -0.8801773607111009756, 23.06368534415484106, 1.068504757029289695E-15 ) ) ;
#84366=CARTESIAN_POINT ( 'NONE',  ( 21.09922568453595559, 42.04030133659708213, -6.408140936763230044 ) ) ;
#84367=CARTESIAN_POINT ( 'NONE',  ( 0.1532563361054100626, 65.80059781766745175, -2.638427012816831230 ) ) ;
#84368=CARTESIAN_POINT ( 'NONE',  ( 2.791683348922237240, 0.3839311510007847872, -7.208316651077763204 ) ) ;
#84372=CARTESIAN_POINT ( 'NONE',  ( 22.26659068614894466, 38.88708216824731068, 7.082119434687054849 ) ) ;
#84373=CARTESIAN_POINT ( 'NONE',  ( 10.00000000000000178, 8.053748834913967869, 14.16423886937410082 ) ) ;
#84374=CARTESIAN_POINT ( 'NONE',  ( 20.88017736071110875, 15.77201867748817143, -2.915334737309920765 ) ) ;
#84375=CARTESIAN_POINT ( 'NONE',  ( 10.00000000000000000, 36.81368534415484106, -10.88017736071110342 ) ) ;
#84378=CARTESIAN_POINT ( 'NONE',  ( 17.96484262340118221, 66.18868534415483396, -7.964842623401177768 ) ) ;
#84379=CARTESIAN_POINT ( 'NONE',  ( -0.8801773607111008646, 63.27201867748817676, 2.915334737309923430 ) ) ;
#84380=CARTESIAN_POINT ( 'NONE',  ( 13.43411237798106583, 27.66530133659708568, -12.81628187352647252 ) ) ;
#84383=CARTESIAN_POINT ( 'NONE',  ( 18.52753015748618282, 8.925597817667451750, -4.923371831947291888 ) ) ;
#84384=CARTESIAN_POINT ( 'NONE',  ( 5.076628168052703671, 41.84226448433411605, 8.527530157486179263 ) ) ;
#84386=CARTESIAN_POINT ( 'NONE',  ( 12.91533473730993009, 11.60535201082150536, -10.88017736071109987 ) ) ;
#84387=CARTESIAN_POINT ( 'NONE',  ( 10.00000000000000000, 37.87363466993041783, -12.81628187352647608 ) ) ;
#84388=CARTESIAN_POINT ( 'NONE',  ( 17.20831665107776587, 14.13393115100078568, -7.208316651077762316 ) ) ;
#84389=CARTESIAN_POINT ( 'NONE',  ( 0.5774900079438607392, 13.48035201082150358, 5.440088680355550821 ) ) ;
#84390=CARTESIAN_POINT ( 'NONE',  ( 7.361572987183169658, 39.96726448433411605, -9.846743663894592657 ) ) ;
#84391=CARTESIAN_POINT ( 'NONE',  ( 19.84674366389459266, 28.71726448433411960, -2.638427012816827677 ) ) ;
#84392=CARTESIAN_POINT ( 'NONE',  ( 2.917880565312950480, 20.97041550158063217, -12.26659068614894821 ) ) ;
#84393=CARTESIAN_POINT ( 'NONE',  ( 20.88017736071110875, 35.77201867748816966, -2.915334737309920765 ) ) ;
#84394=CARTESIAN_POINT ( 'NONE',  ( 4.559911319644449179, 7.230352010821504471, -9.422509992056141925 ) ) ;
#84395=CARTESIAN_POINT ( 'NONE',  ( 17.96484262340118221, 36.18868534415484106, -7.964842623401177768 ) ) ;
#84396=CARTESIAN_POINT ( 'NONE',  ( -0.8801773607110991993, 32.85535201082151247, -2.915334737309923874 ) ) ;
#84398=CARTESIAN_POINT ( 'NONE',  ( 19.42250999205614548, 40.98035201082150536, -5.440088680355545492 ) ) ;
#84399=CARTESIAN_POINT ( 'NONE',  ( 6.565887622018943937, 58.08196800326376064, -12.81628187352647608 ) ) ;
#84400=CARTESIAN_POINT ( 'NONE',  ( -0.8801773607111008646, 43.27201867748817676, 2.915334737309923430 ) ) ;
#84401=CARTESIAN_POINT ( 'NONE',  ( 10.00000000000000000, 51.81368534415484106, -10.88017736071110342 ) ) ;
#84403=VERTEX_POINT ( 'NONE', #91434 ) ;
#84404=CARTESIAN_POINT ( 'NONE',  ( 17.96484262340118221, 51.18868534415483396, -7.964842623401177768 ) ) ;
#84407=CARTESIAN_POINT ( 'NONE',  ( -4.164238869374098151, 66.59541550158060375, -3.795296366450310543 ) ) ;
#84408=CARTESIAN_POINT ( 'NONE',  ( 7.084665262690076126, 69.10535201082151957, 10.88017736071109987 ) ) ;
#84412=CARTESIAN_POINT ( 'NONE',  ( 14.92337183194729988, 39.34226448433412315, -8.527530157486177487 ) ) ;
#84413=ORIENTED_EDGE ( 'NONE', *, *, #36828, .T. ) ;
#84414=CARTESIAN_POINT ( 'NONE',  ( 17.20831665107776587, 34.13393115100078745, -7.208316651077762316 ) ) ;
#84415=COLOUR_RGB ( '', 0.66274510, 0.83137255, 0.94901961) ;
#84416=CARTESIAN_POINT ( 'NONE',  ( 12.91533473730992121, 39.52201867748817676, 10.88017736071110164 ) ) ;
#84417=CARTESIAN_POINT ( 'NONE',  ( 19.84674366389459266, 33.30059781766744464, 2.638427012816836559 ) ) ;
#84418=CARTESIAN_POINT ( 'NONE',  ( 0.6178305044545838731, 24.74863466993042493, 9.382169495545420901 ) ) ;
#84419=CARTESIAN_POINT ( 'NONE',  ( 10.00000000000000178, 69.31368534415484817, 10.88017736071110342 ) ) ;
#84420=CARTESIAN_POINT ( 'NONE',  ( 19.42250999205614193, 60.14701867748817676, 5.440088680355555262 ) ) ;
#84421=CARTESIAN_POINT ( 'NONE',  ( 4.559911319644449179, 48.89701867748817676, 9.422509992056141925 ) ) ;
#84422=CARTESIAN_POINT ( 'NONE',  ( 12.91533473730993009, 6.605352010821504471, -10.88017736071109987 ) ) ;
#84423=CARTESIAN_POINT ( 'NONE',  ( 10.00000000000000178, 63.05374883491396076, 14.16423886937410082 ) ) ;
#84425=CARTESIAN_POINT ( 'NONE',  ( -2.816281873526471635, 18.91530133659708213, -3.434112377981056508 ) ) ;
#84427=ORIENTED_EDGE ( 'NONE', *, *, #51919, .F. ) ;
#84428=CARTESIAN_POINT ( 'NONE',  ( 22.81628187352647785, 16.41530133659708923, 3.434112377981063169 ) ) ;
#84429=CARTESIAN_POINT ( 'NONE',  ( 12.91533473730992121, 24.52201867748816966, 10.88017736071110164 ) ) ;
#84430=CARTESIAN_POINT ( 'NONE',  ( 15.44008868035555260, 54.73035201082150536, 9.422509992056143702 ) ) ;
#84433=CARTESIAN_POINT ( 'NONE',  ( 5.076628168052704559, 5.175597817667451750, -8.527530157486179263 ) ) ;
#84434=CARTESIAN_POINT ( 'NONE',  ( 5.076628168052703671, 51.84226448433412315, 8.527530157486179263 ) ) ;
#84435=CARTESIAN_POINT ( 'NONE',  ( 19.84674366389459621, 33.50893115100078745, 7.409399052514197653E-17 ) ) ;
#84436=CARTESIAN_POINT ( 'NONE',  ( -1.099225684535947600, 63.70696800326376774, -6.408140936763238038 ) ) ;
#84440=CARTESIAN_POINT ( 'NONE',  ( 0.1532563361054083140, 11.00893115100078568, 1.131784320476157264E-15 ) ) ;
#84441=CARTESIAN_POINT ( 'NONE',  ( 0.2751277870542911952, 33.21833443783938122, 6.499999999999992006 ) ) ;
#84443=CARTESIAN_POINT ( 'NONE',  ( 19.84674366389459621, 48.50893115100078745, 7.409399052514197653E-17 ) ) ;
#84446=CARTESIAN_POINT ( 'NONE',  ( 3.591859063236763294, 13.29030133659708746, -11.09922568453595026 ) ) ;
#84447=CARTESIAN_POINT ( 'NONE',  ( 20.88017736071110164, 55.35535201082149825, 2.915334737309930979 ) ) ;
#84448=CARTESIAN_POINT ( 'NONE',  ( 13.79529636645030344, 38.26208216824729647, 14.16423886937410614 ) ) ;
#84449=CARTESIAN_POINT ( 'NONE',  ( 20.00000000000138911, 90.62861641165379467, 5.317662825071818311 ) ) ;
#84450=CARTESIAN_POINT ( 'NONE',  ( 2.917880565312948704, 47.63708216824730357, 12.26659068614894643 ) ) ;
#84451=CARTESIAN_POINT ( 'NONE',  ( 20.36894250292379382, 53.67874883491397497, 10.36894250292379205 ) ) ;
#84452=CARTESIAN_POINT ( 'NONE',  ( 24.16423886937410614, 29.51208216824729647, -3.795296366450302550 ) ) ;
#84453=CARTESIAN_POINT ( 'NONE',  ( -0.3689425029237881626, 27.42874883491397142, 10.36894250292379027 ) ) ;
#84455=CARTESIAN_POINT ( 'NONE',  ( -0.03743638938522369369, 29.25197528031018379, -6.399506433553970197 ) ) ;
#84458=CARTESIAN_POINT ( 'NONE',  ( 12.63842701281683034, 37.46726448433411605, 9.846743663894596210 ) ) ;
#84459=CARTESIAN_POINT ( 'NONE',  ( 17.96484262340118221, 24.93868534415484461, 7.964842623401181321 ) ) ;
#84461=CARTESIAN_POINT ( 'NONE',  ( 12.63842701281683034, 57.46726448433411605, 9.846743663894596210 ) ) ;
#84463=CARTESIAN_POINT ( 'NONE',  ( 2.791683348922237240, 45.38393115100079456, -7.208316651077763204 ) ) ;
#84464=CARTESIAN_POINT ( 'NONE',  ( -2.816281873526473856, 54.12363466993041783, 9.499525473075851096E-16 ) ) ;
#84466=CARTESIAN_POINT ( 'NONE',  ( 2.791683348922237240, 45.38393115100079456, -7.208316651077763204 ) ) ;
#84467=CARTESIAN_POINT ( 'NONE',  ( 7.361572987183170547, 57.05059781766744464, 9.846743663894590881 ) ) ;
#84468=CARTESIAN_POINT ( 'NONE',  ( -4.164238869374099039, 41.80374883491397497, 8.674139862899312516E-16 ) ) ;
#84469=EDGE_CURVE ( 'NONE', #80952, #66014, #1937, .T. ) ;
#84471=CARTESIAN_POINT ( 'NONE',  ( -4.164238869374099039, 16.80374883491396787, 8.674139862899312516E-16 ) ) ;
#84472=CARTESIAN_POINT ( 'NONE',  ( -0.8801773607110991993, 57.85535201082149825, -2.915334737309923874 ) ) ;
#84474=CARTESIAN_POINT ( 'NONE',  ( 10.00000000000000000, 6.813685344154838397, -10.88017736071110342 ) ) ;
#84475=CARTESIAN_POINT ( 'NONE',  ( 6.565887622018943937, 18.08196800326375708, -12.81628187352647608 ) ) ;
#84477=CARTESIAN_POINT ( 'NONE',  ( -0.8801773607111009756, 68.06368534415484817, 1.068504757029289695E-15 ) ) ;
#84478=CARTESIAN_POINT ( 'NONE',  ( 21.92686044187657046, 42.39664270246084499, -3.195792623639524432 ) ) ;
#84480=CARTESIAN_POINT ( 'NONE',  ( 22.26659068614894466, 63.88708216824730357, 7.082119434687054849 ) ) ;
#84482=CARTESIAN_POINT ( 'NONE',  ( -0.8801773607111008646, 33.27201867748817676, 2.915334737309923430 ) ) ;
#84483=CARTESIAN_POINT ( 'NONE',  ( 17.96484262340118221, 24.93868534415484461, 7.964842623401181321 ) ) ;
#84484=CARTESIAN_POINT ( 'NONE',  ( 19.84674366389459266, 58.71726448433411605, -2.638427012816827677 ) ) ;
#84485=CARTESIAN_POINT ( 'NONE',  ( 19.84674366389459266, 53.71726448433411605, -2.638427012816827677 ) ) ;
#84486=CARTESIAN_POINT ( 'NONE',  ( 22.81628187352647785, 46.62363466993041783, 6.195893100308588602E-16 ) ) ;
#84487=LINE ( 'NONE', #77455, #88679 ) ;
#84488=EDGE_LOOP ( 'NONE', ( #35580, #70188, #23789, #13320 ) ) ;
#84489=CARTESIAN_POINT ( 'NONE',  ( 20.88017736071110875, 15.77201867748817143, -2.915334737309920765 ) ) ;
#84490=CARTESIAN_POINT ( 'NONE',  ( -1.099225684535947600, 14.54030133659708568, 6.408140936763237150 ) ) ;
#84493=CARTESIAN_POINT ( 'NONE',  ( 10.00000000000000000, 44.75893115100078745, -9.846743663894594434 ) ) ;
#84494=CARTESIAN_POINT ( 'NONE',  ( 4.559911319644449179, 47.23035201082150536, -9.422509992056141925 ) ) ;
#84495=CARTESIAN_POINT ( 'NONE',  ( -2.816281873526473856, 24.12363466993042138, 9.499525473075851096E-16 ) ) ;
#84496=CARTESIAN_POINT ( 'NONE',  ( 2.035157376598824452, 68.68868534415484817, 7.964842623401179544 ) ) ;
#84499=CARTESIAN_POINT ( 'NONE',  ( -2.816281873526471635, 58.91530133659707502, -3.434112377981056508 ) ) ;
#84502=CARTESIAN_POINT ( 'NONE',  ( 17.96484262340118221, 46.18868534415484106, -7.964842623401177768 ) ) ;
#84503=CARTESIAN_POINT ( 'NONE',  ( 3.591859063236761518, 44.95696800326376064, 11.09922568453594849 ) ) ;
#84504=CARTESIAN_POINT ( 'NONE',  ( 24.16423886937409904, 14.09541550158063217, 3.795296366450317205 ) ) ;
#84505=CARTESIAN_POINT ( 'NONE',  ( 7.361572987183170547, 7.050597817667451750, 9.846743663894590881 ) ) ;
#84508=CARTESIAN_POINT ( 'NONE',  ( 1.472469842513823179, 20.59226448433411960, -4.923371831947296329 ) ) ;
#84510=CARTESIAN_POINT ( 'NONE',  ( 6.204703633549690345, 40.76208216824731778, -14.16423886937410259 ) ) ;
#84511=CARTESIAN_POINT ( 'NONE',  ( 7.084665262690076126, 2.022018677488170990, -10.88017736071110164 ) ) ;
#84514=CARTESIAN_POINT ( 'NONE',  ( 15.44008868035555793, 6.397018677488170546, -9.422509992056140149 ) ) ;
#84516=ORIENTED_EDGE ( 'NONE', *, *, #58859, .T. ) ;
#84518=CARTESIAN_POINT ( 'NONE',  ( 2.035157376598824452, 8.688685344154839285, 7.964842623401179544 ) ) ;
#84519=CARTESIAN_POINT ( 'NONE',  ( -0.8801773607111009756, 8.063685344154837509, 1.068504757029289695E-15 ) ) ;
#84520=CARTESIAN_POINT ( 'NONE',  ( 12.63842701281683922, 44.55059781766745175, -9.846743663894590881 ) ) ;
#84521=CARTESIAN_POINT ( 'NONE',  ( 16.40814093676324603, 32.45696800326375353, -11.09922568453594671 ) ) ;
#84522=CYLINDRICAL_SURFACE ( 'NONE', #10804, 0.5000000000000004441 ) ;
#84523=CARTESIAN_POINT ( 'NONE',  ( 0.2751277870542969683, 2.282175860852373894, -6.500000000000000888 ) ) ;
#84524=CARTESIAN_POINT ( 'NONE',  ( 22.26659068614894466, 8.887082168247300018, 7.082119434687054849 ) ) ;
#84525=CARTESIAN_POINT ( 'NONE',  ( 20.88017736071110875, 30.77201867748816966, -2.915334737309920765 ) ) ;
#84526=CARTESIAN_POINT ( 'NONE',  ( -0.8801773607110991993, 7.855352010821506248, -2.915334737309923874 ) ) ;
#84527=CARTESIAN_POINT ( 'NONE',  ( 2.791683348922240793, 36.63393115100078035, 7.208316651077764092 ) ) ;
#84528=CARTESIAN_POINT ( 'NONE',  ( -25.69000000000001194, 93.50000000000000000, -10.09898361729590199 ) ) ;
#84529=CARTESIAN_POINT ( 'NONE',  ( 17.20831665107776587, 27.88393115100078390, 7.208316651077764980 ) ) ;
#84530=DIRECTION ( 'NONE',  ( -0.000000000000000000, 1.000000000000000000, -0.000000000000000000 ) ) ;
#84534=PRESENTATION_STYLE_ASSIGNMENT (( #8534 ) ) ;
#84535=VERTEX_POINT ( 'NONE', #46426 ) ;
#84536=CARTESIAN_POINT ( 'NONE',  ( 19.84674366389459266, 53.71726448433411605, -2.638427012816827677 ) ) ;
#84537=CARTESIAN_POINT ( 'NONE',  ( 17.96484262340118221, 36.18868534415484106, -7.964842623401177768 ) ) ;
#84538=CARTESIAN_POINT ( 'NONE',  ( 2.035157376598822676, 42.43868534415483396, -7.964842623401177768 ) ) ;
#84539=CARTESIAN_POINT ( 'NONE',  ( 10.00000000000000178, 4.313685344154837509, 10.88017736071110342 ) ) ;
#84540=CARTESIAN_POINT ( 'NONE',  ( -2.816281873526473856, 29.33196800326376064, 3.434112377981055619 ) ) ;
#84541=CARTESIAN_POINT ( 'NONE',  ( 20.36894250292379382, 18.67874883491397142, 10.36894250292379205 ) ) ;
#84542=CARTESIAN_POINT ( 'NONE',  ( 0.6178305044545818747, 43.49863466993042493, -9.382169495545419124 ) ) ;
#84544=CARTESIAN_POINT ( 'NONE',  ( 1.472469842513823179, 51.42559781766745886, 4.923371831947296329 ) ) ;
#84545=CARTESIAN_POINT ( 'NONE',  ( 20.88017736071110519, 50.56368534415484106, 2.639326808657452039E-16 ) ) ;
#84546=CARTESIAN_POINT ( 'NONE',  ( 0.5774900079438607392, 18.48035201082150536, 5.440088680355550821 ) ) ;
#84547=ORIENTED_EDGE ( 'NONE', *, *, #72228, .T. ) ;
#84548=CARTESIAN_POINT ( 'NONE',  ( 20.88017736071110519, 20.56368534415484106, 2.639326808657452039E-16 ) ) ;
#84550=CARTESIAN_POINT ( 'NONE',  ( 2.035157376598822676, 57.43868534415484106, -7.964842623401177768 ) ) ;
#84551=CYLINDRICAL_SURFACE ( 'NONE', #72637, 11.92686044187656513 ) ;
#84552=CARTESIAN_POINT ( 'NONE',  ( 20.88017736071110519, 60.56368534415484106, 2.639326808657452039E-16 ) ) ;
#84553=CARTESIAN_POINT ( 'NONE',  ( 2.791683348922237240, 5.383931151000785675, -7.208316651077763204 ) ) ;
#84554=CARTESIAN_POINT ( 'NONE',  ( -0.8801773607111008646, 63.27201867748817676, 2.915334737309923430 ) ) ;
#84556=EDGE_CURVE ( 'NONE', #49843, #31069, #23939, .T. ) ;
#84557=CARTESIAN_POINT ( 'NONE',  ( -46.75138744620058873, 100.8579332310653598, 9.074091037931069081 ) ) ;
#84558=CARTESIAN_POINT ( 'NONE',  ( 12.63842701281683034, 2.467264484334118269, 9.846743663894596210 ) ) ;
#84559=CARTESIAN_POINT ( 'NONE',  ( 0.1532563361054083140, 46.00893115100079456, 1.131784320476157264E-15 ) ) ;
#84561=EDGE_LOOP ( 'NONE', ( #54719, #82838, #81993, #82168 ) ) ;
#84562=CYLINDRICAL_SURFACE ( 'NONE', #36232, 0.5000000000000004441 ) ;
#84564=CARTESIAN_POINT ( 'NONE',  ( 2.603489959281591659, 10.43575266056827644, -6.500000000000006217 ) ) ;
#84565=AXIS2_PLACEMENT_3D ( 'NONE', #82375, #28875, #59377 ) ;
#84566=CARTESIAN_POINT ( 'NONE',  ( 17.08211943468705130, 23.47041550158063572, 12.26659068614894998 ) ) ;
#84567=CYLINDRICAL_SURFACE ( 'NONE', #20307, 11.92686044187656513 ) ;
#84568=FACE_OUTER_BOUND ( 'NONE', #30758, .T. ) ;
#84569=CARTESIAN_POINT ( 'NONE',  ( -0.8801773607111009756, 58.06368534415484106, 1.068504757029289695E-15 ) ) ;
#84570=CARTESIAN_POINT ( 'NONE',  ( 19.42250999205614548, 20.98035201082150891, -5.440088680355545492 ) ) ;
#84571=CARTESIAN_POINT ( 'NONE',  ( 0.1532563361054083140, 66.00893115100079456, 1.131784320476157264E-15 ) ) ;
#84573=CARTESIAN_POINT ( 'NONE',  ( 2.791683348922240793, 6.633931151000785675, 7.208316651077764092 ) ) ;
#84574=CARTESIAN_POINT ( 'NONE',  ( 18.52753015748618282, 3.925597817667451306, -4.923371831947291888 ) ) ;
#84575=CARTESIAN_POINT ( 'NONE',  ( 22.81628187352647785, 31.41530133659709279, 3.434112377981063169 ) ) ;
#84576=CARTESIAN_POINT ( 'NONE',  ( 0.1532563361054100626, 25.80059781766744820, -2.638427012816831230 ) ) ;
#84579=CARTESIAN_POINT ( 'NONE',  ( 10.00000000000000178, 10.37363466993041961, 12.81628187352647608 ) ) ;
#84581=CARTESIAN_POINT ( 'NONE',  ( 0.1532563361054100626, 5.800597817667452638, -2.638427012816831230 ) ) ;
#84583=ORIENTED_EDGE ( 'NONE', *, *, #20763, .F. ) ;
#84586=CARTESIAN_POINT ( 'NONE',  ( 20.88017736071110875, 20.77201867748816611, -2.915334737309920765 ) ) ;
#84587=CARTESIAN_POINT ( 'NONE',  ( -2.266590686148945544, 16.38708216824730357, -7.082119434687050408 ) ) ;
#84588=CARTESIAN_POINT ( 'NONE',  ( 18.52753015748618282, 38.92559781766745175, -4.923371831947291888 ) ) ;
#84589=CARTESIAN_POINT ( 'NONE',  ( 0.1532563361054100626, 0.8005978176674514168, -2.638427012816831230 ) ) ;
#84590=CARTESIAN_POINT ( 'NONE',  ( 21.09922568453594849, 56.20696800326375353, 6.408140936763242479 ) ) ;
#84592=CARTESIAN_POINT ( 'NONE',  ( 4.559911319644449179, 28.89701867748817321, 9.422509992056141925 ) ) ;
#84596=CARTESIAN_POINT ( 'NONE',  ( 13.43411237798105340, 15.58196800326374998, 12.81628187352647963 ) ) ;
#84597=CARTESIAN_POINT ( 'NONE',  ( 16.40814093676323893, 10.79030133659708923, 11.09922568453595026 ) ) ;
#84598=CARTESIAN_POINT ( 'NONE',  ( 18.52753015748617571, 43.09226448433412315, 4.923371831947298993 ) ) ;
#84600=CARTESIAN_POINT ( 'NONE',  ( 0.6178305044545838731, 54.74863466993042493, 9.382169495545420901 ) ) ;
#84601=CARTESIAN_POINT ( 'NONE',  ( -0.8801773607111009756, 48.06368534415484817, 1.068504757029289695E-15 ) ) ;
#84604=CARTESIAN_POINT ( 'NONE',  ( 15.44008868035555260, 59.73035201082151247, 9.422509992056143702 ) ) ;
#84605=CARTESIAN_POINT ( 'NONE',  ( 12.91533473730992121, 44.52201867748816966, 10.88017736071110164 ) ) ;
#84607=CARTESIAN_POINT ( 'NONE',  ( 7.084665262690076126, 64.10535201082150536, 10.88017736071109987 ) ) ;
#84608=CARTESIAN_POINT ( 'NONE',  ( 12.63842701281683922, 49.55059781766744464, -9.846743663894590881 ) ) ;
#84609=CARTESIAN_POINT ( 'NONE',  ( -0.8801773607111008646, 3.272018677488171434, 2.915334737309923430 ) ) ;
#84611=CARTESIAN_POINT ( 'NONE',  ( 13.43411237798106583, 22.66530133659708923, -12.81628187352647252 ) ) ;
#84612=ORIENTED_EDGE ( 'NONE', *, *, #73376, .T. ) ;
#84613=CARTESIAN_POINT ( 'NONE',  ( 7.084665262690076126, 32.02201867748816966, -10.88017736071110164 ) ) ;
#84614=CARTESIAN_POINT ( 'NONE',  ( -2.816281873526473856, 4.123634669930420493, 9.499525473075851096E-16 ) ) ;
#84615=CARTESIAN_POINT ( 'NONE',  ( 12.91533473730993009, 16.60535201082150891, -10.88017736071109987 ) ) ;
#84616=CARTESIAN_POINT ( 'NONE',  ( -0.8801773607111008646, 33.27201867748817676, 2.915334737309923430 ) ) ;
#84617=CARTESIAN_POINT ( 'NONE',  ( 2.917880565312948704, 37.63708216824731068, 12.26659068614894643 ) ) ;
#84618=CARTESIAN_POINT ( 'NONE',  ( 7.361572987183169658, 24.96726448433412315, -9.846743663894592657 ) ) ;
#84619=CARTESIAN_POINT ( 'NONE',  ( 19.42250999205614548, 55.98035201082150536, -5.440088680355545492 ) ) ;
#84620=CARTESIAN_POINT ( 'NONE',  ( 0.6076426042653103599, 32.37576471608601025, -6.499999999999992006 ) ) ;
#84621=CARTESIAN_POINT ( 'NONE',  ( -0.3689425029237898834, 6.178748834913968757, -10.36894250292378850 ) ) ;
#84623=PRESENTATION_STYLE_ASSIGNMENT (( #69619 ) ) ;
#84624=CARTESIAN_POINT ( 'NONE',  ( 18.52753015748618282, 63.92559781766745886, -4.923371831947291888 ) ) ;
#84627=CARTESIAN_POINT ( 'NONE',  ( 24.16423886937409904, 34.09541550158064638, 3.795296366450317205 ) ) ;
#84628=CARTESIAN_POINT ( 'NONE',  ( 17.08211943468705130, 43.47041550158063927, 12.26659068614894998 ) ) ;
#84629=CARTESIAN_POINT ( 'NONE',  ( 1.472469842513823179, 1.425597817667451528, 4.923371831947296329 ) ) ;
#84630=CARTESIAN_POINT ( 'NONE',  ( 16.40814093676324603, 7.456968003263754419, -11.09922568453594671 ) ) ;
#84631=CARTESIAN_POINT ( 'NONE',  ( 10.00000000000000178, 62.25893115100078745, 9.846743663894594434 ) ) ;
#84633=CARTESIAN_POINT ( 'NONE',  ( 20.88017736071110519, 55.56368534415484817, 2.639326808657452039E-16 ) ) ;
#84634=CARTESIAN_POINT ( 'NONE',  ( 6.565887622018943937, 13.08196800326374998, -12.81628187352647608 ) ) ;
#84635=CARTESIAN_POINT ( 'NONE',  ( 13.79529636645030344, 28.26208216824729647, 14.16423886937410614 ) ) ;
#84636=CARTESIAN_POINT ( 'NONE',  ( 17.96484262340118221, 34.93868534415482685, 7.964842623401181321 ) ) ;
#84637=DIRECTION ( 'NONE',  ( 0.5547001962252290364, 0.8320502943378437211, 0.000000000000000000 ) ) ;
#84638=CARTESIAN_POINT ( 'NONE',  ( 19.42250999205614193, 60.14701867748817676, 5.440088680355555262 ) ) ;
#84646=CARTESIAN_POINT ( 'NONE',  ( -0.3689425029237898834, 6.178748834913968757, -10.36894250292378850 ) ) ;
#84647=CARTESIAN_POINT ( 'NONE',  ( 24.16423886937409904, 59.09541550158063217, 3.795296366450317205 ) ) ;
#84648=CARTESIAN_POINT ( 'NONE',  ( 22.26659068614894466, 58.88708216824729647, 7.082119434687054849 ) ) ;
#84649=CARTESIAN_POINT ( 'NONE',  ( 19.84674366389459266, 33.30059781766744464, 2.638427012816836559 ) ) ;
#84650=CARTESIAN_POINT ( 'NONE',  ( 19.84674366389459266, 63.71726448433412315, -2.638427012816827677 ) ) ;
#84652=CARTESIAN_POINT ( 'NONE',  ( -2.816281873526473856, 4.123634669930420493, 9.499525473075851096E-16 ) ) ;
#84653=VERTEX_POINT ( 'NONE', #22961 ) ;
#84654=CARTESIAN_POINT ( 'NONE',  ( 10.00000000000000000, 50.55374883491396787, -14.16423886937410082 ) ) ;
#84656=CARTESIAN_POINT ( 'NONE',  ( -4.164238869374099039, 41.80374883491397497, 8.674139862899312516E-16 ) ) ;
#84658=CARTESIAN_POINT ( 'NONE',  ( 22.81628187352648496, 51.83196800326376064, -3.434112377981050290 ) ) ;
#84659=VECTOR ( 'NONE', #88253, 1000.000000000000000 ) ;
#84660=CARTESIAN_POINT ( 'NONE',  ( -0.8801773607110991993, 22.85535201082150181, -2.915334737309923874 ) ) ;
#84661=CARTESIAN_POINT ( 'NONE',  ( 12.63842701281683034, 52.46726448433413026, 9.846743663894596210 ) ) ;
#84662=CARTESIAN_POINT ( 'NONE',  ( 4.559911319644449179, 28.89701867748817321, 9.422509992056141925 ) ) ;
#84664=CARTESIAN_POINT ( 'NONE',  ( 2.791683348922240793, 56.63393115100078035, 7.208316651077764092 ) ) ;
#84670=CARTESIAN_POINT ( 'NONE',  ( 0.1532563361054100626, 0.8005978176674514168, -2.638427012816831230 ) ) ;
#84675=CARTESIAN_POINT ( 'NONE',  ( 19.84674366389459621, 28.50893115100078745, 7.409399052514197653E-17 ) ) ;
#84676=EDGE_CURVE ( 'NONE', #20694, #9403, #37797, .T. ) ;
#84678=FACE_OUTER_BOUND ( 'NONE', #78481, .T. ) ;
#84679=DIRECTION ( 'NONE',  ( -0.000000000000000000, -0.000000000000000000, -1.000000000000000000 ) ) ;
#84682=CARTESIAN_POINT ( 'NONE',  ( 19.84674366389459266, 53.71726448433411605, -2.638427012816827677 ) ) ;
#84683=CARTESIAN_POINT ( 'NONE',  ( 22.26659068614895176, 39.72041550158063217, -7.082119434687042414 ) ) ;
#84684=CARTESIAN_POINT ( 'NONE',  ( 18.52753015748617571, 58.09226448433411605, 4.923371831947298993 ) ) ;
#84686=CARTESIAN_POINT ( 'NONE',  ( 7.361572987183170547, 17.05059781766745530, 9.846743663894590881 ) ) ;
#84687=CARTESIAN_POINT ( 'NONE',  ( -2.816281873526473856, 49.33196800326374643, 3.434112377981055619 ) ) ;
#84688=CARTESIAN_POINT ( 'NONE',  ( -4.164238869374099039, 1.803748834913967647, 8.674139862899312516E-16 ) ) ;
#84689=CARTESIAN_POINT ( 'NONE',  ( 3.591859063236763294, -1.709698663402913210, -11.09922568453595026 ) ) ;
#84690=CARTESIAN_POINT ( 'NONE',  ( 10.00000000000000178, 59.31368534415484106, 10.88017736071110342 ) ) ;
#84691=CARTESIAN_POINT ( 'NONE',  ( 19.84674366389459621, 43.50893115100078745, 7.409399052514197653E-17 ) ) ;
#84692=( BOUNDED_SURFACE ( )  B_SPLINE_SURFACE ( 1, 2, ( 
 ( #14413, #5918, #7413, #44883, #75385, #6903, #96940, #29880, #81901, #44396, #22408, #37909, #68397, #14913, #60382, #90880, #13410, #21414, #20923, #74896, #43896, #89407, #52883, #83393, #66905, #51909, #45383, #83885, #98918, #91377, #29387, #30373, #97424, #74395, #60877, #22905, #6394, #7897, #53375, #15414, #45896, #28890, #36909, #59888, #82394, #76382, #66408, #36412, #59395, #28414, #58909, #89898, #13918, #67401, #70370, #92852, #8381, #32346, #17852, #24380, #39864, #78344, #86349, #1888, #423, #38889, #69377, #61861, #16378, #70865, #2381, #85859, #54847, #48338, #17371, #78841, #23402, #8864, #93842, #23892, #62849, #30874, #899, #31361, #92366, #38392, #68895, #55354, #61370, #62347, #39380, #31850, #93347, #25369, #55854, #91880, #53886, #69875, #84392, #24872, #1395, #85361, #46861, #32835, #54358, #15891, #47841, #16873, #47348, #77353, #63337, #84869, #77850, #46376, #9360, #9866, #76865, #40364, #71831, #3340, #79334, #50808, #26324, #88800, #34804, #56346, #12307, #79821, #73299, #57309, #10843, #57801, #64309, #65293, #34298, #64796, #48823, #19806, #95314, #19322, #49806, #40851, #42321, #94329, #87320, #95820, #50296, #80809, #88308, #87801, #27300, #25849, #94820, #63818, #18837, #86841, #33323, #42815, #4334, #41364, #56821, #4823, #27797, #35297, #65790, #41842, #96324, #33802, #18345, #58282, #20310, #49317, #10352, #26816, #80314, #71355, #11323, #72308, #3839, #11814, #2874, #72795, #51294, #96820, #13794, #73788, #12794, #36795, #21298, #14300, #67289, #81780, #75276, #60761, #97817, #82780, #22295, #30258, #44771, #43294, #13295, #43781, #5802, #59282, #14802, #45274, #29764, #29278, #91261, #60272, #22787, #66285, #51790, #37791, #66791, #6787, #5319, #74274, #36294, #97311, #81299, #35798, #98310, #28296, #6293, #82277, #74784, #37301, #68288, #98809, #58789, #89296, #44280, #59774, #89781, #75769, #28784, #90267, #20807, #52282, #21801, #67788, #90771, #52769, #83277, #7290, #93723, #69269, #32720, #77734, #306, #55229, #23779, #17256, #1285, #53763, #1769, #8270, #9245, #77242, #8749, #91763, #62726, #39268, #62234, #92741, #83771, #85250, #38281, #31242, #39755, #93226, #24752, #32225, #31739, #70254, #68776, #38767, #7786, #61738, #30750, #76269, #85744, #47230, #84278, #789, #47731, #70751, #78228, #9741, #84757, #40241, #15778, #61257, #2265, #63219, #92256, #53265, #69757, #24265, #15295, #46267, #54245, #16263, #46746, #45777, #23285, #76751, #54729, #16756, #17743, #55741, #79709, #64192, #57192, #11208, #94210, #19205, #4714, #41727, #26697, #65179, #73175, #87690, #86232 ),
 ( #42213, #80192, #64681, #48219, #25740, #63707, #49687, #40732, #35176, #56232, #95702, #78729, #4216, #94711, #72197, #18725, #26217, #72680, #3726, #57688, #18229, #10239, #27185, #34686, #87201, #34187, #12189, #56710, #71234, #41241, #86727, #48711, #79213, #65677, #71718, #25256, #11703, #2759, #88183, #49205, #19697, #95189, #10724, #50184, #3229, #80695, #42698, #33212, #33694, #6665, #82160, #6175, #36679, #27683, #29154, #81182, #74157, #52167, #37182, #67674, #44660, #44156, #21681, #12682, #51181, #50689, #5691, #43181, #20187, #82660, #90151, #96702, #81663, #14176, #14680, #98184, #22170, #28670, #29641, #28180, #73669, #60148, #75155, #36177, #37667, #13673, #67167, #90645, #58676, #66678, #59163, #13175, #52652, #83155, #66168, #5197, #89668, #88680, #58168, #51681, #97202, #59660, #74665, #89175, #45148, #75653, #97692, #7164, #96200, #35684, #20688, #43671, #21180, #38164, #180, #23163, #54610, #24142, #1158, #674, #9125, #69634, #39640, #22669, #15664, #47112, #61136, #46625, #30136, #76148, #68650, #7673, #1652, #68167, #31619, #70132, #69147, #76633, #38645, #39144, #98687, #60642, #91143, #53146, #31124, #30628, #85127, #61620, #92138, #23662, #83654, #46147, #54124, #91645, #62109, #15170, #92619, #16637, #77124, #84636, #8635, #8152, #77613, #53640, #45651, #16139, #84158, #44482, #51997, #52477, #21500, #82487, #66498, #14004, #29466, #89983, #74984, #6487, #59973, #36994, #58995, #82982, #6006, #67491, #14502, #90467, #59483, #74484, #98012, #60471, #22002, #28501, #44972, #28979, #36501, #66993, #75478, #97516, #90960, #37990, #81990, #6992, #97024, #37496, #67985, #89497, #98512, #29965, #22492, #52965, #68482, #14998, #83477, #21008, #45468, #75969, #43492, #7497, #9, #20512, #58495, #51495, #50997, #89005, #81492, #12995, #35996, #73992, #5518, #13501, #43981, #41548, #20503, #56531, #64501, #72995, #12501, #50989, #4525, #33511, #72013, #3543, #95007, #49504, #5010, #35494, #20000, #57504, #81483, #50501, #12987, #87020, #42037, #27989, #57012, #65492, #64008, #34004, #26515, #87514, #71547, #3057, #88497, #94521, #95514, #72501, #64987, #27497, #58484, #88997, #26040, #18532, #4033, #49023, #57991, #34496, #27007, #80009, #65989, #19027, #11514, #79529, #11029, #88000, #96012, #80998, #19513, #50010, #43000, #80513, #73483, #96516, #12012, #42511, #34988, #66487, #83467, #37487, #82476, #83956, #29456, #82973, #60462, #5998, #51988, #74973, #97505, #14988, #68473, #13492, #58985, #6478, #35985, #73984, #98003, #13996, #75467, #59964, #43971, #91456, #28492, #36492, #44963, #45459, #22982 ) ),
 .UNSPECIFIED., .F., .F., .T. ) 
 B_SPLINE_SURFACE_WITH_KNOTS ( ( 2, 2 ),
 ( 3, 2, 2, 2, 2, 2, 2, 2, 2, 2, 2, 2, 2, 2, 2, 2, 2, 2, 2, 2, 2, 2, 2, 2, 2, 2, 2, 2, 2, 2, 2, 2, 2, 2, 2, 2, 2, 2, 2, 2, 2, 2, 2, 2, 2, 2, 2, 2, 2, 2, 2, 2, 2, 2, 2, 2, 2, 2, 2, 2, 2, 2, 2, 2, 2, 2, 2, 2, 2, 2, 2, 2, 2, 2, 2, 2, 2, 2, 2, 2, 2, 2, 2, 2, 2, 2, 2, 2, 2, 2, 2, 2, 2, 2, 2, 2, 2, 2, 2, 2, 2, 2, 2, 2, 2, 2, 2, 2, 2, 2, 2, 2, 2, 2, 2, 2, 2, 2, 2, 2, 2, 2, 2, 2, 2, 2, 2, 2, 2, 2, 2, 2, 2, 2, 2, 2, 2, 2, 2, 2, 2, 2, 2, 2, 2, 2, 2, 2, 2, 2, 2, 2, 2, 2, 2, 2, 2, 2, 2, 2, 2, 2, 3 ),
 ( 0.000000000000000000, 1.000000000000000000 ),
 ( 0.000000000000000000, 0.005952380952380952051, 0.01190476190476190410, 0.01785714285714285615, 0.02380952380952380820, 0.02976190476190476025, 0.03571428571428571230, 0.04166666666666666435, 0.04761904761904761640, 0.05357142857142856845, 0.05952380952380952051, 0.06547619047619047949, 0.07142857142857142461, 0.07738095238095238360, 0.08333333333333332871, 0.08928571428571428770, 0.09523809523809523281, 0.1011904761904761918, 0.1071428571428571369, 0.1130952380952380959, 0.1190476190476190410, 0.1250000000000000000, 0.1309523809523809590, 0.1369047619047619180, 0.1428571428571428492, 0.1488095238095238082, 0.1547619047619047672, 0.1607142857142857262, 0.1666666666666666574, 0.1726190476190476164, 0.1785714285714285754, 0.1845238095238095344, 0.1904761904761904656, 0.1964285714285714246, 0.2023809523809523836, 0.2083333333333333426, 0.2142857142857142738, 0.2202380952380952328, 0.2261904761904761918, 0.2321428571428571508, 0.2380952380952380820, 0.2440476190476190410, 0.2500000000000000000, 0.2559523809523809312, 0.2619047619047619180, 0.2678571428571428492, 0.2738095238095238360, 0.2797619047619047672, 0.2857142857142856984, 0.2916666666666666852, 0.2976190476190476164, 0.3035714285714285476, 0.3095238095238095344, 0.3154761904761904656, 0.3214285714285714524, 0.3273809523809523836, 0.3333333333333333148, 0.3392857142857143016, 0.3452380952380952328, 0.3511904761904761640, 0.3571428571428571508, 0.3630952380952380820, 0.3690476190476190688, 0.3750000000000000000, 0.3809523809523809312, 0.3869047619047619180, 0.3928571428571428492, 0.3988095238095238360, 0.4047619047619047672, 0.4107142857142856984, 0.4166666666666666852, 0.4226190476190476164, 0.4285714285714285476, 0.4345238095238095344, 0.4404761904761904656, 0.4464285714285714524, 0.4523809523809523836, 0.4583333333333333148, 0.4642857142857143016, 0.4702380952380952328, 0.4761904761904761640, 0.4821428571428571508, 0.4880952380952380820, 0.4940476190476190688, 0.5000000000000000000, 0.5059523809523809312, 0.5119047619047618625, 0.5178571428571429047, 0.5238095238095238360, 0.5297619047619047672, 0.5357142857142856984, 0.5416666666666666297, 0.5476190476190476719, 0.5535714285714286031, 0.5595238095238095344, 0.5654761904761904656, 0.5714285714285713969, 0.5773809523809523281, 0.5833333333333333703, 0.5892857142857143016, 0.5952380952380952328, 0.6011904761904761640, 0.6071428571428570953, 0.6130952380952381375, 0.6190476190476190688, 0.6250000000000000000, 0.6309523809523809312, 0.6369047619047618625, 0.6428571428571429047, 0.6488095238095238360, 0.6547619047619047672, 0.6607142857142856984, 0.6666666666666666297, 0.6726190476190476719, 0.6785714285714286031, 0.6845238095238095344, 0.6904761904761904656, 0.6964285714285713969, 0.7023809523809523281, 0.7083333333333333703, 0.7142857142857143016, 0.7202380952380952328, 0.7261904761904761640, 0.7321428571428570953, 0.7380952380952381375, 0.7440476190476190688, 0.7500000000000000000, 0.7559523809523809312, 0.7619047619047618625, 0.7678571428571429047, 0.7738095238095238360, 0.7797619047619047672, 0.7857142857142856984, 0.7916666666666666297, 0.7976190476190476719, 0.8035714285714286031, 0.8095238095238095344, 0.8154761904761904656, 0.8214285714285713969, 0.8273809523809523281, 0.8333333333333333703, 0.8392857142857143016, 0.8452380952380952328, 0.8511904761904761640, 0.8571428571428570953, 0.8630952380952381375, 0.8690476190476190688, 0.8750000000000000000, 0.8809523809523809312, 0.8869047619047618625, 0.8928571428571429047, 0.8988095238095238360, 0.9047619047619047672, 0.9107142857142856984, 0.9166666666666666297, 0.9226190476190476719, 0.9285714285714286031, 0.9345238095238095344, 0.9404761904761904656, 0.9464285714285713969, 0.9523809523809523281, 0.9583333333333333703, 0.9642857142857143016 ),
 .UNSPECIFIED. ) 
 GEOMETRIC_REPRESENTATION_ITEM ( )  RATIONAL_B_SPLINE_SURFACE ( (
 ( 1.000000000000000000, 0.9659258262890683122, 1.000000000000000000, 0.9659258262890683122, 1.000000000000000000, 0.9659258262890683122, 1.000000000000000000, 0.9659258262890683122, 1.000000000000000000, 0.9659258262890683122, 1.000000000000000000, 0.9659258262890683122, 1.000000000000000000, 0.9659258262890683122, 1.000000000000000000, 0.9659258262890683122, 1.000000000000000000, 0.9659258262890683122, 1.000000000000000000, 0.9659258262890683122, 1.000000000000000000, 0.9659258262890683122, 1.000000000000000000, 0.9659258262890683122, 1.000000000000000000, 0.9659258262890683122, 1.000000000000000000, 0.9659258262890683122, 1.000000000000000000, 0.9659258262890683122, 1.000000000000000000, 0.9659258262890683122, 1.000000000000000000, 0.9659258262890683122, 1.000000000000000000, 0.9659258262890683122, 1.000000000000000000, 0.9659258262890683122, 1.000000000000000000, 0.9659258262890683122, 1.000000000000000000, 0.9659258262890683122, 1.000000000000000000, 0.9659258262890683122, 1.000000000000000000, 0.9659258262890683122, 1.000000000000000000, 0.9659258262890683122, 1.000000000000000000, 0.9659258262890683122, 1.000000000000000000, 0.9659258262890683122, 1.000000000000000000, 0.9659258262890683122, 1.000000000000000000, 0.9659258262890683122, 1.000000000000000000, 0.9659258262890683122, 1.000000000000000000, 0.9659258262890683122, 1.000000000000000000, 0.9659258262890683122, 1.000000000000000000, 0.9659258262890683122, 1.000000000000000000, 0.9659258262890683122, 1.000000000000000000, 0.9659258262890683122, 1.000000000000000000, 0.9659258262890683122, 1.000000000000000000, 0.9659258262890683122, 1.000000000000000000, 0.9659258262890683122, 1.000000000000000000, 0.9659258262890683122, 1.000000000000000000, 0.9659258262890683122, 1.000000000000000000, 0.9659258262890683122, 1.000000000000000000, 0.9659258262890683122, 1.000000000000000000, 0.9659258262890683122, 1.000000000000000000, 0.9659258262890683122, 1.000000000000000000, 0.9659258262890683122, 1.000000000000000000, 0.9659258262890683122, 1.000000000000000000, 0.9659258262890683122, 1.000000000000000000, 0.9659258262890683122, 1.000000000000000000, 0.9659258262890683122, 1.000000000000000000, 0.9659258262890683122, 1.000000000000000000, 0.9659258262890683122, 1.000000000000000000, 0.9659258262890683122, 1.000000000000000000, 0.9659258262890683122, 1.000000000000000000, 0.9659258262890683122, 1.000000000000000000, 0.9659258262890683122, 1.000000000000000000, 0.9659258262890683122, 1.000000000000000000, 0.9659258262890683122, 1.000000000000000000, 0.9659258262890683122, 1.000000000000000000, 0.9659258262890683122, 1.000000000000000000, 0.9659258262890683122, 1.000000000000000000, 0.9659258262890683122, 1.000000000000000000, 0.9659258262890683122, 1.000000000000000000, 0.9659258262890683122, 1.000000000000000000, 0.9659258262890683122, 1.000000000000000000, 0.9659258262890683122, 1.000000000000000000, 0.9659258262890683122, 1.000000000000000000, 0.9659258262890683122, 1.000000000000000000, 0.9659258262890683122, 1.000000000000000000, 0.9659258262890683122, 1.000000000000000000, 0.9659258262890683122, 1.000000000000000000, 0.9659258262890683122, 1.000000000000000000, 0.9659258262890683122, 1.000000000000000000, 0.9659258262890683122, 1.000000000000000000, 0.9659258262890683122, 1.000000000000000000, 0.9659258262890683122, 1.000000000000000000, 0.9659258262890683122, 1.000000000000000000, 0.9659258262890683122, 1.000000000000000000, 0.9659258262890683122, 1.000000000000000000, 0.9659258262890683122, 1.000000000000000000, 0.9659258262890683122, 1.000000000000000000, 0.9659258262890683122, 1.000000000000000000, 0.9659258262890683122, 1.000000000000000000, 0.9659258262890683122, 1.000000000000000000, 0.9659258262890683122, 1.000000000000000000, 0.9659258262890683122, 1.000000000000000000, 0.9659258262890683122, 1.000000000000000000, 0.9659258262890683122, 1.000000000000000000, 0.9659258262890683122, 1.000000000000000000, 0.9659258262890683122, 1.000000000000000000, 0.9659258262890683122, 1.000000000000000000, 0.9659258262890683122, 1.000000000000000000, 0.9659258262890683122, 1.000000000000000000, 0.9659258262890683122, 1.000000000000000000, 0.9659258262890683122, 1.000000000000000000, 0.9659258262890683122, 1.000000000000000000, 0.9659258262890683122, 1.000000000000000000, 0.9659258262890683122, 1.000000000000000000, 0.9659258262890683122, 1.000000000000000000, 0.9659258262890683122, 1.000000000000000000, 0.9659258262890683122, 1.000000000000000000, 0.9659258262890683122, 1.000000000000000000, 0.9659258262890683122, 1.000000000000000000, 0.9659258262890683122, 1.000000000000000000, 0.9659258262890683122, 1.000000000000000000, 0.9659258262890683122, 1.000000000000000000, 0.9659258262890683122, 1.000000000000000000, 0.9659258262890683122, 1.000000000000000000, 0.9659258262890683122, 1.000000000000000000, 0.9659258262890683122, 1.000000000000000000, 0.9659258262890683122, 1.000000000000000000, 0.9659258262890683122, 1.000000000000000000, 0.9659258262890683122, 1.000000000000000000, 0.9659258262890683122, 1.000000000000000000, 0.9659258262890683122, 1.000000000000000000, 0.9659258262890683122, 1.000000000000000000, 0.9659258262890683122, 1.000000000000000000, 0.9659258262890683122, 1.000000000000000000, 0.9659258262890683122, 1.000000000000000000, 0.9659258262890683122, 1.000000000000000000, 0.9659258262890683122, 1.000000000000000000, 0.9659258262890683122, 1.000000000000000000, 0.9659258262890683122, 1.000000000000000000, 0.9659258262890683122, 1.000000000000000000, 0.9659258262890683122, 1.000000000000000000, 0.9659258262890683122, 1.000000000000000000, 0.9659258262890683122, 1.000000000000000000, 0.9659258262890683122, 1.000000000000000000, 0.9659258262890683122, 1.000000000000000000, 0.9659258262890683122, 1.000000000000000000, 0.9659258262890683122, 1.000000000000000000, 0.9659258262890683122, 1.000000000000000000, 0.9659258262890683122, 1.000000000000000000, 0.9659258262890683122, 1.000000000000000000, 0.9659258262890683122, 1.000000000000000000, 0.9659258262890683122, 1.000000000000000000, 0.9659258262890683122, 1.000000000000000000, 0.9659258262890683122, 1.000000000000000000, 0.9659258262890683122, 1.000000000000000000, 0.9659258262890683122, 1.000000000000000000, 0.9659258262890683122, 1.000000000000000000, 0.9659258262890683122, 1.000000000000000000, 0.9659258262890683122, 1.000000000000000000, 0.9659258262890683122, 1.000000000000000000, 0.9659258262890683122, 1.000000000000000000, 0.9659258262890683122, 1.000000000000000000, 0.9659258262890683122, 1.000000000000000000, 0.9659258262890683122, 1.000000000000000000, 0.9659258262890683122, 1.000000000000000000, 0.9659258262890683122, 1.000000000000000000, 0.9659258262890683122, 1.000000000000000000, 0.9659258262890683122, 1.000000000000000000, 0.9659258262890683122, 1.000000000000000000, 0.9659258262890683122, 1.000000000000000000, 0.9659258262890683122, 1.000000000000000000, 0.9659258262890683122, 1.000000000000000000, 0.9659258262890683122, 1.000000000000000000, 0.9659258262890683122, 1.000000000000000000, 0.9659258262890683122, 1.000000000000000000, 0.9659258262890683122, 1.000000000000000000, 0.9659258262890683122, 1.000000000000000000, 0.9659258262890683122, 1.000000000000000000, 0.9659258262890683122, 1.000000000000000000, 0.9659258262890683122, 1.000000000000000000),
 ( 1.000000000000000000, 0.9659258262890683122, 1.000000000000000000, 0.9659258262890683122, 1.000000000000000000, 0.9659258262890683122, 1.000000000000000000, 0.9659258262890683122, 1.000000000000000000, 0.9659258262890683122, 1.000000000000000000, 0.9659258262890683122, 1.000000000000000000, 0.9659258262890683122, 1.000000000000000000, 0.9659258262890683122, 1.000000000000000000, 0.9659258262890683122, 1.000000000000000000, 0.9659258262890683122, 1.000000000000000000, 0.9659258262890683122, 1.000000000000000000, 0.9659258262890683122, 1.000000000000000000, 0.9659258262890683122, 1.000000000000000000, 0.9659258262890683122, 1.000000000000000000, 0.9659258262890683122, 1.000000000000000000, 0.9659258262890683122, 1.000000000000000000, 0.9659258262890683122, 1.000000000000000000, 0.9659258262890683122, 1.000000000000000000, 0.9659258262890683122, 1.000000000000000000, 0.9659258262890683122, 1.000000000000000000, 0.9659258262890683122, 1.000000000000000000, 0.9659258262890683122, 1.000000000000000000, 0.9659258262890683122, 1.000000000000000000, 0.9659258262890683122, 1.000000000000000000, 0.9659258262890683122, 1.000000000000000000, 0.9659258262890683122, 1.000000000000000000, 0.9659258262890683122, 1.000000000000000000, 0.9659258262890683122, 1.000000000000000000, 0.9659258262890683122, 1.000000000000000000, 0.9659258262890683122, 1.000000000000000000, 0.9659258262890683122, 1.000000000000000000, 0.9659258262890683122, 1.000000000000000000, 0.9659258262890683122, 1.000000000000000000, 0.9659258262890683122, 1.000000000000000000, 0.9659258262890683122, 1.000000000000000000, 0.9659258262890683122, 1.000000000000000000, 0.9659258262890683122, 1.000000000000000000, 0.9659258262890683122, 1.000000000000000000, 0.9659258262890683122, 1.000000000000000000, 0.9659258262890683122, 1.000000000000000000, 0.9659258262890683122, 1.000000000000000000, 0.9659258262890683122, 1.000000000000000000, 0.9659258262890683122, 1.000000000000000000, 0.9659258262890683122, 1.000000000000000000, 0.9659258262890683122, 1.000000000000000000, 0.9659258262890683122, 1.000000000000000000, 0.9659258262890683122, 1.000000000000000000, 0.9659258262890683122, 1.000000000000000000, 0.9659258262890683122, 1.000000000000000000, 0.9659258262890683122, 1.000000000000000000, 0.9659258262890683122, 1.000000000000000000, 0.9659258262890683122, 1.000000000000000000, 0.9659258262890683122, 1.000000000000000000, 0.9659258262890683122, 1.000000000000000000, 0.9659258262890683122, 1.000000000000000000, 0.9659258262890683122, 1.000000000000000000, 0.9659258262890683122, 1.000000000000000000, 0.9659258262890683122, 1.000000000000000000, 0.9659258262890683122, 1.000000000000000000, 0.9659258262890683122, 1.000000000000000000, 0.9659258262890683122, 1.000000000000000000, 0.9659258262890683122, 1.000000000000000000, 0.9659258262890683122, 1.000000000000000000, 0.9659258262890683122, 1.000000000000000000, 0.9659258262890683122, 1.000000000000000000, 0.9659258262890683122, 1.000000000000000000, 0.9659258262890683122, 1.000000000000000000, 0.9659258262890683122, 1.000000000000000000, 0.9659258262890683122, 1.000000000000000000, 0.9659258262890683122, 1.000000000000000000, 0.9659258262890683122, 1.000000000000000000, 0.9659258262890683122, 1.000000000000000000, 0.9659258262890683122, 1.000000000000000000, 0.9659258262890683122, 1.000000000000000000, 0.9659258262890683122, 1.000000000000000000, 0.9659258262890683122, 1.000000000000000000, 0.9659258262890683122, 1.000000000000000000, 0.9659258262890683122, 1.000000000000000000, 0.9659258262890683122, 1.000000000000000000, 0.9659258262890683122, 1.000000000000000000, 0.9659258262890683122, 1.000000000000000000, 0.9659258262890683122, 1.000000000000000000, 0.9659258262890683122, 1.000000000000000000, 0.9659258262890683122, 1.000000000000000000, 0.9659258262890683122, 1.000000000000000000, 0.9659258262890683122, 1.000000000000000000, 0.9659258262890683122, 1.000000000000000000, 0.9659258262890683122, 1.000000000000000000, 0.9659258262890683122, 1.000000000000000000, 0.9659258262890683122, 1.000000000000000000, 0.9659258262890683122, 1.000000000000000000, 0.9659258262890683122, 1.000000000000000000, 0.9659258262890683122, 1.000000000000000000, 0.9659258262890683122, 1.000000000000000000, 0.9659258262890683122, 1.000000000000000000, 0.9659258262890683122, 1.000000000000000000, 0.9659258262890683122, 1.000000000000000000, 0.9659258262890683122, 1.000000000000000000, 0.9659258262890683122, 1.000000000000000000, 0.9659258262890683122, 1.000000000000000000, 0.9659258262890683122, 1.000000000000000000, 0.9659258262890683122, 1.000000000000000000, 0.9659258262890683122, 1.000000000000000000, 0.9659258262890683122, 1.000000000000000000, 0.9659258262890683122, 1.000000000000000000, 0.9659258262890683122, 1.000000000000000000, 0.9659258262890683122, 1.000000000000000000, 0.9659258262890683122, 1.000000000000000000, 0.9659258262890683122, 1.000000000000000000, 0.9659258262890683122, 1.000000000000000000, 0.9659258262890683122, 1.000000000000000000, 0.9659258262890683122, 1.000000000000000000, 0.9659258262890683122, 1.000000000000000000, 0.9659258262890683122, 1.000000000000000000, 0.9659258262890683122, 1.000000000000000000, 0.9659258262890683122, 1.000000000000000000, 0.9659258262890683122, 1.000000000000000000, 0.9659258262890683122, 1.000000000000000000, 0.9659258262890683122, 1.000000000000000000, 0.9659258262890683122, 1.000000000000000000, 0.9659258262890683122, 1.000000000000000000, 0.9659258262890683122, 1.000000000000000000, 0.9659258262890683122, 1.000000000000000000, 0.9659258262890683122, 1.000000000000000000, 0.9659258262890683122, 1.000000000000000000, 0.9659258262890683122, 1.000000000000000000, 0.9659258262890683122, 1.000000000000000000, 0.9659258262890683122, 1.000000000000000000, 0.9659258262890683122, 1.000000000000000000, 0.9659258262890683122, 1.000000000000000000, 0.9659258262890683122, 1.000000000000000000, 0.9659258262890683122, 1.000000000000000000, 0.9659258262890683122, 1.000000000000000000, 0.9659258262890683122, 1.000000000000000000, 0.9659258262890683122, 1.000000000000000000, 0.9659258262890683122, 1.000000000000000000, 0.9659258262890683122, 1.000000000000000000, 0.9659258262890683122, 1.000000000000000000, 0.9659258262890683122, 1.000000000000000000, 0.9659258262890683122, 1.000000000000000000, 0.9659258262890683122, 1.000000000000000000, 0.9659258262890683122, 1.000000000000000000, 0.9659258262890683122, 1.000000000000000000, 0.9659258262890683122, 1.000000000000000000, 0.9659258262890683122, 1.000000000000000000, 0.9659258262890683122, 1.000000000000000000, 0.9659258262890683122, 1.000000000000000000, 0.9659258262890683122, 1.000000000000000000, 0.9659258262890683122, 1.000000000000000000, 0.9659258262890683122, 1.000000000000000000, 0.9659258262890683122, 1.000000000000000000, 0.9659258262890683122, 1.000000000000000000, 0.9659258262890683122, 1.000000000000000000, 0.9659258262890683122, 1.000000000000000000, 0.9659258262890683122, 1.000000000000000000, 0.9659258262890683122, 1.000000000000000000, 0.9659258262890683122, 1.000000000000000000, 0.9659258262890683122, 1.000000000000000000, 0.9659258262890683122, 1.000000000000000000, 0.9659258262890683122, 1.000000000000000000, 0.9659258262890683122, 1.000000000000000000, 0.9659258262890683122, 1.000000000000000000) ) ) 
 REPRESENTATION_ITEM ( '' )  SURFACE ( )  );
#84695=EDGE_CURVE ( 'NONE', #39693, #23152, #87374, .T. ) ;
#84696=CARTESIAN_POINT ( 'NONE',  ( -0.8801773607110991993, 57.85535201082149825, -2.915334737309923874 ) ) ;
#84698=CARTESIAN_POINT ( 'NONE',  ( 14.49999999999999822, 11.50000000000000000, 5.000000000000000000 ) ) ;
#84699=CARTESIAN_POINT ( 'NONE',  ( 2.035157376598824452, 28.68868534415484106, 7.964842623401179544 ) ) ;
#84701=CARTESIAN_POINT ( 'NONE',  ( 7.361572987183169658, 64.96726448433412315, -9.846743663894592657 ) ) ;
#84702=CARTESIAN_POINT ( 'NONE',  ( 7.084665262690076126, 59.10535201082150536, 10.88017736071109987 ) ) ;
#84703=CARTESIAN_POINT ( 'NONE',  ( -1.926860441876564023, 62.87045670184114243, 3.195792623639529761 ) ) ;
#84708=CARTESIAN_POINT ( 'NONE',  ( 10.00000000000000178, 34.31368534415484106, 10.88017736071110342 ) ) ;
#84710=CARTESIAN_POINT ( 'NONE',  ( 12.63842701281683922, 34.55059781766745886, -9.846743663894590881 ) ) ;
#84713=CARTESIAN_POINT ( 'NONE',  ( 19.38216949554541557, 2.248634669930420049, -9.382169495545420901 ) ) ;
#84715=CARTESIAN_POINT ( 'NONE',  ( 7.084665262690076126, 17.02201867748817676, -10.88017736071110164 ) ) ;
#84717=CARTESIAN_POINT ( 'NONE',  ( 20.36894250292379738, 24.92874883491396787, -10.36894250292379027 ) ) ;
#84718=CARTESIAN_POINT ( 'NONE',  ( 2.917880565312950480, 65.97041550158063217, -12.26659068614894821 ) ) ;
#84719=CARTESIAN_POINT ( 'NONE',  ( 7.361572987183169658, 29.96726448433411960, -9.846743663894592657 ) ) ;
#84720=CARTESIAN_POINT ( 'NONE',  ( 2.791683348922240793, 21.63393115100078745, 7.208316651077764092 ) ) ;
#84721=FACE_OUTER_BOUND ( 'NONE', #52560, .T. ) ;
#84723=CARTESIAN_POINT ( 'NONE',  ( 14.92337183194729633, 27.67559781766745530, 8.527530157486181039 ) ) ;
#84724=CARTESIAN_POINT ( 'NONE',  ( 20.88017736071110875, 25.77201867748816966, -2.915334737309920765 ) ) ;
#84725=CARTESIAN_POINT ( 'NONE',  ( 2.791683348922237240, 60.38393115100078745, -7.208316651077763204 ) ) ;
#84726=CARTESIAN_POINT ( 'NONE',  ( 6.204703633549690345, 7.845415501580634832, 14.16423886937410082 ) ) ;
#84727=CARTESIAN_POINT ( 'NONE',  ( 5.500000000000000000, 11.50000000000000000, -6.500000000000000888 ) ) ;
#84729=CARTESIAN_POINT ( 'NONE',  ( 2.791683348922240793, 6.633931151000785675, 7.208316651077764092 ) ) ;
#84730=CARTESIAN_POINT ( 'NONE',  ( 10.00000000000000000, 32.87363466993042493, -12.81628187352647608 ) ) ;
#84731=CARTESIAN_POINT ( 'NONE',  ( 14.92337183194729633, 42.67559781766745886, 8.527530157486181039 ) ) ;
#84733=CARTESIAN_POINT ( 'NONE',  ( 1.472469842513823179, 15.59226448433411960, -4.923371831947296329 ) ) ;
#84736=CARTESIAN_POINT ( 'NONE',  ( 20.36894250292379382, 48.67874883491396076, 10.36894250292379205 ) ) ;
#84737=CARTESIAN_POINT ( 'NONE',  ( -0.8801773607111008646, 58.27201867748816966, 2.915334737309923430 ) ) ;
#84739=CARTESIAN_POINT ( 'NONE',  ( 15.44008868035555260, 59.73035201082151247, 9.422509992056143702 ) ) ;
#84740=CARTESIAN_POINT ( 'NONE',  ( 1.472469842513823179, 41.42559781766745886, 4.923371831947296329 ) ) ;
#84741=CARTESIAN_POINT ( 'NONE',  ( 2.035157376598822676, 22.43868534415483396, -7.964842623401177768 ) ) ;
#84743=CARTESIAN_POINT ( 'NONE',  ( 12.63842701281683034, 52.46726448433413026, 9.846743663894596210 ) ) ;
#84745=CARTESIAN_POINT ( 'NONE',  ( 17.96484262340118221, 51.18868534415483396, -7.964842623401177768 ) ) ;
#84750=( LENGTH_UNIT ( ) NAMED_UNIT ( * ) SI_UNIT ( .MILLI., .METRE. ) );
#84751=CARTESIAN_POINT ( 'NONE',  ( 19.84674366389459266, 43.71726448433410894, -2.638427012816827677 ) ) ;
#84752=CARTESIAN_POINT ( 'NONE',  ( 0.1532563361054082862, 16.21726448433411960, 2.638427012816831674 ) ) ;
#84753=CARTESIAN_POINT ( 'NONE',  ( 16.40814093676324603, 52.45696800326375353, -11.09922568453594671 ) ) ;
#84754=CARTESIAN_POINT ( 'NONE',  ( 2.035157376598822676, 22.43868534415483396, -7.964842623401177768 ) ) ;
#84755=CARTESIAN_POINT ( 'NONE',  ( 1.472469842513823179, 51.42559781766745886, 4.923371831947296329 ) ) ;
#84756=CARTESIAN_POINT ( 'NONE',  ( 13.79529636645031943, 30.34541550158063927, -14.16423886937409904 ) ) ;
#84757=CARTESIAN_POINT ( 'NONE',  ( 2.917880565312950480, 60.97041550158063927, -12.26659068614894821 ) ) ;
#84758=CARTESIAN_POINT ( 'NONE',  ( 0.1532563361054083140, 56.00893115100078745, 1.131784320476157264E-15 ) ) ;
#84760=CARTESIAN_POINT ( 'NONE',  ( 19.42250999205614193, 50.14701867748817676, 5.440088680355555262 ) ) ;
#84761=CARTESIAN_POINT ( 'NONE',  ( 10.00000000000000000, 19.75893115100078390, -9.846743663894594434 ) ) ;
#84766=CARTESIAN_POINT ( 'NONE',  ( 0.1532563361054100626, 5.800597817667452638, -2.638427012816831230 ) ) ;
#84768=CARTESIAN_POINT ( 'NONE',  ( 2.917880565312950480, 25.97041550158063572, -12.26659068614894821 ) ) ;
#84769=CARTESIAN_POINT ( 'NONE',  ( 1.472469842513823179, 15.59226448433411960, -4.923371831947296329 ) ) ;
#84770=CARTESIAN_POINT ( 'NONE',  ( -0.8801773607110991993, 42.85535201082150536, -2.915334737309923874 ) ) ;
#84774=CARTESIAN_POINT ( 'NONE',  ( 19.42250999205614548, 25.98035201082150891, -5.440088680355545492 ) ) ;
#84777=CARTESIAN_POINT ( 'NONE',  ( 10.00000000000000178, 8.053748834913967869, 14.16423886937410082 ) ) ;
#84781=CARTESIAN_POINT ( 'NONE',  ( -2.816281873526473856, 14.33196800326375531, 3.434112377981055619 ) ) ;
#84782=CARTESIAN_POINT ( 'NONE',  ( 0.1532563361054100626, 5.800597817667452638, -2.638427012816831230 ) ) ;
#84784=CARTESIAN_POINT ( 'NONE',  ( -0.1503990784575328643, 70.00000000000000000, 6.262539305110068177 ) ) ;
#84785=CARTESIAN_POINT ( 'NONE',  ( 14.92337183194729633, 22.67559781766745175, 8.527530157486181039 ) ) ;
#84786=CARTESIAN_POINT ( 'NONE',  ( 15.44008868035555793, 36.39701867748816966, -9.422509992056140149 ) ) ;
#84787=EDGE_CURVE ( 'NONE', #9539, #94683, #11567, .T. ) ;
#84790=CARTESIAN_POINT ( 'NONE',  ( 20.88017736071110519, 55.56368534415484817, 2.639326808657452039E-16 ) ) ;
#84791=CARTESIAN_POINT ( 'NONE',  ( -46.94000000000001194, 102.9999999999993889, -5.997726559847341932 ) ) ;
#84792=CARTESIAN_POINT ( 'NONE',  ( 19.67858290521088804, 89.00000000000000000, -5.461713021790605360 ) ) ;
#84793=CARTESIAN_POINT ( 'NONE',  ( 10.00000000000000000, 61.81368534415484106, -10.88017736071110342 ) ) ;
#84794=EDGE_CURVE ( 'NONE', #3863, #18606, #49860, .T. ) ;
#84795=CARTESIAN_POINT ( 'NONE',  ( 5.076628168052704559, 65.17559781766745175, -8.527530157486179263 ) ) ;
#84797=CARTESIAN_POINT ( 'NONE',  ( 12.63842701281683034, 27.46726448433411250, 9.846743663894596210 ) ) ;
#84798=CARTESIAN_POINT ( 'NONE',  ( 13.43411237798106583, 52.66530133659708213, -12.81628187352647252 ) ) ;
#84800=CARTESIAN_POINT ( 'NONE',  ( 0.1532563361054083140, 26.00893115100078745, 1.131784320476157264E-15 ) ) ;
#84801=CARTESIAN_POINT ( 'NONE',  ( 13.43411237798106583, 22.66530133659708923, -12.81628187352647252 ) ) ;
#84802=CYLINDRICAL_SURFACE ( 'NONE', #51353, 0.5000000000000004441 ) ;
#84803=CARTESIAN_POINT ( 'NONE',  ( 0.5774900079438590739, 42.64701867748816966, -5.440088680355550821 ) ) ;
#84804=CARTESIAN_POINT ( 'NONE',  ( 0.1532563361054100626, 60.80059781766744464, -2.638427012816831230 ) ) ;
#84809=CARTESIAN_POINT ( 'NONE',  ( 19.84674366389459266, 28.30059781766745886, 2.638427012816836559 ) ) ;
#84810=CARTESIAN_POINT ( 'NONE',  ( 5.076628168052703671, 21.84226448433411960, 8.527530157486179263 ) ) ;
#84811=CARTESIAN_POINT ( 'NONE',  ( 4.559911319644449179, 7.230352010821504471, -9.422509992056141925 ) ) ;
#84812=CARTESIAN_POINT ( 'NONE',  ( 22.81628187352647785, 16.41530133659708923, 3.434112377981063169 ) ) ;
#84816=CARTESIAN_POINT ( 'NONE',  ( 12.91533473730992121, 24.52201867748816966, 10.88017736071110164 ) ) ;
#84818=CARTESIAN_POINT ( 'NONE',  ( 4.559911319644449179, 22.23035201082150536, -9.422509992056141925 ) ) ;
#84819=CARTESIAN_POINT ( 'NONE',  ( 0.8952175423694853640, 12.60160829253885950, -5.990408912944323205 ) ) ;
#84821=CARTESIAN_POINT ( 'NONE',  ( 15.44008868035555260, 34.73035201082151247, 9.422509992056143702 ) ) ;
#84822=CARTESIAN_POINT ( 'NONE',  ( 17.08211943468705840, 60.13708216824729647, -12.26659068614894466 ) ) ;
#84824=CARTESIAN_POINT ( 'NONE',  ( 18.72515096720570327, 6.072280503510315341, -6.499999999999985789 ) ) ;
#84825=CARTESIAN_POINT ( 'NONE',  ( 12.63842701281683922, 24.55059781766745175, -9.846743663894590881 ) ) ;
#84827=CARTESIAN_POINT ( 'NONE',  ( 2.603489959281584998, 6.582109641433292246, 6.499999999999998224 ) ) ;
#84828=CARTESIAN_POINT ( 'NONE',  ( 17.20831665107776587, 62.88393115100078745, 7.208316651077764980 ) ) ;
#84831=CARTESIAN_POINT ( 'NONE',  ( 6.204703633549690345, 20.76208216824730357, -14.16423886937410259 ) ) ;
#84833=CARTESIAN_POINT ( 'NONE',  ( 10.00000000000000000, 39.75893115100078745, -9.846743663894594434 ) ) ;
#84835=CARTESIAN_POINT ( 'NONE',  ( -0.3689425029237898834, 51.17874883491397497, -10.36894250292378850 ) ) ;
#84836=CARTESIAN_POINT ( 'NONE',  ( 19.84674366389459266, 18.30059781766745175, 2.638427012816836559 ) ) ;
#84837=DIRECTION ( 'NONE',  ( 0.8320502943378436100, -0.5547001962252291474, 0.000000000000000000 ) ) ;
#84839=CARTESIAN_POINT ( 'NONE',  ( 20.88017736071110519, 50.56368534415484106, 2.639326808657452039E-16 ) ) ;
#84840=CARTESIAN_POINT ( 'NONE',  ( 13.43411237798106583, 47.66530133659709634, -12.81628187352647252 ) ) ;
#84841=CARTESIAN_POINT ( 'NONE',  ( 0.5774900079438590739, 12.64701867748817143, -5.440088680355550821 ) ) ;
#84842=CARTESIAN_POINT ( 'NONE',  ( 22.81628187352648496, 51.83196800326376064, -3.434112377981050290 ) ) ;
#84844=CARTESIAN_POINT ( 'NONE',  ( 14.92337183194729988, 64.34226448433412315, -8.527530157486177487 ) ) ;
#84845=CARTESIAN_POINT ( 'NONE',  ( 7.361572987183170547, 7.050597817667451750, 9.846743663894590881 ) ) ;
#84848=CARTESIAN_POINT ( 'NONE',  ( 1.697696962861934722, 1.866248959293451470, -6.500000000000000888 ) ) ;
#84849=CARTESIAN_POINT ( 'NONE',  ( -2.266590686148945544, 56.38708216824731068, -7.082119434687050408 ) ) ;
#84850=CARTESIAN_POINT ( 'NONE',  ( 24.16423886937409904, 19.09541550158063927, 3.795296366450317205 ) ) ;
#84851=CARTESIAN_POINT ( 'NONE',  ( 20.88017736071110164, 20.35535201082150891, 2.915334737309930979 ) ) ;
#84852=CARTESIAN_POINT ( 'NONE',  ( 4.559911319644449179, 42.23035201082151247, -9.422509992056141925 ) ) ;
#84855=CARTESIAN_POINT ( 'NONE',  ( 10.00000000000000000, 61.81368534415484106, -10.88017736071110342 ) ) ;
#84856=CARTESIAN_POINT ( 'NONE',  ( -0.8801773607110991993, 57.85535201082149825, -2.915334737309923874 ) ) ;
#84857=CARTESIAN_POINT ( 'NONE',  ( 7.361572987183169658, 14.96726448433411960, -9.846743663894592657 ) ) ;
#84858=CARTESIAN_POINT ( 'NONE',  ( 18.39792806157250382, 19.52224192338640663, 6.499999999999979572 ) ) ;
#84861=CARTESIAN_POINT ( 'NONE',  ( 12.63842701281683922, 4.550597817667451750, -9.846743663894590881 ) ) ;
#84862=CARTESIAN_POINT ( 'NONE',  ( 10.00000000000000178, 32.25893115100078745, 9.846743663894594434 ) ) ;
#84863=CARTESIAN_POINT ( 'NONE',  ( 20.88017736071110519, 20.56368534415484106, 2.639326808657452039E-16 ) ) ;
#84864=CARTESIAN_POINT ( 'NONE',  ( -2.816281873526473856, 34.33196800326376064, 3.434112377981055619 ) ) ;
#84865=CARTESIAN_POINT ( 'NONE',  ( 19.84674366389459266, 8.717264484334116048, -2.638427012816827677 ) ) ;
#84867=CARTESIAN_POINT ( 'NONE',  ( 7.361572987183170547, 47.05059781766745175, 9.846743663894590881 ) ) ;
#84868=CARTESIAN_POINT ( 'NONE',  ( 7.361572987183169658, 34.96726448433411605, -9.846743663894592657 ) ) ;
#84869=CARTESIAN_POINT ( 'NONE',  ( 20.36894250292379382, 23.67874883491397142, 10.36894250292379205 ) ) ;
#84870=CARTESIAN_POINT ( 'NONE',  ( 17.96484262340118221, 31.18868534415483751, -7.964842623401177768 ) ) ;
#84871=CARTESIAN_POINT ( 'NONE',  ( 20.88017736071110875, 15.77201867748817143, -2.915334737309920765 ) ) ;
#84872=CARTESIAN_POINT ( 'NONE',  ( 19.42250999205614548, 50.98035201082151247, -5.440088680355545492 ) ) ;
#84874=CARTESIAN_POINT ( 'NONE',  ( 2.035157376598824452, 33.68868534415484106, 7.964842623401179544 ) ) ;
#84876=CARTESIAN_POINT ( 'NONE',  ( 13.43411237798106583, 37.66530133659708923, -12.81628187352647252 ) ) ;
#84877=CARTESIAN_POINT ( 'NONE',  ( 7.084665262690076126, 34.10535201082151247, 10.88017736071109987 ) ) ;
#84881=CARTESIAN_POINT ( 'NONE',  ( 22.81628187352647785, 56.41530133659708213, 3.434112377981063169 ) ) ;
#84882=CARTESIAN_POINT ( 'NONE',  ( 17.96484262340118221, 54.93868534415484106, 7.964842623401181321 ) ) ;
#84884=CARTESIAN_POINT ( 'NONE',  ( 7.084665262690076126, 52.02201867748816255, -10.88017736071110164 ) ) ;
#84885=PLANE ( 'NONE',  #80113 ) ;
#84887=CARTESIAN_POINT ( 'NONE',  ( 19.42250999205614548, 40.98035201082150536, -5.440088680355545492 ) ) ;
#84888=CARTESIAN_POINT ( 'NONE',  ( -0.2418659066527799606, 25.11633188102327097, 6.114288769123030320 ) ) ;
#84889=CARTESIAN_POINT ( 'NONE',  ( 20.36894250292379738, 59.92874883491397497, -10.36894250292379027 ) ) ;
#84890=CARTESIAN_POINT ( 'NONE',  ( 20.88017736071110164, 65.35535201082150536, 2.915334737309930979 ) ) ;
#84892=LINE ( 'NONE', #60900, #23768 ) ;
#84894=CARTESIAN_POINT ( 'NONE',  ( 7.361572987183170547, 27.05059781766745175, 9.846743663894590881 ) ) ;
#84896=CARTESIAN_POINT ( 'NONE',  ( 0.1532563361054100626, 30.80059781766744820, -2.638427012816831230 ) ) ;
#84897=CARTESIAN_POINT ( 'NONE',  ( 12.91533473730992121, 34.52201867748817676, 10.88017736071110164 ) ) ;
#84898=CARTESIAN_POINT ( 'NONE',  ( 19.84674366389459621, 38.50893115100078745, 7.409399052514197653E-17 ) ) ;
#84900=CARTESIAN_POINT ( 'NONE',  ( 4.559911319644449179, 68.89701867748817676, 9.422509992056141925 ) ) ;
#84901=CARTESIAN_POINT ( 'NONE',  ( 0.5774900079438607392, 48.48035201082150536, 5.440088680355550821 ) ) ;
#84902=CARTESIAN_POINT ( 'NONE',  ( 22.26659068614894466, 58.88708216824729647, 7.082119434687054849 ) ) ;
#84905=CARTESIAN_POINT ( 'NONE',  ( 22.81628187352647785, 16.62363466993042138, 6.195893100308588602E-16 ) ) ;
#84908=CARTESIAN_POINT ( 'NONE',  ( 16.40814093676324603, 27.45696800326375708, -11.09922568453594671 ) ) ;
#84909=CARTESIAN_POINT ( 'NONE',  ( 17.96484262340118221, 26.18868534415483396, -7.964842623401177768 ) ) ;
#84913=CARTESIAN_POINT ( 'NONE',  ( 2.791683348922240793, 6.633931151000785675, 7.208316651077764092 ) ) ;
#84915=CARTESIAN_POINT ( 'NONE',  ( 18.52753015748618282, 43.92559781766745175, -4.923371831947291888 ) ) ;
#84916=CARTESIAN_POINT ( 'NONE',  ( 5.076628168052703671, 41.84226448433411605, 8.527530157486179263 ) ) ;
#84917=CARTESIAN_POINT ( 'NONE',  ( 0.6178305044545838731, 64.74863466993043914, 9.382169495545420901 ) ) ;
#84918=CARTESIAN_POINT ( 'NONE',  ( 19.84674366389459266, 33.30059781766744464, 2.638427012816836559 ) ) ;
#84919=CARTESIAN_POINT ( 'NONE',  ( 20.32896413005680714, 57.60497603579418069, -5.963430220938276349 ) ) ;
#84921=CARTESIAN_POINT ( 'NONE',  ( 19.84674366389459266, 18.71726448433411960, -2.638427012816827677 ) ) ;
#84922=CARTESIAN_POINT ( 'NONE',  ( 1.274849032794231007, 33.57228050351031357, 6.499999999999895195 ) ) ;
#84924=CARTESIAN_POINT ( 'NONE',  ( 12.63842701281683034, 42.46726448433412315, 9.846743663894596210 ) ) ;
#84927=CARTESIAN_POINT ( 'NONE',  ( 13.43411237798105340, 10.58196800326375353, 12.81628187352647963 ) ) ;
#84929=CARTESIAN_POINT ( 'NONE',  ( 12.91533473730992121, 49.52201867748817676, 10.88017736071110164 ) ) ;
#84930=CARTESIAN_POINT ( 'NONE',  ( -4.164238869374099927, 42.01208216824728936, 3.795296366450308767 ) ) ;
#84931=CARTESIAN_POINT ( 'NONE',  ( 19.54721792061764418, 97.02882860391893871, 5.000000000000000888 ) ) ;
#84932=CARTESIAN_POINT ( 'NONE',  ( 10.00000000000000000, 40.55374883491397497, -14.16423886937410082 ) ) ;
#84934=CARTESIAN_POINT ( 'NONE',  ( 6.204703633549690345, 60.76208216824730357, -14.16423886937410259 ) ) ;
#84935=CARTESIAN_POINT ( 'NONE',  ( 24.16423886937409904, 19.09541550158063927, 3.795296366450317205 ) ) ;
#84936=CARTESIAN_POINT ( 'NONE',  ( -4.164238869374099039, 26.80374883491397142, 8.674139862899312516E-16 ) ) ;
#84940=CARTESIAN_POINT ( 'NONE',  ( 18.52753015748618282, 43.92559781766745175, -4.923371831947291888 ) ) ;
#84941=CARTESIAN_POINT ( 'NONE',  ( 20.88017736071110164, 35.35535201082150536, 2.915334737309930979 ) ) ;
#84943=CARTESIAN_POINT ( 'NONE',  ( 5.076628168052703671, 66.84226448433412315, 8.527530157486179263 ) ) ;
#84944=CARTESIAN_POINT ( 'NONE',  ( 19.67370888310397703, 87.37213813211816671, -5.438836974231106680 ) ) ;
#84945=CARTESIAN_POINT ( 'NONE',  ( 2.791683348922237240, 35.38393115100079456, -7.208316651077763204 ) ) ;
#84946=CARTESIAN_POINT ( 'NONE',  ( 19.38216949554541202, 55.99863466993041072, 9.382169495545424454 ) ) ;
#84948=CARTESIAN_POINT ( 'NONE',  ( 0.1532563361054100626, 45.80059781766745886, -2.638427012816831230 ) ) ;
#84949=CARTESIAN_POINT ( 'NONE',  ( 19.84674366389459266, 58.71726448433411605, -2.638427012816827677 ) ) ;
#84950=COLOUR_RGB ( '', 0.31764706, 0.68627451, 0.89019608) ;
#84951=CARTESIAN_POINT ( 'NONE',  ( 10.00000000000000000, 35.55374883491396787, -14.16423886937410082 ) ) ;
#84953=CARTESIAN_POINT ( 'NONE',  ( 2.917880565312950480, 15.97041550158063217, -12.26659068614894821 ) ) ;
#84956=CARTESIAN_POINT ( 'NONE',  ( 2.035157376598824452, 3.688685344154837953, 7.964842623401179544 ) ) ;
#84957=CARTESIAN_POINT ( 'NONE',  ( 10.00000000000000178, 10.37363466993041961, 12.81628187352647608 ) ) ;
#84958=CARTESIAN_POINT ( 'NONE',  ( -0.03447792253739248580, 55.15514106990690379, 6.401564815979742917 ) ) ;
#84959=CARTESIAN_POINT ( 'NONE',  ( 10.00000000000000000, 4.758931151000784787, -9.846743663894594434 ) ) ;
#84962=CARTESIAN_POINT ( 'NONE',  ( -4.164238869374099039, 56.80374883491397497, 8.674139862899312516E-16 ) ) ;
#84964=CARTESIAN_POINT ( 'NONE',  ( 0.5774900079438607392, 28.48035201082150891, 5.440088680355550821 ) ) ;
#84965=CARTESIAN_POINT ( 'NONE',  ( 0.5774900079438607392, 18.48035201082150536, 5.440088680355550821 ) ) ;
#84966=CARTESIAN_POINT ( 'NONE',  ( 2.791683348922240793, 51.63393115100078745, 7.208316651077764092 ) ) ;
#84967=CARTESIAN_POINT ( 'NONE',  ( 2.791683348922240793, 51.63393115100078745, 7.208316651077764092 ) ) ;
#84968=CARTESIAN_POINT ( 'NONE',  ( 5.076628168052704559, 0.1755978176674514724, -8.527530157486179263 ) ) ;
#84970=CARTESIAN_POINT ( 'NONE',  ( 2.035157376598824452, 28.68868534415484106, 7.964842623401179544 ) ) ;
#84971=CARTESIAN_POINT ( 'NONE',  ( 3.591859063236761518, 19.95696800326375353, 11.09922568453594849 ) ) ;
#84974=CARTESIAN_POINT ( 'NONE',  ( 18.52753015748617571, 63.09226448433412315, 4.923371831947298993 ) ) ;
#84975=CARTESIAN_POINT ( 'NONE',  ( 15.44008868035555793, 46.39701867748817676, -9.422509992056140149 ) ) ;
#84976=CARTESIAN_POINT ( 'NONE',  ( 19.84674366389459266, 8.717264484334116048, -2.638427012816827677 ) ) ;
#84977=CARTESIAN_POINT ( 'NONE',  ( 19.38216949554541557, 17.24863466993041783, -9.382169495545420901 ) ) ;
#84978=CIRCLE ( 'NONE', #33919, 7.000000000000005329 ) ;
#84979=CARTESIAN_POINT ( 'NONE',  ( 2.035157376598822676, 57.43868534415484106, -7.964842623401177768 ) ) ;
#84980=CARTESIAN_POINT ( 'NONE',  ( 20.88017736071110519, 15.56368534415483751, 2.639326808657452039E-16 ) ) ;
#84982=VECTOR ( 'NONE', #9773, 1000.000000000000000 ) ;
#84985=CARTESIAN_POINT ( 'NONE',  ( 19.72487221294571214, 24.78217586085238011, 6.499999999999993783 ) ) ;
#84986=CARTESIAN_POINT ( 'NONE',  ( 12.91533473730993009, 46.60535201082150536, -10.88017736071109987 ) ) ;
#84987=CARTESIAN_POINT ( 'NONE',  ( 6.565887622018943937, 43.08196800326374643, -12.81628187352647608 ) ) ;
#84988=CARTESIAN_POINT ( 'NONE',  ( 6.204703633549690345, 12.84541550158063572, 14.16423886937410082 ) ) ;
#84989=CARTESIAN_POINT ( 'NONE',  ( 7.361572987183170547, 22.05059781766745530, 9.846743663894590881 ) ) ;
#84990=AXIS2_PLACEMENT_3D ( 'NONE', #1646, #62597, #85619 ) ;
#84991=CARTESIAN_POINT ( 'NONE',  ( 10.00000000000000178, 62.25893115100078745, 9.846743663894594434 ) ) ;
#84992=CARTESIAN_POINT ( 'NONE',  ( 10.00000000000000178, 17.25893115100078745, 9.846743663894594434 ) ) ;
#84994=CARTESIAN_POINT ( 'NONE',  ( -2.266590686148945544, 56.38708216824731068, -7.082119434687050408 ) ) ;
#84996=CIRCLE ( 'NONE', #11541, 62.50000000000000000 ) ;
#84997=ADVANCED_FACE ( 'NONE', ( #85910 ), #75323, .T. ) ;
#85000=CARTESIAN_POINT ( 'NONE',  ( 20.88017736071110519, 10.56368534415483751, 2.639326808657452039E-16 ) ) ;
#85003=EDGE_LOOP ( 'NONE', ( #16833, #7791, #52303, #34977 ) ) ;
#85005=CARTESIAN_POINT ( 'NONE',  ( 12.91533473730992121, 4.522018677488170546, 10.88017736071110164 ) ) ;
#85006=CARTESIAN_POINT ( 'NONE',  ( 12.91533473730992121, 4.522018677488170546, 10.88017736071110164 ) ) ;
#85007=CARTESIAN_POINT ( 'NONE',  ( 18.52753015748617571, 38.09226448433412315, 4.923371831947298993 ) ) ;
#85008=CARTESIAN_POINT ( 'NONE',  ( -2.816281873526473856, 44.12363466993042493, 9.499525473075851096E-16 ) ) ;
#85011=CARTESIAN_POINT ( 'NONE',  ( 17.08211943468705840, 15.13708216824730179, -12.26659068614894466 ) ) ;
#85012=CARTESIAN_POINT ( 'NONE',  ( 20.88017736071110164, 30.35535201082151247, 2.915334737309930979 ) ) ;
#85013=CARTESIAN_POINT ( 'NONE',  ( 19.42250999205614193, 5.147018677488171434, 5.440088680355555262 ) ) ;
#85014=CARTESIAN_POINT ( 'NONE',  ( 17.20831665107776587, 39.13393115100079456, -7.208316651077762316 ) ) ;
#85016=CARTESIAN_POINT ( 'NONE',  ( 0.1532563361054100626, 30.80059781766744820, -2.638427012816831230 ) ) ;
#85021=CARTESIAN_POINT ( 'NONE',  ( -0.8801773607111008646, 63.27201867748817676, 2.915334737309923430 ) ) ;
#85022=CARTESIAN_POINT ( 'NONE',  ( 17.20831665107776587, 54.13393115100079456, -7.208316651077762316 ) ) ;
#85023=CARTESIAN_POINT ( 'NONE',  ( 4.559911319644449179, 27.23035201082150536, -9.422509992056141925 ) ) ;
#85024=CARTESIAN_POINT ( 'NONE',  ( 12.91533473730992121, 9.522018677488171434, 10.88017736071110164 ) ) ;
#85025=CARTESIAN_POINT ( 'NONE',  ( 6.565887622018943937, 28.08196800326375353, -12.81628187352647608 ) ) ;
#85026=CARTESIAN_POINT ( 'NONE',  ( -0.3689425029237881626, 12.42874883491396609, 10.36894250292379027 ) ) ;
#85029=CARTESIAN_POINT ( 'NONE',  ( 22.81628187352647785, 41.41530133659708923, 3.434112377981063169 ) ) ;
#85031=CARTESIAN_POINT ( 'NONE',  ( 7.361572987183169658, 49.96726448433410894, -9.846743663894592657 ) ) ;
#85032=CARTESIAN_POINT ( 'NONE',  ( 20.88017736071110164, 50.35535201082151247, 2.915334737309930979 ) ) ;
#85034=CARTESIAN_POINT ( 'NONE',  ( 4.559911319644449179, 18.89701867748817321, 9.422509992056141925 ) ) ;
#85036=CARTESIAN_POINT ( 'NONE',  ( 0.5774900079438590739, 17.64701867748817321, -5.440088680355550821 ) ) ;
#85038=CARTESIAN_POINT ( 'NONE',  ( 4.559911319644449179, 62.23035201082150536, -9.422509992056141925 ) ) ;
#85040=CARTESIAN_POINT ( 'NONE',  ( 5.076628168052703671, 6.842264484334118713, 8.527530157486179263 ) ) ;
#85041=CARTESIAN_POINT ( 'NONE',  ( 19.42250999205614548, 65.98035201082151957, -5.440088680355545492 ) ) ;
#85042=CARTESIAN_POINT ( 'NONE',  ( 5.076628168052704559, 5.175597817667451750, -8.527530157486179263 ) ) ;
#85043=AXIS2_PLACEMENT_3D ( 'NONE', #31348, #40837, #16366 ) ;
#85045=CARTESIAN_POINT ( 'NONE',  ( 0.1532563361054082862, 36.21726448433410894, 2.638427012816831674 ) ) ;
#85046=ORIENTED_EDGE ( 'NONE', *, *, #57257, .T. ) ;
#85047=VERTEX_POINT ( 'NONE', #27357 ) ;
#85049=CARTESIAN_POINT ( 'NONE',  ( -4.164238869374099927, 12.01208216824730357, 3.795296366450308767 ) ) ;
#85051=CARTESIAN_POINT ( 'NONE',  ( -1.099225684535947600, 58.70696800326375353, -6.408140936763238038 ) ) ;
#85053=CARTESIAN_POINT ( 'NONE',  ( 24.16423886937409904, 9.095415501580633943, 3.795296366450317205 ) ) ;
#85054=CARTESIAN_POINT ( 'NONE',  ( 6.204703633549690345, 25.76208216824730712, -14.16423886937410259 ) ) ;
#85055=DIRECTION ( 'NONE',  ( 0.000000000000000000, 0.000000000000000000, -1.000000000000000000 ) ) ;
#85057=CARTESIAN_POINT ( 'NONE',  ( 17.96484262340118221, 21.18868534415483396, -7.964842623401177768 ) ) ;
#85058=CARTESIAN_POINT ( 'NONE',  ( 0.9413316022086010149, 68.45508385108956873, 6.499999999999960032 ) ) ;
#85060=CARTESIAN_POINT ( 'NONE',  ( 19.84674366389459266, 8.717264484334116048, -2.638427012816827677 ) ) ;
#85062=CARTESIAN_POINT ( 'NONE',  ( 14.92337183194729633, 7.675597817667451750, 8.527530157486181039 ) ) ;
#85063=CARTESIAN_POINT ( 'NONE',  ( -1.099225684535947600, 38.70696800326375353, -6.408140936763238038 ) ) ;
#85064=CARTESIAN_POINT ( 'NONE',  ( 5.076628168052704559, 30.17559781766745175, -8.527530157486179263 ) ) ;
#85067=CARTESIAN_POINT ( 'NONE',  ( 21.09922568453595559, 22.04030133659708923, -6.408140936763230044 ) ) ;
#85068=CIRCLE ( 'NONE', #41973, 7.000000000000000000 ) ;
#85070=CARTESIAN_POINT ( 'NONE',  ( 0.1532563361054100626, 10.80059781766745175, -2.638427012816831230 ) ) ;
#85071=ORIENTED_EDGE ( 'NONE', *, *, #79370, .T. ) ;
#85073=CARTESIAN_POINT ( 'NONE',  ( 19.42250999205614548, 35.98035201082151247, -5.440088680355545492 ) ) ;
#85074=CARTESIAN_POINT ( 'NONE',  ( 24.16423886937409904, 39.09541550158062506, 3.795296366450317205 ) ) ;
#85075=CARTESIAN_POINT ( 'NONE',  ( 10.00000000000000178, 42.25893115100078745, 9.846743663894594434 ) ) ;
#85076=CARTESIAN_POINT ( 'NONE',  ( 7.361572987183169658, -0.03273551566588185635, -9.846743663894592657 ) ) ;
#85077=CARTESIAN_POINT ( 'NONE',  ( -2.816281873526471635, 53.91530133659709634, -3.434112377981056508 ) ) ;
#85079=CARTESIAN_POINT ( 'NONE',  ( 15.44008868035555793, 31.39701867748817676, -9.422509992056140149 ) ) ;
#85082=CARTESIAN_POINT ( 'NONE',  ( 6.565887622018943937, 8.081968003263751754, -12.81628187352647608 ) ) ;
#85083=CARTESIAN_POINT ( 'NONE',  ( 12.63842701281683922, 39.55059781766744464, -9.846743663894590881 ) ) ;
#85085=CARTESIAN_POINT ( 'NONE',  ( 0.6178305044545818747, 53.49863466993041072, -9.382169495545419124 ) ) ;
#85087=CARTESIAN_POINT ( 'NONE',  ( 12.91533473730993009, 51.60535201082149825, -10.88017736071109987 ) ) ;
#85090=CARTESIAN_POINT ( 'NONE',  ( -42.16485527613927076, 107.5383484153110061, -5.000000000000000000 ) ) ;
#85091=CARTESIAN_POINT ( 'NONE',  ( -0.8801773607110991993, 57.85535201082149825, -2.915334737309923874 ) ) ;
#85093=CARTESIAN_POINT ( 'NONE',  ( -0.8801773607111008646, 58.27201867748816966, 2.915334737309923430 ) ) ;
#85095=CARTESIAN_POINT ( 'NONE',  ( 15.44008868035555260, 64.73035201082151957, 9.422509992056143702 ) ) ;
#85096=CARTESIAN_POINT ( 'NONE',  ( 4.559911319644449179, 7.230352010821505360, -9.422509992056141925 ) ) ;
#85097=CARTESIAN_POINT ( 'NONE',  ( 10.00000000000000178, 47.25893115100078745, 9.846743663894594434 ) ) ;
#85098=CARTESIAN_POINT ( 'NONE',  ( 4.559911319644449179, 27.23035201082150536, -9.422509992056141925 ) ) ;
#85100=CARTESIAN_POINT ( 'NONE',  ( 3.591859063236761518, 29.95696800326375708, 11.09922568453594849 ) ) ;
#85102=CARTESIAN_POINT ( 'NONE',  ( 0.5774900079438590739, 42.64701867748816966, -5.440088680355550821 ) ) ;
#85103=CARTESIAN_POINT ( 'NONE',  ( 22.81628187352648496, 11.83196800326375531, -3.434112377981050290 ) ) ;
#85104=CARTESIAN_POINT ( 'NONE',  ( 0.5774900079438607392, 8.480352010821505360, 5.440088680355550821 ) ) ;
#85105=CARTESIAN_POINT ( 'NONE',  ( 4.559911319644449179, 43.89701867748816966, 9.422509992056141925 ) ) ;
#85106=CARTESIAN_POINT ( 'NONE',  ( -2.266590686148945544, 51.38708216824730357, -7.082119434687050408 ) ) ;
#85107=CARTESIAN_POINT ( 'NONE',  ( 2.791683348922240793, 21.63393115100078745, 7.208316651077764092 ) ) ;
#85108=CARTESIAN_POINT ( 'NONE',  ( 19.42250999205614193, 60.14701867748817676, 5.440088680355555262 ) ) ;
#85110=CARTESIAN_POINT ( 'NONE',  ( -4.164238869374099039, 11.80374883491396965, 8.674139862899312516E-16 ) ) ;
#85111=ADVANCED_FACE ( 'NONE', ( #57851 ), #28348, .T. ) ;
#85115=EDGE_LOOP ( 'NONE', ( #88056, #34507, #19833, #91272 ) ) ;
#85117=CARTESIAN_POINT ( 'NONE',  ( 22.26659068614894466, 38.88708216824731068, 7.082119434687054849 ) ) ;
#85118=CARTESIAN_POINT ( 'NONE',  ( 10.00000000000000000, 35.55374883491396787, -14.16423886937410082 ) ) ;
#85119=CARTESIAN_POINT ( 'NONE',  ( 1.472469842513823179, 0.5922644843341181575, -4.923371831947296329 ) ) ;
#85120=CARTESIAN_POINT ( 'NONE',  ( 19.84674366389459621, 58.50893115100078745, 7.409399052514197653E-17 ) ) ;
#85122=CARTESIAN_POINT ( 'NONE',  ( 17.96484262340118221, 54.93868534415484106, 7.964842623401181321 ) ) ;
#85123=CARTESIAN_POINT ( 'NONE',  ( 22.81628187352647785, 21.41530133659708923, 3.434112377981063169 ) ) ;
#85124=CARTESIAN_POINT ( 'NONE',  ( 24.16423886937410614, 24.51208216824730002, -3.795296366450302550 ) ) ;
#85125=CARTESIAN_POINT ( 'NONE',  ( 0.5774900079438607392, 23.48035201082150536, 5.440088680355550821 ) ) ;
#85127=CARTESIAN_POINT ( 'NONE',  ( 4.559911319644449179, 32.23035201082150536, -9.422509992056141925 ) ) ;
#85130=CARTESIAN_POINT ( 'NONE',  ( 0.5774900079438607392, 58.48035201082151247, 5.440088680355550821 ) ) ;
#85135=CARTESIAN_POINT ( 'NONE',  ( 8.673617379884035472E-16, 78.91966277462714174, 5.000000000000000000 ) ) ;
#85136=MECHANICAL_DESIGN_GEOMETRIC_PRESENTATION_REPRESENTATION('',(#46792),#89908);
#85139=CARTESIAN_POINT ( 'NONE',  ( 20.36894250292379738, 9.928748834913966093, -10.36894250292379027 ) ) ;
#85140=CARTESIAN_POINT ( 'NONE',  ( -2.266590686148945544, 62.22041550158063927, 7.082119434687048631 ) ) ;
#85141=CARTESIAN_POINT ( 'NONE',  ( -4.164238869374099039, 61.80374883491397497, 8.674139862899312516E-16 ) ) ;
#85142=CARTESIAN_POINT ( 'NONE',  ( 10.00000000000000178, 32.25893115100078745, 9.846743663894594434 ) ) ;
#85143=CARTESIAN_POINT ( 'NONE',  ( 0.1532563361054083140, 66.00893115100079456, 1.131784320476157264E-15 ) ) ;
#85145=DIRECTION ( 'NONE',  ( -0.000000000000000000, -0.000000000000000000, 1.000000000000000000 ) ) ;
#85147=CARTESIAN_POINT ( 'NONE',  ( 19.38216949554541202, 10.99863466993042138, 9.382169495545424454 ) ) ;
#85149=CARTESIAN_POINT ( 'NONE',  ( 20.36894250292379738, 49.92874883491396787, -10.36894250292379027 ) ) ;
#85152=CARTESIAN_POINT ( 'NONE',  ( 24.16423886937410614, 44.30374883491397497, 8.672049930838204340E-16 ) ) ;
#85154=CARTESIAN_POINT ( 'NONE',  ( 15.44008868035555793, 21.39701867748817321, -9.422509992056140149 ) ) ;
#85155=CARTESIAN_POINT ( 'NONE',  ( -0.8801773607110991993, 37.85535201082151247, -2.915334737309923874 ) ) ;
#85156=CARTESIAN_POINT ( 'NONE',  ( 0.1532563361054100626, 45.80059781766745886, -2.638427012816831230 ) ) ;
#85157=CARTESIAN_POINT ( 'NONE',  ( -0.8801773607111008646, 38.27201867748816255, 2.915334737309923430 ) ) ;
#85158=DIRECTION ( 'NONE',  ( -0.7385627893568404989, 0.6741846973770935225, 0.000000000000000000 ) ) ;
#85159=CARTESIAN_POINT ( 'NONE',  ( 20.88017736071110164, 65.35535201082150536, 2.915334737309930979 ) ) ;
#85160=CARTESIAN_POINT ( 'NONE',  ( -0.8801773607110991993, 27.85535201082150181, -2.915334737309923874 ) ) ;
#85164=CARTESIAN_POINT ( 'NONE',  ( 0.1532563361054083140, 1.008931151000784787, 1.131784320476157264E-15 ) ) ;
#85168=CARTESIAN_POINT ( 'NONE',  ( 2.791683348922240793, 36.63393115100078035, 7.208316651077764092 ) ) ;
#85169=CARTESIAN_POINT ( 'NONE',  ( -45.94000000000001194, 100.9999999999999858, 9.500000000000000000 ) ) ;
#85170=CARTESIAN_POINT ( 'NONE',  ( -1.099225684535947600, 49.54030133659708923, 6.408140936763237150 ) ) ;
#85171=SURFACE_SIDE_STYLE ('',( #17667 ) ) ;
#85173=CARTESIAN_POINT ( 'NONE',  ( 19.84674366389459621, 63.50893115100078745, 7.409399052514197653E-17 ) ) ;
#85174=CARTESIAN_POINT ( 'NONE',  ( -43.14347499112858486, 107.3164382878165668, 4.970428862813641935 ) ) ;
#85175=CARTESIAN_POINT ( 'NONE',  ( 18.52753015748617571, 48.09226448433412315, 4.923371831947298993 ) ) ;
#85176=CARTESIAN_POINT ( 'NONE',  ( 22.26659068614894466, 43.88708216824729647, 7.082119434687054849 ) ) ;
#85177=CARTESIAN_POINT ( 'NONE',  ( 5.076628168052704559, 65.17559781766745175, -8.527530157486179263 ) ) ;
#85178=CARTESIAN_POINT ( 'NONE',  ( 18.52753015748617571, 13.09226448433411960, 4.923371831947298993 ) ) ;
#85179=CARTESIAN_POINT ( 'NONE',  ( 19.38216949554541557, 52.24863466993041072, -9.382169495545420901 ) ) ;
#85180=CARTESIAN_POINT ( 'NONE',  ( 17.20831665107776587, 62.88393115100078745, 7.208316651077764980 ) ) ;
#85181=CARTESIAN_POINT ( 'NONE',  ( 7.084665262690076126, 57.02201867748817676, -10.88017736071110164 ) ) ;
#85183=CARTESIAN_POINT ( 'NONE',  ( 19.84674366389459621, 48.50893115100078745, 7.409399052514197653E-17 ) ) ;
#85186=CARTESIAN_POINT ( 'NONE',  ( 2.035157376598822676, 57.43868534415484106, -7.964842623401177768 ) ) ;
#85188=ORIENTED_EDGE ( 'NONE', *, *, #79817, .F. ) ;
#85189=CARTESIAN_POINT ( 'NONE',  ( 20.36894250292379382, 48.67874883491396076, 10.36894250292379205 ) ) ;
#85191=CARTESIAN_POINT ( 'NONE',  ( 17.96484262340118221, 24.93868534415484461, 7.964842623401181321 ) ) ;
#85192=CARTESIAN_POINT ( 'NONE',  ( -1.099225684535947600, 14.54030133659708568, 6.408140936763237150 ) ) ;
#85193=CARTESIAN_POINT ( 'NONE',  ( 4.559911319644449179, 62.23035201082150536, -9.422509992056141925 ) ) ;
#85197=CARTESIAN_POINT ( 'NONE',  ( 19.80777595082616216, 10.68878173731741121, -6.500000000000000888 ) ) ;
#85199=CARTESIAN_POINT ( 'NONE',  ( 20.88017736071110875, 50.77201867748817676, -2.915334737309920765 ) ) ;
#85200=CARTESIAN_POINT ( 'NONE',  ( 2.603489959281592991, 11.58210964143329313, 6.500000000000006217 ) ) ;
#85201=CARTESIAN_POINT ( 'NONE',  ( 18.52753015748617571, 38.09226448433412315, 4.923371831947298993 ) ) ;
#85205=CARTESIAN_POINT ( 'NONE',  ( 13.43411237798105340, 10.58196800326375353, 12.81628187352647963 ) ) ;
#85206=CARTESIAN_POINT ( 'NONE',  ( 12.91533473730993009, 11.60535201082150714, -10.88017736071109987 ) ) ;
#85207=FILL_AREA_STYLE_COLOUR ( '', #13805 ) ;
#85208=DIRECTION ( 'NONE',  ( 0.000000000000000000, -1.000000000000000000, 0.000000000000000000 ) ) ;
#85209=CARTESIAN_POINT ( 'NONE',  ( -0.3689425029237898834, 36.17874883491396787, -10.36894250292378850 ) ) ;
#85210=CARTESIAN_POINT ( 'NONE',  ( -2.266590686148945544, 67.22041550158063217, 7.082119434687048631 ) ) ;
#85211=CARTESIAN_POINT ( 'NONE',  ( 5.076628168052703671, 31.84226448433412315, 8.527530157486179263 ) ) ;
#85212=( BOUNDED_SURFACE ( )  B_SPLINE_SURFACE ( 1, 2, ( 
 ( #72427, #54964, #40485, #48946, #93963, #16995, #24502, #32471, #93471, #85982, #47474, #62966, #24998, #18956, #87440, #71945, #32958, #33437, #48458, #63462, #3953, #17493, #92970, #85486, #49433, #2006, #94448, #47958, #55481, #64431, #78468, #70486, #3469, #40976, #25489, #79454, #79937, #94938, #70983, #2988, #55974, #77974, #9481, #78957, #10953, #39984, #10468, #26440, #18461, #41479, #56938, #63934, #11444, #25961, #56462, #62465, #5441, #34424, #74397, #35913, #27425, #42929, #34920, #87926, #51911, #4938, #74898, #64916, #72925, #20430, #73410, #5920, #57433, #4455, #97426, #27912, #73912, #35418, #65912, #59397, #66410, #65417, #88922, #82396, #95442, #57918, #89409, #12423, #95942, #88428, #50917, #19443, #19928, #81413, #20925, #49932, #51414, #80930, #96942, #66907, #28415, #96442, #89900, #13412, #13920, #81903, #44398, #58911, #43898, #26935, #36414, #11938, #58405, #12915, #43412, #42443, #50422, #28892, #21416, #80440, #46378, #68399, #90882, #83887, #53887, #52398, #30376, #98427, #7899, #60879, #97932, #38394, #52885, #61862, #54360, #15416, #75387, #15892, #29882, #6905, #37417, #84870, #44885, #67904, #76866, #45898, #83395, #16379, #8382, #68896, #90381, #98920, #424, #30875, #76384, #46862, #38890, #14915, #37911, #61371, #91379, #91881, #23403, #84393, #60384, #69378, #22907, #53377, #900, #22410, #45385, #31362, #75891, #92367, #23893, #6396, #36911, #67403, #7415, #29389, #14415, #59890, #21919, #82897, #16874, #19688, #40366, #62851, #55856, #27176, #24381, #2383, #70372, #78843, #32837, #69876, #10354, #24874, #35168, #27674, #86352, #47349, #88175, #1889, #77851, #9361, #58159, #39865, #32348, #50175, #17854, #55356, #88669, #80685, #40853, #62349, #70867, #71357, #4206, #48340, #20178, #12181, #85861, #9868, #34676, #63339, #65172, #95692, #57679, #93349, #42687, #93844, #25371, #73166, #17373, #47843, #4705, #78347, #65668, #96190, #77354, #8865, #39381, #1396, #31851, #92853, #54848, #85362, #59153, #21672, #50681, #90636, #52158, #43663, #89660, #51172, #5188, #68158, #21170, #91135, #81173, #89167, #36670, #51673, #22161, #73661, #20678, #14672, #44147, #90142, #82151, #13663, #75644, #82651, #81656, #6166, #98679, #12673, #74149, #6656, #28661, #13165, #5683, #67158, #35675, #36168, #97683, #37172, #66159, #67665, #97193, #14167, #83147, #44651, #74655, #7155, #29631, #30128, #98175, #60634, #75146, #60139, #43173, #52643, #28172, #29145, #66668, #59651, #45138, #96692, #58665, #37659, #39632, #76139, #61612, #93100, #77604, #70122, #16132, #30621, #9613, #15656, #92130, #83646, #47105 ),
 ( #70615, #54603, #9118, #15161, #85119, #173, #46618, #667, #84629, #61128, #76625, #55097, #91637, #23155, #62595, #77115, #8145, #1150, #1644, #68643, #8628, #46139, #24136, #39137, #45641, #16629, #69139, #78107, #2141, #31610, #53630, #32096, #38638, #84149, #31117, #32599, #23655, #54116, #24630, #62102, #69626, #63097, #85616, #17133, #7665, #92611, #47612, #40113, #22660, #53137, #38156, #41114, #26098, #19083, #18594, #64558, #3603, #11577, #33091, #95575, #56593, #49087, #57075, #10600, #33573, #49559, #94093, #11091, #50069, #93598, #34554, #72558, #88060, #86110, #42570, #95066, #41608, #3117, #26572, #25135, #65049, #87571, #86602, #64067, #25614, #48091, #12067, #94582, #35049, #55613, #63584, #79590, #87083, #27062, #17621, #56107, #57561, #72077, #34062, #80071, #42091, #78603, #10113, #18109, #48586, #79087, #40612, #71605, #4090, #80572, #19571, #73054, #4587, #71109, #2637, #36047, #75530, #89053, #96075, #88556, #90520, #5070, #97567, #51050, #35557, #67547, #20564, #73545, #6540, #44035, #97079, #52046, #83037, #37049, #96573, #74536, #28050, #20059, #12561, #58546, #82537, #50562, #5572, #98060, #21556, #14055, #59043, #66047, #52529, #81540, #66551, #27557, #90033, #58049, #43064, #6057, #44537, #81057, #13050, #36555, #43544, #74039, #28551, #67045, #89549, #59539, #75033, #60025, #21058, #51551, #22056, #29517, #82039, #29031, #13550, #14554, #45023, #7043, #65549, #8518, #39020, #16520, #23538, #30512, #85007, #92988, #60524, #76022, #46994, #46031, #54981, #62484, #15546, #8031, #31005, #16016, #77488, #61995, #76515, #92495, #24522, #54492, #17010, #46506, #38530, #54011, #9000, #65, #69026, #560, #61501, #39516, #77006, #23040, #70009, #84520, #1533, #84024, #92009, #69515, #1031, #31492, #24024, #31978, #47488, #30019, #85499, #77991, #37548, #68039, #61015, #98565, #91014, #22547, #53017, #83532, #53513, #15050, #45522, #7553, #38043, #68534, #91526, #41491, #63949, #3483, #56475, #87941, #2024, #55989, #94951, #40993, #62981, #70502, #78484, #40502, #32973, #93486, #9999, #70996, #64931, #34437, #18970, #78971, #79471, #33454, #10481, #19457, #63478, #39997, #32487, #95458, #47975, #71960, #93981, #2519, #11459, #25503, #17510, #49449, #86962, #71491, #26452, #26949, #79953, #86491, #18476, #17990, #25011, #55498, #48473, #56953, #85999, #3005, #41977, #64444, #87455, #94461, #25979, #57450, #48961, #10970, #33940, #72440, #3969, #49950, #9496, #59410, #11953, #50435, #20940, #72938, #34936, #19942, #58927, #42457, #74411, #28908, #74917, #12438, #58420, #36928, #82412, #42946, #51429 ) ),
 .UNSPECIFIED., .F., .F., .F. ) 
 B_SPLINE_SURFACE_WITH_KNOTS ( ( 2, 2 ),
 ( 3, 2, 2, 2, 2, 2, 2, 2, 2, 2, 2, 2, 2, 2, 2, 2, 2, 2, 2, 2, 2, 2, 2, 2, 2, 2, 2, 2, 2, 2, 2, 2, 2, 2, 2, 2, 2, 2, 2, 2, 2, 2, 2, 2, 2, 2, 2, 2, 2, 2, 2, 2, 2, 2, 2, 2, 2, 2, 2, 2, 2, 2, 2, 2, 2, 2, 2, 2, 2, 2, 2, 2, 2, 2, 2, 2, 2, 2, 2, 2, 2, 2, 2, 2, 2, 2, 2, 2, 2, 2, 2, 2, 2, 2, 2, 2, 2, 2, 2, 2, 2, 2, 2, 2, 2, 2, 2, 2, 2, 2, 2, 2, 2, 2, 2, 2, 2, 2, 2, 2, 2, 2, 2, 2, 2, 2, 2, 2, 2, 2, 2, 2, 2, 2, 2, 2, 2, 2, 2, 2, 2, 2, 2, 2, 2, 2, 2, 2, 2, 2, 2, 2, 2, 2, 2, 2, 2, 2, 2, 2, 2, 2, 3 ),
 ( 0.000000000000000000, 1.000000000000000000 ),
 ( 0.000000000000000000, 0.005952380952380952051, 0.01190476190476190410, 0.01785714285714285615, 0.02380952380952380820, 0.02976190476190476025, 0.03571428571428571230, 0.04166666666666666435, 0.04761904761904761640, 0.05357142857142856845, 0.05952380952380952051, 0.06547619047619047949, 0.07142857142857142461, 0.07738095238095238360, 0.08333333333333332871, 0.08928571428571428770, 0.09523809523809523281, 0.1011904761904761918, 0.1071428571428571369, 0.1130952380952380959, 0.1190476190476190410, 0.1250000000000000000, 0.1309523809523809590, 0.1369047619047619180, 0.1428571428571428492, 0.1488095238095238082, 0.1547619047619047672, 0.1607142857142857262, 0.1666666666666666574, 0.1726190476190476164, 0.1785714285714285754, 0.1845238095238095344, 0.1904761904761904656, 0.1964285714285714246, 0.2023809523809523836, 0.2083333333333333426, 0.2142857142857142738, 0.2202380952380952328, 0.2261904761904761918, 0.2321428571428571508, 0.2380952380952380820, 0.2440476190476190410, 0.2500000000000000000, 0.2559523809523809312, 0.2619047619047619180, 0.2678571428571428492, 0.2738095238095238360, 0.2797619047619047672, 0.2857142857142856984, 0.2916666666666666852, 0.2976190476190476164, 0.3035714285714285476, 0.3095238095238095344, 0.3154761904761904656, 0.3214285714285714524, 0.3273809523809523836, 0.3333333333333333148, 0.3392857142857143016, 0.3452380952380952328, 0.3511904761904761640, 0.3571428571428571508, 0.3630952380952380820, 0.3690476190476190688, 0.3750000000000000000, 0.3809523809523809312, 0.3869047619047619180, 0.3928571428571428492, 0.3988095238095238360, 0.4047619047619047672, 0.4107142857142856984, 0.4166666666666666852, 0.4226190476190476164, 0.4285714285714285476, 0.4345238095238095344, 0.4404761904761904656, 0.4464285714285714524, 0.4523809523809523836, 0.4583333333333333148, 0.4642857142857143016, 0.4702380952380952328, 0.4761904761904761640, 0.4821428571428571508, 0.4880952380952380820, 0.4940476190476190688, 0.5000000000000000000, 0.5059523809523809312, 0.5119047619047618625, 0.5178571428571429047, 0.5238095238095238360, 0.5297619047619047672, 0.5357142857142856984, 0.5416666666666666297, 0.5476190476190476719, 0.5535714285714286031, 0.5595238095238095344, 0.5654761904761904656, 0.5714285714285713969, 0.5773809523809523281, 0.5833333333333333703, 0.5892857142857143016, 0.5952380952380952328, 0.6011904761904761640, 0.6071428571428570953, 0.6130952380952381375, 0.6190476190476190688, 0.6250000000000000000, 0.6309523809523809312, 0.6369047619047618625, 0.6428571428571429047, 0.6488095238095238360, 0.6547619047619047672, 0.6607142857142856984, 0.6666666666666666297, 0.6726190476190476719, 0.6785714285714286031, 0.6845238095238095344, 0.6904761904761904656, 0.6964285714285713969, 0.7023809523809523281, 0.7083333333333333703, 0.7142857142857143016, 0.7202380952380952328, 0.7261904761904761640, 0.7321428571428570953, 0.7380952380952381375, 0.7440476190476190688, 0.7500000000000000000, 0.7559523809523809312, 0.7619047619047618625, 0.7678571428571429047, 0.7738095238095238360, 0.7797619047619047672, 0.7857142857142856984, 0.7916666666666666297, 0.7976190476190476719, 0.8035714285714286031, 0.8095238095238095344, 0.8154761904761904656, 0.8214285714285713969, 0.8273809523809523281, 0.8333333333333333703, 0.8392857142857143016, 0.8452380952380952328, 0.8511904761904761640, 0.8571428571428570953, 0.8630952380952381375, 0.8690476190476190688, 0.8750000000000000000, 0.8809523809523809312, 0.8869047619047618625, 0.8928571428571429047, 0.8988095238095238360, 0.9047619047619047672, 0.9107142857142856984, 0.9166666666666666297, 0.9226190476190476719, 0.9285714285714286031, 0.9345238095238095344, 0.9404761904761904656, 0.9464285714285713969, 0.9523809523809523281, 0.9583333333333333703, 0.9642857142857143016 ),
 .UNSPECIFIED. ) 
 GEOMETRIC_REPRESENTATION_ITEM ( )  RATIONAL_B_SPLINE_SURFACE ( (
 ( 1.000000000000000000, 0.9659258262890683122, 1.000000000000000000, 0.9659258262890683122, 1.000000000000000000, 0.9659258262890683122, 1.000000000000000000, 0.9659258262890683122, 1.000000000000000000, 0.9659258262890683122, 1.000000000000000000, 0.9659258262890683122, 1.000000000000000000, 0.9659258262890683122, 1.000000000000000000, 0.9659258262890683122, 1.000000000000000000, 0.9659258262890683122, 1.000000000000000000, 0.9659258262890683122, 1.000000000000000000, 0.9659258262890683122, 1.000000000000000000, 0.9659258262890683122, 1.000000000000000000, 0.9659258262890683122, 1.000000000000000000, 0.9659258262890683122, 1.000000000000000000, 0.9659258262890683122, 1.000000000000000000, 0.9659258262890683122, 1.000000000000000000, 0.9659258262890683122, 1.000000000000000000, 0.9659258262890683122, 1.000000000000000000, 0.9659258262890683122, 1.000000000000000000, 0.9659258262890683122, 1.000000000000000000, 0.9659258262890683122, 1.000000000000000000, 0.9659258262890683122, 1.000000000000000000, 0.9659258262890683122, 1.000000000000000000, 0.9659258262890683122, 1.000000000000000000, 0.9659258262890683122, 1.000000000000000000, 0.9659258262890683122, 1.000000000000000000, 0.9659258262890683122, 1.000000000000000000, 0.9659258262890683122, 1.000000000000000000, 0.9659258262890683122, 1.000000000000000000, 0.9659258262890683122, 1.000000000000000000, 0.9659258262890683122, 1.000000000000000000, 0.9659258262890683122, 1.000000000000000000, 0.9659258262890683122, 1.000000000000000000, 0.9659258262890683122, 1.000000000000000000, 0.9659258262890683122, 1.000000000000000000, 0.9659258262890683122, 1.000000000000000000, 0.9659258262890683122, 1.000000000000000000, 0.9659258262890683122, 1.000000000000000000, 0.9659258262890683122, 1.000000000000000000, 0.9659258262890683122, 1.000000000000000000, 0.9659258262890683122, 1.000000000000000000, 0.9659258262890683122, 1.000000000000000000, 0.9659258262890683122, 1.000000000000000000, 0.9659258262890683122, 1.000000000000000000, 0.9659258262890683122, 1.000000000000000000, 0.9659258262890683122, 1.000000000000000000, 0.9659258262890683122, 1.000000000000000000, 0.9659258262890683122, 1.000000000000000000, 0.9659258262890683122, 1.000000000000000000, 0.9659258262890683122, 1.000000000000000000, 0.9659258262890683122, 1.000000000000000000, 0.9659258262890683122, 1.000000000000000000, 0.9659258262890683122, 1.000000000000000000, 0.9659258262890683122, 1.000000000000000000, 0.9659258262890683122, 1.000000000000000000, 0.9659258262890683122, 1.000000000000000000, 0.9659258262890683122, 1.000000000000000000, 0.9659258262890683122, 1.000000000000000000, 0.9659258262890683122, 1.000000000000000000, 0.9659258262890683122, 1.000000000000000000, 0.9659258262890683122, 1.000000000000000000, 0.9659258262890683122, 1.000000000000000000, 0.9659258262890683122, 1.000000000000000000, 0.9659258262890683122, 1.000000000000000000, 0.9659258262890683122, 1.000000000000000000, 0.9659258262890683122, 1.000000000000000000, 0.9659258262890683122, 1.000000000000000000, 0.9659258262890683122, 1.000000000000000000, 0.9659258262890683122, 1.000000000000000000, 0.9659258262890683122, 1.000000000000000000, 0.9659258262890683122, 1.000000000000000000, 0.9659258262890683122, 1.000000000000000000, 0.9659258262890683122, 1.000000000000000000, 0.9659258262890683122, 1.000000000000000000, 0.9659258262890683122, 1.000000000000000000, 0.9659258262890683122, 1.000000000000000000, 0.9659258262890683122, 1.000000000000000000, 0.9659258262890683122, 1.000000000000000000, 0.9659258262890683122, 1.000000000000000000, 0.9659258262890683122, 1.000000000000000000, 0.9659258262890683122, 1.000000000000000000, 0.9659258262890683122, 1.000000000000000000, 0.9659258262890683122, 1.000000000000000000, 0.9659258262890683122, 1.000000000000000000, 0.9659258262890683122, 1.000000000000000000, 0.9659258262890683122, 1.000000000000000000, 0.9659258262890683122, 1.000000000000000000, 0.9659258262890683122, 1.000000000000000000, 0.9659258262890683122, 1.000000000000000000, 0.9659258262890683122, 1.000000000000000000, 0.9659258262890683122, 1.000000000000000000, 0.9659258262890683122, 1.000000000000000000, 0.9659258262890683122, 1.000000000000000000, 0.9659258262890683122, 1.000000000000000000, 0.9659258262890683122, 1.000000000000000000, 0.9659258262890683122, 1.000000000000000000, 0.9659258262890683122, 1.000000000000000000, 0.9659258262890683122, 1.000000000000000000, 0.9659258262890683122, 1.000000000000000000, 0.9659258262890683122, 1.000000000000000000, 0.9659258262890683122, 1.000000000000000000, 0.9659258262890683122, 1.000000000000000000, 0.9659258262890683122, 1.000000000000000000, 0.9659258262890683122, 1.000000000000000000, 0.9659258262890683122, 1.000000000000000000, 0.9659258262890683122, 1.000000000000000000, 0.9659258262890683122, 1.000000000000000000, 0.9659258262890683122, 1.000000000000000000, 0.9659258262890683122, 1.000000000000000000, 0.9659258262890683122, 1.000000000000000000, 0.9659258262890683122, 1.000000000000000000, 0.9659258262890683122, 1.000000000000000000, 0.9659258262890683122, 1.000000000000000000, 0.9659258262890683122, 1.000000000000000000, 0.9659258262890683122, 1.000000000000000000, 0.9659258262890683122, 1.000000000000000000, 0.9659258262890683122, 1.000000000000000000, 0.9659258262890683122, 1.000000000000000000, 0.9659258262890683122, 1.000000000000000000, 0.9659258262890683122, 1.000000000000000000, 0.9659258262890683122, 1.000000000000000000, 0.9659258262890683122, 1.000000000000000000, 0.9659258262890683122, 1.000000000000000000, 0.9659258262890683122, 1.000000000000000000, 0.9659258262890683122, 1.000000000000000000, 0.9659258262890683122, 1.000000000000000000, 0.9659258262890683122, 1.000000000000000000, 0.9659258262890683122, 1.000000000000000000, 0.9659258262890683122, 1.000000000000000000, 0.9659258262890683122, 1.000000000000000000, 0.9659258262890683122, 1.000000000000000000, 0.9659258262890683122, 1.000000000000000000, 0.9659258262890683122, 1.000000000000000000, 0.9659258262890683122, 1.000000000000000000, 0.9659258262890683122, 1.000000000000000000, 0.9659258262890683122, 1.000000000000000000, 0.9659258262890683122, 1.000000000000000000, 0.9659258262890683122, 1.000000000000000000, 0.9659258262890683122, 1.000000000000000000, 0.9659258262890683122, 1.000000000000000000, 0.9659258262890683122, 1.000000000000000000, 0.9659258262890683122, 1.000000000000000000, 0.9659258262890683122, 1.000000000000000000, 0.9659258262890683122, 1.000000000000000000, 0.9659258262890683122, 1.000000000000000000, 0.9659258262890683122, 1.000000000000000000, 0.9659258262890683122, 1.000000000000000000, 0.9659258262890683122, 1.000000000000000000, 0.9659258262890683122, 1.000000000000000000, 0.9659258262890683122, 1.000000000000000000, 0.9659258262890683122, 1.000000000000000000, 0.9659258262890683122, 1.000000000000000000, 0.9659258262890683122, 1.000000000000000000, 0.9659258262890683122, 1.000000000000000000, 0.9659258262890683122, 1.000000000000000000, 0.9659258262890683122, 1.000000000000000000, 0.9659258262890683122, 1.000000000000000000, 0.9659258262890683122, 1.000000000000000000, 0.9659258262890683122, 1.000000000000000000, 0.9659258262890683122, 1.000000000000000000, 0.9659258262890683122, 1.000000000000000000, 0.9659258262890683122, 1.000000000000000000),
 ( 1.000000000000000000, 0.9659258262890683122, 1.000000000000000000, 0.9659258262890683122, 1.000000000000000000, 0.9659258262890683122, 1.000000000000000000, 0.9659258262890683122, 1.000000000000000000, 0.9659258262890683122, 1.000000000000000000, 0.9659258262890683122, 1.000000000000000000, 0.9659258262890683122, 1.000000000000000000, 0.9659258262890683122, 1.000000000000000000, 0.9659258262890683122, 1.000000000000000000, 0.9659258262890683122, 1.000000000000000000, 0.9659258262890683122, 1.000000000000000000, 0.9659258262890683122, 1.000000000000000000, 0.9659258262890683122, 1.000000000000000000, 0.9659258262890683122, 1.000000000000000000, 0.9659258262890683122, 1.000000000000000000, 0.9659258262890683122, 1.000000000000000000, 0.9659258262890683122, 1.000000000000000000, 0.9659258262890683122, 1.000000000000000000, 0.9659258262890683122, 1.000000000000000000, 0.9659258262890683122, 1.000000000000000000, 0.9659258262890683122, 1.000000000000000000, 0.9659258262890683122, 1.000000000000000000, 0.9659258262890683122, 1.000000000000000000, 0.9659258262890683122, 1.000000000000000000, 0.9659258262890683122, 1.000000000000000000, 0.9659258262890683122, 1.000000000000000000, 0.9659258262890683122, 1.000000000000000000, 0.9659258262890683122, 1.000000000000000000, 0.9659258262890683122, 1.000000000000000000, 0.9659258262890683122, 1.000000000000000000, 0.9659258262890683122, 1.000000000000000000, 0.9659258262890683122, 1.000000000000000000, 0.9659258262890683122, 1.000000000000000000, 0.9659258262890683122, 1.000000000000000000, 0.9659258262890683122, 1.000000000000000000, 0.9659258262890683122, 1.000000000000000000, 0.9659258262890683122, 1.000000000000000000, 0.9659258262890683122, 1.000000000000000000, 0.9659258262890683122, 1.000000000000000000, 0.9659258262890683122, 1.000000000000000000, 0.9659258262890683122, 1.000000000000000000, 0.9659258262890683122, 1.000000000000000000, 0.9659258262890683122, 1.000000000000000000, 0.9659258262890683122, 1.000000000000000000, 0.9659258262890683122, 1.000000000000000000, 0.9659258262890683122, 1.000000000000000000, 0.9659258262890683122, 1.000000000000000000, 0.9659258262890683122, 1.000000000000000000, 0.9659258262890683122, 1.000000000000000000, 0.9659258262890683122, 1.000000000000000000, 0.9659258262890683122, 1.000000000000000000, 0.9659258262890683122, 1.000000000000000000, 0.9659258262890683122, 1.000000000000000000, 0.9659258262890683122, 1.000000000000000000, 0.9659258262890683122, 1.000000000000000000, 0.9659258262890683122, 1.000000000000000000, 0.9659258262890683122, 1.000000000000000000, 0.9659258262890683122, 1.000000000000000000, 0.9659258262890683122, 1.000000000000000000, 0.9659258262890683122, 1.000000000000000000, 0.9659258262890683122, 1.000000000000000000, 0.9659258262890683122, 1.000000000000000000, 0.9659258262890683122, 1.000000000000000000, 0.9659258262890683122, 1.000000000000000000, 0.9659258262890683122, 1.000000000000000000, 0.9659258262890683122, 1.000000000000000000, 0.9659258262890683122, 1.000000000000000000, 0.9659258262890683122, 1.000000000000000000, 0.9659258262890683122, 1.000000000000000000, 0.9659258262890683122, 1.000000000000000000, 0.9659258262890683122, 1.000000000000000000, 0.9659258262890683122, 1.000000000000000000, 0.9659258262890683122, 1.000000000000000000, 0.9659258262890683122, 1.000000000000000000, 0.9659258262890683122, 1.000000000000000000, 0.9659258262890683122, 1.000000000000000000, 0.9659258262890683122, 1.000000000000000000, 0.9659258262890683122, 1.000000000000000000, 0.9659258262890683122, 1.000000000000000000, 0.9659258262890683122, 1.000000000000000000, 0.9659258262890683122, 1.000000000000000000, 0.9659258262890683122, 1.000000000000000000, 0.9659258262890683122, 1.000000000000000000, 0.9659258262890683122, 1.000000000000000000, 0.9659258262890683122, 1.000000000000000000, 0.9659258262890683122, 1.000000000000000000, 0.9659258262890683122, 1.000000000000000000, 0.9659258262890683122, 1.000000000000000000, 0.9659258262890683122, 1.000000000000000000, 0.9659258262890683122, 1.000000000000000000, 0.9659258262890683122, 1.000000000000000000, 0.9659258262890683122, 1.000000000000000000, 0.9659258262890683122, 1.000000000000000000, 0.9659258262890683122, 1.000000000000000000, 0.9659258262890683122, 1.000000000000000000, 0.9659258262890683122, 1.000000000000000000, 0.9659258262890683122, 1.000000000000000000, 0.9659258262890683122, 1.000000000000000000, 0.9659258262890683122, 1.000000000000000000, 0.9659258262890683122, 1.000000000000000000, 0.9659258262890683122, 1.000000000000000000, 0.9659258262890683122, 1.000000000000000000, 0.9659258262890683122, 1.000000000000000000, 0.9659258262890683122, 1.000000000000000000, 0.9659258262890683122, 1.000000000000000000, 0.9659258262890683122, 1.000000000000000000, 0.9659258262890683122, 1.000000000000000000, 0.9659258262890683122, 1.000000000000000000, 0.9659258262890683122, 1.000000000000000000, 0.9659258262890683122, 1.000000000000000000, 0.9659258262890683122, 1.000000000000000000, 0.9659258262890683122, 1.000000000000000000, 0.9659258262890683122, 1.000000000000000000, 0.9659258262890683122, 1.000000000000000000, 0.9659258262890683122, 1.000000000000000000, 0.9659258262890683122, 1.000000000000000000, 0.9659258262890683122, 1.000000000000000000, 0.9659258262890683122, 1.000000000000000000, 0.9659258262890683122, 1.000000000000000000, 0.9659258262890683122, 1.000000000000000000, 0.9659258262890683122, 1.000000000000000000, 0.9659258262890683122, 1.000000000000000000, 0.9659258262890683122, 1.000000000000000000, 0.9659258262890683122, 1.000000000000000000, 0.9659258262890683122, 1.000000000000000000, 0.9659258262890683122, 1.000000000000000000, 0.9659258262890683122, 1.000000000000000000, 0.9659258262890683122, 1.000000000000000000, 0.9659258262890683122, 1.000000000000000000, 0.9659258262890683122, 1.000000000000000000, 0.9659258262890683122, 1.000000000000000000, 0.9659258262890683122, 1.000000000000000000, 0.9659258262890683122, 1.000000000000000000, 0.9659258262890683122, 1.000000000000000000, 0.9659258262890683122, 1.000000000000000000, 0.9659258262890683122, 1.000000000000000000, 0.9659258262890683122, 1.000000000000000000, 0.9659258262890683122, 1.000000000000000000, 0.9659258262890683122, 1.000000000000000000, 0.9659258262890683122, 1.000000000000000000, 0.9659258262890683122, 1.000000000000000000, 0.9659258262890683122, 1.000000000000000000, 0.9659258262890683122, 1.000000000000000000, 0.9659258262890683122, 1.000000000000000000, 0.9659258262890683122, 1.000000000000000000, 0.9659258262890683122, 1.000000000000000000, 0.9659258262890683122, 1.000000000000000000, 0.9659258262890683122, 1.000000000000000000, 0.9659258262890683122, 1.000000000000000000, 0.9659258262890683122, 1.000000000000000000, 0.9659258262890683122, 1.000000000000000000, 0.9659258262890683122, 1.000000000000000000, 0.9659258262890683122, 1.000000000000000000, 0.9659258262890683122, 1.000000000000000000, 0.9659258262890683122, 1.000000000000000000, 0.9659258262890683122, 1.000000000000000000, 0.9659258262890683122, 1.000000000000000000, 0.9659258262890683122, 1.000000000000000000, 0.9659258262890683122, 1.000000000000000000, 0.9659258262890683122, 1.000000000000000000, 0.9659258262890683122, 1.000000000000000000, 0.9659258262890683122, 1.000000000000000000) ) ) 
 REPRESENTATION_ITEM ( '' )  SURFACE ( )  );
#85213=CARTESIAN_POINT ( 'NONE',  ( 14.92337183194729633, 17.67559781766745175, 8.527530157486181039 ) ) ;
#85214=CARTESIAN_POINT ( 'NONE',  ( 4.559911319644449179, 18.89701867748817321, 9.422509992056141925 ) ) ;
#85215=VERTEX_POINT ( 'NONE', #54783 ) ;
#85216=CARTESIAN_POINT ( 'NONE',  ( 19.84674366389459266, 43.71726448433410894, -2.638427012816827677 ) ) ;
#85217=CARTESIAN_POINT ( 'NONE',  ( 7.084665262690076126, 32.02201867748816966, -10.88017736071110164 ) ) ;
#85218=CARTESIAN_POINT ( 'NONE',  ( 12.63842701281683034, 57.46726448433411605, 9.846743663894596210 ) ) ;
#85219=CARTESIAN_POINT ( 'NONE',  ( 24.16423886937409904, 4.095415501580634832, 3.795296366450317205 ) ) ;
#85220=DIRECTION ( 'NONE',  ( -0.000000000000000000, -0.000000000000000000, 1.000000000000000000 ) ) ;
#85223=CARTESIAN_POINT ( 'NONE',  ( 17.20831665107776587, 17.88393115100078745, 7.208316651077764980 ) ) ;
#85224=CARTESIAN_POINT ( 'NONE',  ( -2.816281873526471635, 48.91530133659708213, -3.434112377981056508 ) ) ;
#85225=CARTESIAN_POINT ( 'NONE',  ( 0.1532563361054100626, 55.80059781766745175, -2.638427012816831230 ) ) ;
#85227=CARTESIAN_POINT ( 'NONE',  ( 5.076628168052704559, 15.17559781766745175, -8.527530157486179263 ) ) ;
#85229=CARTESIAN_POINT ( 'NONE',  ( 19.72487221294570858, 70.00000000000000000, 6.500000000000000888 ) ) ;
#85230=CARTESIAN_POINT ( 'NONE',  ( 2.035157376598822676, 2.438685344154838397, -7.964842623401177768 ) ) ;
#85231=CARTESIAN_POINT ( 'NONE',  ( 4.559911319644449179, 48.89701867748817676, 9.422509992056141925 ) ) ;
#85233=CARTESIAN_POINT ( 'NONE',  ( 10.00000000000000178, 54.31368534415484106, 10.88017736071110342 ) ) ;
#85234=CARTESIAN_POINT ( 'NONE',  ( 0.1532563361054083140, 41.00893115100078745, 1.131784320476157264E-15 ) ) ;
#85235=CARTESIAN_POINT ( 'NONE',  ( 19.42250999205614548, 15.98035201082150714, -5.440088680355545492 ) ) ;
#85237=CARTESIAN_POINT ( 'NONE',  ( 19.84674366389459266, 53.30059781766744464, 2.638427012816836559 ) ) ;
#85242=CARTESIAN_POINT ( 'NONE',  ( 12.63842701281683922, 39.55059781766744464, -9.846743663894590881 ) ) ;
#85243=CARTESIAN_POINT ( 'NONE',  ( 2.791683348922240793, 16.63393115100078745, 7.208316651077764092 ) ) ;
#85244=CARTESIAN_POINT ( 'NONE',  ( -2.816281873526471635, 53.91530133659709634, -3.434112377981056508 ) ) ;
#85245=CARTESIAN_POINT ( 'NONE',  ( -0.8801773607111008646, 23.27201867748817676, 2.915334737309923430 ) ) ;
#85246=CARTESIAN_POINT ( 'NONE',  ( 5.076628168052704559, 55.17559781766745175, -8.527530157486179263 ) ) ;
#85249=CARTESIAN_POINT ( 'NONE',  ( 6.204703633549690345, 45.76208216824729647, -14.16423886937410259 ) ) ;
#85250=CARTESIAN_POINT ( 'NONE',  ( -0.3689425029237898834, 56.17874883491396076, -10.36894250292378850 ) ) ;
#85253=CARTESIAN_POINT ( 'NONE',  ( 20.88017736071110875, 45.77201867748816966, -2.915334737309920765 ) ) ;
#85254=CARTESIAN_POINT ( 'NONE',  ( 0.1532563361054082862, 16.21726448433411960, 2.638427012816831674 ) ) ;
#85257=DIRECTION ( 'NONE',  ( 1.000000000000000000, -0.000000000000000000, 0.000000000000000000 ) ) ;
#85260=CARTESIAN_POINT ( 'NONE',  ( 14.92337183194729988, 14.34226448433411782, -8.527530157486177487 ) ) ;
#85262=CARTESIAN_POINT ( 'NONE',  ( 24.16423886937410614, 14.51208216824730179, -3.795296366450302550 ) ) ;
#85263=CARTESIAN_POINT ( 'NONE',  ( 7.361572987183169658, 24.96726448433412315, -9.846743663894592657 ) ) ;
#85264=CARTESIAN_POINT ( 'NONE',  ( 12.91533473730993009, 46.60535201082150536, -10.88017736071109987 ) ) ;
#85267=CARTESIAN_POINT ( 'NONE',  ( 20.88017736071110164, 45.35535201082149115, 2.915334737309930979 ) ) ;
#85271=CARTESIAN_POINT ( 'NONE',  ( 17.08211943468705840, 10.13708216824730179, -12.26659068614894466 ) ) ;
#85272=EDGE_CURVE ( 'NONE', #20606, #45049, #59853, .T. ) ;
#85275=CARTESIAN_POINT ( 'NONE',  ( 19.38216949554541557, 22.24863466993041428, -9.382169495545420901 ) ) ;
#85276=CARTESIAN_POINT ( 'NONE',  ( 7.361572987183169658, 4.967264484334119601, -9.846743663894592657 ) ) ;
#85277=CARTESIAN_POINT ( 'NONE',  ( 20.88017736071110519, 5.563685344154837509, 2.639326808657452039E-16 ) ) ;
#85278=CARTESIAN_POINT ( 'NONE',  ( 18.72515096720570327, 11.07228050351031712, -6.499999999999992006 ) ) ;
#85279=CARTESIAN_POINT ( 'NONE',  ( 5.076628168052703671, 21.84226448433411960, 8.527530157486179263 ) ) ;
#85280=CARTESIAN_POINT ( 'NONE',  ( -0.8801773607111008646, 28.27201867748817321, 2.915334737309923430 ) ) ;
#85283=CARTESIAN_POINT ( 'NONE',  ( 17.96484262340118221, 61.18868534415482685, -7.964842623401177768 ) ) ;
#85284=CARTESIAN_POINT ( 'NONE',  ( 17.85158348494333325, 39.73726573380442773, -6.500000000000027534 ) ) ;
#85285=CARTESIAN_POINT ( 'NONE',  ( 3.591859063236761518, 64.95696800326376774, 11.09922568453594849 ) ) ;
#85286=CARTESIAN_POINT ( 'NONE',  ( -0.8801773607110991993, 57.85535201082149825, -2.915334737309923874 ) ) ;
#85287=( BOUNDED_SURFACE ( )  B_SPLINE_SURFACE ( 1, 2, ( 
 ( #17029, #8049, #71016, #23559, #38549, #15564, #78505, #69044, #92029, #85519, #24540, #32504, #84539, #77025, #39040, #70027, #47995, #69534, #31515, #62014, #55516, #31997, #2538, #578, #86015, #32993, #31023, #54511, #1551, #10018, #92514, #40519, #63002, #63496, #93998, #61519, #47508, #85024, #16036, #46525, #25522, #16537, #47014, #77504, #9018, #39535, #62503, #93006, #55001, #78009, #9516, #40016, #70520, #2043, #88458, #65450, #49466, #64949, #73446, #56494, #27948, #94971, #78992, #86512, #56971, #18493, #27458, #41010, #63969, #80471, #49965, #4972, #25999, #71510, #10990, #26473, #33472, #57466, #35452, #80960, #48489, #87959, #87474, #10497, #41995, #65948, #96475, #86984, #48981, #19475, #18989, #50454, #34458, #79490, #11969, #42472, #72956, #18009, #72459, #41511, #95975, #3993, #19959, #71977, #95477, #3024, #3502, #79972, #11478, #4485, #34952, #57951, #12460, #42965, #94481, #26965, #33959, #64464, #81447, #96975, #37448, #66942, #12948, #43443, #89448, #37942, #98459, #83428, #89933, #90914, #58946, #73944, #29915, #52433, #97462, #98954, #44431, #97963, #75427, #20961, #28927, #21450, #13445, #60420, #14947, #28449, #5473, #51947, #50952, #88954, #13957, #59431, #90412, #74934, #51449, #82931, #68432, #6435, #14449, #58440, #29419, #22444, #20463, #81935, #43932, #74429, #35945, #52916, #59924, #66441, #36946, #7444, #6941, #5957, #67938, #67444, #82432, #36450, #21954, #44919, #45416, #75920, #62376, #15918, #453, #32377, #24415, #76415, #15445, #39411, #85393, #17404, #85890, #78376, #30410, #31390, #45926, #16906, #61890, #92395, #38919, #62882, #47871, #92882, #30903, #47381, #54881, #7930, #23920, #31878, #91415, #9897, #38427, #22941, #60912, #93379, #53409, #68924, #1426, #69906, #77880, #61397, #91908, #23433, #84901, #24906, #84421, #53912, #46409, #70399, #46891, #40401, #83916, #1918, #70895, #76897, #69407, #16414, #55389, #8412, #928, #9392, #39896, #54389, #77382, #8895, #10874, #2903, #55885, #19839, #71862, #42845, #2412, #40887, #94854, #32871, #94361, #25880, #19355, #79853, #34835, #56381, #93874, #4370, #80351, #64344, #11355, #88341, #71390, #63370, #41396, #25400, #86383, #3374, #33353, #42357, #17885, #78874, #95349, #64831, #50328, #63848, #48369, #86870, #57832, #10382, #87356, #26355, #26847, #56856, #18379, #49351, #80840, #57343, #33835, #18870, #41875, #72339, #65328, #3871, #49839, #48858, #34335, #95853, #79367, #87836, #11848, #72832, #27336, #12340, #90293, #20341, #96357, #73329, #97341, #65823, #74811, #20836, #81331, #90799, #36824, #5352, #97841, #74307, #73818 ),
 ( #27828, #58314, #35830, #52799, #14327, #98337, #5832, #6815, #66316, #88830, #44798, #67316, #13328, #14828, #59312, #13828, #21830, #96852, #81809, #36325, #28328, #75303, #29795, #43325, #50838, #66818, #12826, #4854, #28813, #43812, #6317, #89810, #58818, #29306, #83303, #21331, #59801, #35329, #44309, #37331, #89327, #51325, #51820, #82306, #52313, #67821, #82805, #60306, #22325, #93261, #92767, #24785, #24294, #92285, #46293, #75799, #7317, #68313, #70284, #83801, #77268, #30780, #15324, #47260, #39296, #91290, #30287, #54269, #1316, #32255, #1800, #55260, #45304, #76781, #60790, #31767, #8297, #38796, #53793, #77760, #68805, #84308, #22812, #16294, #85775, #39785, #37820, #46775, #15808, #98833, #816, #62757, #53293, #45806, #7814, #8779, #69295, #9275, #23808, #76297, #69787, #62261, #54760, #38309, #31270, #336, #85279, #61770, #61284, #91793, #84785, #23313, #16785, #79244, #10757, #87230, #41757, #18754, #49237, #95220, #95729, #41274, #32750, #57714, #25769, #70779, #40271, #48250, #27214, #57222, #42242, #48738, #49715, #17774, #2295, #87721, #11237, #56263, #17285, #3256, #56738, #34215, #78761, #86756, #71748, #71264, #19234, #72708, #86261, #63247, #33723, #9775, #47762, #64223, #18261, #79740, #94739, #10268, #72227, #78260, #26244, #3757, #93753, #64709, #80225, #25286, #40762, #2789, #33243, #55769, #11729, #26727, #63738, #4244, #65209, #34714, #94238, #67200, #36206, #89206, #19722, #50211, #12217, #14208, #27711, #21210, #73698, #58195, #90182, #82193, #35202, #73206, #97232, #44187, #75184, #44689, #37215, #88214, #20719, #4737, #74697, #51210, #81694, #96730, #21712, #12713, #28206, #65707, #59191, #67703, #82690, #80722, #89697, #58702, #42726, #43701, #6697, #98214, #88706, #50720, #51709, #13206, #52196, #66704, #20216, #13702, #6207, #36709, #29673, #74187, #81213, #97726, #5718, #96232, #43206, #28699, #5232, #35710, #29189, #59687, #66198, #69179, #46178, #76664, #92166, #31648, #211, #14710, #92646, #52684, #37699, #23691, #76179, #8182, #61168, #68197, #38679, #62138, #91676, #702, #60183, #31155, #16172, #22205, #98718, #60673, #22700, #7196, #77152, #61645, #30169, #23195, #90679, #84664, #83185, #8661, #54154, #53669, #45184, #75682, #83684, #91171, #30662, #1189, #46657, #84184, #53178, #15199, #15694, #39173, #69663, #45681, #7699, #38196, #68683, #50547, #51535, #66033, #37035, #82027, #13537, #59030, #83023, #74026, #89536, #96562, #21541, #98553, #45010, #12549, #52032, #21046, #43051, #6044, #68025, #37536, #51036, #13035, #82525, #44021, #14540, #97555, #81529, #14041, #44522 ) ),
 .UNSPECIFIED., .F., .F., .F. ) 
 B_SPLINE_SURFACE_WITH_KNOTS ( ( 2, 2 ),
 ( 3, 2, 2, 2, 2, 2, 2, 2, 2, 2, 2, 2, 2, 2, 2, 2, 2, 2, 2, 2, 2, 2, 2, 2, 2, 2, 2, 2, 2, 2, 2, 2, 2, 2, 2, 2, 2, 2, 2, 2, 2, 2, 2, 2, 2, 2, 2, 2, 2, 2, 2, 2, 2, 2, 2, 2, 2, 2, 2, 2, 2, 2, 2, 2, 2, 2, 2, 2, 2, 2, 2, 2, 2, 2, 2, 2, 2, 2, 2, 2, 2, 2, 2, 2, 2, 2, 2, 2, 2, 2, 2, 2, 2, 2, 2, 2, 2, 2, 2, 2, 2, 2, 2, 2, 2, 2, 2, 2, 2, 2, 2, 2, 2, 2, 2, 2, 2, 2, 2, 2, 2, 2, 2, 2, 2, 2, 2, 2, 2, 2, 2, 2, 2, 2, 2, 2, 2, 2, 2, 2, 2, 2, 2, 2, 2, 2, 2, 2, 2, 2, 2, 2, 2, 2, 2, 2, 2, 2, 2, 2, 2, 2, 3 ),
 ( 0.000000000000000000, 1.000000000000000000 ),
 ( 0.000000000000000000, 0.005952380952380952051, 0.01190476190476190410, 0.01785714285714285615, 0.02380952380952380820, 0.02976190476190476025, 0.03571428571428571230, 0.04166666666666666435, 0.04761904761904761640, 0.05357142857142856845, 0.05952380952380952051, 0.06547619047619047949, 0.07142857142857142461, 0.07738095238095238360, 0.08333333333333332871, 0.08928571428571428770, 0.09523809523809523281, 0.1011904761904761918, 0.1071428571428571369, 0.1130952380952380959, 0.1190476190476190410, 0.1250000000000000000, 0.1309523809523809590, 0.1369047619047619180, 0.1428571428571428492, 0.1488095238095238082, 0.1547619047619047672, 0.1607142857142857262, 0.1666666666666666574, 0.1726190476190476164, 0.1785714285714285754, 0.1845238095238095344, 0.1904761904761904656, 0.1964285714285714246, 0.2023809523809523836, 0.2083333333333333426, 0.2142857142857142738, 0.2202380952380952328, 0.2261904761904761918, 0.2321428571428571508, 0.2380952380952380820, 0.2440476190476190410, 0.2500000000000000000, 0.2559523809523809312, 0.2619047619047619180, 0.2678571428571428492, 0.2738095238095238360, 0.2797619047619047672, 0.2857142857142856984, 0.2916666666666666852, 0.2976190476190476164, 0.3035714285714285476, 0.3095238095238095344, 0.3154761904761904656, 0.3214285714285714524, 0.3273809523809523836, 0.3333333333333333148, 0.3392857142857143016, 0.3452380952380952328, 0.3511904761904761640, 0.3571428571428571508, 0.3630952380952380820, 0.3690476190476190688, 0.3750000000000000000, 0.3809523809523809312, 0.3869047619047619180, 0.3928571428571428492, 0.3988095238095238360, 0.4047619047619047672, 0.4107142857142856984, 0.4166666666666666852, 0.4226190476190476164, 0.4285714285714285476, 0.4345238095238095344, 0.4404761904761904656, 0.4464285714285714524, 0.4523809523809523836, 0.4583333333333333148, 0.4642857142857143016, 0.4702380952380952328, 0.4761904761904761640, 0.4821428571428571508, 0.4880952380952380820, 0.4940476190476190688, 0.5000000000000000000, 0.5059523809523809312, 0.5119047619047618625, 0.5178571428571429047, 0.5238095238095238360, 0.5297619047619047672, 0.5357142857142856984, 0.5416666666666666297, 0.5476190476190476719, 0.5535714285714286031, 0.5595238095238095344, 0.5654761904761904656, 0.5714285714285713969, 0.5773809523809523281, 0.5833333333333333703, 0.5892857142857143016, 0.5952380952380952328, 0.6011904761904761640, 0.6071428571428570953, 0.6130952380952381375, 0.6190476190476190688, 0.6250000000000000000, 0.6309523809523809312, 0.6369047619047618625, 0.6428571428571429047, 0.6488095238095238360, 0.6547619047619047672, 0.6607142857142856984, 0.6666666666666666297, 0.6726190476190476719, 0.6785714285714286031, 0.6845238095238095344, 0.6904761904761904656, 0.6964285714285713969, 0.7023809523809523281, 0.7083333333333333703, 0.7142857142857143016, 0.7202380952380952328, 0.7261904761904761640, 0.7321428571428570953, 0.7380952380952381375, 0.7440476190476190688, 0.7500000000000000000, 0.7559523809523809312, 0.7619047619047618625, 0.7678571428571429047, 0.7738095238095238360, 0.7797619047619047672, 0.7857142857142856984, 0.7916666666666666297, 0.7976190476190476719, 0.8035714285714286031, 0.8095238095238095344, 0.8154761904761904656, 0.8214285714285713969, 0.8273809523809523281, 0.8333333333333333703, 0.8392857142857143016, 0.8452380952380952328, 0.8511904761904761640, 0.8571428571428570953, 0.8630952380952381375, 0.8690476190476190688, 0.8750000000000000000, 0.8809523809523809312, 0.8869047619047618625, 0.8928571428571429047, 0.8988095238095238360, 0.9047619047619047672, 0.9107142857142856984, 0.9166666666666666297, 0.9226190476190476719, 0.9285714285714286031, 0.9345238095238095344, 0.9404761904761904656, 0.9464285714285713969, 0.9523809523809523281, 0.9583333333333333703, 0.9642857142857143016 ),
 .UNSPECIFIED. ) 
 GEOMETRIC_REPRESENTATION_ITEM ( )  RATIONAL_B_SPLINE_SURFACE ( (
 ( 1.000000000000000000, 0.9659258262890683122, 1.000000000000000000, 0.9659258262890683122, 1.000000000000000000, 0.9659258262890683122, 1.000000000000000000, 0.9659258262890683122, 1.000000000000000000, 0.9659258262890683122, 1.000000000000000000, 0.9659258262890683122, 1.000000000000000000, 0.9659258262890683122, 1.000000000000000000, 0.9659258262890683122, 1.000000000000000000, 0.9659258262890683122, 1.000000000000000000, 0.9659258262890683122, 1.000000000000000000, 0.9659258262890683122, 1.000000000000000000, 0.9659258262890683122, 1.000000000000000000, 0.9659258262890683122, 1.000000000000000000, 0.9659258262890683122, 1.000000000000000000, 0.9659258262890683122, 1.000000000000000000, 0.9659258262890683122, 1.000000000000000000, 0.9659258262890683122, 1.000000000000000000, 0.9659258262890683122, 1.000000000000000000, 0.9659258262890683122, 1.000000000000000000, 0.9659258262890683122, 1.000000000000000000, 0.9659258262890683122, 1.000000000000000000, 0.9659258262890683122, 1.000000000000000000, 0.9659258262890683122, 1.000000000000000000, 0.9659258262890683122, 1.000000000000000000, 0.9659258262890683122, 1.000000000000000000, 0.9659258262890683122, 1.000000000000000000, 0.9659258262890683122, 1.000000000000000000, 0.9659258262890683122, 1.000000000000000000, 0.9659258262890683122, 1.000000000000000000, 0.9659258262890683122, 1.000000000000000000, 0.9659258262890683122, 1.000000000000000000, 0.9659258262890683122, 1.000000000000000000, 0.9659258262890683122, 1.000000000000000000, 0.9659258262890683122, 1.000000000000000000, 0.9659258262890683122, 1.000000000000000000, 0.9659258262890683122, 1.000000000000000000, 0.9659258262890683122, 1.000000000000000000, 0.9659258262890683122, 1.000000000000000000, 0.9659258262890683122, 1.000000000000000000, 0.9659258262890683122, 1.000000000000000000, 0.9659258262890683122, 1.000000000000000000, 0.9659258262890683122, 1.000000000000000000, 0.9659258262890683122, 1.000000000000000000, 0.9659258262890683122, 1.000000000000000000, 0.9659258262890683122, 1.000000000000000000, 0.9659258262890683122, 1.000000000000000000, 0.9659258262890683122, 1.000000000000000000, 0.9659258262890683122, 1.000000000000000000, 0.9659258262890683122, 1.000000000000000000, 0.9659258262890683122, 1.000000000000000000, 0.9659258262890683122, 1.000000000000000000, 0.9659258262890683122, 1.000000000000000000, 0.9659258262890683122, 1.000000000000000000, 0.9659258262890683122, 1.000000000000000000, 0.9659258262890683122, 1.000000000000000000, 0.9659258262890683122, 1.000000000000000000, 0.9659258262890683122, 1.000000000000000000, 0.9659258262890683122, 1.000000000000000000, 0.9659258262890683122, 1.000000000000000000, 0.9659258262890683122, 1.000000000000000000, 0.9659258262890683122, 1.000000000000000000, 0.9659258262890683122, 1.000000000000000000, 0.9659258262890683122, 1.000000000000000000, 0.9659258262890683122, 1.000000000000000000, 0.9659258262890683122, 1.000000000000000000, 0.9659258262890683122, 1.000000000000000000, 0.9659258262890683122, 1.000000000000000000, 0.9659258262890683122, 1.000000000000000000, 0.9659258262890683122, 1.000000000000000000, 0.9659258262890683122, 1.000000000000000000, 0.9659258262890683122, 1.000000000000000000, 0.9659258262890683122, 1.000000000000000000, 0.9659258262890683122, 1.000000000000000000, 0.9659258262890683122, 1.000000000000000000, 0.9659258262890683122, 1.000000000000000000, 0.9659258262890683122, 1.000000000000000000, 0.9659258262890683122, 1.000000000000000000, 0.9659258262890683122, 1.000000000000000000, 0.9659258262890683122, 1.000000000000000000, 0.9659258262890683122, 1.000000000000000000, 0.9659258262890683122, 1.000000000000000000, 0.9659258262890683122, 1.000000000000000000, 0.9659258262890683122, 1.000000000000000000, 0.9659258262890683122, 1.000000000000000000, 0.9659258262890683122, 1.000000000000000000, 0.9659258262890683122, 1.000000000000000000, 0.9659258262890683122, 1.000000000000000000, 0.9659258262890683122, 1.000000000000000000, 0.9659258262890683122, 1.000000000000000000, 0.9659258262890683122, 1.000000000000000000, 0.9659258262890683122, 1.000000000000000000, 0.9659258262890683122, 1.000000000000000000, 0.9659258262890683122, 1.000000000000000000, 0.9659258262890683122, 1.000000000000000000, 0.9659258262890683122, 1.000000000000000000, 0.9659258262890683122, 1.000000000000000000, 0.9659258262890683122, 1.000000000000000000, 0.9659258262890683122, 1.000000000000000000, 0.9659258262890683122, 1.000000000000000000, 0.9659258262890683122, 1.000000000000000000, 0.9659258262890683122, 1.000000000000000000, 0.9659258262890683122, 1.000000000000000000, 0.9659258262890683122, 1.000000000000000000, 0.9659258262890683122, 1.000000000000000000, 0.9659258262890683122, 1.000000000000000000, 0.9659258262890683122, 1.000000000000000000, 0.9659258262890683122, 1.000000000000000000, 0.9659258262890683122, 1.000000000000000000, 0.9659258262890683122, 1.000000000000000000, 0.9659258262890683122, 1.000000000000000000, 0.9659258262890683122, 1.000000000000000000, 0.9659258262890683122, 1.000000000000000000, 0.9659258262890683122, 1.000000000000000000, 0.9659258262890683122, 1.000000000000000000, 0.9659258262890683122, 1.000000000000000000, 0.9659258262890683122, 1.000000000000000000, 0.9659258262890683122, 1.000000000000000000, 0.9659258262890683122, 1.000000000000000000, 0.9659258262890683122, 1.000000000000000000, 0.9659258262890683122, 1.000000000000000000, 0.9659258262890683122, 1.000000000000000000, 0.9659258262890683122, 1.000000000000000000, 0.9659258262890683122, 1.000000000000000000, 0.9659258262890683122, 1.000000000000000000, 0.9659258262890683122, 1.000000000000000000, 0.9659258262890683122, 1.000000000000000000, 0.9659258262890683122, 1.000000000000000000, 0.9659258262890683122, 1.000000000000000000, 0.9659258262890683122, 1.000000000000000000, 0.9659258262890683122, 1.000000000000000000, 0.9659258262890683122, 1.000000000000000000, 0.9659258262890683122, 1.000000000000000000, 0.9659258262890683122, 1.000000000000000000, 0.9659258262890683122, 1.000000000000000000, 0.9659258262890683122, 1.000000000000000000, 0.9659258262890683122, 1.000000000000000000, 0.9659258262890683122, 1.000000000000000000, 0.9659258262890683122, 1.000000000000000000, 0.9659258262890683122, 1.000000000000000000, 0.9659258262890683122, 1.000000000000000000, 0.9659258262890683122, 1.000000000000000000, 0.9659258262890683122, 1.000000000000000000, 0.9659258262890683122, 1.000000000000000000, 0.9659258262890683122, 1.000000000000000000, 0.9659258262890683122, 1.000000000000000000, 0.9659258262890683122, 1.000000000000000000, 0.9659258262890683122, 1.000000000000000000, 0.9659258262890683122, 1.000000000000000000, 0.9659258262890683122, 1.000000000000000000, 0.9659258262890683122, 1.000000000000000000, 0.9659258262890683122, 1.000000000000000000, 0.9659258262890683122, 1.000000000000000000, 0.9659258262890683122, 1.000000000000000000, 0.9659258262890683122, 1.000000000000000000, 0.9659258262890683122, 1.000000000000000000, 0.9659258262890683122, 1.000000000000000000, 0.9659258262890683122, 1.000000000000000000, 0.9659258262890683122, 1.000000000000000000, 0.9659258262890683122, 1.000000000000000000, 0.9659258262890683122, 1.000000000000000000, 0.9659258262890683122, 1.000000000000000000, 0.9659258262890683122, 1.000000000000000000),
 ( 1.000000000000000000, 0.9659258262890683122, 1.000000000000000000, 0.9659258262890683122, 1.000000000000000000, 0.9659258262890683122, 1.000000000000000000, 0.9659258262890683122, 1.000000000000000000, 0.9659258262890683122, 1.000000000000000000, 0.9659258262890683122, 1.000000000000000000, 0.9659258262890683122, 1.000000000000000000, 0.9659258262890683122, 1.000000000000000000, 0.9659258262890683122, 1.000000000000000000, 0.9659258262890683122, 1.000000000000000000, 0.9659258262890683122, 1.000000000000000000, 0.9659258262890683122, 1.000000000000000000, 0.9659258262890683122, 1.000000000000000000, 0.9659258262890683122, 1.000000000000000000, 0.9659258262890683122, 1.000000000000000000, 0.9659258262890683122, 1.000000000000000000, 0.9659258262890683122, 1.000000000000000000, 0.9659258262890683122, 1.000000000000000000, 0.9659258262890683122, 1.000000000000000000, 0.9659258262890683122, 1.000000000000000000, 0.9659258262890683122, 1.000000000000000000, 0.9659258262890683122, 1.000000000000000000, 0.9659258262890683122, 1.000000000000000000, 0.9659258262890683122, 1.000000000000000000, 0.9659258262890683122, 1.000000000000000000, 0.9659258262890683122, 1.000000000000000000, 0.9659258262890683122, 1.000000000000000000, 0.9659258262890683122, 1.000000000000000000, 0.9659258262890683122, 1.000000000000000000, 0.9659258262890683122, 1.000000000000000000, 0.9659258262890683122, 1.000000000000000000, 0.9659258262890683122, 1.000000000000000000, 0.9659258262890683122, 1.000000000000000000, 0.9659258262890683122, 1.000000000000000000, 0.9659258262890683122, 1.000000000000000000, 0.9659258262890683122, 1.000000000000000000, 0.9659258262890683122, 1.000000000000000000, 0.9659258262890683122, 1.000000000000000000, 0.9659258262890683122, 1.000000000000000000, 0.9659258262890683122, 1.000000000000000000, 0.9659258262890683122, 1.000000000000000000, 0.9659258262890683122, 1.000000000000000000, 0.9659258262890683122, 1.000000000000000000, 0.9659258262890683122, 1.000000000000000000, 0.9659258262890683122, 1.000000000000000000, 0.9659258262890683122, 1.000000000000000000, 0.9659258262890683122, 1.000000000000000000, 0.9659258262890683122, 1.000000000000000000, 0.9659258262890683122, 1.000000000000000000, 0.9659258262890683122, 1.000000000000000000, 0.9659258262890683122, 1.000000000000000000, 0.9659258262890683122, 1.000000000000000000, 0.9659258262890683122, 1.000000000000000000, 0.9659258262890683122, 1.000000000000000000, 0.9659258262890683122, 1.000000000000000000, 0.9659258262890683122, 1.000000000000000000, 0.9659258262890683122, 1.000000000000000000, 0.9659258262890683122, 1.000000000000000000, 0.9659258262890683122, 1.000000000000000000, 0.9659258262890683122, 1.000000000000000000, 0.9659258262890683122, 1.000000000000000000, 0.9659258262890683122, 1.000000000000000000, 0.9659258262890683122, 1.000000000000000000, 0.9659258262890683122, 1.000000000000000000, 0.9659258262890683122, 1.000000000000000000, 0.9659258262890683122, 1.000000000000000000, 0.9659258262890683122, 1.000000000000000000, 0.9659258262890683122, 1.000000000000000000, 0.9659258262890683122, 1.000000000000000000, 0.9659258262890683122, 1.000000000000000000, 0.9659258262890683122, 1.000000000000000000, 0.9659258262890683122, 1.000000000000000000, 0.9659258262890683122, 1.000000000000000000, 0.9659258262890683122, 1.000000000000000000, 0.9659258262890683122, 1.000000000000000000, 0.9659258262890683122, 1.000000000000000000, 0.9659258262890683122, 1.000000000000000000, 0.9659258262890683122, 1.000000000000000000, 0.9659258262890683122, 1.000000000000000000, 0.9659258262890683122, 1.000000000000000000, 0.9659258262890683122, 1.000000000000000000, 0.9659258262890683122, 1.000000000000000000, 0.9659258262890683122, 1.000000000000000000, 0.9659258262890683122, 1.000000000000000000, 0.9659258262890683122, 1.000000000000000000, 0.9659258262890683122, 1.000000000000000000, 0.9659258262890683122, 1.000000000000000000, 0.9659258262890683122, 1.000000000000000000, 0.9659258262890683122, 1.000000000000000000, 0.9659258262890683122, 1.000000000000000000, 0.9659258262890683122, 1.000000000000000000, 0.9659258262890683122, 1.000000000000000000, 0.9659258262890683122, 1.000000000000000000, 0.9659258262890683122, 1.000000000000000000, 0.9659258262890683122, 1.000000000000000000, 0.9659258262890683122, 1.000000000000000000, 0.9659258262890683122, 1.000000000000000000, 0.9659258262890683122, 1.000000000000000000, 0.9659258262890683122, 1.000000000000000000, 0.9659258262890683122, 1.000000000000000000, 0.9659258262890683122, 1.000000000000000000, 0.9659258262890683122, 1.000000000000000000, 0.9659258262890683122, 1.000000000000000000, 0.9659258262890683122, 1.000000000000000000, 0.9659258262890683122, 1.000000000000000000, 0.9659258262890683122, 1.000000000000000000, 0.9659258262890683122, 1.000000000000000000, 0.9659258262890683122, 1.000000000000000000, 0.9659258262890683122, 1.000000000000000000, 0.9659258262890683122, 1.000000000000000000, 0.9659258262890683122, 1.000000000000000000, 0.9659258262890683122, 1.000000000000000000, 0.9659258262890683122, 1.000000000000000000, 0.9659258262890683122, 1.000000000000000000, 0.9659258262890683122, 1.000000000000000000, 0.9659258262890683122, 1.000000000000000000, 0.9659258262890683122, 1.000000000000000000, 0.9659258262890683122, 1.000000000000000000, 0.9659258262890683122, 1.000000000000000000, 0.9659258262890683122, 1.000000000000000000, 0.9659258262890683122, 1.000000000000000000, 0.9659258262890683122, 1.000000000000000000, 0.9659258262890683122, 1.000000000000000000, 0.9659258262890683122, 1.000000000000000000, 0.9659258262890683122, 1.000000000000000000, 0.9659258262890683122, 1.000000000000000000, 0.9659258262890683122, 1.000000000000000000, 0.9659258262890683122, 1.000000000000000000, 0.9659258262890683122, 1.000000000000000000, 0.9659258262890683122, 1.000000000000000000, 0.9659258262890683122, 1.000000000000000000, 0.9659258262890683122, 1.000000000000000000, 0.9659258262890683122, 1.000000000000000000, 0.9659258262890683122, 1.000000000000000000, 0.9659258262890683122, 1.000000000000000000, 0.9659258262890683122, 1.000000000000000000, 0.9659258262890683122, 1.000000000000000000, 0.9659258262890683122, 1.000000000000000000, 0.9659258262890683122, 1.000000000000000000, 0.9659258262890683122, 1.000000000000000000, 0.9659258262890683122, 1.000000000000000000, 0.9659258262890683122, 1.000000000000000000, 0.9659258262890683122, 1.000000000000000000, 0.9659258262890683122, 1.000000000000000000, 0.9659258262890683122, 1.000000000000000000, 0.9659258262890683122, 1.000000000000000000, 0.9659258262890683122, 1.000000000000000000, 0.9659258262890683122, 1.000000000000000000, 0.9659258262890683122, 1.000000000000000000, 0.9659258262890683122, 1.000000000000000000, 0.9659258262890683122, 1.000000000000000000, 0.9659258262890683122, 1.000000000000000000, 0.9659258262890683122, 1.000000000000000000, 0.9659258262890683122, 1.000000000000000000, 0.9659258262890683122, 1.000000000000000000, 0.9659258262890683122, 1.000000000000000000, 0.9659258262890683122, 1.000000000000000000, 0.9659258262890683122, 1.000000000000000000, 0.9659258262890683122, 1.000000000000000000, 0.9659258262890683122, 1.000000000000000000, 0.9659258262890683122, 1.000000000000000000, 0.9659258262890683122, 1.000000000000000000) ) ) 
 REPRESENTATION_ITEM ( '' )  SURFACE ( )  );
#85290=CARTESIAN_POINT ( 'NONE',  ( 19.84674366389459621, 33.50893115100078745, 7.409399052514197653E-17 ) ) ;
#85291=CARTESIAN_POINT ( 'NONE',  ( 22.81628187352647785, 56.41530133659708213, 3.434112377981063169 ) ) ;
#85292=CARTESIAN_POINT ( 'NONE',  ( 10.00000000000000178, 13.05374883491396787, 14.16423886937410082 ) ) ;
#85293=CARTESIAN_POINT ( 'NONE',  ( 5.076628168052703671, 21.84226448433411960, 8.527530157486179263 ) ) ;
#85294=CARTESIAN_POINT ( 'NONE',  ( 16.40814093676323893, 25.79030133659708923, 11.09922568453595026 ) ) ;
#85296=DIRECTION ( 'NONE',  ( -1.000000000000000000, 0.000000000000000000, 0.000000000000000000 ) ) ;
#85297=CARTESIAN_POINT ( 'NONE',  ( 2.035157376598824452, 53.68868534415484817, 7.964842623401179544 ) ) ;
#85298=CARTESIAN_POINT ( 'NONE',  ( 5.076628168052703671, 61.84226448433412315, 8.527530157486179263 ) ) ;
#85300=CARTESIAN_POINT ( 'NONE',  ( 14.92337183194729988, 34.34226448433411605, -8.527530157486177487 ) ) ;
#85301=CARTESIAN_POINT ( 'NONE',  ( 18.52753015748618282, 18.92559781766745175, -4.923371831947291888 ) ) ;
#85302=CARTESIAN_POINT ( 'NONE',  ( 15.44008868035555260, 14.73035201082150536, 9.422509992056143702 ) ) ;
#85304=CARTESIAN_POINT ( 'NONE',  ( 22.81628187352648496, 21.83196800326374643, -3.434112377981050290 ) ) ;
#85305=CARTESIAN_POINT ( 'NONE',  ( 17.20831665107776587, 27.88393115100078390, 7.208316651077764980 ) ) ;
#85307=CARTESIAN_POINT ( 'NONE',  ( 20.88017736071110875, 15.77201867748817143, -2.915334737309920765 ) ) ;
#85308=CARTESIAN_POINT ( 'NONE',  ( 0.1532563361054100626, 40.80059781766745886, -2.638427012816831230 ) ) ;
#85309=CARTESIAN_POINT ( 'NONE',  ( 0.5774900079438590739, 12.64701867748817321, -5.440088680355550821 ) ) ;
#85311=CARTESIAN_POINT ( 'NONE',  ( 0.5774900079438590739, 37.64701867748817676, -5.440088680355550821 ) ) ;
#85312=CARTESIAN_POINT ( 'NONE',  ( -4.164238869374099927, 62.01208216824728936, 3.795296366450308767 ) ) ;
#85313=CARTESIAN_POINT ( 'NONE',  ( 10.00000000000000000, 19.75893115100078390, -9.846743663894594434 ) ) ;
#85314=CARTESIAN_POINT ( 'NONE',  ( 14.92337183194729988, 44.34226448433412315, -8.527530157486177487 ) ) ;
#85315=CARTESIAN_POINT ( 'NONE',  ( -12.69000000000001371, 93.50000000000000000, 9.500000000000000000 ) ) ;
#85318=CARTESIAN_POINT ( 'NONE',  ( -0.3689425029237898834, 21.17874883491396432, -10.36894250292378850 ) ) ;
#85319=CARTESIAN_POINT ( 'NONE',  ( 0.1532563361054083140, 41.00893115100078745, 1.131784320476157264E-15 ) ) ;
#85322=CARTESIAN_POINT ( 'NONE',  ( -4.164238869374099927, 57.01208216824731068, 3.795296366450308767 ) ) ;
#85323=CARTESIAN_POINT ( 'NONE',  ( 18.52753015748617571, 23.09226448433411960, 4.923371831947298993 ) ) ;
#85326=CARTESIAN_POINT ( 'NONE',  ( 0.5774900079438590739, 52.64701867748817676, -5.440088680355550821 ) ) ;
#85327=CARTESIAN_POINT ( 'NONE',  ( 0.6178305044545818747, 53.49863466993041072, -9.382169495545419124 ) ) ;
#85328=CARTESIAN_POINT ( 'NONE',  ( 2.035157376598824452, 18.68868534415484106, 7.964842623401179544 ) ) ;
#85329=CARTESIAN_POINT ( 'NONE',  ( 22.81628187352647785, 51.62363466993042493, 6.195893100308588602E-16 ) ) ;
#85330=CARTESIAN_POINT ( 'NONE',  ( 10.00000000000000178, 62.25893115100078745, 9.846743663894594434 ) ) ;
#85331=CARTESIAN_POINT ( 'NONE',  ( 5.076628168052704559, 20.17559781766745175, -8.527530157486179263 ) ) ;
#85332=VERTEX_POINT ( 'NONE', #87252 ) ;
#85336=CARTESIAN_POINT ( 'NONE',  ( 10.00000000000000000, 50.55374883491396787, -14.16423886937410082 ) ) ;
#85337=CARTESIAN_POINT ( 'NONE',  ( -4.164238869374099927, 12.01208216824730357, 3.795296366450308767 ) ) ;
#85338=CARTESIAN_POINT ( 'NONE',  ( -0.8801773607111008646, 18.27201867748817321, 2.915334737309923430 ) ) ;
#85339=CARTESIAN_POINT ( 'NONE',  ( 4.559911319644449179, 37.23035201082150536, -9.422509992056141925 ) ) ;
#85341=CARTESIAN_POINT ( 'NONE',  ( -46.82017113615791004, 100.6079546444643569, -9.324761308090124601 ) ) ;
#85342=CARTESIAN_POINT ( 'NONE',  ( 1.472469842513823179, 1.425597817667451528, 4.923371831947296329 ) ) ;
#85344=CARTESIAN_POINT ( 'NONE',  ( 1.472469842513823179, 20.59226448433411960, -4.923371831947296329 ) ) ;
#85345=CARTESIAN_POINT ( 'NONE',  ( 18.28836319691946599, 19.34492782695771140, 6.499999999999979572 ) ) ;
#85347=CARTESIAN_POINT ( 'NONE',  ( 10.00000000000000000, 9.758931151000785675, -9.846743663894594434 ) ) ;
#85348=CARTESIAN_POINT ( 'NONE',  ( 1.472469842513823179, 36.42559781766745175, 4.923371831947296329 ) ) ;
#85349=CARTESIAN_POINT ( 'NONE',  ( 7.084665262690076126, 9.105352010821503583, 10.88017736071109987 ) ) ;
#85351=CARTESIAN_POINT ( 'NONE',  ( 16.40814093676323893, 25.79030133659708923, 11.09922568453595026 ) ) ;
#85352=CARTESIAN_POINT ( 'NONE',  ( 10.00000000000000178, 54.31368534415484106, 10.88017736071110342 ) ) ;
#85353=CARTESIAN_POINT ( 'NONE',  ( 20.36894250292379738, 44.92874883491396787, -10.36894250292379027 ) ) ;
#85354=CARTESIAN_POINT ( 'NONE',  ( 12.63842701281683922, 4.550597817667451750, -9.846743663894590881 ) ) ;
#85356=EDGE_CURVE ( 'NONE', #85047, #24064, #78781, .T. ) ;
#85357=EDGE_CURVE ( 'NONE', #37711, #24202, #60445, .T. ) ;
#85358=CARTESIAN_POINT ( 'NONE',  ( 18.52753015748617571, 48.09226448433412315, 4.923371831947298993 ) ) ;
#85359=CARTESIAN_POINT ( 'NONE',  ( 10.00000000000000178, 37.25893115100078745, 9.846743663894594434 ) ) ;
#85360=CARTESIAN_POINT ( 'NONE',  ( -4.164238869374099927, 12.01208216824730357, 3.795296366450308767 ) ) ;
#85361=CARTESIAN_POINT ( 'NONE',  ( -4.164238869374098151, 21.59541550158063217, -3.795296366450310543 ) ) ;
#85362=CARTESIAN_POINT ( 'NONE',  ( -0.8801773607111008646, 53.27201867748816966, 2.915334737309923430 ) ) ;
#85363=CARTESIAN_POINT ( 'NONE',  ( 20.88017736071110875, 5.772018677488170546, -2.915334737309920765 ) ) ;
#85364=CARTESIAN_POINT ( 'NONE',  ( 10.00000000000000000, 51.81368534415484106, -10.88017736071110342 ) ) ;
#85365=CARTESIAN_POINT ( 'NONE',  ( 10.00000000000000000, 36.81368534415484106, -10.88017736071110342 ) ) ;
#85367=CARTESIAN_POINT ( 'NONE',  ( -2.816281873526471635, 33.91530133659708213, -3.434112377981056508 ) ) ;
#85368=CARTESIAN_POINT ( 'NONE',  ( 4.559911319644449179, 38.89701867748817676, 9.422509992056141925 ) ) ;
#85370=MECHANICAL_DESIGN_GEOMETRIC_PRESENTATION_REPRESENTATION('',(#75801),#90206);
#85371=CARTESIAN_POINT ( 'NONE',  ( -1.099225684535947600, 59.54030133659708923, 6.408140936763237150 ) ) ;
#85372=CARTESIAN_POINT ( 'NONE',  ( 17.96484262340118221, 44.93868534415483396, 7.964842623401181321 ) ) ;
#85374=CARTESIAN_POINT ( 'NONE',  ( 17.96484262340118221, 49.93868534415484106, 7.964842623401181321 ) ) ;
#85375=PRESENTATION_STYLE_ASSIGNMENT (( #71845 ) ) ;
#85376=CARTESIAN_POINT ( 'NONE',  ( 1.602071938427497289, 27.02224192338640663, -6.499999999999968914 ) ) ;
#85377=CARTESIAN_POINT ( 'NONE',  ( 0.1916775849787262787, 37.25868815902071418, -6.499999999999990230 ) ) ;
#85378=CARTESIAN_POINT ( 'NONE',  ( 10.00000000000000000, 60.55374883491397497, -14.16423886937410082 ) ) ;
#85379=CARTESIAN_POINT ( 'NONE',  ( 10.00000000000000000, -0.2410688489992152128, -9.846743663894594434 ) ) ;
#85380=CARTESIAN_POINT ( 'NONE',  ( 2.917880565312950480, 5.970415501580634832, -12.26659068614894821 ) ) ;
#85381=( LENGTH_UNIT ( ) NAMED_UNIT ( * ) SI_UNIT ( .MILLI., .METRE. ) );
#85382=CARTESIAN_POINT ( 'NONE',  ( 20.88017736071110519, 15.56368534415483751, 2.639326808657452039E-16 ) ) ;
#85383=CARTESIAN_POINT ( 'NONE',  ( 5.076628168052703671, 46.84226448433412315, 8.527530157486179263 ) ) ;
#85384=VERTEX_POINT ( 'NONE', #70306 ) ;
#85386=CARTESIAN_POINT ( 'NONE',  ( 0.1532563361054082862, 46.21726448433411605, 2.638427012816831674 ) ) ;
#85387=COLOUR_RGB ( '', 0.66274510, 0.83137255, 0.94901961) ;
#85388=CARTESIAN_POINT ( 'NONE',  ( 19.42250999205614193, 45.14701867748817676, 5.440088680355555262 ) ) ;
#85389=CARTESIAN_POINT ( 'NONE',  ( 14.92337183194729988, 44.34226448433412315, -8.527530157486177487 ) ) ;
#85390=CARTESIAN_POINT ( 'NONE',  ( 19.38216949554541202, 30.99863466993042138, 9.382169495545424454 ) ) ;
#85391=( NAMED_UNIT ( * ) SI_UNIT ( $, .STERADIAN. ) SOLID_ANGLE_UNIT ( ) );
#85392=CARTESIAN_POINT ( 'NONE',  ( 20.15039907845753930, 1.748846992468885198, 6.262539305110068177 ) ) ;
#85393=CARTESIAN_POINT ( 'NONE',  ( 15.44008868035555793, 41.39701867748817676, -9.422509992056140149 ) ) ;
#85394=CARTESIAN_POINT ( 'NONE',  ( -2.266590686148945544, 61.38708216824730357, -7.082119434687050408 ) ) ;
#85397=CARTESIAN_POINT ( 'NONE',  ( -2.816281873526473856, 24.12363466993042138, 9.499525473075851096E-16 ) ) ;
#85400=TOROIDAL_SURFACE ( 'NONE', #18313, 1.000000000000000000, 0.5000000000000000000 ) ;
#85401=CARTESIAN_POINT ( 'NONE',  ( -1.099225684535947600, 28.70696800326375353, -6.408140936763238038 ) ) ;
#85402=CARTESIAN_POINT ( 'NONE',  ( 2.035157376598824452, 18.68868534415484106, 7.964842623401179544 ) ) ;
#85404=CARTESIAN_POINT ( 'NONE',  ( 20.88017736071110875, 65.77201867748817676, -2.915334737309920765 ) ) ;
#85406=CARTESIAN_POINT ( 'NONE',  ( 5.076628168052704559, 45.17559781766745175, -8.527530157486179263 ) ) ;
#85407=CARTESIAN_POINT ( 'NONE',  ( 18.52753015748618282, 8.925597817667451750, -4.923371831947291888 ) ) ;
#85408=CARTESIAN_POINT ( 'NONE',  ( 14.92337183194729633, 37.67559781766745175, 8.527530157486181039 ) ) ;
#85411=CARTESIAN_POINT ( 'NONE',  ( 19.84674366389459266, 28.30059781766745886, 2.638427012816836559 ) ) ;
#85412=CARTESIAN_POINT ( 'NONE',  ( 20.15039907845753220, 56.74884699246889141, 6.262539305110074395 ) ) ;
#85414=CARTESIAN_POINT ( 'NONE',  ( 1.472469842513823179, 25.59226448433412315, -4.923371831947296329 ) ) ;
#85415=CARTESIAN_POINT ( 'NONE',  ( 18.52753015748617571, 3.092264484334118269, 4.923371831947298993 ) ) ;
#85416=CARTESIAN_POINT ( 'NONE',  ( 19.84674366389459266, 48.71726448433413026, -2.638427012816827677 ) ) ;
#85417=ORIENTED_EDGE ( 'NONE', *, *, #71835, .T. ) ;
#85418=CARTESIAN_POINT ( 'NONE',  ( 21.92686044187657046, 17.39664270246083788, -3.195792623639524432 ) ) ;
#85419=CARTESIAN_POINT ( 'NONE',  ( 16.40814093676323893, 30.79030133659708923, 11.09922568453595026 ) ) ;
#85421=DIRECTION ( 'NONE',  ( 0.000000000000000000, 0.000000000000000000, -1.000000000000000000 ) ) ;
#85422=CARTESIAN_POINT ( 'NONE',  ( -4.164238869374099927, 47.01208216824729647, 3.795296366450308767 ) ) ;
#85423=CARTESIAN_POINT ( 'NONE',  ( 10.00000000000000178, 22.25893115100078745, 9.846743663894594434 ) ) ;
#85424=CARTESIAN_POINT ( 'NONE',  ( 19.84674366389459621, 3.508931151000785231, 7.409399052514197653E-17 ) ) ;
#85425=CARTESIAN_POINT ( 'NONE',  ( 19.50000000000000711, 98.59912998021083297, 5.000000000000000888 ) ) ;
#85426=CARTESIAN_POINT ( 'NONE',  ( 22.26659068614895176, 39.72041550158063217, -7.082119434687042414 ) ) ;
#85427=CARTESIAN_POINT ( 'NONE',  ( 12.63842701281683922, 64.55059781766745175, -9.846743663894590881 ) ) ;
#85428=CARTESIAN_POINT ( 'NONE',  ( 13.79529636645030344, 53.26208216824730357, 14.16423886937410614 ) ) ;
#85429=CARTESIAN_POINT ( 'NONE',  ( -4.164238869374099927, 17.01208216824730357, 3.795296366450308767 ) ) ;
#85430=CARTESIAN_POINT ( 'NONE',  ( 20.36894250292379382, 23.67874883491397142, 10.36894250292379205 ) ) ;
#85431=CARTESIAN_POINT ( 'NONE',  ( -42.50369195530269195, 107.9060299417078426, -4.500000000000001776 ) ) ;
#85434=CARTESIAN_POINT ( 'NONE',  ( 1.472469842513823179, 40.59226448433411605, -4.923371831947296329 ) ) ;
#85435=CARTESIAN_POINT ( 'NONE',  ( 12.91533473730992121, 39.52201867748817676, 10.88017736071110164 ) ) ;
#85440=CARTESIAN_POINT ( 'NONE',  ( 2.791683348922240793, 41.63393115100078745, 7.208316651077764092 ) ) ;
#85441=CARTESIAN_POINT ( 'NONE',  ( 6.565887622018943937, 60.16530133659707502, 12.81628187352647430 ) ) ;
#85443=CARTESIAN_POINT ( 'NONE',  ( 0.1532563361054100626, 40.80059781766745886, -2.638427012816831230 ) ) ;
#85444=CARTESIAN_POINT ( 'NONE',  ( 1.472469842513823179, 65.59226448433412315, -4.923371831947296329 ) ) ;
#85447=CARTESIAN_POINT ( 'NONE',  ( 22.26659068614895176, 19.72041550158063572, -7.082119434687042414 ) ) ;
#85448=CARTESIAN_POINT ( 'NONE',  ( 0.2751277870542967463, 69.50000000000000000, -6.500000000000000888 ) ) ;
#85449=CARTESIAN_POINT ( 'NONE',  ( 19.39235739573469175, 44.87576471608600315, 6.499999999999993783 ) ) ;
#85451=CARTESIAN_POINT ( 'NONE',  ( -0.8801773607111009756, 3.063685344154838397, 1.068504757029289695E-15 ) ) ;
#85452=CARTESIAN_POINT ( 'NONE',  ( 10.00000000000000178, 15.37363466993042138, 12.81628187352647608 ) ) ;
#85453=CARTESIAN_POINT ( 'NONE',  ( 10.00000000000000178, 69.31368534415484817, 10.88017736071110342 ) ) ;
#85455=FACE_OUTER_BOUND ( 'NONE', #96602, .T. ) ;
#85457=CARTESIAN_POINT ( 'NONE',  ( 6.204703633549690345, 67.84541550158060375, 14.16423886937410082 ) ) ;
#85458=DIRECTION ( 'NONE',  ( 0.000000000000000000, -1.000000000000000000, 0.000000000000000000 ) ) ;
#85460=CARTESIAN_POINT ( 'NONE',  ( 0.2751277870542965243, 3.218334437839379891, 6.500000000000000888 ) ) ;
#85461=CARTESIAN_POINT ( 'NONE',  ( 20.88017736071110164, 25.35535201082150891, 2.915334737309930979 ) ) ;
#85462=CARTESIAN_POINT ( 'NONE',  ( 7.084665262690076126, 44.10535201082151247, 10.88017736071109987 ) ) ;
#85463=CARTESIAN_POINT ( 'NONE',  ( 22.81628187352647785, 6.415301336597088344, 3.434112377981063169 ) ) ;
#85464=CARTESIAN_POINT ( 'NONE',  ( 14.92337183194729633, 57.67559781766745886, 8.527530157486181039 ) ) ;
#85465=CARTESIAN_POINT ( 'NONE',  ( 10.00000000000000178, 65.37363466993042493, 12.81628187352647608 ) ) ;
#85466=CARTESIAN_POINT ( 'NONE',  ( 18.52753015748617571, 3.092264484334118269, 4.923371831947298993 ) ) ;
#85467=EDGE_CURVE ( 'NONE', #35320, #20878, #71767, .T. ) ;
#85469=CARTESIAN_POINT ( 'NONE',  ( 0.5774900079438590739, 27.64701867748817676, -5.440088680355550821 ) ) ;
#85470=CARTESIAN_POINT ( 'NONE',  ( 19.38216949554541202, 25.99863466993042138, 9.382169495545424454 ) ) ;
#85473=CARTESIAN_POINT ( 'NONE',  ( 0.1532563361054100626, 60.80059781766744464, -2.638427012816831230 ) ) ;
#85474=CARTESIAN_POINT ( 'NONE',  ( 15.44008868035555260, 44.73035201082151247, 9.422509992056143702 ) ) ;
#85475=AXIS2_PLACEMENT_3D ( 'NONE', #21851, #88360, #97359 ) ;
#85477=CARTESIAN_POINT ( 'NONE',  ( 5.076628168052704559, 15.17559781766745175, -8.527530157486179263 ) ) ;
#85478=CARTESIAN_POINT ( 'NONE',  ( 13.43411237798106583, 37.66530133659708923, -12.81628187352647252 ) ) ;
#85479=CARTESIAN_POINT ( 'NONE',  ( 2.035157376598824452, 58.68868534415482685, 7.964842623401179544 ) ) ;
#85480=CARTESIAN_POINT ( 'NONE',  ( 18.72515096720570327, 16.07228050351031712, -6.499999999999992006 ) ) ;
#85481=CARTESIAN_POINT ( 'NONE',  ( 0.1957200283969096621, 50.25733960839543357, 6.499999999999992895 ) ) ;
#85482=CARTESIAN_POINT ( 'NONE',  ( 10.00000000000000178, 60.37363466993041783, 12.81628187352647608 ) ) ;
#85483=ORIENTED_EDGE ( 'NONE', *, *, #81606, .T. ) ;
#85486=CARTESIAN_POINT ( 'NONE',  ( 12.91533473730993009, 6.605352010821504471, -10.88017736071109987 ) ) ;
#85487=CARTESIAN_POINT ( 'NONE',  ( 19.38216949554541202, 45.99863466993041072, 9.382169495545424454 ) ) ;
#85488=CARTESIAN_POINT ( 'NONE',  ( 2.917880565312950480, 15.97041550158063217, -12.26659068614894821 ) ) ;
#85489=CARTESIAN_POINT ( 'NONE',  ( 0.1532563361054083140, 16.00893115100078390, 1.131784320476157264E-15 ) ) ;
#85490=CARTESIAN_POINT ( 'NONE',  ( 2.035157376598824452, 3.688685344154837953, 7.964842623401179544 ) ) ;
#85491=CARTESIAN_POINT ( 'NONE',  ( 0.1532563361054082862, 26.21726448433411605, 2.638427012816831674 ) ) ;
#85492=CARTESIAN_POINT ( 'NONE',  ( 2.917880565312950480, 50.97041550158064638, -12.26659068614894821 ) ) ;
#85493=VERTEX_POINT ( 'NONE', #26259 ) ;
#85494=CARTESIAN_POINT ( 'NONE',  ( 17.96484262340118221, 9.938685344154837509, 7.964842623401181321 ) ) ;
#85495=DIRECTION ( 'NONE',  ( 0.000000000000000000, 0.000000000000000000, -1.000000000000000000 ) ) ;
#85497=CARTESIAN_POINT ( 'NONE',  ( -0.8801773607111009756, 13.06368534415483929, 1.068504757029289695E-15 ) ) ;
#85498=CARTESIAN_POINT ( 'NONE',  ( 20.88017736071110519, 5.563685344154838397, 2.639326808657452039E-16 ) ) ;
#85499=CARTESIAN_POINT ( 'NONE',  ( 5.076628168052703671, 46.84226448433412315, 8.527530157486179263 ) ) ;
#85501=CARTESIAN_POINT ( 'NONE',  ( -1.099225684535947600, 54.54030133659708923, 6.408140936763237150 ) ) ;
#85503=CARTESIAN_POINT ( 'NONE',  ( 19.84674366389459266, 63.30059781766745886, 2.638427012816836559 ) ) ;
#85504=CARTESIAN_POINT ( 'NONE',  ( 22.26659068614894466, 18.88708216824730002, 7.082119434687054849 ) ) ;
#85505=CARTESIAN_POINT ( 'NONE',  ( 7.084665262690076126, 27.02201867748817676, -10.88017736071110164 ) ) ;
#85506=CARTESIAN_POINT ( 'NONE',  ( -0.8801773607111008646, 3.272018677488171434, 2.915334737309923430 ) ) ;
#85507=CARTESIAN_POINT ( 'NONE',  ( 7.361572987183169658, 59.96726448433410894, -9.846743663894592657 ) ) ;
#85509=CARTESIAN_POINT ( 'NONE',  ( 10.00000000000000000, 39.75893115100078745, -9.846743663894594434 ) ) ;
#85515=CARTESIAN_POINT ( 'NONE',  ( 2.035157376598822676, 62.43868534415483396, -7.964842623401177768 ) ) ;
#85516=CARTESIAN_POINT ( 'NONE',  ( 1.472469842513823179, 61.42559781766745175, 4.923371831947296329 ) ) ;
#85517=CARTESIAN_POINT ( 'NONE',  ( -0.8801773607110991993, 52.85535201082151247, -2.915334737309923874 ) ) ;
#85518=CARTESIAN_POINT ( 'NONE',  ( 2.035157376598822676, 47.43868534415484817, -7.964842623401177768 ) ) ;
#85519=CARTESIAN_POINT ( 'NONE',  ( 2.035157376598824452, 3.688685344154837953, 7.964842623401179544 ) ) ;
#85520=CARTESIAN_POINT ( 'NONE',  ( 10.00000000000000000, 37.87363466993041783, -12.81628187352647608 ) ) ;
#85521=CARTESIAN_POINT ( 'NONE',  ( 20.36894250292379382, 13.67874883491396965, 10.36894250292379205 ) ) ;
#85523=CARTESIAN_POINT ( 'NONE',  ( 22.81628187352647785, 51.41530133659708923, 3.434112377981063169 ) ) ;
#85525=CARTESIAN_POINT ( 'NONE',  ( 17.20831665107776587, 54.13393115100079456, -7.208316651077762316 ) ) ;
#85526=CARTESIAN_POINT ( 'NONE',  ( 20.88017736071110875, 15.77201867748817143, -2.915334737309920765 ) ) ;
#85528=CARTESIAN_POINT ( 'NONE',  ( 20.88017736071110164, 25.35535201082150891, 2.915334737309930979 ) ) ;
#85529=VERTEX_POINT ( 'NONE', #80245 ) ;
#85530=CARTESIAN_POINT ( 'NONE',  ( 4.559911319644449179, 68.89701867748817676, 9.422509992056141925 ) ) ;
#85531=CARTESIAN_POINT ( 'NONE',  ( 4.559911319644449179, 67.23035201082150536, -9.422509992056141925 ) ) ;
#85532=LINE ( 'NONE', #2055, #3693 ) ;
#85533=CARTESIAN_POINT ( 'NONE',  ( 18.52753015748617571, 13.09226448433411960, 4.923371831947298993 ) ) ;
#85534=CARTESIAN_POINT ( 'NONE',  ( 20.88017736071110164, 65.35535201082150536, 2.915334737309930979 ) ) ;
#85537=CARTESIAN_POINT ( 'NONE',  ( 7.084665262690076126, 64.10535201082150536, 10.88017736071109987 ) ) ;
#85539=CARTESIAN_POINT ( 'NONE',  ( 10.00000000000000178, 7.258931151000785675, 9.846743663894594434 ) ) ;
#85542=CARTESIAN_POINT ( 'NONE',  ( 19.84674366389459266, 48.71726448433413026, -2.638427012816827677 ) ) ;
#85544=ORIENTED_EDGE ( 'NONE', *, *, #26789, .F. ) ;
#85545=CARTESIAN_POINT ( 'NONE',  ( -46.68456736488007408, 103.6675473310227034, -5.775421524742654356 ) ) ;
#85547=CARTESIAN_POINT ( 'NONE',  ( 2.917880565312950480, 0.9704155015806342766, -12.26659068614894821 ) ) ;
#85548=CARTESIAN_POINT ( 'NONE',  ( -2.816281873526473856, 64.33196800326376774, 3.434112377981055619 ) ) ;
#85549=CARTESIAN_POINT ( 'NONE',  ( 24.16423886937410614, 9.512082168247301794, -3.795296366450302550 ) ) ;
#85550=CARTESIAN_POINT ( 'NONE',  ( 22.26659068614895176, 14.72041550158063572, -7.082119434687042414 ) ) ;
#85552=CARTESIAN_POINT ( 'NONE',  ( 19.05914839598884569, 9.966938638839758724, 6.499999999999981348 ) ) ;
#85553=CARTESIAN_POINT ( 'NONE',  ( 20.88017736071110875, 20.77201867748816611, -2.915334737309920765 ) ) ;
#85554=CARTESIAN_POINT ( 'NONE',  ( 2.603489959281613420, 65.43575266056828355, -6.500000000000031086 ) ) ;
#85556=CARTESIAN_POINT ( 'NONE',  ( 14.92337183194729988, 4.342264484334117824, -8.527530157486177487 ) ) ;
#85557=CARTESIAN_POINT ( 'NONE',  ( 17.20831665107776587, 4.133931151000785675, -7.208316651077762316 ) ) ;
#85558=CARTESIAN_POINT ( 'NONE',  ( 16.40814093676324603, 32.45696800326375353, -11.09922568453594671 ) ) ;
#85559=CARTESIAN_POINT ( 'NONE',  ( 14.92337183194729633, 42.67559781766745886, 8.527530157486181039 ) ) ;
#85562=CARTESIAN_POINT ( 'NONE',  ( 21.09922568453595559, 12.04030133659708746, -6.408140936763230044 ) ) ;
#85564=CARTESIAN_POINT ( 'NONE',  ( 1.472469842513823179, 20.59226448433411960, -4.923371831947296329 ) ) ;
#85566=CARTESIAN_POINT ( 'NONE',  ( 5.076628168052703671, 1.842264484334118047, 8.527530157486179263 ) ) ;
#85569=CARTESIAN_POINT ( 'NONE',  ( 20.88017736071110875, 40.77201867748818387, -2.915334737309920765 ) ) ;
#85570=CARTESIAN_POINT ( 'NONE',  ( 10.00000000000000000, 30.55374883491397142, -14.16423886937410082 ) ) ;
#85571=CARTESIAN_POINT ( 'NONE',  ( 0.1532563361054083140, 41.00893115100078745, 1.131784320476157264E-15 ) ) ;
#85572=CARTESIAN_POINT ( 'NONE',  ( 18.52753015748618282, 3.925597817667451306, -4.923371831947291888 ) ) ;
#85573=CARTESIAN_POINT ( 'NONE',  ( -2.816281873526473856, 49.12363466993042493, 9.499525473075851096E-16 ) ) ;
#85575=CARTESIAN_POINT ( 'NONE',  ( 19.42250999205614193, 30.14701867748817321, 5.440088680355555262 ) ) ;
#85577=CARTESIAN_POINT ( 'NONE',  ( 10.00000000000000178, 25.37363466993041783, 12.81628187352647608 ) ) ;
#85578=CARTESIAN_POINT ( 'NONE',  ( 7.361572987183170547, 37.05059781766744464, 9.846743663894590881 ) ) ;
#85580=CARTESIAN_POINT ( 'NONE',  ( 6.565887622018943937, 43.08196800326374643, -12.81628187352647608 ) ) ;
#85582=CARTESIAN_POINT ( 'NONE',  ( 2.035157376598824452, 48.68868534415483396, 7.964842623401179544 ) ) ;
#85586=CARTESIAN_POINT ( 'NONE',  ( 19.72487221294570858, 69.50000000000000000, 6.500000000000000888 ) ) ;
#85587=CARTESIAN_POINT ( 'NONE',  ( 20.88017736071110164, 55.35535201082149825, 2.915334737309930979 ) ) ;
#85588=CARTESIAN_POINT ( 'NONE',  ( 2.035157376598822676, 52.43868534415483396, -7.964842623401177768 ) ) ;
#85591=CARTESIAN_POINT ( 'NONE',  ( -0.1688089201193209155, 79.91181047996344944, 5.000000000000000000 ) ) ;
#85592=CARTESIAN_POINT ( 'NONE',  ( -0.8801773607111008646, 13.27201867748817321, 2.915334737309923430 ) ) ;
#85593=EDGE_CURVE ( 'NONE', #73005, #5600, #82309, .T. ) ;
#85594=CARTESIAN_POINT ( 'NONE',  ( 17.20831665107776587, 49.13393115100078745, -7.208316651077762316 ) ) ;
#85595=CARTESIAN_POINT ( 'NONE',  ( 2.035157376598824452, 23.68868534415484461, 7.964842623401179544 ) ) ;
#85596=CARTESIAN_POINT ( 'NONE',  ( 18.52753015748618282, 23.92559781766745530, -4.923371831947291888 ) ) ;
#85597=CARTESIAN_POINT ( 'NONE',  ( 0.6178305044545818747, 23.49863466993041783, -9.382169495545419124 ) ) ;
#85598=ORIENTED_EDGE ( 'NONE', *, *, #83788, .F. ) ;
#85599=CARTESIAN_POINT ( 'NONE',  ( -0.8801773607111008646, 33.27201867748817676, 2.915334737309923430 ) ) ;
#85600=CARTESIAN_POINT ( 'NONE',  ( 12.63842701281683922, 39.55059781766744464, -9.846743663894590881 ) ) ;
#85601=CARTESIAN_POINT ( 'NONE',  ( 10.00000000000000000, 12.87363466993042138, -12.81628187352647608 ) ) ;
#85602=CARTESIAN_POINT ( 'NONE',  ( 17.39651004071838969, 39.08210964143329846, -6.500000000000027534 ) ) ;
#85603=CARTESIAN_POINT ( 'NONE',  ( 2.035157376598824452, 18.68868534415484106, 7.964842623401179544 ) ) ;
#85604=CARTESIAN_POINT ( 'NONE',  ( 19.42250999205614193, 45.14701867748817676, 5.440088680355555262 ) ) ;
#85605=CARTESIAN_POINT ( 'NONE',  ( 2.917880565312950480, 45.97041550158063927, -12.26659068614894821 ) ) ;
#85606=CARTESIAN_POINT ( 'NONE',  ( 19.84674366389459266, 38.71726448433412315, -2.638427012816827677 ) ) ;
#85607=CARTESIAN_POINT ( 'NONE',  ( 20.88017736071110519, 60.56368534415484106, 2.639326808657452039E-16 ) ) ;
#85609=CARTESIAN_POINT ( 'NONE',  ( -0.3689425029237881626, 17.42874883491397142, 10.36894250292379027 ) ) ;
#85611=CARTESIAN_POINT ( 'NONE',  ( 18.95785429995053306, 12.24216108172006834, 6.499999999999848121 ) ) ;
#85614=CARTESIAN_POINT ( 'NONE',  ( 13.79529636645030344, 33.26208216824730357, 14.16423886937410614 ) ) ;
#85615=CARTESIAN_POINT ( 'NONE',  ( -2.266590686148945544, 41.38708216824729647, -7.082119434687050408 ) ) ;
#85616=CARTESIAN_POINT ( 'NONE',  ( 19.84674366389459621, 8.508931151000785675, 7.409399052514197653E-17 ) ) ;
#85617=CARTESIAN_POINT ( 'NONE',  ( 21.09922568453594849, 16.20696800326375353, 6.408140936763242479 ) ) ;
#85618=CARTESIAN_POINT ( 'NONE',  ( 14.92337183194729988, 64.34226448433412315, -8.527530157486177487 ) ) ;
#85619=DIRECTION ( 'NONE',  ( 0.000000000000000000, 0.000000000000000000, 1.000000000000000000 ) ) ;
#85620=CARTESIAN_POINT ( 'NONE',  ( 15.44008868035555793, 61.39701867748817676, -9.422509992056140149 ) ) ;
#85621=CARTESIAN_POINT ( 'NONE',  ( 16.40814093676324603, 37.45696800326376064, -11.09922568453594671 ) ) ;
#85622=CARTESIAN_POINT ( 'NONE',  ( 20.36894250292379738, 29.92874883491396432, -10.36894250292379027 ) ) ;
#85623=CARTESIAN_POINT ( 'NONE',  ( 4.559911319644449179, 23.89701867748817321, 9.422509992056141925 ) ) ;
#85624=STYLED_ITEM ( 'NONE', ( #327 ), #86830 ) ;
#85625=DIRECTION ( 'NONE',  ( -0.000000000000000000, 1.000000000000000000, -0.000000000000000000 ) ) ;
#85626=CARTESIAN_POINT ( 'NONE',  ( 1.472469842513823179, 1.425597817667451528, 4.923371831947296329 ) ) ;
#85628=ORIENTED_EDGE ( 'NONE', *, *, #91599, .T. ) ;
#85631=CARTESIAN_POINT ( 'NONE',  ( -0.3689425029237881626, 7.428748834913967869, 10.36894250292379027 ) ) ;
#85632=CARTESIAN_POINT ( 'NONE',  ( 0.5774900079438607392, 3.480352010821504916, 5.440088680355550821 ) ) ;
#85633=CARTESIAN_POINT ( 'NONE',  ( -0.8801773607111009756, 18.06368534415484106, 1.068504757029289695E-15 ) ) ;
#85634=CARTESIAN_POINT ( 'NONE',  ( 10.00000000000000178, 42.25893115100078745, 9.846743663894594434 ) ) ;
#85635=CARTESIAN_POINT ( 'NONE',  ( 2.791683348922240793, 61.63393115100079456, 7.208316651077764092 ) ) ;
#85638=CARTESIAN_POINT ( 'NONE',  ( 21.09922568453594849, 1.206968003263753531, 6.408140936763242479 ) ) ;
#85640=CARTESIAN_POINT ( 'NONE',  ( -0.3689425029237881626, 42.42874883491396787, 10.36894250292379027 ) ) ;
#85642=CARTESIAN_POINT ( 'NONE',  ( 6.204703633549690345, 60.76208216824730357, -14.16423886937410259 ) ) ;
#85644=CARTESIAN_POINT ( 'NONE',  ( 15.44008868035555793, 26.39701867748817321, -9.422509992056140149 ) ) ;
#85645=CARTESIAN_POINT ( 'NONE',  ( 2.035157376598822676, 32.43868534415483396, -7.964842623401177768 ) ) ;
#85646=CARTESIAN_POINT ( 'NONE',  ( 0.1532563361054082862, 46.21726448433411605, 2.638427012816831674 ) ) ;
#85647=CARTESIAN_POINT ( 'NONE',  ( -0.8801773607111008646, 33.27201867748817676, 2.915334737309923430 ) ) ;
#85648=CARTESIAN_POINT ( 'NONE',  ( 19.42250999205614193, 65.14701867748817676, 5.440088680355555262 ) ) ;
#85649=CARTESIAN_POINT ( 'NONE',  ( -0.8801773607110991993, 22.85535201082150181, -2.915334737309923874 ) ) ;
#85652=B_SPLINE_CURVE_WITH_KNOTS ( 'NONE', 3,
 ( #65310, #78751, #94226, #62253, #77751, #56251 ),
 .UNSPECIFIED., .F., .F.,
 ( 4, 2, 4 ),
 ( 0.000000000000000000, 0.0002565770811490988542, 0.0005131541622981977083 ),
 .UNSPECIFIED. ) ;
#85653=CARTESIAN_POINT ( 'NONE',  ( 14.92337183194729633, 7.675597817667451750, 8.527530157486181039 ) ) ;
#85656=LINE ( 'NONE', #47148, #14256 ) ;
#85657=CARTESIAN_POINT ( 'NONE',  ( 2.791683348922240793, 46.63393115100077324, 7.208316651077764092 ) ) ;
#85659=CARTESIAN_POINT ( 'NONE',  ( 6.565887622018943937, 45.16530133659708923, 12.81628187352647430 ) ) ;
#85660=PRESENTATION_STYLE_ASSIGNMENT (( #70666 ) ) ;
#85663=CARTESIAN_POINT ( 'NONE',  ( 5.076628168052703671, 66.84226448433412315, 8.527530157486179263 ) ) ;
#85665=CARTESIAN_POINT ( 'NONE',  ( 0.1532563361054100626, 50.80059781766745175, -2.638427012816831230 ) ) ;
#85666=CARTESIAN_POINT ( 'NONE',  ( 20.36894250292379382, 53.67874883491397497, 10.36894250292379205 ) ) ;
#85667=CARTESIAN_POINT ( 'NONE',  ( 5.076628168052704559, 60.17559781766745175, -8.527530157486179263 ) ) ;
#85668=ORIENTED_EDGE ( 'NONE', *, *, #24292, .F. ) ;
#85670=CARTESIAN_POINT ( 'NONE',  ( 2.791683348922240793, 16.63393115100078745, 7.208316651077764092 ) ) ;
#85671=CARTESIAN_POINT ( 'NONE',  ( 13.43411237798105340, 50.58196800326375353, 12.81628187352647963 ) ) ;
#85673=CARTESIAN_POINT ( 'NONE',  ( 1.472469842513823179, 66.42559781766745175, 4.923371831947296329 ) ) ;
#85674=CARTESIAN_POINT ( 'NONE',  ( 19.42250999205614193, 60.14701867748817676, 5.440088680355555262 ) ) ;
#85679=CARTESIAN_POINT ( 'NONE',  ( 17.08211943468705840, 65.13708216824730357, -12.26659068614894466 ) ) ;
#85681=CARTESIAN_POINT ( 'NONE',  ( 2.035157376598824452, 23.68868534415484461, 7.964842623401179544 ) ) ;
#85682=CARTESIAN_POINT ( 'NONE',  ( 10.00000000000000000, 17.87363466993041783, -12.81628187352647608 ) ) ;
#85683=CARTESIAN_POINT ( 'NONE',  ( 15.44008868035555260, 54.73035201082150536, 9.422509992056143702 ) ) ;
#85685=CARTESIAN_POINT ( 'NONE',  ( 19.10478245763057714, 65.10160829253887016, 5.990408912944228170 ) ) ;
#85689=CARTESIAN_POINT ( 'NONE',  ( 5.076628168052703671, 51.84226448433412315, 8.527530157486179263 ) ) ;
#85690=CARTESIAN_POINT ( 'NONE',  ( 7.361572987183169658, -0.03273551566588185635, -9.846743663894592657 ) ) ;
#85692=CARTESIAN_POINT ( 'NONE',  ( 10.00000000000000178, 15.37363466993042138, 12.81628187352647608 ) ) ;
#85693=CARTESIAN_POINT ( 'NONE',  ( 20.88017736071110875, 15.77201867748817143, -2.915334737309920765 ) ) ;
#85694=CARTESIAN_POINT ( 'NONE',  ( 2.153642693323479129, 66.13791097397319163, -6.500000000000079048 ) ) ;
#85695=STYLED_ITEM ( 'NONE', ( #98420 ), #32379 ) ;
#85697=CARTESIAN_POINT ( 'NONE',  ( -0.3689425029237881626, 42.42874883491396787, 10.36894250292379027 ) ) ;
#85698=COLOUR_RGB ( '', 0.72549020, 0.75294118, 0.79215686) ;
#85699=CARTESIAN_POINT ( 'NONE',  ( 24.16423886937410614, 34.51208216824731068, -3.795296366450302550 ) ) ;
#85700=CARTESIAN_POINT ( 'NONE',  ( 10.00000000000000000, 1.813685344154838175, -10.88017736071110342 ) ) ;
#85702=CARTESIAN_POINT ( 'NONE',  ( 0.1532563361054083140, 21.00893115100078745, 1.131784320476157264E-15 ) ) ;
#85703=CARTESIAN_POINT ( 'NONE',  ( 15.44008868035555260, 19.73035201082150536, 9.422509992056143702 ) ) ;
#85705=CARTESIAN_POINT ( 'NONE',  ( 2.791683348922237240, 40.38393115100078035, -7.208316651077763204 ) ) ;
#85706=VECTOR ( 'NONE', #16078, 1000.000000000000000 ) ;
#85708=CARTESIAN_POINT ( 'NONE',  ( 12.91533473730992121, 39.52201867748817676, 10.88017736071110164 ) ) ;
#85709=CARTESIAN_POINT ( 'NONE',  ( 14.92337183194729988, 59.34226448433412315, -8.527530157486177487 ) ) ;
#85710=CARTESIAN_POINT ( 'NONE',  ( 2.917880565312948704, 22.63708216824730002, 12.26659068614894643 ) ) ;
#85713=CARTESIAN_POINT ( 'NONE',  ( 18.52753015748617571, 8.092264484334117824, 4.923371831947298993 ) ) ;
#85714=CARTESIAN_POINT ( 'NONE',  ( 19.38216949554541202, 50.99863466993042493, 9.382169495545424454 ) ) ;
#85715=CARTESIAN_POINT ( 'NONE',  ( 10.00000000000000000, 59.75893115100078745, -9.846743663894594434 ) ) ;
#85719=CARTESIAN_POINT ( 'NONE',  ( 4.559911319644449179, 3.897018677488171434, 9.422509992056141925 ) ) ;
#85720=CARTESIAN_POINT ( 'NONE',  ( 12.91533473730992121, 54.52201867748816255, 10.88017736071110164 ) ) ;
#85721=CARTESIAN_POINT ( 'NONE',  ( -2.266590686148945544, 17.22041550158063572, 7.082119434687048631 ) ) ;
#85722=CARTESIAN_POINT ( 'NONE',  ( 15.44008868035555260, 54.73035201082150536, 9.422509992056143702 ) ) ;
#85723=CARTESIAN_POINT ( 'NONE',  ( 5.076628168052704559, 40.17559781766745175, -8.527530157486179263 ) ) ;
#85724=CARTESIAN_POINT ( 'NONE',  ( 20.88017736071110164, 20.35535201082150891, 2.915334737309930979 ) ) ;
#85726=CARTESIAN_POINT ( 'NONE',  ( 17.20831665107776587, 59.13393115100078745, -7.208316651077762316 ) ) ;
#85728=CARTESIAN_POINT ( 'NONE',  ( 17.20831665107776587, 2.883931151000785231, 7.208316651077764980 ) ) ;
#85729=CARTESIAN_POINT ( 'NONE',  ( -1.099225684535947600, 64.54030133659709634, 6.408140936763237150 ) ) ;
#85730=VERTEX_POINT ( 'NONE', #4757 ) ;
#85734=PRESENTATION_STYLE_ASSIGNMENT (( #55219 ) ) ;
#85735=CARTESIAN_POINT ( 'NONE',  ( 10.00000000000000178, 43.05374883491397497, 14.16423886937410082 ) ) ;
#85736=CARTESIAN_POINT ( 'NONE',  ( 5.076628168052704559, 40.17559781766745175, -8.527530157486179263 ) ) ;
#85737=CARTESIAN_POINT ( 'NONE',  ( 0.1532563361054082862, 21.21726448433412315, 2.638427012816831674 ) ) ;
#85739=CARTESIAN_POINT ( 'NONE',  ( 19.42250999205614193, 25.14701867748817321, 5.440088680355555262 ) ) ;
#85740=CARTESIAN_POINT ( 'NONE',  ( 17.20831665107776587, 64.13393115100079456, -7.208316651077762316 ) ) ;
#85742=CARTESIAN_POINT ( 'NONE',  ( -0.3689425029237881626, 37.42874883491396787, 10.36894250292379027 ) ) ;
#85744=CARTESIAN_POINT ( 'NONE',  ( 24.16423886937410614, 59.30374883491397497, 8.672049930838204340E-16 ) ) ;
#85747=CARTESIAN_POINT ( 'NONE',  ( 15.44008868035555793, 61.39701867748817676, -9.422509992056140149 ) ) ;
#85748=CARTESIAN_POINT ( 'NONE',  ( 0.1532563361054083140, 21.00893115100078745, 1.131784320476157264E-15 ) ) ;
#85754=CARTESIAN_POINT ( 'NONE',  ( 18.52753015748617571, 13.09226448433411960, 4.923371831947298993 ) ) ;
#85756=CARTESIAN_POINT ( 'NONE',  ( 17.08211943468705130, 23.47041550158063572, 12.26659068614894998 ) ) ;
#85757=CARTESIAN_POINT ( 'NONE',  ( 19.84674366389459266, 18.30059781766745175, 2.638427012816836559 ) ) ;
#85758=CARTESIAN_POINT ( 'NONE',  ( 0.5774900079438607392, 48.48035201082150536, 5.440088680355550821 ) ) ;
#85762=CARTESIAN_POINT ( 'NONE',  ( 7.084665262690076126, 47.02201867748818387, -10.88017736071110164 ) ) ;
#85766=CARTESIAN_POINT ( 'NONE',  ( 17.96484262340118221, 44.93868534415483396, 7.964842623401181321 ) ) ;
#85767=CARTESIAN_POINT ( 'NONE',  ( 2.917880565312948704, 7.637082168247301794, 12.26659068614894643 ) ) ;
#85769=CARTESIAN_POINT ( 'NONE',  ( 10.00000000000000178, 35.37363466993042493, 12.81628187352647608 ) ) ;
#85770=STYLED_ITEM ( 'NONE', ( #27963 ), #11640 ) ;
#85771=CARTESIAN_POINT ( 'NONE',  ( 19.84674366389459266, 3.717264484334118713, -2.638427012816827677 ) ) ;
#85773=CARTESIAN_POINT ( 'NONE',  ( -1.099225684535947600, 43.70696800326375353, -6.408140936763238038 ) ) ;
#85774=CARTESIAN_POINT ( 'NONE',  ( 19.42250999205614548, 10.98035201082150536, -5.440088680355545492 ) ) ;
#85775=CARTESIAN_POINT ( 'NONE',  ( 10.00000000000000178, 17.25893115100078745, 9.846743663894594434 ) ) ;
#85776=CARTESIAN_POINT ( 'NONE',  ( 15.44008868035555260, 49.73035201082150536, 9.422509992056143702 ) ) ;
#85780=CARTESIAN_POINT ( 'NONE',  ( 4.559911319644449179, 53.89701867748817676, 9.422509992056141925 ) ) ;
#85781=CARTESIAN_POINT ( 'NONE',  ( 18.72515096720571393, 41.07228050351032778, -6.499999999999974243 ) ) ;
#85782=CARTESIAN_POINT ( 'NONE',  ( 19.84674366389459621, 8.508931151000785675, 7.409399052514197653E-17 ) ) ;
#85783=CARTESIAN_POINT ( 'NONE',  ( 10.00000000000000000, 12.87363466993042138, -12.81628187352647608 ) ) ;
#85785=CARTESIAN_POINT ( 'NONE',  ( 1.472469842513823179, 36.42559781766745175, 4.923371831947296329 ) ) ;
#85786=CARTESIAN_POINT ( 'NONE',  ( -0.3689425029237898834, 11.17874883491396787, -10.36894250292378850 ) ) ;
#85787=CARTESIAN_POINT ( 'NONE',  ( 0.1532563361054083140, 21.00893115100078745, 1.131784320476157264E-15 ) ) ;
#85788=CARTESIAN_POINT ( 'NONE',  ( 16.40814093676323893, 20.79030133659708923, 11.09922568453595026 ) ) ;
#85789=DIRECTION ( 'NONE',  ( -0.6776733583268309546, 0.7353630527936758643, 0.000000000000000000 ) ) ;
#85790=CARTESIAN_POINT ( 'NONE',  ( 15.44008868035555793, 51.39701867748816966, -9.422509992056140149 ) ) ;
#85791=CARTESIAN_POINT ( 'NONE',  ( 18.52753015748617571, 58.09226448433411605, 4.923371831947298993 ) ) ;
#85793=CARTESIAN_POINT ( 'NONE',  ( 5.076628168052703671, 26.84226448433411960, 8.527530157486179263 ) ) ;
#85794=CARTESIAN_POINT ( 'NONE',  ( 7.361572987183169658, 19.96726448433411960, -9.846743663894592657 ) ) ;
#85795=CARTESIAN_POINT ( 'NONE',  ( 20.88017736071110875, 15.77201867748817143, -2.915334737309920765 ) ) ;
#85797=CARTESIAN_POINT ( 'NONE',  ( 10.00000000000000000, 17.87363466993041783, -12.81628187352647608 ) ) ;
#85798=CARTESIAN_POINT ( 'NONE',  ( 18.52753015748617571, 18.09226448433411960, 4.923371831947298993 ) ) ;
#85800=CARTESIAN_POINT ( 'NONE',  ( 15.44008868035555260, 19.73035201082150536, 9.422509992056143702 ) ) ;
#85802=AXIS2_PLACEMENT_3D ( 'NONE', #31837, #92354, #410 ) ;
#85803=ORIENTED_EDGE ( 'NONE', *, *, #95271, .T. ) ;
#85804=CARTESIAN_POINT ( 'NONE',  ( 19.42250999205614193, 55.14701867748817676, 5.440088680355555262 ) ) ;
#85805=CARTESIAN_POINT ( 'NONE',  ( 12.63842701281683034, 42.46726448433412315, 9.846743663894596210 ) ) ;
#85806=CARTESIAN_POINT ( 'NONE',  ( 10.00000000000000000, 11.81368534415483751, -10.88017736071110342 ) ) ;
#85807=FILL_AREA_STYLE_COLOUR ( '', #53533 ) ;
#85808=CARTESIAN_POINT ( 'NONE',  ( 0.5774900079438590739, 47.64701867748817676, -5.440088680355550821 ) ) ;
#85809=CARTESIAN_POINT ( 'NONE',  ( 7.084665262690076126, 7.022018677488170546, -10.88017736071110164 ) ) ;
#85811=CARTESIAN_POINT ( 'NONE',  ( 19.84674366389459266, 18.30059781766745175, 2.638427012816836559 ) ) ;
#85812=CARTESIAN_POINT ( 'NONE',  ( 2.791683348922240793, 36.63393115100078035, 7.208316651077764092 ) ) ;
#85815=CARTESIAN_POINT ( 'NONE',  ( 2.791683348922240793, 66.63393115100079456, 7.208316651077764092 ) ) ;
#85817=CARTESIAN_POINT ( 'NONE',  ( 13.79529636645031943, 20.34541550158063572, -14.16423886937409904 ) ) ;
#85818=CARTESIAN_POINT ( 'NONE',  ( 0.1532563361054100626, 40.80059781766745886, -2.638427012816831230 ) ) ;
#85819=DIRECTION ( 'NONE',  ( -0.000000000000000000, -1.000000000000000000, 0.000000000000000000 ) ) ;
#85822=CARTESIAN_POINT ( 'NONE',  ( 13.79529636645030344, 58.26208216824728936, 14.16423886937410614 ) ) ;
#85823=CARTESIAN_POINT ( 'NONE',  ( 14.92337183194729988, 24.34226448433411960, -8.527530157486177487 ) ) ;
#85825=CARTESIAN_POINT ( 'NONE',  ( 20.88017736071110875, 45.77201867748816966, -2.915334737309920765 ) ) ;
#85827=CARTESIAN_POINT ( 'NONE',  ( 2.035157376598822676, 22.43868534415483396, -7.964842623401177768 ) ) ;
#85828=CARTESIAN_POINT ( 'NONE',  ( -2.816281873526473856, 49.12363466993042493, 9.499525473075851096E-16 ) ) ;
#85829=CARTESIAN_POINT ( 'NONE',  ( 0.6178305044545818747, 8.498634669930421381, -9.382169495545419124 ) ) ;
#85830=CARTESIAN_POINT ( 'NONE',  ( 0.1532563361054100626, 15.80059781766745353, -2.638427012816831230 ) ) ;
#85835=CARTESIAN_POINT ( 'NONE',  ( 6.204703633549690345, 55.76208216824730357, -14.16423886937410259 ) ) ;
#85836=CARTESIAN_POINT ( 'NONE',  ( 24.16423886937409904, 34.09541550158064638, 3.795296366450317205 ) ) ;
#85837=CARTESIAN_POINT ( 'NONE',  ( 4.559911319644449179, 17.23035201082150536, -9.422509992056141925 ) ) ;
#85839=CARTESIAN_POINT ( 'NONE',  ( 0.5774900079438590739, 47.64701867748817676, -5.440088680355550821 ) ) ;
#85841=CARTESIAN_POINT ( 'NONE',  ( 19.50000000000000355, 70.00000000000000000, -5.000000000000000000 ) ) ;
#85842=CARTESIAN_POINT ( 'NONE',  ( 1.472469842513823179, 0.5922644843341181575, -4.923371831947296329 ) ) ;
#85844=CARTESIAN_POINT ( 'NONE',  ( 14.92337183194729988, 14.34226448433411782, -8.527530157486177487 ) ) ;
#85845=PRESENTATION_STYLE_ASSIGNMENT (( #40836 ) ) ;
#85846=CARTESIAN_POINT ( 'NONE',  ( 19.84674366389459266, 28.71726448433411960, -2.638427012816827677 ) ) ;
#85847=CARTESIAN_POINT ( 'NONE',  ( 7.361572987183170547, 52.05059781766745175, 9.846743663894590881 ) ) ;
#85849=CARTESIAN_POINT ( 'NONE',  ( 17.96484262340118221, 11.18868534415483929, -7.964842623401177768 ) ) ;
#85852=CARTESIAN_POINT ( 'NONE',  ( 19.38216949554541557, 32.24863466993041783, -9.382169495545420901 ) ) ;
#85853=CARTESIAN_POINT ( 'NONE',  ( 4.559911319644449179, 48.89701867748817676, 9.422509992056141925 ) ) ;
#85854=CARTESIAN_POINT ( 'NONE',  ( -0.3689425029237898834, 41.17874883491397497, -10.36894250292378850 ) ) ;
#85855=CARTESIAN_POINT ( 'NONE',  ( 14.92337183194729988, 9.342264484334119601, -8.527530157486177487 ) ) ;
#85857=CARTESIAN_POINT ( 'NONE',  ( 19.84674366389459266, 53.30059781766744464, 2.638427012816836559 ) ) ;
#85858=CARTESIAN_POINT ( 'NONE',  ( 12.63842701281683922, 34.55059781766745886, -9.846743663894590881 ) ) ;
#85859=CARTESIAN_POINT ( 'NONE',  ( 13.79529636645031943, 15.34541550158063750, -14.16423886937409904 ) ) ;
#85860=CARTESIAN_POINT ( 'NONE',  ( 12.63842701281683034, 27.46726448433411250, 9.846743663894596210 ) ) ;
#85861=CARTESIAN_POINT ( 'NONE',  ( -0.8801773607111009756, 48.06368534415484817, 1.068504757029289695E-15 ) ) ;
#85862=CARTESIAN_POINT ( 'NONE',  ( 10.00000000000000000, 16.81368534415483751, -10.88017736071110342 ) ) ;
#85863=CARTESIAN_POINT ( 'NONE',  ( 20.88017736071110519, 45.56368534415484106, 2.639326808657452039E-16 ) ) ;
#85864=CARTESIAN_POINT ( 'NONE',  ( 20.88017736071110875, 25.77201867748816966, -2.915334737309920765 ) ) ;
#85865=VERTEX_POINT ( 'NONE', #52218 ) ;
#85866=CARTESIAN_POINT ( 'NONE',  ( 21.09922568453594849, 31.20696800326375353, 6.408140936763242479 ) ) ;
#85867=CARTESIAN_POINT ( 'NONE',  ( 0.5774900079438590739, 37.64701867748817676, -5.440088680355550821 ) ) ;
#85868=ORIENTED_EDGE ( 'NONE', *, *, #58506, .F. ) ;
#85869=CARTESIAN_POINT ( 'NONE',  ( 10.00000000000000178, 65.37363466993042493, 12.81628187352647608 ) ) ;
#85871=CARTESIAN_POINT ( 'NONE',  ( 17.96484262340118221, 59.93868534415484106, 7.964842623401181321 ) ) ;
#85873=CARTESIAN_POINT ( 'NONE',  ( 4.559911319644449179, 52.23035201082151247, -9.422509992056141925 ) ) ;
#85874=SURFACE_STYLE_FILL_AREA ( #78856 ) ;
#85875=CARTESIAN_POINT ( 'NONE',  ( 19.84674366389459621, 8.508931151000785675, 7.409399052514197653E-17 ) ) ;
#85877=CARTESIAN_POINT ( 'NONE',  ( -2.266590686148945544, 62.22041550158063927, 7.082119434687048631 ) ) ;
#85878=CARTESIAN_POINT ( 'NONE',  ( 17.20831665107776587, 7.883931151000784787, 7.208316651077764980 ) ) ;
#85879=CARTESIAN_POINT ( 'NONE',  ( 17.08211943468705130, 8.470415501580635720, 12.26659068614894998 ) ) ;
#85880=CARTESIAN_POINT ( 'NONE',  ( 14.92337183194729988, 9.342264484334119601, -8.527530157486177487 ) ) ;
#85881=CARTESIAN_POINT ( 'NONE',  ( 17.96484262340118221, 16.18868534415483396, -7.964842623401177768 ) ) ;
#85882=CARTESIAN_POINT ( 'NONE',  ( 19.84674366389459621, 43.50893115100078745, 7.409399052514197653E-17 ) ) ;
#85883=ORIENTED_EDGE ( 'NONE', *, *, #62342, .T. ) ;
#85884=CARTESIAN_POINT ( 'NONE',  ( 14.92337183194729633, 47.67559781766745175, 8.527530157486181039 ) ) ;
#85886=CARTESIAN_POINT ( 'NONE',  ( 4.559911319644449179, 43.89701867748816966, 9.422509992056141925 ) ) ;
#85887=CARTESIAN_POINT ( 'NONE',  ( 0.1532563361054083140, 56.00893115100078745, 1.131784320476157264E-15 ) ) ;
#85888=( LENGTH_UNIT ( ) NAMED_UNIT ( * ) SI_UNIT ( .MILLI., .METRE. ) );
#85890=CARTESIAN_POINT ( 'NONE',  ( 10.00000000000000000, 41.81368534415484106, -10.88017736071110342 ) ) ;
#85891=CARTESIAN_POINT ( 'NONE',  ( 0.5774900079438590739, 2.647018677488171434, -5.440088680355550821 ) ) ;
#85893=CARTESIAN_POINT ( 'NONE',  ( 13.43411237798105340, 20.58196800326374643, 12.81628187352647963 ) ) ;
#85895=EDGE_LOOP ( 'NONE', ( #6413, #29425, #69278, #20668 ) ) ;
#85896=CARTESIAN_POINT ( 'NONE',  ( 16.40814093676324603, 32.45696800326375353, -11.09922568453594671 ) ) ;
#85897=CARTESIAN_POINT ( 'NONE',  ( -0.8801773607111008646, 18.27201867748817321, 2.915334737309923430 ) ) ;
#85898=EDGE_CURVE ( 'NONE', #25477, #86614, #36208, .T. ) ;
#85902=CARTESIAN_POINT ( 'NONE',  ( 1.472469842513823179, 1.425597817667451528, 4.923371831947296329 ) ) ;
#85903=CARTESIAN_POINT ( 'NONE',  ( 10.00000000000000178, 47.25893115100078745, 9.846743663894594434 ) ) ;
#85904=CARTESIAN_POINT ( 'NONE',  ( 0.1532563361054083140, 6.008931151000784787, 1.131784320476157264E-15 ) ) ;
#85905=CARTESIAN_POINT ( 'NONE',  ( 19.84674366389459621, 43.50893115100078745, 7.409399052514197653E-17 ) ) ;
#85908=CARTESIAN_POINT ( 'NONE',  ( 19.84674366389459266, 23.30059781766745530, 2.638427012816836559 ) ) ;
#85910=FACE_OUTER_BOUND ( 'NONE', #78, .T. ) ;
#85911=CARTESIAN_POINT ( 'NONE',  ( 17.20831665107776587, 22.88393115100078745, 7.208316651077764980 ) ) ;
#85912=VECTOR ( 'NONE', #15138, 1000.000000000000000 ) ;
#85913=CARTESIAN_POINT ( 'NONE',  ( 2.791683348922240793, 1.633931151000784565, 7.208316651077764092 ) ) ;
#85915=ADVANCED_FACE ( 'NONE', ( #91700 ), #5566, .T. ) ;
#85916=CARTESIAN_POINT ( 'NONE',  ( 10.00000000000000178, 52.25893115100078745, 9.846743663894594434 ) ) ;
#85920=CARTESIAN_POINT ( 'NONE',  ( 0.6178305044545838731, 29.74863466993042138, 9.382169495545420901 ) ) ;
#85921=EDGE_CURVE ( 'NONE', #25175, #91846, #42534, .T. ) ;
#85923=CARTESIAN_POINT ( 'NONE',  ( -4.164238869374099039, 46.80374883491397497, 8.674139862899312516E-16 ) ) ;
#85924=EDGE_CURVE ( 'NONE', #50559, #27193, #7247, .T. ) ;
#85925=CARTESIAN_POINT ( 'NONE',  ( 5.076628168052703671, 16.84226448433411960, 8.527530157486179263 ) ) ;
#85926=CARTESIAN_POINT ( 'NONE',  ( 7.361572987183169658, 4.967264484334119601, -9.846743663894592657 ) ) ;
#85928=CARTESIAN_POINT ( 'NONE',  ( 10.00000000000000178, 38.05374883491396787, 14.16423886937410082 ) ) ;
#85929=CARTESIAN_POINT ( 'NONE',  ( 7.361572987183170547, 62.05059781766745886, 9.846743663894590881 ) ) ;
#85930=CARTESIAN_POINT ( 'NONE',  ( 20.88017736071110164, 10.35535201082150714, 2.915334737309930979 ) ) ;
#85931=CARTESIAN_POINT ( 'NONE',  ( 24.16423886937410614, 29.30374883491396787, 8.672049930838204340E-16 ) ) ;
#85932=CARTESIAN_POINT ( 'NONE',  ( 17.08211943468705840, 40.13708216824731068, -12.26659068614894466 ) ) ;
#85933=DIRECTION ( 'NONE',  ( -0.000000000000000000, -0.000000000000000000, -1.000000000000000000 ) ) ;
#85935=CARTESIAN_POINT ( 'NONE',  ( 19.84674366389459621, 53.50893115100078745, 7.409399052514197653E-17 ) ) ;
#85936=ORIENTED_EDGE ( 'NONE', *, *, #57943, .T. ) ;
#85937=CARTESIAN_POINT ( 'NONE',  ( 17.96484262340118221, 36.18868534415484106, -7.964842623401177768 ) ) ;
#85940=CARTESIAN_POINT ( 'NONE',  ( 18.52753015748618282, 38.92559781766745175, -4.923371831947291888 ) ) ;
#85941=CARTESIAN_POINT ( 'NONE',  ( 10.00000000000000000, 62.87363466993042493, -12.81628187352647608 ) ) ;
#85943=CARTESIAN_POINT ( 'NONE',  ( 5.076628168052704559, 40.17559781766745175, -8.527530157486179263 ) ) ;
#85945=ORIENTED_EDGE ( 'NONE', *, *, #5339, .F. ) ;
#85947=CARTESIAN_POINT ( 'NONE',  ( 17.08211943468705840, 20.13708216824730357, -12.26659068614894466 ) ) ;
#85949=CARTESIAN_POINT ( 'NONE',  ( 0.1089645850228990742, 68.16234555792571825, 6.479102184480824533 ) ) ;
#85950=CARTESIAN_POINT ( 'NONE',  ( 19.50000000000000711, 105.0000000000000000, 4.500000000000000888 ) ) ;
#85951=CARTESIAN_POINT ( 'NONE',  ( 15.44008868035555260, 4.730352010821505360, 9.422509992056143702 ) ) ;
#85952=CARTESIAN_POINT ( 'NONE',  ( 6.565887622018943937, 30.16530133659708568, 12.81628187352647430 ) ) ;
#85953=CARTESIAN_POINT ( 'NONE',  ( 2.791683348922237240, 0.3839311510007847872, -7.208316651077763204 ) ) ;
#85954=EDGE_CURVE ( 'NONE', #36088, #36584, #41074, .T. ) ;
#85956=CARTESIAN_POINT ( 'NONE',  ( -1.926860441876562025, 9.479976035794173583, -3.195792623639529761 ) ) ;
#85957=CYLINDRICAL_SURFACE ( 'NONE', #35919, 0.5000000000000004441 ) ;
#85958=CARTESIAN_POINT ( 'NONE',  ( 6.204703633549690345, 60.76208216824730357, -14.16423886937410259 ) ) ;
#85960=CARTESIAN_POINT ( 'NONE',  ( 0.2751277870542871429, 42.28217586085238366, -6.499999999999984901 ) ) ;
#85961=CARTESIAN_POINT ( 'NONE',  ( 17.96484262340118221, 24.93868534415484461, 7.964842623401181321 ) ) ;
#85962=CARTESIAN_POINT ( 'NONE',  ( -0.8801773607110991993, 32.85535201082151247, -2.915334737309923874 ) ) ;
#85963=CARTESIAN_POINT ( 'NONE',  ( 12.63842701281683922, 64.55059781766745175, -9.846743663894590881 ) ) ;
#85964=CARTESIAN_POINT ( 'NONE',  ( 12.63842701281683034, 57.46726448433411605, 9.846743663894596210 ) ) ;
#85965=CARTESIAN_POINT ( 'NONE',  ( 16.40814093676323893, 60.79030133659709634, 11.09922568453595026 ) ) ;
#85966=FILL_AREA_STYLE_COLOUR ( '', #42436 ) ;
#85967=ORIENTED_EDGE ( 'NONE', *, *, #58957, .F. ) ;
#85968=CARTESIAN_POINT ( 'NONE',  ( 12.91533473730993009, 36.60535201082151247, -10.88017736071109987 ) ) ;
#85969=CARTESIAN_POINT ( 'NONE',  ( 3.591859063236763294, 28.29030133659708568, -11.09922568453595026 ) ) ;
#85972=CARTESIAN_POINT ( 'NONE',  ( 5.076628168052703671, 61.84226448433412315, 8.527530157486179263 ) ) ;
#85973=CARTESIAN_POINT ( 'NONE',  ( 20.88017736071110875, 45.77201867748816966, -2.915334737309920765 ) ) ;
#85974=CARTESIAN_POINT ( 'NONE',  ( 5.076628168052703671, 11.84226448433411960, 8.527530157486179263 ) ) ;
#85975=CARTESIAN_POINT ( 'NONE',  ( 0.6178305044545838731, 39.74863466993041072, 9.382169495545420901 ) ) ;
#85976=CARTESIAN_POINT ( 'NONE',  ( 4.559911319644449179, 67.23035201082150536, -9.422509992056141925 ) ) ;
#85978=CARTESIAN_POINT ( 'NONE',  ( 22.81628187352647785, 61.41530133659709634, 3.434112377981063169 ) ) ;
#85982=CARTESIAN_POINT ( 'NONE',  ( 2.035157376598824452, 3.688685344154837953, 7.964842623401179544 ) ) ;
#85983=CARTESIAN_POINT ( 'NONE',  ( 22.81628187352647785, 46.62363466993041783, 6.195893100308588602E-16 ) ) ;
#85984=CARTESIAN_POINT ( 'NONE',  ( 13.79529636645030344, 18.26208216824730002, 14.16423886937410614 ) ) ;
#85985=CARTESIAN_POINT ( 'NONE',  ( 19.84674366389459621, 18.50893115100078745, 7.409399052514197653E-17 ) ) ;
#85986=CARTESIAN_POINT ( 'NONE',  ( 4.559911319644449179, 7.230352010821504471, -9.422509992056141925 ) ) ;
#85987=CARTESIAN_POINT ( 'NONE',  ( 1.472469842513823179, 15.59226448433411960, -4.923371831947296329 ) ) ;
#85988=CARTESIAN_POINT ( 'NONE',  ( 20.36894250292379382, 58.67874883491396076, 10.36894250292379205 ) ) ;
#85989=VERTEX_POINT ( 'NONE', #19538 ) ;
#85990=CARTESIAN_POINT ( 'NONE',  ( 10.00000000000000000, 1.813685344154837731, -10.88017736071110342 ) ) ;
#85992=CARTESIAN_POINT ( 'NONE',  ( 7.084665262690076126, 22.02201867748817321, -10.88017736071110164 ) ) ;
#85994=VECTOR ( 'NONE', #71006, 1000.000000000000000 ) ;
#85997=CARTESIAN_POINT ( 'NONE',  ( 2.035157376598822676, 17.43868534415483751, -7.964842623401177768 ) ) ;
#85998=CARTESIAN_POINT ( 'NONE',  ( 2.035157376598824452, 8.688685344154839285, 7.964842623401179544 ) ) ;
#85999=CARTESIAN_POINT ( 'NONE',  ( 1.472469842513823179, 60.59226448433412315, -4.923371831947296329 ) ) ;
#86000=CARTESIAN_POINT ( 'NONE',  ( -2.816281873526473856, 54.12363466993041783, 9.499525473075851096E-16 ) ) ;
#86002=CARTESIAN_POINT ( 'NONE',  ( 22.26659068614895176, 19.72041550158063572, -7.082119434687042414 ) ) ;
#86003=CARTESIAN_POINT ( 'NONE',  ( 15.44008868035555260, 24.73035201082150891, 9.422509992056143702 ) ) ;
#86004=CARTESIAN_POINT ( 'NONE',  ( 20.88017736071110519, 15.56368534415483751, 2.639326808657452039E-16 ) ) ;
#86005=CARTESIAN_POINT ( 'NONE',  ( 14.92337183194729988, 49.34226448433411605, -8.527530157486177487 ) ) ;
#86006=CARTESIAN_POINT ( 'NONE',  ( 7.361572987183169658, 39.96726448433411605, -9.846743663894592657 ) ) ;
#86008=CARTESIAN_POINT ( 'NONE',  ( 2.791683348922237240, 10.38393115100078390, -7.208316651077763204 ) ) ;
#86011=FACE_OUTER_BOUND ( 'NONE', #812, .T. ) ;
#86012=CARTESIAN_POINT ( 'NONE',  ( 0.1532563361054082862, 16.21726448433411960, 2.638427012816831674 ) ) ;
#86013=CARTESIAN_POINT ( 'NONE',  ( 16.40814093676324603, 2.456968003263753531, -11.09922568453594671 ) ) ;
#86014=CARTESIAN_POINT ( 'NONE',  ( -0.8801773607111009756, 53.06368534415484106, 1.068504757029289695E-15 ) ) ;
#86015=CARTESIAN_POINT ( 'NONE',  ( 10.00000000000000000, 6.813685344154838397, -10.88017736071110342 ) ) ;
#86016=CARTESIAN_POINT ( 'NONE',  ( -2.816281873526471635, 43.91530133659708923, -3.434112377981056508 ) ) ;
#86017=CARTESIAN_POINT ( 'NONE',  ( 10.00000000000000178, 18.05374883491396787, 14.16423886937410082 ) ) ;
#86018=CARTESIAN_POINT ( 'NONE',  ( 0.6178305044545838731, 54.74863466993042493, 9.382169495545420901 ) ) ;
#86020=CARTESIAN_POINT ( 'NONE',  ( 17.20831665107776587, 59.13393115100078745, -7.208316651077762316 ) ) ;
#86021=CARTESIAN_POINT ( 'NONE',  ( -0.8801773607110991993, 22.85535201082150181, -2.915334737309923874 ) ) ;
#86023=CARTESIAN_POINT ( 'NONE',  ( 10.00000000000000178, 7.258931151000785675, 9.846743663894594434 ) ) ;
#86024=CARTESIAN_POINT ( 'NONE',  ( 17.96484262340118221, 66.18868534415483396, -7.964842623401177768 ) ) ;
#86026=CARTESIAN_POINT ( 'NONE',  ( 18.52753015748618282, 13.92559781766745175, -4.923371831947291888 ) ) ;
#86028=CARTESIAN_POINT ( 'NONE',  ( 15.44008868035555793, 66.39701867748817676, -9.422509992056140149 ) ) ;
#86030=CARTESIAN_POINT ( 'NONE',  ( 19.42250999205614548, 60.98035201082151247, -5.440088680355545492 ) ) ;
#86032=CARTESIAN_POINT ( 'NONE',  ( 20.88017736071110164, 65.35535201082150536, 2.915334737309930979 ) ) ;
#86033=CARTESIAN_POINT ( 'NONE',  ( 0.1532563361054083140, 6.008931151000784787, 1.131784320476157264E-15 ) ) ;
#86034=VERTEX_POINT ( 'NONE', #37515 ) ;
#86035=EDGE_CURVE ( 'NONE', #24202, #74944, #22652, .T. ) ;
#86037=CARTESIAN_POINT ( 'NONE',  ( 18.52753015748618282, 53.92559781766745175, -4.923371831947291888 ) ) ;
#86041=CARTESIAN_POINT ( 'NONE',  ( 22.26659068614894466, 3.887082168247300906, 7.082119434687054849 ) ) ;
#86043=CARTESIAN_POINT ( 'NONE',  ( 13.43411237798105340, 60.58196800326376064, 12.81628187352647963 ) ) ;
#86044=CARTESIAN_POINT ( 'NONE',  ( 6.204703633549690345, 5.762082168247301794, -14.16423886937410259 ) ) ;
#86045=CARTESIAN_POINT ( 'NONE',  ( 13.79529636645031943, 15.34541550158063750, -14.16423886937409904 ) ) ;
#86046=AXIS2_PLACEMENT_3D ( 'NONE', #58901, #56925, #72912 ) ;
#86048=CARTESIAN_POINT ( 'NONE',  ( 22.26659068614895176, 4.720415501580633943, -7.082119434687042414 ) ) ;
#86049=CARTESIAN_POINT ( 'NONE',  ( 12.91533473730992121, 24.52201867748816966, 10.88017736071110164 ) ) ;
#86051=VERTEX_POINT ( 'NONE', #13519 ) ;
#86052=CARTESIAN_POINT ( 'NONE',  ( 5.076628168052704559, 5.175597817667451750, -8.527530157486179263 ) ) ;
#86053=CARTESIAN_POINT ( 'NONE',  ( 7.361572987183170547, 22.05059781766745530, 9.846743663894590881 ) ) ;
#86054=CARTESIAN_POINT ( 'NONE',  ( 22.81628187352647785, 36.41530133659707502, 3.434112377981063169 ) ) ;
#86055=CARTESIAN_POINT ( 'NONE',  ( 5.076628168052704559, 35.17559781766745175, -8.527530157486179263 ) ) ;
#86058=CARTESIAN_POINT ( 'NONE',  ( 10.00000000000000178, 20.37363466993042138, 12.81628187352647608 ) ) ;
#86060=CARTESIAN_POINT ( 'NONE',  ( 2.791683348922240793, 31.63393115100078745, 7.208316651077764092 ) ) ;
#86061=CARTESIAN_POINT ( 'NONE',  ( 6.204703633549690345, 17.84541550158063217, 14.16423886937410082 ) ) ;
#86064=CARTESIAN_POINT ( 'NONE',  ( 12.91533473730992121, 34.52201867748817676, 10.88017736071110164 ) ) ;
#86065=CARTESIAN_POINT ( 'NONE',  ( 24.16423886937410614, 34.51208216824731068, -3.795296366450302550 ) ) ;
#86066=CARTESIAN_POINT ( 'NONE',  ( 5.076628168052703671, 41.84226448433411605, 8.527530157486179263 ) ) ;
#86067=CARTESIAN_POINT ( 'NONE',  ( 7.361572987183169658, 14.96726448433411960, -9.846743663894592657 ) ) ;
#86068=CARTESIAN_POINT ( 'NONE',  ( 6.565887622018943937, 53.08196800326374643, -12.81628187352647608 ) ) ;
#86069=CARTESIAN_POINT ( 'NONE',  ( 19.72487221294570858, 0.000000000000000000, -6.500000000000000888 ) ) ;
#86070=CARTESIAN_POINT ( 'NONE',  ( 12.91533473730992121, 29.52201867748817321, 10.88017736071110164 ) ) ;
#86072=CARTESIAN_POINT ( 'NONE',  ( 21.09922568453595559, 27.04030133659708568, -6.408140936763230044 ) ) ;
#86073=CARTESIAN_POINT ( 'NONE',  ( 1.472469842513823179, 45.59226448433412315, -4.923371831947296329 ) ) ;
#86075=CARTESIAN_POINT ( 'NONE',  ( 10.00000000000000000, 47.87363466993042493, -12.81628187352647608 ) ) ;
#86076=( BOUNDED_CURVE ( )  B_SPLINE_CURVE ( 2, ( #8446, #53947, #7483, #14487, #75462, #6978, #67972, #15479, #98497 ),
 .UNSPECIFIED., .F., .T. ) 
 B_SPLINE_CURVE_WITH_KNOTS ( ( 3, 2, 2, 2, 3 ),
 ( 0.4401409369402313199, 0.4404761904761904656, 0.4464285714285713969, 0.4523809523809524391, 0.4527162059169115849 ),
 .UNSPECIFIED. ) 
 CURVE ( )  GEOMETRIC_REPRESENTATION_ITEM ( )  RATIONAL_B_SPLINE_CURVE ( ( 0.9963778908391760503, 0.9980808541467920403, 1.000000000000000000, 0.9659258262890682012, 1.000000000000000000, 0.9659258262890682012, 1.000000000000000000, 0.9980808541467920403, 0.9963778908391759392 ) ) 
 REPRESENTATION_ITEM ( '' )  );
#86077=CARTESIAN_POINT ( 'NONE',  ( 2.035157376598824452, 58.68868534415482685, 7.964842623401179544 ) ) ;
#86078=CARTESIAN_POINT ( 'NONE',  ( 20.04068437667223890, 9.719743609177204036, 6.396802510829703969 ) ) ;
#86081=CARTESIAN_POINT ( 'NONE',  ( 12.91533473730992121, 54.52201867748816255, 10.88017736071110164 ) ) ;
#86082=CARTESIAN_POINT ( 'NONE',  ( -0.8801773607111008646, 53.27201867748816966, 2.915334737309923430 ) ) ;
#86083=CARTESIAN_POINT ( 'NONE',  ( 19.72487221294570858, 56.86607318730075633, 6.500000000000000888 ) ) ;
#86085=CARTESIAN_POINT ( 'NONE',  ( 12.91533473730992121, 4.522018677488170546, 10.88017736071110164 ) ) ;
#86086=CARTESIAN_POINT ( 'NONE',  ( 14.92337183194729988, 59.34226448433412315, -8.527530157486177487 ) ) ;
#86087=CARTESIAN_POINT ( 'NONE',  ( 12.91533473730993009, 16.60535201082150891, -10.88017736071109987 ) ) ;
#86089=CARTESIAN_POINT ( 'NONE',  ( 6.565887622018943937, 28.08196800326375353, -12.81628187352647608 ) ) ;
#86091=CARTESIAN_POINT ( 'NONE',  ( -0.8801773607110991993, 57.85535201082149825, -2.915334737309923874 ) ) ;
#86092=CARTESIAN_POINT ( 'NONE',  ( 7.361572987183169658, 39.96726448433411605, -9.846743663894592657 ) ) ;
#86093=CARTESIAN_POINT ( 'NONE',  ( 13.43411237798106583, 12.66530133659708746, -12.81628187352647252 ) ) ;
#86095=CARTESIAN_POINT ( 'NONE',  ( 7.084665262690076126, 17.02201867748817676, -10.88017736071110164 ) ) ;
#86096=CARTESIAN_POINT ( 'NONE',  ( 20.88017736071110875, 35.77201867748816966, -2.915334737309920765 ) ) ;
#86097=CARTESIAN_POINT ( 'NONE',  ( 6.204703633549690345, 50.76208216824730357, -14.16423886937410259 ) ) ;
#86098=CARTESIAN_POINT ( 'NONE',  ( 14.92337183194729988, 44.34226448433412315, -8.527530157486177487 ) ) ;
#86100=CARTESIAN_POINT ( 'NONE',  ( 4.559911319644449179, 53.89701867748817676, 9.422509992056141925 ) ) ;
#86102=CARTESIAN_POINT ( 'NONE',  ( 13.79529636645030344, 13.26208216824729824, 14.16423886937410614 ) ) ;
#86105=CARTESIAN_POINT ( 'NONE',  ( 2.603489959281581889, 20.43575266056827999, -6.499999999999995559 ) ) ;
#86106=ORIENTED_EDGE ( 'NONE', *, *, #96583, .T. ) ;
#86108=CARTESIAN_POINT ( 'NONE',  ( -2.266590686148945544, 42.22041550158063217, 7.082119434687048631 ) ) ;
#86109=CARTESIAN_POINT ( 'NONE',  ( 22.26659068614895176, 39.72041550158063217, -7.082119434687042414 ) ) ;
#86110=CARTESIAN_POINT ( 'NONE',  ( 7.361572987183169658, 14.96726448433411960, -9.846743663894592657 ) ) ;
#86111=CARTESIAN_POINT ( 'NONE',  ( 22.81628187352647785, 16.41530133659708923, 3.434112377981063169 ) ) ;
#86112=CARTESIAN_POINT ( 'NONE',  ( 10.00000000000000178, 67.25893115100079456, 9.846743663894594434 ) ) ;
#86114=CARTESIAN_POINT ( 'NONE',  ( 12.91533473730993009, 56.60535201082151247, -10.88017736071109987 ) ) ;
#86115=CARTESIAN_POINT ( 'NONE',  ( -2.816281873526473856, 39.33196800326374643, 3.434112377981055619 ) ) ;
#86116=CARTESIAN_POINT ( 'NONE',  ( 22.26659068614895176, 29.72041550158063572, -7.082119434687042414 ) ) ;
#86117=CARTESIAN_POINT ( 'NONE',  ( 20.88017736071110519, 20.56368534415484106, 2.639326808657452039E-16 ) ) ;
#86119=CARTESIAN_POINT ( 'NONE',  ( 15.44008868035555793, 66.39701867748817676, -9.422509992056140149 ) ) ;
#86123=ORIENTED_EDGE ( 'NONE', *, *, #12478, .T. ) ;
#86126=VERTEX_POINT ( 'NONE', #22513 ) ;
#86127=CARTESIAN_POINT ( 'NONE',  ( -4.164238869374099039, 1.803748834913967647, 8.674139862899312516E-16 ) ) ;
#86128=CARTESIAN_POINT ( 'NONE',  ( 4.559911319644449179, 7.230352010821505360, -9.422509992056141925 ) ) ;
#86129=CARTESIAN_POINT ( 'NONE',  ( 0.5774900079438607392, 18.48035201082150536, 5.440088680355550821 ) ) ;
#86130=CARTESIAN_POINT ( 'NONE',  ( 5.076628168052704559, 35.17559781766745175, -8.527530157486179263 ) ) ;
#86131=CARTESIAN_POINT ( 'NONE',  ( 0.6178305044545818747, 3.498634669930420049, -9.382169495545419124 ) ) ;
#86135=CARTESIAN_POINT ( 'NONE',  ( 22.81628187352647785, 11.41530133659708390, 3.434112377981063169 ) ) ;
#86137=CARTESIAN_POINT ( 'NONE',  ( 17.08211943468705840, 50.13708216824730357, -12.26659068614894466 ) ) ;
#86139=CARTESIAN_POINT ( 'NONE',  ( -2.266590686148945544, 56.38708216824731068, -7.082119434687050408 ) ) ;
#86141=CARTESIAN_POINT ( 'NONE',  ( 20.88017736071110164, 40.35535201082150536, 2.915334737309930979 ) ) ;
#86143=CARTESIAN_POINT ( 'NONE',  ( 4.559911319644449179, 37.23035201082150536, -9.422509992056141925 ) ) ;
#86144=CARTESIAN_POINT ( 'NONE',  ( 20.88017736071110164, 35.35535201082150536, 2.915334737309930979 ) ) ;
#86145=CARTESIAN_POINT ( 'NONE',  ( -28.94000000000001549, 93.50000000000000000, -9.500000000000000000 ) ) ;
#86146=CARTESIAN_POINT ( 'NONE',  ( 17.96484262340118221, 26.18868534415483396, -7.964842623401177768 ) ) ;
#86148=( BOUNDED_CURVE ( )  B_SPLINE_CURVE ( 2, ( #15504, #22013, #23002, #89995, #13512, #30468, #83491, #82995, #98022 ),
 .UNSPECIFIED., .F., .F. ) 
 B_SPLINE_CURVE_WITH_KNOTS ( ( 3, 2, 2, 2, 3 ),
 ( 0.5829980797973742801, 0.5833333333333333703, 0.5892857142857143016, 0.5952380952380952328, 0.5955733487740544341 ),
 .UNSPECIFIED. ) 
 CURVE ( )  GEOMETRIC_REPRESENTATION_ITEM ( )  RATIONAL_B_SPLINE_CURVE ( ( 0.9963778908391764944, 0.9980808541467923733, 1.000000000000000000, 0.9659258262890682012, 1.000000000000000000, 0.9659258262890682012, 1.000000000000000000, 0.9980808541467918182, 0.9963778908391756062 ) ) 
 REPRESENTATION_ITEM ( '' )  );
#86152=CARTESIAN_POINT ( 'NONE',  ( 1.472469842513823179, 21.42559781766745175, 4.923371831947296329 ) ) ;
#86153=EDGE_LOOP ( 'NONE', ( #51092, #82851, #61262, #14321 ) ) ;
#86154=CARTESIAN_POINT ( 'NONE',  ( 10.00000000000000000, 44.75893115100078745, -9.846743663894594434 ) ) ;
#86159=VERTEX_POINT ( 'NONE', #21519 ) ;
#86161=CARTESIAN_POINT ( 'NONE',  ( 0.2751277870542967463, 70.00000000000000000, -6.500000000000000888 ) ) ;
#86162=CARTESIAN_POINT ( 'NONE',  ( 12.63842701281683034, 57.46726448433411605, 9.846743663894596210 ) ) ;
#86163=CARTESIAN_POINT ( 'NONE',  ( 10.00000000000000178, 48.05374883491396787, 14.16423886937410082 ) ) ;
#86164=CARTESIAN_POINT ( 'NONE',  ( 5.076628168052703671, 66.84226448433412315, 8.527530157486179263 ) ) ;
#86167=CARTESIAN_POINT ( 'NONE',  ( 0.1532563361054083140, 21.00893115100078745, 1.131784320476157264E-15 ) ) ;
#86168=CARTESIAN_POINT ( 'NONE',  ( -2.816281873526471635, 58.91530133659707502, -3.434112377981056508 ) ) ;
#86170=CARTESIAN_POINT ( 'NONE',  ( 12.63842701281683922, 59.55059781766744464, -9.846743663894590881 ) ) ;
#86171=CARTESIAN_POINT ( 'NONE',  ( -0.8801773607111008646, 63.27201867748817676, 2.915334737309923430 ) ) ;
#86172=CARTESIAN_POINT ( 'NONE',  ( 17.20831665107776587, 44.13393115100078745, -7.208316651077762316 ) ) ;
#86173=CARTESIAN_POINT ( 'NONE',  ( 20.15039907845754286, 14.72266099184918531, 6.262539305110064625 ) ) ;
#86176=CARTESIAN_POINT ( 'NONE',  ( -2.266590686148945544, 66.38708216824730357, -7.082119434687050408 ) ) ;
#86178=CARTESIAN_POINT ( 'NONE',  ( 20.88017736071110875, 45.77201867748816966, -2.915334737309920765 ) ) ;
#86179=CARTESIAN_POINT ( 'NONE',  ( 19.38216949554541557, 17.24863466993041783, -9.382169495545420901 ) ) ;
#86180=CARTESIAN_POINT ( 'NONE',  ( -0.8801773607111009756, 68.06368534415484817, 1.068504757029289695E-15 ) ) ;
#86183=EDGE_CURVE ( 'NONE', #51686, #10866, #6025, .T. ) ;
#86186=CARTESIAN_POINT ( 'NONE',  ( 18.52753015748618282, 48.92559781766745886, -4.923371831947291888 ) ) ;
#86187=CARTESIAN_POINT ( 'NONE',  ( 0.1532563361054082862, 6.217264484334118713, 2.638427012816831674 ) ) ;
#86189=CARTESIAN_POINT ( 'NONE',  ( 16.40814093676323893, 10.79030133659708923, 11.09922568453595026 ) ) ;
#86190=CARTESIAN_POINT ( 'NONE',  ( 17.96484262340118221, 9.938685344154839285, 7.964842623401181321 ) ) ;
#86192=CARTESIAN_POINT ( 'NONE',  ( 10.00000000000000178, 33.05374883491396787, 14.16423886937410082 ) ) ;
#86193=CARTESIAN_POINT ( 'NONE',  ( 17.08211943468705130, 28.47041550158063572, 12.26659068614894998 ) ) ;
#86194=CARTESIAN_POINT ( 'NONE',  ( 24.16423886937410614, 59.30374883491397497, 8.672049930838204340E-16 ) ) ;
#86195=CARTESIAN_POINT ( 'NONE',  ( 21.09922568453594849, 36.20696800326375353, 6.408140936763242479 ) ) ;
#86196=CARTESIAN_POINT ( 'NONE',  ( 19.42250999205614548, 10.98035201082150358, -5.440088680355545492 ) ) ;
#86198=CARTESIAN_POINT ( 'NONE',  ( 0.1532563361054083140, 41.00893115100078745, 1.131784320476157264E-15 ) ) ;
#86199=CARTESIAN_POINT ( 'NONE',  ( 10.00000000000000000, 46.81368534415484106, -10.88017736071110342 ) ) ;
#86200=CARTESIAN_POINT ( 'NONE',  ( 17.20831665107776587, 64.13393115100079456, -7.208316651077762316 ) ) ;
#86201=CARTESIAN_POINT ( 'NONE',  ( 13.79529636645031943, 15.34541550158063750, -14.16423886937409904 ) ) ;
#86203=CARTESIAN_POINT ( 'NONE',  ( 18.50749283717776805, 34.69955587570481015, 6.500000000000000888 ) ) ;
#86204=UNCERTAINTY_MEASURE_WITH_UNIT (LENGTH_MEASURE( 1.000000000000000082E-05 ), #63143, 'distance_accuracy_value', 'NONE');
#86205=CARTESIAN_POINT ( 'NONE',  ( 14.92337183194729988, 19.34226448433411960, -8.527530157486177487 ) ) ;
#86206=CARTESIAN_POINT ( 'NONE',  ( 6.565887622018943937, 45.16530133659708923, 12.81628187352647430 ) ) ;
#86207=CARTESIAN_POINT ( 'NONE',  ( 7.361572987183170547, 57.05059781766744464, 9.846743663894590881 ) ) ;
#86211=CARTESIAN_POINT ( 'NONE',  ( 17.96484262340118221, 4.938685344154837509, 7.964842623401181321 ) ) ;
#86212=CARTESIAN_POINT ( 'NONE',  ( 10.00000000000000178, 8.053748834913967869, 14.16423886937410082 ) ) ;
#86213=CARTESIAN_POINT ( 'NONE',  ( 10.00000000000000178, 69.31368534415484817, 10.88017736071110342 ) ) ;
#86214=CARTESIAN_POINT ( 'NONE',  ( 18.52753015748618282, 48.92559781766745886, -4.923371831947291888 ) ) ;
#86215=CARTESIAN_POINT ( 'NONE',  ( 4.559911319644449179, 23.89701867748817321, 9.422509992056141925 ) ) ;
#86216=CARTESIAN_POINT ( 'NONE',  ( 0.1532563361054083140, 61.00893115100078745, 1.131784320476157264E-15 ) ) ;
#86218=PRESENTATION_STYLE_ASSIGNMENT (( #24252 ) ) ;
#86223=CARTESIAN_POINT ( 'NONE',  ( 18.72515096720583827, 30.05509018479937566, 6.499999999999810818 ) ) ;
#86225=CARTESIAN_POINT ( 'NONE',  ( 2.917880565312948704, 37.63708216824731068, 12.26659068614894643 ) ) ;
#86226=CARTESIAN_POINT ( 'NONE',  ( 0.1532563361054083140, 51.00893115100078745, 1.131784320476157264E-15 ) ) ;
#86227=CARTESIAN_POINT ( 'NONE',  ( 5.076628168052703671, 26.84226448433411960, 8.527530157486179263 ) ) ;
#86228=CARTESIAN_POINT ( 'NONE',  ( 20.88017736071110164, 20.35535201082150891, 2.915334737309930979 ) ) ;
#86229=CARTESIAN_POINT ( 'NONE',  ( 19.84674366389459266, 63.71726448433412315, -2.638427012816827677 ) ) ;
#86231=CARTESIAN_POINT ( 'NONE',  ( 17.08211943468705130, 38.47041550158063217, 12.26659068614894998 ) ) ;
#86232=CARTESIAN_POINT ( 'NONE',  ( 10.00000000000000178, 68.05374883491397497, 14.16423886937410082 ) ) ;
#86233=CARTESIAN_POINT ( 'NONE',  ( -42.50369195530268485, 107.9060299417078426, 4.500000000000000888 ) ) ;
#86235=CARTESIAN_POINT ( 'NONE',  ( 19.42250999205614193, 60.14701867748817676, 5.440088680355555262 ) ) ;
#86236=CARTESIAN_POINT ( 'NONE',  ( 5.076628168052704559, 10.17559781766745175, -8.527530157486179263 ) ) ;
#86241=CARTESIAN_POINT ( 'NONE',  ( 17.20831665107776587, 27.88393115100078390, 7.208316651077764980 ) ) ;
#86243=CARTESIAN_POINT ( 'NONE',  ( 20.36894250292379738, 29.92874883491396432, -10.36894250292379027 ) ) ;
#86244=CARTESIAN_POINT ( 'NONE',  ( 17.20831665107776587, 34.13393115100078745, -7.208316651077762316 ) ) ;
#86245=CARTESIAN_POINT ( 'NONE',  ( 2.035157376598824452, 38.68868534415483396, 7.964842623401179544 ) ) ;
#86247=FILL_AREA_STYLE_COLOUR ( '', #7549 ) ;
#86249=CARTESIAN_POINT ( 'NONE',  ( 4.559911319644449179, 37.23035201082150536, -9.422509992056141925 ) ) ;
#86252=VERTEX_POINT ( 'NONE', #54461 ) ;
#86253=CARTESIAN_POINT ( 'NONE',  ( -4.164238869374098151, 11.59541550158063217, -3.795296366450310543 ) ) ;
#86254=ORIENTED_EDGE ( 'NONE', *, *, #97258, .T. ) ;
#86255=EDGE_LOOP ( 'NONE', ( #10653, #1319, #13696, #32044 ) ) ;
#86256=CARTESIAN_POINT ( 'NONE',  ( 16.40814093676324603, 32.45696800326375353, -11.09922568453594671 ) ) ;
#86258=CARTESIAN_POINT ( 'NONE',  ( 19.84674366389459266, 18.30059781766745175, 2.638427012816836559 ) ) ;
#86261=CARTESIAN_POINT ( 'NONE',  ( 1.472469842513823179, 30.59226448433411960, -4.923371831947296329 ) ) ;
#86262=CARTESIAN_POINT ( 'NONE',  ( -0.8801773607111009756, 58.06368534415484106, 1.068504757029289695E-15 ) ) ;
#86266=CARTESIAN_POINT ( 'NONE',  ( 2.035157376598822676, 67.43868534415484817, -7.964842623401177768 ) ) ;
#86269=CARTESIAN_POINT ( 'NONE',  ( 12.63842701281683034, 2.467264484334118269, 9.846743663894596210 ) ) ;
#86270=EDGE_CURVE ( 'NONE', #45712, #55747, #84487, .T. ) ;
#86271=CARTESIAN_POINT ( 'NONE',  ( 13.43411237798106583, 7.665301336597086568, -12.81628187352647252 ) ) ;
#86274=( GEOMETRIC_REPRESENTATION_CONTEXT ( 3 ) GLOBAL_UNCERTAINTY_ASSIGNED_CONTEXT ( ( #17227 ) ) GLOBAL_UNIT_ASSIGNED_CONTEXT ( ( #48315, #33306, #70847 ) ) REPRESENTATION_CONTEXT ( 'NONE', 'WORKASPACE' ) );
#86275=CARTESIAN_POINT ( 'NONE',  ( 18.52753015748617571, 48.09226448433412315, 4.923371831947298993 ) ) ;
#86277=CARTESIAN_POINT ( 'NONE',  ( 22.26659068614894466, 3.887082168247300906, 7.082119434687054849 ) ) ;
#86278=CARTESIAN_POINT ( 'NONE',  ( 0.1532563361054083140, 16.00893115100078390, 1.131784320476157264E-15 ) ) ;
#86279=CARTESIAN_POINT ( 'NONE',  ( -1.099225684535947600, 39.54030133659708923, 6.408140936763237150 ) ) ;
#86282=CARTESIAN_POINT ( 'NONE',  ( 20.88017736071110519, 50.56368534415484106, 2.639326808657452039E-16 ) ) ;
#86284=CARTESIAN_POINT ( 'NONE',  ( 10.00000000000000000, 12.87363466993042138, -12.81628187352647608 ) ) ;
#86285=CARTESIAN_POINT ( 'NONE',  ( 2.603489959281614308, 41.58210964143329846, 6.500000000000031086 ) ) ;
#86286=CARTESIAN_POINT ( 'NONE',  ( 10.00000000000000000, 24.75893115100078745, -9.846743663894594434 ) ) ;
#86287=CARTESIAN_POINT ( 'NONE',  ( 2.035157376598822676, 32.43868534415483396, -7.964842623401177768 ) ) ;
#86288=CARTESIAN_POINT ( 'NONE',  ( 0.6178305044545838731, 34.74863466993042493, 9.382169495545420901 ) ) ;
#86289=CARTESIAN_POINT ( 'NONE',  ( 10.00000000000000178, 17.25893115100078745, 9.846743663894594434 ) ) ;
#86291=LINE ( 'NONE', #8809, #58192 ) ;
#86292=CARTESIAN_POINT ( 'NONE',  ( 7.084665262690076126, 22.02201867748817321, -10.88017736071110164 ) ) ;
#86294=CARTESIAN_POINT ( 'NONE',  ( 20.88017736071110519, 55.56368534415484817, 2.639326808657452039E-16 ) ) ;
#86295=CARTESIAN_POINT ( 'NONE',  ( -0.8801773607110991993, 7.855352010821504471, -2.915334737309923874 ) ) ;
#86296=CARTESIAN_POINT ( 'NONE',  ( 18.52753015748618282, 38.92559781766745175, -4.923371831947291888 ) ) ;
#86297=CARTESIAN_POINT ( 'NONE',  ( 15.44008868035555260, 14.73035201082150536, 9.422509992056143702 ) ) ;
#86299=CARTESIAN_POINT ( 'NONE',  ( 10.00000000000000000, 41.81368534415484106, -10.88017736071110342 ) ) ;
#86300=CARTESIAN_POINT ( 'NONE',  ( 10.00000000000000178, 19.31368534415484106, 10.88017736071110342 ) ) ;
#86301=CARTESIAN_POINT ( 'NONE',  ( 19.89220837332773684, 59.74062864464242040, 6.478736007406005193 ) ) ;
#86303=CARTESIAN_POINT ( 'NONE',  ( 5.076628168052703671, 31.84226448433412315, 8.527530157486179263 ) ) ;
#86307=CARTESIAN_POINT ( 'NONE',  ( 21.09922568453594849, 1.206968003263753531, 6.408140936763242479 ) ) ;
#86309=CARTESIAN_POINT ( 'NONE',  ( 13.79529636645031943, 25.34541550158063572, -14.16423886937409904 ) ) ;
#86311=DIRECTION ( 'NONE',  ( 0.000000000000000000, 0.000000000000000000, -1.000000000000000000 ) ) ;
#86313=CARTESIAN_POINT ( 'NONE',  ( 24.16423886937410614, 64.30374883491396076, 8.672049930838204340E-16 ) ) ;
#86314=CARTESIAN_POINT ( 'NONE',  ( 1.472469842513823179, 21.42559781766745175, 4.923371831947296329 ) ) ;
#86316=CARTESIAN_POINT ( 'NONE',  ( 0.5774900079438607392, 43.48035201082151247, 5.440088680355550821 ) ) ;
#86317=CARTESIAN_POINT ( 'NONE',  ( -2.816281873526471635, 58.91530133659707502, -3.434112377981056508 ) ) ;
#86318=CARTESIAN_POINT ( 'NONE',  ( 20.88017736071110164, 30.35535201082151247, 2.915334737309930979 ) ) ;
#86319=CYLINDRICAL_SURFACE ( 'NONE', #81835, 11.92686044187656513 ) ;
#86320=CARTESIAN_POINT ( 'NONE',  ( 16.40814093676323893, 10.79030133659708923, 11.09922568453595026 ) ) ;
#86321=CARTESIAN_POINT ( 'NONE',  ( 1.472469842513823179, 21.42559781766745175, 4.923371831947296329 ) ) ;
#86325=CARTESIAN_POINT ( 'NONE',  ( -2.266590686148945544, 52.22041550158064638, 7.082119434687048631 ) ) ;
#86326=CARTESIAN_POINT ( 'NONE',  ( 22.26659068614894466, 28.88708216824730357, 7.082119434687054849 ) ) ;
#86327=CARTESIAN_POINT ( 'NONE',  ( 20.88017736071110164, 25.35535201082150891, 2.915334737309930979 ) ) ;
#86328=CARTESIAN_POINT ( 'NONE',  ( 20.88017736071110519, 50.56368534415484106, 2.639326808657452039E-16 ) ) ;
#86331=CARTESIAN_POINT ( 'NONE',  ( 17.20831665107776587, 14.13393115100078568, -7.208316651077762316 ) ) ;
#86333=CARTESIAN_POINT ( 'NONE',  ( 19.84674366389459266, 18.71726448433411960, -2.638427012816827677 ) ) ;
#86335=CARTESIAN_POINT ( 'NONE',  ( 1.472469842513823179, 30.59226448433411960, -4.923371831947296329 ) ) ;
#86336=CARTESIAN_POINT ( 'NONE',  ( 18.52753015748618282, 48.92559781766745886, -4.923371831947291888 ) ) ;
#86337=CARTESIAN_POINT ( 'NONE',  ( 7.084665262690076126, 22.02201867748817321, -10.88017736071110164 ) ) ;
#86338=UNCERTAINTY_MEASURE_WITH_UNIT (LENGTH_MEASURE( 1.000000000000000082E-05 ), #6784, 'distance_accuracy_value', 'NONE');
#86340=CARTESIAN_POINT ( 'NONE',  ( 22.81628187352647785, 36.41530133659707502, 3.434112377981063169 ) ) ;
#86341=CARTESIAN_POINT ( 'NONE',  ( 12.91533473730993009, 56.60535201082151247, -10.88017736071109987 ) ) ;
#86342=CARTESIAN_POINT ( 'NONE',  ( 19.84674366389459266, 23.30059781766745530, 2.638427012816836559 ) ) ;
#86343=CARTESIAN_POINT ( 'NONE',  ( 22.26659068614895176, 39.72041550158063217, -7.082119434687042414 ) ) ;
#86344=CARTESIAN_POINT ( 'NONE',  ( 19.84674366389459266, 28.71726448433411960, -2.638427012816827677 ) ) ;
#86345=CARTESIAN_POINT ( 'NONE',  ( -0.1503990784575329198, 2.222660991849184864, -6.262539305110070842 ) ) ;
#86346=CARTESIAN_POINT ( 'NONE',  ( 10.00000000000000178, 47.25893115100078745, 9.846743663894594434 ) ) ;
#86347=CARTESIAN_POINT ( 'NONE',  ( 5.076628168052703671, 26.84226448433411960, 8.527530157486179263 ) ) ;
#86348=CARTESIAN_POINT ( 'NONE',  ( -4.164238869374098151, 6.595415501580634832, -3.795296366450310543 ) ) ;
#86349=CARTESIAN_POINT ( 'NONE',  ( 17.08211943468705130, 13.47041550158063572, 12.26659068614894998 ) ) ;
#86350=CARTESIAN_POINT ( 'NONE',  ( 17.20831665107776587, 27.88393115100078390, 7.208316651077764980 ) ) ;
#86352=CARTESIAN_POINT ( 'NONE',  ( 0.5774900079438607392, 43.48035201082151247, 5.440088680355550821 ) ) ;
#86353=CARTESIAN_POINT ( 'NONE',  ( 2.035157376598822676, 22.43868534415483396, -7.964842623401177768 ) ) ;
#86355=CARTESIAN_POINT ( 'NONE',  ( 4.559911319644449179, 47.23035201082150536, -9.422509992056141925 ) ) ;
#86356=CARTESIAN_POINT ( 'NONE',  ( 0.5774900079438607392, 33.48035201082150536, 5.440088680355550821 ) ) ;
#86359=CARTESIAN_POINT ( 'NONE',  ( -0.8801773607111009756, 58.06368534415484106, 1.068504757029289695E-15 ) ) ;
#86362=EDGE_CURVE ( 'NONE', #11778, #53014, #50089, .T. ) ;
#86363=CARTESIAN_POINT ( 'NONE',  ( 10.00000000000000000, 61.81368534415484106, -10.88017736071110342 ) ) ;
#86366=CARTESIAN_POINT ( 'NONE',  ( 20.88017736071110875, 5.772018677488170546, -2.915334737309920765 ) ) ;
#86367=CARTESIAN_POINT ( 'NONE',  ( 1.932340009482140353, 26.49127512925449324, -6.499999999999992006 ) ) ;
#86369=CARTESIAN_POINT ( 'NONE',  ( 22.26659068614895176, 59.72041550158063927, -7.082119434687042414 ) ) ;
#86370=CARTESIAN_POINT ( 'NONE',  ( 5.076628168052704559, 5.175597817667451750, -8.527530157486179263 ) ) ;
#86371=CARTESIAN_POINT ( 'NONE',  ( 6.204703633549690345, 0.7620821682473009062, -14.16423886937410259 ) ) ;
#86372=CARTESIAN_POINT ( 'NONE',  ( 17.20831665107776587, 4.133931151000785675, -7.208316651077762316 ) ) ;
#86373=CARTESIAN_POINT ( 'NONE',  ( 19.42250999205614193, 5.147018677488171434, 5.440088680355555262 ) ) ;
#86374=CARTESIAN_POINT ( 'NONE',  ( 18.52753015748617571, 43.09226448433412315, 4.923371831947298993 ) ) ;
#86376=CARTESIAN_POINT ( 'NONE',  ( 1.472469842513823179, 45.59226448433412315, -4.923371831947296329 ) ) ;
#86377=ORIENTED_EDGE ( 'NONE', *, *, #81063, .F. ) ;
#86378=DIRECTION ( 'NONE',  ( 0.000000000000000000, 0.000000000000000000, -1.000000000000000000 ) ) ;
#86379=CARTESIAN_POINT ( 'NONE',  ( 19.42250999205614193, 55.14701867748817676, 5.440088680355555262 ) ) ;
#86380=CARTESIAN_POINT ( 'NONE',  ( 7.361572987183170547, 57.05059781766744464, 9.846743663894590881 ) ) ;
#86381=SURFACE_STYLE_USAGE ( .BOTH. , #1916 ) ;
#86383=CARTESIAN_POINT ( 'NONE',  ( 0.5774900079438607392, 58.48035201082151247, 5.440088680355550821 ) ) ;
#86384=CARTESIAN_POINT ( 'NONE',  ( 7.084665262690076126, 2.022018677488171434, -10.88017736071110164 ) ) ;
#86387=CARTESIAN_POINT ( 'NONE',  ( 19.38216949554541202, 40.99863466993042493, 9.382169495545424454 ) ) ;
#86388=CARTESIAN_POINT ( 'NONE',  ( 0.1143410931637261624, 10.21691075486302580, 6.480892540919854561 ) ) ;
#86390=CARTESIAN_POINT ( 'NONE',  ( 0.6178305044545838731, 29.74863466993042138, 9.382169495545420901 ) ) ;
#86391=CARTESIAN_POINT ( 'NONE',  ( -0.8801773607111008646, 38.27201867748816255, 2.915334737309923430 ) ) ;
#86395=CARTESIAN_POINT ( 'NONE',  ( 19.84674366389459621, 63.50893115100078745, 7.409399052514197653E-17 ) ) ;
#86396=CARTESIAN_POINT ( 'NONE',  ( 7.361572987183170547, 17.05059781766745530, 9.846743663894590881 ) ) ;
#86397=CARTESIAN_POINT ( 'NONE',  ( 7.361572987183170547, 37.05059781766744464, 9.846743663894590881 ) ) ;
#86398=CARTESIAN_POINT ( 'NONE',  ( -0.03932841506543702931, 28.12161441960501307, 6.397827110478937485 ) ) ;
#86400=MECHANICAL_DESIGN_GEOMETRIC_PRESENTATION_REPRESENTATION('',(#8184),#78476);
#86401=CARTESIAN_POINT ( 'NONE',  ( 2.791683348922240793, 36.63393115100078035, 7.208316651077764092 ) ) ;
#86404=CARTESIAN_POINT ( 'NONE',  ( 5.076628168052703671, 21.84226448433411960, 8.527530157486179263 ) ) ;
#86405=FACE_OUTER_BOUND ( 'NONE', #37150, .T. ) ;
#86407=CARTESIAN_POINT ( 'NONE',  ( 5.076628168052703671, 46.84226448433412315, 8.527530157486179263 ) ) ;
#86408=ORIENTED_EDGE ( 'NONE', *, *, #68403, .T. ) ;
#86411=CARTESIAN_POINT ( 'NONE',  ( 16.40814093676323893, 25.79030133659708923, 11.09922568453595026 ) ) ;
#86412=CARTESIAN_POINT ( 'NONE',  ( 18.52753015748617571, 43.09226448433412315, 4.923371831947298993 ) ) ;
#86414=CARTESIAN_POINT ( 'NONE',  ( 22.26659068614894466, 48.88708216824730357, 7.082119434687054849 ) ) ;
#86415=CARTESIAN_POINT ( 'NONE',  ( 14.92337183194729633, 22.67559781766745175, 8.527530157486181039 ) ) ;
#86417=CARTESIAN_POINT ( 'NONE',  ( 1.472469842513823179, 1.425597817667451528, 4.923371831947296329 ) ) ;
#86419=CARTESIAN_POINT ( 'NONE',  ( 20.36894250292379738, 44.92874883491396787, -10.36894250292379027 ) ) ;
#86420=CARTESIAN_POINT ( 'NONE',  ( 10.00000000000000178, 62.25893115100078745, 9.846743663894594434 ) ) ;
#86421=CARTESIAN_POINT ( 'NONE',  ( 20.88017736071110164, 5.355352010821503583, 2.915334737309930979 ) ) ;
#86422=CARTESIAN_POINT ( 'NONE',  ( -0.3689425029237898834, 21.17874883491396432, -10.36894250292378850 ) ) ;
#86423=CARTESIAN_POINT ( 'NONE',  ( 17.08211943468705130, 38.47041550158063217, 12.26659068614894998 ) ) ;
#86426=CARTESIAN_POINT ( 'NONE',  ( 18.52753015748617571, 58.09226448433411605, 4.923371831947298993 ) ) ;
#86428=CARTESIAN_POINT ( 'NONE',  ( -0.8801773607111008646, 38.27201867748816255, 2.915334737309923430 ) ) ;
#86429=CARTESIAN_POINT ( 'NONE',  ( 19.80427997160309417, 22.75733960839544778, -6.499999999999987566 ) ) ;
#86432=CARTESIAN_POINT ( 'NONE',  ( 12.63842701281683034, 42.46726448433412315, 9.846743663894596210 ) ) ;
#86435=CARTESIAN_POINT ( 'NONE',  ( 0.1532563361054082862, 61.21726448433412315, 2.638427012816831674 ) ) ;
#86436=CARTESIAN_POINT ( 'NONE',  ( 0.1532563361054083140, 61.00893115100078745, 1.131784320476157264E-15 ) ) ;
#86438=CARTESIAN_POINT ( 'NONE',  ( 10.00000000000000000, 30.55374883491397142, -14.16423886937410082 ) ) ;
#86439=DIRECTION ( 'NONE',  ( 0.000000000000000000, -0.5943319733994194554, 0.8042198116156749066 ) ) ;
#86441=DIRECTION ( 'NONE',  ( -6.608470384673550777E-17, -1.000000000000000000, 0.000000000000000000 ) ) ;
#86442=CARTESIAN_POINT ( 'NONE',  ( 12.91533473730992121, 4.522018677488170546, 10.88017736071110164 ) ) ;
#86443=CARTESIAN_POINT ( 'NONE',  ( 19.38216949554541557, 22.24863466993041428, -9.382169495545420901 ) ) ;
#86444=CARTESIAN_POINT ( 'NONE',  ( 20.32896413005680003, 1.771642702460841212, 5.963430220938287007 ) ) ;
#86445=CARTESIAN_POINT ( 'NONE',  ( 1.472469842513823179, 16.42559781766745175, 4.923371831947296329 ) ) ;
#86447=ADVANCED_FACE ( 'NONE', ( #7518 ), #29780, .T. ) ;
#86450=CARTESIAN_POINT ( 'NONE',  ( 19.42250999205614193, 15.14701867748817143, 5.440088680355555262 ) ) ;
#86453=CARTESIAN_POINT ( 'NONE',  ( 19.42250999205614548, 30.98035201082150536, -5.440088680355545492 ) ) ;
#86454=CARTESIAN_POINT ( 'NONE',  ( 19.42250999205614193, 40.14701867748817676, 5.440088680355555262 ) ) ;
#86455=CARTESIAN_POINT ( 'NONE',  ( 0.1532563361054082862, 66.21726448433413736, 2.638427012816831674 ) ) ;
#86456=PRESENTATION_STYLE_ASSIGNMENT (( #18941 ) ) ;
#86457=CARTESIAN_POINT ( 'NONE',  ( -43.18663561153960728, 107.2766636452753062, -4.499999999609646473 ) ) ;
#86458=CARTESIAN_POINT ( 'NONE',  ( 0.1532563361054083140, 16.00893115100078390, 1.131784320476157264E-15 ) ) ;
#86460=AXIS2_PLACEMENT_3D ( 'NONE', #58865, #96398, #59849 ) ;
#86461=CARTESIAN_POINT ( 'NONE',  ( 20.88017736071110875, 30.77201867748816966, -2.915334737309920765 ) ) ;
#86462=CARTESIAN_POINT ( 'NONE',  ( 19.38216949554541557, 32.24863466993041783, -9.382169495545420901 ) ) ;
#86464=UNCERTAINTY_MEASURE_WITH_UNIT (LENGTH_MEASURE( 1.000000000000000082E-05 ), #55175, 'distance_accuracy_value', 'NONE');
#86466=CARTESIAN_POINT ( 'NONE',  ( 2.791683348922240793, 61.63393115100079456, 7.208316651077764092 ) ) ;
#86467=CARTESIAN_POINT ( 'NONE',  ( 4.559911319644449179, 67.23035201082150536, -9.422509992056141925 ) ) ;
#86468=CARTESIAN_POINT ( 'NONE',  ( 19.84674366389459266, 18.30059781766745175, 2.638427012816836559 ) ) ;
#86469=CARTESIAN_POINT ( 'NONE',  ( 21.09922568453595559, 32.04030133659708923, -6.408140936763230044 ) ) ;
#86470=CARTESIAN_POINT ( 'NONE',  ( 10.00000000000000000, 66.81368534415484817, -10.88017736071110342 ) ) ;
#86472=( BOUNDED_SURFACE ( )  B_SPLINE_SURFACE ( 1, 2, ( 
 ( #81731, #28738, #81248, #59228, #72748, #57262, #13246, #66236, #80762, #82231, #43245, #73741, #58741, #4281, #50246, #5271, #57752, #43738, #89731, #34755, #87757, #96770, #34250, #72267, #28246, #20755, #21249, #51748, #65245, #41794, #19272, #49755, #88254, #19762, #22245, #36750, #44229, #21755, #82728, #44728, #29228, #253, #98760, #59728, #45225, #53708, #15245, #84228, #45724, #75722, #60226, #13746, #74733, #97763, #15736, #14247, #53221, #98261, #75225, #61212, #83723, #52236, #90223, #30210, #76226, #46219, #6246, #67240, #7237, #6737, #22738, #37253, #7739, #38234, #68724, #67742, #29719, #37744, #90720, #52722, #83227, #14752, #60713, #68243, #91210, #91716, #30701, #23236, #96771, #67743, #65744, #97268, #5759, #6247, #74225, #88751, #59230, #29720, #36751, #21756, #28739, #44729, #43246, #66744, #96273, #66237, #36247, #89732, #82232, #67241, #13747, #44230, #90224, #12747, #60227, #90721, #82729, #35248, #50760, #52237, #20756, #22246, #37255, #89246, #81732, #14248, #98263, #43739, #75226, #73742, #27748, #6739, #97765, #51245, #52723, #21250, #51749, #29229, #5272, #13247, #74734, #28247, #12257, #42765, #81249, #58231, #59729, #4775, #73248, #20261, #35749, #58742, #38719, #53222, #77195, #62677, #69218, #30702, #69704, #15737, #37745, #45226, #83724, #15248, #7741, #60714, #16706, #84710, #91211, #744, #32174, #31689, #93177, #62179, #31197, #84229, #14753, #75724, #7239, #9198, #22739, #16213, #68725, #45725, #85201, #8701, #30211, #68244, #92207, #39218, #70199, #39711, #24703, #76227, #47179, #91717, #54680, #46220, #76705, #23238, #77684, #1718, #38235, #1234, #83228, #98761, #254, #61213, #54195, #53710, #8225, #61690, #23732, #46697, #92689, #24214, #56659, #25690, #19155, #3179, #55687, #87147, #49158, #11157, #65129, #10674, #93674, #25208, #79661, #34630, #41189, #2709, #41677, #86674, #9692, #17209, #86186, #17696, #78680, #32672, #87641, #18672, #63166, #71669, #4162, #3674, #95650, #34136, #33645, #56181, #85689, #47686, #78179, #80142, #48167, #72146, #40684, #10191, #57144, #64628, #2213, #40187, #64141, #95137, #42167, #11652, #55174, #71184, #49634, #63655, #26648, #18179, #48659, #94162, #72630, #70694, #33160, #79161, #94658, #26167, #21633, #88133, #97156, #35634, #19646, #81617, #44614, #14129, #27633, #88626, #28624, #96649, #90108, #74109, #58118, #59111, #21133, #82113, #37130, #13126, #65625, #36636, #43623, #59611, #20135, #5643, #12141, #81128, #89126, #20638, #89621, #51634, #13623, #44105, #6130, #50639, #75110, #6616, #97644, #50138, #96150, #67119, #66120, #67625, #52119 ),
 ( #82613, #74616, #12630, #29108, #27134, #42646, #51127, #57638, #80647, #73122, #35126, #4664, #43129, #73621, #5144, #28128, #58628, #36119, #66627, #37621, #60599, #68117, #30092, #22621, #75606, #31571, #634, #7117, #84103, #47067, #46582, #77565, #77080, #46104, #137, #29595, #60097, #22125, #24097, #98643, #31082, #83610, #91094, #1109, #92088, #45099, #83107, #8106, #54081, #85082, #54566, #9081, #53100, #62066, #7629, #69589, #30586, #61091, #38120, #92573, #16590, #15125, #84597, #39595, #98134, #90598, #52606, #69100, #68608, #14636, #53589, #45600, #76098, #91601, #23117, #61577, #15619, #76588, #38601, #23616, #16095, #8591, #39098, #81385, #25577, #9574, #79552, #56069, #3568, #2102, #86564, #55059, #25091, #33050, #63546, #41070, #94542, #71565, #3077, #49048, #70575, #20404, #50891, #41571, #93063, #40074, #11051, #78563, #88895, #96411, #48049, #40574, #72038, #27887, #2596, #34026, #32561, #24594, #64523, #64030, #10073, #12887, #18067, #10559, #87045, #63059, #71071, #94055, #55574, #58374, #70083, #93557, #85577, #48546, #62559, #1607, #79046, #33535, #26060, #56550, #86072, #18556, #32056, #17091, #17584, #47573, #78069, #96912, #5412, #52859, #29362, #75863, #74365, #97904, #28389, #97398, #6371, #36885, #14387, #67878, #44858, #75362, #22384, #43869, #91351, #22878, #14889, #66379, #81873, #83366, #51885, #60852, #68375, #21388, #13889, #45358, #98894, #74871, #7384, #5894, #58882, #37881, #37388, #82366, #83857, #59865, #82873, #60358, #36386, #44373, #67374, #28867, #30345, #53349, #13385, #89384, #90352, #35883, #73882, #21890, #52368, #6877, #98399, #66881, #29855, #43384, #90853, #89874, #20898, #51387, #59370, #76356, #84366, #46350, #38860, #91855, #47813, #16843, #23370, #1370, #63302, #62819, #93811, #93317, #62319, #16350, #45866, #7871, #38366, #40334, #53856, #47317, #873, #15865, #17343, #9332, #61344, #396, #24355, #70340, #2350, #70837, #25341, #76838, #78313, #23864, #85828, #46832, #77324, #54328, #9833, #32806, #8352, #1858, #55825, #15381, #68865, #30846, #85329, #84842, #69349, #69846, #31332, #61832, #92340, #8838, #77817, #39352, #31821, #92826, #54818, #39834, #32314, #24839, #55322, #41814, #25819, #72281, #56316, #95790, #3811, #19776, #18316, #34267, #71323, #41332, #49291, #79792, #57282, #11785, #87776, #19292, #65261, #86812, #35267, #65763, #57770, #10321, #48796, #27271, #94791, #4790, #12277, #64279, #56793, #88275, #42784, #18808, #50264, #79305, #40823, #80780, #80285, #26293, #27767, #64769, #26784, #4301, #10813, #87288, #11294, #71804, #73269, #96290, #3309 ) ),
 .UNSPECIFIED., .F., .F., .F. ) 
 B_SPLINE_SURFACE_WITH_KNOTS ( ( 2, 2 ),
 ( 3, 2, 2, 2, 2, 2, 2, 2, 2, 2, 2, 2, 2, 2, 2, 2, 2, 2, 2, 2, 2, 2, 2, 2, 2, 2, 2, 2, 2, 2, 2, 2, 2, 2, 2, 2, 2, 2, 2, 2, 2, 2, 2, 2, 2, 2, 2, 2, 2, 2, 2, 2, 2, 2, 2, 2, 2, 2, 2, 2, 2, 2, 2, 2, 2, 2, 2, 2, 2, 2, 2, 2, 2, 2, 2, 2, 2, 2, 2, 2, 2, 2, 2, 2, 2, 2, 2, 2, 2, 2, 2, 2, 2, 2, 2, 2, 2, 2, 2, 2, 2, 2, 2, 2, 2, 2, 2, 2, 2, 2, 2, 2, 2, 2, 2, 2, 2, 2, 2, 2, 2, 2, 2, 2, 2, 2, 2, 2, 2, 2, 2, 2, 2, 2, 2, 2, 2, 2, 2, 2, 2, 2, 2, 2, 2, 2, 2, 2, 2, 2, 2, 2, 2, 2, 2, 2, 2, 2, 2, 2, 2, 2, 3 ),
 ( 0.000000000000000000, 1.000000000000000000 ),
 ( 0.000000000000000000, 0.005952380952380952051, 0.01190476190476190410, 0.01785714285714285615, 0.02380952380952380820, 0.02976190476190476025, 0.03571428571428571230, 0.04166666666666666435, 0.04761904761904761640, 0.05357142857142856845, 0.05952380952380952051, 0.06547619047619047949, 0.07142857142857142461, 0.07738095238095238360, 0.08333333333333332871, 0.08928571428571428770, 0.09523809523809523281, 0.1011904761904761918, 0.1071428571428571369, 0.1130952380952380959, 0.1190476190476190410, 0.1250000000000000000, 0.1309523809523809590, 0.1369047619047619180, 0.1428571428571428492, 0.1488095238095238082, 0.1547619047619047672, 0.1607142857142857262, 0.1666666666666666574, 0.1726190476190476164, 0.1785714285714285754, 0.1845238095238095344, 0.1904761904761904656, 0.1964285714285714246, 0.2023809523809523836, 0.2083333333333333426, 0.2142857142857142738, 0.2202380952380952328, 0.2261904761904761918, 0.2321428571428571508, 0.2380952380952380820, 0.2440476190476190410, 0.2500000000000000000, 0.2559523809523809312, 0.2619047619047619180, 0.2678571428571428492, 0.2738095238095238360, 0.2797619047619047672, 0.2857142857142856984, 0.2916666666666666852, 0.2976190476190476164, 0.3035714285714285476, 0.3095238095238095344, 0.3154761904761904656, 0.3214285714285714524, 0.3273809523809523836, 0.3333333333333333148, 0.3392857142857143016, 0.3452380952380952328, 0.3511904761904761640, 0.3571428571428571508, 0.3630952380952380820, 0.3690476190476190688, 0.3750000000000000000, 0.3809523809523809312, 0.3869047619047619180, 0.3928571428571428492, 0.3988095238095238360, 0.4047619047619047672, 0.4107142857142856984, 0.4166666666666666852, 0.4226190476190476164, 0.4285714285714285476, 0.4345238095238095344, 0.4404761904761904656, 0.4464285714285714524, 0.4523809523809523836, 0.4583333333333333148, 0.4642857142857143016, 0.4702380952380952328, 0.4761904761904761640, 0.4821428571428571508, 0.4880952380952380820, 0.4940476190476190688, 0.5000000000000000000, 0.5059523809523809312, 0.5119047619047618625, 0.5178571428571429047, 0.5238095238095238360, 0.5297619047619047672, 0.5357142857142856984, 0.5416666666666666297, 0.5476190476190476719, 0.5535714285714286031, 0.5595238095238095344, 0.5654761904761904656, 0.5714285714285713969, 0.5773809523809523281, 0.5833333333333333703, 0.5892857142857143016, 0.5952380952380952328, 0.6011904761904761640, 0.6071428571428570953, 0.6130952380952381375, 0.6190476190476190688, 0.6250000000000000000, 0.6309523809523809312, 0.6369047619047618625, 0.6428571428571429047, 0.6488095238095238360, 0.6547619047619047672, 0.6607142857142856984, 0.6666666666666666297, 0.6726190476190476719, 0.6785714285714286031, 0.6845238095238095344, 0.6904761904761904656, 0.6964285714285713969, 0.7023809523809523281, 0.7083333333333333703, 0.7142857142857143016, 0.7202380952380952328, 0.7261904761904761640, 0.7321428571428570953, 0.7380952380952381375, 0.7440476190476190688, 0.7500000000000000000, 0.7559523809523809312, 0.7619047619047618625, 0.7678571428571429047, 0.7738095238095238360, 0.7797619047619047672, 0.7857142857142856984, 0.7916666666666666297, 0.7976190476190476719, 0.8035714285714286031, 0.8095238095238095344, 0.8154761904761904656, 0.8214285714285713969, 0.8273809523809523281, 0.8333333333333333703, 0.8392857142857143016, 0.8452380952380952328, 0.8511904761904761640, 0.8571428571428570953, 0.8630952380952381375, 0.8690476190476190688, 0.8750000000000000000, 0.8809523809523809312, 0.8869047619047618625, 0.8928571428571429047, 0.8988095238095238360, 0.9047619047619047672, 0.9107142857142856984, 0.9166666666666666297, 0.9226190476190476719, 0.9285714285714286031, 0.9345238095238095344, 0.9404761904761904656, 0.9464285714285713969, 0.9523809523809523281, 0.9583333333333333703, 0.9642857142857143016 ),
 .UNSPECIFIED. ) 
 GEOMETRIC_REPRESENTATION_ITEM ( )  RATIONAL_B_SPLINE_SURFACE ( (
 ( 1.000000000000000000, 0.9659258262890683122, 1.000000000000000000, 0.9659258262890683122, 1.000000000000000000, 0.9659258262890683122, 1.000000000000000000, 0.9659258262890683122, 1.000000000000000000, 0.9659258262890683122, 1.000000000000000000, 0.9659258262890683122, 1.000000000000000000, 0.9659258262890683122, 1.000000000000000000, 0.9659258262890683122, 1.000000000000000000, 0.9659258262890683122, 1.000000000000000000, 0.9659258262890683122, 1.000000000000000000, 0.9659258262890683122, 1.000000000000000000, 0.9659258262890683122, 1.000000000000000000, 0.9659258262890683122, 1.000000000000000000, 0.9659258262890683122, 1.000000000000000000, 0.9659258262890683122, 1.000000000000000000, 0.9659258262890683122, 1.000000000000000000, 0.9659258262890683122, 1.000000000000000000, 0.9659258262890683122, 1.000000000000000000, 0.9659258262890683122, 1.000000000000000000, 0.9659258262890683122, 1.000000000000000000, 0.9659258262890683122, 1.000000000000000000, 0.9659258262890683122, 1.000000000000000000, 0.9659258262890683122, 1.000000000000000000, 0.9659258262890683122, 1.000000000000000000, 0.9659258262890683122, 1.000000000000000000, 0.9659258262890683122, 1.000000000000000000, 0.9659258262890683122, 1.000000000000000000, 0.9659258262890683122, 1.000000000000000000, 0.9659258262890683122, 1.000000000000000000, 0.9659258262890683122, 1.000000000000000000, 0.9659258262890683122, 1.000000000000000000, 0.9659258262890683122, 1.000000000000000000, 0.9659258262890683122, 1.000000000000000000, 0.9659258262890683122, 1.000000000000000000, 0.9659258262890683122, 1.000000000000000000, 0.9659258262890683122, 1.000000000000000000, 0.9659258262890683122, 1.000000000000000000, 0.9659258262890683122, 1.000000000000000000, 0.9659258262890683122, 1.000000000000000000, 0.9659258262890683122, 1.000000000000000000, 0.9659258262890683122, 1.000000000000000000, 0.9659258262890683122, 1.000000000000000000, 0.9659258262890683122, 1.000000000000000000, 0.9659258262890683122, 1.000000000000000000, 0.9659258262890683122, 1.000000000000000000, 0.9659258262890683122, 1.000000000000000000, 0.9659258262890683122, 1.000000000000000000, 0.9659258262890683122, 1.000000000000000000, 0.9659258262890683122, 1.000000000000000000, 0.9659258262890683122, 1.000000000000000000, 0.9659258262890683122, 1.000000000000000000, 0.9659258262890683122, 1.000000000000000000, 0.9659258262890683122, 1.000000000000000000, 0.9659258262890683122, 1.000000000000000000, 0.9659258262890683122, 1.000000000000000000, 0.9659258262890683122, 1.000000000000000000, 0.9659258262890683122, 1.000000000000000000, 0.9659258262890683122, 1.000000000000000000, 0.9659258262890683122, 1.000000000000000000, 0.9659258262890683122, 1.000000000000000000, 0.9659258262890683122, 1.000000000000000000, 0.9659258262890683122, 1.000000000000000000, 0.9659258262890683122, 1.000000000000000000, 0.9659258262890683122, 1.000000000000000000, 0.9659258262890683122, 1.000000000000000000, 0.9659258262890683122, 1.000000000000000000, 0.9659258262890683122, 1.000000000000000000, 0.9659258262890683122, 1.000000000000000000, 0.9659258262890683122, 1.000000000000000000, 0.9659258262890683122, 1.000000000000000000, 0.9659258262890683122, 1.000000000000000000, 0.9659258262890683122, 1.000000000000000000, 0.9659258262890683122, 1.000000000000000000, 0.9659258262890683122, 1.000000000000000000, 0.9659258262890683122, 1.000000000000000000, 0.9659258262890683122, 1.000000000000000000, 0.9659258262890683122, 1.000000000000000000, 0.9659258262890683122, 1.000000000000000000, 0.9659258262890683122, 1.000000000000000000, 0.9659258262890683122, 1.000000000000000000, 0.9659258262890683122, 1.000000000000000000, 0.9659258262890683122, 1.000000000000000000, 0.9659258262890683122, 1.000000000000000000, 0.9659258262890683122, 1.000000000000000000, 0.9659258262890683122, 1.000000000000000000, 0.9659258262890683122, 1.000000000000000000, 0.9659258262890683122, 1.000000000000000000, 0.9659258262890683122, 1.000000000000000000, 0.9659258262890683122, 1.000000000000000000, 0.9659258262890683122, 1.000000000000000000, 0.9659258262890683122, 1.000000000000000000, 0.9659258262890683122, 1.000000000000000000, 0.9659258262890683122, 1.000000000000000000, 0.9659258262890683122, 1.000000000000000000, 0.9659258262890683122, 1.000000000000000000, 0.9659258262890683122, 1.000000000000000000, 0.9659258262890683122, 1.000000000000000000, 0.9659258262890683122, 1.000000000000000000, 0.9659258262890683122, 1.000000000000000000, 0.9659258262890683122, 1.000000000000000000, 0.9659258262890683122, 1.000000000000000000, 0.9659258262890683122, 1.000000000000000000, 0.9659258262890683122, 1.000000000000000000, 0.9659258262890683122, 1.000000000000000000, 0.9659258262890683122, 1.000000000000000000, 0.9659258262890683122, 1.000000000000000000, 0.9659258262890683122, 1.000000000000000000, 0.9659258262890683122, 1.000000000000000000, 0.9659258262890683122, 1.000000000000000000, 0.9659258262890683122, 1.000000000000000000, 0.9659258262890683122, 1.000000000000000000, 0.9659258262890683122, 1.000000000000000000, 0.9659258262890683122, 1.000000000000000000, 0.9659258262890683122, 1.000000000000000000, 0.9659258262890683122, 1.000000000000000000, 0.9659258262890683122, 1.000000000000000000, 0.9659258262890683122, 1.000000000000000000, 0.9659258262890683122, 1.000000000000000000, 0.9659258262890683122, 1.000000000000000000, 0.9659258262890683122, 1.000000000000000000, 0.9659258262890683122, 1.000000000000000000, 0.9659258262890683122, 1.000000000000000000, 0.9659258262890683122, 1.000000000000000000, 0.9659258262890683122, 1.000000000000000000, 0.9659258262890683122, 1.000000000000000000, 0.9659258262890683122, 1.000000000000000000, 0.9659258262890683122, 1.000000000000000000, 0.9659258262890683122, 1.000000000000000000, 0.9659258262890683122, 1.000000000000000000, 0.9659258262890683122, 1.000000000000000000, 0.9659258262890683122, 1.000000000000000000, 0.9659258262890683122, 1.000000000000000000, 0.9659258262890683122, 1.000000000000000000, 0.9659258262890683122, 1.000000000000000000, 0.9659258262890683122, 1.000000000000000000, 0.9659258262890683122, 1.000000000000000000, 0.9659258262890683122, 1.000000000000000000, 0.9659258262890683122, 1.000000000000000000, 0.9659258262890683122, 1.000000000000000000, 0.9659258262890683122, 1.000000000000000000, 0.9659258262890683122, 1.000000000000000000, 0.9659258262890683122, 1.000000000000000000, 0.9659258262890683122, 1.000000000000000000, 0.9659258262890683122, 1.000000000000000000, 0.9659258262890683122, 1.000000000000000000, 0.9659258262890683122, 1.000000000000000000, 0.9659258262890683122, 1.000000000000000000, 0.9659258262890683122, 1.000000000000000000, 0.9659258262890683122, 1.000000000000000000, 0.9659258262890683122, 1.000000000000000000, 0.9659258262890683122, 1.000000000000000000, 0.9659258262890683122, 1.000000000000000000, 0.9659258262890683122, 1.000000000000000000, 0.9659258262890683122, 1.000000000000000000, 0.9659258262890683122, 1.000000000000000000, 0.9659258262890683122, 1.000000000000000000, 0.9659258262890683122, 1.000000000000000000, 0.9659258262890683122, 1.000000000000000000, 0.9659258262890683122, 1.000000000000000000, 0.9659258262890683122, 1.000000000000000000, 0.9659258262890683122, 1.000000000000000000, 0.9659258262890683122, 1.000000000000000000),
 ( 1.000000000000000000, 0.9659258262890683122, 1.000000000000000000, 0.9659258262890683122, 1.000000000000000000, 0.9659258262890683122, 1.000000000000000000, 0.9659258262890683122, 1.000000000000000000, 0.9659258262890683122, 1.000000000000000000, 0.9659258262890683122, 1.000000000000000000, 0.9659258262890683122, 1.000000000000000000, 0.9659258262890683122, 1.000000000000000000, 0.9659258262890683122, 1.000000000000000000, 0.9659258262890683122, 1.000000000000000000, 0.9659258262890683122, 1.000000000000000000, 0.9659258262890683122, 1.000000000000000000, 0.9659258262890683122, 1.000000000000000000, 0.9659258262890683122, 1.000000000000000000, 0.9659258262890683122, 1.000000000000000000, 0.9659258262890683122, 1.000000000000000000, 0.9659258262890683122, 1.000000000000000000, 0.9659258262890683122, 1.000000000000000000, 0.9659258262890683122, 1.000000000000000000, 0.9659258262890683122, 1.000000000000000000, 0.9659258262890683122, 1.000000000000000000, 0.9659258262890683122, 1.000000000000000000, 0.9659258262890683122, 1.000000000000000000, 0.9659258262890683122, 1.000000000000000000, 0.9659258262890683122, 1.000000000000000000, 0.9659258262890683122, 1.000000000000000000, 0.9659258262890683122, 1.000000000000000000, 0.9659258262890683122, 1.000000000000000000, 0.9659258262890683122, 1.000000000000000000, 0.9659258262890683122, 1.000000000000000000, 0.9659258262890683122, 1.000000000000000000, 0.9659258262890683122, 1.000000000000000000, 0.9659258262890683122, 1.000000000000000000, 0.9659258262890683122, 1.000000000000000000, 0.9659258262890683122, 1.000000000000000000, 0.9659258262890683122, 1.000000000000000000, 0.9659258262890683122, 1.000000000000000000, 0.9659258262890683122, 1.000000000000000000, 0.9659258262890683122, 1.000000000000000000, 0.9659258262890683122, 1.000000000000000000, 0.9659258262890683122, 1.000000000000000000, 0.9659258262890683122, 1.000000000000000000, 0.9659258262890683122, 1.000000000000000000, 0.9659258262890683122, 1.000000000000000000, 0.9659258262890683122, 1.000000000000000000, 0.9659258262890683122, 1.000000000000000000, 0.9659258262890683122, 1.000000000000000000, 0.9659258262890683122, 1.000000000000000000, 0.9659258262890683122, 1.000000000000000000, 0.9659258262890683122, 1.000000000000000000, 0.9659258262890683122, 1.000000000000000000, 0.9659258262890683122, 1.000000000000000000, 0.9659258262890683122, 1.000000000000000000, 0.9659258262890683122, 1.000000000000000000, 0.9659258262890683122, 1.000000000000000000, 0.9659258262890683122, 1.000000000000000000, 0.9659258262890683122, 1.000000000000000000, 0.9659258262890683122, 1.000000000000000000, 0.9659258262890683122, 1.000000000000000000, 0.9659258262890683122, 1.000000000000000000, 0.9659258262890683122, 1.000000000000000000, 0.9659258262890683122, 1.000000000000000000, 0.9659258262890683122, 1.000000000000000000, 0.9659258262890683122, 1.000000000000000000, 0.9659258262890683122, 1.000000000000000000, 0.9659258262890683122, 1.000000000000000000, 0.9659258262890683122, 1.000000000000000000, 0.9659258262890683122, 1.000000000000000000, 0.9659258262890683122, 1.000000000000000000, 0.9659258262890683122, 1.000000000000000000, 0.9659258262890683122, 1.000000000000000000, 0.9659258262890683122, 1.000000000000000000, 0.9659258262890683122, 1.000000000000000000, 0.9659258262890683122, 1.000000000000000000, 0.9659258262890683122, 1.000000000000000000, 0.9659258262890683122, 1.000000000000000000, 0.9659258262890683122, 1.000000000000000000, 0.9659258262890683122, 1.000000000000000000, 0.9659258262890683122, 1.000000000000000000, 0.9659258262890683122, 1.000000000000000000, 0.9659258262890683122, 1.000000000000000000, 0.9659258262890683122, 1.000000000000000000, 0.9659258262890683122, 1.000000000000000000, 0.9659258262890683122, 1.000000000000000000, 0.9659258262890683122, 1.000000000000000000, 0.9659258262890683122, 1.000000000000000000, 0.9659258262890683122, 1.000000000000000000, 0.9659258262890683122, 1.000000000000000000, 0.9659258262890683122, 1.000000000000000000, 0.9659258262890683122, 1.000000000000000000, 0.9659258262890683122, 1.000000000000000000, 0.9659258262890683122, 1.000000000000000000, 0.9659258262890683122, 1.000000000000000000, 0.9659258262890683122, 1.000000000000000000, 0.9659258262890683122, 1.000000000000000000, 0.9659258262890683122, 1.000000000000000000, 0.9659258262890683122, 1.000000000000000000, 0.9659258262890683122, 1.000000000000000000, 0.9659258262890683122, 1.000000000000000000, 0.9659258262890683122, 1.000000000000000000, 0.9659258262890683122, 1.000000000000000000, 0.9659258262890683122, 1.000000000000000000, 0.9659258262890683122, 1.000000000000000000, 0.9659258262890683122, 1.000000000000000000, 0.9659258262890683122, 1.000000000000000000, 0.9659258262890683122, 1.000000000000000000, 0.9659258262890683122, 1.000000000000000000, 0.9659258262890683122, 1.000000000000000000, 0.9659258262890683122, 1.000000000000000000, 0.9659258262890683122, 1.000000000000000000, 0.9659258262890683122, 1.000000000000000000, 0.9659258262890683122, 1.000000000000000000, 0.9659258262890683122, 1.000000000000000000, 0.9659258262890683122, 1.000000000000000000, 0.9659258262890683122, 1.000000000000000000, 0.9659258262890683122, 1.000000000000000000, 0.9659258262890683122, 1.000000000000000000, 0.9659258262890683122, 1.000000000000000000, 0.9659258262890683122, 1.000000000000000000, 0.9659258262890683122, 1.000000000000000000, 0.9659258262890683122, 1.000000000000000000, 0.9659258262890683122, 1.000000000000000000, 0.9659258262890683122, 1.000000000000000000, 0.9659258262890683122, 1.000000000000000000, 0.9659258262890683122, 1.000000000000000000, 0.9659258262890683122, 1.000000000000000000, 0.9659258262890683122, 1.000000000000000000, 0.9659258262890683122, 1.000000000000000000, 0.9659258262890683122, 1.000000000000000000, 0.9659258262890683122, 1.000000000000000000, 0.9659258262890683122, 1.000000000000000000, 0.9659258262890683122, 1.000000000000000000, 0.9659258262890683122, 1.000000000000000000, 0.9659258262890683122, 1.000000000000000000, 0.9659258262890683122, 1.000000000000000000, 0.9659258262890683122, 1.000000000000000000, 0.9659258262890683122, 1.000000000000000000, 0.9659258262890683122, 1.000000000000000000, 0.9659258262890683122, 1.000000000000000000, 0.9659258262890683122, 1.000000000000000000, 0.9659258262890683122, 1.000000000000000000, 0.9659258262890683122, 1.000000000000000000, 0.9659258262890683122, 1.000000000000000000, 0.9659258262890683122, 1.000000000000000000, 0.9659258262890683122, 1.000000000000000000, 0.9659258262890683122, 1.000000000000000000, 0.9659258262890683122, 1.000000000000000000, 0.9659258262890683122, 1.000000000000000000, 0.9659258262890683122, 1.000000000000000000, 0.9659258262890683122, 1.000000000000000000, 0.9659258262890683122, 1.000000000000000000, 0.9659258262890683122, 1.000000000000000000, 0.9659258262890683122, 1.000000000000000000, 0.9659258262890683122, 1.000000000000000000, 0.9659258262890683122, 1.000000000000000000, 0.9659258262890683122, 1.000000000000000000, 0.9659258262890683122, 1.000000000000000000, 0.9659258262890683122, 1.000000000000000000, 0.9659258262890683122, 1.000000000000000000, 0.9659258262890683122, 1.000000000000000000, 0.9659258262890683122, 1.000000000000000000, 0.9659258262890683122, 1.000000000000000000) ) ) 
 REPRESENTATION_ITEM ( '' )  SURFACE ( )  );
#86473=ORIENTED_EDGE ( 'NONE', *, *, #14994, .T. ) ;
#86476=CARTESIAN_POINT ( 'NONE',  ( -2.816281873526471635, 58.91530133659707502, -3.434112377981056508 ) ) ;
#86477=CARTESIAN_POINT ( 'NONE',  ( 2.917880565312950480, 25.97041550158063572, -12.26659068614894821 ) ) ;
#86478=CARTESIAN_POINT ( 'NONE',  ( 17.20831665107776587, 22.88393115100078745, 7.208316651077764980 ) ) ;
#86480=CARTESIAN_POINT ( 'NONE',  ( 17.96484262340118221, 6.188685344154836621, -7.964842623401177768 ) ) ;
#86481=CARTESIAN_POINT ( 'NONE',  ( 17.20831665107776587, 19.13393115100078035, -7.208316651077762316 ) ) ;
#86482=CARTESIAN_POINT ( 'NONE',  ( -2.266590686148945544, 52.22041550158064638, 7.082119434687048631 ) ) ;
#86483=ORIENTED_EDGE ( 'NONE', *, *, #69317, .F. ) ;
#86484=DIRECTION ( 'NONE',  ( -0.000000000000000000, 1.000000000000000000, 0.000000000000000000 ) ) ;
#86485=ADVANCED_FACE ( 'NONE', ( #72428 ), #71946, .T. ) ;
#86486=CARTESIAN_POINT ( 'NONE',  ( 7.084665262690076126, 27.02201867748817676, -10.88017736071110164 ) ) ;
#86487=CARTESIAN_POINT ( 'NONE',  ( 20.03743638938528449, 46.75197528031019090, 6.399506433553902696 ) ) ;
#86488=CIRCLE ( 'NONE', #40225, 0.5000000000000073275 ) ;
#86490=CARTESIAN_POINT ( 'NONE',  ( 0.5774900079438607392, 28.48035201082150891, 5.440088680355550821 ) ) ;
#86491=CARTESIAN_POINT ( 'NONE',  ( 17.20831665107776587, 59.13393115100078745, -7.208316651077762316 ) ) ;
#86492=CARTESIAN_POINT ( 'NONE',  ( 16.40814093676324603, 52.45696800326375353, -11.09922568453594671 ) ) ;
#86494=CARTESIAN_POINT ( 'NONE',  ( 10.00000000000000000, 20.55374883491396787, -14.16423886937410082 ) ) ;
#86495=CARTESIAN_POINT ( 'NONE',  ( 15.44008868035555260, 39.73035201082150536, 9.422509992056143702 ) ) ;
#86496=CARTESIAN_POINT ( 'NONE',  ( 20.88017736071110875, 10.77201867748817143, -2.915334737309920765 ) ) ;
#86499=CARTESIAN_POINT ( 'NONE',  ( 14.92337183194729633, 57.67559781766745886, 8.527530157486181039 ) ) ;
#86501=CARTESIAN_POINT ( 'NONE',  ( 5.076628168052704559, 30.17559781766745175, -8.527530157486179263 ) ) ;
#86504=CARTESIAN_POINT ( 'NONE',  ( 18.52753015748617571, 8.092264484334117824, 4.923371831947298993 ) ) ;
#86506=ORIENTED_EDGE ( 'NONE', *, *, #39553, .T. ) ;
#86507=CARTESIAN_POINT ( 'NONE',  ( 19.42250999205614193, 5.147018677488171434, 5.440088680355555262 ) ) ;
#86508=CARTESIAN_POINT ( 'NONE',  ( 12.63842701281683922, 14.55059781766744997, -9.846743663894590881 ) ) ;
#86509=EDGE_CURVE ( 'NONE', #26347, #81670, #59398, .T. ) ;
#86510=CARTESIAN_POINT ( 'NONE',  ( 18.52753015748618282, 63.92559781766745886, -4.923371831947291888 ) ) ;
#86511=CARTESIAN_POINT ( 'NONE',  ( 10.00000000000000178, 44.31368534415484106, 10.88017736071110342 ) ) ;
#86512=CARTESIAN_POINT ( 'NONE',  ( 17.96484262340118221, 14.93868534415483751, 7.964842623401181321 ) ) ;
#86513=CARTESIAN_POINT ( 'NONE',  ( 6.565887622018943937, 45.16530133659708923, 12.81628187352647430 ) ) ;
#86514=CARTESIAN_POINT ( 'NONE',  ( -0.3689425029237898834, 36.17874883491396787, -10.36894250292378850 ) ) ;
#86515=CARTESIAN_POINT ( 'NONE',  ( 3.591859063236761518, 54.95696800326376064, 11.09922568453594849 ) ) ;
#86517=CARTESIAN_POINT ( 'NONE',  ( 5.076628168052703671, 56.84226448433412315, 8.527530157486179263 ) ) ;
#86518=CARTESIAN_POINT ( 'NONE',  ( 4.559911319644449179, 28.89701867748817321, 9.422509992056141925 ) ) ;
#86519=EDGE_CURVE ( 'NONE', #96104, #94230, #97427, .T. ) ;
#86521=CARTESIAN_POINT ( 'NONE',  ( 0.1532563361054083140, 1.008931151000784787, 1.131784320476157264E-15 ) ) ;
#86522=CARTESIAN_POINT ( 'NONE',  ( 10.00000000000000178, 7.258931151000785675, 9.846743663894594434 ) ) ;
#86523=CARTESIAN_POINT ( 'NONE',  ( 19.84674366389459266, 3.717264484334118713, -2.638427012816827677 ) ) ;
#86524=CARTESIAN_POINT ( 'NONE',  ( -0.8801773607110991993, 57.85535201082149825, -2.915334737309923874 ) ) ;
#86526=CARTESIAN_POINT ( 'NONE',  ( -0.8801773607111009756, 58.06368534415484106, 1.068504757029289695E-15 ) ) ;
#86527=CARTESIAN_POINT ( 'NONE',  ( 2.791683348922237240, 10.38393115100078390, -7.208316651077763204 ) ) ;
#86528=ORIENTED_EDGE ( 'NONE', *, *, #11878, .F. ) ;
#86531=CARTESIAN_POINT ( 'NONE',  ( 0.1532563361054082862, 56.21726448433411605, 2.638427012816831674 ) ) ;
#86534=CARTESIAN_POINT ( 'NONE',  ( -2.816281873526473856, 64.12363466993042493, 9.499525473075851096E-16 ) ) ;
#86535=CARTESIAN_POINT ( 'NONE',  ( 13.79529636645030344, 3.262082168247301350, 14.16423886937410614 ) ) ;
#86536=CARTESIAN_POINT ( 'NONE',  ( 24.16423886937409904, 29.09541550158063572, 3.795296366450317205 ) ) ;
#86538=CARTESIAN_POINT ( 'NONE',  ( 15.44008868035555793, 26.39701867748817321, -9.422509992056140149 ) ) ;
#86541=CARTESIAN_POINT ( 'NONE',  ( 5.076628168052703671, 11.84226448433411960, 8.527530157486179263 ) ) ;
#86542=CARTESIAN_POINT ( 'NONE',  ( 3.591859063236761518, 44.95696800326376064, 11.09922568453594849 ) ) ;
#86543=CARTESIAN_POINT ( 'NONE',  ( 1.472469842513823179, 36.42559781766745175, 4.923371831947296329 ) ) ;
#86544=CARTESIAN_POINT ( 'NONE',  ( -0.03447792253739276336, 25.15514106990690379, 6.401564815979735812 ) ) ;
#86546=CARTESIAN_POINT ( 'NONE',  ( 2.791683348922240793, 21.63393115100078745, 7.208316651077764092 ) ) ;
#86547=CARTESIAN_POINT ( 'NONE',  ( -1.099225684535947600, 34.54030133659708923, 6.408140936763237150 ) ) ;
#86549=TOROIDAL_SURFACE ( 'NONE', #5104, 0.5000000000000043299, 0.5000000000000000000 ) ;
#86550=CARTESIAN_POINT ( 'NONE',  ( 2.791683348922237240, 25.38393115100078390, -7.208316651077763204 ) ) ;
#86552=CARTESIAN_POINT ( 'NONE',  ( -2.266590686148945544, 7.220415501580634832, 7.082119434687048631 ) ) ;
#86554=CARTESIAN_POINT ( 'NONE',  ( 17.96484262340118221, 34.93868534415482685, 7.964842623401181321 ) ) ;
#86555=CARTESIAN_POINT ( 'NONE',  ( 22.26659068614894466, 28.88708216824730357, 7.082119434687054849 ) ) ;
#86556=CARTESIAN_POINT ( 'NONE',  ( 19.84674366389459621, 48.50893115100078745, 7.409399052514197653E-17 ) ) ;
#86557=CARTESIAN_POINT ( 'NONE',  ( 7.361572987183170547, 7.050597817667451750, 9.846743663894590881 ) ) ;
#86559=CARTESIAN_POINT ( 'NONE',  ( 0.6178305044545838731, 49.74863466993041072, 9.382169495545420901 ) ) ;
#86561=CARTESIAN_POINT ( 'NONE',  ( -0.8801773607111008646, 28.27201867748817321, 2.915334737309923430 ) ) ;
#86564=CARTESIAN_POINT ( 'NONE',  ( 22.81628187352647785, 16.62363466993042138, 6.195893100308588602E-16 ) ) ;
#86565=CARTESIAN_POINT ( 'NONE',  ( 14.92337183194729988, 44.34226448433412315, -8.527530157486177487 ) ) ;
#86568=MECHANICAL_DESIGN_GEOMETRIC_PRESENTATION_REPRESENTATION('',(#24273),#81765);
#86572=CARTESIAN_POINT ( 'NONE',  ( -0.8801773607111009756, 58.06368534415484106, 1.068504757029289695E-15 ) ) ;
#86573=CARTESIAN_POINT ( 'NONE',  ( -0.8801773607111009756, 58.06368534415484106, 1.068504757029289695E-15 ) ) ;
#86574=CARTESIAN_POINT ( 'NONE',  ( 20.10384461210892226, 56.74302437010793199, 6.337995344473749348 ) ) ;
#86576=CARTESIAN_POINT ( 'NONE',  ( 12.91533473730992121, 9.522018677488171434, 10.88017736071110164 ) ) ;
#86577=CARTESIAN_POINT ( 'NONE',  ( 1.472469842513823179, 66.42559781766745175, 4.923371831947296329 ) ) ;
#86578=CARTESIAN_POINT ( 'NONE',  ( 0.5774900079438590739, 27.64701867748817676, -5.440088680355550821 ) ) ;
#86580=CARTESIAN_POINT ( 'NONE',  ( -2.816281873526471635, 18.91530133659708213, -3.434112377981056508 ) ) ;
#86582=CARTESIAN_POINT ( 'NONE',  ( 15.44008868035555793, 56.39701867748817676, -9.422509992056140149 ) ) ;
#86583=CARTESIAN_POINT ( 'NONE',  ( 14.92337183194729988, 34.34226448433411605, -8.527530157486177487 ) ) ;
#86584=CARTESIAN_POINT ( 'NONE',  ( 16.40814093676323893, 0.7903013365970867898, 11.09922568453595026 ) ) ;
#86585=CARTESIAN_POINT ( 'NONE',  ( 0.000000000000000000, 70.00000000000000000, 6.500000000000000888 ) ) ;
#86586=CARTESIAN_POINT ( 'NONE',  ( 7.084665262690076126, 27.02201867748817676, -10.88017736071110164 ) ) ;
#86587=CARTESIAN_POINT ( 'NONE',  ( 15.44008868035555793, 41.39701867748817676, -9.422509992056140149 ) ) ;
#86588=CARTESIAN_POINT ( 'NONE',  ( -2.266590686148945544, 47.22041550158063927, 7.082119434687048631 ) ) ;
#86589=CARTESIAN_POINT ( 'NONE',  ( 1.472469842513823179, 36.42559781766745175, 4.923371831947296329 ) ) ;
#86590=CARTESIAN_POINT ( 'NONE',  ( 10.00000000000000000, 56.81368534415484106, -10.88017736071110342 ) ) ;
#86591=CARTESIAN_POINT ( 'NONE',  ( 7.084665262690076126, 44.10535201082151247, 10.88017736071109987 ) ) ;
#86592=DIRECTION ( 'NONE',  ( 0.000000000000000000, -1.000000000000000000, 0.000000000000000000 ) ) ;
#86593=CARTESIAN_POINT ( 'NONE',  ( 13.79529636645030344, 18.26208216824730002, 14.16423886937410614 ) ) ;
#86594=EDGE_CURVE ( 'NONE', #4978, #95793, #81414, .T. ) ;
#86595=CARTESIAN_POINT ( 'NONE',  ( -16.94000000000001549, 92.00000000000000000, -9.500000000000000000 ) ) ;
#86596=CARTESIAN_POINT ( 'NONE',  ( 20.15039907845753930, 70.00000000000000000, 6.262539305110068177 ) ) ;
#86597=EDGE_CURVE ( 'NONE', #87349, #74857, #16958, .T. ) ;
#86600=CARTESIAN_POINT ( 'NONE',  ( -2.266590686148945544, 46.38708216824730357, -7.082119434687050408 ) ) ;
#86601=CARTESIAN_POINT ( 'NONE',  ( 22.26659068614895176, 34.72041550158063927, -7.082119434687042414 ) ) ;
#86602=CARTESIAN_POINT ( 'NONE',  ( 5.076628168052703671, 16.84226448433411960, 8.527530157486179263 ) ) ;
#86605=CARTESIAN_POINT ( 'NONE',  ( 10.00000000000000000, 66.81368534415484817, -10.88017736071110342 ) ) ;
#86606=CARTESIAN_POINT ( 'NONE',  ( 22.81628187352647785, 31.41530133659709279, 3.434112377981063169 ) ) ;
#86607=CARTESIAN_POINT ( 'NONE',  ( 17.08211943468705840, 50.13708216824730357, -12.26659068614894466 ) ) ;
#86608=ADVANCED_FACE ( 'NONE', ( #43413 ), #40019, .T. ) ;
#86611=CARTESIAN_POINT ( 'NONE',  ( 4.559911319644449179, 67.23035201082150536, -9.422509992056141925 ) ) ;
#86613=CARTESIAN_POINT ( 'NONE',  ( 2.791683348922237240, 5.383931151000785675, -7.208316651077763204 ) ) ;
#86614=VERTEX_POINT ( 'NONE', #45799 ) ;
#86615=CARTESIAN_POINT ( 'NONE',  ( 7.361572987183170547, 22.05059781766745530, 9.846743663894590881 ) ) ;
#86618=CARTESIAN_POINT ( 'NONE',  ( 24.16423886937410614, 4.303748834913967869, 8.672049930838204340E-16 ) ) ;
#86619=CARTESIAN_POINT ( 'NONE',  ( -2.266590686148945544, 67.22041550158063217, 7.082119434687048631 ) ) ;
#86620=CARTESIAN_POINT ( 'NONE',  ( 7.084665262690076126, 12.02201867748817321, -10.88017736071110164 ) ) ;
#86621=CARTESIAN_POINT ( 'NONE',  ( 18.52753015748618282, 33.92559781766745886, -4.923371831947291888 ) ) ;
#86622=CARTESIAN_POINT ( 'NONE',  ( -2.816281873526471635, 3.915301336597087456, -3.434112377981056508 ) ) ;
#86624=CARTESIAN_POINT ( 'NONE',  ( 3.591859063236761518, 14.95696800326375531, 11.09922568453594849 ) ) ;
#86628=CARTESIAN_POINT ( 'NONE',  ( 13.79529636645030344, 53.26208216824730357, 14.16423886937410614 ) ) ;
#86630=ADVANCED_FACE ( 'NONE', ( #45296 ), #61276, .T. ) ;
#86632=CARTESIAN_POINT ( 'NONE',  ( 20.36894250292379738, 59.92874883491397497, -10.36894250292379027 ) ) ;
#86634=CARTESIAN_POINT ( 'NONE',  ( 20.88017736071110519, 35.56368534415484106, 2.639326808657452039E-16 ) ) ;
#86635=CARTESIAN_POINT ( 'NONE',  ( 2.035157376598824452, 33.68868534415484106, 7.964842623401179544 ) ) ;
#86636=CIRCLE ( 'NONE', #38752, 7.000000000000000000 ) ;
#86638=CARTESIAN_POINT ( 'NONE',  ( 17.96484262340118221, 31.18868534415483751, -7.964842623401177768 ) ) ;
#86639=( GEOMETRIC_REPRESENTATION_CONTEXT ( 3 ) GLOBAL_UNCERTAINTY_ASSIGNED_CONTEXT ( ( #84140 ) ) GLOBAL_UNIT_ASSIGNED_CONTEXT ( ( #21266, #68259, #44250 ) ) REPRESENTATION_CONTEXT ( 'NONE', 'WORKASPACE' ) );
#86640=CARTESIAN_POINT ( 'NONE',  ( -0.1042174387088606879, 33.10736173766203905, 6.337391062633419558 ) ) ;
#86641=CARTESIAN_POINT ( 'NONE',  ( 12.63842701281683922, 19.55059781766745175, -9.846743663894590881 ) ) ;
#86645=CARTESIAN_POINT ( 'NONE',  ( 2.791683348922237240, 50.38393115100078035, -7.208316651077763204 ) ) ;
#86646=EDGE_CURVE ( 'NONE', #63634, #54365, #44460, .T. ) ;
#86653=CARTESIAN_POINT ( 'NONE',  ( 6.204703633549690345, 45.76208216824729647, -14.16423886937410259 ) ) ;
#86656=( BOUNDED_SURFACE ( )  B_SPLINE_SURFACE ( 3, 2, ( 
 ( #39061, #60566, #76550 ),
 ( #54046, #7590, #91057 ),
 ( #46545, #24060, #70044 ),
 ( #84065, #8558, #1568 ),
 ( #32017, #15582, #77523 ),
 ( #98606, #45565, #1071 ),
 ( #46065, #600, #61541 ),
 ( #62030, #62520, #84557 ),
 ( #38082, #61051, #103 ),
 ( #9041, #30549, #91564 ) ),
 .UNSPECIFIED., .F., .F., .F. ) 
 B_SPLINE_SURFACE_WITH_KNOTS ( ( 4, 2, 2, 2, 4 ),
 ( 3, 3 ),
 ( 0.000000000000000000, 0.002067014858588510882, 0.003100522287882766324, 0.003617276002529893827, 0.004134029717177021765 ),
 ( 0.000000000000000000, 1.000000000000000000 ),
 .UNSPECIFIED. ) 
 GEOMETRIC_REPRESENTATION_ITEM ( )  RATIONAL_B_SPLINE_SURFACE ( (
 ( 1.000000000000000000, 0.7411386215561424073, 1.000000000000000000),
 ( 1.000000000000000000, 0.7517628147009809414, 1.000000000000000000),
 ( 1.000000000000000000, 0.7644153482607498606, 1.000000000000000000),
 ( 1.000000000000000000, 0.8033584422216667464, 1.000000000000000000),
 ( 1.000000000000000000, 0.8197614970480194829, 1.000000000000000000),
 ( 1.000000000000000000, 0.8550190949536496943, 1.000000000000000000),
 ( 1.000000000000000000, 0.8686037895732486858, 1.000000000000000000),
 ( 1.000000000000000000, 0.9009153382757982831, 1.000000000000000000),
 ( 1.000000000000000000, 0.9197777054298900135, 1.000000000000000000),
 ( 1.000000000000000000, 0.9412039349194007976, 1.000000000000000000) ) ) 
 REPRESENTATION_ITEM ( '' )  SURFACE ( )  );
#86657=CARTESIAN_POINT ( 'NONE',  ( 0.1532563361054082862, 21.21726448433412315, 2.638427012816831674 ) ) ;
#86659=CARTESIAN_POINT ( 'NONE',  ( 0.1532563361054082862, 61.21726448433412315, 2.638427012816831674 ) ) ;
#86660=CARTESIAN_POINT ( 'NONE',  ( 2.035157376598824452, 68.68868534415484817, 7.964842623401179544 ) ) ;
#86661=CARTESIAN_POINT ( 'NONE',  ( 14.92337183194729633, 57.67559781766745886, 8.527530157486181039 ) ) ;
#86662=( BOUNDED_SURFACE ( )  B_SPLINE_SURFACE ( 1, 2, ( 
 ( #56708, #26215, #49685, #79211, #87199, #11702, #50182, #48708, #42694, #41725, #27183, #58166, #88181, #26695, #50688, #73173, #43179, #4712, #73667, #57685, #80692, #56230, #19695, #71716, #87688, #72195, #19202, #18722, #35174, #42211, #11206, #34683, #65675, #34185, #88677, #64677, #20185, #95699, #86724, #12680, #95187, #5194, #35682, #25738, #49204, #10721, #41238, #97689, #66675, #67165, #52165, #98182, #21679, #22667, #29638, #36175, #22168, #60146, #51179, #59658, #67672, #90643, #44658, #45648, #37665, #6663, #83652, #75650, #15167, #37179, #75153, #83153, #5689, #68165, #29151, #90149, #52650, #82158, #6173, #14678, #97200, #82658, #53143, #66166, #7162, #45144, #60640, #58672, #76145, #98685, #14174, #74662, #30134, #96699, #91141, #7671, #59160, #36677, #28668, #20685, #28178, #89174, #81662, #13172, #89666, #43669, #74156, #21177, #51679, #13670, #44154, #70621, #31122, #25142, #16635, #85124, #46145, #55619, #672, #78113, #40120, #61617, #93105, #16137, #92135, #76631, #92617, #23161, #8150, #24141, #24635, #91643, #55102, #84635, #70127, #2146, #32101, #69632, #93604, #17139, #86116, #85622, #17627, #1649, #47618, #178, #62600, #15662, #31616, #46623, #1156, #38643, #23660, #32606, #69144, #54122, #48097, #9619, #77121, #63102, #78610, #53636, #62107, #39638, #38162, #47110, #68648, #30626, #77610, #61133, #84156, #8633, #9123, #39142, #54608, #48591, #12073, #72082, #34069, #72563, #26103, #49093, #34560, #10606, #26578, #65552, #10119, #50073, #88064, #4592, #2643, #58054, #11583, #57081, #18600, #80077, #40617, #80577, #42098, #3121, #79596, #41120, #63591, #27561, #11097, #50566, #71116, #79094, #95073, #41613, #42575, #33097, #27068, #87576, #73058, #33579, #96080, #19088, #49565, #18116, #88561, #71610, #35054, #20064, #64073, #65055, #87090, #94588, #56599, #64563, #94099, #3608, #4097, #95581, #25620, #57566, #19576, #56113, #86607, #75039, #13555, #37555, #60031, #30024, #29524, #60530, #14060, #37055, #43067, #44543, #58550, #74542, #59048, #44041, #89057, #36053, #14559, #51055, #20570, #22061, #6062, #66555, #59545, #90526, #21062, #75535, #89552, #98065, #36561, #73549, #82543, #28555, #68045, #91021, #90040, #81545, #98571, #97084, #67050, #13055, #82043, #97573, #6545, #29036, #81062, #52535, #67554, #74043, #51557, #43549, #35561, #22553, #21563, #12566, #5075, #5578, #52052, #83043, #45028, #66052, #7051, #96579, #28055, #46036, #40004, #31498, #1037, #61020, #70506, #15551, #92994, #54987, #76521, #9006, #31012, #8037, #91532, #8525, #38048, #23047, #39027, #39522, #7559, #70014, #566 ),
 ( #83538, #47001, #1540, #47494, #84031, #61508, #9502, #85506, #38535, #24030, #77012, #53519, #92015, #2030, #77494, #54498, #85013, #31984, #62001, #76028, #16023, #92500, #68540, #69031, #62490, #23545, #32492, #77997, #54017, #84526, #71, #46512, #69522, #30517, #16526, #24528, #17016, #62987, #93493, #53023, #15057, #45530, #41982, #86496, #33459, #56482, #48967, #72446, #3489, #10487, #3976, #80460, #34445, #55996, #79477, #63956, #56958, #10976, #18976, #71966, #4475, #17515, #71496, #11464, #86968, #78491, #86004, #93987, #17996, #48478, #10005, #25509, #78977, #11958, #49955, #64936, #94468, #94957, #26459, #41497, #32979, #25985, #42463, #49454, #87461, #79960, #95464, #33946, #47981, #18482, #64450, #40507, #63483, #26955, #57455, #72945, #34941, #3010, #87948, #71003, #40998, #19463, #2526, #65439, #25016, #55504, #52782, #37314, #38782, #83291, #37804, #15307, #58427, #6800, #29777, #22310, #45792, #75782, #82792, #76283, #53777, #7798, #27934, #14816, #67803, #30273, #45287, #91277, #7305, #76765, #88447, #44784, #83784, #60287, #50442, #57939, #65934, #88941, #21812, #80947, #96463, #52296, #84293, #23299, #38294, #98323, #68301, #98820, #90784, #8285, #14314, #27445, #19947, #15792, #35439, #60775, #75290, #22799, #321, #53277, #4959, #68789, #30763, #61269, #46280, #95963, #12445, #42953, #73432, #91777, #55754, #25271, #39767, #31256, #17269, #9260, #40745, #86245, #17758, #62740, #77256, #56248, #62248, #70267, #61752, #93737, #92270, #46761, #9755, #48235, #803, #39282, #40257, #23794, #54259, #8765, #47744, #84770, #63234, #78744, #63721, #1300, #47246, #25754, #71249, #31753, #16279, #69770, #10252, #77747, #86741, #94224, #1783, #32241, #92754, #85264, #93240, #24279, #78241, #2772, #70764, #24766, #55244, #10738, #85758, #2278, #33226, #54743, #32734, #18243, #48724, #79228, #69281, #16771, #88690, #96713, #20198, #72212, #95713, #80207, #73187, #27196, #35186, #88198, #20700, #33708, #87701, #27694, #72691, #94723, #3242, #11222, #3740, #64693, #26230, #41741, #34200, #28191, #66179, #50700, #11713, #12200, #65191, #42225, #51192, #95204, #71732, #64208, #58686, #79722, #4723, #26709, #57204, #43191, #19217, #49218, #81194, #19707, #96212, #89187, #81674, #41257, #56723, #87215, #18738, #58178, #12695, #4228, #49698, #50194, #34698, #73679, #5211, #35695, #57698, #80705, #42709, #65688, #52181, #74168, #37683, #5702, #89680, #52668, #91158, #43681, #82172, #83170, #36188, #66688, #51693, #90661, #97213, #7180, #60659, #7685, #44171, #90165, #68668, #15186, #74679, #14695, #37199, #21193, #21695 ) ),
 .UNSPECIFIED., .F., .F., .F. ) 
 B_SPLINE_SURFACE_WITH_KNOTS ( ( 2, 2 ),
 ( 3, 2, 2, 2, 2, 2, 2, 2, 2, 2, 2, 2, 2, 2, 2, 2, 2, 2, 2, 2, 2, 2, 2, 2, 2, 2, 2, 2, 2, 2, 2, 2, 2, 2, 2, 2, 2, 2, 2, 2, 2, 2, 2, 2, 2, 2, 2, 2, 2, 2, 2, 2, 2, 2, 2, 2, 2, 2, 2, 2, 2, 2, 2, 2, 2, 2, 2, 2, 2, 2, 2, 2, 2, 2, 2, 2, 2, 2, 2, 2, 2, 2, 2, 2, 2, 2, 2, 2, 2, 2, 2, 2, 2, 2, 2, 2, 2, 2, 2, 2, 2, 2, 2, 2, 2, 2, 2, 2, 2, 2, 2, 2, 2, 2, 2, 2, 2, 2, 2, 2, 2, 2, 2, 2, 2, 2, 2, 2, 2, 2, 2, 2, 2, 2, 2, 2, 2, 2, 2, 2, 2, 2, 2, 2, 2, 2, 2, 2, 2, 2, 2, 2, 2, 2, 2, 2, 2, 2, 2, 2, 2, 2, 3 ),
 ( 0.000000000000000000, 1.000000000000000000 ),
 ( 0.000000000000000000, 0.005952380952380952051, 0.01190476190476190410, 0.01785714285714285615, 0.02380952380952380820, 0.02976190476190476025, 0.03571428571428571230, 0.04166666666666666435, 0.04761904761904761640, 0.05357142857142856845, 0.05952380952380952051, 0.06547619047619047949, 0.07142857142857142461, 0.07738095238095238360, 0.08333333333333332871, 0.08928571428571428770, 0.09523809523809523281, 0.1011904761904761918, 0.1071428571428571369, 0.1130952380952380959, 0.1190476190476190410, 0.1250000000000000000, 0.1309523809523809590, 0.1369047619047619180, 0.1428571428571428492, 0.1488095238095238082, 0.1547619047619047672, 0.1607142857142857262, 0.1666666666666666574, 0.1726190476190476164, 0.1785714285714285754, 0.1845238095238095344, 0.1904761904761904656, 0.1964285714285714246, 0.2023809523809523836, 0.2083333333333333426, 0.2142857142857142738, 0.2202380952380952328, 0.2261904761904761918, 0.2321428571428571508, 0.2380952380952380820, 0.2440476190476190410, 0.2500000000000000000, 0.2559523809523809312, 0.2619047619047619180, 0.2678571428571428492, 0.2738095238095238360, 0.2797619047619047672, 0.2857142857142856984, 0.2916666666666666852, 0.2976190476190476164, 0.3035714285714285476, 0.3095238095238095344, 0.3154761904761904656, 0.3214285714285714524, 0.3273809523809523836, 0.3333333333333333148, 0.3392857142857143016, 0.3452380952380952328, 0.3511904761904761640, 0.3571428571428571508, 0.3630952380952380820, 0.3690476190476190688, 0.3750000000000000000, 0.3809523809523809312, 0.3869047619047619180, 0.3928571428571428492, 0.3988095238095238360, 0.4047619047619047672, 0.4107142857142856984, 0.4166666666666666852, 0.4226190476190476164, 0.4285714285714285476, 0.4345238095238095344, 0.4404761904761904656, 0.4464285714285714524, 0.4523809523809523836, 0.4583333333333333148, 0.4642857142857143016, 0.4702380952380952328, 0.4761904761904761640, 0.4821428571428571508, 0.4880952380952380820, 0.4940476190476190688, 0.5000000000000000000, 0.5059523809523809312, 0.5119047619047618625, 0.5178571428571429047, 0.5238095238095238360, 0.5297619047619047672, 0.5357142857142856984, 0.5416666666666666297, 0.5476190476190476719, 0.5535714285714286031, 0.5595238095238095344, 0.5654761904761904656, 0.5714285714285713969, 0.5773809523809523281, 0.5833333333333333703, 0.5892857142857143016, 0.5952380952380952328, 0.6011904761904761640, 0.6071428571428570953, 0.6130952380952381375, 0.6190476190476190688, 0.6250000000000000000, 0.6309523809523809312, 0.6369047619047618625, 0.6428571428571429047, 0.6488095238095238360, 0.6547619047619047672, 0.6607142857142856984, 0.6666666666666666297, 0.6726190476190476719, 0.6785714285714286031, 0.6845238095238095344, 0.6904761904761904656, 0.6964285714285713969, 0.7023809523809523281, 0.7083333333333333703, 0.7142857142857143016, 0.7202380952380952328, 0.7261904761904761640, 0.7321428571428570953, 0.7380952380952381375, 0.7440476190476190688, 0.7500000000000000000, 0.7559523809523809312, 0.7619047619047618625, 0.7678571428571429047, 0.7738095238095238360, 0.7797619047619047672, 0.7857142857142856984, 0.7916666666666666297, 0.7976190476190476719, 0.8035714285714286031, 0.8095238095238095344, 0.8154761904761904656, 0.8214285714285713969, 0.8273809523809523281, 0.8333333333333333703, 0.8392857142857143016, 0.8452380952380952328, 0.8511904761904761640, 0.8571428571428570953, 0.8630952380952381375, 0.8690476190476190688, 0.8750000000000000000, 0.8809523809523809312, 0.8869047619047618625, 0.8928571428571429047, 0.8988095238095238360, 0.9047619047619047672, 0.9107142857142856984, 0.9166666666666666297, 0.9226190476190476719, 0.9285714285714286031, 0.9345238095238095344, 0.9404761904761904656, 0.9464285714285713969, 0.9523809523809523281, 0.9583333333333333703, 0.9642857142857143016 ),
 .UNSPECIFIED. ) 
 GEOMETRIC_REPRESENTATION_ITEM ( )  RATIONAL_B_SPLINE_SURFACE ( (
 ( 1.000000000000000000, 0.9659258262890683122, 1.000000000000000000, 0.9659258262890683122, 1.000000000000000000, 0.9659258262890683122, 1.000000000000000000, 0.9659258262890683122, 1.000000000000000000, 0.9659258262890683122, 1.000000000000000000, 0.9659258262890683122, 1.000000000000000000, 0.9659258262890683122, 1.000000000000000000, 0.9659258262890683122, 1.000000000000000000, 0.9659258262890683122, 1.000000000000000000, 0.9659258262890683122, 1.000000000000000000, 0.9659258262890683122, 1.000000000000000000, 0.9659258262890683122, 1.000000000000000000, 0.9659258262890683122, 1.000000000000000000, 0.9659258262890683122, 1.000000000000000000, 0.9659258262890683122, 1.000000000000000000, 0.9659258262890683122, 1.000000000000000000, 0.9659258262890683122, 1.000000000000000000, 0.9659258262890683122, 1.000000000000000000, 0.9659258262890683122, 1.000000000000000000, 0.9659258262890683122, 1.000000000000000000, 0.9659258262890683122, 1.000000000000000000, 0.9659258262890683122, 1.000000000000000000, 0.9659258262890683122, 1.000000000000000000, 0.9659258262890683122, 1.000000000000000000, 0.9659258262890683122, 1.000000000000000000, 0.9659258262890683122, 1.000000000000000000, 0.9659258262890683122, 1.000000000000000000, 0.9659258262890683122, 1.000000000000000000, 0.9659258262890683122, 1.000000000000000000, 0.9659258262890683122, 1.000000000000000000, 0.9659258262890683122, 1.000000000000000000, 0.9659258262890683122, 1.000000000000000000, 0.9659258262890683122, 1.000000000000000000, 0.9659258262890683122, 1.000000000000000000, 0.9659258262890683122, 1.000000000000000000, 0.9659258262890683122, 1.000000000000000000, 0.9659258262890683122, 1.000000000000000000, 0.9659258262890683122, 1.000000000000000000, 0.9659258262890683122, 1.000000000000000000, 0.9659258262890683122, 1.000000000000000000, 0.9659258262890683122, 1.000000000000000000, 0.9659258262890683122, 1.000000000000000000, 0.9659258262890683122, 1.000000000000000000, 0.9659258262890683122, 1.000000000000000000, 0.9659258262890683122, 1.000000000000000000, 0.9659258262890683122, 1.000000000000000000, 0.9659258262890683122, 1.000000000000000000, 0.9659258262890683122, 1.000000000000000000, 0.9659258262890683122, 1.000000000000000000, 0.9659258262890683122, 1.000000000000000000, 0.9659258262890683122, 1.000000000000000000, 0.9659258262890683122, 1.000000000000000000, 0.9659258262890683122, 1.000000000000000000, 0.9659258262890683122, 1.000000000000000000, 0.9659258262890683122, 1.000000000000000000, 0.9659258262890683122, 1.000000000000000000, 0.9659258262890683122, 1.000000000000000000, 0.9659258262890683122, 1.000000000000000000, 0.9659258262890683122, 1.000000000000000000, 0.9659258262890683122, 1.000000000000000000, 0.9659258262890683122, 1.000000000000000000, 0.9659258262890683122, 1.000000000000000000, 0.9659258262890683122, 1.000000000000000000, 0.9659258262890683122, 1.000000000000000000, 0.9659258262890683122, 1.000000000000000000, 0.9659258262890683122, 1.000000000000000000, 0.9659258262890683122, 1.000000000000000000, 0.9659258262890683122, 1.000000000000000000, 0.9659258262890683122, 1.000000000000000000, 0.9659258262890683122, 1.000000000000000000, 0.9659258262890683122, 1.000000000000000000, 0.9659258262890683122, 1.000000000000000000, 0.9659258262890683122, 1.000000000000000000, 0.9659258262890683122, 1.000000000000000000, 0.9659258262890683122, 1.000000000000000000, 0.9659258262890683122, 1.000000000000000000, 0.9659258262890683122, 1.000000000000000000, 0.9659258262890683122, 1.000000000000000000, 0.9659258262890683122, 1.000000000000000000, 0.9659258262890683122, 1.000000000000000000, 0.9659258262890683122, 1.000000000000000000, 0.9659258262890683122, 1.000000000000000000, 0.9659258262890683122, 1.000000000000000000, 0.9659258262890683122, 1.000000000000000000, 0.9659258262890683122, 1.000000000000000000, 0.9659258262890683122, 1.000000000000000000, 0.9659258262890683122, 1.000000000000000000, 0.9659258262890683122, 1.000000000000000000, 0.9659258262890683122, 1.000000000000000000, 0.9659258262890683122, 1.000000000000000000, 0.9659258262890683122, 1.000000000000000000, 0.9659258262890683122, 1.000000000000000000, 0.9659258262890683122, 1.000000000000000000, 0.9659258262890683122, 1.000000000000000000, 0.9659258262890683122, 1.000000000000000000, 0.9659258262890683122, 1.000000000000000000, 0.9659258262890683122, 1.000000000000000000, 0.9659258262890683122, 1.000000000000000000, 0.9659258262890683122, 1.000000000000000000, 0.9659258262890683122, 1.000000000000000000, 0.9659258262890683122, 1.000000000000000000, 0.9659258262890683122, 1.000000000000000000, 0.9659258262890683122, 1.000000000000000000, 0.9659258262890683122, 1.000000000000000000, 0.9659258262890683122, 1.000000000000000000, 0.9659258262890683122, 1.000000000000000000, 0.9659258262890683122, 1.000000000000000000, 0.9659258262890683122, 1.000000000000000000, 0.9659258262890683122, 1.000000000000000000, 0.9659258262890683122, 1.000000000000000000, 0.9659258262890683122, 1.000000000000000000, 0.9659258262890683122, 1.000000000000000000, 0.9659258262890683122, 1.000000000000000000, 0.9659258262890683122, 1.000000000000000000, 0.9659258262890683122, 1.000000000000000000, 0.9659258262890683122, 1.000000000000000000, 0.9659258262890683122, 1.000000000000000000, 0.9659258262890683122, 1.000000000000000000, 0.9659258262890683122, 1.000000000000000000, 0.9659258262890683122, 1.000000000000000000, 0.9659258262890683122, 1.000000000000000000, 0.9659258262890683122, 1.000000000000000000, 0.9659258262890683122, 1.000000000000000000, 0.9659258262890683122, 1.000000000000000000, 0.9659258262890683122, 1.000000000000000000, 0.9659258262890683122, 1.000000000000000000, 0.9659258262890683122, 1.000000000000000000, 0.9659258262890683122, 1.000000000000000000, 0.9659258262890683122, 1.000000000000000000, 0.9659258262890683122, 1.000000000000000000, 0.9659258262890683122, 1.000000000000000000, 0.9659258262890683122, 1.000000000000000000, 0.9659258262890683122, 1.000000000000000000, 0.9659258262890683122, 1.000000000000000000, 0.9659258262890683122, 1.000000000000000000, 0.9659258262890683122, 1.000000000000000000, 0.9659258262890683122, 1.000000000000000000, 0.9659258262890683122, 1.000000000000000000, 0.9659258262890683122, 1.000000000000000000, 0.9659258262890683122, 1.000000000000000000, 0.9659258262890683122, 1.000000000000000000, 0.9659258262890683122, 1.000000000000000000, 0.9659258262890683122, 1.000000000000000000, 0.9659258262890683122, 1.000000000000000000, 0.9659258262890683122, 1.000000000000000000, 0.9659258262890683122, 1.000000000000000000, 0.9659258262890683122, 1.000000000000000000, 0.9659258262890683122, 1.000000000000000000, 0.9659258262890683122, 1.000000000000000000, 0.9659258262890683122, 1.000000000000000000, 0.9659258262890683122, 1.000000000000000000, 0.9659258262890683122, 1.000000000000000000, 0.9659258262890683122, 1.000000000000000000, 0.9659258262890683122, 1.000000000000000000, 0.9659258262890683122, 1.000000000000000000, 0.9659258262890683122, 1.000000000000000000, 0.9659258262890683122, 1.000000000000000000, 0.9659258262890683122, 1.000000000000000000, 0.9659258262890683122, 1.000000000000000000, 0.9659258262890683122, 1.000000000000000000, 0.9659258262890683122, 1.000000000000000000, 0.9659258262890683122, 1.000000000000000000),
 ( 1.000000000000000000, 0.9659258262890683122, 1.000000000000000000, 0.9659258262890683122, 1.000000000000000000, 0.9659258262890683122, 1.000000000000000000, 0.9659258262890683122, 1.000000000000000000, 0.9659258262890683122, 1.000000000000000000, 0.9659258262890683122, 1.000000000000000000, 0.9659258262890683122, 1.000000000000000000, 0.9659258262890683122, 1.000000000000000000, 0.9659258262890683122, 1.000000000000000000, 0.9659258262890683122, 1.000000000000000000, 0.9659258262890683122, 1.000000000000000000, 0.9659258262890683122, 1.000000000000000000, 0.9659258262890683122, 1.000000000000000000, 0.9659258262890683122, 1.000000000000000000, 0.9659258262890683122, 1.000000000000000000, 0.9659258262890683122, 1.000000000000000000, 0.9659258262890683122, 1.000000000000000000, 0.9659258262890683122, 1.000000000000000000, 0.9659258262890683122, 1.000000000000000000, 0.9659258262890683122, 1.000000000000000000, 0.9659258262890683122, 1.000000000000000000, 0.9659258262890683122, 1.000000000000000000, 0.9659258262890683122, 1.000000000000000000, 0.9659258262890683122, 1.000000000000000000, 0.9659258262890683122, 1.000000000000000000, 0.9659258262890683122, 1.000000000000000000, 0.9659258262890683122, 1.000000000000000000, 0.9659258262890683122, 1.000000000000000000, 0.9659258262890683122, 1.000000000000000000, 0.9659258262890683122, 1.000000000000000000, 0.9659258262890683122, 1.000000000000000000, 0.9659258262890683122, 1.000000000000000000, 0.9659258262890683122, 1.000000000000000000, 0.9659258262890683122, 1.000000000000000000, 0.9659258262890683122, 1.000000000000000000, 0.9659258262890683122, 1.000000000000000000, 0.9659258262890683122, 1.000000000000000000, 0.9659258262890683122, 1.000000000000000000, 0.9659258262890683122, 1.000000000000000000, 0.9659258262890683122, 1.000000000000000000, 0.9659258262890683122, 1.000000000000000000, 0.9659258262890683122, 1.000000000000000000, 0.9659258262890683122, 1.000000000000000000, 0.9659258262890683122, 1.000000000000000000, 0.9659258262890683122, 1.000000000000000000, 0.9659258262890683122, 1.000000000000000000, 0.9659258262890683122, 1.000000000000000000, 0.9659258262890683122, 1.000000000000000000, 0.9659258262890683122, 1.000000000000000000, 0.9659258262890683122, 1.000000000000000000, 0.9659258262890683122, 1.000000000000000000, 0.9659258262890683122, 1.000000000000000000, 0.9659258262890683122, 1.000000000000000000, 0.9659258262890683122, 1.000000000000000000, 0.9659258262890683122, 1.000000000000000000, 0.9659258262890683122, 1.000000000000000000, 0.9659258262890683122, 1.000000000000000000, 0.9659258262890683122, 1.000000000000000000, 0.9659258262890683122, 1.000000000000000000, 0.9659258262890683122, 1.000000000000000000, 0.9659258262890683122, 1.000000000000000000, 0.9659258262890683122, 1.000000000000000000, 0.9659258262890683122, 1.000000000000000000, 0.9659258262890683122, 1.000000000000000000, 0.9659258262890683122, 1.000000000000000000, 0.9659258262890683122, 1.000000000000000000, 0.9659258262890683122, 1.000000000000000000, 0.9659258262890683122, 1.000000000000000000, 0.9659258262890683122, 1.000000000000000000, 0.9659258262890683122, 1.000000000000000000, 0.9659258262890683122, 1.000000000000000000, 0.9659258262890683122, 1.000000000000000000, 0.9659258262890683122, 1.000000000000000000, 0.9659258262890683122, 1.000000000000000000, 0.9659258262890683122, 1.000000000000000000, 0.9659258262890683122, 1.000000000000000000, 0.9659258262890683122, 1.000000000000000000, 0.9659258262890683122, 1.000000000000000000, 0.9659258262890683122, 1.000000000000000000, 0.9659258262890683122, 1.000000000000000000, 0.9659258262890683122, 1.000000000000000000, 0.9659258262890683122, 1.000000000000000000, 0.9659258262890683122, 1.000000000000000000, 0.9659258262890683122, 1.000000000000000000, 0.9659258262890683122, 1.000000000000000000, 0.9659258262890683122, 1.000000000000000000, 0.9659258262890683122, 1.000000000000000000, 0.9659258262890683122, 1.000000000000000000, 0.9659258262890683122, 1.000000000000000000, 0.9659258262890683122, 1.000000000000000000, 0.9659258262890683122, 1.000000000000000000, 0.9659258262890683122, 1.000000000000000000, 0.9659258262890683122, 1.000000000000000000, 0.9659258262890683122, 1.000000000000000000, 0.9659258262890683122, 1.000000000000000000, 0.9659258262890683122, 1.000000000000000000, 0.9659258262890683122, 1.000000000000000000, 0.9659258262890683122, 1.000000000000000000, 0.9659258262890683122, 1.000000000000000000, 0.9659258262890683122, 1.000000000000000000, 0.9659258262890683122, 1.000000000000000000, 0.9659258262890683122, 1.000000000000000000, 0.9659258262890683122, 1.000000000000000000, 0.9659258262890683122, 1.000000000000000000, 0.9659258262890683122, 1.000000000000000000, 0.9659258262890683122, 1.000000000000000000, 0.9659258262890683122, 1.000000000000000000, 0.9659258262890683122, 1.000000000000000000, 0.9659258262890683122, 1.000000000000000000, 0.9659258262890683122, 1.000000000000000000, 0.9659258262890683122, 1.000000000000000000, 0.9659258262890683122, 1.000000000000000000, 0.9659258262890683122, 1.000000000000000000, 0.9659258262890683122, 1.000000000000000000, 0.9659258262890683122, 1.000000000000000000, 0.9659258262890683122, 1.000000000000000000, 0.9659258262890683122, 1.000000000000000000, 0.9659258262890683122, 1.000000000000000000, 0.9659258262890683122, 1.000000000000000000, 0.9659258262890683122, 1.000000000000000000, 0.9659258262890683122, 1.000000000000000000, 0.9659258262890683122, 1.000000000000000000, 0.9659258262890683122, 1.000000000000000000, 0.9659258262890683122, 1.000000000000000000, 0.9659258262890683122, 1.000000000000000000, 0.9659258262890683122, 1.000000000000000000, 0.9659258262890683122, 1.000000000000000000, 0.9659258262890683122, 1.000000000000000000, 0.9659258262890683122, 1.000000000000000000, 0.9659258262890683122, 1.000000000000000000, 0.9659258262890683122, 1.000000000000000000, 0.9659258262890683122, 1.000000000000000000, 0.9659258262890683122, 1.000000000000000000, 0.9659258262890683122, 1.000000000000000000, 0.9659258262890683122, 1.000000000000000000, 0.9659258262890683122, 1.000000000000000000, 0.9659258262890683122, 1.000000000000000000, 0.9659258262890683122, 1.000000000000000000, 0.9659258262890683122, 1.000000000000000000, 0.9659258262890683122, 1.000000000000000000, 0.9659258262890683122, 1.000000000000000000, 0.9659258262890683122, 1.000000000000000000, 0.9659258262890683122, 1.000000000000000000, 0.9659258262890683122, 1.000000000000000000, 0.9659258262890683122, 1.000000000000000000, 0.9659258262890683122, 1.000000000000000000, 0.9659258262890683122, 1.000000000000000000, 0.9659258262890683122, 1.000000000000000000, 0.9659258262890683122, 1.000000000000000000, 0.9659258262890683122, 1.000000000000000000, 0.9659258262890683122, 1.000000000000000000, 0.9659258262890683122, 1.000000000000000000, 0.9659258262890683122, 1.000000000000000000, 0.9659258262890683122, 1.000000000000000000, 0.9659258262890683122, 1.000000000000000000, 0.9659258262890683122, 1.000000000000000000, 0.9659258262890683122, 1.000000000000000000, 0.9659258262890683122, 1.000000000000000000, 0.9659258262890683122, 1.000000000000000000, 0.9659258262890683122, 1.000000000000000000, 0.9659258262890683122, 1.000000000000000000, 0.9659258262890683122, 1.000000000000000000) ) ) 
 REPRESENTATION_ITEM ( '' )  SURFACE ( )  );
#86666=CARTESIAN_POINT ( 'NONE',  ( -4.164238869374098151, 66.59541550158060375, -3.795296366450310543 ) ) ;
#86668=CARTESIAN_POINT ( 'NONE',  ( 10.00000000000000000, 46.81368534415484106, -10.88017736071110342 ) ) ;
#86669=CARTESIAN_POINT ( 'NONE',  ( -2.816281873526473856, 19.12363466993042138, 9.499525473075851096E-16 ) ) ;
#86670=CARTESIAN_POINT ( 'NONE',  ( 19.42250999205614193, 65.14701867748817676, 5.440088680355555262 ) ) ;
#86673=CARTESIAN_POINT ( 'NONE',  ( 1.821158202401524262, 31.16688879859523453, 6.499999999999990230 ) ) ;
#86674=CARTESIAN_POINT ( 'NONE',  ( 19.84674366389459266, 48.30059781766745175, 2.638427012816836559 ) ) ;
#86675=CARTESIAN_POINT ( 'NONE',  ( 0.1532563361054082862, 1.217264484334117824, 2.638427012816831674 ) ) ;
#86677=CARTESIAN_POINT ( 'NONE',  ( -2.816281873526473856, 9.123634669930421381, 9.499525473075851096E-16 ) ) ;
#86678=CARTESIAN_POINT ( 'NONE',  ( 10.00000000000000000, 11.81368534415483751, -10.88017736071110342 ) ) ;
#86680=DIRECTION ( 'NONE',  ( 1.000000000000000000, -0.000000000000000000, 0.000000000000000000 ) ) ;
#86681=EDGE_CURVE ( 'NONE', #84166, #76088, #67131, .T. ) ;
#86682=CARTESIAN_POINT ( 'NONE',  ( 13.79529636645031943, 30.34541550158063927, -14.16423886937409904 ) ) ;
#86683=CARTESIAN_POINT ( 'NONE',  ( 24.16423886937410614, 29.30374883491396787, 8.672049930838204340E-16 ) ) ;
#86684=CARTESIAN_POINT ( 'NONE',  ( 10.00000000000000000, 65.55374883491396076, -14.16423886937410082 ) ) ;
#86685=CARTESIAN_POINT ( 'NONE',  ( 2.791683348922237240, 45.38393115100079456, -7.208316651077763204 ) ) ;
#86686=CARTESIAN_POINT ( 'NONE',  ( -1.099225684535947600, 43.70696800326375353, -6.408140936763238038 ) ) ;
#86687=CARTESIAN_POINT ( 'NONE',  ( 12.91533473730993009, 11.60535201082150536, -10.88017736071109987 ) ) ;
#86689=CARTESIAN_POINT ( 'NONE',  ( 2.791683348922240793, 31.63393115100078745, 7.208316651077764092 ) ) ;
#86690=CARTESIAN_POINT ( 'NONE',  ( 10.00000000000000178, 44.31368534415484106, 10.88017736071110342 ) ) ;
#86691=CARTESIAN_POINT ( 'NONE',  ( 19.38216949554541202, 5.998634669930420493, 9.382169495545424454 ) ) ;
#86692=CARTESIAN_POINT ( 'NONE',  ( 6.204703633549690345, 22.84541550158062861, 14.16423886937410082 ) ) ;
#86694=CARTESIAN_POINT ( 'NONE',  ( 18.17829156368507171, 34.16792564121897158, 6.500000000000019540 ) ) ;
#86695=CIRCLE ( 'NONE', #24403, 1.000000000000000000 ) ;
#86696=CARTESIAN_POINT ( 'NONE',  ( 18.52753015748618282, 18.92559781766745175, -4.923371831947291888 ) ) ;
#86697=CARTESIAN_POINT ( 'NONE',  ( 10.00000000000000000, 52.87363466993041783, -12.81628187352647608 ) ) ;
#86698=CARTESIAN_POINT ( 'NONE',  ( 1.472469842513823179, 56.42559781766745886, 4.923371831947296329 ) ) ;
#86700=STYLED_ITEM ( 'NONE', ( #49051 ), #93125 ) ;
#86701=CARTESIAN_POINT ( 'NONE',  ( 1.816707512666844604, 35.10290668512023871, -6.499999999999958256 ) ) ;
#86703=CARTESIAN_POINT ( 'NONE',  ( 20.88017736071110164, 5.355352010821503583, 2.915334737309930979 ) ) ;
#86704=CARTESIAN_POINT ( 'NONE',  ( 6.204703633549690345, 5.762082168247301794, -14.16423886937410259 ) ) ;
#86705=CARTESIAN_POINT ( 'NONE',  ( 5.076628168052704559, 5.175597817667451750, -8.527530157486179263 ) ) ;
#86706=CARTESIAN_POINT ( 'NONE',  ( 12.63842701281683922, 44.55059781766745175, -9.846743663894590881 ) ) ;
#86707=CARTESIAN_POINT ( 'NONE',  ( 2.035157376598824452, 18.68868534415484106, 7.964842623401179544 ) ) ;
#86710=CARTESIAN_POINT ( 'NONE',  ( 0.1532563361054082862, 61.21726448433412315, 2.638427012816831674 ) ) ;
#86712=EDGE_CURVE ( 'NONE', #8076, #26237, #13818, .T. ) ;
#86716=CARTESIAN_POINT ( 'NONE',  ( 17.08211943468705840, 15.13708216824730179, -12.26659068614894466 ) ) ;
#86717=CARTESIAN_POINT ( 'NONE',  ( -4.164238869374099927, 2.012082168247300906, 3.795296366450308767 ) ) ;
#86718=CARTESIAN_POINT ( 'NONE',  ( -4.164238869374099927, 47.01208216824729647, 3.795296366450308767 ) ) ;
#86719=CARTESIAN_POINT ( 'NONE',  ( 1.472469842513823179, 55.59226448433412315, -4.923371831947296329 ) ) ;
#86720=CARTESIAN_POINT ( 'NONE',  ( 17.20831665107776587, 19.13393115100078035, -7.208316651077762316 ) ) ;
#86722=CARTESIAN_POINT ( 'NONE',  ( 7.084665262690076126, 22.02201867748817321, -10.88017736071110164 ) ) ;
#86723=CARTESIAN_POINT ( 'NONE',  ( -2.816281873526473856, -0.8763653300695799508, 9.499525473075851096E-16 ) ) ;
#86724=CARTESIAN_POINT ( 'NONE',  ( 17.08211943468705130, 8.470415501580635720, 12.26659068614894998 ) ) ;
#86725=CARTESIAN_POINT ( 'NONE',  ( -4.164238869374098151, 41.59541550158061796, -3.795296366450310543 ) ) ;
#86727=CARTESIAN_POINT ( 'NONE',  ( -0.8801773607111009756, 8.063685344154837509, 1.068504757029289695E-15 ) ) ;
#86730=CARTESIAN_POINT ( 'NONE',  ( 2.035157376598822676, 62.43868534415483396, -7.964842623401177768 ) ) ;
#86731=CARTESIAN_POINT ( 'NONE',  ( 0.1532563361054082862, 11.21726448433411605, 2.638427012816831674 ) ) ;
#86732=AXIS2_PLACEMENT_3D ( 'NONE', #1411, #10369, #63832 ) ;
#86737=CARTESIAN_POINT ( 'NONE',  ( 10.00000000000000178, 17.25893115100078745, 9.846743663894594434 ) ) ;
#86739=CARTESIAN_POINT ( 'NONE',  ( 20.36894250292379738, 34.92874883491396076, -10.36894250292379027 ) ) ;
#86740=CARTESIAN_POINT ( 'NONE',  ( 19.84674366389459266, 33.71726448433410894, -2.638427012816827677 ) ) ;
#86741=CARTESIAN_POINT ( 'NONE',  ( 20.88017736071110519, 45.56368534415484106, 2.639326808657452039E-16 ) ) ;
#86743=CARTESIAN_POINT ( 'NONE',  ( 2.035157376598822676, 47.43868534415484817, -7.964842623401177768 ) ) ;
#86744=VECTOR ( 'NONE', #26374, 1000.000000000000000 ) ;
#86746=ORIENTED_EDGE ( 'NONE', *, *, #17081, .T. ) ;
#86747=CARTESIAN_POINT ( 'NONE',  ( -0.3689425029237881626, 2.428748834913967869, 10.36894250292379027 ) ) ;
#86749=EDGE_CURVE ( 'NONE', #75285, #21162, #48001, .T. ) ;
#86751=CARTESIAN_POINT ( 'NONE',  ( 22.81628187352648496, 26.83196800326374998, -3.434112377981050290 ) ) ;
#86752=CARTESIAN_POINT ( 'NONE',  ( 19.84674366389459621, 28.50893115100078745, 7.409399052514197653E-17 ) ) ;
#86753=CARTESIAN_POINT ( 'NONE',  ( 0.000000000000000000, 81.99999999999992895, 5.000000000000000000 ) ) ;
#86754=CARTESIAN_POINT ( 'NONE',  ( 16.40814093676323893, 45.79030133659708923, 11.09922568453595026 ) ) ;
#86756=CARTESIAN_POINT ( 'NONE',  ( 12.63842701281683922, 29.55059781766745175, -9.846743663894590881 ) ) ;
#86757=CARTESIAN_POINT ( 'NONE',  ( 2.035157376598822676, 57.43868534415484106, -7.964842623401177768 ) ) ;
#86759=CARTESIAN_POINT ( 'NONE',  ( 13.99999999999999822, 11.50000000000000000, -6.500000000000000888 ) ) ;
#86762=CARTESIAN_POINT ( 'NONE',  ( 0.1532563361054100626, 0.8005978176674514168, -2.638427012816831230 ) ) ;
#86764=CARTESIAN_POINT ( 'NONE',  ( 16.40814093676323893, 15.79030133659708746, 11.09922568453595026 ) ) ;
#86767=B_SPLINE_CURVE_WITH_KNOTS ( 'NONE', 3,
 ( #60012, #52517, #20355, #4869 ),
 .UNSPECIFIED., .F., .F.,
 ( 4, 4 ),
 ( 4.336808689942017255E-19, 0.002657014572711318117 ),
 .UNSPECIFIED. ) ;
#86768=CARTESIAN_POINT ( 'NONE',  ( 19.84674366389459621, 48.50893115100078745, 7.409399052514197653E-17 ) ) ;
#86769=CARTESIAN_POINT ( 'NONE',  ( 16.40814093676324603, 62.45696800326376064, -11.09922568453594671 ) ) ;
#86770=CARTESIAN_POINT ( 'NONE',  ( 24.16423886937410614, 4.303748834913967869, 8.672049930838204340E-16 ) ) ;
#86771=CARTESIAN_POINT ( 'NONE',  ( 18.52753015748617571, 38.09226448433412315, 4.923371831947298993 ) ) ;
#86773=CARTESIAN_POINT ( 'NONE',  ( 16.40814093676324603, 32.45696800326375353, -11.09922568453594671 ) ) ;
#86776=CARTESIAN_POINT ( 'NONE',  ( 0.5774900079438590739, 52.64701867748817676, -5.440088680355550821 ) ) ;
#86777=CARTESIAN_POINT ( 'NONE',  ( 16.40814093676323893, 0.7903013365970867898, 11.09922568453595026 ) ) ;
#86779=CARTESIAN_POINT ( 'NONE',  ( 2.791683348922237240, 20.38393115100078745, -7.208316651077763204 ) ) ;
#86780=CARTESIAN_POINT ( 'NONE',  ( 20.88017736071110164, 30.35535201082151247, 2.915334737309930979 ) ) ;
#86781=CARTESIAN_POINT ( 'NONE',  ( -1.099225684535947600, 29.54030133659708923, 6.408140936763237150 ) ) ;
#86782=CARTESIAN_POINT ( 'NONE',  ( 19.84674366389459266, 23.71726448433412315, -2.638427012816827677 ) ) ;
#86785=CARTESIAN_POINT ( 'NONE',  ( 0.5774900079438607392, 38.48035201082150536, 5.440088680355550821 ) ) ;
#86786=ORIENTED_EDGE ( 'NONE', *, *, #86035, .F. ) ;
#86787=CARTESIAN_POINT ( 'NONE',  ( 0.5774900079438590739, 57.64701867748817676, -5.440088680355550821 ) ) ;
#86788=SURFACE_STYLE_USAGE ( .BOTH. , #17802 ) ;
#86789=CARTESIAN_POINT ( 'NONE',  ( 19.84674366389459266, 43.71726448433410894, -2.638427012816827677 ) ) ;
#86790=CARTESIAN_POINT ( 'NONE',  ( 20.88017736071110164, 25.35535201082150891, 2.915334737309930979 ) ) ;
#86792=CARTESIAN_POINT ( 'NONE',  ( 20.88017736071110875, 45.77201867748816966, -2.915334737309920765 ) ) ;
#86793=CARTESIAN_POINT ( 'NONE',  ( 15.44008868035555793, 11.39701867748817143, -9.422509992056140149 ) ) ;
#86794=CARTESIAN_POINT ( 'NONE',  ( 20.15039907845753575, 59.72266099184918176, 6.262539305110074395 ) ) ;
#86796=CARTESIAN_POINT ( 'NONE',  ( 18.52753015748617571, 38.09226448433412315, 4.923371831947298993 ) ) ;
#86797=CARTESIAN_POINT ( 'NONE',  ( 10.00000000000000000, 40.55374883491397497, -14.16423886937410082 ) ) ;
#86799=CARTESIAN_POINT ( 'NONE',  ( 1.711636803080551772, 6.844927826957706074, -6.500000000000008882 ) ) ;
#86802=( NAMED_UNIT ( * ) PLANE_ANGLE_UNIT ( ) SI_UNIT ( $, .RADIAN. ) );
#86803=CARTESIAN_POINT ( 'NONE',  ( 22.26659068614894466, 28.88708216824730357, 7.082119434687054849 ) ) ;
#86805=CARTESIAN_POINT ( 'NONE',  ( 10.00000000000000178, 68.05374883491397497, 14.16423886937410082 ) ) ;
#86806=CARTESIAN_POINT ( 'NONE',  ( 7.361572987183170547, 32.05059781766745175, 9.846743663894590881 ) ) ;
#86807=DIRECTION ( 'NONE',  ( -1.000000000000000000, 0.000000000000000000, 0.000000000000000000 ) ) ;
#86808=DIRECTION ( 'NONE',  ( 1.000000000000000000, 0.000000000000000000, -0.000000000000000000 ) ) ;
#86809=CARTESIAN_POINT ( 'NONE',  ( -0.8801773607111008646, 63.27201867748817676, 2.915334737309923430 ) ) ;
#86810=CARTESIAN_POINT ( 'NONE',  ( 3.591859063236761518, 64.95696800326376774, 11.09922568453594849 ) ) ;
#86811=CARTESIAN_POINT ( 'NONE',  ( 20.88017736071110519, 25.56368534415483751, 2.639326808657452039E-16 ) ) ;
#86812=CARTESIAN_POINT ( 'NONE',  ( -2.816281873526471635, 58.91530133659707502, -3.434112377981056508 ) ) ;
#86813=CARTESIAN_POINT ( 'NONE',  ( 19.38216949554541557, 12.24863466993041961, -9.382169495545420901 ) ) ;
#86814=CARTESIAN_POINT ( 'NONE',  ( 19.84674366389459621, 13.50893115100078568, 7.409399052514197653E-17 ) ) ;
#86818=CARTESIAN_POINT ( 'NONE',  ( 24.16423886937410614, 59.30374883491397497, 8.672049930838204340E-16 ) ) ;
#86819=CARTESIAN_POINT ( 'NONE',  ( -0.3689425029237898834, 31.17874883491396787, -10.36894250292378850 ) ) ;
#86820=CARTESIAN_POINT ( 'NONE',  ( 4.559911319644449179, 33.89701867748817676, 9.422509992056141925 ) ) ;
#86821=CARTESIAN_POINT ( 'NONE',  ( -0.8801773607111009756, 43.06368534415484106, 1.068504757029289695E-15 ) ) ;
#86823=CARTESIAN_POINT ( 'NONE',  ( 1.472469842513823179, 5.592264484334118713, -4.923371831947296329 ) ) ;
#86824=CARTESIAN_POINT ( 'NONE',  ( 14.92337183194729988, 24.34226448433411960, -8.527530157486177487 ) ) ;
#86827=CARTESIAN_POINT ( 'NONE',  ( 18.52753015748617571, 23.09226448433411960, 4.923371831947298993 ) ) ;
#86828=CARTESIAN_POINT ( 'NONE',  ( 18.52753015748617571, 48.09226448433412315, 4.923371831947298993 ) ) ;
#86829=CARTESIAN_POINT ( 'NONE',  ( -0.8801773607111009756, 28.06368534415484106, 1.068504757029289695E-15 ) ) ;
#86830=ADVANCED_FACE ( 'NONE', ( #68796 ), #91704, .T. ) ;
#86831=CARTESIAN_POINT ( 'NONE',  ( 3.591859063236763294, 48.29030133659708923, -11.09922568453595026 ) ) ;
#86833=CARTESIAN_POINT ( 'NONE',  ( 17.96484262340118221, 49.93868534415484106, 7.964842623401181321 ) ) ;
#86834=CARTESIAN_POINT ( 'NONE',  ( 0.1532563361054082862, 31.21726448433412315, 2.638427012816831674 ) ) ;
#86835=CARTESIAN_POINT ( 'NONE',  ( -0.3689425029237898834, 51.17874883491397497, -10.36894250292378850 ) ) ;
#86836=CARTESIAN_POINT ( 'NONE',  ( 7.361572987183170547, 22.05059781766745530, 9.846743663894590881 ) ) ;
#86838=CARTESIAN_POINT ( 'NONE',  ( 12.63842701281683034, 57.46726448433411605, 9.846743663894596210 ) ) ;
#86839=CARTESIAN_POINT ( 'NONE',  ( 10.00000000000000178, 8.053748834913967869, 14.16423886937410082 ) ) ;
#86841=CARTESIAN_POINT ( 'NONE',  ( 6.204703633549690345, 32.84541550158063927, 14.16423886937410082 ) ) ;
#86842=CARTESIAN_POINT ( 'NONE',  ( 10.00000000000000000, 24.75893115100078745, -9.846743663894594434 ) ) ;
#86844=CARTESIAN_POINT ( 'NONE',  ( 7.084665262690076126, 24.10535201082150181, 10.88017736071109987 ) ) ;
#86846=CARTESIAN_POINT ( 'NONE',  ( 15.44008868035555793, 41.39701867748817676, -9.422509992056140149 ) ) ;
#86847=CARTESIAN_POINT ( 'NONE',  ( 0.5774900079438590739, 37.64701867748817676, -5.440088680355550821 ) ) ;
#86848=ORIENTED_EDGE ( 'NONE', *, *, #68674, .F. ) ;
#86849=CARTESIAN_POINT ( 'NONE',  ( 7.084665262690076126, 54.10535201082151247, 10.88017736071109987 ) ) ;
#86852=CARTESIAN_POINT ( 'NONE',  ( 0.5774900079438590739, 67.64701867748817676, -5.440088680355550821 ) ) ;
#86854=CARTESIAN_POINT ( 'NONE',  ( 20.88017736071110164, 60.35535201082151957, 2.915334737309930979 ) ) ;
#86857=CARTESIAN_POINT ( 'NONE',  ( 7.084665262690076126, 9.105352010821503583, 10.88017736071109987 ) ) ;
#86858=CARTESIAN_POINT ( 'NONE',  ( 17.20831665107776587, 12.88393115100078390, 7.208316651077764980 ) ) ;
#86859=CARTESIAN_POINT ( 'NONE',  ( -4.164238869374098151, 6.595415501580634832, -3.795296366450310543 ) ) ;
#86860=CARTESIAN_POINT ( 'NONE',  ( 2.791683348922240793, 1.633931151000784565, 7.208316651077764092 ) ) ;
#86861=CARTESIAN_POINT ( 'NONE',  ( 17.96484262340118221, 9.938685344154837509, 7.964842623401181321 ) ) ;
#86862=CARTESIAN_POINT ( 'NONE',  ( 2.791683348922237240, 40.38393115100078035, -7.208316651077763204 ) ) ;
#86864=CARTESIAN_POINT ( 'NONE',  ( 14.92337183194729988, 54.34226448433412315, -8.527530157486177487 ) ) ;
#86866=CARTESIAN_POINT ( 'NONE',  ( 19.42250999205614193, 50.14701867748817676, 5.440088680355555262 ) ) ;
#86867=CARTESIAN_POINT ( 'NONE',  ( 10.00000000000000178, 52.25893115100078745, 9.846743663894594434 ) ) ;
#86868=CARTESIAN_POINT ( 'NONE',  ( 16.40814093676324603, 27.45696800326375708, -11.09922568453594671 ) ) ;
#86869=CARTESIAN_POINT ( 'NONE',  ( 7.084665262690076126, 67.02201867748817676, -10.88017736071110164 ) ) ;
#86870=CARTESIAN_POINT ( 'NONE',  ( 20.88017736071110875, 60.77201867748817676, -2.915334737309920765 ) ) ;
#86871=CARTESIAN_POINT ( 'NONE',  ( 15.44008868035555793, 6.397018677488171434, -9.422509992056140149 ) ) ;
#86872=CARTESIAN_POINT ( 'NONE',  ( 3.591859063236763294, 43.29030133659708923, -11.09922568453595026 ) ) ;
#86874=ORIENTED_EDGE ( 'NONE', *, *, #1938, .T. ) ;
#86875=CARTESIAN_POINT ( 'NONE',  ( 13.43411237798106583, 22.66530133659708923, -12.81628187352647252 ) ) ;
#86876=CARTESIAN_POINT ( 'NONE',  ( -0.8801773607110991993, 37.85535201082151247, -2.915334737309923874 ) ) ;
#86878=CARTESIAN_POINT ( 'NONE',  ( 10.00000000000000000, 64.75893115100078035, -9.846743663894594434 ) ) ;
#86879=CARTESIAN_POINT ( 'NONE',  ( 5.076628168052704559, 15.17559781766745175, -8.527530157486179263 ) ) ;
#86880=CARTESIAN_POINT ( 'NONE',  ( 0.1532563361054083140, 46.00893115100079456, 1.131784320476157264E-15 ) ) ;
#86882=CARTESIAN_POINT ( 'NONE',  ( 17.20831665107776587, 34.13393115100078745, -7.208316651077762316 ) ) ;
#86885=CARTESIAN_POINT ( 'NONE',  ( 2.791683348922240793, 26.63393115100078745, 7.208316651077764092 ) ) ;
#86887=CARTESIAN_POINT ( 'NONE',  ( 12.63842701281683034, 62.46726448433410894, 9.846743663894596210 ) ) ;
#86890=CARTESIAN_POINT ( 'NONE',  ( 0.6178305044545818747, 23.49863466993041783, -9.382169495545419124 ) ) ;
#86891=CARTESIAN_POINT ( 'NONE',  ( 12.63842701281683034, 47.46726448433412315, 9.846743663894596210 ) ) ;
#86894=CARTESIAN_POINT ( 'NONE',  ( -2.266590686148945544, 47.22041550158063927, 7.082119434687048631 ) ) ;
#86895=CARTESIAN_POINT ( 'NONE',  ( 5.076628168052704559, 20.17559781766745175, -8.527530157486179263 ) ) ;
#86898=CARTESIAN_POINT ( 'NONE',  ( -2.266590686148945544, 61.38708216824730357, -7.082119434687050408 ) ) ;
#86899=CARTESIAN_POINT ( 'NONE',  ( 19.84674366389459266, 53.30059781766744464, 2.638427012816836559 ) ) ;
#86900=CARTESIAN_POINT ( 'NONE',  ( 10.00000000000000178, 4.313685344154837509, 10.88017736071110342 ) ) ;
#86901=CARTESIAN_POINT ( 'NONE',  ( 10.00000000000000178, 33.05374883491396787, 14.16423886937410082 ) ) ;
#86902=CARTESIAN_POINT ( 'NONE',  ( 20.36894250292379382, 43.67874883491397497, 10.36894250292379205 ) ) ;
#86904=CARTESIAN_POINT ( 'NONE',  ( 1.274849032794223680, 28.57228050351031001, 6.499999999999884537 ) ) ;
#86905=CARTESIAN_POINT ( 'NONE',  ( 0.1532563361054082862, 56.21726448433411605, 2.638427012816831674 ) ) ;
#86907=CARTESIAN_POINT ( 'NONE',  ( 12.91533473730993009, 41.60535201082149825, -10.88017736071109987 ) ) ;
#86910=EDGE_CURVE ( 'NONE', #10984, #79104, #97233, .T. ) ;
#86911=CARTESIAN_POINT ( 'NONE',  ( 19.84674366389459266, 53.71726448433411605, -2.638427012816827677 ) ) ;
#86912=CARTESIAN_POINT ( 'NONE',  ( -0.08248232600719085372, 0.1423898869303599768, 6.349449577244200782 ) ) ;
#86915=CARTESIAN_POINT ( 'NONE',  ( 7.361572987183170547, 57.05059781766744464, 9.846743663894590881 ) ) ;
#86916=DIRECTION ( 'NONE',  ( 0.000000000000000000, 1.000000000000000000, -0.000000000000000000 ) ) ;
#86917=ORIENTED_EDGE ( 'NONE', *, *, #51498, .F. ) ;
#86918=CARTESIAN_POINT ( 'NONE',  ( -0.3689425029237881626, 32.42874883491395366, 10.36894250292379027 ) ) ;
#86922=CARTESIAN_POINT ( 'NONE',  ( 2.035157376598824452, 13.68868534415483751, 7.964842623401179544 ) ) ;
#86923=CARTESIAN_POINT ( 'NONE',  ( -2.816281873526473856, 24.12363466993042138, 9.499525473075851096E-16 ) ) ;
#86924=CARTESIAN_POINT ( 'NONE',  ( 0.1532563361054082862, 6.217264484334118713, 2.638427012816831674 ) ) ;
#86925=CARTESIAN_POINT ( 'NONE',  ( 18.72515096720568906, 15.05509018479935612, 6.500000000000002665 ) ) ;
#86926=CARTESIAN_POINT ( 'NONE',  ( 1.472469842513823179, 20.59226448433411960, -4.923371831947296329 ) ) ;
#86928=CARTESIAN_POINT ( 'NONE',  ( 17.96484262340118221, 9.938685344154839285, 7.964842623401181321 ) ) ;
#86930=CARTESIAN_POINT ( 'NONE',  ( 17.96484262340118221, 44.93868534415483396, 7.964842623401181321 ) ) ;
#86931=CARTESIAN_POINT ( 'NONE',  ( -0.8801773607111009756, 33.06368534415484106, 1.068504757029289695E-15 ) ) ;
#86932=CARTESIAN_POINT ( 'NONE',  ( 0.1532563361054083140, 66.00893115100079456, 1.131784320476157264E-15 ) ) ;
#86933=CARTESIAN_POINT ( 'NONE',  ( 5.076628168052703671, 66.84226448433412315, 8.527530157486179263 ) ) ;
#86934=CARTESIAN_POINT ( 'NONE',  ( -42.50369195530268485, 107.9060299417078426, -5.000000000000000888 ) ) ;
#86935=CARTESIAN_POINT ( 'NONE',  ( 19.84674366389459266, 8.300597817667451750, 2.638427012816836559 ) ) ;
#86938=CARTESIAN_POINT ( 'NONE',  ( 7.084665262690076126, 27.02201867748817676, -10.88017736071110164 ) ) ;
#86939=CARTESIAN_POINT ( 'NONE',  ( 0.6178305044545818747, 28.49863466993041783, -9.382169495545419124 ) ) ;
#86940=EDGE_CURVE ( 'NONE', #95286, #45739, #94903, .T. ) ;
#86941=CARTESIAN_POINT ( 'NONE',  ( 1.472469842513823179, 56.42559781766745886, 4.923371831947296329 ) ) ;
#86942=CARTESIAN_POINT ( 'NONE',  ( 0.5774900079438590739, 62.64701867748817676, -5.440088680355550821 ) ) ;
#86943=CARTESIAN_POINT ( 'NONE',  ( 10.00000000000000000, 14.75893115100078568, -9.846743663894594434 ) ) ;
#86944=CARTESIAN_POINT ( 'NONE',  ( 19.38216949554541202, 35.99863466993041072, 9.382169495545424454 ) ) ;
#86945=CARTESIAN_POINT ( 'NONE',  ( 17.20831665107776587, 4.133931151000785675, -7.208316651077762316 ) ) ;
#86948=( NAMED_UNIT ( * ) PLANE_ANGLE_UNIT ( ) SI_UNIT ( $, .RADIAN. ) );
#86949=CARTESIAN_POINT ( 'NONE',  ( 19.38216949554541202, 60.99863466993042493, 9.382169495545424454 ) ) ;
#86950=CARTESIAN_POINT ( 'NONE',  ( -4.164238869374099927, 27.01208216824730357, 3.795296366450308767 ) ) ;
#86951=CARTESIAN_POINT ( 'NONE',  ( 19.84674366389459266, 18.71726448433411960, -2.638427012816827677 ) ) ;
#86952=CARTESIAN_POINT ( 'NONE',  ( 10.00000000000000000, 6.813685344154838397, -10.88017736071110342 ) ) ;
#86953=CARTESIAN_POINT ( 'NONE',  ( 10.00000000000000178, 27.25893115100078390, 9.846743663894594434 ) ) ;
#86954=CARTESIAN_POINT ( 'NONE',  ( 2.917880565312948704, 52.63708216824730357, 12.26659068614894643 ) ) ;
#86956=CARTESIAN_POINT ( 'NONE',  ( 7.084665262690076126, 9.105352010821503583, 10.88017736071109987 ) ) ;
#86957=CARTESIAN_POINT ( 'NONE',  ( -0.8801773607110991993, 17.85535201082150536, -2.915334737309923874 ) ) ;
#86958=CARTESIAN_POINT ( 'NONE',  ( 0.1532563361054083140, 16.00893115100078390, 1.131784320476157264E-15 ) ) ;
#86961=CARTESIAN_POINT ( 'NONE',  ( 2.035157376598824452, 23.68868534415484461, 7.964842623401179544 ) ) ;
#86962=CARTESIAN_POINT ( 'NONE',  ( 18.52753015748617571, 58.09226448433411605, 4.923371831947298993 ) ) ;
#86964=CARTESIAN_POINT ( 'NONE',  ( -0.8801773607111009756, 68.27201867748817676, 2.915334737309923874 ) ) ;
#86966=CARTESIAN_POINT ( 'NONE',  ( 13.79529636645031943, 25.34541550158063572, -14.16423886937409904 ) ) ;
#86967=CARTESIAN_POINT ( 'NONE',  ( 2.035157376598824452, 43.68868534415484106, 7.964842623401179544 ) ) ;
#86968=CARTESIAN_POINT ( 'NONE',  ( 19.42250999205614193, 15.14701867748817143, 5.440088680355555262 ) ) ;
#86969=CARTESIAN_POINT ( 'NONE',  ( 10.00000000000000178, 52.25893115100078745, 9.846743663894594434 ) ) ;
#86972=CARTESIAN_POINT ( 'NONE',  ( 5.076628168052703671, 41.84226448433411605, 8.527530157486179263 ) ) ;
#86975=CARTESIAN_POINT ( 'NONE',  ( 19.84674366389459621, 13.50893115100078568, 7.409399052514197653E-17 ) ) ;
#86979=CARTESIAN_POINT ( 'NONE',  ( 15.44008868035555793, 11.39701867748817143, -9.422509992056140149 ) ) ;
#86980=CARTESIAN_POINT ( 'NONE',  ( 2.791683348922240793, 6.633931151000785675, 7.208316651077764092 ) ) ;
#86981=CARTESIAN_POINT ( 'NONE',  ( 2.791683348922240793, 66.63393115100079456, 7.208316651077764092 ) ) ;
#86982=CARTESIAN_POINT ( 'NONE',  ( -0.8801773607111009756, 43.06368534415484106, 1.068504757029289695E-15 ) ) ;
#86983=CARTESIAN_POINT ( 'NONE',  ( 4.559911319644449179, 48.89701867748817676, 9.422509992056141925 ) ) ;
#86984=CARTESIAN_POINT ( 'NONE',  ( 17.96484262340118221, 19.93868534415484106, 7.964842623401181321 ) ) ;
#86985=CARTESIAN_POINT ( 'NONE',  ( 10.00000000000000178, 50.37363466993042493, 12.81628187352647608 ) ) ;
#86986=CARTESIAN_POINT ( 'NONE',  ( 17.08211943468705840, 35.13708216824730357, -12.26659068614894466 ) ) ;
#86988=CARTESIAN_POINT ( 'NONE',  ( 21.92686044187657046, 12.39664270246084321, -3.195792623639524432 ) ) ;
#86989=AXIS2_PLACEMENT_3D ( 'NONE', #18804, #78309, #86808 ) ;
#86990=CARTESIAN_POINT ( 'NONE',  ( 6.565887622018943937, 63.08196800326376064, -12.81628187352647608 ) ) ;
#86992=CARTESIAN_POINT ( 'NONE',  ( 19.84674366389459266, 63.71726448433412315, -2.638427012816827677 ) ) ;
#86993=CARTESIAN_POINT ( 'NONE',  ( -0.1503990784575328643, 15.12777174578612538, 6.262539305110068177 ) ) ;
#86994=CARTESIAN_POINT ( 'NONE',  ( 12.91533473730993009, 36.60535201082151247, -10.88017736071109987 ) ) ;
#86997=CARTESIAN_POINT ( 'NONE',  ( 2.791683348922240793, 1.633931151000784565, 7.208316651077764092 ) ) ;
#86999=CARTESIAN_POINT ( 'NONE',  ( -0.1491070598754174470, 61.94583914210339515, 4.500000000000000888 ) ) ;
#87000=CARTESIAN_POINT ( 'NONE',  ( 14.92337183194729988, 29.34226448433411960, -8.527530157486177487 ) ) ;
#87001=CARTESIAN_POINT ( 'NONE',  ( 2.791683348922240793, 16.63393115100078745, 7.208316651077764092 ) ) ;
#87002=CARTESIAN_POINT ( 'NONE',  ( 0.5774900079438590739, 62.64701867748817676, -5.440088680355550821 ) ) ;
#87004=CARTESIAN_POINT ( 'NONE',  ( 0.5774900079438607392, 58.48035201082151247, 5.440088680355550821 ) ) ;
#87005=CARTESIAN_POINT ( 'NONE',  ( 18.52753015748617571, 23.09226448433411960, 4.923371831947298993 ) ) ;
#87008=CARTESIAN_POINT ( 'NONE',  ( 0.1532563361054083140, 51.00893115100078745, 1.131784320476157264E-15 ) ) ;
#87009=ORIENTED_EDGE ( 'NONE', *, *, #42450, .F. ) ;
#87012=CARTESIAN_POINT ( 'NONE',  ( 20.36894250292379738, 4.928748834913967869, -10.36894250292379027 ) ) ;
#87013=CARTESIAN_POINT ( 'NONE',  ( 19.72487221294570858, 70.00000000000000000, -6.000000000000000000 ) ) ;
#87014=SURFACE_STYLE_USAGE ( .BOTH. , #70054 ) ;
#87015=CARTESIAN_POINT ( 'NONE',  ( -4.164238869374099039, 36.80374883491396787, 8.674139862899312516E-16 ) ) ;
#87016=SURFACE_STYLE_FILL_AREA ( #27003 ) ;
#87017=CARTESIAN_POINT ( 'NONE',  ( 7.084665262690076126, 39.10535201082150536, 10.88017736071109987 ) ) ;
#87019=CARTESIAN_POINT ( 'NONE',  ( 2.791683348922237240, 15.38393115100078212, -7.208316651077763204 ) ) ;
#87020=CARTESIAN_POINT ( 'NONE',  ( 7.084665262690076126, 54.10535201082151247, 10.88017736071109987 ) ) ;
#87021=CARTESIAN_POINT ( 'NONE',  ( 17.20831665107776587, 12.88393115100078390, 7.208316651077764980 ) ) ;
#87022=CARTESIAN_POINT ( 'NONE',  ( 10.00000000000000178, 45.37363466993041783, 12.81628187352647608 ) ) ;
#87023=CARTESIAN_POINT ( 'NONE',  ( 1.472469842513823179, 31.42559781766745530, 4.923371831947296329 ) ) ;
#87024=CARTESIAN_POINT ( 'NONE',  ( 17.39651004071838969, 59.08210964143329846, -6.500000000000027534 ) ) ;
#87025=CARTESIAN_POINT ( 'NONE',  ( 17.96484262340118221, 54.93868534415484106, 7.964842623401181321 ) ) ;
#87027=CARTESIAN_POINT ( 'NONE',  ( 16.40814093676323893, 25.79030133659708923, 11.09922568453595026 ) ) ;
#87029=CARTESIAN_POINT ( 'NONE',  ( 0.1532563361054082862, 26.21726448433411605, 2.638427012816831674 ) ) ;
#87030=CARTESIAN_POINT ( 'NONE',  ( 10.00000000000000178, 18.05374883491396787, 14.16423886937410082 ) ) ;
#87032=VERTEX_POINT ( 'NONE', #66201 ) ;
#87033=EDGE_CURVE ( 'NONE', #75712, #53231, #62345, .T. ) ;
#87035=CARTESIAN_POINT ( 'NONE',  ( -0.8801773607111009756, 38.06368534415484106, 1.068504757029289695E-15 ) ) ;
#87036=CARTESIAN_POINT ( 'NONE',  ( -0.8801773607111009756, 53.06368534415484106, 1.068504757029289695E-15 ) ) ;
#87037=CARTESIAN_POINT ( 'NONE',  ( 2.917880565312950480, 30.97041550158063572, -12.26659068614894821 ) ) ;
#87038=CARTESIAN_POINT ( 'NONE',  ( 12.63842701281683922, 49.55059781766744464, -9.846743663894590881 ) ) ;
#87040=CARTESIAN_POINT ( 'NONE',  ( 17.20831665107776587, 12.88393115100078390, 7.208316651077764980 ) ) ;
#87043=CARTESIAN_POINT ( 'NONE',  ( 20.88017736071110875, 45.77201867748816966, -2.915334737309920765 ) ) ;
#87045=CARTESIAN_POINT ( 'NONE',  ( -1.099225684535947600, 23.70696800326375708, -6.408140936763238038 ) ) ;
#87046=CARTESIAN_POINT ( 'NONE',  ( 18.52753015748617571, 48.09226448433412315, 4.923371831947298993 ) ) ;
#87048=CARTESIAN_POINT ( 'NONE',  ( -0.8801773607111008646, 3.272018677488171434, 2.915334737309923430 ) ) ;
#87053=CARTESIAN_POINT ( 'NONE',  ( 1.816707512666851265, 15.10290668512023338, -6.499999999999988454 ) ) ;
#87054=CARTESIAN_POINT ( 'NONE',  ( 15.44008868035555260, 64.73035201082151957, 9.422509992056143702 ) ) ;
#87055=CARTESIAN_POINT ( 'NONE',  ( 7.084665262690076126, 59.10535201082150536, 10.88017736071109987 ) ) ;
#87057=CARTESIAN_POINT ( 'NONE',  ( 0.2751277870542871984, 68.21833443783938833, 6.499999999999984901 ) ) ;
#87059=CARTESIAN_POINT ( 'NONE',  ( 18.52753015748618282, 23.92559781766745530, -4.923371831947291888 ) ) ;
#87060=CARTESIAN_POINT ( 'NONE',  ( 20.88017736071110519, 20.56368534415484106, 2.639326808657452039E-16 ) ) ;
#87061=CARTESIAN_POINT ( 'NONE',  ( 12.63842701281683922, 64.55059781766745175, -9.846743663894590881 ) ) ;
#87062=CARTESIAN_POINT ( 'NONE',  ( 20.88017736071110519, 20.56368534415484106, 2.639326808657452039E-16 ) ) ;
#87065=CARTESIAN_POINT ( 'NONE',  ( 22.81628187352647785, 41.62363466993042493, 6.195893100308588602E-16 ) ) ;
#87066=ORIENTED_EDGE ( 'NONE', *, *, #40200, .T. ) ;
#87067=CARTESIAN_POINT ( 'NONE',  ( 0.5774900079438590739, 47.64701867748817676, -5.440088680355550821 ) ) ;
#87068=EDGE_CURVE ( 'NONE', #61681, #24281, #68685, .T. ) ;
#87069=CARTESIAN_POINT ( 'NONE',  ( 22.81628187352648496, 26.83196800326374998, -3.434112377981050290 ) ) ;
#87070=CARTESIAN_POINT ( 'NONE',  ( 20.15039907845753220, 51.74884699246889852, 6.262539305110077059 ) ) ;
#87071=CARTESIAN_POINT ( 'NONE',  ( 4.559911319644449179, 23.89701867748817321, 9.422509992056141925 ) ) ;
#87072=CARTESIAN_POINT ( 'NONE',  ( 22.26659068614894466, 53.88708216824731068, 7.082119434687054849 ) ) ;
#87073=CARTESIAN_POINT ( 'NONE',  ( 10.00000000000000000, 44.75893115100078745, -9.846743663894594434 ) ) ;
#87074=CARTESIAN_POINT ( 'NONE',  ( 0.1532563361054100626, 5.800597817667452638, -2.638427012816831230 ) ) ;
#87075=CARTESIAN_POINT ( 'NONE',  ( 17.96484262340118221, 49.93868534415484106, 7.964842623401181321 ) ) ;
#87077=CARTESIAN_POINT ( 'NONE',  ( -0.3689425029237898834, 16.17874883491396076, -10.36894250292378850 ) ) ;
#87081=CARTESIAN_POINT ( 'NONE',  ( 24.16423886937410614, 44.30374883491397497, 8.672049930838204340E-16 ) ) ;
#87082=CARTESIAN_POINT ( 'NONE',  ( -0.3689425029237898834, 51.17874883491397497, -10.36894250292378850 ) ) ;
#87083=CARTESIAN_POINT ( 'NONE',  ( 18.52753015748618282, 18.92559781766745175, -4.923371831947291888 ) ) ;
#87085=CARTESIAN_POINT ( 'NONE',  ( 6.565887622018943937, 13.08196800326374998, -12.81628187352647608 ) ) ;
#87088=CARTESIAN_POINT ( 'NONE',  ( 7.084665262690076126, 4.105352010821503583, 10.88017736071109987 ) ) ;
#87089=CARTESIAN_POINT ( 'NONE',  ( 13.43411237798105340, 30.58196800326374998, 12.81628187352647963 ) ) ;
#87090=CARTESIAN_POINT ( 'NONE',  ( 2.917880565312948704, 47.63708216824730357, 12.26659068614894643 ) ) ;
#87092=CARTESIAN_POINT ( 'NONE',  ( 12.91533473730992121, 64.52201867748817676, 10.88017736071110164 ) ) ;
#87094=ORIENTED_EDGE ( 'NONE', *, *, #33204, .F. ) ;
#87095=CARTESIAN_POINT ( 'NONE',  ( 0.1532563361054100626, 20.80059781766744464, -2.638427012816831230 ) ) ;
#87097=CARTESIAN_POINT ( 'NONE',  ( 7.084665262690076126, 2.022018677488171434, -10.88017736071110164 ) ) ;
#87098=CARTESIAN_POINT ( 'NONE',  ( 20.88017736071110875, 10.77201867748817143, -2.915334737309920765 ) ) ;
#87099=CARTESIAN_POINT ( 'NONE',  ( 10.00000000000000178, 47.25893115100078745, 9.846743663894594434 ) ) ;
#87100=CARTESIAN_POINT ( 'NONE',  ( 10.00000000000000178, 67.25893115100079456, 9.846743663894594434 ) ) ;
#87104=CARTESIAN_POINT ( 'NONE',  ( 22.81628187352647785, 21.41530133659708923, 3.434112377981063169 ) ) ;
#87105=VERTEX_POINT ( 'NONE', #14212 ) ;
#87106=CARTESIAN_POINT ( 'NONE',  ( 2.917880565312948704, 57.63708216824731068, 12.26659068614894643 ) ) ;
#87107=VERTEX_POINT ( 'NONE', #214 ) ;
#87108=CARTESIAN_POINT ( 'NONE',  ( 2.917880565312950480, 55.97041550158063217, -12.26659068614894821 ) ) ;
#87110=CARTESIAN_POINT ( 'NONE',  ( 12.91533473730993009, 31.60535201082150891, -10.88017736071109987 ) ) ;
#87111=CARTESIAN_POINT ( 'NONE',  ( 7.084665262690076126, 42.02201867748816966, -10.88017736071110164 ) ) ;
#87113=CARTESIAN_POINT ( 'NONE',  ( 19.42250999205614548, 25.98035201082150891, -5.440088680355545492 ) ) ;
#87114=DIRECTION ( 'NONE',  ( 0.000000000000000000, -1.000000000000000000, 0.000000000000000000 ) ) ;
#87116=CARTESIAN_POINT ( 'NONE',  ( 0.1532563361054100626, 15.80059781766745353, -2.638427012816831230 ) ) ;
#87119=CARTESIAN_POINT ( 'NONE',  ( 7.361572987183170547, 47.05059781766745175, 9.846743663894590881 ) ) ;
#87121=CARTESIAN_POINT ( 'NONE',  ( 22.81628187352647785, 56.41530133659708213, 3.434112377981063169 ) ) ;
#87124=CARTESIAN_POINT ( 'NONE',  ( 0.1532563361054082862, 66.21726448433413736, 2.638427012816831674 ) ) ;
#87125=CARTESIAN_POINT ( 'NONE',  ( 6.204703633549690345, 47.84541550158064638, 14.16423886937410082 ) ) ;
#87126=CARTESIAN_POINT ( 'NONE',  ( 19.72487221294570858, 5.718334437839381224, -6.500000000000000888 ) ) ;
#87129=CARTESIAN_POINT ( 'NONE',  ( 19.84674366389459266, 28.71726448433411960, -2.638427012816827677 ) ) ;
#87131=CARTESIAN_POINT ( 'NONE',  ( 6.565887622018943937, 0.1653013365970866511, 12.81628187352647430 ) ) ;
#87132=CARTESIAN_POINT ( 'NONE',  ( 15.44008868035555793, 66.39701867748817676, -9.422509992056140149 ) ) ;
#87134=CARTESIAN_POINT ( 'NONE',  ( 14.92337183194729633, 52.67559781766745175, 8.527530157486181039 ) ) ;
#87139=CARTESIAN_POINT ( 'NONE',  ( 17.08211943468705130, 58.47041550158063927, 12.26659068614894998 ) ) ;
#87140=LINE ( 'NONE', #55678, #35204 ) ;
#87141=CARTESIAN_POINT ( 'NONE',  ( 0.5774900079438607392, 43.48035201082151247, 5.440088680355550821 ) ) ;
#87142=CARTESIAN_POINT ( 'NONE',  ( 6.565887622018943937, 20.16530133659708213, 12.81628187352647430 ) ) ;
#87143=CARTESIAN_POINT ( 'NONE',  ( 10.00000000000000178, 64.31368534415483396, 10.88017736071110342 ) ) ;
#87144=CARTESIAN_POINT ( 'NONE',  ( 7.084665262690076126, 2.022018677488170990, -10.88017736071110164 ) ) ;
#87146=CARTESIAN_POINT ( 'NONE',  ( 19.39235739573469885, 59.87576471608601025, 6.499999999999986677 ) ) ;
#87147=CARTESIAN_POINT ( 'NONE',  ( 0.1532563361054100626, 45.80059781766745886, -2.638427012816831230 ) ) ;
#87148=( NAMED_UNIT ( * ) SI_UNIT ( $, .STERADIAN. ) SOLID_ANGLE_UNIT ( ) );
#87150=CARTESIAN_POINT ( 'NONE',  ( 16.40814093676324603, 17.45696800326375353, -11.09922568453594671 ) ) ;
#87152=CARTESIAN_POINT ( 'NONE',  ( -0.8801773607111009756, 28.06368534415484106, 1.068504757029289695E-15 ) ) ;
#87155=CARTESIAN_POINT ( 'NONE',  ( 24.16423886937409904, 34.09541550158064638, 3.795296366450317205 ) ) ;
#87156=CARTESIAN_POINT ( 'NONE',  ( -2.266590686148945544, 27.22041550158063572, 7.082119434687048631 ) ) ;
#87157=CARTESIAN_POINT ( 'NONE',  ( -0.8801773607111009756, 13.06368534415483929, 1.068504757029289695E-15 ) ) ;
#87159=CARTESIAN_POINT ( 'NONE',  ( 14.92337183194729988, 44.34226448433412315, -8.527530157486177487 ) ) ;
#87160=CARTESIAN_POINT ( 'NONE',  ( 21.09922568453594849, 41.20696800326375353, 6.408140936763242479 ) ) ;
#87161=CARTESIAN_POINT ( 'NONE',  ( 0.5774900079438607392, 8.480352010821505360, 5.440088680355550821 ) ) ;
#87162=VECTOR ( 'NONE', #45160, 1000.000000000000000 ) ;
#87163=CARTESIAN_POINT ( 'NONE',  ( 5.076628168052704559, 40.17559781766745175, -8.527530157486179263 ) ) ;
#87164=CARTESIAN_POINT ( 'NONE',  ( -0.8801773607110991993, 37.85535201082151247, -2.915334737309923874 ) ) ;
#87165=CARTESIAN_POINT ( 'NONE',  ( 0.6178305044545818747, 8.498634669930421381, -9.382169495545419124 ) ) ;
#87166=CARTESIAN_POINT ( 'NONE',  ( -4.164238869374099039, 26.80374883491397142, 8.674139862899312516E-16 ) ) ;
#87168=MECHANICAL_DESIGN_GEOMETRIC_PRESENTATION_REPRESENTATION('',(#5748),#53638);
#87171=CARTESIAN_POINT ( 'NONE',  ( 12.63842701281683922, 19.55059781766745175, -9.846743663894590881 ) ) ;
#87172=CARTESIAN_POINT ( 'NONE',  ( -1.099225684535947600, 54.54030133659708923, 6.408140936763237150 ) ) ;
#87173=CARTESIAN_POINT ( 'NONE',  ( 14.92337183194729988, 54.34226448433412315, -8.527530157486177487 ) ) ;
#87176=DIRECTION ( 'NONE',  ( 0.000000000000000000, -1.000000000000000000, -0.000000000000000000 ) ) ;
#87178=CARTESIAN_POINT ( 'NONE',  ( 20.36894250292379738, 64.92874883491397497, -10.36894250292379027 ) ) ;
#87179=CARTESIAN_POINT ( 'NONE',  ( 13.79529636645030344, 13.26208216824729824, 14.16423886937410614 ) ) ;
#87181=CARTESIAN_POINT ( 'NONE',  ( 2.791683348922237240, 5.383931151000785675, -7.208316651077763204 ) ) ;
#87182=CARTESIAN_POINT ( 'NONE',  ( 17.20831665107776587, 47.88393115100078745, 7.208316651077764980 ) ) ;
#87183=CARTESIAN_POINT ( 'NONE',  ( 19.42250999205614193, 40.14701867748817676, 5.440088680355555262 ) ) ;
#87185=FACE_OUTER_BOUND ( 'NONE', #16391, .T. ) ;
#87186=VERTEX_POINT ( 'NONE', #15698 ) ;
#87188=EDGE_LOOP ( 'NONE', ( #24958, #65503, #15595, #36605, #77470, #72230 ) ) ;
#87191=CARTESIAN_POINT ( 'NONE',  ( 13.79529636645031943, 10.34541550158063394, -14.16423886937409904 ) ) ;
#87192=CARTESIAN_POINT ( 'NONE',  ( 10.00000000000000178, 8.053748834913967869, 14.16423886937410082 ) ) ;
#87193=CARTESIAN_POINT ( 'NONE',  ( 20.36894250292379738, 39.92874883491396787, -10.36894250292379027 ) ) ;
#87194=CARTESIAN_POINT ( 'NONE',  ( 10.00000000000000178, 62.25893115100078745, 9.846743663894594434 ) ) ;
#87195=CARTESIAN_POINT ( 'NONE',  ( 2.791683348922240793, 41.63393115100078745, 7.208316651077764092 ) ) ;
#87197=CARTESIAN_POINT ( 'NONE',  ( -0.8801773607110991993, 27.85535201082150181, -2.915334737309923874 ) ) ;
#87198=CARTESIAN_POINT ( 'NONE',  ( 7.361572987183170547, 57.05059781766744464, 9.846743663894590881 ) ) ;
#87199=CARTESIAN_POINT ( 'NONE',  ( -2.266590686148945544, 1.387082168247301128, -7.082119434687050408 ) ) ;
#87200=CARTESIAN_POINT ( 'NONE',  ( -0.3689425029237898834, 41.17874883491397497, -10.36894250292378850 ) ) ;
#87201=CARTESIAN_POINT ( 'NONE',  ( 10.00000000000000000, 6.813685344154838397, -10.88017736071110342 ) ) ;
#87204=CARTESIAN_POINT ( 'NONE',  ( 20.88017736071110875, 65.77201867748817676, -2.915334737309920765 ) ) ;
#87205=CARTESIAN_POINT ( 'NONE',  ( 19.84674366389459266, 28.71726448433411960, -2.638427012816827677 ) ) ;
#87210=CARTESIAN_POINT ( 'NONE',  ( 1.472469842513823179, 26.42559781766745175, 4.923371831947296329 ) ) ;
#87213=CARTESIAN_POINT ( 'NONE',  ( -2.266590686148945544, 31.38708216824730002, -7.082119434687050408 ) ) ;
#87214=CARTESIAN_POINT ( 'NONE',  ( 5.076628168052704559, 35.17559781766745175, -8.527530157486179263 ) ) ;
#87215=CARTESIAN_POINT ( 'NONE',  ( 20.88017736071110875, 60.77201867748817676, -2.915334737309920765 ) ) ;
#87217=CARTESIAN_POINT ( 'NONE',  ( 10.00000000000000000, 36.81368534415484106, -10.88017736071110342 ) ) ;
#87218=CARTESIAN_POINT ( 'NONE',  ( 2.791683348922240793, 46.63393115100077324, 7.208316651077764092 ) ) ;
#87221=ORIENTED_EDGE ( 'NONE', *, *, #29070, .F. ) ;
#87222=CARTESIAN_POINT ( 'NONE',  ( 24.16423886937409904, 14.09541550158063217, 3.795296366450317205 ) ) ;
#87224=VERTEX_POINT ( 'NONE', #83189 ) ;
#87225=( NAMED_UNIT ( * ) PLANE_ANGLE_UNIT ( ) SI_UNIT ( $, .RADIAN. ) );
#87226=CARTESIAN_POINT ( 'NONE',  ( -1.099225684535947600, 34.54030133659708923, 6.408140936763237150 ) ) ;
#87227=CARTESIAN_POINT ( 'NONE',  ( 12.63842701281683922, 24.55059781766745175, -9.846743663894590881 ) ) ;
#87230=CARTESIAN_POINT ( 'NONE',  ( 19.84674366389459266, 23.71726448433412315, -2.638427012816827677 ) ) ;
#87231=B_SPLINE_CURVE_WITH_KNOTS ( 'NONE', 3,
 ( #71643, #94628, #1689, #26139 ),
 .UNSPECIFIED., .F., .F.,
 ( 4, 4 ),
 ( 7.757919228897728493E-18, 0.002392975128318426507 ),
 .UNSPECIFIED. ) ;
#87235=CARTESIAN_POINT ( 'NONE',  ( 10.00000000000000000, 61.81368534415484106, -10.88017736071110342 ) ) ;
#87239=CARTESIAN_POINT ( 'NONE',  ( 7.084665262690076126, 69.10535201082151957, 10.88017736071109987 ) ) ;
#87240=CARTESIAN_POINT ( 'NONE',  ( 22.81628187352647785, 11.62363466993042138, 6.195893100308588602E-16 ) ) ;
#87242=CARTESIAN_POINT ( 'NONE',  ( 5.076628168052703671, 41.84226448433411605, 8.527530157486179263 ) ) ;
#87243=LINE ( 'NONE', #10770, #2644 ) ;
#87244=CARTESIAN_POINT ( 'NONE',  ( 24.16423886937409904, 14.09541550158063217, 3.795296366450317205 ) ) ;
#87245=CARTESIAN_POINT ( 'NONE',  ( 12.63842701281683034, 37.46726448433411605, 9.846743663894596210 ) ) ;
#87246=CARTESIAN_POINT ( 'NONE',  ( 22.81628187352648496, 31.83196800326375353, -3.434112377981050290 ) ) ;
#87247=CARTESIAN_POINT ( 'NONE',  ( 1.707155281725164508, 17.90189080397290056, 6.499999999999992006 ) ) ;
#87249=CARTESIAN_POINT ( 'NONE',  ( 4.559911319644449179, 67.23035201082150536, -9.422509992056141925 ) ) ;
#87251=CARTESIAN_POINT ( 'NONE',  ( 6.565887622018943937, 5.165301336597086568, 12.81628187352647430 ) ) ;
#87252=CARTESIAN_POINT ( 'NONE',  ( 5.500000000000000000, 60.50000000000000000, -5.000000000000000000 ) ) ;
#87253=CARTESIAN_POINT ( 'NONE',  ( 0.1532563361054083140, 36.00893115100078745, 1.131784320476157264E-15 ) ) ;
#87254=CARTESIAN_POINT ( 'NONE',  ( 0.5774900079438607392, 28.48035201082150891, 5.440088680355550821 ) ) ;
#87255=CARTESIAN_POINT ( 'NONE',  ( 22.81628187352648496, 26.83196800326374998, -3.434112377981050290 ) ) ;
#87261=CARTESIAN_POINT ( 'NONE',  ( 4.559911319644449179, 33.89701867748817676, 9.422509992056141925 ) ) ;
#87264=CARTESIAN_POINT ( 'NONE',  ( 15.44008868035555793, 61.39701867748817676, -9.422509992056140149 ) ) ;
#87265=CARTESIAN_POINT ( 'NONE',  ( 7.084665262690076126, 4.105352010821503583, 10.88017736071109987 ) ) ;
#87266=CARTESIAN_POINT ( 'NONE',  ( 18.52753015748617571, 43.09226448433412315, 4.923371831947298993 ) ) ;
#87267=CARTESIAN_POINT ( 'NONE',  ( 10.00000000000000000, 36.81368534415484106, -10.88017736071110342 ) ) ;
#87268=CARTESIAN_POINT ( 'NONE',  ( -0.8801773607110991993, 42.85535201082150536, -2.915334737309923874 ) ) ;
#87269=CARTESIAN_POINT ( 'NONE',  ( 17.96484262340118221, 16.18868534415483396, -7.964842623401177768 ) ) ;
#87271=CARTESIAN_POINT ( 'NONE',  ( 19.72487221294570858, 0.000000000000000000, -6.500000000000000888 ) ) ;
#87272=CARTESIAN_POINT ( 'NONE',  ( 10.00000000000000000, 34.75893115100078745, -9.846743663894594434 ) ) ;
#87273=CARTESIAN_POINT ( 'NONE',  ( 24.16423886937410614, 54.30374883491396787, 8.672049930838204340E-16 ) ) ;
#87277=CARTESIAN_POINT ( 'NONE',  ( 2.917880565312950480, 35.97041550158063217, -12.26659068614894821 ) ) ;
#87278=DIRECTION ( 'NONE',  ( -0.000000000000000000, -0.000000000000000000, -1.000000000000000000 ) ) ;
#87280=CARTESIAN_POINT ( 'NONE',  ( 4.559911319644449179, 2.230352010821504916, -9.422509992056141925 ) ) ;
#87281=CARTESIAN_POINT ( 'NONE',  ( 14.92337183194729988, 29.34226448433411960, -8.527530157486177487 ) ) ;
#87284=CARTESIAN_POINT ( 'NONE',  ( 17.96484262340118221, 64.93868534415483396, 7.964842623401181321 ) ) ;
#87287=CARTESIAN_POINT ( 'NONE',  ( 2.035157376598822676, 37.43868534415484106, -7.964842623401177768 ) ) ;
#87288=CARTESIAN_POINT ( 'NONE',  ( -2.816281873526473856, 64.33196800326376774, 3.434112377981055619 ) ) ;
#87289=CARTESIAN_POINT ( 'NONE',  ( -2.816281873526471635, 13.91530133659708746, -3.434112377981056508 ) ) ;
#87290=CARTESIAN_POINT ( 'NONE',  ( 1.472469842513823179, 11.42559781766745175, 4.923371831947296329 ) ) ;
#87294=CARTESIAN_POINT ( 'NONE',  ( 0.2751277870542949144, 4.366073187301309666, -6.499999999999997335 ) ) ;
#87295=CARTESIAN_POINT ( 'NONE',  ( 22.26659068614894466, 63.88708216824730357, 7.082119434687054849 ) ) ;
#87296=CARTESIAN_POINT ( 'NONE',  ( 17.08211943468705130, 28.47041550158063572, 12.26659068614894998 ) ) ;
#87297=CARTESIAN_POINT ( 'NONE',  ( -0.8801773607111008646, 38.27201867748816255, 2.915334737309923430 ) ) ;
#87298=CARTESIAN_POINT ( 'NONE',  ( 4.559911319644449179, 48.89701867748817676, 9.422509992056141925 ) ) ;
#87301=CARTESIAN_POINT ( 'NONE',  ( 17.20831665107776587, 9.133931151000787452, -7.208316651077762316 ) ) ;
#87302=( NAMED_UNIT ( * ) PLANE_ANGLE_UNIT ( ) SI_UNIT ( $, .RADIAN. ) );
#87303=CARTESIAN_POINT ( 'NONE',  ( 10.00000000000000178, 27.25893115100078390, 9.846743663894594434 ) ) ;
#87304=CARTESIAN_POINT ( 'NONE',  ( 19.72487221294570858, 56.86607318730075633, 6.500000000000000888 ) ) ;
#87306=CARTESIAN_POINT ( 'NONE',  ( 0.1532563361054082862, 26.21726448433411605, 2.638427012816831674 ) ) ;
#87307=CARTESIAN_POINT ( 'NONE',  ( 5.076628168052703671, 51.84226448433412315, 8.527530157486179263 ) ) ;
#87308=CARTESIAN_POINT ( 'NONE',  ( 15.44008868035555793, 21.39701867748817321, -9.422509992056140149 ) ) ;
#87309=EDGE_CURVE ( 'NONE', #86614, #20501, #45685, .T. ) ;
#87310=( GEOMETRIC_REPRESENTATION_CONTEXT ( 3 ) GLOBAL_UNCERTAINTY_ASSIGNED_CONTEXT ( ( #55197 ) ) GLOBAL_UNIT_ASSIGNED_CONTEXT ( ( #63724, #87702, #18244 ) ) REPRESENTATION_CONTEXT ( 'NONE', 'WORKASPACE' ) );
#87311=CARTESIAN_POINT ( 'NONE',  ( -1.099225684535947600, 49.54030133659708923, 6.408140936763237150 ) ) ;
#87312=CARTESIAN_POINT ( 'NONE',  ( 4.559911319644449179, 62.23035201082150536, -9.422509992056141925 ) ) ;
#87313=CARTESIAN_POINT ( 'NONE',  ( 19.84674366389459621, 28.50893115100078745, 7.409399052514197653E-17 ) ) ;
#87314=CARTESIAN_POINT ( 'NONE',  ( 22.26659068614895176, 54.72041550158063217, -7.082119434687042414 ) ) ;
#87315=CARTESIAN_POINT ( 'NONE',  ( 5.076628168052704559, 25.17559781766745175, -8.527530157486179263 ) ) ;
#87318=CARTESIAN_POINT ( 'NONE',  ( 19.84674366389459266, 63.71726448433412315, -2.638427012816827677 ) ) ;
#87319=CARTESIAN_POINT ( 'NONE',  ( 2.917880565312948704, 7.637082168247301794, 12.26659068614894643 ) ) ;
#87320=CARTESIAN_POINT ( 'NONE',  ( 10.00000000000000000, 30.55374883491397142, -14.16423886937410082 ) ) ;
#87321=CARTESIAN_POINT ( 'NONE',  ( 17.20831665107776587, 32.88393115100078745, 7.208316651077764980 ) ) ;
#87323=CARTESIAN_POINT ( 'NONE',  ( 7.084665262690076126, 29.10535201082150181, 10.88017736071109987 ) ) ;
#87324=CARTESIAN_POINT ( 'NONE',  ( -0.8801773607110991993, 62.85535201082150536, -2.915334737309923874 ) ) ;
#87325=CARTESIAN_POINT ( 'NONE',  ( 7.084665262690076126, 42.02201867748816966, -10.88017736071110164 ) ) ;
#87327=CARTESIAN_POINT ( 'NONE',  ( 19.38216949554541202, 40.99863466993042493, 9.382169495545424454 ) ) ;
#87329=CARTESIAN_POINT ( 'NONE',  ( -0.8801773607110991993, 47.85535201082150536, -2.915334737309923874 ) ) ;
#87331=FILL_AREA_STYLE_COLOUR ( '', #88099 ) ;
#87335=VECTOR ( 'NONE', #69616, 1000.000000000000000 ) ;
#87336=CARTESIAN_POINT ( 'NONE',  ( -0.8801773607111009756, 68.06368534415484817, 1.068504757029289695E-15 ) ) ;
#87337=CARTESIAN_POINT ( 'NONE',  ( 15.44008868035555793, 6.397018677488170546, -9.422509992056140149 ) ) ;
#87341=CARTESIAN_POINT ( 'NONE',  ( 19.42250999205614548, 10.98035201082150536, -5.440088680355545492 ) ) ;
#87342=CARTESIAN_POINT ( 'NONE',  ( 0.1532563361054083140, 11.00893115100078568, 1.131784320476157264E-15 ) ) ;
#87343=CARTESIAN_POINT ( 'NONE',  ( 2.917880565312948704, 2.637082168247300906, 12.26659068614894643 ) ) ;
#87344=CARTESIAN_POINT ( 'NONE',  ( 0.1532563361054100626, 5.800597817667452638, -2.638427012816831230 ) ) ;
#87345=CARTESIAN_POINT ( 'NONE',  ( 20.88017736071110519, 5.563685344154837509, 2.639326808657452039E-16 ) ) ;
#87346=CARTESIAN_POINT ( 'NONE',  ( 10.00000000000000178, 52.25893115100078745, 9.846743663894594434 ) ) ;
#87347=ORIENTED_EDGE ( 'NONE', *, *, #15317, .F. ) ;
#87348=CARTESIAN_POINT ( 'NONE',  ( 2.791683348922240793, 51.63393115100078745, 7.208316651077764092 ) ) ;
#87349=VERTEX_POINT ( 'NONE', #7704 ) ;
#87351=CARTESIAN_POINT ( 'NONE',  ( -0.8801773607110991993, 57.85535201082149825, -2.915334737309923874 ) ) ;
#87352=CARTESIAN_POINT ( 'NONE',  ( 17.20831665107776587, 57.88393115100078745, 7.208316651077764980 ) ) ;
#87353=MECHANICAL_DESIGN_GEOMETRIC_PRESENTATION_REPRESENTATION('',(#95345),#57011);
#87354=CARTESIAN_POINT ( 'NONE',  ( 2.035157376598822676, 2.438685344154837953, -7.964842623401177768 ) ) ;
#87356=CARTESIAN_POINT ( 'NONE',  ( 15.44008868035555793, 61.39701867748817676, -9.422509992056140149 ) ) ;
#87357=CARTESIAN_POINT ( 'NONE',  ( 4.559911319644449179, 3.897018677488171434, 9.422509992056141925 ) ) ;
#87359=CARTESIAN_POINT ( 'NONE',  ( 0.6178305044545818747, 43.49863466993042493, -9.382169495545419124 ) ) ;
#87360=CARTESIAN_POINT ( 'NONE',  ( 19.42250999205614193, 35.14701867748816966, 5.440088680355555262 ) ) ;
#87362=ORIENTED_EDGE ( 'NONE', *, *, #67090, .F. ) ;
#87363=CARTESIAN_POINT ( 'NONE',  ( 3.591859063236761518, 44.95696800326376064, 11.09922568453594849 ) ) ;
#87364=CARTESIAN_POINT ( 'NONE',  ( 17.96484262340118221, 36.18868534415484106, -7.964842623401177768 ) ) ;
#87367=CARTESIAN_POINT ( 'NONE',  ( 12.63842701281683034, 57.46726448433411605, 9.846743663894596210 ) ) ;
#87368=CARTESIAN_POINT ( 'NONE',  ( 17.20831665107776587, 9.133931151000787452, -7.208316651077762316 ) ) ;
#87369=CARTESIAN_POINT ( 'NONE',  ( 0.1532563361054082862, 46.21726448433411605, 2.638427012816831674 ) ) ;
#87370=CARTESIAN_POINT ( 'NONE',  ( -0.1503990784575287842, 28.10158574516642815, 6.262539305110075283 ) ) ;
#87372=CARTESIAN_POINT ( 'NONE',  ( 14.92337183194729633, 37.67559781766745175, 8.527530157486181039 ) ) ;
#87374=LINE ( 'NONE', #3392, #27698 ) ;
#87375=CARTESIAN_POINT ( 'NONE',  ( 19.84674366389459621, 23.50893115100078390, 7.409399052514197653E-17 ) ) ;
#87376=CARTESIAN_POINT ( 'NONE',  ( 1.472469842513823179, 1.425597817667451528, 4.923371831947296329 ) ) ;
#87378=CARTESIAN_POINT ( 'NONE',  ( 1.472469842513823179, 55.59226448433412315, -4.923371831947296329 ) ) ;
#87381=CARTESIAN_POINT ( 'NONE',  ( 22.81628187352647785, 21.62363466993041783, 6.195893100308588602E-16 ) ) ;
#87382=CARTESIAN_POINT ( 'NONE',  ( 1.472469842513823179, 40.59226448433411605, -4.923371831947296329 ) ) ;
#87383=DIRECTION ( 'NONE',  ( 0.000000000000000000, -1.000000000000000000, 0.000000000000000000 ) ) ;
#87384=VECTOR ( 'NONE', #70057, 1000.000000000000000 ) ;
#87385=CARTESIAN_POINT ( 'NONE',  ( 22.26659068614895176, 64.72041550158064638, -7.082119434687042414 ) ) ;
#87386=CARTESIAN_POINT ( 'NONE',  ( 19.84674366389459266, 23.30059781766745530, 2.638427012816836559 ) ) ;
#87388=CARTESIAN_POINT ( 'NONE',  ( -0.1503990784575277295, 39.24884699246889141, -6.262539305110077947 ) ) ;
#87389=CARTESIAN_POINT ( 'NONE',  ( -4.164238869374098151, 56.59541550158063927, -3.795296366450310543 ) ) ;
#87390=CARTESIAN_POINT ( 'NONE',  ( 19.84674366389459266, 53.71726448433411605, -2.638427012816827677 ) ) ;
#87391=CARTESIAN_POINT ( 'NONE',  ( 4.559911319644449179, 3.897018677488171434, 9.422509992056141925 ) ) ;
#87392=CARTESIAN_POINT ( 'NONE',  ( -0.3689425029237898834, 36.17874883491396787, -10.36894250292378850 ) ) ;
#87394=CARTESIAN_POINT ( 'NONE',  ( 6.204703633549690345, 45.76208216824729647, -14.16423886937410259 ) ) ;
#87397=CARTESIAN_POINT ( 'NONE',  ( 5.076628168052704559, 60.17559781766745175, -8.527530157486179263 ) ) ;
#87400=CARTESIAN_POINT ( 'NONE',  ( 15.44008868035555793, 51.39701867748816966, -9.422509992056140149 ) ) ;
#87401=CARTESIAN_POINT ( 'NONE',  ( 20.00000000000000711, 92.18909449964071712, -4.886738312952714658 ) ) ;
#87402=CARTESIAN_POINT ( 'NONE',  ( 14.92337183194729988, 54.34226448433412315, -8.527530157486177487 ) ) ;
#87404=B_SPLINE_CURVE_WITH_KNOTS ( 'NONE', 3,
 ( #7737, #46216, #15241, #45222 ),
 .UNSPECIFIED., .F., .F.,
 ( 4, 4 ),
 ( 0.000000000000000000, 0.0004111141682194737997 ),
 .UNSPECIFIED. ) ;
#87405=CARTESIAN_POINT ( 'NONE',  ( 10.00000000000000178, 57.25893115100078745, 9.846743663894594434 ) ) ;
#87406=CARTESIAN_POINT ( 'NONE',  ( 0.1532563361054083140, 66.00893115100079456, 1.131784320476157264E-15 ) ) ;
#87407=CARTESIAN_POINT ( 'NONE',  ( 6.204703633549690345, 20.76208216824730357, -14.16423886937410259 ) ) ;
#87410=CARTESIAN_POINT ( 'NONE',  ( 4.559911319644449179, 17.23035201082150536, -9.422509992056141925 ) ) ;
#87411=CARTESIAN_POINT ( 'NONE',  ( 13.43411237798105340, 20.58196800326374643, 12.81628187352647963 ) ) ;
#87413=CARTESIAN_POINT ( 'NONE',  ( 0.1532563361054082862, 11.21726448433411605, 2.638427012816831674 ) ) ;
#87415=CARTESIAN_POINT ( 'NONE',  ( 22.26659068614895176, 24.72041550158063572, -7.082119434687042414 ) ) ;
#87417=CARTESIAN_POINT ( 'NONE',  ( 20.15039907845753930, 70.00000000000000000, -6.262539305110068177 ) ) ;
#87418=CARTESIAN_POINT ( 'NONE',  ( 20.88017736071110875, 5.772018677488170546, -2.915334737309920765 ) ) ;
#87421=CARTESIAN_POINT ( 'NONE',  ( 20.88017736071110519, 35.56368534415484106, 2.639326808657452039E-16 ) ) ;
#87422=CARTESIAN_POINT ( 'NONE',  ( 20.88017736071110164, 40.35535201082150536, 2.915334737309930979 ) ) ;
#87423=CARTESIAN_POINT ( 'NONE',  ( 17.20831665107776587, 64.13393115100079456, -7.208316651077762316 ) ) ;
#87424=FILL_AREA_STYLE ('',( #27409 ) ) ;
#87425=CARTESIAN_POINT ( 'NONE',  ( 1.941103589310612554, 1.227327784520227727, 6.500000000000002665 ) ) ;
#87426=CARTESIAN_POINT ( 'NONE',  ( 18.52753015748618282, 8.925597817667451750, -4.923371831947291888 ) ) ;
#87429=CARTESIAN_POINT ( 'NONE',  ( 2.035157376598824452, 48.68868534415483396, 7.964842623401179544 ) ) ;
#87430=UNCERTAINTY_MEASURE_WITH_UNIT (LENGTH_MEASURE( 1.000000000000000082E-05 ), #37746, 'distance_accuracy_value', 'NONE');
#87431=CARTESIAN_POINT ( 'NONE',  ( 21.09922568453595559, 12.04030133659708746, -6.408140936763230044 ) ) ;
#87432=CARTESIAN_POINT ( 'NONE',  ( 7.084665262690076126, 62.02201867748816966, -10.88017736071110164 ) ) ;
#87433=CARTESIAN_POINT ( 'NONE',  ( 5.076628168052703671, 26.84226448433411960, 8.527530157486179263 ) ) ;
#87435=CARTESIAN_POINT ( 'NONE',  ( 10.00000000000000000, 32.87363466993042493, -12.81628187352647608 ) ) ;
#87436=CARTESIAN_POINT ( 'NONE',  ( 1.472469842513823179, 6.425597817667451750, 4.923371831947296329 ) ) ;
#87440=CARTESIAN_POINT ( 'NONE',  ( 15.44008868035555260, 4.730352010821504471, 9.422509992056143702 ) ) ;
#87441=CARTESIAN_POINT ( 'NONE',  ( 21.09922568453594849, 56.20696800326375353, 6.408140936763242479 ) ) ;
#87442=CARTESIAN_POINT ( 'NONE',  ( -2.266590686148945544, 21.38708216824730357, -7.082119434687050408 ) ) ;
#87443=CARTESIAN_POINT ( 'NONE',  ( 19.84674366389459621, 28.50893115100078745, 7.409399052514197653E-17 ) ) ;
#87444=CARTESIAN_POINT ( 'NONE',  ( -0.8801773607111008646, 3.272018677488171434, 2.915334737309923430 ) ) ;
#87446=CARTESIAN_POINT ( 'NONE',  ( 12.91533473730992121, 9.522018677488171434, 10.88017736071110164 ) ) ;
#87448=CARTESIAN_POINT ( 'NONE',  ( 15.44008868035555793, 16.39701867748817321, -9.422509992056140149 ) ) ;
#87449=CARTESIAN_POINT ( 'NONE',  ( 0.5774900079438607392, 23.48035201082150536, 5.440088680355550821 ) ) ;
#87451=AXIS2_PLACEMENT_3D ( 'NONE', #43546, #59541, #44038 ) ;
#87453=CARTESIAN_POINT ( 'NONE',  ( 5.076628168052703671, 61.84226448433412315, 8.527530157486179263 ) ) ;
#87454=CARTESIAN_POINT ( 'NONE',  ( 15.44008868035555793, 21.39701867748817321, -9.422509992056140149 ) ) ;
#87455=CARTESIAN_POINT ( 'NONE',  ( 1.472469842513823179, 61.42559781766745175, 4.923371831947296329 ) ) ;
#87457=CARTESIAN_POINT ( 'NONE',  ( 3.591859063236763294, 53.29030133659708923, -11.09922568453595026 ) ) ;
#87458=CARTESIAN_POINT ( 'NONE',  ( -1.926860441876564023, 4.688309369127507509, 1.004413902775740781E-15 ) ) ;
#87459=CARTESIAN_POINT ( 'NONE',  ( -2.266590686148945544, 32.22041550158063927, 7.082119434687048631 ) ) ;
#87460=CARTESIAN_POINT ( 'NONE',  ( 7.084665262690076126, 42.02201867748816966, -10.88017736071110164 ) ) ;
#87461=CARTESIAN_POINT ( 'NONE',  ( 10.00000000000000178, 19.31368534415484106, 10.88017736071110342 ) ) ;
#87462=CARTESIAN_POINT ( 'NONE',  ( 0.1532563361054083140, 61.00893115100078745, 1.131784320476157264E-15 ) ) ;
#87464=CARTESIAN_POINT ( 'NONE',  ( 5.076628168052704559, 55.17559781766745175, -8.527530157486179263 ) ) ;
#87465=DIRECTION ( 'NONE',  ( -0.000000000000000000, 1.000000000000000000, -0.000000000000000000 ) ) ;
#87466=CARTESIAN_POINT ( 'NONE',  ( 5.076628168052703671, 6.842264484334118713, 8.527530157486179263 ) ) ;
#87470=CARTESIAN_POINT ( 'NONE',  ( 19.42250999205614548, 10.98035201082150358, -5.440088680355545492 ) ) ;
#87471=CARTESIAN_POINT ( 'NONE',  ( 0.1532563361054083140, 6.008931151000784787, 1.131784320476157264E-15 ) ) ;
#87472=CARTESIAN_POINT ( 'NONE',  ( 21.09922568453594849, 1.206968003263753531, 6.408140936763242479 ) ) ;
#87473=CARTESIAN_POINT ( 'NONE',  ( 15.44008868035555793, 51.39701867748816966, -9.422509992056140149 ) ) ;
#87474=CARTESIAN_POINT ( 'NONE',  ( 4.559911319644449179, 18.89701867748817321, 9.422509992056141925 ) ) ;
#87475=CARTESIAN_POINT ( 'NONE',  ( 13.43411237798106583, 37.66530133659708923, -12.81628187352647252 ) ) ;
#87476=CARTESIAN_POINT ( 'NONE',  ( 2.917880565312950480, 35.97041550158063217, -12.26659068614894821 ) ) ;
#87479=CARTESIAN_POINT ( 'NONE',  ( 21.92686044187656691, 12.18830936912750751, 4.562052436263911564E-16 ) ) ;
#87480=CARTESIAN_POINT ( 'NONE',  ( 19.38216949554541557, 52.24863466993041072, -9.382169495545420901 ) ) ;
#87482=CARTESIAN_POINT ( 'NONE',  ( 19.84674366389459266, 53.71726448433411605, -2.638427012816827677 ) ) ;
#87484=CARTESIAN_POINT ( 'NONE',  ( -0.8801773607111008646, 33.27201867748817676, 2.915334737309923430 ) ) ;
#87485=CARTESIAN_POINT ( 'NONE',  ( 18.52753015748618282, 58.92559781766745886, -4.923371831947291888 ) ) ;
#87487=CARTESIAN_POINT ( 'NONE',  ( 0.5774900079438590739, 67.64701867748817676, -5.440088680355550821 ) ) ;
#87490=CARTESIAN_POINT ( 'NONE',  ( 14.92337183194729633, 12.67559781766745353, 8.527530157486181039 ) ) ;
#87491=CARTESIAN_POINT ( 'NONE',  ( 18.52753015748617571, 18.09226448433411960, 4.923371831947298993 ) ) ;
#87492=CARTESIAN_POINT ( 'NONE',  ( 2.791683348922237240, 10.38393115100078390, -7.208316651077763204 ) ) ;
#87493=CARTESIAN_POINT ( 'NONE',  ( 4.559911319644449179, 57.23035201082150536, -9.422509992056141925 ) ) ;
#87494=CARTESIAN_POINT ( 'NONE',  ( 0.8952175423694801459, 37.60160829253886305, -5.990408912944315212 ) ) ;
#87495=CARTESIAN_POINT ( 'NONE',  ( 20.88017736071110519, 65.56368534415483396, 2.639326808657452039E-16 ) ) ;
#87496=CARTESIAN_POINT ( 'NONE',  ( 18.52753015748618282, 23.92559781766745530, -4.923371831947291888 ) ) ;
#87500=CARTESIAN_POINT ( 'NONE',  ( 14.92337183194729988, 59.34226448433412315, -8.527530157486177487 ) ) ;
#87502=CARTESIAN_POINT ( 'NONE',  ( -28.94000000000001549, 93.50000000000000000, 9.500000000000000000 ) ) ;
#87503=CARTESIAN_POINT ( 'NONE',  ( -2.266590686148945544, 21.38708216824730357, -7.082119434687050408 ) ) ;
#87504=ADVANCED_FACE ( 'NONE', ( #55137 ), #77644, .T. ) ;
#87505=UNCERTAINTY_MEASURE_WITH_UNIT (LENGTH_MEASURE( 1.000000000000000082E-05 ), #40885, 'distance_accuracy_value', 'NONE');
#87507=CARTESIAN_POINT ( 'NONE',  ( 10.00000000000000178, 13.05374883491396787, 14.16423886937410082 ) ) ;
#87508=CARTESIAN_POINT ( 'NONE',  ( 20.36894250292379738, 29.92874883491396432, -10.36894250292379027 ) ) ;
#87509=CARTESIAN_POINT ( 'NONE',  ( 12.91533473730992121, 39.52201867748817676, 10.88017736071110164 ) ) ;
#87510=SURFACE_STYLE_USAGE ( .BOTH. , #49019 ) ;
#87511=ORIENTED_EDGE ( 'NONE', *, *, #13948, .F. ) ;
#87512=( BOUNDED_CURVE ( )  B_SPLINE_CURVE ( 2, ( #66543, #22540, #21548, #91517, #23034, #83029, #52039, #15043, #90513 ),
 .UNSPECIFIED., .F., .F. ) 
 B_SPLINE_CURVE_WITH_KNOTS ( ( 3, 2, 2, 2, 3 ),
 ( 0.6187123655116599785, 0.6190476190476190688, 0.6250000000000000000, 0.6309523809523809312, 0.6312876344883400215 ),
 .UNSPECIFIED. ) 
 CURVE ( )  GEOMETRIC_REPRESENTATION_ITEM ( )  RATIONAL_B_SPLINE_CURVE ( ( 0.9963778908391764944, 0.9980808541467923733, 1.000000000000000000, 0.9659258262890682012, 1.000000000000000000, 0.9659258262890682012, 1.000000000000000000, 0.9980808541467922623, 0.9963778908391764944 ) ) 
 REPRESENTATION_ITEM ( '' )  );
#87513=CARTESIAN_POINT ( 'NONE',  ( 0.1532563361054082862, 11.21726448433411605, 2.638427012816831674 ) ) ;
#87514=CARTESIAN_POINT ( 'NONE',  ( 20.88017736071110875, 55.77201867748816966, -2.915334737309920765 ) ) ;
#87515=CARTESIAN_POINT ( 'NONE',  ( 12.63842701281683034, 12.46726448433411782, 9.846743663894596210 ) ) ;
#87516=CARTESIAN_POINT ( 'NONE',  ( -1.099225684535947600, 48.70696800326375353, -6.408140936763238038 ) ) ;
#87517=CARTESIAN_POINT ( 'NONE',  ( 17.20831665107776587, 34.13393115100078745, -7.208316651077762316 ) ) ;
#87518=CARTESIAN_POINT ( 'NONE',  ( 0.1143410931637231370, 25.21691075486303291, 6.480892540919854561 ) ) ;
#87519=CARTESIAN_POINT ( 'NONE',  ( 16.40814093676323893, 30.79030133659708923, 11.09922568453595026 ) ) ;
#87521=CARTESIAN_POINT ( 'NONE',  ( 0.1532563361054100626, 30.80059781766744820, -2.638427012816831230 ) ) ;
#87522=CARTESIAN_POINT ( 'NONE',  ( -4.164238869374099039, 16.80374883491396787, 8.674139862899312516E-16 ) ) ;
#87525=CARTESIAN_POINT ( 'NONE',  ( 2.035157376598824452, 43.68868534415484106, 7.964842623401179544 ) ) ;
#87526=CARTESIAN_POINT ( 'NONE',  ( 15.44008868035555260, 54.73035201082150536, 9.422509992056143702 ) ) ;
#87527=CARTESIAN_POINT ( 'NONE',  ( 24.16423886937409904, 44.09541550158063927, 3.795296366450317205 ) ) ;
#87528=CARTESIAN_POINT ( 'NONE',  ( 10.00000000000000000, 49.75893115100078745, -9.846743663894594434 ) ) ;
#87529=CARTESIAN_POINT ( 'NONE',  ( 7.361572987183170547, 12.05059781766744997, 9.846743663894590881 ) ) ;
#87530=CARTESIAN_POINT ( 'NONE',  ( 0.6178305044545818747, 63.49863466993043204, -9.382169495545419124 ) ) ;
#87532=CARTESIAN_POINT ( 'NONE',  ( 19.42250999205614548, 35.98035201082151247, -5.440088680355545492 ) ) ;
#87535=CARTESIAN_POINT ( 'NONE',  ( 21.09922568453595559, 27.04030133659708568, -6.408140936763230044 ) ) ;
#87536=CARTESIAN_POINT ( 'NONE',  ( 0.1532563361054082862, 56.21726448433411605, 2.638427012816831674 ) ) ;
#87538=CARTESIAN_POINT ( 'NONE',  ( 15.44008868035555260, 4.730352010821504471, 9.422509992056143702 ) ) ;
#87539=CARTESIAN_POINT ( 'NONE',  ( 10.00000000000000178, 69.31368534415484817, 10.88017736071110342 ) ) ;
#87541=VECTOR ( 'NONE', #53425, 1000.000000000000000 ) ;
#87542=CARTESIAN_POINT ( 'NONE',  ( 0.5774900079438590739, 2.647018677488170990, -5.440088680355550821 ) ) ;
#87544=CARTESIAN_POINT ( 'NONE',  ( 7.084665262690076126, 67.02201867748817676, -10.88017736071110164 ) ) ;
#87545=CARTESIAN_POINT ( 'NONE',  ( 14.92337183194729633, 2.675597817667451750, 8.527530157486181039 ) ) ;
#87547=CARTESIAN_POINT ( 'NONE',  ( 0.1532563361054082862, 41.21726448433411605, 2.638427012816831674 ) ) ;
#87548=CARTESIAN_POINT ( 'NONE',  ( 20.88017736071110875, 25.77201867748816966, -2.915334737309920765 ) ) ;
#87549=CARTESIAN_POINT ( 'NONE',  ( 22.81628187352648496, 1.831968003263753753, -3.434112377981050290 ) ) ;
#87550=CARTESIAN_POINT ( 'NONE',  ( -0.8801773607111009756, 33.06368534415484106, 1.068504757029289695E-15 ) ) ;
#87553=CARTESIAN_POINT ( 'NONE',  ( -2.816281873526471635, 38.91530133659708213, -3.434112377981056508 ) ) ;
#87555=CARTESIAN_POINT ( 'NONE',  ( 19.42250999205614548, 45.98035201082150536, -5.440088680355545492 ) ) ;
#87556=CARTESIAN_POINT ( 'NONE',  ( -2.816281873526471635, 23.91530133659708568, -3.434112377981056508 ) ) ;
#87557=( NAMED_UNIT ( * ) SI_UNIT ( $, .STERADIAN. ) SOLID_ANGLE_UNIT ( ) );
#87558=CARTESIAN_POINT ( 'NONE',  ( 17.96484262340118221, 26.18868534415483396, -7.964842623401177768 ) ) ;
#87559=CARTESIAN_POINT ( 'NONE',  ( 7.084665262690076126, 2.022018677488171434, -10.88017736071110164 ) ) ;
#87560=CARTESIAN_POINT ( 'NONE',  ( 7.361572987183170547, 42.05059781766745886, 9.846743663894590881 ) ) ;
#87561=CARTESIAN_POINT ( 'NONE',  ( 0.1532563361054083140, 6.008931151000784787, 1.131784320476157264E-15 ) ) ;
#87562=CARTESIAN_POINT ( 'NONE',  ( -0.8801773607111009756, 63.06368534415484106, 1.068504757029289695E-15 ) ) ;
#87564=CARTESIAN_POINT ( 'NONE',  ( 24.16423886937410614, 24.51208216824730002, -3.795296366450302550 ) ) ;
#87565=DIRECTION ( 'NONE',  ( 0.000000000000000000, 0.000000000000000000, 1.000000000000000000 ) ) ;
#87569=CARTESIAN_POINT ( 'NONE',  ( 17.08211943468705130, 43.47041550158063927, 12.26659068614894998 ) ) ;
#87570=CARTESIAN_POINT ( 'NONE',  ( 20.36894250292379382, 53.67874883491397497, 10.36894250292379205 ) ) ;
#87571=CARTESIAN_POINT ( 'NONE',  ( 2.791683348922240793, 16.63393115100078745, 7.208316651077764092 ) ) ;
#87572=CARTESIAN_POINT ( 'NONE',  ( -2.816281873526473856, 14.12363466993041961, 9.499525473075851096E-16 ) ) ;
#87575=CARTESIAN_POINT ( 'NONE',  ( 3.591859063236763294, 28.29030133659708568, -11.09922568453595026 ) ) ;
#87576=CARTESIAN_POINT ( 'NONE',  ( 20.36894250292379738, 44.92874883491396787, -10.36894250292379027 ) ) ;
#87581=CARTESIAN_POINT ( 'NONE',  ( 5.076628168052704559, 15.17559781766745175, -8.527530157486179263 ) ) ;
#87583=CARTESIAN_POINT ( 'NONE',  ( -4.164238869374099039, 11.80374883491396965, 8.674139862899312516E-16 ) ) ;
#87584=CARTESIAN_POINT ( 'NONE',  ( 7.084665262690076126, 12.02201867748817321, -10.88017736071110164 ) ) ;
#87585=CARTESIAN_POINT ( 'NONE',  ( 7.084665262690076126, 14.10535201082150358, 10.88017736071109987 ) ) ;
#87586=CARTESIAN_POINT ( 'NONE',  ( 5.076628168052703671, 51.84226448433412315, 8.527530157486179263 ) ) ;
#87587=CARTESIAN_POINT ( 'NONE',  ( 19.38216949554541557, 2.248634669930420049, -9.382169495545420901 ) ) ;
#87588=CARTESIAN_POINT ( 'NONE',  ( 19.72487221294570858, 0.000000000000000000, -6.500000000000000888 ) ) ;
#87591=CARTESIAN_POINT ( 'NONE',  ( -2.816281873526473856, 19.12363466993042138, 9.499525473075851096E-16 ) ) ;
#87593=CARTESIAN_POINT ( 'NONE',  ( -0.3689425029237898834, 61.17874883491396076, -10.36894250292378850 ) ) ;
#87595=CARTESIAN_POINT ( 'NONE',  ( -0.3689425029237881626, 57.42874883491397497, 10.36894250292379027 ) ) ;
#87597=CARTESIAN_POINT ( 'NONE',  ( 4.559911319644449179, 32.23035201082150536, -9.422509992056141925 ) ) ;
#87598=CARTESIAN_POINT ( 'NONE',  ( -0.8801773607111009756, 48.06368534415484817, 1.068504757029289695E-15 ) ) ;
#87600=CARTESIAN_POINT ( 'NONE',  ( 0.5774900079438607392, 48.48035201082150536, 5.440088680355550821 ) ) ;
#87601=CARTESIAN_POINT ( 'NONE',  ( 10.00000000000000178, 34.31368534415484106, 10.88017736071110342 ) ) ;
#87602=MECHANICAL_DESIGN_GEOMETRIC_PRESENTATION_REPRESENTATION('',(#22188),#74830);
#87606=CARTESIAN_POINT ( 'NONE',  ( 10.00000000000000000, 14.75893115100078568, -9.846743663894594434 ) ) ;
#87609=CARTESIAN_POINT ( 'NONE',  ( 0.1532563361054083140, 46.00893115100079456, 1.131784320476157264E-15 ) ) ;
#87611=CARTESIAN_POINT ( 'NONE',  ( 21.09922568453595559, 52.04030133659708923, -6.408140936763230044 ) ) ;
#87616=CARTESIAN_POINT ( 'NONE',  ( 14.92337183194729988, 64.34226448433412315, -8.527530157486177487 ) ) ;
#87617=CARTESIAN_POINT ( 'NONE',  ( 18.52753015748617571, 28.09226448433411960, 4.923371831947298993 ) ) ;
#87618=CARTESIAN_POINT ( 'NONE',  ( -2.266590686148945544, 61.38708216824730357, -7.082119434687050408 ) ) ;
#87620=VERTEX_POINT ( 'NONE', #33126 ) ;
#87621=CARTESIAN_POINT ( 'NONE',  ( 1.274849032794292736, 52.55509018479936856, -6.499999999999977796 ) ) ;
#87622=CARTESIAN_POINT ( 'NONE',  ( 17.20831665107776587, 29.13393115100078390, -7.208316651077762316 ) ) ;
#87624=CARTESIAN_POINT ( 'NONE',  ( 22.81628187352647785, 11.41530133659708390, 3.434112377981063169 ) ) ;
#87625=CARTESIAN_POINT ( 'NONE',  ( 10.00000000000000178, 69.31368534415484817, 10.88017736071110342 ) ) ;
#87628=CARTESIAN_POINT ( 'NONE',  ( 12.63842701281683922, 14.55059781766744997, -9.846743663894590881 ) ) ;
#87629=CARTESIAN_POINT ( 'NONE',  ( 7.361572987183169658, 54.96726448433413026, -9.846743663894592657 ) ) ;
#87632=CARTESIAN_POINT ( 'NONE',  ( 13.79529636645030344, 58.26208216824728936, 14.16423886937410614 ) ) ;
#87633=CARTESIAN_POINT ( 'NONE',  ( 10.00000000000000178, 3.053748834913967425, 14.16423886937410082 ) ) ;
#87634=CARTESIAN_POINT ( 'NONE',  ( 0.1532563361054100626, 15.80059781766745353, -2.638427012816831230 ) ) ;
#87635=CARTESIAN_POINT ( 'NONE',  ( 20.88017736071110875, 35.77201867748816966, -2.915334737309920765 ) ) ;
#87636=CARTESIAN_POINT ( 'NONE',  ( 0.6178305044545818747, 23.49863466993041783, -9.382169495545419124 ) ) ;
#87638=CARTESIAN_POINT ( 'NONE',  ( -0.8801773607111009756, 3.063685344154837509, 1.068504757029289695E-15 ) ) ;
#87641=CARTESIAN_POINT ( 'NONE',  ( 10.00000000000000000, 49.75893115100078745, -9.846743663894594434 ) ) ;
#87642=CARTESIAN_POINT ( 'NONE',  ( 10.00000000000000000, 9.758931151000785675, -9.846743663894594434 ) ) ;
#87644=CARTESIAN_POINT ( 'NONE',  ( 3.591859063236761518, 24.95696800326375353, 11.09922568453594849 ) ) ;
#87645=CARTESIAN_POINT ( 'NONE',  ( 2.377183314879991460, 50.78593319516822646, -6.500000000000057732 ) ) ;
#87646=CARTESIAN_POINT ( 'NONE',  ( 10.00000000000000178, 24.31368534415484106, 10.88017736071110342 ) ) ;
#87649=CARTESIAN_POINT ( 'NONE',  ( 24.16423886937410614, 44.51208216824730357, -3.795296366450302550 ) ) ;
#87651=CARTESIAN_POINT ( 'NONE',  ( 17.08211943468705840, 30.13708216824730357, -12.26659068614894466 ) ) ;
#87652=CARTESIAN_POINT ( 'NONE',  ( 14.92337183194729988, 39.34226448433412315, -8.527530157486177487 ) ) ;
#87653=CARTESIAN_POINT ( 'NONE',  ( -1.099225684535947600, 34.54030133659708923, 6.408140936763237150 ) ) ;
#87654=CARTESIAN_POINT ( 'NONE',  ( 20.88017736071110519, 30.56368534415484106, 2.639326808657452039E-16 ) ) ;
#87655=CARTESIAN_POINT ( 'NONE',  ( 7.361572987183170547, 57.05059781766744464, 9.846743663894590881 ) ) ;
#87656=CARTESIAN_POINT ( 'NONE',  ( 20.88017736071110519, 40.56368534415484106, 2.639326808657452039E-16 ) ) ;
#87657=CARTESIAN_POINT ( 'NONE',  ( 16.40814093676324603, 7.456968003263754419, -11.09922568453594671 ) ) ;
#87658=CARTESIAN_POINT ( 'NONE',  ( 17.08211943468705130, 23.47041550158063572, 12.26659068614894998 ) ) ;
#87660=CARTESIAN_POINT ( 'NONE',  ( 19.84674366389459621, 28.50893115100078745, 7.409399052514197653E-17 ) ) ;
#87661=CARTESIAN_POINT ( 'NONE',  ( 2.791683348922240793, 61.63393115100079456, 7.208316651077764092 ) ) ;
#87665=CARTESIAN_POINT ( 'NONE',  ( 10.00000000000000178, 19.31368534415484106, 10.88017736071110342 ) ) ;
#87666=CARTESIAN_POINT ( 'NONE',  ( 15.44008868035555260, 59.73035201082151247, 9.422509992056143702 ) ) ;
#87667=CARTESIAN_POINT ( 'NONE',  ( -4.164238869374099927, 7.012082168247302683, 3.795296366450308767 ) ) ;
#87668=CARTESIAN_POINT ( 'NONE',  ( 5.076628168052703671, 6.842264484334118713, 8.527530157486179263 ) ) ;
#87669=CARTESIAN_POINT ( 'NONE',  ( 1.472469842513823179, 51.42559781766745886, 4.923371831947296329 ) ) ;
#87670=CARTESIAN_POINT ( 'NONE',  ( 4.559911319644449179, 32.23035201082150536, -9.422509992056141925 ) ) ;
#87671=CARTESIAN_POINT ( 'NONE',  ( 18.95386800104995828, 13.23810908735726777, -6.500000000000000888 ) ) ;
#87672=PLANE ( 'NONE',  #32965 ) ;
#87678=ORIENTED_EDGE ( 'NONE', *, *, #78331, .T. ) ;
#87679=LINE ( 'NONE', #11693, #59693 ) ;
#87680=CARTESIAN_POINT ( 'NONE',  ( 17.08211943468705840, 5.137082168247300906, -12.26659068614894466 ) ) ;
#87681=CARTESIAN_POINT ( 'NONE',  ( 24.16423886937410614, 14.30374883491396787, 8.672049930838204340E-16 ) ) ;
#87682=CARTESIAN_POINT ( 'NONE',  ( 17.08211943468705840, 60.13708216824729647, -12.26659068614894466 ) ) ;
#87683=CARTESIAN_POINT ( 'NONE',  ( 5.076628168052703671, 56.84226448433412315, 8.527530157486179263 ) ) ;
#87684=CARTESIAN_POINT ( 'NONE',  ( 7.361572987183170547, 42.05059781766745886, 9.846743663894590881 ) ) ;
#87685=CARTESIAN_POINT ( 'NONE',  ( -1.099225684535947600, 64.54030133659709634, 6.408140936763237150 ) ) ;
#87686=CARTESIAN_POINT ( 'NONE',  ( 7.084665262690076126, 39.10535201082150536, 10.88017736071109987 ) ) ;
#87687=CARTESIAN_POINT ( 'NONE',  ( 17.20831665107776587, 59.13393115100078745, -7.208316651077762316 ) ) ;
#87688=CARTESIAN_POINT ( 'NONE',  ( 10.00000000000000000, 5.553748834913967869, -14.16423886937410082 ) ) ;
#87689=CARTESIAN_POINT ( 'NONE',  ( 6.204703633549690345, 52.84541550158062506, 14.16423886937410082 ) ) ;
#87690=CARTESIAN_POINT ( 'NONE',  ( 6.204703633549690345, 67.84541550158060375, 14.16423886937410082 ) ) ;
#87694=VERTEX_POINT ( 'NONE', #31654 ) ;
#87696=ORIENTED_EDGE ( 'NONE', *, *, #66191, .T. ) ;
#87697=CARTESIAN_POINT ( 'NONE',  ( 19.84674366389459266, 23.30059781766745530, 2.638427012816836559 ) ) ;
#87698=ORIENTED_EDGE ( 'NONE', *, *, #9489, .T. ) ;
#87699=CARTESIAN_POINT ( 'NONE',  ( 17.08211943468705130, 38.47041550158063217, 12.26659068614894998 ) ) ;
#87700=CARTESIAN_POINT ( 'NONE',  ( 7.361572987183170547, 32.05059781766745175, 9.846743663894590881 ) ) ;
#87701=CARTESIAN_POINT ( 'NONE',  ( -0.8801773607111009756, 53.06368534415484106, 1.068504757029289695E-15 ) ) ;
#87702=( NAMED_UNIT ( * ) PLANE_ANGLE_UNIT ( ) SI_UNIT ( $, .RADIAN. ) );
#87703=EDGE_CURVE ( 'NONE', #20606, #51688, #94589, .T. ) ;
#87704=CARTESIAN_POINT ( 'NONE',  ( 15.44008868035555260, 54.73035201082150536, 9.422509992056143702 ) ) ;
#87705=CARTESIAN_POINT ( 'NONE',  ( 14.92337183194729988, 49.34226448433411605, -8.527530157486177487 ) ) ;
#87706=EDGE_CURVE ( 'NONE', #66014, #91084, #7475, .T. ) ;
#87710=CARTESIAN_POINT ( 'NONE',  ( 10.00000000000000000, 20.55374883491396787, -14.16423886937410082 ) ) ;
#87712=ORIENTED_EDGE ( 'NONE', *, *, #85357, .T. ) ;
#87713=CARTESIAN_POINT ( 'NONE',  ( 6.565887622018943937, 28.08196800326375353, -12.81628187352647608 ) ) ;
#87714=DIRECTION ( 'NONE',  ( 0.8320502943378436100, -0.5547001962252291474, 0.000000000000000000 ) ) ;
#87715=CARTESIAN_POINT ( 'NONE',  ( 14.92337183194729633, 22.67559781766745175, 8.527530157486181039 ) ) ;
#87716=CARTESIAN_POINT ( 'NONE',  ( 4.559911319644449179, 18.89701867748817321, 9.422509992056141925 ) ) ;
#87718=CARTESIAN_POINT ( 'NONE',  ( -1.099225684535947600, 48.70696800326375353, -6.408140936763238038 ) ) ;
#87721=CARTESIAN_POINT ( 'NONE',  ( 17.20831665107776587, 27.88393115100078390, 7.208316651077764980 ) ) ;
#87723=CARTESIAN_POINT ( 'NONE',  ( 20.32896413005680714, 22.60497603579417714, -5.963430220938276349 ) ) ;
#87725=CARTESIAN_POINT ( 'NONE',  ( 7.084665262690076126, 64.10535201082150536, 10.88017736071109987 ) ) ;
#87726=CARTESIAN_POINT ( 'NONE',  ( 19.90229974777923161, 69.67742753483354079, 6.500000000000000000 ) ) ;
#87728=CARTESIAN_POINT ( 'NONE',  ( 0.1532563361054082862, 6.217264484334118713, 2.638427012816831674 ) ) ;
#87729=CARTESIAN_POINT ( 'NONE',  ( 3.591859063236761518, 29.95696800326375708, 11.09922568453594849 ) ) ;
#87732=CARTESIAN_POINT ( 'NONE',  ( 7.361572987183170547, 42.05059781766745886, 9.846743663894590881 ) ) ;
#87733=CARTESIAN_POINT ( 'NONE',  ( 19.10478245763047411, 36.02576239577082617, -5.990408912944397812 ) ) ;
#87734=CARTESIAN_POINT ( 'NONE',  ( -2.266590686148945544, 27.22041550158063572, 7.082119434687048631 ) ) ;
#87735=CARTESIAN_POINT ( 'NONE',  ( 12.63842701281683922, 29.55059781766745175, -9.846743663894590881 ) ) ;
#87736=CARTESIAN_POINT ( 'NONE',  ( 3.591859063236763294, 28.29030133659708568, -11.09922568453595026 ) ) ;
#87739=CARTESIAN_POINT ( 'NONE',  ( 15.44008868035555793, 56.39701867748817676, -9.422509992056140149 ) ) ;
#87740=CARTESIAN_POINT ( 'NONE',  ( 3.591859063236761518, 9.956968003263753531, 11.09922568453594849 ) ) ;
#87742=CARTESIAN_POINT ( 'NONE',  ( 10.00000000000000178, 37.25893115100078745, 9.846743663894594434 ) ) ;
#87743=CARTESIAN_POINT ( 'NONE',  ( 15.44008868035555793, 31.39701867748817676, -9.422509992056140149 ) ) ;
#87744=CARTESIAN_POINT ( 'NONE',  ( 21.09922568453594849, 26.20696800326375353, 6.408140936763242479 ) ) ;
#87747=CARTESIAN_POINT ( 'NONE',  ( 17.96484262340118221, 34.93868534415482685, 7.964842623401181321 ) ) ;
#87749=CARTESIAN_POINT ( 'NONE',  ( 7.084665262690076126, 62.02201867748816966, -10.88017736071110164 ) ) ;
#87750=FACE_OUTER_BOUND ( 'NONE', #40962, .T. ) ;
#87751=CARTESIAN_POINT ( 'NONE',  ( 7.361572987183169658, 54.96726448433413026, -9.846743663894592657 ) ) ;
#87752=CARTESIAN_POINT ( 'NONE',  ( 17.96484262340118221, 34.93868534415482685, 7.964842623401181321 ) ) ;
#87754=CARTESIAN_POINT ( 'NONE',  ( 17.96484262340118221, 44.93868534415483396, 7.964842623401181321 ) ) ;
#87755=CARTESIAN_POINT ( 'NONE',  ( -0.8801773607110991993, 22.85535201082150181, -2.915334737309923874 ) ) ;
#87756=CARTESIAN_POINT ( 'NONE',  ( 20.00000000000000711, 88.18949240714751170, -4.994480956901625746 ) ) ;
#87757=CARTESIAN_POINT ( 'NONE',  ( 18.52753015748618282, 3.925597817667451306, -4.923371831947291888 ) ) ;
#87759=CARTESIAN_POINT ( 'NONE',  ( 10.00000000000000178, 57.25893115100078745, 9.846743663894594434 ) ) ;
#87760=CARTESIAN_POINT ( 'NONE',  ( 2.917880565312948704, 57.63708216824731068, 12.26659068614894643 ) ) ;
#87765=CARTESIAN_POINT ( 'NONE',  ( 20.36894250292379738, 34.92874883491396076, -10.36894250292379027 ) ) ;
#87766=CARTESIAN_POINT ( 'NONE',  ( 10.00000000000000178, 5.373634669930420493, 12.81628187352647608 ) ) ;
#87768=ORIENTED_EDGE ( 'NONE', *, *, #9402, .F. ) ;
#87769=CARTESIAN_POINT ( 'NONE',  ( 10.00000000000000178, 63.05374883491396076, 14.16423886937410082 ) ) ;
#87770=CARTESIAN_POINT ( 'NONE',  ( 10.00000000000000178, 32.25893115100078745, 9.846743663894594434 ) ) ;
#87771=CARTESIAN_POINT ( 'NONE',  ( 3.640395162852214650, 89.00000000000000000, -9.500000000000000000 ) ) ;
#87773=CARTESIAN_POINT ( 'NONE',  ( 20.88017736071110519, 65.56368534415483396, 2.639326808657452039E-16 ) ) ;
#87775=CARTESIAN_POINT ( 'NONE',  ( 4.559911319644449179, 28.89701867748817321, 9.422509992056141925 ) ) ;
#87776=CARTESIAN_POINT ( 'NONE',  ( 3.591859063236763294, 58.29030133659708923, -11.09922568453595026 ) ) ;
#87777=CARTESIAN_POINT ( 'NONE',  ( 22.81628187352647785, 11.41530133659708390, 3.434112377981063169 ) ) ;
#87778=CARTESIAN_POINT ( 'NONE',  ( 14.92337183194729633, 32.67559781766745175, 8.527530157486181039 ) ) ;
#87780=( NAMED_UNIT ( * ) PLANE_ANGLE_UNIT ( ) SI_UNIT ( $, .RADIAN. ) );
#87781=CARTESIAN_POINT ( 'NONE',  ( 17.39651004071841811, 2.935752660568277328, 6.500000000000002665 ) ) ;
#87782=CARTESIAN_POINT ( 'NONE',  ( 10.00000000000000178, 63.05374883491396076, 14.16423886937410082 ) ) ;
#87783=CARTESIAN_POINT ( 'NONE',  ( 13.79529636645030344, 33.26208216824730357, 14.16423886937410614 ) ) ;
#87784=CARTESIAN_POINT ( 'NONE',  ( 20.88017736071110875, 35.77201867748816966, -2.915334737309920765 ) ) ;
#87785=CARTESIAN_POINT ( 'NONE',  ( 10.00000000000000178, 54.31368534415484106, 10.88017736071110342 ) ) ;
#87786=DIRECTION ( 'NONE',  ( 0.000000000000000000, 0.000000000000000000, -1.000000000000000000 ) ) ;
#87788=CARTESIAN_POINT ( 'NONE',  ( 0.1532563361054082862, 6.217264484334118713, 2.638427012816831674 ) ) ;
#87789=SURFACE_STYLE_FILL_AREA ( #49304 ) ;
#87791=CARTESIAN_POINT ( 'NONE',  ( 18.52753015748618282, 18.92559781766745175, -4.923371831947291888 ) ) ;
#87792=CARTESIAN_POINT ( 'NONE',  ( 10.00000000000000000, 44.75893115100078745, -9.846743663894594434 ) ) ;
#87793=CARTESIAN_POINT ( 'NONE',  ( 10.00000000000000178, 45.37363466993041783, 12.81628187352647608 ) ) ;
#87795=CARTESIAN_POINT ( 'NONE',  ( -0.8801773607111008646, 68.27201867748817676, 2.915334737309923430 ) ) ;
#87796=CARTESIAN_POINT ( 'NONE',  ( 7.361572987183169658, 34.96726448433411605, -9.846743663894592657 ) ) ;
#87797=CARTESIAN_POINT ( 'NONE',  ( 20.36894250292379738, 59.92874883491397497, -10.36894250292379027 ) ) ;
#87798=CARTESIAN_POINT ( 'NONE',  ( 14.92337183194729988, 19.34226448433411960, -8.527530157486177487 ) ) ;
#87800=CARTESIAN_POINT ( 'NONE',  ( 17.20831665107776587, 64.13393115100079456, -7.208316651077762316 ) ) ;
#87801=CARTESIAN_POINT ( 'NONE',  ( -4.164238869374098151, 31.59541550158063927, -3.795296366450310543 ) ) ;
#87802=CARTESIAN_POINT ( 'NONE',  ( 19.84674366389459266, 43.30059781766744464, 2.638427012816836559 ) ) ;
#87803=CARTESIAN_POINT ( 'NONE',  ( 19.72487221294570858, 12.80223176428831167, -6.500000000000000888 ) ) ;
#87804=CARTESIAN_POINT ( 'NONE',  ( 20.88017736071110164, 30.35535201082151247, 2.915334737309930979 ) ) ;
#87805=B_SPLINE_CURVE_WITH_KNOTS ( 'NONE', 3,
 ( #92362, #46854, #93344, #63330 ),
 .UNSPECIFIED., .F., .F.,
 ( 4, 4 ),
 ( 0.000000000000000000, 0.001036303429213365507 ),
 .UNSPECIFIED. ) ;
#87806=CARTESIAN_POINT ( 'NONE',  ( 0.5774900079438607392, 63.48035201082149825, 5.440088680355550821 ) ) ;
#87807=CARTESIAN_POINT ( 'NONE',  ( 19.10478245763052740, 51.02576239577081907, -5.990408912944300113 ) ) ;
#87808=ORIENTED_EDGE ( 'NONE', *, *, #11199, .T. ) ;
#87809=CARTESIAN_POINT ( 'NONE',  ( 19.38216949554541202, 45.99863466993041072, 9.382169495545424454 ) ) ;
#87811=CARTESIAN_POINT ( 'NONE',  ( 0.5774900079438590739, 57.64701867748817676, -5.440088680355550821 ) ) ;
#87812=ORIENTED_EDGE ( 'NONE', *, *, #81442, .F. ) ;
#87813=CARTESIAN_POINT ( 'NONE',  ( 18.52753015748618282, 63.92559781766745886, -4.923371831947291888 ) ) ;
#87814=CARTESIAN_POINT ( 'NONE',  ( 10.00000000000000000, 66.81368534415484817, -10.88017736071110342 ) ) ;
#87816=CARTESIAN_POINT ( 'NONE',  ( 12.91533473730992121, 64.52201867748817676, 10.88017736071110164 ) ) ;
#87818=CARTESIAN_POINT ( 'NONE',  ( 0.5774900079438590739, 12.64701867748817143, -5.440088680355550821 ) ) ;
#87819=CARTESIAN_POINT ( 'NONE',  ( 1.958556081791334780, 0.5155005897679896254, -5.765297895236029646 ) ) ;
#87821=CARTESIAN_POINT ( 'NONE',  ( 15.44008868035555260, 4.730352010821505360, 9.422509992056143702 ) ) ;
#87822=CARTESIAN_POINT ( 'NONE',  ( 0.1532563361054100626, 5.800597817667452638, -2.638427012816831230 ) ) ;
#87823=CARTESIAN_POINT ( 'NONE',  ( -2.266590686148945544, 12.22041550158063394, 7.082119434687048631 ) ) ;
#87826=CARTESIAN_POINT ( 'NONE',  ( 19.42250999205614193, 25.14701867748817321, 5.440088680355555262 ) ) ;
#87827=CARTESIAN_POINT ( 'NONE',  ( 18.52753015748618282, 58.92559781766745886, -4.923371831947291888 ) ) ;
#87828=ORIENTED_EDGE ( 'NONE', *, *, #46732, .F. ) ;
#87830=CARTESIAN_POINT ( 'NONE',  ( 2.791683348922237240, 55.38393115100078745, -7.208316651077763204 ) ) ;
#87832=CARTESIAN_POINT ( 'NONE',  ( -0.8801773607111008646, 48.27201867748816966, 2.915334737309923430 ) ) ;
#87833=CARTESIAN_POINT ( 'NONE',  ( 1.472469842513823179, 45.59226448433412315, -4.923371831947296329 ) ) ;
#87834=CARTESIAN_POINT ( 'NONE',  ( 19.42250999205614548, 10.98035201082150358, -5.440088680355545492 ) ) ;
#87836=CARTESIAN_POINT ( 'NONE',  ( 20.88017736071110164, 65.35535201082150536, 2.915334737309930979 ) ) ;
#87838=CARTESIAN_POINT ( 'NONE',  ( 17.96484262340118221, 4.938685344154837509, 7.964842623401181321 ) ) ;
#87839=EDGE_CURVE ( 'NONE', #44176, #93746, #57599, .T. ) ;
#87841=CARTESIAN_POINT ( 'NONE',  ( 19.38216949554541202, 35.99863466993041072, 9.382169495545424454 ) ) ;
#87842=CARTESIAN_POINT ( 'NONE',  ( 15.44008868035555793, 36.39701867748816966, -9.422509992056140149 ) ) ;
#87844=ORIENTED_EDGE ( 'NONE', *, *, #25585, .T. ) ;
#87845=CARTESIAN_POINT ( 'NONE',  ( 0.6178305044545838731, 39.74863466993041072, 9.382169495545420901 ) ) ;
#87846=CARTESIAN_POINT ( 'NONE',  ( 7.084665262690076126, 37.02201867748817676, -10.88017736071110164 ) ) ;
#87847=CARTESIAN_POINT ( 'NONE',  ( 18.52753015748618282, 58.92559781766745886, -4.923371831947291888 ) ) ;
#87851=CARTESIAN_POINT ( 'NONE',  ( 17.20831665107776587, 57.88393115100078745, 7.208316651077764980 ) ) ;
#87853=CARTESIAN_POINT ( 'NONE',  ( 5.076628168052703671, 51.84226448433412315, 8.527530157486179263 ) ) ;
#87854=CARTESIAN_POINT ( 'NONE',  ( 7.084665262690076126, 17.02201867748817676, -10.88017736071110164 ) ) ;
#87855=CARTESIAN_POINT ( 'NONE',  ( -28.94000000000001549, 93.50000000000000000, -10.09898361729590199 ) ) ;
#87856=CARTESIAN_POINT ( 'NONE',  ( 1.472469842513823179, 35.59226448433412315, -4.923371831947296329 ) ) ;
#87858=CARTESIAN_POINT ( 'NONE',  ( 0.2751277870542909176, 60.30223176428830101, 6.499999999999992006 ) ) ;
#87859=CARTESIAN_POINT ( 'NONE',  ( 1.472469842513823179, 46.42559781766745175, 4.923371831947296329 ) ) ;
#87860=CARTESIAN_POINT ( 'NONE',  ( 5.076628168052704559, 15.17559781766745175, -8.527530157486179263 ) ) ;
#87861=CARTESIAN_POINT ( 'NONE',  ( 0.9413316022086116730, 8.455083851089586489, 6.499999999999963585 ) ) ;
#87862=CARTESIAN_POINT ( 'NONE',  ( 0.1532563361054083140, 66.00893115100079456, 1.131784320476157264E-15 ) ) ;
#87863=EDGE_LOOP ( 'NONE', ( #94732, #85936, #11591, #74571 ) ) ;
#87865=CARTESIAN_POINT ( 'NONE',  ( 6.565887622018943937, 45.16530133659708923, 12.81628187352647430 ) ) ;
#87866=CARTESIAN_POINT ( 'NONE',  ( 19.84674366389459266, 38.71726448433412315, -2.638427012816827677 ) ) ;
#87868=CARTESIAN_POINT ( 'NONE',  ( 6.204703633549690345, 65.76208216824731778, -14.16423886937410259 ) ) ;
#87869=CARTESIAN_POINT ( 'NONE',  ( 19.84674366389459621, 33.50893115100078745, 7.409399052514197653E-17 ) ) ;
#87871=CARTESIAN_POINT ( 'NONE',  ( -4.164238869374099039, 56.80374883491397497, 8.674139862899312516E-16 ) ) ;
#87873=CARTESIAN_POINT ( 'NONE',  ( -0.8801773607111009756, 3.063685344154838397, 1.068504757029289695E-15 ) ) ;
#87874=CARTESIAN_POINT ( 'NONE',  ( 17.08211943468705840, 35.13708216824730357, -12.26659068614894466 ) ) ;
#87875=CARTESIAN_POINT ( 'NONE',  ( 22.26659068614895176, 39.72041550158063217, -7.082119434687042414 ) ) ;
#87876=DIRECTION ( 'NONE',  ( -0.5547001962252290364, -0.8320502943378437211, 0.000000000000000000 ) ) ;
#87877=CARTESIAN_POINT ( 'NONE',  ( 5.076628168052703671, 16.84226448433411960, 8.527530157486179263 ) ) ;
#87879=CARTESIAN_POINT ( 'NONE',  ( 0.1532563361054082862, 61.21726448433412315, 2.638427012816831674 ) ) ;
#87880=CARTESIAN_POINT ( 'NONE',  ( 0.5774900079438607392, 48.48035201082150536, 5.440088680355550821 ) ) ;
#87882=CARTESIAN_POINT ( 'NONE',  ( 2.791683348922237240, 50.38393115100078035, -7.208316651077763204 ) ) ;
#87883=CARTESIAN_POINT ( 'NONE',  ( 6.565887622018943937, 65.16530133659709634, 12.81628187352647430 ) ) ;
#87884=CARTESIAN_POINT ( 'NONE',  ( 2.791683348922240793, 56.63393115100078035, 7.208316651077764092 ) ) ;
#87887=CARTESIAN_POINT ( 'NONE',  ( -4.164238869374098151, 21.59541550158063217, -3.795296366450310543 ) ) ;
#87888=CARTESIAN_POINT ( 'NONE',  ( 6.000000000000000000, 60.50000000000000711, 5.000000000000000000 ) ) ;
#87890=FACE_OUTER_BOUND ( 'NONE', #94003, .T. ) ;
#87891=CARTESIAN_POINT ( 'NONE',  ( 12.91533473730992121, 24.52201867748816966, 10.88017736071110164 ) ) ;
#87892=CARTESIAN_POINT ( 'NONE',  ( -2.816281873526473856, 19.33196800326375708, 3.434112377981055619 ) ) ;
#87894=CARTESIAN_POINT ( 'NONE',  ( 17.20831665107776587, 7.883931151000784787, 7.208316651077764980 ) ) ;
#87896=CARTESIAN_POINT ( 'NONE',  ( 6.565887622018943937, 48.08196800326375353, -12.81628187352647608 ) ) ;
#87897=VERTEX_POINT ( 'NONE', #27597 ) ;
#87900=CARTESIAN_POINT ( 'NONE',  ( -4.164238869374098151, 26.59541550158063217, -3.795296366450310543 ) ) ;
#87903=CARTESIAN_POINT ( 'NONE',  ( 19.72487221294570858, 61.86607318730076344, 6.500000000000000888 ) ) ;
#87904=CARTESIAN_POINT ( 'NONE',  ( 0.5774900079438607392, 13.48035201082150358, 5.440088680355550821 ) ) ;
#87907=CARTESIAN_POINT ( 'NONE',  ( 20.88017736071110519, 45.56368534415484106, 2.639326808657452039E-16 ) ) ;
#87908=CARTESIAN_POINT ( 'NONE',  ( 4.559911319644449179, 47.23035201082150536, -9.422509992056141925 ) ) ;
#87909=CARTESIAN_POINT ( 'NONE',  ( 21.09922568453595559, 12.04030133659708746, -6.408140936763230044 ) ) ;
#87910=CARTESIAN_POINT ( 'NONE',  ( 1.472469842513823179, 60.59226448433412315, -4.923371831947296329 ) ) ;
#87912=CARTESIAN_POINT ( 'NONE',  ( 2.791683348922237240, 5.383931151000785675, -7.208316651077763204 ) ) ;
#87914=CARTESIAN_POINT ( 'NONE',  ( 17.84635730667658393, 48.63791097397317031, 6.499999999999931610 ) ) ;
#87916=CARTESIAN_POINT ( 'NONE',  ( 15.44008868035555260, 49.73035201082150536, 9.422509992056143702 ) ) ;
#87917=CARTESIAN_POINT ( 'NONE',  ( 6.565887622018943937, 5.165301336597086568, 12.81628187352647430 ) ) ;
#87918=CARTESIAN_POINT ( 'NONE',  ( 20.88017736071110519, 65.56368534415483396, 2.639326808657452039E-16 ) ) ;
#87919=CARTESIAN_POINT ( 'NONE',  ( 2.791683348922240793, 31.63393115100078745, 7.208316651077764092 ) ) ;
#87920=CARTESIAN_POINT ( 'NONE',  ( -2.816281873526473856, 49.33196800326374643, 3.434112377981055619 ) ) ;
#87921=CARTESIAN_POINT ( 'NONE',  ( 10.00000000000000000, 4.758931151000784787, -9.846743663894594434 ) ) ;
#87924=CARTESIAN_POINT ( 'NONE',  ( 1.274849032794278747, 57.55509018479938277, -6.499999999999960032 ) ) ;
#87926=CARTESIAN_POINT ( 'NONE',  ( 17.96484262340118221, 14.93868534415483751, 7.964842623401181321 ) ) ;
#87927=CARTESIAN_POINT ( 'NONE',  ( 16.40814093676324603, 57.45696800326375353, -11.09922568453594671 ) ) ;
#87928=CARTESIAN_POINT ( 'NONE',  ( 12.63842701281683922, 34.55059781766745886, -9.846743663894590881 ) ) ;
#87929=CARTESIAN_POINT ( 'NONE',  ( -0.8801773607110991993, 17.85535201082150536, -2.915334737309923874 ) ) ;
#87930=CARTESIAN_POINT ( 'NONE',  ( 20.88017736071110164, 5.355352010821503583, 2.915334737309930979 ) ) ;
#87933=CARTESIAN_POINT ( 'NONE',  ( 10.00000000000000178, 14.31368534415483751, 10.88017736071110342 ) ) ;
#87934=CARTESIAN_POINT ( 'NONE',  ( 19.42250999205614548, 25.98035201082150891, -5.440088680355545492 ) ) ;
#87936=CARTESIAN_POINT ( 'NONE',  ( 4.559911319644449179, 22.23035201082150536, -9.422509992056141925 ) ) ;
#87937=VERTEX_POINT ( 'NONE', #15583 ) ;
#87939=CARTESIAN_POINT ( 'NONE',  ( 15.44008868035555793, 26.39701867748817321, -9.422509992056140149 ) ) ;
#87941=CARTESIAN_POINT ( 'NONE',  ( 0.1532563361054082862, 51.21726448433412315, 2.638427012816831674 ) ) ;
#87945=CARTESIAN_POINT ( 'NONE',  ( 0.5774900079438590739, 67.64701867748817676, -5.440088680355550821 ) ) ;
#87946=CARTESIAN_POINT ( 'NONE',  ( -2.266590686148945544, 31.38708216824730002, -7.082119434687050408 ) ) ;
#87947=CARTESIAN_POINT ( 'NONE',  ( 19.42250999205614193, 45.14701867748817676, 5.440088680355555262 ) ) ;
#87948=CARTESIAN_POINT ( 'NONE',  ( 4.559911319644449179, 22.23035201082150536, -9.422509992056141925 ) ) ;
#87950=ADVANCED_FACE ( 'NONE', ( #8070 ), #98097, .T. ) ;
#87952=CARTESIAN_POINT ( 'NONE',  ( 17.20831665107776587, 47.88393115100078745, 7.208316651077764980 ) ) ;
#87953=CARTESIAN_POINT ( 'NONE',  ( 17.20831665107776587, 7.883931151000784787, 7.208316651077764980 ) ) ;
#87955=CARTESIAN_POINT ( 'NONE',  ( 20.88017736071110875, 15.77201867748817143, -2.915334737309920765 ) ) ;
#87956=CARTESIAN_POINT ( 'NONE',  ( 0.1532563361054082862, 6.217264484334118713, 2.638427012816831674 ) ) ;
#87957=CARTESIAN_POINT ( 'NONE',  ( 3.591859063236763294, 8.290301336597087456, -11.09922568453595026 ) ) ;
#87958=CARTESIAN_POINT ( 'NONE',  ( 17.96484262340118221, 61.18868534415482685, -7.964842623401177768 ) ) ;
#87959=CARTESIAN_POINT ( 'NONE',  ( 2.035157376598824452, 18.68868534415484106, 7.964842623401179544 ) ) ;
#87960=CARTESIAN_POINT ( 'NONE',  ( -1.099225684535947600, 59.54030133659708923, 6.408140936763237150 ) ) ;
#87961=CARTESIAN_POINT ( 'NONE',  ( 2.917880565312948704, 32.63708216824730357, 12.26659068614894643 ) ) ;
#87962=B_SPLINE_CURVE_WITH_KNOTS ( 'NONE', 3,
 ( #13559, #5583, #81551, #44046, #96083, #36566, #13060, #83046, #58555, #66560 ),
 .UNSPECIFIED., .F., .F.,
 ( 4, 3, 3, 4 ),
 ( 5.003707553108400597E-17, 0.0006253016069560918136, 0.001250604074564953165, 0.002501455912506547405 ),
 .UNSPECIFIED. ) ;
#87963=FILL_AREA_STYLE_COLOUR ( '', #49080 ) ;
#87965=CARTESIAN_POINT ( 'NONE',  ( -2.816281873526473856, 54.12363466993041783, 9.499525473075851096E-16 ) ) ;
#87967=CARTESIAN_POINT ( 'NONE',  ( -1.099225684535947600, 4.540301336597087456, 6.408140936763237150 ) ) ;
#87969=CARTESIAN_POINT ( 'NONE',  ( 20.88017736071110875, 50.77201867748817676, -2.915334737309920765 ) ) ;
#87970=CARTESIAN_POINT ( 'NONE',  ( -0.8801773607111009756, 33.06368534415484106, 1.068504757029289695E-15 ) ) ;
#87972=CARTESIAN_POINT ( 'NONE',  ( 0.1532563361054082862, 66.21726448433413736, 2.638427012816831674 ) ) ;
#87975=CARTESIAN_POINT ( 'NONE',  ( 2.791683348922237240, 15.38393115100078212, -7.208316651077763204 ) ) ;
#87976=STYLED_ITEM ( 'NONE', ( #27421 ), #21696 ) ;
#87977=CARTESIAN_POINT ( 'NONE',  ( 0.1532563361054082862, 16.21726448433411960, 2.638427012816831674 ) ) ;
#87978=CARTESIAN_POINT ( 'NONE',  ( 10.00000000000000178, 12.25893115100078568, 9.846743663894594434 ) ) ;
#87979=CARTESIAN_POINT ( 'NONE',  ( 7.084665262690076126, 59.10535201082150536, 10.88017736071109987 ) ) ;
#87981=CARTESIAN_POINT ( 'NONE',  ( 1.472469842513823179, 10.59226448433411782, -4.923371831947296329 ) ) ;
#87982=CARTESIAN_POINT ( 'NONE',  ( 0.1532563361054100626, 20.80059781766744464, -2.638427012816831230 ) ) ;
#87985=CARTESIAN_POINT ( 'NONE',  ( 22.81628187352648496, 1.831968003263753753, -3.434112377981050290 ) ) ;
#87988=CARTESIAN_POINT ( 'NONE',  ( -0.8801773607111008646, 3.272018677488171434, 2.915334737309923430 ) ) ;
#87989=CARTESIAN_POINT ( 'NONE',  ( 17.08211943468705840, 15.13708216824730179, -12.26659068614894466 ) ) ;
#87991=CARTESIAN_POINT ( 'NONE',  ( 17.08211943468705130, 18.47041550158063572, 12.26659068614894998 ) ) ;
#87993=CARTESIAN_POINT ( 'NONE',  ( -0.3689425029237881626, 27.42874883491397142, 10.36894250292379027 ) ) ;
#87995=CARTESIAN_POINT ( 'NONE',  ( 24.16423886937410614, 4.512082168247300906, -3.795296366450302550 ) ) ;
#87996=CARTESIAN_POINT ( 'NONE',  ( 12.91533473730993009, 31.60535201082150891, -10.88017736071109987 ) ) ;
#87999=CARTESIAN_POINT ( 'NONE',  ( 17.20831665107776587, 17.88393115100078745, 7.208316651077764980 ) ) ;
#88000=CARTESIAN_POINT ( 'NONE',  ( 20.88017736071110875, 60.77201867748817676, -2.915334737309920765 ) ) ;
#88001=CARTESIAN_POINT ( 'NONE',  ( 12.63842701281683922, 9.550597817667449974, -9.846743663894590881 ) ) ;
#88003=VECTOR ( 'NONE', #55305, 1000.000000000000000 ) ;
#88004=CARTESIAN_POINT ( 'NONE',  ( 0.5774900079438590739, 17.64701867748817321, -5.440088680355550821 ) ) ;
#88005=CARTESIAN_POINT ( 'NONE',  ( 22.81628187352647785, 51.41530133659708923, 3.434112377981063169 ) ) ;
#88006=CARTESIAN_POINT ( 'NONE',  ( 12.63842701281683922, 49.55059781766744464, -9.846743663894590881 ) ) ;
#88007=LINE ( 'NONE', #42516, #84148 ) ;
#88008=CARTESIAN_POINT ( 'NONE',  ( 3.591859063236763294, 23.29030133659708568, -11.09922568453595026 ) ) ;
#88010=CARTESIAN_POINT ( 'NONE',  ( 19.84674366389459266, 43.71726448433410894, -2.638427012816827677 ) ) ;
#88012=CARTESIAN_POINT ( 'NONE',  ( -4.164238869374098151, 11.59541550158063217, -3.795296366450310543 ) ) ;
#88015=CARTESIAN_POINT ( 'NONE',  ( 17.96484262340118221, 46.18868534415484106, -7.964842623401177768 ) ) ;
#88016=CARTESIAN_POINT ( 'NONE',  ( 15.44008868035555793, 56.39701867748817676, -9.422509992056140149 ) ) ;
#88017=CARTESIAN_POINT ( 'NONE',  ( -0.3689425029237898834, 51.17874883491397497, -10.36894250292378850 ) ) ;
#88018=CARTESIAN_POINT ( 'NONE',  ( 7.361572987183169658, 59.96726448433410894, -9.846743663894592657 ) ) ;
#88019=CARTESIAN_POINT ( 'NONE',  ( -2.816281873526471635, 63.91530133659708923, -3.434112377981056508 ) ) ;
#88020=CARTESIAN_POINT ( 'NONE',  ( 15.44008868035555260, 34.73035201082151247, 9.422509992056143702 ) ) ;
#88022=CARTESIAN_POINT ( 'NONE',  ( 5.076628168052704559, 50.17559781766745886, -8.527530157486179263 ) ) ;
#88026=ADVANCED_FACE ( 'NONE', ( #31043 ), #32401, .T. ) ;
#88027=CARTESIAN_POINT ( 'NONE',  ( -0.8801773607111009756, 8.063685344154837509, 1.068504757029289695E-15 ) ) ;
#88029=CARTESIAN_POINT ( 'NONE',  ( 7.361572987183169658, -0.03273551566588185635, -9.846743663894592657 ) ) ;
#88031=CARTESIAN_POINT ( 'NONE',  ( 19.84674366389459266, 3.717264484334118713, -2.638427012816827677 ) ) ;
#88033=CARTESIAN_POINT ( 'NONE',  ( 14.92337183194729633, 32.67559781766745175, 8.527530157486181039 ) ) ;
#88034=CARTESIAN_POINT ( 'NONE',  ( 19.42250999205614548, 25.98035201082150891, -5.440088680355545492 ) ) ;
#88035=CARTESIAN_POINT ( 'NONE',  ( 0.6178305044545838731, 14.74863466993041783, 9.382169495545420901 ) ) ;
#88036=CARTESIAN_POINT ( 'NONE',  ( 7.084665262690076126, 39.10535201082150536, 10.88017736071109987 ) ) ;
#88039=AXIS2_PLACEMENT_3D ( 'NONE', #36536, #90012, #42 ) ;
#88040=CARTESIAN_POINT ( 'NONE',  ( 6.565887622018943937, 45.16530133659708923, 12.81628187352647430 ) ) ;
#88041=VERTEX_POINT ( 'NONE', #55781 ) ;
#88042=CARTESIAN_POINT ( 'NONE',  ( -0.8801773607111009756, 48.06368534415484817, 1.068504757029289695E-15 ) ) ;
#88043=CARTESIAN_POINT ( 'NONE',  ( -2.816281873526471635, 18.91530133659708213, -3.434112377981056508 ) ) ;
#88045=DIRECTION ( 'NONE',  ( -0.5547001962252291474, -0.8320502943378437211, -0.000000000000000000 ) ) ;
#88046=CARTESIAN_POINT ( 'NONE',  ( 19.42250999205614548, 30.98035201082150536, -5.440088680355545492 ) ) ;
#88047=CARTESIAN_POINT ( 'NONE',  ( -4.164238869374099039, 66.80374883491396076, 8.674139862899312516E-16 ) ) ;
#88048=CARTESIAN_POINT ( 'NONE',  ( 2.791683348922237240, 55.38393115100078745, -7.208316651077763204 ) ) ;
#88049=CARTESIAN_POINT ( 'NONE',  ( 17.20831665107776587, 9.133931151000787452, -7.208316651077762316 ) ) ;
#88050=CARTESIAN_POINT ( 'NONE',  ( 19.42250999205614193, 65.14701867748817676, 5.440088680355555262 ) ) ;
#88052=CARTESIAN_POINT ( 'NONE',  ( -0.3689425029237898834, 36.17874883491396787, -10.36894250292378850 ) ) ;
#88056=ORIENTED_EDGE ( 'NONE', *, *, #61415, .T. ) ;
#88057=CARTESIAN_POINT ( 'NONE',  ( -4.164238869374099039, 51.80374883491396787, 8.674139862899312516E-16 ) ) ;
#88058=CARTESIAN_POINT ( 'NONE',  ( 2.917880565312950480, 45.97041550158063927, -12.26659068614894821 ) ) ;
#88059=EDGE_CURVE ( 'NONE', #27809, #90918, #2369, .T. ) ;
#88060=CARTESIAN_POINT ( 'NONE',  ( 10.00000000000000000, 14.75893115100078568, -9.846743663894594434 ) ) ;
#88062=LINE ( 'NONE', #65052, #51440 ) ;
#88063=FACE_OUTER_BOUND ( 'NONE', #62206, .T. ) ;
#88064=CARTESIAN_POINT ( 'NONE',  ( 22.26659068614895176, 39.72041550158063217, -7.082119434687042414 ) ) ;
#88067=CARTESIAN_POINT ( 'NONE',  ( 18.52753015748617571, 3.092264484334118269, 4.923371831947298993 ) ) ;
#88070=DIRECTION ( 'NONE',  ( 0.000000000000000000, 0.000000000000000000, -1.000000000000000000 ) ) ;
#88074=CARTESIAN_POINT ( 'NONE',  ( 2.035157376598824452, 23.68868534415484461, 7.964842623401179544 ) ) ;
#88075=CARTESIAN_POINT ( 'NONE',  ( 17.96484262340118221, 21.18868534415483396, -7.964842623401177768 ) ) ;
#88076=CARTESIAN_POINT ( 'NONE',  ( 5.076628168052704559, 50.17559781766745886, -8.527530157486179263 ) ) ;
#88077=CARTESIAN_POINT ( 'NONE',  ( -1.099225684535947600, 23.70696800326375708, -6.408140936763238038 ) ) ;
#88079=VECTOR ( 'NONE', #44236, 1000.000000000000000 ) ;
#88082=CARTESIAN_POINT ( 'NONE',  ( -1.099225684535947600, 23.70696800326375708, -6.408140936763238038 ) ) ;
#88084=CARTESIAN_POINT ( 'NONE',  ( 0.1532563361054100626, 35.80059781766745175, -2.638427012816831230 ) ) ;
#88085=CARTESIAN_POINT ( 'NONE',  ( 24.16423886937410614, 64.51208216824728936, -3.795296366450302550 ) ) ;
#88087=CARTESIAN_POINT ( 'NONE',  ( 17.08211943468705130, 63.47041550158063927, 12.26659068614894998 ) ) ;
#88089=CARTESIAN_POINT ( 'NONE',  ( 20.88017736071110164, 30.35535201082151247, 2.915334737309930979 ) ) ;
#88090=CARTESIAN_POINT ( 'NONE',  ( 12.91533473730992121, 49.52201867748817676, 10.88017736071110164 ) ) ;
#88091=CARTESIAN_POINT ( 'NONE',  ( 7.084665262690076126, 54.10535201082151247, 10.88017736071109987 ) ) ;
#88093=CARTESIAN_POINT ( 'NONE',  ( 19.42250999205614193, 40.14701867748817676, 5.440088680355555262 ) ) ;
#88098=ORIENTED_EDGE ( 'NONE', *, *, #85467, .F. ) ;
#88099=COLOUR_RGB ( '', 0.31764706, 0.68627451, 0.89019608) ;
#88100=CARTESIAN_POINT ( 'NONE',  ( 1.472469842513823179, 20.59226448433411960, -4.923371831947296329 ) ) ;
#88103=CARTESIAN_POINT ( 'NONE',  ( 14.92337183194729633, 62.67559781766745886, 8.527530157486181039 ) ) ;
#88107=FACE_OUTER_BOUND ( 'NONE', #97674, .T. ) ;
#88109=CARTESIAN_POINT ( 'NONE',  ( 10.00000000000000178, 62.25893115100078745, 9.846743663894594434 ) ) ;
#88110=CARTESIAN_POINT ( 'NONE',  ( 7.361572987183170547, 27.05059781766745175, 9.846743663894590881 ) ) ;
#88111=CARTESIAN_POINT ( 'NONE',  ( 22.26659068614894466, 58.88708216824729647, 7.082119434687054849 ) ) ;
#88115=CARTESIAN_POINT ( 'NONE',  ( 18.52753015748618282, 33.92559781766745886, -4.923371831947291888 ) ) ;
#88116=CARTESIAN_POINT ( 'NONE',  ( 13.43411237798105340, 60.58196800326376064, 12.81628187352647963 ) ) ;
#88117=CARTESIAN_POINT ( 'NONE',  ( 13.43411237798106583, 2.665301336597086568, -12.81628187352647252 ) ) ;
#88118=CARTESIAN_POINT ( 'NONE',  ( 0.1532563361054100626, 5.800597817667452638, -2.638427012816831230 ) ) ;
#88119=CARTESIAN_POINT ( 'NONE',  ( 0.1129803114748722526, 4.294273331840908980, -6.480634945678659165 ) ) ;
#88120=CARTESIAN_POINT ( 'NONE',  ( 19.84674366389459621, 3.508931151000785231, 7.409399052514197653E-17 ) ) ;
#88121=CARTESIAN_POINT ( 'NONE',  ( 18.52753015748618282, 63.92559781766745886, -4.923371831947291888 ) ) ;
#88123=VERTEX_POINT ( 'NONE', #56750 ) ;
#88124=CARTESIAN_POINT ( 'NONE',  ( 10.00000000000000178, 9.313685344154839285, 10.88017736071110342 ) ) ;
#88125=CARTESIAN_POINT ( 'NONE',  ( -4.164238869374098151, 6.595415501580634832, -3.795296366450310543 ) ) ;
#88126=CARTESIAN_POINT ( 'NONE',  ( 2.791683348922240793, 16.63393115100078745, 7.208316651077764092 ) ) ;
#88127=CARTESIAN_POINT ( 'NONE',  ( 4.559911319644449179, 47.23035201082150536, -9.422509992056141925 ) ) ;
#88128=CARTESIAN_POINT ( 'NONE',  ( 0.6178305044545818747, 33.49863466993042493, -9.382169495545419124 ) ) ;
#88131=CARTESIAN_POINT ( 'NONE',  ( 19.88565890683628368, 17.71691075486302935, -6.480892540919849232 ) ) ;
#88133=CARTESIAN_POINT ( 'NONE',  ( 19.84674366389459266, 58.30059781766745886, 2.638427012816836559 ) ) ;
#88134=CARTESIAN_POINT ( 'NONE',  ( 5.076628168052704559, 20.17559781766745175, -8.527530157486179263 ) ) ;
#88136=CARTESIAN_POINT ( 'NONE',  ( 21.09922568453595559, 17.04030133659708923, -6.408140936763230044 ) ) ;
#88138=CARTESIAN_POINT ( 'NONE',  ( 4.559911319644449179, 22.23035201082150536, -9.422509992056141925 ) ) ;
#88140=CARTESIAN_POINT ( 'NONE',  ( 2.917880565312950480, 50.97041550158064638, -12.26659068614894821 ) ) ;
#88143=CARTESIAN_POINT ( 'NONE',  ( 7.361572987183170547, 47.05059781766745175, 9.846743663894590881 ) ) ;
#88144=CARTESIAN_POINT ( 'NONE',  ( 19.38216949554541557, 37.24863466993041783, -9.382169495545420901 ) ) ;
#88145=CARTESIAN_POINT ( 'NONE',  ( 12.91533473730993009, 31.60535201082150891, -10.88017736071109987 ) ) ;
#88147=CARTESIAN_POINT ( 'NONE',  ( 5.076628168052704559, 55.17559781766745175, -8.527530157486179263 ) ) ;
#88148=CARTESIAN_POINT ( 'NONE',  ( 0.5774900079438607392, 48.48035201082150536, 5.440088680355550821 ) ) ;
#88149=CARTESIAN_POINT ( 'NONE',  ( 16.40814093676323893, 0.7903013365970867898, 11.09922568453595026 ) ) ;
#88150=CARTESIAN_POINT ( 'NONE',  ( 17.08211943468705130, 33.47041550158063927, 12.26659068614894998 ) ) ;
#88152=CARTESIAN_POINT ( 'NONE',  ( 5.076628168052703671, 21.84226448433411960, 8.527530157486179263 ) ) ;
#88153=CARTESIAN_POINT ( 'NONE',  ( -2.816281873526473856, 64.33196800326376774, 3.434112377981055619 ) ) ;
#88154=B_SPLINE_CURVE_WITH_KNOTS ( 'NONE', 3,
 ( #22537, #45513, #31969, #91515 ),
 .UNSPECIFIED., .F., .F.,
 ( 4, 4 ),
 ( 6.942281208919283290E-19, 7.431658353028133043E-05 ),
 .UNSPECIFIED. ) ;
#88155=CARTESIAN_POINT ( 'NONE',  ( 0.1532563361054082862, 66.21726448433413736, 2.638427012816831674 ) ) ;
#88156=ORIENTED_EDGE ( 'NONE', *, *, #35042, .F. ) ;
#88158=CARTESIAN_POINT ( 'NONE',  ( 7.084665262690076126, 12.02201867748817321, -10.88017736071110164 ) ) ;
#88159=CARTESIAN_POINT ( 'NONE',  ( 24.16423886937410614, 24.51208216824730002, -3.795296366450302550 ) ) ;
#88160=CARTESIAN_POINT ( 'NONE',  ( 18.52753015748618282, 13.92559781766745175, -4.923371831947291888 ) ) ;
#88161=CARTESIAN_POINT ( 'NONE',  ( 7.361572987183169658, 54.96726448433413026, -9.846743663894592657 ) ) ;
#88162=CARTESIAN_POINT ( 'NONE',  ( 2.035157376598822676, 27.43868534415483396, -7.964842623401177768 ) ) ;
#88165=ORIENTED_EDGE ( 'NONE', *, *, #32285, .T. ) ;
#88168=CARTESIAN_POINT ( 'NONE',  ( 7.361572987183170547, 52.05059781766745175, 9.846743663894590881 ) ) ;
#88172=CARTESIAN_POINT ( 'NONE',  ( 20.36894250292379382, 13.67874883491396965, 10.36894250292379205 ) ) ;
#88173=CARTESIAN_POINT ( 'NONE',  ( 24.16423886937410614, 4.303748834913967869, 8.672049930838204340E-16 ) ) ;
#88174=EDGE_CURVE ( 'NONE', #93746, #15284, #87243, .T. ) ;
#88175=CARTESIAN_POINT ( 'NONE',  ( 4.559911319644449179, 43.89701867748816966, 9.422509992056141925 ) ) ;
#88176=CARTESIAN_POINT ( 'NONE',  ( 2.917880565312950480, 60.97041550158063927, -12.26659068614894821 ) ) ;
#88177=CARTESIAN_POINT ( 'NONE',  ( 17.20831665107776587, 59.13393115100078745, -7.208316651077762316 ) ) ;
#88178=CARTESIAN_POINT ( 'NONE',  ( 14.92337183194729988, 29.34226448433411960, -8.527530157486177487 ) ) ;
#88179=CARTESIAN_POINT ( 'NONE',  ( 20.88017736071110164, 35.35535201082150536, 2.915334737309930979 ) ) ;
#88180=CARTESIAN_POINT ( 'NONE',  ( -2.816281873526471635, 8.915301336597083903, -3.434112377981056508 ) ) ;
#88181=CARTESIAN_POINT ( 'NONE',  ( 10.00000000000000178, 3.053748834913967425, 14.16423886937410082 ) ) ;
#88182=CARTESIAN_POINT ( 'NONE',  ( 10.00000000000000000, 50.55374883491396787, -14.16423886937410082 ) ) ;
#88183=CARTESIAN_POINT ( 'NONE',  ( 15.44008868035555260, 9.730352010821505360, 9.422509992056143702 ) ) ;
#88192=CIRCLE ( 'NONE', #70654, 2.999999999999999112 ) ;
#88193=EDGE_LOOP ( 'NONE', ( #9979, #18128, #14818, #55325 ) ) ;
#88194=CARTESIAN_POINT ( 'NONE',  ( 19.84674366389459266, 28.71726448433411960, -2.638427012816827677 ) ) ;
#88196=CARTESIAN_POINT ( 'NONE',  ( 24.16423886937410614, 34.51208216824731068, -3.795296366450302550 ) ) ;
#88197=CARTESIAN_POINT ( 'NONE',  ( 10.00000000000000000, 39.75893115100078745, -9.846743663894594434 ) ) ;
#88198=CARTESIAN_POINT ( 'NONE',  ( 2.035157376598822676, 52.43868534415483396, -7.964842623401177768 ) ) ;
#88201=CARTESIAN_POINT ( 'NONE',  ( 15.44008868035555260, 49.73035201082150536, 9.422509992056143702 ) ) ;
#88202=CARTESIAN_POINT ( 'NONE',  ( 6.565887622018943937, 63.08196800326376064, -12.81628187352647608 ) ) ;
#88205=CARTESIAN_POINT ( 'NONE',  ( 20.36894250292379382, 18.67874883491397142, 10.36894250292379205 ) ) ;
#88206=ORIENTED_EDGE ( 'NONE', *, *, #7616, .T. ) ;
#88207=CARTESIAN_POINT ( 'NONE',  ( 6.565887622018943937, 50.16530133659708213, 12.81628187352647430 ) ) ;
#88209=CARTESIAN_POINT ( 'NONE',  ( 17.96484262340118221, 21.18868534415483396, -7.964842623401177768 ) ) ;
#88210=CARTESIAN_POINT ( 'NONE',  ( 19.84674366389459266, 23.30059781766745530, 2.638427012816836559 ) ) ;
#88211=CARTESIAN_POINT ( 'NONE',  ( 12.91533473730993009, 16.60535201082150891, -10.88017736071109987 ) ) ;
#88212=CARTESIAN_POINT ( 'NONE',  ( -2.816281873526473856, 49.12363466993042493, 9.499525473075851096E-16 ) ) ;
#88214=CARTESIAN_POINT ( 'NONE',  ( 0.1532563361054100626, 40.80059781766745886, -2.638427012816831230 ) ) ;
#88218=CARTESIAN_POINT ( 'NONE',  ( 10.00000000000000000, 66.81368534415484817, -10.88017736071110342 ) ) ;
#88221=CARTESIAN_POINT ( 'NONE',  ( 2.791683348922240793, 21.63393115100078745, 7.208316651077764092 ) ) ;
#88223=CARTESIAN_POINT ( 'NONE',  ( -2.816281873526471635, 18.91530133659708213, -3.434112377981056508 ) ) ;
#88226=CARTESIAN_POINT ( 'NONE',  ( 1.472469842513823179, 46.42559781766745175, 4.923371831947296329 ) ) ;
#88228=CARTESIAN_POINT ( 'NONE',  ( -4.164238869374099039, 16.80374883491396787, 8.674139862899312516E-16 ) ) ;
#88229=CARTESIAN_POINT ( 'NONE',  ( 19.84674366389459266, 38.30059781766745175, 2.638427012816836559 ) ) ;
#88230=CARTESIAN_POINT ( 'NONE',  ( 21.09922568453595559, 37.04030133659708923, -6.408140936763230044 ) ) ;
#88232=CARTESIAN_POINT ( 'NONE',  ( 0.8952175423694819223, 23.52576239577082262, 5.990408912944316100 ) ) ;
#88233=CARTESIAN_POINT ( 'NONE',  ( 0.5774900079438590739, 57.64701867748817676, -5.440088680355550821 ) ) ;
#88234=CARTESIAN_POINT ( 'NONE',  ( 16.40814093676323893, 5.790301336597087456, 11.09922568453595026 ) ) ;
#88237=CARTESIAN_POINT ( 'NONE',  ( 0.1532563361054100626, 35.80059781766745175, -2.638427012816831230 ) ) ;
#88238=CARTESIAN_POINT ( 'NONE',  ( 12.91533473730993009, 31.60535201082150891, -10.88017736071109987 ) ) ;
#88239=CARTESIAN_POINT ( 'NONE',  ( -1.099225684535947600, 34.54030133659708923, 6.408140936763237150 ) ) ;
#88241=CARTESIAN_POINT ( 'NONE',  ( 1.472469842513823179, 35.59226448433412315, -4.923371831947296329 ) ) ;
#88243=CARTESIAN_POINT ( 'NONE',  ( 4.559911319644449179, 37.23035201082150536, -9.422509992056141925 ) ) ;
#88248=CARTESIAN_POINT ( 'NONE',  ( 0.1532563361054082862, 56.21726448433411605, 2.638427012816831674 ) ) ;
#88249=CARTESIAN_POINT ( 'NONE',  ( 17.96484262340118221, 31.18868534415483751, -7.964842623401177768 ) ) ;
#88251=CARTESIAN_POINT ( 'NONE',  ( 20.88017736071110164, 65.35535201082150536, 2.915334737309930979 ) ) ;
#88252=CARTESIAN_POINT ( 'NONE',  ( 10.00000000000000000, 21.81368534415484106, -10.88017736071110342 ) ) ;
#88253=DIRECTION ( 'NONE',  ( -0.000000000000000000, -0.000000000000000000, -1.000000000000000000 ) ) ;
#88254=CARTESIAN_POINT ( 'NONE',  ( 1.472469842513823179, 6.425597817667451750, 4.923371831947296329 ) ) ;
#88257=CARTESIAN_POINT ( 'NONE',  ( 0.1532563361054083140, 56.00893115100078745, 1.131784320476157264E-15 ) ) ;
#88258=CARTESIAN_POINT ( 'NONE',  ( 6.204703633549690345, 57.84541550158063927, 14.16423886937410082 ) ) ;
#88260=DIRECTION ( 'NONE',  ( -0.000000000000000000, -0.000000000000000000, -1.000000000000000000 ) ) ;
#88261=CARTESIAN_POINT ( 'NONE',  ( 13.79529636645031943, 15.34541550158063750, -14.16423886937409904 ) ) ;
#88263=CARTESIAN_POINT ( 'NONE',  ( 13.79529636645031943, 40.34541550158063217, -14.16423886937409904 ) ) ;
#88264=CARTESIAN_POINT ( 'NONE',  ( -1.099225684535947600, 8.706968003263753531, -6.408140936763238038 ) ) ;
#88267=CARTESIAN_POINT ( 'NONE',  ( 2.035157376598824452, 3.688685344154837953, 7.964842623401179544 ) ) ;
#88268=EDGE_CURVE ( 'NONE', #38312, #41376, #43038, .T. ) ;
#88269=CARTESIAN_POINT ( 'NONE',  ( 1.472469842513823179, 41.42559781766745886, 4.923371831947296329 ) ) ;
#88270=( NAMED_UNIT ( * ) PLANE_ANGLE_UNIT ( ) SI_UNIT ( $, .RADIAN. ) );
#88272=CARTESIAN_POINT ( 'NONE',  ( 4.559911319644449179, 57.23035201082150536, -9.422509992056141925 ) ) ;
#88273=LINE ( 'NONE', #11783, #67577 ) ;
#88275=CARTESIAN_POINT ( 'NONE',  ( 22.81628187352647785, 61.41530133659709634, 3.434112377981063169 ) ) ;
#88276=CARTESIAN_POINT ( 'NONE',  ( -1.099225684535947600, 19.54030133659708568, 6.408140936763237150 ) ) ;
#88277=CARTESIAN_POINT ( 'NONE',  ( 0.1532563361054082862, 31.21726448433412315, 2.638427012816831674 ) ) ;
#88279=CARTESIAN_POINT ( 'NONE',  ( 2.791683348922240793, 1.633931151000784565, 7.208316651077764092 ) ) ;
#88280=CARTESIAN_POINT ( 'NONE',  ( 18.06765999051785343, 3.991275129254488796, 6.500000000000000888 ) ) ;
#88281=CARTESIAN_POINT ( 'NONE',  ( 2.917880565312948704, 67.63708216824730357, 12.26659068614894643 ) ) ;
#88282=CARTESIAN_POINT ( 'NONE',  ( 7.084665262690076126, 12.02201867748817143, -10.88017736071110164 ) ) ;
#88284=CARTESIAN_POINT ( 'NONE',  ( 6.204703633549690345, 45.76208216824729647, -14.16423886937410259 ) ) ;
#88285=CARTESIAN_POINT ( 'NONE',  ( 15.44008868035555793, 26.39701867748817321, -9.422509992056140149 ) ) ;
#88286=CARTESIAN_POINT ( 'NONE',  ( 0.5774900079438607392, 68.48035201082150536, 5.440088680355550821 ) ) ;
#88288=CARTESIAN_POINT ( 'NONE',  ( 18.04007052943773459, 49.00257860105350005, -5.767676674365834089 ) ) ;
#88289=CARTESIAN_POINT ( 'NONE',  ( 0.1532563361054082862, 16.21726448433411960, 2.638427012816831674 ) ) ;
#88291=CARTESIAN_POINT ( 'NONE',  ( 12.63842701281683922, 9.550597817667449974, -9.846743663894590881 ) ) ;
#88292=CARTESIAN_POINT ( 'NONE',  ( 18.52753015748618282, 43.92559781766745175, -4.923371831947291888 ) ) ;
#88293=CARTESIAN_POINT ( 'NONE',  ( 7.361572987183170547, 62.05059781766745886, 9.846743663894590881 ) ) ;
#88294=CARTESIAN_POINT ( 'NONE',  ( 12.91533473730992121, 29.52201867748817321, 10.88017736071110164 ) ) ;
#88298=CARTESIAN_POINT ( 'NONE',  ( 13.43411237798106583, 42.66530133659707502, -12.81628187352647252 ) ) ;
#88301=CARTESIAN_POINT ( 'NONE',  ( -0.8801773607111008646, 63.27201867748817676, 2.915334737309923430 ) ) ;
#88302=CARTESIAN_POINT ( 'NONE',  ( -2.816281873526473856, 39.12363466993041783, 9.499525473075851096E-16 ) ) ;
#88303=CARTESIAN_POINT ( 'NONE',  ( -2.266590686148945544, 57.22041550158063217, 7.082119434687048631 ) ) ;
#88304=CARTESIAN_POINT ( 'NONE',  ( 14.92337183194729988, 24.34226448433411960, -8.527530157486177487 ) ) ;
#88307=CARTESIAN_POINT ( 'NONE',  ( -2.266590686148945544, 16.38708216824730357, -7.082119434687050408 ) ) ;
#88308=CARTESIAN_POINT ( 'NONE',  ( -2.266590686148945544, 31.38708216824730002, -7.082119434687050408 ) ) ;
#88309=CARTESIAN_POINT ( 'NONE',  ( 12.63842701281683034, 47.46726448433412315, 9.846743663894596210 ) ) ;
#88311=CARTESIAN_POINT ( 'NONE',  ( 20.88017736071110164, 20.35535201082150891, 2.915334737309930979 ) ) ;
#88312=EDGE_CURVE ( 'NONE', #34886, #65300, #27621, .T. ) ;
#88313=CARTESIAN_POINT ( 'NONE',  ( 10.00000000000000178, 59.31368534415484106, 10.88017736071110342 ) ) ;
#88315=CARTESIAN_POINT ( 'NONE',  ( 16.40814093676323893, 45.79030133659708923, 11.09922568453595026 ) ) ;
#88317=CARTESIAN_POINT ( 'NONE',  ( 12.91533473730992121, 54.52201867748816255, 10.88017736071110164 ) ) ;
#88319=( LENGTH_UNIT ( ) NAMED_UNIT ( * ) SI_UNIT ( .MILLI., .METRE. ) );
#88321=DIRECTION ( 'NONE',  ( 0.6093027842603870869, 0.6796026999251361111, 0.4085220769395525586 ) ) ;
#88322=ORIENTED_EDGE ( 'NONE', *, *, #69692, .F. ) ;
#88323=CARTESIAN_POINT ( 'NONE',  ( 2.035157376598822676, 62.43868534415483396, -7.964842623401177768 ) ) ;
#88324=CARTESIAN_POINT ( 'NONE',  ( 19.42250999205614193, 15.14701867748817143, 5.440088680355555262 ) ) ;
#88326=CARTESIAN_POINT ( 'NONE',  ( 3.558677480090427725, 70.40124509038875544, 5.000000000000000000 ) ) ;
#88327=CARTESIAN_POINT ( 'NONE',  ( 0.5774900079438590739, 7.647018677488171434, -5.440088680355550821 ) ) ;
#88328=CARTESIAN_POINT ( 'NONE',  ( 10.00000000000000178, 27.25893115100078390, 9.846743663894594434 ) ) ;
#88329=CARTESIAN_POINT ( 'NONE',  ( 22.26659068614895176, 19.72041550158063572, -7.082119434687042414 ) ) ;
#88331=CARTESIAN_POINT ( 'NONE',  ( 10.00000000000000178, 19.31368534415484106, 10.88017736071110342 ) ) ;
#88332=CARTESIAN_POINT ( 'NONE',  ( 5.076628168052704559, 65.17559781766745175, -8.527530157486179263 ) ) ;
#88334=CARTESIAN_POINT ( 'NONE',  ( 6.565887622018943937, -1.918031996736246692, -12.81628187352647608 ) ) ;
#88337=CARTESIAN_POINT ( 'NONE',  ( 20.88017736071110519, 50.56368534415484106, 2.639326808657452039E-16 ) ) ;
#88339=CARTESIAN_POINT ( 'NONE',  ( 3.591859063236763294, 38.29030133659708923, -11.09922568453595026 ) ) ;
#88341=CARTESIAN_POINT ( 'NONE',  ( 2.035157376598822676, 57.43868534415484106, -7.964842623401177768 ) ) ;
#88342=CARTESIAN_POINT ( 'NONE',  ( 0.5774900079438590739, 17.64701867748817321, -5.440088680355550821 ) ) ;
#88344=CARTESIAN_POINT ( 'NONE',  ( -2.816281873526471635, 43.91530133659708923, -3.434112377981056508 ) ) ;
#88345=CARTESIAN_POINT ( 'NONE',  ( 4.559911319644449179, 32.23035201082150536, -9.422509992056141925 ) ) ;
#88347=CARTESIAN_POINT ( 'NONE',  ( 6.565887622018943937, 38.08196800326376064, -12.81628187352647608 ) ) ;
#88348=CARTESIAN_POINT ( 'NONE',  ( 12.91533473730992121, 34.52201867748817676, 10.88017736071110164 ) ) ;
#88349=CARTESIAN_POINT ( 'NONE',  ( 17.20831665107776587, 57.88393115100078745, 7.208316651077764980 ) ) ;
#88353=CARTESIAN_POINT ( 'NONE',  ( 19.84674366389459266, 8.300597817667451750, 2.638427012816836559 ) ) ;
#88354=CARTESIAN_POINT ( 'NONE',  ( 7.361572987183169658, 64.96726448433412315, -9.846743663894592657 ) ) ;
#88356=CARTESIAN_POINT ( 'NONE',  ( 17.20831665107776587, 47.88393115100078745, 7.208316651077764980 ) ) ;
#88357=CARTESIAN_POINT ( 'NONE',  ( 7.084665262690076126, 29.10535201082150181, 10.88017736071109987 ) ) ;
#88359=CARTESIAN_POINT ( 'NONE',  ( -0.1038446121089068586, 39.24302437010792488, -6.337995344473776882 ) ) ;
#88360=DIRECTION ( 'NONE',  ( 0.000000000000000000, -1.000000000000000000, 0.000000000000000000 ) ) ;
#88362=CARTESIAN_POINT ( 'NONE',  ( 17.20831665107776587, 39.13393115100079456, -7.208316651077762316 ) ) ;
#88363=CARTESIAN_POINT ( 'NONE',  ( 19.84674366389459266, 3.717264484334118713, -2.638427012816827677 ) ) ;
#88365=CARTESIAN_POINT ( 'NONE',  ( 14.92337183194729988, 64.34226448433412315, -8.527530157486177487 ) ) ;
#88366=VERTEX_POINT ( 'NONE', #11744 ) ;
#88369=CARTESIAN_POINT ( 'NONE',  ( -2.816281873526473856, 34.33196800326376064, 3.434112377981055619 ) ) ;
#88370=CARTESIAN_POINT ( 'NONE',  ( 17.20831665107776587, 44.13393115100078745, -7.208316651077762316 ) ) ;
#88372=CARTESIAN_POINT ( 'NONE',  ( -4.164238869374098151, 56.59541550158063927, -3.795296366450310543 ) ) ;
#88373=CARTESIAN_POINT ( 'NONE',  ( 12.63842701281683922, 34.55059781766745886, -9.846743663894590881 ) ) ;
#88376=CARTESIAN_POINT ( 'NONE',  ( 10.00000000000000178, 58.05374883491397497, 14.16423886937410082 ) ) ;
#88378=CARTESIAN_POINT ( 'NONE',  ( 2.035157376598824452, 18.68868534415484106, 7.964842623401179544 ) ) ;
#88379=CARTESIAN_POINT ( 'NONE',  ( 20.36894250292379738, 29.92874883491396432, -10.36894250292379027 ) ) ;
#88380=CARTESIAN_POINT ( 'NONE',  ( -4.164238869374099039, 46.80374883491397497, 8.674139862899312516E-16 ) ) ;
#88382=CARTESIAN_POINT ( 'NONE',  ( 2.791683348922240793, 16.63393115100078745, 7.208316651077764092 ) ) ;
#88384=CARTESIAN_POINT ( 'NONE',  ( 19.84674366389459266, 63.30059781766745886, 2.638427012816836559 ) ) ;
#88386=CARTESIAN_POINT ( 'NONE',  ( 10.00000000000000178, 44.31368534415484106, 10.88017736071110342 ) ) ;
#88387=CARTESIAN_POINT ( 'NONE',  ( 0.1955144967548739787, 64.32703681773342907, -6.500000000002695622 ) ) ;
#88388=CARTESIAN_POINT ( 'NONE',  ( 17.20831665107776587, 54.13393115100079456, -7.208316651077762316 ) ) ;
#88389=DIRECTION ( 'NONE',  ( 0.6093027842603860877, 0.6796026999251382206, -0.4085220769395505602 ) ) ;
#88390=CARTESIAN_POINT ( 'NONE',  ( 10.00000000000000000, 54.75893115100078745, -9.846743663894594434 ) ) ;
#88391=CARTESIAN_POINT ( 'NONE',  ( 10.00000000000000000, 0.5537488349139675359, -14.16423886937410082 ) ) ;
#88393=CARTESIAN_POINT ( 'NONE',  ( 2.917880565312950480, 20.97041550158063217, -12.26659068614894821 ) ) ;
#88396=FILL_AREA_STYLE_COLOUR ( '', #21529 ) ;
#88399=CARTESIAN_POINT ( 'NONE',  ( 4.559911319644449179, 18.89701867748817321, 9.422509992056141925 ) ) ;
#88400=CARTESIAN_POINT ( 'NONE',  ( 22.81628187352647785, 41.41530133659708923, 3.434112377981063169 ) ) ;
#88401=CARTESIAN_POINT ( 'NONE',  ( 21.92686044187656336, 61.97997603579418069, 3.195792623639536423 ) ) ;
#88402=CARTESIAN_POINT ( 'NONE',  ( 14.92337183194729988, 14.34226448433411782, -8.527530157486177487 ) ) ;
#88405=VECTOR ( 'NONE', #90456, 1000.000000000000000 ) ;
#88407=CARTESIAN_POINT ( 'NONE',  ( 17.08211943468705840, 30.13708216824730357, -12.26659068614894466 ) ) ;
#88408=CARTESIAN_POINT ( 'NONE',  ( 2.035157376598822676, 7.438685344154837509, -7.964842623401177768 ) ) ;
#88411=CARTESIAN_POINT ( 'NONE',  ( 4.559911319644449179, 37.23035201082150536, -9.422509992056141925 ) ) ;
#88412=CARTESIAN_POINT ( 'NONE',  ( 0.5774900079438590739, 47.64701867748817676, -5.440088680355550821 ) ) ;
#88413=CARTESIAN_POINT ( 'NONE',  ( -2.816281873526473856, 14.33196800326375531, 3.434112377981055619 ) ) ;
#88414=CARTESIAN_POINT ( 'NONE',  ( 14.92337183194729633, 62.67559781766745886, 8.527530157486181039 ) ) ;
#88415=CARTESIAN_POINT ( 'NONE',  ( -0.8801773607111009756, 3.063685344154838397, 1.068504757029289695E-15 ) ) ;
#88416=CARTESIAN_POINT ( 'NONE',  ( 0.1532563361054100626, 5.800597817667452638, -2.638427012816831230 ) ) ;
#88418=CARTESIAN_POINT ( 'NONE',  ( 19.42250999205614193, 50.14701867748817676, 5.440088680355555262 ) ) ;
#88419=CARTESIAN_POINT ( 'NONE',  ( 3.591859063236763294, 8.290301336597087456, -11.09922568453595026 ) ) ;
#88421=CARTESIAN_POINT ( 'NONE',  ( 7.084665262690076126, 64.10535201082150536, 10.88017736071109987 ) ) ;
#88422=CARTESIAN_POINT ( 'NONE',  ( 5.076628168052704559, 25.17559781766745175, -8.527530157486179263 ) ) ;
#88423=CARTESIAN_POINT ( 'NONE',  ( 13.43411237798106583, 47.66530133659709634, -12.81628187352647252 ) ) ;
#88424=CARTESIAN_POINT ( 'NONE',  ( 19.84674366389459621, 3.508931151000785231, 7.409399052514197653E-17 ) ) ;
#88427=CARTESIAN_POINT ( 'NONE',  ( 0.9413316022086073431, 28.45508385108958649, 6.499999999999968914 ) ) ;
#88428=CARTESIAN_POINT ( 'NONE',  ( 20.88017736071110164, 20.35535201082150891, 2.915334737309930979 ) ) ;
#88429=CARTESIAN_POINT ( 'NONE',  ( -1.099225684535947600, 64.54030133659709634, 6.408140936763237150 ) ) ;
#88431=CARTESIAN_POINT ( 'NONE',  ( 10.00000000000000000, 24.75893115100078745, -9.846743663894594434 ) ) ;
#88432=CARTESIAN_POINT ( 'NONE',  ( 15.44008868035555260, 24.73035201082150891, 9.422509992056143702 ) ) ;
#88433=CARTESIAN_POINT ( 'NONE',  ( 20.88017736071110519, 5.563685344154838397, 2.639326808657452039E-16 ) ) ;
#88434=ORIENTED_EDGE ( 'NONE', *, *, #17779, .F. ) ;
#88435=CARTESIAN_POINT ( 'NONE',  ( -0.8801773607111008646, 13.27201867748817143, 2.915334737309923430 ) ) ;
#88436=CARTESIAN_POINT ( 'NONE',  ( 20.88017736071110519, 30.56368534415484106, 2.639326808657452039E-16 ) ) ;
#88438=CARTESIAN_POINT ( 'NONE',  ( 10.00000000000000178, 39.31368534415484106, 10.88017736071110342 ) ) ;
#88440=CARTESIAN_POINT ( 'NONE',  ( 5.076628168052704559, 65.17559781766745175, -8.527530157486179263 ) ) ;
#88441=CARTESIAN_POINT ( 'NONE',  ( 12.91533473730992121, 29.52201867748817321, 10.88017736071110164 ) ) ;
#88444=CARTESIAN_POINT ( 'NONE',  ( 13.99999999999999822, 10.49999999999999822, 6.500000000000000888 ) ) ;
#88445=CARTESIAN_POINT ( 'NONE',  ( 22.26659068614894466, 33.88708216824730357, 7.082119434687054849 ) ) ;
#88446=CARTESIAN_POINT ( 'NONE',  ( -0.8801773607111008646, 33.27201867748817676, 2.915334737309923430 ) ) ;
#88447=CARTESIAN_POINT ( 'NONE',  ( 4.559911319644449179, 28.89701867748817321, 9.422509992056141925 ) ) ;
#88448=CARTESIAN_POINT ( 'NONE',  ( 17.20831665107776587, 64.13393115100079456, -7.208316651077762316 ) ) ;
#88449=CYLINDRICAL_SURFACE ( 'NONE', #47718, 0.4999999999999995559 ) ;
#88450=CARTESIAN_POINT ( 'NONE',  ( 0.1532563361054083140, 51.00893115100078745, 1.131784320476157264E-15 ) ) ;
#88451=CARTESIAN_POINT ( 'NONE',  ( 0.2751277870542913062, 29.36607318730131411, -6.499999999999992006 ) ) ;
#88452=CARTESIAN_POINT ( 'NONE',  ( 17.20831665107776587, 17.88393115100078745, 7.208316651077764980 ) ) ;
#88454=CARTESIAN_POINT ( 'NONE',  ( -0.8801773607111008646, 13.27201867748817143, 2.915334737309923430 ) ) ;
#88455=CARTESIAN_POINT ( 'NONE',  ( 19.84674366389459266, 28.71726448433411960, -2.638427012816827677 ) ) ;
#88456=CARTESIAN_POINT ( 'NONE',  ( 16.40814093676324603, 12.45696800326375353, -11.09922568453594671 ) ) ;
#88457=CARTESIAN_POINT ( 'NONE',  ( 7.084665262690076126, 57.02201867748817676, -10.88017736071110164 ) ) ;
#88458=CARTESIAN_POINT ( 'NONE',  ( -0.8801773607111009756, 13.06368534415483929, 1.068504757029289695E-15 ) ) ;
#88459=CARTESIAN_POINT ( 'NONE',  ( 21.09922568453595559, 57.04030133659708923, -6.408140936763230044 ) ) ;
#88460=CARTESIAN_POINT ( 'NONE',  ( 20.36894250292379738, 29.92874883491396432, -10.36894250292379027 ) ) ;
#88463=CARTESIAN_POINT ( 'NONE',  ( 0.6178305044545818747, 8.498634669930421381, -9.382169495545419124 ) ) ;
#88464=FILL_AREA_STYLE ('',( #72470 ) ) ;
#88465=CARTESIAN_POINT ( 'NONE',  ( 2.035157376598822676, 27.43868534415483396, -7.964842623401177768 ) ) ;
#88466=CARTESIAN_POINT ( 'NONE',  ( 7.361572987183170547, 62.05059781766745886, 9.846743663894590881 ) ) ;
#88467=ORIENTED_EDGE ( 'NONE', *, *, #17682, .T. ) ;
#88468=CARTESIAN_POINT ( 'NONE',  ( 17.20831665107776587, 12.88393115100078390, 7.208316651077764980 ) ) ;
#88469=CARTESIAN_POINT ( 'NONE',  ( 7.361572987183169658, 14.96726448433411960, -9.846743663894592657 ) ) ;
#88470=CARTESIAN_POINT ( 'NONE',  ( 19.84674366389459621, 18.50893115100078745, 7.409399052514197653E-17 ) ) ;
#88471=CARTESIAN_POINT ( 'NONE',  ( 17.20831665107776587, 14.13393115100078568, -7.208316651077762316 ) ) ;
#88473=FILL_AREA_STYLE ('',( #11988 ) ) ;
#88476=CARTESIAN_POINT ( 'NONE',  ( 0.5774900079438607392, 68.48035201082150536, 5.440088680355550821 ) ) ;
#88478=CARTESIAN_POINT ( 'NONE',  ( 7.361572987183169658, 4.967264484334119601, -9.846743663894592657 ) ) ;
#88479=CARTESIAN_POINT ( 'NONE',  ( 5.076628168052703671, 16.84226448433411960, 8.527530157486179263 ) ) ;
#88480=VERTEX_POINT ( 'NONE', #13718 ) ;
#88482=CARTESIAN_POINT ( 'NONE',  ( 2.791683348922237240, 65.38393115100078035, -7.208316651077763204 ) ) ;
#88485=CARTESIAN_POINT ( 'NONE',  ( 4.559911319644449179, 2.230352010821504471, -9.422509992056141925 ) ) ;
#88486=CARTESIAN_POINT ( 'NONE',  ( 2.917880565312950480, 25.97041550158063572, -12.26659068614894821 ) ) ;
#88487=PRODUCT_DEFINITION_CONTEXT ( 'detailed design', #83209, 'design' ) ;
#88489=CARTESIAN_POINT ( 'NONE',  ( -2.266590686148945544, 17.22041550158063572, 7.082119434687048631 ) ) ;
#88490=CARTESIAN_POINT ( 'NONE',  ( 17.08211943468705130, 38.47041550158063217, 12.26659068614894998 ) ) ;
#88491=CARTESIAN_POINT ( 'NONE',  ( -4.164238869374099039, 16.80374883491396787, 8.674139862899312516E-16 ) ) ;
#88492=CARTESIAN_POINT ( 'NONE',  ( 10.00000000000000000, 36.81368534415484106, -10.88017736071110342 ) ) ;
#88495=CARTESIAN_POINT ( 'NONE',  ( 2.791683348922237240, 20.38393115100078745, -7.208316651077763204 ) ) ;
#88497=CARTESIAN_POINT ( 'NONE',  ( 15.44008868035555793, 56.39701867748817676, -9.422509992056140149 ) ) ;
#88498=CARTESIAN_POINT ( 'NONE',  ( 2.791683348922237240, 25.38393115100078390, -7.208316651077763204 ) ) ;
#88500=CARTESIAN_POINT ( 'NONE',  ( 12.91533473730993009, 16.60535201082150891, -10.88017736071109987 ) ) ;
#88501=CARTESIAN_POINT ( 'NONE',  ( -2.816281873526471635, 38.91530133659708213, -3.434112377981056508 ) ) ;
#88502=CARTESIAN_POINT ( 'NONE',  ( 7.361572987183169658, 54.96726448433413026, -9.846743663894592657 ) ) ;
#88504=CARTESIAN_POINT ( 'NONE',  ( 10.00000000000000000, 47.87363466993042493, -12.81628187352647608 ) ) ;
#88506=CARTESIAN_POINT ( 'NONE',  ( 12.63842701281683922, 34.55059781766745886, -9.846743663894590881 ) ) ;
#88508=CARTESIAN_POINT ( 'NONE',  ( 20.36894250292379382, 28.67874883491396787, 10.36894250292379205 ) ) ;
#88512=CARTESIAN_POINT ( 'NONE',  ( 20.88017736071110164, 55.35535201082149825, 2.915334737309930979 ) ) ;
#88513=CARTESIAN_POINT ( 'NONE',  ( 17.96484262340118221, 49.93868534415484106, 7.964842623401181321 ) ) ;
#88514=CARTESIAN_POINT ( 'NONE',  ( 24.16423886937410614, 39.51208216824731068, -3.795296366450302550 ) ) ;
#88515=CARTESIAN_POINT ( 'NONE',  ( 0.6178305044545838731, 4.748634669930420493, 9.382169495545420901 ) ) ;
#88516=B_SPLINE_CURVE_WITH_KNOTS ( 'NONE', 3,
 ( #91102, #641, #7638, #98143, #75118, #45107 ),
 .UNSPECIFIED., .F., .F.,
 ( 4, 2, 4 ),
 ( 9.220181747203676555E-18, 0.0002605067024380944827, 0.0005210134048761797497 ),
 .UNSPECIFIED. ) ;
#88517=CARTESIAN_POINT ( 'NONE',  ( 0.2751277870542868098, 57.28217586085237656, -6.499999999999985789 ) ) ;
#88518=CARTESIAN_POINT ( 'NONE',  ( 0.5774900079438607392, 38.48035201082150536, 5.440088680355550821 ) ) ;
#88520=CARTESIAN_POINT ( 'NONE',  ( 12.63842701281683922, 59.55059781766744464, -9.846743663894590881 ) ) ;
#88523=CARTESIAN_POINT ( 'NONE',  ( 20.88017736071110875, 65.77201867748817676, -2.915334737309920765 ) ) ;
#88525=CARTESIAN_POINT ( 'NONE',  ( 19.42250999205614548, 5.980352010821504471, -5.440088680355545492 ) ) ;
#88526=CARTESIAN_POINT ( 'NONE',  ( 19.80777595082616926, 65.68878173731739878, -6.499999999999942268 ) ) ;
#88527=CARTESIAN_POINT ( 'NONE',  ( -0.8801773607111009756, 68.06368534415484817, 1.068504757029289695E-15 ) ) ;
#88528=CARTESIAN_POINT ( 'NONE',  ( 17.20831665107776587, 2.883931151000785231, 7.208316651077764980 ) ) ;
#88529=CARTESIAN_POINT ( 'NONE',  ( 20.15039907845753575, 36.74884699246889141, 6.262539305110075283 ) ) ;
#88531=CARTESIAN_POINT ( 'NONE',  ( 12.63842701281683922, 34.55059781766745886, -9.846743663894590881 ) ) ;
#88532=CARTESIAN_POINT ( 'NONE',  ( 2.035157376598824452, 28.68868534415484106, 7.964842623401179544 ) ) ;
#88533=VECTOR ( 'NONE', #55224, 1000.000000000000000 ) ;
#88534=CARTESIAN_POINT ( 'NONE',  ( 0.6178305044545838731, 4.748634669930420493, 9.382169495545420901 ) ) ;
#88535=CARTESIAN_POINT ( 'NONE',  ( 4.559911319644449179, 32.23035201082150536, -9.422509992056141925 ) ) ;
#88537=CARTESIAN_POINT ( 'NONE',  ( 6.565887622018943937, 33.08196800326374643, -12.81628187352647608 ) ) ;
#88539=CARTESIAN_POINT ( 'NONE',  ( -0.8801773607111008646, 58.27201867748816966, 2.915334737309923430 ) ) ;
#88540=CARTESIAN_POINT ( 'NONE',  ( 0.6178305044545838731, 19.74863466993042138, 9.382169495545420901 ) ) ;
#88543=SURFACE_STYLE_FILL_AREA ( #5055 ) ;
#88544=CARTESIAN_POINT ( 'NONE',  ( 12.91533473730993009, 26.60535201082150536, -10.88017736071109987 ) ) ;
#88545=CARTESIAN_POINT ( 'NONE',  ( 2.917880565312948704, 62.63708216824730357, 12.26659068614894643 ) ) ;
#88546=CARTESIAN_POINT ( 'NONE',  ( 1.472469842513823179, 56.42559781766745886, 4.923371831947296329 ) ) ;
#88547=CARTESIAN_POINT ( 'NONE',  ( 5.076628168052704559, 10.17559781766745175, -8.527530157486179263 ) ) ;
#88548=CARTESIAN_POINT ( 'NONE',  ( 12.91533473730993009, 66.60535201082150536, -10.88017736071109987 ) ) ;
#88550=CARTESIAN_POINT ( 'NONE',  ( 24.16423886937410614, 34.30374883491396787, 8.672049930838204340E-16 ) ) ;
#88554=CARTESIAN_POINT ( 'NONE',  ( 17.08211943468705130, 58.47041550158063927, 12.26659068614894998 ) ) ;
#88555=CARTESIAN_POINT ( 'NONE',  ( -2.266590686148945544, 47.22041550158063927, 7.082119434687048631 ) ) ;
#88556=CARTESIAN_POINT ( 'NONE',  ( 12.63842701281683922, 24.55059781766745175, -9.846743663894590881 ) ) ;
#88558=CARTESIAN_POINT ( 'NONE',  ( 13.43411237798106583, 22.66530133659708923, -12.81628187352647252 ) ) ;
#88561=CARTESIAN_POINT ( 'NONE',  ( -2.266590686148945544, 46.38708216824730357, -7.082119434687050408 ) ) ;
#88563=CARTESIAN_POINT ( 'NONE',  ( 0.1532563361054082862, 6.217264484334118713, 2.638427012816831674 ) ) ;
#88566=EDGE_LOOP ( 'NONE', ( #58797, #11875, #88961, #84192 ) ) ;
#88570=CARTESIAN_POINT ( 'NONE',  ( 19.42250999205614193, 15.14701867748817143, 5.440088680355555262 ) ) ;
#88571=CARTESIAN_POINT ( 'NONE',  ( 15.44008868035555260, 24.73035201082150891, 9.422509992056143702 ) ) ;
#88572=CARTESIAN_POINT ( 'NONE',  ( 2.791683348922237240, 50.38393115100078035, -7.208316651077763204 ) ) ;
#88573=CARTESIAN_POINT ( 'NONE',  ( 3.591859063236761518, 19.95696800326375353, 11.09922568453594849 ) ) ;
#88574=CARTESIAN_POINT ( 'NONE',  ( 15.00000000000000000, 11.50000000000000000, 6.000000000000000000 ) ) ;
#88576=CARTESIAN_POINT ( 'NONE',  ( 3.591859063236763294, 13.29030133659708746, -11.09922568453595026 ) ) ;
#88578=CARTESIAN_POINT ( 'NONE',  ( 7.361572987183169658, 29.96726448433411960, -9.846743663894592657 ) ) ;
#88579=CARTESIAN_POINT ( 'NONE',  ( 13.79529636645031943, 55.34541550158062506, -14.16423886937409904 ) ) ;
#88581=CARTESIAN_POINT ( 'NONE',  ( 10.00000000000000178, 4.313685344154837509, 10.88017736071110342 ) ) ;
#88583=CARTESIAN_POINT ( 'NONE',  ( 12.91533473730993009, 41.60535201082149825, -10.88017736071109987 ) ) ;
#88584=CARTESIAN_POINT ( 'NONE',  ( 2.035157376598824452, 38.68868534415483396, 7.964842623401179544 ) ) ;
#88585=CARTESIAN_POINT ( 'NONE',  ( 17.96484262340118221, 44.93868534415483396, 7.964842623401181321 ) ) ;
#88586=CARTESIAN_POINT ( 'NONE',  ( 19.80777595082615861, 5.688781737317405884, -6.500000000000003553 ) ) ;
#88587=CARTESIAN_POINT ( 'NONE',  ( 0.5774900079438607392, 38.48035201082150536, 5.440088680355550821 ) ) ;
#88591=CARTESIAN_POINT ( 'NONE',  ( 17.20831665107776587, 24.13393115100078035, -7.208316651077762316 ) ) ;
#88593=CARTESIAN_POINT ( 'NONE',  ( 19.84674366389459266, 63.71726448433412315, -2.638427012816827677 ) ) ;
#88594=DIRECTION ( 'NONE',  ( 0.000000000000000000, 0.000000000000000000, -1.000000000000000000 ) ) ;
#88599=CARTESIAN_POINT ( 'NONE',  ( 1.472469842513823179, 35.59226448433412315, -4.923371831947296329 ) ) ;
#88600=CARTESIAN_POINT ( 'NONE',  ( 6.204703633549690345, 60.76208216824730357, -14.16423886937410259 ) ) ;
#88604=CARTESIAN_POINT ( 'NONE',  ( 2.791683348922240793, 26.63393115100078745, 7.208316651077764092 ) ) ;
#88607=CARTESIAN_POINT ( 'NONE',  ( 22.81628187352648496, 6.831968003263753531, -3.434112377981050290 ) ) ;
#88608=CARTESIAN_POINT ( 'NONE',  ( 2.791683348922240793, 11.63393115100078568, 7.208316651077764092 ) ) ;
#88610=CARTESIAN_POINT ( 'NONE',  ( 1.472469842513823179, 6.425597817667451750, 4.923371831947296329 ) ) ;
#88611=CARTESIAN_POINT ( 'NONE',  ( 17.20831665107776587, 52.88393115100078035, 7.208316651077764980 ) ) ;
#88612=CARTESIAN_POINT ( 'NONE',  ( 20.88017736071110164, 20.35535201082150536, 2.915334737309930979 ) ) ;
#88617=CARTESIAN_POINT ( 'NONE',  ( -0.8801773607111008646, 13.27201867748817321, 2.915334737309923430 ) ) ;
#88618=CARTESIAN_POINT ( 'NONE',  ( 10.00000000000000000, 5.553748834913967869, -14.16423886937410082 ) ) ;
#88619=CARTESIAN_POINT ( 'NONE',  ( 18.52753015748617571, 18.09226448433411960, 4.923371831947298993 ) ) ;
#88620=CARTESIAN_POINT ( 'NONE',  ( 15.44008868035555260, 54.73035201082150536, 9.422509992056143702 ) ) ;
#88621=CARTESIAN_POINT ( 'NONE',  ( 22.81628187352648496, 26.83196800326374998, -3.434112377981050290 ) ) ;
#88623=CARTESIAN_POINT ( 'NONE',  ( 12.91533473730992121, 4.522018677488169658, 10.88017736071110164 ) ) ;
#88624=CARTESIAN_POINT ( 'NONE',  ( 20.03447792253738768, 17.65514106990690379, -6.401564815979731371 ) ) ;
#88625=CARTESIAN_POINT ( 'NONE',  ( 19.72487221294570858, 0.5000000000000000000, -6.500000000000000888 ) ) ;
#88626=CARTESIAN_POINT ( 'NONE',  ( 7.361572987183169658, 59.96726448433410894, -9.846743663894592657 ) ) ;
#88627=CARTESIAN_POINT ( 'NONE',  ( 17.20831665107776587, 7.883931151000784787, 7.208316651077764980 ) ) ;
#88629=CARTESIAN_POINT ( 'NONE',  ( -2.816281873526471635, 18.91530133659708213, -3.434112377981056508 ) ) ;
#88631=CARTESIAN_POINT ( 'NONE',  ( 15.44008868035555793, 26.39701867748817321, -9.422509992056140149 ) ) ;
#88635=CARTESIAN_POINT ( 'NONE',  ( -2.266590686148945544, 52.22041550158064638, 7.082119434687048631 ) ) ;
#88638=CARTESIAN_POINT ( 'NONE',  ( 4.559911319644449179, 27.23035201082150536, -9.422509992056141925 ) ) ;
#88639=CARTESIAN_POINT ( 'NONE',  ( 0.1532563361054100626, 55.80059781766745175, -2.638427012816831230 ) ) ;
#88640=CARTESIAN_POINT ( 'NONE',  ( 15.44008868035555260, 54.73035201082150536, 9.422509992056143702 ) ) ;
#88642=CARTESIAN_POINT ( 'NONE',  ( 6.204703633549690345, 32.84541550158063927, 14.16423886937410082 ) ) ;
#88645=CARTESIAN_POINT ( 'NONE',  ( 0.1532563361054082862, 36.21726448433410894, 2.638427012816831674 ) ) ;
#88646=CARTESIAN_POINT ( 'NONE',  ( -1.099225684535947600, 63.70696800326376774, -6.408140936763238038 ) ) ;
#88647=CARTESIAN_POINT ( 'NONE',  ( -1.099225684535947600, 4.540301336597087456, 6.408140936763237150 ) ) ;
#88648=ORIENTED_EDGE ( 'NONE', *, *, #31026, .F. ) ;
#88649=CARTESIAN_POINT ( 'NONE',  ( 12.91533473730993009, 26.60535201082150536, -10.88017736071109987 ) ) ;
#88650=CARTESIAN_POINT ( 'NONE',  ( 20.32896413005680714, 7.604976035794174472, -5.963430220938276349 ) ) ;
#88652=CARTESIAN_POINT ( 'NONE',  ( 4.559911319644449179, 8.897018677488173211, 9.422509992056141925 ) ) ;
#88653=CARTESIAN_POINT ( 'NONE',  ( 4.559911319644449179, 68.89701867748817676, 9.422509992056141925 ) ) ;
#88654=CARTESIAN_POINT ( 'NONE',  ( 24.16423886937410614, 24.30374883491396787, 8.672049930838204340E-16 ) ) ;
#88655=CARTESIAN_POINT ( 'NONE',  ( 10.00000000000000000, 14.75893115100078568, -9.846743663894594434 ) ) ;
#88656=CARTESIAN_POINT ( 'NONE',  ( 19.84674366389459621, 63.50893115100078745, 7.409399052514197653E-17 ) ) ;
#88657=CARTESIAN_POINT ( 'NONE',  ( 4.559911319644449179, 27.23035201082150536, -9.422509992056141925 ) ) ;
#88658=VECTOR ( 'NONE', #96005, 1000.000000000000000 ) ;
#88661=ORIENTED_EDGE ( 'NONE', *, *, #39854, .F. ) ;
#88663=CARTESIAN_POINT ( 'NONE',  ( 7.361572987183170547, 42.05059781766745886, 9.846743663894590881 ) ) ;
#88665=ORIENTED_EDGE ( 'NONE', *, *, #71910, .F. ) ;
#88667=CARTESIAN_POINT ( 'NONE',  ( 24.16423886937410614, 4.512082168247300906, -3.795296366450302550 ) ) ;
#88668=CARTESIAN_POINT ( 'NONE',  ( -4.164238869374099927, 12.01208216824730357, 3.795296366450308767 ) ) ;
#88669=CARTESIAN_POINT ( 'NONE',  ( 19.42250999205614548, 45.98035201082150536, -5.440088680355545492 ) ) ;
#88671=CARTESIAN_POINT ( 'NONE',  ( -2.266590686148945544, 52.22041550158064638, 7.082119434687048631 ) ) ;
#88672=CARTESIAN_POINT ( 'NONE',  ( 22.81628187352647785, 6.415301336597088344, 3.434112377981063169 ) ) ;
#88673=CARTESIAN_POINT ( 'NONE',  ( 14.92337183194729633, 37.67559781766745175, 8.527530157486181039 ) ) ;
#88675=CARTESIAN_POINT ( 'NONE',  ( 10.00000000000000000, 36.81368534415484106, -10.88017736071110342 ) ) ;
#88676=CARTESIAN_POINT ( 'NONE',  ( 19.38216949554541557, 2.248634669930420049, -9.382169495545420901 ) ) ;
#88677=CARTESIAN_POINT ( 'NONE',  ( 2.917880565312948704, 7.637082168247301794, 12.26659068614894643 ) ) ;
#88678=CARTESIAN_POINT ( 'NONE',  ( -2.266590686148945544, 56.38708216824731068, -7.082119434687050408 ) ) ;
#88679=VECTOR ( 'NONE', #30974, 1000.000000000000000 ) ;
#88680=CARTESIAN_POINT ( 'NONE',  ( 7.084665262690076126, 22.02201867748817321, -10.88017736071110164 ) ) ;
#88688=CARTESIAN_POINT ( 'NONE',  ( 24.16423886937410614, 44.51208216824730357, -3.795296366450302550 ) ) ;
#88689=CARTESIAN_POINT ( 'NONE',  ( 10.00000000000000178, 52.25893115100078745, 9.846743663894594434 ) ) ;
#88690=CARTESIAN_POINT ( 'NONE',  ( 20.88017736071110519, 50.56368534415484106, 2.639326808657452039E-16 ) ) ;
#88691=CARTESIAN_POINT ( 'NONE',  ( -41.94000000000001194, 93.50000000000000000, -10.09898361729590199 ) ) ;
#88692=CARTESIAN_POINT ( 'NONE',  ( 4.559911319644449179, 57.23035201082150536, -9.422509992056141925 ) ) ;
#88694=CARTESIAN_POINT ( 'NONE',  ( 19.38216949554541557, 57.24863466993042493, -9.382169495545420901 ) ) ;
#88696=VERTEX_POINT ( 'NONE', #61664 ) ;
#88697=CARTESIAN_POINT ( 'NONE',  ( 24.16423886937410614, 24.51208216824730002, -3.795296366450302550 ) ) ;
#88699=CARTESIAN_POINT ( 'NONE',  ( 16.40814093676323893, 30.79030133659708923, 11.09922568453595026 ) ) ;
#88700=EDGE_LOOP ( 'NONE', ( #64351, #77002, #96467, #70543 ) ) ;
#88701=CARTESIAN_POINT ( 'NONE',  ( 13.43411237798105340, 40.58196800326375353, 12.81628187352647963 ) ) ;
#88702=CARTESIAN_POINT ( 'NONE',  ( 17.20831665107776587, 42.88393115100077324, 7.208316651077764980 ) ) ;
#88703=CARTESIAN_POINT ( 'NONE',  ( 12.91533473730993009, 11.60535201082150536, -10.88017736071109987 ) ) ;
#88704=CARTESIAN_POINT ( 'NONE',  ( 16.40814093676324603, 52.45696800326375353, -11.09922568453594671 ) ) ;
#88706=CARTESIAN_POINT ( 'NONE',  ( 5.076628168052704559, 45.17559781766745175, -8.527530157486179263 ) ) ;
#88713=DIRECTION ( 'NONE',  ( 0.000000000000000000, 0.000000000000000000, -1.000000000000000000 ) ) ;
#88716=CARTESIAN_POINT ( 'NONE',  ( 12.63842701281683034, 22.46726448433411605, 9.846743663894596210 ) ) ;
#88717=CARTESIAN_POINT ( 'NONE',  ( 22.81628187352648496, 21.83196800326374643, -3.434112377981050290 ) ) ;
#88720=CARTESIAN_POINT ( 'NONE',  ( 7.361572987183170547, 62.05059781766745886, 9.846743663894590881 ) ) ;
#88721=CARTESIAN_POINT ( 'NONE',  ( 18.95386800105009328, 28.23810908735718783, -6.499999999999990230 ) ) ;
#88722=CARTESIAN_POINT ( 'NONE',  ( 6.204703633549690345, 17.84541550158063217, 14.16423886937410082 ) ) ;
#88723=CARTESIAN_POINT ( 'NONE',  ( 17.20831665107776587, 29.13393115100078390, -7.208316651077762316 ) ) ;
#88724=CARTESIAN_POINT ( 'NONE',  ( 13.43411237798105340, 45.58196800326374643, 12.81628187352647963 ) ) ;
#88727=CARTESIAN_POINT ( 'NONE',  ( 0.5774900079438607392, 58.48035201082151247, 5.440088680355550821 ) ) ;
#88728=CARTESIAN_POINT ( 'NONE',  ( 0.6178305044545818747, 13.49863466993041783, -9.382169495545419124 ) ) ;
#88730=CARTESIAN_POINT ( 'NONE',  ( 17.20831665107776587, 32.88393115100078745, 7.208316651077764980 ) ) ;
#88731=CARTESIAN_POINT ( 'NONE',  ( 15.44008868035555260, 44.73035201082151247, 9.422509992056143702 ) ) ;
#88732=CARTESIAN_POINT ( 'NONE',  ( 22.81628187352648496, 41.83196800326375353, -3.434112377981050290 ) ) ;
#88734=CARTESIAN_POINT ( 'NONE',  ( 0.1532563361054083140, 36.00893115100078745, 1.131784320476157264E-15 ) ) ;
#88739=CARTESIAN_POINT ( 'NONE',  ( -0.8801773607111008646, 28.27201867748817321, 2.915334737309923430 ) ) ;
#88743=CARTESIAN_POINT ( 'NONE',  ( 19.42250999205614193, 15.14701867748817143, 5.440088680355555262 ) ) ;
#88744=CARTESIAN_POINT ( 'NONE',  ( 10.00000000000000000, 54.75893115100078745, -9.846743663894594434 ) ) ;
#88745=CARTESIAN_POINT ( 'NONE',  ( 7.084665262690076126, 32.02201867748816966, -10.88017736071110164 ) ) ;
#88747=CARTESIAN_POINT ( 'NONE',  ( 12.91533473730992121, 54.52201867748816255, 10.88017736071110164 ) ) ;
#88748=CARTESIAN_POINT ( 'NONE',  ( 4.559911319644449179, 27.23035201082150536, -9.422509992056141925 ) ) ;
#88749=CARTESIAN_POINT ( 'NONE',  ( -0.000000000000000000, 77.78215977002660964, -8.385699614948331160 ) ) ;
#88750=SURFACE_STYLE_USAGE ( .BOTH. , #35748 ) ;
#88751=CARTESIAN_POINT ( 'NONE',  ( 12.63842701281683922, 19.55059781766745175, -9.846743663894590881 ) ) ;
#88754=CARTESIAN_POINT ( 'NONE',  ( 5.076628168052703671, 51.84226448433412315, 8.527530157486179263 ) ) ;
#88755=CARTESIAN_POINT ( 'NONE',  ( -4.164238869374098151, 51.59541550158063217, -3.795296366450310543 ) ) ;
#88756=CARTESIAN_POINT ( 'NONE',  ( 20.24186590665278018, 20.59014588040357197, -6.114288769123027656 ) ) ;
#88757=CARTESIAN_POINT ( 'NONE',  ( -2.266590686148945544, 7.220415501580634832, 7.082119434687048631 ) ) ;
#88758=CARTESIAN_POINT ( 'NONE',  ( 17.08211943468705130, 33.47041550158063927, 12.26659068614894998 ) ) ;
#88759=CARTESIAN_POINT ( 'NONE',  ( -1.099225684535947600, -0.4596986634029132657, 6.408140936763237150 ) ) ;
#88763=CARTESIAN_POINT ( 'NONE',  ( 19.42250999205614193, 15.14701867748817143, 5.440088680355555262 ) ) ;
#88764=CARTESIAN_POINT ( 'NONE',  ( 19.84674366389459621, 33.50893115100078745, 7.409399052514197653E-17 ) ) ;
#88765=( LENGTH_UNIT ( ) NAMED_UNIT ( * ) SI_UNIT ( .MILLI., .METRE. ) );
#88767=CARTESIAN_POINT ( 'NONE',  ( 5.076628168052703671, 1.842264484334118047, 8.527530157486179263 ) ) ;
#88768=CARTESIAN_POINT ( 'NONE',  ( 16.40814093676323893, 20.79030133659708923, 11.09922568453595026 ) ) ;
#88769=CARTESIAN_POINT ( 'NONE',  ( 1.472469842513823179, 26.42559781766745175, 4.923371831947296329 ) ) ;
#88770=ORIENTED_EDGE ( 'NONE', *, *, #60727, .T. ) ;
#88773=CARTESIAN_POINT ( 'NONE',  ( -4.164238869374099039, 61.80374883491397497, 8.674139862899312516E-16 ) ) ;
#88774=CARTESIAN_POINT ( 'NONE',  ( 15.44008868035555793, 16.39701867748817321, -9.422509992056140149 ) ) ;
#88775=CARTESIAN_POINT ( 'NONE',  ( 2.917880565312950480, 35.97041550158063217, -12.26659068614894821 ) ) ;
#88776=CARTESIAN_POINT ( 'NONE',  ( 0.5774900079438590739, 37.64701867748817676, -5.440088680355550821 ) ) ;
#88777=CARTESIAN_POINT ( 'NONE',  ( 20.88017736071110519, 60.56368534415484106, 2.639326808657452039E-16 ) ) ;
#88780=CARTESIAN_POINT ( 'NONE',  ( 20.15039907845753575, 39.72266099184919597, 6.262539305110075283 ) ) ;
#88781=CARTESIAN_POINT ( 'NONE',  ( 17.20831665107776587, 29.13393115100078390, -7.208316651077762316 ) ) ;
#88783=CARTESIAN_POINT ( 'NONE',  ( 7.361572987183169658, 9.967264484334119601, -9.846743663894592657 ) ) ;
#88785=CARTESIAN_POINT ( 'NONE',  ( 1.472469842513823179, 41.42559781766745886, 4.923371831947296329 ) ) ;
#88786=CARTESIAN_POINT ( 'NONE',  ( 14.92337183194729988, 59.34226448433412315, -8.527530157486177487 ) ) ;
#88787=COLOUR_RGB ( '', 0.09019608, 0.27058824, 0.51372549) ;
#88790=CARTESIAN_POINT ( 'NONE',  ( -0.8801773607110991993, 32.85535201082151247, -2.915334737309923874 ) ) ;
#88792=CARTESIAN_POINT ( 'NONE',  ( 19.38216949554541557, 47.24863466993041783, -9.382169495545420901 ) ) ;
#88794=CARTESIAN_POINT ( 'NONE',  ( 2.791683348922237240, 0.3839311510007847872, -7.208316651077763204 ) ) ;
#88795=CARTESIAN_POINT ( 'NONE',  ( -1.099225684535947600, 38.70696800326375353, -6.408140936763238038 ) ) ;
#88796=CARTESIAN_POINT ( 'NONE',  ( 10.00000000000000178, 58.05374883491397497, 14.16423886937410082 ) ) ;
#88797=CARTESIAN_POINT ( 'NONE',  ( 2.791683348922237240, 35.38393115100079456, -7.208316651077763204 ) ) ;
#88799=CARTESIAN_POINT ( 'NONE',  ( 2.791683348922240793, 61.63393115100079456, 7.208316651077764092 ) ) ;
#88800=CARTESIAN_POINT ( 'NONE',  ( -0.3689425029237898834, 26.17874883491396432, -10.36894250292378850 ) ) ;
#88801=CARTESIAN_POINT ( 'NONE',  ( 12.63842701281683922, 39.55059781766744464, -9.846743663894590881 ) ) ;
#88802=CARTESIAN_POINT ( 'NONE',  ( 19.88565890683628368, 12.71691075486302580, -6.480892540919847455 ) ) ;
#88803=CARTESIAN_POINT ( 'NONE',  ( 0.5774900079438607392, 38.48035201082150536, 5.440088680355550821 ) ) ;
#88804=CARTESIAN_POINT ( 'NONE',  ( 15.44008868035555260, 54.73035201082150536, 9.422509992056143702 ) ) ;
#88807=CARTESIAN_POINT ( 'NONE',  ( 0.6178305044545838731, 44.74863466993042493, 9.382169495545420901 ) ) ;
#88808=CARTESIAN_POINT ( 'NONE',  ( 17.20831665107776587, 2.883931151000785231, 7.208316651077764980 ) ) ;
#88810=CARTESIAN_POINT ( 'NONE',  ( 2.917880565312948704, 12.63708216824730179, 12.26659068614894643 ) ) ;
#88811=CARTESIAN_POINT ( 'NONE',  ( 14.92337183194729988, 4.342264484334117824, -8.527530157486177487 ) ) ;
#88812=CARTESIAN_POINT ( 'NONE',  ( 1.250199848463767305, 0.007464128780085518312, -6.094592771028128020 ) ) ;
#88816=CARTESIAN_POINT ( 'NONE',  ( 4.559911319644449179, 8.897018677488171434, 9.422509992056141925 ) ) ;
#88818=CARTESIAN_POINT ( 'NONE',  ( 22.26659068614894466, 18.88708216824730002, 7.082119434687054849 ) ) ;
#88819=COLOUR_RGB ( '', 0.09019608, 0.27058824, 0.51372549) ;
#88820=CARTESIAN_POINT ( 'NONE',  ( 15.44008868035555260, 24.73035201082150891, 9.422509992056143702 ) ) ;
#88821=CARTESIAN_POINT ( 'NONE',  ( 10.00000000000000178, 62.25893115100078745, 9.846743663894594434 ) ) ;
#88823=CARTESIAN_POINT ( 'NONE',  ( 12.63842701281683922, 59.55059781766744464, -9.846743663894590881 ) ) ;
#88825=CARTESIAN_POINT ( 'NONE',  ( 17.96484262340118221, 66.18868534415483396, -7.964842623401177768 ) ) ;
#88826=CARTESIAN_POINT ( 'NONE',  ( 18.52753015748617571, 63.09226448433412315, 4.923371831947298993 ) ) ;
#88827=CARTESIAN_POINT ( 'NONE',  ( 13.43411237798106583, 37.66530133659708923, -12.81628187352647252 ) ) ;
#88828=CARTESIAN_POINT ( 'NONE',  ( 4.559911319644449179, 2.230352010821504471, -9.422509992056141925 ) ) ;
#88830=CARTESIAN_POINT ( 'NONE',  ( 2.791683348922240793, 1.633931151000784565, 7.208316651077764092 ) ) ;
#88831=CARTESIAN_POINT ( 'NONE',  ( 0.5774900079438607392, 18.48035201082150536, 5.440088680355550821 ) ) ;
#88835=EDGE_LOOP ( 'NONE', ( #50066, #26115, #11001, #79347, #63414, #18811 ) ) ;
#88837=CARTESIAN_POINT ( 'NONE',  ( 21.09922568453595559, 52.04030133659708923, -6.408140936763230044 ) ) ;
#88838=CARTESIAN_POINT ( 'NONE',  ( 0.5774900079438607392, 28.48035201082150891, 5.440088680355550821 ) ) ;
#88839=CARTESIAN_POINT ( 'NONE',  ( -46.94000000000000483, 100.6164469616018238, -8.719320056940125241 ) ) ;
#88840=CARTESIAN_POINT ( 'NONE',  ( 13.43411237798106583, 37.66530133659708923, -12.81628187352647252 ) ) ;
#88841=CARTESIAN_POINT ( 'NONE',  ( 4.559911319644449179, 53.89701867748817676, 9.422509992056141925 ) ) ;
#88842=CARTESIAN_POINT ( 'NONE',  ( 17.20831665107776587, 52.88393115100078035, 7.208316651077764980 ) ) ;
#88844=CARTESIAN_POINT ( 'NONE',  ( -0.1038446121089038471, 49.24302437010793909, -6.337995344473782211 ) ) ;
#88845=CARTESIAN_POINT ( 'NONE',  ( 7.361572987183169658, 9.967264484334119601, -9.846743663894592657 ) ) ;
#88846=CARTESIAN_POINT ( 'NONE',  ( 22.81628187352647785, 11.62363466993042138, 6.195893100308588602E-16 ) ) ;
#88848=CARTESIAN_POINT ( 'NONE',  ( 2.791683348922240793, 51.63393115100078745, 7.208316651077764092 ) ) ;
#88849=CARTESIAN_POINT ( 'NONE',  ( 4.559911319644449179, 27.23035201082150536, -9.422509992056141925 ) ) ;
#88850=CARTESIAN_POINT ( 'NONE',  ( 14.92337183194729988, 49.34226448433411605, -8.527530157486177487 ) ) ;
#88854=CARTESIAN_POINT ( 'NONE',  ( 2.791683348922240793, 6.633931151000785675, 7.208316651077764092 ) ) ;
#88855=CARTESIAN_POINT ( 'NONE',  ( 12.63842701281683034, 57.46726448433411605, 9.846743663894596210 ) ) ;
#88856=VERTEX_POINT ( 'NONE', #15218 ) ;
#88859=CARTESIAN_POINT ( 'NONE',  ( 0.6178305044545818747, 43.49863466993042493, -9.382169495545419124 ) ) ;
#88861=CARTESIAN_POINT ( 'NONE',  ( 12.63842701281683922, 29.55059781766745175, -9.846743663894590881 ) ) ;
#88862=CARTESIAN_POINT ( 'NONE',  ( -0.1503990784575407469, 12.22266099184918531, -6.262539305110056631 ) ) ;
#88863=CARTESIAN_POINT ( 'NONE',  ( 10.00000000000000000, 60.55374883491397497, -14.16423886937410082 ) ) ;
#88864=CARTESIAN_POINT ( 'NONE',  ( 18.52753015748617571, 33.09226448433411605, 4.923371831947298993 ) ) ;
#88865=AXIS2_PLACEMENT_3D ( 'NONE', #11954, #42948, #35434 ) ;
#88867=CARTESIAN_POINT ( 'NONE',  ( 19.64232630867105556, 84.97379543201886065, 5.304930624720102017 ) ) ;
#88869=CARTESIAN_POINT ( 'NONE',  ( 20.36894250292379382, 58.67874883491396076, 10.36894250292379205 ) ) ;
#88870=DIRECTION ( 'NONE',  ( -0.000000000000000000, -0.000000000000000000, -1.000000000000000000 ) ) ;
#88871=CARTESIAN_POINT ( 'NONE',  ( 20.88017736071110875, 15.77201867748817143, -2.915334737309920765 ) ) ;
#88872=CARTESIAN_POINT ( 'NONE',  ( -4.164238869374098151, 41.59541550158061796, -3.795296366450310543 ) ) ;
#88873=CARTESIAN_POINT ( 'NONE',  ( 2.917880565312950480, 55.97041550158063217, -12.26659068614894821 ) ) ;
#88875=CARTESIAN_POINT ( 'NONE',  ( 20.88017736071110875, 5.772018677488170546, -2.915334737309920321 ) ) ;
#88876=CARTESIAN_POINT ( 'NONE',  ( 0.1532563361054082862, 6.217264484334118713, 2.638427012816831674 ) ) ;
#88877=CARTESIAN_POINT ( 'NONE',  ( 0.6178305044545818747, -1.501365330069579951, -9.382169495545419124 ) ) ;
#88878=CARTESIAN_POINT ( 'NONE',  ( 17.62281668512002852, 13.28593319516822469, 6.499999999999993783 ) ) ;
#88879=CARTESIAN_POINT ( 'NONE',  ( -0.8801773607111009756, 48.06368534415484817, 1.068504757029289695E-15 ) ) ;
#88881=CARTESIAN_POINT ( 'NONE',  ( 14.92337183194729988, 49.34226448433411605, -8.527530157486177487 ) ) ;
#88885=( NAMED_UNIT ( * ) PLANE_ANGLE_UNIT ( ) SI_UNIT ( $, .RADIAN. ) );
#88887=CARTESIAN_POINT ( 'NONE',  ( -2.266590686148945544, 36.38708216824730357, -7.082119434687050408 ) ) ;
#88889=CARTESIAN_POINT ( 'NONE',  ( 0.9408516040111475354, 37.46693863883976405, -6.499999999999953815 ) ) ;
#88892=CARTESIAN_POINT ( 'NONE',  ( 17.96484262340118221, 21.18868534415483396, -7.964842623401177768 ) ) ;
#88893=CARTESIAN_POINT ( 'NONE',  ( -1.099225684535947600, 43.70696800326375353, -6.408140936763238038 ) ) ;
#88895=CARTESIAN_POINT ( 'NONE',  ( 10.00000000000000178, 20.37363466993042138, 12.81628187352647608 ) ) ;
#88896=CARTESIAN_POINT ( 'NONE',  ( 3.591859063236761518, 64.95696800326376774, 11.09922568453594849 ) ) ;
#88900=CARTESIAN_POINT ( 'NONE',  ( 17.08211943468705130, 28.47041550158063572, 12.26659068614894998 ) ) ;
#88902=CARTESIAN_POINT ( 'NONE',  ( 10.00000000000000178, 24.31368534415484106, 10.88017736071110342 ) ) ;
#88903=CARTESIAN_POINT ( 'NONE',  ( 19.72487221294570858, 70.00000000000000000, 6.500000000000000888 ) ) ;
#88904=CARTESIAN_POINT ( 'NONE',  ( 19.42250999205614193, 40.14701867748817676, 5.440088680355555262 ) ) ;
#88905=CARTESIAN_POINT ( 'NONE',  ( 10.00000000000000000, 46.81368534415484106, -10.88017736071110342 ) ) ;
#88906=CARTESIAN_POINT ( 'NONE',  ( -1.099225684535947600, 14.54030133659708568, 6.408140936763237150 ) ) ;
#88909=CARTESIAN_POINT ( 'NONE',  ( 17.20831665107776587, 17.88393115100078745, 7.208316651077764980 ) ) ;
#88911=CARTESIAN_POINT ( 'NONE',  ( 17.96484262340118221, 46.18868534415484106, -7.964842623401177768 ) ) ;
#88915=CARTESIAN_POINT ( 'NONE',  ( -1.099225684535947600, -0.4596986634029132657, 6.408140936763237150 ) ) ;
#88916=CARTESIAN_POINT ( 'NONE',  ( 1.274849032794278747, 42.55509018479936856, -6.499999999999960032 ) ) ;
#88917=CARTESIAN_POINT ( 'NONE',  ( 10.00000000000000178, 27.25893115100078390, 9.846743663894594434 ) ) ;
#88918=CARTESIAN_POINT ( 'NONE',  ( 10.00000000000000000, 52.87363466993041783, -12.81628187352647608 ) ) ;
#88919=CARTESIAN_POINT ( 'NONE',  ( 2.791683348922240793, 11.63393115100078568, 7.208316651077764092 ) ) ;
#88921=CARTESIAN_POINT ( 'NONE',  ( 2.603489959281582777, 31.58210964143329136, 6.499999999999995559 ) ) ;
#88922=CARTESIAN_POINT ( 'NONE',  ( 4.559911319644449179, 18.89701867748817321, 9.422509992056141925 ) ) ;
#88923=DIRECTION ( 'NONE',  ( 0.000000000000000000, -1.000000000000000000, 0.000000000000000000 ) ) ;
#88924=CARTESIAN_POINT ( 'NONE',  ( 2.791683348922237240, 30.38393115100078390, -7.208316651077763204 ) ) ;
#88925=CARTESIAN_POINT ( 'NONE',  ( 12.91533473730993009, 21.60535201082150536, -10.88017736071109987 ) ) ;
#88926=CARTESIAN_POINT ( 'NONE',  ( 19.42250999205614548, 5.980352010821504471, -5.440088680355545492 ) ) ;
#88928=CARTESIAN_POINT ( 'NONE',  ( 0.5774900079438590739, 32.64701867748816966, -5.440088680355550821 ) ) ;
#88929=CARTESIAN_POINT ( 'NONE',  ( 19.42250999205614548, 40.98035201082150536, -5.440088680355545492 ) ) ;
#88931=CARTESIAN_POINT ( 'NONE',  ( 12.91533473730993009, 41.60535201082149825, -10.88017736071109987 ) ) ;
#88933=CARTESIAN_POINT ( 'NONE',  ( 14.92337183194729633, 62.67559781766745886, 8.527530157486181039 ) ) ;
#88934=CARTESIAN_POINT ( 'NONE',  ( 2.035157376598824452, 38.68868534415483396, 7.964842623401179544 ) ) ;
#88937=CARTESIAN_POINT ( 'NONE',  ( 13.43411237798105340, 60.58196800326376064, 12.81628187352647963 ) ) ;
#88939=CARTESIAN_POINT ( 'NONE',  ( 17.08211943468705840, 30.13708216824730357, -12.26659068614894466 ) ) ;
#88940=CARTESIAN_POINT ( 'NONE',  ( 10.00000000000000000, 51.81368534415484106, -10.88017736071110342 ) ) ;
#88941=CARTESIAN_POINT ( 'NONE',  ( 20.88017736071110164, 30.35535201082151247, 2.915334737309930979 ) ) ;
#88943=CARTESIAN_POINT ( 'NONE',  ( 20.15039907845753220, 27.62777174578613071, -6.262539305110077947 ) ) ;
#88944=CARTESIAN_POINT ( 'NONE',  ( 0.1532563361054083140, 56.00893115100078745, 1.131784320476157264E-15 ) ) ;
#88945=EDGE_CURVE ( 'NONE', #84166, #37561, #21623, .T. ) ;
#88946=ORIENTED_EDGE ( 'NONE', *, *, #44801, .F. ) ;
#88948=CARTESIAN_POINT ( 'NONE',  ( 17.20831665107776587, 19.13393115100078035, -7.208316651077762316 ) ) ;
#88950=CARTESIAN_POINT ( 'NONE',  ( 17.96484262340118221, 9.938685344154837509, 7.964842623401181321 ) ) ;
#88951=CARTESIAN_POINT ( 'NONE',  ( 0.1532563361054100626, 30.80059781766744820, -2.638427012816831230 ) ) ;
#88952=CARTESIAN_POINT ( 'NONE',  ( 13.43411237798105340, 10.58196800326375353, 12.81628187352647963 ) ) ;
#88953=CARTESIAN_POINT ( 'NONE',  ( 0.5774900079438590739, 62.64701867748817676, -5.440088680355550821 ) ) ;
#88954=CARTESIAN_POINT ( 'NONE',  ( -0.8801773607110991993, 32.85535201082151247, -2.915334737309923874 ) ) ;
#88955=CARTESIAN_POINT ( 'NONE',  ( 3.591859063236763294, 58.29030133659708923, -11.09922568453595026 ) ) ;
#88956=CARTESIAN_POINT ( 'NONE',  ( -4.164238869374098151, 51.59541550158063217, -3.795296366450310543 ) ) ;
#88960=EDGE_CURVE ( 'NONE', #78529, #31207, #46432, .T. ) ;
#88961=ORIENTED_EDGE ( 'NONE', *, *, #26094, .T. ) ;
#88962=CARTESIAN_POINT ( 'NONE',  ( 7.361572987183169658, 64.96726448433412315, -9.846743663894592657 ) ) ;
#88963=CARTESIAN_POINT ( 'NONE',  ( 19.42250999205614193, 10.14701867748816966, 5.440088680355555262 ) ) ;
#88964=CARTESIAN_POINT ( 'NONE',  ( 15.44008868035555793, 41.39701867748817676, -9.422509992056140149 ) ) ;
#88965=CARTESIAN_POINT ( 'NONE',  ( 12.63842701281683922, 64.55059781766745175, -9.846743663894590881 ) ) ;
#88967=CARTESIAN_POINT ( 'NONE',  ( 10.00000000000000178, 22.25893115100078745, 9.846743663894594434 ) ) ;
#88969=CARTESIAN_POINT ( 'NONE',  ( 2.791683348922240793, 11.63393115100078568, 7.208316651077764092 ) ) ;
#88970=CARTESIAN_POINT ( 'NONE',  ( 14.92337183194729633, 17.67559781766745175, 8.527530157486181039 ) ) ;
#88971=CARTESIAN_POINT ( 'NONE',  ( 14.92337183194729633, 12.67559781766745353, 8.527530157486181039 ) ) ;
#88972=CARTESIAN_POINT ( 'NONE',  ( 17.20831665107776587, 4.133931151000785675, -7.208316651077762316 ) ) ;
#88974=CARTESIAN_POINT ( 'NONE',  ( 5.076628168052703671, 6.842264484334118713, 8.527530157486179263 ) ) ;
#88977=CARTESIAN_POINT ( 'NONE',  ( 12.63842701281683922, 9.550597817667449974, -9.846743663894590881 ) ) ;
#88978=CARTESIAN_POINT ( 'NONE',  ( 0.1532563361054082862, 16.21726448433411960, 2.638427012816831674 ) ) ;
#88982=CARTESIAN_POINT ( 'NONE',  ( 10.00000000000000178, 0.3736346699304200492, 12.81628187352647608 ) ) ;
#88985=CARTESIAN_POINT ( 'NONE',  ( 0.2751277870542980231, 14.36607318730130878, -6.500000000000002665 ) ) ;
#88986=CARTESIAN_POINT ( 'NONE',  ( 2.917880565312948704, 17.63708216824730357, 12.26659068614894643 ) ) ;
#88989=CARTESIAN_POINT ( 'NONE',  ( -2.266590686148945544, 21.38708216824730357, -7.082119434687050408 ) ) ;
#88990=CARTESIAN_POINT ( 'NONE',  ( 24.16423886937410614, 49.51208216824730357, -3.795296366450302550 ) ) ;
#88992=CARTESIAN_POINT ( 'NONE',  ( -2.266590686148945544, 7.220415501580634832, 7.082119434687048631 ) ) ;
#88993=CARTESIAN_POINT ( 'NONE',  ( 4.559911319644449179, 38.89701867748817676, 9.422509992056141925 ) ) ;
#88996=CARTESIAN_POINT ( 'NONE',  ( 14.92337183194729633, 22.67559781766745175, 8.527530157486181039 ) ) ;
#88997=CARTESIAN_POINT ( 'NONE',  ( -0.8801773607110991993, 57.85535201082149825, -2.915334737309923874 ) ) ;
#88998=CARTESIAN_POINT ( 'NONE',  ( 7.361572987183169658, 34.96726448433411605, -9.846743663894592657 ) ) ;
#88999=CARTESIAN_POINT ( 'NONE',  ( 7.084665262690076126, 9.105352010821503583, 10.88017736071109987 ) ) ;
#89000=CARTESIAN_POINT ( 'NONE',  ( 22.81628187352647785, 61.62363466993041783, 6.195893100308588602E-16 ) ) ;
#89001=CARTESIAN_POINT ( 'NONE',  ( 12.63842701281683034, 47.46726448433412315, 9.846743663894596210 ) ) ;
#89002=DIRECTION ( 'NONE',  ( 1.000000000000000000, 0.000000000000000000, 0.000000000000000000 ) ) ;
#89003=CARTESIAN_POINT ( 'NONE',  ( 6.565887622018943937, 43.08196800326374643, -12.81628187352647608 ) ) ;
#89005=CARTESIAN_POINT ( 'NONE',  ( -0.8801773607111008646, 48.27201867748816966, 2.915334737309923430 ) ) ;
#89006=CARTESIAN_POINT ( 'NONE',  ( 1.472469842513823179, 41.42559781766745886, 4.923371831947296329 ) ) ;
#89007=CARTESIAN_POINT ( 'NONE',  ( -4.164238869374099039, 31.80374883491396432, 8.674139862899312516E-16 ) ) ;
#89009=VECTOR ( 'NONE', #62834, 1000.000000000000000 ) ;
#89010=CARTESIAN_POINT ( 'NONE',  ( 12.91533473730992121, 54.52201867748816255, 10.88017736071110164 ) ) ;
#89011=CARTESIAN_POINT ( 'NONE',  ( 17.96484262340118221, 61.18868534415482685, -7.964842623401177768 ) ) ;
#89012=CARTESIAN_POINT ( 'NONE',  ( -4.164238869374098151, 51.59541550158063217, -3.795296366450310543 ) ) ;
#89013=CARTESIAN_POINT ( 'NONE',  ( 6.565887622018943937, -1.918031996736246692, -12.81628187352647608 ) ) ;
#89014=CARTESIAN_POINT ( 'NONE',  ( 6.000000000000000000, 61.00000000000000711, -5.000000000000000000 ) ) ;
#89015=CARTESIAN_POINT ( 'NONE',  ( 7.084665262690076126, 39.10535201082150536, 10.88017736071109987 ) ) ;
#89017=CARTESIAN_POINT ( 'NONE',  ( 17.20831665107776587, 47.88393115100078745, 7.208316651077764980 ) ) ;
#89020=CARTESIAN_POINT ( 'NONE',  ( 19.42250999205614193, 15.14701867748817143, 5.440088680355555262 ) ) ;
#89023=CARTESIAN_POINT ( 'NONE',  ( 10.00000000000000178, 4.313685344154837509, 10.88017736071110342 ) ) ;
#89025=CARTESIAN_POINT ( 'NONE',  ( -0.8801773607111008646, 68.27201867748817676, 2.915334737309923430 ) ) ;
#89027=CARTESIAN_POINT ( 'NONE',  ( 10.00000000000000178, 69.31368534415484817, 10.88017736071110342 ) ) ;
#89028=CARTESIAN_POINT ( 'NONE',  ( 14.92337183194729988, 29.34226448433411960, -8.527530157486177487 ) ) ;
#89029=CARTESIAN_POINT ( 'NONE',  ( 12.91533473730993009, 16.60535201082150891, -10.88017736071109987 ) ) ;
#89030=CARTESIAN_POINT ( 'NONE',  ( 21.09922568453594849, 11.20696800326375531, 6.408140936763242479 ) ) ;
#89031=CARTESIAN_POINT ( 'NONE',  ( 7.084665262690076126, 37.02201867748817676, -10.88017736071110164 ) ) ;
#89033=CARTESIAN_POINT ( 'NONE',  ( 10.00000000000000178, 35.37363466993042493, 12.81628187352647608 ) ) ;
#89034=ORIENTED_EDGE ( 'NONE', *, *, #53620, .F. ) ;
#89035=CARTESIAN_POINT ( 'NONE',  ( 20.88017736071110164, 60.35535201082151957, 2.915334737309930979 ) ) ;
#89036=CARTESIAN_POINT ( 'NONE',  ( 6.565887622018943937, 25.16530133659708213, 12.81628187352647430 ) ) ;
#89037=FILL_AREA_STYLE_COLOUR ( '', #57384 ) ;
#89038=CARTESIAN_POINT ( 'NONE',  ( 21.92686044187656691, 32.18830936912750929, 4.562052436263911564E-16 ) ) ;
#89039=CARTESIAN_POINT ( 'NONE',  ( 0.5774900079438607392, 33.48035201082150536, 5.440088680355550821 ) ) ;
#89040=CARTESIAN_POINT ( 'NONE',  ( 0.2751277870542979120, 15.30223176428831344, 6.500000000000003553 ) ) ;
#89041=CARTESIAN_POINT ( 'NONE',  ( 2.917880565312948704, 67.63708216824730357, 12.26659068614894643 ) ) ;
#89042=CARTESIAN_POINT ( 'NONE',  ( 10.00000000000000178, 52.25893115100078745, 9.846743663894594434 ) ) ;
#89043=CARTESIAN_POINT ( 'NONE',  ( 10.00000000000000000, -0.2410688489992152128, -9.846743663894594434 ) ) ;
#89044=CARTESIAN_POINT ( 'NONE',  ( 4.559911319644449179, 58.89701867748817676, 9.422509992056141925 ) ) ;
#89045=CARTESIAN_POINT ( 'NONE',  ( 13.79529636645030344, 28.26208216824729647, 14.16423886937410614 ) ) ;
#89047=( NAMED_UNIT ( * ) PLANE_ANGLE_UNIT ( ) SI_UNIT ( $, .RADIAN. ) );
#89048=CARTESIAN_POINT ( 'NONE',  ( 19.65595853167378948, 85.79736161466001931, -5.361990343729008401 ) ) ;
#89051=CARTESIAN_POINT ( 'NONE',  ( -2.266590686148945544, 61.38708216824730357, -7.082119434687050408 ) ) ;
#89052=CARTESIAN_POINT ( 'NONE',  ( 6.204703633549690345, 47.84541550158064638, 14.16423886937410082 ) ) ;
#89053=CARTESIAN_POINT ( 'NONE',  ( 17.20831665107776587, 24.13393115100078035, -7.208316651077762316 ) ) ;
#89056=CARTESIAN_POINT ( 'NONE',  ( 17.96484262340118221, 11.18868534415483929, -7.964842623401177768 ) ) ;
#89057=CARTESIAN_POINT ( 'NONE',  ( 17.08211943468705130, 53.47041550158063217, 12.26659068614894998 ) ) ;
#89058=CARTESIAN_POINT ( 'NONE',  ( 12.63842701281683034, 22.46726448433411605, 9.846743663894596210 ) ) ;
#89060=CARTESIAN_POINT ( 'NONE',  ( 5.076628168052703671, 6.842264484334118713, 8.527530157486179263 ) ) ;
#89061=CARTESIAN_POINT ( 'NONE',  ( 19.84674366389459266, 3.717264484334118713, -2.638427012816827677 ) ) ;
#89063=VERTEX_POINT ( 'NONE', #25665 ) ;
#89065=EDGE_CURVE ( 'NONE', #76154, #56374, #55662, .T. ) ;
#89067=CARTESIAN_POINT ( 'NONE',  ( 20.36894250292379738, 14.92874883491396432, -10.36894250292379027 ) ) ;
#89068=CARTESIAN_POINT ( 'NONE',  ( 2.035157376598824452, 18.68868534415484106, 7.964842623401179544 ) ) ;
#89069=CARTESIAN_POINT ( 'NONE',  ( 17.96484262340118221, 29.93868534415484106, 7.964842623401181321 ) ) ;
#89070=CARTESIAN_POINT ( 'NONE',  ( 0.1532563361054082862, 46.21726448433411605, 2.638427012816831674 ) ) ;
#89071=CARTESIAN_POINT ( 'NONE',  ( 19.38216949554541202, 20.99863466993042138, 9.382169495545424454 ) ) ;
#89072=CARTESIAN_POINT ( 'NONE',  ( 6.204703633549690345, 10.76208216824729824, -14.16423886937410259 ) ) ;
#89074=CARTESIAN_POINT ( 'NONE',  ( -2.816281873526473856, 29.33196800326376064, 3.434112377981055619 ) ) ;
#89077=CARTESIAN_POINT ( 'NONE',  ( 1.472469842513823179, 25.59226448433412315, -4.923371831947296329 ) ) ;
#89078=CARTESIAN_POINT ( 'NONE',  ( -0.3689425029237898834, 66.17874883491396076, -10.36894250292378850 ) ) ;
#89080=CARTESIAN_POINT ( 'NONE',  ( -0.3689425029237898834, 66.17874883491396076, -10.36894250292378850 ) ) ;
#89081=ORIENTED_EDGE ( 'NONE', *, *, #35903, .T. ) ;
#89082=CARTESIAN_POINT ( 'NONE',  ( -0.8801773607111009756, 53.06368534415484106, 1.068504757029289695E-15 ) ) ;
#89083=CARTESIAN_POINT ( 'NONE',  ( 19.42250999205614548, 40.98035201082150536, -5.440088680355545492 ) ) ;
#89084=CARTESIAN_POINT ( 'NONE',  ( -0.8801773607111009756, 53.06368534415484106, 1.068504757029289695E-15 ) ) ;
#89086=CARTESIAN_POINT ( 'NONE',  ( 15.44008868035555793, 41.39701867748817676, -9.422509992056140149 ) ) ;
#89087=CARTESIAN_POINT ( 'NONE',  ( 1.383448333479233794, 47.37718327197428891, -6.499999999999977796 ) ) ;
#89088=DIRECTION ( 'NONE',  ( 0.000000000000000000, -1.000000000000000000, 0.000000000000000000 ) ) ;
#89090=ORIENTED_EDGE ( 'NONE', *, *, #25107, .F. ) ;
#89091=CARTESIAN_POINT ( 'NONE',  ( 19.84674366389459621, 33.50893115100078745, 7.409399052514197653E-17 ) ) ;
#89093=CARTESIAN_POINT ( 'NONE',  ( 18.52753015748618282, 63.92559781766745886, -4.923371831947291888 ) ) ;
#89094=CARTESIAN_POINT ( 'NONE',  ( -0.1038446121089049989, 24.24302437010794264, -6.337995344473780435 ) ) ;
#89096=CARTESIAN_POINT ( 'NONE',  ( 2.917880565312948704, 7.637082168247301794, 12.26659068614894643 ) ) ;
#89098=VERTEX_POINT ( 'NONE', #2190 ) ;
#89101=CARTESIAN_POINT ( 'NONE',  ( -46.91881431881006392, 103.2388046827858545, -5.912160981969285523 ) ) ;
#89102=CARTESIAN_POINT ( 'NONE',  ( 17.08211943468705840, 65.13708216824730357, -12.26659068614894466 ) ) ;
#89106=CARTESIAN_POINT ( 'NONE',  ( 19.84674366389459266, 28.30059781766745886, 2.638427012816836559 ) ) ;
#89108=VERTEX_POINT ( 'NONE', #32149 ) ;
#89109=CARTESIAN_POINT ( 'NONE',  ( 3.591859063236763294, 8.290301336597087456, -11.09922568453595026 ) ) ;
#89110=CARTESIAN_POINT ( 'NONE',  ( 1.472469842513823179, 10.59226448433411782, -4.923371831947296329 ) ) ;
#89112=CARTESIAN_POINT ( 'NONE',  ( 18.52753015748617571, 8.092264484334117824, 4.923371831947298993 ) ) ;
#89113=CARTESIAN_POINT ( 'NONE',  ( 22.81628187352648496, 6.831968003263753531, -3.434112377981050290 ) ) ;
#89114=ADVANCED_FACE ( 'NONE', ( #71159 ), #32999, .T. ) ;
#89115=CYLINDRICAL_SURFACE ( 'NONE', #45684, 62.50000000000000000 ) ;
#89116=ORIENTED_EDGE ( 'NONE', *, *, #35308, .F. ) ;
#89117=CARTESIAN_POINT ( 'NONE',  ( 7.084665262690076126, 12.02201867748817321, -10.88017736071110164 ) ) ;
#89118=CARTESIAN_POINT ( 'NONE',  ( -2.266590686148945544, 6.387082168247300906, -7.082119434687050408 ) ) ;
#89119=CARTESIAN_POINT ( 'NONE',  ( 12.63842701281683034, 27.46726448433411250, 9.846743663894596210 ) ) ;
#89120=CARTESIAN_POINT ( 'NONE',  ( 7.084665262690076126, 57.02201867748817676, -10.88017736071110164 ) ) ;
#89121=CARTESIAN_POINT ( 'NONE',  ( 6.565887622018943937, 25.16530133659708213, 12.81628187352647430 ) ) ;
#89123=CARTESIAN_POINT ( 'NONE',  ( 17.96484262340118221, 4.938685344154837509, 7.964842623401181321 ) ) ;
#89126=CARTESIAN_POINT ( 'NONE',  ( 18.52753015748618282, 63.92559781766745886, -4.923371831947291888 ) ) ;
#89127=CARTESIAN_POINT ( 'NONE',  ( 18.52753015748617571, 18.09226448433411960, 4.923371831947298993 ) ) ;
#89128=B_SPLINE_CURVE_WITH_KNOTS ( 'NONE', 3,
 ( #28946, #82951, #58458, #58967 ),
 .UNSPECIFIED., .F., .F.,
 ( 4, 4 ),
 ( 0.000000000000000000, 0.002657014572711325923 ),
 .UNSPECIFIED. ) ;
#89130=CARTESIAN_POINT ( 'NONE',  ( 16.40814093676323893, 25.79030133659708923, 11.09922568453595026 ) ) ;
#89133=CARTESIAN_POINT ( 'NONE',  ( 15.44008868035555260, 44.73035201082151247, 9.422509992056143702 ) ) ;
#89136=CARTESIAN_POINT ( 'NONE',  ( 20.36894250292379738, 54.92874883491396076, -10.36894250292379027 ) ) ;
#89138=CARTESIAN_POINT ( 'NONE',  ( -0.8801773607111009756, 28.06368534415484106, 1.068504757029289695E-15 ) ) ;
#89139=CARTESIAN_POINT ( 'NONE',  ( 17.20831665107776587, 49.13393115100078745, -7.208316651077762316 ) ) ;
#89140=CARTESIAN_POINT ( 'NONE',  ( 0.5774900079438607392, 53.48035201082151247, 5.440088680355550821 ) ) ;
#89141=CARTESIAN_POINT ( 'NONE',  ( 17.08211943468705130, 28.47041550158063572, 12.26659068614894998 ) ) ;
#89143=CARTESIAN_POINT ( 'NONE',  ( 19.84674366389459621, 43.50893115100078745, 7.409399052514197653E-17 ) ) ;
#89144=CARTESIAN_POINT ( 'NONE',  ( 3.591859063236763294, -1.709698663402913210, -11.09922568453595026 ) ) ;
#89145=EDGE_LOOP ( 'NONE', ( #32925, #95, #87808, #29073 ) ) ;
#89146=CARTESIAN_POINT ( 'NONE',  ( -0.8801773607110991993, 27.85535201082150181, -2.915334737309923874 ) ) ;
#89147=CARTESIAN_POINT ( 'NONE',  ( 20.24186590665275887, 7.616331881023276296, -6.114288769123074729 ) ) ;
#89148=CARTESIAN_POINT ( 'NONE',  ( 4.559911319644449179, 17.23035201082150536, -9.422509992056141925 ) ) ;
#89149=CARTESIAN_POINT ( 'NONE',  ( 17.20831665107776587, 4.133931151000785675, -7.208316651077762316 ) ) ;
#89150=CARTESIAN_POINT ( 'NONE',  ( 17.08211943468705130, 23.47041550158063572, 12.26659068614894998 ) ) ;
#89152=CARTESIAN_POINT ( 'NONE',  ( 19.84674366389459266, 18.71726448433411960, -2.638427012816827677 ) ) ;
#89153=CARTESIAN_POINT ( 'NONE',  ( 19.84674366389459621, 58.50893115100078745, 7.409399052514197653E-17 ) ) ;
#89154=CARTESIAN_POINT ( 'NONE',  ( -0.8801773607111009756, 28.06368534415484106, 1.068504757029289695E-15 ) ) ;
#89159=STYLED_ITEM ( 'NONE', ( #54013 ), #16060 ) ;
#89161=CARTESIAN_POINT ( 'NONE',  ( 10.00000000000000000, 39.75893115100078745, -9.846743663894594434 ) ) ;
#89165=CARTESIAN_POINT ( 'NONE',  ( 2.917880565312948704, 27.63708216824730357, 12.26659068614894643 ) ) ;
#89166=CARTESIAN_POINT ( 'NONE',  ( 20.36894250292379738, 14.92874883491396432, -10.36894250292379027 ) ) ;
#89167=CARTESIAN_POINT ( 'NONE',  ( 17.96484262340118221, 56.18868534415484817, -7.964842623401177768 ) ) ;
#89168=CARTESIAN_POINT ( 'NONE',  ( -0.3689425029237898834, 51.17874883491397497, -10.36894250292378850 ) ) ;
#89169=CARTESIAN_POINT ( 'NONE',  ( 10.00000000000000000, 64.75893115100078035, -9.846743663894594434 ) ) ;
#89170=CARTESIAN_POINT ( 'NONE',  ( 10.00000000000000000, 29.75893115100078745, -9.846743663894594434 ) ) ;
#89171=CARTESIAN_POINT ( 'NONE',  ( -1.028725271592155099, -1.208271517246092823E-15, 4.540618777627624780 ) ) ;
#89172=CARTESIAN_POINT ( 'NONE',  ( 15.44008868035555793, 31.39701867748817676, -9.422509992056140149 ) ) ;
#89173=CARTESIAN_POINT ( 'NONE',  ( 22.81628187352648496, 6.831968003263753531, -3.434112377981050290 ) ) ;
#89174=CARTESIAN_POINT ( 'NONE',  ( -4.164238869374098151, 21.59541550158063217, -3.795296366450310543 ) ) ;
#89175=CARTESIAN_POINT ( 'NONE',  ( -0.8801773607111008646, 23.27201867748817676, 2.915334737309923430 ) ) ;
#89178=CARTESIAN_POINT ( 'NONE',  ( 15.44008868035555260, 44.73035201082151247, 9.422509992056143702 ) ) ;
#89181=ORIENTED_EDGE ( 'NONE', *, *, #77642, .F. ) ;
#89185=CARTESIAN_POINT ( 'NONE',  ( -0.3689425029237898834, 51.17874883491397497, -10.36894250292378850 ) ) ;
#89186=CARTESIAN_POINT ( 'NONE',  ( 19.84674366389459266, 53.71726448433411605, -2.638427012816827677 ) ) ;
#89187=CARTESIAN_POINT ( 'NONE',  ( 17.96484262340118221, 59.93868534415484106, 7.964842623401181321 ) ) ;
#89190=CIRCLE ( 'NONE', #70005, 0.5000000000000004441 ) ;
#89191=CARTESIAN_POINT ( 'NONE',  ( -0.8801773607111009756, 53.06368534415484106, 1.068504757029289695E-15 ) ) ;
#89193=CARTESIAN_POINT ( 'NONE',  ( 10.00000000000000000, 57.87363466993042493, -12.81628187352647608 ) ) ;
#89197=CARTESIAN_POINT ( 'NONE',  ( 17.08211943468705840, 25.13708216824730357, -12.26659068614894466 ) ) ;
#89198=CARTESIAN_POINT ( 'NONE',  ( 10.00000000000000000, 17.87363466993041783, -12.81628187352647608 ) ) ;
#89200=CARTESIAN_POINT ( 'NONE',  ( 22.81628187352647785, 41.41530133659708923, 3.434112377981063169 ) ) ;
#89201=CARTESIAN_POINT ( 'NONE',  ( -0.8801773607111008646, 18.27201867748817321, 2.915334737309923430 ) ) ;
#89202=CARTESIAN_POINT ( 'NONE',  ( 12.63842701281683922, 34.55059781766745886, -9.846743663894590881 ) ) ;
#89203=CARTESIAN_POINT ( 'NONE',  ( 7.084665262690076126, 14.10535201082150358, 10.88017736071109987 ) ) ;
#89204=CARTESIAN_POINT ( 'NONE',  ( 0.6178305044545818747, 58.49863466993042493, -9.382169495545419124 ) ) ;
#89205=CARTESIAN_POINT ( 'NONE',  ( -0.1503990784575328643, 70.00000000000000000, 6.262539305110068177 ) ) ;
#89206=CARTESIAN_POINT ( 'NONE',  ( 7.361572987183170547, 37.05059781766744464, 9.846743663894590881 ) ) ;
#89208=ORIENTED_EDGE ( 'NONE', *, *, #27761, .T. ) ;
#89210=CARTESIAN_POINT ( 'NONE',  ( 1.707155281725185381, 32.90189080397284016, 6.499999999999955591 ) ) ;
#89212=EDGE_CURVE ( 'NONE', #33986, #1529, #83599, .T. ) ;
#89214=CARTESIAN_POINT ( 'NONE',  ( 0.1532563361054082862, 16.21726448433411960, 2.638427012816831674 ) ) ;
#89215=CARTESIAN_POINT ( 'NONE',  ( 10.00000000000000000, 17.87363466993041783, -12.81628187352647608 ) ) ;
#89221=CARTESIAN_POINT ( 'NONE',  ( 0.1532563361054082862, 51.21726448433412315, 2.638427012816831674 ) ) ;
#89223=CARTESIAN_POINT ( 'NONE',  ( -0.3689425029237881626, 17.42874883491397142, 10.36894250292379027 ) ) ;
#89224=CARTESIAN_POINT ( 'NONE',  ( 1.472469842513823179, 41.42559781766745886, 4.923371831947296329 ) ) ;
#89225=CARTESIAN_POINT ( 'NONE',  ( 6.565887622018943937, 48.08196800326375353, -12.81628187352647608 ) ) ;
#89227=CARTESIAN_POINT ( 'NONE',  ( -0.8801773607110991993, 57.85535201082149825, -2.915334737309923874 ) ) ;
#89229=CARTESIAN_POINT ( 'NONE',  ( 7.361572987183169658, 39.96726448433411605, -9.846743663894592657 ) ) ;
#89230=CARTESIAN_POINT ( 'NONE',  ( 4.559911319644449179, 38.89701867748817676, 9.422509992056141925 ) ) ;
#89231=CARTESIAN_POINT ( 'NONE',  ( 13.43411237798105340, 45.58196800326374643, 12.81628187352647963 ) ) ;
#89232=CARTESIAN_POINT ( 'NONE',  ( 0.1532563361054082862, 31.21726448433412315, 2.638427012816831674 ) ) ;
#89235=CARTESIAN_POINT ( 'NONE',  ( 12.91533473730992121, 44.52201867748816966, 10.88017736071110164 ) ) ;
#89239=CARTESIAN_POINT ( 'NONE',  ( 4.559911319644449179, 12.23035201082150536, -9.422509992056141925 ) ) ;
#89240=CARTESIAN_POINT ( 'NONE',  ( 5.076628168052703671, 51.84226448433412315, 8.527530157486179263 ) ) ;
#89241=CARTESIAN_POINT ( 'NONE',  ( -0.8801773607111009756, 43.06368534415484106, 1.068504757029289695E-15 ) ) ;
#89243=CARTESIAN_POINT ( 'NONE',  ( 0.5774900079438607392, 63.48035201082149825, 5.440088680355550821 ) ) ;
#89244=CARTESIAN_POINT ( 'NONE',  ( 4.559911319644449179, 32.23035201082150536, -9.422509992056141925 ) ) ;
#89246=CARTESIAN_POINT ( 'NONE',  ( 2.791683348922237240, 25.38393115100078390, -7.208316651077763204 ) ) ;
#89249=CARTESIAN_POINT ( 'NONE',  ( 2.791683348922237240, 55.38393115100078745, -7.208316651077763204 ) ) ;
#89250=CARTESIAN_POINT ( 'NONE',  ( 13.79529636645031943, 50.34541550158064638, -14.16423886937409904 ) ) ;
#89253=CARTESIAN_POINT ( 'NONE',  ( 22.26659068614894466, 3.887082168247300906, 7.082119434687054849 ) ) ;
#89255=CARTESIAN_POINT ( 'NONE',  ( 13.79529636645031943, 35.34541550158063927, -14.16423886937409904 ) ) ;
#89256=CARTESIAN_POINT ( 'NONE',  ( 3.591859063236761518, -0.04303199673624671928, 11.09922568453594849 ) ) ;
#89258=CARTESIAN_POINT ( 'NONE',  ( 20.88017736071110519, 20.56368534415484106, 2.639326808657452039E-16 ) ) ;
#89259=CARTESIAN_POINT ( 'NONE',  ( 17.20831665107776587, 52.88393115100078035, 7.208316651077764980 ) ) ;
#89260=CARTESIAN_POINT ( 'NONE',  ( 2.831191079880678085, 79.91181047996344944, -9.500000000000000000 ) ) ;
#89263=SURFACE_STYLE_FILL_AREA ( #45243 ) ;
#89264=CARTESIAN_POINT ( 'NONE',  ( 10.00000000000000000, 27.87363466993042138, -12.81628187352647608 ) ) ;
#89265=CARTESIAN_POINT ( 'NONE',  ( 10.00000000000000178, 22.25893115100078745, 9.846743663894594434 ) ) ;
#89267=CARTESIAN_POINT ( 'NONE',  ( 19.84674366389459621, 3.508931151000785231, 7.409399052514197653E-17 ) ) ;
#89270=CARTESIAN_POINT ( 'NONE',  ( 12.91533473730992121, 9.522018677488171434, 10.88017736071110164 ) ) ;
#89271=CARTESIAN_POINT ( 'NONE',  ( -4.164238869374098151, 36.59541550158063217, -3.795296366450310543 ) ) ;
#89272=CARTESIAN_POINT ( 'NONE',  ( 2.035157376598822676, 47.43868534415484817, -7.964842623401177768 ) ) ;
#89273=CARTESIAN_POINT ( 'NONE',  ( 10.00000000000000000, 61.81368534415484106, -10.88017736071110342 ) ) ;
#89275=CARTESIAN_POINT ( 'NONE',  ( 19.72487221294570858, 16.86607318730074567, 6.500000000000000888 ) ) ;
#89276=CARTESIAN_POINT ( 'NONE',  ( 17.20831665107776587, 24.13393115100078035, -7.208316651077762316 ) ) ;
#89277=DIRECTION ( 'NONE',  ( 0.000000000000000000, -1.000000000000000000, -0.000000000000000000 ) ) ;
#89278=CARTESIAN_POINT ( 'NONE',  ( 14.92337183194729988, 9.342264484334119601, -8.527530157486177487 ) ) ;
#89279=( BOUNDED_CURVE ( )  B_SPLINE_CURVE ( 2, ( #58084, #68570, #29069, #37584, #90563, #74576, #75073, #84062, #46063 ),
 .UNSPECIFIED., .F., .F. ) 
 B_SPLINE_CURVE_WITH_KNOTS ( ( 3, 2, 2, 2, 3 ),
 ( 0.2258552226545170460, 0.2261904761904761640, 0.2321428571428572063, 0.2380952380952381375, 0.2384304916311972555 ),
 .UNSPECIFIED. ) 
 CURVE ( )  GEOMETRIC_REPRESENTATION_ITEM ( )  RATIONAL_B_SPLINE_CURVE ( ( 0.9963778908391762723, 0.9980808541467921513, 1.000000000000000000, 0.9659258262890682012, 1.000000000000000000, 0.9659258262890682012, 1.000000000000000000, 0.9980808541467921513, 0.9963778908391762723 ) ) 
 REPRESENTATION_ITEM ( '' )  );
#89281=CARTESIAN_POINT ( 'NONE',  ( 12.63842701281683922, 34.55059781766745886, -9.846743663894590881 ) ) ;
#89282=CARTESIAN_POINT ( 'NONE',  ( 18.52753015748618282, 58.92559781766745886, -4.923371831947291888 ) ) ;
#89284=CARTESIAN_POINT ( 'NONE',  ( 7.084665262690076126, 37.02201867748817676, -10.88017736071110164 ) ) ;
#89285=UNCERTAINTY_MEASURE_WITH_UNIT (LENGTH_MEASURE( 1.000000000000000082E-05 ), #10368, 'distance_accuracy_value', 'NONE');
#89287=CARTESIAN_POINT ( 'NONE',  ( 22.81628187352647785, 61.41530133659709634, 3.434112377981063169 ) ) ;
#89289=CARTESIAN_POINT ( 'NONE',  ( 0.1532563361054082862, 1.217264484334117824, 2.638427012816831674 ) ) ;
#89290=CARTESIAN_POINT ( 'NONE',  ( 3.591859063236761518, 39.95696800326375353, 11.09922568453594849 ) ) ;
#89291=CARTESIAN_POINT ( 'NONE',  ( 17.08211943468705840, 65.13708216824730357, -12.26659068614894466 ) ) ;
#89292=CARTESIAN_POINT ( 'NONE',  ( 0.1532563361054100626, 40.80059781766745886, -2.638427012816831230 ) ) ;
#89293=CARTESIAN_POINT ( 'NONE',  ( 0.2751277870542909731, 47.28217586085238366, -6.499999999999992006 ) ) ;
#89294=CARTESIAN_POINT ( 'NONE',  ( 1.472469842513823179, 1.425597817667451528, 4.923371831947296329 ) ) ;
#89295=CARTESIAN_POINT ( 'NONE',  ( -0.3689425029237898834, 21.17874883491396432, -10.36894250292378850 ) ) ;
#89296=CARTESIAN_POINT ( 'NONE',  ( 20.36894250292379382, 48.67874883491396076, 10.36894250292379205 ) ) ;
#89297=CARTESIAN_POINT ( 'NONE',  ( 17.20831665107776587, 37.88393115100078745, 7.208316651077764980 ) ) ;
#89299=CARTESIAN_POINT ( 'NONE',  ( 19.42250999205614193, 40.14701867748817676, 5.440088680355555262 ) ) ;
#89300=CARTESIAN_POINT ( 'NONE',  ( 19.42250999205614193, 55.14701867748817676, 5.440088680355555262 ) ) ;
#89304=CARTESIAN_POINT ( 'NONE',  ( 21.09922568453594849, 46.20696800326376064, 6.408140936763242479 ) ) ;
#89305=VERTEX_POINT ( 'NONE', #5119 ) ;
#89306=CARTESIAN_POINT ( 'NONE',  ( 7.361572987183169658, -0.03273551566588185635, -9.846743663894592657 ) ) ;
#89307=VERTEX_POINT ( 'NONE', #19128 ) ;
#89308=CARTESIAN_POINT ( 'NONE',  ( 13.79529636645030344, 8.262082168247300018, 14.16423886937410614 ) ) ;
#89309=CARTESIAN_POINT ( 'NONE',  ( 5.076628168052704559, 5.175597817667451750, -8.527530157486179263 ) ) ;
#89312=CARTESIAN_POINT ( 'NONE',  ( 2.035157376598824452, 18.68868534415484106, 7.964842623401179544 ) ) ;
#89315=CARTESIAN_POINT ( 'NONE',  ( 2.917880565312948704, 12.63708216824730179, 12.26659068614894643 ) ) ;
#89318=CARTESIAN_POINT ( 'NONE',  ( 19.42250999205614548, 20.98035201082150891, -5.440088680355545492 ) ) ;
#89319=CARTESIAN_POINT ( 'NONE',  ( 17.20831665107776587, 62.88393115100078745, 7.208316651077764980 ) ) ;
#89321=CARTESIAN_POINT ( 'NONE',  ( 18.52753015748618282, 58.92559781766745886, -4.923371831947291888 ) ) ;
#89323=CARTESIAN_POINT ( 'NONE',  ( 2.035157376598824452, 63.68868534415484106, 7.964842623401179544 ) ) ;
#89325=CARTESIAN_POINT ( 'NONE',  ( -0.8801773607110991993, 12.85535201082150358, -2.915334737309923874 ) ) ;
#89327=CARTESIAN_POINT ( 'NONE',  ( 18.52753015748617571, 8.092264484334117824, 4.923371831947298993 ) ) ;
#89328=CARTESIAN_POINT ( 'NONE',  ( 4.559911319644449179, 13.89701867748817321, 9.422509992056141925 ) ) ;
#89330=EDGE_LOOP ( 'NONE', ( #27088, #69077, #83202, #64315 ) ) ;
#89331=CARTESIAN_POINT ( 'NONE',  ( 4.559911319644449179, 47.23035201082150536, -9.422509992056141925 ) ) ;
#89332=CARTESIAN_POINT ( 'NONE',  ( 19.54819611545892144, 96.99629728834725029, 4.999999999999999112 ) ) ;
#89333=CARTESIAN_POINT ( 'NONE',  ( 3.591859063236763294, 43.29030133659708923, -11.09922568453595026 ) ) ;
#89334=CARTESIAN_POINT ( 'NONE',  ( 7.084665262690076126, 42.02201867748816966, -10.88017736071110164 ) ) ;
#89335=CARTESIAN_POINT ( 'NONE',  ( 5.076628168052704559, 60.17559781766745175, -8.527530157486179263 ) ) ;
#89338=CARTESIAN_POINT ( 'NONE',  ( 2.791683348922240793, 11.63393115100078568, 7.208316651077764092 ) ) ;
#89339=CARTESIAN_POINT ( 'NONE',  ( -1.099225684535947600, 4.540301336597087456, 6.408140936763237150 ) ) ;
#89341=CARTESIAN_POINT ( 'NONE',  ( 2.791683348922237240, 60.38393115100078745, -7.208316651077763204 ) ) ;
#89342=CARTESIAN_POINT ( 'NONE',  ( 2.035157376598824452, 23.68868534415484461, 7.964842623401179544 ) ) ;
#89343=CARTESIAN_POINT ( 'NONE',  ( 10.00000000000000178, 47.25893115100078745, 9.846743663894594434 ) ) ;
#89347=CARTESIAN_POINT ( 'NONE',  ( 5.076628168052703671, 11.84226448433411960, 8.527530157486179263 ) ) ;
#89349=CARTESIAN_POINT ( 'NONE',  ( 0.6178305044545818747, -1.501365330069579951, -9.382169495545419124 ) ) ;
#89350=ORIENTED_EDGE ( 'NONE', *, *, #58920, .F. ) ;
#89352=CARTESIAN_POINT ( 'NONE',  ( 10.00000000000000178, 40.37363466993042493, 12.81628187352647608 ) ) ;
#89353=CARTESIAN_POINT ( 'NONE',  ( 0.1532563361054083140, 36.00893115100078745, 1.131784320476157264E-15 ) ) ;
#89355=CARTESIAN_POINT ( 'NONE',  ( 22.26659068614895176, 54.72041550158063217, -7.082119434687042414 ) ) ;
#89356=CARTESIAN_POINT ( 'NONE',  ( 0.1532563361054082862, 26.21726448433411605, 2.638427012816831674 ) ) ;
#89358=CARTESIAN_POINT ( 'NONE',  ( 0.5774900079438607392, 8.480352010821505360, 5.440088680355550821 ) ) ;
#89360=CARTESIAN_POINT ( 'NONE',  ( 17.96484262340118221, 14.93868534415484106, 7.964842623401181321 ) ) ;
#89361=CARTESIAN_POINT ( 'NONE',  ( -0.3689425029237881626, 47.42874883491396787, 10.36894250292379027 ) ) ;
#89362=CARTESIAN_POINT ( 'NONE',  ( -4.164238869374099927, 47.01208216824729647, 3.795296366450308767 ) ) ;
#89365=CARTESIAN_POINT ( 'NONE',  ( 14.92337183194729988, 14.34226448433411782, -8.527530157486177487 ) ) ;
#89366=CARTESIAN_POINT ( 'NONE',  ( 10.00000000000000000, 64.75893115100078035, -9.846743663894594434 ) ) ;
#89368=CARTESIAN_POINT ( 'NONE',  ( 19.42250999205614193, 50.14701867748817676, 5.440088680355555262 ) ) ;
#89369=CARTESIAN_POINT ( 'NONE',  ( 0.5774900079438590739, 17.64701867748817321, -5.440088680355550821 ) ) ;
#89370=CARTESIAN_POINT ( 'NONE',  ( 10.00000000000000000, 54.75893115100078745, -9.846743663894594434 ) ) ;
#89372=CARTESIAN_POINT ( 'NONE',  ( 17.20831665107776587, 62.88393115100078745, 7.208316651077764980 ) ) ;
#89373=CARTESIAN_POINT ( 'NONE',  ( 20.36894250292379382, 3.678748834913967869, 10.36894250292379205 ) ) ;
#89374=CARTESIAN_POINT ( 'NONE',  ( 10.00000000000000178, 32.25893115100078745, 9.846743663894594434 ) ) ;
#89377=CARTESIAN_POINT ( 'NONE',  ( 13.79529636645030344, 43.26208216824730357, 14.16423886937410614 ) ) ;
#89378=CARTESIAN_POINT ( 'NONE',  ( 10.00000000000000000, -0.2410688489992152128, -9.846743663894594434 ) ) ;
#89380=CARTESIAN_POINT ( 'NONE',  ( 10.00000000000000178, 70.00000000000000000, 0.000000000000000000 ) ) ;
#89381=CARTESIAN_POINT ( 'NONE',  ( 17.96484262340118221, 29.93868534415484106, 7.964842623401181321 ) ) ;
#89382=CARTESIAN_POINT ( 'NONE',  ( 19.38216949554541202, 40.99863466993042493, 9.382169495545424454 ) ) ;
#89383=CARTESIAN_POINT ( 'NONE',  ( 15.44008868035555793, 6.397018677488170546, -9.422509992056140149 ) ) ;
#89384=CARTESIAN_POINT ( 'NONE',  ( 0.6178305044545818747, 38.49863466993042493, -9.382169495545419124 ) ) ;
#89385=CARTESIAN_POINT ( 'NONE',  ( 6.565887622018943937, 58.08196800326376064, -12.81628187352647608 ) ) ;
#89389=CARTESIAN_POINT ( 'NONE',  ( 20.36894250292379738, 29.92874883491396432, -10.36894250292379027 ) ) ;
#89390=CARTESIAN_POINT ( 'NONE',  ( 0.5774900079438607392, 18.48035201082150536, 5.440088680355550821 ) ) ;
#89391=DIRECTION ( 'NONE',  ( -0.5547001962252291474, -0.8320502943378437211, -0.000000000000000000 ) ) ;
#89393=CARTESIAN_POINT ( 'NONE',  ( -0.8801773607111009756, 48.06368534415484817, 1.068504757029289695E-15 ) ) ;
#89394=CARTESIAN_POINT ( 'NONE',  ( 12.91533473730993009, 51.60535201082149825, -10.88017736071109987 ) ) ;
#89395=CARTESIAN_POINT ( 'NONE',  ( 21.09922568453595559, 7.040301336597086568, -6.408140936763230044 ) ) ;
#89396=( NAMED_UNIT ( * ) SI_UNIT ( $, .STERADIAN. ) SOLID_ANGLE_UNIT ( ) );
#89397=CARTESIAN_POINT ( 'NONE',  ( 2.603489959281588106, 1.582109641433292690, 6.500000000000000888 ) ) ;
#89398=CARTESIAN_POINT ( 'NONE',  ( 14.92337183194729633, 22.67559781766745175, 8.527530157486181039 ) ) ;
#89399=CARTESIAN_POINT ( 'NONE',  ( 12.91533473730993009, 41.60535201082149825, -10.88017736071109987 ) ) ;
#89401=CARTESIAN_POINT ( 'NONE',  ( 6.565887622018943937, 10.16530133659708746, 12.81628187352647430 ) ) ;
#89402=CARTESIAN_POINT ( 'NONE',  ( 10.00000000000000000, -0.2410688489992152128, -9.846743663894594434 ) ) ;
#89403=CARTESIAN_POINT ( 'NONE',  ( 7.361572987183169658, 29.96726448433411960, -9.846743663894592657 ) ) ;
#89404=CARTESIAN_POINT ( 'NONE',  ( 6.565887622018943937, 55.16530133659709634, 12.81628187352647430 ) ) ;
#89405=CARTESIAN_POINT ( 'NONE',  ( 18.52753015748617571, 23.09226448433411960, 4.923371831947298993 ) ) ;
#89407=CARTESIAN_POINT ( 'NONE',  ( 20.36894250292379738, 4.928748834913967869, -10.36894250292379027 ) ) ;
#89408=DIRECTION ( 'NONE',  ( 1.000000000000000000, 0.000000000000000000, 0.000000000000000000 ) ) ;
#89409=CARTESIAN_POINT ( 'NONE',  ( 15.44008868035555260, 19.73035201082150536, 9.422509992056143702 ) ) ;
#89410=CARTESIAN_POINT ( 'NONE',  ( 10.00000000000000000, 1.813685344154837731, -10.88017736071110342 ) ) ;
#89411=CARTESIAN_POINT ( 'NONE',  ( -4.164238869374099039, 36.80374883491396787, 8.674139862899312516E-16 ) ) ;
#89412=CARTESIAN_POINT ( 'NONE',  ( 14.92337183194729988, 34.34226448433411605, -8.527530157486177487 ) ) ;
#89414=CARTESIAN_POINT ( 'NONE',  ( 7.084665262690076126, 22.02201867748817321, -10.88017736071110164 ) ) ;
#89415=CARTESIAN_POINT ( 'NONE',  ( -0.8801773607111008646, 18.27201867748817321, 2.915334737309923430 ) ) ;
#89416=ORIENTED_EDGE ( 'NONE', *, *, #35734, .T. ) ;
#89418=CARTESIAN_POINT ( 'NONE',  ( 20.88017736071110164, 20.35535201082150891, 2.915334737309930979 ) ) ;
#89420=CARTESIAN_POINT ( 'NONE',  ( -2.816281873526473856, 44.12363466993042493, 9.499525473075851096E-16 ) ) ;
#89421=CARTESIAN_POINT ( 'NONE',  ( 10.00000000000000178, 39.31368534415484106, 10.88017736071110342 ) ) ;
#89423=CARTESIAN_POINT ( 'NONE',  ( 7.084665262690076126, 42.02201867748816966, -10.88017736071110164 ) ) ;
#89425=CARTESIAN_POINT ( 'NONE',  ( 0.1532563361054100626, 55.80059781766745175, -2.638427012816831230 ) ) ;
#89426=CARTESIAN_POINT ( 'NONE',  ( -0.8801773607111008646, 38.27201867748816255, 2.915334737309923430 ) ) ;
#89428=EDGE_CURVE ( 'NONE', #96626, #71776, #84113, .T. ) ;
#89431=CARTESIAN_POINT ( 'NONE',  ( -4.164238869374098151, 51.59541550158063217, -3.795296366450310543 ) ) ;
#89432=CARTESIAN_POINT ( 'NONE',  ( -0.8801773607110991993, 57.85535201082149825, -2.915334737309923874 ) ) ;
#89436=CARTESIAN_POINT ( 'NONE',  ( 19.84674366389459266, 53.71726448433411605, -2.638427012816827677 ) ) ;
#89437=CARTESIAN_POINT ( 'NONE',  ( 19.84674366389459621, 3.508931151000785231, 7.409399052514197653E-17 ) ) ;
#89438=CARTESIAN_POINT ( 'NONE',  ( 1.472469842513823179, 20.59226448433411960, -4.923371831947296329 ) ) ;
#89439=EDGE_CURVE ( 'NONE', #92463, #48349, #7288, .T. ) ;
#89440=CARTESIAN_POINT ( 'NONE',  ( 1.472469842513823179, 25.59226448433412315, -4.923371831947296329 ) ) ;
#89443=CARTESIAN_POINT ( 'NONE',  ( 0.5774900079438607392, 23.48035201082150536, 5.440088680355550821 ) ) ;
#89444=CARTESIAN_POINT ( 'NONE',  ( 5.076628168052704559, 20.17559781766745175, -8.527530157486179263 ) ) ;
#89445=CARTESIAN_POINT ( 'NONE',  ( 22.81628187352648496, 11.83196800326375531, -3.434112377981050290 ) ) ;
#89446=CARTESIAN_POINT ( 'NONE',  ( -0.8801773607110991993, 62.85535201082150536, -2.915334737309923874 ) ) ;
#89447=CARTESIAN_POINT ( 'NONE',  ( 17.96484262340118221, 51.18868534415483396, -7.964842623401177768 ) ) ;
#89448=CARTESIAN_POINT ( 'NONE',  ( 0.5774900079438590739, 27.64701867748817676, -5.440088680355550821 ) ) ;
#89449=CARTESIAN_POINT ( 'NONE',  ( 3.591859063236761518, 59.95696800326375353, 11.09922568453594849 ) ) ;
#89450=CARTESIAN_POINT ( 'NONE',  ( -4.164238869374099039, 46.80374883491397497, 8.674139862899312516E-16 ) ) ;
#89453=CARTESIAN_POINT ( 'NONE',  ( 3.591859063236763294, -1.709698663402913210, -11.09922568453595026 ) ) ;
#89454=CARTESIAN_POINT ( 'NONE',  ( 12.91533473730993009, 11.60535201082150536, -10.88017736071109987 ) ) ;
#89455=CARTESIAN_POINT ( 'NONE',  ( 0.5774900079438607392, 48.48035201082150536, 5.440088680355550821 ) ) ;
#89456=CARTESIAN_POINT ( 'NONE',  ( 10.00000000000000000, 0.5537488349139675359, -14.16423886937410082 ) ) ;
#89458=CARTESIAN_POINT ( 'NONE',  ( 14.92337183194729988, 19.34226448433411960, -8.527530157486177487 ) ) ;
#89459=CARTESIAN_POINT ( 'NONE',  ( 0.5774900079438590739, 62.64701867748817676, -5.440088680355550821 ) ) ;
#89460=CARTESIAN_POINT ( 'NONE',  ( 17.20831665107776587, 32.88393115100078745, 7.208316651077764980 ) ) ;
#89461=CARTESIAN_POINT ( 'NONE',  ( 10.00000000000000000, 24.75893115100078745, -9.846743663894594434 ) ) ;
#89462=CARTESIAN_POINT ( 'NONE',  ( 1.472469842513823179, 15.59226448433411960, -4.923371831947296329 ) ) ;
#89464=EDGE_CURVE ( 'NONE', #25008, #64876, #18660, .T. ) ;
#89465=CARTESIAN_POINT ( 'NONE',  ( 0.5774900079438590739, 67.64701867748817676, -5.440088680355550821 ) ) ;
#89467=CARTESIAN_POINT ( 'NONE',  ( 2.791683348922237240, 35.38393115100079456, -7.208316651077763204 ) ) ;
#89470=CARTESIAN_POINT ( 'NONE',  ( 13.43411237798105340, 50.58196800326375353, 12.81628187352647963 ) ) ;
#89472=CARTESIAN_POINT ( 'NONE',  ( 1.472469842513823179, 66.42559781766745175, 4.923371831947296329 ) ) ;
#89474=CARTESIAN_POINT ( 'NONE',  ( 13.79529636645031943, 20.34541550158063572, -14.16423886937409904 ) ) ;
#89477=CARTESIAN_POINT ( 'NONE',  ( 1.492507162822248157, 42.19955587570481725, -6.500000000000035527 ) ) ;
#89478=CARTESIAN_POINT ( 'NONE',  ( -4.164238869374098151, 16.59541550158063927, -3.795296366450310543 ) ) ;
#89480=AXIS2_PLACEMENT_3D ( 'NONE', #26303, #24850, #49300 ) ;
#89481=CARTESIAN_POINT ( 'NONE',  ( 17.08211943468705840, 45.13708216824730357, -12.26659068614894466 ) ) ;
#89482=CARTESIAN_POINT ( 'NONE',  ( -0.3689425029237881626, 2.428748834913967869, 10.36894250292379027 ) ) ;
#89483=CARTESIAN_POINT ( 'NONE',  ( -0.3689425029237881626, 12.42874883491396609, 10.36894250292379027 ) ) ;
#89484=CARTESIAN_POINT ( 'NONE',  ( 19.42250999205614193, 45.14701867748817676, 5.440088680355555262 ) ) ;
#89487=CARTESIAN_POINT ( 'NONE',  ( 14.92337183194729633, 27.67559781766745530, 8.527530157486181039 ) ) ;
#89488=CARTESIAN_POINT ( 'NONE',  ( 19.72487221294570858, 61.86607318730076344, 6.500000000000000888 ) ) ;
#89489=CARTESIAN_POINT ( 'NONE',  ( 2.791683348922240793, 31.63393115100078745, 7.208316651077764092 ) ) ;
#89490=VECTOR ( 'NONE', #51209, 1000.000000000000000 ) ;
#89491=CARTESIAN_POINT ( 'NONE',  ( -0.8801773607111008646, 13.27201867748817321, 2.915334737309923430 ) ) ;
#89492=CARTESIAN_POINT ( 'NONE',  ( 13.43411237798106583, 52.66530133659708213, -12.81628187352647252 ) ) ;
#89493=CARTESIAN_POINT ( 'NONE',  ( 18.52753015748617571, 53.09226448433412315, 4.923371831947298993 ) ) ;
#89495=CARTESIAN_POINT ( 'NONE',  ( 22.81628187352647785, 46.41530133659708213, 3.434112377981063169 ) ) ;
#89497=CARTESIAN_POINT ( 'NONE',  ( 12.91533473730992121, 44.52201867748816966, 10.88017736071110164 ) ) ;
#89498=CARTESIAN_POINT ( 'NONE',  ( 5.076628168052703671, 41.84226448433411605, 8.527530157486179263 ) ) ;
#89499=CARTESIAN_POINT ( 'NONE',  ( -0.3689425029237881626, 22.42874883491397142, 10.36894250292379027 ) ) ;
#89501=CARTESIAN_POINT ( 'NONE',  ( -4.164238869374098151, 6.595415501580634832, -3.795296366450310543 ) ) ;
#89502=CARTESIAN_POINT ( 'NONE',  ( 15.44008868035555260, 44.73035201082151247, 9.422509992056143702 ) ) ;
#89503=CARTESIAN_POINT ( 'NONE',  ( 20.88017736071110519, 65.56368534415483396, 2.639326808657452039E-16 ) ) ;
#89504=CARTESIAN_POINT ( 'NONE',  ( -4.164238869374099927, 42.01208216824728936, 3.795296366450308767 ) ) ;
#89505=CARTESIAN_POINT ( 'NONE',  ( 12.63842701281683922, 64.55059781766745175, -9.846743663894590881 ) ) ;
#89507=CARTESIAN_POINT ( 'NONE',  ( 15.44008868035555260, 54.73035201082150536, 9.422509992056143702 ) ) ;
#89510=CARTESIAN_POINT ( 'NONE',  ( 3.591859063236763294, 23.29030133659708568, -11.09922568453595026 ) ) ;
#89511=CARTESIAN_POINT ( 'NONE',  ( 10.00000000000000000, 2.873634669930420049, -12.81628187352647608 ) ) ;
#89513=CARTESIAN_POINT ( 'NONE',  ( 2.035157376598822676, 17.43868534415483751, -7.964842623401177768 ) ) ;
#89514=CARTESIAN_POINT ( 'NONE',  ( 20.88017736071110164, 5.355352010821503583, 2.915334737309930979 ) ) ;
#89520=CARTESIAN_POINT ( 'NONE',  ( 10.00000000000000000, 4.758931151000784787, -9.846743663894594434 ) ) ;
#89522=CARTESIAN_POINT ( 'NONE',  ( 7.361572987183169658, 39.96726448433411605, -9.846743663894592657 ) ) ;
#89523=EDGE_CURVE ( 'NONE', #85047, #97286, #37100, .T. ) ;
#89524=CARTESIAN_POINT ( 'NONE',  ( 7.084665262690076126, 42.02201867748816966, -10.88017736071110164 ) ) ;
#89525=CARTESIAN_POINT ( 'NONE',  ( -1.099225684535947600, 9.540301336597087456, 6.408140936763237150 ) ) ;
#89526=CARTESIAN_POINT ( 'NONE',  ( 12.91533473730992121, 34.52201867748817676, 10.88017736071110164 ) ) ;
#89529=CARTESIAN_POINT ( 'NONE',  ( 0.6178305044545818747, 48.49863466993042493, -9.382169495545419124 ) ) ;
#89530=ORIENTED_EDGE ( 'NONE', *, *, #75635, .F. ) ;
#89531=CARTESIAN_POINT ( 'NONE',  ( 17.96484262340118221, 59.93868534415484106, 7.964842623401181321 ) ) ;
#89532=CARTESIAN_POINT ( 'NONE',  ( 3.591859063236761518, 29.95696800326375708, 11.09922568453594849 ) ) ;
#89533=CARTESIAN_POINT ( 'NONE',  ( 22.26659068614895176, 4.720415501580633943, -7.082119434687042414 ) ) ;
#89534=( NAMED_UNIT ( * ) SI_UNIT ( $, .STERADIAN. ) SOLID_ANGLE_UNIT ( ) );
#89535=CARTESIAN_POINT ( 'NONE',  ( 2.035157376598822676, 42.43868534415483396, -7.964842623401177768 ) ) ;
#89536=CARTESIAN_POINT ( 'NONE',  ( 18.52753015748617571, 63.09226448433412315, 4.923371831947298993 ) ) ;
#89537=CARTESIAN_POINT ( 'NONE',  ( 17.20831665107776587, 47.88393115100078745, 7.208316651077764980 ) ) ;
#89538=CARTESIAN_POINT ( 'NONE',  ( 12.63842701281683922, 19.55059781766745175, -9.846743663894590881 ) ) ;
#89539=CARTESIAN_POINT ( 'NONE',  ( 19.42250999205614548, 60.98035201082151247, -5.440088680355545492 ) ) ;
#89540=CARTESIAN_POINT ( 'NONE',  ( 24.16423886937410614, 29.51208216824729647, -3.795296366450302550 ) ) ;
#89542=CARTESIAN_POINT ( 'NONE',  ( 20.15039907845753930, 70.00000000000000000, 6.262539305110068177 ) ) ;
#89547=CARTESIAN_POINT ( 'NONE',  ( 24.16423886937410614, 64.30374883491396076, 8.672049930838204340E-16 ) ) ;
#89548=CARTESIAN_POINT ( 'NONE',  ( 22.26659068614894466, 63.88708216824730357, 7.082119434687054849 ) ) ;
#89549=CARTESIAN_POINT ( 'NONE',  ( 18.52753015748618282, 33.92559781766745886, -4.923371831947291888 ) ) ;
#89551=CARTESIAN_POINT ( 'NONE',  ( 10.00000000000000178, 14.31368534415483751, 10.88017736071110342 ) ) ;
#89552=CARTESIAN_POINT ( 'NONE',  ( 2.917880565312950480, 55.97041550158063217, -12.26659068614894821 ) ) ;
#89553=CARTESIAN_POINT ( 'NONE',  ( 10.00000000000000000, 34.75893115100078745, -9.846743663894594434 ) ) ;
#89555=CARTESIAN_POINT ( 'NONE',  ( 1.472469842513823179, 10.59226448433411782, -4.923371831947296329 ) ) ;
#89564=CARTESIAN_POINT ( 'NONE',  ( 18.52753015748617571, 43.09226448433412315, 4.923371831947298993 ) ) ;
#89565=CARTESIAN_POINT ( 'NONE',  ( 20.88017736071110875, 15.77201867748817143, -2.915334737309920765 ) ) ;
#89566=CARTESIAN_POINT ( 'NONE',  ( 15.44008868035555793, 21.39701867748817321, -9.422509992056140149 ) ) ;
#89567=CARTESIAN_POINT ( 'NONE',  ( 22.81628187352647785, 21.62363466993041783, 6.195893100308588602E-16 ) ) ;
#89568=CARTESIAN_POINT ( 'NONE',  ( -4.164238869374099927, 2.012082168247300906, 3.795296366450308767 ) ) ;
#89569=CARTESIAN_POINT ( 'NONE',  ( -1.099225684535947600, 34.54030133659708923, 6.408140936763237150 ) ) ;
#89571=CARTESIAN_POINT ( 'NONE',  ( 0.1532563361054083140, 31.00893115100078390, 1.131784320476157264E-15 ) ) ;
#89572=CARTESIAN_POINT ( 'NONE',  ( 10.00000000000000178, 68.05374883491397497, 14.16423886937410082 ) ) ;
#89574=CARTESIAN_POINT ( 'NONE',  ( -0.3689425029237881626, 67.42874883491396076, 10.36894250292379027 ) ) ;
#89576=CARTESIAN_POINT ( 'NONE',  ( 20.88017736071110164, 50.35535201082151247, 2.915334737309930979 ) ) ;
#89577=CARTESIAN_POINT ( 'NONE',  ( -0.8801773607111008646, 63.27201867748817676, 2.915334737309923430 ) ) ;
#89578=CARTESIAN_POINT ( 'NONE',  ( 17.96484262340118221, 56.18868534415484817, -7.964842623401177768 ) ) ;
#89579=CARTESIAN_POINT ( 'NONE',  ( 2.791683348922240793, 1.633931151000784565, 7.208316651077764092 ) ) ;
#89580=CARTESIAN_POINT ( 'NONE',  ( 19.42250999205614193, 45.14701867748817676, 5.440088680355555262 ) ) ;
#89584=EDGE_CURVE ( 'NONE', #31232, #6963, #31166, .T. ) ;
#89586=AXIS2_PLACEMENT_3D ( 'NONE', #36613, #76568, #44590 ) ;
#89587=CARTESIAN_POINT ( 'NONE',  ( 7.361572987183170547, 27.05059781766745175, 9.846743663894590881 ) ) ;
#89589=CARTESIAN_POINT ( 'NONE',  ( 18.52753015748617571, 53.09226448433412315, 4.923371831947298993 ) ) ;
#89591=B_SPLINE_CURVE_WITH_KNOTS ( 'NONE', 3,
 ( #45913, #69395, #29902, #52903 ),
 .UNSPECIFIED., .F., .F.,
 ( 4, 4 ),
 ( 0.000000000000000000, 0.001036303429213365507 ),
 .UNSPECIFIED. ) ;
#89592=CARTESIAN_POINT ( 'NONE',  ( -4.164238869374099039, 11.80374883491396965, 8.674139862899312516E-16 ) ) ;
#89593=ORIENTED_EDGE ( 'NONE', *, *, #5682, .F. ) ;
#89594=CARTESIAN_POINT ( 'NONE',  ( 19.72487221294571569, 50.71833443783938122, -6.499999999999983125 ) ) ;
#89597=CARTESIAN_POINT ( 'NONE',  ( 5.076628168052703671, 36.84226448433412315, 8.527530157486179263 ) ) ;
#89598=CARTESIAN_POINT ( 'NONE',  ( 10.00000000000000178, 63.05374883491396076, 14.16423886937410082 ) ) ;
#89601=CARTESIAN_POINT ( 'NONE',  ( 20.15039907845753575, 62.62777174578612716, -6.262539305110073506 ) ) ;
#89602=CARTESIAN_POINT ( 'NONE',  ( 17.20831665107776587, 42.88393115100077324, 7.208316651077764980 ) ) ;
#89604=CARTESIAN_POINT ( 'NONE',  ( 13.43411237798106583, 22.66530133659708923, -12.81628187352647252 ) ) ;
#89605=CARTESIAN_POINT ( 'NONE',  ( 5.076628168052704559, 10.17559781766745175, -8.527530157486179263 ) ) ;
#89606=DIRECTION ( 'NONE',  ( 0.000000000000000000, -1.000000000000000000, 0.000000000000000000 ) ) ;
#89607=CARTESIAN_POINT ( 'NONE',  ( 0.1532563361054100626, 5.800597817667452638, -2.638427012816831230 ) ) ;
#89608=CARTESIAN_POINT ( 'NONE',  ( -2.816281873526471635, 8.915301336597083903, -3.434112377981056508 ) ) ;
#89609=CARTESIAN_POINT ( 'NONE',  ( 1.472469842513823179, 25.59226448433412315, -4.923371831947296329 ) ) ;
#89611=CARTESIAN_POINT ( 'NONE',  ( 2.035157376598822676, 12.43868534415483751, -7.964842623401177768 ) ) ;
#89612=CARTESIAN_POINT ( 'NONE',  ( 17.08211943468705840, 10.13708216824730179, -12.26659068614894466 ) ) ;
#89613=CARTESIAN_POINT ( 'NONE',  ( 1.472469842513823179, 31.42559781766745530, 4.923371831947296329 ) ) ;
#89614=CARTESIAN_POINT ( 'NONE',  ( 19.42250999205614193, 60.14701867748817676, 5.440088680355555262 ) ) ;
#89615=AXIS2_PLACEMENT_3D ( 'NONE', #45501, #8010, #38019 ) ;
#89616=CARTESIAN_POINT ( 'NONE',  ( 22.81628187352647785, 21.41530133659708923, 3.434112377981063169 ) ) ;
#89618=CARTESIAN_POINT ( 'NONE',  ( 4.559911319644449179, 8.897018677488171434, 9.422509992056141925 ) ) ;
#89621=CARTESIAN_POINT ( 'NONE',  ( 14.92337183194729988, 64.34226448433412315, -8.527530157486177487 ) ) ;
#89622=CARTESIAN_POINT ( 'NONE',  ( 18.52753015748618282, 33.92559781766745886, -4.923371831947291888 ) ) ;
#89624=CARTESIAN_POINT ( 'NONE',  ( 13.43411237798106583, 37.66530133659708923, -12.81628187352647252 ) ) ;
#89626=CARTESIAN_POINT ( 'NONE',  ( 19.42250999205614193, 40.14701867748817676, 5.440088680355555262 ) ) ;
#89629=CARTESIAN_POINT ( 'NONE',  ( 20.88017736071110519, 25.56368534415483751, 2.639326808657452039E-16 ) ) ;
#89630=ADVANCED_FACE ( 'NONE', ( #59585 ), #84567, .T. ) ;
#89631=CARTESIAN_POINT ( 'NONE',  ( 19.42250999205614548, 35.98035201082151247, -5.440088680355545492 ) ) ;
#89632=CARTESIAN_POINT ( 'NONE',  ( 14.92337183194729633, 52.67559781766745175, 8.527530157486181039 ) ) ;
#89633=CARTESIAN_POINT ( 'NONE',  ( 7.084665262690076126, 59.10535201082150536, 10.88017736071109987 ) ) ;
#89634=CARTESIAN_POINT ( 'NONE',  ( 13.79529636645031943, 30.34541550158063927, -14.16423886937409904 ) ) ;
#89637=CARTESIAN_POINT ( 'NONE',  ( 18.52753015748617571, 43.09226448433412315, 4.923371831947298993 ) ) ;
#89638=CARTESIAN_POINT ( 'NONE',  ( 19.38216949554541202, 0.9986346699304200492, 9.382169495545424454 ) ) ;
#89640=CARTESIAN_POINT ( 'NONE',  ( 19.42250999205614548, 20.98035201082150891, -5.440088680355545492 ) ) ;
#89642=CARTESIAN_POINT ( 'NONE',  ( 2.035157376598824452, 18.68868534415484106, 7.964842623401179544 ) ) ;
#89643=CARTESIAN_POINT ( 'NONE',  ( 12.63842701281683034, 2.467264484334118269, 9.846743663894596210 ) ) ;
#89644=CARTESIAN_POINT ( 'NONE',  ( 17.08211943468705840, 30.13708216824730357, -12.26659068614894466 ) ) ;
#89645=CARTESIAN_POINT ( 'NONE',  ( 5.076628168052703671, 11.84226448433411960, 8.527530157486179263 ) ) ;
#89646=CARTESIAN_POINT ( 'NONE',  ( 14.92337183194729988, 64.34226448433412315, -8.527530157486177487 ) ) ;
#89647=CARTESIAN_POINT ( 'NONE',  ( 12.91533473730993009, 46.60535201082150536, -10.88017736071109987 ) ) ;
#89648=CARTESIAN_POINT ( 'NONE',  ( 18.17884179759845509, 38.66688879859523098, -6.500000000000054179 ) ) ;
#89650=EDGE_CURVE ( 'NONE', #63634, #38758, #97783, .T. ) ;
#89652=EDGE_LOOP ( 'NONE', ( #79390, #2699, #4186, #98631, #98597, #53211 ) ) ;
#89654=CARTESIAN_POINT ( 'NONE',  ( 19.84674366389459621, 48.50893115100078745, 7.409399052514197653E-17 ) ) ;
#89658=CARTESIAN_POINT ( 'NONE',  ( -2.266590686148945544, 16.38708216824730357, -7.082119434687050408 ) ) ;
#89659=CARTESIAN_POINT ( 'NONE',  ( 22.26659068614894466, 28.88708216824730357, 7.082119434687054849 ) ) ;
#89660=CARTESIAN_POINT ( 'NONE',  ( 15.44008868035555260, 54.73035201082150536, 9.422509992056143702 ) ) ;
#89661=CARTESIAN_POINT ( 'NONE',  ( 2.917880565312948704, 52.63708216824730357, 12.26659068614894643 ) ) ;
#89662=CARTESIAN_POINT ( 'NONE',  ( 1.472469842513823179, 66.42559781766745175, 4.923371831947296329 ) ) ;
#89663=CARTESIAN_POINT ( 'NONE',  ( 14.92337183194729633, 42.67559781766745886, 8.527530157486181039 ) ) ;
#89664=CARTESIAN_POINT ( 'NONE',  ( 4.559911319644449179, 48.89701867748817676, 9.422509992056141925 ) ) ;
#89665=CARTESIAN_POINT ( 'NONE',  ( 13.43411237798106583, 7.665301336597086568, -12.81628187352647252 ) ) ;
#89666=CARTESIAN_POINT ( 'NONE',  ( -2.266590686148945544, 22.22041550158063572, 7.082119434687048631 ) ) ;
#89667=CARTESIAN_POINT ( 'NONE',  ( -2.266590686148945544, 46.38708216824730357, -7.082119434687050408 ) ) ;
#89668=CARTESIAN_POINT ( 'NONE',  ( 10.00000000000000000, 21.81368534415484106, -10.88017736071110342 ) ) ;
#89669=CARTESIAN_POINT ( 'NONE',  ( 19.84674366389459266, 53.71726448433411605, -2.638427012816827677 ) ) ;
#89670=CARTESIAN_POINT ( 'NONE',  ( 2.035157376598822676, 37.43868534415484106, -7.964842623401177768 ) ) ;
#89672=CARTESIAN_POINT ( 'NONE',  ( 19.38216949554541202, 50.99863466993042493, 9.382169495545424454 ) ) ;
#89678=CARTESIAN_POINT ( 'NONE',  ( 13.79529636645031943, 45.34541550158062506, -14.16423886937409904 ) ) ;
#89679=CARTESIAN_POINT ( 'NONE',  ( 12.63842701281683034, 47.46726448433412315, 9.846743663894596210 ) ) ;
#89680=CARTESIAN_POINT ( 'NONE',  ( 15.44008868035555260, 64.73035201082151957, 9.422509992056143702 ) ) ;
#89682=CARTESIAN_POINT ( 'NONE',  ( 2.035157376598824452, 53.68868534415484817, 7.964842623401179544 ) ) ;
#89687=CARTESIAN_POINT ( 'NONE',  ( -2.266590686148945544, 27.22041550158063572, 7.082119434687048631 ) ) ;
#89688=CARTESIAN_POINT ( 'NONE',  ( 0.6178305044545838731, 24.74863466993042493, 9.382169495545420901 ) ) ;
#89690=CARTESIAN_POINT ( 'NONE',  ( -1.099225684535947600, 38.70696800326375353, -6.408140936763238038 ) ) ;
#89691=CARTESIAN_POINT ( 'NONE',  ( 12.91533473730993009, 16.60535201082150891, -10.88017736071109987 ) ) ;
#89692=CARTESIAN_POINT ( 'NONE',  ( 18.52753015748617571, 38.09226448433412315, 4.923371831947298993 ) ) ;
#89693=CARTESIAN_POINT ( 'NONE',  ( 20.88017736071110164, 15.35535201082150358, 2.915334737309930979 ) ) ;
#89695=CARTESIAN_POINT ( 'NONE',  ( 3.591859063236761518, 64.95696800326376774, 11.09922568453594849 ) ) ;
#89697=CARTESIAN_POINT ( 'NONE',  ( 18.52753015748618282, 43.92559781766745175, -4.923371831947291888 ) ) ;
#89702=CARTESIAN_POINT ( 'NONE',  ( 0.2751277870542868098, 57.28217586085237656, -6.499999999999985789 ) ) ;
#89703=CARTESIAN_POINT ( 'NONE',  ( 7.361572987183170547, 12.05059781766744997, 9.846743663894590881 ) ) ;
#89704=CARTESIAN_POINT ( 'NONE',  ( 21.09922568453594849, 21.20696800326375353, 6.408140936763242479 ) ) ;
#89707=CARTESIAN_POINT ( 'NONE',  ( 10.00000000000000178, 57.25893115100078745, 9.846743663894594434 ) ) ;
#89709=CARTESIAN_POINT ( 'NONE',  ( 13.79529636645031943, 20.34541550158063572, -14.16423886937409904 ) ) ;
#89710=CARTESIAN_POINT ( 'NONE',  ( 5.076628168052703671, 41.84226448433411605, 8.527530157486179263 ) ) ;
#89711=CARTESIAN_POINT ( 'NONE',  ( 6.565887622018943937, 40.16530133659708923, 12.81628187352647430 ) ) ;
#89714=CARTESIAN_POINT ( 'NONE',  ( 7.361572987183169658, 4.967264484334119601, -9.846743663894592657 ) ) ;
#89715=CARTESIAN_POINT ( 'NONE',  ( 21.92686044187656691, 47.18830936912750929, 4.562052436263911564E-16 ) ) ;
#89716=EDGE_CURVE ( 'NONE', #87186, #51568, #1200, .T. ) ;
#89717=CARTESIAN_POINT ( 'NONE',  ( 19.84674366389459266, 48.30059781766745175, 2.638427012816836559 ) ) ;
#89718=CARTESIAN_POINT ( 'NONE',  ( 17.96484262340118221, 46.18868534415484106, -7.964842623401177768 ) ) ;
#89721=AXIS2_PLACEMENT_3D ( 'NONE', #31989, #83542, #68049 ) ;
#89722=CARTESIAN_POINT ( 'NONE',  ( 12.91533473730993009, 41.60535201082149825, -10.88017736071109987 ) ) ;
#89725=CARTESIAN_POINT ( 'NONE',  ( 15.44008868035555793, 11.39701867748817143, -9.422509992056140149 ) ) ;
#89726=CARTESIAN_POINT ( 'NONE',  ( 10.00000000000000178, 57.25893115100078745, 9.846743663894594434 ) ) ;
#89727=CARTESIAN_POINT ( 'NONE',  ( -0.8801773607110991993, 47.85535201082150536, -2.915334737309923874 ) ) ;
#89729=CARTESIAN_POINT ( 'NONE',  ( 7.084665262690076126, 59.10535201082150536, 10.88017736071109987 ) ) ;
#89730=CARTESIAN_POINT ( 'NONE',  ( 19.42250999205614548, 20.98035201082150891, -5.440088680355545492 ) ) ;
#89731=CARTESIAN_POINT ( 'NONE',  ( 19.84674366389459621, 3.508931151000785231, 7.409399052514197653E-17 ) ) ;
#89732=CARTESIAN_POINT ( 'NONE',  ( 7.361572987183170547, 22.05059781766745530, 9.846743663894590881 ) ) ;
#89734=CARTESIAN_POINT ( 'NONE',  ( 1.472469842513823179, 56.42559781766745886, 4.923371831947296329 ) ) ;
#89736=CARTESIAN_POINT ( 'NONE',  ( 6.204703633549690345, 62.84541550158063927, 14.16423886937410082 ) ) ;
#89738=CARTESIAN_POINT ( 'NONE',  ( 10.00000000000000000, 5.553748834913967869, -14.16423886937410082 ) ) ;
#89739=CARTESIAN_POINT ( 'NONE',  ( -4.164238869374098151, 51.59541550158063217, -3.795296366450310543 ) ) ;
#89740=CARTESIAN_POINT ( 'NONE',  ( 19.38216949554541557, 7.248634669930421381, -9.382169495545420901 ) ) ;
#89743=CARTESIAN_POINT ( 'NONE',  ( -0.8801773607111008646, 18.27201867748817321, 2.915334737309923430 ) ) ;
#89744=CARTESIAN_POINT ( 'NONE',  ( 12.63842701281683034, 47.46726448433412315, 9.846743663894596210 ) ) ;
#89745=SURFACE_STYLE_USAGE ( .BOTH. , #65759 ) ;
#89747=EDGE_CURVE ( 'NONE', #65595, #30124, #58429, .T. ) ;
#89749=SURFACE_STYLE_USAGE ( .BOTH. , #66254 ) ;
#89750=CARTESIAN_POINT ( 'NONE',  ( 21.09922568453595559, 22.04030133659708923, -6.408140936763230044 ) ) ;
#89751=CARTESIAN_POINT ( 'NONE',  ( 19.84674366389459266, 28.30059781766745886, 2.638427012816836559 ) ) ;
#89753=CARTESIAN_POINT ( 'NONE',  ( 5.076628168052704559, 10.17559781766745175, -8.527530157486179263 ) ) ;
#89756=CARTESIAN_POINT ( 'NONE',  ( -46.78784730906664180, 100.7327625268226825, -9.217559165526038711 ) ) ;
#89757=CARTESIAN_POINT ( 'NONE',  ( 10.00000000000000178, 14.31368534415483751, 10.88017736071110342 ) ) ;
#89758=CARTESIAN_POINT ( 'NONE',  ( 17.08211943468705840, 35.13708216824730357, -12.26659068614894466 ) ) ;
#89759=CARTESIAN_POINT ( 'NONE',  ( 10.00000000000000000, 41.81368534415484106, -10.88017736071110342 ) ) ;
#89760=CARTESIAN_POINT ( 'NONE',  ( 2.035157376598824452, 63.68868534415484106, 7.964842623401179544 ) ) ;
#89761=CARTESIAN_POINT ( 'NONE',  ( 18.95785429995054372, 17.24216108172007011, 6.499999999999841016 ) ) ;
#89762=CARTESIAN_POINT ( 'NONE',  ( 19.84674366389459621, 23.50893115100078390, 7.409399052514197653E-17 ) ) ;
#89764=CARTESIAN_POINT ( 'NONE',  ( 14.92337183194729988, 4.342264484334117824, -8.527530157486177487 ) ) ;
#89766=CARTESIAN_POINT ( 'NONE',  ( -1.266189978427564089, -7.341591041528217097E-16, 3.630449589664167753 ) ) ;
#89767=CARTESIAN_POINT ( 'NONE',  ( 7.361572987183170547, 32.05059781766745175, 9.846743663894590881 ) ) ;
#89768=CARTESIAN_POINT ( 'NONE',  ( 10.00000000000000000, 64.75893115100078035, -9.846743663894594434 ) ) ;
#89769=CARTESIAN_POINT ( 'NONE',  ( 12.91533473730993009, 31.60535201082150891, -10.88017736071109987 ) ) ;
#89772=CARTESIAN_POINT ( 'NONE',  ( 22.81628187352647785, 56.62363466993042493, 6.195893100308588602E-16 ) ) ;
#89774=CARTESIAN_POINT ( 'NONE',  ( 17.20831665107776587, 14.13393115100078568, -7.208316651077762316 ) ) ;
#89775=CARTESIAN_POINT ( 'NONE',  ( 0.6178305044545818747, 48.49863466993042493, -9.382169495545419124 ) ) ;
#89776=CARTESIAN_POINT ( 'NONE',  ( 10.00000000000000000, 6.813685344154838397, -10.88017736071110342 ) ) ;
#89777=CARTESIAN_POINT ( 'NONE',  ( 12.63842701281683922, 39.55059781766744464, -9.846743663894590881 ) ) ;
#89779=CARTESIAN_POINT ( 'NONE',  ( 7.361572987183169658, -0.03273551566588185635, -9.846743663894592657 ) ) ;
#89780=CARTESIAN_POINT ( 'NONE',  ( -4.164238869374099039, 21.80374883491396787, 8.674139862899312516E-16 ) ) ;
#89781=CARTESIAN_POINT ( 'NONE',  ( 24.16423886937410614, 49.30374883491396787, 8.672049930838204340E-16 ) ) ;
#89782=CARTESIAN_POINT ( 'NONE',  ( 12.63842701281683922, 49.55059781766744464, -9.846743663894590881 ) ) ;
#89784=CARTESIAN_POINT ( 'NONE',  ( 20.88017736071110875, 40.77201867748818387, -2.915334737309920765 ) ) ;
#89786=CARTESIAN_POINT ( 'NONE',  ( 12.63842701281683922, 4.550597817667451750, -9.846743663894590881 ) ) ;
#89789=CARTESIAN_POINT ( 'NONE',  ( -2.816281873526473856, 64.12363466993042493, 9.499525473075851096E-16 ) ) ;
#89790=CARTESIAN_POINT ( 'NONE',  ( 12.91533473730993009, 61.60535201082150536, -10.88017736071109987 ) ) ;
#89792=CARTESIAN_POINT ( 'NONE',  ( 20.36894250292379382, 3.678748834913967869, 10.36894250292379205 ) ) ;
#89793=CARTESIAN_POINT ( 'NONE',  ( 5.076628168052703671, 6.842264484334118713, 8.527530157486179263 ) ) ;
#89796=CARTESIAN_POINT ( 'NONE',  ( 17.96484262340118221, 19.93868534415484106, 7.964842623401181321 ) ) ;
#89799=CARTESIAN_POINT ( 'NONE',  ( -0.8801773607110991993, 27.85535201082150181, -2.915334737309923874 ) ) ;
#89800=CARTESIAN_POINT ( 'NONE',  ( 5.076628168052704559, 55.17559781766745175, -8.527530157486179263 ) ) ;
#89802=CARTESIAN_POINT ( 'NONE',  ( 7.361572987183170547, 57.05059781766744464, 9.846743663894590881 ) ) ;
#89804=CARTESIAN_POINT ( 'NONE',  ( 7.084665262690076126, 62.02201867748816966, -10.88017736071110164 ) ) ;
#89806=CARTESIAN_POINT ( 'NONE',  ( 10.00000000000000000, 64.75893115100078035, -9.846743663894594434 ) ) ;
#89807=CARTESIAN_POINT ( 'NONE',  ( -2.816281873526473856, 34.33196800326376064, 3.434112377981055619 ) ) ;
#89808=CARTESIAN_POINT ( 'NONE',  ( 10.00000000000000000, 26.81368534415484106, -10.88017736071110342 ) ) ;
#89809=CARTESIAN_POINT ( 'NONE',  ( 20.10384461210893292, 6.743024370107935539, 6.337995344473741355 ) ) ;
#89810=CARTESIAN_POINT ( 'NONE',  ( 0.1532563361054082862, 6.217264484334118713, 2.638427012816831674 ) ) ;
#89811=CARTESIAN_POINT ( 'NONE',  ( -0.8801773607111008646, 13.27201867748817321, 2.915334737309923430 ) ) ;
#89814=CARTESIAN_POINT ( 'NONE',  ( -1.099225684535947600, 53.70696800326376064, -6.408140936763238038 ) ) ;
#89815=CARTESIAN_POINT ( 'NONE',  ( 15.44008868035555793, 41.39701867748817676, -9.422509992056140149 ) ) ;
#89817=CARTESIAN_POINT ( 'NONE',  ( -2.816281873526471635, 58.91530133659707502, -3.434112377981056508 ) ) ;
#89818=CARTESIAN_POINT ( 'NONE',  ( 0.5774900079438607392, 48.48035201082150536, 5.440088680355550821 ) ) ;
#89821=CARTESIAN_POINT ( 'NONE',  ( 5.076628168052704559, 50.17559781766745886, -8.527530157486179263 ) ) ;
#89822=CIRCLE ( 'NONE', #49937, 11.92686044187656513 ) ;
#89823=( NAMED_UNIT ( * ) PLANE_ANGLE_UNIT ( ) SI_UNIT ( $, .RADIAN. ) );
#89824=CARTESIAN_POINT ( 'NONE',  ( 18.52753015748618282, 18.92559781766745175, -4.923371831947291888 ) ) ;
#89826=CARTESIAN_POINT ( 'NONE',  ( 22.81628187352648496, 6.831968003263753531, -3.434112377981050290 ) ) ;
#89828=CARTESIAN_POINT ( 'NONE',  ( 0.1532563361054100626, 60.80059781766744464, -2.638427012816831230 ) ) ;
#89829=CARTESIAN_POINT ( 'NONE',  ( 10.00000000000000178, 34.31368534415484106, 10.88017736071110342 ) ) ;
#89830=CARTESIAN_POINT ( 'NONE',  ( 1.472469842513823179, 45.59226448433412315, -4.923371831947296329 ) ) ;
#89832=CARTESIAN_POINT ( 'NONE',  ( 0.1532563361054083140, 6.008931151000784787, 1.131784320476157264E-15 ) ) ;
#89834=CARTESIAN_POINT ( 'NONE',  ( 0.6178305044545818747, 3.498634669930420049, -9.382169495545419124 ) ) ;
#89837=CARTESIAN_POINT ( 'NONE',  ( 6.565887622018943937, 65.16530133659709634, 12.81628187352647430 ) ) ;
#89839=CARTESIAN_POINT ( 'NONE',  ( -1.099225684535947600, 33.70696800326375353, -6.408140936763238038 ) ) ;
#89840=CARTESIAN_POINT ( 'NONE',  ( 10.00000000000000000, 34.75893115100078745, -9.846743663894594434 ) ) ;
#89842=CARTESIAN_POINT ( 'NONE',  ( 0.5774900079438590739, 12.64701867748817321, -5.440088680355550821 ) ) ;
#89843=CARTESIAN_POINT ( 'NONE',  ( 10.00000000000000178, 32.25893115100078745, 9.846743663894594434 ) ) ;
#89844=CARTESIAN_POINT ( 'NONE',  ( 14.49999999999999822, 11.00000000000000000, 6.500000000000000888 ) ) ;
#89845=CARTESIAN_POINT ( 'NONE',  ( 17.96484262340118221, 4.938685344154837509, 7.964842623401181321 ) ) ;
#89847=CARTESIAN_POINT ( 'NONE',  ( -0.8801773607111008646, 13.27201867748817321, 2.915334737309923430 ) ) ;
#89848=CIRCLE ( 'NONE', #91426, 0.5000000000000004441 ) ;
#89849=CARTESIAN_POINT ( 'NONE',  ( 10.00000000000000178, 53.05374883491396787, 14.16423886937410082 ) ) ;
#89850=CARTESIAN_POINT ( 'NONE',  ( -4.164238869374098151, 46.59541550158063927, -3.795296366450310543 ) ) ;
#89853=CARTESIAN_POINT ( 'NONE',  ( 17.20831665107776587, 12.88393115100078390, 7.208316651077764980 ) ) ;
#89854=CARTESIAN_POINT ( 'NONE',  ( 6.565887622018943937, 3.081968003263753531, -12.81628187352647608 ) ) ;
#89856=CARTESIAN_POINT ( 'NONE',  ( -0.1503990784575242878, 64.24884699246891273, -6.262539305110083276 ) ) ;
#89858=( BOUNDED_SURFACE ( )  B_SPLINE_SURFACE ( 1, 2, ( 
 ( #25042, #62514, #93019, #55014, #53371, #14907, #21914, #83881, #91876, #15407, #67397, #90874, #75381, #68393, #22404, #30367, #83389, #15888, #28886, #82892, #22899, #67898, #89892, #97420, #6390, #97923, #59884, #21410, #36905, #29383, #23397, #61366, #45891, #6897, #7407, #60378, #37411, #46373, #90375, #66901, #59390, #53882, #74891, #98914, #52390, #14408, #38387, #44879, #44392, #76378, #45379, #91373, #98421, #7893, #75885, #68888, #84389, #76862, #36407, #51905, #82389, #13913, #418, #30869, #29876, #52879, #37904, #60873, #4871, #73839, #57360, #73344, #3886, #87854, #35348, #5367, #72354, #35846, #65344, #50853, #51343, #12842, #50346, #74324, #96869, #66835, #66333, #97357, #81346, #28345, #79868, #43342, #95363, #12354, #95872, #80857, #26863, #72847, #18885, #20852, #19853, #58835, #42861, #4383, #96371, #89342, #80366, #19372, #81828, #13344, #65842, #11372, #20357, #27354, #5850, #28826, #27844, #49857, #36341, #34848, #58332, #11866, #88849, #43828, #59326, #49366, #41894, #34353, #42373, #64844, #57847, #88357, #83324, #91308, #53311, #68332, #69312, #61302, #30306, #8316, #355, #38820, #60808, #98852, #7833, #29320, #91813, #52816, #14850, #83819, #6834, #29815, #15345, #90312, #7340, #46313, #89829, #30804, #68823, #84325, #82324, #833, #22836, #37841, #98357, #45827, #21346, #23334, #76315, #82822, #60324, #21848, #44326, #31293, #90814, #51837, #13844, #59817, #75819, #22343, #38329, #74827, #53814, #15825, #14342, #45321, #52329, #6331, #36843, #76800, #67331, #97857, #44814, #75321, #37348, #67839, #84803, #78779, #40290, #94258, #54781, #48757, #70798, #9791, #69810, #79265, #24316, #2807, #63753, #16805, #93280, #47779, #17791, #1332, #17304, #46796, #31784, #78277, #48266, #16312, #10285, #9294, #93774, #25785, #55787, #24804, #18277, #40785, #10775, #71284, #41291, #25300, #33262, #23826, #86282, #39315, #55281, #39802, #85790, #62279, #47280, #61793, #56280, #62781, #86776, #2315, #77782, #32769, #71765, #85297, #92785, #3275, #92301, #63265, #54289, #77289, #70303, #8800, #1817, #32273, #3778, #20736, #87739, #65224, #34231, #34733, #19742, #65724, #88233, #89227, #96250, #64728, #88727, #27729, #18775, #27235, #35225, #58210, #12236, #13225, #5252, #73226, #51228, #43225, #81712, #4754, #42744, #50742, #72244, #35730, #95751, #57730, #20238, #49735, #72728, #81231, #95238, #50226, #43722, #33738, #73720, #12729, #28224, #26258, #74207, #66218, #80741, #11255, #96749, #58723, #64240, #26746, #94758, #56755, #87249, #57241, #49258, #79757, #41773, #19251, #80243, #11750, #42258, #4262, #7721 ),
 ( #67223, #44208, #91193, #45702, #29697, #97250, #7218, #52216, #61191, #53689, #83211, #74717, #91697, #59708, #37234, #6229, #6718, #90701, #37718, #60206, #23216, #68222, #36732, #60693, #98742, #89714, #98236, #30192, #22718, #14732, #84208, #76202, #45208, #15715, #15223, #46201, #75707, #53202, #83706, #97746, #38218, #67723, #22229, #68703, #21735, #44708, #235, #29209, #52705, #5739, #36226, #30683, #66726, #28720, #59210, #21228, #51732, #82213, #14229, #13724, #90204, #82711, #75207, #69684, #85178, #77176, #31178, #94143, #47159, #18162, #76685, #16197, #62657, #16689, #17677, #724, #93654, #55156, #10170, #1215, #63636, #85670, #24685, #84686, #25671, #39196, #48151, #78664, #31670, #9177, #93160, #32658, #46678, #32156, #61670, #8683, #17189, #63151, #92188, #25188, #24194, #56165, #86167, #86657, #47670, #78164, #55668, #62160, #40667, #39695, #1699, #40172, #92667, #77663, #2196, #54662, #9674, #33141, #8205, #71165, #2690, #38700, #69199, #23714, #70676, #54175, #70183, #19624, #48640, #88604, #50118, #41659, #57124, #49139, #3162, #66099, #19136, #89106, #79143, #87129, #34611, #87622, #20114, #71654, #65603, #27117, #81109, #72127, #35613, #57616, #95628, #56644, #96628, #11140, #50618, #12610, #3654, #80124, #65107, #4641, #18650, #4146, #33624, #79641, #88115, #35105, #64124, #96131, #95119, #80628, #43111, #42624, #11631, #5125, #27612, #28103, #58098, #58605, #12122, #73598, #10655, #73102, #26150, #42147, #26627, #72611, #34119, #64611, #41170, #94640, #49613, #75587, #82592, #6109, #98111, #68095, #82094, #59093, #7099, #60581, #44591, #13107, #22104, #67101, #76075, #68588, #29573, #89602, #7605, #74595, #52099, #21112, #21614, #6595, #52584, #75089, #38101, #83087, #51611, #37601, #14615, #5623, #14107, #45082, #98623, #60076, #118, #91073, #90578, #30072, #22599, #90087, #81595, #67604, #53077, #30565, #83588, #15105, #37108, #28604, #61070, #13605, #59588, #43602, #45581, #74089, #97134, #20618, #51108, #36099, #44085, #66606, #36614, #97626, #29089, #71422, #23098, #86899, #41429, #87390, #24939, #70932, #49384, #94889, #55421, #63884, #26387, #94396, #33386, #93910, #18409, #25911, #56413, #71890, #93416, #41914, #72376, #64379, #16936, #32414, #3413, #2449, #11392, #18907, #32906, #63405, #47417, #9929, #55921, #9426, #40924, #33874, #2938, #48405, #25438, #34373, #78908, #48892, #10907, #85929, #86420, #17921, #10417, #56887, #79403, #78411, #79885, #3906, #91581, #17439, #53568, #85427, #77920, #39930, #70433, #1950, #62915, #47906, #40433, #51361, #96389, #19388, #26885, #34870, #95893 ) ),
 .UNSPECIFIED., .F., .F., .T. ) 
 B_SPLINE_SURFACE_WITH_KNOTS ( ( 2, 2 ),
 ( 3, 2, 2, 2, 2, 2, 2, 2, 2, 2, 2, 2, 2, 2, 2, 2, 2, 2, 2, 2, 2, 2, 2, 2, 2, 2, 2, 2, 2, 2, 2, 2, 2, 2, 2, 2, 2, 2, 2, 2, 2, 2, 2, 2, 2, 2, 2, 2, 2, 2, 2, 2, 2, 2, 2, 2, 2, 2, 2, 2, 2, 2, 2, 2, 2, 2, 2, 2, 2, 2, 2, 2, 2, 2, 2, 2, 2, 2, 2, 2, 2, 2, 2, 2, 2, 2, 2, 2, 2, 2, 2, 2, 2, 2, 2, 2, 2, 2, 2, 2, 2, 2, 2, 2, 2, 2, 2, 2, 2, 2, 2, 2, 2, 2, 2, 2, 2, 2, 2, 2, 2, 2, 2, 2, 2, 2, 2, 2, 2, 2, 2, 2, 2, 2, 2, 2, 2, 2, 2, 2, 2, 2, 2, 2, 2, 2, 2, 2, 2, 2, 2, 2, 2, 2, 2, 2, 2, 2, 2, 2, 2, 2, 3 ),
 ( 0.000000000000000000, 1.000000000000000000 ),
 ( 0.000000000000000000, 0.005952380952380952051, 0.01190476190476190410, 0.01785714285714285615, 0.02380952380952380820, 0.02976190476190476025, 0.03571428571428571230, 0.04166666666666666435, 0.04761904761904761640, 0.05357142857142856845, 0.05952380952380952051, 0.06547619047619047949, 0.07142857142857142461, 0.07738095238095238360, 0.08333333333333332871, 0.08928571428571428770, 0.09523809523809523281, 0.1011904761904761918, 0.1071428571428571369, 0.1130952380952380959, 0.1190476190476190410, 0.1250000000000000000, 0.1309523809523809590, 0.1369047619047619180, 0.1428571428571428492, 0.1488095238095238082, 0.1547619047619047672, 0.1607142857142857262, 0.1666666666666666574, 0.1726190476190476164, 0.1785714285714285754, 0.1845238095238095344, 0.1904761904761904656, 0.1964285714285714246, 0.2023809523809523836, 0.2083333333333333426, 0.2142857142857142738, 0.2202380952380952328, 0.2261904761904761918, 0.2321428571428571508, 0.2380952380952380820, 0.2440476190476190410, 0.2500000000000000000, 0.2559523809523809312, 0.2619047619047619180, 0.2678571428571428492, 0.2738095238095238360, 0.2797619047619047672, 0.2857142857142856984, 0.2916666666666666852, 0.2976190476190476164, 0.3035714285714285476, 0.3095238095238095344, 0.3154761904761904656, 0.3214285714285714524, 0.3273809523809523836, 0.3333333333333333148, 0.3392857142857143016, 0.3452380952380952328, 0.3511904761904761640, 0.3571428571428571508, 0.3630952380952380820, 0.3690476190476190688, 0.3750000000000000000, 0.3809523809523809312, 0.3869047619047619180, 0.3928571428571428492, 0.3988095238095238360, 0.4047619047619047672, 0.4107142857142856984, 0.4166666666666666852, 0.4226190476190476164, 0.4285714285714285476, 0.4345238095238095344, 0.4404761904761904656, 0.4464285714285714524, 0.4523809523809523836, 0.4583333333333333148, 0.4642857142857143016, 0.4702380952380952328, 0.4761904761904761640, 0.4821428571428571508, 0.4880952380952380820, 0.4940476190476190688, 0.5000000000000000000, 0.5059523809523809312, 0.5119047619047618625, 0.5178571428571429047, 0.5238095238095238360, 0.5297619047619047672, 0.5357142857142856984, 0.5416666666666666297, 0.5476190476190476719, 0.5535714285714286031, 0.5595238095238095344, 0.5654761904761904656, 0.5714285714285713969, 0.5773809523809523281, 0.5833333333333333703, 0.5892857142857143016, 0.5952380952380952328, 0.6011904761904761640, 0.6071428571428570953, 0.6130952380952381375, 0.6190476190476190688, 0.6250000000000000000, 0.6309523809523809312, 0.6369047619047618625, 0.6428571428571429047, 0.6488095238095238360, 0.6547619047619047672, 0.6607142857142856984, 0.6666666666666666297, 0.6726190476190476719, 0.6785714285714286031, 0.6845238095238095344, 0.6904761904761904656, 0.6964285714285713969, 0.7023809523809523281, 0.7083333333333333703, 0.7142857142857143016, 0.7202380952380952328, 0.7261904761904761640, 0.7321428571428570953, 0.7380952380952381375, 0.7440476190476190688, 0.7500000000000000000, 0.7559523809523809312, 0.7619047619047618625, 0.7678571428571429047, 0.7738095238095238360, 0.7797619047619047672, 0.7857142857142856984, 0.7916666666666666297, 0.7976190476190476719, 0.8035714285714286031, 0.8095238095238095344, 0.8154761904761904656, 0.8214285714285713969, 0.8273809523809523281, 0.8333333333333333703, 0.8392857142857143016, 0.8452380952380952328, 0.8511904761904761640, 0.8571428571428570953, 0.8630952380952381375, 0.8690476190476190688, 0.8750000000000000000, 0.8809523809523809312, 0.8869047619047618625, 0.8928571428571429047, 0.8988095238095238360, 0.9047619047619047672, 0.9107142857142856984, 0.9166666666666666297, 0.9226190476190476719, 0.9285714285714286031, 0.9345238095238095344, 0.9404761904761904656, 0.9464285714285713969, 0.9523809523809523281, 0.9583333333333333703, 0.9642857142857143016 ),
 .UNSPECIFIED. ) 
 GEOMETRIC_REPRESENTATION_ITEM ( )  RATIONAL_B_SPLINE_SURFACE ( (
 ( 1.000000000000000000, 0.9659258262890683122, 1.000000000000000000, 0.9659258262890683122, 1.000000000000000000, 0.9659258262890683122, 1.000000000000000000, 0.9659258262890683122, 1.000000000000000000, 0.9659258262890683122, 1.000000000000000000, 0.9659258262890683122, 1.000000000000000000, 0.9659258262890683122, 1.000000000000000000, 0.9659258262890683122, 1.000000000000000000, 0.9659258262890683122, 1.000000000000000000, 0.9659258262890683122, 1.000000000000000000, 0.9659258262890683122, 1.000000000000000000, 0.9659258262890683122, 1.000000000000000000, 0.9659258262890683122, 1.000000000000000000, 0.9659258262890683122, 1.000000000000000000, 0.9659258262890683122, 1.000000000000000000, 0.9659258262890683122, 1.000000000000000000, 0.9659258262890683122, 1.000000000000000000, 0.9659258262890683122, 1.000000000000000000, 0.9659258262890683122, 1.000000000000000000, 0.9659258262890683122, 1.000000000000000000, 0.9659258262890683122, 1.000000000000000000, 0.9659258262890683122, 1.000000000000000000, 0.9659258262890683122, 1.000000000000000000, 0.9659258262890683122, 1.000000000000000000, 0.9659258262890683122, 1.000000000000000000, 0.9659258262890683122, 1.000000000000000000, 0.9659258262890683122, 1.000000000000000000, 0.9659258262890683122, 1.000000000000000000, 0.9659258262890683122, 1.000000000000000000, 0.9659258262890683122, 1.000000000000000000, 0.9659258262890683122, 1.000000000000000000, 0.9659258262890683122, 1.000000000000000000, 0.9659258262890683122, 1.000000000000000000, 0.9659258262890683122, 1.000000000000000000, 0.9659258262890683122, 1.000000000000000000, 0.9659258262890683122, 1.000000000000000000, 0.9659258262890683122, 1.000000000000000000, 0.9659258262890683122, 1.000000000000000000, 0.9659258262890683122, 1.000000000000000000, 0.9659258262890683122, 1.000000000000000000, 0.9659258262890683122, 1.000000000000000000, 0.9659258262890683122, 1.000000000000000000, 0.9659258262890683122, 1.000000000000000000, 0.9659258262890683122, 1.000000000000000000, 0.9659258262890683122, 1.000000000000000000, 0.9659258262890683122, 1.000000000000000000, 0.9659258262890683122, 1.000000000000000000, 0.9659258262890683122, 1.000000000000000000, 0.9659258262890683122, 1.000000000000000000, 0.9659258262890683122, 1.000000000000000000, 0.9659258262890683122, 1.000000000000000000, 0.9659258262890683122, 1.000000000000000000, 0.9659258262890683122, 1.000000000000000000, 0.9659258262890683122, 1.000000000000000000, 0.9659258262890683122, 1.000000000000000000, 0.9659258262890683122, 1.000000000000000000, 0.9659258262890683122, 1.000000000000000000, 0.9659258262890683122, 1.000000000000000000, 0.9659258262890683122, 1.000000000000000000, 0.9659258262890683122, 1.000000000000000000, 0.9659258262890683122, 1.000000000000000000, 0.9659258262890683122, 1.000000000000000000, 0.9659258262890683122, 1.000000000000000000, 0.9659258262890683122, 1.000000000000000000, 0.9659258262890683122, 1.000000000000000000, 0.9659258262890683122, 1.000000000000000000, 0.9659258262890683122, 1.000000000000000000, 0.9659258262890683122, 1.000000000000000000, 0.9659258262890683122, 1.000000000000000000, 0.9659258262890683122, 1.000000000000000000, 0.9659258262890683122, 1.000000000000000000, 0.9659258262890683122, 1.000000000000000000, 0.9659258262890683122, 1.000000000000000000, 0.9659258262890683122, 1.000000000000000000, 0.9659258262890683122, 1.000000000000000000, 0.9659258262890683122, 1.000000000000000000, 0.9659258262890683122, 1.000000000000000000, 0.9659258262890683122, 1.000000000000000000, 0.9659258262890683122, 1.000000000000000000, 0.9659258262890683122, 1.000000000000000000, 0.9659258262890683122, 1.000000000000000000, 0.9659258262890683122, 1.000000000000000000, 0.9659258262890683122, 1.000000000000000000, 0.9659258262890683122, 1.000000000000000000, 0.9659258262890683122, 1.000000000000000000, 0.9659258262890683122, 1.000000000000000000, 0.9659258262890683122, 1.000000000000000000, 0.9659258262890683122, 1.000000000000000000, 0.9659258262890683122, 1.000000000000000000, 0.9659258262890683122, 1.000000000000000000, 0.9659258262890683122, 1.000000000000000000, 0.9659258262890683122, 1.000000000000000000, 0.9659258262890683122, 1.000000000000000000, 0.9659258262890683122, 1.000000000000000000, 0.9659258262890683122, 1.000000000000000000, 0.9659258262890683122, 1.000000000000000000, 0.9659258262890683122, 1.000000000000000000, 0.9659258262890683122, 1.000000000000000000, 0.9659258262890683122, 1.000000000000000000, 0.9659258262890683122, 1.000000000000000000, 0.9659258262890683122, 1.000000000000000000, 0.9659258262890683122, 1.000000000000000000, 0.9659258262890683122, 1.000000000000000000, 0.9659258262890683122, 1.000000000000000000, 0.9659258262890683122, 1.000000000000000000, 0.9659258262890683122, 1.000000000000000000, 0.9659258262890683122, 1.000000000000000000, 0.9659258262890683122, 1.000000000000000000, 0.9659258262890683122, 1.000000000000000000, 0.9659258262890683122, 1.000000000000000000, 0.9659258262890683122, 1.000000000000000000, 0.9659258262890683122, 1.000000000000000000, 0.9659258262890683122, 1.000000000000000000, 0.9659258262890683122, 1.000000000000000000, 0.9659258262890683122, 1.000000000000000000, 0.9659258262890683122, 1.000000000000000000, 0.9659258262890683122, 1.000000000000000000, 0.9659258262890683122, 1.000000000000000000, 0.9659258262890683122, 1.000000000000000000, 0.9659258262890683122, 1.000000000000000000, 0.9659258262890683122, 1.000000000000000000, 0.9659258262890683122, 1.000000000000000000, 0.9659258262890683122, 1.000000000000000000, 0.9659258262890683122, 1.000000000000000000, 0.9659258262890683122, 1.000000000000000000, 0.9659258262890683122, 1.000000000000000000, 0.9659258262890683122, 1.000000000000000000, 0.9659258262890683122, 1.000000000000000000, 0.9659258262890683122, 1.000000000000000000, 0.9659258262890683122, 1.000000000000000000, 0.9659258262890683122, 1.000000000000000000, 0.9659258262890683122, 1.000000000000000000, 0.9659258262890683122, 1.000000000000000000, 0.9659258262890683122, 1.000000000000000000, 0.9659258262890683122, 1.000000000000000000, 0.9659258262890683122, 1.000000000000000000, 0.9659258262890683122, 1.000000000000000000, 0.9659258262890683122, 1.000000000000000000, 0.9659258262890683122, 1.000000000000000000, 0.9659258262890683122, 1.000000000000000000, 0.9659258262890683122, 1.000000000000000000, 0.9659258262890683122, 1.000000000000000000, 0.9659258262890683122, 1.000000000000000000, 0.9659258262890683122, 1.000000000000000000, 0.9659258262890683122, 1.000000000000000000, 0.9659258262890683122, 1.000000000000000000, 0.9659258262890683122, 1.000000000000000000, 0.9659258262890683122, 1.000000000000000000, 0.9659258262890683122, 1.000000000000000000, 0.9659258262890683122, 1.000000000000000000, 0.9659258262890683122, 1.000000000000000000, 0.9659258262890683122, 1.000000000000000000, 0.9659258262890683122, 1.000000000000000000, 0.9659258262890683122, 1.000000000000000000, 0.9659258262890683122, 1.000000000000000000, 0.9659258262890683122, 1.000000000000000000, 0.9659258262890683122, 1.000000000000000000, 0.9659258262890683122, 1.000000000000000000, 0.9659258262890683122, 1.000000000000000000, 0.9659258262890683122, 1.000000000000000000, 0.9659258262890683122, 1.000000000000000000, 0.9659258262890683122, 1.000000000000000000),
 ( 1.000000000000000000, 0.9659258262890683122, 1.000000000000000000, 0.9659258262890683122, 1.000000000000000000, 0.9659258262890683122, 1.000000000000000000, 0.9659258262890683122, 1.000000000000000000, 0.9659258262890683122, 1.000000000000000000, 0.9659258262890683122, 1.000000000000000000, 0.9659258262890683122, 1.000000000000000000, 0.9659258262890683122, 1.000000000000000000, 0.9659258262890683122, 1.000000000000000000, 0.9659258262890683122, 1.000000000000000000, 0.9659258262890683122, 1.000000000000000000, 0.9659258262890683122, 1.000000000000000000, 0.9659258262890683122, 1.000000000000000000, 0.9659258262890683122, 1.000000000000000000, 0.9659258262890683122, 1.000000000000000000, 0.9659258262890683122, 1.000000000000000000, 0.9659258262890683122, 1.000000000000000000, 0.9659258262890683122, 1.000000000000000000, 0.9659258262890683122, 1.000000000000000000, 0.9659258262890683122, 1.000000000000000000, 0.9659258262890683122, 1.000000000000000000, 0.9659258262890683122, 1.000000000000000000, 0.9659258262890683122, 1.000000000000000000, 0.9659258262890683122, 1.000000000000000000, 0.9659258262890683122, 1.000000000000000000, 0.9659258262890683122, 1.000000000000000000, 0.9659258262890683122, 1.000000000000000000, 0.9659258262890683122, 1.000000000000000000, 0.9659258262890683122, 1.000000000000000000, 0.9659258262890683122, 1.000000000000000000, 0.9659258262890683122, 1.000000000000000000, 0.9659258262890683122, 1.000000000000000000, 0.9659258262890683122, 1.000000000000000000, 0.9659258262890683122, 1.000000000000000000, 0.9659258262890683122, 1.000000000000000000, 0.9659258262890683122, 1.000000000000000000, 0.9659258262890683122, 1.000000000000000000, 0.9659258262890683122, 1.000000000000000000, 0.9659258262890683122, 1.000000000000000000, 0.9659258262890683122, 1.000000000000000000, 0.9659258262890683122, 1.000000000000000000, 0.9659258262890683122, 1.000000000000000000, 0.9659258262890683122, 1.000000000000000000, 0.9659258262890683122, 1.000000000000000000, 0.9659258262890683122, 1.000000000000000000, 0.9659258262890683122, 1.000000000000000000, 0.9659258262890683122, 1.000000000000000000, 0.9659258262890683122, 1.000000000000000000, 0.9659258262890683122, 1.000000000000000000, 0.9659258262890683122, 1.000000000000000000, 0.9659258262890683122, 1.000000000000000000, 0.9659258262890683122, 1.000000000000000000, 0.9659258262890683122, 1.000000000000000000, 0.9659258262890683122, 1.000000000000000000, 0.9659258262890683122, 1.000000000000000000, 0.9659258262890683122, 1.000000000000000000, 0.9659258262890683122, 1.000000000000000000, 0.9659258262890683122, 1.000000000000000000, 0.9659258262890683122, 1.000000000000000000, 0.9659258262890683122, 1.000000000000000000, 0.9659258262890683122, 1.000000000000000000, 0.9659258262890683122, 1.000000000000000000, 0.9659258262890683122, 1.000000000000000000, 0.9659258262890683122, 1.000000000000000000, 0.9659258262890683122, 1.000000000000000000, 0.9659258262890683122, 1.000000000000000000, 0.9659258262890683122, 1.000000000000000000, 0.9659258262890683122, 1.000000000000000000, 0.9659258262890683122, 1.000000000000000000, 0.9659258262890683122, 1.000000000000000000, 0.9659258262890683122, 1.000000000000000000, 0.9659258262890683122, 1.000000000000000000, 0.9659258262890683122, 1.000000000000000000, 0.9659258262890683122, 1.000000000000000000, 0.9659258262890683122, 1.000000000000000000, 0.9659258262890683122, 1.000000000000000000, 0.9659258262890683122, 1.000000000000000000, 0.9659258262890683122, 1.000000000000000000, 0.9659258262890683122, 1.000000000000000000, 0.9659258262890683122, 1.000000000000000000, 0.9659258262890683122, 1.000000000000000000, 0.9659258262890683122, 1.000000000000000000, 0.9659258262890683122, 1.000000000000000000, 0.9659258262890683122, 1.000000000000000000, 0.9659258262890683122, 1.000000000000000000, 0.9659258262890683122, 1.000000000000000000, 0.9659258262890683122, 1.000000000000000000, 0.9659258262890683122, 1.000000000000000000, 0.9659258262890683122, 1.000000000000000000, 0.9659258262890683122, 1.000000000000000000, 0.9659258262890683122, 1.000000000000000000, 0.9659258262890683122, 1.000000000000000000, 0.9659258262890683122, 1.000000000000000000, 0.9659258262890683122, 1.000000000000000000, 0.9659258262890683122, 1.000000000000000000, 0.9659258262890683122, 1.000000000000000000, 0.9659258262890683122, 1.000000000000000000, 0.9659258262890683122, 1.000000000000000000, 0.9659258262890683122, 1.000000000000000000, 0.9659258262890683122, 1.000000000000000000, 0.9659258262890683122, 1.000000000000000000, 0.9659258262890683122, 1.000000000000000000, 0.9659258262890683122, 1.000000000000000000, 0.9659258262890683122, 1.000000000000000000, 0.9659258262890683122, 1.000000000000000000, 0.9659258262890683122, 1.000000000000000000, 0.9659258262890683122, 1.000000000000000000, 0.9659258262890683122, 1.000000000000000000, 0.9659258262890683122, 1.000000000000000000, 0.9659258262890683122, 1.000000000000000000, 0.9659258262890683122, 1.000000000000000000, 0.9659258262890683122, 1.000000000000000000, 0.9659258262890683122, 1.000000000000000000, 0.9659258262890683122, 1.000000000000000000, 0.9659258262890683122, 1.000000000000000000, 0.9659258262890683122, 1.000000000000000000, 0.9659258262890683122, 1.000000000000000000, 0.9659258262890683122, 1.000000000000000000, 0.9659258262890683122, 1.000000000000000000, 0.9659258262890683122, 1.000000000000000000, 0.9659258262890683122, 1.000000000000000000, 0.9659258262890683122, 1.000000000000000000, 0.9659258262890683122, 1.000000000000000000, 0.9659258262890683122, 1.000000000000000000, 0.9659258262890683122, 1.000000000000000000, 0.9659258262890683122, 1.000000000000000000, 0.9659258262890683122, 1.000000000000000000, 0.9659258262890683122, 1.000000000000000000, 0.9659258262890683122, 1.000000000000000000, 0.9659258262890683122, 1.000000000000000000, 0.9659258262890683122, 1.000000000000000000, 0.9659258262890683122, 1.000000000000000000, 0.9659258262890683122, 1.000000000000000000, 0.9659258262890683122, 1.000000000000000000, 0.9659258262890683122, 1.000000000000000000, 0.9659258262890683122, 1.000000000000000000, 0.9659258262890683122, 1.000000000000000000, 0.9659258262890683122, 1.000000000000000000, 0.9659258262890683122, 1.000000000000000000, 0.9659258262890683122, 1.000000000000000000, 0.9659258262890683122, 1.000000000000000000, 0.9659258262890683122, 1.000000000000000000, 0.9659258262890683122, 1.000000000000000000, 0.9659258262890683122, 1.000000000000000000, 0.9659258262890683122, 1.000000000000000000, 0.9659258262890683122, 1.000000000000000000, 0.9659258262890683122, 1.000000000000000000, 0.9659258262890683122, 1.000000000000000000, 0.9659258262890683122, 1.000000000000000000, 0.9659258262890683122, 1.000000000000000000, 0.9659258262890683122, 1.000000000000000000, 0.9659258262890683122, 1.000000000000000000, 0.9659258262890683122, 1.000000000000000000, 0.9659258262890683122, 1.000000000000000000, 0.9659258262890683122, 1.000000000000000000, 0.9659258262890683122, 1.000000000000000000, 0.9659258262890683122, 1.000000000000000000, 0.9659258262890683122, 1.000000000000000000, 0.9659258262890683122, 1.000000000000000000, 0.9659258262890683122, 1.000000000000000000, 0.9659258262890683122, 1.000000000000000000, 0.9659258262890683122, 1.000000000000000000) ) ) 
 REPRESENTATION_ITEM ( '' )  SURFACE ( )  );
#89860=CARTESIAN_POINT ( 'NONE',  ( -2.266590686148945544, 1.387082168247301128, -7.082119434687050408 ) ) ;
#89862=CARTESIAN_POINT ( 'NONE',  ( 5.076628168052704559, 25.17559781766745175, -8.527530157486179263 ) ) ;
#89863=EDGE_CURVE ( 'NONE', #31758, #9043, #92542, .T. ) ;
#89866=CARTESIAN_POINT ( 'NONE',  ( 10.00000000000000000, 35.55374883491396787, -14.16423886937410082 ) ) ;
#89867=CARTESIAN_POINT ( 'NONE',  ( 18.52753015748617571, 8.092264484334117824, 4.923371831947298993 ) ) ;
#89868=CARTESIAN_POINT ( 'NONE',  ( -0.03932841506541356197, 63.12161441960502373, 6.397827110479011203 ) ) ;
#89870=CARTESIAN_POINT ( 'NONE',  ( -0.8801773607111008646, 33.27201867748817676, 2.915334737309923430 ) ) ;
#89871=CARTESIAN_POINT ( 'NONE',  ( 3.591859063236761518, 39.95696800326375353, 11.09922568453594849 ) ) ;
#89873=SURFACE_SIDE_STYLE ('',( #28865 ) ) ;
#89874=CARTESIAN_POINT ( 'NONE',  ( 19.38216949554541202, 40.99863466993042493, 9.382169495545424454 ) ) ;
#89875=CARTESIAN_POINT ( 'NONE',  ( 10.00000000000000000, 62.87363466993042493, -12.81628187352647608 ) ) ;
#89876=ORIENTED_EDGE ( 'NONE', *, *, #49595, .F. ) ;
#89879=CARTESIAN_POINT ( 'NONE',  ( -4.164238869374099927, 47.01208216824729647, 3.795296366450308767 ) ) ;
#89880=CARTESIAN_POINT ( 'NONE',  ( 12.91533473730993009, 26.60535201082150536, -10.88017736071109987 ) ) ;
#89883=CARTESIAN_POINT ( 'NONE',  ( 4.559911319644449179, 53.89701867748817676, 9.422509992056141925 ) ) ;
#89884=CARTESIAN_POINT ( 'NONE',  ( 19.42250999205614193, 55.14701867748817676, 5.440088680355555262 ) ) ;
#89885=CARTESIAN_POINT ( 'NONE',  ( 13.43411237798106583, 7.665301336597086568, -12.81628187352647252 ) ) ;
#89888=CARTESIAN_POINT ( 'NONE',  ( 18.52753015748617571, 23.09226448433411960, 4.923371831947298993 ) ) ;
#89889=CARTESIAN_POINT ( 'NONE',  ( 0.5774900079438607392, 63.48035201082149825, 5.440088680355550821 ) ) ;
#89890=CARTESIAN_POINT ( 'NONE',  ( 22.81628187352647785, 16.62363466993042138, 6.195893100308588602E-16 ) ) ;
#89892=CARTESIAN_POINT ( 'NONE',  ( 15.44008868035555793, 6.397018677488170546, -9.422509992056140149 ) ) ;
#89893=CARTESIAN_POINT ( 'NONE',  ( 10.00000000000000000, 44.75893115100078745, -9.846743663894594434 ) ) ;
#89894=CARTESIAN_POINT ( 'NONE',  ( 21.09922568453595559, 42.04030133659708213, -6.408140936763230044 ) ) ;
#89895=TOROIDAL_SURFACE ( 'NONE', #49925, 62.00000000000000000, 0.5000000000000000000 ) ;
#89896=CARTESIAN_POINT ( 'NONE',  ( 5.076628168052703671, 21.84226448433411960, 8.527530157486179263 ) ) ;
#89897=STYLED_ITEM ( 'NONE', ( #23844 ), #49642 ) ;
#89898=CARTESIAN_POINT ( 'NONE',  ( -0.3689425029237898834, 11.17874883491396787, -10.36894250292378850 ) ) ;
#89900=CARTESIAN_POINT ( 'NONE',  ( -0.8801773607111009756, 23.06368534415484106, 1.068504757029289695E-15 ) ) ;
#89902=CARTESIAN_POINT ( 'NONE',  ( 6.204703633549690345, 32.84541550158063927, 14.16423886937410082 ) ) ;
#89903=CARTESIAN_POINT ( 'NONE',  ( 17.20831665107776587, 49.13393115100078745, -7.208316651077762316 ) ) ;
#89905=CARTESIAN_POINT ( 'NONE',  ( 19.42250999205614548, 25.98035201082150891, -5.440088680355545492 ) ) ;
#89906=CARTESIAN_POINT ( 'NONE',  ( -0.8801773607110991993, 17.85535201082150536, -2.915334737309923874 ) ) ;
#89908=( GEOMETRIC_REPRESENTATION_CONTEXT ( 3 ) GLOBAL_UNCERTAINTY_ASSIGNED_CONTEXT ( ( #92225 ) ) GLOBAL_UNIT_ASSIGNED_CONTEXT ( ( #8539, #17528, #76534 ) ) REPRESENTATION_CONTEXT ( 'NONE', 'WORKASPACE' ) );
#89909=CARTESIAN_POINT ( 'NONE',  ( 10.00000000000000178, 29.31368534415483751, 10.88017736071110342 ) ) ;
#89910=CARTESIAN_POINT ( 'NONE',  ( -2.816281873526473856, 49.12363466993042493, 9.499525473075851096E-16 ) ) ;
#89911=CARTESIAN_POINT ( 'NONE',  ( 19.42250999205614193, 35.14701867748816966, 5.440088680355555262 ) ) ;
#89912=CARTESIAN_POINT ( 'NONE',  ( 20.88017736071110164, 35.35535201082150536, 2.915334737309930979 ) ) ;
#89914=CARTESIAN_POINT ( 'NONE',  ( 5.076628168052704559, 55.17559781766745175, -8.527530157486179263 ) ) ;
#89915=CARTESIAN_POINT ( 'NONE',  ( 0.5774900079438590739, 37.64701867748817676, -5.440088680355550821 ) ) ;
#89919=CARTESIAN_POINT ( 'NONE',  ( 2.603489959281613420, 60.43575266056826933, -6.500000000000031086 ) ) ;
#89920=CARTESIAN_POINT ( 'NONE',  ( -0.3689425029237898834, 51.17874883491397497, -10.36894250292378850 ) ) ;
#89921=CARTESIAN_POINT ( 'NONE',  ( 20.88017736071110875, 55.77201867748816966, -2.915334737309920765 ) ) ;
#89922=CARTESIAN_POINT ( 'NONE',  ( 17.39651004071841456, 49.08210964143329136, -6.500000000000001776 ) ) ;
#89924=CARTESIAN_POINT ( 'NONE',  ( 19.84674366389459621, 58.50893115100078745, 7.409399052514197653E-17 ) ) ;
#89925=CARTESIAN_POINT ( 'NONE',  ( 18.52753015748617571, 23.09226448433411960, 4.923371831947298993 ) ) ;
#89927=CARTESIAN_POINT ( 'NONE',  ( 12.63842701281683034, 17.46726448433411250, 9.846743663894596210 ) ) ;
#89929=CARTESIAN_POINT ( 'NONE',  ( -0.8801773607110991993, 32.85535201082151247, -2.915334737309923874 ) ) ;
#89930=CARTESIAN_POINT ( 'NONE',  ( 1.472469842513823179, 20.59226448433411960, -4.923371831947296329 ) ) ;
#89931=CARTESIAN_POINT ( 'NONE',  ( 16.40814093676323893, 10.79030133659708923, 11.09922568453595026 ) ) ;
#89932=CARTESIAN_POINT ( 'NONE',  ( 4.559911319644449179, 58.89701867748817676, 9.422509992056141925 ) ) ;
#89933=CARTESIAN_POINT ( 'NONE',  ( 0.5774900079438607392, 28.48035201082150891, 5.440088680355550821 ) ) ;
#89934=CARTESIAN_POINT ( 'NONE',  ( -2.816281873526473856, 54.33196800326376064, 3.434112377981055619 ) ) ;
#89935=CARTESIAN_POINT ( 'NONE',  ( 10.00000000000000178, 43.05374883491397497, 14.16423886937410082 ) ) ;
#89940=CARTESIAN_POINT ( 'NONE',  ( 19.38216949554541202, 10.99863466993042138, 9.382169495545424454 ) ) ;
#89941=CARTESIAN_POINT ( 'NONE',  ( 10.00000000000000000, 6.813685344154838397, -10.88017736071110342 ) ) ;
#89942=CARTESIAN_POINT ( 'NONE',  ( 2.035157376598822676, 52.43868534415483396, -7.964842623401177768 ) ) ;
#89943=CARTESIAN_POINT ( 'NONE',  ( 18.29284471827479308, 25.40189080397286148, -6.500000000000035527 ) ) ;
#89945=CARTESIAN_POINT ( 'NONE',  ( 4.559911319644449179, 63.89701867748817676, 9.422509992056141925 ) ) ;
#89946=CARTESIAN_POINT ( 'NONE',  ( 18.52753015748617571, 38.09226448433412315, 4.923371831947298993 ) ) ;
#89947=CARTESIAN_POINT ( 'NONE',  ( 18.52753015748618282, 28.92559781766745175, -4.923371831947291888 ) ) ;
#89948=CARTESIAN_POINT ( 'NONE',  ( 17.20831665107776587, 17.88393115100078745, 7.208316651077764980 ) ) ;
#89950=CARTESIAN_POINT ( 'NONE',  ( 6.565887622018943937, 40.16530133659708923, 12.81628187352647430 ) ) ;
#89952=CARTESIAN_POINT ( 'NONE',  ( 2.791683348922240793, 1.633931151000784565, 7.208316651077764092 ) ) ;
#89953=LINE ( 'NONE', #51968, #64285 ) ;
#89955=CARTESIAN_POINT ( 'NONE',  ( 7.361572987183170547, 32.05059781766745175, 9.846743663894590881 ) ) ;
#89957=CARTESIAN_POINT ( 'NONE',  ( 16.40814093676324603, 57.45696800326375353, -11.09922568453594671 ) ) ;
#89959=CARTESIAN_POINT ( 'NONE',  ( 13.43411237798105340, 0.5819680032637533085, 12.81628187352647963 ) ) ;
#89961=CARTESIAN_POINT ( 'NONE',  ( -0.8801773607111008646, 13.27201867748817143, 2.915334737309923430 ) ) ;
#89962=CARTESIAN_POINT ( 'NONE',  ( 20.36894250292379738, 29.92874883491396432, -10.36894250292379027 ) ) ;
#89966=CARTESIAN_POINT ( 'NONE',  ( 20.36894250292379382, 28.67874883491396787, 10.36894250292379205 ) ) ;
#89967=CARTESIAN_POINT ( 'NONE',  ( 24.16423886937410614, 44.51208216824730357, -3.795296366450302550 ) ) ;
#89968=CARTESIAN_POINT ( 'NONE',  ( -2.266590686148945544, 6.387082168247300906, -7.082119434687050408 ) ) ;
#89969=CARTESIAN_POINT ( 'NONE',  ( 24.16423886937409904, 9.095415501580633943, 3.795296366450317205 ) ) ;
#89971=CARTESIAN_POINT ( 'NONE',  ( 7.084665262690076126, 47.02201867748818387, -10.88017736071110164 ) ) ;
#89972=CARTESIAN_POINT ( 'NONE',  ( 0.1532563361054082862, 36.21726448433410894, 2.638427012816831674 ) ) ;
#89974=LINE ( 'NONE', #66984, #59632 ) ;
#89975=CARTESIAN_POINT ( 'NONE',  ( 0.1532563361054083140, 26.00893115100078745, 1.131784320476157264E-15 ) ) ;
#89976=CARTESIAN_POINT ( 'NONE',  ( 12.91533473730992121, 14.52201867748817143, 10.88017736071110164 ) ) ;
#89977=CARTESIAN_POINT ( 'NONE',  ( 6.565887622018943937, 58.08196800326376064, -12.81628187352647608 ) ) ;
#89978=CARTESIAN_POINT ( 'NONE',  ( 12.63842701281683922, 54.55059781766745175, -9.846743663894590881 ) ) ;
#89979=CARTESIAN_POINT ( 'NONE',  ( -0.1503990784575280903, 23.10158574516642815, 6.262539305110076171 ) ) ;
#89980=CARTESIAN_POINT ( 'NONE',  ( 12.63842701281683922, 29.55059781766745175, -9.846743663894590881 ) ) ;
#89981=CARTESIAN_POINT ( 'NONE',  ( 16.40814093676323893, 45.79030133659708923, 11.09922568453595026 ) ) ;
#89983=CARTESIAN_POINT ( 'NONE',  ( -0.8801773607111008646, 38.27201867748816255, 2.915334737309923430 ) ) ;
#89984=CARTESIAN_POINT ( 'NONE',  ( 0.1532563361054100626, 40.80059781766745886, -2.638427012816831230 ) ) ;
#89985=CARTESIAN_POINT ( 'NONE',  ( -0.3689425029237881626, 27.42874883491397142, 10.36894250292379027 ) ) ;
#89988=CARTESIAN_POINT ( 'NONE',  ( 13.79529636645031943, 5.345415501580634832, -14.16423886937409904 ) ) ;
#89989=CARTESIAN_POINT ( 'NONE',  ( 2.035157376598824452, 63.68868534415484106, 7.964842623401179544 ) ) ;
#89990=CARTESIAN_POINT ( 'NONE',  ( 2.035157376598822676, 67.43868534415484817, -7.964842623401177768 ) ) ;
#89991=CARTESIAN_POINT ( 'NONE',  ( 2.917880565312948704, 52.63708216824730357, 12.26659068614894643 ) ) ;
#89992=CARTESIAN_POINT ( 'NONE',  ( 16.40814093676323893, 0.7903013365970867898, 11.09922568453595026 ) ) ;
#89994=CARTESIAN_POINT ( 'NONE',  ( -0.8801773607111008646, 58.27201867748816966, 2.915334737309923430 ) ) ;
#89995=CARTESIAN_POINT ( 'NONE',  ( -1.926860441876564023, 27.87045670184114243, 3.195792623639529761 ) ) ;
#89996=CARTESIAN_POINT ( 'NONE',  ( -1.099225684535947600, 34.54030133659708923, 6.408140936763237150 ) ) ;
#89998=CARTESIAN_POINT ( 'NONE',  ( 17.96484262340118221, 19.93868534415484106, 7.964842623401181321 ) ) ;
#89999=CARTESIAN_POINT ( 'NONE',  ( 7.084665262690076126, 9.105352010821503583, 10.88017736071109987 ) ) ;
#90000=CARTESIAN_POINT ( 'NONE',  ( 2.791683348922240793, 36.63393115100078035, 7.208316651077764092 ) ) ;
#90001=CARTESIAN_POINT ( 'NONE',  ( 6.565887622018943937, 45.16530133659708923, 12.81628187352647430 ) ) ;
#90002=ORIENTED_EDGE ( 'NONE', *, *, #48131, .T. ) ;
#90003=CARTESIAN_POINT ( 'NONE',  ( -0.8801773607110991993, 22.85535201082150181, -2.915334737309923874 ) ) ;
#90004=CARTESIAN_POINT ( 'NONE',  ( 3.591859063236761518, 4.956968003263753531, 11.09922568453594849 ) ) ;
#90006=CARTESIAN_POINT ( 'NONE',  ( 18.52753015748617571, 8.092264484334117824, 4.923371831947298993 ) ) ;
#90007=CARTESIAN_POINT ( 'NONE',  ( 14.92337183194729988, 49.34226448433411605, -8.527530157486177487 ) ) ;
#90008=CARTESIAN_POINT ( 'NONE',  ( 19.42250999205614193, 30.14701867748817321, 5.440088680355555262 ) ) ;
#90009=CARTESIAN_POINT ( 'NONE',  ( 6.565887622018943937, 13.08196800326374998, -12.81628187352647608 ) ) ;
#90010=CARTESIAN_POINT ( 'NONE',  ( 4.559911319644449179, 53.89701867748817676, 9.422509992056141925 ) ) ;
#90012=DIRECTION ( 'NONE',  ( -0.000000000000000000, -0.000000000000000000, 1.000000000000000000 ) ) ;
#90013=CARTESIAN_POINT ( 'NONE',  ( 21.09922568453594849, 46.20696800326376064, 6.408140936763242479 ) ) ;
#90015=CARTESIAN_POINT ( 'NONE',  ( 2.035157376598822676, 62.43868534415483396, -7.964842623401177768 ) ) ;
#90016=CARTESIAN_POINT ( 'NONE',  ( 22.81628187352647785, 36.41530133659707502, 3.434112377981063169 ) ) ;
#90018=CARTESIAN_POINT ( 'NONE',  ( 17.96484262340118221, 44.93868534415483396, 7.964842623401181321 ) ) ;
#90020=CARTESIAN_POINT ( 'NONE',  ( 19.84674366389459621, 48.50893115100078745, 7.409399052514197653E-17 ) ) ;
#90021=CARTESIAN_POINT ( 'NONE',  ( 5.076628168052703671, 21.84226448433411960, 8.527530157486179263 ) ) ;
#90023=CARTESIAN_POINT ( 'NONE',  ( 1.472469842513823179, 11.42559781766745175, 4.923371831947296329 ) ) ;
#90025=CARTESIAN_POINT ( 'NONE',  ( -4.164238869374099039, 46.80374883491397497, 8.674139862899312516E-16 ) ) ;
#90027=ADVANCED_FACE ( 'NONE', ( #27002 ), #53433, .T. ) ;
#90031=CARTESIAN_POINT ( 'NONE',  ( 22.26659068614895176, 59.72041550158063927, -7.082119434687042414 ) ) ;
#90032=CARTESIAN_POINT ( 'NONE',  ( -0.3689425029237881626, 67.42874883491396076, 10.36894250292379027 ) ) ;
#90033=CARTESIAN_POINT ( 'NONE',  ( 1.472469842513823179, 31.42559781766745530, 4.923371831947296329 ) ) ;
#90034=CARTESIAN_POINT ( 'NONE',  ( 13.43411237798105340, 25.58196800326374998, 12.81628187352647963 ) ) ;
#90036=VECTOR ( 'NONE', #46259, 1000.000000000000000 ) ;
#90038=CARTESIAN_POINT ( 'NONE',  ( 13.79529636645030344, 13.26208216824729824, 14.16423886937410614 ) ) ;
#90039=CARTESIAN_POINT ( 'NONE',  ( 19.42250999205614548, 10.98035201082150358, -5.440088680355545492 ) ) ;
#90040=CARTESIAN_POINT ( 'NONE',  ( 2.917880565312948704, 57.63708216824731068, 12.26659068614894643 ) ) ;
#90041=CARTESIAN_POINT ( 'NONE',  ( 7.361572987183169658, 34.96726448433411605, -9.846743663894592657 ) ) ;
#90043=CARTESIAN_POINT ( 'NONE',  ( 1.472469842513823179, 6.425597817667451750, 4.923371831947296329 ) ) ;
#90044=VECTOR ( 'NONE', #15616, 1000.000000000000000 ) ;
#90050=CARTESIAN_POINT ( 'NONE',  ( 0.1532563361054083140, 41.00893115100078745, 1.131784320476157264E-15 ) ) ;
#90051=CARTESIAN_POINT ( 'NONE',  ( 22.26659068614894466, 18.88708216824730002, 7.082119434687054849 ) ) ;
#90052=CARTESIAN_POINT ( 'NONE',  ( 19.42250999205614548, 25.98035201082150891, -5.440088680355545492 ) ) ;
#90053=CARTESIAN_POINT ( 'NONE',  ( 12.91533473730993009, 26.60535201082150536, -10.88017736071109987 ) ) ;
#90054=CARTESIAN_POINT ( 'NONE',  ( 5.076628168052704559, 65.17559781766745175, -8.527530157486179263 ) ) ;
#90055=CARTESIAN_POINT ( 'NONE',  ( -2.816281873526473856, 14.33196800326375531, 3.434112377981055619 ) ) ;
#90056=CARTESIAN_POINT ( 'NONE',  ( -0.3689425029237898834, 1.178748834913967869, -10.36894250292378850 ) ) ;
#90057=CARTESIAN_POINT ( 'NONE',  ( -0.8801773607110991993, 62.85535201082150536, -2.915334737309923874 ) ) ;
#90058=CARTESIAN_POINT ( 'NONE',  ( 6.565887622018943937, 38.08196800326376064, -12.81628187352647608 ) ) ;
#90060=CARTESIAN_POINT ( 'NONE',  ( 10.00000000000000000, 34.75893115100078745, -9.846743663894594434 ) ) ;
#90061=CARTESIAN_POINT ( 'NONE',  ( 10.00000000000000000, 11.81368534415483751, -10.88017736071110342 ) ) ;
#90063=CARTESIAN_POINT ( 'NONE',  ( 0.5774900079438607392, 8.480352010821505360, 5.440088680355550821 ) ) ;
#90065=CARTESIAN_POINT ( 'NONE',  ( 7.084665262690076126, 49.10535201082149825, 10.88017736071109987 ) ) ;
#90066=CARTESIAN_POINT ( 'NONE',  ( -0.8801773607110991993, 57.85535201082149825, -2.915334737309923874 ) ) ;
#90067=CARTESIAN_POINT ( 'NONE',  ( 0.2751277870542871429, 42.28217586085238366, -6.499999999999984901 ) ) ;
#90068=SURFACE_SIDE_STYLE ('',( #75568 ) ) ;
#90069=CARTESIAN_POINT ( 'NONE',  ( 2.035157376598822676, 52.43868534415483396, -7.964842623401177768 ) ) ;
#90072=CARTESIAN_POINT ( 'NONE',  ( 12.63842701281683034, 32.46726448433412315, 9.846743663894596210 ) ) ;
#90073=ORIENTED_EDGE ( 'NONE', *, *, #27524, .T. ) ;
#90074=CARTESIAN_POINT ( 'NONE',  ( 2.791683348922240793, 56.63393115100078035, 7.208316651077764092 ) ) ;
#90078=CARTESIAN_POINT ( 'NONE',  ( 6.204703633549690345, 5.762082168247301794, -14.16423886937410259 ) ) ;
#90079=EDGE_LOOP ( 'NONE', ( #51669, #95063, #14307, #78753 ) ) ;
#90080=CARTESIAN_POINT ( 'NONE',  ( 19.72487221294571214, 44.78217586085236945, 6.499999999999993783 ) ) ;
#90081=DIRECTION ( 'NONE',  ( 0.000000000000000000, 0.000000000000000000, -1.000000000000000000 ) ) ;
#90083=CARTESIAN_POINT ( 'NONE',  ( 10.00000000000000000, 11.81368534415483751, -10.88017736071110342 ) ) ;
#90084=CARTESIAN_POINT ( 'NONE',  ( 18.06765999051789251, 63.99127512925452521, 6.499999999999953815 ) ) ;
#90085=ORIENTED_EDGE ( 'NONE', *, *, #76586, .F. ) ;
#90086=FILL_AREA_STYLE_COLOUR ( '', #78379 ) ;
#90087=CARTESIAN_POINT ( 'NONE',  ( 17.20831665107776587, 47.88393115100078745, 7.208316651077764980 ) ) ;
#90089=CARTESIAN_POINT ( 'NONE',  ( 13.43411237798105340, 15.58196800326374998, 12.81628187352647963 ) ) ;
#90090=CARTESIAN_POINT ( 'NONE',  ( 14.92337183194729988, 9.342264484334119601, -8.527530157486177487 ) ) ;
#90091=CARTESIAN_POINT ( 'NONE',  ( 0.2751277870542913062, 29.36607318730131411, -6.499999999999992006 ) ) ;
#90092=CARTESIAN_POINT ( 'NONE',  ( 19.38216949554541202, 5.998634669930420493, 9.382169495545424454 ) ) ;
#90093=CARTESIAN_POINT ( 'NONE',  ( 0.1532563361054083140, 26.00893115100078745, 1.131784320476157264E-15 ) ) ;
#90097=CARTESIAN_POINT ( 'NONE',  ( 4.559911319644449179, 8.897018677488173211, 9.422509992056141925 ) ) ;
#90098=CARTESIAN_POINT ( 'NONE',  ( 24.16423886937410614, 24.30374883491396787, 8.672049930838204340E-16 ) ) ;
#90099=CARTESIAN_POINT ( 'NONE',  ( 18.52753015748617571, 33.09226448433411605, 4.923371831947298993 ) ) ;
#90100=CARTESIAN_POINT ( 'NONE',  ( 20.88017736071110164, 50.35535201082151247, 2.915334737309930979 ) ) ;
#90101=CARTESIAN_POINT ( 'NONE',  ( 16.40814093676324603, 42.45696800326375353, -11.09922568453594671 ) ) ;
#90102=CARTESIAN_POINT ( 'NONE',  ( 19.42250999205614548, 20.98035201082150891, -5.440088680355545492 ) ) ;
#90103=EDGE_CURVE ( 'NONE', #34211, #91796, #2955, .T. ) ;
#90106=DIRECTION ( 'NONE',  ( -0.000000000000000000, 1.000000000000000000, 0.000000000000000000 ) ) ;
#90108=CARTESIAN_POINT ( 'NONE',  ( 1.472469842513823179, 60.59226448433412315, -4.923371831947296329 ) ) ;
#90109=CARTESIAN_POINT ( 'NONE',  ( 5.076628168052703671, 26.84226448433411960, 8.527530157486179263 ) ) ;
#90111=CARTESIAN_POINT ( 'NONE',  ( 6.565887622018943937, 40.16530133659708923, 12.81628187352647430 ) ) ;
#90113=CARTESIAN_POINT ( 'NONE',  ( 12.91533473730993009, 46.60535201082150536, -10.88017736071109987 ) ) ;
#90116=CARTESIAN_POINT ( 'NONE',  ( 20.88017736071110875, 60.77201867748817676, -2.915334737309920765 ) ) ;
#90117=CARTESIAN_POINT ( 'NONE',  ( 17.96484262340118221, 46.18868534415484106, -7.964842623401177768 ) ) ;
#90118=CARTESIAN_POINT ( 'NONE',  ( 10.00000000000000178, 49.31368534415484106, 10.88017736071110342 ) ) ;
#90120=CARTESIAN_POINT ( 'NONE',  ( 10.00000000000000000, 51.81368534415484106, -10.88017736071110342 ) ) ;
#90121=CARTESIAN_POINT ( 'NONE',  ( 17.20831665107776587, 37.88393115100078745, 7.208316651077764980 ) ) ;
#90122=CARTESIAN_POINT ( 'NONE',  ( 12.91533473730992121, 9.522018677488171434, 10.88017736071110164 ) ) ;
#90123=CARTESIAN_POINT ( 'NONE',  ( 6.565887622018943937, 13.08196800326374998, -12.81628187352647608 ) ) ;
#90125=CARTESIAN_POINT ( 'NONE',  ( 15.44008868035555260, 24.73035201082150891, 9.422509992056143702 ) ) ;
#90126=CARTESIAN_POINT ( 'NONE',  ( 0.5774900079438607392, 23.48035201082150536, 5.440088680355550821 ) ) ;
#90127=CARTESIAN_POINT ( 'NONE',  ( -0.8801773607111008646, 68.27201867748817676, 2.915334737309923430 ) ) ;
#90128=CARTESIAN_POINT ( 'NONE',  ( 6.204703633549690345, 25.76208216824730712, -14.16423886937410259 ) ) ;
#90129=CARTESIAN_POINT ( 'NONE',  ( 17.20831665107776587, 7.883931151000784787, 7.208316651077764980 ) ) ;
#90130=CARTESIAN_POINT ( 'NONE',  ( 10.00000000000000000, 41.81368534415484106, -10.88017736071110342 ) ) ;
#90133=ADVANCED_FACE ( 'NONE', ( #18430 ), #85400, .T. ) ;
#90136=CARTESIAN_POINT ( 'NONE',  ( 0.1532563361054083140, 41.00893115100078745, 1.131784320476157264E-15 ) ) ;
#90140=CARTESIAN_POINT ( 'NONE',  ( 24.16423886937410614, 19.30374883491397142, 8.672049930838204340E-16 ) ) ;
#90141=CARTESIAN_POINT ( 'NONE',  ( 22.26659068614895176, 19.72041550158063572, -7.082119434687042414 ) ) ;
#90142=CARTESIAN_POINT ( 'NONE',  ( -0.8801773607110991993, 57.85535201082149825, -2.915334737309923874 ) ) ;
#90143=CARTESIAN_POINT ( 'NONE',  ( 4.559911319644449179, 2.230352010821504916, -9.422509992056141925 ) ) ;
#90144=CARTESIAN_POINT ( 'NONE',  ( -2.816281873526473856, -0.6680319967362464695, 3.434112377981055619 ) ) ;
#90145=CARTESIAN_POINT ( 'NONE',  ( 10.00000000000000000, 54.75893115100078745, -9.846743663894594434 ) ) ;
#90147=CARTESIAN_POINT ( 'NONE',  ( -0.8801773607110991993, 42.85535201082150536, -2.915334737309923874 ) ) ;
#90148=CARTESIAN_POINT ( 'NONE',  ( 10.00000000000000178, 10.37363466993041961, 12.81628187352647608 ) ) ;
#90149=CARTESIAN_POINT ( 'NONE',  ( -0.3689425029237898834, 16.17874883491396076, -10.36894250292378850 ) ) ;
#90150=CARTESIAN_POINT ( 'NONE',  ( -0.8801773607111008646, 13.27201867748817321, 2.915334737309923430 ) ) ;
#90151=CARTESIAN_POINT ( 'NONE',  ( 15.44008868035555793, 16.39701867748817321, -9.422509992056140149 ) ) ;
#90153=CARTESIAN_POINT ( 'NONE',  ( 7.084665262690076126, 39.10535201082150536, 10.88017736071109987 ) ) ;
#90157=VERTEX_POINT ( 'NONE', #85448 ) ;
#90158=CARTESIAN_POINT ( 'NONE',  ( 1.472469842513823179, 31.42559781766745530, 4.923371831947296329 ) ) ;
#90161=CARTESIAN_POINT ( 'NONE',  ( 13.79529636645030344, 48.26208216824728936, 14.16423886937410614 ) ) ;
#90162=CARTESIAN_POINT ( 'NONE',  ( 15.44008868035555793, 11.39701867748817143, -9.422509992056140149 ) ) ;
#90163=CARTESIAN_POINT ( 'NONE',  ( 0.1532563361054082862, 21.21726448433412315, 2.638427012816831674 ) ) ;
#90164=CARTESIAN_POINT ( 'NONE',  ( 2.791683348922240793, 46.63393115100077324, 7.208316651077764092 ) ) ;
#90165=CARTESIAN_POINT ( 'NONE',  ( -0.8801773607110991993, 67.85535201082151957, -2.915334737309923874 ) ) ;
#90166=CARTESIAN_POINT ( 'NONE',  ( 10.00000000000000000, 4.758931151000784787, -9.846743663894594434 ) ) ;
#90169=ORIENTED_EDGE ( 'NONE', *, *, #64407, .F. ) ;
#90171=CARTESIAN_POINT ( 'NONE',  ( 2.917880565312950480, 35.97041550158063217, -12.26659068614894821 ) ) ;
#90173=CARTESIAN_POINT ( 'NONE',  ( 0.6178305044545818747, 28.49863466993041783, -9.382169495545419124 ) ) ;
#90175=CARTESIAN_POINT ( 'NONE',  ( 3.591859063236763294, 48.29030133659708923, -11.09922568453595026 ) ) ;
#90176=CARTESIAN_POINT ( 'NONE',  ( 17.96484262340118221, 16.18868534415483396, -7.964842623401177768 ) ) ;
#90177=CARTESIAN_POINT ( 'NONE',  ( 7.361572987183169658, 39.96726448433411605, -9.846743663894592657 ) ) ;
#90178=CARTESIAN_POINT ( 'NONE',  ( 2.035157376598822676, 27.43868534415483396, -7.964842623401177768 ) ) ;
#90182=CARTESIAN_POINT ( 'NONE',  ( 18.52753015748618282, 38.92559781766745175, -4.923371831947291888 ) ) ;
#90183=CARTESIAN_POINT ( 'NONE',  ( 7.361572987183169658, 44.96726448433412315, -9.846743663894592657 ) ) ;
#90186=ORIENTED_EDGE ( 'NONE', *, *, #8057, .T. ) ;
#90190=DIRECTION ( 'NONE',  ( 0.000000000000000000, 0.000000000000000000, -1.000000000000000000 ) ) ;
#90192=CARTESIAN_POINT ( 'NONE',  ( 2.791683348922237240, 20.38393115100078745, -7.208316651077763204 ) ) ;
#90194=CARTESIAN_POINT ( 'NONE',  ( 19.38216949554541202, 30.99863466993042138, 9.382169495545424454 ) ) ;
#90197=CARTESIAN_POINT ( 'NONE',  ( 5.076628168052703671, 51.84226448433412315, 8.527530157486179263 ) ) ;
#90198=CARTESIAN_POINT ( 'NONE',  ( 19.72487221294571569, 27.80223176428830811, -6.499999999999990230 ) ) ;
#90199=CARTESIAN_POINT ( 'NONE',  ( 14.92337183194729633, 37.67559781766745175, 8.527530157486181039 ) ) ;
#90200=CARTESIAN_POINT ( 'NONE',  ( 22.26659068614894466, 38.88708216824731068, 7.082119434687054849 ) ) ;
#90201=CARTESIAN_POINT ( 'NONE',  ( 18.52753015748618282, 43.92559781766745175, -4.923371831947291888 ) ) ;
#90202=CARTESIAN_POINT ( 'NONE',  ( 22.81628187352647785, 46.62363466993041783, 6.195893100308588602E-16 ) ) ;
#90204=CARTESIAN_POINT ( 'NONE',  ( 10.00000000000000178, 12.25893115100078568, 9.846743663894594434 ) ) ;
#90206=( GEOMETRIC_REPRESENTATION_CONTEXT ( 3 ) GLOBAL_UNCERTAINTY_ASSIGNED_CONTEXT ( ( #26312 ) ) GLOBAL_UNIT_ASSIGNED_CONTEXT ( ( #27681, #3724, #4213 ) ) REPRESENTATION_CONTEXT ( 'NONE', 'WORKASPACE' ) );
#90207=CARTESIAN_POINT ( 'NONE',  ( 19.84674366389459266, 53.71726448433411605, -2.638427012816827677 ) ) ;
#90208=CARTESIAN_POINT ( 'NONE',  ( 12.91533473730993009, 46.60535201082150536, -10.88017736071109987 ) ) ;
#90210=CARTESIAN_POINT ( 'NONE',  ( 20.10384461210892582, 31.74302437010793199, 6.337995344473749348 ) ) ;
#90211=CARTESIAN_POINT ( 'NONE',  ( 4.559911319644449179, 42.23035201082151247, -9.422509992056141925 ) ) ;
#90214=CARTESIAN_POINT ( 'NONE',  ( 15.44008868035555260, 9.730352010821505360, 9.422509992056143702 ) ) ;
#90215=CARTESIAN_POINT ( 'NONE',  ( 13.43411237798105340, 0.5819680032637533085, 12.81628187352647963 ) ) ;
#90216=CARTESIAN_POINT ( 'NONE',  ( 17.96484262340118221, 46.18868534415484106, -7.964842623401177768 ) ) ;
#90217=CARTESIAN_POINT ( 'NONE',  ( 2.603489959281591659, 15.43575266056827999, -6.500000000000006217 ) ) ;
#90219=CARTESIAN_POINT ( 'NONE',  ( 4.559911319644449179, 53.89701867748817676, 9.422509992056141925 ) ) ;
#90221=CARTESIAN_POINT ( 'NONE',  ( 2.035157376598824452, 43.68868534415484106, 7.964842623401179544 ) ) ;
#90223=CARTESIAN_POINT ( 'NONE',  ( 14.92337183194729633, 12.67559781766745353, 8.527530157486181039 ) ) ;
#90224=CARTESIAN_POINT ( 'NONE',  ( 18.52753015748617571, 23.09226448433411960, 4.923371831947298993 ) ) ;
#90225=PRESENTATION_STYLE_ASSIGNMENT (( #38720 ) ) ;
#90228=CARTESIAN_POINT ( 'NONE',  ( 10.00000000000000000, 59.75893115100078745, -9.846743663894594434 ) ) ;
#90229=CARTESIAN_POINT ( 'NONE',  ( 20.88017736071110519, 5.563685344154838397, 2.639326808657452039E-16 ) ) ;
#90231=CARTESIAN_POINT ( 'NONE',  ( 24.16423886937409904, 29.09541550158063572, 3.795296366450317205 ) ) ;
#90232=CARTESIAN_POINT ( 'NONE',  ( 17.08211943468705130, 53.47041550158063217, 12.26659068614894998 ) ) ;
#90233=CARTESIAN_POINT ( 'NONE',  ( 0.5774900079438607392, 3.480352010821504027, 5.440088680355550821 ) ) ;
#90234=ORIENTED_EDGE ( 'NONE', *, *, #75409, .F. ) ;
#90235=CARTESIAN_POINT ( 'NONE',  ( 10.00000000000000178, 22.25893115100078745, 9.846743663894594434 ) ) ;
#90236=CARTESIAN_POINT ( 'NONE',  ( 0.5774900079438590739, 17.64701867748817321, -5.440088680355550821 ) ) ;
#90237=CARTESIAN_POINT ( 'NONE',  ( 2.791683348922237240, 50.38393115100078035, -7.208316651077763204 ) ) ;
#90243=CARTESIAN_POINT ( 'NONE',  ( 0.6178305044545818747, 18.49863466993041428, -9.382169495545419124 ) ) ;
#90244=CARTESIAN_POINT ( 'NONE',  ( 0.1532563361054100626, 40.80059781766745886, -2.638427012816831230 ) ) ;
#90245=ORIENTED_EDGE ( 'NONE', *, *, #56512, .T. ) ;
#90246=CARTESIAN_POINT ( 'NONE',  ( 18.52753015748617571, 8.092264484334117824, 4.923371831947298993 ) ) ;
#90248=CARTESIAN_POINT ( 'NONE',  ( -0.8801773607111009756, 13.06368534415483929, 1.068504757029289695E-15 ) ) ;
#90249=CARTESIAN_POINT ( 'NONE',  ( 10.00000000000000178, 38.05374883491396787, 14.16423886937410082 ) ) ;
#90250=CARTESIAN_POINT ( 'NONE',  ( 15.44008868035555260, 44.73035201082151247, 9.422509992056143702 ) ) ;
#90251=CARTESIAN_POINT ( 'NONE',  ( 7.084665262690076126, 64.10535201082150536, 10.88017736071109987 ) ) ;
#90252=CARTESIAN_POINT ( 'NONE',  ( 0.1532563361054100626, 25.80059781766744820, -2.638427012816831230 ) ) ;
#90253=CARTESIAN_POINT ( 'NONE',  ( 2.791683348922237240, 5.383931151000785675, -7.208316651077763204 ) ) ;
#90255=CARTESIAN_POINT ( 'NONE',  ( 18.52753015748617571, 43.09226448433412315, 4.923371831947298993 ) ) ;
#90256=CARTESIAN_POINT ( 'NONE',  ( 0.5774900079438590739, 37.64701867748817676, -5.440088680355550821 ) ) ;
#90258=CARTESIAN_POINT ( 'NONE',  ( -1.099225684535947600, 64.54030133659709634, 6.408140936763237150 ) ) ;
#90261=CARTESIAN_POINT ( 'NONE',  ( 1.472469842513823179, 5.592264484334118713, -4.923371831947296329 ) ) ;
#90262=CARTESIAN_POINT ( 'NONE',  ( 19.38216949554541202, 45.99863466993041072, 9.382169495545424454 ) ) ;
#90263=CARTESIAN_POINT ( 'NONE',  ( 4.559911319644449179, 12.23035201082150714, -9.422509992056141925 ) ) ;
#90264=CARTESIAN_POINT ( 'NONE',  ( 7.361572987183170547, 42.05059781766745886, 9.846743663894590881 ) ) ;
#90265=( NAMED_UNIT ( * ) PLANE_ANGLE_UNIT ( ) SI_UNIT ( $, .RADIAN. ) );
#90266=CARTESIAN_POINT ( 'NONE',  ( 20.36894250292379738, 29.92874883491396432, -10.36894250292379027 ) ) ;
#90267=CARTESIAN_POINT ( 'NONE',  ( 20.36894250292379738, 49.92874883491396787, -10.36894250292379027 ) ) ;
#90268=CARTESIAN_POINT ( 'NONE',  ( 1.472469842513823179, 60.59226448433412315, -4.923371831947296329 ) ) ;
#90270=CARTESIAN_POINT ( 'NONE',  ( 20.88017736071110164, 35.35535201082150536, 2.915334737309930979 ) ) ;
#90271=CARTESIAN_POINT ( 'NONE',  ( 10.00000000000000178, 7.258931151000785675, 9.846743663894594434 ) ) ;
#90273=CARTESIAN_POINT ( 'NONE',  ( 16.40814093676324603, 62.45696800326376064, -11.09922568453594671 ) ) ;
#90274=CARTESIAN_POINT ( 'NONE',  ( 7.084665262690076126, 64.10535201082150536, 10.88017736071109987 ) ) ;
#90277=ADVANCED_FACE ( 'NONE', ( #93436 ), #50198, .T. ) ;
#90278=CARTESIAN_POINT ( 'NONE',  ( 22.26659068614894466, 3.887082168247300906, 7.082119434687054849 ) ) ;
#90279=CARTESIAN_POINT ( 'NONE',  ( 14.92337183194729633, 12.67559781766745353, 8.527530157486181039 ) ) ;
#90281=VERTEX_POINT ( 'NONE', #63427 ) ;
#90282=CARTESIAN_POINT ( 'NONE',  ( 2.035157376598824452, 33.68868534415484106, 7.964842623401179544 ) ) ;
#90284=CARTESIAN_POINT ( 'NONE',  ( 0.5774900079438590739, 32.64701867748816966, -5.440088680355550821 ) ) ;
#90285=CARTESIAN_POINT ( 'NONE',  ( 19.80777595082616216, 55.68878173731741299, -6.499999999999961808 ) ) ;
#90288=CARTESIAN_POINT ( 'NONE',  ( 15.44008868035555260, 64.73035201082151957, 9.422509992056143702 ) ) ;
#90289=CARTESIAN_POINT ( 'NONE',  ( 12.63842701281683922, 64.55059781766745175, -9.846743663894590881 ) ) ;
#90291=CARTESIAN_POINT ( 'NONE',  ( -0.8801773607111008646, 18.27201867748817321, 2.915334737309923430 ) ) ;
#90293=CARTESIAN_POINT ( 'NONE',  ( 15.44008868035555793, 66.39701867748817676, -9.422509992056140149 ) ) ;
#90294=CARTESIAN_POINT ( 'NONE',  ( 0.5774900079438607392, 13.48035201082150358, 5.440088680355550821 ) ) ;
#90295=AXIS2_PLACEMENT_3D ( 'NONE', #63945, #17505, #85495 ) ;
#90298=EDGE_LOOP ( 'NONE', ( #50049, #23171, #20209, #76905 ) ) ;
#90299=CARTESIAN_POINT ( 'NONE',  ( 21.09922568453594849, 56.20696800326375353, 6.408140936763242479 ) ) ;
#90300=CARTESIAN_POINT ( 'NONE',  ( 10.00000000000000000, 41.81368534415484106, -10.88017736071110342 ) ) ;
#90302=CARTESIAN_POINT ( 'NONE',  ( 6.565887622018943937, 53.08196800326374643, -12.81628187352647608 ) ) ;
#90303=CARTESIAN_POINT ( 'NONE',  ( 12.91533473730992121, 44.52201867748816966, 10.88017736071110164 ) ) ;
#90304=EDGE_CURVE ( 'NONE', #53168, #89098, #9446, .T. ) ;
#90305=CARTESIAN_POINT ( 'NONE',  ( 13.43411237798106583, 2.665301336597086568, -12.81628187352647252 ) ) ;
#90307=CARTESIAN_POINT ( 'NONE',  ( 5.076628168052703671, 16.84226448433411960, 8.527530157486179263 ) ) ;
#90309=CARTESIAN_POINT ( 'NONE',  ( 16.40814093676323893, 0.7903013365970867898, 11.09922568453595026 ) ) ;
#90311=CARTESIAN_POINT ( 'NONE',  ( 1.472469842513823179, 65.59226448433412315, -4.923371831947296329 ) ) ;
#90312=CARTESIAN_POINT ( 'NONE',  ( 2.035157376598824452, 33.68868534415484106, 7.964842623401179544 ) ) ;
#90313=CARTESIAN_POINT ( 'NONE',  ( 5.076628168052704559, 45.17559781766745175, -8.527530157486179263 ) ) ;
#90314=CARTESIAN_POINT ( 'NONE',  ( 12.63842701281683922, 19.55059781766745175, -9.846743663894590881 ) ) ;
#90315=CARTESIAN_POINT ( 'NONE',  ( 10.00000000000000178, 2.258931151000784787, 9.846743663894594434 ) ) ;
#90316=CARTESIAN_POINT ( 'NONE',  ( 22.81628187352647785, 1.415301336597087012, 3.434112377981063169 ) ) ;
#90317=ORIENTED_EDGE ( 'NONE', *, *, #5682, .T. ) ;
#90318=( NAMED_UNIT ( * ) PLANE_ANGLE_UNIT ( ) SI_UNIT ( $, .RADIAN. ) );
#90319=CARTESIAN_POINT ( 'NONE',  ( 18.52753015748617571, 58.09226448433411605, 4.923371831947298993 ) ) ;
#90321=CARTESIAN_POINT ( 'NONE',  ( 1.472469842513823179, 31.42559781766745530, 4.923371831947296329 ) ) ;
#90323=CARTESIAN_POINT ( 'NONE',  ( -4.164238869374099927, 67.01208216824728936, 3.795296366450308767 ) ) ;
#90324=CARTESIAN_POINT ( 'NONE',  ( 17.20831665107776587, 39.13393115100079456, -7.208316651077762316 ) ) ;
#90325=CARTESIAN_POINT ( 'NONE',  ( 20.15039907845753930, 70.00000000000000000, 6.262539305110068177 ) ) ;
#90326=CARTESIAN_POINT ( 'NONE',  ( 13.79529636645031943, 65.34541550158063217, -14.16423886937409904 ) ) ;
#90329=CARTESIAN_POINT ( 'NONE',  ( 15.44008868035555793, 16.39701867748817321, -9.422509992056140149 ) ) ;
#90330=CARTESIAN_POINT ( 'NONE',  ( 10.00000000000000000, 55.55374883491396787, -14.16423886937410082 ) ) ;
#90331=CARTESIAN_POINT ( 'NONE',  ( -4.164238869374098151, 51.59541550158063217, -3.795296366450310543 ) ) ;
#90332=DIRECTION ( 'NONE',  ( 0.000000000000000000, 0.000000000000000000, -1.000000000000000000 ) ) ;
#90333=SURFACE_STYLE_FILL_AREA ( #23352 ) ;
#90334=CARTESIAN_POINT ( 'NONE',  ( 5.076628168052704559, 25.17559781766745175, -8.527530157486179263 ) ) ;
#90335=CARTESIAN_POINT ( 'NONE',  ( 22.81628187352647785, 6.623634669930420493, 6.195893100308588602E-16 ) ) ;
#90339=CARTESIAN_POINT ( 'NONE',  ( 1.472469842513823179, 60.59226448433412315, -4.923371831947296329 ) ) ;
#90341=EDGE_CURVE ( 'NONE', #58602, #17129, #23107, .T. ) ;
#90343=CARTESIAN_POINT ( 'NONE',  ( 17.08211943468705840, 15.13708216824730179, -12.26659068614894466 ) ) ;
#90344=CARTESIAN_POINT ( 'NONE',  ( 19.84674366389459266, 28.71726448433411960, -2.638427012816827677 ) ) ;
#90345=CARTESIAN_POINT ( 'NONE',  ( 2.917880565312948704, 37.63708216824731068, 12.26659068614894643 ) ) ;
#90346=CARTESIAN_POINT ( 'NONE',  ( 19.84674366389459621, 8.508931151000785675, 7.409399052514197653E-17 ) ) ;
#90349=CARTESIAN_POINT ( 'NONE',  ( 2.035157376598822676, 32.43868534415483396, -7.964842623401177768 ) ) ;
#90350=CARTESIAN_POINT ( 'NONE',  ( 6.565887622018943937, 38.08196800326376064, -12.81628187352647608 ) ) ;
#90351=CARTESIAN_POINT ( 'NONE',  ( 12.91533473730993009, 6.605352010821504471, -10.88017736071109987 ) ) ;
#90352=CARTESIAN_POINT ( 'NONE',  ( -1.099225684535947600, 38.70696800326375353, -6.408140936763238038 ) ) ;
#90353=CARTESIAN_POINT ( 'NONE',  ( 3.591859063236763294, 58.29030133659708923, -11.09922568453595026 ) ) ;
#90354=VERTEX_POINT ( 'NONE', #11907 ) ;
#90357=CARTESIAN_POINT ( 'NONE',  ( 22.26659068614895176, 44.72041550158063927, -7.082119434687042414 ) ) ;
#90358=CARTESIAN_POINT ( 'NONE',  ( 22.26659068614895176, 4.720415501580633943, -7.082119434687042414 ) ) ;
#90359=CARTESIAN_POINT ( 'NONE',  ( 20.88017736071110519, 10.56368534415483751, 2.639326808657452039E-16 ) ) ;
#90360=CARTESIAN_POINT ( 'NONE',  ( 19.42250999205614193, 20.14701867748817321, 5.440088680355555262 ) ) ;
#90363=CARTESIAN_POINT ( 'NONE',  ( 10.00000000000000000, 46.81368534415484106, -10.88017736071110342 ) ) ;
#90364=B_SPLINE_CURVE_WITH_KNOTS ( 'NONE', 3,
 ( #38315, #75806, #61779, #77275 ),
 .UNSPECIFIED., .F., .F.,
 ( 4, 4 ),
 ( 9.697399036122160616E-19, 0.002392975128318514545 ),
 .UNSPECIFIED. ) ;
#90365=CARTESIAN_POINT ( 'NONE',  ( 4.559911319644449179, 62.23035201082150536, -9.422509992056141925 ) ) ;
#90366=CARTESIAN_POINT ( 'NONE',  ( 0.6178305044545818747, 23.49863466993041783, -9.382169495545419124 ) ) ;
#90369=CARTESIAN_POINT ( 'NONE',  ( 7.361572987183170547, 17.05059781766745530, 9.846743663894590881 ) ) ;
#90370=CARTESIAN_POINT ( 'NONE',  ( 19.42250999205614193, 60.14701867748817676, 5.440088680355555262 ) ) ;
#90374=CARTESIAN_POINT ( 'NONE',  ( 13.43411237798106583, 12.66530133659708746, -12.81628187352647252 ) ) ;
#90375=CARTESIAN_POINT ( 'NONE',  ( 15.44008868035555260, 9.730352010821505360, 9.422509992056143702 ) ) ;
#90376=CARTESIAN_POINT ( 'NONE',  ( 0.1532563361054100626, 40.80059781766745886, -2.638427012816831230 ) ) ;
#90378=CARTESIAN_POINT ( 'NONE',  ( 7.361572987183170547, 17.05059781766745530, 9.846743663894590881 ) ) ;
#90379=( LENGTH_UNIT ( ) NAMED_UNIT ( * ) SI_UNIT ( .MILLI., .METRE. ) );
#90380=CARTESIAN_POINT ( 'NONE',  ( 20.88017736071110519, 30.56368534415484106, 2.639326808657452039E-16 ) ) ;
#90381=CARTESIAN_POINT ( 'NONE',  ( -0.8801773607111009756, 33.06368534415484106, 1.068504757029289695E-15 ) ) ;
#90382=CARTESIAN_POINT ( 'NONE',  ( 20.36894250292379738, 34.92874883491396076, -10.36894250292379027 ) ) ;
#90383=CARTESIAN_POINT ( 'NONE',  ( 7.361572987183169658, 44.96726448433412315, -9.846743663894592657 ) ) ;
#90384=CARTESIAN_POINT ( 'NONE',  ( -0.8801773607110991993, 27.85535201082150181, -2.915334737309923874 ) ) ;
#90386=CARTESIAN_POINT ( 'NONE',  ( 2.035157376598824452, 18.68868534415484106, 7.964842623401179544 ) ) ;
#90387=ORIENTED_EDGE ( 'NONE', *, *, #53184, .F. ) ;
#90388=CARTESIAN_POINT ( 'NONE',  ( 20.88017736071110164, 30.35535201082151247, 2.915334737309930979 ) ) ;
#90389=EDGE_CURVE ( 'NONE', #58376, #76182, #94959, .T. ) ;
#90390=CARTESIAN_POINT ( 'NONE',  ( 10.00000000000000000, 47.87363466993042493, -12.81628187352647608 ) ) ;
#90391=CARTESIAN_POINT ( 'NONE',  ( 19.42250999205614193, 30.14701867748817321, 5.440088680355555262 ) ) ;
#90394=CARTESIAN_POINT ( 'NONE',  ( 19.84674366389459266, 58.30059781766745886, 2.638427012816836559 ) ) ;
#90395=CARTESIAN_POINT ( 'NONE',  ( 0.5774900079438607392, 33.48035201082150536, 5.440088680355550821 ) ) ;
#90398=CARTESIAN_POINT ( 'NONE',  ( 2.917880565312948704, 47.63708216824730357, 12.26659068614894643 ) ) ;
#90399=CARTESIAN_POINT ( 'NONE',  ( 10.00000000000000000, 56.81368534415484106, -10.88017736071110342 ) ) ;
#90400=FILL_AREA_STYLE_COLOUR ( '', #3552 ) ;
#90402=CARTESIAN_POINT ( 'NONE',  ( 7.361572987183170547, 67.05059781766746596, 9.846743663894590881 ) ) ;
#90404=CARTESIAN_POINT ( 'NONE',  ( 17.20831665107776587, 32.88393115100078745, 7.208316651077764980 ) ) ;
#90405=CARTESIAN_POINT ( 'NONE',  ( 0.1532563361054082862, 41.21726448433411605, 2.638427012816831674 ) ) ;
#90407=CARTESIAN_POINT ( 'NONE',  ( 10.00000000000000000, 31.81368534415483751, -10.88017736071110342 ) ) ;
#90408=CARTESIAN_POINT ( 'NONE',  ( 7.361572987183170547, 27.05059781766745175, 9.846743663894590881 ) ) ;
#90409=CARTESIAN_POINT ( 'NONE',  ( 22.81628187352648496, 21.83196800326374643, -3.434112377981050290 ) ) ;
#90411=CARTESIAN_POINT ( 'NONE',  ( 10.00000000000000000, 61.81368534415484106, -10.88017736071110342 ) ) ;
#90412=CARTESIAN_POINT ( 'NONE',  ( 0.5774900079438607392, 33.48035201082150536, 5.440088680355550821 ) ) ;
#90413=CARTESIAN_POINT ( 'NONE',  ( 2.035157376598822676, 7.438685344154837509, -7.964842623401177768 ) ) ;
#90414=CARTESIAN_POINT ( 'NONE',  ( -4.164238869374098151, 46.59541550158063927, -3.795296366450310543 ) ) ;
#90419=CARTESIAN_POINT ( 'NONE',  ( -2.816281873526473856, 14.12363466993041961, 9.499525473075851096E-16 ) ) ;
#90420=CARTESIAN_POINT ( 'NONE',  ( 12.91533473730992121, 9.522018677488171434, 10.88017736071110164 ) ) ;
#90422=CARTESIAN_POINT ( 'NONE',  ( -0.8801773607110991993, 52.85535201082151247, -2.915334737309923874 ) ) ;
#90423=PRESENTATION_STYLE_ASSIGNMENT (( #30420 ) ) ;
#90425=CARTESIAN_POINT ( 'NONE',  ( 4.559911319644449179, 53.89701867748817676, 9.422509992056141925 ) ) ;
#90426=CARTESIAN_POINT ( 'NONE',  ( 7.361572987183170547, 32.05059781766745175, 9.846743663894590881 ) ) ;
#90427=CARTESIAN_POINT ( 'NONE',  ( 5.076628168052704559, 25.17559781766745175, -8.527530157486179263 ) ) ;
#90429=CARTESIAN_POINT ( 'NONE',  ( 18.52753015748618282, 13.92559781766745175, -4.923371831947291888 ) ) ;
#90431=CARTESIAN_POINT ( 'NONE',  ( 16.40814093676324603, 37.45696800326376064, -11.09922568453594671 ) ) ;
#90432=CARTESIAN_POINT ( 'NONE',  ( 5.076628168052703671, 1.842264484334118047, 8.527530157486179263 ) ) ;
#90435=CARTESIAN_POINT ( 'NONE',  ( 10.00000000000000178, 32.25893115100078745, 9.846743663894594434 ) ) ;
#90437=CARTESIAN_POINT ( 'NONE',  ( 0.6178305044545818747, 58.49863466993042493, -9.382169495545419124 ) ) ;
#90439=CARTESIAN_POINT ( 'NONE',  ( 16.40814093676324603, 7.456968003263754419, -11.09922568453594671 ) ) ;
#90440=EDGE_CURVE ( 'NONE', #25641, #50375, #11856, .T. ) ;
#90442=CARTESIAN_POINT ( 'NONE',  ( 19.42250999205614193, 55.14701867748817676, 5.440088680355555262 ) ) ;
#90444=CARTESIAN_POINT ( 'NONE',  ( -2.266590686148945544, 31.38708216824730002, -7.082119434687050408 ) ) ;
#90445=UNCERTAINTY_MEASURE_WITH_UNIT (LENGTH_MEASURE( 1.000000000000000082E-05 ), #16978, 'distance_accuracy_value', 'NONE');
#90447=CARTESIAN_POINT ( 'NONE',  ( 22.26659068614894466, 28.88708216824730357, 7.082119434687054849 ) ) ;
#90449=CARTESIAN_POINT ( 'NONE',  ( -4.164238869374099927, 42.01208216824728936, 3.795296366450308767 ) ) ;
#90450=CARTESIAN_POINT ( 'NONE',  ( 17.08211943468705130, 13.47041550158063572, 12.26659068614894998 ) ) ;
#90451=CARTESIAN_POINT ( 'NONE',  ( -4.164238869374099927, 7.012082168247302683, 3.795296366450308767 ) ) ;
#90452=CARTESIAN_POINT ( 'NONE',  ( 15.44008868035555793, 66.39701867748817676, -9.422509992056140149 ) ) ;
#90453=CARTESIAN_POINT ( 'NONE',  ( -0.8801773607110991993, 42.85535201082150536, -2.915334737309923874 ) ) ;
#90455=CARTESIAN_POINT ( 'NONE',  ( 17.20831665107776587, 32.88393115100078745, 7.208316651077764980 ) ) ;
#90456=DIRECTION ( 'NONE',  ( 0.000000000000000000, 1.000000000000000000, -0.000000000000000000 ) ) ;
#90457=CARTESIAN_POINT ( 'NONE',  ( 2.791683348922237240, 30.38393115100078390, -7.208316651077763204 ) ) ;
#90459=CARTESIAN_POINT ( 'NONE',  ( -0.8801773607111008646, 28.27201867748817321, 2.915334737309923430 ) ) ;
#90460=CARTESIAN_POINT ( 'NONE',  ( 21.09922568453594849, 56.20696800326375353, 6.408140936763242479 ) ) ;
#90461=CARTESIAN_POINT ( 'NONE',  ( 1.472469842513823179, 60.59226448433412315, -4.923371831947296329 ) ) ;
#90463=CARTESIAN_POINT ( 'NONE',  ( 19.84674366389459266, 28.30059781766745886, 2.638427012816836559 ) ) ;
#90465=CARTESIAN_POINT ( 'NONE',  ( 3.591859063236763294, 38.29030133659708923, -11.09922568453595026 ) ) ;
#90467=CARTESIAN_POINT ( 'NONE',  ( 20.88017736071110164, 40.35535201082150536, 2.915334737309930979 ) ) ;
#90468=CARTESIAN_POINT ( 'NONE',  ( 2.791683348922240793, 56.63393115100078035, 7.208316651077764092 ) ) ;
#90469=CARTESIAN_POINT ( 'NONE',  ( 2.917880565312950480, 20.97041550158063217, -12.26659068614894821 ) ) ;
#90470=ORIENTED_EDGE ( 'NONE', *, *, #5771, .T. ) ;
#90473=CARTESIAN_POINT ( 'NONE',  ( 4.559911319644449179, 58.89701867748817676, 9.422509992056141925 ) ) ;
#90475=CARTESIAN_POINT ( 'NONE',  ( 13.79529636645030344, 53.26208216824730357, 14.16423886937410614 ) ) ;
#90476=CARTESIAN_POINT ( 'NONE',  ( 19.38216949554541557, 2.248634669930420049, -9.382169495545420901 ) ) ;
#90477=CARTESIAN_POINT ( 'NONE',  ( 0.5774900079438590739, 57.64701867748817676, -5.440088680355550821 ) ) ;
#90481=CARTESIAN_POINT ( 'NONE',  ( 4.559911319644449179, 7.230352010821504471, -9.422509992056141925 ) ) ;
#90482=CARTESIAN_POINT ( 'NONE',  ( 15.44008868035555260, 9.730352010821505360, 9.422509992056143702 ) ) ;
#90483=CARTESIAN_POINT ( 'NONE',  ( 17.20831665107776587, 59.13393115100078745, -7.208316651077762316 ) ) ;
#90485=CARTESIAN_POINT ( 'NONE',  ( 3.591859063236763294, 53.29030133659708923, -11.09922568453595026 ) ) ;
#90486=DIRECTION ( 'NONE',  ( 0.8320502943378436100, -0.5547001962252291474, 0.000000000000000000 ) ) ;
#90488=CARTESIAN_POINT ( 'NONE',  ( 7.084665262690076126, 14.10535201082150358, 10.88017736071109987 ) ) ;
#90489=CARTESIAN_POINT ( 'NONE',  ( 22.81628187352647785, 16.41530133659708923, 3.434112377981063169 ) ) ;
#90491=CARTESIAN_POINT ( 'NONE',  ( 0.1532563361054100626, 5.800597817667452638, -2.638427012816831230 ) ) ;
#90492=VECTOR ( 'NONE', #10150, 1000.000000000000000 ) ;
#90493=CARTESIAN_POINT ( 'NONE',  ( 18.52753015748618282, 48.92559781766745886, -4.923371831947291888 ) ) ;
#90494=CARTESIAN_POINT ( 'NONE',  ( 17.96484262340118221, 34.93868534415482685, 7.964842623401181321 ) ) ;
#90496=CARTESIAN_POINT ( 'NONE',  ( 22.81628187352647785, 26.62363466993042138, 6.195893100308588602E-16 ) ) ;
#90497=CARTESIAN_POINT ( 'NONE',  ( 2.035157376598824452, 43.68868534415484106, 7.964842623401179544 ) ) ;
#90499=FACE_OUTER_BOUND ( 'NONE', #83796, .T. ) ;
#90500=CARTESIAN_POINT ( 'NONE',  ( 22.81628187352647785, 51.41530133659708923, 3.434112377981063169 ) ) ;
#90503=CARTESIAN_POINT ( 'NONE',  ( -0.8801773607111008646, 53.27201867748816966, 2.915334737309923430 ) ) ;
#90504=CARTESIAN_POINT ( 'NONE',  ( -2.816281873526473856, 39.33196800326374643, 3.434112377981055619 ) ) ;
#90505=CARTESIAN_POINT ( 'NONE',  ( 13.79529636645031943, 5.345415501580634832, -14.16423886937409904 ) ) ;
#90506=CARTESIAN_POINT ( 'NONE',  ( 12.91533473730992121, 44.52201867748816966, 10.88017736071110164 ) ) ;
#90508=FILL_AREA_STYLE_COLOUR ( '', #1920 ) ;
#90509=CARTESIAN_POINT ( 'NONE',  ( 12.63842701281683034, 22.46726448433411605, 9.846743663894596210 ) ) ;
#90510=CARTESIAN_POINT ( 'NONE',  ( 10.00000000000000000, 4.758931151000784787, -9.846743663894594434 ) ) ;
#90512=CARTESIAN_POINT ( 'NONE',  ( 13.79529636645031943, 40.34541550158063217, -14.16423886937409904 ) ) ;
#90513=CARTESIAN_POINT ( 'NONE',  ( 20.15039907845753220, 24.72266099184919241, 6.262539305110077947 ) ) ;
#90515=SURFACE_STYLE_FILL_AREA ( #60020 ) ;
#90518=CARTESIAN_POINT ( 'NONE',  ( -4.164238869374098151, 66.59541550158060375, -3.795296366450310543 ) ) ;
#90519=CARTESIAN_POINT ( 'NONE',  ( 10.00000000000000178, 68.05374883491397497, 14.16423886937410082 ) ) ;
#90520=CARTESIAN_POINT ( 'NONE',  ( 10.00000000000000000, 24.75893115100078745, -9.846743663894594434 ) ) ;
#90521=CARTESIAN_POINT ( 'NONE',  ( 6.565887622018943937, 38.08196800326376064, -12.81628187352647608 ) ) ;
#90524=CARTESIAN_POINT ( 'NONE',  ( 20.36894250292379738, 9.928748834913966093, -10.36894250292379027 ) ) ;
#90525=CARTESIAN_POINT ( 'NONE',  ( -0.8801773607111009756, 8.063685344154837509, 1.068504757029289695E-15 ) ) ;
#90526=CARTESIAN_POINT ( 'NONE',  ( 13.79529636645031943, 55.34541550158062506, -14.16423886937409904 ) ) ;
#90528=CARTESIAN_POINT ( 'NONE',  ( 19.84674366389459266, 33.30059781766744464, 2.638427012816836559 ) ) ;
#90529=( BOUNDED_CURVE ( )  B_SPLINE_CURVE ( 2, ( #23813, #61291, #76787, #75310, #7326, #98838, #6821, #22819, #83807 ),
 .UNSPECIFIED., .F., .T. ) 
 B_SPLINE_CURVE_WITH_KNOTS ( ( 3, 2, 2, 2, 3 ),
 ( 0.6544266512259456769, 0.6547619047619047672, 0.6607142857142858094, 0.6666666666666667407, 0.6670019202026259419 ),
 .UNSPECIFIED. ) 
 CURVE ( )  GEOMETRIC_REPRESENTATION_ITEM ( )  RATIONAL_B_SPLINE_CURVE ( ( 0.9963778908391764944, 0.9980808541467923733, 1.000000000000000000, 0.9659258262890682012, 1.000000000000000000, 0.9659258262890682012, 1.000000000000000000, 0.9980808541467917072, 0.9963778908391753841 ) ) 
 REPRESENTATION_ITEM ( '' )  );
#90530=CARTESIAN_POINT ( 'NONE',  ( 19.05866839779139710, 40.95508385108959004, -6.499999999999974243 ) ) ;
#90531=CARTESIAN_POINT ( 'NONE',  ( 5.076628168052703671, 16.84226448433411960, 8.527530157486179263 ) ) ;
#90535=ORIENTED_EDGE ( 'NONE', *, *, #29070, .T. ) ;
#90539=CARTESIAN_POINT ( 'NONE',  ( 7.361572987183170547, 47.05059781766745175, 9.846743663894590881 ) ) ;
#90540=CARTESIAN_POINT ( 'NONE',  ( 20.36894250292379738, 19.92874883491396787, -10.36894250292379027 ) ) ;
#90541=CARTESIAN_POINT ( 'NONE',  ( 2.035157376598824452, 38.68868534415483396, 7.964842623401179544 ) ) ;
#90542=CARTESIAN_POINT ( 'NONE',  ( 7.084665262690076126, 34.10535201082151247, 10.88017736071109987 ) ) ;
#90543=CARTESIAN_POINT ( 'NONE',  ( 19.84674366389459266, 63.71726448433412315, -2.638427012816827677 ) ) ;
#90544=CARTESIAN_POINT ( 'NONE',  ( 10.00000000000000178, 35.37363466993042493, 12.81628187352647608 ) ) ;
#90545=CARTESIAN_POINT ( 'NONE',  ( 24.16423886937409904, 4.095415501580634832, 3.795296366450317205 ) ) ;
#90548=ADVANCED_FACE ( 'NONE', ( #57398 ), #70093, .T. ) ;
#90549=CARTESIAN_POINT ( 'NONE',  ( 22.81628187352648496, 31.83196800326375353, -3.434112377981050290 ) ) ;
#90550=EDGE_LOOP ( 'NONE', ( #84268, #36809, #2549, #26932 ) ) ;
#90551=CARTESIAN_POINT ( 'NONE',  ( 5.076628168052704559, 50.17559781766745886, -8.527530157486179263 ) ) ;
#90553=CARTESIAN_POINT ( 'NONE',  ( 7.084665262690076126, 7.022018677488170546, -10.88017736071110164 ) ) ;
#90554=ORIENTED_EDGE ( 'NONE', *, *, #49841, .F. ) ;
#90555=CARTESIAN_POINT ( 'NONE',  ( 19.42250999205614193, 15.14701867748817143, 5.440088680355555262 ) ) ;
#90557=CARTESIAN_POINT ( 'NONE',  ( -0.8801773607111008646, 48.27201867748816966, 2.915334737309923430 ) ) ;
#90558=CARTESIAN_POINT ( 'NONE',  ( 2.035157376598824452, 58.68868534415482685, 7.964842623401179544 ) ) ;
#90559=CARTESIAN_POINT ( 'NONE',  ( 19.42250999205614193, 65.14701867748817676, 5.440088680355555262 ) ) ;
#90561=CARTESIAN_POINT ( 'NONE',  ( 7.361572987183169658, -0.03273551566588185635, -9.846743663894592657 ) ) ;
#90562=CARTESIAN_POINT ( 'NONE',  ( 17.96484262340118221, 49.93868534415484106, 7.964842623401181321 ) ) ;
#90563=CARTESIAN_POINT ( 'NONE',  ( -1.926860441876563801, 52.66212336850780673, 1.004413902775740978E-15 ) ) ;
#90565=CARTESIAN_POINT ( 'NONE',  ( 2.791683348922237240, 25.38393115100078390, -7.208316651077763204 ) ) ;
#90568=FILL_AREA_STYLE ('',( #98102 ) ) ;
#90569=( GEOMETRIC_REPRESENTATION_CONTEXT ( 3 ) GLOBAL_UNCERTAINTY_ASSIGNED_CONTEXT ( ( #37145 ) ) GLOBAL_UNIT_ASSIGNED_CONTEXT ( ( #97413, #35403, #89396 ) ) REPRESENTATION_CONTEXT ( 'NONE', 'WORKASPACE' ) );
#90570=CARTESIAN_POINT ( 'NONE',  ( -4.164238869374098151, 1.595415501580634388, -3.795296366450310543 ) ) ;
#90571=EDGE_CURVE ( 'NONE', #91132, #57334, #44075, .T. ) ;
#90573=CARTESIAN_POINT ( 'NONE',  ( -46.76851119026090231, 103.5739182654012325, -5.803562628621293129 ) ) ;
#90574=CARTESIAN_POINT ( 'NONE',  ( 6.204703633549690345, 67.84541550158060375, 14.16423886937410082 ) ) ;
#90578=CARTESIAN_POINT ( 'NONE',  ( 10.00000000000000178, 47.25893115100078745, 9.846743663894594434 ) ) ;
#90580=CARTESIAN_POINT ( 'NONE',  ( -1.099225684535947600, 23.70696800326375708, -6.408140936763238038 ) ) ;
#90581=CARTESIAN_POINT ( 'NONE',  ( 18.52753015748618282, 18.92559781766745175, -4.923371831947291888 ) ) ;
#90582=EDGE_CURVE ( 'NONE', #90354, #95793, #9562, .T. ) ;
#90583=CARTESIAN_POINT ( 'NONE',  ( 1.816707512666850599, 30.10290668512023160, -6.499999999999995559 ) ) ;
#90584=CARTESIAN_POINT ( 'NONE',  ( 0.1532563361054083140, 21.00893115100078745, 1.131784320476157264E-15 ) ) ;
#90585=CARTESIAN_POINT ( 'NONE',  ( 22.81628187352647785, 6.623634669930420493, 6.195893100308588602E-16 ) ) ;
#90588=CARTESIAN_POINT ( 'NONE',  ( 15.44008868035555260, 29.73035201082150891, 9.422509992056143702 ) ) ;
#90589=CARTESIAN_POINT ( 'NONE',  ( 17.08211943468705840, 15.13708216824730179, -12.26659068614894466 ) ) ;
#90590=CARTESIAN_POINT ( 'NONE',  ( 18.52753015748617571, 28.09226448433411960, 4.923371831947298993 ) ) ;
#90591=CARTESIAN_POINT ( 'NONE',  ( -0.8801773607111009756, 58.06368534415484106, 1.068504757029289695E-15 ) ) ;
#90592=CARTESIAN_POINT ( 'NONE',  ( 6.565887622018943937, 43.08196800326374643, -12.81628187352647608 ) ) ;
#90594=CARTESIAN_POINT ( 'NONE',  ( 10.00000000000000178, 14.31368534415483751, 10.88017736071110342 ) ) ;
#90598=CARTESIAN_POINT ( 'NONE',  ( 22.81628187352647785, 11.41530133659708390, 3.434112377981063169 ) ) ;
#90599=CARTESIAN_POINT ( 'NONE',  ( 17.20831665107776587, 32.88393115100078745, 7.208316651077764980 ) ) ;
#90601=CARTESIAN_POINT ( 'NONE',  ( 22.81628187352647785, 31.41530133659709279, 3.434112377981063169 ) ) ;
#90603=CARTESIAN_POINT ( 'NONE',  ( 4.559911319644449179, 42.23035201082151247, -9.422509992056141925 ) ) ;
#90609=AXIS2_PLACEMENT_3D ( 'NONE', #53504, #46496, #16508 ) ;
#90610=CARTESIAN_POINT ( 'NONE',  ( -0.8801773607110991993, 37.85535201082151247, -2.915334737309923874 ) ) ;
#90611=CARTESIAN_POINT ( 'NONE',  ( 7.084665262690076126, 47.02201867748818387, -10.88017736071110164 ) ) ;
#90612=CARTESIAN_POINT ( 'NONE',  ( 7.361572987183170547, 67.05059781766746596, 9.846743663894590881 ) ) ;
#90613=CARTESIAN_POINT ( 'NONE',  ( 12.91533473730993009, 61.60535201082150536, -10.88017736071109987 ) ) ;
#90614=CARTESIAN_POINT ( 'NONE',  ( 12.63842701281683034, 37.46726448433411605, 9.846743663894596210 ) ) ;
#90615=CARTESIAN_POINT ( 'NONE',  ( 19.42250999205614548, 10.98035201082150358, -5.440088680355545492 ) ) ;
#90616=CARTESIAN_POINT ( 'NONE',  ( 21.09922568453594849, 16.20696800326375353, 6.408140936763242479 ) ) ;
#90618=CARTESIAN_POINT ( 'NONE',  ( 19.42250999205614193, 30.14701867748817321, 5.440088680355555262 ) ) ;
#90620=CARTESIAN_POINT ( 'NONE',  ( 20.88017736071110164, 25.35535201082150891, 2.915334737309930979 ) ) ;
#90621=CARTESIAN_POINT ( 'NONE',  ( 4.559911319644449179, 63.89701867748817676, 9.422509992056141925 ) ) ;
#90622=CARTESIAN_POINT ( 'NONE',  ( 2.917880565312948704, 32.63708216824730357, 12.26659068614894643 ) ) ;
#90623=CARTESIAN_POINT ( 'NONE',  ( 1.472469842513823179, 30.59226448433411960, -4.923371831947296329 ) ) ;
#90624=CARTESIAN_POINT ( 'NONE',  ( 0.5774900079438607392, 43.48035201082151247, 5.440088680355550821 ) ) ;
#90626=CARTESIAN_POINT ( 'NONE',  ( 20.36894250292379382, 3.678748834913967869, 10.36894250292379205 ) ) ;
#90628=VERTEX_POINT ( 'NONE', #32715 ) ;
#90630=CARTESIAN_POINT ( 'NONE',  ( 1.472469842513823179, 61.42559781766745175, 4.923371831947296329 ) ) ;
#90633=CARTESIAN_POINT ( 'NONE',  ( 1.274849032794292736, 62.55509018479936145, -6.499999999999977796 ) ) ;
#90634=CARTESIAN_POINT ( 'NONE',  ( 13.79529636645031943, 15.34541550158063750, -14.16423886937409904 ) ) ;
#90635=CARTESIAN_POINT ( 'NONE',  ( 2.917880565312948704, 27.63708216824730357, 12.26659068614894643 ) ) ;
#90636=CARTESIAN_POINT ( 'NONE',  ( 7.084665262690076126, 54.10535201082151247, 10.88017736071109987 ) ) ;
#90637=CARTESIAN_POINT ( 'NONE',  ( 17.08211943468705130, 63.47041550158063927, 12.26659068614894998 ) ) ;
#90638=CARTESIAN_POINT ( 'NONE',  ( 14.92337183194729988, 64.34226448433412315, -8.527530157486177487 ) ) ;
#90639=CARTESIAN_POINT ( 'NONE',  ( 1.472469842513823179, 51.42559781766745886, 4.923371831947296329 ) ) ;
#90641=CARTESIAN_POINT ( 'NONE',  ( 19.42250999205614193, 50.14701867748817676, 5.440088680355555262 ) ) ;
#90642=CARTESIAN_POINT ( 'NONE',  ( -2.816281873526473856, 24.33196800326375353, 3.434112377981055619 ) ) ;
#90643=CARTESIAN_POINT ( 'NONE',  ( 13.79529636645030344, 13.26208216824729824, 14.16423886937410614 ) ) ;
#90644=CARTESIAN_POINT ( 'NONE',  ( 17.96484262340118221, 16.18868534415483396, -7.964842623401177768 ) ) ;
#90645=CARTESIAN_POINT ( 'NONE',  ( 17.96484262340118221, 19.93868534415484106, 7.964842623401181321 ) ) ;
#90646=B_SPLINE_CURVE_WITH_KNOTS ( 'NONE', 3,
 ( #92723, #76736, #47716, #24248, #2246, #69254, #54715, #23269, #92238, #1266 ),
 .UNSPECIFIED., .F., .F.,
 ( 4, 3, 3, 4 ),
 ( 7.757919228897728493E-18, 0.0006253016069560782611, 0.001250604074564933433, 0.002501455912506544803 ),
 .UNSPECIFIED. ) ;
#90647=CARTESIAN_POINT ( 'NONE',  ( 20.88017736071110875, 60.77201867748817676, -2.915334737309920765 ) ) ;
#90648=CARTESIAN_POINT ( 'NONE',  ( 22.81628187352647785, 46.41530133659708213, 3.434112377981063169 ) ) ;
#90651=LINE ( 'NONE', #21687, #49132 ) ;
#90657=CARTESIAN_POINT ( 'NONE',  ( -4.164238869374099039, 41.80374883491397497, 8.674139862899312516E-16 ) ) ;
#90658=CARTESIAN_POINT ( 'NONE',  ( 10.00000000000000178, 4.313685344154837509, 10.88017736071110342 ) ) ;
#90659=CARTESIAN_POINT ( 'NONE',  ( 19.84674366389459621, 23.50893115100078390, 7.409399052514197653E-17 ) ) ;
#90660=CARTESIAN_POINT ( 'NONE',  ( 2.791683348922240793, 41.63393115100078745, 7.208316651077764092 ) ) ;
#90661=CARTESIAN_POINT ( 'NONE',  ( 12.91533473730993009, 66.60535201082150536, -10.88017736071109987 ) ) ;
#90663=CARTESIAN_POINT ( 'NONE',  ( 5.076628168052704559, 0.1755978176674514724, -8.527530157486179263 ) ) ;
#90664=EDGE_CURVE ( 'NONE', #64876, #50256, #47727, .T. ) ;
#90668=CARTESIAN_POINT ( 'NONE',  ( 24.16423886937410614, 39.30374883491396787, 8.672049930838204340E-16 ) ) ;
#90670=CARTESIAN_POINT ( 'NONE',  ( 19.38216949554541202, 20.99863466993042138, 9.382169495545424454 ) ) ;
#90672=CARTESIAN_POINT ( 'NONE',  ( 0.6178305044545838731, 54.74863466993042493, 9.382169495545420901 ) ) ;
#90674=CARTESIAN_POINT ( 'NONE',  ( -0.8801773607111008646, 23.27201867748817676, 2.915334737309923430 ) ) ;
#90675=CARTESIAN_POINT ( 'NONE',  ( 1.472469842513823179, 30.59226448433411960, -4.923371831947296329 ) ) ;
#90676=CARTESIAN_POINT ( 'NONE',  ( 0.5774900079438590739, 22.64701867748817321, -5.440088680355550821 ) ) ;
#90679=CARTESIAN_POINT ( 'NONE',  ( 1.472469842513823179, 56.42559781766745886, 4.923371831947296329 ) ) ;
#90680=CARTESIAN_POINT ( 'NONE',  ( 0.1532563361054082862, 46.21726448433411605, 2.638427012816831674 ) ) ;
#90686=DIRECTION ( 'NONE',  ( 1.000000000000000000, 0.000000000000000000, 0.000000000000000000 ) ) ;
#90688=CARTESIAN_POINT ( 'NONE',  ( 10.00000000000000178, 37.25893115100078745, 9.846743663894594434 ) ) ;
#90690=CARTESIAN_POINT ( 'NONE',  ( 19.38216949554541202, 35.99863466993041072, 9.382169495545424454 ) ) ;
#90693=CARTESIAN_POINT ( 'NONE',  ( 5.076628168052703671, 61.84226448433412315, 8.527530157486179263 ) ) ;
#90695=CARTESIAN_POINT ( 'NONE',  ( 19.84674366389459266, 38.71726448433412315, -2.638427012816827677 ) ) ;
#90696=CARTESIAN_POINT ( 'NONE',  ( 20.36894250292379738, 34.92874883491396076, -10.36894250292379027 ) ) ;
#90697=CARTESIAN_POINT ( 'NONE',  ( 10.00000000000000000, 39.75893115100078745, -9.846743663894594434 ) ) ;
#90698=CARTESIAN_POINT ( 'NONE',  ( 22.81628187352647785, 51.62363466993042493, 6.195893100308588602E-16 ) ) ;
#90701=CARTESIAN_POINT ( 'NONE',  ( 19.84674366389459266, 3.300597817667451750, 2.638427012816836559 ) ) ;
#90702=CARTESIAN_POINT ( 'NONE',  ( -2.266590686148945544, 1.387082168247301128, -7.082119434687050408 ) ) ;
#90703=CARTESIAN_POINT ( 'NONE',  ( 17.20831665107776587, 44.13393115100078745, -7.208316651077762316 ) ) ;
#90704=CARTESIAN_POINT ( 'NONE',  ( 19.42250999205614193, 40.14701867748817676, 5.440088680355555262 ) ) ;
#90706=CARTESIAN_POINT ( 'NONE',  ( 17.20831665107776587, 42.88393115100077324, 7.208316651077764980 ) ) ;
#90709=CARTESIAN_POINT ( 'NONE',  ( 0.5774900079438590739, 52.64701867748817676, -5.440088680355550821 ) ) ;
#90712=CARTESIAN_POINT ( 'NONE',  ( -0.8801773607111008646, 18.27201867748817321, 2.915334737309923430 ) ) ;
#90713=CARTESIAN_POINT ( 'NONE',  ( 22.81628187352647785, 1.623634669930420271, 6.195893100308588602E-16 ) ) ;
#90714=CARTESIAN_POINT ( 'NONE',  ( -0.8801773607111008646, 48.27201867748816966, 2.915334737309923430 ) ) ;
#90715=CARTESIAN_POINT ( 'NONE',  ( -1.926860441876562247, 47.45379003517447813, -3.195792623639530650 ) ) ;
#90718=CARTESIAN_POINT ( 'NONE',  ( -0.8801773607110991993, 42.85535201082150536, -2.915334737309923874 ) ) ;
#90720=CARTESIAN_POINT ( 'NONE',  ( 0.1532563361054083140, 16.00893115100078390, 1.131784320476157264E-15 ) ) ;
#90721=CARTESIAN_POINT ( 'NONE',  ( 19.84674366389459266, 23.71726448433412315, -2.638427012816827677 ) ) ;
#90724=CARTESIAN_POINT ( 'NONE',  ( 10.00000000000000178, 62.25893115100078745, 9.846743663894594434 ) ) ;
#90725=CARTESIAN_POINT ( 'NONE',  ( 7.084665262690076126, 2.022018677488171434, -10.88017736071110164 ) ) ;
#90726=CARTESIAN_POINT ( 'NONE',  ( 0.1922240491738544388, 18.18878173731740944, 6.500000000000007105 ) ) ;
#90728=CARTESIAN_POINT ( 'NONE',  ( -4.164238869374099927, 17.01208216824730357, 3.795296366450308767 ) ) ;
#90729=CARTESIAN_POINT ( 'NONE',  ( 2.917880565312950480, 45.97041550158063927, -12.26659068614894821 ) ) ;
#90730=CIRCLE ( 'NONE', #52410, 2.999999999999999112 ) ;
#90731=CARTESIAN_POINT ( 'NONE',  ( 7.084665262690076126, 4.105352010821503583, 10.88017736071109987 ) ) ;
#90732=ORIENTED_EDGE ( 'NONE', *, *, #46756, .T. ) ;
#90733=CARTESIAN_POINT ( 'NONE',  ( 17.20831665107776587, 24.13393115100078035, -7.208316651077762316 ) ) ;
#90734=CARTESIAN_POINT ( 'NONE',  ( -0.8801773607111008646, 23.27201867748817676, 2.915334737309923430 ) ) ;
#90735=CARTESIAN_POINT ( 'NONE',  ( 2.791683348922237240, 55.38393115100078745, -7.208316651077763204 ) ) ;
#90736=CARTESIAN_POINT ( 'NONE',  ( 22.26659068614894466, 8.887082168247300018, 7.082119434687054849 ) ) ;
#90738=FACE_OUTER_BOUND ( 'NONE', #82957, .T. ) ;
#90739=CARTESIAN_POINT ( 'NONE',  ( 21.09922568453595559, 37.04030133659708923, -6.408140936763230044 ) ) ;
#90740=CARTESIAN_POINT ( 'NONE',  ( 2.791683348922237240, 40.38393115100078035, -7.208316651077763204 ) ) ;
#90742=CARTESIAN_POINT ( 'NONE',  ( 2.791683348922237240, 5.383931151000785675, -7.208316651077763204 ) ) ;
#90745=CARTESIAN_POINT ( 'NONE',  ( 12.91533473730992121, 14.52201867748817143, 10.88017736071110164 ) ) ;
#90746=CARTESIAN_POINT ( 'NONE',  ( 24.16423886937409904, 49.09541550158063217, 3.795296366450317205 ) ) ;
#90750=CARTESIAN_POINT ( 'NONE',  ( 17.20831665107776587, 27.88393115100078390, 7.208316651077764980 ) ) ;
#90751=CARTESIAN_POINT ( 'NONE',  ( -0.8801773607110991993, 12.85535201082150358, -2.915334737309923874 ) ) ;
#90752=CARTESIAN_POINT ( 'NONE',  ( 5.076628168052703671, 41.84226448433411605, 8.527530157486179263 ) ) ;
#90754=CARTESIAN_POINT ( 'NONE',  ( 1.472469842513823179, 51.42559781766745886, 4.923371831947296329 ) ) ;
#90756=CARTESIAN_POINT ( 'NONE',  ( 19.42250999205614548, 40.98035201082150536, -5.440088680355545492 ) ) ;
#90758=EDGE_CURVE ( 'NONE', #24281, #84653, #6138, .T. ) ;
#90762=CARTESIAN_POINT ( 'NONE',  ( -2.816281873526473856, 64.12363466993042493, 9.499525473075851096E-16 ) ) ;
#90764=CARTESIAN_POINT ( 'NONE',  ( 10.00000000000000000, 4.758931151000784787, -9.846743663894594434 ) ) ;
#90765=CARTESIAN_POINT ( 'NONE',  ( 22.81628187352647785, 61.41530133659709634, 3.434112377981063169 ) ) ;
#90766=CARTESIAN_POINT ( 'NONE',  ( 17.96484262340118221, 4.938685344154837509, 7.964842623401181321 ) ) ;
#90767=CARTESIAN_POINT ( 'NONE',  ( 1.472469842513823179, 31.42559781766745530, 4.923371831947296329 ) ) ;
#90768=CARTESIAN_POINT ( 'NONE',  ( -12.69000000000001371, 93.50000000000000000, -9.500000000000000000 ) ) ;
#90770=DIRECTION ( 'NONE',  ( 0.000000000000000000, 0.000000000000000000, 1.000000000000000000 ) ) ;
#90771=CARTESIAN_POINT ( 'NONE',  ( 2.917880565312950480, 50.97041550158064638, -12.26659068614894821 ) ) ;
#90772=CARTESIAN_POINT ( 'NONE',  ( 0.1532563361054100626, 50.80059781766745175, -2.638427012816831230 ) ) ;
#90774=CARTESIAN_POINT ( 'NONE',  ( 15.44008868035555260, 34.73035201082151247, 9.422509992056143702 ) ) ;
#90775=CARTESIAN_POINT ( 'NONE',  ( 5.076628168052704559, 5.175597817667451750, -8.527530157486179263 ) ) ;
#90777=CARTESIAN_POINT ( 'NONE',  ( 0.6178305044545838731, 59.74863466993041783, 9.382169495545420901 ) ) ;
#90780=CARTESIAN_POINT ( 'NONE',  ( 7.361572987183170547, 2.050597817667451750, 9.846743663894590881 ) ) ;
#90782=CARTESIAN_POINT ( 'NONE',  ( 2.917880565312950480, 0.9704155015806342766, -12.26659068614894821 ) ) ;
#90783=CARTESIAN_POINT ( 'NONE',  ( 0.1532563361054100626, 5.800597817667452638, -2.638427012816831230 ) ) ;
#90784=CARTESIAN_POINT ( 'NONE',  ( 0.5774900079438590739, 32.64701867748816966, -5.440088680355550821 ) ) ;
#90787=CARTESIAN_POINT ( 'NONE',  ( -0.8801773607111009756, 28.06368534415484106, 1.068504757029289695E-15 ) ) ;
#90789=CARTESIAN_POINT ( 'NONE',  ( 10.00000000000000000, 31.81368534415483751, -10.88017736071110342 ) ) ;
#90791=ORIENTED_EDGE ( 'NONE', *, *, #93727, .F. ) ;
#90794=CARTESIAN_POINT ( 'NONE',  ( 3.591859063236763294, 13.29030133659708746, -11.09922568453595026 ) ) ;
#90795=CARTESIAN_POINT ( 'NONE',  ( 10.00000000000000178, 2.258931151000784787, 9.846743663894594434 ) ) ;
#90797=CARTESIAN_POINT ( 'NONE',  ( 19.42250999205614193, 20.14701867748817321, 5.440088680355555262 ) ) ;
#90798=CARTESIAN_POINT ( 'NONE',  ( 19.80448550324507551, 6.827036817733427299, 6.500000000002767564 ) ) ;
#90799=CARTESIAN_POINT ( 'NONE',  ( -0.8801773607111008646, 68.27201867748817676, 2.915334737309923430 ) ) ;
#90800=CARTESIAN_POINT ( 'NONE',  ( 15.44008868035555793, 31.39701867748817676, -9.422509992056140149 ) ) ;
#90802=CARTESIAN_POINT ( 'NONE',  ( 13.43411237798105340, 50.58196800326375353, 12.81628187352647963 ) ) ;
#90803=CARTESIAN_POINT ( 'NONE',  ( 2.035157376598824452, 48.68868534415483396, 7.964842623401179544 ) ) ;
#90804=CARTESIAN_POINT ( 'NONE',  ( -1.099225684535947600, 49.54030133659708923, 6.408140936763237150 ) ) ;
#90805=CARTESIAN_POINT ( 'NONE',  ( 19.42250999205614193, 45.14701867748817676, 5.440088680355555262 ) ) ;
#90806=CARTESIAN_POINT ( 'NONE',  ( 22.81628187352648496, 1.831968003263753753, -3.434112377981050290 ) ) ;
#90807=SURFACE_SIDE_STYLE ('',( #91300 ) ) ;
#90808=CARTESIAN_POINT ( 'NONE',  ( 0.1532563361054100626, 15.80059781766745353, -2.638427012816831230 ) ) ;
#90809=CARTESIAN_POINT ( 'NONE',  ( 3.591859063236761518, 59.95696800326375353, 11.09922568453594849 ) ) ;
#90811=CARTESIAN_POINT ( 'NONE',  ( 7.361572987183170547, 12.05059781766744997, 9.846743663894590881 ) ) ;
#90812=CARTESIAN_POINT ( 'NONE',  ( 21.09922568453594849, 1.206968003263753531, 6.408140936763242479 ) ) ;
#90813=CARTESIAN_POINT ( 'NONE',  ( 14.92337183194729988, 64.34226448433412315, -8.527530157486177487 ) ) ;
#90814=CARTESIAN_POINT ( 'NONE',  ( -0.8801773607111009756, 38.06368534415484106, 1.068504757029289695E-15 ) ) ;
#90815=CARTESIAN_POINT ( 'NONE',  ( 0.1532563361054082862, 51.21726448433412315, 2.638427012816831674 ) ) ;
#90817=CARTESIAN_POINT ( 'NONE',  ( 19.84674366389459266, 23.71726448433412315, -2.638427012816827677 ) ) ;
#90818=CARTESIAN_POINT ( 'NONE',  ( 1.472469842513823179, 11.42559781766745175, 4.923371831947296329 ) ) ;
#90820=CARTESIAN_POINT ( 'NONE',  ( 13.43411237798105340, 5.581968003263753531, 12.81628187352647963 ) ) ;
#90821=ORIENTED_EDGE ( 'NONE', *, *, #23539, .F. ) ;
#90823=CARTESIAN_POINT ( 'NONE',  ( 19.42250999205614548, 5.980352010821504471, -5.440088680355545492 ) ) ;
#90825=CARTESIAN_POINT ( 'NONE',  ( 17.20831665107776587, 64.13393115100079456, -7.208316651077762316 ) ) ;
#90827=CARTESIAN_POINT ( 'NONE',  ( 20.88017736071110164, 5.355352010821503583, 2.915334737309930979 ) ) ;
#90828=CARTESIAN_POINT ( 'NONE',  ( 10.00000000000000178, 42.25893115100078745, 9.846743663894594434 ) ) ;
#90831=CARTESIAN_POINT ( 'NONE',  ( -2.266590686148945544, 66.38708216824730357, -7.082119434687050408 ) ) ;
#90833=CARTESIAN_POINT ( 'NONE',  ( 19.42250999205614548, 30.98035201082150536, -5.440088680355545492 ) ) ;
#90834=CARTESIAN_POINT ( 'NONE',  ( 10.00000000000000000, 45.55374883491397497, -14.16423886937410082 ) ) ;
#90835=CARTESIAN_POINT ( 'NONE',  ( 0.5774900079438607392, 3.480352010821504916, 5.440088680355550821 ) ) ;
#90837=CARTESIAN_POINT ( 'NONE',  ( 2.791683348922240793, 26.63393115100078745, 7.208316651077764092 ) ) ;
#90838=CARTESIAN_POINT ( 'NONE',  ( 10.00000000000000178, 10.37363466993041961, 12.81628187352647608 ) ) ;
#90842=CARTESIAN_POINT ( 'NONE',  ( -4.164238869374099039, 6.803748834913967869, 8.674139862899312516E-16 ) ) ;
#90843=CARTESIAN_POINT ( 'NONE',  ( 0.1532563361054100626, 25.80059781766744820, -2.638427012816831230 ) ) ;
#90844=B_SPLINE_CURVE_WITH_KNOTS ( 'NONE', 3,
 ( #26767, #21248, #82230, #64749, #95261, #57261, #87756, #19270, #49754, #6736, #15735, #83722, #22737, #30700 ),
 .UNSPECIFIED., .F., .F.,
 ( 4, 2, 2, 2, 2, 2, 4 ),
 ( 0.000000000000000000, 0.004797171936611957510, 0.007195757904917936265, 0.009594343873223915020, 0.01199292984152989378, 0.01439151580983587253, 0.01918868774644783004 ),
 .UNSPECIFIED. ) ;
#90846=CARTESIAN_POINT ( 'NONE',  ( 10.00000000000000000, 45.55374883491397497, -14.16423886937410082 ) ) ;
#90847=CARTESIAN_POINT ( 'NONE',  ( 12.63842701281683922, 14.55059781766744997, -9.846743663894590881 ) ) ;
#90849=FACE_OUTER_BOUND ( 'NONE', #44789, .T. ) ;
#90850=CARTESIAN_POINT ( 'NONE',  ( 10.00000000000000000, 26.81368534415484106, -10.88017736071110342 ) ) ;
#90851=CARTESIAN_POINT ( 'NONE',  ( 21.09922568453595559, 57.04030133659708923, -6.408140936763230044 ) ) ;
#90852=CARTESIAN_POINT ( 'NONE',  ( 15.44008868035555260, 4.730352010821504471, 9.422509992056143702 ) ) ;
#90853=CARTESIAN_POINT ( 'NONE',  ( 16.40814093676323893, 40.79030133659708923, 11.09922568453595026 ) ) ;
#90854=CARTESIAN_POINT ( 'NONE',  ( 14.92337183194729633, 7.675597817667451750, 8.527530157486181039 ) ) ;
#90857=CARTESIAN_POINT ( 'NONE',  ( 19.72487221294570148, 35.71833443783938833, -6.500000000000010658 ) ) ;
#90858=CARTESIAN_POINT ( 'NONE',  ( 17.08211943468705840, 40.13708216824731068, -12.26659068614894466 ) ) ;
#90859=CARTESIAN_POINT ( 'NONE',  ( 20.36894250292379382, 13.67874883491396965, 10.36894250292379205 ) ) ;
#90860=CARTESIAN_POINT ( 'NONE',  ( 20.88017736071110164, 10.35535201082150714, 2.915334737309930979 ) ) ;
#90861=CARTESIAN_POINT ( 'NONE',  ( 7.084665262690076126, 27.02201867748817676, -10.88017736071110164 ) ) ;
#90863=STYLED_ITEM ( 'NONE', ( #79070 ), #3977 ) ;
#90865=CARTESIAN_POINT ( 'NONE',  ( 4.559911319644449179, 52.23035201082151247, -9.422509992056141925 ) ) ;
#90866=CARTESIAN_POINT ( 'NONE',  ( 17.96484262340118221, 61.18868534415482685, -7.964842623401177768 ) ) ;
#90867=CARTESIAN_POINT ( 'NONE',  ( 10.00000000000000178, 20.37363466993042138, 12.81628187352647608 ) ) ;
#90869=CARTESIAN_POINT ( 'NONE',  ( 19.80448550324510038, 26.82703681773341131, 6.500000000002802203 ) ) ;
#90870=CARTESIAN_POINT ( 'NONE',  ( 0.1532563361054082862, 41.21726448433411605, 2.638427012816831674 ) ) ;
#90873=CARTESIAN_POINT ( 'NONE',  ( 21.09922568453594849, 16.20696800326375353, 6.408140936763242479 ) ) ;
#90874=CARTESIAN_POINT ( 'NONE',  ( 7.084665262690076126, 4.105352010821503583, 10.88017736071109987 ) ) ;
#90875=ADVANCED_FACE ( 'NONE', ( #47107 ), #40614, .T. ) ;
#90877=CARTESIAN_POINT ( 'NONE',  ( 14.92337183194729988, 39.34226448433412315, -8.527530157486177487 ) ) ;
#90878=LINE ( 'NONE', #7410, #80210 ) ;
#90879=CARTESIAN_POINT ( 'NONE',  ( 14.92337183194729988, 14.34226448433411782, -8.527530157486177487 ) ) ;
#90880=CARTESIAN_POINT ( 'NONE',  ( 20.36894250292379382, 3.678748834913967869, 10.36894250292379205 ) ) ;
#90881=CARTESIAN_POINT ( 'NONE',  ( 19.42250999205614193, 30.14701867748817321, 5.440088680355555262 ) ) ;
#90882=CARTESIAN_POINT ( 'NONE',  ( 4.559911319644449179, 27.23035201082150536, -9.422509992056141925 ) ) ;
#90884=CARTESIAN_POINT ( 'NONE',  ( 24.16423886937410614, 29.30374883491396787, 8.672049930838204340E-16 ) ) ;
#90885=CARTESIAN_POINT ( 'NONE',  ( 18.52753015748617571, 38.09226448433412315, 4.923371831947298993 ) ) ;
#90886=CARTESIAN_POINT ( 'NONE',  ( 15.44008868035555793, 31.39701867748817676, -9.422509992056140149 ) ) ;
#90887=CARTESIAN_POINT ( 'NONE',  ( 17.96484262340118221, 21.18868534415483396, -7.964842623401177768 ) ) ;
#90888=ORIENTED_EDGE ( 'NONE', *, *, #93713, .F. ) ;
#90889=CARTESIAN_POINT ( 'NONE',  ( 4.559911319644449179, 23.89701867748817321, 9.422509992056141925 ) ) ;
#90890=AXIS2_PLACEMENT_3D ( 'NONE', #7569, #21070, #67563 ) ;
#90891=CARTESIAN_POINT ( 'NONE',  ( -1.099225684535947600, 44.54030133659708923, 6.408140936763237150 ) ) ;
#90892=CARTESIAN_POINT ( 'NONE',  ( 2.035157376598822676, 47.43868534415484817, -7.964842623401177768 ) ) ;
#90894=CARTESIAN_POINT ( 'NONE',  ( 15.44008868035555793, 56.39701867748817676, -9.422509992056140149 ) ) ;
#90895=ORIENTED_EDGE ( 'NONE', *, *, #66820, .F. ) ;
#90896=CARTESIAN_POINT ( 'NONE',  ( 14.92337183194729633, 57.67559781766745886, 8.527530157486181039 ) ) ;
#90897=CARTESIAN_POINT ( 'NONE',  ( 15.44008868035555260, 39.73035201082150536, 9.422509992056143702 ) ) ;
#90901=CARTESIAN_POINT ( 'NONE',  ( -2.266590686148945544, 47.22041550158063927, 7.082119434687048631 ) ) ;
#90902=CARTESIAN_POINT ( 'NONE',  ( 4.559911319644449179, 52.23035201082151247, -9.422509992056141925 ) ) ;
#90904=SURFACE_SIDE_STYLE ('',( #60899 ) ) ;
#90905=CARTESIAN_POINT ( 'NONE',  ( 7.361572987183169658, 59.96726448433410894, -9.846743663894592657 ) ) ;
#90906=CARTESIAN_POINT ( 'NONE',  ( 18.52753015748617571, 28.09226448433411960, 4.923371831947298993 ) ) ;
#90909=CARTESIAN_POINT ( 'NONE',  ( 12.63842701281683034, 32.46726448433412315, 9.846743663894596210 ) ) ;
#90911=CARTESIAN_POINT ( 'NONE',  ( 2.035157376598824452, 23.68868534415484461, 7.964842623401179544 ) ) ;
#90912=CARTESIAN_POINT ( 'NONE',  ( 2.791683348922240793, 41.63393115100078745, 7.208316651077764092 ) ) ;
#90914=CARTESIAN_POINT ( 'NONE',  ( 2.035157376598824452, 28.68868534415484106, 7.964842623401179544 ) ) ;
#90915=CARTESIAN_POINT ( 'NONE',  ( 17.08211943468705130, 43.47041550158063927, 12.26659068614894998 ) ) ;
#90917=CARTESIAN_POINT ( 'NONE',  ( 1.472469842513823179, 51.42559781766745886, 4.923371831947296329 ) ) ;
#90918=VERTEX_POINT ( 'NONE', #2640 ) ;
#90919=CARTESIAN_POINT ( 'NONE',  ( 0.6178305044545818747, 18.49863466993041428, -9.382169495545419124 ) ) ;
#90920=CARTESIAN_POINT ( 'NONE',  ( -0.8801773607111009756, 13.06368534415483929, 1.068504757029289695E-15 ) ) ;
#90921=CARTESIAN_POINT ( 'NONE',  ( 2.035157376598822676, 47.43868534415484817, -7.964842623401177768 ) ) ;
#90922=DIRECTION ( 'NONE',  ( 0.000000000000000000, 0.000000000000000000, -1.000000000000000000 ) ) ;
#90925=CARTESIAN_POINT ( 'NONE',  ( -0.8801773607111009756, 58.06368534415484106, 1.068504757029289695E-15 ) ) ;
#90926=CARTESIAN_POINT ( 'NONE',  ( 0.1532563361054083140, 41.00893115100078745, 1.131784320476157264E-15 ) ) ;
#90927=CARTESIAN_POINT ( 'NONE',  ( 0.1532563361054082862, 21.21726448433412315, 2.638427012816831674 ) ) ;
#90928=CARTESIAN_POINT ( 'NONE',  ( 1.472469842513823179, 11.42559781766745175, 4.923371831947296329 ) ) ;
#90931=CARTESIAN_POINT ( 'NONE',  ( 22.81628187352647785, 41.41530133659708923, 3.434112377981063169 ) ) ;
#90932=CARTESIAN_POINT ( 'NONE',  ( 10.00000000000000000, 19.75893115100078390, -9.846743663894594434 ) ) ;
#90933=CARTESIAN_POINT ( 'NONE',  ( 0.9413316022086128942, 33.45508385108959004, 6.499999999999978684 ) ) ;
#90934=LINE ( 'NONE', #92418, #2660 ) ;
#90935=CARTESIAN_POINT ( 'NONE',  ( 0.1532563361054100626, 35.80059781766745175, -2.638427012816831230 ) ) ;
#90937=CARTESIAN_POINT ( 'NONE',  ( 21.92686044187656691, 17.18830936912750929, 4.562052436263911564E-16 ) ) ;
#90938=CARTESIAN_POINT ( 'NONE',  ( 21.09922568453595559, 12.04030133659708746, -6.408140936763230044 ) ) ;
#90939=CARTESIAN_POINT ( 'NONE',  ( 17.96484262340118221, 49.93868534415484106, 7.964842623401181321 ) ) ;
#90940=CARTESIAN_POINT ( 'NONE',  ( -0.3689425029237898834, 31.17874883491396787, -10.36894250292378850 ) ) ;
#90942=CARTESIAN_POINT ( 'NONE',  ( 6.204703633549690345, 32.84541550158063927, 14.16423886937410082 ) ) ;
#90943=CARTESIAN_POINT ( 'NONE',  ( -4.164238869374099927, 52.01208216824729647, 3.795296366450308767 ) ) ;
#90945=CARTESIAN_POINT ( 'NONE',  ( 17.08211943468705840, 5.137082168247300906, -12.26659068614894466 ) ) ;
#90946=CARTESIAN_POINT ( 'NONE',  ( 6.204703633549690345, 27.84541550158063217, 14.16423886937410082 ) ) ;
#90948=CARTESIAN_POINT ( 'NONE',  ( 20.88017736071110164, 50.35535201082151247, 2.915334737309930979 ) ) ;
#90950=CARTESIAN_POINT ( 'NONE',  ( 1.472469842513823179, 35.59226448433412315, -4.923371831947296329 ) ) ;
#90951=CARTESIAN_POINT ( 'NONE',  ( 18.52753015748617571, 48.09226448433412315, 4.923371831947298993 ) ) ;
#90952=CARTESIAN_POINT ( 'NONE',  ( -0.8801773607110991993, 22.85535201082150181, -2.915334737309923874 ) ) ;
#90953=CARTESIAN_POINT ( 'NONE',  ( 22.81628187352647785, 61.41530133659709634, 3.434112377981063169 ) ) ;
#90955=EDGE_CURVE ( 'NONE', #53414, #88480, #28685, .T. ) ;
#90956=CARTESIAN_POINT ( 'NONE',  ( 20.00000000000000711, 80.90097674908675174, -4.954892789988381452 ) ) ;
#90957=CARTESIAN_POINT ( 'NONE',  ( 17.20831665107776587, 27.88393115100078390, 7.208316651077764980 ) ) ;
#90958=CARTESIAN_POINT ( 'NONE',  ( 22.81628187352648496, 61.83196800326376774, -3.434112377981050290 ) ) ;
#90960=CARTESIAN_POINT ( 'NONE',  ( -0.8801773607111009756, 43.06368534415484106, 1.068504757029289695E-15 ) ) ;
#90961=CARTESIAN_POINT ( 'NONE',  ( 19.84674366389459266, 48.71726448433413026, -2.638427012816827677 ) ) ;
#90962=CARTESIAN_POINT ( 'NONE',  ( 24.16423886937410614, 44.30374883491397497, 8.672049930838204340E-16 ) ) ;
#90963=ORIENTED_EDGE ( 'NONE', *, *, #75189, .T. ) ;
#90964=CARTESIAN_POINT ( 'NONE',  ( -4.164238869374099039, 1.803748834913967647, 8.674139862899312516E-16 ) ) ;
#90965=CARTESIAN_POINT ( 'NONE',  ( 2.035157376598822676, 62.43868534415483396, -7.964842623401177768 ) ) ;
#90966=CARTESIAN_POINT ( 'NONE',  ( 17.96484262340118221, 66.18868534415483396, -7.964842623401177768 ) ) ;
#90967=CARTESIAN_POINT ( 'NONE',  ( 6.204703633549690345, 65.76208216824731778, -14.16423886937410259 ) ) ;
#90968=CARTESIAN_POINT ( 'NONE',  ( 3.591859063236761518, 9.956968003263753531, 11.09922568453594849 ) ) ;
#90970=CARTESIAN_POINT ( 'NONE',  ( -0.8801773607111008646, 53.27201867748816966, 2.915334737309923430 ) ) ;
#90971=CARTESIAN_POINT ( 'NONE',  ( 0.1077916266722474120, 27.24062864464240619, -6.478736007405939468 ) ) ;
#90974=CARTESIAN_POINT ( 'NONE',  ( -2.266590686148945544, 51.38708216824730357, -7.082119434687050408 ) ) ;
#90976=CARTESIAN_POINT ( 'NONE',  ( 20.88017736071110875, 10.77201867748817143, -2.915334737309920765 ) ) ;
#90977=CARTESIAN_POINT ( 'NONE',  ( 20.88017736071110164, 20.35535201082150891, 2.915334737309930979 ) ) ;
#90978=CARTESIAN_POINT ( 'NONE',  ( 17.20831665107776587, 57.88393115100078745, 7.208316651077764980 ) ) ;
#90979=CARTESIAN_POINT ( 'NONE',  ( 0.6178305044545818747, 53.49863466993041072, -9.382169495545419124 ) ) ;
#90983=VECTOR ( 'NONE', #26959, 1000.000000000000000 ) ;
#90984=CARTESIAN_POINT ( 'NONE',  ( 10.00000000000000000, 11.81368534415483751, -10.88017736071110342 ) ) ;
#90985=CARTESIAN_POINT ( 'NONE',  ( 3.591859063236761518, 24.95696800326375353, 11.09922568453594849 ) ) ;
#90986=CARTESIAN_POINT ( 'NONE',  ( 19.72487221294571569, 39.78217586085237656, 6.499999999999986677 ) ) ;
#90987=ADVANCED_FACE ( 'NONE', ( #63587 ), #77607, .F. ) ;
#90988=CARTESIAN_POINT ( 'NONE',  ( 1.472469842513823179, 50.59226448433411605, -4.923371831947296329 ) ) ;
#90989=CARTESIAN_POINT ( 'NONE',  ( 19.42250999205614548, 30.98035201082150536, -5.440088680355545492 ) ) ;
#90991=CARTESIAN_POINT ( 'NONE',  ( 13.43411237798105340, 20.58196800326374643, 12.81628187352647963 ) ) ;
#90992=CARTESIAN_POINT ( 'NONE',  ( 12.91533473730993009, 46.60535201082150536, -10.88017736071109987 ) ) ;
#90994=DIRECTION ( 'NONE',  ( 0.000000000000000000, 1.000000000000000000, 0.000000000000000000 ) ) ;
#90995=CARTESIAN_POINT ( 'NONE',  ( 13.43411237798105340, 50.58196800326375353, 12.81628187352647963 ) ) ;
#90997=CARTESIAN_POINT ( 'NONE',  ( 20.88017736071110875, 50.77201867748817676, -2.915334737309920765 ) ) ;
#90998=CARTESIAN_POINT ( 'NONE',  ( 16.40814093676324603, 32.45696800326375353, -11.09922568453594671 ) ) ;
#90999=CARTESIAN_POINT ( 'NONE',  ( -0.3689425029237898834, 1.178748834913967869, -10.36894250292378850 ) ) ;
#91000=CARTESIAN_POINT ( 'NONE',  ( 17.20831665107776587, 4.133931151000785675, -7.208316651077762316 ) ) ;
#91001=CARTESIAN_POINT ( 'NONE',  ( 0.5774900079438607392, 53.48035201082151247, 5.440088680355550821 ) ) ;
#91003=CARTESIAN_POINT ( 'NONE',  ( 5.076628168052703671, 61.84226448433412315, 8.527530157486179263 ) ) ;
#91004=CARTESIAN_POINT ( 'NONE',  ( 7.361572987183169658, 14.96726448433411960, -9.846743663894592657 ) ) ;
#91005=CARTESIAN_POINT ( 'NONE',  ( 12.63842701281683034, 2.467264484334118269, 9.846743663894596210 ) ) ;
#91007=CARTESIAN_POINT ( 'NONE',  ( 24.16423886937410614, 39.30374883491396787, 8.672049930838204340E-16 ) ) ;
#91009=CARTESIAN_POINT ( 'NONE',  ( -0.8801773607110991993, 2.855352010821504471, -2.915334737309923874 ) ) ;
#91012=CARTESIAN_POINT ( 'NONE',  ( 17.96484262340118221, 6.188685344154837509, -7.964842623401177768 ) ) ;
#91013=CARTESIAN_POINT ( 'NONE',  ( 20.36894250292379738, 64.92874883491397497, -10.36894250292379027 ) ) ;
#91014=CARTESIAN_POINT ( 'NONE',  ( 18.52753015748617571, 48.09226448433412315, 4.923371831947298993 ) ) ;
#91015=CARTESIAN_POINT ( 'NONE',  ( 10.00000000000000178, 40.37363466993042493, 12.81628187352647608 ) ) ;
#91018=CARTESIAN_POINT ( 'NONE',  ( -4.164238869374098151, 6.595415501580634832, -3.795296366450310543 ) ) ;
#91019=CARTESIAN_POINT ( 'NONE',  ( 19.42250999205614193, 15.14701867748817143, 5.440088680355555262 ) ) ;
#91020=ADVANCED_FACE ( 'NONE', ( #25617 ), #56110, .T. ) ;
#91021=CARTESIAN_POINT ( 'NONE',  ( -0.3689425029237881626, 57.42874883491397497, 10.36894250292379027 ) ) ;
#91023=CARTESIAN_POINT ( 'NONE',  ( 5.076628168052703671, 36.84226448433412315, 8.527530157486179263 ) ) ;
#91025=CARTESIAN_POINT ( 'NONE',  ( 17.20831665107776587, 24.13393115100078035, -7.208316651077762316 ) ) ;
#91026=B_SPLINE_CURVE_WITH_KNOTS ( 'NONE', 3,
 ( #5236, #35713, #96735, #28209, #58708, #68686 ),
 .UNSPECIFIED., .F., .F.,
 ( 4, 2, 4 ),
 ( 0.000000000000000000, 0.0002605067024380912843, 0.0005210134048761825686 ),
 .UNSPECIFIED. ) ;
#91027=EDGE_CURVE ( 'NONE', #39498, #58781, #6033, .T. ) ;
#91028=SURFACE_STYLE_FILL_AREA ( #16531 ) ;
#91034=CARTESIAN_POINT ( 'NONE',  ( 12.63842701281683034, 52.46726448433413026, 9.846743663894596210 ) ) ;
#91035=CARTESIAN_POINT ( 'NONE',  ( 10.00000000000000000, 15.55374883491396787, -14.16423886937410082 ) ) ;
#91036=CARTESIAN_POINT ( 'NONE',  ( 2.035157376598824452, 33.68868534415484106, 7.964842623401179544 ) ) ;
#91037=CARTESIAN_POINT ( 'NONE',  ( 12.91533473730992121, 34.52201867748817676, 10.88017736071110164 ) ) ;
#91038=CARTESIAN_POINT ( 'NONE',  ( 12.63842701281683922, 64.55059781766745175, -9.846743663894590881 ) ) ;
#91039=CARTESIAN_POINT ( 'NONE',  ( 21.09922568453595559, 37.04030133659708923, -6.408140936763230044 ) ) ;
#91040=CARTESIAN_POINT ( 'NONE',  ( 22.26659068614895176, 9.720415501580633943, -7.082119434687042414 ) ) ;
#91041=CARTESIAN_POINT ( 'NONE',  ( 7.084665262690076126, 67.02201867748817676, -10.88017736071110164 ) ) ;
#91042=CARTESIAN_POINT ( 'NONE',  ( 19.38216949554541557, 32.24863466993041783, -9.382169495545420901 ) ) ;
#91043=VERTEX_POINT ( 'NONE', #94585 ) ;
#91044=CARTESIAN_POINT ( 'NONE',  ( 10.00000000000000000, 39.75893115100078745, -9.846743663894594434 ) ) ;
#91045=CARTESIAN_POINT ( 'NONE',  ( 7.084665262690076126, 2.022018677488171434, -10.88017736071110164 ) ) ;
#91046=VERTEX_POINT ( 'NONE', #56596 ) ;
#91047=CARTESIAN_POINT ( 'NONE',  ( 4.559911319644449179, 12.23035201082150714, -9.422509992056141925 ) ) ;
#91049=CARTESIAN_POINT ( 'NONE',  ( 7.084665262690076126, 57.02201867748817676, -10.88017736071110164 ) ) ;
#91051=CARTESIAN_POINT ( 'NONE',  ( 12.91533473730993009, 56.60535201082151247, -10.88017736071109987 ) ) ;
#91052=CARTESIAN_POINT ( 'NONE',  ( -0.8801773607111008646, 58.27201867748816966, 2.915334737309923430 ) ) ;
#91053=( NAMED_UNIT ( * ) SI_UNIT ( $, .STERADIAN. ) SOLID_ANGLE_UNIT ( ) );
#91054=CARTESIAN_POINT ( 'NONE',  ( -0.8801773607111009756, 48.06368534415484817, 1.068504757029289695E-15 ) ) ;
#91056=CARTESIAN_POINT ( 'NONE',  ( -46.94000000000001194, 100.4376529975699981, 9.000000000001183054 ) ) ;
#91057=CARTESIAN_POINT ( 'NONE',  ( -46.50435961404672014, 102.7681846068616238, 6.785878169524574233 ) ) ;
#91060=CARTESIAN_POINT ( 'NONE',  ( 18.52753015748617571, 48.09226448433412315, 4.923371831947298993 ) ) ;
#91061=ORIENTED_EDGE ( 'NONE', *, *, #67539, .T. ) ;
#91063=SURFACE_STYLE_USAGE ( .BOTH. , #91571 ) ;
#91064=CARTESIAN_POINT ( 'NONE',  ( 24.16423886937409904, 4.095415501580634832, 3.795296366450317205 ) ) ;
#91067=CARTESIAN_POINT ( 'NONE',  ( 20.88017736071110875, 60.77201867748817676, -2.915334737309920765 ) ) ;
#91068=CARTESIAN_POINT ( 'NONE',  ( 12.91533473730992121, 4.522018677488170546, 10.88017736071110164 ) ) ;
#91070=CARTESIAN_POINT ( 'NONE',  ( -2.816281873526471635, 43.91530133659708923, -3.434112377981056508 ) ) ;
#91073=CARTESIAN_POINT ( 'NONE',  ( 7.361572987183170547, 47.05059781766745175, 9.846743663894590881 ) ) ;
#91074=SURFACE_STYLE_USAGE ( .BOTH. , #92067 ) ;
#91075=CARTESIAN_POINT ( 'NONE',  ( 3.591859063236763294, 23.29030133659708568, -11.09922568453595026 ) ) ;
#91076=CARTESIAN_POINT ( 'NONE',  ( 7.361572987183170547, 22.05059781766745530, 9.846743663894590881 ) ) ;
#91079=CARTESIAN_POINT ( 'NONE',  ( 18.52753015748618282, 18.92559781766745175, -4.923371831947291888 ) ) ;
#91080=CARTESIAN_POINT ( 'NONE',  ( 2.791683348922237240, 65.38393115100078035, -7.208316651077763204 ) ) ;
#91084=VERTEX_POINT ( 'NONE', #95071 ) ;
#91085=CARTESIAN_POINT ( 'NONE',  ( 19.42250999205614193, 20.14701867748817321, 5.440088680355555262 ) ) ;
#91086=CARTESIAN_POINT ( 'NONE',  ( 10.00000000000000178, 23.05374883491397142, 14.16423886937410082 ) ) ;
#91087=CARTESIAN_POINT ( 'NONE',  ( 5.076628168052703671, 26.84226448433411960, 8.527530157486179263 ) ) ;
#91088=CARTESIAN_POINT ( 'NONE',  ( 10.00000000000000000, 4.758931151000784787, -9.846743663894594434 ) ) ;
#91089=CARTESIAN_POINT ( 'NONE',  ( 13.43411237798105340, 40.58196800326375353, 12.81628187352647963 ) ) ;
#91091=CARTESIAN_POINT ( 'NONE',  ( 2.035157376598822676, 17.43868534415483751, -7.964842623401177768 ) ) ;
#91093=CARTESIAN_POINT ( 'NONE',  ( -2.816281873526473856, 9.123634669930421381, 9.499525473075851096E-16 ) ) ;
#91094=CARTESIAN_POINT ( 'NONE',  ( 22.81628187352647785, 6.623634669930420493, 6.195893100308588602E-16 ) ) ;
#91095=CARTESIAN_POINT ( 'NONE',  ( 14.92337183194729633, 32.67559781766745175, 8.527530157486181039 ) ) ;
#91097=CARTESIAN_POINT ( 'NONE',  ( -1.099225684535947600, 39.54030133659708923, 6.408140936763237150 ) ) ;
#91099=CARTESIAN_POINT ( 'NONE',  ( 4.559911319644449179, 38.89701867748817676, 9.422509992056141925 ) ) ;
#91102=CARTESIAN_POINT ( 'NONE',  ( 20.15039907845753220, 20.60158574516643171, -6.262539305110077947 ) ) ;
#91103=CARTESIAN_POINT ( 'NONE',  ( 12.91533473730992121, 39.52201867748817676, 10.88017736071110164 ) ) ;
#91105=CARTESIAN_POINT ( 'NONE',  ( 20.88017736071110519, 40.56368534415484106, 2.639326808657452039E-16 ) ) ;
#91106=CARTESIAN_POINT ( 'NONE',  ( 19.84674366389459266, 58.71726448433411605, -2.638427012816827677 ) ) ;
#91107=ADVANCED_FACE ( 'NONE', ( #57078 ), #70124, .T. ) ;
#91108=CARTESIAN_POINT ( 'NONE',  ( -0.8801773607111009756, 68.06368534415484817, 1.068504757029289695E-15 ) ) ;
#91111=CARTESIAN_POINT ( 'NONE',  ( 7.361572987183170547, 57.05059781766744464, 9.846743663894590881 ) ) ;
#91112=CARTESIAN_POINT ( 'NONE',  ( 4.559911319644449179, 7.230352010821504471, -9.422509992056141925 ) ) ;
#91115=CARTESIAN_POINT ( 'NONE',  ( 16.40814093676323893, 10.79030133659708923, 11.09922568453595026 ) ) ;
#91117=CARTESIAN_POINT ( 'NONE',  ( 0.5774900079438607392, 43.48035201082151247, 5.440088680355550821 ) ) ;
#91118=CARTESIAN_POINT ( 'NONE',  ( 1.274849032794199255, 23.57228050351030646, 6.499999999999850786 ) ) ;
#91119=CARTESIAN_POINT ( 'NONE',  ( 0.5774900079438607392, 3.480352010821504027, 5.440088680355550821 ) ) ;
#91121=CARTESIAN_POINT ( 'NONE',  ( 0.5774900079438607392, 28.48035201082150891, 5.440088680355550821 ) ) ;
#91122=CARTESIAN_POINT ( 'NONE',  ( 19.84674366389459621, 13.50893115100078568, 7.409399052514197653E-17 ) ) ;
#91123=CARTESIAN_POINT ( 'NONE',  ( 20.36894250292379738, 34.92874883491396076, -10.36894250292379027 ) ) ;
#91124=CARTESIAN_POINT ( 'NONE',  ( 0.1532563361054083140, 26.00893115100078745, 1.131784320476157264E-15 ) ) ;
#91125=CARTESIAN_POINT ( 'NONE',  ( 19.42250999205614548, 50.98035201082151247, -5.440088680355545492 ) ) ;
#91127=CARTESIAN_POINT ( 'NONE',  ( 13.79529636645030344, 8.262082168247300018, 14.16423886937410614 ) ) ;
#91130=CARTESIAN_POINT ( 'NONE',  ( 18.52753015748617571, 63.09226448433412315, 4.923371831947298993 ) ) ;
#91132=VERTEX_POINT ( 'NONE', #9616 ) ;
#91133=CARTESIAN_POINT ( 'NONE',  ( 24.16423886937410614, 24.51208216824730002, -3.795296366450302550 ) ) ;
#91134=CARTESIAN_POINT ( 'NONE',  ( -4.164238869374099927, 27.01208216824730357, 3.795296366450308767 ) ) ;
#91135=CARTESIAN_POINT ( 'NONE',  ( 20.88017736071110875, 55.77201867748816966, -2.915334737309920765 ) ) ;
#91136=CARTESIAN_POINT ( 'NONE',  ( 2.035157376598822676, 2.438685344154838397, -7.964842623401177768 ) ) ;
#91137=CARTESIAN_POINT ( 'NONE',  ( 0.1532563361054100626, 50.80059781766745175, -2.638427012816831230 ) ) ;
#91139=CARTESIAN_POINT ( 'NONE',  ( -0.8801773607110991993, 52.85535201082151247, -2.915334737309923874 ) ) ;
#91140=CARTESIAN_POINT ( 'NONE',  ( 0.6178305044545838731, 14.74863466993041783, 9.382169495545420901 ) ) ;
#91141=CARTESIAN_POINT ( 'NONE',  ( 17.08211943468705840, 20.13708216824730357, -12.26659068614894466 ) ) ;
#91142=CARTESIAN_POINT ( 'NONE',  ( 7.084665262690076126, 17.02201867748817676, -10.88017736071110164 ) ) ;
#91143=CARTESIAN_POINT ( 'NONE',  ( 15.44008868035555793, 31.39701867748817676, -9.422509992056140149 ) ) ;
#91144=CARTESIAN_POINT ( 'NONE',  ( 7.084665262690076126, 62.02201867748816966, -10.88017736071110164 ) ) ;
#91145=CARTESIAN_POINT ( 'NONE',  ( 6.565887622018943937, 50.16530133659708213, 12.81628187352647430 ) ) ;
#91148=CARTESIAN_POINT ( 'NONE',  ( 19.89220837332776171, 34.74062864464240619, 6.478736007405959008 ) ) ;
#91149=EDGE_LOOP ( 'NONE', ( #48989, #77616, #68935, #89876 ) ) ;
#91152=CIRCLE ( 'NONE', #71953, 0.5000000000000004441 ) ;
#91154=CARTESIAN_POINT ( 'NONE',  ( 10.00000000000000178, 53.05374883491396787, 14.16423886937410082 ) ) ;
#91155=CARTESIAN_POINT ( 'NONE',  ( 24.16423886937409904, 64.09541550158064638, 3.795296366450317205 ) ) ;
#91156=CARTESIAN_POINT ( 'NONE',  ( 0.1532563361054100626, 25.80059781766744820, -2.638427012816831230 ) ) ;
#91157=CARTESIAN_POINT ( 'NONE',  ( 2.791683348922237240, 65.38393115100078035, -7.208316651077763204 ) ) ;
#91158=CARTESIAN_POINT ( 'NONE',  ( 19.42250999205614193, 65.14701867748817676, 5.440088680355555262 ) ) ;
#91159=EDGE_CURVE ( 'NONE', #64436, #19224, #32603, .T. ) ;
#91163=CARTESIAN_POINT ( 'NONE',  ( 22.26659068614894466, 33.88708216824730357, 7.082119434687054849 ) ) ;
#91164=CARTESIAN_POINT ( 'NONE',  ( -4.164238869374099927, 47.01208216824729647, 3.795296366450308767 ) ) ;
#91166=CARTESIAN_POINT ( 'NONE',  ( 16.40814093676324603, 62.45696800326376064, -11.09922568453594671 ) ) ;
#91167=CARTESIAN_POINT ( 'NONE',  ( 0.1532563361054082862, 56.21726448433411605, 2.638427012816831674 ) ) ;
#91168=CARTESIAN_POINT ( 'NONE',  ( 7.084665262690076126, 27.02201867748817676, -10.88017736071110164 ) ) ;
#91170=CARTESIAN_POINT ( 'NONE',  ( -0.1298530154764001854, 80.39370036920264795, -9.500000000000000000 ) ) ;
#91171=CARTESIAN_POINT ( 'NONE',  ( 19.84674366389459266, 58.30059781766745886, 2.638427012816836559 ) ) ;
#91172=CARTESIAN_POINT ( 'NONE',  ( 19.84674366389459266, 53.30059781766744464, 2.638427012816836559 ) ) ;
#91178=CARTESIAN_POINT ( 'NONE',  ( 17.20831665107776587, 7.883931151000784787, 7.208316651077764980 ) ) ;
#91182=CARTESIAN_POINT ( 'NONE',  ( 18.52753015748618282, 28.92559781766745175, -4.923371831947291888 ) ) ;
#91184=CARTESIAN_POINT ( 'NONE',  ( 6.565887622018943937, 40.16530133659708923, 12.81628187352647430 ) ) ;
#91185=CARTESIAN_POINT ( 'NONE',  ( -13.69000000000001194, 92.00000000000000000, -9.500000000000000000 ) ) ;
#91187=CARTESIAN_POINT ( 'NONE',  ( 19.84674366389459266, 63.71726448433412315, -2.638427012816827677 ) ) ;
#91189=CARTESIAN_POINT ( 'NONE',  ( 14.92337183194729988, 34.34226448433411605, -8.527530157486177487 ) ) ;
#91190=CARTESIAN_POINT ( 'NONE',  ( 6.204703633549690345, 30.76208216824730357, -14.16423886937410259 ) ) ;
#91191=CARTESIAN_POINT ( 'NONE',  ( 2.791683348922237240, 40.38393115100078035, -7.208316651077763204 ) ) ;
#91193=CARTESIAN_POINT ( 'NONE',  ( 5.076628168052704559, 0.1755978176674514724, -8.527530157486179263 ) ) ;
#91194=CARTESIAN_POINT ( 'NONE',  ( 19.84674366389459266, 43.71726448433410894, -2.638427012816827677 ) ) ;
#91195=CARTESIAN_POINT ( 'NONE',  ( 19.42250999205614193, 55.14701867748817676, 5.440088680355555262 ) ) ;
#91197=CARTESIAN_POINT ( 'NONE',  ( 7.361572987183169658, 39.96726448433411605, -9.846743663894592657 ) ) ;
#91199=CARTESIAN_POINT ( 'NONE',  ( 19.42250999205614548, 45.98035201082150536, -5.440088680355545492 ) ) ;
#91202=CARTESIAN_POINT ( 'NONE',  ( 19.42250999205614193, 25.14701867748817321, 5.440088680355555262 ) ) ;
#91203=CARTESIAN_POINT ( 'NONE',  ( 3.591859063236763294, -1.709698663402913210, -11.09922568453595026 ) ) ;
#91204=CARTESIAN_POINT ( 'NONE',  ( 7.084665262690076126, 39.10535201082150536, 10.88017736071109987 ) ) ;
#91206=DIRECTION ( 'NONE',  ( -0.000000000000000000, -1.000000000000000000, 0.000000000000000000 ) ) ;
#91208=CARTESIAN_POINT ( 'NONE',  ( -0.8801773607111009756, 38.06368534415484106, 1.068504757029289695E-15 ) ) ;
#91210=CARTESIAN_POINT ( 'NONE',  ( 10.00000000000000178, 17.25893115100078745, 9.846743663894594434 ) ) ;
#91211=CARTESIAN_POINT ( 'NONE',  ( 10.00000000000000000, 34.75893115100078745, -9.846743663894594434 ) ) ;
#91212=CARTESIAN_POINT ( 'NONE',  ( 19.80427997160309417, 57.75733960839543357, -6.499999999999988454 ) ) ;
#91214=CARTESIAN_POINT ( 'NONE',  ( 22.81628187352647785, 1.623634669930420271, 6.195893100308588602E-16 ) ) ;
#91215=CARTESIAN_POINT ( 'NONE',  ( -2.266590686148945544, 61.38708216824730357, -7.082119434687050408 ) ) ;
#91216=CARTESIAN_POINT ( 'NONE',  ( 20.10239578412225470, 27.63377557478296254, -6.340343622311919169 ) ) ;
#91218=CARTESIAN_POINT ( 'NONE',  ( -4.164238869374099039, 26.80374883491397142, 8.674139862899312516E-16 ) ) ;
#91219=CARTESIAN_POINT ( 'NONE',  ( 2.917880565312948704, 47.63708216824730357, 12.26659068614894643 ) ) ;
#91220=CARTESIAN_POINT ( 'NONE',  ( 12.63842701281683034, 22.46726448433411605, 9.846743663894596210 ) ) ;
#91221=CARTESIAN_POINT ( 'NONE',  ( 3.640395162852214650, 89.00000000000000000, 12.00000000000000000 ) ) ;
#91224=CARTESIAN_POINT ( 'NONE',  ( 12.63842701281683922, 29.55059781766745175, -9.846743663894590881 ) ) ;
#91226=CARTESIAN_POINT ( 'NONE',  ( 0.5774900079438590739, 22.64701867748817321, -5.440088680355550821 ) ) ;
#91227=CARTESIAN_POINT ( 'NONE',  ( 2.791683348922240793, 51.63393115100078745, 7.208316651077764092 ) ) ;
#91228=CARTESIAN_POINT ( 'NONE',  ( 22.26659068614895176, 9.720415501580633943, -7.082119434687042414 ) ) ;
#91231=UNCERTAINTY_MEASURE_WITH_UNIT (LENGTH_MEASURE( 1.000000000000000082E-05 ), #1585, 'distance_accuracy_value', 'NONE');
#91232=CARTESIAN_POINT ( 'NONE',  ( 0.1532563361054100626, 10.80059781766745175, -2.638427012816831230 ) ) ;
#91233=CARTESIAN_POINT ( 'NONE',  ( 10.00000000000000178, 35.37363466993042493, 12.81628187352647608 ) ) ;
#91234=CARTESIAN_POINT ( 'NONE',  ( 19.84674366389459266, 43.71726448433410894, -2.638427012816827677 ) ) ;
#91237=CARTESIAN_POINT ( 'NONE',  ( 0.1532563361054082862, 26.21726448433411605, 2.638427012816831674 ) ) ;
#91240=CARTESIAN_POINT ( 'NONE',  ( 2.917880565312950480, 55.97041550158063217, -12.26659068614894821 ) ) ;
#91241=CARTESIAN_POINT ( 'NONE',  ( 20.88017736071110164, 40.35535201082150536, 2.915334737309930979 ) ) ;
#91242=CARTESIAN_POINT ( 'NONE',  ( -4.164238869374099039, 1.803748834913967647, 8.674139862899312516E-16 ) ) ;
#91243=CARTESIAN_POINT ( 'NONE',  ( 1.472469842513823179, 31.42559781766745530, 4.923371831947296329 ) ) ;
#91244=CARTESIAN_POINT ( 'NONE',  ( -0.8801773607111009756, 13.06368534415483929, 1.068504757029289695E-15 ) ) ;
#91245=CARTESIAN_POINT ( 'NONE',  ( 1.472469842513823179, 36.42559781766745175, 4.923371831947296329 ) ) ;
#91246=CARTESIAN_POINT ( 'NONE',  ( -1.187721892393765133, 1.950157826164673567E-16, -1.468135075551455948 ) ) ;
#91247=CARTESIAN_POINT ( 'NONE',  ( 12.63842701281683034, 57.46726448433411605, 9.846743663894596210 ) ) ;
#91248=CARTESIAN_POINT ( 'NONE',  ( -0.8801773607111008646, 53.27201867748816966, 2.915334737309923430 ) ) ;
#91251=EDGE_LOOP ( 'NONE', ( #2226, #7676, #32354, #54161 ) ) ;
#91252=CARTESIAN_POINT ( 'NONE',  ( 22.81628187352648496, 56.83196800326374643, -3.434112377981050290 ) ) ;
#91254=CARTESIAN_POINT ( 'NONE',  ( 17.20831665107776587, 12.88393115100078390, 7.208316651077764980 ) ) ;
#91255=CARTESIAN_POINT ( 'NONE',  ( 19.38216949554541557, 57.24863466993042493, -9.382169495545420901 ) ) ;
#91256=CARTESIAN_POINT ( 'NONE',  ( 12.91533473730992121, 4.522018677488170546, 10.88017736071110164 ) ) ;
#91257=CARTESIAN_POINT ( 'NONE',  ( 19.84674366389459266, 53.30059781766744464, 2.638427012816836559 ) ) ;
#91258=SURFACE_SIDE_STYLE ('',( #21798 ) ) ;
#91259=CARTESIAN_POINT ( 'NONE',  ( 0.1532563361054083140, 1.008931151000784787, 1.131784320476157264E-15 ) ) ;
#91260=CARTESIAN_POINT ( 'NONE',  ( 17.08211943468705130, 28.47041550158063572, 12.26659068614894998 ) ) ;
#91261=CARTESIAN_POINT ( 'NONE',  ( 22.26659068614894466, 43.88708216824729647, 7.082119434687054849 ) ) ;
#91262=CARTESIAN_POINT ( 'NONE',  ( 0.1532563361054082862, 56.21726448433411605, 2.638427012816831674 ) ) ;
#91265=CARTESIAN_POINT ( 'NONE',  ( 17.96484262340118221, 51.18868534415483396, -7.964842623401177768 ) ) ;
#91266=CARTESIAN_POINT ( 'NONE',  ( 19.84674366389459621, 8.508931151000785675, 7.409399052514197653E-17 ) ) ;
#91270=CARTESIAN_POINT ( 'NONE',  ( 0.6178305044545818747, 53.49863466993041072, -9.382169495545419124 ) ) ;
#91272=ORIENTED_EDGE ( 'NONE', *, *, #81866, .T. ) ;
#91273=CARTESIAN_POINT ( 'NONE',  ( 17.20831665107776587, 9.133931151000787452, -7.208316651077762316 ) ) ;
#91275=CARTESIAN_POINT ( 'NONE',  ( 10.00000000000000178, 13.05374883491396787, 14.16423886937410082 ) ) ;
#91276=CARTESIAN_POINT ( 'NONE',  ( 7.361572987183169658, 19.96726448433411960, -9.846743663894592657 ) ) ;
#91277=CARTESIAN_POINT ( 'NONE',  ( -0.8801773607111008646, 28.27201867748817321, 2.915334737309923430 ) ) ;
#91278=ADVANCED_FACE ( 'NONE', ( #11580 ), #73057, .F. ) ;
#91281=CARTESIAN_POINT ( 'NONE',  ( 12.91533473730992121, 24.52201867748816966, 10.88017736071110164 ) ) ;
#91282=ORIENTED_EDGE ( 'NONE', *, *, #17077, .T. ) ;
#91283=CARTESIAN_POINT ( 'NONE',  ( 10.00000000000000178, 34.31368534415484106, 10.88017736071110342 ) ) ;
#91286=CARTESIAN_POINT ( 'NONE',  ( -2.816281873526471635, 18.91530133659708213, -3.434112377981056508 ) ) ;
#91287=CARTESIAN_POINT ( 'NONE',  ( 10.00000000000000000, 9.758931151000785675, -9.846743663894594434 ) ) ;
#91290=CARTESIAN_POINT ( 'NONE',  ( 19.84674366389459266, 13.30059781766745353, 2.638427012816836559 ) ) ;
#91291=CARTESIAN_POINT ( 'NONE',  ( 12.91533473730993009, 26.60535201082150536, -10.88017736071109987 ) ) ;
#91294=CARTESIAN_POINT ( 'NONE',  ( 16.40814093676323893, 60.79030133659709634, 11.09922568453595026 ) ) ;
#91295=CARTESIAN_POINT ( 'NONE',  ( -0.8801773607111009756, 43.06368534415484106, 1.068504757029289695E-15 ) ) ;
#91296=CARTESIAN_POINT ( 'NONE',  ( -46.85982187872481575, 103.4720723654396721, -5.834173416404226487 ) ) ;
#91297=CARTESIAN_POINT ( 'NONE',  ( 16.40814093676323893, 50.79030133659708923, 11.09922568453595026 ) ) ;
#91298=CARTESIAN_POINT ( 'NONE',  ( -0.8801773607111008646, 58.27201867748816966, 2.915334737309923430 ) ) ;
#91299=CARTESIAN_POINT ( 'NONE',  ( 5.076628168052703671, 66.84226448433412315, 8.527530157486179263 ) ) ;
#91300=SURFACE_STYLE_FILL_AREA ( #22827 ) ;
#91301=CARTESIAN_POINT ( 'NONE',  ( 19.84674366389459266, 33.71726448433410894, -2.638427012816827677 ) ) ;
#91302=CARTESIAN_POINT ( 'NONE',  ( 6.565887622018943937, 48.08196800326375353, -12.81628187352647608 ) ) ;
#91303=CARTESIAN_POINT ( 'NONE',  ( 0.000000000000000000, 78.76819843555267653, 9.368993295344042238 ) ) ;
#91304=CARTESIAN_POINT ( 'NONE',  ( 10.00000000000000178, 12.25893115100078568, 9.846743663894594434 ) ) ;
#91305=CARTESIAN_POINT ( 'NONE',  ( 10.00000000000000000, 17.87363466993041783, -12.81628187352647608 ) ) ;
#91307=CARTESIAN_POINT ( 'NONE',  ( -46.94000000000001194, 100.4376529975699981, 9.000000000001183054 ) ) ;
#91308=CARTESIAN_POINT ( 'NONE',  ( 12.91533473730992121, 29.52201867748817321, 10.88017736071110164 ) ) ;
#91309=CARTESIAN_POINT ( 'NONE',  ( 12.63842701281683034, 62.46726448433410894, 9.846743663894596210 ) ) ;
#91310=CARTESIAN_POINT ( 'NONE',  ( 12.63842701281683922, 24.55059781766745175, -9.846743663894590881 ) ) ;
#91311=CARTESIAN_POINT ( 'NONE',  ( 5.076628168052704559, 5.175597817667451750, -8.527530157486179263 ) ) ;
#91312=EDGE_CURVE ( 'NONE', #23152, #81206, #88062, .T. ) ;
#91313=CARTESIAN_POINT ( 'NONE',  ( 13.43411237798106583, 12.66530133659708746, -12.81628187352647252 ) ) ;
#91316=CARTESIAN_POINT ( 'NONE',  ( 4.559911319644449179, 7.230352010821504471, -9.422509992056141925 ) ) ;
#91319=CARTESIAN_POINT ( 'NONE',  ( -0.8801773607111008646, 3.272018677488171434, 2.915334737309923430 ) ) ;
#91321=CARTESIAN_POINT ( 'NONE',  ( 5.076628168052704559, 40.17559781766745175, -8.527530157486179263 ) ) ;
#91324=CARTESIAN_POINT ( 'NONE',  ( -0.8801773607110991993, 7.855352010821506248, -2.915334737309923874 ) ) ;
#91326=B_SPLINE_CURVE_WITH_KNOTS ( 'NONE', 3,
 ( #98748, #90210, #37240, #52224, #51737, #15723 ),
 .UNSPECIFIED., .F., .F.,
 ( 4, 2, 4 ),
 ( 0.000000000000000000, 0.0002626113303184732001, 0.0005252226606369464002 ),
 .UNSPECIFIED. ) ;
#91327=CARTESIAN_POINT ( 'NONE',  ( 0.5774900079438607392, 33.48035201082150536, 5.440088680355550821 ) ) ;
#91328=CARTESIAN_POINT ( 'NONE',  ( 24.16423886937409904, 49.09541550158063217, 3.795296366450317205 ) ) ;
#91329=CARTESIAN_POINT ( 'NONE',  ( 15.44008868035555260, 4.730352010821505360, 9.422509992056143702 ) ) ;
#91330=FACE_OUTER_BOUND ( 'NONE', #9749, .T. ) ;
#91331=CARTESIAN_POINT ( 'NONE',  ( 7.361572987183170547, 7.050597817667451750, 9.846743663894590881 ) ) ;
#91332=VECTOR ( 'NONE', #70058, 1000.000000000000000 ) ;
#91333=CARTESIAN_POINT ( 'NONE',  ( 12.63842701281683922, 19.55059781766745175, -9.846743663894590881 ) ) ;
#91334=EDGE_CURVE ( 'NONE', #15989, #60007, #13133, .T. ) ;
#91335=CARTESIAN_POINT ( 'NONE',  ( 16.40814093676324603, 17.45696800326375353, -11.09922568453594671 ) ) ;
#91337=CARTESIAN_POINT ( 'NONE',  ( 6.000000000000000000, 60.50000000000000000, -6.500000000000000888 ) ) ;
#91339=CARTESIAN_POINT ( 'NONE',  ( 13.79529636645031943, 15.34541550158063750, -14.16423886937409904 ) ) ;
#91340=CARTESIAN_POINT ( 'NONE',  ( 12.63842701281683922, 19.55059781766745175, -9.846743663894590881 ) ) ;
#91344=CARTESIAN_POINT ( 'NONE',  ( 24.16423886937410614, 59.30374883491397497, 8.672049930838204340E-16 ) ) ;
#91345=CARTESIAN_POINT ( 'NONE',  ( 14.92337183194729633, 7.675597817667451750, 8.527530157486181039 ) ) ;
#91348=CARTESIAN_POINT ( 'NONE',  ( 0.5774900079438607392, 38.48035201082150536, 5.440088680355550821 ) ) ;
#91349=CARTESIAN_POINT ( 'NONE',  ( -1.099225684535947600, 53.70696800326376064, -6.408140936763238038 ) ) ;
#91350=CARTESIAN_POINT ( 'NONE',  ( 7.084665262690076126, 2.022018677488170990, -10.88017736071110164 ) ) ;
#91351=CARTESIAN_POINT ( 'NONE',  ( 21.09922568453595559, 32.04030133659708923, -6.408140936763230044 ) ) ;
#91352=CARTESIAN_POINT ( 'NONE',  ( -1.099225684535947600, 4.540301336597087456, 6.408140936763237150 ) ) ;
#91353=CARTESIAN_POINT ( 'NONE',  ( 17.20831665107776587, 7.883931151000784787, 7.208316651077764980 ) ) ;
#91356=CARTESIAN_POINT ( 'NONE',  ( 1.274849032794305170, 12.55509018479935968, -6.499999999999995559 ) ) ;
#91358=CARTESIAN_POINT ( 'NONE',  ( -0.3689425029237898834, 41.17874883491397497, -10.36894250292378850 ) ) ;
#91359=CARTESIAN_POINT ( 'NONE',  ( -2.266590686148945544, 17.22041550158063572, 7.082119434687048631 ) ) ;
#91360=( NAMED_UNIT ( * ) PLANE_ANGLE_UNIT ( ) SI_UNIT ( $, .RADIAN. ) );
#91361=CARTESIAN_POINT ( 'NONE',  ( 10.00000000000000000, 31.81368534415483751, -10.88017736071110342 ) ) ;
#91364=CARTESIAN_POINT ( 'NONE',  ( 20.88017736071110875, 60.77201867748817676, -2.915334737309920765 ) ) ;
#91365=CARTESIAN_POINT ( 'NONE',  ( 10.00000000000000178, 69.31368534415484817, 10.88017736071110342 ) ) ;
#91366=CARTESIAN_POINT ( 'NONE',  ( 10.00000000000000178, 30.37363466993042138, 12.81628187352647608 ) ) ;
#91367=DIRECTION ( 'NONE',  ( 0.000000000000000000, 0.000000000000000000, 1.000000000000000000 ) ) ;
#91369=CARTESIAN_POINT ( 'NONE',  ( 12.63842701281683034, 32.46726448433412315, 9.846743663894596210 ) ) ;
#91371=CARTESIAN_POINT ( 'NONE',  ( 13.43411237798106583, 22.66530133659708923, -12.81628187352647252 ) ) ;
#91372=CARTESIAN_POINT ( 'NONE',  ( 19.84674366389459266, 13.71726448433411782, -2.638427012816827677 ) ) ;
#91373=CARTESIAN_POINT ( 'NONE',  ( 2.035157376598822676, 12.43868534415483751, -7.964842623401177768 ) ) ;
#91374=CARTESIAN_POINT ( 'NONE',  ( 19.84674366389459266, 33.71726448433410894, -2.638427012816827677 ) ) ;
#91376=CARTESIAN_POINT ( 'NONE',  ( 18.52753015748617571, 13.09226448433411960, 4.923371831947298993 ) ) ;
#91377=CARTESIAN_POINT ( 'NONE',  ( -4.164238869374098151, 6.595415501580634832, -3.795296366450310543 ) ) ;
#91379=CARTESIAN_POINT ( 'NONE',  ( 19.42250999205614193, 35.14701867748816966, 5.440088680355555262 ) ) ;
#91380=CARTESIAN_POINT ( 'NONE',  ( 7.084665262690076126, 12.02201867748817143, -10.88017736071110164 ) ) ;
#91381=CARTESIAN_POINT ( 'NONE',  ( 2.917880565312950480, 40.97041550158063217, -12.26659068614894821 ) ) ;
#91382=CARTESIAN_POINT ( 'NONE',  ( 15.44008868035555260, 29.73035201082150891, 9.422509992056143702 ) ) ;
#91383=CARTESIAN_POINT ( 'NONE',  ( 15.44008868035555793, 11.39701867748817143, -9.422509992056140149 ) ) ;
#91385=CARTESIAN_POINT ( 'NONE',  ( 17.96484262340118221, 44.93868534415483396, 7.964842623401181321 ) ) ;
#91386=CARTESIAN_POINT ( 'NONE',  ( 19.38216949554541557, 42.24863466993041783, -9.382169495545420901 ) ) ;
#91388=CARTESIAN_POINT ( 'NONE',  ( 17.96484262340118221, 49.93868534415484106, 7.964842623401181321 ) ) ;
#91390=CARTESIAN_POINT ( 'NONE',  ( 2.035157376598822676, 52.43868534415483396, -7.964842623401177768 ) ) ;
#91393=CARTESIAN_POINT ( 'NONE',  ( 19.42250999205614548, 55.98035201082150536, -5.440088680355545492 ) ) ;
#91394=FILL_AREA_STYLE_COLOUR ( '', #83338 ) ;
#91396=CARTESIAN_POINT ( 'NONE',  ( 24.16423886937410614, 44.51208216824730357, -3.795296366450302550 ) ) ;
#91397=CARTESIAN_POINT ( 'NONE',  ( -0.8801773607111009756, 68.06368534415484817, 1.068504757029289695E-15 ) ) ;
#91401=CARTESIAN_POINT ( 'NONE',  ( 0.1532563361054083140, 61.00893115100078745, 1.131784320476157264E-15 ) ) ;
#91403=SURFACE_STYLE_FILL_AREA ( #46882 ) ;
#91404=CARTESIAN_POINT ( 'NONE',  ( 2.791683348922240793, 31.63393115100078745, 7.208316651077764092 ) ) ;
#91407=CARTESIAN_POINT ( 'NONE',  ( 19.84674366389459266, 28.30059781766745886, 2.638427012816836559 ) ) ;
#91410=CARTESIAN_POINT ( 'NONE',  ( 20.88017736071110519, 30.56368534415484106, 2.639326808657452039E-16 ) ) ;
#91411=CARTESIAN_POINT ( 'NONE',  ( 12.63842701281683034, 37.46726448433411605, 9.846743663894596210 ) ) ;
#91412=CARTESIAN_POINT ( 'NONE',  ( 19.38216949554541557, 17.24863466993041783, -9.382169495545420901 ) ) ;
#91414=CARTESIAN_POINT ( 'NONE',  ( 0.5774900079438590739, 57.64701867748817676, -5.440088680355550821 ) ) ;
#91415=CARTESIAN_POINT ( 'NONE',  ( 20.88017736071110519, 45.56368534415484106, 2.639326808657452039E-16 ) ) ;
#91416=CARTESIAN_POINT ( 'NONE',  ( 19.42250999205614193, 5.147018677488171434, 5.440088680355555262 ) ) ;
#91417=CARTESIAN_POINT ( 'NONE',  ( 20.36894250292379738, 64.92874883491397497, -10.36894250292379027 ) ) ;
#91419=CARTESIAN_POINT ( 'NONE',  ( 0.6178305044545838731, 19.74863466993042138, 9.382169495545420901 ) ) ;
#91420=DIRECTION ( 'NONE',  ( 1.000000000000000000, -0.000000000000000000, -0.000000000000000000 ) ) ;
#91421=EDGE_LOOP ( 'NONE', ( #1988, #29799, #77553, #2688 ) ) ;
#91422=CARTESIAN_POINT ( 'NONE',  ( 3.591859063236761518, 9.956968003263753531, 11.09922568453594849 ) ) ;
#91423=CARTESIAN_POINT ( 'NONE',  ( 15.44008868035555260, 14.73035201082150536, 9.422509992056143702 ) ) ;
#91424=CARTESIAN_POINT ( 'NONE',  ( 15.44008868035555260, 59.73035201082151247, 9.422509992056143702 ) ) ;
#91426=AXIS2_PLACEMENT_3D ( 'NONE', #29936, #46428, #29439 ) ;
#91427=B_SPLINE_CURVE_WITH_KNOTS ( 'NONE', 3,
 ( #69186, #29681, #76671, #14216 ),
 .UNSPECIFIED., .F., .F.,
 ( 4, 4 ),
 ( 7.757919228897728493E-18, 0.002392975128318548372 ),
 .UNSPECIFIED. ) ;
#91428=CARTESIAN_POINT ( 'NONE',  ( 2.035157376598824452, 63.68868534415484106, 7.964842623401179544 ) ) ;
#91429=CARTESIAN_POINT ( 'NONE',  ( 7.361572987183170547, 42.05059781766745886, 9.846743663894590881 ) ) ;
#91430=CARTESIAN_POINT ( 'NONE',  ( 12.63842701281683922, 24.55059781766745175, -9.846743663894590881 ) ) ;
#91432=CARTESIAN_POINT ( 'NONE',  ( 19.84674366389459621, 18.50893115100078745, 7.409399052514197653E-17 ) ) ;
#91433=CARTESIAN_POINT ( 'NONE',  ( 21.92686044187657046, 57.39664270246084499, -3.195792623639524432 ) ) ;
#91434=CARTESIAN_POINT ( 'NONE',  ( 0.2751277870542982451, 17.28217586085238011, -6.500000000000002665 ) ) ;
#91435=CARTESIAN_POINT ( 'NONE',  ( 21.09922568453595559, 42.04030133659708213, -6.408140936763230044 ) ) ;
#91436=CARTESIAN_POINT ( 'NONE',  ( 12.63842701281683922, 9.550597817667449974, -9.846743663894590881 ) ) ;
#91438=CARTESIAN_POINT ( 'NONE',  ( 21.92686044187657401, 45.37045670184114243, -3.195792623639525765 ) ) ;
#91439=CARTESIAN_POINT ( 'NONE',  ( 10.00000000000000000, 29.75893115100078745, -9.846743663894594434 ) ) ;
#91441=VECTOR ( 'NONE', #77386, 1000.000000000000000 ) ;
#91443=CARTESIAN_POINT ( 'NONE',  ( 6.565887622018943937, 10.16530133659708746, 12.81628187352647430 ) ) ;
#91445=CARTESIAN_POINT ( 'NONE',  ( 10.00000000000000178, 49.31368534415484106, 10.88017736071110342 ) ) ;
#91446=CARTESIAN_POINT ( 'NONE',  ( 20.36894250292379382, 33.67874883491396076, 10.36894250292379205 ) ) ;
#91447=EDGE_CURVE ( 'NONE', #14105, #34568, #78630, .T. ) ;
#91448=( BOUNDED_SURFACE ( )  B_SPLINE_SURFACE ( 3, 2, ( 
 ( #85425, #31420, #47415 ),
 ( #84931, #32412, #16443 ),
 ( #39928, #93414, #78409 ),
 ( #24937, #55419, #484 ),
 ( #30932, #32904, #91938 ),
 ( #63403, #84449, #93908 ),
 ( #15948, #46440, #34371 ),
 ( #26385, #4888, #41427 ),
 ( #42387, #71420, #12371 ),
 ( #64377, #79883, #71888 ),
 ( #88867, #41912, #12859 ),
 ( #73360, #94886, #79401 ),
 ( #10905, #35367, #64861 ),
 ( #72373, #11390, #96387 ) ),
 .UNSPECIFIED., .F., .F., .F. ) 
 B_SPLINE_SURFACE_WITH_KNOTS ( ( 4, 2, 2, 2, 2, 2, 4 ),
 ( 3, 3 ),
 ( 0.000000000000000000, 0.004797171936611957510, 0.007195757904917936265, 0.009594343873223915020, 0.01199292984152989378, 0.01439151580983587253, 0.01918868774644783004 ),
 ( 0.000000000000000000, 1.000000000000000000 ),
 .UNSPECIFIED. ) 
 GEOMETRIC_REPRESENTATION_ITEM ( )  RATIONAL_B_SPLINE_SURFACE ( (
 ( 1.000000000000000000, 0.7071067811865475727, 1.000000000000000000),
 ( 1.000000000000000000, 0.7404680669564855933, 1.000000000000000000),
 ( 1.000000000000000000, 0.7699744256216403127, 1.000000000000000000),
 ( 1.000000000000000000, 0.8013264333395565542, 1.000000000000000000),
 ( 1.000000000000000000, 0.8096066803152818236, 1.000000000000000000),
 ( 1.000000000000000000, 0.8208168491803492506, 1.000000000000000000),
 ( 1.000000000000000000, 0.8237352673350482046, 1.000000000000000000),
 ( 1.000000000000000000, 0.8237872525054150685, 1.000000000000000000),
 ( 1.000000000000000000, 0.8209201555337369838, 1.000000000000000000),
 ( 1.000000000000000000, 0.8097813946838617882, 1.000000000000000000),
 ( 1.000000000000000000, 0.8015207097676279036, 1.000000000000000000),
 ( 1.000000000000000000, 0.7701797223629573974, 1.000000000000000000),
 ( 1.000000000000000000, 0.7406378784107887636, 1.000000000000000000),
 ( 1.000000000000000000, 0.7071067811865475727, 1.000000000000000000) ) ) 
 REPRESENTATION_ITEM ( '' )  SURFACE ( )  );
#91450=CARTESIAN_POINT ( 'NONE',  ( 10.00000000000000000, 30.55374883491397142, -14.16423886937410082 ) ) ;
#91451=CARTESIAN_POINT ( 'NONE',  ( 24.16423886937410614, 64.51208216824728936, -3.795296366450302550 ) ) ;
#91452=CARTESIAN_POINT ( 'NONE',  ( 22.26659068614895176, 14.72041550158063572, -7.082119434687042414 ) ) ;
#91453=CARTESIAN_POINT ( 'NONE',  ( 20.36894250292379738, 24.92874883491396787, -10.36894250292379027 ) ) ;
#91454=CARTESIAN_POINT ( 'NONE',  ( 12.91533473730993009, 41.60535201082149825, -10.88017736071109987 ) ) ;
#91456=CARTESIAN_POINT ( 'NONE',  ( -0.8801773607111008646, 68.27201867748817676, 2.915334737309923430 ) ) ;
#91457=CARTESIAN_POINT ( 'NONE',  ( 5.076628168052703671, 36.84226448433412315, 8.527530157486179263 ) ) ;
#91458=CARTESIAN_POINT ( 'NONE',  ( 20.88017736071110519, 20.56368534415484106, 2.639326808657452039E-16 ) ) ;
#91460=CARTESIAN_POINT ( 'NONE',  ( 1.472469842513823179, 61.42559781766745175, 4.923371831947296329 ) ) ;
#91461=CARTESIAN_POINT ( 'NONE',  ( 19.99999999999863576, 84.95449374057137959, -5.196918121119169065 ) ) ;
#91462=CARTESIAN_POINT ( 'NONE',  ( 10.00000000000000178, 32.25893115100078745, 9.846743663894594434 ) ) ;
#91463=CARTESIAN_POINT ( 'NONE',  ( 13.43411237798105340, 55.58196800326374643, 12.81628187352647963 ) ) ;
#91466=CARTESIAN_POINT ( 'NONE',  ( 5.076628168052703671, 41.84226448433411605, 8.527530157486179263 ) ) ;
#91467=CARTESIAN_POINT ( 'NONE',  ( 2.791683348922237240, 50.38393115100078035, -7.208316651077763204 ) ) ;
#91468=CARTESIAN_POINT ( 'NONE',  ( 24.16423886937410614, 39.51208216824731068, -3.795296366450302550 ) ) ;
#91470=CARTESIAN_POINT ( 'NONE',  ( 17.08211943468705840, 15.13708216824730179, -12.26659068614894466 ) ) ;
#91471=CARTESIAN_POINT ( 'NONE',  ( 20.88017736071110519, 60.56368534415484106, 2.639326808657452039E-16 ) ) ;
#91473=CARTESIAN_POINT ( 'NONE',  ( -0.3689425029237898834, 61.17874883491396076, -10.36894250292378850 ) ) ;
#91475=CARTESIAN_POINT ( 'NONE',  ( 22.81628187352647785, 16.62363466993042138, 6.195893100308588602E-16 ) ) ;
#91478=CARTESIAN_POINT ( 'NONE',  ( 2.035157376598824452, 58.68868534415482685, 7.964842623401179544 ) ) ;
#91482=CARTESIAN_POINT ( 'NONE',  ( 19.38216949554541557, 32.24863466993041783, -9.382169495545420901 ) ) ;
#91483=CARTESIAN_POINT ( 'NONE',  ( 10.00000000000000178, 58.05374883491397497, 14.16423886937410082 ) ) ;
#91485=CARTESIAN_POINT ( 'NONE',  ( 12.91533473730993009, 16.60535201082150891, -10.88017736071109987 ) ) ;
#91486=CARTESIAN_POINT ( 'NONE',  ( 7.084665262690076126, 19.10535201082150181, 10.88017736071109987 ) ) ;
#91488=CARTESIAN_POINT ( 'NONE',  ( 2.791683348922240793, 56.63393115100078035, 7.208316651077764092 ) ) ;
#91489=CARTESIAN_POINT ( 'NONE',  ( 12.63842701281683034, 52.46726448433413026, 9.846743663894596210 ) ) ;
#91490=CARTESIAN_POINT ( 'NONE',  ( -1.099225684535947600, 49.54030133659708923, 6.408140936763237150 ) ) ;
#91491=CARTESIAN_POINT ( 'NONE',  ( 0.1532563361054100626, 0.8005978176674514168, -2.638427012816831230 ) ) ;
#91493=CARTESIAN_POINT ( 'NONE',  ( 15.44008868035555793, 21.39701867748817321, -9.422509992056140149 ) ) ;
#91494=CARTESIAN_POINT ( 'NONE',  ( -1.099225684535947600, 23.70696800326375708, -6.408140936763238038 ) ) ;
#91496=CARTESIAN_POINT ( 'NONE',  ( 19.84674366389459266, 43.30059781766744464, 2.638427012816836559 ) ) ;
#91497=CARTESIAN_POINT ( 'NONE',  ( 15.44008868035555260, 34.73035201082151247, 9.422509992056143702 ) ) ;
#91498=CARTESIAN_POINT ( 'NONE',  ( 16.40814093676323893, 15.79030133659708746, 11.09922568453595026 ) ) ;
#91499=CARTESIAN_POINT ( 'NONE',  ( -0.8801773607111008646, 53.27201867748816966, 2.915334737309923430 ) ) ;
#91502=CARTESIAN_POINT ( 'NONE',  ( 3.591859063236763294, 48.29030133659708923, -11.09922568453595026 ) ) ;
#91503=VERTEX_POINT ( 'NONE', #23044 ) ;
#91504=CARTESIAN_POINT ( 'NONE',  ( 1.472469842513823179, 65.59226448433412315, -4.923371831947296329 ) ) ;
#91506=CARTESIAN_POINT ( 'NONE',  ( 10.00000000000000000, 51.81368534415484106, -10.88017736071110342 ) ) ;
#91507=CARTESIAN_POINT ( 'NONE',  ( 10.00000000000000000, 32.87363466993042493, -12.81628187352647608 ) ) ;
#91508=CARTESIAN_POINT ( 'NONE',  ( -0.3689425029237898834, 16.17874883491396076, -10.36894250292378850 ) ) ;
#91509=CARTESIAN_POINT ( 'NONE',  ( 0.5774900079438590739, 52.64701867748817676, -5.440088680355550821 ) ) ;
#91510=CARTESIAN_POINT ( 'NONE',  ( -2.266590686148945544, 42.22041550158063217, 7.082119434687048631 ) ) ;
#91513=CARTESIAN_POINT ( 'NONE',  ( 19.84674366389459621, 18.50893115100078745, 7.409399052514197653E-17 ) ) ;
#91514=CARTESIAN_POINT ( 'NONE',  ( 19.84674366389459266, 8.300597817667451750, 2.638427012816836559 ) ) ;
#91515=CARTESIAN_POINT ( 'NONE',  ( 2.562013731377108972, 0.5000000000000000000, -6.499999999999999112 ) ) ;
#91516=CARTESIAN_POINT ( 'NONE',  ( 20.36894250292379738, 39.92874883491396787, -10.36894250292379027 ) ) ;
#91517=CARTESIAN_POINT ( 'NONE',  ( 21.92686044187657401, 25.37045670184114243, -3.195792623639525765 ) ) ;
#91518=AXIS2_PLACEMENT_3D ( 'NONE', #26913, #26414, #48433 ) ;
#91519=CARTESIAN_POINT ( 'NONE',  ( 2.035157376598822676, 2.438685344154837953, -7.964842623401177768 ) ) ;
#91524=CARTESIAN_POINT ( 'NONE',  ( 10.00000000000000178, 14.31368534415483929, 10.88017736071110342 ) ) ;
#91525=CARTESIAN_POINT ( 'NONE',  ( 6.204703633549690345, 60.76208216824730357, -14.16423886937410259 ) ) ;
#91526=CARTESIAN_POINT ( 'NONE',  ( 5.076628168052704559, 50.17559781766745886, -8.527530157486179263 ) ) ;
#91527=CARTESIAN_POINT ( 'NONE',  ( 0.6178305044545838731, 39.74863466993041072, 9.382169495545420901 ) ) ;
#91528=CARTESIAN_POINT ( 'NONE',  ( 19.72487221294570858, 64.78217586085237656, 6.499999999999992895 ) ) ;
#91530=CARTESIAN_POINT ( 'NONE',  ( -4.164238869374099927, 2.012082168247300906, 3.795296366450308767 ) ) ;
#91531=CARTESIAN_POINT ( 'NONE',  ( 20.88017736071110519, 30.56368534415484106, 2.639326808657452039E-16 ) ) ;
#91532=CARTESIAN_POINT ( 'NONE',  ( -2.266590686148945544, 66.38708216824730357, -7.082119434687050408 ) ) ;
#91533=CARTESIAN_POINT ( 'NONE',  ( 14.92337183194729988, 44.34226448433412315, -8.527530157486177487 ) ) ;
#91534=CARTESIAN_POINT ( 'NONE',  ( 14.49999999999999822, 61.50000000000000711, 6.500000000000000888 ) ) ;
#91535=CARTESIAN_POINT ( 'NONE',  ( 7.361572987183169658, 19.96726448433411960, -9.846743663894592657 ) ) ;
#91536=( NAMED_UNIT ( * ) PLANE_ANGLE_UNIT ( ) SI_UNIT ( $, .RADIAN. ) );
#91541=CARTESIAN_POINT ( 'NONE',  ( 7.361572987183170547, 57.05059781766744464, 9.846743663894590881 ) ) ;
#91542=CARTESIAN_POINT ( 'NONE',  ( -0.8801773607111009756, 33.06368534415484106, 1.068504757029289695E-15 ) ) ;
#91543=CARTESIAN_POINT ( 'NONE',  ( -0.8801773607110991993, 37.85535201082151247, -2.915334737309923874 ) ) ;
#91544=CARTESIAN_POINT ( 'NONE',  ( 12.63842701281683034, 62.46726448433410894, 9.846743663894596210 ) ) ;
#91545=CARTESIAN_POINT ( 'NONE',  ( -1.099225684535947600, 29.54030133659708923, 6.408140936763237150 ) ) ;
#91546=CARTESIAN_POINT ( 'NONE',  ( 13.79529636645030344, 13.26208216824729824, 14.16423886937410614 ) ) ;
#91548=CARTESIAN_POINT ( 'NONE',  ( -2.816281873526473856, 39.12363466993041783, 9.499525473075851096E-16 ) ) ;
#91551=CARTESIAN_POINT ( 'NONE',  ( 1.472469842513823179, 40.59226448433411605, -4.923371831947296329 ) ) ;
#91552=CARTESIAN_POINT ( 'NONE',  ( 0.5774900079438607392, 13.48035201082150358, 5.440088680355550821 ) ) ;
#91553=ORIENTED_EDGE ( 'NONE', *, *, #9620, .T. ) ;
#91554=CARTESIAN_POINT ( 'NONE',  ( 12.91533473730992121, 14.52201867748817143, 10.88017736071110164 ) ) ;
#91555=VERTEX_POINT ( 'NONE', #1034 ) ;
#91556=CARTESIAN_POINT ( 'NONE',  ( 4.559911319644449179, 67.23035201082150536, -9.422509992056141925 ) ) ;
#91557=CARTESIAN_POINT ( 'NONE',  ( 20.88017736071110519, 55.56368534415484817, 2.639326808657452039E-16 ) ) ;
#91558=CARTESIAN_POINT ( 'NONE',  ( 2.035157376598822676, 67.43868534415484817, -7.964842623401177768 ) ) ;
#91560=CARTESIAN_POINT ( 'NONE',  ( 0.1532563361054082862, 1.217264484334117824, 2.638427012816831674 ) ) ;
#91562=CARTESIAN_POINT ( 'NONE',  ( 17.96484262340118221, 51.18868534415483396, -7.964842623401177768 ) ) ;
#91564=CARTESIAN_POINT ( 'NONE',  ( -46.82586484710777341, 100.5857744218339036, 9.343464521776596143 ) ) ;
#91565=SURFACE_STYLE_FILL_AREA ( #29559 ) ;
#91567=EDGE_CURVE ( 'NONE', #53936, #46415, #54699, .T. ) ;
#91568=CARTESIAN_POINT ( 'NONE',  ( 14.92337183194729633, 37.67559781766745175, 8.527530157486181039 ) ) ;
#91569=EDGE_LOOP ( 'NONE', ( #56861, #40042, #64098, #94733 ) ) ;
#91571=SURFACE_SIDE_STYLE ('',( #30060 ) ) ;
#91573=CARTESIAN_POINT ( 'NONE',  ( 2.917880565312950480, 15.97041550158063217, -12.26659068614894821 ) ) ;
#91574=CARTESIAN_POINT ( 'NONE',  ( 0.1143410931637277583, 35.21691075486304356, 6.480892540919860778 ) ) ;
#91575=CARTESIAN_POINT ( 'NONE',  ( 2.831191079880678085, 79.91181047996344944, 5.000000000000000000 ) ) ;
#91576=CARTESIAN_POINT ( 'NONE',  ( 0.5774900079438607392, 3.480352010821504916, 5.440088680355550821 ) ) ;
#91577=CARTESIAN_POINT ( 'NONE',  ( 20.15039907845753220, 29.72266099184918531, 6.262539305110077947 ) ) ;
#91578=CARTESIAN_POINT ( 'NONE',  ( 22.81628187352647785, 36.62363466993041783, 6.195893100308588602E-16 ) ) ;
#91581=CARTESIAN_POINT ( 'NONE',  ( 18.52753015748618282, 63.92559781766745886, -4.923371831947291888 ) ) ;
#91582=CARTESIAN_POINT ( 'NONE',  ( 0.1532563361054082862, 1.217264484334117824, 2.638427012816831674 ) ) ;
#91583=CARTESIAN_POINT ( 'NONE',  ( 22.81628187352647785, 21.62363466993041783, 6.195893100308588602E-16 ) ) ;
#91584=CARTESIAN_POINT ( 'NONE',  ( 19.84674366389459621, 18.50893115100078745, 7.409399052514197653E-17 ) ) ;
#91586=CARTESIAN_POINT ( 'NONE',  ( 19.84674366389459621, 18.50893115100078745, 7.409399052514197653E-17 ) ) ;
#91587=CARTESIAN_POINT ( 'NONE',  ( 21.09922568453594849, 21.20696800326375353, 6.408140936763242479 ) ) ;
#91589=CARTESIAN_POINT ( 'NONE',  ( 18.52753015748618282, 8.925597817667451750, -4.923371831947291888 ) ) ;
#91592=CARTESIAN_POINT ( 'NONE',  ( 15.44008868035555793, 26.39701867748817321, -9.422509992056140149 ) ) ;
#91593=CARTESIAN_POINT ( 'NONE',  ( 2.917880565312948704, 22.63708216824730002, 12.26659068614894643 ) ) ;
#91594=CARTESIAN_POINT ( 'NONE',  ( 7.361572987183170547, 47.05059781766745175, 9.846743663894590881 ) ) ;
#91595=CARTESIAN_POINT ( 'NONE',  ( -0.8801773607111008646, 68.27201867748817676, 2.915334737309923430 ) ) ;
#91596=CARTESIAN_POINT ( 'NONE',  ( 22.81628187352647785, 36.41530133659707502, 3.434112377981063169 ) ) ;
#91598=CARTESIAN_POINT ( 'NONE',  ( 17.96484262340118221, 9.938685344154837509, 7.964842623401181321 ) ) ;
#91599=EDGE_CURVE ( 'NONE', #86051, #42399, #66869, .T. ) ;
#91601=CARTESIAN_POINT ( 'NONE',  ( 6.565887622018943937, 13.08196800326374998, -12.81628187352647608 ) ) ;
#91602=CARTESIAN_POINT ( 'NONE',  ( 17.20831665107776587, 27.88393115100078390, 7.208316651077764980 ) ) ;
#91604=CARTESIAN_POINT ( 'NONE',  ( 21.09922568453594849, 36.20696800326375353, 6.408140936763242479 ) ) ;
#91605=CARTESIAN_POINT ( 'NONE',  ( 18.39792806157249672, 24.52224192338641373, 6.499999999999999112 ) ) ;
#91606=CARTESIAN_POINT ( 'NONE',  ( -0.8801773607111008646, 53.27201867748816966, 2.915334737309923430 ) ) ;
#91609=CARTESIAN_POINT ( 'NONE',  ( 10.00000000000000000, 66.81368534415484817, -10.88017736071110342 ) ) ;
#91610=CARTESIAN_POINT ( 'NONE',  ( 20.88017736071110519, 35.56368534415484106, 2.639326808657452039E-16 ) ) ;
#91611=CARTESIAN_POINT ( 'NONE',  ( 0.5774900079438607392, 43.48035201082151247, 5.440088680355550821 ) ) ;
#91612=CARTESIAN_POINT ( 'NONE',  ( 12.63842701281683922, 59.55059781766744464, -9.846743663894590881 ) ) ;
#91613=CARTESIAN_POINT ( 'NONE',  ( 20.88017736071110875, 60.77201867748817676, -2.915334737309920765 ) ) ;
#91615=CARTESIAN_POINT ( 'NONE',  ( 18.52753015748618282, 53.92559781766745175, -4.923371831947291888 ) ) ;
#91616=CARTESIAN_POINT ( 'NONE',  ( 2.035157376598822676, 2.438685344154837953, -7.964842623401177768 ) ) ;
#91618=CARTESIAN_POINT ( 'NONE',  ( -1.099225684535947600, 13.70696800326375353, -6.408140936763238038 ) ) ;
#91619=ORIENTED_EDGE ( 'NONE', *, *, #13948, .T. ) ;
#91620=CARTESIAN_POINT ( 'NONE',  ( 15.44008868035555793, 41.39701867748817676, -9.422509992056140149 ) ) ;
#91622=CARTESIAN_POINT ( 'NONE',  ( 12.63842701281683922, 59.55059781766744464, -9.846743663894590881 ) ) ;
#91624=CARTESIAN_POINT ( 'NONE',  ( -0.8801773607111009756, 18.06368534415484106, 1.068504757029289695E-15 ) ) ;
#91625=CARTESIAN_POINT ( 'NONE',  ( 12.91533473730992121, 29.52201867748817321, 10.88017736071110164 ) ) ;
#91626=CARTESIAN_POINT ( 'NONE',  ( 6.204703633549690345, 37.84541550158063927, 14.16423886937410082 ) ) ;
#91627=CARTESIAN_POINT ( 'NONE',  ( 14.92337183194729633, 22.67559781766745175, 8.527530157486181039 ) ) ;
#91628=CARTESIAN_POINT ( 'NONE',  ( 2.035157376598822676, 52.43868534415483396, -7.964842623401177768 ) ) ;
#91629=DIRECTION ( 'NONE',  ( 0.000000000000000000, 0.000000000000000000, -1.000000000000000000 ) ) ;
#91630=( NAMED_UNIT ( * ) SI_UNIT ( $, .STERADIAN. ) SOLID_ANGLE_UNIT ( ) );
#91632=CARTESIAN_POINT ( 'NONE',  ( 2.791683348922240793, 61.63393115100079456, 7.208316651077764092 ) ) ;
#91635=CARTESIAN_POINT ( 'NONE',  ( 22.26659068614895176, 34.72041550158063927, -7.082119434687042414 ) ) ;
#91636=CARTESIAN_POINT ( 'NONE',  ( 24.16423886937410614, 29.51208216824729647, -3.795296366450302550 ) ) ;
#91637=CARTESIAN_POINT ( 'NONE',  ( 10.00000000000000178, 2.258931151000784787, 9.846743663894594434 ) ) ;
#91638=CARTESIAN_POINT ( 'NONE',  ( 0.6178305044545818747, 8.498634669930421381, -9.382169495545419124 ) ) ;
#91639=CARTESIAN_POINT ( 'NONE',  ( 5.076628168052703671, 51.84226448433412315, 8.527530157486179263 ) ) ;
#91641=CARTESIAN_POINT ( 'NONE',  ( 17.96484262340118221, 46.18868534415484106, -7.964842623401177768 ) ) ;
#91642=CARTESIAN_POINT ( 'NONE',  ( 13.43411237798106583, 17.66530133659708923, -12.81628187352647252 ) ) ;
#91643=CARTESIAN_POINT ( 'NONE',  ( 6.204703633549690345, 27.84541550158063217, 14.16423886937410082 ) ) ;
#91644=CARTESIAN_POINT ( 'NONE',  ( 2.035157376598824452, 13.68868534415483751, 7.964842623401179544 ) ) ;
#91645=CARTESIAN_POINT ( 'NONE',  ( 2.035157376598824452, 33.68868534415484106, 7.964842623401179544 ) ) ;
#91646=CARTESIAN_POINT ( 'NONE',  ( 21.92686044187657046, 5.162123368507804066, 4.562052436263912550E-16 ) ) ;
#91647=CARTESIAN_POINT ( 'NONE',  ( -0.8801773607111008646, 63.27201867748817676, 2.915334737309923430 ) ) ;
#91648=CARTESIAN_POINT ( 'NONE',  ( 22.81628187352647785, 51.41530133659708923, 3.434112377981063169 ) ) ;
#91651=FACE_OUTER_BOUND ( 'NONE', #75098, .T. ) ;
#91652=ORIENTED_EDGE ( 'NONE', *, *, #75995, .T. ) ;
#91653=CARTESIAN_POINT ( 'NONE',  ( -0.3289641300567998083, 13.07879003517447103, 5.963430220938281678 ) ) ;
#91656=CARTESIAN_POINT ( 'NONE',  ( 24.16423886937409904, 54.09541550158063217, 3.795296366450317205 ) ) ;
#91657=CARTESIAN_POINT ( 'NONE',  ( -0.8801773607110991993, 2.855352010821504471, -2.915334737309923874 ) ) ;
#91658=CARTESIAN_POINT ( 'NONE',  ( 18.52753015748618282, 23.92559781766745530, -4.923371831947291888 ) ) ;
#91659=CARTESIAN_POINT ( 'NONE',  ( 5.076628168052704559, 60.17559781766745175, -8.527530157486179263 ) ) ;
#91661=ADVANCED_FACE ( 'NONE', ( #24525 ), #95831, .F. ) ;
#91663=CARTESIAN_POINT ( 'NONE',  ( 1.472469842513823179, 10.59226448433411782, -4.923371831947296329 ) ) ;
#91664=CARTESIAN_POINT ( 'NONE',  ( 21.09922568453595559, 7.040301336597086568, -6.408140936763230044 ) ) ;
#91667=CARTESIAN_POINT ( 'NONE',  ( 24.16423886937410614, 29.51208216824729647, -3.795296366450302550 ) ) ;
#91668=CARTESIAN_POINT ( 'NONE',  ( -0.3689425029237881626, 47.42874883491396787, 10.36894250292379027 ) ) ;
#91669=ORIENTED_EDGE ( 'NONE', *, *, #95160, .T. ) ;
#91670=CARTESIAN_POINT ( 'NONE',  ( 22.81628187352648496, 61.83196800326376774, -3.434112377981050290 ) ) ;
#91671=CARTESIAN_POINT ( 'NONE',  ( 4.559911319644449179, 28.89701867748817321, 9.422509992056141925 ) ) ;
#91672=CARTESIAN_POINT ( 'NONE',  ( 2.791683348922240793, 51.63393115100078745, 7.208316651077764092 ) ) ;
#91673=CARTESIAN_POINT ( 'NONE',  ( 15.44008868035555260, 29.73035201082150891, 9.422509992056143702 ) ) ;
#91676=CARTESIAN_POINT ( 'NONE',  ( 19.84674366389459621, 53.50893115100078745, 7.409399052514197653E-17 ) ) ;
#91677=CARTESIAN_POINT ( 'NONE',  ( 12.63842701281683034, 47.46726448433412315, 9.846743663894596210 ) ) ;
#91683=ORIENTED_EDGE ( 'NONE', *, *, #13215, .F. ) ;
#91684=CARTESIAN_POINT ( 'NONE',  ( 2.791683348922240793, 31.63393115100078745, 7.208316651077764092 ) ) ;
#91687=CARTESIAN_POINT ( 'NONE',  ( 13.43411237798105340, 35.58196800326375353, 12.81628187352647963 ) ) ;
#91693=CARTESIAN_POINT ( 'NONE',  ( 18.52753015748617571, 53.09226448433412315, 4.923371831947298993 ) ) ;
#91694=CARTESIAN_POINT ( 'NONE',  ( 10.00000000000000178, 38.05374883491396787, 14.16423886937410082 ) ) ;
#91695=CARTESIAN_POINT ( 'NONE',  ( 1.472469842513823179, 60.59226448433412315, -4.923371831947296329 ) ) ;
#91697=CARTESIAN_POINT ( 'NONE',  ( 10.00000000000000178, 2.258931151000784787, 9.846743663894594434 ) ) ;
#91699=CARTESIAN_POINT ( 'NONE',  ( 0.6178305044545818747, 58.49863466993042493, -9.382169495545419124 ) ) ;
#91700=FACE_OUTER_BOUND ( 'NONE', #80835, .T. ) ;
#91701=CARTESIAN_POINT ( 'NONE',  ( 2.791683348922240793, 51.63393115100078745, 7.208316651077764092 ) ) ;
#91702=CARTESIAN_POINT ( 'NONE',  ( 20.88017736071110875, 50.77201867748817676, -2.915334737309920765 ) ) ;
#91703=CARTESIAN_POINT ( 'NONE',  ( 14.92337183194729633, 47.67559781766745175, 8.527530157486181039 ) ) ;
#91704=( BOUNDED_SURFACE ( )  B_SPLINE_SURFACE ( 1, 2, ( 
 ( #93252, #40264, #56255, #77754, #48731, #2780, #10748, #79235, #16286, #86747, #24285, #10260, #1309, #33716, #16777, #18252, #46766, #63729, #24776, #32745, #78250, #55252, #33236, #63241, #41266, #9268, #77261, #71740, #94229, #47752, #93745, #3249, #54752, #26236, #85767, #8773, #84777, #17278, #47252, #25761, #39289, #62255, #70275, #70771, #39777, #2286, #85271, #55761, #1793, #40754, #25280, #9767, #71257, #86253, #92760, #17767, #64214, #94731, #48242, #69780, #31759, #32247, #62750, #97222, #35701, #87222, #42715, #81203, #58185, #57705, #19715, #42233, #35193, #5222, #26717, #73198, #27205, #72700, #34704, #96221, #4235, #58693, #36198, #80215, #65199, #95212, #12704, #88205, #57213, #27701, #66186, #50202, #80714, #66695, #13197, #20206, #87710, #43198, #50711, #49229, #19226, #49706, #11721, #56731, #18745, #73687, #5709, #12209, #4729, #65697, #96721, #43690, #74177, #79730, #11229, #88697, #72219, #28197, #89197, #20707, #95720, #51200, #81683, #41749, #3749, #34210, #64700, #23185, #89687, #98708, #21702, #97715, #69170, #44680, #8174, #53169, #74686, #30651, #98206, #91667, #75673, #29179, #60662, #22690, #83675, #38667, #83176, #67191, #38187, #14701, #59679, #7690, #53661, #6198, #13693, #6687, #15189, #68673, #45672, #30158, #91163, #200, #44177, #82680, #82182, #37203, #36702, #51701, #76170, #61158, #90171, #14199, #84178, #46171, #15685, #76654, #60173, #28690, #52186, #75175, #59182, #21202, #67694, #29664, #45172, #68188, #90668, #22195, #52674, #7186, #37690, #71136, #25642, #69654, #16163, #32124, #92158, #31147, #55124, #39662, #32626, #85640, #1180, #93627, #79116, #17159, #93128, #31637, #62622, #10629, #61638, #62129, #92638, #24162, #77143, #33115, #2169, #8652, #47639, #48612, #48120, #41141, #77628, #9145, #2664, #9644, #25162, #23682, #78135, #70153, #63124, #40142, #54632, #55637, #693, #70645, #24654, #85149, #86137, #54146, #84654, #16657, #47131, #1671, #39165, #63609, #17651, #78636, #10143, #46645, #40638, #94115, #56135, #86628, #18140, #80598, #65574, #64095, #41633, #3625, #72099, #13077, #71627, #88579, #20591, #95600, #72584, #65075, #27584, #58576, #28078, #51078, #3136, #4117, #87106, #58075, #34581, #27086, #80096, #5094, #95092, #11600, #18621, #42598, #81569, #66073, #33597, #73077, #64583, #34093, #94610, #87593, #26125, #96101, #49112, #73570, #42119, #35584, #19597, #26600, #4613, #20088, #50591, #56617, #57588, #11114, #81082, #88085, #57097, #12585, #96601, #79613, #19103, #49584, #43084, #89078, #50093, #35074, #12096, #22573, #59067, #97598, #97106, #21585, #89572 ),
 ( #83061, #91045, #6568, #37079, #23071, #92, #7074, #13577, #98596, #37576, #28577, #67578, #45051, #5597, #30539, #51580, #36076, #43571, #7581, #74065, #21083, #15082, #66579, #53044, #82569, #90553, #98088, #14083, #60554, #22082, #76051, #36583, #82068, #45553, #83561, #29546, #52557, #61039, #44061, #84053, #52076, #74568, #6082, #44563, #67071, #38069, #29060, #59568, #90061, #60052, #75061, #14582, #75560, #68069, #30046, #68561, #91552, #53539, #9523, #77512, #92038, #62509, #33004, #40024, #47021, #9029, #70034, #85526, #32512, #56019, #93513, #46054, #1558, #70527, #17039, #16546, #39546, #1059, #93014, #63011, #84546, #32005, #85034, #31525, #92522, #55009, #62021, #17536, #94005, #39047, #24047, #54035, #2050, #24551, #16044, #47518, #25039, #78020, #55524, #25528, #71025, #86021, #46533, #48003, #78511, #586, #10026, #40526, #76541, #2548, #23567, #8058, #15573, #63505, #38556, #77035, #69051, #31030, #61530, #8548, #69542, #54518, #42005, #88465, #42973, #71986, #56979, #11485, #4003, #73453, #86518, #27467, #4981, #27956, #94979, #72471, #57961, #79501, #50465, #4496, #12469, #80969, #18016, #19967, #26008, #80481, #3031, #35461, #18501, #11981, #87970, #87484, #49474, #3510, #64959, #34961, #56502, #34467, #18999, #33969, #64472, #26977, #26483, #65957, #96484, #10999, #79982, #86994, #42482, #95486, #48991, #57476, #65459, #19483, #49975, #48498, #79000, #72965, #41519, #95986, #10505, #71521, #41020, #33480, #63976, #94490, #66449, #50959, #58449, #22451, #88964, #35953, #29428, #67451, #75436, #96984, #20971, #51456, #13965, #60428, #14957, #43940, #28935, #82441, #74942, #45424, #20472, #98470, #75929, #98963, #66953, #44440, #29923, #81945, #52924, #6950, #83437, #7454, #81455, #90921, #28461, #52442, #73954, #37951, #89455, #68444, #12956, #37457, #97471, #6445, #51957, #59440, #67945, #36954, #43452, #13455, #5480, #58955, #74439, #21459, #97972, #5964, #36458, #89942, #59933, #90422, #21961, #82940, #14457, #44929, #83925, #7940, #15927, #17775, #84430, #48251, #68933, #2793, #23443, #25770, #78762, #23928, #56264, #92405, #38435, #10270, #49238, #86757, #61898, #54399, #86262, #33245, #48741, #72229, #10760, #60919, #40764, #94740, #91424, #463, #63739, #71266, #79246, #30911, #91918, #53921, #94240, #33725, #87235, #46419, #938, #18262, #41275, #18757, #30419, #71750, #79742, #22952, #38928, #3257, #64224, #76908, #26245, #56739, #11239, #41758, #53418, #15455, #61409, #45934, #76425, #8421, #69415, #31399, #64712, #81696, #42730, #50724, #96233, #73207, #20720, #81214, #36209, #95732, #95221 ) ),
 .UNSPECIFIED., .F., .F., .F. ) 
 B_SPLINE_SURFACE_WITH_KNOTS ( ( 2, 2 ),
 ( 3, 2, 2, 2, 2, 2, 2, 2, 2, 2, 2, 2, 2, 2, 2, 2, 2, 2, 2, 2, 2, 2, 2, 2, 2, 2, 2, 2, 2, 2, 2, 2, 2, 2, 2, 2, 2, 2, 2, 2, 2, 2, 2, 2, 2, 2, 2, 2, 2, 2, 2, 2, 2, 2, 2, 2, 2, 2, 2, 2, 2, 2, 2, 2, 2, 2, 2, 2, 2, 2, 2, 2, 2, 2, 2, 2, 2, 2, 2, 2, 2, 2, 2, 2, 2, 2, 2, 2, 2, 2, 2, 2, 2, 2, 2, 2, 2, 2, 2, 2, 2, 2, 2, 2, 2, 2, 2, 2, 2, 2, 2, 2, 2, 2, 2, 2, 2, 2, 2, 2, 2, 2, 2, 2, 2, 2, 2, 2, 2, 2, 2, 2, 2, 2, 2, 2, 2, 2, 2, 2, 2, 2, 2, 2, 2, 2, 2, 2, 2, 2, 2, 2, 2, 2, 2, 2, 2, 2, 2, 2, 2, 2, 3 ),
 ( 0.000000000000000000, 1.000000000000000000 ),
 ( 0.000000000000000000, 0.005952380952380952051, 0.01190476190476190410, 0.01785714285714285615, 0.02380952380952380820, 0.02976190476190476025, 0.03571428571428571230, 0.04166666666666666435, 0.04761904761904761640, 0.05357142857142856845, 0.05952380952380952051, 0.06547619047619047949, 0.07142857142857142461, 0.07738095238095238360, 0.08333333333333332871, 0.08928571428571428770, 0.09523809523809523281, 0.1011904761904761918, 0.1071428571428571369, 0.1130952380952380959, 0.1190476190476190410, 0.1250000000000000000, 0.1309523809523809590, 0.1369047619047619180, 0.1428571428571428492, 0.1488095238095238082, 0.1547619047619047672, 0.1607142857142857262, 0.1666666666666666574, 0.1726190476190476164, 0.1785714285714285754, 0.1845238095238095344, 0.1904761904761904656, 0.1964285714285714246, 0.2023809523809523836, 0.2083333333333333426, 0.2142857142857142738, 0.2202380952380952328, 0.2261904761904761918, 0.2321428571428571508, 0.2380952380952380820, 0.2440476190476190410, 0.2500000000000000000, 0.2559523809523809312, 0.2619047619047619180, 0.2678571428571428492, 0.2738095238095238360, 0.2797619047619047672, 0.2857142857142856984, 0.2916666666666666852, 0.2976190476190476164, 0.3035714285714285476, 0.3095238095238095344, 0.3154761904761904656, 0.3214285714285714524, 0.3273809523809523836, 0.3333333333333333148, 0.3392857142857143016, 0.3452380952380952328, 0.3511904761904761640, 0.3571428571428571508, 0.3630952380952380820, 0.3690476190476190688, 0.3750000000000000000, 0.3809523809523809312, 0.3869047619047619180, 0.3928571428571428492, 0.3988095238095238360, 0.4047619047619047672, 0.4107142857142856984, 0.4166666666666666852, 0.4226190476190476164, 0.4285714285714285476, 0.4345238095238095344, 0.4404761904761904656, 0.4464285714285714524, 0.4523809523809523836, 0.4583333333333333148, 0.4642857142857143016, 0.4702380952380952328, 0.4761904761904761640, 0.4821428571428571508, 0.4880952380952380820, 0.4940476190476190688, 0.5000000000000000000, 0.5059523809523809312, 0.5119047619047618625, 0.5178571428571429047, 0.5238095238095238360, 0.5297619047619047672, 0.5357142857142856984, 0.5416666666666666297, 0.5476190476190476719, 0.5535714285714286031, 0.5595238095238095344, 0.5654761904761904656, 0.5714285714285713969, 0.5773809523809523281, 0.5833333333333333703, 0.5892857142857143016, 0.5952380952380952328, 0.6011904761904761640, 0.6071428571428570953, 0.6130952380952381375, 0.6190476190476190688, 0.6250000000000000000, 0.6309523809523809312, 0.6369047619047618625, 0.6428571428571429047, 0.6488095238095238360, 0.6547619047619047672, 0.6607142857142856984, 0.6666666666666666297, 0.6726190476190476719, 0.6785714285714286031, 0.6845238095238095344, 0.6904761904761904656, 0.6964285714285713969, 0.7023809523809523281, 0.7083333333333333703, 0.7142857142857143016, 0.7202380952380952328, 0.7261904761904761640, 0.7321428571428570953, 0.7380952380952381375, 0.7440476190476190688, 0.7500000000000000000, 0.7559523809523809312, 0.7619047619047618625, 0.7678571428571429047, 0.7738095238095238360, 0.7797619047619047672, 0.7857142857142856984, 0.7916666666666666297, 0.7976190476190476719, 0.8035714285714286031, 0.8095238095238095344, 0.8154761904761904656, 0.8214285714285713969, 0.8273809523809523281, 0.8333333333333333703, 0.8392857142857143016, 0.8452380952380952328, 0.8511904761904761640, 0.8571428571428570953, 0.8630952380952381375, 0.8690476190476190688, 0.8750000000000000000, 0.8809523809523809312, 0.8869047619047618625, 0.8928571428571429047, 0.8988095238095238360, 0.9047619047619047672, 0.9107142857142856984, 0.9166666666666666297, 0.9226190476190476719, 0.9285714285714286031, 0.9345238095238095344, 0.9404761904761904656, 0.9464285714285713969, 0.9523809523809523281, 0.9583333333333333703, 0.9642857142857143016 ),
 .UNSPECIFIED. ) 
 GEOMETRIC_REPRESENTATION_ITEM ( )  RATIONAL_B_SPLINE_SURFACE ( (
 ( 1.000000000000000000, 0.9659258262890683122, 1.000000000000000000, 0.9659258262890683122, 1.000000000000000000, 0.9659258262890683122, 1.000000000000000000, 0.9659258262890683122, 1.000000000000000000, 0.9659258262890683122, 1.000000000000000000, 0.9659258262890683122, 1.000000000000000000, 0.9659258262890683122, 1.000000000000000000, 0.9659258262890683122, 1.000000000000000000, 0.9659258262890683122, 1.000000000000000000, 0.9659258262890683122, 1.000000000000000000, 0.9659258262890683122, 1.000000000000000000, 0.9659258262890683122, 1.000000000000000000, 0.9659258262890683122, 1.000000000000000000, 0.9659258262890683122, 1.000000000000000000, 0.9659258262890683122, 1.000000000000000000, 0.9659258262890683122, 1.000000000000000000, 0.9659258262890683122, 1.000000000000000000, 0.9659258262890683122, 1.000000000000000000, 0.9659258262890683122, 1.000000000000000000, 0.9659258262890683122, 1.000000000000000000, 0.9659258262890683122, 1.000000000000000000, 0.9659258262890683122, 1.000000000000000000, 0.9659258262890683122, 1.000000000000000000, 0.9659258262890683122, 1.000000000000000000, 0.9659258262890683122, 1.000000000000000000, 0.9659258262890683122, 1.000000000000000000, 0.9659258262890683122, 1.000000000000000000, 0.9659258262890683122, 1.000000000000000000, 0.9659258262890683122, 1.000000000000000000, 0.9659258262890683122, 1.000000000000000000, 0.9659258262890683122, 1.000000000000000000, 0.9659258262890683122, 1.000000000000000000, 0.9659258262890683122, 1.000000000000000000, 0.9659258262890683122, 1.000000000000000000, 0.9659258262890683122, 1.000000000000000000, 0.9659258262890683122, 1.000000000000000000, 0.9659258262890683122, 1.000000000000000000, 0.9659258262890683122, 1.000000000000000000, 0.9659258262890683122, 1.000000000000000000, 0.9659258262890683122, 1.000000000000000000, 0.9659258262890683122, 1.000000000000000000, 0.9659258262890683122, 1.000000000000000000, 0.9659258262890683122, 1.000000000000000000, 0.9659258262890683122, 1.000000000000000000, 0.9659258262890683122, 1.000000000000000000, 0.9659258262890683122, 1.000000000000000000, 0.9659258262890683122, 1.000000000000000000, 0.9659258262890683122, 1.000000000000000000, 0.9659258262890683122, 1.000000000000000000, 0.9659258262890683122, 1.000000000000000000, 0.9659258262890683122, 1.000000000000000000, 0.9659258262890683122, 1.000000000000000000, 0.9659258262890683122, 1.000000000000000000, 0.9659258262890683122, 1.000000000000000000, 0.9659258262890683122, 1.000000000000000000, 0.9659258262890683122, 1.000000000000000000, 0.9659258262890683122, 1.000000000000000000, 0.9659258262890683122, 1.000000000000000000, 0.9659258262890683122, 1.000000000000000000, 0.9659258262890683122, 1.000000000000000000, 0.9659258262890683122, 1.000000000000000000, 0.9659258262890683122, 1.000000000000000000, 0.9659258262890683122, 1.000000000000000000, 0.9659258262890683122, 1.000000000000000000, 0.9659258262890683122, 1.000000000000000000, 0.9659258262890683122, 1.000000000000000000, 0.9659258262890683122, 1.000000000000000000, 0.9659258262890683122, 1.000000000000000000, 0.9659258262890683122, 1.000000000000000000, 0.9659258262890683122, 1.000000000000000000, 0.9659258262890683122, 1.000000000000000000, 0.9659258262890683122, 1.000000000000000000, 0.9659258262890683122, 1.000000000000000000, 0.9659258262890683122, 1.000000000000000000, 0.9659258262890683122, 1.000000000000000000, 0.9659258262890683122, 1.000000000000000000, 0.9659258262890683122, 1.000000000000000000, 0.9659258262890683122, 1.000000000000000000, 0.9659258262890683122, 1.000000000000000000, 0.9659258262890683122, 1.000000000000000000, 0.9659258262890683122, 1.000000000000000000, 0.9659258262890683122, 1.000000000000000000, 0.9659258262890683122, 1.000000000000000000, 0.9659258262890683122, 1.000000000000000000, 0.9659258262890683122, 1.000000000000000000, 0.9659258262890683122, 1.000000000000000000, 0.9659258262890683122, 1.000000000000000000, 0.9659258262890683122, 1.000000000000000000, 0.9659258262890683122, 1.000000000000000000, 0.9659258262890683122, 1.000000000000000000, 0.9659258262890683122, 1.000000000000000000, 0.9659258262890683122, 1.000000000000000000, 0.9659258262890683122, 1.000000000000000000, 0.9659258262890683122, 1.000000000000000000, 0.9659258262890683122, 1.000000000000000000, 0.9659258262890683122, 1.000000000000000000, 0.9659258262890683122, 1.000000000000000000, 0.9659258262890683122, 1.000000000000000000, 0.9659258262890683122, 1.000000000000000000, 0.9659258262890683122, 1.000000000000000000, 0.9659258262890683122, 1.000000000000000000, 0.9659258262890683122, 1.000000000000000000, 0.9659258262890683122, 1.000000000000000000, 0.9659258262890683122, 1.000000000000000000, 0.9659258262890683122, 1.000000000000000000, 0.9659258262890683122, 1.000000000000000000, 0.9659258262890683122, 1.000000000000000000, 0.9659258262890683122, 1.000000000000000000, 0.9659258262890683122, 1.000000000000000000, 0.9659258262890683122, 1.000000000000000000, 0.9659258262890683122, 1.000000000000000000, 0.9659258262890683122, 1.000000000000000000, 0.9659258262890683122, 1.000000000000000000, 0.9659258262890683122, 1.000000000000000000, 0.9659258262890683122, 1.000000000000000000, 0.9659258262890683122, 1.000000000000000000, 0.9659258262890683122, 1.000000000000000000, 0.9659258262890683122, 1.000000000000000000, 0.9659258262890683122, 1.000000000000000000, 0.9659258262890683122, 1.000000000000000000, 0.9659258262890683122, 1.000000000000000000, 0.9659258262890683122, 1.000000000000000000, 0.9659258262890683122, 1.000000000000000000, 0.9659258262890683122, 1.000000000000000000, 0.9659258262890683122, 1.000000000000000000, 0.9659258262890683122, 1.000000000000000000, 0.9659258262890683122, 1.000000000000000000, 0.9659258262890683122, 1.000000000000000000, 0.9659258262890683122, 1.000000000000000000, 0.9659258262890683122, 1.000000000000000000, 0.9659258262890683122, 1.000000000000000000, 0.9659258262890683122, 1.000000000000000000, 0.9659258262890683122, 1.000000000000000000, 0.9659258262890683122, 1.000000000000000000, 0.9659258262890683122, 1.000000000000000000, 0.9659258262890683122, 1.000000000000000000, 0.9659258262890683122, 1.000000000000000000, 0.9659258262890683122, 1.000000000000000000, 0.9659258262890683122, 1.000000000000000000, 0.9659258262890683122, 1.000000000000000000, 0.9659258262890683122, 1.000000000000000000, 0.9659258262890683122, 1.000000000000000000, 0.9659258262890683122, 1.000000000000000000, 0.9659258262890683122, 1.000000000000000000, 0.9659258262890683122, 1.000000000000000000, 0.9659258262890683122, 1.000000000000000000, 0.9659258262890683122, 1.000000000000000000, 0.9659258262890683122, 1.000000000000000000, 0.9659258262890683122, 1.000000000000000000, 0.9659258262890683122, 1.000000000000000000, 0.9659258262890683122, 1.000000000000000000, 0.9659258262890683122, 1.000000000000000000, 0.9659258262890683122, 1.000000000000000000, 0.9659258262890683122, 1.000000000000000000, 0.9659258262890683122, 1.000000000000000000, 0.9659258262890683122, 1.000000000000000000, 0.9659258262890683122, 1.000000000000000000, 0.9659258262890683122, 1.000000000000000000, 0.9659258262890683122, 1.000000000000000000, 0.9659258262890683122, 1.000000000000000000, 0.9659258262890683122, 1.000000000000000000, 0.9659258262890683122, 1.000000000000000000),
 ( 1.000000000000000000, 0.9659258262890683122, 1.000000000000000000, 0.9659258262890683122, 1.000000000000000000, 0.9659258262890683122, 1.000000000000000000, 0.9659258262890683122, 1.000000000000000000, 0.9659258262890683122, 1.000000000000000000, 0.9659258262890683122, 1.000000000000000000, 0.9659258262890683122, 1.000000000000000000, 0.9659258262890683122, 1.000000000000000000, 0.9659258262890683122, 1.000000000000000000, 0.9659258262890683122, 1.000000000000000000, 0.9659258262890683122, 1.000000000000000000, 0.9659258262890683122, 1.000000000000000000, 0.9659258262890683122, 1.000000000000000000, 0.9659258262890683122, 1.000000000000000000, 0.9659258262890683122, 1.000000000000000000, 0.9659258262890683122, 1.000000000000000000, 0.9659258262890683122, 1.000000000000000000, 0.9659258262890683122, 1.000000000000000000, 0.9659258262890683122, 1.000000000000000000, 0.9659258262890683122, 1.000000000000000000, 0.9659258262890683122, 1.000000000000000000, 0.9659258262890683122, 1.000000000000000000, 0.9659258262890683122, 1.000000000000000000, 0.9659258262890683122, 1.000000000000000000, 0.9659258262890683122, 1.000000000000000000, 0.9659258262890683122, 1.000000000000000000, 0.9659258262890683122, 1.000000000000000000, 0.9659258262890683122, 1.000000000000000000, 0.9659258262890683122, 1.000000000000000000, 0.9659258262890683122, 1.000000000000000000, 0.9659258262890683122, 1.000000000000000000, 0.9659258262890683122, 1.000000000000000000, 0.9659258262890683122, 1.000000000000000000, 0.9659258262890683122, 1.000000000000000000, 0.9659258262890683122, 1.000000000000000000, 0.9659258262890683122, 1.000000000000000000, 0.9659258262890683122, 1.000000000000000000, 0.9659258262890683122, 1.000000000000000000, 0.9659258262890683122, 1.000000000000000000, 0.9659258262890683122, 1.000000000000000000, 0.9659258262890683122, 1.000000000000000000, 0.9659258262890683122, 1.000000000000000000, 0.9659258262890683122, 1.000000000000000000, 0.9659258262890683122, 1.000000000000000000, 0.9659258262890683122, 1.000000000000000000, 0.9659258262890683122, 1.000000000000000000, 0.9659258262890683122, 1.000000000000000000, 0.9659258262890683122, 1.000000000000000000, 0.9659258262890683122, 1.000000000000000000, 0.9659258262890683122, 1.000000000000000000, 0.9659258262890683122, 1.000000000000000000, 0.9659258262890683122, 1.000000000000000000, 0.9659258262890683122, 1.000000000000000000, 0.9659258262890683122, 1.000000000000000000, 0.9659258262890683122, 1.000000000000000000, 0.9659258262890683122, 1.000000000000000000, 0.9659258262890683122, 1.000000000000000000, 0.9659258262890683122, 1.000000000000000000, 0.9659258262890683122, 1.000000000000000000, 0.9659258262890683122, 1.000000000000000000, 0.9659258262890683122, 1.000000000000000000, 0.9659258262890683122, 1.000000000000000000, 0.9659258262890683122, 1.000000000000000000, 0.9659258262890683122, 1.000000000000000000, 0.9659258262890683122, 1.000000000000000000, 0.9659258262890683122, 1.000000000000000000, 0.9659258262890683122, 1.000000000000000000, 0.9659258262890683122, 1.000000000000000000, 0.9659258262890683122, 1.000000000000000000, 0.9659258262890683122, 1.000000000000000000, 0.9659258262890683122, 1.000000000000000000, 0.9659258262890683122, 1.000000000000000000, 0.9659258262890683122, 1.000000000000000000, 0.9659258262890683122, 1.000000000000000000, 0.9659258262890683122, 1.000000000000000000, 0.9659258262890683122, 1.000000000000000000, 0.9659258262890683122, 1.000000000000000000, 0.9659258262890683122, 1.000000000000000000, 0.9659258262890683122, 1.000000000000000000, 0.9659258262890683122, 1.000000000000000000, 0.9659258262890683122, 1.000000000000000000, 0.9659258262890683122, 1.000000000000000000, 0.9659258262890683122, 1.000000000000000000, 0.9659258262890683122, 1.000000000000000000, 0.9659258262890683122, 1.000000000000000000, 0.9659258262890683122, 1.000000000000000000, 0.9659258262890683122, 1.000000000000000000, 0.9659258262890683122, 1.000000000000000000, 0.9659258262890683122, 1.000000000000000000, 0.9659258262890683122, 1.000000000000000000, 0.9659258262890683122, 1.000000000000000000, 0.9659258262890683122, 1.000000000000000000, 0.9659258262890683122, 1.000000000000000000, 0.9659258262890683122, 1.000000000000000000, 0.9659258262890683122, 1.000000000000000000, 0.9659258262890683122, 1.000000000000000000, 0.9659258262890683122, 1.000000000000000000, 0.9659258262890683122, 1.000000000000000000, 0.9659258262890683122, 1.000000000000000000, 0.9659258262890683122, 1.000000000000000000, 0.9659258262890683122, 1.000000000000000000, 0.9659258262890683122, 1.000000000000000000, 0.9659258262890683122, 1.000000000000000000, 0.9659258262890683122, 1.000000000000000000, 0.9659258262890683122, 1.000000000000000000, 0.9659258262890683122, 1.000000000000000000, 0.9659258262890683122, 1.000000000000000000, 0.9659258262890683122, 1.000000000000000000, 0.9659258262890683122, 1.000000000000000000, 0.9659258262890683122, 1.000000000000000000, 0.9659258262890683122, 1.000000000000000000, 0.9659258262890683122, 1.000000000000000000, 0.9659258262890683122, 1.000000000000000000, 0.9659258262890683122, 1.000000000000000000, 0.9659258262890683122, 1.000000000000000000, 0.9659258262890683122, 1.000000000000000000, 0.9659258262890683122, 1.000000000000000000, 0.9659258262890683122, 1.000000000000000000, 0.9659258262890683122, 1.000000000000000000, 0.9659258262890683122, 1.000000000000000000, 0.9659258262890683122, 1.000000000000000000, 0.9659258262890683122, 1.000000000000000000, 0.9659258262890683122, 1.000000000000000000, 0.9659258262890683122, 1.000000000000000000, 0.9659258262890683122, 1.000000000000000000, 0.9659258262890683122, 1.000000000000000000, 0.9659258262890683122, 1.000000000000000000, 0.9659258262890683122, 1.000000000000000000, 0.9659258262890683122, 1.000000000000000000, 0.9659258262890683122, 1.000000000000000000, 0.9659258262890683122, 1.000000000000000000, 0.9659258262890683122, 1.000000000000000000, 0.9659258262890683122, 1.000000000000000000, 0.9659258262890683122, 1.000000000000000000, 0.9659258262890683122, 1.000000000000000000, 0.9659258262890683122, 1.000000000000000000, 0.9659258262890683122, 1.000000000000000000, 0.9659258262890683122, 1.000000000000000000, 0.9659258262890683122, 1.000000000000000000, 0.9659258262890683122, 1.000000000000000000, 0.9659258262890683122, 1.000000000000000000, 0.9659258262890683122, 1.000000000000000000, 0.9659258262890683122, 1.000000000000000000, 0.9659258262890683122, 1.000000000000000000, 0.9659258262890683122, 1.000000000000000000, 0.9659258262890683122, 1.000000000000000000, 0.9659258262890683122, 1.000000000000000000, 0.9659258262890683122, 1.000000000000000000, 0.9659258262890683122, 1.000000000000000000, 0.9659258262890683122, 1.000000000000000000, 0.9659258262890683122, 1.000000000000000000, 0.9659258262890683122, 1.000000000000000000, 0.9659258262890683122, 1.000000000000000000, 0.9659258262890683122, 1.000000000000000000, 0.9659258262890683122, 1.000000000000000000, 0.9659258262890683122, 1.000000000000000000, 0.9659258262890683122, 1.000000000000000000, 0.9659258262890683122, 1.000000000000000000, 0.9659258262890683122, 1.000000000000000000, 0.9659258262890683122, 1.000000000000000000, 0.9659258262890683122, 1.000000000000000000, 0.9659258262890683122, 1.000000000000000000) ) ) 
 REPRESENTATION_ITEM ( '' )  SURFACE ( )  );
#91706=CARTESIAN_POINT ( 'NONE',  ( 20.88017736071110164, 55.35535201082149825, 2.915334737309930979 ) ) ;
#91707=ORIENTED_EDGE ( 'NONE', *, *, #24384, .T. ) ;
#91709=CARTESIAN_POINT ( 'NONE',  ( -0.8801773607111008646, 28.27201867748817321, 2.915334737309923430 ) ) ;
#91710=CARTESIAN_POINT ( 'NONE',  ( 2.791683348922240793, 66.63393115100079456, 7.208316651077764092 ) ) ;
#91711=CARTESIAN_POINT ( 'NONE',  ( 20.88017736071110519, 55.56368534415484817, 2.639326808657452039E-16 ) ) ;
#91714=CARTESIAN_POINT ( 'NONE',  ( 15.44008868035555260, 34.73035201082151247, 9.422509992056143702 ) ) ;
#91715=CARTESIAN_POINT ( 'NONE',  ( -46.71039645252511718, 100.6859025094012026, 9.426366605710914115 ) ) ;
#91716=CARTESIAN_POINT ( 'NONE',  ( 12.63842701281683034, 17.46726448433411250, 9.846743663894596210 ) ) ;
#91717=CARTESIAN_POINT ( 'NONE',  ( 2.791683348922237240, 40.38393115100078035, -7.208316651077763204 ) ) ;
#91720=CARTESIAN_POINT ( 'NONE',  ( 5.076628168052704559, 65.17559781766745175, -8.527530157486179263 ) ) ;
#91721=CARTESIAN_POINT ( 'NONE',  ( 24.16423886937409904, 64.09541550158064638, 3.795296366450317205 ) ) ;
#91724=CARTESIAN_POINT ( 'NONE',  ( -2.266590686148945544, 27.22041550158063572, 7.082119434687048631 ) ) ;
#91725=CARTESIAN_POINT ( 'NONE',  ( -2.266590686148945544, 57.22041550158063217, 7.082119434687048631 ) ) ;
#91726=CARTESIAN_POINT ( 'NONE',  ( 10.00000000000000178, 17.25893115100078745, 9.846743663894594434 ) ) ;
#91727=CARTESIAN_POINT ( 'NONE',  ( 4.559911319644449179, 3.897018677488170990, 9.422509992056141925 ) ) ;
#91729=CARTESIAN_POINT ( 'NONE',  ( 2.791683348922237240, 30.38393115100078390, -7.208316651077763204 ) ) ;
#91730=CARTESIAN_POINT ( 'NONE',  ( 7.084665262690076126, 29.10535201082150181, 10.88017736071109987 ) ) ;
#91731=CARTESIAN_POINT ( 'NONE',  ( 10.00000000000000178, 67.25893115100079456, 9.846743663894594434 ) ) ;
#91732=CARTESIAN_POINT ( 'NONE',  ( 17.08211943468705130, 3.470415501580634388, 12.26659068614894998 ) ) ;
#91734=B_SPLINE_CURVE_WITH_KNOTS ( 'NONE', 3,
 ( #49638, #20139, #96653, #80651, #12145, #28628, #74113, #81132, #87645, #5647 ),
 .UNSPECIFIED., .F., .F.,
 ( 4, 3, 3, 4 ),
 ( 0.000000000000000000, 0.0006253016069560992946, 0.001250604074564904376, 0.002501455912506566921 ),
 .UNSPECIFIED. ) ;
#91736=CARTESIAN_POINT ( 'NONE',  ( 0.1532563361054082862, 6.217264484334118713, 2.638427012816831674 ) ) ;
#91737=CARTESIAN_POINT ( 'NONE',  ( 0.6178305044545818747, 38.49863466993042493, -9.382169495545419124 ) ) ;
#91738=CARTESIAN_POINT ( 'NONE',  ( 0.1532563361054100626, 35.80059781766745175, -2.638427012816831230 ) ) ;
#91740=CARTESIAN_POINT ( 'NONE',  ( 18.52753015748617571, 18.09226448433411960, 4.923371831947298993 ) ) ;
#91743=CARTESIAN_POINT ( 'NONE',  ( 6.204703633549690345, 50.76208216824730357, -14.16423886937410259 ) ) ;
#91744=CARTESIAN_POINT ( 'NONE',  ( 7.084665262690076126, 49.10535201082149825, 10.88017736071109987 ) ) ;
#91745=DIRECTION ( 'NONE',  ( -0.000000000000000000, 1.000000000000000000, -0.000000000000000000 ) ) ;
#91746=CARTESIAN_POINT ( 'NONE',  ( 1.472469842513823179, 35.59226448433412315, -4.923371831947296329 ) ) ;
#91747=CARTESIAN_POINT ( 'NONE',  ( 20.88017736071110164, 10.35535201082150714, 2.915334737309930979 ) ) ;
#91748=CARTESIAN_POINT ( 'NONE',  ( 0.1532563361054082862, 41.21726448433411605, 2.638427012816831674 ) ) ;
#91750=CARTESIAN_POINT ( 'NONE',  ( 5.076628168052704559, 45.17559781766745175, -8.527530157486179263 ) ) ;
#91751=CARTESIAN_POINT ( 'NONE',  ( 0.5774900079438590739, 52.64701867748817676, -5.440088680355550821 ) ) ;
#91756=CARTESIAN_POINT ( 'NONE',  ( 12.63842701281683922, 9.550597817667449974, -9.846743663894590881 ) ) ;
#91757=CARTESIAN_POINT ( 'NONE',  ( -2.816281873526473856, 54.12363466993041783, 9.499525473075851096E-16 ) ) ;
#91758=CARTESIAN_POINT ( 'NONE',  ( 17.96484262340118221, 11.18868534415484106, -7.964842623401177768 ) ) ;
#91759=CARTESIAN_POINT ( 'NONE',  ( 0.1532563361054083140, 46.00893115100079456, 1.131784320476157264E-15 ) ) ;
#91761=CARTESIAN_POINT ( 'NONE',  ( -4.164238869374098151, 31.59541550158063927, -3.795296366450310543 ) ) ;
#91763=CARTESIAN_POINT ( 'NONE',  ( 20.36894250292379738, 54.92874883491396076, -10.36894250292379027 ) ) ;
#91764=CARTESIAN_POINT ( 'NONE',  ( 0.1532563361054082862, 61.21726448433412315, 2.638427012816831674 ) ) ;
#91766=CARTESIAN_POINT ( 'NONE',  ( 17.96484262340118221, 46.18868534415484106, -7.964842623401177768 ) ) ;
#91768=CARTESIAN_POINT ( 'NONE',  ( 14.92337183194729633, 2.675597817667451750, 8.527530157486181039 ) ) ;
#91771=CARTESIAN_POINT ( 'NONE',  ( 3.591859063236763294, 63.29030133659708923, -11.09922568453595026 ) ) ;
#91772=EDGE_LOOP ( 'NONE', ( #88946, #88665, #61248, #33446, #91669, #42448, #59699, #98934, #9776, #63374, #36925, #9549, #84310, #66274, #77542, #32369, #98091, #36504, #37193, #67338, #30880, #33524, #13891, #2194, #70074, #47537, #84290, #21612, #91282, #41911, #45811, #13504, #31171, #84583, #97615, #43525, #33954, #34044, #28701, #89530, #23086, #92506, #78955, #74181, #56848, #72185, #98799, #4121, #21309, #79136, #46277, #9902, #44404, #27435, #27485, #83922, #39016, #19704, #92863, #53494, #54746, #26716, #49994, #84145, #24051, #56047, #10868, #28089, #64179, #87221, #80401, #53784, #46273, #86917, #76055, #59739, #33982, #37586, #13880, #65766, #86786, #92637, #93117, #36301, #13309, #82474, #94896, #35955, #78648, #60172, #37564, #13063, #46136, #36238, #4361, #71741, #80277, #56021, #15756, #93233, #89181, #54234, #53133, #73321, #39837, #35987, #83240, #52185, #93243, #61944, #57089 ) ) ;
#91773=CARTESIAN_POINT ( 'NONE',  ( 5.076628168052703671, 6.842264484334118713, 8.527530157486179263 ) ) ;
#91775=CARTESIAN_POINT ( 'NONE',  ( -4.164238869374098151, 16.59541550158063927, -3.795296366450310543 ) ) ;
#91776=CARTESIAN_POINT ( 'NONE',  ( 10.00000000000000000, 24.75893115100078745, -9.846743663894594434 ) ) ;
#91777=CARTESIAN_POINT ( 'NONE',  ( 7.084665262690076126, 37.02201867748817676, -10.88017736071110164 ) ) ;
#91781=CARTESIAN_POINT ( 'NONE',  ( 19.42250999205614548, 30.98035201082150536, -5.440088680355545492 ) ) ;
#91782=AXIS2_PLACEMENT_3D ( 'NONE', #81869, #58878, #72890 ) ;
#91784=CARTESIAN_POINT ( 'NONE',  ( 20.88017736071110519, 30.56368534415484106, 2.639326808657452039E-16 ) ) ;
#91785=CARTESIAN_POINT ( 'NONE',  ( 2.791683348922240793, 66.63393115100079456, 7.208316651077764092 ) ) ;
#91789=CARTESIAN_POINT ( 'NONE',  ( 22.81628187352647785, 11.41530133659708390, 3.434112377981063169 ) ) ;
#91790=CARTESIAN_POINT ( 'NONE',  ( 17.20831665107776587, 4.133931151000785675, -7.208316651077762316 ) ) ;
#91792=CARTESIAN_POINT ( 'NONE',  ( 0.2751277870543045734, 27.28217586085238011, -6.500000000000012434 ) ) ;
#91793=CARTESIAN_POINT ( 'NONE',  ( 12.63842701281683034, 22.46726448433411605, 9.846743663894596210 ) ) ;
#91794=CARTESIAN_POINT ( 'NONE',  ( 19.42250999205614548, 30.98035201082150536, -5.440088680355545492 ) ) ;
#91796=VERTEX_POINT ( 'NONE', #92991 ) ;
#91798=CARTESIAN_POINT ( 'NONE',  ( 21.09922568453594849, 61.20696800326376064, 6.408140936763242479 ) ) ;
#91799=CARTESIAN_POINT ( 'NONE',  ( 15.44008868035555793, 61.39701867748817676, -9.422509992056140149 ) ) ;
#91801=CARTESIAN_POINT ( 'NONE',  ( 10.00000000000000000, 57.87363466993042493, -12.81628187352647608 ) ) ;
#91802=CARTESIAN_POINT ( 'NONE',  ( -0.8801773607111009756, 63.06368534415484106, 1.068504757029289695E-15 ) ) ;
#91803=CARTESIAN_POINT ( 'NONE',  ( 2.791683348922240793, 66.63393115100079456, 7.208316651077764092 ) ) ;
#91804=FACE_OUTER_BOUND ( 'NONE', #54400, .T. ) ;
#91805=CARTESIAN_POINT ( 'NONE',  ( 0.1532563361054083140, 31.00893115100078390, 1.131784320476157264E-15 ) ) ;
#91806=CARTESIAN_POINT ( 'NONE',  ( 3.591859063236763294, 48.29030133659708923, -11.09922568453595026 ) ) ;
#91807=CARTESIAN_POINT ( 'NONE',  ( 0.000000000000000000, 78.33947701945625397, 8.949703107968367988 ) ) ;
#91808=CARTESIAN_POINT ( 'NONE',  ( 17.20831665107776587, 17.88393115100078745, 7.208316651077764980 ) ) ;
#91809=CARTESIAN_POINT ( 'NONE',  ( 3.591859063236761518, 14.95696800326375531, 11.09922568453594849 ) ) ;
#91811=LINE ( 'NONE', #83817, #81909 ) ;
#91813=CARTESIAN_POINT ( 'NONE',  ( 4.559911319644449179, 32.23035201082150536, -9.422509992056141925 ) ) ;
#91814=CARTESIAN_POINT ( 'NONE',  ( 3.591859063236761518, -0.04303199673624671928, 11.09922568453594849 ) ) ;
#91816=CARTESIAN_POINT ( 'NONE',  ( 19.84674366389459266, 23.30059781766745530, 2.638427012816836559 ) ) ;
#91817=CARTESIAN_POINT ( 'NONE',  ( 14.92337183194729633, 2.675597817667451750, 8.527530157486181039 ) ) ;
#91818=CARTESIAN_POINT ( 'NONE',  ( 0.5774900079438607392, 8.480352010821505360, 5.440088680355550821 ) ) ;
#91819=CARTESIAN_POINT ( 'NONE',  ( -2.816281873526471635, 18.91530133659708213, -3.434112377981056508 ) ) ;
#91820=CARTESIAN_POINT ( 'NONE',  ( 2.035157376598822676, 2.438685344154837953, -7.964842623401177768 ) ) ;
#91822=CARTESIAN_POINT ( 'NONE',  ( 7.361572987183170547, 62.05059781766745886, 9.846743663894590881 ) ) ;
#91824=CARTESIAN_POINT ( 'NONE',  ( 22.26659068614895176, 19.72041550158063572, -7.082119434687042414 ) ) ;
#91825=CARTESIAN_POINT ( 'NONE',  ( -0.3689425029237881626, 67.42874883491396076, 10.36894250292379027 ) ) ;
#91826=CARTESIAN_POINT ( 'NONE',  ( 14.92337183194729988, 39.34226448433412315, -8.527530157486177487 ) ) ;
#91828=CARTESIAN_POINT ( 'NONE',  ( -1.926860441876562025, 49.47997603579417358, -3.195792623639529761 ) ) ;
#91829=CARTESIAN_POINT ( 'NONE',  ( 15.44008868035555260, 19.73035201082150536, 9.422509992056143702 ) ) ;
#91830=CARTESIAN_POINT ( 'NONE',  ( -0.8801773607110990882, 12.85535201082150358, -2.915334737309924318 ) ) ;
#91831=CARTESIAN_POINT ( 'NONE',  ( 4.559911319644449179, 28.89701867748817321, 9.422509992056141925 ) ) ;
#91832=CARTESIAN_POINT ( 'NONE',  ( -4.164238869374098151, 66.59541550158060375, -3.795296366450310543 ) ) ;
#91833=DIRECTION ( 'NONE',  ( 0.000000000000000000, -1.000000000000000000, 0.000000000000000000 ) ) ;
#91834=SURFACE_STYLE_USAGE ( .BOTH. , #76818 ) ;
#91836=CARTESIAN_POINT ( 'NONE',  ( 7.361572987183169658, 24.96726448433412315, -9.846743663894592657 ) ) ;
#91837=CARTESIAN_POINT ( 'NONE',  ( 22.81628187352647785, 11.62363466993042138, 6.195893100308588602E-16 ) ) ;
#91838=CARTESIAN_POINT ( 'NONE',  ( -46.44011323352863485, 103.5176347749360133, 6.245517546461054614 ) ) ;
#91841=CARTESIAN_POINT ( 'NONE',  ( 10.00000000000000000, 64.75893115100078035, -9.846743663894594434 ) ) ;
#91843=CARTESIAN_POINT ( 'NONE',  ( 13.79529636645030344, 13.26208216824729824, 14.16423886937410614 ) ) ;
#91844=CARTESIAN_POINT ( 'NONE',  ( 19.84674366389459266, 43.30059781766744464, 2.638427012816836559 ) ) ;
#91846=VERTEX_POINT ( 'NONE', #32489 ) ;
#91848=CARTESIAN_POINT ( 'NONE',  ( 24.16423886937410614, 54.30374883491396787, 8.672049930838204340E-16 ) ) ;
#91849=CARTESIAN_POINT ( 'NONE',  ( 17.20831665107776587, 4.133931151000785675, -7.208316651077762316 ) ) ;
#91852=CARTESIAN_POINT ( 'NONE',  ( 17.96484262340118221, 44.93868534415483396, 7.964842623401181321 ) ) ;
#91853=CARTESIAN_POINT ( 'NONE',  ( -1.099225684535947600, 48.70696800326375353, -6.408140936763238038 ) ) ;
#91854=CARTESIAN_POINT ( 'NONE',  ( 0.5774900079438607392, 18.48035201082150536, 5.440088680355550821 ) ) ;
#91855=CARTESIAN_POINT ( 'NONE',  ( 13.43411237798106583, 42.66530133659707502, -12.81628187352647252 ) ) ;
#91856=CARTESIAN_POINT ( 'NONE',  ( 16.40814093676323893, 0.7903013365970867898, 11.09922568453595026 ) ) ;
#91859=CARTESIAN_POINT ( 'NONE',  ( -0.3689425029237881626, 37.42874883491396787, 10.36894250292379027 ) ) ;
#91860=CARTESIAN_POINT ( 'NONE',  ( 17.08211943468705840, 10.13708216824730179, -12.26659068614894466 ) ) ;
#91861=CARTESIAN_POINT ( 'NONE',  ( -0.8801773607110991993, 22.85535201082150181, -2.915334737309923874 ) ) ;
#91862=CARTESIAN_POINT ( 'NONE',  ( 4.559911319644449179, 32.23035201082150536, -9.422509992056141925 ) ) ;
#91865=CARTESIAN_POINT ( 'NONE',  ( 15.44008868035555793, 66.39701867748817676, -9.422509992056140149 ) ) ;
#91866=CARTESIAN_POINT ( 'NONE',  ( 15.44008868035555260, 59.73035201082151247, 9.422509992056143702 ) ) ;
#91867=CARTESIAN_POINT ( 'NONE',  ( 13.43411237798106583, 22.66530133659708923, -12.81628187352647252 ) ) ;
#91870=CARTESIAN_POINT ( 'NONE',  ( 2.791683348922237240, 40.38393115100078035, -7.208316651077763204 ) ) ;
#91871=( GEOMETRIC_REPRESENTATION_CONTEXT ( 3 ) GLOBAL_UNCERTAINTY_ASSIGNED_CONTEXT ( ( #82264 ) ) GLOBAL_UNIT_ASSIGNED_CONTEXT ( ( #67571, #59559, #98590 ) ) REPRESENTATION_CONTEXT ( 'NONE', 'WORKASPACE' ) );
#91872=CARTESIAN_POINT ( 'NONE',  ( -0.8801773607111009756, 8.063685344154837509, 1.068504757029289695E-15 ) ) ;
#91873=CARTESIAN_POINT ( 'NONE',  ( -1.099225684535947600, 19.54030133659708568, 6.408140936763237150 ) ) ;
#91875=CARTESIAN_POINT ( 'NONE',  ( 12.63842701281683034, 12.46726448433411782, 9.846743663894596210 ) ) ;
#91876=CARTESIAN_POINT ( 'NONE',  ( 0.5774900079438607392, 3.480352010821504027, 5.440088680355550821 ) ) ;
#91877=CARTESIAN_POINT ( 'NONE',  ( 14.92337183194729988, 34.34226448433411605, -8.527530157486177487 ) ) ;
#91878=CARTESIAN_POINT ( 'NONE',  ( -2.816281873526473856, 64.33196800326376774, 3.434112377981055619 ) ) ;
#91879=CARTESIAN_POINT ( 'NONE',  ( 19.84674366389459621, 28.50893115100078745, 7.409399052514197653E-17 ) ) ;
#91880=CARTESIAN_POINT ( 'NONE',  ( 13.79529636645031943, 20.34541550158063572, -14.16423886937409904 ) ) ;
#91881=CARTESIAN_POINT ( 'NONE',  ( 20.88017736071110164, 35.35535201082150536, 2.915334737309930979 ) ) ;
#91882=CARTESIAN_POINT ( 'NONE',  ( 10.00000000000000000, 11.81368534415483751, -10.88017736071110342 ) ) ;
#91883=CARTESIAN_POINT ( 'NONE',  ( 7.084665262690076126, 27.02201867748817676, -10.88017736071110164 ) ) ;
#91884=CARTESIAN_POINT ( 'NONE',  ( 10.00000000000000000, 31.81368534415483751, -10.88017736071110342 ) ) ;
#91885=ORIENTED_EDGE ( 'NONE', *, *, #75170, .F. ) ;
#91886=CARTESIAN_POINT ( 'NONE',  ( 15.44008868035555793, 46.39701867748817676, -9.422509992056140149 ) ) ;
#91887=CARTESIAN_POINT ( 'NONE',  ( 16.40814093676324603, 62.45696800326376064, -11.09922568453594671 ) ) ;
#91888=ADVANCED_FACE ( 'NONE', ( #40504 ), #16371, .T. ) ;
#91889=CARTESIAN_POINT ( 'NONE',  ( 20.88017736071110164, 45.35535201082149115, 2.915334737309930979 ) ) ;
#91890=CARTESIAN_POINT ( 'NONE',  ( 2.035157376598824452, 48.68868534415483396, 7.964842623401179544 ) ) ;
#91893=CARTESIAN_POINT ( 'NONE',  ( 10.00000000000000000, 51.81368534415484106, -10.88017736071110342 ) ) ;
#91894=PRESENTATION_STYLE_ASSIGNMENT (( #30391 ) ) ;
#91895=CARTESIAN_POINT ( 'NONE',  ( 6.204703633549690345, 62.84541550158063927, 14.16423886937410082 ) ) ;
#91896=CARTESIAN_POINT ( 'NONE',  ( 5.076628168052704559, 0.1755978176674514724, -8.527530157486179263 ) ) ;
#91897=DIRECTION ( 'NONE',  ( 0.000000000000000000, 0.000000000000000000, 1.000000000000000000 ) ) ;
#91899=( NAMED_UNIT ( * ) SI_UNIT ( $, .STERADIAN. ) SOLID_ANGLE_UNIT ( ) );
#91900=CARTESIAN_POINT ( 'NONE',  ( 10.00000000000000000, 29.75893115100078745, -9.846743663894594434 ) ) ;
#91901=VERTEX_POINT ( 'NONE', #14447 ) ;
#91902=CARTESIAN_POINT ( 'NONE',  ( 0.1532563361054082862, 31.21726448433412315, 2.638427012816831674 ) ) ;
#91903=CARTESIAN_POINT ( 'NONE',  ( 7.084665262690076126, 44.10535201082151247, 10.88017736071109987 ) ) ;
#91904=CARTESIAN_POINT ( 'NONE',  ( 12.63842701281683922, 34.55059781766745886, -9.846743663894590881 ) ) ;
#91905=CARTESIAN_POINT ( 'NONE',  ( 13.43411237798105340, 15.58196800326374998, 12.81628187352647963 ) ) ;
#91906=CARTESIAN_POINT ( 'NONE',  ( 0.5774900079438590739, 67.64701867748817676, -5.440088680355550821 ) ) ;
#91907=CARTESIAN_POINT ( 'NONE',  ( 15.44008868035555260, 59.73035201082151247, 9.422509992056143702 ) ) ;
#91908=CARTESIAN_POINT ( 'NONE',  ( -0.8801773607111009756, 48.06368534415484817, 1.068504757029289695E-15 ) ) ;
#91909=( NAMED_UNIT ( * ) SI_UNIT ( $, .STERADIAN. ) SOLID_ANGLE_UNIT ( ) );
#91910=CARTESIAN_POINT ( 'NONE',  ( 6.204703633549690345, 62.84541550158063927, 14.16423886937410082 ) ) ;
#91913=CARTESIAN_POINT ( 'NONE',  ( 19.38216949554541557, 22.24863466993041428, -9.382169495545420901 ) ) ;
#91914=DIRECTION ( 'NONE',  ( 0.000000000000000000, 0.000000000000000000, -1.000000000000000000 ) ) ;
#91915=ORIENTED_EDGE ( 'NONE', *, *, #79370, .F. ) ;
#91916=CARTESIAN_POINT ( 'NONE',  ( 3.591859063236763294, 13.29030133659708746, -11.09922568453595026 ) ) ;
#91917=CARTESIAN_POINT ( 'NONE',  ( 17.96484262340118221, 16.18868534415483396, -7.964842623401177768 ) ) ;
#91918=CARTESIAN_POINT ( 'NONE',  ( 19.42250999205614548, 60.98035201082151247, -5.440088680355545492 ) ) ;
#91919=EDGE_CURVE ( 'NONE', #39149, #47405, #89822, .T. ) ;
#91921=CARTESIAN_POINT ( 'NONE',  ( 10.00000000000000000, 4.758931151000784787, -9.846743663894594434 ) ) ;
#91922=CARTESIAN_POINT ( 'NONE',  ( 14.92337183194729633, 47.67559781766745175, 8.527530157486181039 ) ) ;
#91923=CARTESIAN_POINT ( 'NONE',  ( 18.52753015748617571, 38.09226448433412315, 4.923371831947298993 ) ) ;
#91925=CARTESIAN_POINT ( 'NONE',  ( 2.791683348922240793, 26.63393115100078745, 7.208316651077764092 ) ) ;
#91928=CARTESIAN_POINT ( 'NONE',  ( 3.591859063236763294, 43.29030133659708923, -11.09922568453595026 ) ) ;
#91929=CARTESIAN_POINT ( 'NONE',  ( 1.472469842513823179, 20.59226448433411960, -4.923371831947296329 ) ) ;
#91932=CARTESIAN_POINT ( 'NONE',  ( 19.84674366389459266, 43.71726448433410894, -2.638427012816827677 ) ) ;
#91935=CARTESIAN_POINT ( 'NONE',  ( 21.09922568453594849, 16.20696800326375353, 6.408140936763242479 ) ) ;
#91936=CARTESIAN_POINT ( 'NONE',  ( 2.035157376598824452, 53.68868534415484817, 7.964842623401179544 ) ) ;
#91937=CARTESIAN_POINT ( 'NONE',  ( 10.00000000000000178, 28.05374883491396787, 14.16423886937410082 ) ) ;
#91938=CARTESIAN_POINT ( 'NONE',  ( 20.00000000000000711, 92.20777562798905080, 4.885465336749220455 ) ) ;
#91939=CARTESIAN_POINT ( 'NONE',  ( 24.16423886937410614, 29.30374883491396787, 8.672049930838204340E-16 ) ) ;
#91940=CARTESIAN_POINT ( 'NONE',  ( 20.36894250292379738, 59.92874883491397497, -10.36894250292379027 ) ) ;
#91941=CARTESIAN_POINT ( 'NONE',  ( 13.79529636645031943, 15.34541550158063750, -14.16423886937409904 ) ) ;
#91942=CARTESIAN_POINT ( 'NONE',  ( 10.00000000000000000, 25.55374883491396787, -14.16423886937410082 ) ) ;
#91943=DIRECTION ( 'NONE',  ( -1.000000000000000000, 0.000000000000000000, 0.000000000000000000 ) ) ;
#91946=CARTESIAN_POINT ( 'NONE',  ( 14.92337183194729988, 44.34226448433412315, -8.527530157486177487 ) ) ;
#91948=CARTESIAN_POINT ( 'NONE',  ( 20.88017736071110164, 25.35535201082150891, 2.915334737309930979 ) ) ;
#91950=CARTESIAN_POINT ( 'NONE',  ( 18.52753015748618282, 58.92559781766745886, -4.923371831947291888 ) ) ;
#91952=EDGE_CURVE ( 'NONE', #90628, #49115, #59488, .T. ) ;
#91953=CARTESIAN_POINT ( 'NONE',  ( 12.63842701281683922, 44.55059781766745175, -9.846743663894590881 ) ) ;
#91954=CARTESIAN_POINT ( 'NONE',  ( 22.81628187352648496, 56.83196800326374643, -3.434112377981050290 ) ) ;
#91956=VECTOR ( 'NONE', #93410, 1000.000000000000114 ) ;
#91957=CARTESIAN_POINT ( 'NONE',  ( 19.84674366389459266, 43.30059781766744464, 2.638427012816836559 ) ) ;
#91958=CARTESIAN_POINT ( 'NONE',  ( 2.791683348922237240, 55.38393115100078745, -7.208316651077763204 ) ) ;
#91960=CARTESIAN_POINT ( 'NONE',  ( 20.36894250292379738, 39.92874883491396787, -10.36894250292379027 ) ) ;
#91962=CARTESIAN_POINT ( 'NONE',  ( 24.16423886937410614, 14.30374883491396787, 8.672049930838204340E-16 ) ) ;
#91963=AXIS2_PLACEMENT_3D ( 'NONE', #12916, #67905, #66908 ) ;
#91964=CARTESIAN_POINT ( 'NONE',  ( 15.44008868035555260, 59.73035201082151247, 9.422509992056143702 ) ) ;
#91965=CARTESIAN_POINT ( 'NONE',  ( -2.266590686148945544, 56.38708216824731068, -7.082119434687050408 ) ) ;
#91966=CARTESIAN_POINT ( 'NONE',  ( 13.43411237798106583, 17.66530133659708923, -12.81628187352647252 ) ) ;
#91967=CARTESIAN_POINT ( 'NONE',  ( 0.2751277870542911397, 55.30223176428831522, 6.499999999999992006 ) ) ;
#91968=CARTESIAN_POINT ( 'NONE',  ( 17.96484262340118221, 64.93868534415483396, 7.964842623401181321 ) ) ;
#91969=CYLINDRICAL_SURFACE ( 'NONE', #21461, 0.5000000000000004441 ) ;
#91971=CARTESIAN_POINT ( 'NONE',  ( 24.16423886937410614, 64.51208216824728936, -3.795296366450302550 ) ) ;
#91973=CARTESIAN_POINT ( 'NONE',  ( -0.8801773607110991993, 27.85535201082150181, -2.915334737309923874 ) ) ;
#91974=CARTESIAN_POINT ( 'NONE',  ( -0.8801773607111008646, 23.27201867748817676, 2.915334737309923430 ) ) ;
#91975=CARTESIAN_POINT ( 'NONE',  ( 7.361572987183170547, 57.05059781766744464, 9.846743663894590881 ) ) ;
#91976=CARTESIAN_POINT ( 'NONE',  ( 18.52753015748617571, 48.09226448433412315, 4.923371831947298993 ) ) ;
#91977=CARTESIAN_POINT ( 'NONE',  ( 22.81628187352647785, 46.41530133659708213, 3.434112377981063169 ) ) ;
#91980=CARTESIAN_POINT ( 'NONE',  ( 10.00000000000000000, 21.81368534415484106, -10.88017736071110342 ) ) ;
#91981=CARTESIAN_POINT ( 'NONE',  ( -1.099225684535947600, 19.54030133659708568, 6.408140936763237150 ) ) ;
#91982=DIRECTION ( 'NONE',  ( -1.000000000000000000, 0.000000000000000000, 0.000000000000000000 ) ) ;
#91983=CARTESIAN_POINT ( 'NONE',  ( 5.076628168052703671, 51.84226448433412315, 8.527530157486179263 ) ) ;
#91984=CARTESIAN_POINT ( 'NONE',  ( 7.084665262690076126, 44.10535201082151247, 10.88017736071109987 ) ) ;
#91985=CARTESIAN_POINT ( 'NONE',  ( 16.40814093676323893, 20.79030133659708923, 11.09922568453595026 ) ) ;
#91986=CARTESIAN_POINT ( 'NONE',  ( 10.00000000000000178, 54.31368534415484106, 10.88017736071110342 ) ) ;
#91987=CARTESIAN_POINT ( 'NONE',  ( 19.72487221294571569, 55.71833443783938833, -6.499999999999990230 ) ) ;
#91989=SURFACE_STYLE_FILL_AREA ( #39979 ) ;
#91990=ORIENTED_EDGE ( 'NONE', *, *, #37217, .F. ) ;
#91991=CARTESIAN_POINT ( 'NONE',  ( 2.791683348922237240, 60.38393115100078745, -7.208316651077763204 ) ) ;
#91992=CARTESIAN_POINT ( 'NONE',  ( 2.035157376598824452, 43.68868534415484106, 7.964842623401179544 ) ) ;
#91993=CARTESIAN_POINT ( 'NONE',  ( -1.099225684535947600, 43.70696800326375353, -6.408140936763238038 ) ) ;
#91994=CARTESIAN_POINT ( 'NONE',  ( 6.204703633549690345, 10.76208216824729824, -14.16423886937410259 ) ) ;
#91995=CARTESIAN_POINT ( 'NONE',  ( 19.84674366389459266, 8.717264484334116048, -2.638427012816827677 ) ) ;
#91996=CARTESIAN_POINT ( 'NONE',  ( 1.472469842513823179, 66.42559781766745175, 4.923371831947296329 ) ) ;
#91997=CARTESIAN_POINT ( 'NONE',  ( 2.791683348922237240, 0.3839311510007847872, -7.208316651077763204 ) ) ;
#91999=CARTESIAN_POINT ( 'NONE',  ( -4.164238869374099039, 36.80374883491396787, 8.674139862899312516E-16 ) ) ;
#92000=CARTESIAN_POINT ( 'NONE',  ( 12.91533473730993009, 6.605352010821504471, -10.88017736071109987 ) ) ;
#92003=CARTESIAN_POINT ( 'NONE',  ( -0.8801773607111009756, 3.063685344154837509, 1.068504757029289695E-15 ) ) ;
#92005=ORIENTED_EDGE ( 'NONE', *, *, #79097, .T. ) ;
#92006=ORIENTED_EDGE ( 'NONE', *, *, #31026, .T. ) ;
#92007=CARTESIAN_POINT ( 'NONE',  ( 4.559911319644449179, 7.230352010821505360, -9.422509992056141925 ) ) ;
#92008=CARTESIAN_POINT ( 'NONE',  ( 12.91533473730993009, 11.60535201082150714, -10.88017736071109987 ) ) ;
#92009=CARTESIAN_POINT ( 'NONE',  ( 5.076628168052704559, 45.17559781766745175, -8.527530157486179263 ) ) ;
#92010=CARTESIAN_POINT ( 'NONE',  ( -2.816281873526473856, 39.33196800326374643, 3.434112377981055619 ) ) ;
#92011=CARTESIAN_POINT ( 'NONE',  ( 20.15039907845753220, 64.72266099184918176, 6.262539305110077947 ) ) ;
#92013=CARTESIAN_POINT ( 'NONE',  ( 10.00000000000000178, 13.05374883491396787, 14.16423886937410082 ) ) ;
#92014=CARTESIAN_POINT ( 'NONE',  ( 2.035157376598822676, 22.43868534415483396, -7.964842623401177768 ) ) ;
#92015=CARTESIAN_POINT ( 'NONE',  ( 10.00000000000000178, 4.313685344154837509, 10.88017736071110342 ) ) ;
#92016=ADVANCED_FACE ( 'NONE', ( #22939 ), #68430, .F. ) ;
#92017=CARTESIAN_POINT ( 'NONE',  ( 10.00000000000000000, 39.75893115100078745, -9.846743663894594434 ) ) ;
#92020=CARTESIAN_POINT ( 'NONE',  ( 12.63842701281683034, 22.46726448433411605, 9.846743663894596210 ) ) ;
#92026=CARTESIAN_POINT ( 'NONE',  ( 0.1532563361054082862, 61.21726448433412315, 2.638427012816831674 ) ) ;
#92027=CARTESIAN_POINT ( 'NONE',  ( 20.88017736071110164, 35.35535201082150536, 2.915334737309930979 ) ) ;
#92028=CARTESIAN_POINT ( 'NONE',  ( 15.44008868035555793, 41.39701867748817676, -9.422509992056140149 ) ) ;
#92029=CARTESIAN_POINT ( 'NONE',  ( 0.5774900079438607392, 3.480352010821504027, 5.440088680355550821 ) ) ;
#92030=CARTESIAN_POINT ( 'NONE',  ( -1.099225684535947600, 33.70696800326375353, -6.408140936763238038 ) ) ;
#92031=CARTESIAN_POINT ( 'NONE',  ( 22.26659068614894466, 18.88708216824730002, 7.082119434687054849 ) ) ;
#92033=EDGE_CURVE ( 'NONE', #37825, #21097, #55967, .T. ) ;
#92034=AXIS2_PLACEMENT_3D ( 'NONE', #16670, #87114, #46660 ) ;
#92035=CARTESIAN_POINT ( 'NONE',  ( 6.565887622018943937, 40.16530133659708923, 12.81628187352647430 ) ) ;
#92037=CARTESIAN_POINT ( 'NONE',  ( 19.84674366389459621, 38.50893115100078745, 7.409399052514197653E-17 ) ) ;
#92038=CARTESIAN_POINT ( 'NONE',  ( 10.00000000000000178, 14.31368534415483929, 10.88017736071110342 ) ) ;
#92041=CARTESIAN_POINT ( 'NONE',  ( 0.5774900079438590739, 22.64701867748817321, -5.440088680355550821 ) ) ;
#92043=CARTESIAN_POINT ( 'NONE',  ( -0.8801773607111009756, 58.06368534415484106, 1.068504757029289695E-15 ) ) ;
#92044=CARTESIAN_POINT ( 'NONE',  ( 19.42250999205614548, 65.98035201082151957, -5.440088680355545492 ) ) ;
#92045=CARTESIAN_POINT ( 'NONE',  ( 17.96484262340118221, 64.93868534415483396, 7.964842623401181321 ) ) ;
#92046=CARTESIAN_POINT ( 'NONE',  ( 1.472469842513823179, 15.59226448433411960, -4.923371831947296329 ) ) ;
#92047=CARTESIAN_POINT ( 'NONE',  ( 17.20831665107776587, 4.133931151000785675, -7.208316651077762316 ) ) ;
#92051=CARTESIAN_POINT ( 'NONE',  ( 14.92337183194729633, 2.675597817667451750, 8.527530157486181039 ) ) ;
#92053=VECTOR ( 'NONE', #46932, 1000.000000000000000 ) ;
#92055=CARTESIAN_POINT ( 'NONE',  ( 5.076628168052703671, 41.84226448433411605, 8.527530157486179263 ) ) ;
#92056=ORIENTED_EDGE ( 'NONE', *, *, #86270, .F. ) ;
#92059=CARTESIAN_POINT ( 'NONE',  ( 20.20024927138669213, 69.97537705844109723, -6.181741512438952313 ) ) ;
#92060=CARTESIAN_POINT ( 'NONE',  ( 6.204703633549690345, 12.84541550158063572, 14.16423886937410082 ) ) ;
#92061=DIRECTION ( 'NONE',  ( 0.5547001962252290364, 0.8320502943378437211, 0.000000000000000000 ) ) ;
#92062=CARTESIAN_POINT ( 'NONE',  ( 20.30776406404399737, 70.00000000000000000, 6.000000000000270894 ) ) ;
#92063=CARTESIAN_POINT ( 'NONE',  ( 17.96484262340118221, 59.93868534415484106, 7.964842623401181321 ) ) ;
#92064=CARTESIAN_POINT ( 'NONE',  ( 17.96484262340118221, 16.18868534415483396, -7.964842623401177768 ) ) ;
#92066=CARTESIAN_POINT ( 'NONE',  ( 0.1532563361054082862, 1.217264484334117824, 2.638427012816831674 ) ) ;
#92067=SURFACE_SIDE_STYLE ('',( #24578 ) ) ;
#92068=MECHANICAL_DESIGN_GEOMETRIC_PRESENTATION_REPRESENTATION('',(#15448),#18630);
#92069=CARTESIAN_POINT ( 'NONE',  ( 21.09922568453595559, 27.04030133659708568, -6.408140936763230044 ) ) ;
#92070=CARTESIAN_POINT ( 'NONE',  ( 12.63842701281683922, 19.55059781766745175, -9.846743663894590881 ) ) ;
#92073=CARTESIAN_POINT ( 'NONE',  ( 12.63842701281683034, 17.46726448433411250, 9.846743663894596210 ) ) ;
#92074=CARTESIAN_POINT ( 'NONE',  ( 19.38216949554541557, 12.24863466993041961, -9.382169495545420901 ) ) ;
#92077=CARTESIAN_POINT ( 'NONE',  ( 19.84674366389459266, 8.717264484334116048, -2.638427012816827677 ) ) ;
#92079=ORIENTED_EDGE ( 'NONE', *, *, #26520, .F. ) ;
#92080=CARTESIAN_POINT ( 'NONE',  ( -0.8801773607111008646, 28.27201867748817321, 2.915334737309923430 ) ) ;
#92081=CARTESIAN_POINT ( 'NONE',  ( 10.00000000000000000, 25.55374883491396787, -14.16423886937410082 ) ) ;
#92082=CARTESIAN_POINT ( 'NONE',  ( 2.791683348922240793, 46.63393115100077324, 7.208316651077764092 ) ) ;
#92083=CARTESIAN_POINT ( 'NONE',  ( 0.5774900079438590739, 67.64701867748817676, -5.440088680355550821 ) ) ;
#92084=CARTESIAN_POINT ( 'NONE',  ( 16.40814093676323893, 35.79030133659708923, 11.09922568453595026 ) ) ;
#92086=CARTESIAN_POINT ( 'NONE',  ( 10.00000000000000000, 21.81368534415484106, -10.88017736071110342 ) ) ;
#92088=CARTESIAN_POINT ( 'NONE',  ( 21.09922568453595559, 7.040301336597086568, -6.408140936763230044 ) ) ;
#92089=CARTESIAN_POINT ( 'NONE',  ( 19.84674366389459266, 38.71726448433412315, -2.638427012816827677 ) ) ;
#92091=CARTESIAN_POINT ( 'NONE',  ( 6.565887622018943937, 53.08196800326374643, -12.81628187352647608 ) ) ;
#92092=( NAMED_UNIT ( * ) PLANE_ANGLE_UNIT ( ) SI_UNIT ( $, .RADIAN. ) );
#92093=CARTESIAN_POINT ( 'NONE',  ( 10.00000000000000178, 54.31368534415484106, 10.88017736071110342 ) ) ;
#92097=CARTESIAN_POINT ( 'NONE',  ( 17.96484262340118221, 36.18868534415484106, -7.964842623401177768 ) ) ;
#92098=CARTESIAN_POINT ( 'NONE',  ( 20.88017736071110164, 50.35535201082151247, 2.915334737309930979 ) ) ;
#92099=CARTESIAN_POINT ( 'NONE',  ( 0.1532563361054082862, 61.21726448433412315, 2.638427012816831674 ) ) ;
#92100=B_SPLINE_CURVE_WITH_KNOTS ( 'NONE', 3,
 ( #55808, #25322, #86301, #39817, #56300, #86794 ),
 .UNSPECIFIED., .F., .F.,
 ( 4, 2, 4 ),
 ( 0.000000000000000000, 0.0002565770811490931079, 0.0005131541622981862158 ),
 .UNSPECIFIED. ) ;
#92101=CARTESIAN_POINT ( 'NONE',  ( -0.8801773607110991993, 62.85535201082150536, -2.915334737309923874 ) ) ;
#92103=CARTESIAN_POINT ( 'NONE',  ( 19.84674366389459266, 53.71726448433411605, -2.638427012816827677 ) ) ;
#92104=CARTESIAN_POINT ( 'NONE',  ( -0.8801773607110991993, 2.855352010821504471, -2.915334737309923874 ) ) ;
#92105=CARTESIAN_POINT ( 'NONE',  ( 19.84674366389459621, 23.50893115100078390, 7.409399052514197653E-17 ) ) ;
#92106=CARTESIAN_POINT ( 'NONE',  ( 10.00000000000000178, 5.373634669930420493, 12.81628187352647608 ) ) ;
#92108=CARTESIAN_POINT ( 'NONE',  ( 2.035157376598822676, 37.43868534415484106, -7.964842623401177768 ) ) ;
#92109=CARTESIAN_POINT ( 'NONE',  ( 21.09922568453595559, 2.040301336597086568, -6.408140936763230044 ) ) ;
#92111=CARTESIAN_POINT ( 'NONE',  ( 20.88017736071110519, 10.56368534415483751, 2.639326808657452039E-16 ) ) ;
#92112=CARTESIAN_POINT ( 'NONE',  ( -0.8801773607111008646, 23.27201867748817676, 2.915334737309923430 ) ) ;
#92113=CARTESIAN_POINT ( 'NONE',  ( -4.164238869374098151, 36.59541550158063217, -3.795296366450310543 ) ) ;
#92114=CARTESIAN_POINT ( 'NONE',  ( 10.00000000000000000, 24.75893115100078745, -9.846743663894594434 ) ) ;
#92115=CARTESIAN_POINT ( 'NONE',  ( 4.559911319644449179, 57.23035201082150536, -9.422509992056141925 ) ) ;
#92117=CARTESIAN_POINT ( 'NONE',  ( 2.917880565312948704, 7.637082168247301794, 12.26659068614894643 ) ) ;
#92118=EDGE_CURVE ( 'NONE', #84056, #74723, #76146, .T. ) ;
#92122=CARTESIAN_POINT ( 'NONE',  ( 1.472469842513823179, 56.42559781766745886, 4.923371831947296329 ) ) ;
#92125=ORIENTED_EDGE ( 'NONE', *, *, #37611, .T. ) ;
#92127=CARTESIAN_POINT ( 'NONE',  ( -4.164238869374099039, 36.80374883491396787, 8.674139862899312516E-16 ) ) ;
#92128=CARTESIAN_POINT ( 'NONE',  ( 2.917880565312950480, 30.97041550158063572, -12.26659068614894821 ) ) ;
#92130=CARTESIAN_POINT ( 'NONE',  ( 4.559911319644449179, 68.89701867748817676, 9.422509992056141925 ) ) ;
#92131=CARTESIAN_POINT ( 'NONE',  ( 2.791683348922240793, 56.63393115100078035, 7.208316651077764092 ) ) ;
#92133=CARTESIAN_POINT ( 'NONE',  ( 20.88017736071110875, 65.77201867748817676, -2.915334737309920765 ) ) ;
#92134=CARTESIAN_POINT ( 'NONE',  ( 6.565887622018943937, 20.16530133659708213, 12.81628187352647430 ) ) ;
#92135=CARTESIAN_POINT ( 'NONE',  ( -2.266590686148945544, 26.38708216824730357, -7.082119434687050408 ) ) ;
#92136=CARTESIAN_POINT ( 'NONE',  ( 15.44008868035555793, 11.39701867748817143, -9.422509992056140149 ) ) ;
#92138=CARTESIAN_POINT ( 'NONE',  ( 0.5774900079438590739, 32.64701867748816966, -5.440088680355550821 ) ) ;
#92139=LINE ( 'NONE', #32608, #84297 ) ;
#92140=CARTESIAN_POINT ( 'NONE',  ( 15.44008868035555260, 59.73035201082151247, 9.422509992056143702 ) ) ;
#92145=VERTEX_POINT ( 'NONE', #79365 ) ;
#92146=CARTESIAN_POINT ( 'NONE',  ( -4.164238869374098151, 1.595415501580634388, -3.795296366450310543 ) ) ;
#92147=CARTESIAN_POINT ( 'NONE',  ( -0.3689425029237898834, 56.17874883491396076, -10.36894250292378850 ) ) ;
#92148=CARTESIAN_POINT ( 'NONE',  ( 0.5774900079438607392, 3.480352010821504916, 5.440088680355550821 ) ) ;
#92149=CARTESIAN_POINT ( 'NONE',  ( 0.1532563361054082862, 36.21726448433410894, 2.638427012816831674 ) ) ;
#92150=CARTESIAN_POINT ( 'NONE',  ( 10.00000000000000000, 59.75893115100078745, -9.846743663894594434 ) ) ;
#92154=CARTESIAN_POINT ( 'NONE',  ( 10.00000000000000178, 5.373634669930420493, 12.81628187352647608 ) ) ;
#92158=CARTESIAN_POINT ( 'NONE',  ( -2.266590686148945544, 41.38708216824729647, -7.082119434687050408 ) ) ;
#92159=ADVANCED_FACE ( 'NONE', ( #9895 ), #56379, .F. ) ;
#92160=CARTESIAN_POINT ( 'NONE',  ( 22.26659068614895176, 44.72041550158063927, -7.082119434687042414 ) ) ;
#92162=CARTESIAN_POINT ( 'NONE',  ( 0.6178305044545818747, 53.49863466993041072, -9.382169495545419124 ) ) ;
#92163=CARTESIAN_POINT ( 'NONE',  ( 7.361572987183170547, 47.05059781766745175, 9.846743663894590881 ) ) ;
#92164=CARTESIAN_POINT ( 'NONE',  ( 19.42250999205614193, 30.14701867748817321, 5.440088680355555262 ) ) ;
#92165=DIRECTION ( 'NONE',  ( -1.000000000000000000, -2.799047438454523729E-16, 0.000000000000000000 ) ) ;
#92166=CARTESIAN_POINT ( 'NONE',  ( 1.472469842513823179, 50.59226448433411605, -4.923371831947296329 ) ) ;
#92167=CARTESIAN_POINT ( 'NONE',  ( 18.52753015748618282, 43.92559781766745175, -4.923371831947291888 ) ) ;
#92172=CARTESIAN_POINT ( 'NONE',  ( 2.791683348922237240, 5.383931151000785675, -7.208316651077763204 ) ) ;
#92174=ORIENTED_EDGE ( 'NONE', *, *, #9761, .T. ) ;
#92177=CARTESIAN_POINT ( 'NONE',  ( 14.92337183194729633, 27.67559781766745530, 8.527530157486181039 ) ) ;
#92179=CARTESIAN_POINT ( 'NONE',  ( 19.38216949554541557, 37.24863466993041783, -9.382169495545420901 ) ) ;
#92182=DIRECTION ( 'NONE',  ( 1.000000000000000000, 0.000000000000000000, -0.000000000000000000 ) ) ;
#92184=CARTESIAN_POINT ( 'NONE',  ( 14.92337183194729988, 59.34226448433412315, -8.527530157486177487 ) ) ;
#92185=CARTESIAN_POINT ( 'NONE',  ( 17.08211943468705840, 30.13708216824730357, -12.26659068614894466 ) ) ;
#92186=CARTESIAN_POINT ( 'NONE',  ( 12.63842701281683034, 62.46726448433410894, 9.846743663894596210 ) ) ;
#92187=CARTESIAN_POINT ( 'NONE',  ( 0.2751277870542949144, 4.366073187301309666, -6.499999999999997335 ) ) ;
#92188=CARTESIAN_POINT ( 'NONE',  ( 5.076628168052704559, 20.17559781766745175, -8.527530157486179263 ) ) ;
#92190=CARTESIAN_POINT ( 'NONE',  ( 16.40814093676324603, 52.45696800326375353, -11.09922568453594671 ) ) ;
#92191=CARTESIAN_POINT ( 'NONE',  ( 24.16423886937410614, 4.303748834913967869, 8.672049930838204340E-16 ) ) ;
#92192=CARTESIAN_POINT ( 'NONE',  ( 0.1532563361054083140, 61.00893115100078745, 1.131784320476157264E-15 ) ) ;
#92193=CARTESIAN_POINT ( 'NONE',  ( 19.42250999205614193, 50.14701867748817676, 5.440088680355555262 ) ) ;
#92197=CARTESIAN_POINT ( 'NONE',  ( 2.035157376598822676, 62.43868534415483396, -7.964842623401177768 ) ) ;
#92200=CARTESIAN_POINT ( 'NONE',  ( 17.96484262340118221, 26.18868534415483396, -7.964842623401177768 ) ) ;
#92201=CARTESIAN_POINT ( 'NONE',  ( 16.40814093676324603, 2.456968003263753531, -11.09922568453594671 ) ) ;
#92202=CARTESIAN_POINT ( 'NONE',  ( 20.88017736071110875, 55.77201867748816966, -2.915334737309920765 ) ) ;
#92203=CARTESIAN_POINT ( 'NONE',  ( -0.3289641300568009741, 47.24545670184114243, -5.963430220938281678 ) ) ;
#92205=CARTESIAN_POINT ( 'NONE',  ( 2.035157376598824452, 38.68868534415483396, 7.964842623401179544 ) ) ;
#92207=CARTESIAN_POINT ( 'NONE',  ( 18.52753015748618282, 38.92559781766745175, -4.923371831947291888 ) ) ;
#92209=CARTESIAN_POINT ( 'NONE',  ( 0.1532563361054083140, 66.00893115100079456, 1.131784320476157264E-15 ) ) ;
#92210=CARTESIAN_POINT ( 'NONE',  ( -0.8801773607111008646, 8.272018677488171434, 2.915334737309923430 ) ) ;
#92213=CARTESIAN_POINT ( 'NONE',  ( 6.204703633549690345, 17.84541550158063217, 14.16423886937410082 ) ) ;
#92214=CARTESIAN_POINT ( 'NONE',  ( 22.26659068614894466, 58.88708216824729647, 7.082119434687054849 ) ) ;
#92216=CARTESIAN_POINT ( 'NONE',  ( 19.84674366389459266, 23.71726448433412315, -2.638427012816827677 ) ) ;
#92218=CARTESIAN_POINT ( 'NONE',  ( 7.361572987183170547, 22.05059781766745530, 9.846743663894590881 ) ) ;
#92219=CARTESIAN_POINT ( 'NONE',  ( 12.91533473730992121, 24.52201867748816966, 10.88017736071110164 ) ) ;
#92220=CARTESIAN_POINT ( 'NONE',  ( 19.84674366389459621, 63.50893115100078745, 7.409399052514197653E-17 ) ) ;
#92221=CARTESIAN_POINT ( 'NONE',  ( -0.3689425029237898834, 11.17874883491396787, -10.36894250292378850 ) ) ;
#92222=CARTESIAN_POINT ( 'NONE',  ( 18.95386800104996183, 48.23810908735726599, -6.499999999999982236 ) ) ;
#92225=UNCERTAINTY_MEASURE_WITH_UNIT (LENGTH_MEASURE( 1.000000000000000082E-05 ), #8539, 'distance_accuracy_value', 'NONE');
#92226=CARTESIAN_POINT ( 'NONE',  ( 5.076628168052704559, 15.17559781766745175, -8.527530157486179263 ) ) ;
#92227=CARTESIAN_POINT ( 'NONE',  ( 3.591859063236761518, 39.95696800326375353, 11.09922568453594849 ) ) ;
#92228=CARTESIAN_POINT ( 'NONE',  ( 7.361572987183170547, 37.05059781766744464, 9.846743663894590881 ) ) ;
#92230=CARTESIAN_POINT ( 'NONE',  ( 14.92337183194729988, 19.34226448433411960, -8.527530157486177487 ) ) ;
#92231=DIRECTION ( 'NONE',  ( 0.000000000000000000, -1.000000000000000000, 0.000000000000000000 ) ) ;
#92232=CARTESIAN_POINT ( 'NONE',  ( 24.16423886937409904, 59.09541550158063217, 3.795296366450317205 ) ) ;
#92233=CARTESIAN_POINT ( 'NONE',  ( -0.8801773607111009756, 53.06368534415484106, 1.068504757029289695E-15 ) ) ;
#92234=SURFACE_STYLE_FILL_AREA ( #75749 ) ;
#92235=CARTESIAN_POINT ( 'NONE',  ( 20.88017736071110519, 55.56368534415484817, 2.639326808657452039E-16 ) ) ;
#92236=CARTESIAN_POINT ( 'NONE',  ( 1.472469842513823179, 30.59226448433411960, -4.923371831947296329 ) ) ;
#92237=CARTESIAN_POINT ( 'NONE',  ( 19.42250999205614193, 5.147018677488171434, 5.440088680355555262 ) ) ;
#92238=CARTESIAN_POINT ( 'NONE',  ( 17.62281668512001787, 38.28593319516822646, 6.500000000000010658 ) ) ;
#92239=CARTESIAN_POINT ( 'NONE',  ( 18.52753015748618282, 53.92559781766745175, -4.923371831947291888 ) ) ;
#92240=CARTESIAN_POINT ( 'NONE',  ( 19.42250999205614548, 45.98035201082150536, -5.440088680355545492 ) ) ;
#92242=UNCERTAINTY_MEASURE_WITH_UNIT (LENGTH_MEASURE( 1.000000000000000082E-05 ), #4059, 'distance_accuracy_value', 'NONE');
#92244=ADVANCED_FACE ( 'NONE', ( #55883 ), #23393, .T. ) ;
#92249=CARTESIAN_POINT ( 'NONE',  ( 14.92337183194729988, 24.34226448433411960, -8.527530157486177487 ) ) ;
#92250=CARTESIAN_POINT ( 'NONE',  ( 16.40814093676324603, 57.45696800326375353, -11.09922568453594671 ) ) ;
#92251=CARTESIAN_POINT ( 'NONE',  ( 19.42250999205614548, 20.98035201082150891, -5.440088680355545492 ) ) ;
#92252=CARTESIAN_POINT ( 'NONE',  ( 2.791683348922237240, 50.38393115100078035, -7.208316651077763204 ) ) ;
#92254=CARTESIAN_POINT ( 'NONE',  ( -0.3689425029237881626, 32.42874883491395366, 10.36894250292379027 ) ) ;
#92256=CARTESIAN_POINT ( 'NONE',  ( -2.266590686148945544, 62.22041550158063927, 7.082119434687048631 ) ) ;
#92257=CARTESIAN_POINT ( 'NONE',  ( 1.472469842513823179, 56.42559781766745886, 4.923371831947296329 ) ) ;
#92259=CARTESIAN_POINT ( 'NONE',  ( -0.8801773607111009756, 58.06368534415484106, 1.068504757029289695E-15 ) ) ;
#92260=CARTESIAN_POINT ( 'NONE',  ( 17.20831665107776587, 19.13393115100078035, -7.208316651077762316 ) ) ;
#92265=ORIENTED_EDGE ( 'NONE', *, *, #13694, .T. ) ;
#92266=CARTESIAN_POINT ( 'NONE',  ( 19.84674366389459621, 13.50893115100078568, 7.409399052514197653E-17 ) ) ;
#92268=CARTESIAN_POINT ( 'NONE',  ( 24.16423886937410614, 19.30374883491397142, 8.672049930838204340E-16 ) ) ;
#92269=CARTESIAN_POINT ( 'NONE',  ( 0.1532563361054083140, 21.00893115100078745, 1.131784320476157264E-15 ) ) ;
#92270=CARTESIAN_POINT ( 'NONE',  ( 20.88017736071110519, 40.56368534415484106, 2.639326808657452039E-16 ) ) ;
#92274=CARTESIAN_POINT ( 'NONE',  ( -0.8801773607111009756, 33.06368534415484106, 1.068504757029289695E-15 ) ) ;
#92275=ADVANCED_FACE ( 'NONE', ( #44844 ), #14841, .T. ) ;
#92282=CARTESIAN_POINT ( 'NONE',  ( 0.6178305044545818747, 23.49863466993041783, -9.382169495545419124 ) ) ;
#92283=CARTESIAN_POINT ( 'NONE',  ( 0.1532563361054100626, 10.80059781766745175, -2.638427012816831230 ) ) ;
#92284=CARTESIAN_POINT ( 'NONE',  ( 13.99999999999999822, 60.50000000000000000, 6.500000000000000888 ) ) ;
#92285=CARTESIAN_POINT ( 'NONE',  ( 0.1532563361054100626, 10.80059781766745175, -2.638427012816831230 ) ) ;
#92286=CARTESIAN_POINT ( 'NONE',  ( 20.88017736071110519, 35.56368534415484106, 2.639326808657452039E-16 ) ) ;
#92287=ORIENTED_EDGE ( 'NONE', *, *, #43046, .F. ) ;
#92288=CARTESIAN_POINT ( 'NONE',  ( -1.099225684535947600, 64.54030133659709634, 6.408140936763237150 ) ) ;
#92289=CARTESIAN_POINT ( 'NONE',  ( 12.91533473730993009, 51.60535201082149825, -10.88017736071109987 ) ) ;
#92292=CARTESIAN_POINT ( 'NONE',  ( 15.44008868035555793, 61.39701867748817676, -9.422509992056140149 ) ) ;
#92293=CARTESIAN_POINT ( 'NONE',  ( 7.361572987183169658, 64.96726448433412315, -9.846743663894592657 ) ) ;
#92295=CARTESIAN_POINT ( 'NONE',  ( 7.361572987183169658, 24.96726448433412315, -9.846743663894592657 ) ) ;
#92296=CARTESIAN_POINT ( 'NONE',  ( 3.591859063236763294, 53.29030133659708923, -11.09922568453595026 ) ) ;
#92297=CARTESIAN_POINT ( 'NONE',  ( 0.000000000000000000, 76.90945382226833260, 7.553580139337960908 ) ) ;
#92298=CARTESIAN_POINT ( 'NONE',  ( 14.92337183194729988, 24.34226448433411960, -8.527530157486177487 ) ) ;
#92299=CARTESIAN_POINT ( 'NONE',  ( 22.81628187352648496, 16.83196800326374998, -3.434112377981050290 ) ) ;
#92301=CARTESIAN_POINT ( 'NONE',  ( 10.00000000000000178, 54.31368534415484106, 10.88017736071110342 ) ) ;
#92302=CARTESIAN_POINT ( 'NONE',  ( 17.20831665107776587, 64.13393115100079456, -7.208316651077762316 ) ) ;
#92304=CARTESIAN_POINT ( 'NONE',  ( 7.361572987183169658, 24.96726448433412315, -9.846743663894592657 ) ) ;
#92305=CARTESIAN_POINT ( 'NONE',  ( 12.63842701281683922, 14.55059781766744997, -9.846743663894590881 ) ) ;
#92306=CARTESIAN_POINT ( 'NONE',  ( 19.42250999205614193, 10.14701867748816966, 5.440088680355555262 ) ) ;
#92307=CARTESIAN_POINT ( 'NONE',  ( 22.81628187352647785, 16.62363466993042138, 6.195893100308588602E-16 ) ) ;
#92309=CARTESIAN_POINT ( 'NONE',  ( 7.361572987183170547, 67.05059781766746596, 9.846743663894590881 ) ) ;
#92311=CARTESIAN_POINT ( 'NONE',  ( 20.88017736071110164, 25.35535201082150891, 2.915334737309930979 ) ) ;
#92313=CARTESIAN_POINT ( 'NONE',  ( 0.5774900079438607392, 18.48035201082150536, 5.440088680355550821 ) ) ;
#92314=LINE ( 'NONE', #38345, #35962 ) ;
#92315=CARTESIAN_POINT ( 'NONE',  ( 2.035157376598824452, 28.68868534415484106, 7.964842623401179544 ) ) ;
#92317=CARTESIAN_POINT ( 'NONE',  ( 17.96484262340118221, 4.938685344154837509, 7.964842623401181321 ) ) ;
#92319=CARTESIAN_POINT ( 'NONE',  ( 14.92337183194729633, 2.675597817667451750, 8.527530157486181039 ) ) ;
#92320=CARTESIAN_POINT ( 'NONE',  ( 14.92337183194729988, 29.34226448433411960, -8.527530157486177487 ) ) ;
#92321=CARTESIAN_POINT ( 'NONE',  ( 13.43411237798106583, 12.66530133659708746, -12.81628187352647252 ) ) ;
#92325=CARTESIAN_POINT ( 'NONE',  ( 12.63842701281683034, 62.46726448433410894, 9.846743663894596210 ) ) ;
#92328=CARTESIAN_POINT ( 'NONE',  ( -2.266590686148945544, 11.38708216824730179, -7.082119434687050408 ) ) ;
#92330=CARTESIAN_POINT ( 'NONE',  ( 17.20831665107776587, 39.13393115100079456, -7.208316651077762316 ) ) ;
#92333=CARTESIAN_POINT ( 'NONE',  ( 17.08211943468705840, 55.13708216824731068, -12.26659068614894466 ) ) ;
#92334=CARTESIAN_POINT ( 'NONE',  ( 5.076628168052703671, 26.84226448433411960, 8.527530157486179263 ) ) ;
#92336=CARTESIAN_POINT ( 'NONE',  ( -0.1503990784575328643, 25.12777174578613426, 6.262539305110068177 ) ) ;
#92337=CARTESIAN_POINT ( 'NONE',  ( 12.91533473730993009, 46.60535201082150536, -10.88017736071109987 ) ) ;
#92338=CARTESIAN_POINT ( 'NONE',  ( 13.43411237798105340, 45.58196800326374643, 12.81628187352647963 ) ) ;
#92339=CARTESIAN_POINT ( 'NONE',  ( 0.5774900079438590739, 17.64701867748817321, -5.440088680355550821 ) ) ;
#92340=CARTESIAN_POINT ( 'NONE',  ( 10.00000000000000000, 52.87363466993041783, -12.81628187352647608 ) ) ;
#92341=CARTESIAN_POINT ( 'NONE',  ( -1.099225684535947600, -1.293031996736246469, -6.408140936763238038 ) ) ;
#92345=CARTESIAN_POINT ( 'NONE',  ( 13.79529636645031943, 60.34541550158063927, -14.16423886937409904 ) ) ;
#92346=CARTESIAN_POINT ( 'NONE',  ( 2.917880565312948704, 7.637082168247301794, 12.26659068614894643 ) ) ;
#92347=CARTESIAN_POINT ( 'NONE',  ( 19.42250999205614548, 15.98035201082150714, -5.440088680355545492 ) ) ;
#92348=CARTESIAN_POINT ( 'NONE',  ( 20.88017736071110519, 35.56368534415484106, 2.639326808657452039E-16 ) ) ;
#92351=CARTESIAN_POINT ( 'NONE',  ( 12.91533473730993009, 61.60535201082150536, -10.88017736071109987 ) ) ;
#92352=CARTESIAN_POINT ( 'NONE',  ( 12.91533473730993009, 61.60535201082150536, -10.88017736071109987 ) ) ;
#92353=CARTESIAN_POINT ( 'NONE',  ( 22.81628187352647785, 31.41530133659709279, 3.434112377981063169 ) ) ;
#92354=DIRECTION ( 'NONE',  ( -0.000000000000000000, -0.000000000000000000, -1.000000000000000000 ) ) ;
#92356=CARTESIAN_POINT ( 'NONE',  ( 7.361572987183169658, 4.967264484334119601, -9.846743663894592657 ) ) ;
#92357=CARTESIAN_POINT ( 'NONE',  ( 2.791683348922237240, 30.38393115100078390, -7.208316651077763204 ) ) ;
#92358=CARTESIAN_POINT ( 'NONE',  ( 4.559911319644449179, 17.23035201082150536, -9.422509992056141925 ) ) ;
#92360=CARTESIAN_POINT ( 'NONE',  ( 21.09922568453594849, 26.20696800326375353, 6.408140936763242479 ) ) ;
#92361=CARTESIAN_POINT ( 'NONE',  ( 2.791683348922237240, 5.383931151000785675, -7.208316651077763204 ) ) ;
#92362=CARTESIAN_POINT ( 'NONE',  ( 19.72487221294571569, 54.78217586085238366, 6.499999999999995559 ) ) ;
#92363=CARTESIAN_POINT ( 'NONE',  ( 19.84674366389459621, 58.50893115100078745, 7.409399052514197653E-17 ) ) ;
#92364=CARTESIAN_POINT ( 'NONE',  ( 0.1532563361054082862, 31.21726448433412315, 2.638427012816831674 ) ) ;
#92366=CARTESIAN_POINT ( 'NONE',  ( 10.00000000000000178, 18.05374883491396787, 14.16423886937410082 ) ) ;
#92367=CARTESIAN_POINT ( 'NONE',  ( -0.8801773607110991993, 37.85535201082151247, -2.915334737309923874 ) ) ;
#92368=CARTESIAN_POINT ( 'NONE',  ( 0.5774900079438607392, 13.48035201082150358, 5.440088680355550821 ) ) ;
#92369=CARTESIAN_POINT ( 'NONE',  ( 20.88017736071110519, 50.56368534415484106, 2.639326808657452039E-16 ) ) ;
#92370=CARTESIAN_POINT ( 'NONE',  ( 7.084665262690076126, 32.02201867748816966, -10.88017736071110164 ) ) ;
#92372=CARTESIAN_POINT ( 'NONE',  ( 22.81628187352647785, 31.41530133659709279, 3.434112377981063169 ) ) ;
#92373=CARTESIAN_POINT ( 'NONE',  ( 7.084665262690076126, 39.10535201082150536, 10.88017736071109987 ) ) ;
#92376=CARTESIAN_POINT ( 'NONE',  ( 20.88017736071110875, 50.77201867748817676, -2.915334737309920765 ) ) ;
#92378=CARTESIAN_POINT ( 'NONE',  ( 2.035157376598822676, 47.43868534415484817, -7.964842623401177768 ) ) ;
#92381=CARTESIAN_POINT ( 'NONE',  ( -4.164238869374098151, 56.59541550158063927, -3.795296366450310543 ) ) ;
#92382=CARTESIAN_POINT ( 'NONE',  ( 20.88017736071110519, 65.56368534415483396, 2.639326808657452039E-16 ) ) ;
#92385=CARTESIAN_POINT ( 'NONE',  ( 0.5774900079438590739, 2.647018677488170990, -5.440088680355550821 ) ) ;
#92386=CARTESIAN_POINT ( 'NONE',  ( 18.52753015748618282, 28.92559781766745175, -4.923371831947291888 ) ) ;
#92387=B_SPLINE_CURVE_WITH_KNOTS ( 'NONE', 3,
 ( #23984, #2481, #93942, #85460 ),
 .UNSPECIFIED., .F., .F.,
 ( 4, 4 ),
 ( 1.778362592763157239E-16, 0.001060528352561988102 ),
 .UNSPECIFIED. ) ;
#92389=CARTESIAN_POINT ( 'NONE',  ( 14.92337183194729988, 39.34226448433412315, -8.527530157486177487 ) ) ;
#92390=CARTESIAN_POINT ( 'NONE',  ( 19.42250999205614548, 40.98035201082150536, -5.440088680355545492 ) ) ;
#92391=CARTESIAN_POINT ( 'NONE',  ( 10.00000000000000000, 39.75893115100078745, -9.846743663894594434 ) ) ;
#92392=CARTESIAN_POINT ( 'NONE',  ( 22.81628187352647785, 16.62363466993042138, 6.195893100308588602E-16 ) ) ;
#92395=CARTESIAN_POINT ( 'NONE',  ( -0.8801773607111008646, 43.27201867748817676, 2.915334737309923430 ) ) ;
#92396=CARTESIAN_POINT ( 'NONE',  ( -2.266590686148945544, 52.22041550158064638, 7.082119434687048631 ) ) ;
#92400=CARTESIAN_POINT ( 'NONE',  ( 6.565887622018943937, 23.08196800326375708, -12.81628187352647608 ) ) ;
#92403=CARTESIAN_POINT ( 'NONE',  ( 6.565887622018943937, 28.08196800326375353, -12.81628187352647608 ) ) ;
#92404=CARTESIAN_POINT ( 'NONE',  ( 4.559911319644449179, 23.89701867748817321, 9.422509992056141925 ) ) ;
#92405=CARTESIAN_POINT ( 'NONE',  ( 12.91533473730993009, 56.60535201082151247, -10.88017736071109987 ) ) ;
#92409=CARTESIAN_POINT ( 'NONE',  ( 0.1532563361054082862, 6.217264484334118713, 2.638427012816831674 ) ) ;
#92410=CARTESIAN_POINT ( 'NONE',  ( 14.92337183194729633, 52.67559781766745175, 8.527530157486181039 ) ) ;
#92411=CARTESIAN_POINT ( 'NONE',  ( 5.076628168052704559, 35.17559781766745175, -8.527530157486179263 ) ) ;
#92413=CARTESIAN_POINT ( 'NONE',  ( 10.00000000000000178, 32.25893115100078745, 9.846743663894594434 ) ) ;
#92414=CARTESIAN_POINT ( 'NONE',  ( 19.80832241502127644, 54.75868815902071418, 6.499999999999992895 ) ) ;
#92416=CARTESIAN_POINT ( 'NONE',  ( 19.84674366389459266, 13.30059781766745353, 2.638427012816836559 ) ) ;
#92418=CARTESIAN_POINT ( 'NONE',  ( 0.000000000000000000, 69.50000000000000000, -6.500000000000000888 ) ) ;
#92419=CARTESIAN_POINT ( 'NONE',  ( 14.92337183194729633, 47.67559781766745175, 8.527530157486181039 ) ) ;
#92421=CARTESIAN_POINT ( 'NONE',  ( 20.15039907845753220, 17.62777174578612716, -6.262539305110077947 ) ) ;
#92422=CARTESIAN_POINT ( 'NONE',  ( -2.816281873526473856, 14.33196800326375531, 3.434112377981055619 ) ) ;
#92423=CARTESIAN_POINT ( 'NONE',  ( 2.035157376598822676, 57.43868534415484106, -7.964842623401177768 ) ) ;
#92424=CARTESIAN_POINT ( 'NONE',  ( 10.00000000000000178, 48.05374883491396787, 14.16423886937410082 ) ) ;
#92426=CARTESIAN_POINT ( 'NONE',  ( 20.36894250292379382, 43.67874883491397497, 10.36894250292379205 ) ) ;
#92427=CARTESIAN_POINT ( 'NONE',  ( 24.16423886937410614, 54.30374883491396787, 8.672049930838204340E-16 ) ) ;
#92428=CARTESIAN_POINT ( 'NONE',  ( 24.16423886937410614, 19.51208216824729647, -3.795296366450302550 ) ) ;
#92429=CARTESIAN_POINT ( 'NONE',  ( -2.266590686148945544, 26.38708216824730357, -7.082119434687050408 ) ) ;
#92433=CARTESIAN_POINT ( 'NONE',  ( 0.1532563361054083140, 36.00893115100078745, 1.131784320476157264E-15 ) ) ;
#92434=CARTESIAN_POINT ( 'NONE',  ( 0.5774900079438607392, 18.48035201082150536, 5.440088680355550821 ) ) ;
#92437=CARTESIAN_POINT ( 'NONE',  ( 19.67387888393821527, 90.60653825729899324, -5.439610960094903191 ) ) ;
#92439=CARTESIAN_POINT ( 'NONE',  ( 14.92337183194729633, 42.67559781766745886, 8.527530157486181039 ) ) ;
#92440=CARTESIAN_POINT ( 'NONE',  ( 6.565887622018943937, 55.16530133659709634, 12.81628187352647430 ) ) ;
#92442=CARTESIAN_POINT ( 'NONE',  ( 12.63842701281683922, 39.55059781766744464, -9.846743663894590881 ) ) ;
#92443=CARTESIAN_POINT ( 'NONE',  ( 19.84674366389459621, 58.50893115100078745, 7.409399052514197653E-17 ) ) ;
#92444=CARTESIAN_POINT ( 'NONE',  ( 10.00000000000000000, 45.55374883491397497, -14.16423886937410082 ) ) ;
#92446=CARTESIAN_POINT ( 'NONE',  ( 24.16423886937409904, 19.09541550158063927, 3.795296366450317205 ) ) ;
#92450=CARTESIAN_POINT ( 'NONE',  ( 2.035157376598822676, 7.438685344154837509, -7.964842623401177768 ) ) ;
#92451=CARTESIAN_POINT ( 'NONE',  ( -2.816281873526473856, 9.123634669930421381, 9.499525473075851096E-16 ) ) ;
#92452=CARTESIAN_POINT ( 'NONE',  ( 17.96484262340118221, 66.18868534415483396, -7.964842623401177768 ) ) ;
#92455=CARTESIAN_POINT ( 'NONE',  ( -0.3689425029237898834, 66.17874883491396076, -10.36894250292378850 ) ) ;
#92457=CARTESIAN_POINT ( 'NONE',  ( -0.8801773607111009756, 28.06368534415484106, 1.068504757029289695E-15 ) ) ;
#92458=CARTESIAN_POINT ( 'NONE',  ( 12.91533473730993009, 21.60535201082150536, -10.88017736071109987 ) ) ;
#92459=CARTESIAN_POINT ( 'NONE',  ( 1.472469842513823179, 51.42559781766745886, 4.923371831947296329 ) ) ;
#92460=CARTESIAN_POINT ( 'NONE',  ( 18.52753015748618282, 48.92559781766745886, -4.923371831947291888 ) ) ;
#92461=CARTESIAN_POINT ( 'NONE',  ( -2.816281873526473856, 64.33196800326376774, 3.434112377981055619 ) ) ;
#92463=VERTEX_POINT ( 'NONE', #98387 ) ;
#92465=CARTESIAN_POINT ( 'NONE',  ( 0.5774900079438607392, 33.48035201082150536, 5.440088680355550821 ) ) ;
#92466=CARTESIAN_POINT ( 'NONE',  ( 22.81628187352648496, 21.83196800326374643, -3.434112377981050290 ) ) ;
#92467=CARTESIAN_POINT ( 'NONE',  ( 2.059615949176877749E-15, 71.60587665882023600, 5.000000000000000000 ) ) ;
#92470=CARTESIAN_POINT ( 'NONE',  ( 1.472469842513823179, 60.59226448433412315, -4.923371831947296329 ) ) ;
#92471=CARTESIAN_POINT ( 'NONE',  ( 19.42250999205614193, 50.14701867748817676, 5.440088680355555262 ) ) ;
#92472=CARTESIAN_POINT ( 'NONE',  ( 22.81628187352647785, 16.41530133659708923, 3.434112377981063169 ) ) ;
#92473=CARTESIAN_POINT ( 'NONE',  ( 15.44008868035555793, 61.39701867748817676, -9.422509992056140149 ) ) ;
#92474=LINE ( 'NONE', #15998, #43216 ) ;
#92478=EDGE_CURVE ( 'NONE', #78529, #3611, #91734, .T. ) ;
#92479=CARTESIAN_POINT ( 'NONE',  ( 2.035157376598822676, 47.43868534415484817, -7.964842623401177768 ) ) ;
#92480=CARTESIAN_POINT ( 'NONE',  ( 16.40814093676323893, 40.79030133659708923, 11.09922568453595026 ) ) ;
#92481=CARTESIAN_POINT ( 'NONE',  ( 17.08211943468705840, 20.13708216824730357, -12.26659068614894466 ) ) ;
#92482=CARTESIAN_POINT ( 'NONE',  ( 0.1532563361054082862, 61.21726448433412315, 2.638427012816831674 ) ) ;
#92483=CARTESIAN_POINT ( 'NONE',  ( 2.791683348922237240, 25.38393115100078390, -7.208316651077763204 ) ) ;
#92485=CARTESIAN_POINT ( 'NONE',  ( 10.00000000000000178, 63.05374883491396076, 14.16423886937410082 ) ) ;
#92487=( BOUNDED_CURVE ( )  B_SPLINE_CURVE ( 2, ( #79951, #41489, #71488, #72438, #58418, #26947, #95456, #4467, #57448 ),
 .UNSPECIFIED., .F., .T. ) 
 B_SPLINE_CURVE_WITH_KNOTS ( ( 3, 2, 2, 2, 3 ),
 ( 0.5472837940830884707, 0.5476190476190476719, 0.5535714285714286031, 0.5595238095238095344, 0.5598590630597686246 ),
 .UNSPECIFIED. ) 
 CURVE ( )  GEOMETRIC_REPRESENTATION_ITEM ( )  RATIONAL_B_SPLINE_CURVE ( ( 0.9963778908391753841, 0.9980808541467917072, 1.000000000000000000, 0.9659258262890683122, 1.000000000000000000, 0.9659258262890683122, 1.000000000000000000, 0.9980808541467922623, 0.9963778908391764944 ) ) 
 REPRESENTATION_ITEM ( '' )  );
#92488=CARTESIAN_POINT ( 'NONE',  ( 20.88017736071110164, 5.355352010821502695, 2.915334737309930979 ) ) ;
#92489=CARTESIAN_POINT ( 'NONE',  ( 0.5774900079438607392, 8.480352010821505360, 5.440088680355550821 ) ) ;
#92493=CARTESIAN_POINT ( 'NONE',  ( 7.084665262690076126, 9.105352010821503583, 10.88017736071109987 ) ) ;
#92494=CARTESIAN_POINT ( 'NONE',  ( 20.88017736071110164, 5.355352010821503583, 2.915334737309930979 ) ) ;
#92495=CARTESIAN_POINT ( 'NONE',  ( 0.1532563361054082862, 41.21726448433411605, 2.638427012816831674 ) ) ;
#92496=CARTESIAN_POINT ( 'NONE',  ( 10.00000000000000000, 42.87363466993042493, -12.81628187352647608 ) ) ;
#92498=CARTESIAN_POINT ( 'NONE',  ( -4.164238869374098151, 26.59541550158063217, -3.795296366450310543 ) ) ;
#92499=CARTESIAN_POINT ( 'NONE',  ( -0.8801773607111009756, 28.06368534415484106, 1.068504757029289695E-15 ) ) ;
#92500=CARTESIAN_POINT ( 'NONE',  ( 17.96484262340118221, 6.188685344154837509, -7.964842623401177768 ) ) ;
#92501=CARTESIAN_POINT ( 'NONE',  ( 19.84674366389459266, 38.71726448433412315, -2.638427012816827677 ) ) ;
#92503=CARTESIAN_POINT ( 'NONE',  ( 7.361572987183170547, 37.05059781766744464, 9.846743663894590881 ) ) ;
#92506=ORIENTED_EDGE ( 'NONE', *, *, #89212, .F. ) ;
#92509=CARTESIAN_POINT ( 'NONE',  ( -0.8801773607111009756, 3.063685344154837509, 1.068504757029289695E-15 ) ) ;
#92510=CARTESIAN_POINT ( 'NONE',  ( 10.00000000000000000, 61.81368534415484106, -10.88017736071110342 ) ) ;
#92511=CARTESIAN_POINT ( 'NONE',  ( 19.84674366389459266, 58.30059781766745886, 2.638427012816836559 ) ) ;
#92512=CARTESIAN_POINT ( 'NONE',  ( 2.035157376598822676, 37.43868534415484106, -7.964842623401177768 ) ) ;
#92513=CARTESIAN_POINT ( 'NONE',  ( -0.8801773607111008646, 48.27201867748816966, 2.915334737309923430 ) ) ;
#92514=CARTESIAN_POINT ( 'NONE',  ( -0.8801773607111009756, 8.063685344154837509, 1.068504757029289695E-15 ) ) ;
#92515=CARTESIAN_POINT ( 'NONE',  ( 19.38216949554541557, 32.24863466993041783, -9.382169495545420901 ) ) ;
#92516=CARTESIAN_POINT ( 'NONE',  ( 2.917880565312948704, 22.63708216824730002, 12.26659068614894643 ) ) ;
#92518=ORIENTED_EDGE ( 'NONE', *, *, #12529, .F. ) ;
#92519=CARTESIAN_POINT ( 'NONE',  ( 6.565887622018943937, 45.16530133659708923, 12.81628187352647430 ) ) ;
#92521=CARTESIAN_POINT ( 'NONE',  ( 19.84674366389459266, 43.71726448433410894, -2.638427012816827677 ) ) ;
#92522=CARTESIAN_POINT ( 'NONE',  ( 10.00000000000000178, 19.31368534415484106, 10.88017736071110342 ) ) ;
#92523=CARTESIAN_POINT ( 'NONE',  ( -0.8801773607111008646, 13.27201867748817321, 2.915334737309923430 ) ) ;
#92525=CARTESIAN_POINT ( 'NONE',  ( 20.88017736071110875, 60.77201867748817676, -2.915334737309920765 ) ) ;
#92526=DIRECTION ( 'NONE',  ( -0.000000000000000000, -1.000000000000000000, -0.000000000000000000 ) ) ;
#92527=CARTESIAN_POINT ( 'NONE',  ( 19.84674366389459621, 3.508931151000785231, 7.409399052514197653E-17 ) ) ;
#92528=CARTESIAN_POINT ( 'NONE',  ( 2.035157376598822676, 62.43868534415483396, -7.964842623401177768 ) ) ;
#92531=CARTESIAN_POINT ( 'NONE',  ( 18.52753015748617571, 3.092264484334118269, 4.923371831947298993 ) ) ;
#92533=CARTESIAN_POINT ( 'NONE',  ( 2.791683348922237240, 35.38393115100079456, -7.208316651077763204 ) ) ;
#92538=CARTESIAN_POINT ( 'NONE',  ( 21.09922568453595559, 57.04030133659708923, -6.408140936763230044 ) ) ;
#92539=CARTESIAN_POINT ( 'NONE',  ( 17.08211943468705130, 8.470415501580635720, 12.26659068614894998 ) ) ;
#92541=CARTESIAN_POINT ( 'NONE',  ( 20.36894250292379738, 14.92874883491396432, -10.36894250292379027 ) ) ;
#92542=LINE ( 'NONE', #47041, #87384 ) ;
#92544=CARTESIAN_POINT ( 'NONE',  ( 4.559911319644449179, 62.23035201082150536, -9.422509992056141925 ) ) ;
#92545=CARTESIAN_POINT ( 'NONE',  ( 20.88017736071110519, 15.56368534415483751, 2.639326808657452039E-16 ) ) ;
#92546=CARTESIAN_POINT ( 'NONE',  ( 20.00000000000000711, 105.0000000000000000, -4.500000000000001776 ) ) ;
#92548=CARTESIAN_POINT ( 'NONE',  ( 18.52753015748617571, 8.092264484334117824, 4.923371831947298993 ) ) ;
#92549=CARTESIAN_POINT ( 'NONE',  ( 10.00000000000000178, 2.258931151000784787, 9.846743663894594434 ) ) ;
#92551=CARTESIAN_POINT ( 'NONE',  ( 21.09922568453594849, 36.20696800326375353, 6.408140936763242479 ) ) ;
#92552=CARTESIAN_POINT ( 'NONE',  ( 18.52753015748618282, 28.92559781766745175, -4.923371831947291888 ) ) ;
#92555=ADVANCED_FACE ( 'NONE', ( #4166 ), #96154, .F. ) ;
#92556=CARTESIAN_POINT ( 'NONE',  ( 21.09922568453594849, 11.20696800326375531, 6.408140936763242479 ) ) ;
#92558=CARTESIAN_POINT ( 'NONE',  ( 14.92337183194729633, 7.675597817667451750, 8.527530157486181039 ) ) ;
#92562=CARTESIAN_POINT ( 'NONE',  ( 12.91533473730992121, 24.52201867748816966, 10.88017736071110164 ) ) ;
#92563=CARTESIAN_POINT ( 'NONE',  ( 13.79529636645030344, 38.26208216824729647, 14.16423886937410614 ) ) ;
#92564=CARTESIAN_POINT ( 'NONE',  ( 18.52753015748617571, 38.09226448433412315, 4.923371831947298993 ) ) ;
#92565=CARTESIAN_POINT ( 'NONE',  ( 7.084665262690076126, 64.10535201082150536, 10.88017736071109987 ) ) ;
#92566=CARTESIAN_POINT ( 'NONE',  ( 6.565887622018943937, 55.16530133659709634, 12.81628187352647430 ) ) ;
#92568=CARTESIAN_POINT ( 'NONE',  ( 19.42250999205614193, 25.14701867748817321, 5.440088680355555262 ) ) ;
#92571=AXIS2_PLACEMENT_3D ( 'NONE', #53328, #91833, #90332 ) ;
#92572=CARTESIAN_POINT ( 'NONE',  ( -2.816281873526473856, 19.12363466993042138, 9.499525473075851096E-16 ) ) ;
#92573=CARTESIAN_POINT ( 'NONE',  ( 6.565887622018943937, 10.16530133659708746, 12.81628187352647430 ) ) ;
#92574=CARTESIAN_POINT ( 'NONE',  ( 0.1532563361054100626, 35.80059781766745175, -2.638427012816831230 ) ) ;
#92576=CARTESIAN_POINT ( 'NONE',  ( 6.565887622018943937, 50.16530133659708213, 12.81628187352647430 ) ) ;
#92579=CARTESIAN_POINT ( 'NONE',  ( 12.91533473730992121, 59.52201867748816966, 10.88017736071110164 ) ) ;
#92582=CARTESIAN_POINT ( 'NONE',  ( 10.00000000000000178, 69.31368534415484817, 10.88017736071110342 ) ) ;
#92583=CARTESIAN_POINT ( 'NONE',  ( 15.44008868035555260, 54.73035201082150536, 9.422509992056143702 ) ) ;
#92584=CARTESIAN_POINT ( 'NONE',  ( 10.00000000000000000, 51.81368534415484106, -10.88017736071110342 ) ) ;
#92585=DIRECTION ( 'NONE',  ( -0.000000000000000000, 1.000000000000000000, -0.000000000000000000 ) ) ;
#92587=LINE ( 'NONE', #53114, #85912 ) ;
#92588=CARTESIAN_POINT ( 'NONE',  ( 20.88017736071110875, 15.77201867748817143, -2.915334737309920765 ) ) ;
#92589=CARTESIAN_POINT ( 'NONE',  ( 5.076628168052703671, 56.84226448433412315, 8.527530157486179263 ) ) ;
#92590=CARTESIAN_POINT ( 'NONE',  ( -0.8801773607110991993, 17.85535201082150536, -2.915334737309923874 ) ) ;
#92592=CARTESIAN_POINT ( 'NONE',  ( 22.81628187352647785, 31.41530133659709279, 3.434112377981063169 ) ) ;
#92594=CARTESIAN_POINT ( 'NONE',  ( 17.96484262340118221, 39.93868534415484106, 7.964842623401181321 ) ) ;
#92596=CARTESIAN_POINT ( 'NONE',  ( 21.09922568453594849, 6.206968003263753531, 6.408140936763242479 ) ) ;
#92597=CARTESIAN_POINT ( 'NONE',  ( -19.19000000000001194, 93.50000000000000000, 9.500000000000000000 ) ) ;
#92598=CARTESIAN_POINT ( 'NONE',  ( 10.00000000000000000, 16.81368534415483751, -10.88017736071110342 ) ) ;
#92599=CARTESIAN_POINT ( 'NONE',  ( -0.8801773607111008646, 43.27201867748817676, 2.915334737309923430 ) ) ;
#92600=CARTESIAN_POINT ( 'NONE',  ( -2.266590686148945544, 42.22041550158063217, 7.082119434687048631 ) ) ;
#92601=CARTESIAN_POINT ( 'NONE',  ( 17.20831665107776587, 22.88393115100078745, 7.208316651077764980 ) ) ;
#92602=CARTESIAN_POINT ( 'NONE',  ( 10.00000000000000178, 59.31368534415484106, 10.88017736071110342 ) ) ;
#92604=CARTESIAN_POINT ( 'NONE',  ( 2.917880565312948704, 22.63708216824730002, 12.26659068614894643 ) ) ;
#92606=CARTESIAN_POINT ( 'NONE',  ( 2.791683348922237240, 60.38393115100078745, -7.208316651077763204 ) ) ;
#92607=ORIENTED_EDGE ( 'NONE', *, *, #2813, .F. ) ;
#92609=CARTESIAN_POINT ( 'NONE',  ( -2.266590686148945544, 36.38708216824730357, -7.082119434687050408 ) ) ;
#92610=CARTESIAN_POINT ( 'NONE',  ( 20.36894250292379382, 33.67874883491396076, 10.36894250292379205 ) ) ;
#92611=CARTESIAN_POINT ( 'NONE',  ( 17.20831665107776587, 9.133931151000787452, -7.208316651077762316 ) ) ;
#92612=CARTESIAN_POINT ( 'NONE',  ( 19.38216949554541202, 10.99863466993042138, 9.382169495545424454 ) ) ;
#92613=CARTESIAN_POINT ( 'NONE',  ( 7.361572987183169658, 64.96726448433412315, -9.846743663894592657 ) ) ;
#92615=CARTESIAN_POINT ( 'NONE',  ( 0.5774900079438590739, 57.64701867748817676, -5.440088680355550821 ) ) ;
#92616=CARTESIAN_POINT ( 'NONE',  ( 21.09922568453594849, 16.20696800326375353, 6.408140936763242479 ) ) ;
#92617=CARTESIAN_POINT ( 'NONE',  ( -4.164238869374099039, 26.80374883491397142, 8.674139862899312516E-16 ) ) ;
#92618=CARTESIAN_POINT ( 'NONE',  ( 0.5774900079438607392, 33.48035201082150536, 5.440088680355550821 ) ) ;
#92619=CARTESIAN_POINT ( 'NONE',  ( 10.00000000000000178, 34.31368534415484106, 10.88017736071110342 ) ) ;
#92621=CARTESIAN_POINT ( 'NONE',  ( 15.44008868035555260, 54.73035201082150536, 9.422509992056143702 ) ) ;
#92624=ORIENTED_EDGE ( 'NONE', *, *, #71749, .F. ) ;
#92625=CYLINDRICAL_SURFACE ( 'NONE', #81043, 11.92686044187656513 ) ;
#92627=CARTESIAN_POINT ( 'NONE',  ( 10.00000000000000000, 5.553748834913967869, -14.16423886937410082 ) ) ;
#92628=CARTESIAN_POINT ( 'NONE',  ( -2.266590686148945544, 61.38708216824730357, -7.082119434687050408 ) ) ;
#92629=CARTESIAN_POINT ( 'NONE',  ( -2.266590686148945544, 61.38708216824730357, -7.082119434687050408 ) ) ;
#92630=CARTESIAN_POINT ( 'NONE',  ( 14.92337183194729633, 37.67559781766745175, 8.527530157486181039 ) ) ;
#92631=CARTESIAN_POINT ( 'NONE',  ( 5.076628168052703671, 66.84226448433412315, 8.527530157486179263 ) ) ;
#92634=CARTESIAN_POINT ( 'NONE',  ( 6.000000000000000000, 60.50000000000000000, -6.500000000000000888 ) ) ;
#92635=EDGE_CURVE ( 'NONE', #85529, #42599, #53462, .T. ) ;
#92636=CARTESIAN_POINT ( 'NONE',  ( 16.40814093676323893, 0.7903013365970867898, 11.09922568453595026 ) ) ;
#92637=ORIENTED_EDGE ( 'NONE', *, *, #4887, .F. ) ;
#92638=CARTESIAN_POINT ( 'NONE',  ( 22.26659068614895176, 44.72041550158063927, -7.082119434687042414 ) ) ;
#92639=CARTESIAN_POINT ( 'NONE',  ( 2.917880565312948704, 42.63708216824729647, 12.26659068614894643 ) ) ;
#92641=CARTESIAN_POINT ( 'NONE',  ( 17.96484262340118221, 14.93868534415483751, 7.964842623401181321 ) ) ;
#92642=CARTESIAN_POINT ( 'NONE',  ( 3.591859063236763294, 58.29030133659708923, -11.09922568453595026 ) ) ;
#92643=CARTESIAN_POINT ( 'NONE',  ( 18.52753015748618282, 53.92559781766745175, -4.923371831947291888 ) ) ;
#92644=CARTESIAN_POINT ( 'NONE',  ( 15.44008868035555260, 34.73035201082151247, 9.422509992056143702 ) ) ;
#92646=CARTESIAN_POINT ( 'NONE',  ( 1.472469842513823179, 51.42559781766745886, 4.923371831947296329 ) ) ;
#92647=CARTESIAN_POINT ( 'NONE',  ( 7.084665262690076126, 64.10535201082150536, 10.88017736071109987 ) ) ;
#92648=CARTESIAN_POINT ( 'NONE',  ( -0.8801773607110991993, 32.85535201082151247, -2.915334737309923874 ) ) ;
#92651=FACE_OUTER_BOUND ( 'NONE', #62507, .T. ) ;
#92655=CARTESIAN_POINT ( 'NONE',  ( 0.1532563361054083140, 36.00893115100078745, 1.131784320476157264E-15 ) ) ;
#92656=CARTESIAN_POINT ( 'NONE',  ( -46.48928645636215151, 103.2957187381728232, 6.397878122523974476 ) ) ;
#92658=CARTESIAN_POINT ( 'NONE',  ( -12.69000000000001371, 93.50000000000000000, 9.500000000000000000 ) ) ;
#92659=ORIENTED_EDGE ( 'NONE', *, *, #66046, .T. ) ;
#92661=CARTESIAN_POINT ( 'NONE',  ( -42.83934546894332129, 106.9582108035436363, 5.000000000000000888 ) ) ;
#92662=CARTESIAN_POINT ( 'NONE',  ( 12.63842701281683922, 49.55059781766744464, -9.846743663894590881 ) ) ;
#92663=CARTESIAN_POINT ( 'NONE',  ( 6.204703633549690345, 52.84541550158062506, 14.16423886937410082 ) ) ;
#92664=CARTESIAN_POINT ( 'NONE',  ( 10.00000000000000178, 62.25893115100078745, 9.846743663894594434 ) ) ;
#92667=CARTESIAN_POINT ( 'NONE',  ( 18.52753015748617571, 23.09226448433411960, 4.923371831947298993 ) ) ;
#92668=CARTESIAN_POINT ( 'NONE',  ( 22.81628187352647785, 51.41530133659708923, 3.434112377981063169 ) ) ;
#92669=CARTESIAN_POINT ( 'NONE',  ( 0.1532563361054100626, 60.80059781766744464, -2.638427012816831230 ) ) ;
#92670=CARTESIAN_POINT ( 'NONE',  ( 7.084665262690076126, 59.10535201082150536, 10.88017736071109987 ) ) ;
#92671=CARTESIAN_POINT ( 'NONE',  ( 14.92337183194729988, 49.34226448433411605, -8.527530157486177487 ) ) ;
#92672=FACE_OUTER_BOUND ( 'NONE', #66563, .T. ) ;
#92673=EDGE_CURVE ( 'NONE', #98100, #27569, #83111, .T. ) ;
#92674=CARTESIAN_POINT ( 'NONE',  ( 15.44008868035555793, 56.39701867748817676, -9.422509992056140149 ) ) ;
#92679=CARTESIAN_POINT ( 'NONE',  ( 15.44008868035555260, 24.73035201082150891, 9.422509992056143702 ) ) ;
#92680=AXIS2_PLACEMENT_3D ( 'NONE', #28876, #50900, #14397 ) ;
#92681=CARTESIAN_POINT ( 'NONE',  ( 6.565887622018943937, 13.08196800326374998, -12.81628187352647608 ) ) ;
#92682=CARTESIAN_POINT ( 'NONE',  ( 12.91533473730993009, 61.60535201082150536, -10.88017736071109987 ) ) ;
#92687=CARTESIAN_POINT ( 'NONE',  ( 4.559911319644449179, 57.23035201082150536, -9.422509992056141925 ) ) ;
#92689=CARTESIAN_POINT ( 'NONE',  ( 14.92337183194729988, 44.34226448433412315, -8.527530157486177487 ) ) ;
#92690=CARTESIAN_POINT ( 'NONE',  ( 2.791683348922240793, 6.633931151000785675, 7.208316651077764092 ) ) ;
#92692=CARTESIAN_POINT ( 'NONE',  ( -2.816281873526471635, 8.915301336597083903, -3.434112377981056508 ) ) ;
#92693=AXIS2_PLACEMENT_3D ( 'NONE', #74186, #15693, #85158 ) ;
#92694=CARTESIAN_POINT ( 'NONE',  ( 20.88017736071110164, 15.35535201082150358, 2.915334737309930979 ) ) ;
#92695=CARTESIAN_POINT ( 'NONE',  ( 1.602071938427537701, 67.02224192338641728, -6.500000000000075495 ) ) ;
#92697=CARTESIAN_POINT ( 'NONE',  ( -2.266590686148945544, 41.38708216824729647, -7.082119434687050408 ) ) ;
#92698=CARTESIAN_POINT ( 'NONE',  ( -4.164238869374098151, 61.59541550158063217, -3.795296366450310543 ) ) ;
#92699=CARTESIAN_POINT ( 'NONE',  ( 5.076628168052704559, 35.17559781766745175, -8.527530157486179263 ) ) ;
#92700=CARTESIAN_POINT ( 'NONE',  ( 18.52753015748618282, 13.92559781766745175, -4.923371831947291888 ) ) ;
#92701=CARTESIAN_POINT ( 'NONE',  ( 7.084665262690076126, 19.10535201082150181, 10.88017736071109987 ) ) ;
#92703=CARTESIAN_POINT ( 'NONE',  ( 19.84674366389459266, 43.30059781766744464, 2.638427012816836559 ) ) ;
#92704=CARTESIAN_POINT ( 'NONE',  ( 17.96484262340118221, 21.18868534415483396, -7.964842623401177768 ) ) ;
#92705=CARTESIAN_POINT ( 'NONE',  ( 7.361572987183170547, 67.05059781766746596, 9.846743663894590881 ) ) ;
#92706=CARTESIAN_POINT ( 'NONE',  ( -2.266590686148945544, 11.38708216824730179, -7.082119434687050408 ) ) ;
#92709=CARTESIAN_POINT ( 'NONE',  ( 12.63842701281683034, 17.46726448433411250, 9.846743663894596210 ) ) ;
#92710=CARTESIAN_POINT ( 'NONE',  ( 16.40814093676324603, 52.45696800326375353, -11.09922568453594671 ) ) ;
#92711=CARTESIAN_POINT ( 'NONE',  ( 18.52753015748617571, 53.09226448433412315, 4.923371831947298993 ) ) ;
#92713=CARTESIAN_POINT ( 'NONE',  ( 14.92337183194729633, 17.67559781766745175, 8.527530157486181039 ) ) ;
#92715=CARTESIAN_POINT ( 'NONE',  ( 0.2751277870542967463, 70.00000000000000000, -6.000000000000000000 ) ) ;
#92716=CARTESIAN_POINT ( 'NONE',  ( -4.164238869374098151, 56.59541550158063927, -3.795296366450310543 ) ) ;
#92717=CARTESIAN_POINT ( 'NONE',  ( -0.8801773607111008646, 53.27201867748816966, 2.915334737309923430 ) ) ;
#92720=CARTESIAN_POINT ( 'NONE',  ( 12.91533473730992121, 59.52201867748816966, 10.88017736071110164 ) ) ;
#92721=CARTESIAN_POINT ( 'NONE',  ( 19.84674366389459266, 38.71726448433412315, -2.638427012816827677 ) ) ;
#92722=CARTESIAN_POINT ( 'NONE',  ( 7.084665262690076126, 24.10535201082150181, 10.88017736071109987 ) ) ;
#92723=CARTESIAN_POINT ( 'NONE',  ( 18.72515096720572458, 40.05509018479936145, 6.499999999999964473 ) ) ;
#92724=CARTESIAN_POINT ( 'NONE',  ( 0.1532563361054100626, 55.80059781766745175, -2.638427012816831230 ) ) ;
#92726=CARTESIAN_POINT ( 'NONE',  ( 15.44008868035555260, 54.73035201082150536, 9.422509992056143702 ) ) ;
#92728=EDGE_CURVE ( 'NONE', #79104, #52153, #38124, .T. ) ;
#92734=CARTESIAN_POINT ( 'NONE',  ( 14.92337183194729988, 44.34226448433412315, -8.527530157486177487 ) ) ;
#92735=CARTESIAN_POINT ( 'NONE',  ( 12.63842701281683034, 22.46726448433411605, 9.846743663894596210 ) ) ;
#92736=CARTESIAN_POINT ( 'NONE',  ( 22.81628187352648496, 61.83196800326376774, -3.434112377981050290 ) ) ;
#92737=CARTESIAN_POINT ( 'NONE',  ( 4.559911319644449179, 17.23035201082150536, -9.422509992056141925 ) ) ;
#92738=CARTESIAN_POINT ( 'NONE',  ( 17.20831665107776587, 49.13393115100078745, -7.208316651077762316 ) ) ;
#92740=CARTESIAN_POINT ( 'NONE',  ( 20.36894250292379738, 39.92874883491396787, -10.36894250292379027 ) ) ;
#92741=CARTESIAN_POINT ( 'NONE',  ( 6.204703633549690345, 55.76208216824730357, -14.16423886937410259 ) ) ;
#92744=CARTESIAN_POINT ( 'NONE',  ( -0.8801773607111008646, 53.27201867748816966, 2.915334737309923430 ) ) ;
#92745=CARTESIAN_POINT ( 'NONE',  ( 5.076628168052703671, 21.84226448433411960, 8.527530157486179263 ) ) ;
#92750=CARTESIAN_POINT ( 'NONE',  ( 5.076628168052704559, 5.175597817667451750, -8.527530157486179263 ) ) ;
#92752=CARTESIAN_POINT ( 'NONE',  ( 2.917880565312950480, 15.97041550158063217, -12.26659068614894821 ) ) ;
#92753=CARTESIAN_POINT ( 'NONE',  ( 10.00000000000000178, 22.25893115100078745, 9.846743663894594434 ) ) ;
#92754=CARTESIAN_POINT ( 'NONE',  ( 15.44008868035555793, 46.39701867748817676, -9.422509992056140149 ) ) ;
#92755=DIRECTION ( 'NONE',  ( 0.000000000000000000, 1.000000000000000000, -0.000000000000000000 ) ) ;
#92756=EDGE_LOOP ( 'NONE', ( #52555, #67562, #45787, #6117 ) ) ;
#92757=CARTESIAN_POINT ( 'NONE',  ( 7.084665262690076126, 39.10535201082150536, 10.88017736071109987 ) ) ;
#92760=CARTESIAN_POINT ( 'NONE',  ( -4.164238869374099039, 11.80374883491396965, 8.674139862899312516E-16 ) ) ;
#92763=CARTESIAN_POINT ( 'NONE',  ( 6.565887622018943937, 15.16530133659708568, 12.81628187352647430 ) ) ;
#92764=CARTESIAN_POINT ( 'NONE',  ( 2.791683348922240793, 6.633931151000785675, 7.208316651077764092 ) ) ;
#92766=CARTESIAN_POINT ( 'NONE',  ( 20.88017736071110519, 10.56368534415483929, 2.639326808657452039E-16 ) ) ;
#92767=CARTESIAN_POINT ( 'NONE',  ( 5.076628168052704559, 10.17559781766745175, -8.527530157486179263 ) ) ;
#92768=CARTESIAN_POINT ( 'NONE',  ( 4.559911319644449179, 37.23035201082150536, -9.422509992056141925 ) ) ;
#92769=EDGE_CURVE ( 'NONE', #75287, #32729, #45604, .T. ) ;
#92770=ORIENTED_EDGE ( 'NONE', *, *, #3524, .F. ) ;
#92772=CARTESIAN_POINT ( 'NONE',  ( -46.34323875807881166, 103.6109741468810483, 6.190393423093146552 ) ) ;
#92773=CARTESIAN_POINT ( 'NONE',  ( 7.084665262690076126, 59.10535201082150536, 10.88017736071109987 ) ) ;
#92775=CARTESIAN_POINT ( 'NONE',  ( 10.00000000000000000, 62.87363466993042493, -12.81628187352647608 ) ) ;
#92776=CARTESIAN_POINT ( 'NONE',  ( 17.96484262340118221, 54.93868534415484106, 7.964842623401181321 ) ) ;
#92778=CARTESIAN_POINT ( 'NONE',  ( 18.52753015748618282, 33.92559781766745886, -4.923371831947291888 ) ) ;
#92779=CARTESIAN_POINT ( 'NONE',  ( 0.6178305044545818747, 58.49863466993042493, -9.382169495545419124 ) ) ;
#92780=CARTESIAN_POINT ( 'NONE',  ( 10.00000000000000000, 5.553748834913967869, -14.16423886937410082 ) ) ;
#92781=CARTESIAN_POINT ( 'NONE',  ( 2.791683348922237240, 15.38393115100078212, -7.208316651077763204 ) ) ;
#92782=CARTESIAN_POINT ( 'NONE',  ( 10.00000000000000178, 25.37363466993041783, 12.81628187352647608 ) ) ;
#92785=CARTESIAN_POINT ( 'NONE',  ( 4.559911319644449179, 53.89701867748817676, 9.422509992056141925 ) ) ;
#92787=CARTESIAN_POINT ( 'NONE',  ( 7.361572987183170547, 57.05059781766744464, 9.846743663894590881 ) ) ;
#92789=CARTESIAN_POINT ( 'NONE',  ( 19.84674366389459266, 33.71726448433410894, -2.638427012816827677 ) ) ;
#92790=CARTESIAN_POINT ( 'NONE',  ( 5.076628168052703671, 16.84226448433411960, 8.527530157486179263 ) ) ;
#92791=CARTESIAN_POINT ( 'NONE',  ( 20.88017736071110519, 15.56368534415483751, 2.639326808657452039E-16 ) ) ;
#92792=CARTESIAN_POINT ( 'NONE',  ( 21.09922568453594849, 21.20696800326375353, 6.408140936763242479 ) ) ;
#92793=CARTESIAN_POINT ( 'NONE',  ( 12.91533473730992121, 4.522018677488169658, 10.88017736071110164 ) ) ;
#92795=CARTESIAN_POINT ( 'NONE',  ( 18.72515096720577787, 46.07228050351031357, -6.499999999999891642 ) ) ;
#92798=CARTESIAN_POINT ( 'NONE',  ( 20.88017736071110519, 15.56368534415483751, 2.639326808657452039E-16 ) ) ;
#92802=CARTESIAN_POINT ( 'NONE',  ( 0.1532563361054083140, 31.00893115100078390, 1.131784320476157264E-15 ) ) ;
#92803=CARTESIAN_POINT ( 'NONE',  ( 2.035157376598824452, 13.68868534415483751, 7.964842623401179544 ) ) ;
#92805=CARTESIAN_POINT ( 'NONE',  ( -0.8801773607110991993, 37.85535201082151247, -2.915334737309923874 ) ) ;
#92806=CARTESIAN_POINT ( 'NONE',  ( 19.42250999205614548, 5.980352010821504471, -5.440088680355545492 ) ) ;
#92807=CARTESIAN_POINT ( 'NONE',  ( 14.92337183194729988, 19.34226448433411960, -8.527530157486177487 ) ) ;
#92808=CARTESIAN_POINT ( 'NONE',  ( 19.84674366389459266, 33.71726448433410894, -2.638427012816827677 ) ) ;
#92814=CARTESIAN_POINT ( 'NONE',  ( 24.16423886937409904, 19.09541550158063927, 3.795296366450317205 ) ) ;
#92815=CARTESIAN_POINT ( 'NONE',  ( 14.92337183194729633, 37.67559781766745175, 8.527530157486181039 ) ) ;
#92817=CARTESIAN_POINT ( 'NONE',  ( 10.00000000000000178, 53.05374883491396787, 14.16423886937410082 ) ) ;
#92819=CARTESIAN_POINT ( 'NONE',  ( 0.1532563361054100626, 20.80059781766744464, -2.638427012816831230 ) ) ;
#92822=CARTESIAN_POINT ( 'NONE',  ( 4.559911319644449179, 52.23035201082151247, -9.422509992056141925 ) ) ;
#92823=CARTESIAN_POINT ( 'NONE',  ( -2.816281873526473856, 54.33196800326376064, 3.434112377981055619 ) ) ;
#92824=CARTESIAN_POINT ( 'NONE',  ( 20.88017736071110164, 15.35535201082150358, 2.915334737309930979 ) ) ;
#92826=CARTESIAN_POINT ( 'NONE',  ( -2.816281873526471635, 53.91530133659709634, -3.434112377981056508 ) ) ;
#92827=CARTESIAN_POINT ( 'NONE',  ( 5.076628168052703671, 66.84226448433412315, 8.527530157486179263 ) ) ;
#92828=CARTESIAN_POINT ( 'NONE',  ( 7.361572987183169658, -0.03273551566588185635, -9.846743663894592657 ) ) ;
#92829=VERTEX_POINT ( 'NONE', #63549 ) ;
#92833=CARTESIAN_POINT ( 'NONE',  ( -0.3689425029237881626, 52.42874883491396076, 10.36894250292379027 ) ) ;
#92834=CARTESIAN_POINT ( 'NONE',  ( 24.16423886937409904, 14.09541550158063217, 3.795296366450317205 ) ) ;
#92835=CARTESIAN_POINT ( 'NONE',  ( -0.8801773607111009756, 13.06368534415483929, 1.068504757029289695E-15 ) ) ;
#92836=CARTESIAN_POINT ( 'NONE',  ( 15.44008868035555260, 29.73035201082150891, 9.422509992056143702 ) ) ;
#92838=CARTESIAN_POINT ( 'NONE',  ( 10.00000000000000000, -0.2410688489992152128, -9.846743663894594434 ) ) ;
#92839=SURFACE_STYLE_USAGE ( .BOTH. , #93332 ) ;
#92840=CARTESIAN_POINT ( 'NONE',  ( 1.472469842513823179, 16.42559781766745175, 4.923371831947296329 ) ) ;
#92842=AXIS2_PLACEMENT_3D ( 'NONE', #40718, #71220, #26203 ) ;
#92844=CARTESIAN_POINT ( 'NONE',  ( 12.63842701281683922, 14.55059781766744997, -9.846743663894590881 ) ) ;
#92845=CARTESIAN_POINT ( 'NONE',  ( 14.92337183194729633, 37.67559781766745175, 8.527530157486181039 ) ) ;
#92846=CARTESIAN_POINT ( 'NONE',  ( -0.8801773607111008646, 18.27201867748817321, 2.915334737309923430 ) ) ;
#92847=CARTESIAN_POINT ( 'NONE',  ( 22.81628187352647785, 26.41530133659708923, 3.434112377981063169 ) ) ;
#92848=CARTESIAN_POINT ( 'NONE',  ( 17.20831665107776587, 12.88393115100078390, 7.208316651077764980 ) ) ;
#92850=CARTESIAN_POINT ( 'NONE',  ( 10.00000000000000178, 52.25893115100078745, 9.846743663894594434 ) ) ;
#92851=CARTESIAN_POINT ( 'NONE',  ( 12.63842701281683034, 32.46726448433412315, 9.846743663894596210 ) ) ;
#92852=CARTESIAN_POINT ( 'NONE',  ( -4.164238869374099927, 12.01208216824730357, 3.795296366450308767 ) ) ;
#92853=CARTESIAN_POINT ( 'NONE',  ( -0.8801773607110991993, 52.85535201082151247, -2.915334737309923874 ) ) ;
#92854=CARTESIAN_POINT ( 'NONE',  ( 20.88017736071110875, 10.77201867748817143, -2.915334737309920765 ) ) ;
#92855=CARTESIAN_POINT ( 'NONE',  ( 10.00000000000000178, 49.31368534415484106, 10.88017736071110342 ) ) ;
#92856=CARTESIAN_POINT ( 'NONE',  ( 20.88017736071110875, 35.77201867748816966, -2.915334737309920765 ) ) ;
#92859=CARTESIAN_POINT ( 'NONE',  ( -0.8801773607111008646, 43.27201867748817676, 2.915334737309923430 ) ) ;
#92860=EDGE_LOOP ( 'NONE', ( #12466, #98089, #79237, #681 ) ) ;
#92861=CARTESIAN_POINT ( 'NONE',  ( 21.09922568453594849, 61.20696800326376064, 6.408140936763242479 ) ) ;
#92862=CARTESIAN_POINT ( 'NONE',  ( -0.8801773607110991993, 52.85535201082151247, -2.915334737309923874 ) ) ;
#92863=ORIENTED_EDGE ( 'NONE', *, *, #29529, .T. ) ;
#92864=CARTESIAN_POINT ( 'NONE',  ( -0.8801773607110991993, 47.85535201082150536, -2.915334737309923874 ) ) ;
#92866=VECTOR ( 'NONE', #26401, 1000.000000000000000 ) ;
#92867=CARTESIAN_POINT ( 'NONE',  ( 18.04007052943772749, 8.015283700948081957, 5.767676674365838529 ) ) ;
#92868=CARTESIAN_POINT ( 'NONE',  ( -1.926860441876564023, 24.68830936912750929, 1.004413902775740781E-15 ) ) ;
#92869=CARTESIAN_POINT ( 'NONE',  ( 6.204703633549690345, 55.76208216824730357, -14.16423886937410259 ) ) ;
#92870=CARTESIAN_POINT ( 'NONE',  ( 0.5774900079438607392, 68.48035201082150536, 5.440088680355550821 ) ) ;
#92872=CARTESIAN_POINT ( 'NONE',  ( 12.91533473730992121, 14.52201867748817143, 10.88017736071110164 ) ) ;
#92873=CARTESIAN_POINT ( 'NONE',  ( 5.076628168052704559, 50.17559781766745886, -8.527530157486179263 ) ) ;
#92875=CARTESIAN_POINT ( 'NONE',  ( 17.20831665107776587, 42.88393115100077324, 7.208316651077764980 ) ) ;
#92876=CARTESIAN_POINT ( 'NONE',  ( 4.559911319644449179, 67.23035201082150536, -9.422509992056141925 ) ) ;
#92877=CARTESIAN_POINT ( 'NONE',  ( 15.44008868035555793, 36.39701867748816966, -9.422509992056140149 ) ) ;
#92878=CARTESIAN_POINT ( 'NONE',  ( 19.84674366389459266, 43.30059781766744464, 2.638427012816836559 ) ) ;
#92879=CARTESIAN_POINT ( 'NONE',  ( 6.565887622018943937, 28.08196800326375353, -12.81628187352647608 ) ) ;
#92882=CARTESIAN_POINT ( 'NONE',  ( 7.084665262690076126, 44.10535201082151247, 10.88017736071109987 ) ) ;
#92883=CARTESIAN_POINT ( 'NONE',  ( 13.79529636645031943, 60.34541550158063927, -14.16423886937409904 ) ) ;
#92886=CARTESIAN_POINT ( 'NONE',  ( 16.40814093676323893, 25.79030133659708923, 11.09922568453595026 ) ) ;
#92887=CARTESIAN_POINT ( 'NONE',  ( 2.603489959281614308, 51.58210964143330557, 6.500000000000031086 ) ) ;
#92889=CARTESIAN_POINT ( 'NONE',  ( 3.591859063236763294, 23.29030133659708568, -11.09922568453595026 ) ) ;
#92890=CARTESIAN_POINT ( 'NONE',  ( 12.91533473730993009, 26.60535201082150536, -10.88017736071109987 ) ) ;
#92894=CARTESIAN_POINT ( 'NONE',  ( 2.791683348922240793, 1.633931151000784565, 7.208316651077764092 ) ) ;
#92895=STYLED_ITEM ( 'NONE', ( #36041 ), #74512 ) ;
#92896=CARTESIAN_POINT ( 'NONE',  ( 0.1532563361054083140, 51.00893115100078745, 1.131784320476157264E-15 ) ) ;
#92897=CARTESIAN_POINT ( 'NONE',  ( 19.84674366389459621, 8.508931151000785675, 7.409399052514197653E-17 ) ) ;
#92898=CARTESIAN_POINT ( 'NONE',  ( 12.63842701281683922, 34.55059781766745886, -9.846743663894590881 ) ) ;
#92900=CARTESIAN_POINT ( 'NONE',  ( -2.816281873526471635, 63.91530133659708923, -3.434112377981056508 ) ) ;
#92901=CARTESIAN_POINT ( 'NONE',  ( 0.1532563361054082862, 26.21726448433411605, 2.638427012816831674 ) ) ;
#92902=CARTESIAN_POINT ( 'NONE',  ( 0.1143410931637268563, 40.21691075486302225, 6.480892540919860778 ) ) ;
#92904=CARTESIAN_POINT ( 'NONE',  ( 14.92337183194729633, 12.67559781766745353, 8.527530157486181039 ) ) ;
#92905=CYLINDRICAL_SURFACE ( 'NONE', #14807, 0.5000000000000004441 ) ;
#92906=CARTESIAN_POINT ( 'NONE',  ( 5.076628168052704559, 45.17559781766745175, -8.527530157486179263 ) ) ;
#92907=ORIENTED_EDGE ( 'NONE', *, *, #14315, .T. ) ;
#92908=CARTESIAN_POINT ( 'NONE',  ( 6.565887622018943937, 63.08196800326376064, -12.81628187352647608 ) ) ;
#92911=CARTESIAN_POINT ( 'NONE',  ( 0.6178305044545818747, 28.49863466993041783, -9.382169495545419124 ) ) ;
#92912=CYLINDRICAL_SURFACE ( 'NONE', #13729, 0.5000000000000004441 ) ;
#92913=CARTESIAN_POINT ( 'NONE',  ( 22.26659068614894466, 43.88708216824729647, 7.082119434687054849 ) ) ;
#92916=CARTESIAN_POINT ( 'NONE',  ( 6.204703633549690345, 37.84541550158063927, 14.16423886937410082 ) ) ;
#92917=CARTESIAN_POINT ( 'NONE',  ( -2.266590686148945544, 62.22041550158063927, 7.082119434687048631 ) ) ;
#92918=CARTESIAN_POINT ( 'NONE',  ( 2.917880565312950480, 20.97041550158063217, -12.26659068614894821 ) ) ;
#92919=CARTESIAN_POINT ( 'NONE',  ( 22.26659068614894466, 28.88708216824730357, 7.082119434687054849 ) ) ;
#92922=CARTESIAN_POINT ( 'NONE',  ( 5.076628168052704559, 45.17559781766745175, -8.527530157486179263 ) ) ;
#92924=CARTESIAN_POINT ( 'NONE',  ( 19.42250999205614548, 40.98035201082150536, -5.440088680355545492 ) ) ;
#92926=CARTESIAN_POINT ( 'NONE',  ( 19.54721792061789643, 80.97117139608940306, -5.000000000000000888 ) ) ;
#92927=CARTESIAN_POINT ( 'NONE',  ( 16.40814093676323893, 55.79030133659708923, 11.09922568453595026 ) ) ;
#92929=CARTESIAN_POINT ( 'NONE',  ( 2.791683348922237240, 40.38393115100078035, -7.208316651077763204 ) ) ;
#92930=CARTESIAN_POINT ( 'NONE',  ( 10.00000000000000178, 62.25893115100078745, 9.846743663894594434 ) ) ;
#92931=MECHANICAL_DESIGN_GEOMETRIC_PRESENTATION_REPRESENTATION('',(#97751),#56265);
#92932=ORIENTED_EDGE ( 'NONE', *, *, #53955, .F. ) ;
#92933=CARTESIAN_POINT ( 'NONE',  ( -0.3689425029237881626, 7.428748834913967869, 10.36894250292379027 ) ) ;
#92934=DIRECTION ( 'NONE',  ( 1.000000000000000000, 0.000000000000000000, 0.000000000000000000 ) ) ;
#92937=CARTESIAN_POINT ( 'NONE',  ( 2.035157376598822676, 12.43868534415483751, -7.964842623401177768 ) ) ;
#92938=CARTESIAN_POINT ( 'NONE',  ( 10.00000000000000000, 12.87363466993042138, -12.81628187352647608 ) ) ;
#92940=CARTESIAN_POINT ( 'NONE',  ( 0.5774900079438607392, 63.48035201082149825, 5.440088680355550821 ) ) ;
#92943=DIRECTION ( 'NONE',  ( 1.000000000000000000, 0.000000000000000000, 0.000000000000000000 ) ) ;
#92944=CARTESIAN_POINT ( 'NONE',  ( 2.035157376598822676, 2.438685344154838397, -7.964842623401177768 ) ) ;
#92946=CARTESIAN_POINT ( 'NONE',  ( 4.559911319644449179, 22.23035201082150536, -9.422509992056141925 ) ) ;
#92947=CARTESIAN_POINT ( 'NONE',  ( 15.44008868035555260, 29.73035201082150891, 9.422509992056143702 ) ) ;
#92948=CARTESIAN_POINT ( 'NONE',  ( 0.6178305044545818747, 3.498634669930420049, -9.382169495545419124 ) ) ;
#92949=CARTESIAN_POINT ( 'NONE',  ( 1.472469842513823179, 55.59226448433412315, -4.923371831947296329 ) ) ;
#92950=CARTESIAN_POINT ( 'NONE',  ( 22.81628187352648496, 61.83196800326376774, -3.434112377981050290 ) ) ;
#92951=CARTESIAN_POINT ( 'NONE',  ( 2.791683348922237240, 0.3839311510007847872, -7.208316651077763204 ) ) ;
#92952=EDGE_LOOP ( 'NONE', ( #46503, #61028, #2896, #54751 ) ) ;
#92953=CARTESIAN_POINT ( 'NONE',  ( -0.8801773607111009756, 33.06368534415484106, 1.068504757029289695E-15 ) ) ;
#92954=CARTESIAN_POINT ( 'NONE',  ( 16.40814093676323893, 30.79030133659708923, 11.09922568453595026 ) ) ;
#92957=CARTESIAN_POINT ( 'NONE',  ( 12.63842701281683034, 62.46726448433410894, 9.846743663894596210 ) ) ;
#92958=CARTESIAN_POINT ( 'NONE',  ( 10.00000000000000178, 49.31368534415484106, 10.88017736071110342 ) ) ;
#92959=CARTESIAN_POINT ( 'NONE',  ( 19.84674366389459266, 8.300597817667451750, 2.638427012816836559 ) ) ;
#92960=CARTESIAN_POINT ( 'NONE',  ( 21.09922568453595559, 37.04030133659708923, -6.408140936763230044 ) ) ;
#92961=( GEOMETRIC_REPRESENTATION_CONTEXT ( 3 ) GLOBAL_UNCERTAINTY_ASSIGNED_CONTEXT ( ( #40210 ) ) GLOBAL_UNIT_ASSIGNED_CONTEXT ( ( #97851, #89823, #30793 ) ) REPRESENTATION_CONTEXT ( 'NONE', 'WORKASPACE' ) );
#92962=CARTESIAN_POINT ( 'NONE',  ( 10.00000000000000000, 61.81368534415484106, -10.88017736071110342 ) ) ;
#92966=CARTESIAN_POINT ( 'NONE',  ( -2.816281873526473856, 59.12363466993042493, 9.499525473075851096E-16 ) ) ;
#92970=CARTESIAN_POINT ( 'NONE',  ( 15.44008868035555793, 6.397018677488170546, -9.422509992056140149 ) ) ;
#92971=CARTESIAN_POINT ( 'NONE',  ( 0.6178305044545838731, 49.74863466993041072, 9.382169495545420901 ) ) ;
#92972=CARTESIAN_POINT ( 'NONE',  ( -2.266590686148945544, 16.38708216824730357, -7.082119434687050408 ) ) ;
#92973=CARTESIAN_POINT ( 'NONE',  ( 19.84674366389459266, 13.30059781766745353, 2.638427012816836559 ) ) ;
#92975=CARTESIAN_POINT ( 'NONE',  ( 0.5774900079438607392, 8.480352010821505360, 5.440088680355550821 ) ) ;
#92976=CARTESIAN_POINT ( 'NONE',  ( 19.84674366389459266, 13.71726448433411782, -2.638427012816827677 ) ) ;
#92978=CARTESIAN_POINT ( 'NONE',  ( 2.917880565312948704, 62.63708216824730357, 12.26659068614894643 ) ) ;
#92981=CARTESIAN_POINT ( 'NONE',  ( 15.44008868035555260, 9.730352010821505360, 9.422509992056143702 ) ) ;
#92982=CARTESIAN_POINT ( 'NONE',  ( 2.603489959281591659, 15.43575266056827999, -6.500000000000006217 ) ) ;
#92986=CARTESIAN_POINT ( 'NONE',  ( 10.00000000000000000, 11.81368534415483751, -10.88017736071110342 ) ) ;
#92987=CARTESIAN_POINT ( 'NONE',  ( 15.44008868035555793, 16.39701867748817321, -9.422509992056140149 ) ) ;
#92988=CARTESIAN_POINT ( 'NONE',  ( 19.84674366389459266, 38.30059781766745175, 2.638427012816836559 ) ) ;
#92989=CARTESIAN_POINT ( 'NONE',  ( -1.099225684535947600, 53.70696800326376064, -6.408140936763238038 ) ) ;
#92991=CARTESIAN_POINT ( 'NONE',  ( 19.72487221294570858, 16.86607318730074567, 6.500000000000000888 ) ) ;
#92992=CARTESIAN_POINT ( 'NONE',  ( 6.204703633549690345, 20.76208216824730357, -14.16423886937410259 ) ) ;
#92993=CARTESIAN_POINT ( 'NONE',  ( -0.8801773607110991993, 27.85535201082150181, -2.915334737309923874 ) ) ;
#92994=CARTESIAN_POINT ( 'NONE',  ( 17.08211943468705840, 65.13708216824730357, -12.26659068614894466 ) ) ;
#92995=CARTESIAN_POINT ( 'NONE',  ( 10.00000000000000178, 57.25893115100078745, 9.846743663894594434 ) ) ;
#92997=CARTESIAN_POINT ( 'NONE',  ( 1.472469842513823179, 36.42559781766745175, 4.923371831947296329 ) ) ;
#93003=CARTESIAN_POINT ( 'NONE',  ( 12.91533473730993009, 61.60535201082150536, -10.88017736071109987 ) ) ;
#93004=CARTESIAN_POINT ( 'NONE',  ( 1.472469842513823179, 60.59226448433412315, -4.923371831947296329 ) ) ;
#93005=CARTESIAN_POINT ( 'NONE',  ( 4.559911319644449179, 52.23035201082151247, -9.422509992056141925 ) ) ;
#93006=CARTESIAN_POINT ( 'NONE',  ( 12.91533473730993009, 11.60535201082150536, -10.88017736071109987 ) ) ;
#93007=CARTESIAN_POINT ( 'NONE',  ( 6.565887622018943937, 38.08196800326376064, -12.81628187352647608 ) ) ;
#93008=CARTESIAN_POINT ( 'NONE',  ( 2.917880565312948704, 12.63708216824730179, 12.26659068614894643 ) ) ;
#93011=CARTESIAN_POINT ( 'NONE',  ( 19.38216949554541202, 50.99863466993042493, 9.382169495545424454 ) ) ;
#93013=CARTESIAN_POINT ( 'NONE',  ( 17.20831665107776587, 64.13393115100079456, -7.208316651077762316 ) ) ;
#93014=CARTESIAN_POINT ( 'NONE',  ( -0.8801773607111009756, 18.06368534415484106, 1.068504757029289695E-15 ) ) ;
#93016=CARTESIAN_POINT ( 'NONE',  ( 10.00000000000000000, 31.81368534415483751, -10.88017736071110342 ) ) ;
#93018=CARTESIAN_POINT ( 'NONE',  ( 20.88017736071110519, 65.56368534415483396, 2.639326808657452039E-16 ) ) ;
#93019=CARTESIAN_POINT ( 'NONE',  ( 4.559911319644449179, 2.230352010821504471, -9.422509992056141925 ) ) ;
#93020=CARTESIAN_POINT ( 'NONE',  ( 0.6076426042653030324, 42.37576471608601025, -6.499999999999984901 ) ) ;
#93021=CARTESIAN_POINT ( 'NONE',  ( 0.1532563361054082862, 6.217264484334118713, 2.638427012816831674 ) ) ;
#93022=CARTESIAN_POINT ( 'NONE',  ( 19.84674366389459266, 3.300597817667451750, 2.638427012816836559 ) ) ;
#93025=CARTESIAN_POINT ( 'NONE',  ( 19.84674366389459266, 8.717264484334116048, -2.638427012816827677 ) ) ;
#93028=CARTESIAN_POINT ( 'NONE',  ( 0.1532563361054083140, 36.00893115100078745, 1.131784320476157264E-15 ) ) ;
#93032=CARTESIAN_POINT ( 'NONE',  ( 24.16423886937409904, 9.095415501580633943, 3.795296366450317205 ) ) ;
#93035=CARTESIAN_POINT ( 'NONE',  ( -2.816281873526473856, 59.33196800326374643, 3.434112377981055619 ) ) ;
#93036=( GEOMETRIC_REPRESENTATION_CONTEXT ( 3 ) GLOBAL_UNCERTAINTY_ASSIGNED_CONTEXT ( ( #34487 ) ) GLOBAL_UNIT_ASSIGNED_CONTEXT ( ( #88319, #73310, #73799 ) ) REPRESENTATION_CONTEXT ( 'NONE', 'WORKASPACE' ) );
#93037=CARTESIAN_POINT ( 'NONE',  ( 17.08211943468705840, 10.13708216824730179, -12.26659068614894466 ) ) ;
#93038=CARTESIAN_POINT ( 'NONE',  ( 22.26659068614894466, 18.88708216824730002, 7.082119434687054849 ) ) ;
#93041=CARTESIAN_POINT ( 'NONE',  ( 7.084665262690076126, 19.10535201082150181, 10.88017736071109987 ) ) ;
#93045=CARTESIAN_POINT ( 'NONE',  ( 7.361572987183170547, 2.050597817667451750, 9.846743663894590881 ) ) ;
#93046=CARTESIAN_POINT ( 'NONE',  ( 3.591859063236761518, 29.95696800326375708, 11.09922568453594849 ) ) ;
#93047=CARTESIAN_POINT ( 'NONE',  ( 12.63842701281683922, 39.55059781766744464, -9.846743663894590881 ) ) ;
#93048=CARTESIAN_POINT ( 'NONE',  ( 6.565887622018943937, 20.16530133659708213, 12.81628187352647430 ) ) ;
#93050=CARTESIAN_POINT ( 'NONE',  ( 0.1532563361054082862, 31.21726448433412315, 2.638427012816831674 ) ) ;
#93051=CARTESIAN_POINT ( 'NONE',  ( 5.076628168052703671, 11.84226448433411960, 8.527530157486179263 ) ) ;
#93054=CARTESIAN_POINT ( 'NONE',  ( 7.084665262690076126, 32.02201867748816966, -10.88017736071110164 ) ) ;
#93055=CARTESIAN_POINT ( 'NONE',  ( -2.266590686148945544, 27.22041550158063572, 7.082119434687048631 ) ) ;
#93056=CARTESIAN_POINT ( 'NONE',  ( 19.84674366389459621, 43.50893115100078745, 7.409399052514197653E-17 ) ) ;
#93057=CARTESIAN_POINT ( 'NONE',  ( 19.84674366389459266, 3.717264484334118713, -2.638427012816827677 ) ) ;
#93058=CARTESIAN_POINT ( 'NONE',  ( 6.565887622018943937, 50.16530133659708213, 12.81628187352647430 ) ) ;
#93060=CARTESIAN_POINT ( 'NONE',  ( 0.5774900079438590739, 32.64701867748816966, -5.440088680355550821 ) ) ;
#93062=ADVANCED_FACE ( 'NONE', ( #40578 ), #48053, .F. ) ;
#93063=CARTESIAN_POINT ( 'NONE',  ( -1.099225684535947600, 19.54030133659708568, 6.408140936763237150 ) ) ;
#93064=CARTESIAN_POINT ( 'NONE',  ( 1.472469842513823179, 36.42559781766745175, 4.923371831947296329 ) ) ;
#93066=CARTESIAN_POINT ( 'NONE',  ( -1.099225684535947600, 43.70696800326375353, -6.408140936763238038 ) ) ;
#93068=CARTESIAN_POINT ( 'NONE',  ( 2.035157376598824452, 53.68868534415484817, 7.964842623401179544 ) ) ;
#93071=CARTESIAN_POINT ( 'NONE',  ( 13.99999999999999822, 60.50000000000000711, -5.000000000000000000 ) ) ;
#93072=DIRECTION ( 'NONE',  ( 1.000000000000000000, 0.000000000000000000, -0.000000000000000000 ) ) ;
#93073=( BOUNDED_SURFACE ( )  B_SPLINE_SURFACE ( 1, 2, ( 
 ( #21662, #7657, #38150, #16125, #23146, #76618, #53130, #67656, #77108, #52634, #60626, #82642, #15649, #44643, #59642, #90626, #54108, #75137, #29622, #165, #6643, #98166, #60128, #68636, #22151, #53619, #8136, #84621, #14662, #37650, #8621, #61603, #45128, #38629, #92117, #69130, #31109, #91127, #23648, #39130, #69617, #1139, #22650, #83638, #45631, #76130, #54597, #70113, #10591, #40106, #49079, #56587, #9603, #2133, #85110, #47606, #93587, #47097, #78595, #41103, #10107, #86102, #70607, #72070, #17612, #71101, #48579, #93092, #32593, #63088, #55607, #79078, #40604, #17124, #71599, #87077, #3111, #62587, #48082, #25125, #39624, #85609, #31601, #33565, #2627, #86593, #33081, #78100, #63578, #64061, #24623, #1638, #18102, #94573, #94088, #24128, #25607, #56100, #18586, #79582, #26091, #32089, #11082, #41602, #62096, #55089, #92604, #16621, #77595, #9110, #59036, #66039, #72549, #58538, #96568, #87564, #96066, #5063, #28043, #81048, #82032, #74032, #43058, #21051, #13042, #51542, #73537, #12555, #20557, #42086, #5563, #65542, #27548, #89045, #19565, #42560, #51042, #4082, #20051, #89540, #3595, #43538, #13542, #44026, #12059, #58042, #35548, #50553, #73044, #81535, #34054, #36039, #66542, #95566, #4579, #34545, #57063, #64550, #35041, #95057, #26566, #65040, #88550, #97070, #28543, #19074, #49552, #80064, #11569, #27055, #57553, #88052, #50061, #80565, #91999, #37039, #15538, #76509, #29509, #7035, #60515, #30503, #14045, #30009, #59530, #44527, #91007, #61005, #29021, #91516, #23033, #90512, #67538, #84510, #37541, #30995, #53505, #23530, #84016, #54002, #7543, #46021, #36548, #38034, #52037, #68031, #52522, #53009, #75026, #61493, #60017, #98558, #6531, #75519, #22538, #68525, #83524, #16008, #56, #98053, #8023, #38520, #90025, #15042, #76014, #69018, #45514, #74529, #549, #6050, #67038, #97560, #21546, #82529, #22047, #83028, #14545, #45015, #9486, #70492, #9990, #62472, #85492, #70989, #46986, #62972, #2995, #46497, #86482, #33445, #86954, #54971, #2012, #47965, #93477, #17001, #17500, #76997, #17980, #78474, #39508, #47480, #77480, #1022, #63940, #77980, #8509, #39012, #84994, #32477, #39989, #48464, #69506, #63468, #25003, #78961, #69998, #94452, #55488, #85988, #54483, #25968, #8991, #10473, #40982, #1524, #40491, #2511, #32963, #16509, #93970, #31482, #31970, #25494, #55981, #61986, #71479, #56468, #92978, #24509, #92485, #24013, #73917, #96447, #66416, #65918, #96947, #50427, #73416, #79461, #80934, #94943, #11942, #95448, #80445, #26444, #72432, #18467, #20435, #19447, #4943, #42447, #3958, #95946, #27918 ),
 ( #43417, #72930, #12428, #34428, #57439, #42935, #18960, #34925, #5446, #48952, #58410, #35917, #58916, #26939, #4459, #19932, #65423, #87930, #88433, #10959, #88926, #35423, #11449, #49939, #49439, #71951, #28420, #27429, #41483, #3473, #56943, #57923, #50923, #81419, #33930, #12920, #64435, #87446, #41966, #79943, #64920, #37422, #97432, #7904, #51916, #30381, #91383, #44403, #21923, #75392, #45388, #28897, #44889, #74402, #59402, #6911, #75894, #43902, #7419, #37916, #6404, #82400, #429, #52402, #45902, #68404, #38398, #98924, #68900, #22414, #60884, #51418, #52888, #66912, #82903, #67407, #14420, #89906, #74904, #89415, #22913, #90386, #53380, #67909, #36915, #98432, #83891, #13925, #21421, #15420, #76389, #29888, #81907, #90887, #97937, #30879, #20929, #60390, #29393, #13417, #59895, #83400, #14920, #5927, #36419, #93352, #16878, #17857, #24877, #31365, #17377, #55360, #46383, #54852, #62856, #85864, #39868, #40856, #32840, #1893, #78848, #70871, #10357, #32351, #70376, #78350, #904, #63342, #24385, #47353, #47846, #77855, #69879, #9871, #61375, #2387, #40370, #54364, #1399, #61865, #15895, #71361, #31854, #2878, #91884, #92370, #9365, #62353, #93848, #84396, #25375, #55860, #86356, #84874, #48343, #23406, #53890, #69381, #76869, #23896, #8385, #38895, #16382, #92856, #46866, #77358, #8868, #39385, #85365, #71837, #20691, #89670, #86847, #51683, #21183, #50692, #94826, #44662, #66171, #90153, #13675, #82662, #82162, #14178, #66680, #44158, #94336, #97204, #10848, #28183, #12685, #96705, #41369, #87325, #33328, #36681, #35687, #74667, #58679, #18842, #13179, #6177, #26329, #3345, #67169, #97694, #89178, #25853, #36179, #81185, #21683, #75156, #43673, #33808, #52168, #43184, #51183, #64314, #81666, #74160, #28673, #5694, #63822, #59165, #56828, #29157, #59662, #18351, #56350, #48828, #79338, #73671, #5201, #77127, #46149, #24144, #16141, #54612, #76635, #15666, #23664, #45150, #8637, #68653, #30630, #69150, #22670, #45653, #31126, #7166, #23165, #62111, #6667, #46627, #92621, #47114, #15172, #37669, #1160, #37185, #75656, #8154, #98186, #60150, #68169, #84160, #67676, #676, #54126, #31621, #98688, #83656, #85130, #39146, #30137, #38647, #69636, #61622, #92140, #7674, #84638, #16641, #29643, #90647, #60644, #22172, #52654, #83157, #14681, #91144, #53148, #76149, #38166, #182, #61139, #91647, #53643, #93608, #40620, #93110, #25622, #87092, #56114, #33100, #17630, #19090, #63594, #18119, #94591, #40123, #86119, #10123, #2646, #26107, #86611, #63105, #56601, #34072, #18603, #9624, #94100, #48102, #10609, #48593, #71612 ) ),
 .UNSPECIFIED., .F., .F., .T. ) 
 B_SPLINE_SURFACE_WITH_KNOTS ( ( 2, 2 ),
 ( 3, 2, 2, 2, 2, 2, 2, 2, 2, 2, 2, 2, 2, 2, 2, 2, 2, 2, 2, 2, 2, 2, 2, 2, 2, 2, 2, 2, 2, 2, 2, 2, 2, 2, 2, 2, 2, 2, 2, 2, 2, 2, 2, 2, 2, 2, 2, 2, 2, 2, 2, 2, 2, 2, 2, 2, 2, 2, 2, 2, 2, 2, 2, 2, 2, 2, 2, 2, 2, 2, 2, 2, 2, 2, 2, 2, 2, 2, 2, 2, 2, 2, 2, 2, 2, 2, 2, 2, 2, 2, 2, 2, 2, 2, 2, 2, 2, 2, 2, 2, 2, 2, 2, 2, 2, 2, 2, 2, 2, 2, 2, 2, 2, 2, 2, 2, 2, 2, 2, 2, 2, 2, 2, 2, 2, 2, 2, 2, 2, 2, 2, 2, 2, 2, 2, 2, 2, 2, 2, 2, 2, 2, 2, 2, 2, 2, 2, 2, 2, 2, 2, 2, 2, 2, 2, 2, 2, 2, 2, 2, 2, 2, 3 ),
 ( 0.000000000000000000, 1.000000000000000000 ),
 ( 0.000000000000000000, 0.005952380952380952051, 0.01190476190476190410, 0.01785714285714285615, 0.02380952380952380820, 0.02976190476190476025, 0.03571428571428571230, 0.04166666666666666435, 0.04761904761904761640, 0.05357142857142856845, 0.05952380952380952051, 0.06547619047619047949, 0.07142857142857142461, 0.07738095238095238360, 0.08333333333333332871, 0.08928571428571428770, 0.09523809523809523281, 0.1011904761904761918, 0.1071428571428571369, 0.1130952380952380959, 0.1190476190476190410, 0.1250000000000000000, 0.1309523809523809590, 0.1369047619047619180, 0.1428571428571428492, 0.1488095238095238082, 0.1547619047619047672, 0.1607142857142857262, 0.1666666666666666574, 0.1726190476190476164, 0.1785714285714285754, 0.1845238095238095344, 0.1904761904761904656, 0.1964285714285714246, 0.2023809523809523836, 0.2083333333333333426, 0.2142857142857142738, 0.2202380952380952328, 0.2261904761904761918, 0.2321428571428571508, 0.2380952380952380820, 0.2440476190476190410, 0.2500000000000000000, 0.2559523809523809312, 0.2619047619047619180, 0.2678571428571428492, 0.2738095238095238360, 0.2797619047619047672, 0.2857142857142856984, 0.2916666666666666852, 0.2976190476190476164, 0.3035714285714285476, 0.3095238095238095344, 0.3154761904761904656, 0.3214285714285714524, 0.3273809523809523836, 0.3333333333333333148, 0.3392857142857143016, 0.3452380952380952328, 0.3511904761904761640, 0.3571428571428571508, 0.3630952380952380820, 0.3690476190476190688, 0.3750000000000000000, 0.3809523809523809312, 0.3869047619047619180, 0.3928571428571428492, 0.3988095238095238360, 0.4047619047619047672, 0.4107142857142856984, 0.4166666666666666852, 0.4226190476190476164, 0.4285714285714285476, 0.4345238095238095344, 0.4404761904761904656, 0.4464285714285714524, 0.4523809523809523836, 0.4583333333333333148, 0.4642857142857143016, 0.4702380952380952328, 0.4761904761904761640, 0.4821428571428571508, 0.4880952380952380820, 0.4940476190476190688, 0.5000000000000000000, 0.5059523809523809312, 0.5119047619047618625, 0.5178571428571429047, 0.5238095238095238360, 0.5297619047619047672, 0.5357142857142856984, 0.5416666666666666297, 0.5476190476190476719, 0.5535714285714286031, 0.5595238095238095344, 0.5654761904761904656, 0.5714285714285713969, 0.5773809523809523281, 0.5833333333333333703, 0.5892857142857143016, 0.5952380952380952328, 0.6011904761904761640, 0.6071428571428570953, 0.6130952380952381375, 0.6190476190476190688, 0.6250000000000000000, 0.6309523809523809312, 0.6369047619047618625, 0.6428571428571429047, 0.6488095238095238360, 0.6547619047619047672, 0.6607142857142856984, 0.6666666666666666297, 0.6726190476190476719, 0.6785714285714286031, 0.6845238095238095344, 0.6904761904761904656, 0.6964285714285713969, 0.7023809523809523281, 0.7083333333333333703, 0.7142857142857143016, 0.7202380952380952328, 0.7261904761904761640, 0.7321428571428570953, 0.7380952380952381375, 0.7440476190476190688, 0.7500000000000000000, 0.7559523809523809312, 0.7619047619047618625, 0.7678571428571429047, 0.7738095238095238360, 0.7797619047619047672, 0.7857142857142856984, 0.7916666666666666297, 0.7976190476190476719, 0.8035714285714286031, 0.8095238095238095344, 0.8154761904761904656, 0.8214285714285713969, 0.8273809523809523281, 0.8333333333333333703, 0.8392857142857143016, 0.8452380952380952328, 0.8511904761904761640, 0.8571428571428570953, 0.8630952380952381375, 0.8690476190476190688, 0.8750000000000000000, 0.8809523809523809312, 0.8869047619047618625, 0.8928571428571429047, 0.8988095238095238360, 0.9047619047619047672, 0.9107142857142856984, 0.9166666666666666297, 0.9226190476190476719, 0.9285714285714286031, 0.9345238095238095344, 0.9404761904761904656, 0.9464285714285713969, 0.9523809523809523281, 0.9583333333333333703, 0.9642857142857143016 ),
 .UNSPECIFIED. ) 
 GEOMETRIC_REPRESENTATION_ITEM ( )  RATIONAL_B_SPLINE_SURFACE ( (
 ( 1.000000000000000000, 0.9659258262890683122, 1.000000000000000000, 0.9659258262890683122, 1.000000000000000000, 0.9659258262890683122, 1.000000000000000000, 0.9659258262890683122, 1.000000000000000000, 0.9659258262890683122, 1.000000000000000000, 0.9659258262890683122, 1.000000000000000000, 0.9659258262890683122, 1.000000000000000000, 0.9659258262890683122, 1.000000000000000000, 0.9659258262890683122, 1.000000000000000000, 0.9659258262890683122, 1.000000000000000000, 0.9659258262890683122, 1.000000000000000000, 0.9659258262890683122, 1.000000000000000000, 0.9659258262890683122, 1.000000000000000000, 0.9659258262890683122, 1.000000000000000000, 0.9659258262890683122, 1.000000000000000000, 0.9659258262890683122, 1.000000000000000000, 0.9659258262890683122, 1.000000000000000000, 0.9659258262890683122, 1.000000000000000000, 0.9659258262890683122, 1.000000000000000000, 0.9659258262890683122, 1.000000000000000000, 0.9659258262890683122, 1.000000000000000000, 0.9659258262890683122, 1.000000000000000000, 0.9659258262890683122, 1.000000000000000000, 0.9659258262890683122, 1.000000000000000000, 0.9659258262890683122, 1.000000000000000000, 0.9659258262890683122, 1.000000000000000000, 0.9659258262890683122, 1.000000000000000000, 0.9659258262890683122, 1.000000000000000000, 0.9659258262890683122, 1.000000000000000000, 0.9659258262890683122, 1.000000000000000000, 0.9659258262890683122, 1.000000000000000000, 0.9659258262890683122, 1.000000000000000000, 0.9659258262890683122, 1.000000000000000000, 0.9659258262890683122, 1.000000000000000000, 0.9659258262890683122, 1.000000000000000000, 0.9659258262890683122, 1.000000000000000000, 0.9659258262890683122, 1.000000000000000000, 0.9659258262890683122, 1.000000000000000000, 0.9659258262890683122, 1.000000000000000000, 0.9659258262890683122, 1.000000000000000000, 0.9659258262890683122, 1.000000000000000000, 0.9659258262890683122, 1.000000000000000000, 0.9659258262890683122, 1.000000000000000000, 0.9659258262890683122, 1.000000000000000000, 0.9659258262890683122, 1.000000000000000000, 0.9659258262890683122, 1.000000000000000000, 0.9659258262890683122, 1.000000000000000000, 0.9659258262890683122, 1.000000000000000000, 0.9659258262890683122, 1.000000000000000000, 0.9659258262890683122, 1.000000000000000000, 0.9659258262890683122, 1.000000000000000000, 0.9659258262890683122, 1.000000000000000000, 0.9659258262890683122, 1.000000000000000000, 0.9659258262890683122, 1.000000000000000000, 0.9659258262890683122, 1.000000000000000000, 0.9659258262890683122, 1.000000000000000000, 0.9659258262890683122, 1.000000000000000000, 0.9659258262890683122, 1.000000000000000000, 0.9659258262890683122, 1.000000000000000000, 0.9659258262890683122, 1.000000000000000000, 0.9659258262890683122, 1.000000000000000000, 0.9659258262890683122, 1.000000000000000000, 0.9659258262890683122, 1.000000000000000000, 0.9659258262890683122, 1.000000000000000000, 0.9659258262890683122, 1.000000000000000000, 0.9659258262890683122, 1.000000000000000000, 0.9659258262890683122, 1.000000000000000000, 0.9659258262890683122, 1.000000000000000000, 0.9659258262890683122, 1.000000000000000000, 0.9659258262890683122, 1.000000000000000000, 0.9659258262890683122, 1.000000000000000000, 0.9659258262890683122, 1.000000000000000000, 0.9659258262890683122, 1.000000000000000000, 0.9659258262890683122, 1.000000000000000000, 0.9659258262890683122, 1.000000000000000000, 0.9659258262890683122, 1.000000000000000000, 0.9659258262890683122, 1.000000000000000000, 0.9659258262890683122, 1.000000000000000000, 0.9659258262890683122, 1.000000000000000000, 0.9659258262890683122, 1.000000000000000000, 0.9659258262890683122, 1.000000000000000000, 0.9659258262890683122, 1.000000000000000000, 0.9659258262890683122, 1.000000000000000000, 0.9659258262890683122, 1.000000000000000000, 0.9659258262890683122, 1.000000000000000000, 0.9659258262890683122, 1.000000000000000000, 0.9659258262890683122, 1.000000000000000000, 0.9659258262890683122, 1.000000000000000000, 0.9659258262890683122, 1.000000000000000000, 0.9659258262890683122, 1.000000000000000000, 0.9659258262890683122, 1.000000000000000000, 0.9659258262890683122, 1.000000000000000000, 0.9659258262890683122, 1.000000000000000000, 0.9659258262890683122, 1.000000000000000000, 0.9659258262890683122, 1.000000000000000000, 0.9659258262890683122, 1.000000000000000000, 0.9659258262890683122, 1.000000000000000000, 0.9659258262890683122, 1.000000000000000000, 0.9659258262890683122, 1.000000000000000000, 0.9659258262890683122, 1.000000000000000000, 0.9659258262890683122, 1.000000000000000000, 0.9659258262890683122, 1.000000000000000000, 0.9659258262890683122, 1.000000000000000000, 0.9659258262890683122, 1.000000000000000000, 0.9659258262890683122, 1.000000000000000000, 0.9659258262890683122, 1.000000000000000000, 0.9659258262890683122, 1.000000000000000000, 0.9659258262890683122, 1.000000000000000000, 0.9659258262890683122, 1.000000000000000000, 0.9659258262890683122, 1.000000000000000000, 0.9659258262890683122, 1.000000000000000000, 0.9659258262890683122, 1.000000000000000000, 0.9659258262890683122, 1.000000000000000000, 0.9659258262890683122, 1.000000000000000000, 0.9659258262890683122, 1.000000000000000000, 0.9659258262890683122, 1.000000000000000000, 0.9659258262890683122, 1.000000000000000000, 0.9659258262890683122, 1.000000000000000000, 0.9659258262890683122, 1.000000000000000000, 0.9659258262890683122, 1.000000000000000000, 0.9659258262890683122, 1.000000000000000000, 0.9659258262890683122, 1.000000000000000000, 0.9659258262890683122, 1.000000000000000000, 0.9659258262890683122, 1.000000000000000000, 0.9659258262890683122, 1.000000000000000000, 0.9659258262890683122, 1.000000000000000000, 0.9659258262890683122, 1.000000000000000000, 0.9659258262890683122, 1.000000000000000000, 0.9659258262890683122, 1.000000000000000000, 0.9659258262890683122, 1.000000000000000000, 0.9659258262890683122, 1.000000000000000000, 0.9659258262890683122, 1.000000000000000000, 0.9659258262890683122, 1.000000000000000000, 0.9659258262890683122, 1.000000000000000000, 0.9659258262890683122, 1.000000000000000000, 0.9659258262890683122, 1.000000000000000000, 0.9659258262890683122, 1.000000000000000000, 0.9659258262890683122, 1.000000000000000000, 0.9659258262890683122, 1.000000000000000000, 0.9659258262890683122, 1.000000000000000000, 0.9659258262890683122, 1.000000000000000000, 0.9659258262890683122, 1.000000000000000000, 0.9659258262890683122, 1.000000000000000000, 0.9659258262890683122, 1.000000000000000000, 0.9659258262890683122, 1.000000000000000000, 0.9659258262890683122, 1.000000000000000000, 0.9659258262890683122, 1.000000000000000000, 0.9659258262890683122, 1.000000000000000000, 0.9659258262890683122, 1.000000000000000000, 0.9659258262890683122, 1.000000000000000000, 0.9659258262890683122, 1.000000000000000000, 0.9659258262890683122, 1.000000000000000000, 0.9659258262890683122, 1.000000000000000000, 0.9659258262890683122, 1.000000000000000000, 0.9659258262890683122, 1.000000000000000000, 0.9659258262890683122, 1.000000000000000000, 0.9659258262890683122, 1.000000000000000000, 0.9659258262890683122, 1.000000000000000000, 0.9659258262890683122, 1.000000000000000000, 0.9659258262890683122, 1.000000000000000000, 0.9659258262890683122, 1.000000000000000000, 0.9659258262890683122, 1.000000000000000000),
 ( 1.000000000000000000, 0.9659258262890683122, 1.000000000000000000, 0.9659258262890683122, 1.000000000000000000, 0.9659258262890683122, 1.000000000000000000, 0.9659258262890683122, 1.000000000000000000, 0.9659258262890683122, 1.000000000000000000, 0.9659258262890683122, 1.000000000000000000, 0.9659258262890683122, 1.000000000000000000, 0.9659258262890683122, 1.000000000000000000, 0.9659258262890683122, 1.000000000000000000, 0.9659258262890683122, 1.000000000000000000, 0.9659258262890683122, 1.000000000000000000, 0.9659258262890683122, 1.000000000000000000, 0.9659258262890683122, 1.000000000000000000, 0.9659258262890683122, 1.000000000000000000, 0.9659258262890683122, 1.000000000000000000, 0.9659258262890683122, 1.000000000000000000, 0.9659258262890683122, 1.000000000000000000, 0.9659258262890683122, 1.000000000000000000, 0.9659258262890683122, 1.000000000000000000, 0.9659258262890683122, 1.000000000000000000, 0.9659258262890683122, 1.000000000000000000, 0.9659258262890683122, 1.000000000000000000, 0.9659258262890683122, 1.000000000000000000, 0.9659258262890683122, 1.000000000000000000, 0.9659258262890683122, 1.000000000000000000, 0.9659258262890683122, 1.000000000000000000, 0.9659258262890683122, 1.000000000000000000, 0.9659258262890683122, 1.000000000000000000, 0.9659258262890683122, 1.000000000000000000, 0.9659258262890683122, 1.000000000000000000, 0.9659258262890683122, 1.000000000000000000, 0.9659258262890683122, 1.000000000000000000, 0.9659258262890683122, 1.000000000000000000, 0.9659258262890683122, 1.000000000000000000, 0.9659258262890683122, 1.000000000000000000, 0.9659258262890683122, 1.000000000000000000, 0.9659258262890683122, 1.000000000000000000, 0.9659258262890683122, 1.000000000000000000, 0.9659258262890683122, 1.000000000000000000, 0.9659258262890683122, 1.000000000000000000, 0.9659258262890683122, 1.000000000000000000, 0.9659258262890683122, 1.000000000000000000, 0.9659258262890683122, 1.000000000000000000, 0.9659258262890683122, 1.000000000000000000, 0.9659258262890683122, 1.000000000000000000, 0.9659258262890683122, 1.000000000000000000, 0.9659258262890683122, 1.000000000000000000, 0.9659258262890683122, 1.000000000000000000, 0.9659258262890683122, 1.000000000000000000, 0.9659258262890683122, 1.000000000000000000, 0.9659258262890683122, 1.000000000000000000, 0.9659258262890683122, 1.000000000000000000, 0.9659258262890683122, 1.000000000000000000, 0.9659258262890683122, 1.000000000000000000, 0.9659258262890683122, 1.000000000000000000, 0.9659258262890683122, 1.000000000000000000, 0.9659258262890683122, 1.000000000000000000, 0.9659258262890683122, 1.000000000000000000, 0.9659258262890683122, 1.000000000000000000, 0.9659258262890683122, 1.000000000000000000, 0.9659258262890683122, 1.000000000000000000, 0.9659258262890683122, 1.000000000000000000, 0.9659258262890683122, 1.000000000000000000, 0.9659258262890683122, 1.000000000000000000, 0.9659258262890683122, 1.000000000000000000, 0.9659258262890683122, 1.000000000000000000, 0.9659258262890683122, 1.000000000000000000, 0.9659258262890683122, 1.000000000000000000, 0.9659258262890683122, 1.000000000000000000, 0.9659258262890683122, 1.000000000000000000, 0.9659258262890683122, 1.000000000000000000, 0.9659258262890683122, 1.000000000000000000, 0.9659258262890683122, 1.000000000000000000, 0.9659258262890683122, 1.000000000000000000, 0.9659258262890683122, 1.000000000000000000, 0.9659258262890683122, 1.000000000000000000, 0.9659258262890683122, 1.000000000000000000, 0.9659258262890683122, 1.000000000000000000, 0.9659258262890683122, 1.000000000000000000, 0.9659258262890683122, 1.000000000000000000, 0.9659258262890683122, 1.000000000000000000, 0.9659258262890683122, 1.000000000000000000, 0.9659258262890683122, 1.000000000000000000, 0.9659258262890683122, 1.000000000000000000, 0.9659258262890683122, 1.000000000000000000, 0.9659258262890683122, 1.000000000000000000, 0.9659258262890683122, 1.000000000000000000, 0.9659258262890683122, 1.000000000000000000, 0.9659258262890683122, 1.000000000000000000, 0.9659258262890683122, 1.000000000000000000, 0.9659258262890683122, 1.000000000000000000, 0.9659258262890683122, 1.000000000000000000, 0.9659258262890683122, 1.000000000000000000, 0.9659258262890683122, 1.000000000000000000, 0.9659258262890683122, 1.000000000000000000, 0.9659258262890683122, 1.000000000000000000, 0.9659258262890683122, 1.000000000000000000, 0.9659258262890683122, 1.000000000000000000, 0.9659258262890683122, 1.000000000000000000, 0.9659258262890683122, 1.000000000000000000, 0.9659258262890683122, 1.000000000000000000, 0.9659258262890683122, 1.000000000000000000, 0.9659258262890683122, 1.000000000000000000, 0.9659258262890683122, 1.000000000000000000, 0.9659258262890683122, 1.000000000000000000, 0.9659258262890683122, 1.000000000000000000, 0.9659258262890683122, 1.000000000000000000, 0.9659258262890683122, 1.000000000000000000, 0.9659258262890683122, 1.000000000000000000, 0.9659258262890683122, 1.000000000000000000, 0.9659258262890683122, 1.000000000000000000, 0.9659258262890683122, 1.000000000000000000, 0.9659258262890683122, 1.000000000000000000, 0.9659258262890683122, 1.000000000000000000, 0.9659258262890683122, 1.000000000000000000, 0.9659258262890683122, 1.000000000000000000, 0.9659258262890683122, 1.000000000000000000, 0.9659258262890683122, 1.000000000000000000, 0.9659258262890683122, 1.000000000000000000, 0.9659258262890683122, 1.000000000000000000, 0.9659258262890683122, 1.000000000000000000, 0.9659258262890683122, 1.000000000000000000, 0.9659258262890683122, 1.000000000000000000, 0.9659258262890683122, 1.000000000000000000, 0.9659258262890683122, 1.000000000000000000, 0.9659258262890683122, 1.000000000000000000, 0.9659258262890683122, 1.000000000000000000, 0.9659258262890683122, 1.000000000000000000, 0.9659258262890683122, 1.000000000000000000, 0.9659258262890683122, 1.000000000000000000, 0.9659258262890683122, 1.000000000000000000, 0.9659258262890683122, 1.000000000000000000, 0.9659258262890683122, 1.000000000000000000, 0.9659258262890683122, 1.000000000000000000, 0.9659258262890683122, 1.000000000000000000, 0.9659258262890683122, 1.000000000000000000, 0.9659258262890683122, 1.000000000000000000, 0.9659258262890683122, 1.000000000000000000, 0.9659258262890683122, 1.000000000000000000, 0.9659258262890683122, 1.000000000000000000, 0.9659258262890683122, 1.000000000000000000, 0.9659258262890683122, 1.000000000000000000, 0.9659258262890683122, 1.000000000000000000, 0.9659258262890683122, 1.000000000000000000, 0.9659258262890683122, 1.000000000000000000, 0.9659258262890683122, 1.000000000000000000, 0.9659258262890683122, 1.000000000000000000, 0.9659258262890683122, 1.000000000000000000, 0.9659258262890683122, 1.000000000000000000, 0.9659258262890683122, 1.000000000000000000, 0.9659258262890683122, 1.000000000000000000, 0.9659258262890683122, 1.000000000000000000, 0.9659258262890683122, 1.000000000000000000, 0.9659258262890683122, 1.000000000000000000, 0.9659258262890683122, 1.000000000000000000, 0.9659258262890683122, 1.000000000000000000, 0.9659258262890683122, 1.000000000000000000, 0.9659258262890683122, 1.000000000000000000, 0.9659258262890683122, 1.000000000000000000, 0.9659258262890683122, 1.000000000000000000, 0.9659258262890683122, 1.000000000000000000, 0.9659258262890683122, 1.000000000000000000) ) ) 
 REPRESENTATION_ITEM ( '' )  SURFACE ( )  );
#93074=CARTESIAN_POINT ( 'NONE',  ( 2.035157376598824452, 48.68868534415483396, 7.964842623401179544 ) ) ;
#93075=CARTESIAN_POINT ( 'NONE',  ( 17.96484262340118221, 61.18868534415482685, -7.964842623401177768 ) ) ;
#93077=CARTESIAN_POINT ( 'NONE',  ( 17.96484262340118221, 6.188685344154837509, -7.964842623401177768 ) ) ;
#93078=CARTESIAN_POINT ( 'NONE',  ( 0.1532563361054083140, 46.00893115100079456, 1.131784320476157264E-15 ) ) ;
#93079=CARTESIAN_POINT ( 'NONE',  ( 15.44008868035555793, 21.39701867748817321, -9.422509992056140149 ) ) ;
#93080=CARTESIAN_POINT ( 'NONE',  ( 18.52753015748617571, 23.09226448433411960, 4.923371831947298993 ) ) ;
#93081=CARTESIAN_POINT ( 'NONE',  ( 10.00000000000000178, 20.37363466993042138, 12.81628187352647608 ) ) ;
#93082=ORIENTED_EDGE ( 'NONE', *, *, #16714, .F. ) ;
#93083=CARTESIAN_POINT ( 'NONE',  ( 10.00000000000000178, 44.31368534415484106, 10.88017736071110342 ) ) ;
#93084=CARTESIAN_POINT ( 'NONE',  ( 22.81628187352647785, 6.623634669930420493, 6.195893100308588602E-16 ) ) ;
#93085=DIRECTION ( 'NONE',  ( -0.000000000000000000, -0.000000000000000000, 1.000000000000000000 ) ) ;
#93086=CARTESIAN_POINT ( 'NONE',  ( 12.91533473730992121, 9.522018677488171434, 10.88017736071110164 ) ) ;
#93087=CARTESIAN_POINT ( 'NONE',  ( 17.96484262340118221, 44.93868534415483396, 7.964842623401181321 ) ) ;
#93088=CARTESIAN_POINT ( 'NONE',  ( 13.79529636645031943, 50.34541550158064638, -14.16423886937409904 ) ) ;
#93089=CARTESIAN_POINT ( 'NONE',  ( 18.52753015748618282, 38.92559781766745175, -4.923371831947291888 ) ) ;
#93090=CARTESIAN_POINT ( 'NONE',  ( 12.91533473730992121, 54.52201867748816255, 10.88017736071110164 ) ) ;
#93092=CARTESIAN_POINT ( 'NONE',  ( 24.16423886937410614, 14.51208216824730179, -3.795296366450302550 ) ) ;
#93093=UNCERTAINTY_MEASURE_WITH_UNIT (LENGTH_MEASURE( 1.000000000000000082E-05 ), #26035, 'distance_accuracy_value', 'NONE');
#93098=CARTESIAN_POINT ( 'NONE',  ( 20.36894250292379382, 38.67874883491396076, 10.36894250292379205 ) ) ;
#93099=CARTESIAN_POINT ( 'NONE',  ( -4.164238869374098151, 36.59541550158063217, -3.795296366450310543 ) ) ;
#93100=CARTESIAN_POINT ( 'NONE',  ( 2.035157376598822676, 67.43868534415484817, -7.964842623401177768 ) ) ;
#93101=CARTESIAN_POINT ( 'NONE',  ( 0.1532563361054083140, 56.00893115100078745, 1.131784320476157264E-15 ) ) ;
#93103=CARTESIAN_POINT ( 'NONE',  ( -0.8801773607111008646, 58.27201867748816966, 2.915334737309923430 ) ) ;
#93104=CARTESIAN_POINT ( 'NONE',  ( 16.40814093676324603, 27.45696800326375708, -11.09922568453594671 ) ) ;
#93105=CARTESIAN_POINT ( 'NONE',  ( 2.917880565312950480, 25.97041550158063572, -12.26659068614894821 ) ) ;
#93106=CARTESIAN_POINT ( 'NONE',  ( 12.91533473730992121, 24.52201867748816966, 10.88017736071110164 ) ) ;
#93110=CARTESIAN_POINT ( 'NONE',  ( 7.084665262690076126, 64.10535201082150536, 10.88017736071109987 ) ) ;
#93117=ORIENTED_EDGE ( 'NONE', *, *, #86594, .T. ) ;
#93118=CARTESIAN_POINT ( 'NONE',  ( -0.8801773607110991993, 7.855352010821506248, -2.915334737309923874 ) ) ;
#93119=CARTESIAN_POINT ( 'NONE',  ( 2.035157376598822676, 17.43868534415483751, -7.964842623401177768 ) ) ;
#93120=CARTESIAN_POINT ( 'NONE',  ( 0.1532563361054100626, 40.80059781766745886, -2.638427012816831230 ) ) ;
#93121=CARTESIAN_POINT ( 'NONE',  ( 19.84674366389459266, 58.71726448433411605, -2.638427012816827677 ) ) ;
#93125=ADVANCED_FACE ( 'NONE', ( #50525 ), #54031, .T. ) ;
#93126=CARTESIAN_POINT ( 'NONE',  ( 13.43411237798105340, 5.581968003263753531, 12.81628187352647963 ) ) ;
#93128=CARTESIAN_POINT ( 'NONE',  ( 17.08211943468705130, 43.47041550158063927, 12.26659068614894998 ) ) ;
#93130=CARTESIAN_POINT ( 'NONE',  ( -0.3689425029237898834, 46.17874883491397497, -10.36894250292378850 ) ) ;
#93132=CARTESIAN_POINT ( 'NONE',  ( 17.96484262340118221, 26.18868534415483396, -7.964842623401177768 ) ) ;
#93134=CARTESIAN_POINT ( 'NONE',  ( 10.00000000000000000, 36.81368534415484106, -10.88017736071110342 ) ) ;
#93135=CARTESIAN_POINT ( 'NONE',  ( 14.92337183194729633, 52.67559781766745175, 8.527530157486181039 ) ) ;
#93136=CARTESIAN_POINT ( 'NONE',  ( 20.88017736071110875, 35.77201867748816966, -2.915334737309920765 ) ) ;
#93137=CARTESIAN_POINT ( 'NONE',  ( 15.44008868035555793, 61.39701867748817676, -9.422509992056140149 ) ) ;
#93138=CARTESIAN_POINT ( 'NONE',  ( 4.559911319644449179, 33.89701867748817676, 9.422509992056141925 ) ) ;
#93144=CARTESIAN_POINT ( 'NONE',  ( 7.361572987183169658, 4.967264484334119601, -9.846743663894592657 ) ) ;
#93146=ORIENTED_EDGE ( 'NONE', *, *, #18270, .F. ) ;
#93148=CARTESIAN_POINT ( 'NONE',  ( 19.84674366389459266, 43.30059781766744464, 2.638427012816836559 ) ) ;
#93156=CARTESIAN_POINT ( 'NONE',  ( 14.92337183194729633, 47.67559781766745175, 8.527530157486181039 ) ) ;
#93157=CARTESIAN_POINT ( 'NONE',  ( 24.16423886937409904, 49.09541550158063217, 3.795296366450317205 ) ) ;
#93158=CARTESIAN_POINT ( 'NONE',  ( 10.00000000000000178, 57.25893115100078745, 9.846743663894594434 ) ) ;
#93160=CARTESIAN_POINT ( 'NONE',  ( 19.84674366389459621, 18.50893115100078745, 7.409399052514197653E-17 ) ) ;
#93161=CARTESIAN_POINT ( 'NONE',  ( 16.40814093676324603, 57.45696800326375353, -11.09922568453594671 ) ) ;
#93162=CARTESIAN_POINT ( 'NONE',  ( 0.1532563361054083140, 56.00893115100078745, 1.131784320476157264E-15 ) ) ;
#93163=CARTESIAN_POINT ( 'NONE',  ( -0.8801773607111009756, 58.06368534415484106, 1.068504757029289695E-15 ) ) ;
#93164=CARTESIAN_POINT ( 'NONE',  ( 19.39188664607694790, 30.83703382326399378, -6.499999999999962697 ) ) ;
#93166=ORIENTED_EDGE ( 'NONE', *, *, #78458, .T. ) ;
#93167=CARTESIAN_POINT ( 'NONE',  ( -4.164238869374099039, 66.80374883491396076, 8.674139862899312516E-16 ) ) ;
#93169=CARTESIAN_POINT ( 'NONE',  ( 10.00000000000000000, 26.81368534415484106, -10.88017736071110342 ) ) ;
#93170=CARTESIAN_POINT ( 'NONE',  ( 10.00000000000000000, 12.87363466993042138, -12.81628187352647608 ) ) ;
#93171=CARTESIAN_POINT ( 'NONE',  ( 2.035157376598822676, 57.43868534415484106, -7.964842623401177768 ) ) ;
#93172=CARTESIAN_POINT ( 'NONE',  ( -0.3289641300567998083, 63.07879003517447103, 5.963430220938281678 ) ) ;
#93175=CARTESIAN_POINT ( 'NONE',  ( 2.035157376598822676, 52.43868534415483396, -7.964842623401177768 ) ) ;
#93177=CARTESIAN_POINT ( 'NONE',  ( 1.472469842513823179, 35.59226448433412315, -4.923371831947296329 ) ) ;
#93178=CARTESIAN_POINT ( 'NONE',  ( 19.84674366389459621, 3.508931151000785231, 7.409399052514197653E-17 ) ) ;
#93180=CARTESIAN_POINT ( 'NONE',  ( 13.43411237798106583, 2.665301336597086568, -12.81628187352647252 ) ) ;
#93181=CARTESIAN_POINT ( 'NONE',  ( 0.5774900079438607392, 18.48035201082150536, 5.440088680355550821 ) ) ;
#93182=CARTESIAN_POINT ( 'NONE',  ( 1.932340009482190313, 66.49127512925448968, -6.500000000000079048 ) ) ;
#93183=CARTESIAN_POINT ( 'NONE',  ( -4.164238869374099039, 41.80374883491397497, 8.674139862899312516E-16 ) ) ;
#93185=CARTESIAN_POINT ( 'NONE',  ( 22.26659068614894466, 33.88708216824730357, 7.082119434687054849 ) ) ;
#93186=CARTESIAN_POINT ( 'NONE',  ( 0.5774900079438590739, 2.647018677488171434, -5.440088680355550821 ) ) ;
#93187=CARTESIAN_POINT ( 'NONE',  ( 12.63842701281683034, 17.46726448433411250, 9.846743663894596210 ) ) ;
#93188=CARTESIAN_POINT ( 'NONE',  ( 12.91533473730992121, 19.52201867748816611, 10.88017736071110164 ) ) ;
#93190=CARTESIAN_POINT ( 'NONE',  ( 14.92337183194729988, 44.34226448433412315, -8.527530157486177487 ) ) ;
#93191=CARTESIAN_POINT ( 'NONE',  ( 17.96484262340118221, 34.93868534415482685, 7.964842623401181321 ) ) ;
#93192=CARTESIAN_POINT ( 'NONE',  ( 2.791683348922240793, 61.63393115100079456, 7.208316651077764092 ) ) ;
#93193=CARTESIAN_POINT ( 'NONE',  ( 6.204703633549690345, 17.84541550158063217, 14.16423886937410082 ) ) ;
#93194=CARTESIAN_POINT ( 'NONE',  ( 1.959929470562281395, 60.51528370094807485, -5.767676674365853629 ) ) ;
#93196=UNCERTAINTY_MEASURE_WITH_UNIT (LENGTH_MEASURE( 1.000000000000000082E-05 ), #25423, 'distance_accuracy_value', 'NONE');
#93197=CARTESIAN_POINT ( 'NONE',  ( 7.361572987183169658, 9.967264484334119601, -9.846743663894592657 ) ) ;
#93198=CARTESIAN_POINT ( 'NONE',  ( 6.565887622018943937, 50.16530133659708213, 12.81628187352647430 ) ) ;
#93199=CARTESIAN_POINT ( 'NONE',  ( 17.20831665107776587, 54.13393115100079456, -7.208316651077762316 ) ) ;
#93203=CARTESIAN_POINT ( 'NONE',  ( 22.26659068614895176, 64.72041550158064638, -7.082119434687042414 ) ) ;
#93204=CARTESIAN_POINT ( 'NONE',  ( 15.44008868035555260, 54.73035201082150536, 9.422509992056143702 ) ) ;
#93205=CARTESIAN_POINT ( 'NONE',  ( 22.26659068614894466, 8.887082168247300018, 7.082119434687054849 ) ) ;
#93206=CARTESIAN_POINT ( 'NONE',  ( 17.96484262340118221, 61.18868534415482685, -7.964842623401177768 ) ) ;
#93207=CARTESIAN_POINT ( 'NONE',  ( 1.472469842513823179, 36.42559781766745175, 4.923371831947296329 ) ) ;
#93208=CARTESIAN_POINT ( 'NONE',  ( 7.084665262690076126, 14.10535201082150358, 10.88017736071109987 ) ) ;
#93210=CARTESIAN_POINT ( 'NONE',  ( 10.00000000000000000, 59.75893115100078745, -9.846743663894594434 ) ) ;
#93211=CARTESIAN_POINT ( 'NONE',  ( 5.076628168052703671, 1.842264484334118047, 8.527530157486179263 ) ) ;
#93218=CARTESIAN_POINT ( 'NONE',  ( 6.204703633549690345, 47.84541550158064638, 14.16423886937410082 ) ) ;
#93219=CARTESIAN_POINT ( 'NONE',  ( 0.1532563361054083140, 41.00893115100078745, 1.131784320476157264E-15 ) ) ;
#93220=CARTESIAN_POINT ( 'NONE',  ( 7.361572987183169658, 19.96726448433411960, -9.846743663894592657 ) ) ;
#93221=CARTESIAN_POINT ( 'NONE',  ( 0.1089645850229087609, 38.16234555792571115, 6.479102184480833415 ) ) ;
#93222=CARTESIAN_POINT ( 'NONE',  ( 10.00000000000000000, 16.81368534415483751, -10.88017736071110342 ) ) ;
#93223=CARTESIAN_POINT ( 'NONE',  ( 19.84674366389459621, 43.50893115100078745, 7.409399052514197653E-17 ) ) ;
#93225=CARTESIAN_POINT ( 'NONE',  ( 2.917880565312950480, 40.97041550158063217, -12.26659068614894821 ) ) ;
#93226=CARTESIAN_POINT ( 'NONE',  ( -4.164238869374099927, 57.01208216824731068, 3.795296366450308767 ) ) ;
#93227=CARTESIAN_POINT ( 'NONE',  ( 7.361572987183170547, 67.05059781766746596, 9.846743663894590881 ) ) ;
#93230=CARTESIAN_POINT ( 'NONE',  ( -0.8801773607111009756, 48.06368534415484817, 1.068504757029289695E-15 ) ) ;
#93231=CARTESIAN_POINT ( 'NONE',  ( 10.00000000000000000, 9.758931151000785675, -9.846743663894594434 ) ) ;
#93233=ORIENTED_EDGE ( 'NONE', *, *, #42484, .F. ) ;
#93234=CARTESIAN_POINT ( 'NONE',  ( 21.92686044187657046, 30.16212336850780673, 4.562052436263912550E-16 ) ) ;
#93236=CARTESIAN_POINT ( 'NONE',  ( 17.20831665107776587, 12.88393115100078390, 7.208316651077764980 ) ) ;
#93238=CARTESIAN_POINT ( 'NONE',  ( 24.16423886937409904, 24.09541550158063927, 3.795296366450317205 ) ) ;
#93239=CARTESIAN_POINT ( 'NONE',  ( 17.20831665107776587, 22.88393115100078745, 7.208316651077764980 ) ) ;
#93240=CARTESIAN_POINT ( 'NONE',  ( 10.00000000000000000, 46.81368534415484106, -10.88017736071110342 ) ) ;
#93243=ORIENTED_EDGE ( 'NONE', *, *, #82866, .F. ) ;
#93244=CARTESIAN_POINT ( 'NONE',  ( 12.91533473730992121, 44.52201867748816966, 10.88017736071110164 ) ) ;
#93245=CARTESIAN_POINT ( 'NONE',  ( 20.10239578412224759, 37.63377557478296609, -6.340343622311915617 ) ) ;
#93251=CARTESIAN_POINT ( 'NONE',  ( 10.00000000000000000, 46.81368534415484106, -10.88017736071110342 ) ) ;
#93252=CARTESIAN_POINT ( 'NONE',  ( 10.00000000000000000, 0.5537488349139675359, -14.16423886937410082 ) ) ;
#93255=CARTESIAN_POINT ( 'NONE',  ( 10.00000000000000178, 25.37363466993041783, 12.81628187352647608 ) ) ;
#93256=CARTESIAN_POINT ( 'NONE',  ( -2.266590686148945544, 1.387082168247301128, -7.082119434687050408 ) ) ;
#93257=CARTESIAN_POINT ( 'NONE',  ( 17.20831665107776587, 12.88393115100078390, 7.208316651077764980 ) ) ;
#93258=CARTESIAN_POINT ( 'NONE',  ( 15.44008868035555260, 4.730352010821504471, 9.422509992056143702 ) ) ;
#93259=CARTESIAN_POINT ( 'NONE',  ( -2.816281873526473856, 44.33196800326375353, 3.434112377981055619 ) ) ;
#93260=LINE ( 'NONE', #84784, #4855 ) ;
#93261=CARTESIAN_POINT ( 'NONE',  ( 7.361572987183169658, 9.967264484334119601, -9.846743663894592657 ) ) ;
#93262=CARTESIAN_POINT ( 'NONE',  ( 12.91533473730993009, 41.60535201082149825, -10.88017736071109987 ) ) ;
#93266=CARTESIAN_POINT ( 'NONE',  ( 1.711636803080571090, 46.84492782695772206, -6.500000000000077272 ) ) ;
#93267=CARTESIAN_POINT ( 'NONE',  ( 10.00000000000000000, 61.81368534415484106, -10.88017736071110342 ) ) ;
#93269=CARTESIAN_POINT ( 'NONE',  ( -1.099225684535947600, 63.70696800326376774, -6.408140936763238038 ) ) ;
#93270=CARTESIAN_POINT ( 'NONE',  ( 19.42250999205614548, 55.98035201082150536, -5.440088680355545492 ) ) ;
#93271=CARTESIAN_POINT ( 'NONE',  ( 16.40814093676323893, 10.79030133659708923, 11.09922568453595026 ) ) ;
#93274=CARTESIAN_POINT ( 'NONE',  ( 0.1532563361054083140, 26.00893115100078745, 1.131784320476157264E-15 ) ) ;
#93276=CARTESIAN_POINT ( 'NONE',  ( 13.79529636645030344, 8.262082168247300018, 14.16423886937410614 ) ) ;
#93277=CARTESIAN_POINT ( 'NONE',  ( 0.1532563361054082862, 16.21726448433411960, 2.638427012816831674 ) ) ;
#93278=CARTESIAN_POINT ( 'NONE',  ( 19.38216949554541202, 15.99863466993042138, 9.382169495545424454 ) ) ;
#93279=LINE ( 'NONE', #8315, #13090 ) ;
#93280=CARTESIAN_POINT ( 'NONE',  ( 20.88017736071110519, 45.56368534415484106, 2.639326808657452039E-16 ) ) ;
#93281=CARTESIAN_POINT ( 'NONE',  ( 5.076628168052703671, 66.84226448433412315, 8.527530157486179263 ) ) ;
#93282=CARTESIAN_POINT ( 'NONE',  ( -0.1503990784575247319, 32.22266099184917465, -6.262539305110083276 ) ) ;
#93283=CARTESIAN_POINT ( 'NONE',  ( 18.52753015748618282, 33.92559781766745886, -4.923371831947291888 ) ) ;
#93284=CARTESIAN_POINT ( 'NONE',  ( 10.00000000000000178, 22.25893115100078745, 9.846743663894594434 ) ) ;
#93285=CARTESIAN_POINT ( 'NONE',  ( 7.084665262690076126, 19.10535201082150181, 10.88017736071109987 ) ) ;
#93286=CARTESIAN_POINT ( 'NONE',  ( 16.40814093676323893, 10.79030133659708923, 11.09922568453595026 ) ) ;
#93287=CARTESIAN_POINT ( 'NONE',  ( 0.1532563361054082862, 26.21726448433411605, 2.638427012816831674 ) ) ;
#93290=CARTESIAN_POINT ( 'NONE',  ( 7.084665262690076126, 14.10535201082150358, 10.88017736071109987 ) ) ;
#93292=CARTESIAN_POINT ( 'NONE',  ( -0.8801773607111008646, 63.27201867748817676, 2.915334737309923430 ) ) ;
#93293=CARTESIAN_POINT ( 'NONE',  ( -0.2418659066527711621, 49.26028685723175471, -6.114288769123046308 ) ) ;
#93294=CARTESIAN_POINT ( 'NONE',  ( 2.791683348922237240, 45.38393115100079456, -7.208316651077763204 ) ) ;
#93295=CARTESIAN_POINT ( 'NONE',  ( 19.42250999205614548, 10.98035201082150536, -5.440088680355545492 ) ) ;
#93297=CARTESIAN_POINT ( 'NONE',  ( 0.5774900079438607392, 43.48035201082151247, 5.440088680355550821 ) ) ;
#93298=CARTESIAN_POINT ( 'NONE',  ( 20.88017736071110519, 15.56368534415483751, 2.639326808657452039E-16 ) ) ;
#93300=CARTESIAN_POINT ( 'NONE',  ( 10.00000000000000000, 14.75893115100078568, -9.846743663894594434 ) ) ;
#93301=CARTESIAN_POINT ( 'NONE',  ( 10.00000000000000178, 32.25893115100078745, 9.846743663894594434 ) ) ;
#93304=CARTESIAN_POINT ( 'NONE',  ( 18.52753015748618282, 63.92559781766745886, -4.923371831947291888 ) ) ;
#93305=CARTESIAN_POINT ( 'NONE',  ( -4.164238869374099927, 2.012082168247300906, 3.795296366450308767 ) ) ;
#93306=CARTESIAN_POINT ( 'NONE',  ( 24.16423886937410614, 29.30374883491396787, 8.672049930838204340E-16 ) ) ;
#93307=CARTESIAN_POINT ( 'NONE',  ( 14.92337183194729633, 32.67559781766745175, 8.527530157486181039 ) ) ;
#93310=CARTESIAN_POINT ( 'NONE',  ( 13.79529636645031943, 55.34541550158062506, -14.16423886937409904 ) ) ;
#93311=CARTESIAN_POINT ( 'NONE',  ( 17.20831665107776587, 22.88393115100078745, 7.208316651077764980 ) ) ;
#93314=CARTESIAN_POINT ( 'NONE',  ( 4.559911319644449179, 48.89701867748817676, 9.422509992056141925 ) ) ;
#93316=CARTESIAN_POINT ( 'NONE',  ( 20.88017736071110875, 20.77201867748816611, -2.915334737309920765 ) ) ;
#93317=CARTESIAN_POINT ( 'NONE',  ( -2.816281873526473856, 44.33196800326375353, 3.434112377981055619 ) ) ;
#93318=CARTESIAN_POINT ( 'NONE',  ( 13.43411237798106583, 17.66530133659708923, -12.81628187352647252 ) ) ;
#93320=CARTESIAN_POINT ( 'NONE',  ( 12.63842701281683034, 12.46726448433411782, 9.846743663894596210 ) ) ;
#93325=CARTESIAN_POINT ( 'NONE',  ( -2.266590686148945544, 51.38708216824730357, -7.082119434687050408 ) ) ;
#93326=CARTESIAN_POINT ( 'NONE',  ( 13.79529636645030344, 28.26208216824729647, 14.16423886937410614 ) ) ;
#93327=CARTESIAN_POINT ( 'NONE',  ( 0.5774900079438607392, 23.48035201082150536, 5.440088680355550821 ) ) ;
#93328=CARTESIAN_POINT ( 'NONE',  ( 15.44008868035555260, 54.73035201082150536, 9.422509992056143702 ) ) ;
#93329=PLANE ( 'NONE',  #62270 ) ;
#93331=CARTESIAN_POINT ( 'NONE',  ( 0.5774900079438590739, 67.64701867748817676, -5.440088680355550821 ) ) ;
#93332=SURFACE_SIDE_STYLE ('',( #78326 ) ) ;
#93333=CARTESIAN_POINT ( 'NONE',  ( 2.791683348922237240, 25.38393115100078390, -7.208316651077763204 ) ) ;
#93334=CARTESIAN_POINT ( 'NONE',  ( 2.148416515056627674, 62.23726573380440641, 6.499999999999959144 ) ) ;
#93336=CARTESIAN_POINT ( 'NONE',  ( 14.92337183194729633, 22.67559781766745175, 8.527530157486181039 ) ) ;
#93337=CARTESIAN_POINT ( 'NONE',  ( 0.1532563361054100626, 45.80059781766745886, -2.638427012816831230 ) ) ;
#93338=CARTESIAN_POINT ( 'NONE',  ( 10.00000000000000000, 11.81368534415483751, -10.88017736071110342 ) ) ;
#93340=CARTESIAN_POINT ( 'NONE',  ( -1.099225684535947600, 29.54030133659708923, 6.408140936763237150 ) ) ;
#93341=CARTESIAN_POINT ( 'NONE',  ( -0.8801773607111009756, 53.06368534415484106, 1.068504757029289695E-15 ) ) ;
#93342=CARTESIAN_POINT ( 'NONE',  ( 2.917880565312950480, 45.97041550158063927, -12.26659068614894821 ) ) ;
#93343=CARTESIAN_POINT ( 'NONE',  ( 5.076628168052704559, 10.17559781766745175, -8.527530157486179263 ) ) ;
#93344=CARTESIAN_POINT ( 'NONE',  ( 19.05914839598885635, 54.96693863883976405, 6.499999999999962697 ) ) ;
#93345=CARTESIAN_POINT ( 'NONE',  ( 0.1532563361054082862, 51.21726448433412315, 2.638427012816831674 ) ) ;
#93346=CARTESIAN_POINT ( 'NONE',  ( 18.52753015748617571, 38.09226448433412315, 4.923371831947298993 ) ) ;
#93347=CARTESIAN_POINT ( 'NONE',  ( 22.26659068614895176, 19.72041550158063572, -7.082119434687042414 ) ) ;
#93348=CARTESIAN_POINT ( 'NONE',  ( 10.00000000000000000, 34.75893115100078745, -9.846743663894594434 ) ) ;
#93349=CARTESIAN_POINT ( 'NONE',  ( 12.91533473730992121, 49.52201867748817676, 10.88017736071110164 ) ) ;
#93350=CARTESIAN_POINT ( 'NONE',  ( 19.42250999205614193, 10.14701867748816966, 5.440088680355555262 ) ) ;
#93351=CARTESIAN_POINT ( 'NONE',  ( 0.5774900079438607392, 43.48035201082151247, 5.440088680355550821 ) ) ;
#93352=CARTESIAN_POINT ( 'NONE',  ( 2.035157376598824452, 23.68868534415484461, 7.964842623401179544 ) ) ;
#93355=CARTESIAN_POINT ( 'NONE',  ( 20.88017736071110875, 35.77201867748816966, -2.915334737309920765 ) ) ;
#93357=CARTESIAN_POINT ( 'NONE',  ( 6.565887622018943937, 53.08196800326374643, -12.81628187352647608 ) ) ;
#93360=CARTESIAN_POINT ( 'NONE',  ( 17.96484262340118221, 56.18868534415484817, -7.964842623401177768 ) ) ;
#93362=CARTESIAN_POINT ( 'NONE',  ( 2.035157376598822676, 2.438685344154837953, -7.964842623401177768 ) ) ;
#93364=CARTESIAN_POINT ( 'NONE',  ( 24.16423886937409904, 54.09541550158063217, 3.795296366450317205 ) ) ;
#93365=CARTESIAN_POINT ( 'NONE',  ( 2.791683348922240793, 1.633931151000784565, 7.208316651077764092 ) ) ;
#93366=CARTESIAN_POINT ( 'NONE',  ( -2.266590686148945544, 7.220415501580634832, 7.082119434687048631 ) ) ;
#93367=EDGE_CURVE ( 'NONE', #26718, #74552, #74454, .T. ) ;
#93368=CARTESIAN_POINT ( 'NONE',  ( 19.84674366389459621, 3.508931151000785231, 7.409399052514197653E-17 ) ) ;
#93369=CARTESIAN_POINT ( 'NONE',  ( 7.084665262690076126, 14.10535201082150358, 10.88017736071109987 ) ) ;
#93370=CARTESIAN_POINT ( 'NONE',  ( 10.00000000000000000, 44.75893115100078745, -9.846743663894594434 ) ) ;
#93372=CARTESIAN_POINT ( 'NONE',  ( 12.63842701281683034, 52.46726448433413026, 9.846743663894596210 ) ) ;
#93374=( GEOMETRIC_REPRESENTATION_CONTEXT ( 3 ) GLOBAL_UNCERTAINTY_ASSIGNED_CONTEXT ( ( #18201 ) ) GLOBAL_UNIT_ASSIGNED_CONTEXT ( ( #30257, #90265, #28782 ) ) REPRESENTATION_CONTEXT ( 'NONE', 'WORKASPACE' ) );
#93375=CARTESIAN_POINT ( 'NONE',  ( 2.035157376598822676, 42.43868534415483396, -7.964842623401177768 ) ) ;
#93376=CARTESIAN_POINT ( 'NONE',  ( 19.84674366389459621, 53.50893115100078745, 7.409399052514197653E-17 ) ) ;
#93378=CARTESIAN_POINT ( 'NONE',  ( 0.5774900079438590739, 67.64701867748817676, -5.440088680355550821 ) ) ;
#93379=CARTESIAN_POINT ( 'NONE',  ( 12.91533473730993009, 46.60535201082150536, -10.88017736071109987 ) ) ;
#93380=CARTESIAN_POINT ( 'NONE',  ( 13.79529636645030344, 58.26208216824728936, 14.16423886937410614 ) ) ;
#93382=CARTESIAN_POINT ( 'NONE',  ( 6.565887622018943937, 28.08196800326375353, -12.81628187352647608 ) ) ;
#93384=B_SPLINE_CURVE_WITH_KNOTS ( 'NONE', 3,
 ( #18071, #48551, #79556, #81878 ),
 .UNSPECIFIED., .F., .F.,
 ( 4, 4 ),
 ( 0.000000000000000000, 0.002657014572710779919 ),
 .UNSPECIFIED. ) ;
#93387=CARTESIAN_POINT ( 'NONE',  ( 6.565887622018943937, 23.08196800326375708, -12.81628187352647608 ) ) ;
#93388=CARTESIAN_POINT ( 'NONE',  ( 17.96484262340118221, 14.93868534415483751, 7.964842623401181321 ) ) ;
#93391=CARTESIAN_POINT ( 'NONE',  ( 0.5774900079438607392, 68.48035201082150536, 5.440088680355550821 ) ) ;
#93392=CARTESIAN_POINT ( 'NONE',  ( 17.20831665107776587, 47.88393115100078745, 7.208316651077764980 ) ) ;
#93393=CARTESIAN_POINT ( 'NONE',  ( 1.472469842513823179, 16.42559781766745175, 4.923371831947296329 ) ) ;
#93394=CARTESIAN_POINT ( 'NONE',  ( 5.076628168052703671, 36.84226448433412315, 8.527530157486179263 ) ) ;
#93396=CARTESIAN_POINT ( 'NONE',  ( -0.1298530154764001854, 80.39370036920264795, 5.000000000000000000 ) ) ;
#93397=CARTESIAN_POINT ( 'NONE',  ( 0.1532563361054083140, 21.00893115100078745, 1.131784320476157264E-15 ) ) ;
#93400=CARTESIAN_POINT ( 'NONE',  ( 1.472469842513823179, 26.42559781766745175, 4.923371831947296329 ) ) ;
#93401=DIRECTION ( 'NONE',  ( -0.000000000000000000, 1.000000000000000000, -0.000000000000000000 ) ) ;
#93403=CARTESIAN_POINT ( 'NONE',  ( 7.361572987183170547, 42.05059781766745886, 9.846743663894590881 ) ) ;
#93406=CARTESIAN_POINT ( 'NONE',  ( -1.099225684535947600, 64.54030133659709634, 6.408140936763237150 ) ) ;
#93407=CARTESIAN_POINT ( 'NONE',  ( 20.15039907845753575, 7.627771745786129820, -6.262539305110077059 ) ) ;
#93408=CARTESIAN_POINT ( 'NONE',  ( -1.099225684535947600, 28.70696800326375353, -6.408140936763238038 ) ) ;
#93410=DIRECTION ( 'NONE',  ( 0.5547001962252290364, 0.8320502943378437211, 0.000000000000000000 ) ) ;
#93411=CARTESIAN_POINT ( 'NONE',  ( -2.266590686148945544, 42.22041550158063217, 7.082119434687048631 ) ) ;
#93412=CARTESIAN_POINT ( 'NONE',  ( 0.1532563361054083140, 16.00893115100078390, 1.131784320476157264E-15 ) ) ;
#93413=SURFACE_STYLE_USAGE ( .BOTH. , #48402 ) ;
#93414=CARTESIAN_POINT ( 'NONE',  ( 19.99999999999715072, 95.48020498407724688, 5.046714348925600113 ) ) ;
#93415=CARTESIAN_POINT ( 'NONE',  ( -0.3689425029237881626, 47.42874883491396787, 10.36894250292379027 ) ) ;
#93416=CARTESIAN_POINT ( 'NONE',  ( 5.076628168052703671, 56.84226448433412315, 8.527530157486179263 ) ) ;
#93417=CARTESIAN_POINT ( 'NONE',  ( 6.204703633549690345, 62.84541550158063927, 14.16423886937410082 ) ) ;
#93418=CARTESIAN_POINT ( 'NONE',  ( 13.79529636645030344, 18.26208216824730002, 14.16423886937410614 ) ) ;
#93419=CARTESIAN_POINT ( 'NONE',  ( -2.266590686148945544, 37.22041550158063217, 7.082119434687048631 ) ) ;
#93420=CARTESIAN_POINT ( 'NONE',  ( -45.10972591793716191, 105.3622991512831675, -4.928873526103649816 ) ) ;
#93423=CARTESIAN_POINT ( 'NONE',  ( 12.63842701281683034, 62.46726448433410894, 9.846743663894596210 ) ) ;
#93425=CARTESIAN_POINT ( 'NONE',  ( -0.8801773607111009756, 33.06368534415484106, 1.068504757029289695E-15 ) ) ;
#93427=( GEOMETRIC_REPRESENTATION_CONTEXT ( 3 ) GLOBAL_UNCERTAINTY_ASSIGNED_CONTEXT ( ( #36283 ) ) GLOBAL_UNIT_ASSIGNED_CONTEXT ( ( #16551, #2054, #63014 ) ) REPRESENTATION_CONTEXT ( 'NONE', 'WORKASPACE' ) );
#93428=CARTESIAN_POINT ( 'NONE',  ( 19.67858290521089160, 89.80068721897295347, -5.461713021790606248 ) ) ;
#93429=CARTESIAN_POINT ( 'NONE',  ( 14.92337183194729988, 34.34226448433411605, -8.527530157486177487 ) ) ;
#93432=CARTESIAN_POINT ( 'NONE',  ( 17.20831665107776587, 42.88393115100077324, 7.208316651077764980 ) ) ;
#93435=CARTESIAN_POINT ( 'NONE',  ( 17.08211943468705840, 10.13708216824730179, -12.26659068614894466 ) ) ;
#93436=FACE_OUTER_BOUND ( 'NONE', #88193, .T. ) ;
#93439=CARTESIAN_POINT ( 'NONE',  ( 10.00000000000000000, 11.81368534415483751, -10.88017736071110342 ) ) ;
#93440=CARTESIAN_POINT ( 'NONE',  ( 16.40814093676323893, 20.79030133659708923, 11.09922568453595026 ) ) ;
#93442=CARTESIAN_POINT ( 'NONE',  ( 2.035157376598824452, 68.68868534415484817, 7.964842623401179544 ) ) ;
#93443=CARTESIAN_POINT ( 'NONE',  ( -46.48928645636214441, 103.2957187381728232, -6.397878122523972699 ) ) ;
#93446=CARTESIAN_POINT ( 'NONE',  ( -2.266590686148945544, 66.38708216824730357, -7.082119434687050408 ) ) ;
#93448=CARTESIAN_POINT ( 'NONE',  ( 19.42250999205614193, 20.14701867748817321, 5.440088680355555262 ) ) ;
#93449=CARTESIAN_POINT ( 'NONE',  ( 7.084665262690076126, 34.10535201082151247, 10.88017736071109987 ) ) ;
#93450=CARTESIAN_POINT ( 'NONE',  ( 1.472469842513823179, 66.42559781766745175, 4.923371831947296329 ) ) ;
#93451=CARTESIAN_POINT ( 'NONE',  ( 12.63842701281683922, 59.55059781766744464, -9.846743663894590881 ) ) ;
#93452=CARTESIAN_POINT ( 'NONE',  ( 19.38216949554541557, 62.24863466993041072, -9.382169495545420901 ) ) ;
#93454=ORIENTED_EDGE ( 'NONE', *, *, #24581, .T. ) ;
#93456=CARTESIAN_POINT ( 'NONE',  ( 2.035157376598822676, 32.43868534415483396, -7.964842623401177768 ) ) ;
#93457=CARTESIAN_POINT ( 'NONE',  ( 22.81628187352647785, 36.62363466993041783, 6.195893100308588602E-16 ) ) ;
#93458=CARTESIAN_POINT ( 'NONE',  ( 0.000000000000000000, 74.63951520916478444, 5.933331309799314113 ) ) ;
#93459=UNCERTAINTY_MEASURE_WITH_UNIT (LENGTH_MEASURE( 1.000000000000000082E-05 ), #2289, 'distance_accuracy_value', 'NONE');
#93460=CARTESIAN_POINT ( 'NONE',  ( 12.63842701281683922, 59.55059781766744464, -9.846743663894590881 ) ) ;
#93461=CARTESIAN_POINT ( 'NONE',  ( 7.084665262690076126, 47.02201867748818387, -10.88017736071110164 ) ) ;
#93463=CARTESIAN_POINT ( 'NONE',  ( 12.63842701281683034, 7.467264484334118713, 9.846743663894596210 ) ) ;
#93464=CARTESIAN_POINT ( 'NONE',  ( 21.09922568453594849, 31.20696800326375353, 6.408140936763242479 ) ) ;
#93465=CARTESIAN_POINT ( 'NONE',  ( 4.559911319644449179, 62.23035201082150536, -9.422509992056141925 ) ) ;
#93467=CARTESIAN_POINT ( 'NONE',  ( -1.099225684535947600, 59.54030133659708923, 6.408140936763237150 ) ) ;
#93470=CARTESIAN_POINT ( 'NONE',  ( 0.2751277870542983006, 13.21833443783938122, 6.500000000000002665 ) ) ;
#93471=CARTESIAN_POINT ( 'NONE',  ( 0.5774900079438607392, 3.480352010821504027, 5.440088680355550821 ) ) ;
#93472=CARTESIAN_POINT ( 'NONE',  ( 6.565887622018943937, 45.16530133659708923, 12.81628187352647430 ) ) ;
#93473=CARTESIAN_POINT ( 'NONE',  ( 10.00000000000000178, 18.05374883491396787, 14.16423886937410082 ) ) ;
#93474=CARTESIAN_POINT ( 'NONE',  ( 19.84674366389459266, 13.71726448433411782, -2.638427012816827677 ) ) ;
#93475=CARTESIAN_POINT ( 'NONE',  ( 19.42250999205614548, 5.980352010821504471, -5.440088680355545492 ) ) ;
#93476=CARTESIAN_POINT ( 'NONE',  ( 19.84674366389459621, 18.50893115100078745, 7.409399052514197653E-17 ) ) ;
#93477=CARTESIAN_POINT ( 'NONE',  ( 17.08211943468705130, 53.47041550158063217, 12.26659068614894998 ) ) ;
#93480=CARTESIAN_POINT ( 'NONE',  ( 10.00000000000000000, 26.81368534415484106, -10.88017736071110342 ) ) ;
#93483=CARTESIAN_POINT ( 'NONE',  ( 20.88017736071110875, 15.77201867748817143, -2.915334737309920765 ) ) ;
#93484=CARTESIAN_POINT ( 'NONE',  ( 10.00000000000000000, 16.81368534415483751, -10.88017736071110342 ) ) ;
#93485=EDGE_CURVE ( 'NONE', #47944, #11778, #48679, .T. ) ;
#93486=CARTESIAN_POINT ( 'NONE',  ( 19.84674366389459266, 53.30059781766744464, 2.638427012816836559 ) ) ;
#93488=CARTESIAN_POINT ( 'NONE',  ( 19.38216949554541202, 55.99863466993041072, 9.382169495545424454 ) ) ;
#93490=FILL_AREA_STYLE ('',( #34815 ) ) ;
#93491=CARTESIAN_POINT ( 'NONE',  ( 24.16423886937410614, 19.30374883491397142, 8.672049930838204340E-16 ) ) ;
#93492=CARTESIAN_POINT ( 'NONE',  ( -0.8801773607111008646, 28.27201867748817321, 2.915334737309923430 ) ) ;
#93493=CARTESIAN_POINT ( 'NONE',  ( 15.44008868035555260, 9.730352010821505360, 9.422509992056143702 ) ) ;
#93494=CARTESIAN_POINT ( 'NONE',  ( 17.20831665107776587, 52.88393115100078035, 7.208316651077764980 ) ) ;
#93497=CARTESIAN_POINT ( 'NONE',  ( 19.84674366389459266, 38.71726448433412315, -2.638427012816827677 ) ) ;
#93498=CARTESIAN_POINT ( 'NONE',  ( 1.472469842513823179, 10.59226448433411782, -4.923371831947296329 ) ) ;
#93501=CARTESIAN_POINT ( 'NONE',  ( 15.44008868035555260, 4.730352010821504471, 9.422509992056143702 ) ) ;
#93502=CARTESIAN_POINT ( 'NONE',  ( 4.559911319644449179, 62.23035201082150536, -9.422509992056141925 ) ) ;
#93503=CARTESIAN_POINT ( 'NONE',  ( 0.6178305044545838731, 4.748634669930420493, 9.382169495545420901 ) ) ;
#93504=CARTESIAN_POINT ( 'NONE',  ( -0.8801773607111008646, 48.27201867748816966, 2.915334737309923430 ) ) ;
#93505=CARTESIAN_POINT ( 'NONE',  ( 19.38216949554541202, 40.99863466993042493, 9.382169495545424454 ) ) ;
#93506=CARTESIAN_POINT ( 'NONE',  ( 20.36894250292379738, 24.92874883491396787, -10.36894250292379027 ) ) ;
#93507=CIRCLE ( 'NONE', #44027, 0.5000000000000004441 ) ;
#93508=VECTOR ( 'NONE', #35764, 1000.000000000000000 ) ;
#93510=CARTESIAN_POINT ( 'NONE',  ( 3.591859063236761518, 64.95696800326376774, 11.09922568453594849 ) ) ;
#93512=CARTESIAN_POINT ( 'NONE',  ( 19.84674366389459266, 58.30059781766745886, 2.638427012816836559 ) ) ;
#93513=CARTESIAN_POINT ( 'NONE',  ( 15.44008868035555793, 16.39701867748817321, -9.422509992056140149 ) ) ;
#93516=CARTESIAN_POINT ( 'NONE',  ( 2.791683348922240793, 6.633931151000785675, 7.208316651077764092 ) ) ;
#93517=CARTESIAN_POINT ( 'NONE',  ( 19.84674366389459266, 13.71726448433411782, -2.638427012816827677 ) ) ;
#93518=CARTESIAN_POINT ( 'NONE',  ( 2.791683348922240793, 1.633931151000784565, 7.208316651077764092 ) ) ;
#93520=CARTESIAN_POINT ( 'NONE',  ( 19.42250999205614193, 55.14701867748817676, 5.440088680355555262 ) ) ;
#93522=CARTESIAN_POINT ( 'NONE',  ( 10.00000000000000178, 64.31368534415483396, 10.88017736071110342 ) ) ;
#93523=CARTESIAN_POINT ( 'NONE',  ( 18.52753015748617571, 8.092264484334117824, 4.923371831947298993 ) ) ;
#93525=CARTESIAN_POINT ( 'NONE',  ( 19.84674366389459266, 58.71726448433411605, -2.638427012816827677 ) ) ;
#93528=CARTESIAN_POINT ( 'NONE',  ( 6.204703633549690345, 10.76208216824729824, -14.16423886937410259 ) ) ;
#93529=CARTESIAN_POINT ( 'NONE',  ( 6.565887622018943937, 60.16530133659707502, 12.81628187352647430 ) ) ;
#93530=CARTESIAN_POINT ( 'NONE',  ( -4.164238869374099927, 17.01208216824730357, 3.795296366450308767 ) ) ;
#93531=B_SPLINE_CURVE_WITH_KNOTS ( 'NONE', 3,
 ( #14535, #75511, #68021, #2005, #47957, #26439, #62965, #32470, #33925, #10952 ),
 .UNSPECIFIED., .F., .F.,
 ( 4, 3, 3, 4 ),
 ( 8.182674270850422113E-18, 0.0006253016069560709969, 0.001250604074564918905, 0.002501455912506541333 ),
 .UNSPECIFIED. ) ;
#93532=CARTESIAN_POINT ( 'NONE',  ( -0.1023957841222446069, 45.13377557478297319, 6.340343622311912952 ) ) ;
#93534=CARTESIAN_POINT ( 'NONE',  ( 2.035157376598822676, 17.43868534415483751, -7.964842623401177768 ) ) ;
#93535=PLANE ( 'NONE',  #29155 ) ;
#93537=CARTESIAN_POINT ( 'NONE',  ( 10.00000000000000000, 9.758931151000785675, -9.846743663894594434 ) ) ;
#93538=CARTESIAN_POINT ( 'NONE',  ( 2.791683348922240793, 21.63393115100078745, 7.208316651077764092 ) ) ;
#93539=CARTESIAN_POINT ( 'NONE',  ( 16.40814093676324603, 27.45696800326375708, -11.09922568453594671 ) ) ;
#93540=CARTESIAN_POINT ( 'NONE',  ( 12.63842701281683034, 32.46726448433412315, 9.846743663894596210 ) ) ;
#93541=CARTESIAN_POINT ( 'NONE',  ( -19.19000000000001194, 93.50000000000000000, -9.500000000000000000 ) ) ;
#93542=CARTESIAN_POINT ( 'NONE',  ( 6.565887622018943937, 18.08196800326375708, -12.81628187352647608 ) ) ;
#93544=CARTESIAN_POINT ( 'NONE',  ( 10.00000000000000000, 24.75893115100078745, -9.846743663894594434 ) ) ;
#93545=AXIS2_PLACEMENT_3D ( 'NONE', #82727, #68242, #75721 ) ;
#93546=CARTESIAN_POINT ( 'NONE',  ( 5.076628168052703671, 6.842264484334118713, 8.527530157486179263 ) ) ;
#93549=CARTESIAN_POINT ( 'NONE',  ( 17.96484262340118221, 39.93868534415484106, 7.964842623401181321 ) ) ;
#93550=CARTESIAN_POINT ( 'NONE',  ( 20.36894250292379738, 29.92874883491396432, -10.36894250292379027 ) ) ;
#93551=CARTESIAN_POINT ( 'NONE',  ( 12.63842701281683034, 37.46726448433411605, 9.846743663894596210 ) ) ;
#93552=CARTESIAN_POINT ( 'NONE',  ( 19.84674366389459621, 18.50893115100078745, 7.409399052514197653E-17 ) ) ;
#93553=CARTESIAN_POINT ( 'NONE',  ( 21.09922568453595559, 57.04030133659708923, -6.408140936763230044 ) ) ;
#93555=CARTESIAN_POINT ( 'NONE',  ( -0.8801773607110991993, 27.85535201082150181, -2.915334737309923874 ) ) ;
#93557=CARTESIAN_POINT ( 'NONE',  ( 6.565887622018943937, 25.16530133659708213, 12.81628187352647430 ) ) ;
#93558=CARTESIAN_POINT ( 'NONE',  ( 7.361572987183169658, 44.96726448433412315, -9.846743663894592657 ) ) ;
#93560=CARTESIAN_POINT ( 'NONE',  ( 0.6178305044545818747, 48.49863466993042493, -9.382169495545419124 ) ) ;
#93562=CARTESIAN_POINT ( 'NONE',  ( 19.42250999205614193, 55.14701867748817676, 5.440088680355555262 ) ) ;
#93564=ADVANCED_FACE ( 'NONE', ( #42928 ), #73910, .T. ) ;
#93566=DIRECTION ( 'NONE',  ( 0.000000000000000000, -1.000000000000000000, 0.000000000000000000 ) ) ;
#93567=CARTESIAN_POINT ( 'NONE',  ( 20.88017736071110875, 55.77201867748816966, -2.915334737309920765 ) ) ;
#93568=CARTESIAN_POINT ( 'NONE',  ( 12.91533473730993009, 56.60535201082151247, -10.88017736071109987 ) ) ;
#93572=CARTESIAN_POINT ( 'NONE',  ( 15.44008868035555793, 11.39701867748817143, -9.422509992056140149 ) ) ;
#93573=CARTESIAN_POINT ( 'NONE',  ( 19.84674366389459266, 63.30059781766745886, 2.638427012816836559 ) ) ;
#93574=CARTESIAN_POINT ( 'NONE',  ( 15.44008868035555260, 24.73035201082150891, 9.422509992056143702 ) ) ;
#93577=CARTESIAN_POINT ( 'NONE',  ( 3.591859063236763294, 23.29030133659708568, -11.09922568453595026 ) ) ;
#93578=EDGE_LOOP ( 'NONE', ( #52299, #16342, #47720, #2064, #98782, #21071 ) ) ;
#93579=CARTESIAN_POINT ( 'NONE',  ( 7.084665262690076126, 57.02201867748817676, -10.88017736071110164 ) ) ;
#93580=CARTESIAN_POINT ( 'NONE',  ( 14.92337183194729633, 37.67559781766745175, 8.527530157486181039 ) ) ;
#93581=CARTESIAN_POINT ( 'NONE',  ( 0.6178305044545818747, 13.49863466993041783, -9.382169495545419124 ) ) ;
#93582=CARTESIAN_POINT ( 'NONE',  ( 12.91533473730993009, 11.60535201082150536, -10.88017736071109987 ) ) ;
#93583=CARTESIAN_POINT ( 'NONE',  ( 10.00000000000000178, 39.31368534415484106, 10.88017736071110342 ) ) ;
#93584=CARTESIAN_POINT ( 'NONE',  ( -4.164238869374099039, 51.80374883491396787, 8.674139862899312516E-16 ) ) ;
#93585=CARTESIAN_POINT ( 'NONE',  ( 17.20831665107776587, 34.13393115100078745, -7.208316651077762316 ) ) ;
#93586=CARTESIAN_POINT ( 'NONE',  ( 20.88017736071110875, 55.77201867748816966, -2.915334737309920765 ) ) ;
#93587=CARTESIAN_POINT ( 'NONE',  ( -2.266590686148945544, 12.22041550158063394, 7.082119434687048631 ) ) ;
#93590=CARTESIAN_POINT ( 'NONE',  ( 5.076628168052703671, 66.84226448433412315, 8.527530157486179263 ) ) ;
#93595=CARTESIAN_POINT ( 'NONE',  ( 24.16423886937410614, 34.30374883491396787, 8.672049930838204340E-16 ) ) ;
#93596=CARTESIAN_POINT ( 'NONE',  ( -0.3689425029237898834, 36.17874883491396787, -10.36894250292378850 ) ) ;
#93598=CARTESIAN_POINT ( 'NONE',  ( 17.20831665107776587, 14.13393115100078568, -7.208316651077762316 ) ) ;
#93599=CARTESIAN_POINT ( 'NONE',  ( 22.81628187352647785, 11.41530133659708390, 3.434112377981063169 ) ) ;
#93600=CARTESIAN_POINT ( 'NONE',  ( 12.63842701281683922, 64.55059781766745175, -9.846743663894590881 ) ) ;
#93601=DIRECTION ( 'NONE',  ( 0.000000000000000000, -1.000000000000000000, -0.000000000000000000 ) ) ;
#93602=CARTESIAN_POINT ( 'NONE',  ( 19.42250999205614548, 55.98035201082150536, -5.440088680355545492 ) ) ;
#93603=CARTESIAN_POINT ( 'NONE',  ( 22.81628187352647785, 36.62363466993041783, 6.195893100308588602E-16 ) ) ;
#93604=CARTESIAN_POINT ( 'NONE',  ( 24.16423886937410614, 29.30374883491396787, 8.672049930838204340E-16 ) ) ;
#93605=CARTESIAN_POINT ( 'NONE',  ( 19.42250999205614193, 25.14701867748817321, 5.440088680355555262 ) ) ;
#93606=MECHANICAL_DESIGN_GEOMETRIC_PRESENTATION_REPRESENTATION('',(#85624),#20151);
#93608=CARTESIAN_POINT ( 'NONE',  ( 2.035157376598824452, 63.68868534415484106, 7.964842623401179544 ) ) ;
#93610=ORIENTED_EDGE ( 'NONE', *, *, #84556, .F. ) ;
#93611=CARTESIAN_POINT ( 'NONE',  ( 10.00000000000000178, 70.00000000000000000, 0.000000000000000000 ) ) ;
#93612=VERTEX_POINT ( 'NONE', #5439 ) ;
#93615=CARTESIAN_POINT ( 'NONE',  ( 2.917880565312950480, 0.9704155015806342766, -12.26659068614894821 ) ) ;
#93616=CARTESIAN_POINT ( 'NONE',  ( 10.00000000000000000, 1.813685344154838175, -10.88017736071110342 ) ) ;
#93617=CARTESIAN_POINT ( 'NONE',  ( 0.5774900079438590739, 17.64701867748817321, -5.440088680355550821 ) ) ;
#93618=CARTESIAN_POINT ( 'NONE',  ( 17.20831665107776587, 32.88393115100078745, 7.208316651077764980 ) ) ;
#93619=CARTESIAN_POINT ( 'NONE',  ( 6.565887622018943937, 10.16530133659708746, 12.81628187352647430 ) ) ;
#93625=CARTESIAN_POINT ( 'NONE',  ( -1.099225684535947600, 9.540301336597087456, 6.408140936763237150 ) ) ;
#93627=CARTESIAN_POINT ( 'NONE',  ( 6.204703633549690345, 42.84541550158063217, 14.16423886937410082 ) ) ;
#93628=ORIENTED_EDGE ( 'NONE', *, *, #51264, .F. ) ;
#93629=CARTESIAN_POINT ( 'NONE',  ( 20.36894250292379738, 54.92874883491396076, -10.36894250292379027 ) ) ;
#93630=VERTEX_POINT ( 'NONE', #88921 ) ;
#93631=CARTESIAN_POINT ( 'NONE',  ( 19.42250999205614193, 40.14701867748817676, 5.440088680355555262 ) ) ;
#93632=CARTESIAN_POINT ( 'NONE',  ( -0.8801773607111008646, 38.27201867748816255, 2.915334737309923430 ) ) ;
#93634=CARTESIAN_POINT ( 'NONE',  ( 2.035157376598822676, 42.43868534415483396, -7.964842623401177768 ) ) ;
#93635=CARTESIAN_POINT ( 'NONE',  ( 13.99999999999999822, 11.00000000000000000, 5.000000000000000000 ) ) ;
#93636=CARTESIAN_POINT ( 'NONE',  ( 19.42250999205614548, 20.98035201082150891, -5.440088680355545492 ) ) ;
#93637=ADVANCED_FACE ( 'NONE', ( #35911 ), #84692, .T. ) ;
#93639=CARTESIAN_POINT ( 'NONE',  ( 0.1532563361054083140, 16.00893115100078390, 1.131784320476157264E-15 ) ) ;
#93641=ORIENTED_EDGE ( 'NONE', *, *, #9691, .T. ) ;
#93643=CARTESIAN_POINT ( 'NONE',  ( 2.791683348922237240, 40.38393115100078035, -7.208316651077763204 ) ) ;
#93646=VERTEX_POINT ( 'NONE', #44474 ) ;
#93647=DIRECTION ( 'NONE',  ( -1.000000000000000000, 0.000000000000000000, 0.000000000000000000 ) ) ;
#93649=CARTESIAN_POINT ( 'NONE',  ( 1.472469842513823179, 56.42559781766745886, 4.923371831947296329 ) ) ;
#93650=CARTESIAN_POINT ( 'NONE',  ( 22.26659068614895176, 49.72041550158063927, -7.082119434687042414 ) ) ;
#93651=CARTESIAN_POINT ( 'NONE',  ( 19.84674366389459266, 58.30059781766745886, 2.638427012816836559 ) ) ;
#93654=CARTESIAN_POINT ( 'NONE',  ( 1.472469842513823179, 15.59226448433411960, -4.923371831947296329 ) ) ;
#93655=CARTESIAN_POINT ( 'NONE',  ( 3.591859063236763294, 58.29030133659708923, -11.09922568453595026 ) ) ;
#93656=CARTESIAN_POINT ( 'NONE',  ( 5.076628168052704559, 60.17559781766745175, -8.527530157486179263 ) ) ;
#93657=CARTESIAN_POINT ( 'NONE',  ( 5.076628168052703671, 1.842264484334118047, 8.527530157486179263 ) ) ;
#93659=CARTESIAN_POINT ( 'NONE',  ( 18.52753015748618282, 48.92559781766745886, -4.923371831947291888 ) ) ;
#93660=( BOUNDED_SURFACE ( )  B_SPLINE_SURFACE ( 1, 2, ( 
 ( #39642, #70624, #79096, #70134, #1654, #32104, #24638, #55106, #85626, #17142, #47621, #78116, #2150, #32609, #25145, #55622, #88067, #28558, #58056, #67053, #74547, #27564, #20066, #72564, #65554, #12568, #65057, #96582, #59053, #28058, #5077, #88563, #90043, #35564, #89060, #66559, #12074, #20575, #73551, #50570, #59548, #73060, #80079, #4101, #6065, #19579, #81548, #35056, #50076, #51561, #4594, #57568, #89555, #58554, #5582, #36565, #97578, #29039, #34562, #95584, #49568, #36057, #97087, #81066, #11585, #51058, #13058, #42101, #43552, #21065, #43069, #80579, #27070, #42580, #66055, #96082, #74046, #82046, #13558, #44045, #16027, #52055, #90531, #61023, #14064, #75042, #60034, #75, #82548, #15555, #69034, #46515, #52538, #98576, #77016, #23548, #83045, #91535, #54020, #23050, #53523, #22556, #46039, #84034, #76524, #569, #22065, #69525, #1040, #92020, #44546, #14562, #31015, #30027, #39030, #8529, #60534, #91025, #6548, #37558, #83541, #37060, #68543, #61511, #30520, #76031, #53026, #62004, #7564, #8040, #38539, #45031, #15062, #45533, #38051, #84529, #31503, #7054, #21566, #67557, #98068, #75540, #29527, #68048, #25512, #47985, #86501, #40510, #71969, #85016, #40007, #78981, #25020, #47005, #54501, #62493, #24531, #17020, #70019, #25989, #93990, #1543, #18485, #3013, #62991, #63486, #2530, #10490, #31987, #94471, #55507, #17518, #55998, #9506, #32495, #17999, #92997, #10008, #48972, #92503, #33462, #79480, #33949, #2033, #78494, #48481, #71007, #93497, #41001, #24033, #63959, #71500, #85509, #86006, #54991, #77497, #10980, #32984, #16530, #9009, #47497, #56485, #86972, #41500, #39525, #3492, #78000, #70509, #57458, #51435, #42956, #12448, #72449, #81926, #26958, #5464, #66432, #19466, #95966, #50445, #20453, #3980, #19951, #49458, #34447, #80951, #50942, #18979, #81436, #12940, #80463, #87952, #74418, #27449, #20949, #43434, #13434, #73935, #43922, #96466, #35936, #26462, #27938, #41985, #57942, #42466, #88450, #64940, #49958, #64454, #96967, #65442, #28438, #73435, #11960, #4962, #58936, #72948, #95467, #89436, #5948, #35442, #56963, #65939, #4477, #94960, #87464, #58431, #34944, #79963, #88944, #11467, #74924, #82920, #67928, #52904, #37437, #15436, #83415, #44420, #75910, #14936, #89924, #75413, #22433, #45404, #29904, #7919, #60901, #90905, #45915, #98943, #76404, #7435, #91401, #37931, #68420, #14438, #30397, #22930, #53398, #83907, #6422, #38416, #68914, #36438, #59418, #36936, #66931, #44908, #97452, #28917, #6929, #98448, #13944, #60410, #21438, #67428, #51936, #82420, #97952, #29409, #59913, #90402, #21943 ),
 ( #52421, #36256, #44240, #96780, #35758, #43749, #65253, #28750, #88759, #50769, #89256, #42775, #65754, #51255, #27261, #43256, #82241, #26774, #66753, #13754, #67251, #35256, #81260, #28256, #73751, #96280, #58752, #57271, #97277, #20767, #19768, #27757, #57761, #80275, #74744, #58240, #87766, #19280, #95781, #12758, #20271, #59241, #49766, #74235, #5282, #89740, #50254, #6256, #66246, #81741, #34764, #36759, #88264, #21259, #51756, #80771, #13257, #5768, #11776, #12266, #42284, #72756, #73258, #4291, #4783, #91789, #54754, #37325, #68308, #31763, #67815, #7313, #76777, #29789, #90794, #75794, #15803, #98331, #31266, #84781, #62257, #98829, #15319, #92763, #39292, #30283, #60785, #23310, #76293, #69292, #53788, #61766, #84304, #16780, #60301, #83797, #23804, #68801, #22320, #52794, #37814, #91286, #22809, #14824, #69782, #38792, #45299, #24288, #46770, #7807, #8294, #61280, #38305, #47256, #53289, #83299, #45802, #85275, #331, #813, #30775, #46288, #1312, #92282, #54265, #77264, #16290, #8775, #77756, #64704, #57216, #32250, #93255, #26720, #94735, #64217, #78756, #70279, #56258, #86751, #95215, #10750, #26241, #2784, #17281, #87713, #2290, #17770, #1796, #63733, #19229, #9271, #40266, #3752, #39780, #78254, #48733, #62752, #24779, #47755, #18256, #55255, #3251, #56734, #34212, #70774, #86256, #49708, #11232, #32747, #79238, #41751, #41270, #71743, #10264, #33718, #87226, #18748, #49232, #9771, #85769, #63244, #79734, #93747, #25282, #72222, #48246, #55764, #40757, #71260, #33239, #94233, #25765, #43201, #95722, #28200, #89690, #58696, #35705, #20210, #21705, #66190, #20712, #97226, #42720, #88701, #12707, #5226, #28693, #89200, #65700, #59186, #36705, #21206, #97719, #51704, #29183, #51204, #81687, #82186, #19717, #13697, #73691, #96724, #43694, #96226, #50714, #5712, #80717, #13202, #67194, #80219, #44181, #59682, #11723, #81207, #74182, #36201, #66698, #74690, #6201, #42236, #90175, #72702, #73201, #4238, #12213, #34706, #65202, #27207, #57708, #88207, #50205, #4732, #35197, #27704, #58189, #69174, #30655, #84658, #45177, #39169, #61162, #204, #60176, #69658, #14704, #92162, #54149, #7190, #83678, #38190, #8178, #90672, #7693, #37209, #22198, #46174, #15688, #1184, #52678, #38672, #68192, #75677, #62134, #15193, #8656, #31150, #31642, #697, #92642, #84181, #61641, #14202, #76657, #29667, #45675, #30163, #76173, #83179, #37693, #52190, #16167, #53173, #23685, #68677, #98712, #91670, #46651, #60666, #91166, #77147, #82684, #23189, #44683, #53665, #22693, #75179, #6690, #67697, #98209, #12468, #79499, #56978, #24660 ) ),
 .UNSPECIFIED., .F., .F., .T. ) 
 B_SPLINE_SURFACE_WITH_KNOTS ( ( 2, 2 ),
 ( 3, 2, 2, 2, 2, 2, 2, 2, 2, 2, 2, 2, 2, 2, 2, 2, 2, 2, 2, 2, 2, 2, 2, 2, 2, 2, 2, 2, 2, 2, 2, 2, 2, 2, 2, 2, 2, 2, 2, 2, 2, 2, 2, 2, 2, 2, 2, 2, 2, 2, 2, 2, 2, 2, 2, 2, 2, 2, 2, 2, 2, 2, 2, 2, 2, 2, 2, 2, 2, 2, 2, 2, 2, 2, 2, 2, 2, 2, 2, 2, 2, 2, 2, 2, 2, 2, 2, 2, 2, 2, 2, 2, 2, 2, 2, 2, 2, 2, 2, 2, 2, 2, 2, 2, 2, 2, 2, 2, 2, 2, 2, 2, 2, 2, 2, 2, 2, 2, 2, 2, 2, 2, 2, 2, 2, 2, 2, 2, 2, 2, 2, 2, 2, 2, 2, 2, 2, 2, 2, 2, 2, 2, 2, 2, 2, 2, 2, 2, 2, 2, 2, 2, 2, 2, 2, 2, 2, 2, 2, 2, 2, 2, 3 ),
 ( 0.000000000000000000, 1.000000000000000000 ),
 ( 0.000000000000000000, 0.005952380952380952051, 0.01190476190476190410, 0.01785714285714285615, 0.02380952380952380820, 0.02976190476190476025, 0.03571428571428571230, 0.04166666666666666435, 0.04761904761904761640, 0.05357142857142856845, 0.05952380952380952051, 0.06547619047619047949, 0.07142857142857142461, 0.07738095238095238360, 0.08333333333333332871, 0.08928571428571428770, 0.09523809523809523281, 0.1011904761904761918, 0.1071428571428571369, 0.1130952380952380959, 0.1190476190476190410, 0.1250000000000000000, 0.1309523809523809590, 0.1369047619047619180, 0.1428571428571428492, 0.1488095238095238082, 0.1547619047619047672, 0.1607142857142857262, 0.1666666666666666574, 0.1726190476190476164, 0.1785714285714285754, 0.1845238095238095344, 0.1904761904761904656, 0.1964285714285714246, 0.2023809523809523836, 0.2083333333333333426, 0.2142857142857142738, 0.2202380952380952328, 0.2261904761904761918, 0.2321428571428571508, 0.2380952380952380820, 0.2440476190476190410, 0.2500000000000000000, 0.2559523809523809312, 0.2619047619047619180, 0.2678571428571428492, 0.2738095238095238360, 0.2797619047619047672, 0.2857142857142856984, 0.2916666666666666852, 0.2976190476190476164, 0.3035714285714285476, 0.3095238095238095344, 0.3154761904761904656, 0.3214285714285714524, 0.3273809523809523836, 0.3333333333333333148, 0.3392857142857143016, 0.3452380952380952328, 0.3511904761904761640, 0.3571428571428571508, 0.3630952380952380820, 0.3690476190476190688, 0.3750000000000000000, 0.3809523809523809312, 0.3869047619047619180, 0.3928571428571428492, 0.3988095238095238360, 0.4047619047619047672, 0.4107142857142856984, 0.4166666666666666852, 0.4226190476190476164, 0.4285714285714285476, 0.4345238095238095344, 0.4404761904761904656, 0.4464285714285714524, 0.4523809523809523836, 0.4583333333333333148, 0.4642857142857143016, 0.4702380952380952328, 0.4761904761904761640, 0.4821428571428571508, 0.4880952380952380820, 0.4940476190476190688, 0.5000000000000000000, 0.5059523809523809312, 0.5119047619047618625, 0.5178571428571429047, 0.5238095238095238360, 0.5297619047619047672, 0.5357142857142856984, 0.5416666666666666297, 0.5476190476190476719, 0.5535714285714286031, 0.5595238095238095344, 0.5654761904761904656, 0.5714285714285713969, 0.5773809523809523281, 0.5833333333333333703, 0.5892857142857143016, 0.5952380952380952328, 0.6011904761904761640, 0.6071428571428570953, 0.6130952380952381375, 0.6190476190476190688, 0.6250000000000000000, 0.6309523809523809312, 0.6369047619047618625, 0.6428571428571429047, 0.6488095238095238360, 0.6547619047619047672, 0.6607142857142856984, 0.6666666666666666297, 0.6726190476190476719, 0.6785714285714286031, 0.6845238095238095344, 0.6904761904761904656, 0.6964285714285713969, 0.7023809523809523281, 0.7083333333333333703, 0.7142857142857143016, 0.7202380952380952328, 0.7261904761904761640, 0.7321428571428570953, 0.7380952380952381375, 0.7440476190476190688, 0.7500000000000000000, 0.7559523809523809312, 0.7619047619047618625, 0.7678571428571429047, 0.7738095238095238360, 0.7797619047619047672, 0.7857142857142856984, 0.7916666666666666297, 0.7976190476190476719, 0.8035714285714286031, 0.8095238095238095344, 0.8154761904761904656, 0.8214285714285713969, 0.8273809523809523281, 0.8333333333333333703, 0.8392857142857143016, 0.8452380952380952328, 0.8511904761904761640, 0.8571428571428570953, 0.8630952380952381375, 0.8690476190476190688, 0.8750000000000000000, 0.8809523809523809312, 0.8869047619047618625, 0.8928571428571429047, 0.8988095238095238360, 0.9047619047619047672, 0.9107142857142856984, 0.9166666666666666297, 0.9226190476190476719, 0.9285714285714286031, 0.9345238095238095344, 0.9404761904761904656, 0.9464285714285713969, 0.9523809523809523281, 0.9583333333333333703, 0.9642857142857143016 ),
 .UNSPECIFIED. ) 
 GEOMETRIC_REPRESENTATION_ITEM ( )  RATIONAL_B_SPLINE_SURFACE ( (
 ( 1.000000000000000000, 0.9659258262890683122, 1.000000000000000000, 0.9659258262890683122, 1.000000000000000000, 0.9659258262890683122, 1.000000000000000000, 0.9659258262890683122, 1.000000000000000000, 0.9659258262890683122, 1.000000000000000000, 0.9659258262890683122, 1.000000000000000000, 0.9659258262890683122, 1.000000000000000000, 0.9659258262890683122, 1.000000000000000000, 0.9659258262890683122, 1.000000000000000000, 0.9659258262890683122, 1.000000000000000000, 0.9659258262890683122, 1.000000000000000000, 0.9659258262890683122, 1.000000000000000000, 0.9659258262890683122, 1.000000000000000000, 0.9659258262890683122, 1.000000000000000000, 0.9659258262890683122, 1.000000000000000000, 0.9659258262890683122, 1.000000000000000000, 0.9659258262890683122, 1.000000000000000000, 0.9659258262890683122, 1.000000000000000000, 0.9659258262890683122, 1.000000000000000000, 0.9659258262890683122, 1.000000000000000000, 0.9659258262890683122, 1.000000000000000000, 0.9659258262890683122, 1.000000000000000000, 0.9659258262890683122, 1.000000000000000000, 0.9659258262890683122, 1.000000000000000000, 0.9659258262890683122, 1.000000000000000000, 0.9659258262890683122, 1.000000000000000000, 0.9659258262890683122, 1.000000000000000000, 0.9659258262890683122, 1.000000000000000000, 0.9659258262890683122, 1.000000000000000000, 0.9659258262890683122, 1.000000000000000000, 0.9659258262890683122, 1.000000000000000000, 0.9659258262890683122, 1.000000000000000000, 0.9659258262890683122, 1.000000000000000000, 0.9659258262890683122, 1.000000000000000000, 0.9659258262890683122, 1.000000000000000000, 0.9659258262890683122, 1.000000000000000000, 0.9659258262890683122, 1.000000000000000000, 0.9659258262890683122, 1.000000000000000000, 0.9659258262890683122, 1.000000000000000000, 0.9659258262890683122, 1.000000000000000000, 0.9659258262890683122, 1.000000000000000000, 0.9659258262890683122, 1.000000000000000000, 0.9659258262890683122, 1.000000000000000000, 0.9659258262890683122, 1.000000000000000000, 0.9659258262890683122, 1.000000000000000000, 0.9659258262890683122, 1.000000000000000000, 0.9659258262890683122, 1.000000000000000000, 0.9659258262890683122, 1.000000000000000000, 0.9659258262890683122, 1.000000000000000000, 0.9659258262890683122, 1.000000000000000000, 0.9659258262890683122, 1.000000000000000000, 0.9659258262890683122, 1.000000000000000000, 0.9659258262890683122, 1.000000000000000000, 0.9659258262890683122, 1.000000000000000000, 0.9659258262890683122, 1.000000000000000000, 0.9659258262890683122, 1.000000000000000000, 0.9659258262890683122, 1.000000000000000000, 0.9659258262890683122, 1.000000000000000000, 0.9659258262890683122, 1.000000000000000000, 0.9659258262890683122, 1.000000000000000000, 0.9659258262890683122, 1.000000000000000000, 0.9659258262890683122, 1.000000000000000000, 0.9659258262890683122, 1.000000000000000000, 0.9659258262890683122, 1.000000000000000000, 0.9659258262890683122, 1.000000000000000000, 0.9659258262890683122, 1.000000000000000000, 0.9659258262890683122, 1.000000000000000000, 0.9659258262890683122, 1.000000000000000000, 0.9659258262890683122, 1.000000000000000000, 0.9659258262890683122, 1.000000000000000000, 0.9659258262890683122, 1.000000000000000000, 0.9659258262890683122, 1.000000000000000000, 0.9659258262890683122, 1.000000000000000000, 0.9659258262890683122, 1.000000000000000000, 0.9659258262890683122, 1.000000000000000000, 0.9659258262890683122, 1.000000000000000000, 0.9659258262890683122, 1.000000000000000000, 0.9659258262890683122, 1.000000000000000000, 0.9659258262890683122, 1.000000000000000000, 0.9659258262890683122, 1.000000000000000000, 0.9659258262890683122, 1.000000000000000000, 0.9659258262890683122, 1.000000000000000000, 0.9659258262890683122, 1.000000000000000000, 0.9659258262890683122, 1.000000000000000000, 0.9659258262890683122, 1.000000000000000000, 0.9659258262890683122, 1.000000000000000000, 0.9659258262890683122, 1.000000000000000000, 0.9659258262890683122, 1.000000000000000000, 0.9659258262890683122, 1.000000000000000000, 0.9659258262890683122, 1.000000000000000000, 0.9659258262890683122, 1.000000000000000000, 0.9659258262890683122, 1.000000000000000000, 0.9659258262890683122, 1.000000000000000000, 0.9659258262890683122, 1.000000000000000000, 0.9659258262890683122, 1.000000000000000000, 0.9659258262890683122, 1.000000000000000000, 0.9659258262890683122, 1.000000000000000000, 0.9659258262890683122, 1.000000000000000000, 0.9659258262890683122, 1.000000000000000000, 0.9659258262890683122, 1.000000000000000000, 0.9659258262890683122, 1.000000000000000000, 0.9659258262890683122, 1.000000000000000000, 0.9659258262890683122, 1.000000000000000000, 0.9659258262890683122, 1.000000000000000000, 0.9659258262890683122, 1.000000000000000000, 0.9659258262890683122, 1.000000000000000000, 0.9659258262890683122, 1.000000000000000000, 0.9659258262890683122, 1.000000000000000000, 0.9659258262890683122, 1.000000000000000000, 0.9659258262890683122, 1.000000000000000000, 0.9659258262890683122, 1.000000000000000000, 0.9659258262890683122, 1.000000000000000000, 0.9659258262890683122, 1.000000000000000000, 0.9659258262890683122, 1.000000000000000000, 0.9659258262890683122, 1.000000000000000000, 0.9659258262890683122, 1.000000000000000000, 0.9659258262890683122, 1.000000000000000000, 0.9659258262890683122, 1.000000000000000000, 0.9659258262890683122, 1.000000000000000000, 0.9659258262890683122, 1.000000000000000000, 0.9659258262890683122, 1.000000000000000000, 0.9659258262890683122, 1.000000000000000000, 0.9659258262890683122, 1.000000000000000000, 0.9659258262890683122, 1.000000000000000000, 0.9659258262890683122, 1.000000000000000000, 0.9659258262890683122, 1.000000000000000000, 0.9659258262890683122, 1.000000000000000000, 0.9659258262890683122, 1.000000000000000000, 0.9659258262890683122, 1.000000000000000000, 0.9659258262890683122, 1.000000000000000000, 0.9659258262890683122, 1.000000000000000000, 0.9659258262890683122, 1.000000000000000000, 0.9659258262890683122, 1.000000000000000000, 0.9659258262890683122, 1.000000000000000000, 0.9659258262890683122, 1.000000000000000000, 0.9659258262890683122, 1.000000000000000000, 0.9659258262890683122, 1.000000000000000000, 0.9659258262890683122, 1.000000000000000000, 0.9659258262890683122, 1.000000000000000000, 0.9659258262890683122, 1.000000000000000000, 0.9659258262890683122, 1.000000000000000000, 0.9659258262890683122, 1.000000000000000000, 0.9659258262890683122, 1.000000000000000000, 0.9659258262890683122, 1.000000000000000000, 0.9659258262890683122, 1.000000000000000000, 0.9659258262890683122, 1.000000000000000000, 0.9659258262890683122, 1.000000000000000000, 0.9659258262890683122, 1.000000000000000000, 0.9659258262890683122, 1.000000000000000000, 0.9659258262890683122, 1.000000000000000000, 0.9659258262890683122, 1.000000000000000000, 0.9659258262890683122, 1.000000000000000000, 0.9659258262890683122, 1.000000000000000000, 0.9659258262890683122, 1.000000000000000000, 0.9659258262890683122, 1.000000000000000000, 0.9659258262890683122, 1.000000000000000000, 0.9659258262890683122, 1.000000000000000000, 0.9659258262890683122, 1.000000000000000000, 0.9659258262890683122, 1.000000000000000000, 0.9659258262890683122, 1.000000000000000000, 0.9659258262890683122, 1.000000000000000000, 0.9659258262890683122, 1.000000000000000000),
 ( 1.000000000000000000, 0.9659258262890683122, 1.000000000000000000, 0.9659258262890683122, 1.000000000000000000, 0.9659258262890683122, 1.000000000000000000, 0.9659258262890683122, 1.000000000000000000, 0.9659258262890683122, 1.000000000000000000, 0.9659258262890683122, 1.000000000000000000, 0.9659258262890683122, 1.000000000000000000, 0.9659258262890683122, 1.000000000000000000, 0.9659258262890683122, 1.000000000000000000, 0.9659258262890683122, 1.000000000000000000, 0.9659258262890683122, 1.000000000000000000, 0.9659258262890683122, 1.000000000000000000, 0.9659258262890683122, 1.000000000000000000, 0.9659258262890683122, 1.000000000000000000, 0.9659258262890683122, 1.000000000000000000, 0.9659258262890683122, 1.000000000000000000, 0.9659258262890683122, 1.000000000000000000, 0.9659258262890683122, 1.000000000000000000, 0.9659258262890683122, 1.000000000000000000, 0.9659258262890683122, 1.000000000000000000, 0.9659258262890683122, 1.000000000000000000, 0.9659258262890683122, 1.000000000000000000, 0.9659258262890683122, 1.000000000000000000, 0.9659258262890683122, 1.000000000000000000, 0.9659258262890683122, 1.000000000000000000, 0.9659258262890683122, 1.000000000000000000, 0.9659258262890683122, 1.000000000000000000, 0.9659258262890683122, 1.000000000000000000, 0.9659258262890683122, 1.000000000000000000, 0.9659258262890683122, 1.000000000000000000, 0.9659258262890683122, 1.000000000000000000, 0.9659258262890683122, 1.000000000000000000, 0.9659258262890683122, 1.000000000000000000, 0.9659258262890683122, 1.000000000000000000, 0.9659258262890683122, 1.000000000000000000, 0.9659258262890683122, 1.000000000000000000, 0.9659258262890683122, 1.000000000000000000, 0.9659258262890683122, 1.000000000000000000, 0.9659258262890683122, 1.000000000000000000, 0.9659258262890683122, 1.000000000000000000, 0.9659258262890683122, 1.000000000000000000, 0.9659258262890683122, 1.000000000000000000, 0.9659258262890683122, 1.000000000000000000, 0.9659258262890683122, 1.000000000000000000, 0.9659258262890683122, 1.000000000000000000, 0.9659258262890683122, 1.000000000000000000, 0.9659258262890683122, 1.000000000000000000, 0.9659258262890683122, 1.000000000000000000, 0.9659258262890683122, 1.000000000000000000, 0.9659258262890683122, 1.000000000000000000, 0.9659258262890683122, 1.000000000000000000, 0.9659258262890683122, 1.000000000000000000, 0.9659258262890683122, 1.000000000000000000, 0.9659258262890683122, 1.000000000000000000, 0.9659258262890683122, 1.000000000000000000, 0.9659258262890683122, 1.000000000000000000, 0.9659258262890683122, 1.000000000000000000, 0.9659258262890683122, 1.000000000000000000, 0.9659258262890683122, 1.000000000000000000, 0.9659258262890683122, 1.000000000000000000, 0.9659258262890683122, 1.000000000000000000, 0.9659258262890683122, 1.000000000000000000, 0.9659258262890683122, 1.000000000000000000, 0.9659258262890683122, 1.000000000000000000, 0.9659258262890683122, 1.000000000000000000, 0.9659258262890683122, 1.000000000000000000, 0.9659258262890683122, 1.000000000000000000, 0.9659258262890683122, 1.000000000000000000, 0.9659258262890683122, 1.000000000000000000, 0.9659258262890683122, 1.000000000000000000, 0.9659258262890683122, 1.000000000000000000, 0.9659258262890683122, 1.000000000000000000, 0.9659258262890683122, 1.000000000000000000, 0.9659258262890683122, 1.000000000000000000, 0.9659258262890683122, 1.000000000000000000, 0.9659258262890683122, 1.000000000000000000, 0.9659258262890683122, 1.000000000000000000, 0.9659258262890683122, 1.000000000000000000, 0.9659258262890683122, 1.000000000000000000, 0.9659258262890683122, 1.000000000000000000, 0.9659258262890683122, 1.000000000000000000, 0.9659258262890683122, 1.000000000000000000, 0.9659258262890683122, 1.000000000000000000, 0.9659258262890683122, 1.000000000000000000, 0.9659258262890683122, 1.000000000000000000, 0.9659258262890683122, 1.000000000000000000, 0.9659258262890683122, 1.000000000000000000, 0.9659258262890683122, 1.000000000000000000, 0.9659258262890683122, 1.000000000000000000, 0.9659258262890683122, 1.000000000000000000, 0.9659258262890683122, 1.000000000000000000, 0.9659258262890683122, 1.000000000000000000, 0.9659258262890683122, 1.000000000000000000, 0.9659258262890683122, 1.000000000000000000, 0.9659258262890683122, 1.000000000000000000, 0.9659258262890683122, 1.000000000000000000, 0.9659258262890683122, 1.000000000000000000, 0.9659258262890683122, 1.000000000000000000, 0.9659258262890683122, 1.000000000000000000, 0.9659258262890683122, 1.000000000000000000, 0.9659258262890683122, 1.000000000000000000, 0.9659258262890683122, 1.000000000000000000, 0.9659258262890683122, 1.000000000000000000, 0.9659258262890683122, 1.000000000000000000, 0.9659258262890683122, 1.000000000000000000, 0.9659258262890683122, 1.000000000000000000, 0.9659258262890683122, 1.000000000000000000, 0.9659258262890683122, 1.000000000000000000, 0.9659258262890683122, 1.000000000000000000, 0.9659258262890683122, 1.000000000000000000, 0.9659258262890683122, 1.000000000000000000, 0.9659258262890683122, 1.000000000000000000, 0.9659258262890683122, 1.000000000000000000, 0.9659258262890683122, 1.000000000000000000, 0.9659258262890683122, 1.000000000000000000, 0.9659258262890683122, 1.000000000000000000, 0.9659258262890683122, 1.000000000000000000, 0.9659258262890683122, 1.000000000000000000, 0.9659258262890683122, 1.000000000000000000, 0.9659258262890683122, 1.000000000000000000, 0.9659258262890683122, 1.000000000000000000, 0.9659258262890683122, 1.000000000000000000, 0.9659258262890683122, 1.000000000000000000, 0.9659258262890683122, 1.000000000000000000, 0.9659258262890683122, 1.000000000000000000, 0.9659258262890683122, 1.000000000000000000, 0.9659258262890683122, 1.000000000000000000, 0.9659258262890683122, 1.000000000000000000, 0.9659258262890683122, 1.000000000000000000, 0.9659258262890683122, 1.000000000000000000, 0.9659258262890683122, 1.000000000000000000, 0.9659258262890683122, 1.000000000000000000, 0.9659258262890683122, 1.000000000000000000, 0.9659258262890683122, 1.000000000000000000, 0.9659258262890683122, 1.000000000000000000, 0.9659258262890683122, 1.000000000000000000, 0.9659258262890683122, 1.000000000000000000, 0.9659258262890683122, 1.000000000000000000, 0.9659258262890683122, 1.000000000000000000, 0.9659258262890683122, 1.000000000000000000, 0.9659258262890683122, 1.000000000000000000, 0.9659258262890683122, 1.000000000000000000, 0.9659258262890683122, 1.000000000000000000, 0.9659258262890683122, 1.000000000000000000, 0.9659258262890683122, 1.000000000000000000, 0.9659258262890683122, 1.000000000000000000, 0.9659258262890683122, 1.000000000000000000, 0.9659258262890683122, 1.000000000000000000, 0.9659258262890683122, 1.000000000000000000, 0.9659258262890683122, 1.000000000000000000, 0.9659258262890683122, 1.000000000000000000, 0.9659258262890683122, 1.000000000000000000, 0.9659258262890683122, 1.000000000000000000, 0.9659258262890683122, 1.000000000000000000, 0.9659258262890683122, 1.000000000000000000, 0.9659258262890683122, 1.000000000000000000, 0.9659258262890683122, 1.000000000000000000, 0.9659258262890683122, 1.000000000000000000, 0.9659258262890683122, 1.000000000000000000, 0.9659258262890683122, 1.000000000000000000, 0.9659258262890683122, 1.000000000000000000, 0.9659258262890683122, 1.000000000000000000) ) ) 
 REPRESENTATION_ITEM ( '' )  SURFACE ( )  );
#93661=CARTESIAN_POINT ( 'NONE',  ( 20.15039907845753575, 15.60158574516642815, -6.262539305110077059 ) ) ;
#93665=CARTESIAN_POINT ( 'NONE',  ( 22.26659068614895176, 64.72041550158064638, -7.082119434687042414 ) ) ;
#93666=DIRECTION ( 'NONE',  ( -1.000000000000000000, -2.799047438454523729E-16, -0.000000000000000000 ) ) ;
#93667=CARTESIAN_POINT ( 'NONE',  ( 15.44008868035555260, 39.73035201082150536, 9.422509992056143702 ) ) ;
#93668=CARTESIAN_POINT ( 'NONE',  ( 19.38216949554541557, 7.248634669930421381, -9.382169495545420901 ) ) ;
#93669=CARTESIAN_POINT ( 'NONE',  ( 17.96484262340118221, 56.18868534415484817, -7.964842623401177768 ) ) ;
#93674=CARTESIAN_POINT ( 'NONE',  ( 5.076628168052703671, 46.84226448433412315, 8.527530157486179263 ) ) ;
#93676=CARTESIAN_POINT ( 'NONE',  ( 10.00000000000000178, 10.37363466993041961, 12.81628187352647608 ) ) ;
#93677=CARTESIAN_POINT ( 'NONE',  ( 12.91533473730992121, 14.52201867748817143, 10.88017736071110164 ) ) ;
#93680=CARTESIAN_POINT ( 'NONE',  ( 6.204703633549690345, 32.84541550158063927, 14.16423886937410082 ) ) ;
#93681=EDGE_CURVE ( 'NONE', #68278, #94075, #74473, .T. ) ;
#93682=CARTESIAN_POINT ( 'NONE',  ( -4.164238869374099927, 32.01208216824730357, 3.795296366450308767 ) ) ;
#93683=CARTESIAN_POINT ( 'NONE',  ( 6.204703633549690345, 67.84541550158060375, 14.16423886937410082 ) ) ;
#93685=CARTESIAN_POINT ( 'NONE',  ( 0.6178305044545838731, 39.74863466993041072, 9.382169495545420901 ) ) ;
#93686=CARTESIAN_POINT ( 'NONE',  ( 2.035157376598824452, 18.68868534415484106, 7.964842623401179544 ) ) ;
#93688=CARTESIAN_POINT ( 'NONE',  ( 5.076628168052703671, 36.84226448433412315, 8.527530157486179263 ) ) ;
#93689=CARTESIAN_POINT ( 'NONE',  ( 20.88017736071110875, 35.77201867748816966, -2.915334737309920765 ) ) ;
#93690=CARTESIAN_POINT ( 'NONE',  ( 18.52753015748617571, 58.09226448433411605, 4.923371831947298993 ) ) ;
#93691=CARTESIAN_POINT ( 'NONE',  ( 10.00000000000000000, 25.55374883491396787, -14.16423886937410082 ) ) ;
#93692=CARTESIAN_POINT ( 'NONE',  ( -0.2418659066527499291, 17.23410085661204150, -6.114288769123083611 ) ) ;
#93693=CARTESIAN_POINT ( 'NONE',  ( 18.72515096720573879, 35.05509018479936145, 6.499999999999937828 ) ) ;
#93694=CARTESIAN_POINT ( 'NONE',  ( 0.1532563361054082862, 26.21726448433411605, 2.638427012816831674 ) ) ;
#93695=CARTESIAN_POINT ( 'NONE',  ( 16.40814093676323893, 55.79030133659708923, 11.09922568453595026 ) ) ;
#93696=CARTESIAN_POINT ( 'NONE',  ( 0.1532563361054083140, 56.00893115100078745, 1.131784320476157264E-15 ) ) ;
#93697=VERTEX_POINT ( 'NONE', #67976 ) ;
#93699=DIRECTION ( 'NONE',  ( 0.000000000000000000, -1.000000000000000000, 0.000000000000000000 ) ) ;
#93700=CARTESIAN_POINT ( 'NONE',  ( 2.917880565312950480, 65.97041550158063217, -12.26659068614894821 ) ) ;
#93701=CARTESIAN_POINT ( 'NONE',  ( 20.36894250292379738, 14.92874883491396432, -10.36894250292379027 ) ) ;
#93702=CARTESIAN_POINT ( 'NONE',  ( 17.96484262340118221, 66.18868534415483396, -7.964842623401177768 ) ) ;
#93703=CARTESIAN_POINT ( 'NONE',  ( 1.472469842513823179, 56.42559781766745886, 4.923371831947296329 ) ) ;
#93704=CARTESIAN_POINT ( 'NONE',  ( 10.00000000000000178, 24.31368534415484106, 10.88017736071110342 ) ) ;
#93706=CYLINDRICAL_SURFACE ( 'NONE', #39413, 0.5000000000000004441 ) ;
#93707=CARTESIAN_POINT ( 'NONE',  ( 18.52753015748618282, 3.925597817667451306, -4.923371831947291888 ) ) ;
#93708=CARTESIAN_POINT ( 'NONE',  ( 10.00000000000000000, 62.87363466993042493, -12.81628187352647608 ) ) ;
#93709=VERTEX_POINT ( 'NONE', #36982 ) ;
#93711=CARTESIAN_POINT ( 'NONE',  ( 20.15039907845753930, 70.00000000000000000, -6.262539305110068177 ) ) ;
#93713=EDGE_CURVE ( 'NONE', #49375, #34270, #98501, .T. ) ;
#93714=CARTESIAN_POINT ( 'NONE',  ( -0.3689425029237881626, 47.42874883491396787, 10.36894250292379027 ) ) ;
#93715=CARTESIAN_POINT ( 'NONE',  ( 2.791683348922240793, 51.63393115100078745, 7.208316651077764092 ) ) ;
#93716=CARTESIAN_POINT ( 'NONE',  ( 7.361572987183169658, 24.96726448433412315, -9.846743663894592657 ) ) ;
#93718=CARTESIAN_POINT ( 'NONE',  ( 19.42250999205614548, 25.98035201082150891, -5.440088680355545492 ) ) ;
#93719=CARTESIAN_POINT ( 'NONE',  ( 12.63842701281683922, 59.55059781766744464, -9.846743663894590881 ) ) ;
#93721=CARTESIAN_POINT ( 'NONE',  ( -4.164238869374099927, 37.01208216824731068, 3.795296366450308767 ) ) ;
#93723=CARTESIAN_POINT ( 'NONE',  ( -4.164238869374099039, 51.80374883491396787, 8.674139862899312516E-16 ) ) ;
#93724=CYLINDRICAL_SURFACE ( 'NONE', #13072, 0.5000000000000004441 ) ;
#93726=CARTESIAN_POINT ( 'NONE',  ( 12.91533473730992121, 59.52201867748816966, 10.88017736071110164 ) ) ;
#93727=EDGE_CURVE ( 'NONE', #62035, #38580, #89974, .T. ) ;
#93728=CARTESIAN_POINT ( 'NONE',  ( 14.92337183194729988, 14.34226448433411782, -8.527530157486177487 ) ) ;
#93730=ORIENTED_EDGE ( 'NONE', *, *, #55674, .T. ) ;
#93733=CARTESIAN_POINT ( 'NONE',  ( 7.361572987183169658, 29.96726448433411960, -9.846743663894592657 ) ) ;
#93735=CARTESIAN_POINT ( 'NONE',  ( -0.3689425029237881626, 37.42874883491396787, 10.36894250292379027 ) ) ;
#93736=CARTESIAN_POINT ( 'NONE',  ( 17.20831665107776587, 27.88393115100078390, 7.208316651077764980 ) ) ;
#93737=CARTESIAN_POINT ( 'NONE',  ( 20.88017736071110164, 40.35535201082150536, 2.915334737309930979 ) ) ;
#93738=FACE_OUTER_BOUND ( 'NONE', #49212, .T. ) ;
#93740=CARTESIAN_POINT ( 'NONE',  ( -0.8801773607111009756, 43.06368534415484106, 1.068504757029289695E-15 ) ) ;
#93745=CARTESIAN_POINT ( 'NONE',  ( -4.164238869374099039, 6.803748834913967869, 8.674139862899312516E-16 ) ) ;
#93746=VERTEX_POINT ( 'NONE', #21993 ) ;
#93747=CARTESIAN_POINT ( 'NONE',  ( 19.38216949554541202, 35.99863466993041072, 9.382169495545424454 ) ) ;
#93749=( NAMED_UNIT ( * ) SI_UNIT ( $, .STERADIAN. ) SOLID_ANGLE_UNIT ( ) );
#93750=CARTESIAN_POINT ( 'NONE',  ( 12.63842701281683034, 27.46726448433411250, 9.846743663894596210 ) ) ;
#93751=( LENGTH_UNIT ( ) NAMED_UNIT ( * ) SI_UNIT ( .MILLI., .METRE. ) );
#93752=CARTESIAN_POINT ( 'NONE',  ( 20.88017736071110875, 10.77201867748817143, -2.915334737309920321 ) ) ;
#93753=CARTESIAN_POINT ( 'NONE',  ( 19.84674366389459621, 33.50893115100078745, 7.409399052514197653E-17 ) ) ;
#93755=EDGE_CURVE ( 'NONE', #10984, #36088, #16547, .T. ) ;
#93758=ORIENTED_EDGE ( 'NONE', *, *, #32285, .F. ) ;
#93760=CARTESIAN_POINT ( 'NONE',  ( 4.559911319644449179, 58.89701867748817676, 9.422509992056141925 ) ) ;
#93763=CARTESIAN_POINT ( 'NONE',  ( 17.20831665107776587, 7.883931151000784787, 7.208316651077764980 ) ) ;
#93764=CARTESIAN_POINT ( 'NONE',  ( 19.38216949554541557, 12.24863466993041961, -9.382169495545420901 ) ) ;
#93766=EDGE_CURVE ( 'NONE', #76727, #22152, #6982, .T. ) ;
#93767=CARTESIAN_POINT ( 'NONE',  ( 14.92337183194729633, 47.67559781766745175, 8.527530157486181039 ) ) ;
#93769=CARTESIAN_POINT ( 'NONE',  ( 2.917880565312948704, 12.63708216824730179, 12.26659068614894643 ) ) ;
#93770=CARTESIAN_POINT ( 'NONE',  ( 18.52753015748618282, 18.92559781766745175, -4.923371831947291888 ) ) ;
#93771=CARTESIAN_POINT ( 'NONE',  ( 6.565887622018943937, 33.08196800326374643, -12.81628187352647608 ) ) ;
#93774=CARTESIAN_POINT ( 'NONE',  ( -0.8801773607111009756, 48.06368534415484817, 1.068504757029289695E-15 ) ) ;
#93775=CARTESIAN_POINT ( 'NONE',  ( 21.09922568453594849, 11.20696800326375531, 6.408140936763242479 ) ) ;
#93777=CARTESIAN_POINT ( 'NONE',  ( 7.361572987183170547, 22.05059781766745530, 9.846743663894590881 ) ) ;
#93778=CARTESIAN_POINT ( 'NONE',  ( 19.42250999205614548, 30.98035201082150536, -5.440088680355545492 ) ) ;
#93779=CARTESIAN_POINT ( 'NONE',  ( 16.40814093676323893, 25.79030133659708923, 11.09922568453595026 ) ) ;
#93780=CARTESIAN_POINT ( 'NONE',  ( 0.1532563361054100626, 20.80059781766744464, -2.638427012816831230 ) ) ;
#93782=CARTESIAN_POINT ( 'NONE',  ( 0.5774900079438607392, 18.48035201082150536, 5.440088680355550821 ) ) ;
#93783=( GEOMETRIC_REPRESENTATION_CONTEXT ( 3 ) GLOBAL_UNCERTAINTY_ASSIGNED_CONTEXT ( ( #72417 ) ) GLOBAL_UNIT_ASSIGNED_CONTEXT ( ( #64780, #49792, #94310 ) ) REPRESENTATION_CONTEXT ( 'NONE', 'WORKASPACE' ) );
#93785=CARTESIAN_POINT ( 'NONE',  ( 2.035157376598822676, 57.43868534415484106, -7.964842623401177768 ) ) ;
#93787=CARTESIAN_POINT ( 'NONE',  ( 0.1532563361054082862, 41.21726448433411605, 2.638427012816831674 ) ) ;
#93788=CARTESIAN_POINT ( 'NONE',  ( -0.8801773607111009756, 23.06368534415484106, 1.068504757029289695E-15 ) ) ;
#93789=DIRECTION ( 'NONE',  ( 0.000000000000000000, -0.000000000000000000, 1.000000000000000000 ) ) ;
#93790=CARTESIAN_POINT ( 'NONE',  ( 20.88017736071110519, 50.56368534415484106, 2.639326808657452039E-16 ) ) ;
#93791=CARTESIAN_POINT ( 'NONE',  ( 2.035157376598822676, 17.43868534415483751, -7.964842623401177768 ) ) ;
#93793=CARTESIAN_POINT ( 'NONE',  ( 12.63842701281683034, 17.46726448433411250, 9.846743663894596210 ) ) ;
#93794=CARTESIAN_POINT ( 'NONE',  ( 5.076628168052704559, 40.17559781766745175, -8.527530157486179263 ) ) ;
#93796=CARTESIAN_POINT ( 'NONE',  ( 1.602071938427511721, 7.022241923386403961, -6.500000000000008882 ) ) ;
#93797=CARTESIAN_POINT ( 'NONE',  ( 18.52753015748617571, 63.09226448433412315, 4.923371831947298993 ) ) ;
#93798=EDGE_CURVE ( 'NONE', #86051, #83178, #78430, .T. ) ;
#93799=CARTESIAN_POINT ( 'NONE',  ( 10.00000000000000000, 25.55374883491396787, -14.16423886937410082 ) ) ;
#93800=CARTESIAN_POINT ( 'NONE',  ( 1.472469842513823179, 41.42559781766745886, 4.923371831947296329 ) ) ;
#93803=CARTESIAN_POINT ( 'NONE',  ( 10.00000000000000000, 6.813685344154838397, -10.88017736071110342 ) ) ;
#93806=CARTESIAN_POINT ( 'NONE',  ( 7.361572987183170547, 27.05059781766745175, 9.846743663894590881 ) ) ;
#93808=CARTESIAN_POINT ( 'NONE',  ( 15.44008868035555793, 46.39701867748817676, -9.422509992056140149 ) ) ;
#93810=CARTESIAN_POINT ( 'NONE',  ( 17.96484262340118221, 16.18868534415483396, -7.964842623401177768 ) ) ;
#93811=CARTESIAN_POINT ( 'NONE',  ( -2.816281873526473856, 44.12363466993042493, 9.499525473075851096E-16 ) ) ;
#93812=CARTESIAN_POINT ( 'NONE',  ( -1.099225684535947600, 14.54030133659708568, 6.408140936763237150 ) ) ;
#93813=CARTESIAN_POINT ( 'NONE',  ( 0.1532563361054083140, 21.00893115100078745, 1.131784320476157264E-15 ) ) ;
#93815=DIRECTION ( 'NONE',  ( 1.000000000000000000, 0.000000000000000000, 0.000000000000000000 ) ) ;
#93817=CARTESIAN_POINT ( 'NONE',  ( 22.26659068614894466, 48.88708216824730357, 7.082119434687054849 ) ) ;
#93818=CARTESIAN_POINT ( 'NONE',  ( 6.204703633549690345, 22.84541550158062861, 14.16423886937410082 ) ) ;
#93819=CARTESIAN_POINT ( 'NONE',  ( 12.91533473730992121, 24.52201867748816966, 10.88017736071110164 ) ) ;
#93820=COLOUR_RGB ( '', 0.31764706, 0.68627451, 0.89019608) ;
#93821=CARTESIAN_POINT ( 'NONE',  ( 10.00000000000000000, 51.81368534415484106, -10.88017736071110342 ) ) ;
#93822=SURFACE_STYLE_FILL_AREA ( #48806 ) ;
#93824=CARTESIAN_POINT ( 'NONE',  ( 0.1532563361054100626, 10.80059781766745175, -2.638427012816831230 ) ) ;
#93825=CARTESIAN_POINT ( 'NONE',  ( 5.076628168052704559, 15.17559781766745175, -8.527530157486179263 ) ) ;
#93827=CARTESIAN_POINT ( 'NONE',  ( 0.1532563361054082862, 21.21726448433412315, 2.638427012816831674 ) ) ;
#93828=CARTESIAN_POINT ( 'NONE',  ( 17.20831665107776587, 47.88393115100078745, 7.208316651077764980 ) ) ;
#93830=CARTESIAN_POINT ( 'NONE',  ( 0.5774900079438607392, 13.48035201082150358, 5.440088680355550821 ) ) ;
#93833=CARTESIAN_POINT ( 'NONE',  ( 19.38216949554541202, 25.99863466993042138, 9.382169495545424454 ) ) ;
#93834=CARTESIAN_POINT ( 'NONE',  ( 20.88017736071110875, 55.77201867748816966, -2.915334737309920765 ) ) ;
#93835=CARTESIAN_POINT ( 'NONE',  ( 0.1532563361054100626, 30.80059781766744820, -2.638427012816831230 ) ) ;
#93836=CARTESIAN_POINT ( 'NONE',  ( 10.00000000000000000, 50.55374883491396787, -14.16423886937410082 ) ) ;
#93837=CARTESIAN_POINT ( 'NONE',  ( 18.52753015748617571, 28.09226448433411960, 4.923371831947298993 ) ) ;
#93839=CARTESIAN_POINT ( 'NONE',  ( 19.84674366389459266, 48.71726448433413026, -2.638427012816827677 ) ) ;
#93840=CARTESIAN_POINT ( 'NONE',  ( 2.791683348922237240, 35.38393115100079456, -7.208316651077763204 ) ) ;
#93841=CARTESIAN_POINT ( 'NONE',  ( 6.204703633549690345, 15.76208216824730179, -14.16423886937410259 ) ) ;
#93842=CARTESIAN_POINT ( 'NONE',  ( -4.164238869374099039, 16.80374883491396787, 8.674139862899312516E-16 ) ) ;
#93843=CARTESIAN_POINT ( 'NONE',  ( 2.791683348922240793, 36.63393115100078035, 7.208316651077764092 ) ) ;
#93844=CARTESIAN_POINT ( 'NONE',  ( 17.96484262340118221, 49.93868534415484106, 7.964842623401181321 ) ) ;
#93845=CARTESIAN_POINT ( 'NONE',  ( -0.8801773607111009756, 28.06368534415484106, 1.068504757029289695E-15 ) ) ;
#93847=CARTESIAN_POINT ( 'NONE',  ( -0.8801773607110991993, 47.85535201082150536, -2.915334737309923874 ) ) ;
#93848=CARTESIAN_POINT ( 'NONE',  ( 0.5774900079438590739, 32.64701867748816966, -5.440088680355550821 ) ) ;
#93850=CARTESIAN_POINT ( 'NONE',  ( 19.42250999205614193, 50.14701867748817676, 5.440088680355555262 ) ) ;
#93851=VERTEX_POINT ( 'NONE', #46448 ) ;
#93852=CARTESIAN_POINT ( 'NONE',  ( 6.565887622018943937, 60.16530133659707502, 12.81628187352647430 ) ) ;
#93853=CARTESIAN_POINT ( 'NONE',  ( 15.44008868035555260, 59.73035201082151247, 9.422509992056143702 ) ) ;
#93856=CARTESIAN_POINT ( 'NONE',  ( 10.00000000000000000, 1.813685344154837731, -10.88017736071110342 ) ) ;
#93859=CARTESIAN_POINT ( 'NONE',  ( 17.08211943468705840, 55.13708216824731068, -12.26659068614894466 ) ) ;
#93860=CARTESIAN_POINT ( 'NONE',  ( 19.84674366389459266, 8.717264484334116048, -2.638427012816827677 ) ) ;
#93861=CARTESIAN_POINT ( 'NONE',  ( -0.3689425029237881626, 7.428748834913967869, 10.36894250292379027 ) ) ;
#93862=CARTESIAN_POINT ( 'NONE',  ( 19.84674366389459621, 8.508931151000785675, 7.409399052514197653E-17 ) ) ;
#93863=CARTESIAN_POINT ( 'NONE',  ( 12.91533473730993009, 11.60535201082150536, -10.88017736071109987 ) ) ;
#93864=CARTESIAN_POINT ( 'NONE',  ( 7.361572987183170547, 47.05059781766745175, 9.846743663894590881 ) ) ;
#93866=CARTESIAN_POINT ( 'NONE',  ( 17.20831665107776587, 52.88393115100078035, 7.208316651077764980 ) ) ;
#93869=CARTESIAN_POINT ( 'NONE',  ( 20.88017736071110875, 40.77201867748818387, -2.915334737309920765 ) ) ;
#93870=CARTESIAN_POINT ( 'NONE',  ( 14.92337183194729633, 47.67559781766745175, 8.527530157486181039 ) ) ;
#93871=CARTESIAN_POINT ( 'NONE',  ( 21.09922568453594849, 31.20696800326375353, 6.408140936763242479 ) ) ;
#93872=PRESENTATION_STYLE_ASSIGNMENT (( #86381 ) ) ;
#93873=CARTESIAN_POINT ( 'NONE',  ( 19.88701968852526392, 1.794273331840863683, 6.480634945678604986 ) ) ;
#93874=CARTESIAN_POINT ( 'NONE',  ( 15.44008868035555793, 56.39701867748817676, -9.422509992056140149 ) ) ;
#93875=CARTESIAN_POINT ( 'NONE',  ( 12.91533473730992121, 9.522018677488171434, 10.88017736071110164 ) ) ;
#93877=CARTESIAN_POINT ( 'NONE',  ( 10.00000000000000000, 47.87363466993042493, -12.81628187352647608 ) ) ;
#93878=DIRECTION ( 'NONE',  ( 1.000000000000000000, 0.000000000000000000, 0.000000000000000000 ) ) ;
#93880=CARTESIAN_POINT ( 'NONE',  ( -2.816281873526471635, 28.91530133659708213, -3.434112377981056508 ) ) ;
#93881=CARTESIAN_POINT ( 'NONE',  ( -0.8801773607110991993, 27.85535201082150181, -2.915334737309923874 ) ) ;
#93885=CARTESIAN_POINT ( 'NONE',  ( 1.472469842513823179, 0.5922644843341181575, -4.923371831947296329 ) ) ;
#93886=CARTESIAN_POINT ( 'NONE',  ( 10.00000000000000178, 52.25893115100078745, 9.846743663894594434 ) ) ;
#93887=CARTESIAN_POINT ( 'NONE',  ( 10.00000000000000178, 12.25893115100078568, 9.846743663894594434 ) ) ;
#93888=CARTESIAN_POINT ( 'NONE',  ( 18.52753015748617571, 33.09226448433411605, 4.923371831947298993 ) ) ;
#93891=CARTESIAN_POINT ( 'NONE',  ( 5.076628168052704559, 25.17559781766745175, -8.527530157486179263 ) ) ;
#93894=CARTESIAN_POINT ( 'NONE',  ( 2.791683348922237240, 30.38393115100078390, -7.208316651077763204 ) ) ;
#93895=VECTOR ( 'NONE', #69602, 1000.000000000000000 ) ;
#93896=FILL_AREA_STYLE ('',( #40909 ) ) ;
#93898=CARTESIAN_POINT ( 'NONE',  ( 14.92337183194729633, 52.67559781766745175, 8.527530157486181039 ) ) ;
#93902=CARTESIAN_POINT ( 'NONE',  ( 3.591859063236763294, 28.29030133659708568, -11.09922568453595026 ) ) ;
#93903=CARTESIAN_POINT ( 'NONE',  ( 19.84674366389459621, 38.50893115100078745, 7.409399052514197653E-17 ) ) ;
#93904=CARTESIAN_POINT ( 'NONE',  ( -0.1042174387088646015, 8.107361737662019507, 6.337391062633415117 ) ) ;
#93905=CARTESIAN_POINT ( 'NONE',  ( 2.917880565312948704, 42.63708216824729647, 12.26659068614894643 ) ) ;
#93906=CARTESIAN_POINT ( 'NONE',  ( 19.84674366389459266, 18.30059781766745175, 2.638427012816836559 ) ) ;
#93907=CARTESIAN_POINT ( 'NONE',  ( 0.1532563361054082862, 1.217264484334117824, 2.638427012816831674 ) ) ;
#93908=CARTESIAN_POINT ( 'NONE',  ( 20.00000000000000711, 90.60976979464389558, 4.970182471799130752 ) ) ;
#93909=CARTESIAN_POINT ( 'NONE',  ( 17.08211943468705840, 50.13708216824730357, -12.26659068614894466 ) ) ;
#93910=CARTESIAN_POINT ( 'NONE',  ( 0.1532563361054100626, 55.80059781766745175, -2.638427012816831230 ) ) ;
#93911=CARTESIAN_POINT ( 'NONE',  ( 0.5774900079438590739, 12.64701867748817321, -5.440088680355550821 ) ) ;
#93912=CARTESIAN_POINT ( 'NONE',  ( 17.08211943468705840, 25.13708216824730357, -12.26659068614894466 ) ) ;
#93913=CARTESIAN_POINT ( 'NONE',  ( 22.26659068614894466, 33.88708216824730357, 7.082119434687054849 ) ) ;
#93915=EDGE_CURVE ( 'NONE', #86159, #48470, #76939, .T. ) ;
#93917=CARTESIAN_POINT ( 'NONE',  ( 14.92337183194729633, 52.67559781766745175, 8.527530157486181039 ) ) ;
#93920=CARTESIAN_POINT ( 'NONE',  ( -0.8801773607110991993, 32.85535201082151247, -2.915334737309923874 ) ) ;
#93923=CARTESIAN_POINT ( 'NONE',  ( 14.92337183194729988, 44.34226448433412315, -8.527530157486177487 ) ) ;
#93926=CARTESIAN_POINT ( 'NONE',  ( 7.361572987183169658, 49.96726448433410894, -9.846743663894592657 ) ) ;
#93929=ORIENTED_EDGE ( 'NONE', *, *, #89464, .F. ) ;
#93930=CARTESIAN_POINT ( 'NONE',  ( -2.266590686148945544, 27.22041550158063572, 7.082119434687048631 ) ) ;
#93935=CARTESIAN_POINT ( 'NONE',  ( 10.00000000000000178, 9.313685344154839285, 10.88017736071110342 ) ) ;
#93936=CARTESIAN_POINT ( 'NONE',  ( 13.43411237798105340, 30.58196800326374998, 12.81628187352647963 ) ) ;
#93938=CARTESIAN_POINT ( 'NONE',  ( 0.5774900079438590739, 67.64701867748817676, -5.440088680355550821 ) ) ;
#93939=CARTESIAN_POINT ( 'NONE',  ( 20.24186590665277308, 42.61633188102327807, -6.114288769123051637 ) ) ;
#93941=CARTESIAN_POINT ( 'NONE',  ( 12.91533473730992121, 14.52201867748817143, 10.88017736071110164 ) ) ;
#93942=CARTESIAN_POINT ( 'NONE',  ( 0.6081133539230610952, 3.337033823263999111, 6.500000000000004441 ) ) ;
#93943=( BOUNDED_SURFACE ( )  B_SPLINE_SURFACE ( 1, 2, ( 
 ( #18330, #9848, #63317, #6772, #96305, #20293, #67273, #66775, #5303, #67773, #59759, #21281, #42800, #51280, #59263, #51777, #36278, #37283, #29263, #57784, #13277, #50791, #89764, #28769, #97296, #74768, #27782, #90253, #20790, #81764, #82259, #19790, #98294, #28280, #13776, #43768, #58775, #4807, #74258, #75259, #35780, #12781, #21786, #82762, #58267, #5787, #89278, #88291, #50279, #88783, #36782, #73284, #81282, #43279, #73774, #52266, #44262, #6276, #97801, #96804, #14284, #44757, #66269, #80795, #12291, #35281, #65775, #24853, #33310, #78327, #85844, #33787, #25833, #84857, #93825, #1382, #70851, #9847, #55336, #17358, #92840, #78827, #40835, #62333, #40348, #16364, #71336, #71817, #55838, #10337, #46845, #86333, #31836, #47826, #1872, #2364, #24369, #77832, #56331, #54831, #85344, #63804, #2856, #32328, #32818, #16856, #3323, #63316, #17837, #64293, #25355, #77340, #48319, #70353, #79318, #23880, #94309, #47331, #86824, #9344, #39848, #62833, #54344, #93333, #18329, #48810, #10827, #41347, #8852, #39366, #69861, #94805, #87303, #18823, #49303, #26306, #56807, #25217, #23247, #47189, #54203, #24713, #55185, #1729, #9701, #84719, #55698, #54690, #16716, #47696, #53721, #2718, #62189, #70210, #85211, #39227, #10200, #77692, #70705, #48177, #84238, #71195, #33172, #46229, #76715, #38728, #69228, #753, #16223, #69715, #92699, #1242, #78188, #31698, #24223, #40197, #97533, #90000, #64151, #57154, #34146, #6503, #63665, #3190, #43999, #48670, #56670, #94670, #33656, #28992, #87652, #4173, #64640, #3685, #21517, #34642, #26179, #19165, #82502, #25701, #44500, #95149, #74501, #49644, #26659, #75001, #67012, #56191, #65139, #41200, #11663, #80151, #42176, #72640, #87159, #21025, #82006, #18683, #95660, #86685, #13518, #14020, #27145, #51514, #18189, #57647, #71680, #88143, #41687, #6024, #49169, #79671, #59503, #11168, #72157, #36520, #52013, #94170, #79171, #10686, #16483, #27, #68989, #77452, #60975, #29482, #38494, #83498, #92459, #84966, #15511, #7007, #46472, #60489, #37513, #68005, #46958, #75496, #98531, #76968, #45993, #15016, #37011, #38986, #525, #22020, #30474, #30971, #61468, #76482, #67508, #8481, #98027, #91488, #29984, #91975, #7996, #23504, #53975, #90978, #69479, #23008, #53476, #84484, #59990, #90483, #7516, #15985, #83986, #22511, #23987, #997, #52494, #83001, #52983, #31458, #45485, #54458, #61960, #75987, #38007, #14519, #44988, #68500, #33419, #47939, #63918, #94921, #25944, #87423, #17953, #85963, #25473, #56446, #70463, #17472, #40467, #32938, #86932, #86455, #93450, #10937, #33907, #1491, #78940 ),
 ( #78445, #48440, #2485, #24975, #26420, #63439, #18445, #3450, #31944, #56921, #64415, #79439, #9960, #54946, #93946, #18940, #55460, #62947, #41461, #49417, #9461, #55955, #70965, #8966, #39482, #47455, #48927, #92948, #1985, #39962, #77954, #71929, #10450, #40958, #71455, #2969, #69972, #94429, #32451, #62445, #24483, #85463, #16975, #80914, #89395, #35402, #42915, #89885, #81887, #41947, #50903, #57416, #27899, #65895, #12408, #73396, #49915, #35896, #96924, #19423, #96426, #72411, #28402, #28879, #12900, #66391, #3937, #43397, #87909, #4924, #57899, #58388, #80426, #34906, #13399, #11922, #42426, #20911, #58897, #88413, #88906, #72907, #59381, #20417, #73895, #4440, #43882, #5426, #74378, #97412, #21403, #81398, #51400, #79918, #5905, #65402, #36400, #95928, #34406, #26919, #27408, #66893, #64895, #11427, #95423, #19913, #50404, #6889, #90867, #67890, #76852, #82884, #22397, #52380, #83379, #31346, #21903, #75876, #52873, #91867, #6383, #98412, #45881, #90366, #30358, #82379, #76371, #409, #46364, #14400, #29868, #8366, #53870, #44871, #22892, #7397, #59877, #60370, #69365, #61847, #14901, #45372, #23385, #84380, #75374, #61358, #44386, #74885, #37402, #30861, #37895, #886, #38874, #68387, #98907, #60866, #91366, #15880, #7886, #53364, #38378, #92353, #68879, #51897, #83871, #15395, #13901, #36899, #67387, #97916, #29376, #76166, #69167, #66461, #97980, #83935, #7950, #74448, #52935, #37466, #21971, #14967, #67955, #7463, #29933, #61418, #5975, #82952, #22962, #29436, #90431, #74951, #38445, #68452, #14465, #36468, #82451, #13974, #472, #44450, #6454, #59941, #98974, #89950, #59449, #44940, #98478, #30427, #60438, #90931, #22459, #60929, #91435, #53427, #15463, #45944, #76434, #30919, #91928, #23454, #13468, #97481, #28947, #19208, #183, #21684, #37670, #52169, #44159, #6179, #75157, #76150, #74669, #90648, #68170, #98689, #30631, #6668, #29644, #37187, #84162, #60151, #22174, #52655, #83158, #69152, #14682, #30138, #60646, #61140, #67171, #91145, #53150, #97695, #22671, #89672, #15173, #91648, #53644, #23166, #15667, #46152, #76636, #8155, #677, #51684, #73062, #42712, #51697, #13690, #80710, #73194, #5706, #36194, #27202, #43687, #26714, #57210, #72696, #13193, #35190, #82179, #59179, #12205, #96217, #88694, #12700, #81678, #89193, #20202, #20704, #21199, #51197, #44174, #43195, #50706, #81199, #66692, #95717, #73682, #5218, #28194, #97219, #28686, #19712, #34206, #64696, #19222, #95208, #49703, #11717, #42230, #57702, #88202, #50199, #71403, #84436, #92900, #32887, #39428, #1442, #84917, #48385, #62897, #31894 ) ),
 .UNSPECIFIED., .F., .F., .F. ) 
 B_SPLINE_SURFACE_WITH_KNOTS ( ( 2, 2 ),
 ( 3, 2, 2, 2, 2, 2, 2, 2, 2, 2, 2, 2, 2, 2, 2, 2, 2, 2, 2, 2, 2, 2, 2, 2, 2, 2, 2, 2, 2, 2, 2, 2, 2, 2, 2, 2, 2, 2, 2, 2, 2, 2, 2, 2, 2, 2, 2, 2, 2, 2, 2, 2, 2, 2, 2, 2, 2, 2, 2, 2, 2, 2, 2, 2, 2, 2, 2, 2, 2, 2, 2, 2, 2, 2, 2, 2, 2, 2, 2, 2, 2, 2, 2, 2, 2, 2, 2, 2, 2, 2, 2, 2, 2, 2, 2, 2, 2, 2, 2, 2, 2, 2, 2, 2, 2, 2, 2, 2, 2, 2, 2, 2, 2, 2, 2, 2, 2, 2, 2, 2, 2, 2, 2, 2, 2, 2, 2, 2, 2, 2, 2, 2, 2, 2, 2, 2, 2, 2, 2, 2, 2, 2, 2, 2, 2, 2, 2, 2, 2, 2, 2, 2, 2, 2, 2, 2, 2, 2, 2, 2, 2, 2, 3 ),
 ( 0.000000000000000000, 1.000000000000000000 ),
 ( 0.000000000000000000, 0.005952380952380952051, 0.01190476190476190410, 0.01785714285714285615, 0.02380952380952380820, 0.02976190476190476025, 0.03571428571428571230, 0.04166666666666666435, 0.04761904761904761640, 0.05357142857142856845, 0.05952380952380952051, 0.06547619047619047949, 0.07142857142857142461, 0.07738095238095238360, 0.08333333333333332871, 0.08928571428571428770, 0.09523809523809523281, 0.1011904761904761918, 0.1071428571428571369, 0.1130952380952380959, 0.1190476190476190410, 0.1250000000000000000, 0.1309523809523809590, 0.1369047619047619180, 0.1428571428571428492, 0.1488095238095238082, 0.1547619047619047672, 0.1607142857142857262, 0.1666666666666666574, 0.1726190476190476164, 0.1785714285714285754, 0.1845238095238095344, 0.1904761904761904656, 0.1964285714285714246, 0.2023809523809523836, 0.2083333333333333426, 0.2142857142857142738, 0.2202380952380952328, 0.2261904761904761918, 0.2321428571428571508, 0.2380952380952380820, 0.2440476190476190410, 0.2500000000000000000, 0.2559523809523809312, 0.2619047619047619180, 0.2678571428571428492, 0.2738095238095238360, 0.2797619047619047672, 0.2857142857142856984, 0.2916666666666666852, 0.2976190476190476164, 0.3035714285714285476, 0.3095238095238095344, 0.3154761904761904656, 0.3214285714285714524, 0.3273809523809523836, 0.3333333333333333148, 0.3392857142857143016, 0.3452380952380952328, 0.3511904761904761640, 0.3571428571428571508, 0.3630952380952380820, 0.3690476190476190688, 0.3750000000000000000, 0.3809523809523809312, 0.3869047619047619180, 0.3928571428571428492, 0.3988095238095238360, 0.4047619047619047672, 0.4107142857142856984, 0.4166666666666666852, 0.4226190476190476164, 0.4285714285714285476, 0.4345238095238095344, 0.4404761904761904656, 0.4464285714285714524, 0.4523809523809523836, 0.4583333333333333148, 0.4642857142857143016, 0.4702380952380952328, 0.4761904761904761640, 0.4821428571428571508, 0.4880952380952380820, 0.4940476190476190688, 0.5000000000000000000, 0.5059523809523809312, 0.5119047619047618625, 0.5178571428571429047, 0.5238095238095238360, 0.5297619047619047672, 0.5357142857142856984, 0.5416666666666666297, 0.5476190476190476719, 0.5535714285714286031, 0.5595238095238095344, 0.5654761904761904656, 0.5714285714285713969, 0.5773809523809523281, 0.5833333333333333703, 0.5892857142857143016, 0.5952380952380952328, 0.6011904761904761640, 0.6071428571428570953, 0.6130952380952381375, 0.6190476190476190688, 0.6250000000000000000, 0.6309523809523809312, 0.6369047619047618625, 0.6428571428571429047, 0.6488095238095238360, 0.6547619047619047672, 0.6607142857142856984, 0.6666666666666666297, 0.6726190476190476719, 0.6785714285714286031, 0.6845238095238095344, 0.6904761904761904656, 0.6964285714285713969, 0.7023809523809523281, 0.7083333333333333703, 0.7142857142857143016, 0.7202380952380952328, 0.7261904761904761640, 0.7321428571428570953, 0.7380952380952381375, 0.7440476190476190688, 0.7500000000000000000, 0.7559523809523809312, 0.7619047619047618625, 0.7678571428571429047, 0.7738095238095238360, 0.7797619047619047672, 0.7857142857142856984, 0.7916666666666666297, 0.7976190476190476719, 0.8035714285714286031, 0.8095238095238095344, 0.8154761904761904656, 0.8214285714285713969, 0.8273809523809523281, 0.8333333333333333703, 0.8392857142857143016, 0.8452380952380952328, 0.8511904761904761640, 0.8571428571428570953, 0.8630952380952381375, 0.8690476190476190688, 0.8750000000000000000, 0.8809523809523809312, 0.8869047619047618625, 0.8928571428571429047, 0.8988095238095238360, 0.9047619047619047672, 0.9107142857142856984, 0.9166666666666666297, 0.9226190476190476719, 0.9285714285714286031, 0.9345238095238095344, 0.9404761904761904656, 0.9464285714285713969, 0.9523809523809523281, 0.9583333333333333703, 0.9642857142857143016 ),
 .UNSPECIFIED. ) 
 GEOMETRIC_REPRESENTATION_ITEM ( )  RATIONAL_B_SPLINE_SURFACE ( (
 ( 1.000000000000000000, 0.9659258262890683122, 1.000000000000000000, 0.9659258262890683122, 1.000000000000000000, 0.9659258262890683122, 1.000000000000000000, 0.9659258262890683122, 1.000000000000000000, 0.9659258262890683122, 1.000000000000000000, 0.9659258262890683122, 1.000000000000000000, 0.9659258262890683122, 1.000000000000000000, 0.9659258262890683122, 1.000000000000000000, 0.9659258262890683122, 1.000000000000000000, 0.9659258262890683122, 1.000000000000000000, 0.9659258262890683122, 1.000000000000000000, 0.9659258262890683122, 1.000000000000000000, 0.9659258262890683122, 1.000000000000000000, 0.9659258262890683122, 1.000000000000000000, 0.9659258262890683122, 1.000000000000000000, 0.9659258262890683122, 1.000000000000000000, 0.9659258262890683122, 1.000000000000000000, 0.9659258262890683122, 1.000000000000000000, 0.9659258262890683122, 1.000000000000000000, 0.9659258262890683122, 1.000000000000000000, 0.9659258262890683122, 1.000000000000000000, 0.9659258262890683122, 1.000000000000000000, 0.9659258262890683122, 1.000000000000000000, 0.9659258262890683122, 1.000000000000000000, 0.9659258262890683122, 1.000000000000000000, 0.9659258262890683122, 1.000000000000000000, 0.9659258262890683122, 1.000000000000000000, 0.9659258262890683122, 1.000000000000000000, 0.9659258262890683122, 1.000000000000000000, 0.9659258262890683122, 1.000000000000000000, 0.9659258262890683122, 1.000000000000000000, 0.9659258262890683122, 1.000000000000000000, 0.9659258262890683122, 1.000000000000000000, 0.9659258262890683122, 1.000000000000000000, 0.9659258262890683122, 1.000000000000000000, 0.9659258262890683122, 1.000000000000000000, 0.9659258262890683122, 1.000000000000000000, 0.9659258262890683122, 1.000000000000000000, 0.9659258262890683122, 1.000000000000000000, 0.9659258262890683122, 1.000000000000000000, 0.9659258262890683122, 1.000000000000000000, 0.9659258262890683122, 1.000000000000000000, 0.9659258262890683122, 1.000000000000000000, 0.9659258262890683122, 1.000000000000000000, 0.9659258262890683122, 1.000000000000000000, 0.9659258262890683122, 1.000000000000000000, 0.9659258262890683122, 1.000000000000000000, 0.9659258262890683122, 1.000000000000000000, 0.9659258262890683122, 1.000000000000000000, 0.9659258262890683122, 1.000000000000000000, 0.9659258262890683122, 1.000000000000000000, 0.9659258262890683122, 1.000000000000000000, 0.9659258262890683122, 1.000000000000000000, 0.9659258262890683122, 1.000000000000000000, 0.9659258262890683122, 1.000000000000000000, 0.9659258262890683122, 1.000000000000000000, 0.9659258262890683122, 1.000000000000000000, 0.9659258262890683122, 1.000000000000000000, 0.9659258262890683122, 1.000000000000000000, 0.9659258262890683122, 1.000000000000000000, 0.9659258262890683122, 1.000000000000000000, 0.9659258262890683122, 1.000000000000000000, 0.9659258262890683122, 1.000000000000000000, 0.9659258262890683122, 1.000000000000000000, 0.9659258262890683122, 1.000000000000000000, 0.9659258262890683122, 1.000000000000000000, 0.9659258262890683122, 1.000000000000000000, 0.9659258262890683122, 1.000000000000000000, 0.9659258262890683122, 1.000000000000000000, 0.9659258262890683122, 1.000000000000000000, 0.9659258262890683122, 1.000000000000000000, 0.9659258262890683122, 1.000000000000000000, 0.9659258262890683122, 1.000000000000000000, 0.9659258262890683122, 1.000000000000000000, 0.9659258262890683122, 1.000000000000000000, 0.9659258262890683122, 1.000000000000000000, 0.9659258262890683122, 1.000000000000000000, 0.9659258262890683122, 1.000000000000000000, 0.9659258262890683122, 1.000000000000000000, 0.9659258262890683122, 1.000000000000000000, 0.9659258262890683122, 1.000000000000000000, 0.9659258262890683122, 1.000000000000000000, 0.9659258262890683122, 1.000000000000000000, 0.9659258262890683122, 1.000000000000000000, 0.9659258262890683122, 1.000000000000000000, 0.9659258262890683122, 1.000000000000000000, 0.9659258262890683122, 1.000000000000000000, 0.9659258262890683122, 1.000000000000000000, 0.9659258262890683122, 1.000000000000000000, 0.9659258262890683122, 1.000000000000000000, 0.9659258262890683122, 1.000000000000000000, 0.9659258262890683122, 1.000000000000000000, 0.9659258262890683122, 1.000000000000000000, 0.9659258262890683122, 1.000000000000000000, 0.9659258262890683122, 1.000000000000000000, 0.9659258262890683122, 1.000000000000000000, 0.9659258262890683122, 1.000000000000000000, 0.9659258262890683122, 1.000000000000000000, 0.9659258262890683122, 1.000000000000000000, 0.9659258262890683122, 1.000000000000000000, 0.9659258262890683122, 1.000000000000000000, 0.9659258262890683122, 1.000000000000000000, 0.9659258262890683122, 1.000000000000000000, 0.9659258262890683122, 1.000000000000000000, 0.9659258262890683122, 1.000000000000000000, 0.9659258262890683122, 1.000000000000000000, 0.9659258262890683122, 1.000000000000000000, 0.9659258262890683122, 1.000000000000000000, 0.9659258262890683122, 1.000000000000000000, 0.9659258262890683122, 1.000000000000000000, 0.9659258262890683122, 1.000000000000000000, 0.9659258262890683122, 1.000000000000000000, 0.9659258262890683122, 1.000000000000000000, 0.9659258262890683122, 1.000000000000000000, 0.9659258262890683122, 1.000000000000000000, 0.9659258262890683122, 1.000000000000000000, 0.9659258262890683122, 1.000000000000000000, 0.9659258262890683122, 1.000000000000000000, 0.9659258262890683122, 1.000000000000000000, 0.9659258262890683122, 1.000000000000000000, 0.9659258262890683122, 1.000000000000000000, 0.9659258262890683122, 1.000000000000000000, 0.9659258262890683122, 1.000000000000000000, 0.9659258262890683122, 1.000000000000000000, 0.9659258262890683122, 1.000000000000000000, 0.9659258262890683122, 1.000000000000000000, 0.9659258262890683122, 1.000000000000000000, 0.9659258262890683122, 1.000000000000000000, 0.9659258262890683122, 1.000000000000000000, 0.9659258262890683122, 1.000000000000000000, 0.9659258262890683122, 1.000000000000000000, 0.9659258262890683122, 1.000000000000000000, 0.9659258262890683122, 1.000000000000000000, 0.9659258262890683122, 1.000000000000000000, 0.9659258262890683122, 1.000000000000000000, 0.9659258262890683122, 1.000000000000000000, 0.9659258262890683122, 1.000000000000000000, 0.9659258262890683122, 1.000000000000000000, 0.9659258262890683122, 1.000000000000000000, 0.9659258262890683122, 1.000000000000000000, 0.9659258262890683122, 1.000000000000000000, 0.9659258262890683122, 1.000000000000000000, 0.9659258262890683122, 1.000000000000000000, 0.9659258262890683122, 1.000000000000000000, 0.9659258262890683122, 1.000000000000000000, 0.9659258262890683122, 1.000000000000000000, 0.9659258262890683122, 1.000000000000000000, 0.9659258262890683122, 1.000000000000000000, 0.9659258262890683122, 1.000000000000000000, 0.9659258262890683122, 1.000000000000000000, 0.9659258262890683122, 1.000000000000000000, 0.9659258262890683122, 1.000000000000000000, 0.9659258262890683122, 1.000000000000000000, 0.9659258262890683122, 1.000000000000000000, 0.9659258262890683122, 1.000000000000000000, 0.9659258262890683122, 1.000000000000000000, 0.9659258262890683122, 1.000000000000000000, 0.9659258262890683122, 1.000000000000000000, 0.9659258262890683122, 1.000000000000000000, 0.9659258262890683122, 1.000000000000000000, 0.9659258262890683122, 1.000000000000000000, 0.9659258262890683122, 1.000000000000000000),
 ( 1.000000000000000000, 0.9659258262890683122, 1.000000000000000000, 0.9659258262890683122, 1.000000000000000000, 0.9659258262890683122, 1.000000000000000000, 0.9659258262890683122, 1.000000000000000000, 0.9659258262890683122, 1.000000000000000000, 0.9659258262890683122, 1.000000000000000000, 0.9659258262890683122, 1.000000000000000000, 0.9659258262890683122, 1.000000000000000000, 0.9659258262890683122, 1.000000000000000000, 0.9659258262890683122, 1.000000000000000000, 0.9659258262890683122, 1.000000000000000000, 0.9659258262890683122, 1.000000000000000000, 0.9659258262890683122, 1.000000000000000000, 0.9659258262890683122, 1.000000000000000000, 0.9659258262890683122, 1.000000000000000000, 0.9659258262890683122, 1.000000000000000000, 0.9659258262890683122, 1.000000000000000000, 0.9659258262890683122, 1.000000000000000000, 0.9659258262890683122, 1.000000000000000000, 0.9659258262890683122, 1.000000000000000000, 0.9659258262890683122, 1.000000000000000000, 0.9659258262890683122, 1.000000000000000000, 0.9659258262890683122, 1.000000000000000000, 0.9659258262890683122, 1.000000000000000000, 0.9659258262890683122, 1.000000000000000000, 0.9659258262890683122, 1.000000000000000000, 0.9659258262890683122, 1.000000000000000000, 0.9659258262890683122, 1.000000000000000000, 0.9659258262890683122, 1.000000000000000000, 0.9659258262890683122, 1.000000000000000000, 0.9659258262890683122, 1.000000000000000000, 0.9659258262890683122, 1.000000000000000000, 0.9659258262890683122, 1.000000000000000000, 0.9659258262890683122, 1.000000000000000000, 0.9659258262890683122, 1.000000000000000000, 0.9659258262890683122, 1.000000000000000000, 0.9659258262890683122, 1.000000000000000000, 0.9659258262890683122, 1.000000000000000000, 0.9659258262890683122, 1.000000000000000000, 0.9659258262890683122, 1.000000000000000000, 0.9659258262890683122, 1.000000000000000000, 0.9659258262890683122, 1.000000000000000000, 0.9659258262890683122, 1.000000000000000000, 0.9659258262890683122, 1.000000000000000000, 0.9659258262890683122, 1.000000000000000000, 0.9659258262890683122, 1.000000000000000000, 0.9659258262890683122, 1.000000000000000000, 0.9659258262890683122, 1.000000000000000000, 0.9659258262890683122, 1.000000000000000000, 0.9659258262890683122, 1.000000000000000000, 0.9659258262890683122, 1.000000000000000000, 0.9659258262890683122, 1.000000000000000000, 0.9659258262890683122, 1.000000000000000000, 0.9659258262890683122, 1.000000000000000000, 0.9659258262890683122, 1.000000000000000000, 0.9659258262890683122, 1.000000000000000000, 0.9659258262890683122, 1.000000000000000000, 0.9659258262890683122, 1.000000000000000000, 0.9659258262890683122, 1.000000000000000000, 0.9659258262890683122, 1.000000000000000000, 0.9659258262890683122, 1.000000000000000000, 0.9659258262890683122, 1.000000000000000000, 0.9659258262890683122, 1.000000000000000000, 0.9659258262890683122, 1.000000000000000000, 0.9659258262890683122, 1.000000000000000000, 0.9659258262890683122, 1.000000000000000000, 0.9659258262890683122, 1.000000000000000000, 0.9659258262890683122, 1.000000000000000000, 0.9659258262890683122, 1.000000000000000000, 0.9659258262890683122, 1.000000000000000000, 0.9659258262890683122, 1.000000000000000000, 0.9659258262890683122, 1.000000000000000000, 0.9659258262890683122, 1.000000000000000000, 0.9659258262890683122, 1.000000000000000000, 0.9659258262890683122, 1.000000000000000000, 0.9659258262890683122, 1.000000000000000000, 0.9659258262890683122, 1.000000000000000000, 0.9659258262890683122, 1.000000000000000000, 0.9659258262890683122, 1.000000000000000000, 0.9659258262890683122, 1.000000000000000000, 0.9659258262890683122, 1.000000000000000000, 0.9659258262890683122, 1.000000000000000000, 0.9659258262890683122, 1.000000000000000000, 0.9659258262890683122, 1.000000000000000000, 0.9659258262890683122, 1.000000000000000000, 0.9659258262890683122, 1.000000000000000000, 0.9659258262890683122, 1.000000000000000000, 0.9659258262890683122, 1.000000000000000000, 0.9659258262890683122, 1.000000000000000000, 0.9659258262890683122, 1.000000000000000000, 0.9659258262890683122, 1.000000000000000000, 0.9659258262890683122, 1.000000000000000000, 0.9659258262890683122, 1.000000000000000000, 0.9659258262890683122, 1.000000000000000000, 0.9659258262890683122, 1.000000000000000000, 0.9659258262890683122, 1.000000000000000000, 0.9659258262890683122, 1.000000000000000000, 0.9659258262890683122, 1.000000000000000000, 0.9659258262890683122, 1.000000000000000000, 0.9659258262890683122, 1.000000000000000000, 0.9659258262890683122, 1.000000000000000000, 0.9659258262890683122, 1.000000000000000000, 0.9659258262890683122, 1.000000000000000000, 0.9659258262890683122, 1.000000000000000000, 0.9659258262890683122, 1.000000000000000000, 0.9659258262890683122, 1.000000000000000000, 0.9659258262890683122, 1.000000000000000000, 0.9659258262890683122, 1.000000000000000000, 0.9659258262890683122, 1.000000000000000000, 0.9659258262890683122, 1.000000000000000000, 0.9659258262890683122, 1.000000000000000000, 0.9659258262890683122, 1.000000000000000000, 0.9659258262890683122, 1.000000000000000000, 0.9659258262890683122, 1.000000000000000000, 0.9659258262890683122, 1.000000000000000000, 0.9659258262890683122, 1.000000000000000000, 0.9659258262890683122, 1.000000000000000000, 0.9659258262890683122, 1.000000000000000000, 0.9659258262890683122, 1.000000000000000000, 0.9659258262890683122, 1.000000000000000000, 0.9659258262890683122, 1.000000000000000000, 0.9659258262890683122, 1.000000000000000000, 0.9659258262890683122, 1.000000000000000000, 0.9659258262890683122, 1.000000000000000000, 0.9659258262890683122, 1.000000000000000000, 0.9659258262890683122, 1.000000000000000000, 0.9659258262890683122, 1.000000000000000000, 0.9659258262890683122, 1.000000000000000000, 0.9659258262890683122, 1.000000000000000000, 0.9659258262890683122, 1.000000000000000000, 0.9659258262890683122, 1.000000000000000000, 0.9659258262890683122, 1.000000000000000000, 0.9659258262890683122, 1.000000000000000000, 0.9659258262890683122, 1.000000000000000000, 0.9659258262890683122, 1.000000000000000000, 0.9659258262890683122, 1.000000000000000000, 0.9659258262890683122, 1.000000000000000000, 0.9659258262890683122, 1.000000000000000000, 0.9659258262890683122, 1.000000000000000000, 0.9659258262890683122, 1.000000000000000000, 0.9659258262890683122, 1.000000000000000000, 0.9659258262890683122, 1.000000000000000000, 0.9659258262890683122, 1.000000000000000000, 0.9659258262890683122, 1.000000000000000000, 0.9659258262890683122, 1.000000000000000000, 0.9659258262890683122, 1.000000000000000000, 0.9659258262890683122, 1.000000000000000000, 0.9659258262890683122, 1.000000000000000000, 0.9659258262890683122, 1.000000000000000000, 0.9659258262890683122, 1.000000000000000000, 0.9659258262890683122, 1.000000000000000000, 0.9659258262890683122, 1.000000000000000000, 0.9659258262890683122, 1.000000000000000000, 0.9659258262890683122, 1.000000000000000000, 0.9659258262890683122, 1.000000000000000000, 0.9659258262890683122, 1.000000000000000000, 0.9659258262890683122, 1.000000000000000000, 0.9659258262890683122, 1.000000000000000000, 0.9659258262890683122, 1.000000000000000000, 0.9659258262890683122, 1.000000000000000000, 0.9659258262890683122, 1.000000000000000000, 0.9659258262890683122, 1.000000000000000000) ) ) 
 REPRESENTATION_ITEM ( '' )  SURFACE ( )  );
#93944=CARTESIAN_POINT ( 'NONE',  ( 19.42250999205614193, 30.14701867748817321, 5.440088680355555262 ) ) ;
#93945=CARTESIAN_POINT ( 'NONE',  ( 15.44008868035555793, 41.39701867748817676, -9.422509992056140149 ) ) ;
#93946=CARTESIAN_POINT ( 'NONE',  ( 16.40814093676323893, 0.7903013365970867898, 11.09922568453595026 ) ) ;
#93947=SURFACE_STYLE_FILL_AREA ( #87424 ) ;
#93948=CARTESIAN_POINT ( 'NONE',  ( 16.40814093676324603, 62.45696800326376064, -11.09922568453594671 ) ) ;
#93949=CARTESIAN_POINT ( 'NONE',  ( 5.076628168052704559, 15.17559781766745175, -8.527530157486179263 ) ) ;
#93952=CARTESIAN_POINT ( 'NONE',  ( -0.8801773607111008646, 28.27201867748817321, 2.915334737309923430 ) ) ;
#93953=CARTESIAN_POINT ( 'NONE',  ( -1.099225684535947600, 29.54030133659708923, 6.408140936763237150 ) ) ;
#93954=CARTESIAN_POINT ( 'NONE',  ( -0.2418659066527710233, 55.11633188102327807, 6.114288769123046308 ) ) ;
#93956=CARTESIAN_POINT ( 'NONE',  ( 0.1532563361054083140, 61.00893115100078745, 1.131784320476157264E-15 ) ) ;
#93957=CARTESIAN_POINT ( 'NONE',  ( 10.00000000000000178, 54.31368534415484106, 10.88017736071110342 ) ) ;
#93958=CARTESIAN_POINT ( 'NONE',  ( 5.076628168052703671, 16.84226448433411960, 8.527530157486179263 ) ) ;
#93959=CARTESIAN_POINT ( 'NONE',  ( 10.00000000000000178, 30.37363466993042138, 12.81628187352647608 ) ) ;
#93960=CARTESIAN_POINT ( 'NONE',  ( 10.00000000000000178, 59.31368534415484106, 10.88017736071110342 ) ) ;
#93963=CARTESIAN_POINT ( 'NONE',  ( 0.5774900079438590739, 2.647018677488170990, -5.440088680355550821 ) ) ;
#93964=CARTESIAN_POINT ( 'NONE',  ( -2.816281873526473856, 59.12363466993042493, 9.499525473075851096E-16 ) ) ;
#93965=CARTESIAN_POINT ( 'NONE',  ( 20.36894250292379738, 24.92874883491396787, -10.36894250292379027 ) ) ;
#93966=EDGE_CURVE ( 'NONE', #25008, #32248, #17926, .T. ) ;
#93967=CARTESIAN_POINT ( 'NONE',  ( 7.361572987183170547, 17.05059781766745530, 9.846743663894590881 ) ) ;
#93968=CARTESIAN_POINT ( 'NONE',  ( 17.96484262340118221, 9.938685344154837509, 7.964842623401181321 ) ) ;
#93969=CARTESIAN_POINT ( 'NONE',  ( 5.076628168052703671, 16.84226448433411960, 8.527530157486179263 ) ) ;
#93970=CARTESIAN_POINT ( 'NONE',  ( 2.917880565312950480, 60.97041550158063927, -12.26659068614894821 ) ) ;
#93972=CARTESIAN_POINT ( 'NONE',  ( -0.8801773607110991993, 2.855352010821504471, -2.915334737309923874 ) ) ;
#93974=CARTESIAN_POINT ( 'NONE',  ( 17.96484262340118221, 24.93868534415484461, 7.964842623401181321 ) ) ;
#93975=ADVANCED_FACE ( 'NONE', ( #48410 ), #95901, .T. ) ;
#93978=ORIENTED_EDGE ( 'NONE', *, *, #28684, .F. ) ;
#93980=CARTESIAN_POINT ( 'NONE',  ( 19.42250999205614548, 15.98035201082150714, -5.440088680355545492 ) ) ;
#93981=CARTESIAN_POINT ( 'NONE',  ( 5.076628168052703671, 56.84226448433412315, 8.527530157486179263 ) ) ;
#93982=CARTESIAN_POINT ( 'NONE',  ( 19.38216949554541202, 45.99863466993041072, 9.382169495545424454 ) ) ;
#93985=CARTESIAN_POINT ( 'NONE',  ( 13.79529636645030344, 23.26208216824730002, 14.16423886937410614 ) ) ;
#93986=CARTESIAN_POINT ( 'NONE',  ( 15.44008868035555260, 34.73035201082151247, 9.422509992056143702 ) ) ;
#93987=CARTESIAN_POINT ( 'NONE',  ( 20.88017736071110875, 15.77201867748817143, -2.915334737309920765 ) ) ;
#93988=CARTESIAN_POINT ( 'NONE',  ( 14.92337183194729988, 54.34226448433412315, -8.527530157486177487 ) ) ;
#93990=CARTESIAN_POINT ( 'NONE',  ( 18.52753015748617571, 33.09226448433411605, 4.923371831947298993 ) ) ;
#93991=CARTESIAN_POINT ( 'NONE',  ( 10.00000000000000178, 12.25893115100078568, 9.846743663894594434 ) ) ;
#93995=CARTESIAN_POINT ( 'NONE',  ( 2.791683348922237240, 10.38393115100078390, -7.208316651077763204 ) ) ;
#93996=CARTESIAN_POINT ( 'NONE',  ( 19.84674366389459266, 63.71726448433412315, -2.638427012816827677 ) ) ;
#93997=CARTESIAN_POINT ( 'NONE',  ( 0.5774900079438607392, 48.48035201082150536, 5.440088680355550821 ) ) ;
#93998=CARTESIAN_POINT ( 'NONE',  ( 4.559911319644449179, 8.897018677488171434, 9.422509992056141925 ) ) ;
#93999=CARTESIAN_POINT ( 'NONE',  ( -2.816281873526473856, 39.12363466993041783, 9.499525473075851096E-16 ) ) ;
#94000=CARTESIAN_POINT ( 'NONE',  ( 20.36894250292379738, 34.92874883491396076, -10.36894250292379027 ) ) ;
#94002=CARTESIAN_POINT ( 'NONE',  ( 19.38216949554541557, 57.24863466993042493, -9.382169495545420901 ) ) ;
#94003=EDGE_LOOP ( 'NONE', ( #65264, #46762, #96402, #34258 ) ) ;
#94004=CARTESIAN_POINT ( 'NONE',  ( 7.361572987183170547, 62.05059781766745886, 9.846743663894590881 ) ) ;
#94005=CARTESIAN_POINT ( 'NONE',  ( 19.42250999205614193, 20.14701867748817321, 5.440088680355555262 ) ) ;
#94006=ORIENTED_EDGE ( 'NONE', *, *, #3637, .T. ) ;
#94007=CARTESIAN_POINT ( 'NONE',  ( 5.076628168052704559, 5.175597817667451750, -8.527530157486179263 ) ) ;
#94008=DIRECTION ( 'NONE',  ( 1.000000000000000000, 0.000000000000000000, 0.000000000000000000 ) ) ;
#94010=CARTESIAN_POINT ( 'NONE',  ( 7.361572987183170547, 7.050597817667451750, 9.846743663894590881 ) ) ;
#94011=CARTESIAN_POINT ( 'NONE',  ( 0.5774900079438607392, 63.48035201082149825, 5.440088680355550821 ) ) ;
#94014=CARTESIAN_POINT ( 'NONE',  ( -0.8801773607111008646, 53.27201867748816966, 2.915334737309923430 ) ) ;
#94016=CARTESIAN_POINT ( 'NONE',  ( -0.8801773607110991993, 62.85535201082150536, -2.915334737309923874 ) ) ;
#94017=CARTESIAN_POINT ( 'NONE',  ( 5.076628168052704559, 0.1755978176674514724, -8.527530157486179263 ) ) ;
#94020=CARTESIAN_POINT ( 'NONE',  ( 2.791683348922237240, 55.38393115100078745, -7.208316651077763204 ) ) ;
#94021=EDGE_LOOP ( 'NONE', ( #58871, #24930, #72804, #86377, #66883, #33679, #58139 ) ) ;
#94024=CARTESIAN_POINT ( 'NONE',  ( -0.3689425029237881626, 7.428748834913967869, 10.36894250292379027 ) ) ;
#94025=CARTESIAN_POINT ( 'NONE',  ( 16.40814093676324603, 62.45696800326376064, -11.09922568453594671 ) ) ;
#94026=CARTESIAN_POINT ( 'NONE',  ( 22.26659068614894466, 3.887082168247300906, 7.082119434687054849 ) ) ;
#94028=CARTESIAN_POINT ( 'NONE',  ( -2.266590686148945544, 31.38708216824730002, -7.082119434687050408 ) ) ;
#94030=CARTESIAN_POINT ( 'NONE',  ( 18.95785429995050819, 57.24216108172005590, 6.499999999999926281 ) ) ;
#94031=CARTESIAN_POINT ( 'NONE',  ( 13.79529636645031943, 5.345415501580634832, -14.16423886937409904 ) ) ;
#94032=CARTESIAN_POINT ( 'NONE',  ( 15.44008868035555260, 14.73035201082150536, 9.422509992056143702 ) ) ;
#94035=( NAMED_UNIT ( * ) SI_UNIT ( $, .STERADIAN. ) SOLID_ANGLE_UNIT ( ) );
#94036=CARTESIAN_POINT ( 'NONE',  ( 10.00000000000000000, 14.75893115100078568, -9.846743663894594434 ) ) ;
#94037=CARTESIAN_POINT ( 'NONE',  ( 13.43411237798106583, 37.66530133659708923, -12.81628187352647252 ) ) ;
#94038=CARTESIAN_POINT ( 'NONE',  ( 2.791683348922240793, 31.63393115100078745, 7.208316651077764092 ) ) ;
#94039=FACE_OUTER_BOUND ( 'NONE', #9803, .T. ) ;
#94040=CARTESIAN_POINT ( 'NONE',  ( -2.816281873526473856, 34.33196800326376064, 3.434112377981055619 ) ) ;
#94042=CARTESIAN_POINT ( 'NONE',  ( 12.63842701281683922, 24.55059781766745175, -9.846743663894590881 ) ) ;
#94044=CARTESIAN_POINT ( 'NONE',  ( -4.164238869374099927, 17.01208216824730357, 3.795296366450308767 ) ) ;
#94047=CARTESIAN_POINT ( 'NONE',  ( 15.44008868035555260, 34.73035201082151247, 9.422509992056143702 ) ) ;
#94048=CARTESIAN_POINT ( 'NONE',  ( 10.00000000000000178, 28.05374883491396787, 14.16423886937410082 ) ) ;
#94049=CARTESIAN_POINT ( 'NONE',  ( 18.52753015748617571, 58.09226448433411605, 4.923371831947298993 ) ) ;
#94050=CARTESIAN_POINT ( 'NONE',  ( 5.076628168052703671, 6.842264484334118713, 8.527530157486179263 ) ) ;
#94051=CARTESIAN_POINT ( 'NONE',  ( 10.00000000000000000, 57.87363466993042493, -12.81628187352647608 ) ) ;
#94053=CARTESIAN_POINT ( 'NONE',  ( 0.5774900079438607392, 23.48035201082150536, 5.440088680355550821 ) ) ;
#94054=CARTESIAN_POINT ( 'NONE',  ( 22.81628187352648496, 16.83196800326374998, -3.434112377981050290 ) ) ;
#94055=CARTESIAN_POINT ( 'NONE',  ( -2.816281873526473856, 24.33196800326375353, 3.434112377981055619 ) ) ;
#94056=CARTESIAN_POINT ( 'NONE',  ( 10.00000000000000178, 42.25893115100078745, 9.846743663894594434 ) ) ;
#94059=DIRECTION ( 'NONE',  ( -0.000000000000000000, 1.000000000000000000, -0.000000000000000000 ) ) ;
#94064=CARTESIAN_POINT ( 'NONE',  ( 20.88017736071110164, 50.35535201082151247, 2.915334737309930979 ) ) ;
#94065=CARTESIAN_POINT ( 'NONE',  ( 2.035157376598822676, 57.43868534415484106, -7.964842623401177768 ) ) ;
#94068=EDGE_CURVE ( 'NONE', #91046, #29895, #36810, .T. ) ;
#94069=CARTESIAN_POINT ( 'NONE',  ( 20.88017736071110164, 5.355352010821503583, 2.915334737309930979 ) ) ;
#94070=CARTESIAN_POINT ( 'NONE',  ( 21.09922568453594849, 1.206968003263753531, 6.408140936763242479 ) ) ;
#94071=CARTESIAN_POINT ( 'NONE',  ( 20.88017736071110875, 15.77201867748817143, -2.915334737309920765 ) ) ;
#94074=CARTESIAN_POINT ( 'NONE',  ( -2.816281873526473856, 19.33196800326375708, 3.434112377981055619 ) ) ;
#94075=VERTEX_POINT ( 'NONE', #34379 ) ;
#94076=CARTESIAN_POINT ( 'NONE',  ( 12.91533473730993009, 56.60535201082151247, -10.88017736071109987 ) ) ;
#94077=CARTESIAN_POINT ( 'NONE',  ( 19.84674366389459621, 43.50893115100078745, 7.409399052514197653E-17 ) ) ;
#94078=CARTESIAN_POINT ( 'NONE',  ( 10.00000000000000000, 2.873634669930420049, -12.81628187352647608 ) ) ;
#94081=CARTESIAN_POINT ( 'NONE',  ( 7.084665262690076126, 32.02201867748816966, -10.88017736071110164 ) ) ;
#94082=CARTESIAN_POINT ( 'NONE',  ( 4.559911319644449179, 37.23035201082150536, -9.422509992056141925 ) ) ;
#94083=CARTESIAN_POINT ( 'NONE',  ( 22.26659068614895176, 49.72041550158063927, -7.082119434687042414 ) ) ;
#94084=CARTESIAN_POINT ( 'NONE',  ( 0.1532563361054100626, 35.80059781766745175, -2.638427012816831230 ) ) ;
#94085=AXIS2_PLACEMENT_3D ( 'NONE', #46446, #24450, #91943 ) ;
#94086=CARTESIAN_POINT ( 'NONE',  ( -0.8801773607110991993, 62.85535201082150536, -2.915334737309923874 ) ) ;
#94088=CARTESIAN_POINT ( 'NONE',  ( 17.08211943468705840, 20.13708216824730357, -12.26659068614894466 ) ) ;
#94091=CARTESIAN_POINT ( 'NONE',  ( 17.08211943468705840, 45.13708216824730357, -12.26659068614894466 ) ) ;
#94092=CARTESIAN_POINT ( 'NONE',  ( 24.16423886937409904, 39.09541550158062506, 3.795296366450317205 ) ) ;
#94093=CARTESIAN_POINT ( 'NONE',  ( 19.84674366389459621, 13.50893115100078568, 7.409399052514197653E-17 ) ) ;
#94094=CARTESIAN_POINT ( 'NONE',  ( -2.816281873526473856, 19.12363466993042138, 9.499525473075851096E-16 ) ) ;
#94096=DIRECTION ( 'NONE',  ( 0.000000000000000000, 1.000000000000000000, 0.000000000000000000 ) ) ;
#94097=CARTESIAN_POINT ( 'NONE',  ( -0.8801773607110991993, 57.85535201082149825, -2.915334737309923874 ) ) ;
#94098=CARTESIAN_POINT ( 'NONE',  ( 19.38216949554541557, 32.24863466993041783, -9.382169495545420901 ) ) ;
#94099=CARTESIAN_POINT ( 'NONE',  ( 17.08211943468705130, 48.47041550158063927, 12.26659068614894998 ) ) ;
#94100=CARTESIAN_POINT ( 'NONE',  ( 0.5774900079438607392, 68.48035201082150536, 5.440088680355550821 ) ) ;
#94103=DIRECTION ( 'NONE',  ( -0.000000000000000000, 1.000000000000000000, -0.000000000000000000 ) ) ;
#94105=CARTESIAN_POINT ( 'NONE',  ( 13.79529636645031943, 5.345415501580634832, -14.16423886937409904 ) ) ;
#94106=CARTESIAN_POINT ( 'NONE',  ( 4.559911319644449179, 8.897018677488173211, 9.422509992056141925 ) ) ;
#94107=CARTESIAN_POINT ( 'NONE',  ( -0.8801773607111008646, 8.272018677488171434, 2.915334737309923430 ) ) ;
#94108=CARTESIAN_POINT ( 'NONE',  ( 19.84674366389459621, 38.50893115100078745, 7.409399052514197653E-17 ) ) ;
#94109=CARTESIAN_POINT ( 'NONE',  ( 0.6178305044545838731, -0.2513653300695798953, 9.382169495545420901 ) ) ;
#94113=CARTESIAN_POINT ( 'NONE',  ( 13.43411237798105340, 20.58196800326374643, 12.81628187352647963 ) ) ;
#94115=CARTESIAN_POINT ( 'NONE',  ( 6.204703633549690345, 52.84541550158062506, 14.16423886937410082 ) ) ;
#94117=CARTESIAN_POINT ( 'NONE',  ( 24.16423886937410614, 59.51208216824728936, -3.795296366450302550 ) ) ;
#94119=CARTESIAN_POINT ( 'NONE',  ( 17.96484262340118221, 36.18868534415484106, -7.964842623401177768 ) ) ;
#94121=CARTESIAN_POINT ( 'NONE',  ( 17.96484262340118221, 36.18868534415484106, -7.964842623401177768 ) ) ;
#94122=CARTESIAN_POINT ( 'NONE',  ( 17.96484262340118221, 41.18868534415484106, -7.964842623401177768 ) ) ;
#94123=CARTESIAN_POINT ( 'NONE',  ( 15.44008868035555260, 64.73035201082151957, 9.422509992056143702 ) ) ;
#94124=CARTESIAN_POINT ( 'NONE',  ( 17.96484262340118221, 29.93868534415484106, 7.964842623401181321 ) ) ;
#94126=CARTESIAN_POINT ( 'NONE',  ( -0.1503990784575277573, 33.10158574516643171, 6.262539305110076171 ) ) ;
#94127=CARTESIAN_POINT ( 'NONE',  ( 17.20831665107776587, 19.13393115100078035, -7.208316651077762316 ) ) ;
#94131=CARTESIAN_POINT ( 'NONE',  ( 10.00000000000000178, 42.25893115100078745, 9.846743663894594434 ) ) ;
#94133=CARTESIAN_POINT ( 'NONE',  ( 19.38216949554541557, 47.24863466993041783, -9.382169495545420901 ) ) ;
#94136=CARTESIAN_POINT ( 'NONE',  ( -45.94000000000001904, 103.9981609152045507, 5.961202730336936817 ) ) ;
#94137=CARTESIAN_POINT ( 'NONE',  ( 0.5774900079438607392, 53.48035201082151247, 5.440088680355550821 ) ) ;
#94139=CARTESIAN_POINT ( 'NONE',  ( -2.266590686148945544, 46.38708216824730357, -7.082119434687050408 ) ) ;
#94143=CARTESIAN_POINT ( 'NONE',  ( 19.84674366389459266, 13.71726448433411782, -2.638427012816827677 ) ) ;
#94146=CARTESIAN_POINT ( 'NONE',  ( 12.63842701281683034, 57.46726448433411605, 9.846743663894596210 ) ) ;
#94147=CARTESIAN_POINT ( 'NONE',  ( 20.88017736071110519, 65.56368534415483396, 2.639326808657452039E-16 ) ) ;
#94148=CARTESIAN_POINT ( 'NONE',  ( -0.1503990784575328643, 65.12777174578613426, 6.262539305110068177 ) ) ;
#94149=CARTESIAN_POINT ( 'NONE',  ( 19.84674366389459266, 53.71726448433411605, -2.638427012816827677 ) ) ;
#94153=EDGE_CURVE ( 'NONE', #58602, #28561, #87404, .T. ) ;
#94154=CARTESIAN_POINT ( 'NONE',  ( 24.16423886937409904, 64.09541550158064638, 3.795296366450317205 ) ) ;
#94156=CARTESIAN_POINT ( 'NONE',  ( 12.91533473730993009, 41.60535201082149825, -10.88017736071109987 ) ) ;
#94157=CARTESIAN_POINT ( 'NONE',  ( 19.38216949554541557, 12.24863466993041961, -9.382169495545420901 ) ) ;
#94162=CARTESIAN_POINT ( 'NONE',  ( 2.791683348922240793, 56.63393115100078035, 7.208316651077764092 ) ) ;
#94164=CARTESIAN_POINT ( 'NONE',  ( 0.6178305044545818747, 13.49863466993041783, -9.382169495545419124 ) ) ;
#94165=CARTESIAN_POINT ( 'NONE',  ( 4.559911319644449179, 18.89701867748817321, 9.422509992056141925 ) ) ;
#94167=CARTESIAN_POINT ( 'NONE',  ( 17.08211943468705840, 35.13708216824730357, -12.26659068614894466 ) ) ;
#94168=CARTESIAN_POINT ( 'NONE',  ( 24.16423886937410614, 34.30374883491396787, 8.672049930838204340E-16 ) ) ;
#94169=CARTESIAN_POINT ( 'NONE',  ( 10.00000000000000178, 4.313685344154837509, 10.88017736071110342 ) ) ;
#94170=CARTESIAN_POINT ( 'NONE',  ( 17.20831665107776587, 49.13393115100078745, -7.208316651077762316 ) ) ;
#94171=CARTESIAN_POINT ( 'NONE',  ( -1.099225684535947600, 38.70696800326375353, -6.408140936763238038 ) ) ;
#94172=CARTESIAN_POINT ( 'NONE',  ( 12.91533473730992121, 14.52201867748817143, 10.88017736071110164 ) ) ;
#94174=CARTESIAN_POINT ( 'NONE',  ( 12.63842701281683922, 34.55059781766745886, -9.846743663894590881 ) ) ;
#94175=CARTESIAN_POINT ( 'NONE',  ( -0.8801773607110991993, 42.85535201082150536, -2.915334737309923874 ) ) ;
#94176=CARTESIAN_POINT ( 'NONE',  ( 3.591859063236763294, 8.290301336597087456, -11.09922568453595026 ) ) ;
#94177=CARTESIAN_POINT ( 'NONE',  ( 24.16423886937410614, 19.30374883491397142, 8.672049930838204340E-16 ) ) ;
#94180=UNCERTAINTY_MEASURE_WITH_UNIT (LENGTH_MEASURE( 1.000000000000000082E-05 ), #15588, 'distance_accuracy_value', 'NONE');
#94181=CARTESIAN_POINT ( 'NONE',  ( 14.92337183194729988, 29.34226448433411960, -8.527530157486177487 ) ) ;
#94182=CARTESIAN_POINT ( 'NONE',  ( -2.816281873526473856, 49.12363466993042493, 9.499525473075851096E-16 ) ) ;
#94183=CARTESIAN_POINT ( 'NONE',  ( 12.63842701281683034, 52.46726448433413026, 9.846743663894596210 ) ) ;
#94186=CARTESIAN_POINT ( 'NONE',  ( 12.91533473730992121, 4.522018677488170546, 10.88017736071110164 ) ) ;
#94187=CARTESIAN_POINT ( 'NONE',  ( -0.3689425029237881626, 12.42874883491396609, 10.36894250292379027 ) ) ;
#94188=CARTESIAN_POINT ( 'NONE',  ( -0.8801773607110991993, 67.85535201082151957, -2.915334737309923874 ) ) ;
#94189=CARTESIAN_POINT ( 'NONE',  ( 7.361572987183170547, 52.05059781766745175, 9.846743663894590881 ) ) ;
#94190=CARTESIAN_POINT ( 'NONE',  ( 19.42250999205614193, 25.14701867748817321, 5.440088680355555262 ) ) ;
#94191=DIRECTION ( 'NONE',  ( 1.000000000000000000, 0.000000000000000000, 0.000000000000000000 ) ) ;
#94192=CARTESIAN_POINT ( 'NONE',  ( 12.63842701281683922, 64.55059781766745175, -9.846743663894590881 ) ) ;
#94197=VERTEX_POINT ( 'NONE', #22735 ) ;
#94200=CARTESIAN_POINT ( 'NONE',  ( -2.266590686148945544, 6.387082168247300906, -7.082119434687050408 ) ) ;
#94201=CARTESIAN_POINT ( 'NONE',  ( -4.164238869374098151, 1.595415501580634388, -3.795296366450310543 ) ) ;
#94202=CARTESIAN_POINT ( 'NONE',  ( 13.79529636645030344, 48.26208216824728936, 14.16423886937410614 ) ) ;
#94203=CARTESIAN_POINT ( 'NONE',  ( 2.791683348922237240, 60.38393115100078745, -7.208316651077763204 ) ) ;
#94204=CARTESIAN_POINT ( 'NONE',  ( 14.92337183194729633, 27.67559781766745530, 8.527530157486181039 ) ) ;
#94206=CARTESIAN_POINT ( 'NONE',  ( 7.084665262690076126, 14.10535201082150358, 10.88017736071109987 ) ) ;
#94207=CARTESIAN_POINT ( 'NONE',  ( 5.076628168052704559, 65.17559781766745175, -8.527530157486179263 ) ) ;
#94208=FILL_AREA_STYLE ('',( #16261 ) ) ;
#94209=CARTESIAN_POINT ( 'NONE',  ( 22.26659068614894466, 38.88708216824731068, 7.082119434687054849 ) ) ;
#94210=CARTESIAN_POINT ( 'NONE',  ( -2.266590686148945544, 66.38708216824730357, -7.082119434687050408 ) ) ;
#94213=CARTESIAN_POINT ( 'NONE',  ( 4.559911319644449179, 63.89701867748817676, 9.422509992056141925 ) ) ;
#94214=CARTESIAN_POINT ( 'NONE',  ( 1.472469842513823179, 16.42559781766745175, 4.923371831947296329 ) ) ;
#94218=CARTESIAN_POINT ( 'NONE',  ( 21.92686044187657401, 30.37045670184114599, -3.195792623639525765 ) ) ;
#94220=CARTESIAN_POINT ( 'NONE',  ( 19.84674366389459621, 23.50893115100078390, 7.409399052514197653E-17 ) ) ;
#94222=CARTESIAN_POINT ( 'NONE',  ( -4.164238869374099927, 37.01208216824731068, 3.795296366450308767 ) ) ;
#94223=CARTESIAN_POINT ( 'NONE',  ( 7.361572987183169658, 29.96726448433411960, -9.846743663894592657 ) ) ;
#94224=CARTESIAN_POINT ( 'NONE',  ( 20.88017736071110875, 45.77201867748816966, -2.915334737309920765 ) ) ;
#94225=CARTESIAN_POINT ( 'NONE',  ( 19.42250999205614548, 45.98035201082150536, -5.440088680355545492 ) ) ;
#94226=CARTESIAN_POINT ( 'NONE',  ( 0.1077916266722479394, 2.240628644642390643, -6.478736007405952790 ) ) ;
#94229=CARTESIAN_POINT ( 'NONE',  ( -2.266590686148945544, 6.387082168247300906, -7.082119434687050408 ) ) ;
#94230=VERTEX_POINT ( 'NONE', #76702 ) ;
#94232=CARTESIAN_POINT ( 'NONE',  ( 2.791683348922240793, 1.633931151000784565, 7.208316651077764092 ) ) ;
#94233=CARTESIAN_POINT ( 'NONE',  ( 13.43411237798106583, 37.66530133659708923, -12.81628187352647252 ) ) ;
#94234=CARTESIAN_POINT ( 'NONE',  ( -42.70923076923077844, 104.8461538461538396, -9.500000000000000000 ) ) ;
#94235=CARTESIAN_POINT ( 'NONE',  ( 2.791683348922240793, 21.63393115100078745, 7.208316651077764092 ) ) ;
#94238=CARTESIAN_POINT ( 'NONE',  ( 1.472469842513823179, 36.42559781766745175, 4.923371831947296329 ) ) ;
#94240=CARTESIAN_POINT ( 'NONE',  ( 15.44008868035555793, 61.39701867748817676, -9.422509992056140149 ) ) ;
#94243=CARTESIAN_POINT ( 'NONE',  ( 4.559911319644449179, 63.89701867748817676, 9.422509992056141925 ) ) ;
#94246=CARTESIAN_POINT ( 'NONE',  ( 0.1532563361054083140, 11.00893115100078568, 1.131784320476157264E-15 ) ) ;
#94247=CARTESIAN_POINT ( 'NONE',  ( 22.81628187352648496, 6.831968003263753531, -3.434112377981050290 ) ) ;
#94251=CARTESIAN_POINT ( 'NONE',  ( 7.361572987183169658, 44.96726448433412315, -9.846743663894592657 ) ) ;
#94252=CARTESIAN_POINT ( 'NONE',  ( 0.6178305044545838731, 64.74863466993043914, 9.382169495545420901 ) ) ;
#94253=CARTESIAN_POINT ( 'NONE',  ( 17.08211943468705840, 10.13708216824730179, -12.26659068614894466 ) ) ;
#94254=CARTESIAN_POINT ( 'NONE',  ( 1.472469842513823179, 31.42559781766745530, 4.923371831947296329 ) ) ;
#94255=CARTESIAN_POINT ( 'NONE',  ( 22.81628187352647785, 36.41530133659707502, 3.434112377981063169 ) ) ;
#94257=CARTESIAN_POINT ( 'NONE',  ( 0.5774900079438590739, 22.64701867748817321, -5.440088680355550821 ) ) ;
#94258=CARTESIAN_POINT ( 'NONE',  ( -0.8801773607111008646, 43.27201867748817676, 2.915334737309923430 ) ) ;
#94260=CARTESIAN_POINT ( 'NONE',  ( 19.38216949554541202, 0.9986346699304200492, 9.382169495545424454 ) ) ;
#94262=CARTESIAN_POINT ( 'NONE',  ( 12.63842701281683922, 19.55059781766745175, -9.846743663894590881 ) ) ;
#94263=CARTESIAN_POINT ( 'NONE',  ( 7.084665262690076126, 29.10535201082150181, 10.88017736071109987 ) ) ;
#94264=CARTESIAN_POINT ( 'NONE',  ( 19.38216949554541557, 32.24863466993041783, -9.382169495545420901 ) ) ;
#94265=CARTESIAN_POINT ( 'NONE',  ( 7.361572987183169658, 19.96726448433411960, -9.846743663894592657 ) ) ;
#94268=ADVANCED_FACE ( 'NONE', ( #38716 ), #67739, .T. ) ;
#94269=CARTESIAN_POINT ( 'NONE',  ( 0.5774900079438590739, 17.64701867748817321, -5.440088680355550821 ) ) ;
#94270=CARTESIAN_POINT ( 'NONE',  ( 12.91533473730993009, 61.60535201082150536, -10.88017736071109987 ) ) ;
#94271=CARTESIAN_POINT ( 'NONE',  ( 4.559911319644449179, 8.897018677488171434, 9.422509992056141925 ) ) ;
#94272=CARTESIAN_POINT ( 'NONE',  ( 5.076628168052704559, 40.17559781766745175, -8.527530157486179263 ) ) ;
#94273=CARTESIAN_POINT ( 'NONE',  ( 19.42250999205614193, 25.14701867748817321, 5.440088680355555262 ) ) ;
#94275=CARTESIAN_POINT ( 'NONE',  ( 15.44008868035555260, 39.73035201082150536, 9.422509992056143702 ) ) ;
#94276=CARTESIAN_POINT ( 'NONE',  ( 12.91533473730993009, 6.605352010821504471, -10.88017736071109987 ) ) ;
#94277=CARTESIAN_POINT ( 'NONE',  ( -0.3289641300568005855, 19.27164270246084499, -5.963430220938281678 ) ) ;
#94280=CARTESIAN_POINT ( 'NONE',  ( 19.84674366389459266, 38.30059781766745175, 2.638427012816836559 ) ) ;
#94281=CARTESIAN_POINT ( 'NONE',  ( 13.79529636645031943, 45.34541550158062506, -14.16423886937409904 ) ) ;
#94282=CARTESIAN_POINT ( 'NONE',  ( 17.39651004071897589, 34.08210964143323451, -6.499999999999361400 ) ) ;
#94283=CARTESIAN_POINT ( 'NONE',  ( 1.492507162822240385, 7.199555875704810148, -6.500000000000008882 ) ) ;
#94284=CARTESIAN_POINT ( 'NONE',  ( 22.81628187352647785, 6.415301336597088344, 3.434112377981063169 ) ) ;
#94286=CARTESIAN_POINT ( 'NONE',  ( 22.26659068614895176, 29.72041550158063572, -7.082119434687042414 ) ) ;
#94290=CARTESIAN_POINT ( 'NONE',  ( 17.08211943468705130, 63.47041550158063927, 12.26659068614894998 ) ) ;
#94291=CARTESIAN_POINT ( 'NONE',  ( 17.20831665107776587, 24.13393115100078035, -7.208316651077762316 ) ) ;
#94293=CARTESIAN_POINT ( 'NONE',  ( 17.96484262340118221, 56.18868534415484817, -7.964842623401177768 ) ) ;
#94294=CARTESIAN_POINT ( 'NONE',  ( -1.099225684535947600, 58.70696800326375353, -6.408140936763238038 ) ) ;
#94295=CARTESIAN_POINT ( 'NONE',  ( 12.91533473730992121, 29.52201867748817321, 10.88017736071110164 ) ) ;
#94297=CARTESIAN_POINT ( 'NONE',  ( 19.38216949554541202, 10.99863466993042138, 9.382169495545424454 ) ) ;
#94298=CARTESIAN_POINT ( 'NONE',  ( 12.63842701281683034, 17.46726448433411250, 9.846743663894596210 ) ) ;
#94300=CARTESIAN_POINT ( 'NONE',  ( 0.1532563361054100626, 0.8005978176674514168, -2.638427012816831230 ) ) ;
#94301=FACE_OUTER_BOUND ( 'NONE', #84561, .T. ) ;
#94302=CARTESIAN_POINT ( 'NONE',  ( 17.08211943468705130, 58.47041550158063927, 12.26659068614894998 ) ) ;
#94303=CARTESIAN_POINT ( 'NONE',  ( 20.36894250292379738, 24.92874883491396787, -10.36894250292379027 ) ) ;
#94304=CARTESIAN_POINT ( 'NONE',  ( 15.44008868035555260, 49.73035201082150536, 9.422509992056143702 ) ) ;
#94305=CYLINDRICAL_SURFACE ( 'NONE', #67076, 11.92686044187656513 ) ;
#94308=CARTESIAN_POINT ( 'NONE',  ( 2.791683348922240793, 6.633931151000785675, 7.208316651077764092 ) ) ;
#94309=CARTESIAN_POINT ( 'NONE',  ( 18.52753015748618282, 23.92559781766745530, -4.923371831947291888 ) ) ;
#94310=( NAMED_UNIT ( * ) SI_UNIT ( $, .STERADIAN. ) SOLID_ANGLE_UNIT ( ) );
#94312=CARTESIAN_POINT ( 'NONE',  ( 19.84674366389459621, 28.50893115100078745, 7.409399052514197653E-17 ) ) ;
#94313=CARTESIAN_POINT ( 'NONE',  ( 17.20831665107776587, 44.13393115100078745, -7.208316651077762316 ) ) ;
#94319=CARTESIAN_POINT ( 'NONE',  ( 19.38216949554541202, 50.99863466993042493, 9.382169495545424454 ) ) ;
#94320=CARTESIAN_POINT ( 'NONE',  ( 4.559911319644449179, 47.23035201082150536, -9.422509992056141925 ) ) ;
#94321=CARTESIAN_POINT ( 'NONE',  ( 5.076628168052703671, 31.84226448433412315, 8.527530157486179263 ) ) ;
#94322=CARTESIAN_POINT ( 'NONE',  ( 24.16423886937409904, 49.09541550158063217, 3.795296366450317205 ) ) ;
#94323=CARTESIAN_POINT ( 'NONE',  ( 0.1532563361054082862, 21.21726448433412315, 2.638427012816831674 ) ) ;
#94325=CARTESIAN_POINT ( 'NONE',  ( 7.361572987183170547, 57.05059781766744464, 9.846743663894590881 ) ) ;
#94326=CARTESIAN_POINT ( 'NONE',  ( 17.20831665107776587, 42.88393115100077324, 7.208316651077764980 ) ) ;
#94327=CARTESIAN_POINT ( 'NONE',  ( 17.08211943468705840, 10.13708216824730179, -12.26659068614894466 ) ) ;
#94328=( BOUNDED_CURVE ( )  B_SPLINE_CURVE ( 2, ( #66057, #96584, #59054, #6550, #60036, #89061, #74048, #28559, #21066 ),
 .UNSPECIFIED., .F., .T. ) 
 B_SPLINE_CURVE_WITH_KNOTS ( ( 3, 2, 2, 2, 3 ),
 ( 0.04537130733198223298, 0.04761904761904761640, 0.05357142857142856845, 0.05952380952380952051, 0.06177154981087491087 ),
 .UNSPECIFIED. ) 
 CURVE ( )  GEOMETRIC_REPRESENTATION_ITEM ( )  RATIONAL_B_SPLINE_CURVE ( ( 0.9839835555609424134, 0.9871328979762477029, 1.000000000000000000, 0.9659258262890683122, 1.000000000000000000, 0.9659258262890683122, 1.000000000000000000, 0.9871328979762477029, 0.9839835555609424134 ) ) 
 REPRESENTATION_ITEM ( '' )  );
#94329=CARTESIAN_POINT ( 'NONE',  ( 13.79529636645031943, 30.34541550158063927, -14.16423886937409904 ) ) ;
#94330=CARTESIAN_POINT ( 'NONE',  ( 7.361572987183170547, 27.05059781766745175, 9.846743663894590881 ) ) ;
#94332=CARTESIAN_POINT ( 'NONE',  ( 20.88017736071110875, 25.77201867748816966, -2.915334737309920765 ) ) ;
#94333=EDGE_CURVE ( 'NONE', #64921, #13800, #82733, .T. ) ;
#94335=CARTESIAN_POINT ( 'NONE',  ( 19.42250999205614193, 50.14701867748817676, 5.440088680355555262 ) ) ;
#94336=CARTESIAN_POINT ( 'NONE',  ( 20.88017736071110519, 40.56368534415484106, 2.639326808657452039E-16 ) ) ;
#94338=CARTESIAN_POINT ( 'NONE',  ( -2.816281873526473856, 34.12363466993042493, 9.499525473075851096E-16 ) ) ;
#94339=CARTESIAN_POINT ( 'NONE',  ( -0.8801773607111009756, 48.06368534415484817, 1.068504757029289695E-15 ) ) ;
#94340=ORIENTED_EDGE ( 'NONE', *, *, #36949, .T. ) ;
#94341=CARTESIAN_POINT ( 'NONE',  ( 5.076628168052704559, 0.1755978176674514724, -8.527530157486179263 ) ) ;
#94342=CARTESIAN_POINT ( 'NONE',  ( 19.42250999205614548, 60.98035201082151247, -5.440088680355545492 ) ) ;
#94344=CARTESIAN_POINT ( 'NONE',  ( 0.5774900079438607392, 58.48035201082151247, 5.440088680355550821 ) ) ;
#94345=CARTESIAN_POINT ( 'NONE',  ( 4.559911319644449179, 2.230352010821504471, -9.422509992056141925 ) ) ;
#94346=CARTESIAN_POINT ( 'NONE',  ( 2.153642693323432944, 26.13791097397318808, -6.499999999999992006 ) ) ;
#94347=LINE ( 'NONE', #48352, #18516 ) ;
#94348=CARTESIAN_POINT ( 'NONE',  ( 7.084665262690076126, 7.022018677488170546, -10.88017736071110164 ) ) ;
#94349=CARTESIAN_POINT ( 'NONE',  ( 10.00000000000000000, 9.758931151000785675, -9.846743663894594434 ) ) ;
#94350=CARTESIAN_POINT ( 'NONE',  ( 24.16423886937410614, 4.512082168247300906, -3.795296366450302550 ) ) ;
#94351=CARTESIAN_POINT ( 'NONE',  ( 12.63842701281683922, 9.550597817667449974, -9.846743663894590881 ) ) ;
#94352=CARTESIAN_POINT ( 'NONE',  ( -0.8801773607110991993, 7.855352010821504471, -2.915334737309923874 ) ) ;
#94353=CARTESIAN_POINT ( 'NONE',  ( 1.472469842513823179, 41.42559781766745886, 4.923371831947296329 ) ) ;
#94355=CARTESIAN_POINT ( 'NONE',  ( 19.84674366389459266, 53.71726448433411605, -2.638427012816827677 ) ) ;
#94357=CARTESIAN_POINT ( 'NONE',  ( 7.084665262690076126, 57.02201867748817676, -10.88017736071110164 ) ) ;
#94358=CARTESIAN_POINT ( 'NONE',  ( 0.1532563361054100626, 45.80059781766745886, -2.638427012816831230 ) ) ;
#94359=FILL_AREA_STYLE ('',( #54879 ) ) ;
#94361=CARTESIAN_POINT ( 'NONE',  ( 19.42250999205614193, 55.14701867748817676, 5.440088680355555262 ) ) ;
#94362=CARTESIAN_POINT ( 'NONE',  ( -0.3689425029237898834, 66.17874883491396076, -10.36894250292378850 ) ) ;
#94365=CARTESIAN_POINT ( 'NONE',  ( 21.09922568453594849, 46.20696800326376064, 6.408140936763242479 ) ) ;
#94366=CARTESIAN_POINT ( 'NONE',  ( 20.15039907845753930, 70.00000000000000000, 6.262539305110068177 ) ) ;
#94369=CARTESIAN_POINT ( 'NONE',  ( 22.81628187352647785, 31.62363466993042138, 6.195893100308588602E-16 ) ) ;
#94370=CARTESIAN_POINT ( 'NONE',  ( 17.96484262340118221, 31.18868534415483751, -7.964842623401177768 ) ) ;
#94373=CARTESIAN_POINT ( 'NONE',  ( 19.84674366389459266, 63.71726448433412315, -2.638427012816827677 ) ) ;
#94374=CARTESIAN_POINT ( 'NONE',  ( 7.361572987183169658, 9.967264484334119601, -9.846743663894592657 ) ) ;
#94375=CARTESIAN_POINT ( 'NONE',  ( 1.472469842513823179, 56.42559781766745886, 4.923371831947296329 ) ) ;
#94377=FILL_AREA_STYLE_COLOUR ( '', #74664 ) ;
#94378=CARTESIAN_POINT ( 'NONE',  ( 0.1532563361054083140, 36.00893115100078745, 1.131784320476157264E-15 ) ) ;
#94380=CARTESIAN_POINT ( 'NONE',  ( 18.95386800104995473, 58.23810908735727310, -6.499999999999988454 ) ) ;
#94381=CARTESIAN_POINT ( 'NONE',  ( 0.1532563361054083140, 21.00893115100078745, 1.131784320476157264E-15 ) ) ;
#94383=CARTESIAN_POINT ( 'NONE',  ( 0.1532563361054100626, 55.80059781766745175, -2.638427012816831230 ) ) ;
#94386=CARTESIAN_POINT ( 'NONE',  ( 6.565887622018943937, 20.16530133659708213, 12.81628187352647430 ) ) ;
#94388=CARTESIAN_POINT ( 'NONE',  ( 14.92337183194729988, 39.34226448433412315, -8.527530157486177487 ) ) ;
#94389=CARTESIAN_POINT ( 'NONE',  ( -26.67076923076924189, 87.15384615384614619, -9.500000000000000000 ) ) ;
#94390=CARTESIAN_POINT ( 'NONE',  ( 6.204703633549690345, 47.84541550158064638, 14.16423886937410082 ) ) ;
#94391=CARTESIAN_POINT ( 'NONE',  ( 10.00000000000000000, 19.75893115100078390, -9.846743663894594434 ) ) ;
#94395=CARTESIAN_POINT ( 'NONE',  ( 22.26659068614894466, 48.88708216824730357, 7.082119434687054849 ) ) ;
#94396=CARTESIAN_POINT ( 'NONE',  ( 2.791683348922237240, 55.38393115100078745, -7.208316651077763204 ) ) ;
#94397=CARTESIAN_POINT ( 'NONE',  ( 10.00000000000000000, 6.813685344154838397, -10.88017736071110342 ) ) ;
#94398=CARTESIAN_POINT ( 'NONE',  ( 13.79529636645030344, 38.26208216824729647, 14.16423886937410614 ) ) ;
#94399=CARTESIAN_POINT ( 'NONE',  ( -4.164238869374099927, 37.01208216824731068, 3.795296366450308767 ) ) ;
#94400=SURFACE_STYLE_USAGE ( .BOTH. , #63888 ) ;
#94404=CARTESIAN_POINT ( 'NONE',  ( 7.361572987183170547, 57.05059781766744464, 9.846743663894590881 ) ) ;
#94406=CARTESIAN_POINT ( 'NONE',  ( 12.91533473730992121, 34.52201867748817676, 10.88017736071110164 ) ) ;
#94408=CARTESIAN_POINT ( 'NONE',  ( 19.50000000000000355, 98.59912998021083297, -5.000000000000000000 ) ) ;
#94411=CARTESIAN_POINT ( 'NONE',  ( 19.84674366389459621, 53.50893115100078745, 7.409399052514197653E-17 ) ) ;
#94412=CARTESIAN_POINT ( 'NONE',  ( 17.20831665107776587, 64.13393115100079456, -7.208316651077762316 ) ) ;
#94414=CARTESIAN_POINT ( 'NONE',  ( -4.164238869374098151, 31.59541550158063927, -3.795296366450310543 ) ) ;
#94417=CARTESIAN_POINT ( 'NONE',  ( 15.44008868035555260, 9.730352010821505360, 9.422509992056143702 ) ) ;
#94418=CARTESIAN_POINT ( 'NONE',  ( 22.81628187352648496, 21.83196800326374643, -3.434112377981050290 ) ) ;
#94420=CARTESIAN_POINT ( 'NONE',  ( 17.20831665107776587, 17.88393115100078745, 7.208316651077764980 ) ) ;
#94422=CARTESIAN_POINT ( 'NONE',  ( -46.94000000000001194, 100.4344880109628093, -9.014049137172644777 ) ) ;
#94423=CARTESIAN_POINT ( 'NONE',  ( 6.000000000000000000, 60.50000000000000000, -5.000000000000000000 ) ) ;
#94424=CARTESIAN_POINT ( 'NONE',  ( 17.96484262340118221, 16.18868534415483396, -7.964842623401177768 ) ) ;
#94427=CARTESIAN_POINT ( 'NONE',  ( -0.8801773607110991993, 42.85535201082150536, -2.915334737309923874 ) ) ;
#94428=CARTESIAN_POINT ( 'NONE',  ( 7.084665262690076126, 42.02201867748816966, -10.88017736071110164 ) ) ;
#94429=CARTESIAN_POINT ( 'NONE',  ( 13.43411237798105340, 5.581968003263753531, 12.81628187352647963 ) ) ;
#94430=CARTESIAN_POINT ( 'NONE',  ( 10.00000000000000178, 67.25893115100079456, 9.846743663894594434 ) ) ;
#94431=CARTESIAN_POINT ( 'NONE',  ( -45.93038741018368398, 104.4960312484300999, -5.681613179053518259 ) ) ;
#94432=CARTESIAN_POINT ( 'NONE',  ( 10.00000000000000000, 14.75893115100078568, -9.846743663894594434 ) ) ;
#94435=CARTESIAN_POINT ( 'NONE',  ( 12.91533473730992121, 34.52201867748817676, 10.88017736071110164 ) ) ;
#94437=CARTESIAN_POINT ( 'NONE',  ( -1.099225684535947600, 28.70696800326375353, -6.408140936763238038 ) ) ;
#94438=B_SPLINE_CURVE_WITH_KNOTS ( 'NONE', 3,
 ( #35755, #65749, #66242, #28253, #20762, #51252, #43745, #5764, #21256, #54200 ),
 .UNSPECIFIED., .F., .F.,
 ( 4, 3, 3, 4 ),
 ( 0.000000000000000000, 0.0006253016069561002704, 0.001250604074564923892, 0.002501455912506560415 ),
 .UNSPECIFIED. ) ;
#94440=CARTESIAN_POINT ( 'NONE',  ( 2.791683348922237240, 65.38393115100078035, -7.208316651077763204 ) ) ;
#94441=CARTESIAN_POINT ( 'NONE',  ( 0.5774900079438607392, 68.48035201082150536, 5.440088680355550821 ) ) ;
#94442=CARTESIAN_POINT ( 'NONE',  ( 7.361572987183169658, 14.96726448433411960, -9.846743663894592657 ) ) ;
#94443=CARTESIAN_POINT ( 'NONE',  ( 13.43411237798105340, 35.58196800326375353, 12.81628187352647963 ) ) ;
#94444=CARTESIAN_POINT ( 'NONE',  ( 5.076628168052703671, 11.84226448433411960, 8.527530157486179263 ) ) ;
#94448=CARTESIAN_POINT ( 'NONE',  ( 4.559911319644449179, 7.230352010821504471, -9.422509992056141925 ) ) ;
#94449=CARTESIAN_POINT ( 'NONE',  ( 10.00000000000000178, 55.37363466993042493, 12.81628187352647608 ) ) ;
#94450=CARTESIAN_POINT ( 'NONE',  ( 0.1532563361054082862, 11.21726448433411605, 2.638427012816831674 ) ) ;
#94451=CARTESIAN_POINT ( 'NONE',  ( 18.52753015748618282, 18.92559781766745175, -4.923371831947291888 ) ) ;
#94452=CARTESIAN_POINT ( 'NONE',  ( 13.79529636645030344, 58.26208216824728936, 14.16423886937410614 ) ) ;
#94454=CARTESIAN_POINT ( 'NONE',  ( 12.91533473730992121, 19.52201867748816611, 10.88017736071110164 ) ) ;
#94455=CARTESIAN_POINT ( 'NONE',  ( 12.91533473730992121, 24.52201867748816966, 10.88017736071110164 ) ) ;
#94460=CARTESIAN_POINT ( 'NONE',  ( 10.00000000000000000, 26.81368534415484106, -10.88017736071110342 ) ) ;
#94461=CARTESIAN_POINT ( 'NONE',  ( 2.791683348922240793, 61.63393115100079456, 7.208316651077764092 ) ) ;
#94462=VECTOR ( 'NONE', #83818, 1000.000000000000000 ) ;
#94464=CARTESIAN_POINT ( 'NONE',  ( 21.09922568453594849, 46.20696800326376064, 6.408140936763242479 ) ) ;
#94465=CARTESIAN_POINT ( 'NONE',  ( -0.3289641300568005855, 4.271642702460841434, -5.963430220938281678 ) ) ;
#94466=CARTESIAN_POINT ( 'NONE',  ( 17.08211943468705840, 25.13708216824730357, -12.26659068614894466 ) ) ;
#94467=CARTESIAN_POINT ( 'NONE',  ( 4.559911319644449179, 38.89701867748817676, 9.422509992056141925 ) ) ;
#94468=CARTESIAN_POINT ( 'NONE',  ( 0.5774900079438590739, 17.64701867748817321, -5.440088680355550821 ) ) ;
#94469=CARTESIAN_POINT ( 'NONE',  ( 17.20831665107776587, 49.13393115100078745, -7.208316651077762316 ) ) ;
#94471=CARTESIAN_POINT ( 'NONE',  ( 7.361572987183169658, 34.96726448433411605, -9.846743663894592657 ) ) ;
#94474=CARTESIAN_POINT ( 'NONE',  ( 12.63842701281683034, 12.46726448433411782, 9.846743663894596210 ) ) ;
#94478=CARTESIAN_POINT ( 'NONE',  ( 7.084665262690076126, 9.105352010821503583, 10.88017736071109987 ) ) ;
#94479=CARTESIAN_POINT ( 'NONE',  ( 0.1532563361054083140, 16.00893115100078390, 1.131784320476157264E-15 ) ) ;
#94480=CARTESIAN_POINT ( 'NONE',  ( -0.8801773607110991993, 47.85535201082150536, -2.915334737309923874 ) ) ;
#94481=CARTESIAN_POINT ( 'NONE',  ( 20.88017736071110519, 25.56368534415483751, 2.639326808657452039E-16 ) ) ;
#94482=CARTESIAN_POINT ( 'NONE',  ( 3.591859063236761518, 49.95696800326375353, 11.09922568453594849 ) ) ;
#94483=CARTESIAN_POINT ( 'NONE',  ( 6.204703633549690345, 35.76208216824729647, -14.16423886937410259 ) ) ;
#94486=CARTESIAN_POINT ( 'NONE',  ( 13.43411237798106583, 62.66530133659708923, -12.81628187352647252 ) ) ;
#94489=CARTESIAN_POINT ( 'NONE',  ( 5.076628168052704559, 55.17559781766745175, -8.527530157486179263 ) ) ;
#94490=CARTESIAN_POINT ( 'NONE',  ( 20.88017736071110164, 40.35535201082150536, 2.915334737309930979 ) ) ;
#94492=CARTESIAN_POINT ( 'NONE',  ( 18.52753015748618282, 3.925597817667451306, -4.923371831947291888 ) ) ;
#94493=LINE ( 'NONE', #26013, #68729 ) ;
#94495=CARTESIAN_POINT ( 'NONE',  ( 14.92337183194729988, 24.34226448433411960, -8.527530157486177487 ) ) ;
#94496=CARTESIAN_POINT ( 'NONE',  ( 1.472469842513823179, 10.59226448433411782, -4.923371831947296329 ) ) ;
#94497=CARTESIAN_POINT ( 'NONE',  ( 0.1532563361054082862, 6.217264484334118713, 2.638427012816831674 ) ) ;
#94498=CARTESIAN_POINT ( 'NONE',  ( -0.8801773607110991993, 52.85535201082151247, -2.915334737309923874 ) ) ;
#94500=CARTESIAN_POINT ( 'NONE',  ( 7.084665262690076126, 57.02201867748817676, -10.88017736071110164 ) ) ;
#94501=CARTESIAN_POINT ( 'NONE',  ( 17.20831665107776587, 17.88393115100078745, 7.208316651077764980 ) ) ;
#94505=CARTESIAN_POINT ( 'NONE',  ( 1.472469842513823179, 51.42559781766745886, 4.923371831947296329 ) ) ;
#94509=CARTESIAN_POINT ( 'NONE',  ( 24.16423886937409904, 4.095415501580634832, 3.795296366450317205 ) ) ;
#94511=CARTESIAN_POINT ( 'NONE',  ( 22.81628187352648496, 61.83196800326376774, -3.434112377981050290 ) ) ;
#94513=CARTESIAN_POINT ( 'NONE',  ( -2.266590686148945544, 2.220415501580634388, 7.082119434687048631 ) ) ;
#94514=CARTESIAN_POINT ( 'NONE',  ( 10.00000000000000178, 33.05374883491396787, 14.16423886937410082 ) ) ;
#94516=CARTESIAN_POINT ( 'NONE',  ( 6.204703633549690345, 0.7620821682473009062, -14.16423886937410259 ) ) ;
#94517=CARTESIAN_POINT ( 'NONE',  ( 2.035157376598824452, 38.68868534415483396, 7.964842623401179544 ) ) ;
#94518=SURFACE_STYLE_FILL_AREA ( #34000 ) ;
#94519=ORIENTED_EDGE ( 'NONE', *, *, #65112, .F. ) ;
#94520=CARTESIAN_POINT ( 'NONE',  ( 14.92337183194729988, 14.34226448433411782, -8.527530157486177487 ) ) ;
#94521=CARTESIAN_POINT ( 'NONE',  ( 12.91533473730993009, 56.60535201082151247, -10.88017736071109987 ) ) ;
#94522=CARTESIAN_POINT ( 'NONE',  ( 17.20831665107776587, 17.88393115100078745, 7.208316651077764980 ) ) ;
#94523=CARTESIAN_POINT ( 'NONE',  ( 0.6178305044545838731, 44.74863466993042493, 9.382169495545420901 ) ) ;
#94524=CARTESIAN_POINT ( 'NONE',  ( 5.076628168052703671, 36.84226448433412315, 8.527530157486179263 ) ) ;
#94526=CARTESIAN_POINT ( 'NONE',  ( 17.96484262340118221, 59.93868534415484106, 7.964842623401181321 ) ) ;
#94527=CARTESIAN_POINT ( 'NONE',  ( 13.43411237798105340, 25.58196800326374998, 12.81628187352647963 ) ) ;
#94530=CARTESIAN_POINT ( 'NONE',  ( 18.52753015748617571, 23.09226448433411960, 4.923371831947298993 ) ) ;
#94531=CARTESIAN_POINT ( 'NONE',  ( 2.917880565312950480, 10.97041550158063572, -12.26659068614894821 ) ) ;
#94533=CARTESIAN_POINT ( 'NONE',  ( 7.084665262690076126, 37.02201867748817676, -10.88017736071110164 ) ) ;
#94534=CARTESIAN_POINT ( 'NONE',  ( 6.204703633549690345, 30.76208216824730357, -14.16423886937410259 ) ) ;
#94535=CARTESIAN_POINT ( 'NONE',  ( 7.361572987183169658, 54.96726448433413026, -9.846743663894592657 ) ) ;
#94536=CARTESIAN_POINT ( 'NONE',  ( 12.63842701281683034, 7.467264484334118713, 9.846743663894596210 ) ) ;
#94538=CARTESIAN_POINT ( 'NONE',  ( 0.6178305044545838731, 54.74863466993042493, 9.382169495545420901 ) ) ;
#94540=CARTESIAN_POINT ( 'NONE',  ( 12.91533473730992121, 44.52201867748816966, 10.88017736071110164 ) ) ;
#94542=CARTESIAN_POINT ( 'NONE',  ( 10.00000000000000000, 17.87363466993041783, -12.81628187352647608 ) ) ;
#94543=CARTESIAN_POINT ( 'NONE',  ( 19.84674366389459266, 48.30059781766745175, 2.638427012816836559 ) ) ;
#94545=CARTESIAN_POINT ( 'NONE',  ( 2.035157376598822676, 2.438685344154837953, -7.964842623401177768 ) ) ;
#94547=CARTESIAN_POINT ( 'NONE',  ( 0.1922240491738545221, 13.18878173731740766, 6.500000000000007105 ) ) ;
#94552=CARTESIAN_POINT ( 'NONE',  ( 17.96484262340118221, 56.18868534415484817, -7.964842623401177768 ) ) ;
#94553=CARTESIAN_POINT ( 'NONE',  ( 17.96484262340118221, 51.18868534415483396, -7.964842623401177768 ) ) ;
#94556=CARTESIAN_POINT ( 'NONE',  ( 7.361572987183169658, 19.96726448433411960, -9.846743663894592657 ) ) ;
#94557=CARTESIAN_POINT ( 'NONE',  ( 12.91533473730992121, 19.52201867748816611, 10.88017736071110164 ) ) ;
#94558=CARTESIAN_POINT ( 'NONE',  ( -2.816281873526473856, -0.6680319967362464695, 3.434112377981055619 ) ) ;
#94559=CARTESIAN_POINT ( 'NONE',  ( 10.00000000000000178, 19.31368534415484106, 10.88017736071110342 ) ) ;
#94562=CARTESIAN_POINT ( 'NONE',  ( 21.09922568453594849, 26.20696800326375353, 6.408140936763242479 ) ) ;
#94564=CARTESIAN_POINT ( 'NONE',  ( 7.084665262690076126, 54.10535201082151247, 10.88017736071109987 ) ) ;
#94565=CARTESIAN_POINT ( 'NONE',  ( 5.076628168052703671, 46.84226448433412315, 8.527530157486179263 ) ) ;
#94566=CARTESIAN_POINT ( 'NONE',  ( 21.09922568453594849, 26.20696800326375353, 6.408140936763242479 ) ) ;
#94567=CARTESIAN_POINT ( 'NONE',  ( 19.42250999205614193, 25.14701867748817321, 5.440088680355555262 ) ) ;
#94568=CARTESIAN_POINT ( 'NONE',  ( 20.36894250292379382, 48.67874883491396076, 10.36894250292379205 ) ) ;
#94569=CARTESIAN_POINT ( 'NONE',  ( 18.52753015748617571, 43.09226448433412315, 4.923371831947298993 ) ) ;
#94570=CARTESIAN_POINT ( 'NONE',  ( 10.00000000000000178, 69.31368534415484817, 10.88017736071110342 ) ) ;
#94571=CARTESIAN_POINT ( 'NONE',  ( 20.88017736071110875, 50.77201867748817676, -2.915334737309920765 ) ) ;
#94573=CARTESIAN_POINT ( 'NONE',  ( 20.36894250292379738, 19.92874883491396787, -10.36894250292379027 ) ) ;
#94580=CARTESIAN_POINT ( 'NONE',  ( 6.204703633549690345, 50.76208216824730357, -14.16423886937410259 ) ) ;
#94581=CARTESIAN_POINT ( 'NONE',  ( 24.16423886937409904, 49.09541550158063217, 3.795296366450317205 ) ) ;
#94582=CARTESIAN_POINT ( 'NONE',  ( 17.20831665107776587, 17.88393115100078745, 7.208316651077764980 ) ) ;
#94583=CARTESIAN_POINT ( 'NONE',  ( 19.38216949554541557, 17.24863466993041783, -9.382169495545420901 ) ) ;
#94584=CARTESIAN_POINT ( 'NONE',  ( -46.44000000000001194, 103.0000000000000000, 5.997726559847112782 ) ) ;
#94585=CARTESIAN_POINT ( 'NONE',  ( 17.39651004071841456, 9.082109641433294911, -6.500000000000003553 ) ) ;
#94586=CARTESIAN_POINT ( 'NONE',  ( -0.8801773607111009756, 68.06368534415484817, 1.068504757029289695E-15 ) ) ;
#94587=CARTESIAN_POINT ( 'NONE',  ( 0.6178305044545838731, 29.74863466993042138, 9.382169495545420901 ) ) ;
#94588=CARTESIAN_POINT ( 'NONE',  ( 6.204703633549690345, 47.84541550158064638, 14.16423886937410082 ) ) ;
#94589=B_SPLINE_CURVE_WITH_KNOTS ( 'NONE', 3,
 ( #94126, #86640, #24666, #79125, #10637, #3146 ),
 .UNSPECIFIED., .F., .F.,
 ( 4, 2, 4 ),
 ( 0.000000000000000000, 0.0002605067024380841828, 0.0005210134048761683656 ),
 .UNSPECIFIED. ) ;
#94591=CARTESIAN_POINT ( 'NONE',  ( 19.42250999205614548, 65.98035201082151957, -5.440088680355545492 ) ) ;
#94594=DIRECTION ( 'NONE',  ( -0.5547001962252290364, -0.8320502943378437211, 0.000000000000000000 ) ) ;
#94595=CARTESIAN_POINT ( 'NONE',  ( 0.1532563361054100626, 15.80059781766745353, -2.638427012816831230 ) ) ;
#94596=CARTESIAN_POINT ( 'NONE',  ( 20.15039907845753930, 70.00000000000000000, -6.262539305110068177 ) ) ;
#94599=CARTESIAN_POINT ( 'NONE',  ( -0.3689425029237881626, 67.42874883491396076, 10.36894250292379027 ) ) ;
#94600=CARTESIAN_POINT ( 'NONE',  ( 15.44008868035555793, 16.39701867748817321, -9.422509992056140149 ) ) ;
#94601=CARTESIAN_POINT ( 'NONE',  ( 0.1532563361054082862, 51.21726448433412315, 2.638427012816831674 ) ) ;
#94602=CARTESIAN_POINT ( 'NONE',  ( 0.6178305044545818747, -1.501365330069579951, -9.382169495545419124 ) ) ;
#94606=CARTESIAN_POINT ( 'NONE',  ( 3.591859063236763294, 23.29030133659708568, -11.09922568453595026 ) ) ;
#94607=EDGE_CURVE ( 'NONE', #48119, #79733, #15202, .T. ) ;
#94610=CARTESIAN_POINT ( 'NONE',  ( 2.917880565312950480, 60.97041550158063927, -12.26659068614894821 ) ) ;
#94613=CARTESIAN_POINT ( 'NONE',  ( 22.26659068614895176, 59.72041550158063927, -7.082119434687042414 ) ) ;
#94615=CARTESIAN_POINT ( 'NONE',  ( -0.8801773607110991993, 27.85535201082150181, -2.915334737309923874 ) ) ;
#94616=CARTESIAN_POINT ( 'NONE',  ( 19.42250999205614193, 35.14701867748816966, 5.440088680355555262 ) ) ;
#94617=B_SPLINE_CURVE_WITH_KNOTS ( 'NONE', 3,
 ( #7233, #740, #22734, #37740, #85197, #38715 ),
 .UNSPECIFIED., .F., .F.,
 ( 4, 2, 4 ),
 ( 1.608716371138911572E-17, 0.0002605067024381052163, 0.0005210134048761942780 ),
 .UNSPECIFIED. ) ;
#94619=CARTESIAN_POINT ( 'NONE',  ( 20.15039907845753930, 5.601585745166425490, -6.262539305110069954 ) ) ;
#94620=CARTESIAN_POINT ( 'NONE',  ( 2.035157376598824452, 23.68868534415484461, 7.964842623401179544 ) ) ;
#94623=CARTESIAN_POINT ( 'NONE',  ( 0.1532563361054100626, 10.80059781766745175, -2.638427012816831230 ) ) ;
#94627=CARTESIAN_POINT ( 'NONE',  ( 1.472469842513823179, 50.59226448433411605, -4.923371831947296329 ) ) ;
#94628=CARTESIAN_POINT ( 'NONE',  ( 17.85158348494336522, 9.737265733804411738, -6.499999999999984901 ) ) ;
#94633=DIRECTION ( 'NONE',  ( 0.000000000000000000, 1.000000000000000000, -0.000000000000000000 ) ) ;
#94635=CARTESIAN_POINT ( 'NONE',  ( 19.84674366389459266, 63.71726448433412315, -2.638427012816827677 ) ) ;
#94636=CARTESIAN_POINT ( 'NONE',  ( 17.08211943468705840, 50.13708216824730357, -12.26659068614894466 ) ) ;
#94640=CARTESIAN_POINT ( 'NONE',  ( 17.20831665107776587, 39.13393115100079456, -7.208316651077762316 ) ) ;
#94641=CARTESIAN_POINT ( 'NONE',  ( 21.09922568453594849, 61.20696800326376064, 6.408140936763242479 ) ) ;
#94642=CARTESIAN_POINT ( 'NONE',  ( -1.099225684535947600, 9.540301336597087456, 6.408140936763237150 ) ) ;
#94643=CARTESIAN_POINT ( 'NONE',  ( 10.00000000000000178, 64.31368534415483396, 10.88017736071110342 ) ) ;
#94645=CARTESIAN_POINT ( 'NONE',  ( 17.20831665107776587, 57.88393115100078745, 7.208316651077764980 ) ) ;
#94647=CARTESIAN_POINT ( 'NONE',  ( -45.94000000000000483, 92.00000000000000000, 9.000000000000000000 ) ) ;
#94649=( BOUNDED_CURVE ( )  B_SPLINE_CURVE ( 2, ( #85554, #77541, #613, #83584, #84571, #69568, #9059, #23094, #31057 ),
 .UNSPECIFIED., .F., .F. ) 
 B_SPLINE_CURVE_WITH_KNOTS ( ( 3, 2, 2, 2, 3 ),
 ( 0.9382284501891250406, 0.9404761904761904656, 0.9464285714285713969, 0.9523809523809523281, 0.9546286926680177531 ),
 .UNSPECIFIED. ) 
 CURVE ( )  GEOMETRIC_REPRESENTATION_ITEM ( )  RATIONAL_B_SPLINE_CURVE ( ( 0.9839835555609424134, 0.9871328979762474809, 1.000000000000000000, 0.9659258262890683122, 1.000000000000000000, 0.9659258262890683122, 1.000000000000000000, 0.9871328979762477029, 0.9839835555609425244 ) ) 
 REPRESENTATION_ITEM ( '' )  );
#94650=CARTESIAN_POINT ( 'NONE',  ( -2.266590686148945544, 62.22041550158063927, 7.082119434687048631 ) ) ;
#94652=CARTESIAN_POINT ( 'NONE',  ( 15.44008868035555260, 44.73035201082151247, 9.422509992056143702 ) ) ;
#94653=CARTESIAN_POINT ( 'NONE',  ( -2.816281873526471635, 18.91530133659708213, -3.434112377981056508 ) ) ;
#94654=CARTESIAN_POINT ( 'NONE',  ( 2.035157376598824452, 68.68868534415484817, 7.964842623401179544 ) ) ;
#94655=CARTESIAN_POINT ( 'NONE',  ( 4.559911319644449179, 7.230352010821504471, -9.422509992056141925 ) ) ;
#94657=CARTESIAN_POINT ( 'NONE',  ( 17.39651004071897589, 34.08210964143323451, -6.499999999999361400 ) ) ;
#94658=CARTESIAN_POINT ( 'NONE',  ( 14.92337183194729633, 57.67559781766745886, 8.527530157486181039 ) ) ;
#94659=CARTESIAN_POINT ( 'NONE',  ( 15.64039516285221154, 89.00000000000000000, -9.500000000000000000 ) ) ;
#94661=CARTESIAN_POINT ( 'NONE',  ( -1.099225684535947600, 24.54030133659708923, 6.408140936763237150 ) ) ;
#94663=CARTESIAN_POINT ( 'NONE',  ( 7.084665262690076126, 22.02201867748817321, -10.88017736071110164 ) ) ;
#94666=CARTESIAN_POINT ( 'NONE',  ( 24.16423886937410614, 39.30374883491396787, 8.672049930838204340E-16 ) ) ;
#94667=CARTESIAN_POINT ( 'NONE',  ( 17.08211943468705840, 25.13708216824730357, -12.26659068614894466 ) ) ;
#94668=CARTESIAN_POINT ( 'NONE',  ( 19.42250999205614548, 10.98035201082150536, -5.440088680355545492 ) ) ;
#94670=CARTESIAN_POINT ( 'NONE',  ( 19.84674366389459266, 38.71726448433412315, -2.638427012816827677 ) ) ;
#94671=CARTESIAN_POINT ( 'NONE',  ( 3.591859063236763294, 38.29030133659708923, -11.09922568453595026 ) ) ;
#94672=CARTESIAN_POINT ( 'NONE',  ( 7.084665262690076126, 17.02201867748817676, -10.88017736071110164 ) ) ;
#94673=CARTESIAN_POINT ( 'NONE',  ( 12.63842701281683034, 42.46726448433412315, 9.846743663894596210 ) ) ;
#94674=CARTESIAN_POINT ( 'NONE',  ( -0.8801773607111009756, 38.06368534415484106, 1.068504757029289695E-15 ) ) ;
#94675=CARTESIAN_POINT ( 'NONE',  ( 19.38216949554541557, 7.248634669930421381, -9.382169495545420901 ) ) ;
#94676=CARTESIAN_POINT ( 'NONE',  ( -0.3689425029237898834, 26.17874883491396432, -10.36894250292378850 ) ) ;
#94679=COLOUR_RGB ( '', 0.72549020, 0.75294118, 0.79215686) ;
#94680=CARTESIAN_POINT ( 'NONE',  ( 10.00000000000000000, 19.75893115100078390, -9.846743663894594434 ) ) ;
#94681=CARTESIAN_POINT ( 'NONE',  ( 13.43411237798106583, 52.66530133659708213, -12.81628187352647252 ) ) ;
#94682=CARTESIAN_POINT ( 'NONE',  ( 0.1532563361054083140, 61.00893115100078745, 1.131784320476157264E-15 ) ) ;
#94683=VERTEX_POINT ( 'NONE', #27630 ) ;
#94686=PRESENTATION_STYLE_ASSIGNMENT (( #41217 ) ) ;
#94687=CARTESIAN_POINT ( 'NONE',  ( -2.266590686148945544, 67.22041550158063217, 7.082119434687048631 ) ) ;
#94688=CARTESIAN_POINT ( 'NONE',  ( 17.96484262340118221, 59.93868534415484106, 7.964842623401181321 ) ) ;
#94689=CARTESIAN_POINT ( 'NONE',  ( -2.266590686148945544, 12.22041550158063394, 7.082119434687048631 ) ) ;
#94691=CARTESIAN_POINT ( 'NONE',  ( 1.472469842513823179, 5.592264484334118713, -4.923371831947296329 ) ) ;
#94692=CARTESIAN_POINT ( 'NONE',  ( 5.076628168052703671, 46.84226448433412315, 8.527530157486179263 ) ) ;
#94693=CARTESIAN_POINT ( 'NONE',  ( 15.44008868035555793, 21.39701867748817321, -9.422509992056140149 ) ) ;
#94703=CARTESIAN_POINT ( 'NONE',  ( 2.917880565312948704, 2.637082168247300906, 12.26659068614894643 ) ) ;
#94704=CARTESIAN_POINT ( 'NONE',  ( 13.79529636645031943, 5.345415501580634832, -14.16423886937409904 ) ) ;
#94705=CARTESIAN_POINT ( 'NONE',  ( 19.84674366389459621, 58.50893115100078745, 7.409399052514197653E-17 ) ) ;
#94706=CARTESIAN_POINT ( 'NONE',  ( 2.791683348922237240, 40.38393115100078035, -7.208316651077763204 ) ) ;
#94708=CARTESIAN_POINT ( 'NONE',  ( 20.88017736071110519, 35.56368534415484106, 2.639326808657452039E-16 ) ) ;
#94709=CARTESIAN_POINT ( 'NONE',  ( 7.361572987183169658, 64.96726448433412315, -9.846743663894592657 ) ) ;
#94710=CARTESIAN_POINT ( 'NONE',  ( 24.16423886937410614, 44.30374883491397497, 8.672049930838204340E-16 ) ) ;
#94711=CARTESIAN_POINT ( 'NONE',  ( 12.91533473730992121, 4.522018677488170546, 10.88017736071110164 ) ) ;
#94712=DIRECTION ( 'NONE',  ( 0.000000000000000000, 0.000000000000000000, 1.000000000000000000 ) ) ;
#94713=CARTESIAN_POINT ( 'NONE',  ( 10.00000000000000178, 59.31368534415484106, 10.88017736071110342 ) ) ;
#94714=CARTESIAN_POINT ( 'NONE',  ( 7.361572987183169658, 29.96726448433411960, -9.846743663894592657 ) ) ;
#94715=DIRECTION ( 'NONE',  ( 6.608470384673550777E-17, 1.000000000000000000, -0.000000000000000000 ) ) ;
#94719=CARTESIAN_POINT ( 'NONE',  ( 12.63842701281683034, 22.46726448433411605, 9.846743663894596210 ) ) ;
#94721=CARTESIAN_POINT ( 'NONE',  ( 20.36894250292379382, 33.67874883491396076, 10.36894250292379205 ) ) ;
#94722=CARTESIAN_POINT ( 'NONE',  ( 14.92337183194729988, 34.34226448433411605, -8.527530157486177487 ) ) ;
#94723=CARTESIAN_POINT ( 'NONE',  ( 2.035157376598824452, 53.68868534415484817, 7.964842623401179544 ) ) ;
#94724=CARTESIAN_POINT ( 'NONE',  ( 20.88017736071110519, 35.56368534415484106, 2.639326808657452039E-16 ) ) ;
#94725=CIRCLE ( 'NONE', #58019, 0.5000000000000004441 ) ;
#94726=EDGE_CURVE ( 'NONE', #21166, #69569, #50380, .T. ) ;
#94727=CARTESIAN_POINT ( 'NONE',  ( 0.1532563361054083140, 51.00893115100078745, 1.131784320476157264E-15 ) ) ;
#94731=CARTESIAN_POINT ( 'NONE',  ( -0.3689425029237881626, 12.42874883491396609, 10.36894250292379027 ) ) ;
#94732=ORIENTED_EDGE ( 'NONE', *, *, #8057, .F. ) ;
#94733=ORIENTED_EDGE ( 'NONE', *, *, #89584, .T. ) ;
#94734=CARTESIAN_POINT ( 'NONE',  ( 5.076628168052704559, 0.1755978176674514724, -8.527530157486179263 ) ) ;
#94735=CARTESIAN_POINT ( 'NONE',  ( 16.40814093676323893, 25.79030133659708923, 11.09922568453595026 ) ) ;
#94736=CARTESIAN_POINT ( 'NONE',  ( 5.076628168052703671, 16.84226448433411960, 8.527530157486179263 ) ) ;
#94737=CARTESIAN_POINT ( 'NONE',  ( 19.38216949554541557, 47.24863466993041783, -9.382169495545420901 ) ) ;
#94739=CARTESIAN_POINT ( 'NONE',  ( 10.00000000000000178, 32.25893115100078745, 9.846743663894594434 ) ) ;
#94740=CARTESIAN_POINT ( 'NONE',  ( 12.91533473730992121, 59.52201867748816966, 10.88017736071110164 ) ) ;
#94744=CARTESIAN_POINT ( 'NONE',  ( 2.148416515056630782, 2.237265733804437495, 6.499999999999993783 ) ) ;
#94745=CARTESIAN_POINT ( 'NONE',  ( 0.5774900079438607392, 68.48035201082150536, 5.440088680355550821 ) ) ;
#94747=CARTESIAN_POINT ( 'NONE',  ( 3.591859063236761518, 14.95696800326375531, 11.09922568453594849 ) ) ;
#94750=CARTESIAN_POINT ( 'NONE',  ( 10.00000000000000000, 49.75893115100078745, -9.846743663894594434 ) ) ;
#94751=CARTESIAN_POINT ( 'NONE',  ( 13.43411237798106583, 62.66530133659708923, -12.81628187352647252 ) ) ;
#94752=CARTESIAN_POINT ( 'NONE',  ( -4.164238869374098151, 11.59541550158063217, -3.795296366450310543 ) ) ;
#94753=CARTESIAN_POINT ( 'NONE',  ( 2.791683348922240793, 36.63393115100078035, 7.208316651077764092 ) ) ;
#94755=CARTESIAN_POINT ( 'NONE',  ( 16.40814093676323893, 30.79030133659708923, 11.09922568453595026 ) ) ;
#94757=CARTESIAN_POINT ( 'NONE',  ( 20.10421743870887212, 15.60736173766201951, -6.337391062633417782 ) ) ;
#94758=CARTESIAN_POINT ( 'NONE',  ( 10.00000000000000000, 66.81368534415484817, -10.88017736071110342 ) ) ;
#94759=CARTESIAN_POINT ( 'NONE',  ( -2.816281873526473856, 4.123634669930420493, 9.499525473075851096E-16 ) ) ;
#94761=CARTESIAN_POINT ( 'NONE',  ( 19.84674366389459266, 38.30059781766745175, 2.638427012816836559 ) ) ;
#94762=CARTESIAN_POINT ( 'NONE',  ( 10.00000000000000178, 29.31368534415483751, 10.88017736071110342 ) ) ;
#94763=CARTESIAN_POINT ( 'NONE',  ( -2.816281873526473856, 24.33196800326375353, 3.434112377981055619 ) ) ;
#94764=CARTESIAN_POINT ( 'NONE',  ( 17.20831665107776587, 17.88393115100078745, 7.208316651077764980 ) ) ;
#94766=CARTESIAN_POINT ( 'NONE',  ( 2.035157376598824452, 38.68868534415483396, 7.964842623401179544 ) ) ;
#94768=CARTESIAN_POINT ( 'NONE',  ( 0.5774900079438607392, 58.48035201082151247, 5.440088680355550821 ) ) ;
#94769=SURFACE_STYLE_FILL_AREA ( #10788 ) ;
#94770=CARTESIAN_POINT ( 'NONE',  ( 14.92337183194729633, 47.67559781766745175, 8.527530157486181039 ) ) ;
#94771=CARTESIAN_POINT ( 'NONE',  ( -0.8801773607110991993, 27.85535201082150181, -2.915334737309923874 ) ) ;
#94772=CARTESIAN_POINT ( 'NONE',  ( 2.035157376598822676, 47.43868534415484817, -7.964842623401177768 ) ) ;
#94773=CARTESIAN_POINT ( 'NONE',  ( 12.91533473730993009, 11.60535201082150714, -10.88017736071109987 ) ) ;
#94775=CARTESIAN_POINT ( 'NONE',  ( 14.92337183194729633, 42.67559781766745886, 8.527530157486181039 ) ) ;
#94776=CARTESIAN_POINT ( 'NONE',  ( 6.204703633549690345, 47.84541550158064638, 14.16423886937410082 ) ) ;
#94781=CARTESIAN_POINT ( 'NONE',  ( 20.36894250292379382, 43.67874883491397497, 10.36894250292379205 ) ) ;
#94783=VERTEX_POINT ( 'NONE', #95135 ) ;
#94784=CARTESIAN_POINT ( 'NONE',  ( 4.559911319644449179, 3.897018677488171434, 9.422509992056141925 ) ) ;
#94785=CARTESIAN_POINT ( 'NONE',  ( 18.52753015748618282, 38.92559781766745175, -4.923371831947291888 ) ) ;
#94788=CARTESIAN_POINT ( 'NONE',  ( 0.5774900079438607392, 63.48035201082149825, 5.440088680355550821 ) ) ;
#94789=CARTESIAN_POINT ( 'NONE',  ( -1.099225684535947600, 59.54030133659708923, 6.408140936763237150 ) ) ;
#94790=CARTESIAN_POINT ( 'NONE',  ( 12.91533473730993009, 36.60535201082151247, -10.88017736071109987 ) ) ;
#94791=CARTESIAN_POINT ( 'NONE',  ( 10.00000000000000178, 60.37363466993041783, 12.81628187352647608 ) ) ;
#94792=CARTESIAN_POINT ( 'NONE',  ( 13.43411237798105340, 10.58196800326375353, 12.81628187352647963 ) ) ;
#94793=CARTESIAN_POINT ( 'NONE',  ( 0.1532563361054082862, 16.21726448433411960, 2.638427012816831674 ) ) ;
#94795=( LENGTH_UNIT ( ) NAMED_UNIT ( * ) SI_UNIT ( .MILLI., .METRE. ) );
#94797=CARTESIAN_POINT ( 'NONE',  ( 2.035157376598822676, 7.438685344154837509, -7.964842623401177768 ) ) ;
#94798=CARTESIAN_POINT ( 'NONE',  ( -0.3689425029237898834, 21.17874883491396432, -10.36894250292378850 ) ) ;
#94799=CARTESIAN_POINT ( 'NONE',  ( 17.96484262340118221, 29.93868534415484106, 7.964842623401181321 ) ) ;
#94800=CARTESIAN_POINT ( 'NONE',  ( 19.42250999205614548, 50.98035201082151247, -5.440088680355545492 ) ) ;
#94801=CARTESIAN_POINT ( 'NONE',  ( -38.69000000000001194, 93.50000000000000000, -10.09898361729590199 ) ) ;
#94803=CARTESIAN_POINT ( 'NONE',  ( 1.472469842513823179, 6.425597817667451750, 4.923371831947296329 ) ) ;
#94805=CARTESIAN_POINT ( 'NONE',  ( 7.361572987183170547, 27.05059781766745175, 9.846743663894590881 ) ) ;
#94807=CARTESIAN_POINT ( 'NONE',  ( 19.84674366389459621, 23.50893115100078390, 7.409399052514197653E-17 ) ) ;
#94808=CARTESIAN_POINT ( 'NONE',  ( 1.472469842513823179, 46.42559781766745175, 4.923371831947296329 ) ) ;
#94810=CARTESIAN_POINT ( 'NONE',  ( 2.035157376598822676, 22.43868534415483396, -7.964842623401177768 ) ) ;
#94811=CARTESIAN_POINT ( 'NONE',  ( 10.00000000000000000, 42.87363466993042493, -12.81628187352647608 ) ) ;
#94813=CARTESIAN_POINT ( 'NONE',  ( 0.1532563361054100626, 0.8005978176674514168, -2.638427012816831230 ) ) ;
#94814=CARTESIAN_POINT ( 'NONE',  ( 14.92337183194729633, 32.67559781766745175, 8.527530157486181039 ) ) ;
#94815=CARTESIAN_POINT ( 'NONE',  ( 13.79529636645031943, 60.34541550158063927, -14.16423886937409904 ) ) ;
#94816=CARTESIAN_POINT ( 'NONE',  ( 18.52753015748617571, 18.09226448433411960, 4.923371831947298993 ) ) ;
#94818=CARTESIAN_POINT ( 'NONE',  ( -42.80192881254231452, 92.20710678118653902, -9.499999999999998224 ) ) ;
#94819=CARTESIAN_POINT ( 'NONE',  ( -4.164238869374099039, 6.803748834913967869, 8.674139862899312516E-16 ) ) ;
#94820=CARTESIAN_POINT ( 'NONE',  ( -2.266590686148945544, 32.22041550158063927, 7.082119434687048631 ) ) ;
#94821=CARTESIAN_POINT ( 'NONE',  ( 2.791683348922237240, 25.38393115100078390, -7.208316651077763204 ) ) ;
#94823=CARTESIAN_POINT ( 'NONE',  ( 15.44008868035555260, 19.73035201082150536, 9.422509992056143702 ) ) ;
#94825=CARTESIAN_POINT ( 'NONE',  ( 10.00000000000000000, 56.81368534415484106, -10.88017736071110342 ) ) ;
#94826=CARTESIAN_POINT ( 'NONE',  ( 0.5774900079438607392, 38.48035201082150536, 5.440088680355550821 ) ) ;
#94828=CARTESIAN_POINT ( 'NONE',  ( 3.591859063236761518, 44.95696800326376064, 11.09922568453594849 ) ) ;
#94829=CARTESIAN_POINT ( 'NONE',  ( 12.91533473730992121, 49.52201867748817676, 10.88017736071110164 ) ) ;
#94834=CARTESIAN_POINT ( 'NONE',  ( 15.44008868035555793, 61.39701867748817676, -9.422509992056140149 ) ) ;
#94835=CARTESIAN_POINT ( 'NONE',  ( 19.42250999205614548, 5.980352010821504471, -5.440088680355545492 ) ) ;
#94837=CARTESIAN_POINT ( 'NONE',  ( 20.88017736071110164, 40.35535201082150536, 2.915334737309930979 ) ) ;
#94838=DIRECTION ( 'NONE',  ( -0.000000000000000000, -1.000000000000000000, 0.000000000000000000 ) ) ;
#94839=CARTESIAN_POINT ( 'NONE',  ( 10.00000000000000000, 1.813685344154838175, -10.88017736071110342 ) ) ;
#94840=CARTESIAN_POINT ( 'NONE',  ( 14.92337183194729988, 4.342264484334117824, -8.527530157486177487 ) ) ;
#94841=CARTESIAN_POINT ( 'NONE',  ( 22.26659068614894466, 8.887082168247300018, 7.082119434687054849 ) ) ;
#94842=CARTESIAN_POINT ( 'NONE',  ( 5.076628168052704559, 5.175597817667451750, -8.527530157486179263 ) ) ;
#94844=CARTESIAN_POINT ( 'NONE',  ( -0.8801773607111008646, 13.27201867748817143, 2.915334737309923430 ) ) ;
#94845=CARTESIAN_POINT ( 'NONE',  ( 1.472469842513823179, 46.42559781766745175, 4.923371831947296329 ) ) ;
#94847=CARTESIAN_POINT ( 'NONE',  ( 19.84674366389459621, 48.50893115100078745, 7.409399052514197653E-17 ) ) ;
#94850=CARTESIAN_POINT ( 'NONE',  ( 12.91533473730993009, 56.60535201082151247, -10.88017736071109987 ) ) ;
#94851=CARTESIAN_POINT ( 'NONE',  ( 5.076628168052703671, 51.84226448433412315, 8.527530157486179263 ) ) ;
#94852=CARTESIAN_POINT ( 'NONE',  ( 0.5774900079438607392, 3.480352010821504027, 5.440088680355550821 ) ) ;
#94854=CARTESIAN_POINT ( 'NONE',  ( 15.44008868035555260, 54.73035201082150536, 9.422509992056143702 ) ) ;
#94855=CARTESIAN_POINT ( 'NONE',  ( 4.559911319644449179, 7.230352010821505360, -9.422509992056141925 ) ) ;
#94856=CARTESIAN_POINT ( 'NONE',  ( 10.00000000000000000, 37.87363466993041783, -12.81628187352647608 ) ) ;
#94857=CARTESIAN_POINT ( 'NONE',  ( 12.91533473730992121, 34.52201867748817676, 10.88017736071110164 ) ) ;
#94858=CARTESIAN_POINT ( 'NONE',  ( 0.000000000000000000, 69.50000000000000000, 6.000000000000000000 ) ) ;
#94859=EDGE_LOOP ( 'NONE', ( #3313, #7688, #19001, #57577 ) ) ;
#94860=CARTESIAN_POINT ( 'NONE',  ( 16.40814093676323893, 45.79030133659708923, 11.09922568453595026 ) ) ;
#94861=CARTESIAN_POINT ( 'NONE',  ( 0.5774900079438607392, 38.48035201082150536, 5.440088680355550821 ) ) ;
#94862=EDGE_LOOP ( 'NONE', ( #12587, #30769, #38368, #76953 ) ) ;
#94865=CARTESIAN_POINT ( 'NONE',  ( 18.52753015748617571, 8.092264484334117824, 4.923371831947298993 ) ) ;
#94866=CARTESIAN_POINT ( 'NONE',  ( 10.00000000000000178, 62.25893115100078745, 9.846743663894594434 ) ) ;
#94867=CARTESIAN_POINT ( 'NONE',  ( 1.472469842513823179, 6.425597817667451750, 4.923371831947296329 ) ) ;
#94868=CARTESIAN_POINT ( 'NONE',  ( 14.92337183194729633, 57.67559781766745886, 8.527530157486181039 ) ) ;
#94870=CARTESIAN_POINT ( 'NONE',  ( 12.63842701281683922, 39.55059781766744464, -9.846743663894590881 ) ) ;
#94873=EDGE_CURVE ( 'NONE', #72785, #38297, #42165, .T. ) ;
#94874=CARTESIAN_POINT ( 'NONE',  ( 17.20831665107776587, 34.13393115100078745, -7.208316651077762316 ) ) ;
#94875=CARTESIAN_POINT ( 'NONE',  ( 10.00000000000000000, -0.2410688489992152128, -9.846743663894594434 ) ) ;
#94877=CARTESIAN_POINT ( 'NONE',  ( 12.63842701281683922, 59.55059781766744464, -9.846743663894590881 ) ) ;
#94878=EDGE_LOOP ( 'NONE', ( #87768, #39760, #71252, #9144 ) ) ;
#94880=CARTESIAN_POINT ( 'NONE',  ( -2.816281873526473856, 29.12363466993041783, 9.499525473075851096E-16 ) ) ;
#94881=CARTESIAN_POINT ( 'NONE',  ( 12.63842701281683922, 44.55059781766745175, -9.846743663894590881 ) ) ;
#94882=VECTOR ( 'NONE', #8922, 1000.000000000000000 ) ;
#94884=CARTESIAN_POINT ( 'NONE',  ( 20.36894250292379382, 58.67874883491396076, 10.36894250292379205 ) ) ;
#94885=CARTESIAN_POINT ( 'NONE',  ( 1.472469842513823179, 21.42559781766745175, 4.923371831947296329 ) ) ;
#94886=CARTESIAN_POINT ( 'NONE',  ( 20.00000000000000355, 82.53121788603681352, 5.047406989012417355 ) ) ;
#94888=CARTESIAN_POINT ( 'NONE',  ( -4.164238869374098151, 61.59541550158063217, -3.795296366450310543 ) ) ;
#94889=CARTESIAN_POINT ( 'NONE',  ( 12.63842701281683922, 54.55059781766745175, -9.846743663894590881 ) ) ;
#94890=CARTESIAN_POINT ( 'NONE',  ( 7.084665262690076126, 9.105352010821503583, 10.88017736071109987 ) ) ;
#94891=CARTESIAN_POINT ( 'NONE',  ( 24.16423886937410614, 34.30374883491396787, 8.672049930838204340E-16 ) ) ;
#94892=CARTESIAN_POINT ( 'NONE',  ( -4.164238869374099927, 42.01208216824728936, 3.795296366450308767 ) ) ;
#94893=DIRECTION ( 'NONE',  ( -1.000000000000000000, 0.000000000000000000, 0.000000000000000000 ) ) ;
#94894=DIRECTION ( 'NONE',  ( 0.000000000000000000, -1.000000000000000000, 0.000000000000000000 ) ) ;
#94895=CARTESIAN_POINT ( 'NONE',  ( 12.63842701281683034, 52.46726448433413026, 9.846743663894596210 ) ) ;
#94896=ORIENTED_EDGE ( 'NONE', *, *, #22288, .T. ) ;
#94897=CARTESIAN_POINT ( 'NONE',  ( 4.559911319644449179, 32.23035201082150536, -9.422509992056141925 ) ) ;
#94899=CARTESIAN_POINT ( 'NONE',  ( 19.84674366389459621, 53.50893115100078745, 7.409399052514197653E-17 ) ) ;
#94902=CARTESIAN_POINT ( 'NONE',  ( 12.63842701281683034, 52.46726448433413026, 9.846743663894596210 ) ) ;
#94903=( BOUNDED_CURVE ( )  B_SPLINE_CURVE ( 2, ( #65708, #82195, #87723, #72710, #34718, #27215, #80226, #28700, #5233 ),
 .UNSPECIFIED., .F., .F. ) 
 B_SPLINE_CURVE_WITH_KNOTS ( ( 3, 2, 2, 2, 3 ),
 ( 0.6187123655116599785, 0.6190476190476190688, 0.6250000000000000000, 0.6309523809523809312, 0.6312876344883400215 ),
 .UNSPECIFIED. ) 
 CURVE ( )  GEOMETRIC_REPRESENTATION_ITEM ( )  RATIONAL_B_SPLINE_CURVE ( ( 0.9963778908391764944, 0.9980808541467923733, 1.000000000000000000, 0.9659258262890683122, 1.000000000000000000, 0.9659258262890683122, 1.000000000000000000, 0.9980808541467922623, 0.9963778908391764944 ) ) 
 REPRESENTATION_ITEM ( '' )  );
#94904=CARTESIAN_POINT ( 'NONE',  ( 17.20831665107776587, 62.88393115100078745, 7.208316651077764980 ) ) ;
#94905=CARTESIAN_POINT ( 'NONE',  ( 13.79529636645031943, 25.34541550158063572, -14.16423886937409904 ) ) ;
#94908=CARTESIAN_POINT ( 'NONE',  ( -46.68456736488007408, 103.6675473310227034, 5.775421524742653467 ) ) ;
#94909=CARTESIAN_POINT ( 'NONE',  ( 19.42250999205614193, 15.14701867748817143, 5.440088680355555262 ) ) ;
#94910=CARTESIAN_POINT ( 'NONE',  ( 10.00000000000000178, 20.37363466993042138, 12.81628187352647608 ) ) ;
#94912=CARTESIAN_POINT ( 'NONE',  ( 1.472469842513823179, 10.59226448433411782, -4.923371831947296329 ) ) ;
#94914=CARTESIAN_POINT ( 'NONE',  ( 6.204703633549690345, 30.76208216824730357, -14.16423886937410259 ) ) ;
#94916=SURFACE_STYLE_FILL_AREA ( #64410 ) ;
#94917=CARTESIAN_POINT ( 'NONE',  ( 2.035157376598824452, 8.688685344154839285, 7.964842623401179544 ) ) ;
#94919=CARTESIAN_POINT ( 'NONE',  ( 7.084665262690076126, 42.02201867748816966, -10.88017736071110164 ) ) ;
#94920=CARTESIAN_POINT ( 'NONE',  ( 7.084665262690076126, 37.02201867748817676, -10.88017736071110164 ) ) ;
#94921=CARTESIAN_POINT ( 'NONE',  ( 19.84674366389459266, 63.71726448433412315, -2.638427012816827677 ) ) ;
#94922=LINE ( 'NONE', #41462, #26617 ) ;
#94924=CARTESIAN_POINT ( 'NONE',  ( 19.84674366389459266, 8.717264484334116048, -2.638427012816827677 ) ) ;
#94927=CARTESIAN_POINT ( 'NONE',  ( 20.88017736071110875, 40.77201867748818387, -2.915334737309920765 ) ) ;
#94929=CARTESIAN_POINT ( 'NONE',  ( -2.816281873526473856, 4.331968003263754419, 3.434112377981055619 ) ) ;
#94930=CARTESIAN_POINT ( 'NONE',  ( 4.559911319644449179, 58.89701867748817676, 9.422509992056141925 ) ) ;
#94931=CARTESIAN_POINT ( 'NONE',  ( 14.92337183194729633, 22.67559781766745175, 8.527530157486181039 ) ) ;
#94932=CARTESIAN_POINT ( 'NONE',  ( 0.6178305044545838731, 29.74863466993042138, 9.382169495545420901 ) ) ;
#94933=CARTESIAN_POINT ( 'NONE',  ( 0.1532563361054082862, 6.217264484334118713, 2.638427012816831674 ) ) ;
#94938=CARTESIAN_POINT ( 'NONE',  ( 12.91533473730992121, 9.522018677488171434, 10.88017736071110164 ) ) ;
#94939=CARTESIAN_POINT ( 'NONE',  ( 6.565887622018943937, 55.16530133659709634, 12.81628187352647430 ) ) ;
#94940=CARTESIAN_POINT ( 'NONE',  ( 10.00000000000000000, 20.55374883491396787, -14.16423886937410082 ) ) ;
#94941=CARTESIAN_POINT ( 'NONE',  ( 19.84674366389459266, 33.71726448433410894, -2.638427012816827677 ) ) ;
#94942=CARTESIAN_POINT ( 'NONE',  ( 15.44008868035555793, 6.397018677488170546, -9.422509992056140149 ) ) ;
#94943=CARTESIAN_POINT ( 'NONE',  ( 13.79529636645031943, 65.34541550158063217, -14.16423886937409904 ) ) ;
#94945=CARTESIAN_POINT ( 'NONE',  ( 17.96484262340118221, 11.18868534415483929, -7.964842623401177768 ) ) ;
#94946=CARTESIAN_POINT ( 'NONE',  ( -0.8801773607111008646, 23.27201867748817676, 2.915334737309923430 ) ) ;
#94949=CARTESIAN_POINT ( 'NONE',  ( 7.361572987183169658, 64.96726448433412315, -9.846743663894592657 ) ) ;
#94950=CARTESIAN_POINT ( 'NONE',  ( 20.88017736071110875, 20.77201867748816611, -2.915334737309920765 ) ) ;
#94951=CARTESIAN_POINT ( 'NONE',  ( 5.076628168052703671, 51.84226448433412315, 8.527530157486179263 ) ) ;
#94953=CARTESIAN_POINT ( 'NONE',  ( 22.81628187352647785, 51.41530133659708923, 3.434112377981063169 ) ) ;
#94955=CARTESIAN_POINT ( 'NONE',  ( 17.08211943468705840, 40.13708216824731068, -12.26659068614894466 ) ) ;
#94956=CARTESIAN_POINT ( 'NONE',  ( 20.88017736071110519, 40.56368534415484106, 2.639326808657452039E-16 ) ) ;
#94957=CARTESIAN_POINT ( 'NONE',  ( -0.8801773607110991993, 17.85535201082150536, -2.915334737309923874 ) ) ;
#94958=CARTESIAN_POINT ( 'NONE',  ( 2.791683348922237240, 50.38393115100078035, -7.208316651077763204 ) ) ;
#94959=CIRCLE ( 'NONE', #32645, 0.5000000000000004441 ) ;
#94960=CARTESIAN_POINT ( 'NONE',  ( 7.361572987183169658, 54.96726448433413026, -9.846743663894592657 ) ) ;
#94963=CARTESIAN_POINT ( 'NONE',  ( 18.52753015748618282, 3.925597817667451306, -4.923371831947291888 ) ) ;
#94966=CARTESIAN_POINT ( 'NONE',  ( 2.035157376598824452, 18.68868534415484106, 7.964842623401179544 ) ) ;
#94967=CARTESIAN_POINT ( 'NONE',  ( 0.1532563361054100626, 15.80059781766745353, -2.638427012816831230 ) ) ;
#94968=CARTESIAN_POINT ( 'NONE',  ( 13.43411237798106583, 2.665301336597086568, -12.81628187352647252 ) ) ;
#94969=CARTESIAN_POINT ( 'NONE',  ( 19.42250999205614548, 45.98035201082150536, -5.440088680355545492 ) ) ;
#94970=CARTESIAN_POINT ( 'NONE',  ( 0.5774900079438590739, 52.64701867748817676, -5.440088680355550821 ) ) ;
#94971=CARTESIAN_POINT ( 'NONE',  ( 12.91533473730992121, 14.52201867748817143, 10.88017736071110164 ) ) ;
#94972=CARTESIAN_POINT ( 'NONE',  ( 13.43411237798105340, 45.58196800326374643, 12.81628187352647963 ) ) ;
#94973=CARTESIAN_POINT ( 'NONE',  ( 24.16423886937410614, 29.30374883491396787, 8.672049930838204340E-16 ) ) ;
#94976=CARTESIAN_POINT ( 'NONE',  ( 16.40814093676323893, 55.79030133659708923, 11.09922568453595026 ) ) ;
#94978=CARTESIAN_POINT ( 'NONE',  ( 10.00000000000000000, 59.75893115100078745, -9.846743663894594434 ) ) ;
#94979=CARTESIAN_POINT ( 'NONE',  ( 15.44008868035555260, 29.73035201082150891, 9.422509992056143702 ) ) ;
#94981=CARTESIAN_POINT ( 'NONE',  ( 5.076628168052703671, 6.842264484334118713, 8.527530157486179263 ) ) ;
#94983=CARTESIAN_POINT ( 'NONE',  ( 2.791683348922240793, 6.633931151000785675, 7.208316651077764092 ) ) ;
#94984=CARTESIAN_POINT ( 'NONE',  ( 7.361572987183169658, 19.96726448433411960, -9.846743663894592657 ) ) ;
#94985=CARTESIAN_POINT ( 'NONE',  ( 14.92337183194729633, 7.675597817667451750, 8.527530157486181039 ) ) ;
#94986=CARTESIAN_POINT ( 'NONE',  ( 17.20831665107776587, 2.883931151000785231, 7.208316651077764980 ) ) ;
#94989=CARTESIAN_POINT ( 'NONE',  ( 2.035157376598824452, 63.68868534415484106, 7.964842623401179544 ) ) ;
#94990=CARTESIAN_POINT ( 'NONE',  ( 4.559911319644449179, 62.23035201082150536, -9.422509992056141925 ) ) ;
#94991=CARTESIAN_POINT ( 'NONE',  ( 2.791683348922237240, 20.38393115100078745, -7.208316651077763204 ) ) ;
#94993=B_SPLINE_CURVE_WITH_KNOTS ( 'NONE', 3,
 ( #84564, #6717, #96748, #36731 ),
 .UNSPECIFIED., .F., .F.,
 ( 4, 4 ),
 ( 1.321126039445492370E-17, 0.002562518741975311660 ),
 .UNSPECIFIED. ) ;
#94995=CARTESIAN_POINT ( 'NONE',  ( 12.63842701281683922, 59.55059781766744464, -9.846743663894590881 ) ) ;
#94997=CARTESIAN_POINT ( 'NONE',  ( -42.94000000000001194, 92.00000000000000000, -10.09898361729590199 ) ) ;
#94998=CARTESIAN_POINT ( 'NONE',  ( 20.36894250292379382, 3.678748834913967869, 10.36894250292379205 ) ) ;
#95000=CARTESIAN_POINT ( 'NONE',  ( -4.164238869374099927, 12.01208216824730357, 3.795296366450308767 ) ) ;
#95001=CARTESIAN_POINT ( 'NONE',  ( 13.79529636645030344, 28.26208216824729647, 14.16423886937410614 ) ) ;
#95003=CARTESIAN_POINT ( 'NONE',  ( 6.204703633549690345, 2.845415501580634388, 14.16423886937410082 ) ) ;
#95004=CARTESIAN_POINT ( 'NONE',  ( 20.88017736071110164, 35.35535201082150536, 2.915334737309930979 ) ) ;
#95006=CARTESIAN_POINT ( 'NONE',  ( 18.52753015748618282, 18.92559781766745175, -4.923371831947291888 ) ) ;
#95007=CARTESIAN_POINT ( 'NONE',  ( 4.559911319644449179, 52.23035201082151247, -9.422509992056141925 ) ) ;
#95008=CARTESIAN_POINT ( 'NONE',  ( 19.84674366389459266, 13.71726448433411782, -2.638427012816827677 ) ) ;
#95009=CARTESIAN_POINT ( 'NONE',  ( 19.38216949554541202, 40.99863466993042493, 9.382169495545424454 ) ) ;
#95010=CARTESIAN_POINT ( 'NONE',  ( 14.92337183194729988, 39.34226448433412315, -8.527530157486177487 ) ) ;
#95011=DIRECTION ( 'NONE',  ( 1.000000000000000000, -0.000000000000000000, -0.000000000000000000 ) ) ;
#95012=CARTESIAN_POINT ( 'NONE',  ( 21.09922568453594849, 26.20696800326375353, 6.408140936763242479 ) ) ;
#95014=CARTESIAN_POINT ( 'NONE',  ( 2.791683348922237240, 30.38393115100078390, -7.208316651077763204 ) ) ;
#95015=CARTESIAN_POINT ( 'NONE',  ( -2.266590686148945544, 17.22041550158063572, 7.082119434687048631 ) ) ;
#95019=CARTESIAN_POINT ( 'NONE',  ( 20.88017736071110519, 35.56368534415484106, 2.639326808657452039E-16 ) ) ;
#95020=CARTESIAN_POINT ( 'NONE',  ( -0.8801773607110991993, 52.85535201082151247, -2.915334737309923874 ) ) ;
#95021=CARTESIAN_POINT ( 'NONE',  ( -4.164238869374099039, 46.80374883491397497, 8.674139862899312516E-16 ) ) ;
#95022=CARTESIAN_POINT ( 'NONE',  ( 14.92337183194729633, 57.67559781766745886, 8.527530157486181039 ) ) ;
#95023=CARTESIAN_POINT ( 'NONE',  ( 0.1532563361054083140, 6.008931151000784787, 1.131784320476157264E-15 ) ) ;
#95026=CARTESIAN_POINT ( 'NONE',  ( 12.91533473730993009, 46.60535201082150536, -10.88017736071109987 ) ) ;
#95027=DIRECTION ( 'NONE',  ( -0.000000000000000000, -0.000000000000000000, -1.000000000000000000 ) ) ;
#95028=CARTESIAN_POINT ( 'NONE',  ( 21.09922568453594849, 26.20696800326375353, 6.408140936763242479 ) ) ;
#95029=CARTESIAN_POINT ( 'NONE',  ( 19.84674366389459621, 53.50893115100078745, 7.409399052514197653E-17 ) ) ;
#95031=CARTESIAN_POINT ( 'NONE',  ( 10.00000000000000178, 4.313685344154837509, 10.88017736071110342 ) ) ;
#95032=CARTESIAN_POINT ( 'NONE',  ( 0.5774900079438607392, 63.48035201082149825, 5.440088680355550821 ) ) ;
#95035=FACE_OUTER_BOUND ( 'NONE', #72585, .T. ) ;
#95036=CARTESIAN_POINT ( 'NONE',  ( 20.88017736071110875, 65.77201867748817676, -2.915334737309920765 ) ) ;
#95037=CARTESIAN_POINT ( 'NONE',  ( 10.00000000000000000, 66.81368534415484817, -10.88017736071110342 ) ) ;
#95040=CARTESIAN_POINT ( 'NONE',  ( 17.20831665107776587, 37.88393115100078745, 7.208316651077764980 ) ) ;
#95041=EDGE_CURVE ( 'NONE', #48119, #80255, #30585, .T. ) ;
#95042=CARTESIAN_POINT ( 'NONE',  ( 4.559911319644449179, 22.23035201082150536, -9.422509992056141925 ) ) ;
#95043=CARTESIAN_POINT ( 'NONE',  ( 6.565887622018943937, 0.1653013365970866511, 12.81628187352647430 ) ) ;
#95044=CARTESIAN_POINT ( 'NONE',  ( 19.42250999205614548, 35.98035201082151247, -5.440088680355545492 ) ) ;
#95047=CARTESIAN_POINT ( 'NONE',  ( 16.40814093676324603, 32.45696800326375353, -11.09922568453594671 ) ) ;
#95049=CARTESIAN_POINT ( 'NONE',  ( 15.44008868035555793, 51.39701867748816966, -9.422509992056140149 ) ) ;
#95050=CARTESIAN_POINT ( 'NONE',  ( 16.40814093676324603, 22.45696800326375353, -11.09922568453594671 ) ) ;
#95051=CARTESIAN_POINT ( 'NONE',  ( 12.91533473730992121, 24.52201867748816966, 10.88017736071110164 ) ) ;
#95052=CARTESIAN_POINT ( 'NONE',  ( 2.917880565312950480, 65.97041550158063217, -12.26659068614894821 ) ) ;
#95053=CARTESIAN_POINT ( 'NONE',  ( 0.1532563361054100626, 45.80059781766745886, -2.638427012816831230 ) ) ;
#95054=CARTESIAN_POINT ( 'NONE',  ( 19.84674366389459266, 3.300597817667451750, 2.638427012816836559 ) ) ;
#95055=CARTESIAN_POINT ( 'NONE',  ( 15.44008868035555793, 56.39701867748817676, -9.422509992056140149 ) ) ;
#95057=CARTESIAN_POINT ( 'NONE',  ( 20.36894250292379382, 33.67874883491396076, 10.36894250292379205 ) ) ;
#95063=ORIENTED_EDGE ( 'NONE', *, *, #3061, .F. ) ;
#95064=CARTESIAN_POINT ( 'NONE',  ( 22.26659068614894466, 53.88708216824731068, 7.082119434687054849 ) ) ;
#95065=CARTESIAN_POINT ( 'NONE',  ( -0.3689425029237881626, 52.42874883491396076, 10.36894250292379027 ) ) ;
#95066=CARTESIAN_POINT ( 'NONE',  ( 2.791683348922237240, 15.38393115100078212, -7.208316651077763204 ) ) ;
#95069=CARTESIAN_POINT ( 'NONE',  ( 10.00000000000000178, 15.37363466993042138, 12.81628187352647608 ) ) ;
#95071=CARTESIAN_POINT ( 'NONE',  ( 4.999999999999999112, 11.50000000000000000, 6.500000000000000888 ) ) ;
#95072=CARTESIAN_POINT ( 'NONE',  ( 0.6178305044545818747, 28.49863466993041783, -9.382169495545419124 ) ) ;
#95073=CARTESIAN_POINT ( 'NONE',  ( 22.26659068614894466, 43.88708216824729647, 7.082119434687054849 ) ) ;
#95075=( NAMED_UNIT ( * ) SI_UNIT ( $, .STERADIAN. ) SOLID_ANGLE_UNIT ( ) );
#95079=AXIS2_PLACEMENT_3D ( 'NONE', #72005, #11505, #12490 ) ;
#95080=FACE_OUTER_BOUND ( 'NONE', #46028, .T. ) ;
#95081=CARTESIAN_POINT ( 'NONE',  ( 5.076628168052703671, 16.84226448433411960, 8.527530157486179263 ) ) ;
#95083=CARTESIAN_POINT ( 'NONE',  ( 17.96484262340118221, 11.18868534415484106, -7.964842623401177768 ) ) ;
#95084=CARTESIAN_POINT ( 'NONE',  ( 0.5774900079438607392, 8.480352010821505360, 5.440088680355550821 ) ) ;
#95085=CARTESIAN_POINT ( 'NONE',  ( 17.20831665107776587, 54.13393115100079456, -7.208316651077762316 ) ) ;
#95086=CARTESIAN_POINT ( 'NONE',  ( -1.099225684535947600, 3.706968003263753531, -6.408140936763238038 ) ) ;
#95090=CARTESIAN_POINT ( 'NONE',  ( 6.565887622018943937, 15.16530133659708568, 12.81628187352647430 ) ) ;
#95092=CARTESIAN_POINT ( 'NONE',  ( 22.26659068614894466, 58.88708216824729647, 7.082119434687054849 ) ) ;
#95094=CARTESIAN_POINT ( 'NONE',  ( -4.164238869374098151, 61.59541550158063217, -3.795296366450310543 ) ) ;
#95096=CARTESIAN_POINT ( 'NONE',  ( 4.559911319644449179, 28.89701867748817321, 9.422509992056141925 ) ) ;
#95097=CARTESIAN_POINT ( 'NONE',  ( 17.96484262340118221, 41.18868534415484106, -7.964842623401177768 ) ) ;
#95098=CARTESIAN_POINT ( 'NONE',  ( 19.42250999205614548, 55.98035201082150536, -5.440088680355545492 ) ) ;
#95100=CARTESIAN_POINT ( 'NONE',  ( 7.084665262690076126, 47.02201867748818387, -10.88017736071110164 ) ) ;
#95104=CARTESIAN_POINT ( 'NONE',  ( 12.63842701281683034, 12.46726448433411782, 9.846743663894596210 ) ) ;
#95107=CARTESIAN_POINT ( 'NONE',  ( 1.472469842513823179, 41.42559781766745886, 4.923371831947296329 ) ) ;
#95109=CARTESIAN_POINT ( 'NONE',  ( 10.00000000000000178, 50.37363466993042493, 12.81628187352647608 ) ) ;
#95115=CARTESIAN_POINT ( 'NONE',  ( 6.204703633549690345, 65.76208216824731778, -14.16423886937410259 ) ) ;
#95116=CARTESIAN_POINT ( 'NONE',  ( 1.472469842513823179, 66.42559781766745175, 4.923371831947296329 ) ) ;
#95119=CARTESIAN_POINT ( 'NONE',  ( 10.00000000000000000, 34.75893115100078745, -9.846743663894594434 ) ) ;
#95120=CARTESIAN_POINT ( 'NONE',  ( 22.81628187352647785, 61.62363466993041783, 6.195893100308588602E-16 ) ) ;
#95122=CARTESIAN_POINT ( 'NONE',  ( -1.099225684535947600, 3.706968003263753531, -6.408140936763238038 ) ) ;
#95123=CARTESIAN_POINT ( 'NONE',  ( 19.84674366389459266, 3.300597817667451750, 2.638427012816836559 ) ) ;
#95125=CARTESIAN_POINT ( 'NONE',  ( 2.791683348922237240, 15.38393115100078212, -7.208316651077763204 ) ) ;
#95126=CARTESIAN_POINT ( 'NONE',  ( 12.63842701281683034, 52.46726448433413026, 9.846743663894596210 ) ) ;
#95129=CARTESIAN_POINT ( 'NONE',  ( 2.917880565312948704, 62.63708216824730357, 12.26659068614894643 ) ) ;
#95130=CARTESIAN_POINT ( 'NONE',  ( 20.36894250292379382, 8.678748834913967869, 10.36894250292379205 ) ) ;
#95131=CARTESIAN_POINT ( 'NONE',  ( 15.44008868035555793, 41.39701867748817676, -9.422509992056140149 ) ) ;
#95132=CARTESIAN_POINT ( 'NONE',  ( 6.565887622018943937, 28.08196800326375353, -12.81628187352647608 ) ) ;
#95133=CARTESIAN_POINT ( 'NONE',  ( 4.559911319644449179, 67.23035201082150536, -9.422509992056141925 ) ) ;
#95134=SURFACE_STYLE_FILL_AREA ( #19642 ) ;
#95135=CARTESIAN_POINT ( 'NONE',  ( -42.50369195530269195, 107.9060299417078426, -4.500000000000001776 ) ) ;
#95137=CARTESIAN_POINT ( 'NONE',  ( 12.63842701281683922, 54.55059781766745175, -9.846743663894590881 ) ) ;
#95138=CARTESIAN_POINT ( 'NONE',  ( 0.1532563361054100626, 10.80059781766745175, -2.638427012816831230 ) ) ;
#95140=CARTESIAN_POINT ( 'NONE',  ( 21.09922568453594849, 21.20696800326375353, 6.408140936763242479 ) ) ;
#95143=CARTESIAN_POINT ( 'NONE',  ( 17.96484262340118221, 31.18868534415483751, -7.964842623401177768 ) ) ;
#95146=CARTESIAN_POINT ( 'NONE',  ( 22.26659068614895176, 54.72041550158063217, -7.082119434687042414 ) ) ;
#95147=CARTESIAN_POINT ( 'NONE',  ( 2.917880565312950480, 35.97041550158063217, -12.26659068614894821 ) ) ;
#95149=CARTESIAN_POINT ( 'NONE',  ( 2.791683348922240793, 41.63393115100078745, 7.208316651077764092 ) ) ;
#95151=CARTESIAN_POINT ( 'NONE',  ( 21.09922568453594849, 31.20696800326375353, 6.408140936763242479 ) ) ;
#95152=CARTESIAN_POINT ( 'NONE',  ( 20.88017736071110875, 25.77201867748816966, -2.915334737309920765 ) ) ;
#95154=CARTESIAN_POINT ( 'NONE',  ( 7.361572987183169658, 54.96726448433413026, -9.846743663894592657 ) ) ;
#95155=CARTESIAN_POINT ( 'NONE',  ( 7.084665262690076126, 37.02201867748817676, -10.88017736071110164 ) ) ;
#95156=CARTESIAN_POINT ( 'NONE',  ( -2.816281873526473856, 4.123634669930420493, 9.499525473075851096E-16 ) ) ;
#95157=CARTESIAN_POINT ( 'NONE',  ( 2.917880565312950480, 15.97041550158063217, -12.26659068614894821 ) ) ;
#95160=EDGE_CURVE ( 'NONE', #55238, #33937, #22620, .T. ) ;
#95161=CARTESIAN_POINT ( 'NONE',  ( 7.361572987183169658, 19.96726448433411960, -9.846743663894592657 ) ) ;
#95162=FILL_AREA_STYLE_COLOUR ( '', #7319 ) ;
#95163=CARTESIAN_POINT ( 'NONE',  ( 10.00000000000000178, 62.25893115100078745, 9.846743663894594434 ) ) ;
#95167=CARTESIAN_POINT ( 'NONE',  ( 20.36894250292379382, 63.67874883491396787, 10.36894250292379205 ) ) ;
#95168=CARTESIAN_POINT ( 'NONE',  ( 17.08211943468705840, 15.13708216824730179, -12.26659068614894466 ) ) ;
#95169=CARTESIAN_POINT ( 'NONE',  ( 20.88017736071110875, 65.77201867748817676, -2.915334737309920765 ) ) ;
#95170=CARTESIAN_POINT ( 'NONE',  ( 2.791683348922237240, 50.38393115100078035, -7.208316651077763204 ) ) ;
#95171=CARTESIAN_POINT ( 'NONE',  ( 0.5774900079438607392, 33.48035201082150536, 5.440088680355550821 ) ) ;
#95173=CARTESIAN_POINT ( 'NONE',  ( 14.92337183194729633, 57.67559781766745886, 8.527530157486181039 ) ) ;
#95179=CARTESIAN_POINT ( 'NONE',  ( 24.16423886937410614, 9.512082168247301794, -3.795296366450302550 ) ) ;
#95180=CARTESIAN_POINT ( 'NONE',  ( 17.08211943468705840, 10.13708216824730179, -12.26659068614894466 ) ) ;
#95181=CARTESIAN_POINT ( 'NONE',  ( 24.16423886937409904, 59.09541550158063217, 3.795296366450317205 ) ) ;
#95182=CARTESIAN_POINT ( 'NONE',  ( 17.20831665107776587, 62.88393115100078745, 7.208316651077764980 ) ) ;
#95183=CARTESIAN_POINT ( 'NONE',  ( 0.1532563361054083140, 41.00893115100078745, 1.131784320476157264E-15 ) ) ;
#95184=CARTESIAN_POINT ( 'NONE',  ( 14.49999999999999822, 60.50000000000000000, 5.000000000000000000 ) ) ;
#95185=CARTESIAN_POINT ( 'NONE',  ( 20.88017736071110875, 35.77201867748816966, -2.915334737309920765 ) ) ;
#95186=CARTESIAN_POINT ( 'NONE',  ( 10.00000000000000000, 59.75893115100078745, -9.846743663894594434 ) ) ;
#95187=CARTESIAN_POINT ( 'NONE',  ( 22.26659068614894466, 8.887082168247300018, 7.082119434687054849 ) ) ;
#95188=CARTESIAN_POINT ( 'NONE',  ( 10.00000000000000178, 58.05374883491397497, 14.16423886937410082 ) ) ;
#95189=CARTESIAN_POINT ( 'NONE',  ( 20.88017736071110164, 10.35535201082150714, 2.915334737309930979 ) ) ;
#95190=CARTESIAN_POINT ( 'NONE',  ( -0.2418659066527709955, 68.09014588040356841, 6.114288769123044531 ) ) ;
#95192=CARTESIAN_POINT ( 'NONE',  ( -0.8801773607111009756, 63.06368534415484106, 1.068504757029289695E-15 ) ) ;
#95193=EDGE_CURVE ( 'NONE', #74944, #67813, #65972, .T. ) ;
#95194=CARTESIAN_POINT ( 'NONE',  ( 18.52753015748618282, 23.92559781766745530, -4.923371831947291888 ) ) ;
#95196=ORIENTED_EDGE ( 'NONE', *, *, #33169, .F. ) ;
#95199=CARTESIAN_POINT ( 'NONE',  ( 18.52753015748618282, 18.92559781766745175, -4.923371831947291888 ) ) ;
#95202=CARTESIAN_POINT ( 'NONE',  ( -4.164238869374098151, 31.59541550158063927, -3.795296366450310543 ) ) ;
#95203=CARTESIAN_POINT ( 'NONE',  ( 0.1532563361054083140, 31.00893115100078390, 1.131784320476157264E-15 ) ) ;
#95204=CARTESIAN_POINT ( 'NONE',  ( 7.084665262690076126, 57.02201867748817676, -10.88017736071110164 ) ) ;
#95206=CARTESIAN_POINT ( 'NONE',  ( 20.88017736071110519, 50.56368534415484106, 2.639326808657452039E-16 ) ) ;
#95207=CARTESIAN_POINT ( 'NONE',  ( 12.63842701281683922, 49.55059781766744464, -9.846743663894590881 ) ) ;
#95208=CARTESIAN_POINT ( 'NONE',  ( 21.09922568453595559, 62.04030133659709634, -6.408140936763230044 ) ) ;
#95210=MECHANICAL_DESIGN_GEOMETRIC_PRESENTATION_REPRESENTATION('',(#25018),#34528);
#95211=ORIENTED_EDGE ( 'NONE', *, *, #19747, .T. ) ;
#95212=CARTESIAN_POINT ( 'NONE',  ( 13.79529636645030344, 18.26208216824730002, 14.16423886937410614 ) ) ;
#95215=CARTESIAN_POINT ( 'NONE',  ( 21.09922568453595559, 27.04030133659708568, -6.408140936763230044 ) ) ;
#95216=CARTESIAN_POINT ( 'NONE',  ( 18.52753015748617571, 18.09226448433411960, 4.923371831947298993 ) ) ;
#95217=CARTESIAN_POINT ( 'NONE',  ( 20.88017736071110164, 5.355352010821502695, 2.915334737309930979 ) ) ;
#95218=CARTESIAN_POINT ( 'NONE',  ( 0.6178305044545838731, 54.74863466993042493, 9.382169495545420901 ) ) ;
#95220=CARTESIAN_POINT ( 'NONE',  ( 12.63842701281683922, 24.55059781766745175, -9.846743663894590881 ) ) ;
#95221=CARTESIAN_POINT ( 'NONE',  ( 10.00000000000000178, 69.31368534415484817, 10.88017736071110342 ) ) ;
#95224=DIRECTION ( 'NONE',  ( 0.000000000000000000, 0.000000000000000000, 1.000000000000000000 ) ) ;
#95225=CARTESIAN_POINT ( 'NONE',  ( 20.05723567505239302, 69.83236346210667023, 6.413539670616450472 ) ) ;
#95227=CARTESIAN_POINT ( 'NONE',  ( 7.361572987183169658, 4.967264484334119601, -9.846743663894592657 ) ) ;
#95228=CARTESIAN_POINT ( 'NONE',  ( -2.816281873526473856, 29.12363466993041783, 9.499525473075851096E-16 ) ) ;
#95231=CARTESIAN_POINT ( 'NONE',  ( 14.92337183194729988, 49.34226448433411605, -8.527530157486177487 ) ) ;
#95233=CARTESIAN_POINT ( 'NONE',  ( -4.164238869374099039, 21.80374883491396787, 8.674139862899312516E-16 ) ) ;
#95234=CARTESIAN_POINT ( 'NONE',  ( 12.63842701281683922, 34.55059781766745886, -9.846743663894590881 ) ) ;
#95235=CARTESIAN_POINT ( 'NONE',  ( 16.40814093676324603, 37.45696800326376064, -11.09922568453594671 ) ) ;
#95237=FACE_OUTER_BOUND ( 'NONE', #44820, .T. ) ;
#95238=CARTESIAN_POINT ( 'NONE',  ( 0.5774900079438607392, 63.48035201082149825, 5.440088680355550821 ) ) ;
#95239=CARTESIAN_POINT ( 'NONE',  ( -2.816281873526473856, 9.331968003263753531, 3.434112377981055619 ) ) ;
#95241=CARTESIAN_POINT ( 'NONE',  ( 0.1532563361054100626, 40.80059781766745886, -2.638427012816831230 ) ) ;
#95243=CARTESIAN_POINT ( 'NONE',  ( 18.52753015748618282, 28.92559781766745175, -4.923371831947291888 ) ) ;
#95244=CARTESIAN_POINT ( 'NONE',  ( 2.035157376598824452, 28.68868534415484106, 7.964842623401179544 ) ) ;
#95245=CARTESIAN_POINT ( 'NONE',  ( 16.40814093676323893, 30.79030133659708923, 11.09922568453595026 ) ) ;
#95247=CARTESIAN_POINT ( 'NONE',  ( 19.84674366389459621, 23.50893115100078390, 7.409399052514197653E-17 ) ) ;
#95248=STYLED_ITEM ( 'NONE', ( #11873 ), #72940 ) ;
#95252=CARTESIAN_POINT ( 'NONE',  ( 19.42250999205614548, 35.98035201082151247, -5.440088680355545492 ) ) ;
#95254=CARTESIAN_POINT ( 'NONE',  ( 4.559911319644449179, 62.23035201082150536, -9.422509992056141925 ) ) ;
#95255=CARTESIAN_POINT ( 'NONE',  ( 12.91533473730992121, 4.522018677488169658, 10.88017736071110164 ) ) ;
#95256=CARTESIAN_POINT ( 'NONE',  ( 10.00000000000000000, 59.75893115100078745, -9.846743663894594434 ) ) ;
#95257=CARTESIAN_POINT ( 'NONE',  ( 17.96484262340118221, 29.93868534415484106, 7.964842623401181321 ) ) ;
#95258=DIRECTION ( 'NONE',  ( 0.000000000000000000, 0.000000000000000000, -1.000000000000000000 ) ) ;
#95259=CARTESIAN_POINT ( 'NONE',  ( 20.88017736071110164, 50.35535201082151247, 2.915334737309930979 ) ) ;
#95260=CARTESIAN_POINT ( 'NONE',  ( 4.559911319644449179, 12.23035201082150714, -9.422509992056141925 ) ) ;
#95261=CARTESIAN_POINT ( 'NONE',  ( 20.00000000000000711, 85.79222437201613616, -4.885465336098351763 ) ) ;
#95262=CARTESIAN_POINT ( 'NONE',  ( 0.000000000000000000, 81.99999999999992895, -5.000000000000000000 ) ) ;
#95263=CARTESIAN_POINT ( 'NONE',  ( 5.500000000000000000, 11.50000000000000000, -5.000000000000000000 ) ) ;
#95264=CARTESIAN_POINT ( 'NONE',  ( 19.84674366389459266, 58.30059781766745886, 2.638427012816836559 ) ) ;
#95265=CARTESIAN_POINT ( 'NONE',  ( -0.3689425029237881626, 57.42874883491397497, 10.36894250292379027 ) ) ;
#95266=CIRCLE ( 'NONE', #56945, 11.99999999999999645 ) ;
#95269=CARTESIAN_POINT ( 'NONE',  ( -4.164238869374099039, 31.80374883491396432, 8.674139862899312516E-16 ) ) ;
#95271=EDGE_CURVE ( 'NONE', #50559, #69353, #40572, .T. ) ;
#95274=CARTESIAN_POINT ( 'NONE',  ( 2.917880565312948704, 67.63708216824730357, 12.26659068614894643 ) ) ;
#95275=CARTESIAN_POINT ( 'NONE',  ( 18.52753015748618282, 33.92559781766745886, -4.923371831947291888 ) ) ;
#95278=CARTESIAN_POINT ( 'NONE',  ( 10.00000000000000178, 54.31368534415484106, 10.88017736071110342 ) ) ;
#95282=CARTESIAN_POINT ( 'NONE',  ( 15.44008868035555793, 26.39701867748817321, -9.422509992056140149 ) ) ;
#95283=FACE_OUTER_BOUND ( 'NONE', #90550, .T. ) ;
#95284=CARTESIAN_POINT ( 'NONE',  ( 19.38216949554541557, 17.24863466993041783, -9.382169495545420901 ) ) ;
#95285=CARTESIAN_POINT ( 'NONE',  ( 17.20831665107776587, 17.88393115100078745, 7.208316651077764980 ) ) ;
#95286=VERTEX_POINT ( 'NONE', #71069 ) ;
#95289=CARTESIAN_POINT ( 'NONE',  ( -4.164238869374099039, 66.80374883491396076, 8.674139862899312516E-16 ) ) ;
#95290=CARTESIAN_POINT ( 'NONE',  ( -2.266590686148945544, 31.38708216824730002, -7.082119434687050408 ) ) ;
#95291=CARTESIAN_POINT ( 'NONE',  ( -0.8801773607111009756, 28.06368534415484106, 1.068504757029289695E-15 ) ) ;
#95292=CARTESIAN_POINT ( 'NONE',  ( 4.559911319644449179, 47.23035201082150536, -9.422509992056141925 ) ) ;
#95295=CARTESIAN_POINT ( 'NONE',  ( 14.92337183194729988, 9.342264484334119601, -8.527530157486177487 ) ) ;
#95296=CARTESIAN_POINT ( 'NONE',  ( 6.000000000000000000, 10.49999999999999822, -6.500000000000000888 ) ) ;
#95299=CARTESIAN_POINT ( 'NONE',  ( 18.52753015748618282, 23.92559781766745530, -4.923371831947291888 ) ) ;
#95300=CARTESIAN_POINT ( 'NONE',  ( 12.63842701281683922, 49.55059781766744464, -9.846743663894590881 ) ) ;
#95301=CARTESIAN_POINT ( 'NONE',  ( -0.8801773607110991993, 27.85535201082150181, -2.915334737309923874 ) ) ;
#95303=CARTESIAN_POINT ( 'NONE',  ( -2.816281873526471635, 48.91530133659708213, -3.434112377981056508 ) ) ;
#95305=CARTESIAN_POINT ( 'NONE',  ( 10.00000000000000178, 64.31368534415483396, 10.88017736071110342 ) ) ;
#95306=CARTESIAN_POINT ( 'NONE',  ( 12.63842701281683034, 32.46726448433412315, 9.846743663894596210 ) ) ;
#95307=CARTESIAN_POINT ( 'NONE',  ( -4.164238869374098151, 56.59541550158063927, -3.795296366450310543 ) ) ;
#95308=CARTESIAN_POINT ( 'NONE',  ( 0.1532563361054082862, 26.21726448433411605, 2.638427012816831674 ) ) ;
#95312=CARTESIAN_POINT ( 'NONE',  ( 2.791683348922240793, 66.63393115100079456, 7.208316651077764092 ) ) ;
#95313=CARTESIAN_POINT ( 'NONE',  ( -0.3689425029237881626, 7.428748834913967869, 10.36894250292379027 ) ) ;
#95314=CARTESIAN_POINT ( 'NONE',  ( 24.16423886937410614, 29.30374883491396787, 8.672049930838204340E-16 ) ) ;
#95315=CARTESIAN_POINT ( 'NONE',  ( 1.472469842513823179, 31.42559781766745530, 4.923371831947296329 ) ) ;
#95317=CARTESIAN_POINT ( 'NONE',  ( 4.559911319644449179, 28.89701867748817321, 9.422509992056141925 ) ) ;
#95319=CARTESIAN_POINT ( 'NONE',  ( -0.8801773607111009756, 53.06368534415484106, 1.068504757029289695E-15 ) ) ;
#95320=CARTESIAN_POINT ( 'NONE',  ( 19.42250999205614193, 50.14701867748817676, 5.440088680355555262 ) ) ;
#95322=CARTESIAN_POINT ( 'NONE',  ( 10.00000000000000000, 42.87363466993042493, -12.81628187352647608 ) ) ;
#95323=CARTESIAN_POINT ( 'NONE',  ( 10.00000000000000000, 46.81368534415484106, -10.88017736071110342 ) ) ;
#95324=ORIENTED_EDGE ( 'NONE', *, *, #43284, .T. ) ;
#95326=AXIS2_PLACEMENT_3D ( 'NONE', #18034, #41038, #47036 ) ;
#95327=CARTESIAN_POINT ( 'NONE',  ( 7.084665262690076126, 69.10535201082151957, 10.88017736071109987 ) ) ;
#95330=CARTESIAN_POINT ( 'NONE',  ( 19.42250999205614548, 60.98035201082151247, -5.440088680355545492 ) ) ;
#95331=CARTESIAN_POINT ( 'NONE',  ( 20.88017736071110519, 20.56368534415484106, 2.639326808657452039E-16 ) ) ;
#95334=CARTESIAN_POINT ( 'NONE',  ( 15.44008868035555793, 6.397018677488171434, -9.422509992056140149 ) ) ;
#95335=CARTESIAN_POINT ( 'NONE',  ( 5.076628168052704559, 15.17559781766745175, -8.527530157486179263 ) ) ;
#95336=CARTESIAN_POINT ( 'NONE',  ( 13.79529636645030344, 18.26208216824730002, 14.16423886937410614 ) ) ;
#95337=CARTESIAN_POINT ( 'NONE',  ( 7.084665262690076126, 29.10535201082150181, 10.88017736071109987 ) ) ;
#95338=CARTESIAN_POINT ( 'NONE',  ( 0.1532563361054083140, 61.00893115100078745, 1.131784320476157264E-15 ) ) ;
#95340=CARTESIAN_POINT ( 'NONE',  ( 7.361572987183170547, 67.05059781766746596, 9.846743663894590881 ) ) ;
#95343=CARTESIAN_POINT ( 'NONE',  ( 7.084665262690076126, 49.10535201082149825, 10.88017736071109987 ) ) ;
#95344=CARTESIAN_POINT ( 'NONE',  ( 14.92337183194729633, 57.67559781766745886, 8.527530157486181039 ) ) ;
#95345=STYLED_ITEM ( 'NONE', ( #86218 ), #144 ) ;
#95346=CARTESIAN_POINT ( 'NONE',  ( 16.40814093676324603, 32.45696800326375353, -11.09922568453594671 ) ) ;
#95347=CARTESIAN_POINT ( 'NONE',  ( -0.8801773607111009756, 3.063685344154837509, 1.068504757029289695E-15 ) ) ;
#95349=CARTESIAN_POINT ( 'NONE',  ( 15.44008868035555260, 59.73035201082151247, 9.422509992056143702 ) ) ;
#95350=CARTESIAN_POINT ( 'NONE',  ( 6.204703633549690345, 67.84541550158060375, 14.16423886937410082 ) ) ;
#95352=CARTESIAN_POINT ( 'NONE',  ( -2.816281873526471635, 38.91530133659708213, -3.434112377981056508 ) ) ;
#95353=CARTESIAN_POINT ( 'NONE',  ( 20.88017736071110875, 35.77201867748816966, -2.915334737309920765 ) ) ;
#95356=CARTESIAN_POINT ( 'NONE',  ( 22.81628187352647785, 41.41530133659708923, 3.434112377981063169 ) ) ;
#95357=CARTESIAN_POINT ( 'NONE',  ( 4.559911319644449179, 33.89701867748817676, 9.422509992056141925 ) ) ;
#95358=CARTESIAN_POINT ( 'NONE',  ( 0.1532563361054082862, 51.21726448433412315, 2.638427012816831674 ) ) ;
#95360=CARTESIAN_POINT ( 'NONE',  ( 1.472469842513823179, 56.42559781766745886, 4.923371831947296329 ) ) ;
#95362=CARTESIAN_POINT ( 'NONE',  ( 10.00000000000000178, 52.25893115100078745, 9.846743663894594434 ) ) ;
#95363=CARTESIAN_POINT ( 'NONE',  ( 19.42250999205614548, 20.98035201082150891, -5.440088680355545492 ) ) ;
#95364=SURFACE_STYLE_USAGE ( .BOTH. , #3388 ) ;
#95365=CARTESIAN_POINT ( 'NONE',  ( 19.84674366389459621, 38.50893115100078745, 7.409399052514197653E-17 ) ) ;
#95369=CARTESIAN_POINT ( 'NONE',  ( 0.1532563361054100626, 30.80059781766744820, -2.638427012816831230 ) ) ;
#95370=CARTESIAN_POINT ( 'NONE',  ( 12.63842701281683922, 14.55059781766744997, -9.846743663894590881 ) ) ;
#95371=CARTESIAN_POINT ( 'NONE',  ( 5.076628168052704559, 0.1755978176674514724, -8.527530157486179263 ) ) ;
#95372=CARTESIAN_POINT ( 'NONE',  ( 17.20831665107776587, 59.13393115100078745, -7.208316651077762316 ) ) ;
#95374=CARTESIAN_POINT ( 'NONE',  ( -1.099225684535947600, 63.70696800326376774, -6.408140936763238038 ) ) ;
#95376=CARTESIAN_POINT ( 'NONE',  ( 3.591859063236761518, 44.95696800326376064, 11.09922568453594849 ) ) ;
#95377=CARTESIAN_POINT ( 'NONE',  ( 17.20831665107776587, 47.88393115100078745, 7.208316651077764980 ) ) ;
#95378=CARTESIAN_POINT ( 'NONE',  ( 0.2751277870542978565, 12.28217586085238011, -6.500000000000002665 ) ) ;
#95379=CARTESIAN_POINT ( 'NONE',  ( 13.79529636645031943, 65.34541550158063217, -14.16423886937409904 ) ) ;
#95380=CARTESIAN_POINT ( 'NONE',  ( 0.1532563361054100626, 20.80059781766744464, -2.638427012816831230 ) ) ;
#95382=CARTESIAN_POINT ( 'NONE',  ( 20.36894250292379382, 53.67874883491397497, 10.36894250292379205 ) ) ;
#95384=CARTESIAN_POINT ( 'NONE',  ( -0.3689425029237898834, 66.17874883491396076, -10.36894250292378850 ) ) ;
#95385=CARTESIAN_POINT ( 'NONE',  ( 20.36894250292379382, 38.67874883491396076, 10.36894250292379205 ) ) ;
#95386=CARTESIAN_POINT ( 'NONE',  ( 22.26659068614894466, 38.88708216824731068, 7.082119434687054849 ) ) ;
#95387=CARTESIAN_POINT ( 'NONE',  ( -43.84531931158922191, 106.6415101899049915, -4.576679558232020995 ) ) ;
#95389=CARTESIAN_POINT ( 'NONE',  ( 1.472469842513823179, 16.42559781766745175, 4.923371831947296329 ) ) ;
#95391=CARTESIAN_POINT ( 'NONE',  ( 2.791683348922240793, 56.63393115100078035, 7.208316651077764092 ) ) ;
#95394=CARTESIAN_POINT ( 'NONE',  ( 19.42250999205614548, 50.98035201082151247, -5.440088680355545492 ) ) ;
#95396=CARTESIAN_POINT ( 'NONE',  ( 10.00000000000000178, 47.25893115100078745, 9.846743663894594434 ) ) ;
#95398=CARTESIAN_POINT ( 'NONE',  ( 19.72487221294570858, 0.000000000000000000, -6.500000000000000888 ) ) ;
#95400=CARTESIAN_POINT ( 'NONE',  ( 1.472469842513823179, 50.59226448433411605, -4.923371831947296329 ) ) ;
#95401=FILL_AREA_STYLE_COLOUR ( '', #75305 ) ;
#95404=CARTESIAN_POINT ( 'NONE',  ( -0.3689425029237898834, 21.17874883491396432, -10.36894250292378850 ) ) ;
#95408=CARTESIAN_POINT ( 'NONE',  ( 10.00000000000000178, 24.31368534415484106, 10.88017736071110342 ) ) ;
#95409=CARTESIAN_POINT ( 'NONE',  ( 16.40814093676324603, 22.45696800326375353, -11.09922568453594671 ) ) ;
#95412=CARTESIAN_POINT ( 'NONE',  ( 1.472469842513823179, 6.425597817667451750, 4.923371831947296329 ) ) ;
#95413=CARTESIAN_POINT ( 'NONE',  ( 10.00000000000000178, 50.37363466993042493, 12.81628187352647608 ) ) ;
#95417=CARTESIAN_POINT ( 'NONE',  ( 19.80448550324509682, 61.82703681773343618, 6.500000000002703615 ) ) ;
#95418=CARTESIAN_POINT ( 'NONE',  ( 19.42250999205614548, 5.980352010821504471, -5.440088680355545492 ) ) ;
#95421=CARTESIAN_POINT ( 'NONE',  ( 12.91533473730992121, 39.52201867748817676, 10.88017736071110164 ) ) ;
#95422=CARTESIAN_POINT ( 'NONE',  ( 12.91533473730993009, 41.60535201082149825, -10.88017736071109987 ) ) ;
#95423=CARTESIAN_POINT ( 'NONE',  ( -1.099225684535947600, 19.54030133659708568, 6.408140936763237150 ) ) ;
#95426=CARTESIAN_POINT ( 'NONE',  ( 0.1532563361054100626, 15.80059781766745353, -2.638427012816831230 ) ) ;
#95428=CARTESIAN_POINT ( 'NONE',  ( 12.91533473730993009, 46.60535201082150536, -10.88017736071109987 ) ) ;
#95431=( BOUNDED_SURFACE ( )  B_SPLINE_SURFACE ( 1, 2, ( 
 ( #70281, #2293, #63736, #16782, #79241, #49235, #79737, #25284, #2787, #72224, #11234, #33241, #41272, #71747, #93258, #34214, #64707, #95217, #85277, #47258, #1798, #32253, #62754, #12710, #5229, #80222, #95726, #36203, #65702, #74694, #82189, #35199, #27708, #50717, #35707, #5715, #81690, #96229, #13204, #44184, #74184, #36707, #66193, #58191, #73694, #66701, #19719, #88703, #20213, #81210, #97229, #96727, #42723, #28696, #28203, #59188, #4736, #43204, #58699, #89203, #20716, #51207, #43697, #67197, #49711, #89693, #21208, #51706, #11726, #19231, #27210, #88211, #80719, #42239, #57711, #50208, #13699, #6204, #97722, #72705, #12215, #57219, #87716, #4241, #34711, #65206, #73204, #22696, #7697, #76661, #53667, #68194, #84183, #16170, #46177, #8659, #38193, #7193, #45678, #8180, #90676, #37696, #60670, #53175, #38676, #68680, #14706, #700, #76176, #69177, #75679, #83681, #98715, #61165, #15196, #23192, #208, #39172, #21708, #30166, #15692, #91168, #82688, #90178, #98212, #60179, #52681, #14205, #29670, #22202, #84662, #54152, #31153, #30658, #91673, #61643, #92164, #69661, #83182, #59684, #52193, #46654, #67700, #23689, #45180, #77150, #29186, #44686, #37212, #75181, #6693, #85647, #55644, #63615, #78642, #77636, #40149, #9153, #92644, #54639, #39671, #86144, #24169, #93136, #10149, #25168, #17657, #17166, #16665, #33121, #70162, #24663, #31646, #48127, #62136, #85157, #2176, #40644, #1187, #55133, #71142, #1679, #32132, #47647, #2670, #47139, #56141, #62631, #78142, #94122, #25648, #9652, #70653, #32634, #63132, #93634, #98548, #46, #8984, #16002, #61487, #91992, #69500, #39501, #23523, #46012, #38512, #30988, #83019, #45006, #30000, #69010, #22037, #84502, #39005, #84986, #22528, #68517, #46979, #92479, #53000, #53995, #15531, #60507, #30495, #69990, #46490, #76989, #8502, #1016, #1518, #31476, #76501, #541, #14536, #90997, #61979, #60994, #31964, #16502, #91506, #23025, #84007, #24004, #54476, #77473, #53497, #90503, #52512, #75512, #7026, #37532, #8015, #68022, #83514, #15032, #45505, #76005, #7532, #38023, #9476, #63990, #42017, #33979, #72482, #94500, #33492, #41528, #63022, #26494, #86526, #48507, #87004, #40537, #63512, #49002, #25050, #41029, #79993, #24560, #64482, #3521, #19010, #17050, #4016, #26019, #71531, #33013, #56514, #55021, #94990, #18512, #17545, #94016, #55536, #78032, #34477, #25538, #64971, #85537, #93522, #10514, #56029, #56992, #47530, #86032, #87495, #18026, #79509, #79010, #3040, #49486, #11011, #48013, #71996, #9534, #40038, #78522, #11496, #2556, #10034, #71035, #70539, #2061, #32523 ),
 ( #83320, #27969, #49987, #57487, #65469, #27479, #19980, #80494, #95996, #57972, #53307, #22831, #7336, #65969, #66464, #20484, #96496, #7829, #50477, #26988, #19492, #83815, #34973, #29811, #80981, #88478, #98848, #12481, #4507, #37837, #73965, #58461, #14845, #15341, #68328, #42984, #5494, #73465, #11992, #42493, #4992, #45317, #72978, #35473, #30302, #52813, #75814, #88977, #50972, #45824, #81465, #12970, #87981, #22339, #43463, #35966, #98353, #60804, #60320, #90811, #91304, #76311, #38325, #95497, #47276, #352, #62778, #17300, #63261, #830, #46791, #25296, #70794, #31289, #39799, #92781, #76796, #77284, #86278, #93277, #70299, #1814, #47775, #17787, #32269, #24312, #16800, #91808, #8312, #78273, #8795, #48262, #93770, #39312, #69805, #62275, #77777, #9787, #24800, #1328, #55277, #55783, #85787, #78775, #9290, #31780, #85293, #40286, #61788, #54777, #2311, #32766, #10281, #68819, #54285, #30799, #61299, #23330, #92298, #53810, #84321, #15822, #46309, #38815, #69308, #23822, #84800, #16309, #64724, #4258, #56752, #79753, #65220, #41287, #57237, #96246, #40781, #80737, #19738, #35220, #33258, #88723, #42254, #87735, #49253, #11746, #71281, #12232, #72724, #33735, #11251, #71761, #94254, #58206, #41769, #81227, #2803, #79261, #26742, #72240, #42741, #63749, #10772, #4750, #34227, #80238, #3773, #95234, #65720, #34729, #3271, #19247, #20234, #25782, #64236, #95747, #18771, #94753, #26255, #49731, #56276, #87245, #27231, #57726, #86771, #88229, #50223, #73222, #27726, #50738, #18274, #48753, #90697, #60691, #60202, #91191, #44704, #67719, #73715, #75204, #89224, #6224, #89710, #74714, #20733, #66723, #45205, #81708, #51224, #52702, #36728, #97247, #90201, #22226, #67219, #53200, #97742, #30190, #29205, #5248, #14225, #59207, #68218, #22716, #21731, #13222, #83207, #36222, #43718, #74202, #12726, #5736, #28716, #14729, #52213, #21224, #43221, #75704, #6714, #96745, #59704, #37231, #98232, #82707, #35726, #7215, #29693, #66214, #37716, #28221, #98739, #58719, #51728, #82210, #13720, #44204, #23712, #16687, #39194, #77660, #31668, #63149, #76200, #31176, #70180, #16194, #38216, #45700, #53687, #15713, #8203, #68701, #84205, #46199, #40168, #9671, #93158, #54173, #54661, #8682, #84684, #93651, #38698, #15221, #7719, #70673, #23214, #47157, #69197, #76683, #85667, #722, #91695, #24682, #62158, #46676, #1696, #2193, #55153, #61667, #92664, #92186, #233, #30681, #77174, #32152, #61189, #69682, #17187, #39692, #62654, #1213, #24192, #32655, #85177, #9174, #47667, #78161, #25185, #83704, #95116, #34608, #86164, #25668, #26624 ) ),
 .UNSPECIFIED., .F., .F., .F. ) 
 B_SPLINE_SURFACE_WITH_KNOTS ( ( 2, 2 ),
 ( 3, 2, 2, 2, 2, 2, 2, 2, 2, 2, 2, 2, 2, 2, 2, 2, 2, 2, 2, 2, 2, 2, 2, 2, 2, 2, 2, 2, 2, 2, 2, 2, 2, 2, 2, 2, 2, 2, 2, 2, 2, 2, 2, 2, 2, 2, 2, 2, 2, 2, 2, 2, 2, 2, 2, 2, 2, 2, 2, 2, 2, 2, 2, 2, 2, 2, 2, 2, 2, 2, 2, 2, 2, 2, 2, 2, 2, 2, 2, 2, 2, 2, 2, 2, 2, 2, 2, 2, 2, 2, 2, 2, 2, 2, 2, 2, 2, 2, 2, 2, 2, 2, 2, 2, 2, 2, 2, 2, 2, 2, 2, 2, 2, 2, 2, 2, 2, 2, 2, 2, 2, 2, 2, 2, 2, 2, 2, 2, 2, 2, 2, 2, 2, 2, 2, 2, 2, 2, 2, 2, 2, 2, 2, 2, 2, 2, 2, 2, 2, 2, 2, 2, 2, 2, 2, 2, 2, 2, 2, 2, 2, 2, 3 ),
 ( 0.000000000000000000, 1.000000000000000000 ),
 ( 0.000000000000000000, 0.005952380952380952051, 0.01190476190476190410, 0.01785714285714285615, 0.02380952380952380820, 0.02976190476190476025, 0.03571428571428571230, 0.04166666666666666435, 0.04761904761904761640, 0.05357142857142856845, 0.05952380952380952051, 0.06547619047619047949, 0.07142857142857142461, 0.07738095238095238360, 0.08333333333333332871, 0.08928571428571428770, 0.09523809523809523281, 0.1011904761904761918, 0.1071428571428571369, 0.1130952380952380959, 0.1190476190476190410, 0.1250000000000000000, 0.1309523809523809590, 0.1369047619047619180, 0.1428571428571428492, 0.1488095238095238082, 0.1547619047619047672, 0.1607142857142857262, 0.1666666666666666574, 0.1726190476190476164, 0.1785714285714285754, 0.1845238095238095344, 0.1904761904761904656, 0.1964285714285714246, 0.2023809523809523836, 0.2083333333333333426, 0.2142857142857142738, 0.2202380952380952328, 0.2261904761904761918, 0.2321428571428571508, 0.2380952380952380820, 0.2440476190476190410, 0.2500000000000000000, 0.2559523809523809312, 0.2619047619047619180, 0.2678571428571428492, 0.2738095238095238360, 0.2797619047619047672, 0.2857142857142856984, 0.2916666666666666852, 0.2976190476190476164, 0.3035714285714285476, 0.3095238095238095344, 0.3154761904761904656, 0.3214285714285714524, 0.3273809523809523836, 0.3333333333333333148, 0.3392857142857143016, 0.3452380952380952328, 0.3511904761904761640, 0.3571428571428571508, 0.3630952380952380820, 0.3690476190476190688, 0.3750000000000000000, 0.3809523809523809312, 0.3869047619047619180, 0.3928571428571428492, 0.3988095238095238360, 0.4047619047619047672, 0.4107142857142856984, 0.4166666666666666852, 0.4226190476190476164, 0.4285714285714285476, 0.4345238095238095344, 0.4404761904761904656, 0.4464285714285714524, 0.4523809523809523836, 0.4583333333333333148, 0.4642857142857143016, 0.4702380952380952328, 0.4761904761904761640, 0.4821428571428571508, 0.4880952380952380820, 0.4940476190476190688, 0.5000000000000000000, 0.5059523809523809312, 0.5119047619047618625, 0.5178571428571429047, 0.5238095238095238360, 0.5297619047619047672, 0.5357142857142856984, 0.5416666666666666297, 0.5476190476190476719, 0.5535714285714286031, 0.5595238095238095344, 0.5654761904761904656, 0.5714285714285713969, 0.5773809523809523281, 0.5833333333333333703, 0.5892857142857143016, 0.5952380952380952328, 0.6011904761904761640, 0.6071428571428570953, 0.6130952380952381375, 0.6190476190476190688, 0.6250000000000000000, 0.6309523809523809312, 0.6369047619047618625, 0.6428571428571429047, 0.6488095238095238360, 0.6547619047619047672, 0.6607142857142856984, 0.6666666666666666297, 0.6726190476190476719, 0.6785714285714286031, 0.6845238095238095344, 0.6904761904761904656, 0.6964285714285713969, 0.7023809523809523281, 0.7083333333333333703, 0.7142857142857143016, 0.7202380952380952328, 0.7261904761904761640, 0.7321428571428570953, 0.7380952380952381375, 0.7440476190476190688, 0.7500000000000000000, 0.7559523809523809312, 0.7619047619047618625, 0.7678571428571429047, 0.7738095238095238360, 0.7797619047619047672, 0.7857142857142856984, 0.7916666666666666297, 0.7976190476190476719, 0.8035714285714286031, 0.8095238095238095344, 0.8154761904761904656, 0.8214285714285713969, 0.8273809523809523281, 0.8333333333333333703, 0.8392857142857143016, 0.8452380952380952328, 0.8511904761904761640, 0.8571428571428570953, 0.8630952380952381375, 0.8690476190476190688, 0.8750000000000000000, 0.8809523809523809312, 0.8869047619047618625, 0.8928571428571429047, 0.8988095238095238360, 0.9047619047619047672, 0.9107142857142856984, 0.9166666666666666297, 0.9226190476190476719, 0.9285714285714286031, 0.9345238095238095344, 0.9404761904761904656, 0.9464285714285713969, 0.9523809523809523281, 0.9583333333333333703, 0.9642857142857143016 ),
 .UNSPECIFIED. ) 
 GEOMETRIC_REPRESENTATION_ITEM ( )  RATIONAL_B_SPLINE_SURFACE ( (
 ( 1.000000000000000000, 0.9659258262890683122, 1.000000000000000000, 0.9659258262890683122, 1.000000000000000000, 0.9659258262890683122, 1.000000000000000000, 0.9659258262890683122, 1.000000000000000000, 0.9659258262890683122, 1.000000000000000000, 0.9659258262890683122, 1.000000000000000000, 0.9659258262890683122, 1.000000000000000000, 0.9659258262890683122, 1.000000000000000000, 0.9659258262890683122, 1.000000000000000000, 0.9659258262890683122, 1.000000000000000000, 0.9659258262890683122, 1.000000000000000000, 0.9659258262890683122, 1.000000000000000000, 0.9659258262890683122, 1.000000000000000000, 0.9659258262890683122, 1.000000000000000000, 0.9659258262890683122, 1.000000000000000000, 0.9659258262890683122, 1.000000000000000000, 0.9659258262890683122, 1.000000000000000000, 0.9659258262890683122, 1.000000000000000000, 0.9659258262890683122, 1.000000000000000000, 0.9659258262890683122, 1.000000000000000000, 0.9659258262890683122, 1.000000000000000000, 0.9659258262890683122, 1.000000000000000000, 0.9659258262890683122, 1.000000000000000000, 0.9659258262890683122, 1.000000000000000000, 0.9659258262890683122, 1.000000000000000000, 0.9659258262890683122, 1.000000000000000000, 0.9659258262890683122, 1.000000000000000000, 0.9659258262890683122, 1.000000000000000000, 0.9659258262890683122, 1.000000000000000000, 0.9659258262890683122, 1.000000000000000000, 0.9659258262890683122, 1.000000000000000000, 0.9659258262890683122, 1.000000000000000000, 0.9659258262890683122, 1.000000000000000000, 0.9659258262890683122, 1.000000000000000000, 0.9659258262890683122, 1.000000000000000000, 0.9659258262890683122, 1.000000000000000000, 0.9659258262890683122, 1.000000000000000000, 0.9659258262890683122, 1.000000000000000000, 0.9659258262890683122, 1.000000000000000000, 0.9659258262890683122, 1.000000000000000000, 0.9659258262890683122, 1.000000000000000000, 0.9659258262890683122, 1.000000000000000000, 0.9659258262890683122, 1.000000000000000000, 0.9659258262890683122, 1.000000000000000000, 0.9659258262890683122, 1.000000000000000000, 0.9659258262890683122, 1.000000000000000000, 0.9659258262890683122, 1.000000000000000000, 0.9659258262890683122, 1.000000000000000000, 0.9659258262890683122, 1.000000000000000000, 0.9659258262890683122, 1.000000000000000000, 0.9659258262890683122, 1.000000000000000000, 0.9659258262890683122, 1.000000000000000000, 0.9659258262890683122, 1.000000000000000000, 0.9659258262890683122, 1.000000000000000000, 0.9659258262890683122, 1.000000000000000000, 0.9659258262890683122, 1.000000000000000000, 0.9659258262890683122, 1.000000000000000000, 0.9659258262890683122, 1.000000000000000000, 0.9659258262890683122, 1.000000000000000000, 0.9659258262890683122, 1.000000000000000000, 0.9659258262890683122, 1.000000000000000000, 0.9659258262890683122, 1.000000000000000000, 0.9659258262890683122, 1.000000000000000000, 0.9659258262890683122, 1.000000000000000000, 0.9659258262890683122, 1.000000000000000000, 0.9659258262890683122, 1.000000000000000000, 0.9659258262890683122, 1.000000000000000000, 0.9659258262890683122, 1.000000000000000000, 0.9659258262890683122, 1.000000000000000000, 0.9659258262890683122, 1.000000000000000000, 0.9659258262890683122, 1.000000000000000000, 0.9659258262890683122, 1.000000000000000000, 0.9659258262890683122, 1.000000000000000000, 0.9659258262890683122, 1.000000000000000000, 0.9659258262890683122, 1.000000000000000000, 0.9659258262890683122, 1.000000000000000000, 0.9659258262890683122, 1.000000000000000000, 0.9659258262890683122, 1.000000000000000000, 0.9659258262890683122, 1.000000000000000000, 0.9659258262890683122, 1.000000000000000000, 0.9659258262890683122, 1.000000000000000000, 0.9659258262890683122, 1.000000000000000000, 0.9659258262890683122, 1.000000000000000000, 0.9659258262890683122, 1.000000000000000000, 0.9659258262890683122, 1.000000000000000000, 0.9659258262890683122, 1.000000000000000000, 0.9659258262890683122, 1.000000000000000000, 0.9659258262890683122, 1.000000000000000000, 0.9659258262890683122, 1.000000000000000000, 0.9659258262890683122, 1.000000000000000000, 0.9659258262890683122, 1.000000000000000000, 0.9659258262890683122, 1.000000000000000000, 0.9659258262890683122, 1.000000000000000000, 0.9659258262890683122, 1.000000000000000000, 0.9659258262890683122, 1.000000000000000000, 0.9659258262890683122, 1.000000000000000000, 0.9659258262890683122, 1.000000000000000000, 0.9659258262890683122, 1.000000000000000000, 0.9659258262890683122, 1.000000000000000000, 0.9659258262890683122, 1.000000000000000000, 0.9659258262890683122, 1.000000000000000000, 0.9659258262890683122, 1.000000000000000000, 0.9659258262890683122, 1.000000000000000000, 0.9659258262890683122, 1.000000000000000000, 0.9659258262890683122, 1.000000000000000000, 0.9659258262890683122, 1.000000000000000000, 0.9659258262890683122, 1.000000000000000000, 0.9659258262890683122, 1.000000000000000000, 0.9659258262890683122, 1.000000000000000000, 0.9659258262890683122, 1.000000000000000000, 0.9659258262890683122, 1.000000000000000000, 0.9659258262890683122, 1.000000000000000000, 0.9659258262890683122, 1.000000000000000000, 0.9659258262890683122, 1.000000000000000000, 0.9659258262890683122, 1.000000000000000000, 0.9659258262890683122, 1.000000000000000000, 0.9659258262890683122, 1.000000000000000000, 0.9659258262890683122, 1.000000000000000000, 0.9659258262890683122, 1.000000000000000000, 0.9659258262890683122, 1.000000000000000000, 0.9659258262890683122, 1.000000000000000000, 0.9659258262890683122, 1.000000000000000000, 0.9659258262890683122, 1.000000000000000000, 0.9659258262890683122, 1.000000000000000000, 0.9659258262890683122, 1.000000000000000000, 0.9659258262890683122, 1.000000000000000000, 0.9659258262890683122, 1.000000000000000000, 0.9659258262890683122, 1.000000000000000000, 0.9659258262890683122, 1.000000000000000000, 0.9659258262890683122, 1.000000000000000000, 0.9659258262890683122, 1.000000000000000000, 0.9659258262890683122, 1.000000000000000000, 0.9659258262890683122, 1.000000000000000000, 0.9659258262890683122, 1.000000000000000000, 0.9659258262890683122, 1.000000000000000000, 0.9659258262890683122, 1.000000000000000000, 0.9659258262890683122, 1.000000000000000000, 0.9659258262890683122, 1.000000000000000000, 0.9659258262890683122, 1.000000000000000000, 0.9659258262890683122, 1.000000000000000000, 0.9659258262890683122, 1.000000000000000000, 0.9659258262890683122, 1.000000000000000000, 0.9659258262890683122, 1.000000000000000000, 0.9659258262890683122, 1.000000000000000000, 0.9659258262890683122, 1.000000000000000000, 0.9659258262890683122, 1.000000000000000000, 0.9659258262890683122, 1.000000000000000000, 0.9659258262890683122, 1.000000000000000000, 0.9659258262890683122, 1.000000000000000000, 0.9659258262890683122, 1.000000000000000000, 0.9659258262890683122, 1.000000000000000000, 0.9659258262890683122, 1.000000000000000000, 0.9659258262890683122, 1.000000000000000000, 0.9659258262890683122, 1.000000000000000000, 0.9659258262890683122, 1.000000000000000000, 0.9659258262890683122, 1.000000000000000000, 0.9659258262890683122, 1.000000000000000000, 0.9659258262890683122, 1.000000000000000000, 0.9659258262890683122, 1.000000000000000000, 0.9659258262890683122, 1.000000000000000000, 0.9659258262890683122, 1.000000000000000000, 0.9659258262890683122, 1.000000000000000000),
 ( 1.000000000000000000, 0.9659258262890683122, 1.000000000000000000, 0.9659258262890683122, 1.000000000000000000, 0.9659258262890683122, 1.000000000000000000, 0.9659258262890683122, 1.000000000000000000, 0.9659258262890683122, 1.000000000000000000, 0.9659258262890683122, 1.000000000000000000, 0.9659258262890683122, 1.000000000000000000, 0.9659258262890683122, 1.000000000000000000, 0.9659258262890683122, 1.000000000000000000, 0.9659258262890683122, 1.000000000000000000, 0.9659258262890683122, 1.000000000000000000, 0.9659258262890683122, 1.000000000000000000, 0.9659258262890683122, 1.000000000000000000, 0.9659258262890683122, 1.000000000000000000, 0.9659258262890683122, 1.000000000000000000, 0.9659258262890683122, 1.000000000000000000, 0.9659258262890683122, 1.000000000000000000, 0.9659258262890683122, 1.000000000000000000, 0.9659258262890683122, 1.000000000000000000, 0.9659258262890683122, 1.000000000000000000, 0.9659258262890683122, 1.000000000000000000, 0.9659258262890683122, 1.000000000000000000, 0.9659258262890683122, 1.000000000000000000, 0.9659258262890683122, 1.000000000000000000, 0.9659258262890683122, 1.000000000000000000, 0.9659258262890683122, 1.000000000000000000, 0.9659258262890683122, 1.000000000000000000, 0.9659258262890683122, 1.000000000000000000, 0.9659258262890683122, 1.000000000000000000, 0.9659258262890683122, 1.000000000000000000, 0.9659258262890683122, 1.000000000000000000, 0.9659258262890683122, 1.000000000000000000, 0.9659258262890683122, 1.000000000000000000, 0.9659258262890683122, 1.000000000000000000, 0.9659258262890683122, 1.000000000000000000, 0.9659258262890683122, 1.000000000000000000, 0.9659258262890683122, 1.000000000000000000, 0.9659258262890683122, 1.000000000000000000, 0.9659258262890683122, 1.000000000000000000, 0.9659258262890683122, 1.000000000000000000, 0.9659258262890683122, 1.000000000000000000, 0.9659258262890683122, 1.000000000000000000, 0.9659258262890683122, 1.000000000000000000, 0.9659258262890683122, 1.000000000000000000, 0.9659258262890683122, 1.000000000000000000, 0.9659258262890683122, 1.000000000000000000, 0.9659258262890683122, 1.000000000000000000, 0.9659258262890683122, 1.000000000000000000, 0.9659258262890683122, 1.000000000000000000, 0.9659258262890683122, 1.000000000000000000, 0.9659258262890683122, 1.000000000000000000, 0.9659258262890683122, 1.000000000000000000, 0.9659258262890683122, 1.000000000000000000, 0.9659258262890683122, 1.000000000000000000, 0.9659258262890683122, 1.000000000000000000, 0.9659258262890683122, 1.000000000000000000, 0.9659258262890683122, 1.000000000000000000, 0.9659258262890683122, 1.000000000000000000, 0.9659258262890683122, 1.000000000000000000, 0.9659258262890683122, 1.000000000000000000, 0.9659258262890683122, 1.000000000000000000, 0.9659258262890683122, 1.000000000000000000, 0.9659258262890683122, 1.000000000000000000, 0.9659258262890683122, 1.000000000000000000, 0.9659258262890683122, 1.000000000000000000, 0.9659258262890683122, 1.000000000000000000, 0.9659258262890683122, 1.000000000000000000, 0.9659258262890683122, 1.000000000000000000, 0.9659258262890683122, 1.000000000000000000, 0.9659258262890683122, 1.000000000000000000, 0.9659258262890683122, 1.000000000000000000, 0.9659258262890683122, 1.000000000000000000, 0.9659258262890683122, 1.000000000000000000, 0.9659258262890683122, 1.000000000000000000, 0.9659258262890683122, 1.000000000000000000, 0.9659258262890683122, 1.000000000000000000, 0.9659258262890683122, 1.000000000000000000, 0.9659258262890683122, 1.000000000000000000, 0.9659258262890683122, 1.000000000000000000, 0.9659258262890683122, 1.000000000000000000, 0.9659258262890683122, 1.000000000000000000, 0.9659258262890683122, 1.000000000000000000, 0.9659258262890683122, 1.000000000000000000, 0.9659258262890683122, 1.000000000000000000, 0.9659258262890683122, 1.000000000000000000, 0.9659258262890683122, 1.000000000000000000, 0.9659258262890683122, 1.000000000000000000, 0.9659258262890683122, 1.000000000000000000, 0.9659258262890683122, 1.000000000000000000, 0.9659258262890683122, 1.000000000000000000, 0.9659258262890683122, 1.000000000000000000, 0.9659258262890683122, 1.000000000000000000, 0.9659258262890683122, 1.000000000000000000, 0.9659258262890683122, 1.000000000000000000, 0.9659258262890683122, 1.000000000000000000, 0.9659258262890683122, 1.000000000000000000, 0.9659258262890683122, 1.000000000000000000, 0.9659258262890683122, 1.000000000000000000, 0.9659258262890683122, 1.000000000000000000, 0.9659258262890683122, 1.000000000000000000, 0.9659258262890683122, 1.000000000000000000, 0.9659258262890683122, 1.000000000000000000, 0.9659258262890683122, 1.000000000000000000, 0.9659258262890683122, 1.000000000000000000, 0.9659258262890683122, 1.000000000000000000, 0.9659258262890683122, 1.000000000000000000, 0.9659258262890683122, 1.000000000000000000, 0.9659258262890683122, 1.000000000000000000, 0.9659258262890683122, 1.000000000000000000, 0.9659258262890683122, 1.000000000000000000, 0.9659258262890683122, 1.000000000000000000, 0.9659258262890683122, 1.000000000000000000, 0.9659258262890683122, 1.000000000000000000, 0.9659258262890683122, 1.000000000000000000, 0.9659258262890683122, 1.000000000000000000, 0.9659258262890683122, 1.000000000000000000, 0.9659258262890683122, 1.000000000000000000, 0.9659258262890683122, 1.000000000000000000, 0.9659258262890683122, 1.000000000000000000, 0.9659258262890683122, 1.000000000000000000, 0.9659258262890683122, 1.000000000000000000, 0.9659258262890683122, 1.000000000000000000, 0.9659258262890683122, 1.000000000000000000, 0.9659258262890683122, 1.000000000000000000, 0.9659258262890683122, 1.000000000000000000, 0.9659258262890683122, 1.000000000000000000, 0.9659258262890683122, 1.000000000000000000, 0.9659258262890683122, 1.000000000000000000, 0.9659258262890683122, 1.000000000000000000, 0.9659258262890683122, 1.000000000000000000, 0.9659258262890683122, 1.000000000000000000, 0.9659258262890683122, 1.000000000000000000, 0.9659258262890683122, 1.000000000000000000, 0.9659258262890683122, 1.000000000000000000, 0.9659258262890683122, 1.000000000000000000, 0.9659258262890683122, 1.000000000000000000, 0.9659258262890683122, 1.000000000000000000, 0.9659258262890683122, 1.000000000000000000, 0.9659258262890683122, 1.000000000000000000, 0.9659258262890683122, 1.000000000000000000, 0.9659258262890683122, 1.000000000000000000, 0.9659258262890683122, 1.000000000000000000, 0.9659258262890683122, 1.000000000000000000, 0.9659258262890683122, 1.000000000000000000, 0.9659258262890683122, 1.000000000000000000, 0.9659258262890683122, 1.000000000000000000, 0.9659258262890683122, 1.000000000000000000, 0.9659258262890683122, 1.000000000000000000, 0.9659258262890683122, 1.000000000000000000, 0.9659258262890683122, 1.000000000000000000, 0.9659258262890683122, 1.000000000000000000, 0.9659258262890683122, 1.000000000000000000, 0.9659258262890683122, 1.000000000000000000, 0.9659258262890683122, 1.000000000000000000, 0.9659258262890683122, 1.000000000000000000, 0.9659258262890683122, 1.000000000000000000, 0.9659258262890683122, 1.000000000000000000, 0.9659258262890683122, 1.000000000000000000, 0.9659258262890683122, 1.000000000000000000, 0.9659258262890683122, 1.000000000000000000, 0.9659258262890683122, 1.000000000000000000, 0.9659258262890683122, 1.000000000000000000) ) ) 
 REPRESENTATION_ITEM ( '' )  SURFACE ( )  );
#95432=CARTESIAN_POINT ( 'NONE',  ( 21.09922568453594849, 1.206968003263753531, 6.408140936763242479 ) ) ;
#95433=CARTESIAN_POINT ( 'NONE',  ( 15.44008868035555260, 64.73035201082151957, 9.422509992056143702 ) ) ;
#95434=CARTESIAN_POINT ( 'NONE',  ( 19.84674366389459266, 28.71726448433411960, -2.638427012816827677 ) ) ;
#95435=CARTESIAN_POINT ( 'NONE',  ( 22.81628187352647785, 46.41530133659708213, 3.434112377981063169 ) ) ;
#95436=CARTESIAN_POINT ( 'NONE',  ( 10.00000000000000178, 2.258931151000784787, 9.846743663894594434 ) ) ;
#95437=DIRECTION ( 'NONE',  ( -1.000000000000000000, -0.000000000000000000, -0.000000000000000000 ) ) ;
#95439=B_SPLINE_CURVE_WITH_KNOTS ( 'NONE', 3,
 ( #45761, #98794, #76255, #97297 ),
 .UNSPECIFIED., .F., .F.,
 ( 4, 4 ),
 ( 7.269816092100958512E-18, 0.002562518741975552787 ),
 .UNSPECIFIED. ) ;
#95441=CARTESIAN_POINT ( 'NONE',  ( 0.2751277870542980231, 9.366073187301308778, -6.500000000000002665 ) ) ;
#95442=CARTESIAN_POINT ( 'NONE',  ( 10.00000000000000178, 19.31368534415484106, 10.88017736071110342 ) ) ;
#95443=CARTESIAN_POINT ( 'NONE',  ( 6.565887622018943937, 58.08196800326376064, -12.81628187352647608 ) ) ;
#95444=CARTESIAN_POINT ( 'NONE',  ( 20.36894250292379382, 23.67874883491397142, 10.36894250292379205 ) ) ;
#95445=CARTESIAN_POINT ( 'NONE',  ( 10.00000000000000000, 29.75893115100078745, -9.846743663894594434 ) ) ;
#95446=CARTESIAN_POINT ( 'NONE',  ( -0.8801773607110991993, 22.85535201082150181, -2.915334737309923874 ) ) ;
#95447=AXIS2_PLACEMENT_3D ( 'NONE', #12735, #43232, #74214 ) ;
#95448=CARTESIAN_POINT ( 'NONE',  ( 6.204703633549690345, 65.76208216824731778, -14.16423886937410259 ) ) ;
#95450=CARTESIAN_POINT ( 'NONE',  ( 4.559911319644449179, 8.897018677488171434, 9.422509992056141925 ) ) ;
#95452=CARTESIAN_POINT ( 'NONE',  ( 10.00000000000000000, 21.81368534415484106, -10.88017736071110342 ) ) ;
#95454=CARTESIAN_POINT ( 'NONE',  ( 2.035157376598824452, 23.68868534415484461, 7.964842623401179544 ) ) ;
#95456=CARTESIAN_POINT ( 'NONE',  ( 20.32896413005680003, 26.77164270246084499, 5.963430220938287007 ) ) ;
#95457=CARTESIAN_POINT ( 'NONE',  ( -0.8801773607110991993, 17.85535201082150536, -2.915334737309923874 ) ) ;
#95458=CARTESIAN_POINT ( 'NONE',  ( 0.1532563361054082862, 56.21726448433411605, 2.638427012816831674 ) ) ;
#95461=CARTESIAN_POINT ( 'NONE',  ( -20.19000000000000838, 92.00000000000000000, 9.500000000000000000 ) ) ;
#95462=CARTESIAN_POINT ( 'NONE',  ( 17.08211943468705840, 35.13708216824730357, -12.26659068614894466 ) ) ;
#95463=CARTESIAN_POINT ( 'NONE',  ( 4.559911319644449179, 42.23035201082151247, -9.422509992056141925 ) ) ;
#95464=CARTESIAN_POINT ( 'NONE',  ( 15.44008868035555260, 19.73035201082150536, 9.422509992056143702 ) ) ;
#95465=CARTESIAN_POINT ( 'NONE',  ( 19.84674366389459266, 63.71726448433412315, -2.638427012816827677 ) ) ;
#95466=CARTESIAN_POINT ( 'NONE',  ( 18.95785429995053306, 32.24216108172007011, 6.499999999999848121 ) ) ;
#95467=CARTESIAN_POINT ( 'NONE',  ( 19.84674366389459621, 53.50893115100078745, 7.409399052514197653E-17 ) ) ;
#95468=LINE ( 'NONE', #57944, #15990 ) ;
#95469=CARTESIAN_POINT ( 'NONE',  ( 5.076628168052704559, 10.17559781766745175, -8.527530157486179263 ) ) ;
#95472=CARTESIAN_POINT ( 'NONE',  ( 7.084665262690076126, 14.10535201082150358, 10.88017736071109987 ) ) ;
#95473=CARTESIAN_POINT ( 'NONE',  ( 1.472469842513823179, 10.59226448433411782, -4.923371831947296329 ) ) ;
#95475=CARTESIAN_POINT ( 'NONE',  ( 0.1532563361054100626, 65.80059781766745175, -2.638427012816831230 ) ) ;
#95476=CARTESIAN_POINT ( 'NONE',  ( 17.96484262340118221, 64.93868534415483396, 7.964842623401181321 ) ) ;
#95477=CARTESIAN_POINT ( 'NONE',  ( 0.5774900079438607392, 23.48035201082150536, 5.440088680355550821 ) ) ;
#95478=CARTESIAN_POINT ( 'NONE',  ( 21.09922568453594849, 51.20696800326375353, 6.408140936763242479 ) ) ;
#95479=CARTESIAN_POINT ( 'NONE',  ( 17.08211943468705840, 30.13708216824730357, -12.26659068614894466 ) ) ;
#95481=CIRCLE ( 'NONE', #26806, 1.000000000000000000 ) ;
#95482=CARTESIAN_POINT ( 'NONE',  ( -1.099225684535947600, 58.70696800326375353, -6.408140936763238038 ) ) ;
#95483=ORIENTED_EDGE ( 'NONE', *, *, #37611, .F. ) ;
#95484=CARTESIAN_POINT ( 'NONE',  ( 6.565887622018943937, 0.1653013365970866511, 12.81628187352647430 ) ) ;
#95486=CARTESIAN_POINT ( 'NONE',  ( 7.084665262690076126, 37.02201867748817676, -10.88017736071110164 ) ) ;
#95487=CARTESIAN_POINT ( 'NONE',  ( 0.1532563361054082862, 61.21726448433412315, 2.638427012816831674 ) ) ;
#95489=CARTESIAN_POINT ( 'NONE',  ( 14.92337183194729988, 9.342264484334119601, -8.527530157486177487 ) ) ;
#95490=CARTESIAN_POINT ( 'NONE',  ( 0.1532563361054082862, 11.21726448433411605, 2.638427012816831674 ) ) ;
#95491=CARTESIAN_POINT ( 'NONE',  ( 2.791683348922240793, 21.63393115100078745, 7.208316651077764092 ) ) ;
#95492=CARTESIAN_POINT ( 'NONE',  ( 5.076628168052703671, 6.842264484334118713, 8.527530157486179263 ) ) ;
#95493=CARTESIAN_POINT ( 'NONE',  ( 19.84674366389459266, 3.300597817667451750, 2.638427012816836559 ) ) ;
#95495=CARTESIAN_POINT ( 'NONE',  ( 12.91533473730993009, 51.60535201082149825, -10.88017736071109987 ) ) ;
#95497=CARTESIAN_POINT ( 'NONE',  ( 17.20831665107776587, 12.88393115100078390, 7.208316651077764980 ) ) ;
#95498=CARTESIAN_POINT ( 'NONE',  ( 1.472469842513823179, 15.59226448433411960, -4.923371831947296329 ) ) ;
#95501=CARTESIAN_POINT ( 'NONE',  ( 1.472469842513823179, 55.59226448433412315, -4.923371831947296329 ) ) ;
#95503=CARTESIAN_POINT ( 'NONE',  ( 0.2751277870542967463, 70.00000000000000000, -6.500000000000000888 ) ) ;
#95504=CARTESIAN_POINT ( 'NONE',  ( 10.00000000000000000, 15.55374883491396787, -14.16423886937410082 ) ) ;
#95505=UNCERTAINTY_MEASURE_WITH_UNIT (LENGTH_MEASURE( 1.000000000000000082E-05 ), #47072, 'distance_accuracy_value', 'NONE');
#95507=CARTESIAN_POINT ( 'NONE',  ( 22.26659068614895176, 14.72041550158063572, -7.082119434687042414 ) ) ;
#95508=CARTESIAN_POINT ( 'NONE',  ( 20.36894250292379738, 34.92874883491396076, -10.36894250292379027 ) ) ;
#95509=CARTESIAN_POINT ( 'NONE',  ( 13.79529636645030344, 3.262082168247301350, 14.16423886937410614 ) ) ;
#95510=CARTESIAN_POINT ( 'NONE',  ( 20.88017736071110875, 40.77201867748818387, -2.915334737309920765 ) ) ;
#95513=CARTESIAN_POINT ( 'NONE',  ( 2.791683348922240793, 16.63393115100078745, 7.208316651077764092 ) ) ;
#95514=CARTESIAN_POINT ( 'NONE',  ( 10.00000000000000000, 56.81368534415484106, -10.88017736071110342 ) ) ;
#95515=CARTESIAN_POINT ( 'NONE',  ( 5.076628168052704559, 15.17559781766745175, -8.527530157486179263 ) ) ;
#95516=CARTESIAN_POINT ( 'NONE',  ( 10.00000000000000000, 16.81368534415483751, -10.88017736071110342 ) ) ;
#95517=CARTESIAN_POINT ( 'NONE',  ( 19.38216949554541202, 50.99863466993042493, 9.382169495545424454 ) ) ;
#95518=CARTESIAN_POINT ( 'NONE',  ( 14.92337183194729988, 49.34226448433411605, -8.527530157486177487 ) ) ;
#95520=CARTESIAN_POINT ( 'NONE',  ( 0.6178305044545838731, 24.74863466993042493, 9.382169495545420901 ) ) ;
#95523=CARTESIAN_POINT ( 'NONE',  ( 0.1532563361054083140, 46.00893115100079456, 1.131784320476157264E-15 ) ) ;
#95524=CARTESIAN_POINT ( 'NONE',  ( 22.26659068614894466, 18.88708216824730002, 7.082119434687054849 ) ) ;
#95527=ORIENTED_EDGE ( 'NONE', *, *, #14935, .T. ) ;
#95529=CARTESIAN_POINT ( 'NONE',  ( 17.96484262340118221, 51.18868534415483396, -7.964842623401177768 ) ) ;
#95530=CARTESIAN_POINT ( 'NONE',  ( 10.00000000000000000, 56.81368534415484106, -10.88017736071110342 ) ) ;
#95531=CARTESIAN_POINT ( 'NONE',  ( 22.26659068614895176, 39.72041550158063217, -7.082119434687042414 ) ) ;
#95532=CARTESIAN_POINT ( 'NONE',  ( 1.472469842513823179, 60.59226448433412315, -4.923371831947296329 ) ) ;
#95533=CARTESIAN_POINT ( 'NONE',  ( 18.52753015748618282, 8.925597817667451750, -4.923371831947291888 ) ) ;
#95534=CYLINDRICAL_SURFACE ( 'NONE', #73583, 0.5000000000000004441 ) ;
#95535=CARTESIAN_POINT ( 'NONE',  ( 19.42250999205614193, 45.14701867748817676, 5.440088680355555262 ) ) ;
#95538=CARTESIAN_POINT ( 'NONE',  ( 14.92337183194729988, 49.34226448433411605, -8.527530157486177487 ) ) ;
#95540=CARTESIAN_POINT ( 'NONE',  ( -0.8801773607110991993, 2.855352010821504471, -2.915334737309923874 ) ) ;
#95543=CARTESIAN_POINT ( 'NONE',  ( 4.559911319644449179, 2.230352010821504471, -9.422509992056141925 ) ) ;
#95546=CARTESIAN_POINT ( 'NONE',  ( -0.8801773607111008646, 63.27201867748817676, 2.915334737309923430 ) ) ;
#95547=CARTESIAN_POINT ( 'NONE',  ( 5.076628168052703671, 1.842264484334118047, 8.527530157486179263 ) ) ;
#95549=CARTESIAN_POINT ( 'NONE',  ( 19.84674366389459266, 33.71726448433410894, -2.638427012816827677 ) ) ;
#95550=CARTESIAN_POINT ( 'NONE',  ( 19.42250999205614193, 25.14701867748817321, 5.440088680355555262 ) ) ;
#95551=CARTESIAN_POINT ( 'NONE',  ( 19.84674366389459266, 63.71726448433412315, -2.638427012816827677 ) ) ;
#95552=CARTESIAN_POINT ( 'NONE',  ( -0.8801773607111008646, 38.27201867748816255, 2.915334737309923430 ) ) ;
#95554=CARTESIAN_POINT ( 'NONE',  ( -1.099225684535947600, 44.54030133659708923, 6.408140936763237150 ) ) ;
#95556=CARTESIAN_POINT ( 'NONE',  ( 17.96484262340118221, 56.18868534415484817, -7.964842623401177768 ) ) ;
#95557=CARTESIAN_POINT ( 'NONE',  ( 21.09922568453594849, 16.20696800326375353, 6.408140936763242479 ) ) ;
#95558=CARTESIAN_POINT ( 'NONE',  ( 18.52753015748618282, 18.92559781766745175, -4.923371831947291888 ) ) ;
#95559=CARTESIAN_POINT ( 'NONE',  ( 17.20831665107776587, 2.883931151000785231, 7.208316651077764980 ) ) ;
#95560=CARTESIAN_POINT ( 'NONE',  ( 15.44008868035555793, 31.39701867748817676, -9.422509992056140149 ) ) ;
#95561=CARTESIAN_POINT ( 'NONE',  ( 17.08211943468705130, 63.47041550158063927, 12.26659068614894998 ) ) ;
#95562=CARTESIAN_POINT ( 'NONE',  ( 0.1532563361054082862, 51.21726448433412315, 2.638427012816831674 ) ) ;
#95563=CARTESIAN_POINT ( 'NONE',  ( 18.52753015748618282, 8.925597817667451750, -4.923371831947291888 ) ) ;
#95564=CARTESIAN_POINT ( 'NONE',  ( 2.035157376598824452, 63.68868534415484106, 7.964842623401179544 ) ) ;
#95566=CARTESIAN_POINT ( 'NONE',  ( -0.3689425029237881626, 32.42874883491395366, 10.36894250292379027 ) ) ;
#95573=CARTESIAN_POINT ( 'NONE',  ( -0.3689425029237898834, 51.17874883491397497, -10.36894250292378850 ) ) ;
#95574=CARTESIAN_POINT ( 'NONE',  ( 2.917880565312948704, 52.63708216824730357, 12.26659068614894643 ) ) ;
#95575=CARTESIAN_POINT ( 'NONE',  ( 7.361572987183170547, 12.05059781766744997, 9.846743663894590881 ) ) ;
#95576=CARTESIAN_POINT ( 'NONE',  ( 3.591859063236763294, 18.29030133659708568, -11.09922568453595026 ) ) ;
#95580=CARTESIAN_POINT ( 'NONE',  ( -2.816281873526471635, 43.91530133659708923, -3.434112377981056508 ) ) ;
#95581=CARTESIAN_POINT ( 'NONE',  ( 24.16423886937409904, 49.09541550158063217, 3.795296366450317205 ) ) ;
#95584=CARTESIAN_POINT ( 'NONE',  ( 7.361572987183170547, 12.05059781766744997, 9.846743663894590881 ) ) ;
#95587=DIRECTION ( 'NONE',  ( -0.000000000000000000, 1.000000000000000000, 0.000000000000000000 ) ) ;
#95588=CARTESIAN_POINT ( 'NONE',  ( 2.791683348922240793, 21.63393115100078745, 7.208316651077764092 ) ) ;
#95590=CARTESIAN_POINT ( 'NONE',  ( -19.19000000000001194, 93.50000000000000000, 9.500000000000000000 ) ) ;
#95592=CARTESIAN_POINT ( 'NONE',  ( 20.88017736071110164, 20.35535201082150891, 2.915334737309930979 ) ) ;
#95593=CARTESIAN_POINT ( 'NONE',  ( 12.91533473730993009, 31.60535201082150891, -10.88017736071109987 ) ) ;
#95594=CARTESIAN_POINT ( 'NONE',  ( 14.92337183194729988, 49.34226448433411605, -8.527530157486177487 ) ) ;
#95595=CARTESIAN_POINT ( 'NONE',  ( 22.81628187352647785, 1.623634669930420271, 6.195893100308588602E-16 ) ) ;
#95597=CARTESIAN_POINT ( 'NONE',  ( 16.40814093676324603, 22.45696800326375353, -11.09922568453594671 ) ) ;
#95599=CARTESIAN_POINT ( 'NONE',  ( 14.92337183194729988, 29.34226448433411960, -8.527530157486177487 ) ) ;
#95600=CARTESIAN_POINT ( 'NONE',  ( 6.204703633549690345, 55.76208216824730357, -14.16423886937410259 ) ) ;
#95601=CARTESIAN_POINT ( 'NONE',  ( 15.44008868035555260, 9.730352010821505360, 9.422509992056143702 ) ) ;
#95603=CARTESIAN_POINT ( 'NONE',  ( 0.5774900079438607392, 38.48035201082150536, 5.440088680355550821 ) ) ;
#95604=CARTESIAN_POINT ( 'NONE',  ( 20.88017736071110519, 40.56368534415484106, 2.639326808657452039E-16 ) ) ;
#95605=CARTESIAN_POINT ( 'NONE',  ( 20.88017736071110519, 50.56368534415484106, 2.639326808657452039E-16 ) ) ;
#95606=CARTESIAN_POINT ( 'NONE',  ( 19.42250999205614193, 35.14701867748816966, 5.440088680355555262 ) ) ;
#95607=CARTESIAN_POINT ( 'NONE',  ( 2.603489959281613420, 45.43575266056827644, -6.500000000000031086 ) ) ;
#95609=ADVANCED_FACE ( 'NONE', ( #18554 ), #35009, .T. ) ;
#95610=B_SPLINE_CURVE_WITH_KNOTS ( 'NONE', 3,
 ( #14932, #85377, #45399, #54375, #22923, #914 ),
 .UNSPECIFIED., .F., .F.,
 ( 4, 2, 4 ),
 ( 0.000000000000000000, 0.0002565770811490922947, 0.0005131541622981845895 ),
 .UNSPECIFIED. ) ;
#95613=CARTESIAN_POINT ( 'NONE',  ( 5.076628168052704559, 20.17559781766745175, -8.527530157486179263 ) ) ;
#95616=CARTESIAN_POINT ( 'NONE',  ( 7.361572987183170547, 52.05059781766745175, 9.846743663894590881 ) ) ;
#95620=CARTESIAN_POINT ( 'NONE',  ( -46.56032334906372938, 103.8061263278359689, 5.692785474546972146 ) ) ;
#95623=CARTESIAN_POINT ( 'NONE',  ( 0.1532563361054100626, 30.80059781766744820, -2.638427012816831230 ) ) ;
#95624=CARTESIAN_POINT ( 'NONE',  ( -4.164238869374098151, 66.59541550158060375, -3.795296366450310543 ) ) ;
#95627=CARTESIAN_POINT ( 'NONE',  ( 0.2751277870542967463, 70.00000000000000000, -6.500000000000000888 ) ) ;
#95628=CARTESIAN_POINT ( 'NONE',  ( 0.1532563361054083140, 31.00893115100078390, 1.131784320476157264E-15 ) ) ;
#95631=CARTESIAN_POINT ( 'NONE',  ( -2.816281873526473856, -0.6680319967362464695, 3.434112377981055619 ) ) ;
#95632=CARTESIAN_POINT ( 'NONE',  ( 2.791683348922237240, 0.3839311510007847872, -7.208316651077763204 ) ) ;
#95633=CIRCLE ( 'NONE', #98880, 2.999999999999999112 ) ;
#95634=CARTESIAN_POINT ( 'NONE',  ( 0.1532563361054082862, 16.21726448433411960, 2.638427012816831674 ) ) ;
#95635=CARTESIAN_POINT ( 'NONE',  ( 17.20831665107776587, 62.88393115100078745, 7.208316651077764980 ) ) ;
#95637=EDGE_CURVE ( 'NONE', #25751, #12094, #83774, .T. ) ;
#95639=CARTESIAN_POINT ( 'NONE',  ( -0.8801773607111009756, 13.06368534415483929, 1.068504757029289695E-15 ) ) ;
#95640=CARTESIAN_POINT ( 'NONE',  ( 24.16423886937410614, 4.303748834913967869, 8.672049930838204340E-16 ) ) ;
#95641=CARTESIAN_POINT ( 'NONE',  ( 19.84674366389459266, 8.300597817667451750, 2.638427012816836559 ) ) ;
#95642=CARTESIAN_POINT ( 'NONE',  ( 12.91533473730992121, 39.52201867748817676, 10.88017736071110164 ) ) ;
#95643=CARTESIAN_POINT ( 'NONE',  ( 22.81628187352648496, 31.83196800326375353, -3.434112377981050290 ) ) ;
#95644=CARTESIAN_POINT ( 'NONE',  ( 17.96484262340118221, 64.93868534415483396, 7.964842623401181321 ) ) ;
#95645=SURFACE_STYLE_USAGE ( .BOTH. , #11154 ) ;
#95649=AXIS2_PLACEMENT_3D ( 'NONE', #26192, #56684, #11679 ) ;
#95650=CARTESIAN_POINT ( 'NONE',  ( 0.1532563361054083140, 51.00893115100078745, 1.131784320476157264E-15 ) ) ;
#95651=CARTESIAN_POINT ( 'NONE',  ( 10.00000000000000000, 14.75893115100078568, -9.846743663894594434 ) ) ;
#95653=CARTESIAN_POINT ( 'NONE',  ( 0.6178305044545818747, 28.49863466993041783, -9.382169495545419124 ) ) ;
#95655=CARTESIAN_POINT ( 'NONE',  ( 20.88017736071110875, 30.77201867748816966, -2.915334737309920765 ) ) ;
#95658=CARTESIAN_POINT ( 'NONE',  ( 24.16423886937410614, 44.30374883491397497, 8.672049930838204340E-16 ) ) ;
#95660=CARTESIAN_POINT ( 'NONE',  ( 5.076628168052704559, 45.17559781766745175, -8.527530157486179263 ) ) ;
#95661=CARTESIAN_POINT ( 'NONE',  ( -1.099225684535947600, 33.70696800326375353, -6.408140936763238038 ) ) ;
#95662=CARTESIAN_POINT ( 'NONE',  ( 7.084665262690076126, 24.10535201082150181, 10.88017736071109987 ) ) ;
#95663=CARTESIAN_POINT ( 'NONE',  ( 17.20831665107776587, 57.88393115100078745, 7.208316651077764980 ) ) ;
#95664=CARTESIAN_POINT ( 'NONE',  ( 2.035157376598824452, 48.68868534415483396, 7.964842623401179544 ) ) ;
#95665=CARTESIAN_POINT ( 'NONE',  ( 3.591859063236761518, 9.956968003263753531, 11.09922568453594849 ) ) ;
#95666=CARTESIAN_POINT ( 'NONE',  ( 20.36894250292379382, 38.67874883491396076, 10.36894250292379205 ) ) ;
#95668=CARTESIAN_POINT ( 'NONE',  ( 1.472469842513823179, 31.42559781766745530, 4.923371831947296329 ) ) ;
#95669=CARTESIAN_POINT ( 'NONE',  ( 21.09922568453594849, 61.20696800326376064, 6.408140936763242479 ) ) ;
#95670=CARTESIAN_POINT ( 'NONE',  ( 22.81628187352647785, 1.415301336597087012, 3.434112377981063169 ) ) ;
#95671=VERTEX_POINT ( 'NONE', #74003 ) ;
#95673=CARTESIAN_POINT ( 'NONE',  ( 20.88017736071110875, 10.77201867748817143, -2.915334737309920765 ) ) ;
#95675=CARTESIAN_POINT ( 'NONE',  ( -4.164238869374099039, 26.80374883491397142, 8.674139862899312516E-16 ) ) ;
#95677=CARTESIAN_POINT ( 'NONE',  ( 12.91533473730993009, 66.60535201082150536, -10.88017736071109987 ) ) ;
#95678=CARTESIAN_POINT ( 'NONE',  ( 2.791683348922237240, 45.38393115100079456, -7.208316651077763204 ) ) ;
#95679=CARTESIAN_POINT ( 'NONE',  ( 0.5774900079438607392, 28.48035201082150891, 5.440088680355550821 ) ) ;
#95683=ADVANCED_FACE ( 'NONE', ( #4054 ), #72037, .T. ) ;
#95687=ORIENTED_EDGE ( 'NONE', *, *, #87068, .F. ) ;
#95689=CARTESIAN_POINT ( 'NONE',  ( 2.603489959281592991, 11.58210964143329313, 6.500000000000006217 ) ) ;
#95690=CARTESIAN_POINT ( 'NONE',  ( 24.16423886937410614, 4.303748834913967869, 8.672049930838204340E-16 ) ) ;
#95691=CARTESIAN_POINT ( 'NONE',  ( 6.204703633549690345, 5.762082168247301794, -14.16423886937410259 ) ) ;
#95692=CARTESIAN_POINT ( 'NONE',  ( 7.084665262690076126, 49.10535201082149825, 10.88017736071109987 ) ) ;
#95693=CARTESIAN_POINT ( 'NONE',  ( -0.3689425029237898834, 61.17874883491396076, -10.36894250292378850 ) ) ;
#95694=CARTESIAN_POINT ( 'NONE',  ( 14.92337183194729633, 57.67559781766745886, 8.527530157486181039 ) ) ;
#95695=CARTESIAN_POINT ( 'NONE',  ( 7.361572987183170547, 37.05059781766744464, 9.846743663894590881 ) ) ;
#95697=CARTESIAN_POINT ( 'NONE',  ( 7.084665262690076126, 34.10535201082151247, 10.88017736071109987 ) ) ;
#95698=CARTESIAN_POINT ( 'NONE',  ( 1.472469842513823179, 61.42559781766745175, 4.923371831947296329 ) ) ;
#95699=CARTESIAN_POINT ( 'NONE',  ( 13.79529636645030344, 8.262082168247300018, 14.16423886937410614 ) ) ;
#95701=CARTESIAN_POINT ( 'NONE',  ( 2.917880565312950480, 50.97041550158064638, -12.26659068614894821 ) ) ;
#95702=CARTESIAN_POINT ( 'NONE',  ( 4.559911319644449179, 3.897018677488171434, 9.422509992056141925 ) ) ;
#95703=CARTESIAN_POINT ( 'NONE',  ( 5.500000000000000000, 60.50000000000000711, 6.000000000000000000 ) ) ;
#95704=LINE ( 'NONE', #50186, #15629 ) ;
#95709=CARTESIAN_POINT ( 'NONE',  ( 19.84674366389459621, 28.50893115100078745, 7.409399052514197653E-17 ) ) ;
#95711=CARTESIAN_POINT ( 'NONE',  ( 22.26659068614894466, 33.88708216824730357, 7.082119434687054849 ) ) ;
#95712=CARTESIAN_POINT ( 'NONE',  ( 14.92337183194729633, 37.67559781766745175, 8.527530157486181039 ) ) ;
#95713=CARTESIAN_POINT ( 'NONE',  ( 15.44008868035555793, 51.39701867748816966, -9.422509992056140149 ) ) ;
#95716=CARTESIAN_POINT ( 'NONE',  ( 7.084665262690076126, 57.02201867748817676, -10.88017736071110164 ) ) ;
#95717=CARTESIAN_POINT ( 'NONE',  ( 3.591859063236761518, 59.95696800326375353, 11.09922568453594849 ) ) ;
#95720=CARTESIAN_POINT ( 'NONE',  ( 10.00000000000000000, 25.55374883491396787, -14.16423886937410082 ) ) ;
#95722=CARTESIAN_POINT ( 'NONE',  ( 3.591859063236763294, 38.29030133659708923, -11.09922568453595026 ) ) ;
#95724=CARTESIAN_POINT ( 'NONE',  ( 20.88017736071110875, 20.77201867748816611, -2.915334737309920765 ) ) ;
#95725=CARTESIAN_POINT ( 'NONE',  ( 17.20831665107776587, 29.13393115100078390, -7.208316651077762316 ) ) ;
#95726=CARTESIAN_POINT ( 'NONE',  ( 4.559911319644449179, 7.230352010821504471, -9.422509992056141925 ) ) ;
#95727=CARTESIAN_POINT ( 'NONE',  ( 3.591859063236761518, 59.95696800326375353, 11.09922568453594849 ) ) ;
#95729=CARTESIAN_POINT ( 'NONE',  ( 10.00000000000000000, 24.75893115100078745, -9.846743663894594434 ) ) ;
#95731=CARTESIAN_POINT ( 'NONE',  ( 19.42250999205614548, 50.98035201082151247, -5.440088680355545492 ) ) ;
#95732=CARTESIAN_POINT ( 'NONE',  ( 7.084665262690076126, 69.10535201082151957, 10.88017736071109987 ) ) ;
#95734=EDGE_CURVE ( 'NONE', #22423, #73925, #80240, .T. ) ;
#95738=ADVANCED_FACE ( 'NONE', ( #59498 ), #38001, .T. ) ;
#95740=CARTESIAN_POINT ( 'NONE',  ( 19.84674366389459266, 8.300597817667451750, 2.638427012816836559 ) ) ;
#95741=EDGE_CURVE ( 'NONE', #96981, #73925, #86148, .T. ) ;
#95742=CARTESIAN_POINT ( 'NONE',  ( 16.40814093676323893, 30.79030133659708923, 11.09922568453595026 ) ) ;
#95744=CARTESIAN_POINT ( 'NONE',  ( 2.791683348922237240, 40.38393115100078035, -7.208316651077763204 ) ) ;
#95746=CARTESIAN_POINT ( 'NONE',  ( -0.3689425029237898834, 16.17874883491396076, -10.36894250292378850 ) ) ;
#95747=CARTESIAN_POINT ( 'NONE',  ( 0.1532563361054082862, 36.21726448433410894, 2.638427012816831674 ) ) ;
#95748=CARTESIAN_POINT ( 'NONE',  ( 0.6178305044545838731, 34.74863466993042493, 9.382169495545420901 ) ) ;
#95749=CARTESIAN_POINT ( 'NONE',  ( 18.72515096720570327, 16.07228050351031712, -6.499999999999992006 ) ) ;
#95750=DIRECTION ( 'NONE',  ( 6.608470384673550777E-17, 1.000000000000000000, -0.000000000000000000 ) ) ;
#95751=CARTESIAN_POINT ( 'NONE',  ( 4.559911319644449179, 62.23035201082150536, -9.422509992056141925 ) ) ;
#95752=CARTESIAN_POINT ( 'NONE',  ( 22.81628187352647785, 11.41530133659708390, 3.434112377981063169 ) ) ;
#95754=CARTESIAN_POINT ( 'NONE',  ( 14.92337183194729988, 34.34226448433411605, -8.527530157486177487 ) ) ;
#95755=CARTESIAN_POINT ( 'NONE',  ( 20.88017736071110875, 20.77201867748816611, -2.915334737309920765 ) ) ;
#95756=CARTESIAN_POINT ( 'NONE',  ( 13.43411237798106583, 32.66530133659708213, -12.81628187352647252 ) ) ;
#95757=CARTESIAN_POINT ( 'NONE',  ( 10.00000000000000000, 29.75893115100078745, -9.846743663894594434 ) ) ;
#95759=CARTESIAN_POINT ( 'NONE',  ( 7.084665262690076126, 32.02201867748816966, -10.88017736071110164 ) ) ;
#95762=CARTESIAN_POINT ( 'NONE',  ( 15.44008868035555260, 4.730352010821504471, 9.422509992056143702 ) ) ;
#95763=CARTESIAN_POINT ( 'NONE',  ( 0.1532563361054082862, 51.21726448433412315, 2.638427012816831674 ) ) ;
#95764=CARTESIAN_POINT ( 'NONE',  ( 4.559911319644449179, 33.89701867748817676, 9.422509992056141925 ) ) ;
#95767=CARTESIAN_POINT ( 'NONE',  ( 10.00000000000000178, 64.31368534415483396, 10.88017736071110342 ) ) ;
#95769=CARTESIAN_POINT ( 'NONE',  ( 7.084665262690076126, 29.10535201082150181, 10.88017736071109987 ) ) ;
#95770=CARTESIAN_POINT ( 'NONE',  ( 0.000000000000000000, 75.66482536767503575, -6.574273087692857231 ) ) ;
#95771=( NAMED_UNIT ( * ) SI_UNIT ( $, .STERADIAN. ) SOLID_ANGLE_UNIT ( ) );
#95772=LINE ( 'NONE', #36248, #96900 ) ;
#95773=CARTESIAN_POINT ( 'NONE',  ( 18.52753015748617571, 53.09226448433412315, 4.923371831947298993 ) ) ;
#95775=CARTESIAN_POINT ( 'NONE',  ( -4.164238869374099927, 52.01208216824729647, 3.795296366450308767 ) ) ;
#95776=CARTESIAN_POINT ( 'NONE',  ( 21.92686044187656691, 19.95379003517448169, 3.195792623639537755 ) ) ;
#95779=CARTESIAN_POINT ( 'NONE',  ( 17.08211943468705840, 15.13708216824730179, -12.26659068614894466 ) ) ;
#95780=CARTESIAN_POINT ( 'NONE',  ( 24.16423886937409904, 44.09541550158063927, 3.795296366450317205 ) ) ;
#95781=CARTESIAN_POINT ( 'NONE',  ( 16.40814093676323893, 5.790301336597087456, 11.09922568453595026 ) ) ;
#95784=CARTESIAN_POINT ( 'NONE',  ( 10.00000000000000000, 65.55374883491396076, -14.16423886937410082 ) ) ;
#95785=CARTESIAN_POINT ( 'NONE',  ( 12.63842701281683922, 39.55059781766744464, -9.846743663894590881 ) ) ;
#95786=DIRECTION ( 'NONE',  ( 0.000000000000000000, 0.000000000000000000, -1.000000000000000000 ) ) ;
#95788=CARTESIAN_POINT ( 'NONE',  ( 10.00000000000000000, 56.81368534415484106, -10.88017736071110342 ) ) ;
#95790=CARTESIAN_POINT ( 'NONE',  ( 19.38216949554541202, 55.99863466993041072, 9.382169495545424454 ) ) ;
#95791=CARTESIAN_POINT ( 'NONE',  ( 16.40814093676323893, 30.79030133659708923, 11.09922568453595026 ) ) ;
#95792=CARTESIAN_POINT ( 'NONE',  ( 18.52753015748617571, 28.09226448433411960, 4.923371831947298993 ) ) ;
#95793=VERTEX_POINT ( 'NONE', #36513 ) ;
#95796=CARTESIAN_POINT ( 'NONE',  ( -2.266590686148945544, 61.38708216824730357, -7.082119434687050408 ) ) ;
#95797=CARTESIAN_POINT ( 'NONE',  ( -0.8801773607111009756, 18.06368534415484106, 1.068504757029289695E-15 ) ) ;
#95798=CARTESIAN_POINT ( 'NONE',  ( 20.36894250292379382, 43.67874883491397497, 10.36894250292379205 ) ) ;
#95799=CARTESIAN_POINT ( 'NONE',  ( -0.8801773607110991993, 32.85535201082151247, -2.915334737309923874 ) ) ;
#95800=CARTESIAN_POINT ( 'NONE',  ( 0.5774900079438607392, 63.48035201082149825, 5.440088680355550821 ) ) ;
#95804=CARTESIAN_POINT ( 'NONE',  ( 14.92337183194729633, 12.67559781766745353, 8.527530157486181039 ) ) ;
#95805=CARTESIAN_POINT ( 'NONE',  ( 0.2751277870542967463, 0.000000000000000000, 6.500000000000000888 ) ) ;
#95808=CARTESIAN_POINT ( 'NONE',  ( 1.472469842513823179, 40.59226448433411605, -4.923371831947296329 ) ) ;
#95809=CARTESIAN_POINT ( 'NONE',  ( 18.52753015748617571, 58.09226448433411605, 4.923371831947298993 ) ) ;
#95810=CARTESIAN_POINT ( 'NONE',  ( 10.00000000000000178, 29.31368534415483751, 10.88017736071110342 ) ) ;
#95812=CARTESIAN_POINT ( 'NONE',  ( 10.00000000000000178, 50.37363466993042493, 12.81628187352647608 ) ) ;
#95814=CARTESIAN_POINT ( 'NONE',  ( 15.44008868035555260, 59.73035201082151247, 9.422509992056143702 ) ) ;
#95815=CARTESIAN_POINT ( 'NONE',  ( 0.1532563361054083140, 26.00893115100078745, 1.131784320476157264E-15 ) ) ;
#95816=CARTESIAN_POINT ( 'NONE',  ( -2.266590686148945544, 56.38708216824731068, -7.082119434687050408 ) ) ;
#95817=CARTESIAN_POINT ( 'NONE',  ( 5.076628168052704559, 20.17559781766745175, -8.527530157486179263 ) ) ;
#95818=CARTESIAN_POINT ( 'NONE',  ( -0.04068437667222160603, 47.21974360917721469, -6.396802510829771471 ) ) ;
#95819=CARTESIAN_POINT ( 'NONE',  ( 0.1532563361054082862, 61.21726448433412315, 2.638427012816831674 ) ) ;
#95820=CARTESIAN_POINT ( 'NONE',  ( 6.204703633549690345, 30.76208216824730357, -14.16423886937410259 ) ) ;
#95821=CARTESIAN_POINT ( 'NONE',  ( 18.52753015748617571, 38.09226448433412315, 4.923371831947298993 ) ) ;
#95823=CARTESIAN_POINT ( 'NONE',  ( 0.5774900079438590739, 27.64701867748817676, -5.440088680355550821 ) ) ;
#95824=CARTESIAN_POINT ( 'NONE',  ( 17.96484262340118221, 64.93868534415483396, 7.964842623401181321 ) ) ;
#95827=CARTESIAN_POINT ( 'NONE',  ( 21.09922568453594849, 41.20696800326375353, 6.408140936763242479 ) ) ;
#95828=CARTESIAN_POINT ( 'NONE',  ( 10.00000000000000178, 54.31368534415484106, 10.88017736071110342 ) ) ;
#95829=ORIENTED_EDGE ( 'NONE', *, *, #28330, .F. ) ;
#95831=PLANE ( 'NONE',  #33847 ) ;
#95834=CARTESIAN_POINT ( 'NONE',  ( 4.559911319644449179, 63.89701867748817676, 9.422509992056141925 ) ) ;
#95835=CARTESIAN_POINT ( 'NONE',  ( 4.559911319644449179, 13.89701867748817143, 9.422509992056141925 ) ) ;
#95836=CARTESIAN_POINT ( 'NONE',  ( 0.1532563361054083140, 1.008931151000784787, 1.131784320476157264E-15 ) ) ;
#95838=CARTESIAN_POINT ( 'NONE',  ( -0.8801773607111009756, 3.063685344154838397, 1.068504757029289695E-15 ) ) ;
#95839=CARTESIAN_POINT ( 'NONE',  ( 17.20831665107776587, 4.133931151000785675, -7.208316651077762316 ) ) ;
#95840=CARTESIAN_POINT ( 'NONE',  ( -2.266590686148945544, 16.38708216824730357, -7.082119434687050408 ) ) ;
#95841=CARTESIAN_POINT ( 'NONE',  ( 17.96484262340118221, 21.18868534415483396, -7.964842623401177768 ) ) ;
#95842=CARTESIAN_POINT ( 'NONE',  ( 12.63842701281683034, 62.46726448433410894, 9.846743663894596210 ) ) ;
#95844=CARTESIAN_POINT ( 'NONE',  ( 2.791683348922237240, 65.38393115100078035, -7.208316651077763204 ) ) ;
#95846=CARTESIAN_POINT ( 'NONE',  ( 17.96484262340118221, 54.93868534415484106, 7.964842623401181321 ) ) ;
#95848=CARTESIAN_POINT ( 'NONE',  ( 14.92337183194729633, 62.67559781766745886, 8.527530157486181039 ) ) ;
#95850=CARTESIAN_POINT ( 'NONE',  ( 22.81628187352648496, 41.83196800326375353, -3.434112377981050290 ) ) ;
#95851=CARTESIAN_POINT ( 'NONE',  ( 10.00000000000000178, 4.313685344154837509, 10.88017736071110342 ) ) ;
#95853=CARTESIAN_POINT ( 'NONE',  ( 17.96484262340118221, 64.93868534415483396, 7.964842623401181321 ) ) ;
#95855=CARTESIAN_POINT ( 'NONE',  ( 15.44008868035555260, 9.730352010821505360, 9.422509992056143702 ) ) ;
#95857=VERTEX_POINT ( 'NONE', #14514 ) ;
#95858=CARTESIAN_POINT ( 'NONE',  ( 6.565887622018943937, 35.16530133659708923, 12.81628187352647430 ) ) ;
#95859=CARTESIAN_POINT ( 'NONE',  ( 12.91533473730992121, 24.52201867748816966, 10.88017736071110164 ) ) ;
#95860=CARTESIAN_POINT ( 'NONE',  ( 0.9408516040111476464, 47.46693863883976405, -6.499999999999953815 ) ) ;
#95861=ORIENTED_EDGE ( 'NONE', *, *, #23633, .T. ) ;
#95862=CARTESIAN_POINT ( 'NONE',  ( 3.591859063236761518, 39.95696800326375353, 11.09922568453594849 ) ) ;
#95863=CARTESIAN_POINT ( 'NONE',  ( 10.00000000000000000, 31.81368534415483751, -10.88017736071110342 ) ) ;
#95864=EDGE_CURVE ( 'NONE', #93697, #39498, #79004, .T. ) ;
#95865=CARTESIAN_POINT ( 'NONE',  ( 10.00000000000000178, 52.25893115100078745, 9.846743663894594434 ) ) ;
#95866=ORIENTED_EDGE ( 'NONE', *, *, #54420, .T. ) ;
#95869=CARTESIAN_POINT ( 'NONE',  ( 2.791683348922240793, 61.63393115100079456, 7.208316651077764092 ) ) ;
#95870=CARTESIAN_POINT ( 'NONE',  ( 0.2751277870542967463, 70.00000000000000000, -6.000000000000000000 ) ) ;
#95871=CARTESIAN_POINT ( 'NONE',  ( 1.472469842513823179, 51.42559781766745886, 4.923371831947296329 ) ) ;
#95872=CARTESIAN_POINT ( 'NONE',  ( 15.44008868035555793, 21.39701867748817321, -9.422509992056140149 ) ) ;
#95874=CARTESIAN_POINT ( 'NONE',  ( 14.92337183194729988, 39.34226448433412315, -8.527530157486177487 ) ) ;
#95875=CARTESIAN_POINT ( 'NONE',  ( -46.82017113615791004, 100.6079546444643569, -9.324761308090124601 ) ) ;
#95877=CARTESIAN_POINT ( 'NONE',  ( 5.076628168052704559, 40.17559781766745175, -8.527530157486179263 ) ) ;
#95878=CARTESIAN_POINT ( 'NONE',  ( 19.84674366389459621, 13.50893115100078568, 7.409399052514197653E-17 ) ) ;
#95879=CARTESIAN_POINT ( 'NONE',  ( 0.1532563361054100626, 0.8005978176674514168, -2.638427012816831230 ) ) ;
#95880=CARTESIAN_POINT ( 'NONE',  ( 5.076628168052703671, 61.84226448433412315, 8.527530157486179263 ) ) ;
#95882=CARTESIAN_POINT ( 'NONE',  ( 10.00000000000000178, 65.37363466993042493, 12.81628187352647608 ) ) ;
#95885=CARTESIAN_POINT ( 'NONE',  ( 19.38216949554541557, 42.24863466993041783, -9.382169495545420901 ) ) ;
#95886=CARTESIAN_POINT ( 'NONE',  ( 10.00000000000000178, 42.25893115100078745, 9.846743663894594434 ) ) ;
#95888=CARTESIAN_POINT ( 'NONE',  ( 10.00000000000000178, 58.05374883491397497, 14.16423886937410082 ) ) ;
#95889=CARTESIAN_POINT ( 'NONE',  ( 7.361572987183170547, 27.05059781766745175, 9.846743663894590881 ) ) ;
#95890=CARTESIAN_POINT ( 'NONE',  ( 0.1532563361054082862, 6.217264484334118713, 2.638427012816831674 ) ) ;
#95892=CARTESIAN_POINT ( 'NONE',  ( 24.16423886937409904, 59.09541550158063217, 3.795296366450317205 ) ) ;
#95893=CARTESIAN_POINT ( 'NONE',  ( 10.00000000000000178, 67.25893115100079456, 9.846743663894594434 ) ) ;
#95895=CARTESIAN_POINT ( 'NONE',  ( 7.084665262690076126, 7.022018677488170546, -10.88017736071110164 ) ) ;
#95896=CARTESIAN_POINT ( 'NONE',  ( -2.266590686148945544, 37.22041550158063217, 7.082119434687048631 ) ) ;
#95897=CARTESIAN_POINT ( 'NONE',  ( -0.3689425029237898834, 51.17874883491397497, -10.36894250292378850 ) ) ;
#95900=CARTESIAN_POINT ( 'NONE',  ( 7.361572987183169658, 9.967264484334119601, -9.846743663894592657 ) ) ;
#95901=CYLINDRICAL_SURFACE ( 'NONE', #75696, 0.5000000000000004441 ) ;
#95902=CARTESIAN_POINT ( 'NONE',  ( 12.63842701281683922, 64.55059781766745175, -9.846743663894590881 ) ) ;
#95903=CARTESIAN_POINT ( 'NONE',  ( 2.035157376598824452, 48.68868534415483396, 7.964842623401179544 ) ) ;
#95904=CARTESIAN_POINT ( 'NONE',  ( 14.92337183194729633, 47.67559781766745175, 8.527530157486181039 ) ) ;
#95906=CARTESIAN_POINT ( 'NONE',  ( 12.63842701281683922, 59.55059781766744464, -9.846743663894590881 ) ) ;
#95907=PRESENTATION_STYLE_ASSIGNMENT (( #64875 ) ) ;
#95910=CARTESIAN_POINT ( 'NONE',  ( 20.36894250292379382, 23.67874883491397142, 10.36894250292379205 ) ) ;
#95913=CARTESIAN_POINT ( 'NONE',  ( -0.8801773607111008646, 18.27201867748817321, 2.915334737309923430 ) ) ;
#95914=CARTESIAN_POINT ( 'NONE',  ( 19.38216949554541202, 35.99863466993041072, 9.382169495545424454 ) ) ;
#95916=CARTESIAN_POINT ( 'NONE',  ( 18.52753015748618282, 8.925597817667451750, -4.923371831947291888 ) ) ;
#95917=CARTESIAN_POINT ( 'NONE',  ( 19.38216949554541557, 57.24863466993042493, -9.382169495545420901 ) ) ;
#95920=CARTESIAN_POINT ( 'NONE',  ( 20.36894250292379738, 24.92874883491396787, -10.36894250292379027 ) ) ;
#95921=PRESENTATION_STYLE_ASSIGNMENT (( #65888 ) ) ;
#95923=CARTESIAN_POINT ( 'NONE',  ( 20.88017736071110875, 10.77201867748817143, -2.915334737309920765 ) ) ;
#95926=CARTESIAN_POINT ( 'NONE',  ( 10.00000000000000178, 39.31368534415484106, 10.88017736071110342 ) ) ;
#95927=CARTESIAN_POINT ( 'NONE',  ( 20.88017736071110519, 45.56368534415484106, 2.639326808657452039E-16 ) ) ;
#95928=CARTESIAN_POINT ( 'NONE',  ( 6.565887622018943937, 18.08196800326375708, -12.81628187352647608 ) ) ;
#95929=CARTESIAN_POINT ( 'NONE',  ( 7.361572987183170547, 67.05059781766746596, 9.846743663894590881 ) ) ;
#95930=DIRECTION ( 'NONE',  ( 0.000000000000000000, -1.000000000000000000, 0.000000000000000000 ) ) ;
#95931=CARTESIAN_POINT ( 'NONE',  ( 5.076628168052704559, 10.17559781766745175, -8.527530157486179263 ) ) ;
#95933=CARTESIAN_POINT ( 'NONE',  ( 12.91533473730992121, 44.52201867748816966, 10.88017736071110164 ) ) ;
#95934=CARTESIAN_POINT ( 'NONE',  ( 19.38216949554541202, 5.998634669930420493, 9.382169495545424454 ) ) ;
#95935=CARTESIAN_POINT ( 'NONE',  ( 4.559911319644449179, 57.23035201082150536, -9.422509992056141925 ) ) ;
#95936=CARTESIAN_POINT ( 'NONE',  ( 10.00000000000000000, 19.75893115100078390, -9.846743663894594434 ) ) ;
#95937=CARTESIAN_POINT ( 'NONE',  ( 6.565887622018943937, 43.08196800326374643, -12.81628187352647608 ) ) ;
#95938=CARTESIAN_POINT ( 'NONE',  ( 17.20831665107776587, 9.133931151000787452, -7.208316651077762316 ) ) ;
#95941=CARTESIAN_POINT ( 'NONE',  ( 19.72487221294570858, 0.000000000000000000, -6.500000000000000888 ) ) ;
#95942=CARTESIAN_POINT ( 'NONE',  ( 19.42250999205614193, 20.14701867748817321, 5.440088680355555262 ) ) ;
#95943=CARTESIAN_POINT ( 'NONE',  ( -2.816281873526471635, 53.91530133659709634, -3.434112377981056508 ) ) ;
#95944=CARTESIAN_POINT ( 'NONE',  ( 7.361572987183170547, 37.05059781766744464, 9.846743663894590881 ) ) ;
#95945=CARTESIAN_POINT ( 'NONE',  ( 2.035157376598822676, 12.43868534415483751, -7.964842623401177768 ) ) ;
#95946=CARTESIAN_POINT ( 'NONE',  ( 6.204703633549690345, 67.84541550158060375, 14.16423886937410082 ) ) ;
#95948=AXIS2_PLACEMENT_3D ( 'NONE', #64026, #41066, #13375 ) ;
#95949=CARTESIAN_POINT ( 'NONE',  ( 12.91533473730993009, 16.60535201082150891, -10.88017736071109987 ) ) ;
#95951=CARTESIAN_POINT ( 'NONE',  ( 4.559911319644449179, 37.23035201082150536, -9.422509992056141925 ) ) ;
#95952=DIRECTION ( 'NONE',  ( 1.000000000000000000, 0.000000000000000000, 0.000000000000000000 ) ) ;
#95953=CARTESIAN_POINT ( 'NONE',  ( 12.91533473730993009, 21.60535201082150536, -10.88017736071109987 ) ) ;
#95955=CARTESIAN_POINT ( 'NONE',  ( 20.32896413005680714, 10.57879003517447281, -5.963430220938276349 ) ) ;
#95956=CARTESIAN_POINT ( 'NONE',  ( 7.084665262690076126, 19.10535201082150181, 10.88017736071109987 ) ) ;
#95959=CARTESIAN_POINT ( 'NONE',  ( 6.565887622018943937, 63.08196800326376064, -12.81628187352647608 ) ) ;
#95960=DIRECTION ( 'NONE',  ( -0.5547001962252290364, -0.8320502943378437211, 0.000000000000000000 ) ) ;
#95961=CARTESIAN_POINT ( 'NONE',  ( 10.00000000000000178, 28.05374883491396787, 14.16423886937410082 ) ) ;
#95962=CARTESIAN_POINT ( 'NONE',  ( 10.00000000000000178, 39.31368534415484106, 10.88017736071110342 ) ) ;
#95963=CARTESIAN_POINT ( 'NONE',  ( 17.96484262340118221, 36.18868534415484106, -7.964842623401177768 ) ) ;
#95965=CARTESIAN_POINT ( 'NONE',  ( 19.72487221294571569, 60.71833443783937412, -6.499999999999990230 ) ) ;
#95966=CARTESIAN_POINT ( 'NONE',  ( 5.076628168052704559, 45.17559781766745175, -8.527530157486179263 ) ) ;
#95968=CARTESIAN_POINT ( 'NONE',  ( 10.00000000000000178, 22.25893115100078745, 9.846743663894594434 ) ) ;
#95970=CARTESIAN_POINT ( 'NONE',  ( 2.035157376598822676, 7.438685344154837509, -7.964842623401177768 ) ) ;
#95971=CARTESIAN_POINT ( 'NONE',  ( 5.076628168052703671, 11.84226448433411960, 8.527530157486179263 ) ) ;
#95973=CARTESIAN_POINT ( 'NONE',  ( -2.816281873526471635, 13.91530133659708746, -3.434112377981056508 ) ) ;
#95974=CARTESIAN_POINT ( 'NONE',  ( 20.88017736071110519, 55.56368534415484817, 2.639326808657452039E-16 ) ) ;
#95975=CARTESIAN_POINT ( 'NONE',  ( 0.5774900079438590739, 22.64701867748817321, -5.440088680355550821 ) ) ;
#95976=CARTESIAN_POINT ( 'NONE',  ( 13.43411237798105340, 60.58196800326376064, 12.81628187352647963 ) ) ;
#95977=CARTESIAN_POINT ( 'NONE',  ( 22.26659068614894466, 33.88708216824730357, 7.082119434687054849 ) ) ;
#95983=CARTESIAN_POINT ( 'NONE',  ( 6.565887622018943937, 8.081968003263751754, -12.81628187352647608 ) ) ;
#95986=CARTESIAN_POINT ( 'NONE',  ( 7.084665262690076126, 39.10535201082150536, 10.88017736071109987 ) ) ;
#95988=CARTESIAN_POINT ( 'NONE',  ( 7.361572987183169658, 59.96726448433410894, -9.846743663894592657 ) ) ;
#95990=CARTESIAN_POINT ( 'NONE',  ( 2.791683348922240793, 21.63393115100078745, 7.208316651077764092 ) ) ;
#95991=CARTESIAN_POINT ( 'NONE',  ( 17.20831665107776587, 22.88393115100078745, 7.208316651077764980 ) ) ;
#95992=CARTESIAN_POINT ( 'NONE',  ( 0.1532563361054083140, 16.00893115100078390, 1.131784320476157264E-15 ) ) ;
#95993=CARTESIAN_POINT ( 'NONE',  ( 2.791683348922240793, 6.633931151000785675, 7.208316651077764092 ) ) ;
#95994=CARTESIAN_POINT ( 'NONE',  ( 7.361572987183169658, 4.967264484334119601, -9.846743663894592657 ) ) ;
#95995=CARTESIAN_POINT ( 'NONE',  ( -45.94000000000000483, 92.50000000000000000, -9.500000000000000000 ) ) ;
#95996=CARTESIAN_POINT ( 'NONE',  ( 1.472469842513823179, 1.425597817667451528, 4.923371831947296329 ) ) ;
#95997=CARTESIAN_POINT ( 'NONE',  ( 1.472469842513823179, 16.42559781766745175, 4.923371831947296329 ) ) ;
#96000=CARTESIAN_POINT ( 'NONE',  ( 0.6178305044545818747, -1.501365330069579951, -9.382169495545419124 ) ) ;
#96002=SURFACE_SIDE_STYLE ('',( #4514 ) ) ;
#96004=CARTESIAN_POINT ( 'NONE',  ( 20.36894250292379382, 23.67874883491397142, 10.36894250292379205 ) ) ;
#96005=DIRECTION ( 'NONE',  ( -0.000000000000000000, -1.000000000000000000, 0.000000000000000000 ) ) ;
#96006=CARTESIAN_POINT ( 'NONE',  ( 20.36894250292379382, 18.67874883491397142, 10.36894250292379205 ) ) ;
#96007=CARTESIAN_POINT ( 'NONE',  ( 24.16423886937409904, 34.09541550158064638, 3.795296366450317205 ) ) ;
#96009=CARTESIAN_POINT ( 'NONE',  ( 2.035157376598824452, 28.68868534415484106, 7.964842623401179544 ) ) ;
#96011=CARTESIAN_POINT ( 'NONE',  ( 10.00000000000000000, 19.75893115100078390, -9.846743663894594434 ) ) ;
#96012=CARTESIAN_POINT ( 'NONE',  ( 19.42250999205614548, 60.98035201082151247, -5.440088680355545492 ) ) ;
#96013=CARTESIAN_POINT ( 'NONE',  ( 7.361572987183170547, 32.05059781766745175, 9.846743663894590881 ) ) ;
#96014=AXIS2_PLACEMENT_3D ( 'NONE', #33287, #24346, #86311 ) ;
#96016=CARTESIAN_POINT ( 'NONE',  ( 2.035157376598824452, 13.68868534415483751, 7.964842623401179544 ) ) ;
#96017=CARTESIAN_POINT ( 'NONE',  ( 22.81628187352648496, 46.83196800326376064, -3.434112377981050290 ) ) ;
#96018=CARTESIAN_POINT ( 'NONE',  ( 1.472469842513823179, 45.59226448433412315, -4.923371831947296329 ) ) ;
#96020=CARTESIAN_POINT ( 'NONE',  ( 7.361572987183170547, 22.05059781766745530, 9.846743663894590881 ) ) ;
#96021=CARTESIAN_POINT ( 'NONE',  ( 13.43411237798106583, 22.66530133659708923, -12.81628187352647252 ) ) ;
#96023=CARTESIAN_POINT ( 'NONE',  ( 19.84674366389459621, 38.50893115100078745, 7.409399052514197653E-17 ) ) ;
#96025=CARTESIAN_POINT ( 'NONE',  ( 13.79529636645031943, 15.34541550158063750, -14.16423886937409904 ) ) ;
#96027=CARTESIAN_POINT ( 'NONE',  ( 2.035157376598822676, 47.43868534415484817, -7.964842623401177768 ) ) ;
#96028=CARTESIAN_POINT ( 'NONE',  ( -0.8801773607111008646, 53.27201867748816966, 2.915334737309923430 ) ) ;
#96029=CARTESIAN_POINT ( 'NONE',  ( -2.266590686148945544, 41.38708216824729647, -7.082119434687050408 ) ) ;
#96030=CARTESIAN_POINT ( 'NONE',  ( 19.84674366389459266, 53.30059781766744464, 2.638427012816836559 ) ) ;
#96032=CARTESIAN_POINT ( 'NONE',  ( 2.035157376598822676, 42.43868534415483396, -7.964842623401177768 ) ) ;
#96034=CARTESIAN_POINT ( 'NONE',  ( -2.816281873526473856, 24.33196800326375353, 3.434112377981055619 ) ) ;
#96035=CARTESIAN_POINT ( 'NONE',  ( 18.52753015748618282, 58.92559781766745886, -4.923371831947291888 ) ) ;
#96037=CARTESIAN_POINT ( 'NONE',  ( 15.44008868035555793, 6.397018677488170546, -9.422509992056140149 ) ) ;
#96038=CARTESIAN_POINT ( 'NONE',  ( 2.035157376598822676, 62.43868534415483396, -7.964842623401177768 ) ) ;
#96040=EDGE_LOOP ( 'NONE', ( #7172, #77513, #28031, #79443 ) ) ;
#96041=CARTESIAN_POINT ( 'NONE',  ( 0.5774900079438607392, 8.480352010821505360, 5.440088680355550821 ) ) ;
#96043=CARTESIAN_POINT ( 'NONE',  ( 10.00000000000000178, 64.31368534415483396, 10.88017736071110342 ) ) ;
#96044=VECTOR ( 'NONE', #53306, 1000.000000000000000 ) ;
#96045=CARTESIAN_POINT ( 'NONE',  ( 7.084665262690076126, 69.10535201082151957, 10.88017736071109987 ) ) ;
#96047=CARTESIAN_POINT ( 'NONE',  ( 17.20831665107776587, 32.88393115100078745, 7.208316651077764980 ) ) ;
#96048=CARTESIAN_POINT ( 'NONE',  ( 0.5774900079438607392, 28.48035201082150891, 5.440088680355550821 ) ) ;
#96049=CARTESIAN_POINT ( 'NONE',  ( 0.6178305044545838731, 9.748634669930416052, 9.382169495545420901 ) ) ;
#96050=CARTESIAN_POINT ( 'NONE',  ( 15.44008868035555260, 39.73035201082150536, 9.422509992056143702 ) ) ;
#96053=CARTESIAN_POINT ( 'NONE',  ( -1.099225684535947600, 39.54030133659708923, 6.408140936763237150 ) ) ;
#96055=CARTESIAN_POINT ( 'NONE',  ( 0.5774900079438607392, 63.48035201082149825, 5.440088680355550821 ) ) ;
#96056=CARTESIAN_POINT ( 'NONE',  ( -2.816281873526473856, 19.33196800326375708, 3.434112377981055619 ) ) ;
#96057=CARTESIAN_POINT ( 'NONE',  ( 19.88701968852526036, 51.79427333184086990, 6.480634945678620973 ) ) ;
#96058=CARTESIAN_POINT ( 'NONE',  ( 19.84674366389459266, 3.300597817667451750, 2.638427012816836559 ) ) ;
#96059=CARTESIAN_POINT ( 'NONE',  ( 2.035157376598824452, 23.68868534415484461, 7.964842623401179544 ) ) ;
#96060=CARTESIAN_POINT ( 'NONE',  ( 20.36894250292379738, 59.92874883491397497, -10.36894250292379027 ) ) ;
#96061=CARTESIAN_POINT ( 'NONE',  ( 19.84674366389459266, 48.71726448433413026, -2.638427012816827677 ) ) ;
#96062=CARTESIAN_POINT ( 'NONE',  ( 7.361572987183169658, 4.967264484334119601, -9.846743663894592657 ) ) ;
#96063=CARTESIAN_POINT ( 'NONE',  ( 10.00000000000000178, 59.31368534415484106, 10.88017736071110342 ) ) ;
#96064=B_SPLINE_CURVE_WITH_KNOTS ( 'NONE', 3,
 ( #78947, #1005, #8973, #17480 ),
 .UNSPECIFIED., .F., .F.,
 ( 4, 4 ),
 ( 0.000000000000000000, 0.001036303429213342089 ),
 .UNSPECIFIED. ) ;
#96065=CARTESIAN_POINT ( 'NONE',  ( 0.2751277870542981341, 8.218334437839383000, 6.500000000000002665 ) ) ;
#96066=CARTESIAN_POINT ( 'NONE',  ( 22.26659068614895176, 24.72041550158063572, -7.082119434687042414 ) ) ;
#96067=MECHANICAL_DESIGN_GEOMETRIC_PRESENTATION_REPRESENTATION('',(#9849),#6621);
#96068=EDGE_CURVE ( 'NONE', #81670, #93612, #10802, .T. ) ;
#96071=EDGE_LOOP ( 'NONE', ( #43028, #55189, #74310, #92518, #13822, #81471 ) ) ;
#96073=CARTESIAN_POINT ( 'NONE',  ( -0.3689425029237881626, 67.42874883491396076, 10.36894250292379027 ) ) ;
#96074=CARTESIAN_POINT ( 'NONE',  ( 24.16423886937410614, 44.30374883491397497, 8.672049930838204340E-16 ) ) ;
#96075=CARTESIAN_POINT ( 'NONE',  ( 14.92337183194729988, 24.34226448433411960, -8.527530157486177487 ) ) ;
#96076=CARTESIAN_POINT ( 'NONE',  ( 22.81628187352647785, 26.62363466993042138, 6.195893100308588602E-16 ) ) ;
#96080=CARTESIAN_POINT ( 'NONE',  ( 10.00000000000000000, 45.55374883491397497, -14.16423886937410082 ) ) ;
#96082=CARTESIAN_POINT ( 'NONE',  ( 2.791683348922237240, 15.38393115100078212, -7.208316651077763204 ) ) ;
#96083=CARTESIAN_POINT ( 'NONE',  ( 18.28836319691943757, 59.34492782695770074, 6.500000000000035527 ) ) ;
#96085=ORIENTED_EDGE ( 'NONE', *, *, #19153, .F. ) ;
#96089=CARTESIAN_POINT ( 'NONE',  ( 13.79529636645030344, 13.26208216824729824, 14.16423886937410614 ) ) ;
#96090=CARTESIAN_POINT ( 'NONE',  ( -0.8801773607110991993, 17.85535201082150536, -2.915334737309923874 ) ) ;
#96091=CARTESIAN_POINT ( 'NONE',  ( -0.8801773607110991993, 22.85535201082150181, -2.915334737309923874 ) ) ;
#96092=CARTESIAN_POINT ( 'NONE',  ( 17.20831665107776587, 47.88393115100078745, 7.208316651077764980 ) ) ;
#96093=CARTESIAN_POINT ( 'NONE',  ( -2.816281873526473856, 24.12363466993042138, 9.499525473075851096E-16 ) ) ;
#96094=SURFACE_STYLE_USAGE ( .BOTH. , #65568 ) ;
#96095=CARTESIAN_POINT ( 'NONE',  ( 18.04007052943771683, 43.01528370094807485, 5.767676674365856293 ) ) ;
#96098=CARTESIAN_POINT ( 'NONE',  ( 3.591859063236761518, 24.95696800326375353, 11.09922568453594849 ) ) ;
#96099=ORIENTED_EDGE ( 'NONE', *, *, #22498, .T. ) ;
#96100=CARTESIAN_POINT ( 'NONE',  ( 2.791683348922240793, 36.63393115100078035, 7.208316651077764092 ) ) ;
#96101=CARTESIAN_POINT ( 'NONE',  ( -4.164238869374098151, 61.59541550158063217, -3.795296366450310543 ) ) ;
#96103=CARTESIAN_POINT ( 'NONE',  ( 13.79529636645031943, 65.34541550158063217, -14.16423886937409904 ) ) ;
#96104=VERTEX_POINT ( 'NONE', #1977 ) ;
#96105=CARTESIAN_POINT ( 'NONE',  ( 7.084665262690076126, 52.02201867748816255, -10.88017736071110164 ) ) ;
#96106=CARTESIAN_POINT ( 'NONE',  ( 0.5774900079438607392, 43.48035201082151247, 5.440088680355550821 ) ) ;
#96107=CARTESIAN_POINT ( 'NONE',  ( 4.559911319644449179, 47.23035201082150536, -9.422509992056141925 ) ) ;
#96109=CARTESIAN_POINT ( 'NONE',  ( -0.8801773607111008646, 43.27201867748817676, 2.915334737309923430 ) ) ;
#96111=CARTESIAN_POINT ( 'NONE',  ( 3.591859063236761518, 29.95696800326375708, 11.09922568453594849 ) ) ;
#96114=ORIENTED_EDGE ( 'NONE', *, *, #95637, .F. ) ;
#96115=CARTESIAN_POINT ( 'NONE',  ( 17.20831665107776587, 29.13393115100078390, -7.208316651077762316 ) ) ;
#96116=ORIENTED_EDGE ( 'NONE', *, *, #27402, .T. ) ;
#96117=CARTESIAN_POINT ( 'NONE',  ( 2.791683348922237240, 60.38393115100078745, -7.208316651077763204 ) ) ;
#96119=( GEOMETRIC_REPRESENTATION_CONTEXT ( 3 ) GLOBAL_UNCERTAINTY_ASSIGNED_CONTEXT ( ( #71344 ) ) GLOBAL_UNIT_ASSIGNED_CONTEXT ( ( #38409, #33337, #40868 ) ) REPRESENTATION_CONTEXT ( 'NONE', 'WORKASPACE' ) );
#96122=ORIENTED_EDGE ( 'NONE', *, *, #83073, .T. ) ;
#96123=ADVANCED_FACE ( 'NONE', ( #40950 ), #91969, .F. ) ;
#96125=CARTESIAN_POINT ( 'NONE',  ( 7.361572987183170547, 67.05059781766746596, 9.846743663894590881 ) ) ;
#96126=CARTESIAN_POINT ( 'NONE',  ( 17.20831665107776587, 37.88393115100078745, 7.208316651077764980 ) ) ;
#96127=CARTESIAN_POINT ( 'NONE',  ( -4.164238869374099927, 57.01208216824731068, 3.795296366450308767 ) ) ;
#96128=DIRECTION ( 'NONE',  ( -1.000000000000000000, -0.000000000000000000, -0.000000000000000000 ) ) ;
#96131=CARTESIAN_POINT ( 'NONE',  ( 12.63842701281683922, 34.55059781766745886, -9.846743663894590881 ) ) ;
#96132=CARTESIAN_POINT ( 'NONE',  ( 10.00000000000000000, 62.87363466993042493, -12.81628187352647608 ) ) ;
#96133=CARTESIAN_POINT ( 'NONE',  ( 0.6178305044545838731, 4.748634669930420493, 9.382169495545420901 ) ) ;
#96134=CARTESIAN_POINT ( 'NONE',  ( 14.92337183194729988, 4.342264484334117824, -8.527530157486177487 ) ) ;
#96136=CARTESIAN_POINT ( 'NONE',  ( 1.472469842513823179, 5.592264484334118713, -4.923371831947296329 ) ) ;
#96137=CARTESIAN_POINT ( 'NONE',  ( 19.84674366389459621, 53.50893115100078745, 7.409399052514197653E-17 ) ) ;
#96138=CARTESIAN_POINT ( 'NONE',  ( 19.42250999205614548, 20.98035201082150891, -5.440088680355545492 ) ) ;
#96140=CARTESIAN_POINT ( 'NONE',  ( 15.44008868035555260, 14.73035201082150536, 9.422509992056143702 ) ) ;
#96141=CARTESIAN_POINT ( 'NONE',  ( 6.204703633549690345, 0.7620821682473009062, -14.16423886937410259 ) ) ;
#96142=CARTESIAN_POINT ( 'NONE',  ( 19.84674366389459266, 8.717264484334116048, -2.638427012816827677 ) ) ;
#96143=CARTESIAN_POINT ( 'NONE',  ( 17.96484262340118221, 59.93868534415484106, 7.964842623401181321 ) ) ;
#96144=CARTESIAN_POINT ( 'NONE',  ( 22.81628187352647785, 21.62363466993041783, 6.195893100308588602E-16 ) ) ;
#96147=B_SPLINE_CURVE_WITH_KNOTS ( 'NONE', 3,
 ( #89293, #79330, #80807, #95818, #10840, #73296 ),
 .UNSPECIFIED., .F., .F.,
 ( 4, 2, 4 ),
 ( 0.000000000000000000, 0.0002565770811490924574, 0.0005131541622981849148 ),
 .UNSPECIFIED. ) ;
#96148=CARTESIAN_POINT ( 'NONE',  ( -1.926860441876562247, 57.45379003517447813, -3.195792623639530650 ) ) ;
#96149=CARTESIAN_POINT ( 'NONE',  ( 18.72515096720578853, 60.05509018479938277, 6.499999999999877431 ) ) ;
#96150=CARTESIAN_POINT ( 'NONE',  ( 1.472469842513823179, 66.42559781766745175, 4.923371831947296329 ) ) ;
#96151=CARTESIAN_POINT ( 'NONE',  ( 0.1532563361054082862, 11.21726448433411605, 2.638427012816831674 ) ) ;
#96153=CARTESIAN_POINT ( 'NONE',  ( -2.816281873526471635, 23.91530133659708568, -3.434112377981056508 ) ) ;
#96154=PLANE ( 'NONE',  #35654 ) ;
#96155=CARTESIAN_POINT ( 'NONE',  ( 20.88017736071110519, 30.56368534415484106, 2.639326808657452039E-16 ) ) ;
#96157=CARTESIAN_POINT ( 'NONE',  ( 10.00000000000000000, 45.55374883491397497, -14.16423886937410082 ) ) ;
#96159=CARTESIAN_POINT ( 'NONE',  ( 10.00000000000000178, 45.37363466993041783, 12.81628187352647608 ) ) ;
#96160=CARTESIAN_POINT ( 'NONE',  ( -0.8801773607111008646, 33.27201867748817676, 2.915334737309923430 ) ) ;
#96162=CARTESIAN_POINT ( 'NONE',  ( 1.472469842513823179, 56.42559781766745886, 4.923371831947296329 ) ) ;
#96163=CARTESIAN_POINT ( 'NONE',  ( 15.44008868035555260, 59.73035201082151247, 9.422509992056143702 ) ) ;
#96164=CARTESIAN_POINT ( 'NONE',  ( -0.3689425029237898834, 31.17874883491396787, -10.36894250292378850 ) ) ;
#96166=CARTESIAN_POINT ( 'NONE',  ( 14.92337183194729633, 32.67559781766745175, 8.527530157486181039 ) ) ;
#96167=CARTESIAN_POINT ( 'NONE',  ( 10.00000000000000178, 60.37363466993041783, 12.81628187352647608 ) ) ;
#96168=CARTESIAN_POINT ( 'NONE',  ( 3.591859063236761518, -0.04303199673624671928, 11.09922568453594849 ) ) ;
#96170=CARTESIAN_POINT ( 'NONE',  ( 15.44008868035555793, 21.39701867748817321, -9.422509992056140149 ) ) ;
#96173=CARTESIAN_POINT ( 'NONE',  ( 20.88017736071110164, 20.35535201082150891, 2.915334737309930979 ) ) ;
#96174=CARTESIAN_POINT ( 'NONE',  ( -0.3689425029237881626, 27.42874883491397142, 10.36894250292379027 ) ) ;
#96175=CARTESIAN_POINT ( 'NONE',  ( 12.63842701281683034, 12.46726448433411782, 9.846743663894596210 ) ) ;
#96176=CARTESIAN_POINT ( 'NONE',  ( 19.84674366389459266, 58.71726448433411605, -2.638427012816827677 ) ) ;
#96177=CARTESIAN_POINT ( 'NONE',  ( 7.084665262690076126, 27.02201867748817676, -10.88017736071110164 ) ) ;
#96184=CARTESIAN_POINT ( 'NONE',  ( 0.1532563361054100626, 50.80059781766745175, -2.638427012816831230 ) ) ;
#96185=VERTEX_POINT ( 'NONE', #10443 ) ;
#96188=CARTESIAN_POINT ( 'NONE',  ( 2.917880565312948704, 12.63708216824730179, 12.26659068614894643 ) ) ;
#96189=CARTESIAN_POINT ( 'NONE',  ( 13.79529636645030344, 8.262082168247300018, 14.16423886937410614 ) ) ;
#96190=CARTESIAN_POINT ( 'NONE',  ( 12.91533473730993009, 51.60535201082149825, -10.88017736071109987 ) ) ;
#96191=CARTESIAN_POINT ( 'NONE',  ( -4.164238869374099039, 56.80374883491397497, 8.674139862899312516E-16 ) ) ;
#96192=CARTESIAN_POINT ( 'NONE',  ( 7.361572987183170547, 32.05059781766745175, 9.846743663894590881 ) ) ;
#96194=CARTESIAN_POINT ( 'NONE',  ( 2.035157376598824452, 33.68868534415484106, 7.964842623401179544 ) ) ;
#96195=CARTESIAN_POINT ( 'NONE',  ( 6.565887622018943937, 8.081968003263751754, -12.81628187352647608 ) ) ;
#96196=SURFACE_STYLE_USAGE ( .BOTH. , #33692 ) ;
#96198=CARTESIAN_POINT ( 'NONE',  ( -2.266590686148945544, 52.22041550158064638, 7.082119434687048631 ) ) ;
#96199=VECTOR ( 'NONE', #71277, 1000.000000000000114 ) ;
#96200=CARTESIAN_POINT ( 'NONE',  ( 10.00000000000000178, 24.31368534415484106, 10.88017736071110342 ) ) ;
#96202=LINE ( 'NONE', #27685, #2862 ) ;
#96210=CARTESIAN_POINT ( 'NONE',  ( -0.3689425029237881626, 52.42874883491396076, 10.36894250292379027 ) ) ;
#96211=CARTESIAN_POINT ( 'NONE',  ( 19.84674366389459621, 43.50893115100078745, 7.409399052514197653E-17 ) ) ;
#96212=CARTESIAN_POINT ( 'NONE',  ( 15.44008868035555260, 59.73035201082151247, 9.422509992056143702 ) ) ;
#96215=CARTESIAN_POINT ( 'NONE',  ( 20.88017736071110164, 50.35535201082151247, 2.915334737309930979 ) ) ;
#96217=CARTESIAN_POINT ( 'NONE',  ( 21.09922568453595559, 57.04030133659708923, -6.408140936763230044 ) ) ;
#96219=VERTEX_POINT ( 'NONE', #86925 ) ;
#96220=CARTESIAN_POINT ( 'NONE',  ( 12.91533473730992121, 49.52201867748817676, 10.88017736071110164 ) ) ;
#96221=CARTESIAN_POINT ( 'NONE',  ( -4.164238869374099927, 17.01208216824730357, 3.795296366450308767 ) ) ;
#96223=CARTESIAN_POINT ( 'NONE',  ( -2.816281873526473856, 19.12363466993042138, 9.499525473075851096E-16 ) ) ;
#96224=EDGE_LOOP ( 'NONE', ( #31760, #55938, #4399, #12959, #68917 ) ) ;
#96226=CARTESIAN_POINT ( 'NONE',  ( 0.6178305044545838731, 44.74863466993042493, 9.382169495545420901 ) ) ;
#96227=CARTESIAN_POINT ( 'NONE',  ( 15.44008868035555793, 21.39701867748817321, -9.422509992056140149 ) ) ;
#96228=CARTESIAN_POINT ( 'NONE',  ( 10.00000000000000178, 42.25893115100078745, 9.846743663894594434 ) ) ;
#96229=CARTESIAN_POINT ( 'NONE',  ( 12.91533473730992121, 9.522018677488171434, 10.88017736071110164 ) ) ;
#96230=CARTESIAN_POINT ( 'NONE',  ( 3.591859063236763294, 48.29030133659708923, -11.09922568453595026 ) ) ;
#96232=CARTESIAN_POINT ( 'NONE',  ( 19.84674366389459266, 48.30059781766745175, 2.638427012816836559 ) ) ;
#96233=CARTESIAN_POINT ( 'NONE',  ( -0.8801773607111009756, 68.06368534415484817, 1.068504757029289695E-15 ) ) ;
#96237=CARTESIAN_POINT ( 'NONE',  ( 20.15039907845753930, 69.92552686551195507, 6.262539305110068177 ) ) ;
#96239=CARTESIAN_POINT ( 'NONE',  ( 10.00000000000000178, 12.25893115100078568, 9.846743663894594434 ) ) ;
#96240=CARTESIAN_POINT ( 'NONE',  ( 19.38216949554541202, 20.99863466993042138, 9.382169495545424454 ) ) ;
#96243=CARTESIAN_POINT ( 'NONE',  ( 12.63842701281683034, 52.46726448433413026, 9.846743663894596210 ) ) ;
#96245=CARTESIAN_POINT ( 'NONE',  ( 17.08211943468705840, 20.13708216824730357, -12.26659068614894466 ) ) ;
#96246=CARTESIAN_POINT ( 'NONE',  ( 17.20831665107776587, 27.88393115100078390, 7.208316651077764980 ) ) ;
#96247=CARTESIAN_POINT ( 'NONE',  ( 22.81628187352647785, 41.41530133659708923, 3.434112377981063169 ) ) ;
#96250=CARTESIAN_POINT ( 'NONE',  ( -0.8801773607111009756, 58.06368534415484106, 1.068504757029289695E-15 ) ) ;
#96251=CARTESIAN_POINT ( 'NONE',  ( 0.6178305044545838731, 14.74863466993041783, 9.382169495545420901 ) ) ;
#96253=CARTESIAN_POINT ( 'NONE',  ( 19.84674366389459621, 28.50893115100078745, 7.409399052514197653E-17 ) ) ;
#96254=CARTESIAN_POINT ( 'NONE',  ( 2.035157376598822676, 37.43868534415484106, -7.964842623401177768 ) ) ;
#96256=CARTESIAN_POINT ( 'NONE',  ( 13.43411237798105340, 40.58196800326375353, 12.81628187352647963 ) ) ;
#96257=AXIS2_PLACEMENT_3D ( 'NONE', #13606, #81110, #75090 ) ;
#96258=CARTESIAN_POINT ( 'NONE',  ( 7.361572987183170547, 37.05059781766744464, 9.846743663894590881 ) ) ;
#96260=CARTESIAN_POINT ( 'NONE',  ( -0.8801773607111009756, 38.06368534415484106, 1.068504757029289695E-15 ) ) ;
#96266=CARTESIAN_POINT ( 'NONE',  ( 20.88017736071110519, 5.563685344154837509, 2.639326808657452039E-16 ) ) ;
#96267=CARTESIAN_POINT ( 'NONE',  ( 17.20831665107776587, 57.88393115100078745, 7.208316651077764980 ) ) ;
#96268=CARTESIAN_POINT ( 'NONE',  ( 20.88017736071110164, 35.35535201082150536, 2.915334737309930979 ) ) ;
#96270=STYLED_ITEM ( 'NONE', ( #64342 ), #92159 ) ;
#96271=CARTESIAN_POINT ( 'NONE',  ( -0.8801773607111008646, 63.27201867748817676, 2.915334737309923430 ) ) ;
#96272=CARTESIAN_POINT ( 'NONE',  ( 12.91533473730993009, 21.60535201082150536, -10.88017736071109987 ) ) ;
#96273=CARTESIAN_POINT ( 'NONE',  ( 1.472469842513823179, 21.42559781766745175, 4.923371831947296329 ) ) ;
#96276=CARTESIAN_POINT ( 'NONE',  ( 2.791683348922237240, 50.38393115100078035, -7.208316651077763204 ) ) ;
#96277=CARTESIAN_POINT ( 'NONE',  ( 2.917880565312948704, 47.63708216824730357, 12.26659068614894643 ) ) ;
#96278=CARTESIAN_POINT ( 'NONE',  ( 10.00000000000000178, 3.053748834913967425, 14.16423886937410082 ) ) ;
#96279=CARTESIAN_POINT ( 'NONE',  ( -2.266590686148945544, 32.22041550158063927, 7.082119434687048631 ) ) ;
#96280=CARTESIAN_POINT ( 'NONE',  ( 6.565887622018943937, 3.081968003263753531, -12.81628187352647608 ) ) ;
#96282=CARTESIAN_POINT ( 'NONE',  ( 17.96484262340118221, 9.938685344154839285, 7.964842623401181321 ) ) ;
#96283=CARTESIAN_POINT ( 'NONE',  ( 10.00000000000000000, 39.75893115100078745, -9.846743663894594434 ) ) ;
#96284=PRESENTATION_STYLE_ASSIGNMENT (( #89745 ) ) ;
#96286=CARTESIAN_POINT ( 'NONE',  ( -0.8801773607111009756, 58.06368534415484106, 1.068504757029289695E-15 ) ) ;
#96288=UNCERTAINTY_MEASURE_WITH_UNIT (LENGTH_MEASURE( 1.000000000000000082E-05 ), #43868, 'distance_accuracy_value', 'NONE');
#96290=CARTESIAN_POINT ( 'NONE',  ( 6.565887622018943937, 65.16530133659709634, 12.81628187352647430 ) ) ;
#96291=CARTESIAN_POINT ( 'NONE',  ( -2.816281873526473856, 24.33196800326375353, 3.434112377981055619 ) ) ;
#96292=CARTESIAN_POINT ( 'NONE',  ( 19.84674366389459266, 33.71726448433410894, -2.638427012816827677 ) ) ;
#96294=LINE ( 'NONE', #12281, #77391 ) ;
#96296=CARTESIAN_POINT ( 'NONE',  ( 20.88017736071110875, 5.772018677488170546, -2.915334737309920765 ) ) ;
#96297=CARTESIAN_POINT ( 'NONE',  ( -0.8801773607111008646, 8.272018677488171434, 2.915334737309923430 ) ) ;
#96299=CARTESIAN_POINT ( 'NONE',  ( 13.79529636645031943, 40.34541550158063217, -14.16423886937409904 ) ) ;
#96300=CARTESIAN_POINT ( 'NONE',  ( 7.084665262690076126, 37.02201867748817676, -10.88017736071110164 ) ) ;
#96301=CARTESIAN_POINT ( 'NONE',  ( 4.559911319644449179, 57.23035201082150536, -9.422509992056141925 ) ) ;
#96304=CARTESIAN_POINT ( 'NONE',  ( 19.84674366389459266, 18.30059781766745175, 2.638427012816836559 ) ) ;
#96305=CARTESIAN_POINT ( 'NONE',  ( 1.472469842513823179, 0.5922644843341181575, -4.923371831947296329 ) ) ;
#96307=CARTESIAN_POINT ( 'NONE',  ( 14.92337183194729633, 37.67559781766745175, 8.527530157486181039 ) ) ;
#96308=CARTESIAN_POINT ( 'NONE',  ( 0.6178305044545838731, -0.2513653300695798953, 9.382169495545420901 ) ) ;
#96310=CARTESIAN_POINT ( 'NONE',  ( 7.084665262690076126, 39.10535201082150536, 10.88017736071109987 ) ) ;
#96312=UNCERTAINTY_MEASURE_WITH_UNIT (LENGTH_MEASURE( 1.000000000000000082E-05 ), #47990, 'distance_accuracy_value', 'NONE');
#96314=CARTESIAN_POINT ( 'NONE',  ( -1.099225684535947600, 43.70696800326375353, -6.408140936763238038 ) ) ;
#96316=CARTESIAN_POINT ( 'NONE',  ( 10.00000000000000000, 61.81368534415484106, -10.88017736071110342 ) ) ;
#96317=CARTESIAN_POINT ( 'NONE',  ( -2.816281873526473856, 49.33196800326374643, 3.434112377981055619 ) ) ;
#96318=CARTESIAN_POINT ( 'NONE',  ( 20.36894250292379738, 54.92874883491396076, -10.36894250292379027 ) ) ;
#96319=CARTESIAN_POINT ( 'NONE',  ( 14.92337183194729988, 34.34226448433411605, -8.527530157486177487 ) ) ;
#96321=ADVANCED_FACE ( 'NONE', ( #56439 ), #38882, .T. ) ;
#96322=CARTESIAN_POINT ( 'NONE',  ( 0.8801356535991349261, 124.4373638429518962, -4.500000000000001776 ) ) ;
#96323=CARTESIAN_POINT ( 'NONE',  ( -4.164238869374098151, 16.59541550158063927, -3.795296366450310543 ) ) ;
#96324=CARTESIAN_POINT ( 'NONE',  ( 17.08211943468705840, 35.13708216824730357, -12.26659068614894466 ) ) ;
#96325=CARTESIAN_POINT ( 'NONE',  ( 12.63842701281683922, 44.55059781766745175, -9.846743663894590881 ) ) ;
#96327=CARTESIAN_POINT ( 'NONE',  ( 4.559911319644449179, 43.89701867748816966, 9.422509992056141925 ) ) ;
#96328=CARTESIAN_POINT ( 'NONE',  ( 15.44008868035555793, 61.39701867748817676, -9.422509992056140149 ) ) ;
#96330=ORIENTED_EDGE ( 'NONE', *, *, #17682, .F. ) ;
#96331=CARTESIAN_POINT ( 'NONE',  ( 16.40814093676323893, 40.79030133659708923, 11.09922568453595026 ) ) ;
#96333=CARTESIAN_POINT ( 'NONE',  ( -0.8801773607111008646, 63.27201867748817676, 2.915334737309923430 ) ) ;
#96335=CARTESIAN_POINT ( 'NONE',  ( -0.3689425029237881626, 7.428748834913967869, 10.36894250292379027 ) ) ;
#96338=VERTEX_POINT ( 'NONE', #48920 ) ;
#96340=CARTESIAN_POINT ( 'NONE',  ( 0.5774900079438590739, 17.64701867748817321, -5.440088680355550821 ) ) ;
#96341=CARTESIAN_POINT ( 'NONE',  ( 19.42250999205614193, 60.14701867748817676, 5.440088680355555262 ) ) ;
#96343=CARTESIAN_POINT ( 'NONE',  ( -4.164238869374098151, 21.59541550158063217, -3.795296366450310543 ) ) ;
#96345=CARTESIAN_POINT ( 'NONE',  ( 19.42250999205614193, 20.14701867748817321, 5.440088680355555262 ) ) ;
#96346=CARTESIAN_POINT ( 'NONE',  ( 17.20831665107776587, 57.88393115100078745, 7.208316651077764980 ) ) ;
#96350=CARTESIAN_POINT ( 'NONE',  ( 18.52753015748617571, 58.09226448433411605, 4.923371831947298993 ) ) ;
#96353=CARTESIAN_POINT ( 'NONE',  ( 4.559911319644449179, 53.89701867748817676, 9.422509992056141925 ) ) ;
#96354=CARTESIAN_POINT ( 'NONE',  ( 7.361572987183170547, 67.05059781766746596, 9.846743663894590881 ) ) ;
#96355=CARTESIAN_POINT ( 'NONE',  ( 20.88017736071110164, 10.35535201082150714, 2.915334737309930979 ) ) ;
#96357=CARTESIAN_POINT ( 'NONE',  ( 10.00000000000000000, 66.81368534415484817, -10.88017736071110342 ) ) ;
#96358=CARTESIAN_POINT ( 'NONE',  ( 7.084665262690076126, 12.02201867748817321, -10.88017736071110164 ) ) ;
#96360=CARTESIAN_POINT ( 'NONE',  ( 3.591859063236761518, 59.95696800326375353, 11.09922568453594849 ) ) ;
#96361=CARTESIAN_POINT ( 'NONE',  ( 20.88017736071110519, 25.56368534415483751, 2.639326808657452039E-16 ) ) ;
#96363=CARTESIAN_POINT ( 'NONE',  ( 19.38216949554541202, 40.99863466993042493, 9.382169495545424454 ) ) ;
#96364=CARTESIAN_POINT ( 'NONE',  ( -0.8801773607110991993, 52.85535201082151247, -2.915334737309923874 ) ) ;
#96365=CARTESIAN_POINT ( 'NONE',  ( 5.076628168052704559, 55.17559781766745175, -8.527530157486179263 ) ) ;
#96368=CARTESIAN_POINT ( 'NONE',  ( 21.09922568453594849, 11.20696800326375531, 6.408140936763242479 ) ) ;
#96370=CARTESIAN_POINT ( 'NONE',  ( 1.472469842513823179, 46.42559781766745175, 4.923371831947296329 ) ) ;
#96371=CARTESIAN_POINT ( 'NONE',  ( 0.5774900079438607392, 23.48035201082150536, 5.440088680355550821 ) ) ;
#96372=CARTESIAN_POINT ( 'NONE',  ( 12.63842701281683922, 49.55059781766744464, -9.846743663894590881 ) ) ;
#96375=CARTESIAN_POINT ( 'NONE',  ( 1.472469842513823179, 41.42559781766745886, 4.923371831947296329 ) ) ;
#96376=CARTESIAN_POINT ( 'NONE',  ( 5.076628168052704559, 5.175597817667451750, -8.527530157486179263 ) ) ;
#96377=SURFACE_SIDE_STYLE ('',( #42868 ) ) ;
#96378=CARTESIAN_POINT ( 'NONE',  ( 19.84674366389459621, 53.50893115100078745, 7.409399052514197653E-17 ) ) ;
#96381=CARTESIAN_POINT ( 'NONE',  ( 16.40814093676323893, 40.79030133659708923, 11.09922568453595026 ) ) ;
#96382=CARTESIAN_POINT ( 'NONE',  ( 12.63842701281683034, 32.46726448433412315, 9.846743663894596210 ) ) ;
#96383=CARTESIAN_POINT ( 'NONE',  ( -0.04068437667225312249, 12.21974360917720581, -6.396802510829700417 ) ) ;
#96384=CARTESIAN_POINT ( 'NONE',  ( -4.164238869374099039, 61.80374883491397497, 8.674139862899312516E-16 ) ) ;
#96385=CARTESIAN_POINT ( 'NONE',  ( 0.1532563361054100626, 35.80059781766745175, -2.638427012816831230 ) ) ;
#96387=CARTESIAN_POINT ( 'NONE',  ( 20.00000000000000711, 79.40087001978916703, 4.500000000000000000 ) ) ;
#96388=CARTESIAN_POINT ( 'NONE',  ( -0.3689425029237898834, 51.17874883491397497, -10.36894250292378850 ) ) ;
#96389=CARTESIAN_POINT ( 'NONE',  ( 1.472469842513823179, 66.42559781766745175, 4.923371831947296329 ) ) ;
#96390=CARTESIAN_POINT ( 'NONE',  ( 10.00000000000000178, 19.31368534415484106, 10.88017736071110342 ) ) ;
#96391=CARTESIAN_POINT ( 'NONE',  ( 22.26659068614894466, 38.88708216824731068, 7.082119434687054849 ) ) ;
#96392=CARTESIAN_POINT ( 'NONE',  ( 24.16423886937410614, 49.30374883491396787, 8.672049930838204340E-16 ) ) ;
#96394=CARTESIAN_POINT ( 'NONE',  ( 18.52753015748618282, 8.925597817667451750, -4.923371831947291888 ) ) ;
#96395=CARTESIAN_POINT ( 'NONE',  ( 16.40814093676324603, 2.456968003263753531, -11.09922568453594671 ) ) ;
#96397=CARTESIAN_POINT ( 'NONE',  ( 4.559911319644449179, 47.23035201082150536, -9.422509992056141925 ) ) ;
#96398=DIRECTION ( 'NONE',  ( 0.000000000000000000, -1.000000000000000000, 0.000000000000000000 ) ) ;
#96402=ORIENTED_EDGE ( 'NONE', *, *, #3014, .T. ) ;
#96404=CARTESIAN_POINT ( 'NONE',  ( -4.164238869374099039, 41.80374883491397497, 8.674139862899312516E-16 ) ) ;
#96405=( NAMED_UNIT ( * ) SI_UNIT ( $, .STERADIAN. ) SOLID_ANGLE_UNIT ( ) );
#96408=CARTESIAN_POINT ( 'NONE',  ( 20.88017736071110875, 20.77201867748816611, -2.915334737309920765 ) ) ;
#96409=CARTESIAN_POINT ( 'NONE',  ( 0.6178305044545818747, 38.49863466993042493, -9.382169495545419124 ) ) ;
#96411=CARTESIAN_POINT ( 'NONE',  ( 13.43411237798105340, 20.58196800326374643, 12.81628187352647963 ) ) ;
#96412=CARTESIAN_POINT ( 'NONE',  ( 16.40814093676323893, 55.79030133659708923, 11.09922568453595026 ) ) ;
#96417=CARTESIAN_POINT ( 'NONE',  ( 24.16423886937410614, 24.51208216824730002, -3.795296366450302550 ) ) ;
#96418=CARTESIAN_POINT ( 'NONE',  ( 2.917880565312950480, 0.9704155015806342766, -12.26659068614894821 ) ) ;
#96420=CARTESIAN_POINT ( 'NONE',  ( -0.8801773607111008646, 28.27201867748817321, 2.915334737309923430 ) ) ;
#96423=CARTESIAN_POINT ( 'NONE',  ( 2.035157376598822676, 37.43868534415484106, -7.964842623401177768 ) ) ;
#96424=B_SPLINE_CURVE_WITH_KNOTS ( 'NONE', 3,
 ( #42850, #5357, #11853, #4861, #35337, #97347, #89332, #13835 ),
 .UNSPECIFIED., .F., .F.,
 ( 4, 2, 2, 4 ),
 ( 0.009612260643802141014, 0.01201872016511521847, 0.01442517968642829593, 0.01923809872905445084 ),
 .UNSPECIFIED. ) ;
#96425=CARTESIAN_POINT ( 'NONE',  ( 20.88017736071110519, 55.56368534415484817, 2.639326808657452039E-16 ) ) ;
#96426=CARTESIAN_POINT ( 'NONE',  ( 10.00000000000000178, 10.37363466993041961, 12.81628187352647608 ) ) ;
#96427=CARTESIAN_POINT ( 'NONE',  ( 0.9537732071275217827, 0.6838673512643470564, 6.500000000000001776 ) ) ;
#96428=CARTESIAN_POINT ( 'NONE',  ( 18.52753015748618282, 28.92559781766745175, -4.923371831947291888 ) ) ;
#96431=CARTESIAN_POINT ( 'NONE',  ( 7.084665262690076126, 39.10535201082150536, 10.88017736071109987 ) ) ;
#96433=CARTESIAN_POINT ( 'NONE',  ( 10.00000000000000000, 2.873634669930420049, -12.81628187352647608 ) ) ;
#96434=CARTESIAN_POINT ( 'NONE',  ( 15.00000000000000000, 11.50000000000000000, 6.500000000000000888 ) ) ;
#96436=CARTESIAN_POINT ( 'NONE',  ( 2.791683348922240793, 26.63393115100078745, 7.208316651077764092 ) ) ;
#96437=CARTESIAN_POINT ( 'NONE',  ( 21.09922568453594849, 46.20696800326376064, 6.408140936763242479 ) ) ;
#96438=CARTESIAN_POINT ( 'NONE',  ( 10.00000000000000178, 7.258931151000785675, 9.846743663894594434 ) ) ;
#96442=CARTESIAN_POINT ( 'NONE',  ( -0.8801773607110991993, 22.85535201082150181, -2.915334737309923874 ) ) ;
#96444=CARTESIAN_POINT ( 'NONE',  ( 6.204703633549690345, 35.76208216824729647, -14.16423886937410259 ) ) ;
#96445=CARTESIAN_POINT ( 'NONE',  ( 19.84674366389459266, 28.71726448433411960, -2.638427012816827677 ) ) ;
#96446=CARTESIAN_POINT ( 'NONE',  ( 19.42250999205614193, 15.14701867748817143, 5.440088680355555262 ) ) ;
#96447=CARTESIAN_POINT ( 'NONE',  ( 20.36894250292379382, 63.67874883491396787, 10.36894250292379205 ) ) ;
#96449=CARTESIAN_POINT ( 'NONE',  ( 10.00000000000000000, 6.813685344154838397, -10.88017736071110342 ) ) ;
#96450=CARTESIAN_POINT ( 'NONE',  ( 10.00000000000000000, 36.81368534415484106, -10.88017736071110342 ) ) ;
#96452=CARTESIAN_POINT ( 'NONE',  ( 10.00000000000000178, 44.31368534415484106, 10.88017736071110342 ) ) ;
#96454=CARTESIAN_POINT ( 'NONE',  ( 7.361572987183170547, 62.05059781766745886, 9.846743663894590881 ) ) ;
#96455=CARTESIAN_POINT ( 'NONE',  ( 10.00000000000000178, 39.31368534415484106, 10.88017736071110342 ) ) ;
#96458=CARTESIAN_POINT ( 'NONE',  ( 19.38216949554541202, 60.99863466993042493, 9.382169495545424454 ) ) ;
#96460=CARTESIAN_POINT ( 'NONE',  ( 24.16423886937409904, 39.09541550158062506, 3.795296366450317205 ) ) ;
#96461=CARTESIAN_POINT ( 'NONE',  ( 0.5774900079438607392, 48.48035201082150536, 5.440088680355550821 ) ) ;
#96463=CARTESIAN_POINT ( 'NONE',  ( 19.42250999205614548, 30.98035201082150536, -5.440088680355545492 ) ) ;
#96464=CARTESIAN_POINT ( 'NONE',  ( 7.361572987183170547, 67.05059781766746596, 9.846743663894590881 ) ) ;
#96466=CARTESIAN_POINT ( 'NONE',  ( 12.63842701281683922, 49.55059781766744464, -9.846743663894590881 ) ) ;
#96467=ORIENTED_EDGE ( 'NONE', *, *, #17867, .F. ) ;
#96468=EDGE_CURVE ( 'NONE', #62128, #68797, #75466, .T. ) ;
#96469=CARTESIAN_POINT ( 'NONE',  ( 17.20831665107776587, 27.88393115100078390, 7.208316651077764980 ) ) ;
#96471=CARTESIAN_POINT ( 'NONE',  ( 19.42250999205614193, 10.14701867748816966, 5.440088680355555262 ) ) ;
#96472=CARTESIAN_POINT ( 'NONE',  ( 1.472469842513823179, 26.42559781766745175, 4.923371831947296329 ) ) ;
#96473=CARTESIAN_POINT ( 'NONE',  ( 22.81628187352648496, 6.831968003263753531, -3.434112377981050290 ) ) ;
#96474=CARTESIAN_POINT ( 'NONE',  ( 19.42250999205614193, 55.14701867748817676, 5.440088680355555262 ) ) ;
#96475=CARTESIAN_POINT ( 'NONE',  ( 15.44008868035555260, 19.73035201082150536, 9.422509992056143702 ) ) ;
#96476=CARTESIAN_POINT ( 'NONE',  ( 6.565887622018943937, 53.08196800326374643, -12.81628187352647608 ) ) ;
#96477=CARTESIAN_POINT ( 'NONE',  ( 22.26659068614895176, 39.72041550158063217, -7.082119434687042414 ) ) ;
#96480=CARTESIAN_POINT ( 'NONE',  ( -44.76220231628991542, 105.1780506895835998, 5.381450656841352043 ) ) ;
#96481=EDGE_LOOP ( 'NONE', ( #79083, #82643, #10941, #81802, #47882, #73557 ) ) ;
#96482=CARTESIAN_POINT ( 'NONE',  ( 1.472469842513823179, 65.59226448433412315, -4.923371831947296329 ) ) ;
#96483=CARTESIAN_POINT ( 'NONE',  ( 2.035157376598824452, 13.68868534415483751, 7.964842623401179544 ) ) ;
#96484=CARTESIAN_POINT ( 'NONE',  ( 19.42250999205614548, 35.98035201082151247, -5.440088680355545492 ) ) ;
#96485=CARTESIAN_POINT ( 'NONE',  ( 10.00000000000000178, 57.25893115100078745, 9.846743663894594434 ) ) ;
#96488=CARTESIAN_POINT ( 'NONE',  ( 0.1532563361054083140, 21.00893115100078745, 1.131784320476157264E-15 ) ) ;
#96489=CARTESIAN_POINT ( 'NONE',  ( 1.472469842513823179, 15.59226448433411960, -4.923371831947296329 ) ) ;
#96490=CARTESIAN_POINT ( 'NONE',  ( 10.00000000000000178, 17.25893115100078745, 9.846743663894594434 ) ) ;
#96491=CARTESIAN_POINT ( 'NONE',  ( 12.63842701281683922, 4.550597817667451750, -9.846743663894590881 ) ) ;
#96492=CARTESIAN_POINT ( 'NONE',  ( 18.52753015748617571, 3.092264484334118269, 4.923371831947298993 ) ) ;
#96494=CARTESIAN_POINT ( 'NONE',  ( 2.035157376598822676, 67.43868534415484817, -7.964842623401177768 ) ) ;
#96496=CARTESIAN_POINT ( 'NONE',  ( 18.52753015748617571, 3.092264484334118269, 4.923371831947298993 ) ) ;
#96497=CARTESIAN_POINT ( 'NONE',  ( 18.52753015748618282, 18.92559781766745175, -4.923371831947291888 ) ) ;
#96499=CARTESIAN_POINT ( 'NONE',  ( 18.72515096720583827, 56.07228050351029225, -6.499999999999802824 ) ) ;
#96500=CARTESIAN_POINT ( 'NONE',  ( 22.81628187352647785, 1.623634669930420271, 6.195893100308588602E-16 ) ) ;
#96503=CARTESIAN_POINT ( 'NONE',  ( 10.00000000000000178, 18.05374883491396787, 14.16423886937410082 ) ) ;
#96506=CARTESIAN_POINT ( 'NONE',  ( -2.266590686148945544, 16.38708216824730357, -7.082119434687050408 ) ) ;
#96507=CARTESIAN_POINT ( 'NONE',  ( 6.204703633549690345, 45.76208216824729647, -14.16423886937410259 ) ) ;
#96510=CARTESIAN_POINT ( 'NONE',  ( -2.266590686148945544, 6.387082168247300906, -7.082119434687050408 ) ) ;
#96512=CARTESIAN_POINT ( 'NONE',  ( 2.035157376598822676, 37.43868534415484106, -7.964842623401177768 ) ) ;
#96514=ORIENTED_EDGE ( 'NONE', *, *, #86940, .T. ) ;
#96515=CARTESIAN_POINT ( 'NONE',  ( 19.84674366389459266, 13.30059781766745353, 2.638427012816836559 ) ) ;
#96516=CARTESIAN_POINT ( 'NONE',  ( 2.035157376598822676, 62.43868534415483396, -7.964842623401177768 ) ) ;
#96517=CARTESIAN_POINT ( 'NONE',  ( 19.84674366389459266, 28.71726448433411960, -2.638427012816827677 ) ) ;
#96518=CARTESIAN_POINT ( 'NONE',  ( -0.8801773607111009756, 8.063685344154837509, 1.068504757029289695E-15 ) ) ;
#96519=CARTESIAN_POINT ( 'NONE',  ( -1.099225684535947600, 63.70696800326376774, -6.408140936763238038 ) ) ;
#96520=CARTESIAN_POINT ( 'NONE',  ( 0.1532563361054083140, 56.00893115100078745, 1.131784320476157264E-15 ) ) ;
#96523=CARTESIAN_POINT ( 'NONE',  ( 19.38216949554541202, 35.99863466993041072, 9.382169495545424454 ) ) ;
#96525=CARTESIAN_POINT ( 'NONE',  ( 19.84674366389459266, 33.71726448433410894, -2.638427012816827677 ) ) ;
#96526=CARTESIAN_POINT ( 'NONE',  ( -0.3689425029237898834, 31.17874883491396787, -10.36894250292378850 ) ) ;
#96529=CARTESIAN_POINT ( 'NONE',  ( 20.88017736071110164, 45.35535201082149115, 2.915334737309930979 ) ) ;
#96530=CARTESIAN_POINT ( 'NONE',  ( 10.00000000000000000, 61.81368534415484106, -10.88017736071110342 ) ) ;
#96531=CARTESIAN_POINT ( 'NONE',  ( 2.917880565312948704, 42.63708216824729647, 12.26659068614894643 ) ) ;
#96532=CARTESIAN_POINT ( 'NONE',  ( 18.52753015748618282, 63.92559781766745886, -4.923371831947291888 ) ) ;
#96533=CARTESIAN_POINT ( 'NONE',  ( 21.09922568453595559, 62.04030133659709634, -6.408140936763230044 ) ) ;
#96534=CARTESIAN_POINT ( 'NONE',  ( -0.8801773607110991993, 42.85535201082150536, -2.915334737309923874 ) ) ;
#96536=CARTESIAN_POINT ( 'NONE',  ( -1.099225684535947600, 28.70696800326375353, -6.408140936763238038 ) ) ;
#96537=CARTESIAN_POINT ( 'NONE',  ( 2.791683348922240793, 51.63393115100078745, 7.208316651077764092 ) ) ;
#96539=CARTESIAN_POINT ( 'NONE',  ( 19.42250999205614193, 5.147018677488171434, 5.440088680355555262 ) ) ;
#96540=ORIENTED_EDGE ( 'NONE', *, *, #98121, .T. ) ;
#96541=FILL_AREA_STYLE_COLOUR ( '', #16250 ) ;
#96542=CARTESIAN_POINT ( 'NONE',  ( 20.15039907845753575, 65.60158574516643171, -6.262539305110073506 ) ) ;
#96543=CARTESIAN_POINT ( 'NONE',  ( 2.035157376598824452, 68.68868534415484817, 7.964842623401179544 ) ) ;
#96544=CARTESIAN_POINT ( 'NONE',  ( 15.44008868035555260, 64.73035201082151957, 9.422509992056143702 ) ) ;
#96547=VECTOR ( 'NONE', #77407, 1000.000000000000000 ) ;
#96548=CARTESIAN_POINT ( 'NONE',  ( 5.076628168052704559, 35.17559781766745175, -8.527530157486179263 ) ) ;
#96549=CARTESIAN_POINT ( 'NONE',  ( 10.00000000000000178, 19.31368534415484106, 10.88017736071110342 ) ) ;
#96551=CARTESIAN_POINT ( 'NONE',  ( -1.099225684535947600, 3.706968003263753531, -6.408140936763238038 ) ) ;
#96552=CARTESIAN_POINT ( 'NONE',  ( 20.88017736071110164, 30.35535201082151247, 2.915334737309930979 ) ) ;
#96555=CARTESIAN_POINT ( 'NONE',  ( -2.816281873526473856, 39.12363466993041783, 9.499525473075851096E-16 ) ) ;
#96557=CARTESIAN_POINT ( 'NONE',  ( 19.42250999205614548, 65.98035201082151957, -5.440088680355545492 ) ) ;
#96559=CARTESIAN_POINT ( 'NONE',  ( 13.43411237798105340, 15.58196800326374998, 12.81628187352647963 ) ) ;
#96561=CARTESIAN_POINT ( 'NONE',  ( 19.42250999205614548, 35.98035201082151247, -5.440088680355545492 ) ) ;
#96562=CARTESIAN_POINT ( 'NONE',  ( 19.84674366389459266, 63.30059781766745886, 2.638427012816836559 ) ) ;
#96563=CARTESIAN_POINT ( 'NONE',  ( 22.26659068614894466, 63.88708216824730357, 7.082119434687054849 ) ) ;
#96564=CARTESIAN_POINT ( 'NONE',  ( 18.52753015748617571, 48.09226448433412315, 4.923371831947298993 ) ) ;
#96565=CARTESIAN_POINT ( 'NONE',  ( 7.361572987183170547, 7.050597817667451750, 9.846743663894590881 ) ) ;
#96566=CARTESIAN_POINT ( 'NONE',  ( -0.8801773607110991993, 67.85535201082151957, -2.915334737309923874 ) ) ;
#96568=CARTESIAN_POINT ( 'NONE',  ( 24.16423886937410614, 24.30374883491396787, 8.672049930838204340E-16 ) ) ;
#96571=CARTESIAN_POINT ( 'NONE',  ( 2.917880565312948704, 62.63708216824730357, 12.26659068614894643 ) ) ;
#96572=CARTESIAN_POINT ( 'NONE',  ( -2.266590686148945544, 46.38708216824730357, -7.082119434687050408 ) ) ;
#96573=CARTESIAN_POINT ( 'NONE',  ( 14.92337183194729633, 27.67559781766745530, 8.527530157486181039 ) ) ;
#96574=AXIS2_PLACEMENT_3D ( 'NONE', #61828, #37878, #46828 ) ;
#96575=CARTESIAN_POINT ( 'NONE',  ( 6.565887622018943937, 25.16530133659708213, 12.81628187352647430 ) ) ;
#96577=FILL_AREA_STYLE ('',( #67048 ) ) ;
#96578=CARTESIAN_POINT ( 'NONE',  ( 0.5774900079438607392, 13.48035201082150358, 5.440088680355550821 ) ) ;
#96579=CARTESIAN_POINT ( 'NONE',  ( 13.79529636645030344, 63.26208216824730357, 14.16423886937410614 ) ) ;
#96582=CARTESIAN_POINT ( 'NONE',  ( 2.791683348922237240, 5.383931151000785675, -7.208316651077763204 ) ) ;
#96583=EDGE_CURVE ( 'NONE', #94075, #31231, #81963, .T. ) ;
#96584=CARTESIAN_POINT ( 'NONE',  ( 18.04007052943773104, 3.015283700948082402, 5.767676674365838529 ) ) ;
#96591=CARTESIAN_POINT ( 'NONE',  ( 2.035157376598822676, 22.43868534415483396, -7.964842623401177768 ) ) ;
#96592=CARTESIAN_POINT ( 'NONE',  ( 12.91533473730992121, 29.52201867748817321, 10.88017736071110164 ) ) ;
#96593=CARTESIAN_POINT ( 'NONE',  ( 1.472469842513823179, 55.59226448433412315, -4.923371831947296329 ) ) ;
#96594=CARTESIAN_POINT ( 'NONE',  ( 22.81628187352647785, 21.41530133659708923, 3.434112377981063169 ) ) ;
#96595=DIRECTION ( 'NONE',  ( -0.5547001962252291474, -0.8320502943378437211, -0.000000000000000000 ) ) ;
#96597=CARTESIAN_POINT ( 'NONE',  ( 19.38216949554541202, 35.99863466993041072, 9.382169495545424454 ) ) ;
#96598=CARTESIAN_POINT ( 'NONE',  ( 0.1532563361054083140, 1.008931151000784787, 1.131784320476157264E-15 ) ) ;
#96600=CARTESIAN_POINT ( 'NONE',  ( 0.1532563361054100626, 25.80059781766744820, -2.638427012816831230 ) ) ;
#96601=CARTESIAN_POINT ( 'NONE',  ( 17.08211943468705840, 65.13708216824730357, -12.26659068614894466 ) ) ;
#96602=EDGE_LOOP ( 'NONE', ( #36441, #4720, #82311, #37423 ) ) ;
#96603=CARTESIAN_POINT ( 'NONE',  ( 17.08211943468705840, 65.13708216824730357, -12.26659068614894466 ) ) ;
#96605=CARTESIAN_POINT ( 'NONE',  ( 2.035157376598824452, 43.68868534415484106, 7.964842623401179544 ) ) ;
#96606=CARTESIAN_POINT ( 'NONE',  ( 7.084665262690076126, 47.02201867748818387, -10.88017736071110164 ) ) ;
#96607=CARTESIAN_POINT ( 'NONE',  ( 2.035157376598824452, 48.68868534415483396, 7.964842623401179544 ) ) ;
#96609=CARTESIAN_POINT ( 'NONE',  ( 12.91533473730993009, 46.60535201082150536, -10.88017736071109987 ) ) ;
#96610=CARTESIAN_POINT ( 'NONE',  ( 20.15039907845753575, 65.60158574516643171, -6.262539305110073506 ) ) ;
#96614=CARTESIAN_POINT ( 'NONE',  ( 17.20831665107776587, 32.88393115100078745, 7.208316651077764980 ) ) ;
#96616=CARTESIAN_POINT ( 'NONE',  ( 12.63842701281683922, 64.55059781766745175, -9.846743663894590881 ) ) ;
#96618=FILL_AREA_STYLE_COLOUR ( '', #68361 ) ;
#96623=CARTESIAN_POINT ( 'NONE',  ( 18.52753015748617571, 38.09226448433412315, 4.923371831947298993 ) ) ;
#96624=CARTESIAN_POINT ( 'NONE',  ( -2.266590686148945544, 62.22041550158063927, 7.082119434687048631 ) ) ;
#96625=CARTESIAN_POINT ( 'NONE',  ( 18.17829156368510723, 64.16792564121900000, 6.499999999999953815 ) ) ;
#96626=VERTEX_POINT ( 'NONE', #15868 ) ;
#96628=CARTESIAN_POINT ( 'NONE',  ( 1.472469842513823179, 31.42559781766745530, 4.923371831947296329 ) ) ;
#96630=CARTESIAN_POINT ( 'NONE',  ( 0.6178305044545818747, 8.498634669930421381, -9.382169495545419124 ) ) ;
#96631=CARTESIAN_POINT ( 'NONE',  ( 7.361572987183169658, 4.967264484334119601, -9.846743663894592657 ) ) ;
#96633=LINE ( 'NONE', #46084, #85706 ) ;
#96634=CARTESIAN_POINT ( 'NONE',  ( 7.361572987183170547, 7.050597817667451750, 9.846743663894590881 ) ) ;
#96635=CARTESIAN_POINT ( 'NONE',  ( 0.6178305044545818747, 3.498634669930420049, -9.382169495545419124 ) ) ;
#96639=CARTESIAN_POINT ( 'NONE',  ( 17.96484262340118221, 11.18868534415484106, -7.964842623401177768 ) ) ;
#96640=CARTESIAN_POINT ( 'NONE',  ( 13.79529636645030344, 3.262082168247301350, 14.16423886937410614 ) ) ;
#96641=CARTESIAN_POINT ( 'NONE',  ( 2.791683348922237240, 25.38393115100078390, -7.208316651077763204 ) ) ;
#96642=CARTESIAN_POINT ( 'NONE',  ( 4.559911319644449179, 52.23035201082151247, -9.422509992056141925 ) ) ;
#96643=CARTESIAN_POINT ( 'NONE',  ( 3.591859063236761518, 29.95696800326375708, 11.09922568453594849 ) ) ;
#96645=CARTESIAN_POINT ( 'NONE',  ( 20.88017736071110875, 5.772018677488170546, -2.915334737309920765 ) ) ;
#96648=CARTESIAN_POINT ( 'NONE',  ( 0.6178305044545838731, 4.748634669930420493, 9.382169495545420901 ) ) ;
#96649=CARTESIAN_POINT ( 'NONE',  ( 2.791683348922237240, 60.38393115100078745, -7.208316651077763204 ) ) ;
#96650=CARTESIAN_POINT ( 'NONE',  ( 14.92337183194729633, 12.67559781766745353, 8.527530157486181039 ) ) ;
#96652=CARTESIAN_POINT ( 'NONE',  ( 13.43411237798105340, 25.58196800326374998, 12.81628187352647963 ) ) ;
#96653=CARTESIAN_POINT ( 'NONE',  ( 1.492507162822262590, 52.19955587570481725, -6.500000000000077272 ) ) ;
#96654=CARTESIAN_POINT ( 'NONE',  ( 2.035157376598822676, 27.43868534415483396, -7.964842623401177768 ) ) ;
#96657=CARTESIAN_POINT ( 'NONE',  ( 24.16423886937410614, 54.51208216824730357, -3.795296366450302550 ) ) ;
#96659=CARTESIAN_POINT ( 'NONE',  ( 17.96484262340118221, 24.93868534415484461, 7.964842623401181321 ) ) ;
#96660=CARTESIAN_POINT ( 'NONE',  ( 2.791683348922240793, 51.63393115100078745, 7.208316651077764092 ) ) ;
#96662=CARTESIAN_POINT ( 'NONE',  ( 15.44008868035555793, 51.39701867748816966, -9.422509992056140149 ) ) ;
#96664=CARTESIAN_POINT ( 'NONE',  ( 2.917880565312948704, 32.63708216824730357, 12.26659068614894643 ) ) ;
#96667=CARTESIAN_POINT ( 'NONE',  ( 14.92337183194729633, 42.67559781766745886, 8.527530157486181039 ) ) ;
#96668=CARTESIAN_POINT ( 'NONE',  ( -1.099225684535947600, 58.70696800326375353, -6.408140936763238038 ) ) ;
#96669=CARTESIAN_POINT ( 'NONE',  ( 21.09922568453595559, 2.040301336597086568, -6.408140936763230044 ) ) ;
#96671=CARTESIAN_POINT ( 'NONE',  ( 12.91533473730992121, 24.52201867748816966, 10.88017736071110164 ) ) ;
#96672=CARTESIAN_POINT ( 'NONE',  ( 19.88701968852525326, 11.79427333184086635, 6.480634945678620973 ) ) ;
#96673=CARTESIAN_POINT ( 'NONE',  ( 19.42250999205614193, 5.147018677488171434, 5.440088680355555262 ) ) ;
#96674=CARTESIAN_POINT ( 'NONE',  ( -0.8801773607111009756, 8.063685344154837509, 1.068504757029289695E-15 ) ) ;
#96675=CARTESIAN_POINT ( 'NONE',  ( 2.035157376598824452, 63.68868534415484106, 7.964842623401179544 ) ) ;
#96676=CARTESIAN_POINT ( 'NONE',  ( -0.3689425029237898834, 26.17874883491396432, -10.36894250292378850 ) ) ;
#96677=CARTESIAN_POINT ( 'NONE',  ( 5.076628168052704559, 10.17559781766745175, -8.527530157486179263 ) ) ;
#96678=CARTESIAN_POINT ( 'NONE',  ( 1.472469842513823179, 60.59226448433412315, -4.923371831947296329 ) ) ;
#96679=CARTESIAN_POINT ( 'NONE',  ( 17.96484262340118221, 36.18868534415484106, -7.964842623401177768 ) ) ;
#96683=ORIENTED_EDGE ( 'NONE', *, *, #72012, .F. ) ;
#96686=CARTESIAN_POINT ( 'NONE',  ( 5.076628168052704559, 50.17559781766745886, -8.527530157486179263 ) ) ;
#96687=ORIENTED_EDGE ( 'NONE', *, *, #27413, .T. ) ;
#96689=CARTESIAN_POINT ( 'NONE',  ( -0.8801773607110990882, 62.85535201082149825, -2.915334737309924318 ) ) ;
#96690=CARTESIAN_POINT ( 'NONE',  ( -4.164238869374099039, 26.80374883491397142, 8.674139862899312516E-16 ) ) ;
#96691=CARTESIAN_POINT ( 'NONE',  ( 10.00000000000000000, 5.553748834913967869, -14.16423886937410082 ) ) ;
#96692=CARTESIAN_POINT ( 'NONE',  ( 17.96484262340118221, 66.18868534415483396, -7.964842623401177768 ) ) ;
#96693=CARTESIAN_POINT ( 'NONE',  ( 20.36894250292379738, 54.92874883491396076, -10.36894250292379027 ) ) ;
#96694=CARTESIAN_POINT ( 'NONE',  ( 2.791683348922240793, 66.63393115100079456, 7.208316651077764092 ) ) ;
#96695=CARTESIAN_POINT ( 'NONE',  ( 17.20831665107776587, 37.88393115100078745, 7.208316651077764980 ) ) ;
#96697=CARTESIAN_POINT ( 'NONE',  ( 12.91533473730993009, 31.60535201082150891, -10.88017736071109987 ) ) ;
#96698=CARTESIAN_POINT ( 'NONE',  ( 0.6178305044545838731, 4.748634669930420493, 9.382169495545420901 ) ) ;
#96699=CARTESIAN_POINT ( 'NONE',  ( 20.36894250292379738, 19.92874883491396787, -10.36894250292379027 ) ) ;
#96700=CARTESIAN_POINT ( 'NONE',  ( 24.16423886937409904, 54.09541550158063217, 3.795296366450317205 ) ) ;
#96702=CARTESIAN_POINT ( 'NONE',  ( 12.91533473730993009, 16.60535201082150891, -10.88017736071109987 ) ) ;
#96705=CARTESIAN_POINT ( 'NONE',  ( 12.91533473730993009, 41.60535201082149825, -10.88017736071109987 ) ) ;
#96710=ORIENTED_EDGE ( 'NONE', *, *, #891, .F. ) ;
#96711=CARTESIAN_POINT ( 'NONE',  ( 17.08211943468705130, 48.47041550158063927, 12.26659068614894998 ) ) ;
#96712=CARTESIAN_POINT ( 'NONE',  ( 17.20831665107776587, 47.88393115100078745, 7.208316651077764980 ) ) ;
#96713=CARTESIAN_POINT ( 'NONE',  ( 20.88017736071110875, 50.77201867748817676, -2.915334737309920765 ) ) ;
#96716=CARTESIAN_POINT ( 'NONE',  ( 17.96484262340118221, 51.18868534415483396, -7.964842623401177768 ) ) ;
#96721=CARTESIAN_POINT ( 'NONE',  ( 17.08211943468705130, 23.47041550158063572, 12.26659068614894998 ) ) ;
#96722=CARTESIAN_POINT ( 'NONE',  ( 6.565887622018943937, 25.16530133659708213, 12.81628187352647430 ) ) ;
#96724=CARTESIAN_POINT ( 'NONE',  ( -2.816281873526473856, 44.33196800326375353, 3.434112377981055619 ) ) ;
#96725=CARTESIAN_POINT ( 'NONE',  ( 20.88017736071110519, 15.56368534415483751, 2.639326808657452039E-16 ) ) ;
#96726=CARTESIAN_POINT ( 'NONE',  ( 5.076628168052704559, 35.17559781766745175, -8.527530157486179263 ) ) ;
#96727=CARTESIAN_POINT ( 'NONE',  ( 2.035157376598822676, 12.43868534415483751, -7.964842623401177768 ) ) ;
#96728=CARTESIAN_POINT ( 'NONE',  ( 10.00000000000000178, 55.37363466993042493, 12.81628187352647608 ) ) ;
#96730=CARTESIAN_POINT ( 'NONE',  ( 7.361572987183170547, 42.05059781766745886, 9.846743663894590881 ) ) ;
#96735=CARTESIAN_POINT ( 'NONE',  ( -0.03932841506543251903, 3.121614419605014401, 6.397827110478961465 ) ) ;
#96736=CARTESIAN_POINT ( 'NONE',  ( 2.603489959281582777, 31.58210964143329136, 6.499999999999995559 ) ) ;
#96739=CARTESIAN_POINT ( 'NONE',  ( 10.00000000000000000, 19.75893115100078390, -9.846743663894594434 ) ) ;
#96740=CARTESIAN_POINT ( 'NONE',  ( 16.40814093676324603, 22.45696800326375353, -11.09922568453594671 ) ) ;
#96744=CARTESIAN_POINT ( 'NONE',  ( 20.36894250292379382, 18.67874883491397142, 10.36894250292379205 ) ) ;
#96745=CARTESIAN_POINT ( 'NONE',  ( 12.63842701281683922, 49.55059781766744464, -9.846743663894590881 ) ) ;
#96746=CARTESIAN_POINT ( 'NONE',  ( -2.816281873526473856, 44.12363466993042493, 9.499525473075851096E-16 ) ) ;
#96748=CARTESIAN_POINT ( 'NONE',  ( 1.042145700049407431, 9.742161081720029259, -6.499999999999879208 ) ) ;
#96749=CARTESIAN_POINT ( 'NONE',  ( 19.42250999205614548, 65.98035201082151957, -5.440088680355545492 ) ) ;
#96751=CARTESIAN_POINT ( 'NONE',  ( 14.92337183194729633, 32.67559781766745175, 8.527530157486181039 ) ) ;
#96752=CARTESIAN_POINT ( 'NONE',  ( 12.91533473730992121, 34.52201867748817676, 10.88017736071110164 ) ) ;
#96754=CARTESIAN_POINT ( 'NONE',  ( -1.099225684535947600, 39.54030133659708923, 6.408140936763237150 ) ) ;
#96756=CARTESIAN_POINT ( 'NONE',  ( 2.791683348922240793, 31.63393115100078745, 7.208316651077764092 ) ) ;
#96760=CARTESIAN_POINT ( 'NONE',  ( 10.00000000000000178, 34.31368534415484106, 10.88017736071110342 ) ) ;
#96761=VECTOR ( 'NONE', #88923, 1000.000000000000000 ) ;
#96764=CARTESIAN_POINT ( 'NONE',  ( 20.88017736071110875, 15.77201867748817143, -2.915334737309920765 ) ) ;
#96765=CARTESIAN_POINT ( 'NONE',  ( 7.361572987183170547, 62.05059781766745886, 9.846743663894590881 ) ) ;
#96766=CARTESIAN_POINT ( 'NONE',  ( 17.96484262340118221, 41.18868534415484106, -7.964842623401177768 ) ) ;
#96768=CARTESIAN_POINT ( 'NONE',  ( 10.00000000000000178, 59.31368534415484106, 10.88017736071110342 ) ) ;
#96769=CARTESIAN_POINT ( 'NONE',  ( 20.88017736071110875, 25.77201867748816966, -2.915334737309920765 ) ) ;
#96770=CARTESIAN_POINT ( 'NONE',  ( 17.20831665107776587, 4.133931151000785675, -7.208316651077762316 ) ) ;
#96771=CARTESIAN_POINT ( 'NONE',  ( 18.52753015748617571, 18.09226448433411960, 4.923371831947298993 ) ) ;
#96774=CARTESIAN_POINT ( 'NONE',  ( 2.791683348922237240, 45.38393115100079456, -7.208316651077763204 ) ) ;
#96775=CARTESIAN_POINT ( 'NONE',  ( 20.36894250292379382, 53.67874883491397497, 10.36894250292379205 ) ) ;
#96778=CARTESIAN_POINT ( 'NONE',  ( 17.08211943468705130, 8.470415501580635720, 12.26659068614894998 ) ) ;
#96779=CARTESIAN_POINT ( 'NONE',  ( -0.3689425029237881626, 42.42874883491396787, 10.36894250292379027 ) ) ;
#96780=CARTESIAN_POINT ( 'NONE',  ( 0.6178305044545818747, -1.501365330069579951, -9.382169495545419124 ) ) ;
#96783=CARTESIAN_POINT ( 'NONE',  ( 20.88017736071110164, 10.35535201082150714, 2.915334737309930979 ) ) ;
#96784=CARTESIAN_POINT ( 'NONE',  ( 10.00000000000000000, 29.75893115100078745, -9.846743663894594434 ) ) ;
#96788=CARTESIAN_POINT ( 'NONE',  ( 18.52753015748618282, 3.925597817667451306, -4.923371831947291888 ) ) ;
#96789=CARTESIAN_POINT ( 'NONE',  ( 3.591859063236763294, 18.29030133659708568, -11.09922568453595026 ) ) ;
#96790=CARTESIAN_POINT ( 'NONE',  ( 10.00000000000000000, 24.75893115100078745, -9.846743663894594434 ) ) ;
#96793=CARTESIAN_POINT ( 'NONE',  ( 10.00000000000000000, 14.75893115100078568, -9.846743663894594434 ) ) ;
#96795=CARTESIAN_POINT ( 'NONE',  ( 20.36894250292379382, 63.67874883491396787, 10.36894250292379205 ) ) ;
#96796=CARTESIAN_POINT ( 'NONE',  ( 0.5774900079438607392, 13.48035201082150358, 5.440088680355550821 ) ) ;
#96797=CARTESIAN_POINT ( 'NONE',  ( -2.266590686148945544, 41.38708216824729647, -7.082119434687050408 ) ) ;
#96798=CARTESIAN_POINT ( 'NONE',  ( 7.084665262690076126, 47.02201867748818387, -10.88017736071110164 ) ) ;
#96799=CARTESIAN_POINT ( 'NONE',  ( 15.44008868035555793, 56.39701867748817676, -9.422509992056140149 ) ) ;
#96802=CARTESIAN_POINT ( 'NONE',  ( 18.52753015748617571, 28.09226448433411960, 4.923371831947298993 ) ) ;
#96803=SURFACE_STYLE_USAGE ( .BOTH. , #51279 ) ;
#96804=CARTESIAN_POINT ( 'NONE',  ( 7.361572987183170547, 12.05059781766744997, 9.846743663894590881 ) ) ;
#96805=CARTESIAN_POINT ( 'NONE',  ( 17.20831665107776587, 32.88393115100078745, 7.208316651077764980 ) ) ;
#96806=CARTESIAN_POINT ( 'NONE',  ( 19.84674366389459266, 63.30059781766745886, 2.638427012816836559 ) ) ;
#96809=CARTESIAN_POINT ( 'NONE',  ( 19.42250999205614193, 35.14701867748816966, 5.440088680355555262 ) ) ;
#96811=CARTESIAN_POINT ( 'NONE',  ( 22.81628187352647785, 61.62363466993041783, 6.195893100308588602E-16 ) ) ;
#96813=CARTESIAN_POINT ( 'NONE',  ( 4.559911319644449179, 63.89701867748817676, 9.422509992056141925 ) ) ;
#96814=CARTESIAN_POINT ( 'NONE',  ( 16.40814093676324603, 42.45696800326375353, -11.09922568453594671 ) ) ;
#96815=CARTESIAN_POINT ( 'NONE',  ( 2.917880565312948704, 62.63708216824730357, 12.26659068614894643 ) ) ;
#96816=CARTESIAN_POINT ( 'NONE',  ( 17.20831665107776587, 29.13393115100078390, -7.208316651077762316 ) ) ;
#96817=CARTESIAN_POINT ( 'NONE',  ( -19.92076923076924189, 82.65384615384614619, -9.500000000000000000 ) ) ;
#96818=CARTESIAN_POINT ( 'NONE',  ( 7.361572987183170547, 62.05059781766745886, 9.846743663894590881 ) ) ;
#96819=CARTESIAN_POINT ( 'NONE',  ( 2.917880565312950480, 20.97041550158063217, -12.26659068614894821 ) ) ;
#96820=CARTESIAN_POINT ( 'NONE',  ( 20.36894250292379382, 38.67874883491396076, 10.36894250292379205 ) ) ;
#96821=CARTESIAN_POINT ( 'NONE',  ( 10.00000000000000178, 42.25893115100078745, 9.846743663894594434 ) ) ;
#96822=DIRECTION ( 'NONE',  ( 0.000000000000000000, -1.000000000000000000, 0.000000000000000000 ) ) ;
#96823=CARTESIAN_POINT ( 'NONE',  ( 4.559911319644449179, 32.23035201082150536, -9.422509992056141925 ) ) ;
#96824=CARTESIAN_POINT ( 'NONE',  ( 2.035157376598822676, 62.43868534415483396, -7.964842623401177768 ) ) ;
#96825=CARTESIAN_POINT ( 'NONE',  ( -0.1082834614903535886, 0.1165887514553498872, 6.323045919668897952 ) ) ;
#96826=ORIENTED_EDGE ( 'NONE', *, *, #74961, .T. ) ;
#96827=CARTESIAN_POINT ( 'NONE',  ( 22.81628187352648496, 46.83196800326376064, -3.434112377981050290 ) ) ;
#96828=ORIENTED_EDGE ( 'NONE', *, *, #54303, .T. ) ;
#96829=CARTESIAN_POINT ( 'NONE',  ( 2.035157376598822676, 67.43868534415484817, -7.964842623401177768 ) ) ;
#96831=CARTESIAN_POINT ( 'NONE',  ( 6.204703633549690345, 7.845415501580634832, 14.16423886937410082 ) ) ;
#96832=CARTESIAN_POINT ( 'NONE',  ( 14.92337183194729633, 2.675597817667451750, 8.527530157486181039 ) ) ;
#96836=EDGE_LOOP ( 'NONE', ( #60155, #33020, #47088, #47955 ) ) ;
#96838=CARTESIAN_POINT ( 'NONE',  ( -0.8801773607110991993, 12.85535201082150358, -2.915334737309923874 ) ) ;
#96839=CARTESIAN_POINT ( 'NONE',  ( 17.39651004071841456, 9.082109641433294911, -6.500000000000003553 ) ) ;
#96840=CARTESIAN_POINT ( 'NONE',  ( -2.266590686148945544, 22.22041550158063572, 7.082119434687048631 ) ) ;
#96843=CARTESIAN_POINT ( 'NONE',  ( 4.559911319644449179, 23.89701867748817321, 9.422509992056141925 ) ) ;
#96844=CARTESIAN_POINT ( 'NONE',  ( 0.1532563361054083140, 56.00893115100078745, 1.131784320476157264E-15 ) ) ;
#96846=CARTESIAN_POINT ( 'NONE',  ( 0.1532563361054083140, 56.00893115100078745, 1.131784320476157264E-15 ) ) ;
#96848=CARTESIAN_POINT ( 'NONE',  ( 4.559911319644449179, 67.23035201082150536, -9.422509992056141925 ) ) ;
#96849=CARTESIAN_POINT ( 'NONE',  ( 7.361572987183169658, 59.96726448433410894, -9.846743663894592657 ) ) ;
#96850=CARTESIAN_POINT ( 'NONE',  ( 0.5774900079438590739, 12.64701867748817143, -5.440088680355550821 ) ) ;
#96852=CARTESIAN_POINT ( 'NONE',  ( 19.84674366389459266, 3.300597817667451750, 2.638427012816836559 ) ) ;
#96853=CARTESIAN_POINT ( 'NONE',  ( -0.8801773607110991993, 22.85535201082150181, -2.915334737309923874 ) ) ;
#96858=CARTESIAN_POINT ( 'NONE',  ( 4.559911319644449179, 38.89701867748817676, 9.422509992056141925 ) ) ;
#96860=CARTESIAN_POINT ( 'NONE',  ( 22.81628187352647785, 36.62363466993041783, 6.195893100308588602E-16 ) ) ;
#96861=CARTESIAN_POINT ( 'NONE',  ( 2.035157376598824452, 53.68868534415484817, 7.964842623401179544 ) ) ;
#96862=CARTESIAN_POINT ( 'NONE',  ( 14.92337183194729633, 57.67559781766745886, 8.527530157486181039 ) ) ;
#96864=CARTESIAN_POINT ( 'NONE',  ( 0.1955144967548773649, 49.32703681773342197, -6.500000000002692957 ) ) ;
#96865=CARTESIAN_POINT ( 'NONE',  ( 19.84674366389459266, 23.71726448433412315, -2.638427012816827677 ) ) ;
#96866=CARTESIAN_POINT ( 'NONE',  ( 13.43411237798106583, 12.66530133659708746, -12.81628187352647252 ) ) ;
#96869=CARTESIAN_POINT ( 'NONE',  ( 10.00000000000000178, 19.31368534415484106, 10.88017736071110342 ) ) ;
#96870=CARTESIAN_POINT ( 'NONE',  ( 18.52753015748618282, 53.92559781766745175, -4.923371831947291888 ) ) ;
#96873=CARTESIAN_POINT ( 'NONE',  ( 10.00000000000000178, 7.258931151000785675, 9.846743663894594434 ) ) ;
#96874=CARTESIAN_POINT ( 'NONE',  ( 18.04007052943791933, 29.00257860105346097, -5.767676674365512568 ) ) ;
#96876=CARTESIAN_POINT ( 'NONE',  ( 21.09922568453594849, 1.206968003263753531, 6.408140936763242479 ) ) ;
#96880=CARTESIAN_POINT ( 'NONE',  ( 22.81628187352647785, 36.41530133659707502, 3.434112377981063169 ) ) ;
#96881=CARTESIAN_POINT ( 'NONE',  ( 5.076628168052703671, 31.84226448433412315, 8.527530157486179263 ) ) ;
#96883=CARTESIAN_POINT ( 'NONE',  ( 22.26659068614894466, 53.88708216824731068, 7.082119434687054849 ) ) ;
#96884=EDGE_CURVE ( 'NONE', #12573, #43815, #96294, .T. ) ;
#96885=CARTESIAN_POINT ( 'NONE',  ( 17.20831665107776587, 32.88393115100078745, 7.208316651077764980 ) ) ;
#96887=FACE_OUTER_BOUND ( 'NONE', #49267, .T. ) ;
#96888=CARTESIAN_POINT ( 'NONE',  ( 7.084665262690076126, 7.022018677488170546, -10.88017736071110164 ) ) ;
#96889=DIRECTION ( 'NONE',  ( 1.000000000000000000, 0.000000000000000000, 0.000000000000000000 ) ) ;
#96890=CARTESIAN_POINT ( 'NONE',  ( -0.8801773607111009756, 13.06368534415483929, 1.068504757029289695E-15 ) ) ;
#96891=CARTESIAN_POINT ( 'NONE',  ( 20.36894250292379382, 53.67874883491397497, 10.36894250292379205 ) ) ;
#96892=CARTESIAN_POINT ( 'NONE',  ( -2.266590686148945544, 46.38708216824730357, -7.082119434687050408 ) ) ;
#96893=( BOUNDED_CURVE ( )  B_SPLINE_CURVE ( 2, ( #62242, #76759, #47239, #94218, #93234, #77741, #78235, #17263, #2272 ),
 .UNSPECIFIED., .F., .T. ) 
 B_SPLINE_CURVE_WITH_KNOTS ( ( 3, 2, 2, 2, 3 ),
 ( 0.5472837940830884707, 0.5476190476190476719, 0.5535714285714286031, 0.5595238095238095344, 0.5598590630597686246 ),
 .UNSPECIFIED. ) 
 CURVE ( )  GEOMETRIC_REPRESENTATION_ITEM ( )  RATIONAL_B_SPLINE_CURVE ( ( 0.9963778908391753841, 0.9980808541467917072, 1.000000000000000000, 0.9659258262890682012, 1.000000000000000000, 0.9659258262890682012, 1.000000000000000000, 0.9980808541467922623, 0.9963778908391764944 ) ) 
 REPRESENTATION_ITEM ( '' )  );
#96894=CARTESIAN_POINT ( 'NONE',  ( 10.00000000000000178, 7.258931151000785675, 9.846743663894594434 ) ) ;
#96895=CARTESIAN_POINT ( 'NONE',  ( 18.52753015748617571, 63.09226448433412315, 4.923371831947298993 ) ) ;
#96896=CARTESIAN_POINT ( 'NONE',  ( 17.96484262340118221, 44.93868534415483396, 7.964842623401181321 ) ) ;
#96898=CARTESIAN_POINT ( 'NONE',  ( 1.472469842513823179, 61.42559781766745175, 4.923371831947296329 ) ) ;
#96900=VECTOR ( 'NONE', #80268, 1000.000000000000000 ) ;
#96901=CARTESIAN_POINT ( 'NONE',  ( 1.472469842513823179, 65.59226448433412315, -4.923371831947296329 ) ) ;
#96902=CARTESIAN_POINT ( 'NONE',  ( 10.00000000000000178, 3.053748834913967425, 14.16423886937410082 ) ) ;
#96904=CARTESIAN_POINT ( 'NONE',  ( 22.26659068614894466, 33.88708216824730357, 7.082119434687054849 ) ) ;
#96907=CARTESIAN_POINT ( 'NONE',  ( 0.1532563361054100626, 0.8005978176674514168, -2.638427012816831230 ) ) ;
#96910=CARTESIAN_POINT ( 'NONE',  ( 10.00000000000000178, 39.31368534415484106, 10.88017736071110342 ) ) ;
#96911=CARTESIAN_POINT ( 'NONE',  ( 0.6178305044545838731, 44.74863466993042493, 9.382169495545420901 ) ) ;
#96912=CARTESIAN_POINT ( 'NONE',  ( 0.6178305044545818747, 28.49863466993041783, -9.382169495545419124 ) ) ;
#96913=CARTESIAN_POINT ( 'NONE',  ( 13.43411237798106583, 62.66530133659708923, -12.81628187352647252 ) ) ;
#96918=CARTESIAN_POINT ( 'NONE',  ( 13.79529636645031943, 30.34541550158063927, -14.16423886937409904 ) ) ;
#96920=CARTESIAN_POINT ( 'NONE',  ( 20.88017736071110164, 20.35535201082150891, 2.915334737309930979 ) ) ;
#96922=CARTESIAN_POINT ( 'NONE',  ( 0.5774900079438607392, 58.48035201082151247, 5.440088680355550821 ) ) ;
#96923=CARTESIAN_POINT ( 'NONE',  ( 10.00000000000000000, 51.81368534415484106, -10.88017736071110342 ) ) ;
#96924=CARTESIAN_POINT ( 'NONE',  ( 3.591859063236761518, 9.956968003263753531, 11.09922568453594849 ) ) ;
#96925=CARTESIAN_POINT ( 'NONE',  ( -0.03932841506541961962, 48.12161441960502373, 6.397827110479001433 ) ) ;
#96927=CARTESIAN_POINT ( 'NONE',  ( 5.076628168052703671, 16.84226448433411960, 8.527530157486179263 ) ) ;
#96930=CARTESIAN_POINT ( 'NONE',  ( 10.00000000000000000, 41.81368534415484106, -10.88017736071110342 ) ) ;
#96933=CARTESIAN_POINT ( 'NONE',  ( 13.43411237798105340, 5.581968003263753531, 12.81628187352647963 ) ) ;
#96934=CARTESIAN_POINT ( 'NONE',  ( 0.5774900079438607392, 43.48035201082151247, 5.440088680355550821 ) ) ;
#96935=CARTESIAN_POINT ( 'NONE',  ( 12.63842701281683922, 29.55059781766745175, -9.846743663894590881 ) ) ;
#96936=CARTESIAN_POINT ( 'NONE',  ( 21.09922568453594849, 51.20696800326375353, 6.408140936763242479 ) ) ;
#96937=CARTESIAN_POINT ( 'NONE',  ( 7.361572987183169658, 24.96726448433412315, -9.846743663894592657 ) ) ;
#96938=SURFACE_STYLE_USAGE ( .BOTH. , #43894 ) ;
#96939=ORIENTED_EDGE ( 'NONE', *, *, #79732, .T. ) ;
#96940=CARTESIAN_POINT ( 'NONE',  ( -4.164238869374099039, 1.803748834913967647, 8.674139862899312516E-16 ) ) ;
#96941=DIRECTION ( 'NONE',  ( 0.8320502943378436100, -0.5547001962252291474, 0.000000000000000000 ) ) ;
#96942=CARTESIAN_POINT ( 'NONE',  ( 4.559911319644449179, 22.23035201082150536, -9.422509992056141925 ) ) ;
#96944=CARTESIAN_POINT ( 'NONE',  ( 20.36894250292379382, 33.67874883491396076, 10.36894250292379205 ) ) ;
#96945=CARTESIAN_POINT ( 'NONE',  ( 10.00000000000000178, 32.25893115100078745, 9.846743663894594434 ) ) ;
#96946=CARTESIAN_POINT ( 'NONE',  ( 4.559911319644449179, 18.89701867748817321, 9.422509992056141925 ) ) ;
#96947=CARTESIAN_POINT ( 'NONE',  ( 24.16423886937410614, 64.30374883491396076, 8.672049930838204340E-16 ) ) ;
#96950=CARTESIAN_POINT ( 'NONE',  ( 12.91533473730993009, 21.60535201082150536, -10.88017736071109987 ) ) ;
#96951=ADVANCED_FACE ( 'NONE', ( #18812 ), #4392, .T. ) ;
#96952=CARTESIAN_POINT ( 'NONE',  ( 0.5774900079438607392, 38.48035201082150536, 5.440088680355550821 ) ) ;
#96955=CARTESIAN_POINT ( 'NONE',  ( 12.63842701281683922, 59.55059781766744464, -9.846743663894590881 ) ) ;
#96956=CARTESIAN_POINT ( 'NONE',  ( 19.42250999205614193, 40.14701867748817676, 5.440088680355555262 ) ) ;
#96959=CARTESIAN_POINT ( 'NONE',  ( 0.6178305044545838731, 64.74863466993043914, 9.382169495545420901 ) ) ;
#96961=CARTESIAN_POINT ( 'NONE',  ( -4.164238869374099927, 32.01208216824730357, 3.795296366450308767 ) ) ;
#96962=CARTESIAN_POINT ( 'NONE',  ( 2.035157376598822676, 47.43868534415484817, -7.964842623401177768 ) ) ;
#96963=B_SPLINE_CURVE_WITH_KNOTS ( 'NONE', 3,
 ( #71328, #41337, #25824, #77822, #10817, #8843 ),
 .UNSPECIFIED., .F., .F.,
 ( 4, 2, 4 ),
 ( 0.000000000000000000, 0.0002701661927229330592, 0.0005403323854458661184 ),
 .UNSPECIFIED. ) ;
#96964=CARTESIAN_POINT ( 'NONE',  ( 18.29284471827483571, 50.40189080397284016, -6.499999999999912070 ) ) ;
#96967=CARTESIAN_POINT ( 'NONE',  ( 5.076628168052703671, 51.84226448433412315, 8.527530157486179263 ) ) ;
#96968=CARTESIAN_POINT ( 'NONE',  ( 17.20831665107776587, 4.133931151000785675, -7.208316651077762316 ) ) ;
#96969=ORIENTED_EDGE ( 'NONE', *, *, #85356, .T. ) ;
#96970=CARTESIAN_POINT ( 'NONE',  ( 18.52753015748617571, 23.09226448433411960, 4.923371831947298993 ) ) ;
#96972=CARTESIAN_POINT ( 'NONE',  ( 15.44008868035555793, 31.39701867748817676, -9.422509992056140149 ) ) ;
#96973=CARTESIAN_POINT ( 'NONE',  ( 7.361572987183169658, 24.96726448433412315, -9.846743663894592657 ) ) ;
#96974=CARTESIAN_POINT ( 'NONE',  ( 2.035157376598822676, 62.43868534415483396, -7.964842623401177768 ) ) ;
#96975=CARTESIAN_POINT ( 'NONE',  ( 12.91533473730993009, 26.60535201082150536, -10.88017736071109987 ) ) ;
#96976=CARTESIAN_POINT ( 'NONE',  ( -2.816281873526471635, 58.91530133659707502, -3.434112377981056508 ) ) ;
#96977=CARTESIAN_POINT ( 'NONE',  ( 24.16423886937410614, 44.30374883491397497, 8.672049930838204340E-16 ) ) ;
#96981=VERTEX_POINT ( 'NONE', #31233 ) ;
#96982=CARTESIAN_POINT ( 'NONE',  ( 13.43411237798106583, 2.665301336597086568, -12.81628187352647252 ) ) ;
#96983=CARTESIAN_POINT ( 'NONE',  ( 15.44008868035555793, 11.39701867748817143, -9.422509992056140149 ) ) ;
#96984=CARTESIAN_POINT ( 'NONE',  ( 2.035157376598822676, 42.43868534415483396, -7.964842623401177768 ) ) ;
#96985=CARTESIAN_POINT ( 'NONE',  ( 17.20831665107776587, 57.88393115100078745, 7.208316651077764980 ) ) ;
#96987=CARTESIAN_POINT ( 'NONE',  ( 18.52753015748617571, 18.09226448433411960, 4.923371831947298993 ) ) ;
#96988=MECHANICAL_DESIGN_GEOMETRIC_PRESENTATION_REPRESENTATION('',(#85770),#53864);
#96989=CARTESIAN_POINT ( 'NONE',  ( 15.44008868035555260, 54.73035201082150536, 9.422509992056143702 ) ) ;
#96990=CARTESIAN_POINT ( 'NONE',  ( 12.63842701281683922, 34.55059781766745886, -9.846743663894590881 ) ) ;
#96991=CARTESIAN_POINT ( 'NONE',  ( 14.92337183194729633, 27.67559781766745530, 8.527530157486181039 ) ) ;
#96992=CARTESIAN_POINT ( 'NONE',  ( 2.791683348922237240, 20.38393115100078745, -7.208316651077763204 ) ) ;
#96994=CARTESIAN_POINT ( 'NONE',  ( 0.1532563361054082862, 1.217264484334117824, 2.638427012816831674 ) ) ;
#96996=CARTESIAN_POINT ( 'NONE',  ( 19.84674366389459266, 28.71726448433411960, -2.638427012816827677 ) ) ;
#96997=ORIENTED_EDGE ( 'NONE', *, *, #89523, .T. ) ;
#97001=CARTESIAN_POINT ( 'NONE',  ( 18.52753015748618282, 63.92559781766745886, -4.923371831947291888 ) ) ;
#97003=CARTESIAN_POINT ( 'NONE',  ( 2.917880565312950480, 15.97041550158063217, -12.26659068614894821 ) ) ;
#97005=CARTESIAN_POINT ( 'NONE',  ( 2.917880565312948704, 12.63708216824730179, 12.26659068614894643 ) ) ;
#97006=CARTESIAN_POINT ( 'NONE',  ( -2.266590686148945544, 51.38708216824730357, -7.082119434687050408 ) ) ;
#97007=CARTESIAN_POINT ( 'NONE',  ( -2.266590686148945544, 1.387082168247301128, -7.082119434687050408 ) ) ;
#97008=CARTESIAN_POINT ( 'NONE',  ( 20.36894250292379382, 13.67874883491396965, 10.36894250292379205 ) ) ;
#97009=CARTESIAN_POINT ( 'NONE',  ( 20.88017736071110875, 65.77201867748817676, -2.915334737309920765 ) ) ;
#97010=CARTESIAN_POINT ( 'NONE',  ( 19.42250999205614548, 45.98035201082150536, -5.440088680355545492 ) ) ;
#97012=VERTEX_POINT ( 'NONE', #77233 ) ;
#97013=CARTESIAN_POINT ( 'NONE',  ( 12.63842701281683922, 34.55059781766745886, -9.846743663894590881 ) ) ;
#97015=CARTESIAN_POINT ( 'NONE',  ( 18.52753015748618282, 23.92559781766745530, -4.923371831947291888 ) ) ;
#97016=VERTEX_POINT ( 'NONE', #39747 ) ;
#97017=CARTESIAN_POINT ( 'NONE',  ( 4.559911319644449179, 12.23035201082150714, -9.422509992056141925 ) ) ;
#97018=CARTESIAN_POINT ( 'NONE',  ( 0.6178305044545838731, 54.74863466993042493, 9.382169495545420901 ) ) ;
#97019=CARTESIAN_POINT ( 'NONE',  ( 2.791683348922237240, 50.38393115100078035, -7.208316651077763204 ) ) ;
#97021=CARTESIAN_POINT ( 'NONE',  ( 17.20831665107776587, 32.88393115100078745, 7.208316651077764980 ) ) ;
#97022=CARTESIAN_POINT ( 'NONE',  ( 10.00000000000000000, 42.87363466993042493, -12.81628187352647608 ) ) ;
#97024=CARTESIAN_POINT ( 'NONE',  ( 4.559911319644449179, 43.89701867748816966, 9.422509992056141925 ) ) ;
#97025=CARTESIAN_POINT ( 'NONE',  ( 14.92337183194729633, 37.67559781766745175, 8.527530157486181039 ) ) ;
#97026=CARTESIAN_POINT ( 'NONE',  ( 24.16423886937409904, 24.09541550158063927, 3.795296366450317205 ) ) ;
#97028=CARTESIAN_POINT ( 'NONE',  ( 22.26659068614895176, 4.720415501580633943, -7.082119434687042414 ) ) ;
#97030=CARTESIAN_POINT ( 'NONE',  ( 12.91533473730992121, 49.52201867748817676, 10.88017736071110164 ) ) ;
#97031=CARTESIAN_POINT ( 'NONE',  ( 12.91533473730992121, 64.52201867748817676, 10.88017736071110164 ) ) ;
#97032=CARTESIAN_POINT ( 'NONE',  ( -4.164238869374099927, 47.01208216824729647, 3.795296366450308767 ) ) ;
#97033=CARTESIAN_POINT ( 'NONE',  ( -2.816281873526473856, 4.123634669930420493, 9.499525473075851096E-16 ) ) ;
#97035=CARTESIAN_POINT ( 'NONE',  ( 20.88017736071110519, 60.56368534415484106, 2.639326808657452039E-16 ) ) ;
#97038=CARTESIAN_POINT ( 'NONE',  ( 10.00000000000000178, 25.37363466993041783, 12.81628187352647608 ) ) ;
#97039=CARTESIAN_POINT ( 'NONE',  ( 19.84674366389459266, 63.71726448433412315, -2.638427012816827677 ) ) ;
#97041=CARTESIAN_POINT ( 'NONE',  ( 2.035157376598824452, 18.68868534415484106, 7.964842623401179544 ) ) ;
#97042=CARTESIAN_POINT ( 'NONE',  ( 12.91533473730992121, 4.522018677488170546, 10.88017736071110164 ) ) ;
#97046=DIRECTION ( 'NONE',  ( 1.000000000000000000, 4.163336342344333240E-14, 0.000000000000000000 ) ) ;
#97048=CARTESIAN_POINT ( 'NONE',  ( 19.84674366389459266, 3.300597817667451750, 2.638427012816836559 ) ) ;
#97050=CARTESIAN_POINT ( 'NONE',  ( 10.00000000000000178, 32.25893115100078745, 9.846743663894594434 ) ) ;
#97051=CARTESIAN_POINT ( 'NONE',  ( 19.42250999205614548, 40.98035201082150536, -5.440088680355545492 ) ) ;
#97052=CARTESIAN_POINT ( 'NONE',  ( 19.38216949554541202, 10.99863466993042138, 9.382169495545424454 ) ) ;
#97053=CARTESIAN_POINT ( 'NONE',  ( -0.8801773607111008646, 33.27201867748817676, 2.915334737309923430 ) ) ;
#97056=CARTESIAN_POINT ( 'NONE',  ( -1.099225684535947600, 33.70696800326375353, -6.408140936763238038 ) ) ;
#97057=ORIENTED_EDGE ( 'NONE', *, *, #32742, .F. ) ;
#97058=CARTESIAN_POINT ( 'NONE',  ( 2.035157376598822676, 67.43868534415484817, -7.964842623401177768 ) ) ;
#97059=CARTESIAN_POINT ( 'NONE',  ( 22.81628187352648496, 36.83196800326376064, -3.434112377981050290 ) ) ;
#97060=CARTESIAN_POINT ( 'NONE',  ( 13.79529636645030344, 8.262082168247300018, 14.16423886937410614 ) ) ;
#97061=CARTESIAN_POINT ( 'NONE',  ( 21.92686044187656336, 31.97997603579417358, 3.195792623639536423 ) ) ;
#97062=CARTESIAN_POINT ( 'NONE',  ( 15.44008868035555793, 36.39701867748816966, -9.422509992056140149 ) ) ;
#97063=CARTESIAN_POINT ( 'NONE',  ( 6.000000000000000000, 11.00000000000000000, 5.000000000000000000 ) ) ;
#97064=CARTESIAN_POINT ( 'NONE',  ( 13.79529636645031943, 65.34541550158063217, -14.16423886937409904 ) ) ;
#97066=CARTESIAN_POINT ( 'NONE',  ( 14.92337183194729633, 57.67559781766745886, 8.527530157486181039 ) ) ;
#97067=CARTESIAN_POINT ( 'NONE',  ( 12.63842701281683922, 14.55059781766744997, -9.846743663894590881 ) ) ;
#97068=CARTESIAN_POINT ( 'NONE',  ( 7.084665262690076126, 57.02201867748817676, -10.88017736071110164 ) ) ;
#97070=CARTESIAN_POINT ( 'NONE',  ( 24.16423886937410614, 34.51208216824731068, -3.795296366450302550 ) ) ;
#97077=CARTESIAN_POINT ( 'NONE',  ( 10.00000000000000000, 60.55374883491397497, -14.16423886937410082 ) ) ;
#97078=CARTESIAN_POINT ( 'NONE',  ( 0.5774900079438607392, 3.480352010821504916, 5.440088680355550821 ) ) ;
#97079=CARTESIAN_POINT ( 'NONE',  ( 5.076628168052703671, 26.84226448433411960, 8.527530157486179263 ) ) ;
#97080=CARTESIAN_POINT ( 'NONE',  ( -1.099225684535947600, 23.70696800326375708, -6.408140936763238038 ) ) ;
#97082=CARTESIAN_POINT ( 'NONE',  ( -0.1503990784575279516, 43.10158574516643171, 6.262539305110076171 ) ) ;
#97083=CARTESIAN_POINT ( 'NONE',  ( 2.035157376598822676, 7.438685344154837509, -7.964842623401177768 ) ) ;
#97084=CARTESIAN_POINT ( 'NONE',  ( 13.79529636645030344, 58.26208216824728936, 14.16423886937410614 ) ) ;
#97085=CARTESIAN_POINT ( 'NONE',  ( 17.20831665107776587, 32.88393115100078745, 7.208316651077764980 ) ) ;
#97087=CARTESIAN_POINT ( 'NONE',  ( 14.92337183194729633, 12.67559781766745353, 8.527530157486181039 ) ) ;
#97088=B_SPLINE_CURVE_WITH_KNOTS ( 'NONE', 3,
 ( #73438, #34449, #4964, #64941, #57459, #11962 ),
 .UNSPECIFIED., .F., .F.,
 ( 4, 2, 4 ),
 ( 0.000000000000000000, 0.0002565770811490921321, 0.0005131541622981842642 ),
 .UNSPECIFIED. ) ;
#97093=VERTEX_POINT ( 'NONE', #9237 ) ;
#97094=CARTESIAN_POINT ( 'NONE',  ( 0.1532563361054100626, 40.80059781766745886, -2.638427012816831230 ) ) ;
#97095=CARTESIAN_POINT ( 'NONE',  ( -0.3689425029237898834, 16.17874883491396076, -10.36894250292378850 ) ) ;
#97096=CARTESIAN_POINT ( 'NONE',  ( 20.88017736071110875, 20.77201867748816611, -2.915334737309920765 ) ) ;
#97097=CARTESIAN_POINT ( 'NONE',  ( 7.084665262690076126, 24.10535201082150181, 10.88017736071109987 ) ) ;
#97098=SURFACE_SIDE_STYLE ('',( #44556 ) ) ;
#97099=CARTESIAN_POINT ( 'NONE',  ( 6.565887622018943937, 18.08196800326375708, -12.81628187352647608 ) ) ;
#97100=CARTESIAN_POINT ( 'NONE',  ( 10.00000000000000000, 0.5537488349139675359, -14.16423886937410082 ) ) ;
#97102=CARTESIAN_POINT ( 'NONE',  ( 22.81628187352648496, 36.83196800326376064, -3.434112377981050290 ) ) ;
#97103=CARTESIAN_POINT ( 'NONE',  ( 1.472469842513823179, 1.425597817667451528, 4.923371831947296329 ) ) ;
#97105=CARTESIAN_POINT ( 'NONE',  ( 0.1532563361054083140, 26.00893115100078745, 1.131784320476157264E-15 ) ) ;
#97106=CARTESIAN_POINT ( 'NONE',  ( 2.917880565312948704, 67.63708216824730357, 12.26659068614894643 ) ) ;
#97107=VERTEX_POINT ( 'NONE', #70243 ) ;
#97108=CARTESIAN_POINT ( 'NONE',  ( 20.36894250292379382, 63.67874883491396787, 10.36894250292379205 ) ) ;
#97110=CARTESIAN_POINT ( 'NONE',  ( 20.88017736071110875, 45.77201867748816966, -2.915334737309920765 ) ) ;
#97111=CARTESIAN_POINT ( 'NONE',  ( -0.8801773607111009756, 63.06368534415484106, 1.068504757029289695E-15 ) ) ;
#97112=CARTESIAN_POINT ( 'NONE',  ( -0.8801773607111008646, 48.27201867748816966, 2.915334737309923430 ) ) ;
#97113=CARTESIAN_POINT ( 'NONE',  ( 1.472469842513823179, 1.425597817667451528, 4.923371831947296329 ) ) ;
#97114=CARTESIAN_POINT ( 'NONE',  ( 4.559911319644449179, 42.23035201082151247, -9.422509992056141925 ) ) ;
#97119=CARTESIAN_POINT ( 'NONE',  ( 14.92337183194729988, 29.34226448433411960, -8.527530157486177487 ) ) ;
#97121=CARTESIAN_POINT ( 'NONE',  ( 0.1532563361054083140, 56.00893115100078745, 1.131784320476157264E-15 ) ) ;
#97124=CARTESIAN_POINT ( 'NONE',  ( -4.164238869374099039, 1.803748834913967647, 8.674139862899312516E-16 ) ) ;
#97127=CARTESIAN_POINT ( 'NONE',  ( 19.05866839779140776, 50.95508385108959004, -6.499999999999956479 ) ) ;
#97130=CARTESIAN_POINT ( 'NONE',  ( 13.79529636645031943, 55.34541550158062506, -14.16423886937409904 ) ) ;
#97131=CARTESIAN_POINT ( 'NONE',  ( -46.94000000000001194, 103.0000000000000000, 5.000000000000000000 ) ) ;
#97134=CARTESIAN_POINT ( 'NONE',  ( 0.1532563361054083140, 51.00893115100078745, 1.131784320476157264E-15 ) ) ;
#97136=CARTESIAN_POINT ( 'NONE',  ( 22.81628187352647785, 21.41530133659708923, 3.434112377981063169 ) ) ;
#97137=CARTESIAN_POINT ( 'NONE',  ( 2.791683348922237240, 15.38393115100078212, -7.208316651077763204 ) ) ;
#97138=CARTESIAN_POINT ( 'NONE',  ( -33.19000000000001194, 92.00000000000000000, 9.500000000000000000 ) ) ;
#97139=CARTESIAN_POINT ( 'NONE',  ( 19.84674366389459266, 3.717264484334118713, -2.638427012816827677 ) ) ;
#97140=CARTESIAN_POINT ( 'NONE',  ( -1.099225684535947600, 3.706968003263753531, -6.408140936763238038 ) ) ;
#97143=VERTEX_POINT ( 'NONE', #69748 ) ;
#97144=CARTESIAN_POINT ( 'NONE',  ( 20.88017736071110164, 5.355352010821503583, 2.915334737309930979 ) ) ;
#97145=CARTESIAN_POINT ( 'NONE',  ( 10.00000000000000000, 0.5537488349139675359, -14.16423886937410082 ) ) ;
#97146=CARTESIAN_POINT ( 'NONE',  ( 12.63842701281683034, 22.46726448433411605, 9.846743663894596210 ) ) ;
#97147=CARTESIAN_POINT ( 'NONE',  ( 2.035157376598822676, 57.43868534415484106, -7.964842623401177768 ) ) ;
#97148=CARTESIAN_POINT ( 'NONE',  ( -1.099225684535947600, 28.70696800326375353, -6.408140936763238038 ) ) ;
#97150=CARTESIAN_POINT ( 'NONE',  ( 15.44008868035555260, 19.73035201082150536, 9.422509992056143702 ) ) ;
#97155=CARTESIAN_POINT ( 'NONE',  ( -1.099225684535947600, 3.706968003263753531, -6.408140936763238038 ) ) ;
#97156=CARTESIAN_POINT ( 'NONE',  ( 19.84674366389459621, 58.50893115100078745, 7.409399052514197653E-17 ) ) ;
#97157=CARTESIAN_POINT ( 'NONE',  ( 18.52753015748618282, 8.925597817667451750, -4.923371831947291888 ) ) ;
#97159=CARTESIAN_POINT ( 'NONE',  ( 19.38216949554541557, 37.24863466993041783, -9.382169495545420901 ) ) ;
#97161=CARTESIAN_POINT ( 'NONE',  ( 4.559911319644449179, 37.23035201082150536, -9.422509992056141925 ) ) ;
#97164=CARTESIAN_POINT ( 'NONE',  ( -0.8801773607110991993, 22.85535201082150181, -2.915334737309923874 ) ) ;
#97165=CARTESIAN_POINT ( 'NONE',  ( 4.559911319644449179, 33.89701867748817676, 9.422509992056141925 ) ) ;
#97166=CARTESIAN_POINT ( 'NONE',  ( 17.20831665107776587, 47.88393115100078745, 7.208316651077764980 ) ) ;
#97167=CARTESIAN_POINT ( 'NONE',  ( 10.00000000000000178, 54.31368534415484106, 10.88017736071110342 ) ) ;
#97168=CARTESIAN_POINT ( 'NONE',  ( 13.79529636645031943, 35.34541550158063927, -14.16423886937409904 ) ) ;
#97170=CARTESIAN_POINT ( 'NONE',  ( 14.92337183194729988, 44.34226448433412315, -8.527530157486177487 ) ) ;
#97171=CARTESIAN_POINT ( 'NONE',  ( 0.6178305044545838731, 59.74863466993041783, 9.382169495545420901 ) ) ;
#97172=CARTESIAN_POINT ( 'NONE',  ( 16.40814093676323893, 0.7903013365970867898, 11.09922568453595026 ) ) ;
#97174=CARTESIAN_POINT ( 'NONE',  ( 2.035157376598822676, 22.43868534415483396, -7.964842623401177768 ) ) ;
#97175=CARTESIAN_POINT ( 'NONE',  ( 17.96484262340118221, 6.188685344154836621, -7.964842623401177768 ) ) ;
#97176=CARTESIAN_POINT ( 'NONE',  ( 17.96484262340118221, 16.18868534415483396, -7.964842623401177768 ) ) ;
#97177=CARTESIAN_POINT ( 'NONE',  ( 0.1532563361054082862, 1.217264484334117824, 2.638427012816831674 ) ) ;
#97178=CARTESIAN_POINT ( 'NONE',  ( 13.79529636645030344, 18.26208216824730002, 14.16423886937410614 ) ) ;
#97179=CARTESIAN_POINT ( 'NONE',  ( 19.84674366389459266, 8.717264484334116048, -2.638427012816827677 ) ) ;
#97180=CARTESIAN_POINT ( 'NONE',  ( 7.361572987183170547, 62.05059781766745886, 9.846743663894590881 ) ) ;
#97181=CARTESIAN_POINT ( 'NONE',  ( 10.00000000000000178, 39.31368534415484106, 10.88017736071110342 ) ) ;
#97182=CARTESIAN_POINT ( 'NONE',  ( 18.72515096720577787, 46.07228050351031357, -6.499999999999891642 ) ) ;
#97186=CARTESIAN_POINT ( 'NONE',  ( 13.99999999999999822, 11.00000000000000000, 5.000000000000000000 ) ) ;
#97187=CARTESIAN_POINT ( 'NONE',  ( 7.361572987183169658, 44.96726448433412315, -9.846743663894592657 ) ) ;
#97191=CARTESIAN_POINT ( 'NONE',  ( 17.08211943468705130, 28.47041550158063572, 12.26659068614894998 ) ) ;
#97192=CARTESIAN_POINT ( 'NONE',  ( -2.266590686148945544, 21.38708216824730357, -7.082119434687050408 ) ) ;
#97193=CARTESIAN_POINT ( 'NONE',  ( 4.559911319644449179, 62.23035201082150536, -9.422509992056141925 ) ) ;
#97194=CARTESIAN_POINT ( 'NONE',  ( 20.36894250292379382, 58.67874883491396076, 10.36894250292379205 ) ) ;
#97195=CARTESIAN_POINT ( 'NONE',  ( 19.38216949554541202, 0.9986346699304200492, 9.382169495545424454 ) ) ;
#97196=CARTESIAN_POINT ( 'NONE',  ( 2.791683348922237240, 55.38393115100078745, -7.208316651077763204 ) ) ;
#97198=CARTESIAN_POINT ( 'NONE',  ( 7.084665262690076126, 44.10535201082151247, 10.88017736071109987 ) ) ;
#97199=CARTESIAN_POINT ( 'NONE',  ( -2.816281873526473856, 4.331968003263754419, 3.434112377981055619 ) ) ;
#97200=CARTESIAN_POINT ( 'NONE',  ( -2.266590686148945544, 17.22041550158063572, 7.082119434687048631 ) ) ;
#97201=CARTESIAN_POINT ( 'NONE',  ( 6.204703633549690345, 50.76208216824730357, -14.16423886937410259 ) ) ;
#97202=CARTESIAN_POINT ( 'NONE',  ( 0.5774900079438590739, 22.64701867748817321, -5.440088680355550821 ) ) ;
#97203=CARTESIAN_POINT ( 'NONE',  ( 20.24186590665278018, 5.590145880403569301, -6.114288769123027656 ) ) ;
#97204=CARTESIAN_POINT ( 'NONE',  ( 20.88017736071110875, 40.77201867748818387, -2.915334737309920765 ) ) ;
#97205=MECHANICAL_DESIGN_GEOMETRIC_PRESENTATION_REPRESENTATION('',(#9386),#10957);
#97208=CARTESIAN_POINT ( 'NONE',  ( 19.80832241502128355, 4.758688159020694641, 6.500000000000000888 ) ) ;
#97211=CARTESIAN_POINT ( 'NONE',  ( 10.00000000000000178, 43.05374883491397497, 14.16423886937410082 ) ) ;
#97212=CARTESIAN_POINT ( 'NONE',  ( 0.1532563361054083140, 41.00893115100078745, 1.131784320476157264E-15 ) ) ;
#97213=CARTESIAN_POINT ( 'NONE',  ( 10.00000000000000000, 66.81368534415484817, -10.88017736071110342 ) ) ;
#97216=DIRECTION ( 'NONE',  ( 1.000000000000000000, 0.000000000000000000, 0.000000000000000000 ) ) ;
#97218=CARTESIAN_POINT ( 'NONE',  ( 10.00000000000000178, 59.31368534415484106, 10.88017736071110342 ) ) ;
#97219=CARTESIAN_POINT ( 'NONE',  ( 16.40814093676323893, 60.79030133659709634, 11.09922568453595026 ) ) ;
#97222=CARTESIAN_POINT ( 'NONE',  ( 20.36894250292379382, 13.67874883491396965, 10.36894250292379205 ) ) ;
#97224=CARTESIAN_POINT ( 'NONE',  ( 21.09922568453594849, 21.20696800326375353, 6.408140936763242479 ) ) ;
#97226=CARTESIAN_POINT ( 'NONE',  ( 6.565887622018943937, 40.16530133659708923, 12.81628187352647430 ) ) ;
#97228=CARTESIAN_POINT ( 'NONE',  ( 14.92337183194729988, 34.34226448433411605, -8.527530157486177487 ) ) ;
#97229=CARTESIAN_POINT ( 'NONE',  ( 4.559911319644449179, 12.23035201082150536, -9.422509992056141925 ) ) ;
#97230=CARTESIAN_POINT ( 'NONE',  ( 16.40814093676323893, 50.79030133659708923, 11.09922568453595026 ) ) ;
#97232=CARTESIAN_POINT ( 'NONE',  ( 10.00000000000000000, 39.75893115100078745, -9.846743663894594434 ) ) ;
#97233=LINE ( 'NONE', #80724, #68064 ) ;
#97238=CARTESIAN_POINT ( 'NONE',  ( 0.9408516040111476464, 67.46693863883976405, -6.499999999999953815 ) ) ;
#97239=CARTESIAN_POINT ( 'NONE',  ( 5.076628168052704559, 15.17559781766745175, -8.527530157486179263 ) ) ;
#97240=EDGE_CURVE ( 'NONE', #73676, #27464, #61249, .T. ) ;
#97241=CARTESIAN_POINT ( 'NONE',  ( -2.816281873526473856, 19.12363466993042138, 9.499525473075851096E-16 ) ) ;
#97244=CARTESIAN_POINT ( 'NONE',  ( 7.361572987183170547, 57.05059781766744464, 9.846743663894590881 ) ) ;
#97246=CARTESIAN_POINT ( 'NONE',  ( 20.36894250292379382, 23.67874883491397142, 10.36894250292379205 ) ) ;
#97247=CARTESIAN_POINT ( 'NONE',  ( 19.84674366389459266, 43.71726448433410894, -2.638427012816827677 ) ) ;
#97248=CARTESIAN_POINT ( 'NONE',  ( 3.591859063236763294, 48.29030133659708923, -11.09922568453595026 ) ) ;
#97250=CARTESIAN_POINT ( 'NONE',  ( 0.1532563361054100626, 0.8005978176674514168, -2.638427012816831230 ) ) ;
#97252=CARTESIAN_POINT ( 'NONE',  ( 14.92337183194729633, 52.67559781766745175, 8.527530157486181039 ) ) ;
#97253=CARTESIAN_POINT ( 'NONE',  ( 15.44008868035555793, 36.39701867748816966, -9.422509992056140149 ) ) ;
#97254=CARTESIAN_POINT ( 'NONE',  ( 18.52753015748618282, 33.92559781766745886, -4.923371831947291888 ) ) ;
#97257=CARTESIAN_POINT ( 'NONE',  ( 17.96484262340118221, 41.18868534415484106, -7.964842623401177768 ) ) ;
#97258=EDGE_CURVE ( 'NONE', #61157, #37561, #2254, .T. ) ;
#97261=CARTESIAN_POINT ( 'NONE',  ( 12.91533473730992121, 9.522018677488171434, 10.88017736071110164 ) ) ;
#97262=CARTESIAN_POINT ( 'NONE',  ( 18.52753015748618282, 53.92559781766745175, -4.923371831947291888 ) ) ;
#97263=CARTESIAN_POINT ( 'NONE',  ( 15.44008868035555260, 44.73035201082151247, 9.422509992056143702 ) ) ;
#97264=CARTESIAN_POINT ( 'NONE',  ( 7.084665262690076126, 57.02201867748817676, -10.88017736071110164 ) ) ;
#97266=CARTESIAN_POINT ( 'NONE',  ( 20.88017736071110164, 25.35535201082150891, 2.915334737309930979 ) ) ;
#97267=CARTESIAN_POINT ( 'NONE',  ( -0.000000000000000000, 72.78284190987160684, -5.243908048977683478 ) ) ;
#97268=CARTESIAN_POINT ( 'NONE',  ( 19.84674366389459266, 18.71726448433411960, -2.638427012816827677 ) ) ;
#97269=CARTESIAN_POINT ( 'NONE',  ( -46.43542959741873233, 103.9441885970218351, -5.610226944091871282 ) ) ;
#97271=CARTESIAN_POINT ( 'NONE',  ( 19.84674366389459266, 48.30059781766745175, 2.638427012816836559 ) ) ;
#97272=CARTESIAN_POINT ( 'NONE',  ( 2.917880565312948704, 67.63708216824730357, 12.26659068614894643 ) ) ;
#97274=CARTESIAN_POINT ( 'NONE',  ( -4.164238869374099927, 7.012082168247302683, 3.795296366450308767 ) ) ;
#97276=CARTESIAN_POINT ( 'NONE',  ( -2.266590686148945544, 52.22041550158064638, 7.082119434687048631 ) ) ;
#97277=CARTESIAN_POINT ( 'NONE',  ( -1.099225684535947600, 3.706968003263753531, -6.408140936763238038 ) ) ;
#97278=CARTESIAN_POINT ( 'NONE',  ( 2.035157376598822676, 12.43868534415483751, -7.964842623401177768 ) ) ;
#97279=CARTESIAN_POINT ( 'NONE',  ( 10.00000000000000178, 47.25893115100078745, 9.846743663894594434 ) ) ;
#97280=CARTESIAN_POINT ( 'NONE',  ( 2.917880565312950480, 0.9704155015806342766, -12.26659068614894821 ) ) ;
#97284=CARTESIAN_POINT ( 'NONE',  ( -2.816281873526473856, 29.12363466993041783, 9.499525473075851096E-16 ) ) ;
#97285=CARTESIAN_POINT ( 'NONE',  ( 19.84674366389459266, 23.71726448433412315, -2.638427012816827677 ) ) ;
#97286=VERTEX_POINT ( 'NONE', #78719 ) ;
#97287=CARTESIAN_POINT ( 'NONE',  ( 19.84674366389459621, 8.508931151000785675, 7.409399052514197653E-17 ) ) ;
#97289=DIRECTION ( 'NONE',  ( -0.000000000000000000, 1.000000000000000000, -0.000000000000000000 ) ) ;
#97290=CARTESIAN_POINT ( 'NONE',  ( 0.5774900079438607392, 18.48035201082150536, 5.440088680355550821 ) ) ;
#97291=CARTESIAN_POINT ( 'NONE',  ( 13.79529636645030344, 43.26208216824730357, 14.16423886937410614 ) ) ;
#97292=CARTESIAN_POINT ( 'NONE',  ( 20.88017736071110519, 40.56368534415484106, 2.639326808657452039E-16 ) ) ;
#97293=CARTESIAN_POINT ( 'NONE',  ( 20.88017736071110875, 65.77201867748817676, -2.915334737309920765 ) ) ;
#97294=CARTESIAN_POINT ( 'NONE',  ( 0.1532563361054083140, 21.00893115100078745, 1.131784320476157264E-15 ) ) ;
#97296=CARTESIAN_POINT ( 'NONE',  ( 10.00000000000000000, 4.758931151000784787, -9.846743663894594434 ) ) ;
#97297=CARTESIAN_POINT ( 'NONE',  ( 19.72487221294570858, 1.866073187300754110, 6.500000000000000888 ) ) ;
#97298=CARTESIAN_POINT ( 'NONE',  ( 0.1532563361054082862, 41.21726448433411605, 2.638427012816831674 ) ) ;
#97299=CARTESIAN_POINT ( 'NONE',  ( 2.791683348922240793, 61.63393115100079456, 7.208316651077764092 ) ) ;
#97300=CARTESIAN_POINT ( 'NONE',  ( -0.8801773607110991993, 42.85535201082150536, -2.915334737309923874 ) ) ;
#97301=UNCERTAINTY_MEASURE_WITH_UNIT (LENGTH_MEASURE( 1.000000000000000082E-05 ), #32129, 'distance_accuracy_value', 'NONE');
#97302=EDGE_LOOP ( 'NONE', ( #51164, #18449, #17037, #59306, #16032, #58577 ) ) ;
#97303=CARTESIAN_POINT ( 'NONE',  ( 6.565887622018943937, 55.16530133659709634, 12.81628187352647430 ) ) ;
#97305=CARTESIAN_POINT ( 'NONE',  ( 1.472469842513823179, 10.59226448433411782, -4.923371831947296329 ) ) ;
#97306=CARTESIAN_POINT ( 'NONE',  ( 13.43411237798106583, 47.66530133659709634, -12.81628187352647252 ) ) ;
#97307=CARTESIAN_POINT ( 'NONE',  ( 7.084665262690076126, 12.02201867748817321, -10.88017736071110164 ) ) ;
#97308=CARTESIAN_POINT ( 'NONE',  ( 0.1532563361054100626, 30.80059781766744820, -2.638427012816831230 ) ) ;
#97309=CARTESIAN_POINT ( 'NONE',  ( 0.2751277870542911952, 33.21833443783938122, 6.499999999999992006 ) ) ;
#97310=CARTESIAN_POINT ( 'NONE',  ( 10.00000000000000178, 18.05374883491396787, 14.16423886937410082 ) ) ;
#97311=CARTESIAN_POINT ( 'NONE',  ( -0.3689425029237898834, 46.17874883491397497, -10.36894250292378850 ) ) ;
#97312=CARTESIAN_POINT ( 'NONE',  ( 19.84674366389459266, 48.71726448433413026, -2.638427012816827677 ) ) ;
#97314=CARTESIAN_POINT ( 'NONE',  ( 10.00000000000000178, 39.31368534415484106, 10.88017736071110342 ) ) ;
#97315=CARTESIAN_POINT ( 'NONE',  ( 14.92337183194729988, 4.342264484334117824, -8.527530157486177487 ) ) ;
#97316=TOROIDAL_SURFACE ( 'NONE', #94085, 1.000000000000000000, 0.5000000000000000000 ) ;
#97318=CARTESIAN_POINT ( 'NONE',  ( 0.6178305044545818747, 63.49863466993043204, -9.382169495545419124 ) ) ;
#97320=CARTESIAN_POINT ( 'NONE',  ( 7.084665262690076126, 62.02201867748816966, -10.88017736071110164 ) ) ;
#97323=CARTESIAN_POINT ( 'NONE',  ( 20.36894250292379738, 4.928748834913967869, -10.36894250292379027 ) ) ;
#97324=CARTESIAN_POINT ( 'NONE',  ( 18.52753015748617571, 3.092264484334118269, 4.923371831947298993 ) ) ;
#97325=EDGE_CURVE ( 'NONE', #20168, #42200, #84270, .T. ) ;
#97328=CARTESIAN_POINT ( 'NONE',  ( 15.44008868035555793, 16.39701867748817321, -9.422509992056140149 ) ) ;
#97329=CARTESIAN_POINT ( 'NONE',  ( 19.42250999205614548, 60.98035201082151247, -5.440088680355545492 ) ) ;
#97331=CARTESIAN_POINT ( 'NONE',  ( 7.084665262690076126, 27.02201867748817676, -10.88017736071110164 ) ) ;
#97332=CARTESIAN_POINT ( 'NONE',  ( 1.472469842513823179, 56.42559781766745886, 4.923371831947296329 ) ) ;
#97333=ORIENTED_EDGE ( 'NONE', *, *, #82890, .F. ) ;
#97334=CARTESIAN_POINT ( 'NONE',  ( 0.1532563361054082862, 66.21726448433413736, 2.638427012816831674 ) ) ;
#97336=CARTESIAN_POINT ( 'NONE',  ( 0.5774900079438607392, 68.48035201082150536, 5.440088680355550821 ) ) ;
#97337=CARTESIAN_POINT ( 'NONE',  ( 0.1532563361054100626, 60.80059781766744464, -2.638427012816831230 ) ) ;
#97338=CARTESIAN_POINT ( 'NONE',  ( 19.38216949554541202, 40.99863466993042493, 9.382169495545424454 ) ) ;
#97339=CARTESIAN_POINT ( 'NONE',  ( 0.5774900079438607392, 23.48035201082150536, 5.440088680355550821 ) ) ;
#97341=CARTESIAN_POINT ( 'NONE',  ( 4.559911319644449179, 67.23035201082150536, -9.422509992056141925 ) ) ;
#97342=CARTESIAN_POINT ( 'NONE',  ( 12.91533473730993009, 16.60535201082150891, -10.88017736071109987 ) ) ;
#97345=CARTESIAN_POINT ( 'NONE',  ( 10.00000000000000000, 57.87363466993042493, -12.81628187352647608 ) ) ;
#97346=CARTESIAN_POINT ( 'NONE',  ( -0.8801773607110991993, 37.85535201082151247, -2.915334737309923874 ) ) ;
#97347=CARTESIAN_POINT ( 'NONE',  ( 19.59355871817327710, 95.39900665025442095, 5.130928526377548593 ) ) ;
#97348=CARTESIAN_POINT ( 'NONE',  ( 0.6178305044545838731, 54.74863466993042493, 9.382169495545420901 ) ) ;
#97349=CARTESIAN_POINT ( 'NONE',  ( 10.00000000000000178, 49.31368534415484106, 10.88017736071110342 ) ) ;
#97350=CARTESIAN_POINT ( 'NONE',  ( 2.791683348922240793, 61.63393115100079456, 7.208316651077764092 ) ) ;
#97351=DIRECTION ( 'NONE',  ( 0.000000000000000000, -1.000000000000000000, 0.000000000000000000 ) ) ;
#97353=CARTESIAN_POINT ( 'NONE',  ( 10.00000000000000178, 22.25893115100078745, 9.846743663894594434 ) ) ;
#97354=CARTESIAN_POINT ( 'NONE',  ( 22.81628187352647785, 6.415301336597088344, 3.434112377981063169 ) ) ;
#97355=CYLINDRICAL_SURFACE ( 'NONE', #40466, 0.5000000000000004441 ) ;
#97356=CARTESIAN_POINT ( 'NONE',  ( 19.84674366389459266, 58.71726448433411605, -2.638427012816827677 ) ) ;
#97357=CARTESIAN_POINT ( 'NONE',  ( 17.96484262340118221, 19.93868534415484106, 7.964842623401181321 ) ) ;
#97358=CARTESIAN_POINT ( 'NONE',  ( 14.92337183194729988, 54.34226448433412315, -8.527530157486177487 ) ) ;
#97359=DIRECTION ( 'NONE',  ( 0.000000000000000000, 0.000000000000000000, -1.000000000000000000 ) ) ;
#97360=CARTESIAN_POINT ( 'NONE',  ( 18.52753015748618282, 3.925597817667451306, -4.923371831947291888 ) ) ;
#97362=CARTESIAN_POINT ( 'NONE',  ( 0.1532563361054082862, 66.21726448433413736, 2.638427012816831674 ) ) ;
#97366=CARTESIAN_POINT ( 'NONE',  ( 22.81628187352647785, 36.62363466993041783, 6.195893100308588602E-16 ) ) ;
#97367=CARTESIAN_POINT ( 'NONE',  ( 7.361572987183169658, 34.96726448433411605, -9.846743663894592657 ) ) ;
#97368=CARTESIAN_POINT ( 'NONE',  ( 0.1077916266722445254, 12.24062864464239020, -6.478736007405951902 ) ) ;
#97369=CARTESIAN_POINT ( 'NONE',  ( 17.96484262340118221, 6.188685344154837509, -7.964842623401177768 ) ) ;
#97370=CARTESIAN_POINT ( 'NONE',  ( 10.00000000000000178, 37.25893115100078745, 9.846743663894594434 ) ) ;
#97372=CARTESIAN_POINT ( 'NONE',  ( -0.8801773607111009756, 3.063685344154838397, 1.068504757029289695E-15 ) ) ;
#97373=CARTESIAN_POINT ( 'NONE',  ( 1.274849032794102888, 3.572280503510291361, 6.499999999999721112 ) ) ;
#97374=CARTESIAN_POINT ( 'NONE',  ( 2.035157376598824452, 23.68868534415484461, 7.964842623401179544 ) ) ;
#97375=CARTESIAN_POINT ( 'NONE',  ( 22.26659068614894466, 43.88708216824729647, 7.082119434687054849 ) ) ;
#97376=CARTESIAN_POINT ( 'NONE',  ( 20.36894250292379382, 53.67874883491397497, 10.36894250292379205 ) ) ;
#97378=CARTESIAN_POINT ( 'NONE',  ( -0.05723567505238607439, 69.83236346210668444, 6.413539670616451360 ) ) ;
#97380=CARTESIAN_POINT ( 'NONE',  ( 17.20831665107776587, 9.133931151000787452, -7.208316651077762316 ) ) ;
#97381=CARTESIAN_POINT ( 'NONE',  ( -1.099225684535947600, 4.540301336597087456, 6.408140936763237150 ) ) ;
#97382=ORIENTED_EDGE ( 'NONE', *, *, #52405, .F. ) ;
#97383=CARTESIAN_POINT ( 'NONE',  ( 7.084665262690076126, 54.10535201082151247, 10.88017736071109987 ) ) ;
#97388=( LENGTH_UNIT ( ) NAMED_UNIT ( * ) SI_UNIT ( .MILLI., .METRE. ) );
#97389=CARTESIAN_POINT ( 'NONE',  ( 7.361572987183169658, 19.96726448433411960, -9.846743663894592657 ) ) ;
#97391=CARTESIAN_POINT ( 'NONE',  ( 6.204703633549690345, 40.76208216824731778, -14.16423886937410259 ) ) ;
#97392=CARTESIAN_POINT ( 'NONE',  ( 19.84674366389459266, 8.300597817667451750, 2.638427012816836559 ) ) ;
#97394=SURFACE_SIDE_STYLE ('',( #59366 ) ) ;
#97395=CARTESIAN_POINT ( 'NONE',  ( 17.96484262340118221, 26.18868534415483396, -7.964842623401177768 ) ) ;
#97396=CARTESIAN_POINT ( 'NONE',  ( 21.09922568453595559, 37.04030133659708923, -6.408140936763230044 ) ) ;
#97397=CARTESIAN_POINT ( 'NONE',  ( -0.8801773607111009756, 8.063685344154837509, 1.068504757029289695E-15 ) ) ;
#97398=CARTESIAN_POINT ( 'NONE',  ( 6.565887622018943937, 30.16530133659708568, 12.81628187352647430 ) ) ;
#97399=CARTESIAN_POINT ( 'NONE',  ( 22.81628187352648496, 61.83196800326376774, -3.434112377981050290 ) ) ;
#97401=CARTESIAN_POINT ( 'NONE',  ( 1.602071938427518161, 12.02224192338640130, -6.500000000000021316 ) ) ;
#97404=CARTESIAN_POINT ( 'NONE',  ( -4.164238869374099039, 41.80374883491397497, 8.674139862899312516E-16 ) ) ;
#97405=CARTESIAN_POINT ( 'NONE',  ( 20.36894250292379382, 3.678748834913967869, 10.36894250292379205 ) ) ;
#97406=CARTESIAN_POINT ( 'NONE',  ( 12.91533473730992121, 4.522018677488169658, 10.88017736071110164 ) ) ;
#97407=CARTESIAN_POINT ( 'NONE',  ( 10.00000000000000178, 19.31368534415484106, 10.88017736071110342 ) ) ;
#97408=FACE_OUTER_BOUND ( 'NONE', #37655, .T. ) ;
#97410=CARTESIAN_POINT ( 'NONE',  ( 15.44008868035555793, 56.39701867748817676, -9.422509992056140149 ) ) ;
#97411=CARTESIAN_POINT ( 'NONE',  ( 10.00000000000000000, 56.81368534415484106, -10.88017736071110342 ) ) ;
#97412=CARTESIAN_POINT ( 'NONE',  ( 22.81628187352647785, 16.41530133659708923, 3.434112377981063169 ) ) ;
#97413=( LENGTH_UNIT ( ) NAMED_UNIT ( * ) SI_UNIT ( .MILLI., .METRE. ) );
#97415=CARTESIAN_POINT ( 'NONE',  ( 0.1532563361054082862, 26.21726448433411605, 2.638427012816831674 ) ) ;
#97416=CARTESIAN_POINT ( 'NONE',  ( 2.035157376598822676, 57.43868534415484106, -7.964842623401177768 ) ) ;
#97418=CARTESIAN_POINT ( 'NONE',  ( 19.38216949554541557, 17.24863466993041783, -9.382169495545420901 ) ) ;
#97419=FILL_AREA_STYLE_COLOUR ( '', #9038 ) ;
#97420=CARTESIAN_POINT ( 'NONE',  ( 12.91533473730993009, 6.605352010821504471, -10.88017736071109987 ) ) ;
#97421=CARTESIAN_POINT ( 'NONE',  ( 18.52753015748618282, 43.92559781766745175, -4.923371831947291888 ) ) ;
#97422=CARTESIAN_POINT ( 'NONE',  ( 6.565887622018943937, 48.08196800326375353, -12.81628187352647608 ) ) ;
#97423=CARTESIAN_POINT ( 'NONE',  ( 2.791683348922240793, 21.63393115100078745, 7.208316651077764092 ) ) ;
#97424=CARTESIAN_POINT ( 'NONE',  ( -2.266590686148945544, 7.220415501580634832, 7.082119434687048631 ) ) ;
#97426=CARTESIAN_POINT ( 'NONE',  ( 4.559911319644449179, 17.23035201082150536, -9.422509992056141925 ) ) ;
#97427=LINE ( 'NONE', #27913, #96761 ) ;
#97428=CARTESIAN_POINT ( 'NONE',  ( 2.917880565312950480, 30.97041550158063572, -12.26659068614894821 ) ) ;
#97429=CARTESIAN_POINT ( 'NONE',  ( 18.52753015748618282, 48.92559781766745886, -4.923371831947291888 ) ) ;
#97431=CARTESIAN_POINT ( 'NONE',  ( 12.91533473730992121, 19.52201867748816611, 10.88017736071110164 ) ) ;
#97432=CARTESIAN_POINT ( 'NONE',  ( 20.88017736071110519, 10.56368534415483929, 2.639326808657452039E-16 ) ) ;
#97434=AXIS2_PLACEMENT_3D ( 'NONE', #80839, #49350, #27335 ) ;
#97435=CARTESIAN_POINT ( 'NONE',  ( 2.035157376598824452, 28.68868534415484106, 7.964842623401179544 ) ) ;
#97437=CARTESIAN_POINT ( 'NONE',  ( 13.43411237798106583, 47.66530133659709634, -12.81628187352647252 ) ) ;
#97439=CARTESIAN_POINT ( 'NONE',  ( 12.91533473730993009, 31.60535201082150891, -10.88017736071109987 ) ) ;
#97440=CARTESIAN_POINT ( 'NONE',  ( 20.88017736071110519, 35.56368534415484106, 2.639326808657452039E-16 ) ) ;
#97442=CARTESIAN_POINT ( 'NONE',  ( 17.20831665107776587, 52.88393115100078035, 7.208316651077764980 ) ) ;
#97443=CARTESIAN_POINT ( 'NONE',  ( 19.42250999205614548, 30.98035201082150536, -5.440088680355545492 ) ) ;
#97446=CYLINDRICAL_SURFACE ( 'NONE', #76395, 0.5000000000000004441 ) ;
#97447=CARTESIAN_POINT ( 'NONE',  ( -0.3689425029237881626, 52.42874883491396076, 10.36894250292379027 ) ) ;
#97448=CARTESIAN_POINT ( 'NONE',  ( 7.084665262690076126, 57.02201867748817676, -10.88017736071110164 ) ) ;
#97449=EDGE_CURVE ( 'NONE', #63997, #46284, #65169, .T. ) ;
#97450=CARTESIAN_POINT ( 'NONE',  ( 10.00000000000000000, 64.75893115100078035, -9.846743663894594434 ) ) ;
#97452=CARTESIAN_POINT ( 'NONE',  ( 14.92337183194729988, 64.34226448433412315, -8.527530157486177487 ) ) ;
#97453=CARTESIAN_POINT ( 'NONE',  ( 19.84674366389459266, 3.717264484334118713, -2.638427012816827677 ) ) ;
#97454=CARTESIAN_POINT ( 'NONE',  ( 0.1532563361054100626, 25.80059781766744820, -2.638427012816831230 ) ) ;
#97455=VERTEX_POINT ( 'NONE', #95689 ) ;
#97456=CARTESIAN_POINT ( 'NONE',  ( 18.52753015748618282, 23.92559781766745530, -4.923371831947291888 ) ) ;
#97458=CARTESIAN_POINT ( 'NONE',  ( 0.5774900079438590739, 32.64701867748816966, -5.440088680355550821 ) ) ;
#97459=CARTESIAN_POINT ( 'NONE',  ( 17.20831665107776587, 19.13393115100078035, -7.208316651077762316 ) ) ;
#97460=CARTESIAN_POINT ( 'NONE',  ( 20.88017736071110875, 65.77201867748817676, -2.915334737309920765 ) ) ;
#97461=CARTESIAN_POINT ( 'NONE',  ( -0.8801773607110991993, 57.85535201082149825, -2.915334737309923874 ) ) ;
#97462=CARTESIAN_POINT ( 'NONE',  ( 15.44008868035555260, 29.73035201082150891, 9.422509992056143702 ) ) ;
#97463=CARTESIAN_POINT ( 'NONE',  ( 13.43411237798106583, 62.66530133659708923, -12.81628187352647252 ) ) ;
#97464=CARTESIAN_POINT ( 'NONE',  ( 13.79529636645031943, 45.34541550158062506, -14.16423886937409904 ) ) ;
#97467=CARTESIAN_POINT ( 'NONE',  ( 21.92686044187657401, 35.37045670184114243, -3.195792623639525765 ) ) ;
#97469=CARTESIAN_POINT ( 'NONE',  ( 13.43411237798105340, 5.581968003263753531, 12.81628187352647963 ) ) ;
#97470=CARTESIAN_POINT ( 'NONE',  ( 20.88017736071110164, 5.355352010821502695, 2.915334737309930979 ) ) ;
#97471=CARTESIAN_POINT ( 'NONE',  ( 10.00000000000000178, 49.31368534415484106, 10.88017736071110342 ) ) ;
#97472=CARTESIAN_POINT ( 'NONE',  ( 17.85158348494336167, 24.73726573380441351, -6.499999999999992895 ) ) ;
#97475=CARTESIAN_POINT ( 'NONE',  ( 18.52753015748618282, 13.92559781766745175, -4.923371831947291888 ) ) ;
#97476=CARTESIAN_POINT ( 'NONE',  ( 20.88017736071110164, 60.35535201082151957, 2.915334737309930979 ) ) ;
#97477=CARTESIAN_POINT ( 'NONE',  ( 7.361572987183169658, 34.96726448433411605, -9.846743663894592657 ) ) ;
#97478=CARTESIAN_POINT ( 'NONE',  ( 17.20831665107776587, 22.88393115100078745, 7.208316651077764980 ) ) ;
#97479=CARTESIAN_POINT ( 'NONE',  ( 10.00000000000000178, 17.25893115100078745, 9.846743663894594434 ) ) ;
#97480=CARTESIAN_POINT ( 'NONE',  ( 2.603489959281613420, 50.43575266056826933, -6.500000000000031086 ) ) ;
#97481=CARTESIAN_POINT ( 'NONE',  ( -2.816281873526471635, 43.91530133659708923, -3.434112377981056508 ) ) ;
#97482=CARTESIAN_POINT ( 'NONE',  ( 5.076628168052704559, 5.175597817667451750, -8.527530157486179263 ) ) ;
#97485=CARTESIAN_POINT ( 'NONE',  ( 19.84674366389459621, 28.50893115100078745, 7.409399052514197653E-17 ) ) ;
#97488=CARTESIAN_POINT ( 'NONE',  ( 22.81628187352647785, 56.62363466993042493, 6.195893100308588602E-16 ) ) ;
#97490=CARTESIAN_POINT ( 'NONE',  ( 3.591859063236761518, -0.04303199673624671928, 11.09922568453594849 ) ) ;
#97491=CARTESIAN_POINT ( 'NONE',  ( 12.91533473730992121, 4.522018677488169658, 10.88017736071110164 ) ) ;
#97492=CARTESIAN_POINT ( 'NONE',  ( 13.79529636645030344, 18.26208216824730002, 14.16423886937410614 ) ) ;
#97494=UNCERTAINTY_MEASURE_WITH_UNIT (LENGTH_MEASURE( 1.000000000000000082E-05 ), #4906, 'distance_accuracy_value', 'NONE');
#97495=FACE_OUTER_BOUND ( 'NONE', #69154, .T. ) ;
#97496=CARTESIAN_POINT ( 'NONE',  ( -2.266590686148945544, 36.38708216824730357, -7.082119434687050408 ) ) ;
#97498=CARTESIAN_POINT ( 'NONE',  ( 17.08211943468705130, 43.47041550158063927, 12.26659068614894998 ) ) ;
#97499=CARTESIAN_POINT ( 'NONE',  ( -2.266590686148945544, 16.38708216824730357, -7.082119434687050408 ) ) ;
#97500=CARTESIAN_POINT ( 'NONE',  ( 24.16423886937410614, 14.30374883491396787, 8.672049930838204340E-16 ) ) ;
#97502=CARTESIAN_POINT ( 'NONE',  ( 7.084665262690076126, 49.10535201082149825, 10.88017736071109987 ) ) ;
#97504=CARTESIAN_POINT ( 'NONE',  ( 14.92337183194729633, 32.67559781766745175, 8.527530157486181039 ) ) ;
#97505=CARTESIAN_POINT ( 'NONE',  ( 20.88017736071110519, 65.56368534415483396, 2.639326808657452039E-16 ) ) ;
#97506=CARTESIAN_POINT ( 'NONE',  ( 5.076628168052704559, 25.17559781766745175, -8.527530157486179263 ) ) ;
#97508=CARTESIAN_POINT ( 'NONE',  ( 20.88017736071110164, 15.35535201082150358, 2.915334737309930979 ) ) ;
#97509=CARTESIAN_POINT ( 'NONE',  ( 10.00000000000000178, 65.37363466993042493, 12.81628187352647608 ) ) ;
#97510=CARTESIAN_POINT ( 'NONE',  ( 0.1532563361054100626, 50.80059781766745175, -2.638427012816831230 ) ) ;
#97513=CARTESIAN_POINT ( 'NONE',  ( 1.472469842513823179, 25.59226448433412315, -4.923371831947296329 ) ) ;
#97514=CARTESIAN_POINT ( 'NONE',  ( 21.09922568453595559, 42.04030133659708213, -6.408140936763230044 ) ) ;
#97516=CARTESIAN_POINT ( 'NONE',  ( -0.8801773607110991993, 42.85535201082150536, -2.915334737309923874 ) ) ;
#97517=CARTESIAN_POINT ( 'NONE',  ( 14.92337183194729988, 34.34226448433411605, -8.527530157486177487 ) ) ;
#97518=CARTESIAN_POINT ( 'NONE',  ( 24.16423886937410614, 29.30374883491396787, 8.672049930838204340E-16 ) ) ;
#97520=CARTESIAN_POINT ( 'NONE',  ( -4.164238869374099927, 7.012082168247302683, 3.795296366450308767 ) ) ;
#97521=CARTESIAN_POINT ( 'NONE',  ( 2.035157376598822676, 57.43868534415484106, -7.964842623401177768 ) ) ;
#97522=CARTESIAN_POINT ( 'NONE',  ( 15.44008868035555793, 61.39701867748817676, -9.422509992056140149 ) ) ;
#97523=CARTESIAN_POINT ( 'NONE',  ( -0.3689425029237881626, 62.42874883491396787, 10.36894250292379027 ) ) ;
#97524=CARTESIAN_POINT ( 'NONE',  ( -2.816281873526473856, -0.8763653300695799508, 9.499525473075851096E-16 ) ) ;
#97525=CARTESIAN_POINT ( 'NONE',  ( 17.96484262340118221, 56.18868534415484817, -7.964842623401177768 ) ) ;
#97526=CARTESIAN_POINT ( 'NONE',  ( -0.1503990784575263973, 27.22266099184919241, -6.262539305110081500 ) ) ;
#97528=CARTESIAN_POINT ( 'NONE',  ( 16.40814093676324603, 32.45696800326375353, -11.09922568453594671 ) ) ;
#97529=CARTESIAN_POINT ( 'NONE',  ( 19.84674366389459266, 63.30059781766745886, 2.638427012816836559 ) ) ;
#97531=CARTESIAN_POINT ( 'NONE',  ( 10.00000000000000000, 6.813685344154838397, -10.88017736071110342 ) ) ;
#97532=CARTESIAN_POINT ( 'NONE',  ( 20.88017736071110875, 10.77201867748817143, -2.915334737309920765 ) ) ;
#97533=CARTESIAN_POINT ( 'NONE',  ( 1.472469842513823179, 36.42559781766745175, 4.923371831947296329 ) ) ;
#97534=CARTESIAN_POINT ( 'NONE',  ( 2.148416515056618792, 42.23726573380440641, 6.499999999999959144 ) ) ;
#97537=CARTESIAN_POINT ( 'NONE',  ( 10.00000000000000000, 1.813685344154837731, -10.88017736071110342 ) ) ;
#97538=CARTESIAN_POINT ( 'NONE',  ( 16.40814093676323893, 10.79030133659708923, 11.09922568453595026 ) ) ;
#97539=CARTESIAN_POINT ( 'NONE',  ( 2.791683348922237240, 10.38393115100078390, -7.208316651077763204 ) ) ;
#97541=CARTESIAN_POINT ( 'NONE',  ( 10.00000000000000178, 52.25893115100078745, 9.846743663894594434 ) ) ;
#97542=CARTESIAN_POINT ( 'NONE',  ( 0.5774900079438590739, 42.64701867748816966, -5.440088680355550821 ) ) ;
#97543=CARTESIAN_POINT ( 'NONE',  ( -2.816281873526471635, 13.91530133659708746, -3.434112377981056508 ) ) ;
#97544=CARTESIAN_POINT ( 'NONE',  ( 20.88017736071110164, 55.35535201082149825, 2.915334737309930979 ) ) ;
#97545=CARTESIAN_POINT ( 'NONE',  ( 19.72487221294571569, 25.71833443783938478, -6.499999999999989342 ) ) ;
#97548=CARTESIAN_POINT ( 'NONE',  ( 22.81628187352648496, 46.83196800326376064, -3.434112377981050290 ) ) ;
#97550=CARTESIAN_POINT ( 'NONE',  ( 10.00000000000000178, 69.31368534415484817, 10.88017736071110342 ) ) ;
#97551=CARTESIAN_POINT ( 'NONE',  ( 6.565887622018943937, 38.08196800326376064, -12.81628187352647608 ) ) ;
#97552=CARTESIAN_POINT ( 'NONE',  ( 20.36894250292379382, 8.678748834913967869, 10.36894250292379205 ) ) ;
#97554=CARTESIAN_POINT ( 'NONE',  ( 19.42250999205614548, 40.98035201082150536, -5.440088680355545492 ) ) ;
#97555=CARTESIAN_POINT ( 'NONE',  ( 2.791683348922240793, 66.63393115100079456, 7.208316651077764092 ) ) ;
#97556=CARTESIAN_POINT ( 'NONE',  ( 5.076628168052704559, 50.17559781766745886, -8.527530157486179263 ) ) ;
#97557=CARTESIAN_POINT ( 'NONE',  ( 1.472469842513823179, 16.42559781766745175, 4.923371831947296329 ) ) ;
#97558=CARTESIAN_POINT ( 'NONE',  ( 1.472469842513823179, 5.592264484334118713, -4.923371831947296329 ) ) ;
#97560=CARTESIAN_POINT ( 'NONE',  ( 20.36894250292379382, 48.67874883491396076, 10.36894250292379205 ) ) ;
#97563=CARTESIAN_POINT ( 'NONE',  ( 0.2751277870542986892, 7.282175860852375671, -6.500000000000003553 ) ) ;
#97565=CARTESIAN_POINT ( 'NONE',  ( -4.164238869374099039, 61.80374883491397497, 8.674139862899312516E-16 ) ) ;
#97566=CARTESIAN_POINT ( 'NONE',  ( 13.79529636645031943, 60.34541550158063927, -14.16423886937409904 ) ) ;
#97567=CARTESIAN_POINT ( 'NONE',  ( 5.076628168052704559, 25.17559781766745175, -8.527530157486179263 ) ) ;
#97568=CARTESIAN_POINT ( 'NONE',  ( 10.00000000000000178, 25.37363466993041783, 12.81628187352647608 ) ) ;
#97570=CARTESIAN_POINT ( 'NONE',  ( -1.926860441876562247, 42.45379003517447813, -3.195792623639530650 ) ) ;
#97571=CARTESIAN_POINT ( 'NONE',  ( 20.36894250292379382, 3.678748834913967869, 10.36894250292379205 ) ) ;
#97572=CARTESIAN_POINT ( 'NONE',  ( 7.084665262690076126, 17.02201867748817676, -10.88017736071110164 ) ) ;
#97573=CARTESIAN_POINT ( 'NONE',  ( 24.16423886937409904, 59.09541550158063217, 3.795296366450317205 ) ) ;
#97574=EDGE_CURVE ( 'NONE', #1911, #72785, #87679, .T. ) ;
#97576=CARTESIAN_POINT ( 'NONE',  ( 19.84674366389459621, 33.50893115100078745, 7.409399052514197653E-17 ) ) ;
#97578=CARTESIAN_POINT ( 'NONE',  ( 1.472469842513823179, 11.42559781766745175, 4.923371831947296329 ) ) ;
#97585=ORIENTED_EDGE ( 'NONE', *, *, #97325, .T. ) ;
#97586=CARTESIAN_POINT ( 'NONE',  ( 5.076628168052703671, 46.84226448433412315, 8.527530157486179263 ) ) ;
#97587=CARTESIAN_POINT ( 'NONE',  ( -4.164238869374099927, 17.01208216824730357, 3.795296366450308767 ) ) ;
#97588=CARTESIAN_POINT ( 'NONE',  ( 4.559911319644449179, 22.23035201082150536, -9.422509992056141925 ) ) ;
#97589=CARTESIAN_POINT ( 'NONE',  ( 7.084665262690076126, 29.10535201082150181, 10.88017736071109987 ) ) ;
#97590=CARTESIAN_POINT ( 'NONE',  ( 2.791683348922240793, 61.63393115100079456, 7.208316651077764092 ) ) ;
#97591=CARTESIAN_POINT ( 'NONE',  ( 10.00000000000000000, 22.87363466993042138, -12.81628187352647608 ) ) ;
#97592=CARTESIAN_POINT ( 'NONE',  ( 6.204703633549690345, 5.762082168247301794, -14.16423886937410259 ) ) ;
#97593=CARTESIAN_POINT ( 'NONE',  ( 20.88017736071110875, 65.77201867748817676, -2.915334737309920765 ) ) ;
#97594=EDGE_CURVE ( 'NONE', #75712, #63730, #72668, .T. ) ;
#97595=CARTESIAN_POINT ( 'NONE',  ( 21.09922568453594849, 36.20696800326375353, 6.408140936763242479 ) ) ;
#97597=CARTESIAN_POINT ( 'NONE',  ( 14.92337183194729988, 34.34226448433411605, -8.527530157486177487 ) ) ;
#97598=CARTESIAN_POINT ( 'NONE',  ( -0.3689425029237881626, 67.42874883491396076, 10.36894250292379027 ) ) ;
#97601=CARTESIAN_POINT ( 'NONE',  ( 0.5774900079438590739, 7.647018677488171434, -5.440088680355550821 ) ) ;
#97603=CARTESIAN_POINT ( 'NONE',  ( 4.559911319644449179, 53.89701867748817676, 9.422509992056141925 ) ) ;
#97604=CARTESIAN_POINT ( 'NONE',  ( 10.00000000000000178, 64.31368534415483396, 10.88017736071110342 ) ) ;
#97605=CARTESIAN_POINT ( 'NONE',  ( -0.8801773607111009756, 68.06368534415484817, 1.068504757029289695E-15 ) ) ;
#97607=CARTESIAN_POINT ( 'NONE',  ( 12.91533473730992121, 59.52201867748816966, 10.88017736071110164 ) ) ;
#97610=DIRECTION ( 'NONE',  ( 0.000000000000000000, 0.000000000000000000, -1.000000000000000000 ) ) ;
#97614=CARTESIAN_POINT ( 'NONE',  ( 10.00000000000000000, 24.75893115100078745, -9.846743663894594434 ) ) ;
#97615=ORIENTED_EDGE ( 'NONE', *, *, #66486, .F. ) ;
#97616=CARTESIAN_POINT ( 'NONE',  ( 18.52753015748618282, 53.92559781766745175, -4.923371831947291888 ) ) ;
#97617=CARTESIAN_POINT ( 'NONE',  ( -36.44000000000001194, 92.00000000000000000, -9.500000000000000000 ) ) ;
#97618=CARTESIAN_POINT ( 'NONE',  ( -4.164238869374098151, 6.595415501580634832, -3.795296366450310543 ) ) ;
#97620=CARTESIAN_POINT ( 'NONE',  ( 19.89220837332775815, 29.74062864464239553, 6.478736007405959008 ) ) ;
#97622=CARTESIAN_POINT ( 'NONE',  ( 10.00000000000000178, 4.313685344154837509, 10.88017736071110342 ) ) ;
#97624=ORIENTED_EDGE ( 'NONE', *, *, #67090, .T. ) ;
#97626=CARTESIAN_POINT ( 'NONE',  ( 12.63842701281683034, 52.46726448433413026, 9.846743663894596210 ) ) ;
#97627=CARTESIAN_POINT ( 'NONE',  ( 0.6178305044545818747, 13.49863466993041783, -9.382169495545419124 ) ) ;
#97628=CARTESIAN_POINT ( 'NONE',  ( 17.20831665107776587, 12.88393115100078390, 7.208316651077764980 ) ) ;
#97630=CARTESIAN_POINT ( 'NONE',  ( 19.38216949554541202, 0.9986346699304200492, 9.382169495545424454 ) ) ;
#97634=CARTESIAN_POINT ( 'NONE',  ( 7.084665262690076126, 4.105352010821503583, 10.88017736071109987 ) ) ;
#97635=CARTESIAN_POINT ( 'NONE',  ( -4.164238869374099039, 16.80374883491396787, 8.674139862899312516E-16 ) ) ;
#97636=CARTESIAN_POINT ( 'NONE',  ( 14.92337183194729988, 24.34226448433411960, -8.527530157486177487 ) ) ;
#97637=CARTESIAN_POINT ( 'NONE',  ( 17.96484262340118221, 61.18868534415482685, -7.964842623401177768 ) ) ;
#97638=CARTESIAN_POINT ( 'NONE',  ( 3.591859063236763294, 38.29030133659708923, -11.09922568453595026 ) ) ;
#97640=CARTESIAN_POINT ( 'NONE',  ( 10.00000000000000178, 19.31368534415484106, 10.88017736071110342 ) ) ;
#97643=CARTESIAN_POINT ( 'NONE',  ( 16.40814093676324603, 12.45696800326375353, -11.09922568453594671 ) ) ;
#97644=CARTESIAN_POINT ( 'NONE',  ( 0.1532563361054083140, 66.00893115100079456, 1.131784320476157264E-15 ) ) ;
#97645=CARTESIAN_POINT ( 'NONE',  ( 19.84674366389459266, 28.30059781766745886, 2.638427012816836559 ) ) ;
#97647=CARTESIAN_POINT ( 'NONE',  ( -1.099225684535947600, 34.54030133659708923, 6.408140936763237150 ) ) ;
#97648=DIRECTION ( 'NONE',  ( 0.000000000000000000, 1.000000000000000000, -0.000000000000000000 ) ) ;
#97650=CARTESIAN_POINT ( 'NONE',  ( 15.44008868035555793, 46.39701867748817676, -9.422509992056140149 ) ) ;
#97654=CARTESIAN_POINT ( 'NONE',  ( 7.084665262690076126, 44.10535201082151247, 10.88017736071109987 ) ) ;
#97655=CARTESIAN_POINT ( 'NONE',  ( 7.084665262690076126, 34.10535201082151247, 10.88017736071109987 ) ) ;
#97656=CARTESIAN_POINT ( 'NONE',  ( 19.84674366389459266, 63.30059781766745886, 2.638427012816836559 ) ) ;
#97657=CARTESIAN_POINT ( 'NONE',  ( -0.8801773607111008646, 58.27201867748816966, 2.915334737309923430 ) ) ;
#97658=CARTESIAN_POINT ( 'NONE',  ( 5.076628168052703671, 41.84226448433411605, 8.527530157486179263 ) ) ;
#97659=CARTESIAN_POINT ( 'NONE',  ( 15.44008868035555260, 9.730352010821505360, 9.422509992056143702 ) ) ;
#97660=CARTESIAN_POINT ( 'NONE',  ( -2.816281873526473856, 14.12363466993041961, 9.499525473075851096E-16 ) ) ;
#97662=CARTESIAN_POINT ( 'NONE',  ( 10.00000000000000000, 26.81368534415484106, -10.88017736071110342 ) ) ;
#97664=CARTESIAN_POINT ( 'NONE',  ( -0.8801773607111008646, 3.272018677488171434, 2.915334737309923430 ) ) ;
#97665=CARTESIAN_POINT ( 'NONE',  ( 0.5774900079438590739, 22.64701867748817321, -5.440088680355550821 ) ) ;
#97666=CARTESIAN_POINT ( 'NONE',  ( 15.44008868035555793, 66.39701867748817676, -9.422509992056140149 ) ) ;
#97667=CARTESIAN_POINT ( 'NONE',  ( 13.79529636645031943, 20.34541550158063572, -14.16423886937409904 ) ) ;
#97668=CARTESIAN_POINT ( 'NONE',  ( 18.52753015748618282, 18.92559781766745175, -4.923371831947291888 ) ) ;
#97669=CARTESIAN_POINT ( 'NONE',  ( -0.8801773607111009756, 43.06368534415484106, 1.068504757029289695E-15 ) ) ;
#97674=EDGE_LOOP ( 'NONE', ( #57274, #89090, #55495, #9032 ) ) ;
#97676=CARTESIAN_POINT ( 'NONE',  ( 17.20831665107776587, 47.88393115100078745, 7.208316651077764980 ) ) ;
#97678=ORIENTED_EDGE ( 'NONE', *, *, #11165, .T. ) ;
#97681=CARTESIAN_POINT ( 'NONE',  ( 22.26659068614895176, 19.72041550158063572, -7.082119434687042414 ) ) ;
#97682=CARTESIAN_POINT ( 'NONE',  ( -4.164238869374099039, 26.80374883491397142, 8.674139862899312516E-16 ) ) ;
#97683=CARTESIAN_POINT ( 'NONE',  ( 15.44008868035555793, 61.39701867748817676, -9.422509992056140149 ) ) ;
#97684=CARTESIAN_POINT ( 'NONE',  ( 6.204703633549690345, 62.84541550158063927, 14.16423886937410082 ) ) ;
#97685=CARTESIAN_POINT ( 'NONE',  ( 6.565887622018943937, 5.165301336597086568, 12.81628187352647430 ) ) ;
#97686=CARTESIAN_POINT ( 'NONE',  ( 19.84674366389459266, 53.30059781766744464, 2.638427012816836559 ) ) ;
#97687=CARTESIAN_POINT ( 'NONE',  ( 15.44008868035555793, 51.39701867748816966, -9.422509992056140149 ) ) ;
#97688=CARTESIAN_POINT ( 'NONE',  ( 6.565887622018943937, 10.16530133659708746, 12.81628187352647430 ) ) ;
#97689=CARTESIAN_POINT ( 'NONE',  ( 13.79529636645031943, 10.34541550158063394, -14.16423886937409904 ) ) ;
#97690=CARTESIAN_POINT ( 'NONE',  ( -0.8801773607111009756, 13.06368534415483929, 1.068504757029289695E-15 ) ) ;
#97692=CARTESIAN_POINT ( 'NONE',  ( 4.559911319644449179, 23.89701867748817321, 9.422509992056141925 ) ) ;
#97694=CARTESIAN_POINT ( 'NONE',  ( 12.91533473730992121, 44.52201867748816966, 10.88017736071110164 ) ) ;
#97695=CARTESIAN_POINT ( 'NONE',  ( 13.43411237798105340, 50.58196800326375353, 12.81628187352647963 ) ) ;
#97697=EDGE_LOOP ( 'NONE', ( #29708, #85803, #465, #44647 ) ) ;
#97702=CARTESIAN_POINT ( 'NONE',  ( 2.917880565312948704, 47.63708216824730357, 12.26659068614894643 ) ) ;
#97703=CARTESIAN_POINT ( 'NONE',  ( 2.035157376598824452, 8.688685344154839285, 7.964842623401179544 ) ) ;
#97704=CARTESIAN_POINT ( 'NONE',  ( 14.92337183194729988, 24.34226448433411960, -8.527530157486177487 ) ) ;
#97705=CARTESIAN_POINT ( 'NONE',  ( 0.1532563361054100626, 45.80059781766745886, -2.638427012816831230 ) ) ;
#97709=CARTESIAN_POINT ( 'NONE',  ( 19.84674366389459266, 3.717264484334118713, -2.638427012816827677 ) ) ;
#97710=VECTOR ( 'NONE', #23825, 1000.000000000000000 ) ;
#97711=B_SPLINE_CURVE_WITH_KNOTS ( 'NONE', 3,
 ( #26553, #33068, #3584, #41589 ),
 .UNSPECIFIED., .F., .F.,
 ( 4, 4 ),
 ( 1.283695372222837250E-16, 0.001060528352562002848 ),
 .UNSPECIFIED. ) ;
#97715=CARTESIAN_POINT ( 'NONE',  ( 6.204703633549690345, 27.84541550158063217, 14.16423886937410082 ) ) ;
#97717=CARTESIAN_POINT ( 'NONE',  ( 0.6178305044545818747, 18.49863466993041428, -9.382169495545419124 ) ) ;
#97718=ORIENTED_EDGE ( 'NONE', *, *, #14589, .F. ) ;
#97719=CARTESIAN_POINT ( 'NONE',  ( 16.40814093676324603, 42.45696800326375353, -11.09922568453594671 ) ) ;
#97720=CARTESIAN_POINT ( 'NONE',  ( 20.88017736071110875, 15.77201867748817143, -2.915334737309920765 ) ) ;
#97721=CARTESIAN_POINT ( 'NONE',  ( 1.472469842513823179, 40.59226448433411605, -4.923371831947296329 ) ) ;
#97722=CARTESIAN_POINT ( 'NONE',  ( -0.8801773607111009756, 18.06368534415484106, 1.068504757029289695E-15 ) ) ;
#97724=CARTESIAN_POINT ( 'NONE',  ( 6.565887622018943937, 63.08196800326376064, -12.81628187352647608 ) ) ;
#97726=CARTESIAN_POINT ( 'NONE',  ( 17.20831665107776587, 47.88393115100078745, 7.208316651077764980 ) ) ;
#97727=CARTESIAN_POINT ( 'NONE',  ( 0.1532563361054100626, 55.80059781766745175, -2.638427012816831230 ) ) ;
#97735=CARTESIAN_POINT ( 'NONE',  ( 17.20831665107776587, 14.13393115100078568, -7.208316651077762316 ) ) ;
#97736=CARTESIAN_POINT ( 'NONE',  ( 6.565887622018943937, 43.08196800326374643, -12.81628187352647608 ) ) ;
#97738=ORIENTED_EDGE ( 'NONE', *, *, #40647, .F. ) ;
#97739=CARTESIAN_POINT ( 'NONE',  ( 10.00000000000000178, 52.25893115100078745, 9.846743663894594434 ) ) ;
#97741=CARTESIAN_POINT ( 'NONE',  ( 24.16423886937410614, 34.51208216824731068, -3.795296366450302550 ) ) ;
#97742=CARTESIAN_POINT ( 'NONE',  ( 10.00000000000000000, 44.75893115100078745, -9.846743663894594434 ) ) ;
#97743=CARTESIAN_POINT ( 'NONE',  ( 19.38216949554541557, 52.24863466993041072, -9.382169495545420901 ) ) ;
#97746=CARTESIAN_POINT ( 'NONE',  ( 17.20831665107776587, 7.883931151000784787, 7.208316651077764980 ) ) ;
#97748=CARTESIAN_POINT ( 'NONE',  ( 5.076628168052703671, 51.84226448433412315, 8.527530157486179263 ) ) ;
#97749=CARTESIAN_POINT ( 'NONE',  ( 20.88017736071110875, 40.77201867748818387, -2.915334737309920765 ) ) ;
#97751=STYLED_ITEM ( 'NONE', ( #54021 ), #81586 ) ;
#97752=CARTESIAN_POINT ( 'NONE',  ( 10.00000000000000000, 41.81368534415484106, -10.88017736071110342 ) ) ;
#97754=LINE ( 'NONE', #35740, #12242 ) ;
#97755=CARTESIAN_POINT ( 'NONE',  ( 20.88017736071110875, 20.77201867748816611, -2.915334737309920765 ) ) ;
#97756=CARTESIAN_POINT ( 'NONE',  ( 22.81628187352647785, 6.415301336597088344, 3.434112377981063169 ) ) ;
#97757=CARTESIAN_POINT ( 'NONE',  ( 0.5774900079438607392, 38.48035201082150536, 5.440088680355550821 ) ) ;
#97758=CARTESIAN_POINT ( 'NONE',  ( -0.1503990784575294781, 48.10158574516642460, 6.262539305110072618 ) ) ;
#97759=CARTESIAN_POINT ( 'NONE',  ( 19.42250999205614193, 65.14701867748817676, 5.440088680355555262 ) ) ;
#97761=CARTESIAN_POINT ( 'NONE',  ( -0.8801773607110991993, 32.85535201082151247, -2.915334737309923874 ) ) ;
#97762=CARTESIAN_POINT ( 'NONE',  ( -46.76855771576528298, 100.6387111820534415, 9.385180859874349579 ) ) ;
#97763=CARTESIAN_POINT ( 'NONE',  ( 0.1532563361054100626, 10.80059781766745175, -2.638427012816831230 ) ) ;
#97764=EDGE_CURVE ( 'NONE', #26202, #37993, #7612, .T. ) ;
#97765=CARTESIAN_POINT ( 'NONE',  ( 10.00000000000000178, 27.25893115100078390, 9.846743663894594434 ) ) ;
#97767=( BOUNDED_SURFACE ( )  B_SPLINE_SURFACE ( 1, 2, ( 
 ( #51075, #66576, #94734, #73567, #66070, #63732, #96598, #13074, #97103, #94232, #25764, #41269, #36439, #74419, #6424, #28440, #66932, #21439, #89437, #97453, #66433, #96968, #58937, #20950, #51437, #81927, #13435, #86613, #17633, #56116, #78617, #48104, #10126, #79099, #9627, #40623, #71121, #18123, #48595, #40126, #70626, #2154, #53166, #45668, #38661, #30644, #22684, #83670, #53657, #46166, #61153, #76165, #91663, #689, #31142, #7686, #38183, #3996, #72848, #79882, #56409, #62910, #33382, #71419, #17916, #48400, #55417, #41426, #3408, #24935, #40919, #47413, #33869, #34370, #18405, #71887, #77914, #48887, #93412, #78903, #63400, #10412, #85925, #40429, #18904, #17434, #47902, #26384, #64376, #93906, #2935, #78406, #64860, #63880, #79399, #26881, #94391, #9423, #86895, #32901, #41910, #95380, #25907, #9925, #94885, #70925, #2445, #25433, #85423, #55916, #86415, #56883, #10904, #87386, #16933, #49381, #11388, #70428, #72371, #3902, #39926, #1947, #32409, #28838, #57374, #12857, #19869, #89356, #28361, #66346, #74337, #95889, #59340, #20373, #81359, #20866, #19385, #67347, #27857, #35857, #50867, #42876, #44339, #43355, #36356, #51851, #49869, #6345, #21358, #65857, #73853, #58345, #5383, #74845, #4886, #12370, #89843, #82339, #57862, #96885, #88864, #97873, #87869, #27369, #66851, #42386, #50363, #88373, #80872, #13859, #58850, #51357, #81842, #96385, #36856, #13356, #73359, #43841, #5862, #35364, #97370, #80383, #11883, #72863, #4398, #34867, #65360, #61314, #84338, #90324, #91826, #6846, #22848, #7353, #91321, #37358, #83336, #61805, #98369, #67851, #69325, #46325, #37854, #53322, #90828, #10174, #83829, #23344, #71171, #15356, #21863, #30816, #75832, #86172, #78668, #7844, #29825, #38831, #52830, #60335, #22354, #40672, #14860, #45333, #845, #38341, #68344, #29333, #31304, #53826, #14358, #45841, #15840, #76812, #68836, #59831, #93659, #52342, #76325, #98865, #8327, #367, #25195, #55672, #30319, #17681, #48155, #82837, #44827, #75333, #60821, #72133, #80130, #95126, #87134, #88611, #26634, #80633, #96137, #94149, #50624, #65610, #11146, #57132, #3660, #87629, #20121, #49146, #56649, #35111, #27618, #3167, #19143, #34124, #43118, #2696, #41177, #12129, #86661, #94645, #33629, #71658, #58105, #49619, #42152, #64616, #41665, #81115, #72617, #64128, #11637, #12617, #63642, #33148, #4152, #42630, #34617, #10662, #25676, #26155, #56170, #65114, #79149, #95635, #27122, #18658, #18166, #57623, #88121, #19632, #50123, #48646, #73108, #79648, #4649, #91080, #35621, #53083, #74602, #83092, #29095, #81602, #15109, #43609, #68101 ),
 ( #28111, #21118, #67611, #13113, #52106, #5131, #98117, #22110, #98628, #5629, #51617, #30079, #75592, #36107, #44598, #97630, #74096, #82099, #22605, #83594, #13612, #44092, #45087, #7104, #66612, #14621, #66105, #96635, #97140, #52591, #6115, #73606, #60586, #36620, #67106, #59595, #82598, #37607, #29578, #90092, #60082, #58611, #90585, #89113, #14114, #21619, #75094, #20625, #28610, #6601, #37114, #51114, #59099, #89608, #31065, #47556, #70558, #38105, #16577, #1095, #84579, #77548, #31557, #39578, #92556, #25074, #68595, #46566, #85562, #92074, #54064, #38587, #2085, #47052, #16079, #122, #15601, #46086, #32545, #30572, #7611, #78054, #63046, #53573, #23102, #8578, #69575, #62542, #84087, #62053, #39081, #9067, #61564, #76572, #9557, #70070, #40058, #93542, #55556, #17073, #61074, #23600, #1591, #8091, #24082, #76083, #32040, #93048, #86058, #69085, #77065, #45586, #91587, #619, #24582, #54549, #85067, #55043, #34996, #96021, #64015, #26047, #88008, #19520, #10544, #27013, #10059, #40557, #56054, #95520, #56537, #65499, #42518, #94527, #87027, #11035, #95012, #64994, #42043, #18539, #72507, #4532, #34502, #27502, #26521, #49030, #34011, #57511, #79031, #79535, #41557, #72021, #50016, #57017, #3065, #80520, #73001, #71057, #87519, #3550, #64508, #49510, #19033, #11519, #80017, #57998, #2581, #4040, #12018, #17569, #48035, #41054, #78547, #33036, #63532, #94040, #86547, #18054, #25563, #48531, #71553, #33519, #44970, #96523, #65995, #51493, #13499, #6485, #27995, #43978, #81987, #21498, #73989, #58492, #90465, #82484, #22000, #6990, #37494, #21006, #74981, #67982, #29464, #20510, #66991, #50995, #43008, #35500, #81490, #36992, #73490, #74482, #97514, #28977, #59970, #82980, #97022, #89003, #52475, #12993, #28499, #43489, #6004, #98509, #5516, #36499, #58993, #29963, #59480, #66496, #89981, #67488, #35993, #89495, #51995, #14002, #98010, #44479, #14500, #75475, #88504, #81006, #20007, #50508, #12507, #5017, #15962, #54437, #8457, #39941, #52963, #61448, #1470, #7977, #68969, #53455, #16948, #31437, #500, #14996, #30455, #60954, #47433, #45466, #22490, #62424, #77932, #68480, #37988, #23484, #84464, #77430, #6, #46454, #53957, #92440, #45972, #91463, #92927, #84946, #24459, #9440, #70444, #91954, #46937, #1961, #31924, #22989, #38963, #83962, #75966, #7494, #15489, #8942, #76462, #76947, #69456, #974, #54925, #85441, #30949, #38476, #60469, #61938, #23963, #16457, #39461, #90958, #69951, #83474, #2949, #72388, #85941, #78919, #26398, #70945, #10917, #62928, #56898, #79897, #26898, #63421, #10429, #87883, #34385 ) ),
 .UNSPECIFIED., .F., .F., .F. ) 
 B_SPLINE_SURFACE_WITH_KNOTS ( ( 2, 2 ),
 ( 3, 2, 2, 2, 2, 2, 2, 2, 2, 2, 2, 2, 2, 2, 2, 2, 2, 2, 2, 2, 2, 2, 2, 2, 2, 2, 2, 2, 2, 2, 2, 2, 2, 2, 2, 2, 2, 2, 2, 2, 2, 2, 2, 2, 2, 2, 2, 2, 2, 2, 2, 2, 2, 2, 2, 2, 2, 2, 2, 2, 2, 2, 2, 2, 2, 2, 2, 2, 2, 2, 2, 2, 2, 2, 2, 2, 2, 2, 2, 2, 2, 2, 2, 2, 2, 2, 2, 2, 2, 2, 2, 2, 2, 2, 2, 2, 2, 2, 2, 2, 2, 2, 2, 2, 2, 2, 2, 2, 2, 2, 2, 2, 2, 2, 2, 2, 2, 2, 2, 2, 2, 2, 2, 2, 2, 2, 2, 2, 2, 2, 2, 2, 2, 2, 2, 2, 2, 2, 2, 2, 2, 2, 2, 2, 2, 2, 2, 2, 2, 2, 2, 2, 2, 2, 2, 2, 2, 2, 2, 2, 2, 2, 3 ),
 ( 0.000000000000000000, 1.000000000000000000 ),
 ( 0.000000000000000000, 0.005952380952380952051, 0.01190476190476190410, 0.01785714285714285615, 0.02380952380952380820, 0.02976190476190476025, 0.03571428571428571230, 0.04166666666666666435, 0.04761904761904761640, 0.05357142857142856845, 0.05952380952380952051, 0.06547619047619047949, 0.07142857142857142461, 0.07738095238095238360, 0.08333333333333332871, 0.08928571428571428770, 0.09523809523809523281, 0.1011904761904761918, 0.1071428571428571369, 0.1130952380952380959, 0.1190476190476190410, 0.1250000000000000000, 0.1309523809523809590, 0.1369047619047619180, 0.1428571428571428492, 0.1488095238095238082, 0.1547619047619047672, 0.1607142857142857262, 0.1666666666666666574, 0.1726190476190476164, 0.1785714285714285754, 0.1845238095238095344, 0.1904761904761904656, 0.1964285714285714246, 0.2023809523809523836, 0.2083333333333333426, 0.2142857142857142738, 0.2202380952380952328, 0.2261904761904761918, 0.2321428571428571508, 0.2380952380952380820, 0.2440476190476190410, 0.2500000000000000000, 0.2559523809523809312, 0.2619047619047619180, 0.2678571428571428492, 0.2738095238095238360, 0.2797619047619047672, 0.2857142857142856984, 0.2916666666666666852, 0.2976190476190476164, 0.3035714285714285476, 0.3095238095238095344, 0.3154761904761904656, 0.3214285714285714524, 0.3273809523809523836, 0.3333333333333333148, 0.3392857142857143016, 0.3452380952380952328, 0.3511904761904761640, 0.3571428571428571508, 0.3630952380952380820, 0.3690476190476190688, 0.3750000000000000000, 0.3809523809523809312, 0.3869047619047619180, 0.3928571428571428492, 0.3988095238095238360, 0.4047619047619047672, 0.4107142857142856984, 0.4166666666666666852, 0.4226190476190476164, 0.4285714285714285476, 0.4345238095238095344, 0.4404761904761904656, 0.4464285714285714524, 0.4523809523809523836, 0.4583333333333333148, 0.4642857142857143016, 0.4702380952380952328, 0.4761904761904761640, 0.4821428571428571508, 0.4880952380952380820, 0.4940476190476190688, 0.5000000000000000000, 0.5059523809523809312, 0.5119047619047618625, 0.5178571428571429047, 0.5238095238095238360, 0.5297619047619047672, 0.5357142857142856984, 0.5416666666666666297, 0.5476190476190476719, 0.5535714285714286031, 0.5595238095238095344, 0.5654761904761904656, 0.5714285714285713969, 0.5773809523809523281, 0.5833333333333333703, 0.5892857142857143016, 0.5952380952380952328, 0.6011904761904761640, 0.6071428571428570953, 0.6130952380952381375, 0.6190476190476190688, 0.6250000000000000000, 0.6309523809523809312, 0.6369047619047618625, 0.6428571428571429047, 0.6488095238095238360, 0.6547619047619047672, 0.6607142857142856984, 0.6666666666666666297, 0.6726190476190476719, 0.6785714285714286031, 0.6845238095238095344, 0.6904761904761904656, 0.6964285714285713969, 0.7023809523809523281, 0.7083333333333333703, 0.7142857142857143016, 0.7202380952380952328, 0.7261904761904761640, 0.7321428571428570953, 0.7380952380952381375, 0.7440476190476190688, 0.7500000000000000000, 0.7559523809523809312, 0.7619047619047618625, 0.7678571428571429047, 0.7738095238095238360, 0.7797619047619047672, 0.7857142857142856984, 0.7916666666666666297, 0.7976190476190476719, 0.8035714285714286031, 0.8095238095238095344, 0.8154761904761904656, 0.8214285714285713969, 0.8273809523809523281, 0.8333333333333333703, 0.8392857142857143016, 0.8452380952380952328, 0.8511904761904761640, 0.8571428571428570953, 0.8630952380952381375, 0.8690476190476190688, 0.8750000000000000000, 0.8809523809523809312, 0.8869047619047618625, 0.8928571428571429047, 0.8988095238095238360, 0.9047619047619047672, 0.9107142857142856984, 0.9166666666666666297, 0.9226190476190476719, 0.9285714285714286031, 0.9345238095238095344, 0.9404761904761904656, 0.9464285714285713969, 0.9523809523809523281, 0.9583333333333333703, 0.9642857142857143016 ),
 .UNSPECIFIED. ) 
 GEOMETRIC_REPRESENTATION_ITEM ( )  RATIONAL_B_SPLINE_SURFACE ( (
 ( 1.000000000000000000, 0.9659258262890683122, 1.000000000000000000, 0.9659258262890683122, 1.000000000000000000, 0.9659258262890683122, 1.000000000000000000, 0.9659258262890683122, 1.000000000000000000, 0.9659258262890683122, 1.000000000000000000, 0.9659258262890683122, 1.000000000000000000, 0.9659258262890683122, 1.000000000000000000, 0.9659258262890683122, 1.000000000000000000, 0.9659258262890683122, 1.000000000000000000, 0.9659258262890683122, 1.000000000000000000, 0.9659258262890683122, 1.000000000000000000, 0.9659258262890683122, 1.000000000000000000, 0.9659258262890683122, 1.000000000000000000, 0.9659258262890683122, 1.000000000000000000, 0.9659258262890683122, 1.000000000000000000, 0.9659258262890683122, 1.000000000000000000, 0.9659258262890683122, 1.000000000000000000, 0.9659258262890683122, 1.000000000000000000, 0.9659258262890683122, 1.000000000000000000, 0.9659258262890683122, 1.000000000000000000, 0.9659258262890683122, 1.000000000000000000, 0.9659258262890683122, 1.000000000000000000, 0.9659258262890683122, 1.000000000000000000, 0.9659258262890683122, 1.000000000000000000, 0.9659258262890683122, 1.000000000000000000, 0.9659258262890683122, 1.000000000000000000, 0.9659258262890683122, 1.000000000000000000, 0.9659258262890683122, 1.000000000000000000, 0.9659258262890683122, 1.000000000000000000, 0.9659258262890683122, 1.000000000000000000, 0.9659258262890683122, 1.000000000000000000, 0.9659258262890683122, 1.000000000000000000, 0.9659258262890683122, 1.000000000000000000, 0.9659258262890683122, 1.000000000000000000, 0.9659258262890683122, 1.000000000000000000, 0.9659258262890683122, 1.000000000000000000, 0.9659258262890683122, 1.000000000000000000, 0.9659258262890683122, 1.000000000000000000, 0.9659258262890683122, 1.000000000000000000, 0.9659258262890683122, 1.000000000000000000, 0.9659258262890683122, 1.000000000000000000, 0.9659258262890683122, 1.000000000000000000, 0.9659258262890683122, 1.000000000000000000, 0.9659258262890683122, 1.000000000000000000, 0.9659258262890683122, 1.000000000000000000, 0.9659258262890683122, 1.000000000000000000, 0.9659258262890683122, 1.000000000000000000, 0.9659258262890683122, 1.000000000000000000, 0.9659258262890683122, 1.000000000000000000, 0.9659258262890683122, 1.000000000000000000, 0.9659258262890683122, 1.000000000000000000, 0.9659258262890683122, 1.000000000000000000, 0.9659258262890683122, 1.000000000000000000, 0.9659258262890683122, 1.000000000000000000, 0.9659258262890683122, 1.000000000000000000, 0.9659258262890683122, 1.000000000000000000, 0.9659258262890683122, 1.000000000000000000, 0.9659258262890683122, 1.000000000000000000, 0.9659258262890683122, 1.000000000000000000, 0.9659258262890683122, 1.000000000000000000, 0.9659258262890683122, 1.000000000000000000, 0.9659258262890683122, 1.000000000000000000, 0.9659258262890683122, 1.000000000000000000, 0.9659258262890683122, 1.000000000000000000, 0.9659258262890683122, 1.000000000000000000, 0.9659258262890683122, 1.000000000000000000, 0.9659258262890683122, 1.000000000000000000, 0.9659258262890683122, 1.000000000000000000, 0.9659258262890683122, 1.000000000000000000, 0.9659258262890683122, 1.000000000000000000, 0.9659258262890683122, 1.000000000000000000, 0.9659258262890683122, 1.000000000000000000, 0.9659258262890683122, 1.000000000000000000, 0.9659258262890683122, 1.000000000000000000, 0.9659258262890683122, 1.000000000000000000, 0.9659258262890683122, 1.000000000000000000, 0.9659258262890683122, 1.000000000000000000, 0.9659258262890683122, 1.000000000000000000, 0.9659258262890683122, 1.000000000000000000, 0.9659258262890683122, 1.000000000000000000, 0.9659258262890683122, 1.000000000000000000, 0.9659258262890683122, 1.000000000000000000, 0.9659258262890683122, 1.000000000000000000, 0.9659258262890683122, 1.000000000000000000, 0.9659258262890683122, 1.000000000000000000, 0.9659258262890683122, 1.000000000000000000, 0.9659258262890683122, 1.000000000000000000, 0.9659258262890683122, 1.000000000000000000, 0.9659258262890683122, 1.000000000000000000, 0.9659258262890683122, 1.000000000000000000, 0.9659258262890683122, 1.000000000000000000, 0.9659258262890683122, 1.000000000000000000, 0.9659258262890683122, 1.000000000000000000, 0.9659258262890683122, 1.000000000000000000, 0.9659258262890683122, 1.000000000000000000, 0.9659258262890683122, 1.000000000000000000, 0.9659258262890683122, 1.000000000000000000, 0.9659258262890683122, 1.000000000000000000, 0.9659258262890683122, 1.000000000000000000, 0.9659258262890683122, 1.000000000000000000, 0.9659258262890683122, 1.000000000000000000, 0.9659258262890683122, 1.000000000000000000, 0.9659258262890683122, 1.000000000000000000, 0.9659258262890683122, 1.000000000000000000, 0.9659258262890683122, 1.000000000000000000, 0.9659258262890683122, 1.000000000000000000, 0.9659258262890683122, 1.000000000000000000, 0.9659258262890683122, 1.000000000000000000, 0.9659258262890683122, 1.000000000000000000, 0.9659258262890683122, 1.000000000000000000, 0.9659258262890683122, 1.000000000000000000, 0.9659258262890683122, 1.000000000000000000, 0.9659258262890683122, 1.000000000000000000, 0.9659258262890683122, 1.000000000000000000, 0.9659258262890683122, 1.000000000000000000, 0.9659258262890683122, 1.000000000000000000, 0.9659258262890683122, 1.000000000000000000, 0.9659258262890683122, 1.000000000000000000, 0.9659258262890683122, 1.000000000000000000, 0.9659258262890683122, 1.000000000000000000, 0.9659258262890683122, 1.000000000000000000, 0.9659258262890683122, 1.000000000000000000, 0.9659258262890683122, 1.000000000000000000, 0.9659258262890683122, 1.000000000000000000, 0.9659258262890683122, 1.000000000000000000, 0.9659258262890683122, 1.000000000000000000, 0.9659258262890683122, 1.000000000000000000, 0.9659258262890683122, 1.000000000000000000, 0.9659258262890683122, 1.000000000000000000, 0.9659258262890683122, 1.000000000000000000, 0.9659258262890683122, 1.000000000000000000, 0.9659258262890683122, 1.000000000000000000, 0.9659258262890683122, 1.000000000000000000, 0.9659258262890683122, 1.000000000000000000, 0.9659258262890683122, 1.000000000000000000, 0.9659258262890683122, 1.000000000000000000, 0.9659258262890683122, 1.000000000000000000, 0.9659258262890683122, 1.000000000000000000, 0.9659258262890683122, 1.000000000000000000, 0.9659258262890683122, 1.000000000000000000, 0.9659258262890683122, 1.000000000000000000, 0.9659258262890683122, 1.000000000000000000, 0.9659258262890683122, 1.000000000000000000, 0.9659258262890683122, 1.000000000000000000, 0.9659258262890683122, 1.000000000000000000, 0.9659258262890683122, 1.000000000000000000, 0.9659258262890683122, 1.000000000000000000, 0.9659258262890683122, 1.000000000000000000, 0.9659258262890683122, 1.000000000000000000, 0.9659258262890683122, 1.000000000000000000, 0.9659258262890683122, 1.000000000000000000, 0.9659258262890683122, 1.000000000000000000, 0.9659258262890683122, 1.000000000000000000, 0.9659258262890683122, 1.000000000000000000, 0.9659258262890683122, 1.000000000000000000, 0.9659258262890683122, 1.000000000000000000, 0.9659258262890683122, 1.000000000000000000, 0.9659258262890683122, 1.000000000000000000, 0.9659258262890683122, 1.000000000000000000, 0.9659258262890683122, 1.000000000000000000, 0.9659258262890683122, 1.000000000000000000, 0.9659258262890683122, 1.000000000000000000),
 ( 1.000000000000000000, 0.9659258262890683122, 1.000000000000000000, 0.9659258262890683122, 1.000000000000000000, 0.9659258262890683122, 1.000000000000000000, 0.9659258262890683122, 1.000000000000000000, 0.9659258262890683122, 1.000000000000000000, 0.9659258262890683122, 1.000000000000000000, 0.9659258262890683122, 1.000000000000000000, 0.9659258262890683122, 1.000000000000000000, 0.9659258262890683122, 1.000000000000000000, 0.9659258262890683122, 1.000000000000000000, 0.9659258262890683122, 1.000000000000000000, 0.9659258262890683122, 1.000000000000000000, 0.9659258262890683122, 1.000000000000000000, 0.9659258262890683122, 1.000000000000000000, 0.9659258262890683122, 1.000000000000000000, 0.9659258262890683122, 1.000000000000000000, 0.9659258262890683122, 1.000000000000000000, 0.9659258262890683122, 1.000000000000000000, 0.9659258262890683122, 1.000000000000000000, 0.9659258262890683122, 1.000000000000000000, 0.9659258262890683122, 1.000000000000000000, 0.9659258262890683122, 1.000000000000000000, 0.9659258262890683122, 1.000000000000000000, 0.9659258262890683122, 1.000000000000000000, 0.9659258262890683122, 1.000000000000000000, 0.9659258262890683122, 1.000000000000000000, 0.9659258262890683122, 1.000000000000000000, 0.9659258262890683122, 1.000000000000000000, 0.9659258262890683122, 1.000000000000000000, 0.9659258262890683122, 1.000000000000000000, 0.9659258262890683122, 1.000000000000000000, 0.9659258262890683122, 1.000000000000000000, 0.9659258262890683122, 1.000000000000000000, 0.9659258262890683122, 1.000000000000000000, 0.9659258262890683122, 1.000000000000000000, 0.9659258262890683122, 1.000000000000000000, 0.9659258262890683122, 1.000000000000000000, 0.9659258262890683122, 1.000000000000000000, 0.9659258262890683122, 1.000000000000000000, 0.9659258262890683122, 1.000000000000000000, 0.9659258262890683122, 1.000000000000000000, 0.9659258262890683122, 1.000000000000000000, 0.9659258262890683122, 1.000000000000000000, 0.9659258262890683122, 1.000000000000000000, 0.9659258262890683122, 1.000000000000000000, 0.9659258262890683122, 1.000000000000000000, 0.9659258262890683122, 1.000000000000000000, 0.9659258262890683122, 1.000000000000000000, 0.9659258262890683122, 1.000000000000000000, 0.9659258262890683122, 1.000000000000000000, 0.9659258262890683122, 1.000000000000000000, 0.9659258262890683122, 1.000000000000000000, 0.9659258262890683122, 1.000000000000000000, 0.9659258262890683122, 1.000000000000000000, 0.9659258262890683122, 1.000000000000000000, 0.9659258262890683122, 1.000000000000000000, 0.9659258262890683122, 1.000000000000000000, 0.9659258262890683122, 1.000000000000000000, 0.9659258262890683122, 1.000000000000000000, 0.9659258262890683122, 1.000000000000000000, 0.9659258262890683122, 1.000000000000000000, 0.9659258262890683122, 1.000000000000000000, 0.9659258262890683122, 1.000000000000000000, 0.9659258262890683122, 1.000000000000000000, 0.9659258262890683122, 1.000000000000000000, 0.9659258262890683122, 1.000000000000000000, 0.9659258262890683122, 1.000000000000000000, 0.9659258262890683122, 1.000000000000000000, 0.9659258262890683122, 1.000000000000000000, 0.9659258262890683122, 1.000000000000000000, 0.9659258262890683122, 1.000000000000000000, 0.9659258262890683122, 1.000000000000000000, 0.9659258262890683122, 1.000000000000000000, 0.9659258262890683122, 1.000000000000000000, 0.9659258262890683122, 1.000000000000000000, 0.9659258262890683122, 1.000000000000000000, 0.9659258262890683122, 1.000000000000000000, 0.9659258262890683122, 1.000000000000000000, 0.9659258262890683122, 1.000000000000000000, 0.9659258262890683122, 1.000000000000000000, 0.9659258262890683122, 1.000000000000000000, 0.9659258262890683122, 1.000000000000000000, 0.9659258262890683122, 1.000000000000000000, 0.9659258262890683122, 1.000000000000000000, 0.9659258262890683122, 1.000000000000000000, 0.9659258262890683122, 1.000000000000000000, 0.9659258262890683122, 1.000000000000000000, 0.9659258262890683122, 1.000000000000000000, 0.9659258262890683122, 1.000000000000000000, 0.9659258262890683122, 1.000000000000000000, 0.9659258262890683122, 1.000000000000000000, 0.9659258262890683122, 1.000000000000000000, 0.9659258262890683122, 1.000000000000000000, 0.9659258262890683122, 1.000000000000000000, 0.9659258262890683122, 1.000000000000000000, 0.9659258262890683122, 1.000000000000000000, 0.9659258262890683122, 1.000000000000000000, 0.9659258262890683122, 1.000000000000000000, 0.9659258262890683122, 1.000000000000000000, 0.9659258262890683122, 1.000000000000000000, 0.9659258262890683122, 1.000000000000000000, 0.9659258262890683122, 1.000000000000000000, 0.9659258262890683122, 1.000000000000000000, 0.9659258262890683122, 1.000000000000000000, 0.9659258262890683122, 1.000000000000000000, 0.9659258262890683122, 1.000000000000000000, 0.9659258262890683122, 1.000000000000000000, 0.9659258262890683122, 1.000000000000000000, 0.9659258262890683122, 1.000000000000000000, 0.9659258262890683122, 1.000000000000000000, 0.9659258262890683122, 1.000000000000000000, 0.9659258262890683122, 1.000000000000000000, 0.9659258262890683122, 1.000000000000000000, 0.9659258262890683122, 1.000000000000000000, 0.9659258262890683122, 1.000000000000000000, 0.9659258262890683122, 1.000000000000000000, 0.9659258262890683122, 1.000000000000000000, 0.9659258262890683122, 1.000000000000000000, 0.9659258262890683122, 1.000000000000000000, 0.9659258262890683122, 1.000000000000000000, 0.9659258262890683122, 1.000000000000000000, 0.9659258262890683122, 1.000000000000000000, 0.9659258262890683122, 1.000000000000000000, 0.9659258262890683122, 1.000000000000000000, 0.9659258262890683122, 1.000000000000000000, 0.9659258262890683122, 1.000000000000000000, 0.9659258262890683122, 1.000000000000000000, 0.9659258262890683122, 1.000000000000000000, 0.9659258262890683122, 1.000000000000000000, 0.9659258262890683122, 1.000000000000000000, 0.9659258262890683122, 1.000000000000000000, 0.9659258262890683122, 1.000000000000000000, 0.9659258262890683122, 1.000000000000000000, 0.9659258262890683122, 1.000000000000000000, 0.9659258262890683122, 1.000000000000000000, 0.9659258262890683122, 1.000000000000000000, 0.9659258262890683122, 1.000000000000000000, 0.9659258262890683122, 1.000000000000000000, 0.9659258262890683122, 1.000000000000000000, 0.9659258262890683122, 1.000000000000000000, 0.9659258262890683122, 1.000000000000000000, 0.9659258262890683122, 1.000000000000000000, 0.9659258262890683122, 1.000000000000000000, 0.9659258262890683122, 1.000000000000000000, 0.9659258262890683122, 1.000000000000000000, 0.9659258262890683122, 1.000000000000000000, 0.9659258262890683122, 1.000000000000000000, 0.9659258262890683122, 1.000000000000000000, 0.9659258262890683122, 1.000000000000000000, 0.9659258262890683122, 1.000000000000000000, 0.9659258262890683122, 1.000000000000000000, 0.9659258262890683122, 1.000000000000000000, 0.9659258262890683122, 1.000000000000000000, 0.9659258262890683122, 1.000000000000000000, 0.9659258262890683122, 1.000000000000000000, 0.9659258262890683122, 1.000000000000000000, 0.9659258262890683122, 1.000000000000000000, 0.9659258262890683122, 1.000000000000000000, 0.9659258262890683122, 1.000000000000000000, 0.9659258262890683122, 1.000000000000000000, 0.9659258262890683122, 1.000000000000000000, 0.9659258262890683122, 1.000000000000000000) ) ) 
 REPRESENTATION_ITEM ( '' )  SURFACE ( )  );
#97769=CARTESIAN_POINT ( 'NONE',  ( 3.591859063236763294, -1.709698663402913210, -11.09922568453595026 ) ) ;
#97770=CARTESIAN_POINT ( 'NONE',  ( 10.00000000000000000, 65.55374883491396076, -14.16423886937410082 ) ) ;
#97773=CARTESIAN_POINT ( 'NONE',  ( 20.36894250292379738, 4.928748834913967869, -10.36894250292379027 ) ) ;
#97774=CARTESIAN_POINT ( 'NONE',  ( -0.3689425029237881626, 47.42874883491396787, 10.36894250292379027 ) ) ;
#97775=STYLED_ITEM ( 'NONE', ( #52419 ), #64438 ) ;
#97778=CARTESIAN_POINT ( 'NONE',  ( 19.84674366389459621, 23.50893115100078390, 7.409399052514197653E-17 ) ) ;
#97779=CARTESIAN_POINT ( 'NONE',  ( -0.8801773607111008646, 8.272018677488171434, 2.915334737309923430 ) ) ;
#97780=CARTESIAN_POINT ( 'NONE',  ( 1.472469842513823179, 51.42559781766745886, 4.923371831947296329 ) ) ;
#97781=CARTESIAN_POINT ( 'NONE',  ( 0.2751277870542911952, 34.36607318730131055, -6.499999999999992006 ) ) ;
#97783=B_SPLINE_CURVE_WITH_KNOTS ( 'NONE', 3,
 ( #48519, #2571, #47545, #49016, #93532, #48024 ),
 .UNSPECIFIED., .F., .F.,
 ( 4, 2, 4 ),
 ( 0.000000000000000000, 0.0002701661927229356613, 0.0005403323854458713226 ),
 .UNSPECIFIED. ) ;
#97784=CIRCLE ( 'NONE', #37095, 0.5000000000000004441 ) ;
#97786=CARTESIAN_POINT ( 'NONE',  ( 0.1532563361054083140, 1.008931151000784787, 1.131784320476157264E-15 ) ) ;
#97787=CARTESIAN_POINT ( 'NONE',  ( 10.00000000000000000, 22.87363466993042138, -12.81628187352647608 ) ) ;
#97788=CARTESIAN_POINT ( 'NONE',  ( 18.52753015748618282, 43.92559781766745175, -4.923371831947291888 ) ) ;
#97790=CARTESIAN_POINT ( 'NONE',  ( 17.20831665107776587, 9.133931151000787452, -7.208316651077762316 ) ) ;
#97791=STYLED_ITEM ( 'NONE', ( #58052 ), #91278 ) ;
#97793=CARTESIAN_POINT ( 'NONE',  ( 0.2751277870542909176, 59.36607318730130345, -6.499999999999992006 ) ) ;
#97794=CARTESIAN_POINT ( 'NONE',  ( 17.96484262340118221, 11.18868534415483929, -7.964842623401177768 ) ) ;
#97795=CARTESIAN_POINT ( 'NONE',  ( 2.917880565312948704, 37.63708216824731068, 12.26659068614894643 ) ) ;
#97796=CARTESIAN_POINT ( 'NONE',  ( -0.8801773607110991993, 42.85535201082150536, -2.915334737309923874 ) ) ;
#97797=CARTESIAN_POINT ( 'NONE',  ( 4.559911319644449179, 62.23035201082150536, -9.422509992056141925 ) ) ;
#97799=CARTESIAN_POINT ( 'NONE',  ( 0.1532563361054082862, 26.21726448433411605, 2.638427012816831674 ) ) ;
#97800=CARTESIAN_POINT ( 'NONE',  ( 4.559911319644449179, 12.23035201082150536, -9.422509992056141925 ) ) ;
#97801=CARTESIAN_POINT ( 'NONE',  ( 5.076628168052703671, 11.84226448433411960, 8.527530157486179263 ) ) ;
#97803=CARTESIAN_POINT ( 'NONE',  ( -46.67755760958102229, 101.1477792333171664, 8.700766897918562393 ) ) ;
#97804=CARTESIAN_POINT ( 'NONE',  ( 19.84674366389459266, 38.71726448433412315, -2.638427012816827677 ) ) ;
#97805=CARTESIAN_POINT ( 'NONE',  ( 0.5774900079438607392, 38.48035201082150536, 5.440088680355550821 ) ) ;
#97808=ORIENTED_EDGE ( 'NONE', *, *, #14472, .F. ) ;
#97809=CARTESIAN_POINT ( 'NONE',  ( 3.591859063236761518, 59.95696800326375353, 11.09922568453594849 ) ) ;
#97811=CARTESIAN_POINT ( 'NONE',  ( 7.361572987183169658, 9.967264484334119601, -9.846743663894592657 ) ) ;
#97812=CARTESIAN_POINT ( 'NONE',  ( 3.591859063236763294, 48.29030133659708923, -11.09922568453595026 ) ) ;
#97813=CARTESIAN_POINT ( 'NONE',  ( 20.88017736071110164, 10.35535201082150714, 2.915334737309930979 ) ) ;
#97814=CARTESIAN_POINT ( 'NONE',  ( 19.84674366389459266, 38.71726448433412315, -2.638427012816827677 ) ) ;
#97817=CARTESIAN_POINT ( 'NONE',  ( 2.917880565312950480, 40.97041550158063217, -12.26659068614894821 ) ) ;
#97818=CARTESIAN_POINT ( 'NONE',  ( 18.52753015748617571, 43.09226448433412315, 4.923371831947298993 ) ) ;
#97819=CARTESIAN_POINT ( 'NONE',  ( 19.42250999205614548, 40.98035201082150536, -5.440088680355545492 ) ) ;
#97820=CARTESIAN_POINT ( 'NONE',  ( 10.00000000000000178, 2.258931151000784787, 9.846743663894594434 ) ) ;
#97822=VERTEX_POINT ( 'NONE', #78527 ) ;
#97823=CARTESIAN_POINT ( 'NONE',  ( 21.09922568453595559, 57.04030133659708923, -6.408140936763230044 ) ) ;
#97824=CARTESIAN_POINT ( 'NONE',  ( -0.8801773607111009756, 68.06368534415484817, 1.068504757029289695E-15 ) ) ;
#97826=CARTESIAN_POINT ( 'NONE',  ( -2.266590686148945544, 11.38708216824730179, -7.082119434687050408 ) ) ;
#97827=CARTESIAN_POINT ( 'NONE',  ( 1.472469842513823179, 11.42559781766745175, 4.923371831947296329 ) ) ;
#97828=CARTESIAN_POINT ( 'NONE',  ( 14.49999999999999822, 11.00000000000000000, -6.000000000000000000 ) ) ;
#97829=ORIENTED_EDGE ( 'NONE', *, *, #5483, .T. ) ;
#97830=CARTESIAN_POINT ( 'NONE',  ( 12.91533473730993009, 31.60535201082150891, -10.88017736071109987 ) ) ;
#97833=CARTESIAN_POINT ( 'NONE',  ( 15.44008868035555793, 41.39701867748817676, -9.422509992056140149 ) ) ;
#97836=EDGE_LOOP ( 'NONE', ( #48108, #14072, #34671, #36770 ) ) ;
#97837=CARTESIAN_POINT ( 'NONE',  ( 10.00000000000000000, 66.81368534415484817, -10.88017736071110342 ) ) ;
#97838=CARTESIAN_POINT ( 'NONE',  ( 17.20831665107776587, 64.13393115100079456, -7.208316651077762316 ) ) ;
#97839=CARTESIAN_POINT ( 'NONE',  ( 19.42250999205614548, 20.98035201082150891, -5.440088680355545492 ) ) ;
#97840=LINE ( 'NONE', #37330, #17565 ) ;
#97841=CARTESIAN_POINT ( 'NONE',  ( 4.559911319644449179, 68.89701867748817676, 9.422509992056141925 ) ) ;
#97842=CARTESIAN_POINT ( 'NONE',  ( -0.8801773607111009756, 18.06368534415484106, 1.068504757029289695E-15 ) ) ;
#97843=ORIENTED_EDGE ( 'NONE', *, *, #81811, .T. ) ;
#97844=CARTESIAN_POINT ( 'NONE',  ( 22.81628187352648496, 51.83196800326376064, -3.434112377981050290 ) ) ;
#97845=CARTESIAN_POINT ( 'NONE',  ( 19.42250999205614193, 50.14701867748817676, 5.440088680355555262 ) ) ;
#97847=CARTESIAN_POINT ( 'NONE',  ( 19.38216949554541202, 55.99863466993041072, 9.382169495545424454 ) ) ;
#97848=CARTESIAN_POINT ( 'NONE',  ( 19.42250999205614548, 50.98035201082151247, -5.440088680355545492 ) ) ;
#97850=CARTESIAN_POINT ( 'NONE',  ( 10.00000000000000178, 67.25893115100079456, 9.846743663894594434 ) ) ;
#97851=( LENGTH_UNIT ( ) NAMED_UNIT ( * ) SI_UNIT ( .MILLI., .METRE. ) );
#97852=CARTESIAN_POINT ( 'NONE',  ( 1.472469842513823179, 11.42559781766745175, 4.923371831947296329 ) ) ;
#97854=CARTESIAN_POINT ( 'NONE',  ( 3.591859063236761518, 9.956968003263753531, 11.09922568453594849 ) ) ;
#97856=CARTESIAN_POINT ( 'NONE',  ( 7.361572987183170547, 67.05059781766746596, 9.846743663894590881 ) ) ;
#97857=CARTESIAN_POINT ( 'NONE',  ( 12.91533473730993009, 41.60535201082149825, -10.88017736071109987 ) ) ;
#97858=CARTESIAN_POINT ( 'NONE',  ( 0.1532563361054100626, 45.80059781766745886, -2.638427012816831230 ) ) ;
#97860=CARTESIAN_POINT ( 'NONE',  ( 2.791683348922240793, 26.63393115100078745, 7.208316651077764092 ) ) ;
#97861=CARTESIAN_POINT ( 'NONE',  ( 7.361572987183169658, 14.96726448433411960, -9.846743663894592657 ) ) ;
#97862=CARTESIAN_POINT ( 'NONE',  ( -2.816281873526473856, 9.331968003263753531, 3.434112377981055619 ) ) ;
#97863=ORIENTED_EDGE ( 'NONE', *, *, #42129, .F. ) ;
#97865=B_SPLINE_CURVE_WITH_KNOTS ( 'NONE', 3,
 ( #7713, #13217, #38208, #43712 ),
 .UNSPECIFIED., .F., .F.,
 ( 4, 4 ),
 ( 5.989547311264452633E-17, 0.001060528352562006968 ),
 .UNSPECIFIED. ) ;
#97866=SURFACE_SIDE_STYLE ('',( #74837 ) ) ;
#97869=CARTESIAN_POINT ( 'NONE',  ( 6.565887622018943937, 53.08196800326374643, -12.81628187352647608 ) ) ;
#97870=CARTESIAN_POINT ( 'NONE',  ( 7.361572987183170547, 37.05059781766744464, 9.846743663894590881 ) ) ;
#97872=CARTESIAN_POINT ( 'NONE',  ( -0.8801773607110991993, 12.85535201082150358, -2.915334737309923874 ) ) ;
#97873=CARTESIAN_POINT ( 'NONE',  ( 19.84674366389459266, 33.30059781766744464, 2.638427012816836559 ) ) ;
#97875=DIRECTION ( 'NONE',  ( 0.000000000000000000, -1.000000000000000000, -0.000000000000000000 ) ) ;
#97876=CARTESIAN_POINT ( 'NONE',  ( 4.559911319644449179, 8.897018677488173211, 9.422509992056141925 ) ) ;
#97877=CARTESIAN_POINT ( 'NONE',  ( -0.8801773607111009756, 13.06368534415483929, 1.068504757029289695E-15 ) ) ;
#97878=CARTESIAN_POINT ( 'NONE',  ( 20.88017736071110164, 25.35535201082150891, 2.915334737309930979 ) ) ;
#97879=CARTESIAN_POINT ( 'NONE',  ( 24.16423886937410614, 49.30374883491396787, 8.672049930838204340E-16 ) ) ;
#97880=CARTESIAN_POINT ( 'NONE',  ( 6.204703633549690345, 52.84541550158062506, 14.16423886937410082 ) ) ;
#97881=CARTESIAN_POINT ( 'NONE',  ( 2.603489959281614308, 41.58210964143329846, 6.500000000000031086 ) ) ;
#97882=CARTESIAN_POINT ( 'NONE',  ( 19.72487221294570858, 70.00000000000000000, -6.000000000000000000 ) ) ;
#97883=CARTESIAN_POINT ( 'NONE',  ( 7.361572987183169658, 19.96726448433411960, -9.846743663894592657 ) ) ;
#97884=CARTESIAN_POINT ( 'NONE',  ( 21.09922568453595559, 2.040301336597086568, -6.408140936763230044 ) ) ;
#97889=CARTESIAN_POINT ( 'NONE',  ( -46.31228368244003946, 103.3337736655113588, 5.775421524742653467 ) ) ;
#97890=CARTESIAN_POINT ( 'NONE',  ( 0.1532563361054082862, 66.21726448433413736, 2.638427012816831674 ) ) ;
#97891=CARTESIAN_POINT ( 'NONE',  ( 24.16423886937410614, 14.30374883491396787, 8.672049930838204340E-16 ) ) ;
#97893=CARTESIAN_POINT ( 'NONE',  ( 7.361572987183169658, 29.96726448433411960, -9.846743663894592657 ) ) ;
#97897=CARTESIAN_POINT ( 'NONE',  ( -4.164238869374099039, 36.80374883491396787, 8.674139862899312516E-16 ) ) ;
#97898=CARTESIAN_POINT ( 'NONE',  ( 5.076628168052704559, 10.17559781766745175, -8.527530157486179263 ) ) ;
#97900=CARTESIAN_POINT ( 'NONE',  ( 0.2751277870542967463, 70.00000000000000000, -6.500000000000000888 ) ) ;
#97901=CARTESIAN_POINT ( 'NONE',  ( 17.96484262340118221, 34.93868534415482685, 7.964842623401181321 ) ) ;
#97902=CARTESIAN_POINT ( 'NONE',  ( 16.40814093676324603, 37.45696800326376064, -11.09922568453594671 ) ) ;
#97903=CARTESIAN_POINT ( 'NONE',  ( 10.00000000000000178, 4.313685344154837509, 10.88017736071110342 ) ) ;
#97904=CARTESIAN_POINT ( 'NONE',  ( 0.6178305044545838731, 29.74863466993042138, 9.382169495545420901 ) ) ;
#97905=CARTESIAN_POINT ( 'NONE',  ( 16.40814093676324603, 62.45696800326376064, -11.09922568453594671 ) ) ;
#97907=CARTESIAN_POINT ( 'NONE',  ( 19.89103541497709315, 35.66234555792572536, -6.479102184480822757 ) ) ;
#97908=CARTESIAN_POINT ( 'NONE',  ( -2.266590686148945544, 41.38708216824729647, -7.082119434687050408 ) ) ;
#97909=CARTESIAN_POINT ( 'NONE',  ( 6.204703633549690345, 2.845415501580634388, 14.16423886937410082 ) ) ;
#97910=CARTESIAN_POINT ( 'NONE',  ( 4.559911319644449179, 3.897018677488170990, 9.422509992056141925 ) ) ;
#97911=CARTESIAN_POINT ( 'NONE',  ( 7.084665262690076126, 24.10535201082150181, 10.88017736071109987 ) ) ;
#97914=CARTESIAN_POINT ( 'NONE',  ( 7.084665262690076126, 57.02201867748817676, -10.88017736071110164 ) ) ;
#97915=LINE ( 'NONE', #16363, #33747 ) ;
#97916=CARTESIAN_POINT ( 'NONE',  ( 6.565887622018943937, 33.08196800326374643, -12.81628187352647608 ) ) ;
#97918=CARTESIAN_POINT ( 'NONE',  ( 19.84674366389459621, 28.50893115100078745, 7.409399052514197653E-17 ) ) ;
#97919=CARTESIAN_POINT ( 'NONE',  ( 7.084665262690076126, 59.10535201082150536, 10.88017736071109987 ) ) ;
#97921=CARTESIAN_POINT ( 'NONE',  ( 0.6178305044545838731, 19.74863466993042138, 9.382169495545420901 ) ) ;
#97922=CARTESIAN_POINT ( 'NONE',  ( 0.8952175423694743728, 42.60160829253886305, -5.990408912944304554 ) ) ;
#97923=CARTESIAN_POINT ( 'NONE',  ( 7.084665262690076126, 7.022018677488169658, -10.88017736071110164 ) ) ;
#97924=CARTESIAN_POINT ( 'NONE',  ( 17.20831665107776587, 39.13393115100079456, -7.208316651077762316 ) ) ;
#97925=CARTESIAN_POINT ( 'NONE',  ( 10.00000000000000000, 57.87363466993042493, -12.81628187352647608 ) ) ;
#97927=CARTESIAN_POINT ( 'NONE',  ( 2.791683348922240793, 16.63393115100078745, 7.208316651077764092 ) ) ;
#97929=VECTOR ( 'NONE', #57383, 1000.000000000000000 ) ;
#97930=( NAMED_UNIT ( * ) PLANE_ANGLE_UNIT ( ) SI_UNIT ( $, .RADIAN. ) );
#97932=CARTESIAN_POINT ( 'NONE',  ( 4.559911319644449179, 28.89701867748817321, 9.422509992056141925 ) ) ;
#97933=CARTESIAN_POINT ( 'NONE',  ( -0.8801773607111009756, 3.063685344154837509, 1.068504757029289695E-15 ) ) ;
#97934=CARTESIAN_POINT ( 'NONE',  ( 14.92337183194729988, 39.34226448433412315, -8.527530157486177487 ) ) ;
#97936=CARTESIAN_POINT ( 'NONE',  ( 2.035157376598824452, 38.68868534415483396, 7.964842623401179544 ) ) ;
#97937=CARTESIAN_POINT ( 'NONE',  ( 15.44008868035555793, 21.39701867748817321, -9.422509992056140149 ) ) ;
#97938=ORIENTED_EDGE ( 'NONE', *, *, #65588, .T. ) ;
#97939=CARTESIAN_POINT ( 'NONE',  ( 0.5774900079438590739, 27.64701867748817676, -5.440088680355550821 ) ) ;
#97940=CARTESIAN_POINT ( 'NONE',  ( 10.00000000000000178, 40.37363466993042493, 12.81628187352647608 ) ) ;
#97941=CARTESIAN_POINT ( 'NONE',  ( 17.96484262340118221, 36.18868534415484106, -7.964842623401177768 ) ) ;
#97942=CARTESIAN_POINT ( 'NONE',  ( -0.8801773607110991993, 42.85535201082150536, -2.915334737309923874 ) ) ;
#97944=CARTESIAN_POINT ( 'NONE',  ( 1.472469842513823179, 56.42559781766745886, 4.923371831947296329 ) ) ;
#97945=CARTESIAN_POINT ( 'NONE',  ( 4.559911319644449179, 37.23035201082150536, -9.422509992056141925 ) ) ;
#97947=CARTESIAN_POINT ( 'NONE',  ( 4.999999999999999112, 11.00000000000000000, 6.000000000000000000 ) ) ;
#97948=CARTESIAN_POINT ( 'NONE',  ( 13.79529636645030344, 43.26208216824730357, 14.16423886937410614 ) ) ;
#97949=CARTESIAN_POINT ( 'NONE',  ( 20.88017736071110164, 50.35535201082151247, 2.915334737309930979 ) ) ;
#97952=CARTESIAN_POINT ( 'NONE',  ( 1.472469842513823179, 66.42559781766745175, 4.923371831947296329 ) ) ;
#97953=CARTESIAN_POINT ( 'NONE',  ( 7.084665262690076126, 2.022018677488170990, -10.88017736071110164 ) ) ;
#97954=CARTESIAN_POINT ( 'NONE',  ( 2.791683348922240793, 26.63393115100078745, 7.208316651077764092 ) ) ;
#97956=CARTESIAN_POINT ( 'NONE',  ( 5.076628168052704559, 20.17559781766745175, -8.527530157486179263 ) ) ;
#97959=CARTESIAN_POINT ( 'NONE',  ( 20.88017736071110875, 25.77201867748816966, -2.915334737309920765 ) ) ;
#97960=CARTESIAN_POINT ( 'NONE',  ( 14.92337183194729988, 24.34226448433411960, -8.527530157486177487 ) ) ;
#97962=CARTESIAN_POINT ( 'NONE',  ( 0.5774900079438607392, 63.48035201082149825, 5.440088680355550821 ) ) ;
#97963=CARTESIAN_POINT ( 'NONE',  ( 20.88017736071110164, 30.35535201082151247, 2.915334737309930979 ) ) ;
#97964=CARTESIAN_POINT ( 'NONE',  ( 10.00000000000000000, 1.813685344154837731, -10.88017736071110342 ) ) ;
#97965=CARTESIAN_POINT ( 'NONE',  ( 24.16423886937410614, 44.51208216824730357, -3.795296366450302550 ) ) ;
#97970=CARTESIAN_POINT ( 'NONE',  ( 13.43411237798105340, 10.58196800326375353, 12.81628187352647963 ) ) ;
#97971=CARTESIAN_POINT ( 'NONE',  ( 4.559911319644449179, 8.897018677488171434, 9.422509992056141925 ) ) ;
#97972=CARTESIAN_POINT ( 'NONE',  ( 10.00000000000000000, 51.81368534415484106, -10.88017736071110342 ) ) ;
#97973=FACE_OUTER_BOUND ( 'NONE', #13736, .T. ) ;
#97975=CARTESIAN_POINT ( 'NONE',  ( 19.42250999205614548, 55.98035201082150536, -5.440088680355545492 ) ) ;
#97976=CARTESIAN_POINT ( 'NONE',  ( 0.1532563361054100626, 40.80059781766745886, -2.638427012816831230 ) ) ;
#97977=CARTESIAN_POINT ( 'NONE',  ( 19.84674366389459266, 23.30059781766745530, 2.638427012816836559 ) ) ;
#97978=CARTESIAN_POINT ( 'NONE',  ( 12.63842701281683034, 12.46726448433411782, 9.846743663894596210 ) ) ;
#97980=CARTESIAN_POINT ( 'NONE',  ( -2.816281873526473856, 34.12363466993042493, 9.499525473075851096E-16 ) ) ;
#97981=CARTESIAN_POINT ( 'NONE',  ( 1.472469842513823179, 5.592264484334118713, -4.923371831947296329 ) ) ;
#97984=CARTESIAN_POINT ( 'NONE',  ( 12.63842701281683034, 27.46726448433411250, 9.846743663894596210 ) ) ;
#97986=CARTESIAN_POINT ( 'NONE',  ( 21.09922568453594849, 56.20696800326375353, 6.408140936763242479 ) ) ;
#97988=CARTESIAN_POINT ( 'NONE',  ( 10.00000000000000000, -2.126365330069579951, -12.81628187352647608 ) ) ;
#97990=CARTESIAN_POINT ( 'NONE',  ( 6.204703633549690345, 27.84541550158063217, 14.16423886937410082 ) ) ;
#97992=DIRECTION ( 'NONE',  ( 0.000000000000000000, 0.000000000000000000, -1.000000000000000000 ) ) ;
#97994=CARTESIAN_POINT ( 'NONE',  ( -4.164238869374098151, 36.59541550158063217, -3.795296366450310543 ) ) ;
#97995=CARTESIAN_POINT ( 'NONE',  ( 20.36894250292379738, 39.92874883491396787, -10.36894250292379027 ) ) ;
#97996=CARTESIAN_POINT ( 'NONE',  ( 13.79529636645031943, 5.345415501580634832, -14.16423886937409904 ) ) ;
#97997=CARTESIAN_POINT ( 'NONE',  ( 6.204703633549690345, 10.76208216824729824, -14.16423886937410259 ) ) ;
#97998=CARTESIAN_POINT ( 'NONE',  ( -0.8801773607110991993, 67.85535201082151957, -2.915334737309923874 ) ) ;
#97999=CARTESIAN_POINT ( 'NONE',  ( 12.91533473730992121, 44.52201867748816966, 10.88017736071110164 ) ) ;
#98001=CARTESIAN_POINT ( 'NONE',  ( 5.076628168052704559, 30.17559781766745175, -8.527530157486179263 ) ) ;
#98003=CARTESIAN_POINT ( 'NONE',  ( 4.559911319644449179, 67.23035201082150536, -9.422509992056141925 ) ) ;
#98004=CARTESIAN_POINT ( 'NONE',  ( 19.84674366389459266, 33.30059781766744464, 2.638427012816836559 ) ) ;
#98005=CARTESIAN_POINT ( 'NONE',  ( 2.035157376598824452, 23.68868534415484461, 7.964842623401179544 ) ) ;
#98006=CARTESIAN_POINT ( 'NONE',  ( 6.565887622018943937, 53.08196800326374643, -12.81628187352647608 ) ) ;
#98007=CARTESIAN_POINT ( 'NONE',  ( 17.20831665107776587, 62.88393115100078745, 7.208316651077764980 ) ) ;
#98009=CARTESIAN_POINT ( 'NONE',  ( 14.92337183194729633, 22.67559781766745175, 8.527530157486181039 ) ) ;
#98010=CARTESIAN_POINT ( 'NONE',  ( 21.09922568453595559, 47.04030133659708923, -6.408140936763230044 ) ) ;
#98012=CARTESIAN_POINT ( 'NONE',  ( 19.42250999205614548, 40.98035201082150536, -5.440088680355545492 ) ) ;
#98013=CARTESIAN_POINT ( 'NONE',  ( 17.20831665107776587, 52.88393115100078035, 7.208316651077764980 ) ) ;
#98014=CARTESIAN_POINT ( 'NONE',  ( -4.164238869374099927, 32.01208216824730357, 3.795296366450308767 ) ) ;
#98016=SURFACE_SIDE_STYLE ('',( #22006 ) ) ;
#98017=CARTESIAN_POINT ( 'NONE',  ( -0.8801773607110991993, 67.85535201082151957, -2.915334737309923874 ) ) ;
#98018=DIRECTION ( 'NONE',  ( 1.000000000000000000, 1.776356839400250465E-15, 0.000000000000000000 ) ) ;
#98019=CARTESIAN_POINT ( 'NONE',  ( 24.16423886937409904, 64.09541550158064638, 3.795296366450317205 ) ) ;
#98020=CARTESIAN_POINT ( 'NONE',  ( -2.816281873526473856, -0.6680319967362464695, 3.434112377981055619 ) ) ;
#98021=CARTESIAN_POINT ( 'NONE',  ( 19.42250999205614193, 50.14701867748817676, 5.440088680355555262 ) ) ;
#98022=CARTESIAN_POINT ( 'NONE',  ( -0.1503990784575263973, 27.22266099184919241, -6.262539305110081500 ) ) ;
#98023=CARTESIAN_POINT ( 'NONE',  ( 21.09922568453595559, 32.04030133659708923, -6.408140936763230044 ) ) ;
#98025=CARTESIAN_POINT ( 'NONE',  ( 2.035157376598822676, 7.438685344154837509, -7.964842623401177768 ) ) ;
#98026=CARTESIAN_POINT ( 'NONE',  ( 10.00000000000000000, 11.81368534415483751, -10.88017736071110342 ) ) ;
#98027=CARTESIAN_POINT ( 'NONE',  ( 1.472469842513823179, 56.42559781766745886, 4.923371831947296329 ) ) ;
#98028=CARTESIAN_POINT ( 'NONE',  ( 13.43411237798106583, 47.66530133659709634, -12.81628187352647252 ) ) ;
#98031=CARTESIAN_POINT ( 'NONE',  ( 12.91533473730993009, 21.60535201082150536, -10.88017736071109987 ) ) ;
#98032=CARTESIAN_POINT ( 'NONE',  ( 19.38216949554541202, 15.99863466993042138, 9.382169495545424454 ) ) ;
#98034=CARTESIAN_POINT ( 'NONE',  ( 12.63842701281683034, 17.46726448433411250, 9.846743663894596210 ) ) ;
#98036=CARTESIAN_POINT ( 'NONE',  ( 1.472469842513823179, 45.59226448433412315, -4.923371831947296329 ) ) ;
#98037=CARTESIAN_POINT ( 'NONE',  ( 20.88017736071110164, 35.35535201082150536, 2.915334737309930979 ) ) ;
#98038=CARTESIAN_POINT ( 'NONE',  ( 13.43411237798105340, 10.58196800326375353, 12.81628187352647963 ) ) ;
#98039=CARTESIAN_POINT ( 'NONE',  ( 12.91533473730992121, 49.52201867748817676, 10.88017736071110164 ) ) ;
#98041=DIRECTION ( 'NONE',  ( -1.000000000000000000, 6.608470384673545847E-17, 0.000000000000000000 ) ) ;
#98042=CARTESIAN_POINT ( 'NONE',  ( 3.591859063236763294, 58.29030133659708923, -11.09922568453595026 ) ) ;
#98044=CARTESIAN_POINT ( 'NONE',  ( 12.91533473730993009, 61.60535201082150536, -10.88017736071109987 ) ) ;
#98046=CARTESIAN_POINT ( 'NONE',  ( -2.816281873526473856, 39.12363466993041783, 9.499525473075851096E-16 ) ) ;
#98047=CARTESIAN_POINT ( 'NONE',  ( -0.8801773607111009756, 38.06368534415484106, 1.068504757029289695E-15 ) ) ;
#98048=CARTESIAN_POINT ( 'NONE',  ( 14.92337183194729988, 19.34226448433411960, -8.527530157486177487 ) ) ;
#98050=CARTESIAN_POINT ( 'NONE',  ( 10.00000000000000178, 12.25893115100078568, 9.846743663894594434 ) ) ;
#98051=CARTESIAN_POINT ( 'NONE',  ( 7.361572987183170547, 12.05059781766744997, 9.846743663894590881 ) ) ;
#98053=CARTESIAN_POINT ( 'NONE',  ( -0.3689425029237898834, 46.17874883491397497, -10.36894250292378850 ) ) ;
#98058=CARTESIAN_POINT ( 'NONE',  ( 10.00000000000000178, 58.05374883491397497, 14.16423886937410082 ) ) ;
#98059=CARTESIAN_POINT ( 'NONE',  ( 17.08211943468705840, 65.13708216824730357, -12.26659068614894466 ) ) ;
#98060=CARTESIAN_POINT ( 'NONE',  ( 12.63842701281683922, 29.55059781766745175, -9.846743663894590881 ) ) ;
#98061=CARTESIAN_POINT ( 'NONE',  ( -2.816281873526473856, 44.33196800326375353, 3.434112377981055619 ) ) ;
#98062=CARTESIAN_POINT ( 'NONE',  ( 2.603489959281199972, 21.58210964143324873, 6.499999999999559464 ) ) ;
#98063=CARTESIAN_POINT ( 'NONE',  ( 24.16423886937410614, 9.303748834913967869, 8.672049930838204340E-16 ) ) ;
#98064=CARTESIAN_POINT ( 'NONE',  ( 20.88017736071110164, 15.35535201082150358, 2.915334737309930979 ) ) ;
#98065=CARTESIAN_POINT ( 'NONE',  ( -0.3689425029237898834, 56.17874883491396076, -10.36894250292378850 ) ) ;
#98066=CARTESIAN_POINT ( 'NONE',  ( 0.1532563361054083140, 31.00893115100078390, 1.131784320476157264E-15 ) ) ;
#98067=CARTESIAN_POINT ( 'NONE',  ( 18.72515096720571393, 41.07228050351032778, -6.499999999999974243 ) ) ;
#98068=CARTESIAN_POINT ( 'NONE',  ( 18.52753015748618282, 28.92559781766745175, -4.923371831947291888 ) ) ;
#98072=ORIENTED_EDGE ( 'NONE', *, *, #86597, .T. ) ;
#98074=PRESENTATION_STYLE_ASSIGNMENT (( #14071 ) ) ;
#98075=B_SPLINE_CURVE_WITH_KNOTS ( 'NONE', 3,
 ( #32517, #24556, #56507, #17044 ),
 .UNSPECIFIED., .F., .F.,
 ( 4, 4 ),
 ( 0.000000000000000000, 0.0006041882680322483833 ),
 .UNSPECIFIED. ) ;
#98077=CARTESIAN_POINT ( 'NONE',  ( 10.00000000000000178, 42.25893115100078745, 9.846743663894594434 ) ) ;
#98078=CARTESIAN_POINT ( 'NONE',  ( 6.204703633549690345, 15.76208216824730179, -14.16423886937410259 ) ) ;
#98079=CARTESIAN_POINT ( 'NONE',  ( -0.8801773607110991993, 27.85535201082150181, -2.915334737309923874 ) ) ;
#98080=CARTESIAN_POINT ( 'NONE',  ( 19.42250999205614193, 40.14701867748817676, 5.440088680355555262 ) ) ;
#98081=CARTESIAN_POINT ( 'NONE',  ( 0.1532563361054082862, 61.21726448433412315, 2.638427012816831674 ) ) ;
#98082=CARTESIAN_POINT ( 'NONE',  ( 16.40814093676323893, 15.79030133659708746, 11.09922568453595026 ) ) ;
#98084=CARTESIAN_POINT ( 'NONE',  ( -0.8801773607110991993, 67.85535201082151957, -2.915334737309923874 ) ) ;
#98085=CARTESIAN_POINT ( 'NONE',  ( 0.6178305044545818747, 33.49863466993042493, -9.382169495545419124 ) ) ;
#98087=CARTESIAN_POINT ( 'NONE',  ( 1.472469842513823179, 46.42559781766745175, 4.923371831947296329 ) ) ;
#98088=CARTESIAN_POINT ( 'NONE',  ( 4.559911319644449179, 7.230352010821505360, -9.422509992056141925 ) ) ;
#98089=ORIENTED_EDGE ( 'NONE', *, *, #44760, .T. ) ;
#98090=CARTESIAN_POINT ( 'NONE',  ( 17.96484262340118221, 14.93868534415484106, 7.964842623401181321 ) ) ;
#98091=ORIENTED_EDGE ( 'NONE', *, *, #90103, .T. ) ;
#98092=CARTESIAN_POINT ( 'NONE',  ( 19.42250999205614193, 45.14701867748817676, 5.440088680355555262 ) ) ;
#98093=CARTESIAN_POINT ( 'NONE',  ( 2.035157376598822676, 57.43868534415484106, -7.964842623401177768 ) ) ;
#98094=CARTESIAN_POINT ( 'NONE',  ( 10.00000000000000000, 61.81368534415484106, -10.88017736071110342 ) ) ;
#98096=CARTESIAN_POINT ( 'NONE',  ( 0.5774900079438607392, 53.48035201082151247, 5.440088680355550821 ) ) ;
#98097=CYLINDRICAL_SURFACE ( 'NONE', #4250, 0.5000000000000004441 ) ;
#98098=ORIENTED_EDGE ( 'NONE', *, *, #15028, .T. ) ;
#98099=CARTESIAN_POINT ( 'NONE',  ( 14.92337183194729633, 22.67559781766745175, 8.527530157486181039 ) ) ;
#98100=VERTEX_POINT ( 'NONE', #40540 ) ;
#98101=CARTESIAN_POINT ( 'NONE',  ( 1.472469842513823179, 66.42559781766745175, 4.923371831947296329 ) ) ;
#98102=FILL_AREA_STYLE_COLOUR ( '', #57300 ) ;
#98103=CARTESIAN_POINT ( 'NONE',  ( 22.26659068614895176, 4.720415501580633943, -7.082119434687042414 ) ) ;
#98106=CARTESIAN_POINT ( 'NONE',  ( 2.791683348922240793, 36.63393115100078035, 7.208316651077764092 ) ) ;
#98107=CARTESIAN_POINT ( 'NONE',  ( 4.559911319644449179, 13.89701867748817321, 9.422509992056141925 ) ) ;
#98109=VERTEX_POINT ( 'NONE', #74456 ) ;
#98111=CARTESIAN_POINT ( 'NONE',  ( 5.076628168052704559, 40.17559781766745175, -8.527530157486179263 ) ) ;
#98113=CARTESIAN_POINT ( 'NONE',  ( -2.816281873526473856, 14.33196800326375531, 3.434112377981055619 ) ) ;
#98114=CARTESIAN_POINT ( 'NONE',  ( 19.84674366389459266, 13.30059781766745353, 2.638427012816836559 ) ) ;
#98115=CARTESIAN_POINT ( 'NONE',  ( -0.08248232600719085372, 0.1423898869303599768, 6.349449577244200782 ) ) ;
#98117=CARTESIAN_POINT ( 'NONE',  ( -2.816281873526473856, -0.8763653300695799508, 9.499525473075851096E-16 ) ) ;
#98121=EDGE_CURVE ( 'NONE', #82667, #47240, #29444, .T. ) ;
#98122=ORIENTED_EDGE ( 'NONE', *, *, #3524, .T. ) ;
#98123=CARTESIAN_POINT ( 'NONE',  ( 15.44008868035555793, 21.39701867748817321, -9.422509992056140149 ) ) ;
#98124=CARTESIAN_POINT ( 'NONE',  ( -2.266590686148945544, 22.22041550158063572, 7.082119434687048631 ) ) ;
#98125=CARTESIAN_POINT ( 'NONE',  ( 0.1532563361054082862, 31.21726448433412315, 2.638427012816831674 ) ) ;
#98126=CARTESIAN_POINT ( 'NONE',  ( 19.42250999205614548, 60.98035201082151247, -5.440088680355545492 ) ) ;
#98127=CARTESIAN_POINT ( 'NONE',  ( 22.81628187352648496, 41.83196800326375353, -3.434112377981050290 ) ) ;
#98129=CARTESIAN_POINT ( 'NONE',  ( 2.035157376598824452, 13.68868534415483751, 7.964842623401179544 ) ) ;
#98133=CARTESIAN_POINT ( 'NONE',  ( -2.816281873526473856, 14.12363466993041961, 9.499525473075851096E-16 ) ) ;
#98134=CARTESIAN_POINT ( 'NONE',  ( 21.09922568453594849, 11.20696800326375531, 6.408140936763242479 ) ) ;
#98135=CARTESIAN_POINT ( 'NONE',  ( 0.1532563361054082862, 21.21726448433412315, 2.638427012816831674 ) ) ;
#98137=CARTESIAN_POINT ( 'NONE',  ( 21.09922568453594849, 41.20696800326375353, 6.408140936763242479 ) ) ;
#98140=CARTESIAN_POINT ( 'NONE',  ( 17.96484262340118221, 41.18868534415484106, -7.964842623401177768 ) ) ;
#98141=CARTESIAN_POINT ( 'NONE',  ( 5.500000000000000000, 61.00000000000000711, -6.500000000000000888 ) ) ;
#98143=CARTESIAN_POINT ( 'NONE',  ( 19.89103541497711447, 20.66234555792571115, -6.479102184480773907 ) ) ;
#98144=CARTESIAN_POINT ( 'NONE',  ( 4.559911319644449179, 47.23035201082150536, -9.422509992056141925 ) ) ;
#98145=CARTESIAN_POINT ( 'NONE',  ( 17.96484262340118221, 41.18868534415484106, -7.964842623401177768 ) ) ;
#98146=CARTESIAN_POINT ( 'NONE',  ( 18.52753015748618282, 58.92559781766745886, -4.923371831947291888 ) ) ;
#98150=UNCERTAINTY_MEASURE_WITH_UNIT (LENGTH_MEASURE( 1.000000000000000082E-05 ), #7931, 'distance_accuracy_value', 'NONE');
#98151=( BOUNDED_CURVE ( )  B_SPLINE_CURVE ( 2, ( #20188, #27684, #5198, #80193, #34687, #66169, #58169, #27186, #4217 ),
 .UNSPECIFIED., .F., .F. ) 
 B_SPLINE_CURVE_WITH_KNOTS ( ( 3, 2, 2, 2, 3 ),
 ( 0.5453713073319822469, 0.5476190476190476719, 0.5535714285714286031, 0.5595238095238095344, 0.5617715498108749594 ),
 .UNSPECIFIED. ) 
 CURVE ( )  GEOMETRIC_REPRESENTATION_ITEM ( )  RATIONAL_B_SPLINE_CURVE ( ( 0.9839835555609424134, 0.9871328979762477029, 1.000000000000000000, 0.9659258262890683122, 1.000000000000000000, 0.9659258262890683122, 1.000000000000000000, 0.9871328979762474809, 0.9839835555609424134 ) ) 
 REPRESENTATION_ITEM ( '' )  );
#98152=CARTESIAN_POINT ( 'NONE',  ( 17.20831665107776587, 32.88393115100078745, 7.208316651077764980 ) ) ;
#98153=CARTESIAN_POINT ( 'NONE',  ( 17.96484262340118221, 4.938685344154837509, 7.964842623401181321 ) ) ;
#98154=CARTESIAN_POINT ( 'NONE',  ( 22.81628187352648496, 16.83196800326374998, -3.434112377981050290 ) ) ;
#98156=CARTESIAN_POINT ( 'NONE',  ( 10.00000000000000178, 19.31368534415484106, 10.88017736071110342 ) ) ;
#98159=CARTESIAN_POINT ( 'NONE',  ( 10.00000000000000178, 4.313685344154837509, 10.88017736071110342 ) ) ;
#98160=CARTESIAN_POINT ( 'NONE',  ( 7.084665262690076126, 22.02201867748817321, -10.88017736071110164 ) ) ;
#98161=CARTESIAN_POINT ( 'NONE',  ( 7.361572987183169658, -0.03273551566588185635, -9.846743663894592657 ) ) ;
#98162=CARTESIAN_POINT ( 'NONE',  ( 24.16423886937409904, 44.09541550158063927, 3.795296366450317205 ) ) ;
#98163=CARTESIAN_POINT ( 'NONE',  ( 19.84674366389459266, 13.71726448433411782, -2.638427012816827677 ) ) ;
#98164=CARTESIAN_POINT ( 'NONE',  ( 10.00000000000000178, 44.31368534415484106, 10.88017736071110342 ) ) ;
#98165=CARTESIAN_POINT ( 'NONE',  ( 3.059999999999993392, 76.92054879330447648, 9.500000000000000000 ) ) ;
#98166=CARTESIAN_POINT ( 'NONE',  ( 20.36894250292379738, 4.928748834913967869, -10.36894250292379027 ) ) ;
#98168=DIRECTION ( 'NONE',  ( 0.000000000000000000, 0.000000000000000000, -1.000000000000000000 ) ) ;
#98169=CARTESIAN_POINT ( 'NONE',  ( 10.00000000000000178, 57.25893115100078745, 9.846743663894594434 ) ) ;
#98171=ORIENTED_EDGE ( 'NONE', *, *, #17895, .F. ) ;
#98173=CARTESIAN_POINT ( 'NONE',  ( 22.26659068614894466, 18.88708216824730002, 7.082119434687054849 ) ) ;
#98174=CARTESIAN_POINT ( 'NONE',  ( 10.00000000000000000, 25.55374883491396787, -14.16423886937410082 ) ) ;
#98175=CARTESIAN_POINT ( 'NONE',  ( 4.559911319644449179, 63.89701867748817676, 9.422509992056141925 ) ) ;
#98176=CARTESIAN_POINT ( 'NONE',  ( 24.16423886937410614, 64.30374883491396076, 8.672049930838204340E-16 ) ) ;
#98177=CARTESIAN_POINT ( 'NONE',  ( -2.816281873526471635, -1.084698663402913210, -3.434112377981056508 ) ) ;
#98178=CARTESIAN_POINT ( 'NONE',  ( 1.472469842513823179, 45.59226448433412315, -4.923371831947296329 ) ) ;
#98180=CARTESIAN_POINT ( 'NONE',  ( 20.88017736071110519, 45.56368534415484106, 2.639326808657452039E-16 ) ) ;
#98181=CARTESIAN_POINT ( 'NONE',  ( -1.099225684535947600, 23.70696800326375708, -6.408140936763238038 ) ) ;
#98182=CARTESIAN_POINT ( 'NONE',  ( -0.3689425029237898834, 11.17874883491396787, -10.36894250292378850 ) ) ;
#98183=CARTESIAN_POINT ( 'NONE',  ( 17.96484262340118221, 14.93868534415484106, 7.964842623401181321 ) ) ;
#98184=CARTESIAN_POINT ( 'NONE',  ( 2.035157376598822676, 17.43868534415483751, -7.964842623401177768 ) ) ;
#98186=CARTESIAN_POINT ( 'NONE',  ( 15.44008868035555793, 56.39701867748817676, -9.422509992056140149 ) ) ;
#98189=CARTESIAN_POINT ( 'NONE',  ( -45.94000000000001194, 103.9981609152045650, -5.961202730336927047 ) ) ;
#98190=COLOUR_RGB ( '', 0.09019608, 0.27058824, 0.51372549) ;
#98194=SURFACE_SIDE_STYLE ('',( #50313 ) ) ;
#98195=CARTESIAN_POINT ( 'NONE',  ( 17.08211943468705840, 50.13708216824730357, -12.26659068614894466 ) ) ;
#98196=CARTESIAN_POINT ( 'NONE',  ( 13.79529636645031943, 65.34541550158063217, -14.16423886937409904 ) ) ;
#98197=CARTESIAN_POINT ( 'NONE',  ( 19.84674366389459266, 23.30059781766745530, 2.638427012816836559 ) ) ;
#98198=CARTESIAN_POINT ( 'NONE',  ( 12.63842701281683922, 44.55059781766745175, -9.846743663894590881 ) ) ;
#98199=CARTESIAN_POINT ( 'NONE',  ( 20.15039907845753220, 60.60158574516643881, -6.262539305110077947 ) ) ;
#98201=EDGE_CURVE ( 'NONE', #12692, #91503, #13302, .T. ) ;
#98202=CARTESIAN_POINT ( 'NONE',  ( 10.00000000000000000, 66.81368534415484817, -10.88017736071110342 ) ) ;
#98203=B_SPLINE_CURVE_WITH_KNOTS ( 'NONE', 3,
 ( #12163, #19671, #72172, #96672, #27158, #73147 ),
 .UNSPECIFIED., .F., .F.,
 ( 4, 2, 4 ),
 ( 0.000000000000000000, 0.0002626113303184800848, 0.0005252226606369601696 ),
 .UNSPECIFIED. ) ;
#98205=VERTEX_POINT ( 'NONE', #34975 ) ;
#98206=CARTESIAN_POINT ( 'NONE',  ( 24.16423886937410614, 29.30374883491396787, 8.672049930838204340E-16 ) ) ;
#98207=CARTESIAN_POINT ( 'NONE',  ( 13.43411237798106583, 22.66530133659708923, -12.81628187352647252 ) ) ;
#98209=CARTESIAN_POINT ( 'NONE',  ( -1.099225684535947600, 64.54030133659709634, 6.408140936763237150 ) ) ;
#98210=CARTESIAN_POINT ( 'NONE',  ( 17.96484262340118221, 31.18868534415483751, -7.964842623401177768 ) ) ;
#98211=CARTESIAN_POINT ( 'NONE',  ( 2.791683348922240793, 41.63393115100078745, 7.208316651077764092 ) ) ;
#98212=CARTESIAN_POINT ( 'NONE',  ( 0.5774900079438590739, 27.64701867748817676, -5.440088680355550821 ) ) ;
#98213=CARTESIAN_POINT ( 'NONE',  ( 13.43411237798106583, 62.66530133659708923, -12.81628187352647252 ) ) ;
#98214=CARTESIAN_POINT ( 'NONE',  ( 7.361572987183169658, 44.96726448433412315, -9.846743663894592657 ) ) ;
#98215=CARTESIAN_POINT ( 'NONE',  ( 5.076628168052703671, 56.84226448433412315, 8.527530157486179263 ) ) ;
#98219=DIRECTION ( 'NONE',  ( -0.000000000000000000, -0.000000000000000000, 1.000000000000000000 ) ) ;
#98220=LINE ( 'NONE', #51715, #30645 ) ;
#98221=DIRECTION ( 'NONE',  ( 0.000000000000000000, -1.000000000000000000, 0.000000000000000000 ) ) ;
#98223=CARTESIAN_POINT ( 'NONE',  ( 17.20831665107776587, 34.13393115100078745, -7.208316651077762316 ) ) ;
#98225=CARTESIAN_POINT ( 'NONE',  ( 6.565887622018943937, 38.08196800326376064, -12.81628187352647608 ) ) ;
#98227=ORIENTED_EDGE ( 'NONE', *, *, #53620, .T. ) ;
#98228=CARTESIAN_POINT ( 'NONE',  ( 5.076628168052703671, 56.84226448433412315, 8.527530157486179263 ) ) ;
#98230=CARTESIAN_POINT ( 'NONE',  ( 18.52753015748617571, 38.09226448433412315, 4.923371831947298993 ) ) ;
#98231=CARTESIAN_POINT ( 'NONE',  ( 6.204703633549690345, 27.84541550158063217, 14.16423886937410082 ) ) ;
#98232=CARTESIAN_POINT ( 'NONE',  ( 5.076628168052704559, 50.17559781766745886, -8.527530157486179263 ) ) ;
#98233=CARTESIAN_POINT ( 'NONE',  ( 10.00000000000000000, 42.87363466993042493, -12.81628187352647608 ) ) ;
#98236=CARTESIAN_POINT ( 'NONE',  ( 5.076628168052704559, 5.175597817667451750, -8.527530157486179263 ) ) ;
#98238=CARTESIAN_POINT ( 'NONE',  ( 20.24186590665276597, 46.76028685723174760, 6.114288769123062295 ) ) ;
#98239=VECTOR ( 'NONE', #72094, 1000.000000000000000 ) ;
#98240=CARTESIAN_POINT ( 'NONE',  ( 18.52753015748618282, 43.92559781766745175, -4.923371831947291888 ) ) ;
#98241=CARTESIAN_POINT ( 'NONE',  ( 20.88017736071110519, 35.56368534415484106, 2.639326808657452039E-16 ) ) ;
#98242=CARTESIAN_POINT ( 'NONE',  ( 0.1532563361054082862, 41.21726448433411605, 2.638427012816831674 ) ) ;
#98247=CARTESIAN_POINT ( 'NONE',  ( 19.42250999205614548, 50.98035201082151247, -5.440088680355545492 ) ) ;
#98251=CARTESIAN_POINT ( 'NONE',  ( 0.2751277870542909731, 22.28217586085237656, -6.499999999999992006 ) ) ;
#98252=CARTESIAN_POINT ( 'NONE',  ( 4.559911319644449179, 17.23035201082150536, -9.422509992056141925 ) ) ;
#98253=CARTESIAN_POINT ( 'NONE',  ( 19.84674366389459266, 63.71726448433412315, -2.638427012816827677 ) ) ;
#98254=CARTESIAN_POINT ( 'NONE',  ( 15.44008868035555260, 39.73035201082150536, 9.422509992056143702 ) ) ;
#98255=CARTESIAN_POINT ( 'NONE',  ( 2.603489959281115151, 16.58210964143323807, 6.499999999999462652 ) ) ;
#98256=B_SPLINE_CURVE_WITH_KNOTS ( 'NONE', 3,
 ( #5300, #58772, #89761, #89275 ),
 .UNSPECIFIED., .F., .F.,
 ( 4, 4 ),
 ( 0.000000000000000000, 0.002562518741975551920 ),
 .UNSPECIFIED. ) ;
#98259=CARTESIAN_POINT ( 'NONE',  ( 12.91533473730992121, 34.52201867748817676, 10.88017736071110164 ) ) ;
#98261=CARTESIAN_POINT ( 'NONE',  ( 2.791683348922240793, 11.63393115100078568, 7.208316651077764092 ) ) ;
#98263=CARTESIAN_POINT ( 'NONE',  ( 0.1532563361054083140, 26.00893115100078745, 1.131784320476157264E-15 ) ) ;
#98266=CARTESIAN_POINT ( 'NONE',  ( 17.20831665107776587, 64.13393115100079456, -7.208316651077762316 ) ) ;
#98267=CARTESIAN_POINT ( 'NONE',  ( 2.035157376598822676, 2.438685344154838397, -7.964842623401177768 ) ) ;
#98270=CARTESIAN_POINT ( 'NONE',  ( 13.79529636645030344, 18.26208216824730002, 14.16423886937410614 ) ) ;
#98271=CARTESIAN_POINT ( 'NONE',  ( 22.26659068614895176, 54.72041550158063217, -7.082119434687042414 ) ) ;
#98273=CARTESIAN_POINT ( 'NONE',  ( 14.92337183194729988, 19.34226448433411960, -8.527530157486177487 ) ) ;
#98274=CARTESIAN_POINT ( 'NONE',  ( 4.559911319644449179, 8.897018677488173211, 9.422509992056141925 ) ) ;
#98275=CARTESIAN_POINT ( 'NONE',  ( 12.63842701281683034, 52.46726448433413026, 9.846743663894596210 ) ) ;
#98276=CARTESIAN_POINT ( 'NONE',  ( -0.3689425029237881626, 2.428748834913967869, 10.36894250292379027 ) ) ;
#98280=CARTESIAN_POINT ( 'NONE',  ( 14.92337183194729633, 2.675597817667451750, 8.527530157486181039 ) ) ;
#98281=CARTESIAN_POINT ( 'NONE',  ( 22.81628187352647785, 41.41530133659708923, 3.434112377981063169 ) ) ;
#98282=CARTESIAN_POINT ( 'NONE',  ( 5.076628168052703671, 46.84226448433412315, 8.527530157486179263 ) ) ;
#98284=CARTESIAN_POINT ( 'NONE',  ( 0.1532563361054100626, 10.80059781766745175, -2.638427012816831230 ) ) ;
#98288=CARTESIAN_POINT ( 'NONE',  ( 4.559911319644449179, 13.89701867748817321, 9.422509992056141925 ) ) ;
#98289=CARTESIAN_POINT ( 'NONE',  ( 6.204703633549690345, 60.76208216824730357, -14.16423886937410259 ) ) ;
#98292=CARTESIAN_POINT ( 'NONE',  ( 10.00000000000000178, 27.25893115100078390, 9.846743663894594434 ) ) ;
#98293=CARTESIAN_POINT ( 'NONE',  ( 12.91533473730993009, 11.60535201082150536, -10.88017736071109987 ) ) ;
#98294=CARTESIAN_POINT ( 'NONE',  ( 1.472469842513823179, 6.425597817667451750, 4.923371831947296329 ) ) ;
#98295=CARTESIAN_POINT ( 'NONE',  ( 17.20831665107776587, 49.13393115100078745, -7.208316651077762316 ) ) ;
#98296=CARTESIAN_POINT ( 'NONE',  ( 19.42250999205614193, 30.14701867748817321, 5.440088680355555262 ) ) ;
#98299=ORIENTED_EDGE ( 'NONE', *, *, #27562, .T. ) ;
#98300=CARTESIAN_POINT ( 'NONE',  ( 19.38216949554541557, 62.24863466993041072, -9.382169495545420901 ) ) ;
#98303=CARTESIAN_POINT ( 'NONE',  ( 0.1532563361054083140, 11.00893115100078568, 1.131784320476157264E-15 ) ) ;
#98304=CARTESIAN_POINT ( 'NONE',  ( 10.00000000000000178, 45.37363466993041783, 12.81628187352647608 ) ) ;
#98305=CARTESIAN_POINT ( 'NONE',  ( 15.44008868035555260, 4.730352010821505360, 9.422509992056143702 ) ) ;
#98306=CARTESIAN_POINT ( 'NONE',  ( 17.20831665107776587, 34.13393115100078745, -7.208316651077762316 ) ) ;
#98307=CARTESIAN_POINT ( 'NONE',  ( 20.00000000000000711, 98.59912998021083297, 4.500000000000000888 ) ) ;
#98308=DIRECTION ( 'NONE',  ( 1.000000000000000000, 0.000000000000000000, 0.000000000000000000 ) ) ;
#98309=CARTESIAN_POINT ( 'NONE',  ( 22.26659068614895176, 29.72041550158063572, -7.082119434687042414 ) ) ;
#98310=CARTESIAN_POINT ( 'NONE',  ( -4.164238869374099039, 46.80374883491397497, 8.674139862899312516E-16 ) ) ;
#98311=CARTESIAN_POINT ( 'NONE',  ( 14.92337183194729988, 54.34226448433412315, -8.527530157486177487 ) ) ;
#98313=CARTESIAN_POINT ( 'NONE',  ( 2.035157376598824452, 43.68868534415484106, 7.964842623401179544 ) ) ;
#98314=CARTESIAN_POINT ( 'NONE',  ( 5.076628168052703671, 6.842264484334118713, 8.527530157486179263 ) ) ;
#98316=CARTESIAN_POINT ( 'NONE',  ( -1.099225684535947600, 54.54030133659708923, 6.408140936763237150 ) ) ;
#98318=CARTESIAN_POINT ( 'NONE',  ( 0.1532563361054082862, 1.217264484334117824, 2.638427012816831674 ) ) ;
#98321=CARTESIAN_POINT ( 'NONE',  ( 20.36894250292379738, 9.928748834913966093, -10.36894250292379027 ) ) ;
#98322=CARTESIAN_POINT ( 'NONE',  ( 19.84674366389459621, 8.508931151000785675, 7.409399052514197653E-17 ) ) ;
#98323=CARTESIAN_POINT ( 'NONE',  ( 7.084665262690076126, 32.02201867748816966, -10.88017736071110164 ) ) ;
#98325=CARTESIAN_POINT ( 'NONE',  ( -0.8801773607111008646, 28.27201867748817321, 2.915334737309923430 ) ) ;
#98326=VERTEX_POINT ( 'NONE', #68947 ) ;
#98327=CARTESIAN_POINT ( 'NONE',  ( 20.88017736071110519, 35.56368534415484106, 2.639326808657452039E-16 ) ) ;
#98328=CARTESIAN_POINT ( 'NONE',  ( 0.2751277870542876425, 45.30223176428830811, 6.499999999999984901 ) ) ;
#98331=CARTESIAN_POINT ( 'NONE',  ( -2.816281873526471635, 13.91530133659708746, -3.434112377981056508 ) ) ;
#98332=EDGE_CURVE ( 'NONE', #19080, #32896, #22967, .T. ) ;
#98333=CARTESIAN_POINT ( 'NONE',  ( 12.63842701281683034, 2.467264484334118269, 9.846743663894596210 ) ) ;
#98335=CARTESIAN_POINT ( 'NONE',  ( 7.084665262690076126, 19.10535201082150181, 10.88017736071109987 ) ) ;
#98337=CARTESIAN_POINT ( 'NONE',  ( 0.1532563361054100626, 0.8005978176674514168, -2.638427012816831230 ) ) ;
#98338=CARTESIAN_POINT ( 'NONE',  ( 10.00000000000000000, 21.81368534415484106, -10.88017736071110342 ) ) ;
#98341=ORIENTED_EDGE ( 'NONE', *, *, #52504, .F. ) ;
#98342=CARTESIAN_POINT ( 'NONE',  ( 10.00000000000000178, 55.37363466993042493, 12.81628187352647608 ) ) ;
#98343=CARTESIAN_POINT ( 'NONE',  ( 2.035157376598822676, 42.43868534415483396, -7.964842623401177768 ) ) ;
#98345=STYLED_ITEM ( 'NONE', ( #23507 ), #86447 ) ;
#98346=CARTESIAN_POINT ( 'NONE',  ( 19.38216949554541557, 57.24863466993042493, -9.382169495545420901 ) ) ;
#98347=CARTESIAN_POINT ( 'NONE',  ( 12.91533473730993009, 51.60535201082149825, -10.88017736071109987 ) ) ;
#98348=CARTESIAN_POINT ( 'NONE',  ( 18.52753015748617571, 63.09226448433412315, 4.923371831947298993 ) ) ;
#98349=CYLINDRICAL_SURFACE ( 'NONE', #73828, 11.92686044187656513 ) ;
#98350=CARTESIAN_POINT ( 'NONE',  ( 17.20831665107776587, 19.13393115100078035, -7.208316651077762316 ) ) ;
#98351=CARTESIAN_POINT ( 'NONE',  ( 0.6178305044545838731, 59.74863466993041783, 9.382169495545420901 ) ) ;
#98353=CARTESIAN_POINT ( 'NONE',  ( 1.472469842513823179, 11.42559781766745175, 4.923371831947296329 ) ) ;
#98354=CARTESIAN_POINT ( 'NONE',  ( 21.09922568453595559, 2.040301336597086568, -6.408140936763230044 ) ) ;
#98356=CARTESIAN_POINT ( 'NONE',  ( 10.00000000000000178, 62.25893115100078745, 9.846743663894594434 ) ) ;
#98357=CARTESIAN_POINT ( 'NONE',  ( 19.42250999205614548, 35.98035201082151247, -5.440088680355545492 ) ) ;
#98358=CARTESIAN_POINT ( 'NONE',  ( 7.361572987183169658, 44.96726448433412315, -9.846743663894592657 ) ) ;
#98359=CARTESIAN_POINT ( 'NONE',  ( -0.2418659066527486246, 33.09014588040358262, 6.114288769123083611 ) ) ;
#98360=CARTESIAN_POINT ( 'NONE',  ( 17.20831665107776587, 22.88393115100078745, 7.208316651077764980 ) ) ;
#98361=CARTESIAN_POINT ( 'NONE',  ( 19.84674366389459621, 3.508931151000785231, 7.409399052514197653E-17 ) ) ;
#98362=CARTESIAN_POINT ( 'NONE',  ( 16.40814093676324603, 7.456968003263754419, -11.09922568453594671 ) ) ;
#98364=CARTESIAN_POINT ( 'NONE',  ( 1.472469842513823179, 66.42559781766745175, 4.923371831947296329 ) ) ;
#98368=CARTESIAN_POINT ( 'NONE',  ( -0.8801773607111009756, 3.063685344154838397, 1.068504757029289695E-15 ) ) ;
#98369=CARTESIAN_POINT ( 'NONE',  ( 0.1532563361054083140, 41.00893115100078745, 1.131784320476157264E-15 ) ) ;
#98370=EDGE_CURVE ( 'NONE', #39149, #69767, #15470, .T. ) ;
#98371=VERTEX_POINT ( 'NONE', #61425 ) ;
#98373=CARTESIAN_POINT ( 'NONE',  ( -0.8801773607110991993, 2.855352010821504471, -2.915334737309923874 ) ) ;
#98374=CARTESIAN_POINT ( 'NONE',  ( 20.15039907845753930, 69.92552686551195507, -6.262539305110068177 ) ) ;
#98375=CARTESIAN_POINT ( 'NONE',  ( 4.559911319644449179, 23.89701867748817321, 9.422509992056141925 ) ) ;
#98376=CARTESIAN_POINT ( 'NONE',  ( 24.16423886937410614, 54.30374883491396787, 8.672049930838204340E-16 ) ) ;
#98377=CARTESIAN_POINT ( 'NONE',  ( 7.084665262690076126, 2.022018677488171434, -10.88017736071110164 ) ) ;
#98379=CARTESIAN_POINT ( 'NONE',  ( 10.00000000000000000, -0.2410688489992152128, -9.846743663894594434 ) ) ;
#98380=CARTESIAN_POINT ( 'NONE',  ( 0.1532563361054083140, 21.00893115100078745, 1.131784320476157264E-15 ) ) ;
#98381=CARTESIAN_POINT ( 'NONE',  ( 6.565887622018943937, 15.16530133659708568, 12.81628187352647430 ) ) ;
#98385=CARTESIAN_POINT ( 'NONE',  ( 1.472469842513823179, 55.59226448433412315, -4.923371831947296329 ) ) ;
#98387=CARTESIAN_POINT ( 'NONE',  ( 19.72487221294570858, 29.78217586085238366, 6.499999999999992895 ) ) ;
#98388=CARTESIAN_POINT ( 'NONE',  ( 2.917880565312950480, 15.97041550158063217, -12.26659068614894821 ) ) ;
#98389=CARTESIAN_POINT ( 'NONE',  ( 2.791683348922240793, 21.63393115100078745, 7.208316651077764092 ) ) ;
#98391=ORIENTED_EDGE ( 'NONE', *, *, #82079, .T. ) ;
#98392=CARTESIAN_POINT ( 'NONE',  ( 24.16423886937409904, 44.09541550158063927, 3.795296366450317205 ) ) ;
#98393=CARTESIAN_POINT ( 'NONE',  ( 10.00000000000000178, 7.258931151000785675, 9.846743663894594434 ) ) ;
#98394=CARTESIAN_POINT ( 'NONE',  ( -0.1503990784575277573, 63.10158574516643171, 6.262539305110076171 ) ) ;
#98396=CARTESIAN_POINT ( 'NONE',  ( 7.084665262690076126, 34.10535201082151247, 10.88017736071109987 ) ) ;
#98397=CARTESIAN_POINT ( 'NONE',  ( -2.816281873526473856, 54.12363466993041783, 9.499525473075851096E-16 ) ) ;
#98398=CARTESIAN_POINT ( 'NONE',  ( 4.559911319644449179, 8.897018677488171434, 9.422509992056141925 ) ) ;
#98399=CARTESIAN_POINT ( 'NONE',  ( 3.591859063236761518, 39.95696800326375353, 11.09922568453594849 ) ) ;
#98400=CARTESIAN_POINT ( 'NONE',  ( 10.00000000000000178, 7.258931151000785675, 9.846743663894594434 ) ) ;
#98403=CYLINDRICAL_SURFACE ( 'NONE', #57391, 0.5000000000000004441 ) ;
#98404=CARTESIAN_POINT ( 'NONE',  ( 10.00000000000000000, 40.55374883491397497, -14.16423886937410082 ) ) ;
#98405=CARTESIAN_POINT ( 'NONE',  ( 10.00000000000000000, 10.55374883491396787, -14.16423886937410082 ) ) ;
#98406=CARTESIAN_POINT ( 'NONE',  ( 15.44008868035555260, 9.730352010821505360, 9.422509992056143702 ) ) ;
#98407=CARTESIAN_POINT ( 'NONE',  ( 17.96484262340118221, 26.18868534415483396, -7.964842623401177768 ) ) ;
#98410=CARTESIAN_POINT ( 'NONE',  ( -0.8801773607111008646, 58.27201867748816966, 2.915334737309923430 ) ) ;
#98411=CARTESIAN_POINT ( 'NONE',  ( -0.8801773607111009756, 58.06368534415484106, 1.068504757029289695E-15 ) ) ;
#98412=CARTESIAN_POINT ( 'NONE',  ( 6.565887622018943937, 23.08196800326375708, -12.81628187352647608 ) ) ;
#98415=CARTESIAN_POINT ( 'NONE',  ( 19.84674366389459266, 23.30059781766745530, 2.638427012816836559 ) ) ;
#98419=CARTESIAN_POINT ( 'NONE',  ( 10.00000000000000178, 25.37363466993041783, 12.81628187352647608 ) ) ;
#98420=PRESENTATION_STYLE_ASSIGNMENT (( #13912 ) ) ;
#98421=CARTESIAN_POINT ( 'NONE',  ( 0.5774900079438590739, 12.64701867748817143, -5.440088680355550821 ) ) ;
#98422=AXIS2_PLACEMENT_3D ( 'NONE', #82798, #30279, #83296 ) ;
#98423=CARTESIAN_POINT ( 'NONE',  ( 10.00000000000000178, 32.25893115100078745, 9.846743663894594434 ) ) ;
#98424=CARTESIAN_POINT ( 'NONE',  ( 6.565887622018943937, 65.16530133659709634, 12.81628187352647430 ) ) ;
#98425=CARTESIAN_POINT ( 'NONE',  ( 17.20831665107776587, 19.13393115100078035, -7.208316651077762316 ) ) ;
#98427=CARTESIAN_POINT ( 'NONE',  ( -0.8801773607111008646, 28.27201867748817321, 2.915334737309923430 ) ) ;
#98428=( LENGTH_UNIT ( ) NAMED_UNIT ( * ) SI_UNIT ( .MILLI., .METRE. ) );
#98429=CARTESIAN_POINT ( 'NONE',  ( 2.917880565312950480, 35.97041550158063217, -12.26659068614894821 ) ) ;
#98430=CARTESIAN_POINT ( 'NONE',  ( 19.84674366389459266, 48.30059781766745175, 2.638427012816836559 ) ) ;
#98431=CARTESIAN_POINT ( 'NONE',  ( 10.00000000000000178, 29.31368534415483751, 10.88017736071110342 ) ) ;
#98432=CARTESIAN_POINT ( 'NONE',  ( 12.91533473730992121, 19.52201867748816611, 10.88017736071110164 ) ) ;
#98434=CARTESIAN_POINT ( 'NONE',  ( 12.91533473730993009, 31.60535201082150891, -10.88017736071109987 ) ) ;
#98435=CARTESIAN_POINT ( 'NONE',  ( 22.81628187352648496, 51.83196800326376064, -3.434112377981050290 ) ) ;
#98436=CARTESIAN_POINT ( 'NONE',  ( 12.91533473730993009, 41.60535201082149825, -10.88017736071109987 ) ) ;
#98438=CARTESIAN_POINT ( 'NONE',  ( 4.559911319644449179, 37.23035201082150536, -9.422509992056141925 ) ) ;
#98440=CARTESIAN_POINT ( 'NONE',  ( -0.8801773607111008646, 33.27201867748817676, 2.915334737309923430 ) ) ;
#98443=CARTESIAN_POINT ( 'NONE',  ( 19.72487221294570858, 70.00000000000000000, 6.500000000000000888 ) ) ;
#98444=CARTESIAN_POINT ( 'NONE',  ( -2.266590686148945544, 42.22041550158063217, 7.082119434687048631 ) ) ;
#98445=CARTESIAN_POINT ( 'NONE',  ( 7.084665262690076126, 49.10535201082149825, 10.88017736071109987 ) ) ;
#98448=CARTESIAN_POINT ( 'NONE',  ( 7.361572987183169658, 64.96726448433412315, -9.846743663894592657 ) ) ;
#98450=CARTESIAN_POINT ( 'NONE',  ( 7.361572987183170547, 37.05059781766744464, 9.846743663894590881 ) ) ;
#98452=CARTESIAN_POINT ( 'NONE',  ( 18.52753015748617571, 38.09226448433412315, 4.923371831947298993 ) ) ;
#98454=CARTESIAN_POINT ( 'NONE',  ( 19.42250999205614193, 25.14701867748817321, 5.440088680355555262 ) ) ;
#98455=CARTESIAN_POINT ( 'NONE',  ( 17.20831665107776587, 32.88393115100078745, 7.208316651077764980 ) ) ;
#98456=CARTESIAN_POINT ( 'NONE',  ( 22.81628187352648496, 26.83196800326374998, -3.434112377981050290 ) ) ;
#98458=CARTESIAN_POINT ( 'NONE',  ( 4.559911319644449179, 57.23035201082150536, -9.422509992056141925 ) ) ;
#98459=CARTESIAN_POINT ( 'NONE',  ( -0.8801773607111009756, 28.06368534415484106, 1.068504757029289695E-15 ) ) ;
#98460=CARTESIAN_POINT ( 'NONE',  ( 17.96484262340118221, 4.938685344154837509, 7.964842623401181321 ) ) ;
#98461=CARTESIAN_POINT ( 'NONE',  ( 6.204703633549690345, 47.84541550158064638, 14.16423886937410082 ) ) ;
#98462=STYLED_ITEM ( 'NONE', ( #39229 ), #55104 ) ;
#98466=ORIENTED_EDGE ( 'NONE', *, *, #71412, .T. ) ;
#98467=CARTESIAN_POINT ( 'NONE',  ( 13.43411237798105340, 15.58196800326374998, 12.81628187352647963 ) ) ;
#98468=CARTESIAN_POINT ( 'NONE',  ( -0.8801773607111008646, 8.272018677488171434, 2.915334737309923430 ) ) ;
#98470=CARTESIAN_POINT ( 'NONE',  ( 17.96484262340118221, 44.93868534415483396, 7.964842623401181321 ) ) ;
#98472=CARTESIAN_POINT ( 'NONE',  ( 17.96484262340118221, 61.18868534415482685, -7.964842623401177768 ) ) ;
#98473=CARTESIAN_POINT ( 'NONE',  ( 1.472469842513823179, 31.42559781766745530, 4.923371831947296329 ) ) ;
#98474=CARTESIAN_POINT ( 'NONE',  ( 10.00000000000000178, 27.25893115100078390, 9.846743663894594434 ) ) ;
#98475=CARTESIAN_POINT ( 'NONE',  ( 19.84674366389459621, 13.50893115100078568, 7.409399052514197653E-17 ) ) ;
#98478=CARTESIAN_POINT ( 'NONE',  ( 16.40814093676323893, 40.79030133659708923, 11.09922568453595026 ) ) ;
#98479=CARTESIAN_POINT ( 'NONE',  ( 18.52753015748618282, 18.92559781766745175, -4.923371831947291888 ) ) ;
#98480=CARTESIAN_POINT ( 'NONE',  ( 0.6081133539230531015, 33.33703382326400089, 6.499999999999970690 ) ) ;
#98482=AXIS2_PLACEMENT_3D ( 'NONE', #53711, #69219, #745 ) ;
#98483=CARTESIAN_POINT ( 'NONE',  ( 18.52753015748617571, 33.09226448433411605, 4.923371831947298993 ) ) ;
#98487=CARTESIAN_POINT ( 'NONE',  ( 16.40814093676323893, 5.790301336597087456, 11.09922568453595026 ) ) ;
#98488=CARTESIAN_POINT ( 'NONE',  ( 4.559911319644449179, 47.23035201082150536, -9.422509992056141925 ) ) ;
#98489=CARTESIAN_POINT ( 'NONE',  ( -0.3689425029237898834, 26.17874883491396432, -10.36894250292378850 ) ) ;
#98491=EDGE_CURVE ( 'NONE', #69569, #7550, #28018, .T. ) ;
#98493=CARTESIAN_POINT ( 'NONE',  ( 2.917880565312948704, 32.63708216824730357, 12.26659068614894643 ) ) ;
#98494=CARTESIAN_POINT ( 'NONE',  ( 24.16423886937409904, 49.09541550158063217, 3.795296366450317205 ) ) ;
#98495=CARTESIAN_POINT ( 'NONE',  ( 22.26659068614894466, 13.88708216824730179, 7.082119434687054849 ) ) ;
#98496=CARTESIAN_POINT ( 'NONE',  ( 22.26659068614894466, 13.88708216824730179, 7.082119434687054849 ) ) ;
#98497=CARTESIAN_POINT ( 'NONE',  ( -0.1503990784575247319, 37.22266099184918176, -6.262539305110083276 ) ) ;
#98498=CARTESIAN_POINT ( 'NONE',  ( 10.00000000000000178, 44.31368534415484106, 10.88017736071110342 ) ) ;
#98500=CARTESIAN_POINT ( 'NONE',  ( 19.84674366389459266, 33.30059781766744464, 2.638427012816836559 ) ) ;
#98501=LINE ( 'NONE', #5509, #88405 ) ;
#98502=CARTESIAN_POINT ( 'NONE',  ( 2.791683348922240793, 46.63393115100077324, 7.208316651077764092 ) ) ;
#98504=CARTESIAN_POINT ( 'NONE',  ( 2.035157376598824452, 28.68868534415484106, 7.964842623401179544 ) ) ;
#98505=CARTESIAN_POINT ( 'NONE',  ( 13.43411237798106583, 62.66530133659708923, -12.81628187352647252 ) ) ;
#98506=CARTESIAN_POINT ( 'NONE',  ( 12.63842701281683922, 64.55059781766745175, -9.846743663894590881 ) ) ;
#98508=CARTESIAN_POINT ( 'NONE',  ( 18.52753015748618282, 23.92559781766745530, -4.923371831947291888 ) ) ;
#98509=CARTESIAN_POINT ( 'NONE',  ( -2.816281873526473856, 44.33196800326375353, 3.434112377981055619 ) ) ;
#98512=CARTESIAN_POINT ( 'NONE',  ( 15.44008868035555260, 44.73035201082151247, 9.422509992056143702 ) ) ;
#98513=CARTESIAN_POINT ( 'NONE',  ( 18.52753015748617571, 48.09226448433412315, 4.923371831947298993 ) ) ;
#98514=CARTESIAN_POINT ( 'NONE',  ( 13.79529636645030344, 28.26208216824729647, 14.16423886937410614 ) ) ;
#98515=VECTOR ( 'NONE', #74600, 1000.000000000000000 ) ;
#98517=FILL_AREA_STYLE ('',( #74988 ) ) ;
#98518=CARTESIAN_POINT ( 'NONE',  ( 20.88017736071110164, 65.35535201082150536, 2.915334737309930979 ) ) ;
#98519=CARTESIAN_POINT ( 'NONE',  ( -0.8801773607111009756, 68.06368534415484817, 1.068504757029289695E-15 ) ) ;
#98520=CARTESIAN_POINT ( 'NONE',  ( 13.79529636645031943, 65.34541550158063217, -14.16423886937409904 ) ) ;
#98521=CARTESIAN_POINT ( 'NONE',  ( -1.099225684535947600, 3.706968003263753531, -6.408140936763238038 ) ) ;
#98523=CARTESIAN_POINT ( 'NONE',  ( 20.88017736071110875, 50.77201867748817676, -2.915334737309920765 ) ) ;
#98525=CARTESIAN_POINT ( 'NONE',  ( 3.640395162852214650, 89.00000000000000000, 9.500000000000000000 ) ) ;
#98526=CARTESIAN_POINT ( 'NONE',  ( -1.099225684535947600, 29.54030133659708923, 6.408140936763237150 ) ) ;
#98527=CARTESIAN_POINT ( 'NONE',  ( -4.164238869374098151, 51.59541550158063217, -3.795296366450310543 ) ) ;
#98529=CARTESIAN_POINT ( 'NONE',  ( 7.084665262690076126, 7.022018677488169658, -10.88017736071110164 ) ) ;
#98530=CARTESIAN_POINT ( 'NONE',  ( 20.88017736071110519, 20.56368534415484106, 2.639326808657452039E-16 ) ) ;
#98531=CARTESIAN_POINT ( 'NONE',  ( 19.84674366389459621, 53.50893115100078745, 7.409399052514197653E-17 ) ) ;
#98532=CARTESIAN_POINT ( 'NONE',  ( 3.591859063236763294, 48.29030133659708923, -11.09922568453595026 ) ) ;
#98536=CARTESIAN_POINT ( 'NONE',  ( 19.42250999205614548, 20.98035201082150891, -5.440088680355545492 ) ) ;
#98537=CARTESIAN_POINT ( 'NONE',  ( 16.40814093676323893, 15.79030133659708746, 11.09922568453595026 ) ) ;
#98540=CARTESIAN_POINT ( 'NONE',  ( 18.52753015748617571, 48.09226448433412315, 4.923371831947298993 ) ) ;
#98541=CARTESIAN_POINT ( 'NONE',  ( 12.91533473730992121, 34.52201867748817676, 10.88017736071110164 ) ) ;
#98542=CARTESIAN_POINT ( 'NONE',  ( 22.81628187352648496, 21.83196800326374643, -3.434112377981050290 ) ) ;
#98543=CARTESIAN_POINT ( 'NONE',  ( 0.5774900079438607392, 48.48035201082150536, 5.440088680355550821 ) ) ;
#98545=CYLINDRICAL_SURFACE ( 'NONE', #44930, 0.5000000000000004441 ) ;
#98546=CARTESIAN_POINT ( 'NONE',  ( 21.09922568453595559, 47.04030133659708923, -6.408140936763230044 ) ) ;
#98547=VERTEX_POINT ( 'NONE', #6965 ) ;
#98548=CARTESIAN_POINT ( 'NONE',  ( 0.5774900079438590739, 42.64701867748816966, -5.440088680355550821 ) ) ;
#98549=CARTESIAN_POINT ( 'NONE',  ( -2.816281873526473856, 34.12363466993042493, 9.499525473075851096E-16 ) ) ;
#98550=CARTESIAN_POINT ( 'NONE',  ( 2.917880565312950480, 0.9704155015806342766, -12.26659068614894821 ) ) ;
#98551=CARTESIAN_POINT ( 'NONE',  ( 12.63842701281683922, 9.550597817667449974, -9.846743663894590881 ) ) ;
#98552=CARTESIAN_POINT ( 'NONE',  ( 4.559911319644449179, 38.89701867748817676, 9.422509992056141925 ) ) ;
#98553=CARTESIAN_POINT ( 'NONE',  ( 19.84674366389459266, 63.71726448433412315, -2.638427012816827677 ) ) ;
#98554=SURFACE_SIDE_STYLE ('',( #7031 ) ) ;
#98555=CARTESIAN_POINT ( 'NONE',  ( 19.84674366389459621, 23.50893115100078390, 7.409399052514197653E-17 ) ) ;
#98556=CARTESIAN_POINT ( 'NONE',  ( 0.1532563361054100626, 5.800597817667452638, -2.638427012816831230 ) ) ;
#98558=CARTESIAN_POINT ( 'NONE',  ( 24.16423886937410614, 44.51208216824730357, -3.795296366450302550 ) ) ;
#98560=CARTESIAN_POINT ( 'NONE',  ( 10.00000000000000000, 6.813685344154838397, -10.88017736071110342 ) ) ;
#98563=CARTESIAN_POINT ( 'NONE',  ( -0.8801773607111008646, 13.27201867748817321, 2.915334737309923430 ) ) ;
#98564=CARTESIAN_POINT ( 'NONE',  ( -0.3689425029237881626, 62.42874883491396787, 10.36894250292379027 ) ) ;
#98565=CARTESIAN_POINT ( 'NONE',  ( 17.20831665107776587, 47.88393115100078745, 7.208316651077764980 ) ) ;
#98566=CARTESIAN_POINT ( 'NONE',  ( 21.09922568453595559, 37.04030133659708923, -6.408140936763230044 ) ) ;
#98569=CARTESIAN_POINT ( 'NONE',  ( 22.26659068614895176, 4.720415501580633943, -7.082119434687042414 ) ) ;
#98570=CARTESIAN_POINT ( 'NONE',  ( 19.42250999205614193, 10.14701867748816966, 5.440088680355555262 ) ) ;
#98571=CARTESIAN_POINT ( 'NONE',  ( 10.00000000000000178, 58.05374883491397497, 14.16423886937410082 ) ) ;
#98574=CARTESIAN_POINT ( 'NONE',  ( 12.63842701281683922, 39.55059781766744464, -9.846743663894590881 ) ) ;
#98575=CARTESIAN_POINT ( 'NONE',  ( -0.1306922352674164955, 0.1302365040536442309, 6.294480393734140478 ) ) ;
#98576=CARTESIAN_POINT ( 'NONE',  ( 17.20831665107776587, 19.13393115100078035, -7.208316651077762316 ) ) ;
#98577=CARTESIAN_POINT ( 'NONE',  ( 5.076628168052704559, 0.1755978176674514724, -8.527530157486179263 ) ) ;
#98585=CARTESIAN_POINT ( 'NONE',  ( 18.52753015748617571, 53.09226448433412315, 4.923371831947298993 ) ) ;
#98586=CARTESIAN_POINT ( 'NONE',  ( 0.5774900079438590739, 37.64701867748817676, -5.440088680355550821 ) ) ;
#98587=CARTESIAN_POINT ( 'NONE',  ( 7.084665262690076126, 32.02201867748816966, -10.88017736071110164 ) ) ;
#98588=CARTESIAN_POINT ( 'NONE',  ( 10.00000000000000178, 57.25893115100078745, 9.846743663894594434 ) ) ;
#98589=CARTESIAN_POINT ( 'NONE',  ( 19.38216949554541557, 27.24863466993041783, -9.382169495545420901 ) ) ;
#98590=( NAMED_UNIT ( * ) SI_UNIT ( $, .STERADIAN. ) SOLID_ANGLE_UNIT ( ) );
#98593=CARTESIAN_POINT ( 'NONE',  ( 22.81628187352647785, 31.41530133659709279, 3.434112377981063169 ) ) ;
#98595=CARTESIAN_POINT ( 'NONE',  ( 12.63842701281683034, 42.46726448433412315, 9.846743663894596210 ) ) ;
#98596=CARTESIAN_POINT ( 'NONE',  ( 0.5774900079438607392, 3.480352010821504916, 5.440088680355550821 ) ) ;
#98597=ORIENTED_EDGE ( 'NONE', *, *, #58950, .F. ) ;
#98598=CARTESIAN_POINT ( 'NONE',  ( 7.084665262690076126, 12.02201867748817321, -10.88017736071110164 ) ) ;
#98600=CARTESIAN_POINT ( 'NONE',  ( 12.91533473730993009, 66.60535201082150536, -10.88017736071109987 ) ) ;
#98601=CARTESIAN_POINT ( 'NONE',  ( 12.91533473730992121, 54.52201867748816255, 10.88017736071110164 ) ) ;
#98602=CARTESIAN_POINT ( 'NONE',  ( 19.42250999205614548, 60.98035201082151247, -5.440088680355545492 ) ) ;
#98603=PRODUCT ( '1.2 Movable Jaw', '1.2 Movable Jaw', '', ( #80252 ) ) ;
#98604=CARTESIAN_POINT ( 'NONE',  ( 7.084665262690076126, 54.10535201082151247, 10.88017736071109987 ) ) ;
#98605=CARTESIAN_POINT ( 'NONE',  ( -0.1503990784575328643, 30.12777174578613781, 6.262539305110068177 ) ) ;
#98606=CARTESIAN_POINT ( 'NONE',  ( -46.94000000000001194, 100.8028158894829289, 8.422108456579607605 ) ) ;
#98609=CARTESIAN_POINT ( 'NONE',  ( 14.92337183194729633, 47.67559781766745175, 8.527530157486181039 ) ) ;
#98615=CARTESIAN_POINT ( 'NONE',  ( 20.36894250292379382, 3.678748834913967869, 10.36894250292379205 ) ) ;
#98616=ORIENTED_EDGE ( 'NONE', *, *, #59796, .T. ) ;
#98619=CARTESIAN_POINT ( 'NONE',  ( -0.8801773607111009756, 3.063685344154838397, 1.068504757029289695E-15 ) ) ;
#98620=CARTESIAN_POINT ( 'NONE',  ( 13.43411237798106583, 37.66530133659708923, -12.81628187352647252 ) ) ;
#98621=ORIENTED_EDGE ( 'NONE', *, *, #89428, .T. ) ;
#98623=CARTESIAN_POINT ( 'NONE',  ( 1.472469842513823179, 46.42559781766745175, 4.923371831947296329 ) ) ;
#98625=CARTESIAN_POINT ( 'NONE',  ( 19.38216949554541557, 12.24863466993041961, -9.382169495545420901 ) ) ;
#98626=CARTESIAN_POINT ( 'NONE',  ( 7.361572987183169658, 24.96726448433412315, -9.846743663894592657 ) ) ;
#98627=CARTESIAN_POINT ( 'NONE',  ( 1.046131998950049491, 35.73810908735726599, 6.499999999999992006 ) ) ;
#98628=CARTESIAN_POINT ( 'NONE',  ( -1.099225684535947600, -0.4596986634029132657, 6.408140936763237150 ) ) ;
#98631=ORIENTED_EDGE ( 'NONE', *, *, #54420, .F. ) ;
#98632=CARTESIAN_POINT ( 'NONE',  ( 20.88017736071110164, 25.35535201082150891, 2.915334737309930979 ) ) ;
#98633=CARTESIAN_POINT ( 'NONE',  ( 2.917880565312950480, 20.97041550158063217, -12.26659068614894821 ) ) ;
#98634=CARTESIAN_POINT ( 'NONE',  ( 19.84674366389459621, 23.50893115100078390, 7.409399052514197653E-17 ) ) ;
#98635=CARTESIAN_POINT ( 'NONE',  ( 4.559911319644449179, 68.89701867748817676, 9.422509992056141925 ) ) ;
#98636=CARTESIAN_POINT ( 'NONE',  ( -2.816281873526473856, 39.12363466993041783, 9.499525473075851096E-16 ) ) ;
#98637=DIRECTION ( 'NONE',  ( 0.000000000000000000, 0.000000000000000000, -1.000000000000000000 ) ) ;
#98638=CARTESIAN_POINT ( 'NONE',  ( 17.96484262340118221, 16.18868534415483396, -7.964842623401177768 ) ) ;
#98642=CARTESIAN_POINT ( 'NONE',  ( 3.591859063236763294, 13.29030133659708746, -11.09922568453595026 ) ) ;
#98643=CARTESIAN_POINT ( 'NONE',  ( 19.38216949554541202, 5.998634669930420493, 9.382169495545424454 ) ) ;
#98644=CARTESIAN_POINT ( 'NONE',  ( 12.63842701281683922, 29.55059781766745175, -9.846743663894590881 ) ) ;
#98646=CARTESIAN_POINT ( 'NONE',  ( -2.816281873526471635, 38.91530133659708213, -3.434112377981056508 ) ) ;
#98648=CARTESIAN_POINT ( 'NONE',  ( -0.8801773607111009756, 43.06368534415484106, 1.068504757029289695E-15 ) ) ;
#98654=CARTESIAN_POINT ( 'NONE',  ( 7.084665262690076126, 67.02201867748817676, -10.88017736071110164 ) ) ;
#98655=CARTESIAN_POINT ( 'NONE',  ( 20.88017736071110164, 40.35535201082150536, 2.915334737309930979 ) ) ;
#98656=CARTESIAN_POINT ( 'NONE',  ( 4.559911319644449179, 42.23035201082151247, -9.422509992056141925 ) ) ;
#98657=CARTESIAN_POINT ( 'NONE',  ( 1.472469842513823179, 60.59226448433412315, -4.923371831947296329 ) ) ;
#98658=CARTESIAN_POINT ( 'NONE',  ( 2.035157376598824452, 68.68868534415484817, 7.964842623401179544 ) ) ;
#98659=CARTESIAN_POINT ( 'NONE',  ( 19.84674366389459266, 48.30059781766745175, 2.638427012816836559 ) ) ;
#98660=CARTESIAN_POINT ( 'NONE',  ( 20.88017736071110164, 5.355352010821502695, 2.915334737309930979 ) ) ;
#98662=CARTESIAN_POINT ( 'NONE',  ( 19.38216949554541557, 17.24863466993041783, -9.382169495545420901 ) ) ;
#98663=ORIENTED_EDGE ( 'NONE', *, *, #46768, .F. ) ;
#98664=CARTESIAN_POINT ( 'NONE',  ( 12.91533473730993009, 36.60535201082151247, -10.88017736071109987 ) ) ;
#98667=CARTESIAN_POINT ( 'NONE',  ( 20.88017736071110519, 5.563685344154837509, 2.639326808657452039E-16 ) ) ;
#98668=CARTESIAN_POINT ( 'NONE',  ( 15.44008868035555793, 26.39701867748817321, -9.422509992056140149 ) ) ;
#98669=CARTESIAN_POINT ( 'NONE',  ( 20.36894250292379382, 43.67874883491397497, 10.36894250292379205 ) ) ;
#98670=CARTESIAN_POINT ( 'NONE',  ( 0.1532563361054100626, 20.80059781766744464, -2.638427012816831230 ) ) ;
#98671=CARTESIAN_POINT ( 'NONE',  ( 20.88017736071110875, 50.77201867748817676, -2.915334737309920765 ) ) ;
#98672=SURFACE_SIDE_STYLE ('',( #7146 ) ) ;
#98674=CARTESIAN_POINT ( 'NONE',  ( 12.63842701281683034, 62.46726448433410894, 9.846743663894596210 ) ) ;
#98677=CARTESIAN_POINT ( 'NONE',  ( -4.164238869374098151, 16.59541550158063927, -3.795296366450310543 ) ) ;
#98678=CARTESIAN_POINT ( 'NONE',  ( 22.26659068614894466, 23.88708216824730357, 7.082119434687054849 ) ) ;
#98679=CARTESIAN_POINT ( 'NONE',  ( 10.00000000000000178, 59.31368534415484106, 10.88017736071110342 ) ) ;
#98680=CARTESIAN_POINT ( 'NONE',  ( 10.00000000000000178, 68.05374883491397497, 14.16423886937410082 ) ) ;
#98681=CARTESIAN_POINT ( 'NONE',  ( 14.92337183194729633, 47.67559781766745175, 8.527530157486181039 ) ) ;
#98683=CARTESIAN_POINT ( 'NONE',  ( 2.035157376598822676, 42.43868534415483396, -7.964842623401177768 ) ) ;
#98684=CARTESIAN_POINT ( 'NONE',  ( 16.40814093676324603, 17.45696800326375353, -11.09922568453594671 ) ) ;
#98685=CARTESIAN_POINT ( 'NONE',  ( 24.16423886937409904, 19.09541550158063927, 3.795296366450317205 ) ) ;
#98686=CARTESIAN_POINT ( 'NONE',  ( 12.91533473730992121, 9.522018677488171434, 10.88017736071110164 ) ) ;
#98687=CARTESIAN_POINT ( 'NONE',  ( 19.42250999205614548, 30.98035201082150536, -5.440088680355545492 ) ) ;
#98688=CARTESIAN_POINT ( 'NONE',  ( -0.8801773607111009756, 58.06368534415484106, 1.068504757029289695E-15 ) ) ;
#98689=CARTESIAN_POINT ( 'NONE',  ( 22.81628187352648496, 46.83196800326376064, -3.434112377981050290 ) ) ;
#98692=CARTESIAN_POINT ( 'NONE',  ( 19.72487221294571569, 34.78217586085237656, 6.499999999999993783 ) ) ;
#98697=CARTESIAN_POINT ( 'NONE',  ( -0.3689425029237898834, 66.17874883491396076, -10.36894250292378850 ) ) ;
#98698=CARTESIAN_POINT ( 'NONE',  ( -0.3689425029237881626, 67.42874883491396076, 10.36894250292379027 ) ) ;
#98699=CARTESIAN_POINT ( 'NONE',  ( 5.076628168052703671, 16.84226448433411960, 8.527530157486179263 ) ) ;
#98700=CARTESIAN_POINT ( 'NONE',  ( 14.92337183194729988, 54.34226448433412315, -8.527530157486177487 ) ) ;
#98704=CARTESIAN_POINT ( 'NONE',  ( 0.5774900079438590739, 67.64701867748817676, -5.440088680355550821 ) ) ;
#98708=CARTESIAN_POINT ( 'NONE',  ( -0.3689425029237881626, 27.42874883491397142, 10.36894250292379027 ) ) ;
#98710=CARTESIAN_POINT ( 'NONE',  ( 10.00000000000000178, 43.05374883491397497, 14.16423886937410082 ) ) ;
#98712=CARTESIAN_POINT ( 'NONE',  ( 22.81628187352647785, 61.62363466993041783, 6.195893100308588602E-16 ) ) ;
#98713=VECTOR ( 'NONE', #30186, 1000.000000000000000 ) ;
#98714=CARTESIAN_POINT ( 'NONE',  ( 18.52753015748618282, 48.92559781766745886, -4.923371831947291888 ) ) ;
#98715=CARTESIAN_POINT ( 'NONE',  ( 19.42250999205614193, 25.14701867748817321, 5.440088680355555262 ) ) ;
#98716=CARTESIAN_POINT ( 'NONE',  ( 6.565887622018943937, 65.16530133659709634, 12.81628187352647430 ) ) ;
#98718=CARTESIAN_POINT ( 'NONE',  ( 10.00000000000000000, 54.75893115100078745, -9.846743663894594434 ) ) ;
#98719=CARTESIAN_POINT ( 'NONE',  ( 19.84674366389459266, 48.71726448433413026, -2.638427012816827677 ) ) ;
#98725=CARTESIAN_POINT ( 'NONE',  ( 10.00000000000000000, 4.758931151000784787, -9.846743663894594434 ) ) ;
#98727=ORIENTED_EDGE ( 'NONE', *, *, #42576, .F. ) ;
#98728=CARTESIAN_POINT ( 'NONE',  ( 19.67388484268946058, 87.39743296926540950, 5.439657303569386926 ) ) ;
#98729=CARTESIAN_POINT ( 'NONE',  ( 19.84674366389459266, 28.30059781766745886, 2.638427012816836559 ) ) ;
#98731=CARTESIAN_POINT ( 'NONE',  ( 22.81628187352648496, 36.83196800326376064, -3.434112377981050290 ) ) ;
#98732=EDGE_CURVE ( 'NONE', #35821, #4466, #38270, .T. ) ;
#98737=CARTESIAN_POINT ( 'NONE',  ( 10.00000000000000000, 39.75893115100078745, -9.846743663894594434 ) ) ;
#98738=CARTESIAN_POINT ( 'NONE',  ( 24.16423886937410614, 34.30374883491396787, 8.672049930838204340E-16 ) ) ;
#98739=CARTESIAN_POINT ( 'NONE',  ( 5.076628168052703671, 51.84226448433412315, 8.527530157486179263 ) ) ;
#98742=CARTESIAN_POINT ( 'NONE',  ( 10.00000000000000000, 4.758931151000784787, -9.846743663894594434 ) ) ;
#98743=B_SPLINE_CURVE_WITH_KNOTS ( 'NONE', 3,
 ( #66743, #51244, #12256, #5758 ),
 .UNSPECIFIED., .F., .F.,
 ( 4, 4 ),
 ( 0.000000000000000000, 0.001036303429213369194 ),
 .UNSPECIFIED. ) ;
#98744=CARTESIAN_POINT ( 'NONE',  ( 20.32896413005680003, 46.77164270246085209, 5.963430220938287007 ) ) ;
#98745=CARTESIAN_POINT ( 'NONE',  ( 18.52753015748617571, 48.09226448433412315, 4.923371831947298993 ) ) ;
#98746=CARTESIAN_POINT ( 'NONE',  ( 15.44008868035555793, 51.39701867748816966, -9.422509992056140149 ) ) ;
#98747=CARTESIAN_POINT ( 'NONE',  ( 17.20831665107776587, 44.13393115100078745, -7.208316651077762316 ) ) ;
#98748=CARTESIAN_POINT ( 'NONE',  ( 20.15039907845753220, 31.74884699246888786, 6.262539305110077059 ) ) ;
#98749=CARTESIAN_POINT ( 'NONE',  ( -0.8801773607111008646, 43.27201867748817676, 2.915334737309923430 ) ) ;
#98752=CARTESIAN_POINT ( 'NONE',  ( 15.44008868035555260, 19.73035201082150536, 9.422509992056143702 ) ) ;
#98753=CARTESIAN_POINT ( 'NONE',  ( 13.43411237798106583, 2.665301336597086568, -12.81628187352647252 ) ) ;
#98754=CARTESIAN_POINT ( 'NONE',  ( 0.5774900079438590739, 42.64701867748816966, -5.440088680355550821 ) ) ;
#98755=CARTESIAN_POINT ( 'NONE',  ( 0.2751277870542979120, 15.30223176428831344, 6.500000000000003553 ) ) ;
#98756=CARTESIAN_POINT ( 'NONE',  ( 19.84674366389459266, 13.30059781766745175, 2.638427012816836559 ) ) ;
#98758=CARTESIAN_POINT ( 'NONE',  ( 7.084665262690076126, 39.10535201082150536, 10.88017736071109987 ) ) ;
#98759=CARTESIAN_POINT ( 'NONE',  ( 6.000000000000000000, 61.00000000000000711, 6.000000000000000000 ) ) ;
#98760=CARTESIAN_POINT ( 'NONE',  ( 19.84674366389459621, 8.508931151000785675, 7.409399052514197653E-17 ) ) ;
#98761=CARTESIAN_POINT ( 'NONE',  ( 12.63842701281683034, 42.46726448433412315, 9.846743663894596210 ) ) ;
#98762=DIRECTION ( 'NONE',  ( 0.000000000000000000, 0.000000000000000000, 1.000000000000000000 ) ) ;
#98764=CARTESIAN_POINT ( 'NONE',  ( 22.81628187352647785, 1.415301336597087012, 3.434112377981063169 ) ) ;
#98765=CARTESIAN_POINT ( 'NONE',  ( 0.5774900079438607392, 3.480352010821504916, 5.440088680355550821 ) ) ;
#98767=CARTESIAN_POINT ( 'NONE',  ( 17.08211943468705840, 25.13708216824730357, -12.26659068614894466 ) ) ;
#98768=EDGE_CURVE ( 'NONE', #87897, #74488, #14368, .T. ) ;
#98769=CARTESIAN_POINT ( 'NONE',  ( 6.204703633549690345, 50.76208216824730357, -14.16423886937410259 ) ) ;
#98773=CARTESIAN_POINT ( 'NONE',  ( 0.1532563361054083140, 21.00893115100078745, 1.131784320476157264E-15 ) ) ;
#98774=CARTESIAN_POINT ( 'NONE',  ( 15.44008868035555793, 31.39701867748817676, -9.422509992056140149 ) ) ;
#98775=CARTESIAN_POINT ( 'NONE',  ( 0.1532563361054100626, 45.80059781766745886, -2.638427012816831230 ) ) ;
#98776=CARTESIAN_POINT ( 'NONE',  ( 20.36894250292379738, 9.928748834913966093, -10.36894250292379027 ) ) ;
#98780=CARTESIAN_POINT ( 'NONE',  ( -1.099225684535947600, 44.54030133659708923, 6.408140936763237150 ) ) ;
#98781=CARTESIAN_POINT ( 'NONE',  ( 2.791683348922240793, 41.63393115100078745, 7.208316651077764092 ) ) ;
#98782=ORIENTED_EDGE ( 'NONE', *, *, #83216, .T. ) ;
#98783=CARTESIAN_POINT ( 'NONE',  ( 14.92337183194729633, 7.675597817667451750, 8.527530157486181039 ) ) ;
#98786=CARTESIAN_POINT ( 'NONE',  ( 17.08211943468705840, 55.13708216824731068, -12.26659068614894466 ) ) ;
#98787=CARTESIAN_POINT ( 'NONE',  ( 17.96484262340118221, 44.93868534415483396, 7.964842623401181321 ) ) ;
#98788=COLOUR_RGB ( '', 0.31764706, 0.68627451, 0.89019608) ;
#98789=SURFACE_SIDE_STYLE ('',( #92234 ) ) ;
#98791=CARTESIAN_POINT ( 'NONE',  ( 14.92337183194729633, 32.67559781766745175, 8.527530157486181039 ) ) ;
#98792=CARTESIAN_POINT ( 'NONE',  ( 10.00000000000000178, 9.313685344154839285, 10.88017736071110342 ) ) ;
#98793=CARTESIAN_POINT ( 'NONE',  ( 7.361572987183169658, 34.96726448433411605, -9.846743663894592657 ) ) ;
#98794=CARTESIAN_POINT ( 'NONE',  ( 18.18329248733322601, 2.602906685120200070, 6.499999999999992006 ) ) ;
#98795=CARTESIAN_POINT ( 'NONE',  ( 10.00000000000000178, 57.25893115100078745, 9.846743663894594434 ) ) ;
#98796=CARTESIAN_POINT ( 'NONE',  ( 10.00000000000000000, 51.81368534415484106, -10.88017736071110342 ) ) ;
#98799=ORIENTED_EDGE ( 'NONE', *, *, #46871, .F. ) ;
#98800=CARTESIAN_POINT ( 'NONE',  ( 19.38216949554541557, 52.24863466993041072, -9.382169495545420901 ) ) ;
#98802=CARTESIAN_POINT ( 'NONE',  ( 2.791683348922240793, 11.63393115100078568, 7.208316651077764092 ) ) ;
#98803=CARTESIAN_POINT ( 'NONE',  ( 22.81628187352647785, 56.62363466993042493, 6.195893100308588602E-16 ) ) ;
#98804=CARTESIAN_POINT ( 'NONE',  ( 7.084665262690076126, 7.022018677488170546, -10.88017736071110164 ) ) ;
#98805=CARTESIAN_POINT ( 'NONE',  ( 19.84674366389459621, 53.50893115100078745, 7.409399052514197653E-17 ) ) ;
#98806=CARTESIAN_POINT ( 'NONE',  ( 20.00000000000000711, 92.20777562798386384, 4.885465336098351763 ) ) ;
#98807=FILL_AREA_STYLE_COLOUR ( '', #98190 ) ;
#98808=CARTESIAN_POINT ( 'NONE',  ( 13.79529636645031943, 25.34541550158063572, -14.16423886937409904 ) ) ;
#98809=CARTESIAN_POINT ( 'NONE',  ( 13.79529636645030344, 48.26208216824728936, 14.16423886937410614 ) ) ;
#98810=CARTESIAN_POINT ( 'NONE',  ( 12.63842701281683034, 57.46726448433411605, 9.846743663894596210 ) ) ;
#98812=CARTESIAN_POINT ( 'NONE',  ( 15.44008868035555793, 46.39701867748817676, -9.422509992056140149 ) ) ;
#98813=CARTESIAN_POINT ( 'NONE',  ( 17.20831665107776587, 7.883931151000784787, 7.208316651077764980 ) ) ;
#98815=CARTESIAN_POINT ( 'NONE',  ( 3.591859063236761518, 59.95696800326375353, 11.09922568453594849 ) ) ;
#98816=CARTESIAN_POINT ( 'NONE',  ( 10.00000000000000000, 14.75893115100078568, -9.846743663894594434 ) ) ;
#98818=CARTESIAN_POINT ( 'NONE',  ( -4.164238869374099039, 21.80374883491396787, 8.674139862899312516E-16 ) ) ;
#98819=CARTESIAN_POINT ( 'NONE',  ( 10.00000000000000178, 7.258931151000785675, 9.846743663894594434 ) ) ;
#98820=CARTESIAN_POINT ( 'NONE',  ( 2.035157376598822676, 32.43868534415483396, -7.964842623401177768 ) ) ;
#98821=DIRECTION ( 'NONE',  ( -1.000000000000000000, -2.799047438454523236E-16, 0.000000000000000000 ) ) ;
#98823=CARTESIAN_POINT ( 'NONE',  ( 4.559911319644449179, 32.23035201082150536, -9.422509992056141925 ) ) ;
#98829=CARTESIAN_POINT ( 'NONE',  ( 0.6178305044545838731, 14.74863466993041783, 9.382169495545420901 ) ) ;
#98831=CARTESIAN_POINT ( 'NONE',  ( 10.00000000000000178, 69.31368534415484817, 10.88017736071110342 ) ) ;
#98833=CARTESIAN_POINT ( 'NONE',  ( 19.84674366389459266, 18.30059781766745175, 2.638427012816836559 ) ) ;
#98834=CARTESIAN_POINT ( 'NONE',  ( 12.91533473730993009, 31.60535201082150891, -10.88017736071109987 ) ) ;
#98837=CARTESIAN_POINT ( 'NONE',  ( 12.91533473730992121, 39.52201867748817676, 10.88017736071110164 ) ) ;
#98838=CARTESIAN_POINT ( 'NONE',  ( -1.926860441876562247, 22.45379003517447103, -3.195792623639530650 ) ) ;
#98839=CARTESIAN_POINT ( 'NONE',  ( 3.591859063236761518, 49.95696800326375353, 11.09922568453594849 ) ) ;
#98840=CARTESIAN_POINT ( 'NONE',  ( 2.035157376598824452, 63.68868534415484106, 7.964842623401179544 ) ) ;
#98841=CARTESIAN_POINT ( 'NONE',  ( 19.84674366389459621, 63.50893115100078745, 7.409399052514197653E-17 ) ) ;
#98842=EDGE_CURVE ( 'NONE', #26206, #32549, #57857, .T. ) ;
#98845=CARTESIAN_POINT ( 'NONE',  ( 1.472469842513823179, 15.59226448433411960, -4.923371831947296329 ) ) ;
#98846=CARTESIAN_POINT ( 'NONE',  ( -2.816281873526473856, 49.33196800326374643, 3.434112377981055619 ) ) ;
#98848=CARTESIAN_POINT ( 'NONE',  ( 5.076628168052704559, 5.175597817667451750, -8.527530157486179263 ) ) ;
#98849=CARTESIAN_POINT ( 'NONE',  ( 13.43411237798106583, 17.66530133659708923, -12.81628187352647252 ) ) ;
#98851=DIRECTION ( 'NONE',  ( -6.608470384673550777E-17, -1.000000000000000000, 0.000000000000000000 ) ) ;
#98852=CARTESIAN_POINT ( 'NONE',  ( 12.91533473730993009, 31.60535201082150891, -10.88017736071109987 ) ) ;
#98853=CARTESIAN_POINT ( 'NONE',  ( -1.099225684535947600, -1.293031996736246469, -6.408140936763238038 ) ) ;
#98856=CARTESIAN_POINT ( 'NONE',  ( 18.52753015748617571, 18.09226448433411960, 4.923371831947298993 ) ) ;
#98857=CARTESIAN_POINT ( 'NONE',  ( 18.52753015748618282, 13.92559781766745175, -4.923371831947291888 ) ) ;
#98858=CARTESIAN_POINT ( 'NONE',  ( 10.00000000000000000, -2.126365330069579951, -12.81628187352647608 ) ) ;
#98861=CARTESIAN_POINT ( 'NONE',  ( 12.91533473730993009, 6.605352010821504471, -10.88017736071109987 ) ) ;
#98864=CARTESIAN_POINT ( 'NONE',  ( 7.084665262690076126, 9.105352010821503583, 10.88017736071109987 ) ) ;
#98865=CARTESIAN_POINT ( 'NONE',  ( 12.63842701281683922, 49.55059781766744464, -9.846743663894590881 ) ) ;
#98867=LINE ( 'NONE', #90325, #24956 ) ;
#98868=CARTESIAN_POINT ( 'NONE',  ( -0.3689425029237898834, 66.17874883491396076, -10.36894250292378850 ) ) ;
#98869=CARTESIAN_POINT ( 'NONE',  ( 17.96484262340118221, 34.93868534415482685, 7.964842623401181321 ) ) ;
#98870=CARTESIAN_POINT ( 'NONE',  ( 24.16423886937410614, 49.51208216824730357, -3.795296366450302550 ) ) ;
#98871=CARTESIAN_POINT ( 'NONE',  ( 17.08211943468705130, 63.47041550158063927, 12.26659068614894998 ) ) ;
#98873=CARTESIAN_POINT ( 'NONE',  ( 17.20831665107776587, 2.883931151000785231, 7.208316651077764980 ) ) ;
#98874=CARTESIAN_POINT ( 'NONE',  ( 0.1532563361054082862, 26.21726448433411605, 2.638427012816831674 ) ) ;
#98875=CARTESIAN_POINT ( 'NONE',  ( 21.09922568453595559, 17.04030133659708923, -6.408140936763230044 ) ) ;
#98877=ORIENTED_EDGE ( 'NONE', *, *, #65588, .F. ) ;
#98879=CARTESIAN_POINT ( 'NONE',  ( 14.92337183194729633, 57.67559781766745886, 8.527530157486181039 ) ) ;
#98880=AXIS2_PLACEMENT_3D ( 'NONE', #9891, #70890, #63366 ) ;
#98881=FACE_OUTER_BOUND ( 'NONE', #2745, .T. ) ;
#98883=CARTESIAN_POINT ( 'NONE',  ( 6.204703633549690345, 10.76208216824729824, -14.16423886937410259 ) ) ;
#98884=CARTESIAN_POINT ( 'NONE',  ( 18.52753015748618282, 28.92559781766745175, -4.923371831947291888 ) ) ;
#98887=CARTESIAN_POINT ( 'NONE',  ( 24.16423886937409904, 59.09541550158063217, 3.795296366450317205 ) ) ;
#98888=CARTESIAN_POINT ( 'NONE',  ( 19.84674366389459266, 8.717264484334116048, -2.638427012816827677 ) ) ;
#98891=CARTESIAN_POINT ( 'NONE',  ( 0.5774900079438590739, 37.64701867748817676, -5.440088680355550821 ) ) ;
#98892=CARTESIAN_POINT ( 'NONE',  ( 21.09922568453594849, 51.20696800326375353, 6.408140936763242479 ) ) ;
#98893=CARTESIAN_POINT ( 'NONE',  ( 19.42250999205614548, 5.980352010821504471, -5.440088680355545492 ) ) ;
#98894=CARTESIAN_POINT ( 'NONE',  ( -1.099225684535947600, 34.54030133659708923, 6.408140936763237150 ) ) ;
#98895=CARTESIAN_POINT ( 'NONE',  ( 19.84674366389459266, 3.717264484334118713, -2.638427012816827677 ) ) ;
#98899=CARTESIAN_POINT ( 'NONE',  ( 10.00000000000000000, 45.55374883491397497, -14.16423886937410082 ) ) ;
#98900=CARTESIAN_POINT ( 'NONE',  ( -4.164238869374098151, 11.59541550158063217, -3.795296366450310543 ) ) ;
#98901=CARTESIAN_POINT ( 'NONE',  ( 0.5774900079438607392, 8.480352010821505360, 5.440088680355550821 ) ) ;
#98902=CARTESIAN_POINT ( 'NONE',  ( 10.00000000000000000, 41.81368534415484106, -10.88017736071110342 ) ) ;
#98905=CARTESIAN_POINT ( 'NONE',  ( 2.035157376598824452, 48.68868534415483396, 7.964842623401179544 ) ) ;
#98906=CARTESIAN_POINT ( 'NONE',  ( 4.559911319644449179, 68.89701867748817676, 9.422509992056141925 ) ) ;
#98907=CARTESIAN_POINT ( 'NONE',  ( 3.591859063236761518, 29.95696800326375708, 11.09922568453594849 ) ) ;
#98908=CARTESIAN_POINT ( 'NONE',  ( 18.72515096720568550, 20.05509018479935790, 6.500000000000015099 ) ) ;
#98910=CARTESIAN_POINT ( 'NONE',  ( 19.84674366389459621, 38.50893115100078745, 7.409399052514197653E-17 ) ) ;
#98912=CARTESIAN_POINT ( 'NONE',  ( 16.40814093676323893, 20.79030133659708923, 11.09922568453595026 ) ) ;
#98913=CARTESIAN_POINT ( 'NONE',  ( 0.1532563361054082862, 11.21726448433411605, 2.638427012816831674 ) ) ;
#98914=CARTESIAN_POINT ( 'NONE',  ( 20.88017736071110875, 10.77201867748817143, -2.915334737309920765 ) ) ;
#98915=CARTESIAN_POINT ( 'NONE',  ( 19.84674366389459621, 38.50893115100078745, 7.409399052514197653E-17 ) ) ;
#98916=CARTESIAN_POINT ( 'NONE',  ( 13.43411237798106583, 57.66530133659708923, -12.81628187352647252 ) ) ;
#98917=CARTESIAN_POINT ( 'NONE',  ( 19.84674366389459266, 23.30059781766745530, 2.638427012816836559 ) ) ;
#98918=CARTESIAN_POINT ( 'NONE',  ( -2.266590686148945544, 6.387082168247300906, -7.082119434687050408 ) ) ;
#98920=CARTESIAN_POINT ( 'NONE',  ( -0.8801773607111008646, 33.27201867748817676, 2.915334737309923430 ) ) ;
#98921=CARTESIAN_POINT ( 'NONE',  ( 2.035157376598822676, 17.43868534415483751, -7.964842623401177768 ) ) ;
#98923=CARTESIAN_POINT ( 'NONE',  ( 20.88017736071110519, 30.56368534415484106, 2.639326808657452039E-16 ) ) ;
#98924=CARTESIAN_POINT ( 'NONE',  ( 20.88017736071110875, 15.77201867748817143, -2.915334737309920765 ) ) ;
#98928=CARTESIAN_POINT ( 'NONE',  ( 17.96484262340118221, 29.93868534415484106, 7.964842623401181321 ) ) ;
#98930=CARTESIAN_POINT ( 'NONE',  ( -2.816281873526471635, 48.91530133659708213, -3.434112377981056508 ) ) ;
#98931=CARTESIAN_POINT ( 'NONE',  ( 17.96484262340118221, 46.18868534415484106, -7.964842623401177768 ) ) ;
#98932=CARTESIAN_POINT ( 'NONE',  ( 2.603489959281590771, 46.58210964143328425, 6.500000000000003553 ) ) ;
#98933=CARTESIAN_POINT ( 'NONE',  ( 20.88017736071110164, 45.35535201082149115, 2.915334737309930979 ) ) ;
#98934=ORIENTED_EDGE ( 'NONE', *, *, #80963, .F. ) ;
#98935=CARTESIAN_POINT ( 'NONE',  ( 7.084665262690076126, 49.10535201082149825, 10.88017736071109987 ) ) ;
#98936=EDGE_CURVE ( 'NONE', #38297, #74440, #58339, .T. ) ;
#98939=CARTESIAN_POINT ( 'NONE',  ( 22.26659068614894466, 43.88708216824729647, 7.082119434687054849 ) ) ;
#98940=CARTESIAN_POINT ( 'NONE',  ( 12.91533473730992121, 64.52201867748817676, 10.88017736071110164 ) ) ;
#98943=CARTESIAN_POINT ( 'NONE',  ( 2.791683348922237240, 60.38393115100078745, -7.208316651077763204 ) ) ;
#98945=CARTESIAN_POINT ( 'NONE',  ( 12.63842701281683922, 34.55059781766745886, -9.846743663894590881 ) ) ;
#98947=CARTESIAN_POINT ( 'NONE',  ( 14.92337183194729988, 29.34226448433411960, -8.527530157486177487 ) ) ;
#98949=CARTESIAN_POINT ( 'NONE',  ( 15.44008868035555793, 21.39701867748817321, -9.422509992056140149 ) ) ;
#98950=CARTESIAN_POINT ( 'NONE',  ( 5.076628168052703671, 31.84226448433412315, 8.527530157486179263 ) ) ;
#98951=CARTESIAN_POINT ( 'NONE',  ( 10.00000000000000178, 25.37363466993041783, 12.81628187352647608 ) ) ;
#98953=CARTESIAN_POINT ( 'NONE',  ( 2.035157376598824452, 53.68868534415484817, 7.964842623401179544 ) ) ;
#98954=CARTESIAN_POINT ( 'NONE',  ( 17.96484262340118221, 29.93868534415484106, 7.964842623401181321 ) ) ;
#98955=SURFACE_STYLE_USAGE ( .BOTH. , #14450 ) ;
#98956=CARTESIAN_POINT ( 'NONE',  ( 6.204703633549690345, 57.84541550158063927, 14.16423886937410082 ) ) ;
#98958=CARTESIAN_POINT ( 'NONE',  ( 19.38216949554541557, 27.24863466993041783, -9.382169495545420901 ) ) ;
#98961=CARTESIAN_POINT ( 'NONE',  ( 21.09922568453595559, 12.04030133659708746, -6.408140936763230044 ) ) ;
#98962=CARTESIAN_POINT ( 'NONE',  ( 12.91533473730992121, 14.52201867748817143, 10.88017736071110164 ) ) ;
#98963=CARTESIAN_POINT ( 'NONE',  ( 20.88017736071110164, 45.35535201082149115, 2.915334737309930979 ) ) ;
#98968=CARTESIAN_POINT ( 'NONE',  ( -0.8801773607110991993, 62.85535201082150536, -2.915334737309923874 ) ) ;
#98969=CARTESIAN_POINT ( 'NONE',  ( 10.00000000000000000, 29.75893115100078745, -9.846743663894594434 ) ) ;
#98970=CARTESIAN_POINT ( 'NONE',  ( 2.791683348922237240, 30.38393115100078390, -7.208316651077763204 ) ) ;
#98971=CARTESIAN_POINT ( 'NONE',  ( 1.472469842513823179, 10.59226448433411782, -4.923371831947296329 ) ) ;
#98972=FACE_OUTER_BOUND ( 'NONE', #17981, .T. ) ;
#98974=CARTESIAN_POINT ( 'NONE',  ( 3.591859063236761518, 39.95696800326375353, 11.09922568453594849 ) ) ;
#98975=CARTESIAN_POINT ( 'NONE',  ( 7.361572987183169658, 19.96726448433411960, -9.846743663894592657 ) ) ;
#98977=CARTESIAN_POINT ( 'NONE',  ( 20.32896413005680714, 45.57879003517447813, -5.963430220938276349 ) ) ;
#98978=CARTESIAN_POINT ( 'NONE',  ( 10.00000000000000000, 34.75893115100078745, -9.846743663894594434 ) ) ;
#98980=CARTESIAN_POINT ( 'NONE',  ( 21.09922568453595559, 62.04030133659709634, -6.408140936763230044 ) ) ;
#98982=CARTESIAN_POINT ( 'NONE',  ( -1.099225684535947600, 9.540301336597087456, 6.408140936763237150 ) ) ;
#98983=CARTESIAN_POINT ( 'NONE',  ( 0.5774900079438590739, 47.64701867748817676, -5.440088680355550821 ) ) ;
#98984=CARTESIAN_POINT ( 'NONE',  ( 24.16423886937410614, 29.30374883491396787, 8.672049930838204340E-16 ) ) ;
#98986=CARTESIAN_POINT ( 'NONE',  ( 24.16423886937409904, 34.09541550158064638, 3.795296366450317205 ) ) ;
#98987=CARTESIAN_POINT ( 'NONE',  ( 22.26659068614894466, 58.88708216824729647, 7.082119434687054849 ) ) ;
#98988=CARTESIAN_POINT ( 'NONE',  ( 22.26659068614894466, 3.887082168247300906, 7.082119434687054849 ) ) ;
#98989=CARTESIAN_POINT ( 'NONE',  ( 10.00000000000000178, 37.25893115100078745, 9.846743663894594434 ) ) ;
ENDSEC;
END-ISO-10303-21;
